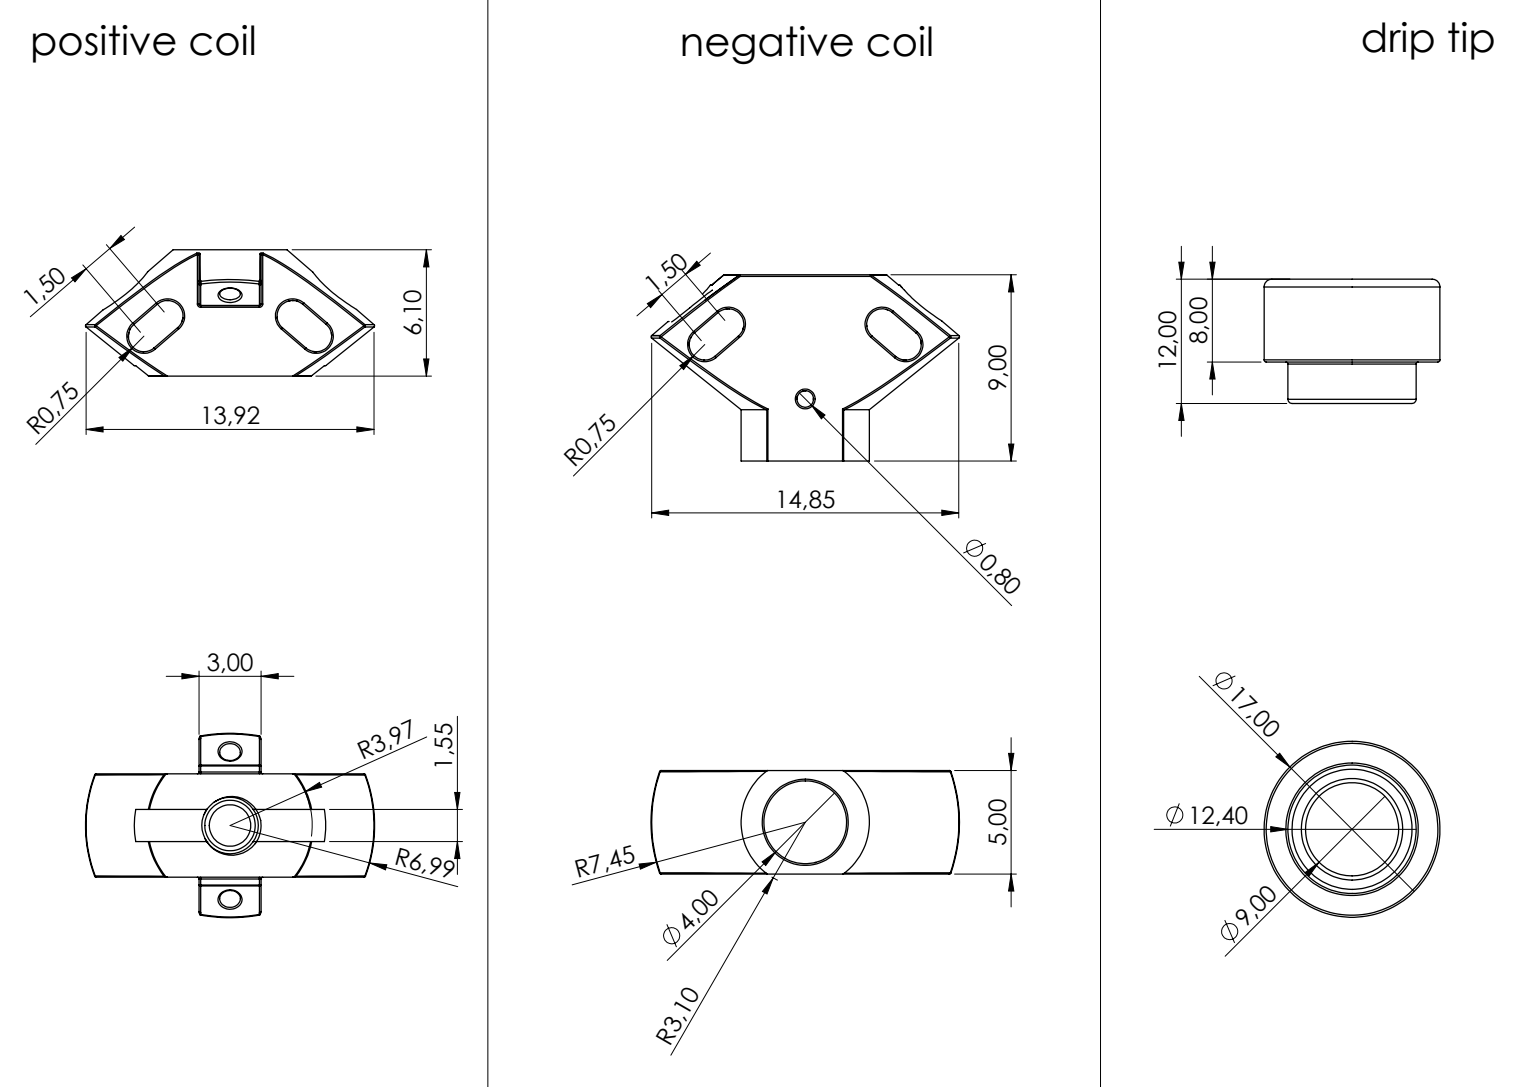
ISO-10303-21;
HEADER;
FILE_DESCRIPTION (('STEP AP214'),
    '1' );
FILE_NAME ('positive coil.step',
    '2026-10-05T20:10:51',
    ( '' ),
    ( '' ),
    'SwSTEP 2.0',
    'SolidWorks 2020',
    '' );
FILE_SCHEMA (( 'AUTOMOTIVE_DESIGN' ));
ENDSEC;

DATA;
#3=ORIENTED_EDGE ( 'NONE', *, *, #96141, .T. ) ;
#13=CARTESIAN_POINT ( 'NONE',  ( -4.869349725602420520, 8.832658446511480577, 1.040834085586084257E-14 ) ) ;
#16=CARTESIAN_POINT ( 'NONE',  ( 5.233084105194869551, 6.167981546557892436, -1.082531754730548412 ) ) ;
#20=CARTESIAN_POINT ( 'NONE',  ( -4.460796234096120472, 5.163016013655583158, 1.199719254218462483 ) ) ;
#28=CARTESIAN_POINT ( 'NONE',  ( -8.474009703741204547, 9.845098394908269768, -1.199719254218446718 ) ) ;
#29=CARTESIAN_POINT ( 'NONE',  ( 5.666418135507635512, 8.698239360479199433, 1.199719254218462483 ) ) ;
#31=CARTESIAN_POINT ( 'NONE',  ( -9.158696461231359720, 10.64389961198009615, 1.199719254218462483 ) ) ;
#33=CARTESIAN_POINT ( 'NONE',  ( 5.118366684358879759, 5.930181538962194132, 1.199719254218462483 ) ) ;
#36=CARTESIAN_POINT ( 'NONE',  ( 0.6823417656249882723, -0.5947916663252492686, 1.181850606188755259 ) ) ;
#39=CARTESIAN_POINT ( 'NONE',  ( 6.954969614130424027, 11.05795561655343384, 1.040834085586084257E-14 ) ) ;
#45=CARTESIAN_POINT ( 'NONE',  ( 10.37162432432990755, 11.20257592124748136, -0.7216878364870257245 ) ) ;
#49=( BOUNDED_SURFACE ( )  B_SPLINE_SURFACE ( 3, 2, ( 
 ( #54801, #106802, #172831 ),
 ( #26553, #190122, #173916 ),
 ( #25490, #91596, #38551 ),
 ( #157648, #9245, #191177 ),
 ( #108952, #72088, #42845 ),
 ( #4939, #71015, #22263 ) ),
 .UNSPECIFIED., .F., .F., .T. ) 
 B_SPLINE_SURFACE_WITH_KNOTS ( ( 4, 2, 4 ),
 ( 3, 3 ),
 ( 0.0001465838689801548850, 0.0002810652682710442613, 0.0004155466675619336647 ),
 ( 0.000000000000000000, 1.000000000000000000 ),
 .UNSPECIFIED. ) 
 GEOMETRIC_REPRESENTATION_ITEM ( )  RATIONAL_B_SPLINE_SURFACE ( (
 ( 1.000000000000000000, 0.8789000212895399233, 1.000000000000000000),
 ( 1.000000000000000000, 0.9073166784884888481, 1.000000000000000000),
 ( 1.000000000000000000, 0.9160359019619195298, 1.000000000000000000),
 ( 1.000000000000000000, 0.8858134948703222378, 1.000000000000000000),
 ( 1.000000000000000000, 0.8506312074210943264, 1.000000000000000000),
 ( 1.000000000000000000, 0.8104931255412257673, 1.000000000000000000) ) ) 
 REPRESENTATION_ITEM ( '' )  SURFACE ( )  );
#64=CARTESIAN_POINT ( 'NONE',  ( 1.499999999999989120, 0.05625000068281565957, 0.000000000000000000 ) ) ;
#71=CARTESIAN_POINT ( 'NONE',  ( 8.540746701604824409, 12.05162268759261224, -1.199719254218446718 ) ) ;
#75=CARTESIAN_POINT ( 'NONE',  ( 4.253507506385319381, 5.985511395581417204, 1.599625672291267398 ) ) ;
#76=CARTESIAN_POINT ( 'NONE',  ( -6.887178846062123938, 8.097758744236356776, -1.082531754730544860 ) ) ;
#77=CARTESIAN_POINT ( 'NONE',  ( -5.762141863986474100, 6.090740110424618159, 0.6348889758391648153 ) ) ;
#80=CARTESIAN_POINT ( 'NONE',  ( -8.830438121202295321, 9.196599317691152464, -0.7998128361456291469 ) ) ;
#81=CARTESIAN_POINT ( 'NONE',  ( -4.460269348771590536, 5.266364330730674226, 1.082531754730558626 ) ) ;
#84=CARTESIAN_POINT ( 'NONE',  ( -0.7500000000000006661, -0.6104166659838470288, -1.299038105676652011 ) ) ;
#91=CARTESIAN_POINT ( 'NONE',  ( -3.592547517496929466, 7.135129837147637488, -0.7216878364870257245 ) ) ;
#94=CARTESIAN_POINT ( 'NONE',  ( 4.014365637759117256, 7.575528411784208771, 0.2883143100938356240 ) ) ;
#99=CARTESIAN_POINT ( 'NONE',  ( -8.859363311525973117, 12.42334206583395328, -1.199719254218446718 ) ) ;
#100=CARTESIAN_POINT ( 'NONE',  ( 8.308449207076147758, 8.587612251210650527, -0.7998128361456281477 ) ) ;
#104=CARTESIAN_POINT ( 'NONE',  ( -0.7500000000000215383, 5.191666666666685082, 1.299038105676671107 ) ) ;
#109=CARTESIAN_POINT ( 'NONE',  ( -8.565000355531095622, 11.01558638625153286, -1.599625672291263179 ) ) ;
#112=ORIENTED_EDGE ( 'NONE', *, *, #89227, .T. ) ;
#114=CARTESIAN_POINT ( 'NONE',  ( 5.843727902690005749, 6.776436293681846301, -1.199719254218445830 ) ) ;
#132=CARTESIAN_POINT ( 'NONE',  ( 6.286176778230493589, 10.48562334124426698, 0.7998128361456462443 ) ) ;
#134=CARTESIAN_POINT ( 'NONE',  ( -5.434120640978981065, 5.234228924097238611, -0.7998128361456221525 ) ) ;
#136=AXIS2_PLACEMENT_3D ( 'NONE', #150027, #130648, #82874 ) ;
#142=CARTESIAN_POINT ( 'NONE',  ( -1.500000000000015099, -0.5479166659838513587, 0.8660254037844403729 ) ) ;
#146=CARTESIAN_POINT ( 'NONE',  ( 4.403700966340357681, 4.032072637018845107, -0.7998128361456211532 ) ) ;
#148=CARTESIAN_POINT ( 'NONE',  ( -3.216308754939891212, 4.775446185561722956, -1.599625672291262513 ) ) ;
#154=CARTESIAN_POINT ( 'NONE',  ( 5.178851490740207453, 5.144340948726102702, 0.7216878364870317197 ) ) ;
#157=CARTESIAN_POINT ( 'NONE',  ( -1.364683531250010295, 5.301041667008085767, -0.7879004041258300672 ) ) ;
#159=CARTESIAN_POINT ( 'NONE',  ( 4.541618270453549044, 5.361271406026338227, -1.082531754730548412 ) ) ;
#167=CARTESIAN_POINT ( 'NONE',  ( -6.137267537028628261, 5.996416355291856348, 0.05987573180751305790 ) ) ;
#170=CARTESIAN_POINT ( 'NONE',  ( 0.6823417656249899377, 5.738541667008087543, -1.181850606188754593 ) ) ;
#177=CARTESIAN_POINT ( 'NONE',  ( 1.499999999999990896, 4.275000000000021672, 1.214306433183764966E-14 ) ) ;
#185=CARTESIAN_POINT ( 'NONE',  ( -1.201851678989727383E-14, 5.009375000341421469, -1.575800808251660134 ) ) ;
#187=CARTESIAN_POINT ( 'NONE',  ( 4.964256800898067645, 8.943383367689749619, 0.7998128361456462443 ) ) ;
#188=CARTESIAN_POINT ( 'NONE',  ( -8.154339323615371171, 11.60081407993821045, 1.199719254218453823 ) ) ;
#194=CARTESIAN_POINT ( 'NONE',  ( -1.402160292154681736E-14, -1.115624999658584082, 1.575800808251672791 ) ) ;
#198=CARTESIAN_POINT ( 'NONE',  ( 3.823036128929238942, 7.404033217152015567, 1.040834085586084257E-14 ) ) ;
#201=CARTESIAN_POINT ( 'NONE',  ( 7.443063144222396232, 11.62739806832741785, 1.040834085586084257E-14 ) ) ;
#206=CARTESIAN_POINT ( 'NONE',  ( -1.500000000000011324, 3.702083334016152971, 0.8660254037844403729 ) ) ;
#208=CARTESIAN_POINT ( 'NONE',  ( -3.554208825076827782, 7.298327395898266623, 0.7998128361456341429 ) ) ;
#209=CARTESIAN_POINT ( 'NONE',  ( 5.300874872818843286, 5.286701561151180506, 0.7216878364870317197 ) ) ;
#217=CARTESIAN_POINT ( 'NONE',  ( 3.011882680530176604, 6.665613560593854459, 0.7998128361456341429 ) ) ;
#221=CARTESIAN_POINT ( 'NONE',  ( 2.706824224222692088, 6.309712028235118453, 0.7998128361456362523 ) ) ;
#232=CARTESIAN_POINT ( 'NONE',  ( 2.279325334093329936, 5.605928279738464859, -0.5932882675315593879 ) ) ;
#233=CARTESIAN_POINT ( 'NONE',  ( 4.809732914444119878, 6.735689552132856583, -1.248430568442916888 ) ) ;
#236=CARTESIAN_POINT ( 'NONE',  ( 9.673906298550626559, 11.24497775551929557, 1.199719254218452047 ) ) ;
#243=CARTESIAN_POINT ( 'NONE',  ( 5.775410249741494972, 8.721433810464993996, -1.082531754730537088 ) ) ;
#244=CARTESIAN_POINT ( 'NONE',  ( -10.49364770729726359, 11.34493653470939023, 0.7216878364870438212 ) ) ;
#250=CARTESIAN_POINT ( 'NONE',  ( -4.009460741339347045, 5.700790169694431420, -1.599625672291256295 ) ) ;
#254=ORIENTED_EDGE ( 'NONE', *, *, #20526, .T. ) ;
#261=ADVANCED_FACE ( 'NONE', ( #76746 ), #62774, .T. ) ;
#263=CARTESIAN_POINT ( 'NONE',  ( 6.114015800945279189, 6.016301931502064271, 0.06476946160361742033 ) ) ;
#270=CARTESIAN_POINT ( 'NONE',  ( -7.537970219518066450, 11.73812298950569044, -0.7216878364870267237 ) ) ;
#274=CARTESIAN_POINT ( 'NONE',  ( 6.805303039055573322, 10.02693841461847057, 1.199719254218460707 ) ) ;
#275=CARTESIAN_POINT ( 'NONE',  ( -4.680589345215810049, 6.483773540883647435, -1.599625672291256517 ) ) ;
#277=CARTESIAN_POINT ( 'NONE',  ( 4.054051625686104998, 4.688480637177271149, -1.199719254218446718 ) ) ;
#279=CARTESIAN_POINT ( 'NONE',  ( -5.063080299699540987, 7.994345218703034384, 1.199719254218464037 ) ) ;
#280=CARTESIAN_POINT ( 'NONE',  ( 4.196412238629597447, 4.854568018944682706, -1.199719254218452047 ) ) ;
#282=CARTESIAN_POINT ( 'NONE',  ( -6.227272627378437342, 6.159572908229946187, -0.7998128361456291469 ) ) ;
#284=ADVANCED_FACE ( 'NONE', ( #194766 ), #46403, .F. ) ;
#286=CARTESIAN_POINT ( 'NONE',  ( 8.809047120577066181, 11.30030761213851953, 1.599625672291281386 ) ) ;
#287=CARTESIAN_POINT ( 'NONE',  ( 0.5718752940412629160, 6.816535892783741168, 3.722047857044940233 ) ) ;
#289=CARTESIAN_POINT ( 'NONE',  ( 4.000033042702237474, 7.827758669039140749, -0.08873751906842038129 ) ) ;
#290=CARTESIAN_POINT ( 'NONE',  ( 6.344852701515477200, 6.504675694630598137, -0.7216878364870257245 ) ) ;
#295=CARTESIAN_POINT ( 'NONE',  ( 1.123270288254022198, 3.158552654332631882, -0.7749999999939810591 ) ) ;
#297=CARTESIAN_POINT ( 'NONE',  ( 7.036318535368067728, 10.19249347702934294, -1.082531754730537976 ) ) ;
#300=CARTESIAN_POINT ( 'NONE',  ( -8.597841969360544567, 13.18256606422934674, 0.7998128361456341429 ) ) ;
#301=CARTESIAN_POINT ( 'NONE',  ( -8.389798128758148010, 8.682519326506312751, 0.7998128361456462443 ) ) ;
#306=DIRECTION ( 'NONE',  ( -5.578564026256490882E-16, -1.000000000000000000, -9.066213480720158442E-32 ) ) ;
#309=CARTESIAN_POINT ( 'NONE',  ( 4.227444969362701421, 3.826440640544909400, 1.214306433183764966E-14 ) ) ;
#314=CARTESIAN_POINT ( 'NONE',  ( 5.034155109375821446, 4.767602470560229122, -0.7998128361456221525 ) ) ;
#318=CARTESIAN_POINT ( 'NONE',  ( -0.7500000000000215383, 3.722916667349487785, 1.299038105676671107 ) ) ;
#324=CARTESIAN_POINT ( 'NONE',  ( -1.500000000000013101, 1.670833333333355153, 0.8660254037844403729 ) ) ;
#325=CARTESIAN_POINT ( 'NONE',  ( 7.149227073107712549, 7.235186428247455837, -0.7998128361456281477 ) ) ;
#326=CARTESIAN_POINT ( 'NONE',  ( 3.348500752450929596, 6.850408611260650815, 0.7216878364870317197 ) ) ;
#329=CARTESIAN_POINT ( 'NONE',  ( 8.758204044748010730, 9.320252261735261001, 0.7216878364870438212 ) ) ;
#333=CARTESIAN_POINT ( 'NONE',  ( -4.548924232584923288, 5.265832011892554121, -1.199719254218446718 ) ) ;
#334=CARTESIAN_POINT ( 'NONE',  ( 1.499999999999990896, 5.306250000682820378, 1.214306433183764966E-14 ) ) ;
#335=CARTESIAN_POINT ( 'NONE',  ( 1.364683531249986537, -0.8447916663252468261, -0.7879004041258309554 ) ) ;
#339=CARTESIAN_POINT ( 'NONE',  ( 3.497113557321089861, 6.167384019261527683, -1.199719254218446718 ) ) ;
#341=CARTESIAN_POINT ( 'NONE',  ( -1.402160292154681736E-14, -1.178124999658576311, 1.575800808251672791 ) ) ;
#349=CARTESIAN_POINT ( 'NONE',  ( -7.039708073993679704, 9.236078724457858158, 1.599625672291283607 ) ) ;
#350=CARTESIAN_POINT ( 'NONE',  ( 5.681030059326015014, 6.586622143090519188, -1.199719254218445830 ) ) ;
#353=CARTESIAN_POINT ( 'NONE',  ( -1.364683531250000748, -0.4906249996585801409, 0.000000000000000000 ) ) ;
#360=CARTESIAN_POINT ( 'NONE',  ( -5.585069213825653023, 8.603332285183535433, -1.199719254218440723 ) ) ;
#364=CARTESIAN_POINT ( 'NONE',  ( 9.378489572351044856, 11.96465713920816043, -1.599625672291262513 ) ) ;
#366=CARTESIAN_POINT ( 'NONE',  ( 9.413438726589914651, 9.876766690643398405, 0.000000000000000000 ) ) ;
#368=CARTESIAN_POINT ( 'NONE',  ( -3.765413976293358278, 5.416068943807445635, 1.599625672291267398 ) ) ;
#369=CARTESIAN_POINT ( 'NONE',  ( -8.532158741701643123, 8.848606708273724308, 0.7998128361456462443 ) ) ;
#372=CARTESIAN_POINT ( 'NONE',  ( -4.265659997730736563, 7.487761795085347671, 1.069252549957976361 ) ) ;
#373=CARTESIAN_POINT ( 'NONE',  ( -1.364683531250014514, 0.4885416670080875434, -0.7879004041258289570 ) ) ;
#377=CARTESIAN_POINT ( 'NONE',  ( 9.083599731475992201, 9.699880562917908122, 0.7216878364870438212 ) ) ;
#380=CARTESIAN_POINT ( 'NONE',  ( 5.005985031943777308, 6.863401842066294556, -1.599625672291256295 ) ) ;
#399=CARTESIAN_POINT ( 'NONE',  ( 9.480175724453529185, 12.08329098332774265, 1.599625672291279388 ) ) ;
#400=CARTESIAN_POINT ( 'NONE',  ( -3.511198596259299087, 6.271927390929313617, -7.499999999999997335 ) ) ;
#403=CARTESIAN_POINT ( 'NONE',  ( -3.899941742225307539, 7.701682465904834629, 0.7998128361456341429 ) ) ;
#409=CARTESIAN_POINT ( 'NONE',  ( -1.500000000000013101, 3.660416667349488673, -0.8660254037844313801 ) ) ;
#410=CARTESIAN_POINT ( 'NONE',  ( 9.413438726589914651, 9.876766690643398405, 0.000000000000000000 ) ) ;
#415=CARTESIAN_POINT ( 'NONE',  ( -9.287498920561160887, 10.79416914786490089, -1.199719254218441611 ) ) ;
#417=CARTESIAN_POINT ( 'NONE',  ( -0.6823417656250003738, 2.467708333674753618, -1.181850606188749264 ) ) ;
#419=CARTESIAN_POINT ( 'NONE',  ( -5.738979324000901272, 5.917037536912919116, 2.440165351842437769 ) ) ;
#423=CARTESIAN_POINT ( 'NONE',  ( -4.464712657601869417, 4.103252943490596216, 0.7998128361456341429 ) ) ;
#428=CARTESIAN_POINT ( 'NONE',  ( 0.6823417656249882723, 1.238541667008083547, -1.181850606188749264 ) ) ;
#429=AXIS2_PLACEMENT_3D ( 'NONE', #143118, #44524, #58621 ) ;
#434=CARTESIAN_POINT ( 'NONE',  ( -1.364683531250014514, 1.488541667008084435, -0.7879004041258289570 ) ) ;
#437=CARTESIAN_POINT ( 'NONE',  ( -5.575427483717760424, 7.527751369135936343, 1.599625672291269396 ) ) ;
#438=CARTESIAN_POINT ( 'NONE',  ( 7.450369105909416589, 8.650851030771185890, -1.199719254218441611 ) ) ;
#439=CARTESIAN_POINT ( 'NONE',  ( -0.9999999999999988898, 5.868705557303652398, -4.125226524755048807 ) ) ;
#441=CARTESIAN_POINT ( 'NONE',  ( 0.7499999999999902300, 3.733333333333352488, 1.299038105676669330 ) ) ;
#442=EDGE_CURVE ( 'NONE', #108282, #170224, #25846, .T. ) ;
#443=CARTESIAN_POINT ( 'NONE',  ( -1.364683531250012516, 2.301041667008087988, -0.7879004041258289570 ) ) ;
#446=CARTESIAN_POINT ( 'NONE',  ( -3.795919822146315514, 7.372397525905186377, -0.7216878364870545903 ) ) ;
#447=CARTESIAN_POINT ( 'NONE',  ( -3.931501358282937009, 7.530575984731317618, 0.7216878364870317197 ) ) ;
#450=CARTESIAN_POINT ( 'NONE',  ( 5.422898255786183341, 7.349800603215774331, -1.443375672974051449 ) ) ;
#453=CARTESIAN_POINT ( 'NONE',  ( -8.045874094706015001, 11.47427131287732927, -1.199719254218446718 ) ) ;
#454=CARTESIAN_POINT ( 'NONE',  ( -9.110716038703348119, 12.61262389758715408, 1.082531754730560403 ) ) ;
#456=CARTESIAN_POINT ( 'NONE',  ( -0.6823417656249969321, 5.217708333674756283, -1.181850606188749264 ) ) ;
#461=CARTESIAN_POINT ( 'NONE',  ( -5.856759170979136897, 9.776710099543576504, 0.000000000000000000 ) ) ;
#463=CARTESIAN_POINT ( 'NONE',  ( 1.364683531249986537, -0.2822916663252520997, -0.7879004041258309554 ) ) ;
#466=CARTESIAN_POINT ( 'NONE',  ( 6.480434237652115570, 10.50433101066207442, 0.7216878364870438212 ) ) ;
#472=CARTESIAN_POINT ( 'NONE',  ( -4.238987453163843178, 3.980249526191325771, 0.4947463914901452098 ) ) ;
#476=AXIS2_PLACEMENT_3D ( 'NONE', #130364, #209367, #32780 ) ;
#483=CARTESIAN_POINT ( 'NONE',  ( 7.474622759835693131, 7.614814729430110951, -0.7998128361456281477 ) ) ;
#484=CARTESIAN_POINT ( 'NONE',  ( -5.579343907223557331, 6.467988298970945849, 1.199719254218450271 ) ) ;
#488=CARTESIAN_POINT ( 'NONE',  ( 6.005898860729467437, 7.069598761348265370, -1.082531754730543083 ) ) ;
#489=CARTESIAN_POINT ( 'NONE',  ( -1.402160292154681736E-14, 0.7593750003414168059, -1.575800808251659024 ) ) ;
#490=CARTESIAN_POINT ( 'NONE',  ( 4.365362273920252889, 4.195270195769483124, 0.7216878364870317197 ) ) ;
#491=CARTESIAN_POINT ( 'NONE',  ( -8.890396042259075315, 11.39521468743417998, -1.599625672291263179 ) ) ;
#507=CARTESIAN_POINT ( 'NONE',  ( 6.877010230629674759, 9.046264573866535486, 1.599625672291281386 ) ) ;
#508=CARTESIAN_POINT ( 'NONE',  ( 6.174848896020108668, 9.291408581077091000, 1.199719254218460707 ) ) ;
#517=CARTESIAN_POINT ( 'NONE',  ( 8.886479618753304166, 12.45497775759917758, -1.199719254218446718 ) ) ;
#519=CARTESIAN_POINT ( 'NONE',  ( -6.087774667736030487, 7.061157519568837415, 1.199719254218450271 ) ) ;
#520=CARTESIAN_POINT ( 'NONE',  ( 1.123270288254022198, 2.908552654332631437, -0.7749999999939810591 ) ) ;
#524=CARTESIAN_POINT ( 'NONE',  ( -1.499999999999997780, 4.681250000682819490, 1.214306433183764966E-14 ) ) ;
#530=CARTESIAN_POINT ( 'NONE',  ( -8.948018195339354719, 12.42280974699582607, 1.082531754730560403 ) ) ;
#533=CARTESIAN_POINT ( 'NONE',  ( 5.666418135507635512, 8.698239360479199433, 1.199719254218462483 ) ) ;
#534=CARTESIAN_POINT ( 'NONE',  ( 1.364683531249990311, 5.363541667008086655, 0.7879004041258499402 ) ) ;
#538=ADVANCED_FACE ( 'NONE', ( #17059 ), #84921, .T. ) ;
#540=CARTESIAN_POINT ( 'NONE',  ( 3.334942598837264960, 6.834590765378040444, 1.214306433183764966E-14 ) ) ;
#541=CARTESIAN_POINT ( 'NONE',  ( -6.693975156845199059, 8.832723654451292816, 1.599625672291283607 ) ) ;
#546=CARTESIAN_POINT ( 'NONE',  ( -7.802881099864745984, 9.062115023719057305, -1.199719254218446718 ) ) ;
#547=CARTESIAN_POINT ( 'NONE',  ( -4.111146893441842920, 5.819424013814012753, 1.599625672291267398 ) ) ;
#555=CARTESIAN_POINT ( 'NONE',  ( 6.959412922516382771, 7.013736585890911535, 0.7998128361456341429 ) ) ;
#568=CARTESIAN_POINT ( 'NONE',  ( -1.364683531250000748, 0.3218750003414205807, 0.000000000000000000 ) ) ;
#569=CARTESIAN_POINT ( 'NONE',  ( 2.496672843210871129, 6.064535417054653266, -0.7998128361456291469 ) ) ;
#570=CARTESIAN_POINT ( 'NONE',  ( 5.681030059326015014, 6.586622143090519188, -1.199719254218445830 ) ) ;
#573=CARTESIAN_POINT ( 'NONE',  ( -7.754900677336769022, 9.110100880723427608, 1.082531754730558626 ) ) ;
#576=CARTESIAN_POINT ( 'NONE',  ( 6.656690234629796699, 6.868486149930637552, 1.040834085586084257E-14 ) ) ;
#577=CARTESIAN_POINT ( 'NONE',  ( -7.659993601596720936, 8.999375959026737704, -1.082531754730543083 ) ) ;
#579=ORIENTED_EDGE ( 'NONE', *, *, #182370, .T. ) ;
#581=CARTESIAN_POINT ( 'NONE',  ( 5.587931867126699537, 9.671004278289832001, -0.7998128361456291469 ) ) ;
#586=CARTESIAN_POINT ( 'NONE',  ( -0.6823417656249969321, 3.217708333674754062, -1.181850606188749264 ) ) ;
#591=CARTESIAN_POINT ( 'NONE',  ( 7.202405917357655341, 9.425892875049191488, 1.599625672291281386 ) ) ;
#595=CARTESIAN_POINT ( 'NONE',  ( -8.015895134177625891, 10.37496362800581018, 1.599625672291295375 ) ) ;
#601=CARTESIAN_POINT ( 'NONE',  ( 9.589694723567584234, 10.08239868711733855, -0.7998128361456281477 ) ) ;
#604=CARTESIAN_POINT ( 'NONE',  ( -8.690940161559884913, 10.09818392903003748, 1.199719254218462483 ) ) ;
#607=CARTESIAN_POINT ( 'NONE',  ( 4.459584003380381745, 7.054591843250856975, -1.127873490090089748 ) ) ;
#608=CARTESIAN_POINT ( 'NONE',  ( -4.288456660624211381, 3.897620947016656956, 1.214306433183764966E-14 ) ) ;
#613=CARTESIAN_POINT ( 'NONE',  ( 5.289652487626049115, 9.323011668872403845, 0.7998128361456462443 ) ) ;
#615=CARTESIAN_POINT ( 'NONE',  ( 4.852928918687680948, 7.749168607522574526, 1.199719254218462483 ) ) ;
#616=CARTESIAN_POINT ( 'NONE',  ( -4.047760499819613500, 7.578451897646762525, -0.3740945913360635977 ) ) ;
#617=CARTESIAN_POINT ( 'NONE',  ( 5.508690485854129903, 5.321227076451600091, 1.040834085586084257E-14 ) ) ;
#619=CARTESIAN_POINT ( 'NONE',  ( -7.754900677336769022, 9.110100880723427608, 1.082531754730558626 ) ) ;
#628=CARTESIAN_POINT ( 'NONE',  ( -4.379705010876359772, 7.173806194452361673, -1.050513582990858064 ) ) ;
#630=ADVANCED_FACE ( 'NONE', ( #146201 ), #63852, .T. ) ;
#632=DIRECTION ( 'NONE',  ( 1.207943261119674327E-30, 2.168404344971008079E-15, 1.000000000000000000 ) ) ;
#633=CARTESIAN_POINT ( 'NONE',  ( 5.355107487717867265, 5.349972945200037522, 1.040834085586084257E-14 ) ) ;
#643=CARTESIAN_POINT ( 'NONE',  ( -8.134528978075012517, 12.43410820782212767, 1.040834085586084257E-14 ) ) ;
#650=CARTESIAN_POINT ( 'NONE',  ( -8.148087131688679818, 12.44992605370473804, -0.7216878364870267237 ) ) ;
#657=CARTESIAN_POINT ( 'NONE',  ( -0.7500000000000215383, 2.722916667349486897, 1.299038105676671107 ) ) ;
#659=CARTESIAN_POINT ( 'NONE',  ( -5.850506979496850057, 6.784345216623154151, -1.199719254218446718 ) ) ;
#663=CARTESIAN_POINT ( 'NONE',  ( -9.508345801885592863, 9.987491611821676329, 0.7998128361456462443 ) ) ;
#667=CARTESIAN_POINT ( 'NONE',  ( 6.311484202361478779, 7.322151976631905868, -1.199719254218446718 ) ) ;
#674=CARTESIAN_POINT ( 'NONE',  ( 7.584896871841365851, 10.93646455286856956, -1.199719254218446718 ) ) ;
#680=CARTESIAN_POINT ( 'NONE',  ( -6.317736394288148816, 8.393778431468064127, 1.443375672974078761 ) ) ;
#683=CARTESIAN_POINT ( 'NONE',  ( 1.284279953904121641, 3.077889714876734573, -0.7749999999999892530 ) ) ;
#686=CARTESIAN_POINT ( 'NONE',  ( -1.364683531250010295, 5.488541667008087543, -0.7879004041258300672 ) ) ;
#690=CARTESIAN_POINT ( 'NONE',  ( -3.511198595814942980, 5.119484333249288532, 1.443375672974064550 ) ) ;
#692=EDGE_CURVE ( 'NONE', #173454, #209728, #53694, .T. ) ;
#693=CARTESIAN_POINT ( 'NONE',  ( 9.694243528971124846, 11.26870452434320491, 1.199719254218450271 ) ) ;
#695=CARTESIAN_POINT ( 'NONE',  ( -9.398826802771548472, 11.98838390803207865, -1.599625672291263179 ) ) ;
#698=CARTESIAN_POINT ( 'NONE',  ( 0.6823417656249882723, 1.676041667008083769, -1.181850606188749264 ) ) ;
#701=CARTESIAN_POINT ( 'NONE',  ( 4.172158584703322681, 5.890604320285754980, -1.599625672291256295 ) ) ;
#706=FACE_OUTER_BOUND ( 'NONE', #213489, .T. ) ;
#707=DIRECTION ( 'NONE',  ( 0.6507913734559627184, 0.7592566023653016805, 0.000000000000000000 ) ) ;
#708=CARTESIAN_POINT ( 'NONE',  ( 9.856414487010592751, 10.60149777770828194, 0.7216878364870438212 ) ) ;
#709=CARTESIAN_POINT ( 'NONE',  ( -1.201851678989727383E-14, 3.993750000682817713, 1.732050807568877637 ) ) ;
#710=CARTESIAN_POINT ( 'NONE',  ( -7.619319141200077361, 9.912291636198670375, 1.443375672974090751 ) ) ;
#712=CARTESIAN_POINT ( 'NONE',  ( 0.4301767877893971637, 8.007958762483859516, 1.954153227243374813 ) ) ;
#714=CARTESIAN_POINT ( 'NONE',  ( -8.670602931139386627, 10.07445716020612103, 1.199719254218462483 ) ) ;
#715=CARTESIAN_POINT ( 'NONE',  ( -3.592547517496929466, 7.135129837147637488, -0.7216878364870257245 ) ) ;
#716=CARTESIAN_POINT ( 'NONE',  ( -0.6823417656250212460, 3.363541667008085323, 1.181850606188767472 ) ) ;
#732=CARTESIAN_POINT ( 'NONE',  ( -1.436838838544753694, 7.449283400311743186, 4.203727439823589762 ) ) ;
#735=CARTESIAN_POINT ( 'NONE',  ( 0.6823417656249899377, 3.988541667008085767, -1.181850606188754593 ) ) ;
#742=CARTESIAN_POINT ( 'NONE',  ( 10.08456733046637765, 10.65975006183261087, 0.000000000000000000 ) ) ;
#745=CARTESIAN_POINT ( 'NONE',  ( -1.201851678989727383E-14, 2.321875000341416584, 1.575800808251672791 ) ) ;
#747=CARTESIAN_POINT ( 'NONE',  ( -7.592202833972775622, 8.920286730132099606, 1.082531754730558626 ) ) ;
#755=CARTESIAN_POINT ( 'NONE',  ( 5.054492339796319733, 4.791329239384148231, -0.7998128361456211532 ) ) ;
#759=CARTESIAN_POINT ( 'NONE',  ( 10.38962578677386084, 11.01565159419135043, 0.000000000000000000 ) ) ;
#763=ORIENTED_EDGE ( 'NONE', *, *, #8087, .T. ) ;
#765=CARTESIAN_POINT ( 'NONE',  ( -8.123306592882240551, 12.62894145833798376, 0.000000000000000000 ) ) ;
#767=CARTESIAN_POINT ( 'NONE',  ( 5.784525094524856748, 9.900363043587685041, 1.040834085586084257E-14 ) ) ;
#769=CARTESIAN_POINT ( 'NONE',  ( 5.327991180046175224, 5.318337252916401248, -0.7216878364870207285 ) ) ;
#778=CARTESIAN_POINT ( 'NONE',  ( -5.409340102172518705, 9.254721185935849803, 0.000000000000000000 ) ) ;
#779=CARTESIAN_POINT ( 'NONE',  ( 4.310602774141044868, 7.116454772218158809, -1.199719254218452047 ) ) ;
#782=CARTESIAN_POINT ( 'NONE',  ( -7.537443334193545397, 10.88110209227943770, -1.199719254218446718 ) ) ;
#787=CARTESIAN_POINT ( 'NONE',  ( -4.620631424159025613, 4.285158171140619032, -0.7998128361456221525 ) ) ;
#791=CARTESIAN_POINT ( 'NONE',  ( 8.235688245297327015, 11.69572115523387268, -1.199719254218446718 ) ) ;
#792=DIRECTION ( 'NONE',  ( -0.5265943820737358783, 0.4485553919928856326, 0.7221470882600643515 ) ) ;
#798=CARTESIAN_POINT ( 'NONE',  ( 3.145128448690309053, 4.692402494937224056, -1.443375672974057666 ) ) ;
#801=CARTESIAN_POINT ( 'NONE',  ( -2.740719608256871442, 6.349256642941639051, 0.7998128361456341429 ) ) ;
#802=CYLINDRICAL_SURFACE ( 'NONE', #123024, 1.250000000000000000 ) ;
#804=CARTESIAN_POINT ( 'NONE',  ( -9.332089804907933939, 9.781859615347734405, 1.040834085586084257E-14 ) ) ;
#808=CARTESIAN_POINT ( 'NONE',  ( 7.131225611108085616, 10.30321839872603462, 1.082531754730558626 ) ) ;
#809=CARTESIAN_POINT ( 'NONE',  ( -1.001543065824772872E-14, 5.634375000341417028, 1.575800808251672791 ) ) ;
#812=CARTESIAN_POINT ( 'NONE',  ( 4.518945272056516416, 4.166524327021037699, 0.7998128361456341429 ) ) ;
#813=CARTESIAN_POINT ( 'NONE',  ( 5.928835565505618632, 6.052265235248638575, -0.5446974197955555264 ) ) ;
#815=CARTESIAN_POINT ( 'NONE',  ( -5.377780486114890124, 9.425827667109372143, 0.000000000000000000 ) ) ;
#818=CARTESIAN_POINT ( 'NONE',  ( 1.123270288250311610, 3.110197346350006331, 0.7749999999993734123 ) ) ;
#827=CARTESIAN_POINT ( 'NONE',  ( -1.364683531250012516, 3.592708333674750509, 0.7879004041258379498 ) ) ;
#828=CARTESIAN_POINT ( 'NONE',  ( 8.971744963941056028, 11.49012176272984931, 1.599625672291281386 ) ) ;
#830=CARTESIAN_POINT ( 'NONE',  ( -5.938108093105513241, 6.030140318152288792, 0.7216878364870317197 ) ) ;
#832=CYLINDRICAL_SURFACE ( 'NONE', #156750, 1.250000000000000000 ) ;
#835=CARTESIAN_POINT ( 'NONE',  ( -4.080641047588907888, 6.744203074620265248, -1.082531754730548412 ) ) ;
#844=CARTESIAN_POINT ( 'NONE',  ( 2.849184837166184536, 6.475799410002530898, 0.7998128361456362523 ) ) ;
#854=CARTESIAN_POINT ( 'NONE',  ( 3.832150974156964818, 7.622593236491780999, 1.040834085586084257E-14 ) ) ;
#859=CARTESIAN_POINT ( 'NONE',  ( -6.144869935491728441, 8.192100896205577243, -1.599625672291263179 ) ) ;
#863=CARTESIAN_POINT ( 'NONE',  ( 7.637320603199683866, 7.804628880021436288, -0.7998128361456281477 ) ) ;
#866=CARTESIAN_POINT ( 'NONE',  ( -4.791917227426195858, 7.677988301050826969, -1.199719254218452047 ) ) ;
#867=CARTESIAN_POINT ( 'NONE',  ( 5.463572716182819811, 8.357623354646536384, 1.082531754730558626 ) ) ;
#868=CARTESIAN_POINT ( 'NONE',  ( -1.402160292154681736E-14, 1.837500000000019895, -1.732050807568863648 ) ) ;
#870=CARTESIAN_POINT ( 'NONE',  ( -2.761056838677368397, 6.372983411765559048, 0.7998128361456341429 ) ) ;
#873=CARTESIAN_POINT ( 'NONE',  ( -6.261168011412601153, 6.199117522936475666, 1.040834085586084257E-14 ) ) ;
#876=CARTESIAN_POINT ( 'NONE',  ( 1.364683531249988535, 3.905208333674751842, -0.7879004041258239610 ) ) ;
#878=CARTESIAN_POINT ( 'NONE',  ( -5.260200412422208593, 7.159986452624450770, -1.443375672974053447 ) ) ;
#884=CARTESIAN_POINT ( 'NONE',  ( 5.005985031943777308, 6.863401842066294556, -1.599625672291256295 ) ) ;
#887=CARTESIAN_POINT ( 'NONE',  ( 1.364683531249988535, 2.176041667008087543, 0.7879004041258500513 ) ) ;
#889=CARTESIAN_POINT ( 'NONE',  ( 2.737856954955798727, 5.281584649835344258, 1.199719254218452047 ) ) ;
#891=CARTESIAN_POINT ( 'NONE',  ( -1.402160292154681736E-14, 0.5093750003414236893, -1.575800808251659024 ) ) ;
#894=CARTESIAN_POINT ( 'NONE',  ( -4.081167932913447594, 4.720116328942494555, -1.199719254218452047 ) ) ;
#895=CARTESIAN_POINT ( 'NONE',  ( -6.439759776366783761, 8.536139043893143707, 1.443375672974078761 ) ) ;
#898=CARTESIAN_POINT ( 'NONE',  ( -1.364683531250012516, 3.530208333674758059, 0.7879004041258379498 ) ) ;
#906=CARTESIAN_POINT ( 'NONE',  ( -6.141480396866151992, 9.148515648777049591, 1.082531754730548412 ) ) ;
#909=CARTESIAN_POINT ( 'NONE',  ( 4.758470758277942636, 5.183766117661583017, 0.9120521451414279612 ) ) ;
#912=CARTESIAN_POINT ( 'NONE',  ( -1.499999999999997780, 5.150000000000022560, 1.214306433183764966E-14 ) ) ;
#914=CARTESIAN_POINT ( 'NONE',  ( -6.765155463094763455, 8.915767345075790828, 1.443375672974078761 ) ) ;
#927=CARTESIAN_POINT ( 'NONE',  ( -5.961834861707238531, 7.978559976790334574, -1.599625672291263179 ) ) ;
#929=CARTESIAN_POINT ( 'NONE',  ( -0.7500000000000006661, -0.8916666666666448471, -1.299038105676652011 ) ) ;
#930=CARTESIAN_POINT ( 'NONE',  ( 9.571693261567954636, 12.19006144329456731, 1.443375672974076540 ) ) ;
#932=EDGE_CURVE ( 'NONE', #104450, #135613, #77272, .T. ) ;
#935=CARTESIAN_POINT ( 'NONE',  ( 4.008406971134620633, 7.828225232965717595, 0.7998128361456321445 ) ) ;
#943=CARTESIAN_POINT ( 'NONE',  ( -3.633221978782299910, 5.261844946711204507, -1.443375672974053447 ) ) ;
#946=CARTESIAN_POINT ( 'NONE',  ( -0.02418498125556165293, 7.070485378046342362, 4.060647170728404198 ) ) ;
#947=CARTESIAN_POINT ( 'NONE',  ( 3.159844690031233583, 6.439914444440794306, -0.7080165339683067716 ) ) ;
#950=CARTESIAN_POINT ( 'NONE',  ( 1.364683531249988535, 2.113541667008087099, 0.7879004041258500513 ) ) ;
#951=CARTESIAN_POINT ( 'NONE',  ( 9.151390499099949949, 12.66007743471656788, -1.082531754730543971 ) ) ;
#952=CARTESIAN_POINT ( 'NONE',  ( -7.283754839039664475, 9.520799950344851936, -1.599625672291263179 ) ) ;
#956=CARTESIAN_POINT ( 'NONE',  ( 7.494959990256193194, 7.638541498254023843, -0.7998128361456281477 ) ) ;
#957=CARTESIAN_POINT ( 'NONE',  ( -7.874588291438845644, 8.081441182967111558, -0.7998128361456291469 ) ) ;
#960=CARTESIAN_POINT ( 'NONE',  ( -1.402160292154681736E-14, -0.5062499993171791779, 1.732050807568877637 ) ) ;
#963=CARTESIAN_POINT ( 'NONE',  ( 8.920901888111997025, 10.47043562662792304, 1.082531754730549967 ) ) ;
#966=CARTESIAN_POINT ( 'NONE',  ( -1.364683531250012516, 1.342708333674755616, 0.7879004041258379498 ) ) ;
#968=CARTESIAN_POINT ( 'NONE',  ( 3.404766800216717737, 6.348112014766642552, 1.069586989871921467 ) ) ;
#969=CARTESIAN_POINT ( 'NONE',  ( 5.897433631820129918, 8.863794422890064695, -1.082531754730537976 ) ) ;
#972=CARTESIAN_POINT ( 'NONE',  ( -3.280709984826970516, 6.771319382366015383, 0.7216878364870317197 ) ) ;
#974=CARTESIAN_POINT ( 'NONE',  ( -1.364683531250010295, 5.238541667008086655, -0.7879004041258300672 ) ) ;
#985=CARTESIAN_POINT ( 'NONE',  ( 7.416473721875251890, 8.611306416064660851, 1.199719254218462483 ) ) ;
#989=CARTESIAN_POINT ( 'NONE',  ( 4.304877467538922531, 4.981110786005563007, 1.199719254218464037 ) ) ;
#995=ORIENTED_EDGE ( 'NONE', *, *, #65741, .T. ) ;
#996=CARTESIAN_POINT ( 'NONE',  ( 4.528060117284222308, 8.226561203566173930, 0.7216878364870438212 ) ) ;
#997=CARTESIAN_POINT ( 'NONE',  ( -1.402160292154681736E-14, 0.7593750003414168059, -1.575800808251659024 ) ) ;
#999=CARTESIAN_POINT ( 'NONE',  ( 9.459838494033030898, 12.05956421450382088, 1.599625672291281386 ) ) ;
#1000=DIRECTION ( 'NONE',  ( 1.207943261119674327E-30, 2.168404344971008079E-15, 1.000000000000000000 ) ) ;
#1002=DIRECTION ( 'NONE',  ( 0.000000000000000000, 0.7999999999999973799, -0.6000000000000034195 ) ) ;
#1004=CARTESIAN_POINT ( 'NONE',  ( -0.7500000000000006661, -0.1416666666666441254, -1.299038105676652011 ) ) ;
#1005=CARTESIAN_POINT ( 'NONE',  ( 8.111855979677986994, 8.358253485912799263, 1.040834085586084257E-14 ) ) ;
#1006=CARTESIAN_POINT ( 'NONE',  ( -8.636707547105197946, 10.03491254549959777, -1.199719254218446718 ) ) ;
#1009=CARTESIAN_POINT ( 'NONE',  ( -1.201851678989727383E-14, 1.321875000341419248, 1.575800808251672791 ) ) ;
#1010=CARTESIAN_POINT ( 'NONE',  ( -0.7500000000000215383, 2.191666666666689078, 1.299038105676671107 ) ) ;
#1012=CARTESIAN_POINT ( 'NONE',  ( 5.007038802148489509, 4.735966778795008381, 0.7998128361456341429 ) ) ;
#1020=CARTESIAN_POINT ( 'NONE',  ( 0.7499999999999867883, -0.9020833326505162120, -1.299038105676652011 ) ) ;
#1021=CARTESIAN_POINT ( 'NONE',  ( -6.482770005628665011, 10.71498210654212002, 0.7998128361456481317 ) ) ;
#1022=CARTESIAN_POINT ( 'NONE',  ( -5.599154252763867134, 5.634694171087028636, 0.000000000000000000 ) ) ;
#1029=ORIENTED_EDGE ( 'NONE', *, *, #159807, .F. ) ;
#1030=CARTESIAN_POINT ( 'NONE',  ( 6.425674737872927089, 9.584038729905381970, -1.199719254218440723 ) ) ;
#1032=DIRECTION ( 'NONE',  ( -5.176899690512889973E-31, 0.6299249119529756191, -0.7766560405359864694 ) ) ;
#1035=CARTESIAN_POINT ( 'NONE',  ( 5.300874872818821082, 9.128178418356554857, 0.7216878364870438212 ) ) ;
#1040=CARTESIAN_POINT ( 'NONE',  ( -5.859094939400033120, 9.987361195942037639, -0.7998128361456231517 ) ) ;
#1041=CARTESIAN_POINT ( 'NONE',  ( 4.813308228051395687, 5.574280006603454574, 1.199719254218462483 ) ) ;
#1047=CARTESIAN_POINT ( 'NONE',  ( 8.839552966430002101, 11.33589776563360019, -1.443375672974052559 ) ) ;
#1048=ORIENTED_EDGE ( 'NONE', *, *, #68958, .F. ) ;
#1056=( BOUNDED_CURVE ( )  B_SPLINE_CURVE ( 2, ( #102050, #170239, #187553, #185416, #85797, #37034, #69520 ),
 .UNSPECIFIED., .F., .T. ) 
 B_SPLINE_CURVE_WITH_KNOTS ( ( 3, 2, 2, 3 ),
 ( 0.000000000000000000, 0.005952380952380876590, 0.01190476190476175318, 0.01785714285714263064 ),
 .UNSPECIFIED. ) 
 CURVE ( )  GEOMETRIC_REPRESENTATION_ITEM ( )  RATIONAL_B_SPLINE_CURVE ( ( 1.000000000000000000, 0.8660254037844387076, 1.000000000000000000, 0.8660254037844387076, 1.000000000000000000, 0.8660254037844438146, 0.9999999999999948930 ) ) 
 REPRESENTATION_ITEM ( '' )  );
#1057=CARTESIAN_POINT ( 'NONE',  ( -4.039966587192274083, 5.736380323189513852, 1.443375672974064550 ) ) ;
#1058=CARTESIAN_POINT ( 'NONE',  ( 9.273413882067330860, 9.921330405274451536, -0.7216878364870257245 ) ) ;
#1061=CARTESIAN_POINT ( 'NONE',  ( -5.311043488251275591, 7.219303374425030562, -1.599625672291256295 ) ) ;
#1067=CARTESIAN_POINT ( 'NONE',  ( -5.181187258716735577, 9.196468901811520880, 0.7998128361456481317 ) ) ;
#1068=CARTESIAN_POINT ( 'NONE',  ( -1.284279953904132077, 2.878360285806111474, -0.7749999999999935829 ) ) ;
#1070=CARTESIAN_POINT ( 'NONE',  ( 5.447384925931444855, 6.422658924545643799, -1.238017914293283228 ) ) ;
#1082=CARTESIAN_POINT ( 'NONE',  ( -5.473741331615264549, 7.409117525016355010, -1.599625672291256295 ) ) ;
#1085=CARTESIAN_POINT ( 'NONE',  ( 4.365362273920244007, 6.116008624372160973, 1.443375672974062551 ) ) ;
#1088=CARTESIAN_POINT ( 'NONE',  ( -3.563261906135796409, 6.332667919118538435, 2.500000000000011102 ) ) ;
#1091=CARTESIAN_POINT ( 'NONE',  ( -3.598799709423620374, 6.286017863381107240, 1.199719254218464037 ) ) ;
#1101=CARTESIAN_POINT ( 'NONE',  ( -8.688077508258798431, 9.030511935923748013, -0.7998128361456291469 ) ) ;
#1102=CARTESIAN_POINT ( 'NONE',  ( 5.124091990960999432, 8.065525525174782828, -1.199719254218452047 ) ) ;
#1105=CARTESIAN_POINT ( 'NONE',  ( -7.472515219426274946, 11.86968485597268064, 0.000000000000000000 ) ) ;
#1106=CARTESIAN_POINT ( 'NONE',  ( 4.310602774141044868, 7.116454772218158809, -1.199719254218452047 ) ) ;
#1109=CARTESIAN_POINT ( 'NONE',  ( -1.402160292154681736E-14, 0.5093750003414236893, -1.575800808251659024 ) ) ;
#1110=VERTEX_POINT ( 'NONE', #18511 ) ;
#1112=CARTESIAN_POINT ( 'NONE',  ( 8.771762198361678031, 9.336070107617867819, 1.040834085586084257E-14 ) ) ;
#1131=CARTESIAN_POINT ( 'NONE',  ( -3.297657676621885692, 4.870353260857385180, 1.599625672291267398 ) ) ;
#1138=CARTESIAN_POINT ( 'NONE',  ( -1.402160292154681736E-14, -0.2562499993171780122, 1.732050807568877637 ) ) ;
#1143=CARTESIAN_POINT ( 'NONE',  ( -1.500000000000001110, 5.379166666666693075, -0.8660254037844372643 ) ) ;
#1144=CARTESIAN_POINT ( 'NONE',  ( -1.270904146967337889, 3.209693569853256268, 0.7750000000000083489 ) ) ;
#1146=CARTESIAN_POINT ( 'NONE',  ( 8.269583629331492602, 11.73526576994040482, 1.199719254218450271 ) ) ;
#1150=CARTESIAN_POINT ( 'NONE',  ( 3.662674053986138656, 7.424870162959149589, 0.7998128361456321445 ) ) ;
#1151=CARTESIAN_POINT ( 'NONE',  ( -5.558479791922849245, 9.428717490644563881, 0.7216878364870458196 ) ) ;
#1152=CARTESIAN_POINT ( 'NONE',  ( -5.907986510169434879, 6.002582827494773454, 0.1128355114666315662 ) ) ;
#1153=CARTESIAN_POINT ( 'NONE',  ( 10.56588178375152864, 11.22128359066528169, -0.7998128361456281477 ) ) ;
#1154=CIRCLE ( 'NONE', #42813, 0.07999999999999994615 ) ;
#1156=CARTESIAN_POINT ( 'NONE',  ( -6.995117189646935962, 10.24838825697502109, 1.199719254218453823 ) ) ;
#1157=CARTESIAN_POINT ( 'NONE',  ( -3.090895833791289071, 6.549869539491048442, 1.040834085586084257E-14 ) ) ;
#1160=CARTESIAN_POINT ( 'NONE',  ( 1.499999999999987121, 0.03541666734948738238, 0.8660254037844524744 ) ) ;
#1167=CARTESIAN_POINT ( 'NONE',  ( -4.568734577680887199, 6.353276312092901890, -1.443375672974051449 ) ) ;
#1170=CARTESIAN_POINT ( 'NONE',  ( 4.010558181858147719, 7.580895019428740333, -0.2605091080661054437 ) ) ;
#1176=CARTESIAN_POINT ( 'NONE',  ( -4.243338890952904841, 5.973648010910253880, -1.443375672974051449 ) ) ;
#1177=CARTESIAN_POINT ( 'NONE',  ( 8.127223016387999266, 11.56917838817298616, 1.199719254218460707 ) ) ;
#1183=EDGE_LOOP ( 'NONE', ( #24674, #45547, #19701, #34320, #64094 ) ) ;
#1185=CARTESIAN_POINT ( 'NONE',  ( -2.252626078164912560, 5.779814191167667481, 0.7998128361456341429 ) ) ;
#1186=CARTESIAN_POINT ( 'NONE',  ( -7.458957065812611198, 11.85386701009007204, 0.7998128361456481317 ) ) ;
#1190=CARTESIAN_POINT ( 'NONE',  ( 5.626797444871351139, 6.523350759560078593, 1.199719254218462483 ) ) ;
#1195=CARTESIAN_POINT ( 'NONE',  ( -1.284279953904156280, 2.921639714193936754, 0.7750000000000117906 ) ) ;
#1198=DIRECTION ( 'NONE',  ( 0.000000000000000000, 8.546850786086437571E-32, 1.000000000000000000 ) ) ;
#1199=VERTEX_POINT ( 'NONE', #148536 ) ;
#1207=CARTESIAN_POINT ( 'NONE',  ( 8.633844893804129228, 8.967240552393299424, -0.7998128361456211532 ) ) ;
#1209=CARTESIAN_POINT ( 'NONE',  ( -3.438964519360665051, 7.163875705896082913, -0.7998128361456281477 ) ) ;
#1215=CARTESIAN_POINT ( 'NONE',  ( -1.402160292154681736E-14, -1.256249999317182953, 1.732050807568877637 ) ) ;
#1219=CARTESIAN_POINT ( 'NONE',  ( 4.856179778084614540, 5.010200168423447842, 0.6077543439236311462 ) ) ;
#1220=CARTESIAN_POINT ( 'NONE',  ( 4.976006071415387311, 5.764094157194782575, 1.199719254218462483 ) ) ;
#1222=CARTESIAN_POINT ( 'NONE',  ( -4.810445574750349174, 4.506608013497163334, 0.7998128361456341429 ) ) ;
#1228=CARTESIAN_POINT ( 'NONE',  ( 4.365362273920230685, 8.036747052974847705, 0.7216878364870298324 ) ) ;
#1231=CARTESIAN_POINT ( 'NONE',  ( 7.659993601596707613, 9.959745173328078849, -1.443375672974058777 ) ) ;
#1232=CARTESIAN_POINT ( 'NONE',  ( 0.6823417656249917140, 4.405208333674755394, 1.181850606188765695 ) ) ;
#1234=CARTESIAN_POINT ( 'NONE',  ( 3.131570294632282092, 5.636953862837537521, -1.082531754730543971 ) ) ;
#1242=CARTESIAN_POINT ( 'NONE',  ( -6.137326611691442224, 5.996379759157309586, -0.05818935505210766357 ) ) ;
#1244=CARTESIAN_POINT ( 'NONE',  ( -1.364683531250010295, 5.342708333674750953, 0.7879004041258379498 ) ) ;
#1252=CARTESIAN_POINT ( 'NONE',  ( -0.7500000000000249800, -1.058333333333314030, 1.299038105676659116 ) ) ;
#1261=CARTESIAN_POINT ( 'NONE',  ( 1.364683531249990311, 4.446875000341417028, 1.214306433183764966E-14 ) ) ;
#1263=CARTESIAN_POINT ( 'NONE',  ( 6.100279051144945619, 9.204410428722734849, -1.199719254218440723 ) ) ;
#1264=CARTESIAN_POINT ( 'NONE',  ( -7.991641480251377772, 11.41099992934688956, 1.199719254218453823 ) ) ;
#1272=CARTESIAN_POINT ( 'NONE',  ( -1.500000000000011324, 4.420833333333352044, 0.8660254037844403729 ) ) ;
#1278=CARTESIAN_POINT ( 'NONE',  ( 8.514157279702022407, 10.95626946445095307, -1.443375672974063439 ) ) ;
#1283=CARTESIAN_POINT ( 'NONE',  ( 1.499999999999987121, 3.327083334016150751, -0.8660254037844262731 ) ) ;
#1285=CARTESIAN_POINT ( 'NONE',  ( -5.576481253922474401, 5.400316305864651056, -0.7998128361456221525 ) ) ;
#1286=CARTESIAN_POINT ( 'NONE',  ( 4.378920427089557421, 5.171457255435017331, -1.082531754730548412 ) ) ;
#1287=CARTESIAN_POINT ( 'NONE',  ( -1.420000000000001039, 6.280000000000042881, -2.899999999999995470 ) ) ;
#1294=CARTESIAN_POINT ( 'NONE',  ( 4.172158584703322681, 5.890604320285754980, -1.599625672291256295 ) ) ;
#1297=CARTESIAN_POINT ( 'NONE',  ( 4.924636110261782385, 6.768494766770632332, 1.599625672291267398 ) ) ;
#1309=CARTESIAN_POINT ( 'NONE',  ( 5.762717851902044330, 6.056246448182416309, -0.5943541797442238872 ) ) ;
#1311=CARTESIAN_POINT ( 'NONE',  ( 9.999301985278609806, 11.62460605670194447, 1.199719254218452047 ) ) ;
#1317=CARTESIAN_POINT ( 'NONE',  ( -1.364683531250014514, -1.219791666325248602, 0.7879004041258379498 ) ) ;
#1319=CARTESIAN_POINT ( 'NONE',  ( 6.399085315970131305, 8.488685506763726352, -1.443375672974057666 ) ) ;
#1320=CARTESIAN_POINT ( 'NONE',  ( -9.653042183249970876, 11.32459930428888306, -1.082531754730539753 ) ) ;
#1326=CARTESIAN_POINT ( 'NONE',  ( -4.939248034080176097, 4.656877549381960080, 1.214306433183764966E-14 ) ) ;
#1338=CARTESIAN_POINT ( 'NONE',  ( 6.115167699822185554, 6.015585554489271125, 0.01814796302670486361 ) ) ;
#1339=CARTESIAN_POINT ( 'NONE',  ( -4.281104764355953662, 5.612007818275039917, -1.265243560071245055 ) ) ;
#1345=CARTESIAN_POINT ( 'NONE',  ( -8.839552966430012759, 10.37552855133225904, -1.082531754730543971 ) ) ;
#1349=CARTESIAN_POINT ( 'NONE',  ( 8.111855979677986994, 8.358253485912799263, 1.040834085586084257E-14 ) ) ;
#1350=CARTESIAN_POINT ( 'NONE',  ( -3.922452899745962451, 7.727945483012266692, -0.5281491603440056082 ) ) ;
#1352=CARTESIAN_POINT ( 'NONE',  ( 4.813308228051395687, 5.574280006603454574, 1.199719254218462483 ) ) ;
#1354=CARTESIAN_POINT ( 'NONE',  ( -4.629219384062206011, 7.488174150459498968, -1.199719254218452047 ) ) ;
#1356=CARTESIAN_POINT ( 'NONE',  ( -6.742482464697739708, 6.760651051769146491, 0.7998128361456341429 ) ) ;
#1359=CARTESIAN_POINT ( 'NONE',  ( 10.06423010004587759, 10.63602329300870153, 0.000000000000000000 ) ) ;
#1360=CARTESIAN_POINT ( 'NONE',  ( 0.4934552264687537271, 6.857579847919138771, 3.660192259447391461 ) ) ;
#1363=CARTESIAN_POINT ( 'NONE',  ( 4.033840454514115770, 7.781623563118116316, -0.4120627063678127255 ) ) ;
#1364=CARTESIAN_POINT ( 'NONE',  ( 6.182154858151487353, 6.314861544039274577, -0.7216878364870257245 ) ) ;
#1366=CARTESIAN_POINT ( 'NONE',  ( -2.081668171172168513E-14, 6.487495393664096888, 3.100011470320013451 ) ) ;
#1368=CARTESIAN_POINT ( 'NONE',  ( -1.198337723683057465, 3.300000000000024691, 0.6661986840810731891 ) ) ;
#1369=CARTESIAN_POINT ( 'NONE',  ( 1.123270288250309834, 3.221052654332833054, -0.7749999999993620881 ) ) ;
#1372=CARTESIAN_POINT ( 'NONE',  ( 8.893785580440313865, 9.478430720042945623, 1.040834085586084257E-14 ) ) ;
#1377=CARTESIAN_POINT ( 'NONE',  ( -7.527801604085656351, 9.805521176231838609, 1.599625672291295375 ) ) ;
#1386=CARTESIAN_POINT ( 'NONE',  ( 9.541187415715040032, 12.15447128979948310, -1.599625672291262513 ) ) ;
#1389=CARTESIAN_POINT ( 'NONE',  ( 5.522248639467795428, 5.337044922334209573, -0.7998128361456231517 ) ) ;
#1392=CARTESIAN_POINT ( 'NONE',  ( 1.499999999999989120, 4.535416667349484676, 0.8660254037844524744 ) ) ;
#1398=CARTESIAN_POINT ( 'NONE',  ( 0.7499999999999902300, 1.983333333333357817, 1.299038105676669330 ) ) ;
#1399=CARTESIAN_POINT ( 'NONE',  ( 5.612185521052973414, 8.634967976948757951, -1.199719254218440723 ) ) ;
#1400=CARTESIAN_POINT ( 'NONE',  ( 4.406036734316882253, 6.163462161501577441, -1.443375672974051449 ) ) ;
#1404=CARTESIAN_POINT ( 'NONE',  ( 8.771762198361678031, 9.336070107617867819, 1.040834085586084257E-14 ) ) ;
#1411=CARTESIAN_POINT ( 'NONE',  ( -5.752737250900127997, 5.605948302338584099, 0.000000000000000000 ) ) ;
#1412=CARTESIAN_POINT ( 'NONE',  ( 1.499999999999989120, 4.285416667349482900, 0.8660254037844524744 ) ) ;
#1413=CARTESIAN_POINT ( 'NONE',  ( -0.6823417656250246877, -0.1989583329919109023, 1.181850606188755259 ) ) ;
#1417=CARTESIAN_POINT ( 'NONE',  ( 5.020596955762157698, 4.751784624677624080, 1.040834085586084257E-14 ) ) ;
#1419=CARTESIAN_POINT ( 'NONE',  ( -1.001543065824772872E-14, 4.884375000341420581, 1.575800808251672791 ) ) ;
#1424=CARTESIAN_POINT ( 'NONE',  ( -3.755245360860945958, 7.324943987738942397, -0.7216878364870454865 ) ) ;
#1426=CARTESIAN_POINT ( 'NONE',  ( -7.714753101375940503, 8.959299025482085455, 1.199719254218462483 ) ) ;
#1427=CARTESIAN_POINT ( 'NONE',  ( 6.114890974963323345, 7.092793211334054604, 1.199719254218462483 ) ) ;
#1430=CARTESIAN_POINT ( 'NONE',  ( -0.6823417656250003738, -0.5322916663252491576, -1.181850606188749264 ) ) ;
#1436=CARTESIAN_POINT ( 'NONE',  ( -5.181187258716735577, 9.196468901811520880, 0.7998128361456481317 ) ) ;
#1441=CARTESIAN_POINT ( 'NONE',  ( 10.22692794340986921, 10.82583744360002243, 0.000000000000000000 ) ) ;
#1443=CARTESIAN_POINT ( 'NONE',  ( -2.981903720001798597, 5.566305875722335372, -1.199719254218446718 ) ) ;
#1444=CARTESIAN_POINT ( 'NONE',  ( -7.670162217029145246, 9.971608557999250166, 1.599625672291295375 ) ) ;
#1447=CARTESIAN_POINT ( 'NONE',  ( -5.011569529345123897, 6.785514760743092566, 1.449221747052743092 ) ) ;
#1452=CARTESIAN_POINT ( 'NONE',  ( 8.622622508611357262, 9.162073802909148412, -0.7216878364870197293 ) ) ;
#1455=CARTESIAN_POINT ( 'NONE',  ( 3.832150974156964818, 7.622593236491780999, 1.040834085586084257E-14 ) ) ;
#1474=ORIENTED_EDGE ( 'NONE', *, *, #92359, .T. ) ;
#1476=CARTESIAN_POINT ( 'NONE',  ( -3.411848212133334446, 7.132240014130862171, 0.7998128361456341429 ) ) ;
#1477=CARTESIAN_POINT ( 'NONE',  ( -7.133561379084627063, 11.47423870890741782, 0.7998128361456481317 ) ) ;
#1478=FACE_OUTER_BOUND ( 'NONE', #174070, .T. ) ;
#1483=CARTESIAN_POINT ( 'NONE',  ( -1.500000000000013101, 2.410416667349482456, -0.8660254037844313801 ) ) ;
#1484=CARTESIAN_POINT ( 'NONE',  ( 10.71502147350184231, 11.39527989537399755, 0.000000000000000000 ) ) ;
#1488=CARTESIAN_POINT ( 'NONE',  ( -9.179033691651859783, 10.66762638080401260, 1.199719254218462483 ) ) ;
#1489=CARTESIAN_POINT ( 'NONE',  ( 1.438880590755393429, 3.300000000000025135, 0.4368907704009279414 ) ) ;
#1490=CARTESIAN_POINT ( 'NONE',  ( -0.6823417656250212460, 2.551041667008084435, 1.181850606188767472 ) ) ;
#1492=FACE_OUTER_BOUND ( 'NONE', #13832, .T. ) ;
#1497=CARTESIAN_POINT ( 'NONE',  ( -10.49364770729726359, 11.34493653470939023, 0.7216878364870438212 ) ) ;
#1501=CARTESIAN_POINT ( 'NONE',  ( -1.201851678989727383E-14, 2.134375000341423689, 1.575800808251672791 ) ) ;
#1506=CARTESIAN_POINT ( 'NONE',  ( -0.6823417656250212460, 1.301041667008083547, 1.181850606188755259 ) ) ;
#1508=CARTESIAN_POINT ( 'NONE',  ( -5.819474248763749635, 7.812472595022922128, -1.599625672291256295 ) ) ;
#1509=CARTESIAN_POINT ( 'NONE',  ( 8.076906825439115423, 10.44614393447756129, -1.599625672291262513 ) ) ;
#1510=CARTESIAN_POINT ( 'NONE',  ( 5.217190183160311356, 4.981143389975473568, -0.7998128361456211532 ) ) ;
#1511=EDGE_CURVE ( 'NONE', #26662, #152681, #56567, .T. ) ;
#1512=CIRCLE ( 'NONE', #164066, 0.7499999999999997780 ) ;
#1514=CARTESIAN_POINT ( 'NONE',  ( -0.7499999999999972244, 3.858333333333359594, -1.299038105676652011 ) ) ;
#1516=CARTESIAN_POINT ( 'NONE',  ( -1.201851678989727383E-14, 3.009375000341419248, -1.575800808251660134 ) ) ;
#1523=CARTESIAN_POINT ( 'NONE',  ( 5.178851490740193242, 8.025448591630130579, 1.082531754730558626 ) ) ;
#1526=CARTESIAN_POINT ( 'NONE',  ( -9.352427035328430449, 9.805586384171650849, 1.040834085586084257E-14 ) ) ;
#1527=CARTESIAN_POINT ( 'NONE',  ( -9.978437869977950569, 11.70422760547153906, -1.082531754730539753 ) ) ;
#1529=CARTESIAN_POINT ( 'NONE',  ( 1.364683531249990311, 4.384375000341417028, 1.214306433183764966E-14 ) ) ;
#1533=DIRECTION ( 'NONE',  ( 1.000000000000000000, -5.578564026256504688E-16, -1.232595164407830946E-31 ) ) ;
#1534=CARTESIAN_POINT ( 'NONE',  ( -7.673551755210395342, 8.054824590608001600, 1.040834085586084257E-14 ) ) ;
#1536=CARTESIAN_POINT ( 'NONE',  ( 1.499999999999990896, 5.025000000000022560, 1.214306433183764966E-14 ) ) ;
#1539=CARTESIAN_POINT ( 'NONE',  ( 7.565086526745395723, 10.80938946696957004, -1.082531754730543083 ) ) ;
#1545=CARTESIAN_POINT ( 'NONE',  ( 3.511198595814932766, 5.119484333249288532, 1.443375672974066548 ) ) ;
#1548=CARTESIAN_POINT ( 'NONE',  ( 8.690413276235306128, 13.08263988900915109, -0.7216878364870267237 ) ) ;
#1555=CARTESIAN_POINT ( 'NONE',  ( 7.287671262545424966, 8.461036880179857889, -1.199719254218451159 ) ) ;
#1557=CARTESIAN_POINT ( 'NONE',  ( -4.880045225915050189, 7.780804299287790826, 1.199719254218464037 ) ) ;
#1561=CARTESIAN_POINT ( 'NONE',  ( 5.951666246274803562, 7.006327377817825663, 1.082531754730558626 ) ) ;
#1562=CARTESIAN_POINT ( 'NONE',  ( -1.201851678989727383E-14, 0.8843750003414173610, 1.575800808251672791 ) ) ;
#1563=CARTESIAN_POINT ( 'NONE',  ( -3.164938793786285842, 5.779846795137578930, -1.199719254218452935 ) ) ;
#1579=CARTESIAN_POINT ( 'NONE',  ( 7.633404179693907388, 8.864391950186421454, -1.199719254218441611 ) ) ;
#1580=CARTESIAN_POINT ( 'NONE',  ( 5.445571254183207088, 9.504916896522420444, -0.7998128361456281477 ) ) ;
#1586=CARTESIAN_POINT ( 'NONE',  ( 1.492681600543877440, 8.694743381153815065, 2.590460435319994481 ) ) ;
#1591=CARTESIAN_POINT ( 'NONE',  ( -4.791917227426195858, 7.677988301050826969, -1.199719254218452047 ) ) ;
#1593=CARTESIAN_POINT ( 'NONE',  ( -4.009460741339347045, 5.700790169694431420, -1.599625672291256295 ) ) ;
#1598=CARTESIAN_POINT ( 'NONE',  ( -1.001543065824772872E-14, 4.743750000682821266, 1.732050807568877637 ) ) ;
#1599=EDGE_CURVE ( 'NONE', #159704, #117563, #86721, .T. ) ;
#1602=AXIS2_PLACEMENT_3D ( 'NONE', #73848, #139942, #205969 ) ;
#1604=CARTESIAN_POINT ( 'NONE',  ( -8.351459436338023679, 12.68719374246231624, -0.7216878364870267237 ) ) ;
#1607=AXIS2_PLACEMENT_3D ( 'NONE', #102862, #87673, #121322 ) ;
#1608=CARTESIAN_POINT ( 'NONE',  ( 6.796715079152391148, 6.823922435299587974, 0.7998128361456341429 ) ) ;
#1609=CARTESIAN_POINT ( 'NONE',  ( 1.364683531249990311, 4.634375000341417916, 1.214306433183764966E-14 ) ) ;
#1615=CARTESIAN_POINT ( 'NONE',  ( 3.999292125906894313, 7.609665213625947722, 0.7216878364870317197 ) ) ;
#1616=CARTESIAN_POINT ( 'NONE',  ( -6.021792782764022078, 10.17717534653336209, -0.7998128361456291469 ) ) ;
#1617=ORIENTED_EDGE ( 'NONE', *, *, #48198, .T. ) ;
#1618=ORIENTED_EDGE ( 'NONE', *, *, #202081, .T. ) ;
#1622=CARTESIAN_POINT ( 'NONE',  ( -8.694856585065634746, 9.038420858865048757, 0.7998128361456462443 ) ) ;
#1623=CARTESIAN_POINT ( 'NONE',  ( -5.250031796989778066, 7.148123067953287446, 1.599625672291267398 ) ) ;
#1630=CARTESIAN_POINT ( 'NONE',  ( 6.693975156845185737, 8.832723654451292816, 1.599625672291281386 ) ) ;
#1637=PLANE ( 'NONE',  #210177 ) ;
#1642=VERTEX_POINT ( 'NONE', #153866 ) ;
#1644=CARTESIAN_POINT ( 'NONE',  ( -1.001543065824772872E-14, 5.712500000000021672, 1.732050807568877637 ) ) ;
#1645=CARTESIAN_POINT ( 'NONE',  ( 3.521367211247359741, 5.131347717920458962, -1.599625672291262513 ) ) ;
#1646=CARTESIAN_POINT ( 'NONE',  ( 4.981731378017507872, 7.899438143407371271, -1.199719254218452047 ) ) ;
#1648=CARTESIAN_POINT ( 'NONE',  ( -7.456621297836087514, 9.722477485607340597, 1.443375672974090751 ) ) ;
#1649=CARTESIAN_POINT ( 'NONE',  ( -2.493766133720152212, 8.265889183060426859, -2.456386456769293236 ) ) ;
#1650=CARTESIAN_POINT ( 'NONE',  ( 6.317736394288140822, 7.433409217166723870, 1.082531754730558626 ) ) ;
#1651=CARTESIAN_POINT ( 'NONE',  ( -8.365017589507372620, 9.821903944922480534, 1.082531754730558626 ) ) ;
#1656=CARTESIAN_POINT ( 'NONE',  ( 6.642605195691581699, 9.837124264027149678, 1.199719254218462483 ) ) ;
#1661=CARTESIAN_POINT ( 'NONE',  ( -2.305169766234572926, 5.485456815665096464, -0.7666753726264395885 ) ) ;
#1662=CARTESIAN_POINT ( 'NONE',  ( -1.201851678989727383E-14, 3.446875000341421469, -1.575800808251660134 ) ) ;
#1669=CARTESIAN_POINT ( 'NONE',  ( 8.392660782059197189, 9.750191319612612872, 1.199719254218462483 ) ) ;
#1673=CARTESIAN_POINT ( 'NONE',  ( -9.040589502214116280, 9.441775928871617651, 0.7998128361456462443 ) ) ;
#1677=CARTESIAN_POINT ( 'NONE',  ( 1.499999999999990896, 4.306250000682819490, 1.214306433183764966E-14 ) ) ;
#1679=CARTESIAN_POINT ( 'NONE',  ( 9.728138913005292210, 11.30824913904973705, -1.199719254218440723 ) ) ;
#1682=CARTESIAN_POINT ( 'NONE',  ( -6.692921386640485082, 10.96015871772258521, -0.7998128361456291469 ) ) ;
#1688=CARTESIAN_POINT ( 'NONE',  ( 5.859090863903361424, 5.997168572722006097, -0.3086645125121977862 ) ) ;
#1689=CARTESIAN_POINT ( 'NONE',  ( -3.898132859128961236, 4.506575409527250997, -1.199719254218452047 ) ) ;
#1694=CARTESIAN_POINT ( 'NONE',  ( 7.637320603199683866, 7.804628880021436288, -0.7998128361456281477 ) ) ;
#1696=CARTESIAN_POINT ( 'NONE',  ( 7.623762449586013901, 7.788811034138823253, 1.040834085586084257E-14 ) ) ;
#1697=CARTESIAN_POINT ( 'NONE',  ( -4.209440762792112878, 7.367024337791516331, -0.8326445619948764643 ) ) ;
#1698=CARTESIAN_POINT ( 'NONE',  ( 3.662674053986138656, 7.424870162959149589, 0.7998128361456321445 ) ) ;
#1700=CARTESIAN_POINT ( 'NONE',  ( -8.026063749610061748, 9.426457798375635022, -1.082531754730543971 ) ) ;
#1707=CARTESIAN_POINT ( 'NONE',  ( -4.018125071768071876, 7.621166010707856486, 0.1319346992594405132 ) ) ;
#1711=CARTESIAN_POINT ( 'NONE',  ( 5.178851490740193242, 8.025448591630130579, 1.082531754730558626 ) ) ;
#1715=CARTESIAN_POINT ( 'NONE',  ( -9.775065565328603157, 11.46695991671396087, -1.082531754730537976 ) ) ;
#1720=CARTESIAN_POINT ( 'NONE',  ( -9.124274191872636663, 11.66807252865000244, -1.443375672974058777 ) ) ;
#1722=ORIENTED_EDGE ( 'NONE', *, *, #196542, .T. ) ;
#1727=CARTESIAN_POINT ( 'NONE',  ( -10.26315909542058336, 11.07603315418659840, -0.7216878364870267237 ) ) ;
#1732=EDGE_LOOP ( 'NONE', ( #72750, #180023, #184227, #175031, #33412, #31755 ) ) ;
#1734=CARTESIAN_POINT ( 'NONE',  ( -0.7500000000000215383, 3.222916667349487341, 1.299038105676671107 ) ) ;
#1736=CARTESIAN_POINT ( 'NONE',  ( -5.042743069279040036, 7.970618449879118828, 1.199719254218464037 ) ) ;
#1739=CARTESIAN_POINT ( 'NONE',  ( -8.402302512167102222, 10.82577223566020841, -1.599625672291263179 ) ) ;
#1740=CARTESIAN_POINT ( 'NONE',  ( 7.084367489069545069E-14, 8.210952333604106812, 2.038660652713624177 ) ) ;
#1744=CARTESIAN_POINT ( 'NONE',  ( 5.438792177376376991, 9.497007973581119700, 1.040834085586084257E-14 ) ) ;
#1749=CARTESIAN_POINT ( 'NONE',  ( 7.750457368506414646, 12.19395069656619945, 0.7998128361456462443 ) ) ;
#1756=CARTESIAN_POINT ( 'NONE',  ( -6.724481002698120768, 9.828683022247721723, -1.082531754730538864 ) ) ;
#1759=CARTESIAN_POINT ( 'NONE',  ( -1.201851678989727383E-14, 5.009375000341421469, -1.575800808251660134 ) ) ;
#1767=CARTESIAN_POINT ( 'NONE',  ( -2.765500147063310266, 6.170241238308400433, 1.040834085586084257E-14 ) ) ;
#1770=CARTESIAN_POINT ( 'NONE',  ( 8.374132434735052755, 12.92157160716627295, -0.7998128361456352531 ) ) ;
#1772=CARTESIAN_POINT ( 'NONE',  ( -1.127943160727153060, 2.800000000000024691, -0.7749999999999935829 ) ) ;
#1776=CARTESIAN_POINT ( 'NONE',  ( 1.364683531249988535, 2.113541667008087099, 0.7879004041258500513 ) ) ;
#1778=CARTESIAN_POINT ( 'NONE',  ( 5.508690485854129903, 5.321227076451600091, 1.040834085586084257E-14 ) ) ;
#1786=DIRECTION ( 'NONE',  ( -5.578564026256490882E-16, -1.000000000000000000, -9.066213480720158442E-32 ) ) ;
#1787=CARTESIAN_POINT ( 'NONE',  ( -5.897433632264490910, 9.824163637709826702, 0.000000000000000000 ) ) ;
#1789=CARTESIAN_POINT ( 'NONE',  ( -0.004619473214107579565, 7.151453204069600389, 1.999995854215794511 ) ) ;
#1792=CARTESIAN_POINT ( 'NONE',  ( -8.320953590485107298, 10.73086516036454618, 1.599625672291269396 ) ) ;
#1793=CARTESIAN_POINT ( 'NONE',  ( -3.565431210269599749, 7.103494145382415859, 0.7216878364870317197 ) ) ;
#1794=CARTESIAN_POINT ( 'NONE',  ( 0.6823417656249899377, 2.655208333674753618, 1.181850606188767472 ) ) ;
#1812=CARTESIAN_POINT ( 'NONE',  ( 0.6823417656249917140, 4.655208333674755394, 1.181850606188765695 ) ) ;
#1820=CARTESIAN_POINT ( 'NONE',  ( 9.260382613333817403, 10.76253345609967660, -1.199719254218446718 ) ) ;
#1823=CARTESIAN_POINT ( 'NONE',  ( 0.6823417656249899377, 2.092708333674753174, 1.181850606188767472 ) ) ;
#1826=CARTESIAN_POINT ( 'NONE',  ( -8.541273586929371220, 9.067166727613487964, 0.7216878364870438212 ) ) ;
#1834=CARTESIAN_POINT ( 'NONE',  ( 5.138703914779377158, 5.953908307786102583, 1.199719254218462483 ) ) ;
#1839=CARTESIAN_POINT ( 'NONE',  ( -0.7500000000000006661, 2.858333333333358706, -1.299038105676652011 ) ) ;
#1843=ORIENTED_EDGE ( 'NONE', *, *, #58178, .F. ) ;
#1845=CARTESIAN_POINT ( 'NONE',  ( -3.490334480514268645, 6.159475096320226939, -1.199719254218452935 ) ) ;
#1846=CARTESIAN_POINT ( 'NONE',  ( 8.132193210098487057, 8.381980254736715708, 1.040834085586084257E-14 ) ) ;
#1848=CARTESIAN_POINT ( 'NONE',  ( 5.151735183068521629, 5.112705256442466428, 1.040834085586084257E-14 ) ) ;
#1857=CARTESIAN_POINT ( 'NONE',  ( -6.209271165378811297, 10.18797409300986878, 0.7216878364870458196 ) ) ;
#1858=CARTESIAN_POINT ( 'NONE',  ( 4.635998460869027227, 7.496083073400806818, -1.199719254218452047 ) ) ;
#1861=CARTESIAN_POINT ( 'NONE',  ( -6.984421689334302741, 11.30024240419870374, 0.000000000000000000 ) ) ;
#1865=CARTESIAN_POINT ( 'NONE',  ( -2.937312835655025101, 6.578615408239493867, 1.040834085586084257E-14 ) ) ;
#1868=CARTESIAN_POINT ( 'NONE',  ( 8.829384350997564468, 11.32403438096243775, 1.599625672291281386 ) ) ;
#1869=CARTESIAN_POINT ( 'NONE',  ( 3.246287715468270108, 5.874753870433235825, 1.199719254218450271 ) ) ;
#1878=CARTESIAN_POINT ( 'NONE',  ( -5.766295404513795297, 5.621766148221195358, 0.7998128361456341429 ) ) ;
#1879=CARTESIAN_POINT ( 'NONE',  ( -1.364683531249997417, 5.759375000341418804, 1.214306433183764966E-14 ) ) ;
#1881=CARTESIAN_POINT ( 'NONE',  ( -8.402302512167102222, 10.82577223566020841, -1.599625672291263179 ) ) ;
#1886=CARTESIAN_POINT ( 'NONE',  ( 8.432808358020029260, 8.940623960552603222, 0.7216878364870438212 ) ) ;
#1889=CARTESIAN_POINT ( 'NONE',  ( 3.499976210622149253, 7.235056012367825140, 0.7998128361456321445 ) ) ;
#1890=CARTESIAN_POINT ( 'NONE',  ( 5.969672231941198781, 6.017005441543672895, -0.3686804784870336693 ) ) ;
#1891=CARTESIAN_POINT ( 'NONE',  ( 5.691725559638619814, 5.534767995866836543, 1.040834085586084257E-14 ) ) ;
#1893=CARTESIAN_POINT ( 'NONE',  ( -5.540478329478883524, 9.615641817700700145, 0.000000000000000000 ) ) ;
#1901=EDGE_CURVE ( 'NONE', #91287, #146442, #53074, .T. ) ;
#1904=CARTESIAN_POINT ( 'NONE',  ( -1.402160292154681736E-14, 2.009375000341422801, -1.575800808251660134 ) ) ;
#1905=CARTESIAN_POINT ( 'NONE',  ( 7.879259827836241570, 12.34422023245099176, 1.040834085586084257E-14 ) ) ;
#1907=CARTESIAN_POINT ( 'NONE',  ( -5.436456409399874623, 5.444880020495701523, 0.000000000000000000 ) ) ;
#1909=CARTESIAN_POINT ( 'NONE',  ( 4.202664430556261266, 4.005456045178151570, 0.7216878364870317197 ) ) ;
#1910=CARTESIAN_POINT ( 'NONE',  ( -5.463572716182839351, 7.397254140345190798, 1.443375672974064550 ) ) ;
#1918=CARTESIAN_POINT ( 'NONE',  ( 5.671388329218120639, 5.511041227042920099, 1.040834085586084257E-14 ) ) ;
#1922=EDGE_CURVE ( 'NONE', #174777, #97759, #198409, .T. ) ;
#1929=CARTESIAN_POINT ( 'NONE',  ( 3.683011284406639607, 7.448596931783069586, 0.7998128361456321445 ) ) ;
#1932=( BOUNDED_CURVE ( )  B_SPLINE_CURVE ( 2, ( #75134, #139079, #40511, #104435, #26365, #138007, #141242 ),
 .UNSPECIFIED., .F., .T. ) 
 B_SPLINE_CURVE_WITH_KNOTS ( ( 3, 2, 2, 3 ),
 ( 0.1874999999999999722, 0.1916666666666665964, 0.1958333333333332205, 0.1999999999999998446 ),
 .UNSPECIFIED. ) 
 CURVE ( )  GEOMETRIC_REPRESENTATION_ITEM ( )  RATIONAL_B_SPLINE_CURVE ( ( 1.000000000000000888, 0.8660254037844378194, 1.000000000000000000, 0.8660254037844387076, 1.000000000000000000, 0.8660254037844440367, 0.9999999999999946709 ) ) 
 REPRESENTATION_ITEM ( '' )  );
#1933=CARTESIAN_POINT ( 'NONE',  ( -5.494078562035765501, 7.432844293840273231, -1.599625672291256295 ) ) ;
#1937=CARTESIAN_POINT ( 'NONE',  ( 6.908042961362778733, 8.018137195466769285, 1.199719254218462483 ) ) ;
#1940=CARTESIAN_POINT ( 'NONE',  ( -5.925076824372040640, 6.871343368977510302, 1.199719254218450271 ) ) ;
#1941=CARTESIAN_POINT ( 'NONE',  ( -1.201851678989727383E-14, 2.837500000000024780, -1.732050807568863648 ) ) ;
#1942=CARTESIAN_POINT ( 'NONE',  ( -3.276266675996675204, 6.974061555304760240, -0.7998128361456281477 ) ) ;
#1945=CARTESIAN_POINT ( 'NONE',  ( -4.574986769607567894, 7.424902766929059261, 1.199719254218464037 ) ) ;
#1947=CARTESIAN_POINT ( 'NONE',  ( -1.364683531250012516, 2.780208333674754506, 0.7879004041258379498 ) ) ;
#1950=CARTESIAN_POINT ( 'NONE',  ( -6.236387472606166327, 6.378132927569716060, -0.7216878364870278340 ) ) ;
#1956=CARTESIAN_POINT ( 'NONE',  ( 3.818592820543298405, 7.606775390609172405, -0.7998128361456221525 ) ) ;
#1958=CARTESIAN_POINT ( 'NONE',  ( 0.6823417656249899377, 2.655208333674753618, 1.181850606188767472 ) ) ;
#1961=CARTESIAN_POINT ( 'NONE',  ( 0.6823417656249864960, -1.011458332991911568, -1.181850606188749264 ) ) ;
#1964=CARTESIAN_POINT ( 'NONE',  ( -4.406563619641430840, 5.099744630125142564, -1.199719254218446718 ) ) ;
#1965=CARTESIAN_POINT ( 'NONE',  ( -7.551528372687420720, 8.872833191965849409, 1.082531754730558626 ) ) ;
#1967=CARTESIAN_POINT ( 'NONE',  ( -1.364683531250012516, 2.488541667008088876, -0.7879004041258289570 ) ) ;
#1975=CARTESIAN_POINT ( 'NONE',  ( -7.009202228140751778, 9.200488570962775725, -1.443375672974058777 ) ) ;
#1981=CARTESIAN_POINT ( 'NONE',  ( -5.192409643909507544, 9.001635651295671892, 0.7216878364870458196 ) ) ;
#1994=CARTESIAN_POINT ( 'NONE',  ( -5.904739593951539689, 6.847616600153594746, 1.199719254218450271 ) ) ;
#1996=CARTESIAN_POINT ( 'NONE',  ( -1.500000000000001332, -0.5999999999999755529, 0.000000000000000000 ) ) ;
#1997=CARTESIAN_POINT ( 'NONE',  ( 2.523789150438203510, 6.096171108819874007, 0.7998128361456462443 ) ) ;
#2001=CARTESIAN_POINT ( 'NONE',  ( 6.765682348419287173, 7.852049813699357728, 1.199719254218462483 ) ) ;
#2007=CARTESIAN_POINT ( 'NONE',  ( -3.443407828190963915, 6.961133532957338943, 0.7216878364870317197 ) ) ;
#2014=CARTESIAN_POINT ( 'NONE',  ( 0.6823417656249899377, 2.592708333674753618, 1.181850606188767472 ) ) ;
#2015=CARTESIAN_POINT ( 'NONE',  ( 9.368320956918608999, 11.95279375453699622, 1.443375672974076540 ) ) ;
#2016=CARTESIAN_POINT ( 'NONE',  ( -7.015454420067433361, 10.27211502579893754, 1.199719254218453823 ) ) ;
#2019=CARTESIAN_POINT ( 'NONE',  ( 7.308008492965924141, 8.484763649003774333, -1.199719254218451159 ) ) ;
#2020=CARTESIAN_POINT ( 'NONE',  ( -5.703176172842872482, 9.805455968292021041, 0.000000000000000000 ) ) ;
#2021=CARTESIAN_POINT ( 'NONE',  ( -1.445184293213162663, 8.696352241143832984, 2.614796098495217436 ) ) ;
#2023=CARTESIAN_POINT ( 'NONE',  ( 0.7499999999999885647, -1.235416665983847473, 1.299038105676657340 ) ) ;
#2025=CARTESIAN_POINT ( 'NONE',  ( 6.792271770766432404, 10.86814146596211472, 1.040834085586084257E-14 ) ) ;
#2028=CARTESIAN_POINT ( 'NONE',  ( 1.364683531249986537, 0.4260416670080872659, 0.7879004041258500513 ) ) ;
#2031=CARTESIAN_POINT ( 'NONE',  ( 7.741342523278707866, 8.133913820021057006, 0.7216878364870458196 ) ) ;
#2033=CARTESIAN_POINT ( 'NONE',  ( -5.924549939491850381, 6.014322472269677533, 0.000000000000000000 ) ) ;
#2035=CARTESIAN_POINT ( 'NONE',  ( -0.6823417656250212460, 3.301041667008085323, 1.181850606188767472 ) ) ;
#2039=CARTESIAN_POINT ( 'NONE',  ( -4.985647801523292344, 6.839675073242382553, -1.599625672291256295 ) ) ;
#2040=CARTESIAN_POINT ( 'NONE',  ( -4.662544117754887196, 7.086110115384146368, -1.393066284953614620 ) ) ;
#2046=CARTESIAN_POINT ( 'NONE',  ( 6.174848896020108668, 9.291408581077091000, 1.199719254218460707 ) ) ;
#2050=CARTESIAN_POINT ( 'NONE',  ( -0.7500000000000006661, 2.858333333333358706, -1.299038105676652011 ) ) ;
#2056=CARTESIAN_POINT ( 'NONE',  ( 6.209271165378815738, 7.306866450105836464, -1.082531754730543083 ) ) ;
#2057=CARTESIAN_POINT ( 'NONE',  ( -1.402160292154681736E-14, 0.5093750003414236893, -1.575800808251659024 ) ) ;
#2061=CARTESIAN_POINT ( 'NONE',  ( 9.378489572351044856, 11.96465713920816043, -1.599625672291262513 ) ) ;
#2062=CARTESIAN_POINT ( 'NONE',  ( -1.201851678989727383E-14, 2.821875000341418360, 1.575800808251672791 ) ) ;
#2068=CARTESIAN_POINT ( 'NONE',  ( -1.500000000000013101, 0.1708333333333560411, 0.8660254037844403729 ) ) ;
#2069=CARTESIAN_POINT ( 'NONE',  ( 5.750629710490689384, 9.860818428881154674, -0.7998128361456291469 ) ) ;
#2070=CARTESIAN_POINT ( 'NONE',  ( -7.991641480251377772, 11.41099992934688956, 1.199719254218453823 ) ) ;
#2072=CARTESIAN_POINT ( 'NONE',  ( 1.364683531249986537, 0.6135416670080880985, 0.7879004041258500513 ) ) ;
#2073=CARTESIAN_POINT ( 'NONE',  ( -1.500000000000011324, 2.920833333333352932, 0.8660254037844403729 ) ) ;
#2075=CARTESIAN_POINT ( 'NONE',  ( 3.928111819657337911, 5.605883094398769195, 1.599625672291267398 ) ) ;
#2082=CARTESIAN_POINT ( 'NONE',  ( -1.402160292154681736E-14, -0.1312499993171854229, -1.732050807568870754 ) ) ;
#2083=CARTESIAN_POINT ( 'NONE',  ( -8.342344591110322227, 8.627156865917170236, -0.7998128361456291469 ) ) ;
#2084=CARTESIAN_POINT ( 'NONE',  ( -4.772106882330241717, 5.630174786549132726, -1.082531754730544860 ) ) ;
#2086=CARTESIAN_POINT ( 'NONE',  ( 6.938893903907228378E-15, 10.64264068711930733, 1.214306433183764966E-14 ) ) ;
#2091=VERTEX_POINT ( 'NONE', #146970 ) ;
#2092=EDGE_CURVE ( 'NONE', #108467, #7144, #178391, .T. ) ;
#2093=CARTESIAN_POINT ( 'NONE',  ( 6.938021921891177612, 9.117444880338284818, -1.599625672291262513 ) ) ;
#2097=CARTESIAN_POINT ( 'NONE',  ( 5.599154252319471503, 9.476171027773981237, -0.7216878364870267237 ) ) ;
#2102=CARTESIAN_POINT ( 'NONE',  ( -8.345207244411405156, 9.694828859023472134, 1.199719254218462483 ) ) ;
#2103=CARTESIAN_POINT ( 'NONE',  ( 5.678167406024951624, 5.518950149984223508, 0.7998128361456341429 ) ) ;
#2107=CARTESIAN_POINT ( 'NONE',  ( 3.995705304526904200, 7.602062626508213405, -0.07732544726959944548 ) ) ;
#2108=CARTESIAN_POINT ( 'NONE',  ( 8.107412671292022921, 12.40247251657532956, 0.7216878364870438212 ) ) ;
#2115=CARTESIAN_POINT ( 'NONE',  ( -5.287316719649550301, 5.270883715786984780, 0.7216878364870317197 ) ) ;
#2116=CARTESIAN_POINT ( 'NONE',  ( 9.408995418203971894, 11.03987807840189816, 1.082531754730549967 ) ) ;
#2119=CARTESIAN_POINT ( 'NONE',  ( -6.566226467720086113, 6.555019055295208119, 1.040834085586084257E-14 ) ) ;
#2125=CARTESIAN_POINT ( 'NONE',  ( -7.832860060393135093, 10.16142270859057462, 1.599625672291295375 ) ) ;
#2128=EDGE_CURVE ( 'NONE', #10132, #104455, #80771, .T. ) ;
#2130=ORIENTED_EDGE ( 'NONE', *, *, #75894, .F. ) ;
#2140=CARTESIAN_POINT ( 'NONE',  ( -4.530395885260773525, 8.437212299446219532, 0.7998128361456481317 ) ) ;
#2143=CARTESIAN_POINT ( 'NONE',  ( 3.863710590214593399, 7.451486755318259547, 1.040834085586084257E-14 ) ) ;
#2149=CARTESIAN_POINT ( 'NONE',  ( -4.517891501851816649, 6.293959390292322986, -1.599625672291256295 ) ) ;
#2152=CARTESIAN_POINT ( 'NONE',  ( 3.946537740505243974, 2.817530495244580102, -0.7749999999999935829 ) ) ;
#2155=CARTESIAN_POINT ( 'NONE',  ( -10.15235809853472126, 10.73883929124566983, -0.7998128361456291469 ) ) ;
#2156=CARTESIAN_POINT ( 'NONE',  ( 7.461064606222022277, 7.598996883547496139, 1.040834085586084257E-14 ) ) ;
#2159=CARTESIAN_POINT ( 'NONE',  ( -7.797910906154257304, 12.24931315715533486, 0.000000000000000000 ) ) ;
#2160=CARTESIAN_POINT ( 'NONE',  ( 5.443762371086860341, 6.309809840144842141, 1.199719254218462483 ) ) ;
#2162=CARTESIAN_POINT ( 'NONE',  ( -1.364683531250000748, -0.1781249996585798634, 0.000000000000000000 ) ) ;
#2164=EDGE_LOOP ( 'NONE', ( #182900, #30650 ) ) ;
#2166=CARTESIAN_POINT ( 'NONE',  ( 7.402388683381404988, 10.61957531637824204, -1.082531754730537976 ) ) ;
#2176=CARTESIAN_POINT ( 'NONE',  ( -0.03975248801529755738, 6.418311689316416491, -3.191082252424501498 ) ) ;
#2195=CARTESIAN_POINT ( 'NONE',  ( -0.7500000000000006661, -0.3604166659838467512, -1.299038105676652011 ) ) ;
#2200=CARTESIAN_POINT ( 'NONE',  ( 1.230761180058546289, 3.021116465842660581, -0.7749999999999874767 ) ) ;
#2201=CARTESIAN_POINT ( 'NONE',  ( 4.175548122884573665, 3.973820352894515295, 1.214306433183764966E-14 ) ) ;
#2203=CARTESIAN_POINT ( 'NONE',  ( 9.240045382913317340, 10.73880668727576015, -1.199719254218446718 ) ) ;
#2204=CARTESIAN_POINT ( 'NONE',  ( 3.469446951953614189E-15, 5.227586206896610577, 1.214306433183764966E-14 ) ) ;
#2208=CARTESIAN_POINT ( 'NONE',  ( 3.472859903394816872, 7.203420320602605287, -0.7998128361456291469 ) ) ;
#2209=CARTESIAN_POINT ( 'NONE',  ( -7.266807147244793263, 8.540658428949452485, 1.082531754730549967 ) ) ;
#2210=CARTESIAN_POINT ( 'NONE',  ( -5.912397865540070185, 5.999963284693008880, 0.01096864257240509621 ) ) ;
#2214=CARTESIAN_POINT ( 'NONE',  ( -6.496328159242330536, 10.73079995242472862, 0.000000000000000000 ) ) ;
#2215=CARTESIAN_POINT ( 'NONE',  ( -4.650083499362882122, 6.448183387388563226, 1.443375672974064550 ) ) ;
#2219=CARTESIAN_POINT ( 'NONE',  ( 1.499999999999987121, 0.07708333401615156955, -0.8660254037844323793 ) ) ;
#2226=CARTESIAN_POINT ( 'NONE',  ( -5.233084104750526322, 5.207612331738130429, 0.000000000000000000 ) ) ;
#2229=CARTESIAN_POINT ( 'NONE',  ( 3.995022045461748217, 7.603044914155053569, 0.06581304817247432548 ) ) ;
#2234=CARTESIAN_POINT ( 'NONE',  ( -4.582292731294565158, 4.448355729372827305, 1.214306433183764966E-14 ) ) ;
#2235=CARTESIAN_POINT ( 'NONE',  ( 9.284636267260101050, 9.726497154758602548, -0.7998128361456281477 ) ) ;
#2244=CARTESIAN_POINT ( 'NONE',  ( -3.952365473583647315, 4.569846793057691592, 1.199719254218462483 ) ) ;
#2246=CARTESIAN_POINT ( 'NONE',  ( -8.727698198895085469, 11.20540053684285553, -1.599625672291263179 ) ) ;
#2251=CARTESIAN_POINT ( 'NONE',  ( 5.705283713252285338, 5.550585841749444249, -0.7998128361456211532 ) ) ;
#2267=CARTESIAN_POINT ( 'NONE',  ( 8.959240580532112475, 9.346868853575953651, -0.7998128361456221525 ) ) ;
#2269=CARTESIAN_POINT ( 'NONE',  ( -3.601662362724658895, 7.353689856487406473, -0.7998128361456281477 ) ) ;
#2275=CARTESIAN_POINT ( 'NONE',  ( -0.7500000000000006661, -1.110416665983847473, -1.299038105676652011 ) ) ;
#2279=CARTESIAN_POINT ( 'NONE',  ( 5.040934186182656873, 4.775511393501539636, 1.040834085586084257E-14 ) ) ;
#2281=CARTESIAN_POINT ( 'NONE',  ( -5.610376637956639101, 5.439860920571172542, 0.000000000000000000 ) ) ;
#2287=CARTESIAN_POINT ( 'NONE',  ( 6.832946231607457399, 7.074118146404578589, -0.7216878364870257245 ) ) ;
#2289=VERTEX_POINT ( 'NONE', #198859 ) ;
#2290=CARTESIAN_POINT ( 'NONE',  ( 8.446366511189332016, 9.916811020218137429, -1.082531754730543083 ) ) ;
#2291=CARTESIAN_POINT ( 'NONE',  ( -1.001543065824772872E-14, 5.134375000341421469, 1.575800808251672791 ) ) ;
#2293=CARTESIAN_POINT ( 'NONE',  ( 3.321384445223597659, 6.818772919495430074, -0.7216878364870267237 ) ) ;
#2297=CARTESIAN_POINT ( 'NONE',  ( 5.358717427693826529, 6.320109463822404905, -1.084804798701855422 ) ) ;
#2301=CARTESIAN_POINT ( 'NONE',  ( -5.796211742468360129, 6.069872997065163922, -0.5622600474686073602 ) ) ;
#2305=CARTESIAN_POINT ( 'NONE',  ( -1.364683531250010295, 5.092708333674757171, 0.7879004041258379498 ) ) ;
#2321=CARTESIAN_POINT ( 'NONE',  ( -0.6823417656249969321, 5.280208333674756283, -1.181850606188749264 ) ) ;
#2323=CARTESIAN_POINT ( 'NONE',  ( 5.438792177376376991, 9.497007973581119700, 1.040834085586084257E-14 ) ) ;
#2325=CARTESIAN_POINT ( 'NONE',  ( -7.669108446824431269, 12.09904362127053545, -0.7998128361456291469 ) ) ;
#2326=CARTESIAN_POINT ( 'NONE',  ( 1.931788062848141441E-13, 7.054063922337705073, -3.955400951015614730 ) ) ;
#2328=DIRECTION ( 'NONE',  ( 0.7071067811865489050, -0.7071067811865462405, -6.410781031902101009E-32 ) ) ;
#2331=CARTESIAN_POINT ( 'NONE',  ( 1.499999999999990896, 4.775000000000022560, 1.214306433183764966E-14 ) ) ;
#2335=DIRECTION ( 'NONE',  ( 1.000000000000000000, 0.000000000000000000, 0.000000000000000000 ) ) ;
#2338=CARTESIAN_POINT ( 'NONE',  ( 8.351459436338029008, 10.76645531385962862, -1.443375672974063439 ) ) ;
#2344=CARTESIAN_POINT ( 'NONE',  ( -0.7500000000000006661, 2.889583334016148974, -1.299038105676652011 ) ) ;
#2346=CARTESIAN_POINT ( 'NONE',  ( -5.199715606040888005, 6.025088614257851027, -1.199719254218446718 ) ) ;
#2347=CARTESIAN_POINT ( 'NONE',  ( 2.670593071767634719, 6.059516317130127838, -0.7216878364870267237 ) ) ;
#2348=CARTESIAN_POINT ( 'NONE',  ( -8.771762197917311710, 13.17754696430482042, 0.7216878364870317197 ) ) ;
#2355=CARTESIAN_POINT ( 'NONE',  ( 2.998324526916512411, 6.649795714711241423, 0.000000000000000000 ) ) ;
#2356=CARTESIAN_POINT ( 'NONE',  ( -1.203941962966158297, 2.947768152887754400, -0.7749999999999944711 ) ) ;
#2358=( BOUNDED_CURVE ( )  B_SPLINE_CURVE ( 2, ( #63130, #78303, #129294, #209348, #192038, #177957, #128227 ),
 .UNSPECIFIED., .F., .T. ) 
 B_SPLINE_CURVE_WITH_KNOTS ( ( 3, 2, 2, 3 ),
 ( 0.1607142857142856152, 0.1666666666666666297, 0.1726190476190476719, 0.1785714285714287142 ),
 .UNSPECIFIED. ) 
 CURVE ( )  GEOMETRIC_REPRESENTATION_ITEM ( )  RATIONAL_B_SPLINE_CURVE ( ( 1.000000000000002442, 0.8660254037844361541, 1.000000000000000000, 0.8660254037844387076, 1.000000000000000000, 0.8660254037844355990, 1.000000000000003109 ) ) 
 REPRESENTATION_ITEM ( '' )  );
#2359=LINE ( 'NONE', #202702, #32917 ) ;
#2360=CARTESIAN_POINT ( 'NONE',  ( 3.194917754314666514, 6.879154480009089134, 0.7998128361456321445 ) ) ;
#2371=CARTESIAN_POINT ( 'NONE',  ( 5.000138648025401977, 6.582195279309941860, -1.237349059142704988 ) ) ;
#2372=AXIS2_PLACEMENT_3D ( 'NONE', #8636, #206834, #154907 ) ;
#2374=CARTESIAN_POINT ( 'NONE',  ( 8.218213668177886788, 12.73966637951625813, 0.7998128361456462443 ) ) ;
#2380=CARTESIAN_POINT ( 'NONE',  ( 6.832946231607457399, 7.074118146404578589, -0.7216878364870257245 ) ) ;
#2381=B_SPLINE_CURVE_WITH_KNOTS ( 'NONE', 3,
 ( #62739, #78993, #77931, #47596, #28118, #113710, #147221 ),
 .UNSPECIFIED., .F., .F.,
 ( 4, 3, 4 ),
 ( 0.000000000000000000, 6.254153400238295828E-05, 0.0001620526076657094038 ),
 .UNSPECIFIED. ) ;
#2382=CARTESIAN_POINT ( 'NONE',  ( -2.279742385392243165, 5.811449882932888222, -0.7998128361456281477 ) ) ;
#2387=CARTESIAN_POINT ( 'NONE',  ( -5.739179097286464248, 5.590130456455974617, -0.7998128361456221525 ) ) ;
#2397=CARTESIAN_POINT ( 'NONE',  ( 8.934986926605834157, 10.38290515491702770, -1.199719254218446718 ) ) ;
#2398=CARTESIAN_POINT ( 'NONE',  ( 6.101957686160805139, 6.023808750328159434, -0.2146407016825630509 ) ) ;
#2400=CARTESIAN_POINT ( 'NONE',  ( 4.578903193113299963, 6.365139696764064325, 1.599625672291267398 ) ) ;
#2406=CARTESIAN_POINT ( 'NONE',  ( -7.998947442382709383, 12.27592974951444660, 0.7216878364870478180 ) ) ;
#2412=CARTESIAN_POINT ( 'NONE',  ( 7.775764792637399836, 9.030479331953833011, -1.199719254218441611 ) ) ;
#2414=CARTESIAN_POINT ( 'NONE',  ( -3.411848212133334446, 7.132240014130863059, 0.7998128361456341429 ) ) ;
#2415=CARTESIAN_POINT ( 'NONE',  ( 2.679707916995359263, 6.278076336469897711, -0.7998128361456291469 ) ) ;
#2417=CARTESIAN_POINT ( 'NONE',  ( -6.250472511100020334, 7.250971670160158311, 1.199719254218450271 ) ) ;
#2418=CARTESIAN_POINT ( 'NONE',  ( 4.304877467538922531, 4.981110786005563007, 1.199719254218464037 ) ) ;
#2421=CARTESIAN_POINT ( 'NONE',  ( 7.242026607993941489, 11.60078147596829901, 0.7998128361456462443 ) ) ;
#2425=CARTESIAN_POINT ( 'NONE',  ( 4.104435073692848768, 7.689436668370499106, -0.6928796192886893524 ) ) ;
#2426=CARTESIAN_POINT ( 'NONE',  ( 6.832946231607457399, 7.074118146404578589, -0.7216878364870257245 ) ) ;
#2428=DIRECTION ( 'NONE',  ( 0.7797859179643625849, -0.6260462619842693810, -1.666848690107906998E-15 ) ) ;
#2435=CARTESIAN_POINT ( 'NONE',  ( 7.659993601596707613, 9.959745173328078849, -1.443375672974058777 ) ) ;
#2439=CARTESIAN_POINT ( 'NONE',  ( -7.153898609505128015, 11.49796547773133604, 0.7998128361456481317 ) ) ;
#2448=CARTESIAN_POINT ( 'NONE',  ( 9.622536337397022521, 12.24937836509514710, 1.599625672291281386 ) ) ;
#2451=CARTESIAN_POINT ( 'NONE',  ( 4.364835388595708743, 7.179726155748598515, 1.199719254218462483 ) ) ;
#2454=CARTESIAN_POINT ( 'NONE',  ( -1.201851678989727383E-14, 3.868750000682817713, -1.732050807568863648 ) ) ;
#2460=CARTESIAN_POINT ( 'NONE',  ( -0.7500000000000006661, 1.108333333333356929, -1.299038105676652011 ) ) ;
#2461=CARTESIAN_POINT ( 'NONE',  ( 5.262536180398716290, 9.291375977107183104, -0.7998128361456291469 ) ) ;
#2462=CARTESIAN_POINT ( 'NONE',  ( 4.433153041544209749, 7.155467067568137551, -1.082531754730548412 ) ) ;
#2466=CARTESIAN_POINT ( 'NONE',  ( 7.782016984564049444, 11.06247500109133064, 1.082531754730557072 ) ) ;
#2473=CARTESIAN_POINT ( 'NONE',  ( -5.928993247877788697, 5.811580298812519807, 0.7998128361456341429 ) ) ;
#2474=CARTESIAN_POINT ( 'NONE',  ( -1.500000000000011324, 3.702083334016152971, 0.8660254037844403729 ) ) ;
#2475=CARTESIAN_POINT ( 'NONE',  ( -0.6823417656250003738, -0.2822916663252489355, -1.181850606188749264 ) ) ;
#2482=CARTESIAN_POINT ( 'NONE',  ( 1.364683531249988535, 4.176041667008081326, 0.7879004041258500513 ) ) ;
#2485=CARTESIAN_POINT ( 'NONE',  ( -4.586165880992525423, 5.350526861157986147, -7.499999999999997335 ) ) ;
#2488=CARTESIAN_POINT ( 'NONE',  ( 5.605114358992040913, 6.317488171369740613, -1.123711807521186490 ) ) ;
#2490=CARTESIAN_POINT ( 'NONE',  ( -8.688077508258798431, 9.030511935923748013, -0.7998128361456291469 ) ) ;
#2491=CARTESIAN_POINT ( 'NONE',  ( 5.982172092127724383, 8.002286745614243912, -1.599625672291262513 ) ) ;
#2494=CARTESIAN_POINT ( 'NONE',  ( 1.364683531249986981, -1.115624999658580752, 0.000000000000000000 ) ) ;
#2496=ORIENTED_EDGE ( 'NONE', *, *, #183589, .T. ) ;
#2500=EDGE_CURVE ( 'NONE', #54417, #1642, #189065, .T. ) ;
#2502=CARTESIAN_POINT ( 'NONE',  ( -6.175902666224832416, 7.163973517805802160, -1.199719254218446718 ) ) ;
#2507=CARTESIAN_POINT ( 'NONE',  ( 8.041957671200231417, 12.53403438304231976, 1.040834085586084257E-14 ) ) ;
#2510=CARTESIAN_POINT ( 'NONE',  ( -2.428882075142555497, 5.985446187641602300, 1.040834085586084257E-14 ) ) ;
#2511=CARTESIAN_POINT ( 'NONE',  ( -8.290974629956718189, 9.631557475493025322, -1.199719254218446718 ) ) ;
#2513=CARTESIAN_POINT ( 'NONE',  ( -4.201283080389795366, 7.561618497949153195, 0.9685097419542560981 ) ) ;
#2514=CARTESIAN_POINT ( 'NONE',  ( -0.6823417656250246877, -0.4489583329919111243, 1.181850606188755259 ) ) ;
#2518=CARTESIAN_POINT ( 'NONE',  ( 9.097157885089661278, 9.715698408800516717, 1.040834085586084257E-14 ) ) ;
#2521=CARTESIAN_POINT ( 'NONE',  ( 4.656335691289526402, 7.519809842224722374, -1.199719254218452047 ) ) ;
#2538=CARTESIAN_POINT ( 'NONE',  ( 4.229780737783593203, 4.037091736943370535, -0.7216878364870188411 ) ) ;
#2542=CARTESIAN_POINT ( 'NONE',  ( -5.274285450916075035, 6.112086766612214284, 1.199719254218450271 ) ) ;
#2543=CARTESIAN_POINT ( 'NONE',  ( -9.006694118179950692, 9.402231314165087284, 1.040834085586084257E-14 ) ) ;
#2548=CARTESIAN_POINT ( 'NONE',  ( -0.7500000000000215383, 1.472916667349486008, 1.299038105676659116 ) ) ;
#2549=CARTESIAN_POINT ( 'NONE',  ( 9.565441069641300587, 11.11843498845840905, -1.199719254218440723 ) ) ;
#2554=CARTESIAN_POINT ( 'NONE',  ( -9.504429378379839477, 11.04725468198666150, 1.199719254218462483 ) ) ;
#2555=CARTESIAN_POINT ( 'NONE',  ( 1.499999999999990896, 5.025000000000022560, 1.214306433183764966E-14 ) ) ;
#2556=CARTESIAN_POINT ( 'NONE',  ( -1.364683531250012516, 2.030208333674750953, 0.7879004041258379498 ) ) ;
#2558=CARTESIAN_POINT ( 'NONE',  ( -5.690973801483992567, 5.856266416790857576, 2.499999999999998668 ) ) ;
#2566=CARTESIAN_POINT ( 'NONE',  ( -3.277320446201389181, 4.846626492033466072, 1.599625672291267398 ) ) ;
#2570=CARTESIAN_POINT ( 'NONE',  ( 1.364683531249988757, 0.6968750003414209138, 0.000000000000000000 ) ) ;
#2577=CARTESIAN_POINT ( 'NONE',  ( 1.364683531249988757, 1.634375000341421691, 0.000000000000000000 ) ) ;
#2579=CARTESIAN_POINT ( 'NONE',  ( -6.575868197828002693, 7.630599971342813426, 1.199719254218450271 ) ) ;
#2580=CARTESIAN_POINT ( 'NONE',  ( 7.079328764629950754, 11.41096732537697633, 0.7998128361456462443 ) ) ;
#2581=CARTESIAN_POINT ( 'NONE',  ( -1.284279953904156280, 2.921639714193936754, 0.7750000000000117906 ) ) ;
#2582=CARTESIAN_POINT ( 'NONE',  ( 4.819033534653518025, 7.709623992816043270, -1.199719254218452047 ) ) ;
#2584=CARTESIAN_POINT ( 'NONE',  ( -0.7500000000000215383, 3.191666666666689967, 1.299038105676671107 ) ) ;
#2586=CARTESIAN_POINT ( 'NONE',  ( -1.364683531250012516, 0.8427083336747532849, 0.7879004041258379498 ) ) ;
#2589=CARTESIAN_POINT ( 'NONE',  ( -3.782361668532609134, 7.356579680022602652, 1.040834085586084257E-14 ) ) ;
#2594=CARTESIAN_POINT ( 'NONE',  ( 5.748293942514166588, 7.729428904398431222, -1.443375672974057666 ) ) ;
#2597=CARTESIAN_POINT ( 'NONE',  ( -8.748035429315585532, 11.22912730566677553, -1.599625672291263179 ) ) ;
#2598=CARTESIAN_POINT ( 'NONE',  ( -2.916975605234527702, 6.554888639415577423, 1.040834085586084257E-14 ) ) ;
#2604=CARTESIAN_POINT ( 'NONE',  ( -6.019457014343129408, 9.966524250134902729, 0.000000000000000000 ) ) ;
#2606=CARTESIAN_POINT ( 'NONE',  ( 0.7499999999999920064, 4.983333333333353821, 1.299038105676669330 ) ) ;
#2609=CARTESIAN_POINT ( 'NONE',  ( 8.934460041725669655, 9.525884258209195821, 1.040834085586084257E-14 ) ) ;
#2614=CARTESIAN_POINT ( 'NONE',  ( -4.217958839219735800, 3.978389137448586244, 0.5316758947214468289 ) ) ;
#2622=CARTESIAN_POINT ( 'NONE',  ( 6.612626235163189925, 8.737816579155630592, -1.599625672291262513 ) ) ;
#2623=CARTESIAN_POINT ( 'NONE',  ( -6.417086777969760902, 6.381022750586497594, 0.7998128361456341429 ) ) ;
#2625=FACE_OUTER_BOUND ( 'NONE', #17021, .T. ) ;
#2627=CARTESIAN_POINT ( 'NONE',  ( 0.6823417656249882723, -0.3447916663252489911, 1.181850606188755259 ) ) ;
#2628=CARTESIAN_POINT ( 'NONE',  ( 2.846849069189655967, 5.304779099821139710, -1.082531754730543083 ) ) ;
#2629=CARTESIAN_POINT ( 'NONE',  ( -2.676845263694313637, 5.210404343363602919, -1.199719254218446718 ) ) ;
#2642=ORIENTED_EDGE ( 'NONE', *, *, #49219, .T. ) ;
#2645=DIRECTION ( 'NONE',  ( -5.578564026256490882E-16, -1.000000000000000000, -9.066213480720158442E-32 ) ) ;
#2646=CARTESIAN_POINT ( 'NONE',  ( 5.282873410819217241, 9.315102745931094219, -0.7998128361456281477 ) ) ;
#2652=CARTESIAN_POINT ( 'NONE',  ( 1.536019160937515116, 8.701056780447510519, 2.509677374737102618 ) ) ;
#2655=DIRECTION ( 'NONE',  ( -7.387867266669436732E-31, -1.000000000000000000, 8.546850786086437571E-32 ) ) ;
#2658=CARTESIAN_POINT ( 'NONE',  ( -4.577849422908604637, 8.492574760035358494, -0.7998128361456281477 ) ) ;
#2659=VECTOR ( 'NONE', #54397, 1000.000000000000000 ) ;
#2661=CARTESIAN_POINT ( 'NONE',  ( -4.253507506385335368, 5.985511395581417204, 1.599625672291267398 ) ) ;
#2671=CARTESIAN_POINT ( 'NONE',  ( -9.002250809794000830, 11.52571191622492464, -1.443375672974059665 ) ) ;
#2675=CARTESIAN_POINT ( 'NONE',  ( 7.447506452608354088, 7.583179037664891098, 0.7998128361456341429 ) ) ;
#2676=CARTESIAN_POINT ( 'NONE',  ( 1.364683531249988535, 4.905208333674756283, -0.7879004041258300672 ) ) ;
#2683=CARTESIAN_POINT ( 'NONE',  ( 5.083944415000174466, 7.914723669933440675, -1.082531754730549078 ) ) ;
#2684=CARTESIAN_POINT ( 'NONE',  ( -6.989391883044787868, 8.113044270762433285, -1.199719254218446718 ) ) ;
#2687=CARTESIAN_POINT ( 'NONE',  ( -7.965578943228732278, 9.251929174310385307, -1.199719254218446718 ) ) ;
#2688=CARTESIAN_POINT ( 'NONE',  ( -3.927058049452637700, 7.733318157670055371, -0.7998128361456281477 ) ) ;
#2696=CARTESIAN_POINT ( 'NONE',  ( 5.940443861082012944, 10.08226827123770697, 0.7998128361456462443 ) ) ;
#2703=CARTESIAN_POINT ( 'NONE',  ( -1.500000000000051514, 3.920833333333356485, 0.8660254037844170583 ) ) ;
#2709=CARTESIAN_POINT ( 'NONE',  ( -1.500000000000011324, 5.629166666666693963, -0.8660254037844313801 ) ) ;
#2710=CARTESIAN_POINT ( 'NONE',  ( 2.361091307074211887, 5.906356958228550447, 0.7998128361456462443 ) ) ;
#2711=CARTESIAN_POINT ( 'NONE',  ( 6.654354466208897811, 6.657835053532175529, 0.7998128361456341429 ) ) ;
#2714=CARTESIAN_POINT ( 'NONE',  ( -6.710922849084449915, 10.77323439066645783, 0.000000000000000000 ) ) ;
#2716=CARTESIAN_POINT ( 'NONE',  ( 5.748293942514166588, 7.729428904398431222, -1.443375672974057666 ) ) ;
#2717=CARTESIAN_POINT ( 'NONE',  ( -9.300530188850304469, 9.952966096521256745, 1.040834085586084257E-14 ) ) ;
#2718=EDGE_CURVE ( 'NONE', #5398, #119510, #136351, .T. ) ;
#2721=CARTESIAN_POINT ( 'NONE',  ( 7.564559641420864899, 10.91273778404466199, -1.199719254218446718 ) ) ;
#2726=CARTESIAN_POINT ( 'NONE',  ( -1.201851678989727383E-14, 4.071875000341425022, 1.575800808251672791 ) ) ;
#2730=B_SPLINE_CURVE_WITH_KNOTS ( 'NONE', 3,
 ( #213653, #83672, #34915, #98882, #85818, #65279, #135648, #200607, #84749, #49067 ),
 .UNSPECIFIED., .F., .F.,
 ( 4, 3, 3, 4 ),
 ( 0.000000000000000000, 4.502046072368915222E-05, 9.004093402560281781E-05, 0.0001800865003231029719 ),
 .UNSPECIFIED. ) ;
#2733=CARTESIAN_POINT ( 'NONE',  ( 8.772289083241844310, 10.19309100432570148, -1.199719254218446718 ) ) ;
#2737=CARTESIAN_POINT ( 'NONE',  ( -8.503988664269602538, 10.94440607977979063, 1.599625672291269396 ) ) ;
#2743=CARTESIAN_POINT ( 'NONE',  ( 9.999301985278609806, 11.62460605670194447, 1.199719254218452047 ) ) ;
#2746=CARTESIAN_POINT ( 'NONE',  ( -7.828943636887387925, 11.22118577875556156, 1.199719254218453823 ) ) ;
#2751=CARTESIAN_POINT ( 'NONE',  ( 5.449628763635895545, 6.258197423388296876, 1.014392677442396806 ) ) ;
#2754=CARTESIAN_POINT ( 'NONE',  ( -4.451154503988200339, 4.087435097607984957, 1.214306433183764966E-14 ) ) ;
#2758=CARTESIAN_POINT ( 'NONE',  ( 7.287671262545424966, 8.461036880179857889, -1.199719254218451159 ) ) ;
#2760=CARTESIAN_POINT ( 'NONE',  ( 7.135668919494039031, 7.219368582364847242, 1.040834085586084257E-14 ) ) ;
#2761=CARTESIAN_POINT ( 'NONE',  ( 4.904298879841284098, 6.744767997946721216, 1.599625672291267398 ) ) ;
#2763=CARTESIAN_POINT ( 'NONE',  ( -7.375272376154081932, 10.58793962461302485, -1.082531754730543971 ) ) ;
#2770=CARTESIAN_POINT ( 'NONE',  ( -4.328009424535094851, 7.229878788426305825, -0.9977569098220413490 ) ) ;
#2771=CARTESIAN_POINT ( 'NONE',  ( -1.364683531250000748, -1.178124999658580752, 0.000000000000000000 ) ) ;
#2774=AXIS2_PLACEMENT_3D ( 'NONE', #61267, #40770, #7156 ) ;
#2775=CARTESIAN_POINT ( 'NONE',  ( 4.636525346193557162, 7.392734756325715750, -1.082531754730549078 ) ) ;
#2784=CARTESIAN_POINT ( 'NONE',  ( -9.666600336419303829, 11.34041714965307968, 1.082531754730558626 ) ) ;
#2792=CARTESIAN_POINT ( 'NONE',  ( -9.788623718942277563, 10.52240854829523187, 1.040834085586084257E-14 ) ) ;
#2799=CARTESIAN_POINT ( 'NONE',  ( -1.201851678989727383E-14, 3.368750000682815049, -1.732050807568863648 ) ) ;
#2801=CARTESIAN_POINT ( 'NONE',  ( -4.706651882238427120, 8.642844295920152575, 1.040834085586084257E-14 ) ) ;
#2804=CARTESIAN_POINT ( 'NONE',  ( -8.320953590485107298, 10.73086516036454618, 1.599625672291269396 ) ) ;
#2808=CARTESIAN_POINT ( 'NONE',  ( 5.937581207780954884, 9.014596278131406848, -1.199719254218440723 ) ) ;
#2812=CARTESIAN_POINT ( 'NONE',  ( 9.585778300061798873, 11.14216175728232550, -1.199719254218440723 ) ) ;
#2815=ADVANCED_FACE ( 'NONE', ( #11520 ), #165360, .T. ) ;
#2819=CARTESIAN_POINT ( 'NONE',  ( -7.537970219518083326, 9.817384560903001045, -1.443375672974059665 ) ) ;
#2822=CARTESIAN_POINT ( 'NONE',  ( -0.6823417656249969321, 5.530208333674756283, -1.181850606188749264 ) ) ;
#2831=CARTESIAN_POINT ( 'NONE',  ( -3.429849674132948500, 5.024577257953626308, -1.443375672974051449 ) ) ;
#2833=CARTESIAN_POINT ( 'NONE',  ( 10.18233705906309972, 11.83814697611718714, 1.199719254218450271 ) ) ;
#2835=CARTESIAN_POINT ( 'NONE',  ( -9.829825065107822724, 11.42688298316931572, 1.199719254218462483 ) ) ;
#2839=CARTESIAN_POINT ( 'NONE',  ( 0.6823417656249882723, 2.426041667008084435, -1.181850606188749264 ) ) ;
#2840=FACE_OUTER_BOUND ( 'NONE', #99831, .T. ) ;
#2841=CARTESIAN_POINT ( 'NONE',  ( 4.955668840994886359, 5.740367388370866131, 1.199719254218462483 ) ) ;
#2850=CARTESIAN_POINT ( 'NONE',  ( -6.805829924380121909, 8.963220883242035697, 1.443375672974078761 ) ) ;
#2855=CARTESIAN_POINT ( 'NONE',  ( -7.700141177557535244, 11.07091624287075859, -1.199719254218446718 ) ) ;
#2856=CARTESIAN_POINT ( 'NONE',  ( -3.863710589770277259, 6.491117540498504646, 1.082531754730560403 ) ) ;
#2857=CARTESIAN_POINT ( 'NONE',  ( 0.6823417656249882723, 1.988541667008083991, -1.181850606188749264 ) ) ;
#2877=CARTESIAN_POINT ( 'NONE',  ( 1.364683531249988535, 3.176041667008084435, 0.7879004041258500513 ) ) ;
#2881=DIRECTION ( 'NONE',  ( 0.7592566023653005702, -0.6507913734559639396, 0.000000000000000000 ) ) ;
#2884=CARTESIAN_POINT ( 'NONE',  ( 9.154780037725547714, 11.70366268214508487, 1.599625672291279388 ) ) ;
#2887=CARTESIAN_POINT ( 'NONE',  ( 1.364683531249988535, 2.363541667008088432, 0.7879004041258500513 ) ) ;
#2895=VERTEX_POINT ( 'NONE', #94937 ) ;
#2897=CARTESIAN_POINT ( 'NONE',  ( 3.330499290451326200, 7.037332938835193730, -0.7998128361456291469 ) ) ;
#2901=CARTESIAN_POINT ( 'NONE',  ( 8.530051201292206287, 13.10347683481629488, 0.000000000000000000 ) ) ;
#2909=CARTESIAN_POINT ( 'NONE',  ( -2.788173145904702555, 6.404619103530779789, -0.7998128361456281477 ) ) ;
#2910=CARTESIAN_POINT ( 'NONE',  ( 8.609591239877852686, 10.00327685373437347, -1.199719254218445830 ) ) ;
#2913=CARTESIAN_POINT ( 'NONE',  ( 4.433153041544209749, 7.155467067568137551, -1.082531754730548412 ) ) ;
#2923=CARTESIAN_POINT ( 'NONE',  ( -5.897433632264490910, 9.824163637709826702, 0.000000000000000000 ) ) ;
#2925=CARTESIAN_POINT ( 'NONE',  ( 3.811813743736467419, 7.598866467667865443, 1.040834085586084257E-14 ) ) ;
#2929=CARTESIAN_POINT ( 'NONE',  ( -8.971744963941075568, 11.49012176272984931, 1.599625672291269396 ) ) ;
#2934=CARTESIAN_POINT ( 'NONE',  ( -4.471491734408701291, 4.111161866431900513, 1.214306433183764966E-14 ) ) ;
#2936=CARTESIAN_POINT ( 'NONE',  ( 9.911173986789782120, 11.52179005846497972, -1.199719254218440723 ) ) ;
#2937=CARTESIAN_POINT ( 'NONE',  ( 2.544126380858701797, 6.119897877643793116, 0.7998128361456462443 ) ) ;
#2939=ORIENTED_EDGE ( 'NONE', *, *, #137004, .T. ) ;
#2943=CARTESIAN_POINT ( 'NONE',  ( 3.633221978782282147, 5.261844946711204507, -1.443375672974057666 ) ) ;
#2946=CARTESIAN_POINT ( 'NONE',  ( -4.069418662396130593, 7.899405539437467816, -0.7998128361456281477 ) ) ;
#2949=CARTESIAN_POINT ( 'NONE',  ( -10.30827686509187835, 10.92074451889568643, 1.040834085586084257E-14 ) ) ;
#2955=CARTESIAN_POINT ( 'NONE',  ( 7.443063144222396232, 11.62739806832741785, 1.040834085586084257E-14 ) ) ;
#2956=CARTESIAN_POINT ( 'NONE',  ( -0.6823417656249969321, 5.280208333674756283, -1.181850606188749264 ) ) ;
#2958=CARTESIAN_POINT ( 'NONE',  ( 5.196852952739813070, 4.957416621151553571, -0.7998128361456221525 ) ) ;
#2960=CARTESIAN_POINT ( 'NONE',  ( 5.854423403002611437, 5.724582146458163656, 1.040834085586084257E-14 ) ) ;
#2962=CARTESIAN_POINT ( 'NONE',  ( -5.876569516519495551, 8.943415971659659292, 1.199719254218452047 ) ) ;
#2974=CARTESIAN_POINT ( 'NONE',  ( -1.364683531250012516, 2.801041667008090652, -0.7879004041258289570 ) ) ;
#2976=CARTESIAN_POINT ( 'NONE',  ( 8.218213668177886788, 12.73966637951625813, 0.7998128361456462443 ) ) ;
#2978=CARTESIAN_POINT ( 'NONE',  ( -4.094199201646926412, 7.720390135322642067, 0.7216878364870317197 ) ) ;
#2980=CARTESIAN_POINT ( 'NONE',  ( -4.243338890952892406, 7.894386439512932618, -0.7216878364870257245 ) ) ;
#2985=EDGE_LOOP ( 'NONE', ( #132684, #96087, #82644, #101049 ) ) ;
#2987=CARTESIAN_POINT ( 'NONE',  ( 5.332434488876471868, 5.115595079977664383, 0.7998128361456341429 ) ) ;
#2996=CARTESIAN_POINT ( 'NONE',  ( 6.602984505055297326, 7.662235663108029726, 1.199719254218462483 ) ) ;
#3000=CARTESIAN_POINT ( 'NONE',  ( -6.413170354464012846, 7.440785820751486312, 1.199719254218450271 ) ) ;
#3004=CARTESIAN_POINT ( 'NONE',  ( 7.019370843573166319, 9.212351955633947043, 1.599625672291281386 ) ) ;
#3006=CARTESIAN_POINT ( 'NONE',  ( -5.331380718671772101, 7.243030143248949670, -1.599625672291256295 ) ) ;
#3007=CARTESIAN_POINT ( 'NONE',  ( 6.927853306458752414, 7.184843067064434763, 0.7216878364870317197 ) ) ;
#3008=CARTESIAN_POINT ( 'NONE',  ( 4.945911955618520928, 6.845357471522081738, 1.424928946000488583 ) ) ;
#3009=CARTESIAN_POINT ( 'NONE',  ( -2.788173145904702555, 6.404619103530779789, -0.7998128361456281477 ) ) ;
#3012=CARTESIAN_POINT ( 'NONE',  ( -4.412288926243578935, 7.235088616337731260, 1.199719254218464037 ) ) ;
#3017=CARTESIAN_POINT ( 'NONE',  ( 1.364683531249986537, 1.905208333674750287, -0.7879004041258239610 ) ) ;
#3019=CARTESIAN_POINT ( 'NONE',  ( -4.256897045010916258, 7.910204285913967404, 0.7216878364870317197 ) ) ;
#3022=ORIENTED_EDGE ( 'NONE', *, *, #119577, .T. ) ;
#3025=CARTESIAN_POINT ( 'NONE',  ( 4.482942347612929979, 8.381849838857084123, 1.040834085586084257E-14 ) ) ;
#3028=CARTESIAN_POINT ( 'NONE',  ( -0.6823417656250003738, 2.530208333674753618, -1.181850606188749264 ) ) ;
#3031=CARTESIAN_POINT ( 'NONE',  ( -1.364683531250000748, -0.9281249996585805295, 0.000000000000000000 ) ) ;
#3035=CARTESIAN_POINT ( 'NONE',  ( -4.295235737431041478, 3.905529869957963029, -0.7998128361456221525 ) ) ;
#3036=CARTESIAN_POINT ( 'NONE',  ( -7.171900071504745178, 9.390302721554109056, -1.443375672974058777 ) ) ;
#3038=CARTESIAN_POINT ( 'NONE',  ( 1.364683531249988535, 3.405208333674749621, -0.7879004041258239610 ) ) ;
#3045=CARTESIAN_POINT ( 'NONE',  ( -8.148087131688699358, 8.608449196499371681, -0.7216878364870267237 ) ) ;
#3050=CARTESIAN_POINT ( 'NONE',  ( -6.846504384776758378, 9.010674420371453053, -1.443375672974058777 ) ) ;
#3062=CARTESIAN_POINT ( 'NONE',  ( -5.259673527097670664, 8.223703984000886535, -1.199719254218446718 ) ) ;
#3064=CARTESIAN_POINT ( 'NONE',  ( -1.500000000000015099, 0.1291666666666918539, -0.8660254037844383745 ) ) ;
#3065=CARTESIAN_POINT ( 'NONE',  ( 4.142179624174931796, 4.791296635414242111, 1.199719254218464037 ) ) ;
#3069=CARTESIAN_POINT ( 'NONE',  ( 6.063521013809720195, 8.097193820909906137, 1.599625672291281386 ) ) ;
#3074=CARTESIAN_POINT ( 'NONE',  ( -4.446711195602252253, 6.210915699667823198, -1.443375672974053447 ) ) ;
#3079=CARTESIAN_POINT ( 'NONE',  ( -0.5167901049056953244, 6.690130572215640115, 3.553507429615057056 ) ) ;
#3080=CARTESIAN_POINT ( 'NONE',  ( 3.194898696050481934, 6.432863918183953089, -0.8190951789856844023 ) ) ;
#3083=CARTESIAN_POINT ( 'NONE',  ( -1.364683531250012516, 2.488541667008088876, -0.7879004041258289570 ) ) ;
#3085=CARTESIAN_POINT ( 'NONE',  ( -8.202846631467911820, 9.528741477256060577, 1.199719254218462483 ) ) ;
#3087=CARTESIAN_POINT ( 'NONE',  ( 6.500244582748090139, 9.671036882259738121, 1.199719254218460707 ) ) ;
#3088=CARTESIAN_POINT ( 'NONE',  ( -7.389357414647957256, 8.579670724299436557, 1.199719254218450271 ) ) ;
#3091=CARTESIAN_POINT ( 'NONE',  ( -1.364683531250010295, 5.738541667008088432, -0.7879004041258300672 ) ) ;
#3094=CARTESIAN_POINT ( 'NONE',  ( 7.782016984564054773, 10.10210578678999482, 1.443375672974076540 ) ) ;
#3097=CARTESIAN_POINT ( 'NONE',  ( -0.6823417656250212460, 0.8635416670080899859, 1.181850606188755259 ) ) ;
#3099=CARTESIAN_POINT ( 'NONE',  ( 6.412643469139427843, 10.42524178073059993, -0.7216878364870267237 ) ) ;
#3102=CARTESIAN_POINT ( 'NONE',  ( -5.910991785878183080, 5.998504626387068051, -0.7216878364870278340 ) ) ;
#3104=CARTESIAN_POINT ( 'NONE',  ( -1.364683531250012516, 3.988541667008088876, -0.7879004041258300672 ) ) ;
#3108=CARTESIAN_POINT ( 'NONE',  ( -5.371001409308059138, 9.417918744168066070, -0.7998128361456231517 ) ) ;
#3109=CARTESIAN_POINT ( 'NONE',  ( -0.6823417656249969321, 5.780208333674756283, -1.181850606188749264 ) ) ;
#3117=CARTESIAN_POINT ( 'NONE',  ( 6.259060471003163428, 10.45398764947904624, -0.7998128361456291469 ) ) ;
#3120=CARTESIAN_POINT ( 'NONE',  ( -1.500000000000013101, 3.129166666666689967, -0.8660254037844313801 ) ) ;
#3126=VERTEX_POINT ( 'NONE', #76233 ) ;
#3127=CARTESIAN_POINT ( 'NONE',  ( 5.016153647376196290, 8.796003655340152605, 0.7216878364870438212 ) ) ;
#3128=CARTESIAN_POINT ( 'NONE',  ( -1.402160292154681736E-14, -0.3656249996585805295, 1.575800808251672791 ) ) ;
#3130=CARTESIAN_POINT ( 'NONE',  ( 3.837121167867449945, 4.435395103055503441, 1.199719254218464037 ) ) ;
#3136=CARTESIAN_POINT ( 'NONE',  ( 1.499999999999987121, 0.7541666666666868579, 0.8660254037844524744 ) ) ;
#3137=CARTESIAN_POINT ( 'NONE',  ( 6.076025397218672630, 10.24044673006381245, -0.7998128361456291469 ) ) ;
#3138=CARTESIAN_POINT ( 'NONE',  ( -9.124801077197171040, 10.60435499727357289, -1.199719254218441611 ) ) ;
#3141=CARTESIAN_POINT ( 'NONE',  ( 0.6823417656249899377, 1.342708333674752508, 1.181850606188755259 ) ) ;
#3143=CARTESIAN_POINT ( 'NONE',  ( -0.7500000000000215383, 1.691666666666688634, 1.299038105676659116 ) ) ;
#3145=CARTESIAN_POINT ( 'NONE',  ( 5.009901455449552010, 5.803638771901306725, -1.199719254218452047 ) ) ;
#3151=CARTESIAN_POINT ( 'NONE',  ( 0.7499999999999885647, -0.9854166659838472508, 1.299038105676657340 ) ) ;
#3152=CARTESIAN_POINT ( 'NONE',  ( -8.532158741701643123, 8.848606708273724308, 0.7998128361456462443 ) ) ;
#3153=CARTESIAN_POINT ( 'NONE',  ( -5.965224400332865606, 7.022145224218852455, 1.082531754730549967 ) ) ;
#3161=CARTESIAN_POINT ( 'NONE',  ( 6.414979237560321401, 10.63589287712906462, 1.040834085586084257E-14 ) ) ;
#3165=CARTESIAN_POINT ( 'NONE',  ( 7.429504990164394584, 7.770103364721017591, 1.040834085586084257E-14 ) ) ;
#3169=CARTESIAN_POINT ( 'NONE',  ( -7.157815033010924921, 10.43820240756634199, 1.199719254218453823 ) ) ;
#3170=CARTESIAN_POINT ( 'NONE',  ( 5.738125327081736060, 7.717565519727259904, 1.599625672291267398 ) ) ;
#3173=CARTESIAN_POINT ( 'NONE',  ( 4.088303131848604721, 7.475188365022519932, -0.6044521916458069910 ) ) ;
#3174=CARTESIAN_POINT ( 'NONE',  ( 2.333974999846879061, 5.874721266463329705, -0.7998128361456291469 ) ) ;
#3182=CARTESIAN_POINT ( 'NONE',  ( -4.446711195602252253, 6.210915699667823198, -1.443375672974053447 ) ) ;
#3183=CARTESIAN_POINT ( 'NONE',  ( 8.812436659202669276, 10.34389285956704363, -1.082531754730543083 ) ) ;
#3186=CARTESIAN_POINT ( 'NONE',  ( -5.687809136132860210, 6.594531066031826150, -1.199719254218446718 ) ) ;
#3192=CARTESIAN_POINT ( 'NONE',  ( -6.170932472514347289, 10.35117165124207972, 0.000000000000000000 ) ) ;
#3196=( BOUNDED_CURVE ( )  B_SPLINE_CURVE ( 2, ( #79841, #46301, #211960, #66750, #180542, #83028, #683 ),
 .UNSPECIFIED., .F., .T. ) 
 B_SPLINE_CURVE_WITH_KNOTS ( ( 3, 2, 2, 3 ),
 ( 0.3602265381971914149, 0.3630952380952380820, 0.3690476190476190688, 0.3719163189456657359 ),
 .UNSPECIFIED. ) 
 CURVE ( )  GEOMETRIC_REPRESENTATION_ITEM ( )  RATIONAL_B_SPLINE_CURVE ( ( 0.9331000818465633451, 0.9354320710352566071, 1.000000000000000000, 0.8660254037844387076, 1.000000000000000000, 0.9354320710352564960, 0.9331000818465632340 ) ) 
 REPRESENTATION_ITEM ( '' )  );
#3199=ORIENTED_EDGE ( 'NONE', *, *, #79298, .T. ) ;
#3209=CARTESIAN_POINT ( 'NONE',  ( -7.705111371268023923, 7.883718109434487253, 1.040834085586084257E-14 ) ) ;
#3213=CARTESIAN_POINT ( 'NONE',  ( 5.178851490740207453, 5.144340948726102702, 0.7216878364870317197 ) ) ;
#3219=CARTESIAN_POINT ( 'NONE',  ( -5.610376637956639101, 5.439860920571172542, 0.000000000000000000 ) ) ;
#3223=CARTESIAN_POINT ( 'NONE',  ( 8.543609354905870035, 13.11929468069890525, 0.7998128361456462443 ) ) ;
#3228=CARTESIAN_POINT ( 'NONE',  ( -7.669108446824431269, 12.09904362127053545, -0.7998128361456291469 ) ) ;
#3229=CARTESIAN_POINT ( 'NONE',  ( 5.750629710490689384, 9.860818428881154674, -0.7998128361456291469 ) ) ;
#3234=CARTESIAN_POINT ( 'NONE',  ( -9.215791728987058562, 11.77484298861683598, -1.599625672291263179 ) ) ;
#3237=CARTESIAN_POINT ( 'NONE',  ( 1.364683531249986537, -0.3239583329919163424, 0.7879004041258500513 ) ) ;
#3239=ORIENTED_EDGE ( 'NONE', *, *, #70073, .T. ) ;
#3241=CARTESIAN_POINT ( 'NONE',  ( 7.429504990608736037, 11.61158022244479682, -0.7216878364870267237 ) ) ;
#3247=CARTESIAN_POINT ( 'NONE',  ( -0.3380113051594444973, 6.991913160484415357, -3.863100633853273624 ) ) ;
#3267=CARTESIAN_POINT ( 'NONE',  ( -1.500000000000001332, -0.5687499993171779566, 0.000000000000000000 ) ) ;
#3271=CARTESIAN_POINT ( 'NONE',  ( 9.836604141914616406, 11.43479190611061647, 1.199719254218452047 ) ) ;
#3276=CARTESIAN_POINT ( 'NONE',  ( 9.836604141914616406, 11.43479190611061647, 1.199719254218452047 ) ) ;
#3281=CARTESIAN_POINT ( 'NONE',  ( 5.118366684358879759, 5.930181538962194132, 1.199719254218462483 ) ) ;
#3282=CARTESIAN_POINT ( 'NONE',  ( -1.364683531249997417, 2.821875000341422801, 1.214306433183764966E-14 ) ) ;
#3284=CARTESIAN_POINT ( 'NONE',  ( -5.877243123607416742, 6.020912620514094371, 0.3151507616369741416 ) ) ;
#3285=CARTESIAN_POINT ( 'NONE',  ( 8.353795204314554468, 12.89784483834236184, -0.7998128361456352531 ) ) ;
#3287=CARTESIAN_POINT ( 'NONE',  ( -8.453672473320708036, 9.821371626084353323, -1.199719254218446718 ) ) ;
#3288=CARTESIAN_POINT ( 'NONE',  ( -3.429849674132936066, 6.945315686556313040, -0.7216878364870257245 ) ) ;
#3291=CARTESIAN_POINT ( 'NONE',  ( -6.728924311084075960, 6.744833205886536120, 1.040834085586084257E-14 ) ) ;
#3293=CARTESIAN_POINT ( 'NONE',  ( -1.402160292154681736E-14, 0.6187500006828180465, -1.732050807568863648 ) ) ;
#3300=CARTESIAN_POINT ( 'NONE',  ( -5.572037945092175981, 5.603058478803387032, 0.7216878364870317197 ) ) ;
#3302=CARTESIAN_POINT ( 'NONE',  ( 4.034853869772982549, 7.546986718285443985, 0.4065704115671017749 ) ) ;
#3306=CARTESIAN_POINT ( 'NONE',  ( -5.070386261386537363, 5.017798181146802428, 1.214306433183764966E-14 ) ) ;
#3307=CARTESIAN_POINT ( 'NONE',  ( 8.235688245297327015, 11.69572115523387268, -1.199719254218446718 ) ) ;
#3317=CARTESIAN_POINT ( 'NONE',  ( -8.286004436246233951, 12.81875560892930466, 1.040834085586084257E-14 ) ) ;
#3322=CARTESIAN_POINT ( 'NONE',  ( 6.505214776458575265, 6.483838748823460563, 1.040834085586084257E-14 ) ) ;
#3325=ORIENTED_EDGE ( 'NONE', *, *, #12700, .F. ) ;
#3326=ORIENTED_EDGE ( 'NONE', *, *, #166535, .F. ) ;
#3328=CARTESIAN_POINT ( 'NONE',  ( 4.729096653068339151, 4.411700938201493116, -0.7998128361456211532 ) ) ;
#3330=VERTEX_POINT ( 'NONE', #125077 ) ;
#3334=CARTESIAN_POINT ( 'NONE',  ( -2.064209525776537379, 8.524375063532971808, 2.459883114193454734 ) ) ;
#3339=CARTESIAN_POINT ( 'NONE',  ( 6.923409998072794558, 11.22906209772695618, 1.040834085586084257E-14 ) ) ;
#3342=CARTESIAN_POINT ( 'NONE',  ( -5.436983294280064882, 6.301900917203534291, 1.199719254218450271 ) ) ;
#3348=CARTESIAN_POINT ( 'NONE',  ( -1.500000000000015099, -0.8395833326505166561, -0.8660254037844383745 ) ) ;
#3351=ORIENTED_EDGE ( 'NONE', *, *, #39947, .F. ) ;
#3352=CARTESIAN_POINT ( 'NONE',  ( -3.946537740505278613, 2.817530495244580102, 0.7750000000000135669 ) ) ;
#3353=CARTESIAN_POINT ( 'NONE',  ( 3.517450787741589036, 6.191110788085444128, -1.199719254218446718 ) ) ;
#3354=CARTESIAN_POINT ( 'NONE',  ( -5.284980951228653190, 5.060232619388524533, 0.000000000000000000 ) ) ;
#3359=ADVANCED_FACE ( 'NONE', ( #193180 ), #42332, .T. ) ;
#3361=CARTESIAN_POINT ( 'NONE',  ( 4.663641653420880218, 8.384739662392275861, -0.7216878364870207285 ) ) ;
#3364=CARTESIAN_POINT ( 'NONE',  ( 7.036318535368067728, 10.19249347702934294, -1.082531754730537976 ) ) ;
#3365=CARTESIAN_POINT ( 'NONE',  ( 1.364683531249990311, 4.946875000341417916, 1.214306433183764966E-14 ) ) ;
#3367=CARTESIAN_POINT ( 'NONE',  ( 5.138177029454847222, 6.057256624861201644, 1.082531754730560403 ) ) ;
#3372=CARTESIAN_POINT ( 'NONE',  ( 5.299301323368958094, 6.361497809228795930, -1.122821758042211959 ) ) ;
#3375=CARTESIAN_POINT ( 'NONE',  ( -4.797329538616279976, 6.965272035667838146, 1.434408638962878957 ) ) ;
#3378=CARTESIAN_POINT ( 'NONE',  ( 1.364683531249988535, 5.467708333674750953, -0.7879004041258300672 ) ) ;
#3382=CARTESIAN_POINT ( 'NONE',  ( -10.01677656239806247, 10.58066083241955901, 0.7998128361456462443 ) ) ;
#3392=CARTESIAN_POINT ( 'NONE',  ( 4.690757960648234359, 4.574898496952131133, 0.7216878364870317197 ) ) ;
#3394=CARTESIAN_POINT ( 'NONE',  ( 0.6823417656249899377, 4.988541667008086655, -1.181850606188754593 ) ) ;
#3396=CARTESIAN_POINT ( 'NONE',  ( 6.479907352327590964, 9.647310113435821677, 1.199719254218462483 ) ) ;
#3397=CARTESIAN_POINT ( 'NONE',  ( -10.31505594189871111, 10.92865344183699428, -0.7998128361456291469 ) ) ;
#3398=CYLINDRICAL_SURFACE ( 'NONE', #154398, 1.500000000000000222 ) ;
#3401=ORIENTED_EDGE ( 'NONE', *, *, #139587, .T. ) ;
#3403=CARTESIAN_POINT ( 'NONE',  ( 1.499999999999990896, 5.025000000000022560, 1.214306433183764966E-14 ) ) ;
#3404=CARTESIAN_POINT ( 'NONE',  ( 5.684946482831785275, 5.526859072925533134, -0.7998128361456231517 ) ) ;
#3407=EDGE_CURVE ( 'NONE', #7144, #39666, #210193, .T. ) ;
#3412=CARTESIAN_POINT ( 'NONE',  ( 7.293923454472077239, 10.49303254931736262, 1.082531754730558626 ) ) ;
#3417=CARTESIAN_POINT ( 'NONE',  ( 1.499999999999989120, 3.035416667349485564, 0.8660254037844524744 ) ) ;
#3419=CARTESIAN_POINT ( 'NONE',  ( -4.554649539187067830, 7.401175998105142817, 1.199719254218464037 ) ) ;
#3420=CARTESIAN_POINT ( 'NONE',  ( 4.541618270453549044, 5.361271406026338227, -1.082531754730548412 ) ) ;
#3421=DIRECTION ( 'NONE',  ( 0.8079921913844798631, -2.168404344971001295E-14, -0.5891931929865669160 ) ) ;
#3429=CARTESIAN_POINT ( 'NONE',  ( 5.933664784275179294, 10.07435934829639912, -0.7998128361456291469 ) ) ;
#3430=CARTESIAN_POINT ( 'NONE',  ( 4.578903193113299963, 6.365139696764064325, 1.599625672291267398 ) ) ;
#3431=CARTESIAN_POINT ( 'NONE',  ( -3.094265954482842140, 2.800000000000024691, -2.490342512183689294 ) ) ;
#3434=CARTESIAN_POINT ( 'NONE',  ( 4.517891501851804215, 6.293959390292322986, -1.599625672291255185 ) ) ;
#3436=ORIENTED_EDGE ( 'NONE', *, *, #120152, .T. ) ;
#3444=DIRECTION ( 'NONE',  ( -1.000000000000000000, 4.984021416236792516E-16, 0.000000000000000000 ) ) ;
#3445=CARTESIAN_POINT ( 'NONE',  ( 5.808322585208748556, 6.028124808163927817, -0.4837759047566763670 ) ) ;
#3447=CARTESIAN_POINT ( 'NONE',  ( 10.37606763316019531, 10.99983374830873650, 0.7998128361456462443 ) ) ;
#3453=CARTESIAN_POINT ( 'NONE',  ( 5.490689023854504747, 9.349628261231513804, 1.040834085586084257E-14 ) ) ;
#3454=CARTESIAN_POINT ( 'NONE',  ( -2.819205876637805641, 5.376491725131008259, -1.199719254218446718 ) ) ;
#3459=CARTESIAN_POINT ( 'NONE',  ( -4.822949958159302497, 6.649860922651058992, -1.599625672291256295 ) ) ;
#3465=B_SPLINE_CURVE_WITH_KNOTS ( 'NONE', 3,
 ( #152853, #149657, #133439, #18570, #199446, #35891, #54290, #84648, #20692, #202640, #150737, #134505, #101968, #4430, #2297, #68374, #151797, #3372 ),
 .UNSPECIFIED., .F., .F.,
 ( 4, 2, 2, 2, 2, 2, 2, 2, 4 ),
 ( 0.7195170131146431114, 0.7275020556221073464, 0.7354870981295715815, 0.7434721406370357055, 0.7514571831444999406, 0.7594422256519641756, 0.7674272681594282997, 0.7754123106668925347, 0.7833973531743566587 ),
 .UNSPECIFIED. ) ;
#3470=CARTESIAN_POINT ( 'NONE',  ( 8.748035429315576650, 11.22912730566677553, -1.599625672291255185 ) ) ;
#3471=CARTESIAN_POINT ( 'NONE',  ( 5.971451247601332391, 6.106144735068791185, -0.6754856502540294017 ) ) ;
#3478=CARTESIAN_POINT ( 'NONE',  ( -8.026063749610043985, 12.30756544127966912, -0.7216878364870267237 ) ) ;
#3480=CARTESIAN_POINT ( 'NONE',  ( 3.511198596259284876, 6.271927390929313617, -1.052294140492317842 ) ) ;
#3482=CARTESIAN_POINT ( 'NONE',  ( 8.599949509769960088, 8.927695937686774386, 1.040834085586084257E-14 ) ) ;
#3486=CARTESIAN_POINT ( 'NONE',  ( -6.911959384868566758, 6.958374125301778790, 1.040834085586084257E-14 ) ) ;
#3490=CARTESIAN_POINT ( 'NONE',  ( 8.218213668177886788, 12.73966637951625813, 0.7998128361456462443 ) ) ;
#3494=CARTESIAN_POINT ( 'NONE',  ( 4.021084497595363239, 7.798870403269500429, 0.3307836955792880507 ) ) ;
#3496=CARTESIAN_POINT ( 'NONE',  ( 5.666945020832177882, 6.674152614801420746, 1.082531754730558626 ) ) ;
#3504=CARTESIAN_POINT ( 'NONE',  ( 9.070041577417981671, 9.684062716516882219, -0.7216878364870197293 ) ) ;
#3507=CARTESIAN_POINT ( 'NONE',  ( -9.013473194986783454, 9.410140237106395134, -0.7998128361456291469 ) ) ;
#3509=CARTESIAN_POINT ( 'NONE',  ( 1.419999999999989049, 6.280000000000042881, -2.873333333333328632 ) ) ;
#3516=CARTESIAN_POINT ( 'NONE',  ( 4.241003122976366058, 3.842258486427521103, -0.7998128361456211532 ) ) ;
#3519=CARTESIAN_POINT ( 'NONE',  ( 4.955668840994886359, 5.740367388370866131, 1.199719254218462483 ) ) ;
#3522=CARTESIAN_POINT ( 'NONE',  ( 1.499999999999989120, 4.285416667349482900, 0.8660254037844524744 ) ) ;
#3528=CARTESIAN_POINT ( 'NONE',  ( 0.7499999999999885647, 1.816666666666688634, -1.299038105676652899 ) ) ;
#3529=CARTESIAN_POINT ( 'NONE',  ( 6.531277313481192337, 8.642909503859968368, 1.599625672291281386 ) ) ;
#3530=CARTESIAN_POINT ( 'NONE',  ( 4.867013957181530515, 5.740899707208986236, -1.082531754730548412 ) ) ;
#3536=CARTESIAN_POINT ( 'NONE',  ( 8.270110514656026979, 10.67154823856396817, 1.443375672974076540 ) ) ;
#3544=CARTESIAN_POINT ( 'NONE',  ( -4.218558352146454915, 8.073401844146177453, 1.040834085586084257E-14 ) ) ;
#3546=CARTESIAN_POINT ( 'NONE',  ( 1.499999999999987121, 3.577083334016152527, -0.8660254037844262731 ) ) ;
#3547=CARTESIAN_POINT ( 'NONE',  ( 0.6823417656249899377, 5.738541667008087543, -1.181850606188754593 ) ) ;
#3552=CARTESIAN_POINT ( 'NONE',  ( 1.364683531249990311, 3.946875000341417028, 1.214306433183764966E-14 ) ) ;
#3555=DIRECTION ( 'NONE',  ( -5.578564026256490882E-16, -1.000000000000000000, -9.066213480720158442E-32 ) ) ;
#3559=CARTESIAN_POINT ( 'NONE',  ( -9.027031348600448979, 9.425958082989001952, 1.040834085586084257E-14 ) ) ;
#3560=CARTESIAN_POINT ( 'NONE',  ( 5.632522751473472589, 8.658694745772667289, -1.199719254218440723 ) ) ;
#3562=CARTESIAN_POINT ( 'NONE',  ( -1.602468905319636405E-14, -1.053124999658583638, -1.575800808251665908 ) ) ;
#3567=CARTESIAN_POINT ( 'NONE',  ( -4.720210035852093533, 8.658662141802762946, -0.7998128361456281477 ) ) ;
#3570=CARTESIAN_POINT ( 'NONE',  ( 10.24048609702354717, 10.84165528948263457, -0.7998128361456281477 ) ) ;
#3573=CARTESIAN_POINT ( 'NONE',  ( 7.567422294721922960, 11.98040977715095323, 0.7998128361456462443 ) ) ;
#3575=CARTESIAN_POINT ( 'NONE',  ( -3.928111819657352566, 5.605883094398769195, 1.599625672291267398 ) ) ;
#3576=CARTESIAN_POINT ( 'NONE',  ( -6.184490626128011925, 10.36698949712469364, -0.7998128361456291469 ) ) ;
#3579=CARTESIAN_POINT ( 'NONE',  ( -4.031038109533945146, 7.773819255970239261, -0.5157005294549130703 ) ) ;
#3584=CARTESIAN_POINT ( 'NONE',  ( 8.446366511633696561, 8.956441806435218922, 1.040834085586084257E-14 ) ) ;
#3600=ORIENTED_EDGE ( 'NONE', *, *, #25641, .F. ) ;
#3613=CARTESIAN_POINT ( 'NONE',  ( -0.7500000000000006661, 2.139583334016155636, -1.299038105676652011 ) ) ;
#3614=CARTESIAN_POINT ( 'NONE',  ( 8.204655514564224816, 12.72384853363364066, 1.040834085586084257E-14 ) ) ;
#3618=CARTESIAN_POINT ( 'NONE',  ( -8.306341666666730461, 12.84248237775322643, 1.040834085586084257E-14 ) ) ;
#3620=CARTESIAN_POINT ( 'NONE',  ( 1.364683531249986537, 1.655208333674748955, -0.7879004041258239610 ) ) ;
#3627=CARTESIAN_POINT ( 'NONE',  ( -9.490344339885973923, 12.09515436799890331, -1.443375672974059665 ) ) ;
#3632=CARTESIAN_POINT ( 'NONE',  ( 1.364683531249986537, 0.4677083336747514530, -0.7879004041258309554 ) ) ;
#3637=CARTESIAN_POINT ( 'NONE',  ( -1.201851678989727383E-14, 1.071875000341418138, 1.575800808251672791 ) ) ;
#3639=CARTESIAN_POINT ( 'NONE',  ( -6.093499974338126179, 9.196501505781426999, -1.199719254218440723 ) ) ;
#3640=CARTESIAN_POINT ( 'NONE',  ( 6.726816770674637347, 10.99970333242910669, -0.7998128361456291469 ) ) ;
#3641=CARTESIAN_POINT ( 'NONE',  ( 5.366329872910639232, 5.155139694684188534, 1.040834085586084257E-14 ) ) ;
#3642=CARTESIAN_POINT ( 'NONE',  ( 6.003563092752934871, 5.898578451166879510, 0.7998128361456341429 ) ) ;
#3644=CARTESIAN_POINT ( 'NONE',  ( 0.7499999999999920064, 4.233333333333352932, 1.299038105676669330 ) ) ;
#3646=CARTESIAN_POINT ( 'NONE',  ( 0.6823417656249882723, 1.988541667008083991, -1.181850606188749264 ) ) ;
#3649=EDGE_CURVE ( 'NONE', #171443, #25476, #165651, .T. ) ;
#3653=CARTESIAN_POINT ( 'NONE',  ( 6.507550544879468823, 6.694489845221929691, -0.7216878364870257245 ) ) ;
#3656=CARTESIAN_POINT ( 'NONE',  ( -7.316596452869116973, 11.68777962832266049, 0.7998128361456481317 ) ) ;
#3657=CARTESIAN_POINT ( 'NONE',  ( -5.603597561149804562, 5.431951997629870910, 0.7998128361456341429 ) ) ;
#3662=CARTESIAN_POINT ( 'NONE',  ( -7.578644679914719795, 9.864838098032418401, 1.443375672974090751 ) ) ;
#3664=CARTESIAN_POINT ( 'NONE',  ( 1.499999999999990896, 5.275000000000022560, 1.214306433183764966E-14 ) ) ;
#3667=CARTESIAN_POINT ( 'NONE',  ( 9.110716038703335684, 9.731516254683127087, -0.7216878364870197293 ) ) ;
#3682=CARTESIAN_POINT ( 'NONE',  ( 8.148087131688683371, 10.52918762510205042, -1.443375672974063439 ) ) ;
#3683=CARTESIAN_POINT ( 'NONE',  ( 7.949158136313996259, 8.168439335321471262, 1.040834085586084257E-14 ) ) ;
#3684=CARTESIAN_POINT ( 'NONE',  ( -4.205000198532790279, 8.057583998263570635, 0.7998128361456341429 ) ) ;
#3687=CARTESIAN_POINT ( 'NONE',  ( 5.572037945092146671, 8.484166121707415797, -1.082531754730543971 ) ) ;
#3688=CARTESIAN_POINT ( 'NONE',  ( 1.364683531249986537, -0.5322916663252452718, -0.7879004041258309554 ) ) ;
#3689=CARTESIAN_POINT ( 'NONE',  ( 2.901081683644319842, 5.368050483351580304, 1.082531754730548412 ) ) ;
#3691=CARTESIAN_POINT ( 'NONE',  ( -10.63367255181986160, 11.30037282007833532, 1.040834085586084257E-14 ) ) ;
#3706=CARTESIAN_POINT ( 'NONE',  ( 8.145751363712157911, 8.397798100619326078, -0.7998128361456281477 ) ) ;
#3709=ORIENTED_EDGE ( 'NONE', *, *, #84508, .T. ) ;
#3718=CARTESIAN_POINT ( 'NONE',  ( -5.331380718671772101, 7.243030143248949670, -1.599625672291256295 ) ) ;
#3719=CIRCLE ( 'NONE', #173397, 1.500000000000000222 ) ;
#3721=CARTESIAN_POINT ( 'NONE',  ( -4.334856428067329404, 6.080418470877079429, -1.599625672291256295 ) ) ;
#3731=CARTESIAN_POINT ( 'NONE',  ( -3.090368948911150770, 5.692848642783215674, 1.199719254218462483 ) ) ;
#3734=CARTESIAN_POINT ( 'NONE',  ( 5.937581207780954884, 9.014596278131406848, -1.199719254218440723 ) ) ;
#3735=CARTESIAN_POINT ( 'NONE',  ( 0.6823417656249899377, 4.926041667008086655, -1.181850606188754593 ) ) ;
#3741=CARTESIAN_POINT ( 'NONE',  ( 4.812781342726850653, 8.558735966582574406, 0.7216878364870438212 ) ) ;
#3742=CARTESIAN_POINT ( 'NONE',  ( -5.696397096036042385, 9.797547045350714967, -0.7998128361456231517 ) ) ;
#3745=CARTESIAN_POINT ( 'NONE',  ( -8.681298431451969222, 9.022603012982438386, 1.040834085586084257E-14 ) ) ;
#3746=CARTESIAN_POINT ( 'NONE',  ( -4.900382456335551140, 7.804531068111707270, 1.199719254218464037 ) ) ;
#3748=B_SPLINE_CURVE_WITH_KNOTS ( 'NONE', 3,
 ( #3480, #53326, #137797, #55461 ),
 .UNSPECIFIED., .F., .F.,
 ( 4, 4 ),
 ( 0.000000000000000000, 0.0007855215049759376551 ),
 .UNSPECIFIED. ) ;
#3754=CARTESIAN_POINT ( 'NONE',  ( 8.260995669428309540, 8.532249790621511565, 0.7998128361456481317 ) ) ;
#3767=CARTESIAN_POINT ( 'NONE',  ( -1.500000000000011324, 5.420833333333356485, 0.8660254037844403729 ) ) ;
#3768=CARTESIAN_POINT ( 'NONE',  ( 4.681643115420508039, 4.356338477612361260, 0.7998128361456341429 ) ) ;
#3769=CARTESIAN_POINT ( 'NONE',  ( 4.482942347612929979, 8.381849838857084123, 1.040834085586084257E-14 ) ) ;
#3772=CARTESIAN_POINT ( 'NONE',  ( -7.782016984564068096, 10.10210578678999482, 1.443375672974090751 ) ) ;
#3773=CARTESIAN_POINT ( 'NONE',  ( 5.666945020832170776, 7.634521829102760115, 1.443375672974062551 ) ) ;
#3775=CARTESIAN_POINT ( 'NONE',  ( -8.148087131688692253, 9.568818410800712826, -1.082531754730543083 ) ) ;
#3779=CARTESIAN_POINT ( 'NONE',  ( 6.753933077901968396, 11.03133902419432566, 0.7998128361456462443 ) ) ;
#3784=CARTESIAN_POINT ( 'NONE',  ( 1.364683531249988535, 2.863541667008082658, 0.7879004041258500513 ) ) ;
#3790=CARTESIAN_POINT ( 'NONE',  ( 8.880754312151170282, 10.31963377138658089, 1.199719254218453823 ) ) ;
#3795=CARTESIAN_POINT ( 'NONE',  ( -7.991641480251377772, 11.41099992934688956, 1.199719254218453823 ) ) ;
#3799=CARTESIAN_POINT ( 'NONE',  ( 1.500000000000001332, 4.285416667349482900, 0.8660254037844450359 ) ) ;
#3801=CARTESIAN_POINT ( 'NONE',  ( 8.516493047678546091, 13.08765898893368629, -0.7998128361456352531 ) ) ;
#3804=CARTESIAN_POINT ( 'NONE',  ( -10.17947440576205054, 10.77047498301088346, 0.7998128361456462443 ) ) ;
#3810=CARTESIAN_POINT ( 'NONE',  ( 5.740253418993177981, 6.070215967746060315, 0.6401420356763661834 ) ) ;
#3812=CARTESIAN_POINT ( 'NONE',  ( -10.48008955368359629, 11.32911868882677986, 1.040834085586084257E-14 ) ) ;
#3817=CARTESIAN_POINT ( 'NONE',  ( 6.642605195691581699, 9.837124264027149678, 1.199719254218462483 ) ) ;
#3819=CARTESIAN_POINT ( 'NONE',  ( 5.425234023762710578, 9.481190127698507553, -0.7998128361456291469 ) ) ;
#3820=CARTESIAN_POINT ( 'NONE',  ( 5.847644326195776010, 5.716673223516856694, -0.7998128361456281477 ) ) ;
#3822=CARTESIAN_POINT ( 'NONE',  ( -8.514157279702033065, 9.995900250149611921, -1.082531754730543971 ) ) ;
#3830=CARTESIAN_POINT ( 'NONE',  ( -4.397708481796120950, 7.154691356138512148, -1.067048916732843411 ) ) ;
#3833=CARTESIAN_POINT ( 'NONE',  ( 5.585596099150174965, 7.539614753807099667, -1.443375672974057666 ) ) ;
#3835=AXIS2_PLACEMENT_3D ( 'NONE', #173719, #205098, #39419 ) ;
#3851=CARTESIAN_POINT ( 'NONE',  ( -8.473482818416657736, 12.82955435488738516, -0.7216878364870267237 ) ) ;
#3856=CARTESIAN_POINT ( 'NONE',  ( 6.825640269476072497, 10.05066518344239412, 1.199719254218460707 ) ) ;
#3860=CARTESIAN_POINT ( 'NONE',  ( -0.7500000000000006661, 2.139583334016155636, -1.299038105676652011 ) ) ;
#3862=CARTESIAN_POINT ( 'NONE',  ( -4.855791571988752331, 8.816840600628864877, 0.7998128361456481317 ) ) ;
#3865=CARTESIAN_POINT ( 'NONE',  ( -9.155833807930273238, 9.576227618873799585, -0.7998128361456291469 ) ) ;
#3866=CARTESIAN_POINT ( 'NONE',  ( -3.307826292054345974, 6.802955074131202373, -0.7216878364870574769 ) ) ;
#3869=CARTESIAN_POINT ( 'NONE',  ( 5.289652487626049115, 9.323011668872403845, 0.7998128361456462443 ) ) ;
#3871=CARTESIAN_POINT ( 'NONE',  ( -5.391338639728555648, 9.441645512991978961, -0.7998128361456231517 ) ) ;
#3873=CARTESIAN_POINT ( 'NONE',  ( 9.531545685607134999, 11.07889037375188401, 1.199719254218450271 ) ) ;
#3874=CARTESIAN_POINT ( 'NONE',  ( 0.6823417656249899377, 5.676041667008087543, -1.181850606188754593 ) ) ;
#3875=CARTESIAN_POINT ( 'NONE',  ( -5.914749137557818059, 6.074338953224275528, -0.6118981238392419142 ) ) ;
#3883=CARTESIAN_POINT ( 'NONE',  ( -6.995644074971465010, 10.14503993989993091, 1.082531754730549967 ) ) ;
#3886=CARTESIAN_POINT ( 'NONE',  ( 1.364683531249990311, 4.676041667008083103, 0.7879004041258500513 ) ) ;
#3891=CARTESIAN_POINT ( 'NONE',  ( -1.001543065824772872E-14, 5.321875000341422357, 1.575800808251672791 ) ) ;
#3893=CARTESIAN_POINT ( 'NONE',  ( -4.297571505407598025, 5.076550180139354218, 1.082531754730558626 ) ) ;
#3895=CARTESIAN_POINT ( 'NONE',  ( 8.224992744984721327, 12.74757530245756243, 1.040834085586084257E-14 ) ) ;
#3896=CARTESIAN_POINT ( 'NONE',  ( -0.6823417656249969321, 5.780208333674756283, -1.181850606188749264 ) ) ;
#3897=CARTESIAN_POINT ( 'NONE',  ( -8.469039510030723861, 13.03229652834454733, 1.040834085586084257E-14 ) ) ;
#3899=CARTESIAN_POINT ( 'NONE',  ( 1.220000000000002194, 5.900000000000022560, 1.214306433183764966E-14 ) ) ;
#3901=ADVANCED_FACE ( 'NONE', ( #93117 ), #122745, .T. ) ;
#3902=CARTESIAN_POINT ( 'NONE',  ( -0.6823417656250212460, 2.051041667008083991, 1.181850606188767472 ) ) ;
#3903=CARTESIAN_POINT ( 'NONE',  ( -4.460269349215930212, 4.305995116947750390, 1.214306433183764966E-14 ) ) ;
#3904=CARTESIAN_POINT ( 'NONE',  ( 5.671388329218120639, 5.511041227042920099, 1.040834085586084257E-14 ) ) ;
#3909=CARTESIAN_POINT ( 'NONE',  ( -3.001048869802147134, 2.786623193720125791, -2.499999999999995115 ) ) ;
#3910=DIRECTION ( 'NONE',  ( 0.000000000000000000, -0.7999999999999973799, -0.6000000000000034195 ) ) ;
#3911=CARTESIAN_POINT ( 'NONE',  ( 9.693716643646590470, 12.33242205571964512, 1.443375672974076540 ) ) ;
#3913=CARTESIAN_POINT ( 'NONE',  ( -7.361714222540411967, 11.53249099303175385, 0.000000000000000000 ) ) ;
#3919=CARTESIAN_POINT ( 'NONE',  ( -9.494787648271923786, 9.971673765939062406, 1.040834085586084257E-14 ) ) ;
#3920=CARTESIAN_POINT ( 'NONE',  ( -5.897433631820158340, 5.982686779986042147, 0.7216878364870317197 ) ) ;
#3921=CARTESIAN_POINT ( 'NONE',  ( -1.364683531250000748, 2.321875000341422357, 1.214306433183764966E-14 ) ) ;
#3922=CARTESIAN_POINT ( 'NONE',  ( -1.001543065824772872E-14, 4.462500000000024336, 1.732050807568877637 ) ) ;
#3935=ORIENTED_EDGE ( 'NONE', *, *, #52342, .F. ) ;
#3939=CARTESIAN_POINT ( 'NONE',  ( 2.034713692888018954, 8.461455076002922127, -2.499999999999988898 ) ) ;
#3944=B_SPLINE_CURVE_WITH_KNOTS ( 'NONE', 3,
 ( #102434, #103511, #37433, #116615, #169570, #166371, #21151, #197796, #87257, #35291 ),
 .UNSPECIFIED., .F., .F.,
 ( 4, 3, 3, 4 ),
 ( 0.000000000000000000, 6.251636445012719089E-05, 0.0001877505388839963824, 0.0003462489540127104736 ),
 .UNSPECIFIED. ) ;
#3945=CARTESIAN_POINT ( 'NONE',  ( 0.6823417656249882723, 2.488541667008084435, -1.181850606188749264 ) ) ;
#3949=DIRECTION ( 'NONE',  ( 0.6507913734559640506, -0.7592566023653004592, 0.000000000000000000 ) ) ;
#3952=CARTESIAN_POINT ( 'NONE',  ( 8.585337585951586803, 11.03931315507545108, -1.599625672291255185 ) ) ;
#3955=CARTESIAN_POINT ( 'NONE',  ( -1.402160292154681736E-14, 1.446875000341420137, -1.575800808251659024 ) ) ;
#3957=ORIENTED_EDGE ( 'NONE', *, *, #138240, .F. ) ;
#3965=CARTESIAN_POINT ( 'NONE',  ( 6.342516933094585418, 6.294024598232139667, 1.040834085586084257E-14 ) ) ;
#3970=CARTESIAN_POINT ( 'NONE',  ( 4.017950238124170959, 5.837568840759415068, 1.364652132238639348 ) ) ;
#3975=VERTEX_POINT ( 'NONE', #81812 ) ;
#3977=CARTESIAN_POINT ( 'NONE',  ( -4.457933580795036654, 4.095344020549286590, -0.7998128361456221525 ) ) ;
#3978=CARTESIAN_POINT ( 'NONE',  ( 6.923409998072794558, 11.22906209772695618, 1.040834085586084257E-14 ) ) ;
#3981=CARTESIAN_POINT ( 'NONE',  ( 5.517805330637495231, 6.500156309574290248, -1.082531754730543083 ) ) ;
#3991=CARTESIAN_POINT ( 'NONE',  ( -8.541273586929371220, 9.067166727613487964, 0.7216878364870438212 ) ) ;
#3993=CARTESIAN_POINT ( 'NONE',  ( 6.311484202361478779, 7.322151976631905868, -1.199719254218446718 ) ) ;
#3996=CARTESIAN_POINT ( 'NONE',  ( -8.622095623286845978, 12.14652976288826913, 1.199719254218462483 ) ) ;
#4001=CARTESIAN_POINT ( 'NONE',  ( -4.810445574750349174, 4.506608013497163334, 0.7998128361456341429 ) ) ;
#4003=CARTESIAN_POINT ( 'NONE',  ( 10.23370702021670020, 10.83374636654133383, 0.7998128361456462443 ) ) ;
#4004=CARTESIAN_POINT ( 'NONE',  ( 3.167801447087334576, 6.847518788243868393, -0.7998128361456291469 ) ) ;
#4006=ORIENTED_EDGE ( 'NONE', *, *, #98111, .F. ) ;
#4010=CARTESIAN_POINT ( 'NONE',  ( 3.877268743828270470, 5.546566172598190292, 1.443375672974062551 ) ) ;
#4013=CARTESIAN_POINT ( 'NONE',  ( -5.752737250900127997, 5.605948302338584099, 0.000000000000000000 ) ) ;
#4016=CARTESIAN_POINT ( 'NONE',  ( -8.299562589859897699, 12.83457345481192036, -0.7998128361456281477 ) ) ;
#4021=CARTESIAN_POINT ( 'NONE',  ( 7.280365300858406385, 11.43758391773608984, 1.040834085586084257E-14 ) ) ;
#4022=CARTESIAN_POINT ( 'NONE',  ( -1.364683531250010740, 5.342708333674750953, 0.7879004041258379498 ) ) ;
#4024=CARTESIAN_POINT ( 'NONE',  ( 3.822509244049070887, 6.547012320444182798, -1.199719254218452047 ) ) ;
#4033=CARTESIAN_POINT ( 'NONE',  ( 3.998552357014331982, 7.829812261164016185, 1.248643980066187585E-14 ) ) ;
#4038=CARTESIAN_POINT ( 'NONE',  ( -1.364683531250012516, 2.842708333674754506, 0.7879004041258379498 ) ) ;
#4040=CARTESIAN_POINT ( 'NONE',  ( 8.594979316059474073, 12.11489407112305372, 1.199719254218450271 ) ) ;
#4043=CARTESIAN_POINT ( 'NONE',  ( -5.016153647376219382, 6.875265226737464985, 1.443375672974064550 ) ) ;
#4045=CARTESIAN_POINT ( 'NONE',  ( -5.056828107772860292, 6.922718763866881453, -1.443375672974051449 ) ) ;
#4050=CARTESIAN_POINT ( 'NONE',  ( 5.443762371086860341, 6.309809840144842141, 1.199719254218462483 ) ) ;
#4060=CARTESIAN_POINT ( 'NONE',  ( 4.984594031318565932, 8.967110136513669616, 0.7998128361456462443 ) ) ;
#4066=CARTESIAN_POINT ( 'NONE',  ( -4.388035272317281077, 8.271124917678806199, 0.7998128361456481317 ) ) ;
#4070=CARTESIAN_POINT ( 'NONE',  ( 6.317209508963599340, 9.457495962844502557, 1.199719254218462483 ) ) ;
#4073=CARTESIAN_POINT ( 'NONE',  ( -5.605406444246153974, 8.627059054007450101, -1.199719254218440723 ) ) ;
#4074=CARTESIAN_POINT ( 'NONE',  ( 6.493992390821439642, 7.639041213122241381, -1.082531754730543971 ) ) ;
#4075=CARTESIAN_POINT ( 'NONE',  ( 4.666586266758273815, 7.089143983547513628, 1.366926838653566012 ) ) ;
#4076=CARTESIAN_POINT ( 'NONE',  ( -3.249150368769345043, 6.942425863539538611, 0.7998128361456341429 ) ) ;
#4079=CARTESIAN_POINT ( 'NONE',  ( -4.089755892816631544, 7.923132308261379819, -0.7998128361456281477 ) ) ;
#4082=CARTESIAN_POINT ( 'NONE',  ( 1.364683531249988757, 2.134375000341422357, 1.214306433183764966E-14 ) ) ;
#4084=CARTESIAN_POINT ( 'NONE',  ( -4.772106882330227506, 7.550913215151819458, -1.082531754730549967 ) ) ;
#4091=CARTESIAN_POINT ( 'NONE',  ( 7.156006149914539982, 7.243095351188763686, 1.040834085586084257E-14 ) ) ;
#4094=CARTESIAN_POINT ( 'NONE',  ( -0.6823417656249969321, 3.280208333674754062, -1.181850606188749264 ) ) ;
#4101=CARTESIAN_POINT ( 'NONE',  ( -4.783329267523015460, 4.474972321731942593, -0.7998128361456221525 ) ) ;
#4102=VECTOR ( 'NONE', #211672, 1000.000000000000000 ) ;
#4103=CARTESIAN_POINT ( 'NONE',  ( -8.310784975052689205, 8.798263347090697906, -0.7216878364870267237 ) ) ;
#4105=CARTESIAN_POINT ( 'NONE',  ( -1.364683531250012516, 2.988541667008091096, -0.7879004041258289570 ) ) ;
#4112=CARTESIAN_POINT ( 'NONE',  ( -5.843201017365469596, 9.760892253660966134, 0.7216878364870458196 ) ) ;
#4114=CARTESIAN_POINT ( 'NONE',  ( -1.201851678989727383E-14, 2.993750000682821266, 1.732050807568877637 ) ) ;
#4116=CARTESIAN_POINT ( 'NONE',  ( -7.497295758232736418, 7.849192594134070333, -0.7216878364870267237 ) ) ;
#4122=CARTESIAN_POINT ( 'NONE',  ( -1.500000000000011324, 5.410416667349489117, -0.8660254037844313801 ) ) ;
#4130=CARTESIAN_POINT ( 'NONE',  ( -6.552668314106420588, 6.539201209412602189, -0.7998128361456291469 ) ) ;
#4133=CARTESIAN_POINT ( 'NONE',  ( 3.714044015139744914, 6.420469553383295391, 1.199719254218462483 ) ) ;
#4138=CARTESIAN_POINT ( 'NONE',  ( 6.993308306550549247, 7.053281200597435685, 1.040834085586084257E-14 ) ) ;
#4142=CARTESIAN_POINT ( 'NONE',  ( -4.555176424511596878, 7.297827681030051750, 1.082531754730560403 ) ) ;
#4148=ORIENTED_EDGE ( 'NONE', *, *, #189189, .F. ) ;
#4151=CARTESIAN_POINT ( 'NONE',  ( 1.364683531249988535, 1.363541667008083769, 0.7879004041258500513 ) ) ;
#4153=CARTESIAN_POINT ( 'NONE',  ( -6.353967546298838087, 10.56471257065732416, 0.000000000000000000 ) ) ;
#4155=CARTESIAN_POINT ( 'NONE',  ( 7.253775878511261155, 8.421492265473332850, 1.199719254218462483 ) ) ;
#4157=CARTESIAN_POINT ( 'NONE',  ( -6.353967546298838087, 10.56471257065732416, 0.000000000000000000 ) ) ;
#4160=CARTESIAN_POINT ( 'NONE',  ( -1.402160292154681736E-14, -0.8812499993171809543, -1.732050807568870754 ) ) ;
#4162=CARTESIAN_POINT ( 'NONE',  ( 7.443063144222396232, 11.62739806832741785, 1.040834085586084257E-14 ) ) ;
#4165=CARTESIAN_POINT ( 'NONE',  ( -0.6823417656250003738, -0.9697916663252494907, -1.181850606188749264 ) ) ;
#4167=CARTESIAN_POINT ( 'NONE',  ( 7.253248993186720561, 10.44557901115111065, 1.082531754730558626 ) ) ;
#4170=CARTESIAN_POINT ( 'NONE',  ( -5.639828713604883248, 6.642516923036197340, 1.082531754730548412 ) ) ;
#4173=CARTESIAN_POINT ( 'NONE',  ( -0.6823417656250212460, 3.051041667008084879, 1.181850606188767472 ) ) ;
#4177=CARTESIAN_POINT ( 'NONE',  ( -5.194745412330402878, 9.212286747694129474, 0.000000000000000000 ) ) ;
#4184=CARTESIAN_POINT ( 'NONE',  ( 7.584896871841365851, 10.93646455286856956, -1.199719254218446718 ) ) ;
#4188=CARTESIAN_POINT ( 'NONE',  ( -1.500000000000013101, 1.920833333333356263, 0.8660254037844403729 ) ) ;
#4194=CARTESIAN_POINT ( 'NONE',  ( 5.287316719649520991, 8.151991358691011769, -1.082531754730549078 ) ) ;
#4195=CARTESIAN_POINT ( 'NONE',  ( 1.364683531249984538, -1.032291666325247714, -0.7879004041258309554 ) ) ;
#4197=CARTESIAN_POINT ( 'NONE',  ( 3.891353782322113375, 4.498666486585943147, -1.199719254218446718 ) ) ;
#4204=CARTESIAN_POINT ( 'NONE',  ( -0.7500000000000006661, 1.108333333333356929, -1.299038105676652011 ) ) ;
#4205=CARTESIAN_POINT ( 'NONE',  ( 7.401861798056875053, 10.72292363345333399, -1.199719254218441611 ) ) ;
#4206=CARTESIAN_POINT ( 'NONE',  ( -7.804689982961090955, 12.25722208009664094, 0.7998128361456481317 ) ) ;
#4208=CARTESIAN_POINT ( 'NONE',  ( -0.6823417656250003738, -0.5322916663252491576, -1.181850606188749264 ) ) ;
#4209=CARTESIAN_POINT ( 'NONE',  ( -1.500000000000013101, 1.379166666666689745, -0.8660254037844313801 ) ) ;
#4211=CARTESIAN_POINT ( 'NONE',  ( 5.443762371086860341, 6.309809840144842141, 1.199719254218462483 ) ) ;
#4218=CARTESIAN_POINT ( 'NONE',  ( -1.364683531250010295, 5.530208333674751842, 0.7879004041258379498 ) ) ;
#4220=CARTESIAN_POINT ( 'NONE',  ( -8.843996274815957293, 9.212417163573759282, 1.040834085586084257E-14 ) ) ;
#4221=CARTESIAN_POINT ( 'NONE',  ( -5.016153647376219382, 6.875265226737464985, 1.443375672974064550 ) ) ;
#4225=CARTESIAN_POINT ( 'NONE',  ( 4.040754838981084340, 7.538853419981225379, -0.4347147375480670539 ) ) ;
#4228=CARTESIAN_POINT ( 'NONE',  ( 6.740374924288304648, 11.01552117831172062, 1.040834085586084257E-14 ) ) ;
#4229=CARTESIAN_POINT ( 'NONE',  ( -4.456559383047711265, 7.083366476587958260, -1.119882773345021842 ) ) ;
#4230=VECTOR ( 'NONE', #185116, 1000.000000000000114 ) ;
#4231=CARTESIAN_POINT ( 'NONE',  ( 6.795661308947685164, 8.951357498570873261, -1.599625672291262513 ) ) ;
#4232=CARTESIAN_POINT ( 'NONE',  ( 6.602457619730760285, 8.725953194484466380, 1.443375672974076540 ) ) ;
#4236=CARTESIAN_POINT ( 'NONE',  ( -9.020252271793614440, 9.418049160047695878, 0.7998128361456462443 ) ) ;
#4237=CARTESIAN_POINT ( 'NONE',  ( 5.518332215962025167, 6.396807992499198292, -1.199719254218445830 ) ) ;
#4239=CARTESIAN_POINT ( 'NONE',  ( 4.065672160753666553, 7.505179260319745360, -0.5311146244057519672 ) ) ;
#4240=CARTESIAN_POINT ( 'NONE',  ( 10.56143847536557878, 11.42402576412244386, 0.000000000000000000 ) ) ;
#4245=VECTOR ( 'NONE', #197041, 1000.000000000000227 ) ;
#4249=CARTESIAN_POINT ( 'NONE',  ( -3.578989364327652467, 6.158942777482099729, 1.082531754730560403 ) ) ;
#4250=CARTESIAN_POINT ( 'NONE',  ( 9.951321562750607086, 11.67259191370631477, -1.082531754730537088 ) ) ;
#4253=CARTESIAN_POINT ( 'NONE',  ( -6.718228810771495141, 7.796687353110217877, 1.199719254218450271 ) ) ;
#4256=CARTESIAN_POINT ( 'NONE',  ( 5.427887300360813683, 4.356806483369909166, 2.440341253675380351 ) ) ;
#4258=CARTESIAN_POINT ( 'NONE',  ( -7.507464373665155399, 9.781794407407920389, 1.599625672291295375 ) ) ;
#4261=CARTESIAN_POINT ( 'NONE',  ( 7.084367489069545069E-14, 8.210952333604106812, 2.038660652713624177 ) ) ;
#4272=CARTESIAN_POINT ( 'NONE',  ( -5.994676475536691029, 10.14553965476814845, 0.7998128361456481317 ) ) ;
#4275=CARTESIAN_POINT ( 'NONE',  ( 5.992340707560163793, 6.093411701682730275, 0.7216878364870317197 ) ) ;
#4277=CIRCLE ( 'NONE', #159863, 0.8299999999999999600 ) ;
#4280=CARTESIAN_POINT ( 'NONE',  ( -3.588104209110990706, 7.337872010604796991, 1.040834085586084257E-14 ) ) ;
#4281=( BOUNDED_SURFACE ( )  B_SPLINE_SURFACE ( 1, 2, ( 
 ( #60722, #125819, #11968, #92201, #191780, #158251, #174510, #8773, #194993, #46627, #45566, #13027, #144166, #43436, #208033, #74856, #109560, #9839, #193920, #140958, #160365, #126885, #175564, #75915, #206969, #94324, #192843, #27155, #210158, #93259, #159293, #10892, #76967, #58599, #112750, #178762, #111683, #79104, #61799, #127968, #124754, #143094, #209087, #145222, #44502, #177690, #29301, #110619, #190714, #176619, #95395, #161447, #129016, #181921, #213352, #214388, #200296, #96461, #197117, #63923, #162511, #84434, #50874, #33551, #116996, #14082, #180869, #182996, #48755, #179819, #64974, #148387, #32490, #51949, #30375, #196073, #98564, #67087, #97517, #147324, #150523, #118071, #80172, #146278, #164625, #66017, #212290, #130078, #2084, #31438, #132166, #47705, #113820, #34613, #149440, #163573, #133221, #15156, #82294, #68157, #81242, #199227, #18356, #49805, #131128, #115931, #114868, #16210, #198172, #99624, #165690, #134291, #17279, #83355, #1022, #100683, #166761, #172096, #121287, #171015, #56205, #120213, #203488, #35676, #19421, #151586, #138534, #86571, #36740, #135343, #187263, #153712, #204557, #188325, #89799, #104974, #37820, #57274, #152634, #102826, #20485, #4221, #154779, #201357, #72432, #39966, #185114, #70290, #168881, #186187, #54077, #52998, #38889, #22612, #103898, #101754, #69224, #88720, #136406, #202422, #184058, #139614, #205636, #169945, #23689, #122369, #21531, #106073, #87641, #155844, #6363, #167821, #85499, #5281, #71358, #137474, #3153, #55141, #7430, #73511, #119134, #58336, #9577, #60457, #126614, #42109, #95120, #26887, #123436, #191513, #207769, #124492, #190451, #160098, #24754, #45295, #78829, #108222, #90856, #177419, #175301, #74590, #189398, #142820, #77775, #144950, #12755, #174247, #161169, #127693, #210956, #44232, #140693, #76703, #25819, #91929, #41040, #110353, #107149, #157989, #143895, #75654, #176356, #141761, #193653, #94057, #173174, #109291, #11701, #27964, #59396, #61527, #125552, #156920, #43178, #92990, #159035, #10628, #8509, #206709, #208827, #192577, #209889, #111415, #29037, #84169, #99367, #100419, #182727, #113549, #166490, #163300, #165419, #97246, #34346, #194719, #63661, #149170, #18081, #179552, #13824, #146007, #31173, #132956, #164362, #114611, #130858, #46358, #150258, #14881, #80975, #147065, #112478, #213086, #79898, #17015, #178487, #131900, #98299, #64716, #212017, #30097, #214124, #32227, #196854, #197907, #129815, #48493, #195797, #47434, #62583, #128745, #96187, #83091, #198959, #49536, #747, #162238, #180602, #15947, #116727, #82030, #115662, #181656, #148124, #65753, #33282, #66813, #50602, #57812, #156394, #187802, #188875, #174795, #67885, #171557, #35411, #134030, #58884, #25306, #7980, #91408, #200037, #155318, #157468, #23153, #154257, #39430, #122917, #6902, #26371, #1826, #170489, #72979, #41591, #71903, #121831, #125039, #92483, #51689, #117811, #139082, #40515, #183801, #101489, #190995, #5830, #106618, #22073, #88185, #9063, #123975, #138012, #107703, #204027, #56752, #42661, #55675, #173729, #207256, #24223, #105523, #90325, #89268, #205109, #172647, #74069, #140162, #108770, #206185, #189942, #75138, #141247, #210454, #146569, #95682, #145518, #30668, #94611, #177981, #10120, #208315, #126101, #113043, #61018, #11182, #109838, #161736, #128251, #179049, #162801, #64226, #79401, #12252, #31733, #127176, #77261, #45859, #62092, #78329, #142304, #114116, #193145, #129318, #175853, #46925, #14378, #159584, #44795, #143375, #160654, #28521, #27442, #13327, #211517, #144451, #76195, #43724, #63153, #110900, #209374, #158523, #180109, #59945, #176906, #212587, #96751, #194214, #80470, #111980, #130368, #195294, #192061, #93540, #29596, #196358, #47999, #65259, #116227, #17569, #199529, #184352, #32786, #198462, #34897, #100970, #16507, #69523, #1320, #97806, #165983, #182218, #98862, #164914, #134588, #213633, #19721, #53300, #82589, #131406, #151880, #149743, #49047, #163869, #117295, #52236, #119432, #201650, #148676, #135630, #102054, #185419, #18651, #115167, #51172, #244, #66316, #15445, #84730, #81534, #132460 ),
 ( #50106, #33841, #67381, #99922, #147615, #197406, #83653, #181162, #133522, #183292, #167059, #150819, #200588, #2382, #3454, #68460, #118363, #35974, #168120, #85800, #157216, #169179, #38122, #123732, #8813, #87935, #202723, #120513, #154008, #107454, #6662, #71655, #20772, #207006, #5575, #58637, #137769, #74890, #170242, #124790, #73817, #140998, #37037, #203787, #103121, #55433, #139911, #121585, #86867, #152933, #104195, #189694, #4510, #187557, #54376, #186491, #39185, #173481, #138836, #89021, #105273, #70582, #136698, #171310, #7732, #21827, #205942, #41346, #22904, #155073, #72739, #204852, #56507, #122668, #188630, #23984, #40261, #106373, #172396, #90087, #156150, #57574, #25058, #91160, #146310, #109595, #30414, #145260, #192881, #79143, #60763, #96498, #161486, #174548, #212324, #27190, #143130, #94360, #158285, #209126, #110654, #78078, #62890, #125856, #77004, #128002, #193956, #175601, #162548, #160402, #190750, #44538, #126924, #191813, #43477, #13064, #92235, #112787, #63963, #93296, #9875, #14118, #28268, #142053, #42414, #210199, #211266, #108519, #80210, #159332, #26123, #195032, #75951, #111720, #208068, #144203, #10928, #176655, #59693, #177728, #12004, #61835, #129058, #45603, #29340, #95433, #46666, #178798, #3186, #115970, #100719, #50910, #114907, #68194, #180905, #113860, #197153, #48790, #85530, #1061, #131162, #130118, #179855, #198207, #196108, #184092, #35711, #31478, #97553, #165728, #181958, #118107, #67126, #117038, #2119, #66056, #149478, #47744, #163611, #15192, #84467, #32528, #98603, #81283, #133259, #99659, #150559, #134326, #101788, #183033, #49842, #147359, #164664, #16246, #82332, #148424, #66031, #213386, #132200, #65010, #18390, #33587, #199266, #17316, #83394, #34649, #166796, #200332, #51982, #167857, #19454, #151620, #37853, #136439, #20520, #69257, #173207, #24787, #23721, #205668, #56240, #106105, #90890, #103932, #4253, #123469, #38921, #122399, #188357, #169976, #135374, #54109, #72467, #105005, #39997, #6394, #21564, #171044, #156949, #201392, #87670, #102859, #53030, #189432, #89828, #138567, #155876, #119163, #5310, #7465, #153742, #70322, #71391, #187295, #137503, #185149, #36773, #86603, #203520, #172127, #202455, #186222, #41074, #168915, #152669, #120244, #55174, #22643, #121319, #88751, #107181, #154808, #204588, #73544, #139647, #57306, #127728, #42141, #111449, #178521, #60488, #62616, #59428, #45330, #210989, #27996, #30131, #126646, #128778, #125586, #177454, #194755, #94093, #96220, #160132, #9609, #8541, #206740, #76735, #74623, #46392, #112509, #58371, #124525, #44264, #192611, #140727, #11731, #209923, #95151, #159067, #77807, #190482, #108256, #174277, #29068, #191546, #75686, #25852, #143928, #110386, #161203, #12789, #91962, #61562, #142853, #158021, #43211, #141796, #109327, #175335, #26917, #207800, #93026, #10663, #78863, #208857, #193686, #176391, #144984, #97282, #63694, #99400, #131934, #130894, #83127, #163337, #196888, #14916, #113584, #162271, #51724, #117846, #116766, #84206, #149207, #198994, #183838, #48526, #81010, #1861, #197944, #782, #66849, #114646, #13858, #147098, #165453, #49572, #132993, #17048, #180639, #115697, #35447, #79935, #32264, #195831, #146040, #67922, #182764, #50640, #34381, #212054, #98331, #100454, #164397, #213122, #15980, #65784, #82065, #129848, #47469, #179586, #148157, #166527, #64752, #214158, #134066, #31208, #181689, #33319, #18118, #150294, #200075, #201134, #7206, #102603, #203271, #52772, #135118, #188104, #6135, #118909, #204327, #155621, #152417, #138312, #89572, #121068, #57054, #187036, #168657, #101527, #85273, #169725, #189182, #73279, #139383, #151360, #2929, #137251, #153488, #205416, #38668, #88495, #39734, #37594, #104747, #167596, #69001, #184892, #55985, #3996, #20262, #36516, #170795, #71133, #122137, #105839, #123218, #22386, #21314, #19195, #70065, #86346, #136178, #202196, #53852, #119985, #185962, #103677, #171866, #87421, #154556, #54917, #5058, #72204, #23460, #10419, #109072, #25604, #208611, #124277, #91716, #190235, #140476, #40819, #193452, #45096, #27751, #77563 ) ),
 .UNSPECIFIED., .F., .F., .T. ) 
 B_SPLINE_SURFACE_WITH_KNOTS ( ( 2, 2 ),
 ( 3, 2, 2, 2, 2, 2, 2, 2, 2, 2, 2, 2, 2, 2, 2, 2, 2, 2, 2, 2, 2, 2, 2, 2, 2, 2, 2, 2, 2, 2, 2, 2, 2, 2, 2, 2, 2, 2, 2, 2, 2, 2, 2, 2, 2, 2, 2, 2, 2, 2, 2, 2, 2, 2, 2, 2, 2, 2, 2, 2, 2, 2, 2, 2, 2, 2, 2, 2, 2, 2, 2, 2, 2, 2, 2, 2, 2, 2, 2, 2, 2, 2, 2, 2, 2, 2, 2, 2, 2, 2, 2, 2, 2, 2, 2, 2, 2, 2, 2, 2, 2, 2, 2, 2, 2, 2, 2, 2, 2, 2, 2, 2, 2, 2, 2, 2, 2, 2, 2, 2, 2, 2, 2, 2, 2, 2, 2, 2, 2, 2, 2, 2, 2, 2, 2, 2, 2, 2, 2, 2, 2, 2, 2, 2, 2, 2, 2, 2, 2, 2, 2, 2, 2, 2, 2, 2, 2, 2, 2, 2, 2, 2, 2, 2, 2, 2, 2, 2, 2, 2, 2, 2, 2, 2, 2, 2, 2, 2, 2, 2, 2, 2, 2, 2, 2, 2, 2, 2, 2, 2, 2, 2, 2, 2, 2, 2, 2, 2, 2, 2, 2, 2, 2, 2, 2, 2, 2, 2, 2, 2, 2, 2, 2, 2, 2, 2, 2, 2, 2, 2, 2, 2, 2, 2, 2, 2, 2, 2, 2, 2, 2, 2, 2, 2, 2, 2, 2, 2, 2, 2, 3 ),
 ( 0.000000000000000000, 1.000000000000000000 ),
 ( 0.000000000000000000, 0.004166666666666666609, 0.008333333333333333218, 0.01250000000000000069, 0.01666666666666666644, 0.02083333333333333218, 0.02500000000000000139, 0.02916666666666666713, 0.03333333333333333287, 0.03749999999999999861, 0.04166666666666666435, 0.04583333333333333010, 0.05000000000000000278, 0.05416666666666666852, 0.05833333333333333426, 0.06250000000000000000, 0.06666666666666666574, 0.07083333333333333148, 0.07499999999999999722, 0.07916666666666666297, 0.08333333333333332871, 0.08749999999999999445, 0.09166666666666666019, 0.09583333333333333981, 0.1000000000000000056, 0.1041666666666666713, 0.1083333333333333370, 0.1125000000000000028, 0.1166666666666666685, 0.1208333333333333343, 0.1250000000000000000, 0.1291666666666666796, 0.1333333333333333315, 0.1375000000000000111, 0.1416666666666666630, 0.1458333333333333426, 0.1499999999999999944, 0.1541666666666666741, 0.1583333333333333259, 0.1625000000000000056, 0.1666666666666666574, 0.1708333333333333370, 0.1749999999999999889, 0.1791666666666666685, 0.1833333333333333204, 0.1875000000000000000, 0.1916666666666666796, 0.1958333333333333315, 0.2000000000000000111, 0.2041666666666666630, 0.2083333333333333426, 0.2124999999999999944, 0.2166666666666666741, 0.2208333333333333259, 0.2250000000000000056, 0.2291666666666666574, 0.2333333333333333370, 0.2374999999999999889, 0.2416666666666666685, 0.2458333333333333204, 0.2500000000000000000, 0.2541666666666666519, 0.2583333333333333592, 0.2625000000000000111, 0.2666666666666666630, 0.2708333333333333148, 0.2750000000000000222, 0.2791666666666666741, 0.2833333333333333259, 0.2874999999999999778, 0.2916666666666666852, 0.2958333333333333370, 0.2999999999999999889, 0.3041666666666666408, 0.3083333333333333481, 0.3125000000000000000, 0.3166666666666666519, 0.3208333333333333592, 0.3250000000000000111, 0.3291666666666666630, 0.3333333333333333148, 0.3375000000000000222, 0.3416666666666666741, 0.3458333333333333259, 0.3499999999999999778, 0.3541666666666666852, 0.3583333333333333370, 0.3624999999999999889, 0.3666666666666666408, 0.3708333333333333481, 0.3750000000000000000, 0.3791666666666666519, 0.3833333333333333592, 0.3875000000000000111, 0.3916666666666666630, 0.3958333333333333148, 0.4000000000000000222, 0.4041666666666666741, 0.4083333333333333259, 0.4124999999999999778, 0.4166666666666666852, 0.4208333333333333370, 0.4249999999999999889, 0.4291666666666666408, 0.4333333333333333481, 0.4375000000000000000, 0.4416666666666666519, 0.4458333333333333592, 0.4500000000000000111, 0.4541666666666666630, 0.4583333333333333148, 0.4625000000000000222, 0.4666666666666666741, 0.4708333333333333259, 0.4749999999999999778, 0.4791666666666666852, 0.4833333333333333370, 0.4874999999999999889, 0.4916666666666666408, 0.4958333333333333481, 0.5000000000000000000, 0.5041666666666666519, 0.5083333333333333037, 0.5124999999999999556, 0.5166666666666667185, 0.5208333333333333703, 0.5250000000000000222, 0.5291666666666666741, 0.5333333333333333259, 0.5374999999999999778, 0.5416666666666666297, 0.5458333333333332815, 0.5500000000000000444, 0.5541666666666666963, 0.5583333333333333481, 0.5625000000000000000, 0.5666666666666666519, 0.5708333333333333037, 0.5749999999999999556, 0.5791666666666667185, 0.5833333333333333703, 0.5875000000000000222, 0.5916666666666666741, 0.5958333333333333259, 0.5999999999999999778, 0.6041666666666666297, 0.6083333333333332815, 0.6125000000000000444, 0.6166666666666666963, 0.6208333333333333481, 0.6250000000000000000, 0.6291666666666666519, 0.6333333333333333037, 0.6374999999999999556, 0.6416666666666667185, 0.6458333333333333703, 0.6500000000000000222, 0.6541666666666666741, 0.6583333333333333259, 0.6624999999999999778, 0.6666666666666666297, 0.6708333333333332815, 0.6750000000000000444, 0.6791666666666666963, 0.6833333333333333481, 0.6875000000000000000, 0.6916666666666666519, 0.6958333333333333037, 0.6999999999999999556, 0.7041666666666667185, 0.7083333333333333703, 0.7125000000000000222, 0.7166666666666666741, 0.7208333333333333259, 0.7249999999999999778, 0.7291666666666666297, 0.7333333333333332815, 0.7375000000000000444, 0.7416666666666666963, 0.7458333333333333481, 0.7500000000000000000, 0.7541666666666666519, 0.7583333333333333037, 0.7624999999999999556, 0.7666666666666667185, 0.7708333333333333703, 0.7750000000000000222, 0.7791666666666666741, 0.7833333333333333259, 0.7874999999999999778, 0.7916666666666666297, 0.7958333333333332815, 0.8000000000000000444, 0.8041666666666666963, 0.8083333333333333481, 0.8125000000000000000, 0.8166666666666666519, 0.8208333333333333037, 0.8249999999999999556, 0.8291666666666667185, 0.8333333333333333703, 0.8375000000000000222, 0.8416666666666666741, 0.8458333333333333259, 0.8499999999999999778, 0.8541666666666666297, 0.8583333333333332815, 0.8625000000000000444, 0.8666666666666666963, 0.8708333333333333481, 0.8750000000000000000, 0.8791666666666666519, 0.8833333333333333037, 0.8874999999999999556, 0.8916666666666667185, 0.8958333333333333703, 0.9000000000000000222, 0.9041666666666666741, 0.9083333333333333259, 0.9124999999999999778, 0.9166666666666666297, 0.9208333333333332815, 0.9250000000000000444, 0.9291666666666666963, 0.9333333333333333481, 0.9375000000000000000, 0.9416666666666666519, 0.9458333333333333037, 0.9499999999999999556, 0.9541666666666667185, 0.9583333333333333703, 0.9625000000000000222, 0.9666666666666666741, 0.9708333333333333259, 0.9749999999999999778, 0.9791666666666666297, 0.9833333333333332815, 0.9875000000000000444, 0.9916666666666666963, 0.9958333333333333481, 1.000000000000000000 ),
 .UNSPECIFIED. ) 
 GEOMETRIC_REPRESENTATION_ITEM ( )  RATIONAL_B_SPLINE_SURFACE ( (
 ( 1.000000000000000000, 0.8660254037844387076, 1.000000000000000000, 0.8660254037844387076, 1.000000000000000000, 0.8660254037844387076, 1.000000000000000000, 0.8660254037844387076, 1.000000000000000000, 0.8660254037844387076, 1.000000000000000000, 0.8660254037844387076, 1.000000000000000000, 0.8660254037844387076, 1.000000000000000000, 0.8660254037844387076, 1.000000000000000000, 0.8660254037844387076, 1.000000000000000000, 0.8660254037844387076, 1.000000000000000000, 0.8660254037844387076, 1.000000000000000000, 0.8660254037844387076, 1.000000000000000000, 0.8660254037844387076, 1.000000000000000000, 0.8660254037844387076, 1.000000000000000000, 0.8660254037844387076, 1.000000000000000000, 0.8660254037844387076, 1.000000000000000000, 0.8660254037844387076, 1.000000000000000000, 0.8660254037844387076, 1.000000000000000000, 0.8660254037844387076, 1.000000000000000000, 0.8660254037844387076, 1.000000000000000000, 0.8660254037844387076, 1.000000000000000000, 0.8660254037844387076, 1.000000000000000000, 0.8660254037844387076, 1.000000000000000000, 0.8660254037844387076, 1.000000000000000000, 0.8660254037844387076, 1.000000000000000000, 0.8660254037844387076, 1.000000000000000000, 0.8660254037844387076, 1.000000000000000000, 0.8660254037844387076, 1.000000000000000000, 0.8660254037844387076, 1.000000000000000000, 0.8660254037844387076, 1.000000000000000000, 0.8660254037844387076, 1.000000000000000000, 0.8660254037844387076, 1.000000000000000000, 0.8660254037844387076, 1.000000000000000000, 0.8660254037844387076, 1.000000000000000000, 0.8660254037844387076, 1.000000000000000000, 0.8660254037844387076, 1.000000000000000000, 0.8660254037844387076, 1.000000000000000000, 0.8660254037844387076, 1.000000000000000000, 0.8660254037844387076, 1.000000000000000000, 0.8660254037844387076, 1.000000000000000000, 0.8660254037844387076, 1.000000000000000000, 0.8660254037844387076, 1.000000000000000000, 0.8660254037844387076, 1.000000000000000000, 0.8660254037844387076, 1.000000000000000000, 0.8660254037844387076, 1.000000000000000000, 0.8660254037844387076, 1.000000000000000000, 0.8660254037844387076, 1.000000000000000000, 0.8660254037844387076, 1.000000000000000000, 0.8660254037844387076, 1.000000000000000000, 0.8660254037844387076, 1.000000000000000000, 0.8660254037844387076, 1.000000000000000000, 0.8660254037844387076, 1.000000000000000000, 0.8660254037844387076, 1.000000000000000000, 0.8660254037844387076, 1.000000000000000000, 0.8660254037844387076, 1.000000000000000000, 0.8660254037844387076, 1.000000000000000000, 0.8660254037844387076, 1.000000000000000000, 0.8660254037844387076, 1.000000000000000000, 0.8660254037844387076, 1.000000000000000000, 0.8660254037844387076, 1.000000000000000000, 0.8660254037844387076, 1.000000000000000000, 0.8660254037844387076, 1.000000000000000000, 0.8660254037844387076, 1.000000000000000000, 0.8660254037844387076, 1.000000000000000000, 0.8660254037844387076, 1.000000000000000000, 0.8660254037844387076, 1.000000000000000000, 0.8660254037844387076, 1.000000000000000000, 0.8660254037844387076, 1.000000000000000000, 0.8660254037844387076, 1.000000000000000000, 0.8660254037844387076, 1.000000000000000000, 0.8660254037844387076, 1.000000000000000000, 0.8660254037844387076, 1.000000000000000000, 0.8660254037844387076, 1.000000000000000000, 0.8660254037844387076, 1.000000000000000000, 0.8660254037844387076, 1.000000000000000000, 0.8660254037844387076, 1.000000000000000000, 0.8660254037844387076, 1.000000000000000000, 0.8660254037844387076, 1.000000000000000000, 0.8660254037844387076, 1.000000000000000000, 0.8660254037844387076, 1.000000000000000000, 0.8660254037844387076, 1.000000000000000000, 0.8660254037844387076, 1.000000000000000000, 0.8660254037844387076, 1.000000000000000000, 0.8660254037844387076, 1.000000000000000000, 0.8660254037844387076, 1.000000000000000000, 0.8660254037844387076, 1.000000000000000000, 0.8660254037844387076, 1.000000000000000000, 0.8660254037844387076, 1.000000000000000000, 0.8660254037844387076, 1.000000000000000000, 0.8660254037844387076, 1.000000000000000000, 0.8660254037844387076, 1.000000000000000000, 0.8660254037844387076, 1.000000000000000000, 0.8660254037844387076, 1.000000000000000000, 0.8660254037844387076, 1.000000000000000000, 0.8660254037844387076, 1.000000000000000000, 0.8660254037844387076, 1.000000000000000000, 0.8660254037844387076, 1.000000000000000000, 0.8660254037844387076, 1.000000000000000000, 0.8660254037844387076, 1.000000000000000000, 0.8660254037844387076, 1.000000000000000000, 0.8660254037844387076, 1.000000000000000000, 0.8660254037844387076, 1.000000000000000000, 0.8660254037844387076, 1.000000000000000000, 0.8660254037844387076, 1.000000000000000000, 0.8660254037844387076, 1.000000000000000000, 0.8660254037844387076, 1.000000000000000000, 0.8660254037844387076, 1.000000000000000000, 0.8660254037844387076, 1.000000000000000000, 0.8660254037844387076, 1.000000000000000000, 0.8660254037844387076, 1.000000000000000000, 0.8660254037844387076, 1.000000000000000000, 0.8660254037844387076, 1.000000000000000000, 0.8660254037844387076, 1.000000000000000000, 0.8660254037844387076, 1.000000000000000000, 0.8660254037844387076, 1.000000000000000000, 0.8660254037844387076, 1.000000000000000000, 0.8660254037844387076, 1.000000000000000000, 0.8660254037844387076, 1.000000000000000000, 0.8660254037844387076, 1.000000000000000000, 0.8660254037844387076, 1.000000000000000000, 0.8660254037844387076, 1.000000000000000000, 0.8660254037844387076, 1.000000000000000000, 0.8660254037844387076, 1.000000000000000000, 0.8660254037844387076, 1.000000000000000000, 0.8660254037844387076, 1.000000000000000000, 0.8660254037844387076, 1.000000000000000000, 0.8660254037844387076, 1.000000000000000000, 0.8660254037844387076, 1.000000000000000000, 0.8660254037844387076, 1.000000000000000000, 0.8660254037844387076, 1.000000000000000000, 0.8660254037844387076, 1.000000000000000000, 0.8660254037844387076, 1.000000000000000000, 0.8660254037844387076, 1.000000000000000000, 0.8660254037844387076, 1.000000000000000000, 0.8660254037844387076, 1.000000000000000000, 0.8660254037844387076, 1.000000000000000000, 0.8660254037844387076, 1.000000000000000000, 0.8660254037844387076, 1.000000000000000000, 0.8660254037844387076, 1.000000000000000000, 0.8660254037844387076, 1.000000000000000000, 0.8660254037844387076, 1.000000000000000000, 0.8660254037844387076, 1.000000000000000000, 0.8660254037844387076, 1.000000000000000000, 0.8660254037844387076, 1.000000000000000000, 0.8660254037844387076, 1.000000000000000000, 0.8660254037844387076, 1.000000000000000000, 0.8660254037844387076, 1.000000000000000000, 0.8660254037844387076, 1.000000000000000000, 0.8660254037844387076, 1.000000000000000000, 0.8660254037844387076, 1.000000000000000000, 0.8660254037844387076, 1.000000000000000000, 0.8660254037844387076, 1.000000000000000000, 0.8660254037844387076, 1.000000000000000000, 0.8660254037844387076, 1.000000000000000000, 0.8660254037844387076, 1.000000000000000000, 0.8660254037844387076, 1.000000000000000000, 0.8660254037844387076, 1.000000000000000000, 0.8660254037844387076, 1.000000000000000000, 0.8660254037844387076, 1.000000000000000000, 0.8660254037844387076, 1.000000000000000000, 0.8660254037844387076, 1.000000000000000000, 0.8660254037844387076, 1.000000000000000000, 0.8660254037844387076, 1.000000000000000000, 0.8660254037844387076, 1.000000000000000000, 0.8660254037844387076, 1.000000000000000000, 0.8660254037844387076, 1.000000000000000000, 0.8660254037844387076, 1.000000000000000000, 0.8660254037844387076, 1.000000000000000000, 0.8660254037844387076, 1.000000000000000000, 0.8660254037844387076, 1.000000000000000000, 0.8660254037844387076, 1.000000000000000000, 0.8660254037844387076, 1.000000000000000000, 0.8660254037844387076, 1.000000000000000000, 0.8660254037844387076, 1.000000000000000000, 0.8660254037844387076, 1.000000000000000000, 0.8660254037844387076, 1.000000000000000000, 0.8660254037844387076, 1.000000000000000000, 0.8660254037844387076, 1.000000000000000000, 0.8660254037844387076, 1.000000000000000000, 0.8660254037844387076, 1.000000000000000000, 0.8660254037844387076, 1.000000000000000000, 0.8660254037844387076, 1.000000000000000000, 0.8660254037844387076, 1.000000000000000000, 0.8660254037844387076, 1.000000000000000000, 0.8660254037844387076, 1.000000000000000000, 0.8660254037844387076, 1.000000000000000000, 0.8660254037844387076, 1.000000000000000000, 0.8660254037844387076, 1.000000000000000000, 0.8660254037844387076, 1.000000000000000000, 0.8660254037844387076, 1.000000000000000000, 0.8660254037844387076, 1.000000000000000000, 0.8660254037844387076, 1.000000000000000000, 0.8660254037844387076, 1.000000000000000000, 0.8660254037844387076, 1.000000000000000000, 0.8660254037844387076, 1.000000000000000000, 0.8660254037844387076, 1.000000000000000000, 0.8660254037844387076, 1.000000000000000000, 0.8660254037844387076, 1.000000000000000000, 0.8660254037844387076, 1.000000000000000000, 0.8660254037844387076, 1.000000000000000000, 0.8660254037844387076, 1.000000000000000000, 0.8660254037844387076, 1.000000000000000000, 0.8660254037844387076, 1.000000000000000000, 0.8660254037844387076, 1.000000000000000000, 0.8660254037844387076, 1.000000000000000000, 0.8660254037844387076, 1.000000000000000000, 0.8660254037844387076, 1.000000000000000000, 0.8660254037844387076, 1.000000000000000000, 0.8660254037844387076, 1.000000000000000000, 0.8660254037844387076, 1.000000000000000000, 0.8660254037844387076, 1.000000000000000000, 0.8660254037844387076, 1.000000000000000000, 0.8660254037844387076, 1.000000000000000000, 0.8660254037844387076, 1.000000000000000000, 0.8660254037844387076, 1.000000000000000000, 0.8660254037844387076, 1.000000000000000000, 0.8660254037844387076, 1.000000000000000000, 0.8660254037844387076, 1.000000000000000000, 0.8660254037844387076, 1.000000000000000000, 0.8660254037844387076, 1.000000000000000000, 0.8660254037844387076, 1.000000000000000000, 0.8660254037844387076, 1.000000000000000000, 0.8660254037844387076, 1.000000000000000000, 0.8660254037844387076, 1.000000000000000000, 0.8660254037844387076, 1.000000000000000000, 0.8660254037844387076, 1.000000000000000000, 0.8660254037844387076, 1.000000000000000000, 0.8660254037844387076, 1.000000000000000000, 0.8660254037844387076, 1.000000000000000000, 0.8660254037844387076, 1.000000000000000000, 0.8660254037844387076, 1.000000000000000000, 0.8660254037844387076, 1.000000000000000000, 0.8660254037844387076, 1.000000000000000000, 0.8660254037844387076, 1.000000000000000000, 0.8660254037844387076, 1.000000000000000000, 0.8660254037844387076, 1.000000000000000000, 0.8660254037844387076, 1.000000000000000000, 0.8660254037844387076, 1.000000000000000000, 0.8660254037844387076, 1.000000000000000000, 0.8660254037844387076, 1.000000000000000000),
 ( 1.000000000000000000, 0.8660254037844387076, 1.000000000000000000, 0.8660254037844387076, 1.000000000000000000, 0.8660254037844387076, 1.000000000000000000, 0.8660254037844387076, 1.000000000000000000, 0.8660254037844387076, 1.000000000000000000, 0.8660254037844387076, 1.000000000000000000, 0.8660254037844387076, 1.000000000000000000, 0.8660254037844387076, 1.000000000000000000, 0.8660254037844387076, 1.000000000000000000, 0.8660254037844387076, 1.000000000000000000, 0.8660254037844387076, 1.000000000000000000, 0.8660254037844387076, 1.000000000000000000, 0.8660254037844387076, 1.000000000000000000, 0.8660254037844387076, 1.000000000000000000, 0.8660254037844387076, 1.000000000000000000, 0.8660254037844387076, 1.000000000000000000, 0.8660254037844387076, 1.000000000000000000, 0.8660254037844387076, 1.000000000000000000, 0.8660254037844387076, 1.000000000000000000, 0.8660254037844387076, 1.000000000000000000, 0.8660254037844387076, 1.000000000000000000, 0.8660254037844387076, 1.000000000000000000, 0.8660254037844387076, 1.000000000000000000, 0.8660254037844387076, 1.000000000000000000, 0.8660254037844387076, 1.000000000000000000, 0.8660254037844387076, 1.000000000000000000, 0.8660254037844387076, 1.000000000000000000, 0.8660254037844387076, 1.000000000000000000, 0.8660254037844387076, 1.000000000000000000, 0.8660254037844387076, 1.000000000000000000, 0.8660254037844387076, 1.000000000000000000, 0.8660254037844387076, 1.000000000000000000, 0.8660254037844387076, 1.000000000000000000, 0.8660254037844387076, 1.000000000000000000, 0.8660254037844387076, 1.000000000000000000, 0.8660254037844387076, 1.000000000000000000, 0.8660254037844387076, 1.000000000000000000, 0.8660254037844387076, 1.000000000000000000, 0.8660254037844387076, 1.000000000000000000, 0.8660254037844387076, 1.000000000000000000, 0.8660254037844387076, 1.000000000000000000, 0.8660254037844387076, 1.000000000000000000, 0.8660254037844387076, 1.000000000000000000, 0.8660254037844387076, 1.000000000000000000, 0.8660254037844387076, 1.000000000000000000, 0.8660254037844387076, 1.000000000000000000, 0.8660254037844387076, 1.000000000000000000, 0.8660254037844387076, 1.000000000000000000, 0.8660254037844387076, 1.000000000000000000, 0.8660254037844387076, 1.000000000000000000, 0.8660254037844387076, 1.000000000000000000, 0.8660254037844387076, 1.000000000000000000, 0.8660254037844387076, 1.000000000000000000, 0.8660254037844387076, 1.000000000000000000, 0.8660254037844387076, 1.000000000000000000, 0.8660254037844387076, 1.000000000000000000, 0.8660254037844387076, 1.000000000000000000, 0.8660254037844387076, 1.000000000000000000, 0.8660254037844387076, 1.000000000000000000, 0.8660254037844387076, 1.000000000000000000, 0.8660254037844387076, 1.000000000000000000, 0.8660254037844387076, 1.000000000000000000, 0.8660254037844387076, 1.000000000000000000, 0.8660254037844387076, 1.000000000000000000, 0.8660254037844387076, 1.000000000000000000, 0.8660254037844387076, 1.000000000000000000, 0.8660254037844387076, 1.000000000000000000, 0.8660254037844387076, 1.000000000000000000, 0.8660254037844387076, 1.000000000000000000, 0.8660254037844387076, 1.000000000000000000, 0.8660254037844387076, 1.000000000000000000, 0.8660254037844387076, 1.000000000000000000, 0.8660254037844387076, 1.000000000000000000, 0.8660254037844387076, 1.000000000000000000, 0.8660254037844387076, 1.000000000000000000, 0.8660254037844387076, 1.000000000000000000, 0.8660254037844387076, 1.000000000000000000, 0.8660254037844387076, 1.000000000000000000, 0.8660254037844387076, 1.000000000000000000, 0.8660254037844387076, 1.000000000000000000, 0.8660254037844387076, 1.000000000000000000, 0.8660254037844387076, 1.000000000000000000, 0.8660254037844387076, 1.000000000000000000, 0.8660254037844387076, 1.000000000000000000, 0.8660254037844387076, 1.000000000000000000, 0.8660254037844387076, 1.000000000000000000, 0.8660254037844387076, 1.000000000000000000, 0.8660254037844387076, 1.000000000000000000, 0.8660254037844387076, 1.000000000000000000, 0.8660254037844387076, 1.000000000000000000, 0.8660254037844387076, 1.000000000000000000, 0.8660254037844387076, 1.000000000000000000, 0.8660254037844387076, 1.000000000000000000, 0.8660254037844387076, 1.000000000000000000, 0.8660254037844387076, 1.000000000000000000, 0.8660254037844387076, 1.000000000000000000, 0.8660254037844387076, 1.000000000000000000, 0.8660254037844387076, 1.000000000000000000, 0.8660254037844387076, 1.000000000000000000, 0.8660254037844387076, 1.000000000000000000, 0.8660254037844387076, 1.000000000000000000, 0.8660254037844387076, 1.000000000000000000, 0.8660254037844387076, 1.000000000000000000, 0.8660254037844387076, 1.000000000000000000, 0.8660254037844387076, 1.000000000000000000, 0.8660254037844387076, 1.000000000000000000, 0.8660254037844387076, 1.000000000000000000, 0.8660254037844387076, 1.000000000000000000, 0.8660254037844387076, 1.000000000000000000, 0.8660254037844387076, 1.000000000000000000, 0.8660254037844387076, 1.000000000000000000, 0.8660254037844387076, 1.000000000000000000, 0.8660254037844387076, 1.000000000000000000, 0.8660254037844387076, 1.000000000000000000, 0.8660254037844387076, 1.000000000000000000, 0.8660254037844387076, 1.000000000000000000, 0.8660254037844387076, 1.000000000000000000, 0.8660254037844387076, 1.000000000000000000, 0.8660254037844387076, 1.000000000000000000, 0.8660254037844387076, 1.000000000000000000, 0.8660254037844387076, 1.000000000000000000, 0.8660254037844387076, 1.000000000000000000, 0.8660254037844387076, 1.000000000000000000, 0.8660254037844387076, 1.000000000000000000, 0.8660254037844387076, 1.000000000000000000, 0.8660254037844387076, 1.000000000000000000, 0.8660254037844387076, 1.000000000000000000, 0.8660254037844387076, 1.000000000000000000, 0.8660254037844387076, 1.000000000000000000, 0.8660254037844387076, 1.000000000000000000, 0.8660254037844387076, 1.000000000000000000, 0.8660254037844387076, 1.000000000000000000, 0.8660254037844387076, 1.000000000000000000, 0.8660254037844387076, 1.000000000000000000, 0.8660254037844387076, 1.000000000000000000, 0.8660254037844387076, 1.000000000000000000, 0.8660254037844387076, 1.000000000000000000, 0.8660254037844387076, 1.000000000000000000, 0.8660254037844387076, 1.000000000000000000, 0.8660254037844387076, 1.000000000000000000, 0.8660254037844387076, 1.000000000000000000, 0.8660254037844387076, 1.000000000000000000, 0.8660254037844387076, 1.000000000000000000, 0.8660254037844387076, 1.000000000000000000, 0.8660254037844387076, 1.000000000000000000, 0.8660254037844387076, 1.000000000000000000, 0.8660254037844387076, 1.000000000000000000, 0.8660254037844387076, 1.000000000000000000, 0.8660254037844387076, 1.000000000000000000, 0.8660254037844387076, 1.000000000000000000, 0.8660254037844387076, 1.000000000000000000, 0.8660254037844387076, 1.000000000000000000, 0.8660254037844387076, 1.000000000000000000, 0.8660254037844387076, 1.000000000000000000, 0.8660254037844387076, 1.000000000000000000, 0.8660254037844387076, 1.000000000000000000, 0.8660254037844387076, 1.000000000000000000, 0.8660254037844387076, 1.000000000000000000, 0.8660254037844387076, 1.000000000000000000, 0.8660254037844387076, 1.000000000000000000, 0.8660254037844387076, 1.000000000000000000, 0.8660254037844387076, 1.000000000000000000, 0.8660254037844387076, 1.000000000000000000, 0.8660254037844387076, 1.000000000000000000, 0.8660254037844387076, 1.000000000000000000, 0.8660254037844387076, 1.000000000000000000, 0.8660254037844387076, 1.000000000000000000, 0.8660254037844387076, 1.000000000000000000, 0.8660254037844387076, 1.000000000000000000, 0.8660254037844387076, 1.000000000000000000, 0.8660254037844387076, 1.000000000000000000, 0.8660254037844387076, 1.000000000000000000, 0.8660254037844387076, 1.000000000000000000, 0.8660254037844387076, 1.000000000000000000, 0.8660254037844387076, 1.000000000000000000, 0.8660254037844387076, 1.000000000000000000, 0.8660254037844387076, 1.000000000000000000, 0.8660254037844387076, 1.000000000000000000, 0.8660254037844387076, 1.000000000000000000, 0.8660254037844387076, 1.000000000000000000, 0.8660254037844387076, 1.000000000000000000, 0.8660254037844387076, 1.000000000000000000, 0.8660254037844387076, 1.000000000000000000, 0.8660254037844387076, 1.000000000000000000, 0.8660254037844387076, 1.000000000000000000, 0.8660254037844387076, 1.000000000000000000, 0.8660254037844387076, 1.000000000000000000, 0.8660254037844387076, 1.000000000000000000, 0.8660254037844387076, 1.000000000000000000, 0.8660254037844387076, 1.000000000000000000, 0.8660254037844387076, 1.000000000000000000, 0.8660254037844387076, 1.000000000000000000, 0.8660254037844387076, 1.000000000000000000, 0.8660254037844387076, 1.000000000000000000, 0.8660254037844387076, 1.000000000000000000, 0.8660254037844387076, 1.000000000000000000, 0.8660254037844387076, 1.000000000000000000, 0.8660254037844387076, 1.000000000000000000, 0.8660254037844387076, 1.000000000000000000, 0.8660254037844387076, 1.000000000000000000, 0.8660254037844387076, 1.000000000000000000, 0.8660254037844387076, 1.000000000000000000, 0.8660254037844387076, 1.000000000000000000, 0.8660254037844387076, 1.000000000000000000, 0.8660254037844387076, 1.000000000000000000, 0.8660254037844387076, 1.000000000000000000, 0.8660254037844387076, 1.000000000000000000, 0.8660254037844387076, 1.000000000000000000, 0.8660254037844387076, 1.000000000000000000, 0.8660254037844387076, 1.000000000000000000, 0.8660254037844387076, 1.000000000000000000, 0.8660254037844387076, 1.000000000000000000, 0.8660254037844387076, 1.000000000000000000, 0.8660254037844387076, 1.000000000000000000, 0.8660254037844387076, 1.000000000000000000, 0.8660254037844387076, 1.000000000000000000, 0.8660254037844387076, 1.000000000000000000, 0.8660254037844387076, 1.000000000000000000, 0.8660254037844387076, 1.000000000000000000, 0.8660254037844387076, 1.000000000000000000, 0.8660254037844387076, 1.000000000000000000, 0.8660254037844387076, 1.000000000000000000, 0.8660254037844387076, 1.000000000000000000, 0.8660254037844387076, 1.000000000000000000, 0.8660254037844387076, 1.000000000000000000, 0.8660254037844387076, 1.000000000000000000, 0.8660254037844387076, 1.000000000000000000, 0.8660254037844387076, 1.000000000000000000, 0.8660254037844387076, 1.000000000000000000, 0.8660254037844387076, 1.000000000000000000, 0.8660254037844387076, 1.000000000000000000, 0.8660254037844387076, 1.000000000000000000, 0.8660254037844387076, 1.000000000000000000, 0.8660254037844387076, 1.000000000000000000, 0.8660254037844387076, 1.000000000000000000, 0.8660254037844387076, 1.000000000000000000, 0.8660254037844387076, 1.000000000000000000, 0.8660254037844387076, 1.000000000000000000, 0.8660254037844387076, 1.000000000000000000, 0.8660254037844387076, 1.000000000000000000) ) ) 
 REPRESENTATION_ITEM ( '' )  SURFACE ( )  );
#4289=CARTESIAN_POINT ( 'NONE',  ( -7.492852449846775897, 11.89341162479659531, 0.000000000000000000 ) ) ;
#4290=CARTESIAN_POINT ( 'NONE',  ( 7.637320603199683866, 7.804628880021436288, -0.7998128361456281477 ) ) ;
#4294=CARTESIAN_POINT ( 'NONE',  ( -10.64723070543352712, 11.31619066596094392, 0.7998128361456462443 ) ) ;
#4297=CARTESIAN_POINT ( 'NONE',  ( 1.364683531249986537, -0.5322916663252452718, -0.7879004041258309554 ) ) ;
#4301=CARTESIAN_POINT ( 'NONE',  ( 9.083599731475988648, 10.66024977721925104, 1.082531754730549967 ) ) ;
#4307=CARTESIAN_POINT ( 'NONE',  ( -0.5161058020549844638, 6.726351010739881175, -3.601801347653132090 ) ) ;
#4315=VERTEX_POINT ( 'NONE', #187828 ) ;
#4328=CARTESIAN_POINT ( 'NONE',  ( 0.7499999999999885647, -0.7354166659838470288, 1.299038105676657340 ) ) ;
#4332=CARTESIAN_POINT ( 'NONE',  ( 8.028399517586572998, 12.51821653715971472, -0.7998128361456352531 ) ) ;
#4334=CARTESIAN_POINT ( 'NONE',  ( 4.175484721775176489, 3.976419294354625933, -0.06592222766770190756 ) ) ;
#4337=CARTESIAN_POINT ( 'NONE',  ( 3.728655938958122196, 4.308852335994623139, -1.199719254218446718 ) ) ;
#4338=EDGE_CURVE ( 'NONE', #17872, #210292, #167413, .T. ) ;
#4343=CARTESIAN_POINT ( 'NONE',  ( 4.150767584078112193, 7.994312614733129152, 0.7998128361456321445 ) ) ;
#4344=CARTESIAN_POINT ( 'NONE',  ( 0.6823417656249899377, 3.238541667008085323, -1.181850606188754593 ) ) ;
#4345=CARTESIAN_POINT ( 'NONE',  ( -5.899175937014327076, 6.007822909898694164, -0.1935691424272238670 ) ) ;
#4348=CARTESIAN_POINT ( 'NONE',  ( -6.509886312855995172, 10.74661779830734254, -0.7998128361456291469 ) ) ;
#4349=CARTESIAN_POINT ( 'NONE',  ( -4.568734577680887199, 6.353276312092901890, -1.443375672974051449 ) ) ;
#4352=CARTESIAN_POINT ( 'NONE',  ( -4.882907879216086933, 8.848476292394087395, -0.7998128361456281477 ) ) ;
#4354=CARTESIAN_POINT ( 'NONE',  ( 0.7499999999999885647, 0.3479166673494848983, -1.299038105676652899 ) ) ;
#4362=CARTESIAN_POINT ( 'NONE',  ( -3.538314903042294457, 6.111489239315849531, 1.082531754730560403 ) ) ;
#4366=CARTESIAN_POINT ( 'NONE',  ( -3.917943204224921150, 5.594019709727598766, -1.443375672974051449 ) ) ;
#4368=CARTESIAN_POINT ( 'NONE',  ( 7.262363838414439776, 11.62450824479221900, 0.7998128361456462443 ) ) ;
#4382=CARTESIAN_POINT ( 'NONE',  ( 5.681030059326015014, 6.586622143090519188, -1.199719254218445830 ) ) ;
#4388=CARTESIAN_POINT ( 'NONE',  ( 2.679707916995359263, 6.278076336469897711, -0.7998128361456291469 ) ) ;
#4398=CARTESIAN_POINT ( 'NONE',  ( 8.392660782059197189, 9.750191319612612872, 1.199719254218462483 ) ) ;
#4400=CARTESIAN_POINT ( 'NONE',  ( -5.922214171070950606, 5.803671375871217286, -0.7998128361456291469 ) ) ;
#4401=CARTESIAN_POINT ( 'NONE',  ( -4.911285141672522059, 4.693790260148114513, 0.3511878651327460243 ) ) ;
#4402=CARTESIAN_POINT ( 'NONE',  ( 1.166320357434693644, 2.840374313856441013, 0.7750000000000117906 ) ) ;
#4407=CARTESIAN_POINT ( 'NONE',  ( -1.001543065824772872E-14, 5.571875000341416140, 1.575800808251672791 ) ) ;
#4409=ORIENTED_EDGE ( 'NONE', *, *, #182370, .F. ) ;
#4411=CARTESIAN_POINT ( 'NONE',  ( 4.487912541323413329, 5.194651705420806564, 1.199719254218462483 ) ) ;
#4412=CARTESIAN_POINT ( 'NONE',  ( -4.303823697334223652, 7.108545849276850959, -1.199719254218452047 ) ) ;
#4418=CARTESIAN_POINT ( 'NONE',  ( 6.507550544879468823, 6.694489845221929691, -0.7216878364870257245 ) ) ;
#4422=CARTESIAN_POINT ( 'NONE',  ( 8.893785580440313865, 9.478430720042945623, 1.040834085586084257E-14 ) ) ;
#4423=CARTESIAN_POINT ( 'NONE',  ( -1.364683531250012516, 3.801041667008087099, -0.7879004041258300672 ) ) ;
#4425=CARTESIAN_POINT ( 'NONE',  ( 5.490689023410166847, 5.508151403507724808, -0.7216878364870207285 ) ) ;
#4430=CARTESIAN_POINT ( 'NONE',  ( 5.374112064994988280, 6.309506852805883526, -1.073983825876674514 ) ) ;
#4433=CARTESIAN_POINT ( 'NONE',  ( -4.670247306389155639, 7.079074041166477649, 1.395957953274113983 ) ) ;
#4439=CARTESIAN_POINT ( 'NONE',  ( -9.667127221743832877, 11.23706883257798772, 1.199719254218462483 ) ) ;
#4449=CARTESIAN_POINT ( 'NONE',  ( 3.606105671554957759, 4.269840040644637291, -1.082531754730543083 ) ) ;
#4450=CARTESIAN_POINT ( 'NONE',  ( -1.201851678989727383E-14, 3.259375000341420581, -1.575800808251660134 ) ) ;
#4452=CARTESIAN_POINT ( 'NONE',  ( 7.287671262545424966, 8.461036880179857889, -1.199719254218451159 ) ) ;
#4453=CARTESIAN_POINT ( 'NONE',  ( -10.17947440576205054, 10.77047498301088346, 0.7998128361456462443 ) ) ;
#4459=CARTESIAN_POINT ( 'NONE',  ( 1.499999999999987121, 4.795833333333353821, -0.8660254037844323793 ) ) ;
#4460=CARTESIAN_POINT ( 'NONE',  ( 4.822949958159288286, 6.649860922651058992, -1.599625672291256295 ) ) ;
#4465=CARTESIAN_POINT ( 'NONE',  ( 8.107412671292031803, 11.44210330227398487, 1.082531754730557072 ) ) ;
#4471=CARTESIAN_POINT ( 'NONE',  ( -0.7500000000000215383, 3.972916667349481123, 1.299038105676671107 ) ) ;
#4473=CARTESIAN_POINT ( 'NONE',  ( -3.906720819032141190, 7.709591388846142479, -0.7998128361456281477 ) ) ;
#4474=CARTESIAN_POINT ( 'NONE',  ( 2.860407222358956503, 6.280966159486672140, 0.7216878364870338292 ) ) ;
#4483=CARTESIAN_POINT ( 'NONE',  ( 8.606728586576791074, 8.935604860628076906, 0.7998128361456462443 ) ) ;
#4484=CARTESIAN_POINT ( 'NONE',  ( 3.499976210622149253, 7.235056012367825140, 0.7998128361456321445 ) ) ;
#4485=CARTESIAN_POINT ( 'NONE',  ( -1.420000000000077423, 7.240846818246208905, 4.154462424328226433 ) ) ;
#4488=CARTESIAN_POINT ( 'NONE',  ( 5.529027716274630855, 5.344953845275508542, 1.040834085586084257E-14 ) ) ;
#4495=ORIENTED_EDGE ( 'NONE', *, *, #87710, .F. ) ;
#4496=CARTESIAN_POINT ( 'NONE',  ( 9.134442807305049428, 11.67993591332117376, 1.599625672291281386 ) ) ;
#4501=CARTESIAN_POINT ( 'NONE',  ( 5.096651299933133039, 6.508523278119453082, -1.213691435513279293 ) ) ;
#4507=CARTESIAN_POINT ( 'NONE',  ( -0.7500000000000215383, 3.191666666666689967, 1.299038105676671107 ) ) ;
#4509=CARTESIAN_POINT ( 'NONE',  ( 7.307481608085759639, 7.627742752295940676, 1.040834085586084257E-14 ) ) ;
#4510=CARTESIAN_POINT ( 'NONE',  ( -4.386226389220933441, 5.076017861301227008, -1.199719254218446718 ) ) ;
#4516=CARTESIAN_POINT ( 'NONE',  ( -5.416646063859567484, 6.278174148379618735, 1.199719254218450271 ) ) ;
#4522=ORIENTED_EDGE ( 'NONE', *, *, #24691, .F. ) ;
#4527=CARTESIAN_POINT ( 'NONE',  ( 8.235688245297327015, 11.69572115523387268, -1.199719254218446718 ) ) ;
#4528=CARTESIAN_POINT ( 'NONE',  ( 6.006184860439112150, 6.084034629330242971, -0.5924424362405518174 ) ) ;
#4530=AXIS2_PLACEMENT_3D ( 'NONE', #162845, #130413, #147660 ) ;
#4535=CARTESIAN_POINT ( 'NONE',  ( -9.869972641068651242, 11.57768483841065787, 1.082531754730558626 ) ) ;
#4539=CARTESIAN_POINT ( 'NONE',  ( 8.749089199520284410, 9.101692242395490240, 0.7998128361456481317 ) ) ;
#4543=CARTESIAN_POINT ( 'NONE',  ( 4.864678189204997949, 4.569879397027603929, 0.7998128361456341429 ) ) ;
#4545=CARTESIAN_POINT ( 'NONE',  ( -6.925517538482230506, 6.974191971184389160, 0.7998128361456341429 ) ) ;
#4546=CARTESIAN_POINT ( 'NONE',  ( 3.499976210622149253, 7.235056012367825140, 0.7998128361456321445 ) ) ;
#4551=CARTESIAN_POINT ( 'NONE',  ( 8.191097360950562845, 12.70803068775103739, -0.7998128361456352531 ) ) ;
#4555=CARTESIAN_POINT ( 'NONE',  ( 4.414360472080629094, 7.100309700288360837, -1.094782333960819809 ) ) ;
#4557=CARTESIAN_POINT ( 'NONE',  ( 6.046573322014824114, 7.117052299514516456, -1.082531754730543083 ) ) ;
#4564=CARTESIAN_POINT ( 'NONE',  ( 8.934460041281305109, 10.48625347199211966, -1.082531754730543083 ) ) ;
#4567=ORIENTED_EDGE ( 'NONE', *, *, #168015, .F. ) ;
#4570=CARTESIAN_POINT ( 'NONE',  ( -8.864333505236459132, 9.236143932397675727, 1.040834085586084257E-14 ) ) ;
#4578=AXIS2_PLACEMENT_3D ( 'NONE', #160731, #176983, #30744 ) ;
#4579=CARTESIAN_POINT ( 'NONE',  ( 10.55232363013785246, 11.20546574478267132, 0.000000000000000000 ) ) ;
#4583=CARTESIAN_POINT ( 'NONE',  ( 4.684505768721569652, 5.424010470718658716, -1.199719254218452047 ) ) ;
#4586=CARTESIAN_POINT ( 'NONE',  ( 1.499999999999989120, 2.285416667349482012, 0.8660254037844524744 ) ) ;
#4590=VERTEX_POINT ( 'NONE', #141275 ) ;
#4592=CARTESIAN_POINT ( 'NONE',  ( 1.499999999999987121, 1.795833333333355819, -0.8660254037844253849 ) ) ;
#4593=CARTESIAN_POINT ( 'NONE',  ( 8.776205506747620788, 9.133327934160710981, -0.7998128361456221525 ) ) ;
#4594=CARTESIAN_POINT ( 'NONE',  ( 4.270455198180219902, 6.965652916976816655, -1.082531754730548412 ) ) ;
#4598=CARTESIAN_POINT ( 'NONE',  ( 7.754900677336718395, 11.99120852362745460, -0.7216878364870267237 ) ) ;
#4603=CARTESIAN_POINT ( 'NONE',  ( -5.739179097286464248, 5.590130456455974617, -0.7998128361456221525 ) ) ;
#4604=CARTESIAN_POINT ( 'NONE',  ( -1.201851678989727383E-14, 3.368750000682815049, -1.732050807568863648 ) ) ;
#4606=CARTESIAN_POINT ( 'NONE',  ( 0.6823417656249899377, 4.988541667008086655, -1.181850606188754593 ) ) ;
#4611=CARTESIAN_POINT ( 'NONE',  ( -1.364683531250012516, 3.551041667008086211, -0.7879004041258300672 ) ) ;
#4614=EDGE_CURVE ( 'NONE', #59123, #6715, #158549, .T. ) ;
#4620=CARTESIAN_POINT ( 'NONE',  ( -7.181014916732457287, 11.52960116949655678, -0.7998128361456291469 ) ) ;
#4621=CARTESIAN_POINT ( 'NONE',  ( 7.156006149914539982, 7.243095351188763686, 1.040834085586084257E-14 ) ) ;
#4629=CARTESIAN_POINT ( 'NONE',  ( -5.696397096036042385, 9.797547045350714967, -0.7998128361456231517 ) ) ;
#4632=CARTESIAN_POINT ( 'NONE',  ( 10.22692794340986921, 10.82583744360002243, 0.000000000000000000 ) ) ;
#4634=CARTESIAN_POINT ( 'NONE',  ( 10.06423010004587759, 10.63602329300870153, 0.000000000000000000 ) ) ;
#4638=CARTESIAN_POINT ( 'NONE',  ( -3.730464822054482710, 7.503959392372201442, 1.040834085586084257E-14 ) ) ;
#4640=CARTESIAN_POINT ( 'NONE',  ( -6.984421689334302741, 11.30024240419870374, 0.000000000000000000 ) ) ;
#4644=CARTESIAN_POINT ( 'NONE',  ( -4.021356766390437265, 7.786759281977493785, -0.4705729632344165525 ) ) ;
#4651=CARTESIAN_POINT ( 'NONE',  ( 6.491656622844908853, 6.468020902940851968, 0.7998128361456341429 ) ) ;
#4664=ORIENTED_EDGE ( 'NONE', *, *, #12460, .T. ) ;
#4673=CARTESIAN_POINT ( 'NONE',  ( -9.508345801885592863, 9.987491611821676329, 0.7998128361456462443 ) ) ;
#4674=DIRECTION ( 'NONE',  ( -0.01538971728768980148, -0.9998815712882226370, 0.000000000000000000 ) ) ;
#4678=CARTESIAN_POINT ( 'NONE',  ( -1.500000000000013101, 1.702083334016151417, 0.8660254037844403729 ) ) ;
#4679=CARTESIAN_POINT ( 'NONE',  ( 10.56588178375152864, 11.22128359066528169, -0.7998128361456281477 ) ) ;
#4683=CARTESIAN_POINT ( 'NONE',  ( -9.561524646135538319, 12.17819805862340310, -1.599625672291263179 ) ) ;
#4685=CARTESIAN_POINT ( 'NONE',  ( -1.364683531250000748, 1.509375000341421691, 0.000000000000000000 ) ) ;
#4689=CARTESIAN_POINT ( 'NONE',  ( -4.277761160311629673, 4.949475094240346706, 1.199719254218462483 ) ) ;
#4691=CYLINDRICAL_SURFACE ( 'NONE', #142641, 0.07999999999999998779 ) ;
#4694=CARTESIAN_POINT ( 'NONE',  ( -0.6823417656250246877, 0.6135416670080897639, 1.181850606188755259 ) ) ;
#4699=CARTESIAN_POINT ( 'NONE',  ( 0.6823417656249882723, -0.07395833299191079124, -1.181850606188749264 ) ) ;
#4701=CIRCLE ( 'NONE', #32417, 0.08000000000000016820 ) ;
#4703=CARTESIAN_POINT ( 'NONE',  ( -7.250913225210214641, 7.353820272367037170, 0.7998128361456341429 ) ) ;
#4704=CARTESIAN_POINT ( 'NONE',  ( 7.076466111328892694, 10.34329533227067799, -1.199719254218441611 ) ) ;
#4706=CARTESIAN_POINT ( 'NONE',  ( 4.981731378017507872, 7.899438143407371271, -1.199719254218452047 ) ) ;
#4708=CARTESIAN_POINT ( 'NONE',  ( -1.201851678989727383E-14, 3.337500000000019007, -1.732050807568863648 ) ) ;
#4711=CARTESIAN_POINT ( 'NONE',  ( 1.364683531249986537, 1.176041667008082658, 0.7879004041258500513 ) ) ;
#4717=CARTESIAN_POINT ( 'NONE',  ( 6.155038550924150087, 7.243595066575396757, 1.082531754730558626 ) ) ;
#4720=CARTESIAN_POINT ( 'NONE',  ( -9.203287345578106127, 9.631590079462940324, 0.7998128361456462443 ) ) ;
#4721=CARTESIAN_POINT ( 'NONE',  ( -3.928111819657352566, 5.605883094398769195, 1.599625672291267398 ) ) ;
#4725=CARTESIAN_POINT ( 'NONE',  ( 6.938893903907228378E-15, 10.64264068711930733, 1.214306433183764966E-14 ) ) ;
#4726=CARTESIAN_POINT ( 'NONE',  ( -7.171900071504729191, 11.31104115015678779, -0.7216878364870267237 ) ) ;
#4728=CARTESIAN_POINT ( 'NONE',  ( -1.201851678989727383E-14, 4.837500000000018119, -1.732050807568863648 ) ) ;
#4732=CARTESIAN_POINT ( 'NONE',  ( 9.734391104931955141, 10.45913716528321125, 0.7216878364870438212 ) ) ;
#4738=CARTESIAN_POINT ( 'NONE',  ( -1.408440994509095656, 7.230285460703086642, -4.273713947604043994 ) ) ;
#4743=DIRECTION ( 'NONE',  ( -7.387867266669436732E-31, 1.000000000000000000, 8.546850786086424434E-32 ) ) ;
#4744=CARTESIAN_POINT ( 'NONE',  ( 6.588899466117086767, 10.63087377720454363, 1.040834085586084257E-14 ) ) ;
#4746=CARTESIAN_POINT ( 'NONE',  ( 7.124973419181436007, 8.271222729588529887, -1.199719254218446718 ) ) ;
#4747=CARTESIAN_POINT ( 'NONE',  ( -4.283486466913726254, 7.084819080452935403, -1.199719254218452047 ) ) ;
#4752=CARTESIAN_POINT ( 'NONE',  ( 4.202664430556257713, 4.965825259479493603, 1.082531754730560403 ) ) ;
#4754=CARTESIAN_POINT ( 'NONE',  ( -2.611917148927046295, 6.198987107056845858, 1.040834085586084257E-14 ) ) ;
#4768=CARTESIAN_POINT ( 'NONE',  ( 8.229962938695207342, 9.560377169021284871, 1.199719254218462483 ) ) ;
#4772=EDGE_CURVE ( 'NONE', #10129, #60515, #159749, .T. ) ;
#4780=CARTESIAN_POINT ( 'NONE',  ( -4.062639585589296942, 7.891496616496157301, 0.7998128361456341429 ) ) ;
#4782=CARTESIAN_POINT ( 'NONE',  ( -5.427341564172148303, 5.226320001155936090, 0.000000000000000000 ) ) ;
#4786=CARTESIAN_POINT ( 'NONE',  ( -4.865483722010302436, 4.987817560565853903, 0.6172052690934929364 ) ) ;
#4791=CARTESIAN_POINT ( 'NONE',  ( -4.600294193738529103, 4.261431402316699035, -0.7998128361456221525 ) ) ;
#4794=CARTESIAN_POINT ( 'NONE',  ( 7.070740804726770357, 8.207951346058097286, 1.199719254218462483 ) ) ;
#4795=CARTESIAN_POINT ( 'NONE',  ( -1.001543065824772872E-14, 4.321875000341417916, 1.575800808251672791 ) ) ;
#4801=CARTESIAN_POINT ( 'NONE',  ( 6.304178240230120522, 6.457222156464352381, -0.7216878364870257245 ) ) ;
#4803=CARTESIAN_POINT ( 'NONE',  ( -6.995117189646935962, 10.24838825697502109, 1.199719254218453823 ) ) ;
#4806=CARTESIAN_POINT ( 'NONE',  ( -5.994676475536691029, 10.14553965476814845, 0.7998128361456481317 ) ) ;
#4807=CARTESIAN_POINT ( 'NONE',  ( -4.466521540698216164, 7.298359999868178960, -1.199719254218452047 ) ) ;
#4815=CARTESIAN_POINT ( 'NONE',  ( 7.263417608619159083, 9.497073181520933716, -1.599625672291262513 ) ) ;
#4831=CARTESIAN_POINT ( 'NONE',  ( -1.402160292154681736E-14, -0.9906249996585834161, -1.575800808251665908 ) ) ;
#4832=CARTESIAN_POINT ( 'NONE',  ( 3.714044015139744914, 6.420469553383295391, 1.199719254218462483 ) ) ;
#4833=CARTESIAN_POINT ( 'NONE',  ( 5.575427483717746213, 7.527751369135936343, 1.599625672291267398 ) ) ;
#4835=CARTESIAN_POINT ( 'NONE',  ( -7.348156068926747331, 11.51667314714914347, 0.7216878364870458196 ) ) ;
#4837=CARTESIAN_POINT ( 'NONE',  ( 4.853455804012203778, 8.606189504748821051, 0.7216878364870438212 ) ) ;
#4838=CARTESIAN_POINT ( 'NONE',  ( -8.310784975052682100, 10.71900177569337487, -1.443375672974058777 ) ) ;
#4842=CARTESIAN_POINT ( 'NONE',  ( 8.586391356156291010, 8.911878091804165791, 0.7998128361456481317 ) ) ;
#4849=CARTESIAN_POINT ( 'NONE',  ( 1.364683531249988757, 2.134375000341422357, 1.214306433183764966E-14 ) ) ;
#4855=EDGE_CURVE ( 'NONE', #38245, #21699, #58544, .T. ) ;
#4856=CARTESIAN_POINT ( 'NONE',  ( 7.248805684800777804, 11.60869039890961218, 1.040834085586084257E-14 ) ) ;
#4859=CARTESIAN_POINT ( 'NONE',  ( -8.045874094706015001, 11.47427131287732927, -1.199719254218446718 ) ) ;
#4863=CARTESIAN_POINT ( 'NONE',  ( 5.299301323368958094, 6.361497809228795930, -1.122821758042211959 ) ) ;
#4865=CARTESIAN_POINT ( 'NONE',  ( 9.541187415715040032, 12.15447128979948310, -1.599625672291262513 ) ) ;
#4869=CARTESIAN_POINT ( 'NONE',  ( -8.992082194361570302, 11.51384853155376220, 1.599625672291269396 ) ) ;
#4871=CARTESIAN_POINT ( 'NONE',  ( -4.911894908834722351, 4.738238661368090909, 0.4458799699701230246 ) ) ;
#4874=CARTESIAN_POINT ( 'NONE',  ( 5.490683550995299811, 6.230756917952954055, 0.9772120879164881702 ) ) ;
#4876=CARTESIAN_POINT ( 'NONE',  ( -2.930533758848195447, 6.570706485298192234, -0.7998128361456281477 ) ) ;
#4880=CARTESIAN_POINT ( 'NONE',  ( 6.775324078527185989, 8.927630729746953264, -1.599625672291262513 ) ) ;
#4882=CARTESIAN_POINT ( 'NONE',  ( 6.474182045725470402, 7.511966127223233869, -1.199719254218446718 ) ) ;
#4884=CARTESIAN_POINT ( 'NONE',  ( 3.486418057008484617, 7.219238166485217434, 1.040834085586084257E-14 ) ) ;
#4886=CARTESIAN_POINT ( 'NONE',  ( -8.351459436338041442, 9.806086099558291025, -1.082531754730543971 ) ) ;
#4894=CARTESIAN_POINT ( 'NONE',  ( -5.603170282960403092, 6.190551086330195574, -0.8764620106105174280 ) ) ;
#4897=CARTESIAN_POINT ( 'NONE',  ( 4.039966587192250103, 7.657118751792200584, 0.7216878364870298324 ) ) ;
#4918=CARTESIAN_POINT ( 'NONE',  ( 6.286176778230493589, 10.48562334124426698, 0.7998128361456462443 ) ) ;
#4920=ORIENTED_EDGE ( 'NONE', *, *, #33691, .F. ) ;
#4922=CARTESIAN_POINT ( 'NONE',  ( -0.7500000000000215383, 1.722916667349486008, 1.299038105676659116 ) ) ;
#4923=PLANE ( 'NONE',  #80079 ) ;
#4924=CARTESIAN_POINT ( 'NONE',  ( -4.720210035852093533, 8.658662141802762946, -0.7998128361456281477 ) ) ;
#4928=CARTESIAN_POINT ( 'NONE',  ( -7.974166903131914452, 12.45494515362926435, -0.7998128361456281477 ) ) ;
#4929=CARTESIAN_POINT ( 'NONE',  ( -1.500000000000079936, 7.240846818246208905, 4.154462424328226433 ) ) ;
#4932=CARTESIAN_POINT ( 'NONE',  ( 5.913327553854682783, 10.05063257947248800, -0.7998128361456291469 ) ) ;
#4934=CARTESIAN_POINT ( 'NONE',  ( -7.226659571283968297, 8.389856573708110332, 1.199719254218450271 ) ) ;
#4936=CARTESIAN_POINT ( 'NONE',  ( 7.747594715205354809, 11.12627870345989756, -1.199719254218446718 ) ) ;
#4939=CARTESIAN_POINT ( 'NONE',  ( -1.499999999998184563, 8.627523663849279600, 2.580000000000257643 ) ) ;
#4943=CARTESIAN_POINT ( 'NONE',  ( -6.887178846062116833, 9.058127958537705027, -1.443375672974059665 ) ) ;
#4946=CARTESIAN_POINT ( 'NONE',  ( 0.6823417656249917140, 4.405208333674755394, 1.181850606188765695 ) ) ;
#4955=CARTESIAN_POINT ( 'NONE',  ( -3.077337680177623103, 6.534051693608437184, 0.7216878364870317197 ) ) ;
#4957=CARTESIAN_POINT ( 'NONE',  ( 2.833290915131624566, 6.249330467721451399, -0.7216878364870267237 ) ) ;
#4958=CARTESIAN_POINT ( 'NONE',  ( 0.6823417656249917140, 5.655208333674749177, 1.181850606188765695 ) ) ;
#4959=CARTESIAN_POINT ( 'NONE',  ( 8.283668668269706714, 8.766627655843896250, 1.040834085586084257E-14 ) ) ;
#4963=CARTESIAN_POINT ( 'NONE',  ( 1.364683531249986537, 0.6135416670080880985, 0.7879004041258500513 ) ) ;
#4964=CARTESIAN_POINT ( 'NONE',  ( -4.311129659465605002, 4.131998812239033647, 0.7216878364870317197 ) ) ;
#4965=CARTESIAN_POINT ( 'NONE',  ( 4.822949958159288286, 6.649860922651058992, -1.599625672291256295 ) ) ;
#4971=CARTESIAN_POINT ( 'NONE',  ( 3.307826292054301121, 4.882216645528547616, -1.443375672974057666 ) ) ;
#4974=CARTESIAN_POINT ( 'NONE',  ( -7.537970219518066450, 11.73812298950569044, -0.7216878364870267237 ) ) ;
#4979=CARTESIAN_POINT ( 'NONE',  ( -7.971304249830880373, 11.38727316052296601, 1.199719254218453823 ) ) ;
#4981=CARTESIAN_POINT ( 'NONE',  ( -4.568734577680875653, 8.274014740695587733, -0.7216878364870257245 ) ) ;
#4982=CARTESIAN_POINT ( 'NONE',  ( -0.6823417656250212460, 1.613541667008083769, 1.181850606188755259 ) ) ;
#5000=ORIENTED_EDGE ( 'NONE', *, *, #203502, .F. ) ;
#5002=EDGE_CURVE ( 'NONE', #213175, #71915, #22342, .T. ) ;
#5009=AXIS2_PLACEMENT_3D ( 'NONE', #84193, #213107, #67910 ) ;
#5010=CARTESIAN_POINT ( 'NONE',  ( 0.6823417656249882723, 2.988541667008084879, -1.181850606188754593 ) ) ;
#5012=B_SPLINE_CURVE_WITH_KNOTS ( 'NONE', 3,
 ( #205696, #87693, #55201, #187322, #71419 ),
 .UNSPECIFIED., .F., .F.,
 ( 4, 1, 4 ),
 ( 0.003096135707997031087, 0.003151720136792417887, 0.003207304565587804253 ),
 .UNSPECIFIED. ) ;
#5021=CARTESIAN_POINT ( 'NONE',  ( -1.201851678989727383E-14, 1.071875000341418138, 1.575800808251672791 ) ) ;
#5023=EDGE_LOOP ( 'NONE', ( #156828, #125984, #201892, #90334 ) ) ;
#5029=ORIENTED_EDGE ( 'NONE', *, *, #163609, .T. ) ;
#5031=CARTESIAN_POINT ( 'NONE',  ( 3.994848817520957773, 7.812407387083109001, 1.040834085586084257E-14 ) ) ;
#5041=CARTESIAN_POINT ( 'NONE',  ( -3.623053363349869382, 5.249981562040033189, 1.599625672291267398 ) ) ;
#5042=CARTESIAN_POINT ( 'NONE',  ( 7.639129486296027061, 10.99973593639901814, 1.199719254218460707 ) ) ;
#5054=CARTESIAN_POINT ( 'NONE',  ( -6.399085315970132193, 10.40942393536641397, -0.7216878364870278340 ) ) ;
#5058=CARTESIAN_POINT ( 'NONE',  ( -9.459838494033043332, 12.05956421450382088, 1.599625672291281386 ) ) ;
#5063=CARTESIAN_POINT ( 'NONE',  ( -4.135400547368138113, 4.783387712472935149, 1.199719254218462483 ) ) ;
#5065=CARTESIAN_POINT ( 'NONE',  ( 8.550388431712704573, 13.12720360364021133, 0.000000000000000000 ) ) ;
#5067=CARTESIAN_POINT ( 'NONE',  ( 5.203632029546647608, 4.965325544092860532, 1.040834085586084257E-14 ) ) ;
#5073=CARTESIAN_POINT ( 'NONE',  ( 4.528060117284244512, 4.385084346360807572, 0.7216878364870317197 ) ) ;
#5075=CARTESIAN_POINT ( 'NONE',  ( -3.581325132304157943, 7.329963087663487364, -0.7998128361456281477 ) ) ;
#5078=CARTESIAN_POINT ( 'NONE',  ( -8.622095623286845978, 12.14652976288826913, 1.199719254218462483 ) ) ;
#5084=CARTESIAN_POINT ( 'NONE',  ( 9.246297574839983824, 9.889694713509232571, 0.7216878364870438212 ) ) ;
#5085=CARTESIAN_POINT ( 'NONE',  ( -1.364683531249997417, 3.571875000341423245, 1.214306433183764966E-14 ) ) ;
#5087=CARTESIAN_POINT ( 'NONE',  ( 5.820528018968444961, 5.685037531751635953, 0.7998128361456341429 ) ) ;
#5096=DIRECTION ( 'NONE',  ( 1.000000000000000000, 0.000000000000000000, 0.000000000000000000 ) ) ;
#5100=CARTESIAN_POINT ( 'NONE',  ( -1.402160292154681736E-14, 2.259375000341416140, -1.575800808251660134 ) ) ;
#5102=CARTESIAN_POINT ( 'NONE',  ( 2.205172540517054802, 5.724451730578533848, 1.040834085586084257E-14 ) ) ;
#5104=CARTESIAN_POINT ( 'NONE',  ( -4.934804725694231564, 5.819988937140460727, -1.082531754730544860 ) ) ;
#5105=DIRECTION ( 'NONE',  ( 0.7592566023653005702, 0.6507913734559639396, 0.000000000000000000 ) ) ;
#5107=CARTESIAN_POINT ( 'NONE',  ( -4.067082893975237035, 7.688754443039000464, 1.040834085586084257E-14 ) ) ;
#5111=CARTESIAN_POINT ( 'NONE',  ( 4.137209430464448445, 7.978494768850520558, 1.040834085586084257E-14 ) ) ;
#5123=CARTESIAN_POINT ( 'NONE',  ( 5.494078562035752178, 7.432844293840273231, -1.599625672291262513 ) ) ;
#5126=CARTESIAN_POINT ( 'NONE',  ( -2.117044542028253318, 5.621635732341564662, -0.7998128361456281477 ) ) ;
#5128=CARTESIAN_POINT ( 'NONE',  ( -5.117312914154178216, 8.057616602233474978, -1.199719254218452047 ) ) ;
#5132=CARTESIAN_POINT ( 'NONE',  ( 5.777746017718023097, 9.892454120646377191, 0.7998128361456462443 ) ) ;
#5134=CARTESIAN_POINT ( 'NONE',  ( -7.335124800193271177, 8.516399340768996851, -1.199719254218452935 ) ) ;
#5135=CARTESIAN_POINT ( 'NONE',  ( 6.765155463094759014, 7.955398130774449683, 1.082531754730558626 ) ) ;
#5136=CARTESIAN_POINT ( 'NONE',  ( 4.765179230921094522, 7.000095391635957398, 1.399907146243694722 ) ) ;
#5137=CARTESIAN_POINT ( 'NONE',  ( -4.249591082879585535, 7.045274465746411252, 1.199719254218464037 ) ) ;
#5140=CARTESIAN_POINT ( 'NONE',  ( -6.226218857173722476, 8.287007971501239467, 1.599625672291283607 ) ) ;
#5144=CARTESIAN_POINT ( 'NONE',  ( 1.364683531249988535, 1.613541667008084879, 0.7879004041258500513 ) ) ;
#5146=CARTESIAN_POINT ( 'NONE',  ( -4.555176424511596878, 7.297827681030051750, 1.082531754730560403 ) ) ;
#5152=CARTESIAN_POINT ( 'NONE',  ( 6.830610463186557624, 6.863467050006115677, 1.040834085586084257E-14 ) ) ;
#5155=CARTESIAN_POINT ( 'NONE',  ( -5.911504460181634002, 6.000493611234613667, 0.05175081109743372154 ) ) ;
#5156=CARTESIAN_POINT ( 'NONE',  ( 1.364683531249988535, 1.926041667008086211, 0.7879004041258500513 ) ) ;
#5158=DIRECTION ( 'NONE',  ( -5.578564026256490882E-16, -1.000000000000000000, -9.066213480720158442E-32 ) ) ;
#5159=CARTESIAN_POINT ( 'NONE',  ( -0.4963857527936129665, 7.354535952643655783, 1.939768365030048125 ) ) ;
#5164=CARTESIAN_POINT ( 'NONE',  ( -5.610376637956639101, 5.439860920571172542, 0.000000000000000000 ) ) ;
#5166=CARTESIAN_POINT ( 'NONE',  ( -7.985389288324710400, 8.418635045908049008, -0.7216878364870267237 ) ) ;
#5175=CARTESIAN_POINT ( 'NONE',  ( -7.171900071504729191, 11.31104115015678779, -0.7216878364870267237 ) ) ;
#5179=CARTESIAN_POINT ( 'NONE',  ( -6.277061933002790362, 8.346324893301817482, 1.443375672974078761 ) ) ;
#5182=ORIENTED_EDGE ( 'NONE', *, *, #52572, .T. ) ;
#5185=CARTESIAN_POINT ( 'NONE',  ( -0.7500000000000215383, 5.222916667349482012, 1.299038105676671107 ) ) ;
#5193=CARTESIAN_POINT ( 'NONE',  ( -4.394814349124112951, 8.279033840620114049, -0.7998128361456281477 ) ) ;
#5196=CARTESIAN_POINT ( 'NONE',  ( 4.708759422647839976, 4.387974169377582001, -0.7998128361456211532 ) ) ;
#5200=CARTESIAN_POINT ( 'NONE',  ( 5.849453209292126310, 8.911780279894442103, 1.199719254218462483 ) ) ;
#5206=CARTESIAN_POINT ( 'NONE',  ( -3.958617665510266725, 7.562211676496538360, -0.7216878364870267237 ) ) ;
#5213=CARTESIAN_POINT ( 'NONE',  ( -1.364683531250014514, 0.7385416670080887647, -0.7879004041258289570 ) ) ;
#5214=CARTESIAN_POINT ( 'NONE',  ( 2.280903940472752467, 5.594607745005274246, -0.6109567437776646237 ) ) ;
#5215=CARTESIAN_POINT ( 'NONE',  ( -7.330154606482786050, 11.70359747420527619, 0.000000000000000000 ) ) ;
#5217=CARTESIAN_POINT ( 'NONE',  ( 7.202405917357655341, 9.425892875049191488, 1.599625672291281386 ) ) ;
#5219=CARTESIAN_POINT ( 'NONE',  ( -8.552495972122143186, 8.872333477097637200, 0.7998128361456462443 ) ) ;
#5222=CARTESIAN_POINT ( 'NONE',  ( -1.364683531249997417, 4.509375000341424133, 1.214306433183764966E-14 ) ) ;
#5225=CARTESIAN_POINT ( 'NONE',  ( 9.083599731475988648, 10.66024977721925104, 1.082531754730549967 ) ) ;
#5228=CARTESIAN_POINT ( 'NONE',  ( -1.402160292154681736E-14, -0.6156249996585817508, 1.575800808251672791 ) ) ;
#5230=CARTESIAN_POINT ( 'NONE',  ( 8.744645890689993095, 9.304434415334227992, -0.7216878364870197293 ) ) ;
#5233=CARTESIAN_POINT ( 'NONE',  ( -4.880572111239580124, 7.677455982212699759, 1.082531754730560403 ) ) ;
#5235=CARTESIAN_POINT ( 'NONE',  ( -1.364683531250012516, 2.988541667008091096, -0.7879004041258289570 ) ) ;
#5239=CARTESIAN_POINT ( 'NONE',  ( -6.742482464697739708, 6.760651051769146491, 0.7998128361456341429 ) ) ;
#5247=CARTESIAN_POINT ( 'NONE',  ( 6.774270308322468459, 11.05506579301824743, 0.7998128361456462443 ) ) ;
#5253=EDGE_LOOP ( 'NONE', ( #32865, #102273, #31606, #108392, #176513 ) ) ;
#5254=CARTESIAN_POINT ( 'NONE',  ( 6.317736394288135493, 8.393778431468064127, 1.443375672974076540 ) ) ;
#5263=CARTESIAN_POINT ( 'NONE',  ( 1.499999999999989120, 0.5250000000000185629, 0.000000000000000000 ) ) ;
#5264=CARTESIAN_POINT ( 'NONE',  ( 7.588813295347141441, 9.876701482703580837, -1.599625672291262513 ) ) ;
#5265=CARTESIAN_POINT ( 'NONE',  ( -9.450196763925152510, 10.98398329845622001, -1.199719254218441611 ) ) ;
#5267=CARTESIAN_POINT ( 'NONE',  ( -1.364683531250000748, -0.7406249996585803075, 0.000000000000000000 ) ) ;
#5268=CARTESIAN_POINT ( 'NONE',  ( -1.500000000000001332, 1.400000000000019229, 0.000000000000000000 ) ) ;
#5270=CARTESIAN_POINT ( 'NONE',  ( 4.904298879841284098, 6.744767997946721216, 1.599625672291267398 ) ) ;
#5278=CARTESIAN_POINT ( 'NONE',  ( -1.201851678989727383E-14, 5.196875000341422357, -1.575800808251660134 ) ) ;
#5280=CARTESIAN_POINT ( 'NONE',  ( -7.914208982075130905, 10.25632978388623684, -1.599625672291263179 ) ) ;
#5281=CARTESIAN_POINT ( 'NONE',  ( -6.399085315970155285, 6.567947078161039620, -0.7216878364870278340 ) ) ;
#5288=CARTESIAN_POINT ( 'NONE',  ( 8.450809820019639318, 8.753699632978056755, -0.7998128361456291469 ) ) ;
#5292=CARTESIAN_POINT ( 'NONE',  ( 7.917598520256366790, 8.339545816494993602, 1.040834085586084257E-14 ) ) ;
#5295=CARTESIAN_POINT ( 'NONE',  ( -6.984421689334302741, 11.30024240419870374, 0.000000000000000000 ) ) ;
#5296=CARTESIAN_POINT ( 'NONE',  ( 6.681470773436232413, 6.689470745297396270, -0.7998128361456281477 ) ) ;
#5299=CARTESIAN_POINT ( 'NONE',  ( 2.737856954955798727, 5.281584649835344258, 1.199719254218452047 ) ) ;
#5305=CARTESIAN_POINT ( 'NONE',  ( -4.609409038966234995, 7.361099064560491456, -1.082531754730549967 ) ) ;
#5307=CARTESIAN_POINT ( 'NONE',  ( 9.490344339885973923, 12.09515436799890331, -1.443375672974057666 ) ) ;
#5310=CARTESIAN_POINT ( 'NONE',  ( -7.043624497499477499, 8.176315654292865887, 1.199719254218450271 ) ) ;
#5315=CARTESIAN_POINT ( 'NONE',  ( -6.496328159242330536, 10.73079995242472862, 0.000000000000000000 ) ) ;
#5320=ORIENTED_EDGE ( 'NONE', *, *, #70130, .T. ) ;
#5331=CARTESIAN_POINT ( 'NONE',  ( -7.881367368245678406, 8.089350105908421185, 0.7998128361456602331 ) ) ;
#5334=CARTESIAN_POINT ( 'NONE',  ( 5.748293942514166588, 7.729428904398431222, -1.443375672974057666 ) ) ;
#5335=ORIENTED_EDGE ( 'NONE', *, *, #197116, .T. ) ;
#5339=CARTESIAN_POINT ( 'NONE',  ( -4.843287188579803448, 6.673587691474970107, -1.599625672291256295 ) ) ;
#5342=CARTESIAN_POINT ( 'NONE',  ( -6.126860945727902852, 6.002842251083519542, -0.2255282439200041456 ) ) ;
#5344=CARTESIAN_POINT ( 'NONE',  ( -6.287230548435221777, 8.358188277972981695, -1.599625672291263179 ) ) ;
#5345=CARTESIAN_POINT ( 'NONE',  ( -5.913158477246164502, 5.999510931274985026, -0.08576477159101922321 ) ) ;
#5350=CARTESIAN_POINT ( 'NONE',  ( -9.667127221743832877, 11.23706883257798772, 1.199719254218462483 ) ) ;
#5351=CARTESIAN_POINT ( 'NONE',  ( 5.926885707468349196, 10.06645042535509660, 1.040834085586084257E-14 ) ) ;
#5354=CARTESIAN_POINT ( 'NONE',  ( -9.646789991323334590, 11.21334206375407305, 1.199719254218462483 ) ) ;
#5362=CARTESIAN_POINT ( 'NONE',  ( 8.242994207428692377, 12.56065097540143327, -0.7216878364870328300 ) ) ;
#5369=ORIENTED_EDGE ( 'NONE', *, *, #11637, .F. ) ;
#5386=CARTESIAN_POINT ( 'NONE',  ( -3.704402285031864306, 5.344888637335695414, -1.599625672291256295 ) ) ;
#5393=CARTESIAN_POINT ( 'NONE',  ( 0.7499999999999867883, -0.6520833326505159899, -1.299038105676652899 ) ) ;
#5398=VERTEX_POINT ( 'NONE', #94559 ) ;
#5399=CARTESIAN_POINT ( 'NONE',  ( 1.483013432599449732, 7.294277089886982424, -4.259227663826814059 ) ) ;
#5401=CARTESIAN_POINT ( 'NONE',  ( -3.633221978782290140, 6.222214161012547429, -1.082531754730549967 ) ) ;
#5402=CARTESIAN_POINT ( 'NONE',  ( 3.785751206713845018, 5.439795712631356750, 1.599625672291267398 ) ) ;
#5403=LINE ( 'NONE', #55263, #76976 ) ;
#5404=DIRECTION ( 'NONE',  ( 1.000000000000000000, 0.000000000000000000, 0.000000000000000000 ) ) ;
#5407=CARTESIAN_POINT ( 'NONE',  ( 4.798696304233017074, 7.685897223992134819, -1.199719254218452047 ) ) ;
#5408=CARTESIAN_POINT ( 'NONE',  ( -1.364683531250012516, 2.801041667008090652, -0.7879004041258289570 ) ) ;
#5409=CARTESIAN_POINT ( 'NONE',  ( -4.361599125657974696, 7.193191237876310318, 1.033186747995703758 ) ) ;
#5410=CARTESIAN_POINT ( 'NONE',  ( 4.371348721082305211, 3.994328350884451151, -0.09103173162486978554 ) ) ;
#5412=CARTESIAN_POINT ( 'NONE',  ( -8.616370316684697883, 10.01118577667568132, -1.199719254218446718 ) ) ;
#5414=CARTESIAN_POINT ( 'NONE',  ( -3.267151830768946663, 6.755501535964989479, -0.7216878364870257245 ) ) ;
#5417=CARTESIAN_POINT ( 'NONE',  ( -6.175902666224832416, 7.163973517805802160, -1.199719254218446718 ) ) ;
#5419=CARTESIAN_POINT ( 'NONE',  ( -0.6823417656249969321, 5.467708333674756283, -1.181850606188749264 ) ) ;
#5427=CARTESIAN_POINT ( 'NONE',  ( -5.870317324592821073, 6.911420302522161663, -1.082531754730543083 ) ) ;
#5431=CARTESIAN_POINT ( 'NONE',  ( -4.907688418022547516, 4.827984030555475314, 1.214306433183764966E-14 ) ) ;
#5433=CARTESIAN_POINT ( 'NONE',  ( 9.745613490124728884, 10.26430391476735338, 0.7998128361456462443 ) ) ;
#5443=CARTESIAN_POINT ( 'NONE',  ( -2.819205876637805641, 5.376491725131008259, -1.199719254218446718 ) ) ;
#5444=CARTESIAN_POINT ( 'NONE',  ( -10.13202086811422475, 10.71511252242175161, -0.7998128361456291469 ) ) ;
#5449=CARTESIAN_POINT ( 'NONE',  ( 6.226218857173709154, 8.287007971501239467, 1.599625672291281386 ) ) ;
#5453=DIRECTION ( 'NONE',  ( -1.000000000000000000, 5.782411586589355667E-16, 0.000000000000000000 ) ) ;
#5454=CARTESIAN_POINT ( 'NONE',  ( 2.706824224222692088, 6.309712028235118453, 0.7998128361456362523 ) ) ;
#5464=CARTESIAN_POINT ( 'NONE',  ( 7.747594715205354809, 11.12627870345989756, -1.199719254218446718 ) ) ;
#5465=CARTESIAN_POINT ( 'NONE',  ( -5.870844209917351009, 6.808071985447069707, -1.199719254218446718 ) ) ;
#5472=AXIS2_PLACEMENT_3D ( 'NONE', #139402, #59195, #174049 ) ;
#5473=CARTESIAN_POINT ( 'NONE',  ( -1.364683531249997417, 4.509375000341424133, 1.214306433183764966E-14 ) ) ;
#5478=CARTESIAN_POINT ( 'NONE',  ( 3.167801447087334576, 6.847518788243868393, -0.7998128361456291469 ) ) ;
#5479=CARTESIAN_POINT ( 'NONE',  ( -5.447678794592645701, 5.250046769979851646, 0.000000000000000000 ) ) ;
#5485=CARTESIAN_POINT ( 'NONE',  ( 6.805829924380118356, 7.042482454639357847, 0.7216878364870317197 ) ) ;
#5487=CARTESIAN_POINT ( 'NONE',  ( 7.253248993186724114, 9.485209796849769504, 1.443375672974076540 ) ) ;
#5488=CARTESIAN_POINT ( 'NONE',  ( -0.6823417656249969321, 4.030208333674754506, -1.181850606188749264 ) ) ;
#5490=CARTESIAN_POINT ( 'NONE',  ( 4.406036734316882253, 6.163462161501577441, -1.443375672974051449 ) ) ;
#5494=CARTESIAN_POINT ( 'NONE',  ( 4.161361007603033180, 7.399433999391101580, -0.7812420967184935394 ) ) ;
#5497=CARTESIAN_POINT ( 'NONE',  ( -4.201283080389795366, 7.561618497949153195, 0.9685097419542560981 ) ) ;
#5502=VECTOR ( 'NONE', #213164, 1000.000000000000000 ) ;
#5504=CARTESIAN_POINT ( 'NONE',  ( -9.022061154889962964, 12.61315621642528129, -1.199719254218446718 ) ) ;
#5513=CARTESIAN_POINT ( 'NONE',  ( 4.365362273920252889, 4.195270195769483124, 0.7216878364870317197 ) ) ;
#5514=EDGE_CURVE ( 'NONE', #6079, #59123, #30565, .T. ) ;
#5515=CARTESIAN_POINT ( 'NONE',  ( -1.364683531250012516, 3.092708333674755838, 0.7879004041258379498 ) ) ;
#5517=CARTESIAN_POINT ( 'NONE',  ( 7.450369105909416589, 8.650851030771185890, -1.199719254218441611 ) ) ;
#5523=CARTESIAN_POINT ( 'NONE',  ( 1.499999999999989120, 5.004166666666691299, 0.8660254037844524744 ) ) ;
#5524=CARTESIAN_POINT ( 'NONE',  ( 4.741601036477289810, 6.554953847355395880, 1.599625672291267398 ) ) ;
#5527=CARTESIAN_POINT ( 'NONE',  ( 0.6823417656249899377, 2.905208333674754062, 1.181850606188765695 ) ) ;
#5528=CARTESIAN_POINT ( 'NONE',  ( 1.364683531249988535, 3.655208333674750509, -0.7879004041258239610 ) ) ;
#5531=CARTESIAN_POINT ( 'NONE',  ( 10.39874063200158893, 11.23421161353111586, 0.000000000000000000 ) ) ;
#5536=CARTESIAN_POINT ( 'NONE',  ( -1.201851678989727383E-14, 2.243750000682818158, 1.732050807568877637 ) ) ;
#5538=CARTESIAN_POINT ( 'NONE',  ( -5.530836599371015794, 8.540060901653093950, 1.199719254218452047 ) ) ;
#5539=CARTESIAN_POINT ( 'NONE',  ( 5.463572716182834910, 5.476515711742504067, 0.7216878364870317197 ) ) ;
#5547=CARTESIAN_POINT ( 'NONE',  ( 7.039708073993665494, 9.236078724457858158, 1.599625672291281386 ) ) ;
#5548=CARTESIAN_POINT ( 'NONE',  ( 4.147904930777053245, 6.926640621626830807, -1.199719254218452047 ) ) ;
#5549=DIRECTION ( 'NONE',  ( 1.000000000000000000, 0.000000000000000000, 0.000000000000000000 ) ) ;
#5552=CARTESIAN_POINT ( 'NONE',  ( 4.599240423533799138, 6.388866465587984322, 1.599625672291267398 ) ) ;
#5554=VERTEX_POINT ( 'NONE', #31681 ) ;
#5560=CARTESIAN_POINT ( 'NONE',  ( 10.22692794340986921, 10.82583744360002243, 0.000000000000000000 ) ) ;
#5566=CARTESIAN_POINT ( 'NONE',  ( 5.421662447778366811, 6.277071961296246450, 1.037714289653376198 ) ) ;
#5572=CARTESIAN_POINT ( 'NONE',  ( 1.084637062511528693, 3.242628807292008197, 1.105835307554807301 ) ) ;
#5574=CARTESIAN_POINT ( 'NONE',  ( 7.632877294813741109, 8.007371053478589573, 1.040834085586084257E-14 ) ) ;
#5575=CARTESIAN_POINT ( 'NONE',  ( -3.090368948911150770, 5.692848642783215674, 1.199719254218462483 ) ) ;
#5580=CARTESIAN_POINT ( 'NONE',  ( -4.229253852459088137, 7.021547696922494808, 1.199719254218464037 ) ) ;
#5588=CARTESIAN_POINT ( 'NONE',  ( -1.201851678989727383E-14, 3.243750000682814161, 1.732050807568877637 ) ) ;
#5593=CARTESIAN_POINT ( 'NONE',  ( 9.073431116043567002, 11.60875560684942265, -1.599625672291262513 ) ) ;
#5600=CARTESIAN_POINT ( 'NONE',  ( -9.815740026613960723, 11.51441345488021106, -1.082531754730539753 ) ) ;
#5604=CARTESIAN_POINT ( 'NONE',  ( 8.320953590485093088, 10.73086516036454618, 1.599625672291281386 ) ) ;
#5608=CARTESIAN_POINT ( 'NONE',  ( -6.847031270101295419, 7.946956888995021728, -1.199719254218446718 ) ) ;
#5609=CARTESIAN_POINT ( 'NONE',  ( 3.714044015139744914, 6.420469553383295391, 1.199719254218462483 ) ) ;
#5611=AXIS2_PLACEMENT_3D ( 'NONE', #38582, #22291, #88404 ) ;
#5614=CARTESIAN_POINT ( 'NONE',  ( 10.40318394038753702, 11.03146944007395724, -0.7998128361456281477 ) ) ;
#5615=FACE_OUTER_BOUND ( 'NONE', #172724, .T. ) ;
#5616=ORIENTED_EDGE ( 'NONE', *, *, #174895, .T. ) ;
#5619=CARTESIAN_POINT ( 'NONE',  ( 1.364683531249986537, 2.717708333674754062, -0.7879004041258239610 ) ) ;
#5622=CARTESIAN_POINT ( 'NONE',  ( 7.158341918335438869, 7.453746447587225710, -0.7216878364870257245 ) ) ;
#5629=CARTESIAN_POINT ( 'NONE',  ( 8.744645890689993095, 9.304434415334227992, -0.7216878364870197293 ) ) ;
#5630=ORIENTED_EDGE ( 'NONE', *, *, #14825, .T. ) ;
#5633=CARTESIAN_POINT ( 'NONE',  ( -9.352427035328430449, 9.805586384171650849, 1.040834085586084257E-14 ) ) ;
#5639=ADVANCED_FACE ( 'NONE', ( #29543 ), #18874, .T. ) ;
#5643=CARTESIAN_POINT ( 'NONE',  ( 4.379447312414087357, 5.068108938359919158, -1.199719254218452047 ) ) ;
#5647=CARTESIAN_POINT ( 'NONE',  ( 4.497554271431305040, 6.270232621468402989, -1.599625672291256295 ) ) ;
#5650=AXIS2_PLACEMENT_3D ( 'NONE', #135606, #134562, #118340 ) ;
#5651=CARTESIAN_POINT ( 'NONE',  ( -1.499999999999997780, 3.431250000682818602, 1.214306433183764966E-14 ) ) ;
#5657=CARTESIAN_POINT ( 'NONE',  ( -1.500000000000001332, -0.09999999999997510880, 0.000000000000000000 ) ) ;
#5658=CARTESIAN_POINT ( 'NONE',  ( 6.642605195691581699, 9.837124264027149678, 1.199719254218462483 ) ) ;
#5659=CARTESIAN_POINT ( 'NONE',  ( 6.168596704093459060, 7.259412911939593371, -1.082531754730543083 ) ) ;
#5662=VECTOR ( 'NONE', #18240, 1000.000000000000000 ) ;
#5664=CARTESIAN_POINT ( 'NONE',  ( 10.07334494527360569, 10.85458331234846696, 0.000000000000000000 ) ) ;
#5669=CARTESIAN_POINT ( 'NONE',  ( -5.915435094264120508, 5.795762452929912101, 0.000000000000000000 ) ) ;
#5671=CARTESIAN_POINT ( 'NONE',  ( 1.499999999999987121, 2.327083334016154303, -0.8660254037844262731 ) ) ;
#5672=CARTESIAN_POINT ( 'NONE',  ( 1.364683531249986537, -1.136458332991912235, 0.7879004041258500513 ) ) ;
#5677=CARTESIAN_POINT ( 'NONE',  ( 0.6823417656249917140, 4.155208333674755394, 1.181850606188765695 ) ) ;
#5687=CARTESIAN_POINT ( 'NONE',  ( -7.018317073368468328, 11.33978701890523233, -0.7998128361456291469 ) ) ;
#5688=CARTESIAN_POINT ( 'NONE',  ( 5.307127064745490230, 8.279066444590018392, -1.199719254218452935 ) ) ;
#5697=CARTESIAN_POINT ( 'NONE',  ( -8.030507057996002729, 8.263346410617135263, 1.040834085586084257E-14 ) ) ;
#5702=CARTESIAN_POINT ( 'NONE',  ( 7.716561984472250835, 12.15440608185967086, 1.040834085586084257E-14 ) ) ;
#5705=CARTESIAN_POINT ( 'NONE',  ( -4.765854690403601879, 5.518917546014321829, 1.199719254218462483 ) ) ;
#5706=CARTESIAN_POINT ( 'NONE',  ( -8.350932551013499960, 11.83017284523606172, -1.199719254218446718 ) ) ;
#5709=CARTESIAN_POINT ( 'NONE',  ( -4.002915605954192380, 7.811702849818844108, -0.3674259761444337302 ) ) ;
#5716=CARTESIAN_POINT ( 'NONE',  ( 6.993308306550549247, 7.053281200597435685, 1.040834085586084257E-14 ) ) ;
#5719=CARTESIAN_POINT ( 'NONE',  ( 5.905025204062885003, 4.805319369733568102, 2.500000000000011102 ) ) ;
#5736=ORIENTED_EDGE ( 'NONE', *, *, #67524, .T. ) ;
#5738=( BOUNDED_SURFACE ( )  B_SPLINE_SURFACE ( 1, 2, ( 
 ( #81026, #99416, #83145, #798, #64770, #15996, #197961, #133011, #49590, #165470, #130912, #116782, #101542, #182779, #17066, #34397, #18132, #134080, #200088, #117860, #183852, #35464, #39750, #85288, #208365, #126149, #201149, #154573, #151374, #153503, #204342, #6149, #92533, #38683, #175902, #5073, #71148, #169739, #26421, #2943, #137265, #21328, #86360, #168672, #174844, #192112, #37609, #202212, #203285, #105855, #158573, #185976, #59996, #87435, #20276, #188119, #69015, #4010, #10172, #53866, #54932, #142355, #76246, #43776, #72219, #109889, #135132, #138326, #119999, #56000, #121084, #52787, #118926, #184906, #88511, #36530, #152431, #122151, #102617, #187051, #104762, #170811, #22402, #70080, #136194, #103690, #61067, #147663, #46972, #209422, #144498, #143426, #110949, #146613, #211564, #63198, #195340, #113088, #127226, #159637, #162848, #179094, #112026, #77313, #196404, #161783, #30716, #93593, #45908, #212631, #15492, #114162, #145565, #12297, #14426, #78377, #176956, #193195, #178028, #27493, #44843, #28572, #31781, #94660, #131452, #130417, #81580, #210505, #29646, #95731, #129362, #64272, #96799, #160703, #11234, #62140, #128300, #194262, #13374, #79448, #80516, #48049, #180155, #97853, #163916, #115214, #213680, #65303, #197453, #49094, #199575, #136742, #181204, #149790, #3496, #70631, #51219, #1364, #66361, #54419, #202769, #148720, #103165, #183340, #119478, #67426, #32832, #98909, #134631, #290, #169226, #168166, #167108, #133569, #20818, #86914, #164961, #118412, #68503, #16553, #132507, #152982, #4557, #50150, #85846, #82636, #198506, #116274, #185466, #182263, #150864, #184397, #36017, #33888, #117343, #34945, #102096, #101017, #18695, #99966, #19764, #166031, #151923, #84777, #52283, #2426, #200635, #69566, #17616, #37086, #135676, #201701, #53344, #83702, #21874, #122715, #156198, #170286, #92284, #157263, #104240, #74933, #186538, #87981, #38167, #71703, #40311, #141043, #190796, #5622, #139960, #124829, #42456, #137815, #188677, #121633, #154055, #203834, #55480, #106418, #187602, #171358, #39229, #90131, #108564, #205983, #174592, #75996, #73865, #158329, #25100, #138883, #58682, #204901, #26166, #173527, #9922, #57619, #105321, #7774, #123776, #56555, #189736, #6706, #22952, #89066, #172441, #41388, #155124, #142101, #24028, #8854, #72783, #120560, #208114, #207050, #107499, #91202, #210243, #78120, #95481, #96543, #13114, #60809, #191860, #159377, #125902, #93341, #160445, #44584, #12052, #176697, #175647, #126970, #61879, #147405, #110697, #109644, #28310, #195079, #14164, #59743, #179901, #97598, #27233, #129105, #43521, #128044, #178846, #46717, #64012, #79192, #10976, #193999, #45648, #144250, #212371, #77049, #111765, #177772, #192928, #143179, #146358, #163657, #29387, #94406, #161529, #80259, #130160, #145307, #31524, #211312, #209171, #162590, #62937, #112830, #196152, #30457, #47792, #113906, #15239, #81326, #134377, #119216, #65054, #200381, #33634, #118155, #1112, #131210, #185199, #180951, #2166, #213431, #39, #52029, #167906, #67173, #18441, #149526, #117083, #36824, #32574, #184139, #98650, #102905, #84518, #164707, #116017, #114951, #82380, #35763, #183082, #34694, #166845, #150606, #16295, #197198, #101838, #68243, #83446, #48837, #19504, #133308, #85580, #148471, #17362, #151670, #201440, #3241, #100763, #198253, #69307, #49893, #66103, #132245, #199313, #182003, #99707, #165779, #135419, #50959, #168964, #53081, #20568, #86651, #4301, #54159, #70372, #103983, #72522, #173260, #8592, #37907, #172183, #157006, #74674, #170026, #154862, #153793, #136487, #120298, #202509, #6444, #186271, #203574, #21612, #122452, #140777, #23773, #206792, #108309, #106157, #190538, #57357, #171099, #90940, #22690, #58424, #205722, #124577, #89878, #137556, #40048, #155930, #88803, #7515, #38975, #87720, #5362, #138618, #73597, #71444, #42194, #204641, #41127, #55225, #152719, #107239, #174329, #121371, #187346, #56292, #25905, #105061, #188411, #189484, #139699, #123520, #24841, #191599, #179643, #195887, #59481, #13910, #94147, #30186, #192664, #92015, #9661, #45387 ),
 ( #175386, #211043, #158073, #125638, #113638, #96276, #75737, #61616, #29121, #161257, #26972, #110440, #44318, #12844, #176442, #11787, #43261, #95208, #47525, #78918, #77861, #177509, #143984, #209975, #127786, #142911, #162326, #60545, #126703, #145040, #141850, #207855, #160186, #193741, #109379, #79992, #62669, #111503, #28054, #146096, #212107, #93077, #128828, #194810, #159119, #10720, #63744, #129903, #76789, #46446, #208911, #112567, #178578, #183892, #118965, #844, #182823, #100512, #180693, #49628, #198002, #166587, #131993, #165512, #196943, #34439, #201189, #18176, #17104, #116821, #83182, #149265, #66909, #82120, #101581, #214215, #65844, #84263, #31263, #147152, #33374, #133049, #81066, #2987, #67977, #14969, #200129, #97337, #213177, #163395, #48583, #199051, #51782, #167649, #130953, #50697, #35504, #19250, #114699, #99455, #32318, #64806, #98386, #164450, #150348, #16037, #148213, #115753, #1918, #85330, #134120, #151413, #52828, #117899, #69054, #135174, #181744, #123273, #203322, #106979, #23518, #173004, #56040, #169779, #72259, #204384, #54973, #122196, #71188, #20317, #4050, #170849, #138367, #36570, #40874, #187089, #73334, #87476, #184943, #139437, #189235, #21368, #86403, #121125, #140528, #102656, #153542, #7258, #74428, #38723, #5111, #70120, #58170, #206540, #152470, #24585, #104804, #90692, #137305, #168713, #136231, #188158, #202254, #53905, #120040, #186014, #156754, #37650, #154611, #39791, #105898, #103728, #22439, #88550, #6190, #8343, #171922, #89624, #155676, #205472, #57104, #28873, #193503, #128594, #77613, #211865, #192416, #44071, #208664, #62431, #124328, #110190, #60295, #125383, #207606, #210806, #162081, #76543, #26727, #176200, #144799, #78673, #10469, #29945, #126453, #59225, #12601, #190288, #43014, #194560, #92829, #27801, #178336, #46205, #13670, #45144, #96030, #41945, #111256, #158873, #94958, #93899, #108058, #79742, #91765, #127531, #174083, #191349, #177259, #112321, #159938, #143736, #11543, #209730, #145859, #157821, #161006, #9417, #25655, #61373, #75488, #142654, #141599, #109127, #175141, #33127, #99207, #16849, #82932, #97093, #195642, #198795, #149005, #147960, #113390, #17910, #197747, #581, #129658, #81876, #182556, #51514, #150085, #181499, #48340, #50444, #114451, #146912, #163146, #213973, #63504, #14730, #80822, #67713, #212930, #167394, #166321, #117639, #32067, #65593, #131742, #165256, #100252, #66647, #64566, #47278, #130709, #179399, #196700, #164203, #180450, #98156, #34180, #31019, #15790, #85066, #1656, #151152, #132792, #116563, #83996, #133864, #49385, #115504, #183631, #199871, #35238, #101313, #18985, #172737, #154342, #137032, #88277, #203059, #120852, #38456, #53635, #73068, #185748, #37381, #204114, #90419, #118699, #4842, #104533, #52568, #188964, #39519, #200920, #171648, #68793, #184685, #134913, #168451, #54702, #23245, #139167, #102384, #22162, #6988, #205198, #20050, #70921, #3779, #36305, #86138, #152209, #186826, #69853, #119768, #135963, #170579, #56839, #5920, #123012, #24313, #71992, #40606, #121924, #21099, #155405, #87202, #106711, #55766, #2721, #138104, #201979, #187891, #105619, #153267, #89357, #103456, #169518, #190032, #142397, #43818, #8077, #12340, #158617, #44887, #58974, #156488, #110993, #160745, #141340, #57903, #174886, #112069, #74165, #125129, #193240, #45949, #26466, #191087, #41685, #29688, #178070, #124067, #78420, #10214, #94704, #42756, #140258, #206280, #109933, #107796, #144542, #143469, #208405, #108860, #210549, #62185, #173821, #93633, #175942, #25399, #91499, #128342, #194308, #157560, #76288, #60039, #92575, #9153, #75230, #126192, #192155, #207354, #27538, #28614, #159675, #11277, #77356, #209466, #176998, #61109, #127269, #4332, #180201, #179137, #201471, #186303, #14470, #102938, #212672, #97899, #152750, #119247, #136520, #19537, #70401, #161828, #85614, #130458, #3271, #163958, #13415, #202538, #63241, #98953, #95771, #96840, #151702, #53114, #15536, #115256, #31823, #213723, #54187, #129403, #69338, #195383, #120327, #181249, #47015, #64313, #211605, #30760, #135449, #65346, #131493 ) ),
 .UNSPECIFIED., .F., .F., .T. ) 
 B_SPLINE_SURFACE_WITH_KNOTS ( ( 2, 2 ),
 ( 3, 2, 2, 2, 2, 2, 2, 2, 2, 2, 2, 2, 2, 2, 2, 2, 2, 2, 2, 2, 2, 2, 2, 2, 2, 2, 2, 2, 2, 2, 2, 2, 2, 2, 2, 2, 2, 2, 2, 2, 2, 2, 2, 2, 2, 2, 2, 2, 2, 2, 2, 2, 2, 2, 2, 2, 2, 2, 2, 2, 2, 2, 2, 2, 2, 2, 2, 2, 2, 2, 2, 2, 2, 2, 2, 2, 2, 2, 2, 2, 2, 2, 2, 2, 2, 2, 2, 2, 2, 2, 2, 2, 2, 2, 2, 2, 2, 2, 2, 2, 2, 2, 2, 2, 2, 2, 2, 2, 2, 2, 2, 2, 2, 2, 2, 2, 2, 2, 2, 2, 2, 2, 2, 2, 2, 2, 2, 2, 2, 2, 2, 2, 2, 2, 2, 2, 2, 2, 2, 2, 2, 2, 2, 2, 2, 2, 2, 2, 2, 2, 2, 2, 2, 2, 2, 2, 2, 2, 2, 2, 2, 2, 2, 2, 2, 2, 2, 2, 2, 2, 2, 2, 2, 2, 2, 2, 2, 2, 2, 2, 2, 2, 2, 2, 2, 2, 2, 2, 2, 2, 2, 2, 2, 2, 2, 2, 2, 2, 2, 2, 2, 2, 2, 2, 2, 2, 2, 2, 2, 2, 2, 2, 2, 2, 2, 2, 2, 2, 2, 2, 2, 2, 2, 2, 2, 2, 2, 2, 2, 2, 2, 2, 2, 2, 2, 2, 2, 2, 2, 2, 3 ),
 ( 0.000000000000000000, 1.000000000000000000 ),
 ( 0.000000000000000000, 0.004166666666666666609, 0.008333333333333333218, 0.01250000000000000069, 0.01666666666666666644, 0.02083333333333333218, 0.02500000000000000139, 0.02916666666666666713, 0.03333333333333333287, 0.03749999999999999861, 0.04166666666666666435, 0.04583333333333333010, 0.05000000000000000278, 0.05416666666666666852, 0.05833333333333333426, 0.06250000000000000000, 0.06666666666666666574, 0.07083333333333333148, 0.07499999999999999722, 0.07916666666666666297, 0.08333333333333332871, 0.08749999999999999445, 0.09166666666666666019, 0.09583333333333333981, 0.1000000000000000056, 0.1041666666666666713, 0.1083333333333333370, 0.1125000000000000028, 0.1166666666666666685, 0.1208333333333333343, 0.1250000000000000000, 0.1291666666666666796, 0.1333333333333333315, 0.1375000000000000111, 0.1416666666666666630, 0.1458333333333333426, 0.1499999999999999944, 0.1541666666666666741, 0.1583333333333333259, 0.1625000000000000056, 0.1666666666666666574, 0.1708333333333333370, 0.1749999999999999889, 0.1791666666666666685, 0.1833333333333333204, 0.1875000000000000000, 0.1916666666666666796, 0.1958333333333333315, 0.2000000000000000111, 0.2041666666666666630, 0.2083333333333333426, 0.2124999999999999944, 0.2166666666666666741, 0.2208333333333333259, 0.2250000000000000056, 0.2291666666666666574, 0.2333333333333333370, 0.2374999999999999889, 0.2416666666666666685, 0.2458333333333333204, 0.2500000000000000000, 0.2541666666666666519, 0.2583333333333333592, 0.2625000000000000111, 0.2666666666666666630, 0.2708333333333333148, 0.2750000000000000222, 0.2791666666666666741, 0.2833333333333333259, 0.2874999999999999778, 0.2916666666666666852, 0.2958333333333333370, 0.2999999999999999889, 0.3041666666666666408, 0.3083333333333333481, 0.3125000000000000000, 0.3166666666666666519, 0.3208333333333333592, 0.3250000000000000111, 0.3291666666666666630, 0.3333333333333333148, 0.3375000000000000222, 0.3416666666666666741, 0.3458333333333333259, 0.3499999999999999778, 0.3541666666666666852, 0.3583333333333333370, 0.3624999999999999889, 0.3666666666666666408, 0.3708333333333333481, 0.3750000000000000000, 0.3791666666666666519, 0.3833333333333333592, 0.3875000000000000111, 0.3916666666666666630, 0.3958333333333333148, 0.4000000000000000222, 0.4041666666666666741, 0.4083333333333333259, 0.4124999999999999778, 0.4166666666666666852, 0.4208333333333333370, 0.4249999999999999889, 0.4291666666666666408, 0.4333333333333333481, 0.4375000000000000000, 0.4416666666666666519, 0.4458333333333333592, 0.4500000000000000111, 0.4541666666666666630, 0.4583333333333333148, 0.4625000000000000222, 0.4666666666666666741, 0.4708333333333333259, 0.4749999999999999778, 0.4791666666666666852, 0.4833333333333333370, 0.4874999999999999889, 0.4916666666666666408, 0.4958333333333333481, 0.5000000000000000000, 0.5041666666666666519, 0.5083333333333333037, 0.5124999999999999556, 0.5166666666666667185, 0.5208333333333333703, 0.5250000000000000222, 0.5291666666666666741, 0.5333333333333333259, 0.5374999999999999778, 0.5416666666666666297, 0.5458333333333332815, 0.5500000000000000444, 0.5541666666666666963, 0.5583333333333333481, 0.5625000000000000000, 0.5666666666666666519, 0.5708333333333333037, 0.5749999999999999556, 0.5791666666666667185, 0.5833333333333333703, 0.5875000000000000222, 0.5916666666666666741, 0.5958333333333333259, 0.5999999999999999778, 0.6041666666666666297, 0.6083333333333332815, 0.6125000000000000444, 0.6166666666666666963, 0.6208333333333333481, 0.6250000000000000000, 0.6291666666666666519, 0.6333333333333333037, 0.6374999999999999556, 0.6416666666666667185, 0.6458333333333333703, 0.6500000000000000222, 0.6541666666666666741, 0.6583333333333333259, 0.6624999999999999778, 0.6666666666666666297, 0.6708333333333332815, 0.6750000000000000444, 0.6791666666666666963, 0.6833333333333333481, 0.6875000000000000000, 0.6916666666666666519, 0.6958333333333333037, 0.6999999999999999556, 0.7041666666666667185, 0.7083333333333333703, 0.7125000000000000222, 0.7166666666666666741, 0.7208333333333333259, 0.7249999999999999778, 0.7291666666666666297, 0.7333333333333332815, 0.7375000000000000444, 0.7416666666666666963, 0.7458333333333333481, 0.7500000000000000000, 0.7541666666666666519, 0.7583333333333333037, 0.7624999999999999556, 0.7666666666666667185, 0.7708333333333333703, 0.7750000000000000222, 0.7791666666666666741, 0.7833333333333333259, 0.7874999999999999778, 0.7916666666666666297, 0.7958333333333332815, 0.8000000000000000444, 0.8041666666666666963, 0.8083333333333333481, 0.8125000000000000000, 0.8166666666666666519, 0.8208333333333333037, 0.8249999999999999556, 0.8291666666666667185, 0.8333333333333333703, 0.8375000000000000222, 0.8416666666666666741, 0.8458333333333333259, 0.8499999999999999778, 0.8541666666666666297, 0.8583333333333332815, 0.8625000000000000444, 0.8666666666666666963, 0.8708333333333333481, 0.8750000000000000000, 0.8791666666666666519, 0.8833333333333333037, 0.8874999999999999556, 0.8916666666666667185, 0.8958333333333333703, 0.9000000000000000222, 0.9041666666666666741, 0.9083333333333333259, 0.9124999999999999778, 0.9166666666666666297, 0.9208333333333332815, 0.9250000000000000444, 0.9291666666666666963, 0.9333333333333333481, 0.9375000000000000000, 0.9416666666666666519, 0.9458333333333333037, 0.9499999999999999556, 0.9541666666666667185, 0.9583333333333333703, 0.9625000000000000222, 0.9666666666666666741, 0.9708333333333333259, 0.9749999999999999778, 0.9791666666666666297, 0.9833333333333332815, 0.9875000000000000444, 0.9916666666666666963, 0.9958333333333333481, 1.000000000000000000 ),
 .UNSPECIFIED. ) 
 GEOMETRIC_REPRESENTATION_ITEM ( )  RATIONAL_B_SPLINE_SURFACE ( (
 ( 1.000000000000000000, 0.8660254037844387076, 1.000000000000000000, 0.8660254037844387076, 1.000000000000000000, 0.8660254037844387076, 1.000000000000000000, 0.8660254037844387076, 1.000000000000000000, 0.8660254037844387076, 1.000000000000000000, 0.8660254037844387076, 1.000000000000000000, 0.8660254037844387076, 1.000000000000000000, 0.8660254037844387076, 1.000000000000000000, 0.8660254037844387076, 1.000000000000000000, 0.8660254037844387076, 1.000000000000000000, 0.8660254037844387076, 1.000000000000000000, 0.8660254037844387076, 1.000000000000000000, 0.8660254037844387076, 1.000000000000000000, 0.8660254037844387076, 1.000000000000000000, 0.8660254037844387076, 1.000000000000000000, 0.8660254037844387076, 1.000000000000000000, 0.8660254037844387076, 1.000000000000000000, 0.8660254037844387076, 1.000000000000000000, 0.8660254037844387076, 1.000000000000000000, 0.8660254037844387076, 1.000000000000000000, 0.8660254037844387076, 1.000000000000000000, 0.8660254037844387076, 1.000000000000000000, 0.8660254037844387076, 1.000000000000000000, 0.8660254037844387076, 1.000000000000000000, 0.8660254037844387076, 1.000000000000000000, 0.8660254037844387076, 1.000000000000000000, 0.8660254037844387076, 1.000000000000000000, 0.8660254037844387076, 1.000000000000000000, 0.8660254037844387076, 1.000000000000000000, 0.8660254037844387076, 1.000000000000000000, 0.8660254037844387076, 1.000000000000000000, 0.8660254037844387076, 1.000000000000000000, 0.8660254037844387076, 1.000000000000000000, 0.8660254037844387076, 1.000000000000000000, 0.8660254037844387076, 1.000000000000000000, 0.8660254037844387076, 1.000000000000000000, 0.8660254037844387076, 1.000000000000000000, 0.8660254037844387076, 1.000000000000000000, 0.8660254037844387076, 1.000000000000000000, 0.8660254037844387076, 1.000000000000000000, 0.8660254037844387076, 1.000000000000000000, 0.8660254037844387076, 1.000000000000000000, 0.8660254037844387076, 1.000000000000000000, 0.8660254037844387076, 1.000000000000000000, 0.8660254037844387076, 1.000000000000000000, 0.8660254037844387076, 1.000000000000000000, 0.8660254037844387076, 1.000000000000000000, 0.8660254037844387076, 1.000000000000000000, 0.8660254037844387076, 1.000000000000000000, 0.8660254037844387076, 1.000000000000000000, 0.8660254037844387076, 1.000000000000000000, 0.8660254037844387076, 1.000000000000000000, 0.8660254037844387076, 1.000000000000000000, 0.8660254037844387076, 1.000000000000000000, 0.8660254037844387076, 1.000000000000000000, 0.8660254037844387076, 1.000000000000000000, 0.8660254037844387076, 1.000000000000000000, 0.8660254037844387076, 1.000000000000000000, 0.8660254037844387076, 1.000000000000000000, 0.8660254037844387076, 1.000000000000000000, 0.8660254037844387076, 1.000000000000000000, 0.8660254037844387076, 1.000000000000000000, 0.8660254037844387076, 1.000000000000000000, 0.8660254037844387076, 1.000000000000000000, 0.8660254037844387076, 1.000000000000000000, 0.8660254037844387076, 1.000000000000000000, 0.8660254037844387076, 1.000000000000000000, 0.8660254037844387076, 1.000000000000000000, 0.8660254037844387076, 1.000000000000000000, 0.8660254037844387076, 1.000000000000000000, 0.8660254037844387076, 1.000000000000000000, 0.8660254037844387076, 1.000000000000000000, 0.8660254037844387076, 1.000000000000000000, 0.8660254037844387076, 1.000000000000000000, 0.8660254037844387076, 1.000000000000000000, 0.8660254037844387076, 1.000000000000000000, 0.8660254037844387076, 1.000000000000000000, 0.8660254037844387076, 1.000000000000000000, 0.8660254037844387076, 1.000000000000000000, 0.8660254037844387076, 1.000000000000000000, 0.8660254037844387076, 1.000000000000000000, 0.8660254037844387076, 1.000000000000000000, 0.8660254037844387076, 1.000000000000000000, 0.8660254037844387076, 1.000000000000000000, 0.8660254037844387076, 1.000000000000000000, 0.8660254037844387076, 1.000000000000000000, 0.8660254037844387076, 1.000000000000000000, 0.8660254037844387076, 1.000000000000000000, 0.8660254037844387076, 1.000000000000000000, 0.8660254037844387076, 1.000000000000000000, 0.8660254037844387076, 1.000000000000000000, 0.8660254037844387076, 1.000000000000000000, 0.8660254037844387076, 1.000000000000000000, 0.8660254037844387076, 1.000000000000000000, 0.8660254037844387076, 1.000000000000000000, 0.8660254037844387076, 1.000000000000000000, 0.8660254037844387076, 1.000000000000000000, 0.8660254037844387076, 1.000000000000000000, 0.8660254037844387076, 1.000000000000000000, 0.8660254037844387076, 1.000000000000000000, 0.8660254037844387076, 1.000000000000000000, 0.8660254037844387076, 1.000000000000000000, 0.8660254037844387076, 1.000000000000000000, 0.8660254037844387076, 1.000000000000000000, 0.8660254037844387076, 1.000000000000000000, 0.8660254037844387076, 1.000000000000000000, 0.8660254037844387076, 1.000000000000000000, 0.8660254037844387076, 1.000000000000000000, 0.8660254037844387076, 1.000000000000000000, 0.8660254037844387076, 1.000000000000000000, 0.8660254037844387076, 1.000000000000000000, 0.8660254037844387076, 1.000000000000000000, 0.8660254037844387076, 1.000000000000000000, 0.8660254037844387076, 1.000000000000000000, 0.8660254037844387076, 1.000000000000000000, 0.8660254037844387076, 1.000000000000000000, 0.8660254037844387076, 1.000000000000000000, 0.8660254037844387076, 1.000000000000000000, 0.8660254037844387076, 1.000000000000000000, 0.8660254037844387076, 1.000000000000000000, 0.8660254037844387076, 1.000000000000000000, 0.8660254037844387076, 1.000000000000000000, 0.8660254037844387076, 1.000000000000000000, 0.8660254037844387076, 1.000000000000000000, 0.8660254037844387076, 1.000000000000000000, 0.8660254037844387076, 1.000000000000000000, 0.8660254037844387076, 1.000000000000000000, 0.8660254037844387076, 1.000000000000000000, 0.8660254037844387076, 1.000000000000000000, 0.8660254037844387076, 1.000000000000000000, 0.8660254037844387076, 1.000000000000000000, 0.8660254037844387076, 1.000000000000000000, 0.8660254037844387076, 1.000000000000000000, 0.8660254037844387076, 1.000000000000000000, 0.8660254037844387076, 1.000000000000000000, 0.8660254037844387076, 1.000000000000000000, 0.8660254037844387076, 1.000000000000000000, 0.8660254037844387076, 1.000000000000000000, 0.8660254037844387076, 1.000000000000000000, 0.8660254037844387076, 1.000000000000000000, 0.8660254037844387076, 1.000000000000000000, 0.8660254037844387076, 1.000000000000000000, 0.8660254037844387076, 1.000000000000000000, 0.8660254037844387076, 1.000000000000000000, 0.8660254037844387076, 1.000000000000000000, 0.8660254037844387076, 1.000000000000000000, 0.8660254037844387076, 1.000000000000000000, 0.8660254037844387076, 1.000000000000000000, 0.8660254037844387076, 1.000000000000000000, 0.8660254037844387076, 1.000000000000000000, 0.8660254037844387076, 1.000000000000000000, 0.8660254037844387076, 1.000000000000000000, 0.8660254037844387076, 1.000000000000000000, 0.8660254037844387076, 1.000000000000000000, 0.8660254037844387076, 1.000000000000000000, 0.8660254037844387076, 1.000000000000000000, 0.8660254037844387076, 1.000000000000000000, 0.8660254037844387076, 1.000000000000000000, 0.8660254037844387076, 1.000000000000000000, 0.8660254037844387076, 1.000000000000000000, 0.8660254037844387076, 1.000000000000000000, 0.8660254037844387076, 1.000000000000000000, 0.8660254037844387076, 1.000000000000000000, 0.8660254037844387076, 1.000000000000000000, 0.8660254037844387076, 1.000000000000000000, 0.8660254037844387076, 1.000000000000000000, 0.8660254037844387076, 1.000000000000000000, 0.8660254037844387076, 1.000000000000000000, 0.8660254037844387076, 1.000000000000000000, 0.8660254037844387076, 1.000000000000000000, 0.8660254037844387076, 1.000000000000000000, 0.8660254037844387076, 1.000000000000000000, 0.8660254037844387076, 1.000000000000000000, 0.8660254037844387076, 1.000000000000000000, 0.8660254037844387076, 1.000000000000000000, 0.8660254037844387076, 1.000000000000000000, 0.8660254037844387076, 1.000000000000000000, 0.8660254037844387076, 1.000000000000000000, 0.8660254037844387076, 1.000000000000000000, 0.8660254037844387076, 1.000000000000000000, 0.8660254037844387076, 1.000000000000000000, 0.8660254037844387076, 1.000000000000000000, 0.8660254037844387076, 1.000000000000000000, 0.8660254037844387076, 1.000000000000000000, 0.8660254037844387076, 1.000000000000000000, 0.8660254037844387076, 1.000000000000000000, 0.8660254037844387076, 1.000000000000000000, 0.8660254037844387076, 1.000000000000000000, 0.8660254037844387076, 1.000000000000000000, 0.8660254037844387076, 1.000000000000000000, 0.8660254037844387076, 1.000000000000000000, 0.8660254037844387076, 1.000000000000000000, 0.8660254037844387076, 1.000000000000000000, 0.8660254037844387076, 1.000000000000000000, 0.8660254037844387076, 1.000000000000000000, 0.8660254037844387076, 1.000000000000000000, 0.8660254037844387076, 1.000000000000000000, 0.8660254037844387076, 1.000000000000000000, 0.8660254037844387076, 1.000000000000000000, 0.8660254037844387076, 1.000000000000000000, 0.8660254037844387076, 1.000000000000000000, 0.8660254037844387076, 1.000000000000000000, 0.8660254037844387076, 1.000000000000000000, 0.8660254037844387076, 1.000000000000000000, 0.8660254037844387076, 1.000000000000000000, 0.8660254037844387076, 1.000000000000000000, 0.8660254037844387076, 1.000000000000000000, 0.8660254037844387076, 1.000000000000000000, 0.8660254037844387076, 1.000000000000000000, 0.8660254037844387076, 1.000000000000000000, 0.8660254037844387076, 1.000000000000000000, 0.8660254037844387076, 1.000000000000000000, 0.8660254037844387076, 1.000000000000000000, 0.8660254037844387076, 1.000000000000000000, 0.8660254037844387076, 1.000000000000000000, 0.8660254037844387076, 1.000000000000000000, 0.8660254037844387076, 1.000000000000000000, 0.8660254037844387076, 1.000000000000000000, 0.8660254037844387076, 1.000000000000000000, 0.8660254037844387076, 1.000000000000000000, 0.8660254037844387076, 1.000000000000000000, 0.8660254037844387076, 1.000000000000000000, 0.8660254037844387076, 1.000000000000000000, 0.8660254037844387076, 1.000000000000000000, 0.8660254037844387076, 1.000000000000000000, 0.8660254037844387076, 1.000000000000000000, 0.8660254037844387076, 1.000000000000000000, 0.8660254037844387076, 1.000000000000000000, 0.8660254037844387076, 1.000000000000000000, 0.8660254037844387076, 1.000000000000000000, 0.8660254037844387076, 1.000000000000000000, 0.8660254037844387076, 1.000000000000000000, 0.8660254037844387076, 1.000000000000000000, 0.8660254037844387076, 1.000000000000000000, 0.8660254037844387076, 1.000000000000000000, 0.8660254037844387076, 1.000000000000000000, 0.8660254037844387076, 1.000000000000000000, 0.8660254037844387076, 1.000000000000000000, 0.8660254037844387076, 1.000000000000000000, 0.8660254037844387076, 1.000000000000000000),
 ( 1.000000000000000000, 0.8660254037844387076, 1.000000000000000000, 0.8660254037844387076, 1.000000000000000000, 0.8660254037844387076, 1.000000000000000000, 0.8660254037844387076, 1.000000000000000000, 0.8660254037844387076, 1.000000000000000000, 0.8660254037844387076, 1.000000000000000000, 0.8660254037844387076, 1.000000000000000000, 0.8660254037844387076, 1.000000000000000000, 0.8660254037844387076, 1.000000000000000000, 0.8660254037844387076, 1.000000000000000000, 0.8660254037844387076, 1.000000000000000000, 0.8660254037844387076, 1.000000000000000000, 0.8660254037844387076, 1.000000000000000000, 0.8660254037844387076, 1.000000000000000000, 0.8660254037844387076, 1.000000000000000000, 0.8660254037844387076, 1.000000000000000000, 0.8660254037844387076, 1.000000000000000000, 0.8660254037844387076, 1.000000000000000000, 0.8660254037844387076, 1.000000000000000000, 0.8660254037844387076, 1.000000000000000000, 0.8660254037844387076, 1.000000000000000000, 0.8660254037844387076, 1.000000000000000000, 0.8660254037844387076, 1.000000000000000000, 0.8660254037844387076, 1.000000000000000000, 0.8660254037844387076, 1.000000000000000000, 0.8660254037844387076, 1.000000000000000000, 0.8660254037844387076, 1.000000000000000000, 0.8660254037844387076, 1.000000000000000000, 0.8660254037844387076, 1.000000000000000000, 0.8660254037844387076, 1.000000000000000000, 0.8660254037844387076, 1.000000000000000000, 0.8660254037844387076, 1.000000000000000000, 0.8660254037844387076, 1.000000000000000000, 0.8660254037844387076, 1.000000000000000000, 0.8660254037844387076, 1.000000000000000000, 0.8660254037844387076, 1.000000000000000000, 0.8660254037844387076, 1.000000000000000000, 0.8660254037844387076, 1.000000000000000000, 0.8660254037844387076, 1.000000000000000000, 0.8660254037844387076, 1.000000000000000000, 0.8660254037844387076, 1.000000000000000000, 0.8660254037844387076, 1.000000000000000000, 0.8660254037844387076, 1.000000000000000000, 0.8660254037844387076, 1.000000000000000000, 0.8660254037844387076, 1.000000000000000000, 0.8660254037844387076, 1.000000000000000000, 0.8660254037844387076, 1.000000000000000000, 0.8660254037844387076, 1.000000000000000000, 0.8660254037844387076, 1.000000000000000000, 0.8660254037844387076, 1.000000000000000000, 0.8660254037844387076, 1.000000000000000000, 0.8660254037844387076, 1.000000000000000000, 0.8660254037844387076, 1.000000000000000000, 0.8660254037844387076, 1.000000000000000000, 0.8660254037844387076, 1.000000000000000000, 0.8660254037844387076, 1.000000000000000000, 0.8660254037844387076, 1.000000000000000000, 0.8660254037844387076, 1.000000000000000000, 0.8660254037844387076, 1.000000000000000000, 0.8660254037844387076, 1.000000000000000000, 0.8660254037844387076, 1.000000000000000000, 0.8660254037844387076, 1.000000000000000000, 0.8660254037844387076, 1.000000000000000000, 0.8660254037844387076, 1.000000000000000000, 0.8660254037844387076, 1.000000000000000000, 0.8660254037844387076, 1.000000000000000000, 0.8660254037844387076, 1.000000000000000000, 0.8660254037844387076, 1.000000000000000000, 0.8660254037844387076, 1.000000000000000000, 0.8660254037844387076, 1.000000000000000000, 0.8660254037844387076, 1.000000000000000000, 0.8660254037844387076, 1.000000000000000000, 0.8660254037844387076, 1.000000000000000000, 0.8660254037844387076, 1.000000000000000000, 0.8660254037844387076, 1.000000000000000000, 0.8660254037844387076, 1.000000000000000000, 0.8660254037844387076, 1.000000000000000000, 0.8660254037844387076, 1.000000000000000000, 0.8660254037844387076, 1.000000000000000000, 0.8660254037844387076, 1.000000000000000000, 0.8660254037844387076, 1.000000000000000000, 0.8660254037844387076, 1.000000000000000000, 0.8660254037844387076, 1.000000000000000000, 0.8660254037844387076, 1.000000000000000000, 0.8660254037844387076, 1.000000000000000000, 0.8660254037844387076, 1.000000000000000000, 0.8660254037844387076, 1.000000000000000000, 0.8660254037844387076, 1.000000000000000000, 0.8660254037844387076, 1.000000000000000000, 0.8660254037844387076, 1.000000000000000000, 0.8660254037844387076, 1.000000000000000000, 0.8660254037844387076, 1.000000000000000000, 0.8660254037844387076, 1.000000000000000000, 0.8660254037844387076, 1.000000000000000000, 0.8660254037844387076, 1.000000000000000000, 0.8660254037844387076, 1.000000000000000000, 0.8660254037844387076, 1.000000000000000000, 0.8660254037844387076, 1.000000000000000000, 0.8660254037844387076, 1.000000000000000000, 0.8660254037844387076, 1.000000000000000000, 0.8660254037844387076, 1.000000000000000000, 0.8660254037844387076, 1.000000000000000000, 0.8660254037844387076, 1.000000000000000000, 0.8660254037844387076, 1.000000000000000000, 0.8660254037844387076, 1.000000000000000000, 0.8660254037844387076, 1.000000000000000000, 0.8660254037844387076, 1.000000000000000000, 0.8660254037844387076, 1.000000000000000000, 0.8660254037844387076, 1.000000000000000000, 0.8660254037844387076, 1.000000000000000000, 0.8660254037844387076, 1.000000000000000000, 0.8660254037844387076, 1.000000000000000000, 0.8660254037844387076, 1.000000000000000000, 0.8660254037844387076, 1.000000000000000000, 0.8660254037844387076, 1.000000000000000000, 0.8660254037844387076, 1.000000000000000000, 0.8660254037844387076, 1.000000000000000000, 0.8660254037844387076, 1.000000000000000000, 0.8660254037844387076, 1.000000000000000000, 0.8660254037844387076, 1.000000000000000000, 0.8660254037844387076, 1.000000000000000000, 0.8660254037844387076, 1.000000000000000000, 0.8660254037844387076, 1.000000000000000000, 0.8660254037844387076, 1.000000000000000000, 0.8660254037844387076, 1.000000000000000000, 0.8660254037844387076, 1.000000000000000000, 0.8660254037844387076, 1.000000000000000000, 0.8660254037844387076, 1.000000000000000000, 0.8660254037844387076, 1.000000000000000000, 0.8660254037844387076, 1.000000000000000000, 0.8660254037844387076, 1.000000000000000000, 0.8660254037844387076, 1.000000000000000000, 0.8660254037844387076, 1.000000000000000000, 0.8660254037844387076, 1.000000000000000000, 0.8660254037844387076, 1.000000000000000000, 0.8660254037844387076, 1.000000000000000000, 0.8660254037844387076, 1.000000000000000000, 0.8660254037844387076, 1.000000000000000000, 0.8660254037844387076, 1.000000000000000000, 0.8660254037844387076, 1.000000000000000000, 0.8660254037844387076, 1.000000000000000000, 0.8660254037844387076, 1.000000000000000000, 0.8660254037844387076, 1.000000000000000000, 0.8660254037844387076, 1.000000000000000000, 0.8660254037844387076, 1.000000000000000000, 0.8660254037844387076, 1.000000000000000000, 0.8660254037844387076, 1.000000000000000000, 0.8660254037844387076, 1.000000000000000000, 0.8660254037844387076, 1.000000000000000000, 0.8660254037844387076, 1.000000000000000000, 0.8660254037844387076, 1.000000000000000000, 0.8660254037844387076, 1.000000000000000000, 0.8660254037844387076, 1.000000000000000000, 0.8660254037844387076, 1.000000000000000000, 0.8660254037844387076, 1.000000000000000000, 0.8660254037844387076, 1.000000000000000000, 0.8660254037844387076, 1.000000000000000000, 0.8660254037844387076, 1.000000000000000000, 0.8660254037844387076, 1.000000000000000000, 0.8660254037844387076, 1.000000000000000000, 0.8660254037844387076, 1.000000000000000000, 0.8660254037844387076, 1.000000000000000000, 0.8660254037844387076, 1.000000000000000000, 0.8660254037844387076, 1.000000000000000000, 0.8660254037844387076, 1.000000000000000000, 0.8660254037844387076, 1.000000000000000000, 0.8660254037844387076, 1.000000000000000000, 0.8660254037844387076, 1.000000000000000000, 0.8660254037844387076, 1.000000000000000000, 0.8660254037844387076, 1.000000000000000000, 0.8660254037844387076, 1.000000000000000000, 0.8660254037844387076, 1.000000000000000000, 0.8660254037844387076, 1.000000000000000000, 0.8660254037844387076, 1.000000000000000000, 0.8660254037844387076, 1.000000000000000000, 0.8660254037844387076, 1.000000000000000000, 0.8660254037844387076, 1.000000000000000000, 0.8660254037844387076, 1.000000000000000000, 0.8660254037844387076, 1.000000000000000000, 0.8660254037844387076, 1.000000000000000000, 0.8660254037844387076, 1.000000000000000000, 0.8660254037844387076, 1.000000000000000000, 0.8660254037844387076, 1.000000000000000000, 0.8660254037844387076, 1.000000000000000000, 0.8660254037844387076, 1.000000000000000000, 0.8660254037844387076, 1.000000000000000000, 0.8660254037844387076, 1.000000000000000000, 0.8660254037844387076, 1.000000000000000000, 0.8660254037844387076, 1.000000000000000000, 0.8660254037844387076, 1.000000000000000000, 0.8660254037844387076, 1.000000000000000000, 0.8660254037844387076, 1.000000000000000000, 0.8660254037844387076, 1.000000000000000000, 0.8660254037844387076, 1.000000000000000000, 0.8660254037844387076, 1.000000000000000000, 0.8660254037844387076, 1.000000000000000000, 0.8660254037844387076, 1.000000000000000000, 0.8660254037844387076, 1.000000000000000000, 0.8660254037844387076, 1.000000000000000000, 0.8660254037844387076, 1.000000000000000000, 0.8660254037844387076, 1.000000000000000000, 0.8660254037844387076, 1.000000000000000000, 0.8660254037844387076, 1.000000000000000000, 0.8660254037844387076, 1.000000000000000000, 0.8660254037844387076, 1.000000000000000000, 0.8660254037844387076, 1.000000000000000000, 0.8660254037844387076, 1.000000000000000000, 0.8660254037844387076, 1.000000000000000000, 0.8660254037844387076, 1.000000000000000000, 0.8660254037844387076, 1.000000000000000000, 0.8660254037844387076, 1.000000000000000000, 0.8660254037844387076, 1.000000000000000000, 0.8660254037844387076, 1.000000000000000000, 0.8660254037844387076, 1.000000000000000000, 0.8660254037844387076, 1.000000000000000000, 0.8660254037844387076, 1.000000000000000000, 0.8660254037844387076, 1.000000000000000000, 0.8660254037844387076, 1.000000000000000000, 0.8660254037844387076, 1.000000000000000000, 0.8660254037844387076, 1.000000000000000000, 0.8660254037844387076, 1.000000000000000000, 0.8660254037844387076, 1.000000000000000000, 0.8660254037844387076, 1.000000000000000000, 0.8660254037844387076, 1.000000000000000000, 0.8660254037844387076, 1.000000000000000000, 0.8660254037844387076, 1.000000000000000000, 0.8660254037844387076, 1.000000000000000000, 0.8660254037844387076, 1.000000000000000000, 0.8660254037844387076, 1.000000000000000000, 0.8660254037844387076, 1.000000000000000000, 0.8660254037844387076, 1.000000000000000000, 0.8660254037844387076, 1.000000000000000000, 0.8660254037844387076, 1.000000000000000000, 0.8660254037844387076, 1.000000000000000000, 0.8660254037844387076, 1.000000000000000000, 0.8660254037844387076, 1.000000000000000000, 0.8660254037844387076, 1.000000000000000000, 0.8660254037844387076, 1.000000000000000000, 0.8660254037844387076, 1.000000000000000000, 0.8660254037844387076, 1.000000000000000000) ) ) 
 REPRESENTATION_ITEM ( '' )  SURFACE ( )  );
#5739=CARTESIAN_POINT ( 'NONE',  ( -8.299562589859897699, 12.83457345481192036, -0.7998128361456281477 ) ) ;
#5745=CARTESIAN_POINT ( 'NONE',  ( 1.499999999999987121, 1.535416667349486453, 0.8660254037844524744 ) ) ;
#5746=CARTESIAN_POINT ( 'NONE',  ( 9.836604141914616406, 11.43479190611061647, 1.199719254218452047 ) ) ;
#5750=CYLINDRICAL_SURFACE ( 'NONE', #104934, 0.08000000000000020983 ) ;
#5752=CARTESIAN_POINT ( 'NONE',  ( 1.364683531249988757, 0.3843750003414206362, 0.000000000000000000 ) ) ;
#5758=CARTESIAN_POINT ( 'NONE',  ( -3.741160322367112379, 6.452105245148518797, 1.199719254218464037 ) ) ;
#5760=CARTESIAN_POINT ( 'NONE',  ( 1.579999999999985860, -1.099999999999982991, -2.579999999999990301 ) ) ;
#5763=CARTESIAN_POINT ( 'NONE',  ( -0.6823417656250003738, -0.2197916663252488800, -1.181850606188749264 ) ) ;
#5769=CARTESIAN_POINT ( 'NONE',  ( 0.6823417656249882723, 0.9260416670080831025, -1.181850606188749264 ) ) ;
#5770=AXIS2_PLACEMENT_3D ( 'NONE', #198618, #116383, #196517 ) ;
#5772=CARTESIAN_POINT ( 'NONE',  ( -7.063961727919978451, 8.200042423116789436, 1.199719254218450271 ) ) ;
#5773=CARTESIAN_POINT ( 'NONE',  ( 7.130698725783555680, 10.40656671580112658, 1.199719254218460707 ) ) ;
#5774=CARTESIAN_POINT ( 'NONE',  ( 4.436542580169809291, 6.199052314996659874, 1.599625672291267175 ) ) ;
#5778=CARTESIAN_POINT ( 'NONE',  ( -0.6823417656250212460, 1.613541667008083769, 1.181850606188755259 ) ) ;
#5785=CARTESIAN_POINT ( 'NONE',  ( 7.022760382198770301, 8.255937203062467589, -1.082531754730543083 ) ) ;
#5788=CARTESIAN_POINT ( 'NONE',  ( -6.744291347794091784, 9.955758108146730123, -1.199719254218440723 ) ) ;
#5789=CARTESIAN_POINT ( 'NONE',  ( -4.711622075948912247, 5.455646162483875017, -1.199719254218446718 ) ) ;
#5790=CARTESIAN_POINT ( 'NONE',  ( -4.199533704925234368, 7.510932310329544670, -0.9222493318717175370 ) ) ;
#5794=CARTESIAN_POINT ( 'NONE',  ( 5.382223794500827552, 7.302347065049529462, -1.443375672974051449 ) ) ;
#5795=CARTESIAN_POINT ( 'NONE',  ( -7.904040366642703930, 10.24446639921506552, 1.443375672974090751 ) ) ;
#5797=CARTESIAN_POINT ( 'NONE',  ( -1.201851678989727383E-14, 5.087500000000019007, -1.732050807568863648 ) ) ;
#5801=CARTESIAN_POINT ( 'NONE',  ( 9.897088948295946764, 10.64895131587453569, 0.7216878364870438212 ) ) ;
#5807=AXIS2_PLACEMENT_3D ( 'NONE', #106904, #86320, #6112 ) ;
#5813=ADVANCED_FACE ( 'NONE', ( #155960 ), #129697, .T. ) ;
#5818=CARTESIAN_POINT ( 'NONE',  ( 8.554831740098663317, 9.082984572977682802, 0.7216878364870458196 ) ) ;
#5819=CARTESIAN_POINT ( 'NONE',  ( 6.252281394196331554, 10.44607872653774372, 1.040834085586084257E-14 ) ) ;
#5820=CARTESIAN_POINT ( 'NONE',  ( -5.961834861707238531, 7.978559976790334574, -1.599625672291263179 ) ) ;
#5825=EDGE_CURVE ( 'NONE', #57442, #6079, #12173, .T. ) ;
#5827=CARTESIAN_POINT ( 'NONE',  ( 4.148431816101584957, 6.823292304551739740, -1.082531754730548412 ) ) ;
#5829=CARTESIAN_POINT ( 'NONE',  ( -3.785751206713858785, 5.439795712631356750, 1.599625672291267398 ) ) ;
#5830=CARTESIAN_POINT ( 'NONE',  ( -7.321039761699444703, 10.52466824108257804, 1.082531754730549967 ) ) ;
#5833=EDGE_CURVE ( 'NONE', #17518, #146015, #43134, .T. ) ;
#5848=CARTESIAN_POINT ( 'NONE',  ( 6.435316467980822353, 10.65961964595298817, 1.040834085586084257E-14 ) ) ;
#5858=CARTESIAN_POINT ( 'NONE',  ( -6.898401231254901234, 6.942556279419168419, -0.7998128361456291469 ) ) ;
#5860=CARTESIAN_POINT ( 'NONE',  ( -2.605138072120212200, 6.191078184115536232, -0.7998128361456281477 ) ) ;
#5864=CARTESIAN_POINT ( 'NONE',  ( -4.812789021178021542, 5.101776157678782120, 0.9029685044427698815 ) ) ;
#5869=CARTESIAN_POINT ( 'NONE',  ( -3.066115294984855133, 6.728884944124295053, 0.7998128361456341429 ) ) ;
#5872=CARTESIAN_POINT ( 'NONE',  ( 8.450809820019639318, 8.753699632978056755, -0.7998128361456291469 ) ) ;
#5873=CARTESIAN_POINT ( 'NONE',  ( -1.364683531250010740, 4.030208333674752730, 0.7879004041258379498 ) ) ;
#5879=CARTESIAN_POINT ( 'NONE',  ( 6.277061933002788585, 6.425586464699131639, 0.7216878364870317197 ) ) ;
#5880=CARTESIAN_POINT ( 'NONE',  ( -6.886651960737580680, 10.12184548991413457, -1.199719254218440723 ) ) ;
#5883=CARTESIAN_POINT ( 'NONE',  ( -6.997979842947967377, 11.31606025008131233, -0.7998128361456291469 ) ) ;
#5885=CARTESIAN_POINT ( 'NONE',  ( -4.412288926243578935, 7.235088616337731260, 1.199719254218464037 ) ) ;
#5893=CARTESIAN_POINT ( 'NONE',  ( 6.317209508963599340, 9.457495962844502557, 1.199719254218462483 ) ) ;
#5903=CARTESIAN_POINT ( 'NONE',  ( -0.2871295479482242619, 7.105992221059546310, -1.980474574527449239 ) ) ;
#5906=ORIENTED_EDGE ( 'NONE', *, *, #198196, .F. ) ;
#5908=CARTESIAN_POINT ( 'NONE',  ( -0.6823417656250246877, -1.136458332991911790, 1.181850606188755259 ) ) ;
#5909=CARTESIAN_POINT ( 'NONE',  ( 6.159481859310094620, 6.080483678816896109, 1.040834085586084257E-14 ) ) ;
#5910=CARTESIAN_POINT ( 'NONE',  ( 6.277588818327314080, 7.282607361925381717, 1.199719254218462483 ) ) ;
#5912=CARTESIAN_POINT ( 'NONE',  ( -8.866669273657352690, 9.446795028796142191, 0.7216878364870438212 ) ) ;
#5914=CARTESIAN_POINT ( 'NONE',  ( 6.968527767744104651, 8.192665819532020777, 1.082531754730558626 ) ) ;
#5915=CARTESIAN_POINT ( 'NONE',  ( -7.659993601596710278, 10.92011438762942355, -1.082531754730543083 ) ) ;
#5918=ORIENTED_EDGE ( 'NONE', *, *, #36887, .T. ) ;
#5920=CARTESIAN_POINT ( 'NONE',  ( 6.889514614038635187, 11.18951748302043114, -0.7998128361456291469 ) ) ;
#5926=CARTESIAN_POINT ( 'NONE',  ( -1.364683531250000748, 2.009375000341421913, 1.214306433183764966E-14 ) ) ;
#5932=CARTESIAN_POINT ( 'NONE',  ( 9.094822116668764167, 9.505047312402055582, 0.7998128361456462443 ) ) ;
#5936=CARTESIAN_POINT ( 'NONE',  ( -10.34217224912604571, 10.96028913360221502, 0.7998128361456462443 ) ) ;
#5942=CARTESIAN_POINT ( 'NONE',  ( 9.028840231696797503, 12.62106513936658203, -1.199719254218446718 ) ) ;
#5946=CARTESIAN_POINT ( 'NONE',  ( -9.854078719034067291, 10.39084668182823634, 0.7998128361456462443 ) ) ;
#5951=CARTESIAN_POINT ( 'NONE',  ( 5.378845419373885051, 6.306261619127770501, 1.070519943709395960 ) ) ;
#5953=CARTESIAN_POINT ( 'NONE',  ( -3.066115294984855133, 6.728884944124295053, 0.7998128361456341429 ) ) ;
#5957=CARTESIAN_POINT ( 'NONE',  ( 7.610204295972345712, 7.772993188256215547, 0.7998128361456341429 ) ) ;
#5959=CARTESIAN_POINT ( 'NONE',  ( 5.587931867126699537, 9.671004278289832001, -0.7998128361456291469 ) ) ;
#5962=AXIS2_PLACEMENT_3D ( 'NONE', #45770, #62003, #127084 ) ;
#5963=CARTESIAN_POINT ( 'NONE',  ( -7.809133291791416909, 11.09411069285655493, 1.082531754730549967 ) ) ;
#5971=CARTESIAN_POINT ( 'NONE',  ( -5.796211742468360129, 6.069872997065163922, -0.5622600474686073602 ) ) ;
#5973=CARTESIAN_POINT ( 'NONE',  ( 4.934804725694211136, 6.780358151441803649, -1.443375672974051449 ) ) ;
#5977=ADVANCED_FACE ( 'NONE', ( #194125 ), #211187, .F. ) ;
#5986=ORIENTED_EDGE ( 'NONE', *, *, #186211, .T. ) ;
#5996=CARTESIAN_POINT ( 'NONE',  ( 6.760712154708803823, 11.03924794713562818, 1.040834085586084257E-14 ) ) ;
#6000=CARTESIAN_POINT ( 'NONE',  ( -0.7500000000000006661, 1.139583334016154526, -1.299038105676652011 ) ) ;
#6001=FACE_OUTER_BOUND ( 'NONE', #149072, .T. ) ;
#6002=CARTESIAN_POINT ( 'NONE',  ( -5.194745412330402878, 9.212286747694129474, 0.000000000000000000 ) ) ;
#6006=CARTESIAN_POINT ( 'NONE',  ( -9.917953063596627317, 11.52969898140628047, -1.199719254218441611 ) ) ;
#6007=CARTESIAN_POINT ( 'NONE',  ( -1.490514837427357131, 7.209629588552680879, 4.246172784736861772 ) ) ;
#6010=CARTESIAN_POINT ( 'NONE',  ( 0.7499999999999920064, 5.514583334016151639, 1.299038105676669330 ) ) ;
#6011=CARTESIAN_POINT ( 'NONE',  ( 7.019370843573166319, 9.212351955633947043, 1.599625672291281386 ) ) ;
#6015=CARTESIAN_POINT ( 'NONE',  ( -5.540478329478883524, 9.615641817700700145, 0.000000000000000000 ) ) ;
#6017=CARTESIAN_POINT ( 'NONE',  ( 5.111635199556411102, 6.706590097621358382, -1.441599559997795321 ) ) ;
#6018=CARTESIAN_POINT ( 'NONE',  ( -5.070386261386537363, 5.017798181146802428, 1.214306433183764966E-14 ) ) ;
#6023=CARTESIAN_POINT ( 'NONE',  ( -7.131225611108100715, 9.342849184424693476, 1.443375672974078761 ) ) ;
#6028=CARTESIAN_POINT ( 'NONE',  ( 1.364683531249988535, 3.967708333674751842, -0.7879004041258239610 ) ) ;
#6034=CARTESIAN_POINT ( 'NONE',  ( -0.6823417656250212460, 4.551041667008086655, 1.181850606188767472 ) ) ;
#6037=CARTESIAN_POINT ( 'NONE',  ( 4.338245966248566177, 4.163634503485842409, 1.214306433183764966E-14 ) ) ;
#6038=CARTESIAN_POINT ( 'NONE',  ( -1.201851678989727383E-14, 5.509375000341415252, -1.575800808251660134 ) ) ;
#6044=CARTESIAN_POINT ( 'NONE',  ( -1.364683531250014514, 1.238541667008091096, -0.7879004041258289570 ) ) ;
#6045=CARTESIAN_POINT ( 'NONE',  ( -2.494337075234348777, 5.853884321174607663, -0.7216878364870267237 ) ) ;
#6046=CARTESIAN_POINT ( 'NONE',  ( 5.820528018968444961, 5.685037531751635953, 0.7998128361456341429 ) ) ;
#6050=FACE_OUTER_BOUND ( 'NONE', #40063, .T. ) ;
#6053=CARTESIAN_POINT ( 'NONE',  ( 5.029711800989886683, 4.970344644017389513, 1.040834085586084257E-14 ) ) ;
#6056=CARTESIAN_POINT ( 'NONE',  ( -9.002250809794013264, 9.604973487622245898, -0.7216878364870267237 ) ) ;
#6061=CARTESIAN_POINT ( 'NONE',  ( -8.459397779922852578, 11.95671561229694824, 1.199719254218453823 ) ) ;
#6063=CARTESIAN_POINT ( 'NONE',  ( -6.710922848640111127, 6.931757532942661726, 0.7216878364870317197 ) ) ;
#6065=CARTESIAN_POINT ( 'NONE',  ( 1.364683531249986537, 2.717708333674754062, -0.7879004041258239610 ) ) ;
#6079=VERTEX_POINT ( 'NONE', #186414 ) ;
#6083=CARTESIAN_POINT ( 'NONE',  ( -3.789667630219657912, 4.380032642466370696, 1.199719254218462483 ) ) ;
#6087=CARTESIAN_POINT ( 'NONE',  ( -1.201851678989727383E-14, 2.634375000341417916, 1.575800808251672791 ) ) ;
#6098=CARTESIAN_POINT ( 'NONE',  ( 1.364683531249986537, 0.6552083336747522857, -0.7879004041258239610 ) ) ;
#6107=CARTESIAN_POINT ( 'NONE',  ( 5.867981556616276073, 5.740399992340775803, -0.7998128361456281477 ) ) ;
#6110=ORIENTED_EDGE ( 'NONE', *, *, #176940, .T. ) ;
#6112=DIRECTION ( 'NONE',  ( 0.1674078377056216482, 0.000000000000000000, 0.9858877298530133171 ) ) ;
#6114=CARTESIAN_POINT ( 'NONE',  ( 8.606728586576791074, 8.935604860628076906, 0.7998128361456462443 ) ) ;
#6119=CARTESIAN_POINT ( 'NONE',  ( 7.476431642932036326, 10.80992178580769014, 1.199719254218460707 ) ) ;
#6125=ORIENTED_EDGE ( 'NONE', *, *, #20625, .T. ) ;
#6127=CYLINDRICAL_SURFACE ( 'NONE', #144539, 1.500000000000000222 ) ;
#6131=CARTESIAN_POINT ( 'NONE',  ( -8.188761592974058701, 8.655902734665618325, -0.7216878364870278340 ) ) ;
#6135=CARTESIAN_POINT ( 'NONE',  ( -8.727698198895085469, 11.20540053684285553, -1.599625672291263179 ) ) ;
#6139=CARTESIAN_POINT ( 'NONE',  ( -3.276266675996675204, 6.974061555304760240, -0.7998128361456281477 ) ) ;
#6141=CARTESIAN_POINT ( 'NONE',  ( 8.452618703115982512, 11.94880668935564216, 1.199719254218450271 ) ) ;
#6143=CARTESIAN_POINT ( 'NONE',  ( 5.840865249388943248, 5.708764300575555062, 0.7998128361456341429 ) ) ;
#6149=CARTESIAN_POINT ( 'NONE',  ( 2.575685996916329046, 5.948791396470269888, 0.7216878364870438212 ) ) ;
#6151=CARTESIAN_POINT ( 'NONE',  ( -5.901876940650454095, 5.779944607047298177, -0.7998128361456291469 ) ) ;
#6154=B_SPLINE_CURVE_WITH_KNOTS ( 'NONE', 3,
 ( #90588, #58065, #41844, #107956, #208558, #175039, #76445, #91666, #9314, #75390 ),
 .UNSPECIFIED., .F., .F.,
 ( 4, 3, 3, 4 ),
 ( 0.000000000000000000, 4.502046072369012122E-05, 9.004093402560476938E-05, 0.0001800865003230942441 ),
 .UNSPECIFIED. ) ;
#6155=CARTESIAN_POINT ( 'NONE',  ( -9.809487834687324437, 11.40315621434539395, 1.199719254218462483 ) ) ;
#6161=CARTESIAN_POINT ( 'NONE',  ( 9.422553571817644524, 10.09532670998316384, 0.000000000000000000 ) ) ;
#6162=CARTESIAN_POINT ( 'NONE',  ( -1.364683531250012516, 3.551041667008085323, -0.7879004041258300672 ) ) ;
#6164=CARTESIAN_POINT ( 'NONE',  ( 3.147464216666835402, 6.823792019419957278, -0.7998128361456291469 ) ) ;
#6168=( BOUNDED_CURVE ( )  B_SPLINE_CURVE ( 2, ( #149856, #1424, #202829, #120623, #183402, #82696, #35006 ),
 .UNSPECIFIED., .F., .T. ) 
 B_SPLINE_CURVE_WITH_KNOTS ( ( 3, 2, 2, 3 ),
 ( 0.2250000000000001998, 0.2291666666666668517, 0.2333333333333335313, 0.2375000000000001832 ),
 .UNSPECIFIED. ) 
 CURVE ( )  GEOMETRIC_REPRESENTATION_ITEM ( )  RATIONAL_B_SPLINE_CURVE ( ( 0.9999999999999937828, 0.8660254037844449249, 1.000000000000000000, 0.8660254037844387076, 1.000000000000000000, 0.8660254037844324904, 1.000000000000006217 ) ) 
 REPRESENTATION_ITEM ( '' )  );
#6180=CARTESIAN_POINT ( 'NONE',  ( -1.201851678989727383E-14, 2.134375000341423689, 1.575800808251672791 ) ) ;
#6182=CARTESIAN_POINT ( 'NONE',  ( 3.460355519985863548, 5.060167411448709629, 1.599625672291267398 ) ) ;
#6184=CARTESIAN_POINT ( 'NONE',  ( -6.236387472606166327, 6.378132927569716060, -0.7216878364870278340 ) ) ;
#6185=CARTESIAN_POINT ( 'NONE',  ( 3.551873057100287223, 5.166937871415542283, 1.443375672974062551 ) ) ;
#6186=CARTESIAN_POINT ( 'NONE',  ( -6.548225005276122168, 6.741943382351338165, 0.7216878364870317197 ) ) ;
#6187=DIRECTION ( 'NONE',  ( 5.578564026256490882E-16, 1.000000000000000000, 9.066213480720158442E-32 ) ) ;
#6190=CARTESIAN_POINT ( 'NONE',  ( 4.462605117192430804, 8.358123070033169455, 1.040834085586084257E-14 ) ) ;
#6200=CARTESIAN_POINT ( 'NONE',  ( 6.440286661691305703, 7.472421512516709718, 1.199719254218462483 ) ) ;
#6201=SURFACE_SIDE_STYLE ('',( #206551 ) ) ;
#6205=CARTESIAN_POINT ( 'NONE',  ( -5.554036483092550824, 9.631459663583308739, -0.7998128361456231517 ) ) ;
#6209=CARTESIAN_POINT ( 'NONE',  ( 6.968000882419564945, 10.21675256520979858, 1.199719254218460707 ) ) ;
#6211=CARTESIAN_POINT ( 'NONE',  ( -5.228640796364566690, 9.251831362400652736, -0.7998128361456231517 ) ) ;
#6212=CARTESIAN_POINT ( 'NONE',  ( 6.765155463094751909, 8.915767345075790828, 1.443375672974076540 ) ) ;
#6213=CARTESIAN_POINT ( 'NONE',  ( 4.247106804623488330, 7.517614509530361033, 0.9983198370346995087 ) ) ;
#6215=CARTESIAN_POINT ( 'NONE',  ( -4.086893239515592136, 6.855460315155083251, 1.199719254218464037 ) ) ;
#6219=CARTESIAN_POINT ( 'NONE',  ( -6.413170354464012846, 7.440785820751486312, 1.199719254218450271 ) ) ;
#6222=CARTESIAN_POINT ( 'NONE',  ( 1.364683531249986537, 1.405208333674755838, -0.7879004041258239610 ) ) ;
#6224=CARTESIAN_POINT ( 'NONE',  ( -5.694061328059534688, 8.626526735169329996, 1.082531754730548412 ) ) ;
#6230=CARTESIAN_POINT ( 'NONE',  ( 7.006866460164219212, 7.069099046480051385, -0.7998128361456281477 ) ) ;
#6232=FACE_OUTER_BOUND ( 'NONE', #129039, .T. ) ;
#6233=CARTESIAN_POINT ( 'NONE',  ( -1.402160292154681736E-14, 1.009375000341417916, -1.575800808251659024 ) ) ;
#6237=CARTESIAN_POINT ( 'NONE',  ( 4.067082894419602468, 3.847277586352047862, -0.7216878364870188411 ) ) ;
#6240=EDGE_CURVE ( 'NONE', #180436, #147186, #129871, .T. ) ;
#6241=CARTESIAN_POINT ( 'NONE',  ( -3.262708522383007903, 6.958243709422141876, 1.040834085586084257E-14 ) ) ;
#6242=CARTESIAN_POINT ( 'NONE',  ( -7.687109908824056426, 8.070642436490613747, 0.7216878364870438212 ) ) ;
#6252=CARTESIAN_POINT ( 'NONE',  ( -8.148087131688692253, 10.52918762510205042, -1.443375672974058777 ) ) ;
#6254=CARTESIAN_POINT ( 'NONE',  ( -7.334597915313094241, 9.580116872663850813, 1.040834085586084257E-14 ) ) ;
#6256=CARTESIAN_POINT ( 'NONE',  ( -8.636180661780672452, 9.177891648273343250, -0.7216878364870267237 ) ) ;
#6262=CARTESIAN_POINT ( 'NONE',  ( -0.7499999999999972244, 5.389583334016151639, -1.299038105676652899 ) ) ;
#6270=CARTESIAN_POINT ( 'NONE',  ( -7.393273838153706201, 7.519907654134449615, 0.7998128361456341429 ) ) ;
#6273=CARTESIAN_POINT ( 'NONE',  ( 3.659811400685081040, 6.357198169852855685, -1.199719254218446718 ) ) ;
#6277=CARTESIAN_POINT ( 'NONE',  ( 6.440286661691305703, 7.472421512516709718, 1.199719254218462483 ) ) ;
#6282=CARTESIAN_POINT ( 'NONE',  ( -3.619663825168619731, 7.166765529431275539, 1.040834085586084257E-14 ) ) ;
#6289=LINE ( 'NONE', #205566, #12324 ) ;
#6292=CARTESIAN_POINT ( 'NONE',  ( -0.6823417656250212460, 1.051041667008083325, 1.181850606188755259 ) ) ;
#6294=CARTESIAN_POINT ( 'NONE',  ( -9.203287345578106127, 9.631590079462940324, 0.7998128361456462443 ) ) ;
#6296=CARTESIAN_POINT ( 'NONE',  ( 8.633844893804129228, 8.967240552393299424, -0.7998128361456211532 ) ) ;
#6298=CARTESIAN_POINT ( 'NONE',  ( -7.316596452869116973, 11.68777962832266049, 0.7998128361456481317 ) ) ;
#6301=B_SPLINE_CURVE_WITH_KNOTS ( 'NONE', 3,
 ( #149473, #168910, #166791, #150553, #202449, #74359, #67121, #54104, #50905, #35706, #84462, #172938, #186217, #140462, #115963, #100714, #99654, #165723, #133254, #117033, #183028, #34644, #18385, #68188, #200326, #101783, #167850, #138143 ),
 .UNSPECIFIED., .F., .F.,
 ( 4, 3, 3, 3, 3, 3, 3, 3, 3, 4 ),
 ( 0.000000000000000000, 1.600956980237147682E-05, 1.644526376030698057E-05, 3.791386034648869355E-05, 4.420234518516011314E-05, 5.951836916331200894E-05, 6.580566471116502784E-05, 8.237066101204505307E-05, 0.0001137110868648263224, 0.0001607716038169918046 ),
 .UNSPECIFIED. ) ;
#6302=CARTESIAN_POINT ( 'NONE',  ( -0.6823417656249969321, 5.217708333674756283, -1.181850606188749264 ) ) ;
#6304=CARTESIAN_POINT ( 'NONE',  ( 9.408995418203971894, 11.03987807840189816, 1.082531754730549967 ) ) ;
#6308=CARTESIAN_POINT ( 'NONE',  ( -1.499999999999997780, 5.900000000000023448, 1.214306433183764966E-14 ) ) ;
#6310=CARTESIAN_POINT ( 'NONE',  ( -2.081668171172168513E-14, 2.800000000000024691, 2.500000000000011102 ) ) ;
#6311=CARTESIAN_POINT ( 'NONE',  ( 6.249945625775433555, 10.23542763013927726, -0.7216878364870267237 ) ) ;
#6314=CARTESIAN_POINT ( 'NONE',  ( -4.921246572080546500, 8.685278734161874681, 1.214306433183764966E-14 ) ) ;
#6316=CARTESIAN_POINT ( 'NONE',  ( 1.364683531249990311, 2.884375000341422801, 1.214306433183764966E-14 ) ) ;
#6320=CARTESIAN_POINT ( 'NONE',  ( -7.217017841176048165, 7.314275657660511243, 1.040834085586084257E-14 ) ) ;
#6327=CARTESIAN_POINT ( 'NONE',  ( 7.690499447449630210, 9.995335326823163058, 1.599625672291281386 ) ) ;
#6330=CARTESIAN_POINT ( 'NONE',  ( -0.7500000000000006661, 1.358333333333357151, -1.299038105676652011 ) ) ;
#6332=VECTOR ( 'NONE', #120431, 1000.000000000000000 ) ;
#6337=CARTESIAN_POINT ( 'NONE',  ( 6.805829924380118356, 7.042482454639357847, 0.7216878364870317197 ) ) ;
#6338=CARTESIAN_POINT ( 'NONE',  ( -1.364683531250000748, -1.178124999658580752, 0.000000000000000000 ) ) ;
#6340=CARTESIAN_POINT ( 'NONE',  ( 3.029357257649615054, 5.621668336311468117, -1.199719254218446718 ) ) ;
#6345=CARTESIAN_POINT ( 'NONE',  ( 6.428537391173986038, 10.65171072301167854, 0.7998128361456462443 ) ) ;
#6346=CARTESIAN_POINT ( 'NONE',  ( -8.829384350997580455, 11.32403438096243775, 1.599625672291269396 ) ) ;
#6348=EDGE_CURVE ( 'NONE', #47677, #152385, #64088, .T. ) ;
#6349=CARTESIAN_POINT ( 'NONE',  ( -1.402160292154681736E-14, 0.07187500034142156602, 1.575800808251672791 ) ) ;
#6350=CARTESIAN_POINT ( 'NONE',  ( 0.7499999999999885647, 0.9833333333333569293, 1.299038105676657340 ) ) ;
#6352=CARTESIAN_POINT ( 'NONE',  ( 4.985647801523278133, 6.839675073242382553, -1.599625672291256295 ) ) ;
#6357=( BOUNDED_SURFACE ( )  B_SPLINE_SURFACE ( 1, 2, ( 
 ( #155486, #185829, #87284, #186904, #171728, #54784, #37460, #140335, #122004, #71000, #137113, #205278, #106787, #56917, #172815, #203142, #206354, #38536, #24387, #57981, #124144, #63317, #107871, #76362, #144612, #211681, #126272, #142469, #207424, #195460, #129478, #9230, #173897, #60113, #145683, #11349, #75302, #59043, #108937, #25473, #160823, #141417, #43892, #91580, #78495, #111067, #157632, #174958, #125201, #191164, #26540, #92648, #178147, #44959, #177073, #61183, #158690, #42831, #10288, #208477, #192229, #77430, #110006, #79564, #176019, #193313, #27611, #12415, #161902, #93711, #143547, #29761, #159752, #209541, #94775, #127343, #28689, #210627, #62253, #128414, #194381, #46024, #112144, #95846, #13489, #132615, #48164, #212751, #181323, #67543, #117461, #146733, #66475, #51335, #183454, #1476, #34005, #165081, #148830, #35059, #49212, #197568, #80641, #50269, #114276, #101130, #180273, #167218, #18805, #31897, #16672, #198622, #133685, #84890, #150977, #65418, #2542, #100079, #68617, #149909, #116387, #96914, #97974, #131567, #182375, #147779, #162965, #134742, #115332, #196521, #164033, #403, #199690, #32951, #99025, #14544, #47089, #15608, #113207, #64385, #82757, #179212, #30837, #81696, #83816, #130530, #166141, #213795, #17728, #76895, #93189, #105168, #200749, #156032, #27081, #107342, #171206, #88914, #204748, #52398, #42300, #22800, #139805, #118525, #174437, #206896, #159221, #56399, #39082, #10821, #122560, #188522, #59587, #187454, #40153, #154968, #6553, #72631, #141949, #138730, #173364, #106266, #172288, #207961, #23876, #24946, #140884, #58527, #157111, #89982, #7622, #73708, #205833, #57466, #91050, #123625, #175494, #189589, #74784, #41235, #108414, #43364, #8700, #124682, #125744, #190640, #26013, #92124, #158176, #9769, #75842, #191705, #109486, #146202, #11895, #144091, #64910, #180799, #14012, #210087, #94253, #62778, #163499, #213284, #28157, #162436, #147252, #131059, #97443, #130009, #46556, #30299, #197047, #145148, #79032, #176547, #212217, #61726, #48684, #127894, #114800, #32424, #193845, #112676, #80098, #15082, #98491, #164555, #161372, #16140, #196000, #143019, #31367, #63853, #192769, #45495, #12954, #47634, #29231, #44428, #209014, #211154, #77969, #111611, #96384, #81173, #128941, #194918, #110545, #60650, #177622, #126813, #160292, #178686, #95323, #113745, #179749, #119065, #186121, #100614, #50801, #181847, #169876, #37755, #198105, #82225, #34544, #120143, #200230, #49734, #33484, #83285, #148316, #135276, #115862, #18281, #214315, #52931, #85432, #103828, #149370, #132095, #65947, #952, #67018, #152566, #99556, #133154, #165621, #36671, #136335, #151517, #4153, #166690, #199156, #17209, #185047, #116929, #182928, #201290, #84364, #150455, #2016, #68085, #134220, #51880, #118003, #183992, #35606, #101683, #167752, #19352, #3085, #168815, #70224, #69156, #102760, #20419, #202355, #86501, #54005, #91871, #154713, #141704, #89732, #155780, #7365, #106009, #174187, #21466, #73442, #172031, #22547, #139546, #9520, #170947, #187195, #74530, #205572, #57210, #71290, #122302, #207715, #23623, #104907, #124432, #109234, #6294, #25758, #123370, #90793, #38823, #189337, #40976, #88653, #107087, #173109, #72368, #43119, #153645, #24689, #156857, #138469, #157927, #5215, #75592, #140630, #8442, #137402, #206643, #58276, #190390, #42048, #108159, #59338, #125492, #203420, #191454, #87575, #55076, #204491, #121225, #56141, #188259, #39900, #142763, #47381, #196800, #61470, #45242, #147011, #209833, #95063, #10574, #129760, #161112, #46307, #26830, #193600, #79847, #163249, #113494, #78776, #160041, #162185, #213035, #128694, #12698, #11645, #211966, #145956, #144897, #77716, #63605, #143838, #110294, #127635, #13771, #210905, #62532, #76648, #111359, #80922, #177364, #44174, #195744, #48442, #94002, #179500, #194662, #30043, #192520, #112423, #178437, #176302, #96132, #31122, #28978, #175244, #92933, #97196, #14831, #126560, #64664, #158977, #130810, #208768, #60396, #27905, #116669, #133971, #50547, #18022, #167498, #35351, #19096, #98248, #20159, #199979, #81977, #16955 ),
 ( #34289, #51626, #180550, #132897, #85175, #102496, #201033, #84108, #99312, #101427, #86246, #67824, #166431, #165362, #151259, #2831, #150197, #83036, #68900, #149111, #49485, #690, #135019, #168560, #117751, #36418, #66756, #33229, #164304, #52676, #136075, #202091, #118807, #198901, #182667, #100361, #1767, #15893, #115606, #183741, #114557, #184792, #32171, #152316, #3893, #69965, #148065, #214071, #65697, #131844, #197854, #181601, #53749, #71033, #137146, #37495, #119882, #87316, #153383, #4955, #21212, #185860, #103571, #169629, #50689, #149258, #131986, #164442, #30177, #112558, #214207, #147144, #64799, #211036, #47518, #66902, #31256, #96267, #49621, #34432, #79985, #165504, #48576, #16029, #178571, #213170, #130943, #162319, #114692, #180685, #212100, #182815, #78909, #163388, #32311, #13904, #17097, #145033, #835, #65837, #82113, #62662, #14961, #98378, #97330, #196936, #197994, #148206, #115746, #128821, #133042, #181735, #194803, #63737, #33367, #83175, #81059, #99448, #46439, #199042, #161250, #113629, #116814, #12837, #195880, #146088, #129895, #179636, #20311, #186009, #166580, #118960, #5107, #88545, #187085, #4045, #85324, #87471, #72255, #53899, #152465, #151407, #137301, #71183, #70114, #2980, #203318, #69049, #35497, #135169, #54968, #154607, #103723, #22435, #52823, #19244, #84256, #121121, #122190, #188155, #153537, #201184, #184938, #36565, #102651, #1910, #101575, #168707, #100505, #86397, #18168, #120035, #136226, #202248, #38718, #6186, #150341, #37644, #169773, #138362, #67969, #104799, #170845, #21363, #204380, #56036, #134112, #200121, #51775, #117893, #183885, #167643, #205467, #44067, #25650, #27797, #189231, #208660, #190284, #91761, #89619, #159934, #40870, #142650, #155672, #58166, #209725, #39787, #8338, #76539, #143732, #124324, #74423, #139432, #127527, #61369, #7254, #105893, #206536, #77607, #157815, #73330, #57100, #106975, #171918, #92824, #123267, #41941, #23514, #10465, #43009, #173000, #24581, #90688, #156749, #140523, #108054, #110185, #174079, #9413, #75484, #141595, #207602, #192412, #59221, #125379, #191344, #109122, #175136, #26723, #158869, #60290, #126449, #176196, #93895, #11538, #165252, #46200, #64561, #211861, #32062, #33123, #112317, #163142, #49381, #162077, #13666, #180446, #80817, #212926, #82928, #181494, #164198, #196696, #62425, #194556, #115499, #16845, #130705, #178332, #144795, #113386, #213969, #99202, #78669, #48336, #197743, #149000, #147956, #98150, #97089, #146907, #577, #195638, #129653, #12596, #114446, #29940, #66643, #96026, #193498, #45140, #79738, #14725, #15786, #65589, #111252, #177255, #63499, #28869, #81871, #94954, #131737, #161002, #210802, #145854, #47272, #128590, #179395, #31015, #120849, #134909, #67709, #35234, #20047, #100248, #104530, #199867, #3775, #151148, #185744, #186822, #51510, #102379, #203054, #101309, #167390, #119765, #86134, #152206, #22157, #38450, #103453, #135960, #1651, #133858, #54698, #170576, #69850, #117635, #83992, #52564, #153263, #88272, #17906, #201975, #137028, #154339, #87199, #37378, #36302, #53632, #5915, #200916, #68790, #166316, #169513, #183626, #132787, #18980, #198790, #50439, #85063, #168448, #21095, #4838, #116559, #182552, #2717, #34176, #70917, #150080, #118695, #184680, #121919, #205194, #90415, #9150, #172734, #187887, #60035, #74160, #6985, #188961, #173818, #26462, #8074, #124064, #39515, #192151, #73065, #174882, #105614, #156485, #27535, #71989, #40602, #108856, #175939, #140254, #106708, #171644, #159672, #93630, #23241, #138100, #24310, #109928, #190029, #89353, #155402, #139164, #204111, #125126, #56835, #206277, #55763, #42752, #75226, #123007, #57899, #41682, #107792, #25396, #91495, #142393, #157555, #141337, #207351, #58971, #191084, #10211, #92571, #158614, #76285, #208402, #126188, #43815, #28611, #94701, #61106, #194304, #195379, #179132, #63238, #210546, #48088, #196443, #129400, #62181, #114200, #128339, #160741, #45946, #180198, #65343, #14465, #147701, #178066, #144537, #209462, #31819, #32872, #98949, #64309, #112066, #29684, #95768, #161823, #127265, #12336 ) ),
 .UNSPECIFIED., .F., .F., .T. ) 
 B_SPLINE_SURFACE_WITH_KNOTS ( ( 2, 2 ),
 ( 3, 2, 2, 2, 2, 2, 2, 2, 2, 2, 2, 2, 2, 2, 2, 2, 2, 2, 2, 2, 2, 2, 2, 2, 2, 2, 2, 2, 2, 2, 2, 2, 2, 2, 2, 2, 2, 2, 2, 2, 2, 2, 2, 2, 2, 2, 2, 2, 2, 2, 2, 2, 2, 2, 2, 2, 2, 2, 2, 2, 2, 2, 2, 2, 2, 2, 2, 2, 2, 2, 2, 2, 2, 2, 2, 2, 2, 2, 2, 2, 2, 2, 2, 2, 2, 2, 2, 2, 2, 2, 2, 2, 2, 2, 2, 2, 2, 2, 2, 2, 2, 2, 2, 2, 2, 2, 2, 2, 2, 2, 2, 2, 2, 2, 2, 2, 2, 2, 2, 2, 2, 2, 2, 2, 2, 2, 2, 2, 2, 2, 2, 2, 2, 2, 2, 2, 2, 2, 2, 2, 2, 2, 2, 2, 2, 2, 2, 2, 2, 2, 2, 2, 2, 2, 2, 2, 2, 2, 2, 2, 2, 2, 2, 2, 2, 2, 2, 2, 2, 2, 2, 2, 2, 2, 2, 2, 2, 2, 2, 2, 2, 2, 2, 2, 2, 2, 2, 2, 2, 2, 2, 2, 2, 2, 2, 2, 2, 2, 2, 2, 2, 2, 2, 2, 2, 2, 2, 2, 2, 2, 2, 2, 2, 2, 2, 2, 2, 2, 2, 2, 2, 2, 2, 2, 2, 2, 2, 2, 2, 2, 2, 2, 2, 2, 2, 2, 2, 2, 2, 2, 3 ),
 ( 0.000000000000000000, 1.000000000000000000 ),
 ( 0.000000000000000000, 0.004166666666666666609, 0.008333333333333333218, 0.01250000000000000069, 0.01666666666666666644, 0.02083333333333333218, 0.02500000000000000139, 0.02916666666666666713, 0.03333333333333333287, 0.03749999999999999861, 0.04166666666666666435, 0.04583333333333333010, 0.05000000000000000278, 0.05416666666666666852, 0.05833333333333333426, 0.06250000000000000000, 0.06666666666666666574, 0.07083333333333333148, 0.07499999999999999722, 0.07916666666666666297, 0.08333333333333332871, 0.08749999999999999445, 0.09166666666666666019, 0.09583333333333333981, 0.1000000000000000056, 0.1041666666666666713, 0.1083333333333333370, 0.1125000000000000028, 0.1166666666666666685, 0.1208333333333333343, 0.1250000000000000000, 0.1291666666666666796, 0.1333333333333333315, 0.1375000000000000111, 0.1416666666666666630, 0.1458333333333333426, 0.1499999999999999944, 0.1541666666666666741, 0.1583333333333333259, 0.1625000000000000056, 0.1666666666666666574, 0.1708333333333333370, 0.1749999999999999889, 0.1791666666666666685, 0.1833333333333333204, 0.1875000000000000000, 0.1916666666666666796, 0.1958333333333333315, 0.2000000000000000111, 0.2041666666666666630, 0.2083333333333333426, 0.2124999999999999944, 0.2166666666666666741, 0.2208333333333333259, 0.2250000000000000056, 0.2291666666666666574, 0.2333333333333333370, 0.2374999999999999889, 0.2416666666666666685, 0.2458333333333333204, 0.2500000000000000000, 0.2541666666666666519, 0.2583333333333333592, 0.2625000000000000111, 0.2666666666666666630, 0.2708333333333333148, 0.2750000000000000222, 0.2791666666666666741, 0.2833333333333333259, 0.2874999999999999778, 0.2916666666666666852, 0.2958333333333333370, 0.2999999999999999889, 0.3041666666666666408, 0.3083333333333333481, 0.3125000000000000000, 0.3166666666666666519, 0.3208333333333333592, 0.3250000000000000111, 0.3291666666666666630, 0.3333333333333333148, 0.3375000000000000222, 0.3416666666666666741, 0.3458333333333333259, 0.3499999999999999778, 0.3541666666666666852, 0.3583333333333333370, 0.3624999999999999889, 0.3666666666666666408, 0.3708333333333333481, 0.3750000000000000000, 0.3791666666666666519, 0.3833333333333333592, 0.3875000000000000111, 0.3916666666666666630, 0.3958333333333333148, 0.4000000000000000222, 0.4041666666666666741, 0.4083333333333333259, 0.4124999999999999778, 0.4166666666666666852, 0.4208333333333333370, 0.4249999999999999889, 0.4291666666666666408, 0.4333333333333333481, 0.4375000000000000000, 0.4416666666666666519, 0.4458333333333333592, 0.4500000000000000111, 0.4541666666666666630, 0.4583333333333333148, 0.4625000000000000222, 0.4666666666666666741, 0.4708333333333333259, 0.4749999999999999778, 0.4791666666666666852, 0.4833333333333333370, 0.4874999999999999889, 0.4916666666666666408, 0.4958333333333333481, 0.5000000000000000000, 0.5041666666666666519, 0.5083333333333333037, 0.5124999999999999556, 0.5166666666666667185, 0.5208333333333333703, 0.5250000000000000222, 0.5291666666666666741, 0.5333333333333333259, 0.5374999999999999778, 0.5416666666666666297, 0.5458333333333332815, 0.5500000000000000444, 0.5541666666666666963, 0.5583333333333333481, 0.5625000000000000000, 0.5666666666666666519, 0.5708333333333333037, 0.5749999999999999556, 0.5791666666666667185, 0.5833333333333333703, 0.5875000000000000222, 0.5916666666666666741, 0.5958333333333333259, 0.5999999999999999778, 0.6041666666666666297, 0.6083333333333332815, 0.6125000000000000444, 0.6166666666666666963, 0.6208333333333333481, 0.6250000000000000000, 0.6291666666666666519, 0.6333333333333333037, 0.6374999999999999556, 0.6416666666666667185, 0.6458333333333333703, 0.6500000000000000222, 0.6541666666666666741, 0.6583333333333333259, 0.6624999999999999778, 0.6666666666666666297, 0.6708333333333332815, 0.6750000000000000444, 0.6791666666666666963, 0.6833333333333333481, 0.6875000000000000000, 0.6916666666666666519, 0.6958333333333333037, 0.6999999999999999556, 0.7041666666666667185, 0.7083333333333333703, 0.7125000000000000222, 0.7166666666666666741, 0.7208333333333333259, 0.7249999999999999778, 0.7291666666666666297, 0.7333333333333332815, 0.7375000000000000444, 0.7416666666666666963, 0.7458333333333333481, 0.7500000000000000000, 0.7541666666666666519, 0.7583333333333333037, 0.7624999999999999556, 0.7666666666666667185, 0.7708333333333333703, 0.7750000000000000222, 0.7791666666666666741, 0.7833333333333333259, 0.7874999999999999778, 0.7916666666666666297, 0.7958333333333332815, 0.8000000000000000444, 0.8041666666666666963, 0.8083333333333333481, 0.8125000000000000000, 0.8166666666666666519, 0.8208333333333333037, 0.8249999999999999556, 0.8291666666666667185, 0.8333333333333333703, 0.8375000000000000222, 0.8416666666666666741, 0.8458333333333333259, 0.8499999999999999778, 0.8541666666666666297, 0.8583333333333332815, 0.8625000000000000444, 0.8666666666666666963, 0.8708333333333333481, 0.8750000000000000000, 0.8791666666666666519, 0.8833333333333333037, 0.8874999999999999556, 0.8916666666666667185, 0.8958333333333333703, 0.9000000000000000222, 0.9041666666666666741, 0.9083333333333333259, 0.9124999999999999778, 0.9166666666666666297, 0.9208333333333332815, 0.9250000000000000444, 0.9291666666666666963, 0.9333333333333333481, 0.9375000000000000000, 0.9416666666666666519, 0.9458333333333333037, 0.9499999999999999556, 0.9541666666666667185, 0.9583333333333333703, 0.9625000000000000222, 0.9666666666666666741, 0.9708333333333333259, 0.9749999999999999778, 0.9791666666666666297, 0.9833333333333332815, 0.9875000000000000444, 0.9916666666666666963, 0.9958333333333333481, 1.000000000000000000 ),
 .UNSPECIFIED. ) 
 GEOMETRIC_REPRESENTATION_ITEM ( )  RATIONAL_B_SPLINE_SURFACE ( (
 ( 1.000000000000000000, 0.8660254037844387076, 1.000000000000000000, 0.8660254037844387076, 1.000000000000000000, 0.8660254037844387076, 1.000000000000000000, 0.8660254037844387076, 1.000000000000000000, 0.8660254037844387076, 1.000000000000000000, 0.8660254037844387076, 1.000000000000000000, 0.8660254037844387076, 1.000000000000000000, 0.8660254037844387076, 1.000000000000000000, 0.8660254037844387076, 1.000000000000000000, 0.8660254037844387076, 1.000000000000000000, 0.8660254037844387076, 1.000000000000000000, 0.8660254037844387076, 1.000000000000000000, 0.8660254037844387076, 1.000000000000000000, 0.8660254037844387076, 1.000000000000000000, 0.8660254037844387076, 1.000000000000000000, 0.8660254037844387076, 1.000000000000000000, 0.8660254037844387076, 1.000000000000000000, 0.8660254037844387076, 1.000000000000000000, 0.8660254037844387076, 1.000000000000000000, 0.8660254037844387076, 1.000000000000000000, 0.8660254037844387076, 1.000000000000000000, 0.8660254037844387076, 1.000000000000000000, 0.8660254037844387076, 1.000000000000000000, 0.8660254037844387076, 1.000000000000000000, 0.8660254037844387076, 1.000000000000000000, 0.8660254037844387076, 1.000000000000000000, 0.8660254037844387076, 1.000000000000000000, 0.8660254037844387076, 1.000000000000000000, 0.8660254037844387076, 1.000000000000000000, 0.8660254037844387076, 1.000000000000000000, 0.8660254037844387076, 1.000000000000000000, 0.8660254037844387076, 1.000000000000000000, 0.8660254037844387076, 1.000000000000000000, 0.8660254037844387076, 1.000000000000000000, 0.8660254037844387076, 1.000000000000000000, 0.8660254037844387076, 1.000000000000000000, 0.8660254037844387076, 1.000000000000000000, 0.8660254037844387076, 1.000000000000000000, 0.8660254037844387076, 1.000000000000000000, 0.8660254037844387076, 1.000000000000000000, 0.8660254037844387076, 1.000000000000000000, 0.8660254037844387076, 1.000000000000000000, 0.8660254037844387076, 1.000000000000000000, 0.8660254037844387076, 1.000000000000000000, 0.8660254037844387076, 1.000000000000000000, 0.8660254037844387076, 1.000000000000000000, 0.8660254037844387076, 1.000000000000000000, 0.8660254037844387076, 1.000000000000000000, 0.8660254037844387076, 1.000000000000000000, 0.8660254037844387076, 1.000000000000000000, 0.8660254037844387076, 1.000000000000000000, 0.8660254037844387076, 1.000000000000000000, 0.8660254037844387076, 1.000000000000000000, 0.8660254037844387076, 1.000000000000000000, 0.8660254037844387076, 1.000000000000000000, 0.8660254037844387076, 1.000000000000000000, 0.8660254037844387076, 1.000000000000000000, 0.8660254037844387076, 1.000000000000000000, 0.8660254037844387076, 1.000000000000000000, 0.8660254037844387076, 1.000000000000000000, 0.8660254037844387076, 1.000000000000000000, 0.8660254037844387076, 1.000000000000000000, 0.8660254037844387076, 1.000000000000000000, 0.8660254037844387076, 1.000000000000000000, 0.8660254037844387076, 1.000000000000000000, 0.8660254037844387076, 1.000000000000000000, 0.8660254037844387076, 1.000000000000000000, 0.8660254037844387076, 1.000000000000000000, 0.8660254037844387076, 1.000000000000000000, 0.8660254037844387076, 1.000000000000000000, 0.8660254037844387076, 1.000000000000000000, 0.8660254037844387076, 1.000000000000000000, 0.8660254037844387076, 1.000000000000000000, 0.8660254037844387076, 1.000000000000000000, 0.8660254037844387076, 1.000000000000000000, 0.8660254037844387076, 1.000000000000000000, 0.8660254037844387076, 1.000000000000000000, 0.8660254037844387076, 1.000000000000000000, 0.8660254037844387076, 1.000000000000000000, 0.8660254037844387076, 1.000000000000000000, 0.8660254037844387076, 1.000000000000000000, 0.8660254037844387076, 1.000000000000000000, 0.8660254037844387076, 1.000000000000000000, 0.8660254037844387076, 1.000000000000000000, 0.8660254037844387076, 1.000000000000000000, 0.8660254037844387076, 1.000000000000000000, 0.8660254037844387076, 1.000000000000000000, 0.8660254037844387076, 1.000000000000000000, 0.8660254037844387076, 1.000000000000000000, 0.8660254037844387076, 1.000000000000000000, 0.8660254037844387076, 1.000000000000000000, 0.8660254037844387076, 1.000000000000000000, 0.8660254037844387076, 1.000000000000000000, 0.8660254037844387076, 1.000000000000000000, 0.8660254037844387076, 1.000000000000000000, 0.8660254037844387076, 1.000000000000000000, 0.8660254037844387076, 1.000000000000000000, 0.8660254037844387076, 1.000000000000000000, 0.8660254037844387076, 1.000000000000000000, 0.8660254037844387076, 1.000000000000000000, 0.8660254037844387076, 1.000000000000000000, 0.8660254037844387076, 1.000000000000000000, 0.8660254037844387076, 1.000000000000000000, 0.8660254037844387076, 1.000000000000000000, 0.8660254037844387076, 1.000000000000000000, 0.8660254037844387076, 1.000000000000000000, 0.8660254037844387076, 1.000000000000000000, 0.8660254037844387076, 1.000000000000000000, 0.8660254037844387076, 1.000000000000000000, 0.8660254037844387076, 1.000000000000000000, 0.8660254037844387076, 1.000000000000000000, 0.8660254037844387076, 1.000000000000000000, 0.8660254037844387076, 1.000000000000000000, 0.8660254037844387076, 1.000000000000000000, 0.8660254037844387076, 1.000000000000000000, 0.8660254037844387076, 1.000000000000000000, 0.8660254037844387076, 1.000000000000000000, 0.8660254037844387076, 1.000000000000000000, 0.8660254037844387076, 1.000000000000000000, 0.8660254037844387076, 1.000000000000000000, 0.8660254037844387076, 1.000000000000000000, 0.8660254037844387076, 1.000000000000000000, 0.8660254037844387076, 1.000000000000000000, 0.8660254037844387076, 1.000000000000000000, 0.8660254037844387076, 1.000000000000000000, 0.8660254037844387076, 1.000000000000000000, 0.8660254037844387076, 1.000000000000000000, 0.8660254037844387076, 1.000000000000000000, 0.8660254037844387076, 1.000000000000000000, 0.8660254037844387076, 1.000000000000000000, 0.8660254037844387076, 1.000000000000000000, 0.8660254037844387076, 1.000000000000000000, 0.8660254037844387076, 1.000000000000000000, 0.8660254037844387076, 1.000000000000000000, 0.8660254037844387076, 1.000000000000000000, 0.8660254037844387076, 1.000000000000000000, 0.8660254037844387076, 1.000000000000000000, 0.8660254037844387076, 1.000000000000000000, 0.8660254037844387076, 1.000000000000000000, 0.8660254037844387076, 1.000000000000000000, 0.8660254037844387076, 1.000000000000000000, 0.8660254037844387076, 1.000000000000000000, 0.8660254037844387076, 1.000000000000000000, 0.8660254037844387076, 1.000000000000000000, 0.8660254037844387076, 1.000000000000000000, 0.8660254037844387076, 1.000000000000000000, 0.8660254037844387076, 1.000000000000000000, 0.8660254037844387076, 1.000000000000000000, 0.8660254037844387076, 1.000000000000000000, 0.8660254037844387076, 1.000000000000000000, 0.8660254037844387076, 1.000000000000000000, 0.8660254037844387076, 1.000000000000000000, 0.8660254037844387076, 1.000000000000000000, 0.8660254037844387076, 1.000000000000000000, 0.8660254037844387076, 1.000000000000000000, 0.8660254037844387076, 1.000000000000000000, 0.8660254037844387076, 1.000000000000000000, 0.8660254037844387076, 1.000000000000000000, 0.8660254037844387076, 1.000000000000000000, 0.8660254037844387076, 1.000000000000000000, 0.8660254037844387076, 1.000000000000000000, 0.8660254037844387076, 1.000000000000000000, 0.8660254037844387076, 1.000000000000000000, 0.8660254037844387076, 1.000000000000000000, 0.8660254037844387076, 1.000000000000000000, 0.8660254037844387076, 1.000000000000000000, 0.8660254037844387076, 1.000000000000000000, 0.8660254037844387076, 1.000000000000000000, 0.8660254037844387076, 1.000000000000000000, 0.8660254037844387076, 1.000000000000000000, 0.8660254037844387076, 1.000000000000000000, 0.8660254037844387076, 1.000000000000000000, 0.8660254037844387076, 1.000000000000000000, 0.8660254037844387076, 1.000000000000000000, 0.8660254037844387076, 1.000000000000000000, 0.8660254037844387076, 1.000000000000000000, 0.8660254037844387076, 1.000000000000000000, 0.8660254037844387076, 1.000000000000000000, 0.8660254037844387076, 1.000000000000000000, 0.8660254037844387076, 1.000000000000000000, 0.8660254037844387076, 1.000000000000000000, 0.8660254037844387076, 1.000000000000000000, 0.8660254037844387076, 1.000000000000000000, 0.8660254037844387076, 1.000000000000000000, 0.8660254037844387076, 1.000000000000000000, 0.8660254037844387076, 1.000000000000000000, 0.8660254037844387076, 1.000000000000000000, 0.8660254037844387076, 1.000000000000000000, 0.8660254037844387076, 1.000000000000000000, 0.8660254037844387076, 1.000000000000000000, 0.8660254037844387076, 1.000000000000000000, 0.8660254037844387076, 1.000000000000000000, 0.8660254037844387076, 1.000000000000000000, 0.8660254037844387076, 1.000000000000000000, 0.8660254037844387076, 1.000000000000000000, 0.8660254037844387076, 1.000000000000000000, 0.8660254037844387076, 1.000000000000000000, 0.8660254037844387076, 1.000000000000000000, 0.8660254037844387076, 1.000000000000000000, 0.8660254037844387076, 1.000000000000000000, 0.8660254037844387076, 1.000000000000000000, 0.8660254037844387076, 1.000000000000000000, 0.8660254037844387076, 1.000000000000000000, 0.8660254037844387076, 1.000000000000000000, 0.8660254037844387076, 1.000000000000000000, 0.8660254037844387076, 1.000000000000000000, 0.8660254037844387076, 1.000000000000000000, 0.8660254037844387076, 1.000000000000000000, 0.8660254037844387076, 1.000000000000000000, 0.8660254037844387076, 1.000000000000000000, 0.8660254037844387076, 1.000000000000000000, 0.8660254037844387076, 1.000000000000000000, 0.8660254037844387076, 1.000000000000000000, 0.8660254037844387076, 1.000000000000000000, 0.8660254037844387076, 1.000000000000000000, 0.8660254037844387076, 1.000000000000000000, 0.8660254037844387076, 1.000000000000000000, 0.8660254037844387076, 1.000000000000000000, 0.8660254037844387076, 1.000000000000000000, 0.8660254037844387076, 1.000000000000000000, 0.8660254037844387076, 1.000000000000000000, 0.8660254037844387076, 1.000000000000000000, 0.8660254037844387076, 1.000000000000000000, 0.8660254037844387076, 1.000000000000000000, 0.8660254037844387076, 1.000000000000000000, 0.8660254037844387076, 1.000000000000000000, 0.8660254037844387076, 1.000000000000000000, 0.8660254037844387076, 1.000000000000000000, 0.8660254037844387076, 1.000000000000000000, 0.8660254037844387076, 1.000000000000000000, 0.8660254037844387076, 1.000000000000000000, 0.8660254037844387076, 1.000000000000000000, 0.8660254037844387076, 1.000000000000000000, 0.8660254037844387076, 1.000000000000000000, 0.8660254037844387076, 1.000000000000000000, 0.8660254037844387076, 1.000000000000000000, 0.8660254037844387076, 1.000000000000000000, 0.8660254037844387076, 1.000000000000000000, 0.8660254037844387076, 1.000000000000000000, 0.8660254037844387076, 1.000000000000000000),
 ( 1.000000000000000000, 0.8660254037844387076, 1.000000000000000000, 0.8660254037844387076, 1.000000000000000000, 0.8660254037844387076, 1.000000000000000000, 0.8660254037844387076, 1.000000000000000000, 0.8660254037844387076, 1.000000000000000000, 0.8660254037844387076, 1.000000000000000000, 0.8660254037844387076, 1.000000000000000000, 0.8660254037844387076, 1.000000000000000000, 0.8660254037844387076, 1.000000000000000000, 0.8660254037844387076, 1.000000000000000000, 0.8660254037844387076, 1.000000000000000000, 0.8660254037844387076, 1.000000000000000000, 0.8660254037844387076, 1.000000000000000000, 0.8660254037844387076, 1.000000000000000000, 0.8660254037844387076, 1.000000000000000000, 0.8660254037844387076, 1.000000000000000000, 0.8660254037844387076, 1.000000000000000000, 0.8660254037844387076, 1.000000000000000000, 0.8660254037844387076, 1.000000000000000000, 0.8660254037844387076, 1.000000000000000000, 0.8660254037844387076, 1.000000000000000000, 0.8660254037844387076, 1.000000000000000000, 0.8660254037844387076, 1.000000000000000000, 0.8660254037844387076, 1.000000000000000000, 0.8660254037844387076, 1.000000000000000000, 0.8660254037844387076, 1.000000000000000000, 0.8660254037844387076, 1.000000000000000000, 0.8660254037844387076, 1.000000000000000000, 0.8660254037844387076, 1.000000000000000000, 0.8660254037844387076, 1.000000000000000000, 0.8660254037844387076, 1.000000000000000000, 0.8660254037844387076, 1.000000000000000000, 0.8660254037844387076, 1.000000000000000000, 0.8660254037844387076, 1.000000000000000000, 0.8660254037844387076, 1.000000000000000000, 0.8660254037844387076, 1.000000000000000000, 0.8660254037844387076, 1.000000000000000000, 0.8660254037844387076, 1.000000000000000000, 0.8660254037844387076, 1.000000000000000000, 0.8660254037844387076, 1.000000000000000000, 0.8660254037844387076, 1.000000000000000000, 0.8660254037844387076, 1.000000000000000000, 0.8660254037844387076, 1.000000000000000000, 0.8660254037844387076, 1.000000000000000000, 0.8660254037844387076, 1.000000000000000000, 0.8660254037844387076, 1.000000000000000000, 0.8660254037844387076, 1.000000000000000000, 0.8660254037844387076, 1.000000000000000000, 0.8660254037844387076, 1.000000000000000000, 0.8660254037844387076, 1.000000000000000000, 0.8660254037844387076, 1.000000000000000000, 0.8660254037844387076, 1.000000000000000000, 0.8660254037844387076, 1.000000000000000000, 0.8660254037844387076, 1.000000000000000000, 0.8660254037844387076, 1.000000000000000000, 0.8660254037844387076, 1.000000000000000000, 0.8660254037844387076, 1.000000000000000000, 0.8660254037844387076, 1.000000000000000000, 0.8660254037844387076, 1.000000000000000000, 0.8660254037844387076, 1.000000000000000000, 0.8660254037844387076, 1.000000000000000000, 0.8660254037844387076, 1.000000000000000000, 0.8660254037844387076, 1.000000000000000000, 0.8660254037844387076, 1.000000000000000000, 0.8660254037844387076, 1.000000000000000000, 0.8660254037844387076, 1.000000000000000000, 0.8660254037844387076, 1.000000000000000000, 0.8660254037844387076, 1.000000000000000000, 0.8660254037844387076, 1.000000000000000000, 0.8660254037844387076, 1.000000000000000000, 0.8660254037844387076, 1.000000000000000000, 0.8660254037844387076, 1.000000000000000000, 0.8660254037844387076, 1.000000000000000000, 0.8660254037844387076, 1.000000000000000000, 0.8660254037844387076, 1.000000000000000000, 0.8660254037844387076, 1.000000000000000000, 0.8660254037844387076, 1.000000000000000000, 0.8660254037844387076, 1.000000000000000000, 0.8660254037844387076, 1.000000000000000000, 0.8660254037844387076, 1.000000000000000000, 0.8660254037844387076, 1.000000000000000000, 0.8660254037844387076, 1.000000000000000000, 0.8660254037844387076, 1.000000000000000000, 0.8660254037844387076, 1.000000000000000000, 0.8660254037844387076, 1.000000000000000000, 0.8660254037844387076, 1.000000000000000000, 0.8660254037844387076, 1.000000000000000000, 0.8660254037844387076, 1.000000000000000000, 0.8660254037844387076, 1.000000000000000000, 0.8660254037844387076, 1.000000000000000000, 0.8660254037844387076, 1.000000000000000000, 0.8660254037844387076, 1.000000000000000000, 0.8660254037844387076, 1.000000000000000000, 0.8660254037844387076, 1.000000000000000000, 0.8660254037844387076, 1.000000000000000000, 0.8660254037844387076, 1.000000000000000000, 0.8660254037844387076, 1.000000000000000000, 0.8660254037844387076, 1.000000000000000000, 0.8660254037844387076, 1.000000000000000000, 0.8660254037844387076, 1.000000000000000000, 0.8660254037844387076, 1.000000000000000000, 0.8660254037844387076, 1.000000000000000000, 0.8660254037844387076, 1.000000000000000000, 0.8660254037844387076, 1.000000000000000000, 0.8660254037844387076, 1.000000000000000000, 0.8660254037844387076, 1.000000000000000000, 0.8660254037844387076, 1.000000000000000000, 0.8660254037844387076, 1.000000000000000000, 0.8660254037844387076, 1.000000000000000000, 0.8660254037844387076, 1.000000000000000000, 0.8660254037844387076, 1.000000000000000000, 0.8660254037844387076, 1.000000000000000000, 0.8660254037844387076, 1.000000000000000000, 0.8660254037844387076, 1.000000000000000000, 0.8660254037844387076, 1.000000000000000000, 0.8660254037844387076, 1.000000000000000000, 0.8660254037844387076, 1.000000000000000000, 0.8660254037844387076, 1.000000000000000000, 0.8660254037844387076, 1.000000000000000000, 0.8660254037844387076, 1.000000000000000000, 0.8660254037844387076, 1.000000000000000000, 0.8660254037844387076, 1.000000000000000000, 0.8660254037844387076, 1.000000000000000000, 0.8660254037844387076, 1.000000000000000000, 0.8660254037844387076, 1.000000000000000000, 0.8660254037844387076, 1.000000000000000000, 0.8660254037844387076, 1.000000000000000000, 0.8660254037844387076, 1.000000000000000000, 0.8660254037844387076, 1.000000000000000000, 0.8660254037844387076, 1.000000000000000000, 0.8660254037844387076, 1.000000000000000000, 0.8660254037844387076, 1.000000000000000000, 0.8660254037844387076, 1.000000000000000000, 0.8660254037844387076, 1.000000000000000000, 0.8660254037844387076, 1.000000000000000000, 0.8660254037844387076, 1.000000000000000000, 0.8660254037844387076, 1.000000000000000000, 0.8660254037844387076, 1.000000000000000000, 0.8660254037844387076, 1.000000000000000000, 0.8660254037844387076, 1.000000000000000000, 0.8660254037844387076, 1.000000000000000000, 0.8660254037844387076, 1.000000000000000000, 0.8660254037844387076, 1.000000000000000000, 0.8660254037844387076, 1.000000000000000000, 0.8660254037844387076, 1.000000000000000000, 0.8660254037844387076, 1.000000000000000000, 0.8660254037844387076, 1.000000000000000000, 0.8660254037844387076, 1.000000000000000000, 0.8660254037844387076, 1.000000000000000000, 0.8660254037844387076, 1.000000000000000000, 0.8660254037844387076, 1.000000000000000000, 0.8660254037844387076, 1.000000000000000000, 0.8660254037844387076, 1.000000000000000000, 0.8660254037844387076, 1.000000000000000000, 0.8660254037844387076, 1.000000000000000000, 0.8660254037844387076, 1.000000000000000000, 0.8660254037844387076, 1.000000000000000000, 0.8660254037844387076, 1.000000000000000000, 0.8660254037844387076, 1.000000000000000000, 0.8660254037844387076, 1.000000000000000000, 0.8660254037844387076, 1.000000000000000000, 0.8660254037844387076, 1.000000000000000000, 0.8660254037844387076, 1.000000000000000000, 0.8660254037844387076, 1.000000000000000000, 0.8660254037844387076, 1.000000000000000000, 0.8660254037844387076, 1.000000000000000000, 0.8660254037844387076, 1.000000000000000000, 0.8660254037844387076, 1.000000000000000000, 0.8660254037844387076, 1.000000000000000000, 0.8660254037844387076, 1.000000000000000000, 0.8660254037844387076, 1.000000000000000000, 0.8660254037844387076, 1.000000000000000000, 0.8660254037844387076, 1.000000000000000000, 0.8660254037844387076, 1.000000000000000000, 0.8660254037844387076, 1.000000000000000000, 0.8660254037844387076, 1.000000000000000000, 0.8660254037844387076, 1.000000000000000000, 0.8660254037844387076, 1.000000000000000000, 0.8660254037844387076, 1.000000000000000000, 0.8660254037844387076, 1.000000000000000000, 0.8660254037844387076, 1.000000000000000000, 0.8660254037844387076, 1.000000000000000000, 0.8660254037844387076, 1.000000000000000000, 0.8660254037844387076, 1.000000000000000000, 0.8660254037844387076, 1.000000000000000000, 0.8660254037844387076, 1.000000000000000000, 0.8660254037844387076, 1.000000000000000000, 0.8660254037844387076, 1.000000000000000000, 0.8660254037844387076, 1.000000000000000000, 0.8660254037844387076, 1.000000000000000000, 0.8660254037844387076, 1.000000000000000000, 0.8660254037844387076, 1.000000000000000000, 0.8660254037844387076, 1.000000000000000000, 0.8660254037844387076, 1.000000000000000000, 0.8660254037844387076, 1.000000000000000000, 0.8660254037844387076, 1.000000000000000000, 0.8660254037844387076, 1.000000000000000000, 0.8660254037844387076, 1.000000000000000000, 0.8660254037844387076, 1.000000000000000000, 0.8660254037844387076, 1.000000000000000000, 0.8660254037844387076, 1.000000000000000000, 0.8660254037844387076, 1.000000000000000000, 0.8660254037844387076, 1.000000000000000000, 0.8660254037844387076, 1.000000000000000000, 0.8660254037844387076, 1.000000000000000000, 0.8660254037844387076, 1.000000000000000000, 0.8660254037844387076, 1.000000000000000000, 0.8660254037844387076, 1.000000000000000000, 0.8660254037844387076, 1.000000000000000000, 0.8660254037844387076, 1.000000000000000000, 0.8660254037844387076, 1.000000000000000000, 0.8660254037844387076, 1.000000000000000000, 0.8660254037844387076, 1.000000000000000000, 0.8660254037844387076, 1.000000000000000000, 0.8660254037844387076, 1.000000000000000000, 0.8660254037844387076, 1.000000000000000000, 0.8660254037844387076, 1.000000000000000000, 0.8660254037844387076, 1.000000000000000000, 0.8660254037844387076, 1.000000000000000000, 0.8660254037844387076, 1.000000000000000000, 0.8660254037844387076, 1.000000000000000000, 0.8660254037844387076, 1.000000000000000000, 0.8660254037844387076, 1.000000000000000000, 0.8660254037844387076, 1.000000000000000000, 0.8660254037844387076, 1.000000000000000000, 0.8660254037844387076, 1.000000000000000000, 0.8660254037844387076, 1.000000000000000000, 0.8660254037844387076, 1.000000000000000000, 0.8660254037844387076, 1.000000000000000000, 0.8660254037844387076, 1.000000000000000000, 0.8660254037844387076, 1.000000000000000000, 0.8660254037844387076, 1.000000000000000000, 0.8660254037844387076, 1.000000000000000000, 0.8660254037844387076, 1.000000000000000000, 0.8660254037844387076, 1.000000000000000000, 0.8660254037844387076, 1.000000000000000000, 0.8660254037844387076, 1.000000000000000000, 0.8660254037844387076, 1.000000000000000000, 0.8660254037844387076, 1.000000000000000000, 0.8660254037844387076, 1.000000000000000000) ) ) 
 REPRESENTATION_ITEM ( '' )  SURFACE ( )  );
#6360=CARTESIAN_POINT ( 'NONE',  ( -1.364683531250010295, 5.030208333674757171, 0.7879004041258379498 ) ) ;
#6362=CARTESIAN_POINT ( 'NONE',  ( -8.507905087775398556, 9.884643009614800135, 1.199719254218462483 ) ) ;
#6363=CARTESIAN_POINT ( 'NONE',  ( -4.934804725694220906, 7.740727365743146571, -1.082531754730549967 ) ) ;
#6371=VERTEX_POINT ( 'NONE', #122593 ) ;
#6372=CARTESIAN_POINT ( 'NONE',  ( 6.968000882419564945, 10.21675256520979858, 1.199719254218460707 ) ) ;
#6374=EDGE_CURVE ( 'NONE', #25036, #199311, #105200, .T. ) ;
#6376=CARTESIAN_POINT ( 'NONE',  ( 7.578644679914713578, 8.904468883731073703, 1.082531754730558626 ) ) ;
#6379=CARTESIAN_POINT ( 'NONE',  ( -7.507464373665155399, 9.781794407407920389, 1.599625672291295375 ) ) ;
#6380=CARTESIAN_POINT ( 'NONE',  ( 3.994848817520957773, 7.812407387083109001, 1.040834085586084257E-14 ) ) ;
#6384=CARTESIAN_POINT ( 'NONE',  ( 3.871016551901614200, 4.474939717762034697, -1.199719254218446718 ) ) ;
#6387=CARTESIAN_POINT ( 'NONE',  ( -4.036335974549790429, 7.671137949187412985, -0.4422704879359267149 ) ) ;
#6390=CARTESIAN_POINT ( 'NONE',  ( -4.609409038966245653, 6.400729850259146758, -1.443375672974053447 ) ) ;
#6391=CARTESIAN_POINT ( 'NONE',  ( 9.327646496521982300, 11.90534021740758064, -1.443375672974057666 ) ) ;
#6394=CARTESIAN_POINT ( 'NONE',  ( -7.393273838153706201, 7.519907654134449615, 0.7998128361456341429 ) ) ;
#6399=CARTESIAN_POINT ( 'NONE',  ( -7.309817376062285099, 11.67987070538135264, 0.000000000000000000 ) ) ;
#6401=DIRECTION ( 'NONE',  ( -0.6507913734559640506, -0.7592566023653004592, 0.000000000000000000 ) ) ;
#6404=CARTESIAN_POINT ( 'NONE',  ( 4.904298879841284098, 6.744767997946721216, 1.599625672291267398 ) ) ;
#6416=CARTESIAN_POINT ( 'NONE',  ( -6.531277313481209212, 8.642909503859968368, 1.599625672291283607 ) ) ;
#6419=CARTESIAN_POINT ( 'NONE',  ( 4.690757960648213931, 8.416375354157496602, 0.7216878364870438212 ) ) ;
#6424=CARTESIAN_POINT ( 'NONE',  ( -4.141125853970233806, 6.918731698685530063, -1.199719254218452047 ) ) ;
#6428=CARTESIAN_POINT ( 'NONE',  ( -6.663996196316808174, 7.733415969579778171, -1.199719254218446718 ) ) ;
#6434=CARTESIAN_POINT ( 'NONE',  ( -7.828943636887387925, 11.22118577875556156, 1.199719254218453823 ) ) ;
#6435=CARTESIAN_POINT ( 'NONE',  ( 7.124973419181436007, 8.271222729588529887, -1.199719254218446718 ) ) ;
#6437=CARTESIAN_POINT ( 'NONE',  ( -3.850152436600983386, 4.554561266531622188, 1.082531754730560403 ) ) ;
#6438=CARTESIAN_POINT ( 'NONE',  ( -8.784793466650835825, 12.33634391347959713, 1.199719254218462483 ) ) ;
#6440=CARTESIAN_POINT ( 'NONE',  ( -1.402160292154681736E-14, -0.9906249996585834161, -1.575800808251665908 ) ) ;
#6444=CARTESIAN_POINT ( 'NONE',  ( 8.839552966430002101, 11.33589776563360019, -1.443375672974052559 ) ) ;
#6451=EDGE_CURVE ( 'NONE', #135502, #92250, #102553, .T. ) ;
#6465=CARTESIAN_POINT ( 'NONE',  ( -3.623053363349869382, 5.249981562040033189, 1.599625672291267398 ) ) ;
#6469=CARTESIAN_POINT ( 'NONE',  ( -3.972702704004144714, 4.593573561881607148, 1.199719254218462483 ) ) ;
#6473=CARTESIAN_POINT ( 'NONE',  ( 1.499999999999987121, -0.7145833326505161009, 0.8660254037844524744 ) ) ;
#6476=CARTESIAN_POINT ( 'NONE',  ( -2.819732761962335577, 5.273143408055916304, -1.082531754730543971 ) ) ;
#6478=CARTESIAN_POINT ( 'NONE',  ( 2.833104737058811384, 6.457039293210589115, -0.1487728517625390434 ) ) ;
#6479=ORIENTED_EDGE ( 'NONE', *, *, #122849, .F. ) ;
#6482=CARTESIAN_POINT ( 'NONE',  ( 4.552840656090682891, 4.206068941727564514, 1.214306433183764966E-14 ) ) ;
#6483=CARTESIAN_POINT ( 'NONE',  ( -3.416291520519271874, 6.929497840673697340, 1.040834085586084257E-14 ) ) ;
#6487=CARTESIAN_POINT ( 'NONE',  ( 10.34450801710256584, 11.17094022948226240, 0.7216878364870438212 ) ) ;
#6490=CARTESIAN_POINT ( 'NONE',  ( -1.201851678989727383E-14, 3.259375000341420581, -1.575800808251660134 ) ) ;
#6493=CARTESIAN_POINT ( 'NONE',  ( -8.483651433849100698, 10.92067931095586886, 1.599625672291269396 ) ) ;
#6494=CARTESIAN_POINT ( 'NONE',  ( -4.406036734316898240, 6.163462161501577441, -1.443375672974051449 ) ) ;
#6496=CARTESIAN_POINT ( 'NONE',  ( -6.013204822860843457, 6.974159367214481264, -1.199719254218446718 ) ) ;
#6498=CARTESIAN_POINT ( 'NONE',  ( -1.364683531250010295, 5.238541667008086655, -0.7879004041258300672 ) ) ;
#6506=CARTESIAN_POINT ( 'NONE',  ( -5.002595493318215070, 7.819816594637776674, 1.082531754730560403 ) ) ;
#6511=CARTESIAN_POINT ( 'NONE',  ( -3.728129053633589152, 7.293308295973741195, 0.7216878364870317197 ) ) ;
#6513=CARTESIAN_POINT ( 'NONE',  ( 10.07100917685271035, 10.64393221595000938, 0.7998128361456462443 ) ) ;
#6518=ORIENTED_EDGE ( 'NONE', *, *, #122619, .T. ) ;
#6522=CARTESIAN_POINT ( 'NONE',  ( -4.386226389220933441, 5.076017861301227008, -1.199719254218446718 ) ) ;
#6523=CARTESIAN_POINT ( 'NONE',  ( -8.947491310014823895, 12.52615806407091803, 1.199719254218462483 ) ) ;
#6528=CARTESIAN_POINT ( 'NONE',  ( 5.198661835836162481, 8.152523677529138979, 1.199719254218462483 ) ) ;
#6533=CARTESIAN_POINT ( 'NONE',  ( 4.241003122976366058, 3.842258486427521103, -0.7998128361456211532 ) ) ;
#6544=CARTESIAN_POINT ( 'NONE',  ( 7.422199028477372451, 10.74665040227725044, -1.199719254218441611 ) ) ;
#6545=CARTESIAN_POINT ( 'NONE',  ( -4.303823697334223652, 7.108545849276850959, -1.199719254218452047 ) ) ;
#6547=CARTESIAN_POINT ( 'NONE',  ( 0.7499999999999902300, 4.097916667349481123, -1.299038105676658228 ) ) ;
#6551=CARTESIAN_POINT ( 'NONE',  ( 1.364683531249990311, 4.634375000341417916, 1.214306433183764966E-14 ) ) ;
#6553=CARTESIAN_POINT ( 'NONE',  ( -6.087774667736030487, 7.061157519568837415, 1.199719254218450271 ) ) ;
#6556=CARTESIAN_POINT ( 'NONE',  ( 4.924636110261782385, 6.768494766770632332, 1.599625672291267398 ) ) ;
#6557=CARTESIAN_POINT ( 'NONE',  ( -3.601662362724658895, 7.353689856487406473, -0.7998128361456281477 ) ) ;
#6563=CARTESIAN_POINT ( 'NONE',  ( 7.646435448427411963, 8.023188899361205273, -0.7216878364870257245 ) ) ;
#6566=CARTESIAN_POINT ( 'NONE',  ( 6.263503779389103521, 10.25124547602188763, 1.040834085586084257E-14 ) ) ;
#6567=CARTESIAN_POINT ( 'NONE',  ( 1.364683531249988535, 2.967708333674755394, -0.7879004041258239610 ) ) ;
#6569=CARTESIAN_POINT ( 'NONE',  ( 4.650083499362864359, 7.408552601689905259, 1.082531754730558626 ) ) ;
#6577=CARTESIAN_POINT ( 'NONE',  ( -4.265659997730736563, 7.487761795085347671, 1.069252549957976361 ) ) ;
#6580=AXIS2_PLACEMENT_3D ( 'NONE', #81953, #126534, #44147 ) ;
#6584=CARTESIAN_POINT ( 'NONE',  ( -9.450196763925152510, 10.98398329845622001, -1.199719254218441611 ) ) ;
#6589=CARTESIAN_POINT ( 'NONE',  ( -2.676845263694313637, 5.210404343363602919, -1.199719254218446718 ) ) ;
#6594=CARTESIAN_POINT ( 'NONE',  ( 3.389175213736292047, 5.937492935125556315, 1.082531754730558626 ) ) ;
#6595=CARTESIAN_POINT ( 'NONE',  ( -1.364683531250012516, 3.801041667008087099, -0.7879004041258300672 ) ) ;
#6597=CARTESIAN_POINT ( 'NONE',  ( 8.437251666405968464, 8.737881787095446384, 1.040834085586084257E-14 ) ) ;
#6605=CARTESIAN_POINT ( 'NONE',  ( 1.499999999999987121, 3.295833333333354709, -0.8660254037844262731 ) ) ;
#6606=CARTESIAN_POINT ( 'NONE',  ( 4.039439701867726384, 6.800097854565950506, 1.199719254218462483 ) ) ;
#6609=CARTESIAN_POINT ( 'NONE',  ( -0.9486429539237359876, 2.855410930033766004, 1.028101543438980858 ) ) ;
#6611=CARTESIAN_POINT ( 'NONE',  ( -0.6823417656250212460, 4.301041667008085767, 1.181850606188767472 ) ) ;
#6613=CARTESIAN_POINT ( 'NONE',  ( 8.080296364064698977, 12.37083682481011060, -0.7216878364870328300 ) ) ;
#6618=CARTESIAN_POINT ( 'NONE',  ( 0.7499999999999902300, 2.264583334016148530, 1.299038105676669330 ) ) ;
#6620=CARTESIAN_POINT ( 'NONE',  ( -5.636439174979254396, 7.598931675607687453, -1.599625672291256295 ) ) ;
#6622=CARTESIAN_POINT ( 'NONE',  ( 5.626270559546826533, 5.666329862333828515, 0.7216878364870317197 ) ) ;
#6629=EDGE_LOOP ( 'NONE', ( #142802, #100215, #187967, #175350, #153356, #26686 ) ) ;
#6631=CARTESIAN_POINT ( 'NONE',  ( 7.904567251967224095, 9.180748867838630645, 1.199719254218462483 ) ) ;
#6632=CARTESIAN_POINT ( 'NONE',  ( 3.988069740714122791, 7.804498464141805592, 0.7998128361456321445 ) ) ;
#6633=DIRECTION ( 'NONE',  ( -0.000000000000000000, -8.546850786086437571E-32, -1.000000000000000000 ) ) ;
#6636=CARTESIAN_POINT ( 'NONE',  ( 4.482942347612929979, 8.381849838857084123, 1.040834085586084257E-14 ) ) ;
#6638=EDGE_LOOP ( 'NONE', ( #124575, #65665, #31410, #32397, #104320, #120467, #203236, #199464, #168970 ) ) ;
#6644=CARTESIAN_POINT ( 'NONE',  ( 9.541187415715040032, 12.15447128979948310, -1.599625672291262513 ) ) ;
#6650=CARTESIAN_POINT ( 'NONE',  ( 5.197613018050254219, 6.434050360596694773, 1.175743713691650871 ) ) ;
#6661=CARTESIAN_POINT ( 'NONE',  ( 7.049876689426101350, 9.247942109129029475, -1.443375672974057666 ) ) ;
#6662=CARTESIAN_POINT ( 'NONE',  ( -4.613852347352193739, 4.277249248199312071, 1.214306433183764966E-14 ) ) ;
#6666=CARTESIAN_POINT ( 'NONE',  ( -6.078132937628113908, 5.985576603521232109, 1.040834085586084257E-14 ) ) ;
#6674=CARTESIAN_POINT ( 'NONE',  ( -1.123270288250342919, 3.096052654332833054, 0.7749999999993751887 ) ) ;
#6679=CARTESIAN_POINT ( 'NONE',  ( 8.992082194361556091, 11.51384853155376220, 1.599625672291279388 ) ) ;
#6682=VERTEX_POINT ( 'NONE', #90015 ) ;
#6688=CARTESIAN_POINT ( 'NONE',  ( -10.49364770729726359, 11.34493653470939023, 0.7216878364870438212 ) ) ;
#6693=CARTESIAN_POINT ( 'NONE',  ( 7.727257484784855635, 11.10255193463598111, -1.199719254218446718 ) ) ;
#6697=CARTESIAN_POINT ( 'NONE',  ( -6.388916700537716764, 8.476822122092563916, 1.599625672291283607 ) ) ;
#6698=CARTESIAN_POINT ( 'NONE',  ( 3.472859903394816872, 7.203420320602605287, -0.7998128361456291469 ) ) ;
#6704=CARTESIAN_POINT ( 'NONE',  ( -1.364683531250012516, 2.301041667008087988, -0.7879004041258289570 ) ) ;
#6706=CARTESIAN_POINT ( 'NONE',  ( 7.619319141200072920, 7.991553207595983643, 0.7216878364870317197 ) ) ;
#6713=VERTEX_POINT ( 'NONE', #10856 ) ;
#6714=CARTESIAN_POINT ( 'NONE',  ( 9.558135107509954764, 10.25350516829085379, -0.7216878364870257245 ) ) ;
#6715=VERTEX_POINT ( 'NONE', #191743 ) ;
#6718=CARTESIAN_POINT ( 'NONE',  ( -8.130085669689073313, 12.63685038127928806, 0.7998128361456481317 ) ) ;
#6726=CARTESIAN_POINT ( 'NONE',  ( 4.325214697959421706, 5.004837554829479451, 1.199719254218462483 ) ) ;
#6732=CARTESIAN_POINT ( 'NONE',  ( 4.798696304233017074, 7.685897223992134819, -1.199719254218452047 ) ) ;
#6735=CARTESIAN_POINT ( 'NONE',  ( 0.7499999999999902300, 2.764583334016148974, 1.299038105676669330 ) ) ;
#6741=CARTESIAN_POINT ( 'NONE',  ( 1.499999999999987566, 0.02500000000001806333, 0.000000000000000000 ) ) ;
#6742=CARTESIAN_POINT ( 'NONE',  ( 7.182068686937156166, 9.402166106225269715, 1.599625672291281386 ) ) ;
#6743=CARTESIAN_POINT ( 'NONE',  ( 1.364683531249986537, -0.09479166632524321789, -0.7879004041258309554 ) ) ;
#6746=EDGE_CURVE ( 'NONE', #154836, #212421, #35941, .T. ) ;
#6747=CARTESIAN_POINT ( 'NONE',  ( 9.598809568795314107, 10.30095870645710754, -0.7216878364870257245 ) ) ;
#6753=CARTESIAN_POINT ( 'NONE',  ( -5.259673527097670664, 8.223703984000886535, -1.199719254218446718 ) ) ;
#6754=( BOUNDED_SURFACE ( )  B_SPLINE_SURFACE ( 3, 2, ( 
 ( #121485, #174439, #123627 ),
 ( #71557, #189591, #42302 ),
 ( #108417, #41237, #122562 ),
 ( #43366, #24950, #107344 ) ),
 .UNSPECIFIED., .F., .F., .T. ) 
 B_SPLINE_SURFACE_WITH_KNOTS ( ( 4, 4 ),
 ( 3, 3 ),
 ( 5.985662991026288423E-05, 0.0001887152224066689804 ),
 ( 0.000000000000000000, 1.000000000000000000 ),
 .UNSPECIFIED. ) 
 GEOMETRIC_REPRESENTATION_ITEM ( )  RATIONAL_B_SPLINE_SURFACE ( (
 ( 1.000000000000000000, 0.8739472344185998942, 1.000000000000000000),
 ( 1.000000000000000000, 0.8497613059193734886, 1.000000000000000000),
 ( 1.000000000000000000, 0.8164163343283138419, 1.000000000000000000),
 ( 1.000000000000000000, 0.7779734834199523164, 1.000000000000000000) ) ) 
 REPRESENTATION_ITEM ( '' )  SURFACE ( )  );
#6755=CARTESIAN_POINT ( 'NONE',  ( -0.7500000000000006661, 2.389583334016155636, -1.299038105676652011 ) ) ;
#6756=CARTESIAN_POINT ( 'NONE',  ( -1.364683531250010295, 4.842708333674756283, 0.7879004041258379498 ) ) ;
#6761=CARTESIAN_POINT ( 'NONE',  ( 1.364683531249988535, 3.717708333674750953, -0.7879004041258239610 ) ) ;
#6768=CARTESIAN_POINT ( 'NONE',  ( -8.259941899223614215, 10.65968485389279508, -1.599625672291263179 ) ) ;
#6769=CARTESIAN_POINT ( 'NONE',  ( 5.309989718046547402, 9.346738437696316737, 0.7998128361456462443 ) ) ;
#6772=ORIENTED_EDGE ( 'NONE', *, *, #124997, .T. ) ;
#6776=CARTESIAN_POINT ( 'NONE',  ( -6.775324078527193983, 8.927630729746953264, -1.599625672291263179 ) ) ;
#6781=CARTESIAN_POINT ( 'NONE',  ( 3.999819011231439347, 4.625209253646830554, 1.199719254218464037 ) ) ;
#6784=CARTESIAN_POINT ( 'NONE',  ( -3.581325132304157943, 7.329963087663487364, -0.7998128361456281477 ) ) ;
#6785=CARTESIAN_POINT ( 'NONE',  ( -7.971304249830880373, 11.38727316052296601, 1.199719254218453823 ) ) ;
#6788=CARTESIAN_POINT ( 'NONE',  ( -4.351531800032816477, 7.393666969396889499, -1.175081553336376317 ) ) ;
#6795=CARTESIAN_POINT ( 'NONE',  ( 4.469384193999260901, 8.366031992974468423, -0.7998128361456231517 ) ) ;
#6796=VECTOR ( 'NONE', #78584, 1000.000000000000000 ) ;
#6814=CARTESIAN_POINT ( 'NONE',  ( 3.633221978782282147, 5.261844946711204507, -1.443375672974057666 ) ) ;
#6818=CARTESIAN_POINT ( 'NONE',  ( -9.104463846776669200, 10.58062822844965645, -1.199719254218441611 ) ) ;
#6824=CARTESIAN_POINT ( 'NONE',  ( 1.499999999999989120, 1.785416667349487563, 0.8660254037844524744 ) ) ;
#6826=DIRECTION ( 'NONE',  ( 0.000000000000000000, 8.546850786086437571E-32, 1.000000000000000000 ) ) ;
#6829=CARTESIAN_POINT ( 'NONE',  ( -8.292783513053063160, 12.82666453187061073, 0.7998128361456481317 ) ) ;
#6831=CARTESIAN_POINT ( 'NONE',  ( -1.402160292154681736E-14, 0.9468750003414176941, -1.575800808251659024 ) ) ;
#6832=CARTESIAN_POINT ( 'NONE',  ( -1.001543065824772872E-14, 5.462500000000020783, 1.732050807568877637 ) ) ;
#6838=CARTESIAN_POINT ( 'NONE',  ( -3.958090780185743451, 6.705190779270287393, -1.199719254218452047 ) ) ;
#6843=CARTESIAN_POINT ( 'NONE',  ( 1.364683531249986537, -0.03229166632525094088, -0.7879004041258309554 ) ) ;
#6848=CARTESIAN_POINT ( 'NONE',  ( 1.364683531249986537, 0.1552083336747499542, -0.7879004041258309554 ) ) ;
#6850=CARTESIAN_POINT ( 'NONE',  ( -7.823218330285243383, 9.085841792542966644, -1.199719254218446718 ) ) ;
#6851=CARTESIAN_POINT ( 'NONE',  ( 9.565441069641300587, 11.11843498845840905, -1.199719254218440723 ) ) ;
#6855=CARTESIAN_POINT ( 'NONE',  ( 1.364683531249988757, 1.696875000341414808, 0.000000000000000000 ) ) ;
#6863=CARTESIAN_POINT ( 'NONE',  ( 7.321039761699430493, 7.643560598178549270, -0.7216878364870257245 ) ) ;
#6866=CARTESIAN_POINT ( 'NONE',  ( -3.578462479003122976, 6.262291094557191684, 1.199719254218464037 ) ) ;
#6867=CARTESIAN_POINT ( 'NONE',  ( -4.213005119291713285, 7.494488749433884323, -0.9457084323257232139 ) ) ;
#6868=CARTESIAN_POINT ( 'NONE',  ( -1.201851678989727383E-14, 5.618750000682818602, -1.732050807568863648 ) ) ;
#6871=ADVANCED_FACE ( 'NONE', ( #110582 ), #56223, .T. ) ;
#6872=CARTESIAN_POINT ( 'NONE',  ( 6.616015773344440021, 6.821032611764393572, 1.040834085586084257E-14 ) ) ;
#6873=CARTESIAN_POINT ( 'NONE',  ( -7.158341917891067219, 11.29522330427417565, 0.000000000000000000 ) ) ;
#6875=CARTESIAN_POINT ( 'NONE',  ( -1.499999999999997780, 3.900000000000021672, 1.214306433183764966E-14 ) ) ;
#6879=CARTESIAN_POINT ( 'NONE',  ( 7.917598520700710019, 12.18102267421877727, -0.7216878364870328300 ) ) ;
#6891=CARTESIAN_POINT ( 'NONE',  ( 6.927853306458731986, 11.02631992426980112, 0.7216878364870438212 ) ) ;
#6893=CARTESIAN_POINT ( 'NONE',  ( 8.158255747121103241, 10.54105100977322174, 1.599625672291281386 ) ) ;
#6894=CARTESIAN_POINT ( 'NONE',  ( -5.555090253297260361, 7.504024600312024340, 1.599625672291269396 ) ) ;
#6900=CARTESIAN_POINT ( 'NONE',  ( 4.365362273920244007, 6.116008624372160973, 1.443375672974062551 ) ) ;
#6901=VERTEX_POINT ( 'NONE', #90103 ) ;
#6902=CARTESIAN_POINT ( 'NONE',  ( -8.514157279702036618, 9.035531035848267223, -0.7216878364870278340 ) ) ;
#6929=CARTESIAN_POINT ( 'NONE',  ( -5.982172092127739482, 8.002286745614243912, -1.599625672291263179 ) ) ;
#6934=CARTESIAN_POINT ( 'NONE',  ( -4.786163832636268545, 5.147994549525747310, 0.9918565312223650565 ) ) ;
#6940=CARTESIAN_POINT ( 'NONE',  ( -5.115504031057831469, 4.862509545855891346, 0.7998128361456341429 ) ) ;
#6943=CARTESIAN_POINT ( 'NONE',  ( 7.263417608619159083, 9.497073181520933716, -1.599625672291262513 ) ) ;
#6946=CARTESIAN_POINT ( 'NONE',  ( 6.055847235078346991, 6.052673195394750572, 0.4411178842869938888 ) ) ;
#6951=CARTESIAN_POINT ( 'NONE',  ( 5.965224399888476192, 6.061776009399090448, 1.040834085586084257E-14 ) ) ;
#6952=CARTESIAN_POINT ( 'NONE',  ( -7.857113714319432063, 9.125386407249497012, 1.199719254218462483 ) ) ;
#6955=CARTESIAN_POINT ( 'NONE',  ( -9.006694118179950692, 9.402231314165087284, 1.040834085586084257E-14 ) ) ;
#6956=CARTESIAN_POINT ( 'NONE',  ( -6.911959384868566758, 6.958374125301778790, 1.040834085586084257E-14 ) ) ;
#6960=CARTESIAN_POINT ( 'NONE',  ( 1.499999999999995115, 3.327083334016150307, -0.8660254037844217212 ) ) ;
#6963=CARTESIAN_POINT ( 'NONE',  ( 8.751951852821344247, 10.16936423550178503, -1.199719254218446718 ) ) ;
#6964=CARTESIAN_POINT ( 'NONE',  ( -2.163990585822766377, 5.468480083527750502, -0.4581612399152222848 ) ) ;
#6970=DIRECTION ( 'NONE',  ( 0.7592566023652994600, 0.6507913734559651608, 0.000000000000000000 ) ) ;
#6973=CARTESIAN_POINT ( 'NONE',  ( -0.3461162505576212411, 7.159215625956849571, -1.970439023737479811 ) ) ;
#6976=VERTEX_POINT ( 'NONE', #122685 ) ;
#6977=CARTESIAN_POINT ( 'NONE',  ( 0.7499999999999920064, 4.483333333333352932, 1.299038105676669330 ) ) ;
#6978=CARTESIAN_POINT ( 'NONE',  ( 5.066996723205273057, 6.934582148538044777, 1.599625672291267398 ) ) ;
#6979=CARTESIAN_POINT ( 'NONE',  ( 6.765682348419287173, 7.852049813699357728, 1.199719254218462483 ) ) ;
#6981=CARTESIAN_POINT ( 'NONE',  ( -9.192064960385334160, 9.826423329978791088, 0.7216878364870438212 ) ) ;
#6984=CARTESIAN_POINT ( 'NONE',  ( 6.399085315970131305, 8.488685506763726352, -1.443375672974057666 ) ) ;
#6985=CARTESIAN_POINT ( 'NONE',  ( -9.015808962963337336, 10.58116054728778366, 1.082531754730558626 ) ) ;
#6988=CARTESIAN_POINT ( 'NONE',  ( 7.751511138711133064, 10.06651563329490529, -1.599625672291262513 ) ) ;
#6994=CARTESIAN_POINT ( 'NONE',  ( 1.364683531249986537, 1.905208333674750287, -0.7879004041258239610 ) ) ;
#7001=CARTESIAN_POINT ( 'NONE',  ( 8.992082194361556091, 11.51384853155376220, 1.599625672291279388 ) ) ;
#7005=CARTESIAN_POINT ( 'NONE',  ( -8.859363311525973117, 12.42334206583395328, -1.199719254218446718 ) ) ;
#7013=CARTESIAN_POINT ( 'NONE',  ( 4.403700966340357681, 4.032072637018845107, -0.7998128361456211532 ) ) ;
#7016=CARTESIAN_POINT ( 'NONE',  ( -9.179033691651859783, 10.66762638080401260, 1.199719254218462483 ) ) ;
#7019=CARTESIAN_POINT ( 'NONE',  ( 7.235247531187115833, 11.59287255302699648, -0.7998128361456291469 ) ) ;
#7021=CARTESIAN_POINT ( 'NONE',  ( 4.574835874639041400, 6.943354005153362429, 1.191215277921169324 ) ) ;
#7022=CARTESIAN_POINT ( 'NONE',  ( 1.123270288250309834, 3.221052654332833054, -0.7749999999993620881 ) ) ;
#7023=CARTESIAN_POINT ( 'NONE',  ( -5.427341564172148303, 5.226320001155936090, 0.000000000000000000 ) ) ;
#7027=CARTESIAN_POINT ( 'NONE',  ( 8.101160479365381306, 9.410107633136481908, -1.199719254218446718 ) ) ;
#7029=CARTESIAN_POINT ( 'NONE',  ( 7.613066949273408213, 8.840665181362512115, -1.199719254218441611 ) ) ;
#7031=CARTESIAN_POINT ( 'NONE',  ( -8.297226821883391779, 11.66355314463053006, 1.082531754730549967 ) ) ;
#7039=CARTESIAN_POINT ( 'NONE',  ( -4.595871994550918771, 6.958256438637705266, -1.193191807407071536 ) ) ;
#7040=EDGE_CURVE ( 'NONE', #45871, #120076, #40428, .T. ) ;
#7042=CARTESIAN_POINT ( 'NONE',  ( 6.561783159334121152, 8.678499657355050800, -1.443375672974057666 ) ) ;
#7044=CARTESIAN_POINT ( 'NONE',  ( 9.908311333488716954, 10.45411806535867782, 0.7998128361456462443 ) ) ;
#7064=CARTESIAN_POINT ( 'NONE',  ( 6.584456157731144899, 10.83361595066169514, -0.7998128361456291469 ) ) ;
#7066=VERTEX_POINT ( 'NONE', #97574 ) ;
#7068=CARTESIAN_POINT ( 'NONE',  ( 0.7499999999999885647, 1.597916667349486008, -1.299038105676652899 ) ) ;
#7070=CARTESIAN_POINT ( 'NONE',  ( -5.343885102080728977, 9.386283052402845328, 0.7998128361456481317 ) ) ;
#7072=ORIENTED_EDGE ( 'NONE', *, *, #63358, .T. ) ;
#7073=CARTESIAN_POINT ( 'NONE',  ( -10.64723070543352712, 11.31619066596094392, 0.7998128361456462443 ) ) ;
#7074=CARTESIAN_POINT ( 'NONE',  ( -1.420000000000079865, 7.176846818246208848, 4.202462424328226476 ) ) ;
#7078=CARTESIAN_POINT ( 'NONE',  ( 8.423693512792301163, 8.722063941212843119, 0.7998128361456481317 ) ) ;
#7082=CARTESIAN_POINT ( 'NONE',  ( -8.199983978166823562, 8.461069484149769337, -0.7998128361456291469 ) ) ;
#7084=CARTESIAN_POINT ( 'NONE',  ( -0.6823417656250212460, 4.051041667008085767, 1.181850606188767472 ) ) ;
#7090=CARTESIAN_POINT ( 'NONE',  ( -7.022760382198764084, 11.13704484596649635, 0.7216878364870458196 ) ) ;
#7094=CARTESIAN_POINT ( 'NONE',  ( -0.6823417656249969321, 4.780208333674755394, -1.181850606188749264 ) ) ;
#7095=AXIS2_PLACEMENT_3D ( 'NONE', #116290, #164979, #97873 ) ;
#7101=CARTESIAN_POINT ( 'NONE',  ( 0.6823417656249899377, 4.676041667008086655, -1.181850606188754593 ) ) ;
#7102=CARTESIAN_POINT ( 'NONE',  ( -5.274285450916075035, 6.112086766612214284, 1.199719254218450271 ) ) ;
#7103=CARTESIAN_POINT ( 'NONE',  ( 6.474182045725470402, 7.511966127223233869, -1.199719254218446718 ) ) ;
#7106=CARTESIAN_POINT ( 'NONE',  ( 4.378920427089557421, 5.171457255435017331, -1.082531754730548412 ) ) ;
#7107=CARTESIAN_POINT ( 'NONE',  ( -1.364683531250010295, 5.592708333674750953, 0.7879004041258379498 ) ) ;
#7111=DIRECTION ( 'NONE',  ( 5.578564026256490882E-16, 1.000000000000000000, 9.066213480720158442E-32 ) ) ;
#7113=CARTESIAN_POINT ( 'NONE',  ( -0.6823417656250212460, 1.301041667008083547, 1.181850606188755259 ) ) ;
#7114=CARTESIAN_POINT ( 'NONE',  ( -3.307826292054316664, 4.882216645528547616, -1.443375672974059665 ) ) ;
#7115=CARTESIAN_POINT ( 'NONE',  ( 5.148345644887269756, 7.029489223833707001, -1.599625672291256295 ) ) ;
#7116=EDGE_LOOP ( 'NONE', ( #145175, #143722, #160934, #141114, #2642, #68990 ) ) ;
#7121=CARTESIAN_POINT ( 'NONE',  ( 4.867013957625893283, 4.780530493426062399, 1.040834085586084257E-14 ) ) ;
#7124=CARTESIAN_POINT ( 'NONE',  ( -7.944714827928056167, 10.29191993738131927, 1.443375672974090751 ) ) ;
#7129=CARTESIAN_POINT ( 'NONE',  ( -10.08065090696061716, 11.71951313199760136, -1.199719254218441611 ) ) ;
#7131=CARTESIAN_POINT ( 'NONE',  ( -4.731432421044865499, 8.463828891286912182, -0.7216878364870257245 ) ) ;
#7133=CARTESIAN_POINT ( 'NONE',  ( 1.364683531249988757, 0.9468750003414211358, 0.000000000000000000 ) ) ;
#7134=CARTESIAN_POINT ( 'NONE',  ( -1.420000000000001039, 6.120000000000041851, -2.579999999999995630 ) ) ;
#7142=CARTESIAN_POINT ( 'NONE',  ( 10.40996301719436090, 11.03937836301526687, 0.000000000000000000 ) ) ;
#7144=VERTEX_POINT ( 'NONE', #78096 ) ;
#7156=DIRECTION ( 'NONE',  ( -1.000000000000000000, 6.505213034913026604E-16, 0.000000000000000000 ) ) ;
#7158=CARTESIAN_POINT ( 'NONE',  ( 1.364683531249986537, 2.717708333674754062, -0.7879004041258239610 ) ) ;
#7160=ORIENTED_EDGE ( 'NONE', *, *, #59177, .F. ) ;
#7169=CARTESIAN_POINT ( 'NONE',  ( -1.364683531250012516, 0.7802083336747528408, 0.7879004041258379498 ) ) ;
#7174=ORIENTED_EDGE ( 'NONE', *, *, #42629, .F. ) ;
#7178=CARTESIAN_POINT ( 'NONE',  ( 4.843287188579786573, 6.673587691474970107, -1.599625672291256295 ) ) ;
#7186=CARTESIAN_POINT ( 'NONE',  ( 7.633404179693907388, 8.864391950186421454, -1.199719254218441611 ) ) ;
#7187=CARTESIAN_POINT ( 'NONE',  ( 4.080641032480825103, 5.783833874167997102, -1.249999999999999334 ) ) ;
#7189=CARTESIAN_POINT ( 'NONE',  ( 7.086107841436786181, 11.41887624831828418, 1.040834085586084257E-14 ) ) ;
#7191=CARTESIAN_POINT ( 'NONE',  ( 1.522480120926855029, 8.691153603980712461, -2.524399069149761310 ) ) ;
#7197=ADVANCED_FACE ( 'NONE', ( #129079 ), #61913, .T. ) ;
#7201=CARTESIAN_POINT ( 'NONE',  ( -7.321039761699444703, 10.52466824108257804, 1.082531754730549967 ) ) ;
#7206=CARTESIAN_POINT ( 'NONE',  ( -8.646349277213090545, 11.11049346154719508, 1.599625672291269396 ) ) ;
#7208=CARTESIAN_POINT ( 'NONE',  ( -4.180211397942203533, 3.976498670287245130, -0.5934635338003064753 ) ) ;
#7212=CARTESIAN_POINT ( 'NONE',  ( 8.563946585326370098, 13.14302144952281814, 0.7998128361456462443 ) ) ;
#7214=CARTESIAN_POINT ( 'NONE',  ( 3.734381245560244089, 6.444196322207211836, 1.199719254218462483 ) ) ;
#7221=CARTESIAN_POINT ( 'NONE',  ( -6.878064000834399394, 6.918829510595249310, -0.7998128361456291469 ) ) ;
#7223=CARTESIAN_POINT ( 'NONE',  ( -8.890396042259075315, 11.39521468743417998, -1.599625672291263179 ) ) ;
#7229=CARTESIAN_POINT ( 'NONE',  ( 9.436111725431318931, 10.11114455586577776, -0.7216878364870257245 ) ) ;
#7230=CARTESIAN_POINT ( 'NONE',  ( -1.201851678989727383E-14, 4.134375000341417028, 1.575800808251672791 ) ) ;
#7232=VECTOR ( 'NONE', #21262, 1000.000000000000114 ) ;
#7233=CARTESIAN_POINT ( 'NONE',  ( 6.498435699651741615, 6.475929825882159818, -0.7998128361456281477 ) ) ;
#7234=CARTESIAN_POINT ( 'NONE',  ( 5.477130869796502211, 5.492333557625114437, 1.040834085586084257E-14 ) ) ;
#7247=CARTESIAN_POINT ( 'NONE',  ( -0.6823417656250212460, 1.863541667008083991, 1.181850606188755259 ) ) ;
#7249=CARTESIAN_POINT ( 'NONE',  ( 3.999819011231439347, 4.625209253646830554, 1.199719254218464037 ) ) ;
#7252=CARTESIAN_POINT ( 'NONE',  ( -6.290620087060847965, 7.401773525401500464, 1.082531754730549967 ) ) ;
#7253=CARTESIAN_POINT ( 'NONE',  ( 5.029711800989886683, 4.970344644017389513, 1.040834085586084257E-14 ) ) ;
#7254=CARTESIAN_POINT ( 'NONE',  ( -5.205967797523171292, 9.017453497178271604, 0.000000000000000000 ) ) ;
#7258=CARTESIAN_POINT ( 'NONE',  ( 5.148345644887269756, 7.029489223833707001, -1.599625672291256295 ) ) ;
#7264=CARTESIAN_POINT ( 'NONE',  ( -1.364683531249997417, 5.759375000341418804, 1.214306433183764966E-14 ) ) ;
#7269=CARTESIAN_POINT ( 'NONE',  ( 6.169123589417988995, 7.156064594864501416, -1.199719254218445830 ) ) ;
#7270=FILL_AREA_STYLE_COLOUR ( '', #179735 ) ;
#7272=CARTESIAN_POINT ( 'NONE',  ( -7.549192604710863286, 7.701812881784464437, -0.7998128361456291469 ) ) ;
#7276=CARTESIAN_POINT ( 'NONE',  ( 8.125414133291656071, 8.374071331795406081, -0.7998128361456291469 ) ) ;
#7279=CARTESIAN_POINT ( 'NONE',  ( -6.256197817702116026, 9.386315656372753224, -1.199719254218440723 ) ) ;
#7280=CARTESIAN_POINT ( 'NONE',  ( 5.287316719205157334, 9.112360572473935605, 1.040834085586084257E-14 ) ) ;
#7281=CARTESIAN_POINT ( 'NONE',  ( 4.279786810092509164, 7.480689796721937235, 1.046525044888670486 ) ) ;
#7282=CARTESIAN_POINT ( 'NONE',  ( -6.098470168048611306, 6.009303372345148553, 1.040834085586084257E-14 ) ) ;
#7285=CARTESIAN_POINT ( 'NONE',  ( -5.656776405399756236, 7.622658444431597680, -1.599625672291256295 ) ) ;
#7291=CARTESIAN_POINT ( 'NONE',  ( 0.6823417656249882723, 1.926041667008083991, -1.181850606188749264 ) ) ;
#7293=CARTESIAN_POINT ( 'NONE',  ( -5.666945020832185875, 7.634521829102760115, 1.443375672974064550 ) ) ;
#7298=CARTESIAN_POINT ( 'NONE',  ( 6.657217119509961201, 7.725507046638470321, -1.199719254218446718 ) ) ;
#7301=VECTOR ( 'NONE', #176467, 1000.000000000000000 ) ;
#7302=CARTESIAN_POINT ( 'NONE',  ( -5.833005281931015418, 6.047509994665502653, 0.4702358434125544773 ) ) ;
#7303=CARTESIAN_POINT ( 'NONE',  ( 1.364683531249986537, 1.467708333674748289, -0.7879004041258239610 ) ) ;
#7306=CARTESIAN_POINT ( 'NONE',  ( 3.958617665510264949, 5.641473247893851628, -1.443375672974051449 ) ) ;
#7309=CARTESIAN_POINT ( 'NONE',  ( -3.588104209110990706, 7.337872010604796991, 1.040834085586084257E-14 ) ) ;
#7311=CARTESIAN_POINT ( 'NONE',  ( -8.500599125644013654, 9.019713189447241319, 0.7216878364870438212 ) ) ;
#7320=CARTESIAN_POINT ( 'NONE',  ( -6.954969613686107444, 10.09758640173367894, 1.082531754730549967 ) ) ;
#7323=CARTESIAN_POINT ( 'NONE',  ( -1.084637062511556005, 2.963621193390831632, 1.105835307554803082 ) ) ;
#7326=CARTESIAN_POINT ( 'NONE',  ( -7.985389288324703294, 9.379004260209384825, -1.082531754730543083 ) ) ;
#7332=CARTESIAN_POINT ( 'NONE',  ( 1.499999999999991118, 5.535416667349481123, 0.8660254037844524744 ) ) ;
#7334=CARTESIAN_POINT ( 'NONE',  ( -0.7499999999999972244, 5.139583334016151639, -1.299038105676652899 ) ) ;
#7340=CARTESIAN_POINT ( 'NONE',  ( -7.691553217654356622, 7.867900263551875994, -0.7998128361456291469 ) ) ;
#7343=CARTESIAN_POINT ( 'NONE',  ( 3.497113557321089861, 6.167384019261527683, -1.199719254218446718 ) ) ;
#7347=CARTESIAN_POINT ( 'NONE',  ( 7.820355676984174664, 8.018169799436671852, -0.7998128361456281477 ) ) ;
#7352=CARTESIAN_POINT ( 'NONE',  ( -5.802526556968872207, 6.832331073627524454, 1.082531754730548412 ) ) ;
#7363=CARTESIAN_POINT ( 'NONE',  ( -1.364683531250012516, 0.5302083336747518416, 0.7879004041258379498 ) ) ;
#7365=CARTESIAN_POINT ( 'NONE',  ( -7.340850106795412167, 10.65174332698158643, 1.199719254218453823 ) ) ;
#7367=CARTESIAN_POINT ( 'NONE',  ( 6.936968151686458306, 11.24487994360957188, 0.7998128361456462443 ) ) ;
#7369=CARTESIAN_POINT ( 'NONE',  ( -7.004758919754800139, 11.32396917302262018, 0.000000000000000000 ) ) ;
#7372=CARTESIAN_POINT ( 'NONE',  ( -1.364683531250010295, 5.280208333674758059, 0.7879004041258379498 ) ) ;
#7374=CARTESIAN_POINT ( 'NONE',  ( 7.782016984564043227, 12.02284421539267356, 0.7216878364870438212 ) ) ;
#7377=CARTESIAN_POINT ( 'NONE',  ( -1.201851678989727383E-14, 5.837500000000023448, -1.732050807568863648 ) ) ;
#7380=CARTESIAN_POINT ( 'NONE',  ( 7.958272981097359811, 9.347368568444167636, -1.082531754730537976 ) ) ;
#7383=CARTESIAN_POINT ( 'NONE',  ( -4.419594888374909658, 8.100018436505289188, 0.7216878364870458196 ) ) ;
#7385=CARTESIAN_POINT ( 'NONE',  ( 0.6823417656249899377, 1.842708333674752952, 1.181850606188755259 ) ) ;
#7389=CARTESIAN_POINT ( 'NONE',  ( -6.205881626753225966, 8.263281202677319470, 1.599625672291283607 ) ) ;
#7390=CARTESIAN_POINT ( 'NONE',  ( 0.6823417656249917140, 4.905208333674755394, 1.181850606188765695 ) ) ;
#7396=CARTESIAN_POINT ( 'NONE',  ( 8.945682426918439845, 9.331051007693339727, 1.040834085586084257E-14 ) ) ;
#7399=CARTESIAN_POINT ( 'NONE',  ( 1.499999999999987121, 1.254166666666689300, 0.8660254037844524744 ) ) ;
#7402=CARTESIAN_POINT ( 'NONE',  ( 1.284279953904121641, 3.284610286488902187, 0.7750000000000135669 ) ) ;
#7405=CARTESIAN_POINT ( 'NONE',  ( 7.293923454472080792, 9.532663335016016148, 1.443375672974076540 ) ) ;
#7406=AXIS2_PLACEMENT_3D ( 'NONE', #155832, #139600, #188311 ) ;
#7413=CARTESIAN_POINT ( 'NONE',  ( 8.749089199520284410, 9.101692242395490240, 0.7998128361456481317 ) ) ;
#7414=CARTESIAN_POINT ( 'NONE',  ( -10.65400978224035811, 11.32409958890225710, 1.040834085586084257E-14 ) ) ;
#7416=DIRECTION ( 'NONE',  ( -0.6507913734559640506, -0.7592566023653004592, 0.000000000000000000 ) ) ;
#7417=CARTESIAN_POINT ( 'NONE',  ( -1.364683531250014514, 0.2802083336747505649, 0.7879004041258379498 ) ) ;
#7418=CARTESIAN_POINT ( 'NONE',  ( -1.500000000000013101, 1.170833333333352710, 0.8660254037844403729 ) ) ;
#7420=CARTESIAN_POINT ( 'NONE',  ( 4.150767584078112193, 7.994312614733129152, 0.7998128361456321445 ) ) ;
#7423=CARTESIAN_POINT ( 'NONE',  ( 3.563261906135759993, 6.332667919118538435, -2.500000000000000444 ) ) ;
#7427=CARTESIAN_POINT ( 'NONE',  ( -1.364683531250012516, 4.488541667008090208, -0.7879004041258300672 ) ) ;
#7429=CARTESIAN_POINT ( 'NONE',  ( -8.402302512167102222, 10.82577223566020841, -1.599625672291263179 ) ) ;
#7430=CARTESIAN_POINT ( 'NONE',  ( -5.043269954603569083, 7.867270132804026872, 1.082531754730560403 ) ) ;
#7439=CARTESIAN_POINT ( 'NONE',  ( 8.098297826064319693, 8.342435640030188893, 0.7998128361456481317 ) ) ;
#7440=CARTESIAN_POINT ( 'NONE',  ( -3.917943204224951348, 7.514758138330256187, -0.7216878364870535911 ) ) ;
#7443=CARTESIAN_POINT ( 'NONE',  ( 6.602457619730756733, 9.686322408785807525, 1.082531754730558626 ) ) ;
#7447=CARTESIAN_POINT ( 'NONE',  ( -9.671043645249580933, 10.17730576241299900, 0.7998128361456462443 ) ) ;
#7449=CARTESIAN_POINT ( 'NONE',  ( 6.667912619822566000, 6.673652899414787676, 1.040834085586084257E-14 ) ) ;
#7452=CARTESIAN_POINT ( 'NONE',  ( 2.521453382017309952, 5.885520012421409319, 0.000000000000000000 ) ) ;
#7454=CARTESIAN_POINT ( 'NONE',  ( 2.672928840188529609, 6.270167413528593414, 0.000000000000000000 ) ) ;
#7461=CARTESIAN_POINT ( 'NONE',  ( -5.748293942514186128, 6.769059690097084747, -1.082531754730544860 ) ) ;
#7462=CARTESIAN_POINT ( 'NONE',  ( 2.347533153460546806, 5.890539112345938300, 0.000000000000000000 ) ) ;
#7465=CARTESIAN_POINT ( 'NONE',  ( -6.531277313481209212, 8.642909503859968368, 1.599625672291283607 ) ) ;
#7470=CARTESIAN_POINT ( 'NONE',  ( -8.158255747121117452, 10.54105100977322174, 1.599625672291295375 ) ) ;
#7472=FACE_OUTER_BOUND ( 'NONE', #34916, .T. ) ;
#7474=CARTESIAN_POINT ( 'NONE',  ( 5.606460214450851964, 6.499623990736163037, 1.199719254218462483 ) ) ;
#7475=CARTESIAN_POINT ( 'NONE',  ( -3.733524485140106819, 7.410126666105433024, -2.499999999999995559 ) ) ;
#7485=CARTESIAN_POINT ( 'NONE',  ( -5.910464900553636269, 8.982960586366182554, -1.199719254218440723 ) ) ;
#7488=CARTESIAN_POINT ( 'NONE',  ( 4.528060117284222308, 8.226561203566173930, 0.7216878364870438212 ) ) ;
#7492=CARTESIAN_POINT ( 'NONE',  ( -5.925076824372040640, 6.871343368977510302, 1.199719254218450271 ) ) ;
#7496=CARTESIAN_POINT ( 'NONE',  ( -6.501298352952815662, 7.543601818988450169, -1.199719254218446718 ) ) ;
#7501=DIRECTION ( 'NONE',  ( -5.578564026256490882E-16, -1.000000000000000000, -9.066213480720158442E-32 ) ) ;
#7502=CARTESIAN_POINT ( 'NONE',  ( -10.64045162862669081, 11.30828174301964140, -0.7998128361456221525 ) ) ;
#7503=CARTESIAN_POINT ( 'NONE',  ( 7.344766530301147789, 9.591980256816594164, 1.599625672291281386 ) ) ;
#7508=CARTESIAN_POINT ( 'NONE',  ( -5.590823505525904125, 6.198478227408987351, -0.8910005059661347815 ) ) ;
#7511=CARTESIAN_POINT ( 'NONE',  ( -1.364683531250000748, -1.178124999658580752, 0.000000000000000000 ) ) ;
#7515=CARTESIAN_POINT ( 'NONE',  ( 9.625925876022625616, 11.29296361252366765, -1.082531754730537088 ) ) ;
#7521=CARTESIAN_POINT ( 'NONE',  ( -5.618132639473230050, 6.180982067432974070, -0.8581683403942765853 ) ) ;
#7535=CARTESIAN_POINT ( 'NONE',  ( -3.541704441667874903, 5.155074486744371853, -1.599625672291256295 ) ) ;
#7538=CARTESIAN_POINT ( 'NONE',  ( -2.272963308585411735, 5.803540959991587478, 0.7998128361456341429 ) ) ;
#7543=CARTESIAN_POINT ( 'NONE',  ( -1.402160292154681736E-14, -0.5062499993171791779, 1.732050807568877637 ) ) ;
#7546=CARTESIAN_POINT ( 'NONE',  ( -2.168941388506379742, 5.474256019991960542, -0.7216878364870267237 ) ) ;
#7549=ORIENTED_EDGE ( 'NONE', *, *, #36887, .F. ) ;
#7552=CARTESIAN_POINT ( 'NONE',  ( 2.866659414285625651, 5.431854185720147221, -1.199719254218446718 ) ) ;
#7555=CARTESIAN_POINT ( 'NONE',  ( 9.693716643646595799, 11.37205284141829686, 1.082531754730548412 ) ) ;
#7558=CARTESIAN_POINT ( 'NONE',  ( -1.201851678989727383E-14, 3.134375000341420137, 1.575800808251672791 ) ) ;
#7561=CARTESIAN_POINT ( 'NONE',  ( -7.995557903757128493, 10.35123685918189729, 1.599625672291295375 ) ) ;
#7562=CARTESIAN_POINT ( 'NONE',  ( -6.534666851662457532, 6.726125536468730459, 1.040834085586084257E-14 ) ) ;
#7564=CARTESIAN_POINT ( 'NONE',  ( -5.045605722580076780, 9.038290442985410067, -0.7998128361456231517 ) ) ;
#7566=CARTESIAN_POINT ( 'NONE',  ( -1.364683531249997417, 5.759375000341418804, 1.214306433183764966E-14 ) ) ;
#7575=CARTESIAN_POINT ( 'NONE',  ( -5.382223794500845315, 6.341977850748185652, -1.082531754730543971 ) ) ;
#7580=CARTESIAN_POINT ( 'NONE',  ( -3.429849674132936066, 6.945315686556313040, -0.7216878364870257245 ) ) ;
#7582=CARTESIAN_POINT ( 'NONE',  ( 10.24726517383036928, 10.84956421242393887, 0.000000000000000000 ) ) ;
#7591=CARTESIAN_POINT ( 'NONE',  ( -4.762992037102518950, 4.451245552908022596, -0.7998128361456221525 ) ) ;
#7592=DIRECTION ( 'NONE',  ( -5.578564026256483980E-16, -1.000000000000000000, 2.168404344971008079E-15 ) ) ;
#7597=CARTESIAN_POINT ( 'NONE',  ( 8.188761592974039161, 10.57664116326830595, -1.443375672974063439 ) ) ;
#7598=CARTESIAN_POINT ( 'NONE',  ( 5.819474248763732760, 7.812472595022922128, -1.599625672291262513 ) ) ;
#7603=CARTESIAN_POINT ( 'NONE',  ( 4.566398809704347528, 4.221886787610169556, -0.7998128361456211532 ) ) ;
#7606=ORIENTED_EDGE ( 'NONE', *, *, #7783, .F. ) ;
#7615=CARTESIAN_POINT ( 'NONE',  ( -4.726989112658928072, 8.666571064744069020, 1.040834085586084257E-14 ) ) ;
#7620=CARTESIAN_POINT ( 'NONE',  ( 1.364683531249990311, 4.884375000341417916, 1.214306433183764966E-14 ) ) ;
#7622=CARTESIAN_POINT ( 'NONE',  ( -5.225778143063529946, 8.184159369294361497, 1.199719254218452047 ) ) ;
#7625=CARTESIAN_POINT ( 'NONE',  ( 5.005985031943777308, 6.863401842066294556, -1.599625672291256295 ) ) ;
#7626=CARTESIAN_POINT ( 'NONE',  ( -6.247609857798938293, 6.183299677053865295, -0.7998128361456291469 ) ) ;
#7632=CARTESIAN_POINT ( 'NONE',  ( 7.456621297836082185, 7.801739057004660971, 0.7216878364870317197 ) ) ;
#7634=( BOUNDED_CURVE ( )  B_SPLINE_CURVE ( 3, ( #196803, #35354, #132900, #198905 ),
 .UNSPECIFIED., .F., .T. ) 
 B_SPLINE_CURVE_WITH_KNOTS ( ( 4, 4 ),
 ( 4.082329036743152173, 4.712388980384690562 ),
 .UNSPECIFIED. ) 
 CURVE ( )  GEOMETRIC_REPRESENTATION_ITEM ( )  RATIONAL_B_SPLINE_CURVE ( ( 1.000000000000000000, 0.9671913951488351202, 0.9671913951488351202, 1.000000000000000000 ) ) 
 REPRESENTATION_ITEM ( '' )  );
#7635=CARTESIAN_POINT ( 'NONE',  ( 6.439759776366765998, 9.496508258194486629, 1.082531754730558626 ) ) ;
#7636=CARTESIAN_POINT ( 'NONE',  ( 1.364683531249988535, 3.676041667008087099, 0.7879004041258500513 ) ) ;
#7638=CARTESIAN_POINT ( 'NONE',  ( 5.965224399888476192, 6.061776009399090448, 1.040834085586084257E-14 ) ) ;
#7648=CARTESIAN_POINT ( 'NONE',  ( -4.902910567894817717, 6.875085367926331514, 1.448488056007392721 ) ) ;
#7656=CARTESIAN_POINT ( 'NONE',  ( -10.47775378526269918, 11.11846759242831872, -0.7998128361456221525 ) ) ;
#7658=CARTESIAN_POINT ( 'NONE',  ( 2.737856954955798727, 5.281584649835344258, 1.199719254218452047 ) ) ;
#7666=CARTESIAN_POINT ( 'NONE',  ( 2.711267533052988732, 6.106969855296372707, -0.7216878364870267237 ) ) ;
#7667=CARTESIAN_POINT ( 'NONE',  ( 1.364683531249988535, 3.926041667008087543, 0.7879004041258500513 ) ) ;
#7669=CARTESIAN_POINT ( 'NONE',  ( 7.130698725783555680, 10.40656671580112658, 1.199719254218460707 ) ) ;
#7670=CARTESIAN_POINT ( 'NONE',  ( -9.317477881089553549, 11.89347683273641820, 1.599625672291281386 ) ) ;
#7672=CARTESIAN_POINT ( 'NONE',  ( -3.228813138348844536, 6.918699094715619502, 0.7998128361456341429 ) ) ;
#7677=CARTESIAN_POINT ( 'NONE',  ( -1.201851678989727383E-14, 3.462500000000019895, 1.732050807568877637 ) ) ;
#7678=CARTESIAN_POINT ( 'NONE',  ( 6.322179702674084467, 6.270297829408224111, 1.040834085586084257E-14 ) ) ;
#7681=CARTESIAN_POINT ( 'NONE',  ( 1.499999999999990896, 8.627523663848672086, 2.580000000000004068 ) ) ;
#7682=CARTESIAN_POINT ( 'NONE',  ( 0.6823417656249899377, 4.426041667008086655, -1.181850606188754593 ) ) ;
#7684=CARTESIAN_POINT ( 'NONE',  ( 8.256552361042350796, 12.57646882128404187, 1.040834085586084257E-14 ) ) ;
#7690=CARTESIAN_POINT ( 'NONE',  ( -1.500000000000013101, 1.452083334016150085, 0.8660254037844403729 ) ) ;
#7692=CARTESIAN_POINT ( 'NONE',  ( -6.891622154448065807, 6.934647356477856128, 1.040834085586084257E-14 ) ) ;
#7701=CARTESIAN_POINT ( 'NONE',  ( 7.955937213120826357, 8.176348258262782664, 0.7998128361456481317 ) ) ;
#7702=CARTESIAN_POINT ( 'NONE',  ( 5.657830175604453338, 5.495223381160312393, 0.7998128361456341429 ) ) ;
#7707=CARTESIAN_POINT ( 'NONE',  ( 4.819033534653518025, 7.709623992816043270, -1.199719254218452047 ) ) ;
#7709=ORIENTED_EDGE ( 'NONE', *, *, #85341, .T. ) ;
#7714=CARTESIAN_POINT ( 'NONE',  ( 10.16199982864259788, 11.81442020729326536, 1.199719254218452047 ) ) ;
#7719=CARTESIAN_POINT ( 'NONE',  ( 4.911299649074239326, 6.652374229206746037, 1.248453844233877286 ) ) ;
#7731=CARTESIAN_POINT ( 'NONE',  ( 6.155038550924139429, 9.164333495178082600, 1.082531754730558626 ) ) ;
#7732=CARTESIAN_POINT ( 'NONE',  ( -4.548924232584923288, 5.265832011892554121, -1.199719254218446718 ) ) ;
#7735=CARTESIAN_POINT ( 'NONE',  ( -6.067437437315529536, 7.037430750744921859, 1.199719254218450271 ) ) ;
#7748=DIRECTION ( 'NONE',  ( 5.578564026256490882E-16, 1.000000000000000000, 2.168404344971008079E-15 ) ) ;
#7749=CARTESIAN_POINT ( 'NONE',  ( 9.236128959407556849, 11.79856975744075598, -1.599625672291262513 ) ) ;
#7752=CARTESIAN_POINT ( 'NONE',  ( 3.145128448690309053, 4.692402494937224056, -1.443375672974057666 ) ) ;
#7757=CARTESIAN_POINT ( 'NONE',  ( -9.002250809794000830, 11.52571191622492464, -1.443375672974059665 ) ) ;
#7760=CARTESIAN_POINT ( 'NONE',  ( 7.401861798056875053, 10.72292363345333399, -1.199719254218441611 ) ) ;
#7764=CARTESIAN_POINT ( 'NONE',  ( -5.768104287610143821, 8.816873204598778102, -1.199719254218440723 ) ) ;
#7765=CARTESIAN_POINT ( 'NONE',  ( 5.183294799126148433, 4.941598775268944976, 1.040834085586084257E-14 ) ) ;
#7767=CARTESIAN_POINT ( 'NONE',  ( 10.71502147350184231, 11.39527989537399755, 0.000000000000000000 ) ) ;
#7768=CARTESIAN_POINT ( 'NONE',  ( -3.687454593236990430, 4.364747115940301292, 1.082531754730560403 ) ) ;
#7771=CARTESIAN_POINT ( 'NONE',  ( -0.6823417656250003738, 3.030208333674754062, -1.181850606188749264 ) ) ;
#7774=CARTESIAN_POINT ( 'NONE',  ( 5.666945020832160118, 9.555260257705446847, 0.7216878364870438212 ) ) ;
#7782=CARTESIAN_POINT ( 'NONE',  ( 10.19536832735223975, 10.99694392477354477, 0.000000000000000000 ) ) ;
#7783=EDGE_CURVE ( 'NONE', #179842, #192556, #181951, .T. ) ;
#7788=CARTESIAN_POINT ( 'NONE',  ( -9.504429378379839477, 11.04725468198666150, 1.199719254218462483 ) ) ;
#7789=CARTESIAN_POINT ( 'NONE',  ( 3.511198596259284876, 6.271927390929313617, -1.052294140492317842 ) ) ;
#7797=CARTESIAN_POINT ( 'NONE',  ( 5.366329872910639232, 5.155139694684188534, 1.040834085586084257E-14 ) ) ;
#7804=CARTESIAN_POINT ( 'NONE',  ( 4.852928918687680948, 7.749168607522574526, 1.199719254218462483 ) ) ;
#7807=CARTESIAN_POINT ( 'NONE',  ( 1.499999999999989120, 3.056250000682818158, 1.214306433183764966E-14 ) ) ;
#7813=CARTESIAN_POINT ( 'NONE',  ( 0.7499999999999885647, 1.066666666666687968, -1.299038105676652899 ) ) ;
#7814=CARTESIAN_POINT ( 'NONE',  ( 8.586391356156291010, 8.911878091804165791, 0.7998128361456481317 ) ) ;
#7815=CARTESIAN_POINT ( 'NONE',  ( -1.364683531250000748, -0.2406249996585799189, 0.000000000000000000 ) ) ;
#7818=CARTESIAN_POINT ( 'NONE',  ( 9.585251415181632595, 10.28514086057449184, 0.000000000000000000 ) ) ;
#7824=CARTESIAN_POINT ( 'NONE',  ( -5.205440912643032547, 8.160432600470439723, 1.199719254218452047 ) ) ;
#7825=CARTESIAN_POINT ( 'NONE',  ( -1.500000000000011324, 3.202083334016150307, 0.8660254037844403729 ) ) ;
#7826=CARTESIAN_POINT ( 'NONE',  ( -0.6823417656250246877, -1.198958332991911790, 1.181850606188755259 ) ) ;
#7830=EDGE_CURVE ( 'NONE', #166540, #80549, #114491, .T. ) ;
#7843=CARTESIAN_POINT ( 'NONE',  ( -9.352427035328430449, 9.805586384171650849, 1.040834085586084257E-14 ) ) ;
#7844=CARTESIAN_POINT ( 'NONE',  ( 5.296431564432884542, 9.330920591813708143, 1.040834085586084257E-14 ) ) ;
#7852=CARTESIAN_POINT ( 'NONE',  ( -7.694415870955439551, 8.935572256658169010, 1.199719254218462483 ) ) ;
#7858=CARTESIAN_POINT ( 'NONE',  ( 10.53876547652418338, 11.18964789890005918, 0.7998128361456462443 ) ) ;
#7861=CARTESIAN_POINT ( 'NONE',  ( -4.391951695823077984, 7.211361847513815704, 1.199719254218464037 ) ) ;
#7862=CARTESIAN_POINT ( 'NONE',  ( -7.645908563102897126, 11.00764485934031889, 1.199719254218453823 ) ) ;
#7865=CARTESIAN_POINT ( 'NONE',  ( -4.212224785787594961, 7.548845203666256332, -0.9872405639642158892 ) ) ;
#7872=CARTESIAN_POINT ( 'NONE',  ( 4.821896187954575197, 8.777295985922343391, 0.7998128361456462443 ) ) ;
#7874=CARTESIAN_POINT ( 'NONE',  ( 3.642672431166742886, 3.097590952613315185, 2.447572309175040761 ) ) ;
#7889=CARTESIAN_POINT ( 'NONE',  ( 6.471393748265519719, 5.229711127717882491, -2.419999999999995932 ) ) ;
#7891=CARTESIAN_POINT ( 'NONE',  ( 2.399429999938675007, 5.743159399996332404, 0.000000000000000000 ) ) ;
#7895=CARTESIAN_POINT ( 'NONE',  ( -9.643927338022246332, 10.14567007064778004, -0.7998128361456291469 ) ) ;
#7900=CARTESIAN_POINT ( 'NONE',  ( -1.402160292154681736E-14, 0.3687500006828169363, -1.732050807568870754 ) ) ;
#7905=CARTESIAN_POINT ( 'NONE',  ( -8.482597663644387609, 13.04811437422715414, -0.7998128361456281477 ) ) ;
#7907=CARTESIAN_POINT ( 'NONE',  ( 1.364683531249986537, 0.3635416670080869328, 0.7879004041258500513 ) ) ;
#7908=CARTESIAN_POINT ( 'NONE',  ( -2.482948226198870678, 5.072301959192136778, -2.419999999999995044 ) ) ;
#7916=CARTESIAN_POINT ( 'NONE',  ( -4.009460741339347045, 5.700790169694431420, -1.599625672291256295 ) ) ;
#7918=CARTESIAN_POINT ( 'NONE',  ( 1.499999999989245048, 7.854386371692742230, -3.680172642288968010 ) ) ;
#7920=CARTESIAN_POINT ( 'NONE',  ( -0.7500000000000249800, -0.3083333333333132531, 1.299038105676659116 ) ) ;
#7922=CARTESIAN_POINT ( 'NONE',  ( -1.364683531250014514, -0.6989583329919100141, -0.7879004041258359514 ) ) ;
#7927=CARTESIAN_POINT ( 'NONE',  ( -1.402160292154681736E-14, 0.4468750003414233563, -1.575800808251665908 ) ) ;
#7929=CARTESIAN_POINT ( 'NONE',  ( -8.040148788103921973, 9.338927326664741457, 1.199719254218462483 ) ) ;
#7930=CARTESIAN_POINT ( 'NONE',  ( 7.892817981449907982, 12.36003807833360391, 0.7998128361456462443 ) ) ;
#7931=CARTESIAN_POINT ( 'NONE',  ( 4.976006071415387311, 5.764094157194782575, 1.199719254218462483 ) ) ;
#7934=CARTESIAN_POINT ( 'NONE',  ( 0.6823417656249864960, -0.5114583329919111243, -1.181850606188749264 ) ) ;
#7942=CARTESIAN_POINT ( 'NONE',  ( 6.263503779833467178, 9.290876262238963790, -1.082531754730537088 ) ) ;
#7945=CARTESIAN_POINT ( 'NONE',  ( -5.148345644887285744, 7.029489223833707001, -1.599625672291256295 ) ) ;
#7946=CARTESIAN_POINT ( 'NONE',  ( -4.251504296082277534, 7.448701262369814557, -1.004931253576486272 ) ) ;
#7949=FACE_OUTER_BOUND ( 'NONE', #105805, .T. ) ;
#7950=CARTESIAN_POINT ( 'NONE',  ( -7.307481607641392429, 11.46921960898288972, 0.7216878364870458196 ) ) ;
#7952=CARTESIAN_POINT ( 'NONE',  ( -1.001543065824772872E-14, 4.212500000000023448, 1.732050807568877637 ) ) ;
#7956=CARTESIAN_POINT ( 'NONE',  ( 7.443063144222396232, 11.62739806832741785, 1.040834085586084257E-14 ) ) ;
#7967=CARTESIAN_POINT ( 'NONE',  ( -2.398572866711294438, 5.287202466803544887, -0.8077998227820496480 ) ) ;
#7970=CARTESIAN_POINT ( 'NONE',  ( 8.419250203962011625, 8.924806114151579095, -0.7216878364870267237 ) ) ;
#7971=CARTESIAN_POINT ( 'NONE',  ( 8.535021395002688749, 9.916278701380017324, 1.199719254218462483 ) ) ;
#7975=CARTESIAN_POINT ( 'NONE',  ( 4.690757960648231695, 5.535267711253469614, 1.082531754730560403 ) ) ;
#7978=CARTESIAN_POINT ( 'NONE',  ( 4.528060117284240071, 5.345453560662148718, 1.082531754730560403 ) ) ;
#7980=CARTESIAN_POINT ( 'NONE',  ( -7.917598520700757980, 9.299915031314755609, 1.082531754730558626 ) ) ;
#8000=EDGE_LOOP ( 'NONE', ( #169777, #110513, #206840, #203741 ) ) ;
#8005=DIRECTION ( 'NONE',  ( -4.336808689941987759E-15, -0.6000000000000035305, -0.7999999999999976019 ) ) ;
#8007=CARTESIAN_POINT ( 'NONE',  ( -0.07432994781761058378, 7.051017997671326754, -3.950880802765572408 ) ) ;
#8009=CARTESIAN_POINT ( 'NONE',  ( -5.930802130974132780, 9.006687355190106103, -1.199719254218440723 ) ) ;
#8012=CARTESIAN_POINT ( 'NONE',  ( 6.498435699651741615, 6.475929825882159818, -0.7998128361456281477 ) ) ;
#8021=CARTESIAN_POINT ( 'NONE',  ( -2.916975605234527702, 6.554888639415577423, 1.040834085586084257E-14 ) ) ;
#8025=CARTESIAN_POINT ( 'NONE',  ( 7.935599982700328958, 8.152621489438862667, 0.7998128361456481317 ) ) ;
#8026=CARTESIAN_POINT ( 'NONE',  ( 1.364683531249990311, 3.384375000341416140, 1.214306433183764966E-14 ) ) ;
#8028=CARTESIAN_POINT ( 'NONE',  ( 5.430717995911492402, 6.471920874811950775, 1.294091166901890633 ) ) ;
#8034=CARTESIAN_POINT ( 'NONE',  ( 6.439759776366775768, 7.575769829591800786, 1.082531754730558626 ) ) ;
#8035=CARTESIAN_POINT ( 'NONE',  ( -6.821723845970312894, 11.11042825360738284, 0.000000000000000000 ) ) ;
#8039=CARTESIAN_POINT ( 'NONE',  ( -8.345207244411405156, 9.694828859023472134, 1.199719254218462483 ) ) ;
#8041=CARTESIAN_POINT ( 'NONE',  ( -5.551173829791513192, 8.563787670477010394, 1.199719254218452047 ) ) ;
#8048=B_SPLINE_CURVE_WITH_KNOTS ( 'NONE', 3,
 ( #16100, #150411, #909, #66978 ),
 .UNSPECIFIED., .F., .F.,
 ( 4, 4 ),
 ( 0.000000000000000000, 0.0003450753579246922977 ),
 .UNSPECIFIED. ) ;
#8049=CARTESIAN_POINT ( 'NONE',  ( 7.456094412511537151, 10.78619501698377370, 1.199719254218460707 ) ) ;
#8067=CARTESIAN_POINT ( 'NONE',  ( 1.499999999999987121, 4.545833333333352932, -0.8660254037844323793 ) ) ;
#8068=CARTESIAN_POINT ( 'NONE',  ( 5.332434488876471868, 5.115595079977664383, 0.7998128361456341429 ) ) ;
#8069=CARTESIAN_POINT ( 'NONE',  ( 6.982612806237943559, 8.105135347821125436, -1.199719254218446718 ) ) ;
#8071=CARTESIAN_POINT ( 'NONE',  ( -7.863365906246061243, 10.19701286208565705, -1.443375672974059665 ) ) ;
#8073=CARTESIAN_POINT ( 'NONE',  ( 5.327991180490514012, 9.159814110640187579, 1.040834085586084257E-14 ) ) ;
#8074=CARTESIAN_POINT ( 'NONE',  ( -7.646435447983039424, 11.86466575604815787, 0.000000000000000000 ) ) ;
#8077=CARTESIAN_POINT ( 'NONE',  ( 7.727257484784855635, 11.10255193463598111, -1.199719254218446718 ) ) ;
#8082=CARTESIAN_POINT ( 'NONE',  ( -2.314109536355652530, 5.457892750589173225, -0.8025987720412944837 ) ) ;
#8083=CARTESIAN_POINT ( 'NONE',  ( 1.364683531249988535, 2.363541667008088432, 0.7879004041258500513 ) ) ;
#8087=EDGE_CURVE ( 'NONE', #191425, #2091, #133614, .T. ) ;
#8089=CARTESIAN_POINT ( 'NONE',  ( -0.6823417656250003738, -0.7822916663252423852, -1.181850606188749264 ) ) ;
#8091=CARTESIAN_POINT ( 'NONE',  ( 8.940712233207955606, 12.51824914112961729, 1.199719254218450271 ) ) ;
#8094=CARTESIAN_POINT ( 'NONE',  ( -10.49131193887636826, 11.13428543831092909, 1.040834085586084257E-14 ) ) ;
#8100=CARTESIAN_POINT ( 'NONE',  ( 3.571683402196252910, 6.254382171615883834, 1.199719254218462483 ) ) ;
#8104=CARTESIAN_POINT ( 'NONE',  ( -8.154339323615371171, 11.60081407993821045, 1.199719254218453823 ) ) ;
#8106=EDGE_CURVE ( 'NONE', #179696, #186824, #27111, .T. ) ;
#8108=CARTESIAN_POINT ( 'NONE',  ( 8.127223016387999266, 11.56917838817298616, 1.199719254218460707 ) ) ;
#8110=CARTESIAN_POINT ( 'NONE',  ( 4.768780016659259324, 6.770301073365750710, 1.244442160714388068 ) ) ;
#8112=CARTESIAN_POINT ( 'NONE',  ( -4.939248034080176097, 4.656877549381960080, 1.214306433183764966E-14 ) ) ;
#8116=CARTESIAN_POINT ( 'NONE',  ( 8.749089199520284410, 9.101692242395490240, 0.7998128361456481317 ) ) ;
#8118=CARTESIAN_POINT ( 'NONE',  ( 8.125414133291656071, 8.374071331795406081, -0.7998128361456291469 ) ) ;
#8121=CARTESIAN_POINT ( 'NONE',  ( -8.351459436338030784, 11.72682452816096976, -1.082531754730543971 ) ) ;
#8129=CARTESIAN_POINT ( 'NONE',  ( -4.639453055371920875, 6.917948375795638150, -1.210149155198399828 ) ) ;
#8130=CARTESIAN_POINT ( 'NONE',  ( -0.6823417656250212460, 1.301041667008083547, 1.181850606188755259 ) ) ;
#8132=CARTESIAN_POINT ( 'NONE',  ( 5.002595493762530765, 8.780185809457538681, 1.040834085586084257E-14 ) ) ;
#8142=CIRCLE ( 'NONE', #91200, 6.959052028703005099 ) ;
#8152=CARTESIAN_POINT ( 'NONE',  ( -4.559605246071192219, 3.300000000000025135, -0.7749999999999935829 ) ) ;
#8154=CARTESIAN_POINT ( 'NONE',  ( 9.935427640716063991, 10.48575375712389679, -0.7998128361456281477 ) ) ;
#8156=ORIENTED_EDGE ( 'NONE', *, *, #203953, .T. ) ;
#8159=CARTESIAN_POINT ( 'NONE',  ( -7.206322340863467346, 8.366129804884193888, 1.199719254218450271 ) ) ;
#8162=CARTESIAN_POINT ( 'NONE',  ( -7.811469059767924605, 12.26513100303794168, -0.7998128361456281477 ) ) ;
#8163=CARTESIAN_POINT ( 'NONE',  ( -1.468321960012643590, 7.242494692102438236, 4.289992922803264719 ) ) ;
#8167=CARTESIAN_POINT ( 'NONE',  ( 6.265839547809997079, 10.46189657242035587, 0.7998128361456462443 ) ) ;
#8170=CARTESIAN_POINT ( 'NONE',  ( -6.714312387265696458, 8.856450423275211037, 1.599625672291283607 ) ) ;
#8172=CARTESIAN_POINT ( 'NONE',  ( -1.364683531250010295, 5.030208333674757171, 0.7879004041258379498 ) ) ;
#8175=CARTESIAN_POINT ( 'NONE',  ( 2.889785579457926801, 6.440540434672812786, -0.3822207396134719715 ) ) ;
#8178=CARTESIAN_POINT ( 'NONE',  ( -8.866669273657352690, 9.446795028796142191, 0.7216878364870438212 ) ) ;
#8182=CARTESIAN_POINT ( 'NONE',  ( -1.364683531249997417, 4.071875000341417028, 1.214306433183764966E-14 ) ) ;
#8188=CARTESIAN_POINT ( 'NONE',  ( 1.364683531249988535, 4.113541667008088432, 0.7879004041258500513 ) ) ;
#8189=CARTESIAN_POINT ( 'NONE',  ( -3.249150368769345043, 6.942425863539538611, 0.7998128361456341429 ) ) ;
#8190=CARTESIAN_POINT ( 'NONE',  ( 7.298366762858032430, 7.409182732956175244, 1.040834085586084257E-14 ) ) ;
#8193=CARTESIAN_POINT ( 'NONE',  ( 3.836594282542914236, 5.499112634431936542, 1.443375672974062551 ) ) ;
#8194=CARTESIAN_POINT ( 'NONE',  ( 1.364683531249988535, 3.926041667008087543, 0.7879004041258500513 ) ) ;
#8198=CARTESIAN_POINT ( 'NONE',  ( -1.364683531250014514, 0.2385416670080863499, -0.7879004041258359514 ) ) ;
#8199=CARTESIAN_POINT ( 'NONE',  ( -5.585596099150199834, 5.618876325204420930, -0.7216878364870207285 ) ) ;
#8200=CARTESIAN_POINT ( 'NONE',  ( 4.313465427442102929, 8.184126765324453601, 0.7998128361456462443 ) ) ;
#8203=CARTESIAN_POINT ( 'NONE',  ( 2.273349394227877074, 5.683342515206170731, 0.4597581080974435519 ) ) ;
#8204=CARTESIAN_POINT ( 'NONE',  ( 3.714570900464274850, 6.317121236308204324, 1.082531754730558626 ) ) ;
#8207=CARTESIAN_POINT ( 'NONE',  ( -7.185458225562757484, 11.32685899655781903, 0.7216878364870458196 ) ) ;
#8212=CARTESIAN_POINT ( 'NONE',  ( -8.272446282632566650, 12.80293776304669962, 0.7998128361456481317 ) ) ;
#8213=CARTESIAN_POINT ( 'NONE',  ( -4.839897649954225223, 7.630002444046455778, 1.082531754730560403 ) ) ;
#8215=CARTESIAN_POINT ( 'NONE',  ( -1.201851678989727383E-14, 1.384375000341419693, 1.575800808251672791 ) ) ;
#8225=CARTESIAN_POINT ( 'NONE',  ( 9.642873567817520808, 12.27310513391906532, 1.599625672291279388 ) ) ;
#8229=CARTESIAN_POINT ( 'NONE',  ( 8.934460041281305109, 10.48625347199211966, -1.082531754730543083 ) ) ;
#8236=EDGE_CURVE ( 'NONE', #60515, #145094, #31973, .T. ) ;
#8239=CARTESIAN_POINT ( 'NONE',  ( -2.656508033273816238, 5.186677574539687363, -1.199719254218446718 ) ) ;
#8240=DIRECTION ( 'NONE',  ( 0.000000000000000000, 8.546850786086437571E-32, 1.000000000000000000 ) ) ;
#8242=CARTESIAN_POINT ( 'NONE',  ( -1.364683531250000748, 1.321875000341421469, 0.000000000000000000 ) ) ;
#8251=CARTESIAN_POINT ( 'NONE',  ( -0.6823417656250003738, 1.717708333674752730, -1.181850606188749264 ) ) ;
#8261=CARTESIAN_POINT ( 'NONE',  ( 4.330940004561544043, 7.140181541042074365, -1.199719254218452047 ) ) ;
#8267=CARTESIAN_POINT ( 'NONE',  ( 4.650083499807235121, 5.295740330745369207, 1.082471891955963716 ) ) ;
#8269=CARTESIAN_POINT ( 'NONE',  ( 8.457588896826466751, 8.761608555919362828, 1.040834085586084257E-14 ) ) ;
#8272=CARTESIAN_POINT ( 'NONE',  ( 7.425061681778431399, 11.81432239538354345, 0.7998128361456462443 ) ) ;
#8274=CARTESIAN_POINT ( 'NONE',  ( 1.530444406200885954, 8.694995975526813581, -2.517029436271772003 ) ) ;
#8277=ORIENTED_EDGE ( 'NONE', *, *, #163792, .T. ) ;
#8284=CARTESIAN_POINT ( 'NONE',  ( -7.537970219518075332, 10.77775377520434574, -1.082531754730543971 ) ) ;
#8296=CARTESIAN_POINT ( 'NONE',  ( 2.670593071767634719, 6.059516317130127838, -0.7216878364870267237 ) ) ;
#8298=CARTESIAN_POINT ( 'NONE',  ( 5.138703914779377158, 5.953908307786102583, 1.199719254218462483 ) ) ;
#8306=CARTESIAN_POINT ( 'NONE',  ( -5.850506979496850057, 6.784345216623154151, -1.199719254218446718 ) ) ;
#8308=CARTESIAN_POINT ( 'NONE',  ( -4.135400547368138113, 4.783387712472935149, 1.199719254218462483 ) ) ;
#8314=CARTESIAN_POINT ( 'NONE',  ( 9.571693261567965294, 10.26932301469188857, 0.7216878364870438212 ) ) ;
#8316=CARTESIAN_POINT ( 'NONE',  ( -1.364683531250012516, 4.051041667008088432, -0.7879004041258300672 ) ) ;
#8318=CARTESIAN_POINT ( 'NONE',  ( 4.852928918687680948, 7.749168607522574526, 1.199719254218462483 ) ) ;
#8332=CARTESIAN_POINT ( 'NONE',  ( 1.364683531249988535, 1.426041667008083991, 0.7879004041258500513 ) ) ;
#8334=CARTESIAN_POINT ( 'NONE',  ( 3.785751206713845018, 5.439795712631356750, 1.599625672291267398 ) ) ;
#8336=CARTESIAN_POINT ( 'NONE',  ( -4.419594888374909658, 8.100018436505289188, 0.7216878364870458196 ) ) ;
#8337=CARTESIAN_POINT ( 'NONE',  ( 2.548569689688999329, 5.917155704705049146, -0.7216878364870267237 ) ) ;
#8338=CARTESIAN_POINT ( 'NONE',  ( -6.521108698048783126, 7.670676904887464786, -1.082531754730543083 ) ) ;
#8343=CARTESIAN_POINT ( 'NONE',  ( 4.476163270806094552, 8.373940915915776273, 0.7998128361456462443 ) ) ;
#8348=FACE_OUTER_BOUND ( 'NONE', #113636, .T. ) ;
#8352=CARTESIAN_POINT ( 'NONE',  ( 6.500244582748090139, 9.671036882259738121, 1.199719254218460707 ) ) ;
#8355=CARTESIAN_POINT ( 'NONE',  ( -5.703176172842872482, 9.805455968292021041, 0.000000000000000000 ) ) ;
#8359=CARTESIAN_POINT ( 'NONE',  ( 9.101601193475611140, 9.512956235343358102, -0.7998128361456221525 ) ) ;
#8362=CARTESIAN_POINT ( 'NONE',  ( -5.551173829791513192, 8.563787670477010394, 1.199719254218452047 ) ) ;
#8364=CARTESIAN_POINT ( 'NONE',  ( 7.090551149822728938, 10.25576486055978442, 1.082531754730558626 ) ) ;
#8365=CARTESIAN_POINT ( 'NONE',  ( 4.051511279158463985, 7.758049153162790645, -0.5006740859710266944 ) ) ;
#8366=CARTESIAN_POINT ( 'NONE',  ( -4.761938266897808525, 6.578680616179308771, 1.599625672291267398 ) ) ;
#8372=CARTESIAN_POINT ( 'NONE',  ( 8.757677159423465696, 12.30470822171437284, 1.199719254218450271 ) ) ;
#8373=FACE_OUTER_BOUND ( 'NONE', #100184, .T. ) ;
#8374=CARTESIAN_POINT ( 'NONE',  ( 1.364683531249986537, 0.3635416670080869328, 0.7879004041258500513 ) ) ;
#8376=CARTESIAN_POINT ( 'NONE',  ( -4.772106882330223954, 8.511282429453158827, -0.7216878364870267237 ) ) ;
#8383=CARTESIAN_POINT ( 'NONE',  ( -5.911556925646939575, 6.000462466000660022, -0.05029327469607651480 ) ) ;
#8384=CARTESIAN_POINT ( 'NONE',  ( -0.6823417656250212460, 0.8635416670080899859, 1.181850606188755259 ) ) ;
#8387=CARTESIAN_POINT ( 'NONE',  ( 2.223174002961016082, 5.537527403522402025, -0.7216878364870267237 ) ) ;
#8390=CARTESIAN_POINT ( 'NONE',  ( -5.434120640978981065, 5.234228924097238611, -0.7998128361456221525 ) ) ;
#8392=CARTESIAN_POINT ( 'NONE',  ( -8.798878505144665851, 9.367705798864669475, -0.7216878364870267237 ) ) ;
#8399=CARTESIAN_POINT ( 'NONE',  ( -6.832946231163084860, 10.91559500309152675, 0.000000000000000000 ) ) ;
#8404=CARTESIAN_POINT ( 'NONE',  ( -8.310784975052685652, 9.758632561392040827, -1.082531754730543083 ) ) ;
#8410=CARTESIAN_POINT ( 'NONE',  ( 1.499999999999989120, 5.327083334016152527, -0.8660254037844323793 ) ) ;
#8412=CARTESIAN_POINT ( 'NONE',  ( 1.499999999999964695, 5.077083334016150751, -0.8660254037844461461 ) ) ;
#8418=CARTESIAN_POINT ( 'NONE',  ( -5.845536785786364931, 9.971543350059432598, 0.000000000000000000 ) ) ;
#8421=CARTESIAN_POINT ( 'NONE',  ( 4.364835388595708743, 7.179726155748598515, 1.199719254218462483 ) ) ;
#8425=CARTESIAN_POINT ( 'NONE',  ( 7.121056995675668411, 9.330985799753529264, -1.599625672291262513 ) ) ;
#8430=CARTESIAN_POINT ( 'NONE',  ( -4.270455198624581783, 7.926022131796578662, 1.040834085586084257E-14 ) ) ;
#8440=CARTESIAN_POINT ( 'NONE',  ( -1.364683531250012516, 1.280208333674755172, 0.7879004041258379498 ) ) ;
#8442=CARTESIAN_POINT ( 'NONE',  ( -8.422639742587602285, 10.84949900448412841, -1.599625672291263179 ) ) ;
#8445=CARTESIAN_POINT ( 'NONE',  ( 8.959240580532112475, 9.346868853575953651, -0.7998128361456221525 ) ) ;
#8447=CARTESIAN_POINT ( 'NONE',  ( -9.352427035328430449, 9.805586384171650849, 1.040834085586084257E-14 ) ) ;
#8450=CARTESIAN_POINT ( 'NONE',  ( 1.364683531249990311, 5.113541667008084879, 0.7879004041258500513 ) ) ;
#8451=CARTESIAN_POINT ( 'NONE',  ( 8.242994207428692377, 12.56065097540143327, -0.7216878364870328300 ) ) ;
#8454=CARTESIAN_POINT ( 'NONE',  ( 0.6823417656249864960, -0.5114583329919111243, -1.181850606188749264 ) ) ;
#8457=CARTESIAN_POINT ( 'NONE',  ( 9.042925270190638187, 9.652427024751663254, 0.7216878364870458196 ) ) ;
#8461=CARTESIAN_POINT ( 'NONE',  ( -5.260200412422200600, 8.120355666925794580, -1.082531754730544860 ) ) ;
#8463=CARTESIAN_POINT ( 'NONE',  ( 1.364683531249986537, 1.655208333674748955, -0.7879004041258239610 ) ) ;
#8465=FACE_OUTER_BOUND ( 'NONE', #74080, .T. ) ;
#8467=CARTESIAN_POINT ( 'NONE',  ( -8.179646747746328828, 8.437342715325849341, -0.7998128361456291469 ) ) ;
#8468=CARTESIAN_POINT ( 'NONE',  ( -1.201851678989727383E-14, 5.009375000341421469, -1.575800808251660134 ) ) ;
#8473=CARTESIAN_POINT ( 'NONE',  ( 7.099665995050449041, 11.43469409420089455, 0.7998128361456462443 ) ) ;
#8477=CARTESIAN_POINT ( 'NONE',  ( -1.500000000000013101, 1.170833333333352710, 0.8660254037844403729 ) ) ;
#8480=CARTESIAN_POINT ( 'NONE',  ( -0.4241069589250067162, 7.990617654048622676, -1.998204128839461191 ) ) ;
#8483=CARTESIAN_POINT ( 'NONE',  ( 7.348156068926750883, 8.635565504245116486, -1.082531754730537976 ) ) ;
#8485=CARTESIAN_POINT ( 'NONE',  ( 10.07100917685271035, 10.64393221595000938, 0.7998128361456462443 ) ) ;
#8493=CARTESIAN_POINT ( 'NONE',  ( 8.646349277213076334, 11.11049346154719508, 1.599625672291281386 ) ) ;
#8494=CARTESIAN_POINT ( 'NONE',  ( -9.992522908471816123, 11.61669713376064372, 1.199719254218462483 ) ) ;
#8497=CARTESIAN_POINT ( 'NONE',  ( -1.402160292154681736E-14, 0.5718750003414239114, 1.575800808251672791 ) ) ;
#8498=CARTESIAN_POINT ( 'NONE',  ( -1.402160292154681736E-14, 0.4625000000000214495, 1.732050807568877637 ) ) ;
#8507=CARTESIAN_POINT ( 'NONE',  ( -1.201851678989727383E-14, 4.696875000341419693, -1.575800808251660134 ) ) ;
#8509=CARTESIAN_POINT ( 'NONE',  ( -5.856759171423528088, 8.816340885760650892, 1.082531754730548412 ) ) ;
#8518=CARTESIAN_POINT ( 'NONE',  ( 9.237182729612253951, 9.671134694169463586, 0.7998128361456462443 ) ) ;
#8519=CARTESIAN_POINT ( 'NONE',  ( -6.080807945883922372, 5.988697446486341391, 0.1578021610283755760 ) ) ;
#8524=CARTESIAN_POINT ( 'NONE',  ( -7.133561379084627063, 11.47423870890741782, 0.7998128361456481317 ) ) ;
#8525=CARTESIAN_POINT ( 'NONE',  ( 5.147291874682557555, 9.156924287104992288, 0.7998128361456462443 ) ) ;
#8526=CARTESIAN_POINT ( 'NONE',  ( 0.007473969438204840048, 8.279395425053873936, 1.999986034896453324 ) ) ;
#8527=CARTESIAN_POINT ( 'NONE',  ( 3.511198595814932766, 5.119484333249288532, 1.443375672974066548 ) ) ;
#8530=CARTESIAN_POINT ( 'NONE',  ( 3.985207087413062066, 6.736826471035503694, -1.199719254218452047 ) ) ;
#8536=CARTESIAN_POINT ( 'NONE',  ( -4.880572111239580124, 7.677455982212699759, 1.082531754730560403 ) ) ;
#8537=CARTESIAN_POINT ( 'NONE',  ( 10.38518247838791986, 11.21839376764850726, 0.7216878364870438212 ) ) ;
#8541=CARTESIAN_POINT ( 'NONE',  ( -7.694415870955439551, 8.935572256658169010, 1.199719254218462483 ) ) ;
#8546=CARTESIAN_POINT ( 'NONE',  ( -6.984421689334302741, 11.30024240419870374, 0.000000000000000000 ) ) ;
#8547=ADVANCED_FACE ( 'NONE', ( #163769 ), #81440, .F. ) ;
#8552=CARTESIAN_POINT ( 'NONE',  ( 4.741601036477289810, 6.554953847355395880, 1.599625672291267398 ) ) ;
#8563=CARTESIAN_POINT ( 'NONE',  ( -6.008234629150358330, 10.16135750065076060, 0.000000000000000000 ) ) ;
#8566=CARTESIAN_POINT ( 'NONE',  ( 6.317736394288140822, 7.433409217166723870, 1.082531754730558626 ) ) ;
#8568=CARTESIAN_POINT ( 'NONE',  ( -1.436717746206722213, 7.422220963915807879, 4.237135035833794916 ) ) ;
#8569=DIRECTION ( 'NONE',  ( 1.000000000000000000, 0.000000000000000000, 0.000000000000000000 ) ) ;
#8570=CARTESIAN_POINT ( 'NONE',  ( 5.352771719296971042, 5.139321848801576387, 0.7998128361456341429 ) ) ;
#8572=CARTESIAN_POINT ( 'NONE',  ( -6.247609857798938293, 6.183299677053865295, -0.7998128361456291469 ) ) ;
#8581=CARTESIAN_POINT ( 'NONE',  ( -9.642873567817536795, 12.27310513391906532, 1.599625672291281386 ) ) ;
#8582=CARTESIAN_POINT ( 'NONE',  ( 7.564559641420864899, 10.91273778404466199, -1.199719254218446718 ) ) ;
#8584=CARTESIAN_POINT ( 'NONE',  ( -2.168941388506379742, 5.474256019991960542, -0.7216878364870267237 ) ) ;
#8586=CARTESIAN_POINT ( 'NONE',  ( -4.822091459260241741, 6.758233420496813082, -1.248138317850192580 ) ) ;
#8588=CARTESIAN_POINT ( 'NONE',  ( 2.280903940472752467, 5.594607745005274246, -0.6109567437776646237 ) ) ;
#8592=CARTESIAN_POINT ( 'NONE',  ( 8.215877900201359552, 11.56864606933486606, -1.082531754730543083 ) ) ;
#8611=CARTESIAN_POINT ( 'NONE',  ( -2.923754682041362241, 6.562797562356882608, 0.7998128361456341429 ) ) ;
#8613=CARTESIAN_POINT ( 'NONE',  ( -1.500000000000011324, 3.670833333333356485, 0.8660254037844403729 ) ) ;
#8615=CARTESIAN_POINT ( 'NONE',  ( -3.460355519985875983, 5.060167411448709629, 1.599625672291267398 ) ) ;
#8619=CARTESIAN_POINT ( 'NONE',  ( 0.6823417656249917140, 5.092708333674749177, 1.181850606188765695 ) ) ;
#8622=AXIS2_PLACEMENT_3D ( 'NONE', #210944, #14869, #130846 ) ;
#8623=CARTESIAN_POINT ( 'NONE',  ( -2.304522924643024773, 5.632434478818063361, 0.7216878364870317197 ) ) ;
#8629=CARTESIAN_POINT ( 'NONE',  ( 2.218730694130720771, 5.740269576461138890, 0.7998128361456462443 ) ) ;
#8633=CARTESIAN_POINT ( 'NONE',  ( 9.205623113554612047, 12.72334881824701469, 1.082531754730546636 ) ) ;
#8635=CARTESIAN_POINT ( 'NONE',  ( -1.364683531250014514, 1.801041667008085767, -0.7879004041258289570 ) ) ;
#8636=CARTESIAN_POINT ( 'NONE',  ( 1.419999999999990603, 6.280000000000042881, 2.873333333333337070 ) ) ;
#8637=EDGE_CURVE ( 'NONE', #190586, #5554, #143562, .T. ) ;
#8639=CARTESIAN_POINT ( 'NONE',  ( -8.402302512167102222, 10.82577223566020841, -1.599625672291263179 ) ) ;
#8640=CARTESIAN_POINT ( 'NONE',  ( -5.463572716182839351, 7.397254140345190798, 1.443375672974064550 ) ) ;
#8645=CARTESIAN_POINT ( 'NONE',  ( -1.402160292154681736E-14, -1.006249999317181620, 1.732050807568877637 ) ) ;
#8653=CARTESIAN_POINT ( 'NONE',  ( -4.514501963226242864, 7.250374142863800664, 1.082531754730560403 ) ) ;
#8655=CARTESIAN_POINT ( 'NONE',  ( -0.4644214298786696893, 7.369507887681775671, -4.459343850242297513 ) ) ;
#8659=CARTESIAN_POINT ( 'NONE',  ( -3.917943204224914933, 6.554388924028945240, -1.082531754730548412 ) ) ;
#8661=CARTESIAN_POINT ( 'NONE',  ( 8.940712233207955606, 12.51824914112961729, 1.199719254218450271 ) ) ;
#8669=CARTESIAN_POINT ( 'NONE',  ( -3.255929445576174697, 6.950334786480840243, -0.7998128361456281477 ) ) ;
#8670=CARTESIAN_POINT ( 'NONE',  ( -6.114675100508033978, 6.010327456751344499, 0.3238074992715953559 ) ) ;
#8675=CARTESIAN_POINT ( 'NONE',  ( 7.592202833972727660, 11.80139437303613015, -0.7216878364870267237 ) ) ;
#8676=CARTESIAN_POINT ( 'NONE',  ( 5.133733721068893807, 9.141106441222381918, 1.040834085586084257E-14 ) ) ;
#8681=CARTESIAN_POINT ( 'NONE',  ( 5.190073875932979419, 4.949507698210251938, 0.7998128361456341429 ) ) ;
#8690=CARTESIAN_POINT ( 'NONE',  ( 8.127223016387999266, 11.56917838817298616, 1.199719254218460707 ) ) ;
#8691=CARTESIAN_POINT ( 'NONE',  ( -6.413170354464012846, 7.440785820751486312, 1.199719254218450271 ) ) ;
#8692=ADVANCED_FACE ( 'NONE', ( #31634 ), #41057, .T. ) ;
#8695=DIRECTION ( 'NONE',  ( 0.000000000000000000, 8.546850786086437571E-32, 1.000000000000000000 ) ) ;
#8698=CARTESIAN_POINT ( 'NONE',  ( 1.364683531249990311, 4.384375000341417028, 1.214306433183764966E-14 ) ) ;
#8699=CARTESIAN_POINT ( 'NONE',  ( 8.717529583462646059, 11.19353715217169309, 1.443375672974076540 ) ) ;
#8700=CARTESIAN_POINT ( 'NONE',  ( -5.388475986427523345, 8.373973519885682393, 1.199719254218452047 ) ) ;
#8703=CARTESIAN_POINT ( 'NONE',  ( 3.994848817520957773, 7.812407387083109001, 1.040834085586084257E-14 ) ) ;
#8704=CARTESIAN_POINT ( 'NONE',  ( -5.762378981008047241, 6.681529218386182301, 1.199719254218450271 ) ) ;
#8710=CARTESIAN_POINT ( 'NONE',  ( 6.155038550924144758, 8.203964280876741455, 1.443375672974076540 ) ) ;
#8712=CARTESIAN_POINT ( 'NONE',  ( 6.927853306458743532, 9.105581495667113501, 1.443375672974076540 ) ) ;
#8713=CARTESIAN_POINT ( 'NONE',  ( 0.6823417656249899377, 3.988541667008085767, -1.181850606188754593 ) ) ;
#8715=CARTESIAN_POINT ( 'NONE',  ( 4.460269348771534581, 8.147471973634706544, -0.7216878364870207285 ) ) ;
#8718=CARTESIAN_POINT ( 'NONE',  ( -4.148431816101615155, 3.942184661647709198, 0.7216878364870317197 ) ) ;
#8721=AXIS2_PLACEMENT_3D ( 'NONE', #55363, #53229, #151811 ) ;
#8728=CARTESIAN_POINT ( 'NONE',  ( -4.212224785787594961, 7.548845203666256332, -0.9872405639642158892 ) ) ;
#8736=CARTESIAN_POINT ( 'NONE',  ( 5.464099601507359516, 6.333536608968757697, 1.199719254218462483 ) ) ;
#8738=CARTESIAN_POINT ( 'NONE',  ( -3.050221372950322252, 5.542046787541873520, 1.082531754730560403 ) ) ;
#8747=CARTESIAN_POINT ( 'NONE',  ( 3.714570900464269076, 7.277490450609545469, 0.7216878364870298324 ) ) ;
#8748=CARTESIAN_POINT ( 'NONE',  ( 1.364683531249988535, 2.926041667008082658, 0.7879004041258500513 ) ) ;
#8750=CARTESIAN_POINT ( 'NONE',  ( 7.832860060393120882, 10.16142270859057462, 1.599625672291281386 ) ) ;
#8751=CARTESIAN_POINT ( 'NONE',  ( -10.15522075183580419, 11.80651128435196462, 1.199719254218462483 ) ) ;
#8758=CARTESIAN_POINT ( 'NONE',  ( 1.499999999999989120, 2.775000000000020339, 1.214306433183764966E-14 ) ) ;
#8759=CARTESIAN_POINT ( 'NONE',  ( 5.099838337034727331, 9.101561826515851550, -0.7998128361456281477 ) ) ;
#8763=CARTESIAN_POINT ( 'NONE',  ( 1.364683531249988535, 3.405208333674749621, -0.7879004041258239610 ) ) ;
#8766=CARTESIAN_POINT ( 'NONE',  ( 7.944714827928033962, 12.21265836598400689, 0.7216878364870438212 ) ) ;
#8770=CARTESIAN_POINT ( 'NONE',  ( 1.499999999999987121, 1.827083334016151861, -0.8660254037844253849 ) ) ;
#8772=CARTESIAN_POINT ( 'NONE',  ( -6.742482464697739708, 6.760651051769146491, 0.7998128361456341429 ) ) ;
#8773=CARTESIAN_POINT ( 'NONE',  ( -4.148431816101615155, 3.942184661647709198, 0.7216878364870317197 ) ) ;
#8781=CARTESIAN_POINT ( 'NONE',  ( 6.484877546038077867, 6.460111979999551224, 1.040834085586084257E-14 ) ) ;
#8782=DIRECTION ( 'NONE',  ( 4.462851221005182648E-16, 0.7999999999999986011, 0.6000000000000019762 ) ) ;
#8786=CARTESIAN_POINT ( 'NONE',  ( 6.681470773436232413, 6.689470745297396270, -0.7998128361456281477 ) ) ;
#8793=CARTESIAN_POINT ( 'NONE',  ( 4.227444969362701421, 3.826440640544909400, 1.214306433183764966E-14 ) ) ;
#8798=CARTESIAN_POINT ( 'NONE',  ( 5.702249273124194495, 6.094009171513759426, 0.7094654760324905496 ) ) ;
#8804=FACE_OUTER_BOUND ( 'NONE', #114369, .T. ) ;
#8808=CARTESIAN_POINT ( 'NONE',  ( -1.519470924986878968, 8.761764328395900137, -2.483655442635856136 ) ) ;
#8810=CARTESIAN_POINT ( 'NONE',  ( 5.992340707560141588, 9.934888558888093968, 0.7216878364870438212 ) ) ;
#8813=CARTESIAN_POINT ( 'NONE',  ( -2.428882075142555497, 5.985446187641602300, 1.040834085586084257E-14 ) ) ;
#8818=CARTESIAN_POINT ( 'NONE',  ( -5.368138756007025947, 8.350246751061767725, 1.199719254218452047 ) ) ;
#8837=CARTESIAN_POINT ( 'NONE',  ( -2.819205876637805641, 5.376491725131008259, -1.199719254218446718 ) ) ;
#8840=CARTESIAN_POINT ( 'NONE',  ( 9.023114925094663619, 10.48572115315399245, 1.199719254218453823 ) ) ;
#8844=CARTESIAN_POINT ( 'NONE',  ( -7.202405917357668663, 9.425892875049191488, 1.599625672291295375 ) ) ;
#8845=CARTESIAN_POINT ( 'NONE',  ( 5.169736645512481132, 4.925780929386339935, 0.7998128361456341429 ) ) ;
#8847=CARTESIAN_POINT ( 'NONE',  ( 3.323720213644492993, 7.029424015893889433, 1.040834085586084257E-14 ) ) ;
#8848=CARTESIAN_POINT ( 'NONE',  ( -2.304522924643024773, 5.632434478818063361, 0.7216878364870317197 ) ) ;
#8851=CARTESIAN_POINT ( 'NONE',  ( -0.6823417656250003738, 2.280208333674753174, -1.181850606188749264 ) ) ;
#8852=VERTEX_POINT ( 'NONE', #183553 ) ;
#8854=CARTESIAN_POINT ( 'NONE',  ( 5.829642864196151741, 9.745074408296771296, 0.7216878364870438212 ) ) ;
#8861=ORIENTED_EDGE ( 'NONE', *, *, #44771, .T. ) ;
#8862=CARTESIAN_POINT ( 'NONE',  ( 7.727784369665023689, 11.95957283134381477, 1.040834085586084257E-14 ) ) ;
#8867=CARTESIAN_POINT ( 'NONE',  ( -7.883176251342026042, 11.28445716228600126, -1.199719254218446718 ) ) ;
#8884=CARTESIAN_POINT ( 'NONE',  ( -0.7500000000000006661, 3.139583334016149418, -1.299038105676652011 ) ) ;
#8888=EDGE_LOOP ( 'NONE', ( #204730, #101929, #36498, #178099 ) ) ;
#8890=CARTESIAN_POINT ( 'NONE',  ( 0.7499999999999885647, 0.7333333333333567072, 1.299038105676657340 ) ) ;
#8891=CARTESIAN_POINT ( 'NONE',  ( 8.749089199520284410, 9.101692242395490240, 0.7998128361456481317 ) ) ;
#8892=CARTESIAN_POINT ( 'NONE',  ( 0.6823417656249864960, -0.5739583329919112353, -1.181850606188749264 ) ) ;
#8895=CARTESIAN_POINT ( 'NONE',  ( 9.734391104931951588, 11.41950637958454706, 1.082531754730548412 ) ) ;
#8896=CARTESIAN_POINT ( 'NONE',  ( -6.155038550924159857, 8.203964280876741455, 1.443375672974078761 ) ) ;
#8901=CARTESIAN_POINT ( 'NONE',  ( -5.392392409933270514, 7.314210449720692786, 1.599625672291269396 ) ) ;
#8904=CARTESIAN_POINT ( 'NONE',  ( -0.7500000000000006661, 3.139583334016149418, -1.299038105676652011 ) ) ;
#8905=CARTESIAN_POINT ( 'NONE',  ( 1.364683531249988535, 3.967708333674751842, -0.7879004041258239610 ) ) ;
#8913=LINE ( 'NONE', #74994, #118908 ) ;
#8918=CARTESIAN_POINT ( 'NONE',  ( -9.826962411806732689, 10.35921099006301382, -0.7998128361456291469 ) ) ;
#8920=CARTESIAN_POINT ( 'NONE',  ( 7.806797523370503811, 8.002351953554066810, 1.040834085586084257E-14 ) ) ;
#8921=CARTESIAN_POINT ( 'NONE',  ( 1.419999999999999485, 7.140846818246212813, 4.154462424328221104 ) ) ;
#8927=CARTESIAN_POINT ( 'NONE',  ( -8.616370316684697883, 10.01118577667568132, -1.199719254218446718 ) ) ;
#8930=ADVANCED_FACE ( 'NONE', ( #200843 ), #104458, .F. ) ;
#8933=CARTESIAN_POINT ( 'NONE',  ( 2.205172540517054802, 5.724451730578533848, 1.040834085586084257E-14 ) ) ;
#8936=ORIENTED_EDGE ( 'NONE', *, *, #6348, .T. ) ;
#8937=CARTESIAN_POINT ( 'NONE',  ( -5.440899717785814715, 5.242137847038546461, 0.7998128361456341429 ) ) ;
#8938=CARTESIAN_POINT ( 'NONE',  ( -8.188234707649510113, 11.64035869464474082, -1.199719254218446718 ) ) ;
#8948=CARTESIAN_POINT ( 'NONE',  ( 5.147291874682557555, 9.156924287104992288, 0.7998128361456462443 ) ) ;
#8949=EDGE_CURVE ( 'NONE', #43706, #168291, #35160, .T. ) ;
#8972=CARTESIAN_POINT ( 'NONE',  ( 4.690757960648234359, 4.574898496952131133, 0.7216878364870317197 ) ) ;
#8976=CARTESIAN_POINT ( 'NONE',  ( -9.982881178363895103, 10.54111621771303753, 1.040834085586084257E-14 ) ) ;
#8979=CARTESIAN_POINT ( 'NONE',  ( 9.368847842243145152, 10.88907622316056312, 1.199719254218453823 ) ) ;
#8983=CARTESIAN_POINT ( 'NONE',  ( 5.096922329222960180, 6.645262723539179461, 1.370935683266294003 ) ) ;
#8987=CARTESIAN_POINT ( 'NONE',  ( 4.363950690066983107, 4.004001632660354915, -0.1812806842866887536 ) ) ;
#8988=CARTESIAN_POINT ( 'NONE',  ( -1.364683531250014514, 0.2802083336747505649, 0.7879004041258379498 ) ) ;
#8994=CARTESIAN_POINT ( 'NONE',  ( -5.278201874421821316, 5.052323696447222900, 0.7998128361456341429 ) ) ;
#8997=CARTESIAN_POINT ( 'NONE',  ( -1.402160292154681736E-14, 0.2125000000000202283, 1.732050807568877637 ) ) ;
#8999=CARTESIAN_POINT ( 'NONE',  ( 0.7499999999999920064, 5.733333333333353821, 1.299038105676669330 ) ) ;
#9004=CARTESIAN_POINT ( 'NONE',  ( 1.364683531249986537, 0.6135416670080880985, 0.7879004041258500513 ) ) ;
#9006=CARTESIAN_POINT ( 'NONE',  ( -7.335124800193271177, 8.516399340768996851, -1.199719254218452935 ) ) ;
#9007=CARTESIAN_POINT ( 'NONE',  ( 7.404724451357931336, 11.79059562655963056, 0.7998128361456462443 ) ) ;
#9012=CARTESIAN_POINT ( 'NONE',  ( 1.364683531249986537, -0.5739583329919174526, 0.7879004041258500513 ) ) ;
#9023=CARTESIAN_POINT ( 'NONE',  ( 7.646435448427411963, 8.023188899361205273, -0.7216878364870257245 ) ) ;
#9026=CARTESIAN_POINT ( 'NONE',  ( -5.362413449404877852, 6.214902764849178141, -1.199719254218446718 ) ) ;
#9031=CARTESIAN_POINT ( 'NONE',  ( -2.103486388414573138, 5.605817886458954291, 1.040834085586084257E-14 ) ) ;
#9032=CARTESIAN_POINT ( 'NONE',  ( 4.473827502385202770, 8.163289819517311585, 1.040834085586084257E-14 ) ) ;
#9033=CARTESIAN_POINT ( 'NONE',  ( -7.497295758232712437, 11.69066945133944380, -0.7216878364870267237 ) ) ;
#9035=CARTESIAN_POINT ( 'NONE',  ( 0.7499999999999902300, 3.816666666666690411, -1.299038105676658228 ) ) ;
#9039=CARTESIAN_POINT ( 'NONE',  ( 9.259855728453651125, 9.905512559391842942, 1.040834085586084257E-14 ) ) ;
#9053=CARTESIAN_POINT ( 'NONE',  ( 7.849807752188022292, 11.14156422998596696, -1.082531754730543083 ) ) ;
#9056=CARTESIAN_POINT ( 'NONE',  ( 8.697719238366680372, 10.10609285197134533, 1.199719254218462483 ) ) ;
#9060=CARTESIAN_POINT ( 'NONE',  ( 4.609409038966229666, 6.400729850259146758, -1.443375672974051449 ) ) ;
#9061=ORIENTED_EDGE ( 'NONE', *, *, #16612, .F. ) ;
#9063=CARTESIAN_POINT ( 'NONE',  ( -7.375272376154081932, 10.58793962461302485, -1.082531754730543971 ) ) ;
#9067=CARTESIAN_POINT ( 'NONE',  ( -3.521367211247373508, 5.131347717920458962, -1.599625672291256295 ) ) ;
#9091=CARTESIAN_POINT ( 'NONE',  ( -7.549192604710863286, 7.701812881784464437, -0.7998128361456291469 ) ) ;
#9092=CIRCLE ( 'NONE', #5650, 0.1599999999999999756 ) ;
#9094=CARTESIAN_POINT ( 'NONE',  ( 1.257518954444996062, 2.841479010054028365, -0.7749999999999926947 ) ) ;
#9096=CARTESIAN_POINT ( 'NONE',  ( 5.799137018343234473, 7.788745826199009237, -1.599625672291262513 ) ) ;
#9104=CARTESIAN_POINT ( 'NONE',  ( -5.590039407536138150, 5.416134151747256986, 0.000000000000000000 ) ) ;
#9107=CARTESIAN_POINT ( 'NONE',  ( 6.938021921891177612, 9.117444880338284818, -1.599625672291262513 ) ) ;
#9108=CARTESIAN_POINT ( 'NONE',  ( 6.520158902582592120, 5.290451655907108197, -2.438235897557449849 ) ) ;
#9110=CARTESIAN_POINT ( 'NONE',  ( 5.577782935947014131, 6.368007920784547693, 1.193350709755973682 ) ) ;
#9117=CARTESIAN_POINT ( 'NONE',  ( 5.734735788456138295, 8.673980272298743799, -1.082531754730537976 ) ) ;
#9118=CARTESIAN_POINT ( 'NONE',  ( -7.212047647465563038, 10.50147379109678880, -1.199719254218446718 ) ) ;
#9121=CARTESIAN_POINT ( 'NONE',  ( -7.320512876374914768, 10.62801655815766999, 1.199719254218453823 ) ) ;
#9122=CARTESIAN_POINT ( 'NONE',  ( -6.358937740009323214, 7.377514437221045718, -1.199719254218446718 ) ) ;
#9130=CARTESIAN_POINT ( 'NONE',  ( 7.995557903757111617, 10.35123685918189729, 1.599625672291281386 ) ) ;
#9145=CARTESIAN_POINT ( 'NONE',  ( -1.499999999999997780, 4.400000000000021672, 1.214306433183764966E-14 ) ) ;
#9146=CARTESIAN_POINT ( 'NONE',  ( 5.996784015946103885, 5.890669528225568996, 1.040834085586084257E-14 ) ) ;
#9147=CARTESIAN_POINT ( 'NONE',  ( 5.296431564432884542, 9.330920591813708143, 1.040834085586084257E-14 ) ) ;
#9149=CARTESIAN_POINT ( 'NONE',  ( 6.073689629242148058, 8.109057205581079231, -1.443375672974057666 ) ) ;
#9150=CARTESIAN_POINT ( 'NONE',  ( -8.473482818416670170, 10.90881592628469932, -1.443375672974058777 ) ) ;
#9153=CARTESIAN_POINT ( 'NONE',  ( 8.890396042259068210, 11.39521468743417998, -1.599625672291257406 ) ) ;
#9158=CARTESIAN_POINT ( 'NONE',  ( -1.201851678989727383E-14, 0.8218750003414171390, 1.575800808251672791 ) ) ;
#9163=CARTESIAN_POINT ( 'NONE',  ( -0.6823417656250246877, -0.6989583329919113464, 1.181850606188755259 ) ) ;
#9165=CARTESIAN_POINT ( 'NONE',  ( 10.55910270694468345, 11.21337466772398095, 0.7998128361456462443 ) ) ;
#9169=CARTESIAN_POINT ( 'NONE',  ( -8.371269781434001800, 11.85389961405997816, -1.199719254218446718 ) ) ;
#9175=CARTESIAN_POINT ( 'NONE',  ( 4.891794496432329886, 4.601515088792824670, -0.7998128361456211532 ) ) ;
#9179=AXIS2_PLACEMENT_3D ( 'NONE', #210281, #64048, #29426 ) ;
#9180=B_SPLINE_CURVE_WITH_KNOTS ( 'NONE', 3,
 ( #116797, #165484, #67950, #813, #1890, #66881, #86378, #133025, #33348, #17081 ),
 .UNSPECIFIED., .F., .F.,
 ( 4, 2, 2, 2, 4 ),
 ( 0.000000000000000000, 0.0005402298572614764672, 0.001080459714522952934, 0.001620689571784429510, 0.002160919429045905869 ),
 .UNSPECIFIED. ) ;
#9181=CARTESIAN_POINT ( 'NONE',  ( -4.134873662043608178, 4.886736029548026217, 1.082531754730558626 ) ) ;
#9184=CARTESIAN_POINT ( 'NONE',  ( 9.935427640716063991, 10.48575375712389679, -0.7998128361456281477 ) ) ;
#9186=CARTESIAN_POINT ( 'NONE',  ( 4.285325189395043033, 7.238007417033815116, 0.9681492361576886641 ) ) ;
#9188=CARTESIAN_POINT ( 'NONE',  ( -5.413783410558481002, 5.210502155273325720, -0.7998128361456221525 ) ) ;
#9192=CARTESIAN_POINT ( 'NONE',  ( 6.428537391173986038, 10.65171072301167854, 0.7998128361456462443 ) ) ;
#9194=CARTESIAN_POINT ( 'NONE',  ( 7.775764792637399836, 9.030479331953833011, -1.199719254218441611 ) ) ;
#9197=CARTESIAN_POINT ( 'NONE',  ( -8.188761592974040937, 11.53701037756964887, -1.082531754730543971 ) ) ;
#9199=FACE_OUTER_BOUND ( 'NONE', #151864, .T. ) ;
#9204=CARTESIAN_POINT ( 'NONE',  ( -5.077710034904439951, 6.555083676148210081, -1.223860624452234980 ) ) ;
#9205=CARTESIAN_POINT ( 'NONE',  ( -1.402160292154681736E-14, 1.446875000341420137, -1.575800808251659024 ) ) ;
#9207=CARTESIAN_POINT ( 'NONE',  ( 6.100805936469477331, 9.101062111647635788, -1.082531754730537088 ) ) ;
#9221=CARTESIAN_POINT ( 'NONE',  ( -10.15469386651127515, 11.90985960142705657, 1.082531754730558626 ) ) ;
#9226=CARTESIAN_POINT ( 'NONE',  ( 8.772289083241844310, 10.19309100432570148, -1.199719254218446718 ) ) ;
#9228=ORIENTED_EDGE ( 'NONE', *, *, #160649, .T. ) ;
#9230=CARTESIAN_POINT ( 'NONE',  ( -4.647747731386360215, 4.316793862905830892, 0.7998128361456341429 ) ) ;
#9231=CARTESIAN_POINT ( 'NONE',  ( -5.845536785786364931, 9.971543350059432598, 0.000000000000000000 ) ) ;
#9234=CARTESIAN_POINT ( 'NONE',  ( -9.001723924469462901, 12.58942944760136484, -1.199719254218446718 ) ) ;
#9237=CARTESIAN_POINT ( 'NONE',  ( -0.7500000000000215383, 4.222916667349481123, 1.299038105676671107 ) ) ;
#9238=CARTESIAN_POINT ( 'NONE',  ( 8.101160479365381306, 9.410107633136481908, -1.199719254218446718 ) ) ;
#9241=CARTESIAN_POINT ( 'NONE',  ( -7.690499447449645309, 9.995335326823163058, 1.599625672291295375 ) ) ;
#9243=CARTESIAN_POINT ( 'NONE',  ( -0.6823417656249969321, 4.467708333674755394, -1.181850606188749264 ) ) ;
#9245=CARTESIAN_POINT ( 'NONE',  ( -1.495221130952461897, 8.717880658893493617, 2.557745341056316679 ) ) ;
#9250=CARTESIAN_POINT ( 'NONE',  ( -7.049876689426097798, 11.16868053773170821, -0.7216878364870267237 ) ) ;
#9254=CARTESIAN_POINT ( 'NONE',  ( -1.364683531250012516, 2.842708333674754506, 0.7879004041258379498 ) ) ;
#9261=CARTESIAN_POINT ( 'NONE',  ( 1.364683531249990311, 4.384375000341417028, 1.214306433183764966E-14 ) ) ;
#9262=CARTESIAN_POINT ( 'NONE',  ( -4.355193658487827690, 6.104145239700998538, -1.599625672291256295 ) ) ;
#9263=CARTESIAN_POINT ( 'NONE',  ( 6.799577732453452761, 7.891594428405881878, -1.199719254218446718 ) ) ;
#9266=CARTESIAN_POINT ( 'NONE',  ( -0.6823417656250212460, 4.363541667008085767, 1.181850606188767472 ) ) ;
#9271=CARTESIAN_POINT ( 'NONE',  ( -1.402160292154681736E-14, -0.4281249996585808071, 1.575800808251672791 ) ) ;
#9273=CARTESIAN_POINT ( 'NONE',  ( -4.067082894419624672, 6.728385229256075739, 1.082531754730560403 ) ) ;
#9274=CARTESIAN_POINT ( 'NONE',  ( 3.825371897350130723, 7.614684313550482031, 0.7998128361456321445 ) ) ;
#9279=CARTESIAN_POINT ( 'NONE',  ( 3.470524135418292300, 5.072030796119872953, -1.443375672974057666 ) ) ;
#9282=CARTESIAN_POINT ( 'NONE',  ( -8.337901282724359930, 12.67137589657970409, 1.040834085586084257E-14 ) ) ;
#9287=CARTESIAN_POINT ( 'NONE',  ( -10.63367255181986160, 11.30037282007833532, 1.040834085586084257E-14 ) ) ;
#9288=CARTESIAN_POINT ( 'NONE',  ( -6.087247782411500552, 7.164505836643929371, 1.082531754730549967 ) ) ;
#9290=CARTESIAN_POINT ( 'NONE',  ( 1.364683531249988535, 1.426041667008083991, 0.7879004041258500513 ) ) ;
#9300=ORIENTED_EDGE ( 'NONE', *, *, #159807, .T. ) ;
#9302=CARTESIAN_POINT ( 'NONE',  ( 7.551528372687370094, 11.75394083486988528, -0.7216878364870267237 ) ) ;
#9306=ORIENTED_EDGE ( 'NONE', *, *, #154040, .F. ) ;
#9310=CARTESIAN_POINT ( 'NONE',  ( 2.869522067586683711, 6.499526178826442013, 0.7998128361456362523 ) ) ;
#9312=CARTESIAN_POINT ( 'NONE',  ( -2.578021764892882040, 6.159442492350315490, 0.7998128361456341429 ) ) ;
#9314=CARTESIAN_POINT ( 'NONE',  ( 1.150196859685076012, 3.185958678954800227, 0.7750000000000135669 ) ) ;
#9316=CARTESIAN_POINT ( 'NONE',  ( -1.364683531250012516, 1.092708333674754506, 0.7879004041258379498 ) ) ;
#9326=( BOUNDED_CURVE ( )  B_SPLINE_CURVE ( 2, ( #61882, #147407, #146360, #179903, #211315, #78123, #80261 ),
 .UNSPECIFIED., .F., .T. ) 
 B_SPLINE_CURVE_WITH_KNOTS ( ( 3, 2, 2, 3 ),
 ( 0.2125000000000000222, 0.2166666666666667573, 0.2208333333333334647, 0.2250000000000001998 ),
 .UNSPECIFIED. ) 
 CURVE ( )  GEOMETRIC_REPRESENTATION_ITEM ( )  RATIONAL_B_SPLINE_CURVE ( ( 0.9999999999999991118, 0.8660254037844395958, 1.000000000000000000, 0.8660254037844387076, 1.000000000000000000, 0.8660254037844324904, 1.000000000000006217 ) ) 
 REPRESENTATION_ITEM ( '' )  );
#9337=CARTESIAN_POINT ( 'NONE',  ( 6.993308306550549247, 7.053281200597435685, 1.040834085586084257E-14 ) ) ;
#9340=ORIENTED_EDGE ( 'NONE', *, *, #45325, .T. ) ;
#9344=CARTESIAN_POINT ( 'NONE',  ( 8.118635056484817980, 8.366162408854107113, 0.7998128361456481317 ) ) ;
#9348=CARTESIAN_POINT ( 'NONE',  ( 8.992082194361556091, 11.51384853155376220, 1.599625672291279388 ) ) ;
#9359=CARTESIAN_POINT ( 'NONE',  ( -7.348156068926747331, 11.51667314714914347, 0.7216878364870458196 ) ) ;
#9372=CARTESIAN_POINT ( 'NONE',  ( 2.521453382017309952, 5.885520012421409319, 0.000000000000000000 ) ) ;
#9380=CARTESIAN_POINT ( 'NONE',  ( -4.855791571988752331, 8.816840600628864877, 0.7998128361456481317 ) ) ;
#9382=CARTESIAN_POINT ( 'NONE',  ( -3.327636637150278798, 5.969660945728899826, -1.199719254218452935 ) ) ;
#9389=CARTESIAN_POINT ( 'NONE',  ( 1.364683531249990311, 3.696875000341416584, 1.214306433183764966E-14 ) ) ;
#9391=CARTESIAN_POINT ( 'NONE',  ( 6.159481859310094620, 6.080483678816896109, 1.040834085586084257E-14 ) ) ;
#9406=CARTESIAN_POINT ( 'NONE',  ( 1.364683531249986537, 0.7177083336747527298, -0.7879004041258239610 ) ) ;
#9408=CARTESIAN_POINT ( 'NONE',  ( 4.192495815123822744, 5.914331089109666983, -1.599625672291255185 ) ) ;
#9409=CIRCLE ( 'NONE', #158169, 0.07999999999999993228 ) ;
#9411=CARTESIAN_POINT ( 'NONE',  ( -5.260200412422200600, 8.120355666925794580, -1.082531754730544860 ) ) ;
#9412=CARTESIAN_POINT ( 'NONE',  ( 4.717874267875568961, 4.606534188717351874, -0.7216878364870188411 ) ) ;
#9413=CARTESIAN_POINT ( 'NONE',  ( -5.517805330637490790, 9.381263952478319013, 0.7216878364870458196 ) ) ;
#9415=ORIENTED_EDGE ( 'NONE', *, *, #36946, .F. ) ;
#9417=CARTESIAN_POINT ( 'NONE',  ( 6.368579470117202490, 8.453095353268645695, 1.599625672291281386 ) ) ;
#9427=CARTESIAN_POINT ( 'NONE',  ( 5.147291874682557555, 9.156924287104992288, 0.7998128361456462443 ) ) ;
#9430=CARTESIAN_POINT ( 'NONE',  ( -5.364222332501225488, 9.410009821226765325, 0.7998128361456481317 ) ) ;
#9434=CARTESIAN_POINT ( 'NONE',  ( 8.320953590485093088, 10.73086516036454618, 1.599625672291281386 ) ) ;
#9436=CARTESIAN_POINT ( 'NONE',  ( -7.365103760721662951, 9.615707025640515937, 1.599625672291295375 ) ) ;
#9437=CYLINDRICAL_SURFACE ( 'NONE', #140955, 1.500000000000000222 ) ;
#9438=CARTESIAN_POINT ( 'NONE',  ( 8.066738210006686671, 9.473911335505048825, 1.082531754730558626 ) ) ;
#9439=CARTESIAN_POINT ( 'NONE',  ( 4.000033042702237474, 7.827758669039140749, -0.08873751906842038129 ) ) ;
#9440=CARTESIAN_POINT ( 'NONE',  ( -4.843287188579803448, 6.673587691474970107, -1.599625672291256295 ) ) ;
#9444=CARTESIAN_POINT ( 'NONE',  ( 4.123651276850781144, 7.962676922967908411, -0.7998128361456221525 ) ) ;
#9446=CARTESIAN_POINT ( 'NONE',  ( 8.540746701604824409, 12.05162268759261224, -1.199719254218446718 ) ) ;
#9447=CARTESIAN_POINT ( 'NONE',  ( -5.028543871580710700, 6.592580098690584478, 1.235119876028653918 ) ) ;
#9448=CARTESIAN_POINT ( 'NONE',  ( -3.913718639709061087, 2.801499522163740430, -0.7749999999999944711 ) ) ;
#9449=CARTESIAN_POINT ( 'NONE',  ( 1.364683531249986537, 0.4052083336747511200, -0.7879004041258309554 ) ) ;
#9451=CARTESIAN_POINT ( 'NONE',  ( -6.588899466561478846, 6.789396920517583922, 0.7216878364870317197 ) ) ;
#9458=CARTESIAN_POINT ( 'NONE',  ( -5.532833371615617502, 6.236068886146576951, 0.9535701153140889730 ) ) ;
#9459=CARTESIAN_POINT ( 'NONE',  ( 1.364683531249986537, 1.176041667008082658, 0.7879004041258500513 ) ) ;
#9462=CARTESIAN_POINT ( 'NONE',  ( 2.711267533052988732, 6.106969855296372707, -0.7216878364870267237 ) ) ;
#9467=CARTESIAN_POINT ( 'NONE',  ( -9.151390499099978371, 9.778969791812544443, 0.7216878364870438212 ) ) ;
#9474=CARTESIAN_POINT ( 'NONE',  ( -8.812436658758329600, 9.383523644747281622, 1.040834085586084257E-14 ) ) ;
#9475=CARTESIAN_POINT ( 'NONE',  ( -1.150222622689996532, 3.108395032273046255, 0.7749999999993751887 ) ) ;
#9478=DIRECTION ( 'NONE',  ( 1.000000000000000000, 0.000000000000000000, 0.000000000000000000 ) ) ;
#9480=VERTEX_POINT ( 'NONE', #213114 ) ;
#9481=CARTESIAN_POINT ( 'NONE',  ( -7.985389288324710400, 8.418635045908049008, -0.7216878364870267237 ) ) ;
#9486=CARTESIAN_POINT ( 'NONE',  ( 1.499999999999990896, 4.806250000682819490, 1.214306433183764966E-14 ) ) ;
#9495=CARTESIAN_POINT ( 'NONE',  ( -6.938021921891187382, 9.117444880338284818, -1.599625672291263179 ) ) ;
#9499=CARTESIAN_POINT ( 'NONE',  ( 4.473300617505036492, 7.306268922809479704, -1.199719254218452047 ) ) ;
#9504=CARTESIAN_POINT ( 'NONE',  ( 8.308449207076147758, 8.587612251210650527, -0.7998128361456281477 ) ) ;
#9511=CARTESIAN_POINT ( 'NONE',  ( -6.588899466561478846, 6.789396920517583922, 0.7216878364870317197 ) ) ;
#9520=CARTESIAN_POINT ( 'NONE',  ( -9.027031348600448979, 9.425958082989001952, 1.040834085586084257E-14 ) ) ;
#9522=CARTESIAN_POINT ( 'NONE',  ( 8.932124273304774320, 9.315233161810734686, 0.7998128361456462443 ) ) ;
#9523=CARTESIAN_POINT ( 'NONE',  ( -1.402160292154681736E-14, -0.2874999999999741096, 1.732050807568877637 ) ) ;
#9524=CARTESIAN_POINT ( 'NONE',  ( -6.991200766141138168, 11.30815132714001159, 0.7998128361456481317 ) ) ;
#9527=CARTESIAN_POINT ( 'NONE',  ( 1.364683531249988535, 4.363541667008090208, 0.7879004041258500513 ) ) ;
#9528=CARTESIAN_POINT ( 'NONE',  ( 8.866669273657322492, 12.32790267170016207, -1.082531754730543083 ) ) ;
#9531=CARTESIAN_POINT ( 'NONE',  ( -1.500000000000011324, 5.629166666666693963, -0.8660254037844313801 ) ) ;
#9533=CARTESIAN_POINT ( 'NONE',  ( 8.229436053370669413, 10.62409470039771442, 1.443375672974076540 ) ) ;
#9536=CARTESIAN_POINT ( 'NONE',  ( -6.317736394288148816, 8.393778431468064127, 1.443375672974078761 ) ) ;
#9538=CARTESIAN_POINT ( 'NONE',  ( 1.364683531249988535, 1.363541667008083769, 0.7879004041258500513 ) ) ;
#9540=FACE_OUTER_BOUND ( 'NONE', #165967, .T. ) ;
#9543=CARTESIAN_POINT ( 'NONE',  ( -5.669280788808708671, 9.765911353585494226, 0.7998128361456481317 ) ) ;
#9544=CARTESIAN_POINT ( 'NONE',  ( 1.364683531249990311, 5.196875000341417916, 1.214306433183764966E-14 ) ) ;
#9550=CARTESIAN_POINT ( 'NONE',  ( 8.235688245297327015, 11.69572115523387268, -1.199719254218446718 ) ) ;
#9553=CARTESIAN_POINT ( 'NONE',  ( 0.7499999999999902300, 1.733333333333357595, 1.299038105676657340 ) ) ;
#9556=CARTESIAN_POINT ( 'NONE',  ( -0.3124725659140401568, 7.215207000027771045, -2.082817582596259154 ) ) ;
#9558=CARTESIAN_POINT ( 'NONE',  ( 5.992340707560141588, 9.934888558888093968, 0.7216878364870438212 ) ) ;
#9565=CARTESIAN_POINT ( 'NONE',  ( 7.404724451357931336, 11.79059562655963056, 0.7998128361456462443 ) ) ;
#9566=CARTESIAN_POINT ( 'NONE',  ( -10.47775378526269918, 11.11846759242831872, -0.7998128361456221525 ) ) ;
#9569=CARTESIAN_POINT ( 'NONE',  ( 0.6823417656249882723, -1.157291666325249713, 1.181850606188755259 ) ) ;
#9575=CARTESIAN_POINT ( 'NONE',  ( -0.6823417656250212460, 4.051041667008085767, 1.181850606188767472 ) ) ;
#9577=CARTESIAN_POINT ( 'NONE',  ( -5.097502569058210753, 7.930541516334467467, -1.082531754730549967 ) ) ;
#9587=CARTESIAN_POINT ( 'NONE',  ( 7.727257484784855635, 11.10255193463598111, -1.199719254218446718 ) ) ;
#9588=CARTESIAN_POINT ( 'NONE',  ( 6.471393748265519719, 5.229711127717882491, -2.499999999999995115 ) ) ;
#9589=CARTESIAN_POINT ( 'NONE',  ( 5.299301323368958094, 6.361497809228795930, -1.122821758042211959 ) ) ;
#9593=CARTESIAN_POINT ( 'NONE',  ( -8.158255747121117452, 10.54105100977322174, 1.599625672291295375 ) ) ;
#9594=CARTESIAN_POINT ( 'NONE',  ( 7.156006149914539982, 7.243095351188763686, 1.040834085586084257E-14 ) ) ;
#9597=CARTESIAN_POINT ( 'NONE',  ( 3.714044015139744914, 6.420469553383295391, 1.199719254218462483 ) ) ;
#9601=CARTESIAN_POINT ( 'NONE',  ( -4.143499164831425219, 7.564990639293021957, -0.8130116771524699137 ) ) ;
#9605=CARTESIAN_POINT ( 'NONE',  ( -5.151735183512911043, 6.073074471262228435, 1.082531754730548412 ) ) ;
#9606=CARTESIAN_POINT ( 'NONE',  ( 4.521807925357579805, 5.234196320127330715, -1.199719254218452047 ) ) ;
#9609=CARTESIAN_POINT ( 'NONE',  ( -8.206763054973658100, 8.468978407091068306, 0.7998128361456602331 ) ) ;
#9614=CARTESIAN_POINT ( 'NONE',  ( -7.808606406466886973, 11.19745900993164511, 1.199719254218453823 ) ) ;
#9617=CARTESIAN_POINT ( 'NONE',  ( 8.229962938695207342, 9.560377169021284871, 1.199719254218462483 ) ) ;
#9618=CARTESIAN_POINT ( 'NONE',  ( 5.769158057814842699, 6.689438141327490150, 1.199719254218462483 ) ) ;
#9629=CARTESIAN_POINT ( 'NONE',  ( -8.681298431451969222, 9.022603012982438386, 1.040834085586084257E-14 ) ) ;
#9632=CARTESIAN_POINT ( 'NONE',  ( 5.450014563013511726, 8.341805509282339770, -1.082531754730543083 ) ) ;
#9634=CARTESIAN_POINT ( 'NONE',  ( -1.440240048133426987, 7.355731858844955617, 4.317885097512588644 ) ) ;
#9637=CARTESIAN_POINT ( 'NONE',  ( -5.168682875307782254, 7.053215992657626110, -1.599625672291256295 ) ) ;
#9647=CARTESIAN_POINT ( 'NONE',  ( -8.455481356417053007, 13.01647868246193518, 0.7998128361456341429 ) ) ;
#9648=CARTESIAN_POINT ( 'NONE',  ( 7.130698725783555680, 10.40656671580112658, 1.199719254218460707 ) ) ;
#9650=CARTESIAN_POINT ( 'NONE',  ( -4.311129659465605002, 4.131998812239033647, 0.7216878364870317197 ) ) ;
#9652=CARTESIAN_POINT ( 'NONE',  ( -5.312752313518235958, 6.384578190230367767, -1.125208257168613502 ) ) ;
#9661=CARTESIAN_POINT ( 'NONE',  ( 10.54788032175191326, 11.40820791823982994, 0.7216878364870317197 ) ) ;
#9680=CARTESIAN_POINT ( 'NONE',  ( -3.653032323878261600, 6.349289246911547835, -1.199719254218452047 ) ) ;
#9681=CARTESIAN_POINT ( 'NONE',  ( 4.812781342726855982, 7.598366752281232372, 1.082531754730558626 ) ) ;
#9682=CARTESIAN_POINT ( 'NONE',  ( -1.201851678989727383E-14, 4.087500000000022560, -1.732050807568863648 ) ) ;
#9684=CARTESIAN_POINT ( 'NONE',  ( -2.625475302540713152, 6.214804952939456228, -0.7998128361456281477 ) ) ;
#9689=CARTESIAN_POINT ( 'NONE',  ( 1.364683531249988535, 5.155208333674749177, -0.7879004041258300672 ) ) ;
#9692=CARTESIAN_POINT ( 'NONE',  ( -3.470524135418306511, 5.072030796119872953, -1.443375672974053447 ) ) ;
#9697=CARTESIAN_POINT ( 'NONE',  ( 5.678167406024951624, 5.518950149984223508, 0.7998128361456341429 ) ) ;
#9699=CYLINDRICAL_SURFACE ( 'NONE', #69895, 0.08000000000000041800 ) ;
#9701=CARTESIAN_POINT ( 'NONE',  ( 10.37162432432990755, 11.20257592124748136, -0.7216878364870257245 ) ) ;
#9704=CARTESIAN_POINT ( 'NONE',  ( -1.364683531250000748, 1.071875000341421247, 0.000000000000000000 ) ) ;
#9708=CARTESIAN_POINT ( 'NONE',  ( -8.296699936558862731, 11.76690146170562201, 1.199719254218453823 ) ) ;
#9709=CARTESIAN_POINT ( 'NONE',  ( -4.378920427089552092, 8.052564898339037214, 0.7216878364870317197 ) ) ;
#9713=CARTESIAN_POINT ( 'NONE',  ( -1.402160292154681736E-14, -0.8812499993171809543, -1.732050807568870754 ) ) ;
#9721=CARTESIAN_POINT ( 'NONE',  ( -5.870317324592829067, 5.951051088220814300, -0.7216878364870197293 ) ) ;
#9726=CARTESIAN_POINT ( 'NONE',  ( -3.890826896997578999, 7.483122446565064756, 0.7216878364870317197 ) ) ;
#9728=CARTESIAN_POINT ( 'NONE',  ( 9.480175724453529185, 12.08329098332774265, 1.599625672291279388 ) ) ;
#9737=CARTESIAN_POINT ( 'NONE',  ( -4.925689880466507908, 4.641059703499347044, -0.7998128361456221525 ) ) ;
#9738=CARTESIAN_POINT ( 'NONE',  ( -6.025283891683315574, 6.066383424671776936, 0.6274445299816646671 ) ) ;
#9744=CARTESIAN_POINT ( 'NONE',  ( 7.782016984564043227, 12.02284421539267356, 0.7216878364870438212 ) ) ;
#9745=CARTESIAN_POINT ( 'NONE',  ( 5.795220594837462436, 8.848508896363995291, -1.199719254218440723 ) ) ;
#9749=CARTESIAN_POINT ( 'NONE',  ( 4.192495815123822744, 5.914331089109666983, -1.599625672291255185 ) ) ;
#9750=CARTESIAN_POINT ( 'NONE',  ( -0.3138284133838390444, 8.211984188054007205, -1.978018658440992006 ) ) ;
#9751=ORIENTED_EDGE ( 'NONE', *, *, #107896, .F. ) ;
#9760=CARTESIAN_POINT ( 'NONE',  ( -6.847031270101295419, 7.946956888995021728, -1.199719254218446718 ) ) ;
#9766=CARTESIAN_POINT ( 'NONE',  ( 1.364683531249988535, 4.905208333674756283, -0.7879004041258300672 ) ) ;
#9767=CARTESIAN_POINT ( 'NONE',  ( 9.205623113554628034, 9.842241175342985926, 0.7216878364870458196 ) ) ;
#9769=CARTESIAN_POINT ( 'NONE',  ( -7.061099074618889304, 7.132370430010492868, -0.7998128361456291469 ) ) ;
#9772=CARTESIAN_POINT ( 'NONE',  ( 4.171104814498611368, 8.018039383557042044, 0.7998128361456321445 ) ) ;
#9773=CARTESIAN_POINT ( 'NONE',  ( -4.737684612971557740, 7.614716917520386374, 1.199719254218464037 ) ) ;
#9780=CARTESIAN_POINT ( 'NONE',  ( 5.002595493762530765, 8.780185809457538681, 1.040834085586084257E-14 ) ) ;
#9782=CARTESIAN_POINT ( 'NONE',  ( 0.6823417656249882723, 1.488541667008083547, -1.181850606188749264 ) ) ;
#9784=CARTESIAN_POINT ( 'NONE',  ( 5.409340101728155936, 8.294351971116089572, -1.082531754730543971 ) ) ;
#9786=CARTESIAN_POINT ( 'NONE',  ( -2.331639231870358930, 5.664070170583284103, -0.7216878364870267237 ) ) ;
#9792=CARTESIAN_POINT ( 'NONE',  ( -3.975603406396657213, 7.849426279905078019, -0.02588959144292704573 ) ) ;
#9799=CARTESIAN_POINT ( 'NONE',  ( 6.817052309572890323, 6.847649204123507083, 0.7998128361456341429 ) ) ;
#9810=CARTESIAN_POINT ( 'NONE',  ( 4.853455804012228647, 4.764712647543454693, 0.7216878364870317197 ) ) ;
#9811=CARTESIAN_POINT ( 'NONE',  ( -1.364683531250012516, 2.551041667008089320, -0.7879004041258289570 ) ) ;
#9813=CARTESIAN_POINT ( 'NONE',  ( 8.101160479365381306, 9.410107633136481908, -1.199719254218446718 ) ) ;
#9814=CARTESIAN_POINT ( 'NONE',  ( -10.65400978224035811, 11.32409958890225710, 1.040834085586084257E-14 ) ) ;
#9816=CARTESIAN_POINT ( 'NONE',  ( 3.008927249609713250, 6.454239524612553680, -0.03298405530798137475 ) ) ;
#9821=CARTESIAN_POINT ( 'NONE',  ( -1.499999999999997780, 3.150000000000020783, 1.214306433183764966E-14 ) ) ;
#9822=CARTESIAN_POINT ( 'NONE',  ( 6.986529229743720926, 7.045372277656132276, -0.7998128361456281477 ) ) ;
#9823=CARTESIAN_POINT ( 'NONE',  ( -7.874588291438845644, 8.081441182967111558, -0.7998128361456291469 ) ) ;
#9827=CARTESIAN_POINT ( 'NONE',  ( 0.6823417656249882723, 2.426041667008084435, -1.181850606188749264 ) ) ;
#9829=CARTESIAN_POINT ( 'NONE',  ( 3.195971524519376494, 4.751719416737803847, -1.599625672291262513 ) ) ;
#9834=CARTESIAN_POINT ( 'NONE',  ( -3.294268138440636928, 6.787137228248626641, 1.040834085586084257E-14 ) ) ;
#9835=CARTESIAN_POINT ( 'NONE',  ( 1.499999999999989120, 2.056250000682817269, 1.214306433183764966E-14 ) ) ;
#9838=CARTESIAN_POINT ( 'NONE',  ( -6.501298352952815662, 7.543601818988450169, -1.199719254218446718 ) ) ;
#9839=CARTESIAN_POINT ( 'NONE',  ( -4.284013352238274841, 4.100363120473813794, -0.7216878364870207285 ) ) ;
#9848=CARTESIAN_POINT ( 'NONE',  ( 6.311484202361478779, 7.322151976631905868, -1.199719254218446718 ) ) ;
#9852=CARTESIAN_POINT ( 'NONE',  ( 5.789495288235341874, 6.713164910151406595, 1.199719254218462483 ) ) ;
#9857=CARTESIAN_POINT ( 'NONE',  ( 4.729096653068339151, 4.411700938201493116, -0.7998128361456211532 ) ) ;
#9861=CARTESIAN_POINT ( 'NONE',  ( 5.726377019126981160, 6.078880280049443918, 0.6665230057388837892 ) ) ;
#9862=CIRCLE ( 'NONE', #82522, 1.250000000000000222 ) ;
#9872=CARTESIAN_POINT ( 'NONE',  ( -4.140316941461365197, 3.976524957527992843, 0.4412079600669023272 ) ) ;
#9873=CARTESIAN_POINT ( 'NONE',  ( 7.293923454472080792, 9.532663335016016148, 1.443375672974076540 ) ) ;
#9875=CARTESIAN_POINT ( 'NONE',  ( -3.730464822054482710, 7.503959392372201442, 1.040834085586084257E-14 ) ) ;
#9876=CARTESIAN_POINT ( 'NONE',  ( -0.4786071537202271076, 6.664221364234077960, 3.365248248540958276 ) ) ;
#9878=CARTESIAN_POINT ( 'NONE',  ( 8.281332899848809603, 8.555976559445431562, 0.7998128361456481317 ) ) ;
#9880=CARTESIAN_POINT ( 'NONE',  ( -5.473741331615264549, 7.409117525016355010, -1.599625672291256295 ) ) ;
#9881=EDGE_CURVE ( 'NONE', #124240, #145532, #176599, .T. ) ;
#9893=CARTESIAN_POINT ( 'NONE',  ( 9.480175724453529185, 12.08329098332774265, 1.599625672291279388 ) ) ;
#9894=CARTESIAN_POINT ( 'NONE',  ( -3.958090780185743451, 6.705190779270287393, -1.199719254218452047 ) ) ;
#9897=CARTESIAN_POINT ( 'NONE',  ( 3.063779527008304360, 6.518233848244248563, 0.7216878364870317197 ) ) ;
#9900=DIRECTION ( 'NONE',  ( -4.462851221005182648E-16, -0.7999999999999986011, 0.6000000000000019762 ) ) ;
#9903=CARTESIAN_POINT ( 'NONE',  ( -2.927671105547157371, 5.503034492191895666, 1.199719254218462483 ) ) ;
#9906=CARTESIAN_POINT ( 'NONE',  ( 7.456094412511537151, 10.78619501698377370, 1.199719254218460707 ) ) ;
#9911=CARTESIAN_POINT ( 'NONE',  ( -8.376239975144482486, 8.666701480623698828, 1.040834085586084257E-14 ) ) ;
#9912=CARTESIAN_POINT ( 'NONE',  ( 5.847644326195776010, 5.716673223516856694, -0.7998128361456281477 ) ) ;
#9915=( BOUNDED_SURFACE ( )  B_SPLINE_SURFACE ( 1, 2, ( 
 ( #122541, #6533, #136575, #154949, #20650, #72612, #138711, #56378, #185290, #35848, #156016, #36913, #135505, #188502, #202596, #151757, #106244, #203663, #105148, #170114, #137644, #169053, #172270, #23856, #89964, #7603, #186361, #54248, #52115, #55314, #118242, #184225, #19598, #167993, #101927, #86740, #70459, #3328, #201528, #171188, #152809, #4388, #120386, #5454, #37996, #104068, #21701, #87813, #153885, #121463, #187433, #22777, #39062, #27062, #75823, #10805, #177602, #110529, #76879, #109467, #24927, #159204, #144074, #210069, #43347, #74763, #61709, #175474, #95304, #91031, #108394, #8681, #205813, #143000, #123605, #9749, #57445, #25994, #208998, #92103, #140865, #191687, #206878, #125726, #124665, #127877, #190622, #157092, #58510, #193827, #189570, #42281, #60634, #59566, #28141, #192752, #174418, #41215, #158157, #141932, #126797, #45476, #207945, #93167, #44409, #161353, #176529, #94236, #160274, #11877, #77953, #111592, #29214, #173346, #12935, #139786, #107322, #211138, #30281, #212199, #147239, #164538, #15062, #16124, #62760, #163480, #145131, #179734, #98473, #31352, #13998, #131041, #146184, #64894, #63836, #83267, #129994, #96368, #195983, #935, #128920, #47615, #82207, #213267, #181831, #132080, #113729, #194901, #97427, #80083, #214298, #67002, #81154, #197030, #48667, #100599, #114784, #180782, #162421, #32407, #148301, #65931, #198089, #112660, #149355, #99539, #49716, #46539, #115845, #33464, #165603, #17192, #133139, #199138, #50783, #116911, #182911, #34527, #166675, #79015, #178669, #121209, #52915, #38806, #187178, #170930, #85416, #68066, #188241, #151499, #101668, #22527, #168798, #117986, #88636, #21452, #137389, #202337, #169863, #135262, #104888, #154694, #6277, #72349, #4138, #86486, #138451, #87560, #204472, #56125, #51864, #200212, #122283, #3069, #102743, #134202, #105992, #203405, #150438, #18265, #183978, #37738, #84349, #35589, #167737, #39881, #2001, #153628, #20405, #55058, #19337, #120130, #152551, #103814, #69139, #201275, #5200, #53989, #119048, #71275, #185032, #36658, #136319, #70206, #186106, #207698, #127619, #57192, #140615, #40957, #23604, #77699, #205553, #139527, #11625, #156838, #42031, #73426, #45227, #142745, #89713, #172012, #123352, #191436, #155763, #7347, #189319, #209817, #107065, #26813, #108143, #208753, #143820, #59319, #174169, #43103, #61452, #60379, #109217, #141685, #173090, #175228, #176285, #27887, #75576, #24671, #93984, #125476, #193583, #90777, #206627, #8425, #74511, #92915, #58257, #25741, #124413, #190371, #158961, #91852, #157909, #9504, #10556, #76630, #126542, #160026, #192504, #44155, #110276, #33212, #28959, #13756, #114539, #31106, #214054, #164288, #96113, #95044, #79830, #112407, #32155, #99296, #113477, #63587, #145940, #132883, #47363, #179484, #128679, #194648, #46290, #64650, #195727, #144883, #115589, #131829, #178418, #161094, #62514, #30028, #97179, #196785, #163233, #49470, #15876, #81961, #14815, #180533, #165343, #197838, #80906, #65682, #211952, #181583, #16938, #83019, #162169, #12683, #66740, #129744, #146997, #149092, #213014, #210889, #674, #98233, #148046, #130790, #48426, #198885, #111342, #177347, #78759, #137125, #36401, #118789, #4936, #119863, #203154, #41505, #54798, #102479, #184775, #71012, #185841, #120947, #173650, #84094, #18004, #107619, #35332, #135003, #166409, #141167, #21193, #182651, #50531, #150181, #69946, #116654, #100345, #67806, #91327, #34273, #37473, #201014, #87296, #25224, #152300, #52661, #136058, #157387, #153365, #202071, #20142, #1749, #53731, #189862, #8979, #168545, #199962, #75053, #86229, #133955, #51610, #19079, #117734, #183723, #103551, #101411, #3873, #167484, #151243, #169611, #2812, #85160, #68884, #59866, #193055, #191978, #211436, #43645, #10042, #126018, #129235, #124955, #109759, #210370, #127092, #95604, #45777, #175768, #190917, #27361, #208234, #128166, #195207, #209288, #159501, #93462, #14290, #143297, #60935, #76116, #142221, #11099, #160567, #77175, #26288, #63067, #13247, #44709, #42581, #158441, #110816, #176821, #78247, #28436, #145436, #111894, #177898 ),
 ( #62010, #30584, #46844, #112958, #94529, #12175, #29511, #108685, #144370, #194127, #161652, #58800, #79320, #80385, #178969, #96666, #162718, #207176, #174714, #92402, #81454, #82503, #64141, #181078, #83571, #212500, #134502, #213552, #1234, #149653, #132373, #148590, #164833, #184262, #130285, #116140, #97724, #68370, #31647, #196273, #114032, #99835, #100888, #98778, #65175, #47920, #117210, #67296, #35888, #200506, #150733, #163782, #165901, #199442, #180026, #182129, #48964, #133435, #15361, #115082, #198375, #52149, #159, #118277, #147531, #131330, #18566, #183207, #33758, #101964, #34813, #17485, #197324, #84642, #16423, #168030, #32696, #2293, #19634, #146481, #66226, #50016, #51085, #166975, #203700, #169089, #138745, #5490, #135542, #56415, #204763, #36954, #201567, #152850, #171221, #188538, #173380, #4425, #89998, #106282, #87849, #137679, #202636, #70495, #71571, #55346, #3367, #54286, #41250, #73723, #103034, #53213, #22816, #172303, #121498, #139819, #122576, #153920, #104104, #69436, #186397, #151793, #88929, #38034, #154984, #20688, #40168, #86779, #23892, #85705, #170154, #156049, #7638, #205849, #187470, #120423, #136611, #21740, #57482, #185331, #6569, #119344, #123641, #39100, #72649, #189604, #105185, #107358, #43379, #62795, #157126, #209031, #190655, #161390, #124697, #91066, #206912, #192786, #193862, #191723, #158193, #8715, #210103, #94269, #128957, #12973, #29248, #42316, #44444, #77986, #74800, #60666, #141964, #160309, #140901, #207976, #10836, #145165, #27097, #211170, #174452, #26028, #111627, #61743, #126829, #79049, #127910, #110562, #92138, #177640, #109500, #194936, #108432, #95340, #46573, #112692, #9784, #58542, #144109, #45511, #143036, #75856, #24964, #159235, #59603, #125761, #175507, #93204, #76910, #176564, #28173, #11913, #51894, #97459, #182943, #199171, #180813, #16155, #81189, #163514, #164570, #82240, #96402, #147267, #134236, #166706, #130025, #80114, #49751, #50817, #98508, #18297, #969, #32440, #197063, #162452, #64926, #30317, #115878, #131075, #33499, #196016, #67034, #113763, #133171, #178703, #48701, #116943, #149386, #34559, #148331, #213299, #179767, #31383, #100629, #63870, #114815, #14028, #15101, #132112, #84383, #150470, #214331, #2031, #65963, #198120, #146219, #181863, #99572, #165636, #47652, #17224, #83301, #68100, #200244, #212237, #122318, #138484, #52944, #35620, #69170, #36687, #186135, #203437, #54021, #56155, #22563, #170963, #202372, #187210, #39915, #204506, #120160, #6311, #152581, #188275, #72385, #106024, #185062, #167769, #73460, #102773, #201304, #172046, #37770, #3099, #23639, #121240, #88669, #87590, #55091, #20433, #89747, #155796, #7380, #139561, #103844, #169892, #205588, #38839, #118017, #184006, #151531, #85446, #101699, #168829, #21481, #19366, #135290, #154728, #119082, #86516, #4167, #137418, #70237, #136352, #153662, #5230, #71305, #104922, #141718, #27921, #177378, #158992, #207727, #142777, #95078, #94016, #208783, #26843, #156871, #76663, #61485, #127650, #175258, #206657, #193614, #92947, #12714, #8457, #25773, #140644, #123385, #60413, #40990, #59350, #189350, #157941, #126574, #9533, #58290, #109250, #124446, #43136, #42061, #45255, #108175, #74545, #190405, #111374, #107101, #174201, #192534, #191469, #160055, #110308, #91886, #173124, #75607, #125506, #44188, #28992, #10588, #176316, #11659, #78788, #77732, #24705, #57225, #90807, #143854, #144911, #209846, #161127, #34304, #62544, #65712, #80934, #181615, #116685, #98261, #147024, #81991, #100378, #33244, #148079, #180563, #96147, #15908, #708, #66772, #114571, #145968, #132913, #32185, #166449, #162198, #179515, #79859, #128707, #214084, #194676, #213048, #46320, #97210, #131860, #163262, #211980, #48458, #63619, #196815, #195756, #198918, #47394, #13785, #129774, #50564, #112436, #113507, #197867, #130823, #99326, #49499, #31135, #178449, #14844, #64676, #115619, #182684, #164318, #165377, #16970, #18040, #83051, #149126, #84127, #210918, #30057, #103588, #20176, #183759, #154476, #170710, #85192, #67842, #101443, #68917, #3911, #21230, #86263, #88408 ) ),
 .UNSPECIFIED., .F., .F., .T. ) 
 B_SPLINE_SURFACE_WITH_KNOTS ( ( 2, 2 ),
 ( 3, 2, 2, 2, 2, 2, 2, 2, 2, 2, 2, 2, 2, 2, 2, 2, 2, 2, 2, 2, 2, 2, 2, 2, 2, 2, 2, 2, 2, 2, 2, 2, 2, 2, 2, 2, 2, 2, 2, 2, 2, 2, 2, 2, 2, 2, 2, 2, 2, 2, 2, 2, 2, 2, 2, 2, 2, 2, 2, 2, 2, 2, 2, 2, 2, 2, 2, 2, 2, 2, 2, 2, 2, 2, 2, 2, 2, 2, 2, 2, 2, 2, 2, 2, 2, 2, 2, 2, 2, 2, 2, 2, 2, 2, 2, 2, 2, 2, 2, 2, 2, 2, 2, 2, 2, 2, 2, 2, 2, 2, 2, 2, 2, 2, 2, 2, 2, 2, 2, 2, 2, 2, 2, 2, 2, 2, 2, 2, 2, 2, 2, 2, 2, 2, 2, 2, 2, 2, 2, 2, 2, 2, 2, 2, 2, 2, 2, 2, 2, 2, 2, 2, 2, 2, 2, 2, 2, 2, 2, 2, 2, 2, 2, 2, 2, 2, 2, 2, 2, 2, 2, 2, 2, 2, 2, 2, 2, 2, 2, 2, 2, 2, 2, 2, 2, 2, 2, 2, 2, 2, 2, 2, 2, 2, 2, 2, 2, 2, 2, 2, 2, 2, 2, 2, 2, 2, 2, 2, 2, 2, 2, 2, 2, 2, 2, 2, 2, 2, 2, 2, 2, 2, 2, 2, 2, 2, 2, 2, 2, 2, 2, 2, 2, 2, 2, 2, 2, 2, 2, 2, 3 ),
 ( 0.000000000000000000, 1.000000000000000000 ),
 ( 0.000000000000000000, 0.004166666666666666609, 0.008333333333333333218, 0.01250000000000000069, 0.01666666666666666644, 0.02083333333333333218, 0.02500000000000000139, 0.02916666666666666713, 0.03333333333333333287, 0.03749999999999999861, 0.04166666666666666435, 0.04583333333333333010, 0.05000000000000000278, 0.05416666666666666852, 0.05833333333333333426, 0.06250000000000000000, 0.06666666666666666574, 0.07083333333333333148, 0.07499999999999999722, 0.07916666666666666297, 0.08333333333333332871, 0.08749999999999999445, 0.09166666666666666019, 0.09583333333333333981, 0.1000000000000000056, 0.1041666666666666713, 0.1083333333333333370, 0.1125000000000000028, 0.1166666666666666685, 0.1208333333333333343, 0.1250000000000000000, 0.1291666666666666796, 0.1333333333333333315, 0.1375000000000000111, 0.1416666666666666630, 0.1458333333333333426, 0.1499999999999999944, 0.1541666666666666741, 0.1583333333333333259, 0.1625000000000000056, 0.1666666666666666574, 0.1708333333333333370, 0.1749999999999999889, 0.1791666666666666685, 0.1833333333333333204, 0.1875000000000000000, 0.1916666666666666796, 0.1958333333333333315, 0.2000000000000000111, 0.2041666666666666630, 0.2083333333333333426, 0.2124999999999999944, 0.2166666666666666741, 0.2208333333333333259, 0.2250000000000000056, 0.2291666666666666574, 0.2333333333333333370, 0.2374999999999999889, 0.2416666666666666685, 0.2458333333333333204, 0.2500000000000000000, 0.2541666666666666519, 0.2583333333333333592, 0.2625000000000000111, 0.2666666666666666630, 0.2708333333333333148, 0.2750000000000000222, 0.2791666666666666741, 0.2833333333333333259, 0.2874999999999999778, 0.2916666666666666852, 0.2958333333333333370, 0.2999999999999999889, 0.3041666666666666408, 0.3083333333333333481, 0.3125000000000000000, 0.3166666666666666519, 0.3208333333333333592, 0.3250000000000000111, 0.3291666666666666630, 0.3333333333333333148, 0.3375000000000000222, 0.3416666666666666741, 0.3458333333333333259, 0.3499999999999999778, 0.3541666666666666852, 0.3583333333333333370, 0.3624999999999999889, 0.3666666666666666408, 0.3708333333333333481, 0.3750000000000000000, 0.3791666666666666519, 0.3833333333333333592, 0.3875000000000000111, 0.3916666666666666630, 0.3958333333333333148, 0.4000000000000000222, 0.4041666666666666741, 0.4083333333333333259, 0.4124999999999999778, 0.4166666666666666852, 0.4208333333333333370, 0.4249999999999999889, 0.4291666666666666408, 0.4333333333333333481, 0.4375000000000000000, 0.4416666666666666519, 0.4458333333333333592, 0.4500000000000000111, 0.4541666666666666630, 0.4583333333333333148, 0.4625000000000000222, 0.4666666666666666741, 0.4708333333333333259, 0.4749999999999999778, 0.4791666666666666852, 0.4833333333333333370, 0.4874999999999999889, 0.4916666666666666408, 0.4958333333333333481, 0.5000000000000000000, 0.5041666666666666519, 0.5083333333333333037, 0.5124999999999999556, 0.5166666666666667185, 0.5208333333333333703, 0.5250000000000000222, 0.5291666666666666741, 0.5333333333333333259, 0.5374999999999999778, 0.5416666666666666297, 0.5458333333333332815, 0.5500000000000000444, 0.5541666666666666963, 0.5583333333333333481, 0.5625000000000000000, 0.5666666666666666519, 0.5708333333333333037, 0.5749999999999999556, 0.5791666666666667185, 0.5833333333333333703, 0.5875000000000000222, 0.5916666666666666741, 0.5958333333333333259, 0.5999999999999999778, 0.6041666666666666297, 0.6083333333333332815, 0.6125000000000000444, 0.6166666666666666963, 0.6208333333333333481, 0.6250000000000000000, 0.6291666666666666519, 0.6333333333333333037, 0.6374999999999999556, 0.6416666666666667185, 0.6458333333333333703, 0.6500000000000000222, 0.6541666666666666741, 0.6583333333333333259, 0.6624999999999999778, 0.6666666666666666297, 0.6708333333333332815, 0.6750000000000000444, 0.6791666666666666963, 0.6833333333333333481, 0.6875000000000000000, 0.6916666666666666519, 0.6958333333333333037, 0.6999999999999999556, 0.7041666666666667185, 0.7083333333333333703, 0.7125000000000000222, 0.7166666666666666741, 0.7208333333333333259, 0.7249999999999999778, 0.7291666666666666297, 0.7333333333333332815, 0.7375000000000000444, 0.7416666666666666963, 0.7458333333333333481, 0.7500000000000000000, 0.7541666666666666519, 0.7583333333333333037, 0.7624999999999999556, 0.7666666666666667185, 0.7708333333333333703, 0.7750000000000000222, 0.7791666666666666741, 0.7833333333333333259, 0.7874999999999999778, 0.7916666666666666297, 0.7958333333333332815, 0.8000000000000000444, 0.8041666666666666963, 0.8083333333333333481, 0.8125000000000000000, 0.8166666666666666519, 0.8208333333333333037, 0.8249999999999999556, 0.8291666666666667185, 0.8333333333333333703, 0.8375000000000000222, 0.8416666666666666741, 0.8458333333333333259, 0.8499999999999999778, 0.8541666666666666297, 0.8583333333333332815, 0.8625000000000000444, 0.8666666666666666963, 0.8708333333333333481, 0.8750000000000000000, 0.8791666666666666519, 0.8833333333333333037, 0.8874999999999999556, 0.8916666666666667185, 0.8958333333333333703, 0.9000000000000000222, 0.9041666666666666741, 0.9083333333333333259, 0.9124999999999999778, 0.9166666666666666297, 0.9208333333333332815, 0.9250000000000000444, 0.9291666666666666963, 0.9333333333333333481, 0.9375000000000000000, 0.9416666666666666519, 0.9458333333333333037, 0.9499999999999999556, 0.9541666666666667185, 0.9583333333333333703, 0.9625000000000000222, 0.9666666666666666741, 0.9708333333333333259, 0.9749999999999999778, 0.9791666666666666297, 0.9833333333333332815, 0.9875000000000000444, 0.9916666666666666963, 0.9958333333333333481, 1.000000000000000000 ),
 .UNSPECIFIED. ) 
 GEOMETRIC_REPRESENTATION_ITEM ( )  RATIONAL_B_SPLINE_SURFACE ( (
 ( 1.000000000000000000, 0.8660254037844387076, 1.000000000000000000, 0.8660254037844387076, 1.000000000000000000, 0.8660254037844387076, 1.000000000000000000, 0.8660254037844387076, 1.000000000000000000, 0.8660254037844387076, 1.000000000000000000, 0.8660254037844387076, 1.000000000000000000, 0.8660254037844387076, 1.000000000000000000, 0.8660254037844387076, 1.000000000000000000, 0.8660254037844387076, 1.000000000000000000, 0.8660254037844387076, 1.000000000000000000, 0.8660254037844387076, 1.000000000000000000, 0.8660254037844387076, 1.000000000000000000, 0.8660254037844387076, 1.000000000000000000, 0.8660254037844387076, 1.000000000000000000, 0.8660254037844387076, 1.000000000000000000, 0.8660254037844387076, 1.000000000000000000, 0.8660254037844387076, 1.000000000000000000, 0.8660254037844387076, 1.000000000000000000, 0.8660254037844387076, 1.000000000000000000, 0.8660254037844387076, 1.000000000000000000, 0.8660254037844387076, 1.000000000000000000, 0.8660254037844387076, 1.000000000000000000, 0.8660254037844387076, 1.000000000000000000, 0.8660254037844387076, 1.000000000000000000, 0.8660254037844387076, 1.000000000000000000, 0.8660254037844387076, 1.000000000000000000, 0.8660254037844387076, 1.000000000000000000, 0.8660254037844387076, 1.000000000000000000, 0.8660254037844387076, 1.000000000000000000, 0.8660254037844387076, 1.000000000000000000, 0.8660254037844387076, 1.000000000000000000, 0.8660254037844387076, 1.000000000000000000, 0.8660254037844387076, 1.000000000000000000, 0.8660254037844387076, 1.000000000000000000, 0.8660254037844387076, 1.000000000000000000, 0.8660254037844387076, 1.000000000000000000, 0.8660254037844387076, 1.000000000000000000, 0.8660254037844387076, 1.000000000000000000, 0.8660254037844387076, 1.000000000000000000, 0.8660254037844387076, 1.000000000000000000, 0.8660254037844387076, 1.000000000000000000, 0.8660254037844387076, 1.000000000000000000, 0.8660254037844387076, 1.000000000000000000, 0.8660254037844387076, 1.000000000000000000, 0.8660254037844387076, 1.000000000000000000, 0.8660254037844387076, 1.000000000000000000, 0.8660254037844387076, 1.000000000000000000, 0.8660254037844387076, 1.000000000000000000, 0.8660254037844387076, 1.000000000000000000, 0.8660254037844387076, 1.000000000000000000, 0.8660254037844387076, 1.000000000000000000, 0.8660254037844387076, 1.000000000000000000, 0.8660254037844387076, 1.000000000000000000, 0.8660254037844387076, 1.000000000000000000, 0.8660254037844387076, 1.000000000000000000, 0.8660254037844387076, 1.000000000000000000, 0.8660254037844387076, 1.000000000000000000, 0.8660254037844387076, 1.000000000000000000, 0.8660254037844387076, 1.000000000000000000, 0.8660254037844387076, 1.000000000000000000, 0.8660254037844387076, 1.000000000000000000, 0.8660254037844387076, 1.000000000000000000, 0.8660254037844387076, 1.000000000000000000, 0.8660254037844387076, 1.000000000000000000, 0.8660254037844387076, 1.000000000000000000, 0.8660254037844387076, 1.000000000000000000, 0.8660254037844387076, 1.000000000000000000, 0.8660254037844387076, 1.000000000000000000, 0.8660254037844387076, 1.000000000000000000, 0.8660254037844387076, 1.000000000000000000, 0.8660254037844387076, 1.000000000000000000, 0.8660254037844387076, 1.000000000000000000, 0.8660254037844387076, 1.000000000000000000, 0.8660254037844387076, 1.000000000000000000, 0.8660254037844387076, 1.000000000000000000, 0.8660254037844387076, 1.000000000000000000, 0.8660254037844387076, 1.000000000000000000, 0.8660254037844387076, 1.000000000000000000, 0.8660254037844387076, 1.000000000000000000, 0.8660254037844387076, 1.000000000000000000, 0.8660254037844387076, 1.000000000000000000, 0.8660254037844387076, 1.000000000000000000, 0.8660254037844387076, 1.000000000000000000, 0.8660254037844387076, 1.000000000000000000, 0.8660254037844387076, 1.000000000000000000, 0.8660254037844387076, 1.000000000000000000, 0.8660254037844387076, 1.000000000000000000, 0.8660254037844387076, 1.000000000000000000, 0.8660254037844387076, 1.000000000000000000, 0.8660254037844387076, 1.000000000000000000, 0.8660254037844387076, 1.000000000000000000, 0.8660254037844387076, 1.000000000000000000, 0.8660254037844387076, 1.000000000000000000, 0.8660254037844387076, 1.000000000000000000, 0.8660254037844387076, 1.000000000000000000, 0.8660254037844387076, 1.000000000000000000, 0.8660254037844387076, 1.000000000000000000, 0.8660254037844387076, 1.000000000000000000, 0.8660254037844387076, 1.000000000000000000, 0.8660254037844387076, 1.000000000000000000, 0.8660254037844387076, 1.000000000000000000, 0.8660254037844387076, 1.000000000000000000, 0.8660254037844387076, 1.000000000000000000, 0.8660254037844387076, 1.000000000000000000, 0.8660254037844387076, 1.000000000000000000, 0.8660254037844387076, 1.000000000000000000, 0.8660254037844387076, 1.000000000000000000, 0.8660254037844387076, 1.000000000000000000, 0.8660254037844387076, 1.000000000000000000, 0.8660254037844387076, 1.000000000000000000, 0.8660254037844387076, 1.000000000000000000, 0.8660254037844387076, 1.000000000000000000, 0.8660254037844387076, 1.000000000000000000, 0.8660254037844387076, 1.000000000000000000, 0.8660254037844387076, 1.000000000000000000, 0.8660254037844387076, 1.000000000000000000, 0.8660254037844387076, 1.000000000000000000, 0.8660254037844387076, 1.000000000000000000, 0.8660254037844387076, 1.000000000000000000, 0.8660254037844387076, 1.000000000000000000, 0.8660254037844387076, 1.000000000000000000, 0.8660254037844387076, 1.000000000000000000, 0.8660254037844387076, 1.000000000000000000, 0.8660254037844387076, 1.000000000000000000, 0.8660254037844387076, 1.000000000000000000, 0.8660254037844387076, 1.000000000000000000, 0.8660254037844387076, 1.000000000000000000, 0.8660254037844387076, 1.000000000000000000, 0.8660254037844387076, 1.000000000000000000, 0.8660254037844387076, 1.000000000000000000, 0.8660254037844387076, 1.000000000000000000, 0.8660254037844387076, 1.000000000000000000, 0.8660254037844387076, 1.000000000000000000, 0.8660254037844387076, 1.000000000000000000, 0.8660254037844387076, 1.000000000000000000, 0.8660254037844387076, 1.000000000000000000, 0.8660254037844387076, 1.000000000000000000, 0.8660254037844387076, 1.000000000000000000, 0.8660254037844387076, 1.000000000000000000, 0.8660254037844387076, 1.000000000000000000, 0.8660254037844387076, 1.000000000000000000, 0.8660254037844387076, 1.000000000000000000, 0.8660254037844387076, 1.000000000000000000, 0.8660254037844387076, 1.000000000000000000, 0.8660254037844387076, 1.000000000000000000, 0.8660254037844387076, 1.000000000000000000, 0.8660254037844387076, 1.000000000000000000, 0.8660254037844387076, 1.000000000000000000, 0.8660254037844387076, 1.000000000000000000, 0.8660254037844387076, 1.000000000000000000, 0.8660254037844387076, 1.000000000000000000, 0.8660254037844387076, 1.000000000000000000, 0.8660254037844387076, 1.000000000000000000, 0.8660254037844387076, 1.000000000000000000, 0.8660254037844387076, 1.000000000000000000, 0.8660254037844387076, 1.000000000000000000, 0.8660254037844387076, 1.000000000000000000, 0.8660254037844387076, 1.000000000000000000, 0.8660254037844387076, 1.000000000000000000, 0.8660254037844387076, 1.000000000000000000, 0.8660254037844387076, 1.000000000000000000, 0.8660254037844387076, 1.000000000000000000, 0.8660254037844387076, 1.000000000000000000, 0.8660254037844387076, 1.000000000000000000, 0.8660254037844387076, 1.000000000000000000, 0.8660254037844387076, 1.000000000000000000, 0.8660254037844387076, 1.000000000000000000, 0.8660254037844387076, 1.000000000000000000, 0.8660254037844387076, 1.000000000000000000, 0.8660254037844387076, 1.000000000000000000, 0.8660254037844387076, 1.000000000000000000, 0.8660254037844387076, 1.000000000000000000, 0.8660254037844387076, 1.000000000000000000, 0.8660254037844387076, 1.000000000000000000, 0.8660254037844387076, 1.000000000000000000, 0.8660254037844387076, 1.000000000000000000, 0.8660254037844387076, 1.000000000000000000, 0.8660254037844387076, 1.000000000000000000, 0.8660254037844387076, 1.000000000000000000, 0.8660254037844387076, 1.000000000000000000, 0.8660254037844387076, 1.000000000000000000, 0.8660254037844387076, 1.000000000000000000, 0.8660254037844387076, 1.000000000000000000, 0.8660254037844387076, 1.000000000000000000, 0.8660254037844387076, 1.000000000000000000, 0.8660254037844387076, 1.000000000000000000, 0.8660254037844387076, 1.000000000000000000, 0.8660254037844387076, 1.000000000000000000, 0.8660254037844387076, 1.000000000000000000, 0.8660254037844387076, 1.000000000000000000, 0.8660254037844387076, 1.000000000000000000, 0.8660254037844387076, 1.000000000000000000, 0.8660254037844387076, 1.000000000000000000, 0.8660254037844387076, 1.000000000000000000, 0.8660254037844387076, 1.000000000000000000, 0.8660254037844387076, 1.000000000000000000, 0.8660254037844387076, 1.000000000000000000, 0.8660254037844387076, 1.000000000000000000, 0.8660254037844387076, 1.000000000000000000, 0.8660254037844387076, 1.000000000000000000, 0.8660254037844387076, 1.000000000000000000, 0.8660254037844387076, 1.000000000000000000, 0.8660254037844387076, 1.000000000000000000, 0.8660254037844387076, 1.000000000000000000, 0.8660254037844387076, 1.000000000000000000, 0.8660254037844387076, 1.000000000000000000, 0.8660254037844387076, 1.000000000000000000, 0.8660254037844387076, 1.000000000000000000, 0.8660254037844387076, 1.000000000000000000, 0.8660254037844387076, 1.000000000000000000, 0.8660254037844387076, 1.000000000000000000, 0.8660254037844387076, 1.000000000000000000, 0.8660254037844387076, 1.000000000000000000, 0.8660254037844387076, 1.000000000000000000, 0.8660254037844387076, 1.000000000000000000, 0.8660254037844387076, 1.000000000000000000, 0.8660254037844387076, 1.000000000000000000, 0.8660254037844387076, 1.000000000000000000, 0.8660254037844387076, 1.000000000000000000, 0.8660254037844387076, 1.000000000000000000, 0.8660254037844387076, 1.000000000000000000, 0.8660254037844387076, 1.000000000000000000, 0.8660254037844387076, 1.000000000000000000, 0.8660254037844387076, 1.000000000000000000, 0.8660254037844387076, 1.000000000000000000, 0.8660254037844387076, 1.000000000000000000, 0.8660254037844387076, 1.000000000000000000, 0.8660254037844387076, 1.000000000000000000, 0.8660254037844387076, 1.000000000000000000, 0.8660254037844387076, 1.000000000000000000, 0.8660254037844387076, 1.000000000000000000, 0.8660254037844387076, 1.000000000000000000, 0.8660254037844387076, 1.000000000000000000, 0.8660254037844387076, 1.000000000000000000, 0.8660254037844387076, 1.000000000000000000, 0.8660254037844387076, 1.000000000000000000, 0.8660254037844387076, 1.000000000000000000, 0.8660254037844387076, 1.000000000000000000, 0.8660254037844387076, 1.000000000000000000, 0.8660254037844387076, 1.000000000000000000),
 ( 1.000000000000000000, 0.8660254037844387076, 1.000000000000000000, 0.8660254037844387076, 1.000000000000000000, 0.8660254037844387076, 1.000000000000000000, 0.8660254037844387076, 1.000000000000000000, 0.8660254037844387076, 1.000000000000000000, 0.8660254037844387076, 1.000000000000000000, 0.8660254037844387076, 1.000000000000000000, 0.8660254037844387076, 1.000000000000000000, 0.8660254037844387076, 1.000000000000000000, 0.8660254037844387076, 1.000000000000000000, 0.8660254037844387076, 1.000000000000000000, 0.8660254037844387076, 1.000000000000000000, 0.8660254037844387076, 1.000000000000000000, 0.8660254037844387076, 1.000000000000000000, 0.8660254037844387076, 1.000000000000000000, 0.8660254037844387076, 1.000000000000000000, 0.8660254037844387076, 1.000000000000000000, 0.8660254037844387076, 1.000000000000000000, 0.8660254037844387076, 1.000000000000000000, 0.8660254037844387076, 1.000000000000000000, 0.8660254037844387076, 1.000000000000000000, 0.8660254037844387076, 1.000000000000000000, 0.8660254037844387076, 1.000000000000000000, 0.8660254037844387076, 1.000000000000000000, 0.8660254037844387076, 1.000000000000000000, 0.8660254037844387076, 1.000000000000000000, 0.8660254037844387076, 1.000000000000000000, 0.8660254037844387076, 1.000000000000000000, 0.8660254037844387076, 1.000000000000000000, 0.8660254037844387076, 1.000000000000000000, 0.8660254037844387076, 1.000000000000000000, 0.8660254037844387076, 1.000000000000000000, 0.8660254037844387076, 1.000000000000000000, 0.8660254037844387076, 1.000000000000000000, 0.8660254037844387076, 1.000000000000000000, 0.8660254037844387076, 1.000000000000000000, 0.8660254037844387076, 1.000000000000000000, 0.8660254037844387076, 1.000000000000000000, 0.8660254037844387076, 1.000000000000000000, 0.8660254037844387076, 1.000000000000000000, 0.8660254037844387076, 1.000000000000000000, 0.8660254037844387076, 1.000000000000000000, 0.8660254037844387076, 1.000000000000000000, 0.8660254037844387076, 1.000000000000000000, 0.8660254037844387076, 1.000000000000000000, 0.8660254037844387076, 1.000000000000000000, 0.8660254037844387076, 1.000000000000000000, 0.8660254037844387076, 1.000000000000000000, 0.8660254037844387076, 1.000000000000000000, 0.8660254037844387076, 1.000000000000000000, 0.8660254037844387076, 1.000000000000000000, 0.8660254037844387076, 1.000000000000000000, 0.8660254037844387076, 1.000000000000000000, 0.8660254037844387076, 1.000000000000000000, 0.8660254037844387076, 1.000000000000000000, 0.8660254037844387076, 1.000000000000000000, 0.8660254037844387076, 1.000000000000000000, 0.8660254037844387076, 1.000000000000000000, 0.8660254037844387076, 1.000000000000000000, 0.8660254037844387076, 1.000000000000000000, 0.8660254037844387076, 1.000000000000000000, 0.8660254037844387076, 1.000000000000000000, 0.8660254037844387076, 1.000000000000000000, 0.8660254037844387076, 1.000000000000000000, 0.8660254037844387076, 1.000000000000000000, 0.8660254037844387076, 1.000000000000000000, 0.8660254037844387076, 1.000000000000000000, 0.8660254037844387076, 1.000000000000000000, 0.8660254037844387076, 1.000000000000000000, 0.8660254037844387076, 1.000000000000000000, 0.8660254037844387076, 1.000000000000000000, 0.8660254037844387076, 1.000000000000000000, 0.8660254037844387076, 1.000000000000000000, 0.8660254037844387076, 1.000000000000000000, 0.8660254037844387076, 1.000000000000000000, 0.8660254037844387076, 1.000000000000000000, 0.8660254037844387076, 1.000000000000000000, 0.8660254037844387076, 1.000000000000000000, 0.8660254037844387076, 1.000000000000000000, 0.8660254037844387076, 1.000000000000000000, 0.8660254037844387076, 1.000000000000000000, 0.8660254037844387076, 1.000000000000000000, 0.8660254037844387076, 1.000000000000000000, 0.8660254037844387076, 1.000000000000000000, 0.8660254037844387076, 1.000000000000000000, 0.8660254037844387076, 1.000000000000000000, 0.8660254037844387076, 1.000000000000000000, 0.8660254037844387076, 1.000000000000000000, 0.8660254037844387076, 1.000000000000000000, 0.8660254037844387076, 1.000000000000000000, 0.8660254037844387076, 1.000000000000000000, 0.8660254037844387076, 1.000000000000000000, 0.8660254037844387076, 1.000000000000000000, 0.8660254037844387076, 1.000000000000000000, 0.8660254037844387076, 1.000000000000000000, 0.8660254037844387076, 1.000000000000000000, 0.8660254037844387076, 1.000000000000000000, 0.8660254037844387076, 1.000000000000000000, 0.8660254037844387076, 1.000000000000000000, 0.8660254037844387076, 1.000000000000000000, 0.8660254037844387076, 1.000000000000000000, 0.8660254037844387076, 1.000000000000000000, 0.8660254037844387076, 1.000000000000000000, 0.8660254037844387076, 1.000000000000000000, 0.8660254037844387076, 1.000000000000000000, 0.8660254037844387076, 1.000000000000000000, 0.8660254037844387076, 1.000000000000000000, 0.8660254037844387076, 1.000000000000000000, 0.8660254037844387076, 1.000000000000000000, 0.8660254037844387076, 1.000000000000000000, 0.8660254037844387076, 1.000000000000000000, 0.8660254037844387076, 1.000000000000000000, 0.8660254037844387076, 1.000000000000000000, 0.8660254037844387076, 1.000000000000000000, 0.8660254037844387076, 1.000000000000000000, 0.8660254037844387076, 1.000000000000000000, 0.8660254037844387076, 1.000000000000000000, 0.8660254037844387076, 1.000000000000000000, 0.8660254037844387076, 1.000000000000000000, 0.8660254037844387076, 1.000000000000000000, 0.8660254037844387076, 1.000000000000000000, 0.8660254037844387076, 1.000000000000000000, 0.8660254037844387076, 1.000000000000000000, 0.8660254037844387076, 1.000000000000000000, 0.8660254037844387076, 1.000000000000000000, 0.8660254037844387076, 1.000000000000000000, 0.8660254037844387076, 1.000000000000000000, 0.8660254037844387076, 1.000000000000000000, 0.8660254037844387076, 1.000000000000000000, 0.8660254037844387076, 1.000000000000000000, 0.8660254037844387076, 1.000000000000000000, 0.8660254037844387076, 1.000000000000000000, 0.8660254037844387076, 1.000000000000000000, 0.8660254037844387076, 1.000000000000000000, 0.8660254037844387076, 1.000000000000000000, 0.8660254037844387076, 1.000000000000000000, 0.8660254037844387076, 1.000000000000000000, 0.8660254037844387076, 1.000000000000000000, 0.8660254037844387076, 1.000000000000000000, 0.8660254037844387076, 1.000000000000000000, 0.8660254037844387076, 1.000000000000000000, 0.8660254037844387076, 1.000000000000000000, 0.8660254037844387076, 1.000000000000000000, 0.8660254037844387076, 1.000000000000000000, 0.8660254037844387076, 1.000000000000000000, 0.8660254037844387076, 1.000000000000000000, 0.8660254037844387076, 1.000000000000000000, 0.8660254037844387076, 1.000000000000000000, 0.8660254037844387076, 1.000000000000000000, 0.8660254037844387076, 1.000000000000000000, 0.8660254037844387076, 1.000000000000000000, 0.8660254037844387076, 1.000000000000000000, 0.8660254037844387076, 1.000000000000000000, 0.8660254037844387076, 1.000000000000000000, 0.8660254037844387076, 1.000000000000000000, 0.8660254037844387076, 1.000000000000000000, 0.8660254037844387076, 1.000000000000000000, 0.8660254037844387076, 1.000000000000000000, 0.8660254037844387076, 1.000000000000000000, 0.8660254037844387076, 1.000000000000000000, 0.8660254037844387076, 1.000000000000000000, 0.8660254037844387076, 1.000000000000000000, 0.8660254037844387076, 1.000000000000000000, 0.8660254037844387076, 1.000000000000000000, 0.8660254037844387076, 1.000000000000000000, 0.8660254037844387076, 1.000000000000000000, 0.8660254037844387076, 1.000000000000000000, 0.8660254037844387076, 1.000000000000000000, 0.8660254037844387076, 1.000000000000000000, 0.8660254037844387076, 1.000000000000000000, 0.8660254037844387076, 1.000000000000000000, 0.8660254037844387076, 1.000000000000000000, 0.8660254037844387076, 1.000000000000000000, 0.8660254037844387076, 1.000000000000000000, 0.8660254037844387076, 1.000000000000000000, 0.8660254037844387076, 1.000000000000000000, 0.8660254037844387076, 1.000000000000000000, 0.8660254037844387076, 1.000000000000000000, 0.8660254037844387076, 1.000000000000000000, 0.8660254037844387076, 1.000000000000000000, 0.8660254037844387076, 1.000000000000000000, 0.8660254037844387076, 1.000000000000000000, 0.8660254037844387076, 1.000000000000000000, 0.8660254037844387076, 1.000000000000000000, 0.8660254037844387076, 1.000000000000000000, 0.8660254037844387076, 1.000000000000000000, 0.8660254037844387076, 1.000000000000000000, 0.8660254037844387076, 1.000000000000000000, 0.8660254037844387076, 1.000000000000000000, 0.8660254037844387076, 1.000000000000000000, 0.8660254037844387076, 1.000000000000000000, 0.8660254037844387076, 1.000000000000000000, 0.8660254037844387076, 1.000000000000000000, 0.8660254037844387076, 1.000000000000000000, 0.8660254037844387076, 1.000000000000000000, 0.8660254037844387076, 1.000000000000000000, 0.8660254037844387076, 1.000000000000000000, 0.8660254037844387076, 1.000000000000000000, 0.8660254037844387076, 1.000000000000000000, 0.8660254037844387076, 1.000000000000000000, 0.8660254037844387076, 1.000000000000000000, 0.8660254037844387076, 1.000000000000000000, 0.8660254037844387076, 1.000000000000000000, 0.8660254037844387076, 1.000000000000000000, 0.8660254037844387076, 1.000000000000000000, 0.8660254037844387076, 1.000000000000000000, 0.8660254037844387076, 1.000000000000000000, 0.8660254037844387076, 1.000000000000000000, 0.8660254037844387076, 1.000000000000000000, 0.8660254037844387076, 1.000000000000000000, 0.8660254037844387076, 1.000000000000000000, 0.8660254037844387076, 1.000000000000000000, 0.8660254037844387076, 1.000000000000000000, 0.8660254037844387076, 1.000000000000000000, 0.8660254037844387076, 1.000000000000000000, 0.8660254037844387076, 1.000000000000000000, 0.8660254037844387076, 1.000000000000000000, 0.8660254037844387076, 1.000000000000000000, 0.8660254037844387076, 1.000000000000000000, 0.8660254037844387076, 1.000000000000000000, 0.8660254037844387076, 1.000000000000000000, 0.8660254037844387076, 1.000000000000000000, 0.8660254037844387076, 1.000000000000000000, 0.8660254037844387076, 1.000000000000000000, 0.8660254037844387076, 1.000000000000000000, 0.8660254037844387076, 1.000000000000000000, 0.8660254037844387076, 1.000000000000000000, 0.8660254037844387076, 1.000000000000000000, 0.8660254037844387076, 1.000000000000000000, 0.8660254037844387076, 1.000000000000000000, 0.8660254037844387076, 1.000000000000000000, 0.8660254037844387076, 1.000000000000000000, 0.8660254037844387076, 1.000000000000000000, 0.8660254037844387076, 1.000000000000000000, 0.8660254037844387076, 1.000000000000000000, 0.8660254037844387076, 1.000000000000000000, 0.8660254037844387076, 1.000000000000000000, 0.8660254037844387076, 1.000000000000000000, 0.8660254037844387076, 1.000000000000000000, 0.8660254037844387076, 1.000000000000000000) ) ) 
 REPRESENTATION_ITEM ( '' )  SURFACE ( )  );
#9919=CARTESIAN_POINT ( 'NONE',  ( -0.6823417656250003738, 2.030208333674753174, -1.181850606188749264 ) ) ;
#9922=CARTESIAN_POINT ( 'NONE',  ( 6.100805936469477331, 9.101062111647635788, -1.082531754730537088 ) ) ;
#9930=CARTESIAN_POINT ( 'NONE',  ( 9.869972640624258275, 10.61731562359089587, 0.000000000000000000 ) ) ;
#9935=CARTESIAN_POINT ( 'NONE',  ( -7.818248136574758256, 12.27303992597924420, 0.000000000000000000 ) ) ;
#9951=CARTESIAN_POINT ( 'NONE',  ( -1.402160292154681736E-14, 0.8687500006828192678, -1.732050807568863648 ) ) ;
#9956=CARTESIAN_POINT ( 'NONE',  ( -1.402160292154681736E-14, 0.08750000000001964540, -1.732050807568870754 ) ) ;
#9957=CARTESIAN_POINT ( 'NONE',  ( 9.074484886248265880, 9.481320543578137361, 0.7998128361456462443 ) ) ;
#9958=ADVANCED_FACE ( 'NONE', ( #60171 ), #27673, .T. ) ;
#9959=CARTESIAN_POINT ( 'NONE',  ( 0.6823417656249882723, -0.9072916663252494907, 1.181850606188755259 ) ) ;
#9962=CARTESIAN_POINT ( 'NONE',  ( 2.683624340501134853, 5.218313266304903664, -1.199719254218446718 ) ) ;
#9963=CARTESIAN_POINT ( 'NONE',  ( -5.748293942514180799, 7.729428904398431222, -1.443375672974052559 ) ) ;
#9968=CARTESIAN_POINT ( 'NONE',  ( -6.718228810771495141, 7.796687353110217877, 1.199719254218450271 ) ) ;
#9970=CARTESIAN_POINT ( 'NONE',  ( -1.500000000000013101, 2.702083334016155636, 0.8660254037844403729 ) ) ;
#9983=CARTESIAN_POINT ( 'NONE',  ( -9.450196763925152510, 10.98398329845622001, -1.199719254218441611 ) ) ;
#9984=CARTESIAN_POINT ( 'NONE',  ( 5.933664784275179294, 10.07435934829639912, -0.7998128361456291469 ) ) ;
#9992=CARTESIAN_POINT ( 'NONE',  ( -8.182509401047415309, 9.505014708432145909, 1.199719254218462483 ) ) ;
#9998=CARTESIAN_POINT ( 'NONE',  ( 2.679707916995359263, 6.278076336469897711, -0.7998128361456291469 ) ) ;
#10002=( BOUNDED_CURVE ( )  B_SPLINE_CURVE ( 2, ( #183760, #167517, #32186, #709, #65713, #15909, #67843 ),
 .UNSPECIFIED., .F., .T. ) 
 B_SPLINE_CURVE_WITH_KNOTS ( ( 3, 2, 2, 3 ),
 ( 0.2321428571428570953, 0.2380952380952381098, 0.2440476190476191798, 0.2500000000000002220 ),
 .UNSPECIFIED. ) 
 CURVE ( )  GEOMETRIC_REPRESENTATION_ITEM ( )  RATIONAL_B_SPLINE_CURVE ( ( 1.000000000000001332, 0.8660254037844374864, 1.000000000000000000, 0.8660254037844387076, 1.000000000000000000, 0.8660254037844337116, 1.000000000000005107 ) ) 
 REPRESENTATION_ITEM ( '' )  );
#10003=CARTESIAN_POINT ( 'NONE',  ( -7.808606406466886973, 11.19745900993164511, 1.199719254218453823 ) ) ;
#10006=CARTESIAN_POINT ( 'NONE',  ( -5.768665591941109838, 6.232869020846472097, -1.039980349891131972 ) ) ;
#10013=CARTESIAN_POINT ( 'NONE',  ( 7.481401836642521452, 7.622723652371411696, 1.040834085586084257E-14 ) ) ;
#10015=CIRCLE ( 'NONE', #162180, 0.07999999999999990452 ) ;
#10032=CARTESIAN_POINT ( 'NONE',  ( -1.580000000000001625, -1.099999999999976108, -2.499999999999989342 ) ) ;
#10034=CARTESIAN_POINT ( 'NONE',  ( 3.050221373394638835, 6.502416002361635528, 0.000000000000000000 ) ) ;
#10039=CARTESIAN_POINT ( 'NONE',  ( -8.646349277213090545, 11.11049346154719508, 1.599625672291269396 ) ) ;
#10042=CARTESIAN_POINT ( 'NONE',  ( 9.694243528971124846, 11.26870452434320491, 1.199719254218450271 ) ) ;
#10045=DIRECTION ( 'NONE',  ( 0.1431542804991169926, 0.000000000000000000, 0.9897003849523248187 ) ) ;
#10051=CARTESIAN_POINT ( 'NONE',  ( -0.6823417656250246877, 0.05104166700808931978, 1.181850606188755259 ) ) ;
#10055=CARTESIAN_POINT ( 'NONE',  ( -4.497554271431319250, 6.270232621468402989, -1.599625672291256295 ) ) ;
#10059=CARTESIAN_POINT ( 'NONE',  ( -0.7500000000000006661, 0.3583333333333563187, -1.299038105676652011 ) ) ;
#10061=CARTESIAN_POINT ( 'NONE',  ( -1.364683531250014514, -0.9489583329919112353, -0.7879004041258359514 ) ) ;
#10066=CARTESIAN_POINT ( 'NONE',  ( -1.364683531250014514, -0.9697916663252473812, 0.7879004041258379498 ) ) ;
#10068=CARTESIAN_POINT ( 'NONE',  ( -6.042130013184518589, 10.20090211535728031, -0.7998128361456291469 ) ) ;
#10069=CARTESIAN_POINT ( 'NONE',  ( 7.214910300766615769, 11.56914578420308715, -0.7998128361456291469 ) ) ;
#10073=VERTEX_POINT ( 'NONE', #160883 ) ;
#10075=CARTESIAN_POINT ( 'NONE',  ( -1.364683531250014514, 0.3010416670080866552, -0.7879004041258359514 ) ) ;
#10084=CARTESIAN_POINT ( 'NONE',  ( 5.775410249741494972, 8.721433810464993996, -1.082531754730537088 ) ) ;
#10087=CARTESIAN_POINT ( 'NONE',  ( -6.403528624356093601, 6.365204904703887223, 1.040834085586084257E-14 ) ) ;
#10089=CARTESIAN_POINT ( 'NONE',  ( 0.7499999999999920064, 5.514583334016151639, 1.299038105676669330 ) ) ;
#10091=CARTESIAN_POINT ( 'NONE',  ( -4.437596350374534815, 4.071617251725375475, -0.7998128361456221525 ) ) ;
#10092=CARTESIAN_POINT ( 'NONE',  ( 6.114364089638795186, 7.196141528409145671, 1.082531754730558626 ) ) ;
#10093=CARTESIAN_POINT ( 'NONE',  ( -8.419250203962027612, 11.80591375705560608, 1.082531754730549967 ) ) ;
#10098=CARTESIAN_POINT ( 'NONE',  ( 4.369805582306193870, 3.992528022312320957, 1.214306433183764966E-14 ) ) ;
#10103=CIRCLE ( 'NONE', #17033, 4.624999999999993783 ) ;
#10114=CARTESIAN_POINT ( 'NONE',  ( 7.670162217029129259, 9.971608557999250166, 1.599625672291281386 ) ) ;
#10116=CARTESIAN_POINT ( 'NONE',  ( -4.038971567461725698, 3.986455684509185193, -0.5169845646830102392 ) ) ;
#10118=CARTESIAN_POINT ( 'NONE',  ( 5.043269954603547767, 4.986162489899998995, -0.7216878364870197293 ) ) ;
#10120=CARTESIAN_POINT ( 'NONE',  ( -8.731087737520713432, 10.24898578427137963, 1.082531754730558626 ) ) ;
#10129=VERTEX_POINT ( 'NONE', #40745 ) ;
#10132=VERTEX_POINT ( 'NONE', #150779 ) ;
#10134=ORIENTED_EDGE ( 'NONE', *, *, #77070, .F. ) ;
#10148=CARTESIAN_POINT ( 'NONE',  ( -6.684333426737305572, 7.757142738403693727, -1.199719254218446718 ) ) ;
#10153=CARTESIAN_POINT ( 'NONE',  ( 6.471319392424407901, 6.444294134116939077, 0.7998128361456341429 ) ) ;
#10159=CARTESIAN_POINT ( 'NONE',  ( -3.411848212133334446, 7.132240014130862171, 0.7998128361456341429 ) ) ;
#10163=ADVANCED_FACE ( 'NONE', ( #183253 ), #132422, .F. ) ;
#10165=CARTESIAN_POINT ( 'NONE',  ( -5.928993247877788697, 5.811580298812519807, 0.7998128361456341429 ) ) ;
#10168=CARTESIAN_POINT ( 'NONE',  ( 8.925345196497941558, 9.307324238869423283, 1.040834085586084257E-14 ) ) ;
#10169=CARTESIAN_POINT ( 'NONE',  ( -0.6823417656250212460, 3.301041667008085323, 1.181850606188767472 ) ) ;
#10171=CARTESIAN_POINT ( 'NONE',  ( 5.529887635128906354, 6.401445659467410287, 1.229860404580757072 ) ) ;
#10172=CARTESIAN_POINT ( 'NONE',  ( 4.365362273920250225, 5.155639410070820716, 1.082531754730560403 ) ) ;
#10178=CARTESIAN_POINT ( 'NONE',  ( 5.463572716182812705, 9.317992568947877530, 0.7216878364870438212 ) ) ;
#10179=CARTESIAN_POINT ( 'NONE',  ( -8.134002093194872884, 11.57708731111429401, 1.199719254218453823 ) ) ;
#10183=CARTESIAN_POINT ( 'NONE',  ( -8.830438121202295321, 9.196599317691152464, -0.7998128361456291469 ) ) ;
#10184=CARTESIAN_POINT ( 'NONE',  ( -5.819474248763749635, 7.812472595022922128, -1.599625672291256295 ) ) ;
#10191=CARTESIAN_POINT ( 'NONE',  ( 7.507464373665139412, 9.781794407407920389, 1.599625672291281386 ) ) ;
#10199=CARTESIAN_POINT ( 'NONE',  ( -1.499999999999997780, 5.181250000682820378, 1.214306433183764966E-14 ) ) ;
#10203=EDGE_LOOP ( 'NONE', ( #213866, #160272, #58142, #76607 ) ) ;
#10204=CARTESIAN_POINT ( 'NONE',  ( 0.7499999999999920064, 4.733333333333352932, 1.299038105676669330 ) ) ;
#10205=CARTESIAN_POINT ( 'NONE',  ( 3.988069740714122791, 7.804498464141805592, 0.7998128361456321445 ) ) ;
#10206=CARTESIAN_POINT ( 'NONE',  ( 5.635385404774530649, 9.726366738878972740, 0.7998128361456462443 ) ) ;
#10210=CARTESIAN_POINT ( 'NONE',  ( 6.805829924380108586, 8.963220883242035697, 1.443375672974076540 ) ) ;
#10211=CARTESIAN_POINT ( 'NONE',  ( -9.205623113554631587, 11.76297960394566466, 1.443375672974076540 ) ) ;
#10214=CARTESIAN_POINT ( 'NONE',  ( 8.565000355531088516, 11.01558638625153286, -1.599625672291257406 ) ) ;
#10217=CARTESIAN_POINT ( 'NONE',  ( -2.442440228756222353, 6.001264033524212671, -0.7998128361456281477 ) ) ;
#10220=CARTESIAN_POINT ( 'NONE',  ( -1.364683531250014514, 0.4885416670080875434, -0.7879004041258289570 ) ) ;
#10225=CARTESIAN_POINT ( 'NONE',  ( 0.6823417656249882723, -0.07395833299191079124, -1.181850606188749264 ) ) ;
#10228=CARTESIAN_POINT ( 'NONE',  ( 8.075853055234393452, 12.57357899774884658, 0.7998128361456462443 ) ) ;
#10231=CARTESIAN_POINT ( 'NONE',  ( -9.667127221743832877, 11.23706883257798772, 1.199719254218462483 ) ) ;
#10236=CARTESIAN_POINT ( 'NONE',  ( 4.111146893441827821, 5.819424013814004759, 1.599625672291267398 ) ) ;
#10243=CARTESIAN_POINT ( 'NONE',  ( 9.433775957010412938, 9.900493459467314850, 0.000000000000000000 ) ) ;
#10246=CARTESIAN_POINT ( 'NONE',  ( -4.717347382551060342, 7.590990148696470818, 1.199719254218464037 ) ) ;
#10250=CARTESIAN_POINT ( 'NONE',  ( 6.968000882419564945, 10.21675256520979858, 1.199719254218460707 ) ) ;
#10252=CARTESIAN_POINT ( 'NONE',  ( 6.089583550832340819, 10.25626457594641749, 1.040834085586084257E-14 ) ) ;
#10257=CARTESIAN_POINT ( 'NONE',  ( -9.002250809793991948, 12.48608113052627289, -1.082531754730543971 ) ) ;
#10263=CARTESIAN_POINT ( 'NONE',  ( -6.123425537405413621, 6.005001634332811200, 0.2246051741978810634 ) ) ;
#10264=CARTESIAN_POINT ( 'NONE',  ( -0.6823417656250003738, 1.217708333674752286, -1.181850606188749264 ) ) ;
#10266=CARTESIAN_POINT ( 'NONE',  ( 5.829642864196157070, 8.784705193995428374, 1.082531754730558626 ) ) ;
#10284=CARTESIAN_POINT ( 'NONE',  ( 9.433775957010412938, 9.900493459467314850, 0.000000000000000000 ) ) ;
#10288=CARTESIAN_POINT ( 'NONE',  ( -3.436101866059630527, 6.096203712789787232, 1.199719254218462483 ) ) ;
#10289=CARTESIAN_POINT ( 'NONE',  ( -6.124532705071231931, 8.168374127381657246, -1.599625672291263179 ) ) ;
#10294=CARTESIAN_POINT ( 'NONE',  ( -0.7500000000000215383, 4.722916667349482012, 1.299038105676671107 ) ) ;
#10295=CARTESIAN_POINT ( 'NONE',  ( 8.938903350111612411, 9.323142084752035430, -0.7998128361456221525 ) ) ;
#10299=CARTESIAN_POINT ( 'NONE',  ( -6.679363233026820446, 10.94434087183997129, 0.000000000000000000 ) ) ;
#10301=CARTESIAN_POINT ( 'NONE',  ( 0.6823417656249899377, 5.176041667008086655, -1.181850606188754593 ) ) ;
#10306=CARTESIAN_POINT ( 'NONE',  ( -7.700668062882072284, 10.00719871149432549, -1.443375672974059665 ) ) ;
#10310=CARTESIAN_POINT ( 'NONE',  ( 0.6823417656249882723, 2.738541667008084879, -1.181850606188749264 ) ) ;
#10318=CARTESIAN_POINT ( 'NONE',  ( 1.364683531249990311, 3.884375000341417028, 1.214306433183764966E-14 ) ) ;
#10319=CARTESIAN_POINT ( 'NONE',  ( -4.111146893441842920, 5.819424013814012753, 1.599625672291267398 ) ) ;
#10320=CARTESIAN_POINT ( 'NONE',  ( 7.311924916471702396, 7.425000578838787391, -0.7998128361456281477 ) ) ;
#10323=CARTESIAN_POINT ( 'NONE',  ( -1.201851678989727383E-14, 3.884375000341423689, 1.575800808251672791 ) ) ;
#10326=CARTESIAN_POINT ( 'NONE',  ( -1.402160292154681736E-14, -0.05312499965857903073, -1.575800808251665908 ) ) ;
#10327=CARTESIAN_POINT ( 'NONE',  ( -4.229780737783618072, 6.918199379847403740, 1.082531754730560403 ) ) ;
#10330=CARTESIAN_POINT ( 'NONE',  ( 4.717874267875568961, 4.606534188717351874, -0.7216878364870188411 ) ) ;
#10333=CARTESIAN_POINT ( 'NONE',  ( -9.544576954340667996, 11.19805653722800365, 1.082531754730558626 ) ) ;
#10337=CARTESIAN_POINT ( 'NONE',  ( -10.32183501870554387, 10.93656236477829502, 0.7998128361456462443 ) ) ;
#10338=CARTESIAN_POINT ( 'NONE',  ( -5.219525951136837705, 9.033271343060892633, -0.7216878364870207285 ) ) ;
#10340=CARTESIAN_POINT ( 'NONE',  ( 0.6823417656249882723, 1.238541667008083547, -1.181850606188749264 ) ) ;
#10347=CARTESIAN_POINT ( 'NONE',  ( -1.402160292154681736E-14, -0.7406249996585823059, -1.575800808251665908 ) ) ;
#10350=ADVANCED_FACE ( 'NONE', ( #105229 ), #71614, .T. ) ;
#10351=CARTESIAN_POINT ( 'NONE',  ( 2.372313692266983853, 5.711523707712699682, 0.7216878364870438212 ) ) ;
#10356=CARTESIAN_POINT ( 'NONE',  ( 8.473482818416664841, 10.90881592628469932, -1.443375672974063439 ) ) ;
#10366=CARTESIAN_POINT ( 'NONE',  ( -3.684065054611367351, 5.321161868511784299, -1.599625672291256295 ) ) ;
#10368=FACE_OUTER_BOUND ( 'NONE', #10203, .T. ) ;
#10369=CARTESIAN_POINT ( 'NONE',  ( 1.364683531249988535, 1.676041667008085101, 0.7879004041258500513 ) ) ;
#10377=CARTESIAN_POINT ( 'NONE',  ( -1.499999999999997780, 5.650000000000023448, 1.214306433183764966E-14 ) ) ;
#10390=CARTESIAN_POINT ( 'NONE',  ( 5.819474248763732760, 7.812472595022922128, -1.599625672291262513 ) ) ;
#10393=ORIENTED_EDGE ( 'NONE', *, *, #121074, .F. ) ;
#10398=CARTESIAN_POINT ( 'NONE',  ( 7.072549687823125097, 11.40305840243567381, -0.7998128361456291469 ) ) ;
#10401=CARTESIAN_POINT ( 'NONE',  ( 9.935427640716063991, 10.48575375712389679, -0.7998128361456281477 ) ) ;
#10403=CARTESIAN_POINT ( 'NONE',  ( -3.045082456892887812, 6.452177443058107364, 0.6540759397886571902 ) ) ;
#10406=ORIENTED_EDGE ( 'NONE', *, *, #104659, .T. ) ;
#10407=LINE ( 'NONE', #28811, #27850 ) ;
#10410=CARTESIAN_POINT ( 'NONE',  ( -0.5511734105799743766, 7.507429961897361892, 1.922562588595814415 ) ) ;
#10414=CARTESIAN_POINT ( 'NONE',  ( -7.212574532790087645, 11.35849468832304154, -0.7216878364870267237 ) ) ;
#10419=CARTESIAN_POINT ( 'NONE',  ( -8.448702279610222021, 13.00856975952063088, 1.040834085586084257E-14 ) ) ;
#10420=CARTESIAN_POINT ( 'NONE',  ( 5.497994985541524215, 6.373081223675282736, -1.199719254218445830 ) ) ;
#10426=CARTESIAN_POINT ( 'NONE',  ( 2.358755538653318773, 5.695705861830088423, 1.040834085586084257E-14 ) ) ;
#10435=CARTESIAN_POINT ( 'NONE',  ( -6.715366157470410435, 6.729015360003925750, -0.7998128361456291469 ) ) ;
#10437=CARTESIAN_POINT ( 'NONE',  ( -4.243865776277440993, 4.909930479533815451, -1.199719254218446718 ) ) ;
#10442=CARTESIAN_POINT ( 'NONE',  ( 1.419999999999990603, 6.280000000000042881, 2.500000000000000444 ) ) ;
#10445=CARTESIAN_POINT ( 'NONE',  ( 6.010342169559767633, 5.906487374108181143, -0.7998128361456281477 ) ) ;
#10447=CARTESIAN_POINT ( 'NONE',  ( 1.567286081490169902, 8.684911043814580012, 2.501016734198271418 ) ) ;
#10459=CARTESIAN_POINT ( 'NONE',  ( -1.201851678989727383E-14, 1.884375000341422135, 1.575800808251672791 ) ) ;
#10461=CARTESIAN_POINT ( 'NONE',  ( 3.083589872104280705, 5.684939719841914929, 1.199719254218450271 ) ) ;
#10463=CARTESIAN_POINT ( 'NONE',  ( -7.049876689426121779, 7.327203680526343632, -0.7216878364870278340 ) ) ;
#10464=CARTESIAN_POINT ( 'NONE',  ( 4.121315508874254796, 5.831287398485176077, -1.443375672974051449 ) ) ;
#10465=CARTESIAN_POINT ( 'NONE',  ( -5.382223794500827552, 9.223085493652217082, -0.7216878364870207285 ) ) ;
#10469=CARTESIAN_POINT ( 'NONE',  ( 6.419949431270806528, 7.448694743692793274, 1.199719254218462483 ) ) ;
#10474=CARTESIAN_POINT ( 'NONE',  ( 1.364683531249990311, 5.134375000341417916, 1.214306433183764966E-14 ) ) ;
#10479=CARTESIAN_POINT ( 'NONE',  ( 6.283314124929436417, 9.417951348137970413, -1.199719254218440723 ) ) ;
#10480=SHAPE_REPRESENTATION_RELATIONSHIP ( 'NONE' , 'NONE' ,  #113740, #127801 ) ;
#10482=CARTESIAN_POINT ( 'NONE',  ( -7.386494761346872551, 7.511998731193139989, -0.7998128361456291469 ) ) ;
#10488=CARTESIAN_POINT ( 'NONE',  ( 7.391166297744269365, 11.77477778067701664, 1.040834085586084257E-14 ) ) ;
#10491=CARTESIAN_POINT ( 'NONE',  ( -8.552495972122143186, 8.872333477097637200, 0.7998128361456462443 ) ) ;
#10493=CARTESIAN_POINT ( 'NONE',  ( 7.253248993186724114, 9.485209796849769504, 1.443375672974076540 ) ) ;
#10494=CARTESIAN_POINT ( 'NONE',  ( 4.166517013042797757, 7.612504677086913141, -0.8493068020909979587 ) ) ;
#10495=CARTESIAN_POINT ( 'NONE',  ( -8.514157279702020631, 11.91663867875229776, -1.082531754730543971 ) ) ;
#10500=CARTESIAN_POINT ( 'NONE',  ( 3.811813743736467419, 7.598866467667865443, 1.040834085586084257E-14 ) ) ;
#10502=CARTESIAN_POINT ( 'NONE',  ( 8.378048858240820351, 11.86180853700128601, -1.199719254218446718 ) ) ;
#10503=CARTESIAN_POINT ( 'NONE',  ( -5.724176140219916498, 6.114206214821067853, 0.7043541215260868960 ) ) ;
#10505=CARTESIAN_POINT ( 'NONE',  ( 1.364683531249988757, 0.6343750003414208027, 0.000000000000000000 ) ) ;
#10507=CARTESIAN_POINT ( 'NONE',  ( -7.076992996653451939, 7.358839372291564374, 0.7216878364870317197 ) ) ;
#10513=CARTESIAN_POINT ( 'NONE',  ( -4.409122955247444686, 7.142713865425108111, 1.076920909521961622 ) ) ;
#10514=CARTESIAN_POINT ( 'NONE',  ( 1.364683531249988757, -0.5531249996585801965, 0.000000000000000000 ) ) ;
#10517=CARTESIAN_POINT ( 'NONE',  ( 3.145128448690309053, 4.692402494937224056, -1.443375672974057666 ) ) ;
#10522=CARTESIAN_POINT ( 'NONE',  ( -7.497295758232720431, 10.73030023703809555, -1.082531754730543083 ) ) ;
#10528=CARTESIAN_POINT ( 'NONE',  ( -8.961576348508641487, 11.47825837805867799, -1.443375672974058777 ) ) ;
#10529=ADVANCED_FACE ( 'NONE', ( #92194 ), #212283, .F. ) ;
#10535=CARTESIAN_POINT ( 'NONE',  ( -7.009202228140739344, 11.12122699956546334, -0.7216878364870267237 ) ) ;
#10539=CARTESIAN_POINT ( 'NONE',  ( 1.364683531249990311, 5.676041667008088432, 0.7879004041258500513 ) ) ;
#10540=CARTESIAN_POINT ( 'NONE',  ( -0.7500000000000215383, 3.972916667349481123, 1.299038105676671107 ) ) ;
#10541=CARTESIAN_POINT ( 'NONE',  ( 5.889294496748854968, 6.159041356224602026, -0.8323295365256941913 ) ) ;
#10547=CARTESIAN_POINT ( 'NONE',  ( -5.533699252672048985, 9.607732894759390518, -0.7998128361456231517 ) ) ;
#10548=CARTESIAN_POINT ( 'NONE',  ( -3.009396220815599321, 6.452359640394901952, 0.6004564335717228474 ) ) ;
#10551=CARTESIAN_POINT ( 'NONE',  ( 5.229694566569264680, 7.124396299129368337, 1.599625672291267398 ) ) ;
#10556=CARTESIAN_POINT ( 'NONE',  ( 7.796102023057898123, 9.054206100777749455, -1.199719254218441611 ) ) ;
#10563=CARTESIAN_POINT ( 'NONE',  ( -5.260200412422200600, 8.120355666925794580, -1.082531754730544860 ) ) ;
#10574=CARTESIAN_POINT ( 'NONE',  ( -9.826962411806732689, 10.35921099006301382, -0.7998128361456291469 ) ) ;
#10576=CARTESIAN_POINT ( 'NONE',  ( 9.257519960032755790, 9.694861462993381807, 0.7998128361456462443 ) ) ;
#10577=CARTESIAN_POINT ( 'NONE',  ( -0.7500000000000215383, 0.1916666666666871910, 1.299038105676659116 ) ) ;
#10578=CARTESIAN_POINT ( 'NONE',  ( -9.176171038350775078, 9.599954387697719582, -0.7998128361456291469 ) ) ;
#10581=CARTESIAN_POINT ( 'NONE',  ( -0.6823417656249969321, 3.217708333674754062, -1.181850606188749264 ) ) ;
#10582=CARTESIAN_POINT ( 'NONE',  ( 2.900554798319789906, 5.471398800426671372, 1.199719254218452047 ) ) ;
#10585=CARTESIAN_POINT ( 'NONE',  ( -1.001543065824772872E-14, 5.462500000000020783, 1.732050807568877637 ) ) ;
#10588=CARTESIAN_POINT ( 'NONE',  ( 8.066738210006674237, 11.39464976410773467, 1.082531754730558626 ) ) ;
#10590=CARTESIAN_POINT ( 'NONE',  ( -7.212574532790102744, 8.477387045419011002, -1.082531754730550855 ) ) ;
#10592=CARTESIAN_POINT ( 'NONE',  ( -1.364683531250012516, 2.488541667008088876, -0.7879004041258289570 ) ) ;
#10596=CARTESIAN_POINT ( 'NONE',  ( -8.342344591110322227, 8.627156865917170236, -0.7998128361456291469 ) ) ;
#10597=CARTESIAN_POINT ( 'NONE',  ( -1.364683531249997417, 5.321875000341417916, 1.214306433183764966E-14 ) ) ;
#10601=( BOUNDED_SURFACE ( )  B_SPLINE_SURFACE ( 1, 2, ( 
 ( #75386, #139333, #8239, #24473, #125285, #60191, #126351, #73226, #6083, #122087, #138263, #74322, #56997, #191245, #140419, #109018, #206437, #104693, #106872, #172899, #175037, #55932, #90587, #154505, #192311, #124227, #190186, #41842, #207508, #107954, #170744, #157715, #173981, #25553, #42909, #9312, #141500, #26623, #158771, #10366, #22329, #72154, #188049, #39680, #105789, #171815, #78573, #15691, #45040, #159833, #47175, #176097, #93794, #195538, #212829, #12501, #196597, #31974, #110085, #129553, #30918, #98053, #11433, #178229, #127424, #77509, #14625, #96994, #144693, #43970, #27697, #211762, #143629, #130609, #80720, #48240, #210706, #128493, #114353, #163046, #209624, #81777, #164107, #62334, #147859, #213875, #193396, #146811, #161981, #180349, #61265, #194461, #111153, #113288, #112222, #13572, #63400, #28771, #177153, #94853, #160904, #29844, #65497, #46104, #179295, #95926, #131645, #79645, #145761, #64467, #67618, #84968, #53536, #19953, #52473, #101211, #70822, #99106, #199770, #82835, #118599, #165157, #4747, #50344, #184587, #116465, #103359, #36205, #167297, #100157, #16750, #117536, #66551, #148910, #168358, #102281, #83894, #197647, #115410, #151060, #484, #69761, #86037, #135867, #166220, #133762, #201886, #152113, #132693, #169422, #37286, #149984, #185655, #21005, #198700, #3684, #18883, #119668, #33028, #17810, #182457, #134817, #51415, #2623, #68694, #34085, #1557, #183531, #35137, #200822, #87102, #153172, #49294, #181403, #29318, #136938, #155311, #6894, #72972, #24215, #210176, #176636, #209102, #40508, #13044, #38354, #139077, #172639, #205101, #90317, #110634, #56742, #10908, #39422, #202965, #105516, #122910, #159311, #120753, #193937, #188868, #45584, #187794, #28248, #94341, #61816, #106612, #5820, #76984, #143110, #111701, #60740, #138003, #186731, #71895, #104432, #88177, #95413, #204020, #126902, #44518, #171550, #170480, #78060, #160383, #22065, #55668, #11983, #23145, #177708, #54605, #89261, #192860, #144185, #127984, #161464, #154248, #121824, #214404, #183013, #63942, #164644, #113840, #212307, #14100, #197133, #99639, #97534, #162527, #163591, #147340, #50891, #16227, #80190, #62869, #146295, #195012, #30392, #34630, #130097, #82310, #198188, #179836, #112768, #17296, #181938, #46645, #196091, #49823, #47723, #117014, #145239, #31457, #64989, #81261, #213368, #165707, #1040, #79123, #66034, #100700, #15174, #148405, #131144, #48771, #114886, #180885, #83373, #178780, #132182, #96480, #166777, #32507, #115948, #98582, #199244, #33568, #149457, #67103, #133239, #211244, #129036, #51965, #203504, #71374, #119149, #18373, #150538, #186203, #134306, #104989, #55156, #171030, #201374, #102842, #22626, #137489, #118088, #204573, #72450, #185131, #6379, #138550, #101769, #121303, #136422, #88736, #68176, #53015, #184074, #169959, #86586, #202438, #37838, #3169, #200314, #69240, #35693, #152652, #154792, #167837, #87657, #84450, #122385, #2102, #36757, #168898, #20501, #120230, #56222, #187277, #153726, #54093, #106090, #19435, #4236, #103914, #70306, #21546, #38905, #5295, #188342, #135357, #85515, #39981, #151601, #207784, #155860, #11716, #9593, #77790, #8524, #208842, #126629, #94073, #160114, #73527, #26902, #172112, #61542, #23705, #190466, #42125, #108238, #59411, #27980, #60472, #93006, #75669, #45312, #139629, #174262, #125568, #25834, #191529, #142836, #91943, #43193, #74605, #89815, #140709, #158005, #109306, #7447, #143911, #141777, #209904, #206724, #192593, #44247, #127708, #175316, #41056, #159051, #10643, #193669, #76719, #173190, #205652, #107165, #57289, #123452, #189414, #24770, #110368, #176374, #58351, #90873, #156935, #124507, #12771, #112492, #82047, #79915, #83110, #177435, #162252, #97262, #113565, #179568, #131915, #33299, #111430, #32243, #765, #96203, #196870, #146023, #30113, #46373, #14898, #197924, #210971, #98314, #78845, #132975, #178503, #164378, #13839, #17032, #15963, #80992, #212034, #144965, #31189, #194735, #62599, #148140, #214142, #63676, #29052, #95135, #64733, #128761, #49552, #65768, #115678, #129830, #195813, #181672, #99384 ),
 ( #165436, #47450, #163316, #198977, #161185, #149190, #147080, #213102, #130877, #48508, #66832, #114628, #180618, #68981, #53835, #118889, #71117, #3977, #85252, #36500, #185943, #102578, #86326, #151340, #152398, #20241, #202178, #19177, #52754, #70045, #54898, #184874, #35431, #5041, #67904, #100439, #136160, #116748, #34365, #168639, #119966, #101508, #37576, #21297, #182747, #103656, #169707, #153468, #167578, #2909, #137233, #87402, #134049, #203255, #50622, #51708, #200058, #166510, #18100, #84188, #150275, #135100, #1845, #201114, #117829, #183820, #92677, #157664, #76393, #10319, #11383, #143579, #106820, #142502, #141451, #110038, #73174, #58011, #123122, #174988, #91614, #207457, #42861, #8189, #139282, #74274, #56950, #9262, #159782, #205312, #158722, #23358, #127374, #89468, #41793, #107906, #173933, #125236, #93743, #60144, #208510, #59076, #111099, #189081, #25505, #191195, #75333, #108969, #126302, #26573, #192261, #140367, #155521, #206385, #43923, #176050, #7102, #77461, #27643, #209572, #124176, #61217, #193346, #44990, #40714, #172849, #24420, #90533, #156597, #190139, #178180, #160856, #46055, #78526, #128446, #66507, #113241, #130562, #147812, #30869, #48195, #79597, #177105, #145716, #96947, #212782, #12448, #16704, #14578, #82790, #13525, #213831, #131599, #99057, #195490, #112175, #47125, #162997, #148863, #114307, #29795, #144643, #95879, #210659, #194412, #132648, #161934, #180305, #81730, #211714, #62286, #115366, #65449, #63351, #129509, #197601, #179245, #437, #28721, #80674, #146764, #64418, #196552, #49244, #165112, #94807, #98008, #198652, #31927, #164063, #15642, #181355, #32981, #50301, #136891, #1508, #37243, #83850, #137959, #183484, #103314, #35093, #22023, #169376, #19910, #18837, #149940, #36162, #199724, #67574, #87058, #20960, #2579, #116419, #34039, #69718, #17762, #202918, #153130, #54562, #84922, #200780, #120708, #4703, #185612, #102241, #70777, #186683, #104388, #88132, #51370, #38311, #85995, #170435, #166173, #151010, #133719, #53490, #184542, #152069, #135821, #101164, #117493, #167251, #68649, #168313, #154203, #134772, #5772, #182410, #71851, #100112, #52432, #118558, #3639, #201846, #203979, #119627, #124983, #173678, #143323, #171508, #57764, #91354, #157415, #93488, #42607, #206134, #9006, #142247, #75081, #190943, #140107, #108715, #58829, #158468, #123925, #25253, #174742, #55626, #141194, #90275, #27388, #56700, #23101, #26316, #187750, #105475, #207205, #10068, #24172, #208260, #43670, #121783, #92428, #76144, #175796, #156344, #189893, #159527, #59893, #122867, #126043, #39379, #6850, #155269, #192005, #109788, #41535, #11126, #188828, #77204, #89217, #72928, #139034, #205058, #107646, #40463, #106566, #172594, #7929, #74017, #95633, #213582, #112988, #80415, #14323, #211462, #96702, #180055, #128196, #63097, #82534, #60963, #97755, #16453, #210399, #31677, #64171, #147560, #131357, #115112, #163813, #48994, #32726, #197352, #178998, #146513, #161682, #212531, #12202, #209316, #129266, #79350, #62043, #65205, #194157, #46874, #45805, #15390, #127120, #130314, #81483, #181110, #29541, #30613, #195237, #98807, #164860, #193088, #111926, #110844, #78272, #28464, #162750, #177927, #44738, #196302, #176850, #47948, #94557, #114063, #160597, #144398, #13276, #145467, #198406, #186427, #118305, #150762, #68400, #36982, #99866, #38066, #1264, #151824, #53243, #183237, #182157, #86809, #103065, #50050, #149683, #119373, #117237, #120452, #188, #199470, #134528, #2325, #200534, #169121, #70523, #148620, #69466, #104135, #133467, #19663, #34841, #67323, #83601, #52180, #20716, #33787, #135571, #116171, #170181, #51112, #201595, #100916, #54314, #185360, #184292, #167004, #165929, #35917, #17514, #18595, #152875, #4453, #84674, #66256, #132404, #101993, #168061, #136640, #202664, #21769, #85739, #3397, #174484, #140932, #157160, #7670, #206946, #74833, #75890, #208011, #171250, #58576, #205880, #26061, #137707, #122605, #187499, #24996, #156084, #57514, #107393, #72679, #203728, #138775, #121530, #73756, #9814, #55375, #8751, #87877, #191755, #153950, #106311 ) ),
 .UNSPECIFIED., .F., .F., .F. ) 
 B_SPLINE_SURFACE_WITH_KNOTS ( ( 2, 2 ),
 ( 3, 2, 2, 2, 2, 2, 2, 2, 2, 2, 2, 2, 2, 2, 2, 2, 2, 2, 2, 2, 2, 2, 2, 2, 2, 2, 2, 2, 2, 2, 2, 2, 2, 2, 2, 2, 2, 2, 2, 2, 2, 2, 2, 2, 2, 2, 2, 2, 2, 2, 2, 2, 2, 2, 2, 2, 2, 2, 2, 2, 2, 2, 2, 2, 2, 2, 2, 2, 2, 2, 2, 2, 2, 2, 2, 2, 2, 2, 2, 2, 2, 2, 2, 2, 2, 2, 2, 2, 2, 2, 2, 2, 2, 2, 2, 2, 2, 2, 2, 2, 2, 2, 2, 2, 2, 2, 2, 2, 2, 2, 2, 2, 2, 2, 2, 2, 2, 2, 2, 2, 2, 2, 2, 2, 2, 2, 2, 2, 2, 2, 2, 2, 2, 2, 2, 2, 2, 2, 2, 2, 2, 2, 2, 2, 2, 2, 2, 2, 2, 2, 2, 2, 2, 2, 2, 2, 2, 2, 2, 2, 2, 2, 2, 2, 2, 2, 2, 2, 2, 2, 2, 2, 2, 2, 2, 2, 2, 2, 2, 2, 2, 2, 2, 2, 2, 2, 2, 2, 2, 2, 2, 2, 2, 2, 2, 2, 2, 2, 2, 2, 2, 2, 2, 2, 2, 2, 2, 2, 2, 2, 2, 2, 2, 2, 2, 2, 2, 2, 2, 2, 2, 2, 2, 2, 2, 2, 2, 2, 2, 2, 2, 2, 2, 2, 2, 2, 2, 2, 2, 2, 3 ),
 ( 0.000000000000000000, 1.000000000000000000 ),
 ( 0.000000000000000000, 0.004166666666666666609, 0.008333333333333333218, 0.01250000000000000069, 0.01666666666666666644, 0.02083333333333333218, 0.02500000000000000139, 0.02916666666666666713, 0.03333333333333333287, 0.03749999999999999861, 0.04166666666666666435, 0.04583333333333333010, 0.05000000000000000278, 0.05416666666666666852, 0.05833333333333333426, 0.06250000000000000000, 0.06666666666666666574, 0.07083333333333333148, 0.07499999999999999722, 0.07916666666666666297, 0.08333333333333332871, 0.08749999999999999445, 0.09166666666666666019, 0.09583333333333333981, 0.1000000000000000056, 0.1041666666666666713, 0.1083333333333333370, 0.1125000000000000028, 0.1166666666666666685, 0.1208333333333333343, 0.1250000000000000000, 0.1291666666666666796, 0.1333333333333333315, 0.1375000000000000111, 0.1416666666666666630, 0.1458333333333333426, 0.1499999999999999944, 0.1541666666666666741, 0.1583333333333333259, 0.1625000000000000056, 0.1666666666666666574, 0.1708333333333333370, 0.1749999999999999889, 0.1791666666666666685, 0.1833333333333333204, 0.1875000000000000000, 0.1916666666666666796, 0.1958333333333333315, 0.2000000000000000111, 0.2041666666666666630, 0.2083333333333333426, 0.2124999999999999944, 0.2166666666666666741, 0.2208333333333333259, 0.2250000000000000056, 0.2291666666666666574, 0.2333333333333333370, 0.2374999999999999889, 0.2416666666666666685, 0.2458333333333333204, 0.2500000000000000000, 0.2541666666666666519, 0.2583333333333333592, 0.2625000000000000111, 0.2666666666666666630, 0.2708333333333333148, 0.2750000000000000222, 0.2791666666666666741, 0.2833333333333333259, 0.2874999999999999778, 0.2916666666666666852, 0.2958333333333333370, 0.2999999999999999889, 0.3041666666666666408, 0.3083333333333333481, 0.3125000000000000000, 0.3166666666666666519, 0.3208333333333333592, 0.3250000000000000111, 0.3291666666666666630, 0.3333333333333333148, 0.3375000000000000222, 0.3416666666666666741, 0.3458333333333333259, 0.3499999999999999778, 0.3541666666666666852, 0.3583333333333333370, 0.3624999999999999889, 0.3666666666666666408, 0.3708333333333333481, 0.3750000000000000000, 0.3791666666666666519, 0.3833333333333333592, 0.3875000000000000111, 0.3916666666666666630, 0.3958333333333333148, 0.4000000000000000222, 0.4041666666666666741, 0.4083333333333333259, 0.4124999999999999778, 0.4166666666666666852, 0.4208333333333333370, 0.4249999999999999889, 0.4291666666666666408, 0.4333333333333333481, 0.4375000000000000000, 0.4416666666666666519, 0.4458333333333333592, 0.4500000000000000111, 0.4541666666666666630, 0.4583333333333333148, 0.4625000000000000222, 0.4666666666666666741, 0.4708333333333333259, 0.4749999999999999778, 0.4791666666666666852, 0.4833333333333333370, 0.4874999999999999889, 0.4916666666666666408, 0.4958333333333333481, 0.5000000000000000000, 0.5041666666666666519, 0.5083333333333333037, 0.5124999999999999556, 0.5166666666666667185, 0.5208333333333333703, 0.5250000000000000222, 0.5291666666666666741, 0.5333333333333333259, 0.5374999999999999778, 0.5416666666666666297, 0.5458333333333332815, 0.5500000000000000444, 0.5541666666666666963, 0.5583333333333333481, 0.5625000000000000000, 0.5666666666666666519, 0.5708333333333333037, 0.5749999999999999556, 0.5791666666666667185, 0.5833333333333333703, 0.5875000000000000222, 0.5916666666666666741, 0.5958333333333333259, 0.5999999999999999778, 0.6041666666666666297, 0.6083333333333332815, 0.6125000000000000444, 0.6166666666666666963, 0.6208333333333333481, 0.6250000000000000000, 0.6291666666666666519, 0.6333333333333333037, 0.6374999999999999556, 0.6416666666666667185, 0.6458333333333333703, 0.6500000000000000222, 0.6541666666666666741, 0.6583333333333333259, 0.6624999999999999778, 0.6666666666666666297, 0.6708333333333332815, 0.6750000000000000444, 0.6791666666666666963, 0.6833333333333333481, 0.6875000000000000000, 0.6916666666666666519, 0.6958333333333333037, 0.6999999999999999556, 0.7041666666666667185, 0.7083333333333333703, 0.7125000000000000222, 0.7166666666666666741, 0.7208333333333333259, 0.7249999999999999778, 0.7291666666666666297, 0.7333333333333332815, 0.7375000000000000444, 0.7416666666666666963, 0.7458333333333333481, 0.7500000000000000000, 0.7541666666666666519, 0.7583333333333333037, 0.7624999999999999556, 0.7666666666666667185, 0.7708333333333333703, 0.7750000000000000222, 0.7791666666666666741, 0.7833333333333333259, 0.7874999999999999778, 0.7916666666666666297, 0.7958333333333332815, 0.8000000000000000444, 0.8041666666666666963, 0.8083333333333333481, 0.8125000000000000000, 0.8166666666666666519, 0.8208333333333333037, 0.8249999999999999556, 0.8291666666666667185, 0.8333333333333333703, 0.8375000000000000222, 0.8416666666666666741, 0.8458333333333333259, 0.8499999999999999778, 0.8541666666666666297, 0.8583333333333332815, 0.8625000000000000444, 0.8666666666666666963, 0.8708333333333333481, 0.8750000000000000000, 0.8791666666666666519, 0.8833333333333333037, 0.8874999999999999556, 0.8916666666666667185, 0.8958333333333333703, 0.9000000000000000222, 0.9041666666666666741, 0.9083333333333333259, 0.9124999999999999778, 0.9166666666666666297, 0.9208333333333332815, 0.9250000000000000444, 0.9291666666666666963, 0.9333333333333333481, 0.9375000000000000000, 0.9416666666666666519, 0.9458333333333333037, 0.9499999999999999556, 0.9541666666666667185, 0.9583333333333333703, 0.9625000000000000222, 0.9666666666666666741, 0.9708333333333333259, 0.9749999999999999778, 0.9791666666666666297, 0.9833333333333332815, 0.9875000000000000444, 0.9916666666666666963, 0.9958333333333333481, 1.000000000000000000 ),
 .UNSPECIFIED. ) 
 GEOMETRIC_REPRESENTATION_ITEM ( )  RATIONAL_B_SPLINE_SURFACE ( (
 ( 1.000000000000000000, 0.8660254037844387076, 1.000000000000000000, 0.8660254037844387076, 1.000000000000000000, 0.8660254037844387076, 1.000000000000000000, 0.8660254037844387076, 1.000000000000000000, 0.8660254037844387076, 1.000000000000000000, 0.8660254037844387076, 1.000000000000000000, 0.8660254037844387076, 1.000000000000000000, 0.8660254037844387076, 1.000000000000000000, 0.8660254037844387076, 1.000000000000000000, 0.8660254037844387076, 1.000000000000000000, 0.8660254037844387076, 1.000000000000000000, 0.8660254037844387076, 1.000000000000000000, 0.8660254037844387076, 1.000000000000000000, 0.8660254037844387076, 1.000000000000000000, 0.8660254037844387076, 1.000000000000000000, 0.8660254037844387076, 1.000000000000000000, 0.8660254037844387076, 1.000000000000000000, 0.8660254037844387076, 1.000000000000000000, 0.8660254037844387076, 1.000000000000000000, 0.8660254037844387076, 1.000000000000000000, 0.8660254037844387076, 1.000000000000000000, 0.8660254037844387076, 1.000000000000000000, 0.8660254037844387076, 1.000000000000000000, 0.8660254037844387076, 1.000000000000000000, 0.8660254037844387076, 1.000000000000000000, 0.8660254037844387076, 1.000000000000000000, 0.8660254037844387076, 1.000000000000000000, 0.8660254037844387076, 1.000000000000000000, 0.8660254037844387076, 1.000000000000000000, 0.8660254037844387076, 1.000000000000000000, 0.8660254037844387076, 1.000000000000000000, 0.8660254037844387076, 1.000000000000000000, 0.8660254037844387076, 1.000000000000000000, 0.8660254037844387076, 1.000000000000000000, 0.8660254037844387076, 1.000000000000000000, 0.8660254037844387076, 1.000000000000000000, 0.8660254037844387076, 1.000000000000000000, 0.8660254037844387076, 1.000000000000000000, 0.8660254037844387076, 1.000000000000000000, 0.8660254037844387076, 1.000000000000000000, 0.8660254037844387076, 1.000000000000000000, 0.8660254037844387076, 1.000000000000000000, 0.8660254037844387076, 1.000000000000000000, 0.8660254037844387076, 1.000000000000000000, 0.8660254037844387076, 1.000000000000000000, 0.8660254037844387076, 1.000000000000000000, 0.8660254037844387076, 1.000000000000000000, 0.8660254037844387076, 1.000000000000000000, 0.8660254037844387076, 1.000000000000000000, 0.8660254037844387076, 1.000000000000000000, 0.8660254037844387076, 1.000000000000000000, 0.8660254037844387076, 1.000000000000000000, 0.8660254037844387076, 1.000000000000000000, 0.8660254037844387076, 1.000000000000000000, 0.8660254037844387076, 1.000000000000000000, 0.8660254037844387076, 1.000000000000000000, 0.8660254037844387076, 1.000000000000000000, 0.8660254037844387076, 1.000000000000000000, 0.8660254037844387076, 1.000000000000000000, 0.8660254037844387076, 1.000000000000000000, 0.8660254037844387076, 1.000000000000000000, 0.8660254037844387076, 1.000000000000000000, 0.8660254037844387076, 1.000000000000000000, 0.8660254037844387076, 1.000000000000000000, 0.8660254037844387076, 1.000000000000000000, 0.8660254037844387076, 1.000000000000000000, 0.8660254037844387076, 1.000000000000000000, 0.8660254037844387076, 1.000000000000000000, 0.8660254037844387076, 1.000000000000000000, 0.8660254037844387076, 1.000000000000000000, 0.8660254037844387076, 1.000000000000000000, 0.8660254037844387076, 1.000000000000000000, 0.8660254037844387076, 1.000000000000000000, 0.8660254037844387076, 1.000000000000000000, 0.8660254037844387076, 1.000000000000000000, 0.8660254037844387076, 1.000000000000000000, 0.8660254037844387076, 1.000000000000000000, 0.8660254037844387076, 1.000000000000000000, 0.8660254037844387076, 1.000000000000000000, 0.8660254037844387076, 1.000000000000000000, 0.8660254037844387076, 1.000000000000000000, 0.8660254037844387076, 1.000000000000000000, 0.8660254037844387076, 1.000000000000000000, 0.8660254037844387076, 1.000000000000000000, 0.8660254037844387076, 1.000000000000000000, 0.8660254037844387076, 1.000000000000000000, 0.8660254037844387076, 1.000000000000000000, 0.8660254037844387076, 1.000000000000000000, 0.8660254037844387076, 1.000000000000000000, 0.8660254037844387076, 1.000000000000000000, 0.8660254037844387076, 1.000000000000000000, 0.8660254037844387076, 1.000000000000000000, 0.8660254037844387076, 1.000000000000000000, 0.8660254037844387076, 1.000000000000000000, 0.8660254037844387076, 1.000000000000000000, 0.8660254037844387076, 1.000000000000000000, 0.8660254037844387076, 1.000000000000000000, 0.8660254037844387076, 1.000000000000000000, 0.8660254037844387076, 1.000000000000000000, 0.8660254037844387076, 1.000000000000000000, 0.8660254037844387076, 1.000000000000000000, 0.8660254037844387076, 1.000000000000000000, 0.8660254037844387076, 1.000000000000000000, 0.8660254037844387076, 1.000000000000000000, 0.8660254037844387076, 1.000000000000000000, 0.8660254037844387076, 1.000000000000000000, 0.8660254037844387076, 1.000000000000000000, 0.8660254037844387076, 1.000000000000000000, 0.8660254037844387076, 1.000000000000000000, 0.8660254037844387076, 1.000000000000000000, 0.8660254037844387076, 1.000000000000000000, 0.8660254037844387076, 1.000000000000000000, 0.8660254037844387076, 1.000000000000000000, 0.8660254037844387076, 1.000000000000000000, 0.8660254037844387076, 1.000000000000000000, 0.8660254037844387076, 1.000000000000000000, 0.8660254037844387076, 1.000000000000000000, 0.8660254037844387076, 1.000000000000000000, 0.8660254037844387076, 1.000000000000000000, 0.8660254037844387076, 1.000000000000000000, 0.8660254037844387076, 1.000000000000000000, 0.8660254037844387076, 1.000000000000000000, 0.8660254037844387076, 1.000000000000000000, 0.8660254037844387076, 1.000000000000000000, 0.8660254037844387076, 1.000000000000000000, 0.8660254037844387076, 1.000000000000000000, 0.8660254037844387076, 1.000000000000000000, 0.8660254037844387076, 1.000000000000000000, 0.8660254037844387076, 1.000000000000000000, 0.8660254037844387076, 1.000000000000000000, 0.8660254037844387076, 1.000000000000000000, 0.8660254037844387076, 1.000000000000000000, 0.8660254037844387076, 1.000000000000000000, 0.8660254037844387076, 1.000000000000000000, 0.8660254037844387076, 1.000000000000000000, 0.8660254037844387076, 1.000000000000000000, 0.8660254037844387076, 1.000000000000000000, 0.8660254037844387076, 1.000000000000000000, 0.8660254037844387076, 1.000000000000000000, 0.8660254037844387076, 1.000000000000000000, 0.8660254037844387076, 1.000000000000000000, 0.8660254037844387076, 1.000000000000000000, 0.8660254037844387076, 1.000000000000000000, 0.8660254037844387076, 1.000000000000000000, 0.8660254037844387076, 1.000000000000000000, 0.8660254037844387076, 1.000000000000000000, 0.8660254037844387076, 1.000000000000000000, 0.8660254037844387076, 1.000000000000000000, 0.8660254037844387076, 1.000000000000000000, 0.8660254037844387076, 1.000000000000000000, 0.8660254037844387076, 1.000000000000000000, 0.8660254037844387076, 1.000000000000000000, 0.8660254037844387076, 1.000000000000000000, 0.8660254037844387076, 1.000000000000000000, 0.8660254037844387076, 1.000000000000000000, 0.8660254037844387076, 1.000000000000000000, 0.8660254037844387076, 1.000000000000000000, 0.8660254037844387076, 1.000000000000000000, 0.8660254037844387076, 1.000000000000000000, 0.8660254037844387076, 1.000000000000000000, 0.8660254037844387076, 1.000000000000000000, 0.8660254037844387076, 1.000000000000000000, 0.8660254037844387076, 1.000000000000000000, 0.8660254037844387076, 1.000000000000000000, 0.8660254037844387076, 1.000000000000000000, 0.8660254037844387076, 1.000000000000000000, 0.8660254037844387076, 1.000000000000000000, 0.8660254037844387076, 1.000000000000000000, 0.8660254037844387076, 1.000000000000000000, 0.8660254037844387076, 1.000000000000000000, 0.8660254037844387076, 1.000000000000000000, 0.8660254037844387076, 1.000000000000000000, 0.8660254037844387076, 1.000000000000000000, 0.8660254037844387076, 1.000000000000000000, 0.8660254037844387076, 1.000000000000000000, 0.8660254037844387076, 1.000000000000000000, 0.8660254037844387076, 1.000000000000000000, 0.8660254037844387076, 1.000000000000000000, 0.8660254037844387076, 1.000000000000000000, 0.8660254037844387076, 1.000000000000000000, 0.8660254037844387076, 1.000000000000000000, 0.8660254037844387076, 1.000000000000000000, 0.8660254037844387076, 1.000000000000000000, 0.8660254037844387076, 1.000000000000000000, 0.8660254037844387076, 1.000000000000000000, 0.8660254037844387076, 1.000000000000000000, 0.8660254037844387076, 1.000000000000000000, 0.8660254037844387076, 1.000000000000000000, 0.8660254037844387076, 1.000000000000000000, 0.8660254037844387076, 1.000000000000000000, 0.8660254037844387076, 1.000000000000000000, 0.8660254037844387076, 1.000000000000000000, 0.8660254037844387076, 1.000000000000000000, 0.8660254037844387076, 1.000000000000000000, 0.8660254037844387076, 1.000000000000000000, 0.8660254037844387076, 1.000000000000000000, 0.8660254037844387076, 1.000000000000000000, 0.8660254037844387076, 1.000000000000000000, 0.8660254037844387076, 1.000000000000000000, 0.8660254037844387076, 1.000000000000000000, 0.8660254037844387076, 1.000000000000000000, 0.8660254037844387076, 1.000000000000000000, 0.8660254037844387076, 1.000000000000000000, 0.8660254037844387076, 1.000000000000000000, 0.8660254037844387076, 1.000000000000000000, 0.8660254037844387076, 1.000000000000000000, 0.8660254037844387076, 1.000000000000000000, 0.8660254037844387076, 1.000000000000000000, 0.8660254037844387076, 1.000000000000000000, 0.8660254037844387076, 1.000000000000000000, 0.8660254037844387076, 1.000000000000000000, 0.8660254037844387076, 1.000000000000000000, 0.8660254037844387076, 1.000000000000000000, 0.8660254037844387076, 1.000000000000000000, 0.8660254037844387076, 1.000000000000000000, 0.8660254037844387076, 1.000000000000000000, 0.8660254037844387076, 1.000000000000000000, 0.8660254037844387076, 1.000000000000000000, 0.8660254037844387076, 1.000000000000000000, 0.8660254037844387076, 1.000000000000000000, 0.8660254037844387076, 1.000000000000000000, 0.8660254037844387076, 1.000000000000000000, 0.8660254037844387076, 1.000000000000000000, 0.8660254037844387076, 1.000000000000000000, 0.8660254037844387076, 1.000000000000000000, 0.8660254037844387076, 1.000000000000000000, 0.8660254037844387076, 1.000000000000000000, 0.8660254037844387076, 1.000000000000000000, 0.8660254037844387076, 1.000000000000000000, 0.8660254037844387076, 1.000000000000000000, 0.8660254037844387076, 1.000000000000000000, 0.8660254037844387076, 1.000000000000000000, 0.8660254037844387076, 1.000000000000000000, 0.8660254037844387076, 1.000000000000000000, 0.8660254037844387076, 1.000000000000000000, 0.8660254037844387076, 1.000000000000000000, 0.8660254037844387076, 1.000000000000000000, 0.8660254037844387076, 1.000000000000000000, 0.8660254037844387076, 1.000000000000000000, 0.8660254037844387076, 1.000000000000000000),
 ( 1.000000000000000000, 0.8660254037844387076, 1.000000000000000000, 0.8660254037844387076, 1.000000000000000000, 0.8660254037844387076, 1.000000000000000000, 0.8660254037844387076, 1.000000000000000000, 0.8660254037844387076, 1.000000000000000000, 0.8660254037844387076, 1.000000000000000000, 0.8660254037844387076, 1.000000000000000000, 0.8660254037844387076, 1.000000000000000000, 0.8660254037844387076, 1.000000000000000000, 0.8660254037844387076, 1.000000000000000000, 0.8660254037844387076, 1.000000000000000000, 0.8660254037844387076, 1.000000000000000000, 0.8660254037844387076, 1.000000000000000000, 0.8660254037844387076, 1.000000000000000000, 0.8660254037844387076, 1.000000000000000000, 0.8660254037844387076, 1.000000000000000000, 0.8660254037844387076, 1.000000000000000000, 0.8660254037844387076, 1.000000000000000000, 0.8660254037844387076, 1.000000000000000000, 0.8660254037844387076, 1.000000000000000000, 0.8660254037844387076, 1.000000000000000000, 0.8660254037844387076, 1.000000000000000000, 0.8660254037844387076, 1.000000000000000000, 0.8660254037844387076, 1.000000000000000000, 0.8660254037844387076, 1.000000000000000000, 0.8660254037844387076, 1.000000000000000000, 0.8660254037844387076, 1.000000000000000000, 0.8660254037844387076, 1.000000000000000000, 0.8660254037844387076, 1.000000000000000000, 0.8660254037844387076, 1.000000000000000000, 0.8660254037844387076, 1.000000000000000000, 0.8660254037844387076, 1.000000000000000000, 0.8660254037844387076, 1.000000000000000000, 0.8660254037844387076, 1.000000000000000000, 0.8660254037844387076, 1.000000000000000000, 0.8660254037844387076, 1.000000000000000000, 0.8660254037844387076, 1.000000000000000000, 0.8660254037844387076, 1.000000000000000000, 0.8660254037844387076, 1.000000000000000000, 0.8660254037844387076, 1.000000000000000000, 0.8660254037844387076, 1.000000000000000000, 0.8660254037844387076, 1.000000000000000000, 0.8660254037844387076, 1.000000000000000000, 0.8660254037844387076, 1.000000000000000000, 0.8660254037844387076, 1.000000000000000000, 0.8660254037844387076, 1.000000000000000000, 0.8660254037844387076, 1.000000000000000000, 0.8660254037844387076, 1.000000000000000000, 0.8660254037844387076, 1.000000000000000000, 0.8660254037844387076, 1.000000000000000000, 0.8660254037844387076, 1.000000000000000000, 0.8660254037844387076, 1.000000000000000000, 0.8660254037844387076, 1.000000000000000000, 0.8660254037844387076, 1.000000000000000000, 0.8660254037844387076, 1.000000000000000000, 0.8660254037844387076, 1.000000000000000000, 0.8660254037844387076, 1.000000000000000000, 0.8660254037844387076, 1.000000000000000000, 0.8660254037844387076, 1.000000000000000000, 0.8660254037844387076, 1.000000000000000000, 0.8660254037844387076, 1.000000000000000000, 0.8660254037844387076, 1.000000000000000000, 0.8660254037844387076, 1.000000000000000000, 0.8660254037844387076, 1.000000000000000000, 0.8660254037844387076, 1.000000000000000000, 0.8660254037844387076, 1.000000000000000000, 0.8660254037844387076, 1.000000000000000000, 0.8660254037844387076, 1.000000000000000000, 0.8660254037844387076, 1.000000000000000000, 0.8660254037844387076, 1.000000000000000000, 0.8660254037844387076, 1.000000000000000000, 0.8660254037844387076, 1.000000000000000000, 0.8660254037844387076, 1.000000000000000000, 0.8660254037844387076, 1.000000000000000000, 0.8660254037844387076, 1.000000000000000000, 0.8660254037844387076, 1.000000000000000000, 0.8660254037844387076, 1.000000000000000000, 0.8660254037844387076, 1.000000000000000000, 0.8660254037844387076, 1.000000000000000000, 0.8660254037844387076, 1.000000000000000000, 0.8660254037844387076, 1.000000000000000000, 0.8660254037844387076, 1.000000000000000000, 0.8660254037844387076, 1.000000000000000000, 0.8660254037844387076, 1.000000000000000000, 0.8660254037844387076, 1.000000000000000000, 0.8660254037844387076, 1.000000000000000000, 0.8660254037844387076, 1.000000000000000000, 0.8660254037844387076, 1.000000000000000000, 0.8660254037844387076, 1.000000000000000000, 0.8660254037844387076, 1.000000000000000000, 0.8660254037844387076, 1.000000000000000000, 0.8660254037844387076, 1.000000000000000000, 0.8660254037844387076, 1.000000000000000000, 0.8660254037844387076, 1.000000000000000000, 0.8660254037844387076, 1.000000000000000000, 0.8660254037844387076, 1.000000000000000000, 0.8660254037844387076, 1.000000000000000000, 0.8660254037844387076, 1.000000000000000000, 0.8660254037844387076, 1.000000000000000000, 0.8660254037844387076, 1.000000000000000000, 0.8660254037844387076, 1.000000000000000000, 0.8660254037844387076, 1.000000000000000000, 0.8660254037844387076, 1.000000000000000000, 0.8660254037844387076, 1.000000000000000000, 0.8660254037844387076, 1.000000000000000000, 0.8660254037844387076, 1.000000000000000000, 0.8660254037844387076, 1.000000000000000000, 0.8660254037844387076, 1.000000000000000000, 0.8660254037844387076, 1.000000000000000000, 0.8660254037844387076, 1.000000000000000000, 0.8660254037844387076, 1.000000000000000000, 0.8660254037844387076, 1.000000000000000000, 0.8660254037844387076, 1.000000000000000000, 0.8660254037844387076, 1.000000000000000000, 0.8660254037844387076, 1.000000000000000000, 0.8660254037844387076, 1.000000000000000000, 0.8660254037844387076, 1.000000000000000000, 0.8660254037844387076, 1.000000000000000000, 0.8660254037844387076, 1.000000000000000000, 0.8660254037844387076, 1.000000000000000000, 0.8660254037844387076, 1.000000000000000000, 0.8660254037844387076, 1.000000000000000000, 0.8660254037844387076, 1.000000000000000000, 0.8660254037844387076, 1.000000000000000000, 0.8660254037844387076, 1.000000000000000000, 0.8660254037844387076, 1.000000000000000000, 0.8660254037844387076, 1.000000000000000000, 0.8660254037844387076, 1.000000000000000000, 0.8660254037844387076, 1.000000000000000000, 0.8660254037844387076, 1.000000000000000000, 0.8660254037844387076, 1.000000000000000000, 0.8660254037844387076, 1.000000000000000000, 0.8660254037844387076, 1.000000000000000000, 0.8660254037844387076, 1.000000000000000000, 0.8660254037844387076, 1.000000000000000000, 0.8660254037844387076, 1.000000000000000000, 0.8660254037844387076, 1.000000000000000000, 0.8660254037844387076, 1.000000000000000000, 0.8660254037844387076, 1.000000000000000000, 0.8660254037844387076, 1.000000000000000000, 0.8660254037844387076, 1.000000000000000000, 0.8660254037844387076, 1.000000000000000000, 0.8660254037844387076, 1.000000000000000000, 0.8660254037844387076, 1.000000000000000000, 0.8660254037844387076, 1.000000000000000000, 0.8660254037844387076, 1.000000000000000000, 0.8660254037844387076, 1.000000000000000000, 0.8660254037844387076, 1.000000000000000000, 0.8660254037844387076, 1.000000000000000000, 0.8660254037844387076, 1.000000000000000000, 0.8660254037844387076, 1.000000000000000000, 0.8660254037844387076, 1.000000000000000000, 0.8660254037844387076, 1.000000000000000000, 0.8660254037844387076, 1.000000000000000000, 0.8660254037844387076, 1.000000000000000000, 0.8660254037844387076, 1.000000000000000000, 0.8660254037844387076, 1.000000000000000000, 0.8660254037844387076, 1.000000000000000000, 0.8660254037844387076, 1.000000000000000000, 0.8660254037844387076, 1.000000000000000000, 0.8660254037844387076, 1.000000000000000000, 0.8660254037844387076, 1.000000000000000000, 0.8660254037844387076, 1.000000000000000000, 0.8660254037844387076, 1.000000000000000000, 0.8660254037844387076, 1.000000000000000000, 0.8660254037844387076, 1.000000000000000000, 0.8660254037844387076, 1.000000000000000000, 0.8660254037844387076, 1.000000000000000000, 0.8660254037844387076, 1.000000000000000000, 0.8660254037844387076, 1.000000000000000000, 0.8660254037844387076, 1.000000000000000000, 0.8660254037844387076, 1.000000000000000000, 0.8660254037844387076, 1.000000000000000000, 0.8660254037844387076, 1.000000000000000000, 0.8660254037844387076, 1.000000000000000000, 0.8660254037844387076, 1.000000000000000000, 0.8660254037844387076, 1.000000000000000000, 0.8660254037844387076, 1.000000000000000000, 0.8660254037844387076, 1.000000000000000000, 0.8660254037844387076, 1.000000000000000000, 0.8660254037844387076, 1.000000000000000000, 0.8660254037844387076, 1.000000000000000000, 0.8660254037844387076, 1.000000000000000000, 0.8660254037844387076, 1.000000000000000000, 0.8660254037844387076, 1.000000000000000000, 0.8660254037844387076, 1.000000000000000000, 0.8660254037844387076, 1.000000000000000000, 0.8660254037844387076, 1.000000000000000000, 0.8660254037844387076, 1.000000000000000000, 0.8660254037844387076, 1.000000000000000000, 0.8660254037844387076, 1.000000000000000000, 0.8660254037844387076, 1.000000000000000000, 0.8660254037844387076, 1.000000000000000000, 0.8660254037844387076, 1.000000000000000000, 0.8660254037844387076, 1.000000000000000000, 0.8660254037844387076, 1.000000000000000000, 0.8660254037844387076, 1.000000000000000000, 0.8660254037844387076, 1.000000000000000000, 0.8660254037844387076, 1.000000000000000000, 0.8660254037844387076, 1.000000000000000000, 0.8660254037844387076, 1.000000000000000000, 0.8660254037844387076, 1.000000000000000000, 0.8660254037844387076, 1.000000000000000000, 0.8660254037844387076, 1.000000000000000000, 0.8660254037844387076, 1.000000000000000000, 0.8660254037844387076, 1.000000000000000000, 0.8660254037844387076, 1.000000000000000000, 0.8660254037844387076, 1.000000000000000000, 0.8660254037844387076, 1.000000000000000000, 0.8660254037844387076, 1.000000000000000000, 0.8660254037844387076, 1.000000000000000000, 0.8660254037844387076, 1.000000000000000000, 0.8660254037844387076, 1.000000000000000000, 0.8660254037844387076, 1.000000000000000000, 0.8660254037844387076, 1.000000000000000000, 0.8660254037844387076, 1.000000000000000000, 0.8660254037844387076, 1.000000000000000000, 0.8660254037844387076, 1.000000000000000000, 0.8660254037844387076, 1.000000000000000000, 0.8660254037844387076, 1.000000000000000000, 0.8660254037844387076, 1.000000000000000000, 0.8660254037844387076, 1.000000000000000000, 0.8660254037844387076, 1.000000000000000000, 0.8660254037844387076, 1.000000000000000000, 0.8660254037844387076, 1.000000000000000000, 0.8660254037844387076, 1.000000000000000000, 0.8660254037844387076, 1.000000000000000000, 0.8660254037844387076, 1.000000000000000000, 0.8660254037844387076, 1.000000000000000000, 0.8660254037844387076, 1.000000000000000000, 0.8660254037844387076, 1.000000000000000000, 0.8660254037844387076, 1.000000000000000000, 0.8660254037844387076, 1.000000000000000000, 0.8660254037844387076, 1.000000000000000000, 0.8660254037844387076, 1.000000000000000000, 0.8660254037844387076, 1.000000000000000000, 0.8660254037844387076, 1.000000000000000000, 0.8660254037844387076, 1.000000000000000000, 0.8660254037844387076, 1.000000000000000000, 0.8660254037844387076, 1.000000000000000000) ) ) 
 REPRESENTATION_ITEM ( '' )  SURFACE ( )  );
#10603=CARTESIAN_POINT ( 'NONE',  ( 7.560643217915098191, 11.97250085420964716, -0.7998128361456291469 ) ) ;
#10606=CARTESIAN_POINT ( 'NONE',  ( 1.499999999999989120, 1.025000000000019007, 0.000000000000000000 ) ) ;
#10611=CARTESIAN_POINT ( 'NONE',  ( 8.062294901620731480, 12.55776115186623620, 1.040834085586084257E-14 ) ) ;
#10617=CARTESIAN_POINT ( 'NONE',  ( -5.070386261386537363, 5.017798181146802428, 1.214306433183764966E-14 ) ) ;
#10620=CARTESIAN_POINT ( 'NONE',  ( 0.6823417656249864960, -1.073958332991911568, -1.181850606188749264 ) ) ;
#10626=CARTESIAN_POINT ( 'NONE',  ( 1.364683531249988535, 4.363541667008090208, 0.7879004041258500513 ) ) ;
#10628=CARTESIAN_POINT ( 'NONE',  ( -6.317736394288148816, 8.393778431468064127, 1.443375672974078761 ) ) ;
#10637=CARTESIAN_POINT ( 'NONE',  ( 7.914208982075123799, 10.25632978388623684, -1.599625672291262513 ) ) ;
#10638=CARTESIAN_POINT ( 'NONE',  ( 6.520158902582594784, 5.290451655907107309, -2.438235897557449405 ) ) ;
#10643=CARTESIAN_POINT ( 'NONE',  ( -9.820183334999905256, 10.35130206712171130, 1.040834085586084257E-14 ) ) ;
#10644=( BOUNDED_SURFACE ( )  B_SPLINE_SURFACE ( 3, 1, ( 
 ( #149942, #116421 ),
 ( #439, #65451 ),
 ( #66508, #100114 ),
 ( #148865, #49245 ),
 ( #132649, #50303 ),
 ( #81732, #198654 ),
 ( #85997, #147814 ) ),
 .UNSPECIFIED., .T., .F., .T. ) 
 B_SPLINE_SURFACE_WITH_KNOTS ( ( 4, 3, 4 ),
 ( 2, 2 ),
 ( 0.000000000000000000, 0.5000000000000000000, 1.000000000000000000 ),
 ( 0.000000000000000000, 1.000000000000000000 ),
 .UNSPECIFIED. ) 
 GEOMETRIC_REPRESENTATION_ITEM ( )  RATIONAL_B_SPLINE_SURFACE ( (
 ( 1.000000000000000000, 1.000000000000000000),
 ( 0.3333333333333333703, 0.3333333333333333703),
 ( 0.3333333333333333703, 0.3333333333333333703),
 ( 1.000000000000000000, 1.000000000000000000),
 ( 0.3333333333333333703, 0.3333333333333333703),
 ( 0.3333333333333333703, 0.3333333333333333703),
 ( 1.000000000000000000, 1.000000000000000000) ) ) 
 REPRESENTATION_ITEM ( '' )  SURFACE ( )  );
#10645=CARTESIAN_POINT ( 'NONE',  ( 5.686755365928134687, 8.721966129303114101, 1.199719254218462483 ) ) ;
#10647=CARTESIAN_POINT ( 'NONE',  ( 3.755245360860917536, 5.404205559136275205, -1.443375672974051449 ) ) ;
#10649=CARTESIAN_POINT ( 'NONE',  ( 3.822509244049070887, 6.547012320444182798, -1.199719254218452047 ) ) ;
#10652=EDGE_CURVE ( 'NONE', #108753, #32719, #85310, .T. ) ;
#10659=CARTESIAN_POINT ( 'NONE',  ( -4.921246572080546500, 8.685278734161874681, 1.214306433183764966E-14 ) ) ;
#10660=CARTESIAN_POINT ( 'NONE',  ( 3.928111819657337911, 5.605883094398769195, 1.599625672291267398 ) ) ;
#10663=CARTESIAN_POINT ( 'NONE',  ( -7.157815033010924921, 10.43820240756634199, 1.199719254218453823 ) ) ;
#10668=CARTESIAN_POINT ( 'NONE',  ( -8.507905087775398556, 9.884643009614800135, 1.199719254218462483 ) ) ;
#10672=CARTESIAN_POINT ( 'NONE',  ( 6.123478934866503742, 10.29580919065294431, 0.7998128361456462443 ) ) ;
#10674=CARTESIAN_POINT ( 'NONE',  ( 4.985647801523278133, 6.839675073242382553, -1.599625672291256295 ) ) ;
#10686=CARTESIAN_POINT ( 'NONE',  ( -7.640183256500752584, 8.872300873127729304, -1.199719254218446718 ) ) ;
#10690=CARTESIAN_POINT ( 'NONE',  ( 6.534666852106798096, 7.686494751288491578, -1.082531754730543083 ) ) ;
#10695=CARTESIAN_POINT ( 'NONE',  ( -6.762819695118240659, 6.784377820593065600, 0.7998128361456341429 ) ) ;
#10707=LINE ( 'NONE', #189472, #61281 ) ;
#10709=CARTESIAN_POINT ( 'NONE',  ( 6.913768267964901071, 10.15348118167935709, -1.199719254218441611 ) ) ;
#10713=CARTESIAN_POINT ( 'NONE',  ( -4.869203491162207520, 6.719169366249152731, -1.250126817991310757 ) ) ;
#10720=CARTESIAN_POINT ( 'NONE',  ( 3.765413976293345844, 5.416068943807445635, 1.599625672291267398 ) ) ;
#10726=CARTESIAN_POINT ( 'NONE',  ( -5.697837992078444991, 6.130623284354489222, -0.7472135431472062272 ) ) ;
#10739=CARTESIAN_POINT ( 'NONE',  ( -3.411848212133334446, 7.132240014130862171, 0.7998128361456341429 ) ) ;
#10740=CARTESIAN_POINT ( 'NONE',  ( 4.487385655998873624, 7.218738451098584363, 1.082531754730558626 ) ) ;
#10741=CARTESIAN_POINT ( 'NONE',  ( -1.500000000000013101, 3.379166666666691299, -0.8660254037844313801 ) ) ;
#10743=CARTESIAN_POINT ( 'NONE',  ( -3.653032323878261600, 6.349289246911547835, -1.199719254218452047 ) ) ;
#10744=DIRECTION ( 'NONE',  ( 0.7592566023653005702, 0.6507913734559639396, 0.000000000000000000 ) ) ;
#10747=CARTESIAN_POINT ( 'NONE',  ( -1.364683531250010295, 4.780208333674755394, 0.7879004041258379498 ) ) ;
#10750=CARTESIAN_POINT ( 'NONE',  ( -3.145128448690317935, 5.652771709238564313, -1.082531754730549967 ) ) ;
#10753=CARTESIAN_POINT ( 'NONE',  ( 1.499999999999821032, 7.388542872122531691, -4.154462424328212222 ) ) ;
#10754=CARTESIAN_POINT ( 'NONE',  ( 4.436542580169809291, 6.199052314996659874, 1.599625672291267398 ) ) ;
#10759=CARTESIAN_POINT ( 'NONE',  ( -1.364683531250012516, 1.592708333674756727, 0.7879004041258379498 ) ) ;
#10762=CARTESIAN_POINT ( 'NONE',  ( -8.286004436246233951, 12.81875560892930466, 1.040834085586084257E-14 ) ) ;
#10763=CARTESIAN_POINT ( 'NONE',  ( -5.707619481228822345, 7.681975366232176583, -1.443375672974051449 ) ) ;
#10767=CARTESIAN_POINT ( 'NONE',  ( 0.6823417656249917140, 4.342708333674755394, 1.181850606188765695 ) ) ;
#10776=CARTESIAN_POINT ( 'NONE',  ( -5.165293336682207581, 8.009630745229104676, 1.082531754730548412 ) ) ;
#10780=CARTESIAN_POINT ( 'NONE',  ( -6.060131475184148186, 6.172500930577367484, 0.7216878364870317197 ) ) ;
#10783=CARTESIAN_POINT ( 'NONE',  ( 8.992082194361556091, 11.51384853155376220, 1.599625672291279388 ) ) ;
#10788=FACE_OUTER_BOUND ( 'NONE', #93961, .T. ) ;
#10793=CARTESIAN_POINT ( 'NONE',  ( -3.418627288940168096, 7.140148937072163804, -0.7998128361456281477 ) ) ;
#10796=CARTESIAN_POINT ( 'NONE',  ( 1.499999999999985123, 0.2958333333333566517, -0.8660254037844323793 ) ) ;
#10797=ORIENTED_EDGE ( 'NONE', *, *, #174895, .F. ) ;
#10799=CARTESIAN_POINT ( 'NONE',  ( 9.408995418203971894, 11.03987807840189816, 1.082531754730549967 ) ) ;
#10800=CARTESIAN_POINT ( 'NONE',  ( 7.741869408603235136, 8.990934717247309749, 1.199719254218462483 ) ) ;
#10803=VERTEX_POINT ( 'NONE', #7423 ) ;
#10805=CARTESIAN_POINT ( 'NONE',  ( 2.869522067586683711, 6.499526178826442013, 0.7998128361456362523 ) ) ;
#10813=CARTESIAN_POINT ( 'NONE',  ( -6.144869935491728441, 8.192100896205577243, -1.599625672291263179 ) ) ;
#10819=CARTESIAN_POINT ( 'NONE',  ( -1.201851678989727383E-14, 2.946875000341419248, -1.575800808251660134 ) ) ;
#10820=CARTESIAN_POINT ( 'NONE',  ( 9.056483423804305488, 9.668244870634271848, 1.040834085586084257E-14 ) ) ;
#10821=CARTESIAN_POINT ( 'NONE',  ( -4.415151579544611238, 8.302760609444034046, -0.7998128361456281477 ) ) ;
#10824=CARTESIAN_POINT ( 'NONE',  ( 4.761938266897790761, 6.578680616179308771, 1.599625672291267398 ) ) ;
#10825=CARTESIAN_POINT ( 'NONE',  ( -6.437424008390261854, 6.404749519410410485, 0.7998128361456341429 ) ) ;
#10831=CARTESIAN_POINT ( 'NONE',  ( 5.666945020832167224, 8.594891043404107478, 1.082531754730558626 ) ) ;
#10834=CARTESIAN_POINT ( 'NONE',  ( 1.364683531249986537, 1.717708333674749399, -0.7879004041258239610 ) ) ;
#10836=CARTESIAN_POINT ( 'NONE',  ( 5.138177029454836564, 7.977995053463880382, 1.082531754730558626 ) ) ;
#10838=CARTESIAN_POINT ( 'NONE',  ( -2.494337075234348777, 5.853884321174607663, -0.7216878364870267237 ) ) ;
#10845=CARTESIAN_POINT ( 'NONE',  ( -3.992976280936286759, 7.825322551632388546, 0.2949607357299148802 ) ) ;
#10851=CIRCLE ( 'NONE', #104268, 0.08000000000000020983 ) ;
#10853=CARTESIAN_POINT ( 'NONE',  ( 5.524057522564145728, 8.532151978711786100, 1.199719254218462483 ) ) ;
#10856=CARTESIAN_POINT ( 'NONE',  ( -3.337985173046072340, 6.383183490859034137, 0.8077998227833966816 ) ) ;
#10864=CARTESIAN_POINT ( 'NONE',  ( 4.202664430556254160, 5.926194473780837413, 1.443375672974062551 ) ) ;
#10865=CARTESIAN_POINT ( 'NONE',  ( 1.364683531249988757, 2.196875000341415252, 1.214306433183764966E-14 ) ) ;
#10867=CARTESIAN_POINT ( 'NONE',  ( 7.076466111328892694, 10.34329533227067799, -1.199719254218441611 ) ) ;
#10869=CARTESIAN_POINT ( 'NONE',  ( 0.6823417656249899377, 3.176041667008085323, -1.181850606188754593 ) ) ;
#10870=CARTESIAN_POINT ( 'NONE',  ( -3.879604511804807032, 7.677955697080921738, 0.7998128361456341429 ) ) ;
#10874=CARTESIAN_POINT ( 'NONE',  ( -0.7499999999999972244, 3.358333333333359150, -1.299038105676652011 ) ) ;
#10875=CARTESIAN_POINT ( 'NONE',  ( 4.638861114170084399, 8.563755066507100722, 0.7998128361456462443 ) ) ;
#10876=CARTESIAN_POINT ( 'NONE',  ( -7.202405917357668663, 9.425892875049191488, 1.599625672291295375 ) ) ;
#10879=CARTESIAN_POINT ( 'NONE',  ( -3.084802633888621859, 6.542760806271256335, 0.3243353321068309092 ) ) ;
#10880=CARTESIAN_POINT ( 'NONE',  ( -1.201851678989727383E-14, 3.071875000341420137, 1.575800808251672791 ) ) ;
#10882=CARTESIAN_POINT ( 'NONE',  ( 10.05978679165993483, 11.79913468076720306, 1.082531754730548412 ) ) ;
#10888=CARTESIAN_POINT ( 'NONE',  ( -0.7500000000000215383, 0.4729166673494850093, 1.299038105676659116 ) ) ;
#10891=CARTESIAN_POINT ( 'NONE',  ( -7.393273838153706201, 7.519907654134449615, 0.7998128361456341429 ) ) ;
#10892=CARTESIAN_POINT ( 'NONE',  ( -4.473827502829599290, 4.321812962830357208, 0.7216878364870317197 ) ) ;
#10900=CARTESIAN_POINT ( 'NONE',  ( 6.661133543015731462, 6.665743976473484267, -0.7998128361456281477 ) ) ;
#10903=CARTESIAN_POINT ( 'NONE',  ( 6.342516933094585418, 6.294024598232139667, 1.040834085586084257E-14 ) ) ;
#10908=CARTESIAN_POINT ( 'NONE',  ( -4.706651882238427120, 8.642844295920152575, 1.040834085586084257E-14 ) ) ;
#10910=CARTESIAN_POINT ( 'NONE',  ( 4.891794496432329886, 4.601515088792824670, -0.7998128361456211532 ) ) ;
#10914=CARTESIAN_POINT ( 'NONE',  ( -4.650083499807243115, 5.295740330745369207, -1.052294140492322283 ) ) ;
#10915=CARTESIAN_POINT ( 'NONE',  ( 4.632932323280743780, 6.889805956345480986, 1.213532624337316124 ) ) ;
#10925=CARTESIAN_POINT ( 'NONE',  ( -4.559605246071217088, 3.300000000000025135, 0.7750000000000135669 ) ) ;
#10926=CARTESIAN_POINT ( 'NONE',  ( 9.083599731475992201, 9.699880562917908122, 0.7216878364870438212 ) ) ;
#10928=CARTESIAN_POINT ( 'NONE',  ( -5.525111292768871252, 6.404716915440499037, -1.199719254218446718 ) ) ;
#10929=DIRECTION ( 'NONE',  ( 1.000000000000000000, 0.000000000000000000, 0.000000000000000000 ) ) ;
#10931=CARTESIAN_POINT ( 'NONE',  ( 8.959240580532112475, 9.346868853575953651, -0.7998128361456221525 ) ) ;
#10933=CARTESIAN_POINT ( 'NONE',  ( -5.205440912643032547, 8.160432600470439723, 1.199719254218452047 ) ) ;
#10946=DIRECTION ( 'NONE',  ( 0.000000000000000000, -2.168404344971008079E-15, 1.000000000000000000 ) ) ;
#10947=CARTESIAN_POINT ( 'NONE',  ( 8.238550898598388628, 12.76339314834017102, 0.7998128361456462443 ) ) ;
#10948=CARTESIAN_POINT ( 'NONE',  ( -4.120788623549732854, 6.895004929861607401, -1.199719254218452047 ) ) ;
#10951=CARTESIAN_POINT ( 'NONE',  ( 4.690757960648234359, 4.574898496952131133, 0.7216878364870317197 ) ) ;
#10956=CARTESIAN_POINT ( 'NONE',  ( 4.867013957181530515, 5.740899707208986236, -1.082531754730548412 ) ) ;
#10957=CARTESIAN_POINT ( 'NONE',  ( -3.602716132929368875, 5.226254793216122074, 1.599625672291267398 ) ) ;
#10960=CARTESIAN_POINT ( 'NONE',  ( 7.730120138085914583, 12.17022392774227768, 0.7998128361456462443 ) ) ;
#10964=VECTOR ( 'NONE', #31462, 1000.000000000000000 ) ;
#10966=CARTESIAN_POINT ( 'NONE',  ( -7.497822643557261024, 8.706213491360317747, -1.199719254218446718 ) ) ;
#10967=CARTESIAN_POINT ( 'NONE',  ( 5.823390672269506574, 6.752709524857930745, -1.199719254218446718 ) ) ;
#10969=CARTESIAN_POINT ( 'NONE',  ( 4.955668840994886359, 5.740367388370866131, 1.199719254218462483 ) ) ;
#10973=CARTESIAN_POINT ( 'NONE',  ( 1.364683531249986537, 1.217708333674754950, -0.7879004041258239610 ) ) ;
#10976=CARTESIAN_POINT ( 'NONE',  ( 8.283668668269706714, 8.766627655843892697, 1.040834085586084257E-14 ) ) ;
#10983=CARTESIAN_POINT ( 'NONE',  ( 8.392133896734652154, 12.73464727959172293, 0.7216878364870438212 ) ) ;
#10989=CARTESIAN_POINT ( 'NONE',  ( -8.962103233833181193, 10.41454084668224489, -1.199719254218446718 ) ) ;
#11007=CARTESIAN_POINT ( 'NONE',  ( 0.7499999999999902300, 1.264583334016147642, 1.299038105676657340 ) ) ;
#11013=AXIS2_PLACEMENT_3D ( 'NONE', #208059, #142044, #22898 ) ;
#11014=CARTESIAN_POINT ( 'NONE',  ( -0.7500000000000006661, -0.6416666666666446250, -1.299038105676652011 ) ) ;
#11015=CARTESIAN_POINT ( 'NONE',  ( 8.320953590485093088, 10.73086516036454618, 1.599625672291281386 ) ) ;
#11016=CARTESIAN_POINT ( 'NONE',  ( -1.402160292154681736E-14, -0.4281249996585808071, 1.575800808251672791 ) ) ;
#11019=CARTESIAN_POINT ( 'NONE',  ( 4.695201269034174452, 4.372156323494968966, 1.214306433183764966E-14 ) ) ;
#11020=CARTESIAN_POINT ( 'NONE',  ( -5.585596099150182958, 8.499983968108443477, -1.082531754730544860 ) ) ;
#11024=CARTESIAN_POINT ( 'NONE',  ( -7.718669524881690336, 7.899535955317097624, 0.7998128361456462443 ) ) ;
#11025=EDGE_LOOP ( 'NONE', ( #127296, #55478, #5029, #135031, #55241 ) ) ;
#11026=CARTESIAN_POINT ( 'NONE',  ( -1.500000000000013101, 1.452083334016150085, 0.8660254037844403729 ) ) ;
#11038=CARTESIAN_POINT ( 'NONE',  ( -2.931280137532493946, 6.571577260429871892, 0.3558765841190729140 ) ) ;
#11039=CARTESIAN_POINT ( 'NONE',  ( -9.365985188942097750, 9.821404230054264772, 0.7998128361456462443 ) ) ;
#11040=CARTESIAN_POINT ( 'NONE',  ( 7.467843683028853263, 7.606905806488803101, 0.7998128361456341429 ) ) ;
#11044=ORIENTED_EDGE ( 'NONE', *, *, #114672, .F. ) ;
#11048=CARTESIAN_POINT ( 'NONE',  ( -9.155833807930273238, 9.576227618873799585, -0.7998128361456291469 ) ) ;
#11055=CARTESIAN_POINT ( 'NONE',  ( 4.701980345841006326, 4.380065246436280368, 0.7998128361456341429 ) ) ;
#11060=CARTESIAN_POINT ( 'NONE',  ( -5.687809136132860210, 6.594531066031826150, -1.199719254218446718 ) ) ;
#11061=CARTESIAN_POINT ( 'NONE',  ( -10.62011439820619429, 11.28455497419572318, -0.7998128361456221525 ) ) ;
#11064=CARTESIAN_POINT ( 'NONE',  ( -5.789674969154799733, 6.218922551941099108, -1.014761583188450000 ) ) ;
#11072=CARTESIAN_POINT ( 'NONE',  ( 7.253775878511261155, 8.421492265473332850, 1.199719254218462483 ) ) ;
#11075=DIRECTION ( 'NONE',  ( 1.000000000000000000, 0.000000000000000000, 0.000000000000000000 ) ) ;
#11077=VECTOR ( 'NONE', #8695, 1000.000000000000000 ) ;
#11082=CARTESIAN_POINT ( 'NONE',  ( -1.201851678989727383E-14, 1.743750000682815493, 1.732050807568877637 ) ) ;
#11093=CARTESIAN_POINT ( 'NONE',  ( 3.877268743828276243, 4.586196958296845594, 1.082531754730560403 ) ) ;
#11096=ORIENTED_EDGE ( 'NONE', *, *, #111969, .T. ) ;
#11097=CARTESIAN_POINT ( 'NONE',  ( -9.972185678051314284, 11.59297036493672017, 1.199719254218462483 ) ) ;
#11099=CARTESIAN_POINT ( 'NONE',  ( 9.480175724453529185, 12.08329098332774265, 1.599625672291279388 ) ) ;
#11109=CARTESIAN_POINT ( 'NONE',  ( -1.364683531250014514, -1.219791666325248602, 0.7879004041258379498 ) ) ;
#11114=CARTESIAN_POINT ( 'NONE',  ( -5.915435094264120508, 5.795762452929912101, 0.000000000000000000 ) ) ;
#11117=CARTESIAN_POINT ( 'NONE',  ( 0.7499999999999885647, -0.5166666666666444030, 1.299038105676657340 ) ) ;
#11119=CARTESIAN_POINT ( 'NONE',  ( -1.402160292154681736E-14, -0.4906249996585810846, -1.575800808251665908 ) ) ;
#11124=CARTESIAN_POINT ( 'NONE',  ( -0.6823417656250246877, -0.4489583329919111243, 1.181850606188755259 ) ) ;
#11126=CARTESIAN_POINT ( 'NONE',  ( -7.365103760721662951, 9.615707025640515937, 1.599625672291295375 ) ) ;
#11128=CARTESIAN_POINT ( 'NONE',  ( 9.915090410295563927, 10.46202698829998567, -0.7998128361456281477 ) ) ;
#11132=ORIENTED_EDGE ( 'NONE', *, *, #47186, .F. ) ;
#11134=CARTESIAN_POINT ( 'NONE',  ( 1.364683531249986537, -0.2822916663252520997, -0.7879004041258309554 ) ) ;
#11141=CARTESIAN_POINT ( 'NONE',  ( 6.805829924380105034, 9.923590097543378619, 1.082531754730558626 ) ) ;
#11144=CARTESIAN_POINT ( 'NONE',  ( -4.069418662396130593, 7.899405539437467816, -0.7998128361456281477 ) ) ;
#11146=CARTESIAN_POINT ( 'NONE',  ( -0.7500000000000215383, 4.472916667349482012, 1.299038105676671107 ) ) ;
#11149=CARTESIAN_POINT ( 'NONE',  ( 6.358410854684775515, 8.441231968597481483, -1.443375672974058777 ) ) ;
#11150=CARTESIAN_POINT ( 'NONE',  ( -7.971831134711019118, 12.24429405723079967, 0.000000000000000000 ) ) ;
#11156=CARTESIAN_POINT ( 'NONE',  ( 4.383363735919856730, 4.008345868194933104, -0.7998128361456211532 ) ) ;
#11161=CIRCLE ( 'NONE', #159920, 3.971937515251341644 ) ;
#11172=EDGE_CURVE ( 'NONE', #205805, #2289, #107528, .T. ) ;
#11174=CARTESIAN_POINT ( 'NONE',  ( 7.426115451983150706, 9.686887332112256388, -1.599625672291262513 ) ) ;
#11180=CARTESIAN_POINT ( 'NONE',  ( 6.493992391265805075, 6.678671999339316656, 1.040834085586084257E-14 ) ) ;
#11182=CARTESIAN_POINT ( 'NONE',  ( -7.375272376154077492, 11.54830883891436422, -0.7216878364870267237 ) ) ;
#11203=CARTESIAN_POINT ( 'NONE',  ( 4.499531974119707733, 7.248992493261455117, -1.273121237324711386 ) ) ;
#11212=CARTESIAN_POINT ( 'NONE',  ( -8.853111120043687166, 9.430977182913531820, 1.040834085586084257E-14 ) ) ;
#11216=CARTESIAN_POINT ( 'NONE',  ( 6.634017235788401301, 6.634108284708264414, 0.7998128361456341429 ) ) ;
#11218=CARTESIAN_POINT ( 'NONE',  ( 2.218730694130720771, 5.740269576461138890, 0.7998128361456462443 ) ) ;
#11220=CARTESIAN_POINT ( 'NONE',  ( -3.249150368769345043, 6.942425863539538611, 0.7998128361456341429 ) ) ;
#11225=CARTESIAN_POINT ( 'NONE',  ( -5.037017762676898158, 5.835274463666530131, -1.199719254218446718 ) ) ;
#11229=CARTESIAN_POINT ( 'NONE',  ( 8.749089199520284410, 9.101692242395490240, 0.7998128361456481317 ) ) ;
#11230=CARTESIAN_POINT ( 'NONE',  ( 0.02270195696656561457, 6.343288419976386372, 3.091051226635131322 ) ) ;
#11233=CARTESIAN_POINT ( 'NONE',  ( 4.556571072163061231, 7.192851904033680910, 1.311937382574361877 ) ) ;
#11234=CARTESIAN_POINT ( 'NONE',  ( 5.395781948558860286, 6.357795697149212444, -1.082531754730542195 ) ) ;
#11242=CARTESIAN_POINT ( 'NONE',  ( 7.429504990164394584, 7.770103364721017591, 1.040834085586084257E-14 ) ) ;
#11243=CARTESIAN_POINT ( 'NONE',  ( -7.995557903757128493, 10.35123685918189729, 1.599625672291295375 ) ) ;
#11246=CARTESIAN_POINT ( 'NONE',  ( -10.30827686509187835, 10.92074451889568643, 1.040834085586084257E-14 ) ) ;
#11247=CARTESIAN_POINT ( 'NONE',  ( -6.684333426737305572, 7.757142738403693727, -1.199719254218446718 ) ) ;
#11255=CARTESIAN_POINT ( 'NONE',  ( 7.130698725783555680, 10.40656671580112658, 1.199719254218460707 ) ) ;
#11258=( BOUNDED_CURVE ( )  B_SPLINE_CURVE ( 2, ( #117538, #83897, #184589, #186733, #101214, #103361, #38356 ),
 .UNSPECIFIED., .F., .T. ) 
 B_SPLINE_CURVE_WITH_KNOTS ( ( 3, 2, 2, 3 ),
 ( 0.1071428571428572341, 0.1130952380952381098, 0.1190476190476189855, 0.1249999999999998612 ),
 .UNSPECIFIED. ) 
 CURVE ( )  GEOMETRIC_REPRESENTATION_ITEM ( )  RATIONAL_B_SPLINE_CURVE ( ( 0.9999999999999977796, 0.8660254037844409281, 1.000000000000000000, 0.8660254037844387076, 1.000000000000000000, 0.8660254037844418162, 0.9999999999999968914 ) ) 
 REPRESENTATION_ITEM ( '' )  );
#11263=CARTESIAN_POINT ( 'NONE',  ( -1.500000000000011324, 5.452083334016153415, 0.8660254037844403729 ) ) ;
#11269=CARTESIAN_POINT ( 'NONE',  ( -1.500000000000011324, 2.920833333333352932, 0.8660254037844403729 ) ) ;
#11270=CARTESIAN_POINT ( 'NONE',  ( 5.931855901178834323, 6.879252291918818152, 1.199719254218462483 ) ) ;
#11273=CARTESIAN_POINT ( 'NONE',  ( 7.619319141200063150, 9.912291636198670375, 1.443375672974076540 ) ) ;
#11277=CARTESIAN_POINT ( 'NONE',  ( 10.05067194643221207, 10.62020544712608938, 0.7998128361456462443 ) ) ;
#11280=DIRECTION ( 'NONE',  ( 0.000000000000000000, 8.546850786086437571E-32, 1.000000000000000000 ) ) ;
#11282=CARTESIAN_POINT ( 'NONE',  ( -0.6823417656250212460, 1.301041667008083547, 1.181850606188755259 ) ) ;
#11287=CARTESIAN_POINT ( 'NONE',  ( 1.364683531249986537, -0.6364583329919177856, 0.7879004041258500513 ) ) ;
#11289=CARTESIAN_POINT ( 'NONE',  ( 9.423080456697809026, 10.95234760669099749, -1.199719254218446718 ) ) ;
#11292=CARTESIAN_POINT ( 'NONE',  ( -2.941756144040970522, 5.415504020480993219, -1.082531754730543083 ) ) ;
#11295=CARTESIAN_POINT ( 'NONE',  ( -6.911959384868566758, 6.958374125301778790, 1.040834085586084257E-14 ) ) ;
#11298=CARTESIAN_POINT ( 'NONE',  ( 4.355193658487811703, 6.104145239700998538, -1.599625672291255185 ) ) ;
#11305=CARTESIAN_POINT ( 'NONE',  ( 9.759171643738394408, 10.28012176064996197, 0.000000000000000000 ) ) ;
#11308=CARTESIAN_POINT ( 'NONE',  ( -4.283486466913726254, 7.084819080452935403, -1.199719254218452047 ) ) ;
#11312=CARTESIAN_POINT ( 'NONE',  ( 9.887974103068218668, 10.43039129653476493, 0.7998128361456462443 ) ) ;
#11314=CARTESIAN_POINT ( 'NONE',  ( 6.968000882419564945, 10.21675256520979858, 1.199719254218460707 ) ) ;
#11315=CARTESIAN_POINT ( 'NONE',  ( 4.879410147971470657, 4.944948943068641967, -0.7687999843507594688 ) ) ;
#11317=CARTESIAN_POINT ( 'NONE',  ( -4.288456660624211381, 3.897620947016656956, 1.214306433183764966E-14 ) ) ;
#11325=CARTESIAN_POINT ( 'NONE',  ( -6.131443063645894753, 6.000026256920684808, -0.1528826387674747100 ) ) ;
#11326=CARTESIAN_POINT ( 'NONE',  ( -1.364683531250014514, 1.738541667008085545, -0.7879004041258289570 ) ) ;
#11329=CARTESIAN_POINT ( 'NONE',  ( 6.832946231607457399, 7.074118146404578589, -0.7216878364870257245 ) ) ;
#11345=CARTESIAN_POINT ( 'NONE',  ( 9.610031953988080744, 10.10612545594124967, -0.7998128361456281477 ) ) ;
#11347=VERTEX_POINT ( 'NONE', #171008 ) ;
#11349=CARTESIAN_POINT ( 'NONE',  ( -2.598358995313378550, 6.183169261174235487, 0.7998128361456341429 ) ) ;
#11350=CARTESIAN_POINT ( 'NONE',  ( -6.509886312855995172, 10.74661779830734254, -0.7998128361456291469 ) ) ;
#11355=CARTESIAN_POINT ( 'NONE',  ( -1.500000000000011324, 4.702083334016148974, 0.8660254037844403729 ) ) ;
#11356=CARTESIAN_POINT ( 'NONE',  ( 7.239163954692881653, 10.53310948286200599, -1.199719254218441611 ) ) ;
#11358=ORIENTED_EDGE ( 'NONE', *, *, #33313, .T. ) ;
#11361=CARTESIAN_POINT ( 'NONE',  ( -6.340409392685171674, 10.54889472477470846, 0.7998128361456481317 ) ) ;
#11363=CARTESIAN_POINT ( 'NONE',  ( -1.364683531250010295, 4.030208333674751842, 0.7879004041258379498 ) ) ;
#11368=CARTESIAN_POINT ( 'NONE',  ( -8.188761592974040937, 11.53701037756964887, -1.082531754730543971 ) ) ;
#11372=CARTESIAN_POINT ( 'NONE',  ( -1.364683531250012516, 2.592708333674753174, 0.7879004041258379498 ) ) ;
#11380=CARTESIAN_POINT ( 'NONE',  ( -0.6823417656250212460, 3.051041667008084879, 1.181850606188767472 ) ) ;
#11383=CARTESIAN_POINT ( 'NONE',  ( -3.598799709423620374, 6.286017863381107240, 1.199719254218464037 ) ) ;
#11384=CARTESIAN_POINT ( 'NONE',  ( 6.449928391799196525, 8.548002428564306143, -1.599625672291262513 ) ) ;
#11387=CARTESIAN_POINT ( 'NONE',  ( -0.6823417656250212460, 3.613541667008085767, 1.181850606188767472 ) ) ;
#11390=CARTESIAN_POINT ( 'NONE',  ( -0.6823417656250246877, 0.05104166700808931978, 1.181850606188755259 ) ) ;
#11391=CARTESIAN_POINT ( 'NONE',  ( -5.273758566035884776, 5.255065869904374409, 0.000000000000000000 ) ) ;
#11395=CARTESIAN_POINT ( 'NONE',  ( 5.694061328059515148, 5.745419092265303007, -0.7216878364870207285 ) ) ;
#11398=CARTESIAN_POINT ( 'NONE',  ( -6.690058733339450114, 9.892486724616283311, 1.199719254218452047 ) ) ;
#11399=CARTESIAN_POINT ( 'NONE',  ( -8.026063749610047537, 11.34719622697832264, -1.082531754730543971 ) ) ;
#11405=B_SPLINE_CURVE_WITH_KNOTS ( 'NONE', 3,
 ( #7967, #139073, #56739, #123964 ),
 .UNSPECIFIED., .F., .F.,
 ( 4, 4 ),
 ( 0.002059939351769829192, 0.002341702326271049867 ),
 .UNSPECIFIED. ) ;
#11406=CARTESIAN_POINT ( 'NONE',  ( -9.001723924469462901, 12.58942944760136484, -1.199719254218446718 ) ) ;
#11407=CARTESIAN_POINT ( 'NONE',  ( -7.063434842595444962, 8.303390740191881392, 1.082531754730549967 ) ) ;
#11409=CARTESIAN_POINT ( 'NONE',  ( 1.364683531249986537, 0.9260416670080896528, 0.7879004041258500513 ) ) ;
#11423=CARTESIAN_POINT ( 'NONE',  ( 8.880227426826646564, 9.462612874160329923, 0.7216878364870458196 ) ) ;
#11431=CARTESIAN_POINT ( 'NONE',  ( 4.310602774141044868, 7.116454772218158809, -1.199719254218452047 ) ) ;
#11433=CARTESIAN_POINT ( 'NONE',  ( -3.469997250093771246, 6.135748327496311383, -1.199719254218452935 ) ) ;
#11436=CARTESIAN_POINT ( 'NONE',  ( 1.403499169903295263, 7.376709478543810761, -4.304123474983216902 ) ) ;
#11437=CARTESIAN_POINT ( 'NONE',  ( 1.364683531249986537, 1.217708333674754950, -0.7879004041258239610 ) ) ;
#11439=CARTESIAN_POINT ( 'NONE',  ( -8.239604668803112375, 10.63595808506888396, -1.599625672291263179 ) ) ;
#11443=EDGE_CURVE ( 'NONE', #166897, #157452, #130929, .T. ) ;
#11457=CARTESIAN_POINT ( 'NONE',  ( 2.276512373593124305, 5.629777788065645439, 0.5132344841170741745 ) ) ;
#11460=CARTESIAN_POINT ( 'NONE',  ( 5.120175567455225618, 9.125288595339771547, -0.7998128361456281477 ) ) ;
#11467=CARTESIAN_POINT ( 'NONE',  ( 9.094822116668764167, 9.505047312402055582, 0.7998128361456462443 ) ) ;
#11472=CARTESIAN_POINT ( 'NONE',  ( 7.886038904643079661, 12.35212915539230139, -0.7998128361456352531 ) ) ;
#11478=CARTESIAN_POINT ( 'NONE',  ( 9.480175724453529185, 12.08329098332774265, 1.599625672291279388 ) ) ;
#11480=CARTESIAN_POINT ( 'NONE',  ( -0.4491468415841158301, 7.944909564338812125, 1.993991491228178869 ) ) ;
#11485=CARTESIAN_POINT ( 'NONE',  ( -9.666600336863641729, 10.38004793587015584, 1.040834085586084257E-14 ) ) ;
#11491=CARTESIAN_POINT ( 'NONE',  ( 3.960953433486789521, 7.772862772376584850, -0.7998128361456221525 ) ) ;
#11497=EDGE_CURVE ( 'NONE', #109299, #83910, #150502, .T. ) ;
#11499=CARTESIAN_POINT ( 'NONE',  ( 5.002595493318194642, 4.938708951733754127, -0.7216878364870197293 ) ) ;
#11507=CARTESIAN_POINT ( 'NONE',  ( -4.205000198532790279, 8.057583998263570635, 0.7998128361456341429 ) ) ;
#11509=CARTESIAN_POINT ( 'NONE',  ( -3.948449050077848632, 5.629609863222681199, 1.599625672291267398 ) ) ;
#11514=CARTESIAN_POINT ( 'NONE',  ( 2.359223927328457648E-13, 7.078193277237625480, 2.121339347286388843 ) ) ;
#11517=AXIS2_PLACEMENT_3D ( 'NONE', #25231, #45785, #141173 ) ;
#11518=CARTESIAN_POINT ( 'NONE',  ( 6.322179702674084467, 6.270297829408224111, 1.040834085586084257E-14 ) ) ;
#11520=FACE_OUTER_BOUND ( 'NONE', #148034, .T. ) ;
#11531=CARTESIAN_POINT ( 'NONE',  ( 1.364683531249986537, 1.967708333674750731, -0.7879004041258239610 ) ) ;
#11532=CARTESIAN_POINT ( 'NONE',  ( 3.871016551901614200, 4.474939717762034697, -1.199719254218446718 ) ) ;
#11533=CARTESIAN_POINT ( 'NONE',  ( 5.203632029546647608, 4.965325544092860532, 1.040834085586084257E-14 ) ) ;
#11535=CARTESIAN_POINT ( 'NONE',  ( -6.561783159334137139, 8.678499657355050800, -1.443375672974059665 ) ) ;
#11536=CARTESIAN_POINT ( 'NONE',  ( 4.039966587192257208, 6.696749537490852333, 1.082531754730558626 ) ) ;
#11538=CARTESIAN_POINT ( 'NONE',  ( -6.683806541412768532, 8.820860269780128604, -1.443375672974058777 ) ) ;
#11543=CARTESIAN_POINT ( 'NONE',  ( 5.774883364416965037, 8.824782127540085952, -1.199719254218440723 ) ) ;
#11545=CARTESIAN_POINT ( 'NONE',  ( 6.471393748265540147, 5.229711127717882491, 2.420000000000010587 ) ) ;
#11548=CARTESIAN_POINT ( 'NONE',  ( 0.6823417656249917140, 4.842708333674755394, 1.181850606188765695 ) ) ;
#11552=CARTESIAN_POINT ( 'NONE',  ( 7.983053520348166288, 8.207983950027992748, -0.7998128361456281477 ) ) ;
#11556=CARTESIAN_POINT ( 'NONE',  ( -8.525379664894808585, 8.840697785332414682, -0.7998128361456291469 ) ) ;
#11561=CARTESIAN_POINT ( 'NONE',  ( 8.483651433849084711, 10.92067931095586886, 1.599625672291281386 ) ) ;
#11564=CARTESIAN_POINT ( 'NONE',  ( -6.177711549321182716, 10.35908057418338402, 0.7998128361456481317 ) ) ;
#11565=DIRECTION ( 'NONE',  ( 1.000000000000000000, 0.000000000000000000, 0.000000000000000000 ) ) ;
#11566=CARTESIAN_POINT ( 'NONE',  ( 8.568389893712330618, 9.098802418860289620, 1.040834085586084257E-14 ) ) ;
#11567=CARTESIAN_POINT ( 'NONE',  ( 4.250508905105749413, 7.277302409985156650, -0.9232175757047023090 ) ) ;
#11568=CARTESIAN_POINT ( 'NONE',  ( -8.758204044748012507, 11.24099069033793974, 1.443375672974064550 ) ) ;
#11573=CARTESIAN_POINT ( 'NONE',  ( 4.473300617505036492, 7.306268922809479704, -1.199719254218452047 ) ) ;
#11575=CARTESIAN_POINT ( 'NONE',  ( 8.594979316059474073, 12.11489407112305372, 1.199719254218450271 ) ) ;
#11576=CARTESIAN_POINT ( 'NONE',  ( -5.638288519115033814, 6.168138913823901781, 0.8326226707794943671 ) ) ;
#11577=CARTESIAN_POINT ( 'NONE',  ( -1.364683531250014514, 0.2385416670080863499, -0.7879004041258359514 ) ) ;
#11579=CARTESIAN_POINT ( 'NONE',  ( -6.670248388243482651, 9.765411638717282017, 1.082531754730548412 ) ) ;
#11584=CARTESIAN_POINT ( 'NONE',  ( -4.653572958549120564, 6.905085616583060748, 1.214936962016188726 ) ) ;
#11585=CARTESIAN_POINT ( 'NONE',  ( -1.364683531250014514, -0.1572916663252435232, 0.7879004041258379498 ) ) ;
#11588=CARTESIAN_POINT ( 'NONE',  ( 2.684151225825664788, 5.114964949229812596, -1.082531754730543083 ) ) ;
#11592=CARTESIAN_POINT ( 'NONE',  ( -8.527715432871366019, 10.01171809551380143, 1.082531754730558626 ) ) ;
#11597=CARTESIAN_POINT ( 'NONE',  ( -9.178506806327330736, 10.77097469787910455, 1.082531754730558626 ) ) ;
#11603=ORIENTED_EDGE ( 'NONE', *, *, #137720, .T. ) ;
#11604=CARTESIAN_POINT ( 'NONE',  ( -8.148087131688683371, 11.48955683940339867, -1.082531754730543083 ) ) ;
#11608=CARTESIAN_POINT ( 'NONE',  ( 1.364683531249988535, 5.717708333674752730, -0.7879004041258300672 ) ) ;
#11609=CARTESIAN_POINT ( 'NONE',  ( -0.7499999999999972244, 3.639583334016149863, -1.299038105676652011 ) ) ;
#11610=CARTESIAN_POINT ( 'NONE',  ( 5.997902985473373860, 6.089292839903872157, -0.6134941253506603909 ) ) ;
#11616=CARTESIAN_POINT ( 'NONE',  ( -7.507464373665155399, 9.781794407407920389, 1.599625672291295375 ) ) ;
#11619=CARTESIAN_POINT ( 'NONE',  ( 3.798255590122797898, 7.583048621785260401, -0.7998128361456221525 ) ) ;
#11625=CARTESIAN_POINT ( 'NONE',  ( 7.145310649601935182, 8.294949498412453437, -1.199719254218446718 ) ) ;
#11626=CARTESIAN_POINT ( 'NONE',  ( -4.911920813620073822, 4.715216669348689216, 0.3991582675463816177 ) ) ;
#11634=CARTESIAN_POINT ( 'NONE',  ( -6.290620087060847965, 7.401773525401500464, 1.082531754730549967 ) ) ;
#11637=EDGE_CURVE ( 'NONE', #69998, #31219, #69047, .T. ) ;
#11638=CARTESIAN_POINT ( 'NONE',  ( -4.498292041426138255, 5.425847295072050436, 1.271850428444160963 ) ) ;
#11645=CARTESIAN_POINT ( 'NONE',  ( -9.504429378379839477, 11.04725468198666150, 1.199719254218462483 ) ) ;
#11647=CARTESIAN_POINT ( 'NONE',  ( 9.271078113646423091, 9.710679308875986848, 1.040834085586084257E-14 ) ) ;
#11648=CARTESIAN_POINT ( 'NONE',  ( 0.7499999999999867883, -0.4333333333333133641, -1.299038105676652899 ) ) ;
#11649=CARTESIAN_POINT ( 'NONE',  ( -7.343712760096452463, 11.71941532008788833, -0.7998128361456291469 ) ) ;
#11652=CARTESIAN_POINT ( 'NONE',  ( -1.364683531250012516, 3.280208333674756727, 0.7879004041258379498 ) ) ;
#11653=CARTESIAN_POINT ( 'NONE',  ( 4.304877467538922531, 4.981110786005563007, 1.199719254218464037 ) ) ;
#11656=CARTESIAN_POINT ( 'NONE',  ( 0.7499999999999920064, 5.233333333333353821, 1.299038105676669330 ) ) ;
#11659=CARTESIAN_POINT ( 'NONE',  ( 9.042925270190632858, 10.61279623905300085, 1.082531754730549967 ) ) ;
#11662=CARTESIAN_POINT ( 'NONE',  ( -5.409340102172518705, 9.254721185935849803, 0.000000000000000000 ) ) ;
#11663=CARTESIAN_POINT ( 'NONE',  ( -0.6823417656250003738, 1.967708333674753174, -1.181850606188749264 ) ) ;
#11667=CARTESIAN_POINT ( 'NONE',  ( -6.989391883044787868, 8.113044270762433285, -1.199719254218446718 ) ) ;
#11668=CARTESIAN_POINT ( 'NONE',  ( -1.201851678989727383E-14, 4.134375000341417028, 1.575800808251672791 ) ) ;
#11673=CARTESIAN_POINT ( 'NONE',  ( 8.880754312151170282, 10.31963377138658089, 1.199719254218453823 ) ) ;
#11676=CARTESIAN_POINT ( 'NONE',  ( 1.499999999999985123, 0.5458333333333577064, -0.8660254037844253849 ) ) ;
#11680=ORIENTED_EDGE ( 'NONE', *, *, #196609, .F. ) ;
#11681=CARTESIAN_POINT ( 'NONE',  ( 9.911173986789782120, 11.52179005846497972, -1.199719254218440723 ) ) ;
#11684=AXIS2_PLACEMENT_3D ( 'NONE', #22954, #191862, #43523 ) ;
#11686=CARTESIAN_POINT ( 'NONE',  ( 7.727257484784855635, 11.10255193463598111, -1.199719254218446718 ) ) ;
#11687=CARTESIAN_POINT ( 'NONE',  ( -1.538487831126141625, 8.695753106490483830, 2.511613306591230721 ) ) ;
#11691=CARTESIAN_POINT ( 'NONE',  ( -1.001543065824772872E-14, 5.384375000341415252, 1.575800808251672791 ) ) ;
#11696=CARTESIAN_POINT ( 'NONE',  ( 8.503988664269582998, 10.94440607977979063, 1.599625672291281386 ) ) ;
#11699=CARTESIAN_POINT ( 'NONE',  ( -1.364683531250012516, 3.530208333674758059, 0.7879004041258379498 ) ) ;
#11701=CARTESIAN_POINT ( 'NONE',  ( -5.246642258808529746, 9.064907035344523578, 0.000000000000000000 ) ) ;
#11707=CARTESIAN_POINT ( 'NONE',  ( 3.460355519985863548, 5.060167411448709629, 1.599625672291267398 ) ) ;
#11710=CARTESIAN_POINT ( 'NONE',  ( 9.185812768458653466, 10.67553530374532045, 1.199719254218453823 ) ) ;
#11711=CARTESIAN_POINT ( 'NONE',  ( 6.511106444361000278, 5.279176164185798825, -2.499999999999995559 ) ) ;
#11716=CARTESIAN_POINT ( 'NONE',  ( -8.670602931139386627, 10.07445716020612103, 1.199719254218462483 ) ) ;
#11717=CARTESIAN_POINT ( 'NONE',  ( 6.657217119509961201, 7.725507046638470321, -1.199719254218446718 ) ) ;
#11720=CARTESIAN_POINT ( 'NONE',  ( 3.659811400685081040, 6.357198169852855685, -1.199719254218446718 ) ) ;
#11727=CARTESIAN_POINT ( 'NONE',  ( -5.083944415444539899, 8.875092884753202682, 0.000000000000000000 ) ) ;
#11728=CARTESIAN_POINT ( 'NONE',  ( 2.822068529938852155, 6.444163718237301275, -0.7998128361456291469 ) ) ;
#11731=CARTESIAN_POINT ( 'NONE',  ( -8.369460898337653276, 8.658792557682392754, 0.7998128361456462443 ) ) ;
#11738=CARTESIAN_POINT ( 'NONE',  ( -9.809487834687324437, 11.40315621434539395, 1.199719254218462483 ) ) ;
#11742=CARTESIAN_POINT ( 'NONE',  ( 8.959240580532112475, 9.346868853575953651, -0.7998128361456221525 ) ) ;
#11745=VERTEX_POINT ( 'NONE', #158635 ) ;
#11755=CARTESIAN_POINT ( 'NONE',  ( -8.843996274815957293, 9.212417163573759282, 1.040834085586084257E-14 ) ) ;
#11759=CARTESIAN_POINT ( 'NONE',  ( 5.938108093105483931, 8.911247961056314892, -1.082531754730537088 ) ) ;
#11761=CARTESIAN_POINT ( 'NONE',  ( -1.451998047846444262, 7.315968950355187239, 4.301760722574934803 ) ) ;
#11764=CARTESIAN_POINT ( 'NONE',  ( -5.656776405399756236, 7.622658444431597680, -1.599625672291256295 ) ) ;
#11774=CARTESIAN_POINT ( 'NONE',  ( 0.7499999999999902300, 5.566666666666685082, -1.299038105676658228 ) ) ;
#11775=CARTESIAN_POINT ( 'NONE',  ( 9.101601193475611140, 9.512956235343358102, -0.7998128361456221525 ) ) ;
#11777=CARTESIAN_POINT ( 'NONE',  ( -4.284013352238262407, 6.021101549076499637, -1.443375672974053447 ) ) ;
#11780=CARTESIAN_POINT ( 'NONE',  ( -5.157125652413038885, 6.495829312680758250, -1.199528311315662510 ) ) ;
#11787=CARTESIAN_POINT ( 'NONE',  ( 3.358669367883368118, 4.941533567329135401, -1.599625672291262513 ) ) ;
#11794=CARTESIAN_POINT ( 'NONE',  ( 5.054492339796319733, 4.791329239384148231, -0.7998128361456211532 ) ) ;
#11799=CARTESIAN_POINT ( 'NONE',  ( -1.364683531250012516, 3.551041667008086211, -0.7879004041258300672 ) ) ;
#11804=CARTESIAN_POINT ( 'NONE',  ( 4.449046963578762615, 8.342305224150557308, -0.7998128361456231517 ) ) ;
#11808=CARTESIAN_POINT ( 'NONE',  ( -5.111587607552082524, 5.922272616020886282, 1.199719254218450271 ) ) ;
#11809=CARTESIAN_POINT ( 'NONE',  ( 6.114364089638798738, 6.235772314107808079, 0.7216878364870317197 ) ) ;
#11810=CARTESIAN_POINT ( 'NONE',  ( 0.7499999999999902300, 4.066666666666690411, -1.299038105676658228 ) ) ;
#11812=CARTESIAN_POINT ( 'NONE',  ( -3.815730167242251003, 6.539103397502874948, -1.199719254218452047 ) ) ;
#11813=CARTESIAN_POINT ( 'NONE',  ( -0.007473969438131279966, 8.279395425053861501, -1.999986034896452436 ) ) ;
#11815=CARTESIAN_POINT ( 'NONE',  ( -1.201851678989727383E-14, 4.946875000341420581, -1.575800808251660134 ) ) ;
#11818=CARTESIAN_POINT ( 'NONE',  ( -2.982430605326321427, 6.423326772948587227, -0.7216878364870267237 ) ) ;
#11822=CARTESIAN_POINT ( 'NONE',  ( 5.203632029546647608, 4.965325544092860532, 1.040834085586084257E-14 ) ) ;
#11825=CARTESIAN_POINT ( 'NONE',  ( 4.911089278408375947, 4.764320510802636299, 0.1685941148131786249 ) ) ;
#11827=CARTESIAN_POINT ( 'NONE',  ( -1.201851678989727383E-14, 1.884375000341422135, 1.575800808251672791 ) ) ;
#11831=CARTESIAN_POINT ( 'NONE',  ( -8.136864746495904299, 12.64475930422059768, -0.7998128361456281477 ) ) ;
#11832=CARTESIAN_POINT ( 'NONE',  ( -4.053524740361572398, 7.672936597156388316, 0.7216878364870317197 ) ) ;
#11835=VERTEX_POINT ( 'NONE', #209484 ) ;
#11836=CARTESIAN_POINT ( 'NONE',  ( 0.6823417656249917140, 3.842708333674754506, 1.181850606188765695 ) ) ;
#11839=AXIS2_PLACEMENT_3D ( 'NONE', #150815, #54373, #120511 ) ;
#11845=CARTESIAN_POINT ( 'NONE',  ( -6.710922848640111127, 6.931757532942661726, 0.7216878364870317197 ) ) ;
#11847=CARTESIAN_POINT ( 'NONE',  ( -2.193105066167322370, 5.702484939155337607, -2.500000000000000444 ) ) ;
#11851=CARTESIAN_POINT ( 'NONE',  ( -6.222829318548141586, 6.362315081168691044, 0.7216878364870317197 ) ) ;
#11855=PLANE ( 'NONE',  #28189 ) ;
#11865=CARTESIAN_POINT ( 'NONE',  ( -5.148345644887285744, 7.029489223833707001, -1.599625672291256295 ) ) ;
#11866=CARTESIAN_POINT ( 'NONE',  ( -5.958368452836739770, 6.108636665014236300, 0.7718718275001738016 ) ) ;
#11868=CARTESIAN_POINT ( 'NONE',  ( 1.499999999999987121, 0.7958333333333510451, -0.8660254037844253849 ) ) ;
#11870=CARTESIAN_POINT ( 'NONE',  ( 9.761507412159302177, 10.49077285704843199, -0.7216878364870257245 ) ) ;
#11871=CARTESIAN_POINT ( 'NONE',  ( 5.960781091502512119, 10.10599504006161986, 0.7998128361456462443 ) ) ;
#11876=FACE_OUTER_BOUND ( 'NONE', #59289, .T. ) ;
#11877=CARTESIAN_POINT ( 'NONE',  ( 5.705283713252285338, 5.550585841749444249, -0.7998128361456211532 ) ) ;
#11878=CARTESIAN_POINT ( 'NONE',  ( -0.5528008270655216938, 7.812676398891195362, -1.922238454054859824 ) ) ;
#11885=CARTESIAN_POINT ( 'NONE',  ( -4.889686956022917919, 8.856385215335397021, 1.214306433183764966E-14 ) ) ;
#11893=CARTESIAN_POINT ( 'NONE',  ( 1.364683531249988535, 3.863541667008087543, 0.7879004041258500513 ) ) ;
#11894=CARTESIAN_POINT ( 'NONE',  ( 8.934460041281305109, 10.48625347199211966, -1.082531754730543083 ) ) ;
#11895=CARTESIAN_POINT ( 'NONE',  ( -5.551173829791513192, 8.563787670477010394, 1.199719254218452047 ) ) ;
#11898=CARTESIAN_POINT ( 'NONE',  ( 6.307567778855705853, 8.381915046796901692, -1.599625672291262513 ) ) ;
#11899=CARTESIAN_POINT ( 'NONE',  ( -4.466521540698216164, 7.298359999868178960, -1.199719254218452047 ) ) ;
#11903=CARTESIAN_POINT ( 'NONE',  ( 1.499999999999987121, 0.2854166673494805684, 0.8660254037844524744 ) ) ;
#11907=CARTESIAN_POINT ( 'NONE',  ( 7.375272376154084597, 9.627570410311676596, -1.443375672974057666 ) ) ;
#11911=CARTESIAN_POINT ( 'NONE',  ( 1.364683531249988535, 2.426041667008088432, 0.7879004041258500513 ) ) ;
#11913=CARTESIAN_POINT ( 'NONE',  ( 5.138177029454829459, 8.938364267765221527, 0.7216878364870438212 ) ) ;
#11916=CARTESIAN_POINT ( 'NONE',  ( -2.982430605326328532, 5.462957558647244305, -1.082531754730543971 ) ) ;
#11918=CARTESIAN_POINT ( 'NONE',  ( -1.364683531250010295, 5.530208333674751842, 0.7879004041258379498 ) ) ;
#11923=VERTEX_POINT ( 'NONE', #126211 ) ;
#11924=CARTESIAN_POINT ( 'NONE',  ( -4.338732707277040745, 7.407397761066524922, -1.160996969951762159 ) ) ;
#11930=( BOUNDED_CURVE ( )  B_SPLINE_CURVE ( 2, ( #138777, #188571, #106313, #55377, #172336, #185362, #136642, #23925, #202666, #20718, #54316, #121532, #21770, #39131, #90030, #7672, #139852, #205882, #105214, #173417, #24998, #120454, #87879, #186429, #69468, #53245, #137709, #104137, #170183, #36984, #135573, #71600, #152877, #155015, #171252, #57516, #22847, #123674, #189636, #41287, #107395, #201597, #11947, #209063, #46607, #124733, #194970, #58578, #190692, #59637, #61779, #143069, #96437, #210136, #125795, #94303, #176598, #76944, #108466, #191757, #159270, #174486, #127946, #10870, #126864, #30352, #13006 ),
 .UNSPECIFIED., .F., .T. ) 
 B_SPLINE_CURVE_WITH_KNOTS ( ( 3, 2, 2, 2, 2, 2, 2, 2, 2, 2, 2, 2, 2, 2, 2, 2, 2, 2, 2, 2, 2, 2, 2, 2, 2, 2, 2, 2, 2, 2, 2, 2, 2, 3 ),
 ( 0.1422369605164285622, 0.1458333333333333426, 0.1499999999999999944, 0.1541666666666666741, 0.1583333333333333259, 0.1625000000000000056, 0.1666666666666666574, 0.1708333333333333370, 0.1749999999999999889, 0.1791666666666666685, 0.1833333333333333204, 0.1875000000000000000, 0.1916666666666666796, 0.1958333333333333315, 0.2000000000000000111, 0.2041666666666666630, 0.2083333333333333426, 0.2124999999999999944, 0.2166666666666666741, 0.2208333333333333259, 0.2250000000000000056, 0.2291666666666666574, 0.2333333333333333370, 0.2374999999999999889, 0.2416666666666666685, 0.2458333333333333204, 0.2500000000000000000, 0.2541666666666666519, 0.2583333333333333592, 0.2625000000000000111, 0.2666666666666666630, 0.2708333333333333148, 0.2750000000000000222, 0.2785089426034975113 ),
 .UNSPECIFIED. ) 
 CURVE ( )  GEOMETRIC_REPRESENTATION_ITEM ( )  RATIONAL_B_SPLINE_CURVE ( ( 0.9683452906431839757, 0.8843625769634950728, 1.000000000000000000, 0.8660254037844387076, 1.000000000000000000, 0.8660254037844387076, 1.000000000000000000, 0.8660254037844387076, 1.000000000000000000, 0.8660254037844387076, 1.000000000000000000, 0.8660254037844387076, 1.000000000000000000, 0.8660254037844387076, 1.000000000000000000, 0.8660254037844387076, 1.000000000000000000, 0.8660254037844387076, 1.000000000000000000, 0.8660254037844387076, 1.000000000000000000, 0.8660254037844387076, 1.000000000000000000, 0.8660254037844387076, 1.000000000000000000, 0.8660254037844387076, 1.000000000000000000, 0.8660254037844387076, 1.000000000000000000, 0.8660254037844387076, 1.000000000000000000, 0.8660254037844387076, 1.000000000000000000, 0.8660254037844387076, 1.000000000000000000, 0.8660254037844387076, 1.000000000000000000, 0.8660254037844387076, 1.000000000000000000, 0.8660254037844387076, 1.000000000000000000, 0.8660254037844387076, 1.000000000000000000, 0.8660254037844387076, 1.000000000000000000, 0.8660254037844387076, 1.000000000000000000, 0.8660254037844387076, 1.000000000000000000, 0.8660254037844387076, 1.000000000000000000, 0.8660254037844387076, 1.000000000000000000, 0.8660254037844387076, 1.000000000000000000, 0.8660254037844387076, 1.000000000000000000, 0.8660254037844387076, 1.000000000000000000, 0.8660254037844387076, 1.000000000000000000, 0.8660254037844387076, 1.000000000000000000, 0.8660254037844387076, 1.000000000000000000, 0.8871737995726820536, 0.9643799166510427234 ) ) 
 REPRESENTATION_ITEM ( '' )  );
#11940=ORIENTED_EDGE ( 'NONE', *, *, #26674, .T. ) ;
#11942=CARTESIAN_POINT ( 'NONE',  ( 5.192409644353875642, 5.160158794608717514, 1.040834085586084257E-14 ) ) ;
#11943=CARTESIAN_POINT ( 'NONE',  ( -1.402160292154681736E-14, 1.759375000341421469, -1.575800808251659024 ) ) ;
#11944=CARTESIAN_POINT ( 'NONE',  ( 8.158255747121103241, 10.54105100977322174, 1.599625672291281386 ) ) ;
#11946=CARTESIAN_POINT ( 'NONE',  ( 1.499999999999990896, 3.806250000682819046, 1.214306433183764966E-14 ) ) ;
#11947=CARTESIAN_POINT ( 'NONE',  ( -4.120788623549732854, 6.895004929861607401, -1.199719254218452047 ) ) ;
#11950=CARTESIAN_POINT ( 'NONE',  ( 1.499999999999989120, 2.025000000000019895, 1.214306433183764966E-14 ) ) ;
#11951=CARTESIAN_POINT ( 'NONE',  ( 6.419949431270806528, 7.448694743692793274, 1.199719254218462483 ) ) ;
#11952=CARTESIAN_POINT ( 'NONE',  ( -7.660520486921249983, 8.896027641951645748, -1.199719254218446718 ) ) ;
#11956=CARTESIAN_POINT ( 'NONE',  ( 0.6823417656249899377, 2.342708333674753618, 1.181850606188767472 ) ) ;
#11959=CARTESIAN_POINT ( 'NONE',  ( 4.369805582306193870, 3.992528022312320957, 1.214306433183764966E-14 ) ) ;
#11965=CARTESIAN_POINT ( 'NONE',  ( -0.7500000000000006661, 0.3895833340161539149, -1.299038105676652011 ) ) ;
#11967=CARTESIAN_POINT ( 'NONE',  ( -7.230575994789712801, 7.330093503543126054, 0.7998128361456341429 ) ) ;
#11968=CARTESIAN_POINT ( 'NONE',  ( -2.657034918598345730, 5.083329257464595408, -1.082531754730543971 ) ) ;
#11976=CARTESIAN_POINT ( 'NONE',  ( 4.638861114170084399, 8.563755066507100722, 0.7998128361456462443 ) ) ;
#11980=CARTESIAN_POINT ( 'NONE',  ( 6.602984505055297326, 7.662235663108029726, 1.199719254218462483 ) ) ;
#11981=DIRECTION ( 'NONE',  ( 1.207943261119674327E-30, 2.168404344971008079E-15, 1.000000000000000000 ) ) ;
#11983=CARTESIAN_POINT ( 'NONE',  ( -5.181187258716735577, 9.196468901811520880, 0.7998128361456481317 ) ) ;
#11985=CARTESIAN_POINT ( 'NONE',  ( 4.542145155778077203, 5.257923088951247159, -1.199719254218452047 ) ) ;
#11991=CARTESIAN_POINT ( 'NONE',  ( 4.139348914150634329, 7.410017372392475821, 0.7316189255667099323 ) ) ;
#11997=CARTESIAN_POINT ( 'NONE',  ( -3.931501358282930791, 7.530575984731325612, 0.7216878364870262796 ) ) ;
#11999=CARTESIAN_POINT ( 'NONE',  ( 1.419999999999990603, 8.627523663848661428, -2.579999999999989413 ) ) ;
#12002=CARTESIAN_POINT ( 'NONE',  ( 6.792271770766432404, 10.86814146596211472, 1.040834085586084257E-14 ) ) ;
#12004=CARTESIAN_POINT ( 'NONE',  ( -5.579343907223557331, 6.467988298970945849, 1.199719254218450271 ) ) ;
#12008=CARTESIAN_POINT ( 'NONE',  ( 7.283754839039659146, 9.520799950344851936, -1.599625672291262513 ) ) ;
#12010=CARTESIAN_POINT ( 'NONE',  ( -6.417086777969760902, 6.381022750586497594, 0.7998128361456341429 ) ) ;
#12026=CARTESIAN_POINT ( 'NONE',  ( -4.985647801523292344, 6.839675073242382553, -1.599625672291256295 ) ) ;
#12029=CARTESIAN_POINT ( 'NONE',  ( 5.016153647376217606, 4.954526798134778254, 0.7216878364870317197 ) ) ;
#12032=CARTESIAN_POINT ( 'NONE',  ( -4.457933580795036654, 4.095344020549286590, -0.7998128361456221525 ) ) ;
#12033=CARTESIAN_POINT ( 'NONE',  ( -5.088387723830502196, 4.830873854090670605, -0.7998128361456221525 ) ) ;
#12036=( GEOMETRIC_REPRESENTATION_CONTEXT ( 3 ) GLOBAL_UNCERTAINTY_ASSIGNED_CONTEXT ( ( #66933 ) ) GLOBAL_UNIT_ASSIGNED_CONTEXT ( ( #170220, #120491, #168099 ) ) REPRESENTATION_CONTEXT ( 'NONE', 'WORKASPACE' ) );
#12037=CARTESIAN_POINT ( 'NONE',  ( 7.703003830858588863, 12.13858823597705872, -0.7998128361456291469 ) ) ;
#12040=CARTESIAN_POINT ( 'NONE',  ( -5.865874016206865882, 9.995270118883347266, 0.000000000000000000 ) ) ;
#12041=CARTESIAN_POINT ( 'NONE',  ( 6.498435699651741615, 6.475929825882159818, -0.7998128361456281477 ) ) ;
#12047=CARTESIAN_POINT ( 'NONE',  ( -1.402160292154681736E-14, 1.509375000341420359, -1.575800808251659024 ) ) ;
#12049=ORIENTED_EDGE ( 'NONE', *, *, #172459, .F. ) ;
#12052=CARTESIAN_POINT ( 'NONE',  ( 7.510853912290742507, 8.825379654836435606, -1.082531754730537976 ) ) ;
#12060=AXIS2_PLACEMENT_3D ( 'NONE', #146329, #96517, #65028 ) ;
#12061=CARTESIAN_POINT ( 'NONE',  ( 8.554831740098642001, 12.92446143018304916, 0.7216878364870438212 ) ) ;
#12068=CARTESIAN_POINT ( 'NONE',  ( -10.50487009249003378, 11.15010328419353947, 0.7998128361456462443 ) ) ;
#12069=CARTESIAN_POINT ( 'NONE',  ( 3.284841267552055299, 6.405332120898776793, -0.9495590844852130896 ) ) ;
#12077=CARTESIAN_POINT ( 'NONE',  ( 1.284279953904121641, 3.300000000000018030, -0.7749999999999892530 ) ) ;
#12084=CARTESIAN_POINT ( 'NONE',  ( -1.500000000000013101, 1.952083334016152527, 0.8660254037844403729 ) ) ;
#12090=CARTESIAN_POINT ( 'NONE',  ( 1.499999999999987566, -0.4749999999999823808, 0.000000000000000000 ) ) ;
#12091=CARTESIAN_POINT ( 'NONE',  ( 9.250740883225924804, 9.686952540052077509, 1.040834085586084257E-14 ) ) ;
#12095=CARTESIAN_POINT ( 'NONE',  ( 2.496672843210871129, 6.064535417054653266, -0.7998128361456291469 ) ) ;
#12096=CARTESIAN_POINT ( 'NONE',  ( -6.073689629242160493, 8.109057205581079231, -1.443375672974059665 ) ) ;
#12100=CARTESIAN_POINT ( 'NONE',  ( -6.612626235163205024, 8.737816579155630592, -1.599625672291263179 ) ) ;
#12101=VERTEX_POINT ( 'NONE', #105638 ) ;
#12102=CARTESIAN_POINT ( 'NONE',  ( -1.500000000000013101, 1.702083334016151417, 0.8660254037844403729 ) ) ;
#12114=CARTESIAN_POINT ( 'NONE',  ( -2.440104460335327463, 5.790612937125752424, 1.040834085586084257E-14 ) ) ;
#12115=CARTESIAN_POINT ( 'NONE',  ( 6.286176778230493589, 10.48562334124426698, 0.7998128361456462443 ) ) ;
#12119=ORIENTED_EDGE ( 'NONE', *, *, #82075, .T. ) ;
#12123=CARTESIAN_POINT ( 'NONE',  ( -6.496328159242330536, 10.73079995242472862, 0.000000000000000000 ) ) ;
#12130=CARTESIAN_POINT ( 'NONE',  ( 3.357615597678655917, 7.068968630600412695, 0.7998128361456321445 ) ) ;
#12135=CARTESIAN_POINT ( 'NONE',  ( -9.378489572351046633, 11.96465713920816043, -1.599625672291263179 ) ) ;
#12138=CARTESIAN_POINT ( 'NONE',  ( -4.764280463835226520, 6.994423760310605864, -1.426210198329436851 ) ) ;
#12147=CARTESIAN_POINT ( 'NONE',  ( 5.957918438201454059, 9.038323046955323292, -1.199719254218440723 ) ) ;
#12149=VERTEX_POINT ( 'NONE', #205215 ) ;
#12158=CARTESIAN_POINT ( 'NONE',  ( -1.500000000000013101, 0.2020833340161521663, 0.8660254037844403729 ) ) ;
#12161=CARTESIAN_POINT ( 'NONE',  ( -4.115954692286631023, 7.559005856764831499, 0.7081028429081294151 ) ) ;
#12170=CARTESIAN_POINT ( 'NONE',  ( 5.016153647376205171, 6.875265226737464985, 1.443375672974062551 ) ) ;
#12172=VERTEX_POINT ( 'NONE', #175960 ) ;
#12173=LINE ( 'NONE', #128164, #133224 ) ;
#12175=CARTESIAN_POINT ( 'NONE',  ( 2.345197385039651472, 5.679888015947478941, -0.7216878364870267237 ) ) ;
#12184=CARTESIAN_POINT ( 'NONE',  ( 1.364683531249986537, -0.5947916663252456049, -0.7879004041258309554 ) ) ;
#12189=CARTESIAN_POINT ( 'NONE',  ( -5.148345644887285744, 7.029489223833707001, -1.599625672291256295 ) ) ;
#12192=CARTESIAN_POINT ( 'NONE',  ( 1.499999999999987566, 0.02500000000001806333, 0.000000000000000000 ) ) ;
#12194=CARTESIAN_POINT ( 'NONE',  ( -1.500000000000011324, 5.670833333333358262, 0.8660254037844403729 ) ) ;
#12200=CARTESIAN_POINT ( 'NONE',  ( 1.364683531249986537, -0.8447916663252468261, -0.7879004041258309554 ) ) ;
#12202=CARTESIAN_POINT ( 'NONE',  ( -7.395082721250053837, 10.71501471051202614, -1.199719254218446718 ) ) ;
#12208=CARTESIAN_POINT ( 'NONE',  ( 1.364683531249986537, 0.2177083336747502595, -0.7879004041258309554 ) ) ;
#12212=CARTESIAN_POINT ( 'NONE',  ( -4.907894938888499148, 6.474487383728022571, 2.499999999999999112 ) ) ;
#12215=CARTESIAN_POINT ( 'NONE',  ( 7.293923454472080792, 9.532663335016016148, 1.443375672974076540 ) ) ;
#12219=CARTESIAN_POINT ( 'NONE',  ( -0.7500000000000215383, 4.222916667349481123, 1.299038105676671107 ) ) ;
#12221=CARTESIAN_POINT ( 'NONE',  ( -3.079673448598517549, 6.744702790006905424, 1.040834085586084257E-14 ) ) ;
#12222=CARTESIAN_POINT ( 'NONE',  ( 7.104109303436412226, 7.390475063538369582, 1.040834085586084257E-14 ) ) ;
#12223=CARTESIAN_POINT ( 'NONE',  ( -7.958272981097355370, 12.22847621134819285, 0.7216878364870458196 ) ) ;
#12229=CARTESIAN_POINT ( 'NONE',  ( 9.897088948295943212, 11.60932053017587506, 1.082531754730548412 ) ) ;
#12231=CARTESIAN_POINT ( 'NONE',  ( 2.378026000468616452, 5.267601517901375097, 0.8449283794987967333 ) ) ;
#12242=ORIENTED_EDGE ( 'NONE', *, *, #7783, .T. ) ;
#12244=CARTESIAN_POINT ( 'NONE',  ( 7.889955328148847258, 11.29236608522730911, -1.199719254218446718 ) ) ;
#12249=CARTESIAN_POINT ( 'NONE',  ( -1.402160292154681736E-14, -0.1781249996585796136, 1.575800808251672791 ) ) ;
#12250=CARTESIAN_POINT ( 'NONE',  ( 4.636525346193557162, 7.392734756325715750, -1.082531754730549078 ) ) ;
#12251=ORIENTED_EDGE ( 'NONE', *, *, #442, .T. ) ;
#12252=CARTESIAN_POINT ( 'NONE',  ( -8.432808358020034589, 10.86136238915529084, 1.443375672974064550 ) ) ;
#12264=VERTEX_POINT ( 'NONE', #173837 ) ;
#12271=CARTESIAN_POINT ( 'NONE',  ( 4.675513026854819287, 7.080785086760167601, -1.371149936167876282 ) ) ;
#12278=CARTESIAN_POINT ( 'NONE',  ( -7.619319141200077361, 9.912291636198670375, 1.443375672974090751 ) ) ;
#12280=DIRECTION ( 'NONE',  ( -0.8002608041566210417, 0.5996521035822340862, 0.000000000000000000 ) ) ;
#12282=CARTESIAN_POINT ( 'NONE',  ( 7.284808609244363353, 7.393364887073558656, 0.7998128361456341429 ) ) ;
#12284=CARTESIAN_POINT ( 'NONE',  ( -5.447678794592645701, 5.250046769979851646, 0.000000000000000000 ) ) ;
#12285=CARTESIAN_POINT ( 'NONE',  ( -5.000000000000000888, 0.2350621082554960051, -0.7749999999999935829 ) ) ;
#12288=CARTESIAN_POINT ( 'NONE',  ( -5.752737250900127997, 5.605948302338584099, 0.000000000000000000 ) ) ;
#12292=CARTESIAN_POINT ( 'NONE',  ( 4.059776932288224671, 6.823824623389866950, 1.199719254218462483 ) ) ;
#12293=CARTESIAN_POINT ( 'NONE',  ( 9.088043039861931405, 9.497138389460751284, 1.040834085586084257E-14 ) ) ;
#12294=CARTESIAN_POINT ( 'NONE',  ( 4.650083499807233345, 5.295740330745369207, -7.499999999999997335 ) ) ;
#12296=CARTESIAN_POINT ( 'NONE',  ( 5.132834705836428313, 6.694876404991986441, 1.408819685294822932 ) ) ;
#12297=CARTESIAN_POINT ( 'NONE',  ( 3.687454593236936251, 7.245854758844324728, -0.7216878364870267237 ) ) ;
#12304=CARTESIAN_POINT ( 'NONE',  ( 7.104109303436412226, 7.390475063538369582, 1.040834085586084257E-14 ) ) ;
#12305=CARTESIAN_POINT ( 'NONE',  ( -8.296699936558862731, 11.76690146170562201, 1.199719254218453823 ) ) ;
#12308=CARTESIAN_POINT ( 'NONE',  ( -9.429859533504656000, 10.96025652963230534, -1.199719254218441611 ) ) ;
#12309=CARTESIAN_POINT ( 'NONE',  ( -6.042130013184518589, 10.20090211535728031, -0.7998128361456291469 ) ) ;
#12314=CARTESIAN_POINT ( 'NONE',  ( 1.566565198595117892, 8.754658464387805594, -2.463935442259830744 ) ) ;
#12317=CARTESIAN_POINT ( 'NONE',  ( 9.185812768458653466, 10.67553530374532045, 1.199719254218453823 ) ) ;
#12321=CARTESIAN_POINT ( 'NONE',  ( 3.171717870593107058, 5.787755718078879674, -1.199719254218446718 ) ) ;
#12324=VECTOR ( 'NONE', #175241, 1000.000000000000000 ) ;
#12325=CARTESIAN_POINT ( 'NONE',  ( 1.499999999999990896, 5.306250000682820378, 1.214306433183764966E-14 ) ) ;
#12331=CARTESIAN_POINT ( 'NONE',  ( -1.500000000000011324, 3.420833333333355597, 0.8660254037844403729 ) ) ;
#12332=CARTESIAN_POINT ( 'NONE',  ( 6.972971076130050072, 7.029554431773520129, 1.040834085586084257E-14 ) ) ;
#12335=CARTESIAN_POINT ( 'NONE',  ( 7.619319141200070256, 8.951922421897323900, 1.082531754730558626 ) ) ;
#12336=CARTESIAN_POINT ( 'NONE',  ( -8.785320351530977234, 13.19336481018743079, 1.040834085586084257E-14 ) ) ;
#12340=CARTESIAN_POINT ( 'NONE',  ( 7.214910300766615769, 11.56914578420308715, -0.7998128361456291469 ) ) ;
#12343=CARTESIAN_POINT ( 'NONE',  ( -3.307299406729781399, 5.945934176904983381, -1.199719254218452935 ) ) ;
#12344=CARTESIAN_POINT ( 'NONE',  ( -0.7499999999999972244, 4.889583334016150751, -1.299038105676652899 ) ) ;
#12345=CARTESIAN_POINT ( 'NONE',  ( -1.402160292154681736E-14, 0.6968750003414164729, -1.575800808251659024 ) ) ;
#12350=CARTESIAN_POINT ( 'NONE',  ( -1.364683531250014514, -0.2614583329919080157, -0.7879004041258359514 ) ) ;
#12356=CARTESIAN_POINT ( 'NONE',  ( -3.375617059678305054, 5.921675088724528635, 1.082531754730560403 ) ) ;
#12360=CARTESIAN_POINT ( 'NONE',  ( -7.549192604710863286, 7.701812881784464437, -0.7998128361456291469 ) ) ;
#12363=CARTESIAN_POINT ( 'NONE',  ( 5.515469562660962666, 5.329135999392899947, 0.7998128361456341429 ) ) ;
#12370=CARTESIAN_POINT ( 'NONE',  ( 10.07387183015377197, 11.71160420905630062, -1.199719254218440723 ) ) ;
#12373=CARTESIAN_POINT ( 'NONE',  ( -5.555090253297260361, 7.504024600312024340, 1.599625672291269396 ) ) ;
#12377=CARTESIAN_POINT ( 'NONE',  ( 9.399880572976245574, 9.860948844760784482, 0.7998128361456462443 ) ) ;
#12379=CARTESIAN_POINT ( 'NONE',  ( 7.751511138711133064, 10.06651563329490529, -1.599625672291262513 ) ) ;
#12382=CARTESIAN_POINT ( 'NONE',  ( -3.789667630219657912, 4.380032642466370696, 1.199719254218462483 ) ) ;
#12385=CARTESIAN_POINT ( 'NONE',  ( -6.531277313481209212, 8.642909503859968368, 1.599625672291283607 ) ) ;
#12389=CARTESIAN_POINT ( 'NONE',  ( -6.024621019446552594, 6.066914679173425640, 0.6088392743194663836 ) ) ;
#12390=CARTESIAN_POINT ( 'NONE',  ( 1.364683531249986537, -0.1364583329919154264, 0.7879004041258500513 ) ) ;
#12393=CARTESIAN_POINT ( 'NONE',  ( 7.131225611108096274, 8.382479970123348778, 1.082531754730558626 ) ) ;
#12411=CARTESIAN_POINT ( 'NONE',  ( 7.248805684800777804, 11.60869039890961218, 1.040834085586084257E-14 ) ) ;
#12415=CARTESIAN_POINT ( 'NONE',  ( -5.135841261478327979, 4.886236314679810455, 0.7998128361456341429 ) ) ;
#12416=CARTESIAN_POINT ( 'NONE',  ( -8.830438121202295321, 9.196599317691152464, -0.7998128361456291469 ) ) ;
#12418=ORIENTED_EDGE ( 'NONE', *, *, #20075, .F. ) ;
#12421=CARTESIAN_POINT ( 'NONE',  ( -1.001543065824772872E-14, 4.243750000682819490, 1.732050807568877637 ) ) ;
#12422=CARTESIAN_POINT ( 'NONE',  ( 9.101601193475611140, 9.512956235343358102, -0.7998128361456221525 ) ) ;
#12425=CARTESIAN_POINT ( 'NONE',  ( -8.715193815486133033, 9.062147627688959872, 0.7998128361456462443 ) ) ;
#12427=CARTESIAN_POINT ( 'NONE',  ( -1.201851678989727383E-14, 3.696875000341422801, -1.575800808251660134 ) ) ;
#12433=CARTESIAN_POINT ( 'NONE',  ( -9.815740026613967828, 10.55404424057886636, -0.7216878364870267237 ) ) ;
#12438=CARTESIAN_POINT ( 'NONE',  ( -1.402160292154681736E-14, 2.259375000341416140, -1.575800808251660134 ) ) ;
#12445=CARTESIAN_POINT ( 'NONE',  ( -1.201851678989727383E-14, 2.696875000341417916, -1.575800808251660134 ) ) ;
#12448=CARTESIAN_POINT ( 'NONE',  ( -4.629219384062206011, 7.488174150459498968, -1.199719254218452047 ) ) ;
#12449=CARTESIAN_POINT ( 'NONE',  ( 7.613066949273408213, 8.840665181362512115, -1.199719254218441611 ) ) ;
#12451=( BOUNDED_CURVE ( )  B_SPLINE_CURVE ( 2, ( #177571, #78985, #154125, #123848, #23024 ),
 .UNSPECIFIED., .F., .T. ) 
 B_SPLINE_CURVE_WITH_KNOTS ( ( 3, 2, 3 ),
 ( 0.01092446968156909545, 0.01250000000000000069, 0.01386088777671199215 ),
 .UNSPECIFIED. ) 
 CURVE ( )  GEOMETRIC_REPRESENTATION_ITEM ( )  RATIONAL_B_SPLINE_CURVE ( ( 0.9369925407309220855, 0.9493405508230827738, 1.000000000000000000, 0.9562421463088763840, 0.9410680661649857282 ) ) 
 REPRESENTATION_ITEM ( '' )  );
#12454=ADVANCED_FACE ( 'NONE', ( #206049 ), #109701, .T. ) ;
#12455=CARTESIAN_POINT ( 'NONE',  ( 0.6823417656249917140, 4.405208333674755394, 1.181850606188765695 ) ) ;
#12458=CARTESIAN_POINT ( 'NONE',  ( 1.364683531249988757, 0.1343750003414204142, 0.000000000000000000 ) ) ;
#12459=CARTESIAN_POINT ( 'NONE',  ( -4.934804725694236893, 4.859619722839116918, -0.7216878364870207285 ) ) ;
#12460=EDGE_CURVE ( 'NONE', #141559, #71915, #153009, .T. ) ;
#12463=CARTESIAN_POINT ( 'NONE',  ( 5.368665641331531013, 5.365790791082654998, -0.7216878364870207285 ) ) ;
#12466=CARTESIAN_POINT ( 'NONE',  ( -8.311311860377216476, 9.655284244316948872, -1.199719254218446718 ) ) ;
#12467=CARTESIAN_POINT ( 'NONE',  ( -9.083599731475995753, 11.62061899152058686, 1.443375672974064550 ) ) ;
#12469=CARTESIAN_POINT ( 'NONE',  ( 1.364683531249990311, 5.613541667008087543, 0.7879004041258500513 ) ) ;
#12475=CARTESIAN_POINT ( 'NONE',  ( -6.195713011320790109, 9.211787032307496403, -1.082531754730537976 ) ) ;
#12477=CARTESIAN_POINT ( 'NONE',  ( -1.364683531250000748, -0.9281249996585805295, 0.000000000000000000 ) ) ;
#12490=CARTESIAN_POINT ( 'NONE',  ( 1.499999999999987121, -0.2458333333333099502, 0.8660254037844524744 ) ) ;
#12491=CARTESIAN_POINT ( 'NONE',  ( 7.578644679914702031, 10.82520731233375955, 1.082531754730558626 ) ) ;
#12495=VERTEX_POINT ( 'NONE', #106481 ) ;
#12499=CARTESIAN_POINT ( 'NONE',  ( 5.636439174979242850, 7.598931675607687453, -1.599625672291262513 ) ) ;
#12501=CARTESIAN_POINT ( 'NONE',  ( -4.952806187693842510, 4.672695395264567786, 0.7998128361456341429 ) ) ;
#12503=CARTESIAN_POINT ( 'NONE',  ( 1.499999999999981126, 3.504166666666683749, 0.8660254037844571373 ) ) ;
#12504=CARTESIAN_POINT ( 'NONE',  ( 5.020596955762157698, 4.751784624677624080, 1.040834085586084257E-14 ) ) ;
#12505=CARTESIAN_POINT ( 'NONE',  ( -1.364683531250000748, 2.071875000341422357, 1.214306433183764966E-14 ) ) ;
#12507=CARTESIAN_POINT ( 'NONE',  ( -9.671043645249580933, 10.17730576241299900, 0.7998128361456462443 ) ) ;
#12513=LINE ( 'NONE', #129565, #6796 ) ;
#12521=ORIENTED_EDGE ( 'NONE', *, *, #31725, .F. ) ;
#12525=CARTESIAN_POINT ( 'NONE',  ( 5.147291874682557555, 9.156924287104992288, 0.7998128361456462443 ) ) ;
#12534=( BOUNDED_SURFACE ( )  B_SPLINE_SURFACE ( 3, 2, ( 
 ( #121731, #72874, #172539 ),
 ( #5719, #71796, #138980 ),
 ( #124930, #205003, #56649 ),
 ( #122811, #156290, #188770 ),
 ( #24124, #90226, #7874 ),
 ( #73962, #140056, #123870 ) ),
 .UNSPECIFIED., .F., .F., .T. ) 
 B_SPLINE_SURFACE_WITH_KNOTS ( ( 4, 2, 4 ),
 ( 3, 3 ),
 ( 0.000000000000000000, 0.002122857551078452965, 0.004245715102156905930 ),
 ( 0.000000000000000000, 1.000000000000000000 ),
 .UNSPECIFIED. ) 
 GEOMETRIC_REPRESENTATION_ITEM ( )  RATIONAL_B_SPLINE_SURFACE ( (
 ( 1.000000000000000000, 0.7806433624857582743, 1.000000000000000000),
 ( 1.000000000000000000, 0.7860453980259710649, 1.000000000000000000),
 ( 1.000000000000000000, 0.7924770197564218188, 1.000000000000000000),
 ( 1.000000000000000000, 0.8094762427233131996, 1.000000000000000000),
 ( 1.000000000000000000, 0.8200718518785218292, 1.000000000000000000),
 ( 1.000000000000000000, 0.8343063410434344851, 1.000000000000000000) ) ) 
 REPRESENTATION_ITEM ( '' )  SURFACE ( )  );
#12535=CARTESIAN_POINT ( 'NONE',  ( 7.913155211870404493, 12.38376484715752213, 0.7998128361456462443 ) ) ;
#12544=CARTESIAN_POINT ( 'NONE',  ( -9.842856333841300653, 10.58567993234409421, 0.7216878364870438212 ) ) ;
#12549=CARTESIAN_POINT ( 'NONE',  ( 4.473300617505036492, 7.306268922809479704, -1.199719254218452047 ) ) ;
#12556=CARTESIAN_POINT ( 'NONE',  ( 3.185802909086937973, 6.660594460669327255, 0.7216878364870317197 ) ) ;
#12564=CARTESIAN_POINT ( 'NONE',  ( -5.682838942422375084, 9.781729199468104596, 0.000000000000000000 ) ) ;
#12565=DIRECTION ( 'NONE',  ( 1.224646799147360603E-16, 1.000000000000000000, -8.546850786086437571E-32 ) ) ;
#12567=CARTESIAN_POINT ( 'NONE',  ( -4.308793891044708779, 3.921347715840572956, 1.214306433183764966E-14 ) ) ;
#12575=CARTESIAN_POINT ( 'NONE',  ( 6.531277313481192337, 8.642909503859968368, 1.599625672291281386 ) ) ;
#12583=CARTESIAN_POINT ( 'NONE',  ( -1.123270288254055060, 3.033552654332631437, 0.7749999999939940487 ) ) ;
#12588=CARTESIAN_POINT ( 'NONE',  ( 1.364683531249986537, -0.3239583329919163424, 0.7879004041258500513 ) ) ;
#12590=CARTESIAN_POINT ( 'NONE',  ( 3.867100128395839942, 5.534702787927018974, -1.599625672291255185 ) ) ;
#12592=CARTESIAN_POINT ( 'NONE',  ( -6.019457014787517046, 9.006155036351978893, 1.082531754730548412 ) ) ;
#12595=CARTESIAN_POINT ( 'NONE',  ( 5.680503174445848735, 5.729601246382692636, 1.040834085586084257E-14 ) ) ;
#12596=CARTESIAN_POINT ( 'NONE',  ( -8.175203438916030407, 8.640084888264587093, 0.7216878364870578100 ) ) ;
#12601=CARTESIAN_POINT ( 'NONE',  ( 6.474182045725470402, 7.511966127223233869, -1.199719254218446718 ) ) ;
#12606=CARTESIAN_POINT ( 'NONE',  ( -1.364683531249997417, 4.759375000341424133, 1.214306433183764966E-14 ) ) ;
#12610=CARTESIAN_POINT ( 'NONE',  ( 6.388916700537700777, 8.476822122092563916, 1.599625672291281386 ) ) ;
#12614=CARTESIAN_POINT ( 'NONE',  ( -7.985916173649233230, 9.275655943134292869, -1.199719254218446718 ) ) ;
#12619=CARTESIAN_POINT ( 'NONE',  ( 8.426556166093362776, 9.789735934319136135, -1.199719254218446718 ) ) ;
#12622=CARTESIAN_POINT ( 'NONE',  ( -6.581593504430098385, 9.765943957555402122, -1.199719254218440723 ) ) ;
#12624=CARTESIAN_POINT ( 'NONE',  ( 3.404766800216717737, 6.348112014766642552, 1.069586989871921467 ) ) ;
#12625=CARTESIAN_POINT ( 'NONE',  ( 8.392133896734671694, 8.893170422386358354, 0.7216878364870458196 ) ) ;
#12626=CARTESIAN_POINT ( 'NONE',  ( 4.005937425286727027, 7.819599604358462130, 0.1919598339409686050 ) ) ;
#12627=CARTESIAN_POINT ( 'NONE',  ( -9.978437869977959451, 10.74385839117019614, -0.7216878364870267237 ) ) ;
#12630=CARTESIAN_POINT ( 'NONE',  ( 3.250441568315368457, 6.417235977211314335, -0.9123035412251535581 ) ) ;
#12632=CARTESIAN_POINT ( 'NONE',  ( 5.666418135507635512, 8.698239360479199433, 1.199719254218462483 ) ) ;
#12634=CARTESIAN_POINT ( 'NONE',  ( 5.286789834324991055, 8.255339675766103724, -1.199719254218452935 ) ) ;
#12635=CARTESIAN_POINT ( 'NONE',  ( -5.155981903556834389, 6.496760599866445496, 1.199444197134313272 ) ) ;
#12636=CARTESIAN_POINT ( 'NONE',  ( 4.630273154266905777, 5.360739087188218122, 1.199719254218464037 ) ) ;
#12639=CARTESIAN_POINT ( 'NONE',  ( -6.561783159334137139, 8.678499657355050800, -1.443375672974059665 ) ) ;
#12645=CARTESIAN_POINT ( 'NONE',  ( -4.609732581575539889, 6.945374051331699938, 1.198810113796699328 ) ) ;
#12646=CARTESIAN_POINT ( 'NONE',  ( 0.6823417656249882723, -0.2614583329919109578, -1.181850606188749264 ) ) ;
#12649=CARTESIAN_POINT ( 'NONE',  ( 3.863710590214593399, 7.451486755318259547, 1.040834085586084257E-14 ) ) ;
#12653=CARTESIAN_POINT ( 'NONE',  ( -7.971831134711019118, 12.24429405723079967, 0.000000000000000000 ) ) ;
#12657=CARTESIAN_POINT ( 'NONE',  ( -8.636180661780660017, 11.09863007687603087, -1.443375672974058777 ) ) ;
#12664=CARTESIAN_POINT ( 'NONE',  ( -7.605760987142072160, 10.85684300409898384, 1.082531754730549967 ) ) ;
#12668=CARTESIAN_POINT ( 'NONE',  ( -1.500000000000013101, 3.660416667349488673, -0.8660254037844313801 ) ) ;
#12669=CARTESIAN_POINT ( 'NONE',  ( 5.018332763094478288, 6.785885375482345161, -1.424093192218821136 ) ) ;
#12672=ORIENTED_EDGE ( 'NONE', *, *, #61478, .T. ) ;
#12674=CARTESIAN_POINT ( 'NONE',  ( -8.019811557683421910, 9.315200557840817908, 1.199719254218462483 ) ) ;
#12678=CARTESIAN_POINT ( 'NONE',  ( 3.499976210622149253, 7.235056012367825140, 0.7998128361456321445 ) ) ;
#12683=CARTESIAN_POINT ( 'NONE',  ( 8.015895134177609904, 10.37496362800581018, 1.599625672291281386 ) ) ;
#12690=CARTESIAN_POINT ( 'NONE',  ( -5.409340102172518705, 9.254721185935849803, 0.000000000000000000 ) ) ;
#12693=CARTESIAN_POINT ( 'NONE',  ( -5.908535366263003574, 4.807949608181244727, -2.499999999999995115 ) ) ;
#12698=CARTESIAN_POINT ( 'NONE',  ( -10.01677656239806247, 10.58066083241955901, 0.7998128361456462443 ) ) ;
#12700=EDGE_CURVE ( 'NONE', #95577, #60775, #94466, .T. ) ;
#12701=CARTESIAN_POINT ( 'NONE',  ( 9.420217803396747414, 9.884675613584706255, 0.7998128361456462443 ) ) ;
#12702=CARTESIAN_POINT ( 'NONE',  ( 0.7499999999999867883, -0.9333333333333138082, -1.299038105676652011 ) ) ;
#12703=CARTESIAN_POINT ( 'NONE',  ( -9.341731535015849630, 10.85744053139533349, 1.199719254218462483 ) ) ;
#12706=CARTESIAN_POINT ( 'NONE',  ( -0.6823417656250212460, 3.801041667008085767, 1.181850606188767472 ) ) ;
#12708=CARTESIAN_POINT ( 'NONE',  ( 2.659370686574860976, 6.254349567645977714, -0.7998128361456291469 ) ) ;
#12712=DIRECTION ( 'NONE',  ( -0.7592566023653016805, -0.6507913734559627184, 0.000000000000000000 ) ) ;
#12714=CARTESIAN_POINT ( 'NONE',  ( 8.554831740098659765, 10.04335378727902395, 1.082531754730558626 ) ) ;
#12717=CARTESIAN_POINT ( 'NONE',  ( -7.375272376154101472, 7.706831981708990753, -0.7216878364870278340 ) ) ;
#12719=CARTESIAN_POINT ( 'NONE',  ( -1.364683531250000748, 1.009375000341421247, 0.000000000000000000 ) ) ;
#12723=CARTESIAN_POINT ( 'NONE',  ( -7.694415870955439551, 8.935572256658169010, 1.199719254218462483 ) ) ;
#12724=CARTESIAN_POINT ( 'NONE',  ( -4.758548728272219641, 4.653987725846768342, 0.7216878364870317197 ) ) ;
#12725=CARTESIAN_POINT ( 'NONE',  ( -1.364683531250012516, 3.051041667008083547, -0.7879004041258289570 ) ) ;
#12730=CARTESIAN_POINT ( 'NONE',  ( 8.585337585951586803, 11.03931315507545108, -1.599625672291255185 ) ) ;
#12736=CARTESIAN_POINT ( 'NONE',  ( 9.748476143425788720, 11.33197590787365172, -1.199719254218440723 ) ) ;
#12741=CARTESIAN_POINT ( 'NONE',  ( 9.752392566931574081, 10.27221283770866300, -0.7998128361456281477 ) ) ;
#12742=CARTESIAN_POINT ( 'NONE',  ( -1.573645197550657349, 8.680485584337372273, 2.500000000000011102 ) ) ;
#12746=CARTESIAN_POINT ( 'NONE',  ( -1.364683531250012516, 5.051041667008085767, -0.7879004041258300672 ) ) ;
#12750=CARTESIAN_POINT ( 'NONE',  ( 7.086107841436786181, 11.41887624831828418, 1.040834085586084257E-14 ) ) ;
#12753=CARTESIAN_POINT ( 'NONE',  ( 0.6823417656249917140, 3.592708333674754506, 1.181850606188765695 ) ) ;
#12755=CARTESIAN_POINT ( 'NONE',  ( -5.422898255786193111, 8.310169817517122581, -1.082531754730544860 ) ) ;
#12757=CARTESIAN_POINT ( 'NONE',  ( 1.474199074347493310, 7.377996015708387034, 4.279257749350846574 ) ) ;
#12761=CARTESIAN_POINT ( 'NONE',  ( 2.517010073631369860, 6.088262185878572375, -0.7998128361456281477 ) ) ;
#12764=CARTESIAN_POINT ( 'NONE',  ( 7.553864141108259211, 11.96459193126834464, 1.040834085586084257E-14 ) ) ;
#12765=CARTESIAN_POINT ( 'NONE',  ( 4.957044826796043857, 6.512741263610869247, -2.500000000000437428 ) ) ;
#12771=CARTESIAN_POINT ( 'NONE',  ( -8.459397779922852578, 11.95671561229694824, 1.199719254218453823 ) ) ;
#12772=CARTESIAN_POINT ( 'NONE',  ( 5.900823170445728572, 7.907379670318584353, 1.599625672291267398 ) ) ;
#12774=CARTESIAN_POINT ( 'NONE',  ( 4.650083499362880346, 4.527444958785877382, 0.7216878364870317197 ) ) ;
#12776=CARTESIAN_POINT ( 'NONE',  ( 5.847644326195776010, 5.716673223516856694, -0.7998128361456281477 ) ) ;
#12785=CARTESIAN_POINT ( 'NONE',  ( -7.049876689426121779, 7.327203680526343632, -0.7216878364870278340 ) ) ;
#12786=CARTESIAN_POINT ( 'NONE',  ( 3.497113557321089861, 6.167384019261527683, -1.199719254218446718 ) ) ;
#12789=CARTESIAN_POINT ( 'NONE',  ( -6.995117189646935962, 10.24838825697502109, 1.199719254218453823 ) ) ;
#12795=CARTESIAN_POINT ( 'NONE',  ( -9.622536337397040285, 12.24937836509514710, 1.599625672291281386 ) ) ;
#12796=CARTESIAN_POINT ( 'NONE',  ( 1.150222622689965446, 3.097854968409793130, 0.7749999999993734123 ) ) ;
#12799=CARTESIAN_POINT ( 'NONE',  ( 6.936968151686458306, 11.24487994360957188, 0.7998128361456462443 ) ) ;
#12800=CARTESIAN_POINT ( 'NONE',  ( 4.774442650306744085, 8.721933525333202653, -0.7998128361456281477 ) ) ;
#12812=CARTESIAN_POINT ( 'NONE',  ( -6.835281999583978418, 11.12624609948998966, -0.7998128361456291469 ) ) ;
#12816=CARTESIAN_POINT ( 'NONE',  ( 7.321039761699430493, 7.643560598178549270, -0.7216878364870257245 ) ) ;
#12818=DIRECTION ( 'NONE',  ( 0.000000000000000000, 8.546850786086437571E-32, 1.000000000000000000 ) ) ;
#12820=CARTESIAN_POINT ( 'NONE',  ( -6.600121851754250812, 6.594563670001734046, 0.7998128361456341429 ) ) ;
#12824=DIRECTION ( 'NONE',  ( 0.6507913734559627184, -0.7592566023653016805, 0.000000000000000000 ) ) ;
#12830=CARTESIAN_POINT ( 'NONE',  ( 0.6823417656249917140, 4.155208333674755394, 1.181850606188765695 ) ) ;
#12831=CARTESIAN_POINT ( 'NONE',  ( 3.998264212729667033, 7.812795105822084807, 0.04491226807220529554 ) ) ;
#12832=CARTESIAN_POINT ( 'NONE',  ( 6.726816770674637347, 10.99970333242910669, -0.7998128361456291469 ) ) ;
#12834=CARTESIAN_POINT ( 'NONE',  ( -3.145128448690317935, 5.652771709238564313, -1.082531754730549967 ) ) ;
#12837=CARTESIAN_POINT ( 'NONE',  ( -4.894130264408866893, 6.732904613275549899, -1.443375672974051449 ) ) ;
#12844=CARTESIAN_POINT ( 'NONE',  ( 4.383363735919856730, 4.008345868194933104, -0.7998128361456211532 ) ) ;
#12851=CARTESIAN_POINT ( 'NONE',  ( 3.246287715468270108, 5.874753870433235825, 1.199719254218450271 ) ) ;
#12856=CARTESIAN_POINT ( 'NONE',  ( -0.6823417656249969321, 4.530208333674755394, -1.181850606188749264 ) ) ;
#12862=CARTESIAN_POINT ( 'NONE',  ( 6.661133543015731462, 6.665743976473484267, -0.7998128361456281477 ) ) ;
#12866=CARTESIAN_POINT ( 'NONE',  ( -4.894657149733403045, 5.669187081899118574, -1.199719254218446718 ) ) ;
#12867=CARTESIAN_POINT ( 'NONE',  ( 5.138177029454836564, 7.977995053463880382, 1.082531754730558626 ) ) ;
#12868=CARTESIAN_POINT ( 'NONE',  ( -1.499999999999997780, 4.150000000000021672, 1.214306433183764966E-14 ) ) ;
#12870=CARTESIAN_POINT ( 'NONE',  ( -5.610376637956639101, 5.439860920571172542, 0.000000000000000000 ) ) ;
#12873=CARTESIAN_POINT ( 'NONE',  ( 0.6823417656249917140, 4.842708333674755394, 1.181850606188765695 ) ) ;
#12876=CARTESIAN_POINT ( 'NONE',  ( -3.741687207691642314, 6.348756928073427730, 1.082531754730560403 ) ) ;
#12879=ORIENTED_EDGE ( 'NONE', *, *, #207859, .T. ) ;
#12881=DIRECTION ( 'NONE',  ( 0.7797859179643623628, 0.6260462619842697141, 0.000000000000000000 ) ) ;
#12882=CARTESIAN_POINT ( 'NONE',  ( 5.691725559638619814, 5.534767995866836543, 1.040834085586084257E-14 ) ) ;
#12885=CARTESIAN_POINT ( 'NONE',  ( -1.364683531250012516, 3.592708333674750509, 0.7879004041258379498 ) ) ;
#12889=CARTESIAN_POINT ( 'NONE',  ( 0.6823417656249882723, 1.238541667008083547, -1.181850606188749264 ) ) ;
#12891=CARTESIAN_POINT ( 'NONE',  ( -8.947491310014823895, 12.52615806407091803, 1.199719254218462483 ) ) ;
#12892=CARTESIAN_POINT ( 'NONE',  ( -7.185458225118419584, 7.485382138834033583, 1.040834085586084257E-14 ) ) ;
#12896=CARTESIAN_POINT ( 'NONE',  ( 1.364683531249990311, 4.134375000341417028, 1.214306433183764966E-14 ) ) ;
#12904=CARTESIAN_POINT ( 'NONE',  ( -7.348156068482412095, 7.675196289425353591, 1.040834085586084257E-14 ) ) ;
#12911=CARTESIAN_POINT ( 'NONE',  ( -6.209271164934474285, 6.346497235286081562, 1.040834085586084257E-14 ) ) ;
#12922=CARTESIAN_POINT ( 'NONE',  ( 4.132297641190314508, 7.622816840561035256, -0.7610026044957002300 ) ) ;
#12924=CARTESIAN_POINT ( 'NONE',  ( -6.091691091241777656, 6.001394449403842479, 0.7998128361456341429 ) ) ;
#12926=CARTESIAN_POINT ( 'NONE',  ( 0.7499999999999885647, 1.066666666666687968, -1.299038105676652899 ) ) ;
#12928=CARTESIAN_POINT ( 'NONE',  ( 8.703971430293332645, 12.13808852110884118, -1.082531754730543083 ) ) ;
#12929=CARTESIAN_POINT ( 'NONE',  ( 7.145310649601935182, 8.294949498412453437, -1.199719254218446718 ) ) ;
#12934=DIRECTION ( 'NONE',  ( -0.9755242178752412396, 0.1319352118352180581, 0.1759136157802891343 ) ) ;
#12935=CARTESIAN_POINT ( 'NONE',  ( 3.669453130792974971, 7.432779085900453886, 1.040834085586084257E-14 ) ) ;
#12937=CARTESIAN_POINT ( 'NONE',  ( -0.2914054381963274709, 8.170846587879108114, -1.980990740193308675 ) ) ;
#12938=EDGE_LOOP ( 'NONE', ( #193587, #178495, #123906, #201563, #24468, #210579 ) ) ;
#12944=CARTESIAN_POINT ( 'NONE',  ( -4.039966587192274083, 5.736380323189513852, 1.443375672974064550 ) ) ;
#12946=AXIS2_PLACEMENT_3D ( 'NONE', #173418, #193900, #126865 ) ;
#12949=CARTESIAN_POINT ( 'NONE',  ( 5.335766472694944973, 4.384919054141800387, -2.499999999999995115 ) ) ;
#12952=CARTESIAN_POINT ( 'NONE',  ( -1.201851678989727383E-14, 3.071875000341420137, 1.575800808251672791 ) ) ;
#12953=CARTESIAN_POINT ( 'NONE',  ( 7.876924059415351564, 12.13356913605253240, -0.7216878364870267237 ) ) ;
#12954=CARTESIAN_POINT ( 'NONE',  ( -7.172426956829277778, 8.326585190177668849, -1.199719254218452935 ) ) ;
#12958=CARTESIAN_POINT ( 'NONE',  ( 5.900823170445728572, 7.907379670318584353, 1.599625672291267398 ) ) ;
#12959=CARTESIAN_POINT ( 'NONE',  ( -5.065942953000576843, 9.062017211809330064, -0.7998128361456231517 ) ) ;
#12964=CARTESIAN_POINT ( 'NONE',  ( 0.7499999999999885647, 0.3479166673494848983, -1.299038105676652899 ) ) ;
#12968=CARTESIAN_POINT ( 'NONE',  ( 7.971831135155394321, 8.402817200543854170, -0.7216878364870267237 ) ) ;
#12971=CARTESIAN_POINT ( 'NONE',  ( 1.364683531249986537, 2.467708333674753174, -0.7879004041258239610 ) ) ;
#12973=CARTESIAN_POINT ( 'NONE',  ( 5.463572716182824252, 7.397254140345190798, 1.443375672974062551 ) ) ;
#12976=CARTESIAN_POINT ( 'NONE',  ( -4.609409038966253647, 4.479991421656468908, -0.7216878364870207285 ) ) ;
#12984=CARTESIAN_POINT ( 'NONE',  ( -4.031038109533945146, 7.773819255970239261, -0.5157005294549130703 ) ) ;
#12990=CARTESIAN_POINT ( 'NONE',  ( 5.133733721068893807, 9.141106441222381918, 1.040834085586084257E-14 ) ) ;
#12993=CARTESIAN_POINT ( 'NONE',  ( 2.361091307074211887, 5.906356958228550447, 0.7998128361456462443 ) ) ;
#13001=CARTESIAN_POINT ( 'NONE',  ( 3.212919216758630014, 6.692230152952963529, 0.000000000000000000 ) ) ;
#13002=CARTESIAN_POINT ( 'NONE',  ( 1.364683531249986537, 1.967708333674750731, -0.7879004041258239610 ) ) ;
#13003=CARTESIAN_POINT ( 'NONE',  ( 9.023114925094663619, 10.48572115315399245, 1.199719254218453823 ) ) ;
#13005=CARTESIAN_POINT ( 'NONE',  ( 0.9486429539266817423, 3.167910930033676298, -1.028101543437250465 ) ) ;
#13006=CARTESIAN_POINT ( 'NONE',  ( -4.303094902415906198, 7.389312076987425648, -1.073240500945132236 ) ) ;
#13009=CARTESIAN_POINT ( 'NONE',  ( -0.7500000000000215383, 1.941666666666688634, 1.299038105676659116 ) ) ;
#13010=CARTESIAN_POINT ( 'NONE',  ( 6.498435699651741615, 6.475929825882159818, -0.7998128361456281477 ) ) ;
#13011=CARTESIAN_POINT ( 'NONE',  ( -6.551614543901706611, 8.666636272683888365, 1.599625672291283607 ) ) ;
#13015=CARTESIAN_POINT ( 'NONE',  ( -0.6823417656249969321, 3.217708333674754062, -1.181850606188749264 ) ) ;
#13016=CARTESIAN_POINT ( 'NONE',  ( -1.500000000000013101, 3.879166666666685970, -0.8660254037844313801 ) ) ;
#13018=CARTESIAN_POINT ( 'NONE',  ( 3.816783937446950770, 4.411668334231586996, 1.199719254218464037 ) ) ;
#13024=CARTESIAN_POINT ( 'NONE',  ( -1.500000000000013101, 0.2020833340161521663, 0.8660254037844403729 ) ) ;
#13026=CARTESIAN_POINT ( 'NONE',  ( -6.775324078527193983, 8.927630729746953264, -1.599625672291263179 ) ) ;
#13027=CARTESIAN_POINT ( 'NONE',  ( -2.304522924643024773, 5.632434478818063361, 0.7216878364870317197 ) ) ;
#13035=CARTESIAN_POINT ( 'NONE',  ( 4.625302960556422427, 8.547937220624488575, 1.040834085586084257E-14 ) ) ;
#13038=CARTESIAN_POINT ( 'NONE',  ( 6.993308306550549247, 7.053281200597435685, 1.040834085586084257E-14 ) ) ;
#13044=CARTESIAN_POINT ( 'NONE',  ( -6.175902666224832416, 7.163973517805802160, -1.199719254218446718 ) ) ;
#13046=CARTESIAN_POINT ( 'NONE',  ( 3.517450787741589036, 6.191110788085444128, -1.199719254218446718 ) ) ;
#13050=CARTESIAN_POINT ( 'NONE',  ( -4.711399975388157024, 5.243183351676022674, -1.000706908094962433 ) ) ;
#13052=CARTESIAN_POINT ( 'NONE',  ( 4.847318722290685500, 6.704483692258053296, 1.249926399124022147 ) ) ;
#13061=CARTESIAN_POINT ( 'NONE',  ( -4.117449517434937256, 3.977532912766735151, 0.4210360159884243281 ) ) ;
#13062=CARTESIAN_POINT ( 'NONE',  ( 8.432808358020025707, 9.900993174853955026, 1.082531754730558626 ) ) ;
#13064=CARTESIAN_POINT ( 'NONE',  ( -5.766295404513795297, 5.621766148221195358, 0.7998128361456341429 ) ) ;
#13069=CARTESIAN_POINT ( 'NONE',  ( -6.398558430645608475, 9.552403038140164782, -1.199719254218440723 ) ) ;
#13084=CARTESIAN_POINT ( 'NONE',  ( 4.065119107856408398, 3.982580166312400749, -0.7566012008942292200 ) ) ;
#13085=CARTESIAN_POINT ( 'NONE',  ( -3.554208825076827782, 7.298327395898266623, 0.7998128361456341429 ) ) ;
#13088=B_SPLINE_CURVE_WITH_KNOTS ( 'NONE', 3,
 ( #43907, #194396, #79581, #82776 ),
 .UNSPECIFIED., .F., .F.,
 ( 4, 4 ),
 ( 2.669248499352272927E-16, 7.241384396125430216E-05 ),
 .UNSPECIFIED. ) ;
#13089=CARTESIAN_POINT ( 'NONE',  ( 2.901081683644312736, 6.328419697652925002, 0.7216878364870338292 ) ) ;
#13093=CARTESIAN_POINT ( 'NONE',  ( -3.002240950422295995, 5.590032644546251817, -1.199719254218452935 ) ) ;
#13094=CARTESIAN_POINT ( 'NONE',  ( -3.578462479003122976, 6.262291094557191684, 1.199719254218464037 ) ) ;
#13098=CARTESIAN_POINT ( 'NONE',  ( 8.971744963941056028, 11.49012176272984931, 1.599625672291281386 ) ) ;
#13103=CARTESIAN_POINT ( 'NONE',  ( -8.864333505236459132, 9.236143932397675727, 1.040834085586084257E-14 ) ) ;
#13104=CARTESIAN_POINT ( 'NONE',  ( 5.555090253297246150, 7.504024600312024340, 1.599625672291267398 ) ) ;
#13108=CARTESIAN_POINT ( 'NONE',  ( 4.684505768721569652, 5.424010470718658716, -1.199719254218452047 ) ) ;
#13110=CARTESIAN_POINT ( 'NONE',  ( -4.624999999999992895, 3.300000000000025135, 1.214306433183764966E-14 ) ) ;
#13111=CARTESIAN_POINT ( 'NONE',  ( 1.364683531249988757, 1.196875000341421469, 0.000000000000000000 ) ) ;
#13112=ORIENTED_EDGE ( 'NONE', *, *, #188476, .F. ) ;
#13114=CARTESIAN_POINT ( 'NONE',  ( 5.978782553946477840, 9.919070713005490703, 1.040834085586084257E-14 ) ) ;
#13121=CARTESIAN_POINT ( 'NONE',  ( 4.690757960648224589, 6.495636925554817864, 1.443375672974062551 ) ) ;
#13128=CARTESIAN_POINT ( 'NONE',  ( -3.325722479477156934, 7.699077257575940081, 2.499999999999999112 ) ) ;
#13130=CARTESIAN_POINT ( 'NONE',  ( -8.292783513053063160, 12.82666453187061073, 0.7998128361456481317 ) ) ;
#13138=AXIS2_PLACEMENT_3D ( 'NONE', #37985, #7592, #185280 ) ;
#13147=CARTESIAN_POINT ( 'NONE',  ( -1.500000000000013101, 2.160416667349489561, -0.8660254037844313801 ) ) ;
#13153=CARTESIAN_POINT ( 'NONE',  ( -1.500000000000015099, -0.6208333333333116988, -0.8660254037844383745 ) ) ;
#13154=CARTESIAN_POINT ( 'NONE',  ( 7.214910300766615769, 11.56914578420308715, -0.7998128361456291469 ) ) ;
#13155=CARTESIAN_POINT ( 'NONE',  ( 0.6823417656249882723, -1.157291666325249713, 1.181850606188755259 ) ) ;
#13159=CARTESIAN_POINT ( 'NONE',  ( 2.900554798319789906, 5.471398800426671372, 1.199719254218452047 ) ) ;
#13160=CARTESIAN_POINT ( 'NONE',  ( -7.239690840017442675, 7.548653522882887934, 0.7216878364870317197 ) ) ;
#13164=CARTESIAN_POINT ( 'NONE',  ( -5.669280788808708671, 9.765911353585494226, 0.7998128361456481317 ) ) ;
#13167=CARTESIAN_POINT ( 'NONE',  ( -1.402160292154681736E-14, 1.618750000682814827, -1.732050807568863648 ) ) ;
#13175=CARTESIAN_POINT ( 'NONE',  ( -2.779058300676980675, 5.225689869889666106, -1.082531754730543083 ) ) ;
#13179=CARTESIAN_POINT ( 'NONE',  ( 4.618273733618881494, 6.903169301580018846, 1.208453198238930382 ) ) ;
#13184=CARTESIAN_POINT ( 'NONE',  ( -9.480175724453545172, 12.08329098332774265, 1.599625672291281386 ) ) ;
#13185=CARTESIAN_POINT ( 'NONE',  ( 7.690499447449630210, 9.995335326823163058, 1.599625672291281386 ) ) ;
#13193=CARTESIAN_POINT ( 'NONE',  ( -6.835281999583978418, 11.12624609948998966, -0.7998128361456291469 ) ) ;
#13199=CARTESIAN_POINT ( 'NONE',  ( 4.599240423533799138, 6.388866465587984322, 1.599625672291267398 ) ) ;
#13205=CARTESIAN_POINT ( 'NONE',  ( -9.001723924469462901, 12.58942944760136484, -1.199719254218446718 ) ) ;
#13209=CARTESIAN_POINT ( 'NONE',  ( -5.969600656924041182, 6.101865228085409321, -0.7346798775042752139 ) ) ;
#13218=CARTESIAN_POINT ( 'NONE',  ( 6.632963465583686435, 8.761543347979550589, -1.599625672291262513 ) ) ;
#13228=CARTESIAN_POINT ( 'NONE',  ( 0.7499999999999885647, 0.01458333401615358182, 1.299038105676657340 ) ) ;
#13233=CARTESIAN_POINT ( 'NONE',  ( 7.334597915313080918, 9.580116872663850813, 1.040834085586084257E-14 ) ) ;
#13235=CARTESIAN_POINT ( 'NONE',  ( -3.623053363349869382, 5.249981562040033189, 1.599625672291267398 ) ) ;
#13240=FACE_OUTER_BOUND ( 'NONE', #186738, .T. ) ;
#13242=CARTESIAN_POINT ( 'NONE',  ( 5.368665641331531013, 5.365790791082654998, -0.7216878364870207285 ) ) ;
#13245=CARTESIAN_POINT ( 'NONE',  ( 1.364683531249988535, 5.717708333674752730, -0.7879004041258300672 ) ) ;
#13247=CARTESIAN_POINT ( 'NONE',  ( 10.07387183015377197, 11.71160420905630062, -1.199719254218440723 ) ) ;
#13257=CARTESIAN_POINT ( 'NONE',  ( -1.402160292154681736E-14, -0.5531249996585814177, -1.575800808251665908 ) ) ;
#13261=CARTESIAN_POINT ( 'NONE',  ( -6.579784621333750749, 6.570836901177822931, 0.7998128361456341429 ) ) ;
#13265=CARTESIAN_POINT ( 'NONE',  ( 0.7499999999999920064, 5.233333333333353821, 1.299038105676669330 ) ) ;
#13273=CARTESIAN_POINT ( 'NONE',  ( -1.402160292154681736E-14, -0.5531249996585814177, -1.575800808251665908 ) ) ;
#13275=CARTESIAN_POINT ( 'NONE',  ( 6.986529229743720926, 7.045372277656132276, -0.7998128361456281477 ) ) ;
#13276=CARTESIAN_POINT ( 'NONE',  ( -7.330154606482786050, 11.70359747420527619, 0.000000000000000000 ) ) ;
#13279=ADVANCED_FACE ( 'NONE', ( #131843 ), #136074, .T. ) ;
#13280=CARTESIAN_POINT ( 'NONE',  ( -1.420000000000021911, 6.280000000000042881, 2.873333333333347728 ) ) ;
#13284=CARTESIAN_POINT ( 'NONE',  ( 1.364683531249986537, -1.073958332991911790, 0.7879004041258500513 ) ) ;
#13291=CARTESIAN_POINT ( 'NONE',  ( 7.375272376154084597, 9.627570410311676596, -1.443375672974057666 ) ) ;
#13295=CARTESIAN_POINT ( 'NONE',  ( -1.500000000000011324, 4.702083334016148974, 0.8660254037844403729 ) ) ;
#13297=CARTESIAN_POINT ( 'NONE',  ( -3.684065054611367351, 5.321161868511784299, -1.599625672291256295 ) ) ;
#13298=CARTESIAN_POINT ( 'NONE',  ( 6.493992390821439642, 7.639041213122241381, -1.082531754730543971 ) ) ;
#13299=CARTESIAN_POINT ( 'NONE',  ( -9.951321562306267410, 10.71222269888655987, 1.040834085586084257E-14 ) ) ;
#13305=CARTESIAN_POINT ( 'NONE',  ( 9.571693261567961741, 11.22969222899322617, 1.082531754730548412 ) ) ;
#13307=CARTESIAN_POINT ( 'NONE',  ( 4.650610384687404952, 5.384465856012134566, 1.199719254218462483 ) ) ;
#13317=CARTESIAN_POINT ( 'NONE',  ( -1.201851678989727383E-14, 3.259375000341420581, -1.575800808251660134 ) ) ;
#13319=ORIENTED_EDGE ( 'NONE', *, *, #200558, .T. ) ;
#13321=CARTESIAN_POINT ( 'NONE',  ( 8.646349277213076334, 11.11049346154719508, 1.599625672291281386 ) ) ;
#13324=CARTESIAN_POINT ( 'NONE',  ( -0.6823417656250003738, 0.4677083336747517306, -1.181850606188749264 ) ) ;
#13325=CARTESIAN_POINT ( 'NONE',  ( 4.338245966692901412, 8.005111361209628740, -0.7216878364870197293 ) ) ;
#13327=CARTESIAN_POINT ( 'NONE',  ( -9.653042183249972652, 10.36423008998754192, -0.7216878364870267237 ) ) ;
#13332=CARTESIAN_POINT ( 'NONE',  ( -5.101945877444165944, 4.846691699973280976, 0.000000000000000000 ) ) ;
#13334=( BOUNDED_SURFACE ( )  B_SPLINE_SURFACE ( 3, 2, ( 
 ( #16974, #1789, #47401 ),
 ( #113513, #34307, #129781 ),
 ( #114576, #63627, #15914 ),
 ( #64682, #150217, #130828 ),
 ( #81997, #79865, #132917 ),
 ( #182689, #33248, #131865 ),
 ( #196820, #148084, #48462 ),
 ( #145974, #214089, #198922 ),
 ( #195762, #194684, #100382 ),
 ( #49504, #112442, #147031 ),
 ( #96153, #712, #128713 ),
 ( #166454, #163267, #180568 ),
 ( #83055, #32190, #65717 ),
 ( #213053, #99332, #116690 ) ),
 .UNSPECIFIED., .F., .F., .T. ) 
 B_SPLINE_SURFACE_WITH_KNOTS ( ( 4, 2, 2, 2, 2, 2, 4 ),
 ( 3, 3 ),
 ( 0.000000000000000000, 0.0002390010041311323369, 0.0004780020082622646739, 0.0009560040165245293478, 0.001195005020655661712, 0.001434006024786793967, 0.001912008033049058696 ),
 ( 0.000000000000000000, 1.000000000000000000 ),
 .UNSPECIFIED. ) 
 GEOMETRIC_REPRESENTATION_ITEM ( )  RATIONAL_B_SPLINE_SURFACE ( (
 ( 1.000000000000000000, 0.4915962107220576138, 1.000000000000000000),
 ( 1.000000000000000000, 0.4903111309377842786, 1.000000000000000000),
 ( 1.000000000000000000, 0.5057854813392340665, 1.000000000000000000),
 ( 1.000000000000000000, 0.5532305778937406382, 1.000000000000000000),
 ( 1.000000000000000000, 0.5846576190772416748, 1.000000000000000000),
 ( 1.000000000000000000, 0.6796638612371262989, 1.000000000000000000),
 ( 1.000000000000000000, 0.7435379557940102746, 1.000000000000000000),
 ( 1.000000000000000000, 0.8106661767825046327, 1.000000000000000000),
 ( 1.000000000000000000, 0.8285023559304793839, 1.000000000000000000),
 ( 1.000000000000000000, 0.8541358093762889681, 1.000000000000000000),
 ( 1.000000000000000000, 0.8615977546921151919, 1.000000000000000000),
 ( 1.000000000000000000, 0.8740883989870674720, 1.000000000000000000),
 ( 1.000000000000000000, 0.8700938199806586004, 1.000000000000000000),
 ( 1.000000000000000000, 0.8708456909032173954, 1.000000000000000000) ) ) 
 REPRESENTATION_ITEM ( '' )  SURFACE ( )  );
#13346=CARTESIAN_POINT ( 'NONE',  ( 4.800107077129743161, 6.969409711611327829, -1.408023891483715317 ) ) ;
#13351=CARTESIAN_POINT ( 'NONE',  ( -4.495875322732098667, 7.242909153342021789, -1.312876762094741245 ) ) ;
#13354=CARTESIAN_POINT ( 'NONE',  ( -7.375272376154081932, 10.58793962461302485, -1.082531754730543971 ) ) ;
#13359=CARTESIAN_POINT ( 'NONE',  ( 6.856673000209174695, 9.022537805042615489, 1.599625672291281386 ) ) ;
#13363=CARTESIAN_POINT ( 'NONE',  ( -4.141125853970233806, 6.918731698685530063, -1.199719254218452047 ) ) ;
#13367=CARTESIAN_POINT ( 'NONE',  ( -4.283486466913726254, 7.084819080452935403, -1.199719254218452047 ) ) ;
#13370=CARTESIAN_POINT ( 'NONE',  ( 7.588813295347141441, 9.876701482703580837, -1.599625672291262513 ) ) ;
#13373=CARTESIAN_POINT ( 'NONE',  ( 4.401803827585060169, 7.348580664174646060, 1.190671039528957253 ) ) ;
#13374=CARTESIAN_POINT ( 'NONE',  ( 4.026408433578586354, 7.641300905909586660, 1.040834085586084257E-14 ) ) ;
#13381=CARTESIAN_POINT ( 'NONE',  ( 6.385527161912102123, 9.433236874664039817, -1.082531754730537976 ) ) ;
#13384=CARTESIAN_POINT ( 'NONE',  ( -9.053093885623068715, 11.58502883802551153, -1.599625672291263179 ) ) ;
#13385=CARTESIAN_POINT ( 'NONE',  ( -7.874588291438845644, 8.081441182967111558, -0.7998128361456291469 ) ) ;
#13392=CARTESIAN_POINT ( 'NONE',  ( 7.703003830858588863, 12.13858823597705872, -0.7998128361456291469 ) ) ;
#13393=TOROIDAL_SURFACE ( 'NONE', #155201, 0.8300000000000010703, 0.08000000000000000167 ) ;
#13397=CARTESIAN_POINT ( 'NONE',  ( 3.440018289565364817, 5.036440642624797626, 1.599625672291267398 ) ) ;
#13400=CARTESIAN_POINT ( 'NONE',  ( -1.201851678989727383E-14, 5.118750000682815937, -1.732050807568863648 ) ) ;
#13406=CARTESIAN_POINT ( 'NONE',  ( -1.500000000000013101, 2.420833333333359150, 0.8660254037844403729 ) ) ;
#13407=CARTESIAN_POINT ( 'NONE',  ( 4.476163270806094552, 8.373940915915776273, 0.7998128361456462443 ) ) ;
#13410=CARTESIAN_POINT ( 'NONE',  ( 7.456621297836072415, 9.722477485607340597, 1.443375672974076540 ) ) ;
#13411=CIRCLE ( 'NONE', #82676, 0.07999999999999971023 ) ;
#13415=CARTESIAN_POINT ( 'NONE',  ( 10.38962578677386084, 11.01565159419135043, 0.000000000000000000 ) ) ;
#13417=CARTESIAN_POINT ( 'NONE',  ( 1.499999999999964695, 5.295833333333357373, -0.8660254037844461461 ) ) ;
#13418=CARTESIAN_POINT ( 'NONE',  ( -3.765413976293358278, 5.416068943807445635, 1.599625672291267398 ) ) ;
#13419=CARTESIAN_POINT ( 'NONE',  ( -1.500000000000011324, 5.410416667349489117, -0.8660254037844313801 ) ) ;
#13420=CARTESIAN_POINT ( 'NONE',  ( 1.364683531249986537, 0.3635416670080869328, 0.7879004041258500513 ) ) ;
#13424=CARTESIAN_POINT ( 'NONE',  ( 5.007038802148489509, 4.735966778795008381, 0.7998128361456341429 ) ) ;
#13426=CARTESIAN_POINT ( 'NONE',  ( -0.6823417656250212460, 5.613541667008087543, 1.181850606188767472 ) ) ;
#13428=CARTESIAN_POINT ( 'NONE',  ( 5.055452015064900273, 6.750733944905253914, 1.449865234212225351 ) ) ;
#13435=CARTESIAN_POINT ( 'NONE',  ( -8.064402442030170093, 8.302891025323665630, 0.7998128361456602331 ) ) ;
#13438=CARTESIAN_POINT ( 'NONE',  ( 4.157546660884947620, 8.002221537674429896, 1.040834085586084257E-14 ) ) ;
#13441=B_SPLINE_CURVE_WITH_KNOTS ( 'NONE', 3,
 ( #76491, #176151, #111205, #106927 ),
 .UNSPECIFIED., .F., .F.,
 ( 4, 4 ),
 ( 0.001235641190896625326, 0.001582017824277171924 ),
 .UNSPECIFIED. ) ;
#13443=ORIENTED_EDGE ( 'NONE', *, *, #49082, .F. ) ;
#13445=CARTESIAN_POINT ( 'NONE',  ( 9.531545685607134999, 11.07889037375188401, 1.199719254218450271 ) ) ;
#13449=CARTESIAN_POINT ( 'NONE',  ( -5.928993247877788697, 5.811580298812519807, 0.7998128361456341429 ) ) ;
#13453=CARTESIAN_POINT ( 'NONE',  ( 9.901532256681887745, 10.44620914241737530, 0.000000000000000000 ) ) ;
#13455=CARTESIAN_POINT ( 'NONE',  ( 8.483651433849084711, 10.92067931095586886, 1.599625672291281386 ) ) ;
#13456=CARTESIAN_POINT ( 'NONE',  ( 4.081882008079450230, 3.980588341361369853, -0.7346435760097062007 ) ) ;
#13458=CARTESIAN_POINT ( 'NONE',  ( -9.490344339885977476, 11.13478515369756217, -1.082531754730539753 ) ) ;
#13459=CARTESIAN_POINT ( 'NONE',  ( -6.449928391799210736, 8.548002428564306143, -1.599625672291263179 ) ) ;
#13463=CARTESIAN_POINT ( 'NONE',  ( -6.127725819454865608, 6.002332559294505820, -0.1884722350499398735 ) ) ;
#13464=CARTESIAN_POINT ( 'NONE',  ( -1.364683531250012516, 0.5302083336747518416, 0.7879004041258379498 ) ) ;
#13467=CARTESIAN_POINT ( 'NONE',  ( 7.212574532790092974, 9.437756259720353924, -1.443375672974057666 ) ) ;
#13485=CARTESIAN_POINT ( 'NONE',  ( 9.585778300061798873, 11.14216175728232550, -1.199719254218440723 ) ) ;
#13489=CARTESIAN_POINT ( 'NONE',  ( -3.262708522383007903, 6.958243709422141876, 1.040834085586084257E-14 ) ) ;
#13490=CARTESIAN_POINT ( 'NONE',  ( -8.044065211609668253, 8.279164256499745633, 0.7998128361456602331 ) ) ;
#13497=CARTESIAN_POINT ( 'NONE',  ( -0.7500000000000215383, 3.722916667349487785, 1.299038105676671107 ) ) ;
#13498=CARTESIAN_POINT ( 'NONE',  ( 7.404724451357931336, 11.79059562655963056, 0.7998128361456462443 ) ) ;
#13503=CARTESIAN_POINT ( 'NONE',  ( -7.340850106795412167, 10.65174332698158643, 1.199719254218453823 ) ) ;
#13505=CARTESIAN_POINT ( 'NONE',  ( 1.364683531249990311, 3.134375000341423245, 1.214306433183764966E-14 ) ) ;
#13511=CARTESIAN_POINT ( 'NONE',  ( -7.687109909268394325, 11.91211929421440097, 0.000000000000000000 ) ) ;
#13515=CARTESIAN_POINT ( 'NONE',  ( -1.201851678989727383E-14, 1.634375000341421025, 1.575800808251672791 ) ) ;
#13522=CARTESIAN_POINT ( 'NONE',  ( -1.201851678989727383E-14, 3.571875000341422357, 1.575800808251672791 ) ) ;
#13525=CARTESIAN_POINT ( 'NONE',  ( -6.261168011412601153, 6.199117522936475666, 1.040834085586084257E-14 ) ) ;
#13526=CARTESIAN_POINT ( 'NONE',  ( 7.935599982700328958, 8.152621489438862667, 0.7998128361456481317 ) ) ;
#13531=CARTESIAN_POINT ( 'NONE',  ( 0.6823417656249899377, 2.655208333674753618, 1.181850606188767472 ) ) ;
#13534=CARTESIAN_POINT ( 'NONE',  ( -0.6823417656250246877, -0.9489583329919115684, 1.181850606188755259 ) ) ;
#13535=CARTESIAN_POINT ( 'NONE',  ( -4.433153041988574294, 8.115836282387899558, 1.040834085586084257E-14 ) ) ;
#13538=CARTESIAN_POINT ( 'NONE',  ( 5.531363484695522637, 5.555604941673978558, -0.7216878364870207285 ) ) ;
#13541=CARTESIAN_POINT ( 'NONE',  ( -6.530223543276495235, 10.77034456713125188, -0.7998128361456291469 ) ) ;
#13542=CARTESIAN_POINT ( 'NONE',  ( -8.622622508611375025, 12.04318144581317895, 1.082531754730560403 ) ) ;
#13547=CARTESIAN_POINT ( 'NONE',  ( -5.368665640887164692, 9.207267647769599606, 0.000000000000000000 ) ) ;
#13549=CARTESIAN_POINT ( 'NONE',  ( -1.402160292154681736E-14, -0.7406249996585823059, -1.575800808251665908 ) ) ;
#13552=CARTESIAN_POINT ( 'NONE',  ( 8.134528978519385944, 8.592631351135175066, -0.7216878364870267237 ) ) ;
#13563=CARTESIAN_POINT ( 'NONE',  ( 10.18181017373857600, 10.98112607889092907, 0.7216878364870438212 ) ) ;
#13567=ORIENTED_EDGE ( 'NONE', *, *, #109130, .T. ) ;
#13571=CARTESIAN_POINT ( 'NONE',  ( 4.611744806942754238, 8.532119374741881757, -0.7998128361456231517 ) ) ;
#13572=CARTESIAN_POINT ( 'NONE',  ( -3.391510981712833939, 7.108513245306943062, 0.7998128361456341429 ) ) ;
#13576=CARTESIAN_POINT ( 'NONE',  ( 5.870317324592803310, 7.871789516823500144, -1.443375672974057666 ) ) ;
#13577=CARTESIAN_POINT ( 'NONE',  ( -0.6823417656250246877, 0.6135416670080897639, 1.181850606188755259 ) ) ;
#13579=CARTESIAN_POINT ( 'NONE',  ( -10.13202086811422475, 10.71511252242175161, -0.7998128361456291469 ) ) ;
#13596=CARTESIAN_POINT ( 'NONE',  ( 4.957477724091233995, 8.935474444748447098, -0.7998128361456281477 ) ) ;
#13599=VERTEX_POINT ( 'NONE', #72105 ) ;
#13605=CARTESIAN_POINT ( 'NONE',  ( 10.55910270694468345, 11.21337466772398095, 0.7998128361456462443 ) ) ;
#13607=CARTESIAN_POINT ( 'NONE',  ( -3.789667630219657912, 4.380032642466370696, 1.199719254218462483 ) ) ;
#13613=CARTESIAN_POINT ( 'NONE',  ( -0.1598595594940371567, 7.033953395470809333, 1.994736385849470883 ) ) ;
#13619=CARTESIAN_POINT ( 'NONE',  ( -9.056483424248693126, 10.62861408545402675, 1.082531754730558626 ) ) ;
#13623=CARTESIAN_POINT ( 'NONE',  ( 4.449046963578762615, 8.342305224150557308, -0.7998128361456231517 ) ) ;
#13629=CARTESIAN_POINT ( 'NONE',  ( 4.975479186090852046, 6.827811688571220117, 1.443375672974062551 ) ) ;
#13637=CARTESIAN_POINT ( 'NONE',  ( -5.520141099058386125, 9.591915048876776595, 0.000000000000000000 ) ) ;
#13638=CARTESIAN_POINT ( 'NONE',  ( -3.262708522383007903, 6.958243709422141876, 1.040834085586084257E-14 ) ) ;
#13639=LINE ( 'NONE', #130678, #154252 ) ;
#13646=CARTESIAN_POINT ( 'NONE',  ( 6.419949431270806528, 7.448694743692793274, 1.199719254218462483 ) ) ;
#13648=CARTESIAN_POINT ( 'NONE',  ( 1.530509776559449753, 8.694755902745800569, 2.517145264428167106 ) ) ;
#13660=CARTESIAN_POINT ( 'NONE',  ( 0.6823417656249882723, -0.2614583329919109578, -1.181850606188749264 ) ) ;
#13662=CARTESIAN_POINT ( 'NONE',  ( 5.867981556616276073, 5.740399992340775803, -0.7998128361456281477 ) ) ;
#13664=CARTESIAN_POINT ( 'NONE',  ( -5.734735788900501952, 9.634349487118505806, 0.000000000000000000 ) ) ;
#13665=CARTESIAN_POINT ( 'NONE',  ( 5.504247177468186258, 6.484338464210099851, 1.082531754730558626 ) ) ;
#13666=CARTESIAN_POINT ( 'NONE',  ( -6.358410854684783509, 9.401601182898824405, -1.082531754730537976 ) ) ;
#13670=CARTESIAN_POINT ( 'NONE',  ( 6.582647274634798151, 7.638508894284114170, 1.199719254218462483 ) ) ;
#13677=CARTESIAN_POINT ( 'NONE',  ( 1.364683531249988535, 4.363541667008090208, 0.7879004041258500513 ) ) ;
#13681=CARTESIAN_POINT ( 'NONE',  ( 7.609150525767641504, 9.900428251527500834, -1.599625672291262513 ) ) ;
#13685=CARTESIAN_POINT ( 'NONE',  ( -8.148614017013223076, 9.465470093725620870, -1.199719254218446718 ) ) ;
#13690=CARTESIAN_POINT ( 'NONE',  ( 7.703003830858588863, 12.13858823597705872, -0.7998128361456291469 ) ) ;
#13693=CARTESIAN_POINT ( 'NONE',  ( -7.121056995675673740, 9.330985799753529264, -1.599625672291263179 ) ) ;
#13694=CARTESIAN_POINT ( 'NONE',  ( 0.4082588578520087719, 6.973322098160817717, 3.931096130881035489 ) ) ;
#13696=CARTESIAN_POINT ( 'NONE',  ( 5.611280047485872835, 6.151892252731265387, -0.8436193503846599606 ) ) ;
#13697=CARTESIAN_POINT ( 'NONE',  ( -8.337901282724359930, 12.67137589657970409, 1.040834085586084257E-14 ) ) ;
#13699=CARTESIAN_POINT ( 'NONE',  ( 3.284841267552055299, 6.405332120898776793, -0.9495590844852130896 ) ) ;
#13702=CARTESIAN_POINT ( 'NONE',  ( 6.311484202361478779, 7.322151976631905868, -1.199719254218446718 ) ) ;
#13704=CARTESIAN_POINT ( 'NONE',  ( 6.311484202361478779, 7.322151976631905868, -1.199719254218446718 ) ) ;
#13705=CARTESIAN_POINT ( 'NONE',  ( -4.305726085941478765, 7.254707473775878768, 0.9719050602644065950 ) ) ;
#13706=CARTESIAN_POINT ( 'NONE',  ( 4.359110081993588182, 5.044382169536003602, -1.199719254218452047 ) ) ;
#13708=CARTESIAN_POINT ( 'NONE',  ( -6.968527767744110868, 9.153035033833367251, 1.443375672974078761 ) ) ;
#13713=CARTESIAN_POINT ( 'NONE',  ( -4.235850332497944848, 7.335353122692886529, 0.8760575672057471230 ) ) ;
#13714=CARTESIAN_POINT ( 'NONE',  ( -1.364683531250012516, 0.5927083336747520637, 0.7879004041258379498 ) ) ;
#13717=CARTESIAN_POINT ( 'NONE',  ( 3.212919216758630014, 6.692230152952963529, 0.000000000000000000 ) ) ;
#13722=CARTESIAN_POINT ( 'NONE',  ( -9.788623718942277563, 10.52240854829523187, 1.040834085586084257E-14 ) ) ;
#13728=CARTESIAN_POINT ( 'NONE',  ( -9.625925875578284163, 10.33259439770390564, 1.040834085586084257E-14 ) ) ;
#13735=CARTESIAN_POINT ( 'NONE',  ( -7.307481607641392429, 11.46921960898288972, 0.7216878364870458196 ) ) ;
#13740=CARTESIAN_POINT ( 'NONE',  ( 0.7499999999999902300, 4.347916667349481123, -1.299038105676658228 ) ) ;
#13741=CARTESIAN_POINT ( 'NONE',  ( 5.389300372041062381, 6.501875383066589187, -1.316743393031569509 ) ) ;
#13744=VERTEX_POINT ( 'NONE', #123124 ) ;
#13746=CARTESIAN_POINT ( 'NONE',  ( -8.453672473320708036, 9.821371626084353323, -1.199719254218446718 ) ) ;
#13748=DIRECTION ( 'NONE',  ( -5.578564026256490882E-16, -1.000000000000000000, -9.066213480720158442E-32 ) ) ;
#13751=CARTESIAN_POINT ( 'NONE',  ( 4.313465427442102929, 8.184126765324453601, 0.7998128361456462443 ) ) ;
#13756=CARTESIAN_POINT ( 'NONE',  ( 8.444030743212801227, 8.745790710036752458, 0.7998128361456462443 ) ) ;
#13761=CARTESIAN_POINT ( 'NONE',  ( -6.616015773788831211, 7.781401826584148473, 1.082531754730549967 ) ) ;
#13768=CARTESIAN_POINT ( 'NONE',  ( 3.551873057100290776, 7.087676300018209474, 0.7216878364870409346 ) ) ;
#13771=CARTESIAN_POINT ( 'NONE',  ( -10.15235809853472126, 10.73883929124566983, -0.7998128361456291469 ) ) ;
#13773=B_SPLINE_CURVE_WITH_KNOTS ( 'NONE', 3,
 ( #52355, #101086, #54487, #18762, #17687, #103239 ),
 .UNSPECIFIED., .F., .F.,
 ( 4, 2, 4 ),
 ( 0.000000000000000000, 0.0004994260320849895846, 0.0009988520641699791692 ),
 .UNSPECIFIED. ) ;
#13774=CARTESIAN_POINT ( 'NONE',  ( 9.121938423896107651, 9.536683004167278099, -0.7998128361456221525 ) ) ;
#13775=CARTESIAN_POINT ( 'NONE',  ( -0.7500000000000006661, -0.1416666666666441254, -1.299038105676652011 ) ) ;
#13776=CARTESIAN_POINT ( 'NONE',  ( -9.515124878692420296, 9.995400534762978850, 1.040834085586084257E-14 ) ) ;
#13777=LINE ( 'NONE', #171770, #34015 ) ;
#13779=CARTESIAN_POINT ( 'NONE',  ( 0.6823417656249917140, 4.092708333674755394, 1.181850606188765695 ) ) ;
#13780=CARTESIAN_POINT ( 'NONE',  ( 4.518945272056516416, 4.166524327021037699, 0.7998128361456341429 ) ) ;
#13782=DIRECTION ( 'NONE',  ( -5.578564026256490882E-16, -1.000000000000000000, -9.066213480720158442E-32 ) ) ;
#13785=CARTESIAN_POINT ( 'NONE',  ( 10.19536832735223975, 10.99694392477354477, 0.000000000000000000 ) ) ;
#13788=CARTESIAN_POINT ( 'NONE',  ( -7.212574532790110737, 7.517017831117667193, -0.7216878364870278340 ) ) ;
#13789=CARTESIAN_POINT ( 'NONE',  ( 0.6823417656249882723, 0.9260416670080831025, -1.181850606188749264 ) ) ;
#13793=CARTESIAN_POINT ( 'NONE',  ( -8.843996274815957293, 9.212417163573759282, 1.040834085586084257E-14 ) ) ;
#13794=CARTESIAN_POINT ( 'NONE',  ( -3.429849674132942727, 5.984946472254969230, -1.082531754730549078 ) ) ;
#13795=CARTESIAN_POINT ( 'NONE',  ( -0.6823417656249969321, 4.030208333674754506, -1.181850606188749264 ) ) ;
#13802=CARTESIAN_POINT ( 'NONE',  ( 9.935427640716063991, 10.48575375712389679, -0.7998128361456281477 ) ) ;
#13805=EDGE_CURVE ( 'NONE', #54853, #69998, #61985, .T. ) ;
#13816=CARTESIAN_POINT ( 'NONE',  ( 0.6823417656249917140, 3.905208333674754950, 1.181850606188765695 ) ) ;
#13819=CARTESIAN_POINT ( 'NONE',  ( 1.123270288250309834, 2.971052654332832610, -0.7749999999993620881 ) ) ;
#13820=CARTESIAN_POINT ( 'NONE',  ( 9.447334110624092673, 9.916311305349925220, -0.7998128361456281477 ) ) ;
#13822=CARTESIAN_POINT ( 'NONE',  ( 1.364683531249988535, 3.655208333674750509, -0.7879004041258239610 ) ) ;
#13824=CARTESIAN_POINT ( 'NONE',  ( -7.104109303880803417, 8.350844278358124484, 1.082531754730549967 ) ) ;
#13826=CARTESIAN_POINT ( 'NONE',  ( 1.485618637124549890, 7.335443175656853221, 4.255655007286210711 ) ) ;
#13830=CARTESIAN_POINT ( 'NONE',  ( 2.191614386903386613, 5.708633884695917260, -0.7998128361456281477 ) ) ;
#13832=EDGE_LOOP ( 'NONE', ( #176733, #106427, #67677, #90976, #85784, #12418 ) ) ;
#13833=CARTESIAN_POINT ( 'NONE',  ( 10.37606763316019531, 10.99983374830873650, 0.7998128361456462443 ) ) ;
#13839=CARTESIAN_POINT ( 'NONE',  ( -8.839026081105473054, 12.39961529701003684, -1.199719254218446718 ) ) ;
#13840=CARTESIAN_POINT ( 'NONE',  ( 7.308008492965924141, 8.484763649003774333, -1.199719254218451159 ) ) ;
#13842=CARTESIAN_POINT ( 'NONE',  ( 4.826339496340538382, 4.733076955259818419, 1.040834085586084257E-14 ) ) ;
#13846=ORIENTED_EDGE ( 'NONE', *, *, #144073, .F. ) ;
#13854=CARTESIAN_POINT ( 'NONE',  ( -6.575341312947811545, 6.773579074634973551, 1.040834085586084257E-14 ) ) ;
#13855=CARTESIAN_POINT ( 'NONE',  ( 4.467575310902914154, 5.170924936596891008, 1.199719254218464037 ) ) ;
#13858=CARTESIAN_POINT ( 'NONE',  ( -9.155833807930273238, 9.576227618873799585, -0.7998128361456291469 ) ) ;
#13862=CARTESIAN_POINT ( 'NONE',  ( -9.134442807305063639, 11.67993591332117376, 1.599625672291281386 ) ) ;
#13867=CARTESIAN_POINT ( 'NONE',  ( 8.121497709785879593, 9.433834401960398353, -1.199719254218445830 ) ) ;
#13868=CARTESIAN_POINT ( 'NONE',  ( 6.094553744542824170, 7.069066442510145265, 1.199719254218462483 ) ) ;
#13879=CARTESIAN_POINT ( 'NONE',  ( -6.984421689334302741, 11.30024240419870374, 0.000000000000000000 ) ) ;
#13883=CARTESIAN_POINT ( 'NONE',  ( 5.666945020832160118, 9.555260257705446847, 0.7216878364870438212 ) ) ;
#13885=CARTESIAN_POINT ( 'NONE',  ( 4.695201269034174452, 4.372156323494968966, 1.214306433183764966E-14 ) ) ;
#13888=CARTESIAN_POINT ( 'NONE',  ( -6.911959384868566758, 6.958374125301778790, 1.040834085586084257E-14 ) ) ;
#13897=CARTESIAN_POINT ( 'NONE',  ( -1.001543065824772872E-14, 4.384375000341417916, 1.575800808251672791 ) ) ;
#13898=CARTESIAN_POINT ( 'NONE',  ( 5.738979324004444216, 5.917037536917005625, 2.440165351819284290 ) ) ;
#13899=CARTESIAN_POINT ( 'NONE',  ( 8.809047120577066181, 11.30030761213851953, 1.599625672291281386 ) ) ;
#13902=CARTESIAN_POINT ( 'NONE',  ( -4.609409038966253647, 4.479991421656468908, -0.7216878364870207285 ) ) ;
#13903=CARTESIAN_POINT ( 'NONE',  ( -6.385527162356468445, 10.39360608948380538, 1.040834085586084257E-14 ) ) ;
#13904=CARTESIAN_POINT ( 'NONE',  ( -3.565431210269599749, 7.103494145382415859, 0.7216878364870317197 ) ) ;
#13910=CARTESIAN_POINT ( 'NONE',  ( 8.581948047770334043, 12.95609712246668899, 0.000000000000000000 ) ) ;
#13919=CARTESIAN_POINT ( 'NONE',  ( 4.680589345215795838, 6.483773540883647435, -1.599625672291256295 ) ) ;
#13923=CARTESIAN_POINT ( 'NONE',  ( 0.6823417656249899377, 3.738541667008085767, -1.181850606188754593 ) ) ;
#13928=CARTESIAN_POINT ( 'NONE',  ( 5.148345644887269756, 7.029489223833707001, -1.599625672291256295 ) ) ;
#13931=CARTESIAN_POINT ( 'NONE',  ( -5.434120640978981065, 5.234228924097238611, -0.7998128361456221525 ) ) ;
#13932=CARTESIAN_POINT ( 'NONE',  ( -1.201851678989727383E-14, 1.962500000000020783, 1.732050807568877637 ) ) ;
#13934=CARTESIAN_POINT ( 'NONE',  ( -4.599240423533815125, 6.388866465587984322, 1.599625672291267398 ) ) ;
#13935=CARTESIAN_POINT ( 'NONE',  ( 0.2718889520039936558, 8.158259021453691417, -2.022062967018519064 ) ) ;
#13937=CARTESIAN_POINT ( 'NONE',  ( 0.6823417656249899377, 2.842708333674753618, 1.181850606188765695 ) ) ;
#13940=CARTESIAN_POINT ( 'NONE',  ( -4.365362273920257330, 6.116008624372160973, 1.443375672974064550 ) ) ;
#13946=CARTESIAN_POINT ( 'NONE',  ( 5.054492339796319733, 4.791329239384148231, -0.7998128361456211532 ) ) ;
#13949=CARTESIAN_POINT ( 'NONE',  ( 0.5451294565930948632, 6.857673063737054875, -3.776897418316011557 ) ) ;
#13950=CARTESIAN_POINT ( 'NONE',  ( -1.364683531250012516, 4.301041667008089320, -0.7879004041258300672 ) ) ;
#13952=CARTESIAN_POINT ( 'NONE',  ( 5.205967797967502975, 5.175976640491358083, -0.7216878364870503715 ) ) ;
#13954=CARTESIAN_POINT ( 'NONE',  ( -1.364683531250000748, 0.5718750003414208027, 0.000000000000000000 ) ) ;
#13956=CARTESIAN_POINT ( 'NONE',  ( -10.63367255181986160, 11.30037282007833532, 1.040834085586084257E-14 ) ) ;
#13957=CARTESIAN_POINT ( 'NONE',  ( -4.894130264408858899, 8.653643041878236630, -0.7216878364870207285 ) ) ;
#13961=CARTESIAN_POINT ( 'NONE',  ( -1.001543065824772872E-14, 4.321875000341417916, 1.575800808251672791 ) ) ;
#13969=CARTESIAN_POINT ( 'NONE',  ( -5.368665640887164692, 9.207267647769599606, 0.000000000000000000 ) ) ;
#13974=CARTESIAN_POINT ( 'NONE',  ( -6.697364695026446491, 6.915939687060050467, 1.040834085586084257E-14 ) ) ;
#13980=EDGE_CURVE ( 'NONE', #73877, #17090, #13411, .T. ) ;
#13984=CARTESIAN_POINT ( 'NONE',  ( 1.458514304043815102, 8.731595392684152301, -2.560210433951503273 ) ) ;
#13988=CARTESIAN_POINT ( 'NONE',  ( -4.205000198532790279, 8.057583998263570635, 0.7998128361456341429 ) ) ;
#13991=CARTESIAN_POINT ( 'NONE',  ( -1.500000000000001332, 0.4000000000000253353, 0.000000000000000000 ) ) ;
#13993=CARTESIAN_POINT ( 'NONE',  ( 4.369805582306193870, 3.992528022312320957, 1.214306433183764966E-14 ) ) ;
#13994=CARTESIAN_POINT ( 'NONE',  ( 8.118635056484817980, 8.366162408854107113, 0.7998128361456481317 ) ) ;
#13997=CARTESIAN_POINT ( 'NONE',  ( -2.428612866367529932E-14, 2.800000000000024691, 0.7750000000000117906 ) ) ;
#13998=CARTESIAN_POINT ( 'NONE',  ( 5.464099601507359516, 6.333536608968757697, 1.199719254218462483 ) ) ;
#13999=CARTESIAN_POINT ( 'NONE',  ( -0.4680205011783908353, 8.035366863023629236, -1.945178226287664902 ) ) ;
#14004=CARTESIAN_POINT ( 'NONE',  ( -4.121315508874269007, 5.831287398485176077, -1.443375672974053447 ) ) ;
#14006=CARTESIAN_POINT ( 'NONE',  ( 3.642672431166743330, 3.097590952613315185, -2.447572309175019889 ) ) ;
#14010=CARTESIAN_POINT ( 'NONE',  ( 1.364683531249988535, 3.155208333674756283, -0.7879004041258239610 ) ) ;
#14012=CARTESIAN_POINT ( 'NONE',  ( -5.605406444246153974, 8.627059054007450101, -1.199719254218440723 ) ) ;
#14015=CARTESIAN_POINT ( 'NONE',  ( 6.169123589417988995, 7.156064594864501416, -1.199719254218445830 ) ) ;
#14016=CARTESIAN_POINT ( 'NONE',  ( -6.039267359883488950, 9.133230122250985517, 1.199719254218452047 ) ) ;
#14019=CARTESIAN_POINT ( 'NONE',  ( 1.499999999999989120, -0.1937499993171845625, 0.000000000000000000 ) ) ;
#14023=CARTESIAN_POINT ( 'NONE',  ( 7.293923454472080792, 9.532663335016016148, 1.443375672974076540 ) ) ;
#14026=CARTESIAN_POINT ( 'NONE',  ( 1.364683531249988535, 1.676041667008085101, 0.7879004041258500513 ) ) ;
#14028=CARTESIAN_POINT ( 'NONE',  ( 5.761852095683461350, 9.665985178365305686, -0.7216878364870267237 ) ) ;
#14031=CARTESIAN_POINT ( 'NONE',  ( -3.850152436600983386, 4.554561266531622188, 1.082531754730560403 ) ) ;
#14033=CARTESIAN_POINT ( 'NONE',  ( -0.6823417656249969321, 4.217708333674755394, -1.181850606188749264 ) ) ;
#14038=CARTESIAN_POINT ( 'NONE',  ( -4.613696345000219523, 7.131516869168907924, -1.371494837298018243 ) ) ;
#14044=CARTESIAN_POINT ( 'NONE',  ( 5.296431564432884542, 9.330920591813708143, 1.040834085586084257E-14 ) ) ;
#14047=CARTESIAN_POINT ( 'NONE',  ( 3.171717870593107058, 5.787755718078879674, -1.199719254218446718 ) ) ;
#14053=VERTEX_POINT ( 'NONE', #98010 ) ;
#14055=CARTESIAN_POINT ( 'NONE',  ( 3.850152436600926542, 7.435668909435648288, -0.7216878364870197293 ) ) ;
#14056=TOROIDAL_SURFACE ( 'NONE', #114504, 0.8299999999999998490, 0.08000000000000000167 ) ;
#14057=CARTESIAN_POINT ( 'NONE',  ( -0.6823417656250003738, 1.530208333674752730, -1.181850606188749264 ) ) ;
#14058=CARTESIAN_POINT ( 'NONE',  ( 9.576136569953906275, 10.06658084123472641, 0.000000000000000000 ) ) ;
#14061=CARTESIAN_POINT ( 'NONE',  ( -0.6823417656249969321, 3.217708333674754062, -1.181850606188749264 ) ) ;
#14065=CARTESIAN_POINT ( 'NONE',  ( -0.7500000000000215383, 2.441666666666689078, 1.299038105676671107 ) ) ;
#14066=CARTESIAN_POINT ( 'NONE',  ( 6.449928391799196525, 8.548002428564306143, -1.599625672291262513 ) ) ;
#14067=CARTESIAN_POINT ( 'NONE',  ( -8.040148788103921973, 9.338927326664741457, 1.199719254218462483 ) ) ;
#14070=CARTESIAN_POINT ( 'NONE',  ( 1.364683531249986537, 2.655208333674754062, -0.7879004041258239610 ) ) ;
#14071=CARTESIAN_POINT ( 'NONE',  ( -1.402160292154681736E-14, 2.587500000000023892, -1.732050807568863648 ) ) ;
#14073=CARTESIAN_POINT ( 'NONE',  ( 3.765413976293345844, 5.416068943807445635, 1.599625672291267398 ) ) ;
#14078=FACE_OUTER_BOUND ( 'NONE', #25305, .T. ) ;
#14079=CARTESIAN_POINT ( 'NONE',  ( 0.7499999999999902300, 1.264583334016147642, 1.299038105676657340 ) ) ;
#14081=CARTESIAN_POINT ( 'NONE',  ( -5.856232286098998152, 8.919689202835742847, 1.199719254218452047 ) ) ;
#14082=CARTESIAN_POINT ( 'NONE',  ( -4.934804725694236893, 4.859619722839116918, -0.7216878364870207285 ) ) ;
#14088=VERTEX_POINT ( 'NONE', #134774 ) ;
#14089=CARTESIAN_POINT ( 'NONE',  ( 5.113396490648394632, 9.117379672398465473, 1.040834085586084257E-14 ) ) ;
#14091=EDGE_CURVE ( 'NONE', #80549, #69931, #47329, .T. ) ;
#14094=CARTESIAN_POINT ( 'NONE',  ( 7.142447996300871793, 7.227277505306155092, 0.7998128361456341429 ) ) ;
#14095=CARTESIAN_POINT ( 'NONE',  ( 8.500599125643985232, 11.90082083235127008, -1.082531754730543083 ) ) ;
#14100=CARTESIAN_POINT ( 'NONE',  ( -6.989391883044787868, 8.113044270762433285, -1.199719254218446718 ) ) ;
#14101=CARTESIAN_POINT ( 'NONE',  ( 4.701980345841006326, 4.380065246436280368, 0.7998128361456341429 ) ) ;
#14107=CARTESIAN_POINT ( 'NONE',  ( 4.863282293121215183, 6.691362709583676072, 1.250037515303052738 ) ) ;
#14108=CARTESIAN_POINT ( 'NONE',  ( 10.08690309888728187, 10.87040115823107911, -0.7216878364870257245 ) ) ;
#14113=CARTESIAN_POINT ( 'NONE',  ( 5.048048446811987944, 4.783811364235761587, -0.4196793407983526181 ) ) ;
#14115=CARTESIAN_POINT ( 'NONE',  ( -3.714570900464290393, 5.356752022006865843, 1.443375672974064550 ) ) ;
#14116=CARTESIAN_POINT ( 'NONE',  ( 7.104109303880752790, 11.23195192126214970, -0.7216878364870267237 ) ) ;
#14118=CARTESIAN_POINT ( 'NONE',  ( -3.744022975668147790, 7.519777238254810925, -0.7998128361456281477 ) ) ;
#14124=CARTESIAN_POINT ( 'NONE',  ( -7.881367368245678406, 8.089350105908421185, 0.7998128361456602331 ) ) ;
#14139=CARTESIAN_POINT ( 'NONE',  ( 1.485661138090796918, 7.335467742080692410, -4.255596723435695949 ) ) ;
#14140=CARTESIAN_POINT ( 'NONE',  ( -6.555530967407501741, 7.606873202518897870, 1.199719254218450271 ) ) ;
#14143=CARTESIAN_POINT ( 'NONE',  ( 4.555176424511575561, 4.416720038126027426, -0.7216878364870188411 ) ) ;
#14144=ORIENTED_EDGE ( 'NONE', *, *, #16612, .T. ) ;
#14146=DIRECTION ( 'NONE',  ( -0.6507913734559640506, -0.7592566023653004592, 0.000000000000000000 ) ) ;
#14148=ADVANCED_FACE ( 'NONE', ( #165114 ), #10644, .T. ) ;
#14152=CARTESIAN_POINT ( 'NONE',  ( 7.879259827836241570, 12.34422023245099176, 1.040834085586084257E-14 ) ) ;
#14155=CARTESIAN_POINT ( 'NONE',  ( -7.015454420067433361, 10.27211502579893754, 1.199719254218453823 ) ) ;
#14156=CARTESIAN_POINT ( 'NONE',  ( 4.462605117192430804, 8.358123070033169455, 1.040834085586084257E-14 ) ) ;
#14159=CARTESIAN_POINT ( 'NONE',  ( 3.662674053986138656, 7.424870162959149589, 0.7998128361456321445 ) ) ;
#14161=CARTESIAN_POINT ( 'NONE',  ( 0.6823417656249899377, 1.655208333674752730, 1.181850606188755259 ) ) ;
#14164=CARTESIAN_POINT ( 'NONE',  ( 8.120970824905713314, 8.576813505252564696, 1.040834085586084257E-14 ) ) ;
#14168=EDGE_CURVE ( 'NONE', #23324, #85368, #93570, .T. ) ;
#14172=CARTESIAN_POINT ( 'NONE',  ( 10.68346185744421462, 11.56638637654751989, 0.000000000000000000 ) ) ;
#14179=CARTESIAN_POINT ( 'NONE',  ( -2.060660350337629509, 8.500464906089689521, 2.499999999999999556 ) ) ;
#14195=CARTESIAN_POINT ( 'NONE',  ( -1.500000000000015099, 0.9104166673494835660, -0.8660254037844313801 ) ) ;
#14201=CARTESIAN_POINT ( 'NONE',  ( 1.499999999999987121, -0.9958333333333134751, 0.8660254037844524744 ) ) ;
#14202=CARTESIAN_POINT ( 'NONE',  ( 7.079328764629950754, 11.41096732537697633, 0.7998128361456462443 ) ) ;
#14206=CARTESIAN_POINT ( 'NONE',  ( 2.347533153460546806, 5.890539112345938300, 0.000000000000000000 ) ) ;
#14207=CARTESIAN_POINT ( 'NONE',  ( -6.073689629242151611, 10.02979563418376685, -0.7216878364870278340 ) ) ;
#14211=CARTESIAN_POINT ( 'NONE',  ( -5.194745412330402878, 9.212286747694129474, 0.000000000000000000 ) ) ;
#14214=CARTESIAN_POINT ( 'NONE',  ( -1.499999999999997780, 1.681250000682817047, 0.000000000000000000 ) ) ;
#14221=CARTESIAN_POINT ( 'NONE',  ( -9.642873567817536795, 12.27310513391906532, 1.599625672291281386 ) ) ;
#14223=CARTESIAN_POINT ( 'NONE',  ( 4.244147651705390878, 7.284590634535035747, 0.9143829328417275581 ) ) ;
#14228=CARTESIAN_POINT ( 'NONE',  ( -8.292783513053063160, 12.82666453187061073, 0.7998128361456481317 ) ) ;
#14229=CARTESIAN_POINT ( 'NONE',  ( 6.923409998072794558, 11.22906209772695618, 1.040834085586084257E-14 ) ) ;
#14233=DIRECTION ( 'NONE',  ( 1.000000000000000000, -4.985516615831701596E-16, 0.000000000000000000 ) ) ;
#14238=CARTESIAN_POINT ( 'NONE',  ( -8.483651433849100698, 10.92067931095586886, 1.599625672291269396 ) ) ;
#14244=CARTESIAN_POINT ( 'NONE',  ( 4.436542580169809291, 6.199052314996659874, 1.599625672291267398 ) ) ;
#14266=CARTESIAN_POINT ( 'NONE',  ( -5.623934791570306402, 5.455678766453782913, 0.7998128361456341429 ) ) ;
#14273=CARTESIAN_POINT ( 'NONE',  ( -0.7500000000000249800, -0.2770833326505156569, 1.299038105676659116 ) ) ;
#14277=CARTESIAN_POINT ( 'NONE',  ( 2.367870383881045981, 5.914265881169853856, 0.000000000000000000 ) ) ;
#14279=CARTESIAN_POINT ( 'NONE',  ( -2.300079615812729905, 5.835176651756807331, -0.7998128361456281477 ) ) ;
#14285=CARTESIAN_POINT ( 'NONE',  ( 3.714570900464274850, 6.317121236308204324, 1.082531754730558626 ) ) ;
#14288=CARTESIAN_POINT ( 'NONE',  ( 0.6823417656249899377, 5.488541667008087543, -1.181850606188754593 ) ) ;
#14290=CARTESIAN_POINT ( 'NONE',  ( 8.886479618753304166, 12.45497775759917758, -1.199719254218446718 ) ) ;
#14298=CARTESIAN_POINT ( 'NONE',  ( -5.679923764332232672, 6.292470487948599533, 1.134535232271353999 ) ) ;
#14302=CARTESIAN_POINT ( 'NONE',  ( 1.364683531249986537, -0.8864583329919110133, 0.7879004041258500513 ) ) ;
#14306=CARTESIAN_POINT ( 'NONE',  ( -6.403528624356093601, 6.365204904703887223, 1.040834085586084257E-14 ) ) ;
#14310=CARTESIAN_POINT ( 'NONE',  ( 1.499999999999990896, 4.775000000000022560, 1.214306433183764966E-14 ) ) ;
#14316=EDGE_LOOP ( 'NONE', ( #108492, #41932, #194808, #161749 ) ) ;
#14319=CARTESIAN_POINT ( 'NONE',  ( 1.364683531249986981, -1.115624999658580752, 0.000000000000000000 ) ) ;
#14321=CARTESIAN_POINT ( 'NONE',  ( 5.829115978871627135, 8.888053511070525659, 1.199719254218462483 ) ) ;
#14323=CARTESIAN_POINT ( 'NONE',  ( -7.069687034522070590, 10.33538640932937724, -1.199719254218440723 ) ) ;
#14324=CARTESIAN_POINT ( 'NONE',  ( 10.21336978979620191, 10.81001959771741205, 0.7998128361456462443 ) ) ;
#14327=CARTESIAN_POINT ( 'NONE',  ( 0.9999999999999833467, 8.600000000000013856, 0.4000000000000014655 ) ) ;
#14332=CARTESIAN_POINT ( 'NONE',  ( -0.7499999999999972244, 5.358333333333353821, -1.299038105676652011 ) ) ;
#14338=ORIENTED_EDGE ( 'NONE', *, *, #36355, .F. ) ;
#14341=CARTESIAN_POINT ( 'NONE',  ( 6.616015773788773480, 10.66250946948817813, -0.7216878364870267237 ) ) ;
#14346=CARTESIAN_POINT ( 'NONE',  ( 1.499999999999990896, 5.056250000682820378, 1.214306433183764966E-14 ) ) ;
#14348=CARTESIAN_POINT ( 'NONE',  ( -4.603156847039612920, 5.329103395422994716, 1.199719254218462483 ) ) ;
#14349=CARTESIAN_POINT ( 'NONE',  ( 5.300874872818828187, 8.167809204055208383, 1.082531754730558626 ) ) ;
#14350=CARTESIAN_POINT ( 'NONE',  ( -7.795575137733361970, 12.03866206075687018, 0.7216878364870458196 ) ) ;
#14356=CARTESIAN_POINT ( 'NONE',  ( 10.39874063200158893, 11.23421161353111586, 0.000000000000000000 ) ) ;
#14357=AXIS2_PLACEMENT_3D ( 'NONE', #75561, #209803, #77685 ) ;
#14362=ORIENTED_EDGE ( 'NONE', *, *, #14825, .F. ) ;
#14372=CARTESIAN_POINT ( 'NONE',  ( 9.725276259704228821, 10.24057714594344048, 0.7998128361456462443 ) ) ;
#14374=CARTESIAN_POINT ( 'NONE',  ( -1.364683531249997417, 5.821875000341418804, 1.214306433183764966E-14 ) ) ;
#14376=CARTESIAN_POINT ( 'NONE',  ( 0.6823417656249882723, -0.6572916663252492686, 1.181850606188755259 ) ) ;
#14377=CARTESIAN_POINT ( 'NONE',  ( 5.422898255786183341, 7.349800603215774331, -1.443375672974051449 ) ) ;
#14378=CARTESIAN_POINT ( 'NONE',  ( -8.134528978519403708, 11.47373899403920205, 1.082531754730549967 ) ) ;
#14383=CARTESIAN_POINT ( 'NONE',  ( -4.790108344329849110, 4.482881244673243337, 0.7998128361456341429 ) ) ;
#14398=CARTESIAN_POINT ( 'NONE',  ( 4.983022828693913553, 6.814620138096638691, -1.425645453754071257 ) ) ;
#14401=CARTESIAN_POINT ( 'NONE',  ( 5.671388329218120639, 5.511041227042920099, 1.040834085586084257E-14 ) ) ;
#14404=( BOUNDED_SURFACE ( )  B_SPLINE_SURFACE ( 3, 1, ( 
 ( #189815, #93415 ),
 ( #41465, #209242 ),
 ( #158396, #60886 ),
 ( #125974, #54755 ),
 ( #76072, #44658 ),
 ( #27311, #110773 ),
 ( #142171, #59821 ) ),
 .UNSPECIFIED., .T., .F., .T. ) 
 B_SPLINE_SURFACE_WITH_KNOTS ( ( 4, 3, 4 ),
 ( 2, 2 ),
 ( 0.000000000000000000, 0.5000000000000000000, 1.000000000000000000 ),
 ( 0.000000000000000000, 1.000000000000000000 ),
 .UNSPECIFIED. ) 
 GEOMETRIC_REPRESENTATION_ITEM ( )  RATIONAL_B_SPLINE_SURFACE ( (
 ( 1.000000000000000000, 1.000000000000000000),
 ( 0.3333333333333333703, 0.3333333333333333703),
 ( 0.3333333333333333703, 0.3333333333333333703),
 ( 1.000000000000000000, 1.000000000000000000),
 ( 0.3333333333333333703, 0.3333333333333333703),
 ( 0.3333333333333333703, 0.3333333333333333703),
 ( 1.000000000000000000, 1.000000000000000000) ) ) 
 REPRESENTATION_ITEM ( '' )  SURFACE ( )  );
#14407=CARTESIAN_POINT ( 'NONE',  ( -7.537970219518083326, 9.817384560903001045, -1.443375672974059665 ) ) ;
#14412=CARTESIAN_POINT ( 'NONE',  ( 6.799577732453452761, 7.891594428405881878, -1.199719254218446718 ) ) ;
#14414=CARTESIAN_POINT ( 'NONE',  ( -5.759516327706960759, 5.613857225279885732, -0.7998128361456221525 ) ) ;
#14416=CARTESIAN_POINT ( 'NONE',  ( -6.410307701162927252, 6.373113827645189744, -0.7998128361456291469 ) ) ;
#14419=CARTESIAN_POINT ( 'NONE',  ( -6.389970470742427189, 6.349387058821269747, -0.7998128361456291469 ) ) ;
#14422=CARTESIAN_POINT ( 'NONE',  ( 7.239163954692881653, 10.53310948286200599, -1.199719254218441611 ) ) ;
#14423=CARTESIAN_POINT ( 'NONE',  ( -0.7500000000000215383, 3.472916667349487785, 1.299038105676671107 ) ) ;
#14425=CARTESIAN_POINT ( 'NONE',  ( 4.954777096267108050, 6.838018505022927407, 1.425084580847448379 ) ) ;
#14426=CARTESIAN_POINT ( 'NONE',  ( 3.701012746850603996, 7.261672604726938651, 1.040834085586084257E-14 ) ) ;
#14434=CARTESIAN_POINT ( 'NONE',  ( 6.114364089638775646, 10.07724917131317355, 0.7216878364870438212 ) ) ;
#14437=CARTESIAN_POINT ( 'NONE',  ( -9.267161690140662600, 10.77044237904097734, -1.199719254218441611 ) ) ;
#14438=CARTESIAN_POINT ( 'NONE',  ( -7.739006755302186846, 7.923262724141010516, 0.7998128361456462443 ) ) ;
#14444=CARTESIAN_POINT ( 'NONE',  ( 1.579999999999990523, 8.674529973577531194, -2.499999999999989342 ) ) ;
#14447=CARTESIAN_POINT ( 'NONE',  ( 9.077347539549325717, 10.54899253668443393, -1.199719254218446718 ) ) ;
#14451=CARTESIAN_POINT ( 'NONE',  ( 4.521807925357579805, 5.234196320127330715, -1.199719254218452047 ) ) ;
#14454=CARTESIAN_POINT ( 'NONE',  ( -1.500000000000011324, 4.910416667349486453, -0.8660254037844313801 ) ) ;
#14460=CARTESIAN_POINT ( 'NONE',  ( -1.500000000000013101, 3.629166666666692187, -0.8660254037844313801 ) ) ;
#14461=CARTESIAN_POINT ( 'NONE',  ( 6.148786358997489820, 7.132337826040578754, -1.199719254218446718 ) ) ;
#14463=CARTESIAN_POINT ( 'NONE',  ( -0.7499999999999972244, 4.858333333333353821, -1.299038105676652011 ) ) ;
#14464=CARTESIAN_POINT ( 'NONE',  ( 6.968527767744093993, 10.11340424813470662, 1.082531754730558626 ) ) ;
#14465=CARTESIAN_POINT ( 'NONE',  ( -9.070041577417988776, 12.56517035942090388, 1.082531754730558626 ) ) ;
#14470=CARTESIAN_POINT ( 'NONE',  ( 9.673906298550626559, 11.24497775551929557, 1.199719254218452047 ) ) ;
#14473=CARTESIAN_POINT ( 'NONE',  ( -3.795392936821753604, 6.515376628678959392, -1.199719254218452047 ) ) ;
#14474=CARTESIAN_POINT ( 'NONE',  ( -1.001543065824772872E-14, 5.243750000682815937, 1.732050807568877637 ) ) ;
#14475=CARTESIAN_POINT ( 'NONE',  ( -1.364683531250000748, -0.2406249996585799189, 0.000000000000000000 ) ) ;
#14479=CARTESIAN_POINT ( 'NONE',  ( 3.659811400685081040, 6.357198169852855685, -1.199719254218446718 ) ) ;
#14481=CARTESIAN_POINT ( 'NONE',  ( 0.6823417656249899377, 5.238541667008086655, -1.181850606188754593 ) ) ;
#14490=CARTESIAN_POINT ( 'NONE',  ( -7.202405917357668663, 9.425892875049191488, 1.599625672291295375 ) ) ;
#14493=CARTESIAN_POINT ( 'NONE',  ( 5.005985031943777308, 6.863401842066294556, -1.599625672291256295 ) ) ;
#14499=CARTESIAN_POINT ( 'NONE',  ( 8.778014389843965759, 12.32843499053828928, 1.199719254218450271 ) ) ;
#14502=CARTESIAN_POINT ( 'NONE',  ( -4.904298879841297421, 6.744767997946721216, 1.599625672291267398 ) ) ;
#14507=CARTESIAN_POINT ( 'NONE',  ( 9.752392566931574081, 10.27221283770866300, -0.7998128361456281477 ) ) ;
#14509=CARTESIAN_POINT ( 'NONE',  ( 7.052212457402625922, 11.37933163361175382, -0.7998128361456291469 ) ) ;
#14512=CARTESIAN_POINT ( 'NONE',  ( -8.948018195339354719, 12.42280974699582607, 1.082531754730560403 ) ) ;
#14513=CARTESIAN_POINT ( 'NONE',  ( -6.398558430645608475, 9.552403038140164782, -1.199719254218440723 ) ) ;
#14517=CARTESIAN_POINT ( 'NONE',  ( -5.364460139690476304, 6.514416944181776081, 1.355983593732257741 ) ) ;
#14518=CARTESIAN_POINT ( 'NONE',  ( -0.6823417656250003738, 0.4677083336747517306, -1.181850606188749264 ) ) ;
#14522=CARTESIAN_POINT ( 'NONE',  ( 6.751597309925441159, 9.860318714012938912, -1.082531754730537088 ) ) ;
#14540=CARTESIAN_POINT ( 'NONE',  ( 9.561524646135536543, 12.17819805862340310, -1.599625672291262513 ) ) ;
#14544=CARTESIAN_POINT ( 'NONE',  ( -5.005985031943793295, 6.863401842066301661, -1.599625672291256295 ) ) ;
#14545=CARTESIAN_POINT ( 'NONE',  ( -6.157374318900681764, 10.33535380535947290, 0.7998128361456481317 ) ) ;
#14549=B_SPLINE_CURVE_WITH_KNOTS ( 'NONE', 3,
 ( #147638, #45883, #95706, #65282, #112004, #82613, #13351, #63176, #129341, #195319, #46950, #213656 ),
 .UNSPECIFIED., .F., .F.,
 ( 4, 2, 2, 2, 2, 4 ),
 ( 0.0001305756608390105640, 0.1066250804225375576, 0.2131195851842360989, 0.2663668375650854458, 0.3196140899459348206, 0.4261085947076337366 ),
 .UNSPECIFIED. ) ;
#14552=CARTESIAN_POINT ( 'NONE',  ( 1.499999999999989120, 3.285416667349486897, 0.8660254037844524744 ) ) ;
#14553=CARTESIAN_POINT ( 'NONE',  ( 8.320953590485093088, 10.73086516036454618, 1.599625672291281386 ) ) ;
#14555=CARTESIAN_POINT ( 'NONE',  ( -7.831806290188425557, 12.28885777186185990, -0.7998128361456281477 ) ) ;
#14557=CARTESIAN_POINT ( 'NONE',  ( 0.6823417656249917140, 3.842708333674754506, 1.181850606188765695 ) ) ;
#14564=CARTESIAN_POINT ( 'NONE',  ( -10.16825202056928390, 10.96530823352674133, 0.7216878364870438212 ) ) ;
#14568=CARTESIAN_POINT ( 'NONE',  ( 0.6823417656249882723, 0.9885416670080832136, -1.181850606188749264 ) ) ;
#14576=CARTESIAN_POINT ( 'NONE',  ( -1.364683531249997417, 3.259375000341423245, 1.214306433183764966E-14 ) ) ;
#14578=CARTESIAN_POINT ( 'NONE',  ( -5.708146366553361162, 6.618257834855742594, -1.199719254218446718 ) ) ;
#14581=CARTESIAN_POINT ( 'NONE',  ( 0.6823417656249899377, 2.905208333674754062, 1.181850606188765695 ) ) ;
#14585=DIRECTION ( 'NONE',  ( -0.6507913734559642727, -0.7592566023653003482, -2.775557561562895049E-17 ) ) ;
#14586=CARTESIAN_POINT ( 'NONE',  ( -4.717874267875590277, 7.487641831621378863, 1.082531754730560403 ) ) ;
#14587=EDGE_CURVE ( 'NONE', #57016, #37648, #11930, .T. ) ;
#14590=CARTESIAN_POINT ( 'NONE',  ( 5.233084105194869551, 6.167981546557892436, -1.082531754730548412 ) ) ;
#14594=CARTESIAN_POINT ( 'NONE',  ( -6.353967546298838087, 10.56471257065732416, 0.000000000000000000 ) ) ;
#14595=CARTESIAN_POINT ( 'NONE',  ( -4.302014814237876017, 3.913438792899272212, 0.7998128361456341429 ) ) ;
#14596=CARTESIAN_POINT ( 'NONE',  ( 0.6823417656249899377, 5.426041667008087543, -1.181850606188754593 ) ) ;
#14601=CARTESIAN_POINT ( 'NONE',  ( -7.036318535368094373, 7.311385834125318617, 0.7216878364870317197 ) ) ;
#14603=CARTESIAN_POINT ( 'NONE',  ( 1.364683531249984538, -1.032291666325247714, -0.7879004041258309554 ) ) ;
#14607=CARTESIAN_POINT ( 'NONE',  ( 6.141480397310468575, 10.10888486359680982, 1.040834085586084257E-14 ) ) ;
#14617=CARTESIAN_POINT ( 'NONE',  ( 8.825994812371966702, 12.28044913353391898, -1.082531754730543083 ) ) ;
#14621=ORIENTED_EDGE ( 'NONE', *, *, #185057, .F. ) ;
#14624=CARTESIAN_POINT ( 'NONE',  ( 6.043183783389218355, 8.073467052085995022, 1.599625672291267398 ) ) ;
#14625=CARTESIAN_POINT ( 'NONE',  ( -5.101945877444165944, 4.846691699973280976, 0.000000000000000000 ) ) ;
#14629=CARTESIAN_POINT ( 'NONE',  ( 1.484505139761094883, 7.334797934598051405, 4.257182005875050024 ) ) ;
#14630=CARTESIAN_POINT ( 'NONE',  ( 4.460269348771534581, 8.147471973634706544, -0.7216878364870207285 ) ) ;
#14631=CARTESIAN_POINT ( 'NONE',  ( -0.6823417656250003738, 0.5302083336747518416, -1.181850606188749264 ) ) ;
#14632=LINE ( 'NONE', #62339, #18849 ) ;
#14633=CARTESIAN_POINT ( 'NONE',  ( -9.053093885623068715, 11.58502883802551153, -1.599625672291263179 ) ) ;
#14653=CARTESIAN_POINT ( 'NONE',  ( 7.644099680006512187, 7.812537802962739697, 1.040834085586084257E-14 ) ) ;
#14660=CARTESIAN_POINT ( 'NONE',  ( 9.121938423896107651, 9.536683004167278099, -0.7998128361456221525 ) ) ;
#14664=CARTESIAN_POINT ( 'NONE',  ( 8.224992744984721327, 12.74757530245756243, 1.040834085586084257E-14 ) ) ;
#14666=CARTESIAN_POINT ( 'NONE',  ( -2.266184231778562541, 5.795632037050281404, 1.040834085586084257E-14 ) ) ;
#14670=CARTESIAN_POINT ( 'NONE',  ( -0.4829820140311024135, 7.516281308464804134, 1.942130999994731377 ) ) ;
#14675=CARTESIAN_POINT ( 'NONE',  ( -8.514157279702020631, 11.91663867875229776, -1.082531754730543971 ) ) ;
#14679=CARTESIAN_POINT ( 'NONE',  ( 5.986088515633498197, 6.942523675449257858, -1.199719254218446718 ) ) ;
#14686=CARTESIAN_POINT ( 'NONE',  ( 4.270455198180219902, 6.965652916976816655, -1.082531754730548412 ) ) ;
#14690=ORIENTED_EDGE ( 'NONE', *, *, #149161, .F. ) ;
#14694=CARTESIAN_POINT ( 'NONE',  ( -5.696397096036042385, 9.797547045350714967, -0.7998128361456231517 ) ) ;
#14695=CARTESIAN_POINT ( 'NONE',  ( -4.731959306369413198, 5.479372931307791461, -1.199719254218446718 ) ) ;
#14705=CARTESIAN_POINT ( 'NONE',  ( 6.474182045725470402, 7.511966127223233869, -1.199719254218446718 ) ) ;
#14719=CARTESIAN_POINT ( 'NONE',  ( 0.6823417656249882723, -0.09479166632524876901, 1.181850606188755259 ) ) ;
#14721=CARTESIAN_POINT ( 'NONE',  ( 4.168242161197552420, 6.950367390450747251, -1.199719254218452047 ) ) ;
#14723=CARTESIAN_POINT ( 'NONE',  ( -6.724481002698130538, 7.907944593645035880, -1.082531754730544860 ) ) ;
#14724=CARTESIAN_POINT ( 'NONE',  ( 4.189106276942576201, 7.831115056500907556, 1.040834085586084257E-14 ) ) ;
#14725=CARTESIAN_POINT ( 'NONE',  ( -7.334597914868735025, 9.580116872145431728, -1.443375672974058777 ) ) ;
#14730=CARTESIAN_POINT ( 'NONE',  ( 5.777746017718023097, 9.892454120646377191, 0.7998128361456462443 ) ) ;
#14734=B_SPLINE_CURVE_WITH_KNOTS ( 'NONE', 3,
 ( #17284, #70295, #67092, #4225, #164631, #54082, #150528, #165695, #53003, #16215 ),
 .UNSPECIFIED., .F., .F.,
 ( 4, 2, 2, 2, 4 ),
 ( 0.03215845547981503738, 0.04524000524079174745, 0.05832155500176845753, 0.08448465452372194706, 0.1368108535676289816 ),
 .UNSPECIFIED. ) ;
#14735=CARTESIAN_POINT ( 'NONE',  ( -5.097502569058221411, 6.009803087731781623, -1.082531754730544860 ) ) ;
#14736=CARTESIAN_POINT ( 'NONE',  ( 1.364683531249992088, 5.634375000341417916, 1.214306433183764966E-14 ) ) ;
#14740=CARTESIAN_POINT ( 'NONE',  ( 8.281332899848809603, 8.555976559445431562, 0.7998128361456481317 ) ) ;
#14744=CARTESIAN_POINT ( 'NONE',  ( -7.446452682403657874, 9.710614100936176385, -1.599625672291263179 ) ) ;
#14750=CARTESIAN_POINT ( 'NONE',  ( 8.106885785967500979, 11.54545161934907682, 1.199719254218460707 ) ) ;
#14751=CYLINDRICAL_SURFACE ( 'NONE', #162988, 0.07999999999999998779 ) ;
#14753=CARTESIAN_POINT ( 'NONE',  ( -7.340850106795412167, 10.65174332698158643, 1.199719254218453823 ) ) ;
#14757=CARTESIAN_POINT ( 'NONE',  ( 5.815065281910236195, 6.023992952839542170, -0.4647386070683479642 ) ) ;
#14758=CARTESIAN_POINT ( 'NONE',  ( -10.30383355670593737, 11.12348669235284504, -0.7216878364870267237 ) ) ;
#14763=CARTESIAN_POINT ( 'NONE',  ( 6.257251587906815793, 7.258880593101466161, 1.199719254218462483 ) ) ;
#14765=CARTESIAN_POINT ( 'NONE',  ( 5.066996723205273057, 6.934582148538044777, 1.599625672291267398 ) ) ;
#14766=CARTESIAN_POINT ( 'NONE',  ( -4.014213326890253342, 7.626914324717730231, 0.01912188359321290165 ) ) ;
#14767=CARTESIAN_POINT ( 'NONE',  ( 3.602716132929354664, 5.226254793216122074, 1.599625672291267398 ) ) ;
#14769=CARTESIAN_POINT ( 'NONE',  ( -7.049876689426113785, 8.287572894827684777, -1.082531754730544860 ) ) ;
#14774=CARTESIAN_POINT ( 'NONE',  ( -4.159863475130535448, 7.428450666093093346, 0.7365534166655554049 ) ) ;
#14775=CARTESIAN_POINT ( 'NONE',  ( 0.6823417656249882723, -0.09479166632524876901, 1.181850606188755259 ) ) ;
#14778=CARTESIAN_POINT ( 'NONE',  ( 4.284013352238246419, 6.021101549076499637, -1.443375672974051449 ) ) ;
#14779=CARTESIAN_POINT ( 'NONE',  ( 1.499999999999987121, 3.577083334016152971, -0.8660254037844263841 ) ) ;
#14782=CARTESIAN_POINT ( 'NONE',  ( -8.310784975052669665, 12.63974020429606249, -0.7216878364870267237 ) ) ;
#14784=AXIS2_PLACEMENT_3D ( 'NONE', #48429, #132885, #183726 ) ;
#14788=CARTESIAN_POINT ( 'NONE',  ( -8.880227426826648340, 11.38335130276301754, 1.443375672974064550 ) ) ;
#14794=ORIENTED_EDGE ( 'NONE', *, *, #95866, .F. ) ;
#14795=CARTESIAN_POINT ( 'NONE',  ( -6.982085920913410071, 11.08959130780024260, 0.7216878364870458196 ) ) ;
#14800=CARTESIAN_POINT ( 'NONE',  ( -0.6823417656249969321, 4.780208333674755394, -1.181850606188749264 ) ) ;
#14801=CARTESIAN_POINT ( 'NONE',  ( -1.499999999999997780, 2.681250000682818158, 1.214306433183764966E-14 ) ) ;
#14806=CARTESIAN_POINT ( 'NONE',  ( -6.157374318900681764, 10.33535380535947290, 0.7998128361456481317 ) ) ;
#14809=CARTESIAN_POINT ( 'NONE',  ( 4.611744806942754238, 8.532119374741881757, -0.7998128361456231517 ) ) ;
#14815=CARTESIAN_POINT ( 'NONE',  ( 8.392660782059197189, 9.750191319612612872, 1.199719254218462483 ) ) ;
#14818=CYLINDRICAL_SURFACE ( 'NONE', #208509, 0.08000000000000020983 ) ;
#14821=CARTESIAN_POINT ( 'NONE',  ( -7.388830529767770550, 7.722649827591604677, 1.040834085586084257E-14 ) ) ;
#14824=CARTESIAN_POINT ( 'NONE',  ( -1.364683531250010295, 5.551041667008087543, -0.7879004041258300672 ) ) ;
#14825=EDGE_CURVE ( 'NONE', #58688, #185939, #54952, .T. ) ;
#14831=CARTESIAN_POINT ( 'NONE',  ( -10.47775378526269918, 11.11846759242831872, -0.7998128361456221525 ) ) ;
#14833=CARTESIAN_POINT ( 'NONE',  ( 7.574201371528760163, 11.98831870009225931, 1.040834085586084257E-14 ) ) ;
#14835=CARTESIAN_POINT ( 'NONE',  ( -9.826962411806732689, 10.35921099006301382, -0.7998128361456291469 ) ) ;
#14838=CARTESIAN_POINT ( 'NONE',  ( -1.364683531249997417, 3.759375000341423689, 1.214306433183764966E-14 ) ) ;
#14839=CARTESIAN_POINT ( 'NONE',  ( 9.029367117021314115, 12.51771682229149008, -1.082531754730543083 ) ) ;
#14844=CARTESIAN_POINT ( 'NONE',  ( 10.34450801710256584, 11.17094022948226240, 0.7216878364870438212 ) ) ;
#14846=CARTESIAN_POINT ( 'NONE',  ( -7.429504990608782222, 8.730472579540773381, 1.082531754730549967 ) ) ;
#14847=CARTESIAN_POINT ( 'NONE',  ( -1.402160292154681736E-14, 0.6968750003414164729, -1.575800808251659024 ) ) ;
#14851=CARTESIAN_POINT ( 'NONE',  ( -7.751511138711140170, 10.06651563329490529, -1.599625672291263179 ) ) ;
#14852=CARTESIAN_POINT ( 'NONE',  ( -4.921246571636213929, 4.843801876438091902, 0.7216878364870317197 ) ) ;
#14853=CARTESIAN_POINT ( 'NONE',  ( 1.364683531249990311, 3.446875000341416584, 1.214306433183764966E-14 ) ) ;
#14862=ORIENTED_EDGE ( 'NONE', *, *, #48534, .F. ) ;
#14869=DIRECTION ( 'NONE',  ( -1.735552045436534953E-14, 0.6004703560067730095, 0.7996470168499969500 ) ) ;
#14871=CARTESIAN_POINT ( 'NONE',  ( -1.001543065824772872E-14, 4.384375000341417916, 1.575800808251672791 ) ) ;
#14876=CARTESIAN_POINT ( 'NONE',  ( 8.555358625423188812, 9.940005470203933768, 1.199719254218462483 ) ) ;
#14879=CARTESIAN_POINT ( 'NONE',  ( 1.364683531249988535, 3.113541667008083991, 0.7879004041258500513 ) ) ;
#14881=CARTESIAN_POINT ( 'NONE',  ( -7.700668062882084719, 8.086460282891644979, -0.7216878364870278340 ) ) ;
#14887=CARTESIAN_POINT ( 'NONE',  ( 3.785751206713845018, 5.439795712631356750, 1.599625672291267398 ) ) ;
#14889=ORIENTED_EDGE ( 'NONE', *, *, #91598, .T. ) ;
#14890=CARTESIAN_POINT ( 'NONE',  ( 8.727698198895078363, 11.20540053684285553, -1.599625672291257406 ) ) ;
#14898=CARTESIAN_POINT ( 'NONE',  ( -10.30827686509187835, 10.92074451889568643, 1.040834085586084257E-14 ) ) ;
#14899=CARTESIAN_POINT ( 'NONE',  ( 6.608709811657416999, 9.797579649320619311, -1.199719254218440723 ) ) ;
#14901=CARTESIAN_POINT ( 'NONE',  ( 5.355107487273504496, 6.310342158982962246, -1.082531754730543083 ) ) ;
#14912=CARTESIAN_POINT ( 'NONE',  ( -5.694061328059534688, 8.626526735169329996, 1.082531754730548412 ) ) ;
#14913=CARTESIAN_POINT ( 'NONE',  ( 3.337278367258157630, 7.045241861776501580, 0.7998128361456341429 ) ) ;
#14916=CARTESIAN_POINT ( 'NONE',  ( -6.821723845970312894, 11.11042825360738284, 0.000000000000000000 ) ) ;
#14918=DIRECTION ( 'NONE',  ( -5.578564026256490882E-16, -1.000000000000000000, -9.066213480720158442E-32 ) ) ;
#14921=CARTESIAN_POINT ( 'NONE',  ( -9.996439331977562404, 10.55693406359564790, 0.7998128361456462443 ) ) ;
#14922=DIRECTION ( 'NONE',  ( -0.7592566023652994600, 0.6507913734559651608, 0.000000000000000000 ) ) ;
#14923=CARTESIAN_POINT ( 'NONE',  ( 5.531363484695498656, 5.555604941674001651, -0.7216878364870402685 ) ) ;
#14924=CARTESIAN_POINT ( 'NONE',  ( 9.772729797352075920, 10.29593960653257234, -0.7998128361456281477 ) ) ;
#14925=DIRECTION ( 'NONE',  ( 0.7592566023653005702, -0.6507913734559639396, 0.000000000000000000 ) ) ;
#14931=DIRECTION ( 'NONE',  ( 6.314299915563594049E-62, 8.546850786086437571E-32, 1.000000000000000000 ) ) ;
#14936=CARTESIAN_POINT ( 'NONE',  ( -9.481229494658258261, 9.955855920056455588, -0.7998128361456291469 ) ) ;
#14941=CARTESIAN_POINT ( 'NONE',  ( 7.782016984564065432, 8.181367358187307204, 0.7216878364870458196 ) ) ;
#14943=CARTESIAN_POINT ( 'NONE',  ( 2.171277156482887882, 5.684907115872006145, -0.7998128361456291469 ) ) ;
#14944=CARTESIAN_POINT ( 'NONE',  ( -5.599154252763867134, 5.634694171087028636, 0.000000000000000000 ) ) ;
#14946=CARTESIAN_POINT ( 'NONE',  ( -6.196239896645333367, 7.187700286629718605, -1.199719254218446718 ) ) ;
#14955=CARTESIAN_POINT ( 'NONE',  ( -1.364683531249997417, 3.571875000341423245, 1.214306433183764966E-14 ) ) ;
#14957=CARTESIAN_POINT ( 'NONE',  ( 7.567422294721922960, 11.98040977715095323, 0.7998128361456462443 ) ) ;
#14959=CARTESIAN_POINT ( 'NONE',  ( -5.111060722671894929, 5.065251719313053513, 0.000000000000000000 ) ) ;
#14960=DIRECTION ( 'NONE',  ( 0.6507913734559640506, -0.7592566023653004592, 0.000000000000000000 ) ) ;
#14961=CARTESIAN_POINT ( 'NONE',  ( -5.558479791478509568, 5.587240632920778438, 0.000000000000000000 ) ) ;
#14962=( BOUNDED_CURVE ( )  B_SPLINE_CURVE ( 2, ( #137176, #72136, #55909, #3922, #203200, #86274, #74301 ),
 .UNSPECIFIED., .F., .T. ) 
 B_SPLINE_CURVE_WITH_KNOTS ( ( 3, 2, 2, 3 ),
 ( 0.1964285714285713413, 0.2023809523809523836, 0.2083333333333334536, 0.2142857142857144681 ),
 .UNSPECIFIED. ) 
 CURVE ( )  GEOMETRIC_REPRESENTATION_ITEM ( )  RATIONAL_B_SPLINE_CURVE ( ( 1.000000000000001776, 0.8660254037844368202, 1.000000000000000000, 0.8660254037844387076, 1.000000000000000000, 0.8660254037844343777, 1.000000000000004441 ) ) 
 REPRESENTATION_ITEM ( '' )  );
#14969=CARTESIAN_POINT ( 'NONE',  ( 5.359550796103802028, 5.147230771742885125, -0.7998128361456231517 ) ) ;
#14974=B_SPLINE_CURVE_WITH_KNOTS ( 'NONE', 3,
 ( #194320, #161840, #15547, #13428, #181262, #146671, #49153, #113144, #79504, #115270, #211618, #179150, #30774, #64328 ),
 .UNSPECIFIED., .F., .F.,
 ( 4, 2, 2, 2, 2, 2, 4 ),
 ( 0.5002398796579472506, 0.5986944666282260075, 0.6971490535985047643, 0.7956036405687834101, 0.8202172873113531271, 0.8448309340539227330, 0.8940582275390620559 ),
 .UNSPECIFIED. ) ;
#14978=CARTESIAN_POINT ( 'NONE',  ( 3.981290663907289140, 7.796589541200495965, -0.7998128361456221525 ) ) ;
#14983=CARTESIAN_POINT ( 'NONE',  ( 1.364683531249990311, 3.696875000341416584, 1.214306433183764966E-14 ) ) ;
#14989=CARTESIAN_POINT ( 'NONE',  ( 6.287230548435207567, 8.358188277972981695, -1.599625672291262513 ) ) ;
#14991=CARTESIAN_POINT ( 'NONE',  ( -6.358937740009323214, 7.377514437221045718, -1.199719254218446718 ) ) ;
#14993=CARTESIAN_POINT ( 'NONE',  ( -0.7500000000000006661, 1.858333333333357595, -1.299038105676652011 ) ) ;
#14996=CARTESIAN_POINT ( 'NONE',  ( -4.436542580169821726, 6.199052314996659874, 1.599625672291267398 ) ) ;
#15001=CARTESIAN_POINT ( 'NONE',  ( -1.364683531250012516, 2.738541667008090208, -0.7879004041258289570 ) ) ;
#15003=CARTESIAN_POINT ( 'NONE',  ( -3.118012141462980669, 6.581505231774690046, 0.7216878364870317197 ) ) ;
#15010=CARTESIAN_POINT ( 'NONE',  ( 6.328958779480917229, 6.278206752349526631, 0.7998128361456341429 ) ) ;
#15015=CARTESIAN_POINT ( 'NONE',  ( -0.6823417656250212460, 4.363541667008085767, 1.181850606188767472 ) ) ;
#15019=CARTESIAN_POINT ( 'NONE',  ( -0.6823417656250246877, -0.3864583329919110688, 1.181850606188755259 ) ) ;
#15022=CARTESIAN_POINT ( 'NONE',  ( -9.484092147959342967, 11.02352791316275216, 1.199719254218462483 ) ) ;
#15023=CARTESIAN_POINT ( 'NONE',  ( -5.870317324592811303, 8.832158731124840401, -1.082531754730537976 ) ) ;
#15027=CARTESIAN_POINT ( 'NONE',  ( -0.6823417656249969321, 4.967708333674755394, -1.181850606188749264 ) ) ;
#15035=CARTESIAN_POINT ( 'NONE',  ( -5.870317324592812191, 7.871789516823500144, -1.443375672974051449 ) ) ;
#15041=CARTESIAN_POINT ( 'NONE',  ( -5.300874872818844175, 7.207439989753867238, 1.443375672974064550 ) ) ;
#15044=CARTESIAN_POINT ( 'NONE',  ( -2.130563195606704152, 5.637407494849765222, -0.3975762604357975238 ) ) ;
#15045=CARTESIAN_POINT ( 'NONE',  ( -1.420000000000077423, 7.388542872122504157, 4.154462424328221104 ) ) ;
#15052=CARTESIAN_POINT ( 'NONE',  ( 4.057778671964185513, 7.726788352570485685, -0.5270377139656738930 ) ) ;
#15054=CARTESIAN_POINT ( 'NONE',  ( 0.5086597423466597823, 6.727065972568171404, -3.461085622288095021 ) ) ;
#15055=CARTESIAN_POINT ( 'NONE',  ( -5.766295404513795297, 5.621766148221195358, 0.7998128361456341429 ) ) ;
#15057=CARTESIAN_POINT ( 'NONE',  ( -0.7500000000000006661, -0.3916666666666443475, -1.299038105676652011 ) ) ;
#15058=CARTESIAN_POINT ( 'NONE',  ( 9.734391104931951588, 11.41950637958454706, 1.082531754730548412 ) ) ;
#15059=CARTESIAN_POINT ( 'NONE',  ( 7.630541526392844887, 7.796719957080126662, 0.7998128361456341429 ) ) ;
#15062=CARTESIAN_POINT ( 'NONE',  ( 5.355634372598031767, 6.206993841907870291, -1.199719254218445830 ) ) ;
#15070=CARTESIAN_POINT ( 'NONE',  ( -3.958617665510283601, 4.681104033592509595, -1.082531754730549967 ) ) ;
#15074=CARTESIAN_POINT ( 'NONE',  ( 3.642287698956710340, 3.120124397464730581, -2.499999999999995115 ) ) ;
#15075=VECTOR ( 'NONE', #63072, 1000.000000000000227 ) ;
#15076=CARTESIAN_POINT ( 'NONE',  ( -0.3986307598441150568, 6.926362299646860343, 3.868483066195463227 ) ) ;
#15080=CARTESIAN_POINT ( 'NONE',  ( 1.364683531249990311, 3.884375000341417028, 1.214306433183764966E-14 ) ) ;
#15081=CARTESIAN_POINT ( 'NONE',  ( 9.531018800282598846, 12.14260790512831889, 1.443375672974076540 ) ) ;
#15082=CARTESIAN_POINT ( 'NONE',  ( -7.549192604710863286, 7.701812881784464437, -0.7998128361456291469 ) ) ;
#15086=CARTESIAN_POINT ( 'NONE',  ( 6.063521013809720195, 8.097193820909906137, 1.599625672291281386 ) ) ;
#15087=CARTESIAN_POINT ( 'NONE',  ( -5.364222332501225488, 9.410009821226765325, 0.7998128361456481317 ) ) ;
#15088=CARTESIAN_POINT ( 'NONE',  ( -1.445103857048130047, 8.688264192037886247, 2.625611233228264840 ) ) ;
#15090=CARTESIAN_POINT ( 'NONE',  ( -1.500000000000001332, -0.06874999931718445145, 0.000000000000000000 ) ) ;
#15094=CARTESIAN_POINT ( 'NONE',  ( 6.629573927402440781, 10.67832731537079383, 1.040834085586084257E-14 ) ) ;
#15098=CARTESIAN_POINT ( 'NONE',  ( 1.364683531249986537, 1.217708333674754950, -0.7879004041258239610 ) ) ;
#15101=CARTESIAN_POINT ( 'NONE',  ( 5.775410249297131315, 9.681803024247919609, 1.040834085586084257E-14 ) ) ;
#15104=CARTESIAN_POINT ( 'NONE',  ( -4.961921032921567054, 4.891255414604337659, 0.7216878364870317197 ) ) ;
#15106=CARTESIAN_POINT ( 'NONE',  ( 1.364683531249988535, 4.405208333674754506, -0.7879004041258300672 ) ) ;
#15110=CARTESIAN_POINT ( 'NONE',  ( -5.657660137730037953, 6.307591819868396676, -1.155748867827746995 ) ) ;
#15116=CARTESIAN_POINT ( 'NONE',  ( 7.156006149914539982, 7.243095351188763686, 1.040834085586084257E-14 ) ) ;
#15119=CARTESIAN_POINT ( 'NONE',  ( 4.684505768721569652, 5.424010470718658716, -1.199719254218452047 ) ) ;
#15120=EDGE_CURVE ( 'NONE', #23582, #57442, #17256, .T. ) ;
#15128=CARTESIAN_POINT ( 'NONE',  ( 4.365362273920238678, 7.076377838673507448, 1.082531754730558626 ) ) ;
#15129=CARTESIAN_POINT ( 'NONE',  ( 1.364683531249988757, 0.6968750003414209138, 0.000000000000000000 ) ) ;
#15135=CARTESIAN_POINT ( 'NONE',  ( 1.499999999999987121, 1.295833333333353377, -0.8660254037844253849 ) ) ;
#15136=CARTESIAN_POINT ( 'NONE',  ( 5.289652487626049115, 9.323011668872403845, 0.7998128361456462443 ) ) ;
#15137=CARTESIAN_POINT ( 'NONE',  ( -8.311311860377216476, 9.655284244316948872, -1.199719254218446718 ) ) ;
#15140=EDGE_CURVE ( 'NONE', #62825, #21505, #10015, .T. ) ;
#15141=B_SPLINE_CURVE_WITH_KNOTS ( 'NONE', 3,
 ( #55799, #155437, #104566, #204144, #173851, #108894, #191119, #124100, #43850, #93666, #26497, #172770 ),
 .UNSPECIFIED., .F., .F.,
 ( 4, 2, 2, 2, 2, 4 ),
 ( 2.082684362675771891E-18, 0.0006884729345724524986, 0.001376945869144903046, 0.002065418803717353376, 0.002409655271003578649, 0.002753891738289803923 ),
 .UNSPECIFIED. ) ;
#15143=CARTESIAN_POINT ( 'NONE',  ( 1.364683531249988757, 1.134375000341421247, 0.000000000000000000 ) ) ;
#15145=CARTESIAN_POINT ( 'NONE',  ( -1.500000000000013101, 3.129166666666689967, -0.8660254037844313801 ) ) ;
#15147=CARTESIAN_POINT ( 'NONE',  ( 4.955668840994886359, 5.740367388370866131, 1.199719254218462483 ) ) ;
#15154=CARTESIAN_POINT ( 'NONE',  ( 0.7499999999999885647, -0.4854166659838468623, 1.299038105676657340 ) ) ;
#15155=CARTESIAN_POINT ( 'NONE',  ( -7.477485413136760073, 8.682486722536401302, -1.199719254218446718 ) ) ;
#15156=CARTESIAN_POINT ( 'NONE',  ( -3.470524135418294520, 6.992769224722559684, -0.7216878364870267237 ) ) ;
#15163=CARTESIAN_POINT ( 'NONE',  ( 6.908042961362778733, 8.018137195466769285, 1.199719254218462483 ) ) ;
#15167=CARTESIAN_POINT ( 'NONE',  ( 7.806797523370503811, 8.002351953554066810, 1.040834085586084257E-14 ) ) ;
#15168=CARTESIAN_POINT ( 'NONE',  ( 7.415946836550703303, 11.59576237604377091, 0.7216878364870438212 ) ) ;
#15174=CARTESIAN_POINT ( 'NONE',  ( -8.016948904382338981, 8.247528564734524892, -0.7998128361456291469 ) ) ;
#15175=CARTESIAN_POINT ( 'NONE',  ( 5.138703914779377158, 5.953908307786102583, 1.199719254218462483 ) ) ;
#15179=CARTESIAN_POINT ( 'NONE',  ( 4.895304229855391043, 6.665267352516039523, 1.249363049274658799 ) ) ;
#15180=CARTESIAN_POINT ( 'NONE',  ( 9.897088948295946764, 10.64895131587453569, 0.7216878364870438212 ) ) ;
#15185=CARTESIAN_POINT ( 'NONE',  ( 4.879410147971469769, 4.944948943068641967, -0.7687999843507594688 ) ) ;
#15188=CARTESIAN_POINT ( 'NONE',  ( -2.480778921620681921, 5.838066475291996404, 1.040834085586084257E-14 ) ) ;
#15189=CARTESIAN_POINT ( 'NONE',  ( 8.270110514656026979, 10.67154823856396817, 1.443375672974076540 ) ) ;
#15192=CARTESIAN_POINT ( 'NONE',  ( -4.530395885260773525, 8.437212299446219532, 0.7998128361456481317 ) ) ;
#15198=CARTESIAN_POINT ( 'NONE',  ( -5.357443255694392725, 9.402100898285455699, 0.000000000000000000 ) ) ;
#15212=FACE_OUTER_BOUND ( 'NONE', #194035, .T. ) ;
#15214=CARTESIAN_POINT ( 'NONE',  ( -6.124532705071231931, 8.168374127381657246, -1.599625672291263179 ) ) ;
#15218=CARTESIAN_POINT ( 'NONE',  ( 5.205967797967541166, 5.175976640491323444, -0.7216878364870197293 ) ) ;
#15222=CARTESIAN_POINT ( 'NONE',  ( -2.839543107058306592, 5.400218493954923815, -1.199719254218446718 ) ) ;
#15225=CARTESIAN_POINT ( 'NONE',  ( 8.041957671200231417, 12.53403438304231976, 1.040834085586084257E-14 ) ) ;
#15228=CARTESIAN_POINT ( 'NONE',  ( -9.040589502214116280, 9.441775928871617651, 0.7998128361456462443 ) ) ;
#15229=CARTESIAN_POINT ( 'NONE',  ( 4.937140493670735708, 8.911747675924535983, -0.7998128361456281477 ) ) ;
#15233=CARTESIAN_POINT ( 'NONE',  ( 4.578903193113299963, 6.365139696764064325, 1.599625672291267175 ) ) ;
#15236=CARTESIAN_POINT ( 'NONE',  ( 0.6823417656249882723, 1.238541667008083547, -1.181850606188749264 ) ) ;
#15239=CARTESIAN_POINT ( 'NONE',  ( 7.239690840017413365, 10.42976116578691403, -1.082531754730537976 ) ) ;
#15246=CARTESIAN_POINT ( 'NONE',  ( 8.717529583462633624, 13.11427558077437894, 0.7216878364870438212 ) ) ;
#15247=EDGE_CURVE ( 'NONE', #28244, #23747, #137843, .T. ) ;
#15249=CARTESIAN_POINT ( 'NONE',  ( 4.800089777832203808, 5.120415418395356077, -0.7784788408505428636 ) ) ;
#15267=CARTESIAN_POINT ( 'NONE',  ( -0.7500000000000006661, 0.1395833340161536928, -1.299038105676652011 ) ) ;
#15273=CARTESIAN_POINT ( 'NONE',  ( -1.402160292154681736E-14, -0.4124999999999747202, -1.732050807568870754 ) ) ;
#15274=CARTESIAN_POINT ( 'NONE',  ( 9.890836756369282057, 11.49806328964105617, -1.199719254218440723 ) ) ;
#15279=CARTESIAN_POINT ( 'NONE',  ( 4.039439701867726384, 6.800097854565950506, 1.199719254218462483 ) ) ;
#15280=CARTESIAN_POINT ( 'NONE',  ( -5.721177635286839092, 9.618531641235897212, 0.7216878364870458196 ) ) ;
#15281=EDGE_CURVE ( 'NONE', #14053, #135613, #88336, .T. ) ;
#15285=CARTESIAN_POINT ( 'NONE',  ( -6.287230548435221777, 8.358188277972981695, -1.599625672291263179 ) ) ;
#15289=CARTESIAN_POINT ( 'NONE',  ( -1.500000000000015099, 0.6604166673494823447, -0.8660254037844313801 ) ) ;
#15296=CARTESIAN_POINT ( 'NONE',  ( -3.592547517496941900, 5.214391408544949869, -1.443375672974051449 ) ) ;
#15302=CARTESIAN_POINT ( 'NONE',  ( -2.941756144040970522, 5.415504020480993219, -1.082531754730543083 ) ) ;
#15303=CARTESIAN_POINT ( 'NONE',  ( 6.272618624616828953, 10.46980549536166016, 1.040834085586084257E-14 ) ) ;
#15308=ORIENTED_EDGE ( 'NONE', *, *, #52716, .T. ) ;
#15311=CARTESIAN_POINT ( 'NONE',  ( -7.700141177557535244, 11.07091624287075859, -1.199719254218446718 ) ) ;
#15317=CARTESIAN_POINT ( 'NONE',  ( 4.273844736805816780, 6.009238164405336313, 1.599625672291267398 ) ) ;
#15321=CARTESIAN_POINT ( 'NONE',  ( -9.459838494033043332, 12.05956421450382088, 1.599625672291281386 ) ) ;
#15325=VERTEX_POINT ( 'NONE', #148364 ) ;
#15334=CARTESIAN_POINT ( 'NONE',  ( 6.934105498385400246, 10.17720795050327354, -1.199719254218441611 ) ) ;
#15336=CARTESIAN_POINT ( 'NONE',  ( -4.111146893441842920, 5.819424013814012753, 1.599625672291267398 ) ) ;
#15343=CARTESIAN_POINT ( 'NONE',  ( -1.402160292154681736E-14, -0.3812499993171785673, -1.732050807568870754 ) ) ;
#15347=CARTESIAN_POINT ( 'NONE',  ( 3.297657676621871925, 4.870353260857385180, 1.599625672291267398 ) ) ;
#15349=CARTESIAN_POINT ( 'NONE',  ( -3.110706179331648169, 5.716575411607132118, 1.199719254218462483 ) ) ;
#15356=CARTESIAN_POINT ( 'NONE',  ( 4.690757960648224589, 6.495636925554817864, 1.443375672974062551 ) ) ;
#15359=CARTESIAN_POINT ( 'NONE',  ( -0.6823417656249969321, 5.780208333674756283, -1.181850606188749264 ) ) ;
#15361=CARTESIAN_POINT ( 'NONE',  ( 4.487385655998885170, 5.298000022495898520, 1.082531754730560403 ) ) ;
#15369=CARTESIAN_POINT ( 'NONE',  ( -5.656850995454980158, 6.308143005704411443, 1.156498089891801140 ) ) ;
#15371=CARTESIAN_POINT ( 'NONE',  ( 0.6823417656249882723, -1.157291666325249713, 1.181850606188755259 ) ) ;
#15378=CARTESIAN_POINT ( 'NONE',  ( 1.499999999999987121, 4.295833333333352044, -0.8660254037844323793 ) ) ;
#15386=CARTESIAN_POINT ( 'NONE',  ( -1.364683531250012516, 4.051041667008088432, -0.7879004041258300672 ) ) ;
#15388=CARTESIAN_POINT ( 'NONE',  ( 4.950698647284403009, 8.927565521807144577, 1.040834085586084257E-14 ) ) ;
#15390=CARTESIAN_POINT ( 'NONE',  ( -6.991200766141138168, 11.30815132714001159, 0.7998128361456481317 ) ) ;
#15392=CARTESIAN_POINT ( 'NONE',  ( 10.40318394038753702, 11.03146944007395724, -0.7998128361456281477 ) ) ;
#15398=CARTESIAN_POINT ( 'NONE',  ( -1.499999999999997780, 5.650000000000023448, 1.214306433183764966E-14 ) ) ;
#15403=CARTESIAN_POINT ( 'NONE',  ( 4.161361007603033180, 7.399433999391101580, -0.7812420967184935394 ) ) ;
#15406=CARTESIAN_POINT ( 'NONE',  ( 8.161645285746708112, 9.584636257201740506, -1.082531754730543083 ) ) ;
#15411=CARTESIAN_POINT ( 'NONE',  ( -1.500000000000011324, 5.202083334016151639, 0.8660254037844403729 ) ) ;
#15413=CARTESIAN_POINT ( 'NONE',  ( -4.765854690403601879, 5.518917546014321829, 1.199719254218462483 ) ) ;
#15414=CARTESIAN_POINT ( 'NONE',  ( 6.277061933002777927, 8.346324893301817482, 1.443375672974076540 ) ) ;
#15415=CARTESIAN_POINT ( 'NONE',  ( -9.693716643646601128, 12.33242205571964512, 1.443375672974076540 ) ) ;
#15422=CARTESIAN_POINT ( 'NONE',  ( 4.334856428067313416, 6.080418470877079429, -1.599625672291256295 ) ) ;
#15424=CARTESIAN_POINT ( 'NONE',  ( 2.693266070609028784, 6.293894182352508970, 0.000000000000000000 ) ) ;
#15436=CARTESIAN_POINT ( 'NONE',  ( 2.275802642753376404, 5.638713387891790774, -0.5397176953658294751 ) ) ;
#15439=CARTESIAN_POINT ( 'NONE',  ( 7.879259827836241570, 12.34422023245099176, 1.040834085586084257E-14 ) ) ;
#15443=CARTESIAN_POINT ( 'NONE',  ( 0.6823417656249864960, -0.5739583329919112353, -1.181850606188749264 ) ) ;
#15444=CARTESIAN_POINT ( 'NONE',  ( 4.473827502829567315, 7.202920605734387749, -1.082531754730548412 ) ) ;
#15445=CARTESIAN_POINT ( 'NONE',  ( -9.571693261567968847, 12.19006144329456731, 1.443375672974076540 ) ) ;
#15451=CARTESIAN_POINT ( 'NONE',  ( -2.903417451620861289, 6.539070793532962611, 0.7998128361456341429 ) ) ;
#15465=CARTESIAN_POINT ( 'NONE',  ( 5.722549628727856330, 6.269105753387675506, -1.057781258018471782 ) ) ;
#15469=CARTESIAN_POINT ( 'NONE',  ( 5.522248639467795428, 5.337044922334209573, -0.7998128361456231517 ) ) ;
#15474=CARTESIAN_POINT ( 'NONE',  ( -7.212574532790092974, 10.39812547402169862, -1.082531754730543971 ) ) ;
#15478=CARTESIAN_POINT ( 'NONE',  ( 7.287671262545424966, 8.461036880179857889, -1.199719254218451159 ) ) ;
#15479=CYLINDRICAL_SURFACE ( 'NONE', #152461, 0.08000000000000041800 ) ;
#15481=CARTESIAN_POINT ( 'NONE',  ( -4.574986769607567894, 7.424902766929059261, 1.199719254218464037 ) ) ;
#15482=CARTESIAN_POINT ( 'NONE',  ( 3.440018289565364817, 5.036440642624797626, 1.599625672291267398 ) ) ;
#15485=CARTESIAN_POINT ( 'NONE',  ( -6.566226467720086113, 6.555019055295208119, 1.040834085586084257E-14 ) ) ;
#15488=CARTESIAN_POINT ( 'NONE',  ( 8.540746701604824409, 12.05162268759261224, -1.199719254218446718 ) ) ;
#15491=CARTESIAN_POINT ( 'NONE',  ( 4.170588824514860349, 7.607689953969209995, 0.8569815457360376865 ) ) ;
#15492=CARTESIAN_POINT ( 'NONE',  ( 5.070386261830877928, 5.978167395966564435, -1.082531754730548412 ) ) ;
#15496=CARTESIAN_POINT ( 'NONE',  ( 3.946537740505224878, 2.817530495244566335, 0.7750000000000135669 ) ) ;
#15499=CARTESIAN_POINT ( 'NONE',  ( 7.904040366642695048, 9.284097184913720824, 1.082531754730558626 ) ) ;
#15502=CARTESIAN_POINT ( 'NONE',  ( -9.917953063596627317, 11.52969898140628047, -1.199719254218441611 ) ) ;
#15503=CARTESIAN_POINT ( 'NONE',  ( -7.172426956829277778, 8.326585190177668849, -1.199719254218452935 ) ) ;
#15509=CARTESIAN_POINT ( 'NONE',  ( 2.189521126745244128, 5.706191747844753692, 0.2764223219648713759 ) ) ;
#15513=CARTESIAN_POINT ( 'NONE',  ( 8.914649696185335870, 10.35917838609310593, -1.199719254218446718 ) ) ;
#15517=CARTESIAN_POINT ( 'NONE',  ( 4.857899112398166075, 4.561970474086296079, 1.040834085586084257E-14 ) ) ;
#15520=CARTESIAN_POINT ( 'NONE',  ( -1.201851678989727383E-14, 3.993750000682817713, 1.732050807568877637 ) ) ;
#15526=CARTESIAN_POINT ( 'NONE',  ( 1.499999999999989120, 3.025000000000020783, 1.214306433183764966E-14 ) ) ;
#15527=CARTESIAN_POINT ( 'NONE',  ( 5.124091990960999432, 8.065525525174782828, -1.199719254218452047 ) ) ;
#15531=CARTESIAN_POINT ( 'NONE',  ( 6.643132081016111634, 9.733775946952057723, 1.082531754730558626 ) ) ;
#15536=CARTESIAN_POINT ( 'NONE',  ( 8.920375002787457319, 12.49452237230570084, 1.199719254218450271 ) ) ;
#15538=CARTESIAN_POINT ( 'NONE',  ( -4.603156847039612920, 5.329103395422994716, 1.199719254218462483 ) ) ;
#15539=CARTESIAN_POINT ( 'NONE',  ( 1.364683531249986537, -0.09479166632524321789, -0.7879004041258309554 ) ) ;
#15543=CARTESIAN_POINT ( 'NONE',  ( 4.681643115420508039, 4.356338477612361260, 0.7998128361456341429 ) ) ;
#15545=CARTESIAN_POINT ( 'NONE',  ( -0.6823417656249969321, 4.780208333674755394, -1.181850606188749264 ) ) ;
#15547=CARTESIAN_POINT ( 'NONE',  ( 5.499899648425819798, 6.417811729657633357, 1.282877755774240791 ) ) ;
#15552=CARTESIAN_POINT ( 'NONE',  ( -7.121056995675673740, 9.330985799753529264, -1.599625672291263179 ) ) ;
#15554=CARTESIAN_POINT ( 'NONE',  ( 4.924636110261782385, 6.768494766770632332, 1.599625672291267398 ) ) ;
#15557=CARTESIAN_POINT ( 'NONE',  ( 1.364683531249986537, 0.1135416670080857532, 0.7879004041258500513 ) ) ;
#15561=CARTESIAN_POINT ( 'NONE',  ( 8.536830278099042602, 13.11138575775759563, -0.7998128361456352531 ) ) ;
#15564=CARTESIAN_POINT ( 'NONE',  ( -5.910464900553636269, 8.982960586366182554, -1.199719254218440723 ) ) ;
#15568=CARTESIAN_POINT ( 'NONE',  ( 8.483651433849084711, 10.92067931095586886, 1.599625672291281386 ) ) ;
#15570=CARTESIAN_POINT ( 'NONE',  ( 8.402302512167096893, 10.82577223566020841, -1.599625672291268286 ) ) ;
#15572=CARTESIAN_POINT ( 'NONE',  ( -2.930533758848195447, 6.570706485298192234, -0.7998128361456281477 ) ) ;
#15573=CARTESIAN_POINT ( 'NONE',  ( -6.693975156845199059, 8.832723654451292816, 1.599625672291283607 ) ) ;
#15577=CARTESIAN_POINT ( 'NONE',  ( -4.081306271799089558, 7.708262650413779227, 0.6970576149333465032 ) ) ;
#15578=CARTESIAN_POINT ( 'NONE',  ( 0.6823417656249882723, 0.09270833367475139752, 1.181850606188755259 ) ) ;
#15582=CARTESIAN_POINT ( 'NONE',  ( 6.643132081016117851, 8.773406732650713025, 1.443375672974076540 ) ) ;
#15585=CARTESIAN_POINT ( 'NONE',  ( 3.845709127770629010, 7.638411082374393146, 0.7998128361456321445 ) ) ;
#15604=CARTESIAN_POINT ( 'NONE',  ( 8.238550898598388628, 12.76339314834017102, 0.7998128361456462443 ) ) ;
#15608=CARTESIAN_POINT ( 'NONE',  ( -6.084912014434944894, 5.993485526462540847, -0.7998128361456291469 ) ) ;
#15609=CARTESIAN_POINT ( 'NONE',  ( -8.193204901359996128, 8.453160561208463264, 1.040834085586084257E-14 ) ) ;
#15611=ORIENTED_EDGE ( 'NONE', *, *, #136238, .T. ) ;
#15615=CARTESIAN_POINT ( 'NONE',  ( -1.201851678989727383E-14, 2.868750000682821266, -1.732050807568863648 ) ) ;
#15616=CARTESIAN_POINT ( 'NONE',  ( 8.727698198895078363, 11.20540053684285553, -1.599625672291257406 ) ) ;
#15620=CARTESIAN_POINT ( 'NONE',  ( -7.330154606482786050, 11.70359747420527619, 0.000000000000000000 ) ) ;
#15622=CARTESIAN_POINT ( 'NONE',  ( -1.201851678989727383E-14, 3.196875000341420137, -1.575800808251660134 ) ) ;
#15628=CARTESIAN_POINT ( 'NONE',  ( -5.558479791478509568, 5.587240632920778438, 0.000000000000000000 ) ) ;
#15631=CARTESIAN_POINT ( 'NONE',  ( -8.622622508611375025, 12.04318144581317895, 1.082531754730560403 ) ) ;
#15635=CARTESIAN_POINT ( 'NONE',  ( -1.364683531250012516, 1.842708333674749843, 0.7879004041258379498 ) ) ;
#15640=CARTESIAN_POINT ( 'NONE',  ( 0.6823417656249899377, 2.592708333674753618, 1.181850606188767472 ) ) ;
#15642=CARTESIAN_POINT ( 'NONE',  ( -5.225778143063529946, 8.184159369294361497, 1.199719254218452047 ) ) ;
#15643=CARTESIAN_POINT ( 'NONE',  ( 7.396136491454752715, 8.587579647240744407, 1.199719254218462483 ) ) ;
#15644=CARTESIAN_POINT ( 'NONE',  ( -1.244150428499027239, 2.902476754118171520, 0.7750000000000117906 ) ) ;
#15646=CARTESIAN_POINT ( 'NONE',  ( 1.499999999999989120, 4.504166666666688634, 0.8660254037844524744 ) ) ;
#15647=CARTESIAN_POINT ( 'NONE',  ( -1.201851678989727383E-14, 3.134375000341420137, 1.575800808251672791 ) ) ;
#15652=CARTESIAN_POINT ( 'NONE',  ( -5.043269954603569083, 7.867270132804026872, 1.082531754730560403 ) ) ;
#15656=CARTESIAN_POINT ( 'NONE',  ( 3.524756749872944628, 7.056040608253000279, -0.7216878364870267237 ) ) ;
#15659=CARTESIAN_POINT ( 'NONE',  ( -7.934546212495630968, 10.28005655271014795, -1.599625672291263179 ) ) ;
#15660=CARTESIAN_POINT ( 'NONE',  ( -8.487040972474682476, 12.84537220128841817, 0.7216878364870338292 ) ) ;
#15662=CARTESIAN_POINT ( 'NONE',  ( -1.364683531249997417, 5.259375000341425022, 1.214306433183764966E-14 ) ) ;
#15667=CARTESIAN_POINT ( 'NONE',  ( -8.161645285302366659, 8.624267042381978499, 1.040834085586084257E-14 ) ) ;
#15669=CARTESIAN_POINT ( 'NONE',  ( 0.6823417656249864960, -0.7614583329919113464, -1.181850606188749264 ) ) ;
#15672=CARTESIAN_POINT ( 'NONE',  ( 8.622622508611357262, 9.162073802909148412, -0.7216878364870197293 ) ) ;
#15682=CARTESIAN_POINT ( 'NONE',  ( 8.175203438916005538, 11.52119253116861586, -1.082531754730543083 ) ) ;
#15690=CARTESIAN_POINT ( 'NONE',  ( 6.661133543015731462, 6.665743976473484267, -0.7998128361456281477 ) ) ;
#15691=CARTESIAN_POINT ( 'NONE',  ( -2.740719608256871442, 6.349256642941639051, 0.7998128361456341429 ) ) ;
#15693=CARTESIAN_POINT ( 'NONE',  ( -1.499999999999997780, 3.400000000000021227, 1.214306433183764966E-14 ) ) ;
#15695=CIRCLE ( 'NONE', #136790, 0.7499999999999997780 ) ;
#15696=CARTESIAN_POINT ( 'NONE',  ( 4.812781342726850653, 8.558735966582574406, 0.7216878364870438212 ) ) ;
#15697=CARTESIAN_POINT ( 'NONE',  ( -0.6823417656250212460, 0.8635416670080899859, 1.181850606188755259 ) ) ;
#15699=CARTESIAN_POINT ( 'NONE',  ( -9.917953063596627317, 11.52969898140628047, -1.199719254218441611 ) ) ;
#15713=DIRECTION ( 'NONE',  ( 1.000000000000000000, -7.387867266669436732E-31, 0.000000000000000000 ) ) ;
#15717=CARTESIAN_POINT ( 'NONE',  ( 7.091078035147269532, 8.231678114882006625, 1.199719254218462483 ) ) ;
#15718=CARTESIAN_POINT ( 'NONE',  ( 5.608269097547198712, 9.694731047113750222, -0.7998128361456281477 ) ) ;
#15729=CARTESIAN_POINT ( 'NONE',  ( -2.927671105547157371, 5.503034492191895666, 1.199719254218462483 ) ) ;
#15740=CARTESIAN_POINT ( 'NONE',  ( -9.544576954340667996, 11.19805653722800365, 1.082531754730558626 ) ) ;
#15743=CARTESIAN_POINT ( 'NONE',  ( 6.972971076130050072, 7.029554431773520129, 1.040834085586084257E-14 ) ) ;
#15750=CARTESIAN_POINT ( 'NONE',  ( 3.484082288587588838, 7.008587070086755411, -0.7216878364870267237 ) ) ;
#15757=CARTESIAN_POINT ( 'NONE',  ( -6.826694039680798021, 7.923230120171105284, -1.199719254218446718 ) ) ;
#15758=CARTESIAN_POINT ( 'NONE',  ( -3.411848212133334446, 7.132240014130862171, 0.7998128361456341429 ) ) ;
#15767=CARTESIAN_POINT ( 'NONE',  ( 5.829115978871627135, 8.888053511070525659, 1.199719254218462483 ) ) ;
#15778=CARTESIAN_POINT ( 'NONE',  ( -1.402160292154681736E-14, 0.2593750003414224681, -1.575800808251665908 ) ) ;
#15779=CARTESIAN_POINT ( 'NONE',  ( 4.005544317833563461, 6.760553239859419250, -1.199719254218452047 ) ) ;
#15782=CARTESIAN_POINT ( 'NONE',  ( -6.643132081016132062, 8.773406732650713025, 1.443375672974078761 ) ) ;
#15784=CARTESIAN_POINT ( 'NONE',  ( 4.473827502829567315, 7.202920605734387749, -1.082531754730548412 ) ) ;
#15785=B_SPLINE_CURVE_WITH_KNOTS ( 'NONE', 3,
 ( #148899, #51405, #19942, #18872, #472, #16737, #200813, #84956, #199761, #2614 ),
 .UNSPECIFIED., .F., .F.,
 ( 4, 3, 3, 4 ),
 ( 1.661478437462647650E-14, 3.125169445508157778E-05, 5.676984422619956599E-05, 8.229491417181853481E-05 ),
 .UNSPECIFIED. ) ;
#15786=CARTESIAN_POINT ( 'NONE',  ( -7.822691444960713447, 9.189190109618056823, -1.082531754730543083 ) ) ;
#15790=CARTESIAN_POINT ( 'NONE',  ( 6.089583550832340819, 10.25626457594641749, 1.040834085586084257E-14 ) ) ;
#15795=CARTESIAN_POINT ( 'NONE',  ( -0.6823417656250212460, 3.551041667008085323, 1.181850606188767472 ) ) ;
#15799=CARTESIAN_POINT ( 'NONE',  ( 8.620286740190458374, 8.951422706510690830, 1.040834085586084257E-14 ) ) ;
#15803=CARTESIAN_POINT ( 'NONE',  ( -6.530223543276495235, 10.77034456713125188, -0.7998128361456291469 ) ) ;
#15809=CARTESIAN_POINT ( 'NONE',  ( 9.185812768458653466, 10.67553530374532045, 1.199719254218453823 ) ) ;
#15812=CARTESIAN_POINT ( 'NONE',  ( -8.341290820905609138, 10.75459192918846618, 1.599625672291269396 ) ) ;
#15815=CARTESIAN_POINT ( 'NONE',  ( 5.373129273518238769, 6.310201232541126970, -1.074510414011679016 ) ) ;
#15816=CARTESIAN_POINT ( 'NONE',  ( -4.060830702492950195, 4.696389560118578999, -1.199719254218452047 ) ) ;
#15821=CARTESIAN_POINT ( 'NONE',  ( 5.612185521052973414, 8.634967976948757951, -1.199719254218440723 ) ) ;
#15823=CARTESIAN_POINT ( 'NONE',  ( 4.150767584078112193, 7.994312614733129152, 0.7998128361456321445 ) ) ;
#15824=CARTESIAN_POINT ( 'NONE',  ( -4.037324417950741484, 7.593329901778307800, 0.3124507474575183297 ) ) ;
#15825=CARTESIAN_POINT ( 'NONE',  ( 2.672928840188529609, 6.270167413528593414, 0.000000000000000000 ) ) ;
#15827=CARTESIAN_POINT ( 'NONE',  ( -6.344852701515500293, 9.385783337534627790, 1.082531754730548412 ) ) ;
#15833=CARTESIAN_POINT ( 'NONE',  ( -4.145235801320589886, 7.447099624555288067, -0.7035710955675591460 ) ) ;
#15834=CARTESIAN_POINT ( 'NONE',  ( -1.402160292154681736E-14, -0.9906249996585834161, -1.575800808251665908 ) ) ;
#15837=CARTESIAN_POINT ( 'NONE',  ( 3.701012746850603996, 7.261672604726938651, 1.040834085586084257E-14 ) ) ;
#15842=CARTESIAN_POINT ( 'NONE',  ( -8.554831740098665094, 11.00372300158037042, 1.443375672974064550 ) ) ;
#15848=CARTESIAN_POINT ( 'NONE',  ( -9.232739420781982176, 12.75498451001223010, 1.082531754730558626 ) ) ;
#15856=CARTESIAN_POINT ( 'NONE',  ( -8.880227426826648340, 11.38335130276301754, 1.443375672974064550 ) ) ;
#15861=( BOUNDED_CURVE ( )  B_SPLINE_CURVE ( 2, ( #42415, #161487, #126925 ),
 .UNSPECIFIED., .F., .T. ) 
 B_SPLINE_CURVE_WITH_KNOTS ( ( 3, 3 ),
 ( 0.1249999999999998751, 0.1276624645066395392 ),
 .UNSPECIFIED. ) 
 CURVE ( )  GEOMETRIC_REPRESENTATION_ITEM ( )  RATIONAL_B_SPLINE_CURVE ( ( 1.000000000000003997, 0.9143913742683281720, 0.9381891137235824907 ) ) 
 REPRESENTATION_ITEM ( '' )  );
#15863=CARTESIAN_POINT ( 'NONE',  ( 1.499999999999989120, 2.535416667349483344, 0.8660254037844524744 ) ) ;
#15867=CARTESIAN_POINT ( 'NONE',  ( -8.681298431451969222, 9.022603012982438386, 1.040834085586084257E-14 ) ) ;
#15871=CARTESIAN_POINT ( 'NONE',  ( 7.122110765880372618, 7.203550736482235095, 0.7998128361456341429 ) ) ;
#15873=CARTESIAN_POINT ( 'NONE',  ( 1.499999999999987566, 6.120000000000041851, -2.499999999999995115 ) ) ;
#15876=CARTESIAN_POINT ( 'NONE',  ( 7.313733799568044702, 10.62010763521636214, 1.199719254218460707 ) ) ;
#15880=CIRCLE ( 'NONE', #136973, 0.7500000000000011102 ) ;
#15883=CARTESIAN_POINT ( 'NONE',  ( -5.558479791922849245, 9.428717490644563881, 0.7216878364870458196 ) ) ;
#15886=CARTESIAN_POINT ( 'NONE',  ( -1.364683531250010295, 5.301041667008085767, -0.7879004041258300672 ) ) ;
#15889=FACE_OUTER_BOUND ( 'NONE', #110188, .T. ) ;
#15893=CARTESIAN_POINT ( 'NONE',  ( -2.779058300676974014, 6.186059084191009916, -0.7216878364870257245 ) ) ;
#15895=CARTESIAN_POINT ( 'NONE',  ( 9.748476143425788720, 11.33197590787365172, -1.199719254218440723 ) ) ;
#15897=CARTESIAN_POINT ( 'NONE',  ( -9.236128959407555072, 11.79856975744075598, -1.599625672291263179 ) ) ;
#15901=CARTESIAN_POINT ( 'NONE',  ( 1.364683531249988757, 2.134375000341422357, 1.214306433183764966E-14 ) ) ;
#15903=CARTESIAN_POINT ( 'NONE',  ( 3.472859903394816872, 7.203420320602605287, -0.7998128361456291469 ) ) ;
#15908=CARTESIAN_POINT ( 'NONE',  ( 9.368320956918614328, 10.99242454023565507, 1.082531754730549967 ) ) ;
#15909=CARTESIAN_POINT ( 'NONE',  ( -1.500000000000043299, 3.952083334016152971, 0.8660254037844216102 ) ) ;
#15910=CARTESIAN_POINT ( 'NONE',  ( -5.910991785878158211, 9.839981483592442402, -0.7216878364870278340 ) ) ;
#15912=CARTESIAN_POINT ( 'NONE',  ( -1.364683531250014514, 0.2802083336747505649, 0.7879004041258379498 ) ) ;
#15914=CARTESIAN_POINT ( 'NONE',  ( 0.1471985351164479261, 7.029189141431359644, 1.995741298138908659 ) ) ;
#15916=CARTESIAN_POINT ( 'NONE',  ( -7.537443334193545397, 10.88110209227943770, -1.199719254218446718 ) ) ;
#15917=CARTESIAN_POINT ( 'NONE',  ( -3.755245360860939297, 4.443836344834937613, -1.082531754730548412 ) ) ;
#15918=CARTESIAN_POINT ( 'NONE',  ( -1.364683531249997417, 4.071875000341417028, 1.214306433183764966E-14 ) ) ;
#15931=EDGE_CURVE ( 'NONE', #108458, #76077, #15785, .T. ) ;
#15935=CARTESIAN_POINT ( 'NONE',  ( -1.566570994388993832, 8.685985410138266971, 2.500753655585676416 ) ) ;
#15936=CARTESIAN_POINT ( 'NONE',  ( 1.364683531249988535, 4.217708333674752730, -0.7879004041258239610 ) ) ;
#15941=CARTESIAN_POINT ( 'NONE',  ( 7.736899214892750010, 12.17813285068358020, 1.040834085586084257E-14 ) ) ;
#15944=CARTESIAN_POINT ( 'NONE',  ( -0.6823417656250003738, 2.467708333674753618, -1.181850606188749264 ) ) ;
#15947=CARTESIAN_POINT ( 'NONE',  ( -6.209271165378811297, 10.18797409300986878, 0.7216878364870458196 ) ) ;
#15953=CARTESIAN_POINT ( 'NONE',  ( 3.897079088924235712, 6.634010472798538949, 1.199719254218462483 ) ) ;
#15956=CARTESIAN_POINT ( 'NONE',  ( 10.55232363013785246, 11.20546574478267132, 0.000000000000000000 ) ) ;
#15963=CARTESIAN_POINT ( 'NONE',  ( -9.917953063596627317, 11.52969898140628047, -1.199719254218441611 ) ) ;
#15964=CARTESIAN_POINT ( 'NONE',  ( 8.294891053462476904, 8.571794405328034827, 1.040834085586084257E-14 ) ) ;
#15966=CARTESIAN_POINT ( 'NONE',  ( 5.300874872818840622, 6.247070775452521652, 1.082531754730560403 ) ) ;
#15974=LINE ( 'NONE', #47463, #199100 ) ;
#15975=CARTESIAN_POINT ( 'NONE',  ( -6.344852701515500293, 9.385783337534627790, 1.082531754730548412 ) ) ;
#15977=CARTESIAN_POINT ( 'NONE',  ( 3.472859903394816872, 7.203420320602605287, -0.7998128361456291469 ) ) ;
#15980=CARTESIAN_POINT ( 'NONE',  ( -8.402302512167102222, 10.82577223566020841, -1.599625672291263179 ) ) ;
#15985=CARTESIAN_POINT ( 'NONE',  ( -7.784352752540590004, 12.23349531127272094, 0.7998128361456481317 ) ) ;
#15989=CARTESIAN_POINT ( 'NONE',  ( 9.610031953988080744, 10.10612545594124967, -0.7998128361456281477 ) ) ;
#15990=CARTESIAN_POINT ( 'NONE',  ( -3.325722479476970861, 7.699077257576049327, -2.499999999999995115 ) ) ;
#15996=CARTESIAN_POINT ( 'NONE',  ( 2.223174002961016082, 5.537527403522402025, -0.7216878364870267237 ) ) ;
#15999=CARTESIAN_POINT ( 'NONE',  ( -4.129789846611330972, 3.920435697242382833, -0.2706067644339962830 ) ) ;
#16001=CARTESIAN_POINT ( 'NONE',  ( -9.643927338022246332, 10.14567007064778004, -0.7998128361456291469 ) ) ;
#16005=CARTESIAN_POINT ( 'NONE',  ( 6.588899466561449536, 9.670504563421618016, -1.082531754730537088 ) ) ;
#16007=CARTESIAN_POINT ( 'NONE',  ( 4.857899112398166075, 4.561970474086296079, 1.040834085586084257E-14 ) ) ;
#16009=CARTESIAN_POINT ( 'NONE',  ( 5.192936529234042808, 6.017179691316550283, -1.199719254218452047 ) ) ;
#16011=CARTESIAN_POINT ( 'NONE',  ( -6.364663046611467756, 9.512858423433634414, 1.199719254218452047 ) ) ;
#16014=AXIS2_PLACEMENT_3D ( 'NONE', #40234, #6633, #5549 ) ;
#16021=CARTESIAN_POINT ( 'NONE',  ( -1.364683531249997417, 4.321875000341417028, 1.214306433183764966E-14 ) ) ;
#16022=CARTESIAN_POINT ( 'NONE',  ( -4.312804375668592982, 3.926026614568435935, 0.2365836213946782007 ) ) ;
#16023=CARTESIAN_POINT ( 'NONE',  ( 8.860417081730671995, 10.29590700256267155, 1.199719254218453823 ) ) ;
#16027=CARTESIAN_POINT ( 'NONE',  ( -2.806174608348664723, 6.217694776474651519, 1.040834085586084257E-14 ) ) ;
#16029=CARTESIAN_POINT ( 'NONE',  ( -3.402733366905605905, 6.913679994791092298, 0.7216878364870317197 ) ) ;
#16033=ORIENTED_EDGE ( 'NONE', *, *, #99218, .T. ) ;
#16037=CARTESIAN_POINT ( 'NONE',  ( 4.578903193113299963, 6.365139696764064325, 1.599625672291267398 ) ) ;
#16046=CARTESIAN_POINT ( 'NONE',  ( 5.515469562660962666, 5.329135999392899947, 0.7998128361456341429 ) ) ;
#16050=CARTESIAN_POINT ( 'NONE',  ( -1.364683531250010295, 3.842708333674751398, 0.7879004041258379498 ) ) ;
#16055=CARTESIAN_POINT ( 'NONE',  ( 5.276094334012385367, 9.307193822989793475, 1.040834085586084257E-14 ) ) ;
#16057=CARTESIAN_POINT ( 'NONE',  ( -5.762378981008047241, 6.681529218386182301, 1.199719254218450271 ) ) ;
#16058=CARTESIAN_POINT ( 'NONE',  ( 6.792271770322100721, 7.026664608238323950, -0.7216878364870257245 ) ) ;
#16059=CARTESIAN_POINT ( 'NONE',  ( 1.499999999999989120, 2.775000000000020339, 1.214306433183764966E-14 ) ) ;
#16062=CARTESIAN_POINT ( 'NONE',  ( -4.415151579544611238, 8.302760609444034046, -0.7998128361456281477 ) ) ;
#16065=CARTESIAN_POINT ( 'NONE',  ( 1.364683531249988535, 3.363541667008084879, 0.7879004041258500513 ) ) ;
#16067=CARTESIAN_POINT ( 'NONE',  ( -3.714570900464290393, 5.356752022006865843, 1.443375672974064550 ) ) ;
#16070=ORIENTED_EDGE ( 'NONE', *, *, #32218, .T. ) ;
#16072=CARTESIAN_POINT ( 'NONE',  ( -1.451998047843676476, 7.315968950353781253, 4.301760722578348073 ) ) ;
#16073=CARTESIAN_POINT ( 'NONE',  ( 3.845709127770629010, 7.638411082374393146, 0.7998128361456321445 ) ) ;
#16074=CARTESIAN_POINT ( 'NONE',  ( 0.7499999999999885647, 3.066666666666689522, -1.299038105676658228 ) ) ;
#16077=CARTESIAN_POINT ( 'NONE',  ( -1.364683531250010295, 3.842708333674751398, 0.7879004041258379498 ) ) ;
#16079=CARTESIAN_POINT ( 'NONE',  ( 3.195971524519376494, 4.751719416737803847, -1.599625672291262513 ) ) ;
#16081=CARTESIAN_POINT ( 'NONE',  ( -1.364683531250012516, 0.5927083336747520637, 0.7879004041258379498 ) ) ;
#16084=CARTESIAN_POINT ( 'NONE',  ( -2.937312835655025101, 6.578615408239493867, 1.040834085586084257E-14 ) ) ;
#16085=CARTESIAN_POINT ( 'NONE',  ( -5.816084710138169633, 8.768887347594400694, 1.082531754730548412 ) ) ;
#16088=EDGE_LOOP ( 'NONE', ( #104066, #153254, #75735 ) ) ;
#16089=CARTESIAN_POINT ( 'NONE',  ( -1.364683531250012516, 3.238541667008084879, -0.7879004041258289570 ) ) ;
#16097=CARTESIAN_POINT ( 'NONE',  ( -6.927853306458756855, 9.105581495667113501, 1.443375672974078761 ) ) ;
#16100=CARTESIAN_POINT ( 'NONE',  ( 4.650083499807235121, 5.295740330745369207, 1.082471891955963716 ) ) ;
#16104=CARTESIAN_POINT ( 'NONE',  ( -6.033015167956805591, 8.061603667414825480, -1.443375672974058777 ) ) ;
#16111=CONICAL_SURFACE ( 'NONE', #68053, 4.000000000000000000, 0.8960553845713404852 ) ;
#16112=DIRECTION ( 'NONE',  ( 0.000000000000000000, 8.546850786086437571E-32, 1.000000000000000000 ) ) ;
#16113=EDGE_LOOP ( 'NONE', ( #16490, #12251, #70332, #82896 ) ) ;
#16117=CARTESIAN_POINT ( 'NONE',  ( -5.915435094264120508, 5.795762452929912101, 0.000000000000000000 ) ) ;
#16119=CARTESIAN_POINT ( 'NONE',  ( 0.7499999999999885647, -0.7666666666666446250, 1.299038105676657340 ) ) ;
#16120=CARTESIAN_POINT ( 'NONE',  ( 2.171277156482887882, 5.684907115872006145, -0.7998128361456291469 ) ) ;
#16121=CARTESIAN_POINT ( 'NONE',  ( 8.444030743212801227, 8.745790710036752458, 0.7998128361456462443 ) ) ;
#16123=CARTESIAN_POINT ( 'NONE',  ( 4.111308439460083619, 3.971718457827854376, 0.3900462783498518937 ) ) ;
#16124=CARTESIAN_POINT ( 'NONE',  ( 4.843287188579786573, 6.673587691474970107, -1.599625672291256295 ) ) ;
#16130=CARTESIAN_POINT ( 'NONE',  ( -4.460269349215930212, 4.305995116947750390, 1.214306433183764966E-14 ) ) ;
#16132=AXIS2_PLACEMENT_3D ( 'NONE', #53453, #200745, #84886 ) ;
#16138=CARTESIAN_POINT ( 'NONE',  ( 1.364683531249988757, 2.384375000341422357, 1.214306433183764966E-14 ) ) ;
#16139=CARTESIAN_POINT ( 'NONE',  ( 9.612367721964607981, 12.23751498042398289, -1.443375672974058777 ) ) ;
#16140=CARTESIAN_POINT ( 'NONE',  ( -6.551614543901706611, 8.666636272683888365, 1.599625672291283607 ) ) ;
#16143=CARTESIAN_POINT ( 'NONE',  ( 7.305145839664861640, 7.417091655897478653, 0.7998128361456341429 ) ) ;
#16144=CARTESIAN_POINT ( 'NONE',  ( -6.911959384868566758, 6.958374125301778790, 1.040834085586084257E-14 ) ) ;
#16147=CARTESIAN_POINT ( 'NONE',  ( -0.7500000000000249800, -1.027083332650516212, 1.299038105676659116 ) ) ;
#16150=CARTESIAN_POINT ( 'NONE',  ( 7.456621297836072415, 9.722477485607340597, 1.443375672974076540 ) ) ;
#16153=CARTESIAN_POINT ( 'NONE',  ( -1.402160292154681736E-14, 0.7593750003414168059, -1.575800808251659024 ) ) ;
#16155=CARTESIAN_POINT ( 'NONE',  ( 7.117667457050084856, 7.406292909420979953, -0.7216878364870257245 ) ) ;
#16158=CARTESIAN_POINT ( 'NONE',  ( -4.934804725694231564, 5.819988937140460727, -1.082531754730544860 ) ) ;
#16161=CARTESIAN_POINT ( 'NONE',  ( 1.364683531249990311, 4.863541667008084879, 0.7879004041258500513 ) ) ;
#16165=CARTESIAN_POINT ( 'NONE',  ( -5.688173390364544169, 6.286868445634342883, -1.126660468825124273 ) ) ;
#16172=CARTESIAN_POINT ( 'NONE',  ( 8.308449207076147758, 8.587612251210650527, -0.7998128361456281477 ) ) ;
#16175=CARTESIAN_POINT ( 'NONE',  ( 4.172158584703322681, 5.890604320285754980, -1.599625672291256295 ) ) ;
#16182=CARTESIAN_POINT ( 'NONE',  ( 6.019457014787495730, 6.125047393447951016, -0.7216878364870257245 ) ) ;
#16184=CARTESIAN_POINT ( 'NONE',  ( -1.364683531250014514, 0.3427083336747508424, 0.7879004041258379498 ) ) ;
#16186=CARTESIAN_POINT ( 'NONE',  ( 10.05353459973327368, 11.68787744023238417, -1.199719254218440723 ) ) ;
#16192=CARTESIAN_POINT ( 'NONE',  ( -1.402160292154681736E-14, 1.837500000000019895, -1.732050807568863648 ) ) ;
#16193=CARTESIAN_POINT ( 'NONE',  ( 6.962275575817444384, 8.081408578997208991, -1.199719254218446718 ) ) ;
#16194=CARTESIAN_POINT ( 'NONE',  ( -7.527801604085656351, 9.805521176231838609, 1.599625672291295375 ) ) ;
#16198=CARTESIAN_POINT ( 'NONE',  ( 1.364683531249988535, 1.363541667008083769, 0.7879004041258500513 ) ) ;
#16199=CARTESIAN_POINT ( 'NONE',  ( -1.500000000000013101, 2.379166666666686414, -0.8660254037844313801 ) ) ;
#16201=CARTESIAN_POINT ( 'NONE',  ( 3.659811400685081040, 6.357198169852855685, -1.199719254218446718 ) ) ;
#16204=CARTESIAN_POINT ( 'NONE',  ( -1.001543065824772872E-14, 4.493750000682820378, 1.732050807568877637 ) ) ;
#16208=CARTESIAN_POINT ( 'NONE',  ( -1.402160292154681736E-14, -0.006249999317184824418, 1.732050807568877637 ) ) ;
#16209=CARTESIAN_POINT ( 'NONE',  ( -6.509886312855995172, 10.74661779830734254, -0.7998128361456291469 ) ) ;
#16210=CARTESIAN_POINT ( 'NONE',  ( -3.606105671554953318, 7.150947683548662503, 0.7216878364870317197 ) ) ;
#16215=CARTESIAN_POINT ( 'NONE',  ( 4.008199524592567897, 7.584238231759597326, 0.2402771892247856922 ) ) ;
#16218=CARTESIAN_POINT ( 'NONE',  ( 5.750629710490689384, 9.860818428881154674, -0.7998128361456291469 ) ) ;
#16222=CARTESIAN_POINT ( 'NONE',  ( 7.253775878511261155, 8.421492265473332850, 1.199719254218462483 ) ) ;
#16223=CARTESIAN_POINT ( 'NONE',  ( 8.798878505144646311, 11.28844422746735532, -1.443375672974052559 ) ) ;
#16227=CARTESIAN_POINT ( 'NONE',  ( -5.520141099058386125, 9.591915048876776595, 0.000000000000000000 ) ) ;
#16228=CARTESIAN_POINT ( 'NONE',  ( 3.330499290451326200, 7.037332938835193730, -0.7998128361456291469 ) ) ;
#16233=LINE ( 'NONE', #148410, #62770 ) ;
#16235=CARTESIAN_POINT ( 'NONE',  ( 8.242994207428692377, 12.56065097540143327, -0.7216878364870328300 ) ) ;
#16242=CARTESIAN_POINT ( 'NONE',  ( -3.280709984826970516, 6.771319382366015383, 0.7216878364870317197 ) ) ;
#16243=CARTESIAN_POINT ( 'NONE',  ( 9.259855728453651125, 9.905512559391842942, 1.040834085586084257E-14 ) ) ;
#16246=CARTESIAN_POINT ( 'NONE',  ( -4.720210035852093533, 8.658662141802762946, -0.7998128361456281477 ) ) ;
#16253=CARTESIAN_POINT ( 'NONE',  ( -7.542413527904030524, 7.693903958843159252, 1.040834085586084257E-14 ) ) ;
#16259=ORIENTED_EDGE ( 'NONE', *, *, #137350, .F. ) ;
#16268=CARTESIAN_POINT ( 'NONE',  ( -6.403528624356093601, 6.365204904703887223, 1.040834085586084257E-14 ) ) ;
#16271=CARTESIAN_POINT ( 'NONE',  ( 5.192409644353875642, 5.160158794608717514, 1.040834085586084257E-14 ) ) ;
#16275=( BOUNDED_CURVE ( )  B_SPLINE_CURVE ( 2, ( #155853, #7440, #153721, #4229, #203497 ),
 .UNSPECIFIED., .F., .T. ) 
 B_SPLINE_CURVE_WITH_KNOTS ( ( 3, 2, 3 ),
 ( 0.2500000000000002776, 0.2541666666666667074, 0.2546568312040279891 ),
 .UNSPECIFIED. ) 
 CURVE ( )  GEOMETRIC_REPRESENTATION_ITEM ( )  RATIONAL_B_SPLINE_CURVE ( ( 0.9999999999999911182, 0.8660254037844475894, 1.000000000000000000, 0.9842392969666786673, 0.9721867560345496262 ) ) 
 REPRESENTATION_ITEM ( '' )  );
#16277=CARTESIAN_POINT ( 'NONE',  ( -3.948449050077848632, 5.629609863222681199, 1.599625672291267398 ) ) ;
#16283=CARTESIAN_POINT ( 'NONE',  ( -6.516665389662827934, 10.75452672124865217, 0.000000000000000000 ) ) ;
#16284=CARTESIAN_POINT ( 'NONE',  ( 5.276094334012385367, 9.307193822989793475, 1.040834085586084257E-14 ) ) ;
#16287=CARTESIAN_POINT ( 'NONE',  ( -7.645908563102897126, 11.00764485934031889, 1.199719254218453823 ) ) ;
#16289=CARTESIAN_POINT ( 'NONE',  ( 3.649115900372475796, 7.409052317076538330, 1.040834085586084257E-14 ) ) ;
#16292=CARTESIAN_POINT ( 'NONE',  ( 1.364683531249986537, -0.5739583329919174526, 0.7879004041258500513 ) ) ;
#16295=CARTESIAN_POINT ( 'NONE',  ( 7.727784370109387346, 10.99920361756089093, -1.082531754730543083 ) ) ;
#16304=CARTESIAN_POINT ( 'NONE',  ( -6.007394966791244961, 6.077829431809393945, -0.6506939885215150543 ) ) ;
#16315=CARTESIAN_POINT ( 'NONE',  ( -2.123823618835070537, 5.629544655282869847, 1.040834085586084257E-14 ) ) ;
#16324=CARTESIAN_POINT ( 'NONE',  ( 1.499999999999987121, 0.5770833340161539704, -0.8660254037844253849 ) ) ;
#16331=CARTESIAN_POINT ( 'NONE',  ( 8.204655514564224816, 12.72384853363364066, 1.040834085586084257E-14 ) ) ;
#16332=EDGE_CURVE ( 'NONE', #110797, #23962, #158502, .T. ) ;
#16333=CARTESIAN_POINT ( 'NONE',  ( -0.7500000000000215383, 5.222916667349482012, 1.299038105676671107 ) ) ;
#16338=CARTESIAN_POINT ( 'NONE',  ( 4.416205349749311004, 6.175325546172740765, 1.599625672291267398 ) ) ;
#16339=CARTESIAN_POINT ( 'NONE',  ( -7.131225611108100715, 9.342849184424693476, 1.443375672974078761 ) ) ;
#16340=CARTESIAN_POINT ( 'NONE',  ( -5.890076507333620981, 6.013243542187837853, -0.2543948676220365024 ) ) ;
#16343=CARTESIAN_POINT ( 'NONE',  ( -8.681298431451969222, 9.022603012982438386, 1.040834085586084257E-14 ) ) ;
#16344=CARTESIAN_POINT ( 'NONE',  ( -4.907688418022547516, 4.827984030555475314, 1.214306433183764966E-14 ) ) ;
#16347=CARTESIAN_POINT ( 'NONE',  ( 1.499999999999989120, 0.05625000068281565957, 0.000000000000000000 ) ) ;
#16356=CARTESIAN_POINT ( 'NONE',  ( -3.348500752450953577, 4.929670182657964084, 1.443375672974062551 ) ) ;
#16364=CARTESIAN_POINT ( 'NONE',  ( -10.34217224912604571, 10.96028913360221502, 0.7998128361456462443 ) ) ;
#16365=CARTESIAN_POINT ( 'NONE',  ( 8.067265095331215718, 9.370563018429956870, 1.199719254218462483 ) ) ;
#16375=CARTESIAN_POINT ( 'NONE',  ( -9.104463846776669200, 10.58062822844965645, -1.199719254218441611 ) ) ;
#16380=CARTESIAN_POINT ( 'NONE',  ( 4.320244504248938355, 8.192035688265757898, 1.040834085586084257E-14 ) ) ;
#16383=ORIENTED_EDGE ( 'NONE', *, *, #115804, .T. ) ;
#16398=CARTESIAN_POINT ( 'NONE',  ( 7.416473721875251890, 8.611306416064660851, 1.199719254218462483 ) ) ;
#16400=CARTESIAN_POINT ( 'NONE',  ( -4.273844736805832767, 6.009238164405336313, 1.599625672291267398 ) ) ;
#16406=CARTESIAN_POINT ( 'NONE',  ( 0.7499999999999885647, -1.235416665983847473, 1.299038105676657340 ) ) ;
#16409=CARTESIAN_POINT ( 'NONE',  ( -1.558944071570950163, 8.694263516232775046, -2.499999999999761080 ) ) ;
#16410=CARTESIAN_POINT ( 'NONE',  ( 2.517010073631369860, 6.088262185878572375, -0.7998128361456281477 ) ) ;
#16412=CARTESIAN_POINT ( 'NONE',  ( -4.973143418114339021, 4.696422164088486895, 0.7998128361456341429 ) ) ;
#16418=CARTESIAN_POINT ( 'NONE',  ( 5.694061328059515148, 5.745419092265303007, -0.7216878364870207285 ) ) ;
#16421=CARTESIAN_POINT ( 'NONE',  ( -1.364683531250010295, 5.342708333674750953, 0.7879004041258379498 ) ) ;
#16423=CARTESIAN_POINT ( 'NONE',  ( 4.704316113817540668, 5.551085556617666228, -1.082531754730548412 ) ) ;
#16433=CARTESIAN_POINT ( 'NONE',  ( -6.121777486219434294, 6.006025806897081765, -0.2357381234046468377 ) ) ;
#16435=CARTESIAN_POINT ( 'NONE',  ( 0.6823417656249899377, 5.238541667008086655, -1.181850606188754593 ) ) ;
#16442=CARTESIAN_POINT ( 'NONE',  ( 0.7499999999999920064, 4.733333333333352932, 1.299038105676669330 ) ) ;
#16449=CARTESIAN_POINT ( 'NONE',  ( -1.201851678989727383E-14, 4.759375000341419693, -1.575800808251660134 ) ) ;
#16452=CARTESIAN_POINT ( 'NONE',  ( 5.799137018343234473, 7.788745826199009237, -1.599625672291262513 ) ) ;
#16453=CARTESIAN_POINT ( 'NONE',  ( -6.665805079413154921, 10.92852302595736447, 0.7998128361456481317 ) ) ;
#16460=CARTESIAN_POINT ( 'NONE',  ( 1.499999999999989120, 5.254166666666684193, 0.8660254037844524744 ) ) ;
#16468=CARTESIAN_POINT ( 'NONE',  ( 7.456621297836061757, 11.64321591421002644, 0.7216878364870438212 ) ) ;
#16473=CARTESIAN_POINT ( 'NONE',  ( -1.499999999999997780, 3.181250000682818602, 1.214306433183764966E-14 ) ) ;
#16475=CARTESIAN_POINT ( 'NONE',  ( -4.613852347352193739, 4.277249248199312071, 1.214306433183764966E-14 ) ) ;
#16476=CARTESIAN_POINT ( 'NONE',  ( 3.023105065722948126, 6.470780310077995701, 0.7216878364870338292 ) ) ;
#16484=CARTESIAN_POINT ( 'NONE',  ( 2.835626683552519012, 6.459981564119914310, 0.000000000000000000 ) ) ;
#16485=CARTESIAN_POINT ( 'NONE',  ( -1.230761180058552950, 2.935133534840178804, -0.7749999999999988010 ) ) ;
#16487=CARTESIAN_POINT ( 'NONE',  ( 2.679707916995359263, 6.278076336469897711, -0.7998128361456291469 ) ) ;
#16490=ORIENTED_EDGE ( 'NONE', *, *, #103236, .F. ) ;
#16498=CARTESIAN_POINT ( 'NONE',  ( 5.237746300327911442, 6.405127287353401755, -1.156737470277836355 ) ) ;
#16502=CARTESIAN_POINT ( 'NONE',  ( 9.134442807305049428, 11.67993591332117376, 1.599625672291281386 ) ) ;
#16505=CARTESIAN_POINT ( 'NONE',  ( -1.364683531250000748, 0.2593750003414205252, 0.000000000000000000 ) ) ;
#16506=CARTESIAN_POINT ( 'NONE',  ( 5.327991180490514012, 9.159814110640187579, 1.040834085586084257E-14 ) ) ;
#16507=CARTESIAN_POINT ( 'NONE',  ( -8.676855123066012254, 12.10645282934361866, -1.082531754730543971 ) ) ;
#16513=CARTESIAN_POINT ( 'NONE',  ( -3.144601563365788444, 5.756120026313656268, -1.199719254218452935 ) ) ;
#16525=CARTESIAN_POINT ( 'NONE',  ( 6.001708393183096568, 6.086876045059843143, 0.6039332608892417076 ) ) ;
#16529=CARTESIAN_POINT ( 'NONE',  ( 5.332434488876471868, 5.115595079977664383, 0.7998128361456341429 ) ) ;
#16531=DIRECTION ( 'NONE',  ( -5.578564026256490882E-16, -1.000000000000000000, -9.066213480720158442E-32 ) ) ;
#16534=CARTESIAN_POINT ( 'NONE',  ( -7.212574532790087645, 11.35849468832304154, -0.7216878364870267237 ) ) ;
#16538=CARTESIAN_POINT ( 'NONE',  ( 5.262536180398716290, 9.291375977107183104, -0.7998128361456291469 ) ) ;
#16539=CARTESIAN_POINT ( 'NONE',  ( -5.220052836461385404, 6.048815383081766583, -1.199719254218446718 ) ) ;
#16543=CARTESIAN_POINT ( 'NONE',  ( -4.238895582566952314, 8.097128612970093897, 1.040834085586084257E-14 ) ) ;
#16544=CARTESIAN_POINT ( 'NONE',  ( 3.009020027229115879, 5.597941567487558778, -1.199719254218446718 ) ) ;
#16546=CARTESIAN_POINT ( 'NONE',  ( -5.042743069279040036, 7.970618449879118828, 1.199719254218464037 ) ) ;
#16549=CARTESIAN_POINT ( 'NONE',  ( 8.483651433849084711, 10.92067931095586886, 1.599625672291281386 ) ) ;
#16552=CARTESIAN_POINT ( 'NONE',  ( 4.193481561896174270, 7.343914482741291216, -0.8359065270147625348 ) ) ;
#16553=CARTESIAN_POINT ( 'NONE',  ( 6.480434237652135998, 6.662854153456708950, 0.7216878364870317197 ) ) ;
#16555=LINE ( 'NONE', #161785, #177448 ) ;
#16558=CARTESIAN_POINT ( 'NONE',  ( 6.938893903907228378E-15, 10.64264068711930733, 1.214306433183764966E-14 ) ) ;
#16561=CARTESIAN_POINT ( 'NONE',  ( 8.093854517234030155, 8.545177812968924869, -0.7216878364870267237 ) ) ;
#16566=CARTESIAN_POINT ( 'NONE',  ( -6.177711549321182716, 10.35908057418338402, 0.7998128361456481317 ) ) ;
#16570=CARTESIAN_POINT ( 'NONE',  ( 4.074186250656476993, 7.493853916489129574, -0.5595503573846259959 ) ) ;
#16574=CARTESIAN_POINT ( 'NONE',  ( 9.673906298550626559, 11.24497775551929557, 1.199719254218452047 ) ) ;
#16578=CARTESIAN_POINT ( 'NONE',  ( 4.467575310902914154, 5.170924936596891008, 1.199719254218464037 ) ) ;
#16582=CARTESIAN_POINT ( 'NONE',  ( 1.499999999999990896, 4.306250000682819490, 1.214306433183764966E-14 ) ) ;
#16588=CARTESIAN_POINT ( 'NONE',  ( 1.499999999999987121, 1.545833333333354487, -0.8660254037844253849 ) ) ;
#16589=CARTESIAN_POINT ( 'NONE',  ( 6.205881626753210867, 8.263281202677319470, 1.599625672291281386 ) ) ;
#16590=CARTESIAN_POINT ( 'NONE',  ( 5.002595493318194642, 4.938708951733754127, -0.7216878364870197293 ) ) ;
#16593=CARTESIAN_POINT ( 'NONE',  ( 8.948018195339340508, 9.541702104091804415, -0.7216878364870197293 ) ) ;
#16600=CARTESIAN_POINT ( 'NONE',  ( -4.416205349749324327, 6.175325546172740765, 1.599625672291267398 ) ) ;
#16601=CARTESIAN_POINT ( 'NONE',  ( -1.500000000000011324, 5.202083334016151639, 0.8660254037844403729 ) ) ;
#16603=CARTESIAN_POINT ( 'NONE',  ( -0.6823417656250003738, -0.03229166632524871350, -1.181850606188749264 ) ) ;
#16607=CARTESIAN_POINT ( 'NONE',  ( 4.359110081993588182, 5.044382169536003602, -1.199719254218452047 ) ) ;
#16609=CARTESIAN_POINT ( 'NONE',  ( -1.364683531250000748, -1.240624999658580752, 0.000000000000000000 ) ) ;
#16612=EDGE_CURVE ( 'NONE', #6901, #173454, #104421, .T. ) ;
#16613=CARTESIAN_POINT ( 'NONE',  ( 10.73535870392234237, 11.41900666419791399, 0.000000000000000000 ) ) ;
#16617=CARTESIAN_POINT ( 'NONE',  ( -6.201965203247477909, 9.323044272842313518, 1.199719254218452047 ) ) ;
#16619=CARTESIAN_POINT ( 'NONE',  ( 4.680589345215795838, 6.483773540883647435, -1.599625672291256295 ) ) ;
#16622=CARTESIAN_POINT ( 'NONE',  ( 1.364683531249986537, -0.5947916663252456049, -0.7879004041258309554 ) ) ;
#16626=CARTESIAN_POINT ( 'NONE',  ( 8.910733272679570049, 11.41894145625809820, -1.599625672291255185 ) ) ;
#16629=CARTESIAN_POINT ( 'NONE',  ( -5.961834861707238531, 7.978559976790334574, -1.599625672291263179 ) ) ;
#16633=CARTESIAN_POINT ( 'NONE',  ( 9.541187415715040032, 12.15447128979948310, -1.599625672291262513 ) ) ;
#16635=CARTESIAN_POINT ( 'NONE',  ( 8.925345196497941558, 9.307324238869423283, 1.040834085586084257E-14 ) ) ;
#16637=AXIS2_PLACEMENT_3D ( 'NONE', #21550, #87660, #55160 ) ;
#16638=CARTESIAN_POINT ( 'NONE',  ( -4.451154503988200339, 4.087435097607984957, 1.214306433183764966E-14 ) ) ;
#16639=CARTESIAN_POINT ( 'NONE',  ( -8.016948904382338981, 8.247528564734524892, -0.7998128361456291469 ) ) ;
#16642=CARTESIAN_POINT ( 'NONE',  ( -4.565105001785453531, 7.177652750280781646, 1.346018956990787885 ) ) ;
#16643=CARTESIAN_POINT ( 'NONE',  ( -0.6823417656250003738, 0.9677083336747521747, -1.181850606188749264 ) ) ;
#16647=CARTESIAN_POINT ( 'NONE',  ( 5.816084710582486217, 9.729256562414162701, 1.040834085586084257E-14 ) ) ;
#16650=CARTESIAN_POINT ( 'NONE',  ( 5.843727902690005749, 6.776436293681846301, -1.199719254218445830 ) ) ;
#16669=CARTESIAN_POINT ( 'NONE',  ( 10.73535870392234237, 11.41900666419791399, 0.000000000000000000 ) ) ;
#16672=CARTESIAN_POINT ( 'NONE',  ( -4.141125853970233806, 6.918731698685530063, -1.199719254218452047 ) ) ;
#16673=CARTESIAN_POINT ( 'NONE',  ( -7.320512876374914768, 10.62801655815766999, 1.199719254218453823 ) ) ;
#16679=CARTESIAN_POINT ( 'NONE',  ( 0.7499999999999902300, 3.597916667349487785, -1.299038105676658228 ) ) ;
#16680=CARTESIAN_POINT ( 'NONE',  ( 9.077347539549325717, 10.54899253668443393, -1.199719254218446718 ) ) ;
#16684=CARTESIAN_POINT ( 'NONE',  ( -9.016335848287868160, 10.47781223021269170, 1.199719254218462483 ) ) ;
#16686=CARTESIAN_POINT ( 'NONE',  ( -1.364683531250012516, 2.738541667008090208, -0.7879004041258289570 ) ) ;
#16688=DIRECTION ( 'NONE',  ( 1.000000000000000000, 0.000000000000000000, 0.000000000000000000 ) ) ;
#16692=CARTESIAN_POINT ( 'NONE',  ( -3.735435015764967837, 4.316761258935923884, -1.199719254218452047 ) ) ;
#16697=CARTESIAN_POINT ( 'NONE',  ( 1.364683531249986537, 1.217708333674754950, -0.7879004041258239610 ) ) ;
#16702=CARTESIAN_POINT ( 'NONE',  ( -1.402160292154681736E-14, 1.696875000341421469, -1.575800808251659024 ) ) ;
#16704=CARTESIAN_POINT ( 'NONE',  ( -5.168682875307782254, 7.053215992657626110, -1.599625672291256295 ) ) ;
#16705=CARTESIAN_POINT ( 'NONE',  ( 7.800018446563675489, 7.994443030612759848, -0.7998128361456281477 ) ) ;
#16706=CARTESIAN_POINT ( 'NONE',  ( -1.257539916218630927, 2.908837156058346807, 0.7750000000000117906 ) ) ;
#16708=CARTESIAN_POINT ( 'NONE',  ( 1.499999999999987121, 4.795833333333353821, -0.8660254037844323793 ) ) ;
#16709=CARTESIAN_POINT ( 'NONE',  ( 1.364683531249988535, 2.426041667008088432, 0.7879004041258500513 ) ) ;
#16713=CARTESIAN_POINT ( 'NONE',  ( -5.910991785878175975, 6.958873840688411860, -1.082531754730544860 ) ) ;
#16716=CARTESIAN_POINT ( 'NONE',  ( 4.799223189557548785, 7.582548906917042864, -1.082531754730549078 ) ) ;
#16719=CARTESIAN_POINT ( 'NONE',  ( -9.016335848287868160, 10.47781223021269170, 1.199719254218462483 ) ) ;
#16720=CARTESIAN_POINT ( 'NONE',  ( -10.03267048443264109, 11.76749898900197877, 1.082531754730558626 ) ) ;
#16721=CARTESIAN_POINT ( 'NONE',  ( 1.579999999999989413, 6.280000000000042881, -2.579999999999995630 ) ) ;
#16722=CARTESIAN_POINT ( 'NONE',  ( -1.364683531250010295, 5.488541667008087543, -0.7879004041258300672 ) ) ;
#16727=CARTESIAN_POINT ( 'NONE',  ( -6.168596704093453731, 10.14052055484361325, 0.7216878364870458196 ) ) ;
#16729=CARTESIAN_POINT ( 'NONE',  ( -1.402160292154681736E-14, -0.1156249996585793222, 1.575800808251672791 ) ) ;
#16732=CARTESIAN_POINT ( 'NONE',  ( 7.456621297836067086, 10.68284669990868174, 1.082531754730558626 ) ) ;
#16734=CARTESIAN_POINT ( 'NONE',  ( -3.402733366905634327, 6.913679994791067429, 0.7216878364870540352 ) ) ;
#16737=CARTESIAN_POINT ( 'NONE',  ( -4.234859498635395347, 3.979834430640218468, 0.5021729129214658194 ) ) ;
#16741=CARTESIAN_POINT ( 'NONE',  ( 8.039621902779343188, 12.32338328664385507, -0.7216878364870328300 ) ) ;
#16749=CARTESIAN_POINT ( 'NONE',  ( 7.447506452608354088, 7.583179037664891098, 0.7998128361456341429 ) ) ;
#16750=CARTESIAN_POINT ( 'NONE',  ( -4.391951695823077984, 7.211361847513815704, 1.199719254218464037 ) ) ;
#16755=CARTESIAN_POINT ( 'NONE',  ( 6.466876083594112146, 6.647036307055676829, -0.7216878364870257245 ) ) ;
#16756=CARTESIAN_POINT ( 'NONE',  ( -1.402160292154681736E-14, 0.2593750003414224681, -1.575800808251665908 ) ) ;
#16757=CARTESIAN_POINT ( 'NONE',  ( 4.216222584169931231, 4.021273891060765493, 1.214306433183764966E-14 ) ) ;
#16758=CARTESIAN_POINT ( 'NONE',  ( -7.797910906154257304, 12.24931315715533486, 0.000000000000000000 ) ) ;
#16775=CARTESIAN_POINT ( 'NONE',  ( 8.118635056484817980, 8.366162408854107113, 0.7998128361456481317 ) ) ;
#16776=CARTESIAN_POINT ( 'NONE',  ( 6.795661308947685164, 8.951357498570873261, -1.599625672291262513 ) ) ;
#16779=VERTEX_POINT ( 'NONE', #94588 ) ;
#16787=CARTESIAN_POINT ( 'NONE',  ( -3.899941742225307539, 7.701682465904834629, 0.7998128361456341429 ) ) ;
#16797=CARTESIAN_POINT ( 'NONE',  ( -10.03267048443264109, 11.76749898900197877, 1.082531754730558626 ) ) ;
#16800=CARTESIAN_POINT ( 'NONE',  ( 7.122110765880372618, 7.203550736482235095, 0.7998128361456341429 ) ) ;
#16806=CARTESIAN_POINT ( 'NONE',  ( 3.673896439178918172, 6.269667698141953238, 1.082531754730558626 ) ) ;
#16808=CARTESIAN_POINT ( 'NONE',  ( -6.531277313481209212, 8.642909503859968368, 1.599625672291283607 ) ) ;
#16814=CARTESIAN_POINT ( 'NONE',  ( -5.194745412330402878, 9.212286747694129474, 0.000000000000000000 ) ) ;
#16815=CARTESIAN_POINT ( 'NONE',  ( -4.680589345215810049, 6.483773540883647435, -1.599625672291256295 ) ) ;
#16822=VECTOR ( 'NONE', #209264, 1000.000000000000114 ) ;
#16823=CARTESIAN_POINT ( 'NONE',  ( 6.311484202361478779, 7.322151976631905868, -1.199719254218446718 ) ) ;
#16838=CARTESIAN_POINT ( 'NONE',  ( -1.364683531250014514, 0.05104166700808546175, -0.7879004041258359514 ) ) ;
#16839=CARTESIAN_POINT ( 'NONE',  ( 3.765413976293345844, 5.416068943807445635, 1.599625672291267398 ) ) ;
#16840=CARTESIAN_POINT ( 'NONE',  ( 3.493197133815315603, 7.227147089426516402, -0.7998128361456291469 ) ) ;
#16842=CARTESIAN_POINT ( 'NONE',  ( -8.541273586929371220, 9.067166727613487964, 0.7216878364870438212 ) ) ;
#16844=CARTESIAN_POINT ( 'NONE',  ( 4.690757960648213931, 8.416375354157496602, 0.7216878364870438212 ) ) ;
#16845=CARTESIAN_POINT ( 'NONE',  ( -6.033015167956794933, 9.982342096017511324, -0.7216878364870267237 ) ) ;
#16849=CARTESIAN_POINT ( 'NONE',  ( 5.452350330990040739, 9.512825819463730070, 0.7998128361456462443 ) ) ;
#16856=CARTESIAN_POINT ( 'NONE',  ( -1.364683531249997417, 3.259375000341423245, 1.214306433183764966E-14 ) ) ;
#16862=CARTESIAN_POINT ( 'NONE',  ( 7.771848369131631351, 10.09024240211882351, -1.599625672291262513 ) ) ;
#16866=CARTESIAN_POINT ( 'NONE',  ( -9.124801077197171040, 10.60435499727357289, -1.199719254218441611 ) ) ;
#16871=CARTESIAN_POINT ( 'NONE',  ( 9.297140650669039275, 11.86975006391249643, 1.599625672291281386 ) ) ;
#16874=CARTESIAN_POINT ( 'NONE',  ( -7.557780564614042795, 10.90482886110335414, -1.199719254218446718 ) ) ;
#16877=CARTESIAN_POINT ( 'NONE',  ( 4.825424889954152086, 6.722588627200480893, -1.249340337910074705 ) ) ;
#16878=CARTESIAN_POINT ( 'NONE',  ( -3.358669367883384105, 4.941533567329135401, -1.599625672291262513 ) ) ;
#16881=CARTESIAN_POINT ( 'NONE',  ( -1.500000000000079270, 7.360305807095733677, 4.205660139708331080 ) ) ;
#16883=CARTESIAN_POINT ( 'NONE',  ( 5.099838337034727331, 9.101561826515851550, -0.7998128361456281477 ) ) ;
#16885=CARTESIAN_POINT ( 'NONE',  ( 4.313465427442102929, 8.184126765324453601, 0.7998128361456462443 ) ) ;
#16886=CARTESIAN_POINT ( 'NONE',  ( -4.055583655087145800, 7.567422049930973671, -0.4132208808486706464 ) ) ;
#16887=CARTESIAN_POINT ( 'NONE',  ( 4.334856428067313416, 6.080418470877079429, -1.599625672291256295 ) ) ;
#16889=CARTESIAN_POINT ( 'NONE',  ( -7.022760382198764084, 11.13704484596649635, 0.7216878364870458196 ) ) ;
#16896=CARTESIAN_POINT ( 'NONE',  ( -4.295541959788370612, 7.266047401097770475, -0.9601269197386901322 ) ) ;
#16897=CARTESIAN_POINT ( 'NONE',  ( 0.6823417656249882723, -0.8447916663252494907, 1.181850606188755259 ) ) ;
#16900=CARTESIAN_POINT ( 'NONE',  ( 4.853455804012222430, 5.725081861844796727, 1.082531754730560403 ) ) ;
#16904=CARTESIAN_POINT ( 'NONE',  ( -8.961576348508641487, 11.47825837805867799, -1.443375672974058777 ) ) ;
#16909=DIRECTION ( 'NONE',  ( 1.000000000000000000, 0.000000000000000000, 0.000000000000000000 ) ) ;
#16911=CARTESIAN_POINT ( 'NONE',  ( -10.10046125205659173, 10.88621900359527572, -0.7216878364870267237 ) ) ;
#16917=CARTESIAN_POINT ( 'NONE',  ( -7.809133291347029271, 12.05447990663947877, 0.000000000000000000 ) ) ;
#16921=VERTEX_POINT ( 'NONE', #161716 ) ;
#16923=CARTESIAN_POINT ( 'NONE',  ( -1.201851678989727383E-14, 2.493750000682819046, 1.732050807568877637 ) ) ;
#16925=CARTESIAN_POINT ( 'NONE',  ( -5.205440912643032547, 8.160432600470439723, 1.199719254218452047 ) ) ;
#16929=CARTESIAN_POINT ( 'NONE',  ( -7.537443334193545397, 10.88110209227943770, -1.199719254218446718 ) ) ;
#16932=CARTESIAN_POINT ( 'NONE',  ( 5.717788096661236885, 7.693838750903348789, 1.599625672291267398 ) ) ;
#16938=CARTESIAN_POINT ( 'NONE',  ( 6.923409998072794558, 11.22906209772695618, 1.040834085586084257E-14 ) ) ;
#16941=CARTESIAN_POINT ( 'NONE',  ( -4.821467422361007671, 5.083637263933393768, -0.9394917190213262215 ) ) ;
#16945=CARTESIAN_POINT ( 'NONE',  ( -7.714226216495749355, 8.102278128774251797, 1.040834085586084257E-14 ) ) ;
#16948=CARTESIAN_POINT ( 'NONE',  ( 1.364683531249988535, 5.467708333674750953, -0.7879004041258300672 ) ) ;
#16955=CARTESIAN_POINT ( 'NONE',  ( -8.631737353394710155, 13.22211067893587533, 1.040834085586084257E-14 ) ) ;
#16957=CARTESIAN_POINT ( 'NONE',  ( 8.561083932025322696, 12.07534945641652158, -1.199719254218446718 ) ) ;
#16962=CARTESIAN_POINT ( 'NONE',  ( -0.6823417656250212460, 2.301041667008084435, 1.181850606188767472 ) ) ;
#16963=CARTESIAN_POINT ( 'NONE',  ( 4.521807925357579805, 5.234196320127330715, -1.199719254218452047 ) ) ;
#16970=CARTESIAN_POINT ( 'NONE',  ( 8.527715432871318058, 12.89282573841782664, -0.7216878364870338292 ) ) ;
#16972=CARTESIAN_POINT ( 'NONE',  ( -8.365017589951714072, 8.861534731139549592, 1.040834085586084257E-14 ) ) ;
#16974=CARTESIAN_POINT ( 'NONE',  ( -0.006158830626143650504, 7.078243236992579845, 2.121324627965421872 ) ) ;
#16976=CARTESIAN_POINT ( 'NONE',  ( -6.659026002606323047, 10.92061410301605662, 0.000000000000000000 ) ) ;
#16977=CARTESIAN_POINT ( 'NONE',  ( -4.243338890952901288, 6.934017225211593249, -1.082531754730548412 ) ) ;
#16978=CARTESIAN_POINT ( 'NONE',  ( 1.364683531249988535, 3.676041667008087099, 0.7879004041258500513 ) ) ;
#16981=EDGE_CURVE ( 'NONE', #80197, #96352, #199150, .T. ) ;
#16991=ORIENTED_EDGE ( 'NONE', *, *, #170571, .T. ) ;
#16995=EDGE_CURVE ( 'NONE', #54853, #25107, #50771, .T. ) ;
#17003=CARTESIAN_POINT ( 'NONE',  ( -1.364683531250012516, 4.051041667008088432, -0.7879004041258300672 ) ) ;
#17010=CARTESIAN_POINT ( 'NONE',  ( 8.666686507633574621, 11.13422023037111330, 1.599625672291281386 ) ) ;
#17011=CARTESIAN_POINT ( 'NONE',  ( -5.436456409399874623, 5.444880020495701523, 0.000000000000000000 ) ) ;
#17013=CARTESIAN_POINT ( 'NONE',  ( 1.364683531249986537, 1.905208333674750287, -0.7879004041258239610 ) ) ;
#17015=CARTESIAN_POINT ( 'NONE',  ( -5.883875478650828050, 9.808345791827219884, 0.7216878364870458196 ) ) ;
#17021=EDGE_LOOP ( 'NONE', ( #64383, #144286, #151370 ) ) ;
#17023=CARTESIAN_POINT ( 'NONE',  ( 4.192495815123822744, 5.914331089109666983, -1.599625672291255185 ) ) ;
#17025=CARTESIAN_POINT ( 'NONE',  ( 9.728138913005292210, 11.30824913904973705, -1.199719254218440723 ) ) ;
#17026=CARTESIAN_POINT ( 'NONE',  ( -1.201851678989727383E-14, 2.837500000000024336, -1.732050807568863648 ) ) ;
#17032=CARTESIAN_POINT ( 'NONE',  ( -9.378489572351046633, 11.96465713920816043, -1.599625672291263179 ) ) ;
#17033=AXIS2_PLACEMENT_3D ( 'NONE', #135425, #185207, #52036 ) ;
#17034=CARTESIAN_POINT ( 'NONE',  ( 7.741869408603235136, 8.990934717247309749, 1.199719254218462483 ) ) ;
#17036=CARTESIAN_POINT ( 'NONE',  ( 4.568734577680873876, 6.353276312092901890, -1.443375672974051449 ) ) ;
#17044=CARTESIAN_POINT ( 'NONE',  ( -7.212574532790102744, 8.477387045419011002, -1.082531754730550855 ) ) ;
#17045=CARTESIAN_POINT ( 'NONE',  ( 3.323720213644492993, 7.029424015893889433, 1.040834085586084257E-14 ) ) ;
#17048=CARTESIAN_POINT ( 'NONE',  ( -7.645908563102897126, 11.00764485934031889, 1.199719254218453823 ) ) ;
#17053=CARTESIAN_POINT ( 'NONE',  ( -4.647747731386360215, 4.316793862905830892, 0.7998128361456341429 ) ) ;
#17055=FACE_OUTER_BOUND ( 'NONE', #20642, .T. ) ;
#17057=CARTESIAN_POINT ( 'NONE',  ( 9.745613490124728884, 10.26430391476735338, 0.7998128361456462443 ) ) ;
#17059=FACE_OUTER_BOUND ( 'NONE', #62667, .T. ) ;
#17062=ORIENTED_EDGE ( 'NONE', *, *, #43825, .F. ) ;
#17066=CARTESIAN_POINT ( 'NONE',  ( 3.768803514918948938, 4.459654191235965293, -1.082531754730543083 ) ) ;
#17069=CARTESIAN_POINT ( 'NONE',  ( -4.765854690403601879, 5.518917546014321829, 1.199719254218462483 ) ) ;
#17072=CARTESIAN_POINT ( 'NONE',  ( -8.134002093194872884, 11.57708731111429401, 1.199719254218453823 ) ) ;
#17076=CARTESIAN_POINT ( 'NONE',  ( 7.076992996653421741, 10.23994701519558781, -1.082531754730537976 ) ) ;
#17077=CARTESIAN_POINT ( 'NONE',  ( 1.364683531249990311, 5.426041667008087543, 0.7879004041258499402 ) ) ;
#17080=CARTESIAN_POINT ( 'NONE',  ( 2.361091307074211887, 5.906356958228550447, 0.7998128361456462443 ) ) ;
#17081=CARTESIAN_POINT ( 'NONE',  ( 5.756345505848640798, 6.148709499980903992, 0.8262799378709930753 ) ) ;
#17083=CARTESIAN_POINT ( 'NONE',  ( -6.093499974338126179, 9.196501505781426999, -1.199719254218440723 ) ) ;
#17090=VERTEX_POINT ( 'NONE', #80449 ) ;
#17092=CARTESIAN_POINT ( 'NONE',  ( 1.364683531249988535, 4.176041667008081326, 0.7879004041258500513 ) ) ;
#17093=CARTESIAN_POINT ( 'NONE',  ( 7.892817981449907982, 12.36003807833360391, 0.7998128361456462443 ) ) ;
#17095=CARTESIAN_POINT ( 'NONE',  ( -4.989037340148921196, 5.883260320670900434, 1.082531754730560403 ) ) ;
#17097=CARTESIAN_POINT ( 'NONE',  ( -3.578989363883261277, 7.119311991265024453, 1.040834085586084257E-14 ) ) ;
#17104=CARTESIAN_POINT ( 'NONE',  ( 3.551346171775753735, 6.230655402791975384, 1.199719254218462483 ) ) ;
#17114=CARTESIAN_POINT ( 'NONE',  ( 5.789495288235341874, 6.713164910151406595, 1.199719254218462483 ) ) ;
#17119=CARTESIAN_POINT ( 'NONE',  ( -4.415151579544611238, 8.302760609444034046, -0.7998128361456281477 ) ) ;
#17124=CARTESIAN_POINT ( 'NONE',  ( 5.829115978871627135, 8.888053511070525659, 1.199719254218462483 ) ) ;
#17125=EDGE_CURVE ( 'NONE', #108467, #143793, #102559, .T. ) ;
#17128=CARTESIAN_POINT ( 'NONE',  ( -4.388035272317281077, 8.271124917678806199, 0.7998128361456481317 ) ) ;
#17129=CARTESIAN_POINT ( 'NONE',  ( -0.7500000000000006661, 1.608333333333357373, -1.299038105676652011 ) ) ;
#17130=CARTESIAN_POINT ( 'NONE',  ( -5.284980951228653190, 5.060232619388524533, 0.000000000000000000 ) ) ;
#17133=CARTESIAN_POINT ( 'NONE',  ( -5.949330478298285207, 5.835307067636438028, 0.7998128361456341429 ) ) ;
#17136=CARTESIAN_POINT ( 'NONE',  ( 0.6823417656249917140, 3.592708333674754506, 1.181850606188765695 ) ) ;
#17138=CARTESIAN_POINT ( 'NONE',  ( -4.853455804012230423, 6.685451076146141425, 1.443375672974064550 ) ) ;
#17144=CARTESIAN_POINT ( 'NONE',  ( 4.143988507271280319, 7.986403691791820414, -0.7998128361456221525 ) ) ;
#17147=CARTESIAN_POINT ( 'NONE',  ( -1.201851678989727383E-14, 2.634375000341417916, 1.575800808251672791 ) ) ;
#17149=CARTESIAN_POINT ( 'NONE',  ( 2.333974999846879061, 5.874721266463329705, -0.7998128361456291469 ) ) ;
#17151=CARTESIAN_POINT ( 'NONE',  ( -1.364683531250014514, -0.6572916663252459379, 0.7879004041258379498 ) ) ;
#17152=DIRECTION ( 'NONE',  ( 0.000000000000000000, 0.000000000000000000, 1.000000000000000000 ) ) ;
#17155=CARTESIAN_POINT ( 'NONE',  ( -2.839543107058306592, 5.400218493954923815, -1.199719254218446718 ) ) ;
#17157=CARTESIAN_POINT ( 'NONE',  ( -7.524412065460066579, 7.880828285899290186, 0.7216878364870317197 ) ) ;
#17161=CARTESIAN_POINT ( 'NONE',  ( -0.6823417656250212460, 3.301041667008085323, 1.181850606188767472 ) ) ;
#17169=CARTESIAN_POINT ( 'NONE',  ( -6.466876083594135238, 9.528143949959703818, 1.082531754730548412 ) ) ;
#17175=CARTESIAN_POINT ( 'NONE',  ( -6.005898860729463884, 9.950706404252290582, 0.7216878364870458196 ) ) ;
#17186=CARTESIAN_POINT ( 'NONE',  ( -5.368138756007025947, 8.350246751061767725, 1.199719254218452047 ) ) ;
#17188=CARTESIAN_POINT ( 'NONE',  ( -1.402160292154681736E-14, -0.6624999999999758860, -1.732050807568870754 ) ) ;
#17189=CARTESIAN_POINT ( 'NONE',  ( 10.56143847536557878, 11.42402576412244386, 0.000000000000000000 ) ) ;
#17192=CARTESIAN_POINT ( 'NONE',  ( 5.494078562035752178, 7.432844293840273231, -1.599625672291262513 ) ) ;
#17199=CARTESIAN_POINT ( 'NONE',  ( -2.494337075234348777, 5.853884321174607663, -0.7216878364870267237 ) ) ;
#17207=CARTESIAN_POINT ( 'NONE',  ( -1.364683531250012516, 2.238541667008087988, -0.7879004041258289570 ) ) ;
#17208=CARTESIAN_POINT ( 'NONE',  ( 9.747949258101261449, 11.43532422494874368, -1.082531754730537088 ) ) ;
#17209=CARTESIAN_POINT ( 'NONE',  ( -7.446452682403657874, 9.710614100936176385, -1.599625672291263179 ) ) ;
#17212=CARTESIAN_POINT ( 'NONE',  ( 6.877010230629674759, 9.046264573866535486, 1.599625672291281386 ) ) ;
#17213=CARTESIAN_POINT ( 'NONE',  ( -5.377780486114890124, 9.425827667109372143, 0.000000000000000000 ) ) ;
#17216=CARTESIAN_POINT ( 'NONE',  ( -0.7500000000000006661, -0.6104166659838470288, -1.299038105676652011 ) ) ;
#17219=CARTESIAN_POINT ( 'NONE',  ( 7.266807147244743526, 11.42176607185347414, -0.7216878364870267237 ) ) ;
#17222=CARTESIAN_POINT ( 'NONE',  ( -1.201851678989727383E-14, 0.8843750003414173610, 1.575800808251672791 ) ) ;
#17224=CARTESIAN_POINT ( 'NONE',  ( 5.951666246274784910, 9.887435020721849099, 0.7216878364870438212 ) ) ;
#17228=CARTESIAN_POINT ( 'NONE',  ( -4.121315508874262790, 6.791656612786516334, -1.082531754730549967 ) ) ;
#17230=CARTESIAN_POINT ( 'NONE',  ( -1.001543065824772872E-14, 4.321875000341417916, 1.575800808251672791 ) ) ;
#17234=CARTESIAN_POINT ( 'NONE',  ( -5.856132087369688044, 6.175168335346238990, -0.9273813317931516309 ) ) ;
#17241=CARTESIAN_POINT ( 'NONE',  ( 6.109920781252839994, 10.27999134477033216, 1.040834085586084257E-14 ) ) ;
#17244=CARTESIAN_POINT ( 'NONE',  ( 4.857899112398166075, 4.561970474086296079, 1.040834085586084257E-14 ) ) ;
#17249=VERTEX_POINT ( 'NONE', #212567 ) ;
#17250=CARTESIAN_POINT ( 'NONE',  ( 6.182154858151487353, 6.314861544039274577, -0.7216878364870257245 ) ) ;
#17252=CARTESIAN_POINT ( 'NONE',  ( 1.364683531249986537, 1.217708333674754950, -0.7879004041258239610 ) ) ;
#17255=CARTESIAN_POINT ( 'NONE',  ( 8.367353357928214663, 12.91366268422496688, 1.040834085586084257E-14 ) ) ;
#17256=LINE ( 'NONE', #164601, #107026 ) ;
#17260=CARTESIAN_POINT ( 'NONE',  ( -0.7500000000000006661, 0.1083333333333560966, -1.299038105676652011 ) ) ;
#17261=CARTESIAN_POINT ( 'NONE',  ( 7.786460292950004636, 7.978625184730144149, 1.040834085586084257E-14 ) ) ;
#17262=CARTESIAN_POINT ( 'NONE',  ( -8.148614017013223076, 9.465470093725620870, -1.199719254218446718 ) ) ;
#17266=CARTESIAN_POINT ( 'NONE',  ( -1.402160292154681736E-14, 1.196875000341419026, -1.575800808251659024 ) ) ;
#17267=CARTESIAN_POINT ( 'NONE',  ( -1.201851678989727383E-14, 2.462500000000023004, 1.732050807568877637 ) ) ;
#17269=CARTESIAN_POINT ( 'NONE',  ( 4.009460741339333723, 5.700790169694431420, -1.599625672291256295 ) ) ;
#17277=CARTESIAN_POINT ( 'NONE',  ( -1.500000000000001332, -0.06874999931718445145, 0.000000000000000000 ) ) ;
#17278=CARTESIAN_POINT ( 'NONE',  ( -6.886651960737580680, 10.12184548991413457, -1.199719254218440723 ) ) ;
#17279=CARTESIAN_POINT ( 'NONE',  ( -5.097502569058221411, 6.009803087731781623, -1.082531754730544860 ) ) ;
#17284=CARTESIAN_POINT ( 'NONE',  ( 4.074186250656476993, 7.493853916489129574, -0.5595503573846259959 ) ) ;
#17287=CARTESIAN_POINT ( 'NONE',  ( 5.601490020740366838, 9.686822124172440596, 1.040834085586084257E-14 ) ) ;
#17289=PLANE ( 'NONE',  #106917 ) ;
#17291=CARTESIAN_POINT ( 'NONE',  ( 7.416473721875251890, 8.611306416064660851, 1.199719254218462483 ) ) ;
#17292=CARTESIAN_POINT ( 'NONE',  ( 7.443063143778065438, 7.785921210603627962, -0.7216878364870257245 ) ) ;
#17296=CARTESIAN_POINT ( 'NONE',  ( -5.682838942422375084, 9.781729199468104596, 0.000000000000000000 ) ) ;
#17297=CARTESIAN_POINT ( 'NONE',  ( 4.005544317833563461, 6.760553239859419250, -1.199719254218452047 ) ) ;
#17302=CARTESIAN_POINT ( 'NONE',  ( 4.008122245411202655, 7.584344604122328803, -0.2404964666735086298 ) ) ;
#17303=CARTESIAN_POINT ( 'NONE',  ( 8.920901888111989919, 11.43080484092926241, 1.443375672974076540 ) ) ;
#17304=VERTEX_POINT ( 'NONE', #186466 ) ;
#17312=CARTESIAN_POINT ( 'NONE',  ( -3.877268743828284681, 5.546566172598190292, 1.443375672974064550 ) ) ;
#17313=CARTESIAN_POINT ( 'NONE',  ( 9.408995418203975447, 10.07950886410055524, 0.7216878364870438212 ) ) ;
#17316=CARTESIAN_POINT ( 'NONE',  ( -4.855791571988752331, 8.816840600628864877, 0.7998128361456481317 ) ) ;
#17321=CARTESIAN_POINT ( 'NONE',  ( -7.206322340863467346, 8.366129804884193888, 1.199719254218450271 ) ) ;
#17336=CARTESIAN_POINT ( 'NONE',  ( -5.422371370461663176, 8.413518134592214537, -1.199719254218446718 ) ) ;
#17339=CARTESIAN_POINT ( 'NONE',  ( 3.701012746850603996, 7.261672604726938651, 1.040834085586084257E-14 ) ) ;
#17342=CARTESIAN_POINT ( 'NONE',  ( 3.022498986271238586, 2.800000000000017586, -2.499999999999995115 ) ) ;
#17344=CARTESIAN_POINT ( 'NONE',  ( -4.731959306369413198, 5.479372931307791461, -1.199719254218446718 ) ) ;
#17351=CARTESIAN_POINT ( 'NONE',  ( -7.853197290813634268, 10.18514947741448573, 1.599625672291295375 ) ) ;
#17352=CARTESIAN_POINT ( 'NONE',  ( 5.289652487626049115, 9.323011668872403845, 0.7998128361456462443 ) ) ;
#17355=CARTESIAN_POINT ( 'NONE',  ( -8.320953590485107298, 10.73086516036454618, 1.599625672291269396 ) ) ;
#17356=CARTESIAN_POINT ( 'NONE',  ( 4.364835388595708743, 7.179726155748598515, 1.199719254218462483 ) ) ;
#17358=CARTESIAN_POINT ( 'NONE',  ( 2.064209525776505849, 8.524375063532966479, -2.459883114193431197 ) ) ;
#17359=CARTESIAN_POINT ( 'NONE',  ( -1.402160292154681736E-14, 0.2593750003414224681, -1.575800808251665908 ) ) ;
#17362=CARTESIAN_POINT ( 'NONE',  ( 8.812436659202669276, 10.34389285956704363, -1.082531754730543083 ) ) ;
#17378=EDGE_CURVE ( 'NONE', #82863, #33705, #209850, .T. ) ;
#17389=CARTESIAN_POINT ( 'NONE',  ( -1.402160292154681736E-14, 0.6187500006828180465, -1.732050807568863648 ) ) ;
#17395=CARTESIAN_POINT ( 'NONE',  ( 8.378048858240820351, 11.86180853700128601, -1.199719254218446718 ) ) ;
#17400=CARTESIAN_POINT ( 'NONE',  ( 4.660252114795294887, 6.460046772059735432, -1.599625672291256295 ) ) ;
#17401=CARTESIAN_POINT ( 'NONE',  ( -8.202319746587722449, 8.671720580548228696, 1.040834085586084257E-14 ) ) ;
#17402=CARTESIAN_POINT ( 'NONE',  ( -5.908080316777766683, 6.002527095666024159, -0.1116623552285273685 ) ) ;
#17403=CARTESIAN_POINT ( 'NONE',  ( 10.16199982864259788, 11.81442020729326536, 1.199719254218452047 ) ) ;
#17405=CARTESIAN_POINT ( 'NONE',  ( -7.802881099864745984, 9.062115023719057305, -1.199719254218446718 ) ) ;
#17407=CARTESIAN_POINT ( 'NONE',  ( -3.999292125906916073, 5.688926785023260102, 1.443375672974064550 ) ) ;
#17410=CARTESIAN_POINT ( 'NONE',  ( -1.402160292154681736E-14, 0.2437500006828163535, 1.732050807568877637 ) ) ;
#17417=CARTESIAN_POINT ( 'NONE',  ( -3.917943204224914933, 6.554388924028945240, -1.082531754730548412 ) ) ;
#17421=CARTESIAN_POINT ( 'NONE',  ( 4.038955833855768063, 7.541343398062151593, 0.4257906834902285276 ) ) ;
#17426=CARTESIAN_POINT ( 'NONE',  ( -4.744990574658554117, 4.638169879964154418, 1.214306433183764966E-14 ) ) ;
#17427=CARTESIAN_POINT ( 'NONE',  ( 7.584896871841365851, 10.93646455286856956, -1.199719254218446718 ) ) ;
#17436=CARTESIAN_POINT ( 'NONE',  ( -7.808606406466886973, 11.19745900993164511, 1.199719254218453823 ) ) ;
#17441=CARTESIAN_POINT ( 'NONE',  ( 6.017121246366603060, 5.914396297049491658, 1.040834085586084257E-14 ) ) ;
#17442=AXIS2_PLACEMENT_3D ( 'NONE', #29341, #96499, #10929 ) ;
#17446=ORIENTED_EDGE ( 'NONE', *, *, #140681, .F. ) ;
#17447=CARTESIAN_POINT ( 'NONE',  ( 2.892933200463445154, 6.441114558253461908, 0.3893011784570130640 ) ) ;
#17450=CARTESIAN_POINT ( 'NONE',  ( 1.499999999999990896, 5.275000000000022560, 1.214306433183764966E-14 ) ) ;
#17459=CARTESIAN_POINT ( 'NONE',  ( 8.067265095331215718, 9.370563018429956870, 1.199719254218462483 ) ) ;
#17461=CARTESIAN_POINT ( 'NONE',  ( -3.411848212133334446, 7.132240014130862171, 0.7998128361456341429 ) ) ;
#17462=EDGE_LOOP ( 'NONE', ( #99648, #51992, #11358, #213136 ) ) ;
#17468=CARTESIAN_POINT ( 'NONE',  ( 1.499999999999987566, -0.6937499993171849511, 0.000000000000000000 ) ) ;
#17471=CARTESIAN_POINT ( 'NONE',  ( -5.586852281741751192, 6.234037913494448802, 1.005928974618113481 ) ) ;
#17472=CARTESIAN_POINT ( 'NONE',  ( 3.344057444064992168, 7.053150784717805877, 1.040834085586084257E-14 ) ) ;
#17474=CARTESIAN_POINT ( 'NONE',  ( -4.029797971759847997, 5.724516938518342535, -1.599625672291256295 ) ) ;
#17480=CARTESIAN_POINT ( 'NONE',  ( 6.155038550924150087, 7.243595066575396757, 1.082531754730558626 ) ) ;
#17483=CARTESIAN_POINT ( 'NONE',  ( -1.364683531250012516, 4.551041667008082214, -0.7879004041258300672 ) ) ;
#17485=CARTESIAN_POINT ( 'NONE',  ( 5.138177029454852551, 5.096887410559856946, 0.7216878364870317197 ) ) ;
#17493=CARTESIAN_POINT ( 'NONE',  ( -5.747036748294815922, 6.247280920146251582, 1.064921034751656226 ) ) ;
#17496=CARTESIAN_POINT ( 'NONE',  ( -1.364683531249997417, 5.071875000341417916, 1.214306433183764966E-14 ) ) ;
#17511=CARTESIAN_POINT ( 'NONE',  ( 1.364683531249990311, 4.926041667008083991, 0.7879004041258500513 ) ) ;
#17513=CARTESIAN_POINT ( 'NONE',  ( 4.937140493670735708, 8.911747675924535983, -0.7998128361456281477 ) ) ;
#17514=CARTESIAN_POINT ( 'NONE',  ( -9.612894607289142357, 11.17379744904754801, -1.199719254218441611 ) ) ;
#17518=VERTEX_POINT ( 'NONE', #171291 ) ;
#17520=CARTESIAN_POINT ( 'NONE',  ( -1.364683531250000748, -0.9281249996585805295, 0.000000000000000000 ) ) ;
#17527=CARTESIAN_POINT ( 'NONE',  ( 8.920901888111997025, 10.47043562662792304, 1.082531754730549967 ) ) ;
#17531=CARTESIAN_POINT ( 'NONE',  ( 0.7499999999999902300, 3.514583334016149863, 1.299038105676669330 ) ) ;
#17533=CARTESIAN_POINT ( 'NONE',  ( -4.741601036477307574, 6.554953847355395880, 1.599625672291267398 ) ) ;
#17534=CARTESIAN_POINT ( 'NONE',  ( 3.158686601859607368, 6.628958768904106513, -0.7216878364870267237 ) ) ;
#17542=CARTESIAN_POINT ( 'NONE',  ( 5.196852952739813070, 4.957416621151553571, -0.7998128361456221525 ) ) ;
#17546=CARTESIAN_POINT ( 'NONE',  ( -1.123270288250339366, 3.283552654332833054, 0.7749999999993804067 ) ) ;
#17547=CARTESIAN_POINT ( 'NONE',  ( 3.669453130792974971, 7.432779085900453886, 1.040834085586084257E-14 ) ) ;
#17557=FACE_OUTER_BOUND ( 'NONE', #140145, .T. ) ;
#17558=B_SPLINE_CURVE_WITH_KNOTS ( 'NONE', 3,
 ( #11514, #94932, #128566, #61344, #212905 ),
 .UNSPECIFIED., .F., .F.,
 ( 4, 1, 4 ),
 ( 0.000000000000000000, 3.079525422856393096E-06, 6.159050845712786192E-06 ),
 .UNSPECIFIED. ) ;
#17559=CARTESIAN_POINT ( 'NONE',  ( 5.298667053604809496, 6.361919491657284986, -1.123377533431538566 ) ) ;
#17561=CARTESIAN_POINT ( 'NONE',  ( 8.594979316059474073, 12.11489407112305372, 1.199719254218450271 ) ) ;
#17568=CARTESIAN_POINT ( 'NONE',  ( 5.829642864196157070, 8.784705193995428374, 1.082531754730558626 ) ) ;
#17569=CARTESIAN_POINT ( 'NONE',  ( -10.00555417720528872, 10.77549408293541866, 0.7216878364870438212 ) ) ;
#17575=CARTESIAN_POINT ( 'NONE',  ( -3.602716132929368875, 5.226254793216122074, 1.599625672291267398 ) ) ;
#17577=CARTESIAN_POINT ( 'NONE',  ( -4.183485216215332869, 3.563207579971354289, 2.499999999999998668 ) ) ;
#17587=CARTESIAN_POINT ( 'NONE',  ( 5.756168354352870331, 6.246635012430203027, 1.018728318139457523 ) ) ;
#17591=CARTESIAN_POINT ( 'NONE',  ( 3.310162060030825248, 7.013606170011280838, -0.7998128361456291469 ) ) ;
#17596=CARTESIAN_POINT ( 'NONE',  ( -8.026063749610047537, 11.34719622697832264, -1.082531754730543971 ) ) ;
#17601=CARTESIAN_POINT ( 'NONE',  ( 8.437251666405968464, 8.737881787095446384, 1.040834085586084257E-14 ) ) ;
#17602=CARTESIAN_POINT ( 'NONE',  ( -4.436542580169821726, 6.199052314996659874, 1.599625672291267175 ) ) ;
#17604=CARTESIAN_POINT ( 'NONE',  ( 4.355193658487811703, 6.104145239700998538, -1.599625672291255185 ) ) ;
#17606=CARTESIAN_POINT ( 'NONE',  ( -6.423865854776591000, 6.388931673527803667, 1.040834085586084257E-14 ) ) ;
#17608=CARTESIAN_POINT ( 'NONE',  ( -4.042302355168801320, 7.867769847672247074, 0.7998128361456341429 ) ) ;
#17611=CARTESIAN_POINT ( 'NONE',  ( 8.052653171512838881, 11.48218023581863001, -1.199719254218446718 ) ) ;
#17615=CARTESIAN_POINT ( 'NONE',  ( 4.513260471453858003, 7.001907027245110271, -1.160773635454902530 ) ) ;
#17616=CARTESIAN_POINT ( 'NONE',  ( 5.450014563013511726, 8.341805509282339770, -1.082531754730543083 ) ) ;
#17620=DIRECTION ( 'NONE',  ( 1.000000000000000000, 0.000000000000000000, 0.000000000000000000 ) ) ;
#17621=CARTESIAN_POINT ( 'NONE',  ( -1.387358672536802340, 7.315968950354509559, 4.254625267136455058 ) ) ;
#17624=CARTESIAN_POINT ( 'NONE',  ( 6.100805936025112786, 10.06143132543056673, 1.040834085586084257E-14 ) ) ;
#17628=CARTESIAN_POINT ( 'NONE',  ( -8.311311860377216476, 9.655284244316948872, -1.199719254218446718 ) ) ;
#17632=CARTESIAN_POINT ( 'NONE',  ( 4.008199524592567897, 7.584238231759597326, 0.2402771892247856922 ) ) ;
#17637=CARTESIAN_POINT ( 'NONE',  ( 3.029357257649615054, 5.621668336311468117, -1.199719254218446718 ) ) ;
#17640=CARTESIAN_POINT ( 'NONE',  ( -6.775324078527193983, 8.927630729746953264, -1.599625672291263179 ) ) ;
#17642=CARTESIAN_POINT ( 'NONE',  ( 5.332434488876471868, 5.115595079977664383, 0.7998128361456341429 ) ) ;
#17646=CARTESIAN_POINT ( 'NONE',  ( 1.499999999999989120, 4.785416667349486453, 0.8660254037844524744 ) ) ;
#17653=CARTESIAN_POINT ( 'NONE',  ( -1.500000000000013101, 2.170833333333357373, 0.8660254037844403729 ) ) ;
#17654=CARTESIAN_POINT ( 'NONE',  ( 6.856673000209174695, 9.022537805042615489, 1.599625672291281386 ) ) ;
#17655=CARTESIAN_POINT ( 'NONE',  ( 3.484082288587588838, 7.008587070086755411, -0.7216878364870267237 ) ) ;
#17659=CARTESIAN_POINT ( 'NONE',  ( 7.429504990608736037, 11.61158022244479682, -0.7216878364870267237 ) ) ;
#17664=CARTESIAN_POINT ( 'NONE',  ( -5.742041750587549842, 6.657802449562273850, 1.199719254218450271 ) ) ;
#17665=CARTESIAN_POINT ( 'NONE',  ( 0.7499999999999902300, 4.597916667349482012, -1.299038105676658228 ) ) ;
#17666=CARTESIAN_POINT ( 'NONE',  ( -1.364683531250014514, 0.03020833367475737191, 0.7879004041258379498 ) ) ;
#17670=CARTESIAN_POINT ( 'NONE',  ( 5.009901455449552010, 5.803638771901306725, -1.199719254218452047 ) ) ;
#17672=CARTESIAN_POINT ( 'NONE',  ( 1.364683531249990311, 5.676041667008088432, 0.7879004041258500513 ) ) ;
#17679=CARTESIAN_POINT ( 'NONE',  ( -6.364663046611467756, 9.512858423433634414, 1.199719254218452047 ) ) ;
#17680=CARTESIAN_POINT ( 'NONE',  ( 3.655894977179307226, 7.416961240017848844, -0.7998128361456291469 ) ) ;
#17683=CARTESIAN_POINT ( 'NONE',  ( 0.6823417656249882723, -0.4072916663252490466, 1.181850606188755259 ) ) ;
#17685=ORIENTED_EDGE ( 'NONE', *, *, #82075, .F. ) ;
#17687=CARTESIAN_POINT ( 'NONE',  ( 2.272459710430874580, 5.681424495331688362, -0.3682267578792697282 ) ) ;
#17689=CARTESIAN_POINT ( 'NONE',  ( -6.663996196316808174, 7.733415969579778171, -1.199719254218446718 ) ) ;
#17692=CARTESIAN_POINT ( 'NONE',  ( 10.05353459973327368, 11.68787744023238417, -1.199719254218440723 ) ) ;
#17694=CARTESIAN_POINT ( 'NONE',  ( 9.053093885623066939, 11.58502883802551153, -1.599625672291262513 ) ) ;
#17696=CARTESIAN_POINT ( 'NONE',  ( -2.266184231778562541, 5.795632037050281404, 1.040834085586084257E-14 ) ) ;
#17697=CARTESIAN_POINT ( 'NONE',  ( -7.212047647465563038, 10.50147379109678880, -1.199719254218446718 ) ) ;
#17700=CARTESIAN_POINT ( 'NONE',  ( -4.670247306389155639, 7.079074041166477649, 1.395957953274113983 ) ) ;
#17701=CARTESIAN_POINT ( 'NONE',  ( -1.402160292154681736E-14, -0.9281249996585830830, 1.575800808251672791 ) ) ;
#17705=CARTESIAN_POINT ( 'NONE',  ( 8.026063749610047537, 10.38682701267698150, -1.443375672974057666 ) ) ;
#17709=CARTESIAN_POINT ( 'NONE',  ( 0.003079562121058774214, 7.078201604703558303, -2.121336893758704711 ) ) ;
#17711=VECTOR ( 'NONE', #30583, 1000.000000000000000 ) ;
#17724=CARTESIAN_POINT ( 'NONE',  ( 10.08456733046637765, 10.65975006183261087, 0.000000000000000000 ) ) ;
#17728=CARTESIAN_POINT ( 'NONE',  ( -5.708146366553361162, 6.618257834855742594, -1.199719254218446718 ) ) ;
#17733=CARTESIAN_POINT ( 'NONE',  ( -0.7499999999999972244, 3.639583334016149863, -1.299038105676652011 ) ) ;
#17734=CARTESIAN_POINT ( 'NONE',  ( 8.530051201292206287, 13.10347683481629488, 0.000000000000000000 ) ) ;
#17739=CARTESIAN_POINT ( 'NONE',  ( -7.167456763118792651, 11.51378332361394818, 0.000000000000000000 ) ) ;
#17741=CARTESIAN_POINT ( 'NONE',  ( 1.364683531249986537, 2.405208333674752286, -0.7879004041258239610 ) ) ;
#17744=VERTEX_POINT ( 'NONE', #137748 ) ;
#17748=CARTESIAN_POINT ( 'NONE',  ( -2.656508033273816238, 5.186677574539687363, -1.199719254218446718 ) ) ;
#17753=CARTESIAN_POINT ( 'NONE',  ( -1.201851678989727383E-14, 0.8843750003414173610, 1.575800808251672791 ) ) ;
#17760=CARTESIAN_POINT ( 'NONE',  ( 1.364683531249986537, 1.905208333674750287, -0.7879004041258239610 ) ) ;
#17762=CARTESIAN_POINT ( 'NONE',  ( -5.052384799386910430, 9.046199365926717917, 1.214306433183764966E-14 ) ) ;
#17763=CARTESIAN_POINT ( 'NONE',  ( 9.088043039861931405, 9.497138389460751284, 1.040834085586084257E-14 ) ) ;
#17764=CARTESIAN_POINT ( 'NONE',  ( 5.203632029546647608, 4.965325544092860532, 1.040834085586084257E-14 ) ) ;
#17766=CARTESIAN_POINT ( 'NONE',  ( -1.201851678989727383E-14, 3.587500000000020339, -1.732050807568863648 ) ) ;
#17768=CARTESIAN_POINT ( 'NONE',  ( -1.364683531250000748, 2.321875000341422357, 1.214306433183764966E-14 ) ) ;
#17775=CARTESIAN_POINT ( 'NONE',  ( 4.528060117284222308, 8.226561203566173930, 0.7216878364870438212 ) ) ;
#17778=CARTESIAN_POINT ( 'NONE',  ( -7.181014916732457287, 11.52960116949655678, -0.7998128361456291469 ) ) ;
#17779=CARTESIAN_POINT ( 'NONE',  ( -2.252626078164912560, 5.779814191167667481, 0.7998128361456341429 ) ) ;
#17781=CARTESIAN_POINT ( 'NONE',  ( -1.364683531250010295, 3.780208333674750953, 0.7879004041258379498 ) ) ;
#17786=CARTESIAN_POINT ( 'NONE',  ( -8.310784975052689205, 8.798263347090697906, -0.7216878364870267237 ) ) ;
#17788=CARTESIAN_POINT ( 'NONE',  ( -0.7500000000000215383, 5.691666666666685082, 1.299038105676671107 ) ) ;
#17791=CARTESIAN_POINT ( 'NONE',  ( 8.026063749610047537, 10.38682701267698150, -1.443375672974057666 ) ) ;
#17798=B_SPLINE_CURVE_WITH_KNOTS ( 'NONE', 3,
 ( #202185, #87413, #102590, #20252 ),
 .UNSPECIFIED., .F., .F.,
 ( 4, 4 ),
 ( 8.516827915682558025E-05, 0.0002597075693988114926 ),
 .UNSPECIFIED. ) ;
#17801=CIRCLE ( 'NONE', #104275, 6.961139734775127152 ) ;
#17802=CARTESIAN_POINT ( 'NONE',  ( 8.392133896734652154, 12.73464727959172293, 0.7216878364870438212 ) ) ;
#17809=CARTESIAN_POINT ( 'NONE',  ( 6.775324078527185989, 8.927630729746953264, -1.599625672291262513 ) ) ;
#17810=CARTESIAN_POINT ( 'NONE',  ( -5.311043488251275591, 7.219303374425030562, -1.599625672291256295 ) ) ;
#17812=DIRECTION ( 'NONE',  ( 0.6507913734559640506, -0.7592566023653004592, 0.000000000000000000 ) ) ;
#17813=CARTESIAN_POINT ( 'NONE',  ( 5.246642258364164313, 8.104537820524768676, -1.082531754730549078 ) ) ;
#17814=EDGE_CURVE ( 'NONE', #67975, #189420, #118890, .T. ) ;
#17816=CARTESIAN_POINT ( 'NONE',  ( 1.364683531249986537, 0.6760416670080884316, 0.7879004041258500513 ) ) ;
#17817=CARTESIAN_POINT ( 'NONE',  ( 3.307826292054301121, 4.882216645528547616, -1.443375672974057666 ) ) ;
#17818=CARTESIAN_POINT ( 'NONE',  ( -8.136864746495904299, 12.64475930422059768, -0.7998128361456281477 ) ) ;
#17827=ORIENTED_EDGE ( 'NONE', *, *, #2718, .F. ) ;
#17835=CARTESIAN_POINT ( 'NONE',  ( 5.621827251160867789, 9.710548892996357040, 1.040834085586084257E-14 ) ) ;
#17836=CARTESIAN_POINT ( 'NONE',  ( 7.644099680006512187, 7.812537802962739697, 1.040834085586084257E-14 ) ) ;
#17847=CARTESIAN_POINT ( 'NONE',  ( -5.762378981008047241, 6.681529218386182301, 1.199719254218450271 ) ) ;
#17849=CARTESIAN_POINT ( 'NONE',  ( -2.578021764892882040, 6.159442492350315490, 0.7998128361456341429 ) ) ;
#17860=CARTESIAN_POINT ( 'NONE',  ( -9.490344339885973923, 12.09515436799890331, -1.443375672974059665 ) ) ;
#17863=CARTESIAN_POINT ( 'NONE',  ( 5.449487677688982679, 8.445153826357429949, -1.199719254218446718 ) ) ;
#17864=CARTESIAN_POINT ( 'NONE',  ( -1.364683531249997417, 5.009375000341425022, 1.214306433183764966E-14 ) ) ;
#17870=CARTESIAN_POINT ( 'NONE',  ( 3.972175818679561043, 7.578029521860726092, -0.7216878364870197293 ) ) ;
#17871=CARTESIAN_POINT ( 'NONE',  ( -5.994676475536691029, 10.14553965476814845, 0.7998128361456481317 ) ) ;
#17872=VERTEX_POINT ( 'NONE', #167721 ) ;
#17873=ORIENTED_EDGE ( 'NONE', *, *, #6374, .F. ) ;
#17876=CARTESIAN_POINT ( 'NONE',  ( -6.509886312855995172, 10.74661779830734254, -0.7998128361456291469 ) ) ;
#17878=CARTESIAN_POINT ( 'NONE',  ( -5.117312914154178216, 8.057616602233474978, -1.199719254218452047 ) ) ;
#17885=CARTESIAN_POINT ( 'NONE',  ( 6.089583550832340819, 10.25626457594641749, 1.040834085586084257E-14 ) ) ;
#17898=CARTESIAN_POINT ( 'NONE',  ( 0.7499999999999902300, 5.566666666666685082, -1.299038105676658228 ) ) ;
#17899=CARTESIAN_POINT ( 'NONE',  ( 3.225950485047770933, 5.851027101609320269, 1.199719254218450271 ) ) ;
#17900=CARTESIAN_POINT ( 'NONE',  ( 5.192936529234042808, 6.017179691316550283, -1.199719254218452047 ) ) ;
#17903=CARTESIAN_POINT ( 'NONE',  ( -8.378575743565381373, 8.877352577022161739, 0.7216878364870438212 ) ) ;
#17905=CARTESIAN_POINT ( 'NONE',  ( 5.666945020832177882, 6.674152614801420746, 1.082531754730558626 ) ) ;
#17906=CARTESIAN_POINT ( 'NONE',  ( -8.975134502122321223, 9.573337795338607847, 1.040834085586084257E-14 ) ) ;
#17910=CARTESIAN_POINT ( 'NONE',  ( 6.612626235163189925, 8.737816579155630592, -1.599625672291262513 ) ) ;
#17915=CARTESIAN_POINT ( 'NONE',  ( -1.364683531249997417, 3.759375000341423689, 1.214306433183764966E-14 ) ) ;
#17922=CARTESIAN_POINT ( 'NONE',  ( 7.313733799568044702, 10.62010763521636214, 1.199719254218460707 ) ) ;
#17926=CARTESIAN_POINT ( 'NONE',  ( -8.178592977541617515, 10.56477777859713463, 1.599625672291295375 ) ) ;
#17931=CARTESIAN_POINT ( 'NONE',  ( 10.06423010004587759, 10.63602329300870153, 0.000000000000000000 ) ) ;
#17934=CARTESIAN_POINT ( 'NONE',  ( -9.501566725078754772, 9.979582688880366703, -0.7998128361456291469 ) ) ;
#17939=CARTESIAN_POINT ( 'NONE',  ( 5.786614514570532997, 6.041473168147688533, -0.5398422057949890940 ) ) ;
#17940=CARTESIAN_POINT ( 'NONE',  ( -2.103486388414573138, 5.605817886458954291, 1.040834085586084257E-14 ) ) ;
#17945=CARTESIAN_POINT ( 'NONE',  ( 7.070740804726770357, 8.207951346058097286, 1.199719254218462483 ) ) ;
#17947=CARTESIAN_POINT ( 'NONE',  ( 6.043183783389218355, 8.073467052085995022, 1.599625672291267398 ) ) ;
#17948=CARTESIAN_POINT ( 'NONE',  ( -4.167783244592077274, 7.418453011031667543, -0.7534271236282058526 ) ) ;
#17949=CARTESIAN_POINT ( 'NONE',  ( 3.147464216666835402, 6.823792019419957278, -0.7998128361456291469 ) ) ;
#17951=CARTESIAN_POINT ( 'NONE',  ( -8.514157279702036618, 9.035531035848267223, -0.7216878364870278340 ) ) ;
#17952=AXIS2_PLACEMENT_3D ( 'NONE', #170064, #50998, #153834 ) ;
#17960=CARTESIAN_POINT ( 'NONE',  ( -4.072711641797504001, 7.543564457389225986, 0.4874124537386469447 ) ) ;
#17961=CARTESIAN_POINT ( 'NONE',  ( 0.6823417656249864960, -1.011458332991911568, -1.181850606188749264 ) ) ;
#17964=CARTESIAN_POINT ( 'NONE',  ( 5.843201017809841247, 5.919415396974013532, 1.040834085586084257E-14 ) ) ;
#17974=CARTESIAN_POINT ( 'NONE',  ( -9.531018800282611281, 12.14260790512831889, 1.443375672974076540 ) ) ;
#17981=CARTESIAN_POINT ( 'NONE',  ( -9.449669878600623463, 11.08733161553131197, -1.082531754730537976 ) ) ;
#17988=CARTESIAN_POINT ( 'NONE',  ( 1.499999999999987121, 3.327083334016150751, -0.8660254037844262731 ) ) ;
#17990=CARTESIAN_POINT ( 'NONE',  ( -5.799137018343247796, 7.788745826199009237, -1.599625672291256295 ) ) ;
#17992=ORIENTED_EDGE ( 'NONE', *, *, #38172, .F. ) ;
#17994=CARTESIAN_POINT ( 'NONE',  ( -7.648771216403934758, 12.07531685244661723, -0.7998128361456291469 ) ) ;
#17998=CARTESIAN_POINT ( 'NONE',  ( 6.471319392424407901, 6.444294134116939077, 0.7998128361456341429 ) ) ;
#18004=CARTESIAN_POINT ( 'NONE',  ( 7.910292558569346433, 11.31609285405122556, -1.199719254218446718 ) ) ;
#18006=CARTESIAN_POINT ( 'NONE',  ( 3.673896439623290266, 4.156855427197417185, 1.000000000000011324 ) ) ;
#18011=CARTESIAN_POINT ( 'NONE',  ( -7.456621297836087514, 9.722477485607340597, 1.443375672974090751 ) ) ;
#18014=CARTESIAN_POINT ( 'NONE',  ( -0.6823417656250212460, 5.113541667008086655, 1.181850606188767472 ) ) ;
#18022=CARTESIAN_POINT ( 'NONE',  ( -10.10098813738111545, 11.74323990082152491, -1.199719254218441611 ) ) ;
#18024=CARTESIAN_POINT ( 'NONE',  ( 10.26082332744404368, 10.86538205830655279, -0.7998128361456281477 ) ) ;
#18026=CARTESIAN_POINT ( 'NONE',  ( -8.455481356417053007, 13.01647868246193518, 0.7998128361456341429 ) ) ;
#18030=CARTESIAN_POINT ( 'NONE',  ( -1.364683531250014514, 1.988541667008086655, -0.7879004041258289570 ) ) ;
#18032=CARTESIAN_POINT ( 'NONE',  ( 3.337278367258157630, 7.045241861776501580, 0.7998128361456341429 ) ) ;
#18039=CARTESIAN_POINT ( 'NONE',  ( 2.901081683644319842, 5.368050483351580304, 1.082531754730548412 ) ) ;
#18040=CARTESIAN_POINT ( 'NONE',  ( 8.541273586484978253, 12.90864358430044589, 0.000000000000000000 ) ) ;
#18042=CARTESIAN_POINT ( 'NONE',  ( -7.131225611108100715, 9.342849184424693476, 1.443375672974078761 ) ) ;
#18044=FACE_OUTER_BOUND ( 'NONE', #77963, .T. ) ;
#18047=CARTESIAN_POINT ( 'NONE',  ( -8.833300774503376473, 10.26427131079744193, 1.199719254218462483 ) ) ;
#18048=CARTESIAN_POINT ( 'NONE',  ( -5.273758565591545988, 6.215435083687305351, 1.082531754730546636 ) ) ;
#18049=CARTESIAN_POINT ( 'NONE',  ( 0.6823417656249882723, 2.238541667008084435, -1.181850606188749264 ) ) ;
#18054=ADVANCED_FACE ( 'NONE', ( #162152 ), #60635, .F. ) ;
#18060=EDGE_LOOP ( 'NONE', ( #148558, #78337, #41757, #56181 ) ) ;
#18068=EDGE_CURVE ( 'NONE', #85365, #116525, #109609, .T. ) ;
#18069=CARTESIAN_POINT ( 'NONE',  ( -0.6823417656249969321, 4.780208333674755394, -1.181850606188749264 ) ) ;
#18073=ADVANCED_FACE ( 'NONE', ( #146392 ), #16111, .T. ) ;
#18077=CARTESIAN_POINT ( 'NONE',  ( 9.043452155515161905, 10.50944792197790889, 1.199719254218453823 ) ) ;
#18079=CARTESIAN_POINT ( 'NONE',  ( -1.364683531249997417, 2.509375000341422357, 1.214306433183764966E-14 ) ) ;
#18081=CARTESIAN_POINT ( 'NONE',  ( -7.551528373131759508, 7.912463978182924684, 1.040834085586084257E-14 ) ) ;
#18089=CARTESIAN_POINT ( 'NONE',  ( 3.357615597678655917, 7.068968630600412695, 0.7998128361456321445 ) ) ;
#18093=CARTESIAN_POINT ( 'NONE',  ( 8.809047120577066181, 11.30030761213851953, 1.599625672291281386 ) ) ;
#18100=CARTESIAN_POINT ( 'NONE',  ( -3.436101866059630527, 6.096203712789787232, 1.199719254218462483 ) ) ;
#18102=CARTESIAN_POINT ( 'NONE',  ( 8.444030743212801227, 8.745790710036752458, 0.7998128361456462443 ) ) ;
#18105=CARTESIAN_POINT ( 'NONE',  ( 3.782361668088245921, 6.396210465202840645, -1.082531754730548412 ) ) ;
#18114=CARTESIAN_POINT ( 'NONE',  ( -7.537970219518089543, 8.857015346601659900, -1.082531754730543971 ) ) ;
#18115=CARTESIAN_POINT ( 'NONE',  ( 5.671388329218120639, 5.511041227042920099, 1.040834085586084257E-14 ) ) ;
#18118=CARTESIAN_POINT ( 'NONE',  ( -9.643927338022246332, 10.14567007064778004, -0.7998128361456291469 ) ) ;
#18123=CARTESIAN_POINT ( 'NONE',  ( -4.460796234096120472, 5.163016013655583158, 1.199719254218462483 ) ) ;
#18125=CARTESIAN_POINT ( 'NONE',  ( 8.289920859751990889, 11.75899253876431416, 1.199719254218450271 ) ) ;
#18126=CARTESIAN_POINT ( 'NONE',  ( 3.032219910950674890, 6.689340329417765574, 0.7998128361456321445 ) ) ;
#18132=CARTESIAN_POINT ( 'NONE',  ( 2.846849069189655967, 5.304779099821139710, -1.082531754730543083 ) ) ;
#18135=CARTESIAN_POINT ( 'NONE',  ( -4.120788623549732854, 6.895004929861607401, -1.199719254218452047 ) ) ;
#18138=CARTESIAN_POINT ( 'NONE',  ( -7.160677686311960777, 11.50587440067263678, -0.7998128361456291469 ) ) ;
#18144=CARTESIAN_POINT ( 'NONE',  ( 6.914295153289432783, 10.05013286460426691, -1.082531754730537976 ) ) ;
#18148=CARTESIAN_POINT ( 'NONE',  ( 3.358669367883368118, 4.941533567329135401, -1.599625672291262513 ) ) ;
#18150=CARTESIAN_POINT ( 'NONE',  ( 3.655894977179307226, 7.416961240017848844, -0.7998128361456291469 ) ) ;
#18152=CARTESIAN_POINT ( 'NONE',  ( -7.711890448074853133, 7.891627032375787998, -0.7998128361456291469 ) ) ;
#18162=CARTESIAN_POINT ( 'NONE',  ( -1.364683531250012516, 2.092708333674750953, 0.7879004041258379498 ) ) ;
#18163=CARTESIAN_POINT ( 'NONE',  ( 9.399880572976245574, 9.860948844760784482, 0.7998128361456462443 ) ) ;
#18165=CARTESIAN_POINT ( 'NONE',  ( -3.456965981804629884, 6.976951378839947537, 1.040834085586084257E-14 ) ) ;
#18166=DIRECTION ( 'NONE',  ( 0.6507913734559640506, -0.7592566023653004592, 0.000000000000000000 ) ) ;
#18168=CARTESIAN_POINT ( 'NONE',  ( -5.056828107772852299, 7.883087978168217269, -1.082531754730548412 ) ) ;
#18176=CARTESIAN_POINT ( 'NONE',  ( 3.011882680530176604, 6.665613560593854459, 0.7998128361456341429 ) ) ;
#18186=CARTESIAN_POINT ( 'NONE',  ( 3.493197133815315603, 7.227147089426516402, -0.7998128361456291469 ) ) ;
#18191=CARTESIAN_POINT ( 'NONE',  ( -6.749261541504576911, 6.768559974710451677, 1.040834085586084257E-14 ) ) ;
#18195=CARTESIAN_POINT ( 'NONE',  ( 4.950698647284403009, 8.927565521807144577, 1.040834085586084257E-14 ) ) ;
#18198=CARTESIAN_POINT ( 'NONE',  ( -5.738125327081750271, 7.717565519727259904, 1.599625672291269396 ) ) ;
#18199=CARTESIAN_POINT ( 'NONE',  ( 1.499999999999989120, 1.525000000000019451, 0.000000000000000000 ) ) ;
#18202=CARTESIAN_POINT ( 'NONE',  ( -4.243865776277440993, 4.909930479533815451, -1.199719254218446718 ) ) ;
#18205=CARTESIAN_POINT ( 'NONE',  ( -5.494078562035765501, 7.432844293840273231, -1.599625672291256295 ) ) ;
#18207=( BOUNDED_SURFACE ( )  B_SPLINE_SURFACE ( 3, 2, ( 
 ( #210225, #48819, #195059 ),
 ( #145290, #161512, #78104 ),
 ( #113889, #192909, #213415 ),
 ( #144231, #44565, #131194 ) ),
 .UNSPECIFIED., .F., .F., .F. ) 
 B_SPLINE_SURFACE_WITH_KNOTS ( ( 4, 4 ),
 ( 3, 3 ),
 ( 3.059570999471135089, 3.223614307708988491 ),
 ( 0.000000000000000000, 1.000000000000000000 ),
 .UNSPECIFIED. ) 
 GEOMETRIC_REPRESENTATION_ITEM ( )  RATIONAL_B_SPLINE_SURFACE ( (
 ( 1.000000000000000000, 0.6179932349766422695, 1.000000000000000000),
 ( 1.000000000000000000, 0.6282795510881240553, 1.000000000000000000),
 ( 1.000000000000000000, 0.6282795510880839762, 1.000000000000000000),
 ( 1.000000000000000000, 0.6179932349765423494, 1.000000000000000000) ) ) 
 REPRESENTATION_ITEM ( '' )  SURFACE ( )  );
#18208=CARTESIAN_POINT ( 'NONE',  ( 1.364683531249988535, 3.113541667008083991, 0.7879004041258500513 ) ) ;
#18210=CARTESIAN_POINT ( 'NONE',  ( -4.392478581147607031, 7.108013530438723748, 1.082531754730560403 ) ) ;
#18216=CARTESIAN_POINT ( 'NONE',  ( 6.518772930072240790, 6.499656594706071822, -0.7998128361456281477 ) ) ;
#18218=CARTESIAN_POINT ( 'NONE',  ( -0.6823417656250212460, 2.363541667008084435, 1.181850606188767472 ) ) ;
#18220=CARTESIAN_POINT ( 'NONE',  ( 4.356247428692526569, 3.976710176429713250, 0.7998128361456341429 ) ) ;
#18227=CARTESIAN_POINT ( 'NONE',  ( -3.541704441667874903, 5.155074486744371853, -1.599625672291256295 ) ) ;
#18228=CARTESIAN_POINT ( 'NONE',  ( -7.009202228140751778, 9.200488570962775725, -1.443375672974058777 ) ) ;
#18230=CARTESIAN_POINT ( 'NONE',  ( -0.6823417656250003738, 2.717708333674753618, -1.181850606188749264 ) ) ;
#18238=CARTESIAN_POINT ( 'NONE',  ( -7.334597914868741242, 8.619747657844088806, -1.082531754730543083 ) ) ;
#18240=DIRECTION ( 'NONE',  ( 7.387867266669436732E-31, -1.000000000000000000, -8.546850786086424434E-32 ) ) ;
#18244=CARTESIAN_POINT ( 'NONE',  ( -5.856759170979136897, 9.776710099543576504, 0.000000000000000000 ) ) ;
#18250=CARTESIAN_POINT ( 'NONE',  ( 1.579999999999989413, 6.280000000000042881, -2.499999999999995115 ) ) ;
#18253=CARTESIAN_POINT ( 'NONE',  ( 1.452308200714679032, 8.721976639181708180, -2.576600914284014276 ) ) ;
#18258=CARTESIAN_POINT ( 'NONE',  ( -6.043183783389232566, 8.073467052085995022, 1.599625672291269396 ) ) ;
#18260=CARTESIAN_POINT ( 'NONE',  ( -1.402160292154681736E-14, -1.037499999999977662, 1.732050807568877637 ) ) ;
#18261=CARTESIAN_POINT ( 'NONE',  ( 2.737856954955798727, 5.281584649835344258, 1.199719254218452047 ) ) ;
#18265=CARTESIAN_POINT ( 'NONE',  ( 6.144869935491714230, 8.192100896205568361, -1.599625672291262513 ) ) ;
#18273=CARTESIAN_POINT ( 'NONE',  ( -5.097502569058221411, 6.009803087731781623, -1.082531754730544860 ) ) ;
#18276=CARTESIAN_POINT ( 'NONE',  ( 0.1100172516835694753, 7.047065462479300990, 3.945011421254984718 ) ) ;
#18279=CARTESIAN_POINT ( 'NONE',  ( 1.364683531249986537, 1.905208333674750287, -0.7879004041258239610 ) ) ;
#18280=CARTESIAN_POINT ( 'NONE',  ( 10.20892648096591770, 11.01276177065614981, -0.7216878364870257245 ) ) ;
#18281=CARTESIAN_POINT ( 'NONE',  ( -8.227100285394159940, 8.492705175914988303, 0.7998128361456602331 ) ) ;
#18284=CARTESIAN_POINT ( 'NONE',  ( 6.174848896020108668, 9.291408581077091000, 1.199719254218460707 ) ) ;
#18285=CARTESIAN_POINT ( 'NONE',  ( -7.877450944739929461, 9.149113176073413456, 1.199719254218462483 ) ) ;
#18286=CARTESIAN_POINT ( 'NONE',  ( -1.448804818547335449, 8.711467014680348342, 2.592604518246293122 ) ) ;
#18288=CARTESIAN_POINT ( 'NONE',  ( -0.7500000000000006661, -1.110416665983847473, -1.299038105676652011 ) ) ;
#18290=CARTESIAN_POINT ( 'NONE',  ( 7.700668062882064291, 10.00719871149432549, -1.443375672974057666 ) ) ;
#18294=CARTESIAN_POINT ( 'NONE',  ( 0.6823417656249882723, 0.7385416670080829915, -1.181850606188749264 ) ) ;
#18297=CARTESIAN_POINT ( 'NONE',  ( 6.358410854684775515, 8.441231968597481483, -1.443375672974058777 ) ) ;
#18300=CARTESIAN_POINT ( 'NONE',  ( -5.273758566035884776, 5.255065869904374409, 0.000000000000000000 ) ) ;
#18302=CARTESIAN_POINT ( 'NONE',  ( -1.201851678989727383E-14, 3.821875000341423689, 1.575800808251672791 ) ) ;
#18304=LINE ( 'NONE', #179773, #32426 ) ;
#18306=CARTESIAN_POINT ( 'NONE',  ( -5.752737250900127997, 5.605948302338584099, 0.000000000000000000 ) ) ;
#18307=CARTESIAN_POINT ( 'NONE',  ( -6.007394967034264788, 6.077829431587280062, -0.6506939886842719734 ) ) ;
#18312=EDGE_CURVE ( 'NONE', #46131, #158010, #140792, .T. ) ;
#18316=CARTESIAN_POINT ( 'NONE',  ( 7.633404179693907388, 8.864391950186421454, -1.199719254218441611 ) ) ;
#18320=CARTESIAN_POINT ( 'NONE',  ( -1.402160292154681736E-14, 2.087500000000021227, -1.732050807568863648 ) ) ;
#18326=CARTESIAN_POINT ( 'NONE',  ( 6.480434237652124452, 8.583592582059388576, 1.443375672974076540 ) ) ;
#18327=CARTESIAN_POINT ( 'NONE',  ( 0.6823417656249899377, 0.9052083336747520637, 1.181850606188755259 ) ) ;
#18329=CARTESIAN_POINT ( 'NONE',  ( 10.56588178375152864, 11.22128359066528169, -0.7998128361456281477 ) ) ;
#18330=CARTESIAN_POINT ( 'NONE',  ( 0.6823417656249899377, 2.842708333674753618, 1.181850606188765695 ) ) ;
#18337=CARTESIAN_POINT ( 'NONE',  ( 1.499999999999985123, 0.5458333333333577064, -0.8660254037844253849 ) ) ;
#18338=CARTESIAN_POINT ( 'NONE',  ( 6.100279051144945619, 9.204410428722734849, -1.199719254218440723 ) ) ;
#18339=CARTESIAN_POINT ( 'NONE',  ( -6.367525699912501835, 10.58053041653993098, -0.7998128361456291469 ) ) ;
#18342=CARTESIAN_POINT ( 'NONE',  ( 0.6823417656249882723, 0.6760416670080898749, -1.181850606188749264 ) ) ;
#18343=CARTESIAN_POINT ( 'NONE',  ( -1.500000000000013101, 2.629166666666687746, -0.8660254037844313801 ) ) ;
#18345=CARTESIAN_POINT ( 'NONE',  ( 3.337278367258157630, 7.045241861776501580, 0.7998128361456341429 ) ) ;
#18349=CARTESIAN_POINT ( 'NONE',  ( -1.499999999999997780, 4.431250000682819490, 1.214306433183764966E-14 ) ) ;
#18354=CARTESIAN_POINT ( 'NONE',  ( -1.402160292154681736E-14, -1.256249999317182953, 1.732050807568877637 ) ) ;
#18355=CARTESIAN_POINT ( 'NONE',  ( -6.561256274009600986, 9.742217188731485678, -1.199719254218440723 ) ) ;
#18356=CARTESIAN_POINT ( 'NONE',  ( -5.436456409399874623, 5.444880020495701523, 0.000000000000000000 ) ) ;
#18364=CARTESIAN_POINT ( 'NONE',  ( 7.935599982700328958, 8.152621489438862667, 0.7998128361456481317 ) ) ;
#18369=CARTESIAN_POINT ( 'NONE',  ( 6.548225005276093746, 9.623051025255367819, -1.082531754730537976 ) ) ;
#18370=FACE_OUTER_BOUND ( 'NONE', #201264, .T. ) ;
#18373=CARTESIAN_POINT ( 'NONE',  ( -8.355902744723985975, 8.642974711799791265, 1.040834085586084257E-14 ) ) ;
#18374=CARTESIAN_POINT ( 'NONE',  ( 5.366329872910639232, 5.155139694684188534, 1.040834085586084257E-14 ) ) ;
#18378=CARTESIAN_POINT ( 'NONE',  ( 9.571693261567961741, 11.22969222899322617, 1.082531754730548412 ) ) ;
#18385=CARTESIAN_POINT ( 'NONE',  ( -1.510809298642995957, 8.679800937805021377, -2.538927604451439723 ) ) ;
#18386=CARTESIAN_POINT ( 'NONE',  ( -4.365362273920257330, 6.116008624372160973, 1.443375672974064550 ) ) ;
#18387=CARTESIAN_POINT ( 'NONE',  ( 8.270110514656021650, 11.63191745286530576, 1.082531754730557072 ) ) ;
#18390=CARTESIAN_POINT ( 'NONE',  ( -6.392833124043511894, 7.417059051927569868, 1.199719254218450271 ) ) ;
#18396=CARTESIAN_POINT ( 'NONE',  ( -6.021792782764022078, 10.17717534653336209, -0.7998128361456291469 ) ) ;
#18401=VERTEX_POINT ( 'NONE', #166883 ) ;
#18410=DIRECTION ( 'NONE',  ( 1.000000000000000000, 0.000000000000000000, 0.000000000000000000 ) ) ;
#18412=CARTESIAN_POINT ( 'NONE',  ( -5.018489415352746619, 9.006654751220198207, 0.7998128361456481317 ) ) ;
#18416=CARTESIAN_POINT ( 'NONE',  ( 4.012850279964918165, 7.625483060026979842, -0.7216878364870197293 ) ) ;
#18421=CARTESIAN_POINT ( 'NONE',  ( -3.867100128395853709, 5.534702787927018974, -1.599625672291256295 ) ) ;
#18430=CARTESIAN_POINT ( 'NONE',  ( -8.585337585951595685, 11.03931315507545108, -1.599625672291263179 ) ) ;
#18431=CARTESIAN_POINT ( 'NONE',  ( 5.829115978871627135, 8.888053511070525659, 1.199719254218462483 ) ) ;
#18434=CARTESIAN_POINT ( 'NONE',  ( -8.109748439268576803, 12.61312361245537517, 0.7998128361456481317 ) ) ;
#18438=CARTESIAN_POINT ( 'NONE',  ( -0.6823417656250003738, 0.2802083336747515641, -1.181850606188749264 ) ) ;
#18441=CARTESIAN_POINT ( 'NONE',  ( 8.432808358020025707, 9.900993174853955026, 1.082531754730558626 ) ) ;
#18466=CARTESIAN_POINT ( 'NONE',  ( 0.7499999999999885647, 0.5979166673494851203, -1.299038105676652899 ) ) ;
#18471=CARTESIAN_POINT ( 'NONE',  ( 1.284279953904119864, 3.046639714193936754, -0.7749999999999910294 ) ) ;
#18472=CARTESIAN_POINT ( 'NONE',  ( -1.203907071533418582, 3.243479746939698316, 0.7750000000000100142 ) ) ;
#18474=CARTESIAN_POINT ( 'NONE',  ( 10.22692794340986921, 10.82583744360002243, 0.000000000000000000 ) ) ;
#18475=CARTESIAN_POINT ( 'NONE',  ( 1.500000000000018430, 5.285416667349480235, 0.8660254037844364872 ) ) ;
#18479=CARTESIAN_POINT ( 'NONE',  ( 5.281064527722868718, 6.119995689553514140, 1.199719254218462483 ) ) ;
#18480=CARTESIAN_POINT ( 'NONE',  ( -7.402388683381436074, 7.738467673474211495, 0.7216878364870317197 ) ) ;
#18481=CARTESIAN_POINT ( 'NONE',  ( -5.826669560333386677, 6.051347404617407832, -0.4878656478981869826 ) ) ;
#18486=CARTESIAN_POINT ( 'NONE',  ( -6.723954117373590833, 9.932031339322813679, -1.199719254218440723 ) ) ;
#18487=CARTESIAN_POINT ( 'NONE',  ( -5.233084104750526322, 5.207612331738130429, 0.000000000000000000 ) ) ;
#18490=CARTESIAN_POINT ( 'NONE',  ( -1.500000000000013101, 0.4520833340161533598, 0.8660254037844403729 ) ) ;
#18498=CARTESIAN_POINT ( 'NONE',  ( -5.056828107772866510, 5.962349549565537643, -1.082531754730543971 ) ) ;
#18501=CARTESIAN_POINT ( 'NONE',  ( 4.018854549923576158, 7.569224129587659888, 0.3183394790292719545 ) ) ;
#18507=CARTESIAN_POINT ( 'NONE',  ( -3.253593677155282471, 6.739683690082376444, 1.040834085586084257E-14 ) ) ;
#18508=CARTESIAN_POINT ( 'NONE',  ( 8.910733272679570049, 11.41894145625809820, -1.599625672291255185 ) ) ;
#18511=CARTESIAN_POINT ( 'NONE',  ( -0.1021852871783679312, 7.053056311350174745, -4.037408415133499240 ) ) ;
#18518=CARTESIAN_POINT ( 'NONE',  ( -8.971744963941075568, 11.49012176272984931, 1.599625672291269396 ) ) ;
#18523=CARTESIAN_POINT ( 'NONE',  ( 5.301401758143367893, 6.143722458377430584, 1.199719254218462483 ) ) ;
#18526=VERTEX_POINT ( 'NONE', #152754 ) ;
#18539=CARTESIAN_POINT ( 'NONE',  ( 7.609150525767641504, 9.900428251527500834, -1.599625672291262513 ) ) ;
#18541=CARTESIAN_POINT ( 'NONE',  ( -4.086893239515592136, 6.855460315155083251, 1.199719254218464037 ) ) ;
#18547=CARTESIAN_POINT ( 'NONE',  ( -1.402160292154681736E-14, -0.7562499993171803991, 1.732050807568877637 ) ) ;
#18551=CARTESIAN_POINT ( 'NONE',  ( 5.366329872910639232, 5.155139694684188534, 1.040834085586084257E-14 ) ) ;
#18553=CARTESIAN_POINT ( 'NONE',  ( -5.122283107864663343, 4.870418468797203637, 0.000000000000000000 ) ) ;
#18559=CARTESIAN_POINT ( 'NONE',  ( 5.666945020832170776, 7.634521829102760115, 1.443375672974062551 ) ) ;
#18560=EDGE_CURVE ( 'NONE', #18526, #210539, #142283, .T. ) ;
#18563=CARTESIAN_POINT ( 'NONE',  ( 8.256552360598020002, 8.734991963560254646, -0.7216878364870267237 ) ) ;
#18564=CARTESIAN_POINT ( 'NONE',  ( 0.6823417656249917140, 4.155208333674755394, 1.181850606188765695 ) ) ;
#18566=CARTESIAN_POINT ( 'NONE',  ( 3.172244755473273781, 6.644776614786712443, 0.000000000000000000 ) ) ;
#18570=CARTESIAN_POINT ( 'NONE',  ( 5.583956936972517937, 6.169539715420659931, -0.8775874851904285068 ) ) ;
#18573=CARTESIAN_POINT ( 'NONE',  ( -5.998154408198820953, 6.083692137903044639, 0.6724663025347333845 ) ) ;
#18576=CARTESIAN_POINT ( 'NONE',  ( 0.6823417656249899377, 4.738541667008086655, -1.181850606188754593 ) ) ;
#18589=ORIENTED_EDGE ( 'NONE', *, *, #125125, .F. ) ;
#18592=CARTESIAN_POINT ( 'NONE',  ( -1.364683531250010295, 4.342708333674753618, 0.7879004041258379498 ) ) ;
#18594=CARTESIAN_POINT ( 'NONE',  ( 7.949158136313996259, 8.168439335321471262, 1.040834085586084257E-14 ) ) ;
#18595=CARTESIAN_POINT ( 'NONE',  ( -10.15235809853472126, 10.73883929124566983, -0.7998128361456291469 ) ) ;
#18596=CARTESIAN_POINT ( 'NONE',  ( 1.445377862185226014, 8.715816065047345518, 2.588769565374623660 ) ) ;
#18602=CARTESIAN_POINT ( 'NONE',  ( -1.201851678989727383E-14, 3.837500000000021227, -1.732050807568863648 ) ) ;
#18606=CYLINDRICAL_SURFACE ( 'NONE', #160072, 1.500000000000000222 ) ;
#18609=CARTESIAN_POINT ( 'NONE',  ( 9.246297574839983824, 9.889694713509232571, 0.7216878364870438212 ) ) ;
#18614=CARTESIAN_POINT ( 'NONE',  ( -1.500000000000011324, 3.202083334016150307, 0.8660254037844403729 ) ) ;
#18616=CARTESIAN_POINT ( 'NONE',  ( -5.752737250900127997, 5.605948302338584099, 0.000000000000000000 ) ) ;
#18618=CARTESIAN_POINT ( 'NONE',  ( 4.975479186090860928, 4.907073259968533385, 0.7216878364870317197 ) ) ;
#18626=CARTESIAN_POINT ( 'NONE',  ( 3.388648328411762556, 6.040841252200647382, 1.199719254218462483 ) ) ;
#18630=CARTESIAN_POINT ( 'NONE',  ( 6.017121246366603060, 5.914396297049491658, 1.040834085586084257E-14 ) ) ;
#18632=CARTESIAN_POINT ( 'NONE',  ( 7.334597915313080918, 9.580116872663850813, 1.040834085586084257E-14 ) ) ;
#18641=CARTESIAN_POINT ( 'NONE',  ( 4.731797659388218946, 6.802130194288283249, -1.238660871931380303 ) ) ;
#18643=CARTESIAN_POINT ( 'NONE',  ( 8.204655514564224816, 12.72384853363364066, 1.040834085586084257E-14 ) ) ;
#18648=ADVANCED_FACE ( 'NONE', ( #190306 ), #9437, .F. ) ;
#18649=CARTESIAN_POINT ( 'NONE',  ( 4.839897650398541806, 8.590371658866210680, 1.040834085586084257E-14 ) ) ;
#18651=CARTESIAN_POINT ( 'NONE',  ( -9.978437869977950569, 11.70422760547153906, -1.082531754730539753 ) ) ;
#18656=CARTESIAN_POINT ( 'NONE',  ( -5.915435094264120508, 5.795762452929912101, 0.000000000000000000 ) ) ;
#18667=CARTESIAN_POINT ( 'NONE',  ( 8.289920859751990889, 11.75899253876431416, 1.199719254218450271 ) ) ;
#18668=CARTESIAN_POINT ( 'NONE',  ( 6.025359521845701671, 6.071890788804434891, 0.5399204162177869692 ) ) ;
#18673=CARTESIAN_POINT ( 'NONE',  ( 3.499976210622149253, 7.235056012367825140, 0.7998128361456321445 ) ) ;
#18678=CARTESIAN_POINT ( 'NONE',  ( -7.361714222540411967, 11.53249099303175385, 0.000000000000000000 ) ) ;
#18682=CARTESIAN_POINT ( 'NONE',  ( 5.940443861082012944, 10.08226827123770697, 0.7998128361456462443 ) ) ;
#18685=CARTESIAN_POINT ( 'NONE',  ( -5.708146366553361162, 6.618257834855742594, -1.199719254218446718 ) ) ;
#18686=CARTESIAN_POINT ( 'NONE',  ( 2.347533153460546806, 5.890539112345938300, 0.000000000000000000 ) ) ;
#18690=CARTESIAN_POINT ( 'NONE',  ( 7.391166297744269365, 11.77477778067701664, 1.040834085586084257E-14 ) ) ;
#18694=CARTESIAN_POINT ( 'NONE',  ( 4.007117460063951420, 7.817974094756804604, -0.2064290434495383852 ) ) ;
#18695=CARTESIAN_POINT ( 'NONE',  ( 4.839897650398541806, 8.590371658866210680, 1.040834085586084257E-14 ) ) ;
#18697=CARTESIAN_POINT ( 'NONE',  ( 0.4267829560204765005, 6.608306969908364081, 3.280653110164307495 ) ) ;
#18700=ORIENTED_EDGE ( 'NONE', *, *, #181594, .F. ) ;
#18701=CARTESIAN_POINT ( 'NONE',  ( 7.524412065460039933, 10.76193592880331984, -1.082531754730537976 ) ) ;
#18705=CARTESIAN_POINT ( 'NONE',  ( -7.720478407978036195, 11.09464301169468037, -1.199719254218446718 ) ) ;
#18713=CARTESIAN_POINT ( 'NONE',  ( 2.703961570921634028, 5.242040035128820108, -1.199719254218446718 ) ) ;
#18717=CARTESIAN_POINT ( 'NONE',  ( 4.822949958159288286, 6.649860922651058992, -1.599625672291256295 ) ) ;
#18720=CARTESIAN_POINT ( 'NONE',  ( -0.7499999999999972244, 3.889583334016149863, -1.299038105676652011 ) ) ;
#18726=CARTESIAN_POINT ( 'NONE',  ( -1.500000000000013101, 1.920833333333356263, 0.8660254037844403729 ) ) ;
#18727=CARTESIAN_POINT ( 'NONE',  ( 6.636879889089462026, 7.701780277814560982, -1.199719254218446718 ) ) ;
#18728=CARTESIAN_POINT ( 'NONE',  ( 5.816084710138150093, 5.887779704690372817, -0.7216878364870257245 ) ) ;
#18733=CARTESIAN_POINT ( 'NONE',  ( 8.595506201384008449, 11.05117653974661529, 1.443375672974076540 ) ) ;
#18739=CARTESIAN_POINT ( 'NONE',  ( -4.066556009095094737, 6.831733546331167695, 1.199719254218464037 ) ) ;
#18740=CARTESIAN_POINT ( 'NONE',  ( -1.500000000000013101, 3.910416667349482012, -0.8660254037844313801 ) ) ;
#18741=CARTESIAN_POINT ( 'NONE',  ( -1.364683531250000748, -0.4906249996585801409, 0.000000000000000000 ) ) ;
#18745=CARTESIAN_POINT ( 'NONE',  ( 10.50720586046655391, 11.36075438007358507, 0.7216878364870438212 ) ) ;
#18747=CARTESIAN_POINT ( 'NONE',  ( 0.6823417656249917140, 3.655208333674754506, 1.181850606188765695 ) ) ;
#18750=CARTESIAN_POINT ( 'NONE',  ( 1.499999999999990896, 5.056250000682820378, 1.214306433183764966E-14 ) ) ;
#18755=CARTESIAN_POINT ( 'NONE',  ( -7.527801604085656351, 9.805521176231838609, 1.599625672291295375 ) ) ;
#18756=CARTESIAN_POINT ( 'NONE',  ( 5.819474248763732760, 7.812472595022922128, -1.599625672291262513 ) ) ;
#18758=CARTESIAN_POINT ( 'NONE',  ( 0.6823417656249882723, -0.6572916663252492686, 1.181850606188755259 ) ) ;
#18762=CARTESIAN_POINT ( 'NONE',  ( 2.273078772964581606, 5.704048046545305617, -0.2041365465368546461 ) ) ;
#18765=CARTESIAN_POINT ( 'NONE',  ( -5.368138756007025947, 8.350246751061767725, 1.199719254218452047 ) ) ;
#18770=CARTESIAN_POINT ( 'NONE',  ( 10.07778825365955733, 10.65184113889131012, -0.7998128361456281477 ) ) ;
#18772=CARTESIAN_POINT ( 'NONE',  ( -4.440459003675619520, 5.139289244831666714, 1.199719254218462483 ) ) ;
#18773=CARTESIAN_POINT ( 'NONE',  ( -6.672584156219988571, 10.93643194889866521, -0.7998128361456291469 ) ) ;
#18775=CARTESIAN_POINT ( 'NONE',  ( -4.645415345243833372, 7.101964347008438594, 1.385782282575825919 ) ) ;
#18776=CARTESIAN_POINT ( 'NONE',  ( -1.402160292154681736E-14, -0.3031249996585801965, -1.575800808251665908 ) ) ;
#18780=CARTESIAN_POINT ( 'NONE',  ( 8.948018195339340508, 9.541702104091804415, -0.7216878364870197293 ) ) ;
#18783=CARTESIAN_POINT ( 'NONE',  ( 4.306686350635271054, 8.176217842383143974, -0.7998128361456221525 ) ) ;
#18789=CIRCLE ( 'NONE', #139908, 6.959052028703005099 ) ;
#18802=CARTESIAN_POINT ( 'NONE',  ( 4.202664430556261266, 4.005456045178151570, 0.7216878364870317197 ) ) ;
#18805=CARTESIAN_POINT ( 'NONE',  ( -3.588104209110990706, 7.337872010604796991, 1.040834085586084257E-14 ) ) ;
#18810=CARTESIAN_POINT ( 'NONE',  ( -0.7499999999999972244, 3.389583334016149863, -1.299038105676652011 ) ) ;
#18811=CARTESIAN_POINT ( 'NONE',  ( 8.971744963941056028, 11.49012176272984931, 1.599625672291281386 ) ) ;
#18815=CARTESIAN_POINT ( 'NONE',  ( -10.00321840878439339, 10.56484298653695397, 1.040834085586084257E-14 ) ) ;
#18817=CARTESIAN_POINT ( 'NONE',  ( -1.402160292154681736E-14, 2.446875000341416584, -1.575800808251660134 ) ) ;
#18819=( BOUNDED_CURVE ( )  B_SPLINE_CURVE ( 2, ( #24188, #205075, #23117, #71867, #168333, #69736, #170455 ),
 .UNSPECIFIED., .F., .T. ) 
 B_SPLINE_CURVE_WITH_KNOTS ( ( 3, 2, 2, 3 ),
 ( 0.3784226669537131271, 0.3809523809523809312, 0.3869047619047619180, 0.3894344759034296666 ),
 .UNSPECIFIED. ) 
 CURVE ( )  GEOMETRIC_REPRESENTATION_ITEM ( )  RATIONAL_B_SPLINE_CURVE ( ( 0.9345202395942608931, 0.9430618748659213013, 1.000000000000000000, 0.8660254037844387076, 1.000000000000000000, 0.9430618748659225226, 0.9345202395942613371 ) ) 
 REPRESENTATION_ITEM ( '' )  );
#18821=ORIENTED_EDGE ( 'NONE', *, *, #137465, .T. ) ;
#18826=CARTESIAN_POINT ( 'NONE',  ( -2.117044542028253318, 5.621635732341564662, -0.7998128361456281477 ) ) ;
#18830=CARTESIAN_POINT ( 'NONE',  ( 1.364683531249986537, 0.1760416670080860446, 0.7879004041258500513 ) ) ;
#18835=CARTESIAN_POINT ( 'NONE',  ( -1.364683531250012516, 1.780208333674757615, 0.7879004041258379498 ) ) ;
#18837=CARTESIAN_POINT ( 'NONE',  ( -4.903245109636583443, 8.872203061218007392, -0.7998128361456281477 ) ) ;
#18838=CARTESIAN_POINT ( 'NONE',  ( 6.903072767652295383, 11.20533532890304684, 1.040834085586084257E-14 ) ) ;
#18840=CARTESIAN_POINT ( 'NONE',  ( 5.843727902690005749, 6.776436293681846301, -1.199719254218445830 ) ) ;
#18843=CARTESIAN_POINT ( 'NONE',  ( 1.499999999999989120, 3.254166666666690855, 0.8660254037844524744 ) ) ;
#18845=CARTESIAN_POINT ( 'NONE',  ( 1.364683531249988757, 1.946875000341415030, 0.000000000000000000 ) ) ;
#18848=DIRECTION ( 'NONE',  ( -5.578564026256490882E-16, -1.000000000000000000, -9.066213480720158442E-32 ) ) ;
#18849=VECTOR ( 'NONE', #45045, 1000.000000000000000 ) ;
#18852=CARTESIAN_POINT ( 'NONE',  ( 4.853455804012203778, 8.606189504748821051, 0.7216878364870438212 ) ) ;
#18855=CARTESIAN_POINT ( 'NONE',  ( -6.991200766141138168, 11.30815132714001159, 0.7998128361456481317 ) ) ;
#18856=CARTESIAN_POINT ( 'NONE',  ( -4.060830702492950195, 4.696389560118578999, -1.199719254218452047 ) ) ;
#18862=CARTESIAN_POINT ( 'NONE',  ( -7.998947441938374148, 8.434452891790657603, 1.040834085586084257E-14 ) ) ;
#18864=CARTESIAN_POINT ( 'NONE',  ( 0.7499999999999920064, 4.733333333333352932, 1.299038105676669330 ) ) ;
#18867=CARTESIAN_POINT ( 'NONE',  ( 7.117667457494414762, 11.24776976714476184, 1.040834085586084257E-14 ) ) ;
#18872=CARTESIAN_POINT ( 'NONE',  ( -4.243057018770354460, 3.980691995439412878, 0.4872899543362524954 ) ) ;
#18873=CARTESIAN_POINT ( 'NONE',  ( 4.514501963226220660, 4.369266499959774563, -0.7216878364870197293 ) ) ;
#18874=( BOUNDED_SURFACE ( )  B_SPLINE_SURFACE ( 3, 1, ( 
 ( #27392, #112989 ),
 ( #93492, #179001 ),
 ( #30616, #96705 ),
 ( #128200, #159532 ),
 ( #95635, #79353 ),
 ( #162754, #14327 ),
 ( #145471, #211466 ) ),
 .UNSPECIFIED., .T., .F., .T. ) 
 B_SPLINE_SURFACE_WITH_KNOTS ( ( 4, 3, 4 ),
 ( 2, 2 ),
 ( 0.000000000000000000, 0.5000000000000000000, 1.000000000000000000 ),
 ( 0.000000000000000000, 1.000000000000000000 ),
 .UNSPECIFIED. ) 
 GEOMETRIC_REPRESENTATION_ITEM ( )  RATIONAL_B_SPLINE_SURFACE ( (
 ( 1.000000000000000000, 1.000000000000000000),
 ( 0.3333333333333333703, 0.3333333333333333703),
 ( 0.3333333333333333703, 0.3333333333333333703),
 ( 1.000000000000000000, 1.000000000000000000),
 ( 0.3333333333333333703, 0.3333333333333333703),
 ( 0.3333333333333333703, 0.3333333333333333703),
 ( 1.000000000000000000, 1.000000000000000000) ) ) 
 REPRESENTATION_ITEM ( '' )  SURFACE ( )  );
#18882=CARTESIAN_POINT ( 'NONE',  ( 6.089583550832340819, 10.25626457594641749, 1.040834085586084257E-14 ) ) ;
#18883=CARTESIAN_POINT ( 'NONE',  ( -4.218558352146454915, 8.073401844146177453, 1.040834085586084257E-14 ) ) ;
#18888=CARTESIAN_POINT ( 'NONE',  ( 6.439759776366775768, 7.575769829591800786, 1.082531754730558626 ) ) ;
#18889=CARTESIAN_POINT ( 'NONE',  ( -1.402160292154681736E-14, -0.9906249996585834161, -1.575800808251665908 ) ) ;
#18890=CARTESIAN_POINT ( 'NONE',  ( 2.738383840280328663, 5.178236332760252303, 1.082531754730548412 ) ) ;
#18891=CARTESIAN_POINT ( 'NONE',  ( -9.622536337397040285, 12.24937836509514710, 1.599625672291281386 ) ) ;
#18907=CARTESIAN_POINT ( 'NONE',  ( 7.793239369756836510, 7.986534107671458216, 0.7998128361456341429 ) ) ;
#18917=CARTESIAN_POINT ( 'NONE',  ( -0.5341596719058562259, 6.871489935936940796, 3.795319914582534704 ) ) ;
#18919=CARTESIAN_POINT ( 'NONE',  ( -5.382750679825375251, 6.238629533673094585, -1.199719254218446718 ) ) ;
#18921=CARTESIAN_POINT ( 'NONE',  ( -5.278201874421821316, 5.052323696447222900, 0.7998128361456341429 ) ) ;
#18931=CARTESIAN_POINT ( 'NONE',  ( -8.514157279702017078, 12.87700789305364069, -0.7216878364870267237 ) ) ;
#18935=CARTESIAN_POINT ( 'NONE',  ( 6.419949431270806528, 7.448694743692793274, 1.199719254218462483 ) ) ;
#18936=CARTESIAN_POINT ( 'NONE',  ( 1.364683531249990311, 4.134375000341417028, 1.214306433183764966E-14 ) ) ;
#18941=B_SPLINE_CURVE_WITH_KNOTS ( 'NONE', 1,
 ( #202880, #21987 ),
 .UNSPECIFIED., .F., .F.,
 ( 2, 2 ),
 ( 0.000000000000000000, 0.9297416518164913768 ),
 .UNSPECIFIED. ) ;
#18943=CARTESIAN_POINT ( 'NONE',  ( 4.161989969270883272, 7.799479364217271282, 0.7216878364870317197 ) ) ;
#18944=CARTESIAN_POINT ( 'NONE',  ( -6.775324078527193983, 8.927630729746953264, -1.599625672291263179 ) ) ;
#18947=VECTOR ( 'NONE', #81634, 1000.000000000000000 ) ;
#18949=CARTESIAN_POINT ( 'NONE',  ( -6.832419346282942563, 10.05857410638369487, 1.199719254218453823 ) ) ;
#18950=CARTESIAN_POINT ( 'NONE',  ( -6.437424008390261854, 6.404749519410410485, 0.7998128361456341429 ) ) ;
#18957=CARTESIAN_POINT ( 'NONE',  ( 7.019370843573166319, 9.212351955633947043, 1.599625672291281386 ) ) ;
#18965=CARTESIAN_POINT ( 'NONE',  ( 0.7499999999999902300, 3.983333333333352488, 1.299038105676669330 ) ) ;
#18972=CARTESIAN_POINT ( 'NONE',  ( -1.001543065824772872E-14, 5.212500000000019895, 1.732050807568877637 ) ) ;
#18973=CARTESIAN_POINT ( 'NONE',  ( 4.844340958784499662, 4.546152628203684820, 0.7998128361456341429 ) ) ;
#18974=CARTESIAN_POINT ( 'NONE',  ( 5.198661835836162481, 8.152523677529138979, 1.199719254218462483 ) ) ;
#18976=CARTESIAN_POINT ( 'NONE',  ( -7.619319141200077361, 9.912291636198670375, 1.443375672974090751 ) ) ;
#18979=CARTESIAN_POINT ( 'NONE',  ( 6.507550544879468823, 6.694489845221929691, -0.7216878364870257245 ) ) ;
#18980=CARTESIAN_POINT ( 'NONE',  ( -8.229436053370685400, 10.62409470039771442, 1.443375672974090751 ) ) ;
#18982=AXIS2_PLACEMENT_3D ( 'NONE', #16721, #148882, #151030 ) ;
#18983=ORIENTED_EDGE ( 'NONE', *, *, #122619, .F. ) ;
#18985=CARTESIAN_POINT ( 'NONE',  ( 6.805303039055573322, 10.02693841461847057, 1.199719254218460707 ) ) ;
#18990=CARTESIAN_POINT ( 'NONE',  ( -1.364683531250010295, 4.030208333674751842, 0.7879004041258379498 ) ) ;
#18998=CARTESIAN_POINT ( 'NONE',  ( 8.259941899223605333, 10.65968485389279508, -1.599625672291268286 ) ) ;
#19001=CARTESIAN_POINT ( 'NONE',  ( -7.343712760096452463, 11.71941532008788833, -0.7998128361456291469 ) ) ;
#19007=CARTESIAN_POINT ( 'NONE',  ( 10.05353459973327368, 11.68787744023238417, -1.199719254218440723 ) ) ;
#19010=CARTESIAN_POINT ( 'NONE',  ( -7.181014916732457287, 11.52960116949655678, -0.7998128361456291469 ) ) ;
#19016=CARTESIAN_POINT ( 'NONE',  ( 5.892130686423356245, 5.977214202646935703, -0.03562020706840245132 ) ) ;
#19017=CARTESIAN_POINT ( 'NONE',  ( -4.790108344329849110, 4.482881244673243337, 0.7998128361456341429 ) ) ;
#19021=CARTESIAN_POINT ( 'NONE',  ( 5.587931867126699537, 9.671004278289832001, -0.7998128361456291469 ) ) ;
#19023=CARTESIAN_POINT ( 'NONE',  ( 5.452350330990040739, 9.512825819463730070, 0.7998128361456462443 ) ) ;
#19024=CARTESIAN_POINT ( 'NONE',  ( 4.310602774141044868, 7.116454772218158809, -1.199719254218452047 ) ) ;
#19026=CARTESIAN_POINT ( 'NONE',  ( -7.321039761699444703, 10.52466824108257804, 1.082531754730549967 ) ) ;
#19033=CARTESIAN_POINT ( 'NONE',  ( -4.053570677780473197, 7.570253647979210854, -0.4034679714342986889 ) ) ;
#19034=EDGE_CURVE ( 'NONE', #59141, #16779, #45477, .T. ) ;
#19035=CARTESIAN_POINT ( 'NONE',  ( -1.364683531250014514, -0.9489583329919112353, -0.7879004041258359514 ) ) ;
#19039=CARTESIAN_POINT ( 'NONE',  ( 6.670248388243460447, 6.884303995813253252, -0.7216878364870257245 ) ) ;
#19049=CARTESIAN_POINT ( 'NONE',  ( -8.771762197917311710, 13.17754696430482042, 0.7216878364870317197 ) ) ;
#19052=EDGE_CURVE ( 'NONE', #210292, #17872, #80252, .T. ) ;
#19058=CARTESIAN_POINT ( 'NONE',  ( -9.124274191872636663, 11.66807252865000244, -1.443375672974058777 ) ) ;
#19063=ORIENTED_EDGE ( 'NONE', *, *, #192235, .F. ) ;
#19065=CARTESIAN_POINT ( 'NONE',  ( -1.500000000000011324, 3.202083334016150307, 0.8660254037844403729 ) ) ;
#19067=CARTESIAN_POINT ( 'NONE',  ( -5.392392409933270514, 7.314210449720692786, 1.599625672291269396 ) ) ;
#19070=CARTESIAN_POINT ( 'NONE',  ( -8.483651433849100698, 10.92067931095586886, 1.599625672291269396 ) ) ;
#19075=CARTESIAN_POINT ( 'NONE',  ( 7.935599982700328958, 8.152621489438862667, 0.7998128361456481317 ) ) ;
#19079=CARTESIAN_POINT ( 'NONE',  ( 7.886038904643079661, 12.35212915539230139, -0.7998128361456352531 ) ) ;
#19086=CARTESIAN_POINT ( 'NONE',  ( -6.887178846062109727, 10.01849717283904262, -1.082531754730537976 ) ) ;
#19089=CARTESIAN_POINT ( 'NONE',  ( 1.364683531249990311, 5.176041667008085767, 0.7879004041258500513 ) ) ;
#19093=CARTESIAN_POINT ( 'NONE',  ( -1.001543065824772872E-14, 5.571875000341416140, 1.575800808251672791 ) ) ;
#19096=CARTESIAN_POINT ( 'NONE',  ( -10.66756793585402363, 11.33991743478486391, 0.7998128361456462443 ) ) ;
#19099=CARTESIAN_POINT ( 'NONE',  ( 8.563946585326370098, 13.14302144952281814, 0.7998128361456462443 ) ) ;
#19100=CARTESIAN_POINT ( 'NONE',  ( 1.403499169903295263, 7.376709478543810761, -4.304123474983216902 ) ) ;
#19101=CARTESIAN_POINT ( 'NONE',  ( -9.480175724453545172, 12.08329098332774265, 1.599625672291281386 ) ) ;
#19105=CARTESIAN_POINT ( 'NONE',  ( -1.364683531250000748, 1.759375000341421913, 0.000000000000000000 ) ) ;
#19106=CARTESIAN_POINT ( 'NONE',  ( -2.304522924643024773, 5.632434478818063361, 0.7216878364870317197 ) ) ;
#19107=CARTESIAN_POINT ( 'NONE',  ( 4.009460741339333723, 5.700790169694431420, -1.599625672291256295 ) ) ;
#19114=CARTESIAN_POINT ( 'NONE',  ( -2.282425430171015623, 5.569261388197155327, -0.5172846513131660329 ) ) ;
#19115=CARTESIAN_POINT ( 'NONE',  ( -6.832946231607472498, 9.955225789308602913, 1.082531754730549967 ) ) ;
#19117=CARTESIAN_POINT ( 'NONE',  ( 4.151089631643987587, 2.978105173886053336, 0.7750000000000117906 ) ) ;
#19120=CARTESIAN_POINT ( 'NONE',  ( -9.345647958521597687, 9.797677461230342999, 0.7998128361456462443 ) ) ;
#19122=CARTESIAN_POINT ( 'NONE',  ( -4.894130264408866893, 6.732904613275549899, -1.443375672974051449 ) ) ;
#19123=CARTESIAN_POINT ( 'NONE',  ( -1.364683531250014514, 2.051041667008086655, -0.7879004041258289570 ) ) ;
#19145=CARTESIAN_POINT ( 'NONE',  ( 0.6823417656249899377, 3.488541667008085323, -1.181850606188754593 ) ) ;
#19154=CARTESIAN_POINT ( 'NONE',  ( 8.062294901620731480, 12.55776115186623620, 1.040834085586084257E-14 ) ) ;
#19157=CARTESIAN_POINT ( 'NONE',  ( 0.6823417656249899377, 2.592708333674753618, 1.181850606188767472 ) ) ;
#19167=CARTESIAN_POINT ( 'NONE',  ( 5.691725559638619814, 5.534767995866836543, 1.040834085586084257E-14 ) ) ;
#19177=CARTESIAN_POINT ( 'NONE',  ( -3.541704441667874903, 5.155074486744371853, -1.599625672291256295 ) ) ;
#19178=CARTESIAN_POINT ( 'NONE',  ( 7.259501185113382604, 10.55683625168592243, -1.199719254218441611 ) ) ;
#19181=CARTESIAN_POINT ( 'NONE',  ( 5.463572716182829581, 6.436884926043849653, 1.082531754730560403 ) ) ;
#19187=ADVANCED_FACE ( 'NONE', ( #146937 ), #182583, .F. ) ;
#19190=CARTESIAN_POINT ( 'NONE',  ( -7.876924059859742755, 8.292092279365579799, 1.040834085586084257E-14 ) ) ;
#19192=CARTESIAN_POINT ( 'NONE',  ( 4.364835388595708743, 7.179726155748598515, 1.199719254218462483 ) ) ;
#19195=CARTESIAN_POINT ( 'NONE',  ( -9.809487834687324437, 11.40315621434539395, 1.199719254218462483 ) ) ;
#19200=CARTESIAN_POINT ( 'NONE',  ( -4.322352044658376968, 3.937165561723182883, 0.7998128361456341429 ) ) ;
#19202=CARTESIAN_POINT ( 'NONE',  ( 10.26082332744404368, 10.86538205830655279, -0.7998128361456281477 ) ) ;
#19203=CARTESIAN_POINT ( 'NONE',  ( 5.054492339796319733, 4.791329239384148231, -0.7998128361456211532 ) ) ;
#19212=CARTESIAN_POINT ( 'NONE',  ( -5.427341564172148303, 5.226320001155936090, 0.000000000000000000 ) ) ;
#19215=CARTESIAN_POINT ( 'NONE',  ( -8.350932551013499960, 11.83017284523606172, -1.199719254218446718 ) ) ;
#19221=CARTESIAN_POINT ( 'NONE',  ( 8.270110514656037637, 8.750809809961280550, 0.7216878364870458196 ) ) ;
#19222=CARTESIAN_POINT ( 'NONE',  ( -1.364683531249997417, 5.821875000341418804, 1.214306433183764966E-14 ) ) ;
#19224=CARTESIAN_POINT ( 'NONE',  ( 3.551346171775753735, 6.230655402791975384, 1.199719254218462483 ) ) ;
#19226=CARTESIAN_POINT ( 'NONE',  ( 4.680589345215795838, 6.483773540883647435, -1.599625672291256295 ) ) ;
#19228=CARTESIAN_POINT ( 'NONE',  ( -7.497822643557261024, 8.706213491360317747, -1.199719254218446718 ) ) ;
#19230=CARTESIAN_POINT ( 'NONE',  ( -1.426546532658534927, 7.396047039057213723, 4.272878514717270093 ) ) ;
#19236=EDGE_CURVE ( 'NONE', #214357, #6682, #162749, .T. ) ;
#19239=CARTESIAN_POINT ( 'NONE',  ( -0.6823417656250212460, 2.613541667008084879, 1.181850606188767472 ) ) ;
#19240=CARTESIAN_POINT ( 'NONE',  ( 9.378489572351044856, 11.96465713920816043, -1.599625672291262513 ) ) ;
#19242=CARTESIAN_POINT ( 'NONE',  ( -5.612712406377534435, 5.650512016969639895, 0.7216878364870317197 ) ) ;
#19244=CARTESIAN_POINT ( 'NONE',  ( -4.378920427089552092, 8.052564898339037214, 0.7216878364870317197 ) ) ;
#19250=CARTESIAN_POINT ( 'NONE',  ( 5.522248639467795428, 5.337044922334209573, -0.7998128361456231517 ) ) ;
#19260=CARTESIAN_POINT ( 'NONE',  ( 5.307127064745490230, 8.279066444590018392, -1.199719254218452935 ) ) ;
#19264=CARTESIAN_POINT ( 'NONE',  ( -6.033542053281340856, 6.997886136038390603, -1.199719254218446718 ) ) ;
#19268=CARTESIAN_POINT ( 'NONE',  ( 7.076466111328892694, 10.34329533227067799, -1.199719254218441611 ) ) ;
#19271=CARTESIAN_POINT ( 'NONE',  ( -4.225337428953291230, 8.081310767087481750, 0.7998128361456341429 ) ) ;
#19272=CARTESIAN_POINT ( 'NONE',  ( 6.114364089638782751, 9.116879957011832403, 1.082531754730558626 ) ) ;
#19273=CARTESIAN_POINT ( 'NONE',  ( 5.061713581663421557, 6.751138122384800155, 1.419579013000639378 ) ) ;
#19274=CARTESIAN_POINT ( 'NONE',  ( -5.298539104842322267, 5.076050465271134016, 0.7998128361456341429 ) ) ;
#19277=CARTESIAN_POINT ( 'NONE',  ( -5.545448523189368650, 6.428443684264421698, -1.199719254218446718 ) ) ;
#19280=CARTESIAN_POINT ( 'NONE',  ( 1.364683531249988535, 2.113541667008087099, 0.7879004041258500513 ) ) ;
#19283=CARTESIAN_POINT ( 'NONE',  ( -5.585596099150199834, 5.618876325204420930, -0.7216878364870207285 ) ) ;
#19289=CARTESIAN_POINT ( 'NONE',  ( 6.179819089730593795, 6.104210447640811665, 1.040834085586084257E-14 ) ) ;
#19292=CARTESIAN_POINT ( 'NONE',  ( -1.201851678989727383E-14, 3.384375000341421469, 1.575800808251672791 ) ) ;
#19298=CARTESIAN_POINT ( 'NONE',  ( -2.611917148927046295, 6.198987107056845858, 1.040834085586084257E-14 ) ) ;
#19299=AXIS2_PLACEMENT_3D ( 'NONE', #141920, #189557, #140853 ) ;
#19300=CARTESIAN_POINT ( 'NONE',  ( -6.521108698048772467, 9.591415333490143524, -1.082531754730537976 ) ) ;
#19303=CARTESIAN_POINT ( 'NONE',  ( 1.364683531249988535, 3.113541667008083991, 0.7879004041258500513 ) ) ;
#19311=CARTESIAN_POINT ( 'NONE',  ( -7.253248993186740989, 9.485209796849769504, 1.443375672974090751 ) ) ;
#19318=CARTESIAN_POINT ( 'NONE',  ( -5.870317324592811303, 8.832158731124840401, -1.082531754730537976 ) ) ;
#19327=VERTEX_POINT ( 'NONE', #4871 ) ;
#19330=CARTESIAN_POINT ( 'NONE',  ( -5.799137018343247796, 7.788745826199009237, -1.599625672291256295 ) ) ;
#19333=CARTESIAN_POINT ( 'NONE',  ( 5.034155109375821446, 4.767602470560229122, -0.7998128361456221525 ) ) ;
#19337=CARTESIAN_POINT ( 'NONE',  ( 6.819914962873951936, 7.915321197229798322, -1.199719254218446718 ) ) ;
#19342=CARTESIAN_POINT ( 'NONE',  ( -4.989037340148921196, 5.883260320670900434, 1.082531754730560403 ) ) ;
#19346=CARTESIAN_POINT ( 'NONE',  ( -0.4925365349140243265, 6.683082350101194002, 3.393863156617258792 ) ) ;
#19350=CARTESIAN_POINT ( 'NONE',  ( -1.364683531250014514, 1.488541667008084435, -0.7879004041258289570 ) ) ;
#19352=CARTESIAN_POINT ( 'NONE',  ( -8.715193815486133033, 9.062147627688959872, 0.7998128361456462443 ) ) ;
#19354=CARTESIAN_POINT ( 'NONE',  ( 7.969495366734495434, 8.192166104145387706, 1.040834085586084257E-14 ) ) ;
#19355=CARTESIAN_POINT ( 'NONE',  ( -7.714753101375940503, 8.959299025482085455, 1.199719254218462483 ) ) ;
#19358=CARTESIAN_POINT ( 'NONE',  ( -1.500000000000015099, -0.3395833326505143801, -0.8660254037844383745 ) ) ;
#19360=CARTESIAN_POINT ( 'NONE',  ( 8.026063749610047537, 10.38682701267698150, -1.443375672974057666 ) ) ;
#19363=CARTESIAN_POINT ( 'NONE',  ( 1.364683531249988757, 0.4468750003414206917, 0.000000000000000000 ) ) ;
#19366=CARTESIAN_POINT ( 'NONE',  ( 7.659993601596707613, 9.959745173328078849, -1.443375672974058777 ) ) ;
#19369=CARTESIAN_POINT ( 'NONE',  ( -4.609409038966245653, 6.400729850259146758, -1.443375672974053447 ) ) ;
#19371=CARTESIAN_POINT ( 'NONE',  ( 0.6823417656249899377, 3.092708333674754062, 1.181850606188765695 ) ) ;
#19375=CARTESIAN_POINT ( 'NONE',  ( -5.343885102080728977, 9.386283052402845328, 0.7998128361456481317 ) ) ;
#19376=CARTESIAN_POINT ( 'NONE',  ( -0.6823417656250212460, 5.613541667008087543, 1.181850606188767472 ) ) ;
#19383=CARTESIAN_POINT ( 'NONE',  ( 7.793239369756836510, 7.986534107671458216, 0.7998128361456341429 ) ) ;
#19386=CARTESIAN_POINT ( 'NONE',  ( -1.499999999999997780, 2.150000000000019895, 1.214306433183764966E-14 ) ) ;
#19392=CARTESIAN_POINT ( 'NONE',  ( 5.829642864196157070, 8.784705193995428374, 1.082531754730558626 ) ) ;
#19393=CARTESIAN_POINT ( 'NONE',  ( 0.6823417656249882723, 0.2385416670080825474, -1.181850606188749264 ) ) ;
#19394=VECTOR ( 'NONE', #184475, 1000.000000000000000 ) ;
#19396=CARTESIAN_POINT ( 'NONE',  ( 2.218730694130720771, 5.740269576461138890, 0.7998128361456462443 ) ) ;
#19404=CARTESIAN_POINT ( 'NONE',  ( -1.402160292154681736E-14, 0.2125000000000202283, 1.732050807568877637 ) ) ;
#19405=CARTESIAN_POINT ( 'NONE',  ( 8.925345196497941558, 9.307324238869423283, 1.040834085586084257E-14 ) ) ;
#19406=CARTESIAN_POINT ( 'NONE',  ( -9.854078719034067291, 10.39084668182823634, 0.7998128361456462443 ) ) ;
#19408=CARTESIAN_POINT ( 'NONE',  ( 1.364683531249988757, 1.884375000341421913, 0.000000000000000000 ) ) ;
#19409=ORIENTED_EDGE ( 'NONE', *, *, #153621, .T. ) ;
#19410=CARTESIAN_POINT ( 'NONE',  ( -0.7500000000000006661, 1.608333333333357373, -1.299038105676652011 ) ) ;
#19412=CARTESIAN_POINT ( 'NONE',  ( 3.714044015139744914, 6.420469553383295391, 1.199719254218462483 ) ) ;
#19419=CARTESIAN_POINT ( 'NONE',  ( 0.7499999999999885647, 0.01458333401615358182, 1.299038105676657340 ) ) ;
#19420=CARTESIAN_POINT ( 'NONE',  ( -7.670162217029145246, 9.971608557999250166, 1.599625672291295375 ) ) ;
#19421=CARTESIAN_POINT ( 'NONE',  ( -5.260200412422213923, 6.199617238323108737, -1.082531754730544860 ) ) ;
#19428=CARTESIAN_POINT ( 'NONE',  ( 7.884230021546724920, 9.157022099014721306, 1.199719254218462483 ) ) ;
#19431=CARTESIAN_POINT ( 'NONE',  ( 5.287316719205157334, 9.112360572473935605, 1.040834085586084257E-14 ) ) ;
#19435=CARTESIAN_POINT ( 'NONE',  ( -9.006694118179950692, 9.402231314165087284, 1.040834085586084257E-14 ) ) ;
#19436=CARTESIAN_POINT ( 'NONE',  ( 3.493197133815315603, 7.227147089426516402, -0.7998128361456291469 ) ) ;
#19439=CARTESIAN_POINT ( 'NONE',  ( 4.003835517601626925, 7.590433450137844318, -0.2001945245787856709 ) ) ;
#19440=CARTESIAN_POINT ( 'NONE',  ( 2.849184837166184536, 6.475799410002530898, 0.7998128361456362523 ) ) ;
#19441=ORIENTED_EDGE ( 'NONE', *, *, #159575, .T. ) ;
#19450=CARTESIAN_POINT ( 'NONE',  ( -5.260200412422220140, 5.239248024021764039, -0.7216878364870207285 ) ) ;
#19451=CARTESIAN_POINT ( 'NONE',  ( 8.053180056837369705, 11.37883191874353805, -1.082531754730543083 ) ) ;
#19454=CARTESIAN_POINT ( 'NONE',  ( -7.054319997812058318, 7.124461507069184130, 1.040834085586084257E-14 ) ) ;
#19455=CARTESIAN_POINT ( 'NONE',  ( 0.000000000000000000, 2.880000000000021210, 1.214306433183764966E-14 ) ) ;
#19459=CARTESIAN_POINT ( 'NONE',  ( 4.322341018716207017, 3.567520274870273678, 2.444429072473035536 ) ) ;
#19461=CARTESIAN_POINT ( 'NONE',  ( -7.374745490829552885, 10.69128794168811680, -1.199719254218446718 ) ) ;
#19464=CARTESIAN_POINT ( 'NONE',  ( 5.493163732433528068, 6.391633739925519642, -1.208849031437130961 ) ) ;
#19475=CARTESIAN_POINT ( 'NONE',  ( -6.856673000209188906, 9.022537805042615489, 1.599625672291283607 ) ) ;
#19479=CARTESIAN_POINT ( 'NONE',  ( 4.446711195602238931, 6.210915699667823198, -1.443375672974051449 ) ) ;
#19484=CARTESIAN_POINT ( 'NONE',  ( -4.111146893441842920, 5.819424013814012753, 1.599625672291267398 ) ) ;
#19493=CARTESIAN_POINT ( 'NONE',  ( -10.16591625214838679, 10.75465713712827487, 1.040834085586084257E-14 ) ) ;
#19494=CARTESIAN_POINT ( 'NONE',  ( 5.286789834324991055, 8.255339675766103724, -1.199719254218452935 ) ) ;
#19497=CARTESIAN_POINT ( 'NONE',  ( -8.448702279610222021, 13.00856975952063088, 1.040834085586084257E-14 ) ) ;
#19500=CARTESIAN_POINT ( 'NONE',  ( 0.6823417656249882723, 0.4052083336747516751, 1.181850606188755259 ) ) ;
#19504=CARTESIAN_POINT ( 'NONE',  ( 8.758204044748005401, 10.28062147603659504, 1.082531754730549967 ) ) ;
#19510=EDGE_CURVE ( 'NONE', #137701, #137589, #67164, .T. ) ;
#19512=CARTESIAN_POINT ( 'NONE',  ( -0.08896015503664653212, 7.049507384514471120, -3.948637857580538313 ) ) ;
#19519=VERTEX_POINT ( 'NONE', #120880 ) ;
#19533=CARTESIAN_POINT ( 'NONE',  ( 1.499999999999987121, -0.4645833326505149907, 0.8660254037844524744 ) ) ;
#19537=CARTESIAN_POINT ( 'NONE',  ( 8.191097360950562845, 12.70803068775103739, -0.7998128361456352531 ) ) ;
#19542=CARTESIAN_POINT ( 'NONE',  ( 10.07778825365955733, 10.65184113889131012, -0.7998128361456281477 ) ) ;
#19547=CARTESIAN_POINT ( 'NONE',  ( 2.849184837166184536, 6.475799410002530898, 0.7998128361456362523 ) ) ;
#19548=CARTESIAN_POINT ( 'NONE',  ( -1.201851678989727383E-14, 2.134375000341423689, 1.575800808251672791 ) ) ;
#19549=CARTESIAN_POINT ( 'NONE',  ( -5.881612045648562770, 6.018300081020916181, 0.2952277700727298781 ) ) ;
#19553=CARTESIAN_POINT ( 'NONE',  ( -6.821723845970312894, 11.11042825360738284, 0.000000000000000000 ) ) ;
#19554=CARTESIAN_POINT ( 'NONE',  ( -3.755245360860925086, 6.364574773437617239, -1.082531754730548412 ) ) ;
#19559=CARTESIAN_POINT ( 'NONE',  ( -1.500000000000015099, -0.5895833326505155458, -0.8660254037844383745 ) ) ;
#19568=CARTESIAN_POINT ( 'NONE',  ( -4.731432421044883263, 5.582721248382882528, -1.082531754730543971 ) ) ;
#19571=CARTESIAN_POINT ( 'NONE',  ( 4.012968703617612931, 7.577496623363801476, 0.2782505873175616373 ) ) ;
#19576=CARTESIAN_POINT ( 'NONE',  ( -4.460269348771590536, 5.266364330730674226, 1.082531754730558626 ) ) ;
#19577=CARTESIAN_POINT ( 'NONE',  ( 8.341290820905593151, 10.75459192918846618, 1.599625672291281386 ) ) ;
#19586=CARTESIAN_POINT ( 'NONE',  ( -4.060830702492950195, 4.696389560118578999, -1.199719254218452047 ) ) ;
#19587=CARTESIAN_POINT ( 'NONE',  ( -8.611400122974211868, 13.19838391011195888, 1.040834085586084257E-14 ) ) ;
#19592=CARTESIAN_POINT ( 'NONE',  ( 5.331380718671758778, 7.243030143248949670, -1.599625672291256295 ) ) ;
#19598=CARTESIAN_POINT ( 'NONE',  ( 3.083589872104280705, 5.684939719841914929, 1.199719254218450271 ) ) ;
#19609=CARTESIAN_POINT ( 'NONE',  ( 9.271078113646423091, 9.710679308875986848, 1.040834085586084257E-14 ) ) ;
#19611=CARTESIAN_POINT ( 'NONE',  ( -4.466521540698216164, 7.298359999868178960, -1.199719254218452047 ) ) ;
#19616=CARTESIAN_POINT ( 'NONE',  ( 1.364683531249990311, 5.363541667008086655, 0.7879004041258500513 ) ) ;
#19620=CARTESIAN_POINT ( 'NONE',  ( 4.878236342818665250, 4.585697242910212523, 1.040834085586084257E-14 ) ) ;
#19621=CARTESIAN_POINT ( 'NONE',  ( -5.786632634934295361, 5.645492917045106473, 0.7998128361456341429 ) ) ;
#19628=CARTESIAN_POINT ( 'NONE',  ( 5.585596099150174965, 7.539614753807099667, -1.443375672974057666 ) ) ;
#19631=CARTESIAN_POINT ( 'NONE',  ( 8.120970824461352322, 9.537182719035495637, -1.082531754730543083 ) ) ;
#19632=CARTESIAN_POINT ( 'NONE',  ( -0.6823417656250212460, 4.113541667008085767, 1.181850606188767472 ) ) ;
#19634=CARTESIAN_POINT ( 'NONE',  ( 3.334942598837264960, 6.834590765378040444, 1.214306433183764966E-14 ) ) ;
#19636=CARTESIAN_POINT ( 'NONE',  ( -5.599154252763867134, 5.634694171087028636, 0.000000000000000000 ) ) ;
#19642=CARTESIAN_POINT ( 'NONE',  ( -4.338283617754775889, 7.407916770541659091, 1.160293660280581785 ) ) ;
#19644=CARTESIAN_POINT ( 'NONE',  ( -1.364683531250010295, 4.842708333674756283, 0.7879004041258379498 ) ) ;
#19647=EDGE_CURVE ( 'NONE', #143793, #163734, #175460, .T. ) ;
#19649=CARTESIAN_POINT ( 'NONE',  ( -8.371269781434001800, 11.85389961405997816, -1.199719254218446718 ) ) ;
#19659=CARTESIAN_POINT ( 'NONE',  ( 4.541618270897912701, 4.400902192243413502, 1.214306433183764966E-14 ) ) ;
#19660=CARTESIAN_POINT ( 'NONE',  ( -1.364683531250010295, 4.842708333674756283, 0.7879004041258379498 ) ) ;
#19662=CARTESIAN_POINT ( 'NONE',  ( 5.615048174354031474, 9.702639970055050966, 0.7998128361456462443 ) ) ;
#19663=CARTESIAN_POINT ( 'NONE',  ( -8.829384350997580455, 11.32403438096243775, 1.599625672291269396 ) ) ;
#19669=CARTESIAN_POINT ( 'NONE',  ( 1.499999999999987121, 4.545833333333352932, -0.8660254037844323793 ) ) ;
#19670=CARTESIAN_POINT ( 'NONE',  ( 5.769158057814842699, 6.689438141327490150, 1.199719254218462483 ) ) ;
#19673=CARTESIAN_POINT ( 'NONE',  ( -0.7499999999999972244, 5.858333333333353821, -1.299038105676652011 ) ) ;
#19675=CARTESIAN_POINT ( 'NONE',  ( 7.280365300858406385, 11.43758391773608984, 1.040834085586084257E-14 ) ) ;
#19680=( BOUNDED_CURVE ( )  B_SPLINE_CURVE ( 2, ( #121893, #139139, #55738, #171621, #56809, #6960, #169489 ),
 .UNSPECIFIED., .F., .T. ) 
 B_SPLINE_CURVE_WITH_KNOTS ( ( 3, 2, 2, 3 ),
 ( 0.3214285714285716744, 0.3273809523809525501, 0.3333333333333334259, 0.3392857142857143571 ),
 .UNSPECIFIED. ) 
 CURVE ( )  GEOMETRIC_REPRESENTATION_ITEM ( )  RATIONAL_B_SPLINE_CURVE ( ( 0.9999999999999950040, 0.8660254037844437036, 1.000000000000000000, 0.8660254037844387076, 1.000000000000000000, 0.8660254037844374864, 1.000000000000001332 ) ) 
 REPRESENTATION_ITEM ( '' )  );
#19681=CARTESIAN_POINT ( 'NONE',  ( -0.7499999999999972244, 3.389583334016149863, -1.299038105676652011 ) ) ;
#19684=CARTESIAN_POINT ( 'NONE',  ( -5.525111292768871252, 6.404716915440499037, -1.199719254218446718 ) ) ;
#19685=CARTESIAN_POINT ( 'NONE',  ( 3.836594282542914236, 5.499112634431936542, 1.443375672974062551 ) ) ;
#19686=CARTESIAN_POINT ( 'NONE',  ( -10.29027540264791440, 11.10766884595181203, 0.7216878364870438212 ) ) ;
#19694=CARTESIAN_POINT ( 'NONE',  ( 7.121056995675668411, 9.330985799753529264, -1.599625672291262513 ) ) ;
#19695=CARTESIAN_POINT ( 'NONE',  ( 4.359110081993588182, 5.044382169536003602, -1.199719254218452047 ) ) ;
#19696=DIRECTION ( 'NONE',  ( 0.000000000000000000, 0.7999999999999973799, -0.6000000000000034195 ) ) ;
#19699=CARTESIAN_POINT ( 'NONE',  ( 4.976006071415387311, 5.764094157194782575, 1.199719254218462483 ) ) ;
#19701=ORIENTED_EDGE ( 'NONE', *, *, #126447, .F. ) ;
#19711=CARTESIAN_POINT ( 'NONE',  ( 5.191320393234815533, 6.438618948542633724, -1.178512179637403623 ) ) ;
#19714=EDGE_CURVE ( 'NONE', #164705, #138703, #64510, .T. ) ;
#19720=CARTESIAN_POINT ( 'NONE',  ( 4.853455804012203778, 8.606189504748821051, 0.7216878364870438212 ) ) ;
#19721=CARTESIAN_POINT ( 'NONE',  ( -8.337901282724359930, 12.67137589657970409, 1.040834085586084257E-14 ) ) ;
#19726=CARTESIAN_POINT ( 'NONE',  ( -3.391510981712833939, 7.108513245306943062, 0.7998128361456341429 ) ) ;
#19729=CARTESIAN_POINT ( 'NONE',  ( -5.335766472694970730, 4.384919054141817263, 2.499999999999998668 ) ) ;
#19737=CARTESIAN_POINT ( 'NONE',  ( 9.759171643738394408, 10.28012176064996197, 0.000000000000000000 ) ) ;
#19738=CARTESIAN_POINT ( 'NONE',  ( 5.922464229660435286, 6.137557782886555735, -0.7752440879994120237 ) ) ;
#19739=FACE_OUTER_BOUND ( 'NONE', #21516, .T. ) ;
#19744=CARTESIAN_POINT ( 'NONE',  ( -7.199016379176422120, 11.34267684244042584, 0.000000000000000000 ) ) ;
#19749=CARTESIAN_POINT ( 'NONE',  ( 8.046927864910717432, 9.346836249606042202, 1.199719254218462483 ) ) ;
#19752=CARTESIAN_POINT ( 'NONE',  ( 3.408985558832261731, 6.064568021024562938, 1.199719254218462483 ) ) ;
#19754=CARTESIAN_POINT ( 'NONE',  ( -5.876569516519495551, 8.943415971659659292, 1.199719254218452047 ) ) ;
#19755=CARTESIAN_POINT ( 'NONE',  ( 3.358669367883368118, 4.941533567329135401, -1.599625672291262513 ) ) ;
#19758=CARTESIAN_POINT ( 'NONE',  ( 8.971744963941056028, 11.49012176272984931, 1.599625672291281386 ) ) ;
#19759=CARTESIAN_POINT ( 'NONE',  ( 0.7499999999999885647, 3.566666666666690411, -1.299038105676658228 ) ) ;
#19762=CARTESIAN_POINT ( 'NONE',  ( 4.085089063302896228, 7.714230733137671159, -0.6301764584765887633 ) ) ;
#19764=CARTESIAN_POINT ( 'NONE',  ( 5.341549334104184865, 8.215262742221458581, 1.082531754730558626 ) ) ;
#19768=VECTOR ( 'NONE', #210248, 1000.000000000000000 ) ;
#19772=CARTESIAN_POINT ( 'NONE',  ( 9.056483423804305488, 9.668244870634271848, 1.040834085586084257E-14 ) ) ;
#19776=CARTESIAN_POINT ( 'NONE',  ( -7.018317073368468328, 11.33978701890523233, -0.7998128361456291469 ) ) ;
#19782=CARTESIAN_POINT ( 'NONE',  ( -1.420000000000001039, 7.176846818246207960, -4.202462424328208712 ) ) ;
#19785=CARTESIAN_POINT ( 'NONE',  ( 8.757677159423465696, 12.30470822171437284, 1.199719254218450271 ) ) ;
#19789=CARTESIAN_POINT ( 'NONE',  ( 5.281064527722868718, 6.119995689553514140, 1.199719254218462483 ) ) ;
#19792=CARTESIAN_POINT ( 'NONE',  ( -1.201851678989727383E-14, 4.618750000682821266, -1.732050807568863648 ) ) ;
#19798=CARTESIAN_POINT ( 'NONE',  ( -0.7500000000000006661, 2.108333333333357817, -1.299038105676652011 ) ) ;
#19799=CARTESIAN_POINT ( 'NONE',  ( 5.587931867126699537, 9.671004278289832001, -0.7998128361456291469 ) ) ;
#19800=CARTESIAN_POINT ( 'NONE',  ( 5.490689023410166847, 5.508151403507724808, -0.7216878364870207285 ) ) ;
#19804=CARTESIAN_POINT ( 'NONE',  ( 8.432808358020016826, 10.86136238915529084, 1.443375672974076540 ) ) ;
#19810=CARTESIAN_POINT ( 'NONE',  ( -6.227272627378437342, 6.159572908229946187, -0.7998128361456291469 ) ) ;
#19811=CARTESIAN_POINT ( 'NONE',  ( 0.7499999999999902300, 3.847916667349481123, -1.299038105676658228 ) ) ;
#19812=CARTESIAN_POINT ( 'NONE',  ( -1.364683531250000748, -0.9906249996585805295, 0.000000000000000000 ) ) ;
#19816=CARTESIAN_POINT ( 'NONE',  ( 8.541273586484978253, 12.90864358430044589, 0.000000000000000000 ) ) ;
#19819=CARTESIAN_POINT ( 'NONE',  ( 1.364683531249988535, 3.467708333674749621, -0.7879004041258239610 ) ) ;
#19826=CARTESIAN_POINT ( 'NONE',  ( -8.877891658850122880, 9.251961778280284321, 0.7998128361456462443 ) ) ;
#19827=CARTESIAN_POINT ( 'NONE',  ( 6.830610463186557624, 6.863467050006115677, 1.040834085586084257E-14 ) ) ;
#19830=CARTESIAN_POINT ( 'NONE',  ( -1.402160292154681736E-14, -0.8031249996585825279, -1.575800808251665908 ) ) ;
#19836=CARTESIAN_POINT ( 'NONE',  ( -5.422371370461663176, 8.413518134592214537, -1.199719254218446718 ) ) ;
#19839=CARTESIAN_POINT ( 'NONE',  ( 9.297140650669039275, 11.86975006391249643, 1.599625672291281386 ) ) ;
#19841=CARTESIAN_POINT ( 'NONE',  ( 9.887974103068218668, 10.43039129653476493, 0.7998128361456462443 ) ) ;
#19844=CARTESIAN_POINT ( 'NONE',  ( -3.253066792275140173, 5.882662793374543675, 1.199719254218462483 ) ) ;
#19845=CARTESIAN_POINT ( 'NONE',  ( -8.507905087775398556, 9.884643009614800135, 1.199719254218462483 ) ) ;
#19848=CARTESIAN_POINT ( 'NONE',  ( -4.103288207896339301, 7.680416417065718093, 0.7589585138018557497 ) ) ;
#19849=CARTESIAN_POINT ( 'NONE',  ( -1.364683531250014514, -1.011458332991911568, -0.7879004041258359514 ) ) ;
#19853=CARTESIAN_POINT ( 'NONE',  ( 7.131225611108085616, 10.30321839872603462, 1.082531754730558626 ) ) ;
#19856=CARTESIAN_POINT ( 'NONE',  ( 4.794779880727245036, 8.745660294157122649, -0.7998128361456281477 ) ) ;
#19879=CARTESIAN_POINT ( 'NONE',  ( -8.320953590485107298, 10.73086516036454618, 1.599625672291269396 ) ) ;
#19884=CARTESIAN_POINT ( 'NONE',  ( 1.499999999999987121, 1.827083334016151861, -0.8660254037844253849 ) ) ;
#19885=CARTESIAN_POINT ( 'NONE',  ( 9.915090410295563927, 10.46202698829998567, -0.7998128361456281477 ) ) ;
#19890=LINE ( 'NONE', #201825, #193665 ) ;
#19891=CARTESIAN_POINT ( 'NONE',  ( -1.402160292154681736E-14, 1.696875000341421469, -1.575800808251659024 ) ) ;
#19893=ORIENTED_EDGE ( 'NONE', *, *, #141538, .F. ) ;
#19897=CARTESIAN_POINT ( 'NONE',  ( -3.090368948911150770, 5.692848642783215674, 1.199719254218462483 ) ) ;
#19899=CARTESIAN_POINT ( 'NONE',  ( 1.500000000000001110, 7.438721522839136568, -4.195160983902596286 ) ) ;
#19902=CARTESIAN_POINT ( 'NONE',  ( -0.6823417656250246877, -0.1364583329919108468, 1.181850606188755259 ) ) ;
#19908=CARTESIAN_POINT ( 'NONE',  ( -1.364683531250012516, 1.530208333674756505, 0.7879004041258379498 ) ) ;
#19910=CARTESIAN_POINT ( 'NONE',  ( -4.889686956022917919, 8.856385215335397021, 1.214306433183764966E-14 ) ) ;
#19911=CARTESIAN_POINT ( 'NONE',  ( 7.670162217029129259, 9.971608557999250166, 1.599625672291281386 ) ) ;
#19912=CARTESIAN_POINT ( 'NONE',  ( -1.203941962966186052, 2.883481847795091202, 0.7750000000000083489 ) ) ;
#19913=CARTESIAN_POINT ( 'NONE',  ( 4.157546660884947620, 8.002221537674429896, 1.040834085586084257E-14 ) ) ;
#19915=CARTESIAN_POINT ( 'NONE',  ( -1.001543065824772872E-14, 4.212500000000023448, 1.732050807568877637 ) ) ;
#19917=CARTESIAN_POINT ( 'NONE',  ( -1.364683531250014514, 1.551041667008084435, -0.7879004041258289570 ) ) ;
#19923=CARTESIAN_POINT ( 'NONE',  ( 4.202664430556241726, 7.846932902383524144, 0.7216878364870298324 ) ) ;
#19926=CARTESIAN_POINT ( 'NONE',  ( -8.341290820905609138, 10.75459192918846618, 1.599625672291269396 ) ) ;
#19927=CARTESIAN_POINT ( 'NONE',  ( -2.903417451620861289, 6.539070793532962611, 0.7998128361456341429 ) ) ;
#19930=FACE_OUTER_BOUND ( 'NONE', #64730, .T. ) ;
#19931=B_SPLINE_CURVE_WITH_KNOTS ( 'NONE', 3,
 ( #1366, #86916, #182265, #18697, #200637, #134633, #84779, #37088, #152984, #199577 ),
 .UNSPECIFIED., .F., .F.,
 ( 4, 2, 2, 2, 4 ),
 ( 0.000000000000000000, 0.0003729762227911204739, 0.0007459524455822409477, 0.001118928668373361367, 0.001491904891164481895 ),
 .UNSPECIFIED. ) ;
#19932=CARTESIAN_POINT ( 'NONE',  ( -7.497295758232731089, 8.809561808435409702, -1.082531754730543083 ) ) ;
#19934=CARTESIAN_POINT ( 'NONE',  ( -0.7499999999999972244, 4.858333333333353821, -1.299038105676652011 ) ) ;
#19937=CARTESIAN_POINT ( 'NONE',  ( 9.097157885089661278, 9.715698408800516717, 1.040834085586084257E-14 ) ) ;
#19942=CARTESIAN_POINT ( 'NONE',  ( -4.248040861160308879, 3.981233870717535872, 0.4781583390340860551 ) ) ;
#19951=CARTESIAN_POINT ( 'NONE',  ( 9.070041577417981671, 9.684062716516882219, -0.7216878364870197293 ) ) ;
#19952=CARTESIAN_POINT ( 'NONE',  ( 7.800018446563675489, 7.994443030612759848, -0.7998128361456281477 ) ) ;
#19953=CARTESIAN_POINT ( 'NONE',  ( -5.739179097286464248, 5.590130456455974617, -0.7998128361456221525 ) ) ;
#19955=DIRECTION ( 'NONE',  ( 0.7592566023653005702, 0.6507913734559639396, 0.000000000000000000 ) ) ;
#19957=CARTESIAN_POINT ( 'NONE',  ( -1.364683531250014514, -0.6572916663252459379, 0.7879004041258379498 ) ) ;
#19958=CARTESIAN_POINT ( 'NONE',  ( 2.684151225825664788, 5.114964949229812596, -1.082531754730543083 ) ) ;
#19961=CARTESIAN_POINT ( 'NONE',  ( -4.457933580795036654, 4.095344020549286590, -0.7998128361456221525 ) ) ;
#19967=ADVANCED_FACE ( 'NONE', ( #123507 ), #92000, .F. ) ;
#19977=CARTESIAN_POINT ( 'NONE',  ( 5.957918438201454059, 9.038323046955323292, -1.199719254218440723 ) ) ;
#19989=CARTESIAN_POINT ( 'NONE',  ( -4.737684612971557740, 7.614716917520386374, 1.199719254218464037 ) ) ;
#19992=CARTESIAN_POINT ( 'NONE',  ( -3.255929445576174697, 6.950334786480840243, -0.7998128361456281477 ) ) ;
#20001=CARTESIAN_POINT ( 'NONE',  ( -4.437596350374534815, 4.071617251725375475, -0.7998128361456221525 ) ) ;
#20005=CARTESIAN_POINT ( 'NONE',  ( 4.625302960556422427, 8.547937220624488575, 1.040834085586084257E-14 ) ) ;
#20006=CARTESIAN_POINT ( 'NONE',  ( 1.364683531249990311, 5.113541667008084879, 0.7879004041258499402 ) ) ;
#20012=CARTESIAN_POINT ( 'NONE',  ( 5.707619481228810798, 7.681975366232176583, -1.443375672974057666 ) ) ;
#20013=CARTESIAN_POINT ( 'NONE',  ( -6.368579470117215813, 8.453095353268645695, 1.599625672291283607 ) ) ;
#20016=CARTESIAN_POINT ( 'NONE',  ( -8.182509401047415309, 9.505014708432145909, 1.199719254218462483 ) ) ;
#20017=CARTESIAN_POINT ( 'NONE',  ( -6.410307701162927252, 6.373113827645189744, -0.7998128361456291469 ) ) ;
#20024=CARTESIAN_POINT ( 'NONE',  ( 6.076025397218672630, 10.24044673006381245, -0.7998128361456291469 ) ) ;
#20040=CARTESIAN_POINT ( 'NONE',  ( -0.6823417656250246877, -0.8864583329919115684, 1.181850606188755259 ) ) ;
#20041=CARTESIAN_POINT ( 'NONE',  ( 2.686486993802192913, 6.285985259411197568, 0.7998128361456362523 ) ) ;
#20042=CARTESIAN_POINT ( 'NONE',  ( 4.957477724091233995, 8.935474444748447098, -0.7998128361456281477 ) ) ;
#20044=CARTESIAN_POINT ( 'NONE',  ( -8.703971430293361067, 9.256980878204810637, 0.7216878364870438212 ) ) ;
#20046=CARTESIAN_POINT ( 'NONE',  ( 6.480434237652135998, 6.662854153456708950, 0.7216878364870317197 ) ) ;
#20047=CARTESIAN_POINT ( 'NONE',  ( -6.670248387799091461, 10.72578085250020585, 0.000000000000000000 ) ) ;
#20050=CARTESIAN_POINT ( 'NONE',  ( 6.726816770674637347, 10.99970333242910669, -0.7998128361456291469 ) ) ;
#20055=CARTESIAN_POINT ( 'NONE',  ( -1.402160292154681736E-14, 1.946875000341422579, -1.575800808251660134 ) ) ;
#20060=CARTESIAN_POINT ( 'NONE',  ( 8.446893396513862839, 9.813462703143045474, -1.199719254218445830 ) ) ;
#20064=CARTESIAN_POINT ( 'NONE',  ( -8.528242318195895066, 9.908369778438709474, 1.199719254218462483 ) ) ;
#20068=CARTESIAN_POINT ( 'NONE',  ( -1.001543065824772872E-14, 4.243750000682819490, 1.732050807568877637 ) ) ;
#20070=CARTESIAN_POINT ( 'NONE',  ( 2.544126380858701797, 6.119897877643793116, 0.7998128361456462443 ) ) ;
#20073=CARTESIAN_POINT ( 'NONE',  ( -8.208571938070008400, 11.66408546346865016, -1.199719254218446718 ) ) ;
#20075=EDGE_CURVE ( 'NONE', #204725, #33202, #10707, .T. ) ;
#20079=CARTESIAN_POINT ( 'NONE',  ( 5.841717777309253457, 6.007722996832359996, 0.3783690319567531435 ) ) ;
#20081=AXIS2_PLACEMENT_3D ( 'NONE', #49852, #150567, #181967 ) ;
#20082=CARTESIAN_POINT ( 'NONE',  ( -3.307299406729781399, 5.945934176904983381, -1.199719254218452935 ) ) ;
#20086=CARTESIAN_POINT ( 'NONE',  ( 8.288111976655649471, 8.563885482386732306, -0.7998128361456291469 ) ) ;
#20088=CARTESIAN_POINT ( 'NONE',  ( 6.449928391799196525, 8.548002428564306143, -1.599625672291262513 ) ) ;
#20090=CARTESIAN_POINT ( 'NONE',  ( 5.522248639467795428, 5.337044922334209573, -0.7998128361456231517 ) ) ;
#20092=CARTESIAN_POINT ( 'NONE',  ( -8.690413276679693766, 9.241163032322203819, 1.040834085586084257E-14 ) ) ;
#20099=CARTESIAN_POINT ( 'NONE',  ( -4.362038794589177648, 7.192753374110822051, -1.033456106840037192 ) ) ;
#20103=CARTESIAN_POINT ( 'NONE',  ( 4.338245966692901412, 8.005111361209628740, -0.7216878364870197293 ) ) ;
#20107=CARTESIAN_POINT ( 'NONE',  ( -9.531018800282611281, 12.14260790512831889, 1.443375672974076540 ) ) ;
#20113=CARTESIAN_POINT ( 'NONE',  ( -8.297226821439000588, 12.62392235841345389, 1.040834085586084257E-14 ) ) ;
#20121=CARTESIAN_POINT ( 'NONE',  ( -8.310784975052669665, 12.63974020429606249, -0.7216878364870267237 ) ) ;
#20125=CARTESIAN_POINT ( 'NONE',  ( 6.909851844459134362, 11.21324425184434936, -0.7998128361456291469 ) ) ;
#20129=CARTESIAN_POINT ( 'NONE',  ( 0.7499999999999885647, 1.097916667349485564, -1.299038105676652899 ) ) ;
#20131=CARTESIAN_POINT ( 'NONE',  ( -4.381256195510448315, 8.263215994737505454, 1.040834085586084257E-14 ) ) ;
#20134=CARTESIAN_POINT ( 'NONE',  ( -7.458957065812611198, 11.85386701009007204, 0.7998128361456481317 ) ) ;
#20135=CARTESIAN_POINT ( 'NONE',  ( -5.260200412422217475, 5.239248024021766703, -0.7216878364870237261 ) ) ;
#20138=CARTESIAN_POINT ( 'NONE',  ( 5.425234023762710578, 9.481190127698507553, -0.7998128361456291469 ) ) ;
#20140=CARTESIAN_POINT ( 'NONE',  ( -5.377780486114890124, 9.425827667109372143, 0.000000000000000000 ) ) ;
#20142=CARTESIAN_POINT ( 'NONE',  ( 7.736899214892750010, 12.17813285068358020, 1.040834085586084257E-14 ) ) ;
#20150=CARTESIAN_POINT ( 'NONE',  ( -6.670248388243482651, 9.765411638717282017, 1.082531754730548412 ) ) ;
#20153=CARTESIAN_POINT ( 'NONE',  ( -0.6823417656249969321, 4.280208333674755394, -1.181850606188749264 ) ) ;
#20157=CARTESIAN_POINT ( 'NONE',  ( -0.6823417656249969321, 5.217708333674756283, -1.181850606188749264 ) ) ;
#20159=CARTESIAN_POINT ( 'NONE',  ( -9.642873567817536795, 12.27310513391906532, 1.599625672291281386 ) ) ;
#20161=CARTESIAN_POINT ( 'NONE',  ( 4.189106276498237413, 3.989638198777126110, -0.7216878364870188411 ) ) ;
#20162=CARTESIAN_POINT ( 'NONE',  ( -0.6823417656250212460, 4.863541667008086655, 1.181850606188767472 ) ) ;
#20165=DIRECTION ( 'NONE',  ( 0.7592566023653016805, -0.6507913734559627184, 0.000000000000000000 ) ) ;
#20167=CARTESIAN_POINT ( 'NONE',  ( -1.364683531250014514, 1.488541667008084435, -0.7879004041258289570 ) ) ;
#20168=CARTESIAN_POINT ( 'NONE',  ( -4.121315508874276112, 4.870918184183829602, -1.082531754730549967 ) ) ;
#20169=CARTESIAN_POINT ( 'NONE',  ( 5.657830175604453338, 5.495223381160312393, 0.7998128361456341429 ) ) ;
#20172=DIRECTION ( 'NONE',  ( 5.176899690512889973E-31, -0.6000000000000035305, 0.7999999999999974909 ) ) ;
#20174=CARTESIAN_POINT ( 'NONE',  ( -3.600749563572677836, 3.160087278256992427, -2.499999999999995115 ) ) ;
#20175=CARTESIAN_POINT ( 'NONE',  ( 4.229780737783593203, 4.037091736943370535, -0.7216878364870188411 ) ) ;
#20176=CARTESIAN_POINT ( 'NONE',  ( 10.53432216769390095, 11.39239007183880581, -0.7216878364870257245 ) ) ;
#20178=CARTESIAN_POINT ( 'NONE',  ( -8.568389894156720032, 10.05917163368005163, 1.082531754730558626 ) ) ;
#20180=CARTESIAN_POINT ( 'NONE',  ( 4.559605246071184226, 3.300000000000025135, 0.7750000000000135669 ) ) ;
#20183=CARTESIAN_POINT ( 'NONE',  ( -9.481229494658258261, 9.955855920056455588, -0.7998128361456291469 ) ) ;
#20184=CARTESIAN_POINT ( 'NONE',  ( -3.402733366905605905, 6.913679994791092298, 0.7216878364870317197 ) ) ;
#20185=CARTESIAN_POINT ( 'NONE',  ( -1.201851678989727383E-14, 1.884375000341422135, 1.575800808251672791 ) ) ;
#20194=ORIENTED_EDGE ( 'NONE', *, *, #121776, .F. ) ;
#20204=CARTESIAN_POINT ( 'NONE',  ( -7.334597915313094241, 9.580116872663850813, 1.040834085586084257E-14 ) ) ;
#20209=CARTESIAN_POINT ( 'NONE',  ( -0.6823417656250212460, 3.363541667008085323, 1.181850606188767472 ) ) ;
#20216=CARTESIAN_POINT ( 'NONE',  ( 9.745613490124728884, 10.26430391476735338, 0.7998128361456462443 ) ) ;
#20219=CARTESIAN_POINT ( 'NONE',  ( 0.6823417656249882723, 0.9260416670080831025, -1.181850606188749264 ) ) ;
#20230=CARTESIAN_POINT ( 'NONE',  ( 3.867100128395839942, 5.534702787927018974, -1.599625672291255185 ) ) ;
#20234=CARTESIAN_POINT ( 'NONE',  ( 10.71502147350184231, 11.39527989537399755, 0.000000000000000000 ) ) ;
#20241=CARTESIAN_POINT ( 'NONE',  ( -2.462777459176719308, 6.024990802348131780, -0.7998128361456281477 ) ) ;
#20242=CARTESIAN_POINT ( 'NONE',  ( 7.853197290813620945, 10.18514947741448573, 1.599625672291281386 ) ) ;
#20245=CARTESIAN_POINT ( 'NONE',  ( 5.978782553502139940, 6.077593855281705260, -0.7216878364870257245 ) ) ;
#20250=ORIENTED_EDGE ( 'NONE', *, *, #29169, .T. ) ;
#20252=CARTESIAN_POINT ( 'NONE',  ( 1.499999999999821032, 7.388542872122531691, -4.154462424328212222 ) ) ;
#20255=FACE_OUTER_BOUND ( 'NONE', #177544, .T. ) ;
#20256=CARTESIAN_POINT ( 'NONE',  ( -7.890482213473404727, 8.307910125248191946, 0.7216878364870578100 ) ) ;
#20258=CARTESIAN_POINT ( 'NONE',  ( 6.322179702674084467, 6.270297829408224111, 1.040834085586084257E-14 ) ) ;
#20262=CARTESIAN_POINT ( 'NONE',  ( -8.109748439268576803, 12.61312361245537517, 0.7998128361456481317 ) ) ;
#20267=CARTESIAN_POINT ( 'NONE',  ( -2.435661151949389147, 5.993355110582911038, 0.7998128361456341429 ) ) ;
#20269=CARTESIAN_POINT ( 'NONE',  ( 9.423080456697809026, 10.95234760669099749, -1.199719254218446718 ) ) ;
#20270=CARTESIAN_POINT ( 'NONE',  ( 3.541704441667858472, 5.155074486744371853, -1.599625672291262513 ) ) ;
#20276=CARTESIAN_POINT ( 'NONE',  ( 2.887523530030648988, 6.312601851770308414, 0.000000000000000000 ) ) ;
#20279=CARTESIAN_POINT ( 'NONE',  ( -4.741601036477307574, 6.554953847355395880, 1.599625672291267398 ) ) ;
#20282=CARTESIAN_POINT ( 'NONE',  ( -9.110189153378817295, 12.71597221466224603, 1.199719254218462483 ) ) ;
#20288=CARTESIAN_POINT ( 'NONE',  ( 7.293923454472077239, 10.49303254931736262, 1.082531754730558626 ) ) ;
#20291=CARTESIAN_POINT ( 'NONE',  ( 3.798255590122797898, 7.583048621785260401, -0.7998128361456221525 ) ) ;
#20305=CARTESIAN_POINT ( 'NONE',  ( -1.201851678989727383E-14, 2.634375000341417916, 1.575800808251672791 ) ) ;
#20307=CARTESIAN_POINT ( 'NONE',  ( 10.40318394038753702, 11.03146944007395724, -0.7998128361456281477 ) ) ;
#20309=CARTESIAN_POINT ( 'NONE',  ( -5.097502569058215194, 6.970172302033127210, -1.443375672974053447 ) ) ;
#20311=CARTESIAN_POINT ( 'NONE',  ( -5.436456408955534947, 6.405249234278626247, 1.082531754730546636 ) ) ;
#20317=CARTESIAN_POINT ( 'NONE',  ( 4.904298879841284098, 6.744767997946721216, 1.599625672291267398 ) ) ;
#20327=CARTESIAN_POINT ( 'NONE',  ( 6.681470773436232413, 6.689470745297396270, -0.7998128361456281477 ) ) ;
#20331=CARTESIAN_POINT ( 'NONE',  ( -6.063521013809733518, 8.097193820909906137, 1.599625672291283607 ) ) ;
#20335=CARTESIAN_POINT ( 'NONE',  ( 8.098297826064319693, 8.342435640030188893, 0.7998128361456481317 ) ) ;
#20337=CARTESIAN_POINT ( 'NONE',  ( -6.632963465583701534, 8.761543347979550589, -1.599625672291263179 ) ) ;
#20340=CARTESIAN_POINT ( 'NONE',  ( 6.602457619730767391, 7.765583980183128787, 1.082531754730558626 ) ) ;
#20341=CARTESIAN_POINT ( 'NONE',  ( 4.388746605030885206, 7.362284722717403085, 1.177686187499202619 ) ) ;
#20342=CARTESIAN_POINT ( 'NONE',  ( -4.647747731386360215, 4.316793862905830892, 0.7998128361456341429 ) ) ;
#20345=CARTESIAN_POINT ( 'NONE',  ( -4.564291269294938225, 8.476756914152748124, 1.040834085586084257E-14 ) ) ;
#20349=CARTESIAN_POINT ( 'NONE',  ( 0.6823417656249899377, 2.592708333674753618, 1.181850606188767472 ) ) ;
#20351=CARTESIAN_POINT ( 'NONE',  ( -5.924549939491850381, 6.014322472269677533, 0.000000000000000000 ) ) ;
#20356=CARTESIAN_POINT ( 'NONE',  ( 4.559605246071182449, 3.300000000000025135, -0.7749999999999944711 ) ) ;
#20357=CARTESIAN_POINT ( 'NONE',  ( 6.817052309572890323, 6.847649204123507083, 0.7998128361456341429 ) ) ;
#20361=CARTESIAN_POINT ( 'NONE',  ( 0.6823417656249882723, 2.238541667008084435, -1.181850606188749264 ) ) ;
#20368=CARTESIAN_POINT ( 'NONE',  ( -4.029797971759847997, 5.724516938518342535, -1.599625672291256295 ) ) ;
#20369=CARTESIAN_POINT ( 'NONE',  ( -6.683806541412762314, 9.781229484081471526, -1.082531754730537976 ) ) ;
#20371=CARTESIAN_POINT ( 'NONE',  ( -0.6823417656249969321, 3.217708333674754062, -1.181850606188749264 ) ) ;
#20378=CARTESIAN_POINT ( 'NONE',  ( -7.673551755210395342, 8.054824590608001600, 1.040834085586084257E-14 ) ) ;
#20383=CARTESIAN_POINT ( 'NONE',  ( -6.900736999231456004, 8.113576589600553390, 1.082531754730549967 ) ) ;
#20393=ORIENTED_EDGE ( 'NONE', *, *, #50263, .F. ) ;
#20397=CARTESIAN_POINT ( 'NONE',  ( -5.042743069279040036, 7.970618449879118828, 1.199719254218464037 ) ) ;
#20400=TOROIDAL_SURFACE ( 'NONE', #148296, 0.8299999999999998490, 0.08000000000000000167 ) ;
#20401=CARTESIAN_POINT ( 'NONE',  ( 4.844340958784499662, 4.546152628203684820, 0.7998128361456341429 ) ) ;
#20403=CARTESIAN_POINT ( 'NONE',  ( -1.483456582845284810, 7.293967155395466584, -4.258619948150268009 ) ) ;
#20405=CARTESIAN_POINT ( 'NONE',  ( 7.318703993278529829, 7.432909501780090800, 1.040834085586084257E-14 ) ) ;
#20409=CARTESIAN_POINT ( 'NONE',  ( -5.422898255786209099, 5.429062174613087599, -0.7216878364870207285 ) ) ;
#20414=CARTESIAN_POINT ( 'NONE',  ( 3.100381309523608131, 6.448533663283696704, -0.4548243241709319928 ) ) ;
#20417=CARTESIAN_POINT ( 'NONE',  ( -0.6823417656250212460, 2.051041667008083991, 1.181850606188767472 ) ) ;
#20419=CARTESIAN_POINT ( 'NONE',  ( -6.692921386640485082, 10.96015871772258521, -0.7998128361456291469 ) ) ;
#20421=CARTESIAN_POINT ( 'NONE',  ( 6.608709811657416999, 9.797579649320619311, -1.199719254218440723 ) ) ;
#20423=CARTESIAN_POINT ( 'NONE',  ( -8.040148788103921973, 9.338927326664741457, 1.199719254218462483 ) ) ;
#20426=CARTESIAN_POINT ( 'NONE',  ( 1.499999999999987566, -1.193749999317185395, 0.000000000000000000 ) ) ;
#20428=CARTESIAN_POINT ( 'NONE',  ( 9.097157885089661278, 9.715698408800516717, 1.040834085586084257E-14 ) ) ;
#20430=CARTESIAN_POINT ( 'NONE',  ( 0.6823417656249882723, -0.8447916663252494907, 1.181850606188755259 ) ) ;
#20433=CARTESIAN_POINT ( 'NONE',  ( 8.392133896734671694, 8.893170422386358354, 0.7216878364870458196 ) ) ;
#20436=CARTESIAN_POINT ( 'NONE',  ( -5.910991785878175975, 6.958873840688411860, -1.082531754730544860 ) ) ;
#20438=CARTESIAN_POINT ( 'NONE',  ( -0.6823417656250212460, 3.551041667008085323, 1.181850606188767472 ) ) ;
#20443=CARTESIAN_POINT ( 'NONE',  ( -4.543954038874438162, 8.453030145328826350, 1.040834085586084257E-14 ) ) ;
#20444=FACE_OUTER_BOUND ( 'NONE', #41048, .T. ) ;
#20450=CARTESIAN_POINT ( 'NONE',  ( 8.284195553149872993, 9.623648552551724578, -1.199719254218445830 ) ) ;
#20453=CARTESIAN_POINT ( 'NONE',  ( 0.7499999999999885647, 3.066666666666689522, -1.299038105676658228 ) ) ;
#20455=EDGE_CURVE ( 'NONE', #78710, #163734, #138660, .T. ) ;
#20457=CARTESIAN_POINT ( 'NONE',  ( 1.499999999999961586, 5.327083334016154303, -0.8660254037844482555 ) ) ;
#20460=CARTESIAN_POINT ( 'NONE',  ( 5.504247177468175600, 8.405076892812779477, 1.082531754730558626 ) ) ;
#20461=CARTESIAN_POINT ( 'NONE',  ( 0.6823417656249882723, -1.094791666325249713, 1.181850606188755259 ) ) ;
#20463=CARTESIAN_POINT ( 'NONE',  ( 10.53876547652418338, 11.18964789890005918, 0.7998128361456462443 ) ) ;
#20467=CARTESIAN_POINT ( 'NONE',  ( -0.7500000000000215383, 0.4416666666666874130, 1.299038105676659116 ) ) ;
#20468=CARTESIAN_POINT ( 'NONE',  ( 7.832860060393120882, 10.16142270859057462, 1.599625672291281386 ) ) ;
#20469=CARTESIAN_POINT ( 'NONE',  ( -8.154339323615371171, 11.60081407993821045, 1.199719254218453823 ) ) ;
#20471=CARTESIAN_POINT ( 'NONE',  ( -0.6823417656250246877, -0.1989583329919109023, 1.181850606188755259 ) ) ;
#20472=CARTESIAN_POINT ( 'NONE',  ( 1.499999999999985123, 0.5458333333333577064, -0.8660254037844253849 ) ) ;
#20475=CARTESIAN_POINT ( 'NONE',  ( 6.634017235788401301, 6.634108284708264414, 0.7998128361456341429 ) ) ;
#20482=CARTESIAN_POINT ( 'NONE',  ( 0.6823417656249917140, 5.342708333674749177, 1.181850606188765695 ) ) ;
#20484=CARTESIAN_POINT ( 'NONE',  ( -7.263417608619167076, 9.497073181520933716, -1.599625672291263179 ) ) ;
#20485=CARTESIAN_POINT ( 'NONE',  ( -5.477130870240893401, 6.452702772444876445, 1.082531754730548412 ) ) ;
#20493=CARTESIAN_POINT ( 'NONE',  ( 8.263858322729371153, 9.599921783727809910, -1.199719254218446718 ) ) ;
#20494=CARTESIAN_POINT ( 'NONE',  ( -3.470524135418306066, 6.992769224722549914, -0.7216878364870351614 ) ) ;
#20497=CARTESIAN_POINT ( 'NONE',  ( 6.385527161912102123, 9.433236874664039817, -1.082531754730537976 ) ) ;
#20501=CARTESIAN_POINT ( 'NONE',  ( -6.808165692356648258, 11.09461040772476714, 0.7998128361456481317 ) ) ;
#20502=CARTESIAN_POINT ( 'NONE',  ( 5.464099601507359516, 6.333536608968757697, 1.199719254218462483 ) ) ;
#20505=CARTESIAN_POINT ( 'NONE',  ( 4.010558181858147719, 7.580895019428740333, -0.2605091080661054437 ) ) ;
#20506=CARTESIAN_POINT ( 'NONE',  ( 3.009020027229115879, 5.597941567487558778, -1.199719254218446718 ) ) ;
#20507=VERTEX_POINT ( 'NONE', #59517 ) ;
#20514=CARTESIAN_POINT ( 'NONE',  ( -4.121315508874269007, 5.831287398485176077, -1.443375672974053447 ) ) ;
#20515=CARTESIAN_POINT ( 'NONE',  ( 9.734391104931951588, 11.41950637958454706, 1.082531754730548412 ) ) ;
#20520=CARTESIAN_POINT ( 'NONE',  ( -5.530836599371015794, 8.540060901653093950, 1.199719254218452047 ) ) ;
#20525=CARTESIAN_POINT ( 'NONE',  ( -6.184490626128011925, 10.36698949712469364, -0.7998128361456291469 ) ) ;
#20526=EDGE_CURVE ( 'NONE', #56362, #6371, #108347, .T. ) ;
#20540=CARTESIAN_POINT ( 'NONE',  ( -6.449928391799210736, 8.548002428564306143, -1.599625672291263179 ) ) ;
#20543=CARTESIAN_POINT ( 'NONE',  ( 5.829642864196168617, 6.863966765392747860, 1.082531754730558626 ) ) ;
#20548=CARTESIAN_POINT ( 'NONE',  ( -3.924195396151603177, 6.665646164563756138, 1.199719254218464037 ) ) ;
#20556=CARTESIAN_POINT ( 'NONE',  ( -9.528683032306089373, 10.01121838064558744, 0.7998128361456462443 ) ) ;
#20557=CARTESIAN_POINT ( 'NONE',  ( 7.721532178182734185, 8.967207948423393304, 1.199719254218462483 ) ) ;
#20561=CARTESIAN_POINT ( 'NONE',  ( -10.63367255181986160, 11.30037282007833532, 1.040834085586084257E-14 ) ) ;
#20564=CARTESIAN_POINT ( 'NONE',  ( -1.402160292154681736E-14, -0.2406249996585799189, -1.575800808251665908 ) ) ;
#20568=CARTESIAN_POINT ( 'NONE',  ( 8.107412671292031803, 11.44210330227398487, 1.082531754730557072 ) ) ;
#20593=CARTESIAN_POINT ( 'NONE',  ( -1.001543065824772872E-14, 5.321875000341422357, 1.575800808251672791 ) ) ;
#20597=DIRECTION ( 'NONE',  ( 0.000000000000000000, 8.546850786086437571E-32, 1.000000000000000000 ) ) ;
#20598=ORIENTED_EDGE ( 'NONE', *, *, #27948, .T. ) ;
#20601=CARTESIAN_POINT ( 'NONE',  ( 9.083072846151447166, 12.68433652289702884, 1.199719254218450271 ) ) ;
#20606=CARTESIAN_POINT ( 'NONE',  ( 5.606460214450851964, 6.499623990736163037, 1.199719254218462483 ) ) ;
#20607=CARTESIAN_POINT ( 'NONE',  ( 1.364683531249988535, 2.676041667008082214, 0.7879004041258500513 ) ) ;
#20608=CARTESIAN_POINT ( 'NONE',  ( 10.53876547652418338, 11.18964789890005918, 0.7998128361456462443 ) ) ;
#20610=CARTESIAN_POINT ( 'NONE',  ( -9.006694118179950692, 9.402231314165087284, 1.040834085586084257E-14 ) ) ;
#20611=CARTESIAN_POINT ( 'NONE',  ( -3.592547517496929466, 7.135129837147637488, -0.7216878364870257245 ) ) ;
#20614=CARTESIAN_POINT ( 'NONE',  ( -7.230575994789712801, 7.330093503543126054, 0.7998128361456341429 ) ) ;
#20616=CARTESIAN_POINT ( 'NONE',  ( 0.7499999999999885647, -0.4854166659838468623, 1.299038105676657340 ) ) ;
#20623=CARTESIAN_POINT ( 'NONE',  ( -3.836594282542926226, 5.499112634431936542, 1.443375672974064550 ) ) ;
#20625=EDGE_CURVE ( 'NONE', #119323, #138593, #180742, .T. ) ;
#20628=CARTESIAN_POINT ( 'NONE',  ( -5.246642258364192735, 5.223430177620739023, 0.7216878364870317197 ) ) ;
#20630=CARTESIAN_POINT ( 'NONE',  ( 8.748035429315576650, 11.22912730566677553, -1.599625672291255185 ) ) ;
#20639=CARTESIAN_POINT ( 'NONE',  ( -9.215791728987058562, 11.77484298861683598, -1.599625672291263179 ) ) ;
#20642=EDGE_LOOP ( 'NONE', ( #93306, #213462, #168074, #204382 ) ) ;
#20644=CARTESIAN_POINT ( 'NONE',  ( 4.873266149108180123, 7.772895376346490970, 1.199719254218462483 ) ) ;
#20650=CARTESIAN_POINT ( 'NONE',  ( 2.703961570921634028, 5.242040035128820108, -1.199719254218446718 ) ) ;
#20652=ORIENTED_EDGE ( 'NONE', *, *, #148219, .T. ) ;
#20660=CARTESIAN_POINT ( 'NONE',  ( 6.774270308322468459, 11.05506579301824743, 0.7998128361456462443 ) ) ;
#20662=CARTESIAN_POINT ( 'NONE',  ( -6.410307701162927252, 6.373113827645189744, -0.7998128361456291469 ) ) ;
#20663=AXIS2_PLACEMENT_3D ( 'NONE', #117657, #67729, #133880 ) ;
#20666=CARTESIAN_POINT ( 'NONE',  ( -5.558479791478509568, 5.587240632920778438, 0.000000000000000000 ) ) ;
#20670=CARTESIAN_POINT ( 'NONE',  ( 1.499999999999985123, -0.6729166659838520248, -0.8660254037844323793 ) ) ;
#20675=CARTESIAN_POINT ( 'NONE',  ( 2.869522067586683711, 6.499526178826442013, 0.7998128361456362523 ) ) ;
#20676=CARTESIAN_POINT ( 'NONE',  ( -3.764360206088648297, 7.543504007078730922, -0.7998128361456281477 ) ) ;
#20682=CARTESIAN_POINT ( 'NONE',  ( 4.338245966692901412, 8.005111361209628740, -0.7216878364870197293 ) ) ;
#20685=CARTESIAN_POINT ( 'NONE',  ( 6.900736999231407154, 10.99468423250458038, -0.7216878364870267237 ) ) ;
#20686=CARTESIAN_POINT ( 'NONE',  ( 1.364683531249990311, 3.696875000341416584, 1.214306433183764966E-14 ) ) ;
#20688=CARTESIAN_POINT ( 'NONE',  ( 3.972175818679561043, 7.578029521860726092, -0.7216878364870197293 ) ) ;
#20692=CARTESIAN_POINT ( 'NONE',  ( 5.491164291198047387, 6.230432265623782939, -0.9768187426044780963 ) ) ;
#20695=CARTESIAN_POINT ( 'NONE',  ( -4.232483270035822365, 7.525443216328503659, 1.020073867034466675 ) ) ;
#20701=CARTESIAN_POINT ( 'NONE',  ( -9.989660255170729641, 10.54902514065433827, -0.7998128361456291469 ) ) ;
#20706=DIRECTION ( 'NONE',  ( -0.4243160830846597342, 0.9055141421511274658, 0.000000000000000000 ) ) ;
#20711=CARTESIAN_POINT ( 'NONE',  ( 3.551873057100287223, 5.166937871415542283, 1.443375672974062551 ) ) ;
#20713=CARTESIAN_POINT ( 'NONE',  ( -1.201851678989727383E-14, 2.759375000341417916, -1.575800808251660134 ) ) ;
#20715=CARTESIAN_POINT ( 'NONE',  ( 5.601490020740366838, 9.686822124172440596, 1.040834085586084257E-14 ) ) ;
#20716=CARTESIAN_POINT ( 'NONE',  ( -8.371269781434001800, 11.85389961405997816, -1.199719254218446718 ) ) ;
#20718=CARTESIAN_POINT ( 'NONE',  ( -5.251085567194492043, 5.020688004682003047, -0.7998128361456221525 ) ) ;
#20719=VERTEX_POINT ( 'NONE', #22730 ) ;
#20721=CARTESIAN_POINT ( 'NONE',  ( -0.7499999999999972244, 5.108333333333353821, -1.299038105676652011 ) ) ;
#20722=CARTESIAN_POINT ( 'NONE',  ( 4.497554271431305040, 6.270232621468402989, -1.599625672291256295 ) ) ;
#20728=CARTESIAN_POINT ( 'NONE',  ( 9.422553571817644524, 10.09532670998316384, 0.000000000000000000 ) ) ;
#20733=CARTESIAN_POINT ( 'NONE',  ( 0.7499999999999902300, 3.847916667349481123, -1.299038105676658228 ) ) ;
#20735=CARTESIAN_POINT ( 'NONE',  ( -4.578903193113314174, 6.365139696764064325, 1.599625672291267398 ) ) ;
#20736=CARTESIAN_POINT ( 'NONE',  ( 2.833290915131624566, 6.249330467721451399, -0.7216878364870267237 ) ) ;
#20745=CARTESIAN_POINT ( 'NONE',  ( 6.988338112840064120, 10.24047933403371502, 1.199719254218460707 ) ) ;
#20746=CARTESIAN_POINT ( 'NONE',  ( 4.527533231959700366, 7.369540306339926516, 1.199719254218462483 ) ) ;
#20750=CARTESIAN_POINT ( 'NONE',  ( 3.493197133815315603, 7.227147089426516402, -0.7998128361456291469 ) ) ;
#20759=CARTESIAN_POINT ( 'NONE',  ( 9.728138913005292210, 11.30824913904973705, -1.199719254218440723 ) ) ;
#20764=CARTESIAN_POINT ( 'NONE',  ( 5.794097129154974546, 6.036864960932135205, -0.5213279746436976225 ) ) ;
#20768=CARTESIAN_POINT ( 'NONE',  ( -5.775410249741537605, 5.840326167560951909, 0.7216878364870206175 ) ) ;
#20770=CARTESIAN_POINT ( 'NONE',  ( 5.992340707560147806, 8.974519344586754599, 1.082531754730558626 ) ) ;
#20771=EDGE_CURVE ( 'NONE', #106155, #173996, #152598, .T. ) ;
#20772=CARTESIAN_POINT ( 'NONE',  ( -4.115063316947640715, 4.759660943649018705, 1.199719254218462483 ) ) ;
#20777=CARTESIAN_POINT ( 'NONE',  ( -3.716906668440817185, 7.488141546489591072, 0.7998128361456341429 ) ) ;
#20780=CARTESIAN_POINT ( 'NONE',  ( -4.222669843016490177, 3.519858668466411267, 2.499999999999998668 ) ) ;
#20790=CARTESIAN_POINT ( 'NONE',  ( 7.750457368506414646, 12.19395069656619945, 0.7998128361456462443 ) ) ;
#20791=CARTESIAN_POINT ( 'NONE',  ( 5.809489818682099127, 6.211223759639540987, 0.9523037572534819306 ) ) ;
#20798=CARTESIAN_POINT ( 'NONE',  ( -9.327646496521992958, 9.984601788804893019, -0.7216878364870267237 ) ) ;
#20802=CARTESIAN_POINT ( 'NONE',  ( 7.507464373665139412, 9.781794407407920389, 1.599625672291281386 ) ) ;
#20805=CARTESIAN_POINT ( 'NONE',  ( 3.517450787741589036, 6.191110788085444128, -1.199719254218446718 ) ) ;
#20807=CARTESIAN_POINT ( 'NONE',  ( -7.386494761346872551, 7.511998731193139989, -0.7998128361456291469 ) ) ;
#20808=CARTESIAN_POINT ( 'NONE',  ( 3.310162060030825248, 7.013606170011280838, -0.7998128361456291469 ) ) ;
#20812=CARTESIAN_POINT ( 'NONE',  ( 10.53876547652418338, 11.18964789890005918, 0.7998128361456462443 ) ) ;
#20816=CARTESIAN_POINT ( 'NONE',  ( 4.166517013042797757, 7.612504677086913141, -0.8493068020909979587 ) ) ;
#20818=CARTESIAN_POINT ( 'NONE',  ( 4.514501963670558560, 8.210743357683563559, 1.040834085586084257E-14 ) ) ;
#20824=CARTESIAN_POINT ( 'NONE',  ( 8.148087131688683371, 10.52918762510205042, -1.443375672974063439 ) ) ;
#20828=CARTESIAN_POINT ( 'NONE',  ( -8.853638004923878313, 10.28799807962136548, 1.199719254218462483 ) ) ;
#20837=CARTESIAN_POINT ( 'NONE',  ( 2.354312230267378236, 5.898448035287240820, -0.7998128361456281477 ) ) ;
#20841=CARTESIAN_POINT ( 'NONE',  ( 4.473300617505036492, 7.306268922809479704, -1.199719254218452047 ) ) ;
#20844=CARTESIAN_POINT ( 'NONE',  ( -0.7499999999999972244, 3.389583334016149863, -1.299038105676652011 ) ) ;
#20850=CARTESIAN_POINT ( 'NONE',  ( -1.500000000000013101, 1.379166666666689745, -0.8660254037844313801 ) ) ;
#20851=CARTESIAN_POINT ( 'NONE',  ( 7.786460292950004636, 7.978625184730144149, 1.040834085586084257E-14 ) ) ;
#20852=CARTESIAN_POINT ( 'NONE',  ( 5.463572716182834910, 5.476515711742504067, 0.7216878364870317197 ) ) ;
#20856=CARTESIAN_POINT ( 'NONE',  ( 7.293923454472069245, 11.45340176361870199, 0.7216878364870438212 ) ) ;
#20862=CARTESIAN_POINT ( 'NONE',  ( -3.879604511804807032, 7.677955697080923514, 0.7998128361456341429 ) ) ;
#20863=CARTESIAN_POINT ( 'NONE',  ( -0.7500000000000215383, 3.472916667349487785, 1.299038105676671107 ) ) ;
#20864=CARTESIAN_POINT ( 'NONE',  ( -1.364683531249997417, 5.821875000341418804, 1.214306433183764966E-14 ) ) ;
#20869=CARTESIAN_POINT ( 'NONE',  ( -0.6823417656250212460, 3.363541667008085323, 1.181850606188767472 ) ) ;
#20876=CARTESIAN_POINT ( 'NONE',  ( -7.153898609505128015, 11.49796547773133604, 0.7998128361456481317 ) ) ;
#20877=CARTESIAN_POINT ( 'NONE',  ( 6.331821432781979730, 7.345878745455822312, -1.199719254218445830 ) ) ;
#20879=CARTESIAN_POINT ( 'NONE',  ( -0.6823417656250246877, -0.9489583329919115684, 1.181850606188755259 ) ) ;
#20886=CARTESIAN_POINT ( 'NONE',  ( -7.369020184227459858, 8.555943955475521889, 1.199719254218450271 ) ) ;
#20889=ADVANCED_FACE ( 'NONE', ( #194853 ), #171337, .T. ) ;
#20890=CARTESIAN_POINT ( 'NONE',  ( 8.530051201292206287, 13.10347683481629488, 0.000000000000000000 ) ) ;
#20892=CARTESIAN_POINT ( 'NONE',  ( 8.378048858240820351, 11.86180853700128601, -1.199719254218446718 ) ) ;
#20894=CARTESIAN_POINT ( 'NONE',  ( -4.172158584703340445, 5.890604320285754980, -1.599625672291256295 ) ) ;
#20895=CARTESIAN_POINT ( 'NONE',  ( -7.483210719738908168, 10.81783070874899799, 1.199719254218453823 ) ) ;
#20898=CARTESIAN_POINT ( 'NONE',  ( -4.244195945626527688, 7.512047922924973697, -1.038054094898384294 ) ) ;
#20899=CARTESIAN_POINT ( 'NONE',  ( -1.402160292154681736E-14, -0.6781249996585819728, 1.575800808251672791 ) ) ;
#20903=CARTESIAN_POINT ( 'NONE',  ( 8.161645285746708112, 9.584636257201740506, -1.082531754730543083 ) ) ;
#20906=CARTESIAN_POINT ( 'NONE',  ( 4.632082037363250748, 8.555846143565791095, -0.7998128361456231517 ) ) ;
#20930=CARTESIAN_POINT ( 'NONE',  ( -9.332089804907933939, 9.781859615347734405, 1.040834085586084257E-14 ) ) ;
#20935=CARTESIAN_POINT ( 'NONE',  ( -1.201851678989727383E-14, 1.743750000682815493, 1.732050807568877637 ) ) ;
#20936=CARTESIAN_POINT ( 'NONE',  ( 7.892817981449907982, 12.36003807833360391, 0.7998128361456462443 ) ) ;
#20941=CARTESIAN_POINT ( 'NONE',  ( -9.398826802771548472, 11.98838390803207865, -1.599625672291263179 ) ) ;
#20943=CARTESIAN_POINT ( 'NONE',  ( -1.364683531250000748, 1.759375000341421913, 0.000000000000000000 ) ) ;
#20945=ORIENTED_EDGE ( 'NONE', *, *, #85279, .T. ) ;
#20948=CARTESIAN_POINT ( 'NONE',  ( -9.978437869977950569, 11.70422760547153906, -1.082531754730539753 ) ) ;
#20953=CARTESIAN_POINT ( 'NONE',  ( -1.364683531250000748, -0.1781249996585798634, 0.000000000000000000 ) ) ;
#20958=CARTESIAN_POINT ( 'NONE',  ( -0.6823417656250003738, 1.217708333674752286, -1.181850606188749264 ) ) ;
#20960=CARTESIAN_POINT ( 'NONE',  ( -7.088215381846223906, 7.164006121775713609, 0.7998128361456341429 ) ) ;
#20961=CARTESIAN_POINT ( 'NONE',  ( 6.414979237560321401, 10.63589287712906462, 1.040834085586084257E-14 ) ) ;
#20962=CARTESIAN_POINT ( 'NONE',  ( 4.843287188579786573, 6.673587691474970107, -1.599625672291256517 ) ) ;
#20964=CARTESIAN_POINT ( 'NONE',  ( 6.179819089730593795, 6.104210447640811665, 1.040834085586084257E-14 ) ) ;
#20966=CARTESIAN_POINT ( 'NONE',  ( -1.201851678989727383E-14, 4.087500000000022560, -1.732050807568863648 ) ) ;
#20968=CARTESIAN_POINT ( 'NONE',  ( 0.6823417656249899377, 1.655208333674752730, 1.181850606188755259 ) ) ;
#20975=CARTESIAN_POINT ( 'NONE',  ( 4.677199807034550183, 8.400557508274889784, 1.040834085586084257E-14 ) ) ;
#20978=CARTESIAN_POINT ( 'NONE',  ( -7.503547950159405566, 10.84155747757291266, 1.199719254218453823 ) ) ;
#20979=CARTESIAN_POINT ( 'NONE',  ( -4.578903193113314174, 6.365139696764064325, 1.599625672291267398 ) ) ;
#20982=CARTESIAN_POINT ( 'NONE',  ( -1.126385703232235747, 3.299232110657536410, -0.7749999999999935829 ) ) ;
#20984=CARTESIAN_POINT ( 'NONE',  ( -8.066738210006693777, 10.43428054980638997, 1.443375672974090751 ) ) ;
#20986=CARTESIAN_POINT ( 'NONE',  ( -1.001543065824772872E-14, 4.712500000000017231, 1.732050807568877637 ) ) ;
#20990=CARTESIAN_POINT ( 'NONE',  ( 7.768458830950378591, 12.00702636951006497, 1.040834085586084257E-14 ) ) ;
#20991=CARTESIAN_POINT ( 'NONE',  ( -6.120066830577914452, 5.977401641919705355, -0.003186534051367873044 ) ) ;
#20992=AXIS2_PLACEMENT_3D ( 'NONE', #108520, #208069, #209127 ) ;
#21003=CARTESIAN_POINT ( 'NONE',  ( 8.229436053370669413, 10.62409470039771442, 1.443375672974076540 ) ) ;
#21004=CARTESIAN_POINT ( 'NONE',  ( 7.786460292950004636, 7.978625184730144149, 1.040834085586084257E-14 ) ) ;
#21005=CARTESIAN_POINT ( 'NONE',  ( -5.229694566569281555, 7.124396299129368337, 1.599625672291267398 ) ) ;
#21008=CARTESIAN_POINT ( 'NONE',  ( -1.402160292154681736E-14, -0.6156249996585817508, 1.575800808251672791 ) ) ;
#21009=CARTESIAN_POINT ( 'NONE',  ( 2.575685996916329046, 5.948791396470269888, 0.7216878364870438212 ) ) ;
#21011=CARTESIAN_POINT ( 'NONE',  ( -2.435661151949389147, 5.993355110582911038, 0.7998128361456341429 ) ) ;
#21029=CARTESIAN_POINT ( 'NONE',  ( 8.015895134177609904, 10.37496362800581018, 1.599625672291281386 ) ) ;
#21041=CARTESIAN_POINT ( 'NONE',  ( -5.656776405399756236, 7.622658444431597680, -1.599625672291256295 ) ) ;
#21044=CARTESIAN_POINT ( 'NONE',  ( -4.548924232584923288, 5.265832011892554121, -1.199719254218446718 ) ) ;
#21049=DIRECTION ( 'NONE',  ( 0.000000000000000000, 1.000000000000000000, 0.000000000000000000 ) ) ;
#21053=CARTESIAN_POINT ( 'NONE',  ( -4.925689880466507908, 4.641059703499347044, -0.7998128361456221525 ) ) ;
#21056=CARTESIAN_POINT ( 'NONE',  ( 7.775764792637399836, 9.030479331953833011, -1.199719254218441611 ) ) ;
#21057=CARTESIAN_POINT ( 'NONE',  ( -1.364683531250010740, 4.780208333674755394, 0.7879004041258379498 ) ) ;
#21063=CARTESIAN_POINT ( 'NONE',  ( 5.843201017365476702, 6.879784610756938257, -1.082531754730543083 ) ) ;
#21064=CARTESIAN_POINT ( 'NONE',  ( -6.344325816190970357, 9.489131654609717970, 1.199719254218452047 ) ) ;
#21067=CARTESIAN_POINT ( 'NONE',  ( -6.669721502918952716, 9.868759955792373972, 1.199719254218452047 ) ) ;
#21068=CARTESIAN_POINT ( 'NONE',  ( -6.247609857798938293, 6.183299677053865295, -0.7998128361456291469 ) ) ;
#21074=CARTESIAN_POINT ( 'NONE',  ( 7.949158136313996259, 8.168439335321471262, 1.040834085586084257E-14 ) ) ;
#21088=CARTESIAN_POINT ( 'NONE',  ( -1.364683531250014514, -1.157291666325248158, 0.7879004041258379498 ) ) ;
#21089=CARTESIAN_POINT ( 'NONE',  ( 3.497113557321089861, 6.167384019261527683, -1.199719254218446718 ) ) ;
#21090=CARTESIAN_POINT ( 'NONE',  ( 5.738125327081736060, 7.717565519727259904, 1.599625672291267398 ) ) ;
#21092=CARTESIAN_POINT ( 'NONE',  ( -8.405692050792730186, 9.869357483088723626, 1.082531754730558626 ) ) ;
#21094=CARTESIAN_POINT ( 'NONE',  ( 6.832946231607457399, 7.074118146404578589, -0.7216878364870257245 ) ) ;
#21095=CARTESIAN_POINT ( 'NONE',  ( -7.822691444960700125, 11.10992853822074444, -1.082531754730543083 ) ) ;
#21099=CARTESIAN_POINT ( 'NONE',  ( 9.074484886248265880, 9.481320543578137361, 0.7998128361456462443 ) ) ;
#21104=CARTESIAN_POINT ( 'NONE',  ( -1.402160292154681736E-14, 2.196875000341423689, -1.575800808251660134 ) ) ;
#21110=CARTESIAN_POINT ( 'NONE',  ( 8.178592977541601527, 10.56477777859713463, 1.599625672291281386 ) ) ;
#21113=CARTESIAN_POINT ( 'NONE',  ( -6.991200766141138168, 11.30815132714001159, 0.7998128361456481317 ) ) ;
#21117=CARTESIAN_POINT ( 'NONE',  ( -0.4634916963857253491, 7.369626292149035862, -4.459501722865316431 ) ) ;
#21119=CARTESIAN_POINT ( 'NONE',  ( 9.459838494033030898, 12.05956421450382088, 1.599625672291281386 ) ) ;
#21123=CARTESIAN_POINT ( 'NONE',  ( -10.00321840878439339, 10.56484298653695397, 1.040834085586084257E-14 ) ) ;
#21130=CARTESIAN_POINT ( 'NONE',  ( 5.849792259110643933, 6.002811869646802911, -0.3480847251615213356 ) ) ;
#21131=CARTESIAN_POINT ( 'NONE',  ( 1.244150428498992600, 3.277476754118171964, -0.7749999999999874767 ) ) ;
#21132=CARTESIAN_POINT ( 'NONE',  ( -3.567766978690493307, 7.314145241780881435, 1.040834085586084257E-14 ) ) ;
#21137=CARTESIAN_POINT ( 'NONE',  ( 5.777746017718023097, 9.892454120646377191, 0.7998128361456462443 ) ) ;
#21139=CARTESIAN_POINT ( 'NONE',  ( 6.612626235163189925, 8.737816579155630592, -1.599625672291262513 ) ) ;
#21140=CARTESIAN_POINT ( 'NONE',  ( 5.684946482831785275, 5.526859072925533134, -0.7998128361456231517 ) ) ;
#21142=CARTESIAN_POINT ( 'NONE',  ( -7.700668062882072284, 10.00719871149432549, -1.443375672974059665 ) ) ;
#21149=CARTESIAN_POINT ( 'NONE',  ( -5.251027302601237956, 6.428042375187708934, -1.158707231040608576 ) ) ;
#21151=CARTESIAN_POINT ( 'NONE',  ( 4.015246738442954211, 7.790260991562450776, 0.2862651747304548744 ) ) ;
#21152=CARTESIAN_POINT ( 'NONE',  ( 6.005898861173831094, 6.109229547565340646, 1.040834085586084257E-14 ) ) ;
#21158=CARTESIAN_POINT ( 'NONE',  ( -10.26315909542058336, 11.07603315418659840, -0.7216878364870267237 ) ) ;
#21165=ORIENTED_EDGE ( 'NONE', *, *, #202366, .T. ) ;
#21176=CARTESIAN_POINT ( 'NONE',  ( 8.959240580532112475, 9.346868853575953651, -0.7998128361456221525 ) ) ;
#21178=ORIENTED_EDGE ( 'NONE', *, *, #206094, .T. ) ;
#21180=CARTESIAN_POINT ( 'NONE',  ( -1.500000000000013101, 1.910416667349488451, -0.8660254037844313801 ) ) ;
#21182=CARTESIAN_POINT ( 'NONE',  ( -4.530395885260773525, 8.437212299446219532, 0.7998128361456481317 ) ) ;
#21186=CARTESIAN_POINT ( 'NONE',  ( -10.15913717534155047, 10.74674821418697057, 0.7998128361456462443 ) ) ;
#21189=CARTESIAN_POINT ( 'NONE',  ( 6.287230548435207567, 8.358188277972981695, -1.599625672291262513 ) ) ;
#21191=CARTESIAN_POINT ( 'NONE',  ( -7.888146445052511169, 8.097259028849730811, 1.040834085586084257E-14 ) ) ;
#21193=CARTESIAN_POINT ( 'NONE',  ( 9.043452155515161905, 10.50944792197790889, 1.199719254218453823 ) ) ;
#21194=CARTESIAN_POINT ( 'NONE',  ( -1.364683531250010295, 5.530208333674751842, 0.7879004041258379498 ) ) ;
#21196=CARTESIAN_POINT ( 'NONE',  ( -4.816538118508267630, 5.092449105792602460, -0.9495590845017554127 ) ) ;
#21201=CARTESIAN_POINT ( 'NONE',  ( -8.080296364064746939, 9.489729181906076505, 1.082531754730558626 ) ) ;
#21204=CARTESIAN_POINT ( 'NONE',  ( 1.364683531249988535, 4.217708333674752730, -0.7879004041258239610 ) ) ;
#21212=CARTESIAN_POINT ( 'NONE',  ( -3.090895833791289071, 6.549869539491048442, 1.040834085586084257E-14 ) ) ;
#21214=CARTESIAN_POINT ( 'NONE',  ( 3.429849674132933846, 5.024577257953626308, -1.443375672974058777 ) ) ;
#21215=CARTESIAN_POINT ( 'NONE',  ( -1.364683531250012516, 5.051041667008085767, -0.7879004041258300672 ) ) ;
#21216=CARTESIAN_POINT ( 'NONE',  ( -8.967828540435322182, 12.54988483289483980, 1.199719254218462483 ) ) ;
#21220=CARTESIAN_POINT ( 'NONE',  ( -1.201851678989727383E-14, 1.071875000341418138, 1.575800808251672791 ) ) ;
#21221=CARTESIAN_POINT ( 'NONE',  ( -4.785665035943912571, 4.685623418130398399, 1.214306433183764966E-14 ) ) ;
#21222=CARTESIAN_POINT ( 'NONE',  ( 5.847644326195776010, 5.716673223516856694, -0.7998128361456281477 ) ) ;
#21225=CARTESIAN_POINT ( 'NONE',  ( 4.772106882330221289, 6.590544000850480089, -1.443375672974051449 ) ) ;
#21229=CARTESIAN_POINT ( 'NONE',  ( 3.226477370372305753, 4.787309570232886280, 1.443375672974062551 ) ) ;
#21230=CARTESIAN_POINT ( 'NONE',  ( 10.18181017373857067, 11.94149529319227909, 1.082531754730548412 ) ) ;
#21232=CARTESIAN_POINT ( 'NONE',  ( -9.015808963407680565, 9.620791333504852716, 1.040834085586084257E-14 ) ) ;
#21237=CARTESIAN_POINT ( 'NONE',  ( -9.833741488613570780, 10.36711991300432345, 0.7998128361456462443 ) ) ;
#21238=CARTESIAN_POINT ( 'NONE',  ( -5.056828107772866510, 5.962349549565537643, -1.082531754730543971 ) ) ;
#21239=CARTESIAN_POINT ( 'NONE',  ( 0.6823417656249899377, 1.655208333674752730, 1.181850606188755259 ) ) ;
#21245=CARTESIAN_POINT ( 'NONE',  ( 9.911173986789782120, 11.52179005846497972, -1.199719254218440723 ) ) ;
#21247=ORIENTED_EDGE ( 'NONE', *, *, #191462, .F. ) ;
#21260=CARTESIAN_POINT ( 'NONE',  ( 2.535011536075336913, 5.133042487381361596, -2.419999999999995044 ) ) ;
#21262=DIRECTION ( 'NONE',  ( -0.7592566023653004592, -0.6507913734559639396, -0.000000000000000000 ) ) ;
#21263=CARTESIAN_POINT ( 'NONE',  ( -1.364683531249997417, 3.071875000341423245, 1.214306433183764966E-14 ) ) ;
#21265=ADVANCED_FACE ( 'NONE', ( #6232 ), #72939, .T. ) ;
#21272=CARTESIAN_POINT ( 'NONE',  ( 0.000000000000000000, 2.800000000000024691, -0.7749999999999935829 ) ) ;
#21274=CARTESIAN_POINT ( 'NONE',  ( -1.364683531250000748, 1.259375000341421469, 0.000000000000000000 ) ) ;
#21283=ORIENTED_EDGE ( 'NONE', *, *, #113401, .T. ) ;
#21285=CARTESIAN_POINT ( 'NONE',  ( 4.547870462380197765, 7.393267075163835855, 1.199719254218462483 ) ) ;
#21293=CARTESIAN_POINT ( 'NONE',  ( 6.662942426112080874, 9.860851032851066122, 1.199719254218460707 ) ) ;
#21295=ORIENTED_EDGE ( 'NONE', *, *, #201653, .T. ) ;
#21297=CARTESIAN_POINT ( 'NONE',  ( -4.810445574750349174, 4.506608013497163334, 0.7998128361456341429 ) ) ;
#21298=CARTESIAN_POINT ( 'NONE',  ( 7.609150525767641504, 9.900428251527500834, -1.599625672291262513 ) ) ;
#21310=CARTESIAN_POINT ( 'NONE',  ( -7.700668062882072284, 10.00719871149432549, -1.443375672974059665 ) ) ;
#21314=CARTESIAN_POINT ( 'NONE',  ( -10.32183501870554387, 10.93656236477829502, 0.7998128361456462443 ) ) ;
#21319=CARTESIAN_POINT ( 'NONE',  ( -3.110706179331648169, 5.716575411607132118, 1.199719254218462483 ) ) ;
#21321=CARTESIAN_POINT ( 'NONE',  ( 7.886038904643079661, 12.35212915539230139, -0.7998128361456352531 ) ) ;
#21322=CARTESIAN_POINT ( 'NONE',  ( 5.040934186182656873, 4.775511393501539636, 1.040834085586084257E-14 ) ) ;
#21328=CARTESIAN_POINT ( 'NONE',  ( 2.711267533052988732, 6.106969855296372707, -0.7216878364870267237 ) ) ;
#21331=CARTESIAN_POINT ( 'NONE',  ( -4.578903193113314174, 6.365139696764064325, 1.599625672291267398 ) ) ;
#21334=CARTESIAN_POINT ( 'NONE',  ( -9.053093885623068715, 11.58502883802551153, -1.599625672291263179 ) ) ;
#21339=CARTESIAN_POINT ( 'NONE',  ( 6.954969614130424027, 11.05795561655343384, 1.040834085586084257E-14 ) ) ;
#21340=CARTESIAN_POINT ( 'NONE',  ( -0.6823417656250212460, 3.613541667008085767, 1.181850606188767472 ) ) ;
#21342=CARTESIAN_POINT ( 'NONE',  ( 5.183294799126148433, 4.941598775268944976, 1.040834085586084257E-14 ) ) ;
#21348=CARTESIAN_POINT ( 'NONE',  ( 1.123270288250311610, 3.172697346350006331, 0.7749999999993734123 ) ) ;
#21352=CARTESIAN_POINT ( 'NONE',  ( 4.161989969715272686, 4.726297878971393196, 2.420000000000010587 ) ) ;
#21355=ORIENTED_EDGE ( 'NONE', *, *, #65262, .F. ) ;
#21357=CARTESIAN_POINT ( 'NONE',  ( -1.364683531250012516, 3.092708333674755838, 0.7879004041258379498 ) ) ;
#21359=CARTESIAN_POINT ( 'NONE',  ( 8.516493047678546091, 13.08765898893368629, -0.7998128361456352531 ) ) ;
#21361=CARTESIAN_POINT ( 'NONE',  ( -5.599154252763867134, 5.634694171087028636, 0.000000000000000000 ) ) ;
#21363=CARTESIAN_POINT ( 'NONE',  ( -5.707619481228822345, 7.681975366232176583, -1.443375672974051449 ) ) ;
#21368=CARTESIAN_POINT ( 'NONE',  ( 5.066996723205273057, 6.934582148538044777, 1.599625672291267398 ) ) ;
#21374=DIRECTION ( 'NONE',  ( 1.000000000000000000, -5.578564026256504688E-16, 0.000000000000000000 ) ) ;
#21378=CARTESIAN_POINT ( 'NONE',  ( 4.333802657862601215, 8.207853534148366492, 0.7998128361456462443 ) ) ;
#21383=CARTESIAN_POINT ( 'NONE',  ( -7.223796917982883592, 7.322184580601816428, -0.7998128361456291469 ) ) ;
#21387=CARTESIAN_POINT ( 'NONE',  ( 7.613066949273408213, 8.840665181362512115, -1.199719254218441611 ) ) ;
#21390=CARTESIAN_POINT ( 'NONE',  ( -6.551614543901706611, 8.666636272683888365, 1.599625672291283607 ) ) ;
#21391=CARTESIAN_POINT ( 'NONE',  ( 5.612712405933139692, 9.491988873656591608, 1.040834085586084257E-14 ) ) ;
#21392=CARTESIAN_POINT ( 'NONE',  ( 4.798800619506367049, 6.970516071510092893, 1.407892184351482889 ) ) ;
#21393=CARTESIAN_POINT ( 'NONE',  ( -3.164938793786285842, 5.779846795137578930, -1.199719254218452935 ) ) ;
#21396=CARTESIAN_POINT ( 'NONE',  ( -5.738125327081750271, 7.717565519727259904, 1.599625672291269396 ) ) ;
#21400=CARTESIAN_POINT ( 'NONE',  ( -1.364683531250012516, 1.780208333674757615, 0.7879004041258379498 ) ) ;
#21402=CARTESIAN_POINT ( 'NONE',  ( -5.761852096127856981, 5.824508321678349532, 0.000000000000000000 ) ) ;
#21408=CARTESIAN_POINT ( 'NONE',  ( 4.808338034340912337, 8.761478140039733020, 1.040834085586084257E-14 ) ) ;
#21410=CARTESIAN_POINT ( 'NONE',  ( -5.912397865540070185, 5.999963284693008880, 0.01096864257240509621 ) ) ;
#21411=CARTESIAN_POINT ( 'NONE',  ( 1.364683531249990311, 3.196875000341416140, 1.214306433183764966E-14 ) ) ;
#21414=CARTESIAN_POINT ( 'NONE',  ( 1.364683531249986537, -0.8239583329919186738, 0.7879004041258500513 ) ) ;
#21418=CARTESIAN_POINT ( 'NONE',  ( -4.731959306369413198, 5.479372931307791461, -1.199719254218446718 ) ) ;
#21419=CARTESIAN_POINT ( 'NONE',  ( -6.033015167956794933, 9.982342096017511324, -0.7216878364870267237 ) ) ;
#21427=CARTESIAN_POINT ( 'NONE',  ( -8.324343128666356506, 8.814081192973304724, 1.040834085586084257E-14 ) ) ;
#21431=CARTESIAN_POINT ( 'NONE',  ( -7.822691444960716112, 8.228820895316715678, -0.7216878364870267237 ) ) ;
#21445=CARTESIAN_POINT ( 'NONE',  ( -4.367698041896780126, 8.247398148854895084, 0.7998128361456481317 ) ) ;
#21446=CARTESIAN_POINT ( 'NONE',  ( 3.023105066167310895, 5.702484939155337607, -2.419999999999995044 ) ) ;
#21447=CARTESIAN_POINT ( 'NONE',  ( 4.009460741339333723, 5.700790169694431420, -1.599625672291256295 ) ) ;
#21448=CIRCLE ( 'NONE', #142580, 0.07999999999999991840 ) ;
#21452=CARTESIAN_POINT ( 'NONE',  ( 5.819474248763732760, 7.812472595022922128, -1.599625672291262513 ) ) ;
#21457=CARTESIAN_POINT ( 'NONE',  ( -3.945059511896602089, 7.546393830613923548, 1.040834085586084257E-14 ) ) ;
#21460=CARTESIAN_POINT ( 'NONE',  ( -4.278334434596112068, 3.985349064379731576, -0.2033706498285611231 ) ) ;
#21464=CARTESIAN_POINT ( 'NONE',  ( -1.201851678989727383E-14, 1.071875000341418138, 1.575800808251672791 ) ) ;
#21465=CARTESIAN_POINT ( 'NONE',  ( -6.471393748265538370, 5.229711127717889596, -2.419999999999995044 ) ) ;
#21466=CARTESIAN_POINT ( 'NONE',  ( -6.855619230004478482, 11.14997286831390788, -0.7998128361456291469 ) ) ;
#21468=CARTESIAN_POINT ( 'NONE',  ( 6.096362627639171805, 10.26417349888772179, -0.7998128361456291469 ) ) ;
#21470=CARTESIAN_POINT ( 'NONE',  ( -8.227100285394159940, 8.492705175914988303, 0.7998128361456602331 ) ) ;
#21473=CARTESIAN_POINT ( 'NONE',  ( -1.201851678989727383E-14, 4.946875000341420581, -1.575800808251660134 ) ) ;
#21475=CARTESIAN_POINT ( 'NONE',  ( 6.954969614130424027, 11.05795561655343384, 1.040834085586084257E-14 ) ) ;
#21478=CARTESIAN_POINT ( 'NONE',  ( 0.6823417656249882723, -0.09479166632524876901, 1.181850606188755259 ) ) ;
#21481=CARTESIAN_POINT ( 'NONE',  ( 8.120970824461352322, 9.537182719035495637, -1.082531754730543083 ) ) ;
#21483=CARTESIAN_POINT ( 'NONE',  ( 6.520158902582616101, 5.290451655907108197, 2.438235897557466281 ) ) ;
#21484=CARTESIAN_POINT ( 'NONE',  ( -5.178851490740209229, 7.065079377328788546, 1.443375672974064550 ) ) ;
#21486=CARTESIAN_POINT ( 'NONE',  ( -1.364683531250012516, 3.238541667008084879, -0.7879004041258289570 ) ) ;
#21490=CARTESIAN_POINT ( 'NONE',  ( -4.530395885260773525, 8.437212299446219532, 0.7998128361456481317 ) ) ;
#21491=CARTESIAN_POINT ( 'NONE',  ( -1.201851678989727383E-14, 5.759375000341417028, -1.575800808251660801 ) ) ;
#21499=CARTESIAN_POINT ( 'NONE',  ( 7.934546212495622086, 10.28005655271014795, -1.599625672291262513 ) ) ;
#21505=VERTEX_POINT ( 'NONE', #97687 ) ;
#21506=CARTESIAN_POINT ( 'NONE',  ( 6.697364695470787943, 7.876308901879812474, -1.082531754730543083 ) ) ;
#21511=CARTESIAN_POINT ( 'NONE',  ( 1.499999999999987121, 0.7958333333333510451, -0.8660254037844253849 ) ) ;
#21512=CARTESIAN_POINT ( 'NONE',  ( 6.913768267964901071, 10.15348118167935709, -1.199719254218441611 ) ) ;
#21513=CARTESIAN_POINT ( 'NONE',  ( -8.045874094706015001, 11.47427131287732927, -1.199719254218446718 ) ) ;
#21515=CARTESIAN_POINT ( 'NONE',  ( -1.402160292154681736E-14, -0.6781249996585819728, 1.575800808251672791 ) ) ;
#21516=EDGE_LOOP ( 'NONE', ( #109719, #67136, #1048, #182706 ) ) ;
#21517=CARTESIAN_POINT ( 'NONE',  ( -0.7500000000000215383, 0.9416666666666878571, 1.299038105676659116 ) ) ;
#21519=CARTESIAN_POINT ( 'NONE',  ( 3.811813743736467419, 7.598866467667865443, 1.040834085586084257E-14 ) ) ;
#21527=CARTESIAN_POINT ( 'NONE',  ( -1.201851678989727383E-14, 5.696875000341416140, -1.575800808251660134 ) ) ;
#21530=CARTESIAN_POINT ( 'NONE',  ( -8.320953590485107298, 10.73086516036454618, 1.599625672291269396 ) ) ;
#21531=CARTESIAN_POINT ( 'NONE',  ( -4.880572111239580124, 7.677455982212699759, 1.082531754730560403 ) ) ;
#21540=CARTESIAN_POINT ( 'NONE',  ( 6.588372581236919601, 9.773852880496709972, -1.199719254218440723 ) ) ;
#21543=CARTESIAN_POINT ( 'NONE',  ( 7.904040366642699489, 8.323727970612377902, 0.7216878364870458196 ) ) ;
#21546=CARTESIAN_POINT ( 'NONE',  ( -7.483210719738908168, 10.81783070874899799, 1.199719254218453823 ) ) ;
#21547=CARTESIAN_POINT ( 'NONE',  ( 5.035963992472171746, 7.962709526937818083, 1.199719254218462483 ) ) ;
#21548=PLANE ( 'NONE',  #204533 ) ;
#21549=CARTESIAN_POINT ( 'NONE',  ( 4.351804119862229037, 4.179452349368450115, -0.7216878364870188411 ) ) ;
#21550=CARTESIAN_POINT ( 'NONE',  ( -1.420000000000056550, 7.388542872122504157, -4.154462424328204229 ) ) ;
#21551=CARTESIAN_POINT ( 'NONE',  ( 4.220665892555866883, 3.818531717603609987, -0.7998128361456211532 ) ) ;
#21552=VERTEX_POINT ( 'NONE', #32659 ) ;
#21559=EDGE_CURVE ( 'NONE', #189420, #63704, #191329, .T. ) ;
#21560=CARTESIAN_POINT ( 'NONE',  ( -4.107757355260591936, 7.736207981205250661, 1.040834085586084257E-14 ) ) ;
#21561=CARTESIAN_POINT ( 'NONE',  ( 9.029367117021314115, 12.51771682229149008, -1.082531754730543083 ) ) ;
#21564=CARTESIAN_POINT ( 'NONE',  ( -6.880926654135487652, 7.986501503701545879, 1.199719254218450271 ) ) ;
#21568=CARTESIAN_POINT ( 'NONE',  ( -7.857113714319432063, 9.125386407249497012, 1.199719254218462483 ) ) ;
#21583=CARTESIAN_POINT ( 'NONE',  ( -5.696397096036042385, 9.797547045350714967, -0.7998128361456231517 ) ) ;
#21586=CARTESIAN_POINT ( 'NONE',  ( 6.670248388243460447, 6.884303995813253252, -0.7216878364870257245 ) ) ;
#21592=CARTESIAN_POINT ( 'NONE',  ( -5.005985031943793295, 6.863401842066301661, -1.599625672291256295 ) ) ;
#21596=CARTESIAN_POINT ( 'NONE',  ( -6.392833124043511894, 7.417059051927569868, 1.199719254218450271 ) ) ;
#21597=CARTESIAN_POINT ( 'NONE',  ( 1.084637062511527361, 3.307371192708035590, -1.105835307554789759 ) ) ;
#21602=CARTESIAN_POINT ( 'NONE',  ( -9.124801077197171040, 10.60435499727357289, -1.199719254218441611 ) ) ;
#21603=CARTESIAN_POINT ( 'NONE',  ( 5.764187864104357573, 9.876636274763768597, 1.040834085586084257E-14 ) ) ;
#21606=CARTESIAN_POINT ( 'NONE',  ( -9.378489572351046633, 11.96465713920816043, -1.599625672291263179 ) ) ;
#21610=VERTEX_POINT ( 'NONE', #17450 ) ;
#21612=CARTESIAN_POINT ( 'NONE',  ( 7.931156674314368438, 12.19684052010138586, 1.040834085586084257E-14 ) ) ;
#21620=CARTESIAN_POINT ( 'NONE',  ( -0.5448033855394223135, 6.555371112116565868, -3.373828149488691253 ) ) ;
#21631=CARTESIAN_POINT ( 'NONE',  ( -4.731959306369413198, 5.479372931307791461, -1.199719254218446718 ) ) ;
#21639=CARTESIAN_POINT ( 'NONE',  ( 1.499999999999987121, -0.9645833326505173222, 0.8660254037844524744 ) ) ;
#21643=CARTESIAN_POINT ( 'NONE',  ( 2.838652716839808576, 6.463511936288419690, 0.1785095769484796591 ) ) ;
#21645=CARTESIAN_POINT ( 'NONE',  ( 1.499999999999819256, 7.176846818246210624, -4.202462424328214041 ) ) ;
#21648=CARTESIAN_POINT ( 'NONE',  ( -3.131570295076647525, 6.597323077657299528, 1.040834085586084257E-14 ) ) ;
#21649=CARTESIAN_POINT ( 'NONE',  ( 4.566398809704347528, 4.221886787610169556, -0.7998128361456211532 ) ) ;
#21654=CARTESIAN_POINT ( 'NONE',  ( 5.983225862332436584, 5.874851682342960402, 0.7998128361456341429 ) ) ;
#21655=CARTESIAN_POINT ( 'NONE',  ( -0.6823417656250003738, 2.280208333674753174, -1.181850606188749264 ) ) ;
#21656=ADVANCED_FACE ( 'NONE', ( #65140 ), #13393, .T. ) ;
#21657=CARTESIAN_POINT ( 'NONE',  ( -4.409122955247444686, 7.142713865425108111, 1.076920909521961622 ) ) ;
#21658=CARTESIAN_POINT ( 'NONE',  ( 9.459838494033030898, 12.05956421450382088, 1.599625672291281386 ) ) ;
#21660=CARTESIAN_POINT ( 'NONE',  ( -8.941766003412679353, 10.39081407785832845, -1.199719254218446718 ) ) ;
#21661=CARTESIAN_POINT ( 'NONE',  ( -5.734735788456164940, 5.792872629394710593, 0.7216878364870317197 ) ) ;
#21664=CARTESIAN_POINT ( 'NONE',  ( -6.566226467720086113, 6.555019055295208119, 1.040834085586084257E-14 ) ) ;
#21666=CARTESIAN_POINT ( 'NONE',  ( 1.499999999999985123, -0.9229166659838452524, -0.8660254037844323793 ) ) ;
#21674=CARTESIAN_POINT ( 'NONE',  ( -4.378920427089552092, 8.052564898339037214, 0.7216878364870317197 ) ) ;
#21675=DIRECTION ( 'NONE',  ( -0.6507913734559640506, -0.7592566023653004592, 0.000000000000000000 ) ) ;
#21676=FACE_OUTER_BOUND ( 'NONE', #108148, .T. ) ;
#21678=CARTESIAN_POINT ( 'NONE',  ( -3.755245360860925086, 6.364574773437617239, -1.082531754730548412 ) ) ;
#21680=CARTESIAN_POINT ( 'NONE',  ( 9.420217803396747414, 9.884675613584706255, 0.7998128361456462443 ) ) ;
#21686=ORIENTED_EDGE ( 'NONE', *, *, #186211, .F. ) ;
#21690=CARTESIAN_POINT ( 'NONE',  ( -9.646789991323334590, 11.21334206375407305, 1.199719254218462483 ) ) ;
#21696=CARTESIAN_POINT ( 'NONE',  ( 6.063521013809720195, 8.097193820909906137, 1.599625672291281386 ) ) ;
#21699=VERTEX_POINT ( 'NONE', #48926 ) ;
#21700=CYLINDRICAL_SURFACE ( 'NONE', #190671, 0.08000000000000041800 ) ;
#21701=CARTESIAN_POINT ( 'NONE',  ( 4.325214697959421706, 5.004837554829479451, 1.199719254218462483 ) ) ;
#21712=CARTESIAN_POINT ( 'NONE',  ( 9.284636267260101050, 9.726497154758602548, -0.7998128361456281477 ) ) ;
#21714=CARTESIAN_POINT ( 'NONE',  ( -4.062639585589296942, 7.891496616496157301, 0.7998128361456341429 ) ) ;
#21721=CARTESIAN_POINT ( 'NONE',  ( 1.364683531249990311, 5.134375000341417916, 1.214306433183764966E-14 ) ) ;
#21726=DIRECTION ( 'NONE',  ( 0.7592566023653004592, 0.6507913734559639396, 0.000000000000000000 ) ) ;
#21727=CARTESIAN_POINT ( 'NONE',  ( 4.813308228051395687, 5.574280006603454574, 1.199719254218462483 ) ) ;
#21728=CARTESIAN_POINT ( 'NONE',  ( -3.249150368769345043, 6.942425863539538611, 0.7998128361456341429 ) ) ;
#21729=CARTESIAN_POINT ( 'NONE',  ( 3.019342412789784547, 6.452475500722323787, 0.1501914610189964416 ) ) ;
#21735=CARTESIAN_POINT ( 'NONE',  ( 5.260200412422194383, 7.159986452624450770, -1.443375672974051449 ) ) ;
#21737=CARTESIAN_POINT ( 'NONE',  ( 6.426201622753093368, 10.44105962661321563, 1.040834085586084257E-14 ) ) ;
#21738=CARTESIAN_POINT ( 'NONE',  ( 0.6823417656249899377, 3.488541667008085323, -1.181850606188754593 ) ) ;
#21740=CARTESIAN_POINT ( 'NONE',  ( 4.134873662043553111, 7.767843672452050541, -0.7216878364870197293 ) ) ;
#21742=CARTESIAN_POINT ( 'NONE',  ( -0.02984615528259876305, 7.053682067332115224, -3.954834431657083371 ) ) ;
#21749=CARTESIAN_POINT ( 'NONE',  ( -5.328671718129330159, 6.540706332611327944, 1.372188321006672540 ) ) ;
#21755=CARTESIAN_POINT ( 'NONE',  ( -8.992082194361570302, 11.51384853155376220, 1.599625672291269396 ) ) ;
#21760=FACE_OUTER_BOUND ( 'NONE', #172155, .T. ) ;
#21763=EDGE_LOOP ( 'NONE', ( #111698, #171731, #28810, #155056, #176706 ) ) ;
#21765=CARTESIAN_POINT ( 'NONE',  ( 2.548569689688999329, 5.917155704705049146, -0.7216878364870267237 ) ) ;
#21766=CARTESIAN_POINT ( 'NONE',  ( 0.6823417656249899377, 3.488541667008085323, -1.181850606188754593 ) ) ;
#21768=CARTESIAN_POINT ( 'NONE',  ( 7.613066949273408213, 8.840665181362512115, -1.199719254218441611 ) ) ;
#21769=CARTESIAN_POINT ( 'NONE',  ( -9.236128959407555072, 11.79856975744075598, -1.599625672291263179 ) ) ;
#21770=CARTESIAN_POINT ( 'NONE',  ( -4.765854690403601879, 5.518917546014321829, 1.199719254218462483 ) ) ;
#21771=LINE ( 'NONE', #55378, #206684 ) ;
#21774=CARTESIAN_POINT ( 'NONE',  ( -0.7500000000000215383, 4.191666666666690411, 1.299038105676671107 ) ) ;
#21775=CARTESIAN_POINT ( 'NONE',  ( 5.983225862332436584, 5.874851682342960402, 0.7998128361456341429 ) ) ;
#21778=DIRECTION ( 'NONE',  ( 1.000000000000000000, 0.000000000000000000, 0.000000000000000000 ) ) ;
#21779=CARTESIAN_POINT ( 'NONE',  ( 1.364683531249988535, 3.363541667008084879, 0.7879004041258500513 ) ) ;
#21782=CARTESIAN_POINT ( 'NONE',  ( 7.931156674314368438, 12.19684052010138586, 1.040834085586084257E-14 ) ) ;
#21787=CARTESIAN_POINT ( 'NONE',  ( 1.499999999999987121, 1.535416667349486453, 0.8660254037844524744 ) ) ;
#21789=CARTESIAN_POINT ( 'NONE',  ( -6.043183783389232566, 8.073467052085995022, 1.599625672291269396 ) ) ;
#21790=CARTESIAN_POINT ( 'NONE',  ( 5.653386866774156694, 5.697965554099049257, -0.7216878364870207285 ) ) ;
#21800=CARTESIAN_POINT ( 'NONE',  ( 7.470706336329915764, 8.674577799595093452, -1.199719254218441611 ) ) ;
#21801=CARTESIAN_POINT ( 'NONE',  ( 5.834086172582112262, 5.700855377634248100, 1.040834085586084257E-14 ) ) ;
#21805=CARTESIAN_POINT ( 'NONE',  ( 5.352771719296971042, 5.139321848801576387, 0.7998128361456341429 ) ) ;
#21813=CARTESIAN_POINT ( 'NONE',  ( 8.757677159423465696, 12.30470822171437284, 1.199719254218450271 ) ) ;
#21818=CARTESIAN_POINT ( 'NONE',  ( 5.782412516234797017, 6.044064802175099338, 0.5499171889626064402 ) ) ;
#21824=CARTESIAN_POINT ( 'NONE',  ( -5.896220218617790110, 6.102442225045867197, -0.7164689422466080648 ) ) ;
#21825=CARTESIAN_POINT ( 'NONE',  ( 6.290620087060792009, 10.28288116830553101, -0.7216878364870267237 ) ) ;
#21827=CARTESIAN_POINT ( 'NONE',  ( -5.088387723830502196, 4.830873854090670605, -0.7998128361456221525 ) ) ;
#21832=CARTESIAN_POINT ( 'NONE',  ( -6.064574784014443942, 5.969758757638621738, -0.7998128361456291469 ) ) ;
#21834=CARTESIAN_POINT ( 'NONE',  ( -3.600749563572741785, 3.160087278256925813, 2.499999999999998668 ) ) ;
#21839=CARTESIAN_POINT ( 'NONE',  ( -3.941149012854040290, 4.002721280689181427, -0.7037892630772435432 ) ) ;
#21844=CARTESIAN_POINT ( 'NONE',  ( 7.899597058256738968, 12.36794700127490820, 1.040834085586084257E-14 ) ) ;
#21848=AXIS2_PLACEMENT_3D ( 'NONE', #51394, #202940, #88153 ) ;
#21853=CARTESIAN_POINT ( 'NONE',  ( -10.14113571334194930, 10.93367254176152059, -0.7216878364870267237 ) ) ;
#21857=CARTESIAN_POINT ( 'NONE',  ( 7.914208982075123799, 10.25632978388623684, -1.599625672291262513 ) ) ;
#21861=CARTESIAN_POINT ( 'NONE',  ( -7.576308911938196999, 7.733448573549685179, 0.7998128361456462443 ) ) ;
#21862=CARTESIAN_POINT ( 'NONE',  ( 2.998324526916512411, 6.649795714711241423, 0.000000000000000000 ) ) ;
#21868=CARTESIAN_POINT ( 'NONE',  ( 8.543609354905870035, 13.11929468069890525, 0.7998128361456462443 ) ) ;
#21869=CARTESIAN_POINT ( 'NONE',  ( -4.297571505851936813, 4.116180966356429494, 1.214306433183764966E-14 ) ) ;
#21872=CARTESIAN_POINT ( 'NONE',  ( -0.6823417656250212460, 2.363541667008084435, 1.181850606188767472 ) ) ;
#21874=CARTESIAN_POINT ( 'NONE',  ( 6.480434237652132445, 7.623223367758051872, 1.082531754730558626 ) ) ;
#21882=CARTESIAN_POINT ( 'NONE',  ( 8.731087737076324018, 9.288616569451617622, 1.040834085586084257E-14 ) ) ;
#21886=CARTESIAN_POINT ( 'NONE',  ( -6.842061076390810292, 11.13415502243129218, 0.000000000000000000 ) ) ;
#21895=CARTESIAN_POINT ( 'NONE',  ( 10.16199982864259788, 11.81442020729326536, 1.199719254218452047 ) ) ;
#21899=CARTESIAN_POINT ( 'NONE',  ( 3.161022370280501814, 6.839609865302569425, 0.000000000000000000 ) ) ;
#21902=CARTESIAN_POINT ( 'NONE',  ( -1.201851678989727383E-14, 2.993750000682821266, 1.732050807568877637 ) ) ;
#21908=CARTESIAN_POINT ( 'NONE',  ( -1.402160292154681736E-14, -0.03749999999998095135, 1.732050807568877637 ) ) ;
#21909=CARTESIAN_POINT ( 'NONE',  ( 8.450809820019639318, 8.753699632978056755, -0.7998128361456291469 ) ) ;
#21910=CARTESIAN_POINT ( 'NONE',  ( 6.616015773344440021, 6.821032611764393572, 1.040834085586084257E-14 ) ) ;
#21914=CARTESIAN_POINT ( 'NONE',  ( 10.41229878561526512, 11.25002945941372623, -0.7216878364870257245 ) ) ;
#21919=CARTESIAN_POINT ( 'NONE',  ( -5.416646063859567484, 6.278174148379618735, 1.199719254218450271 ) ) ;
#21921=CARTESIAN_POINT ( 'NONE',  ( -1.500000000000013101, 4.160416667349482900, -0.8660254037844313801 ) ) ;
#21922=CARTESIAN_POINT ( 'NONE',  ( 1.364683531249984538, -1.094791666325247936, -0.7879004041258309554 ) ) ;
#21927=CARTESIAN_POINT ( 'NONE',  ( -1.364683531250012516, 4.301041667008089320, -0.7879004041258300672 ) ) ;
#21930=EDGE_CURVE ( 'NONE', #196589, #192824, #157450, .T. ) ;
#21931=FACE_OUTER_BOUND ( 'NONE', #84845, .T. ) ;
#21936=CARTESIAN_POINT ( 'NONE',  ( -7.853197290813634268, 10.18514947741448573, 1.599625672291295375 ) ) ;
#21937=CARTESIAN_POINT ( 'NONE',  ( 5.795220594837462436, 8.848508896363995291, -1.199719254218440723 ) ) ;
#21945=CARTESIAN_POINT ( 'NONE',  ( -7.705111371268023923, 7.883718109434487253, 1.040834085586084257E-14 ) ) ;
#21950=CARTESIAN_POINT ( 'NONE',  ( 7.553864141108259211, 11.96459193126834464, 1.040834085586084257E-14 ) ) ;
#21952=ORIENTED_EDGE ( 'NONE', *, *, #101780, .F. ) ;
#21954=CARTESIAN_POINT ( 'NONE',  ( -5.576481253922474401, 5.400316305864651056, -0.7998128361456221525 ) ) ;
#21956=CARTESIAN_POINT ( 'NONE',  ( -8.239604668803112375, 10.63595808506888396, -1.599625672291263179 ) ) ;
#21960=CARTESIAN_POINT ( 'NONE',  ( -4.061770719603903679, 7.733366158448967909, -0.6361108440643822304 ) ) ;
#21961=CARTESIAN_POINT ( 'NONE',  ( -0.6823417656250246877, -0.6989583329919113464, 1.181850606188755259 ) ) ;
#21967=CARTESIAN_POINT ( 'NONE',  ( 5.144429221381498607, 8.089252293998699272, -1.199719254218452047 ) ) ;
#21984=DIRECTION ( 'NONE',  ( 0.3502638921866464417, -1.953969548649013438E-16, 0.9366510587354618389 ) ) ;
#21987=CARTESIAN_POINT ( 'NONE',  ( 4.161361007603033180, 7.399433999391101580, -0.7812420967184935394 ) ) ;
#21988=ORIENTED_EDGE ( 'NONE', *, *, #119470, .F. ) ;
#21990=CARTESIAN_POINT ( 'NONE',  ( -8.286004436246233951, 12.81875560892930466, 1.040834085586084257E-14 ) ) ;
#21996=CARTESIAN_POINT ( 'NONE',  ( -1.500000000000001332, 1.181250000682816603, 0.000000000000000000 ) ) ;
#21997=CARTESIAN_POINT ( 'NONE',  ( 8.432281472695482449, 11.92507992053172572, 1.199719254218450271 ) ) ;
#22003=CARTESIAN_POINT ( 'NONE',  ( -1.201851678989727383E-14, 2.321875000341416584, 1.575800808251672791 ) ) ;
#22005=ORIENTED_EDGE ( 'NONE', *, *, #207859, .F. ) ;
#22010=CARTESIAN_POINT ( 'NONE',  ( -4.066556009095094737, 6.831733546331167695, 1.199719254218464037 ) ) ;
#22015=CARTESIAN_POINT ( 'NONE',  ( -1.364683531250014514, 0.8010416670080889867, -0.7879004041258289570 ) ) ;
#22020=CARTESIAN_POINT ( 'NONE',  ( -1.364683531250012516, 0.7802083336747528408, 0.7879004041258379498 ) ) ;
#22023=CARTESIAN_POINT ( 'NONE',  ( -5.388475986427523345, 8.373973519885682393, 1.199719254218452047 ) ) ;
#22024=CARTESIAN_POINT ( 'NONE',  ( 7.426115451983150706, 9.686887332112256388, -1.599625672291262513 ) ) ;
#22025=CARTESIAN_POINT ( 'NONE',  ( 4.222474775652216294, 7.013638773981186958, 1.199719254218462483 ) ) ;
#22026=CARTESIAN_POINT ( 'NONE',  ( -1.001543065824772872E-14, 4.462500000000024336, 1.732050807568877637 ) ) ;
#22029=CARTESIAN_POINT ( 'NONE',  ( 0.6823417656249882723, 1.238541667008083547, -1.181850606188749264 ) ) ;
#22035=CARTESIAN_POINT ( 'NONE',  ( 7.795575138177731844, 8.197185204069915798, 1.040834085586084257E-14 ) ) ;
#22038=CARTESIAN_POINT ( 'NONE',  ( -6.042130013184518589, 10.20090211535728031, -0.7998128361456291469 ) ) ;
#22039=CARTESIAN_POINT ( 'NONE',  ( -3.415764635639130020, 6.072476943965863683, 1.199719254218462483 ) ) ;
#22044=CARTESIAN_POINT ( 'NONE',  ( -8.975134502122321223, 9.573337795338607847, 1.040834085586084257E-14 ) ) ;
#22046=CARTESIAN_POINT ( 'NONE',  ( -1.001543065824772872E-14, 5.212500000000019895, 1.732050807568877637 ) ) ;
#22050=CARTESIAN_POINT ( 'NONE',  ( 9.761507412159302177, 10.49077285704843199, -0.7216878364870257245 ) ) ;
#22057=CARTESIAN_POINT ( 'NONE',  ( -1.483013432599996628, 7.294277089886567644, -4.259227663825902788 ) ) ;
#22063=CARTESIAN_POINT ( 'NONE',  ( 8.880227426826646564, 9.462612874160329923, 0.7216878364870458196 ) ) ;
#22064=CARTESIAN_POINT ( 'NONE',  ( 7.263417608619159083, 9.497073181520933716, -1.599625672291262513 ) ) ;
#22065=CARTESIAN_POINT ( 'NONE',  ( -6.205881626753225966, 8.263281202677319470, 1.599625672291283607 ) ) ;
#22068=LINE ( 'NONE', #23148, #97424 ) ;
#22069=CARTESIAN_POINT ( 'NONE',  ( 0.6823417656249882723, -1.094791666325249713, 1.181850606188755259 ) ) ;
#22070=CARTESIAN_POINT ( 'NONE',  ( 3.375617060122621194, 6.882044303544283537, 1.040834085586084257E-14 ) ) ;
#22072=CARTESIAN_POINT ( 'NONE',  ( -4.647747731386360215, 4.316793862905830892, 0.7998128361456341429 ) ) ;
#22073=CARTESIAN_POINT ( 'NONE',  ( -6.873620692448438874, 10.96304854125777695, 0.000000000000000000 ) ) ;
#22088=CARTESIAN_POINT ( 'NONE',  ( 6.760712154708803823, 11.03924794713562818, 1.040834085586084257E-14 ) ) ;
#22100=CARTESIAN_POINT ( 'NONE',  ( -6.307567778855718288, 8.381915046796901692, -1.599625672291263179 ) ) ;
#22102=CARTESIAN_POINT ( 'NONE',  ( -4.277761160311629673, 4.949475094240346706, 1.199719254218462483 ) ) ;
#22114=CARTESIAN_POINT ( 'NONE',  ( -2.767835915484202047, 6.380892334706859792, -0.7998128361456281477 ) ) ;
#22117=CARTESIAN_POINT ( 'NONE',  ( 5.601490020740366838, 9.686822124172440596, 1.040834085586084257E-14 ) ) ;
#22118=CARTESIAN_POINT ( 'NONE',  ( -1.201851678989727383E-14, 4.071875000341425022, 1.575800808251672791 ) ) ;
#22124=CARTESIAN_POINT ( 'NONE',  ( 4.134873662043553111, 7.767843672452050541, -0.7216878364870197293 ) ) ;
#22125=CARTESIAN_POINT ( 'NONE',  ( -6.832419346282942563, 10.05857410638369487, 1.199719254218453823 ) ) ;
#22128=CARTESIAN_POINT ( 'NONE',  ( -8.044065211609668253, 8.279164256499745633, 0.7998128361456602331 ) ) ;
#22129=CARTESIAN_POINT ( 'NONE',  ( -5.494078562035765501, 7.432844293840273231, -1.599625672291256295 ) ) ;
#22136=CARTESIAN_POINT ( 'NONE',  ( 7.935599982700328958, 8.152621489438862667, 0.7998128361456481317 ) ) ;
#22137=CARTESIAN_POINT ( 'NONE',  ( -2.398572866711294438, 5.287202466803545775, -0.8077998227820496480 ) ) ;
#22150=CARTESIAN_POINT ( 'NONE',  ( 1.364683531249986537, -0.8239583329919186738, 0.7879004041258500513 ) ) ;
#22151=CARTESIAN_POINT ( 'NONE',  ( 6.145923705696426431, 6.064665832934283962, 0.7998128361456341429 ) ) ;
#22152=CARTESIAN_POINT ( 'NONE',  ( 4.645640190976921602, 8.571663989448405019, 1.040834085586084257E-14 ) ) ;
#22154=CARTESIAN_POINT ( 'NONE',  ( -9.164948653158003111, 9.794787638213568570, -0.7216878364870267237 ) ) ;
#22156=CARTESIAN_POINT ( 'NONE',  ( 7.144783764721768904, 7.437928601704619780, 1.040834085586084257E-14 ) ) ;
#22157=CARTESIAN_POINT ( 'NONE',  ( -8.310784975052685652, 9.758632561392040827, -1.082531754730543083 ) ) ;
#22162=CARTESIAN_POINT ( 'NONE',  ( 8.263858322729371153, 9.599921783727809910, -1.199719254218446718 ) ) ;
#22169=CARTESIAN_POINT ( 'NONE',  ( -0.6823417656250003738, 2.967708333674754062, -1.181850606188749264 ) ) ;
#22176=CARTESIAN_POINT ( 'NONE',  ( 7.411503528164766763, 11.79850454950093841, 1.040834085586084257E-14 ) ) ;
#22180=CARTESIAN_POINT ( 'NONE',  ( -8.696665468161981494, 12.23352791524263239, -1.199719254218446718 ) ) ;
#22185=( BOUNDED_CURVE ( )  B_SPLINE_CURVE ( 2, ( #78018, #210135, #14061, #113793, #10869, #13005, #63900 ),
 .UNSPECIFIED., .F., .T. ) 
 B_SPLINE_CURVE_WITH_KNOTS ( ( 3, 2, 2, 3 ),
 ( 0.3605655240965703334, 0.3630952380952380820, 0.3690476190476190688, 0.3715773330463134627 ),
 .UNSPECIFIED. ) 
 CURVE ( )  GEOMETRIC_REPRESENTATION_ITEM ( )  RATIONAL_B_SPLINE_CURVE ( ( 0.9345202395942613371, 0.9430618748659225226, 1.000000000000000000, 0.8660254037844387076, 1.000000000000000000, 0.9430618748653227801, 0.9345202395940813700 ) ) 
 REPRESENTATION_ITEM ( '' )  );
#22187=CARTESIAN_POINT ( 'NONE',  ( 9.083072846151447166, 12.68433652289702884, 1.199719254218450271 ) ) ;
#22191=CARTESIAN_POINT ( 'NONE',  ( -9.775592450653132204, 11.36361159963886891, -1.199719254218441611 ) ) ;
#22197=CARTESIAN_POINT ( 'NONE',  ( 5.886971415934090679, 5.980320297827544707, -0.1280069804882408846 ) ) ;
#22198=CARTESIAN_POINT ( 'NONE',  ( 1.284279953904119864, 3.296639714193937198, -0.7749999999999910294 ) ) ;
#22199=CARTESIAN_POINT ( 'NONE',  ( -5.101945877444165944, 4.846691699973280976, 0.000000000000000000 ) ) ;
#22203=CARTESIAN_POINT ( 'NONE',  ( 7.623762449586013901, 7.788811034138823253, 1.040834085586084257E-14 ) ) ;
#22205=CARTESIAN_POINT ( 'NONE',  ( 5.615048174354031474, 9.702639970055050966, 0.7998128361456462443 ) ) ;
#22208=CARTESIAN_POINT ( 'NONE',  ( -8.595506201384022660, 11.05117653974661529, 1.443375672974064550 ) ) ;
#22216=CARTESIAN_POINT ( 'NONE',  ( -5.013591113304329383, 6.604120902668014992, -1.237928687022475494 ) ) ;
#22218=CARTESIAN_POINT ( 'NONE',  ( 4.799223189557548785, 7.582548906917042864, -1.082531754730549078 ) ) ;
#22241=LINE ( 'NONE', #189041, #28887 ) ;
#22243=CARTESIAN_POINT ( 'NONE',  ( 7.796102023057898123, 9.054206100777749455, -1.199719254218441611 ) ) ;
#22247=CARTESIAN_POINT ( 'NONE',  ( -1.500000000000013101, 1.452083334016150085, 0.8660254037844403729 ) ) ;
#22249=CARTESIAN_POINT ( 'NONE',  ( -6.612626235163205024, 8.737816579155630592, -1.599625672291263179 ) ) ;
#22252=CARTESIAN_POINT ( 'NONE',  ( -8.272446282632566650, 12.80293776304669962, 0.7998128361456481317 ) ) ;
#22256=CARTESIAN_POINT ( 'NONE',  ( 1.499999999999989120, 5.577083334016153415, -0.8660254037844323793 ) ) ;
#22257=CARTESIAN_POINT ( 'NONE',  ( 6.317209508963599340, 9.457495962844502557, 1.199719254218462483 ) ) ;
#22260=CARTESIAN_POINT ( 'NONE',  ( -7.711890448074853133, 7.891627032375787998, -0.7998128361456291469 ) ) ;
#22262=CARTESIAN_POINT ( 'NONE',  ( 6.015607636943825831, 6.078019264660407650, -0.5714835875584244329 ) ) ;
#22263=CARTESIAN_POINT ( 'NONE',  ( -1.445103857046265317, 8.688264192038502642, 2.625611233228785313 ) ) ;
#22267=CARTESIAN_POINT ( 'NONE',  ( -6.724481002698115439, 10.78905223654906109, -0.7216878364870267237 ) ) ;
#22271=CARTESIAN_POINT ( 'NONE',  ( 0.6823417656249899377, 3.988541667008085767, -1.181850606188754593 ) ) ;
#22277=CARTESIAN_POINT ( 'NONE',  ( -0.6823417656250212460, 4.051041667008085767, 1.181850606188767472 ) ) ;
#22280=CARTESIAN_POINT ( 'NONE',  ( 2.521453382017309952, 5.885520012421409319, 0.000000000000000000 ) ) ;
#22286=CARTESIAN_POINT ( 'NONE',  ( -1.364683531250000748, 0.7593750003414210248, 0.000000000000000000 ) ) ;
#22287=CARTESIAN_POINT ( 'NONE',  ( -2.480778921620681921, 5.838066475291996404, 1.040834085586084257E-14 ) ) ;
#22288=CARTESIAN_POINT ( 'NONE',  ( 6.173040012923759257, 6.096301524699504704, -0.7998128361456281477 ) ) ;
#22291=DIRECTION ( 'NONE',  ( 0.5038915848679205167, -0.5182601445718857391, 0.6910135260959974213 ) ) ;
#22294=CARTESIAN_POINT ( 'NONE',  ( 3.714570900464285064, 4.396382807705524698, 1.082531754730560403 ) ) ;
#22297=CARTESIAN_POINT ( 'NONE',  ( -7.537970219518075332, 10.77775377520434574, -1.082531754730543971 ) ) ;
#22304=CARTESIAN_POINT ( 'NONE',  ( -9.996439331977562404, 10.55693406359564790, 0.7998128361456462443 ) ) ;
#22305=CARTESIAN_POINT ( 'NONE',  ( -5.165293336682207581, 8.009630745229104676, 1.082531754730548412 ) ) ;
#22307=CARTESIAN_POINT ( 'NONE',  ( 0.6823417656249882723, 1.488541667008083547, -1.181850606188749264 ) ) ;
#22314=CARTESIAN_POINT ( 'NONE',  ( 9.480175724453529185, 12.08329098332774265, 1.599625672291279388 ) ) ;
#22329=CARTESIAN_POINT ( 'NONE',  ( -4.223528545856940042, 4.886203710709899006, -1.199719254218446718 ) ) ;
#22331=CARTESIAN_POINT ( 'NONE',  ( -3.931431380944478082, 2.807600633707135529, 0.7750000000000135669 ) ) ;
#22333=CARTESIAN_POINT ( 'NONE',  ( -1.201851678989727383E-14, 2.759375000341417916, -1.575800808251660134 ) ) ;
#22342=B_SPLINE_CURVE_WITH_KNOTS ( 'NONE', 3,
 ( #145167, #146221, #30319, #164573, #194938, #47654 ),
 .UNSPECIFIED., .F., .F.,
 ( 4, 2, 4 ),
 ( 7.273049277091636640E-18, 9.878339706010669664E-05, 0.0001975667941202061020 ),
 .UNSPECIFIED. ) ;
#22344=CARTESIAN_POINT ( 'NONE',  ( -0.6823417656250212460, 1.801041667008083991, 1.181850606188755259 ) ) ;
#22351=ORIENTED_EDGE ( 'NONE', *, *, #175516, .F. ) ;
#22356=CARTESIAN_POINT ( 'NONE',  ( 5.681030059326015014, 6.586622143090519188, -1.199719254218445830 ) ) ;
#22359=ORIENTED_EDGE ( 'NONE', *, *, #121776, .T. ) ;
#22363=CARTESIAN_POINT ( 'NONE',  ( 6.435316467980822353, 10.65961964595298817, 1.040834085586084257E-14 ) ) ;
#22366=CARTESIAN_POINT ( 'NONE',  ( 7.248805684800777804, 11.60869039890961218, 1.040834085586084257E-14 ) ) ;
#22373=ORIENTED_EDGE ( 'NONE', *, *, #119838, .T. ) ;
#22381=CARTESIAN_POINT ( 'NONE',  ( -6.860062538834774237, 10.94723069537516302, 0.7216878364870458196 ) ) ;
#22386=CARTESIAN_POINT ( 'NONE',  ( -10.30827686509187835, 10.92074451889568643, 1.040834085586084257E-14 ) ) ;
#22390=CARTESIAN_POINT ( 'NONE',  ( -3.978428010606240850, 6.728917548094202949, -1.199719254218452047 ) ) ;
#22393=CARTESIAN_POINT ( 'NONE',  ( 3.267151830768944443, 4.834763107362302748, -1.443375672974058777 ) ) ;
#22394=ADVANCED_FACE ( 'NONE', ( #194639 ), #162160, .F. ) ;
#22396=CARTESIAN_POINT ( 'NONE',  ( 4.487912541323413329, 5.194651705420806564, 1.199719254218462483 ) ) ;
#22402=CARTESIAN_POINT ( 'NONE',  ( 4.690757960648231695, 5.535267711253469614, 1.082531754730560403 ) ) ;
#22404=CARTESIAN_POINT ( 'NONE',  ( -3.795392936821753604, 6.515376628678959392, -1.199719254218452047 ) ) ;
#22407=CARTESIAN_POINT ( 'NONE',  ( -8.947491310014823895, 12.52615806407091803, 1.199719254218462483 ) ) ;
#22413=CARTESIAN_POINT ( 'NONE',  ( 7.456621297836061757, 11.64321591421002644, 0.7216878364870438212 ) ) ;
#22414=CARTESIAN_POINT ( 'NONE',  ( -1.201851678989727383E-14, 3.759375000341423245, -1.575800808251660134 ) ) ;
#22416=CARTESIAN_POINT ( 'NONE',  ( 4.147904930777053245, 6.926640621626830807, -1.199719254218452047 ) ) ;
#22424=DIRECTION ( 'NONE',  ( -0.6507913734559642727, -0.7592566023653003482, -2.775557561562895049E-17 ) ) ;
#22429=CARTESIAN_POINT ( 'NONE',  ( 1.364683531249988535, 2.176041667008087543, 0.7879004041258500513 ) ) ;
#22431=CARTESIAN_POINT ( 'NONE',  ( 10.05353459973327368, 11.68787744023238417, -1.199719254218440723 ) ) ;
#22433=CARTESIAN_POINT ( 'NONE',  ( -5.260200412422208593, 7.159986452624450770, -1.443375672974053447 ) ) ;
#22434=CARTESIAN_POINT ( 'NONE',  ( 4.216222584169931231, 4.021273891060765493, 1.214306433183764966E-14 ) ) ;
#22435=CARTESIAN_POINT ( 'NONE',  ( -5.300874872818844175, 7.207439989753867238, 1.443375672974064550 ) ) ;
#22439=CARTESIAN_POINT ( 'NONE',  ( 4.961394147597008697, 7.875711374583454827, -1.199719254218452047 ) ) ;
#22441=CARTESIAN_POINT ( 'NONE',  ( -2.965583170617148046, 6.450339737514259930, -0.2656679274986517014 ) ) ;
#22449=EDGE_CURVE ( 'NONE', #86628, #54687, #193576, .T. ) ;
#22450=CARTESIAN_POINT ( 'NONE',  ( 5.900823170445728572, 7.907379670318584353, 1.599625672291267398 ) ) ;
#22453=CARTESIAN_POINT ( 'NONE',  ( -2.279742385392243165, 5.811449882932888222, -0.7998128361456281477 ) ) ;
#22455=CARTESIAN_POINT ( 'NONE',  ( -6.039267359883488950, 9.133230122250985517, 1.199719254218452047 ) ) ;
#22459=CARTESIAN_POINT ( 'NONE',  ( 6.414979237560321401, 10.63589287712906462, 1.040834085586084257E-14 ) ) ;
#22462=CARTESIAN_POINT ( 'NONE',  ( -5.982172092127739482, 8.002286745614243912, -1.599625672291263179 ) ) ;
#22463=CARTESIAN_POINT ( 'NONE',  ( 6.195713011320782115, 8.251417818006149929, -1.443375672974057666 ) ) ;
#22464=CARTESIAN_POINT ( 'NONE',  ( 5.379472278790374595, 6.509029678566758292, 1.321781506194243727 ) ) ;
#22465=CARTESIAN_POINT ( 'NONE',  ( -4.791917227426195858, 7.677988301050826969, -1.199719254218452047 ) ) ;
#22469=CARTESIAN_POINT ( 'NONE',  ( -6.738566041191992539, 7.820414121934134322, 1.199719254218450271 ) ) ;
#22472=CARTESIAN_POINT ( 'NONE',  ( -1.364683531250014514, 1.488541667008084435, -0.7879004041258289570 ) ) ;
#22474=CARTESIAN_POINT ( 'NONE',  ( -6.155038550924159857, 8.203964280876741455, 1.443375672974078761 ) ) ;
#22478=ORIENTED_EDGE ( 'NONE', *, *, #46917, .T. ) ;
#22480=CARTESIAN_POINT ( 'NONE',  ( 6.494519276145969577, 7.535692896047149425, -1.199719254218446718 ) ) ;
#22482=CARTESIAN_POINT ( 'NONE',  ( -5.912409256564314930, 5.999956524776160371, -0.009440138123966573813 ) ) ;
#22483=CARTESIAN_POINT ( 'NONE',  ( -1.364683531250000748, 1.071875000341421247, 0.000000000000000000 ) ) ;
#22486=CARTESIAN_POINT ( 'NONE',  ( -0.08635228504281292072, 7.011029804986348424, 1.999717945518313611 ) ) ;
#22489=CARTESIAN_POINT ( 'NONE',  ( -5.135841261478327979, 4.886236314679810455, 0.7998128361456341429 ) ) ;
#22490=CARTESIAN_POINT ( 'NONE',  ( -6.168596704093453731, 10.14052055484361325, 0.7216878364870458196 ) ) ;
#22499=CARTESIAN_POINT ( 'NONE',  ( -7.117667457050096402, 10.28740055232499984, 1.082531754730549967 ) ) ;
#22500=EDGE_CURVE ( 'NONE', #11347, #121606, #103548, .T. ) ;
#22506=CARTESIAN_POINT ( 'NONE',  ( -6.629573926958124197, 9.717958100551031819, 1.082531754730548412 ) ) ;
#22512=FACE_OUTER_BOUND ( 'NONE', #134740, .T. ) ;
#22516=VERTEX_POINT ( 'NONE', #79820 ) ;
#22520=CARTESIAN_POINT ( 'NONE',  ( -5.994676475536691029, 10.14553965476814845, 0.7998128361456481317 ) ) ;
#22523=CARTESIAN_POINT ( 'NONE',  ( 3.337278367258157630, 7.045241861776501580, 0.7998128361456341429 ) ) ;
#22527=CARTESIAN_POINT ( 'NONE',  ( 6.817052309572890323, 6.847649204123507083, 0.7998128361456341429 ) ) ;
#22533=CARTESIAN_POINT ( 'NONE',  ( -5.938108093105513241, 6.030140318152288792, 0.7216878364870317197 ) ) ;
#22545=CARTESIAN_POINT ( 'NONE',  ( -0.6823417656250246877, 0.5510416670080897639, 1.181850606188755259 ) ) ;
#22546=DIRECTION ( 'NONE',  ( -1.000000000000000000, 7.109522442527899011E-16, 0.000000000000000000 ) ) ;
#22547=CARTESIAN_POINT ( 'NONE',  ( -8.474009703741204547, 9.845098394908269768, -1.199719254218446718 ) ) ;
#22549=CARTESIAN_POINT ( 'NONE',  ( 6.747154001095143627, 11.02343010125301959, -0.7998128361456291469 ) ) ;
#22551=CARTESIAN_POINT ( 'NONE',  ( -6.877010230629689858, 9.046264573866535486, 1.599625672291283607 ) ) ;
#22554=CARTESIAN_POINT ( 'NONE',  ( 0.6823417656249899377, 5.176041667008086655, -1.181850606188754593 ) ) ;
#22555=AXIS2_PLACEMENT_3D ( 'NONE', #16558, #149795, #183345 ) ;
#22557=CARTESIAN_POINT ( 'NONE',  ( 9.734391104931951588, 11.41950637958454706, 1.082531754730548412 ) ) ;
#22560=CARTESIAN_POINT ( 'NONE',  ( 1.364683531249988757, -0.8031249996585804185, 0.000000000000000000 ) ) ;
#22563=CARTESIAN_POINT ( 'NONE',  ( 7.578644679914713578, 8.904468883731073703, 1.082531754730558626 ) ) ;
#22566=CARTESIAN_POINT ( 'NONE',  ( -6.290620087060847965, 7.401773525401500464, 1.082531754730549967 ) ) ;
#22568=CARTESIAN_POINT ( 'NONE',  ( -1.364683531250012516, 2.738541667008090208, -0.7879004041258289570 ) ) ;
#22572=CARTESIAN_POINT ( 'NONE',  ( -5.018489415352746619, 9.006654751220198207, 0.7998128361456481317 ) ) ;
#22578=CARTESIAN_POINT ( 'NONE',  ( 9.284636267260101050, 9.726497154758602548, -0.7998128361456281477 ) ) ;
#22581=CARTESIAN_POINT ( 'NONE',  ( -0.7500000000000215383, 2.441666666666689078, 1.299038105676671107 ) ) ;
#22584=CARTESIAN_POINT ( 'NONE',  ( -0.7499999999999972244, 5.389583334016151639, -1.299038105676652899 ) ) ;
#22587=CARTESIAN_POINT ( 'NONE',  ( 5.938108093105483931, 8.911247961056314892, -1.082531754730537088 ) ) ;
#22588=CARTESIAN_POINT ( 'NONE',  ( -1.364683531250014514, -0.4072916663252447167, 0.7879004041258379498 ) ) ;
#22590=CARTESIAN_POINT ( 'NONE',  ( 3.460355519985863548, 5.060167411448709629, 1.599625672291267398 ) ) ;
#22596=CARTESIAN_POINT ( 'NONE',  ( -1.500000000000001332, -0.5999999999999755529, 0.000000000000000000 ) ) ;
#22597=CARTESIAN_POINT ( 'NONE',  ( 7.344766530301147789, 9.591980256816594164, 1.599625672291281386 ) ) ;
#22598=CARTESIAN_POINT ( 'NONE',  ( -10.15235809853472126, 10.73883929124566983, -0.7998128361456291469 ) ) ;
#22600=CARTESIAN_POINT ( 'NONE',  ( 1.364683531249988757, 0.3843750003414206362, 0.000000000000000000 ) ) ;
#22601=CARTESIAN_POINT ( 'NONE',  ( 1.499999999999987121, 0.7541666666666868579, 0.8660254037844524744 ) ) ;
#22603=CARTESIAN_POINT ( 'NONE',  ( 6.335737856287750880, 6.286115675290828264, -0.7998128361456281477 ) ) ;
#22609=CARTESIAN_POINT ( 'NONE',  ( -1.364683531250010295, 5.280208333674758059, 0.7879004041258379498 ) ) ;
#22611=CARTESIAN_POINT ( 'NONE',  ( -7.320512876374914768, 10.62801655815766999, 1.199719254218453823 ) ) ;
#22612=CARTESIAN_POINT ( 'NONE',  ( -5.178851490740209229, 7.065079377328788546, 1.443375672974064550 ) ) ;
#22620=CARTESIAN_POINT ( 'NONE',  ( 8.288111976655649471, 8.563885482386732306, -0.7998128361456291469 ) ) ;
#22624=( BOUNDED_SURFACE ( )  B_SPLINE_SURFACE ( 3, 2, ( 
 ( #113739, #35600, #18276 ),
 ( #946, #69149, #97438 ),
 ( #67011, #133147, #199149 ),
 ( #50794, #15076, #31362 ),
 ( #84358, #182922, #34537 ),
 ( #101676, #3079, #47629 ),
 ( #167746, #100608, #19346 ),
 ( #81166, #131054, #170939 ),
 ( #73436, #135268, #156851 ),
 ( #139539, #86495, #203415 ) ),
 .UNSPECIFIED., .F., .F., .F. ) 
 B_SPLINE_SURFACE_WITH_KNOTS ( ( 4, 2, 2, 2, 4 ),
 ( 3, 3 ),
 ( 0.001823043507466968506, 0.002278804384346605483, 0.002734565261226242026, 0.003190326138105878569, 0.003646087014985515545 ),
 ( 0.000000000000000000, 1.000000000000000000 ),
 .UNSPECIFIED. ) 
 GEOMETRIC_REPRESENTATION_ITEM ( )  RATIONAL_B_SPLINE_SURFACE ( (
 ( 1.000000000000000000, 0.8267197332287864464, 1.000000000000000000),
 ( 1.000000000000000000, 0.8323584916099276976, 1.000000000000000000),
 ( 1.000000000000000000, 0.8280586474256576013, 1.000000000000000000),
 ( 1.000000000000000000, 0.7975649039268305485, 1.000000000000000000),
 ( 1.000000000000000000, 0.7708027761888249785, 1.000000000000000000),
 ( 1.000000000000000000, 0.7027005163579342906, 1.000000000000000000),
 ( 1.000000000000000000, 0.6615630608851112981, 1.000000000000000000),
 ( 1.000000000000000000, 0.5955151780456100497, 1.000000000000000000),
 ( 1.000000000000000000, 0.5705924789361177529, 1.000000000000000000),
 ( 1.000000000000000000, 0.5626093260850774103, 1.000000000000000000) ) ) 
 REPRESENTATION_ITEM ( '' )  SURFACE ( )  );
#22626=CARTESIAN_POINT ( 'NONE',  ( -7.426115451983156923, 9.686887332112256388, -1.599625672291263179 ) ) ;
#22627=CARTESIAN_POINT ( 'NONE',  ( 4.710568305744190276, 7.583081225755162968, 1.199719254218462483 ) ) ;
#22629=DIRECTION ( 'NONE',  ( 0.6507913734559651608, 0.7592566023652994600, 1.725633230170963543E-31 ) ) ;
#22630=CARTESIAN_POINT ( 'NONE',  ( 4.708759422647839976, 4.387974169377582001, -0.7998128361456211532 ) ) ;
#22631=ORIENTED_EDGE ( 'NONE', *, *, #65958, .F. ) ;
#22638=CARTESIAN_POINT ( 'NONE',  ( -5.775410249741523394, 5.840326167560965231, 0.7216878364870317197 ) ) ;
#22640=CARTESIAN_POINT ( 'NONE',  ( 2.184835310096557404, 5.700724961754617404, 1.040834085586084257E-14 ) ) ;
#22643=CARTESIAN_POINT ( 'NONE',  ( -6.775324078527193983, 8.927630729746953264, -1.599625672291263179 ) ) ;
#22647=CARTESIAN_POINT ( 'NONE',  ( -6.669721502918952716, 9.868759955792373972, 1.199719254218452047 ) ) ;
#22651=CARTESIAN_POINT ( 'NONE',  ( 5.148345644887269756, 7.029489223833707001, -1.599625672291256295 ) ) ;
#22652=ORIENTED_EDGE ( 'NONE', *, *, #5514, .F. ) ;
#22663=CARTESIAN_POINT ( 'NONE',  ( -6.989391883044787868, 8.113044270762433285, -1.199719254218446718 ) ) ;
#22666=CARTESIAN_POINT ( 'NONE',  ( 5.260200412422194383, 7.159986452624450770, -1.443375672974051449 ) ) ;
#22670=CARTESIAN_POINT ( 'NONE',  ( -3.737243898861318137, 7.511868315313511069, 0.7998128361456341429 ) ) ;
#22674=CARTESIAN_POINT ( 'NONE',  ( -5.530836599371015794, 8.540060901653093950, 1.199719254218452047 ) ) ;
#22680=CARTESIAN_POINT ( 'NONE',  ( -8.829384350997580455, 11.32403438096243775, 1.599625672291269396 ) ) ;
#22681=CARTESIAN_POINT ( 'NONE',  ( 7.775764792637399836, 9.030479331953833011, -1.199719254218441611 ) ) ;
#22683=CARTESIAN_POINT ( 'NONE',  ( -2.480778921620681921, 5.838066475291996404, 1.040834085586084257E-14 ) ) ;
#22684=CARTESIAN_POINT ( 'NONE',  ( -7.784352752540590004, 12.23349531127272094, 0.7998128361456481317 ) ) ;
#22688=ORIENTED_EDGE ( 'NONE', *, *, #20771, .F. ) ;
#22690=CARTESIAN_POINT ( 'NONE',  ( 8.080296364064698977, 12.37083682481011060, -0.7216878364870328300 ) ) ;
#22694=DIRECTION ( 'NONE',  ( 0.000000000000000000, 8.546850786086437571E-32, 1.000000000000000000 ) ) ;
#22697=AXIS2_PLACEMENT_3D ( 'NONE', #27581, #93679, #159721 ) ;
#22711=B_SPLINE_CURVE_WITH_KNOTS ( 'NONE', 3,
 ( #166807, #1070, #183042, #202464, #19464, #35721, #200340, #115979, #201401, #169984 ),
 .UNSPECIFIED., .F., .F.,
 ( 4, 3, 3, 4 ),
 ( 2.763748478102358283E-14, 6.251571079173980452E-05, 0.0001250313277099753971, 0.0002424569244162144992 ),
 .UNSPECIFIED. ) ;
#22713=CARTESIAN_POINT ( 'NONE',  ( -4.081167932913447594, 4.720116328942494555, -1.199719254218452047 ) ) ;
#22716=CARTESIAN_POINT ( 'NONE',  ( -4.457933580795036654, 4.095344020549286590, -0.7998128361456221525 ) ) ;
#22720=CARTESIAN_POINT ( 'NONE',  ( -1.402160292154681736E-14, -0.8812499993171809543, -1.732050807568870754 ) ) ;
#22725=ORIENTED_EDGE ( 'NONE', *, *, #117255, .T. ) ;
#22728=CARTESIAN_POINT ( 'NONE',  ( 4.390142812726693045, 4.016254791136236513, 1.214306433183764966E-14 ) ) ;
#22730=CARTESIAN_POINT ( 'NONE',  ( 1.284279953904119864, 3.046639714193936754, -0.7749999999999910294 ) ) ;
#22732=CARTESIAN_POINT ( 'NONE',  ( 5.473741331615251227, 7.409117525016355010, -1.599625672291262513 ) ) ;
#22733=CARTESIAN_POINT ( 'NONE',  ( -1.364683531250012516, 3.051041667008083547, -0.7879004041258289570 ) ) ;
#22736=CARTESIAN_POINT ( 'NONE',  ( -7.323375529675950624, 11.69568855126397011, -0.7998128361456291469 ) ) ;
#22737=CARTESIAN_POINT ( 'NONE',  ( -3.904385050611244079, 7.498940292447679568, 1.040834085586084257E-14 ) ) ;
#22739=CARTESIAN_POINT ( 'NONE',  ( -5.422371370461663176, 8.413518134592214537, -1.199719254218446718 ) ) ;
#22741=CARTESIAN_POINT ( 'NONE',  ( -1.364683531249997417, 5.259375000341425022, 1.214306433183764966E-14 ) ) ;
#22749=CARTESIAN_POINT ( 'NONE',  ( -4.351804119862249465, 7.060559992272473551, 1.082531754730560403 ) ) ;
#22754=CARTESIAN_POINT ( 'NONE',  ( -3.741687207247254676, 7.309126141856352454, 1.040834085586084257E-14 ) ) ;
#22757=CARTESIAN_POINT ( 'NONE',  ( 3.673896439623286714, 4.156855427197417185, -2.419999999999995044 ) ) ;
#22763=ORIENTED_EDGE ( 'NONE', *, *, #178800, .F. ) ;
#22766=EDGE_CURVE ( 'NONE', #121840, #148633, #160275, .T. ) ;
#22767=CARTESIAN_POINT ( 'NONE',  ( 1.931788062848141441E-13, 7.054063922337705073, -3.955400951015614730 ) ) ;
#22768=CARTESIAN_POINT ( 'NONE',  ( -4.711622075948912247, 5.455646162483875017, -1.199719254218446718 ) ) ;
#22769=CARTESIAN_POINT ( 'NONE',  ( -9.809487834687324437, 11.40315621434539395, 1.199719254218462483 ) ) ;
#22773=CARTESIAN_POINT ( 'NONE',  ( 5.144429221381498607, 8.089252293998699272, -1.199719254218452047 ) ) ;
#22777=CARTESIAN_POINT ( 'NONE',  ( 3.867100128395839942, 5.534702787927018974, -1.599625672291255185 ) ) ;
#22780=ORIENTED_EDGE ( 'NONE', *, *, #34390, .F. ) ;
#22788=CARTESIAN_POINT ( 'NONE',  ( 8.284195553149872993, 9.623648552551724578, -1.199719254218445830 ) ) ;
#22789=CARTESIAN_POINT ( 'NONE',  ( -5.786632634934295361, 5.645492917045106473, 0.7998128361456341429 ) ) ;
#22792=CARTESIAN_POINT ( 'NONE',  ( 1.499999999999990896, 4.056250000682819490, 1.214306433183764966E-14 ) ) ;
#22797=CARTESIAN_POINT ( 'NONE',  ( -1.201851678989727383E-14, 4.946875000341420581, -1.575800808251660134 ) ) ;
#22800=CARTESIAN_POINT ( 'NONE',  ( -6.410307701162927252, 6.373113827645189744, -0.7998128361456291469 ) ) ;
#22803=CARTESIAN_POINT ( 'NONE',  ( 4.222474775652216294, 7.013638773981186958, 1.199719254218462483 ) ) ;
#22804=CARTESIAN_POINT ( 'NONE',  ( -3.978428010606240850, 6.728917548094202949, -1.199719254218452047 ) ) ;
#22810=CARTESIAN_POINT ( 'NONE',  ( 7.632877294813741109, 8.007371053478589573, 1.040834085586084257E-14 ) ) ;
#22812=( BOUNDED_CURVE ( )  B_SPLINE_CURVE ( 2, ( #83134, #144991, #114652, #82071, #214165, #162277, #46398 ),
 .UNSPECIFIED., .F., .T. ) 
 B_SPLINE_CURVE_WITH_KNOTS ( ( 3, 2, 2, 3 ),
 ( 0.3784226669537131271, 0.3809523809523809312, 0.3869047619047619180, 0.3894344759034563674 ),
 .UNSPECIFIED. ) 
 CURVE ( )  GEOMETRIC_REPRESENTATION_ITEM ( )  RATIONAL_B_SPLINE_CURVE ( ( 0.9345202395942608931, 0.9430618748659213013, 1.000000000000000000, 0.8660254037844387076, 1.000000000000000000, 0.9430618748653214478, 0.9345202395940808149 ) ) 
 REPRESENTATION_ITEM ( '' )  );
#22813=CARTESIAN_POINT ( 'NONE',  ( 5.761852095683461350, 9.665985178365305686, -0.7216878364870267237 ) ) ;
#22814=CARTESIAN_POINT ( 'NONE',  ( 1.364683531249990311, 3.946875000341417028, 1.214306433183764966E-14 ) ) ;
#22816=CARTESIAN_POINT ( 'NONE',  ( 4.270455198180219902, 6.965652916976816655, -1.082531754730548412 ) ) ;
#22824=CARTESIAN_POINT ( 'NONE',  ( -5.364460139690476304, 6.514416944181776081, 1.355983593732257741 ) ) ;
#22831=CARTESIAN_POINT ( 'NONE',  ( -7.818248136574758256, 12.27303992597924420, 0.000000000000000000 ) ) ;
#22836=CARTESIAN_POINT ( 'NONE',  ( -3.216308754939891212, 4.775446185561722956, -1.599625672291262513 ) ) ;
#22841=CARTESIAN_POINT ( 'NONE',  ( 4.704316114261903436, 4.590716342834741504, 1.214306433183764966E-14 ) ) ;
#22842=CARTESIAN_POINT ( 'NONE',  ( -0.6823417656249969321, 3.530208333674754506, -1.181850606188749264 ) ) ;
#22844=CARTESIAN_POINT ( 'NONE',  ( 5.764187864104357573, 9.876636274763768597, 1.040834085586084257E-14 ) ) ;
#22845=LINE ( 'NONE', #204794, #191991 ) ;
#22847=CARTESIAN_POINT ( 'NONE',  ( -5.091250377131585125, 5.898545847196970726, 1.199719254218450271 ) ) ;
#22850=ORIENTED_EDGE ( 'NONE', *, *, #66705, .F. ) ;
#22852=CARTESIAN_POINT ( 'NONE',  ( 0.7499999999999902300, 5.066666666666684193, -1.299038105676658228 ) ) ;
#22853=CARTESIAN_POINT ( 'NONE',  ( 5.671388329218120639, 5.511041227042920099, 1.040834085586084257E-14 ) ) ;
#22856=CARTESIAN_POINT ( 'NONE',  ( 1.364683531249990311, 4.134375000341417028, 1.214306433183764966E-14 ) ) ;
#22860=CARTESIAN_POINT ( 'NONE',  ( 8.920901888111989919, 11.43080484092926241, 1.443375672974076540 ) ) ;
#22865=CARTESIAN_POINT ( 'NONE',  ( -0.7500000000000215383, 1.472916667349486008, 1.299038105676659116 ) ) ;
#22867=CARTESIAN_POINT ( 'NONE',  ( -4.530395885260773525, 8.437212299446219532, 0.7998128361456481317 ) ) ;
#22868=CARTESIAN_POINT ( 'NONE',  ( 4.161989969270892153, 6.839110149915929249, 1.082531754730558626 ) ) ;
#22876=CARTESIAN_POINT ( 'NONE',  ( 6.421758314367153275, 10.64380180007036891, -0.7998128361456291469 ) ) ;
#22877=CARTESIAN_POINT ( 'NONE',  ( 5.820528018968444961, 5.685037531751635953, 0.7998128361456341429 ) ) ;
#22878=DIRECTION ( 'NONE',  ( 5.176899690512889097E-31, -0.6000000000000018652, 0.7999999999999984901 ) ) ;
#22881=CARTESIAN_POINT ( 'NONE',  ( 5.361359679200154105, 8.342337828120466980, 1.199719254218462483 ) ) ;
#22888=CARTESIAN_POINT ( 'NONE',  ( 10.53876547652418338, 11.18964789890005918, 0.7998128361456462443 ) ) ;
#22893=CARTESIAN_POINT ( 'NONE',  ( 5.543269800280802073, 6.196057874731542015, 0.9238780061134096444 ) ) ;
#22894=EDGE_CURVE ( 'NONE', #178259, #184579, #127154, .T. ) ;
#22898=DIRECTION ( 'NONE',  ( 0.9366510587354612838, 0.000000000000000000, -0.3502638921866474409 ) ) ;
#22903=CARTESIAN_POINT ( 'NONE',  ( 6.561783159334121152, 8.678499657355050800, -1.443375672974057666 ) ) ;
#22904=CARTESIAN_POINT ( 'NONE',  ( -4.603156847039612920, 5.329103395422994716, 1.199719254218462483 ) ) ;
#22910=CARTESIAN_POINT ( 'NONE',  ( -3.906720819032141190, 7.709591388846142479, -0.7998128361456281477 ) ) ;
#22923=CARTESIAN_POINT ( 'NONE',  ( 7.235247531187115833, 11.59287255302699648, -0.7998128361456291469 ) ) ;
#22925=CARTESIAN_POINT ( 'NONE',  ( 2.684151225825664788, 5.114964949229812596, -1.082531754730543083 ) ) ;
#22931=CARTESIAN_POINT ( 'NONE',  ( -9.408995418203979000, 12.00024729270324286, 1.443375672974076540 ) ) ;
#22935=CARTESIAN_POINT ( 'NONE',  ( 6.903072767652295383, 11.20533532890304684, 1.040834085586084257E-14 ) ) ;
#22940=CARTESIAN_POINT ( 'NONE',  ( -4.889686956022917919, 8.856385215335397021, 1.214306433183764966E-14 ) ) ;
#22941=CARTESIAN_POINT ( 'NONE',  ( 5.007038802148489509, 4.735966778795008381, 0.7998128361456341429 ) ) ;
#22945=CARTESIAN_POINT ( 'NONE',  ( 9.541187415715040032, 12.15447128979948310, -1.599625672291262513 ) ) ;
#22950=CARTESIAN_POINT ( 'NONE',  ( 0.6823417656249882723, 2.988541667008084879, -1.181850606188754593 ) ) ;
#22952=CARTESIAN_POINT ( 'NONE',  ( 7.632877294813741109, 8.007371053478589573, 1.040834085586084257E-14 ) ) ;
#22954=CARTESIAN_POINT ( 'NONE',  ( 3.621833129746810265, 4.096114899008192367, -2.419999999999995044 ) ) ;
#22960=CARTESIAN_POINT ( 'NONE',  ( 7.741342523278686549, 11.97539067722642869, 0.7216878364870438212 ) ) ;
#22961=ORIENTED_EDGE ( 'NONE', *, *, #202925, .T. ) ;
#22964=CARTESIAN_POINT ( 'NONE',  ( -7.669108446824431269, 12.09904362127053545, -0.7998128361456291469 ) ) ;
#22972=CARTESIAN_POINT ( 'NONE',  ( 3.005103603723342953, 6.657704637652544832, -0.7998128361456291469 ) ) ;
#22978=CARTESIAN_POINT ( 'NONE',  ( 5.717788096661236885, 7.693838750903348789, 1.599625672291267398 ) ) ;
#22981=CARTESIAN_POINT ( 'NONE',  ( 0.7499999999999885647, 3.097916667349487341, -1.299038105676658228 ) ) ;
#22985=ORIENTED_EDGE ( 'NONE', *, *, #51647, .T. ) ;
#22987=CARTESIAN_POINT ( 'NONE',  ( -0.7500000000000006661, 0.6083333333333564852, -1.299038105676652011 ) ) ;
#22988=CARTESIAN_POINT ( 'NONE',  ( 6.751070424600909448, 9.963667031088037973, -1.199719254218441611 ) ) ;
#22989=CARTESIAN_POINT ( 'NONE',  ( 1.364683531249986537, -0.3447916663252443836, -0.7879004041258309554 ) ) ;
#22993=CARTESIAN_POINT ( 'NONE',  ( 8.378575743565351175, 11.75846021992619406, -1.082531754730543083 ) ) ;
#22998=CARTESIAN_POINT ( 'NONE',  ( -7.054319997812058318, 7.124461507069184130, 1.040834085586084257E-14 ) ) ;
#22999=CARTESIAN_POINT ( 'NONE',  ( 0.7499999999999902300, 2.514583334016148974, 1.299038105676669330 ) ) ;
#23000=CARTESIAN_POINT ( 'NONE',  ( 0.6823417656249917140, 5.655208333674749177, 1.181850606188765695 ) ) ;
#23005=CARTESIAN_POINT ( 'NONE',  ( -0.6823417656249969321, 3.780208333674754506, -1.181850606188749264 ) ) ;
#23014=CARTESIAN_POINT ( 'NONE',  ( -3.129460678718345878, 6.444905630999884671, -0.7687999843507524744 ) ) ;
#23015=CARTESIAN_POINT ( 'NONE',  ( -6.503107236049161521, 10.73870887536603291, 0.7998128361456481317 ) ) ;
#23016=CARTESIAN_POINT ( 'NONE',  ( 6.662942426112080874, 9.860851032851066122, 1.199719254218460707 ) ) ;
#23024=CARTESIAN_POINT ( 'NONE',  ( 2.273349394227877074, 5.683342515206170731, 0.4597581080974435519 ) ) ;
#23026=CARTESIAN_POINT ( 'NONE',  ( -5.845536785786364931, 9.971543350059432598, 0.000000000000000000 ) ) ;
#23031=CARTESIAN_POINT ( 'NONE',  ( 10.55232363013785246, 11.20546574478267132, 0.000000000000000000 ) ) ;
#23034=CARTESIAN_POINT ( 'NONE',  ( -3.632695093457760649, 6.325562478087638496, -1.199719254218452047 ) ) ;
#23035=CARTESIAN_POINT ( 'NONE',  ( -8.158255747121117452, 10.54105100977322174, 1.599625672291295375 ) ) ;
#23038=CARTESIAN_POINT ( 'NONE',  ( -3.976739547089790161, 7.847837856468413698, 0.08243740857501527519 ) ) ;
#23045=CARTESIAN_POINT ( 'NONE',  ( 6.602984505055297326, 7.662235663108029726, 1.199719254218462483 ) ) ;
#23060=ADVANCED_FACE ( 'NONE', ( #104618 ), #125884, .T. ) ;
#23065=CARTESIAN_POINT ( 'NONE',  ( 3.877268743828270470, 5.546566172598190292, 1.443375672974062551 ) ) ;
#23069=CARTESIAN_POINT ( 'NONE',  ( -8.971744963941075568, 11.49012176272984931, 1.599625672291269396 ) ) ;
#23075=CARTESIAN_POINT ( 'NONE',  ( -1.402160292154681736E-14, 1.368750000682821710, -1.732050807568863648 ) ) ;
#23080=CARTESIAN_POINT ( 'NONE',  ( -10.34217224912604571, 10.96028913360221502, 0.7998128361456462443 ) ) ;
#23081=CARTESIAN_POINT ( 'NONE',  ( -3.701970883082869701, 7.364863713882350282, -2.499999999999995559 ) ) ;
#23082=CARTESIAN_POINT ( 'NONE',  ( -1.402160292154681736E-14, 1.196875000341419026, -1.575800808251659024 ) ) ;
#23088=CARTESIAN_POINT ( 'NONE',  ( -3.093231602212184850, 6.760520635889515795, -0.7998128361456281477 ) ) ;
#23090=CARTESIAN_POINT ( 'NONE',  ( 4.132297641190314508, 7.622816840561035256, -0.7610026044957002300 ) ) ;
#23093=CARTESIAN_POINT ( 'NONE',  ( 1.364683531249988757, 0.4468750003414206917, 0.000000000000000000 ) ) ;
#23099=CARTESIAN_POINT ( 'NONE',  ( -1.364683531250000748, 0.5093750003414208027, 0.000000000000000000 ) ) ;
#23101=CARTESIAN_POINT ( 'NONE',  ( -7.552055258011950656, 8.769484874890757453, 1.199719254218462483 ) ) ;
#23102=CARTESIAN_POINT ( 'NONE',  ( 10.07778825365955733, 10.65184113889131012, -0.7998128361456281477 ) ) ;
#23103=CARTESIAN_POINT ( 'NONE',  ( 3.845709127770629010, 7.638411082374393146, 0.7998128361456321445 ) ) ;
#23107=CARTESIAN_POINT ( 'NONE',  ( 1.364683531249988535, 1.426041667008083991, 0.7879004041258500513 ) ) ;
#23113=CARTESIAN_POINT ( 'NONE',  ( 5.666945020832167224, 8.594891043404107478, 1.082531754730558626 ) ) ;
#23116=CARTESIAN_POINT ( 'NONE',  ( -3.903858165731105778, 6.641919395739846799, 1.199719254218464037 ) ) ;
#23117=CARTESIAN_POINT ( 'NONE',  ( 0.6823417656249899377, 3.155208333674754062, 1.181850606188765695 ) ) ;
#23121=CARTESIAN_POINT ( 'NONE',  ( 6.141480396866128899, 6.267408005873028820, -0.7216878364870257245 ) ) ;
#23122=CARTESIAN_POINT ( 'NONE',  ( -7.443063143778079649, 10.66702885350765584, 1.082531754730549967 ) ) ;
#23124=CARTESIAN_POINT ( 'NONE',  ( 0.7499999999999902300, 4.316666666666691299, -1.299038105676658228 ) ) ;
#23128=CARTESIAN_POINT ( 'NONE',  ( 8.595506201384008449, 11.05117653974661529, 1.443375672974076540 ) ) ;
#23142=CARTESIAN_POINT ( 'NONE',  ( 7.199016378732056687, 10.38230762762066384, -1.082531754730537976 ) ) ;
#23144=CARTESIAN_POINT ( 'NONE',  ( 7.401861798056875053, 10.72292363345333399, -1.199719254218441611 ) ) ;
#23145=CARTESIAN_POINT ( 'NONE',  ( -5.194745412330402878, 9.212286747694129474, 0.000000000000000000 ) ) ;
#23148=CARTESIAN_POINT ( 'NONE',  ( -1.580000000000022276, 8.758163473637745611, 2.500000000000011102 ) ) ;
#23149=CARTESIAN_POINT ( 'NONE',  ( 6.954969613686092345, 7.216478758829655504, -0.7216878364870257245 ) ) ;
#23151=CARTESIAN_POINT ( 'NONE',  ( 3.212919216758630014, 6.692230152952963529, 0.000000000000000000 ) ) ;
#23153=CARTESIAN_POINT ( 'NONE',  ( -6.561783159334121152, 10.59923808595773664, -0.7216878364870278340 ) ) ;
#23170=CARTESIAN_POINT ( 'NONE',  ( 8.294891053462476904, 8.571794405328034827, 1.040834085586084257E-14 ) ) ;
#23180=CARTESIAN_POINT ( 'NONE',  ( -6.925517538482230506, 6.974191971184389160, 0.7998128361456341429 ) ) ;
#23182=CARTESIAN_POINT ( 'NONE',  ( -5.766295404513795297, 5.621766148221195358, 0.7998128361456341429 ) ) ;
#23191=CARTESIAN_POINT ( 'NONE',  ( -3.684065054611367351, 5.321161868511784299, -1.599625672291256295 ) ) ;
#23195=CARTESIAN_POINT ( 'NONE',  ( 7.613066949273408213, 8.840665181362512115, -1.199719254218441611 ) ) ;
#23196=CARTESIAN_POINT ( 'NONE',  ( -1.364683531250012516, 3.530208333674758059, 0.7879004041258379498 ) ) ;
#23199=CARTESIAN_POINT ( 'NONE',  ( 6.114332400817464652, 6.016105027659348181, -0.05221600309115309591 ) ) ;
#23205=CARTESIAN_POINT ( 'NONE',  ( 5.626270559546821204, 6.626699076635176766, 1.082531754730560403 ) ) ;
#23206=CARTESIAN_POINT ( 'NONE',  ( -7.320512876374914768, 10.62801655815766999, 1.199719254218453823 ) ) ;
#23210=CARTESIAN_POINT ( 'NONE',  ( -7.751511138711140170, 10.06651563329490529, -1.599625672291263179 ) ) ;
#23211=CARTESIAN_POINT ( 'NONE',  ( -7.009729113465285266, 8.136771039586342624, -1.199719254218446718 ) ) ;
#23215=CARTESIAN_POINT ( 'NONE',  ( 4.901740149399201663, 4.849955969763177777, 0.6350953998956505586 ) ) ;
#23218=CARTESIAN_POINT ( 'NONE',  ( 8.372323551638698902, 9.726464550788689323, 1.199719254218462483 ) ) ;
#23233=ORIENTED_EDGE ( 'NONE', *, *, #77263, .F. ) ;
#23235=CARTESIAN_POINT ( 'NONE',  ( -0.7499999999999972244, 4.358333333333352932, -1.299038105676652011 ) ) ;
#23236=CARTESIAN_POINT ( 'NONE',  ( 5.522248639467795428, 5.337044922334209573, -0.7998128361456231517 ) ) ;
#23237=CARTESIAN_POINT ( 'NONE',  ( 6.063521013809720195, 8.097193820909906137, 1.599625672291281386 ) ) ;
#23239=CARTESIAN_POINT ( 'NONE',  ( -7.199016379176422120, 11.34267684244042584, 0.000000000000000000 ) ) ;
#23240=CARTESIAN_POINT ( 'NONE',  ( 6.887178846062110615, 9.058127958537705027, -1.443375672974057666 ) ) ;
#23241=CARTESIAN_POINT ( 'NONE',  ( -9.788623718942277563, 10.52240854829523187, 1.040834085586084257E-14 ) ) ;
#23245=CARTESIAN_POINT ( 'NONE',  ( 8.749089199520284410, 9.101692242395490240, 0.7998128361456481317 ) ) ;
#23250=CARTESIAN_POINT ( 'NONE',  ( -0.6823417656250003738, 1.967708333674753174, -1.181850606188749264 ) ) ;
#23256=CARTESIAN_POINT ( 'NONE',  ( 7.639129486296027061, 10.99973593639901814, 1.199719254218460707 ) ) ;
#23260=CARTESIAN_POINT ( 'NONE',  ( -8.306341666666730461, 12.84248237775322643, 1.040834085586084257E-14 ) ) ;
#23266=CARTESIAN_POINT ( 'NONE',  ( 3.891353782322113375, 4.498666486585943147, -1.199719254218446718 ) ) ;
#23270=CARTESIAN_POINT ( 'NONE',  ( -7.804689982961090955, 12.25722208009664094, 0.7998128361456481317 ) ) ;
#23274=CARTESIAN_POINT ( 'NONE',  ( 7.584896871841365851, 10.93646455286856956, -1.199719254218446718 ) ) ;
#23276=CARTESIAN_POINT ( 'NONE',  ( 5.681948419994366617, 6.106813310819505070, 0.7427411415691799190 ) ) ;
#23278=CARTESIAN_POINT ( 'NONE',  ( -4.253507506385335368, 5.985511395581417204, 1.599625672291267398 ) ) ;
#23282=CARTESIAN_POINT ( 'NONE',  ( 9.237182729612253951, 9.671134694169463586, 0.7998128361456462443 ) ) ;
#23284=CARTESIAN_POINT ( 'NONE',  ( 6.588372581236919601, 9.773852880496709972, -1.199719254218440723 ) ) ;
#23288=CARTESIAN_POINT ( 'NONE',  ( -9.680158490477310806, 10.39586578175276266, 0.7216878364870438212 ) ) ;
#23297=CARTESIAN_POINT ( 'NONE',  ( -5.219871119622601086, 6.450327202623305389, -1.173442693870077935 ) ) ;
#23299=CARTESIAN_POINT ( 'NONE',  ( 6.236387472606139681, 8.298871356172400127, -1.443375672974057666 ) ) ;
#23301=VECTOR ( 'NONE', #2328, 1000.000000000000000 ) ;
#23304=DIRECTION ( 'NONE',  ( 0.000000000000000000, 8.546850786086437571E-32, 1.000000000000000000 ) ) ;
#23318=CARTESIAN_POINT ( 'NONE',  ( -9.612367721964606204, 12.23751498042398289, -1.443375672974058777 ) ) ;
#23320=DIRECTION ( 'NONE',  ( 0.9829311923673916818, -0.1839735607939843032, 0.000000000000000000 ) ) ;
#23322=CARTESIAN_POINT ( 'NONE',  ( 9.108380270282433244, 9.520865158284665952, 1.040834085586084257E-14 ) ) ;
#23324=VERTEX_POINT ( 'NONE', #141169 ) ;
#23326=CARTESIAN_POINT ( 'NONE',  ( 1.499999999999987121, 1.827083334016151861, -0.8660254037844253849 ) ) ;
#23327=CARTESIAN_POINT ( 'NONE',  ( -7.366157530926372488, 7.488271962369228874, -0.7998128361456291469 ) ) ;
#23330=CARTESIAN_POINT ( 'NONE',  ( -8.296699936558862731, 11.76690146170562201, 1.199719254218453823 ) ) ;
#23333=CARTESIAN_POINT ( 'NONE',  ( -1.201851678989727383E-14, 5.368750000682816825, -1.732050807568863648 ) ) ;
#23334=CARTESIAN_POINT ( 'NONE',  ( 5.829115978871627135, 8.888053511070525659, 1.199719254218462483 ) ) ;
#23337=CARTESIAN_POINT ( 'NONE',  ( -7.660520486921249983, 8.896027641951645748, -1.199719254218446718 ) ) ;
#23339=CARTESIAN_POINT ( 'NONE',  ( 0.6823417656249917140, 5.092708333674749177, 1.181850606188765695 ) ) ;
#23345=CARTESIAN_POINT ( 'NONE',  ( -8.839552966430023417, 9.415159337030921449, -0.7216878364870267237 ) ) ;
#23350=CARTESIAN_POINT ( 'NONE',  ( 0.6823417656249899377, 4.488541667008086655, -1.181850606188754593 ) ) ;
#23357=CARTESIAN_POINT ( 'NONE',  ( -1.001543065824772872E-14, 4.821875000341419693, 1.575800808251672791 ) ) ;
#23358=CARTESIAN_POINT ( 'NONE',  ( -5.461236948206312114, 5.265864615862458464, 0.7998128361456341429 ) ) ;
#23359=CARTESIAN_POINT ( 'NONE',  ( 5.615048174354031474, 9.702639970055050966, 0.7998128361456462443 ) ) ;
#23362=CARTESIAN_POINT ( 'NONE',  ( 4.826339496340538382, 4.733076955259818419, 1.040834085586084257E-14 ) ) ;
#23363=CARTESIAN_POINT ( 'NONE',  ( 0.6823417656249917140, 5.155208333674749177, 1.181850606188765695 ) ) ;
#23369=CARTESIAN_POINT ( 'NONE',  ( -0.6823417656250246877, 0.5510416670080897639, 1.181850606188755259 ) ) ;
#23370=CARTESIAN_POINT ( 'NONE',  ( -4.121315508874280553, 3.910548969882488901, -0.7216878364870207285 ) ) ;
#23371=CARTESIAN_POINT ( 'NONE',  ( 4.310602774141044868, 7.116454772218158809, -1.199719254218452047 ) ) ;
#23377=CARTESIAN_POINT ( 'NONE',  ( 4.880572111239557920, 4.796348339308675435, -0.7216878364870197293 ) ) ;
#23380=CARTESIAN_POINT ( 'NONE',  ( -8.839552966430023417, 9.415159337030921449, -0.7216878364870267237 ) ) ;
#23384=CARTESIAN_POINT ( 'NONE',  ( -8.947491310014823895, 12.52615806407091803, 1.199719254218462483 ) ) ;
#23385=CARTESIAN_POINT ( 'NONE',  ( -5.599154252319524794, 6.595063384869953360, 1.082531754730546636 ) ) ;
#23387=CARTESIAN_POINT ( 'NONE',  ( 0.6823417656249882723, 0.1552083336747514530, 1.181850606188755259 ) ) ;
#23388=B_SPLINE_CURVE_WITH_KNOTS ( 'NONE', 3,
 ( #193811, #128905, #177584, #207927, #161336, #194886, #93150, #140849, #159187, #141915, #76863, #126779, #142982, #13984, #18253, #164526, #50772, #64882, #98462 ),
 .UNSPECIFIED., .F., .F.,
 ( 4, 3, 3, 3, 3, 3, 4 ),
 ( 0.000000000000000000, 4.552787399504174405E-05, 9.164501444053742372E-05, 0.0001336247809766562765, 0.0001748474261958513174, 0.0002334031072667115464, 0.0002737127687883765038 ),
 .UNSPECIFIED. ) ;
#23404=CARTESIAN_POINT ( 'NONE',  ( 3.294945724223596883, 7.655198976062512983, -2.499999999999994671 ) ) ;
#23411=CARTESIAN_POINT ( 'NONE',  ( -1.364683531250012516, 3.551041667008086211, -0.7879004041258300672 ) ) ;
#23421=CARTESIAN_POINT ( 'NONE',  ( 1.364683531249988757, 1.134375000341421247, 0.000000000000000000 ) ) ;
#23431=CARTESIAN_POINT ( 'NONE',  ( 4.819033534653518025, 7.709623992816043270, -1.199719254218452047 ) ) ;
#23439=CARTESIAN_POINT ( 'NONE',  ( 8.145751363712157911, 8.397798100619326078, -0.7998128361456281477 ) ) ;
#23444=CARTESIAN_POINT ( 'NONE',  ( 6.909851844459134362, 11.21324425184434936, -0.7998128361456291469 ) ) ;
#23446=CARTESIAN_POINT ( 'NONE',  ( -3.040408649313822931, 6.452285303259204241, 0.6472276285178559796 ) ) ;
#23455=CARTESIAN_POINT ( 'NONE',  ( -8.405692050792730186, 9.869357483088723626, 1.082531754730558626 ) ) ;
#23460=CARTESIAN_POINT ( 'NONE',  ( -8.435144125996554720, 12.99275191363802229, 0.7998128361456341429 ) ) ;
#23467=CARTESIAN_POINT ( 'NONE',  ( -5.108724954250998707, 4.854600622914589714, -0.7998128361456221525 ) ) ;
#23470=CARTESIAN_POINT ( 'NONE',  ( 9.935427640716063991, 10.48575375712389679, -0.7998128361456281477 ) ) ;
#23472=CARTESIAN_POINT ( 'NONE',  ( 3.344057444064992168, 7.053150784717805877, 1.040834085586084257E-14 ) ) ;
#23474=( BOUNDED_CURVE ( )  B_SPLINE_CURVE ( 2, ( #156716, #91732, #26692 ),
 .UNSPECIFIED., .F., .T. ) 
 B_SPLINE_CURVE_WITH_KNOTS ( ( 3, 3 ),
 ( 0.2750000000000000777, 0.2780234451730101974 ),
 .UNSPECIFIED. ) 
 CURVE ( )  GEOMETRIC_REPRESENTATION_ITEM ( )  RATIONAL_B_SPLINE_CURVE ( ( 0.9999999999999982236, 0.9027844369038582339, 0.9466533178002750626 ) ) 
 REPRESENTATION_ITEM ( '' )  );
#23480=CARTESIAN_POINT ( 'NONE',  ( -6.728924311084075960, 6.744833205886536120, 1.040834085586084257E-14 ) ) ;
#23483=CARTESIAN_POINT ( 'NONE',  ( -8.462260433223891098, 13.02438760540324481, -0.7998128361456281477 ) ) ;
#23484=CYLINDRICAL_SURFACE ( 'NONE', #5472, 0.07999999999999998779 ) ;
#23489=CARTESIAN_POINT ( 'NONE',  ( 8.812436659202669276, 10.34389285956704363, -1.082531754730543083 ) ) ;
#23491=CARTESIAN_POINT ( 'NONE',  ( -1.364683531249997417, 4.571875000341417028, 1.214306433183764966E-14 ) ) ;
#23493=CARTESIAN_POINT ( 'NONE',  ( 3.472859903394816872, 7.203420320602605287, -0.7998128361456291469 ) ) ;
#23494=CARTESIAN_POINT ( 'NONE',  ( 6.959052028703007764, 5.167241622962437830, 1.214306433183764966E-14 ) ) ;
#23508=CARTESIAN_POINT ( 'NONE',  ( -1.364683531250012516, 0.8427083336747532849, 0.7879004041258379498 ) ) ;
#23510=CARTESIAN_POINT ( 'NONE',  ( 2.920892028740289081, 5.495125569250587816, 1.199719254218452047 ) ) ;
#23512=CARTESIAN_POINT ( 'NONE',  ( -6.588899466561478846, 6.789396920517583922, 0.7216878364870317197 ) ) ;
#23513=CARTESIAN_POINT ( 'NONE',  ( 3.714570900464278846, 5.356752022006865843, 1.443375672974062551 ) ) ;
#23514=CARTESIAN_POINT ( 'NONE',  ( -5.368665640887164692, 9.207267647769599606, 0.000000000000000000 ) ) ;
#23518=CARTESIAN_POINT ( 'NONE',  ( 5.834086172582112262, 5.700855377634248100, 1.040834085586084257E-14 ) ) ;
#23527=CARTESIAN_POINT ( 'NONE',  ( 5.952193131599331721, 6.902979060742733708, 1.199719254218462483 ) ) ;
#23529=CARTESIAN_POINT ( 'NONE',  ( -7.562750758324527922, 7.717630727667075696, 1.040834085586084257E-14 ) ) ;
#23533=CARTESIAN_POINT ( 'NONE',  ( 6.856673000209174695, 9.022537805042615489, 1.599625672291281386 ) ) ;
#23535=CARTESIAN_POINT ( 'NONE',  ( -6.201965203247477909, 9.323044272842313518, 1.199719254218452047 ) ) ;
#23536=CARTESIAN_POINT ( 'NONE',  ( 6.602457619730760285, 8.725953194484466380, 1.443375672974076540 ) ) ;
#23537=CARTESIAN_POINT ( 'NONE',  ( 5.430717995911492402, 6.471920874811950775, 1.294091166901890633 ) ) ;
#23538=CARTESIAN_POINT ( 'NONE',  ( -5.949330478298285207, 5.835307067636438028, 0.7998128361456341429 ) ) ;
#23541=CARTESIAN_POINT ( 'NONE',  ( -6.144869935491728441, 8.192100896205577243, -1.599625672291263179 ) ) ;
#23546=CARTESIAN_POINT ( 'NONE',  ( -1.201851678989727383E-14, 2.321875000341416584, 1.575800808251672791 ) ) ;
#23549=CARTESIAN_POINT ( 'NONE',  ( -6.399085315970151733, 7.528316292462387871, -1.082531754730544860 ) ) ;
#23556=CARTESIAN_POINT ( 'NONE',  ( 6.993308306550549247, 7.053281200597435685, 1.040834085586084257E-14 ) ) ;
#23558=CARTESIAN_POINT ( 'NONE',  ( -5.894595317363360287, 6.010551413984606128, 0.2245382864616944640 ) ) ;
#23559=CARTESIAN_POINT ( 'NONE',  ( 1.364683531249988757, 1.946875000341415030, 0.000000000000000000 ) ) ;
#23562=CARTESIAN_POINT ( 'NONE',  ( 4.704316114261903436, 4.590716342834741504, 1.214306433183764966E-14 ) ) ;
#23565=CARTESIAN_POINT ( 'NONE',  ( -5.623934791570306402, 5.455678766453782913, 0.7998128361456341429 ) ) ;
#23567=CARTESIAN_POINT ( 'NONE',  ( -8.812436658758329600, 9.383523644747281622, 1.040834085586084257E-14 ) ) ;
#23577=CARTESIAN_POINT ( 'NONE',  ( -7.171900071504738072, 10.35067193585544665, -1.082531754730543083 ) ) ;
#23582=VERTEX_POINT ( 'NONE', #87029 ) ;
#23583=CARTESIAN_POINT ( 'NONE',  ( -7.415946836550729948, 9.675023947441092176, 1.443375672974090751 ) ) ;
#23590=CARTESIAN_POINT ( 'NONE',  ( 4.612443543746578278, 7.139628114692022187, -1.342220757880496995 ) ) ;
#23593=ORIENTED_EDGE ( 'NONE', *, *, #66049, .F. ) ;
#23596=CARTESIAN_POINT ( 'NONE',  ( -7.043624497499477499, 8.176315654292865887, 1.199719254218450271 ) ) ;
#23599=CARTESIAN_POINT ( 'NONE',  ( 4.681643115420508039, 4.356338477612361260, 0.7998128361456341429 ) ) ;
#23604=CARTESIAN_POINT ( 'NONE',  ( 7.091078035147269532, 8.231678114882006625, 1.199719254218462483 ) ) ;
#23609=CARTESIAN_POINT ( 'NONE',  ( -6.236387472606158333, 7.338502141871059870, -1.082531754730544860 ) ) ;
#23621=CARTESIAN_POINT ( 'NONE',  ( -1.364683531250014514, 0.9885416670080898749, -0.7879004041258289570 ) ) ;
#23623=CARTESIAN_POINT ( 'NONE',  ( -8.097244055859620815, 10.46987070330147063, -1.599625672291263179 ) ) ;
#23626=CARTESIAN_POINT ( 'NONE',  ( 8.308449207076147758, 8.587612251210650527, -0.7998128361456281477 ) ) ;
#23628=CARTESIAN_POINT ( 'NONE',  ( -8.528242318195895066, 9.908369778438709474, 1.199719254218462483 ) ) ;
#23631=CARTESIAN_POINT ( 'NONE',  ( -1.364683531250010295, 4.280208333674753618, 0.7879004041258379498 ) ) ;
#23633=CARTESIAN_POINT ( 'NONE',  ( 7.931156674314368438, 12.19684052010138586, 1.040834085586084257E-14 ) ) ;
#23636=CARTESIAN_POINT ( 'NONE',  ( 1.364683531249986537, -0.07395833299191513499, 0.7879004041258500513 ) ) ;
#23638=DIRECTION ( 'NONE',  ( 1.000000000000000000, -6.165071176878339540E-16, 0.000000000000000000 ) ) ;
#23639=CARTESIAN_POINT ( 'NONE',  ( 6.426201622753093368, 10.44105962661321563, 1.040834085586084257E-14 ) ) ;
#23642=CARTESIAN_POINT ( 'NONE',  ( -4.094199201646926412, 7.720390135322642067, 0.7216878364870317197 ) ) ;
#23644=CARTESIAN_POINT ( 'NONE',  ( -1.364683531250012516, 1.530208333674756505, 0.7879004041258379498 ) ) ;
#23648=CARTESIAN_POINT ( 'NONE',  ( -4.882907879216086933, 8.848476292394087395, -0.7998128361456281477 ) ) ;
#23650=AXIS2_PLACEMENT_3D ( 'NONE', #81982, #31127, #64669 ) ;
#23655=CARTESIAN_POINT ( 'NONE',  ( 8.959240580532112475, 9.346868853575953651, -0.7998128361456221525 ) ) ;
#23658=CARTESIAN_POINT ( 'NONE',  ( -1.500000000000015099, 0.8791666666666874130, -0.8660254037844313801 ) ) ;
#23662=CARTESIAN_POINT ( 'NONE',  ( -1.499999999999997780, 5.431250000682820378, 1.214306433183764966E-14 ) ) ;
#23664=ORIENTED_EDGE ( 'NONE', *, *, #81050, .T. ) ;
#23665=CARTESIAN_POINT ( 'NONE',  ( 6.968527767744104651, 8.192665819532020777, 1.082531754730558626 ) ) ;
#23667=ORIENTED_EDGE ( 'NONE', *, *, #11443, .F. ) ;
#23672=CARTESIAN_POINT ( 'NONE',  ( 6.252281394196331554, 10.44607872653774372, 1.040834085586084257E-14 ) ) ;
#23673=CARTESIAN_POINT ( 'NONE',  ( -7.343712760096452463, 11.71941532008788833, -0.7998128361456291469 ) ) ;
#23676=CARTESIAN_POINT ( 'NONE',  ( 1.364683531249986537, -0.5947916663252456049, -0.7879004041258309554 ) ) ;
#23677=CARTESIAN_POINT ( 'NONE',  ( -1.201851678989727383E-14, 0.7125000000000225597, 1.732050807568877637 ) ) ;
#23679=CARTESIAN_POINT ( 'NONE',  ( 3.974511587100456822, 7.788680618259193444, 1.040834085586084257E-14 ) ) ;
#23686=CARTESIAN_POINT ( 'NONE',  ( 1.364683531249990311, 4.884375000341417916, 1.214306433183764966E-14 ) ) ;
#23688=CARTESIAN_POINT ( 'NONE',  ( -7.832860060393135093, 10.16142270859057462, 1.599625672291295375 ) ) ;
#23689=CARTESIAN_POINT ( 'NONE',  ( -5.802526556968872207, 6.832331073627524454, 1.082531754730548412 ) ) ;
#23698=CARTESIAN_POINT ( 'NONE',  ( 8.274553823041976841, 8.548067636504127265, 1.040834085586084257E-14 ) ) ;
#23700=CARTESIAN_POINT ( 'NONE',  ( 2.889785579457927245, 6.440540434672811898, -0.3822207396134719715 ) ) ;
#23702=CARTESIAN_POINT ( 'NONE',  ( 6.873620692004076105, 10.00267932643801672, -1.082531754730537976 ) ) ;
#23705=CARTESIAN_POINT ( 'NONE',  ( -8.833300774503376473, 10.26427131079744193, 1.199719254218462483 ) ) ;
#23707=CARTESIAN_POINT ( 'NONE',  ( 6.505214776458575265, 6.483838748823460563, 1.040834085586084257E-14 ) ) ;
#23709=CARTESIAN_POINT ( 'NONE',  ( 2.507895228403643539, 5.869702166538802501, -0.7216878364870267237 ) ) ;
#23711=CARTESIAN_POINT ( 'NONE',  ( 3.171717870593107058, 5.787755718078879674, -1.199719254218446718 ) ) ;
#23714=CARTESIAN_POINT ( 'NONE',  ( -3.131570295076647525, 6.597323077657299528, 1.040834085586084257E-14 ) ) ;
#23717=CARTESIAN_POINT ( 'NONE',  ( -4.392478581147607031, 7.108013530438723748, 1.082531754730560403 ) ) ;
#23718=CARTESIAN_POINT ( 'NONE',  ( 3.708318708537623021, 4.285125567170706695, -1.199719254218446718 ) ) ;
#23721=CARTESIAN_POINT ( 'NONE',  ( -5.585069213825653023, 8.603332285183535433, -1.199719254218440723 ) ) ;
#23727=CARTESIAN_POINT ( 'NONE',  ( -7.296259222448620463, 11.66405285949874759, 0.7998128361456481317 ) ) ;
#23732=CARTESIAN_POINT ( 'NONE',  ( 4.123651276850781144, 7.962676922967908411, -0.7998128361456221525 ) ) ;
#23743=CARTESIAN_POINT ( 'NONE',  ( -5.181187258716735577, 9.196468901811520880, 0.7998128361456481317 ) ) ;
#23746=CARTESIAN_POINT ( 'NONE',  ( 6.493992391265805075, 6.678671999339316656, 1.040834085586084257E-14 ) ) ;
#23747=VERTEX_POINT ( 'NONE', #209290 ) ;
#23752=CARTESIAN_POINT ( 'NONE',  ( -5.250031796989778066, 7.148123067953287446, 1.599625672291267398 ) ) ;
#23755=CARTESIAN_POINT ( 'NONE',  ( 3.895595285070167169, 2.800000000000017586, -0.7749999999999935829 ) ) ;
#23756=CARTESIAN_POINT ( 'NONE',  ( -7.366157530926372488, 7.488271962369228874, -0.7998128361456291469 ) ) ;
#23762=FACE_OUTER_BOUND ( 'NONE', #36121, .T. ) ;
#23763=CARTESIAN_POINT ( 'NONE',  ( 7.019370843573166319, 9.212351955633947043, 1.599625672291281386 ) ) ;
#23773=CARTESIAN_POINT ( 'NONE',  ( 8.920901888111989919, 11.43080484092926241, 1.443375672974076540 ) ) ;
#23779=CARTESIAN_POINT ( 'NONE',  ( -3.240269673027908137, 6.421702286726624465, 0.6780825091596647258 ) ) ;
#23792=CARTESIAN_POINT ( 'NONE',  ( -3.948449050077848632, 5.629609863222681199, 1.599625672291267398 ) ) ;
#23796=CARTESIAN_POINT ( 'NONE',  ( -2.785310492603665367, 5.336947110424484109, 1.199719254218462483 ) ) ;
#23800=CARTESIAN_POINT ( 'NONE',  ( -1.500000000000001332, -1.318749999317178734, 0.000000000000000000 ) ) ;
#23803=CARTESIAN_POINT ( 'NONE',  ( -3.633221978782304351, 4.301475732409860697, -1.082531754730549967 ) ) ;
#23808=CARTESIAN_POINT ( 'NONE',  ( 2.530568227245037605, 6.104080031761181857, 0.000000000000000000 ) ) ;
#23813=CARTESIAN_POINT ( 'NONE',  ( 1.419999999999989049, 6.280000000000042881, -2.579999999999995630 ) ) ;
#23815=CARTESIAN_POINT ( 'NONE',  ( -0.6823417656250003738, 2.530208333674753618, -1.181850606188749264 ) ) ;
#23816=PLANE ( 'NONE',  #95825 ) ;
#23818=CARTESIAN_POINT ( 'NONE',  ( -9.267161690140662600, 10.77044237904097734, -1.199719254218441611 ) ) ;
#23819=CARTESIAN_POINT ( 'NONE',  ( -5.897433631820158340, 5.982686779986042147, 0.7216878364870317197 ) ) ;
#23821=CARTESIAN_POINT ( 'NONE',  ( -5.530836599371015794, 8.540060901653093950, 1.199719254218452047 ) ) ;
#23823=CARTESIAN_POINT ( 'NONE',  ( -1.500000000000001332, -1.068749999317178290, 0.000000000000000000 ) ) ;
#23831=CARTESIAN_POINT ( 'NONE',  ( -4.080641047588902559, 7.704572288921609058, -0.7216878364870257245 ) ) ;
#23835=CARTESIAN_POINT ( 'NONE',  ( -4.026408433134269771, 6.680931691089825541, 1.082531754730560403 ) ) ;
#23837=CARTESIAN_POINT ( 'NONE',  ( 8.401248741962376698, 12.95320729893149370, 0.7998128361456462443 ) ) ;
#23846=CARTESIAN_POINT ( 'NONE',  ( -4.009460741339347045, 5.700790169694431420, -1.599625672291256295 ) ) ;
#23847=CARTESIAN_POINT ( 'NONE',  ( -8.299562589859897699, 12.83457345481192036, -0.7998128361456281477 ) ) ;
#23852=CARTESIAN_POINT ( 'NONE',  ( 6.667912619822566000, 6.673652899414787676, 1.040834085586084257E-14 ) ) ;
#23856=CARTESIAN_POINT ( 'NONE',  ( 4.539282502477016479, 4.190251095844947926, 0.7998128361456341429 ) ) ;
#23867=CARTESIAN_POINT ( 'NONE',  ( 7.397945374551106568, 11.78268670361832093, -0.7998128361456291469 ) ) ;
#23868=CARTESIAN_POINT ( 'NONE',  ( -5.494078562035765501, 7.432844293840273231, -1.599625672291256295 ) ) ;
#23874=CARTESIAN_POINT ( 'NONE',  ( 1.364683531249990311, 5.113541667008084879, 0.7879004041258500513 ) ) ;
#23876=CARTESIAN_POINT ( 'NONE',  ( -6.196239896645333367, 7.187700286629718605, -1.199719254218446718 ) ) ;
#23879=CARTESIAN_POINT ( 'NONE',  ( 4.599240423533799138, 6.388866465587984322, 1.599625672291267398 ) ) ;
#23880=CARTESIAN_POINT ( 'NONE',  ( -5.412729640353771465, 7.337937218544611895, 1.599625672291269396 ) ) ;
#23886=CARTESIAN_POINT ( 'NONE',  ( 6.155038550924139429, 9.164333495178082600, 1.082531754730558626 ) ) ;
#23889=CARTESIAN_POINT ( 'NONE',  ( 7.605760987142057061, 7.975735361194951523, -0.7216878364870267237 ) ) ;
#23890=CARTESIAN_POINT ( 'NONE',  ( -0.6823417656250212460, 3.113541667008084879, 1.181850606188767472 ) ) ;
#23892=CARTESIAN_POINT ( 'NONE',  ( 4.487385655998873624, 7.218738451098584363, 1.082531754730558626 ) ) ;
#23900=CARTESIAN_POINT ( 'NONE',  ( -5.391143034427437364, 6.494952464278877180, 1.342996321926675396 ) ) ;
#23906=( BOUNDED_SURFACE ( )  B_SPLINE_SURFACE ( 1, 2, ( 
 ( #47775, #193982, #110680, #129087, #31508, #45630, #128028, #94387, #80242, #46698, #97583, #81312, #197182, #212354, #15222, #114935, #111747, #12032, #177753, #95463, #147388, #178829, #112815, #211294, #60792, #32555, #13093, #179884, #79173, #65037, #180933, #62919, #30441, #96526, #162574, #146340, #63994, #130146, #196136, #98631, #143159, #176680, #164691, #77030, #126951, #103961, #186249, #37884, #149507, #70351, #185180, #18421, #119194, #100745, #136468, #201421, #20, #16277, #67153, #183062, #134356, #198236, #34675, #150586, #118135, #102887, #165759, #117064, #167884, #19484, #1091, #202487, #200361, #82361, #84496, #166827, #17344, #83426, #53059, #132227, #152699, #148451, #133289, #49873, #54139, #68225, #181986, #66084, #35741, #36804, #115998, #120275, #199295, #33618, #20548, #99688, #151649, #50940, #184121, #2149, #52009, #101816, #3219, #85560, #69286, #168946, #135398, #86632, #4280, #206768, #6424, #141829, #158051, #42172, #38954, #107215, #191576, #72498, #153771, #22670, #88782, #139677, #204620, #5339, #125617, #138597, #43239, #56272, #207831, #154839, #170004, #58402, #59459, #75715, #122430, #21592, #188387, #124557, #40024, #87696, #71422, #171074, #156983, #190515, #137533, #106136, #105036, #9637, #205700, #8572, #74652, #172159, #203549, #23752, #173237, #57335, #140757, #24817, #89856, #123499, #55204, #121349, #155907, #187325, #7492, #73576, #108288, #90919, #174307, #189463, #41106, #25882, #91992, #44296, #77838, #12820, #111479, #130926, #109356, #60520, #177486, #146071, #176421, #11764, #14946, #196919, #175367, #10695, #29100, #145017, #76766, #208889, #81043, #110418, #211022, #126681, #142888, #195863, #13888, #192643, #212084, #64784, #161233, #163371, #160164, #63722, #97312, #128805, #26949, #194787, #28028, #93057, #159095, #95184, #94126, #147128, #213154, #143960, #209955, #62646, #78894, #61592, #127763, #193719, #45362, #96250, #79967, #46423, #112540, #178552, #129880, #30162, #162303, #47504, #113613, #179618, #31238, #167627, #2962, #150326, #815, #118944, #33351, #131965, #115730, #99433, #181721, #180670, #165486, #82096, #117878, #32296, #1893, #182797, #17083, #65818, #98362, #18152, #116799, #83160, #67952, #197977, #149240, #49606, #148189, #48558, #201166, #52806, #35483, #85306, #114677, #66883, #164427, #133027, #16011, #199026, #214191, #50673, #34416, #100488, #19228, #166563, #135150, #84239, #134097, #200105, #183868, #51756, #101560, #151392, #69033, #193361, #111116, #78541, #98024, #129524, #79611, #95896, #11398, #197615, #210673, #212796, #45006, #130578, #31940, #28736, #62301, #94821, #29811, #112190, #177119, #179262, #14594, #161949, #93756, #127388, #30884, #128460, #144658, #115380, #49259, #27661, #160872, #81746, #196568, #13541, #48210, #178194, #147828, #64434, #77476, #159795, #194428, #46069, #145730, #209587, #211730, #63368, #195504, #114322, #12466, #47140, #96963, #163011, #113257, #213847, #80690, #143595, #146781, #180320, #164079, #15659, #65465, #61233, #131616, #136908, #34054, #148880, #20978, #18855, #132664, #181374, #200797, #135838, #202935, #70795, #166189, #4720, #185627, #153145, #102257, #198669, #134790, #17778, #100127, #54578, #168331, #99075, #1526, #201863, #67590, #19926, #83866, #3656, #149957, #32998, #169393, #53509, #50316, #118574, #165128, #133735, #16719, #199742, #51388, #151028, #117509, #82804, #453, #183502, #66521, #37260, #116434, #86012, #182427, #52448, #35110, #101181, #167270, #152086, #84939, #2597, #119644, #68666, #69734, #184560, #103330, #36181, #87075, #202651, #22831, #169104, #19649, #104120, #6584, #20701, #119358, #3382, #55361, #21755, #72663, #56432, #172319, #187485, #120438, #139837, #86794, #185346, #103051, #152861, #4439, #35903, #70509, #69451, #154999, #101978, #121513, #87863, #136624, #201581, #168047, #203713, #153935, #54300, #39115, #53227, #186412, #36968, #135557, #52164, #156069, #7656, #138761, #188554, #105198, #88945, #73740, #38049, #170167, #106298, #5504, #171235, #204778, #71584, #118291, #137693, #122591, #40185, #23909, #90013, #184277 ),
 ( #85722, #151809, #112445, #210927, #15917, #205865, #157145, #62553, #31144, #58562, #111384, #114580, #82000, #57499, #107377, #128716, #30067, #173400, #91085, #180571, #206933, #96157, #8738, #24982, #80942, #113516, #74819, #97218, #164327, #46330, #124716, #45264, #29001, #177387, #189621, #161136, #140919, #163270, #41269, #63630, #162208, #95088, #190675, #12724, #145977, #178458, #78797, #129784, #144920, #194688, #13794, #79868, #123658, #98269, #211989, #14852, #130831, #195765, #147034, #47404, #179524, #213056, #48465, #64686, #196823, #32193, #116693, #214092, #132920, #151285, #183767, #201059, #85201, #182692, #117776, #103596, #65720, #100386, #181622, #131868, #202117, #168584, #2856, #20184, #197876, #84135, #86271, #166457, #83058, #34310, #51653, #150223, #169653, #148087, #99335, #1793, #184817, #715, #50571, #53777, #21238, #49507, #115627, #67850, #35377, #33251, #165384, #119910, #149134, #101452, #16977, #66780, #152342, #52700, #198925, #36447, #18048, #200004, #185886, #133998, #102522, #136101, #167524, #19122, #68925, #135046, #118831, #3920, #69989, #37520, #141473, #207480, #137174, #203198, #123150, #139309, #75361, #24449, #74298, #173957, #23385, #58037, #204255, #54845, #205338, #41819, #55906, #154484, #38594, #90562, #56976, #107932, #91638, #59100, #8213, #155551, #175010, #122063, #72133, #156623, #189107, #140394, #206413, #188027, #40740, #42884, #153411, #39657, #120995, #4981, #125260, #25530, #124201, #157690, #71058, #89497, #9288, #105765, #22305, #171790, #106846, #7131, #108993, #87344, #104671, #73203, #190165, #6063, #172877, #191220, #186962, #170719, #88417, #138241, #62309, #208531, #126324, #146789, #27669, #128468, #192283, #60167, #113266, #145738, #43943, #129532, #196576, #78550, #80698, #77484, #63376, #14601, #46077, #48218, #112197, #93764, #26597, #10338, #94828, #114331, #212805, #64442, #76412, #142522, #194436, #144667, #130586, #178203, #13547, #179270, #177127, #211738, #143603, #110059, #210680, #195513, #209596, #159803, #176071, #29820, #95904, #47149, #30894, #92698, #161957, #160880, #158744, #61240, #11407, #127397, #193369, #45014, #111124, #28744, #12475, #96971, #79619, #163019, #1534, #148888, #115388, #81754, #117515, #149965, #461, #101188, #181382, #66530, #33005, #131624, #180326, #69739, #135844, #134796, #102262, #167277, #2604, #201867, #132672, #99084, #19932, #67596, #18862, #84946, #198678, #31948, #165136, #16727, #50323, #82811, #164086, #116441, #197623, #68673, #15667, #35117, #133742, #182435, #34062, #147836, #183508, #199750, #100133, #151035, #166195, #17786, #83873, #49267, #98032, #53515, #213853, #200802, #168337, #52453, #118578, #65474, #51395, #184566, #86018, #36186, #152091, #3662, #88155, #185633, #104410, #122890, #155290, #172617, #56722, #154223, #89239, #75107, #37266, #71872, #153151, #103336, #173702, #140132, #188849, #206158, #169398, #55648, #57786, #137982, #54585, #5795, #23122, #121804, #141218, #119649, #70801, #187771, #156366, #186705, #22044, #25277, #207228, #20984, #87081, #39403, #6873, #4726, #136914, #91379, #120732, #72951, #202941, #38333, #123946, #24193, #170459, #7950, #203999, #171529, #157439, #105497, #74042, #107673, #139053, #205080, #40485, #106589, #90296, #189915, #41560, #9033, #113012, #179021, #108740, #174767, #94579, #110871, #46897, #210423, #45827, #145491, #209341, #29564, #175821, #26342, #109812, #42631, #126071, #192032, #28488, #93512, #92455, #14350, #27414, #80440, #159553, #96723, #43695, #146539, #162772, #63123, #30639, #194182, #10093, #12223, #11150, #77227, #58852, #111948, #190965, #143346, #13299, #60989, #177950, #127142, #129287, #95656, #125008, #44763, #161707, #79372, #193114, #211486, #176876, #158494, #160622, #78296, #144421, #62065, #76167, #142272, #128220, #208283, #195263, #59914, #131379, #19686, #34863, #35938, #118329, #49016, #102018, #98833, #100937, #32751, #184314, #130338, #213602, #84698, #168086, #115135, #163836, #81505, #181130, #68424, #99889, #50075, #66281, #196327, #85764, #164883, #183259, #15415, #167024, #2348, #65228 ) ),
 .UNSPECIFIED., .F., .F., .F. ) 
 B_SPLINE_SURFACE_WITH_KNOTS ( ( 2, 2 ),
 ( 3, 2, 2, 2, 2, 2, 2, 2, 2, 2, 2, 2, 2, 2, 2, 2, 2, 2, 2, 2, 2, 2, 2, 2, 2, 2, 2, 2, 2, 2, 2, 2, 2, 2, 2, 2, 2, 2, 2, 2, 2, 2, 2, 2, 2, 2, 2, 2, 2, 2, 2, 2, 2, 2, 2, 2, 2, 2, 2, 2, 2, 2, 2, 2, 2, 2, 2, 2, 2, 2, 2, 2, 2, 2, 2, 2, 2, 2, 2, 2, 2, 2, 2, 2, 2, 2, 2, 2, 2, 2, 2, 2, 2, 2, 2, 2, 2, 2, 2, 2, 2, 2, 2, 2, 2, 2, 2, 2, 2, 2, 2, 2, 2, 2, 2, 2, 2, 2, 2, 2, 2, 2, 2, 2, 2, 2, 2, 2, 2, 2, 2, 2, 2, 2, 2, 2, 2, 2, 2, 2, 2, 2, 2, 2, 2, 2, 2, 2, 2, 2, 2, 2, 2, 2, 2, 2, 2, 2, 2, 2, 2, 2, 2, 2, 2, 2, 2, 2, 2, 2, 2, 2, 2, 2, 2, 2, 2, 2, 2, 2, 2, 2, 2, 2, 2, 2, 2, 2, 2, 2, 2, 2, 2, 2, 2, 2, 2, 2, 2, 2, 2, 2, 2, 2, 2, 2, 2, 2, 2, 2, 2, 2, 2, 2, 2, 2, 2, 2, 2, 2, 2, 2, 2, 2, 2, 2, 2, 2, 2, 2, 2, 2, 2, 2, 2, 2, 2, 2, 2, 2, 3 ),
 ( 0.000000000000000000, 1.000000000000000000 ),
 ( 0.000000000000000000, 0.004166666666666666609, 0.008333333333333333218, 0.01250000000000000069, 0.01666666666666666644, 0.02083333333333333218, 0.02500000000000000139, 0.02916666666666666713, 0.03333333333333333287, 0.03749999999999999861, 0.04166666666666666435, 0.04583333333333333010, 0.05000000000000000278, 0.05416666666666666852, 0.05833333333333333426, 0.06250000000000000000, 0.06666666666666666574, 0.07083333333333333148, 0.07499999999999999722, 0.07916666666666666297, 0.08333333333333332871, 0.08749999999999999445, 0.09166666666666666019, 0.09583333333333333981, 0.1000000000000000056, 0.1041666666666666713, 0.1083333333333333370, 0.1125000000000000028, 0.1166666666666666685, 0.1208333333333333343, 0.1250000000000000000, 0.1291666666666666796, 0.1333333333333333315, 0.1375000000000000111, 0.1416666666666666630, 0.1458333333333333426, 0.1499999999999999944, 0.1541666666666666741, 0.1583333333333333259, 0.1625000000000000056, 0.1666666666666666574, 0.1708333333333333370, 0.1749999999999999889, 0.1791666666666666685, 0.1833333333333333204, 0.1875000000000000000, 0.1916666666666666796, 0.1958333333333333315, 0.2000000000000000111, 0.2041666666666666630, 0.2083333333333333426, 0.2124999999999999944, 0.2166666666666666741, 0.2208333333333333259, 0.2250000000000000056, 0.2291666666666666574, 0.2333333333333333370, 0.2374999999999999889, 0.2416666666666666685, 0.2458333333333333204, 0.2500000000000000000, 0.2541666666666666519, 0.2583333333333333592, 0.2625000000000000111, 0.2666666666666666630, 0.2708333333333333148, 0.2750000000000000222, 0.2791666666666666741, 0.2833333333333333259, 0.2874999999999999778, 0.2916666666666666852, 0.2958333333333333370, 0.2999999999999999889, 0.3041666666666666408, 0.3083333333333333481, 0.3125000000000000000, 0.3166666666666666519, 0.3208333333333333592, 0.3250000000000000111, 0.3291666666666666630, 0.3333333333333333148, 0.3375000000000000222, 0.3416666666666666741, 0.3458333333333333259, 0.3499999999999999778, 0.3541666666666666852, 0.3583333333333333370, 0.3624999999999999889, 0.3666666666666666408, 0.3708333333333333481, 0.3750000000000000000, 0.3791666666666666519, 0.3833333333333333592, 0.3875000000000000111, 0.3916666666666666630, 0.3958333333333333148, 0.4000000000000000222, 0.4041666666666666741, 0.4083333333333333259, 0.4124999999999999778, 0.4166666666666666852, 0.4208333333333333370, 0.4249999999999999889, 0.4291666666666666408, 0.4333333333333333481, 0.4375000000000000000, 0.4416666666666666519, 0.4458333333333333592, 0.4500000000000000111, 0.4541666666666666630, 0.4583333333333333148, 0.4625000000000000222, 0.4666666666666666741, 0.4708333333333333259, 0.4749999999999999778, 0.4791666666666666852, 0.4833333333333333370, 0.4874999999999999889, 0.4916666666666666408, 0.4958333333333333481, 0.5000000000000000000, 0.5041666666666666519, 0.5083333333333333037, 0.5124999999999999556, 0.5166666666666667185, 0.5208333333333333703, 0.5250000000000000222, 0.5291666666666666741, 0.5333333333333333259, 0.5374999999999999778, 0.5416666666666666297, 0.5458333333333332815, 0.5500000000000000444, 0.5541666666666666963, 0.5583333333333333481, 0.5625000000000000000, 0.5666666666666666519, 0.5708333333333333037, 0.5749999999999999556, 0.5791666666666667185, 0.5833333333333333703, 0.5875000000000000222, 0.5916666666666666741, 0.5958333333333333259, 0.5999999999999999778, 0.6041666666666666297, 0.6083333333333332815, 0.6125000000000000444, 0.6166666666666666963, 0.6208333333333333481, 0.6250000000000000000, 0.6291666666666666519, 0.6333333333333333037, 0.6374999999999999556, 0.6416666666666667185, 0.6458333333333333703, 0.6500000000000000222, 0.6541666666666666741, 0.6583333333333333259, 0.6624999999999999778, 0.6666666666666666297, 0.6708333333333332815, 0.6750000000000000444, 0.6791666666666666963, 0.6833333333333333481, 0.6875000000000000000, 0.6916666666666666519, 0.6958333333333333037, 0.6999999999999999556, 0.7041666666666667185, 0.7083333333333333703, 0.7125000000000000222, 0.7166666666666666741, 0.7208333333333333259, 0.7249999999999999778, 0.7291666666666666297, 0.7333333333333332815, 0.7375000000000000444, 0.7416666666666666963, 0.7458333333333333481, 0.7500000000000000000, 0.7541666666666666519, 0.7583333333333333037, 0.7624999999999999556, 0.7666666666666667185, 0.7708333333333333703, 0.7750000000000000222, 0.7791666666666666741, 0.7833333333333333259, 0.7874999999999999778, 0.7916666666666666297, 0.7958333333333332815, 0.8000000000000000444, 0.8041666666666666963, 0.8083333333333333481, 0.8125000000000000000, 0.8166666666666666519, 0.8208333333333333037, 0.8249999999999999556, 0.8291666666666667185, 0.8333333333333333703, 0.8375000000000000222, 0.8416666666666666741, 0.8458333333333333259, 0.8499999999999999778, 0.8541666666666666297, 0.8583333333333332815, 0.8625000000000000444, 0.8666666666666666963, 0.8708333333333333481, 0.8750000000000000000, 0.8791666666666666519, 0.8833333333333333037, 0.8874999999999999556, 0.8916666666666667185, 0.8958333333333333703, 0.9000000000000000222, 0.9041666666666666741, 0.9083333333333333259, 0.9124999999999999778, 0.9166666666666666297, 0.9208333333333332815, 0.9250000000000000444, 0.9291666666666666963, 0.9333333333333333481, 0.9375000000000000000, 0.9416666666666666519, 0.9458333333333333037, 0.9499999999999999556, 0.9541666666666667185, 0.9583333333333333703, 0.9625000000000000222, 0.9666666666666666741, 0.9708333333333333259, 0.9749999999999999778, 0.9791666666666666297, 0.9833333333333332815, 0.9875000000000000444, 0.9916666666666666963, 0.9958333333333333481, 1.000000000000000000 ),
 .UNSPECIFIED. ) 
 GEOMETRIC_REPRESENTATION_ITEM ( )  RATIONAL_B_SPLINE_SURFACE ( (
 ( 1.000000000000000000, 0.8660254037844387076, 1.000000000000000000, 0.8660254037844387076, 1.000000000000000000, 0.8660254037844387076, 1.000000000000000000, 0.8660254037844387076, 1.000000000000000000, 0.8660254037844387076, 1.000000000000000000, 0.8660254037844387076, 1.000000000000000000, 0.8660254037844387076, 1.000000000000000000, 0.8660254037844387076, 1.000000000000000000, 0.8660254037844387076, 1.000000000000000000, 0.8660254037844387076, 1.000000000000000000, 0.8660254037844387076, 1.000000000000000000, 0.8660254037844387076, 1.000000000000000000, 0.8660254037844387076, 1.000000000000000000, 0.8660254037844387076, 1.000000000000000000, 0.8660254037844387076, 1.000000000000000000, 0.8660254037844387076, 1.000000000000000000, 0.8660254037844387076, 1.000000000000000000, 0.8660254037844387076, 1.000000000000000000, 0.8660254037844387076, 1.000000000000000000, 0.8660254037844387076, 1.000000000000000000, 0.8660254037844387076, 1.000000000000000000, 0.8660254037844387076, 1.000000000000000000, 0.8660254037844387076, 1.000000000000000000, 0.8660254037844387076, 1.000000000000000000, 0.8660254037844387076, 1.000000000000000000, 0.8660254037844387076, 1.000000000000000000, 0.8660254037844387076, 1.000000000000000000, 0.8660254037844387076, 1.000000000000000000, 0.8660254037844387076, 1.000000000000000000, 0.8660254037844387076, 1.000000000000000000, 0.8660254037844387076, 1.000000000000000000, 0.8660254037844387076, 1.000000000000000000, 0.8660254037844387076, 1.000000000000000000, 0.8660254037844387076, 1.000000000000000000, 0.8660254037844387076, 1.000000000000000000, 0.8660254037844387076, 1.000000000000000000, 0.8660254037844387076, 1.000000000000000000, 0.8660254037844387076, 1.000000000000000000, 0.8660254037844387076, 1.000000000000000000, 0.8660254037844387076, 1.000000000000000000, 0.8660254037844387076, 1.000000000000000000, 0.8660254037844387076, 1.000000000000000000, 0.8660254037844387076, 1.000000000000000000, 0.8660254037844387076, 1.000000000000000000, 0.8660254037844387076, 1.000000000000000000, 0.8660254037844387076, 1.000000000000000000, 0.8660254037844387076, 1.000000000000000000, 0.8660254037844387076, 1.000000000000000000, 0.8660254037844387076, 1.000000000000000000, 0.8660254037844387076, 1.000000000000000000, 0.8660254037844387076, 1.000000000000000000, 0.8660254037844387076, 1.000000000000000000, 0.8660254037844387076, 1.000000000000000000, 0.8660254037844387076, 1.000000000000000000, 0.8660254037844387076, 1.000000000000000000, 0.8660254037844387076, 1.000000000000000000, 0.8660254037844387076, 1.000000000000000000, 0.8660254037844387076, 1.000000000000000000, 0.8660254037844387076, 1.000000000000000000, 0.8660254037844387076, 1.000000000000000000, 0.8660254037844387076, 1.000000000000000000, 0.8660254037844387076, 1.000000000000000000, 0.8660254037844387076, 1.000000000000000000, 0.8660254037844387076, 1.000000000000000000, 0.8660254037844387076, 1.000000000000000000, 0.8660254037844387076, 1.000000000000000000, 0.8660254037844387076, 1.000000000000000000, 0.8660254037844387076, 1.000000000000000000, 0.8660254037844387076, 1.000000000000000000, 0.8660254037844387076, 1.000000000000000000, 0.8660254037844387076, 1.000000000000000000, 0.8660254037844387076, 1.000000000000000000, 0.8660254037844387076, 1.000000000000000000, 0.8660254037844387076, 1.000000000000000000, 0.8660254037844387076, 1.000000000000000000, 0.8660254037844387076, 1.000000000000000000, 0.8660254037844387076, 1.000000000000000000, 0.8660254037844387076, 1.000000000000000000, 0.8660254037844387076, 1.000000000000000000, 0.8660254037844387076, 1.000000000000000000, 0.8660254037844387076, 1.000000000000000000, 0.8660254037844387076, 1.000000000000000000, 0.8660254037844387076, 1.000000000000000000, 0.8660254037844387076, 1.000000000000000000, 0.8660254037844387076, 1.000000000000000000, 0.8660254037844387076, 1.000000000000000000, 0.8660254037844387076, 1.000000000000000000, 0.8660254037844387076, 1.000000000000000000, 0.8660254037844387076, 1.000000000000000000, 0.8660254037844387076, 1.000000000000000000, 0.8660254037844387076, 1.000000000000000000, 0.8660254037844387076, 1.000000000000000000, 0.8660254037844387076, 1.000000000000000000, 0.8660254037844387076, 1.000000000000000000, 0.8660254037844387076, 1.000000000000000000, 0.8660254037844387076, 1.000000000000000000, 0.8660254037844387076, 1.000000000000000000, 0.8660254037844387076, 1.000000000000000000, 0.8660254037844387076, 1.000000000000000000, 0.8660254037844387076, 1.000000000000000000, 0.8660254037844387076, 1.000000000000000000, 0.8660254037844387076, 1.000000000000000000, 0.8660254037844387076, 1.000000000000000000, 0.8660254037844387076, 1.000000000000000000, 0.8660254037844387076, 1.000000000000000000, 0.8660254037844387076, 1.000000000000000000, 0.8660254037844387076, 1.000000000000000000, 0.8660254037844387076, 1.000000000000000000, 0.8660254037844387076, 1.000000000000000000, 0.8660254037844387076, 1.000000000000000000, 0.8660254037844387076, 1.000000000000000000, 0.8660254037844387076, 1.000000000000000000, 0.8660254037844387076, 1.000000000000000000, 0.8660254037844387076, 1.000000000000000000, 0.8660254037844387076, 1.000000000000000000, 0.8660254037844387076, 1.000000000000000000, 0.8660254037844387076, 1.000000000000000000, 0.8660254037844387076, 1.000000000000000000, 0.8660254037844387076, 1.000000000000000000, 0.8660254037844387076, 1.000000000000000000, 0.8660254037844387076, 1.000000000000000000, 0.8660254037844387076, 1.000000000000000000, 0.8660254037844387076, 1.000000000000000000, 0.8660254037844387076, 1.000000000000000000, 0.8660254037844387076, 1.000000000000000000, 0.8660254037844387076, 1.000000000000000000, 0.8660254037844387076, 1.000000000000000000, 0.8660254037844387076, 1.000000000000000000, 0.8660254037844387076, 1.000000000000000000, 0.8660254037844387076, 1.000000000000000000, 0.8660254037844387076, 1.000000000000000000, 0.8660254037844387076, 1.000000000000000000, 0.8660254037844387076, 1.000000000000000000, 0.8660254037844387076, 1.000000000000000000, 0.8660254037844387076, 1.000000000000000000, 0.8660254037844387076, 1.000000000000000000, 0.8660254037844387076, 1.000000000000000000, 0.8660254037844387076, 1.000000000000000000, 0.8660254037844387076, 1.000000000000000000, 0.8660254037844387076, 1.000000000000000000, 0.8660254037844387076, 1.000000000000000000, 0.8660254037844387076, 1.000000000000000000, 0.8660254037844387076, 1.000000000000000000, 0.8660254037844387076, 1.000000000000000000, 0.8660254037844387076, 1.000000000000000000, 0.8660254037844387076, 1.000000000000000000, 0.8660254037844387076, 1.000000000000000000, 0.8660254037844387076, 1.000000000000000000, 0.8660254037844387076, 1.000000000000000000, 0.8660254037844387076, 1.000000000000000000, 0.8660254037844387076, 1.000000000000000000, 0.8660254037844387076, 1.000000000000000000, 0.8660254037844387076, 1.000000000000000000, 0.8660254037844387076, 1.000000000000000000, 0.8660254037844387076, 1.000000000000000000, 0.8660254037844387076, 1.000000000000000000, 0.8660254037844387076, 1.000000000000000000, 0.8660254037844387076, 1.000000000000000000, 0.8660254037844387076, 1.000000000000000000, 0.8660254037844387076, 1.000000000000000000, 0.8660254037844387076, 1.000000000000000000, 0.8660254037844387076, 1.000000000000000000, 0.8660254037844387076, 1.000000000000000000, 0.8660254037844387076, 1.000000000000000000, 0.8660254037844387076, 1.000000000000000000, 0.8660254037844387076, 1.000000000000000000, 0.8660254037844387076, 1.000000000000000000, 0.8660254037844387076, 1.000000000000000000, 0.8660254037844387076, 1.000000000000000000, 0.8660254037844387076, 1.000000000000000000, 0.8660254037844387076, 1.000000000000000000, 0.8660254037844387076, 1.000000000000000000, 0.8660254037844387076, 1.000000000000000000, 0.8660254037844387076, 1.000000000000000000, 0.8660254037844387076, 1.000000000000000000, 0.8660254037844387076, 1.000000000000000000, 0.8660254037844387076, 1.000000000000000000, 0.8660254037844387076, 1.000000000000000000, 0.8660254037844387076, 1.000000000000000000, 0.8660254037844387076, 1.000000000000000000, 0.8660254037844387076, 1.000000000000000000, 0.8660254037844387076, 1.000000000000000000, 0.8660254037844387076, 1.000000000000000000, 0.8660254037844387076, 1.000000000000000000, 0.8660254037844387076, 1.000000000000000000, 0.8660254037844387076, 1.000000000000000000, 0.8660254037844387076, 1.000000000000000000, 0.8660254037844387076, 1.000000000000000000, 0.8660254037844387076, 1.000000000000000000, 0.8660254037844387076, 1.000000000000000000, 0.8660254037844387076, 1.000000000000000000, 0.8660254037844387076, 1.000000000000000000, 0.8660254037844387076, 1.000000000000000000, 0.8660254037844387076, 1.000000000000000000, 0.8660254037844387076, 1.000000000000000000, 0.8660254037844387076, 1.000000000000000000, 0.8660254037844387076, 1.000000000000000000, 0.8660254037844387076, 1.000000000000000000, 0.8660254037844387076, 1.000000000000000000, 0.8660254037844387076, 1.000000000000000000, 0.8660254037844387076, 1.000000000000000000, 0.8660254037844387076, 1.000000000000000000, 0.8660254037844387076, 1.000000000000000000, 0.8660254037844387076, 1.000000000000000000, 0.8660254037844387076, 1.000000000000000000, 0.8660254037844387076, 1.000000000000000000, 0.8660254037844387076, 1.000000000000000000, 0.8660254037844387076, 1.000000000000000000, 0.8660254037844387076, 1.000000000000000000, 0.8660254037844387076, 1.000000000000000000, 0.8660254037844387076, 1.000000000000000000, 0.8660254037844387076, 1.000000000000000000, 0.8660254037844387076, 1.000000000000000000, 0.8660254037844387076, 1.000000000000000000, 0.8660254037844387076, 1.000000000000000000, 0.8660254037844387076, 1.000000000000000000, 0.8660254037844387076, 1.000000000000000000, 0.8660254037844387076, 1.000000000000000000, 0.8660254037844387076, 1.000000000000000000, 0.8660254037844387076, 1.000000000000000000, 0.8660254037844387076, 1.000000000000000000, 0.8660254037844387076, 1.000000000000000000, 0.8660254037844387076, 1.000000000000000000, 0.8660254037844387076, 1.000000000000000000, 0.8660254037844387076, 1.000000000000000000, 0.8660254037844387076, 1.000000000000000000, 0.8660254037844387076, 1.000000000000000000, 0.8660254037844387076, 1.000000000000000000, 0.8660254037844387076, 1.000000000000000000, 0.8660254037844387076, 1.000000000000000000, 0.8660254037844387076, 1.000000000000000000, 0.8660254037844387076, 1.000000000000000000, 0.8660254037844387076, 1.000000000000000000, 0.8660254037844387076, 1.000000000000000000, 0.8660254037844387076, 1.000000000000000000, 0.8660254037844387076, 1.000000000000000000, 0.8660254037844387076, 1.000000000000000000, 0.8660254037844387076, 1.000000000000000000, 0.8660254037844387076, 1.000000000000000000, 0.8660254037844387076, 1.000000000000000000),
 ( 1.000000000000000000, 0.8660254037844387076, 1.000000000000000000, 0.8660254037844387076, 1.000000000000000000, 0.8660254037844387076, 1.000000000000000000, 0.8660254037844387076, 1.000000000000000000, 0.8660254037844387076, 1.000000000000000000, 0.8660254037844387076, 1.000000000000000000, 0.8660254037844387076, 1.000000000000000000, 0.8660254037844387076, 1.000000000000000000, 0.8660254037844387076, 1.000000000000000000, 0.8660254037844387076, 1.000000000000000000, 0.8660254037844387076, 1.000000000000000000, 0.8660254037844387076, 1.000000000000000000, 0.8660254037844387076, 1.000000000000000000, 0.8660254037844387076, 1.000000000000000000, 0.8660254037844387076, 1.000000000000000000, 0.8660254037844387076, 1.000000000000000000, 0.8660254037844387076, 1.000000000000000000, 0.8660254037844387076, 1.000000000000000000, 0.8660254037844387076, 1.000000000000000000, 0.8660254037844387076, 1.000000000000000000, 0.8660254037844387076, 1.000000000000000000, 0.8660254037844387076, 1.000000000000000000, 0.8660254037844387076, 1.000000000000000000, 0.8660254037844387076, 1.000000000000000000, 0.8660254037844387076, 1.000000000000000000, 0.8660254037844387076, 1.000000000000000000, 0.8660254037844387076, 1.000000000000000000, 0.8660254037844387076, 1.000000000000000000, 0.8660254037844387076, 1.000000000000000000, 0.8660254037844387076, 1.000000000000000000, 0.8660254037844387076, 1.000000000000000000, 0.8660254037844387076, 1.000000000000000000, 0.8660254037844387076, 1.000000000000000000, 0.8660254037844387076, 1.000000000000000000, 0.8660254037844387076, 1.000000000000000000, 0.8660254037844387076, 1.000000000000000000, 0.8660254037844387076, 1.000000000000000000, 0.8660254037844387076, 1.000000000000000000, 0.8660254037844387076, 1.000000000000000000, 0.8660254037844387076, 1.000000000000000000, 0.8660254037844387076, 1.000000000000000000, 0.8660254037844387076, 1.000000000000000000, 0.8660254037844387076, 1.000000000000000000, 0.8660254037844387076, 1.000000000000000000, 0.8660254037844387076, 1.000000000000000000, 0.8660254037844387076, 1.000000000000000000, 0.8660254037844387076, 1.000000000000000000, 0.8660254037844387076, 1.000000000000000000, 0.8660254037844387076, 1.000000000000000000, 0.8660254037844387076, 1.000000000000000000, 0.8660254037844387076, 1.000000000000000000, 0.8660254037844387076, 1.000000000000000000, 0.8660254037844387076, 1.000000000000000000, 0.8660254037844387076, 1.000000000000000000, 0.8660254037844387076, 1.000000000000000000, 0.8660254037844387076, 1.000000000000000000, 0.8660254037844387076, 1.000000000000000000, 0.8660254037844387076, 1.000000000000000000, 0.8660254037844387076, 1.000000000000000000, 0.8660254037844387076, 1.000000000000000000, 0.8660254037844387076, 1.000000000000000000, 0.8660254037844387076, 1.000000000000000000, 0.8660254037844387076, 1.000000000000000000, 0.8660254037844387076, 1.000000000000000000, 0.8660254037844387076, 1.000000000000000000, 0.8660254037844387076, 1.000000000000000000, 0.8660254037844387076, 1.000000000000000000, 0.8660254037844387076, 1.000000000000000000, 0.8660254037844387076, 1.000000000000000000, 0.8660254037844387076, 1.000000000000000000, 0.8660254037844387076, 1.000000000000000000, 0.8660254037844387076, 1.000000000000000000, 0.8660254037844387076, 1.000000000000000000, 0.8660254037844387076, 1.000000000000000000, 0.8660254037844387076, 1.000000000000000000, 0.8660254037844387076, 1.000000000000000000, 0.8660254037844387076, 1.000000000000000000, 0.8660254037844387076, 1.000000000000000000, 0.8660254037844387076, 1.000000000000000000, 0.8660254037844387076, 1.000000000000000000, 0.8660254037844387076, 1.000000000000000000, 0.8660254037844387076, 1.000000000000000000, 0.8660254037844387076, 1.000000000000000000, 0.8660254037844387076, 1.000000000000000000, 0.8660254037844387076, 1.000000000000000000, 0.8660254037844387076, 1.000000000000000000, 0.8660254037844387076, 1.000000000000000000, 0.8660254037844387076, 1.000000000000000000, 0.8660254037844387076, 1.000000000000000000, 0.8660254037844387076, 1.000000000000000000, 0.8660254037844387076, 1.000000000000000000, 0.8660254037844387076, 1.000000000000000000, 0.8660254037844387076, 1.000000000000000000, 0.8660254037844387076, 1.000000000000000000, 0.8660254037844387076, 1.000000000000000000, 0.8660254037844387076, 1.000000000000000000, 0.8660254037844387076, 1.000000000000000000, 0.8660254037844387076, 1.000000000000000000, 0.8660254037844387076, 1.000000000000000000, 0.8660254037844387076, 1.000000000000000000, 0.8660254037844387076, 1.000000000000000000, 0.8660254037844387076, 1.000000000000000000, 0.8660254037844387076, 1.000000000000000000, 0.8660254037844387076, 1.000000000000000000, 0.8660254037844387076, 1.000000000000000000, 0.8660254037844387076, 1.000000000000000000, 0.8660254037844387076, 1.000000000000000000, 0.8660254037844387076, 1.000000000000000000, 0.8660254037844387076, 1.000000000000000000, 0.8660254037844387076, 1.000000000000000000, 0.8660254037844387076, 1.000000000000000000, 0.8660254037844387076, 1.000000000000000000, 0.8660254037844387076, 1.000000000000000000, 0.8660254037844387076, 1.000000000000000000, 0.8660254037844387076, 1.000000000000000000, 0.8660254037844387076, 1.000000000000000000, 0.8660254037844387076, 1.000000000000000000, 0.8660254037844387076, 1.000000000000000000, 0.8660254037844387076, 1.000000000000000000, 0.8660254037844387076, 1.000000000000000000, 0.8660254037844387076, 1.000000000000000000, 0.8660254037844387076, 1.000000000000000000, 0.8660254037844387076, 1.000000000000000000, 0.8660254037844387076, 1.000000000000000000, 0.8660254037844387076, 1.000000000000000000, 0.8660254037844387076, 1.000000000000000000, 0.8660254037844387076, 1.000000000000000000, 0.8660254037844387076, 1.000000000000000000, 0.8660254037844387076, 1.000000000000000000, 0.8660254037844387076, 1.000000000000000000, 0.8660254037844387076, 1.000000000000000000, 0.8660254037844387076, 1.000000000000000000, 0.8660254037844387076, 1.000000000000000000, 0.8660254037844387076, 1.000000000000000000, 0.8660254037844387076, 1.000000000000000000, 0.8660254037844387076, 1.000000000000000000, 0.8660254037844387076, 1.000000000000000000, 0.8660254037844387076, 1.000000000000000000, 0.8660254037844387076, 1.000000000000000000, 0.8660254037844387076, 1.000000000000000000, 0.8660254037844387076, 1.000000000000000000, 0.8660254037844387076, 1.000000000000000000, 0.8660254037844387076, 1.000000000000000000, 0.8660254037844387076, 1.000000000000000000, 0.8660254037844387076, 1.000000000000000000, 0.8660254037844387076, 1.000000000000000000, 0.8660254037844387076, 1.000000000000000000, 0.8660254037844387076, 1.000000000000000000, 0.8660254037844387076, 1.000000000000000000, 0.8660254037844387076, 1.000000000000000000, 0.8660254037844387076, 1.000000000000000000, 0.8660254037844387076, 1.000000000000000000, 0.8660254037844387076, 1.000000000000000000, 0.8660254037844387076, 1.000000000000000000, 0.8660254037844387076, 1.000000000000000000, 0.8660254037844387076, 1.000000000000000000, 0.8660254037844387076, 1.000000000000000000, 0.8660254037844387076, 1.000000000000000000, 0.8660254037844387076, 1.000000000000000000, 0.8660254037844387076, 1.000000000000000000, 0.8660254037844387076, 1.000000000000000000, 0.8660254037844387076, 1.000000000000000000, 0.8660254037844387076, 1.000000000000000000, 0.8660254037844387076, 1.000000000000000000, 0.8660254037844387076, 1.000000000000000000, 0.8660254037844387076, 1.000000000000000000, 0.8660254037844387076, 1.000000000000000000, 0.8660254037844387076, 1.000000000000000000, 0.8660254037844387076, 1.000000000000000000, 0.8660254037844387076, 1.000000000000000000, 0.8660254037844387076, 1.000000000000000000, 0.8660254037844387076, 1.000000000000000000, 0.8660254037844387076, 1.000000000000000000, 0.8660254037844387076, 1.000000000000000000, 0.8660254037844387076, 1.000000000000000000, 0.8660254037844387076, 1.000000000000000000, 0.8660254037844387076, 1.000000000000000000, 0.8660254037844387076, 1.000000000000000000, 0.8660254037844387076, 1.000000000000000000, 0.8660254037844387076, 1.000000000000000000, 0.8660254037844387076, 1.000000000000000000, 0.8660254037844387076, 1.000000000000000000, 0.8660254037844387076, 1.000000000000000000, 0.8660254037844387076, 1.000000000000000000, 0.8660254037844387076, 1.000000000000000000, 0.8660254037844387076, 1.000000000000000000, 0.8660254037844387076, 1.000000000000000000, 0.8660254037844387076, 1.000000000000000000, 0.8660254037844387076, 1.000000000000000000, 0.8660254037844387076, 1.000000000000000000, 0.8660254037844387076, 1.000000000000000000, 0.8660254037844387076, 1.000000000000000000, 0.8660254037844387076, 1.000000000000000000, 0.8660254037844387076, 1.000000000000000000, 0.8660254037844387076, 1.000000000000000000, 0.8660254037844387076, 1.000000000000000000, 0.8660254037844387076, 1.000000000000000000, 0.8660254037844387076, 1.000000000000000000, 0.8660254037844387076, 1.000000000000000000, 0.8660254037844387076, 1.000000000000000000, 0.8660254037844387076, 1.000000000000000000, 0.8660254037844387076, 1.000000000000000000, 0.8660254037844387076, 1.000000000000000000, 0.8660254037844387076, 1.000000000000000000, 0.8660254037844387076, 1.000000000000000000, 0.8660254037844387076, 1.000000000000000000, 0.8660254037844387076, 1.000000000000000000, 0.8660254037844387076, 1.000000000000000000, 0.8660254037844387076, 1.000000000000000000, 0.8660254037844387076, 1.000000000000000000, 0.8660254037844387076, 1.000000000000000000, 0.8660254037844387076, 1.000000000000000000, 0.8660254037844387076, 1.000000000000000000, 0.8660254037844387076, 1.000000000000000000, 0.8660254037844387076, 1.000000000000000000, 0.8660254037844387076, 1.000000000000000000, 0.8660254037844387076, 1.000000000000000000, 0.8660254037844387076, 1.000000000000000000, 0.8660254037844387076, 1.000000000000000000, 0.8660254037844387076, 1.000000000000000000, 0.8660254037844387076, 1.000000000000000000, 0.8660254037844387076, 1.000000000000000000, 0.8660254037844387076, 1.000000000000000000, 0.8660254037844387076, 1.000000000000000000, 0.8660254037844387076, 1.000000000000000000, 0.8660254037844387076, 1.000000000000000000, 0.8660254037844387076, 1.000000000000000000, 0.8660254037844387076, 1.000000000000000000, 0.8660254037844387076, 1.000000000000000000, 0.8660254037844387076, 1.000000000000000000, 0.8660254037844387076, 1.000000000000000000, 0.8660254037844387076, 1.000000000000000000, 0.8660254037844387076, 1.000000000000000000, 0.8660254037844387076, 1.000000000000000000, 0.8660254037844387076, 1.000000000000000000, 0.8660254037844387076, 1.000000000000000000, 0.8660254037844387076, 1.000000000000000000, 0.8660254037844387076, 1.000000000000000000, 0.8660254037844387076, 1.000000000000000000, 0.8660254037844387076, 1.000000000000000000) ) ) 
 REPRESENTATION_ITEM ( '' )  SURFACE ( )  );
#23909=CARTESIAN_POINT ( 'NONE',  ( -9.130526383799315582, 12.73969898348616070, 1.199719254218462483 ) ) ;
#23918=CARTESIAN_POINT ( 'NONE',  ( 3.307826292054301121, 4.882216645528547616, -1.443375672974057666 ) ) ;
#23919=CARTESIAN_POINT ( 'NONE',  ( -1.201851678989727383E-14, 3.134375000341420137, 1.575800808251672791 ) ) ;
#23921=CARTESIAN_POINT ( 'NONE',  ( 6.238723240582662477, 10.43026088065513513, -0.7998128361456291469 ) ) ;
#23925=CARTESIAN_POINT ( 'NONE',  ( -4.172158584703340445, 5.890604320285754980, -1.599625672291256517 ) ) ;
#23929=CARTESIAN_POINT ( 'NONE',  ( -1.201851678989727383E-14, 3.087500000000026112, -1.732050807568863648 ) ) ;
#23930=CARTESIAN_POINT ( 'NONE',  ( 4.286349120214771879, 8.152491073559232859, -0.7998128361456221525 ) ) ;
#23933=CARTESIAN_POINT ( 'NONE',  ( -1.499999999999997780, 5.900000000000023448, 1.214306433183764966E-14 ) ) ;
#23935=CARTESIAN_POINT ( 'NONE',  ( 1.364683531249988535, 4.113541667008088432, 0.7879004041258500513 ) ) ;
#23937=CARTESIAN_POINT ( 'NONE',  ( 10.05978679165993839, 10.83876546646586014, 0.7216878364870438212 ) ) ;
#23942=CARTESIAN_POINT ( 'NONE',  ( 1.499999999999989120, 2.556250000682817713, 1.214306433183764966E-14 ) ) ;
#23944=CARTESIAN_POINT ( 'NONE',  ( -6.338600509588822263, 7.353787668397130162, -1.199719254218446718 ) ) ;
#23945=CARTESIAN_POINT ( 'NONE',  ( 4.324687812634882000, 7.028924300507257250, 1.082531754730558626 ) ) ;
#23946=DIRECTION ( 'NONE',  ( -1.000000000000000000, 8.673617379884035472E-16, 0.000000000000000000 ) ) ;
#23955=CARTESIAN_POINT ( 'NONE',  ( 7.202405917357655341, 9.425892875049191488, 1.599625672291281386 ) ) ;
#23956=CARTESIAN_POINT ( 'NONE',  ( 5.118366684358879759, 5.930181538962194132, 1.199719254218462483 ) ) ;
#23960=CARTESIAN_POINT ( 'NONE',  ( 4.547870462380197765, 7.393267075163835855, 1.199719254218462483 ) ) ;
#23962=VERTEX_POINT ( 'NONE', #81711 ) ;
#23967=CARTESIAN_POINT ( 'NONE',  ( 10.40318394038753702, 11.03146944007395724, -0.7998128361456281477 ) ) ;
#23972=CARTESIAN_POINT ( 'NONE',  ( 5.007133299032078710, 6.576657384445655730, 1.236533897214306066 ) ) ;
#23983=CARTESIAN_POINT ( 'NONE',  ( 6.480434237652121787, 9.543961796360731498, 1.082531754730558626 ) ) ;
#23984=CARTESIAN_POINT ( 'NONE',  ( -4.172158584703340445, 5.890604320285754980, -1.599625672291256295 ) ) ;
#23988=CARTESIAN_POINT ( 'NONE',  ( -5.880485940025243607, 7.883652901494672349, 1.599625672291269396 ) ) ;
#23994=ORIENTED_EDGE ( 'NONE', *, *, #126096, .T. ) ;
#23999=CARTESIAN_POINT ( 'NONE',  ( 1.579999999999991189, 8.674529973577531194, 2.420000000000000373 ) ) ;
#24005=ORIENTED_EDGE ( 'NONE', *, *, #143969, .F. ) ;
#24007=CARTESIAN_POINT ( 'NONE',  ( 4.214603523450839440, 3.811458953647739900, -0.4421859227901690503 ) ) ;
#24010=CARTESIAN_POINT ( 'NONE',  ( -2.764973262183167968, 5.313220341600567664, 1.199719254218462483 ) ) ;
#24014=CARTESIAN_POINT ( 'NONE',  ( 7.052212457402625922, 11.37933163361175382, -0.7998128361456291469 ) ) ;
#24016=CARTESIAN_POINT ( 'NONE',  ( -0.5569645644277303465, 2.800000000000026468, 1.258719724711860666 ) ) ;
#24018=CARTESIAN_POINT ( 'NONE',  ( -6.521635583373313061, 7.567328587812373719, -1.199719254218446718 ) ) ;
#24019=CARTESIAN_POINT ( 'NONE',  ( 3.388648328411762556, 6.040841252200647382, 1.199719254218462483 ) ) ;
#24023=CARTESIAN_POINT ( 'NONE',  ( 8.757677159423465696, 12.30470822171437284, 1.199719254218450271 ) ) ;
#24026=CARTESIAN_POINT ( 'NONE',  ( -1.364683531249997417, 3.321875000341423245, 1.214306433183764966E-14 ) ) ;
#24028=CARTESIAN_POINT ( 'NONE',  ( 5.816084710582486217, 9.729256562414162701, 1.040834085586084257E-14 ) ) ;
#24036=CARTESIAN_POINT ( 'NONE',  ( 8.500599125643985232, 11.90082083235127008, -1.082531754730543083 ) ) ;
#24037=VERTEX_POINT ( 'NONE', #2555 ) ;
#24041=CARTESIAN_POINT ( 'NONE',  ( -10.16591625214838679, 10.75465713712827487, 1.040834085586084257E-14 ) ) ;
#24046=B_SPLINE_CURVE_WITH_KNOTS ( 'NONE', 3,
 ( #156683, #141534, #208595, #190220, #91700, #41879, #105825, #74358, #60227, #7191, #58102, #209661, #39718, #8274, #76476, #143668, #124261, #140461, #139369, #127464, #61302, #207542, #157752, #24514, #142587 ),
 .UNSPECIFIED., .F., .F.,
 ( 4, 3, 3, 3, 3, 3, 3, 3, 4 ),
 ( 0.000000000000000000, 2.847723191052623255E-05, 6.630505566358953792E-05, 8.958118362427201905E-05, 9.621695898307930904E-05, 0.0001106671188294701110, 0.0001194291616091197475, 0.0001339184197518206642, 0.0001602236158699481391 ),
 .UNSPECIFIED. ) ;
#24050=CARTESIAN_POINT ( 'NONE',  ( 3.194917754314666514, 6.879154480009089134, 0.7998128361456321445 ) ) ;
#24058=CARTESIAN_POINT ( 'NONE',  ( 5.473741331615251227, 7.409117525016355010, -1.599625672291262513 ) ) ;
#24061=CARTESIAN_POINT ( 'NONE',  ( -1.499999999999997780, 2.431250000682817713, 1.214306433183764966E-14 ) ) ;
#24067=CARTESIAN_POINT ( 'NONE',  ( -1.201851678989727383E-14, 0.7125000000000225597, 1.732050807568877637 ) ) ;
#24068=CARTESIAN_POINT ( 'NONE',  ( 8.046927864910717432, 9.346836249606042202, 1.199719254218462483 ) ) ;
#24069=CARTESIAN_POINT ( 'NONE',  ( 1.364683531249986537, 0.1552083336747499542, -0.7879004041258309554 ) ) ;
#24072=CARTESIAN_POINT ( 'NONE',  ( 9.463228032658635769, 11.10314946193233965, -1.082531754730543083 ) ) ;
#24078=CARTESIAN_POINT ( 'NONE',  ( -6.742482464697739708, 6.760651051769146491, 0.7998128361456341429 ) ) ;
#24079=CARTESIAN_POINT ( 'NONE',  ( 1.499999999999987121, 3.077083334016149863, -0.8660254037844262731 ) ) ;
#24080=CARTESIAN_POINT ( 'NONE',  ( -1.364683531250010295, 5.592708333674750953, 0.7879004041258379498 ) ) ;
#24093=CARTESIAN_POINT ( 'NONE',  ( -8.317037166979361018, 11.79062823052953668, 1.199719254218453823 ) ) ;
#24094=( BOUNDED_CURVE ( )  B_SPLINE_CURVE ( 2, ( #158557, #44828, #211550, #142340, #59980, #210488, #28555, #78361, #125075, #62125, #195327, #128285, #112012, #79434, #191031, #179081, #101004, #198493, #166017, #114148, #148706, #84763, #98894, #32820, #130402, #99952, #97838, #167093, #163903, #17602, #180140, #2414, #117327, #131437, #83687, #213666, #68491, #116260, #64258, #65290, #212618, #82622, #50137, #162835, #182249, #51205, #164947, #275, #16539, #14414, #197440, #183325, #196391, #115200, #52268, #96784, #49081, #133553, #200621, #181193, #66348, #81563, #149775, #134619, #33874, #132491, #147647, #199561, #67412, #1350, #34931 ),
 .UNSPECIFIED., .F., .T. ) 
 B_SPLINE_CURVE_WITH_KNOTS ( ( 3, 2, 2, 2, 2, 2, 2, 2, 2, 2, 2, 2, 2, 2, 2, 2, 2, 2, 2, 2, 2, 2, 2, 2, 2, 2, 2, 2, 2, 2, 2, 2, 2, 2, 2, 3 ),
 ( 0.1345121972684862333, 0.1375000000000000111, 0.1416666666666666630, 0.1458333333333333426, 0.1499999999999999944, 0.1541666666666666741, 0.1583333333333333259, 0.1625000000000000056, 0.1666666666666666574, 0.1708333333333333370, 0.1749999999999999889, 0.1791666666666666685, 0.1833333333333333204, 0.1875000000000000000, 0.1916666666666666796, 0.1958333333333333315, 0.2000000000000000111, 0.2041666666666666630, 0.2083333333333333426, 0.2124999999999999944, 0.2166666666666666741, 0.2208333333333333259, 0.2250000000000000056, 0.2291666666666666574, 0.2333333333333333370, 0.2374999999999999889, 0.2416666666666666685, 0.2458333333333333204, 0.2500000000000000000, 0.2541666666666666519, 0.2583333333333333592, 0.2625000000000000111, 0.2666666666666666630, 0.2708333333333333148, 0.2750000000000000222, 0.2778825950481893514 ),
 .UNSPECIFIED. ) 
 CURVE ( )  GEOMETRIC_REPRESENTATION_ITEM ( )  RATIONAL_B_SPLINE_CURVE ( ( 0.9456386119408557445, 0.9039304805136860743, 1.000000000000000000, 0.8660254037844387076, 1.000000000000000000, 0.8660254037844387076, 1.000000000000000000, 0.8660254037844387076, 1.000000000000000000, 0.8660254037844387076, 1.000000000000000000, 0.8660254037844387076, 1.000000000000000000, 0.8660254037844387076, 1.000000000000000000, 0.8660254037844387076, 1.000000000000000000, 0.8660254037844387076, 1.000000000000000000, 0.8660254037844387076, 1.000000000000000000, 0.8660254037844387076, 1.000000000000000000, 0.8660254037844387076, 1.000000000000000000, 0.8660254037844387076, 1.000000000000000000, 0.8660254037844387076, 1.000000000000000000, 0.8660254037844387076, 1.000000000000000000, 0.8660254037844387076, 1.000000000000000000, 0.8660254037844387076, 1.000000000000000000, 0.8660254037844387076, 1.000000000000000000, 0.8660254037844387076, 1.000000000000000000, 0.8660254037844387076, 1.000000000000000000, 0.8660254037844387076, 1.000000000000000000, 0.8660254037844387076, 1.000000000000000000, 0.8660254037844387076, 1.000000000000000000, 0.8660254037844387076, 1.000000000000000000, 0.8660254037844387076, 1.000000000000000000, 0.8660254037844387076, 1.000000000000000000, 0.8660254037844387076, 1.000000000000000000, 0.8660254037844387076, 1.000000000000000000, 0.8660254037844387076, 1.000000000000000000, 0.8660254037844387076, 1.000000000000000000, 0.8660254037844387076, 1.000000000000000000, 0.8660254037844387076, 1.000000000000000000, 0.8660254037844387076, 1.000000000000000000, 0.8660254037844387076, 1.000000000000000000, 0.9073133181678055825, 0.9428721579752517012 ) ) 
 REPRESENTATION_ITEM ( '' )  );
#24095=CARTESIAN_POINT ( 'NONE',  ( 6.388916700537700777, 8.476822122092563916, 1.599625672291281386 ) ) ;
#24102=CARTESIAN_POINT ( 'NONE',  ( -6.531277313481209212, 8.642909503859968368, 1.599625672291283607 ) ) ;
#24107=CARTESIAN_POINT ( 'NONE',  ( 4.241003122976366058, 3.842258486427521103, -0.7998128361456211532 ) ) ;
#24108=CYLINDRICAL_SURFACE ( 'NONE', #112877, 2.000000000000000000 ) ;
#24110=CARTESIAN_POINT ( 'NONE',  ( -4.578903193113314174, 6.365139696764064325, 1.599625672291267398 ) ) ;
#24111=CARTESIAN_POINT ( 'NONE',  ( -8.809047120577080392, 11.30030761213851953, 1.599625672291269396 ) ) ;
#24114=CARTESIAN_POINT ( 'NONE',  ( -4.119491766144414591, 7.660190618428146081, -0.8001636830725885607 ) ) ;
#24124=CARTESIAN_POINT ( 'NONE',  ( 3.600749563572445133, 3.160087278257350807, 2.499999999999998668 ) ) ;
#24139=CARTESIAN_POINT ( 'NONE',  ( 2.887523530030648988, 6.312601851770308414, 0.000000000000000000 ) ) ;
#24143=CARTESIAN_POINT ( 'NONE',  ( -8.565000355531095622, 11.01558638625153286, -1.599625672291263179 ) ) ;
#24147=CARTESIAN_POINT ( 'NONE',  ( -1.402160292154681736E-14, 2.368750000682818602, -1.732050807568863648 ) ) ;
#24149=CARTESIAN_POINT ( 'NONE',  ( -1.420000000000021911, 6.120000000000041851, 2.500000000000011102 ) ) ;
#24152=CARTESIAN_POINT ( 'NONE',  ( -10.50487009249003378, 11.15010328419353947, 0.7998128361456462443 ) ) ;
#24154=CARTESIAN_POINT ( 'NONE',  ( -1.364683531250014514, 0.4885416670080875434, -0.7879004041258289570 ) ) ;
#24160=CARTESIAN_POINT ( 'NONE',  ( -5.101945877444165944, 4.846691699973280976, 0.000000000000000000 ) ) ;
#24162=CARTESIAN_POINT ( 'NONE',  ( 1.499999999999990896, 8.627523663848663205, -2.579999999999991189 ) ) ;
#24165=CARTESIAN_POINT ( 'NONE',  ( 0.6823417656249882723, -1.094791666325249713, 1.181850606188755259 ) ) ;
#24170=CARTESIAN_POINT ( 'NONE',  ( 0.6823417656249882723, -0.1572916663252488245, 1.181850606188755259 ) ) ;
#24172=CARTESIAN_POINT ( 'NONE',  ( -6.581593504430098385, 9.765943957555402122, -1.199719254218440723 ) ) ;
#24173=CARTESIAN_POINT ( 'NONE',  ( 9.562578416340237197, 10.05076299535211781, 0.7998128361456462443 ) ) ;
#24174=CARTESIAN_POINT ( 'NONE',  ( 5.691725559638619814, 5.534767995866836543, 1.040834085586084257E-14 ) ) ;
#24178=CARTESIAN_POINT ( 'NONE',  ( -0.6823417656250003738, -0.2197916663252488800, -1.181850606188749264 ) ) ;
#24184=CARTESIAN_POINT ( 'NONE',  ( 6.480434237652124452, 8.583592582059388576, 1.443375672974076540 ) ) ;
#24187=CARTESIAN_POINT ( 'NONE',  ( -4.985647801523292344, 6.839675073242382553, -1.599625672291256295 ) ) ;
#24188=CARTESIAN_POINT ( 'NONE',  ( 1.123270288250311610, 3.172697346350006331, 0.7749999999993734123 ) ) ;
#24189=CARTESIAN_POINT ( 'NONE',  ( -1.500000000000011324, 5.452083334016153415, 0.8660254037844403729 ) ) ;
#24192=CARTESIAN_POINT ( 'NONE',  ( 6.439759776366780208, 6.615400615290456088, 0.7216878364870317197 ) ) ;
#24193=CARTESIAN_POINT ( 'NONE',  ( -8.229436053370685400, 10.62409470039771442, 1.443375672974090751 ) ) ;
#24195=CARTESIAN_POINT ( 'NONE',  ( -1.499999999999997780, 4.400000000000021672, 1.214306433183764966E-14 ) ) ;
#24199=CARTESIAN_POINT ( 'NONE',  ( 9.585251415181632595, 10.28514086057449184, 0.000000000000000000 ) ) ;
#24212=CARTESIAN_POINT ( 'NONE',  ( 7.904040366642689719, 10.24446639921506552, 1.443375672974076540 ) ) ;
#24214=CARTESIAN_POINT ( 'NONE',  ( 8.776205506747620788, 9.133327934160710981, -0.7998128361456221525 ) ) ;
#24215=CARTESIAN_POINT ( 'NONE',  ( -4.530395885260773525, 8.437212299446219532, 0.7998128361456481317 ) ) ;
#24219=CARTESIAN_POINT ( 'NONE',  ( 9.103410076571945453, 12.70806329172093818, 1.199719254218450271 ) ) ;
#24221=CARTESIAN_POINT ( 'NONE',  ( 3.985733972737593778, 6.633478153960411738, -1.082531754730548412 ) ) ;
#24223=CARTESIAN_POINT ( 'NONE',  ( -7.036318535812428721, 11.15286269184909784, 0.000000000000000000 ) ) ;
#24241=EDGE_CURVE ( 'NONE', #52497, #71497, #180577, .T. ) ;
#24247=CARTESIAN_POINT ( 'NONE',  ( 1.284279953904125193, 3.003360285806104368, 0.7750000000000065725 ) ) ;
#24251=CARTESIAN_POINT ( 'NONE',  ( -6.388916700537716764, 8.476822122092563916, 1.599625672291283607 ) ) ;
#24254=CARTESIAN_POINT ( 'NONE',  ( 5.931855901178834323, 6.879252291918818152, 1.199719254218462483 ) ) ;
#24264=CARTESIAN_POINT ( 'NONE',  ( -2.591579918506545344, 6.175260338232929413, 1.040834085586084257E-14 ) ) ;
#24267=CARTESIAN_POINT ( 'NONE',  ( 8.423693512792301163, 8.722063941212843119, 0.7998128361456481317 ) ) ;
#24268=CARTESIAN_POINT ( 'NONE',  ( 0.6823417656249899377, 3.426041667008085323, -1.181850606188754593 ) ) ;
#24270=CARTESIAN_POINT ( 'NONE',  ( 5.545980446453017798, 6.390169355917580951, 1.218016560845627483 ) ) ;
#24275=CARTESIAN_POINT ( 'NONE',  ( 6.114364089638782751, 9.116879957011832403, 1.082531754730558626 ) ) ;
#24276=CARTESIAN_POINT ( 'NONE',  ( -6.723954117373590833, 9.932031339322813679, -1.199719254218440723 ) ) ;
#24279=CARTESIAN_POINT ( 'NONE',  ( -8.507905087775398556, 9.884643009614800135, 1.199719254218462483 ) ) ;
#24280=CARTESIAN_POINT ( 'NONE',  ( -6.144869935491728441, 8.192100896205577243, -1.599625672291263179 ) ) ;
#24287=CARTESIAN_POINT ( 'NONE',  ( 7.914208982075123799, 10.25632978388623684, -1.599625672291262513 ) ) ;
#24303=CARTESIAN_POINT ( 'NONE',  ( -1.201851678989727383E-14, 3.962500000000022116, 1.732050807568877637 ) ) ;
#24304=CARTESIAN_POINT ( 'NONE',  ( 5.847644326195776010, 5.716673223516856694, -0.7998128361456281477 ) ) ;
#24305=CARTESIAN_POINT ( 'NONE',  ( 6.012151052656117933, 9.101594430485762999, 1.199719254218460707 ) ) ;
#24307=CARTESIAN_POINT ( 'NONE',  ( -7.524412065904404479, 11.72230514362308185, 0.000000000000000000 ) ) ;
#24309=CARTESIAN_POINT ( 'NONE',  ( 5.802526556968819804, 9.713438716531550554, -0.7216878364870267237 ) ) ;
#24310=CARTESIAN_POINT ( 'NONE',  ( -9.341204649691320583, 10.96078884847042545, 1.082531754730558626 ) ) ;
#24313=CARTESIAN_POINT ( 'NONE',  ( 6.916630921265960019, 11.22115317478565188, 0.7998128361456462443 ) ) ;
#24319=CARTESIAN_POINT ( 'NONE',  ( 1.364683531249990311, 2.634375000341422801, 1.214306433183764966E-14 ) ) ;
#24325=CARTESIAN_POINT ( 'NONE',  ( 10.23370702021670020, 10.83374636654133383, 0.7998128361456462443 ) ) ;
#24329=CARTESIAN_POINT ( 'NONE',  ( -9.154780037725563702, 11.70366268214508487, 1.599625672291281386 ) ) ;
#24335=CARTESIAN_POINT ( 'NONE',  ( 4.192495815123822744, 5.914331089109666983, -1.599625672291255185 ) ) ;
#24338=CARTESIAN_POINT ( 'NONE',  ( -7.994504133552415404, 12.47867192245318435, -0.7998128361456281477 ) ) ;
#24341=CARTESIAN_POINT ( 'NONE',  ( 8.609591239877852686, 10.00327685373437347, -1.199719254218445830 ) ) ;
#24343=CARTESIAN_POINT ( 'NONE',  ( 4.839368334287259543, 6.711050605271530856, 1.249743143419468350 ) ) ;
#24345=CARTESIAN_POINT ( 'NONE',  ( -4.440459003675619520, 5.139289244831666714, 1.199719254218462483 ) ) ;
#24349=CARTESIAN_POINT ( 'NONE',  ( 7.076466111328892694, 10.34329533227067799, -1.199719254218441611 ) ) ;
#24351=CARTESIAN_POINT ( 'NONE',  ( 7.507464373665139412, 9.781794407407920389, 1.599625672291281386 ) ) ;
#24354=CARTESIAN_POINT ( 'NONE',  ( -7.863365906246048809, 12.11775129068834289, -0.7216878364870267237 ) ) ;
#24361=CARTESIAN_POINT ( 'NONE',  ( -5.061731940678604325, 6.567192784585701659, -1.227863150880079246 ) ) ;
#24362=CARTESIAN_POINT ( 'NONE',  ( -1.201851678989727383E-14, 2.071875000341422801, 1.575800808251672791 ) ) ;
#24364=CARTESIAN_POINT ( 'NONE',  ( 5.992340707560147806, 8.974519344586754599, 1.082531754730558626 ) ) ;
#24379=CARTESIAN_POINT ( 'NONE',  ( 3.511198596259283544, 6.271927390929313617, -7.499999999999997335 ) ) ;
#24383=CARTESIAN_POINT ( 'NONE',  ( 8.666686507633574621, 11.13422023037111330, 1.599625672291281386 ) ) ;
#24385=ORIENTED_EDGE ( 'NONE', *, *, #96265, .F. ) ;
#24387=CARTESIAN_POINT ( 'NONE',  ( -4.471491734408701291, 4.111161866431900513, 1.214306433183764966E-14 ) ) ;
#24388=CARTESIAN_POINT ( 'NONE',  ( -6.205881626753225966, 8.263281202677319470, 1.599625672291283607 ) ) ;
#24391=CARTESIAN_POINT ( 'NONE',  ( -7.947050595904583403, 12.42330946186405249, 0.7998128361456481317 ) ) ;
#24395=FACE_OUTER_BOUND ( 'NONE', #27943, .T. ) ;
#24396=CARTESIAN_POINT ( 'NONE',  ( 8.586391356156291010, 8.911878091804165791, 0.7998128361456481317 ) ) ;
#24399=CARTESIAN_POINT ( 'NONE',  ( -6.690058733339450114, 9.892486724616283311, 1.199719254218452047 ) ) ;
#24401=CARTESIAN_POINT ( 'NONE',  ( -0.6823417656250212460, 5.301041667008086655, 1.181850606188767472 ) ) ;
#24407=CARTESIAN_POINT ( 'NONE',  ( -8.676855123066030018, 9.225345186439589895, -0.7216878364870267237 ) ) ;
#24412=CARTESIAN_POINT ( 'NONE',  ( -1.201851678989727383E-14, 4.509375000341417916, -1.575800808251660134 ) ) ;
#24419=CARTESIAN_POINT ( 'NONE',  ( 0.6823417656249917140, 4.842708333674755394, 1.181850606188765695 ) ) ;
#24420=CARTESIAN_POINT ( 'NONE',  ( -5.935772324684618795, 5.819489221753827657, 0.000000000000000000 ) ) ;
#24421=CARTESIAN_POINT ( 'NONE',  ( 7.623762449586013901, 7.788811034138823253, 1.040834085586084257E-14 ) ) ;
#24425=CARTESIAN_POINT ( 'NONE',  ( 4.487385655998885170, 5.298000022495898520, 1.082531754730560403 ) ) ;
#24426=CARTESIAN_POINT ( 'NONE',  ( -1.364683531250010295, 5.092708333674757171, 0.7879004041258379498 ) ) ;
#24432=CARTESIAN_POINT ( 'NONE',  ( 1.364683531249988757, 1.134375000341421247, 0.000000000000000000 ) ) ;
#24433=CARTESIAN_POINT ( 'NONE',  ( -3.470524135418294520, 6.992769224722559684, -0.7216878364870267237 ) ) ;
#24435=CARTESIAN_POINT ( 'NONE',  ( 4.299907273828439180, 8.168308919441841454, 1.040834085586084257E-14 ) ) ;
#24439=CARTESIAN_POINT ( 'NONE',  ( 4.853455804012228647, 4.764712647543454693, 0.7216878364870317197 ) ) ;
#24442=CARTESIAN_POINT ( 'NONE',  ( -8.026063749610056419, 10.38682701267698150, -1.443375672974059665 ) ) ;
#24447=B_SPLINE_CURVE_WITH_KNOTS ( 'NONE', 3,
 ( #24792, #12796, #143935, #205674, #26923, #142861, #126653, #90895, #107188, #209930 ),
 .UNSPECIFIED., .F., .F.,
 ( 4, 3, 3, 4 ),
 ( 0.000000000000000000, 8.893179197954895123E-05, 0.0001334007970840213895, 0.0001778705873658962123 ),
 .UNSPECIFIED. ) ;
#24448=CARTESIAN_POINT ( 'NONE',  ( -9.755255220232635693, 11.33988483081495957, -1.199719254218441611 ) ) ;
#24449=CARTESIAN_POINT ( 'NONE',  ( -6.033015167956818026, 6.140865238812146742, -0.7216878364870267237 ) ) ;
#24451=CARTESIAN_POINT ( 'NONE',  ( -0.6823417656250003738, 1.030208333674752286, -1.181850606188749264 ) ) ;
#24463=CARTESIAN_POINT ( 'NONE',  ( 7.415946836550703303, 11.59576237604377091, 0.7216878364870438212 ) ) ;
#24468=ORIENTED_EDGE ( 'NONE', *, *, #113441, .T. ) ;
#24473=CARTESIAN_POINT ( 'NONE',  ( -3.195971524519394702, 4.751719416737803847, -1.599625672291262513 ) ) ;
#24476=CARTESIAN_POINT ( 'NONE',  ( -1.364683531250014514, 2.051041667008086655, -0.7879004041258289570 ) ) ;
#24487=CARTESIAN_POINT ( 'NONE',  ( 0.6823417656249899377, 1.592708333674752730, 1.181850606188755259 ) ) ;
#24499=CARTESIAN_POINT ( 'NONE',  ( 4.306686350635271054, 8.176217842383143974, -0.7998128361456221525 ) ) ;
#24501=EDGE_CURVE ( 'NONE', #209728, #173454, #200462, .T. ) ;
#24508=CARTESIAN_POINT ( 'NONE',  ( 8.444030743212801227, 8.745790710036752458, 0.7998128361456462443 ) ) ;
#24512=CARTESIAN_POINT ( 'NONE',  ( 7.587759525142423911, 12.00413654597487501, 0.7998128361456462443 ) ) ;
#24514=CARTESIAN_POINT ( 'NONE',  ( 1.573645197550626484, 8.680485584337372273, -2.499999999999989342 ) ) ;
#24517=VERTEX_POINT ( 'NONE', #102224 ) ;
#24525=CARTESIAN_POINT ( 'NONE',  ( -7.036318535812428721, 11.15286269184909784, 0.000000000000000000 ) ) ;
#24533=CARTESIAN_POINT ( 'NONE',  ( -4.185765024244170185, 3.976674809167545011, -0.5846519713818258968 ) ) ;
#24537=CARTESIAN_POINT ( 'NONE',  ( 3.917943204224906939, 5.594019709727598766, -1.443375672974051449 ) ) ;
#24539=CARTESIAN_POINT ( 'NONE',  ( 4.436542580169809291, 6.199052314996659874, 1.599625672291267398 ) ) ;
#24546=CARTESIAN_POINT ( 'NONE',  ( -6.403528624356093601, 6.365204904703887223, 1.040834085586084257E-14 ) ) ;
#24548=CARTESIAN_POINT ( 'NONE',  ( -3.755772246185468788, 4.340488027759846545, -1.199719254218452047 ) ) ;
#24554=CARTESIAN_POINT ( 'NONE',  ( 9.585251415181632595, 10.28514086057449184, 0.000000000000000000 ) ) ;
#24555=ORIENTED_EDGE ( 'NONE', *, *, #41976, .F. ) ;
#24556=CARTESIAN_POINT ( 'NONE',  ( -1.364683531249997417, 4.821875000341417916, 1.214306433183764966E-14 ) ) ;
#24559=CARTESIAN_POINT ( 'NONE',  ( 5.717788096661236885, 7.693838750903348789, 1.599625672291267398 ) ) ;
#24574=CARTESIAN_POINT ( 'NONE',  ( -0.6823417656250003738, 0.7802083336747520637, -1.181850606188749264 ) ) ;
#24576=CARTESIAN_POINT ( 'NONE',  ( 2.530568227245037605, 6.104080031761181857, 0.000000000000000000 ) ) ;
#24578=CARTESIAN_POINT ( 'NONE',  ( -4.595850885352567694, 8.305650432979225783, 1.040834085586084257E-14 ) ) ;
#24579=EDGE_CURVE ( 'NONE', #154420, #6976, #19890, .T. ) ;
#24580=CARTESIAN_POINT ( 'NONE',  ( 4.202664430556257713, 4.965825259479493603, 1.082531754730560403 ) ) ;
#24581=CARTESIAN_POINT ( 'NONE',  ( -6.846504384776765484, 8.050305206070113684, -1.082531754730543083 ) ) ;
#24585=CARTESIAN_POINT ( 'NONE',  ( 6.308621549060418054, 6.254479983525607523, 0.7998128361456341429 ) ) ;
#24595=CARTESIAN_POINT ( 'NONE',  ( 6.226218857173709154, 8.287007971501239467, 1.599625672291281386 ) ) ;
#24598=CARTESIAN_POINT ( 'NONE',  ( -7.009729113465285266, 8.136771039586342624, -1.199719254218446718 ) ) ;
#24602=CARTESIAN_POINT ( 'NONE',  ( 9.088043039861931405, 9.497138389460751284, 1.040834085586084257E-14 ) ) ;
#24604=CARTESIAN_POINT ( 'NONE',  ( -7.549192604710863286, 7.701812881784464437, -0.7998128361456291469 ) ) ;
#24606=CARTESIAN_POINT ( 'NONE',  ( 6.087247782411444597, 10.04561347954795281, -0.7216878364870267237 ) ) ;
#24607=CARTESIAN_POINT ( 'NONE',  ( 4.009205846845453003, 7.815100513429686480, -0.2297154615349787654 ) ) ;
#24608=CARTESIAN_POINT ( 'NONE',  ( -5.087333953625788219, 6.958308917361963886, 1.599625672291267398 ) ) ;
#24615=CARTESIAN_POINT ( 'NONE',  ( 8.191097360950562845, 12.70803068775103739, -0.7998128361456352531 ) ) ;
#24616=CARTESIAN_POINT ( 'NONE',  ( 4.227444969362701421, 3.826440640544909400, 1.214306433183764966E-14 ) ) ;
#24617=CARTESIAN_POINT ( 'NONE',  ( 0.6823417656249899377, 0.5927083336747518416, 1.181850606188755259 ) ) ;
#24619=CARTESIAN_POINT ( 'NONE',  ( -5.504247177468192476, 7.444707678511436555, 1.443375672974064550 ) ) ;
#24626=CARTESIAN_POINT ( 'NONE',  ( -5.693503466768185639, 6.133329901302775333, 0.7540896269448340572 ) ) ;
#24627=CARTESIAN_POINT ( 'NONE',  ( -1.201851678989727383E-14, 1.134375000341418582, 1.575800808251672791 ) ) ;
#24630=CARTESIAN_POINT ( 'NONE',  ( 4.202664430556261266, 4.005456045178151570, 0.7216878364870317197 ) ) ;
#24633=CARTESIAN_POINT ( 'NONE',  ( -3.737243898861318137, 7.511868315313511069, 0.7998128361456341429 ) ) ;
#24635=CARTESIAN_POINT ( 'NONE',  ( -6.846504384776750385, 10.93141284897413890, -0.7216878364870267237 ) ) ;
#24642=CARTESIAN_POINT ( 'NONE',  ( -7.985389288324697965, 10.33937347451072775, -1.443375672974058777 ) ) ;
#24646=EDGE_CURVE ( 'NONE', #77611, #155158, #170223, .T. ) ;
#24649=CARTESIAN_POINT ( 'NONE',  ( -6.819388077549415783, 10.89977715720891815, 0.7216878364870458196 ) ) ;
#24655=CARTESIAN_POINT ( 'NONE',  ( -1.499999999999997780, 5.181250000682820378, 1.214306433183764966E-14 ) ) ;
#24663=CARTESIAN_POINT ( 'NONE',  ( -6.775324078527193983, 8.927630729746953264, -1.599625672291263179 ) ) ;
#24666=CARTESIAN_POINT ( 'NONE',  ( 4.822949958159288286, 6.649860922651058992, -1.599625672291256295 ) ) ;
#24671=CARTESIAN_POINT ( 'NONE',  ( 7.039708073993665494, 9.236078724457858158, 1.599625672291281386 ) ) ;
#24674=ORIENTED_EDGE ( 'NONE', *, *, #41280, .F. ) ;
#24677=CARTESIAN_POINT ( 'NONE',  ( -6.575341312947811545, 6.773579074634973551, 1.040834085586084257E-14 ) ) ;
#24680=CARTESIAN_POINT ( 'NONE',  ( 0.006768871532346317291, 8.210909518262139883, 2.038649385027042626 ) ) ;
#24687=CARTESIAN_POINT ( 'NONE',  ( -1.364683531250012516, 0.7802083336747528408, 0.7879004041258379498 ) ) ;
#24689=CARTESIAN_POINT ( 'NONE',  ( -8.853638004923878313, 10.28799807962136548, 1.199719254218462483 ) ) ;
#24691=EDGE_CURVE ( 'NONE', #179842, #145502, #201276, .T. ) ;
#24692=CARTESIAN_POINT ( 'NONE',  ( 7.796102023057898123, 9.054206100777749455, -1.199719254218441611 ) ) ;
#24694=CARTESIAN_POINT ( 'NONE',  ( -7.720478407978036195, 11.09464301169468037, -1.199719254218446718 ) ) ;
#24697=CARTESIAN_POINT ( 'NONE',  ( 1.364683531249988535, 5.405208333674750953, -0.7879004041258300672 ) ) ;
#24699=CARTESIAN_POINT ( 'NONE',  ( 7.605760987586388744, 11.81721221891873697, 1.040834085586084257E-14 ) ) ;
#24702=CARTESIAN_POINT ( 'NONE',  ( -1.364683531250014514, -0.1989583329919157317, -0.7879004041258359514 ) ) ;
#24705=CARTESIAN_POINT ( 'NONE',  ( 9.558135107509954764, 10.25350516829085379, -0.7216878364870257245 ) ) ;
#24708=CARTESIAN_POINT ( 'NONE',  ( -6.426201623197489887, 6.599582769926260362, 0.7216878364870317197 ) ) ;
#24710=CARTESIAN_POINT ( 'NONE',  ( -1.364683531250012516, 2.530208333674753174, 0.7879004041258379498 ) ) ;
#24714=CARTESIAN_POINT ( 'NONE',  ( -6.693975156845199059, 8.832723654451292816, 1.599625672291283607 ) ) ;
#24715=CARTESIAN_POINT ( 'NONE',  ( -0.6823417656250212460, 4.613541667008086655, 1.181850606188767472 ) ) ;
#24721=CARTESIAN_POINT ( 'NONE',  ( 7.771848369131631351, 10.09024240211882351, -1.599625672291262513 ) ) ;
#24724=CARTESIAN_POINT ( 'NONE',  ( 0.7499999999999902300, 1.233333333333357151, 1.299038105676657340 ) ) ;
#24729=VERTEX_POINT ( 'NONE', #105454 ) ;
#24730=CARTESIAN_POINT ( 'NONE',  ( 6.263503779833467178, 9.290876262238963790, -1.082531754730537088 ) ) ;
#24732=CARTESIAN_POINT ( 'NONE',  ( 8.886479618753304166, 12.45497775759917758, -1.199719254218446718 ) ) ;
#24734=CARTESIAN_POINT ( 'NONE',  ( 4.162516854595432747, 4.815023404238158555, 1.199719254218464037 ) ) ;
#24735=ORIENTED_EDGE ( 'NONE', *, *, #211914, .F. ) ;
#24740=CARTESIAN_POINT ( 'NONE',  ( 7.703003830858588863, 12.13858823597705872, -0.7998128361456291469 ) ) ;
#24741=CARTESIAN_POINT ( 'NONE',  ( -1.510814038188236452, 8.678413394653590629, 2.539834060596353638 ) ) ;
#24744=CARTESIAN_POINT ( 'NONE',  ( -1.364683531250014514, -0.2614583329919080157, -0.7879004041258359514 ) ) ;
#24745=CARTESIAN_POINT ( 'NONE',  ( 1.499999999999987121, 0.5041666666666856367, 0.8660254037844524744 ) ) ;
#24752=CARTESIAN_POINT ( 'NONE',  ( -1.364683531250010295, 4.780208333674755394, 0.7879004041258379498 ) ) ;
#24754=CARTESIAN_POINT ( 'NONE',  ( -5.260200412422200600, 8.120355666925794580, -1.082531754730544860 ) ) ;
#24762=ORIENTED_EDGE ( 'NONE', *, *, #162536, .T. ) ;
#24763=CARTESIAN_POINT ( 'NONE',  ( 8.535021395002688749, 9.916278701380017324, 1.199719254218462483 ) ) ;
#24767=CARTESIAN_POINT ( 'NONE',  ( 6.412643469139427843, 10.42524178073059993, -0.7216878364870267237 ) ) ;
#24770=CARTESIAN_POINT ( 'NONE',  ( -8.890396042259075315, 11.39521468743417998, -1.599625672291263179 ) ) ;
#24771=CARTESIAN_POINT ( 'NONE',  ( 5.133733721068893807, 9.141106441222381918, 1.040834085586084257E-14 ) ) ;
#24774=CARTESIAN_POINT ( 'NONE',  ( 3.348500752450942031, 4.929670182657964084, 1.443375672974066548 ) ) ;
#24776=CARTESIAN_POINT ( 'NONE',  ( 4.955668840994886359, 5.740367388370866131, 1.199719254218462483 ) ) ;
#24783=CARTESIAN_POINT ( 'NONE',  ( -3.795919822146277767, 7.372397525905215687, -0.7216878364870267237 ) ) ;
#24784=CARTESIAN_POINT ( 'NONE',  ( 3.277320446201373638, 4.846626492033466072, 1.599625672291267398 ) ) ;
#24787=CARTESIAN_POINT ( 'NONE',  ( -5.045605722580076780, 9.038290442985410067, -0.7998128361456231517 ) ) ;
#24791=CARTESIAN_POINT ( 'NONE',  ( -9.806625181386236179, 10.33548422123910449, -0.7998128361456291469 ) ) ;
#24792=CARTESIAN_POINT ( 'NONE',  ( 1.123270288250311610, 3.110197346350006331, 0.7749999999993734123 ) ) ;
#24796=CARTESIAN_POINT ( 'NONE',  ( 4.150767584078112193, 7.994312614733129152, 0.7998128361456321445 ) ) ;
#24808=CARTESIAN_POINT ( 'NONE',  ( -6.170932472514347289, 10.35117165124207972, 0.000000000000000000 ) ) ;
#24811=CARTESIAN_POINT ( 'NONE',  ( 5.422898255786183341, 7.349800603215774331, -1.443375672974051449 ) ) ;
#24812=ORIENTED_EDGE ( 'NONE', *, *, #117742, .F. ) ;
#24814=CARTESIAN_POINT ( 'NONE',  ( -1.474248253921377483, 7.378028154548616158, 4.279201940598175824 ) ) ;
#24817=CARTESIAN_POINT ( 'NONE',  ( -4.252453736180621391, 8.112946458852704268, -0.7998128361456281477 ) ) ;
#24827=DIRECTION ( 'NONE',  ( 6.314299915563594049E-62, 8.546850786086437571E-32, 1.000000000000000000 ) ) ;
#24828=CARTESIAN_POINT ( 'NONE',  ( -8.859363311525973117, 12.42334206583395328, -1.199719254218446718 ) ) ;
#24829=CARTESIAN_POINT ( 'NONE',  ( 6.642605195691581699, 9.837124264027149678, 1.199719254218462483 ) ) ;
#24833=CARTESIAN_POINT ( 'NONE',  ( -1.500000000000022204, 10.00000000000000178, 4.154462424328226433 ) ) ;
#24834=CARTESIAN_POINT ( 'NONE',  ( -4.362038794589177648, 7.192753374110822051, -1.033456106840037192 ) ) ;
#24837=CARTESIAN_POINT ( 'NONE',  ( 0.6823417656249864960, -0.7614583329919113464, -1.181850606188749264 ) ) ;
#24841=CARTESIAN_POINT ( 'NONE',  ( 10.41229878561526512, 11.25002945941372623, -0.7216878364870257245 ) ) ;
#24847=CARTESIAN_POINT ( 'NONE',  ( -5.689683820183289775, 6.135727912364857595, -0.7597814889456652176 ) ) ;
#24858=CARTESIAN_POINT ( 'NONE',  ( -2.839543107058306592, 5.400218493954923815, -1.199719254218446718 ) ) ;
#24859=CARTESIAN_POINT ( 'NONE',  ( 0.7499999999999885647, 3.066666666666689522, -1.299038105676658228 ) ) ;
#24862=CARTESIAN_POINT ( 'NONE',  ( -3.327636637150278798, 5.969660945728899826, -1.199719254218452935 ) ) ;
#24866=CARTESIAN_POINT ( 'NONE',  ( -1.500000000000001332, -1.068749999317178290, 0.000000000000000000 ) ) ;
#24869=CARTESIAN_POINT ( 'NONE',  ( -4.121315508874280553, 3.910548969882488901, -0.7216878364870207285 ) ) ;
#24874=CARTESIAN_POINT ( 'NONE',  ( 2.354312230267378236, 5.898448035287240820, -0.7998128361456281477 ) ) ;
#24877=CARTESIAN_POINT ( 'NONE',  ( -1.499999999999993339, 10.64264068711930733, 1.232676135170975238E-14 ) ) ;
#24878=CARTESIAN_POINT ( 'NONE',  ( 10.07334494482924292, 11.81495252613139257, -1.082531754730537088 ) ) ;
#24880=CARTESIAN_POINT ( 'NONE',  ( 1.364683531249986537, 0.6760416670080884316, 0.7879004041258500513 ) ) ;
#24883=CARTESIAN_POINT ( 'NONE',  ( -6.984421689334302741, 11.30024240419870374, 0.000000000000000000 ) ) ;
#24884=CARTESIAN_POINT ( 'NONE',  ( -5.707619481228832115, 6.721606151930833661, -1.082531754730543971 ) ) ;
#24886=CARTESIAN_POINT ( 'NONE',  ( -7.217017841176048165, 7.314275657660511243, 1.040834085586084257E-14 ) ) ;
#24888=CARTESIAN_POINT ( 'NONE',  ( 1.364683531249988535, 5.155208333674749177, -0.7879004041258300672 ) ) ;
#24896=CARTESIAN_POINT ( 'NONE',  ( -5.544921637864833386, 7.492161215640853023, -1.443375672974051449 ) ) ;
#24898=EDGE_CURVE ( 'NONE', #210539, #197889, #154889, .T. ) ;
#24900=DIRECTION ( 'NONE',  ( 0.000000000000000000, 0.000000000000000000, -1.000000000000000000 ) ) ;
#24902=CARTESIAN_POINT ( 'NONE',  ( -3.904385050611244079, 7.498940292447679568, 1.040834085586084257E-14 ) ) ;
#24904=CARTESIAN_POINT ( 'NONE',  ( 8.211434591371064684, 12.73175745657494851, -0.7998128361456352531 ) ) ;
#24915=CARTESIAN_POINT ( 'NONE',  ( -3.253066792275140173, 5.882662793374543675, 1.199719254218462483 ) ) ;
#24916=CARTESIAN_POINT ( 'NONE',  ( -4.285806009943333272, 7.464806705703632694, 1.099619435331932404 ) ) ;
#24920=CARTESIAN_POINT ( 'NONE',  ( 7.605760987586388744, 11.81721221891873697, 1.040834085586084257E-14 ) ) ;
#24921=CARTESIAN_POINT ( 'NONE',  ( 6.144869935491714230, 8.192100896205568361, -1.599625672291262513 ) ) ;
#24927=CARTESIAN_POINT ( 'NONE',  ( 5.040934186182656873, 4.775511393501539636, 1.040834085586084257E-14 ) ) ;
#24938=CARTESIAN_POINT ( 'NONE',  ( -7.386494761346872551, 7.511998731193139989, -0.7998128361456291469 ) ) ;
#24944=CARTESIAN_POINT ( 'NONE',  ( -0.6823417656250212460, 4.051041667008085767, 1.181850606188767472 ) ) ;
#24945=CARTESIAN_POINT ( 'NONE',  ( 9.259855728009286580, 10.86588177317476855, -1.082531754730543083 ) ) ;
#24946=CARTESIAN_POINT ( 'NONE',  ( -6.735703387890906946, 6.752742128827836865, -0.7998128361456291469 ) ) ;
#24948=B_SPLINE_CURVE_WITH_KNOTS ( 'NONE', 3,
 ( #181619, #66776, #80939, #165381, #178455, #50568, #46326, #30064 ),
 .UNSPECIFIED., .F., .F.,
 ( 4, 2, 2, 4 ),
 ( 0.000000000000000000, 0.0006693095108161682119, 0.001003964266224251396, 0.001338619021632334689 ),
 .UNSPECIFIED. ) ;
#24950=CARTESIAN_POINT ( 'NONE',  ( -1.500000000000057288, 7.438721522839117029, -4.195160983902607832 ) ) ;
#24951=CARTESIAN_POINT ( 'NONE',  ( 5.867981556616276073, 5.740399992340775803, -0.7998128361456281477 ) ) ;
#24952=CARTESIAN_POINT ( 'NONE',  ( -4.791917227426195858, 7.677988301050826969, -1.199719254218452047 ) ) ;
#24957=EDGE_CURVE ( 'NONE', #205506, #104139, #169891, .T. ) ;
#24959=CARTESIAN_POINT ( 'NONE',  ( 5.666945020832160118, 9.555260257705446847, 0.7216878364870438212 ) ) ;
#24961=CARTESIAN_POINT ( 'NONE',  ( 7.768458830506048685, 8.165549511786275971, -0.7216878364870267237 ) ) ;
#24962=CARTESIAN_POINT ( 'NONE',  ( 1.364683531249988535, 3.467708333674749621, -0.7879004041258239610 ) ) ;
#24964=CARTESIAN_POINT ( 'NONE',  ( 6.439759776366775768, 7.575769829591800786, 1.082531754730558626 ) ) ;
#24966=CARTESIAN_POINT ( 'NONE',  ( -4.121315508874280553, 3.910548969882488901, -0.7216878364870207285 ) ) ;
#24968=CARTESIAN_POINT ( 'NONE',  ( 0.6823417656249899377, 5.426041667008087543, -1.181850606188754593 ) ) ;
#24973=CARTESIAN_POINT ( 'NONE',  ( -4.002466101043451019, 7.812316210466456745, 0.3644823170804913914 ) ) ;
#24974=DIRECTION ( 'NONE',  ( 0.000000000000000000, 8.546850786086437571E-32, 1.000000000000000000 ) ) ;
#24980=CARTESIAN_POINT ( 'NONE',  ( 4.547870462380197765, 7.393267075163835855, 1.199719254218462483 ) ) ;
#24982=CARTESIAN_POINT ( 'NONE',  ( -2.589244150085650009, 5.964609241834465614, 0.7216878364870317197 ) ) ;
#24987=CARTESIAN_POINT ( 'NONE',  ( -4.620631424159025613, 4.285158171140619032, -0.7998128361456221525 ) ) ;
#24992=CARTESIAN_POINT ( 'NONE',  ( 5.666945020832181434, 5.713783400500082266, 0.7216878364870317197 ) ) ;
#24993=CARTESIAN_POINT ( 'NONE',  ( -1.364683531250012516, 3.551041667008086211, -0.7879004041258300672 ) ) ;
#24995=CARTESIAN_POINT ( 'NONE',  ( 6.564118927310645724, 10.80988918183778225, -0.7998128361456291469 ) ) ;
#24996=CARTESIAN_POINT ( 'NONE',  ( -9.480175724453545172, 12.08329098332774265, 1.599625672291281386 ) ) ;
#24997=CARTESIAN_POINT ( 'NONE',  ( 1.519470924986870308, 8.761764328395914347, 2.483655442635868571 ) ) ;
#24998=CARTESIAN_POINT ( 'NONE',  ( -4.874319919312905647, 5.645460313075203018, -1.199719254218446718 ) ) ;
#25003=CARTESIAN_POINT ( 'NONE',  ( -1.499999999999997780, 2.900000000000020783, 1.214306433183764966E-14 ) ) ;
#25004=CARTESIAN_POINT ( 'NONE',  ( 7.149227073107712549, 7.235186428247455837, -0.7998128361456281477 ) ) ;
#25008=CARTESIAN_POINT ( 'NONE',  ( 1.364683531249990311, 3.634375000341416584, 1.214306433183764966E-14 ) ) ;
#25010=CARTESIAN_POINT ( 'NONE',  ( 9.734391104931951588, 11.41950637958454706, 1.082531754730548412 ) ) ;
#25015=CARTESIAN_POINT ( 'NONE',  ( -0.7500000000000006661, 2.389583334016155636, -1.299038105676652011 ) ) ;
#25017=CARTESIAN_POINT ( 'NONE',  ( -5.096975683733680818, 8.033889833409558534, -1.199719254218452047 ) ) ;
#25027=CARTESIAN_POINT ( 'NONE',  ( 7.135668919494039031, 7.219368582364847242, 1.040834085586084257E-14 ) ) ;
#25032=CARTESIAN_POINT ( 'NONE',  ( 6.179819089730593795, 6.104210447640811665, 1.040834085586084257E-14 ) ) ;
#25036=VERTEX_POINT ( 'NONE', #184005 ) ;
#25039=CARTESIAN_POINT ( 'NONE',  ( 8.703444544968814256, 12.24143683818393313, -1.199719254218446718 ) ) ;
#25044=CARTESIAN_POINT ( 'NONE',  ( 5.744750223003346257, 6.067414509003485001, 0.6312745094601609486 ) ) ;
#25054=CARTESIAN_POINT ( 'NONE',  ( -1.445377862185231344, 8.715816065047343741, -2.588769565374613002 ) ) ;
#25056=CARTESIAN_POINT ( 'NONE',  ( 7.131225611108088280, 9.342849184424693476, 1.443375672974076540 ) ) ;
#25058=CARTESIAN_POINT ( 'NONE',  ( -3.741160322367112379, 6.452105245148518797, 1.199719254218464037 ) ) ;
#25062=CARTESIAN_POINT ( 'NONE',  ( -7.054319997812058318, 7.124461507069184130, 1.040834085586084257E-14 ) ) ;
#25066=ORIENTED_EDGE ( 'NONE', *, *, #77767, .T. ) ;
#25074=CARTESIAN_POINT ( 'NONE',  ( 10.58621901417202515, 11.24501035948919991, -0.7998128361456281477 ) ) ;
#25080=CARTESIAN_POINT ( 'NONE',  ( -3.277320446201389181, 4.846626492033466072, 1.599625672291267398 ) ) ;
#25084=CARTESIAN_POINT ( 'NONE',  ( 8.914649696185335870, 10.35917838609310593, -1.199719254218446718 ) ) ;
#25085=CIRCLE ( 'NONE', #114987, 1.500000000000000222 ) ;
#25090=CARTESIAN_POINT ( 'NONE',  ( -6.581593504430098385, 9.765943957555402122, -1.199719254218440723 ) ) ;
#25091=CARTESIAN_POINT ( 'NONE',  ( 4.172158584703322681, 5.890604320285754980, -1.599625672291256295 ) ) ;
#25093=( BOUNDED_CURVE ( )  B_SPLINE_CURVE ( 2, ( #97409, #15044, #94213 ),
 .UNSPECIFIED., .F., .T. ) 
 B_SPLINE_CURVE_WITH_KNOTS ( ( 3, 3 ),
 ( 0.000000000000000000, 0.002220828379238357509 ),
 .UNSPECIFIED. ) 
 CURVE ( )  GEOMETRIC_REPRESENTATION_ITEM ( )  RATIONAL_B_SPLINE_CURVE ( ( 1.000000000000000000, 0.9285916995105956140, 0.9333044775364149892 ) ) 
 REPRESENTATION_ITEM ( '' )  );
#25094=CARTESIAN_POINT ( 'NONE',  ( 3.147464216666835402, 6.823792019419957278, -0.7998128361456291469 ) ) ;
#25095=CARTESIAN_POINT ( 'NONE',  ( -3.226477370372317743, 4.787309570232886280, 1.443375672974064550 ) ) ;
#25098=CARTESIAN_POINT ( 'NONE',  ( 1.364683531249988757, 2.446875000341415696, 1.214306433183764966E-14 ) ) ;
#25100=CARTESIAN_POINT ( 'NONE',  ( 6.968527767744104651, 8.192665819532020777, 1.082531754730558626 ) ) ;
#25107=VERTEX_POINT ( 'NONE', #51893 ) ;
#25108=CARTESIAN_POINT ( 'NONE',  ( 8.961576348508637935, 11.47825837805867799, -1.443375672974052559 ) ) ;
#25114=CARTESIAN_POINT ( 'NONE',  ( -7.980945979938748103, 12.46285407657057220, 0.000000000000000000 ) ) ;
#25129=CARTESIAN_POINT ( 'NONE',  ( 6.810273232766058449, 6.839740281182199233, 1.040834085586084257E-14 ) ) ;
#25132=CARTESIAN_POINT ( 'NONE',  ( 1.499999999999989120, 2.806250000682818158, 1.214306433183764966E-14 ) ) ;
#25138=CARTESIAN_POINT ( 'NONE',  ( 1.499999999999987121, 0.7541666666666868579, 0.8660254037844524744 ) ) ;
#25139=CARTESIAN_POINT ( 'NONE',  ( 7.884230021546724920, 9.157022099014721306, 1.199719254218462483 ) ) ;
#25140=CARTESIAN_POINT ( 'NONE',  ( -1.364683531250014514, 0.03020833367475737191, 0.7879004041258379498 ) ) ;
#25143=CARTESIAN_POINT ( 'NONE',  ( 8.703971430293332645, 12.13808852110884118, -1.082531754730543083 ) ) ;
#25144=CARTESIAN_POINT ( 'NONE',  ( -5.205967797967562483, 8.057084283395347768, 1.082531754730548412 ) ) ;
#25150=CARTESIAN_POINT ( 'NONE',  ( -5.045605722580076780, 9.038290442985410067, -0.7998128361456231517 ) ) ;
#25151=VERTEX_POINT ( 'NONE', #168828 ) ;
#25152=CARTESIAN_POINT ( 'NONE',  ( -1.500000000000013101, 2.660416667349483788, -0.8660254037844313801 ) ) ;
#25153=CARTESIAN_POINT ( 'NONE',  ( -0.6823417656250212460, 4.113541667008085767, 1.181850606188767472 ) ) ;
#25169=CARTESIAN_POINT ( 'NONE',  ( -7.804689982961090955, 12.25722208009664094, 0.7998128361456481317 ) ) ;
#25170=CARTESIAN_POINT ( 'NONE',  ( 7.481401836642521452, 7.622723652371411696, 1.040834085586084257E-14 ) ) ;
#25178=CARTESIAN_POINT ( 'NONE',  ( -7.528855374290365887, 7.678086112960552434, -0.7998128361456291469 ) ) ;
#25184=CARTESIAN_POINT ( 'NONE',  ( 10.05353459973327368, 11.68787744023238417, -1.199719254218440723 ) ) ;
#25185=CARTESIAN_POINT ( 'NONE',  ( -3.906720819032141190, 7.709591388846142479, -0.7998128361456281477 ) ) ;
#25187=CARTESIAN_POINT ( 'NONE',  ( -8.646349277213090545, 11.11049346154719508, 1.599625672291269396 ) ) ;
#25214=DIRECTION ( 'NONE',  ( 0.9366510587354612838, 0.000000000000000000, -0.3502638921866474409 ) ) ;
#25216=CARTESIAN_POINT ( 'NONE',  ( 2.385871846325007706, 5.727341554113725586, -0.7216878364870267237 ) ) ;
#25221=CARTESIAN_POINT ( 'NONE',  ( -9.267161690140662600, 10.77044237904097734, -1.199719254218441611 ) ) ;
#25222=CARTESIAN_POINT ( 'NONE',  ( -1.500000000000043299, 4.170833333333358262, 0.8660254037844216102 ) ) ;
#25224=CARTESIAN_POINT ( 'NONE',  ( 9.745613490124728884, 10.26430391476735338, 0.7998128361456462443 ) ) ;
#25227=ADVANCED_FACE ( 'NONE', ( #141717 ), #204006, .T. ) ;
#25231=CARTESIAN_POINT ( 'NONE',  ( 6.938893903907228378E-15, 10.64264068711930733, 1.214306433183764966E-14 ) ) ;
#25233=CARTESIAN_POINT ( 'NONE',  ( -0.6823417656250003738, 0.9677083336747521747, -1.181850606188749264 ) ) ;
#25241=CARTESIAN_POINT ( 'NONE',  ( -5.264643720808155791, 5.036505850564608089, 0.000000000000000000 ) ) ;
#25244=CARTESIAN_POINT ( 'NONE',  ( -1.500000000000001332, -0.09999999999997510880, 0.000000000000000000 ) ) ;
#25246=CARTESIAN_POINT ( 'NONE',  ( -1.201851678989727383E-14, 5.837500000000023448, -1.732050807568863648 ) ) ;
#25251=CARTESIAN_POINT ( 'NONE',  ( -1.364683531250014514, 0.4885416670080875434, -0.7879004041258289570 ) ) ;
#25253=CARTESIAN_POINT ( 'NONE',  ( -5.879432169820529630, 10.01108796476595764, -0.7998128361456221525 ) ) ;
#25254=CARTESIAN_POINT ( 'NONE',  ( 7.703003830858588863, 12.13858823597705872, -0.7998128361456291469 ) ) ;
#25260=CARTESIAN_POINT ( 'NONE',  ( -1.402160292154681736E-14, -0.1156249996585793222, 1.575800808251672791 ) ) ;
#25268=CARTESIAN_POINT ( 'NONE',  ( 5.314433026876846711, 9.143996264757578984, -0.7216878364870267237 ) ) ;
#25271=CARTESIAN_POINT ( 'NONE',  ( -4.232116505760120440, 8.089219690028791376, -0.7998128361456281477 ) ) ;
#25276=CARTESIAN_POINT ( 'NONE',  ( 5.680503174001485078, 6.689970460165617361, -1.082531754730543083 ) ) ;
#25277=CARTESIAN_POINT ( 'NONE',  ( -8.988692655735990300, 9.589155641221221771, 0.7216878364870438212 ) ) ;
#25279=CARTESIAN_POINT ( 'NONE',  ( 1.499999999999990896, 3.775000000000021227, 1.214306433183764966E-14 ) ) ;
#25284=CARTESIAN_POINT ( 'NONE',  ( 9.571693261567965294, 10.26932301469188857, 0.7216878364870438212 ) ) ;
#25295=CARTESIAN_POINT ( 'NONE',  ( -1.364683531249997417, 5.790625000341422357, 1.214306433183764966E-14 ) ) ;
#25297=CARTESIAN_POINT ( 'NONE',  ( 9.259855728009286580, 10.86588177317476855, -1.082531754730543083 ) ) ;
#25299=CARTESIAN_POINT ( 'NONE',  ( 8.589254009457354400, 9.979550084910457031, -1.199719254218446718 ) ) ;
#25302=CARTESIAN_POINT ( 'NONE',  ( -4.133872419145380839, 3.976560215030992662, -0.5735765104555013982 ) ) ;
#25303=DIRECTION ( 'NONE',  ( 0.6507913734559652719, 0.7592566023652995710, 1.725633230170963762E-31 ) ) ;
#25304=CARTESIAN_POINT ( 'NONE',  ( 5.016153647376212277, 5.914896012436124728, 1.082531754730558626 ) ) ;
#25305=EDGE_LOOP ( 'NONE', ( #169051, #142565, #213254 ) ) ;
#25306=CARTESIAN_POINT ( 'NONE',  ( -8.378575743565381373, 8.877352577022161739, 0.7216878364870438212 ) ) ;
#25310=CARTESIAN_POINT ( 'NONE',  ( -2.927671105547157371, 5.503034492191895666, 1.199719254218462483 ) ) ;
#25312=VECTOR ( 'NONE', #25466, 1000.000000000000000 ) ;
#25335=CARTESIAN_POINT ( 'NONE',  ( -6.470265622219711688, 8.571729197388226140, -1.599625672291263179 ) ) ;
#25337=CARTESIAN_POINT ( 'NONE',  ( 1.270904146967301473, 2.834693569853255823, -0.7749999999999910294 ) ) ;
#25339=CARTESIAN_POINT ( 'NONE',  ( 6.796715079152391148, 6.823922435299587974, 0.7998128361456341429 ) ) ;
#25340=DIRECTION ( 'NONE',  ( -5.578564026256490882E-16, -1.000000000000000000, -9.066213480720158442E-32 ) ) ;
#25348=CARTESIAN_POINT ( 'NONE',  ( -5.264643720808155791, 5.036505850564608089, 0.000000000000000000 ) ) ;
#25351=CARTESIAN_POINT ( 'NONE',  ( 5.777746017718023097, 9.892454120646377191, 0.7998128361456462443 ) ) ;
#25352=CARTESIAN_POINT ( 'NONE',  ( -1.364683531249997417, 3.759375000341423689, 1.214306433183764966E-14 ) ) ;
#25354=CARTESIAN_POINT ( 'NONE',  ( 5.379472278790374595, 6.509029678566758292, 1.321781506194243727 ) ) ;
#25356=CARTESIAN_POINT ( 'NONE',  ( 1.387358672534390935, 7.315968950353690659, -4.254625267138188782 ) ) ;
#25360=CARTESIAN_POINT ( 'NONE',  ( 5.138177029454829459, 8.938364267765221527, 0.7216878364870438212 ) ) ;
#25361=CARTESIAN_POINT ( 'NONE',  ( -6.333630315878337136, 10.54098580183340772, 0.000000000000000000 ) ) ;
#25365=CARTESIAN_POINT ( 'NONE',  ( -6.835281999583978418, 11.12624609948998966, -0.7998128361456291469 ) ) ;
#25366=CARTESIAN_POINT ( 'NONE',  ( -5.713871673155502151, 8.753601821068331290, 1.199719254218452047 ) ) ;
#25373=CARTESIAN_POINT ( 'NONE',  ( 7.781490099239519509, 11.16582331816642260, 1.199719254218460707 ) ) ;
#25389=CARTESIAN_POINT ( 'NONE',  ( 1.499999999999990896, 4.275000000000021672, 1.214306433183764966E-14 ) ) ;
#25390=CARTESIAN_POINT ( 'NONE',  ( 5.443762371086860341, 6.309809840144842141, 1.199719254218462483 ) ) ;
#25391=CARTESIAN_POINT ( 'NONE',  ( 7.657657833620182153, 7.828355648845348291, -0.7998128361456281477 ) ) ;
#25393=CARTESIAN_POINT ( 'NONE',  ( -8.514157279702033065, 9.995900250149611921, -1.082531754730543971 ) ) ;
#25395=CARTESIAN_POINT ( 'NONE',  ( 7.321039761699430493, 7.643560598178549270, -0.7216878364870257245 ) ) ;
#25396=CARTESIAN_POINT ( 'NONE',  ( -8.148087131688679818, 12.44992605370473804, -0.7216878364870267237 ) ) ;
#25399=CARTESIAN_POINT ( 'NONE',  ( 7.730120138085914583, 12.17022392774227768, 0.7998128361456462443 ) ) ;
#25402=CARTESIAN_POINT ( 'NONE',  ( 1.364683531249988757, 1.134375000341421247, 0.000000000000000000 ) ) ;
#25407=CARTESIAN_POINT ( 'NONE',  ( 0.6823417656249864960, -1.073958332991911568, -1.181850606188749264 ) ) ;
#25409=CARTESIAN_POINT ( 'NONE',  ( 8.778014389843965759, 12.32843499053828928, 1.199719254218450271 ) ) ;
#25412=CARTESIAN_POINT ( 'NONE',  ( -10.65400978224035811, 11.32409958890225710, 1.040834085586084257E-14 ) ) ;
#25418=CARTESIAN_POINT ( 'NONE',  ( 5.030238685870051185, 5.827365540725222282, -1.199719254218452047 ) ) ;
#25421=CARTESIAN_POINT ( 'NONE',  ( -9.561524646135538319, 12.17819805862340310, -1.599625672291263179 ) ) ;
#25424=CARTESIAN_POINT ( 'NONE',  ( 8.097244055859613709, 10.46987070330147063, -1.599625672291262513 ) ) ;
#25426=CARTESIAN_POINT ( 'NONE',  ( 4.847318722290685500, 6.704483692258053296, 1.249926399124022147 ) ) ;
#25428=CARTESIAN_POINT ( 'NONE',  ( -3.554208825076827782, 7.298327395898266623, 0.7998128361456341429 ) ) ;
#25432=CARTESIAN_POINT ( 'NONE',  ( 6.903072767652295383, 11.20533532890304684, 1.040834085586084257E-14 ) ) ;
#25434=CARTESIAN_POINT ( 'NONE',  ( 7.935599982700328958, 8.152621489438862667, 0.7998128361456481317 ) ) ;
#25437=CARTESIAN_POINT ( 'NONE',  ( -9.327646496521989405, 10.94497100310623594, -1.082531754730539753 ) ) ;
#25439=DIRECTION ( 'NONE',  ( 1.000000000000000000, 0.000000000000000000, 0.000000000000000000 ) ) ;
#25444=CARTESIAN_POINT ( 'NONE',  ( -5.526577223899823643, 6.240148858909590146, -0.9599604131041916677 ) ) ;
#25445=CARTESIAN_POINT ( 'NONE',  ( -0.6823417656250003738, 1.717708333674752730, -1.181850606188749264 ) ) ;
#25447=CARTESIAN_POINT ( 'NONE',  ( 7.022760382198770301, 8.255937203062467589, -1.082531754730543083 ) ) ;
#25454=CIRCLE ( 'NONE', #73857, 0.08000000000000020983 ) ;
#25466=DIRECTION ( 'NONE',  ( 0.6507913734559640506, -0.7592566023653004592, 0.000000000000000000 ) ) ;
#25468=CARTESIAN_POINT ( 'NONE',  ( 8.178592977541601527, 10.56477777859713463, 1.599625672291281386 ) ) ;
#25473=CARTESIAN_POINT ( 'NONE',  ( -3.704402285031864306, 5.344888637335695414, -1.599625672291256295 ) ) ;
#25474=CARTESIAN_POINT ( 'NONE',  ( -5.585069213825653023, 8.603332285183535433, -1.199719254218440723 ) ) ;
#25476=VERTEX_POINT ( 'NONE', #114570 ) ;
#25477=CARTESIAN_POINT ( 'NONE',  ( -9.622536337397040285, 12.24937836509514710, 1.599625672291281386 ) ) ;
#25482=CARTESIAN_POINT ( 'NONE',  ( -1.500000000000013101, 4.160416667349482900, -0.8660254037844313801 ) ) ;
#25483=CARTESIAN_POINT ( 'NONE',  ( 6.968000882419564945, 10.21675256520979858, 1.199719254218460707 ) ) ;
#25486=CARTESIAN_POINT ( 'NONE',  ( -8.525379664894808585, 8.840697785332414682, -0.7998128361456291469 ) ) ;
#25488=CARTESIAN_POINT ( 'NONE',  ( -1.364683531249997417, 4.509375000341424133, 1.214306433183764966E-14 ) ) ;
#25490=CARTESIAN_POINT ( 'NONE',  ( -1.536181705502190908, 8.701161256998856786, 2.509509933406568472 ) ) ;
#25494=CARTESIAN_POINT ( 'NONE',  ( -8.270110514656041190, 10.67154823856396817, 1.443375672974090751 ) ) ;
#25498=CARTESIAN_POINT ( 'NONE',  ( 1.364683531249988535, 3.176041667008084435, 0.7879004041258500513 ) ) ;
#25504=CARTESIAN_POINT ( 'NONE',  ( -1.201851678989727383E-14, 4.696875000341419693, -1.575800808251660134 ) ) ;
#25505=CARTESIAN_POINT ( 'NONE',  ( -5.111587607552082524, 5.922272616020886282, 1.199719254218450271 ) ) ;
#25506=CARTESIAN_POINT ( 'NONE',  ( 6.124532705071213279, 8.168374127381657246, -1.599625672291262513 ) ) ;
#25510=CARTESIAN_POINT ( 'NONE',  ( -1.201851678989727383E-14, 4.509375000341417916, -1.575800808251660134 ) ) ;
#25511=CARTESIAN_POINT ( 'NONE',  ( -1.284279953904132077, 3.159610286488902187, -0.7749999999999935829 ) ) ;
#25515=CARTESIAN_POINT ( 'NONE',  ( 1.364683531249986537, 0.1552083336747499542, -0.7879004041258309554 ) ) ;
#25516=CARTESIAN_POINT ( 'NONE',  ( -4.365362273920257330, 6.116008624372160973, 1.443375672974064550 ) ) ;
#25517=CARTESIAN_POINT ( 'NONE',  ( 5.996784015946103885, 5.890669528225568996, 1.040834085586084257E-14 ) ) ;
#25521=CARTESIAN_POINT ( 'NONE',  ( 5.178851490740207453, 5.144340948726102702, 0.7216878364870317197 ) ) ;
#25524=CARTESIAN_POINT ( 'NONE',  ( -9.666600336863641729, 10.38004793587015584, 1.040834085586084257E-14 ) ) ;
#25529=CARTESIAN_POINT ( 'NONE',  ( -8.448702279610222021, 13.00856975952063088, 1.040834085586084257E-14 ) ) ;
#25530=CARTESIAN_POINT ( 'NONE',  ( -5.544921637864833386, 7.492161215640853023, -1.443375672974051449 ) ) ;
#25532=CARTESIAN_POINT ( 'NONE',  ( -0.6823417656250003738, 0.5302083336747518416, -1.181850606188749264 ) ) ;
#25544=CARTESIAN_POINT ( 'NONE',  ( 8.446366511189332016, 9.916811020218137429, -1.082531754730543083 ) ) ;
#25551=CARTESIAN_POINT ( 'NONE',  ( 3.192055101013606233, 5.811482486902795230, -1.199719254218446718 ) ) ;
#25553=CARTESIAN_POINT ( 'NONE',  ( -3.602716132929368875, 5.226254793216122074, 1.599625672291267398 ) ) ;
#25557=CARTESIAN_POINT ( 'NONE',  ( -1.364683531250012516, 2.092708333674750953, 0.7879004041258379498 ) ) ;
#25576=CARTESIAN_POINT ( 'NONE',  ( 4.171104814498611368, 8.018039383557042044, 0.7998128361456321445 ) ) ;
#25583=CARTESIAN_POINT ( 'NONE',  ( 6.584456157731144899, 10.83361595066169514, -0.7998128361456291469 ) ) ;
#25586=CARTESIAN_POINT ( 'NONE',  ( 7.411503528164766763, 11.79850454950093841, 1.040834085586084257E-14 ) ) ;
#25588=CARTESIAN_POINT ( 'NONE',  ( -3.049795748596713985, 6.452024942755530290, 0.6608969203207606391 ) ) ;
#25593=EDGE_CURVE ( 'NONE', #44776, #189774, #207435, .T. ) ;
#25598=CARTESIAN_POINT ( 'NONE',  ( -8.188761592974046266, 10.57664116326830595, -1.443375672974059665 ) ) ;
#25604=CARTESIAN_POINT ( 'NONE',  ( -9.001723924469462901, 12.58942944760136484, -1.199719254218446718 ) ) ;
#25611=CARTESIAN_POINT ( 'NONE',  ( 2.345197385039651472, 5.679888015947478941, -0.7216878364870267237 ) ) ;
#25619=CARTESIAN_POINT ( 'NONE',  ( -5.880485940025243607, 7.883652901494672349, 1.599625672291269396 ) ) ;
#25621=CARTESIAN_POINT ( 'NONE',  ( -2.774614992291035698, 6.388801257648172971, 1.040834085586084257E-14 ) ) ;
#25628=CARTESIAN_POINT ( 'NONE',  ( 0.6823417656249899377, 3.738541667008085767, -1.181850606188754593 ) ) ;
#25630=CARTESIAN_POINT ( 'NONE',  ( 4.137209430464448445, 7.978494768850520558, 1.040834085586084257E-14 ) ) ;
#25632=CARTESIAN_POINT ( 'NONE',  ( 1.501328131443582459, 8.653248444470666101, 2.562127481693529774 ) ) ;
#25641=EDGE_CURVE ( 'NONE', #16921, #112218, #141773, .T. ) ;
#25644=CARTESIAN_POINT ( 'NONE',  ( -1.402160292154681736E-14, 0.7593750003414168059, -1.575800808251659024 ) ) ;
#25646=CARTESIAN_POINT ( 'NONE',  ( 5.217190183160311356, 4.981143389975473568, -0.7998128361456211532 ) ) ;
#25648=CARTESIAN_POINT ( 'NONE',  ( -6.914295153289458540, 7.169025221700239925, 0.7216878364870317197 ) ) ;
#25649=CARTESIAN_POINT ( 'NONE',  ( 3.877268743828270470, 5.546566172598190292, 1.443375672974062551 ) ) ;
#25650=CARTESIAN_POINT ( 'NONE',  ( -5.382223794500835545, 8.262716279350872384, -1.082531754730543971 ) ) ;
#25655=CARTESIAN_POINT ( 'NONE',  ( 6.908042961362778733, 8.018137195466769285, 1.199719254218462483 ) ) ;
#25665=CARTESIAN_POINT ( 'NONE',  ( 6.470265622219697477, 8.571729197388226140, -1.599625672291262513 ) ) ;
#25666=FILL_AREA_STYLE ('',( #7270 ) ) ;
#25669=CARTESIAN_POINT ( 'NONE',  ( -6.958359152311683893, 9.141171649162195934, -1.599625672291263179 ) ) ;
#25673=CARTESIAN_POINT ( 'NONE',  ( 9.264299036839600987, 9.702770385934682551, -0.7998128361456281477 ) ) ;
#25676=CARTESIAN_POINT ( 'NONE',  ( -8.037286134802835491, 8.271255333558444889, -0.7998128361456291469 ) ) ;
#25678=CARTESIAN_POINT ( 'NONE',  ( 8.242994206984347372, 8.719174117677642499, 1.040834085586084257E-14 ) ) ;
#25679=CARTESIAN_POINT ( 'NONE',  ( 3.999262108721039155, 7.828827674157968985, 0.07552679838754294828 ) ) ;
#25680=CARTESIAN_POINT ( 'NONE',  ( -4.599240423533815125, 6.388866465587984322, 1.599625672291267398 ) ) ;
#25687=CARTESIAN_POINT ( 'NONE',  ( 7.716561984472250835, 12.15440608185967086, 1.040834085586084257E-14 ) ) ;
#25688=CARTESIAN_POINT ( 'NONE',  ( -5.076477019373391464, 6.555905325687263030, 1.224675693024103174 ) ) ;
#25690=CARTESIAN_POINT ( 'NONE',  ( 1.364683531249986537, 1.113541667008082658, 0.7879004041258500513 ) ) ;
#25692=CARTESIAN_POINT ( 'NONE',  ( -6.724481002698138532, 6.947575379343695623, -0.7216878364870278340 ) ) ;
#25699=CARTESIAN_POINT ( 'NONE',  ( -5.906331710381417466, 6.003565991635761989, -0.1321356564752910190 ) ) ;
#25700=CARTESIAN_POINT ( 'NONE',  ( 0.6823417656249899377, 1.405208333674752508, 1.181850606188755259 ) ) ;
#25703=CARTESIAN_POINT ( 'NONE',  ( 4.039966587192267866, 4.776011108888172707, 1.082531754730560403 ) ) ;
#25708=CARTESIAN_POINT ( 'NONE',  ( -7.659993601596710278, 10.92011438762942355, -1.082531754730543083 ) ) ;
#25715=CARTESIAN_POINT ( 'NONE',  ( -6.656690234185426824, 10.70996300661758660, 0.7216878364870458196 ) ) ;
#25718=CARTESIAN_POINT ( 'NONE',  ( 6.938893903907228378E-15, 10.64264068711930733, 1.214306433183764966E-14 ) ) ;
#25721=CARTESIAN_POINT ( 'NONE',  ( -6.521108698048772467, 9.591415333490143524, -1.082531754730537976 ) ) ;
#25726=CARTESIAN_POINT ( 'NONE',  ( -1.499999999999997780, 3.681250000682819046, 1.214306433183764966E-14 ) ) ;
#25733=CARTESIAN_POINT ( 'NONE',  ( -7.379715684540041565, 7.504089808251839244, 1.040834085586084257E-14 ) ) ;
#25735=CARTESIAN_POINT ( 'NONE',  ( -1.499999999999993339, 10.64264068711930733, 1.232676135170975238E-14 ) ) ;
#25738=CARTESIAN_POINT ( 'NONE',  ( 3.811813743736467419, 7.598866467667865443, 1.040834085586084257E-14 ) ) ;
#25741=CARTESIAN_POINT ( 'NONE',  ( 6.123478934866503742, 10.29580919065294431, 0.7998128361456462443 ) ) ;
#25748=CARTESIAN_POINT ( 'NONE',  ( -4.744990575102892905, 8.479646737687938085, 0.7216878364870458196 ) ) ;
#25751=CARTESIAN_POINT ( 'NONE',  ( -4.543684818008837389, 5.386939200858302357, 1.243851604716961212 ) ) ;
#25753=ADVANCED_FACE ( 'NONE', ( #83050 ), #115618, .T. ) ;
#25758=CARTESIAN_POINT ( 'NONE',  ( -8.690940161559884913, 10.09818392903003748, 1.199719254218462483 ) ) ;
#25761=CARTESIAN_POINT ( 'NONE',  ( 6.923409998072794558, 11.22906209772695618, 1.040834085586084257E-14 ) ) ;
#25762=CARTESIAN_POINT ( 'NONE',  ( -1.500000000000015099, 0.1291666666666918539, -0.8660254037844383745 ) ) ;
#25763=CARTESIAN_POINT ( 'NONE',  ( -6.828502922777144768, 11.11833717654868892, 0.7998128361456481317 ) ) ;
#25766=CARTESIAN_POINT ( 'NONE',  ( -1.201851678989727383E-14, 4.196875000341417028, -1.575800808251660134 ) ) ;
#25768=CARTESIAN_POINT ( 'NONE',  ( 10.05978679165993839, 10.83876546646586014, 0.7216878364870438212 ) ) ;
#25771=CARTESIAN_POINT ( 'NONE',  ( -1.500000000000011324, 5.670833333333358262, 0.8660254037844403729 ) ) ;
#25773=CARTESIAN_POINT ( 'NONE',  ( 9.056483423804305488, 9.668244870634271848, 1.040834085586084257E-14 ) ) ;
#25777=CARTESIAN_POINT ( 'NONE',  ( -7.076992996653451939, 7.358839372291564374, 0.7216878364870317197 ) ) ;
#25779=CARTESIAN_POINT ( 'NONE',  ( -1.364683531250000748, 1.759375000341421913, 0.000000000000000000 ) ) ;
#25783=CARTESIAN_POINT ( 'NONE',  ( -7.542413527904030524, 7.693903958843159252, 1.040834085586084257E-14 ) ) ;
#25785=CARTESIAN_POINT ( 'NONE',  ( 1.364683531249990311, 4.946875000341417916, 1.214306433183764966E-14 ) ) ;
#25791=CARTESIAN_POINT ( 'NONE',  ( 8.829384350997564468, 11.32403438096243775, 1.599625672291281386 ) ) ;
#25795=CARTESIAN_POINT ( 'NONE',  ( -0.7500000000000215383, 1.191666666666688190, 1.299038105676659116 ) ) ;
#25800=CARTESIAN_POINT ( 'NONE',  ( 6.100805936469477331, 9.101062111647635788, -1.082531754730537088 ) ) ;
#25807=CARTESIAN_POINT ( 'NONE',  ( 9.101601193475611140, 9.512956235343358102, -0.7998128361456221525 ) ) ;
#25808=CARTESIAN_POINT ( 'NONE',  ( -10.49131193887636826, 11.13428543831092909, 1.040834085586084257E-14 ) ) ;
#25810=CARTESIAN_POINT ( 'NONE',  ( 0.6823417656249917140, 5.655208333674749177, 1.181850606188765695 ) ) ;
#25817=CARTESIAN_POINT ( 'NONE',  ( 1.364683531249990311, 4.134375000341417028, 1.214306433183764966E-14 ) ) ;
#25819=CARTESIAN_POINT ( 'NONE',  ( -5.531363484695544841, 8.436712584578003771, 1.082531754730548412 ) ) ;
#25828=CARTESIAN_POINT ( 'NONE',  ( 7.456094412511537151, 10.78619501698377370, 1.199719254218460707 ) ) ;
#25834=CARTESIAN_POINT ( 'NONE',  ( -8.483651433849100698, 10.92067931095586886, 1.599625672291269396 ) ) ;
#25836=CARTESIAN_POINT ( 'NONE',  ( 6.331821432781979730, 7.345878745455822312, -1.199719254218445830 ) ) ;
#25838=B_SPLINE_CURVE_WITH_KNOTS ( 'NONE', 3,
 ( #116827, #182829, #168720, #114705, #34444, #100519, #115759, #131999, #135180, #86409 ),
 .UNSPECIFIED., .F., .F.,
 ( 4, 3, 3, 4 ),
 ( 0.000000000000000000, 4.502046072368877275E-05, 9.004093402560205887E-05, 0.0001800865003231008306 ),
 .UNSPECIFIED. ) ;
#25841=CARTESIAN_POINT ( 'NONE',  ( 4.497554271431305040, 6.270232621468402989, -1.599625672291256295 ) ) ;
#25845=CARTESIAN_POINT ( 'NONE',  ( -4.199533704925234368, 7.510932310329544670, -0.9222493318717175370 ) ) ;
#25846=CIRCLE ( 'NONE', #146962, 0.07999999999999994615 ) ;
#25848=CARTESIAN_POINT ( 'NONE',  ( -5.599154252763867134, 5.634694171087028636, 0.000000000000000000 ) ) ;
#25849=CARTESIAN_POINT ( 'NONE',  ( 3.171717870593107058, 5.787755718078879674, -1.199719254218446718 ) ) ;
#25852=CARTESIAN_POINT ( 'NONE',  ( -8.518600588087975822, 8.832788862391110385, 1.040834085586084257E-14 ) ) ;
#25857=CARTESIAN_POINT ( 'NONE',  ( -6.970863535720637216, 11.28442455831609337, 0.7998128361456481317 ) ) ;
#25861=CARTESIAN_POINT ( 'NONE',  ( 7.365103760721646076, 9.615707025640515937, 1.599625672291281386 ) ) ;
#25862=CARTESIAN_POINT ( 'NONE',  ( 3.960953433486789521, 7.772862772376584850, -0.7998128361456221525 ) ) ;
#25865=ORIENTED_EDGE ( 'NONE', *, *, #200558, .F. ) ;
#25872=PLANE ( 'NONE',  #212739 ) ;
#25873=CARTESIAN_POINT ( 'NONE',  ( -8.369460898337653276, 8.658792557682392754, 0.7998128361456462443 ) ) ;
#25877=CARTESIAN_POINT ( 'NONE',  ( 7.022760382198770301, 8.255937203062467589, -1.082531754730543083 ) ) ;
#25882=CARTESIAN_POINT ( 'NONE',  ( -5.494078562035765501, 7.432844293840273231, -1.599625672291256295 ) ) ;
#25891=CARTESIAN_POINT ( 'NONE',  ( -8.469039510030723861, 13.03229652834454733, 1.040834085586084257E-14 ) ) ;
#25892=CARTESIAN_POINT ( 'NONE',  ( 7.618792255875527886, 10.97600916757510170, 1.199719254218460707 ) ) ;
#25894=CARTESIAN_POINT ( 'NONE',  ( -3.633221978782304351, 4.301475732409860697, -1.082531754730549967 ) ) ;
#25897=CARTESIAN_POINT ( 'NONE',  ( -4.553630449417391368, 6.998240405024593436, -1.173447104293420473 ) ) ;
#25900=CARTESIAN_POINT ( 'NONE',  ( 1.364683531249986537, -1.073958332991911790, 0.7879004041258500513 ) ) ;
#25905=CARTESIAN_POINT ( 'NONE',  ( 8.432808358020004391, 12.78210081775797669, 0.7216878364870438212 ) ) ;
#25911=CARTESIAN_POINT ( 'NONE',  ( -4.161989969715295778, 4.726297878971393196, 2.420000000000010587 ) ) ;
#25926=CARTESIAN_POINT ( 'NONE',  ( -4.783329267523015460, 4.474972321731942593, -0.7998128361456221525 ) ) ;
#25928=CARTESIAN_POINT ( 'NONE',  ( 4.134873662043553111, 7.767843672452050541, -0.7216878364870197293 ) ) ;
#25929=CARTESIAN_POINT ( 'NONE',  ( -1.201851678989727383E-14, 3.462500000000019895, 1.732050807568877637 ) ) ;
#25931=CARTESIAN_POINT ( 'NONE',  ( -4.634189577772691138, 4.300976017023221409, 1.214306433183764966E-14 ) ) ;
#25935=CARTESIAN_POINT ( 'NONE',  ( 1.364683531249990311, 4.863541667008084879, 0.7879004041258500513 ) ) ;
#25939=CARTESIAN_POINT ( 'NONE',  ( -2.467220768007014176, 5.822248629409386922, 0.7216878364870317197 ) ) ;
#25944=CARTESIAN_POINT ( 'NONE',  ( 5.542585869888291938, 5.360771691158120689, -0.7998128361456211532 ) ) ;
#25948=CARTESIAN_POINT ( 'NONE',  ( 9.042925270190622200, 12.53353466765568669, 1.082531754730546636 ) ) ;
#25950=CARTESIAN_POINT ( 'NONE',  ( 1.364683531249988535, 1.426041667008083991, 0.7879004041258500513 ) ) ;
#25953=CARTESIAN_POINT ( 'NONE',  ( -9.155833807930273238, 9.576227618873799585, -0.7998128361456291469 ) ) ;
#25954=CARTESIAN_POINT ( 'NONE',  ( -4.568734577680880093, 7.313645526394248364, -1.082531754730548412 ) ) ;
#25959=CARTESIAN_POINT ( 'NONE',  ( 0.6823417656249899377, 5.676041667008087543, -1.181850606188754593 ) ) ;
#25967=CARTESIAN_POINT ( 'NONE',  ( -3.917943204224913156, 7.514758138330285497, -0.7216878364870257245 ) ) ;
#25972=CARTESIAN_POINT ( 'NONE',  ( -4.894130264408866893, 6.732904613275549899, -1.443375672974051449 ) ) ;
#25974=CARTESIAN_POINT ( 'NONE',  ( 9.317477881089539338, 11.89347683273640932, 1.599625672291279388 ) ) ;
#25983=CARTESIAN_POINT ( 'NONE',  ( -2.754277761870538299, 6.365074488824250309, 1.040834085586084257E-14 ) ) ;
#25984=CARTESIAN_POINT ( 'NONE',  ( -5.163658976018723479, 6.664880576339902163, 1.429021111749773532 ) ) ;
#25989=CARTESIAN_POINT ( 'NONE',  ( 9.300530189294644146, 10.91333531134101165, -1.082531754730543083 ) ) ;
#25990=CARTESIAN_POINT ( 'NONE',  ( 7.318703993278529829, 7.432909501780090800, 1.040834085586084257E-14 ) ) ;
#25994=CARTESIAN_POINT ( 'NONE',  ( 3.167801447087334576, 6.847518788243868393, -0.7998128361456291469 ) ) ;
#25995=CARTESIAN_POINT ( 'NONE',  ( -0.4210486379899329723, 7.995128625469242856, -1.998698746375223045 ) ) ;
#26003=CARTESIAN_POINT ( 'NONE',  ( -7.061099074618889304, 7.132370430010492868, -0.7998128361456291469 ) ) ;
#26011=CARTESIAN_POINT ( 'NONE',  ( -1.201851678989727383E-14, 4.696875000341419693, -1.575800808251660134 ) ) ;
#26012=CARTESIAN_POINT ( 'NONE',  ( 7.253248993186713456, 11.40594822545244824, 0.7216878364870438212 ) ) ;
#26013=CARTESIAN_POINT ( 'NONE',  ( -5.442708600882160574, 8.437244903416123876, -1.199719254218446718 ) ) ;
#26016=CARTESIAN_POINT ( 'NONE',  ( 4.680589345215795838, 6.483773540883647435, -1.599625672291256295 ) ) ;
#26017=CARTESIAN_POINT ( 'NONE',  ( -4.564291269294938225, 8.476756914152748124, 1.040834085586084257E-14 ) ) ;
#26023=CARTESIAN_POINT ( 'NONE',  ( 5.653386867218496370, 9.539442411822841805, 1.040834085586084257E-14 ) ) ;
#26025=CARTESIAN_POINT ( 'NONE',  ( 8.080296363620359301, 8.529359967086321603, 1.040834085586084257E-14 ) ) ;
#26026=CARTESIAN_POINT ( 'NONE',  ( -1.364683531250014514, 1.551041667008084435, -0.7879004041258289570 ) ) ;
#26028=CARTESIAN_POINT ( 'NONE',  ( 6.629573926958101993, 6.836850457647000390, -0.7216878364870257245 ) ) ;
#26032=CARTESIAN_POINT ( 'NONE',  ( -1.364683531250010295, 5.488541667008087543, -0.7879004041258300672 ) ) ;
#26037=CARTESIAN_POINT ( 'NONE',  ( -4.021356766390437265, 7.786759281977493785, -0.4705729632344165525 ) ) ;
#26044=CARTESIAN_POINT ( 'NONE',  ( 4.333802657862601215, 8.207853534148366492, 0.7998128361456462443 ) ) ;
#26050=EDGE_CURVE ( 'NONE', #108697, #163734, #79575, .T. ) ;
#26056=CARTESIAN_POINT ( 'NONE',  ( 5.043269954603547767, 4.986162489899998995, -0.7216878364870197293 ) ) ;
#26057=CARTESIAN_POINT ( 'NONE',  ( 0.6823417656249882723, 2.488541667008084435, -1.181850606188749264 ) ) ;
#26059=CARTESIAN_POINT ( 'NONE',  ( 8.599949509769960088, 8.927695937686774386, 1.040834085586084257E-14 ) ) ;
#26060=ADVANCED_FACE ( 'NONE', ( #84126 ), #119901, .F. ) ;
#26061=CARTESIAN_POINT ( 'NONE',  ( -10.47775378526269918, 11.11846759242831872, -0.7998128361456221525 ) ) ;
#26068=CARTESIAN_POINT ( 'NONE',  ( -1.500000000000011324, 2.920833333333352932, 0.8660254037844403729 ) ) ;
#26069=CARTESIAN_POINT ( 'NONE',  ( 6.823831386379729302, 6.855558127064808716, -0.7998128361456281477 ) ) ;
#26070=CARTESIAN_POINT ( 'NONE',  ( -6.795661308947694934, 8.951357498570873261, -1.599625672291263179 ) ) ;
#26074=CARTESIAN_POINT ( 'NONE',  ( -1.364683531250012516, 3.238541667008084879, -0.7879004041258289570 ) ) ;
#26077=CARTESIAN_POINT ( 'NONE',  ( 10.38518247838791986, 11.21839376764850726, 0.7216878364870438212 ) ) ;
#26081=CARTESIAN_POINT ( 'NONE',  ( -4.663641653420935285, 5.503632019488245319, 1.082531754730560403 ) ) ;
#26082=CARTESIAN_POINT ( 'NONE',  ( -0.7500000000000006661, 1.639583334016154970, -1.299038105676652011 ) ) ;
#26085=CARTESIAN_POINT ( 'NONE',  ( -5.961834861707238531, 7.978559976790334574, -1.599625672291263179 ) ) ;
#26094=CARTESIAN_POINT ( 'NONE',  ( 4.313465427442102929, 8.184126765324453601, 0.7998128361456462443 ) ) ;
#26098=CARTESIAN_POINT ( 'NONE',  ( 6.830610463186557624, 6.863467050006115677, 1.040834085586084257E-14 ) ) ;
#26105=CARTESIAN_POINT ( 'NONE',  ( 2.367870383881045981, 5.914265881169853856, 0.000000000000000000 ) ) ;
#26110=CARTESIAN_POINT ( 'NONE',  ( 5.449628763635895545, 6.258197423388296876, 1.014392677442396806 ) ) ;
#26116=AXIS2_PLACEMENT_3D ( 'NONE', #48784, #98595, #150551 ) ;
#26121=CARTESIAN_POINT ( 'NONE',  ( 6.643132081016111634, 9.733775946952057723, 1.082531754730558626 ) ) ;
#26123=CARTESIAN_POINT ( 'NONE',  ( -4.391951695823077984, 7.211361847513815704, 1.199719254218464037 ) ) ;
#26125=AXIS2_PLACEMENT_3D ( 'NONE', #32040, #36276, #182524 ) ;
#26128=CARTESIAN_POINT ( 'NONE',  ( -6.555530967407501741, 7.606873202518897870, 1.199719254218450271 ) ) ;
#26131=ADVANCED_FACE ( 'NONE', ( #117767 ), #183758, .F. ) ;
#26143=CARTESIAN_POINT ( 'NONE',  ( 4.041704886938696006, 3.985977791876626597, -0.7864694415971177355 ) ) ;
#26146=CARTESIAN_POINT ( 'NONE',  ( 3.389175213736292047, 5.937492935125556315, 1.082531754730558626 ) ) ;
#26152=CARTESIAN_POINT ( 'NONE',  ( -3.090368948911150770, 5.692848642783215674, 1.199719254218462483 ) ) ;
#26155=CARTESIAN_POINT ( 'NONE',  ( 8.697719238366680372, 10.10609285197134533, 1.199719254218462483 ) ) ;
#26159=CARTESIAN_POINT ( 'NONE',  ( -8.525379664894808585, 8.840697785332414682, -0.7998128361456291469 ) ) ;
#26160=CARTESIAN_POINT ( 'NONE',  ( 4.690231075323689325, 7.559354456931247412, 1.199719254218462483 ) ) ;
#26162=CARTESIAN_POINT ( 'NONE',  ( 5.332434488876471868, 5.115595079977664383, 0.7998128361456341429 ) ) ;
#26164=CARTESIAN_POINT ( 'NONE',  ( -0.6823417656250212460, 2.113541667008083991, 1.181850606188767472 ) ) ;
#26166=CARTESIAN_POINT ( 'NONE',  ( 7.022760382198770301, 8.255937203062467589, -1.082531754730543083 ) ) ;
#26171=ADVANCED_FACE ( 'NONE', ( #168574 ), #113223, .T. ) ;
#26172=B_SPLINE_CURVE_WITH_KNOTS ( 'NONE', 3,
 ( #49136, #44884, #211601, #47011, #110990, #30757, #96836, #176994, #162885, #80556, #146655, #212668, #130455, #69610 ),
 .UNSPECIFIED., .F., .F.,
 ( 4, 2, 2, 2, 2, 2, 4 ),
 ( 0.001720018798322700722, 0.002147110083253294267, 0.002360655725718589087, 0.002574201368183881306, 0.003001292653114468779, 0.003214838295579761432, 0.003428383938045054084 ),
 .UNSPECIFIED. ) ;
#26176=CARTESIAN_POINT ( 'NONE',  ( 9.205623113554615600, 11.76297960394566466, 1.443375672974076540 ) ) ;
#26182=CARTESIAN_POINT ( 'NONE',  ( -10.00321840878439339, 10.56484298653695397, 1.040834085586084257E-14 ) ) ;
#26199=CARTESIAN_POINT ( 'NONE',  ( -1.499999999999997780, 1.681250000682817047, 0.000000000000000000 ) ) ;
#26203=ORIENTED_EDGE ( 'NONE', *, *, #24579, .T. ) ;
#26205=CARTESIAN_POINT ( 'NONE',  ( -1.402160292154681736E-14, 0.2125000000000202283, 1.732050807568877637 ) ) ;
#26206=CARTESIAN_POINT ( 'NONE',  ( 7.263417608619159083, 9.497073181520933716, -1.599625672291262513 ) ) ;
#26207=CARTESIAN_POINT ( 'NONE',  ( 1.364683531249988757, -0.6156249996585803075, 0.000000000000000000 ) ) ;
#26210=CARTESIAN_POINT ( 'NONE',  ( 8.866669273657322492, 12.32790267170016207, -1.082531754730543083 ) ) ;
#26211=CARTESIAN_POINT ( 'NONE',  ( -5.422898255786193111, 8.310169817517122581, -1.082531754730544860 ) ) ;
#26214=VECTOR ( 'NONE', #13782, 1000.000000000000000 ) ;
#26216=CARTESIAN_POINT ( 'NONE',  ( -5.042743069279040036, 7.970618449879118828, 1.199719254218464037 ) ) ;
#26219=CARTESIAN_POINT ( 'NONE',  ( -1.201851678989727383E-14, 1.993750000682816381, 1.732050807568877637 ) ) ;
#26231=CARTESIAN_POINT ( 'NONE',  ( -9.287498920561160887, 10.79416914786490089, -1.199719254218441611 ) ) ;
#26232=CARTESIAN_POINT ( 'NONE',  ( 5.947222937888848371, 10.09017719417900416, 1.040834085586084257E-14 ) ) ;
#26239=CARTESIAN_POINT ( 'NONE',  ( -8.670602931139386627, 10.07445716020612103, 1.199719254218462483 ) ) ;
#26244=CARTESIAN_POINT ( 'NONE',  ( 8.530051201292206287, 13.10347683481629488, 0.000000000000000000 ) ) ;
#26248=CARTESIAN_POINT ( 'NONE',  ( -7.147119532698295252, 11.49005655479003174, 0.000000000000000000 ) ) ;
#26252=CARTESIAN_POINT ( 'NONE',  ( -5.703190497605960196, 6.276721696052339539, -1.111643793752248754 ) ) ;
#26256=B_SPLINE_CURVE_WITH_KNOTS ( 'NONE', 3,
 ( #175143, #60297, #22441, #98158, #61375, #97095 ),
 .UNSPECIFIED., .F., .F.,
 ( 4, 2, 4 ),
 ( 0.000000000000000000, 0.0006533415270788660040, 0.001306683054157732008 ),
 .UNSPECIFIED. ) ;
#26260=CARTESIAN_POINT ( 'NONE',  ( 7.145310649601935182, 8.294949498412453437, -1.199719254218446718 ) ) ;
#26281=CARTESIAN_POINT ( 'NONE',  ( 4.528060117284244512, 4.385084346360807572, 0.7216878364870317197 ) ) ;
#26286=CARTESIAN_POINT ( 'NONE',  ( -8.459397779922852578, 11.95671561229694824, 1.199719254218453823 ) ) ;
#26288=CARTESIAN_POINT ( 'NONE',  ( 10.57266086055835075, 11.22919251360659310, 0.000000000000000000 ) ) ;
#26291=CARTESIAN_POINT ( 'NONE',  ( 4.892426280589802445, 6.808304349406905764, 1.389186069060392104 ) ) ;
#26296=CARTESIAN_POINT ( 'NONE',  ( -0.6823417656250003738, 1.217708333674752286, -1.181850606188749264 ) ) ;
#26298=EDGE_LOOP ( 'NONE', ( #159425, #60743 ) ) ;
#26302=CARTESIAN_POINT ( 'NONE',  ( -3.228813138348844536, 6.918699094715619502, 0.7998128361456341429 ) ) ;
#26303=CARTESIAN_POINT ( 'NONE',  ( 3.609978820808554811, 4.211641957610042120, 2.420000000000023022 ) ) ;
#26305=CARTESIAN_POINT ( 'NONE',  ( -0.7500000000000249800, -0.05833333333331303105, 1.299038105676659116 ) ) ;
#26307=CARTESIAN_POINT ( 'NONE',  ( -1.364683531250000748, -0.9281249996585805295, 0.000000000000000000 ) ) ;
#26313=CARTESIAN_POINT ( 'NONE',  ( 0.6823417656249882723, -0.3239583329919110133, -1.181850606188749264 ) ) ;
#26316=CARTESIAN_POINT ( 'NONE',  ( -7.039708073993679704, 9.236078724457858158, 1.599625672291283607 ) ) ;
#26317=CARTESIAN_POINT ( 'NONE',  ( 9.725276259704228821, 10.24057714594344048, 0.7998128361456462443 ) ) ;
#26322=CARTESIAN_POINT ( 'NONE',  ( -0.6823417656250003738, 0.5302083336747518416, -1.181850606188749264 ) ) ;
#26328=PRODUCT ( 'positive coil', 'positive coil', '', ( #166342 ) ) ;
#26332=CARTESIAN_POINT ( 'NONE',  ( 6.399085315970131305, 8.488685506763726352, -1.443375672974057666 ) ) ;
#26335=CARTESIAN_POINT ( 'NONE',  ( -5.850506979496850057, 6.784345216623154151, -1.199719254218446718 ) ) ;
#26341=CARTESIAN_POINT ( 'NONE',  ( 4.622967192135525316, 8.337286124226029216, -0.7216878364870207285 ) ) ;
#26342=CARTESIAN_POINT ( 'NONE',  ( -8.636180661780660017, 11.09863007687603087, -1.443375672974058777 ) ) ;
#26347=CARTESIAN_POINT ( 'NONE',  ( 4.207107738942202246, 3.802713871720993399, 1.214306433183764966E-14 ) ) ;
#26352=ORIENTED_EDGE ( 'NONE', *, *, #129464, .F. ) ;
#26359=CARTESIAN_POINT ( 'NONE',  ( 8.961576348508637935, 11.47825837805867799, -1.443375672974052559 ) ) ;
#26362=CARTESIAN_POINT ( 'NONE',  ( 8.925345196497941558, 9.307324238869423283, 1.040834085586084257E-14 ) ) ;
#26365=CARTESIAN_POINT ( 'NONE',  ( -4.026408433134269771, 6.680931691089825541, 1.082531754730560403 ) ) ;
#26367=AXIS2_PLACEMENT_3D ( 'NONE', #37386, #151156, #154347 ) ;
#26368=DIRECTION ( 'NONE',  ( -1.000000000000000000, 7.109522442527899011E-16, 0.000000000000000000 ) ) ;
#26369=CARTESIAN_POINT ( 'NONE',  ( 5.666945020832181434, 5.713783400500082266, 0.7216878364870317197 ) ) ;
#26371=CARTESIAN_POINT ( 'NONE',  ( -8.527715433315703919, 9.051348881730875817, 1.040834085586084257E-14 ) ) ;
#26375=CARTESIAN_POINT ( 'NONE',  ( -2.764973262183167968, 5.313220341600567664, 1.199719254218462483 ) ) ;
#26381=ORIENTED_EDGE ( 'NONE', *, *, #24691, .T. ) ;
#26397=CARTESIAN_POINT ( 'NONE',  ( 0.1639926229446086736, 8.277376109547596172, 1.999401122995874358 ) ) ;
#26401=CARTESIAN_POINT ( 'NONE',  ( -5.819474248763749635, 7.812472595022922128, -1.599625672291256295 ) ) ;
#26405=CARTESIAN_POINT ( 'NONE',  ( 4.449046963578762615, 8.342305224150557308, -0.7998128361456231517 ) ) ;
#26408=AXIS2_PLACEMENT_3D ( 'NONE', #72582, #21675, #155988 ) ;
#26409=CARTESIAN_POINT ( 'NONE',  ( 3.728655938958122196, 4.308852335994623139, -1.199719254218446718 ) ) ;
#26414=CARTESIAN_POINT ( 'NONE',  ( -4.416205349749324327, 6.175325546172740765, 1.599625672291267398 ) ) ;
#26417=CARTESIAN_POINT ( 'NONE',  ( 7.751511138711133064, 10.06651563329490529, -1.599625672291262513 ) ) ;
#26418=CARTESIAN_POINT ( 'NONE',  ( -1.201851678989727383E-14, 3.321875000341421025, 1.575800808251672791 ) ) ;
#26420=CARTESIAN_POINT ( 'NONE',  ( 5.966167892564917530, 6.109520806784549229, 0.6870465322655286977 ) ) ;
#26421=CARTESIAN_POINT ( 'NONE',  ( 4.094199201646931741, 4.839282492418613302, -1.082531754730543083 ) ) ;
#26429=CARTESIAN_POINT ( 'NONE',  ( 6.765155463094759014, 7.955398130774449683, 1.082531754730558626 ) ) ;
#26430=CARTESIAN_POINT ( 'NONE',  ( -8.646349277213090545, 11.11049346154719508, 1.599625672291269396 ) ) ;
#26433=CARTESIAN_POINT ( 'NONE',  ( -8.025536864285518490, 11.45054454405341282, -1.199719254218446718 ) ) ;
#26434=CARTESIAN_POINT ( 'NONE',  ( -5.228640796364566690, 9.251831362400652736, -0.7998128361456231517 ) ) ;
#26442=CARTESIAN_POINT ( 'NONE',  ( 8.076906825439115423, 10.44614393447756129, -1.599625672291262513 ) ) ;
#26448=CARTESIAN_POINT ( 'NONE',  ( 2.198393463710220264, 5.716542807637226886, 0.7998128361456462443 ) ) ;
#26456=CARTESIAN_POINT ( 'NONE',  ( 1.499999999999989120, 4.754166666666689522, 0.8660254037844524744 ) ) ;
#26457=CARTESIAN_POINT ( 'NONE',  ( 3.662674053986138656, 7.424870162959149589, 0.7998128361456321445 ) ) ;
#26458=CARTESIAN_POINT ( 'NONE',  ( 7.156006149914539982, 7.243095351188763686, 1.040834085586084257E-14 ) ) ;
#26461=CARTESIAN_POINT ( 'NONE',  ( 7.470179451449751262, 7.817556902887268677, 1.040834085586084257E-14 ) ) ;
#26462=CARTESIAN_POINT ( 'NONE',  ( -7.632877294369372123, 11.84884791016554573, 0.7216878364870458196 ) ) ;
#26466=CARTESIAN_POINT ( 'NONE',  ( 7.944187942603509356, 11.35563746875774882, 1.199719254218460707 ) ) ;
#26470=DIRECTION ( 'NONE',  ( 0.000000000000000000, 8.546850786086437571E-32, 1.000000000000000000 ) ) ;
#26471=CARTESIAN_POINT ( 'NONE',  ( -0.6823417656250003738, 0.7177083336747519526, -1.181850606188749264 ) ) ;
#26476=CARTESIAN_POINT ( 'NONE',  ( 0.6823417656249882723, -0.3239583329919110133, -1.181850606188749264 ) ) ;
#26478=CARTESIAN_POINT ( 'NONE',  ( 9.103410076571945453, 12.70806329172093818, 1.199719254218450271 ) ) ;
#26482=CARTESIAN_POINT ( 'NONE',  ( -9.561524646135538319, 12.17819805862340310, -1.599625672291263179 ) ) ;
#26487=CARTESIAN_POINT ( 'NONE',  ( 5.203632029546647608, 4.965325544092860532, 1.040834085586084257E-14 ) ) ;
#26495=CARTESIAN_POINT ( 'NONE',  ( 8.718056468787178659, 10.12981962079525289, 1.199719254218462483 ) ) ;
#26497=CARTESIAN_POINT ( 'NONE',  ( 1.145612256460542211, 2.800000000000024247, -0.9666182179050045731 ) ) ;
#26498=CARTESIAN_POINT ( 'NONE',  ( -4.822949958159302497, 6.649860922651058992, -1.599625672291256295 ) ) ;
#26502=CARTESIAN_POINT ( 'NONE',  ( 9.101601193475611140, 9.512956235343358102, -0.7998128361456221525 ) ) ;
#26504=CARTESIAN_POINT ( 'NONE',  ( 6.428537391173986038, 10.65171072301167854, 0.7998128361456462443 ) ) ;
#26507=CARTESIAN_POINT ( 'NONE',  ( -9.056483424248693126, 10.62861408545402675, 1.082531754730558626 ) ) ;
#26513=ADVANCED_FACE ( 'NONE', ( #100685 ), #182998, .T. ) ;
#26515=CARTESIAN_POINT ( 'NONE',  ( -6.118227108790639690, 6.008232112836603633, 0.2598000991895776934 ) ) ;
#26516=CARTESIAN_POINT ( 'NONE',  ( 1.364683531249988757, 1.384375000341421469, 0.000000000000000000 ) ) ;
#26518=CARTESIAN_POINT ( 'NONE',  ( 6.643132081016124069, 7.813037518349371879, 1.082531754730558626 ) ) ;
#26536=CARTESIAN_POINT ( 'NONE',  ( 7.072549687823125097, 11.40305840243567381, -0.7998128361456291469 ) ) ;
#26538=ORIENTED_EDGE ( 'NONE', *, *, #175957, .T. ) ;
#26540=CARTESIAN_POINT ( 'NONE',  ( -3.327636637150278798, 5.969660945728899826, -1.199719254218452935 ) ) ;
#26541=CARTESIAN_POINT ( 'NONE',  ( -5.693534442735004752, 8.729875052244421951, 1.199719254218452047 ) ) ;
#26546=CARTESIAN_POINT ( 'NONE',  ( -1.499999999999997780, 3.931250000682819046, 1.214306433183764966E-14 ) ) ;
#26547=CARTESIAN_POINT ( 'NONE',  ( 8.911787042884274257, 9.291506392986812912, 0.7998128361456462443 ) ) ;
#26550=CARTESIAN_POINT ( 'NONE',  ( -6.852756576703439961, 10.08230087520760954, 1.199719254218453823 ) ) ;
#26552=CARTESIAN_POINT ( 'NONE',  ( -1.201851678989727383E-14, 4.696875000341419693, -1.575800808251660134 ) ) ;
#26553=CARTESIAN_POINT ( 'NONE',  ( -1.558973042057849590, 8.694236233169934991, 2.500000000000010658 ) ) ;
#26554=CARTESIAN_POINT ( 'NONE',  ( 2.861609313207599925, 6.434901926071078471, -0.3141389326147243088 ) ) ;
#26558=CARTESIAN_POINT ( 'NONE',  ( -9.354762803749327560, 10.01623748057011376, 0.7216878364870438212 ) ) ;
#26562=CARTESIAN_POINT ( 'NONE',  ( 1.364683531249988535, 3.467708333674749621, -0.7879004041258239610 ) ) ;
#26571=CARTESIAN_POINT ( 'NONE',  ( 1.364683531249990311, 4.884375000341417916, 1.214306433183764966E-14 ) ) ;
#26573=CARTESIAN_POINT ( 'NONE',  ( -3.601662362724658895, 7.353689856487406473, -0.7998128361456281477 ) ) ;
#26574=CARTESIAN_POINT ( 'NONE',  ( 6.986529229743720926, 7.045372277656132276, -0.7998128361456281477 ) ) ;
#26578=CARTESIAN_POINT ( 'NONE',  ( -1.364683531249997417, 4.071875000341417028, 1.214306433183764966E-14 ) ) ;
#26582=CARTESIAN_POINT ( 'NONE',  ( -1.402160292154681736E-14, -0.1781249996585796136, 1.575800808251672791 ) ) ;
#26584=CARTESIAN_POINT ( 'NONE',  ( -2.982430605326321427, 6.423326772948587227, -0.7216878364870267237 ) ) ;
#26588=CARTESIAN_POINT ( 'NONE',  ( 3.226477370372302644, 5.747678784534228313, 1.082531754730546636 ) ) ;
#26591=CARTESIAN_POINT ( 'NONE',  ( -9.815740026613967828, 10.55404424057886636, -0.7216878364870267237 ) ) ;
#26597=CARTESIAN_POINT ( 'NONE',  ( -5.205967797523171292, 9.017453497178271604, 0.000000000000000000 ) ) ;
#26599=CARTESIAN_POINT ( 'NONE',  ( -1.364683531250012516, 1.342708333674755616, 0.7879004041258379498 ) ) ;
#26605=CARTESIAN_POINT ( 'NONE',  ( -0.6823417656250003738, 0.03020833367475134201, -1.181850606188749264 ) ) ;
#26609=CARTESIAN_POINT ( 'NONE',  ( 3.728129053633592704, 4.412200653069714207, -1.082531754730543083 ) ) ;
#26613=CARTESIAN_POINT ( 'NONE',  ( 1.499999999999985123, -0.9541666666666493990, -0.8660254037844323793 ) ) ;
#26614=CARTESIAN_POINT ( 'NONE',  ( 9.219181267168295335, 9.858059021225592744, 1.040834085586084257E-14 ) ) ;
#26623=CARTESIAN_POINT ( 'NONE',  ( -2.605138072120212200, 6.191078184115536232, -0.7998128361456281477 ) ) ;
#26626=CARTESIAN_POINT ( 'NONE',  ( -3.895595285070201808, 2.800000000000024691, 0.7750000000000135669 ) ) ;
#26627=CARTESIAN_POINT ( 'NONE',  ( 1.364683531249988535, 1.926041667008086211, 0.7879004041258500513 ) ) ;
#26641=CARTESIAN_POINT ( 'NONE',  ( -0.5451172737955251035, 6.555825640206980331, -3.374434186942578684 ) ) ;
#26648=CARTESIAN_POINT ( 'NONE',  ( 6.063521013809720195, 8.097193820909906137, 1.599625672291281386 ) ) ;
#26653=CARTESIAN_POINT ( 'NONE',  ( 3.009610312849396951, 6.452363523749469643, -0.06592220986071165023 ) ) ;
#26657=CARTESIAN_POINT ( 'NONE',  ( 7.574201371528760163, 11.98831870009225931, 1.040834085586084257E-14 ) ) ;
#26662=VERTEX_POINT ( 'NONE', #34615 ) ;
#26663=CARTESIAN_POINT ( 'NONE',  ( 10.55910270694468345, 11.21337466772398095, 0.7998128361456462443 ) ) ;
#26665=LINE ( 'NONE', #90629, #134168 ) ;
#26669=CARTESIAN_POINT ( 'NONE',  ( -9.192064960385334160, 9.826423329978791088, 0.7216878364870438212 ) ) ;
#26674=EDGE_CURVE ( 'NONE', #45840, #15325, #53000, .T. ) ;
#26677=CARTESIAN_POINT ( 'NONE',  ( 3.798255590122797898, 7.583048621785260401, -0.7998128361456221525 ) ) ;
#26683=CARTESIAN_POINT ( 'NONE',  ( 4.487385655998888723, 4.337630808194552934, 0.7216878364870317197 ) ) ;
#26686=ORIENTED_EDGE ( 'NONE', *, *, #212483, .F. ) ;
#26691=CARTESIAN_POINT ( 'NONE',  ( -5.259673527097670664, 8.223703984000886535, -1.199719254218446718 ) ) ;
#26692=CARTESIAN_POINT ( 'NONE',  ( -4.229020061460118107, 7.343517960532632394, -0.8650006913940473385 ) ) ;
#26693=CARTESIAN_POINT ( 'NONE',  ( -4.810445574750349174, 4.506608013497163334, 0.7998128361456341429 ) ) ;
#26699=CARTESIAN_POINT ( 'NONE',  ( 1.084637062511532246, 2.992628807292006865, 1.105835307554805524 ) ) ;
#26700=CARTESIAN_POINT ( 'NONE',  ( -1.364683531250012516, 3.342708333674756727, 0.7879004041258379498 ) ) ;
#26702=CARTESIAN_POINT ( 'NONE',  ( 5.473741331615251227, 7.409117525016355010, -1.599625672291262513 ) ) ;
#26704=CARTESIAN_POINT ( 'NONE',  ( 1.534404370307017595, 8.695807324171010322, 2.514078760162040904 ) ) ;
#26716=CARTESIAN_POINT ( 'NONE',  ( 0.6823417656249899377, 1.655208333674752730, 1.181850606188755259 ) ) ;
#26718=CARTESIAN_POINT ( 'NONE',  ( 4.650610384687404952, 5.384465856012134566, 1.199719254218462483 ) ) ;
#26719=AXIS2_PLACEMENT_3D ( 'NONE', #191667, #174400, #96351 ) ;
#26721=CARTESIAN_POINT ( 'NONE',  ( -5.802526556968872207, 6.832331073627524454, 1.082531754730548412 ) ) ;
#26722=CARTESIAN_POINT ( 'NONE',  ( 3.172244755917638770, 5.684407401003788607, -1.082531754730543083 ) ) ;
#26723=CARTESIAN_POINT ( 'NONE',  ( -6.602457619730773608, 8.725953194484466380, 1.443375672974078761 ) ) ;
#26724=ADVANCED_FACE ( 'NONE', ( #70292 ), #202424, .F. ) ;
#26727=CARTESIAN_POINT ( 'NONE',  ( 4.788000803920411386, 8.737751371215816576, 1.040834085586084257E-14 ) ) ;
#26732=CARTESIAN_POINT ( 'NONE',  ( 1.364683531249988535, 5.655208333674751842, -0.7879004041258300672 ) ) ;
#26737=CARTESIAN_POINT ( 'NONE',  ( 7.467843683028853263, 7.606905806488803101, 0.7998128361456341429 ) ) ;
#26739=CARTESIAN_POINT ( 'NONE',  ( -6.527360889975461156, 9.702672574024962415, 1.199719254218452047 ) ) ;
#26744=CARTESIAN_POINT ( 'NONE',  ( 8.697719238366680372, 10.10609285197134533, 1.199719254218462483 ) ) ;
#26748=CARTESIAN_POINT ( 'NONE',  ( -8.538937818508475885, 8.856515631215026829, 1.040834085586084257E-14 ) ) ;
#26750=CARTESIAN_POINT ( 'NONE',  ( 6.927853306458743532, 9.105581495667113501, 1.443375672974076540 ) ) ;
#26751=CARTESIAN_POINT ( 'NONE',  ( 4.078932850288060408, 7.722175824222965446, -0.6089670364913578604 ) ) ;
#26752=CARTESIAN_POINT ( 'NONE',  ( -3.438964519360665051, 7.163875705896082913, -0.7998128361456281477 ) ) ;
#26756=CARTESIAN_POINT ( 'NONE',  ( 6.484877546038077867, 6.460111979999551224, 1.040834085586084257E-14 ) ) ;
#26758=CARTESIAN_POINT ( 'NONE',  ( 8.890396042259068210, 11.39521468743417998, -1.599625672291257406 ) ) ;
#26759=CARTESIAN_POINT ( 'NONE',  ( -4.774234299259712877, 6.798759937490593153, 1.242976086189879759 ) ) ;
#26761=CARTESIAN_POINT ( 'NONE',  ( 1.364683531249988757, 0.3843750003414206362, 0.000000000000000000 ) ) ;
#26763=CARTESIAN_POINT ( 'NONE',  ( -5.097502569058207200, 8.890910730635814829, -0.7216878364870207285 ) ) ;
#26770=CARTESIAN_POINT ( 'NONE',  ( -5.028543871580710700, 6.592580098690584478, 1.235119876028653918 ) ) ;
#26771=CARTESIAN_POINT ( 'NONE',  ( -1.402160292154681736E-14, 0.6343750003414162508, 1.575800808251672791 ) ) ;
#26773=CARTESIAN_POINT ( 'NONE',  ( 3.334942599281629949, 5.874221551595115720, -1.082531754730543083 ) ) ;
#26777=CARTESIAN_POINT ( 'NONE',  ( -8.487040972030346353, 9.003895343564625620, 1.040834085586084257E-14 ) ) ;
#26782=CARTESIAN_POINT ( 'NONE',  ( -8.554831740098665094, 11.00372300158037042, 1.443375672974064550 ) ) ;
#26783=CARTESIAN_POINT ( 'NONE',  ( -1.217358635584816495, 3.139784080462332927, 0.7750000000000083489 ) ) ;
#26784=EDGE_LOOP ( 'NONE', ( #63024, #33922, #49454, #195898 ) ) ;
#26788=VERTEX_POINT ( 'NONE', #68160 ) ;
#26789=CARTESIAN_POINT ( 'NONE',  ( -8.324343128666356506, 8.814081192973304724, 1.040834085586084257E-14 ) ) ;
#26793=CARTESIAN_POINT ( 'NONE',  ( -1.364683531249997417, 5.571875000341417916, 1.214306433183764966E-14 ) ) ;
#26794=CARTESIAN_POINT ( 'NONE',  ( -1.201851678989727383E-14, 4.118750000682818602, -1.732050807568863648 ) ) ;
#26795=CARTESIAN_POINT ( 'NONE',  ( 4.408913874118179699, 7.341020650511065782, -1.198271334459002802 ) ) ;
#26804=CARTESIAN_POINT ( 'NONE',  ( -5.506582945444718824, 9.576097202994168001, 0.7998128361456481317 ) ) ;
#26808=CARTESIAN_POINT ( 'NONE',  ( 5.497994985541524215, 6.373081223675282736, -1.199719254218445830 ) ) ;
#26813=CARTESIAN_POINT ( 'NONE',  ( 5.770966940911189447, 9.884545197705074671, -0.7998128361456291469 ) ) ;
#26819=CARTESIAN_POINT ( 'NONE',  ( -5.205967797967562483, 8.057084283395347768, 1.082531754730548412 ) ) ;
#26826=DIRECTION ( 'NONE',  ( 1.000000000000000000, 0.000000000000000000, 0.000000000000000000 ) ) ;
#26830=CARTESIAN_POINT ( 'NONE',  ( -8.829384350997580455, 11.32403438096243775, 1.599625672291269396 ) ) ;
#26832=CARTESIAN_POINT ( 'NONE',  ( 6.272618624616828953, 10.46980549536166016, 1.040834085586084257E-14 ) ) ;
#26833=CARTESIAN_POINT ( 'NONE',  ( 0.7499999999999885647, -0.5166666666666444030, 1.299038105676657340 ) ) ;
#26834=CARTESIAN_POINT ( 'NONE',  ( -7.557780564614042795, 10.90482886110335414, -1.199719254218446718 ) ) ;
#26837=CARTESIAN_POINT ( 'NONE',  ( 0.6823417656249917140, 3.842708333674754506, 1.181850606188765695 ) ) ;
#26838=CARTESIAN_POINT ( 'NONE',  ( 4.356247428692526569, 3.976710176429713250, 0.7998128361456341429 ) ) ;
#26841=CARTESIAN_POINT ( 'NONE',  ( -1.001543065824772872E-14, 5.212500000000019895, 1.732050807568877637 ) ) ;
#26843=CARTESIAN_POINT ( 'NONE',  ( 8.907343734053986495, 9.494248565925552441, -0.7216878364870197293 ) ) ;
#26846=CARTESIAN_POINT ( 'NONE',  ( -5.748293942514169252, 9.650167333001109071, -0.7216878364870207285 ) ) ;
#26848=CARTESIAN_POINT ( 'NONE',  ( 0.6823417656249882723, 2.676041667008084879, -1.181850606188749264 ) ) ;
#26850=CYLINDRICAL_SURFACE ( 'NONE', #195076, 0.7499999999999997780 ) ;
#26852=CARTESIAN_POINT ( 'NONE',  ( -6.449928391799210736, 8.548002428564306143, -1.599625672291263179 ) ) ;
#26853=CARTESIAN_POINT ( 'NONE',  ( -0.6823417656250212460, 5.363541667008087543, 1.181850606188767472 ) ) ;
#26859=CARTESIAN_POINT ( 'NONE',  ( 9.097684769969825780, 10.57271930550834860, -1.199719254218446718 ) ) ;
#26862=CARTESIAN_POINT ( 'NONE',  ( 1.499999999999987121, 1.295833333333353377, -0.8660254037844253849 ) ) ;
#26866=ORIENTED_EDGE ( 'NONE', *, *, #124486, .T. ) ;
#26867=CARTESIAN_POINT ( 'NONE',  ( 6.588899466561449536, 9.670504563421618016, -1.082531754730537088 ) ) ;
#26868=AXIS2_PLACEMENT_3D ( 'NONE', #115909, #165667, #194971 ) ;
#26869=CARTESIAN_POINT ( 'NONE',  ( 9.073431116043567002, 11.60875560684942265, -1.599625672291262513 ) ) ;
#26874=CARTESIAN_POINT ( 'NONE',  ( 7.944187942603509356, 11.35563746875774882, 1.199719254218460707 ) ) ;
#26875=CARTESIAN_POINT ( 'NONE',  ( -5.056828107772880720, 5.001980335264189392, -0.7216878364870142892 ) ) ;
#26877=EDGE_CURVE ( 'NONE', #182051, #73782, #170053, .T. ) ;
#26879=CARTESIAN_POINT ( 'NONE',  ( -1.201851678989727383E-14, 5.509375000341415252, -1.575800808251660134 ) ) ;
#26885=CARTESIAN_POINT ( 'NONE',  ( -1.364683531249997417, 4.009375000341424133, 1.214306433183764966E-14 ) ) ;
#26887=CARTESIAN_POINT ( 'NONE',  ( -6.588899466561478846, 6.789396920517583922, 0.7216878364870317197 ) ) ;
#26893=CARTESIAN_POINT ( 'NONE',  ( 3.891353782322113375, 4.498666486585943147, -1.199719254218446718 ) ) ;
#26896=CARTESIAN_POINT ( 'NONE',  ( 8.925345196497941558, 9.307324238869423283, 1.040834085586084257E-14 ) ) ;
#26902=CARTESIAN_POINT ( 'NONE',  ( -9.318531651294266638, 9.766041769465124034, -0.7998128361456291469 ) ) ;
#26903=CARTESIAN_POINT ( 'NONE',  ( 4.808338034340912337, 8.761478140039733020, 1.040834085586084257E-14 ) ) ;
#26905=CARTESIAN_POINT ( 'NONE',  ( 4.677199806590210507, 4.559080650551097236, -0.7216878364870197293 ) ) ;
#26906=CARTESIAN_POINT ( 'NONE',  ( 4.090809663021327758, 5.795697244990093644, 1.599625672291267398 ) ) ;
#26913=CARTESIAN_POINT ( 'NONE',  ( -5.748293942514180799, 7.729428904398431222, -1.443375672974052559 ) ) ;
#26914=CARTESIAN_POINT ( 'NONE',  ( 3.009020027229115879, 5.597941567487558778, -1.199719254218446718 ) ) ;
#26917=CARTESIAN_POINT ( 'NONE',  ( -8.694856585065634746, 9.038420858865048757, 0.7998128361456462443 ) ) ;
#26920=CARTESIAN_POINT ( 'NONE',  ( -1.123270288250318494, 3.235197346350006331, -0.7749999999993560929 ) ) ;
#26922=CARTESIAN_POINT ( 'NONE',  ( -8.995998617867369873, 10.45408546138876993, 1.199719254218462483 ) ) ;
#26923=CARTESIAN_POINT ( 'NONE',  ( 1.217358635584785631, 3.066465920220505570, 0.7750000000000065725 ) ) ;
#26926=CARTESIAN_POINT ( 'NONE',  ( 8.294891053462476904, 8.571794405328034827, 1.040834085586084257E-14 ) ) ;
#26927=CARTESIAN_POINT ( 'NONE',  ( 6.010342169559767633, 5.906487374108181143, -0.7998128361456281477 ) ) ;
#26939=CARTESIAN_POINT ( 'NONE',  ( -6.832419346282942563, 10.05857410638369487, 1.199719254218453823 ) ) ;
#26944=CARTESIAN_POINT ( 'NONE',  ( 5.666945020832167224, 8.594891043404107478, 1.082531754730558626 ) ) ;
#26946=CARTESIAN_POINT ( 'NONE',  ( -4.080641048033267992, 5.783833860837341412, 1.214306433183764966E-14 ) ) ;
#26949=CARTESIAN_POINT ( 'NONE',  ( -6.521635583373313061, 7.567328587812373719, -1.199719254218446718 ) ) ;
#26958=CARTESIAN_POINT ( 'NONE',  ( 8.372323551638698902, 9.726464550788689323, 1.199719254218462483 ) ) ;
#26962=CARTESIAN_POINT ( 'NONE',  ( -5.125485847170801357, 6.519186964134095597, -1.210412105186658094 ) ) ;
#26972=CARTESIAN_POINT ( 'NONE',  ( 3.816783937446950770, 4.411668334231586996, 1.199719254218464037 ) ) ;
#26978=CARTESIAN_POINT ( 'NONE',  ( -5.651877628014641886, 6.159505484824964405, -0.8148192377588457935 ) ) ;
#26989=CARTESIAN_POINT ( 'NONE',  ( -6.084912014434944894, 5.993485526462540847, -0.7998128361456291469 ) ) ;
#26990=CARTESIAN_POINT ( 'NONE',  ( 5.951666246274807115, 6.045958163516475636, 0.7216878364870317197 ) ) ;
#26991=CARTESIAN_POINT ( 'NONE',  ( 1.499999999999990896, 3.775000000000021227, 1.214306433183764966E-14 ) ) ;
#26994=CYLINDRICAL_SURFACE ( 'NONE', #201710, 1.250000000000000000 ) ;
#26998=CARTESIAN_POINT ( 'NONE',  ( -0.6823417656249969321, 4.717708333674755394, -1.181850606188749264 ) ) ;
#27001=CARTESIAN_POINT ( 'NONE',  ( -4.121315508874276112, 4.870918184183829602, -1.082531754730549967 ) ) ;
#27006=CARTESIAN_POINT ( 'NONE',  ( 2.842405760359353106, 6.467890487061221272, -0.7998128361456291469 ) ) ;
#27007=CARTESIAN_POINT ( 'NONE',  ( -1.284279953904135407, 3.128360285806111474, -0.7749999999999892530 ) ) ;
#27008=DIRECTION ( 'NONE',  ( -0.6507913734559658270, 0.7592566023652989049, 0.000000000000000000 ) ) ;
#27013=CARTESIAN_POINT ( 'NONE',  ( 0.6823417656249882723, 1.738541667008083991, -1.181850606188749264 ) ) ;
#27016=CARTESIAN_POINT ( 'NONE',  ( -10.13202086811422475, 10.71511252242175161, -0.7998128361456291469 ) ) ;
#27017=CARTESIAN_POINT ( 'NONE',  ( -5.165293336682207581, 8.009630745229104676, 1.082531754730548412 ) ) ;
#27021=CARTESIAN_POINT ( 'NONE',  ( -1.364683531249997417, 4.759375000341424133, 1.214306433183764966E-14 ) ) ;
#27029=CARTESIAN_POINT ( 'NONE',  ( -5.056828107772848746, 8.843457192469559303, -0.7216878364870207285 ) ) ;
#27034=CARTESIAN_POINT ( 'NONE',  ( -5.707619481228832115, 6.721606151930833661, -1.082531754730543971 ) ) ;
#27036=CARTESIAN_POINT ( 'NONE',  ( 10.01963921569910632, 11.64833282552586091, 1.199719254218450271 ) ) ;
#27044=CARTESIAN_POINT ( 'NONE',  ( 4.108043207509617822, 7.655708725298683071, -0.6976724544028364283 ) ) ;
#27047=CARTESIAN_POINT ( 'NONE',  ( -4.277761160311629673, 4.949475094240346706, 1.199719254218462483 ) ) ;
#27050=CARTESIAN_POINT ( 'NONE',  ( 1.499999999999989120, 0.5250000000000185629, 0.000000000000000000 ) ) ;
#27054=CARTESIAN_POINT ( 'NONE',  ( 9.422553571817644524, 10.09532670998316384, 0.000000000000000000 ) ) ;
#27055=CARTESIAN_POINT ( 'NONE',  ( 6.096362627639171805, 10.26417349888772179, -0.7998128361456291469 ) ) ;
#27060=( BOUNDED_CURVE ( )  B_SPLINE_CURVE ( 2, ( #154230, #206965, #26081, #118585, #92196, #158245, #9834 ),
 .UNSPECIFIED., .F., .T. ) 
 B_SPLINE_CURVE_WITH_KNOTS ( ( 3, 2, 2, 3 ),
 ( 0.1625000000000003941, 0.1666666666666670182, 0.1708333333333336701, 0.1750000000000002942 ),
 .UNSPECIFIED. ) 
 CURVE ( )  GEOMETRIC_REPRESENTATION_ITEM ( )  RATIONAL_B_SPLINE_CURVE ( ( 0.9999999999999874545, 0.8660254037844512531, 1.000000000000000000, 0.8660254037844387076, 1.000000000000000000, 0.8660254037844289376, 1.000000000000009770 ) ) 
 REPRESENTATION_ITEM ( '' )  );
#27062=CARTESIAN_POINT ( 'NONE',  ( 2.842405760359353106, 6.467890487061221272, -0.7998128361456291469 ) ) ;
#27063=CARTESIAN_POINT ( 'NONE',  ( -0.06360284778254256255, 7.077111424250725591, -2.121658048144599018 ) ) ;
#27072=CARTESIAN_POINT ( 'NONE',  ( -6.388916700537716764, 8.476822122092563916, 1.599625672291283607 ) ) ;
#27079=CARTESIAN_POINT ( 'NONE',  ( -1.364683531250012516, 3.280208333674756727, 0.7879004041258379498 ) ) ;
#27080=CARTESIAN_POINT ( 'NONE',  ( 7.904040366642678173, 12.16520482781775137, 0.7216878364870438212 ) ) ;
#27081=CARTESIAN_POINT ( 'NONE',  ( -4.737684612971557740, 7.614716917520386374, 1.199719254218464037 ) ) ;
#27084=CARTESIAN_POINT ( 'NONE',  ( 4.333802657862601215, 8.207853534148366492, 0.7998128361456462443 ) ) ;
#27085=CARTESIAN_POINT ( 'NONE',  ( -5.168682875307782254, 7.053215992657626110, -1.599625672291256295 ) ) ;
#27092=CARTESIAN_POINT ( 'NONE',  ( 5.639828713604826405, 9.523624565940227882, -0.7216878364870267237 ) ) ;
#27095=CARTESIAN_POINT ( 'NONE',  ( -1.364683531250012516, 2.592708333674753174, 0.7879004041258379498 ) ) ;
#27097=CARTESIAN_POINT ( 'NONE',  ( 6.114364089638795186, 7.196141528409145671, 1.082531754730558626 ) ) ;
#27099=CARTESIAN_POINT ( 'NONE',  ( -4.500943810056945438, 5.313817868896925312, 1.082531754730560403 ) ) ;
#27101=CARTESIAN_POINT ( 'NONE',  ( 1.364683531249990311, 5.363541667008086655, 0.7879004041258500513 ) ) ;
#27106=CARTESIAN_POINT ( 'NONE',  ( -4.144866890078757748, 7.628995377423835045, -0.8586628004631415845 ) ) ;
#27111=( BOUNDED_CURVE ( )  B_SPLINE_CURVE ( 2, ( #41203, #204716, #87800, #203650, #107310, #56365, #173334 ),
 .UNSPECIFIED., .F., .T. ) 
 B_SPLINE_CURVE_WITH_KNOTS ( ( 3, 2, 2, 3 ),
 ( 0.1500000000000002165, 0.1541666666666668961, 0.1583333333333335480, 0.1625000000000002276 ),
 .UNSPECIFIED. ) 
 CURVE ( )  GEOMETRIC_REPRESENTATION_ITEM ( )  RATIONAL_B_SPLINE_CURVE ( ( 0.9999999999999928946, 0.8660254037844458130, 1.000000000000000000, 0.8660254037844387076, 1.000000000000000000, 0.8660254037844316022, 1.000000000000007105 ) ) 
 REPRESENTATION_ITEM ( '' )  );
#27114=CARTESIAN_POINT ( 'NONE',  ( 5.469824908109481854, 8.468880595181346393, -1.199719254218446718 ) ) ;
#27117=CARTESIAN_POINT ( 'NONE',  ( 4.220665892555866883, 3.818531717603609987, -0.7998128361456211532 ) ) ;
#27125=CARTESIAN_POINT ( 'NONE',  ( 5.178851490740207453, 5.144340948726102702, 0.7216878364870317197 ) ) ;
#27126=CARTESIAN_POINT ( 'NONE',  ( -1.364683531250012516, 2.342708333674752286, 0.7879004041258379498 ) ) ;
#27128=CARTESIAN_POINT ( 'NONE',  ( 8.938903350111612411, 9.323142084752035430, -0.7998128361456221525 ) ) ;
#27135=CARTESIAN_POINT ( 'NONE',  ( 0.7499999999999885647, 2.566666666666689522, -1.299038105676658228 ) ) ;
#27136=CARTESIAN_POINT ( 'NONE',  ( 6.124532705071213279, 8.168374127381657246, -1.599625672291262513 ) ) ;
#27137=CARTESIAN_POINT ( 'NONE',  ( -6.527360889975461156, 9.702672574024962415, 1.199719254218452047 ) ) ;
#27142=CARTESIAN_POINT ( 'NONE',  ( 1.364683531249990311, 3.134375000341423245, 1.214306433183764966E-14 ) ) ;
#27145=CARTESIAN_POINT ( 'NONE',  ( 2.737856954955798727, 5.281584649835344258, 1.199719254218452047 ) ) ;
#27151=CARTESIAN_POINT ( 'NONE',  ( 1.499999999999987121, 0.7854166673494828999, 0.8660254037844524744 ) ) ;
#27154=CARTESIAN_POINT ( 'NONE',  ( -7.043624497499477499, 8.176315654292865887, 1.199719254218450271 ) ) ;
#27155=CARTESIAN_POINT ( 'NONE',  ( -3.470524135418306511, 5.072030796119872953, -1.443375672974053447 ) ) ;
#27161=VERTEX_POINT ( 'NONE', #60459 ) ;
#27163=CARTESIAN_POINT ( 'NONE',  ( 6.308621549060418054, 6.254479983525607523, 0.7998128361456341429 ) ) ;
#27167=CARTESIAN_POINT ( 'NONE',  ( 4.008406971134620633, 7.828225232965717595, 0.7998128361456321445 ) ) ;
#27171=CARTESIAN_POINT ( 'NONE',  ( 2.544126380858701797, 6.119897877643793116, 0.7998128361456462443 ) ) ;
#27172=ORIENTED_EDGE ( 'NONE', *, *, #692, .F. ) ;
#27177=CARTESIAN_POINT ( 'NONE',  ( 4.006694938150886287, 7.586369203660299654, 0.2279062292016853508 ) ) ;
#27187=CARTESIAN_POINT ( 'NONE',  ( -3.226477370372317743, 4.787309570232886280, 1.443375672974064550 ) ) ;
#27188=CARTESIAN_POINT ( 'NONE',  ( 8.595506201384013778, 10.09080732544527592, 1.082531754730558626 ) ) ;
#27190=CARTESIAN_POINT ( 'NONE',  ( -3.391510981712833939, 7.108513245306943062, 0.7998128361456341429 ) ) ;
#27191=CYLINDRICAL_SURFACE ( 'NONE', #17442, 1.500000000000000222 ) ;
#27193=CARTESIAN_POINT ( 'NONE',  ( 8.945682426918439845, 9.331051007693339727, 1.040834085586084257E-14 ) ) ;
#27195=CARTESIAN_POINT ( 'NONE',  ( -4.934277840369690971, 7.844075682818238526, -1.199719254218452047 ) ) ;
#27209=CARTESIAN_POINT ( 'NONE',  ( -4.069418662396130593, 7.899405539437467816, -0.7998128361456281477 ) ) ;
#27212=CARTESIAN_POINT ( 'NONE',  ( 4.378920427533921078, 4.211088041652093494, 1.214306433183764966E-14 ) ) ;
#27216=DIRECTION ( 'NONE',  ( -5.176899690512889973E-31, 0.6299249119529756191, 0.7766560405359864694 ) ) ;
#27217=CARTESIAN_POINT ( 'NONE',  ( -3.765413976293358278, 5.416068943807445635, 1.599625672291267398 ) ) ;
#27220=CARTESIAN_POINT ( 'NONE',  ( 9.887974103068218668, 10.43039129653476493, 0.7998128361456462443 ) ) ;
#27223=CIRCLE ( 'NONE', #58311, 0.1599999999999999756 ) ;
#27225=CARTESIAN_POINT ( 'NONE',  ( -7.725448601688521322, 7.907444878258402809, 1.040834085586084257E-14 ) ) ;
#27226=CARTESIAN_POINT ( 'NONE',  ( 4.286349120214771879, 8.152491073559232859, -0.7998128361456221525 ) ) ;
#27228=CARTESIAN_POINT ( 'NONE',  ( 4.253507506385319381, 5.985511395581417204, 1.599625672291267175 ) ) ;
#27230=CARTESIAN_POINT ( 'NONE',  ( 0.6823417656249882723, 0.9885416670080832136, -1.181850606188749264 ) ) ;
#27233=CARTESIAN_POINT ( 'NONE',  ( 6.751597309925441159, 9.860318714012938912, -1.082531754730537088 ) ) ;
#27236=B_SPLINE_CURVE_WITH_KNOTS ( 'NONE', 3,
 ( #54114, #71395, #4256, #19459, #200335, #203523 ),
 .UNSPECIFIED., .F., .F.,
 ( 4, 2, 4 ),
 ( 0.000000000000000000, 0.002037565947615824213, 0.004075131895231648427 ),
 .UNSPECIFIED. ) ;
#27241=CARTESIAN_POINT ( 'NONE',  ( 8.825994812371966702, 12.28044913353391898, -1.082531754730543083 ) ) ;
#27247=CARTESIAN_POINT ( 'NONE',  ( -10.17947440576205054, 10.77047498301088346, 0.7998128361456462443 ) ) ;
#27264=CARTESIAN_POINT ( 'NONE',  ( -1.500000000000013101, 1.452083334016150085, 0.8660254037844403729 ) ) ;
#27268=ORIENTED_EDGE ( 'NONE', *, *, #47118, .T. ) ;
#27271=CARTESIAN_POINT ( 'NONE',  ( 7.889955328148847258, 11.29236608522730911, -1.199719254218446718 ) ) ;
#27272=CARTESIAN_POINT ( 'NONE',  ( -1.364683531250000748, -0.9906249996585805295, 0.000000000000000000 ) ) ;
#27275=CARTESIAN_POINT ( 'NONE',  ( 10.05978679165993483, 11.79913468076720306, 1.082531754730548412 ) ) ;
#27276=CARTESIAN_POINT ( 'NONE',  ( -5.246642258808529746, 9.064907035344523578, 0.000000000000000000 ) ) ;
#27278=CARTESIAN_POINT ( 'NONE',  ( 1.220000000000003526, 6.400000000000022560, 1.229247124133362667E-14 ) ) ;
#27282=CARTESIAN_POINT ( 'NONE',  ( -6.566226467720086113, 6.555019055295208119, 1.040834085586084257E-14 ) ) ;
#27284=CARTESIAN_POINT ( 'NONE',  ( -1.499999999999997780, 2.681250000682818158, 1.214306433183764966E-14 ) ) ;
#27297=CARTESIAN_POINT ( 'NONE',  ( -7.479294296233107708, 11.87759377891399204, 0.7998128361456481317 ) ) ;
#27298=CARTESIAN_POINT ( 'NONE',  ( 7.644099680006512187, 7.812537802962739697, 1.040834085586084257E-14 ) ) ;
#27299=CARTESIAN_POINT ( 'NONE',  ( -6.471393748265538370, 5.229711127717889596, -2.499999999999995115 ) ) ;
#27301=B_SPLINE_CURVE_WITH_KNOTS ( 'NONE', 3,
 ( #65400, #85945, #17709, #82739, #167198 ),
 .UNSPECIFIED., .F., .F.,
 ( 4, 1, 4 ),
 ( 7.342161860471412858E-17, 3.079525422763246153E-06, 6.159050845453070644E-06 ),
 .UNSPECIFIED. ) ;
#27307=CARTESIAN_POINT ( 'NONE',  ( -8.505042434474312074, 8.816971016508505343, -0.7998128361456291469 ) ) ;
#27311=CARTESIAN_POINT ( 'NONE',  ( -1.000000000000017097, 5.868705557303652398, 4.125226524755080781 ) ) ;
#27314=CARTESIAN_POINT ( 'NONE',  ( 8.367353357928214663, 12.91366268422496688, 1.040834085586084257E-14 ) ) ;
#27320=CARTESIAN_POINT ( 'NONE',  ( -4.055860508782465068, 7.883587693554856557, 1.040834085586084257E-14 ) ) ;
#27321=CARTESIAN_POINT ( 'NONE',  ( -10.14557902172788495, 10.73093036830436553, 1.040834085586084257E-14 ) ) ;
#27324=CARTESIAN_POINT ( 'NONE',  ( -5.775737613422593952, 6.228167737865282660, -1.031624843267029190 ) ) ;
#27332=CARTESIAN_POINT ( 'NONE',  ( 7.494959990256193194, 7.638541498254023843, -0.7998128361456281477 ) ) ;
#27341=CARTESIAN_POINT ( 'NONE',  ( 1.499999999999989120, 1.806250000682817269, 0.000000000000000000 ) ) ;
#27352=ADVANCED_FACE ( 'NONE', ( #95122 ), #214299, .T. ) ;
#27353=DIRECTION ( 'NONE',  ( 0.000000000000000000, 0.000000000000000000, -1.000000000000000000 ) ) ;
#27355=CARTESIAN_POINT ( 'NONE',  ( 4.039966587192259873, 5.736380323189513852, 1.443375672974062551 ) ) ;
#27359=CARTESIAN_POINT ( 'NONE',  ( 0.6823417656249917140, 5.655208333674749177, 1.181850606188765695 ) ) ;
#27361=CARTESIAN_POINT ( 'NONE',  ( 9.317477881089539338, 11.89347683273640932, 1.599625672291279388 ) ) ;
#27365=CARTESIAN_POINT ( 'NONE',  ( -3.094265954482870118, 2.800000000000024691, 2.490342512183699508 ) ) ;
#27371=CARTESIAN_POINT ( 'NONE',  ( -1.364683531250000748, 0.5093750003414208027, 0.000000000000000000 ) ) ;
#27376=CARTESIAN_POINT ( 'NONE',  ( -4.608882153641705059, 7.464447381635583412, -1.199719254218452047 ) ) ;
#27378=CARTESIAN_POINT ( 'NONE',  ( 0.7499999999999885647, -0.2666666666666442365, 1.299038105676657340 ) ) ;
#27380=CARTESIAN_POINT ( 'NONE',  ( -0.7500000000000215383, 5.691666666666685082, 1.299038105676671107 ) ) ;
#27386=CARTESIAN_POINT ( 'NONE',  ( 0.6823417656249899377, 5.488541667008087543, -1.181850606188754593 ) ) ;
#27388=CARTESIAN_POINT ( 'NONE',  ( -8.050844288416501016, 8.287073179441051707, 1.040834085586084257E-14 ) ) ;
#27390=CARTESIAN_POINT ( 'NONE',  ( 8.646349277213076334, 11.11049346154719508, 1.599625672291281386 ) ) ;
#27392=CARTESIAN_POINT ( 'NONE',  ( 0.000000000000000000, 5.868705557303649734, -4.125226524755057689 ) ) ;
#27396=CARTESIAN_POINT ( 'NONE',  ( 0.6823417656249882723, 0.1552083336747514530, 1.181850606188755259 ) ) ;
#27402=EDGE_CURVE ( 'NONE', #159043, #103805, #203550, .T. ) ;
#27405=CARTESIAN_POINT ( 'NONE',  ( 7.456621297836078632, 8.762108271306003004, 1.082531754730558626 ) ) ;
#27408=CARTESIAN_POINT ( 'NONE',  ( -3.906720819032141190, 7.709591388846142479, -0.7998128361456281477 ) ) ;
#27410=CARTESIAN_POINT ( 'NONE',  ( -1.499999999999997780, 4.931250000682820378, 1.214306433183764966E-14 ) ) ;
#27413=CARTESIAN_POINT ( 'NONE',  ( 5.138177029454829459, 8.938364267765221527, 0.7216878364870438212 ) ) ;
#27414=CARTESIAN_POINT ( 'NONE',  ( -7.809133291347029271, 12.05447990663947877, 0.000000000000000000 ) ) ;
#27419=CARTESIAN_POINT ( 'NONE',  ( 2.184835310096557404, 5.700724961754617404, 1.040834085586084257E-14 ) ) ;
#27420=CARTESIAN_POINT ( 'NONE',  ( -1.499999999999997780, 3.931250000682819046, 1.214306433183764966E-14 ) ) ;
#27422=DIRECTION ( 'NONE',  ( 0.9366510587354612838, 2.168404344971001926E-14, 0.3502638921866474409 ) ) ;
#27435=CARTESIAN_POINT ( 'NONE',  ( 7.995557903757111617, 10.35123685918189729, 1.599625672291281386 ) ) ;
#27437=CARTESIAN_POINT ( 'NONE',  ( 4.202664430556254160, 5.926194473780837413, 1.443375672974062551 ) ) ;
#27440=CARTESIAN_POINT ( 'NONE',  ( 4.514501963670558560, 8.210743357683563559, 1.040834085586084257E-14 ) ) ;
#27442=CARTESIAN_POINT ( 'NONE',  ( -9.164948653157999559, 10.75515685251491504, -1.082531754730539753 ) ) ;
#27446=CARTESIAN_POINT ( 'NONE',  ( -4.060830702492950195, 4.696389560118578999, -1.199719254218452047 ) ) ;
#27451=ORIENTED_EDGE ( 'NONE', *, *, #180525, .T. ) ;
#27468=CARTESIAN_POINT ( 'NONE',  ( 0.007473969438204840048, 8.279395425053873936, 1.999986034896453324 ) ) ;
#27471=CARTESIAN_POINT ( 'NONE',  ( -6.548225005720456515, 10.58342024007512983, 0.000000000000000000 ) ) ;
#27476=CARTESIAN_POINT ( 'NONE',  ( 5.636439174979242850, 7.598931675607687453, -1.599625672291262513 ) ) ;
#27477=FACE_OUTER_BOUND ( 'NONE', #63136, .T. ) ;
#27479=CARTESIAN_POINT ( 'NONE',  ( 3.297657676621871925, 4.870353260857385180, 1.599625672291267398 ) ) ;
#27481=CARTESIAN_POINT ( 'NONE',  ( -4.894657149733403045, 5.669187081899118574, -1.199719254218446718 ) ) ;
#27486=CARTESIAN_POINT ( 'NONE',  ( -3.879604511804807032, 7.677955697080923514, 0.7998128361456341429 ) ) ;
#27489=CARTESIAN_POINT ( 'NONE',  ( 8.101160479365381306, 9.410107633136481908, -1.199719254218446718 ) ) ;
#27490=CARTESIAN_POINT ( 'NONE',  ( -1.201851678989727383E-14, 3.821875000341422801, 1.575800808251672791 ) ) ;
#27492=CARTESIAN_POINT ( 'NONE',  ( 5.327099315257549428, 6.547468694062620997, 1.346473575380419563 ) ) ;
#27493=CARTESIAN_POINT ( 'NONE',  ( 5.666945020832181434, 5.713783400500082266, 0.7216878364870317197 ) ) ;
#27500=CARTESIAN_POINT ( 'NONE',  ( 7.117667457050084856, 7.406292909420979953, -0.7216878364870257245 ) ) ;
#27501=CARTESIAN_POINT ( 'NONE',  ( -8.727698198895085469, 11.20540053684285553, -1.599625672291263179 ) ) ;
#27504=CARTESIAN_POINT ( 'NONE',  ( -8.239604668803112375, 10.63595808506888396, -1.599625672291263179 ) ) ;
#27505=CARTESIAN_POINT ( 'NONE',  ( -5.364222332501225488, 9.410009821226765325, 0.7998128361456481317 ) ) ;
#27513=CARTESIAN_POINT ( 'NONE',  ( 7.228468454380276853, 11.58496363008569574, 1.040834085586084257E-14 ) ) ;
#27518=DIRECTION ( 'NONE',  ( -0.7592566023652971285, -0.6507913734559680474, 0.000000000000000000 ) ) ;
#27521=CARTESIAN_POINT ( 'NONE',  ( -1.001543065824772872E-14, 5.243750000682815937, 1.732050807568877637 ) ) ;
#27525=VERTEX_POINT ( 'NONE', #141516 ) ;
#27526=CARTESIAN_POINT ( 'NONE',  ( -1.001543065824772872E-14, 4.212500000000023448, 1.732050807568877637 ) ) ;
#27527=CARTESIAN_POINT ( 'NONE',  ( 4.801558957534076022, 8.753569217098425170, 0.7998128361456462443 ) ) ;
#27528=B_SPLINE_CURVE_WITH_KNOTS ( 'NONE', 3,
 ( #79666, #211784, #160928, #28792, #63422, #131665, #78595, #197668, #11457, #178252 ),
 .UNSPECIFIED., .F., .F.,
 ( 4, 3, 3, 4 ),
 ( 1.626303258728287225E-19, 4.381009615557519019E-05, 0.0001116909227615702350, 0.0001805408983559123135 ),
 .UNSPECIFIED. ) ;
#27529=EDGE_CURVE ( 'NONE', #1110, #188860, #115784, .T. ) ;
#27533=CARTESIAN_POINT ( 'NONE',  ( 8.120970824905713314, 8.576813505252564696, 1.040834085586084257E-14 ) ) ;
#27534=ADVANCED_FACE ( 'NONE', ( #92741 ), #57018, .T. ) ;
#27535=CARTESIAN_POINT ( 'NONE',  ( -9.178506806327330736, 10.77097469787910455, 1.082531754730558626 ) ) ;
#27538=CARTESIAN_POINT ( 'NONE',  ( 8.432281472695482449, 11.92507992053172572, 1.199719254218450271 ) ) ;
#27541=CARTESIAN_POINT ( 'NONE',  ( -3.602716132929368875, 5.226254793216122074, 1.599625672291267398 ) ) ;
#27543=CARTESIAN_POINT ( 'NONE',  ( -1.201851678989727383E-14, 1.571875000341420581, 1.575800808251672791 ) ) ;
#27548=CARTESIAN_POINT ( 'NONE',  ( 1.364683531249986537, -0.3864583329919166199, 0.7879004041258500513 ) ) ;
#27550=CARTESIAN_POINT ( 'NONE',  ( 9.368847842243145152, 10.88907622316056312, 1.199719254218453823 ) ) ;
#27554=CARTESIAN_POINT ( 'NONE',  ( -3.809477975315625375, 4.507107728365378208, 1.082531754730558626 ) ) ;
#27557=CARTESIAN_POINT ( 'NONE',  ( -4.889686956022917919, 8.856385215335397021, 1.214306433183764966E-14 ) ) ;
#27560=CARTESIAN_POINT ( 'NONE',  ( 3.167801447087334576, 6.847518788243868393, -0.7998128361456291469 ) ) ;
#27566=CARTESIAN_POINT ( 'NONE',  ( 9.260382613333817403, 10.76253345609967660, -1.199719254218446718 ) ) ;
#27569=CARTESIAN_POINT ( 'NONE',  ( -4.741601036477307574, 6.554953847355395880, 1.599625672291267398 ) ) ;
#27573=CARTESIAN_POINT ( 'NONE',  ( 6.414979237560321401, 10.63589287712906462, 1.040834085586084257E-14 ) ) ;
#27575=CARTESIAN_POINT ( 'NONE',  ( 8.101160479365381306, 9.410107633136481908, -1.199719254218446718 ) ) ;
#27578=CARTESIAN_POINT ( 'NONE',  ( -4.274898507010545856, 3.881803101134051470, -0.7998128361456221525 ) ) ;
#27581=CARTESIAN_POINT ( 'NONE',  ( -3.023105066167326882, 5.702484939155337607, -7.499999999999997335 ) ) ;
#27586=CARTESIAN_POINT ( 'NONE',  ( -5.789194372615304118, 6.219231786955013774, 1.015549131865096211 ) ) ;
#27587=CARTESIAN_POINT ( 'NONE',  ( -1.364683531250014514, 1.238541667008091096, -0.7879004041258289570 ) ) ;
#27590=CARTESIAN_POINT ( 'NONE',  ( 5.775410249741494972, 8.721433810464993996, -1.082531754730537088 ) ) ;
#27607=CARTESIAN_POINT ( 'NONE',  ( 8.503988664269582998, 10.94440607977979063, 1.599625672291281386 ) ) ;
#27611=CARTESIAN_POINT ( 'NONE',  ( -5.122283107864663343, 4.870418468797203637, 0.000000000000000000 ) ) ;
#27612=CARTESIAN_POINT ( 'NONE',  ( -8.182509401047415309, 9.505014708432145909, 1.199719254218462483 ) ) ;
#27614=ORIENTED_EDGE ( 'NONE', *, *, #40619, .F. ) ;
#27617=CARTESIAN_POINT ( 'NONE',  ( -1.201851678989727383E-14, 4.368750000682820378, -1.732050807568863648 ) ) ;
#27618=CARTESIAN_POINT ( 'NONE',  ( 6.414979237560321401, 10.63589287712906462, 1.040834085586084257E-14 ) ) ;
#27622=CARTESIAN_POINT ( 'NONE',  ( -7.069687034522070590, 10.33538640932937724, -1.199719254218440723 ) ) ;
#27624=CARTESIAN_POINT ( 'NONE',  ( 1.364683531249990311, 4.134375000341417028, 1.214306433183764966E-14 ) ) ;
#27629=CARTESIAN_POINT ( 'NONE',  ( -9.490344339885981029, 10.17441593939621924, -0.7216878364870267237 ) ) ;
#27633=CARTESIAN_POINT ( 'NONE',  ( -1.364683531250012516, 2.301041667008087988, -0.7879004041258289570 ) ) ;
#27641=CARTESIAN_POINT ( 'NONE',  ( 0.6823417656249899377, 2.342708333674753618, 1.181850606188767472 ) ) ;
#27643=CARTESIAN_POINT ( 'NONE',  ( -4.249591082879585535, 7.045274465746411252, 1.199719254218464037 ) ) ;
#27644=CARTESIAN_POINT ( 'NONE',  ( 6.100279051144945619, 9.204410428722734849, -1.199719254218440723 ) ) ;
#27648=CARTESIAN_POINT ( 'NONE',  ( 1.364683531249990311, 3.696875000341416584, 1.214306433183764966E-14 ) ) ;
#27653=CARTESIAN_POINT ( 'NONE',  ( 1.364683531249986981, -1.115624999658580752, 0.000000000000000000 ) ) ;
#27654=CARTESIAN_POINT ( 'NONE',  ( -4.446711195602252253, 6.210915699667823198, -1.443375672974053447 ) ) ;
#27658=CARTESIAN_POINT ( 'NONE',  ( 4.378920427533921078, 4.211088041652093494, 1.214306433183764966E-14 ) ) ;
#27661=CARTESIAN_POINT ( 'NONE',  ( -7.527801604085656351, 9.805521176231838609, 1.599625672291295375 ) ) ;
#27662=CARTESIAN_POINT ( 'NONE',  ( -10.30383355670593737, 11.12348669235284504, -0.7216878364870267237 ) ) ;
#27668=CARTESIAN_POINT ( 'NONE',  ( -9.809487834687324437, 11.40315621434539395, 1.199719254218462483 ) ) ;
#27669=CARTESIAN_POINT ( 'NONE',  ( -6.860062538390436337, 7.105753837651378468, 1.040834085586084257E-14 ) ) ;
#27671=CARTESIAN_POINT ( 'NONE',  ( -1.402160292154681736E-14, 0.7593750003414168059, -1.575800808251659024 ) ) ;
#27673=PLANE ( 'NONE',  #176250 ) ;
#27677=CARTESIAN_POINT ( 'NONE',  ( -0.6823417656250003738, -0.9697916663252494907, -1.181850606188749264 ) ) ;
#27684=CARTESIAN_POINT ( 'NONE',  ( -0.7500000000000249800, -0.5583333333333134751, 1.299038105676659116 ) ) ;
#27685=CARTESIAN_POINT ( 'NONE',  ( 7.361714222096048310, 10.57212177821199184, -1.082531754730537976 ) ) ;
#27689=ORIENTED_EDGE ( 'NONE', *, *, #82128, .F. ) ;
#27692=AXIS2_PLACEMENT_3D ( 'NONE', #12285, #62128, #142345 ) ;
#27694=CARTESIAN_POINT ( 'NONE',  ( 5.015626762051672571, 7.938982758113895422, 1.199719254218462483 ) ) ;
#27697=CARTESIAN_POINT ( 'NONE',  ( -3.578462479003122976, 6.262291094557191684, 1.199719254218464037 ) ) ;
#27701=CARTESIAN_POINT ( 'NONE',  ( 1.364683531249988535, 1.426041667008083991, 0.7879004041258500513 ) ) ;
#27703=CARTESIAN_POINT ( 'NONE',  ( -7.486073373039941359, 11.88550270185529278, -0.7998128361456291469 ) ) ;
#27719=CARTESIAN_POINT ( 'NONE',  ( -4.299226640135908717, 7.262029271172127487, -0.9639859114825770625 ) ) ;
#27722=CARTESIAN_POINT ( 'NONE',  ( 6.819914962873951936, 7.915321197229798322, -1.199719254218446718 ) ) ;
#27729=CARTESIAN_POINT ( 'NONE',  ( 7.313733799568044702, 10.62010763521636214, 1.199719254218460707 ) ) ;
#27730=CARTESIAN_POINT ( 'NONE',  ( -5.886439722289627419, 6.118937485343679761, -0.7679415244158314113 ) ) ;
#27732=( BOUNDED_SURFACE ( )  B_SPLINE_SURFACE ( 1, 2, ( 
 ( #156997, #8584, #206781, #59471, #25894, #125630, #43250, #58414, #126694, #175377, #142901, #92004, #188401, #124568, #190528, #108299, #44308, #158064, #88795, #9650, #6437, #109369, #93067, #204633, #22683, #154853, #72513, #56284, #40038, #106149, #172173, #131983, #161248, #94138, #177500, #29113, #48573, #197991, #12834, #130941, #111493, #13902, #179632, #97329, #95196, #110430, #147142, #148204, #16027, #78908, #214204, #211034, #180683, #79983, #145030, #96264, #62660, #196934, #82111, #128818, #61606, #193732, #194801, #32309, #212098, #162316, #178568, #160177, #31254, #65835, #46437, #195878, #112555, #146086, #176434, #30175, #163385, #164439, #14959, #81057, #47516, #213168, #63735, #28045, #129893, #113628, #77850, #11777, #143973, #209966, #127776, #64797, #45377, #114691, #98376, #152463, #18165, #166578, #184937, #69046, #5104, #100503, #1907, #167640, #17095, #67967, #183883, #151405, #136224, #199039, #150339, #201182, #52820, #182813, #21361, #19242, #102649, #118958, #36561, #168705, #50687, #86394, #165502, #186007, #71180, #103720, #83174, #202245, #117891, #116812, #200119, #70111, #134110, #34429, #84253, #85322, #51772, #137299, #49619, #830, #35495, #4043, #101573, #2978, #169771, #115744, #135166, #20309, #53896, #120032, #149257, #66900, #87468, #37642, #153535, #133040, #181733, #33365, #99447, #22433, #39785, #6184, #138360, #106973, #26721, #188153, #191340, #8336, #158867, #74421, #204378, #203316, #187083, #57098, #76537, #43006, #109119, #38716, #41939, #105890, #24578, #171916, #56034, #73328, #54966, #190281, #174076, #23512, #170843, #40868, #157812, #89617, #122187, #154605, #9411, #108051, #175133, #155668, #206534, #172997, #7252, #139430, #205465, #123264, #189229, #90685, #156746, #104796, #140520, #72252, #88543, #25648, #207599, #58164, #124322, #91759, #75482, #141593, #59219, #125377, #92822, #10463, #121118, #209721, #93893, #142648, #161000, #179392, #159932, #94952, #29938, #28865, #14723, #178330, #31012, #80814, #126446, #112315, #129651, #111250, #208657, #127525, #193496, #210800, #45138, #61367, #177253, #96022, #98146, #60287, #12592, #176194, #192409, #164195, #44065, #11535, #62423, #97087, #78666, #144793, #48332, #15782, #162074, #128588, #13664, #194554, #110183, #27795, #114442, #143728, #79736, #77605, #46197, #146905, #145852, #211859, #63496, #195636, #47269, #113384, #180443, #163140, #130702, #212924, #64558, #196693, #32059, #81867, #65586, #150076, #169510, #135957, #201972, #131733, #134907, #198787, #117632, #66639, #148997, #166313, #147953, #68787, #52561, #50436, #49378, #133854, #36299, #116555, #573, #33120, #102375, #200913, #53630, #132784, #85060, #51507, #182549, #34173, #100245, #17903, #83988, #1648, #67706, #197739, #199864, #99198, #115496, #118693, #86131, #183623, #35231, #16842, #181491, #18976, #101306, #167386, #2714, #82924, #151146, #184677, #165249, #213966, #168445, #20044, #152204, #3772, #69846, #119762, #185741, #37375, #103450, #8071, #153260, #89351, #40599, #5912, #21092, #88269, #154337, #39513, #71986, #138095, #204108, #155399, #25393, #87196, #121916, #120845, #137025, #107789, #54694, #206273, #23239, #55760, #105611, #140251, #187885, #22154, #171642, #6981, #73062, #170573, #188959, #4835, #139161, #203052, #205191, #56832, #124061, #70915, #123003, #173814, #106705, #172729, #74157, #57897, #24307, #186819, #41678, #38447, #104527, #90412, #156482, #190026, #91492, #79769, #47304, #110216, #127558, #93923, #60318, #96055, #128620, #193527, #145883, #159963, #45169, #11568, #176223, #158899, #177286, #195669, #27825, #111281, #46232, #28901, #31045, #194586, #113418, #97121, #142679, #112349, #211892, #94986, #10495, #143760, #209755, #12627, #61396, #77638, #161032, #178362, #114479, #76568, #78698, #192441, #208690, #212955, #126477, #163173, #144825, #210832, #62457, #179425, #29969, #162108, #13697, #63531, #129685, #180477, #44096, #14758, #80849, #146940, #64594, #130733, #196726, #32094, #48366, #100283, #199900, #166349, #65620, #197773, #3812, #99235, #51546, #49410, #131769, #184713, #181526 ),
 ( #17940, #185780, #152240, #69884, #147989, #151182, #608, #133893, #82959, #165284, #182587, #164228, #85097, #68823, #118728, #16878, #1689, #167425, #2754, #149032, #119801, #134945, #135996, #202010, #66675, #53669, #198827, #35267, #15816, #117670, #200951, #132823, #36337, #98180, #50472, #115531, #33154, #116593, #168483, #183663, #150116, #84026, #81901, #19017, #213999, #34210, #101344, #67743, #52600, #102415, #20082, #86170, #91534, #90455, #8112, #188998, #24345, #171681, #103490, #170612, #55800, #4876, #75259, #125161, #207384, #59005, #22199, #157593, #206313, #39552, #140294, #5953, #154376, #172771, #56871, #37414, #88312, #204145, #155438, #70955, #121955, #23278, #139200, #124102, #186859, #138136, #40641, #106744, #72024, #9188, #7023, #156521, #74200, #57937, #190065, #38489, #41717, #153300, #173852, #169551, #104567, #137065, #141373, #89390, #187921, #73099, #107827, #25428, #21132, #87236, #205230, #203090, #54735, #120885, #105653, #123047, #144571, #27569, #43851, #162922, #112102, #108895, #11308, #26498, #79525, #178105, #158648, #13449, #93667, #14502, #179169, #63274, #60070, #128372, #212706, #159709, #174918, #109965, #175976, #129436, #64347, #77386, #80594, #94734, #29721, #194339, #95803, #45981, #126226, #145643, #92605, #113165, #146690, #143502, #10246, #30793, #177030, #209499, #28647, #161859, #211638, #195419, #47049, #111025, #191120, #96872, #42786, #76322, #142427, #210585, #61139, #127301, #208436, #192187, #193272, #44917, #160780, #12373, #78453, #62215, #167176, #181279, #102170, #118485, #2502, #213754, #67501, #151995, #32905, #114234, #197526, #49170, #68574, #3567, #98983, #150939, #131523, #33963, #199646, #117418, #115288, #130493, #18765, #168237, #36086, #165036, #19836, #16629, #133647, #196480, #149868, #183415, #82713, #134701, #85922, #148790, #81651, #65377, #360, #200706, #17689, #182335, #198578, #180232, #51293, #48122, #66432, #1436, #132575, #166103, #31855, #50225, #35018, #184469, #101089, #84849, #52357, #97931, #116344, #163989, #100040, #83775, #15564, #147738, #157339, #25178, #91280, #202841, #123850, #24102, #71774, #172517, #38238, #186612, #204979, #89141, #69641, #120634, #21945, #187673, #37164, #88055, #203909, #171436, #156270, #4629, #170360, #6776, #72851, #54490, #41463, #104311, #20886, #153053, #154127, #140033, #23026, #121711, #137890, #53413, #138958, #107572, #5697, #155195, #55556, #105398, #189813, #39303, #56624, #173606, #122789, #40387, #188748, #106491, #90206, #135749, #7852, #73939, #103242, #201773, #119550, #185536, #169302, #206058, #86983, #57693, #70701, #136814, #191929, #125972, #144322, #28384, #178919, #59818, #175715, #127042, #190869, #27307, #143249, #110769, #95552, #158394, #109711, #160519, #12123, #142169, #195160, #193002, #61957, #78195, #210320, #128115, #9992, #45726, #124906, #145387, #30534, #76069, #42533, #63012, #209239, #93412, #60883, #194073, #111845, #177850, #29462, #44655, #46795, #13193, #112908, #161604, #174665, #176769, #43593, #208185, #96614, #79270, #141117, #159450, #58754, #211386, #129182, #108637, #8927, #11048, #75008, #207128, #26239, #92356, #77127, #94479, #213505, #146433, #15311, #81400, #100839, #184215, #65126, #183162, #163730, #66176, #17436, #149601, #147483, #35838, #199390, #200456, #68322, #131284, #52102, #48911, #99785, #14238, #182076, #1186, #197271, #34766, #49967, #109, #16375, #212447, #83520, #118231, #115031, #33708, #181030, #198327, #134453, #32647, #67250, #2246, #133385, #51036, #165851, #117159, #82454, #80332, #98724, #164783, #130233, #162668, #64091, #196226, #47868, #148543, #113979, #166924, #132321, #18518, #116086, #84596, #150684, #179976, #31597, #97673, #54237, #5444, #69386, #120375, #21690, #203653, #188492, #36902, #202585, #39053, #105138, #20639, #73676, #71523, #154939, #171178, #22769, #88885, #102984, #138700, #3317, #23847, #57433, #169042, #135494, #156005, #87802, #186350, #153875, #72600, #6523, #204718, #122531, #137634, #139775, #106234, #205802, #56368, #53165, #55303, #152798, #86728, #123594, #40124, #19587 ) ),
 .UNSPECIFIED., .F., .F., .T. ) 
 B_SPLINE_SURFACE_WITH_KNOTS ( ( 2, 2 ),
 ( 3, 2, 2, 2, 2, 2, 2, 2, 2, 2, 2, 2, 2, 2, 2, 2, 2, 2, 2, 2, 2, 2, 2, 2, 2, 2, 2, 2, 2, 2, 2, 2, 2, 2, 2, 2, 2, 2, 2, 2, 2, 2, 2, 2, 2, 2, 2, 2, 2, 2, 2, 2, 2, 2, 2, 2, 2, 2, 2, 2, 2, 2, 2, 2, 2, 2, 2, 2, 2, 2, 2, 2, 2, 2, 2, 2, 2, 2, 2, 2, 2, 2, 2, 2, 2, 2, 2, 2, 2, 2, 2, 2, 2, 2, 2, 2, 2, 2, 2, 2, 2, 2, 2, 2, 2, 2, 2, 2, 2, 2, 2, 2, 2, 2, 2, 2, 2, 2, 2, 2, 2, 2, 2, 2, 2, 2, 2, 2, 2, 2, 2, 2, 2, 2, 2, 2, 2, 2, 2, 2, 2, 2, 2, 2, 2, 2, 2, 2, 2, 2, 2, 2, 2, 2, 2, 2, 2, 2, 2, 2, 2, 2, 2, 2, 2, 2, 2, 2, 2, 2, 2, 2, 2, 2, 2, 2, 2, 2, 2, 2, 2, 2, 2, 2, 2, 2, 2, 2, 2, 2, 2, 2, 2, 2, 2, 2, 2, 2, 2, 2, 2, 2, 2, 2, 2, 2, 2, 2, 2, 2, 2, 2, 2, 2, 2, 2, 2, 2, 2, 2, 2, 2, 2, 2, 2, 2, 2, 2, 2, 2, 2, 2, 2, 2, 2, 2, 2, 2, 2, 2, 3 ),
 ( 0.000000000000000000, 1.000000000000000000 ),
 ( 0.000000000000000000, 0.004166666666666666609, 0.008333333333333333218, 0.01250000000000000069, 0.01666666666666666644, 0.02083333333333333218, 0.02500000000000000139, 0.02916666666666666713, 0.03333333333333333287, 0.03749999999999999861, 0.04166666666666666435, 0.04583333333333333010, 0.05000000000000000278, 0.05416666666666666852, 0.05833333333333333426, 0.06250000000000000000, 0.06666666666666666574, 0.07083333333333333148, 0.07499999999999999722, 0.07916666666666666297, 0.08333333333333332871, 0.08749999999999999445, 0.09166666666666666019, 0.09583333333333333981, 0.1000000000000000056, 0.1041666666666666713, 0.1083333333333333370, 0.1125000000000000028, 0.1166666666666666685, 0.1208333333333333343, 0.1250000000000000000, 0.1291666666666666796, 0.1333333333333333315, 0.1375000000000000111, 0.1416666666666666630, 0.1458333333333333426, 0.1499999999999999944, 0.1541666666666666741, 0.1583333333333333259, 0.1625000000000000056, 0.1666666666666666574, 0.1708333333333333370, 0.1749999999999999889, 0.1791666666666666685, 0.1833333333333333204, 0.1875000000000000000, 0.1916666666666666796, 0.1958333333333333315, 0.2000000000000000111, 0.2041666666666666630, 0.2083333333333333426, 0.2124999999999999944, 0.2166666666666666741, 0.2208333333333333259, 0.2250000000000000056, 0.2291666666666666574, 0.2333333333333333370, 0.2374999999999999889, 0.2416666666666666685, 0.2458333333333333204, 0.2500000000000000000, 0.2541666666666666519, 0.2583333333333333592, 0.2625000000000000111, 0.2666666666666666630, 0.2708333333333333148, 0.2750000000000000222, 0.2791666666666666741, 0.2833333333333333259, 0.2874999999999999778, 0.2916666666666666852, 0.2958333333333333370, 0.2999999999999999889, 0.3041666666666666408, 0.3083333333333333481, 0.3125000000000000000, 0.3166666666666666519, 0.3208333333333333592, 0.3250000000000000111, 0.3291666666666666630, 0.3333333333333333148, 0.3375000000000000222, 0.3416666666666666741, 0.3458333333333333259, 0.3499999999999999778, 0.3541666666666666852, 0.3583333333333333370, 0.3624999999999999889, 0.3666666666666666408, 0.3708333333333333481, 0.3750000000000000000, 0.3791666666666666519, 0.3833333333333333592, 0.3875000000000000111, 0.3916666666666666630, 0.3958333333333333148, 0.4000000000000000222, 0.4041666666666666741, 0.4083333333333333259, 0.4124999999999999778, 0.4166666666666666852, 0.4208333333333333370, 0.4249999999999999889, 0.4291666666666666408, 0.4333333333333333481, 0.4375000000000000000, 0.4416666666666666519, 0.4458333333333333592, 0.4500000000000000111, 0.4541666666666666630, 0.4583333333333333148, 0.4625000000000000222, 0.4666666666666666741, 0.4708333333333333259, 0.4749999999999999778, 0.4791666666666666852, 0.4833333333333333370, 0.4874999999999999889, 0.4916666666666666408, 0.4958333333333333481, 0.5000000000000000000, 0.5041666666666666519, 0.5083333333333333037, 0.5124999999999999556, 0.5166666666666667185, 0.5208333333333333703, 0.5250000000000000222, 0.5291666666666666741, 0.5333333333333333259, 0.5374999999999999778, 0.5416666666666666297, 0.5458333333333332815, 0.5500000000000000444, 0.5541666666666666963, 0.5583333333333333481, 0.5625000000000000000, 0.5666666666666666519, 0.5708333333333333037, 0.5749999999999999556, 0.5791666666666667185, 0.5833333333333333703, 0.5875000000000000222, 0.5916666666666666741, 0.5958333333333333259, 0.5999999999999999778, 0.6041666666666666297, 0.6083333333333332815, 0.6125000000000000444, 0.6166666666666666963, 0.6208333333333333481, 0.6250000000000000000, 0.6291666666666666519, 0.6333333333333333037, 0.6374999999999999556, 0.6416666666666667185, 0.6458333333333333703, 0.6500000000000000222, 0.6541666666666666741, 0.6583333333333333259, 0.6624999999999999778, 0.6666666666666666297, 0.6708333333333332815, 0.6750000000000000444, 0.6791666666666666963, 0.6833333333333333481, 0.6875000000000000000, 0.6916666666666666519, 0.6958333333333333037, 0.6999999999999999556, 0.7041666666666667185, 0.7083333333333333703, 0.7125000000000000222, 0.7166666666666666741, 0.7208333333333333259, 0.7249999999999999778, 0.7291666666666666297, 0.7333333333333332815, 0.7375000000000000444, 0.7416666666666666963, 0.7458333333333333481, 0.7500000000000000000, 0.7541666666666666519, 0.7583333333333333037, 0.7624999999999999556, 0.7666666666666667185, 0.7708333333333333703, 0.7750000000000000222, 0.7791666666666666741, 0.7833333333333333259, 0.7874999999999999778, 0.7916666666666666297, 0.7958333333333332815, 0.8000000000000000444, 0.8041666666666666963, 0.8083333333333333481, 0.8125000000000000000, 0.8166666666666666519, 0.8208333333333333037, 0.8249999999999999556, 0.8291666666666667185, 0.8333333333333333703, 0.8375000000000000222, 0.8416666666666666741, 0.8458333333333333259, 0.8499999999999999778, 0.8541666666666666297, 0.8583333333333332815, 0.8625000000000000444, 0.8666666666666666963, 0.8708333333333333481, 0.8750000000000000000, 0.8791666666666666519, 0.8833333333333333037, 0.8874999999999999556, 0.8916666666666667185, 0.8958333333333333703, 0.9000000000000000222, 0.9041666666666666741, 0.9083333333333333259, 0.9124999999999999778, 0.9166666666666666297, 0.9208333333333332815, 0.9250000000000000444, 0.9291666666666666963, 0.9333333333333333481, 0.9375000000000000000, 0.9416666666666666519, 0.9458333333333333037, 0.9499999999999999556, 0.9541666666666667185, 0.9583333333333333703, 0.9625000000000000222, 0.9666666666666666741, 0.9708333333333333259, 0.9749999999999999778, 0.9791666666666666297, 0.9833333333333332815, 0.9875000000000000444, 0.9916666666666666963, 0.9958333333333333481, 1.000000000000000000 ),
 .UNSPECIFIED. ) 
 GEOMETRIC_REPRESENTATION_ITEM ( )  RATIONAL_B_SPLINE_SURFACE ( (
 ( 1.000000000000000000, 0.8660254037844387076, 1.000000000000000000, 0.8660254037844387076, 1.000000000000000000, 0.8660254037844387076, 1.000000000000000000, 0.8660254037844387076, 1.000000000000000000, 0.8660254037844387076, 1.000000000000000000, 0.8660254037844387076, 1.000000000000000000, 0.8660254037844387076, 1.000000000000000000, 0.8660254037844387076, 1.000000000000000000, 0.8660254037844387076, 1.000000000000000000, 0.8660254037844387076, 1.000000000000000000, 0.8660254037844387076, 1.000000000000000000, 0.8660254037844387076, 1.000000000000000000, 0.8660254037844387076, 1.000000000000000000, 0.8660254037844387076, 1.000000000000000000, 0.8660254037844387076, 1.000000000000000000, 0.8660254037844387076, 1.000000000000000000, 0.8660254037844387076, 1.000000000000000000, 0.8660254037844387076, 1.000000000000000000, 0.8660254037844387076, 1.000000000000000000, 0.8660254037844387076, 1.000000000000000000, 0.8660254037844387076, 1.000000000000000000, 0.8660254037844387076, 1.000000000000000000, 0.8660254037844387076, 1.000000000000000000, 0.8660254037844387076, 1.000000000000000000, 0.8660254037844387076, 1.000000000000000000, 0.8660254037844387076, 1.000000000000000000, 0.8660254037844387076, 1.000000000000000000, 0.8660254037844387076, 1.000000000000000000, 0.8660254037844387076, 1.000000000000000000, 0.8660254037844387076, 1.000000000000000000, 0.8660254037844387076, 1.000000000000000000, 0.8660254037844387076, 1.000000000000000000, 0.8660254037844387076, 1.000000000000000000, 0.8660254037844387076, 1.000000000000000000, 0.8660254037844387076, 1.000000000000000000, 0.8660254037844387076, 1.000000000000000000, 0.8660254037844387076, 1.000000000000000000, 0.8660254037844387076, 1.000000000000000000, 0.8660254037844387076, 1.000000000000000000, 0.8660254037844387076, 1.000000000000000000, 0.8660254037844387076, 1.000000000000000000, 0.8660254037844387076, 1.000000000000000000, 0.8660254037844387076, 1.000000000000000000, 0.8660254037844387076, 1.000000000000000000, 0.8660254037844387076, 1.000000000000000000, 0.8660254037844387076, 1.000000000000000000, 0.8660254037844387076, 1.000000000000000000, 0.8660254037844387076, 1.000000000000000000, 0.8660254037844387076, 1.000000000000000000, 0.8660254037844387076, 1.000000000000000000, 0.8660254037844387076, 1.000000000000000000, 0.8660254037844387076, 1.000000000000000000, 0.8660254037844387076, 1.000000000000000000, 0.8660254037844387076, 1.000000000000000000, 0.8660254037844387076, 1.000000000000000000, 0.8660254037844387076, 1.000000000000000000, 0.8660254037844387076, 1.000000000000000000, 0.8660254037844387076, 1.000000000000000000, 0.8660254037844387076, 1.000000000000000000, 0.8660254037844387076, 1.000000000000000000, 0.8660254037844387076, 1.000000000000000000, 0.8660254037844387076, 1.000000000000000000, 0.8660254037844387076, 1.000000000000000000, 0.8660254037844387076, 1.000000000000000000, 0.8660254037844387076, 1.000000000000000000, 0.8660254037844387076, 1.000000000000000000, 0.8660254037844387076, 1.000000000000000000, 0.8660254037844387076, 1.000000000000000000, 0.8660254037844387076, 1.000000000000000000, 0.8660254037844387076, 1.000000000000000000, 0.8660254037844387076, 1.000000000000000000, 0.8660254037844387076, 1.000000000000000000, 0.8660254037844387076, 1.000000000000000000, 0.8660254037844387076, 1.000000000000000000, 0.8660254037844387076, 1.000000000000000000, 0.8660254037844387076, 1.000000000000000000, 0.8660254037844387076, 1.000000000000000000, 0.8660254037844387076, 1.000000000000000000, 0.8660254037844387076, 1.000000000000000000, 0.8660254037844387076, 1.000000000000000000, 0.8660254037844387076, 1.000000000000000000, 0.8660254037844387076, 1.000000000000000000, 0.8660254037844387076, 1.000000000000000000, 0.8660254037844387076, 1.000000000000000000, 0.8660254037844387076, 1.000000000000000000, 0.8660254037844387076, 1.000000000000000000, 0.8660254037844387076, 1.000000000000000000, 0.8660254037844387076, 1.000000000000000000, 0.8660254037844387076, 1.000000000000000000, 0.8660254037844387076, 1.000000000000000000, 0.8660254037844387076, 1.000000000000000000, 0.8660254037844387076, 1.000000000000000000, 0.8660254037844387076, 1.000000000000000000, 0.8660254037844387076, 1.000000000000000000, 0.8660254037844387076, 1.000000000000000000, 0.8660254037844387076, 1.000000000000000000, 0.8660254037844387076, 1.000000000000000000, 0.8660254037844387076, 1.000000000000000000, 0.8660254037844387076, 1.000000000000000000, 0.8660254037844387076, 1.000000000000000000, 0.8660254037844387076, 1.000000000000000000, 0.8660254037844387076, 1.000000000000000000, 0.8660254037844387076, 1.000000000000000000, 0.8660254037844387076, 1.000000000000000000, 0.8660254037844387076, 1.000000000000000000, 0.8660254037844387076, 1.000000000000000000, 0.8660254037844387076, 1.000000000000000000, 0.8660254037844387076, 1.000000000000000000, 0.8660254037844387076, 1.000000000000000000, 0.8660254037844387076, 1.000000000000000000, 0.8660254037844387076, 1.000000000000000000, 0.8660254037844387076, 1.000000000000000000, 0.8660254037844387076, 1.000000000000000000, 0.8660254037844387076, 1.000000000000000000, 0.8660254037844387076, 1.000000000000000000, 0.8660254037844387076, 1.000000000000000000, 0.8660254037844387076, 1.000000000000000000, 0.8660254037844387076, 1.000000000000000000, 0.8660254037844387076, 1.000000000000000000, 0.8660254037844387076, 1.000000000000000000, 0.8660254037844387076, 1.000000000000000000, 0.8660254037844387076, 1.000000000000000000, 0.8660254037844387076, 1.000000000000000000, 0.8660254037844387076, 1.000000000000000000, 0.8660254037844387076, 1.000000000000000000, 0.8660254037844387076, 1.000000000000000000, 0.8660254037844387076, 1.000000000000000000, 0.8660254037844387076, 1.000000000000000000, 0.8660254037844387076, 1.000000000000000000, 0.8660254037844387076, 1.000000000000000000, 0.8660254037844387076, 1.000000000000000000, 0.8660254037844387076, 1.000000000000000000, 0.8660254037844387076, 1.000000000000000000, 0.8660254037844387076, 1.000000000000000000, 0.8660254037844387076, 1.000000000000000000, 0.8660254037844387076, 1.000000000000000000, 0.8660254037844387076, 1.000000000000000000, 0.8660254037844387076, 1.000000000000000000, 0.8660254037844387076, 1.000000000000000000, 0.8660254037844387076, 1.000000000000000000, 0.8660254037844387076, 1.000000000000000000, 0.8660254037844387076, 1.000000000000000000, 0.8660254037844387076, 1.000000000000000000, 0.8660254037844387076, 1.000000000000000000, 0.8660254037844387076, 1.000000000000000000, 0.8660254037844387076, 1.000000000000000000, 0.8660254037844387076, 1.000000000000000000, 0.8660254037844387076, 1.000000000000000000, 0.8660254037844387076, 1.000000000000000000, 0.8660254037844387076, 1.000000000000000000, 0.8660254037844387076, 1.000000000000000000, 0.8660254037844387076, 1.000000000000000000, 0.8660254037844387076, 1.000000000000000000, 0.8660254037844387076, 1.000000000000000000, 0.8660254037844387076, 1.000000000000000000, 0.8660254037844387076, 1.000000000000000000, 0.8660254037844387076, 1.000000000000000000, 0.8660254037844387076, 1.000000000000000000, 0.8660254037844387076, 1.000000000000000000, 0.8660254037844387076, 1.000000000000000000, 0.8660254037844387076, 1.000000000000000000, 0.8660254037844387076, 1.000000000000000000, 0.8660254037844387076, 1.000000000000000000, 0.8660254037844387076, 1.000000000000000000, 0.8660254037844387076, 1.000000000000000000, 0.8660254037844387076, 1.000000000000000000, 0.8660254037844387076, 1.000000000000000000, 0.8660254037844387076, 1.000000000000000000, 0.8660254037844387076, 1.000000000000000000, 0.8660254037844387076, 1.000000000000000000, 0.8660254037844387076, 1.000000000000000000, 0.8660254037844387076, 1.000000000000000000, 0.8660254037844387076, 1.000000000000000000, 0.8660254037844387076, 1.000000000000000000, 0.8660254037844387076, 1.000000000000000000, 0.8660254037844387076, 1.000000000000000000, 0.8660254037844387076, 1.000000000000000000, 0.8660254037844387076, 1.000000000000000000, 0.8660254037844387076, 1.000000000000000000, 0.8660254037844387076, 1.000000000000000000, 0.8660254037844387076, 1.000000000000000000, 0.8660254037844387076, 1.000000000000000000, 0.8660254037844387076, 1.000000000000000000, 0.8660254037844387076, 1.000000000000000000, 0.8660254037844387076, 1.000000000000000000, 0.8660254037844387076, 1.000000000000000000, 0.8660254037844387076, 1.000000000000000000, 0.8660254037844387076, 1.000000000000000000, 0.8660254037844387076, 1.000000000000000000, 0.8660254037844387076, 1.000000000000000000, 0.8660254037844387076, 1.000000000000000000, 0.8660254037844387076, 1.000000000000000000, 0.8660254037844387076, 1.000000000000000000, 0.8660254037844387076, 1.000000000000000000, 0.8660254037844387076, 1.000000000000000000, 0.8660254037844387076, 1.000000000000000000, 0.8660254037844387076, 1.000000000000000000, 0.8660254037844387076, 1.000000000000000000, 0.8660254037844387076, 1.000000000000000000, 0.8660254037844387076, 1.000000000000000000, 0.8660254037844387076, 1.000000000000000000, 0.8660254037844387076, 1.000000000000000000, 0.8660254037844387076, 1.000000000000000000, 0.8660254037844387076, 1.000000000000000000, 0.8660254037844387076, 1.000000000000000000, 0.8660254037844387076, 1.000000000000000000, 0.8660254037844387076, 1.000000000000000000, 0.8660254037844387076, 1.000000000000000000, 0.8660254037844387076, 1.000000000000000000, 0.8660254037844387076, 1.000000000000000000, 0.8660254037844387076, 1.000000000000000000, 0.8660254037844387076, 1.000000000000000000, 0.8660254037844387076, 1.000000000000000000, 0.8660254037844387076, 1.000000000000000000, 0.8660254037844387076, 1.000000000000000000, 0.8660254037844387076, 1.000000000000000000, 0.8660254037844387076, 1.000000000000000000, 0.8660254037844387076, 1.000000000000000000, 0.8660254037844387076, 1.000000000000000000, 0.8660254037844387076, 1.000000000000000000, 0.8660254037844387076, 1.000000000000000000, 0.8660254037844387076, 1.000000000000000000, 0.8660254037844387076, 1.000000000000000000, 0.8660254037844387076, 1.000000000000000000, 0.8660254037844387076, 1.000000000000000000, 0.8660254037844387076, 1.000000000000000000, 0.8660254037844387076, 1.000000000000000000, 0.8660254037844387076, 1.000000000000000000, 0.8660254037844387076, 1.000000000000000000, 0.8660254037844387076, 1.000000000000000000, 0.8660254037844387076, 1.000000000000000000, 0.8660254037844387076, 1.000000000000000000, 0.8660254037844387076, 1.000000000000000000, 0.8660254037844387076, 1.000000000000000000, 0.8660254037844387076, 1.000000000000000000, 0.8660254037844387076, 1.000000000000000000, 0.8660254037844387076, 1.000000000000000000, 0.8660254037844387076, 1.000000000000000000, 0.8660254037844387076, 1.000000000000000000, 0.8660254037844387076, 1.000000000000000000),
 ( 1.000000000000000000, 0.8660254037844387076, 1.000000000000000000, 0.8660254037844387076, 1.000000000000000000, 0.8660254037844387076, 1.000000000000000000, 0.8660254037844387076, 1.000000000000000000, 0.8660254037844387076, 1.000000000000000000, 0.8660254037844387076, 1.000000000000000000, 0.8660254037844387076, 1.000000000000000000, 0.8660254037844387076, 1.000000000000000000, 0.8660254037844387076, 1.000000000000000000, 0.8660254037844387076, 1.000000000000000000, 0.8660254037844387076, 1.000000000000000000, 0.8660254037844387076, 1.000000000000000000, 0.8660254037844387076, 1.000000000000000000, 0.8660254037844387076, 1.000000000000000000, 0.8660254037844387076, 1.000000000000000000, 0.8660254037844387076, 1.000000000000000000, 0.8660254037844387076, 1.000000000000000000, 0.8660254037844387076, 1.000000000000000000, 0.8660254037844387076, 1.000000000000000000, 0.8660254037844387076, 1.000000000000000000, 0.8660254037844387076, 1.000000000000000000, 0.8660254037844387076, 1.000000000000000000, 0.8660254037844387076, 1.000000000000000000, 0.8660254037844387076, 1.000000000000000000, 0.8660254037844387076, 1.000000000000000000, 0.8660254037844387076, 1.000000000000000000, 0.8660254037844387076, 1.000000000000000000, 0.8660254037844387076, 1.000000000000000000, 0.8660254037844387076, 1.000000000000000000, 0.8660254037844387076, 1.000000000000000000, 0.8660254037844387076, 1.000000000000000000, 0.8660254037844387076, 1.000000000000000000, 0.8660254037844387076, 1.000000000000000000, 0.8660254037844387076, 1.000000000000000000, 0.8660254037844387076, 1.000000000000000000, 0.8660254037844387076, 1.000000000000000000, 0.8660254037844387076, 1.000000000000000000, 0.8660254037844387076, 1.000000000000000000, 0.8660254037844387076, 1.000000000000000000, 0.8660254037844387076, 1.000000000000000000, 0.8660254037844387076, 1.000000000000000000, 0.8660254037844387076, 1.000000000000000000, 0.8660254037844387076, 1.000000000000000000, 0.8660254037844387076, 1.000000000000000000, 0.8660254037844387076, 1.000000000000000000, 0.8660254037844387076, 1.000000000000000000, 0.8660254037844387076, 1.000000000000000000, 0.8660254037844387076, 1.000000000000000000, 0.8660254037844387076, 1.000000000000000000, 0.8660254037844387076, 1.000000000000000000, 0.8660254037844387076, 1.000000000000000000, 0.8660254037844387076, 1.000000000000000000, 0.8660254037844387076, 1.000000000000000000, 0.8660254037844387076, 1.000000000000000000, 0.8660254037844387076, 1.000000000000000000, 0.8660254037844387076, 1.000000000000000000, 0.8660254037844387076, 1.000000000000000000, 0.8660254037844387076, 1.000000000000000000, 0.8660254037844387076, 1.000000000000000000, 0.8660254037844387076, 1.000000000000000000, 0.8660254037844387076, 1.000000000000000000, 0.8660254037844387076, 1.000000000000000000, 0.8660254037844387076, 1.000000000000000000, 0.8660254037844387076, 1.000000000000000000, 0.8660254037844387076, 1.000000000000000000, 0.8660254037844387076, 1.000000000000000000, 0.8660254037844387076, 1.000000000000000000, 0.8660254037844387076, 1.000000000000000000, 0.8660254037844387076, 1.000000000000000000, 0.8660254037844387076, 1.000000000000000000, 0.8660254037844387076, 1.000000000000000000, 0.8660254037844387076, 1.000000000000000000, 0.8660254037844387076, 1.000000000000000000, 0.8660254037844387076, 1.000000000000000000, 0.8660254037844387076, 1.000000000000000000, 0.8660254037844387076, 1.000000000000000000, 0.8660254037844387076, 1.000000000000000000, 0.8660254037844387076, 1.000000000000000000, 0.8660254037844387076, 1.000000000000000000, 0.8660254037844387076, 1.000000000000000000, 0.8660254037844387076, 1.000000000000000000, 0.8660254037844387076, 1.000000000000000000, 0.8660254037844387076, 1.000000000000000000, 0.8660254037844387076, 1.000000000000000000, 0.8660254037844387076, 1.000000000000000000, 0.8660254037844387076, 1.000000000000000000, 0.8660254037844387076, 1.000000000000000000, 0.8660254037844387076, 1.000000000000000000, 0.8660254037844387076, 1.000000000000000000, 0.8660254037844387076, 1.000000000000000000, 0.8660254037844387076, 1.000000000000000000, 0.8660254037844387076, 1.000000000000000000, 0.8660254037844387076, 1.000000000000000000, 0.8660254037844387076, 1.000000000000000000, 0.8660254037844387076, 1.000000000000000000, 0.8660254037844387076, 1.000000000000000000, 0.8660254037844387076, 1.000000000000000000, 0.8660254037844387076, 1.000000000000000000, 0.8660254037844387076, 1.000000000000000000, 0.8660254037844387076, 1.000000000000000000, 0.8660254037844387076, 1.000000000000000000, 0.8660254037844387076, 1.000000000000000000, 0.8660254037844387076, 1.000000000000000000, 0.8660254037844387076, 1.000000000000000000, 0.8660254037844387076, 1.000000000000000000, 0.8660254037844387076, 1.000000000000000000, 0.8660254037844387076, 1.000000000000000000, 0.8660254037844387076, 1.000000000000000000, 0.8660254037844387076, 1.000000000000000000, 0.8660254037844387076, 1.000000000000000000, 0.8660254037844387076, 1.000000000000000000, 0.8660254037844387076, 1.000000000000000000, 0.8660254037844387076, 1.000000000000000000, 0.8660254037844387076, 1.000000000000000000, 0.8660254037844387076, 1.000000000000000000, 0.8660254037844387076, 1.000000000000000000, 0.8660254037844387076, 1.000000000000000000, 0.8660254037844387076, 1.000000000000000000, 0.8660254037844387076, 1.000000000000000000, 0.8660254037844387076, 1.000000000000000000, 0.8660254037844387076, 1.000000000000000000, 0.8660254037844387076, 1.000000000000000000, 0.8660254037844387076, 1.000000000000000000, 0.8660254037844387076, 1.000000000000000000, 0.8660254037844387076, 1.000000000000000000, 0.8660254037844387076, 1.000000000000000000, 0.8660254037844387076, 1.000000000000000000, 0.8660254037844387076, 1.000000000000000000, 0.8660254037844387076, 1.000000000000000000, 0.8660254037844387076, 1.000000000000000000, 0.8660254037844387076, 1.000000000000000000, 0.8660254037844387076, 1.000000000000000000, 0.8660254037844387076, 1.000000000000000000, 0.8660254037844387076, 1.000000000000000000, 0.8660254037844387076, 1.000000000000000000, 0.8660254037844387076, 1.000000000000000000, 0.8660254037844387076, 1.000000000000000000, 0.8660254037844387076, 1.000000000000000000, 0.8660254037844387076, 1.000000000000000000, 0.8660254037844387076, 1.000000000000000000, 0.8660254037844387076, 1.000000000000000000, 0.8660254037844387076, 1.000000000000000000, 0.8660254037844387076, 1.000000000000000000, 0.8660254037844387076, 1.000000000000000000, 0.8660254037844387076, 1.000000000000000000, 0.8660254037844387076, 1.000000000000000000, 0.8660254037844387076, 1.000000000000000000, 0.8660254037844387076, 1.000000000000000000, 0.8660254037844387076, 1.000000000000000000, 0.8660254037844387076, 1.000000000000000000, 0.8660254037844387076, 1.000000000000000000, 0.8660254037844387076, 1.000000000000000000, 0.8660254037844387076, 1.000000000000000000, 0.8660254037844387076, 1.000000000000000000, 0.8660254037844387076, 1.000000000000000000, 0.8660254037844387076, 1.000000000000000000, 0.8660254037844387076, 1.000000000000000000, 0.8660254037844387076, 1.000000000000000000, 0.8660254037844387076, 1.000000000000000000, 0.8660254037844387076, 1.000000000000000000, 0.8660254037844387076, 1.000000000000000000, 0.8660254037844387076, 1.000000000000000000, 0.8660254037844387076, 1.000000000000000000, 0.8660254037844387076, 1.000000000000000000, 0.8660254037844387076, 1.000000000000000000, 0.8660254037844387076, 1.000000000000000000, 0.8660254037844387076, 1.000000000000000000, 0.8660254037844387076, 1.000000000000000000, 0.8660254037844387076, 1.000000000000000000, 0.8660254037844387076, 1.000000000000000000, 0.8660254037844387076, 1.000000000000000000, 0.8660254037844387076, 1.000000000000000000, 0.8660254037844387076, 1.000000000000000000, 0.8660254037844387076, 1.000000000000000000, 0.8660254037844387076, 1.000000000000000000, 0.8660254037844387076, 1.000000000000000000, 0.8660254037844387076, 1.000000000000000000, 0.8660254037844387076, 1.000000000000000000, 0.8660254037844387076, 1.000000000000000000, 0.8660254037844387076, 1.000000000000000000, 0.8660254037844387076, 1.000000000000000000, 0.8660254037844387076, 1.000000000000000000, 0.8660254037844387076, 1.000000000000000000, 0.8660254037844387076, 1.000000000000000000, 0.8660254037844387076, 1.000000000000000000, 0.8660254037844387076, 1.000000000000000000, 0.8660254037844387076, 1.000000000000000000, 0.8660254037844387076, 1.000000000000000000, 0.8660254037844387076, 1.000000000000000000, 0.8660254037844387076, 1.000000000000000000, 0.8660254037844387076, 1.000000000000000000, 0.8660254037844387076, 1.000000000000000000, 0.8660254037844387076, 1.000000000000000000, 0.8660254037844387076, 1.000000000000000000, 0.8660254037844387076, 1.000000000000000000, 0.8660254037844387076, 1.000000000000000000, 0.8660254037844387076, 1.000000000000000000, 0.8660254037844387076, 1.000000000000000000, 0.8660254037844387076, 1.000000000000000000, 0.8660254037844387076, 1.000000000000000000, 0.8660254037844387076, 1.000000000000000000, 0.8660254037844387076, 1.000000000000000000, 0.8660254037844387076, 1.000000000000000000, 0.8660254037844387076, 1.000000000000000000, 0.8660254037844387076, 1.000000000000000000, 0.8660254037844387076, 1.000000000000000000, 0.8660254037844387076, 1.000000000000000000, 0.8660254037844387076, 1.000000000000000000, 0.8660254037844387076, 1.000000000000000000, 0.8660254037844387076, 1.000000000000000000, 0.8660254037844387076, 1.000000000000000000, 0.8660254037844387076, 1.000000000000000000, 0.8660254037844387076, 1.000000000000000000, 0.8660254037844387076, 1.000000000000000000, 0.8660254037844387076, 1.000000000000000000, 0.8660254037844387076, 1.000000000000000000, 0.8660254037844387076, 1.000000000000000000, 0.8660254037844387076, 1.000000000000000000, 0.8660254037844387076, 1.000000000000000000, 0.8660254037844387076, 1.000000000000000000, 0.8660254037844387076, 1.000000000000000000, 0.8660254037844387076, 1.000000000000000000, 0.8660254037844387076, 1.000000000000000000, 0.8660254037844387076, 1.000000000000000000, 0.8660254037844387076, 1.000000000000000000, 0.8660254037844387076, 1.000000000000000000, 0.8660254037844387076, 1.000000000000000000, 0.8660254037844387076, 1.000000000000000000, 0.8660254037844387076, 1.000000000000000000, 0.8660254037844387076, 1.000000000000000000, 0.8660254037844387076, 1.000000000000000000, 0.8660254037844387076, 1.000000000000000000, 0.8660254037844387076, 1.000000000000000000, 0.8660254037844387076, 1.000000000000000000, 0.8660254037844387076, 1.000000000000000000, 0.8660254037844387076, 1.000000000000000000, 0.8660254037844387076, 1.000000000000000000, 0.8660254037844387076, 1.000000000000000000, 0.8660254037844387076, 1.000000000000000000, 0.8660254037844387076, 1.000000000000000000) ) ) 
 REPRESENTATION_ITEM ( '' )  SURFACE ( )  );
#27733=CARTESIAN_POINT ( 'NONE',  ( 7.910292558569346433, 11.31609285405122556, -1.199719254218446718 ) ) ;
#27735=CARTESIAN_POINT ( 'NONE',  ( -3.026510298046701575, 6.452477208712732448, 0.6266050759124314196 ) ) ;
#27739=CARTESIAN_POINT ( 'NONE',  ( 10.01963921569910632, 11.64833282552586091, 1.199719254218450271 ) ) ;
#27740=DIRECTION ( 'NONE',  ( -1.000000000000000000, 5.578564026256504688E-16, 0.000000000000000000 ) ) ;
#27746=CARTESIAN_POINT ( 'NONE',  ( -7.646435448427427062, 10.90429654226522693, 1.082531754730549967 ) ) ;
#27751=CARTESIAN_POINT ( 'NONE',  ( -8.597841969360544567, 13.18256606422934674, 0.7998128361456341429 ) ) ;
#27752=CARTESIAN_POINT ( 'NONE',  ( 6.647575389402066826, 6.649926130590872120, 1.040834085586084257E-14 ) ) ;
#27758=CARTESIAN_POINT ( 'NONE',  ( 4.514501963226220660, 4.369266499959774563, -0.7216878364870197293 ) ) ;
#27766=CARTESIAN_POINT ( 'NONE',  ( -6.742482464697739708, 6.760651051769146491, 0.7998128361456341429 ) ) ;
#27768=CARTESIAN_POINT ( 'NONE',  ( -4.973143418114339021, 4.696422164088486895, 0.7998128361456341429 ) ) ;
#27773=DIRECTION ( 'NONE',  ( 0.000000000000000000, 8.546850786086437571E-32, 1.000000000000000000 ) ) ;
#27776=CARTESIAN_POINT ( 'NONE',  ( 6.661133543015731462, 6.665743976473484267, -0.7998128361456281477 ) ) ;
#27778=CARTESIAN_POINT ( 'NONE',  ( 1.571977147778452544, 8.681624870483057421, 2.500282472944442613 ) ) ;
#27790=CARTESIAN_POINT ( 'NONE',  ( 0.6823417656249882723, 0.9885416670080832136, -1.181850606188749264 ) ) ;
#27792=CARTESIAN_POINT ( 'NONE',  ( 3.005103603723342953, 6.657704637652544832, -0.7998128361456291469 ) ) ;
#27795=CARTESIAN_POINT ( 'NONE',  ( -6.724481002698126098, 8.868313807946373473, -1.443375672974059665 ) ) ;
#27796=CARTESIAN_POINT ( 'NONE',  ( 3.470524135418292300, 5.072030796119872953, -1.443375672974057666 ) ) ;
#27797=CARTESIAN_POINT ( 'NONE',  ( -5.870317324592812191, 7.871789516823500144, -1.443375672974051449 ) ) ;
#27799=ORIENTED_EDGE ( 'NONE', *, *, #159108, .F. ) ;
#27801=CARTESIAN_POINT ( 'NONE',  ( 4.964256800898067645, 8.943383367689749619, 0.7998128361456462443 ) ) ;
#27806=CARTESIAN_POINT ( 'NONE',  ( 1.364683531249990311, 4.634375000341417916, 1.214306433183764966E-14 ) ) ;
#27810=CARTESIAN_POINT ( 'NONE',  ( 6.446011968293428041, 9.607765498729298415, -1.199719254218440723 ) ) ;
#27814=CARTESIAN_POINT ( 'NONE',  ( -6.204827856548512877, 10.39071626594860476, -0.7998128361456291469 ) ) ;
#27819=CARTESIAN_POINT ( 'NONE',  ( 7.832860060393120882, 10.16142270859057462, 1.599625672291281386 ) ) ;
#27821=CARTESIAN_POINT ( 'NONE',  ( -6.530223543276495235, 10.77034456713125188, -0.7998128361456291469 ) ) ;
#27822=DIRECTION ( 'NONE',  ( -5.578564026256490882E-16, -1.000000000000000000, -9.066213480720158442E-32 ) ) ;
#27823=CARTESIAN_POINT ( 'NONE',  ( 6.426201622753093368, 10.44105962661321563, 1.040834085586084257E-14 ) ) ;
#27824=CARTESIAN_POINT ( 'NONE',  ( 4.184706906298553797, 7.590773377710720915, -0.8858016571234141878 ) ) ;
#27825=CARTESIAN_POINT ( 'NONE',  ( -8.351459436338030784, 11.72682452816096976, -1.082531754730543971 ) ) ;
#27831=CARTESIAN_POINT ( 'NONE',  ( 6.173040012923759257, 6.096301524699504704, -0.7998128361456281477 ) ) ;
#27833=CARTESIAN_POINT ( 'NONE',  ( 8.106885785967500979, 11.54545161934907682, 1.199719254218460707 ) ) ;
#27834=CARTESIAN_POINT ( 'NONE',  ( -5.443780329924999606, 6.294985656096041993, 1.034245658874383578 ) ) ;
#27835=CARTESIAN_POINT ( 'NONE',  ( 4.356247428692526569, 3.976710176429713250, 0.7998128361456341429 ) ) ;
#27836=CARTESIAN_POINT ( 'NONE',  ( -0.6823417656250246877, 0.3010416670080895418, 1.181850606188755259 ) ) ;
#27838=CARTESIAN_POINT ( 'NONE',  ( -5.572037945536512105, 9.444535336527177805, 0.000000000000000000 ) ) ;
#27839=ORIENTED_EDGE ( 'NONE', *, *, #61445, .T. ) ;
#27844=CARTESIAN_POINT ( 'NONE',  ( -4.638859928512265363, 6.918491158249495676, 1.209939204767721987 ) ) ;
#27845=CARTESIAN_POINT ( 'NONE',  ( -0.6823417656250246877, 0.6135416670080897639, 1.181850606188755259 ) ) ;
#27848=CARTESIAN_POINT ( 'NONE',  ( 2.901081683644312736, 6.328419697652925002, 0.7216878364870338292 ) ) ;
#27850=VECTOR ( 'NONE', #128531, 1000.000000000000114 ) ;
#27853=CARTESIAN_POINT ( 'NONE',  ( -7.578644679914719795, 9.864838098032418401, 1.443375672974090751 ) ) ;
#27858=CARTESIAN_POINT ( 'NONE',  ( -7.985389288324692636, 11.29974268881207067, -1.082531754730543083 ) ) ;
#27862=CARTESIAN_POINT ( 'NONE',  ( 8.283668668269706714, 8.766627655843896250, 1.040834085586084257E-14 ) ) ;
#27865=CARTESIAN_POINT ( 'NONE',  ( -8.148087131688692253, 10.52918762510205042, -1.443375672974058777 ) ) ;
#27870=CARTESIAN_POINT ( 'NONE',  ( -1.364683531250010295, 4.842708333674756283, 0.7879004041258379498 ) ) ;
#27871=CARTESIAN_POINT ( 'NONE',  ( -1.201851678989727383E-14, 3.743750000682817269, 1.732050807568877637 ) ) ;
#27872=CARTESIAN_POINT ( 'NONE',  ( 5.302928268938337020, 6.565392180301311775, -1.356678214699511775 ) ) ;
#27876=ORIENTED_EDGE ( 'NONE', *, *, #97341, .T. ) ;
#27878=CARTESIAN_POINT ( 'NONE',  ( -8.843996274815957293, 9.212417163573759282, 1.040834085586084257E-14 ) ) ;
#27879=DIRECTION ( 'NONE',  ( 0.000000000000000000, 8.546850786086437571E-32, 1.000000000000000000 ) ) ;
#27882=CARTESIAN_POINT ( 'NONE',  ( 5.847644326195776010, 5.716673223516856694, -0.7998128361456281477 ) ) ;
#27884=CARTESIAN_POINT ( 'NONE',  ( 3.673896439623286714, 4.156855427197417185, -0.9999999999999940048 ) ) ;
#27887=CARTESIAN_POINT ( 'NONE',  ( 5.960781091502512119, 10.10599504006161986, 0.7998128361456462443 ) ) ;
#27896=CARTESIAN_POINT ( 'NONE',  ( -5.910991785878170646, 7.919243054989755670, -1.443375672974059665 ) ) ;
#27899=LINE ( 'NONE', #127629, #57661 ) ;
#27902=CYLINDRICAL_SURFACE ( 'NONE', #116300, 1.250000000000000000 ) ;
#27905=CARTESIAN_POINT ( 'NONE',  ( -8.469039510030723861, 13.03229652834454733, 1.040834085586084257E-14 ) ) ;
#27907=CARTESIAN_POINT ( 'NONE',  ( 9.908311333488716954, 10.45411806535867782, 0.7998128361456462443 ) ) ;
#27908=CARTESIAN_POINT ( 'NONE',  ( 1.499999999999989120, 0.2750000000000182854, 0.000000000000000000 ) ) ;
#27909=CARTESIAN_POINT ( 'NONE',  ( -9.528683032306089373, 10.01121838064558744, 0.7998128361456462443 ) ) ;
#27913=CARTESIAN_POINT ( 'NONE',  ( 1.364683531249988535, 4.113541667008088432, 0.7879004041258500513 ) ) ;
#27914=CARTESIAN_POINT ( 'NONE',  ( 4.220665892555866883, 3.818531717603609987, -0.7998128361456211532 ) ) ;
#27917=CARTESIAN_POINT ( 'NONE',  ( -1.500000000000011324, 4.879166666666690411, -0.8660254037844313801 ) ) ;
#27921=CARTESIAN_POINT ( 'NONE',  ( 6.900736999231407154, 10.99468423250458038, -0.7216878364870267237 ) ) ;
#27924=CARTESIAN_POINT ( 'NONE',  ( -6.155038550924159857, 8.203964280876741455, 1.443375672974078761 ) ) ;
#27926=CARTESIAN_POINT ( 'NONE',  ( -0.6823417656250003738, 2.217708333674753174, -1.181850606188749264 ) ) ;
#27930=CARTESIAN_POINT ( 'NONE',  ( -7.854251061018346469, 8.057714414143200443, -0.7998128361456291469 ) ) ;
#27932=CARTESIAN_POINT ( 'NONE',  ( 1.364683531249990311, 4.196875000341417028, 1.214306433183764966E-14 ) ) ;
#27937=CARTESIAN_POINT ( 'NONE',  ( 8.934986926605834157, 10.38290515491702770, -1.199719254218446718 ) ) ;
#27940=CARTESIAN_POINT ( 'NONE',  ( 1.499999999999987121, 0.7541666666666868579, 0.8660254037844524744 ) ) ;
#27943=EDGE_LOOP ( 'NONE', ( #92721, #122147, #75961, #69505 ) ) ;
#27944=CARTESIAN_POINT ( 'NONE',  ( 9.935427640716063991, 10.48575375712389679, -0.7998128361456281477 ) ) ;
#27948=EDGE_CURVE ( 'NONE', #169987, #179933, #149191, .T. ) ;
#27951=CARTESIAN_POINT ( 'NONE',  ( 7.065770611016287006, 11.39514947949436774, 1.040834085586084257E-14 ) ) ;
#27952=CARTESIAN_POINT ( 'NONE',  ( -9.829825065107822724, 11.42688298316931572, 1.199719254218462483 ) ) ;
#27955=CARTESIAN_POINT ( 'NONE',  ( -1.364683531249997417, 5.821875000341418804, 1.214306433183764966E-14 ) ) ;
#27959=CARTESIAN_POINT ( 'NONE',  ( 7.964525173024008531, 11.37936423758166526, 1.199719254218460707 ) ) ;
#27962=CARTESIAN_POINT ( 'NONE',  ( 1.364683531249988535, 3.613541667008086211, 0.7879004041258500513 ) ) ;
#27964=CARTESIAN_POINT ( 'NONE',  ( -5.260200412422196159, 9.080724881227137502, -0.7216878364870207285 ) ) ;
#27973=CARTESIAN_POINT ( 'NONE',  ( 7.564559641420864899, 10.91273778404466199, -1.199719254218446718 ) ) ;
#27974=CARTESIAN_POINT ( 'NONE',  ( 4.856179778084614540, 5.010200168423447842, 0.6077543439236311462 ) ) ;
#27976=VECTOR ( 'NONE', #131648, 1000.000000000000000 ) ;
#27980=CARTESIAN_POINT ( 'NONE',  ( -7.323375529675950624, 11.69568855126397011, -0.7998128361456291469 ) ) ;
#27981=CARTESIAN_POINT ( 'NONE',  ( 7.494959990256193194, 7.638541498254023843, -0.7998128361456281477 ) ) ;
#27984=CARTESIAN_POINT ( 'NONE',  ( 4.467575310902914154, 5.170924936596891008, 1.199719254218464037 ) ) ;
#27986=AXIS2_PLACEMENT_3D ( 'NONE', #167124, #306, #69583 ) ;
#27992=CARTESIAN_POINT ( 'NONE',  ( -5.260200412422200600, 8.120355666925794580, -1.082531754730544860 ) ) ;
#27993=CARTESIAN_POINT ( 'NONE',  ( 4.684505768721569652, 5.424010470718658716, -1.199719254218452047 ) ) ;
#27996=CARTESIAN_POINT ( 'NONE',  ( -7.019370843573183194, 9.212351955633947043, 1.599625672291283607 ) ) ;
#28002=CARTESIAN_POINT ( 'NONE',  ( -8.670602931139386627, 10.07445716020612103, 1.199719254218462483 ) ) ;
#28006=CARTESIAN_POINT ( 'NONE',  ( 7.796102023057898123, 9.054206100777749455, -1.199719254218441611 ) ) ;
#28007=CARTESIAN_POINT ( 'NONE',  ( -6.471393748263779777, 5.229711127719298247, -2.499999999999995115 ) ) ;
#28018=CARTESIAN_POINT ( 'NONE',  ( -7.049349804101573191, 10.31165964050546258, -1.199719254218440723 ) ) ;
#28023=CARTESIAN_POINT ( 'NONE',  ( 5.165293337126522388, 8.969999960048859577, 1.040834085586084257E-14 ) ) ;
#28025=CARTESIAN_POINT ( 'NONE',  ( -1.436838838544810093, 7.449283400311735193, 4.203727439823581769 ) ) ;
#28028=CARTESIAN_POINT ( 'NONE',  ( -7.074657228232555717, 7.148188275893099686, 1.040834085586084257E-14 ) ) ;
#28031=CARTESIAN_POINT ( 'NONE',  ( -1.499999999999998002, 8.226407212580417294, -3.114167208185186553 ) ) ;
#28042=CARTESIAN_POINT ( 'NONE',  ( 8.938903350111612411, 9.323142084752035430, -0.7998128361456221525 ) ) ;
#28045=CARTESIAN_POINT ( 'NONE',  ( -3.280709984826970516, 6.771319382366015383, 0.7216878364870317197 ) ) ;
#28046=LINE ( 'NONE', #24833, #28564 ) ;
#28047=CARTESIAN_POINT ( 'NONE',  ( -5.029675114306419559, 6.591709307070120261, -1.234896939913838754 ) ) ;
#28054=CARTESIAN_POINT ( 'NONE',  ( 4.196412238629597447, 4.854568018944682706, -1.199719254218452047 ) ) ;
#28061=CARTESIAN_POINT ( 'NONE',  ( 5.203632029546647608, 4.965325544092860532, 1.040834085586084257E-14 ) ) ;
#28072=CARTESIAN_POINT ( 'NONE',  ( -3.438964519360665051, 7.163875705896082913, -0.7998128361456281477 ) ) ;
#28074=CARTESIAN_POINT ( 'NONE',  ( 6.466876083594112146, 6.647036307055676829, -0.7216878364870257245 ) ) ;
#28075=CARTESIAN_POINT ( 'NONE',  ( -1.499999999999997780, 3.150000000000020783, 1.214306433183764966E-14 ) ) ;
#28077=CARTESIAN_POINT ( 'NONE',  ( -3.249150368769345043, 6.942425863539538611, 0.7998128361456341429 ) ) ;
#28079=CARTESIAN_POINT ( 'NONE',  ( 1.364683531249990311, 4.613541667008083103, 0.7879004041258500513 ) ) ;
#28082=CARTESIAN_POINT ( 'NONE',  ( -4.012850279964973232, 4.744375417122949301, 1.082531754730560403 ) ) ;
#28087=CARTESIAN_POINT ( 'NONE',  ( 5.529027716274630855, 5.344953845275508542, 1.040834085586084257E-14 ) ) ;
#28090=CARTESIAN_POINT ( 'NONE',  ( 0.2198916526692429596, 6.505559487570201860, -3.126830488621899384 ) ) ;
#28093=CARTESIAN_POINT ( 'NONE',  ( -1.364683531250000748, 1.571875000341421691, 0.000000000000000000 ) ) ;
#28096=CARTESIAN_POINT ( 'NONE',  ( -8.784793466650835825, 12.33634391347959713, 1.199719254218462483 ) ) ;
#28098=CARTESIAN_POINT ( 'NONE',  ( -6.249945625775490399, 7.354319987235250267, 1.082531754730549967 ) ) ;
#28102=CARTESIAN_POINT ( 'NONE',  ( 1.364683531249988535, 3.863541667008087543, 0.7879004041258500513 ) ) ;
#28110=CARTESIAN_POINT ( 'NONE',  ( -5.870317324592811303, 8.832158731124840401, -1.082531754730537976 ) ) ;
#28116=CARTESIAN_POINT ( 'NONE',  ( -4.378920427089552092, 8.052564898339037214, 0.7216878364870317197 ) ) ;
#28118=CARTESIAN_POINT ( 'NONE',  ( -4.707509334217570007, 5.241700920597089031, 1.110557563554106952 ) ) ;
#28129=CARTESIAN_POINT ( 'NONE',  ( -5.752737250900127997, 5.605948302338584099, 0.000000000000000000 ) ) ;
#28130=CARTESIAN_POINT ( 'NONE',  ( -5.792162442946777290, 6.216820166843662676, 1.023959129923063260 ) ) ;
#28132=CARTESIAN_POINT ( 'NONE',  ( -1.500000000000015099, 0.6291666666666863028, -0.8660254037844313801 ) ) ;
#28134=CARTESIAN_POINT ( 'NONE',  ( 7.768458830950378591, 12.00702636951006497, 1.040834085586084257E-14 ) ) ;
#28135=CARTESIAN_POINT ( 'NONE',  ( 6.123478934866503742, 10.29580919065294431, 0.7998128361456462443 ) ) ;
#28141=CARTESIAN_POINT ( 'NONE',  ( 4.976006071415387311, 5.764094157194782575, 1.199719254218462483 ) ) ;
#28142=CARTESIAN_POINT ( 'NONE',  ( -0.4909524369919514020, 7.516007857510251355, -2.014442075801170073 ) ) ;
#28149=CARTESIAN_POINT ( 'NONE',  ( -5.201524489137236529, 9.220195670635433771, 0.7998128361456481317 ) ) ;
#28155=CARTESIAN_POINT ( 'NONE',  ( -0.6823417656249969321, 3.967708333674754950, -1.181850606188749264 ) ) ;
#28156=CARTESIAN_POINT ( 'NONE',  ( 8.148087131688683371, 10.52918762510205042, -1.443375672974063439 ) ) ;
#28157=CARTESIAN_POINT ( 'NONE',  ( -6.738566041191992539, 7.820414121934134322, 1.199719254218450271 ) ) ;
#28160=CARTESIAN_POINT ( 'NONE',  ( 7.318703993278529829, 7.432909501780090800, 1.040834085586084257E-14 ) ) ;
#28161=CARTESIAN_POINT ( 'NONE',  ( -4.089755892816631544, 7.923132308261379819, -0.7998128361456281477 ) ) ;
#28165=CARTESIAN_POINT ( 'NONE',  ( -1.500000000000015099, -0.08958333265051321437, -0.8660254037844383745 ) ) ;
#28168=CARTESIAN_POINT ( 'NONE',  ( 7.348156068926750883, 8.635565504245116486, -1.082531754730537976 ) ) ;
#28171=CARTESIAN_POINT ( 'NONE',  ( -1.364683531250012516, 2.342708333674752286, 0.7879004041258379498 ) ) ;
#28173=CARTESIAN_POINT ( 'NONE',  ( 5.124618875841165710, 8.922546421882614709, 1.040834085586084257E-14 ) ) ;
#28175=CARTESIAN_POINT ( 'NONE',  ( -3.633221978782299910, 5.261844946711204507, -1.443375672974053447 ) ) ;
#28178=CARTESIAN_POINT ( 'NONE',  ( 1.364683531249988535, 5.655208333674751842, -0.7879004041258300672 ) ) ;
#28184=CARTESIAN_POINT ( 'NONE',  ( -3.976739547089790161, 7.847837856468413698, 0.08243740857501527519 ) ) ;
#28189=AXIS2_PLACEMENT_3D ( 'NONE', #125705, #210049, #175453 ) ;
#28192=CARTESIAN_POINT ( 'NONE',  ( 4.984594031318565932, 8.967110136513669616, 0.7998128361456462443 ) ) ;
#28204=CARTESIAN_POINT ( 'NONE',  ( 4.609409038966229666, 6.400729850259146758, -1.443375672974051449 ) ) ;
#28205=CARTESIAN_POINT ( 'NONE',  ( -1.364683531250012516, 2.592708333674753174, 0.7879004041258379498 ) ) ;
#28206=CARTESIAN_POINT ( 'NONE',  ( 7.884230021546724920, 9.157022099014721306, 1.199719254218462483 ) ) ;
#28210=FACE_OUTER_BOUND ( 'NONE', #8888, .T. ) ;
#28211=EDGE_CURVE ( 'NONE', #38245, #152353, #33045, .T. ) ;
#28214=CARTESIAN_POINT ( 'NONE',  ( -1.500000000000013101, 3.629166666666692187, -0.8660254037844313801 ) ) ;
#28215=CARTESIAN_POINT ( 'NONE',  ( 5.880485940025228508, 7.883652901494672349, 1.599625672291267398 ) ) ;
#28216=CARTESIAN_POINT ( 'NONE',  ( -6.714312387265696458, 8.856450423275211037, 1.599625672291283607 ) ) ;
#28220=CARTESIAN_POINT ( 'NONE',  ( -1.201851678989727383E-14, 3.196875000341420137, -1.575800808251660134 ) ) ;
#28222=CARTESIAN_POINT ( 'NONE',  ( 4.033714395265605823, 4.664753868353354704, -1.199719254218446718 ) ) ;
#28228=CARTESIAN_POINT ( 'NONE',  ( 1.499999999999989120, 0.5562500006828161592, 0.000000000000000000 ) ) ;
#28230=CARTESIAN_POINT ( 'NONE',  ( -5.506582945444718824, 9.576097202994168001, 0.7998128361456481317 ) ) ;
#28239=CARTESIAN_POINT ( 'NONE',  ( 5.229694566569264680, 7.124396299129368337, 1.599625672291267398 ) ) ;
#28243=CARTESIAN_POINT ( 'NONE',  ( 7.657657833620182153, 7.828355648845348291, -0.7998128361456281477 ) ) ;
#28244=VERTEX_POINT ( 'NONE', #184605 ) ;
#28248=CARTESIAN_POINT ( 'NONE',  ( -4.855791571988752331, 8.816840600628864877, 0.7998128361456481317 ) ) ;
#28249=EDGE_LOOP ( 'NONE', ( #44108, #63980, #98141, #104247, #95306, #50558 ) ) ;
#28250=CARTESIAN_POINT ( 'NONE',  ( 3.837121167867449945, 4.435395103055503441, 1.199719254218464037 ) ) ;
#28256=CARTESIAN_POINT ( 'NONE',  ( 4.002655450416458649, 7.592114961386800864, 0.1875155472659401079 ) ) ;
#28265=CARTESIAN_POINT ( 'NONE',  ( -4.297571505851936813, 4.116180966356429494, 1.214306433183764966E-14 ) ) ;
#28266=CARTESIAN_POINT ( 'NONE',  ( 8.270110514656034084, 9.711179024262627024, 1.082531754730558626 ) ) ;
#28268=CARTESIAN_POINT ( 'NONE',  ( -4.283486466913726254, 7.084819080452935403, -1.199719254218452047 ) ) ;
#28271=CARTESIAN_POINT ( 'NONE',  ( 6.611572464958476836, 10.86525164242692298, 0.7998128361456462443 ) ) ;
#28273=CARTESIAN_POINT ( 'NONE',  ( -5.799137018343247796, 7.788745826199009237, -1.599625672291256295 ) ) ;
#28284=CARTESIAN_POINT ( 'NONE',  ( 10.72180055030867329, 11.40318881831530540, 0.7998128361456341429 ) ) ;
#28285=CARTESIAN_POINT ( 'NONE',  ( -5.590039407536138150, 5.416134151747256986, 0.000000000000000000 ) ) ;
#28288=CARTESIAN_POINT ( 'NONE',  ( 3.633221978782282147, 5.261844946711204507, -1.443375672974057666 ) ) ;
#28293=CARTESIAN_POINT ( 'NONE',  ( -4.009460741339347045, 5.700790169694431420, -1.599625672291256295 ) ) ;
#28296=CARTESIAN_POINT ( 'NONE',  ( 10.06423010004587759, 10.63602329300870153, 0.000000000000000000 ) ) ;
#28300=CARTESIAN_POINT ( 'NONE',  ( -8.362681821530818738, 8.650883634741092010, -0.7998128361456291469 ) ) ;
#28301=CARTESIAN_POINT ( 'NONE',  ( 6.335737856287750880, 6.286115675290828264, -0.7998128361456281477 ) ) ;
#28304=CARTESIAN_POINT ( 'NONE',  ( 5.345992642490140057, 5.131412925860272090, 1.040834085586084257E-14 ) ) ;
#28307=CARTESIAN_POINT ( 'NONE',  ( -1.364683531250000748, 0.8218750003414210248, 0.000000000000000000 ) ) ;
#28308=ORIENTED_EDGE ( 'NONE', *, *, #22894, .F. ) ;
#28310=CARTESIAN_POINT ( 'NONE',  ( 7.619319141200070256, 8.951922421897323900, 1.082531754730558626 ) ) ;
#28311=ORIENTED_EDGE ( 'NONE', *, *, #51004, .T. ) ;
#28317=CARTESIAN_POINT ( 'NONE',  ( 10.34450801710256584, 11.17094022948226240, 0.7216878364870438212 ) ) ;
#28325=CARTESIAN_POINT ( 'NONE',  ( -10.15522075183580419, 11.80651128435196462, 1.199719254218462483 ) ) ;
#28334=CARTESIAN_POINT ( 'NONE',  ( -1.123270288249905713, 3.300000000000025135, 0.7750000000000119016 ) ) ;
#28343=CARTESIAN_POINT ( 'NONE',  ( 0.7499999999999885647, 1.597916667349486008, -1.299038105676652899 ) ) ;
#28348=CARTESIAN_POINT ( 'NONE',  ( -1.402160292154681736E-14, -0.6624999999999758860, -1.732050807568870754 ) ) ;
#28349=CARTESIAN_POINT ( 'NONE',  ( 7.242026607993941489, 11.60078147596829901, 0.7998128361456462443 ) ) ;
#28354=CARTESIAN_POINT ( 'NONE',  ( 3.358669367883368118, 4.941533567329135401, -1.599625672291262513 ) ) ;
#28355=CARTESIAN_POINT ( 'NONE',  ( -5.585596099150191840, 7.539614753807099667, -1.443375672974052559 ) ) ;
#28359=CARTESIAN_POINT ( 'NONE',  ( -7.555971681517696936, 7.709721804725773175, 0.7998128361456462443 ) ) ;
#28361=CARTESIAN_POINT ( 'NONE',  ( 1.499999999999989120, 1.785416667349487563, 0.8660254037844524744 ) ) ;
#28376=CARTESIAN_POINT ( 'NONE',  ( -8.666686507633592385, 11.13422023037111330, 1.599625672291269396 ) ) ;
#28377=CARTESIAN_POINT ( 'NONE',  ( 8.444030743212801227, 8.745790710036752458, 0.7998128361456462443 ) ) ;
#28384=CARTESIAN_POINT ( 'NONE',  ( -6.320072162264675164, 10.52516795595079557, 0.7998128361456481317 ) ) ;
#28392=CARTESIAN_POINT ( 'NONE',  ( 3.330499290451326200, 7.037332938835193730, -0.7998128361456291469 ) ) ;
#28396=ORIENTED_EDGE ( 'NONE', *, *, #95435, .T. ) ;
#28397=CARTESIAN_POINT ( 'NONE',  ( -10.30827686509187835, 10.92074451889568643, 1.040834085586084257E-14 ) ) ;
#28400=CARTESIAN_POINT ( 'NONE',  ( -5.194998520284300980, 6.641152480062820551, -1.419077516013200313 ) ) ;
#28401=ORIENTED_EDGE ( 'NONE', *, *, #99577, .F. ) ;
#28409=CARTESIAN_POINT ( 'NONE',  ( 6.174848896020108668, 9.291408581077091000, 1.199719254218460707 ) ) ;
#28419=CARTESIAN_POINT ( 'NONE',  ( 1.499999999999987121, 0.8270833340161471980, -0.8660254037844253849 ) ) ;
#28431=CARTESIAN_POINT ( 'NONE',  ( 3.362058906508953449, 6.866226457661676719, -0.7216878364870267237 ) ) ;
#28436=CARTESIAN_POINT ( 'NONE',  ( 9.642873567817520808, 12.27310513391906532, 1.599625672291279388 ) ) ;
#28446=CARTESIAN_POINT ( 'NONE',  ( 1.364683531249986981, -1.115624999658580752, 0.000000000000000000 ) ) ;
#28451=CARTESIAN_POINT ( 'NONE',  ( -4.394814349124112951, 8.279033840620114049, -0.7998128361456281477 ) ) ;
#28453=CARTESIAN_POINT ( 'NONE',  ( -1.402160292154681736E-14, -0.6624999999999758860, -1.732050807568870754 ) ) ;
#28455=CARTESIAN_POINT ( 'NONE',  ( -1.201851678989727383E-14, 5.337500000000020783, -1.732050807568863648 ) ) ;
#28461=CARTESIAN_POINT ( 'NONE',  ( -1.001543065824772872E-14, 5.384375000341415252, 1.575800808251672791 ) ) ;
#28464=CARTESIAN_POINT ( 'NONE',  ( -7.181014916732457287, 11.52960116949655678, -0.7998128361456291469 ) ) ;
#28471=CARTESIAN_POINT ( 'NONE',  ( -1.402160292154681736E-14, 0.1343750003414218575, 1.575800808251672791 ) ) ;
#28479=CARTESIAN_POINT ( 'NONE',  ( 8.283668668269706714, 8.766627655843892697, 1.040834085586084257E-14 ) ) ;
#28482=CARTESIAN_POINT ( 'NONE',  ( -5.687809136132860210, 6.594531066031826150, -1.199719254218446718 ) ) ;
#28484=CARTESIAN_POINT ( 'NONE',  ( 1.499999999999989120, 5.035416667349487341, 0.8660254037844524744 ) ) ;
#28486=CARTESIAN_POINT ( 'NONE',  ( -4.009460741339347045, 5.700790169694431420, -1.599625672291256295 ) ) ;
#28487=CARTESIAN_POINT ( 'NONE',  ( 5.788968402910802169, 8.737251655829183505, 1.082531754730558626 ) ) ;
#28488=CARTESIAN_POINT ( 'NONE',  ( -9.178506806327330736, 10.77097469787910455, 1.082531754730558626 ) ) ;
#28494=CARTESIAN_POINT ( 'NONE',  ( 2.900554798319789906, 5.471398800426671372, 1.199719254218452047 ) ) ;
#28498=TOROIDAL_SURFACE ( 'NONE', #166873, 0.8299999999999998490, 0.08000000000000000167 ) ;
#28509=EDGE_LOOP ( 'NONE', ( #176987, #95263, #69460, #132137 ) ) ;
#28512=CARTESIAN_POINT ( 'NONE',  ( 9.752392566931574081, 10.27221283770866300, -0.7998128361456281477 ) ) ;
#28514=CARTESIAN_POINT ( 'NONE',  ( -1.500000000000021760, 7.809254910133661909, 3.635752117228817859 ) ) ;
#28517=CARTESIAN_POINT ( 'NONE',  ( -1.364683531250000748, -0.4906249996585801409, 0.000000000000000000 ) ) ;
#28518=CARTESIAN_POINT ( 'NONE',  ( 5.395781948558860286, 6.357795697149212444, -1.082531754730542195 ) ) ;
#28521=CARTESIAN_POINT ( 'NONE',  ( -8.676855123066019360, 11.14608361504227574, -1.443375672974059665 ) ) ;
#28541=CARTESIAN_POINT ( 'NONE',  ( 5.337709665475443011, 6.539638787446115487, -1.341754179669167213 ) ) ;
#28550=CARTESIAN_POINT ( 'NONE',  ( -8.378575743565381373, 8.877352577022161739, 0.7216878364870438212 ) ) ;
#28554=CARTESIAN_POINT ( 'NONE',  ( 6.745345117998789775, 7.828323044875442172, 1.199719254218462483 ) ) ;
#28555=CARTESIAN_POINT ( 'NONE',  ( -3.598799709423620374, 6.286017863381107240, 1.199719254218464037 ) ) ;
#28558=CARTESIAN_POINT ( 'NONE',  ( -5.057354993097396445, 5.859001232490445688, -1.199719254218446718 ) ) ;
#28563=CARTESIAN_POINT ( 'NONE',  ( -5.440899717785814715, 5.242137847038546461, 0.7998128361456341429 ) ) ;
#28564=VECTOR ( 'NONE', #190529, 1000.000000000000000 ) ;
#28567=CARTESIAN_POINT ( 'NONE',  ( 4.517891501851804215, 6.293959390292322986, -1.599625672291255185 ) ) ;
#28568=CARTESIAN_POINT ( 'NONE',  ( 7.401861798056875053, 10.72292363345333399, -1.199719254218441611 ) ) ;
#28571=CARTESIAN_POINT ( 'NONE',  ( 4.081185262901700028, 7.719248740676039056, 0.6171906885068592086 ) ) ;
#28572=CARTESIAN_POINT ( 'NONE',  ( 5.694061328059515148, 5.745419092265303007, -0.7216878364870207285 ) ) ;
#28579=CARTESIAN_POINT ( 'NONE',  ( 6.602457619730767391, 7.765583980183128787, 1.082531754730558626 ) ) ;
#28581=CARTESIAN_POINT ( 'NONE',  ( -9.345647958521597687, 9.797677461230342999, 0.7998128361456462443 ) ) ;
#28584=CARTESIAN_POINT ( 'NONE',  ( -9.321394304595349567, 10.83371376257142416, 1.199719254218462483 ) ) ;
#28585=CARTESIAN_POINT ( 'NONE',  ( -7.823218330285243383, 9.085841792542966644, -1.199719254218446718 ) ) ;
#28594=CARTESIAN_POINT ( 'NONE',  ( 9.240045382913317340, 10.73880668727576015, -1.199719254218446718 ) ) ;
#28598=CARTESIAN_POINT ( 'NONE',  ( 2.900554798319789906, 5.471398800426671372, 1.199719254218452047 ) ) ;
#28601=CARTESIAN_POINT ( 'NONE',  ( 1.499999999999990896, 5.556250000682820378, 1.214306433183764966E-14 ) ) ;
#28607=CARTESIAN_POINT ( 'NONE',  ( 1.499999999999987121, 2.545833333333351156, -0.8660254037844262731 ) ) ;
#28608=CARTESIAN_POINT ( 'NONE',  ( 5.229694566569264680, 7.124396299129368337, 1.599625672291267398 ) ) ;
#28610=CARTESIAN_POINT ( 'NONE',  ( 7.131225611108085616, 10.30321839872603462, 1.082531754730558626 ) ) ;
#28611=CARTESIAN_POINT ( 'NONE',  ( -9.775065565328603157, 11.46695991671396087, -1.082531754730537976 ) ) ;
#28614=CARTESIAN_POINT ( 'NONE',  ( 8.971744963941056028, 11.49012176272984931, 1.599625672291281386 ) ) ;
#28617=CARTESIAN_POINT ( 'NONE',  ( -4.440459003675619520, 5.139289244831666714, 1.199719254218462483 ) ) ;
#28618=CARTESIAN_POINT ( 'NONE',  ( 0.7499999999999902300, 5.097916667349482012, -1.299038105676658228 ) ) ;
#28619=EDGE_CURVE ( 'NONE', #180436, #179865, #149607, .T. ) ;
#28620=CARTESIAN_POINT ( 'NONE',  ( 1.364683531249986537, 1.655208333674748955, -0.7879004041258239610 ) ) ;
#28625=CARTESIAN_POINT ( 'NONE',  ( -0.6823417656250003738, -1.032291666325242607, -1.181850606188749264 ) ) ;
#28628=CARTESIAN_POINT ( 'NONE',  ( 9.073431116043567002, 11.60875560684942265, -1.599625672291262513 ) ) ;
#28632=CARTESIAN_POINT ( 'NONE',  ( -4.297571505407598025, 5.076550180139354218, 1.082531754730558626 ) ) ;
#28635=CARTESIAN_POINT ( 'NONE',  ( -5.388475986427523345, 8.373973519885682393, 1.199719254218452047 ) ) ;
#28638=CARTESIAN_POINT ( 'NONE',  ( 4.379447312414087357, 5.068108938359919158, -1.199719254218452047 ) ) ;
#28642=ORIENTED_EDGE ( 'NONE', *, *, #100675, .F. ) ;
#28644=CARTESIAN_POINT ( 'NONE',  ( 9.480175724453529185, 12.08329098332774265, 1.599625672291279388 ) ) ;
#28647=CARTESIAN_POINT ( 'NONE',  ( -4.771579997005698459, 7.654261532226910525, -1.199719254218452047 ) ) ;
#28651=CARTESIAN_POINT ( 'NONE',  ( 7.892817981449907982, 12.36003807833360391, 0.7998128361456462443 ) ) ;
#28653=CARTESIAN_POINT ( 'NONE',  ( 7.391166297744269365, 11.77477778067701664, 1.040834085586084257E-14 ) ) ;
#28654=CARTESIAN_POINT ( 'NONE',  ( 4.888763274855682184, 4.911624973226616397, -0.7238686217227735531 ) ) ;
#28657=CARTESIAN_POINT ( 'NONE',  ( -2.117044542028253318, 5.621635732341564662, -0.7998128361456281477 ) ) ;
#28660=CARTESIAN_POINT ( 'NONE',  ( -7.694415870955439551, 8.935572256658169010, 1.199719254218462483 ) ) ;
#28663=AXIS2_PLACEMENT_3D ( 'NONE', #103076, #201605, #185370 ) ;
#28665=CARTESIAN_POINT ( 'NONE',  ( -6.126391799051042142, 6.003160260013642890, 0.2011063304240209848 ) ) ;
#28666=CARTESIAN_POINT ( 'NONE',  ( 0.6823417656249882723, 1.426041667008083547, -1.181850606188749264 ) ) ;
#28669=CARTESIAN_POINT ( 'NONE',  ( 6.968527767744093993, 10.11340424813470662, 1.082531754730558626 ) ) ;
#28685=CARTESIAN_POINT ( 'NONE',  ( 7.411503528164766763, 11.79850454950093841, 1.040834085586084257E-14 ) ) ;
#28689=CARTESIAN_POINT ( 'NONE',  ( -4.731959306369413198, 5.479372931307791461, -1.199719254218446718 ) ) ;
#28690=CARTESIAN_POINT ( 'NONE',  ( -8.355902744723985975, 8.642974711799791265, 1.040834085586084257E-14 ) ) ;
#28695=CARTESIAN_POINT ( 'NONE',  ( 0.7499999999999920064, 4.764583334016150751, 1.299038105676669330 ) ) ;
#28696=CARTESIAN_POINT ( 'NONE',  ( 8.697719238366680372, 10.10609285197134533, 1.199719254218462483 ) ) ;
#28700=CARTESIAN_POINT ( 'NONE',  ( -8.701635661872465732, 9.046329781806354831, 1.040834085586084257E-14 ) ) ;
#28702=CARTESIAN_POINT ( 'NONE',  ( -0.6823417656250212460, 3.801041667008085767, 1.181850606188767472 ) ) ;
#28705=CARTESIAN_POINT ( 'NONE',  ( -3.741687207247254676, 7.309126141856352454, 1.040834085586084257E-14 ) ) ;
#28707=CARTESIAN_POINT ( 'NONE',  ( -7.998947442382709383, 12.27592974951444660, 0.7216878364870478180 ) ) ;
#28711=CARTESIAN_POINT ( 'NONE',  ( -1.201851678989727383E-14, 3.384375000341421469, 1.575800808251672791 ) ) ;
#28718=CARTESIAN_POINT ( 'NONE',  ( -1.201851678989727383E-14, 3.446875000341421469, -1.575800808251660134 ) ) ;
#28721=CARTESIAN_POINT ( 'NONE',  ( -5.063080299699540987, 7.994345218703034384, 1.199719254218464037 ) ) ;
#28722=CARTESIAN_POINT ( 'NONE',  ( 6.425674737872927089, 9.584038729905381970, -1.199719254218440723 ) ) ;
#28725=CARTESIAN_POINT ( 'NONE',  ( -1.364683531249997417, 3.821875000341416584, 1.214306433183764966E-14 ) ) ;
#28728=CARTESIAN_POINT ( 'NONE',  ( 1.364683531249986537, -0.3447916663252443836, -0.7879004041258309554 ) ) ;
#28729=CARTESIAN_POINT ( 'NONE',  ( -4.772106882330241717, 5.630174786549132726, -1.082531754730544860 ) ) ;
#28733=CARTESIAN_POINT ( 'NONE',  ( 4.446711195602238931, 6.210915699667823198, -1.443375672974051449 ) ) ;
#28736=CARTESIAN_POINT ( 'NONE',  ( -8.362681821530818738, 8.650883634741092010, -0.7998128361456291469 ) ) ;
#28737=CARTESIAN_POINT ( 'NONE',  ( -9.680158490477310806, 10.39586578175276266, 0.7216878364870438212 ) ) ;
#28739=CARTESIAN_POINT ( 'NONE',  ( -0.7500000000000215383, 4.941666666666684193, 1.299038105676671107 ) ) ;
#28744=CARTESIAN_POINT ( 'NONE',  ( -5.707619481228814351, 9.602713794834864203, -0.7216878364870207285 ) ) ;
#28746=CARTESIAN_POINT ( 'NONE',  ( 1.364683531249986537, -0.5739583329919174526, 0.7879004041258500513 ) ) ;
#28759=CARTESIAN_POINT ( 'NONE',  ( -1.402160292154681736E-14, -0.5374999999999753308, 1.732050807568877637 ) ) ;
#28760=CARTESIAN_POINT ( 'NONE',  ( 7.090551149822722721, 11.21613407486112379, 0.7216878364870438212 ) ) ;
#28770=CARTESIAN_POINT ( 'NONE',  ( 6.823831386379729302, 6.855558127064808716, -0.7998128361456281477 ) ) ;
#28771=CARTESIAN_POINT ( 'NONE',  ( -3.418627288940168096, 7.140148937072163804, -0.7998128361456281477 ) ) ;
#28775=CARTESIAN_POINT ( 'NONE',  ( -1.201851678989727383E-14, 1.634375000341421025, 1.575800808251672791 ) ) ;
#28777=CARTESIAN_POINT ( 'NONE',  ( -9.104463846776669200, 10.58062822844965645, -1.199719254218441611 ) ) ;
#28785=B_SPLINE_CURVE_WITH_KNOTS ( 'NONE', 3,
 ( #56690, #57753, #140096, #136880, #123913, #120698, #40452, #54551, #206123, #152059 ),
 .UNSPECIFIED., .F., .F.,
 ( 4, 2, 2, 2, 4 ),
 ( 0.000000000000000000, 0.0003777850654088144890, 0.0007555701308176289779, 0.001133355196226443467, 0.001511140261635257956 ),
 .UNSPECIFIED. ) ;
#28792=CARTESIAN_POINT ( 'NONE',  ( 2.288037425052380058, 5.553570322680376314, 0.4296897185159433974 ) ) ;
#28795=CARTESIAN_POINT ( 'NONE',  ( 6.388916700537700777, 8.476822122092563916, 1.599625672291281386 ) ) ;
#28801=CARTESIAN_POINT ( 'NONE',  ( 8.769426429940780920, 9.125419011219408461, 0.7998128361456462443 ) ) ;
#28804=CARTESIAN_POINT ( 'NONE',  ( 9.260382613333817403, 10.76253345609967660, -1.199719254218446718 ) ) ;
#28810=ORIENTED_EDGE ( 'NONE', *, *, #120432, .F. ) ;
#28811=CARTESIAN_POINT ( 'NONE',  ( -1.499999999999997780, 6.344000000000043826, -2.958666666666662337 ) ) ;
#28813=CARTESIAN_POINT ( 'NONE',  ( -0.004619473214107579565, 7.151453204069600389, 1.999995854215794511 ) ) ;
#28818=CARTESIAN_POINT ( 'NONE',  ( -9.829298180227631576, 10.56986208646148384, 1.040834085586084257E-14 ) ) ;
#28823=CARTESIAN_POINT ( 'NONE',  ( 4.798696304233017074, 7.685897223992134819, -1.199719254218452047 ) ) ;
#28828=CARTESIAN_POINT ( 'NONE',  ( 4.053524740361575063, 4.791828954252362216, -1.082531754730543083 ) ) ;
#28832=ORIENTED_EDGE ( 'NONE', *, *, #186592, .T. ) ;
#28837=CARTESIAN_POINT ( 'NONE',  ( -6.205881626753225966, 8.263281202677319470, 1.599625672291283607 ) ) ;
#28839=CARTESIAN_POINT ( 'NONE',  ( -2.300079615812729905, 5.835176651756807331, -0.7998128361456281477 ) ) ;
#28844=CARTESIAN_POINT ( 'NONE',  ( 0.006800380015298257419, 7.009756401597622144, -1.999988438674496383 ) ) ;
#28847=CARTESIAN_POINT ( 'NONE',  ( 6.449928391799196525, 8.548002428564306143, -1.599625672291262513 ) ) ;
#28859=ORIENTED_EDGE ( 'NONE', *, *, #99914, .T. ) ;
#28861=CARTESIAN_POINT ( 'NONE',  ( 0.6823417656249882723, -0.01145833299191073573, -1.181850606188749264 ) ) ;
#28863=CARTESIAN_POINT ( 'NONE',  ( 2.842405760359353106, 6.467890487061221272, -0.7998128361456291469 ) ) ;
#28865=CARTESIAN_POINT ( 'NONE',  ( -6.236387472606153892, 8.298871356172400127, -1.443375672974059665 ) ) ;
#28866=CARTESIAN_POINT ( 'NONE',  ( 5.517805331081858888, 5.539787095791365523, 1.040834085586084257E-14 ) ) ;
#28869=CARTESIAN_POINT ( 'NONE',  ( -7.415946836550729948, 9.675023947441092176, 1.443375672974090751 ) ) ;
#28873=CARTESIAN_POINT ( 'NONE',  ( 6.661133543015731462, 6.665743976473484267, -0.7998128361456281477 ) ) ;
#28880=CARTESIAN_POINT ( 'NONE',  ( -1.364683531250010295, 5.238541667008086655, -0.7879004041258300672 ) ) ;
#28885=CARTESIAN_POINT ( 'NONE',  ( 5.472687561410540802, 9.536552588287639409, 0.7998128361456462443 ) ) ;
#28887=VECTOR ( 'NONE', #23320, 999.9999999999998863 ) ;
#28889=CARTESIAN_POINT ( 'NONE',  ( -6.852756576703439961, 10.08230087520760954, 1.199719254218453823 ) ) ;
#28894=CARTESIAN_POINT ( 'NONE',  ( 7.130698725783555680, 10.40656671580112658, 1.199719254218460707 ) ) ;
#28897=CARTESIAN_POINT ( 'NONE',  ( -8.202846631467911820, 9.528741477256060577, 1.199719254218462483 ) ) ;
#28899=CARTESIAN_POINT ( 'NONE',  ( 8.066738210006692000, 8.513542121203711233, 0.7216878364870458196 ) ) ;
#28900=CARTESIAN_POINT ( 'NONE',  ( 4.046752668985390322, 7.764364035880440440, -0.4786816536347000550 ) ) ;
#28901=CARTESIAN_POINT ( 'NONE',  ( -9.815740026613967828, 10.55404424057886636, -0.7216878364870267237 ) ) ;
#28906=CARTESIAN_POINT ( 'NONE',  ( 5.286789834324991055, 8.255339675766103724, -1.199719254218452935 ) ) ;
#28908=CARTESIAN_POINT ( 'NONE',  ( 8.218213668177886788, 12.73966637951625813, 0.7998128361456462443 ) ) ;
#28909=CARTESIAN_POINT ( 'NONE',  ( -4.525130642185515306, 7.025754810433701536, 1.158151338111103046 ) ) ;
#28910=CARTESIAN_POINT ( 'NONE',  ( 3.551346171775753735, 6.230655402791975384, 1.199719254218462483 ) ) ;
#28912=CARTESIAN_POINT ( 'NONE',  ( -6.317736394288148816, 8.393778431468064127, 1.443375672974078761 ) ) ;
#28918=CARTESIAN_POINT ( 'NONE',  ( -4.322081814030608982, 7.236479734952984799, 0.9908985150933833363 ) ) ;
#28919=CARTESIAN_POINT ( 'NONE',  ( 0.6823417656249882723, 0.7385416670080829915, -1.181850606188749264 ) ) ;
#28922=CARTESIAN_POINT ( 'NONE',  ( 3.714570900464269076, 7.277490450609545469, 0.7216878364870298324 ) ) ;
#28926=CARTESIAN_POINT ( 'NONE',  ( -8.148087131688679818, 12.44992605370473804, -0.7216878364870267237 ) ) ;
#28932=CARTESIAN_POINT ( 'NONE',  ( -9.286972035236635392, 9.937148250638648150, -0.7216878364870267237 ) ) ;
#28939=CARTESIAN_POINT ( 'NONE',  ( -8.798878505144658746, 10.32807501316600884, -1.082531754730543083 ) ) ;
#28943=CARTESIAN_POINT ( 'NONE',  ( -1.364683531249997417, 5.821875000341418804, 1.214306433183764966E-14 ) ) ;
#28944=CARTESIAN_POINT ( 'NONE',  ( 0.7499999999999902300, 3.764583334016149863, 1.299038105676669330 ) ) ;
#28945=CARTESIAN_POINT ( 'NONE',  ( 4.912861335034773624, 6.872882102868723919, -1.423633489635463878 ) ) ;
#28950=CARTESIAN_POINT ( 'NONE',  ( -8.179646747746328828, 8.437342715325849341, -0.7998128361456291469 ) ) ;
#28951=CARTESIAN_POINT ( 'NONE',  ( -1.499999999999997780, 6.280000000000042881, -2.499999999999995115 ) ) ;
#28954=CARTESIAN_POINT ( 'NONE',  ( 4.660252114795294887, 6.460046772059735432, -1.599625672291256295 ) ) ;
#28959=CARTESIAN_POINT ( 'NONE',  ( 7.904567251967224095, 9.180748867838630645, 1.199719254218462483 ) ) ;
#28960=CARTESIAN_POINT ( 'NONE',  ( 1.499999999999990896, 3.556250000682818602, 1.214306433183764966E-14 ) ) ;
#28968=CARTESIAN_POINT ( 'NONE',  ( -7.076992996653451939, 7.358839372291564374, 0.7216878364870317197 ) ) ;
#28974=DIRECTION ( 'NONE',  ( 0.7592566023653005702, 0.6507913734559639396, 0.000000000000000000 ) ) ;
#28978=CARTESIAN_POINT ( 'NONE',  ( -8.319899820280397762, 12.85830022363583147, -0.7998128361456281477 ) ) ;
#28980=CARTESIAN_POINT ( 'NONE',  ( 8.666686507633574621, 11.13422023037111330, 1.599625672291281386 ) ) ;
#28981=CARTESIAN_POINT ( 'NONE',  ( -1.402160292154681736E-14, -0.03749999999998095135, 1.732050807568877637 ) ) ;
#28982=CARTESIAN_POINT ( 'NONE',  ( -7.669108446824431269, 12.09904362127053545, -0.7998128361456291469 ) ) ;
#28985=CARTESIAN_POINT ( 'NONE',  ( -1.364683531250010295, 3.780208333674750953, 0.7879004041258379498 ) ) ;
#28986=CARTESIAN_POINT ( 'NONE',  ( 10.38518247838791986, 11.21839376764850726, 0.7216878364870438212 ) ) ;
#28989=CARTESIAN_POINT ( 'NONE',  ( 1.499999999999987121, 4.545833333333352932, -0.8660254037844323793 ) ) ;
#28992=CARTESIAN_POINT ( 'NONE',  ( 7.578644679914694926, 11.78557652663510424, 0.7216878364870438212 ) ) ;
#28995=CARTESIAN_POINT ( 'NONE',  ( -6.887178846062128379, 7.137389529935019183, -0.7216878364870278340 ) ) ;
#28996=CARTESIAN_POINT ( 'NONE',  ( 1.364683531249986537, 0.6552083336747522857, -0.7879004041258239610 ) ) ;
#29000=CARTESIAN_POINT ( 'NONE',  ( -6.561256274009600986, 9.742217188731485678, -1.199719254218440723 ) ) ;
#29001=CARTESIAN_POINT ( 'NONE',  ( -4.134873662043608178, 4.886736029548026217, 1.082531754730558626 ) ) ;
#29002=CARTESIAN_POINT ( 'NONE',  ( 0.6823417656249899377, 4.738541667008086655, -1.181850606188754593 ) ) ;
#29008=CARTESIAN_POINT ( 'NONE',  ( 9.531545685607134999, 11.07889037375188401, 1.199719254218450271 ) ) ;
#29012=CARTESIAN_POINT ( 'NONE',  ( -0.07118442604936793539, 7.078193277237627257, -2.121339347286375965 ) ) ;
#29016=CARTESIAN_POINT ( 'NONE',  ( 8.374132434735052755, 12.92157160716627295, -0.7998128361456352531 ) ) ;
#29022=CARTESIAN_POINT ( 'NONE',  ( 7.567422294721922960, 11.98040977715095323, 0.7998128361456462443 ) ) ;
#29023=CARTESIAN_POINT ( 'NONE',  ( -1.541006503187426269, 8.695732182938039401, 2.510084419394989386 ) ) ;
#29025=CONICAL_SURFACE ( 'NONE', #184688, 1.219999999999999751, 0.7853981633974463916 ) ;
#29027=CARTESIAN_POINT ( 'NONE',  ( -1.602468905319636405E-14, -1.053124999658583638, -1.575800808251665908 ) ) ;
#29030=ADVANCED_FACE ( 'NONE', ( #180907 ), #47746, .F. ) ;
#29032=CARTESIAN_POINT ( 'NONE',  ( 7.853197290813620945, 10.18514947741448573, 1.599625672291281386 ) ) ;
#29035=CARTESIAN_POINT ( 'NONE',  ( -0.6823417656250212460, 3.301041667008085323, 1.181850606188767472 ) ) ;
#29037=CARTESIAN_POINT ( 'NONE',  ( -6.887178846062123938, 8.097758744236356776, -1.082531754730544860 ) ) ;
#29046=CARTESIAN_POINT ( 'NONE',  ( 9.074484886248265880, 9.481320543578137361, 0.7998128361456462443 ) ) ;
#29047=CARTESIAN_POINT ( 'NONE',  ( 5.738979324002048799, 5.917037536914529383, -2.440165351833862850 ) ) ;
#29052=CARTESIAN_POINT ( 'NONE',  ( -9.001723924469462901, 12.58942944760136484, -1.199719254218446718 ) ) ;
#29053=CARTESIAN_POINT ( 'NONE',  ( 7.006866460164219212, 7.069099046480051385, -0.7998128361456281477 ) ) ;
#29056=CARTESIAN_POINT ( 'NONE',  ( 4.253507506385319381, 5.985511395581417204, 1.599625672291267398 ) ) ;
#29063=VECTOR ( 'NONE', #81964, 1000.000000000000000 ) ;
#29064=CARTESIAN_POINT ( 'NONE',  ( -6.236387472606153892, 8.298871356172400127, -1.443375672974059665 ) ) ;
#29065=CARTESIAN_POINT ( 'NONE',  ( 3.388648328411762556, 6.040841252200647382, 1.199719254218462483 ) ) ;
#29068=CARTESIAN_POINT ( 'NONE',  ( -7.426115451983156923, 9.686887332112256388, -1.599625672291263179 ) ) ;
#29074=CARTESIAN_POINT ( 'NONE',  ( -7.974166903131914452, 12.45494515362926435, -0.7998128361456281477 ) ) ;
#29078=CARTESIAN_POINT ( 'NONE',  ( 6.448874621594486989, 10.67543749183559143, 0.7998128361456462443 ) ) ;
#29080=CARTESIAN_POINT ( 'NONE',  ( 6.311484202361478779, 7.322151976631905868, -1.199719254218446718 ) ) ;
#29083=ORIENTED_EDGE ( 'NONE', *, *, #76301, .T. ) ;
#29090=CARTESIAN_POINT ( 'NONE',  ( -4.138764970217294170, 3.930906674782672194, 0.2071306710573931620 ) ) ;
#29092=CARTESIAN_POINT ( 'NONE',  ( -8.667740277838301921, 9.006785167099828016, -0.7998128361456291469 ) ) ;
#29096=CARTESIAN_POINT ( 'NONE',  ( 7.619319141200072920, 7.991553207595983643, 0.7216878364870317197 ) ) ;
#29098=CARTESIAN_POINT ( 'NONE',  ( -5.612712406377478480, 5.650512016969688744, 0.7216878364870735751 ) ) ;
#29100=CARTESIAN_POINT ( 'NONE',  ( -6.250472511100020334, 7.250971670160158311, 1.199719254218450271 ) ) ;
#29104=CARTESIAN_POINT ( 'NONE',  ( -1.484505139761352455, 7.334797934598009661, -4.257182005874962094 ) ) ;
#29110=CARTESIAN_POINT ( 'NONE',  ( 3.999470987966422086, 7.812499711282003823, 0.08775337862014347123 ) ) ;
#29111=CARTESIAN_POINT ( 'NONE',  ( 8.589254009457354400, 9.979550084910457031, -1.199719254218446718 ) ) ;
#29113=CARTESIAN_POINT ( 'NONE',  ( -2.629918611371007575, 6.012062780000711371, 0.7216878364870317197 ) ) ;
#29115=CARTESIAN_POINT ( 'NONE',  ( -5.486276195386677657, 6.266678140956847720, -0.9979454321464575894 ) ) ;
#29121=CARTESIAN_POINT ( 'NONE',  ( 2.737856954955798727, 5.281584649835344258, 1.199719254218452047 ) ) ;
#29128=CARTESIAN_POINT ( 'NONE',  ( 4.162516854595432747, 4.815023404238158555, 1.199719254218464037 ) ) ;
#29132=CARTESIAN_POINT ( 'NONE',  ( -1.364683531250012516, 3.342708333674756727, 0.7879004041258379498 ) ) ;
#29137=CARTESIAN_POINT ( 'NONE',  ( 5.636439174979242850, 7.598931675607687453, -1.599625672291262513 ) ) ;
#29142=CARTESIAN_POINT ( 'NONE',  ( -4.843287188579803448, 6.673587691474970107, -1.599625672291256295 ) ) ;
#29143=CARTESIAN_POINT ( 'NONE',  ( 5.463572716182824252, 7.397254140345190798, 1.443375672974062551 ) ) ;
#29144=CARTESIAN_POINT ( 'NONE',  ( -1.499999999999997780, 3.900000000000021672, 1.214306433183764966E-14 ) ) ;
#29146=CARTESIAN_POINT ( 'NONE',  ( -3.978428010606240850, 6.728917548094202949, -1.199719254218452047 ) ) ;
#29147=CARTESIAN_POINT ( 'NONE',  ( -0.006768871532362320982, 8.210909518262125673, -2.038649385027043071 ) ) ;
#29149=CARTESIAN_POINT ( 'NONE',  ( -1.201851678989727383E-14, 3.946875000341423689, -1.575800808251660134 ) ) ;
#29152=CARTESIAN_POINT ( 'NONE',  ( -3.958617665510279160, 5.641473247893851628, -1.443375672974053447 ) ) ;
#29157=CARTESIAN_POINT ( 'NONE',  ( 3.517450787741589036, 6.191110788085444128, -1.199719254218446718 ) ) ;
#29159=CARTESIAN_POINT ( 'NONE',  ( 0.5972946108512422470, 6.677937114322130441, -3.537249485762780310 ) ) ;
#29160=CARTESIAN_POINT ( 'NONE',  ( 1.364683531249990311, 4.696875000341417916, 1.214306433183764966E-14 ) ) ;
#29162=CARTESIAN_POINT ( 'NONE',  ( 3.823036129373602154, 6.443664003369091731, -1.082531754730548412 ) ) ;
#29164=CARTESIAN_POINT ( 'NONE',  ( -1.402160292154681736E-14, 1.259375000341419248, -1.575800808251659024 ) ) ;
#29168=CARTESIAN_POINT ( 'NONE',  ( -9.972185678051314284, 11.59297036493672017, 1.199719254218462483 ) ) ;
#29169=EDGE_CURVE ( 'NONE', #71915, #192824, #118494, .T. ) ;
#29170=CARTESIAN_POINT ( 'NONE',  ( -7.510853911846401942, 7.865010440016681592, 1.040834085586084257E-14 ) ) ;
#29174=CARTESIAN_POINT ( 'NONE',  ( 1.364683531249990311, 4.863541667008084879, 0.7879004041258500513 ) ) ;
#29183=CARTESIAN_POINT ( 'NONE',  ( -5.043269954159181445, 8.827639346586952485, 1.214306433183764966E-14 ) ) ;
#29189=CARTESIAN_POINT ( 'NONE',  ( -5.544921637864833386, 7.492161215640853023, -1.443375672974051449 ) ) ;
#29193=( BOUNDED_CURVE ( )  B_SPLINE_CURVE ( 2, ( #114272, #162961, #80637, #146729, #130526 ),
 .UNSPECIFIED., .F., .T. ) 
 B_SPLINE_CURVE_WITH_KNOTS ( ( 3, 2, 3 ),
 ( 0.1113702160535958580, 0.1125000000000000028, 0.1138193015819521647 ),
 .UNSPECIFIED. ) 
 CURVE ( )  GEOMETRIC_REPRESENTATION_ITEM ( )  RATIONAL_B_SPLINE_CURVE ( ( 0.9470460506485154362, 0.9636730364727235099, 1.000000000000000000, 0.9575793047851379747, 0.9420221409164253323 ) ) 
 REPRESENTATION_ITEM ( '' )  );
#29199=ORIENTED_EDGE ( 'NONE', *, *, #81687, .F. ) ;
#29202=CARTESIAN_POINT ( 'NONE',  ( 0.2498445108307164875, 7.025621425018297117, -3.913348414359987704 ) ) ;
#29203=CARTESIAN_POINT ( 'NONE',  ( -3.730464822054482710, 7.503959392372201442, 1.040834085586084257E-14 ) ) ;
#29206=CARTESIAN_POINT ( 'NONE',  ( 0.7499999999999885647, 1.316666666666688190, -1.299038105676652899 ) ) ;
#29208=CARTESIAN_POINT ( 'NONE',  ( 8.595506201384004896, 12.01154575404795466, 1.082531754730546636 ) ) ;
#29209=CARTESIAN_POINT ( 'NONE',  ( 5.933664784275179294, 10.07435934829639912, -0.7998128361456291469 ) ) ;
#29212=EDGE_LOOP ( 'NONE', ( #53456, #56487, #144213, #37866 ) ) ;
#29213=CARTESIAN_POINT ( 'NONE',  ( -0.1263102688159843667, 6.427441598446242743, 3.069922131261606513 ) ) ;
#29214=CARTESIAN_POINT ( 'NONE',  ( 4.168242161197552420, 6.950367390450747251, -1.199719254218452047 ) ) ;
#29215=CARTESIAN_POINT ( 'NONE',  ( -0.2638905955354677868, 7.233311467405415307, -1.984662505942582422 ) ) ;
#29222=CARTESIAN_POINT ( 'NONE',  ( -5.063080299699540987, 7.994345218703034384, 1.199719254218464037 ) ) ;
#29225=CARTESIAN_POINT ( 'NONE',  ( 5.946383829937739840, 4.757679660029577207, -2.499999999999690470 ) ) ;
#29229=CARTESIAN_POINT ( 'NONE',  ( 1.364683531249990311, 2.884375000341422801, 1.214306433183764966E-14 ) ) ;
#29230=CARTESIAN_POINT ( 'NONE',  ( 7.402388682937041331, 11.57994453016116587, 1.040834085586084257E-14 ) ) ;
#29231=CARTESIAN_POINT ( 'NONE',  ( -7.725448601688521322, 7.907444878258402809, 1.040834085586084257E-14 ) ) ;
#29234=CARTESIAN_POINT ( 'NONE',  ( 7.006866460164219212, 7.069099046480051385, -0.7998128361456281477 ) ) ;
#29235=CARTESIAN_POINT ( 'NONE',  ( -5.819474248763749635, 7.812472595022922128, -1.599625672291256295 ) ) ;
#29239=CARTESIAN_POINT ( 'NONE',  ( 1.499999999999987121, 0.7854166673494828999, 0.8660254037844524744 ) ) ;
#29243=CARTESIAN_POINT ( 'NONE',  ( 7.619319141200070256, 8.951922421897323900, 1.082531754730558626 ) ) ;
#29246=CARTESIAN_POINT ( 'NONE',  ( 1.364683531249988535, 1.926041667008086211, 0.7879004041258500513 ) ) ;
#29248=CARTESIAN_POINT ( 'NONE',  ( 5.951666246274803562, 7.006327377817825663, 1.082531754730558626 ) ) ;
#29250=CARTESIAN_POINT ( 'NONE',  ( -4.460269349215930212, 4.305995116947750390, 1.214306433183764966E-14 ) ) ;
#29258=CARTESIAN_POINT ( 'NONE',  ( -3.976064435573588796, 7.848781721302746206, 0.05846302465613295585 ) ) ;
#29264=CARTESIAN_POINT ( 'NONE',  ( 5.849453209292126310, 8.911780279894442103, 1.199719254218462483 ) ) ;
#29267=CARTESIAN_POINT ( 'NONE',  ( 4.090809663021327758, 5.795697244990093644, 1.599625672291267398 ) ) ;
#29275=CARTESIAN_POINT ( 'NONE',  ( 4.202664430556247055, 6.886563688082179446, 1.082531754730558626 ) ) ;
#29277=CARTESIAN_POINT ( 'NONE',  ( 1.364683531249986537, 2.217708333674751398, -0.7879004041258239610 ) ) ;
#29278=CARTESIAN_POINT ( 'NONE',  ( 7.377608144130607393, 11.75895993479440982, -0.7998128361456291469 ) ) ;
#29279=CARTESIAN_POINT ( 'NONE',  ( -1.420000000000001039, 6.200000000000045475, -2.873333333333329520 ) ) ;
#29283=CARTESIAN_POINT ( 'NONE',  ( -0.7500000000000215383, 1.691666666666688634, 1.299038105676659116 ) ) ;
#29284=CARTESIAN_POINT ( 'NONE',  ( 5.931855901178834323, 6.879252291918818152, 1.199719254218462483 ) ) ;
#29285=CARTESIAN_POINT ( 'NONE',  ( -5.865874016206865882, 9.995270118883347266, 0.000000000000000000 ) ) ;
#29288=CARTESIAN_POINT ( 'NONE',  ( 5.477130869796502211, 5.492333557625114437, 1.040834085586084257E-14 ) ) ;
#29289=CARTESIAN_POINT ( 'NONE',  ( 1.364683531249986537, 2.155208333674751398, -0.7879004041258239610 ) ) ;
#29291=CARTESIAN_POINT ( 'NONE',  ( 0.7499999999999885647, 3.316666666666689967, -1.299038105676658228 ) ) ;
#29293=CARTESIAN_POINT ( 'NONE',  ( 3.063252641683779753, 5.661212951017999373, 1.199719254218450271 ) ) ;
#29298=CARTESIAN_POINT ( 'NONE',  ( -1.500000000000013101, 0.4520833340161533598, 0.8660254037844403729 ) ) ;
#29300=CARTESIAN_POINT ( 'NONE',  ( -6.235860587281615075, 9.362588887548838557, -1.199719254218440723 ) ) ;
#29301=CARTESIAN_POINT ( 'NONE',  ( -3.253593677599670109, 5.779314476299451719, 1.082531754730560403 ) ) ;
#29307=ORIENTED_EDGE ( 'NONE', *, *, #183234, .F. ) ;
#29309=CARTESIAN_POINT ( 'NONE',  ( 6.043183783389218355, 8.073467052085995022, 1.599625672291267398 ) ) ;
#29313=CARTESIAN_POINT ( 'NONE',  ( 5.309989718046547402, 9.346738437696316737, 0.7998128361456462443 ) ) ;
#29318=CARTESIAN_POINT ( 'NONE',  ( -6.566226467720086113, 6.555019055295208119, 1.040834085586084257E-14 ) ) ;
#29320=CARTESIAN_POINT ( 'NONE',  ( 2.706824224222692088, 6.309712028235118453, 0.7998128361456362523 ) ) ;
#29326=CARTESIAN_POINT ( 'NONE',  ( 4.196871964084724738, 7.339766560697110975, 0.8424661700066529146 ) ) ;
#29333=LINE ( 'NONE', #78071, #133470 ) ;
#29336=CARTESIAN_POINT ( 'NONE',  ( -4.105300466841341311, 3.978332001433686926, 0.4115170502265364516 ) ) ;
#29338=CARTESIAN_POINT ( 'NONE',  ( 6.629573927402440781, 10.67832731537079383, 1.040834085586084257E-14 ) ) ;
#29340=CARTESIAN_POINT ( 'NONE',  ( -4.055860508782465068, 7.883587693554856557, 1.040834085586084257E-14 ) ) ;
#29341=CARTESIAN_POINT ( 'NONE',  ( 6.938893903907228378E-15, 10.64264068711930733, 1.214306433183764966E-14 ) ) ;
#29345=CARTESIAN_POINT ( 'NONE',  ( -5.194745412330402878, 9.212286747694129474, 0.000000000000000000 ) ) ;
#29361=CARTESIAN_POINT ( 'NONE',  ( -6.227272627378437342, 6.159572908229946187, -0.7998128361456291469 ) ) ;
#29364=CARTESIAN_POINT ( 'NONE',  ( 2.711267533052988732, 6.106969855296372707, -0.7216878364870267237 ) ) ;
#29368=FACE_OUTER_BOUND ( 'NONE', #145751, .T. ) ;
#29369=CARTESIAN_POINT ( 'NONE',  ( -4.762992037102518950, 4.451245552908022596, -0.7998128361456221525 ) ) ;
#29373=CARTESIAN_POINT ( 'NONE',  ( 9.728138913005292210, 11.30824913904973705, -1.199719254218440723 ) ) ;
#29376=CARTESIAN_POINT ( 'NONE',  ( -7.823218330285243383, 9.085841792542966644, -1.199719254218446718 ) ) ;
#29377=CARTESIAN_POINT ( 'NONE',  ( 4.449046963578762615, 8.342305224150557308, -0.7998128361456231517 ) ) ;
#29380=CARTESIAN_POINT ( 'NONE',  ( 4.053524740805938720, 3.831459740469437936, 1.214306433183764966E-14 ) ) ;
#29384=CARTESIAN_POINT ( 'NONE',  ( 1.364683531249986537, 0.7177083336747527298, -0.7879004041258239610 ) ) ;
#29387=CARTESIAN_POINT ( 'NONE',  ( 8.446366511633696561, 8.956441806435218922, 1.040834085586084257E-14 ) ) ;
#29388=ORIENTED_EDGE ( 'NONE', *, *, #103873, .F. ) ;
#29396=CARTESIAN_POINT ( 'NONE',  ( 3.701012746850603996, 7.261672604726938651, 1.040834085586084257E-14 ) ) ;
#29402=LINE ( 'NONE', #81340, #191209 ) ;
#29405=CARTESIAN_POINT ( 'NONE',  ( 1.284279953904126748, 10.64264068711930733, 0.7750000000000013545 ) ) ;
#29420=CARTESIAN_POINT ( 'NONE',  ( -0.7500000000000215383, 1.722916667349486008, 1.299038105676659116 ) ) ;
#29426=DIRECTION ( 'NONE',  ( 0.000000000000000000, 0.000000000000000000, 1.000000000000000000 ) ) ;
#29427=CARTESIAN_POINT ( 'NONE',  ( 8.751951852821344247, 10.16936423550178503, -1.199719254218446718 ) ) ;
#29431=CARTESIAN_POINT ( 'NONE',  ( 3.277320446201373638, 4.846626492033466072, 1.599625672291267398 ) ) ;
#29432=CARTESIAN_POINT ( 'NONE',  ( -5.694061328059534688, 8.626526735169329996, 1.082531754730548412 ) ) ;
#29436=CARTESIAN_POINT ( 'NONE',  ( -5.533699252672048985, 9.607732894759390518, -0.7998128361456231517 ) ) ;
#29440=CARTESIAN_POINT ( 'NONE',  ( 1.499999999999989120, 1.806250000682817269, 0.000000000000000000 ) ) ;
#29447=CARTESIAN_POINT ( 'NONE',  ( -10.49131193887636826, 11.13428543831092909, 1.040834085586084257E-14 ) ) ;
#29449=CARTESIAN_POINT ( 'NONE',  ( 4.525353972290461435, 6.990290696447242880, 1.167197606177571734 ) ) ;
#29454=CARTESIAN_POINT ( 'NONE',  ( -10.49131193887636826, 11.13428543831092909, 1.040834085586084257E-14 ) ) ;
#29455=CARTESIAN_POINT ( 'NONE',  ( 8.633844893804129228, 8.967240552393299424, -0.7998128361456211532 ) ) ;
#29462=CARTESIAN_POINT ( 'NONE',  ( -7.320512876374914768, 10.62801655815766999, 1.199719254218453823 ) ) ;
#29467=CARTESIAN_POINT ( 'NONE',  ( 5.678167406024951624, 5.518950149984223508, 0.7998128361456341429 ) ) ;
#29473=CARTESIAN_POINT ( 'NONE',  ( -9.592557376868645846, 11.15007068022363157, -1.199719254218441611 ) ) ;
#29476=CARTESIAN_POINT ( 'NONE',  ( -5.904496024515287544, 6.143719773163115683, -0.8530293227379917020 ) ) ;
#29493=CARTESIAN_POINT ( 'NONE',  ( -1.402160292154681736E-14, 0.1187500006828157706, -1.732050807568870754 ) ) ;
#29499=CARTESIAN_POINT ( 'NONE',  ( -4.308793891044708779, 3.921347715840572956, 1.214306433183764966E-14 ) ) ;
#29506=CARTESIAN_POINT ( 'NONE',  ( 5.504247177468186258, 6.484338464210099851, 1.082531754730558626 ) ) ;
#29508=ORIENTED_EDGE ( 'NONE', *, *, #53132, .T. ) ;
#29509=DIRECTION ( 'NONE',  ( -1.000000000000000000, 5.578564026256504688E-16, 1.479114197289397135E-31 ) ) ;
#29511=CARTESIAN_POINT ( 'NONE',  ( 2.358755538653318773, 5.695705861830088423, 1.040834085586084257E-14 ) ) ;
#29520=CARTESIAN_POINT ( 'NONE',  ( -0.6823417656250246877, -0.4489583329919111243, 1.181850606188755259 ) ) ;
#29525=CARTESIAN_POINT ( 'NONE',  ( -3.744022975668147790, 7.519777238254810925, -0.7998128361456281477 ) ) ;
#29526=LINE ( 'NONE', #26303, #177245 ) ;
#29528=CARTESIAN_POINT ( 'NONE',  ( -1.402160292154681736E-14, -0.2874999999999741096, 1.732050807568877637 ) ) ;
#29530=CARTESIAN_POINT ( 'NONE',  ( -1.500000000000011324, 4.879166666666690411, -0.8660254037844313801 ) ) ;
#29538=CARTESIAN_POINT ( 'NONE',  ( -1.201851678989727383E-14, 5.759375000341417028, -1.575800808251660801 ) ) ;
#29540=CARTESIAN_POINT ( 'NONE',  ( 6.311484202361478779, 7.322151976631905868, -1.199719254218446718 ) ) ;
#29541=CARTESIAN_POINT ( 'NONE',  ( -8.636707547105197946, 10.03491254549959777, -1.199719254218446718 ) ) ;
#29543=FACE_OUTER_BOUND ( 'NONE', #79119, .T. ) ;
#29547=CARTESIAN_POINT ( 'NONE',  ( -1.364683531250014514, -0.6572916663252459379, 0.7879004041258379498 ) ) ;
#29552=ORIENTED_EDGE ( 'NONE', *, *, #69670, .F. ) ;
#29556=CARTESIAN_POINT ( 'NONE',  ( 7.958272981541723468, 8.386999354661243800, 1.040834085586084257E-14 ) ) ;
#29560=CARTESIAN_POINT ( 'NONE',  ( 1.499999999999989120, 4.285416667349482900, 0.8660254037844524744 ) ) ;
#29562=CARTESIAN_POINT ( 'NONE',  ( -3.415764635639130020, 6.072476943965863683, 1.199719254218462483 ) ) ;
#29563=CARTESIAN_POINT ( 'NONE',  ( 6.060131475184119765, 9.053608573481392696, -1.082531754730537976 ) ) ;
#29564=CARTESIAN_POINT ( 'NONE',  ( -7.659993601596706725, 11.88048360193076647, -0.7216878364870267237 ) ) ;
#29570=CARTESIAN_POINT ( 'NONE',  ( 4.532503425670185493, 4.182342172903648070, 1.214306433183764966E-14 ) ) ;
#29572=CARTESIAN_POINT ( 'NONE',  ( 3.018661757337009810, 6.673522483535157868, 0.000000000000000000 ) ) ;
#29579=DIRECTION ( 'NONE',  ( -0.6507913734559640506, -0.7592566023653004592, 0.000000000000000000 ) ) ;
#29583=CARTESIAN_POINT ( 'NONE',  ( -0.9486429539237212216, 3.288339070649073381, -1.028101543438966425 ) ) ;
#29587=CARTESIAN_POINT ( 'NONE',  ( 9.915090410295563927, 10.46202698829998567, -0.7998128361456281477 ) ) ;
#29593=CARTESIAN_POINT ( 'NONE',  ( 1.364683531249986537, -0.3864583329919166199, 0.7879004041258500513 ) ) ;
#29594=CARTESIAN_POINT ( 'NONE',  ( 4.799223189557548785, 7.582548906917042864, -1.082531754730549078 ) ) ;
#29596=CARTESIAN_POINT ( 'NONE',  ( -8.514157279702020631, 11.91663867875229776, -1.082531754730543971 ) ) ;
#29601=CARTESIAN_POINT ( 'NONE',  ( -4.437596350374534815, 4.071617251725375475, -0.7998128361456221525 ) ) ;
#29606=ORIENTED_EDGE ( 'NONE', *, *, #146212, .T. ) ;
#29615=CARTESIAN_POINT ( 'NONE',  ( 5.285422529909848066, 6.578444217690160301, -1.363614577128515082 ) ) ;
#29616=DIRECTION ( 'NONE',  ( -5.578564026256490882E-16, -1.000000000000000000, -9.066213480720158442E-32 ) ) ;
#29625=CARTESIAN_POINT ( 'NONE',  ( -7.917598520700757980, 9.299915031314755609, 1.082531754730558626 ) ) ;
#29629=CARTESIAN_POINT ( 'NONE',  ( 6.908042961362778733, 8.018137195466769285, 1.199719254218462483 ) ) ;
#29632=CARTESIAN_POINT ( 'NONE',  ( -4.599240423533815125, 6.388866465587984322, 1.599625672291267398 ) ) ;
#29635=AXIS2_PLACEMENT_3D ( 'NONE', #106432, #135689, #169241 ) ;
#29637=CARTESIAN_POINT ( 'NONE',  ( -3.405069135326500351, 7.124331091189553433, 1.040834085586084257E-14 ) ) ;
#29640=CARTESIAN_POINT ( 'NONE',  ( 4.273844736805816780, 6.009238164405336313, 1.599625672291267398 ) ) ;
#29642=CARTESIAN_POINT ( 'NONE',  ( 9.250740883225924804, 9.686952540052077509, 1.040834085586084257E-14 ) ) ;
#29645=CARTESIAN_POINT ( 'NONE',  ( 4.093767505759832837, 7.703081727663242617, 0.6588811006658854552 ) ) ;
#29646=CARTESIAN_POINT ( 'NONE',  ( 4.365362273920238678, 7.076377838673507448, 1.082531754730558626 ) ) ;
#29653=CARTESIAN_POINT ( 'NONE',  ( 7.578644679914706472, 9.864838098032418401, 1.443375672974076540 ) ) ;
#29656=CARTESIAN_POINT ( 'NONE',  ( -9.996439331977562404, 10.55693406359564790, 0.7998128361456462443 ) ) ;
#29657=CARTESIAN_POINT ( 'NONE',  ( -6.958359152311683893, 9.141171649162195934, -1.599625672291263179 ) ) ;
#29663=FACE_OUTER_BOUND ( 'NONE', #170730, .T. ) ;
#29666=CARTESIAN_POINT ( 'NONE',  ( 7.716561984472250835, 12.15440608185967086, 1.040834085586084257E-14 ) ) ;
#29670=CARTESIAN_POINT ( 'NONE',  ( 2.361091307074211887, 5.906356958228550447, 0.7998128361456462443 ) ) ;
#29673=CARTESIAN_POINT ( 'NONE',  ( -0.7500000000000215383, 5.222916667349482012, 1.299038105676671107 ) ) ;
#29679=CARTESIAN_POINT ( 'NONE',  ( 0.7499999999999902300, 2.483333333333351156, 1.299038105676669330 ) ) ;
#29680=CARTESIAN_POINT ( 'NONE',  ( 5.636439174979242850, 7.598931675607687453, -1.599625672291262513 ) ) ;
#29683=CARTESIAN_POINT ( 'NONE',  ( 7.212574532790092974, 9.437756259720353924, -1.443375672974057666 ) ) ;
#29684=CARTESIAN_POINT ( 'NONE',  ( -10.15469386651127515, 11.90985960142705657, 1.082531754730558626 ) ) ;
#29688=CARTESIAN_POINT ( 'NONE',  ( 9.562578416340237197, 10.05076299535211781, 0.7998128361456462443 ) ) ;
#29691=CARTESIAN_POINT ( 'NONE',  ( -4.762992037102518950, 4.451245552908022596, -0.7998128361456221525 ) ) ;
#29692=B_SPLINE_CURVE_WITH_KNOTS ( 'NONE', 3,
 ( #164537, #49715, #131040, #65930, #132079, #16123, #133137, #148300 ),
 .UNSPECIFIED., .F., .F.,
 ( 4, 2, 2, 4 ),
 ( 2.179219396325681589E-18, 0.0002925934901276173745, 0.0005851869802552325806, 0.001170373960510463426 ),
 .UNSPECIFIED. ) ;
#29693=CARTESIAN_POINT ( 'NONE',  ( 1.499999999999989120, 5.077083334016151639, -0.8660254037844323793 ) ) ;
#29694=CARTESIAN_POINT ( 'NONE',  ( 0.6823417656249899377, 1.092708333674752286, 1.181850606188755259 ) ) ;
#29699=CARTESIAN_POINT ( 'NONE',  ( -1.364683531250010295, 5.801041667008088432, -0.7879004041258300672 ) ) ;
#29709=CARTESIAN_POINT ( 'NONE',  ( -6.714312387265696458, 8.856450423275211037, 1.599625672291283607 ) ) ;
#29712=CARTESIAN_POINT ( 'NONE',  ( 5.355634372598031767, 6.206993841907870291, -1.199719254218445830 ) ) ;
#29716=ORIENTED_EDGE ( 'NONE', *, *, #87363, .F. ) ;
#29721=CARTESIAN_POINT ( 'NONE',  ( -4.055860508782465068, 7.883587693554856557, 1.040834085586084257E-14 ) ) ;
#29725=CARTESIAN_POINT ( 'NONE',  ( 8.890396042259068210, 11.39521468743417998, -1.599625672291257406 ) ) ;
#29727=CARTESIAN_POINT ( 'NONE',  ( 7.404724451357931336, 11.79059562655963056, 0.7998128361456462443 ) ) ;
#29730=CARTESIAN_POINT ( 'NONE',  ( -9.815740026613960723, 11.51441345488021106, -1.082531754730539753 ) ) ;
#29731=CARTESIAN_POINT ( 'NONE',  ( -5.669280788808708671, 9.765911353585494226, 0.7998128361456481317 ) ) ;
#29735=CARTESIAN_POINT ( 'NONE',  ( -6.131331467106510225, 6.000095466447766590, 0.1540833971661673130 ) ) ;
#29736=CARTESIAN_POINT ( 'NONE',  ( -1.364683531250012516, 0.7802083336747528408, 0.7879004041258379498 ) ) ;
#29739=CARTESIAN_POINT ( 'NONE',  ( 6.480434237652121787, 9.543961796360731498, 1.082531754730558626 ) ) ;
#29757=CARTESIAN_POINT ( 'NONE',  ( 10.07100917685271035, 10.64393221595000938, 0.7998128361456462443 ) ) ;
#29759=ORIENTED_EDGE ( 'NONE', *, *, #51124, .T. ) ;
#29761=CARTESIAN_POINT ( 'NONE',  ( -3.086452525405351643, 6.752611712948207057, 0.7998128361456341429 ) ) ;
#29762=CARTESIAN_POINT ( 'NONE',  ( -7.426115451983156923, 9.686887332112256388, -1.599625672291263179 ) ) ;
#29768=CARTESIAN_POINT ( 'NONE',  ( 1.499999999999989120, 4.577083334016148974, -0.8660254037844323793 ) ) ;
#29769=CARTESIAN_POINT ( 'NONE',  ( 9.426996880203592610, 9.892584536526015881, -0.7998128361456281477 ) ) ;
#29773=CARTESIAN_POINT ( 'NONE',  ( -7.557780564614042795, 10.90482886110335414, -1.199719254218446718 ) ) ;
#29775=CARTESIAN_POINT ( 'NONE',  ( -1.364683531249997417, 3.259375000341423245, 1.214306433183764966E-14 ) ) ;
#29778=CARTESIAN_POINT ( 'NONE',  ( -4.650083499362883011, 6.448183387388563226, 1.443375672974064550 ) ) ;
#29780=CARTESIAN_POINT ( 'NONE',  ( -9.056483424248693126, 10.62861408545402675, 1.082531754730558626 ) ) ;
#29785=CARTESIAN_POINT ( 'NONE',  ( 1.364683531249988535, 2.926041667008082658, 0.7879004041258500513 ) ) ;
#29792=CARTESIAN_POINT ( 'NONE',  ( -1.364683531250012516, 2.530208333674753174, 0.7879004041258379498 ) ) ;
#29795=CARTESIAN_POINT ( 'NONE',  ( -5.870844209917351009, 6.808071985447069707, -1.199719254218446718 ) ) ;
#29796=CARTESIAN_POINT ( 'NONE',  ( 7.100719765255169236, 9.307259030929609267, -1.599625672291262513 ) ) ;
#29799=CARTESIAN_POINT ( 'NONE',  ( 1.364683531249990311, 3.196875000341416140, 1.214306433183764966E-14 ) ) ;
#29802=CARTESIAN_POINT ( 'NONE',  ( 0.6823417656249864960, -0.8239583329919114574, -1.181850606188749264 ) ) ;
#29803=CARTESIAN_POINT ( 'NONE',  ( -4.419594888374909658, 8.100018436505289188, 0.7216878364870458196 ) ) ;
#29804=EDGE_CURVE ( 'NONE', #140464, #188755, #170307, .T. ) ;
#29807=CARTESIAN_POINT ( 'NONE',  ( 4.473827502829567315, 7.202920605734387749, -1.082531754730548412 ) ) ;
#29811=CARTESIAN_POINT ( 'NONE',  ( -7.877450944739929461, 9.149113176073413456, 1.199719254218462483 ) ) ;
#29812=CARTESIAN_POINT ( 'NONE',  ( -10.16825202056928390, 10.96530823352674133, 0.7216878364870438212 ) ) ;
#29815=CARTESIAN_POINT ( 'NONE',  ( -0.6823417656250212460, 5.051041667008086655, 1.181850606188767472 ) ) ;
#29820=CARTESIAN_POINT ( 'NONE',  ( -5.517805330637490790, 9.381263952478319013, 0.7216878364870458196 ) ) ;
#29822=CARTESIAN_POINT ( 'NONE',  ( -0.6823417656250246877, -0.3864583329919110688, 1.181850606188755259 ) ) ;
#29835=CARTESIAN_POINT ( 'NONE',  ( 9.883530794237934458, 10.63313346947350269, -0.7216878364870257245 ) ) ;
#29843=CARTESIAN_POINT ( 'NONE',  ( 6.796715079152391148, 6.823922435299587974, 0.7998128361456341429 ) ) ;
#29844=CARTESIAN_POINT ( 'NONE',  ( -5.576481253922474401, 5.400316305864651056, -0.7998128361456221525 ) ) ;
#29849=CARTESIAN_POINT ( 'NONE',  ( 1.364683531249986537, 0.9260416670080896528, 0.7879004041258500513 ) ) ;
#29850=CARTESIAN_POINT ( 'NONE',  ( 6.004977026901663351, 6.084690627017792508, 0.6157370554833795362 ) ) ;
#29851=CARTESIAN_POINT ( 'NONE',  ( -10.08065090696061716, 11.71951313199760136, -1.199719254218441611 ) ) ;
#29869=CARTESIAN_POINT ( 'NONE',  ( 5.469824908109481854, 8.468880595181346393, -1.199719254218446718 ) ) ;
#29875=CARTESIAN_POINT ( 'NONE',  ( 8.015895134177609904, 10.37496362800581018, 1.599625672291281386 ) ) ;
#29876=CARTESIAN_POINT ( 'NONE',  ( -3.094265954482870118, 2.800000000000024691, 2.490342512183699508 ) ) ;
#29878=CARTESIAN_POINT ( 'NONE',  ( 9.480175724453529185, 12.08329098332774265, 1.599625672291279388 ) ) ;
#29880=CARTESIAN_POINT ( 'NONE',  ( -2.103486388414573138, 5.605817886458954291, 1.040834085586084257E-14 ) ) ;
#29884=CARTESIAN_POINT ( 'NONE',  ( 3.987613135628201633, 7.732542241470636846, 0.05202909940443302406 ) ) ;
#29885=CARTESIAN_POINT ( 'NONE',  ( -0.4229270055063389377, 8.019365653748030454, 1.955756443285257218 ) ) ;
#29890=CARTESIAN_POINT ( 'NONE',  ( -7.510853912290736289, 11.70648729774046792, 0.7216878364870458196 ) ) ;
#29894=CARTESIAN_POINT ( 'NONE',  ( 4.476163270806094552, 8.373940915915776273, 0.7998128361456462443 ) ) ;
#29901=CARTESIAN_POINT ( 'NONE',  ( 4.487385655998873624, 7.218738451098584363, 1.082531754730558626 ) ) ;
#29909=CARTESIAN_POINT ( 'NONE',  ( -5.530836599371015794, 8.540060901653093950, 1.199719254218452047 ) ) ;
#29912=CARTESIAN_POINT ( 'NONE',  ( -5.461236948206312114, 5.265864615862458464, 0.7998128361456341429 ) ) ;
#29920=CARTESIAN_POINT ( 'NONE',  ( 6.287230548435207567, 8.358188277972981695, -1.599625672291262513 ) ) ;
#29934=CARTESIAN_POINT ( 'NONE',  ( 1.364683531249986537, 0.4677083336747514530, -0.7879004041258309554 ) ) ;
#29936=CARTESIAN_POINT ( 'NONE',  ( 5.854423403002611437, 5.724582146458163656, 1.040834085586084257E-14 ) ) ;
#29938=CARTESIAN_POINT ( 'NONE',  ( -5.748293942514172805, 8.689798118699771479, -1.082531754730538864 ) ) ;
#29939=CARTESIAN_POINT ( 'NONE',  ( 5.856759171423504107, 5.935233242856626568, -0.7216878364870257245 ) ) ;
#29940=CARTESIAN_POINT ( 'NONE',  ( -7.253248993186740989, 9.485209796849769504, 1.443375672974090751 ) ) ;
#29945=CARTESIAN_POINT ( 'NONE',  ( 6.959412922516382771, 7.013736585890911535, 0.7998128361456341429 ) ) ;
#29950=CARTESIAN_POINT ( 'NONE',  ( -0.6823417656250212460, 4.551041667008086655, 1.181850606188767472 ) ) ;
#29954=CARTESIAN_POINT ( 'NONE',  ( 8.229962938695207342, 9.560377169021284871, 1.199719254218462483 ) ) ;
#29957=CARTESIAN_POINT ( 'NONE',  ( -7.690499447449645309, 9.995335326823163058, 1.599625672291295375 ) ) ;
#29962=CARTESIAN_POINT ( 'NONE',  ( 9.915090410295563927, 10.46202698829998567, -0.7998128361456281477 ) ) ;
#29964=CARTESIAN_POINT ( 'NONE',  ( -6.503107236049161521, 10.73870887536603291, 0.7998128361456481317 ) ) ;
#29968=CARTESIAN_POINT ( 'NONE',  ( 5.458613854904844409, 6.252117202148153474, -1.007154897844428687 ) ) ;
#29969=CARTESIAN_POINT ( 'NONE',  ( -8.785320351975364872, 12.23299559640450518, 1.082531754730560403 ) ) ;
#29974=CARTESIAN_POINT ( 'NONE',  ( 5.438792177376376991, 9.497007973581119700, 1.040834085586084257E-14 ) ) ;
#29976=CARTESIAN_POINT ( 'NONE',  ( 4.788000803920411386, 8.737751371215816576, 1.040834085586084257E-14 ) ) ;
#29977=CARTESIAN_POINT ( 'NONE',  ( -4.295139169456660078, 7.266651303919805294, 0.9588947021764819834 ) ) ;
#29978=CARTESIAN_POINT ( 'NONE',  ( 3.011882680530176604, 6.665613560593854459, 0.7998128361456341429 ) ) ;
#29981=CARTESIAN_POINT ( 'NONE',  ( -7.375272376154096143, 8.667201196010339004, -1.082531754730544860 ) ) ;
#29986=CARTESIAN_POINT ( 'NONE',  ( -4.338815981289680934, 7.218015932674029855, 1.009429000442535918 ) ) ;
#29987=CARTESIAN_POINT ( 'NONE',  ( 0.6823417656249899377, 0.6552083336747518416, 1.181850606188755259 ) ) ;
#29990=CARTESIAN_POINT ( 'NONE',  ( 4.202664430556254160, 5.926194473780837413, 1.443375672974062551 ) ) ;
#29993=ADVANCED_FACE ( 'NONE', ( #179588 ), #46394, .F. ) ;
#29995=CARTESIAN_POINT ( 'NONE',  ( -7.632877294369372123, 11.84884791016554573, 0.7216878364870458196 ) ) ;
#30001=CARTESIAN_POINT ( 'NONE',  ( -8.093854517234044366, 11.42628545587295186, 1.082531754730549967 ) ) ;
#30009=CARTESIAN_POINT ( 'NONE',  ( -9.124274191872640216, 10.70770331434866485, -1.082531754730537976 ) ) ;
#30014=CARTESIAN_POINT ( 'NONE',  ( -0.7500000000000215383, 4.472916667349482012, 1.299038105676671107 ) ) ;
#30015=CARTESIAN_POINT ( 'NONE',  ( 5.841900715481964212, 6.189949835993628469, -0.9061318016433889122 ) ) ;
#30019=CARTESIAN_POINT ( 'NONE',  ( -8.355902744723985975, 8.642974711799791265, 1.040834085586084257E-14 ) ) ;
#30022=CARTESIAN_POINT ( 'NONE',  ( 4.625302960556422427, 8.547937220624488575, 1.040834085586084257E-14 ) ) ;
#30028=CARTESIAN_POINT ( 'NONE',  ( 7.771848369131631351, 10.09024240211882351, -1.599625672291262513 ) ) ;
#30034=CARTESIAN_POINT ( 'NONE',  ( -5.246642258808529746, 9.064907035344523578, 0.000000000000000000 ) ) ;
#30037=CARTESIAN_POINT ( 'NONE',  ( -3.619250341048971809, 3.172667246362773863, -2.499999999999999556 ) ) ;
#30040=CARTESIAN_POINT ( 'NONE',  ( 3.538314903486612817, 7.071858454135611538, 1.040834085586084257E-14 ) ) ;
#30043=CARTESIAN_POINT ( 'NONE',  ( -10.32861409551237486, 10.94447128771960287, 1.040834085586084257E-14 ) ) ;
#30045=CARTESIAN_POINT ( 'NONE',  ( 9.759171643738394408, 10.28012176064996197, 0.000000000000000000 ) ) ;
#30046=CARTESIAN_POINT ( 'NONE',  ( -1.500000000000001332, -0.5999999999999755529, 0.000000000000000000 ) ) ;
#30047=CARTESIAN_POINT ( 'NONE',  ( -8.829384350997580455, 11.32403438096243775, 1.599625672291269396 ) ) ;
#30050=CARTESIAN_POINT ( 'NONE',  ( -0.6823417656250003738, 2.967708333674754062, -1.181850606188749264 ) ) ;
#30051=CARTESIAN_POINT ( 'NONE',  ( 8.595506201383999567, 12.97191496834930113, 0.7216878364870438212 ) ) ;
#30057=CARTESIAN_POINT ( 'NONE',  ( 10.50720586046655391, 11.36075438007358507, 0.7216878364870438212 ) ) ;
#30060=CARTESIAN_POINT ( 'NONE',  ( -5.531363484695544841, 8.436712584578003771, 1.082531754730548412 ) ) ;
#30062=CARTESIAN_POINT ( 'NONE',  ( 1.364683531249986537, 1.113541667008082658, 0.7879004041258500513 ) ) ;
#30064=CARTESIAN_POINT ( 'NONE',  ( -3.511198596259319960, 6.271927390929313617, 1.082471891955974153 ) ) ;
#30066=CARTESIAN_POINT ( 'NONE',  ( -6.821723845970312894, 11.11042825360738284, 0.000000000000000000 ) ) ;
#30067=CARTESIAN_POINT ( 'NONE',  ( -3.917943204224928699, 4.633650495426258509, -1.082531754730548412 ) ) ;
#30068=CARTESIAN_POINT ( 'NONE',  ( 0.6823417656249899377, 3.988541667008085767, -1.181850606188754593 ) ) ;
#30074=CARTESIAN_POINT ( 'NONE',  ( 7.574201371528760163, 11.98831870009225931, 1.040834085586084257E-14 ) ) ;
#30078=CARTESIAN_POINT ( 'NONE',  ( -0.1400748609342543360, 7.098713645440452247, -2.115199198882514953 ) ) ;
#30088=CARTESIAN_POINT ( 'NONE',  ( -1.402160292154681736E-14, -0.9281249996585830830, 1.575800808251672791 ) ) ;
#30090=EDGE_CURVE ( 'NONE', #135613, #80197, #150485, .T. ) ;
#30092=CARTESIAN_POINT ( 'NONE',  ( -4.037141169473096980, 7.765219724388391143, 0.5542112752373774542 ) ) ;
#30093=CARTESIAN_POINT ( 'NONE',  ( 8.097244055859613709, 10.46987070330147063, -1.599625672291262513 ) ) ;
#30095=CARTESIAN_POINT ( 'NONE',  ( -1.364683531250012516, 3.238541667008084879, -0.7879004041258289570 ) ) ;
#30097=CARTESIAN_POINT ( 'NONE',  ( -7.863365906246074566, 8.276274433482971205, -0.7216878364870278340 ) ) ;
#30103=CARTESIAN_POINT ( 'NONE',  ( 4.241003122976366058, 3.842258486427521103, -0.7998128361456211532 ) ) ;
#30106=CARTESIAN_POINT ( 'NONE',  ( 9.215791728987056786, 11.77484298861683598, -1.599625672291262513 ) ) ;
#30113=CARTESIAN_POINT ( 'NONE',  ( -9.755255220232635693, 11.33988483081495957, -1.199719254218441611 ) ) ;
#30114=CARTESIAN_POINT ( 'NONE',  ( 7.969495366734495434, 8.192166104145387706, 1.040834085586084257E-14 ) ) ;
#30116=CARTESIAN_POINT ( 'NONE',  ( 4.812781342726870193, 4.717259109377208048, 0.7216878364870317197 ) ) ;
#30127=CARTESIAN_POINT ( 'NONE',  ( -5.965224400332865606, 7.022145224218852455, 1.082531754730549967 ) ) ;
#30128=CARTESIAN_POINT ( 'NONE',  ( 4.334856428067313416, 6.080418470877079429, -1.599625672291256295 ) ) ;
#30131=CARTESIAN_POINT ( 'NONE',  ( -6.507023659554960204, 9.678945805201045971, 1.199719254218452047 ) ) ;
#30137=CARTESIAN_POINT ( 'NONE',  ( -9.429859533504656000, 10.96025652963230534, -1.199719254218441611 ) ) ;
#30141=CARTESIAN_POINT ( 'NONE',  ( 6.771407655021410399, 9.987393799911945536, -1.199719254218441611 ) ) ;
#30153=CARTESIAN_POINT ( 'NONE',  ( -8.646349277213090545, 11.11049346154719508, 1.599625672291269396 ) ) ;
#30157=CARTESIAN_POINT ( 'NONE',  ( 5.829642864196157070, 8.784705193995428374, 1.082531754730558626 ) ) ;
#30159=CARTESIAN_POINT ( 'NONE',  ( 4.142179624174931796, 4.791296635414242111, 1.199719254218464037 ) ) ;
#30160=LINE ( 'NONE', #78892, #130930 ) ;
#30162=CARTESIAN_POINT ( 'NONE',  ( -6.307567778855718288, 8.381915046796901692, -1.599625672291263179 ) ) ;
#30171=CARTESIAN_POINT ( 'NONE',  ( 0.6823417656249899377, 4.238541667008085767, -1.181850606188754593 ) ) ;
#30173=CARTESIAN_POINT ( 'NONE',  ( 7.228468454380276853, 11.58496363008569574, 1.040834085586084257E-14 ) ) ;
#30175=CARTESIAN_POINT ( 'NONE',  ( -4.121315508874269007, 5.831287398485176077, -1.443375672974053447 ) ) ;
#30177=CARTESIAN_POINT ( 'NONE',  ( -4.622967192135580383, 5.456178481322002227, 1.082531754730558626 ) ) ;
#30182=VERTEX_POINT ( 'NONE', #51726 ) ;
#30186=CARTESIAN_POINT ( 'NONE',  ( 9.083599731475976213, 12.58098820582193689, 1.082531754730546636 ) ) ;
#30194=CARTESIAN_POINT ( 'NONE',  ( 3.408985558832261731, 6.064568021024562938, 1.199719254218462483 ) ) ;
#30199=CARTESIAN_POINT ( 'NONE',  ( -1.364683531249997417, 3.821875000341416584, 1.214306433183764966E-14 ) ) ;
#30206=CARTESIAN_POINT ( 'NONE',  ( 5.286789834324991055, 8.255339675766103724, -1.199719254218452935 ) ) ;
#30209=CARTESIAN_POINT ( 'NONE',  ( -4.412288926243578935, 7.235088616337731260, 1.199719254218464037 ) ) ;
#30211=CARTESIAN_POINT ( 'NONE',  ( -1.499999999999997780, 2.400000000000020339, 1.214306433183764966E-14 ) ) ;
#30214=CARTESIAN_POINT ( 'NONE',  ( -5.298539104842322267, 5.076050465271134016, 0.7998128361456341429 ) ) ;
#30218=CARTESIAN_POINT ( 'NONE',  ( 0.6823417656249899377, 5.176041667008086655, -1.181850606188754593 ) ) ;
#30221=CARTESIAN_POINT ( 'NONE',  ( -2.819732761962332024, 6.233512622357263666, -0.7216878364870267237 ) ) ;
#30224=ORIENTED_EDGE ( 'NONE', *, *, #204793, .F. ) ;
#30227=CARTESIAN_POINT ( 'NONE',  ( 3.344057444064992168, 7.053150784717805877, 1.040834085586084257E-14 ) ) ;
#30229=CARTESIAN_POINT ( 'NONE',  ( 0.4131705840078804814, 6.915508634455322046, -3.854011512607138812 ) ) ;
#30230=CARTESIAN_POINT ( 'NONE',  ( -1.364683531250010295, 4.592708333674755394, 0.7879004041258379498 ) ) ;
#30235=CARTESIAN_POINT ( 'NONE',  ( -1.364683531250000748, 0.07187500034142035865, 0.000000000000000000 ) ) ;
#30239=CARTESIAN_POINT ( 'NONE',  ( -10.32183501870554387, 10.93656236477829502, 0.7998128361456462443 ) ) ;
#30240=CARTESIAN_POINT ( 'NONE',  ( -5.544921637864824504, 8.452530429942200385, -1.082531754730543971 ) ) ;
#30244=CARTESIAN_POINT ( 'NONE',  ( 0.6823417656249917140, 4.092708333674755394, 1.181850606188765695 ) ) ;
#30252=CARTESIAN_POINT ( 'NONE',  ( -5.205967797523171292, 9.017453497178271604, 0.000000000000000000 ) ) ;
#30257=CARTESIAN_POINT ( 'NONE',  ( -6.358410854684796831, 6.520493539994793863, -0.7216878364870267237 ) ) ;
#30270=CARTESIAN_POINT ( 'NONE',  ( -4.660252114795309097, 6.460046772059735432, -1.599625672291256295 ) ) ;
#30274=CARTESIAN_POINT ( 'NONE',  ( 0.7499999999999867883, 0.3166666666666873020, -1.299038105676652899 ) ) ;
#30276=CARTESIAN_POINT ( 'NONE',  ( 2.683624340501134853, 5.218313266304903664, -1.199719254218446718 ) ) ;
#30277=CARTESIAN_POINT ( 'NONE',  ( 7.470706336329915764, 8.674577799595093452, -1.199719254218441611 ) ) ;
#30280=SPHERICAL_SURFACE ( 'NONE', #176783, 0.08000000000000000167 ) ;
#30281=CARTESIAN_POINT ( 'NONE',  ( 5.301401758143367893, 6.143722458377430584, 1.199719254218462483 ) ) ;
#30283=( BOUNDED_CURVE ( )  B_SPLINE_CURVE ( 2, ( #63454, #62381, #33083, #179350, #97047, #131695, #115462, #98107, #144749, #128545, #165211, #212886, #82885, #64517, #130662, #48292, #148962, #114404, #164159, #534, #66601, #193454, #154298, #132747, #83947, #200877, #169472, #168409, #150038, #166272, #135916, #20006, #134870, #86090, #52522, #100206, #17864, #38408, #133812, #152166, #3735, #2676, #118654, #85021, #184640, #103411, #201934, #21057, #153225, #36258, #186782, #136988, #183582, #53591, #1609, #69810, #35189, #199826, #104490, #119725, #50397, #182507, #185704, #102337, #37338, #87154, #51467, #68748, #198750, #4795, #70874, #101265, #67668, #203015, #167349, #54657, #120805, #117591, #18936, #170533, #151110, #22118, #88230, #5873, #116517, #34137, #93590, #108817, #109886, #192109, #122962, #175899, #172690, #27490, #73025, #158570, #25352, #41637, #39472, #56793, #139123, #107751, #40559, #207305, #205150, #106665, #188921, #23196, #71946, #90373, #174841, #89312, #24268, #156442, #8026, #74116, #59993, #26418, #10169, #55721, #173777 ),
 .UNSPECIFIED., .F., .T. ) 
 B_SPLINE_CURVE_WITH_KNOTS ( ( 3, 2, 2, 2, 2, 2, 2, 2, 2, 2, 2, 2, 2, 2, 2, 2, 2, 2, 2, 2, 2, 2, 2, 2, 2, 2, 2, 2, 2, 2, 2, 2, 2, 2, 2, 2, 2, 2, 2, 2, 2, 2, 2, 2, 2, 2, 2, 2, 2, 2, 2, 2, 2, 2, 2, 2, 2, 2, 2, 2, 3 ),
 ( 0.000000000000000000, 0.005952380952380951183, 0.01190476190476190237, 0.01785714285714285615, 0.02380952380952380473, 0.02976190476190476025, 0.03571428571428571230, 0.04166666666666666435, 0.04761904761904760947, 0.05357142857142856845, 0.05952380952380952051, 0.06547619047619047949, 0.07142857142857142461, 0.07738095238095238360, 0.08333333333333332871, 0.08928571428571428770, 0.09523809523809521893, 0.1011904761904762057, 0.1071428571428571369, 0.1130952380952380959, 0.1190476190476190410, 0.1250000000000000000, 0.1309523809523809590, 0.1369047619047619180, 0.1428571428571428492, 0.1488095238095238082, 0.1547619047619047672, 0.1607142857142857262, 0.1666666666666666574, 0.1726190476190476164, 0.1785714285714285754, 0.1845238095238095621, 0.1904761904761904379, 0.1964285714285714246, 0.2023809523809524114, 0.2083333333333333426, 0.2142857142857142738, 0.2202380952380952328, 0.2261904761904761918, 0.2321428571428571508, 0.2380952380952380820, 0.2440476190476190133, 0.2500000000000000000, 0.2559523809523809312, 0.2619047619047619180, 0.2678571428571428492, 0.2738095238095238360, 0.2797619047619047672, 0.2857142857142856984, 0.2916666666666666852, 0.2976190476190476164, 0.3035714285714285476, 0.3095238095238095344, 0.3154761904761904656, 0.3214285714285714524, 0.3273809523809523836, 0.3333333333333333148, 0.3392857142857143016, 0.3452380952380952328, 0.3511904761904761640, 0.3537201901891439126 ),
 .UNSPECIFIED. ) 
 CURVE ( )  GEOMETRIC_REPRESENTATION_ITEM ( )  RATIONAL_B_SPLINE_CURVE ( ( 1.000000000000000000, 0.8660254037844387076, 1.000000000000000000, 0.8660254037844387076, 1.000000000000000000, 0.8660254037844387076, 1.000000000000000000, 0.8660254037844387076, 1.000000000000000000, 0.8660254037844387076, 1.000000000000000000, 0.8660254037844387076, 1.000000000000000000, 0.8660254037844387076, 1.000000000000000000, 0.8660254037844387076, 1.000000000000000000, 0.8660254037844387076, 1.000000000000000000, 0.8660254037844387076, 1.000000000000000000, 0.8660254037844387076, 1.000000000000000000, 0.8660254037844387076, 1.000000000000000000, 0.8660254037844387076, 1.000000000000000000, 0.8660254037844387076, 1.000000000000000000, 0.8660254037844387076, 1.000000000000000000, 0.8660254037844387076, 1.000000000000000000, 0.8660254037844387076, 1.000000000000000000, 0.8660254037844387076, 1.000000000000000000, 0.8660254037844387076, 1.000000000000000000, 0.8660254037844387076, 1.000000000000000000, 0.8660254037844387076, 1.000000000000000000, 0.8660254037844387076, 1.000000000000000000, 0.8660254037844387076, 1.000000000000000000, 0.8660254037844387076, 1.000000000000000000, 0.8660254037844387076, 1.000000000000000000, 0.8660254037844387076, 1.000000000000000000, 0.8660254037844387076, 1.000000000000000000, 0.8660254037844387076, 1.000000000000000000, 0.8660254037844387076, 1.000000000000000000, 0.8660254037844387076, 1.000000000000000000, 0.8660254037844387076, 1.000000000000000000, 0.8660254037844387076, 1.000000000000000000, 0.8660254037844387076, 1.000000000000000000, 0.8660254037844387076, 1.000000000000000000, 0.8660254037844387076, 1.000000000000000000, 0.8660254037844387076, 1.000000000000000000, 0.8660254037844387076, 1.000000000000000000, 0.8660254037844387076, 1.000000000000000000, 0.8660254037844387076, 1.000000000000000000, 0.8660254037844387076, 1.000000000000000000, 0.8660254037844387076, 1.000000000000000000, 0.8660254037844387076, 1.000000000000000000, 0.8660254037844387076, 1.000000000000000000, 0.8660254037844387076, 1.000000000000000000, 0.8660254037844387076, 1.000000000000000000, 0.8660254037844387076, 1.000000000000000000, 0.8660254037844387076, 1.000000000000000000, 0.8660254037844387076, 1.000000000000000000, 0.8660254037844387076, 1.000000000000000000, 0.8660254037844387076, 1.000000000000000000, 0.8660254037844387076, 1.000000000000000000, 0.8660254037844387076, 1.000000000000000000, 0.8660254037844387076, 1.000000000000000000, 0.8660254037844387076, 1.000000000000000000, 0.8660254037844387076, 1.000000000000000000, 0.8660254037844387076, 1.000000000000000000, 0.8660254037844387076, 1.000000000000000000, 0.8660254037844387076, 1.000000000000000000, 0.8660254037844387076, 1.000000000000000000, 0.9430618748659230777, 0.9345202395942615592 ) ) 
 REPRESENTATION_ITEM ( '' )  );
#30284=CARTESIAN_POINT ( 'NONE',  ( -0.5029403714634873568, 7.727853499550840333, -1.993913793680506696 ) ) ;
#30285=ORIENTED_EDGE ( 'NONE', *, *, #63218, .F. ) ;
#30290=CARTESIAN_POINT ( 'NONE',  ( -2.467220768007014176, 5.822248629409386922, 0.7216878364870317197 ) ) ;
#30297=CARTESIAN_POINT ( 'NONE',  ( -0.6823417656249969321, 3.467708333674754506, -1.181850606188749264 ) ) ;
#30298=CARTESIAN_POINT ( 'NONE',  ( 10.03267048398825168, 10.80712977418221676, 0.000000000000000000 ) ) ;
#30299=CARTESIAN_POINT ( 'NONE',  ( -6.307567778855718288, 8.381915046796901692, -1.599625672291263179 ) ) ;
#30302=CARTESIAN_POINT ( 'NONE',  ( 6.331821432781979730, 7.345878745455822312, -1.199719254218445830 ) ) ;
#30303=CARTESIAN_POINT ( 'NONE',  ( -7.063961727919978451, 8.200042423116789436, 1.199719254218450271 ) ) ;
#30308=CARTESIAN_POINT ( 'NONE',  ( 0.7499999999999867883, -0.1520833326505155458, -1.299038105676652899 ) ) ;
#30311=CARTESIAN_POINT ( 'NONE',  ( 8.595506201384020883, 9.130438111143927671, 0.7216878364870438212 ) ) ;
#30315=CARTESIAN_POINT ( 'NONE',  ( -1.402160292154681736E-14, 1.759375000341421469, -1.575800808251659024 ) ) ;
#30317=CARTESIAN_POINT ( 'NONE',  ( 6.439759776366769550, 8.536139043893143707, 1.443375672974076540 ) ) ;
#30319=CARTESIAN_POINT ( 'NONE',  ( -3.256827568602408185, 6.415910372102921144, -0.7556650801423603347 ) ) ;
#30320=CARTESIAN_POINT ( 'NONE',  ( -4.622967192579922724, 4.495809267539077503, 1.214306433183764966E-14 ) ) ;
#30322=CARTESIAN_POINT ( 'NONE',  ( -1.364683531250012516, 4.238541667008090208, -0.7879004041258300672 ) ) ;
#30329=CARTESIAN_POINT ( 'NONE',  ( -5.409091473909686698, 6.481950958801420803, -1.333638828535830045 ) ) ;
#30335=CARTESIAN_POINT ( 'NONE',  ( 5.282873410819217241, 9.315102745931094219, -0.7998128361456281477 ) ) ;
#30338=CARTESIAN_POINT ( 'NONE',  ( 3.011882680530176604, 6.665613560593854459, 0.7998128361456341429 ) ) ;
#30347=CARTESIAN_POINT ( 'NONE',  ( 5.856759171423504107, 5.935233242856626568, -0.7216878364870257245 ) ) ;
#30348=CARTESIAN_POINT ( 'NONE',  ( 0.6823417656249899377, 2.405208333674753618, 1.181850606188767472 ) ) ;
#30349=CARTESIAN_POINT ( 'NONE',  ( 9.562578416340237197, 10.05076299535211781, 0.7998128361456462443 ) ) ;
#30352=CARTESIAN_POINT ( 'NONE',  ( -3.904308432943693230, 7.706776938409620747, -0.6575030929269864988 ) ) ;
#30355=CARTESIAN_POINT ( 'NONE',  ( 1.499999999999987121, 2.045833333333356929, -0.8660254037844262731 ) ) ;
#30356=CARTESIAN_POINT ( 'NONE',  ( 5.764187864104357573, 9.876636274763768597, 1.040834085586084257E-14 ) ) ;
#30357=CARTESIAN_POINT ( 'NONE',  ( -9.027031348600448979, 9.425958082989001952, 1.040834085586084257E-14 ) ) ;
#30361=EDGE_CURVE ( 'NONE', #11347, #185972, #49413, .T. ) ;
#30362=CARTESIAN_POINT ( 'NONE',  ( 0.6823417656249899377, 2.842708333674753618, 1.181850606188765695 ) ) ;
#30363=CARTESIAN_POINT ( 'NONE',  ( -1.500000000000013101, 4.129166666666687746, -0.8660254037844313801 ) ) ;
#30365=CARTESIAN_POINT ( 'NONE',  ( 2.686486993802192913, 6.285985259411197568, 0.7998128361456362523 ) ) ;
#30371=CARTESIAN_POINT ( 'NONE',  ( -0.7500000000000006661, 1.139583334016154526, -1.299038105676652011 ) ) ;
#30373=CARTESIAN_POINT ( 'NONE',  ( -6.856673000209188906, 9.022537805042615489, 1.599625672291283607 ) ) ;
#30375=CARTESIAN_POINT ( 'NONE',  ( -3.633221978782290140, 6.222214161012547429, -1.082531754730549967 ) ) ;
#30382=CARTESIAN_POINT ( 'NONE',  ( 7.311924916471702396, 7.425000578838787391, -0.7998128361456281477 ) ) ;
#30386=CARTESIAN_POINT ( 'NONE',  ( 6.012151052656117933, 9.101594430485762999, 1.199719254218460707 ) ) ;
#30387=CARTESIAN_POINT ( 'NONE',  ( 8.934460041281305109, 10.48625347199211966, -1.082531754730543083 ) ) ;
#30392=CARTESIAN_POINT ( 'NONE',  ( -7.691553217654356622, 7.867900263551875994, -0.7998128361456291469 ) ) ;
#30395=CARTESIAN_POINT ( 'NONE',  ( 4.552840656090682891, 4.206068941727564514, 1.214306433183764966E-14 ) ) ;
#30401=CARTESIAN_POINT ( 'NONE',  ( 4.307253300151457687, 7.213791655154011551, 0.9935852123437900474 ) ) ;
#30411=CARTESIAN_POINT ( 'NONE',  ( -2.657034918598345730, 5.083329257464595408, -1.082531754730543971 ) ) ;
#30412=CARTESIAN_POINT ( 'NONE',  ( 6.466876084038451822, 10.48851316477946582, 1.040834085586084257E-14 ) ) ;
#30414=CARTESIAN_POINT ( 'NONE',  ( -3.795392936821753604, 6.515376628678959392, -1.199719254218452047 ) ) ;
#30418=CARTESIAN_POINT ( 'NONE',  ( -6.880926654135487652, 7.986501503701545879, 1.199719254218450271 ) ) ;
#30423=ORIENTED_EDGE ( 'NONE', *, *, #140820, .T. ) ;
#30433=CARTESIAN_POINT ( 'NONE',  ( -4.232116505760120440, 8.089219690028791376, -0.7998128361456281477 ) ) ;
#30436=CARTESIAN_POINT ( 'NONE',  ( 3.009546912553647147, 5.494593250412460606, -1.082531754730543083 ) ) ;
#30441=CARTESIAN_POINT ( 'NONE',  ( -4.135400547368138113, 4.783387712472935149, 1.199719254218462483 ) ) ;
#30445=CARTESIAN_POINT ( 'NONE',  ( 8.218213668177886788, 12.73966637951625813, 0.7998128361456462443 ) ) ;
#30449=CARTESIAN_POINT ( 'NONE',  ( -7.503547950159405566, 10.84155747757291266, 1.199719254218453823 ) ) ;
#30450=CARTESIAN_POINT ( 'NONE',  ( 4.299907273828439180, 8.168308919441841454, 1.040834085586084257E-14 ) ) ;
#30454=CARTESIAN_POINT ( 'NONE',  ( -1.364683531250012516, 1.592708333674756727, 0.7879004041258379498 ) ) ;
#30457=CARTESIAN_POINT ( 'NONE',  ( 8.622622508611357262, 9.162073802909148412, -0.7216878364870197293 ) ) ;
#30473=CARTESIAN_POINT ( 'NONE',  ( -8.306341666666730461, 12.84248237775322643, 1.040834085586084257E-14 ) ) ;
#30481=CARTESIAN_POINT ( 'NONE',  ( 5.120175567455225618, 9.125288595339771547, -0.7998128361456281477 ) ) ;
#30488=CARTESIAN_POINT ( 'NONE',  ( 1.499999999999989120, 2.056250000682817269, 1.214306433183764966E-14 ) ) ;
#30492=VERTEX_POINT ( 'NONE', #175090 ) ;
#30494=CARTESIAN_POINT ( 'NONE',  ( -1.500000000000001332, -0.3499999999999753308, 0.000000000000000000 ) ) ;
#30495=CARTESIAN_POINT ( 'NONE',  ( 7.995557903757111617, 10.35123685918189729, 1.599625672291281386 ) ) ;
#30502=CARTESIAN_POINT ( 'NONE',  ( 3.171717870593107058, 5.787755718078879674, -1.199719254218446718 ) ) ;
#30503=CARTESIAN_POINT ( 'NONE',  ( -5.734735788900501952, 9.634349487118505806, 0.000000000000000000 ) ) ;
#30507=CARTESIAN_POINT ( 'NONE',  ( -5.859094939400033120, 9.987361195942037639, -0.7998128361456231517 ) ) ;
#30510=CARTESIAN_POINT ( 'NONE',  ( -0.7500000000000006661, 1.139583334016154526, -1.299038105676652011 ) ) ;
#30517=CARTESIAN_POINT ( 'NONE',  ( -3.755245360860939297, 4.443836344834937613, -1.082531754730548412 ) ) ;
#30519=CARTESIAN_POINT ( 'NONE',  ( 4.307253300151457687, 7.213791655154011551, 0.9935852123437900474 ) ) ;
#30522=EDGE_CURVE ( 'NONE', #61877, #96829, #123009, .T. ) ;
#30525=CARTESIAN_POINT ( 'NONE',  ( -8.306341666666730461, 12.84248237775322643, 1.040834085586084257E-14 ) ) ;
#30526=CARTESIAN_POINT ( 'NONE',  ( 7.422199028477372451, 10.74665040227725044, -1.199719254218441611 ) ) ;
#30527=DIRECTION ( 'NONE',  ( 5.578564026256490882E-16, 1.000000000000000000, 9.066213480720158442E-32 ) ) ;
#30534=CARTESIAN_POINT ( 'NONE',  ( -6.659026002606323047, 10.92061410301605662, 0.000000000000000000 ) ) ;
#30540=CARTESIAN_POINT ( 'NONE',  ( 4.704842999142070603, 5.447737239542574272, -1.199719254218452047 ) ) ;
#30544=EDGE_LOOP ( 'NONE', ( #42490, #193144, #178946, #88016 ) ) ;
#30545=CARTESIAN_POINT ( 'NONE',  ( -4.069418662396130593, 7.899405539437467816, -0.7998128361456281477 ) ) ;
#30546=CARTESIAN_POINT ( 'NONE',  ( -8.109748439268576803, 12.61312361245537517, 0.7998128361456481317 ) ) ;
#30557=CARTESIAN_POINT ( 'NONE',  ( 6.825640269476072497, 10.05066518344239412, 1.199719254218460707 ) ) ;
#30559=CARTESIAN_POINT ( 'NONE',  ( -3.653032323878261600, 6.349289246911547835, -1.199719254218452047 ) ) ;
#30562=CARTESIAN_POINT ( 'NONE',  ( 5.630352418794719149, 6.139657267270441920, -0.8181431533968346326 ) ) ;
#30565=CIRCLE ( 'NONE', #85893, 0.08000000000000020983 ) ;
#30567=CARTESIAN_POINT ( 'NONE',  ( 0.7499999999999885647, -0.2354166659838466402, 1.299038105676657340 ) ) ;
#30573=CARTESIAN_POINT ( 'NONE',  ( -2.137381772448751605, 5.645362501165475777, -0.7998128361456281477 ) ) ;
#30579=CARTESIAN_POINT ( 'NONE',  ( 5.341549334104200852, 5.334155099317434257, 0.7216878364870317197 ) ) ;
#30582=CARTESIAN_POINT ( 'NONE',  ( -1.364683531250010295, 5.592708333674750953, 0.7879004041258379498 ) ) ;
#30583=DIRECTION ( 'NONE',  ( 5.578564026256490882E-16, 1.000000000000000000, 9.066213480720158442E-32 ) ) ;
#30584=CARTESIAN_POINT ( 'NONE',  ( 4.189106276498237413, 3.989638198777126110, -0.7216878364870188411 ) ) ;
#30594=CARTESIAN_POINT ( 'NONE',  ( -1.364683531250014514, -0.5114583329919092369, -0.7879004041258359514 ) ) ;
#30598=CARTESIAN_POINT ( 'NONE',  ( -3.879604511804807032, 7.677955697080923514, 0.7998128361456341429 ) ) ;
#30602=CARTESIAN_POINT ( 'NONE',  ( -1.500000000000011324, 4.629166666666689522, -0.8660254037844313801 ) ) ;
#30610=CARTESIAN_POINT ( 'NONE',  ( 1.364683531249984538, -1.094791666325247936, -0.7879004041258309554 ) ) ;
#30612=CARTESIAN_POINT ( 'NONE',  ( 6.908042961362778733, 8.018137195466769285, 1.199719254218462483 ) ) ;
#30613=CARTESIAN_POINT ( 'NONE',  ( -9.176171038350775078, 9.599954387697719582, -0.7998128361456291469 ) ) ;
#30616=CARTESIAN_POINT ( 'NONE',  ( -0.9999999999999988898, 6.468705557303653819, -4.925226524755048629 ) ) ;
#30620=CARTESIAN_POINT ( 'NONE',  ( -0.7500000000000215383, 5.441666666666685082, 1.299038105676671107 ) ) ;
#30624=CARTESIAN_POINT ( 'NONE',  ( 4.465192238825641979, 7.096428296808035441, -1.166435484173217629 ) ) ;
#30626=EDGE_LOOP ( 'NONE', ( #180949, #134007, #137222, #70638 ) ) ;
#30627=ORIENTED_EDGE ( 'NONE', *, *, #27402, .T. ) ;
#30629=CARTESIAN_POINT ( 'NONE',  ( 6.480434237652115570, 10.50433101066207442, 0.7216878364870438212 ) ) ;
#30634=CARTESIAN_POINT ( 'NONE',  ( 0.7499999999999902300, 5.347916667349482012, -1.299038105676658228 ) ) ;
#30636=CARTESIAN_POINT ( 'NONE',  ( -3.090368948911150770, 5.692848642783215674, 1.199719254218462483 ) ) ;
#30638=CARTESIAN_POINT ( 'NONE',  ( 5.246642258364164313, 8.104537820524768676, -1.082531754730549078 ) ) ;
#30639=CARTESIAN_POINT ( 'NONE',  ( -9.341204649691320583, 10.96078884847042545, 1.082531754730558626 ) ) ;
#30645=CARTESIAN_POINT ( 'NONE',  ( 3.358669367883368118, 4.941533567329135401, -1.599625672291262513 ) ) ;
#30650=ORIENTED_EDGE ( 'NONE', *, *, #70571, .T. ) ;
#30661=CARTESIAN_POINT ( 'NONE',  ( 8.751951852821344247, 10.16936423550178503, -1.199719254218446718 ) ) ;
#30666=CARTESIAN_POINT ( 'NONE',  ( 1.364683531249986537, 0.1552083336747499542, -0.7879004041258309554 ) ) ;
#30667=CARTESIAN_POINT ( 'NONE',  ( 4.772106882330221289, 6.590544000850479200, -1.443375672974051449 ) ) ;
#30668=CARTESIAN_POINT ( 'NONE',  ( -9.164948653158003111, 9.794787638213568570, -0.7216878364870267237 ) ) ;
#30673=CARTESIAN_POINT ( 'NONE',  ( -4.277761160311629673, 4.949475094240346706, 1.199719254218462483 ) ) ;
#30681=ORIENTED_EDGE ( 'NONE', *, *, #7830, .F. ) ;
#30688=B_SPLINE_CURVE_WITH_KNOTS ( 'NONE', 3,
 ( #91695, #107986, #123201, #27730 ),
 .UNSPECIFIED., .F., .F.,
 ( 4, 4 ),
 ( 0.0009695358052320346897, 0.001130783094531867799 ),
 .UNSPECIFIED. ) ;
#30689=CARTESIAN_POINT ( 'NONE',  ( 5.178766244632133642, 6.659365504414815895, -1.397763381526682336 ) ) ;
#30692=CARTESIAN_POINT ( 'NONE',  ( 5.657830175604453338, 5.495223381160312393, 0.7998128361456341429 ) ) ;
#30697=CARTESIAN_POINT ( 'NONE',  ( -8.690413276679693766, 9.241163032322203819, 1.040834085586084257E-14 ) ) ;
#30702=CARTESIAN_POINT ( 'NONE',  ( 5.612185521052973414, 8.634967976948757951, -1.199719254218440723 ) ) ;
#30703=CARTESIAN_POINT ( 'NONE',  ( 3.023105066167310895, 5.702484939155337607, -2.419999999999995044 ) ) ;
#30705=CARTESIAN_POINT ( 'NONE',  ( -6.600121851754250812, 6.594563670001734046, 0.7998128361456341429 ) ) ;
#30708=CARTESIAN_POINT ( 'NONE',  ( -5.742041750587549842, 6.657802449562273850, 1.199719254218450271 ) ) ;
#30712=CARTESIAN_POINT ( 'NONE',  ( 6.401421083946654100, 10.62007503124645957, -0.7998128361456291469 ) ) ;
#30715=CARTESIAN_POINT ( 'NONE',  ( 5.061713581663421557, 6.751138122384800155, 1.419579013000639378 ) ) ;
#30716=CARTESIAN_POINT ( 'NONE',  ( 5.016153647376212277, 5.914896012436124728, 1.082531754730558626 ) ) ;
#30724=CARTESIAN_POINT ( 'NONE',  ( 7.415946836550722843, 8.714654733139752807, 1.082531754730558626 ) ) ;
#30727=CARTESIAN_POINT ( 'NONE',  ( -8.296699936558862731, 11.76690146170562201, 1.199719254218453823 ) ) ;
#30728=CARTESIAN_POINT ( 'NONE',  ( -8.050844288416501016, 8.287073179441051707, 1.040834085586084257E-14 ) ) ;
#30736=CARTESIAN_POINT ( 'NONE',  ( 8.646349277213076334, 11.11049346154719508, 1.599625672291281386 ) ) ;
#30741=CARTESIAN_POINT ( 'NONE',  ( 4.871457266011829823, 4.577788319968905562, -0.7998128361456221525 ) ) ;
#30744=DIRECTION ( 'NONE',  ( 1.000000000000000000, 0.000000000000000000, 0.000000000000000000 ) ) ;
#30750=CARTESIAN_POINT ( 'NONE',  ( -0.7500000000000215383, 2.941666666666689522, 1.299038105676671107 ) ) ;
#30751=CARTESIAN_POINT ( 'NONE',  ( 4.123651276850781144, 7.962676922967908411, -0.7998128361456221525 ) ) ;
#30755=CARTESIAN_POINT ( 'NONE',  ( 6.805829924380097040, 10.88395931184472154, 0.7216878364870438212 ) ) ;
#30757=CARTESIAN_POINT ( 'NONE',  ( 0.4967775439448678942, 7.792564024146675372, 1.990974371293808165 ) ) ;
#30760=CARTESIAN_POINT ( 'NONE',  ( 9.622536337397022521, 12.24937836509514710, 1.599625672291281386 ) ) ;
#30763=CARTESIAN_POINT ( 'NONE',  ( -3.255929445576174697, 6.950334786480840243, -0.7998128361456281477 ) ) ;
#30764=CARTESIAN_POINT ( 'NONE',  ( -1.201851678989727383E-14, 5.118750000682815937, -1.732050807568863648 ) ) ;
#30765=CARTESIAN_POINT ( 'NONE',  ( -1.364683531250014514, -0.5114583329919092369, -0.7879004041258359514 ) ) ;
#30769=CARTESIAN_POINT ( 'NONE',  ( 2.835626683552519012, 6.459981564119914310, 0.000000000000000000 ) ) ;
#30770=B_SPLINE_CURVE_WITH_KNOTS ( 'NONE', 3,
 ( #100742, #81310, #150583, #179881, #66081, #198233, #147386, #49869 ),
 .UNSPECIFIED., .F., .F.,
 ( 4, 2, 2, 4 ),
 ( 0.000000000000000000, 0.002997375907120273901, 0.004496063860680410418, 0.005994751814240547802 ),
 .UNSPECIFIED. ) ;
#30772=CARTESIAN_POINT ( 'NONE',  ( 1.364683531249990311, 5.196875000341417916, 1.214306433183764966E-14 ) ) ;
#30774=CARTESIAN_POINT ( 'NONE',  ( 3.998552503512865730, 7.829812139846150210, 0.1485553033222472286 ) ) ;
#30781=CARTESIAN_POINT ( 'NONE',  ( -6.527360889975461156, 9.702672574024962415, 1.199719254218452047 ) ) ;
#30784=CARTESIAN_POINT ( 'NONE',  ( 3.981290663907289140, 7.796589541200495965, -0.7998128361456221525 ) ) ;
#30790=CARTESIAN_POINT ( 'NONE',  ( 10.01963921569910632, 11.64833282552586091, 1.199719254218450271 ) ) ;
#30793=CARTESIAN_POINT ( 'NONE',  ( -4.205000198532790279, 8.057583998263570635, 0.7998128361456341429 ) ) ;
#30797=CARTESIAN_POINT ( 'NONE',  ( 7.781490099239519509, 11.16582331816642260, 1.199719254218460707 ) ) ;
#30799=CARTESIAN_POINT ( 'NONE',  ( 7.214910300766615769, 11.56914578420308715, -0.7998128361456291469 ) ) ;
#30802=CARTESIAN_POINT ( 'NONE',  ( -9.707274797704657843, 11.38787068781932987, 1.082531754730558626 ) ) ;
#30803=CARTESIAN_POINT ( 'NONE',  ( -6.775324078527193983, 8.927630729746953264, -1.599625672291263179 ) ) ;
#30807=CARTESIAN_POINT ( 'NONE',  ( -5.867374215541069304, 6.167859493020809047, 0.9100554989533160555 ) ) ;
#30808=CARTESIAN_POINT ( 'NONE',  ( 1.364683531249986537, 0.4052083336747511200, -0.7879004041258309554 ) ) ;
#30813=CARTESIAN_POINT ( 'NONE',  ( 7.131225611108088280, 9.342849184424693476, 1.443375672974076540 ) ) ;
#30816=CARTESIAN_POINT ( 'NONE',  ( 6.030679399980265920, 5.930214142932100252, -0.7998128361456281477 ) ) ;
#30821=EDGE_CURVE ( 'NONE', #201912, #84679, #205772, .T. ) ;
#30833=CARTESIAN_POINT ( 'NONE',  ( 8.062294901620731480, 12.55776115186623620, 1.040834085586084257E-14 ) ) ;
#30837=CARTESIAN_POINT ( 'NONE',  ( -4.574986769607567894, 7.424902766929059261, 1.199719254218464037 ) ) ;
#30838=CARTESIAN_POINT ( 'NONE',  ( -6.669721502918952716, 9.868759955792373972, 1.199719254218452047 ) ) ;
#30844=CARTESIAN_POINT ( 'NONE',  ( 0.7499999999999885647, 3.347916667349487341, -1.299038105676658228 ) ) ;
#30845=CARTESIAN_POINT ( 'NONE',  ( 7.618792255875527886, 10.97600916757510170, 1.199719254218460707 ) ) ;
#30848=CARTESIAN_POINT ( 'NONE',  ( -7.492852449846775897, 11.89341162479659531, 0.000000000000000000 ) ) ;
#30850=CARTESIAN_POINT ( 'NONE',  ( -1.364683531249997417, 3.009375000341422801, 1.214306433183764966E-14 ) ) ;
#30856=CARTESIAN_POINT ( 'NONE',  ( -9.829298180227631576, 10.56986208646148384, 1.040834085586084257E-14 ) ) ;
#30860=CARTESIAN_POINT ( 'NONE',  ( -0.6823417656250212460, 1.113541667008083325, 1.181850606188755259 ) ) ;
#30867=CARTESIAN_POINT ( 'NONE',  ( -0.6823417656250212460, 3.551041667008085323, 1.181850606188767472 ) ) ;
#30869=CARTESIAN_POINT ( 'NONE',  ( -6.112028321662274166, 6.025121218227761588, 0.7998128361456341429 ) ) ;
#30870=CARTESIAN_POINT ( 'NONE',  ( 6.479907352327590964, 9.647310113435821677, 1.199719254218462483 ) ) ;
#30873=CARTESIAN_POINT ( 'NONE',  ( 1.364683531249988535, 2.967708333674755394, -0.7879004041258239610 ) ) ;
#30877=CARTESIAN_POINT ( 'NONE',  ( 1.364683531249988757, -0.3656249996585800299, 0.000000000000000000 ) ) ;
#30878=CARTESIAN_POINT ( 'NONE',  ( -4.121315508874255684, 7.752025827087861920, -0.7216878364870267237 ) ) ;
#30881=CARTESIAN_POINT ( 'NONE',  ( 4.609409038966229666, 6.400729850259146758, -1.443375672974051449 ) ) ;
#30884=CARTESIAN_POINT ( 'NONE',  ( -7.985916173649233230, 9.275655943134292869, -1.199719254218446718 ) ) ;
#30886=CARTESIAN_POINT ( 'NONE',  ( -2.578021764892882040, 6.159442492350315490, 0.7998128361456341429 ) ) ;
#30888=CARTESIAN_POINT ( 'NONE',  ( 1.364683531249990311, 5.363541667008086655, 0.7879004041258500513 ) ) ;
#30894=CARTESIAN_POINT ( 'NONE',  ( -6.033015167956800262, 9.021972881716168402, -1.082531754730537976 ) ) ;
#30896=CARTESIAN_POINT ( 'NONE',  ( 1.364683531249988757, -0.5531249996585801965, 0.000000000000000000 ) ) ;
#30899=CARTESIAN_POINT ( 'NONE',  ( 7.022760382198770301, 8.255937203062467589, -1.082531754730543083 ) ) ;
#30904=( BOUNDED_SURFACE ( )  B_SPLINE_SURFACE ( 1, 2, ( 
 ( #137579, #207879, #205745, #125659, #204665, #190560, #203597, #124600, #71466, #188436, #23796, #7538, #191621, #90963, #43283, #174352, #107260, #22716, #171122, #109404, #6469, #8615, #58446, #40070, #187369, #92039, #108332, #75761, #55249, #139722, #25931, #56314, #72545, #88830, #57377, #155953, #73622, #9684, #153818, #74697, #123541, #121396, #106181, #138643, #172206, #89901, #189505, #38999, #41151, #173280, #24862, #140801, #206812, #141870, #208934, #146120, #192688, #96299, #160211, #210001, #45411, #77888, #176464, #126727, #63769, #212133, #193765, #147177, #145068, #213203, #144009, #129928, #76814, #195916, #10743, #61643, #177534, #161284, #64832, #30214, #130978, #113664, #46470, #28077, #44342, #196969, #11812, #162354, #47553, #127811, #110464, #31287, #179668, #14996, #142933, #78943, #97363, #111528, #29146, #94171, #211071, #95235, #12870, #163421, #48606, #13934, #62694, #180721, #128855, #194836, #112593, #178605, #80017, #60568, #81089, #114724, #93100, #159141, #132019, #136261, #148238, #85359, #198029, #35533, #99482, #149292, #199078, #17133, #115781, #65870, #3012, #151441, #133080, #32345, #164475, #200155, #19277, #69082, #53934, #66938, #181770, #86431, #1945, #135202, #49658, #4079, #152496, #50724, #34469, #201219, #873, #52860, #116849, #68007, #202281, #98411, #33403, #183921, #100540, #150375, #51809, #83209, #82146, #182850, #165540, #166615, #168742, #214240, #101609, #16062, #120070, #18205, #84289, #167676, #134147, #117927, #118993, #184972, #36597, #102684, #20345, #70150, #188185, #7285, #122225, #139468, #159696, #39820, #153571, #21396, #60058, #126213, #105928, #73362, #169807, #103758, #208424, #175962, #11295, #210569, #6219, #121153, #28635, #155704, #27557, #71216, #160765, #94722, #72288, #171952, #93653, #154638, #77374, #138396, #192175, #144559, #37681, #137333, #43836, #23541, #89650, #109952, #170877, #87507, #22469, #5140, #143489, #111013, #203349, #209486, #186046, #78439, #55002, #204414, #61127, #187118, #38750, #104832, #127287, #193258, #88580, #62203, #56068, #44905, #177018, #12360, #81639, #98971, #196467, #95790, #178091, #213741, #65364, #48109, #163977, #112090, #182324, #180220, #33953, #179157, #165023, #29709, #16617, #45969, #96860, #212693, #114221, #100028, #131511, #166091, #148779, #147724, #211626, #79511, #17679, #195406, #197514, #32893, #162908, #161847, #66422, #82698, #50215, #13435, #31842, #349, #30781, #47036, #145629, #97918, #130476, #15552, #132565, #83765, #49158, #115274, #1426, #14490, #113151, #80580, #146678, #64335, #63261, #181267, #129423, #198566, #116334, #149858, #128359, #194327, #120625, #167168, #54479, #55546, #118475, #52347, #171427, #70692, #68565, #136805, #67489, #18755, #84839, #23015, #202831, #134692, #186601, #133635, #150929, #2490, #71764, #170351, #137880, #200696, #36078, #184460, #69631, #151985, #102161, #38228, #168229, #104302, #185526, #19826, #199637, #21936, #39293, #155186, #89132, #51283, #85911, #135740, #169291, #88046, #3559, #201762, #117408, #183404, #154117, #35008, #53403, #5687, #203900, #121700, #187664, #105388, #101079, #119541, #86975, #37151, #103231, #20876, #153045, #4620, #124898, #6768, #75000, #91270, #7843, #11039, #140024, #58745, #206050, #90198, #60875, #159441, #73931, #191920, #41454, #190861, #141109, #175707, #176760, #110761, #57685, #27297, #42524, #107562, #108629, #123841, #93404, #174656, #77118, #143241, #72844, #28376, #209230, #127034, #172509, #207120, #56616, #44647, #26231, #8918, #92348, #208176, #189803, #173597, #24093, #25169, #204970, #157327, #158387, #142160, #9983, #76061, #59809, #125964, #94470, #43585, #138949, #109702, #122780, #192993, #188740, #40379, #106482, #156262, #46785, #82442, #61948, #78188, #164774, #33698, #144314, #210312, #213495, #147474, #148532, #211377, #145379, #16364, #113970, #64080, #160511, #14228, #30525, #161595, #99, #79262, #212438, #63003, #29454, #66165, #98715, #13184, #131273, #195151, #130223, #80323, #115021, #116076, #49957, #129174, #181018, #196217, #112899, #47858, #178910, #32638, #179967 ),
 ( #197261, #132310, #128107, #146424, #198317, #96605, #162657, #111837, #31589, #97664, #163722, #182066, #12114, #81390, #15302, #194065, #65117, #48901, #45718, #177840, #95544, #83509, #52091, #51026, #35827, #134442, #199379, #203639, #101905, #120363, #2234, #54225, #166913, #68311, #118218, #84586, #183151, #133374, #70436, #152786, #200445, #99775, #17426, #53153, #86717, #136552, #121440, #184204, #34754, #153862, #69376, #4366, #117147, #71510, #5431, #167970, #19576, #202573, #85649, #186338, #151736, #135484, #55290, #165840, #100828, #36891, #3306, #201506, #119282, #150673, #149592, #185268, #18507, #102973, #21678, #1176, #169031, #67240, #187409, #20628, #37973, #104046, #170092, #87788, #137622, #7580, #8659, #208975, #105125, #138688, #190600, #107300, #157070, #58487, #23835, #88872, #89942, #72587, #173324, #175450, #154926, #108371, #39040, #142974, #171165, #57420, #174394, #6511, #22754, #204705, #124643, #42258, #56355, #126770, #122518, #41193, #74738, #189545, #206855, #9726, #24902, #188481, #40111, #25972, #92078, #91008, #140843, #106222, #93142, #158135, #159179, #155993, #75801, #172248, #141909, #73665, #139764, #123582, #207921, #10780, #59541, #76855, #125702, #191661, #205790, #43325, #60611, #109443, #27034, #97406, #12911, #11851, #131020, #15041, #114765, #28116, #178646, #147219, #95279, #45452, #144049, #30257, #194878, #46514, #213244, #98454, #113708, #112637, #65913, #161327, #111568, #29189, #78991, #145107, #176504, #211113, #210045, #128897, #62737, #77929, #82188, #96343, #64874, #162398, #197012, #177576, #13974, #80061, #146162, #61684, #127853, #163461, #31329, #212177, #192728, #110504, #63812, #179712, #81133, #214280, #129972, #193803, #32389, #195959, #48648, #47593, #164519, #16104, #180762, #148281, #44382, #94210, #160250, #199118, #134182, #1981, #149334, #119028, #83249, #185010, #35567, #84328, #198070, #36637, #103794, #5179, #87539, #153608, #50761, #200191, #19318, #102721, #116891, #51844, #132060, #49698, #20383, #115826, #133119, #168778, #201254, #70185, #53969, #37716, #86467, #4116, #151480, #182890, #117963, #152531, #136297, #85394, #101648, #181813, #183957, #68045, #34507, #202319, #100580, #167715, #166653, #914, #186085, #120106, #18244, #169844, #150414, #3050, #69119, #21431, #33445, #99522, #135240, #165581, #52894, #17175, #66981, #56105, #25721, #107041, #75553, #9481, #71254, #92894, #91830, #141664, #22506, #139506, #121187, #109195, #40936, #73403, #205533, #58235, #122262, #188220, #88616, #39860, #55038, #138433, #204451, #206606, #155741, #140595, #74489, #105969, #26789, #171991, #175207, #23583, #158939, #108121, #137368, #191415, #89690, #203385, #7326, #207675, #187156, #38785, #59294, #104866, #170911, #154671, #124392, #190350, #125453, #57170, #123332, #6256, #42012, #72327, #174148, #189296, #173068, #24649, #43082, #157889, #90756, #156817, #8404, #194625, #45207, #62494, #209796, #179461, #46268, #14795, #163213, #10535, #32135, #31085, #80886, #176264, #78738, #60358, #48408, #112385, #12664, #144862, #211932, #61431, #127598, #27865, #193564, #208731, #77678, #143799, #145920, #95023, #79808, #13735, #111321, #180515, #177325, #114520, #28939, #98216, #47342, #76608, #130770, #161073, #142722, #210869, #146976, #126521, #192482, #212993, #44134, #110255, #93962, #63566, #129723, #64631, #128659, #178397, #160003, #195707, #11604, #113456, #30009, #96093, #162148, #196765, #97158, #168523, #165323, #132860, #16917, #166390, #34250, #181564, #151223, #115568, #2792, #67784, #116633, #15856, #68863, #136036, #37451, #119842, #185820, #82997, #17981, #51587, #134982, #149073, #84070, #164267, #81942, #52638, #148026, #650, #200992, #19058, #102457, #86207, #69924, #118766, #36379, #183702, #66716, #150159, #184751, #20121, #117711, #133934, #214036, #1727, #100323, #198864, #152278, #50511, #199939, #182628, #33192, #3851, #202049, #35310, #53709, #101387, #167462, #85136, #65661, #131809, #197818, #49449, #99275, #189038, #40676, #23318, #139237, #87274, #157624, #155477, #9221, #154413, #140327, #153342, #74234 ) ),
 .UNSPECIFIED., .F., .F., .T. ) 
 B_SPLINE_SURFACE_WITH_KNOTS ( ( 2, 2 ),
 ( 3, 2, 2, 2, 2, 2, 2, 2, 2, 2, 2, 2, 2, 2, 2, 2, 2, 2, 2, 2, 2, 2, 2, 2, 2, 2, 2, 2, 2, 2, 2, 2, 2, 2, 2, 2, 2, 2, 2, 2, 2, 2, 2, 2, 2, 2, 2, 2, 2, 2, 2, 2, 2, 2, 2, 2, 2, 2, 2, 2, 2, 2, 2, 2, 2, 2, 2, 2, 2, 2, 2, 2, 2, 2, 2, 2, 2, 2, 2, 2, 2, 2, 2, 2, 2, 2, 2, 2, 2, 2, 2, 2, 2, 2, 2, 2, 2, 2, 2, 2, 2, 2, 2, 2, 2, 2, 2, 2, 2, 2, 2, 2, 2, 2, 2, 2, 2, 2, 2, 2, 2, 2, 2, 2, 2, 2, 2, 2, 2, 2, 2, 2, 2, 2, 2, 2, 2, 2, 2, 2, 2, 2, 2, 2, 2, 2, 2, 2, 2, 2, 2, 2, 2, 2, 2, 2, 2, 2, 2, 2, 2, 2, 2, 2, 2, 2, 2, 2, 2, 2, 2, 2, 2, 2, 2, 2, 2, 2, 2, 2, 2, 2, 2, 2, 2, 2, 2, 2, 2, 2, 2, 2, 2, 2, 2, 2, 2, 2, 2, 2, 2, 2, 2, 2, 2, 2, 2, 2, 2, 2, 2, 2, 2, 2, 2, 2, 2, 2, 2, 2, 2, 2, 2, 2, 2, 2, 2, 2, 2, 2, 2, 2, 2, 2, 2, 2, 2, 2, 2, 2, 3 ),
 ( 0.000000000000000000, 1.000000000000000000 ),
 ( 0.000000000000000000, 0.004166666666666666609, 0.008333333333333333218, 0.01250000000000000069, 0.01666666666666666644, 0.02083333333333333218, 0.02500000000000000139, 0.02916666666666666713, 0.03333333333333333287, 0.03749999999999999861, 0.04166666666666666435, 0.04583333333333333010, 0.05000000000000000278, 0.05416666666666666852, 0.05833333333333333426, 0.06250000000000000000, 0.06666666666666666574, 0.07083333333333333148, 0.07499999999999999722, 0.07916666666666666297, 0.08333333333333332871, 0.08749999999999999445, 0.09166666666666666019, 0.09583333333333333981, 0.1000000000000000056, 0.1041666666666666713, 0.1083333333333333370, 0.1125000000000000028, 0.1166666666666666685, 0.1208333333333333343, 0.1250000000000000000, 0.1291666666666666796, 0.1333333333333333315, 0.1375000000000000111, 0.1416666666666666630, 0.1458333333333333426, 0.1499999999999999944, 0.1541666666666666741, 0.1583333333333333259, 0.1625000000000000056, 0.1666666666666666574, 0.1708333333333333370, 0.1749999999999999889, 0.1791666666666666685, 0.1833333333333333204, 0.1875000000000000000, 0.1916666666666666796, 0.1958333333333333315, 0.2000000000000000111, 0.2041666666666666630, 0.2083333333333333426, 0.2124999999999999944, 0.2166666666666666741, 0.2208333333333333259, 0.2250000000000000056, 0.2291666666666666574, 0.2333333333333333370, 0.2374999999999999889, 0.2416666666666666685, 0.2458333333333333204, 0.2500000000000000000, 0.2541666666666666519, 0.2583333333333333592, 0.2625000000000000111, 0.2666666666666666630, 0.2708333333333333148, 0.2750000000000000222, 0.2791666666666666741, 0.2833333333333333259, 0.2874999999999999778, 0.2916666666666666852, 0.2958333333333333370, 0.2999999999999999889, 0.3041666666666666408, 0.3083333333333333481, 0.3125000000000000000, 0.3166666666666666519, 0.3208333333333333592, 0.3250000000000000111, 0.3291666666666666630, 0.3333333333333333148, 0.3375000000000000222, 0.3416666666666666741, 0.3458333333333333259, 0.3499999999999999778, 0.3541666666666666852, 0.3583333333333333370, 0.3624999999999999889, 0.3666666666666666408, 0.3708333333333333481, 0.3750000000000000000, 0.3791666666666666519, 0.3833333333333333592, 0.3875000000000000111, 0.3916666666666666630, 0.3958333333333333148, 0.4000000000000000222, 0.4041666666666666741, 0.4083333333333333259, 0.4124999999999999778, 0.4166666666666666852, 0.4208333333333333370, 0.4249999999999999889, 0.4291666666666666408, 0.4333333333333333481, 0.4375000000000000000, 0.4416666666666666519, 0.4458333333333333592, 0.4500000000000000111, 0.4541666666666666630, 0.4583333333333333148, 0.4625000000000000222, 0.4666666666666666741, 0.4708333333333333259, 0.4749999999999999778, 0.4791666666666666852, 0.4833333333333333370, 0.4874999999999999889, 0.4916666666666666408, 0.4958333333333333481, 0.5000000000000000000, 0.5041666666666666519, 0.5083333333333333037, 0.5124999999999999556, 0.5166666666666667185, 0.5208333333333333703, 0.5250000000000000222, 0.5291666666666666741, 0.5333333333333333259, 0.5374999999999999778, 0.5416666666666666297, 0.5458333333333332815, 0.5500000000000000444, 0.5541666666666666963, 0.5583333333333333481, 0.5625000000000000000, 0.5666666666666666519, 0.5708333333333333037, 0.5749999999999999556, 0.5791666666666667185, 0.5833333333333333703, 0.5875000000000000222, 0.5916666666666666741, 0.5958333333333333259, 0.5999999999999999778, 0.6041666666666666297, 0.6083333333333332815, 0.6125000000000000444, 0.6166666666666666963, 0.6208333333333333481, 0.6250000000000000000, 0.6291666666666666519, 0.6333333333333333037, 0.6374999999999999556, 0.6416666666666667185, 0.6458333333333333703, 0.6500000000000000222, 0.6541666666666666741, 0.6583333333333333259, 0.6624999999999999778, 0.6666666666666666297, 0.6708333333333332815, 0.6750000000000000444, 0.6791666666666666963, 0.6833333333333333481, 0.6875000000000000000, 0.6916666666666666519, 0.6958333333333333037, 0.6999999999999999556, 0.7041666666666667185, 0.7083333333333333703, 0.7125000000000000222, 0.7166666666666666741, 0.7208333333333333259, 0.7249999999999999778, 0.7291666666666666297, 0.7333333333333332815, 0.7375000000000000444, 0.7416666666666666963, 0.7458333333333333481, 0.7500000000000000000, 0.7541666666666666519, 0.7583333333333333037, 0.7624999999999999556, 0.7666666666666667185, 0.7708333333333333703, 0.7750000000000000222, 0.7791666666666666741, 0.7833333333333333259, 0.7874999999999999778, 0.7916666666666666297, 0.7958333333333332815, 0.8000000000000000444, 0.8041666666666666963, 0.8083333333333333481, 0.8125000000000000000, 0.8166666666666666519, 0.8208333333333333037, 0.8249999999999999556, 0.8291666666666667185, 0.8333333333333333703, 0.8375000000000000222, 0.8416666666666666741, 0.8458333333333333259, 0.8499999999999999778, 0.8541666666666666297, 0.8583333333333332815, 0.8625000000000000444, 0.8666666666666666963, 0.8708333333333333481, 0.8750000000000000000, 0.8791666666666666519, 0.8833333333333333037, 0.8874999999999999556, 0.8916666666666667185, 0.8958333333333333703, 0.9000000000000000222, 0.9041666666666666741, 0.9083333333333333259, 0.9124999999999999778, 0.9166666666666666297, 0.9208333333333332815, 0.9250000000000000444, 0.9291666666666666963, 0.9333333333333333481, 0.9375000000000000000, 0.9416666666666666519, 0.9458333333333333037, 0.9499999999999999556, 0.9541666666666667185, 0.9583333333333333703, 0.9625000000000000222, 0.9666666666666666741, 0.9708333333333333259, 0.9749999999999999778, 0.9791666666666666297, 0.9833333333333332815, 0.9875000000000000444, 0.9916666666666666963, 0.9958333333333333481, 1.000000000000000000 ),
 .UNSPECIFIED. ) 
 GEOMETRIC_REPRESENTATION_ITEM ( )  RATIONAL_B_SPLINE_SURFACE ( (
 ( 1.000000000000000000, 0.8660254037844387076, 1.000000000000000000, 0.8660254037844387076, 1.000000000000000000, 0.8660254037844387076, 1.000000000000000000, 0.8660254037844387076, 1.000000000000000000, 0.8660254037844387076, 1.000000000000000000, 0.8660254037844387076, 1.000000000000000000, 0.8660254037844387076, 1.000000000000000000, 0.8660254037844387076, 1.000000000000000000, 0.8660254037844387076, 1.000000000000000000, 0.8660254037844387076, 1.000000000000000000, 0.8660254037844387076, 1.000000000000000000, 0.8660254037844387076, 1.000000000000000000, 0.8660254037844387076, 1.000000000000000000, 0.8660254037844387076, 1.000000000000000000, 0.8660254037844387076, 1.000000000000000000, 0.8660254037844387076, 1.000000000000000000, 0.8660254037844387076, 1.000000000000000000, 0.8660254037844387076, 1.000000000000000000, 0.8660254037844387076, 1.000000000000000000, 0.8660254037844387076, 1.000000000000000000, 0.8660254037844387076, 1.000000000000000000, 0.8660254037844387076, 1.000000000000000000, 0.8660254037844387076, 1.000000000000000000, 0.8660254037844387076, 1.000000000000000000, 0.8660254037844387076, 1.000000000000000000, 0.8660254037844387076, 1.000000000000000000, 0.8660254037844387076, 1.000000000000000000, 0.8660254037844387076, 1.000000000000000000, 0.8660254037844387076, 1.000000000000000000, 0.8660254037844387076, 1.000000000000000000, 0.8660254037844387076, 1.000000000000000000, 0.8660254037844387076, 1.000000000000000000, 0.8660254037844387076, 1.000000000000000000, 0.8660254037844387076, 1.000000000000000000, 0.8660254037844387076, 1.000000000000000000, 0.8660254037844387076, 1.000000000000000000, 0.8660254037844387076, 1.000000000000000000, 0.8660254037844387076, 1.000000000000000000, 0.8660254037844387076, 1.000000000000000000, 0.8660254037844387076, 1.000000000000000000, 0.8660254037844387076, 1.000000000000000000, 0.8660254037844387076, 1.000000000000000000, 0.8660254037844387076, 1.000000000000000000, 0.8660254037844387076, 1.000000000000000000, 0.8660254037844387076, 1.000000000000000000, 0.8660254037844387076, 1.000000000000000000, 0.8660254037844387076, 1.000000000000000000, 0.8660254037844387076, 1.000000000000000000, 0.8660254037844387076, 1.000000000000000000, 0.8660254037844387076, 1.000000000000000000, 0.8660254037844387076, 1.000000000000000000, 0.8660254037844387076, 1.000000000000000000, 0.8660254037844387076, 1.000000000000000000, 0.8660254037844387076, 1.000000000000000000, 0.8660254037844387076, 1.000000000000000000, 0.8660254037844387076, 1.000000000000000000, 0.8660254037844387076, 1.000000000000000000, 0.8660254037844387076, 1.000000000000000000, 0.8660254037844387076, 1.000000000000000000, 0.8660254037844387076, 1.000000000000000000, 0.8660254037844387076, 1.000000000000000000, 0.8660254037844387076, 1.000000000000000000, 0.8660254037844387076, 1.000000000000000000, 0.8660254037844387076, 1.000000000000000000, 0.8660254037844387076, 1.000000000000000000, 0.8660254037844387076, 1.000000000000000000, 0.8660254037844387076, 1.000000000000000000, 0.8660254037844387076, 1.000000000000000000, 0.8660254037844387076, 1.000000000000000000, 0.8660254037844387076, 1.000000000000000000, 0.8660254037844387076, 1.000000000000000000, 0.8660254037844387076, 1.000000000000000000, 0.8660254037844387076, 1.000000000000000000, 0.8660254037844387076, 1.000000000000000000, 0.8660254037844387076, 1.000000000000000000, 0.8660254037844387076, 1.000000000000000000, 0.8660254037844387076, 1.000000000000000000, 0.8660254037844387076, 1.000000000000000000, 0.8660254037844387076, 1.000000000000000000, 0.8660254037844387076, 1.000000000000000000, 0.8660254037844387076, 1.000000000000000000, 0.8660254037844387076, 1.000000000000000000, 0.8660254037844387076, 1.000000000000000000, 0.8660254037844387076, 1.000000000000000000, 0.8660254037844387076, 1.000000000000000000, 0.8660254037844387076, 1.000000000000000000, 0.8660254037844387076, 1.000000000000000000, 0.8660254037844387076, 1.000000000000000000, 0.8660254037844387076, 1.000000000000000000, 0.8660254037844387076, 1.000000000000000000, 0.8660254037844387076, 1.000000000000000000, 0.8660254037844387076, 1.000000000000000000, 0.8660254037844387076, 1.000000000000000000, 0.8660254037844387076, 1.000000000000000000, 0.8660254037844387076, 1.000000000000000000, 0.8660254037844387076, 1.000000000000000000, 0.8660254037844387076, 1.000000000000000000, 0.8660254037844387076, 1.000000000000000000, 0.8660254037844387076, 1.000000000000000000, 0.8660254037844387076, 1.000000000000000000, 0.8660254037844387076, 1.000000000000000000, 0.8660254037844387076, 1.000000000000000000, 0.8660254037844387076, 1.000000000000000000, 0.8660254037844387076, 1.000000000000000000, 0.8660254037844387076, 1.000000000000000000, 0.8660254037844387076, 1.000000000000000000, 0.8660254037844387076, 1.000000000000000000, 0.8660254037844387076, 1.000000000000000000, 0.8660254037844387076, 1.000000000000000000, 0.8660254037844387076, 1.000000000000000000, 0.8660254037844387076, 1.000000000000000000, 0.8660254037844387076, 1.000000000000000000, 0.8660254037844387076, 1.000000000000000000, 0.8660254037844387076, 1.000000000000000000, 0.8660254037844387076, 1.000000000000000000, 0.8660254037844387076, 1.000000000000000000, 0.8660254037844387076, 1.000000000000000000, 0.8660254037844387076, 1.000000000000000000, 0.8660254037844387076, 1.000000000000000000, 0.8660254037844387076, 1.000000000000000000, 0.8660254037844387076, 1.000000000000000000, 0.8660254037844387076, 1.000000000000000000, 0.8660254037844387076, 1.000000000000000000, 0.8660254037844387076, 1.000000000000000000, 0.8660254037844387076, 1.000000000000000000, 0.8660254037844387076, 1.000000000000000000, 0.8660254037844387076, 1.000000000000000000, 0.8660254037844387076, 1.000000000000000000, 0.8660254037844387076, 1.000000000000000000, 0.8660254037844387076, 1.000000000000000000, 0.8660254037844387076, 1.000000000000000000, 0.8660254037844387076, 1.000000000000000000, 0.8660254037844387076, 1.000000000000000000, 0.8660254037844387076, 1.000000000000000000, 0.8660254037844387076, 1.000000000000000000, 0.8660254037844387076, 1.000000000000000000, 0.8660254037844387076, 1.000000000000000000, 0.8660254037844387076, 1.000000000000000000, 0.8660254037844387076, 1.000000000000000000, 0.8660254037844387076, 1.000000000000000000, 0.8660254037844387076, 1.000000000000000000, 0.8660254037844387076, 1.000000000000000000, 0.8660254037844387076, 1.000000000000000000, 0.8660254037844387076, 1.000000000000000000, 0.8660254037844387076, 1.000000000000000000, 0.8660254037844387076, 1.000000000000000000, 0.8660254037844387076, 1.000000000000000000, 0.8660254037844387076, 1.000000000000000000, 0.8660254037844387076, 1.000000000000000000, 0.8660254037844387076, 1.000000000000000000, 0.8660254037844387076, 1.000000000000000000, 0.8660254037844387076, 1.000000000000000000, 0.8660254037844387076, 1.000000000000000000, 0.8660254037844387076, 1.000000000000000000, 0.8660254037844387076, 1.000000000000000000, 0.8660254037844387076, 1.000000000000000000, 0.8660254037844387076, 1.000000000000000000, 0.8660254037844387076, 1.000000000000000000, 0.8660254037844387076, 1.000000000000000000, 0.8660254037844387076, 1.000000000000000000, 0.8660254037844387076, 1.000000000000000000, 0.8660254037844387076, 1.000000000000000000, 0.8660254037844387076, 1.000000000000000000, 0.8660254037844387076, 1.000000000000000000, 0.8660254037844387076, 1.000000000000000000, 0.8660254037844387076, 1.000000000000000000, 0.8660254037844387076, 1.000000000000000000, 0.8660254037844387076, 1.000000000000000000, 0.8660254037844387076, 1.000000000000000000, 0.8660254037844387076, 1.000000000000000000, 0.8660254037844387076, 1.000000000000000000, 0.8660254037844387076, 1.000000000000000000, 0.8660254037844387076, 1.000000000000000000, 0.8660254037844387076, 1.000000000000000000, 0.8660254037844387076, 1.000000000000000000, 0.8660254037844387076, 1.000000000000000000, 0.8660254037844387076, 1.000000000000000000, 0.8660254037844387076, 1.000000000000000000, 0.8660254037844387076, 1.000000000000000000, 0.8660254037844387076, 1.000000000000000000, 0.8660254037844387076, 1.000000000000000000, 0.8660254037844387076, 1.000000000000000000, 0.8660254037844387076, 1.000000000000000000, 0.8660254037844387076, 1.000000000000000000, 0.8660254037844387076, 1.000000000000000000, 0.8660254037844387076, 1.000000000000000000, 0.8660254037844387076, 1.000000000000000000, 0.8660254037844387076, 1.000000000000000000, 0.8660254037844387076, 1.000000000000000000, 0.8660254037844387076, 1.000000000000000000, 0.8660254037844387076, 1.000000000000000000, 0.8660254037844387076, 1.000000000000000000, 0.8660254037844387076, 1.000000000000000000, 0.8660254037844387076, 1.000000000000000000, 0.8660254037844387076, 1.000000000000000000, 0.8660254037844387076, 1.000000000000000000, 0.8660254037844387076, 1.000000000000000000, 0.8660254037844387076, 1.000000000000000000, 0.8660254037844387076, 1.000000000000000000, 0.8660254037844387076, 1.000000000000000000, 0.8660254037844387076, 1.000000000000000000, 0.8660254037844387076, 1.000000000000000000, 0.8660254037844387076, 1.000000000000000000, 0.8660254037844387076, 1.000000000000000000, 0.8660254037844387076, 1.000000000000000000, 0.8660254037844387076, 1.000000000000000000, 0.8660254037844387076, 1.000000000000000000, 0.8660254037844387076, 1.000000000000000000, 0.8660254037844387076, 1.000000000000000000, 0.8660254037844387076, 1.000000000000000000, 0.8660254037844387076, 1.000000000000000000, 0.8660254037844387076, 1.000000000000000000, 0.8660254037844387076, 1.000000000000000000, 0.8660254037844387076, 1.000000000000000000, 0.8660254037844387076, 1.000000000000000000, 0.8660254037844387076, 1.000000000000000000, 0.8660254037844387076, 1.000000000000000000, 0.8660254037844387076, 1.000000000000000000, 0.8660254037844387076, 1.000000000000000000, 0.8660254037844387076, 1.000000000000000000, 0.8660254037844387076, 1.000000000000000000, 0.8660254037844387076, 1.000000000000000000, 0.8660254037844387076, 1.000000000000000000, 0.8660254037844387076, 1.000000000000000000, 0.8660254037844387076, 1.000000000000000000, 0.8660254037844387076, 1.000000000000000000, 0.8660254037844387076, 1.000000000000000000, 0.8660254037844387076, 1.000000000000000000, 0.8660254037844387076, 1.000000000000000000, 0.8660254037844387076, 1.000000000000000000, 0.8660254037844387076, 1.000000000000000000, 0.8660254037844387076, 1.000000000000000000, 0.8660254037844387076, 1.000000000000000000, 0.8660254037844387076, 1.000000000000000000, 0.8660254037844387076, 1.000000000000000000, 0.8660254037844387076, 1.000000000000000000, 0.8660254037844387076, 1.000000000000000000, 0.8660254037844387076, 1.000000000000000000, 0.8660254037844387076, 1.000000000000000000, 0.8660254037844387076, 1.000000000000000000),
 ( 1.000000000000000000, 0.8660254037844387076, 1.000000000000000000, 0.8660254037844387076, 1.000000000000000000, 0.8660254037844387076, 1.000000000000000000, 0.8660254037844387076, 1.000000000000000000, 0.8660254037844387076, 1.000000000000000000, 0.8660254037844387076, 1.000000000000000000, 0.8660254037844387076, 1.000000000000000000, 0.8660254037844387076, 1.000000000000000000, 0.8660254037844387076, 1.000000000000000000, 0.8660254037844387076, 1.000000000000000000, 0.8660254037844387076, 1.000000000000000000, 0.8660254037844387076, 1.000000000000000000, 0.8660254037844387076, 1.000000000000000000, 0.8660254037844387076, 1.000000000000000000, 0.8660254037844387076, 1.000000000000000000, 0.8660254037844387076, 1.000000000000000000, 0.8660254037844387076, 1.000000000000000000, 0.8660254037844387076, 1.000000000000000000, 0.8660254037844387076, 1.000000000000000000, 0.8660254037844387076, 1.000000000000000000, 0.8660254037844387076, 1.000000000000000000, 0.8660254037844387076, 1.000000000000000000, 0.8660254037844387076, 1.000000000000000000, 0.8660254037844387076, 1.000000000000000000, 0.8660254037844387076, 1.000000000000000000, 0.8660254037844387076, 1.000000000000000000, 0.8660254037844387076, 1.000000000000000000, 0.8660254037844387076, 1.000000000000000000, 0.8660254037844387076, 1.000000000000000000, 0.8660254037844387076, 1.000000000000000000, 0.8660254037844387076, 1.000000000000000000, 0.8660254037844387076, 1.000000000000000000, 0.8660254037844387076, 1.000000000000000000, 0.8660254037844387076, 1.000000000000000000, 0.8660254037844387076, 1.000000000000000000, 0.8660254037844387076, 1.000000000000000000, 0.8660254037844387076, 1.000000000000000000, 0.8660254037844387076, 1.000000000000000000, 0.8660254037844387076, 1.000000000000000000, 0.8660254037844387076, 1.000000000000000000, 0.8660254037844387076, 1.000000000000000000, 0.8660254037844387076, 1.000000000000000000, 0.8660254037844387076, 1.000000000000000000, 0.8660254037844387076, 1.000000000000000000, 0.8660254037844387076, 1.000000000000000000, 0.8660254037844387076, 1.000000000000000000, 0.8660254037844387076, 1.000000000000000000, 0.8660254037844387076, 1.000000000000000000, 0.8660254037844387076, 1.000000000000000000, 0.8660254037844387076, 1.000000000000000000, 0.8660254037844387076, 1.000000000000000000, 0.8660254037844387076, 1.000000000000000000, 0.8660254037844387076, 1.000000000000000000, 0.8660254037844387076, 1.000000000000000000, 0.8660254037844387076, 1.000000000000000000, 0.8660254037844387076, 1.000000000000000000, 0.8660254037844387076, 1.000000000000000000, 0.8660254037844387076, 1.000000000000000000, 0.8660254037844387076, 1.000000000000000000, 0.8660254037844387076, 1.000000000000000000, 0.8660254037844387076, 1.000000000000000000, 0.8660254037844387076, 1.000000000000000000, 0.8660254037844387076, 1.000000000000000000, 0.8660254037844387076, 1.000000000000000000, 0.8660254037844387076, 1.000000000000000000, 0.8660254037844387076, 1.000000000000000000, 0.8660254037844387076, 1.000000000000000000, 0.8660254037844387076, 1.000000000000000000, 0.8660254037844387076, 1.000000000000000000, 0.8660254037844387076, 1.000000000000000000, 0.8660254037844387076, 1.000000000000000000, 0.8660254037844387076, 1.000000000000000000, 0.8660254037844387076, 1.000000000000000000, 0.8660254037844387076, 1.000000000000000000, 0.8660254037844387076, 1.000000000000000000, 0.8660254037844387076, 1.000000000000000000, 0.8660254037844387076, 1.000000000000000000, 0.8660254037844387076, 1.000000000000000000, 0.8660254037844387076, 1.000000000000000000, 0.8660254037844387076, 1.000000000000000000, 0.8660254037844387076, 1.000000000000000000, 0.8660254037844387076, 1.000000000000000000, 0.8660254037844387076, 1.000000000000000000, 0.8660254037844387076, 1.000000000000000000, 0.8660254037844387076, 1.000000000000000000, 0.8660254037844387076, 1.000000000000000000, 0.8660254037844387076, 1.000000000000000000, 0.8660254037844387076, 1.000000000000000000, 0.8660254037844387076, 1.000000000000000000, 0.8660254037844387076, 1.000000000000000000, 0.8660254037844387076, 1.000000000000000000, 0.8660254037844387076, 1.000000000000000000, 0.8660254037844387076, 1.000000000000000000, 0.8660254037844387076, 1.000000000000000000, 0.8660254037844387076, 1.000000000000000000, 0.8660254037844387076, 1.000000000000000000, 0.8660254037844387076, 1.000000000000000000, 0.8660254037844387076, 1.000000000000000000, 0.8660254037844387076, 1.000000000000000000, 0.8660254037844387076, 1.000000000000000000, 0.8660254037844387076, 1.000000000000000000, 0.8660254037844387076, 1.000000000000000000, 0.8660254037844387076, 1.000000000000000000, 0.8660254037844387076, 1.000000000000000000, 0.8660254037844387076, 1.000000000000000000, 0.8660254037844387076, 1.000000000000000000, 0.8660254037844387076, 1.000000000000000000, 0.8660254037844387076, 1.000000000000000000, 0.8660254037844387076, 1.000000000000000000, 0.8660254037844387076, 1.000000000000000000, 0.8660254037844387076, 1.000000000000000000, 0.8660254037844387076, 1.000000000000000000, 0.8660254037844387076, 1.000000000000000000, 0.8660254037844387076, 1.000000000000000000, 0.8660254037844387076, 1.000000000000000000, 0.8660254037844387076, 1.000000000000000000, 0.8660254037844387076, 1.000000000000000000, 0.8660254037844387076, 1.000000000000000000, 0.8660254037844387076, 1.000000000000000000, 0.8660254037844387076, 1.000000000000000000, 0.8660254037844387076, 1.000000000000000000, 0.8660254037844387076, 1.000000000000000000, 0.8660254037844387076, 1.000000000000000000, 0.8660254037844387076, 1.000000000000000000, 0.8660254037844387076, 1.000000000000000000, 0.8660254037844387076, 1.000000000000000000, 0.8660254037844387076, 1.000000000000000000, 0.8660254037844387076, 1.000000000000000000, 0.8660254037844387076, 1.000000000000000000, 0.8660254037844387076, 1.000000000000000000, 0.8660254037844387076, 1.000000000000000000, 0.8660254037844387076, 1.000000000000000000, 0.8660254037844387076, 1.000000000000000000, 0.8660254037844387076, 1.000000000000000000, 0.8660254037844387076, 1.000000000000000000, 0.8660254037844387076, 1.000000000000000000, 0.8660254037844387076, 1.000000000000000000, 0.8660254037844387076, 1.000000000000000000, 0.8660254037844387076, 1.000000000000000000, 0.8660254037844387076, 1.000000000000000000, 0.8660254037844387076, 1.000000000000000000, 0.8660254037844387076, 1.000000000000000000, 0.8660254037844387076, 1.000000000000000000, 0.8660254037844387076, 1.000000000000000000, 0.8660254037844387076, 1.000000000000000000, 0.8660254037844387076, 1.000000000000000000, 0.8660254037844387076, 1.000000000000000000, 0.8660254037844387076, 1.000000000000000000, 0.8660254037844387076, 1.000000000000000000, 0.8660254037844387076, 1.000000000000000000, 0.8660254037844387076, 1.000000000000000000, 0.8660254037844387076, 1.000000000000000000, 0.8660254037844387076, 1.000000000000000000, 0.8660254037844387076, 1.000000000000000000, 0.8660254037844387076, 1.000000000000000000, 0.8660254037844387076, 1.000000000000000000, 0.8660254037844387076, 1.000000000000000000, 0.8660254037844387076, 1.000000000000000000, 0.8660254037844387076, 1.000000000000000000, 0.8660254037844387076, 1.000000000000000000, 0.8660254037844387076, 1.000000000000000000, 0.8660254037844387076, 1.000000000000000000, 0.8660254037844387076, 1.000000000000000000, 0.8660254037844387076, 1.000000000000000000, 0.8660254037844387076, 1.000000000000000000, 0.8660254037844387076, 1.000000000000000000, 0.8660254037844387076, 1.000000000000000000, 0.8660254037844387076, 1.000000000000000000, 0.8660254037844387076, 1.000000000000000000, 0.8660254037844387076, 1.000000000000000000, 0.8660254037844387076, 1.000000000000000000, 0.8660254037844387076, 1.000000000000000000, 0.8660254037844387076, 1.000000000000000000, 0.8660254037844387076, 1.000000000000000000, 0.8660254037844387076, 1.000000000000000000, 0.8660254037844387076, 1.000000000000000000, 0.8660254037844387076, 1.000000000000000000, 0.8660254037844387076, 1.000000000000000000, 0.8660254037844387076, 1.000000000000000000, 0.8660254037844387076, 1.000000000000000000, 0.8660254037844387076, 1.000000000000000000, 0.8660254037844387076, 1.000000000000000000, 0.8660254037844387076, 1.000000000000000000, 0.8660254037844387076, 1.000000000000000000, 0.8660254037844387076, 1.000000000000000000, 0.8660254037844387076, 1.000000000000000000, 0.8660254037844387076, 1.000000000000000000, 0.8660254037844387076, 1.000000000000000000, 0.8660254037844387076, 1.000000000000000000, 0.8660254037844387076, 1.000000000000000000, 0.8660254037844387076, 1.000000000000000000, 0.8660254037844387076, 1.000000000000000000, 0.8660254037844387076, 1.000000000000000000, 0.8660254037844387076, 1.000000000000000000, 0.8660254037844387076, 1.000000000000000000, 0.8660254037844387076, 1.000000000000000000, 0.8660254037844387076, 1.000000000000000000, 0.8660254037844387076, 1.000000000000000000, 0.8660254037844387076, 1.000000000000000000, 0.8660254037844387076, 1.000000000000000000, 0.8660254037844387076, 1.000000000000000000, 0.8660254037844387076, 1.000000000000000000, 0.8660254037844387076, 1.000000000000000000, 0.8660254037844387076, 1.000000000000000000, 0.8660254037844387076, 1.000000000000000000, 0.8660254037844387076, 1.000000000000000000, 0.8660254037844387076, 1.000000000000000000, 0.8660254037844387076, 1.000000000000000000, 0.8660254037844387076, 1.000000000000000000, 0.8660254037844387076, 1.000000000000000000, 0.8660254037844387076, 1.000000000000000000, 0.8660254037844387076, 1.000000000000000000, 0.8660254037844387076, 1.000000000000000000, 0.8660254037844387076, 1.000000000000000000, 0.8660254037844387076, 1.000000000000000000, 0.8660254037844387076, 1.000000000000000000, 0.8660254037844387076, 1.000000000000000000, 0.8660254037844387076, 1.000000000000000000, 0.8660254037844387076, 1.000000000000000000, 0.8660254037844387076, 1.000000000000000000, 0.8660254037844387076, 1.000000000000000000, 0.8660254037844387076, 1.000000000000000000, 0.8660254037844387076, 1.000000000000000000, 0.8660254037844387076, 1.000000000000000000, 0.8660254037844387076, 1.000000000000000000, 0.8660254037844387076, 1.000000000000000000, 0.8660254037844387076, 1.000000000000000000, 0.8660254037844387076, 1.000000000000000000, 0.8660254037844387076, 1.000000000000000000, 0.8660254037844387076, 1.000000000000000000, 0.8660254037844387076, 1.000000000000000000, 0.8660254037844387076, 1.000000000000000000, 0.8660254037844387076, 1.000000000000000000, 0.8660254037844387076, 1.000000000000000000, 0.8660254037844387076, 1.000000000000000000, 0.8660254037844387076, 1.000000000000000000, 0.8660254037844387076, 1.000000000000000000, 0.8660254037844387076, 1.000000000000000000, 0.8660254037844387076, 1.000000000000000000, 0.8660254037844387076, 1.000000000000000000) ) ) 
 REPRESENTATION_ITEM ( '' )  SURFACE ( )  );
#30910=EDGE_LOOP ( 'NONE', ( #50609, #100398, #203760, #160946, #3436, #102690 ) ) ;
#30917=CARTESIAN_POINT ( 'NONE',  ( 5.099838337034727331, 9.101561826515851550, -0.7998128361456281477 ) ) ;
#30918=CARTESIAN_POINT ( 'NONE',  ( -2.916975605234527702, 6.554888639415577423, 1.040834085586084257E-14 ) ) ;
#30922=CARTESIAN_POINT ( 'NONE',  ( 4.758548728272192108, 7.535095368750792666, -1.082531754730549078 ) ) ;
#30923=CARTESIAN_POINT ( 'NONE',  ( 1.364683531249986537, -0.07395833299191513499, 0.7879004041258500513 ) ) ;
#30925=CARTESIAN_POINT ( 'NONE',  ( -7.974166903131914452, 12.45494515362926435, -0.7998128361456281477 ) ) ;
#30939=CARTESIAN_POINT ( 'NONE',  ( -4.229020061460118107, 7.343517960532633282, -0.8650006913940473385 ) ) ;
#30943=CARTESIAN_POINT ( 'NONE',  ( 7.481401836642521452, 7.622723652371411696, 1.040834085586084257E-14 ) ) ;
#30950=CARTESIAN_POINT ( 'NONE',  ( 8.959240580532112475, 9.346868853575953651, -0.7998128361456221525 ) ) ;
#30954=CARTESIAN_POINT ( 'NONE',  ( 10.42352117080803708, 11.05519620889787724, -0.7998128361456281477 ) ) ;
#30956=CARTESIAN_POINT ( 'NONE',  ( 1.499999999999987121, 3.795833333333357373, -0.8660254037844263841 ) ) ;
#30962=CARTESIAN_POINT ( 'NONE',  ( -0.4996389044604229723, 7.815212647110488575, 1.937417588921823919 ) ) ;
#30967=CARTESIAN_POINT ( 'NONE',  ( -10.33094986393327197, 11.15512238411806578, 0.7216878364870438212 ) ) ;
#30971=CARTESIAN_POINT ( 'NONE',  ( 6.335737856287750880, 6.286115675290828264, -0.7998128361456281477 ) ) ;
#30977=CARTESIAN_POINT ( 'NONE',  ( 5.490689023410166847, 5.508151403507724808, -0.7216878364870207285 ) ) ;
#30985=CARTESIAN_POINT ( 'NONE',  ( -6.612626235163205024, 8.737816579155630592, -1.599625672291263179 ) ) ;
#30986=CARTESIAN_POINT ( 'NONE',  ( -5.382750679825375251, 6.238629533673094585, -1.199719254218446718 ) ) ;
#30991=CARTESIAN_POINT ( 'NONE',  ( 0.5512317429218656084, 7.510131493957763915, -1.922545642343834738 ) ) ;
#30995=CARTESIAN_POINT ( 'NONE',  ( 6.368579470117202490, 8.453095353268645695, 1.599625672291281386 ) ) ;
#31008=CARTESIAN_POINT ( 'NONE',  ( -0.6823417656250246877, 0.3635416670080895973, 1.181850606188755259 ) ) ;
#31010=CARTESIAN_POINT ( 'NONE',  ( 3.330499290451326200, 7.037332938835193730, -0.7998128361456291469 ) ) ;
#31012=CARTESIAN_POINT ( 'NONE',  ( -7.226132686403777150, 7.532835677000276675, 1.040834085586084257E-14 ) ) ;
#31014=CARTESIAN_POINT ( 'NONE',  ( 3.362058906508953449, 6.866226457661676719, -0.7216878364870267237 ) ) ;
#31015=CARTESIAN_POINT ( 'NONE',  ( -8.500599125644013654, 9.019713189447241319, 0.7216878364870438212 ) ) ;
#31017=EDGE_LOOP ( 'NONE', ( #116832, #45027, #165860, #134297, #63937 ) ) ;
#31019=CARTESIAN_POINT ( 'NONE',  ( 6.076025397218672630, 10.24044673006381245, -0.7998128361456291469 ) ) ;
#31024=CARTESIAN_POINT ( 'NONE',  ( 1.364683531249990311, 5.613541667008087543, 0.7879004041258500513 ) ) ;
#31029=CARTESIAN_POINT ( 'NONE',  ( 7.958799866421889746, 9.244020251369077457, -1.199719254218441611 ) ) ;
#31033=CARTESIAN_POINT ( 'NONE',  ( -6.906989191158078079, 10.14557225873805812, -1.199719254218440723 ) ) ;
#31039=CARTESIAN_POINT ( 'NONE',  ( 8.565000355531088516, 11.01558638625153286, -1.599625672291257406 ) ) ;
#31041=CARTESIAN_POINT ( 'NONE',  ( -9.016335848287868160, 10.47781223021269170, 1.199719254218462483 ) ) ;
#31044=CARTESIAN_POINT ( 'NONE',  ( 5.808322585208748556, 6.028124808163927817, -0.4837759047566763670 ) ) ;
#31045=CARTESIAN_POINT ( 'NONE',  ( -9.829298180227631576, 10.56986208646148384, 1.040834085586084257E-14 ) ) ;
#31050=CARTESIAN_POINT ( 'NONE',  ( 5.961834861707224320, 7.978559976790334574, -1.599625672291262513 ) ) ;
#31052=CARTESIAN_POINT ( 'NONE',  ( 5.392392409933256303, 7.314210449720692786, 1.599625672291267398 ) ) ;
#31053=CARTESIAN_POINT ( 'NONE',  ( -4.073306942994160629, 7.542743630792291043, -0.4897309385070089394 ) ) ;
#31054=CARTESIAN_POINT ( 'NONE',  ( 2.659370686574860976, 6.254349567645977714, -0.7998128361456291469 ) ) ;
#31056=CARTESIAN_POINT ( 'NONE',  ( -7.429504990608782222, 8.730472579540773381, 1.082531754730549967 ) ) ;
#31061=CARTESIAN_POINT ( 'NONE',  ( -5.076477019373391464, 6.555905325687263030, 1.224675693024103174 ) ) ;
#31063=CARTESIAN_POINT ( 'NONE',  ( -1.364683531250000748, -0.1781249996585798634, 0.000000000000000000 ) ) ;
#31066=CARTESIAN_POINT ( 'NONE',  ( 4.202664430556247055, 6.886563688082179446, 1.082531754730558626 ) ) ;
#31070=CARTESIAN_POINT ( 'NONE',  ( -9.015808962963337336, 10.58116054728778366, 1.082531754730558626 ) ) ;
#31077=CARTESIAN_POINT ( 'NONE',  ( -9.802181872555943087, 10.53822639417784046, 0.7216878364870438212 ) ) ;
#31078=DIRECTION ( 'NONE',  ( -0.9055141421511233579, 0.4243160830846685050, -2.454401000341485681E-15 ) ) ;
#31079=ORIENTED_EDGE ( 'NONE', *, *, #198311, .T. ) ;
#31081=EDGE_CURVE ( 'NONE', #136958, #93339, #30283, .T. ) ;
#31085=CARTESIAN_POINT ( 'NONE',  ( -7.985389288324697965, 10.33937347451072775, -1.443375672974058777 ) ) ;
#31090=CARTESIAN_POINT ( 'NONE',  ( -1.364683531250010295, 5.342708333674750953, 0.7879004041258379498 ) ) ;
#31091=CARTESIAN_POINT ( 'NONE',  ( -1.500000000000013101, 2.702083334016155636, 0.8660254037844403729 ) ) ;
#31092=CARTESIAN_POINT ( 'NONE',  ( 5.354985324346148268, 6.526937442883553153, -1.333766491515418817 ) ) ;
#31097=CARTESIAN_POINT ( 'NONE',  ( -6.886651960737580680, 10.12184548991413457, -1.199719254218440723 ) ) ;
#31100=CARTESIAN_POINT ( 'NONE',  ( 6.484877546038077867, 6.460111979999551224, 1.040834085586084257E-14 ) ) ;
#31101=ORIENTED_EDGE ( 'NONE', *, *, #101284, .T. ) ;
#31106=CARTESIAN_POINT ( 'NONE',  ( 8.471147050440139381, 8.777426401801974976, -0.7998128361456281477 ) ) ;
#31112=CARTESIAN_POINT ( 'NONE',  ( -5.992340707560165569, 8.014150130285418783, 1.443375672974064550 ) ) ;
#31115=CARTESIAN_POINT ( 'NONE',  ( -1.364683531249997417, 5.321875000341417916, 1.214306433183764966E-14 ) ) ;
#31116=CIRCLE ( 'NONE', #152157, 0.08000000000000020983 ) ;
#31119=CARTESIAN_POINT ( 'NONE',  ( -5.426287360647527258, 6.306760859481674864, -1.047964138152550406 ) ) ;
#31122=CARTESIAN_POINT ( 'NONE',  ( -8.306341666666730461, 12.84248237775322643, 1.040834085586084257E-14 ) ) ;
#31124=CARTESIAN_POINT ( 'NONE',  ( 7.639129486296027061, 10.99973593639901814, 1.199719254218460707 ) ) ;
#31126=CARTESIAN_POINT ( 'NONE',  ( -8.479735010343349089, 11.98044238112085758, 1.199719254218453823 ) ) ;
#31127=DIRECTION ( 'NONE',  ( -0.7592566023653005702, 0.6507913734559640506, 0.000000000000000000 ) ) ;
#31129=CARTESIAN_POINT ( 'NONE',  ( 1.364683531249990311, 4.134375000341417028, 1.214306433183764966E-14 ) ) ;
#31130=CARTESIAN_POINT ( 'NONE',  ( 4.695201269034174452, 4.372156323494968966, 1.214306433183764966E-14 ) ) ;
#31135=CARTESIAN_POINT ( 'NONE',  ( 9.368320956918608999, 11.95279375453699622, 1.443375672974076540 ) ) ;
#31137=CARTESIAN_POINT ( 'NONE',  ( -6.222829318992474157, 10.20379193889247382, 0.000000000000000000 ) ) ;
#31138=CARTESIAN_POINT ( 'NONE',  ( -1.364683531250012516, 1.030208333674754062, 0.7879004041258379498 ) ) ;
#31142=CARTESIAN_POINT ( 'NONE',  ( -8.857554428429624593, 9.228235009456373206, 0.7998128361456462443 ) ) ;
#31144=CARTESIAN_POINT ( 'NONE',  ( -3.809477975315625375, 4.507107728365378208, 1.082531754730558626 ) ) ;
#31145=CARTESIAN_POINT ( 'NONE',  ( 0.6823417656249899377, 3.155208333674754062, 1.181850606188765695 ) ) ;
#31163=CARTESIAN_POINT ( 'NONE',  ( -1.364683531250012516, 4.551041667008082214, -0.7879004041258300672 ) ) ;
#31168=CARTESIAN_POINT ( 'NONE',  ( 7.934546212495622086, 10.28005655271014795, -1.599625672291262513 ) ) ;
#31171=CARTESIAN_POINT ( 'NONE',  ( 1.364683531249986537, 2.655208333674754062, -0.7879004041258239610 ) ) ;
#31173=CARTESIAN_POINT ( 'NONE',  ( -6.182154858151506893, 9.195969186943299789, 1.082531754730548412 ) ) ;
#31175=CARTESIAN_POINT ( 'NONE',  ( 1.436838838544552299, 7.449283400311791148, 4.203727439823582657 ) ) ;
#31179=CARTESIAN_POINT ( 'NONE',  ( 2.530568227245037605, 6.104080031761181857, 0.000000000000000000 ) ) ;
#31182=CARTESIAN_POINT ( 'NONE',  ( 9.378489572351044856, 11.96465713920816043, -1.599625672291262513 ) ) ;
#31183=CARTESIAN_POINT ( 'NONE',  ( -1.499999999999993339, 10.64264068711930733, 1.232676135170975238E-14 ) ) ;
#31189=CARTESIAN_POINT ( 'NONE',  ( -9.972185678051314284, 11.59297036493672017, 1.199719254218462483 ) ) ;
#31190=CARTESIAN_POINT ( 'NONE',  ( 7.955937213120826357, 8.176348258262782664, 0.7998128361456481317 ) ) ;
#31204=CARTESIAN_POINT ( 'NONE',  ( -6.887178846062128379, 7.137389529935019183, -0.7216878364870278340 ) ) ;
#31205=CARTESIAN_POINT ( 'NONE',  ( 6.173040012923759257, 6.096301524699504704, -0.7998128361456281477 ) ) ;
#31208=CARTESIAN_POINT ( 'NONE',  ( -8.025536864285518490, 11.45054454405341282, -1.199719254218446718 ) ) ;
#31212=CARTESIAN_POINT ( 'NONE',  ( -1.499999999999993339, 10.64264068711930733, 1.232676135170975238E-14 ) ) ;
#31213=CARTESIAN_POINT ( 'NONE',  ( -10.47097470845587175, 11.11055866948701443, 1.040834085586084257E-14 ) ) ;
#31215=CARTESIAN_POINT ( 'NONE',  ( -4.303094902415906198, 7.389312076987425648, -1.073240500945132236 ) ) ;
#31216=CARTESIAN_POINT ( 'NONE',  ( 8.178592977541601527, 10.56477777859713463, 1.599625672291281386 ) ) ;
#31219=VERTEX_POINT ( 'NONE', #9108 ) ;
#31228=CARTESIAN_POINT ( 'NONE',  ( -9.158696461231359720, 10.64389961198009615, 1.199719254218462483 ) ) ;
#31232=CARTESIAN_POINT ( 'NONE',  ( 6.805829924380105034, 9.923590097543378619, 1.082531754730558626 ) ) ;
#31235=CARTESIAN_POINT ( 'NONE',  ( 3.979481780810941949, 4.601482484822914998, 1.199719254218464037 ) ) ;
#31238=CARTESIAN_POINT ( 'NONE',  ( -6.901263884555985051, 8.010228272525461435, 1.199719254218450271 ) ) ;
#31249=CARTESIAN_POINT ( 'NONE',  ( -0.6823417656249969321, 3.780208333674754506, -1.181850606188749264 ) ) ;
#31251=CARTESIAN_POINT ( 'NONE',  ( 8.320953590485093088, 10.73086516036454618, 1.599625672291281386 ) ) ;
#31254=CARTESIAN_POINT ( 'NONE',  ( -4.500943810056945438, 5.313817868896925312, 1.082531754730560403 ) ) ;
#31256=CARTESIAN_POINT ( 'NONE',  ( -4.731432421044883263, 5.582721248382882528, -1.082531754730543971 ) ) ;
#31263=CARTESIAN_POINT ( 'NONE',  ( 3.161022370280501814, 6.839609865302569425, 0.000000000000000000 ) ) ;
#31271=EDGE_CURVE ( 'NONE', #43706, #30492, #74559, .T. ) ;
#31272=CARTESIAN_POINT ( 'NONE',  ( 4.171104814498611368, 8.018039383557042044, 0.7998128361456321445 ) ) ;
#31276=CARTESIAN_POINT ( 'NONE',  ( 0.6823417656249899377, 4.238541667008085767, -1.181850606188754593 ) ) ;
#31281=CARTESIAN_POINT ( 'NONE',  ( 6.986529229743720926, 7.045372277656132276, -0.7998128361456281477 ) ) ;
#31283=CARTESIAN_POINT ( 'NONE',  ( -4.355193658487827690, 6.104145239700998538, -1.599625672291256295 ) ) ;
#31284=CARTESIAN_POINT ( 'NONE',  ( 0.7499999999999902300, 1.983333333333357817, 1.299038105676669330 ) ) ;
#31287=CARTESIAN_POINT ( 'NONE',  ( -5.461236948206312114, 5.265864615862458464, 0.7998128361456341429 ) ) ;
#31291=CARTESIAN_POINT ( 'NONE',  ( 1.364683531249988535, 2.613541667008089764, 0.7879004041258500513 ) ) ;
#31293=CARTESIAN_POINT ( 'NONE',  ( -4.948362879307902418, 4.875437568721725512, 1.214306433183764966E-14 ) ) ;
#31299=CARTESIAN_POINT ( 'NONE',  ( 6.342516933094585418, 6.294024598232139667, 1.040834085586084257E-14 ) ) ;
#31303=CARTESIAN_POINT ( 'NONE',  ( -0.6823417656249969321, 4.530208333674755394, -1.181850606188749264 ) ) ;
#31306=CARTESIAN_POINT ( 'NONE',  ( -1.402160292154681736E-14, 0.3843750003414230232, 1.575800808251672791 ) ) ;
#31308=CARTESIAN_POINT ( 'NONE',  ( -9.001723924469462901, 12.58942944760136484, -1.199719254218446718 ) ) ;
#31309=CARTESIAN_POINT ( 'NONE',  ( -5.368665640887164692, 9.207267647769599606, 0.000000000000000000 ) ) ;
#31311=CARTESIAN_POINT ( 'NONE',  ( -1.403499169902660437, 7.376709478543006071, -4.304123474984413278 ) ) ;
#31313=CARTESIAN_POINT ( 'NONE',  ( -1.364683531249997417, 4.009375000341424133, 1.214306433183764966E-14 ) ) ;
#31323=CARTESIAN_POINT ( 'NONE',  ( -5.327991180046197428, 8.199444895820425572, 1.082531754730548412 ) ) ;
#31325=EDGE_CURVE ( 'NONE', #24517, #153088, #195337, .T. ) ;
#31329=CARTESIAN_POINT ( 'NONE',  ( -4.880572110795192486, 8.637825195995631589, 1.214306433183764966E-14 ) ) ;
#31343=CARTESIAN_POINT ( 'NONE',  ( 0.08888683327021307257, 6.492044364012829583, -3.106763327641859362 ) ) ;
#31344=CARTESIAN_POINT ( 'NONE',  ( -3.893162665418476109, 7.693773542963529444, 1.040834085586084257E-14 ) ) ;
#31347=CARTESIAN_POINT ( 'NONE',  ( -1.402160292154681736E-14, 1.337500000000025446, -1.732050807568863648 ) ) ;
#31348=CARTESIAN_POINT ( 'NONE',  ( 9.246297574839974942, 11.81043314211192019, 1.443375672974076540 ) ) ;
#31349=CARTESIAN_POINT ( 'NONE',  ( 6.877010230629674759, 9.046264573866535486, 1.599625672291281386 ) ) ;
#31352=CARTESIAN_POINT ( 'NONE',  ( 4.924636110261782385, 6.768494766770632332, 1.599625672291267398 ) ) ;
#31358=CARTESIAN_POINT ( 'NONE',  ( -2.955314298098991266, 6.391691081183366485, 0.7216878364870317197 ) ) ;
#31361=CARTESIAN_POINT ( 'NONE',  ( 4.222669843016465308, 3.519858668466394835, -2.499999999999995115 ) ) ;
#31362=CARTESIAN_POINT ( 'NONE',  ( -0.3833105440376022299, 6.967102400362891856, 3.825703835310487300 ) ) ;
#31365=CARTESIAN_POINT ( 'NONE',  ( -1.201851678989727383E-14, 2.696875000341417916, -1.575800808251660134 ) ) ;
#31366=CARTESIAN_POINT ( 'NONE',  ( 10.04622863760192963, 10.82294762006482713, -0.7216878364870257245 ) ) ;
#31367=CARTESIAN_POINT ( 'NONE',  ( -5.540478329478883524, 9.615641817700700145, 0.000000000000000000 ) ) ;
#31370=CARTESIAN_POINT ( 'NONE',  ( 5.819474248763732760, 7.812472595022922128, -1.599625672291262513 ) ) ;
#31371=CARTESIAN_POINT ( 'NONE',  ( -7.223796917982883592, 7.322184580601816428, -0.7998128361456291469 ) ) ;
#31375=CARTESIAN_POINT ( 'NONE',  ( 1.499999999999987121, 0.5354166673494816786, 0.8660254037844524744 ) ) ;
#31378=CARTESIAN_POINT ( 'NONE',  ( 8.459924665247367415, 8.972259652317825740, -0.7216878364870267237 ) ) ;
#31381=CARTESIAN_POINT ( 'NONE',  ( 0.6823417656249882723, 0.2385416670080825474, -1.181850606188749264 ) ) ;
#31383=CARTESIAN_POINT ( 'NONE',  ( 7.605760987142057061, 7.975735361194951523, -0.7216878364870267237 ) ) ;
#31386=CARTESIAN_POINT ( 'NONE',  ( -4.785665035943912571, 4.685623418130398399, 1.214306433183764966E-14 ) ) ;
#31388=CARTESIAN_POINT ( 'NONE',  ( 0.6823417656249899377, 4.426041667008086655, -1.181850606188754593 ) ) ;
#31392=CARTESIAN_POINT ( 'NONE',  ( -5.338497050760650176, 6.533440992188984886, -1.368045069562271010 ) ) ;
#31400=B_SPLINE_CURVE_WITH_KNOTS ( 'NONE', 3,
 ( #76121, #205032, #40440, #174718, #43648, #8983, #26291, #58805, #89193, #190921, #41510, #59869 ),
 .UNSPECIFIED., .F., .F.,
 ( 4, 2, 2, 2, 2, 4 ),
 ( 0.002160919429045905869, 0.002539139494017131175, 0.002917359558988356916, 0.003673799688930807529, 0.004430239818873258142, 0.005186679948815707888 ),
 .UNSPECIFIED. ) ;
#31401=CARTESIAN_POINT ( 'NONE',  ( 7.657657833620182153, 7.828355648845348291, -0.7998128361456281477 ) ) ;
#31404=CARTESIAN_POINT ( 'NONE',  ( 5.034155109375821446, 4.767602470560229122, -0.7998128361456221525 ) ) ;
#31410=ORIENTED_EDGE ( 'NONE', *, *, #43730, .F. ) ;
#31412=CARTESIAN_POINT ( 'NONE',  ( 4.663641653420880218, 8.384739662392275861, -0.7216878364870207285 ) ) ;
#31413=CARTESIAN_POINT ( 'NONE',  ( 1.364683531249986537, 0.4677083336747514530, -0.7879004041258309554 ) ) ;
#31419=CARTESIAN_POINT ( 'NONE',  ( -1.499999999999997780, 1.650000000000019451, 0.000000000000000000 ) ) ;
#31420=CARTESIAN_POINT ( 'NONE',  ( 5.937581207780954884, 9.014596278131406848, -1.199719254218440723 ) ) ;
#31421=CARTESIAN_POINT ( 'NONE',  ( -7.690499447449645309, 9.995335326823163058, 1.599625672291295375 ) ) ;
#31425=CARTESIAN_POINT ( 'NONE',  ( -0.6823417656250003738, 1.217708333674752286, -1.181850606188749264 ) ) ;
#31427=CARTESIAN_POINT ( 'NONE',  ( -1.402160292154681736E-14, 2.337500000000022560, -1.732050807568863648 ) ) ;
#31429=CARTESIAN_POINT ( 'NONE',  ( 4.359110081993588182, 5.044382169536003602, -1.199719254218452047 ) ) ;
#31436=CARTESIAN_POINT ( 'NONE',  ( -1.402160292154681736E-14, 1.118750000682820378, -1.732050807568863648 ) ) ;
#31437=CARTESIAN_POINT ( 'NONE',  ( -6.398558430645608475, 9.552403038140164782, -1.199719254218440723 ) ) ;
#31438=CARTESIAN_POINT ( 'NONE',  ( -5.260200412422220140, 5.239248024021764039, -0.7216878364870207285 ) ) ;
#31444=ORIENTED_EDGE ( 'NONE', *, *, #186498, .T. ) ;
#31445=CARTESIAN_POINT ( 'NONE',  ( 5.099838337034727331, 9.101561826515851550, -0.7998128361456281477 ) ) ;
#31450=CARTESIAN_POINT ( 'NONE',  ( 6.714312387265682247, 8.856450423275211037, 1.599625672291281386 ) ) ;
#31451=CARTESIAN_POINT ( 'NONE',  ( 7.714226216051361718, 11.94375498546120795, -0.7216878364870267237 ) ) ;
#31457=CARTESIAN_POINT ( 'NONE',  ( -7.369020184227459858, 8.555943955475521889, 1.199719254218450271 ) ) ;
#31458=CARTESIAN_POINT ( 'NONE',  ( 3.832150974156964818, 7.622593236491780999, 1.040834085586084257E-14 ) ) ;
#31462=DIRECTION ( 'NONE',  ( 1.207943261119674327E-30, 2.168404344971008079E-15, -1.000000000000000000 ) ) ;
#31463=CARTESIAN_POINT ( 'NONE',  ( 4.067670533747345551, 7.502496534258641603, 0.5382987142239087364 ) ) ;
#31464=CARTESIAN_POINT ( 'NONE',  ( 7.944714827928033962, 12.21265836598400689, 0.7216878364870438212 ) ) ;
#31465=EDGE_LOOP ( 'NONE', ( #155483, #128240, #20598, #120185 ) ) ;
#31474=CARTESIAN_POINT ( 'NONE',  ( -2.494337075234348777, 5.853884321174607663, -0.7216878364870267237 ) ) ;
#31475=CARTESIAN_POINT ( 'NONE',  ( 8.649738815838679429, 10.15407870897571563, -1.082531754730543083 ) ) ;
#31478=CARTESIAN_POINT ( 'NONE',  ( -4.367698041896780126, 8.247398148854895084, 0.7998128361456481317 ) ) ;
#31479=CARTESIAN_POINT ( 'NONE',  ( -5.083944415000194894, 5.033616027029421680, 0.7216878364870371598 ) ) ;
#31484=CARTESIAN_POINT ( 'NONE',  ( -5.693534442735004752, 8.729875052244421951, 1.199719254218452047 ) ) ;
#31491=( BOUNDED_CURVE ( )  B_SPLINE_CURVE ( 2, ( #81099, #113674, #213213, #64842, #114733, #32356, #77898 ),
 .UNSPECIFIED., .F., .T. ) 
 B_SPLINE_CURVE_WITH_KNOTS ( ( 3, 2, 2, 3 ),
 ( 0.1874999999999999722, 0.1916666666666666796, 0.1958333333333333870, 0.2000000000000000944 ),
 .UNSPECIFIED. ) 
 CURVE ( )  GEOMETRIC_REPRESENTATION_ITEM ( )  RATIONAL_B_SPLINE_CURVE ( ( 1.000000000000000888, 0.8660254037844378194, 1.000000000000000000, 0.8660254037844387076, 1.000000000000000000, 0.8660254037844360431, 1.000000000000002665 ) ) 
 REPRESENTATION_ITEM ( '' )  );
#31492=ORIENTED_EDGE ( 'NONE', *, *, #166617, .F. ) ;
#31501=CARTESIAN_POINT ( 'NONE',  ( -6.043183783389232566, 8.073467052085995022, 1.599625672291269396 ) ) ;
#31504=CARTESIAN_POINT ( 'NONE',  ( 3.985733972737593778, 6.633478153960411738, -1.082531754730548412 ) ) ;
#31506=( BOUNDED_CURVE ( )  B_SPLINE_CURVE ( 2, ( #120740, #100140, #202949, #54593, #186714, #16734, #82820 ),
 .UNSPECIFIED., .F., .T. ) 
 B_SPLINE_CURVE_WITH_KNOTS ( ( 3, 2, 2, 3 ),
 ( 0.1625000000000001443, 0.1666666666666666852, 0.1708333333333332260, 0.1749999999999997669 ),
 .UNSPECIFIED. ) 
 CURVE ( )  GEOMETRIC_REPRESENTATION_ITEM ( )  RATIONAL_B_SPLINE_CURVE ( ( 0.9999999999999955591, 0.8660254037844431485, 1.000000000000000000, 0.8660254037844387076, 1.000000000000000000, 0.8660254037844458130, 0.9999999999999928946 ) ) 
 REPRESENTATION_ITEM ( '' )  );
#31508=CARTESIAN_POINT ( 'NONE',  ( -3.755772246185468788, 4.340488027759846545, -1.199719254218452047 ) ) ;
#31510=CARTESIAN_POINT ( 'NONE',  ( 3.673896439623286714, 4.156855427197417185, -7.499999999999997335 ) ) ;
#31511=CARTESIAN_POINT ( 'NONE',  ( 8.757677159423465696, 12.30470822171437284, 1.199719254218450271 ) ) ;
#31514=CARTESIAN_POINT ( 'NONE',  ( -9.352427035328430449, 9.805586384171650849, 1.040834085586084257E-14 ) ) ;
#31515=CARTESIAN_POINT ( 'NONE',  ( 5.799137018343234473, 7.788745826199009237, -1.599625672291262513 ) ) ;
#31517=AXIS2_PLACEMENT_3D ( 'NONE', #132563, #102159, #168227 ) ;
#31518=CARTESIAN_POINT ( 'NONE',  ( 3.499976210622149253, 7.235056012367826028, 0.7998128361456321445 ) ) ;
#31521=CARTESIAN_POINT ( 'NONE',  ( 1.364683531249988535, 1.926041667008086211, 0.7879004041258500513 ) ) ;
#31524=CARTESIAN_POINT ( 'NONE',  ( 6.629573927402440781, 10.67832731537079383, 1.040834085586084257E-14 ) ) ;
#31531=CARTESIAN_POINT ( 'NONE',  ( 8.880227426826630577, 12.34372051706435869, 1.082531754730546636 ) ) ;
#31539=CARTESIAN_POINT ( 'NONE',  ( -9.775592450653132204, 11.36361159963886891, -1.199719254218441611 ) ) ;
#31546=CARTESIAN_POINT ( 'NONE',  ( -4.510196435976065565, 7.040407170307378060, -1.149263043085164915 ) ) ;
#31553=CARTESIAN_POINT ( 'NONE',  ( -0.7500000000000215383, 0.7229166673494852313, 1.299038105676659116 ) ) ;
#31560=CARTESIAN_POINT ( 'NONE',  ( 7.914208982075123799, 10.25632978388623684, -1.599625672291262513 ) ) ;
#31562=CARTESIAN_POINT ( 'NONE',  ( 1.364683531249984538, -1.094791666325247936, -0.7879004041258309554 ) ) ;
#31565=CARTESIAN_POINT ( 'NONE',  ( 9.083599731475976213, 12.58098820582193689, 1.082531754730546636 ) ) ;
#31566=CARTESIAN_POINT ( 'NONE',  ( -6.073689629242158716, 9.069426419882418600, -1.082531754730538864 ) ) ;
#31570=CARTESIAN_POINT ( 'NONE',  ( -5.747767057189642870, 8.793146435774861658, -1.199719254218440723 ) ) ;
#31573=CARTESIAN_POINT ( 'NONE',  ( -0.7500000000000006661, 0.8895833340161543035, -1.299038105676652011 ) ) ;
#31581=CARTESIAN_POINT ( 'NONE',  ( -4.419594887930571758, 4.258541578781506409, 1.214306433183764966E-14 ) ) ;
#31584=EDGE_CURVE ( 'NONE', #138847, #162407, #139411, .T. ) ;
#31585=CARTESIAN_POINT ( 'NONE',  ( 4.159596813995052322, 7.384974941181836172, -0.7733407813514819873 ) ) ;
#31589=CARTESIAN_POINT ( 'NONE',  ( -3.809477975315625375, 4.507107728365378208, 1.082531754730558626 ) ) ;
#31590=CARTESIAN_POINT ( 'NONE',  ( 8.294891053462476904, 8.571794405328034827, 1.040834085586084257E-14 ) ) ;
#31597=CARTESIAN_POINT ( 'NONE',  ( -8.513630394377489807, 12.01998699582738972, -1.199719254218446718 ) ) ;
#31602=CARTESIAN_POINT ( 'NONE',  ( 2.869522067586683711, 6.499526178826442013, 0.7998128361456362523 ) ) ;
#31606=ORIENTED_EDGE ( 'NONE', *, *, #51124, .F. ) ;
#31608=CARTESIAN_POINT ( 'NONE',  ( -10.45741655484220267, 11.09474082360439873, -0.7998128361456221525 ) ) ;
#31622=CARTESIAN_POINT ( 'NONE',  ( 6.662942426112080874, 9.860851032851066122, 1.199719254218460707 ) ) ;
#31624=CARTESIAN_POINT ( 'NONE',  ( -4.959585264500673496, 4.680604318205876524, 1.214306433183764966E-14 ) ) ;
#31626=CARTESIAN_POINT ( 'NONE',  ( 5.516820392445955790, 6.318161192665863624, -1.127043001766608432 ) ) ;
#31630=CARTESIAN_POINT ( 'NONE',  ( 0.7499999999999885647, 0.7645833340161543035, 1.299038105676657340 ) ) ;
#31633=CARTESIAN_POINT ( 'NONE',  ( -1.458525620005792334, 8.740196138359387135, -2.548959422809881747 ) ) ;
#31634=FACE_OUTER_BOUND ( 'NONE', #172255, .T. ) ;
#31636=CARTESIAN_POINT ( 'NONE',  ( -3.297657676621885692, 4.870353260857385180, 1.599625672291267398 ) ) ;
#31642=CARTESIAN_POINT ( 'NONE',  ( 5.517805331081858888, 5.539787095791365523, 1.040834085586084257E-14 ) ) ;
#31645=CARTESIAN_POINT ( 'NONE',  ( 1.364683531249992088, 5.446875000341417916, 1.214306433183764966E-14 ) ) ;
#31647=CARTESIAN_POINT ( 'NONE',  ( 4.216222583725566686, 4.981643104843690217, -1.082531754730548412 ) ) ;
#31651=ADVANCED_FACE ( 'NONE', ( #210502 ), #141026, .T. ) ;
#31656=CARTESIAN_POINT ( 'NONE',  ( -6.082092046053040768, 6.030765914320626919, 0.4329532585971782033 ) ) ;
#31658=CARTESIAN_POINT ( 'NONE',  ( 1.364683531249984538, -1.094791666325247936, -0.7879004041258309554 ) ) ;
#31666=CARTESIAN_POINT ( 'NONE',  ( -0.7500000000000215383, 5.191666666666685082, 1.299038105676671107 ) ) ;
#31674=CARTESIAN_POINT ( 'NONE',  ( -1.364683531249997417, 4.821875000341417916, 1.214306433183764966E-14 ) ) ;
#31676=CARTESIAN_POINT ( 'NONE',  ( 5.774883364416965037, 8.824782127540085952, -1.199719254218440723 ) ) ;
#31677=CARTESIAN_POINT ( 'NONE',  ( -6.692921386640485082, 10.96015871772258521, -0.7998128361456291469 ) ) ;
#31678=DIRECTION ( 'NONE',  ( -0.8079921913640178976, 0.000000000000000000, -0.5891931930146276919 ) ) ;
#31681=CARTESIAN_POINT ( 'NONE',  ( 5.151735183068521629, 5.112705256442466428, 1.040834085586084257E-14 ) ) ;
#31683=ORIENTED_EDGE ( 'NONE', *, *, #203502, .T. ) ;
#31685=CARTESIAN_POINT ( 'NONE',  ( -1.364683531250014514, -1.157291666325248158, 0.7879004041258379498 ) ) ;
#31689=DIRECTION ( 'NONE',  ( -5.578564026256490882E-16, -1.000000000000000000, -9.066213480720158442E-32 ) ) ;
#31693=CARTESIAN_POINT ( 'NONE',  ( 6.480434237652121787, 9.543961796360731498, 1.082531754730558626 ) ) ;
#31697=CARTESIAN_POINT ( 'NONE',  ( -1.500000000000011324, 4.452083334016148086, 0.8660254037844403729 ) ) ;
#31699=CARTESIAN_POINT ( 'NONE',  ( -2.754277761870538299, 6.365074488824250309, 1.040834085586084257E-14 ) ) ;
#31700=CARTESIAN_POINT ( 'NONE',  ( 5.111060722227499298, 8.906728576000002562, -0.7216878364870267237 ) ) ;
#31707=CARTESIAN_POINT ( 'NONE',  ( 0.000000000000000000, -1.099999999999982991, -2.499999999999995115 ) ) ;
#31708=CARTESIAN_POINT ( 'NONE',  ( 2.523789150438203510, 6.096171108819874007, 0.7998128361456462443 ) ) ;
#31716=ORIENTED_EDGE ( 'NONE', *, *, #121204, .T. ) ;
#31721=CARTESIAN_POINT ( 'NONE',  ( 2.280077068888842540, 5.600296667721481825, -0.6021448391562183033 ) ) ;
#31725=EDGE_CURVE ( 'NONE', #102537, #168291, #185226, .T. ) ;
#31727=CARTESIAN_POINT ( 'NONE',  ( 9.887974103068218668, 10.43039129653476493, 0.7998128361456462443 ) ) ;
#31731=CARTESIAN_POINT ( 'NONE',  ( -1.364683531250014514, 0.03020833367475737191, 0.7879004041258379498 ) ) ;
#31732=CARTESIAN_POINT ( 'NONE',  ( 5.829642864196171281, 5.903597551091405826, 0.7216878364870317197 ) ) ;
#31733=CARTESIAN_POINT ( 'NONE',  ( -7.971831135155409420, 11.28392484344787405, 1.082531754730549967 ) ) ;
#31738=CARTESIAN_POINT ( 'NONE',  ( -3.093231602212184850, 6.760520635889515795, -0.7998128361456281477 ) ) ;
#31746=ORIENTED_EDGE ( 'NONE', *, *, #196609, .T. ) ;
#31753=CARTESIAN_POINT ( 'NONE',  ( 4.860569815253008130, 6.917139861862701800, -1.418536646215622365 ) ) ;
#31755=ORIENTED_EDGE ( 'NONE', *, *, #52269, .T. ) ;
#31757=CARTESIAN_POINT ( 'NONE',  ( 3.714044015139744914, 6.420469553383295391, 1.199719254218462483 ) ) ;
#31762=CARTESIAN_POINT ( 'NONE',  ( -9.029367117021344313, 9.636609179387466639, 0.7216878364870438212 ) ) ;
#31767=CARTESIAN_POINT ( 'NONE',  ( 6.775324078527185989, 8.927630729746953264, -1.599625672291262513 ) ) ;
#31768=FACE_OUTER_BOUND ( 'NONE', #56104, .T. ) ;
#31770=CARTESIAN_POINT ( 'NONE',  ( -3.899941742225307539, 7.701682465904834629, 0.7998128361456341429 ) ) ;
#31771=CARTESIAN_POINT ( 'NONE',  ( 3.521367211247359741, 5.131347717920458962, -1.599625672291262513 ) ) ;
#31774=CARTESIAN_POINT ( 'NONE',  ( -6.254388934605767503, 6.191208599995166040, 0.7998128361456341429 ) ) ;
#31777=CARTESIAN_POINT ( 'NONE',  ( 9.402743226277308963, 10.92862083786708816, -1.199719254218446718 ) ) ;
#31778=CARTESIAN_POINT ( 'NONE',  ( -1.499999999999997780, 3.431250000682818602, 1.214306433183764966E-14 ) ) ;
#31780=CARTESIAN_POINT ( 'NONE',  ( 4.291011075107065587, 7.468133931351726318, 1.062205608224401576 ) ) ;
#31781=CARTESIAN_POINT ( 'NONE',  ( 5.233084105194869551, 6.167981546557892436, -1.082531754730548412 ) ) ;
#31788=CARTESIAN_POINT ( 'NONE',  ( 6.765155463094746580, 9.876136559377135526, 1.082531754730558626 ) ) ;
#31792=CARTESIAN_POINT ( 'NONE',  ( -8.286004436246233951, 12.81875560892930466, 1.040834085586084257E-14 ) ) ;
#31793=CARTESIAN_POINT ( 'NONE',  ( -8.376239975144482486, 8.666701480623698828, 1.040834085586084257E-14 ) ) ;
#31798=CARTESIAN_POINT ( 'NONE',  ( 2.184835310096557404, 5.700724961754617404, 1.040834085586084257E-14 ) ) ;
#31801=CARTESIAN_POINT ( 'NONE',  ( 7.553864141108259211, 11.96459193126834464, 1.040834085586084257E-14 ) ) ;
#31805=CARTESIAN_POINT ( 'NONE',  ( 5.169736645512481132, 4.925780929386339935, 0.7998128361456341429 ) ) ;
#31808=CARTESIAN_POINT ( 'NONE',  ( -0.7499999999999972244, 3.639583334016149863, -1.299038105676652011 ) ) ;
#31814=CARTESIAN_POINT ( 'NONE',  ( 1.499999999999989120, 3.275000000000020783, 1.214306433183764966E-14 ) ) ;
#31815=CARTESIAN_POINT ( 'NONE',  ( 5.555090253297246150, 7.504024600312024340, 1.599625672291267398 ) ) ;
#31818=CARTESIAN_POINT ( 'NONE',  ( 6.968527767744098433, 9.153035033833367251, 1.443375672974076540 ) ) ;
#31819=CARTESIAN_POINT ( 'NONE',  ( -9.612367721964606204, 12.23751498042398289, -1.443375672974058777 ) ) ;
#31823=CARTESIAN_POINT ( 'NONE',  ( 9.999301985278609806, 11.62460605670194447, 1.199719254218452047 ) ) ;
#31825=CARTESIAN_POINT ( 'NONE',  ( -2.591579918506545344, 6.175260338232929413, 1.040834085586084257E-14 ) ) ;
#31826=CARTESIAN_POINT ( 'NONE',  ( -1.500000000000011324, 5.660416667349481123, -0.8660254037844313801 ) ) ;
#31827=CARTESIAN_POINT ( 'NONE',  ( 1.364683531249988757, -0.8656249996585805295, 0.000000000000000000 ) ) ;
#31831=CARTESIAN_POINT ( 'NONE',  ( 4.334856428067313416, 6.080418470877079429, -1.599625672291256295 ) ) ;
#31834=CARTESIAN_POINT ( 'NONE',  ( -1.364683531250010295, 5.301041667008085767, -0.7879004041258300672 ) ) ;
#31842=CARTESIAN_POINT ( 'NONE',  ( -7.552055258011950656, 8.769484874890757453, 1.199719254218462483 ) ) ;
#31844=CARTESIAN_POINT ( 'NONE',  ( 4.710568305744190276, 7.583081225755162968, 1.199719254218462483 ) ) ;
#31847=CARTESIAN_POINT ( 'NONE',  ( -1.402160292154681736E-14, 0.9468750003414176941, -1.575800808251659024 ) ) ;
#31852=CARTESIAN_POINT ( 'NONE',  ( 9.561524646135536543, 12.17819805862340310, -1.599625672291262513 ) ) ;
#31855=CARTESIAN_POINT ( 'NONE',  ( -5.747767057189642870, 8.793146435774861658, -1.199719254218440723 ) ) ;
#31860=CARTESIAN_POINT ( 'NONE',  ( 8.106885785967500979, 11.54545161934907682, 1.199719254218460707 ) ) ;
#31862=CARTESIAN_POINT ( 'NONE',  ( 7.781490099239519509, 11.16582331816642260, 1.199719254218460707 ) ) ;
#31863=CARTESIAN_POINT ( 'NONE',  ( 1.387358672531572079, 7.315968950354051259, 4.254625267138675504 ) ) ;
#31864=CARTESIAN_POINT ( 'NONE',  ( -8.337901282724359930, 12.67137589657970409, 1.040834085586084257E-14 ) ) ;
#31865=CARTESIAN_POINT ( 'NONE',  ( -6.008234629150358330, 10.16135750065076060, 0.000000000000000000 ) ) ;
#31868=CARTESIAN_POINT ( 'NONE',  ( -4.300870446666812619, 7.448604017583265957, 1.116033750828262949 ) ) ;
#31869=CARTESIAN_POINT ( 'NONE',  ( -1.364683531250014514, 0.9885416670080898749, -0.7879004041258289570 ) ) ;
#31873=CARTESIAN_POINT ( 'NONE',  ( 6.290620087060792009, 10.28288116830553101, -0.7216878364870267237 ) ) ;
#31876=CARTESIAN_POINT ( 'NONE',  ( 4.493637847925535667, 7.329995691633395261, -1.199719254218452047 ) ) ;
#31889=CARTESIAN_POINT ( 'NONE',  ( -4.080641047588907888, 6.744203074620265248, -1.082531754730548412 ) ) ;
#31897=CARTESIAN_POINT ( 'NONE',  ( -3.601662362724658895, 7.353689856487406473, -0.7998128361456281477 ) ) ;
#31898=CARTESIAN_POINT ( 'NONE',  ( -6.496328159242330536, 10.73079995242472862, 0.000000000000000000 ) ) ;
#31904=CARTESIAN_POINT ( 'NONE',  ( 1.499999999999987121, 2.827083334016148530, -0.8660254037844262731 ) ) ;
#31905=CARTESIAN_POINT ( 'NONE',  ( 9.074484886248265880, 9.481320543578137361, 0.7998128361456462443 ) ) ;
#31909=CARTESIAN_POINT ( 'NONE',  ( -8.422639742587602285, 10.84949900448412841, -1.599625672291263179 ) ) ;
#31911=CARTESIAN_POINT ( 'NONE',  ( -1.364683531250012516, 3.280208333674756727, 0.7879004041258379498 ) ) ;
#31913=CARTESIAN_POINT ( 'NONE',  ( -6.511106444361044687, 5.279176164185805042, 2.499999999999998668 ) ) ;
#31916=CARTESIAN_POINT ( 'NONE',  ( -9.517460647113315630, 10.20605163116143821, 0.7216878364870438212 ) ) ;
#31920=CARTESIAN_POINT ( 'NONE',  ( -0.6823417656250003738, 2.030208333674753174, -1.181850606188749264 ) ) ;
#31925=CARTESIAN_POINT ( 'NONE',  ( 1.364683531249990311, 3.134375000341423245, 1.214306433183764966E-14 ) ) ;
#31927=CARTESIAN_POINT ( 'NONE',  ( -6.250472511100020334, 7.250971670160158311, 1.199719254218450271 ) ) ;
#31928=CARTESIAN_POINT ( 'NONE',  ( 5.777746017718023097, 9.892454120646377191, 0.7998128361456462443 ) ) ;
#31930=CARTESIAN_POINT ( 'NONE',  ( -1.201851678989727383E-14, 2.634375000341417916, 1.575800808251672791 ) ) ;
#31934=CARTESIAN_POINT ( 'NONE',  ( -5.260200412422208593, 7.159986452624450770, -1.443375672974053447 ) ) ;
#31937=CARTESIAN_POINT ( 'NONE',  ( 3.877268743828266029, 6.506935386899531437, 1.082531754730558626 ) ) ;
#31940=CARTESIAN_POINT ( 'NONE',  ( -7.823218330285243383, 9.085841792542966644, -1.199719254218446718 ) ) ;
#31941=CARTESIAN_POINT ( 'NONE',  ( -2.117044542028253318, 5.621635732341564662, -0.7998128361456281477 ) ) ;
#31943=CARTESIAN_POINT ( 'NONE',  ( -0.6823417656249969321, 5.717708333674756283, -1.181850606188749264 ) ) ;
#31948=CARTESIAN_POINT ( 'NONE',  ( -7.090551149822745813, 9.295395646258437949, 1.443375672974078761 ) ) ;
#31950=CARTESIAN_POINT ( 'NONE',  ( -1.364683531250014514, -0.1989583329919157317, -0.7879004041258359514 ) ) ;
#31954=CARTESIAN_POINT ( 'NONE',  ( 7.727784370109387346, 10.99920361756089093, -1.082531754730543083 ) ) ;
#31963=CARTESIAN_POINT ( 'NONE',  ( 9.856414487010592751, 10.60149777770828194, 0.7216878364870438212 ) ) ;
#31970=EDGE_CURVE ( 'NONE', #40394, #99491, #208638, .T. ) ;
#31971=CARTESIAN_POINT ( 'NONE',  ( 6.647575389402066826, 6.649926130590872120, 1.040834085586084257E-14 ) ) ;
#31973=B_SPLINE_CURVE_WITH_KNOTS ( 'NONE', 3,
 ( #22767, #128909, #29202, #194890, #95292, #15054, #61696, #94224, #80071, #31343 ),
 .UNSPECIFIED., .F., .F.,
 ( 4, 2, 2, 2, 4 ),
 ( 0.001600703253539966127, 0.001978746783904330314, 0.002356790314268694501, 0.002734833844633058689, 0.003112877374997422876 ),
 .UNSPECIFIED. ) ;
#31974=CARTESIAN_POINT ( 'NONE',  ( -3.928111819657352566, 5.605883094398769195, 1.599625672291267398 ) ) ;
#31979=CARTESIAN_POINT ( 'NONE',  ( 5.409340101728155936, 8.294351971116089572, -1.082531754730543971 ) ) ;
#31980=CARTESIAN_POINT ( 'NONE',  ( 1.364683531249986537, 0.9677083336747538400, -0.7879004041258239610 ) ) ;
#31982=CARTESIAN_POINT ( 'NONE',  ( -8.513630394377489807, 12.01998699582738972, -1.199719254218446718 ) ) ;
#31993=CARTESIAN_POINT ( 'NONE',  ( -4.251935539942575559, 7.316435789055923955, -0.9001278212061183392 ) ) ;
#31997=CARTESIAN_POINT ( 'NONE',  ( 7.470706336329915764, 8.674577799595093452, -1.199719254218441611 ) ) ;
#31998=CARTESIAN_POINT ( 'NONE',  ( 6.120616281565444794, 9.228137197546649517, -1.199719254218440723 ) ) ;
#32001=ORIENTED_EDGE ( 'NONE', *, *, #209714, .T. ) ;
#32007=CARTESIAN_POINT ( 'NONE',  ( 8.238550898598388628, 12.76339314834017102, 0.7998128361456462443 ) ) ;
#32012=LINE ( 'NONE', #66591, #96992 ) ;
#32013=CARTESIAN_POINT ( 'NONE',  ( 0.000000000000000000, 2.800000000000024691, 1.214306433183764966E-14 ) ) ;
#32014=CARTESIAN_POINT ( 'NONE',  ( -0.2935777296395137848, 7.111227605955122044, 1.979479841891082170 ) ) ;
#32018=CARTESIAN_POINT ( 'NONE',  ( -8.188761592974033832, 12.49737959187099179, -0.7216878364870267237 ) ) ;
#32021=CARTESIAN_POINT ( 'NONE',  ( 5.799137018343234473, 7.788745826199009237, -1.599625672291262513 ) ) ;
#32027=CARTESIAN_POINT ( 'NONE',  ( 5.029711800545521250, 5.930713857800314237, -1.082531754730549078 ) ) ;
#32034=CARTESIAN_POINT ( 'NONE',  ( -7.043624497499477499, 8.176315654292865887, 1.199719254218450271 ) ) ;
#32035=CARTESIAN_POINT ( 'NONE',  ( -3.276266675996675204, 6.974061555304760240, -0.7998128361456281477 ) ) ;
#32040=CARTESIAN_POINT ( 'NONE',  ( 0.000000000000000000, 2.880000000000021210, 1.214306433183764966E-14 ) ) ;
#32044=CARTESIAN_POINT ( 'NONE',  ( 5.774883364416965037, 8.824782127540085952, -1.199719254218440723 ) ) ;
#32049=CARTESIAN_POINT ( 'NONE',  ( 1.217323170181688008, 3.111755683774203085, -0.7749999999999910294 ) ) ;
#32055=CARTESIAN_POINT ( 'NONE',  ( -1.364683531250014514, 0.3427083336747508424, 0.7879004041258379498 ) ) ;
#32056=CARTESIAN_POINT ( 'NONE',  ( 2.171277156482887882, 5.684907115872006145, -0.7998128361456291469 ) ) ;
#32057=CARTESIAN_POINT ( 'NONE',  ( 5.355634372598031767, 6.206993841907870291, -1.199719254218445830 ) ) ;
#32059=CARTESIAN_POINT ( 'NONE',  ( -6.507550544879489252, 9.575597488125954015, 1.082531754730548412 ) ) ;
#32060=CARTESIAN_POINT ( 'NONE',  ( -5.796211742350026341, 6.069872996917573538, -0.5622600474562855499 ) ) ;
#32061=CARTESIAN_POINT ( 'NONE',  ( 5.016153647376212277, 5.914896012436124728, 1.082531754730558626 ) ) ;
#32062=CARTESIAN_POINT ( 'NONE',  ( -7.226132685959434809, 8.493204890783200511, 1.082531754730549967 ) ) ;
#32067=CARTESIAN_POINT ( 'NONE',  ( 7.450369105909416589, 8.650851030771185890, -1.199719254218441611 ) ) ;
#32070=ADVANCED_FACE ( 'NONE', ( #5615 ), #117619, .T. ) ;
#32073=CARTESIAN_POINT ( 'NONE',  ( -1.201851678989727383E-14, 3.696875000341422801, -1.575800808251660134 ) ) ;
#32077=CARTESIAN_POINT ( 'NONE',  ( 8.782984583554449998, 9.141236857102018831, 1.040834085586084257E-14 ) ) ;
#32080=CARTESIAN_POINT ( 'NONE',  ( -8.227100285394159940, 8.492705175914988303, 0.7998128361456602331 ) ) ;
#32086=CARTESIAN_POINT ( 'NONE',  ( 8.269583629331492602, 11.73526576994040482, 1.199719254218450271 ) ) ;
#32087=CARTESIAN_POINT ( 'NONE',  ( 4.122904863638303219, 7.664607755345567597, -0.7618067034359333745 ) ) ;
#32089=CARTESIAN_POINT ( 'NONE',  ( -6.679363233026820446, 10.94434087183997129, 0.000000000000000000 ) ) ;
#32093=CARTESIAN_POINT ( 'NONE',  ( 5.387724311900628393, 6.300193624175450147, -1.063853923354351361 ) ) ;
#32094=CARTESIAN_POINT ( 'NONE',  ( -8.487040972474682476, 12.84537220128841817, 0.7216878364870338292 ) ) ;
#32100=CARTESIAN_POINT ( 'NONE',  ( 6.908042961362778733, 8.018137195466769285, 1.199719254218462483 ) ) ;
#32102=CARTESIAN_POINT ( 'NONE',  ( 4.462605117192430804, 8.358123070033169455, 1.040834085586084257E-14 ) ) ;
#32103=CARTESIAN_POINT ( 'NONE',  ( -4.338815981289680934, 7.218015932674029855, 1.009429000442535918 ) ) ;
#32104=CARTESIAN_POINT ( 'NONE',  ( 4.033714395265605823, 4.664753868353354704, -1.199719254218446718 ) ) ;
#32106=CARTESIAN_POINT ( 'NONE',  ( -7.537970219518089543, 8.857015346601659900, -1.082531754730543971 ) ) ;
#32112=CARTESIAN_POINT ( 'NONE',  ( -4.014146127519945928, 7.627013291057631150, 0.008764090477326666462 ) ) ;
#32113=CARTESIAN_POINT ( 'NONE',  ( 1.364683531249986537, -0.8239583329919186738, 0.7879004041258500513 ) ) ;
#32116=CARTESIAN_POINT ( 'NONE',  ( 3.551873057100283226, 6.127307085716883428, 1.082531754730558626 ) ) ;
#32121=CARTESIAN_POINT ( 'NONE',  ( -9.449669878600623463, 11.08733161553131197, -1.082531754730537976 ) ) ;
#32128=CARTESIAN_POINT ( 'NONE',  ( -8.148087131688679818, 12.44992605370473804, -0.7216878364870267237 ) ) ;
#32135=CARTESIAN_POINT ( 'NONE',  ( -7.497295758232720431, 10.73030023703809555, -1.082531754730543083 ) ) ;
#32141=CARTESIAN_POINT ( 'NONE',  ( -0.7500000000000006661, 2.639583334016156080, -1.299038105676652011 ) ) ;
#32145=CARTESIAN_POINT ( 'NONE',  ( -7.640183256500752584, 8.872300873127729304, -1.199719254218446718 ) ) ;
#32149=CARTESIAN_POINT ( 'NONE',  ( 4.964256800898067645, 8.943383367689749619, 0.7998128361456462443 ) ) ;
#32152=CARTESIAN_POINT ( 'NONE',  ( -4.293142477272898994, 3.903087733106795021, 0.2764223219648706542 ) ) ;
#32155=CARTESIAN_POINT ( 'NONE',  ( 6.988338112840064120, 10.24047933403371502, 1.199719254218460707 ) ) ;
#32159=CARTESIAN_POINT ( 'NONE',  ( -2.200615117903204077, 5.615171720908647579, 1.040834085586084257E-14 ) ) ;
#32162=CARTESIAN_POINT ( 'NONE',  ( -7.049876689426113785, 8.287572894827684777, -1.082531754730544860 ) ) ;
#32165=CARTESIAN_POINT ( 'NONE',  ( 0.6823417656249899377, 4.988541667008086655, -1.181850606188754593 ) ) ;
#32168=CARTESIAN_POINT ( 'NONE',  ( -1.387358672527355008, 7.251968950354660493, 4.302625267139497112 ) ) ;
#32171=CARTESIAN_POINT ( 'NONE',  ( -4.744990574658554117, 4.638169879964154418, 1.214306433183764966E-14 ) ) ;
#32173=CARTESIAN_POINT ( 'NONE',  ( 8.829384350997564468, 11.32403438096243775, 1.599625672291281386 ) ) ;
#32175=CARTESIAN_POINT ( 'NONE',  ( -8.157201976916404362, 12.66848607304450702, -0.7998128361456281477 ) ) ;
#32178=CARTESIAN_POINT ( 'NONE',  ( -1.201851678989727383E-14, 2.071875000341422801, 1.575800808251672791 ) ) ;
#32179=CARTESIAN_POINT ( 'NONE',  ( 4.630273154266905777, 5.360739087188218122, 1.199719254218464037 ) ) ;
#32183=CARTESIAN_POINT ( 'NONE',  ( -6.509799877575631832, 5.178456542363093718, -2.499999999999995115 ) ) ;
#32185=CARTESIAN_POINT ( 'NONE',  ( 8.500599125643985232, 11.90082083235127008, -1.082531754730543083 ) ) ;
#32186=CARTESIAN_POINT ( 'NONE',  ( 0.7499999999999920064, 4.014583334016149863, 1.299038105676669330 ) ) ;
#32187=CARTESIAN_POINT ( 'NONE',  ( -7.863365906246068349, 9.236643647784308797, -1.082531754730543971 ) ) ;
#32188=CARTESIAN_POINT ( 'NONE',  ( 1.364683531249988757, 0.8843750003414210248, 0.000000000000000000 ) ) ;
#32190=CARTESIAN_POINT ( 'NONE',  ( 0.1495493664682667478, 8.232402834745700559, 1.999498275786589119 ) ) ;
#32192=CARTESIAN_POINT ( 'NONE',  ( -7.995557903757128493, 10.35123685918189729, 1.599625672291295375 ) ) ;
#32193=CARTESIAN_POINT ( 'NONE',  ( -5.056828107772872727, 5.001980335264194721, -0.7216878364870197293 ) ) ;
#32194=CARTESIAN_POINT ( 'NONE',  ( -1.364683531250010295, 3.842708333674751398, 0.7879004041258379498 ) ) ;
#32206=VERTEX_POINT ( 'NONE', #34061 ) ;
#32216=CARTESIAN_POINT ( 'NONE',  ( 1.364683531249990311, 4.196875000341417028, 1.214306433183764966E-14 ) ) ;
#32218=EDGE_CURVE ( 'NONE', #162762, #201902, #71870, .T. ) ;
#32222=CARTESIAN_POINT ( 'NONE',  ( 8.392660782059197189, 9.750191319612612872, 1.199719254218462483 ) ) ;
#32225=CARTESIAN_POINT ( 'NONE',  ( -1.364683531250000748, 2.259375000341422357, 1.214306433183764966E-14 ) ) ;
#32227=CARTESIAN_POINT ( 'NONE',  ( -7.890482213473404727, 8.307910125248191946, 0.7216878364870578100 ) ) ;
#32233=CARTESIAN_POINT ( 'NONE',  ( 3.167801447087334576, 6.847518788243868393, -0.7998128361456291469 ) ) ;
#32236=CARTESIAN_POINT ( 'NONE',  ( 10.24048609702354717, 10.84165528948263457, -0.7998128361456281477 ) ) ;
#32243=CARTESIAN_POINT ( 'NONE',  ( -8.109748439268576803, 12.61312361245537517, 0.7998128361456481317 ) ) ;
#32244=CARTESIAN_POINT ( 'NONE',  ( 7.579171565239241737, 8.801120566655981747, 1.199719254218462483 ) ) ;
#32246=CARTESIAN_POINT ( 'NONE',  ( 3.836594282542909795, 6.459481848733281240, 1.082531754730558626 ) ) ;
#32259=CARTESIAN_POINT ( 'NONE',  ( -6.480434237652138663, 8.583592582059388576, 1.443375672974078761 ) ) ;
#32260=CARTESIAN_POINT ( 'NONE',  ( 4.985647801523278133, 6.839675073242382553, -1.599625672291256295 ) ) ;
#32264=CARTESIAN_POINT ( 'NONE',  ( -8.239604668803112375, 10.63595808506888396, -1.599625672291263179 ) ) ;
#32269=CARTESIAN_POINT ( 'NONE',  ( -9.969323024750229578, 10.52529837183042716, -0.7998128361456291469 ) ) ;
#32273=CARTESIAN_POINT ( 'NONE',  ( 7.910292558569346433, 11.31609285405122556, -1.199719254218446718 ) ) ;
#32286=CARTESIAN_POINT ( 'NONE',  ( -8.995998617867369873, 10.45408546138876993, 1.199719254218462483 ) ) ;
#32290=CARTESIAN_POINT ( 'NONE',  ( 7.375272376154084597, 9.627570410311676596, -1.443375672974057666 ) ) ;
#32292=CARTESIAN_POINT ( 'NONE',  ( 2.737856954955798727, 5.281584649835344258, 1.199719254218452047 ) ) ;
#32294=CARTESIAN_POINT ( 'NONE',  ( 3.520313441042647540, 7.258782781191745137, 0.7998128361456321445 ) ) ;
#32296=CARTESIAN_POINT ( 'NONE',  ( -5.526920175865215334, 9.599823971818089774, 0.7998128361456481317 ) ) ;
#32299=LINE ( 'NONE', #164429, #169323 ) ;
#32305=CARTESIAN_POINT ( 'NONE',  ( 1.364683531249988535, 3.467708333674749621, -0.7879004041258239610 ) ) ;
#32306=CARTESIAN_POINT ( 'NONE',  ( -4.308793891044708779, 3.921347715840572956, 1.214306433183764966E-14 ) ) ;
#32307=CARTESIAN_POINT ( 'NONE',  ( 7.944187942603509356, 11.35563746875774882, 1.199719254218460707 ) ) ;
#32309=CARTESIAN_POINT ( 'NONE',  ( -3.958617665510279160, 5.641473247893851628, -1.443375672974053447 ) ) ;
#32311=CARTESIAN_POINT ( 'NONE',  ( -4.026408433134269771, 6.680931691089825541, 1.082531754730560403 ) ) ;
#32318=CARTESIAN_POINT ( 'NONE',  ( 3.985207087413062066, 6.736826471035503694, -1.199719254218452047 ) ) ;
#32326=CARTESIAN_POINT ( 'NONE',  ( 4.599240423533799138, 6.388866465587984322, 1.599625672291267398 ) ) ;
#32331=CARTESIAN_POINT ( 'NONE',  ( -1.364683531250012516, 4.551041667008082214, -0.7879004041258300672 ) ) ;
#32336=CARTESIAN_POINT ( 'NONE',  ( 7.124973419181436007, 8.271222729588529887, -1.199719254218446718 ) ) ;
#32338=CARTESIAN_POINT ( 'NONE',  ( -6.250472511100020334, 7.250971670160158311, 1.199719254218450271 ) ) ;
#32339=EDGE_CURVE ( 'NONE', #52497, #33202, #212030, .T. ) ;
#32341=CARTESIAN_POINT ( 'NONE',  ( 4.812781342726850653, 8.558735966582574406, 0.7216878364870438212 ) ) ;
#32342=CARTESIAN_POINT ( 'NONE',  ( -1.500000000000013101, 2.129166666666693519, -0.8660254037844313801 ) ) ;
#32345=CARTESIAN_POINT ( 'NONE',  ( -3.927058049452637700, 7.733318157670055371, -0.7998128361456281477 ) ) ;
#32346=CARTESIAN_POINT ( 'NONE',  ( 0.4996389044603895546, 7.815212647110186595, -1.937417588921664047 ) ) ;
#32349=CARTESIAN_POINT ( 'NONE',  ( -0.6823417656250212460, 3.801041667008085767, 1.181850606188767472 ) ) ;
#32351=CARTESIAN_POINT ( 'NONE',  ( -5.111060722671894929, 5.065251719313053513, 0.000000000000000000 ) ) ;
#32356=CARTESIAN_POINT ( 'NONE',  ( -3.443407828190952813, 6.961133532957347825, 0.7216878364870233931 ) ) ;
#32358=CARTESIAN_POINT ( 'NONE',  ( 5.626797444871351139, 6.523350759560078593, 1.199719254218462483 ) ) ;
#32362=CARTESIAN_POINT ( 'NONE',  ( -1.201851678989727383E-14, 4.134375000341417028, 1.575800808251672791 ) ) ;
#32364=CARTESIAN_POINT ( 'NONE',  ( 4.532503425670185493, 4.182342172903648070, 1.214306433183764966E-14 ) ) ;
#32366=CARTESIAN_POINT ( 'NONE',  ( 0.6823417656249864960, -0.5114583329919111243, -1.181850606188749264 ) ) ;
#32369=CARTESIAN_POINT ( 'NONE',  ( -2.950870989268691957, 6.594433254122103349, -0.7998128361456281477 ) ) ;
#32371=CARTESIAN_POINT ( 'NONE',  ( -5.219525951136837705, 9.033271343060892633, -0.7216878364870207285 ) ) ;
#32375=CARTESIAN_POINT ( 'NONE',  ( -1.201851678989727383E-14, 2.571875000341417472, 1.575800808251672791 ) ) ;
#32383=CARTESIAN_POINT ( 'NONE',  ( -7.998947441938374148, 8.434452891790657603, 1.040834085586084257E-14 ) ) ;
#32389=CARTESIAN_POINT ( 'NONE',  ( -5.490689023410187275, 8.389259046411751797, 1.082531754730548412 ) ) ;
#32397=ORIENTED_EDGE ( 'NONE', *, *, #124309, .T. ) ;
#32400=CARTESIAN_POINT ( 'NONE',  ( -5.687809136132860210, 6.594531066031826150, -1.199719254218446718 ) ) ;
#32402=CARTESIAN_POINT ( 'NONE',  ( 1.499999999999985123, -0.7041666666666481778, -0.8660254037844323793 ) ) ;
#32403=CARTESIAN_POINT ( 'NONE',  ( 10.54788032175191326, 11.40820791823982994, 0.7216878364870317197 ) ) ;
#32404=CARTESIAN_POINT ( 'NONE',  ( 7.958799866421889746, 9.244020251369077457, -1.199719254218441611 ) ) ;
#32407=CARTESIAN_POINT ( 'NONE',  ( 5.331380718671758778, 7.243030143248949670, -1.599625672291256295 ) ) ;
#32413=CARTESIAN_POINT ( 'NONE',  ( -3.551873057100300990, 5.166937871415542283, 1.443375672974064550 ) ) ;
#32415=ADVANCED_FACE ( 'NONE', ( #19930 ), #83872, .F. ) ;
#32417=AXIS2_PLACEMENT_3D ( 'NONE', #92406, #158445, #10045 ) ;
#32422=CARTESIAN_POINT ( 'NONE',  ( 1.364683531249988757, 2.134375000341422357, 1.214306433183764966E-14 ) ) ;
#32424=CARTESIAN_POINT ( 'NONE',  ( -5.391338639728555648, 9.441645512991978961, -0.7998128361456231517 ) ) ;
#32426=VECTOR ( 'NONE', #114822, 1000.000000000000000 ) ;
#32428=CARTESIAN_POINT ( 'NONE',  ( 6.226218857173709154, 8.287007971501239467, 1.599625672291281386 ) ) ;
#32429=CARTESIAN_POINT ( 'NONE',  ( -6.388916700537716764, 8.476822122092563916, 1.599625672291283607 ) ) ;
#32432=CARTESIAN_POINT ( 'NONE',  ( -1.500000000000013101, 0.9520833340161557468, 0.8660254037844403729 ) ) ;
#32435=CARTESIAN_POINT ( 'NONE',  ( 7.456621297836078632, 8.762108271306003004, 1.082531754730558626 ) ) ;
#32438=CARTESIAN_POINT ( 'NONE',  ( -1.402160292154681736E-14, 0.2593750003414224681, -1.575800808251665908 ) ) ;
#32440=CARTESIAN_POINT ( 'NONE',  ( 5.436456408955479880, 9.286356877182658565, -0.7216878364870267237 ) ) ;
#32443=CARTESIAN_POINT ( 'NONE',  ( -5.477130870240893401, 6.452702772444876445, 1.082531754730548412 ) ) ;
#32445=CARTESIAN_POINT ( 'NONE',  ( 0.6823417656249899377, 4.926041667008086655, -1.181850606188754593 ) ) ;
#32455=CARTESIAN_POINT ( 'NONE',  ( 6.120616281565444794, 9.228137197546649517, -1.199719254218440723 ) ) ;
#32458=CARTESIAN_POINT ( 'NONE',  ( 4.871457266011829823, 4.577788319968905562, -0.7998128361456221525 ) ) ;
#32465=CARTESIAN_POINT ( 'NONE',  ( 5.843201017809841247, 5.919415396974013532, 1.040834085586084257E-14 ) ) ;
#32466=CARTESIAN_POINT ( 'NONE',  ( -1.364683531250012516, 1.092708333674754506, 0.7879004041258379498 ) ) ;
#32471=CARTESIAN_POINT ( 'NONE',  ( -1.201851678989727383E-14, 1.712500000000019229, 1.732050807568877637 ) ) ;
#32472=CARTESIAN_POINT ( 'NONE',  ( 7.474622759835693131, 7.614814729430110951, -0.7998128361456281477 ) ) ;
#32473=CARTESIAN_POINT ( 'NONE',  ( -8.365544474831901667, 9.718555627847388578, 1.199719254218462483 ) ) ;
#32477=CARTESIAN_POINT ( 'NONE',  ( -1.201851678989727383E-14, 1.571875000341420581, 1.575800808251672791 ) ) ;
#32478=CARTESIAN_POINT ( 'NONE',  ( -1.500000000000013101, 1.879166666666692187, -0.8660254037844313801 ) ) ;
#32481=CARTESIAN_POINT ( 'NONE',  ( 4.253507506385319381, 5.985511395581417204, 1.599625672291267398 ) ) ;
#32488=CARTESIAN_POINT ( 'NONE',  ( -0.7500000000000006661, -0.1104166659838465292, -1.299038105676652011 ) ) ;
#32489=CARTESIAN_POINT ( 'NONE',  ( -8.345207244411405156, 9.694828859023472134, 1.199719254218462483 ) ) ;
#32490=CARTESIAN_POINT ( 'NONE',  ( -3.131570295076647525, 6.597323077657299528, 1.040834085586084257E-14 ) ) ;
#32498=CARTESIAN_POINT ( 'NONE',  ( 7.233438648090761980, 8.397765496649418182, 1.199719254218462483 ) ) ;
#32501=CARTESIAN_POINT ( 'NONE',  ( -1.436838838544753694, 7.449283400311743186, 4.203727439823589762 ) ) ;
#32502=CARTESIAN_POINT ( 'NONE',  ( 5.849453209292126310, 8.911780279894442103, 1.199719254218462483 ) ) ;
#32503=CARTESIAN_POINT ( 'NONE',  ( 10.04622863760192963, 10.82294762006482713, -0.7216878364870257245 ) ) ;
#32507=CARTESIAN_POINT ( 'NONE',  ( -7.640183256500752584, 8.872300873127729304, -1.199719254218446718 ) ) ;
#32508=CARTESIAN_POINT ( 'NONE',  ( 4.222474775652216294, 7.013638773981186958, 1.199719254218462483 ) ) ;
#32514=CARTESIAN_POINT ( 'NONE',  ( 7.782016984564043227, 12.02284421539267356, 0.7216878364870438212 ) ) ;
#32523=CARTESIAN_POINT ( 'NONE',  ( -4.663641653420935285, 5.503632019488245319, 1.082531754730560403 ) ) ;
#32524=CARTESIAN_POINT ( 'NONE',  ( 7.605760987586388744, 11.81721221891873697, 1.040834085586084257E-14 ) ) ;
#32528=CARTESIAN_POINT ( 'NONE',  ( -4.557512192488103686, 8.468847991211438497, -0.7998128361456281477 ) ) ;
#32534=CARTESIAN_POINT ( 'NONE',  ( -5.669280788808708671, 9.765911353585494226, 0.7998128361456481317 ) ) ;
#32538=ORIENTED_EDGE ( 'NONE', *, *, #101958, .T. ) ;
#32547=CARTESIAN_POINT ( 'NONE',  ( -5.555090253297260361, 7.504024600312024340, 1.599625672291269396 ) ) ;
#32550=CARTESIAN_POINT ( 'NONE',  ( 4.907688418466886304, 5.788353245375237321, -1.082531754730548412 ) ) ;
#32555=CARTESIAN_POINT ( 'NONE',  ( -2.462777459176719308, 6.024990802348131780, -0.7998128361456281477 ) ) ;
#32561=CARTESIAN_POINT ( 'NONE',  ( -7.178152263431422320, 10.46192917639026554, 1.199719254218453823 ) ) ;
#32562=CARTESIAN_POINT ( 'NONE',  ( 6.124532705071213279, 8.168374127381657246, -1.599625672291262513 ) ) ;
#32566=CARTESIAN_POINT ( 'NONE',  ( -8.670602931139386627, 10.07445716020612103, 1.199719254218462483 ) ) ;
#32570=CARTESIAN_POINT ( 'NONE',  ( 1.364683531249988757, 0.1968750003414204697, 0.000000000000000000 ) ) ;
#32574=CARTESIAN_POINT ( 'NONE',  ( 8.487040972474689582, 9.964264558384387627, -1.082531754730543083 ) ) ;
#32602=CARTESIAN_POINT ( 'NONE',  ( -1.402160292154681736E-14, 0.3687500006828169363, -1.732050807568870754 ) ) ;
#32609=CARTESIAN_POINT ( 'NONE',  ( 8.971744963941056028, 11.49012176272984931, 1.599625672291281386 ) ) ;
#32612=CARTESIAN_POINT ( 'NONE',  ( 5.009901455449552010, 5.803638771901306725, -1.199719254218452047 ) ) ;
#32613=CARTESIAN_POINT ( 'NONE',  ( -6.561783159334130922, 9.638868871656395498, -1.082531754730538864 ) ) ;
#32617=CARTESIAN_POINT ( 'NONE',  ( -6.235860587281615075, 9.362588887548838557, -1.199719254218440723 ) ) ;
#32618=CARTESIAN_POINT ( 'NONE',  ( -4.270455198180246548, 4.084545274072787890, 0.7216878364870317197 ) ) ;
#32622=CARTESIAN_POINT ( 'NONE',  ( -1.500000000000015099, 1.160416667349484898, -0.8660254037844313801 ) ) ;
#32629=CARTESIAN_POINT ( 'NONE',  ( -2.765500147063310266, 6.170241238308400433, 1.040834085586084257E-14 ) ) ;
#32630=AXIS2_PLACEMENT_3D ( 'NONE', #91669, #76448, #142555 ) ;
#32634=CARTESIAN_POINT ( 'NONE',  ( 4.073938026035560434, 7.494178044256873505, -0.5588469191320240004 ) ) ;
#32638=CARTESIAN_POINT ( 'NONE',  ( -8.618179199781044630, 13.20629283305325963, 0.7998128361456341429 ) ) ;
#32639=CARTESIAN_POINT ( 'NONE',  ( 6.598014311344812199, 10.84943379654430906, 1.040834085586084257E-14 ) ) ;
#32647=CARTESIAN_POINT ( 'NONE',  ( -7.648771216403934758, 12.07531685244661723, -0.7998128361456291469 ) ) ;
#32652=CARTESIAN_POINT ( 'NONE',  ( 5.515469562660962666, 5.329135999392899947, 0.7998128361456341429 ) ) ;
#32659=CARTESIAN_POINT ( 'NONE',  ( 1.499999999999990896, 8.627523663848661428, -2.579999999999989413 ) ) ;
#32660=ORIENTED_EDGE ( 'NONE', *, *, #6374, .T. ) ;
#32668=CARTESIAN_POINT ( 'NONE',  ( 6.109920781252839994, 10.27999134477033216, 1.040834085586084257E-14 ) ) ;
#32671=CARTESIAN_POINT ( 'NONE',  ( -4.460796234096120472, 5.163016013655583158, 1.199719254218462483 ) ) ;
#32679=CARTESIAN_POINT ( 'NONE',  ( -1.201851678989727383E-14, 0.7437500006828187127, 1.732050807568877637 ) ) ;
#32682=CARTESIAN_POINT ( 'NONE',  ( -1.566597853259662276, 8.754643479813401186, -2.463935000415734322 ) ) ;
#32683=CARTESIAN_POINT ( 'NONE',  ( 3.460355519985863548, 5.060167411448709629, 1.599625672291267398 ) ) ;
#32685=CARTESIAN_POINT ( 'NONE',  ( -4.959585264500673496, 4.680604318205876524, 1.214306433183764966E-14 ) ) ;
#32691=CARTESIAN_POINT ( 'NONE',  ( 5.843201017809841247, 5.919415396974013532, 1.040834085586084257E-14 ) ) ;
#32694=CARTESIAN_POINT ( 'NONE',  ( -0.6823417656249969321, 4.280208333674755394, -1.181850606188749264 ) ) ;
#32696=CARTESIAN_POINT ( 'NONE',  ( 3.782361668088245921, 6.396210465202840645, -1.082531754730548412 ) ) ;
#32704=CARTESIAN_POINT ( 'NONE',  ( -5.988731108142371085, 6.089685199429741402, 0.6933981374793452002 ) ) ;
#32707=CARTESIAN_POINT ( 'NONE',  ( 0.6823417656249917140, 5.155208333674749177, 1.181850606188765695 ) ) ;
#32714=CARTESIAN_POINT ( 'NONE',  ( -1.001543065824772872E-14, 4.712500000000017231, 1.732050807568877637 ) ) ;
#32719=VERTEX_POINT ( 'NONE', #171527 ) ;
#32721=CARTESIAN_POINT ( 'NONE',  ( 1.499999999999990896, 4.275000000000021672, 1.214306433183764966E-14 ) ) ;
#32722=CARTESIAN_POINT ( 'NONE',  ( -1.364683531250012516, 5.051041667008085767, -0.7879004041258300672 ) ) ;
#32724=CARTESIAN_POINT ( 'NONE',  ( 5.636439174979242850, 7.598931675607687453, -1.599625672291262513 ) ) ;
#32726=CARTESIAN_POINT ( 'NONE',  ( -8.365544474831901667, 9.718555627847388578, 1.199719254218462483 ) ) ;
#32728=CARTESIAN_POINT ( 'NONE',  ( 8.594979316059474073, 12.11489407112305372, 1.199719254218450271 ) ) ;
#32734=CARTESIAN_POINT ( 'NONE',  ( 1.364683531249986537, -0.8239583329919186738, 0.7879004041258500513 ) ) ;
#32738=CARTESIAN_POINT ( 'NONE',  ( 5.097642140193346272, 6.530873256209153155, -1.245904388912087324 ) ) ;
#32739=VERTEX_POINT ( 'NONE', #187769 ) ;
#32742=CARTESIAN_POINT ( 'NONE',  ( 8.948018195339340508, 9.541702104091804415, -0.7216878364870197293 ) ) ;
#32747=CARTESIAN_POINT ( 'NONE',  ( -1.201851678989727383E-14, 3.868750000682817713, -1.732050807568863648 ) ) ;
#32749=CARTESIAN_POINT ( 'NONE',  ( -4.334856428067329404, 6.080418470877079429, -1.599625672291256295 ) ) ;
#32750=CARTESIAN_POINT ( 'NONE',  ( 2.995988758495615745, 6.439144618312774959, -0.7216878364870267237 ) ) ;
#32751=CARTESIAN_POINT ( 'NONE',  ( -9.449669878600616357, 12.04770082983265844, -1.443375672974058777 ) ) ;
#32758=CARTESIAN_POINT ( 'NONE',  ( 3.765413976293345844, 5.416068943807445635, 1.599625672291267398 ) ) ;
#32761=ADVANCED_FACE ( 'NONE', ( #7949 ), #161870, .T. ) ;
#32763=CARTESIAN_POINT ( 'NONE',  ( 4.542145155778077203, 5.257923088951247159, -1.199719254218452047 ) ) ;
#32778=CARTESIAN_POINT ( 'NONE',  ( 10.05067194643221207, 10.62020544712608938, 0.7998128361456462443 ) ) ;
#32780=DIRECTION ( 'NONE',  ( -1.000000000000000000, 5.578564026256490882E-16, 2.058387550816952846E-48 ) ) ;
#32783=CARTESIAN_POINT ( 'NONE',  ( 0.6823417656249882723, -0.4072916663252490466, 1.181850606188755259 ) ) ;
#32784=CARTESIAN_POINT ( 'NONE',  ( 5.165293337126522388, 8.969999960048859577, 1.040834085586084257E-14 ) ) ;
#32786=CARTESIAN_POINT ( 'NONE',  ( -8.622622508611375025, 12.04318144581317895, 1.082531754730560403 ) ) ;
#32793=CARTESIAN_POINT ( 'NONE',  ( -5.413783410558481002, 5.210502155273325720, -0.7998128361456221525 ) ) ;
#32806=CARTESIAN_POINT ( 'NONE',  ( 4.757767692435503015, 7.006667324785019524, -1.397933448811568224 ) ) ;
#32809=CARTESIAN_POINT ( 'NONE',  ( 4.147904930777053245, 6.926640621626830807, -1.199719254218452047 ) ) ;
#32814=CARTESIAN_POINT ( 'NONE',  ( -7.700668062882065179, 10.96756792579566664, -1.082531754730543971 ) ) ;
#32819=CARTESIAN_POINT ( 'NONE',  ( 6.938021921891177612, 9.117444880338284818, -1.599625672291262513 ) ) ;
#32820=CARTESIAN_POINT ( 'NONE',  ( -4.355193658487826802, 6.104145239700998538, -1.599625672291256517 ) ) ;
#32822=CARTESIAN_POINT ( 'NONE',  ( -5.575427483717760424, 7.527751369135936343, 1.599625672291269396 ) ) ;
#32823=CARTESIAN_POINT ( 'NONE',  ( 4.220665892555866883, 3.818531717603609987, -0.7998128361456211532 ) ) ;
#32825=CARTESIAN_POINT ( 'NONE',  ( -4.706651882238427120, 8.642844295920152575, 1.040834085586084257E-14 ) ) ;
#32828=CARTESIAN_POINT ( 'NONE',  ( 7.944187942603509356, 11.35563746875774882, 1.199719254218460707 ) ) ;
#32831=CARTESIAN_POINT ( 'NONE',  ( 4.137223920935246824, 7.648466568186386816, 0.7801199165378830402 ) ) ;
#32832=CARTESIAN_POINT ( 'NONE',  ( 5.829642864196168617, 6.863966765392747860, 1.082531754730558626 ) ) ;
#32834=CARTESIAN_POINT ( 'NONE',  ( 5.639828713160493834, 5.682147708216442439, 1.040834085586084257E-14 ) ) ;
#32840=CARTESIAN_POINT ( 'NONE',  ( 6.873620692004076105, 10.00267932643801672, -1.082531754730537976 ) ) ;
#32843=CARTESIAN_POINT ( 'NONE',  ( -8.435144125996554720, 12.99275191363802229, 0.7998128361456341429 ) ) ;
#32844=CARTESIAN_POINT ( 'NONE',  ( -5.879432169820529630, 10.01108796476595764, -0.7998128361456221525 ) ) ;
#32846=ADVANCED_FACE ( 'NONE', ( #154182 ), #5750, .T. ) ;
#32851=CARTESIAN_POINT ( 'NONE',  ( 8.283668668269706714, 8.766627655843896250, 1.040834085586084257E-14 ) ) ;
#32854=CARTESIAN_POINT ( 'NONE',  ( 8.860417081730671995, 10.29590700256267155, 1.199719254218453823 ) ) ;
#32858=CARTESIAN_POINT ( 'NONE',  ( 4.532503425670185493, 4.182342172903648070, 1.214306433183764966E-14 ) ) ;
#32861=CARTESIAN_POINT ( 'NONE',  ( 0.7499999999999920064, 4.264583334016150751, 1.299038105676669330 ) ) ;
#32865=ORIENTED_EDGE ( 'NONE', *, *, #27529, .F. ) ;
#32867=CARTESIAN_POINT ( 'NONE',  ( -0.7500000000000215383, 3.691666666666690411, 1.299038105676671107 ) ) ;
#32868=CARTESIAN_POINT ( 'NONE',  ( 5.991813822235618758, 9.077867661661846554, 1.199719254218462483 ) ) ;
#32871=CARTESIAN_POINT ( 'NONE',  ( 7.605760987586388744, 11.81721221891873697, 1.040834085586084257E-14 ) ) ;
#32872=CARTESIAN_POINT ( 'NONE',  ( -10.10046125205658463, 11.84658821789661509, -1.082531754730537976 ) ) ;
#32873=CIRCLE ( 'NONE', #181598, 0.07999999999999994615 ) ;
#32878=CARTESIAN_POINT ( 'NONE',  ( -4.386226389220933441, 5.076017861301227008, -1.199719254218446718 ) ) ;
#32880=CARTESIAN_POINT ( 'NONE',  ( 1.364683531249986537, 0.1135416670080857532, 0.7879004041258500513 ) ) ;
#32884=CARTESIAN_POINT ( 'NONE',  ( 5.495132332240461714, 5.305409230568988832, 0.7998128361456341429 ) ) ;
#32886=CARTESIAN_POINT ( 'NONE',  ( 1.364683531249986537, -1.136458332991912235, 0.7879004041258500513 ) ) ;
#32893=CARTESIAN_POINT ( 'NONE',  ( -5.879432169820529630, 10.01108796476595764, -0.7998128361456221525 ) ) ;
#32895=CARTESIAN_POINT ( 'NONE',  ( 4.168242161197552420, 6.950367390450747251, -1.199719254218452047 ) ) ;
#32898=CARTESIAN_POINT ( 'NONE',  ( -0.6823417656250246877, -0.4489583329919111243, 1.181850606188755259 ) ) ;
#32902=CARTESIAN_POINT ( 'NONE',  ( 9.103410076571945453, 12.70806329172093818, 1.199719254218450271 ) ) ;
#32905=CARTESIAN_POINT ( 'NONE',  ( -6.230135280679522936, 7.227244901336242755, 1.199719254218450271 ) ) ;
#32910=CARTESIAN_POINT ( 'NONE',  ( 8.646349277213076334, 11.11049346154719508, 1.599625672291281386 ) ) ;
#32912=CARTESIAN_POINT ( 'NONE',  ( 8.076906825439115423, 10.44614393447756129, -1.599625672291262513 ) ) ;
#32914=CARTESIAN_POINT ( 'NONE',  ( -2.754277761870538299, 6.365074488824250309, 1.040834085586084257E-14 ) ) ;
#32915=CARTESIAN_POINT ( 'NONE',  ( -7.718669524881690336, 7.899535955317097624, 0.7998128361456462443 ) ) ;
#32917=VECTOR ( 'NONE', #165961, 1000.000000000000000 ) ;
#32919=CARTESIAN_POINT ( 'NONE',  ( -4.612682051294048513, 7.132468998681293471, 1.371008595254997964 ) ) ;
#32920=CARTESIAN_POINT ( 'NONE',  ( 1.364683531249988757, 0.6343750003414208027, 0.000000000000000000 ) ) ;
#32924=CARTESIAN_POINT ( 'NONE',  ( 5.992340707560141588, 9.934888558888093968, 0.7216878364870438212 ) ) ;
#32927=ADVANCED_FACE ( 'NONE', ( #191985 ), #41513, .F. ) ;
#32947=CARTESIAN_POINT ( 'NONE',  ( 10.07387183015377197, 11.71160420905630062, -1.199719254218440723 ) ) ;
#32951=CARTESIAN_POINT ( 'NONE',  ( -3.927058049452637700, 7.733318157670055371, -0.7998128361456281477 ) ) ;
#32952=CARTESIAN_POINT ( 'NONE',  ( -8.995998617867369873, 10.45408546138876993, 1.199719254218462483 ) ) ;
#32958=CARTESIAN_POINT ( 'NONE',  ( 1.499999999999987121, 2.577083334016147198, -0.8660254037844262731 ) ) ;
#32959=CARTESIAN_POINT ( 'NONE',  ( 7.377608144130607393, 11.75895993479440982, -0.7998128361456291469 ) ) ;
#32962=CARTESIAN_POINT ( 'NONE',  ( -9.691380875670077444, 10.20103253123691189, 0.7998128361456462443 ) ) ;
#32964=CARTESIAN_POINT ( 'NONE',  ( -1.364683531249997417, 3.759375000341423689, 1.214306433183764966E-14 ) ) ;
#32970=CARTESIAN_POINT ( 'NONE',  ( -7.700668062882059850, 11.92793714009701311, -0.7216878364870267237 ) ) ;
#32974=CARTESIAN_POINT ( 'NONE',  ( -1.364683531250014514, 2.051041667008086655, -0.7879004041258289570 ) ) ;
#32979=CARTESIAN_POINT ( 'NONE',  ( -1.364683531250000748, 1.759375000341421913, 0.000000000000000000 ) ) ;
#32981=CARTESIAN_POINT ( 'NONE',  ( -4.726989112658928072, 8.666571064744069020, 1.040834085586084257E-14 ) ) ;
#32982=CARTESIAN_POINT ( 'NONE',  ( 7.558834334818744338, 8.777393797832065303, 1.199719254218462483 ) ) ;
#32983=CARTESIAN_POINT ( 'NONE',  ( -1.230761180058581372, 2.896116465842660137, 0.7750000000000117906 ) ) ;
#32985=CARTESIAN_POINT ( 'NONE',  ( 0.7499999999999902300, 5.566666666666685082, -1.299038105676658228 ) ) ;
#32986=CARTESIAN_POINT ( 'NONE',  ( 1.364683531249986537, 2.717708333674754062, -0.7879004041258239610 ) ) ;
#32990=CARTESIAN_POINT ( 'NONE',  ( -5.748293942514186128, 6.769059690097084747, -1.082531754730544860 ) ) ;
#32995=CARTESIAN_POINT ( 'NONE',  ( 5.843201017809841247, 5.919415396974013532, 1.040834085586084257E-14 ) ) ;
#32998=CARTESIAN_POINT ( 'NONE',  ( -7.343712760096452463, 11.71941532008788833, -0.7998128361456291469 ) ) ;
#32999=CARTESIAN_POINT ( 'NONE',  ( -4.277761160311629673, 4.949475094240346706, 1.199719254218462483 ) ) ;
#33001=CARTESIAN_POINT ( 'NONE',  ( 1.364683531249988535, 5.655208333674751842, -0.7879004041258300672 ) ) ;
#33005=CARTESIAN_POINT ( 'NONE',  ( -7.334597914868741242, 8.619747657844088806, -1.082531754730543083 ) ) ;
#33007=CARTESIAN_POINT ( 'NONE',  ( -0.6823417656250003738, -0.2197916663252488800, -1.181850606188749264 ) ) ;
#33010=CARTESIAN_POINT ( 'NONE',  ( 6.792271770766432404, 10.86814146596211472, 1.040834085586084257E-14 ) ) ;
#33016=CARTESIAN_POINT ( 'NONE',  ( 2.507895228403643539, 5.869702166538802501, -0.7216878364870267237 ) ) ;
#33020=CARTESIAN_POINT ( 'NONE',  ( 8.337901282279995385, 11.71100668175994386, -1.082531754730543083 ) ) ;
#33027=CARTESIAN_POINT ( 'NONE',  ( 6.124532705071213279, 8.168374127381657246, -1.599625672291262513 ) ) ;
#33028=CARTESIAN_POINT ( 'NONE',  ( -4.771579997005698459, 7.654261532226910525, -1.199719254218452047 ) ) ;
#33032=CARTESIAN_POINT ( 'NONE',  ( 4.487385655998867406, 8.179107665399927285, 0.7216878364870438212 ) ) ;
#33033=CARTESIAN_POINT ( 'NONE',  ( -1.364683531250014514, 0.8010416670080889867, -0.7879004041258289570 ) ) ;
#33035=CARTESIAN_POINT ( 'NONE',  ( -7.784352752540590004, 12.23349531127272094, 0.7998128361456481317 ) ) ;
#33045=LINE ( 'NONE', #83911, #187624 ) ;
#33054=CARTESIAN_POINT ( 'NONE',  ( 5.960781091502512119, 10.10599504006161986, 0.7998128361456462443 ) ) ;
#33055=CARTESIAN_POINT ( 'NONE',  ( 5.472687561410540802, 9.536552588287639409, 0.7998128361456462443 ) ) ;
#33066=CARTESIAN_POINT ( 'NONE',  ( -4.225337428953291230, 8.081310767087481750, 0.7998128361456341429 ) ) ;
#33067=CARTESIAN_POINT ( 'NONE',  ( -4.274898507010545856, 3.881803101134051470, -0.7998128361456221525 ) ) ;
#33072=CARTESIAN_POINT ( 'NONE',  ( 1.483013432599452175, 7.294277089886983312, 4.259227663826820276 ) ) ;
#33079=CARTESIAN_POINT ( 'NONE',  ( -8.026063749610043985, 12.30756544127966912, -0.7216878364870267237 ) ) ;
#33082=CARTESIAN_POINT ( 'NONE',  ( 5.612185521052973414, 8.634967976948757951, -1.199719254218440723 ) ) ;
#33083=CARTESIAN_POINT ( 'NONE',  ( -0.6823417656249969321, 5.717708333674756283, -1.181850606188749264 ) ) ;
#33089=CARTESIAN_POINT ( 'NONE',  ( 4.704316113817540668, 5.551085556617666228, -1.082531754730548412 ) ) ;
#33090=CARTESIAN_POINT ( 'NONE',  ( -5.747767057189642870, 8.793146435774861658, -1.199719254218440723 ) ) ;
#33095=CARTESIAN_POINT ( 'NONE',  ( -7.555971681517696936, 7.709721804725773175, 0.7998128361456462443 ) ) ;
#33096=CARTESIAN_POINT ( 'NONE',  ( -3.598799709423620374, 6.286017863381107240, 1.199719254218464037 ) ) ;
#33101=CARTESIAN_POINT ( 'NONE',  ( -8.283668668269720925, 8.766627655843896250, 1.056142170575426150E-14 ) ) ;
#33104=CARTESIAN_POINT ( 'NONE',  ( 5.449487677688982679, 8.445153826357429949, -1.199719254218446718 ) ) ;
#33116=CARTESIAN_POINT ( 'NONE',  ( -0.6823417656250246877, -0.3864583329919110688, 1.181850606188755259 ) ) ;
#33117=CARTESIAN_POINT ( 'NONE',  ( 3.928111819657337911, 5.605883094398769195, 1.599625672291267398 ) ) ;
#33118=CARTESIAN_POINT ( 'NONE',  ( 6.030679399980265920, 5.930214142932100252, -0.7998128361456281477 ) ) ;
#33120=CARTESIAN_POINT ( 'NONE',  ( -7.293923454472094114, 9.532663335016016148, 1.443375672974090751 ) ) ;
#33122=CARTESIAN_POINT ( 'NONE',  ( 5.504247177468179153, 7.444707678511436555, 1.443375672974062551 ) ) ;
#33123=CARTESIAN_POINT ( 'NONE',  ( -6.765155463094763455, 8.915767345075790828, 1.443375672974078761 ) ) ;
#33127=CARTESIAN_POINT ( 'NONE',  ( 5.425234023762710578, 9.481190127698507553, -0.7998128361456291469 ) ) ;
#33132=CARTESIAN_POINT ( 'NONE',  ( -1.201851678989727383E-14, 3.321875000341421025, 1.575800808251672791 ) ) ;
#33137=CARTESIAN_POINT ( 'NONE',  ( 7.904567251967224095, 9.180748867838630645, 1.199719254218462483 ) ) ;
#33141=CARTESIAN_POINT ( 'NONE',  ( -9.826962411806732689, 10.35921099006301382, -0.7998128361456291469 ) ) ;
#33147=CARTESIAN_POINT ( 'NONE',  ( 8.703444544968814256, 12.24143683818393313, -1.199719254218446718 ) ) ;
#33148=CARTESIAN_POINT ( 'NONE',  ( 1.499999999999821032, 7.240846818246208905, -4.154462424328212222 ) ) ;
#33150=CARTESIAN_POINT ( 'NONE',  ( -9.203287345578106127, 9.631590079462940324, 0.7998128361456462443 ) ) ;
#33153=CARTESIAN_POINT ( 'NONE',  ( 5.678179657697552507, 6.109196432984326464, -0.7486794562398890740 ) ) ;
#33154=CARTESIAN_POINT ( 'NONE',  ( -2.591579918506545344, 6.175260338232929413, 1.040834085586084257E-14 ) ) ;
#33159=CARTESIAN_POINT ( 'NONE',  ( 6.810273232766058449, 6.839740281182199233, 1.040834085586084257E-14 ) ) ;
#33161=CARTESIAN_POINT ( 'NONE',  ( 5.880485940025228508, 7.883652901494672349, 1.599625672291267398 ) ) ;
#33162=CARTESIAN_POINT ( 'NONE',  ( -4.015022313999534909, 7.625723350685065682, -0.07359193599470841007 ) ) ;
#33163=CARTESIAN_POINT ( 'NONE',  ( 3.171717870593107058, 5.787755718078879674, -1.199719254218446718 ) ) ;
#33165=CARTESIAN_POINT ( 'NONE',  ( -6.873620692448438874, 10.96304854125777695, 0.000000000000000000 ) ) ;
#33172=CARTESIAN_POINT ( 'NONE',  ( -4.068573627943592008, 7.549288226164498461, -0.4708643921484123585 ) ) ;
#33173=CARTESIAN_POINT ( 'NONE',  ( -1.364683531250014514, -0.6989583329919100141, -0.7879004041258359514 ) ) ;
#33176=CARTESIAN_POINT ( 'NONE',  ( 5.666945020832181434, 5.713783400500082266, 0.7216878364870317197 ) ) ;
#33181=CARTESIAN_POINT ( 'NONE',  ( -7.985389288324685531, 12.26011190311341537, -0.7216878364870267237 ) ) ;
#33186=CARTESIAN_POINT ( 'NONE',  ( -8.609064354553318310, 12.98773281371349775, 0.7216878364870317197 ) ) ;
#33192=CARTESIAN_POINT ( 'NONE',  ( -8.459924664802993988, 12.81373650900478189, 1.040834085586084257E-14 ) ) ;
#33199=CARTESIAN_POINT ( 'NONE',  ( 1.499999999999989120, 2.785416667349484676, 0.8660254037844524744 ) ) ;
#33200=CARTESIAN_POINT ( 'NONE',  ( 5.029711800989886683, 4.970344644017389513, 1.040834085586084257E-14 ) ) ;
#33202=VERTEX_POINT ( 'NONE', #135551 ) ;
#33204=CARTESIAN_POINT ( 'NONE',  ( -7.133561379084627063, 11.47423870890741782, 0.7998128361456481317 ) ) ;
#33205=CARTESIAN_POINT ( 'NONE',  ( -4.772106882330241717, 5.630174786549132726, -1.082531754730544860 ) ) ;
#33207=CARTESIAN_POINT ( 'NONE',  ( 4.299907273828439180, 8.168308919441841454, 1.040834085586084257E-14 ) ) ;
#33212=CARTESIAN_POINT ( 'NONE',  ( 7.365103760721646076, 9.615707025640515937, 1.599625672291281386 ) ) ;
#33213=CARTESIAN_POINT ( 'NONE',  ( -3.023105066167323329, 5.702484939155337607, -2.500000000000000444 ) ) ;
#33215=FACE_OUTER_BOUND ( 'NONE', #120667, .T. ) ;
#33219=CARTESIAN_POINT ( 'NONE',  ( -7.212574532790102744, 8.477387045419011002, -1.082531754730550855 ) ) ;
#33222=CARTESIAN_POINT ( 'NONE',  ( 1.364683531249988535, 5.717708333674752730, -0.7879004041258300672 ) ) ;
#33225=CARTESIAN_POINT ( 'NONE',  ( -1.364683531249997417, 5.509375000341417916, 1.214306433183764966E-14 ) ) ;
#33229=CARTESIAN_POINT ( 'NONE',  ( -3.592547517496941900, 5.214391408544949869, -1.443375672974051449 ) ) ;
#33231=CARTESIAN_POINT ( 'NONE',  ( 9.561524646135536543, 12.17819805862340310, -1.599625672291262513 ) ) ;
#33236=CARTESIAN_POINT ( 'NONE',  ( -1.364683531250014514, 1.738541667008085545, -0.7879004041258289570 ) ) ;
#33237=VECTOR ( 'NONE', #56520, 1000.000000000000000 ) ;
#33238=CARTESIAN_POINT ( 'NONE',  ( 5.009901455449552010, 5.803638771901306725, -1.199719254218452047 ) ) ;
#33242=CARTESIAN_POINT ( 'NONE',  ( -6.518203450479830963, 5.167241622962447600, -2.437504649502885812 ) ) ;
#33243=DIRECTION ( 'NONE',  ( 0.6507913734559627184, -0.7592566023653016805, 0.000000000000000000 ) ) ;
#33244=CARTESIAN_POINT ( 'NONE',  ( 7.890482213029013536, 12.14938698193514277, 1.040834085586084257E-14 ) ) ;
#33246=CARTESIAN_POINT ( 'NONE',  ( -8.514157279702036618, 9.035531035848267223, -0.7216878364870278340 ) ) ;
#33248=CARTESIAN_POINT ( 'NONE',  ( 0.4020909550005648536, 7.366597533580820034, 1.962779437971595931 ) ) ;
#33250=CARTESIAN_POINT ( 'NONE',  ( -8.667740277838301921, 9.006785167099828016, -0.7998128361456291469 ) ) ;
#33251=CARTESIAN_POINT ( 'NONE',  ( -4.650083499362882122, 6.448183387388563226, 1.443375672974064550 ) ) ;
#33252=CARTESIAN_POINT ( 'NONE',  ( -1.364683531249997417, 2.821875000341422801, 1.214306433183764966E-14 ) ) ;
#33271=CARTESIAN_POINT ( 'NONE',  ( 1.364683531249990311, 4.696875000341417916, 1.214306433183764966E-14 ) ) ;
#33275=CARTESIAN_POINT ( 'NONE',  ( -6.518203450479830963, 5.167241622962448488, -2.437504649502885368 ) ) ;
#33278=CARTESIAN_POINT ( 'NONE',  ( 9.073431116043567002, 11.60875560684942265, -1.599625672291262513 ) ) ;
#33280=CARTESIAN_POINT ( 'NONE',  ( -1.364683531250012516, 2.030208333674750953, 0.7879004041258379498 ) ) ;
#33282=CARTESIAN_POINT ( 'NONE',  ( -8.202319746587722449, 8.671720580548228696, 1.040834085586084257E-14 ) ) ;
#33289=CARTESIAN_POINT ( 'NONE',  ( 3.354752944377597856, 6.001296637494123232, -1.199719254218446718 ) ) ;
#33292=CARTESIAN_POINT ( 'NONE',  ( 8.594979316059474073, 12.11489407112305372, 1.199719254218450271 ) ) ;
#33293=CARTESIAN_POINT ( 'NONE',  ( -1.284279953904132077, 2.878360285806111474, -0.7749999999999936939 ) ) ;
#33299=CARTESIAN_POINT ( 'NONE',  ( -9.134442807305063639, 11.67993591332117376, 1.599625672291281386 ) ) ;
#33300=CARTESIAN_POINT ( 'NONE',  ( 7.806797523370503811, 8.002351953554066810, 1.040834085586084257E-14 ) ) ;
#33302=CARTESIAN_POINT ( 'NONE',  ( 3.985733972293228344, 7.593847367743336463, 1.040834085586084257E-14 ) ) ;
#33313=EDGE_CURVE ( 'NONE', #171893, #109221, #72658, .T. ) ;
#33314=CARTESIAN_POINT ( 'NONE',  ( -5.572037945536512105, 9.444535336527177805, 0.000000000000000000 ) ) ;
#33315=AXIS2_PLACEMENT_3D ( 'NONE', #194564, #178340, #96034 ) ;
#33316=CARTESIAN_POINT ( 'NONE',  ( 4.741601036477289810, 6.554953847355395880, 1.599625672291267398 ) ) ;
#33319=CARTESIAN_POINT ( 'NONE',  ( -9.104463846776669200, 10.58062822844965645, -1.199719254218441611 ) ) ;
#33324=CARTESIAN_POINT ( 'NONE',  ( -10.48453286206953727, 11.12637651536962125, 0.7998128361456462443 ) ) ;
#33327=CARTESIAN_POINT ( 'NONE',  ( 8.585337585951586803, 11.03931315507545108, -1.599625672291255185 ) ) ;
#33328=CARTESIAN_POINT ( 'NONE',  ( 4.390142812726693045, 4.016254791136236513, 1.214306433183764966E-14 ) ) ;
#33330=ORIENTED_EDGE ( 'NONE', *, *, #199925, .F. ) ;
#33334=DIRECTION ( 'NONE',  ( -0.6507913734559642727, 0.7592566023653003482, 2.775557561562893816E-17 ) ) ;
#33337=CARTESIAN_POINT ( 'NONE',  ( -3.469997250093771246, 6.135748327496311383, -1.199719254218452935 ) ) ;
#33340=CARTESIAN_POINT ( 'NONE',  ( -8.727698198895085469, 11.20540053684285553, -1.599625672291263179 ) ) ;
#33344=CARTESIAN_POINT ( 'NONE',  ( 5.992340707560141588, 9.934888558888093968, 0.7216878364870438212 ) ) ;
#33345=CARTESIAN_POINT ( 'NONE',  ( -0.6823417656250212460, 5.113541667008086655, 1.181850606188767472 ) ) ;
#33347=CARTESIAN_POINT ( 'NONE',  ( 3.195971524519376494, 4.751719416737803847, -1.599625672291262513 ) ) ;
#33348=CARTESIAN_POINT ( 'NONE',  ( 5.843238758086321205, 6.086642049024201917, 0.6823498365625046969 ) ) ;
#33349=CARTESIAN_POINT ( 'NONE',  ( 4.976006071415387311, 5.764094157194782575, 1.199719254218462483 ) ) ;
#33351=CARTESIAN_POINT ( 'NONE',  ( -5.930802130974132780, 9.006687355190106103, -1.199719254218440723 ) ) ;
#33355=CIRCLE ( 'NONE', #16014, 0.7500000000000011102 ) ;
#33361=CARTESIAN_POINT ( 'NONE',  ( 0.6823417656249899377, 4.488541667008086655, -1.181850606188754593 ) ) ;
#33362=CARTESIAN_POINT ( 'NONE',  ( 7.703003830858588863, 12.13858823597705872, -0.7998128361456291469 ) ) ;
#33365=CARTESIAN_POINT ( 'NONE',  ( -4.284013352238250860, 7.941839977679187257, -0.7216878364870267237 ) ) ;
#33367=CARTESIAN_POINT ( 'NONE',  ( -5.721177634842498527, 5.777054783512106440, 0.000000000000000000 ) ) ;
#33374=CARTESIAN_POINT ( 'NONE',  ( 3.714044015139744914, 6.420469553383295391, 1.199719254218462483 ) ) ;
#33384=CARTESIAN_POINT ( 'NONE',  ( 6.003563092752934871, 5.898578451166879510, 0.7998128361456341429 ) ) ;
#33385=VERTEX_POINT ( 'NONE', #186406 ) ;
#33390=CARTESIAN_POINT ( 'NONE',  ( -1.364683531250010295, 4.592708333674755394, 0.7879004041258379498 ) ) ;
#33395=CARTESIAN_POINT ( 'NONE',  ( 7.233438648090761980, 8.397765496649418182, 1.199719254218462483 ) ) ;
#33397=CARTESIAN_POINT ( 'NONE',  ( -4.713430959045263435, 8.650753218861462202, 0.7998128361456481317 ) ) ;
#33398=CARTESIAN_POINT ( 'NONE',  ( 4.975479186090839612, 8.748550117173898855, 0.7216878364870438212 ) ) ;
#33399=CARTESIAN_POINT ( 'NONE',  ( 1.499999999999987121, 1.754166666666691521, 0.8660254037844524744 ) ) ;
#33400=CARTESIAN_POINT ( 'NONE',  ( -4.796887421136680985, 4.490790167614548523, 1.214306433183764966E-14 ) ) ;
#33403=CARTESIAN_POINT ( 'NONE',  ( -4.238895582566952314, 8.097128612970093897, 1.040834085586084257E-14 ) ) ;
#33407=CARTESIAN_POINT ( 'NONE',  ( -1.364683531250012516, 3.280208333674756727, 0.7879004041258379498 ) ) ;
#33409=CARTESIAN_POINT ( 'NONE',  ( -2.968872451712654126, 6.407508927065978632, 1.040834085586084257E-14 ) ) ;
#33412=ORIENTED_EDGE ( 'NONE', *, *, #101217, .T. ) ;
#33415=CARTESIAN_POINT ( 'NONE',  ( 4.843287188579786573, 6.673587691474970107, -1.599625672291256295 ) ) ;
#33417=UNCERTAINTY_MEASURE_WITH_UNIT (LENGTH_MEASURE( 1.000000000000000082E-05 ), #37663, 'distance_accuracy_value', 'NONE');
#33419=CARTESIAN_POINT ( 'NONE',  ( -0.6823417656250212460, 2.863541667008084879, 1.181850606188767472 ) ) ;
#33421=CARTESIAN_POINT ( 'NONE',  ( 2.184835310096557404, 5.700724961754617404, 1.040834085586084257E-14 ) ) ;
#33423=CARTESIAN_POINT ( 'NONE',  ( -1.402160292154681736E-14, -0.6156249996585817508, 1.575800808251672791 ) ) ;
#33424=DIRECTION ( 'NONE',  ( -1.000000000000000000, 5.578564026256504688E-16, -1.232595164407830946E-31 ) ) ;
#33427=CARTESIAN_POINT ( 'NONE',  ( -2.300079615812729905, 5.835176651756807331, -0.7998128361456281477 ) ) ;
#33428=CARTESIAN_POINT ( 'NONE',  ( -7.497295758232736418, 7.849192594134070333, -0.7216878364870267237 ) ) ;
#33432=CARTESIAN_POINT ( 'NONE',  ( 1.364683531249988535, 3.613541667008086211, 0.7879004041258500513 ) ) ;
#33440=CARTESIAN_POINT ( 'NONE',  ( -7.171900071504748730, 8.429933507252760805, -1.082531754730549078 ) ) ;
#33442=LINE ( 'NONE', #195955, #5662 ) ;
#33445=CARTESIAN_POINT ( 'NONE',  ( -7.836249598574384301, 8.244638741199329601, 1.040834085586084257E-14 ) ) ;
#33458=CARTESIAN_POINT ( 'NONE',  ( -4.530395885260773525, 8.437212299446219532, 0.7998128361456481317 ) ) ;
#33460=CARTESIAN_POINT ( 'NONE',  ( -1.402160292154681736E-14, -0.9124999999999769962, -1.732050807568870754 ) ) ;
#33461=CARTESIAN_POINT ( 'NONE',  ( 2.361091307074211887, 5.906356958228550447, 0.7998128361456462443 ) ) ;
#33464=CARTESIAN_POINT ( 'NONE',  ( 6.518772930072240790, 6.499656594706071822, -0.7998128361456281477 ) ) ;
#33472=CARTESIAN_POINT ( 'NONE',  ( -4.311129659465605002, 4.131998812239033647, 0.7216878364870317197 ) ) ;
#33481=CARTESIAN_POINT ( 'NONE',  ( 1.364683531249990311, 2.634375000341422801, 1.214306433183764966E-14 ) ) ;
#33482=CARTESIAN_POINT ( 'NONE',  ( 9.205623113554615600, 11.76297960394566466, 1.443375672974076540 ) ) ;
#33484=CARTESIAN_POINT ( 'NONE',  ( -6.581593504430098385, 9.765943957555402122, -1.199719254218440723 ) ) ;
#33487=CARTESIAN_POINT ( 'NONE',  ( 7.470706336329915764, 8.674577799595093452, -1.199719254218441611 ) ) ;
#33488=CARTESIAN_POINT ( 'NONE',  ( -7.088215381846223906, 7.164006121775713609, 0.7998128361456341429 ) ) ;
#33489=CARTESIAN_POINT ( 'NONE',  ( -1.452308200714708342, 8.721976639181708180, 2.576600914284036037 ) ) ;
#33491=CARTESIAN_POINT ( 'NONE',  ( -0.6823417656249969321, 5.717708333674756283, -1.181850606188749264 ) ) ;
#33494=CARTESIAN_POINT ( 'NONE',  ( 6.805829924380097040, 10.88395931184472154, 0.7216878364870438212 ) ) ;
#33497=CARTESIAN_POINT ( 'NONE',  ( 1.364683531249988757, 0.9468750003414211358, 0.000000000000000000 ) ) ;
#33499=CARTESIAN_POINT ( 'NONE',  ( 7.429504990164394584, 7.770103364721017591, 1.040834085586084257E-14 ) ) ;
#33503=CARTESIAN_POINT ( 'NONE',  ( -3.456965981804629884, 6.976951378839947537, 1.040834085586084257E-14 ) ) ;
#33505=CARTESIAN_POINT ( 'NONE',  ( -1.364683531250010295, 4.530208333674754506, 0.7879004041258379498 ) ) ;
#33509=CARTESIAN_POINT ( 'NONE',  ( -5.594971466091354095, 6.350553869658721595, -1.210626573312810761 ) ) ;
#33516=CARTESIAN_POINT ( 'NONE',  ( 6.662942426112080874, 9.860851032851066122, 1.199719254218460707 ) ) ;
#33519=CARTESIAN_POINT ( 'NONE',  ( 4.546061579283848353, 4.198160018786257552, -0.7998128361456211532 ) ) ;
#33525=CARTESIAN_POINT ( 'NONE',  ( 5.341549334104188418, 7.254893527920112994, 1.443375672974062551 ) ) ;
#33526=AXIS2_PLACEMENT_3D ( 'NONE', #63822, #16112, #117973 ) ;
#33527=CARTESIAN_POINT ( 'NONE',  ( -1.364683531250000748, 0.3218750003414205807, 0.000000000000000000 ) ) ;
#33533=CARTESIAN_POINT ( 'NONE',  ( 1.499999999999985123, 0.2958333333333566517, -0.8660254037844323793 ) ) ;
#33534=CARTESIAN_POINT ( 'NONE',  ( 7.311924916471702396, 7.425000578838787391, -0.7998128361456281477 ) ) ;
#33535=CARTESIAN_POINT ( 'NONE',  ( -6.828502922777144768, 11.11833717654868892, 0.7998128361456481317 ) ) ;
#33539=CARTESIAN_POINT ( 'NONE',  ( -1.364683531250000748, 1.009375000341421247, 0.000000000000000000 ) ) ;
#33540=CARTESIAN_POINT ( 'NONE',  ( -1.201851678989727383E-14, 2.962500000000025224, 1.732050807568877637 ) ) ;
#33542=CARTESIAN_POINT ( 'NONE',  ( 5.118366684358879759, 5.930181538962194132, 1.199719254218462483 ) ) ;
#33549=CARTESIAN_POINT ( 'NONE',  ( 0.7499999999999867883, -1.152083332650516434, -1.299038105676652011 ) ) ;
#33550=CARTESIAN_POINT ( 'NONE',  ( -8.019811557683421910, 9.315200557840817908, 1.199719254218462483 ) ) ;
#33551=CARTESIAN_POINT ( 'NONE',  ( -3.958617665510279160, 5.641473247893851628, -1.443375672974053447 ) ) ;
#33560=CARTESIAN_POINT ( 'NONE',  ( 5.829115978871627135, 8.888053511070525659, 1.199719254218462483 ) ) ;
#33564=CARTESIAN_POINT ( 'NONE',  ( 5.924549939047454750, 9.855799328956630134, -0.7216878364870267237 ) ) ;
#33568=CARTESIAN_POINT ( 'NONE',  ( -7.694415870955439551, 8.935572256658169010, 1.199719254218462483 ) ) ;
#33569=CARTESIAN_POINT ( 'NONE',  ( 3.842846474469570062, 6.570739089268092137, -1.199719254218452047 ) ) ;
#33575=CARTESIAN_POINT ( 'NONE',  ( 9.083599731475983319, 11.62061899152058686, 1.443375672974076540 ) ) ;
#33582=CARTESIAN_POINT ( 'NONE',  ( -3.470524135418300737, 6.032400010421219427, -1.082531754730549967 ) ) ;
#33583=CARTESIAN_POINT ( 'NONE',  ( 8.432808358020015049, 11.82173160345663376, 1.082531754730546636 ) ) ;
#33585=B_SPLINE_CURVE_WITH_KNOTS ( 'NONE', 3,
 ( #97028, #116500, #51449, #118636, #200856, #81811, #134850, #101247 ),
 .UNSPECIFIED., .F., .F.,
 ( 4, 2, 2, 4 ),
 ( 1.951563910473858677E-18, 0.0002925934901276177539, 0.0005851869802552335563, 0.001170373960510464294 ),
 .UNSPECIFIED. ) ;
#33587=CARTESIAN_POINT ( 'NONE',  ( -5.880485940025243607, 7.883652901494672349, 1.599625672291269396 ) ) ;
#33593=CARTESIAN_POINT ( 'NONE',  ( -6.989391883044787868, 8.113044270762433285, -1.199719254218446718 ) ) ;
#33599=CYLINDRICAL_SURFACE ( 'NONE', #37536, 0.08000000000000020983 ) ;
#33610=CARTESIAN_POINT ( 'NONE',  ( -6.392833124043511894, 7.417059051927569868, 1.199719254218450271 ) ) ;
#33613=CARTESIAN_POINT ( 'NONE',  ( 5.016153647376212277, 5.914896012436124728, 1.082531754730558626 ) ) ;
#33618=CARTESIAN_POINT ( 'NONE',  ( -4.436542580169821726, 6.199052314996659874, 1.599625672291267398 ) ) ;
#33622=CARTESIAN_POINT ( 'NONE',  ( 9.622536337397022521, 12.24937836509514710, 1.599625672291281386 ) ) ;
#33625=CARTESIAN_POINT ( 'NONE',  ( -8.799405390469187793, 10.22472669609091689, -1.199719254218446718 ) ) ;
#33626=CARTESIAN_POINT ( 'NONE',  ( 5.449487677688982679, 8.445153826357429949, -1.199719254218446718 ) ) ;
#33628=CARTESIAN_POINT ( 'NONE',  ( -6.984421689334302741, 11.30024240419870374, 0.000000000000000000 ) ) ;
#33631=CARTESIAN_POINT ( 'NONE',  ( 1.364683531249986537, -0.03229166632525094088, -0.7879004041258309554 ) ) ;
#33634=CARTESIAN_POINT ( 'NONE',  ( 8.270110514656034084, 9.711179024262627024, 1.082531754730558626 ) ) ;
#33639=CARTESIAN_POINT ( 'NONE',  ( -5.593146208820614973, 6.196971745715879720, -0.8885217884838312319 ) ) ;
#33658=AXIS2_PLACEMENT_3D ( 'NONE', #7889, #21984, #25214 ) ;
#33659=CARTESIAN_POINT ( 'NONE',  ( -1.500000000000015099, 0.1604166673494879791, -0.8660254037844383745 ) ) ;
#33666=CARTESIAN_POINT ( 'NONE',  ( 7.567422294721922960, 11.98040977715095323, 0.7998128361456462443 ) ) ;
#33672=CARTESIAN_POINT ( 'NONE',  ( 5.172599298813543633, 5.993452922492633839, -1.199719254218452047 ) ) ;
#33673=CARTESIAN_POINT ( 'NONE',  ( -5.585596099150174965, 9.460353182409786399, -0.7216878364870207285 ) ) ;
#33675=CARTESIAN_POINT ( 'NONE',  ( -5.892944143475336460, 6.011535633345318708, 0.2346759862181871381 ) ) ;
#33678=CARTESIAN_POINT ( 'NONE',  ( -8.019811557683421910, 9.315200557840817908, 1.199719254218462483 ) ) ;
#33679=CARTESIAN_POINT ( 'NONE',  ( -4.758548728272219641, 4.653987725846768342, 0.7216878364870317197 ) ) ;
#33682=CARTESIAN_POINT ( 'NONE',  ( -0.7500000000000006661, 0.1395833340161536928, -1.299038105676652011 ) ) ;
#33690=CARTESIAN_POINT ( 'NONE',  ( -5.558479791478509568, 5.587240632920778438, 0.000000000000000000 ) ) ;
#33691=EDGE_CURVE ( 'NONE', #179865, #133314, #105193, .T. ) ;
#33698=CARTESIAN_POINT ( 'NONE',  ( -8.130085669689073313, 12.63685038127928806, 0.7998128361456481317 ) ) ;
#33699=CARTESIAN_POINT ( 'NONE',  ( 9.271078113646423091, 9.710679308875986848, 1.040834085586084257E-14 ) ) ;
#33705=VERTEX_POINT ( 'NONE', #204772 ) ;
#33707=CARTESIAN_POINT ( 'NONE',  ( -1.608462485350629301, 8.735270501766756013, 2.463594439587650342 ) ) ;
#33708=CARTESIAN_POINT ( 'NONE',  ( -8.646349277213090545, 11.11049346154719508, 1.599625672291269396 ) ) ;
#33713=CARTESIAN_POINT ( 'NONE',  ( 3.994848817520957773, 7.812407387083109001, 1.040834085586084257E-14 ) ) ;
#33718=CARTESIAN_POINT ( 'NONE',  ( -3.619250341049077946, 3.172667246362661064, 2.500000000000011102 ) ) ;
#33731=CARTESIAN_POINT ( 'NONE',  ( 7.527801604085637699, 9.805521176231838609, 1.599625672291281386 ) ) ;
#33733=CARTESIAN_POINT ( 'NONE',  ( -4.436542580169821726, 6.199052314996659874, 1.599625672291267398 ) ) ;
#33738=CARTESIAN_POINT ( 'NONE',  ( -1.500000000000015099, -0.5895833326505155458, -0.8660254037844383745 ) ) ;
#33743=CARTESIAN_POINT ( 'NONE',  ( 5.352771719296971042, 5.139321848801576387, 0.7998128361456341429 ) ) ;
#33745=CARTESIAN_POINT ( 'NONE',  ( -2.950870989268691957, 6.594433254122103349, -0.7998128361456281477 ) ) ;
#33752=CARTESIAN_POINT ( 'NONE',  ( 6.005898861173831094, 6.109229547565340646, 1.040834085586084257E-14 ) ) ;
#33755=CARTESIAN_POINT ( 'NONE',  ( 7.076992996209058973, 11.20031622897851165, 1.040834085586084257E-14 ) ) ;
#33756=CARTESIAN_POINT ( 'NONE',  ( -0.6823417656249969321, 4.780208333674755394, -1.181850606188749264 ) ) ;
#33758=CARTESIAN_POINT ( 'NONE',  ( 3.673896439178918172, 6.269667698141953238, 1.082531754730558626 ) ) ;
#33766=CARTESIAN_POINT ( 'NONE',  ( -5.641245921709659328, 6.318796091258308323, 1.170641968482153850 ) ) ;
#33769=CARTESIAN_POINT ( 'NONE',  ( -0.6823417656250212460, 5.113541667008086655, 1.181850606188767472 ) ) ;
#33784=CARTESIAN_POINT ( 'NONE',  ( -1.201851678989727383E-14, 4.259375000341417028, -1.575800808251660134 ) ) ;
#33786=CARTESIAN_POINT ( 'NONE',  ( 7.311924916471702396, 7.425000578838787391, -0.7998128361456281477 ) ) ;
#33787=CARTESIAN_POINT ( 'NONE',  ( -8.910733272679575379, 11.41894145625809820, -1.599625672291263179 ) ) ;
#33794=CARTESIAN_POINT ( 'NONE',  ( 1.499999999999989120, 5.795833333333350268, -0.8660254037844323793 ) ) ;
#33799=ORIENTED_EDGE ( 'NONE', *, *, #442, .F. ) ;
#33801=CARTESIAN_POINT ( 'NONE',  ( 7.944714827928039291, 11.25228915168265864, 1.082531754730557072 ) ) ;
#33804=CARTESIAN_POINT ( 'NONE',  ( 7.334597915313080918, 9.580116872663850813, 1.040834085586084257E-14 ) ) ;
#33806=CARTESIAN_POINT ( 'NONE',  ( -1.201851678989727383E-14, 3.743750000682817269, 1.732050807568877637 ) ) ;
#33808=CARTESIAN_POINT ( 'NONE',  ( -4.822949958159302497, 6.649860922651058992, -1.599625672291256295 ) ) ;
#33809=CARTESIAN_POINT ( 'NONE',  ( 3.999292125906905859, 5.688926785023260102, 1.443375672974062551 ) ) ;
#33818=CARTESIAN_POINT ( 'NONE',  ( 2.849184837166184536, 6.475799410002530898, 0.7998128361456362523 ) ) ;
#33825=DIRECTION ( 'NONE',  ( -0.6507913734559640506, -0.7592566023653004592, 0.000000000000000000 ) ) ;
#33833=CARTESIAN_POINT ( 'NONE',  ( 5.206864636422387171, 6.427350532134703087, -1.171562478298654231 ) ) ;
#33836=CARTESIAN_POINT ( 'NONE',  ( 10.70146331988817323, 11.37946204949139251, 0.7998128361456341429 ) ) ;
#33839=CARTESIAN_POINT ( 'NONE',  ( -1.364683531250014514, -1.011458332991911568, -0.7879004041258359514 ) ) ;
#33840=CARTESIAN_POINT ( 'NONE',  ( 6.155038550924150087, 7.243595066575396757, 1.082531754730558626 ) ) ;
#33841=CARTESIAN_POINT ( 'NONE',  ( -2.117044542028253318, 5.621635732341564662, -0.7998128361456281477 ) ) ;
#33847=CARTESIAN_POINT ( 'NONE',  ( -3.228813138348844536, 6.918699094715619502, 0.7998128361456341429 ) ) ;
#33859=CARTESIAN_POINT ( 'NONE',  ( 5.904500254309781759, 6.149185751451256898, 0.8064407133735688182 ) ) ;
#33860=CARTESIAN_POINT ( 'NONE',  ( -1.420000000000001039, 6.200000000000045475, -2.899999999999995470 ) ) ;
#33864=CARTESIAN_POINT ( 'NONE',  ( 3.822509244049070887, 6.547012320444182798, -1.199719254218452047 ) ) ;
#33869=CARTESIAN_POINT ( 'NONE',  ( -9.164948653157999559, 10.75515685251491504, -1.082531754730539753 ) ) ;
#33873=CARTESIAN_POINT ( 'NONE',  ( 8.423693512792301163, 8.722063941212843119, 0.7998128361456481317 ) ) ;
#33874=CARTESIAN_POINT ( 'NONE',  ( -5.436983294280064882, 6.301900917203534291, 1.199719254218450271 ) ) ;
#33877=CARTESIAN_POINT ( 'NONE',  ( -4.225337428953291230, 8.081310767087481750, 0.7998128361456341429 ) ) ;
#33881=CARTESIAN_POINT ( 'NONE',  ( -4.717347382551060342, 7.590990148696470818, 1.199719254218464037 ) ) ;
#33884=CARTESIAN_POINT ( 'NONE',  ( 7.865701674222579598, 12.32840238656838139, -0.7998128361456352531 ) ) ;
#33885=CARTESIAN_POINT ( 'NONE',  ( 0.5337978311145309407, 6.541559214916611076, 3.355412286555431667 ) ) ;
#33887=CARTESIAN_POINT ( 'NONE',  ( 3.999262108721039155, 7.828827674157968985, 0.07552679838754294828 ) ) ;
#33888=CARTESIAN_POINT ( 'NONE',  ( 6.670248388243460447, 6.884303995813253252, -0.7216878364870257245 ) ) ;
#33892=DIRECTION ( 'NONE',  ( -0.000000000000000000, -8.546850786086437571E-32, -1.000000000000000000 ) ) ;
#33896=CARTESIAN_POINT ( 'NONE',  ( 7.009202228140744673, 9.200488570962775725, -1.443375672974058777 ) ) ;
#33899=CARTESIAN_POINT ( 'NONE',  ( 5.974412749747233242, 4.760129193867229880, -2.438793960827100094 ) ) ;
#33900=CARTESIAN_POINT ( 'NONE',  ( -9.027031348600448979, 9.425958082989001952, 1.040834085586084257E-14 ) ) ;
#33909=CARTESIAN_POINT ( 'NONE',  ( 2.367870383881045981, 5.914265881169853856, 0.000000000000000000 ) ) ;
#33914=CARTESIAN_POINT ( 'NONE',  ( 5.508690485854129903, 5.321227076451600091, 1.040834085586084257E-14 ) ) ;
#33918=CARTESIAN_POINT ( 'NONE',  ( 1.499999999999987121, 4.077083334016147198, -0.8660254037844323793 ) ) ;
#33922=ORIENTED_EDGE ( 'NONE', *, *, #125247, .T. ) ;
#33924=B_SPLINE_CURVE_WITH_KNOTS ( 'NONE', 3,
 ( #108060, #174085, #141601, #109129 ),
 .UNSPECIFIED., .F., .F.,
 ( 4, 4 ),
 ( 0.001582017824277145253, 0.002341702326271046831 ),
 .UNSPECIFIED. ) ;
#33925=CARTESIAN_POINT ( 'NONE',  ( 1.499999999999989120, 2.025000000000019895, 1.214306433183764966E-14 ) ) ;
#33926=CARTESIAN_POINT ( 'NONE',  ( 6.317209508963599340, 9.457495962844502557, 1.199719254218462483 ) ) ;
#33927=CARTESIAN_POINT ( 'NONE',  ( 3.646780131951580461, 7.198401220678078971, -0.7216878364870267237 ) ) ;
#33930=CARTESIAN_POINT ( 'NONE',  ( 8.785320351975350661, 9.351887953500479966, -0.7216878364870197293 ) ) ;
#33937=CARTESIAN_POINT ( 'NONE',  ( -4.985647801523292344, 6.839675073242382553, -1.599625672291256295 ) ) ;
#33938=CARTESIAN_POINT ( 'NONE',  ( 1.499999999999987121, 3.327083334016150751, -0.8660254037844262731 ) ) ;
#33939=CARTESIAN_POINT ( 'NONE',  ( -1.364683531250014514, -0.4697916663252449943, 0.7879004041258379498 ) ) ;
#33943=CARTESIAN_POINT ( 'NONE',  ( 3.714044015139744914, 6.420469553383295391, 1.199719254218462483 ) ) ;
#33945=CARTESIAN_POINT ( 'NONE',  ( 0.6823417656249899377, 5.738541667008087543, -1.181850606188754593 ) ) ;
#33949=CARTESIAN_POINT ( 'NONE',  ( 3.469446951953614189E-15, 6.400000000000023448, 1.214306433183764966E-14 ) ) ;
#33953=CARTESIAN_POINT ( 'NONE',  ( -7.725448601688521322, 7.907444878258402809, 1.040834085586084257E-14 ) ) ;
#33954=CARTESIAN_POINT ( 'NONE',  ( 4.819033534653518025, 7.709623992816043270, -1.199719254218452047 ) ) ;
#33957=CARTESIAN_POINT ( 'NONE',  ( 1.364683531249988757, -0.3656249996585800299, 0.000000000000000000 ) ) ;
#33963=CARTESIAN_POINT ( 'NONE',  ( -6.878064000834399394, 6.918829510595249310, -0.7998128361456291469 ) ) ;
#33966=CARTESIAN_POINT ( 'NONE',  ( 9.890836756369282057, 11.49806328964105617, -1.199719254218440723 ) ) ;
#33968=CARTESIAN_POINT ( 'NONE',  ( 9.077347539549325717, 10.54899253668443393, -1.199719254218446718 ) ) ;
#33972=CARTESIAN_POINT ( 'NONE',  ( -3.090368948911150770, 5.692848642783215674, 1.199719254218462483 ) ) ;
#33973=CARTESIAN_POINT ( 'NONE',  ( -6.320072162264675164, 10.52516795595079557, 0.7998128361456481317 ) ) ;
#33976=CARTESIAN_POINT ( 'NONE',  ( -4.144643181316929770, 7.629267798522465505, 0.8581763667485035052 ) ) ;
#33977=CARTESIAN_POINT ( 'NONE',  ( -0.6823417656250212460, 1.051041667008083325, 1.181850606188755259 ) ) ;
#33981=CARTESIAN_POINT ( 'NONE',  ( 8.487040972474689582, 9.964264558384387627, -1.082531754730543083 ) ) ;
#33983=CARTESIAN_POINT ( 'NONE',  ( 5.168682875307768931, 7.053215992657626110, -1.599625672291256295 ) ) ;
#34001=CARTESIAN_POINT ( 'NONE',  ( 10.09812548408005384, 10.67556790771522124, -0.7998128361456281477 ) ) ;
#34005=CARTESIAN_POINT ( 'NONE',  ( -3.425406365747000859, 7.148057860013469877, 1.040834085586084257E-14 ) ) ;
#34006=CARTESIAN_POINT ( 'NONE',  ( -9.169391961543940539, 9.592045464756413509, 1.040834085586084257E-14 ) ) ;
#34011=CARTESIAN_POINT ( 'NONE',  ( 1.499999999999989120, 2.785416667349484676, 0.8660254037844524744 ) ) ;
#34012=CARTESIAN_POINT ( 'NONE',  ( 8.866142388332804103, 12.43125098877526113, -1.199719254218446718 ) ) ;
#34015=VECTOR ( 'NONE', #7111, 1000.000000000000000 ) ;
#34017=CARTESIAN_POINT ( 'NONE',  ( -7.479294296233107708, 11.87759377891399204, 0.7998128361456481317 ) ) ;
#34019=CARTESIAN_POINT ( 'NONE',  ( 0.6823417656249882723, 1.926041667008083991, -1.181850606188749264 ) ) ;
#34027=CARTESIAN_POINT ( 'NONE',  ( -10.46653140006992899, 11.31330084294416771, -0.7216878364870267237 ) ) ;
#34030=CIRCLE ( 'NONE', #124121, 0.7500000000000011102 ) ;
#34032=CARTESIAN_POINT ( 'NONE',  ( 1.364683531249986537, 1.717708333674749399, -0.7879004041258239610 ) ) ;
#34037=CARTESIAN_POINT ( 'NONE',  ( 0.6823417656249899377, 1.592708333674752730, 1.181850606188755259 ) ) ;
#34039=CARTESIAN_POINT ( 'NONE',  ( -5.551173829791513192, 8.563787670477010394, 1.199719254218452047 ) ) ;
#34040=CARTESIAN_POINT ( 'NONE',  ( 8.925345196497941558, 9.307324238869423283, 1.040834085586084257E-14 ) ) ;
#34041=CARTESIAN_POINT ( 'NONE',  ( 4.111146893441827821, 5.819424013814004759, 1.599625672291267175 ) ) ;
#34043=CARTESIAN_POINT ( 'NONE',  ( -1.499999999999997780, 4.400000000000021672, 1.214306433183764966E-14 ) ) ;
#34045=CARTESIAN_POINT ( 'NONE',  ( 0.6823417656249899377, 3.238541667008085323, -1.181850606188754593 ) ) ;
#34051=CARTESIAN_POINT ( 'NONE',  ( 6.656690234629796699, 6.868486149930637552, 1.040834085586084257E-14 ) ) ;
#34054=CARTESIAN_POINT ( 'NONE',  ( -8.528242318195895066, 9.908369778438709474, 1.199719254218462483 ) ) ;
#34055=CARTESIAN_POINT ( 'NONE',  ( -10.48008955368359629, 11.32911868882677986, 1.040834085586084257E-14 ) ) ;
#34057=CARTESIAN_POINT ( 'NONE',  ( 0.6823417656249917140, 4.842708333674755394, 1.181850606188765695 ) ) ;
#34061=CARTESIAN_POINT ( 'NONE',  ( 1.387358672525639269, 7.251968950354889643, 4.302625267139791987 ) ) ;
#34062=CARTESIAN_POINT ( 'NONE',  ( -6.792271770322117597, 9.907772251142352715, 1.082531754730549967 ) ) ;
#34064=CARTESIAN_POINT ( 'NONE',  ( -1.201851678989727383E-14, 5.837500000000023448, -1.732050807568863648 ) ) ;
#34067=CARTESIAN_POINT ( 'NONE',  ( 8.432808358020029260, 8.940623960552603222, 0.7216878364870438212 ) ) ;
#34077=CARTESIAN_POINT ( 'NONE',  ( 9.042925270190632858, 10.61279623905300085, 1.082531754730549967 ) ) ;
#34084=CARTESIAN_POINT ( 'NONE',  ( 7.935599982700328958, 8.152621489438862667, 0.7998128361456481317 ) ) ;
#34085=CARTESIAN_POINT ( 'NONE',  ( -5.392392409933270514, 7.314210449720692786, 1.599625672291269396 ) ) ;
#34090=CARTESIAN_POINT ( 'NONE',  ( 6.114364089638798738, 6.235772314107808079, 0.7216878364870317197 ) ) ;
#34091=CARTESIAN_POINT ( 'NONE',  ( -1.364683531250014514, 0.05104166700808546175, -0.7879004041258359514 ) ) ;
#34092=CARTESIAN_POINT ( 'NONE',  ( 3.470524135418292300, 5.072030796119872953, -1.443375672974057666 ) ) ;
#34093=CARTESIAN_POINT ( 'NONE',  ( -9.646789991323334590, 11.21334206375407305, 1.199719254218462483 ) ) ;
#34108=CARTESIAN_POINT ( 'NONE',  ( 5.947222937888848371, 10.09017719417900416, 1.040834085586084257E-14 ) ) ;
#34109=CARTESIAN_POINT ( 'NONE',  ( 5.296431564432884542, 9.330920591813708143, 1.040834085586084257E-14 ) ) ;
#34119=CARTESIAN_POINT ( 'NONE',  ( 10.07387183015377197, 11.71160420905630062, -1.199719254218440723 ) ) ;
#34121=CARTESIAN_POINT ( 'NONE',  ( -4.303823697334223652, 7.108545849276850959, -1.199719254218452047 ) ) ;
#34122=CARTESIAN_POINT ( 'NONE',  ( -2.930533758848195447, 6.570706485298192234, -0.7998128361456281477 ) ) ;
#34128=CARTESIAN_POINT ( 'NONE',  ( 1.451998047839293315, 7.315968950356647404, 4.301760722583980900 ) ) ;
#34133=CARTESIAN_POINT ( 'NONE',  ( -4.288456660624211381, 3.897620947016656956, 1.214306433183764966E-14 ) ) ;
#34136=CARTESIAN_POINT ( 'NONE',  ( 6.986529229743720926, 7.045372277656132276, -0.7998128361456281477 ) ) ;
#34137=CARTESIAN_POINT ( 'NONE',  ( -1.364683531250012516, 3.988541667008088432, -0.7879004041258300672 ) ) ;
#34143=CARTESIAN_POINT ( 'NONE',  ( 3.836594282542902246, 7.419851063034623273, 0.7216878364870317197 ) ) ;
#34144=CARTESIAN_POINT ( 'NONE',  ( -5.682838942422375084, 9.781729199468104596, 0.000000000000000000 ) ) ;
#34146=VERTEX_POINT ( 'NONE', #205859 ) ;
#34149=CARTESIAN_POINT ( 'NONE',  ( -7.507464373665155399, 9.781794407407920389, 1.599625672291295375 ) ) ;
#34150=CARTESIAN_POINT ( 'NONE',  ( -5.274285450916075035, 6.112086766612214284, 1.199719254218450271 ) ) ;
#34151=FACE_OUTER_BOUND ( 'NONE', #195204, .T. ) ;
#34158=CARTESIAN_POINT ( 'NONE',  ( 8.111855979677986994, 8.358253485912799263, 1.040834085586084257E-14 ) ) ;
#34164=CARTESIAN_POINT ( 'NONE',  ( -1.217323170181719538, 2.986755683774202197, 0.7750000000000152323 ) ) ;
#34169=CARTESIAN_POINT ( 'NONE',  ( -1.500000000000011324, 5.379166666666692187, -0.8660254037844313801 ) ) ;
#34170=CARTESIAN_POINT ( 'NONE',  ( 3.063252641683779753, 5.661212951017999373, 1.199719254218450271 ) ) ;
#34171=CARTESIAN_POINT ( 'NONE',  ( 4.157546660884947620, 8.002221537674429896, 1.040834085586084257E-14 ) ) ;
#34173=CARTESIAN_POINT ( 'NONE',  ( -8.351459436338048548, 8.845716885256940998, -0.7216878364870278340 ) ) ;
#34174=CARTESIAN_POINT ( 'NONE',  ( -5.914749137557818059, 6.074338953224275528, -0.6118981238392419142 ) ) ;
#34175=CARTESIAN_POINT ( 'NONE',  ( 5.287316719649520991, 8.151991358691011769, -1.082531754730549078 ) ) ;
#34176=CARTESIAN_POINT ( 'NONE',  ( -9.314088342463968218, 9.968783942403868892, 0.7216878364870438212 ) ) ;
#34180=CARTESIAN_POINT ( 'NONE',  ( 6.588372581236919601, 9.773852880496709972, -1.199719254218440723 ) ) ;
#34183=CARTESIAN_POINT ( 'NONE',  ( -2.301756715112211360, 5.497064121812672788, -0.7511966642406193717 ) ) ;
#34184=CARTESIAN_POINT ( 'NONE',  ( 1.364683531249988535, 3.155208333674756283, -0.7879004041258239610 ) ) ;
#34190=ADVANCED_FACE ( 'NONE', ( #206924 ), #61754, .T. ) ;
#34191=CARTESIAN_POINT ( 'NONE',  ( 6.760712154708803823, 11.03924794713562818, 1.040834085586084257E-14 ) ) ;
#34194=CARTESIAN_POINT ( 'NONE',  ( -8.636707547105197946, 10.03491254549959777, -1.199719254218446718 ) ) ;
#34200=CARTESIAN_POINT ( 'NONE',  ( 10.07778825365955733, 10.65184113889131012, -0.7998128361456281477 ) ) ;
#34201=CARTESIAN_POINT ( 'NONE',  ( -1.580000000000001625, -1.099999999999982991, -2.579999999999989413 ) ) ;
#34203=CARTESIAN_POINT ( 'NONE',  ( -9.040589502214116280, 9.441775928871617651, 0.7998128361456462443 ) ) ;
#34209=CARTESIAN_POINT ( 'NONE',  ( 4.739561450132447007, 6.795411536013346243, -1.240012687728889951 ) ) ;
#34210=CARTESIAN_POINT ( 'NONE',  ( -3.765413976293358278, 5.416068943807445635, 1.599625672291267398 ) ) ;
#34215=CARTESIAN_POINT ( 'NONE',  ( 6.938021921891177612, 9.117444880338284818, -1.599625672291262513 ) ) ;
#34217=CARTESIAN_POINT ( 'NONE',  ( 4.299907273828439180, 8.168308919441841454, 1.040834085586084257E-14 ) ) ;
#34218=CARTESIAN_POINT ( 'NONE',  ( -4.124570878694319376, 7.473888947179561981, -0.6522657496016289747 ) ) ;
#34219=CARTESIAN_POINT ( 'NONE',  ( 5.657830175604453338, 5.495223381160312393, 0.7998128361456341429 ) ) ;
#34221=CARTESIAN_POINT ( 'NONE',  ( -6.832946231607472498, 9.955225789308602913, 1.082531754730549967 ) ) ;
#34229=CARTESIAN_POINT ( 'NONE',  ( -4.236586233130071655, 7.334480220043515075, -0.8772045297030308664 ) ) ;
#34230=CARTESIAN_POINT ( 'NONE',  ( -1.402160292154681736E-14, -1.115624999658584082, 1.575800808251672791 ) ) ;
#34232=CARTESIAN_POINT ( 'NONE',  ( -1.419999999999997708, 6.280000000000035776, -3.469446951953614189E-15 ) ) ;
#34233=CARTESIAN_POINT ( 'NONE',  ( 6.019457014787495730, 6.125047393447951016, -0.7216878364870257245 ) ) ;
#34237=CARTESIAN_POINT ( 'NONE',  ( -10.58855478214856660, 11.45566145536924552, -0.7216878364870217277 ) ) ;
#34244=CARTESIAN_POINT ( 'NONE',  ( -10.12757755928392456, 10.91785469536048758, 0.7216878364870438212 ) ) ;
#34246=EDGE_CURVE ( 'NONE', #202349, #152273, #34030, .T. ) ;
#34250=CARTESIAN_POINT ( 'NONE',  ( -8.310784975052671442, 11.67937098999472667, -1.082531754730543083 ) ) ;
#34256=ORIENTED_EDGE ( 'NONE', *, *, #20771, .T. ) ;
#34258=CARTESIAN_POINT ( 'NONE',  ( 1.499999999999989120, 2.285416667349482012, 0.8660254037844524744 ) ) ;
#34260=CARTESIAN_POINT ( 'NONE',  ( -6.043183783389232566, 8.073467052085995022, 1.599625672291269396 ) ) ;
#34263=CARTESIAN_POINT ( 'NONE',  ( -9.671043645249580933, 10.17730576241299900, 0.7998128361456462443 ) ) ;
#34265=CARTESIAN_POINT ( 'NONE',  ( -1.499999999999990896, 4.410416667349482900, -0.8660254037844429265 ) ) ;
#34266=CARTESIAN_POINT ( 'NONE',  ( 5.666418135507635512, 8.698239360479199433, 1.199719254218462483 ) ) ;
#34273=CARTESIAN_POINT ( 'NONE',  ( 7.587759525142423911, 12.00413654597487501, 0.7998128361456462443 ) ) ;
#34278=CARTESIAN_POINT ( 'NONE',  ( -5.897433632264490910, 9.824163637709826702, 0.000000000000000000 ) ) ;
#34281=CARTESIAN_POINT ( 'NONE',  ( -1.001543065824772872E-14, 5.134375000341421469, 1.575800808251672791 ) ) ;
#34285=CARTESIAN_POINT ( 'NONE',  ( 0.6823417656249917140, 5.092708333674749177, 1.181850606188765695 ) ) ;
#34289=CARTESIAN_POINT ( 'NONE',  ( -2.277406616971334508, 5.600798786534425311, 1.040834085586084257E-14 ) ) ;
#34291=CARTESIAN_POINT ( 'NONE',  ( 9.911173986789782120, 11.52179005846497972, -1.199719254218440723 ) ) ;
#34293=DIRECTION ( 'NONE',  ( -1.000000000000000000, 5.459311322609750190E-16, -1.776356839400250465E-15 ) ) ;
#34296=CARTESIAN_POINT ( 'NONE',  ( -1.364683531250012516, 2.280208333674751842, 0.7879004041258379498 ) ) ;
#34298=CARTESIAN_POINT ( 'NONE',  ( 5.007038802148489509, 4.735966778795008381, 0.7998128361456341429 ) ) ;
#34304=CARTESIAN_POINT ( 'NONE',  ( 8.229436053370667636, 11.58446391469906267, 1.082531754730558626 ) ) ;
#34305=CARTESIAN_POINT ( 'NONE',  ( -7.266807147244793263, 8.540658428949452485, 1.082531754730549967 ) ) ;
#34307=CARTESIAN_POINT ( 'NONE',  ( 0.04711431077958990604, 7.150937050890798119, 2.000088718513667541 ) ) ;
#34309=CARTESIAN_POINT ( 'NONE',  ( -7.965578943228732278, 9.251929174310385307, -1.199719254218446718 ) ) ;
#34310=CARTESIAN_POINT ( 'NONE',  ( -5.382223794500852421, 5.381608636446842731, -0.7216878364870197293 ) ) ;
#34311=CARTESIAN_POINT ( 'NONE',  ( -1.201851678989727383E-14, 3.134375000341420137, 1.575800808251672791 ) ) ;
#34317=ADVANCED_FACE ( 'NONE', ( #706 ), #102363, .T. ) ;
#34320=ORIENTED_EDGE ( 'NONE', *, *, #49219, .F. ) ;
#34333=CARTESIAN_POINT ( 'NONE',  ( -1.364683531249997417, 3.821875000341416584, 1.214306433183764966E-14 ) ) ;
#34341=CARTESIAN_POINT ( 'NONE',  ( 8.238550898598388628, 12.76339314834017102, 0.7998128361456462443 ) ) ;
#34344=CARTESIAN_POINT ( 'NONE',  ( -0.6823417656250003738, 2.717708333674753618, -1.181850606188749264 ) ) ;
#34346=CARTESIAN_POINT ( 'NONE',  ( -6.073689629242158716, 9.069426419882418600, -1.082531754730538864 ) ) ;
#34354=CARTESIAN_POINT ( 'NONE',  ( 3.018661757337009810, 6.673522483535157868, 0.000000000000000000 ) ) ;
#34358=CARTESIAN_POINT ( 'NONE',  ( 9.752392566931574081, 10.27221283770866300, -0.7998128361456281477 ) ) ;
#34365=CARTESIAN_POINT ( 'NONE',  ( -3.164938793786285842, 5.779846795137578930, -1.199719254218452935 ) ) ;
#34366=CARTESIAN_POINT ( 'NONE',  ( 6.096362627639171805, 10.26417349888772179, -0.7998128361456291469 ) ) ;
#34368=CARTESIAN_POINT ( 'NONE',  ( 5.490689023410166847, 5.508151403507724808, -0.7216878364870207285 ) ) ;
#34372=EDGE_LOOP ( 'NONE', ( #209373, #178150, #31079 ) ) ;
#34377=CARTESIAN_POINT ( 'NONE',  ( -6.046573322014817897, 9.998159942418544333, 0.7216878364870458196 ) ) ;
#34378=CARTESIAN_POINT ( 'NONE',  ( 3.499976210622149253, 7.235056012367825140, 0.7998128361456321445 ) ) ;
#34381=CARTESIAN_POINT ( 'NONE',  ( -8.320953590485107298, 10.73086516036454618, 1.599625672291269396 ) ) ;
#34386=CARTESIAN_POINT ( 'NONE',  ( -4.959585264500673496, 4.680604318205876524, 1.214306433183764966E-14 ) ) ;
#34389=CARTESIAN_POINT ( 'NONE',  ( 9.121938423896107651, 9.536683004167278099, -0.7998128361456221525 ) ) ;
#34390=EDGE_CURVE ( 'NONE', #11745, #81936, #27223, .T. ) ;
#34391=CARTESIAN_POINT ( 'NONE',  ( 2.381428537494710618, 5.930083727052461562, 0.7998128361456462443 ) ) ;
#34397=CARTESIAN_POINT ( 'NONE',  ( 3.307826292054301121, 4.882216645528547616, -1.443375672974057666 ) ) ;
#34400=CARTESIAN_POINT ( 'NONE',  ( -5.579343907223557331, 6.467988298970945849, 1.199719254218450271 ) ) ;
#34403=CARTESIAN_POINT ( 'NONE',  ( -6.970863535720637216, 11.28442455831609337, 0.7998128361456481317 ) ) ;
#34408=CARTESIAN_POINT ( 'NONE',  ( 7.510853912290742507, 8.825379654836435606, -1.082531754730537976 ) ) ;
#34409=CARTESIAN_POINT ( 'NONE',  ( -1.201851678989727383E-14, 5.009375000341421469, -1.575800808251660134 ) ) ;
#34412=CARTESIAN_POINT ( 'NONE',  ( 4.383363735919856730, 4.008345868194933104, -0.7998128361456211532 ) ) ;
#34414=CARTESIAN_POINT ( 'NONE',  ( 3.506755287428983792, 7.242964935309132990, 1.040834085586084257E-14 ) ) ;
#34416=CARTESIAN_POINT ( 'NONE',  ( -6.418895661066105873, 9.576129806964074120, -1.199719254218440723 ) ) ;
#34424=ORIENTED_EDGE ( 'NONE', *, *, #59430, .F. ) ;
#34426=CARTESIAN_POINT ( 'NONE',  ( -1.364683531249997417, 3.321875000341423245, 1.214306433183764966E-14 ) ) ;
#34427=CARTESIAN_POINT ( 'NONE',  ( 9.589694723567584234, 10.08239868711733855, -0.7998128361456281477 ) ) ;
#34429=CARTESIAN_POINT ( 'NONE',  ( -3.958617665510266725, 7.562211676496538360, -0.7216878364870267237 ) ) ;
#34431=FACE_OUTER_BOUND ( 'NONE', #41439, .T. ) ;
#34432=CARTESIAN_POINT ( 'NONE',  ( -5.246642258364192735, 5.223430177620739023, 0.7216878364870317197 ) ) ;
#34439=CARTESIAN_POINT ( 'NONE',  ( 2.984766373302843778, 6.633977868828633717, -0.7998128361456291469 ) ) ;
#34444=CARTESIAN_POINT ( 'NONE',  ( 1.230728480726492879, 2.976239941806479550, 0.7750000000000100142 ) ) ;
#34448=EDGE_CURVE ( 'NONE', #48080, #83910, #107231, .T. ) ;
#34449=CARTESIAN_POINT ( 'NONE',  ( 4.059776932288224671, 6.823824623389866950, 1.199719254218462483 ) ) ;
#34455=CARTESIAN_POINT ( 'NONE',  ( -6.521635583373313061, 7.567328587812373719, -1.199719254218446718 ) ) ;
#34460=CARTESIAN_POINT ( 'NONE',  ( 6.419949431270806528, 7.448694743692793274, 1.199719254218462483 ) ) ;
#34463=CARTESIAN_POINT ( 'NONE',  ( -4.574986769607567894, 7.424902766929059261, 1.199719254218464037 ) ) ;
#34465=CARTESIAN_POINT ( 'NONE',  ( -1.499999999999997780, 1.650000000000019451, 0.000000000000000000 ) ) ;
#34466=CARTESIAN_POINT ( 'NONE',  ( -3.110706179331648169, 5.716575411607132118, 1.199719254218462483 ) ) ;
#34469=CARTESIAN_POINT ( 'NONE',  ( -5.708146366553361162, 6.618257834855742594, -1.199719254218446718 ) ) ;
#34471=CARTESIAN_POINT ( 'NONE',  ( 1.364683531249988535, 2.863541667008082658, 0.7879004041258500513 ) ) ;
#34473=CARTESIAN_POINT ( 'NONE',  ( -5.314433026876900001, 6.262888621853549331, 1.082531754730548412 ) ) ;
#34476=EDGE_LOOP ( 'NONE', ( #163636, #29606, #89777, #64062 ) ) ;
#34479=CARTESIAN_POINT ( 'NONE',  ( 3.994848817520957773, 7.812407387083109001, 1.040834085586084257E-14 ) ) ;
#34481=CARTESIAN_POINT ( 'NONE',  ( 0.6823417656249899377, 2.155208333674753174, 1.181850606188767472 ) ) ;
#34483=CARTESIAN_POINT ( 'NONE',  ( 4.142179624174931796, 4.791296635414242111, 1.199719254218464037 ) ) ;
#34485=CARTESIAN_POINT ( 'NONE',  ( 0.6823417656249882723, 0.4885416670080827695, -1.181850606188749264 ) ) ;
#34488=CARTESIAN_POINT ( 'NONE',  ( -2.774614992291035698, 6.388801257648172971, 1.040834085586084257E-14 ) ) ;
#34489=CARTESIAN_POINT ( 'NONE',  ( -5.843201017365469596, 9.760892253660966134, 0.7216878364870458196 ) ) ;
#34492=CARTESIAN_POINT ( 'NONE',  ( 0.6823417656249899377, 2.592708333674753618, 1.181850606188767472 ) ) ;
#34500=CARTESIAN_POINT ( 'NONE',  ( -7.009202228140755331, 8.240119356661432803, -1.082531754730543083 ) ) ;
#34507=CARTESIAN_POINT ( 'NONE',  ( -7.171900071504748730, 8.429933507252760805, -1.082531754730549078 ) ) ;
#34520=CARTESIAN_POINT ( 'NONE',  ( -4.882907879216086933, 8.848476292394087395, -0.7998128361456281477 ) ) ;
#34522=CARTESIAN_POINT ( 'NONE',  ( 0.7499999999999867883, -0.6833333333333135862, -1.299038105676652899 ) ) ;
#34523=CARTESIAN_POINT ( 'NONE',  ( 4.546061579283848353, 4.198160018786257552, -0.7998128361456211532 ) ) ;
#34527=CARTESIAN_POINT ( 'NONE',  ( 5.575427483717746213, 7.527751369135936343, 1.599625672291267398 ) ) ;
#34534=CARTESIAN_POINT ( 'NONE',  ( -4.948362879307902418, 4.875437568721725512, 1.214306433183764966E-14 ) ) ;
#34537=CARTESIAN_POINT ( 'NONE',  ( -0.4612990374432109908, 6.901512110099052855, 3.726810127985829446 ) ) ;
#34538=CARTESIAN_POINT ( 'NONE',  ( 3.176271558300056697, 6.436868453234527720, -0.7638679071477995075 ) ) ;
#34542=CARTESIAN_POINT ( 'NONE',  ( -1.364683531249997417, 2.509375000341422357, 1.214306433183764966E-14 ) ) ;
#34543=CARTESIAN_POINT ( 'NONE',  ( 9.042925270190625753, 11.57316545335434199, 1.443375672974076540 ) ) ;
#34544=CARTESIAN_POINT ( 'NONE',  ( -6.527360889975461156, 9.702672574024962415, 1.199719254218452047 ) ) ;
#34547=CARTESIAN_POINT ( 'NONE',  ( 5.472687561410540802, 9.536552588287639409, 0.7998128361456462443 ) ) ;
#34548=CARTESIAN_POINT ( 'NONE',  ( -6.744291347794091784, 9.955758108146730123, -1.199719254218440723 ) ) ;
#34551=CARTESIAN_POINT ( 'NONE',  ( 0.7499999999999867883, -0.9020833326505162120, -1.299038105676652011 ) ) ;
#34553=CARTESIAN_POINT ( 'NONE',  ( 7.280365300858406385, 11.43758391773608984, 1.040834085586084257E-14 ) ) ;
#34556=CARTESIAN_POINT ( 'NONE',  ( 0.6823417656249882723, 1.238541667008083547, -1.181850606188749264 ) ) ;
#34559=CARTESIAN_POINT ( 'NONE',  ( 6.602457619730760285, 8.725953194484466380, 1.443375672974076540 ) ) ;
#34562=CARTESIAN_POINT ( 'NONE',  ( -3.958617665510266725, 7.562211676496538360, -0.7216878364870267237 ) ) ;
#34564=CARTESIAN_POINT ( 'NONE',  ( -1.201851678989727383E-14, 4.696875000341419693, -1.575800808251660134 ) ) ;
#34568=CARTESIAN_POINT ( 'NONE',  ( -5.766295404513795297, 5.621766148221195358, 0.7998128361456341429 ) ) ;
#34575=CARTESIAN_POINT ( 'NONE',  ( 5.608269097547198712, 9.694731047113750222, -0.7998128361456281477 ) ) ;
#34579=CARTESIAN_POINT ( 'NONE',  ( 0.7499999999999902300, 2.983333333333351600, 1.299038105676669330 ) ) ;
#34584=ORIENTED_EDGE ( 'NONE', *, *, #184415, .F. ) ;
#34585=CARTESIAN_POINT ( 'NONE',  ( 5.992340707560160240, 7.053780915984068756, 1.082531754730558626 ) ) ;
#34586=CARTESIAN_POINT ( 'NONE',  ( 1.364683531249988757, 1.196875000341421469, 0.000000000000000000 ) ) ;
#34589=CARTESIAN_POINT ( 'NONE',  ( 10.55232363013785246, 11.20546574478267132, 0.000000000000000000 ) ) ;
#34591=VERTEX_POINT ( 'NONE', #8203 ) ;
#34594=( BOUNDED_CURVE ( )  B_SPLINE_CURVE ( 2, ( #113648, #198012, #98396, #82130, #61626 ),
 .UNSPECIFIED., .F., .T. ) 
 B_SPLINE_CURVE_WITH_KNOTS ( ( 3, 2, 3 ),
 ( 0.1116300932268876750, 0.1125000000000000028, 0.1135379806157290616 ),
 .UNSPECIFIED. ) 
 CURVE ( )  GEOMETRIC_REPRESENTATION_ITEM ( )  RATIONAL_B_SPLINE_CURVE ( ( 0.9557375992087471239, 0.9720291019185025583, 1.000000000000000000, 0.9666248718707487475, 0.9498782570434030070 ) ) 
 REPRESENTATION_ITEM ( '' )  );
#34597=CARTESIAN_POINT ( 'NONE',  ( 1.499999999999987121, 1.045833333333352266, -0.8660254037844253849 ) ) ;
#34598=CARTESIAN_POINT ( 'NONE',  ( 6.262976894508937242, 9.394224579314053969, -1.199719254218440723 ) ) ;
#34599=CARTESIAN_POINT ( 'NONE',  ( -8.538937818508475885, 8.856515631215026829, 1.040834085586084257E-14 ) ) ;
#34601=CARTESIAN_POINT ( 'NONE',  ( -1.364683531250014514, 0.7385416670080887647, -0.7879004041258289570 ) ) ;
#34602=CARTESIAN_POINT ( 'NONE',  ( -1.500000000000013101, 2.129166666666693519, -0.8660254037844313801 ) ) ;
#34604=CARTESIAN_POINT ( 'NONE',  ( 3.161022370280501814, 6.839609865302569425, 0.000000000000000000 ) ) ;
#34611=CARTESIAN_POINT ( 'NONE',  ( 1.499999999999987566, -1.193749999317185395, 0.000000000000000000 ) ) ;
#34612=CARTESIAN_POINT ( 'NONE',  ( -8.206763054973658100, 8.468978407091068306, 0.7998128361456602331 ) ) ;
#34613=CARTESIAN_POINT ( 'NONE',  ( -4.365362273920257330, 6.116008624372160973, 1.443375672974064550 ) ) ;
#34615=CARTESIAN_POINT ( 'NONE',  ( -1.123270288250342919, 3.096052654332833054, 0.7749999999993751887 ) ) ;
#34622=CARTESIAN_POINT ( 'NONE',  ( 7.637320603199683866, 7.804628880021436288, -0.7998128361456281477 ) ) ;
#34623=FACE_OUTER_BOUND ( 'NONE', #87542, .T. ) ;
#34626=CARTESIAN_POINT ( 'NONE',  ( 7.280365300414074703, 7.596107060012304402, -0.7216878364870257245 ) ) ;
#34630=CARTESIAN_POINT ( 'NONE',  ( -7.705111371268023923, 7.883718109434487253, 1.040834085586084257E-14 ) ) ;
#34631=CARTESIAN_POINT ( 'NONE',  ( 3.167801447087334576, 6.847518788243868393, -0.7998128361456291469 ) ) ;
#34635=CARTESIAN_POINT ( 'NONE',  ( 4.025675347721991315, 7.559696154190033823, -0.3592088497781486534 ) ) ;
#34636=CARTESIAN_POINT ( 'NONE',  ( 8.093854517678360949, 12.38665467069271386, 1.040834085586084257E-14 ) ) ;
#34644=CARTESIAN_POINT ( 'NONE',  ( -1.515977770626737664, 8.685538819012460721, -2.532029653471351338 ) ) ;
#34645=CARTESIAN_POINT ( 'NONE',  ( -4.785665035943912571, 4.685623418130398399, 1.214306433183764966E-14 ) ) ;
#34646=CARTESIAN_POINT ( 'NONE',  ( 9.585251415181632595, 10.28514086057449184, 0.000000000000000000 ) ) ;
#34649=CARTESIAN_POINT ( 'NONE',  ( -4.882907879216086933, 8.848476292394087395, -0.7998128361456281477 ) ) ;
#34655=CARTESIAN_POINT ( 'NONE',  ( -6.659026002606323047, 10.92061410301605662, 0.000000000000000000 ) ) ;
#34658=CARTESIAN_POINT ( 'NONE',  ( -0.2656570211550942084, 7.171539594011602681, 2.094714161149640042 ) ) ;
#34668=CARTESIAN_POINT ( 'NONE',  ( -4.394814349124112951, 8.279033840620114049, -0.7998128361456281477 ) ) ;
#34671=CARTESIAN_POINT ( 'NONE',  ( 4.934804725694211136, 6.780358151441803649, -1.443375672974051449 ) ) ;
#34675=CARTESIAN_POINT ( 'NONE',  ( -3.490334480514268645, 6.159475096320226939, -1.199719254218452935 ) ) ;
#34683=CARTESIAN_POINT ( 'NONE',  ( -9.027031348600448979, 9.425958082989001952, 1.040834085586084257E-14 ) ) ;
#34684=CARTESIAN_POINT ( 'NONE',  ( 6.449928391799196525, 8.548002428564306143, -1.599625672291262513 ) ) ;
#34687=CARTESIAN_POINT ( 'NONE',  ( -8.459397779922852578, 11.95671561229694824, 1.199719254218453823 ) ) ;
#34691=CARTESIAN_POINT ( 'NONE',  ( -1.402160292154681736E-14, 0.009375000341421267647, -1.575800808251665908 ) ) ;
#34694=CARTESIAN_POINT ( 'NONE',  ( 9.110716038703335684, 9.731516254683127087, -0.7216878364870197293 ) ) ;
#34713=CARTESIAN_POINT ( 'NONE',  ( -2.300079615812729905, 5.835176651756807331, -0.7998128361456281477 ) ) ;
#34719=CARTESIAN_POINT ( 'NONE',  ( 1.499999999999989120, 0.8062500006828163812, 0.000000000000000000 ) ) ;
#34726=CARTESIAN_POINT ( 'NONE',  ( 9.673906298550626559, 11.24497775551929557, 1.199719254218452047 ) ) ;
#34731=CARTESIAN_POINT ( 'NONE',  ( 3.310162060030825248, 7.013606170011280838, -0.7998128361456291469 ) ) ;
#34732=CARTESIAN_POINT ( 'NONE',  ( -7.551528373131759508, 7.912463978182924684, 1.040834085586084257E-14 ) ) ;
#34734=CARTESIAN_POINT ( 'NONE',  ( 4.363950690066983107, 4.004001632660354915, -0.1812806842866887536 ) ) ;
#34736=CARTESIAN_POINT ( 'NONE',  ( -7.212047647465563038, 10.50147379109678880, -1.199719254218446718 ) ) ;
#34737=CARTESIAN_POINT ( 'NONE',  ( -3.511198595814942980, 5.119484333249288532, 1.443375672974064550 ) ) ;
#34740=CARTESIAN_POINT ( 'NONE',  ( 0.7499999999999885647, 0.5145833340161540814, 1.299038105676657340 ) ) ;
#34747=CARTESIAN_POINT ( 'NONE',  ( -3.741687207247254676, 7.309126141856352454, 1.040834085586084257E-14 ) ) ;
#34754=CARTESIAN_POINT ( 'NONE',  ( -2.928197990427299668, 6.360055388899728435, 1.040834085586084257E-14 ) ) ;
#34755=CARTESIAN_POINT ( 'NONE',  ( 7.964525173024008531, 11.37936423758166526, 1.199719254218460707 ) ) ;
#34766=CARTESIAN_POINT ( 'NONE',  ( -7.486073373039941359, 11.88550270185529278, -0.7998128361456291469 ) ) ;
#34769=ORIENTED_EDGE ( 'NONE', *, *, #165987, .F. ) ;
#34771=CARTESIAN_POINT ( 'NONE',  ( 4.330940004561544043, 7.140181541042074365, -1.199719254218452047 ) ) ;
#34779=ORIENTED_EDGE ( 'NONE', *, *, #87971, .F. ) ;
#34787=CARTESIAN_POINT ( 'NONE',  ( 7.446452682403650769, 9.710614100936176385, -1.599625672291262513 ) ) ;
#34789=CARTESIAN_POINT ( 'NONE',  ( -4.623494077460110319, 5.352830164246910272, 1.199719254218462483 ) ) ;
#34796=CARTESIAN_POINT ( 'NONE',  ( -0.6823417656249969321, 5.467708333674756283, -1.181850606188749264 ) ) ;
#34799=CARTESIAN_POINT ( 'NONE',  ( 4.517891501851804215, 6.293959390292322986, -1.599625672291255185 ) ) ;
#34801=CARTESIAN_POINT ( 'NONE',  ( -3.113568832632681360, 6.784247404713427798, -0.7998128361456281477 ) ) ;
#34807=CARTESIAN_POINT ( 'NONE',  ( 4.677199807034550183, 8.400557508274889784, 1.040834085586084257E-14 ) ) ;
#34809=ORIENTED_EDGE ( 'NONE', *, *, #75894, .T. ) ;
#34810=CARTESIAN_POINT ( 'NONE',  ( 7.199016378732056687, 10.38230762762066384, -1.082531754730537976 ) ) ;
#34811=CARTESIAN_POINT ( 'NONE',  ( 1.364683531249988535, 4.217708333674752730, -0.7879004041258239610 ) ) ;
#34813=CARTESIAN_POINT ( 'NONE',  ( 4.650083499362875017, 5.487814173087225633, 1.082531754730560403 ) ) ;
#34819=CARTESIAN_POINT ( 'NONE',  ( -6.138273485042783584, 5.995793210058552702, 0.01269068828805425264 ) ) ;
#34822=CARTESIAN_POINT ( 'NONE',  ( -1.364683531249997417, 4.821875000341417916, 1.214306433183764966E-14 ) ) ;
#34838=CARTESIAN_POINT ( 'NONE',  ( 1.364683531249990311, 5.196875000341417916, 1.214306433183764966E-14 ) ) ;
#34840=CARTESIAN_POINT ( 'NONE',  ( 7.623762449586013901, 7.788811034138823253, 1.040834085586084257E-14 ) ) ;
#34841=CARTESIAN_POINT ( 'NONE',  ( -8.317037166979361018, 11.79062823052953668, 1.199719254218453823 ) ) ;
#34847=CARTESIAN_POINT ( 'NONE',  ( 0.7499999999999902300, 4.816666666666684193, -1.299038105676658228 ) ) ;
#34853=CARTESIAN_POINT ( 'NONE',  ( 9.110716038703335684, 9.731516254683127087, -0.7216878364870197293 ) ) ;
#34859=CARTESIAN_POINT ( 'NONE',  ( -1.201851678989727383E-14, 2.993750000682821266, 1.732050807568877637 ) ) ;
#34861=CARTESIAN_POINT ( 'NONE',  ( -5.928993247877788697, 5.811580298812519807, 0.7998128361456341429 ) ) ;
#34862=CARTESIAN_POINT ( 'NONE',  ( 4.406036734316882253, 6.163462161501577441, -1.443375672974051449 ) ) ;
#34863=CARTESIAN_POINT ( 'NONE',  ( -9.829298179783291900, 11.53023130024440768, 1.082531754730558626 ) ) ;
#34870=CARTESIAN_POINT ( 'NONE',  ( 5.345992642490140057, 5.131412925860272090, 1.040834085586084257E-14 ) ) ;
#34874=CARTESIAN_POINT ( 'NONE',  ( 5.515469562660962666, 5.329135999392899947, 0.7998128361456341429 ) ) ;
#34876=ORIENTED_EDGE ( 'NONE', *, *, #68027, .T. ) ;
#34886=CARTESIAN_POINT ( 'NONE',  ( 4.968100067739229075, 6.607231601306259527, -1.242533411653036879 ) ) ;
#34890=CARTESIAN_POINT ( 'NONE',  ( 9.028840231696797503, 12.62106513936658203, -1.199719254218446718 ) ) ;
#34895=CARTESIAN_POINT ( 'NONE',  ( 0.6823417656249864960, -1.073958332991911568, -1.181850606188749264 ) ) ;
#34896=CARTESIAN_POINT ( 'NONE',  ( 5.910991785878156435, 7.919243054989755670, -1.443375672974057666 ) ) ;
#34897=CARTESIAN_POINT ( 'NONE',  ( -8.175203439360366531, 12.48156174598837787, 1.040834085586084257E-14 ) ) ;
#34903=CARTESIAN_POINT ( 'NONE',  ( -5.576481253922474401, 5.400316305864651056, -0.7998128361456221525 ) ) ;
#34905=CARTESIAN_POINT ( 'NONE',  ( -3.001048869802169783, 2.786623193720129343, 2.499999999999998668 ) ) ;
#34913=CARTESIAN_POINT ( 'NONE',  ( 9.596473800374404561, 10.09030761005864285, 0.000000000000000000 ) ) ;
#34914=CARTESIAN_POINT ( 'NONE',  ( 6.095406204355903412, 6.027892130464396203, -0.2603320317973931153 ) ) ;
#34915=CARTESIAN_POINT ( 'NONE',  ( -1.257518954445011827, 3.114770990628817682, -0.7749999999999918066 ) ) ;
#34916=EDGE_LOOP ( 'NONE', ( #190349, #208983 ) ) ;
#34924=CARTESIAN_POINT ( 'NONE',  ( -9.327646496521989405, 10.94497100310623594, -1.082531754730539753 ) ) ;
#34928=CARTESIAN_POINT ( 'NONE',  ( 6.103141704446003679, 10.27208242182903142, 0.7998128361456462443 ) ) ;
#34931=CARTESIAN_POINT ( 'NONE',  ( -4.199533704925234368, 7.510932310329544670, -0.9222493318717175370 ) ) ;
#34932=AXIS2_PLACEMENT_3D ( 'NONE', #149730, #132453, #116218 ) ;
#34933=CARTESIAN_POINT ( 'NONE',  ( 4.704842999142070603, 5.447737239542574272, -1.199719254218452047 ) ) ;
#34935=CARTESIAN_POINT ( 'NONE',  ( -6.749261541504576911, 6.768559974710451677, 1.040834085586084257E-14 ) ) ;
#34936=CARTESIAN_POINT ( 'NONE',  ( 3.708318708537623021, 4.285125567170706695, -1.199719254218446718 ) ) ;
#34939=CARTESIAN_POINT ( 'NONE',  ( 9.901532256681887745, 10.44620914241737530, 0.000000000000000000 ) ) ;
#34944=CARTESIAN_POINT ( 'NONE',  ( 4.026147685736890303, 7.792003671190927960, 0.3652107146706294882 ) ) ;
#34945=CARTESIAN_POINT ( 'NONE',  ( 5.748293942514166588, 7.729428904398431222, -1.443375672974057666 ) ) ;
#34948=CARTESIAN_POINT ( 'NONE',  ( -1.352264364406415176, 3.300000000000026024, -0.2254051929223724882 ) ) ;
#34952=CARTESIAN_POINT ( 'NONE',  ( 7.741342523278692767, 11.01502146292508044, 1.082531754730558626 ) ) ;
#34955=CARTESIAN_POINT ( 'NONE',  ( -10.13488352141530768, 11.78278451552804817, 1.199719254218462483 ) ) ;
#34956=CARTESIAN_POINT ( 'NONE',  ( -6.828502922777144768, 11.11833717654868892, 0.7998128361456481317 ) ) ;
#34966=CARTESIAN_POINT ( 'NONE',  ( 2.866659414285625651, 5.431854185720147221, -1.199719254218446718 ) ) ;
#34970=CARTESIAN_POINT ( 'NONE',  ( 5.834086172582112262, 5.700855377634248100, 1.040834085586084257E-14 ) ) ;
#34974=CARTESIAN_POINT ( 'NONE',  ( -1.500000000000013101, 4.160416667349482900, -0.8660254037844313801 ) ) ;
#34981=CARTESIAN_POINT ( 'NONE',  ( 1.499999999999989120, 1.275000000000019229, 0.000000000000000000 ) ) ;
#34982=CARTESIAN_POINT ( 'NONE',  ( 5.452350330990040739, 9.512825819463730070, 0.7998128361456462443 ) ) ;
#34983=CARTESIAN_POINT ( 'NONE',  ( 3.158686601859607368, 6.628958768904106513, -0.7216878364870267237 ) ) ;
#34987=CARTESIAN_POINT ( 'NONE',  ( 7.592202833972727660, 11.80139437303613015, -0.7216878364870267237 ) ) ;
#34993=CARTESIAN_POINT ( 'NONE',  ( -4.741601036477307574, 6.554953847355395880, 1.599625672291267398 ) ) ;
#34994=CARTESIAN_POINT ( 'NONE',  ( 1.499999999999990896, 3.806250000682819046, 1.214306433183764966E-14 ) ) ;
#34995=CARTESIAN_POINT ( 'NONE',  ( -1.364683531250000748, -0.7406249996585803075, 0.000000000000000000 ) ) ;
#34999=CARTESIAN_POINT ( 'NONE',  ( 4.009460741339333723, 5.700790169694431420, -1.599625672291256295 ) ) ;
#35001=CARTESIAN_POINT ( 'NONE',  ( 1.364683531249988535, 3.676041667008087099, 0.7879004041258500513 ) ) ;
#35006=CARTESIAN_POINT ( 'NONE',  ( -5.721177634842498527, 5.777054783512106440, 0.000000000000000000 ) ) ;
#35008=CARTESIAN_POINT ( 'NONE',  ( -6.991200766141138168, 11.30815132714001159, 0.7998128361456481317 ) ) ;
#35009=CARTESIAN_POINT ( 'NONE',  ( 5.198661835836162481, 8.152523677529138979, 1.199719254218462483 ) ) ;
#35011=CARTESIAN_POINT ( 'NONE',  ( -1.364683531250014514, -0.9697916663252473812, 0.7879004041258379498 ) ) ;
#35018=CARTESIAN_POINT ( 'NONE',  ( -6.826694039680798021, 7.923230120171105284, -1.199719254218446718 ) ) ;
#35023=CARTESIAN_POINT ( 'NONE',  ( 8.565000355531088516, 11.01558638625153286, -1.599625672291257406 ) ) ;
#35025=CARTESIAN_POINT ( 'NONE',  ( -4.925689880466507908, 4.641059703499347044, -0.7998128361456221525 ) ) ;
#35026=CARTESIAN_POINT ( 'NONE',  ( -6.832419346282942563, 10.05857410638369487, 1.199719254218453823 ) ) ;
#35028=CARTESIAN_POINT ( 'NONE',  ( -5.229776604766065873, 6.614552831964506829, 1.409540066939333425 ) ) ;
#35029=CARTESIAN_POINT ( 'NONE',  ( 0.6823417656249882723, -0.3239583329919110133, -1.181850606188749264 ) ) ;
#35033=CARTESIAN_POINT ( 'NONE',  ( 7.863365906246055914, 10.19701286208565705, -1.443375672974057666 ) ) ;
#35036=CARTESIAN_POINT ( 'NONE',  ( 5.464099601507359516, 6.333536608968757697, 1.199719254218462483 ) ) ;
#35055=CARTESIAN_POINT ( 'NONE',  ( 3.606105671554957759, 4.269840040644637291, -1.082531754730543083 ) ) ;
#35059=CARTESIAN_POINT ( 'NONE',  ( -4.517891501851816649, 6.293959390292322986, -1.599625672291256295 ) ) ;
#35060=CARTESIAN_POINT ( 'NONE',  ( -6.835281999583978418, 11.12624609948998966, -0.7998128361456291469 ) ) ;
#35065=CARTESIAN_POINT ( 'NONE',  ( 0.7499999999999885647, 3.097916667349487341, -1.299038105676658228 ) ) ;
#35066=CARTESIAN_POINT ( 'NONE',  ( 8.378048858240820351, 11.86180853700128601, -1.199719254218446718 ) ) ;
#35071=CARTESIAN_POINT ( 'NONE',  ( -8.371269781434001800, 11.85389961405997816, -1.199719254218446718 ) ) ;
#35073=CARTESIAN_POINT ( 'NONE',  ( -1.364683531250012516, 2.530208333674753174, 0.7879004041258379498 ) ) ;
#35080=CARTESIAN_POINT ( 'NONE',  ( -3.195971524519394702, 4.751719416737803847, -1.599625672291262513 ) ) ;
#35084=CARTESIAN_POINT ( 'NONE',  ( 1.364683531249986537, 1.467708333674748289, -0.7879004041258239610 ) ) ;
#35085=AXIS2_PLACEMENT_3D ( 'NONE', #112466, #86034, #193643 ) ;
#35091=CARTESIAN_POINT ( 'NONE',  ( 0.6823417656249899377, 2.092708333674753174, 1.181850606188767472 ) ) ;
#35093=CARTESIAN_POINT ( 'NONE',  ( -5.900823170445743671, 7.907379670318584353, 1.599625672291269396 ) ) ;
#35094=CARTESIAN_POINT ( 'NONE',  ( 8.776205506747620788, 9.133327934160710981, -0.7998128361456221525 ) ) ;
#35096=CARTESIAN_POINT ( 'NONE',  ( 5.412729640353754590, 7.337937218544611895, 1.599625672291267398 ) ) ;
#35098=CARTESIAN_POINT ( 'NONE',  ( -0.7499999999999972244, 3.358333333333359150, -1.299038105676652011 ) ) ;
#35100=CARTESIAN_POINT ( 'NONE',  ( -0.6823417656250212460, 1.863541667008083991, 1.181850606188755259 ) ) ;
#35103=CARTESIAN_POINT ( 'NONE',  ( -1.015412733742047324, 2.800000000000017586, 0.9313266920541376503 ) ) ;
#35107=CARTESIAN_POINT ( 'NONE',  ( 5.666945020832170776, 7.634521829102760115, 1.443375672974062551 ) ) ;
#35110=CARTESIAN_POINT ( 'NONE',  ( -8.154339323615371171, 11.60081407993821045, 1.199719254218453823 ) ) ;
#35111=CARTESIAN_POINT ( 'NONE',  ( -9.490344339885973923, 12.09515436799890331, -1.443375672974059665 ) ) ;
#35117=CARTESIAN_POINT ( 'NONE',  ( -8.175203438916030407, 8.640084888264587093, 0.7216878364870578100 ) ) ;
#35119=CARTESIAN_POINT ( 'NONE',  ( -0.7499999999999972244, 5.858333333333353821, -1.299038105676652011 ) ) ;
#35122=CARTESIAN_POINT ( 'NONE',  ( 7.104109303880752790, 11.23195192126214970, -0.7216878364870267237 ) ) ;
#35124=CARTESIAN_POINT ( 'NONE',  ( -4.218512253981381299, 3.978430757497701364, -0.5307291018261834914 ) ) ;
#35136=CARTESIAN_POINT ( 'NONE',  ( 6.588372581236919601, 9.773852880496709972, -1.199719254218440723 ) ) ;
#35137=CARTESIAN_POINT ( 'NONE',  ( -4.381256195510448315, 8.263215994737505454, 1.040834085586084257E-14 ) ) ;
#35139=CARTESIAN_POINT ( 'NONE',  ( -1.420000000000021911, 6.280000000000042881, 2.580000000000011173 ) ) ;
#35141=CARTESIAN_POINT ( 'NONE',  ( 6.941411460072420603, 7.200660912947041581, 1.040834085586084257E-14 ) ) ;
#35142=CARTESIAN_POINT ( 'NONE',  ( -0.6823417656250246877, -0.3864583329919110688, 1.181850606188755259 ) ) ;
#35143=CARTESIAN_POINT ( 'NONE',  ( 3.714570900464285064, 4.396382807705524698, 1.082531754730560403 ) ) ;
#35144=CARTESIAN_POINT ( 'NONE',  ( -8.611400122974211868, 13.19838391011195888, 1.040834085586084257E-14 ) ) ;
#35157=ORIENTED_EDGE ( 'NONE', *, *, #154124, .F. ) ;
#35160=LINE ( 'NONE', #39444, #186151 ) ;
#35161=CARTESIAN_POINT ( 'NONE',  ( 6.795661308947685164, 8.951357498570873261, -1.599625672291262513 ) ) ;
#35162=CARTESIAN_POINT ( 'NONE',  ( 6.958359152311676787, 9.141171649162195934, -1.599625672291262513 ) ) ;
#35171=CARTESIAN_POINT ( 'NONE',  ( -0.4421172008954280530, 6.952755576498319989, 3.903674101997708146 ) ) ;
#35173=CARTESIAN_POINT ( 'NONE',  ( -5.575427483717760424, 7.527751369135936343, 1.599625672291269396 ) ) ;
#35175=CARTESIAN_POINT ( 'NONE',  ( -3.632695093457760649, 6.325562478087638496, -1.199719254218452047 ) ) ;
#35180=CARTESIAN_POINT ( 'NONE',  ( 1.387358672530662584, 7.251968950356647348, 4.302625267142138554 ) ) ;
#35183=PRODUCT_DEFINITION_CONTEXT ( 'detailed design', #51947, 'design' ) ;
#35185=CARTESIAN_POINT ( 'NONE',  ( -2.764973262183167968, 5.313220341600567664, 1.199719254218462483 ) ) ;
#35188=CARTESIAN_POINT ( 'NONE',  ( 7.149227073107712549, 7.235186428247455837, -0.7998128361456281477 ) ) ;
#35189=CARTESIAN_POINT ( 'NONE',  ( 0.6823417656249917140, 4.592708333674755394, 1.181850606188765695 ) ) ;
#35197=CARTESIAN_POINT ( 'NONE',  ( 4.622967192135525316, 8.337286124226029216, -0.7216878364870207285 ) ) ;
#35198=CARTESIAN_POINT ( 'NONE',  ( -6.008234629150358330, 10.16135750065076060, 0.000000000000000000 ) ) ;
#35199=ORIENTED_EDGE ( 'NONE', *, *, #137619, .F. ) ;
#35202=CARTESIAN_POINT ( 'NONE',  ( -7.182068686937172153, 9.402166106225269715, 1.599625672291283607 ) ) ;
#35203=CARTESIAN_POINT ( 'NONE',  ( -5.738125327081750271, 7.717565519727259904, 1.599625672291269396 ) ) ;
#35212=CARTESIAN_POINT ( 'NONE',  ( 6.262976894508937242, 9.394224579314053969, -1.199719254218440723 ) ) ;
#35226=CARTESIAN_POINT ( 'NONE',  ( -1.364683531250000748, -1.178124999658580752, 0.000000000000000000 ) ) ;
#35227=CARTESIAN_POINT ( 'NONE',  ( 3.388648328411762556, 6.040841252200647382, 1.199719254218462483 ) ) ;
#35228=CARTESIAN_POINT ( 'NONE',  ( 5.331380718671758778, 7.243030143248949670, -1.599625672291256295 ) ) ;
#35231=CARTESIAN_POINT ( 'NONE',  ( -8.527715433315703919, 9.051348881730875817, 1.040834085586084257E-14 ) ) ;
#35233=CARTESIAN_POINT ( 'NONE',  ( 4.528060117284222308, 8.226561203566173930, 0.7216878364870438212 ) ) ;
#35234=CARTESIAN_POINT ( 'NONE',  ( -6.656690234185426824, 10.70996300661758660, 0.7216878364870458196 ) ) ;
#35238=CARTESIAN_POINT ( 'NONE',  ( 6.252281394196331554, 10.44607872653774372, 1.040834085586084257E-14 ) ) ;
#35243=CARTESIAN_POINT ( 'NONE',  ( -0.6823417656250212460, 3.051041667008084879, 1.181850606188767472 ) ) ;
#35249=CARTESIAN_POINT ( 'NONE',  ( 8.503988664269582998, 10.94440607977979063, 1.599625672291281386 ) ) ;
#35252=CARTESIAN_POINT ( 'NONE',  ( -8.962103233833181193, 10.41454084668224489, -1.199719254218446718 ) ) ;
#35258=CARTESIAN_POINT ( 'NONE',  ( 8.543609354905870035, 13.11929468069890525, 0.7998128361456462443 ) ) ;
#35261=CARTESIAN_POINT ( 'NONE',  ( -7.004758919754800139, 11.32396917302262018, 0.000000000000000000 ) ) ;
#35266=CARTESIAN_POINT ( 'NONE',  ( 5.790052644182137165, 6.039355072771209088, 0.5314338945540015846 ) ) ;
#35267=CARTESIAN_POINT ( 'NONE',  ( -3.521367211247373508, 5.131347717920458962, -1.599625672291256295 ) ) ;
#35272=CARTESIAN_POINT ( 'NONE',  ( 5.452350330990040739, 9.512825819463730070, 0.7998128361456462443 ) ) ;
#35274=CARTESIAN_POINT ( 'NONE',  ( 6.775324078527185989, 8.927630729746953264, -1.599625672291262513 ) ) ;
#35275=CARTESIAN_POINT ( 'NONE',  ( -4.339127873110165901, 7.217636166161084610, -1.009937615098016606 ) ) ;
#35277=CARTESIAN_POINT ( 'NONE',  ( 5.497994985541524215, 6.373081223675282736, -1.199719254218445830 ) ) ;
#35279=CARTESIAN_POINT ( 'NONE',  ( -6.399085315970132193, 10.40942393536641397, -0.7216878364870278340 ) ) ;
#35288=CARTESIAN_POINT ( 'NONE',  ( -4.054949276293840832, 7.568305524423037056, 0.4105793130844727079 ) ) ;
#35289=CARTESIAN_POINT ( 'NONE',  ( 4.232984923718338344, 7.533997312158466464, -0.9744250676351111640 ) ) ;
#35291=CARTESIAN_POINT ( 'NONE',  ( 4.001749955438753226, 7.811071542261023737, 0.1299566359906061952 ) ) ;
#35292=CARTESIAN_POINT ( 'NONE',  ( 5.260200412422194383, 7.159986452624450770, -1.443375672974051449 ) ) ;
#35296=CARTESIAN_POINT ( 'NONE',  ( -10.61567108937589765, 11.48729714713446803, 0.7216878364870438212 ) ) ;
#35302=CARTESIAN_POINT ( 'NONE',  ( -8.622622508166983835, 13.00355065959610279, 1.040834085586084257E-14 ) ) ;
#35310=CARTESIAN_POINT ( 'NONE',  ( -9.449669878600616357, 12.04770082983265844, -1.443375672974058777 ) ) ;
#35317=CARTESIAN_POINT ( 'NONE',  ( 1.499999999999989120, 3.535416667349488229, 0.8660254037844524744 ) ) ;
#35318=CARTESIAN_POINT ( 'NONE',  ( -6.175902666224832416, 7.163973517805802160, -1.199719254218446718 ) ) ;
#35322=CARTESIAN_POINT ( 'NONE',  ( -8.507905087775398556, 9.884643009614800135, 1.199719254218462483 ) ) ;
#35326=CARTESIAN_POINT ( 'NONE',  ( 7.450369105909416589, 8.650851030771185890, -1.199719254218441611 ) ) ;
#35332=CARTESIAN_POINT ( 'NONE',  ( 7.411503528164766763, 11.79850454950093841, 1.040834085586084257E-14 ) ) ;
#35338=CARTESIAN_POINT ( 'NONE',  ( -8.053180056837398126, 8.497724275839514618, 0.7216878364870578100 ) ) ;
#35342=CARTESIAN_POINT ( 'NONE',  ( -0.6823417656249969321, 5.780208333674756283, -1.181850606188749264 ) ) ;
#35347=CARTESIAN_POINT ( 'NONE',  ( -0.6823417656250212460, 5.551041667008087543, 1.181850606188767472 ) ) ;
#35351=CARTESIAN_POINT ( 'NONE',  ( -10.65400978224035811, 11.32409958890225710, 1.040834085586084257E-14 ) ) ;
#35353=CARTESIAN_POINT ( 'NONE',  ( 8.536830278099042602, 13.11138575775759563, -0.7998128361456352531 ) ) ;
#35354=CARTESIAN_POINT ( 'NONE',  ( 1.483456582845025240, 7.293967155395495006, 4.258619948150350609 ) ) ;
#35355=CARTESIAN_POINT ( 'NONE',  ( -10.65400978224035811, 11.32409958890225710, 1.040834085586084257E-14 ) ) ;
#35357=DIRECTION ( 'NONE',  ( 0.6507913734559627184, 0.7592566023653016805, 0.000000000000000000 ) ) ;
#35359=CARTESIAN_POINT ( 'NONE',  ( -0.6823417656250212460, 1.801041667008083991, 1.181850606188755259 ) ) ;
#35360=CARTESIAN_POINT ( 'NONE',  ( -2.765500147507697459, 5.209872024525476597, 1.082531754730560403 ) ) ;
#35361=CARTESIAN_POINT ( 'NONE',  ( 3.334415713957098681, 5.977569868670206787, -1.199719254218446718 ) ) ;
#35370=CARTESIAN_POINT ( 'NONE',  ( -7.714226216495749355, 8.102278128774251797, 1.040834085586084257E-14 ) ) ;
#35376=CARTESIAN_POINT ( 'NONE',  ( -7.645908563102897126, 11.00764485934031889, 1.199719254218453823 ) ) ;
#35377=CARTESIAN_POINT ( 'NONE',  ( -5.111060722227552588, 6.025620933095978238, 1.082531754730546636 ) ) ;
#35378=CARTESIAN_POINT ( 'NONE',  ( 1.364683531249990311, 2.696875000341415696, 1.214306433183764966E-14 ) ) ;
#35396=CARTESIAN_POINT ( 'NONE',  ( -3.621833129746846680, 4.096114899008192367, 2.500000000000011102 ) ) ;
#35397=CARTESIAN_POINT ( 'NONE',  ( -1.364683531249997417, 4.071875000341417028, 1.214306433183764966E-14 ) ) ;
#35401=CARTESIAN_POINT ( 'NONE',  ( -4.322341018716196359, 3.567520274870279007, -2.444429072473030651 ) ) ;
#35405=CARTESIAN_POINT ( 'NONE',  ( 9.759171643738394408, 10.28012176064996197, 0.000000000000000000 ) ) ;
#35408=CARTESIAN_POINT ( 'NONE',  ( -1.201851678989727383E-14, 1.821875000341421691, 1.575800808251672791 ) ) ;
#35411=CARTESIAN_POINT ( 'NONE',  ( -7.863365906246068349, 9.236643647784308797, -1.082531754730543971 ) ) ;
#35417=EDGE_LOOP ( 'NONE', ( #16033, #128581, #169667 ) ) ;
#35419=CARTESIAN_POINT ( 'NONE',  ( 4.379447312414087357, 5.068108938359919158, -1.199719254218452047 ) ) ;
#35431=CARTESIAN_POINT ( 'NONE',  ( -4.135400547368138113, 4.783387712472935149, 1.199719254218462483 ) ) ;
#35435=CARTESIAN_POINT ( 'NONE',  ( 4.487385655998873624, 7.218738451098584363, 1.082531754730558626 ) ) ;
#35442=CARTESIAN_POINT ( 'NONE',  ( -7.537970219518091319, 7.896646132300314314, -0.7216878364870278340 ) ) ;
#35444=CARTESIAN_POINT ( 'NONE',  ( 5.495132332240461714, 5.305409230568988832, 0.7998128361456341429 ) ) ;
#35447=CARTESIAN_POINT ( 'NONE',  ( -7.160677686311960777, 11.50587440067263678, -0.7998128361456291469 ) ) ;
#35449=CARTESIAN_POINT ( 'NONE',  ( 2.295757763869426871, 5.519548059767960702, 0.4031905389056070765 ) ) ;
#35453=CARTESIAN_POINT ( 'NONE',  ( -2.286521462199063492, 5.819358805874190743, 1.040834085586084257E-14 ) ) ;
#35456=CARTESIAN_POINT ( 'NONE',  ( 7.397945374551106568, 11.78268670361832093, -0.7998128361456291469 ) ) ;
#35458=CARTESIAN_POINT ( 'NONE',  ( 2.530568227245037605, 6.104080031761181857, 0.000000000000000000 ) ) ;
#35464=CARTESIAN_POINT ( 'NONE',  ( 3.389175213736297820, 4.977123720824209840, 1.443375672974062551 ) ) ;
#35467=CARTESIAN_POINT ( 'NONE',  ( -3.879604511804807032, 7.677955697080923514, 0.7998128361456341429 ) ) ;
#35470=CARTESIAN_POINT ( 'NONE',  ( -8.971744963941075568, 11.49012176272984931, 1.599625672291269396 ) ) ;
#35475=CARTESIAN_POINT ( 'NONE',  ( 7.131225611108088280, 9.342849184424693476, 1.443375672974076540 ) ) ;
#35478=AXIS2_PLACEMENT_3D ( 'NONE', #97284, #14918, #147100 ) ;
#35479=CARTESIAN_POINT ( 'NONE',  ( 3.161022370280501814, 6.839609865302569425, 0.000000000000000000 ) ) ;
#35481=CARTESIAN_POINT ( 'NONE',  ( 5.030238685870051185, 5.827365540725222282, -1.199719254218452047 ) ) ;
#35483=CARTESIAN_POINT ( 'NONE',  ( -7.335124800193271177, 8.516399340768996851, -1.199719254218452935 ) ) ;
#35492=CARTESIAN_POINT ( 'NONE',  ( -1.201851678989727383E-14, 2.884375000341418804, 1.575800808251672791 ) ) ;
#35493=CARTESIAN_POINT ( 'NONE',  ( 8.380911511541880188, 12.92948053010758258, 0.7998128361456462443 ) ) ;
#35495=CARTESIAN_POINT ( 'NONE',  ( -5.477130870240893401, 6.452702772444876445, 1.082531754730548412 ) ) ;
#35496=CARTESIAN_POINT ( 'NONE',  ( 3.389175213736297820, 4.977123720824209840, 1.443375672974062551 ) ) ;
#35497=CARTESIAN_POINT ( 'NONE',  ( -5.707619481228832115, 6.721606151930833661, -1.082531754730543971 ) ) ;
#35504=CARTESIAN_POINT ( 'NONE',  ( 5.508690485854129903, 5.321227076451600091, 1.040834085586084257E-14 ) ) ;
#35513=CARTESIAN_POINT ( 'NONE',  ( 5.524057522564145728, 8.532151978711786100, 1.199719254218462483 ) ) ;
#35518=CARTESIAN_POINT ( 'NONE',  ( -6.925517538482230506, 6.974191971184389160, 0.7998128361456341429 ) ) ;
#35522=CARTESIAN_POINT ( 'NONE',  ( 7.447506452608354088, 7.583179037664891098, 0.7998128361456341429 ) ) ;
#35524=ADVANCED_FACE ( 'NONE', ( #195003 ), #212299, .F. ) ;
#35526=CARTESIAN_POINT ( 'NONE',  ( -4.401593425930945713, 8.286942763561420122, 1.040834085586084257E-14 ) ) ;
#35527=CARTESIAN_POINT ( 'NONE',  ( 6.033015167956792268, 8.061603667414825480, -1.443375672974057666 ) ) ;
#35528=CARTESIAN_POINT ( 'NONE',  ( 4.469394083494863779, 7.278994484577430590, 1.251062204184281379 ) ) ;
#35530=CARTESIAN_POINT ( 'NONE',  ( -4.946027110887008860, 4.664786472323266153, -0.7998128361456221525 ) ) ;
#35533=CARTESIAN_POINT ( 'NONE',  ( -4.843287188579803448, 6.673587691474970107, -1.599625672291256295 ) ) ;
#35536=CARTESIAN_POINT ( 'NONE',  ( 1.364683531249986537, 2.155208333674751398, -0.7879004041258239610 ) ) ;
#35538=CARTESIAN_POINT ( 'NONE',  ( -4.880572111239580124, 7.677455982212699759, 1.082531754730560403 ) ) ;
#35544=CARTESIAN_POINT ( 'NONE',  ( 4.469384193999260901, 8.366031992974468423, -0.7998128361456231517 ) ) ;
#35546=CARTESIAN_POINT ( 'NONE',  ( -1.201851678989727383E-14, 3.134375000341420137, 1.575800808251672791 ) ) ;
#35549=CARTESIAN_POINT ( 'NONE',  ( 1.364683531249986981, -1.053124999658580752, 0.000000000000000000 ) ) ;
#35552=CARTESIAN_POINT ( 'NONE',  ( -4.620631424159025613, 4.285158171140619032, -0.7998128361456221525 ) ) ;
#35553=CARTESIAN_POINT ( 'NONE',  ( -7.388830529323428209, 8.683019041374528513, 1.082531754730549967 ) ) ;
#35555=CARTESIAN_POINT ( 'NONE',  ( 1.364683531249990311, 3.134375000341423245, 1.214306433183764966E-14 ) ) ;
#35562=CARTESIAN_POINT ( 'NONE',  ( -7.659993601596720936, 8.999375959026737704, -1.082531754730543083 ) ) ;
#35567=CARTESIAN_POINT ( 'NONE',  ( -6.683806541412776525, 7.860491055478785682, -1.082531754730543083 ) ) ;
#35578=ORIENTED_EDGE ( 'NONE', *, *, #31325, .F. ) ;
#35582=CARTESIAN_POINT ( 'NONE',  ( -5.045605722580076780, 9.038290442985410067, -0.7998128361456231517 ) ) ;
#35584=CARTESIAN_POINT ( 'NONE',  ( -1.500000000000001332, -1.099999999999976108, 0.000000000000000000 ) ) ;
#35585=CARTESIAN_POINT ( 'NONE',  ( 5.196852952739813070, 4.957416621151553571, -0.7998128361456221525 ) ) ;
#35589=CARTESIAN_POINT ( 'NONE',  ( 5.147291874682557555, 9.156924287104992288, 0.7998128361456462443 ) ) ;
#35595=CARTESIAN_POINT ( 'NONE',  ( -3.795919822146277767, 7.372397525905215687, -0.7216878364870267237 ) ) ;
#35600=CARTESIAN_POINT ( 'NONE',  ( 0.1144128442461203460, 7.018241394329717942, 3.990988525772905859 ) ) ;
#35601=CARTESIAN_POINT ( 'NONE',  ( 3.132295304332796348, 6.444579696763526933, -0.6078999513244928155 ) ) ;
#35604=CARTESIAN_POINT ( 'NONE',  ( 1.364683531249988535, 1.863541667008086211, 0.7879004041258500513 ) ) ;
#35606=CARTESIAN_POINT ( 'NONE',  ( -8.148614017013223076, 9.465470093725620870, -1.199719254218446718 ) ) ;
#35608=CARTESIAN_POINT ( 'NONE',  ( 5.784525094524856748, 9.900363043587685041, 1.040834085586084257E-14 ) ) ;
#35609=CARTESIAN_POINT ( 'NONE',  ( -8.064402442030170093, 8.302891025323665630, 0.7998128361456602331 ) ) ;
#35612=CARTESIAN_POINT ( 'NONE',  ( 0.6823417656249899377, 5.676041667008087543, -1.181850606188754593 ) ) ;
#35614=CARTESIAN_POINT ( 'NONE',  ( 8.785320351975350661, 9.351887953500479966, -0.7216878364870197293 ) ) ;
#35618=CARTESIAN_POINT ( 'NONE',  ( -1.364683531250014514, 0.3010416670080866552, -0.7879004041258359514 ) ) ;
#35620=CARTESIAN_POINT ( 'NONE',  ( 7.009202228140744673, 9.200488570962775725, -1.443375672974058777 ) ) ;
#35623=CARTESIAN_POINT ( 'NONE',  ( -5.450014563013544588, 5.460697866378308341, 0.7216878364870317197 ) ) ;
#35625=CARTESIAN_POINT ( 'NONE',  ( -1.364683531249997417, 3.009375000341422801, 1.214306433183764966E-14 ) ) ;
#35629=CARTESIAN_POINT ( 'NONE',  ( -5.693534442735004752, 8.729875052244421951, 1.199719254218452047 ) ) ;
#35637=CARTESIAN_POINT ( 'NONE',  ( 6.272618624616828953, 10.46980549536166016, 1.040834085586084257E-14 ) ) ;
#35641=CARTESIAN_POINT ( 'NONE',  ( 1.499999999999989120, 2.504166666666687302, 0.8660254037844524744 ) ) ;
#35647=CARTESIAN_POINT ( 'NONE',  ( 6.073689629242148058, 8.109057205581079231, -1.443375672974057666 ) ) ;
#35648=CARTESIAN_POINT ( 'NONE',  ( -0.6823417656250003738, 0.7802083336747520637, -1.181850606188749264 ) ) ;
#35657=CARTESIAN_POINT ( 'NONE',  ( -1.500000000000013101, 0.6708333333333583726, 0.8660254037844403729 ) ) ;
#35658=CARTESIAN_POINT ( 'NONE',  ( 7.751511138711133064, 10.06651563329490529, -1.599625672291262513 ) ) ;
#35659=CARTESIAN_POINT ( 'NONE',  ( -8.479735010343349089, 11.98044238112085758, 1.199719254218453823 ) ) ;
#35661=CARTESIAN_POINT ( 'NONE',  ( -1.201851678989727383E-14, 0.8218750003414171390, 1.575800808251672791 ) ) ;
#35663=CARTESIAN_POINT ( 'NONE',  ( -1.500000000000013101, 2.420833333333359150, 0.8660254037844403729 ) ) ;
#35665=CARTESIAN_POINT ( 'NONE',  ( 4.039439701867726384, 6.800097854565950506, 1.199719254218462483 ) ) ;
#35674=CARTESIAN_POINT ( 'NONE',  ( 1.499999999999987566, -0.6937499993171849511, 0.000000000000000000 ) ) ;
#35675=CARTESIAN_POINT ( 'NONE',  ( -8.182509401047415309, 9.505014708432145909, 1.199719254218462483 ) ) ;
#35676=CARTESIAN_POINT ( 'NONE',  ( -4.772106882330234612, 6.590544000850479200, -1.443375672974053447 ) ) ;
#35684=CARTESIAN_POINT ( 'NONE',  ( 7.558834334818744338, 8.777393797832065303, 1.199719254218462483 ) ) ;
#35685=CIRCLE ( 'NONE', #184419, 0.07999999999999998779 ) ;
#35689=CARTESIAN_POINT ( 'NONE',  ( 7.307481607641395094, 8.588111966078864512, -1.082531754730537976 ) ) ;
#35690=DIRECTION ( 'NONE',  ( -5.578564026256490882E-16, -1.000000000000000000, -9.066213480720158442E-32 ) ) ;
#35693=CARTESIAN_POINT ( 'NONE',  ( -6.672584156219988571, 10.93643194889866521, -0.7998128361456291469 ) ) ;
#35694=CARTESIAN_POINT ( 'NONE',  ( 4.059776932288224671, 6.823824623389866950, 1.199719254218462483 ) ) ;
#35699=CARTESIAN_POINT ( 'NONE',  ( 10.23604278863759909, 11.04439746293979496, 0.000000000000000000 ) ) ;
#35705=CARTESIAN_POINT ( 'NONE',  ( 2.274369412726469530, 5.658954245771043112, 0.5045856980266817393 ) ) ;
#35706=CARTESIAN_POINT ( 'NONE',  ( -1.548913609767783806, 8.694120146927671655, -2.506286796689249030 ) ) ;
#35707=CARTESIAN_POINT ( 'NONE',  ( -3.443407828190963915, 6.961133532957338943, 0.7216878364870317197 ) ) ;
#35708=CARTESIAN_POINT ( 'NONE',  ( 8.080296364064698977, 12.37083682481011060, -0.7216878364870328300 ) ) ;
#35711=CARTESIAN_POINT ( 'NONE',  ( -4.880045225915050189, 7.780804299287790826, 1.199719254218464037 ) ) ;
#35718=CARTESIAN_POINT ( 'NONE',  ( -8.681298431451969222, 9.022603012982438386, 1.040834085586084257E-14 ) ) ;
#35721=CARTESIAN_POINT ( 'NONE',  ( 5.508226607891452353, 6.381517327172165466, -1.198580242432255583 ) ) ;
#35733=CARTESIAN_POINT ( 'NONE',  ( -4.880045225915050189, 7.780804299287790826, 1.199719254218464037 ) ) ;
#35736=CARTESIAN_POINT ( 'NONE',  ( 4.853455804012216213, 6.685451076146141425, 1.443375672974062551 ) ) ;
#35741=CARTESIAN_POINT ( 'NONE',  ( -4.894657149733403045, 5.669187081899118574, -1.199719254218446718 ) ) ;
#35751=CARTESIAN_POINT ( 'NONE',  ( -8.748035429315585532, 11.22912730566677553, -1.599625672291263179 ) ) ;
#35752=CARTESIAN_POINT ( 'NONE',  ( 4.611744806942754238, 8.532119374741881757, -0.7998128361456231517 ) ) ;
#35755=CARTESIAN_POINT ( 'NONE',  ( -8.435144125996554720, 12.99275191363802229, 0.7998128361456341429 ) ) ;
#35759=CARTESIAN_POINT ( 'NONE',  ( 1.364683531249988757, -0.3031249996585799744, 0.000000000000000000 ) ) ;
#35763=CARTESIAN_POINT ( 'NONE',  ( 9.083599731475992201, 9.699880562917908122, 0.7216878364870438212 ) ) ;
#35771=CARTESIAN_POINT ( 'NONE',  ( -0.4536928783070027782, 6.573802805905836877, -3.398403741207694395 ) ) ;
#35789=CARTESIAN_POINT ( 'NONE',  ( -1.402160292154681736E-14, 0.1187500006828157706, -1.732050807568870754 ) ) ;
#35795=CARTESIAN_POINT ( 'NONE',  ( -1.244123718695710368, 3.223244533904601195, 0.7750000000000100142 ) ) ;
#35797=CARTESIAN_POINT ( 'NONE',  ( 8.041957671200231417, 12.53403438304231976, 1.040834085586084257E-14 ) ) ;
#35802=CARTESIAN_POINT ( 'NONE',  ( 3.011882680530176604, 6.665613560593854459, 0.7998128361456341429 ) ) ;
#35803=CARTESIAN_POINT ( 'NONE',  ( -1.201851678989727383E-14, 2.384375000341416584, 1.575800808251672791 ) ) ;
#35808=CARTESIAN_POINT ( 'NONE',  ( -7.832860060393135093, 10.16142270859057462, 1.599625672291295375 ) ) ;
#35809=CARTESIAN_POINT ( 'NONE',  ( -5.070386261386537363, 5.017798181146802428, 1.214306433183764966E-14 ) ) ;
#35812=ORIENTED_EDGE ( 'NONE', *, *, #50840, .F. ) ;
#35813=CARTESIAN_POINT ( 'NONE',  ( -0.7500000000000249800, -0.5270833326505158789, 1.299038105676659116 ) ) ;
#35821=CARTESIAN_POINT ( 'NONE',  ( -3.267151830768946663, 6.755501535964989479, -0.7216878364870257245 ) ) ;
#35823=CARTESIAN_POINT ( 'NONE',  ( 4.128490713069958851, 7.423566268403333446, -0.7082486411538677640 ) ) ;
#35827=CARTESIAN_POINT ( 'NONE',  ( -2.602802303699316866, 5.980427087717073320, 1.040834085586084257E-14 ) ) ;
#35828=CARTESIAN_POINT ( 'NONE',  ( 7.099665995050449041, 11.43469409420089455, 0.7998128361456462443 ) ) ;
#35835=ORIENTED_EDGE ( 'NONE', *, *, #109210, .F. ) ;
#35837=CARTESIAN_POINT ( 'NONE',  ( -3.440018289565379028, 5.036440642624797626, 1.599625672291267398 ) ) ;
#35838=CARTESIAN_POINT ( 'NONE',  ( -7.323375529675950624, 11.69568855126397011, -0.7998128361456291469 ) ) ;
#35842=CARTESIAN_POINT ( 'NONE',  ( 6.193377243344257543, 6.120028293523423812, -0.7998128361456281477 ) ) ;
#35845=EDGE_LOOP ( 'NONE', ( #51045, #178776, #21247, #35835 ) ) ;
#35847=CARTESIAN_POINT ( 'NONE',  ( -6.471393748265563239, 5.229711127717889596, 2.499999999999998668 ) ) ;
#35848=CARTESIAN_POINT ( 'NONE',  ( 3.297657676621871925, 4.870353260857385180, 1.599625672291267398 ) ) ;
#35859=CARTESIAN_POINT ( 'NONE',  ( 8.718056468787178659, 10.12981962079525289, 1.199719254218462483 ) ) ;
#35861=CARTESIAN_POINT ( 'NONE',  ( -3.764360206088648297, 7.543504007078730922, -0.7998128361456281477 ) ) ;
#35862=ORIENTED_EDGE ( 'NONE', *, *, #16332, .T. ) ;
#35871=CARTESIAN_POINT ( 'NONE',  ( 1.364683531249988535, 5.405208333674750953, -0.7879004041258300672 ) ) ;
#35874=CARTESIAN_POINT ( 'NONE',  ( -5.272649268605510642, 6.486664981949695985, 1.286175789206098319 ) ) ;
#35875=CARTESIAN_POINT ( 'NONE',  ( 3.520313441042647540, 7.258782781191745137, 0.7998128361456321445 ) ) ;
#35876=CARTESIAN_POINT ( 'NONE',  ( -4.141125853970233806, 6.918731698685530063, -1.199719254218452047 ) ) ;
#35882=CARTESIAN_POINT ( 'NONE',  ( 4.189106276942576201, 7.831115056500907556, 1.040834085586084257E-14 ) ) ;
#35885=CARTESIAN_POINT ( 'NONE',  ( 7.334597914868727919, 9.580116872145431728, -1.443375672974058777 ) ) ;
#35886=CARTESIAN_POINT ( 'NONE',  ( -1.364683531250010295, 4.092708333674751842, 0.7879004041258379498 ) ) ;
#35888=CARTESIAN_POINT ( 'NONE',  ( 4.826339496340538382, 4.733076955259818419, 1.040834085586084257E-14 ) ) ;
#35891=CARTESIAN_POINT ( 'NONE',  ( 5.545987530334119953, 6.194280231554463612, -0.9208864965579254269 ) ) ;
#35894=CARTESIAN_POINT ( 'NONE',  ( -4.695247098932518348, 7.056227087241170537, 1.405392365797274445 ) ) ;
#35897=CARTESIAN_POINT ( 'NONE',  ( 1.364683531249988535, 4.967708333674756283, -0.7879004041258300672 ) ) ;
#35903=CARTESIAN_POINT ( 'NONE',  ( -9.154780037725563702, 11.70366268214508487, 1.599625672291281386 ) ) ;
#35913=CARTESIAN_POINT ( 'NONE',  ( 3.389175213736297820, 4.977123720824209840, 1.443375672974062551 ) ) ;
#35914=CARTESIAN_POINT ( 'NONE',  ( 1.364683531249988535, 4.426041667008082214, 0.7879004041258500513 ) ) ;
#35916=CARTESIAN_POINT ( 'NONE',  ( 6.642605195691581699, 9.837124264027149678, 1.199719254218462483 ) ) ;
#35917=CARTESIAN_POINT ( 'NONE',  ( -9.073431116043565225, 11.60875560684942265, -1.599625672291263179 ) ) ;
#35923=CARTESIAN_POINT ( 'NONE',  ( 0.7499999999999920064, 4.233333333333352932, 1.299038105676669330 ) ) ;
#35927=CARTESIAN_POINT ( 'NONE',  ( 1.441115678601017747, 8.287243072884294293, 3.161846531485674738 ) ) ;
#35929=CARTESIAN_POINT ( 'NONE',  ( 8.920901888112002354, 9.510066412326583674, 0.7216878364870438212 ) ) ;
#35934=CARTESIAN_POINT ( 'NONE',  ( 0.7499999999999885647, 3.097916667349487341, -1.299038105676658228 ) ) ;
#35936=CARTESIAN_POINT ( 'NONE',  ( -3.893162665418476109, 7.693773542963529444, 1.040834085586084257E-14 ) ) ;
#35937=CARTESIAN_POINT ( 'NONE',  ( 2.697709378994964879, 6.091152008895348580, 0.7216878364870338292 ) ) ;
#35938=CARTESIAN_POINT ( 'NONE',  ( -9.368320956918621434, 11.95279375453699622, 1.443375672974076540 ) ) ;
#35941=CIRCLE ( 'NONE', #42934, 6.959052028703005099 ) ;
#35947=CARTESIAN_POINT ( 'NONE',  ( 7.969495366734495434, 8.192166104145387706, 1.040834085586084257E-14 ) ) ;
#35948=CARTESIAN_POINT ( 'NONE',  ( 2.984766373302843778, 6.633977868828633717, -0.7998128361456291469 ) ) ;
#35952=CARTESIAN_POINT ( 'NONE',  ( 4.059776932288224671, 6.823824623389866950, 1.199719254218462483 ) ) ;
#35954=ORIENTED_EDGE ( 'NONE', *, *, #41280, .T. ) ;
#35965=CARTESIAN_POINT ( 'NONE',  ( 5.737025562671778545, 6.072208551910874164, -0.6475843906825241580 ) ) ;
#35967=CARTESIAN_POINT ( 'NONE',  ( 8.543609354905870035, 13.11929468069890525, 0.7998128361456462443 ) ) ;
#35971=CARTESIAN_POINT ( 'NONE',  ( 1.284279953904121641, 3.253360285806104812, 0.7750000000000135669 ) ) ;
#35973=CARTESIAN_POINT ( 'NONE',  ( 6.073689629242148058, 8.109057205581079231, -1.443375672974057666 ) ) ;
#35974=CARTESIAN_POINT ( 'NONE',  ( -4.437596350374534815, 4.071617251725375475, -0.7998128361456221525 ) ) ;
#35979=CARTESIAN_POINT ( 'NONE',  ( -4.218558352146454915, 8.073401844146177453, 1.040834085586084257E-14 ) ) ;
#35989=ADVANCED_FACE ( 'NONE', ( #167831 ), #17289, .F. ) ;
#35990=CARTESIAN_POINT ( 'NONE',  ( 7.801827329660018684, 11.18955008699033726, 1.199719254218460707 ) ) ;
#35991=CARTESIAN_POINT ( 'NONE',  ( 6.080382892099663650, 6.037283676876850969, 0.3399492115118609714 ) ) ;
#35993=DIRECTION ( 'NONE',  ( 0.000000000000000000, 8.546850786086437571E-32, 1.000000000000000000 ) ) ;
#35996=CARTESIAN_POINT ( 'NONE',  ( -9.842856333841300653, 10.58567993234409421, 0.7216878364870438212 ) ) ;
#36000=CARTESIAN_POINT ( 'NONE',  ( 7.263417608619159083, 9.497073181520933716, -1.599625672291262513 ) ) ;
#36003=CARTESIAN_POINT ( 'NONE',  ( 4.216749469050096621, 4.878294787768598262, -1.199719254218452047 ) ) ;
#36005=CARTESIAN_POINT ( 'NONE',  ( -5.052384799386910430, 9.046199365926717917, 1.214306433183764966E-14 ) ) ;
#36006=CARTESIAN_POINT ( 'NONE',  ( 2.496672843210871129, 6.064535417054653266, -0.7998128361456291469 ) ) ;
#36011=CARTESIAN_POINT ( 'NONE',  ( 8.041957671200231417, 12.53403438304231976, 1.040834085586084257E-14 ) ) ;
#36012=CARTESIAN_POINT ( 'NONE',  ( 1.499999999999989120, 3.525000000000021227, 1.214306433183764966E-14 ) ) ;
#36015=CARTESIAN_POINT ( 'NONE',  ( 4.016789712308713511, 7.804715019974644008, -0.2988979438510626085 ) ) ;
#36017=CARTESIAN_POINT ( 'NONE',  ( 6.656690234629796699, 6.868486149930637552, 1.040834085586084257E-14 ) ) ;
#36025=CARTESIAN_POINT ( 'NONE',  ( 8.392133896734662812, 10.81390885098904420, 1.443375672974076540 ) ) ;
#36028=CARTESIAN_POINT ( 'NONE',  ( -6.503107236049161521, 10.73870887536603291, 0.7998128361456481317 ) ) ;
#36037=CARTESIAN_POINT ( 'NONE',  ( 8.516493047678546091, 13.08765898893368629, -0.7998128361456352531 ) ) ;
#36041=CARTESIAN_POINT ( 'NONE',  ( 5.996784015946103885, 5.890669528225568996, 1.040834085586084257E-14 ) ) ;
#36044=CARTESIAN_POINT ( 'NONE',  ( 1.499999999999989120, 4.327083334016148086, -0.8660254037844323793 ) ) ;
#36050=CARTESIAN_POINT ( 'NONE',  ( -1.500000000000013101, 1.879166666666692187, -0.8660254037844313801 ) ) ;
#36051=CARTESIAN_POINT ( 'NONE',  ( 7.311924916471702396, 7.425000578838787391, -0.7998128361456281477 ) ) ;
#36052=CARTESIAN_POINT ( 'NONE',  ( 3.172244755473273781, 6.644776614786712443, 0.000000000000000000 ) ) ;
#36056=CARTESIAN_POINT ( 'NONE',  ( 7.619319141200057821, 10.87266085050000974, 1.082531754730557072 ) ) ;
#36063=CARTESIAN_POINT ( 'NONE',  ( -6.254388934605767503, 6.191208599995166040, 0.7998128361456341429 ) ) ;
#36064=CARTESIAN_POINT ( 'NONE',  ( 1.499999999999990896, 4.056250000682819490, 1.214306433183764966E-14 ) ) ;
#36065=CARTESIAN_POINT ( 'NONE',  ( 0.6823417656249917140, 5.155208333674749177, 1.181850606188765695 ) ) ;
#36069=CARTESIAN_POINT ( 'NONE',  ( 9.124274191872634887, 11.66807252865000244, -1.443375672974058777 ) ) ;
#36071=CARTESIAN_POINT ( 'NONE',  ( -1.364683531250010295, 4.342708333674753618, 0.7879004041258379498 ) ) ;
#36078=CARTESIAN_POINT ( 'NONE',  ( -7.178152263431422320, 10.46192917639026554, 1.199719254218453823 ) ) ;
#36079=CARTESIAN_POINT ( 'NONE',  ( 7.142447996300871793, 7.227277505306155092, 0.7998128361456341429 ) ) ;
#36081=CARTESIAN_POINT ( 'NONE',  ( 1.364683531249988757, -0.1156249996585798079, 0.000000000000000000 ) ) ;
#36086=CARTESIAN_POINT ( 'NONE',  ( -4.869349725602420520, 8.832658446511480577, 1.040834085586084257E-14 ) ) ;
#36089=CARTESIAN_POINT ( 'NONE',  ( 9.083072846151447166, 12.68433652289702884, 1.199719254218450271 ) ) ;
#36091=CARTESIAN_POINT ( 'NONE',  ( 9.378489572351044856, 11.96465713920816043, -1.599625672291262513 ) ) ;
#36093=EDGE_LOOP ( 'NONE', ( #167937, #17062, #7606 ) ) ;
#36094=CARTESIAN_POINT ( 'NONE',  ( -3.440018289565379028, 5.036440642624797626, 1.599625672291267398 ) ) ;
#36095=CARTESIAN_POINT ( 'NONE',  ( -6.333630315878337136, 10.54098580183340772, 0.000000000000000000 ) ) ;
#36097=CARTESIAN_POINT ( 'NONE',  ( -4.061425534073997312, 7.733864674645915649, 0.6335290845049870168 ) ) ;
#36098=CARTESIAN_POINT ( 'NONE',  ( -1.364683531250000748, -1.240624999658580752, 0.000000000000000000 ) ) ;
#36102=CARTESIAN_POINT ( 'NONE',  ( 7.782016984564049444, 11.06247500109133064, 1.082531754730557072 ) ) ;
#36105=CARTESIAN_POINT ( 'NONE',  ( 7.156006149914539982, 7.243095351188763686, 1.040834085586084257E-14 ) ) ;
#36121=EDGE_LOOP ( 'NONE', ( #144154, #198195, #38278, #71698 ) ) ;
#36129=CARTESIAN_POINT ( 'NONE',  ( -7.914208982075130905, 10.25632978388623684, -1.599625672291263179 ) ) ;
#36131=CYLINDRICAL_SURFACE ( 'NONE', #75128, 1.250000000000000000 ) ;
#36135=CARTESIAN_POINT ( 'NONE',  ( -1.201851678989727383E-14, 1.243750000682821044, 1.732050807568877637 ) ) ;
#36136=CARTESIAN_POINT ( 'NONE',  ( 8.218213668177886788, 12.73966637951625813, 0.7998128361456462443 ) ) ;
#36140=CARTESIAN_POINT ( 'NONE',  ( -8.618179199781044630, 13.20629283305325963, 0.7998128361456341429 ) ) ;
#36141=DIRECTION ( 'NONE',  ( -1.000000000000000000, 7.109522442527899011E-16, 0.000000000000000000 ) ) ;
#36142=CARTESIAN_POINT ( 'NONE',  ( -1.364683531250000748, 2.009375000341421913, 1.214306433183764966E-14 ) ) ;
#36150=CARTESIAN_POINT ( 'NONE',  ( -4.600294193738529103, 4.261431402316699035, -0.7998128361456221525 ) ) ;
#36155=CARTESIAN_POINT ( 'NONE',  ( 1.364683531249986537, 0.7177083336747527298, -0.7879004041258239610 ) ) ;
#36160=CARTESIAN_POINT ( 'NONE',  ( -0.6823417656250003738, 1.967708333674753174, -1.181850606188749264 ) ) ;
#36162=CARTESIAN_POINT ( 'NONE',  ( -5.982172092127739482, 8.002286745614243912, -1.599625672291263179 ) ) ;
#36163=CARTESIAN_POINT ( 'NONE',  ( 6.968000882419564945, 10.21675256520979858, 1.199719254218460707 ) ) ;
#36164=CARTESIAN_POINT ( 'NONE',  ( 4.273844736805817668, 6.009238164405336313, 1.599625672291267175 ) ) ;
#36165=CARTESIAN_POINT ( 'NONE',  ( 5.789495288235341874, 6.713164910151406595, 1.199719254218462483 ) ) ;
#36168=CARTESIAN_POINT ( 'NONE',  ( -0.7500000000000215383, 3.941666666666690411, 1.299038105676671107 ) ) ;
#36171=CARTESIAN_POINT ( 'NONE',  ( 0.6823417656249882723, 0.7385416670080829915, -1.181850606188749264 ) ) ;
#36174=CARTESIAN_POINT ( 'NONE',  ( -1.123270288249902160, 2.800000000000024691, 0.7750000000000117906 ) ) ;
#36178=CARTESIAN_POINT ( 'NONE',  ( 5.666945020832177882, 6.674152614801420746, 1.082531754730558626 ) ) ;
#36181=CARTESIAN_POINT ( 'NONE',  ( -8.829384350997580455, 11.32403438096243775, 1.599625672291269396 ) ) ;
#36182=CARTESIAN_POINT ( 'NONE',  ( -5.037017762676898158, 5.835274463666530131, -1.199719254218446718 ) ) ;
#36186=CARTESIAN_POINT ( 'NONE',  ( -8.500599125644013654, 9.019713189447241319, 0.7216878364870438212 ) ) ;
#36188=CARTESIAN_POINT ( 'NONE',  ( 1.499999999999989120, 5.295833333333356485, -0.8660254037844323793 ) ) ;
#36191=CARTESIAN_POINT ( 'NONE',  ( 8.948018195339340508, 9.541702104091804415, -0.7216878364870197293 ) ) ;
#36199=CARTESIAN_POINT ( 'NONE',  ( 10.50720586046655391, 11.36075438007358507, 0.7216878364870438212 ) ) ;
#36204=CARTESIAN_POINT ( 'NONE',  ( 5.615048174354031474, 9.702639970055050966, 0.7998128361456462443 ) ) ;
#36205=CARTESIAN_POINT ( 'NONE',  ( -5.928993247877788697, 5.811580298812519807, 0.7998128361456341429 ) ) ;
#36209=CARTESIAN_POINT ( 'NONE',  ( 5.124618875841165710, 8.922546421882614709, 1.040834085586084257E-14 ) ) ;
#36210=CARTESIAN_POINT ( 'NONE',  ( -1.402160292154681736E-14, -0.8656249996585829720, 1.575800808251672791 ) ) ;
#36211=CARTESIAN_POINT ( 'NONE',  ( 3.633221978782282147, 5.261844946711204507, -1.443375672974057666 ) ) ;
#36213=CARTESIAN_POINT ( 'NONE',  ( -4.471491734408701291, 4.111161866431900513, 1.214306433183764966E-14 ) ) ;
#36228=CARTESIAN_POINT ( 'NONE',  ( 7.467843683028853263, 7.606905806488803101, 0.7998128361456341429 ) ) ;
#36241=CARTESIAN_POINT ( 'NONE',  ( -5.949330478298285207, 5.835307067636438028, 0.7998128361456341429 ) ) ;
#36243=CARTESIAN_POINT ( 'NONE',  ( -3.602716132929368875, 5.226254793216122074, 1.599625672291267398 ) ) ;
#36253=CARTESIAN_POINT ( 'NONE',  ( -2.428882075142555497, 5.985446187641602300, 1.040834085586084257E-14 ) ) ;
#36257=CARTESIAN_POINT ( 'NONE',  ( 5.276094334012385367, 9.307193822989793475, 1.040834085586084257E-14 ) ) ;
#36258=CARTESIAN_POINT ( 'NONE',  ( -1.364683531250012516, 4.738541667008091984, -0.7879004041258300672 ) ) ;
#36260=B_SPLINE_CURVE_WITH_KNOTS ( 'NONE', 3,
 ( #25845, #9601, #188349, #6387, #39988, #156943, #190475, #106098, #172120, #63434 ),
 .UNSPECIFIED., .F., .F.,
 ( 4, 2, 2, 2, 4 ),
 ( 0.000000000000000000, 0.0003993275742951113514, 0.0007986551485902227028, 0.001197982722885334054, 0.001597310297180445406 ),
 .UNSPECIFIED. ) ;
#36264=EDGE_CURVE ( 'NONE', #11923, #121448, #160579, .T. ) ;
#36266=CARTESIAN_POINT ( 'NONE',  ( 4.148431815657221300, 7.783661518334664464, 1.040834085586084257E-14 ) ) ;
#36267=CARTESIAN_POINT ( 'NONE',  ( -7.881367368245678406, 8.089350105908421185, 0.7998128361456602331 ) ) ;
#36269=AXIS2_PLACEMENT_3D ( 'NONE', #2485, #208170, #191914 ) ;
#36271=CARTESIAN_POINT ( 'NONE',  ( -8.667740277838301921, 9.006785167099828016, -0.7998128361456291469 ) ) ;
#36272=CARTESIAN_POINT ( 'NONE',  ( -5.436983294280064882, 6.301900917203534291, 1.199719254218450271 ) ) ;
#36276=DIRECTION ( 'NONE',  ( 5.578564026256490882E-16, 1.000000000000000000, 9.066213480720158442E-32 ) ) ;
#36279=CARTESIAN_POINT ( 'NONE',  ( 6.154511665599609493, 9.267681812253174556, 1.199719254218462483 ) ) ;
#36289=VECTOR ( 'NONE', #203220, 1000.000000000000114 ) ;
#36295=CARTESIAN_POINT ( 'NONE',  ( 1.364683531249986981, -1.053124999658580752, 0.000000000000000000 ) ) ;
#36296=CARTESIAN_POINT ( 'NONE',  ( 4.708759422647839976, 4.387974169377582001, -0.7998128361456211532 ) ) ;
#36297=CARTESIAN_POINT ( 'NONE',  ( 6.518772930072240790, 6.499656594706071822, -0.7998128361456281477 ) ) ;
#36299=CARTESIAN_POINT ( 'NONE',  ( -8.202319746587722449, 8.671720580548228696, 1.040834085586084257E-14 ) ) ;
#36301=CARTESIAN_POINT ( 'NONE',  ( 4.365362273920230685, 8.036747052974847705, 0.7216878364870298324 ) ) ;
#36302=CARTESIAN_POINT ( 'NONE',  ( -7.158341917891067219, 11.29522330427417565, 0.000000000000000000 ) ) ;
#36305=CARTESIAN_POINT ( 'NONE',  ( 7.293396569147545527, 10.59638086639245280, 1.199719254218460707 ) ) ;
#36310=CARTESIAN_POINT ( 'NONE',  ( -0.6823417656250212460, 4.301041667008085767, 1.181850606188767472 ) ) ;
#36317=CARTESIAN_POINT ( 'NONE',  ( 7.560643217915098191, 11.97250085420964716, -0.7998128361456291469 ) ) ;
#36320=CARTESIAN_POINT ( 'NONE',  ( -8.585337585951595685, 11.03931315507545108, -1.599625672291263179 ) ) ;
#36326=CARTESIAN_POINT ( 'NONE',  ( 4.566398809704347528, 4.221886787610169556, -0.7998128361456211532 ) ) ;
#36329=CARTESIAN_POINT ( 'NONE',  ( -8.371269781434001800, 11.85389961405997816, -1.199719254218446718 ) ) ;
#36335=CARTESIAN_POINT ( 'NONE',  ( 5.757945239960298167, 6.059206896687658883, 0.6045188873357760784 ) ) ;
#36337=CARTESIAN_POINT ( 'NONE',  ( -4.115063316947640715, 4.759660943649018705, 1.199719254218462483 ) ) ;
#36341=CARTESIAN_POINT ( 'NONE',  ( 8.274553823041976841, 8.548067636504127265, 1.040834085586084257E-14 ) ) ;
#36343=CARTESIAN_POINT ( 'NONE',  ( 5.262536180398716290, 9.291375977107183104, -0.7998128361456291469 ) ) ;
#36344=CARTESIAN_POINT ( 'NONE',  ( 3.337278367258157630, 7.045241861776501580, 0.7998128361456341429 ) ) ;
#36346=CARTESIAN_POINT ( 'NONE',  ( -7.483737605063437215, 10.71448239167390604, 1.082531754730549967 ) ) ;
#36353=B_SPLINE_CURVE_WITH_KNOTS ( 'NONE', 3,
 ( #198629, #102220, #185587, #149917 ),
 .UNSPECIFIED., .F., .F.,
 ( 4, 4 ),
 ( 4.091847515137629478E-16, 0.0006466603606995657751 ),
 .UNSPECIFIED. ) ;
#36354=CARTESIAN_POINT ( 'NONE',  ( -4.192242263785030509, 7.388029550104924681, -0.8017062249071702507 ) ) ;
#36355=EDGE_CURVE ( 'NONE', #112883, #70347, #58099, .T. ) ;
#36358=CARTESIAN_POINT ( 'NONE',  ( 4.514501963670558560, 8.210743357683563559, 1.040834085586084257E-14 ) ) ;
#36360=CARTESIAN_POINT ( 'NONE',  ( 7.723341061279088038, 12.16231500480096983, -0.7998128361456291469 ) ) ;
#36370=CARTESIAN_POINT ( 'NONE',  ( -8.581948047326017459, 11.99572790764693409, 1.082531754730558626 ) ) ;
#36379=CARTESIAN_POINT ( 'NONE',  ( -9.666600336419303829, 11.34041714965307968, 1.082531754730558626 ) ) ;
#36383=CARTESIAN_POINT ( 'NONE',  ( 7.690499447449630210, 9.995335326823163058, 1.599625672291281386 ) ) ;
#36387=CARTESIAN_POINT ( 'NONE',  ( 1.499999999999989120, 1.306250000682816825, 0.000000000000000000 ) ) ;
#36389=CARTESIAN_POINT ( 'NONE',  ( -6.905180308061733996, 6.950465202360470052, 0.7998128361456341429 ) ) ;
#36392=CARTESIAN_POINT ( 'NONE',  ( -9.006694118179950692, 9.402231314165087284, 1.040834085586084257E-14 ) ) ;
#36397=CARTESIAN_POINT ( 'NONE',  ( 7.786460292950004636, 7.978625184730144149, 1.040834085586084257E-14 ) ) ;
#36401=CARTESIAN_POINT ( 'NONE',  ( 8.772289083241844310, 10.19309100432570148, -1.199719254218446718 ) ) ;
#36404=CARTESIAN_POINT ( 'NONE',  ( -4.830635273601783020, 5.066023441139620331, -0.9190199222270474255 ) ) ;
#36408=CARTESIAN_POINT ( 'NONE',  ( -6.046573322014817897, 9.998159942418544333, 0.7216878364870458196 ) ) ;
#36411=CARTESIAN_POINT ( 'NONE',  ( -1.201851678989727383E-14, 4.134375000341417028, 1.575800808251672791 ) ) ;
#36415=CARTESIAN_POINT ( 'NONE',  ( 0.6823417656249917140, 5.342708333674749177, 1.181850606188765695 ) ) ;
#36418=CARTESIAN_POINT ( 'NONE',  ( -2.616360457312984167, 5.996244933599686355, -0.7216878364870257245 ) ) ;
#36421=ADVANCED_FACE ( 'NONE', ( #133530 ), #132772, .T. ) ;
#36422=CARTESIAN_POINT ( 'NONE',  ( 10.24726517383036928, 10.84956421242393887, 0.000000000000000000 ) ) ;
#36423=CARTESIAN_POINT ( 'NONE',  ( -1.001543065824772872E-14, 4.884375000341420581, 1.575800808251672791 ) ) ;
#36428=CARTESIAN_POINT ( 'NONE',  ( 0.6823417656249882723, 1.926041667008083991, -1.181850606188749264 ) ) ;
#36429=CARTESIAN_POINT ( 'NONE',  ( -3.226477370372317743, 4.787309570232886280, 1.443375672974064550 ) ) ;
#36431=CARTESIAN_POINT ( 'NONE',  ( 3.499976210622149253, 7.235056012367825140, 0.7998128361456321445 ) ) ;
#36436=DIRECTION ( 'NONE',  ( 0.000000000000000000, 8.546850786086437571E-32, 1.000000000000000000 ) ) ;
#36437=CARTESIAN_POINT ( 'NONE',  ( 4.202664430556261266, 4.005456045178151570, 0.7216878364870317197 ) ) ;
#36440=CARTESIAN_POINT ( 'NONE',  ( -7.863365906246061243, 10.19701286208565705, -1.443375672974059665 ) ) ;
#36446=CARTESIAN_POINT ( 'NONE',  ( -8.727698198895085469, 11.20540053684285553, -1.599625672291263179 ) ) ;
#36447=CARTESIAN_POINT ( 'NONE',  ( -5.734735788456164940, 5.792872629394710593, 0.7216878364870317197 ) ) ;
#36448=CARTESIAN_POINT ( 'NONE',  ( 1.364683531249988535, 2.176041667008087543, 0.7879004041258500513 ) ) ;
#36462=ORIENTED_EDGE ( 'NONE', *, *, #175516, .T. ) ;
#36464=CARTESIAN_POINT ( 'NONE',  ( 1.483456582844651095, 7.293967155396083868, -4.258619948151496359 ) ) ;
#36470=CARTESIAN_POINT ( 'NONE',  ( 0.6823417656249899377, 2.655208333674753618, 1.181850606188767472 ) ) ;
#36478=CARTESIAN_POINT ( 'NONE',  ( 9.317477881089539338, 11.89347683273640932, 1.599625672291279388 ) ) ;
#36481=CARTESIAN_POINT ( 'NONE',  ( 1.364683531249988535, 1.613541667008084879, 0.7879004041258500513 ) ) ;
#36488=ORIENTED_EDGE ( 'NONE', *, *, #159575, .F. ) ;
#36490=CARTESIAN_POINT ( 'NONE',  ( 3.680148631105580215, 6.380924938676771241, -1.199719254218446718 ) ) ;
#36494=CARTESIAN_POINT ( 'NONE',  ( 10.16199982864259788, 11.81442020729326536, 1.199719254218452047 ) ) ;
#36498=ORIENTED_EDGE ( 'NONE', *, *, #85279, .F. ) ;
#36500=CARTESIAN_POINT ( 'NONE',  ( -4.485049888022365927, 4.126979712314507331, 0.7998128361456341429 ) ) ;
#36501=CARTESIAN_POINT ( 'NONE',  ( 6.774270308322468459, 11.05506579301824743, 0.7998128361456462443 ) ) ;
#36504=CARTESIAN_POINT ( 'NONE',  ( 4.243338890952890630, 5.973648010910253880, -1.443375672974051449 ) ) ;
#36510=CYLINDRICAL_SURFACE ( 'NONE', #46543, 1.250000000000000000 ) ;
#36511=CARTESIAN_POINT ( 'NONE',  ( -7.551528373131759508, 7.912463978182924684, 1.040834085586084257E-14 ) ) ;
#36513=CARTESIAN_POINT ( 'NONE',  ( 6.308621549060418054, 6.254479983525607523, 0.7998128361456341429 ) ) ;
#36516=CARTESIAN_POINT ( 'NONE',  ( -8.123306592882240551, 12.62894145833798376, 0.000000000000000000 ) ) ;
#36521=CARTESIAN_POINT ( 'NONE',  ( -3.623053363349869382, 5.249981562040033189, 1.599625672291267398 ) ) ;
#36523=CARTESIAN_POINT ( 'NONE',  ( 7.913155211870404493, 12.38376484715752213, 0.7998128361456462443 ) ) ;
#36524=CARTESIAN_POINT ( 'NONE',  ( 4.729096653068339151, 4.411700938201493116, -0.7998128361456211532 ) ) ;
#36530=CARTESIAN_POINT ( 'NONE',  ( 4.121315508874254796, 5.831287398485176077, -1.443375672974051449 ) ) ;
#36533=CARTESIAN_POINT ( 'NONE',  ( -5.739179097286464248, 5.590130456455974617, -0.7998128361456221525 ) ) ;
#36536=CARTESIAN_POINT ( 'NONE',  ( -9.622536337397040285, 12.24937836509514710, 1.599625672291281386 ) ) ;
#36541=CARTESIAN_POINT ( 'NONE',  ( 7.266807147244743526, 11.42176607185347414, -0.7216878364870267237 ) ) ;
#36542=CARTESIAN_POINT ( 'NONE',  ( -1.364683531250010740, 5.551041667008087543, -0.7879004041258300672 ) ) ;
#36544=CARTESIAN_POINT ( 'NONE',  ( 4.741601036477289810, 6.554953847355395880, 1.599625672291267398 ) ) ;
#36557=CARTESIAN_POINT ( 'NONE',  ( 1.364683531249986537, 2.467708333674753174, -0.7879004041258239610 ) ) ;
#36559=CARTESIAN_POINT ( 'NONE',  ( 9.083072846151447166, 12.68433652289702884, 1.199719254218450271 ) ) ;
#36561=CARTESIAN_POINT ( 'NONE',  ( -4.229780737783618072, 6.918199379847403740, 1.082531754730560403 ) ) ;
#36565=CARTESIAN_POINT ( 'NONE',  ( -6.385527161912131433, 6.552129231760014605, 0.7216878364870317197 ) ) ;
#36568=ORIENTED_EDGE ( 'NONE', *, *, #60217, .F. ) ;
#36570=CARTESIAN_POINT ( 'NONE',  ( 6.010342169559767633, 5.906487374108181143, -0.7998128361456281477 ) ) ;
#36580=CARTESIAN_POINT ( 'NONE',  ( 5.656776405399742025, 7.622658444431597680, -1.599625672291262513 ) ) ;
#36582=CARTESIAN_POINT ( 'NONE',  ( -2.103486388414573138, 5.605817886458954291, 1.040834085586084257E-14 ) ) ;
#36584=CARTESIAN_POINT ( 'NONE',  ( -7.074657228232555717, 7.148188275893099686, 1.040834085586084257E-14 ) ) ;
#36588=CARTESIAN_POINT ( 'NONE',  ( 7.935599982700328958, 8.152621489438862667, 0.7998128361456481317 ) ) ;
#36591=CARTESIAN_POINT ( 'NONE',  ( -5.819474248763749635, 7.812472595022922128, -1.599625672291256295 ) ) ;
#36592=CARTESIAN_POINT ( 'NONE',  ( 6.954969613686092345, 7.216478758829655504, -0.7216878364870257245 ) ) ;
#36593=CARTESIAN_POINT ( 'NONE',  ( 4.170588824514860349, 7.607689953969209995, 0.8569815457360376865 ) ) ;
#36594=CARTESIAN_POINT ( 'NONE',  ( -4.111146893441842920, 5.819424013814012753, 1.599625672291267398 ) ) ;
#36597=CARTESIAN_POINT ( 'NONE',  ( -5.063080299699540987, 7.994345218703034384, 1.199719254218464037 ) ) ;
#36600=CARTESIAN_POINT ( 'NONE',  ( -1.364683531249997417, 2.509375000341422357, 1.214306433183764966E-14 ) ) ;
#36603=CARTESIAN_POINT ( 'NONE',  ( -4.433153041988574294, 8.115836282387899558, 1.040834085586084257E-14 ) ) ;
#36610=CARTESIAN_POINT ( 'NONE',  ( 5.147291874682557555, 9.156924287104992288, 0.7998128361456462443 ) ) ;
#36613=CARTESIAN_POINT ( 'NONE',  ( -0.6823417656250003738, 2.280208333674753174, -1.181850606188749264 ) ) ;
#36616=CARTESIAN_POINT ( 'NONE',  ( 1.364683531249984538, -1.032291666325247714, -0.7879004041258309554 ) ) ;
#36617=CARTESIAN_POINT ( 'NONE',  ( 5.843201017809841247, 5.919415396974013532, 1.040834085586084257E-14 ) ) ;
#36619=CARTESIAN_POINT ( 'NONE',  ( -4.298098390732130625, 4.973201863064262263, 1.199719254218462483 ) ) ;
#36621=CARTESIAN_POINT ( 'NONE',  ( -7.714226216051410567, 9.062647342557177410, 1.082531754730558626 ) ) ;
#36624=CARTESIAN_POINT ( 'NONE',  ( -0.6823417656249969321, 3.467708333674754506, -1.181850606188749264 ) ) ;
#36631=CARTESIAN_POINT ( 'NONE',  ( -6.792271770322117597, 9.907772251142352715, 1.082531754730549967 ) ) ;
#36635=EDGE_CURVE ( 'NONE', #65489, #108697, #146700, .T. ) ;
#36637=CARTESIAN_POINT ( 'NONE',  ( -7.199016378732087773, 7.501199984716642177, 0.7216878364870317197 ) ) ;
#36650=CARTESIAN_POINT ( 'NONE',  ( -6.718228810771495141, 7.796687353110217877, 1.199719254218450271 ) ) ;
#36652=CARTESIAN_POINT ( 'NONE',  ( -1.500000000000013101, -0.07916666666664513852, 0.8660254037844403729 ) ) ;
#36653=CARTESIAN_POINT ( 'NONE',  ( 2.984766373302843778, 6.633977868828633717, -0.7998128361456291469 ) ) ;
#36655=ADVANCED_FACE ( 'NONE', ( #42421 ), #125864, .F. ) ;
#36658=CARTESIAN_POINT ( 'NONE',  ( 7.494959990256193194, 7.638541498254023843, -0.7998128361456281477 ) ) ;
#36662=CARTESIAN_POINT ( 'NONE',  ( -5.016153647376219382, 6.875265226737464985, 1.443375672974064550 ) ) ;
#36669=CARTESIAN_POINT ( 'NONE',  ( 0.6823417656249882723, 1.426041667008083547, -1.181850606188749264 ) ) ;
#36671=CARTESIAN_POINT ( 'NONE',  ( -7.365103760721662951, 9.615707025640515937, 1.599625672291295375 ) ) ;
#36674=CARTESIAN_POINT ( 'NONE',  ( 8.145751363712157911, 8.397798100619326078, -0.7998128361456281477 ) ) ;
#36676=CARTESIAN_POINT ( 'NONE',  ( -7.446452682403657874, 9.710614100936176385, -1.599625672291263179 ) ) ;
#36679=CARTESIAN_POINT ( 'NONE',  ( -0.6823417656250212460, 5.551041667008087543, 1.181850606188767472 ) ) ;
#36682=CARTESIAN_POINT ( 'NONE',  ( 7.565086526745395723, 10.80938946696957004, -1.082531754730543083 ) ) ;
#36684=CARTESIAN_POINT ( 'NONE',  ( -1.364683531250014514, -0.6989583329919100141, -0.7879004041258359514 ) ) ;
#36687=CARTESIAN_POINT ( 'NONE',  ( 6.087247782411444597, 10.04561347954795281, -0.7216878364870267237 ) ) ;
#36690=CARTESIAN_POINT ( 'NONE',  ( -3.619663825168619731, 7.166765529431275539, 1.040834085586084257E-14 ) ) ;
#36693=CARTESIAN_POINT ( 'NONE',  ( -1.364683531249997417, 3.759375000341423689, 1.214306433183764966E-14 ) ) ;
#36697=CARTESIAN_POINT ( 'NONE',  ( -5.799137018343247796, 7.788745826199009237, -1.599625672291256295 ) ) ;
#36698=DIRECTION ( 'NONE',  ( -0.3502638921866460531, 1.953969548649011466E-16, -0.9366510587354619499 ) ) ;
#36704=CARTESIAN_POINT ( 'NONE',  ( 7.820355676984174664, 8.018169799436671852, -0.7998128361456281477 ) ) ;
#36707=CARTESIAN_POINT ( 'NONE',  ( 1.499999999999989120, 3.004166666666689522, 0.8660254037844524744 ) ) ;
#36713=CARTESIAN_POINT ( 'NONE',  ( 5.829642864196162400, 7.824335979694092558, 1.443375672974062551 ) ) ;
#36714=CARTESIAN_POINT ( 'NONE',  ( 1.364683531249986537, -0.2822916663252520997, -0.7879004041258309554 ) ) ;
#36715=CIRCLE ( 'NONE', #5611, 0.08000000000000004330 ) ;
#36717=CARTESIAN_POINT ( 'NONE',  ( 8.530051201292206287, 13.10347683481629488, 0.000000000000000000 ) ) ;
#36722=CARTESIAN_POINT ( 'NONE',  ( -1.402160292154681736E-14, 1.087500000000024336, -1.732050807568863648 ) ) ;
#36723=CARTESIAN_POINT ( 'NONE',  ( 7.076466111328892694, 10.34329533227067799, -1.199719254218441611 ) ) ;
#36724=CARTESIAN_POINT ( 'NONE',  ( -8.341290820905609138, 10.75459192918846618, 1.599625672291269396 ) ) ;
#36726=CARTESIAN_POINT ( 'NONE',  ( 1.364683531249986537, 0.1135416670080857532, 0.7879004041258500513 ) ) ;
#36727=CARTESIAN_POINT ( 'NONE',  ( 0.7499999999999885647, 0.5666666666666875241, -1.299038105676652899 ) ) ;
#36729=CARTESIAN_POINT ( 'NONE',  ( 5.522248639467795428, 5.337044922334209573, -0.7998128361456231517 ) ) ;
#36737=CARTESIAN_POINT ( 'NONE',  ( -1.500000000000015099, -0.3395833326505143801, -0.8660254037844383745 ) ) ;
#36739=CARTESIAN_POINT ( 'NONE',  ( -7.751511138711140170, 10.06651563329490529, -1.599625672291263179 ) ) ;
#36740=CARTESIAN_POINT ( 'NONE',  ( -5.314433026876900001, 6.262888621853549331, 1.082531754730548412 ) ) ;
#36742=DIRECTION ( 'NONE',  ( 7.387867266669436732E-31, -1.000000000000000000, -8.546850786086424434E-32 ) ) ;
#36748=CARTESIAN_POINT ( 'NONE',  ( 7.670162217029129259, 9.971608557999250166, 1.599625672291281386 ) ) ;
#36752=CARTESIAN_POINT ( 'NONE',  ( 6.656690234185433042, 7.828855363713562276, -1.082531754730543971 ) ) ;
#36757=CARTESIAN_POINT ( 'NONE',  ( -7.832860060393135093, 10.16142270859057462, 1.599625672291295375 ) ) ;
#36758=CARTESIAN_POINT ( 'NONE',  ( 4.493637847925535667, 7.329995691633395261, -1.199719254218452047 ) ) ;
#36760=CARTESIAN_POINT ( 'NONE',  ( 4.050410598061423784, 7.525715715152009544, -0.4746587800704554772 ) ) ;
#36761=CARTESIAN_POINT ( 'NONE',  ( 3.440018289565364817, 5.036440642624797626, 1.599625672291267398 ) ) ;
#36769=CARTESIAN_POINT ( 'NONE',  ( -3.606105671554953318, 7.150947683548662503, 0.7216878364870317197 ) ) ;
#36770=CARTESIAN_POINT ( 'NONE',  ( 9.137832345930652522, 10.72352116074969075, -1.082531754730543083 ) ) ;
#36773=CARTESIAN_POINT ( 'NONE',  ( -7.152089726408780379, 8.302858421353754181, -1.199719254218446718 ) ) ;
#36776=AXIS2_PLACEMENT_3D ( 'NONE', #123488, #204609, #141818 ) ;
#36779=CARTESIAN_POINT ( 'NONE',  ( -8.179646747746328828, 8.437342715325849341, -0.7998128361456291469 ) ) ;
#36795=CARTESIAN_POINT ( 'NONE',  ( -5.845536785786364931, 9.971543350059432598, 0.000000000000000000 ) ) ;
#36798=CARTESIAN_POINT ( 'NONE',  ( 6.019457014787495730, 6.125047393447951016, -0.7216878364870257245 ) ) ;
#36801=CARTESIAN_POINT ( 'NONE',  ( -3.122962944146551845, 6.587281168238894757, 0.4581612399161954507 ) ) ;
#36804=CARTESIAN_POINT ( 'NONE',  ( -5.434120640978981065, 5.234228924097238611, -0.7998128361456221525 ) ) ;
#36812=CARTESIAN_POINT ( 'NONE',  ( -9.016335848287868160, 10.47781223021269170, 1.199719254218462483 ) ) ;
#36813=CARTESIAN_POINT ( 'NONE',  ( 7.396136491454752715, 8.587579647240744407, 1.199719254218462483 ) ) ;
#36817=CARTESIAN_POINT ( 'NONE',  ( -10.47097470845587175, 11.11055866948701443, 1.040834085586084257E-14 ) ) ;
#36820=CARTESIAN_POINT ( 'NONE',  ( -0.6823417656250003738, 0.03020833367475134201, -1.181850606188749264 ) ) ;
#36824=CARTESIAN_POINT ( 'NONE',  ( 8.948018195339340508, 9.541702104091804415, -0.7216878364870197293 ) ) ;
#36835=DIRECTION ( 'NONE',  ( 0.6507913734559640506, -0.7592566023653004592, 0.000000000000000000 ) ) ;
#36838=ORIENTED_EDGE ( 'NONE', *, *, #144102, .F. ) ;
#36843=CARTESIAN_POINT ( 'NONE',  ( -3.216308754939891212, 4.775446185561722956, -1.599625672291262513 ) ) ;
#36850=CARTESIAN_POINT ( 'NONE',  ( 1.499999999999987566, -0.6937499993171849511, 0.000000000000000000 ) ) ;
#36854=FACE_OUTER_BOUND ( 'NONE', #144248, .T. ) ;
#36857=CARTESIAN_POINT ( 'NONE',  ( -1.257518954445032477, 3.216479010054028809, 0.7750000000000100142 ) ) ;
#36859=CARTESIAN_POINT ( 'NONE',  ( 4.864678189204997949, 4.569879397027603929, 0.7998128361456341429 ) ) ;
#36864=CARTESIAN_POINT ( 'NONE',  ( 4.313465427442102929, 8.184126765324453601, 0.7998128361456462443 ) ) ;
#36865=CARTESIAN_POINT ( 'NONE',  ( -0.6823417656250003738, 2.780208333674753618, -1.181850606188749264 ) ) ;
#36866=CARTESIAN_POINT ( 'NONE',  ( -5.901845825571131243, 6.006233656505717278, 0.1738135011533047114 ) ) ;
#36870=CARTESIAN_POINT ( 'NONE',  ( -8.532158741701643123, 8.848606708273724308, 0.7998128361456462443 ) ) ;
#36871=CARTESIAN_POINT ( 'NONE',  ( -5.246642258364192735, 5.223430177620739023, 0.7216878364870317197 ) ) ;
#36875=CARTESIAN_POINT ( 'NONE',  ( -6.043183783389232566, 8.073467052085995022, 1.599625672291269396 ) ) ;
#36877=CARTESIAN_POINT ( 'NONE',  ( 0.7499999999999867883, -0.1520833326505155458, -1.299038105676652899 ) ) ;
#36884=CARTESIAN_POINT ( 'NONE',  ( -2.941756144040963417, 6.375873234782333476, -0.7216878364870257245 ) ) ;
#36887=EDGE_CURVE ( 'NONE', #168810, #69998, #78087, .T. ) ;
#36891=CARTESIAN_POINT ( 'NONE',  ( -5.056828107772872727, 5.001980335264194721, -0.7216878364870197293 ) ) ;
#36893=CARTESIAN_POINT ( 'NONE',  ( 9.423080456697809026, 10.95234760669099749, -1.199719254218446718 ) ) ;
#36901=CARTESIAN_POINT ( 'NONE',  ( -3.358669367883384105, 4.941533567329135401, -1.599625672291262513 ) ) ;
#36902=CARTESIAN_POINT ( 'NONE',  ( -8.109748439268576803, 12.61312361245537517, 0.7998128361456481317 ) ) ;
#36907=CARTESIAN_POINT ( 'NONE',  ( 4.656335691289526402, 7.519809842224722374, -1.199719254218452047 ) ) ;
#36913=CARTESIAN_POINT ( 'NONE',  ( 4.376584659113025744, 4.000436945253625254, 0.7998128361456341429 ) ) ;
#36924=CARTESIAN_POINT ( 'NONE',  ( 8.229962938695207342, 9.560377169021284871, 1.199719254218462483 ) ) ;
#36926=CARTESIAN_POINT ( 'NONE',  ( -4.924636110261798372, 6.768494766770632332, 1.599625672291267398 ) ) ;
#36933=CARTESIAN_POINT ( 'NONE',  ( -1.602468905319636405E-14, -1.131249999317182064, -1.732050807568870754 ) ) ;
#36938=CARTESIAN_POINT ( 'NONE',  ( 1.262825079187945398, 3.294887467576579798, 0.7750000000000100142 ) ) ;
#36939=CARTESIAN_POINT ( 'NONE',  ( 2.679707916995359263, 6.278076336469897711, -0.7998128361456291469 ) ) ;
#36940=CARTESIAN_POINT ( 'NONE',  ( -5.111587607552082524, 5.922272616020886282, 1.199719254218450271 ) ) ;
#36946=EDGE_CURVE ( 'NONE', #116745, #121840, #87170, .T. ) ;
#36948=CARTESIAN_POINT ( 'NONE',  ( 5.883875478650832491, 6.927238148923188454, -1.082531754730543083 ) ) ;
#36951=CARTESIAN_POINT ( 'NONE',  ( 8.419250203962011625, 8.924806114151579095, -0.7216878364870267237 ) ) ;
#36952=CARTESIAN_POINT ( 'NONE',  ( -1.001543065824772872E-14, 4.884375000341420581, 1.575800808251672791 ) ) ;
#36954=CARTESIAN_POINT ( 'NONE',  ( 3.511198595814921219, 7.040222761851976152, 0.7216878364870317197 ) ) ;
#36958=EDGE_CURVE ( 'NONE', #211239, #85368, #22711, .T. ) ;
#36961=CARTESIAN_POINT ( 'NONE',  ( 1.499999999999990896, 5.775000000000023448, 1.040834085586084257E-14 ) ) ;
#36962=CARTESIAN_POINT ( 'NONE',  ( -4.867404985860277478, 6.905081695904778272, 1.445136279841979121 ) ) ;
#36964=CARTESIAN_POINT ( 'NONE',  ( 1.364683531249990311, 5.676041667008088432, 0.7879004041258500513 ) ) ;
#36968=CARTESIAN_POINT ( 'NONE',  ( -8.319899820280397762, 12.85830022363583147, -0.7998128361456281477 ) ) ;
#36978=CARTESIAN_POINT ( 'NONE',  ( 2.562127843302666186, 5.932973550587659517, 0.000000000000000000 ) ) ;
#36979=CARTESIAN_POINT ( 'NONE',  ( 0.6823417656249899377, 2.905208333674754062, 1.181850606188765695 ) ) ;
#36981=CARTESIAN_POINT ( 'NONE',  ( 7.019370843573166319, 9.212351955633947043, 1.599625672291281386 ) ) ;
#36982=CARTESIAN_POINT ( 'NONE',  ( -9.528683032306089373, 10.01121838064558744, 0.7998128361456462443 ) ) ;
#36983=DIRECTION ( 'NONE',  ( 1.000000000000000000, 0.000000000000000000, 0.000000000000000000 ) ) ;
#36984=CARTESIAN_POINT ( 'NONE',  ( -3.418627288940168096, 7.140148937072163804, -0.7998128361456282587 ) ) ;
#36989=CARTESIAN_POINT ( 'NONE',  ( -1.500000000000011324, 4.170833333333359150, 0.8660254037844403729 ) ) ;
#36990=CARTESIAN_POINT ( 'NONE',  ( 4.147904930777053245, 6.926640621626830807, -1.199719254218452047 ) ) ;
#36994=CARTESIAN_POINT ( 'NONE',  ( 8.053180056837369705, 11.37883191874353805, -1.082531754730543083 ) ) ;
#36999=CARTESIAN_POINT ( 'NONE',  ( -0.7500000000000006661, 3.139583334016149418, -1.299038105676652011 ) ) ;
#37002=CARTESIAN_POINT ( 'NONE',  ( -5.091250377131585125, 5.898545847196970726, 1.199719254218450271 ) ) ;
#37003=CARTESIAN_POINT ( 'NONE',  ( 3.619663824724254741, 6.206396314611513532, -1.082531754730543971 ) ) ;
#37011=CARTESIAN_POINT ( 'NONE',  ( 7.096803341749390981, 10.36702210109460154, -1.199719254218441611 ) ) ;
#37012=CARTESIAN_POINT ( 'NONE',  ( 3.798255590122797898, 7.583048621785260401, -0.7998128361456221525 ) ) ;
#37013=CARTESIAN_POINT ( 'NONE',  ( -1.150222622689967888, 2.972854968409793575, -0.7749999999993613109 ) ) ;
#37015=DIRECTION ( 'NONE',  ( -5.578564026256490882E-16, -1.000000000000000000, -9.066213480720158442E-32 ) ) ;
#37017=ORIENTED_EDGE ( 'NONE', *, *, #56788, .T. ) ;
#37022=CARTESIAN_POINT ( 'NONE',  ( 9.887974103068218668, 10.43039129653476493, 0.7998128361456462443 ) ) ;
#37023=DIRECTION ( 'NONE',  ( -7.387867266669436732E-31, 1.000000000000000000, -8.546850786086437571E-32 ) ) ;
#37027=CARTESIAN_POINT ( 'NONE',  ( 5.770924896911269641, 6.051163903260999177, -0.5763553215429690901 ) ) ;
#37033=CIRCLE ( 'NONE', #175432, 0.08000000000000020983 ) ;
#37034=CARTESIAN_POINT ( 'NONE',  ( 1.499999999999956257, 5.577083334016155192, -0.8660254037844512531 ) ) ;
#37036=CARTESIAN_POINT ( 'NONE',  ( 6.982085921357777281, 7.248114451113292667, 1.040834085586084257E-14 ) ) ;
#37037=CARTESIAN_POINT ( 'NONE',  ( -4.776550190716183586, 4.467063398790632966, 1.214306433183764966E-14 ) ) ;
#37043=CARTESIAN_POINT ( 'NONE',  ( -5.752737250900127997, 5.605948302338584099, 0.000000000000000000 ) ) ;
#37056=CARTESIAN_POINT ( 'NONE',  ( 7.964525173024008531, 11.37936423758166526, 1.199719254218460707 ) ) ;
#37057=CARTESIAN_POINT ( 'NONE',  ( 5.951559787436734084, 6.118878616701469042, 0.7174803059855124898 ) ) ;
#37064=CARTESIAN_POINT ( 'NONE',  ( -8.676855123066019360, 11.14608361504227574, -1.443375672974059665 ) ) ;
#37069=CARTESIAN_POINT ( 'NONE',  ( 7.130698725783555680, 10.40656671580112658, 1.199719254218460707 ) ) ;
#37073=EDGE_CURVE ( 'NONE', #69090, #92214, #40847, .T. ) ;
#37074=CARTESIAN_POINT ( 'NONE',  ( 4.542145155778077203, 5.257923088951247159, -1.199719254218452047 ) ) ;
#37076=CARTESIAN_POINT ( 'NONE',  ( -7.237355071596549116, 7.338002426484427687, 1.040834085586084257E-14 ) ) ;
#37077=CARTESIAN_POINT ( 'NONE',  ( 5.684946482831785275, 5.526859072925533134, -0.7998128361456231517 ) ) ;
#37080=CARTESIAN_POINT ( 'NONE',  ( 10.55232363013785246, 11.20546574478267132, 0.000000000000000000 ) ) ;
#37084=CARTESIAN_POINT ( 'NONE',  ( 4.024405658984873568, 7.794362949307388710, 0.3537781459504486525 ) ) ;
#37086=CARTESIAN_POINT ( 'NONE',  ( 4.989037340148863464, 8.764367963574922982, -0.7216878364870257245 ) ) ;
#37088=CARTESIAN_POINT ( 'NONE',  ( 0.3384194684227018746, 6.989896059384769877, 3.860023792759414096 ) ) ;
#37095=CARTESIAN_POINT ( 'NONE',  ( 8.392133896734668141, 9.853539636687704828, 1.082531754730558626 ) ) ;
#37100=CARTESIAN_POINT ( 'NONE',  ( -9.365985188942097750, 9.821404230054264772, 0.7998128361456462443 ) ) ;
#37110=CARTESIAN_POINT ( 'NONE',  ( 2.381428537494710618, 5.930083727052461562, 0.7998128361456462443 ) ) ;
#37114=CARTESIAN_POINT ( 'NONE',  ( 5.497994985541524215, 6.373081223675282736, -1.199719254218445830 ) ) ;
#37117=CARTESIAN_POINT ( 'NONE',  ( 1.499999999999990896, 3.306250000682818602, 1.214306433183764966E-14 ) ) ;
#37123=CARTESIAN_POINT ( 'NONE',  ( 1.499999999999989120, 2.275000000000019895, 1.214306433183764966E-14 ) ) ;
#37124=CARTESIAN_POINT ( 'NONE',  ( 6.962275575817444384, 8.081408578997208991, -1.199719254218446718 ) ) ;
#37125=CARTESIAN_POINT ( 'NONE',  ( 4.650083499362867911, 6.448183387388563226, 1.443375672974062551 ) ) ;
#37129=CARTESIAN_POINT ( 'NONE',  ( 7.117667457494414762, 11.24776976714476184, 1.040834085586084257E-14 ) ) ;
#37134=CARTESIAN_POINT ( 'NONE',  ( -5.850506979496850057, 6.784345216623154151, -1.199719254218446718 ) ) ;
#37136=CARTESIAN_POINT ( 'NONE',  ( 1.499999999999990896, 4.556250000682819490, 1.214306433183764966E-14 ) ) ;
#37137=CARTESIAN_POINT ( 'NONE',  ( -1.364683531250012516, 5.051041667008085767, -0.7879004041258300672 ) ) ;
#37142=CARTESIAN_POINT ( 'NONE',  ( -1.364683531249997417, 3.571875000341423245, 1.214306433183764966E-14 ) ) ;
#37145=CARTESIAN_POINT ( 'NONE',  ( 1.419999999999989049, 6.120000000000041851, -2.579999999999995630 ) ) ;
#37151=CARTESIAN_POINT ( 'NONE',  ( -8.178592977541617515, 10.56477777859713463, 1.599625672291295375 ) ) ;
#37153=CARTESIAN_POINT ( 'NONE',  ( 5.686755365928134687, 8.721966129303114101, 1.199719254218462483 ) ) ;
#37157=CARTESIAN_POINT ( 'NONE',  ( 1.364683531249988757, -0.6156249996585803075, 0.000000000000000000 ) ) ;
#37164=CARTESIAN_POINT ( 'NONE',  ( -7.206322340863467346, 8.366129804884193888, 1.199719254218450271 ) ) ;
#37167=CARTESIAN_POINT ( 'NONE',  ( 9.728138913005292210, 11.30824913904973705, -1.199719254218440723 ) ) ;
#37169=CARTESIAN_POINT ( 'NONE',  ( 9.215791728987056786, 11.77484298861683598, -1.599625672291262513 ) ) ;
#37170=( BOUNDED_SURFACE ( )  B_SPLINE_SURFACE ( 3, 1, ( 
 ( #91947, #137492 ),
 ( #173193, #41061 ),
 ( #202441, #120233 ),
 ( #58356, #190469 ),
 ( #172116, #171033 ),
 ( #140713, #107168 ),
 ( #38909, #203508 ) ),
 .UNSPECIFIED., .T., .F., .F. ) 
 B_SPLINE_SURFACE_WITH_KNOTS ( ( 4, 3, 4 ),
 ( 2, 2 ),
 ( 0.000000000000000000, 0.5000000000000000000, 1.000000000000000000 ),
 ( 0.000000000000000000, 1.000000000000000000 ),
 .UNSPECIFIED. ) 
 GEOMETRIC_REPRESENTATION_ITEM ( )  RATIONAL_B_SPLINE_SURFACE ( (
 ( 1.000000000000000000, 1.000000000000000000),
 ( 0.3333333333333333703, 0.3333333333333333703),
 ( 0.3333333333333333703, 0.3333333333333333703),
 ( 1.000000000000000000, 1.000000000000000000),
 ( 0.3333333333333333703, 0.3333333333333333703),
 ( 0.3333333333333333703, 0.3333333333333333703),
 ( 1.000000000000000000, 1.000000000000000000) ) ) 
 REPRESENTATION_ITEM ( '' )  SURFACE ( )  );
#37174=CARTESIAN_POINT ( 'NONE',  ( -4.090809663021341969, 5.795697244990093644, 1.599625672291267398 ) ) ;
#37175=CARTESIAN_POINT ( 'NONE',  ( -7.507464373665155399, 9.781794407407920389, 1.599625672291295375 ) ) ;
#37178=CARTESIAN_POINT ( 'NONE',  ( -4.277728075731661583, 7.474117497184462167, -1.086723757153153835 ) ) ;
#37179=CARTESIAN_POINT ( 'NONE',  ( -1.364683531250014514, -1.219791666325248602, 0.7879004041258379498 ) ) ;
#37183=CARTESIAN_POINT ( 'NONE',  ( 8.649738815838679429, 10.15407870897571563, -1.082531754730543083 ) ) ;
#37209=CARTESIAN_POINT ( 'NONE',  ( -9.494787648271923786, 9.971673765939062406, 1.040834085586084257E-14 ) ) ;
#37215=CARTESIAN_POINT ( 'NONE',  ( -1.500000000000013101, 2.202083334016153859, 0.8660254037844403729 ) ) ;
#37216=CARTESIAN_POINT ( 'NONE',  ( 9.378489572351044856, 11.96465713920816043, -1.599625672291262513 ) ) ;
#37220=CARTESIAN_POINT ( 'NONE',  ( -9.154780037725563702, 11.70366268214508487, 1.599625672291281386 ) ) ;
#37222=CARTESIAN_POINT ( 'NONE',  ( 0.6823417656249882723, 2.426041667008084435, -1.181850606188749264 ) ) ;
#37224=ORIENTED_EDGE ( 'NONE', *, *, #52716, .F. ) ;
#37230=CARTESIAN_POINT ( 'NONE',  ( -4.223528545856940042, 4.886203710709899006, -1.199719254218446718 ) ) ;
#37235=CARTESIAN_POINT ( 'NONE',  ( -1.364683531250000748, -0.4281249996585800854, 0.000000000000000000 ) ) ;
#37241=CARTESIAN_POINT ( 'NONE',  ( 0.6823417656249882723, 1.426041667008083547, -1.181850606188749264 ) ) ;
#37243=CARTESIAN_POINT ( 'NONE',  ( -6.358937740009323214, 7.377514437221045718, -1.199719254218446718 ) ) ;
#37244=CARTESIAN_POINT ( 'NONE',  ( 8.423693512792301163, 8.722063941212843119, 0.7998128361456481317 ) ) ;
#37245=CARTESIAN_POINT ( 'NONE',  ( 5.355634372598031767, 6.206993841907870291, -1.199719254218445830 ) ) ;
#37247=CARTESIAN_POINT ( 'NONE',  ( 5.005985031943777308, 6.863401842066294556, -1.599625672291256295 ) ) ;
#37249=CARTESIAN_POINT ( 'NONE',  ( 1.499999999999987121, 3.545833333333356041, -0.8660254037844262731 ) ) ;
#37251=CARTESIAN_POINT ( 'NONE',  ( 1.364683531249986537, 1.217708333674754950, -0.7879004041258239610 ) ) ;
#37257=CARTESIAN_POINT ( 'NONE',  ( 6.493992391265805075, 6.678671999339316656, 1.040834085586084257E-14 ) ) ;
#37260=CARTESIAN_POINT ( 'NONE',  ( -9.664264568442742842, 10.16939683947169115, -0.7998128361456291469 ) ) ;
#37261=CARTESIAN_POINT ( 'NONE',  ( -3.567766978690493307, 7.314145241780881435, 1.040834085586084257E-14 ) ) ;
#37266=CARTESIAN_POINT ( 'NONE',  ( -8.202319746143382773, 9.632089794331152532, 1.082531754730558626 ) ) ;
#37268=CARTESIAN_POINT ( 'NONE',  ( -1.500000000000011324, 4.670833333333353821, 0.8660254037844403729 ) ) ;
#37271=CARTESIAN_POINT ( 'NONE',  ( 7.605760987586388744, 11.81721221891873697, 1.040834085586084257E-14 ) ) ;
#37279=CARTESIAN_POINT ( 'NONE',  ( 8.541273586484978253, 12.90864358430044589, 0.000000000000000000 ) ) ;
#37284=CARTESIAN_POINT ( 'NONE',  ( 6.602457619730749627, 10.64669162308715222, 0.7216878364870438212 ) ) ;
#37285=CARTESIAN_POINT ( 'NONE',  ( 5.587931867126699537, 9.671004278289832001, -0.7998128361456291469 ) ) ;
#37286=CARTESIAN_POINT ( 'NONE',  ( -6.240830780992103755, 6.175390754112560110, 1.040834085586084257E-14 ) ) ;
#37291=CARTESIAN_POINT ( 'NONE',  ( 2.887523530030648988, 6.312601851770308414, 0.000000000000000000 ) ) ;
#37293=CARTESIAN_POINT ( 'NONE',  ( -3.623053363349869382, 5.249981562040033189, 1.599625672291267398 ) ) ;
#37308=CARTESIAN_POINT ( 'NONE',  ( 6.774270308322468459, 11.05506579301824743, 0.7998128361456462443 ) ) ;
#37313=CARTESIAN_POINT ( 'NONE',  ( 1.495402192688908727, 8.717956978849549898, 2.557532308801792720 ) ) ;
#37319=CARTESIAN_POINT ( 'NONE',  ( -3.913499895838973508, 7.717500311787445000, 1.040834085586084257E-14 ) ) ;
#37320=CIRCLE ( 'NONE', #182655, 0.07999999999999994615 ) ;
#37322=CARTESIAN_POINT ( 'NONE',  ( -4.874319919312905647, 5.645460313075203018, -1.199719254218446718 ) ) ;
#37324=CARTESIAN_POINT ( 'NONE',  ( 6.938893903907228378E-15, 10.64264068711930733, 1.214306433183764966E-14 ) ) ;
#37332=CARTESIAN_POINT ( 'NONE',  ( -3.469997250093771246, 6.135748327496311383, -1.199719254218452935 ) ) ;
#37337=CARTESIAN_POINT ( 'NONE',  ( 8.260995669428309540, 8.532249790621511565, 0.7998128361456481317 ) ) ;
#37338=CARTESIAN_POINT ( 'NONE',  ( 0.6823417656249899377, 4.426041667008086655, -1.181850606188754593 ) ) ;
#37344=CARTESIAN_POINT ( 'NONE',  ( 6.792271770322100721, 7.026664608238323950, -0.7216878364870257245 ) ) ;
#37345=CARTESIAN_POINT ( 'NONE',  ( -5.371001409308059138, 9.417918744168066070, -0.7998128361456231517 ) ) ;
#37348=CARTESIAN_POINT ( 'NONE',  ( -6.723954117373590833, 9.932031339322813679, -1.199719254218440723 ) ) ;
#37349=CARTESIAN_POINT ( 'NONE',  ( -4.577849422908604637, 8.492574760035358494, -0.7998128361456281477 ) ) ;
#37350=CYLINDRICAL_SURFACE ( 'NONE', #67917, 0.7500000000000011102 ) ;
#37353=CARTESIAN_POINT ( 'NONE',  ( 1.499999999999822586, 7.388542872122531691, 4.154462424328221104 ) ) ;
#37356=CARTESIAN_POINT ( 'NONE',  ( 6.913768267964901071, 10.15348118167935709, -1.199719254218441611 ) ) ;
#37370=CARTESIAN_POINT ( 'NONE',  ( 1.499999999999990896, 5.275000000000022560, 1.214306433183764966E-14 ) ) ;
#37371=CARTESIAN_POINT ( 'NONE',  ( 4.172158584703322681, 5.890604320285754980, -1.599625672291256295 ) ) ;
#37372=CARTESIAN_POINT ( 'NONE',  ( 5.952193131599331721, 6.902979060742733708, 1.199719254218462483 ) ) ;
#37373=VECTOR ( 'NONE', #35690, 1000.000000000000000 ) ;
#37375=CARTESIAN_POINT ( 'NONE',  ( -6.887178846062105286, 10.97886638714038554, -0.7216878364870267237 ) ) ;
#37377=CARTESIAN_POINT ( 'NONE',  ( 6.643132081016125845, 6.852668304048034287, 0.7216878364870317197 ) ) ;
#37378=CARTESIAN_POINT ( 'NONE',  ( -7.144783764277399030, 11.27940545839156528, 0.7216878364870458196 ) ) ;
#37381=CARTESIAN_POINT ( 'NONE',  ( 6.428537391173986038, 10.65171072301167854, 0.7998128361456462443 ) ) ;
#37386=CARTESIAN_POINT ( 'NONE',  ( 4.161989969715248705, 4.726297878971393196, -2.500000000000000444 ) ) ;
#37387=CARTESIAN_POINT ( 'NONE',  ( -1.364683531250012516, 2.488541667008088876, -0.7879004041258289570 ) ) ;
#37393=CARTESIAN_POINT ( 'NONE',  ( 7.235247531187115833, 11.59287255302699648, -0.7998128361456291469 ) ) ;
#37396=CARTESIAN_POINT ( 'NONE',  ( -9.664264568442742842, 10.16939683947169115, -0.7998128361456291469 ) ) ;
#37401=( BOUNDED_CURVE ( )  B_SPLINE_CURVE ( 2, ( #24616, #41977, #56073 ),
 .UNSPECIFIED., .F., .T. ) 
 B_SPLINE_CURVE_WITH_KNOTS ( ( 3, 3 ),
 ( 0.000000000000000000, 0.002220828379238361412 ),
 .UNSPECIFIED. ) 
 CURVE ( )  GEOMETRIC_REPRESENTATION_ITEM ( )  RATIONAL_B_SPLINE_CURVE ( ( 1.000000000000000000, 0.9285916995105953919, 0.9333044775364149892 ) ) 
 REPRESENTATION_ITEM ( '' )  );
#37403=CARTESIAN_POINT ( 'NONE',  ( 8.866142388332804103, 12.43125098877526113, -1.199719254218446718 ) ) ;
#37407=CARTESIAN_POINT ( 'NONE',  ( -8.859363311525973117, 12.42334206583395328, -1.199719254218446718 ) ) ;
#37412=CARTESIAN_POINT ( 'NONE',  ( 5.639205186016292615, 6.133955845365204773, 0.8069632701028349731 ) ) ;
#37414=CARTESIAN_POINT ( 'NONE',  ( -4.172158584703340445, 5.890604320285754980, -1.599625672291256295 ) ) ;
#37418=CARTESIAN_POINT ( 'NONE',  ( 6.262976894508937242, 9.394224579314053969, -1.199719254218440723 ) ) ;
#37420=CARTESIAN_POINT ( 'NONE',  ( 5.612185521052973414, 8.634967976948757951, -1.199719254218440723 ) ) ;
#37421=CARTESIAN_POINT ( 'NONE',  ( 3.811813743736467419, 7.598866467667865443, 1.040834085586084257E-14 ) ) ;
#37423=CARTESIAN_POINT ( 'NONE',  ( -7.537970219518083326, 9.817384560903001045, -1.443375672974059665 ) ) ;
#37431=CARTESIAN_POINT ( 'NONE',  ( -5.704936041347759001, 6.126156357109620032, -0.7369488182252960096 ) ) ;
#37433=CARTESIAN_POINT ( 'NONE',  ( 4.036703073083682369, 7.757870032734638599, 0.4269520307091502209 ) ) ;
#37435=CARTESIAN_POINT ( 'NONE',  ( 5.341549334104188418, 7.254893527920112994, 1.443375672974062551 ) ) ;
#37451=CARTESIAN_POINT ( 'NONE',  ( -7.971831134711019118, 12.24429405723079967, 0.000000000000000000 ) ) ;
#37455=CARTESIAN_POINT ( 'NONE',  ( 9.094822116668764167, 9.505047312402055582, 0.7998128361456462443 ) ) ;
#37459=CARTESIAN_POINT ( 'NONE',  ( -1.500000000000013101, 2.160416667349489561, -0.8660254037844313801 ) ) ;
#37460=CARTESIAN_POINT ( 'NONE',  ( -4.308793891044708779, 3.921347715840572956, 1.214306433183764966E-14 ) ) ;
#37461=CARTESIAN_POINT ( 'NONE',  ( -6.013204822860843457, 6.974159367214481264, -1.199719254218446718 ) ) ;
#37464=CARTESIAN_POINT ( 'NONE',  ( -9.169391961543940539, 9.592045464756413509, 1.040834085586084257E-14 ) ) ;
#37467=EDGE_CURVE ( 'NONE', #180436, #115335, #190491, .T. ) ;
#37469=CARTESIAN_POINT ( 'NONE',  ( 7.949158136313996259, 8.168439335321471262, 1.040834085586084257E-14 ) ) ;
#37471=CARTESIAN_POINT ( 'NONE',  ( -6.039267359883488950, 9.133230122250985517, 1.199719254218452047 ) ) ;
#37473=CARTESIAN_POINT ( 'NONE',  ( 8.127223016387999266, 11.56917838817298616, 1.199719254218460707 ) ) ;
#37474=CARTESIAN_POINT ( 'NONE',  ( -1.364683531250010295, 5.488541667008087543, -0.7879004041258300672 ) ) ;
#37476=CARTESIAN_POINT ( 'NONE',  ( -4.837049282416619356, 5.053169767094015441, -0.9039271902641244916 ) ) ;
#37481=CARTESIAN_POINT ( 'NONE',  ( -8.541273586929371220, 9.067166727613487964, 0.7216878364870438212 ) ) ;
#37484=CARTESIAN_POINT ( 'NONE',  ( -0.6823417656250212460, 4.613541667008086655, 1.181850606188767472 ) ) ;
#37490=CARTESIAN_POINT ( 'NONE',  ( -1.001543065824772872E-14, 5.071875000341421469, 1.575800808251672791 ) ) ;
#37495=CARTESIAN_POINT ( 'NONE',  ( -4.921246571636213929, 4.843801876438091902, 0.7216878364870317197 ) ) ;
#37497=CARTESIAN_POINT ( 'NONE',  ( 3.890826896997583884, 4.602014803661035103, -1.082531754730543083 ) ) ;
#37498=CARTESIAN_POINT ( 'NONE',  ( -1.364683531249997417, 5.071875000341417916, 1.214306433183764966E-14 ) ) ;
#37503=CARTESIAN_POINT ( 'NONE',  ( 0.6823417656249882723, 1.176041667008083325, -1.181850606188749264 ) ) ;
#37504=CARTESIAN_POINT ( 'NONE',  ( -2.819732761962332024, 6.233512622357263666, -0.7216878364870267237 ) ) ;
#37505=CARTESIAN_POINT ( 'NONE',  ( 4.449046963578762615, 8.342305224150557308, -0.7998128361456231517 ) ) ;
#37508=CARTESIAN_POINT ( 'NONE',  ( 4.311129659465574804, 7.013106455143060636, -1.082531754730548412 ) ) ;
#37514=CARTESIAN_POINT ( 'NONE',  ( -7.971831135155409420, 11.28392484344787405, 1.082531754730549967 ) ) ;
#37519=CARTESIAN_POINT ( 'NONE',  ( -9.104463846776669200, 10.58062822844965645, -1.199719254218441611 ) ) ;
#37520=CARTESIAN_POINT ( 'NONE',  ( -4.975479186090865369, 6.827811688571220117, 1.443375672974064550 ) ) ;
#37521=CARTESIAN_POINT ( 'NONE',  ( -0.6823417656250003738, 1.780208333674752952, -1.181850606188749264 ) ) ;
#37536=AXIS2_PLACEMENT_3D ( 'NONE', #148434, #66067, #166809 ) ;
#37544=CARTESIAN_POINT ( 'NONE',  ( -1.201851678989727383E-14, 3.259375000341420581, -1.575800808251660134 ) ) ;
#37551=CARTESIAN_POINT ( 'NONE',  ( 10.23370702021670020, 10.83374636654133383, 0.7998128361456462443 ) ) ;
#37554=CARTESIAN_POINT ( 'NONE',  ( -1.364683531250014514, 1.488541667008084435, -0.7879004041258289570 ) ) ;
#37560=ORIENTED_EDGE ( 'NONE', *, *, #113892, .T. ) ;
#37565=CARTESIAN_POINT ( 'NONE',  ( 5.494078562035752178, 7.432844293840273231, -1.599625672291262513 ) ) ;
#37568=ORIENTED_EDGE ( 'NONE', *, *, #8637, .T. ) ;
#37572=CARTESIAN_POINT ( 'NONE',  ( 6.272618624616828953, 10.46980549536166016, 1.040834085586084257E-14 ) ) ;
#37576=CARTESIAN_POINT ( 'NONE',  ( -4.796887421136680985, 4.490790167614548523, 1.214306433183764966E-14 ) ) ;
#37577=CARTESIAN_POINT ( 'NONE',  ( 8.945682426918439845, 9.331051007693339727, 1.040834085586084257E-14 ) ) ;
#37582=ORIENTED_EDGE ( 'NONE', *, *, #38322, .F. ) ;
#37590=CARTESIAN_POINT ( 'NONE',  ( -6.887178846062105286, 10.97886638714038554, -0.7216878364870267237 ) ) ;
#37594=CARTESIAN_POINT ( 'NONE',  ( -9.592557376868645846, 11.15007068022363157, -1.199719254218441611 ) ) ;
#37599=CARTESIAN_POINT ( 'NONE',  ( -2.611917148927046295, 6.198987107056845858, 1.040834085586084257E-14 ) ) ;
#37602=CARTESIAN_POINT ( 'NONE',  ( 10.18233705906309972, 11.83814697611718714, 1.199719254218450271 ) ) ;
#37603=CARTESIAN_POINT ( 'NONE',  ( 3.354752944377597856, 6.001296637494123232, -1.199719254218446718 ) ) ;
#37609=CARTESIAN_POINT ( 'NONE',  ( 4.202664430556257713, 4.965825259479493603, 1.082531754730560403 ) ) ;
#37612=CARTESIAN_POINT ( 'NONE',  ( -4.066556009095094737, 6.831733546331167695, 1.199719254218464037 ) ) ;
#37615=CARTESIAN_POINT ( 'NONE',  ( -10.13202086811422475, 10.71511252242175161, -0.7998128361456291469 ) ) ;
#37620=CARTESIAN_POINT ( 'NONE',  ( 8.649738815838679429, 10.15407870897571563, -1.082531754730543083 ) ) ;
#37621=CARTESIAN_POINT ( 'NONE',  ( 1.364683531249992088, 5.446875000341417916, 1.214306433183764966E-14 ) ) ;
#37623=CARTESIAN_POINT ( 'NONE',  ( 4.310602774141044868, 7.116454772218158809, -1.199719254218452047 ) ) ;
#37638=CARTESIAN_POINT ( 'NONE',  ( -0.6823417656250003738, 2.280208333674753174, -1.181850606188749264 ) ) ;
#37640=CARTESIAN_POINT ( 'NONE',  ( 2.866659414285625651, 5.431854185720147221, -1.199719254218446718 ) ) ;
#37642=CARTESIAN_POINT ( 'NONE',  ( -5.178851490740209229, 7.065079377328788546, 1.443375672974064550 ) ) ;
#37644=CARTESIAN_POINT ( 'NONE',  ( -5.626270559546828309, 7.587068290936515247, 1.443375672974064550 ) ) ;
#37648=VERTEX_POINT ( 'NONE', #31215 ) ;
#37650=CARTESIAN_POINT ( 'NONE',  ( 6.471319392424407901, 6.444294134116939077, 0.7998128361456341429 ) ) ;
#37662=CARTESIAN_POINT ( 'NONE',  ( 5.738125327081736060, 7.717565519727259904, 1.599625672291267398 ) ) ;
#37663=( LENGTH_UNIT ( ) NAMED_UNIT ( * ) SI_UNIT ( .MILLI., .METRE. ) );
#37665=CARTESIAN_POINT ( 'NONE',  ( -3.952365473583647315, 4.569846793057691592, 1.199719254218462483 ) ) ;
#37667=CARTESIAN_POINT ( 'NONE',  ( -5.412729640353771465, 7.337937218544611895, 1.599625672291269396 ) ) ;
#37671=CARTESIAN_POINT ( 'NONE',  ( 7.182068686937156166, 9.402166106225269715, 1.599625672291281386 ) ) ;
#37674=CARTESIAN_POINT ( 'NONE',  ( -7.237355071596549116, 7.338002426484427687, 1.040834085586084257E-14 ) ) ;
#37675=CARTESIAN_POINT ( 'NONE',  ( 5.300874872818821082, 9.128178418356554857, 0.7216878364870438212 ) ) ;
#37676=CARTESIAN_POINT ( 'NONE',  ( 4.867170269011318773, 6.911508770089412224, 1.419371323323643130 ) ) ;
#37677=CARTESIAN_POINT ( 'NONE',  ( -4.406563619641430840, 5.099744630125142564, -1.199719254218446718 ) ) ;
#37681=CARTESIAN_POINT ( 'NONE',  ( -5.052384799386910430, 9.046199365926717917, 1.214306433183764966E-14 ) ) ;
#37684=CARTESIAN_POINT ( 'NONE',  ( -1.364683531250012516, 2.488541667008088876, -0.7879004041258289570 ) ) ;
#37686=CARTESIAN_POINT ( 'NONE',  ( -4.270455198624581783, 7.926022131796578662, 1.040834085586084257E-14 ) ) ;
#37693=CARTESIAN_POINT ( 'NONE',  ( 6.114890974963323345, 7.092793211334054604, 1.199719254218462483 ) ) ;
#37697=CARTESIAN_POINT ( 'NONE',  ( 1.364683531249988757, 2.446875000341415696, 1.214306433183764966E-14 ) ) ;
#37704=CARTESIAN_POINT ( 'NONE',  ( -5.596818484342970912, 5.424043074688562172, -0.7998128361456221525 ) ) ;
#37705=CARTESIAN_POINT ( 'NONE',  ( -6.019457014343129408, 9.966524250134902729, 0.000000000000000000 ) ) ;
#37713=CARTESIAN_POINT ( 'NONE',  ( -6.819388077549415783, 10.89977715720891815, 0.7216878364870458196 ) ) ;
#37716=CARTESIAN_POINT ( 'NONE',  ( -6.521108698048779573, 8.631046119188804155, -1.443375672974058777 ) ) ;
#37729=CARTESIAN_POINT ( 'NONE',  ( -4.855791571988752331, 8.816840600628864877, 0.7998128361456481317 ) ) ;
#37734=CARTESIAN_POINT ( 'NONE',  ( 4.172158584703322681, 5.890604320285754980, -1.599625672291256295 ) ) ;
#37738=CARTESIAN_POINT ( 'NONE',  ( 5.120175567455225618, 9.125288595339771547, -0.7998128361456281477 ) ) ;
#37744=CARTESIAN_POINT ( 'NONE',  ( -5.273758566035884776, 5.255065869904374409, 0.000000000000000000 ) ) ;
#37752=CARTESIAN_POINT ( 'NONE',  ( -1.364683531250000748, 1.009375000341421247, 0.000000000000000000 ) ) ;
#37754=B_SPLINE_CURVE_WITH_KNOTS ( 'NONE', 3,
 ( #70798, #136911, #74037, #139049 ),
 .UNSPECIFIED., .F., .F.,
 ( 4, 4 ),
 ( 0.000000000000000000, 0.002003498272494338549 ),
 .UNSPECIFIED. ) ;
#37755=CARTESIAN_POINT ( 'NONE',  ( -8.064402442030170093, 8.302891025323665630, 0.7998128361456602331 ) ) ;
#37757=CARTESIAN_POINT ( 'NONE',  ( 6.446011968293428041, 9.607765498729298415, -1.199719254218440723 ) ) ;
#37759=CARTESIAN_POINT ( 'NONE',  ( -6.256197817702116026, 9.386315656372753224, -1.199719254218440723 ) ) ;
#37762=CARTESIAN_POINT ( 'NONE',  ( 0.6823417656249899377, 4.676041667008086655, -1.181850606188754593 ) ) ;
#37765=CARTESIAN_POINT ( 'NONE',  ( 7.944714827928039291, 11.25228915168265864, 1.082531754730557072 ) ) ;
#37768=CARTESIAN_POINT ( 'NONE',  ( -1.402160292154681736E-14, -0.4906249996585810846, -1.575800808251665908 ) ) ;
#37770=CARTESIAN_POINT ( 'NONE',  ( 6.873620692004076105, 10.00267932643801672, -1.082531754730537976 ) ) ;
#37773=CARTESIAN_POINT ( 'NONE',  ( -6.412643469583822586, 6.583764924043652655, 1.040834085586084257E-14 ) ) ;
#37775=CARTESIAN_POINT ( 'NONE',  ( -1.364683531249997417, 4.009375000341424133, 1.214306433183764966E-14 ) ) ;
#37779=CARTESIAN_POINT ( 'NONE',  ( -5.880485940025243607, 7.883652901494672349, 1.599625672291269396 ) ) ;
#37780=CARTESIAN_POINT ( 'NONE',  ( -1.364683531250010295, 5.551041667008087543, -0.7879004041258300672 ) ) ;
#37787=CARTESIAN_POINT ( 'NONE',  ( 6.611572464958476836, 10.86525164242692298, 0.7998128361456462443 ) ) ;
#37790=CARTESIAN_POINT ( 'NONE',  ( 1.499999999999989120, 2.525000000000020339, 1.214306433183764966E-14 ) ) ;
#37793=FACE_OUTER_BOUND ( 'NONE', #66991, .T. ) ;
#37796=CARTESIAN_POINT ( 'NONE',  ( 4.989037340148863464, 8.764367963574922982, -0.7216878364870257245 ) ) ;
#37797=CARTESIAN_POINT ( 'NONE',  ( 1.364683531249986537, -0.8239583329919186738, 0.7879004041258500513 ) ) ;
#37804=CARTESIAN_POINT ( 'NONE',  ( 0.7499999999999885647, 0.8166666666666877461, -1.299038105676652899 ) ) ;
#37805=CARTESIAN_POINT ( 'NONE',  ( 8.288111976655649471, 8.563885482386732306, -0.7998128361456291469 ) ) ;
#37806=CARTESIAN_POINT ( 'NONE',  ( -10.00321840878439339, 10.56484298653695397, 1.040834085586084257E-14 ) ) ;
#37808=CARTESIAN_POINT ( 'NONE',  ( 0.6823417656249864960, -0.5739583329919112353, -1.181850606188749264 ) ) ;
#37809=CARTESIAN_POINT ( 'NONE',  ( 1.499999999999989120, 1.775000000000019673, 0.000000000000000000 ) ) ;
#37811=CARTESIAN_POINT ( 'NONE',  ( 6.322179702674084467, 6.270297829408224111, 1.040834085586084257E-14 ) ) ;
#37817=CARTESIAN_POINT ( 'NONE',  ( -1.364683531249997417, 5.759375000341418804, 1.214306433183764966E-14 ) ) ;
#37819=CARTESIAN_POINT ( 'NONE',  ( -8.076906825439122528, 10.44614393447756129, -1.599625672291263179 ) ) ;
#37820=CARTESIAN_POINT ( 'NONE',  ( -5.422898255786203769, 6.389431388914436738, -1.082531754730544860 ) ) ;
#37828=CARTESIAN_POINT ( 'NONE',  ( 6.238723240582662477, 10.43026088065513513, -0.7998128361456291469 ) ) ;
#37833=CARTESIAN_POINT ( 'NONE',  ( 5.770966940911189447, 9.884545197705074671, -0.7998128361456291469 ) ) ;
#37834=CARTESIAN_POINT ( 'NONE',  ( 6.277061933002774374, 9.306694107603160404, 1.082531754730558626 ) ) ;
#37836=( BOUNDED_SURFACE ( )  B_SPLINE_SURFACE ( 1, 2, ( 
 ( #89235, #75103, #172613, #6868, #190961, #122886, #42626, #188845, #10089, #76163, #40481, #24189, #90292, #57782, #123943, #60984, #30634, #209336, #96719, #161702, #210419, #109808, #162768, #15411, #131374, #213598, #65224, #176872, #45823, #145487, #14346, #28484, #111944, #43691, #175817, #146535, #27410, #44759, #80436, #113007, #196323, #180074, #163832, #212554, #81501, #127138, #93508, #13295, #64193, #47967, #211482, #79368, #159549, #177946, #128216, #110867, #193110, #130334, #11146, #31697, #94575, #97772, #114083, #160618, #147579, #78290, #95652, #29560, #77223, #143342, #12219, #144417, #62061, #63118, #194178, #129283, #195258, #46893, #179017, #201612, #135591, #197370, #4471, #151840, #53261, #148640, #51134, #32747, #20733, #167020, #199488, #117256, #184310, #33806, #99885, #206, #165947, #181126, #50071, #116192, #66276, #183255, #198425, #182177, #17531, #152892, #83620, #86828, #149702, #70542, #19681, #49012, #103082, #1283, #115131, #67341, #98829, #164878, #169138, #18614, #16473, #200551, #36999, #82553, #35934, #132424, #102013, #3417, #84694, #34859, #133486, #100933, #85760, #150781, #2344, #68420, #134547, #52198, #118324, #168082, #69483, #119392, #185380, #139869, #190710, #186447, #189653, #71616, #41304, #91117, #23942, #188588, #204813, #120474, #57534, #153969, #205900, #87896, #25015, #140954, #137729, #105231, #203749, #138793, #6618, #5536, #123691, #55393, #107412, #40220, #88978, #202686, #173436, #108482, #9835, #92197, #158246, #121548, #56464, #90046, #157176, #187519, #122626, #136661, #54335, #8770, #38083, #39150, #74853, #206966, #58595, #124750, #42371, #174506, #26082, #171272, #104155, #106330, #170203, #21787, #156105, #172352, #22865, #7690, #72698, #155033, #73773, #112747, #191776, #212286, #159289, #130076, #14079, #143090, #46624, #110616, #127965, #210154, #30371, #31436, #179817, #60719, #96458, #45563, #176616, #193917, #126882, #162508, #111680, #80169, #146275, #75911, #97514, #63920, #196071, #27151, #144162, #125814, #113817, #177687, #78038, #61796, #62851, #192840, #44499, #93255, #28228, #59657, #209082, #94321, #10888, #29298, #76963, #160362, #11965, #163571, #95392, #142014, #43432, #129013, #161443, #194990, #47703, #13024, #79101, #145219, #109556, #211225, #178759, #208029, #175560, #118069, #19419, #16208, #198170, #82291, #17277, #99622, #32488, #2082, #180867, #68155, #133219, #181917, #81240, #134289, #201354, #102823, #185111, #36737, #148384, #83353, #116994, #200294, #214385, #149438, #15154, #147322, #184055, #213349, #66015, #51946, #84432, #167819, #151584, #135340, #35674, #52995, #98562, #64972, #199225, #101752, #85497, #182994, #50872, #131125, #1020, #165688, #132164, #164623, #3151, #197114, #69221, #49803, #119131, #48753, #115929, #114866, #33549, #67085, #34611, #100680, #166758, #18354, #150521, #189395, #138531 ),
 ( #37817, #120209, #58334, #21527, #172094, #73508, #203485, #202419, #107147, #205633, #90854, #4218, #154776, #123433, #71355, #87638, #186184, #57271, #136403, #70287, #20482, #74588, #89796, #22609, #42107, #137471, #153709, #5278, #55138, #121283, #152631, #187259, #103894, #122366, #140691, #6360, #168878, #41037, #124490, #169942, #190449, #38886, #23686, #139611, #104971, #54074, #173173, #24752, #156918, #171012, #72429, #8507, #88717, #204554, #56203, #206707, #188322, #39962, #86569, #106070, #155842, #7427, #195794, #76701, #175299, #159033, #142818, #10626, #91927, #60455, #59394, #61525, #79896, #94055, #108220, #128743, #63659, #157987, #25817, #208825, #62581, #174245, #9575, #126612, #26885, #125550, #75652, #46356, #192575, #141759, #176354, #95118, #144948, #129813, #44230, #43176, #162236, #77773, #161167, #207767, #146005, #13822, #110351, #27962, #12753, #160096, #78827, #11699, #143893, #191511, #109289, #92988, #45293, #209887, #127691, #193651, #111413, #177417, #29035, #210954, #194717, #30095, #112476, #178485, #96185, #212015, #47432, #14879, #85230, #198957, #116725, #80972, #132954, #50600, #97244, #135079, #163298, #49534, #83089, #147063, #213083, #167556, #48491, #64714, #130857, #182725, #34344, #181654, #149168, #31171, #101486, #99365, #19157, #98297, #84167, #196853, #18079, #179550, #15944, #131897, #115660, #151319, #100417, #2887, #67881, #745, #114609, #180600, #32225, #150255, #164360, #183798, #82028, #68959, #200034, #148121, #1823, #214122, #165417, #33280, #134027, #113547, #65751, #197905, #51686, #17013, #66811, #166488, #117808, #35408, #22344, #205376, #139346, #201092, #8251, #155584, #57013, #152376, #54878, #36481, #24487, #170756, #203234, #121032, #188063, #37554, #103634, #3955, #169686, #184853, #53814, #119943, #70022, #186999, #202154, #185919, #21274, #156659, #87380, #90599, #153448, #77258, #23421, #52733, #106887, #5021, #118867, #71095, #102556, #168617, #172913, #88457, #20219, #204289, #40781, #86306, #39692, #136138, #105803, #7169, #154517, #38630, #104707, #137212, #122099, #6098, #55946, #72167, #89532, #123183, #138275, #171827, #73239, #189143, #13324, #160651, #130366, #94608, #196356, #46923, #95679, #209371, #47997, #115165, #16505, #98860, #164912, #62089, #145515, #30666, #114114, #128247, #211514, #143372, #61015, #31731, #127173, #144448, #180107, #212585, #81532, #65257, #49045, #97804, #181159, #12249, #193142, #113041, #163865, #147613, #96749, #179047, #44791, #63151, #79398, #29593, #32783, #110897, #176903, #162799, #28517, #146566, #197404, #78326, #15443, #210451, #213631, #131404, #14376, #195291, #129315, #194211, #64224, #45856, #111977, #177978, #161733, #80466, #83651, #51170, #149740, #84728, #167057, #99920, #69521, #33839, #135628, #200586, #34895, #148674, #201648, #54374, #170240, #38120, #104192, #1317, #150816 ) ),
 .UNSPECIFIED., .F., .F., .T. ) 
 B_SPLINE_SURFACE_WITH_KNOTS ( ( 2, 2 ),
 ( 3, 2, 2, 2, 2, 2, 2, 2, 2, 2, 2, 2, 2, 2, 2, 2, 2, 2, 2, 2, 2, 2, 2, 2, 2, 2, 2, 2, 2, 2, 2, 2, 2, 2, 2, 2, 2, 2, 2, 2, 2, 2, 2, 2, 2, 2, 2, 2, 2, 2, 2, 2, 2, 2, 2, 2, 2, 2, 2, 2, 2, 2, 2, 2, 2, 2, 2, 2, 2, 2, 2, 2, 2, 2, 2, 2, 2, 2, 2, 2, 2, 2, 2, 2, 2, 2, 2, 2, 2, 2, 2, 2, 2, 2, 2, 2, 2, 2, 2, 2, 2, 2, 2, 2, 2, 2, 2, 2, 2, 2, 2, 2, 2, 2, 2, 2, 2, 2, 2, 2, 2, 2, 2, 2, 2, 2, 2, 2, 2, 2, 2, 2, 2, 2, 2, 2, 2, 2, 2, 2, 2, 2, 2, 2, 2, 2, 2, 2, 2, 2, 2, 2, 2, 2, 2, 2, 2, 2, 2, 2, 2, 2, 2, 2, 2, 2, 2, 2, 3 ),
 ( 0.000000000000000000, 1.000000000000000000 ),
 ( 0.000000000000000000, 0.005952380952380952051, 0.01190476190476190410, 0.01785714285714285615, 0.02380952380952380820, 0.02976190476190476025, 0.03571428571428571230, 0.04166666666666666435, 0.04761904761904761640, 0.05357142857142856845, 0.05952380952380952051, 0.06547619047619047949, 0.07142857142857142461, 0.07738095238095238360, 0.08333333333333332871, 0.08928571428571428770, 0.09523809523809523281, 0.1011904761904761918, 0.1071428571428571369, 0.1130952380952380959, 0.1190476190476190410, 0.1250000000000000000, 0.1309523809523809590, 0.1369047619047619180, 0.1428571428571428492, 0.1488095238095238082, 0.1547619047619047672, 0.1607142857142857262, 0.1666666666666666574, 0.1726190476190476164, 0.1785714285714285754, 0.1845238095238095344, 0.1904761904761904656, 0.1964285714285714246, 0.2023809523809523836, 0.2083333333333333426, 0.2142857142857142738, 0.2202380952380952328, 0.2261904761904761918, 0.2321428571428571508, 0.2380952380952380820, 0.2440476190476190410, 0.2500000000000000000, 0.2559523809523809312, 0.2619047619047619180, 0.2678571428571428492, 0.2738095238095238360, 0.2797619047619047672, 0.2857142857142856984, 0.2916666666666666852, 0.2976190476190476164, 0.3035714285714285476, 0.3095238095238095344, 0.3154761904761904656, 0.3214285714285714524, 0.3273809523809523836, 0.3333333333333333148, 0.3392857142857143016, 0.3452380952380952328, 0.3511904761904761640, 0.3571428571428571508, 0.3630952380952380820, 0.3690476190476190688, 0.3750000000000000000, 0.3809523809523809312, 0.3869047619047619180, 0.3928571428571428492, 0.3988095238095238360, 0.4047619047619047672, 0.4107142857142856984, 0.4166666666666666852, 0.4226190476190476164, 0.4285714285714285476, 0.4345238095238095344, 0.4404761904761904656, 0.4464285714285714524, 0.4523809523809523836, 0.4583333333333333148, 0.4642857142857143016, 0.4702380952380952328, 0.4761904761904761640, 0.4821428571428571508, 0.4880952380952380820, 0.4940476190476190688, 0.5000000000000000000, 0.5059523809523809312, 0.5119047619047618625, 0.5178571428571429047, 0.5238095238095238360, 0.5297619047619047672, 0.5357142857142856984, 0.5416666666666666297, 0.5476190476190476719, 0.5535714285714286031, 0.5595238095238095344, 0.5654761904761904656, 0.5714285714285713969, 0.5773809523809523281, 0.5833333333333333703, 0.5892857142857143016, 0.5952380952380952328, 0.6011904761904761640, 0.6071428571428570953, 0.6130952380952381375, 0.6190476190476190688, 0.6250000000000000000, 0.6309523809523809312, 0.6369047619047618625, 0.6428571428571429047, 0.6488095238095238360, 0.6547619047619047672, 0.6607142857142856984, 0.6666666666666666297, 0.6726190476190476719, 0.6785714285714286031, 0.6845238095238095344, 0.6904761904761904656, 0.6964285714285713969, 0.7023809523809523281, 0.7083333333333333703, 0.7142857142857143016, 0.7202380952380952328, 0.7261904761904761640, 0.7321428571428570953, 0.7380952380952381375, 0.7440476190476190688, 0.7500000000000000000, 0.7559523809523809312, 0.7619047619047618625, 0.7678571428571429047, 0.7738095238095238360, 0.7797619047619047672, 0.7857142857142856984, 0.7916666666666666297, 0.7976190476190476719, 0.8035714285714286031, 0.8095238095238095344, 0.8154761904761904656, 0.8214285714285713969, 0.8273809523809523281, 0.8333333333333333703, 0.8392857142857143016, 0.8452380952380952328, 0.8511904761904761640, 0.8571428571428570953, 0.8630952380952381375, 0.8690476190476190688, 0.8750000000000000000, 0.8809523809523809312, 0.8869047619047618625, 0.8928571428571429047, 0.8988095238095238360, 0.9047619047619047672, 0.9107142857142856984, 0.9166666666666666297, 0.9226190476190476719, 0.9285714285714286031, 0.9345238095238095344, 0.9404761904761904656, 0.9464285714285713969, 0.9523809523809523281, 0.9583333333333333703, 0.9642857142857143016, 0.9702380952380952328, 0.9761904761904761640, 0.9821428571428570953, 0.9880952380952381375, 0.9940476190476190688, 1.000000000000000000 ),
 .UNSPECIFIED. ) 
 GEOMETRIC_REPRESENTATION_ITEM ( )  RATIONAL_B_SPLINE_SURFACE ( (
 ( 1.000000000000000000, 0.8660254037844387076, 1.000000000000000000, 0.8660254037844387076, 1.000000000000000000, 0.8660254037844387076, 1.000000000000000000, 0.8660254037844387076, 1.000000000000000000, 0.8660254037844387076, 1.000000000000000000, 0.8660254037844387076, 1.000000000000000000, 0.8660254037844387076, 1.000000000000000000, 0.8660254037844387076, 1.000000000000000000, 0.8660254037844387076, 1.000000000000000000, 0.8660254037844387076, 1.000000000000000000, 0.8660254037844387076, 1.000000000000000000, 0.8660254037844387076, 1.000000000000000000, 0.8660254037844387076, 1.000000000000000000, 0.8660254037844387076, 1.000000000000000000, 0.8660254037844387076, 1.000000000000000000, 0.8660254037844387076, 1.000000000000000000, 0.8660254037844387076, 1.000000000000000000, 0.8660254037844387076, 1.000000000000000000, 0.8660254037844387076, 1.000000000000000000, 0.8660254037844387076, 1.000000000000000000, 0.8660254037844387076, 1.000000000000000000, 0.8660254037844387076, 1.000000000000000000, 0.8660254037844387076, 1.000000000000000000, 0.8660254037844387076, 1.000000000000000000, 0.8660254037844387076, 1.000000000000000000, 0.8660254037844387076, 1.000000000000000000, 0.8660254037844387076, 1.000000000000000000, 0.8660254037844387076, 1.000000000000000000, 0.8660254037844387076, 1.000000000000000000, 0.8660254037844387076, 1.000000000000000000, 0.8660254037844387076, 1.000000000000000000, 0.8660254037844387076, 1.000000000000000000, 0.8660254037844387076, 1.000000000000000000, 0.8660254037844387076, 1.000000000000000000, 0.8660254037844387076, 1.000000000000000000, 0.8660254037844387076, 1.000000000000000000, 0.8660254037844387076, 1.000000000000000000, 0.8660254037844387076, 1.000000000000000000, 0.8660254037844387076, 1.000000000000000000, 0.8660254037844387076, 1.000000000000000000, 0.8660254037844387076, 1.000000000000000000, 0.8660254037844387076, 1.000000000000000000, 0.8660254037844387076, 1.000000000000000000, 0.8660254037844387076, 1.000000000000000000, 0.8660254037844387076, 1.000000000000000000, 0.8660254037844387076, 1.000000000000000000, 0.8660254037844387076, 1.000000000000000000, 0.8660254037844387076, 1.000000000000000000, 0.8660254037844387076, 1.000000000000000000, 0.8660254037844387076, 1.000000000000000000, 0.8660254037844387076, 1.000000000000000000, 0.8660254037844387076, 1.000000000000000000, 0.8660254037844387076, 1.000000000000000000, 0.8660254037844387076, 1.000000000000000000, 0.8660254037844387076, 1.000000000000000000, 0.8660254037844387076, 1.000000000000000000, 0.8660254037844387076, 1.000000000000000000, 0.8660254037844387076, 1.000000000000000000, 0.8660254037844387076, 1.000000000000000000, 0.8660254037844387076, 1.000000000000000000, 0.8660254037844387076, 1.000000000000000000, 0.8660254037844387076, 1.000000000000000000, 0.8660254037844387076, 1.000000000000000000, 0.8660254037844387076, 1.000000000000000000, 0.8660254037844387076, 1.000000000000000000, 0.8660254037844387076, 1.000000000000000000, 0.8660254037844387076, 1.000000000000000000, 0.8660254037844387076, 1.000000000000000000, 0.8660254037844387076, 1.000000000000000000, 0.8660254037844387076, 1.000000000000000000, 0.8660254037844387076, 1.000000000000000000, 0.8660254037844387076, 1.000000000000000000, 0.8660254037844387076, 1.000000000000000000, 0.8660254037844387076, 1.000000000000000000, 0.8660254037844387076, 1.000000000000000000, 0.8660254037844387076, 1.000000000000000000, 0.8660254037844387076, 1.000000000000000000, 0.8660254037844387076, 1.000000000000000000, 0.8660254037844387076, 1.000000000000000000, 0.8660254037844387076, 1.000000000000000000, 0.8660254037844387076, 1.000000000000000000, 0.8660254037844387076, 1.000000000000000000, 0.8660254037844387076, 1.000000000000000000, 0.8660254037844387076, 1.000000000000000000, 0.8660254037844387076, 1.000000000000000000, 0.8660254037844387076, 1.000000000000000000, 0.8660254037844387076, 1.000000000000000000, 0.8660254037844387076, 1.000000000000000000, 0.8660254037844387076, 1.000000000000000000, 0.8660254037844387076, 1.000000000000000000, 0.8660254037844387076, 1.000000000000000000, 0.8660254037844387076, 1.000000000000000000, 0.8660254037844387076, 1.000000000000000000, 0.8660254037844387076, 1.000000000000000000, 0.8660254037844387076, 1.000000000000000000, 0.8660254037844387076, 1.000000000000000000, 0.8660254037844387076, 1.000000000000000000, 0.8660254037844387076, 1.000000000000000000, 0.8660254037844387076, 1.000000000000000000, 0.8660254037844387076, 1.000000000000000000, 0.8660254037844387076, 1.000000000000000000, 0.8660254037844387076, 1.000000000000000000, 0.8660254037844387076, 1.000000000000000000, 0.8660254037844387076, 1.000000000000000000, 0.8660254037844387076, 1.000000000000000000, 0.8660254037844387076, 1.000000000000000000, 0.8660254037844387076, 1.000000000000000000, 0.8660254037844387076, 1.000000000000000000, 0.8660254037844387076, 1.000000000000000000, 0.8660254037844387076, 1.000000000000000000, 0.8660254037844387076, 1.000000000000000000, 0.8660254037844387076, 1.000000000000000000, 0.8660254037844387076, 1.000000000000000000, 0.8660254037844387076, 1.000000000000000000, 0.8660254037844387076, 1.000000000000000000, 0.8660254037844387076, 1.000000000000000000, 0.8660254037844387076, 1.000000000000000000, 0.8660254037844387076, 1.000000000000000000, 0.8660254037844387076, 1.000000000000000000, 0.8660254037844387076, 1.000000000000000000, 0.8660254037844387076, 1.000000000000000000, 0.8660254037844387076, 1.000000000000000000, 0.8660254037844387076, 1.000000000000000000, 0.8660254037844387076, 1.000000000000000000, 0.8660254037844387076, 1.000000000000000000, 0.8660254037844387076, 1.000000000000000000, 0.8660254037844387076, 1.000000000000000000, 0.8660254037844387076, 1.000000000000000000, 0.8660254037844387076, 1.000000000000000000, 0.8660254037844387076, 1.000000000000000000, 0.8660254037844387076, 1.000000000000000000, 0.8660254037844387076, 1.000000000000000000, 0.8660254037844387076, 1.000000000000000000, 0.8660254037844387076, 1.000000000000000000, 0.8660254037844387076, 1.000000000000000000, 0.8660254037844387076, 1.000000000000000000, 0.8660254037844387076, 1.000000000000000000, 0.8660254037844387076, 1.000000000000000000, 0.8660254037844387076, 1.000000000000000000, 0.8660254037844387076, 1.000000000000000000, 0.8660254037844387076, 1.000000000000000000, 0.8660254037844387076, 1.000000000000000000, 0.8660254037844387076, 1.000000000000000000, 0.8660254037844387076, 1.000000000000000000, 0.8660254037844387076, 1.000000000000000000, 0.8660254037844387076, 1.000000000000000000, 0.8660254037844387076, 1.000000000000000000, 0.8660254037844387076, 1.000000000000000000, 0.8660254037844387076, 1.000000000000000000, 0.8660254037844387076, 1.000000000000000000, 0.8660254037844387076, 1.000000000000000000, 0.8660254037844387076, 1.000000000000000000, 0.8660254037844387076, 1.000000000000000000, 0.8660254037844387076, 1.000000000000000000, 0.8660254037844387076, 1.000000000000000000, 0.8660254037844387076, 1.000000000000000000, 0.8660254037844387076, 1.000000000000000000, 0.8660254037844387076, 1.000000000000000000, 0.8660254037844387076, 1.000000000000000000, 0.8660254037844387076, 1.000000000000000000, 0.8660254037844387076, 1.000000000000000000, 0.8660254037844387076, 1.000000000000000000, 0.8660254037844387076, 1.000000000000000000, 0.8660254037844387076, 1.000000000000000000, 0.8660254037844387076, 1.000000000000000000, 0.8660254037844387076, 1.000000000000000000, 0.8660254037844387076, 1.000000000000000000, 0.8660254037844387076, 1.000000000000000000),
 ( 1.000000000000000000, 0.8660254037844387076, 1.000000000000000000, 0.8660254037844387076, 1.000000000000000000, 0.8660254037844387076, 1.000000000000000000, 0.8660254037844387076, 1.000000000000000000, 0.8660254037844387076, 1.000000000000000000, 0.8660254037844387076, 1.000000000000000000, 0.8660254037844387076, 1.000000000000000000, 0.8660254037844387076, 1.000000000000000000, 0.8660254037844387076, 1.000000000000000000, 0.8660254037844387076, 1.000000000000000000, 0.8660254037844387076, 1.000000000000000000, 0.8660254037844387076, 1.000000000000000000, 0.8660254037844387076, 1.000000000000000000, 0.8660254037844387076, 1.000000000000000000, 0.8660254037844387076, 1.000000000000000000, 0.8660254037844387076, 1.000000000000000000, 0.8660254037844387076, 1.000000000000000000, 0.8660254037844387076, 1.000000000000000000, 0.8660254037844387076, 1.000000000000000000, 0.8660254037844387076, 1.000000000000000000, 0.8660254037844387076, 1.000000000000000000, 0.8660254037844387076, 1.000000000000000000, 0.8660254037844387076, 1.000000000000000000, 0.8660254037844387076, 1.000000000000000000, 0.8660254037844387076, 1.000000000000000000, 0.8660254037844387076, 1.000000000000000000, 0.8660254037844387076, 1.000000000000000000, 0.8660254037844387076, 1.000000000000000000, 0.8660254037844387076, 1.000000000000000000, 0.8660254037844387076, 1.000000000000000000, 0.8660254037844387076, 1.000000000000000000, 0.8660254037844387076, 1.000000000000000000, 0.8660254037844387076, 1.000000000000000000, 0.8660254037844387076, 1.000000000000000000, 0.8660254037844387076, 1.000000000000000000, 0.8660254037844387076, 1.000000000000000000, 0.8660254037844387076, 1.000000000000000000, 0.8660254037844387076, 1.000000000000000000, 0.8660254037844387076, 1.000000000000000000, 0.8660254037844387076, 1.000000000000000000, 0.8660254037844387076, 1.000000000000000000, 0.8660254037844387076, 1.000000000000000000, 0.8660254037844387076, 1.000000000000000000, 0.8660254037844387076, 1.000000000000000000, 0.8660254037844387076, 1.000000000000000000, 0.8660254037844387076, 1.000000000000000000, 0.8660254037844387076, 1.000000000000000000, 0.8660254037844387076, 1.000000000000000000, 0.8660254037844387076, 1.000000000000000000, 0.8660254037844387076, 1.000000000000000000, 0.8660254037844387076, 1.000000000000000000, 0.8660254037844387076, 1.000000000000000000, 0.8660254037844387076, 1.000000000000000000, 0.8660254037844387076, 1.000000000000000000, 0.8660254037844387076, 1.000000000000000000, 0.8660254037844387076, 1.000000000000000000, 0.8660254037844387076, 1.000000000000000000, 0.8660254037844387076, 1.000000000000000000, 0.8660254037844387076, 1.000000000000000000, 0.8660254037844387076, 1.000000000000000000, 0.8660254037844387076, 1.000000000000000000, 0.8660254037844387076, 1.000000000000000000, 0.8660254037844387076, 1.000000000000000000, 0.8660254037844387076, 1.000000000000000000, 0.8660254037844387076, 1.000000000000000000, 0.8660254037844387076, 1.000000000000000000, 0.8660254037844387076, 1.000000000000000000, 0.8660254037844387076, 1.000000000000000000, 0.8660254037844387076, 1.000000000000000000, 0.8660254037844387076, 1.000000000000000000, 0.8660254037844387076, 1.000000000000000000, 0.8660254037844387076, 1.000000000000000000, 0.8660254037844387076, 1.000000000000000000, 0.8660254037844387076, 1.000000000000000000, 0.8660254037844387076, 1.000000000000000000, 0.8660254037844387076, 1.000000000000000000, 0.8660254037844387076, 1.000000000000000000, 0.8660254037844387076, 1.000000000000000000, 0.8660254037844387076, 1.000000000000000000, 0.8660254037844387076, 1.000000000000000000, 0.8660254037844387076, 1.000000000000000000, 0.8660254037844387076, 1.000000000000000000, 0.8660254037844387076, 1.000000000000000000, 0.8660254037844387076, 1.000000000000000000, 0.8660254037844387076, 1.000000000000000000, 0.8660254037844387076, 1.000000000000000000, 0.8660254037844387076, 1.000000000000000000, 0.8660254037844387076, 1.000000000000000000, 0.8660254037844387076, 1.000000000000000000, 0.8660254037844387076, 1.000000000000000000, 0.8660254037844387076, 1.000000000000000000, 0.8660254037844387076, 1.000000000000000000, 0.8660254037844387076, 1.000000000000000000, 0.8660254037844387076, 1.000000000000000000, 0.8660254037844387076, 1.000000000000000000, 0.8660254037844387076, 1.000000000000000000, 0.8660254037844387076, 1.000000000000000000, 0.8660254037844387076, 1.000000000000000000, 0.8660254037844387076, 1.000000000000000000, 0.8660254037844387076, 1.000000000000000000, 0.8660254037844387076, 1.000000000000000000, 0.8660254037844387076, 1.000000000000000000, 0.8660254037844387076, 1.000000000000000000, 0.8660254037844387076, 1.000000000000000000, 0.8660254037844387076, 1.000000000000000000, 0.8660254037844387076, 1.000000000000000000, 0.8660254037844387076, 1.000000000000000000, 0.8660254037844387076, 1.000000000000000000, 0.8660254037844387076, 1.000000000000000000, 0.8660254037844387076, 1.000000000000000000, 0.8660254037844387076, 1.000000000000000000, 0.8660254037844387076, 1.000000000000000000, 0.8660254037844387076, 1.000000000000000000, 0.8660254037844387076, 1.000000000000000000, 0.8660254037844387076, 1.000000000000000000, 0.8660254037844387076, 1.000000000000000000, 0.8660254037844387076, 1.000000000000000000, 0.8660254037844387076, 1.000000000000000000, 0.8660254037844387076, 1.000000000000000000, 0.8660254037844387076, 1.000000000000000000, 0.8660254037844387076, 1.000000000000000000, 0.8660254037844387076, 1.000000000000000000, 0.8660254037844387076, 1.000000000000000000, 0.8660254037844387076, 1.000000000000000000, 0.8660254037844387076, 1.000000000000000000, 0.8660254037844387076, 1.000000000000000000, 0.8660254037844387076, 1.000000000000000000, 0.8660254037844387076, 1.000000000000000000, 0.8660254037844387076, 1.000000000000000000, 0.8660254037844387076, 1.000000000000000000, 0.8660254037844387076, 1.000000000000000000, 0.8660254037844387076, 1.000000000000000000, 0.8660254037844387076, 1.000000000000000000, 0.8660254037844387076, 1.000000000000000000, 0.8660254037844387076, 1.000000000000000000, 0.8660254037844387076, 1.000000000000000000, 0.8660254037844387076, 1.000000000000000000, 0.8660254037844387076, 1.000000000000000000, 0.8660254037844387076, 1.000000000000000000, 0.8660254037844387076, 1.000000000000000000, 0.8660254037844387076, 1.000000000000000000, 0.8660254037844387076, 1.000000000000000000, 0.8660254037844387076, 1.000000000000000000, 0.8660254037844387076, 1.000000000000000000, 0.8660254037844387076, 1.000000000000000000, 0.8660254037844387076, 1.000000000000000000, 0.8660254037844387076, 1.000000000000000000, 0.8660254037844387076, 1.000000000000000000, 0.8660254037844387076, 1.000000000000000000, 0.8660254037844387076, 1.000000000000000000, 0.8660254037844387076, 1.000000000000000000, 0.8660254037844387076, 1.000000000000000000, 0.8660254037844387076, 1.000000000000000000, 0.8660254037844387076, 1.000000000000000000, 0.8660254037844387076, 1.000000000000000000, 0.8660254037844387076, 1.000000000000000000, 0.8660254037844387076, 1.000000000000000000, 0.8660254037844387076, 1.000000000000000000, 0.8660254037844387076, 1.000000000000000000, 0.8660254037844387076, 1.000000000000000000, 0.8660254037844387076, 1.000000000000000000, 0.8660254037844387076, 1.000000000000000000, 0.8660254037844387076, 1.000000000000000000, 0.8660254037844387076, 1.000000000000000000, 0.8660254037844387076, 1.000000000000000000, 0.8660254037844387076, 1.000000000000000000, 0.8660254037844387076, 1.000000000000000000, 0.8660254037844387076, 1.000000000000000000) ) ) 
 REPRESENTATION_ITEM ( '' )  SURFACE ( )  );
#37838=CARTESIAN_POINT ( 'NONE',  ( -7.670162217029145246, 9.971608557999250166, 1.599625672291295375 ) ) ;
#37839=CARTESIAN_POINT ( 'NONE',  ( 4.482942347612929979, 8.381849838857084123, 1.040834085586084257E-14 ) ) ;
#37841=DIRECTION ( 'NONE',  ( -0.7592566023652994600, 0.6507913734559651608, 0.000000000000000000 ) ) ;
#37842=CARTESIAN_POINT ( 'NONE',  ( 2.683624340501134853, 5.218313266304903664, -1.199719254218446718 ) ) ;
#37847=CARTESIAN_POINT ( 'NONE',  ( -1.284279953904125193, 10.64264068711930733, 0.7750000000000117906 ) ) ;
#37849=CARTESIAN_POINT ( 'NONE',  ( -3.931501358282937009, 7.530575984731317618, 0.7216878364870317197 ) ) ;
#37850=CARTESIAN_POINT ( 'NONE',  ( 8.595506201383999567, 12.97191496834930113, 0.7216878364870438212 ) ) ;
#37853=CARTESIAN_POINT ( 'NONE',  ( -6.555530967407501741, 7.606873202518897870, 1.199719254218450271 ) ) ;
#37857=CARTESIAN_POINT ( 'NONE',  ( 3.913718639709028668, 2.801499522163732880, 0.7750000000000135669 ) ) ;
#37859=CARTESIAN_POINT ( 'NONE',  ( -7.670162217029145246, 9.971608557999250166, 1.599625672291295375 ) ) ;
#37864=ORIENTED_EDGE ( 'NONE', *, *, #11497, .F. ) ;
#37866=ORIENTED_EDGE ( 'NONE', *, *, #109624, .F. ) ;
#37877=CARTESIAN_POINT ( 'NONE',  ( -7.206322340863467346, 8.366129804884193888, 1.199719254218450271 ) ) ;
#37880=CARTESIAN_POINT ( 'NONE',  ( 5.666945020832170776, 7.634521829102760115, 1.443375672974062551 ) ) ;
#37884=CARTESIAN_POINT ( 'NONE',  ( -2.761056838677368397, 6.372983411765559048, 0.7998128361456341429 ) ) ;
#37888=CARTESIAN_POINT ( 'NONE',  ( -4.869349725602420520, 8.832658446511480577, 1.040834085586084257E-14 ) ) ;
#37894=CARTESIAN_POINT ( 'NONE',  ( -7.883176251342026042, 11.28445716228600126, -1.199719254218446718 ) ) ;
#37895=CARTESIAN_POINT ( 'NONE',  ( 6.317209508963599340, 9.457495962844502557, 1.199719254218462483 ) ) ;
#37899=CARTESIAN_POINT ( 'NONE',  ( -10.15913717534155047, 10.74674821418697057, 0.7998128361456462443 ) ) ;
#37902=CARTESIAN_POINT ( 'NONE',  ( 1.364683531249986537, -0.7822916663252464931, -0.7879004041258309554 ) ) ;
#37907=CARTESIAN_POINT ( 'NONE',  ( 7.754900677336718395, 11.99120852362745460, -0.7216878364870267237 ) ) ;
#37913=CARTESIAN_POINT ( 'NONE',  ( -5.473998445134435009, 6.274837103192765220, -1.008633756803478443 ) ) ;
#37916=CARTESIAN_POINT ( 'NONE',  ( -0.5637493975453833350, 6.831070374499072173, -3.741427165998697291 ) ) ;
#37928=CARTESIAN_POINT ( 'NONE',  ( -3.867100128395853709, 5.534702787927018974, -1.599625672291256295 ) ) ;
#37935=CARTESIAN_POINT ( 'NONE',  ( 0.7499999999999867883, -1.152083332650516434, -1.299038105676652011 ) ) ;
#37944=CARTESIAN_POINT ( 'NONE',  ( 3.192055101013606233, 5.811482486902795230, -1.199719254218446718 ) ) ;
#37949=CARTESIAN_POINT ( 'NONE',  ( 5.148345644887269756, 7.029489223833707001, -1.599625672291256295 ) ) ;
#37950=CARTESIAN_POINT ( 'NONE',  ( -0.6823417656250212460, 2.363541667008084435, 1.181850606188767472 ) ) ;
#37951=CARTESIAN_POINT ( 'NONE',  ( -4.964471428385745178, 6.642511170548884181, 1.245120630419704888 ) ) ;
#37954=CARTESIAN_POINT ( 'NONE',  ( -8.369460898337653276, 8.658792557682392754, 0.7998128361456462443 ) ) ;
#37955=CARTESIAN_POINT ( 'NONE',  ( -5.707619481228834779, 5.761236937629489852, -0.7216878364870197293 ) ) ;
#37958=CARTESIAN_POINT ( 'NONE',  ( -6.905180308061733996, 6.950465202360470052, 0.7998128361456341429 ) ) ;
#37960=CARTESIAN_POINT ( 'NONE',  ( 1.499999999999987566, -0.9437499993171851731, 0.000000000000000000 ) ) ;
#37968=CARTESIAN_POINT ( 'NONE',  ( -4.026408433134269771, 6.680931691089825541, 1.082531754730560403 ) ) ;
#37969=FACE_OUTER_BOUND ( 'NONE', #60819, .T. ) ;
#37973=CARTESIAN_POINT ( 'NONE',  ( -4.785665035499573783, 5.645992631913323123, 1.082531754730558626 ) ) ;
#37975=CARTESIAN_POINT ( 'NONE',  ( 9.206149998879153529, 10.69926207256923689, 1.199719254218453823 ) ) ;
#37984=CARTESIAN_POINT ( 'NONE',  ( -2.279742385392243165, 5.811449882932888222, -0.7998128361456281477 ) ) ;
#37985=CARTESIAN_POINT ( 'NONE',  ( 8.499999999999980460, 6.200000000000038369, 2.900000000000013678 ) ) ;
#37990=CARTESIAN_POINT ( 'NONE',  ( 5.494078562035752178, 7.432844293840273231, -1.599625672291262513 ) ) ;
#37996=CARTESIAN_POINT ( 'NONE',  ( 3.246287715468270108, 5.874753870433235825, 1.199719254218450271 ) ) ;
#37998=ORIENTED_EDGE ( 'NONE', *, *, #70571, .F. ) ;
#38006=CARTESIAN_POINT ( 'NONE',  ( 7.476431642932036326, 10.80992178580769014, 1.199719254218460707 ) ) ;
#38008=CARTESIAN_POINT ( 'NONE',  ( -4.574986769607567894, 7.424902766929059261, 1.199719254218464037 ) ) ;
#38015=CARTESIAN_POINT ( 'NONE',  ( -0.7500000000000249800, -1.027083332650516212, 1.299038105676659116 ) ) ;
#38019=B_SPLINE_CURVE_WITH_KNOTS ( 'NONE', 3,
 ( #72736, #25054, #108516, #8808, #74886, #122664 ),
 .UNSPECIFIED., .F., .F.,
 ( 4, 2, 4 ),
 ( 0.000000000000000000, 0.0001363166885564070553, 0.0002726333771128141106 ),
 .UNSPECIFIED. ) ;
#38021=CARTESIAN_POINT ( 'NONE',  ( 3.194917754314666514, 6.879154480009089134, 0.7998128361456321445 ) ) ;
#38022=CARTESIAN_POINT ( 'NONE',  ( -5.773074481320628948, 5.629675071162500544, 0.000000000000000000 ) ) ;
#38028=CARTESIAN_POINT ( 'NONE',  ( 6.046573322014824114, 7.117052299514516456, -1.082531754730543083 ) ) ;
#38031=CARTESIAN_POINT ( 'NONE',  ( 7.524412065460039933, 10.76193592880331984, -1.082531754730537976 ) ) ;
#38032=CARTESIAN_POINT ( 'NONE',  ( -1.201851678989727383E-14, 4.009375000341416140, -1.575800808251660134 ) ) ;
#38033=CARTESIAN_POINT ( 'NONE',  ( 1.419999999999990603, 6.120000000000041851, 2.500000000000000444 ) ) ;
#38034=CARTESIAN_POINT ( 'NONE',  ( 4.894130264408854458, 6.732904613275549899, -1.443375672974051449 ) ) ;
#38042=CARTESIAN_POINT ( 'NONE',  ( -5.120997767102647202, 6.698429628811411796, 1.435921996857256300 ) ) ;
#38043=ADVANCED_FACE ( 'NONE', ( #189476 ), #27732, .T. ) ;
#38049=CARTESIAN_POINT ( 'NONE',  ( -8.455481356417053007, 13.01647868246193518, 0.7998128361456341429 ) ) ;
#38060=CARTESIAN_POINT ( 'NONE',  ( 4.202664430556261266, 4.005456045178151570, 0.7216878364870317197 ) ) ;
#38062=CARTESIAN_POINT ( 'NONE',  ( 0.6823417656249899377, 3.155208333674754062, 1.181850606188765695 ) ) ;
#38064=CARTESIAN_POINT ( 'NONE',  ( 7.396136491454752715, 8.587579647240744407, 1.199719254218462483 ) ) ;
#38066=CARTESIAN_POINT ( 'NONE',  ( -8.503988664269602538, 10.94440607977979063, 1.599625672291269396 ) ) ;
#38071=CARTESIAN_POINT ( 'NONE',  ( -0.7500000000000215383, 3.941666666666690411, 1.299038105676671107 ) ) ;
#38072=CARTESIAN_POINT ( 'NONE',  ( 5.229694566569264680, 7.124396299129368337, 1.599625672291267398 ) ) ;
#38075=CARTESIAN_POINT ( 'NONE',  ( 1.364683531249990311, 3.384375000341416140, 1.214306433183764966E-14 ) ) ;
#38078=CARTESIAN_POINT ( 'NONE',  ( 9.747949258545622442, 10.47495501116581984, 0.000000000000000000 ) ) ;
#38083=CARTESIAN_POINT ( 'NONE',  ( 1.499999999999989120, 1.806250000682817269, 0.000000000000000000 ) ) ;
#38085=CARTESIAN_POINT ( 'NONE',  ( -6.227272627378437342, 6.159572908229946187, -0.7998128361456291469 ) ) ;
#38087=CARTESIAN_POINT ( 'NONE',  ( 3.823036128929238942, 7.404033217152015567, 1.040834085586084257E-14 ) ) ;
#38096=CARTESIAN_POINT ( 'NONE',  ( 6.283314124929436417, 9.417951348137970413, -1.199719254218440723 ) ) ;
#38097=CARTESIAN_POINT ( 'NONE',  ( 5.522248639467795428, 5.337044922334209573, -0.7998128361456231517 ) ) ;
#38100=CARTESIAN_POINT ( 'NONE',  ( 1.123270288250308280, 2.922697346350005887, 0.7749999999993786304 ) ) ;
#38101=CARTESIAN_POINT ( 'NONE',  ( 4.761938266897790761, 6.578680616179308771, 1.599625672291267398 ) ) ;
#38107=ORIENTED_EDGE ( 'NONE', *, *, #146747, .T. ) ;
#38108=CARTESIAN_POINT ( 'NONE',  ( 9.565441069641300587, 11.11843498845840905, -1.199719254218440723 ) ) ;
#38113=CARTESIAN_POINT ( 'NONE',  ( 5.890517129559706078, 5.978185313570312687, -0.07684424279984919393 ) ) ;
#38117=DIRECTION ( 'NONE',  ( 5.578564026256490882E-16, 1.000000000000000000, 9.066213480720158442E-32 ) ) ;
#38118=CARTESIAN_POINT ( 'NONE',  ( -4.392478581147607031, 7.108013530438723748, 1.082531754730560403 ) ) ;
#38120=CARTESIAN_POINT ( 'NONE',  ( -1.402160292154681736E-14, -1.178124999658576311, 1.575800808251672791 ) ) ;
#38121=CARTESIAN_POINT ( 'NONE',  ( 7.619319141200072920, 7.991553207595983643, 0.7216878364870317197 ) ) ;
#38122=CARTESIAN_POINT ( 'NONE',  ( -2.927671105547157371, 5.503034492191895666, 1.199719254218462483 ) ) ;
#38127=CARTESIAN_POINT ( 'NONE',  ( -5.525111292768871252, 6.404716915440499037, -1.199719254218446718 ) ) ;
#38129=ADVANCED_FACE ( 'NONE', ( #121452 ), #167982, .T. ) ;
#38134=EDGE_LOOP ( 'NONE', ( #213338, #5000 ) ) ;
#38135=CARTESIAN_POINT ( 'NONE',  ( 1.084637062511528693, 3.273878807974804683, 1.105835307554807301 ) ) ;
#38140=CARTESIAN_POINT ( 'NONE',  ( 8.585337585951586803, 11.03931315507545108, -1.599625672291255185 ) ) ;
#38144=LINE ( 'NONE', #87957, #2659 ) ;
#38149=CARTESIAN_POINT ( 'NONE',  ( -10.00555417720528872, 10.77549408293541866, 0.7216878364870438212 ) ) ;
#38153=CARTESIAN_POINT ( 'NONE',  ( 6.753933077901968396, 11.03133902419432566, 0.7998128361456462443 ) ) ;
#38155=CARTESIAN_POINT ( 'NONE',  ( -0.02374884625625755044, 2.800000000000025135, 1.413344025506580337 ) ) ;
#38157=CARTESIAN_POINT ( 'NONE',  ( -6.901263884555985051, 8.010228272525461435, 1.199719254218450271 ) ) ;
#38158=CARTESIAN_POINT ( 'NONE',  ( 3.551346171775753735, 6.230655402791975384, 1.199719254218462483 ) ) ;
#38161=CARTESIAN_POINT ( 'NONE',  ( 10.21336978979620191, 10.81001959771741205, 0.7998128361456462443 ) ) ;
#38162=CARTESIAN_POINT ( 'NONE',  ( 0.3697396242580934245, 6.943430631093202798, 3.891240841457444866 ) ) ;
#38165=CARTESIAN_POINT ( 'NONE',  ( 4.499659979152191625, 7.015106111828595559, -1.153029749421132566 ) ) ;
#38167=CARTESIAN_POINT ( 'NONE',  ( 5.666945020832167224, 8.594891043404107478, 1.082531754730558626 ) ) ;
#38172=EDGE_CURVE ( 'NONE', #83910, #154420, #58803, .T. ) ;
#38175=ORIENTED_EDGE ( 'NONE', *, *, #178570, .F. ) ;
#38176=CARTESIAN_POINT ( 'NONE',  ( 7.415946836550712185, 10.63539316174243865, 1.082531754730558626 ) ) ;
#38180=CARTESIAN_POINT ( 'NONE',  ( -8.552495972122143186, 8.872333477097637200, 0.7998128361456462443 ) ) ;
#38181=CYLINDRICAL_SURFACE ( 'NONE', #29635, 0.7499999999999997780 ) ;
#38189=CARTESIAN_POINT ( 'NONE',  ( 2.758194185376297902, 5.305311418659259814, 1.199719254218452047 ) ) ;
#38193=CARTESIAN_POINT ( 'NONE',  ( 5.359550796103802028, 5.147230771742885125, -0.7998128361456231517 ) ) ;
#38196=CARTESIAN_POINT ( 'NONE',  ( -1.499999999999997780, 2.181250000682817713, 1.214306433183764966E-14 ) ) ;
#38202=CARTESIAN_POINT ( 'NONE',  ( 0.7499999999999902300, 1.733333333333357595, 1.299038105676657340 ) ) ;
#38203=CARTESIAN_POINT ( 'NONE',  ( 8.288111976655649471, 8.563885482386732306, -0.7998128361456291469 ) ) ;
#38204=CARTESIAN_POINT ( 'NONE',  ( 4.650083499362875017, 5.487814173087225633, 1.082531754730560403 ) ) ;
#38209=CARTESIAN_POINT ( 'NONE',  ( 8.242994207428692377, 12.56065097540143327, -0.7216878364870328300 ) ) ;
#38214=CARTESIAN_POINT ( 'NONE',  ( -3.906720819032141190, 7.709591388846142479, -0.7998128361456281477 ) ) ;
#38215=CARTESIAN_POINT ( 'NONE',  ( -1.201851678989727383E-14, 3.743750000682817269, 1.732050807568877637 ) ) ;
#38216=CARTESIAN_POINT ( 'NONE',  ( -0.6823417656250212460, 5.613541667008087543, 1.181850606188767472 ) ) ;
#38221=CARTESIAN_POINT ( 'NONE',  ( 0.6823417656249899377, 4.488541667008086655, -1.181850606188754593 ) ) ;
#38228=CARTESIAN_POINT ( 'NONE',  ( -7.771848369131641121, 10.09024240211882351, -1.599625672291263179 ) ) ;
#38229=CARTESIAN_POINT ( 'NONE',  ( 6.819914962873951936, 7.915321197229798322, -1.199719254218446718 ) ) ;
#38238=CARTESIAN_POINT ( 'NONE',  ( -5.520141099058386125, 9.591915048876776595, 0.000000000000000000 ) ) ;
#38243=CARTESIAN_POINT ( 'NONE',  ( 10.05067194643221207, 10.62020544712608938, 0.7998128361456462443 ) ) ;
#38245=VERTEX_POINT ( 'NONE', #69425 ) ;
#38246=CARTESIAN_POINT ( 'NONE',  ( -3.418627288940168096, 7.140148937072163804, -0.7998128361456281477 ) ) ;
#38247=CARTESIAN_POINT ( 'NONE',  ( -8.505042434474312074, 8.816971016508505343, -0.7998128361456291469 ) ) ;
#38251=CARTESIAN_POINT ( 'NONE',  ( -4.371234765837696656, 7.372762773471292164, -1.195546268109607846 ) ) ;
#38252=CARTESIAN_POINT ( 'NONE',  ( 1.364683531249988757, -0.6156249996585803075, 0.000000000000000000 ) ) ;
#38258=CARTESIAN_POINT ( 'NONE',  ( 5.952193131599331721, 6.902979060742733708, 1.199719254218462483 ) ) ;
#38278=ORIENTED_EDGE ( 'NONE', *, *, #113945, .F. ) ;
#38280=CARTESIAN_POINT ( 'NONE',  ( -7.635213062790267458, 12.05949900656400686, 0.000000000000000000 ) ) ;
#38285=CARTESIAN_POINT ( 'NONE',  ( -0.7500000000000215383, 1.222916667349485564, 1.299038105676659116 ) ) ;
#38286=CARTESIAN_POINT ( 'NONE',  ( 10.05353459973327368, 11.68787744023238417, -1.199719254218440723 ) ) ;
#38292=CARTESIAN_POINT ( 'NONE',  ( 1.364683531249988757, 1.384375000341421469, 0.000000000000000000 ) ) ;
#38298=CARTESIAN_POINT ( 'NONE',  ( -2.754277761870538299, 6.365074488824250309, 1.040834085586084257E-14 ) ) ;
#38303=CARTESIAN_POINT ( 'NONE',  ( 1.364683531249988757, -0.05312499965857975237, 0.000000000000000000 ) ) ;
#38309=CARTESIAN_POINT ( 'NONE',  ( -1.402160292154681736E-14, 0.5718750003414239114, 1.575800808251672791 ) ) ;
#38311=CARTESIAN_POINT ( 'NONE',  ( -6.307567778855718288, 8.381915046796901692, -1.599625672291263179 ) ) ;
#38312=CARTESIAN_POINT ( 'NONE',  ( 7.456094412511537151, 10.78619501698377370, 1.199719254218460707 ) ) ;
#38313=CARTESIAN_POINT ( 'NONE',  ( 4.168242161197552420, 6.950367390450747251, -1.199719254218452047 ) ) ;
#38315=CARTESIAN_POINT ( 'NONE',  ( 6.030679399980265920, 5.930214142932100252, -0.7998128361456281477 ) ) ;
#38316=CARTESIAN_POINT ( 'NONE',  ( 1.499999999999989120, 4.004166666666685970, 0.8660254037844524744 ) ) ;
#38318=CARTESIAN_POINT ( 'NONE',  ( -1.402160292154681736E-14, 1.009375000341417916, -1.575800808251659024 ) ) ;
#38322=EDGE_CURVE ( 'NONE', #70347, #185939, #159703, .T. ) ;
#38325=CARTESIAN_POINT ( 'NONE',  ( 6.805829924380108586, 8.963220883242035697, 1.443375672974076540 ) ) ;
#38328=CARTESIAN_POINT ( 'NONE',  ( -7.389357414647957256, 8.579670724299436557, 1.199719254218450271 ) ) ;
#38329=CARTESIAN_POINT ( 'NONE',  ( -5.251085567194491155, 5.020688004682002159, -0.7998128361456221525 ) ) ;
#38333=CARTESIAN_POINT ( 'NONE',  ( -9.151390499099978371, 9.778969791812544443, 0.7216878364870438212 ) ) ;
#38335=CARTESIAN_POINT ( 'NONE',  ( -0.7499999999999972244, 5.358333333333353821, -1.299038105676652011 ) ) ;
#38340=CARTESIAN_POINT ( 'NONE',  ( 9.910647101909615841, 10.66476916175714607, 0.000000000000000000 ) ) ;
#38348=CARTESIAN_POINT ( 'NONE',  ( 9.693716643646590470, 12.33242205571964512, 1.443375672974076540 ) ) ;
#38352=CARTESIAN_POINT ( 'NONE',  ( 9.205623113554628034, 9.842241175342985926, 0.7216878364870458196 ) ) ;
#38353=CARTESIAN_POINT ( 'NONE',  ( 8.288111976655649471, 8.563885482386732306, -0.7998128361456291469 ) ) ;
#38354=CARTESIAN_POINT ( 'NONE',  ( -6.715366157470410435, 6.729015360003925750, -0.7998128361456291469 ) ) ;
#38356=CARTESIAN_POINT ( 'NONE',  ( 1.499999999999990896, 5.025000000000022560, 1.214306433183765124E-14 ) ) ;
#38358=CARTESIAN_POINT ( 'NONE',  ( 1.364683531249988757, -0.5531249996585801965, 0.000000000000000000 ) ) ;
#38359=CARTESIAN_POINT ( 'NONE',  ( 2.250290310188348464, 5.569163095287620990, 0.7216878364870438212 ) ) ;
#38361=CARTESIAN_POINT ( 'NONE',  ( -2.625475302540713152, 6.214804952939456228, -0.7998128361456281477 ) ) ;
#38378=CARTESIAN_POINT ( 'NONE',  ( 7.958799866421889746, 9.244020251369077457, -1.199719254218441611 ) ) ;
#38383=CARTESIAN_POINT ( 'NONE',  ( -1.284279953904152949, 2.952889714876734573, 0.7750000000000152323 ) ) ;
#38390=CARTESIAN_POINT ( 'NONE',  ( -4.889686956022917919, 8.856385215335397021, 1.214306433183764966E-14 ) ) ;
#38393=CARTESIAN_POINT ( 'NONE',  ( -3.903858165731105778, 6.641919395739846799, 1.199719254218464037 ) ) ;
#38404=CARTESIAN_POINT ( 'NONE',  ( -2.754277761870538299, 6.365074488824250309, 1.040834085586084257E-14 ) ) ;
#38407=CARTESIAN_POINT ( 'NONE',  ( 6.238723240582662477, 10.43026088065513513, -0.7998128361456291469 ) ) ;
#38408=CARTESIAN_POINT ( 'NONE',  ( -1.364683531250012516, 4.988541667008084879, -0.7879004041258300672 ) ) ;
#38415=CARTESIAN_POINT ( 'NONE',  ( 6.331294547457450683, 7.449227062530913379, -1.082531754730543083 ) ) ;
#38416=CARTESIAN_POINT ( 'NONE',  ( -8.993135964566285168, 9.386413468282476913, -0.7998128361456291469 ) ) ;
#38418=( BOUNDED_CURVE ( )  B_SPLINE_CURVE ( 2, ( #190798, #39231, #71704, #187604, #172443, #142103, #123778 ),
 .UNSPECIFIED., .F., .T. ) 
 B_SPLINE_CURVE_WITH_KNOTS ( ( 3, 2, 2, 3 ),
 ( 0.1428571428571429880, 0.1488095238095238637, 0.1547619047619047394, 0.1607142857142856152 ),
 .UNSPECIFIED. ) 
 CURVE ( )  GEOMETRIC_REPRESENTATION_ITEM ( )  RATIONAL_B_SPLINE_CURVE ( ( 0.9999999999999968914, 0.8660254037844418162, 1.000000000000000000, 0.8660254037844387076, 1.000000000000000000, 0.8660254037844412611, 0.9999999999999974465 ) ) 
 REPRESENTATION_ITEM ( '' )  );
#38420=CARTESIAN_POINT ( 'NONE',  ( -6.507023659554960204, 9.678945805201045971, 1.199719254218452047 ) ) ;
#38421=CARTESIAN_POINT ( 'NONE',  ( -4.737684612971557740, 7.614716917520386374, 1.199719254218464037 ) ) ;
#38426=CARTESIAN_POINT ( 'NONE',  ( -2.334365499475838046, 5.399177108899520405, -0.7827922733892430651 ) ) ;
#38429=CARTESIAN_POINT ( 'NONE',  ( 7.344766530301147789, 9.591980256816594164, 1.599625672291281386 ) ) ;
#38432=( BOUNDED_CURVE ( )  B_SPLINE_CURVE ( 2, ( #59468, #155918, #160174, #125627, #11774, #74661, #208899 ),
 .UNSPECIFIED., .F., .T. ) 
 B_SPLINE_CURVE_WITH_KNOTS ( ( 3, 2, 2, 3 ),
 ( 0.03571428571428574700, 0.04166666666666662272, 0.04761904761904750538, 0.05357142857142838110 ),
 .UNSPECIFIED. ) 
 CURVE ( )  GEOMETRIC_REPRESENTATION_ITEM ( )  RATIONAL_B_SPLINE_CURVE ( ( 0.9999999999999992228, 0.8660254037844394848, 1.000000000000000000, 0.8660254037844387076, 1.000000000000000000, 0.8660254037844429265, 0.9999999999999957812 ) ) 
 REPRESENTATION_ITEM ( '' )  );
#38443=CARTESIAN_POINT ( 'NONE',  ( 0.7499999999999920064, 5.733333333333353821, 1.299038105676669330 ) ) ;
#38444=CARTESIAN_POINT ( 'NONE',  ( 4.364835388595708743, 7.179726155748598515, 1.199719254218462483 ) ) ;
#38445=CARTESIAN_POINT ( 'NONE',  ( 6.979750152936881058, 7.037463354714830643, 0.7998128361456341429 ) ) ;
#38447=CARTESIAN_POINT ( 'NONE',  ( -8.514157279702027736, 10.95626946445095307, -1.443375672974059665 ) ) ;
#38448=LINE ( 'NONE', #88270, #156679 ) ;
#38449=CARTESIAN_POINT ( 'NONE',  ( 5.639828713604826405, 9.523624565940227882, -0.7216878364870267237 ) ) ;
#38450=CARTESIAN_POINT ( 'NONE',  ( -8.798878505144665851, 9.367705798864669475, -0.7216878364870267237 ) ) ;
#38451=CIRCLE ( 'NONE', #180396, 0.07999999999999998779 ) ;
#38456=CARTESIAN_POINT ( 'NONE',  ( 7.426115451983150706, 9.686887332112256388, -1.599625672291262513 ) ) ;
#38462=CARTESIAN_POINT ( 'NONE',  ( -1.364683531250012516, 2.280208333674751842, 0.7879004041258379498 ) ) ;
#38469=CARTESIAN_POINT ( 'NONE',  ( 8.127223016387999266, 11.56917838817298616, 1.199719254218460707 ) ) ;
#38473=CARTESIAN_POINT ( 'NONE',  ( -7.831806290188425557, 12.28885777186185990, -0.7998128361456281477 ) ) ;
#38479=CARTESIAN_POINT ( 'NONE',  ( 3.192055101013606233, 5.811482486902795230, -1.199719254218446718 ) ) ;
#38483=CARTESIAN_POINT ( 'NONE',  ( -9.398826802771548472, 11.98838390803207865, -1.599625672291263179 ) ) ;
#38488=CARTESIAN_POINT ( 'NONE',  ( 5.890592889100787488, 5.978139607520936316, 0.07745371066007235294 ) ) ;
#38489=CARTESIAN_POINT ( 'NONE',  ( -3.391510981712833939, 7.108513245306943062, 0.7998128361456341429 ) ) ;
#38493=CARTESIAN_POINT ( 'NONE',  ( 7.721532178182734185, 8.967207948423393304, 1.199719254218462483 ) ) ;
#38495=CARTESIAN_POINT ( 'NONE',  ( 6.908042961362778733, 8.018137195466769285, 1.199719254218462483 ) ) ;
#38496=CARTESIAN_POINT ( 'NONE',  ( 3.472859903394816872, 7.203420320602605287, -0.7998128361456291469 ) ) ;
#38498=CARTESIAN_POINT ( 'NONE',  ( -8.188761592974046266, 10.57664116326830595, -1.443375672974059665 ) ) ;
#38507=CARTESIAN_POINT ( 'NONE',  ( -4.684235067853224521, 6.877467941869524815, -1.224209591347114046 ) ) ;
#38509=CARTESIAN_POINT ( 'NONE',  ( 6.155038550924150087, 7.243595066575396757, 1.082531754730558626 ) ) ;
#38531=CARTESIAN_POINT ( 'NONE',  ( 7.771848369131631351, 10.09024240211882351, -1.599625672291262513 ) ) ;
#38535=CARTESIAN_POINT ( 'NONE',  ( -1.500000000000013101, 1.410416667349486008, -0.8660254037844313801 ) ) ;
#38536=CARTESIAN_POINT ( 'NONE',  ( -4.457933580795036654, 4.095344020549286590, -0.7998128361456221525 ) ) ;
#38537=CARTESIAN_POINT ( 'NONE',  ( -6.555530967407501741, 7.606873202518897870, 1.199719254218450271 ) ) ;
#38539=ORIENTED_EDGE ( 'NONE', *, *, #185325, .T. ) ;
#38540=CARTESIAN_POINT ( 'NONE',  ( -10.29471871147821282, 10.90492667301307605, -0.7998128361456291469 ) ) ;
#38544=CARTESIAN_POINT ( 'NONE',  ( -1.499999999999997780, 5.681250000682820378, 1.214306433183764966E-14 ) ) ;
#38545=CARTESIAN_POINT ( 'NONE',  ( 7.396136491454752715, 8.587579647240744407, 1.199719254218462483 ) ) ;
#38547=CARTESIAN_POINT ( 'NONE',  ( -7.576308911938196999, 7.733448573549685179, 0.7998128361456462443 ) ) ;
#38549=CARTESIAN_POINT ( 'NONE',  ( 0.6823417656249899377, 5.426041667008087543, -1.181850606188754593 ) ) ;
#38550=CARTESIAN_POINT ( 'NONE',  ( 1.284279953904121641, 3.253360285806104812, 0.7750000000000135669 ) ) ;
#38551=CARTESIAN_POINT ( 'NONE',  ( -1.519536625744598579, 8.761901799250109590, 2.483436355453746192 ) ) ;
#38557=CARTESIAN_POINT ( 'NONE',  ( -7.592202833972775622, 8.920286730132099606, 1.082531754730558626 ) ) ;
#38561=CARTESIAN_POINT ( 'NONE',  ( -1.201851678989727383E-14, 4.759375000341419693, -1.575800808251660134 ) ) ;
#38568=CARTESIAN_POINT ( 'NONE',  ( 1.364683531249990311, 4.634375000341417916, 1.214306433183764966E-14 ) ) ;
#38572=CARTESIAN_POINT ( 'NONE',  ( 2.860407222358963608, 5.320596945185329218, 1.082531754730548412 ) ) ;
#38573=CARTESIAN_POINT ( 'NONE',  ( 0.6823417656249917140, 5.405208333674749177, 1.181850606188765695 ) ) ;
#38578=CARTESIAN_POINT ( 'NONE',  ( 1.364683531249988757, 0.8843750003414210248, 0.000000000000000000 ) ) ;
#38579=CARTESIAN_POINT ( 'NONE',  ( -2.657034918598338180, 6.043698471765932112, -0.7216878364870267237 ) ) ;
#38580=CARTESIAN_POINT ( 'NONE',  ( 5.769158057814842699, 6.689438141327490150, 1.199719254218462483 ) ) ;
#38582=CARTESIAN_POINT ( 'NONE',  ( 1.387358672533454351, 7.315968950353815892, -4.254625267138348654 ) ) ;
#38585=CARTESIAN_POINT ( 'NONE',  ( 4.053524740805938720, 3.831459740469437936, 1.214306433183764966E-14 ) ) ;
#38588=CARTESIAN_POINT ( 'NONE',  ( -7.782016984564068096, 10.10210578678999482, 1.443375672974090751 ) ) ;
#38593=CARTESIAN_POINT ( 'NONE',  ( -9.969323024750229578, 10.52529837183042716, -0.7998128361456291469 ) ) ;
#38594=CARTESIAN_POINT ( 'NONE',  ( -5.707619481228832115, 6.721606151930833661, -1.082531754730543971 ) ) ;
#38595=CARTESIAN_POINT ( 'NONE',  ( -1.364683531250012516, 1.842708333674749843, 0.7879004041258379498 ) ) ;
#38616=CARTESIAN_POINT ( 'NONE',  ( -1.445103857048130047, 8.688264192037886247, 2.625611233228264840 ) ) ;
#38618=CARTESIAN_POINT ( 'NONE',  ( -1.499999999999997780, 4.650000000000022560, 1.214306433183764966E-14 ) ) ;
#38619=CARTESIAN_POINT ( 'NONE',  ( -1.364683531249997417, 3.571875000341423245, 1.214306433183764966E-14 ) ) ;
#38630=CARTESIAN_POINT ( 'NONE',  ( -1.364683531250014514, 0.7385416670080887647, -0.7879004041258289570 ) ) ;
#38638=ORIENTED_EDGE ( 'NONE', *, *, #206116, .F. ) ;
#38640=CARTESIAN_POINT ( 'NONE',  ( 4.493637847925535667, 7.329995691633395261, -1.199719254218452047 ) ) ;
#38648=CARTESIAN_POINT ( 'NONE',  ( 6.109920781252839994, 10.27999134477033216, 1.040834085586084257E-14 ) ) ;
#38651=CARTESIAN_POINT ( 'NONE',  ( 7.747594715205354809, 11.12627870345989756, -1.199719254218446718 ) ) ;
#38664=CARTESIAN_POINT ( 'NONE',  ( -6.995644074971465010, 10.14503993989993091, 1.082531754730549967 ) ) ;
#38668=CARTESIAN_POINT ( 'NONE',  ( -7.974166903131914452, 12.45494515362926435, -0.7998128361456281477 ) ) ;
#38673=CARTESIAN_POINT ( 'NONE',  ( -3.113568832632681360, 6.784247404713427798, -0.7998128361456281477 ) ) ;
#38675=CARTESIAN_POINT ( 'NONE',  ( 10.73535870392234237, 11.41900666419791399, 0.000000000000000000 ) ) ;
#38677=CARTESIAN_POINT ( 'NONE',  ( 2.354312230267378236, 5.898448035287240820, -0.7998128361456281477 ) ) ;
#38683=CARTESIAN_POINT ( 'NONE',  ( 3.551873057100287223, 5.166937871415542283, 1.443375672974062551 ) ) ;
#38685=CARTESIAN_POINT ( 'NONE',  ( -4.391951695823077984, 7.211361847513815704, 1.199719254218464037 ) ) ;
#38686=DIRECTION ( 'NONE',  ( 0.7592566023653005702, -0.6507913734559639396, 0.000000000000000000 ) ) ;
#38688=CARTESIAN_POINT ( 'NONE',  ( -8.784793466650835825, 12.33634391347959713, 1.199719254218462483 ) ) ;
#38695=CARTESIAN_POINT ( 'NONE',  ( 8.595506201384020883, 9.130438111143927671, 0.7216878364870438212 ) ) ;
#38696=CARTESIAN_POINT ( 'NONE',  ( 1.364683531249988535, 4.467708333674754506, -0.7879004041258300672 ) ) ;
#38698=CARTESIAN_POINT ( 'NONE',  ( 5.281064527722868718, 6.119995689553514140, 1.199719254218462483 ) ) ;
#38712=CARTESIAN_POINT ( 'NONE',  ( 0.6823417656249882723, 2.988541667008084879, -1.181850606188754593 ) ) ;
#38714=CARTESIAN_POINT ( 'NONE',  ( 2.758194185376297902, 5.305311418659259814, 1.199719254218452047 ) ) ;
#38716=CARTESIAN_POINT ( 'NONE',  ( -5.504247177468192476, 7.444707678511436555, 1.443375672974064550 ) ) ;
#38717=CARTESIAN_POINT ( 'NONE',  ( 3.606105671554957759, 4.269840040644637291, -1.082531754730543083 ) ) ;
#38718=CARTESIAN_POINT ( 'NONE',  ( -6.534666851662457532, 6.726125536468730459, 1.040834085586084257E-14 ) ) ;
#38723=CARTESIAN_POINT ( 'NONE',  ( 4.123651276850781144, 7.962676922967908411, -0.7998128361456221525 ) ) ;
#38729=CYLINDRICAL_SURFACE ( 'NONE', #123781, 0.08000000000000020983 ) ;
#38733=CARTESIAN_POINT ( 'NONE',  ( 6.817052309572890323, 6.847649204123507083, 0.7998128361456341429 ) ) ;
#38735=CARTESIAN_POINT ( 'NONE',  ( -3.735435015764967837, 4.316761258935923884, -1.199719254218452047 ) ) ;
#38737=CARTESIAN_POINT ( 'NONE',  ( -5.388475986427523345, 8.373973519885682393, 1.199719254218452047 ) ) ;
#38741=CARTESIAN_POINT ( 'NONE',  ( 7.287671262545424966, 8.461036880179857889, -1.199719254218451159 ) ) ;
#38743=CARTESIAN_POINT ( 'NONE',  ( -7.250913225210214641, 7.353820272367037170, 0.7998128361456341429 ) ) ;
#38745=CARTESIAN_POINT ( 'NONE',  ( 6.114364089638786304, 8.156510742710487705, 1.443375672974076540 ) ) ;
#38746=CARTESIAN_POINT ( 'NONE',  ( 4.602920755658417740, 7.148668813305413039, 1.337190490212318839 ) ) ;
#38747=CARTESIAN_POINT ( 'NONE',  ( -4.737684612971557740, 7.614716917520386374, 1.199719254218464037 ) ) ;
#38750=CARTESIAN_POINT ( 'NONE',  ( -6.901263884555985051, 8.010228272525461435, 1.199719254218450271 ) ) ;
#38754=CARTESIAN_POINT ( 'NONE',  ( 0.6823417656249882723, 1.676041667008083769, -1.181850606188749264 ) ) ;
#38756=CARTESIAN_POINT ( 'NONE',  ( -5.083944415444539899, 8.875092884753202682, 0.000000000000000000 ) ) ;
#38761=CARTESIAN_POINT ( 'NONE',  ( 6.331821432781979730, 7.345878745455822312, -1.199719254218445830 ) ) ;
#38763=CARTESIAN_POINT ( 'NONE',  ( -5.890076507333620981, 6.013243542187837853, -0.2543948676220365024 ) ) ;
#38764=CARTESIAN_POINT ( 'NONE',  ( 1.364683531249986537, 0.9677083336747538400, -0.7879004041258239610 ) ) ;
#38767=CARTESIAN_POINT ( 'NONE',  ( -1.402160292154681736E-14, -0.7406249996585823059, -1.575800808251665908 ) ) ;
#38770=CARTESIAN_POINT ( 'NONE',  ( -5.057354993097396445, 5.859001232490445688, -1.199719254218446718 ) ) ;
#38772=CARTESIAN_POINT ( 'NONE',  ( -7.659993601596726265, 8.039006744725394782, -0.7216878364870267237 ) ) ;
#38780=CARTESIAN_POINT ( 'NONE',  ( -7.659993601596713830, 9.959745173328078849, -1.443375672974058777 ) ) ;
#38785=CARTESIAN_POINT ( 'NONE',  ( -8.500599125644013654, 9.019713189447241319, 0.7216878364870438212 ) ) ;
#38791=CARTESIAN_POINT ( 'NONE',  ( 0.7499999999999920064, 5.514583334016151639, 1.299038105676669330 ) ) ;
#38792=CARTESIAN_POINT ( 'NONE',  ( 4.298292216229534723, 7.460037067547172107, -1.072071942351945584 ) ) ;
#38793=FACE_OUTER_BOUND ( 'NONE', #43723, .T. ) ;
#38796=ORIENTED_EDGE ( 'NONE', *, *, #43620, .T. ) ;
#38799=CARTESIAN_POINT ( 'NONE',  ( -6.287230548435221777, 8.358188277972981695, -1.599625672291263179 ) ) ;
#38801=CARTESIAN_POINT ( 'NONE',  ( 3.310162060030825248, 7.013606170011280838, -0.7998128361456291469 ) ) ;
#38804=CARTESIAN_POINT ( 'NONE',  ( 4.882711408206717785, 4.933808380148556161, 0.6288647573781755984 ) ) ;
#38806=CARTESIAN_POINT ( 'NONE',  ( 5.656776405399742025, 7.622658444431597680, -1.599625672291262513 ) ) ;
#38809=CARTESIAN_POINT ( 'NONE',  ( -5.599154252763867134, 5.634694171087028636, 0.000000000000000000 ) ) ;
#38815=CARTESIAN_POINT ( 'NONE',  ( -4.218512253981381299, 3.978430757497701364, -0.5307291018261834914 ) ) ;
#38821=CARTESIAN_POINT ( 'NONE',  ( -0.6823417656250003738, 0.7177083336747519526, -1.181850606188749264 ) ) ;
#38823=CARTESIAN_POINT ( 'NONE',  ( -7.153898609505128015, 11.49796547773133604, 0.7998128361456481317 ) ) ;
#38825=CARTESIAN_POINT ( 'NONE',  ( 7.934546212495622086, 10.28005655271014795, -1.599625672291262513 ) ) ;
#38827=CARTESIAN_POINT ( 'NONE',  ( -6.906989191158078079, 10.14557225873805812, -1.199719254218440723 ) ) ;
#38830=CARTESIAN_POINT ( 'NONE',  ( -1.364683531249997417, 4.759375000341424133, 1.214306433183764966E-14 ) ) ;
#38831=EDGE_CURVE ( 'NONE', #62825, #17090, #135887, .T. ) ;
#38833=CARTESIAN_POINT ( 'NONE',  ( 8.703971430293332645, 12.13808852110884118, -1.082531754730543083 ) ) ;
#38836=CARTESIAN_POINT ( 'NONE',  ( 1.364683531249986537, -0.2822916663252520997, -0.7879004041258309554 ) ) ;
#38839=CARTESIAN_POINT ( 'NONE',  ( 6.602457619730749627, 10.64669162308715222, 0.7216878364870438212 ) ) ;
#38842=CARTESIAN_POINT ( 'NONE',  ( -5.829642864196175722, 7.824335979694092558, 1.443375672974064550 ) ) ;
#38844=CARTESIAN_POINT ( 'NONE',  ( -1.364683531250012516, 2.780208333674754506, 0.7879004041258379498 ) ) ;
#38848=CARTESIAN_POINT ( 'NONE',  ( -6.555530967407501741, 7.606873202518897870, 1.199719254218450271 ) ) ;
#38855=CARTESIAN_POINT ( 'NONE',  ( 6.923409998072794558, 11.22906209772695618, 1.040834085586084257E-14 ) ) ;
#38858=CARTESIAN_POINT ( 'NONE',  ( -1.201851678989727383E-14, 2.712500000000023892, 1.732050807568877637 ) ) ;
#38865=CARTESIAN_POINT ( 'NONE',  ( 5.178851490740187913, 8.985817805931475277, 0.7216878364870438212 ) ) ;
#38866=CARTESIAN_POINT ( 'NONE',  ( 0.6823417656249864960, -0.7614583329919113464, -1.181850606188749264 ) ) ;
#38872=CARTESIAN_POINT ( 'NONE',  ( -0.7500000000000249800, -0.8083333333333136972, 1.299038105676659116 ) ) ;
#38873=CARTESIAN_POINT ( 'NONE',  ( 7.775764792637399836, 9.030479331953833011, -1.199719254218441611 ) ) ;
#38874=CARTESIAN_POINT ( 'NONE',  ( -9.515124878692420296, 9.995400534762978850, 1.040834085586084257E-14 ) ) ;
#38877=CARTESIAN_POINT ( 'NONE',  ( -1.364683531250014514, 0.03020833367475737191, 0.7879004041258379498 ) ) ;
#38878=CARTESIAN_POINT ( 'NONE',  ( -1.500000000000013101, 1.629166666666691077, -0.8660254037844313801 ) ) ;
#38880=CARTESIAN_POINT ( 'NONE',  ( 5.497994985541524215, 6.373081223675282736, -1.199719254218445830 ) ) ;
#38886=CARTESIAN_POINT ( 'NONE',  ( 1.364683531249988535, 4.905208333674756283, -0.7879004041258300672 ) ) ;
#38888=CARTESIAN_POINT ( 'NONE',  ( -8.670602931139386627, 10.07445716020612103, 1.199719254218462483 ) ) ;
#38889=CARTESIAN_POINT ( 'NONE',  ( -5.639828713604883248, 6.642516923036197340, 1.082531754730548412 ) ) ;
#38897=CARTESIAN_POINT ( 'NONE',  ( 7.293396569147545527, 10.59638086639245280, 1.199719254218460707 ) ) ;
#38902=CARTESIAN_POINT ( 'NONE',  ( 7.632877294369377452, 8.967740267261513409, -1.082531754730537976 ) ) ;
#38905=CARTESIAN_POINT ( 'NONE',  ( -6.970863535720637216, 11.28442455831609337, 0.7998128361456481317 ) ) ;
#38906=CARTESIAN_POINT ( 'NONE',  ( 5.952193131599331721, 6.902979060742733708, 1.199719254218462483 ) ) ;
#38909=CARTESIAN_POINT ( 'NONE',  ( -2.081668171172168513E-14, 5.868705557303649734, 4.125226524755077229 ) ) ;
#38910=CARTESIAN_POINT ( 'NONE',  ( 2.510230996824538430, 6.080353262937265413, 0.000000000000000000 ) ) ;
#38916=CARTESIAN_POINT ( 'NONE',  ( 2.273753298029672187, 5.671309185932734032, 0.4822658753677200871 ) ) ;
#38917=CARTESIAN_POINT ( 'NONE',  ( -4.284013352238255301, 6.981470763377843447, -1.082531754730549967 ) ) ;
#38918=CARTESIAN_POINT ( 'NONE',  ( 2.737856954955798727, 5.281584649835344258, 1.199719254218452047 ) ) ;
#38921=CARTESIAN_POINT ( 'NONE',  ( -5.693534442735004752, 8.729875052244421951, 1.199719254218452047 ) ) ;
#38926=CARTESIAN_POINT ( 'NONE',  ( -7.426115451983156923, 9.686887332112256388, -1.599625672291263179 ) ) ;
#38931=CARTESIAN_POINT ( 'NONE',  ( 5.996784015946103885, 5.890669528225568996, 1.040834085586084257E-14 ) ) ;
#38944=CARTESIAN_POINT ( 'NONE',  ( -8.044065211609668253, 8.279164256499745633, 0.7998128361456602331 ) ) ;
#38948=CARTESIAN_POINT ( 'NONE',  ( 5.016153647376201619, 7.835634441038803466, 1.082531754730558626 ) ) ;
#38954=CARTESIAN_POINT ( 'NONE',  ( -5.773074481320628948, 5.629675071162500544, 0.000000000000000000 ) ) ;
#38958=CARTESIAN_POINT ( 'NONE',  ( -7.230575994789712801, 7.330093503543126054, 0.7998128361456341429 ) ) ;
#38964=CARTESIAN_POINT ( 'NONE',  ( -9.664264568442742842, 10.16939683947169115, -0.7998128361456291469 ) ) ;
#38965=CARTESIAN_POINT ( 'NONE',  ( 7.949158136313996259, 8.168439335321471262, 1.040834085586084257E-14 ) ) ;
#38968=CARTESIAN_POINT ( 'NONE',  ( -10.62011439820619429, 11.28455497419572318, -0.7998128361456221525 ) ) ;
#38971=CARTESIAN_POINT ( 'NONE',  ( -1.364683531250014514, -1.157291666325248158, 0.7879004041258379498 ) ) ;
#38973=EDGE_LOOP ( 'NONE', ( #133862, #116237 ) ) ;
#38975=CARTESIAN_POINT ( 'NONE',  ( 9.164948653157988900, 11.71552606681625619, -1.443375672974057666 ) ) ;
#38984=CARTESIAN_POINT ( 'NONE',  ( -0.2214363961139278192, 7.035828811087419865, -3.928328033908623507 ) ) ;
#38996=CARTESIAN_POINT ( 'NONE',  ( -4.471491734408701291, 4.111161866431900513, 1.214306433183764966E-14 ) ) ;
#38999=CARTESIAN_POINT ( 'NONE',  ( -2.761056838677368397, 6.372983411765559048, 0.7998128361456341429 ) ) ;
#39004=CARTESIAN_POINT ( 'NONE',  ( -0.6823417656250212460, 5.551041667008087543, 1.181850606188767472 ) ) ;
#39012=CARTESIAN_POINT ( 'NONE',  ( 9.541187415715040032, 12.15447128979948310, -1.599625672291262513 ) ) ;
#39013=DIRECTION ( 'NONE',  ( -0.7592566023652994600, -0.6507913734559651608, -0.000000000000000000 ) ) ;
#39017=CARTESIAN_POINT ( 'NONE',  ( 5.986088515633498197, 6.942523675449257858, -1.199719254218446718 ) ) ;
#39018=CARTESIAN_POINT ( 'NONE',  ( -0.6823417656250212460, 2.613541667008084879, 1.181850606188767472 ) ) ;
#39022=CARTESIAN_POINT ( 'NONE',  ( -7.537443334193545397, 10.88110209227943770, -1.199719254218446718 ) ) ;
#39023=CARTESIAN_POINT ( 'NONE',  ( -5.219525951136856357, 6.152163700156858539, -1.082531754730543971 ) ) ;
#39025=CARTESIAN_POINT ( 'NONE',  ( -6.715366157470410435, 6.729015360003925750, -0.7998128361456291469 ) ) ;
#39027=CARTESIAN_POINT ( 'NONE',  ( -1.500000000000015099, -1.047916665983845919, 0.8660254037844403729 ) ) ;
#39035=CARTESIAN_POINT ( 'NONE',  ( -6.371969008298464132, 6.536311385877402458, 1.040834085586084257E-14 ) ) ;
#39040=CARTESIAN_POINT ( 'NONE',  ( -5.558479791478509568, 5.587240632920778438, 0.000000000000000000 ) ) ;
#39042=CARTESIAN_POINT ( 'NONE',  ( 9.561524646135536543, 12.17819805862340310, -1.599625672291262513 ) ) ;
#39044=DIRECTION ( 'NONE',  ( -5.578564026256490882E-16, -1.000000000000000000, -9.066213480720158442E-32 ) ) ;
#39053=CARTESIAN_POINT ( 'NONE',  ( -8.136864746495904299, 12.64475930422059768, -0.7998128361456281477 ) ) ;
#39057=CARTESIAN_POINT ( 'NONE',  ( 6.440286661691305703, 7.472421512516709718, 1.199719254218462483 ) ) ;
#39061=SPHERICAL_SURFACE ( 'NONE', #83374, 0.08000000000000000167 ) ;
#39062=CARTESIAN_POINT ( 'NONE',  ( 3.354752944377597856, 6.001296637494123232, -1.199719254218446718 ) ) ;
#39073=CARTESIAN_POINT ( 'NONE',  ( 6.584456157731144899, 10.83361595066169514, -0.7998128361456291469 ) ) ;
#39074=CARTESIAN_POINT ( 'NONE',  ( -6.261168011412601153, 6.199117522936475666, 1.040834085586084257E-14 ) ) ;
#39076=CARTESIAN_POINT ( 'NONE',  ( -1.499999999999984901, 4.160416667349482900, -0.8660254037844477004 ) ) ;
#39080=CARTESIAN_POINT ( 'NONE',  ( -1.201851678989727383E-14, 4.446875000341417916, -1.575800808251660134 ) ) ;
#39082=CARTESIAN_POINT ( 'NONE',  ( -4.401593425930945713, 8.286942763561420122, 1.040834085586084257E-14 ) ) ;
#39086=CARTESIAN_POINT ( 'NONE',  ( 4.306686350635271054, 8.176217842383143974, -0.7998128361456221525 ) ) ;
#39087=CARTESIAN_POINT ( 'NONE',  ( -4.599240423533815125, 6.388866465587984322, 1.599625672291267398 ) ) ;
#39094=CARTESIAN_POINT ( 'NONE',  ( 4.989037340148863464, 8.764367963574922982, -0.7216878364870257245 ) ) ;
#39097=CARTESIAN_POINT ( 'NONE',  ( 5.938108092661121162, 9.871617174839238729, 1.040834085586084257E-14 ) ) ;
#39098=CARTESIAN_POINT ( 'NONE',  ( -1.364683531250012516, 3.342708333674756727, 0.7879004041258379498 ) ) ;
#39100=CARTESIAN_POINT ( 'NONE',  ( 6.114364089638798738, 6.235772314107808079, 0.7216878364870317197 ) ) ;
#39108=CARTESIAN_POINT ( 'NONE',  ( -4.243318646243602998, 7.513047557524930475, 1.036732258902311354 ) ) ;
#39115=CARTESIAN_POINT ( 'NONE',  ( -8.805130697071332335, 12.36007068230351358, 1.199719254218462483 ) ) ;
#39120=CARTESIAN_POINT ( 'NONE',  ( -2.123823618835070537, 5.629544655282869847, 1.040834085586084257E-14 ) ) ;
#39125=CARTESIAN_POINT ( 'NONE',  ( 3.226477370372302644, 5.747678784534228313, 1.082531754730546636 ) ) ;
#39126=CARTESIAN_POINT ( 'NONE',  ( -0.6823417656249969321, 3.780208333674754506, -1.181850606188749264 ) ) ;
#39128=CARTESIAN_POINT ( 'NONE',  ( 7.721532178182734185, 8.967207948423393304, 1.199719254218462483 ) ) ;
#39130=CARTESIAN_POINT ( 'NONE',  ( 1.566537053174811955, 8.754671357082440153, 2.463935854687016480 ) ) ;
#39131=CARTESIAN_POINT ( 'NONE',  ( -4.253507506385334480, 5.985511395581417204, 1.599625672291267175 ) ) ;
#39132=CARTESIAN_POINT ( 'NONE',  ( 1.000000000000003553, 6.120000000000020535, 1.214306433183764966E-14 ) ) ;
#39135=CARTESIAN_POINT ( 'NONE',  ( -1.201851678989727383E-14, 4.587500000000025224, -1.732050807568863648 ) ) ;
#39136=CARTESIAN_POINT ( 'NONE',  ( 4.904298879841284098, 6.744767997946721216, 1.599625672291267398 ) ) ;
#39141=CARTESIAN_POINT ( 'NONE',  ( -1.001543065824772872E-14, 4.571875000341418804, 1.575800808251672791 ) ) ;
#39145=CARTESIAN_POINT ( 'NONE',  ( 9.300530189294644146, 10.91333531134101165, -1.082531754730543083 ) ) ;
#39150=CARTESIAN_POINT ( 'NONE',  ( 1.499999999999989120, 1.785416667349487563, 0.8660254037844524744 ) ) ;
#39152=CARTESIAN_POINT ( 'NONE',  ( -7.054319997812058318, 7.124461507069184130, 1.040834085586084257E-14 ) ) ;
#39153=CARTESIAN_POINT ( 'NONE',  ( 4.975479186090857375, 5.867442474269873642, 1.082531754730560403 ) ) ;
#39161=CARTESIAN_POINT ( 'NONE',  ( 8.444030743212801227, 8.745790710036752458, 0.7998128361456462443 ) ) ;
#39162=CARTESIAN_POINT ( 'NONE',  ( 4.202137545231717120, 6.989912005157271402, 1.199719254218462483 ) ) ;
#39165=CARTESIAN_POINT ( 'NONE',  ( 6.166260936116925606, 6.088392601758203071, 0.7998128361456341429 ) ) ;
#39171=ORIENTED_EDGE ( 'NONE', *, *, #100675, .T. ) ;
#39172=CARTESIAN_POINT ( 'NONE',  ( 10.07778825365955733, 10.65184113889131012, -0.7998128361456281477 ) ) ;
#39177=CARTESIAN_POINT ( 'NONE',  ( 5.228900738148710481, 6.411469580122314049, 1.161126877744517838 ) ) ;
#39183=CARTESIAN_POINT ( 'NONE',  ( -1.284279953904152949, 3.171639714193937198, 0.7750000000000152323 ) ) ;
#39184=CARTESIAN_POINT ( 'NONE',  ( 5.653386867218496370, 9.539442411822841805, 1.040834085586084257E-14 ) ) ;
#39185=CARTESIAN_POINT ( 'NONE',  ( -4.440459003675619520, 5.139289244831666714, 1.199719254218462483 ) ) ;
#39189=CARTESIAN_POINT ( 'NONE',  ( -6.240830780992103755, 6.175390754112560110, 1.040834085586084257E-14 ) ) ;
#39200=CARTESIAN_POINT ( 'NONE',  ( 10.07100917685271035, 10.64393221595000938, 0.7998128361456462443 ) ) ;
#39203=ORIENTED_EDGE ( 'NONE', *, *, #190382, .F. ) ;
#39208=CARTESIAN_POINT ( 'NONE',  ( 3.484082288587600384, 7.008587070086744752, -0.7216878364870351614 ) ) ;
#39209=CARTESIAN_POINT ( 'NONE',  ( -8.175203439360366531, 12.48156174598837787, 1.040834085586084257E-14 ) ) ;
#39213=CARTESIAN_POINT ( 'NONE',  ( 9.250740883225924804, 9.686952540052077509, 1.040834085586084257E-14 ) ) ;
#39215=CARTESIAN_POINT ( 'NONE',  ( -0.6385288935052398918, 2.800000000000018474, 1.214618717626907207 ) ) ;
#39217=CARTESIAN_POINT ( 'NONE',  ( -7.088215381846223906, 7.164006121775713609, 0.7998128361456341429 ) ) ;
#39218=CARTESIAN_POINT ( 'NONE',  ( 4.416205349749311004, 6.175325546172740765, 1.599625672291267398 ) ) ;
#39223=CARTESIAN_POINT ( 'NONE',  ( 8.367353357928214663, 12.91366268422496688, 1.040834085586084257E-14 ) ) ;
#39227=CARTESIAN_POINT ( 'NONE',  ( -0.6823417656250003738, 2.530208333674753618, -1.181850606188749264 ) ) ;
#39229=CARTESIAN_POINT ( 'NONE',  ( 6.860062538834778678, 8.066123052471139587, -1.082531754730543083 ) ) ;
#39231=CARTESIAN_POINT ( 'NONE',  ( -1.499999999999990896, 4.660416667349485564, -0.8660254037844429265 ) ) ;
#39237=CARTESIAN_POINT ( 'NONE',  ( 8.229436053370669413, 10.62409470039771442, 1.443375672974076540 ) ) ;
#39242=CARTESIAN_POINT ( 'NONE',  ( -8.910733272679575379, 11.41894145625809820, -1.599625672291263179 ) ) ;
#39251=CARTESIAN_POINT ( 'NONE',  ( 3.018661757337009810, 6.673522483535157868, 0.000000000000000000 ) ) ;
#39256=CARTESIAN_POINT ( 'NONE',  ( 5.311043488251262268, 7.219303374425030562, -1.599625672291256295 ) ) ;
#39259=CARTESIAN_POINT ( 'NONE',  ( -0.7500000000000006661, 2.639583334016156080, -1.299038105676652011 ) ) ;
#39265=CARTESIAN_POINT ( 'NONE',  ( -0.7500000000000215383, 0.9416666666666878571, 1.299038105676659116 ) ) ;
#39266=CARTESIAN_POINT ( 'NONE',  ( 8.260995669428309540, 8.532249790621511565, 0.7998128361456481317 ) ) ;
#39267=CARTESIAN_POINT ( 'NONE',  ( -1.364683531250014514, -0.4697916663252449943, 0.7879004041258379498 ) ) ;
#39271=CARTESIAN_POINT ( 'NONE',  ( 9.734391104931955141, 10.45913716528321125, 0.7216878364870438212 ) ) ;
#39276=CARTESIAN_POINT ( 'NONE',  ( -5.473741331615264549, 7.409117525016355010, -1.599625672291256295 ) ) ;
#39277=CARTESIAN_POINT ( 'NONE',  ( 1.499999999999989120, 2.535416667349483344, 0.8660254037844524744 ) ) ;
#39278=CARTESIAN_POINT ( 'NONE',  ( -0.6823417656249969321, 5.530208333674756283, -1.181850606188749264 ) ) ;
#39283=CARTESIAN_POINT ( 'NONE',  ( -0.6823417656250212460, 4.613541667008086655, 1.181850606188767472 ) ) ;
#39284=B_SPLINE_CURVE_WITH_KNOTS ( 'NONE', 3,
 ( #130056, #178737, #196050, #96436, #145200, #209062, #60699, #47682, #176597, #211206 ),
 .UNSPECIFIED., .F., .F.,
 ( 4, 2, 2, 2, 4 ),
 ( 0.0001025101613542923196, 0.0005630481886794980444, 0.001023586216004703647, 0.001484124243329909250, 0.001944662270655115070 ),
 .UNSPECIFIED. ) ;
#39293=CARTESIAN_POINT ( 'NONE',  ( -7.340850106795412167, 10.65174332698158643, 1.199719254218453823 ) ) ;
#39295=CARTESIAN_POINT ( 'NONE',  ( 5.147291874682557555, 9.156924287104992288, 0.7998128361456462443 ) ) ;
#39303=CARTESIAN_POINT ( 'NONE',  ( -5.994676475536691029, 10.14553965476814845, 0.7998128361456481317 ) ) ;
#39308=CARTESIAN_POINT ( 'NONE',  ( 3.379006598303866848, 4.965260336153046516, -1.599625672291262513 ) ) ;
#39311=CARTESIAN_POINT ( 'NONE',  ( -5.199715606040888005, 6.025088614257851027, -1.199719254218446718 ) ) ;
#39313=CARTESIAN_POINT ( 'NONE',  ( -7.648771216403934758, 12.07531685244661723, -0.7998128361456291469 ) ) ;
#39316=CARTESIAN_POINT ( 'NONE',  ( -4.127707017443506210, 7.650024674618332021, -0.8198546088712642677 ) ) ;
#39323=CARTESIAN_POINT ( 'NONE',  ( 4.984594031318565932, 8.967110136513669616, 0.7998128361456462443 ) ) ;
#39352=CARTESIAN_POINT ( 'NONE',  ( 0.7499999999999885647, 2.347916667349486453, -1.299038105676652899 ) ) ;
#39354=CARTESIAN_POINT ( 'NONE',  ( -3.189213936345698830, 2.817530495244580102, 2.450448857954578230 ) ) ;
#39357=CARTESIAN_POINT ( 'NONE',  ( -9.022061154889962964, 12.61315621642528129, -1.199719254218446718 ) ) ;
#39358=CARTESIAN_POINT ( 'NONE',  ( -3.294945724223601768, 7.655198976062505878, -2.499999999999995115 ) ) ;
#39359=CARTESIAN_POINT ( 'NONE',  ( 0.6823417656249899377, 1.342708333674752508, 1.181850606188755259 ) ) ;
#39366=CARTESIAN_POINT ( 'NONE',  ( -4.090809663021341969, 5.795697244990093644, 1.599625672291267398 ) ) ;
#39371=CARTESIAN_POINT ( 'NONE',  ( 0.6823417656249882723, 0.7385416670080829915, -1.181850606188749264 ) ) ;
#39376=CARTESIAN_POINT ( 'NONE',  ( -1.402160292154681736E-14, 0.6968750003414164729, -1.575800808251659024 ) ) ;
#39379=CARTESIAN_POINT ( 'NONE',  ( -7.283754839039664475, 9.520799950344851936, -1.599625672291263179 ) ) ;
#39380=CARTESIAN_POINT ( 'NONE',  ( 9.511208455186636712, 11.05516360492796935, 1.199719254218453823 ) ) ;
#39384=CARTESIAN_POINT ( 'NONE',  ( -1.201851678989727383E-14, 0.8843750003414173610, 1.575800808251672791 ) ) ;
#39392=CARTESIAN_POINT ( 'NONE',  ( 6.805829924380114804, 8.002851668940699881, 1.082531754730558626 ) ) ;
#39395=CARTESIAN_POINT ( 'NONE',  ( -7.335124800193271177, 8.516399340768996851, -1.199719254218452935 ) ) ;
#39396=CARTESIAN_POINT ( 'NONE',  ( -4.090809663021341969, 5.795697244990093644, 1.599625672291267398 ) ) ;
#39398=FACE_OUTER_BOUND ( 'NONE', #83528, .T. ) ;
#39401=CARTESIAN_POINT ( 'NONE',  ( -2.428882075142555497, 5.985446187641602300, 1.040834085586084257E-14 ) ) ;
#39402=CARTESIAN_POINT ( 'NONE',  ( 6.277061933002788585, 6.425586464699131639, 0.7216878364870317197 ) ) ;
#39403=CARTESIAN_POINT ( 'NONE',  ( -7.144783764277399030, 11.27940545839156528, 0.7216878364870458196 ) ) ;
#39405=CARTESIAN_POINT ( 'NONE',  ( -1.201851678989727383E-14, 4.337500000000023448, -1.732050807568863648 ) ) ;
#39409=CARTESIAN_POINT ( 'NONE',  ( 8.053180056837369705, 11.37883191874353805, -1.082531754730543083 ) ) ;
#39419=DIRECTION ( 'NONE',  ( 0.6507913734559627184, -0.7592566023653016805, 0.000000000000000000 ) ) ;
#39420=CARTESIAN_POINT ( 'NONE',  ( 8.893785580440313865, 9.478430720042945623, 1.040834085586084257E-14 ) ) ;
#39421=CARTESIAN_POINT ( 'NONE',  ( 8.263858322729371153, 9.599921783727809910, -1.199719254218446718 ) ) ;
#39422=CARTESIAN_POINT ( 'NONE',  ( -4.720210035852093533, 8.658662141802762946, -0.7998128361456281477 ) ) ;
#39424=CARTESIAN_POINT ( 'NONE',  ( -3.673896439623302257, 4.156855427197417185, -0.9999999999999991118 ) ) ;
#39426=CARTESIAN_POINT ( 'NONE',  ( 6.033015167956792268, 8.061603667414825480, -1.443375672974057666 ) ) ;
#39427=CARTESIAN_POINT ( 'NONE',  ( 1.364683531249986537, -0.5739583329919174526, 0.7879004041258500513 ) ) ;
#39428=CARTESIAN_POINT ( 'NONE',  ( 3.050221373394638835, 6.502416002361635528, 0.000000000000000000 ) ) ;
#39430=CARTESIAN_POINT ( 'NONE',  ( -7.537970219518083326, 9.817384560903001045, -1.443375672974059665 ) ) ;
#39444=CARTESIAN_POINT ( 'NONE',  ( 1.500000000000007105, 10.64264068711930733, 1.214306433183764966E-14 ) ) ;
#39445=CARTESIAN_POINT ( 'NONE',  ( 7.609150525767641504, 9.900428251527500834, -1.599625672291262513 ) ) ;
#39456=CARTESIAN_POINT ( 'NONE',  ( -6.226218857173722476, 8.287007971501239467, 1.599625672291283607 ) ) ;
#39459=CARTESIAN_POINT ( 'NONE',  ( -4.608882153641705059, 7.464447381635583412, -1.199719254218452047 ) ) ;
#39468=CARTESIAN_POINT ( 'NONE',  ( -5.088387723830502196, 4.830873854090670605, -0.7998128361456221525 ) ) ;
#39471=CARTESIAN_POINT ( 'NONE',  ( 7.019370843573166319, 9.212351955633947043, 1.599625672291281386 ) ) ;
#39472=CARTESIAN_POINT ( 'NONE',  ( -0.6823417656249969321, 3.717708333674754506, -1.181850606188749264 ) ) ;
#39474=CARTESIAN_POINT ( 'NONE',  ( 5.756168354352870331, 6.246635012430203027, 1.018728318139457523 ) ) ;
#39479=CARTESIAN_POINT ( 'NONE',  ( 5.951666246274803562, 7.006327377817825663, 1.082531754730558626 ) ) ;
#39480=CARTESIAN_POINT ( 'NONE',  ( -7.182068686937172153, 9.402166106225269715, 1.599625672291283607 ) ) ;
#39484=CARTESIAN_POINT ( 'NONE',  ( -8.565000355531095622, 11.01558638625153286, -1.599625672291263179 ) ) ;
#39485=CARTESIAN_POINT ( 'NONE',  ( -6.250472511100020334, 7.250971670160158311, 1.199719254218450271 ) ) ;
#39489=CARTESIAN_POINT ( 'NONE',  ( 4.903883154387664867, 4.836367890058183683, 0.6143738762558150768 ) ) ;
#39493=CARTESIAN_POINT ( 'NONE',  ( 7.242026607993941489, 11.60078147596829901, 0.7998128361456462443 ) ) ;
#39508=CARTESIAN_POINT ( 'NONE',  ( -1.500000000000011324, 4.629166666666689522, -0.8660254037844313801 ) ) ;
#39509=CARTESIAN_POINT ( 'NONE',  ( 4.334856428067313416, 6.080418470877079429, -1.599625672291256295 ) ) ;
#39510=CARTESIAN_POINT ( 'NONE',  ( 6.681470773436232413, 6.689470745297396270, -0.7998128361456281477 ) ) ;
#39513=CARTESIAN_POINT ( 'NONE',  ( -7.022760382198764084, 11.13704484596649635, 0.7216878364870458196 ) ) ;
#39514=CARTESIAN_POINT ( 'NONE',  ( 5.178851490740187913, 8.985817805931475277, 0.7216878364870438212 ) ) ;
#39515=CARTESIAN_POINT ( 'NONE',  ( -8.148087131688683371, 11.48955683940339867, -1.082531754730543083 ) ) ;
#39519=CARTESIAN_POINT ( 'NONE',  ( 7.588813295347141441, 9.876701482703580837, -1.599625672291262513 ) ) ;
#39526=CARTESIAN_POINT ( 'NONE',  ( 1.364683531249986537, 2.655208333674754062, -0.7879004041258239610 ) ) ;
#39532=CARTESIAN_POINT ( 'NONE',  ( 8.609591239877852686, 10.00327685373437347, -1.199719254218445830 ) ) ;
#39535=CARTESIAN_POINT ( 'NONE',  ( -10.16591625214838679, 10.75465713712827487, 1.040834085586084257E-14 ) ) ;
#39541=CARTESIAN_POINT ( 'NONE',  ( 10.70146331988817323, 11.37946204949139251, 0.7998128361456341429 ) ) ;
#39545=CARTESIAN_POINT ( 'NONE',  ( -10.16591625214838679, 10.75465713712827487, 1.040834085586084257E-14 ) ) ;
#39547=CARTESIAN_POINT ( 'NONE',  ( 4.816116650875026828, 5.094466954826537552, -0.7651464576672448725 ) ) ;
#39548=CARTESIAN_POINT ( 'NONE',  ( 9.206149998879153529, 10.69926207256923689, 1.199719254218453823 ) ) ;
#39550=CARTESIAN_POINT ( 'NONE',  ( 5.869075745953527878, 5.991122463535357490, 0.2593076673842714119 ) ) ;
#39551=CARTESIAN_POINT ( 'NONE',  ( 1.203941962966152968, 3.258481847795084541, -0.7749999999999840350 ) ) ;
#39552=CARTESIAN_POINT ( 'NONE',  ( -4.090809663021341969, 5.795697244990093644, 1.599625672291267398 ) ) ;
#39556=CARTESIAN_POINT ( 'NONE',  ( 6.740374924288304648, 11.01552117831172062, 1.040834085586084257E-14 ) ) ;
#39558=CARTESIAN_POINT ( 'NONE',  ( 6.205881626753210867, 8.263281202677319470, 1.599625672291281386 ) ) ;
#39561=CARTESIAN_POINT ( 'NONE',  ( -8.514157279702027736, 10.95626946445095307, -1.443375672974059665 ) ) ;
#39569=CARTESIAN_POINT ( 'NONE',  ( -5.552734181323573992, 6.223089306236814444, -0.9332588772281782408 ) ) ;
#39571=CARTESIAN_POINT ( 'NONE',  ( 6.480434237652124452, 8.583592582059388576, 1.443375672974076540 ) ) ;
#39591=ADVANCED_FACE ( 'NONE', ( #196805 ), #115611, .T. ) ;
#39593=CARTESIAN_POINT ( 'NONE',  ( 6.988338112840064120, 10.24047933403371502, 1.199719254218460707 ) ) ;
#39597=CARTESIAN_POINT ( 'NONE',  ( 0.7499999999999902300, 1.014583334016154526, 1.299038105676657340 ) ) ;
#39598=CARTESIAN_POINT ( 'NONE',  ( -5.357443255694392725, 9.402100898285455699, 0.000000000000000000 ) ) ;
#39600=ORIENTED_EDGE ( 'NONE', *, *, #157816, .T. ) ;
#39601=CARTESIAN_POINT ( 'NONE',  ( -10.13488352141530768, 11.78278451552804817, 1.199719254218462483 ) ) ;
#39605=CARTESIAN_POINT ( 'NONE',  ( 8.111855979677986994, 8.358253485912799263, 1.040834085586084257E-14 ) ) ;
#39609=CARTESIAN_POINT ( 'NONE',  ( -7.039708073993679704, 9.236078724457858158, 1.599625672291283607 ) ) ;
#39611=CARTESIAN_POINT ( 'NONE',  ( 1.364683531249988535, 4.405208333674754506, -0.7879004041258300672 ) ) ;
#39616=CARTESIAN_POINT ( 'NONE',  ( -7.036318535812428721, 11.15286269184909784, 0.000000000000000000 ) ) ;
#39620=CARTESIAN_POINT ( 'NONE',  ( -1.364683531249997417, 4.821875000341417916, 1.214306433183764966E-14 ) ) ;
#39626=CARTESIAN_POINT ( 'NONE',  ( 1.364683531249988535, 3.655208333674750509, -0.7879004041258239610 ) ) ;
#39630=CARTESIAN_POINT ( 'NONE',  ( 3.755245360860917536, 5.404205559136275205, -1.443375672974051449 ) ) ;
#39631=CARTESIAN_POINT ( 'NONE',  ( 1.364683531249988535, 5.217708333674750065, -0.7879004041258300672 ) ) ;
#39638=CARTESIAN_POINT ( 'NONE',  ( -1.364683531250012516, 1.030208333674754062, 0.7879004041258379498 ) ) ;
#39639=CARTESIAN_POINT ( 'NONE',  ( -3.416291520963659512, 5.969128626890772615, 1.082531754730560403 ) ) ;
#39640=CARTESIAN_POINT ( 'NONE',  ( 4.202137545231717120, 6.989912005157271402, 1.199719254218462483 ) ) ;
#39643=CARTESIAN_POINT ( 'NONE',  ( -1.500000000000001332, -1.099999999999982991, 0.000000000000000000 ) ) ;
#39646=CARTESIAN_POINT ( 'NONE',  ( 5.043269954603547767, 4.986162489899998995, -0.7216878364870197293 ) ) ;
#39649=CARTESIAN_POINT ( 'NONE',  ( -7.199016379176422120, 11.34267684244042584, 0.000000000000000000 ) ) ;
#39655=CARTESIAN_POINT ( 'NONE',  ( -8.350932551013499960, 11.83017284523606172, -1.199719254218446718 ) ) ;
#39657=CARTESIAN_POINT ( 'NONE',  ( -4.541618270453545492, 8.242379048930368768, 0.7216878364870458196 ) ) ;
#39659=CARTESIAN_POINT ( 'NONE',  ( 1.364683531249986537, 0.2177083336747502595, -0.7879004041258309554 ) ) ;
#39666=VERTEX_POINT ( 'NONE', #48448 ) ;
#39674=ORIENTED_EDGE ( 'NONE', *, *, #34390, .T. ) ;
#39680=CARTESIAN_POINT ( 'NONE',  ( -4.790108344329849110, 4.482881244673243337, 0.7998128361456341429 ) ) ;
#39683=CARTESIAN_POINT ( 'NONE',  ( -1.364683531249997417, 3.321875000341423245, 1.214306433183764966E-14 ) ) ;
#39692=CARTESIAN_POINT ( 'NONE',  ( 0.6823417656249899377, 0.8427083336747520637, 1.181850606188755259 ) ) ;
#39703=CARTESIAN_POINT ( 'NONE',  ( 5.250031796989762967, 7.148123067953287446, 1.599625672291267398 ) ) ;
#39711=CARTESIAN_POINT ( 'NONE',  ( 7.579171565239241737, 8.801120566655981747, 1.199719254218462483 ) ) ;
#39715=CARTESIAN_POINT ( 'NONE',  ( 7.771848369131631351, 10.09024240211882351, -1.599625672291262513 ) ) ;
#39718=CARTESIAN_POINT ( 'NONE',  ( 1.527007413433539407, 8.693555224946434734, -2.520068491016797196 ) ) ;
#39729=CARTESIAN_POINT ( 'NONE',  ( -8.839552966430023417, 9.415159337030921449, -0.7216878364870267237 ) ) ;
#39734=CARTESIAN_POINT ( 'NONE',  ( -9.053093885623068715, 11.58502883802551153, -1.599625672291263179 ) ) ;
#39739=CARTESIAN_POINT ( 'NONE',  ( -4.843287188579803448, 6.673587691474970107, -1.599625672291256295 ) ) ;
#39742=CARTESIAN_POINT ( 'NONE',  ( 8.886479618753304166, 12.45497775759917758, -1.199719254218446718 ) ) ;
#39744=CARTESIAN_POINT ( 'NONE',  ( 4.924636110261782385, 6.768494766770632332, 1.599625672291267398 ) ) ;
#39750=CARTESIAN_POINT ( 'NONE',  ( 3.877268743828276243, 4.586196958296845594, 1.082531754730560403 ) ) ;
#39752=CARTESIAN_POINT ( 'NONE',  ( -4.232116505760120440, 8.089219690028791376, -0.7998128361456281477 ) ) ;
#39755=CARTESIAN_POINT ( 'NONE',  ( -8.839026081105473054, 12.39961529701003684, -1.199719254218446718 ) ) ;
#39761=CARTESIAN_POINT ( 'NONE',  ( 6.941411460516762943, 11.04213777067082702, -0.7216878364870267237 ) ) ;
#39762=ORIENTED_EDGE ( 'NONE', *, *, #116366, .T. ) ;
#39763=CARTESIAN_POINT ( 'NONE',  ( -0.6823417656249969321, 4.780208333674755394, -1.181850606188749264 ) ) ;
#39765=CARTESIAN_POINT ( 'NONE',  ( 3.876741858503734761, 6.610283703974623393, 1.199719254218462483 ) ) ;
#39780=CARTESIAN_POINT ( 'NONE',  ( -1.364683531250014514, 1.051041667008090208, -0.7879004041258289570 ) ) ;
#39782=CARTESIAN_POINT ( 'NONE',  ( 2.703961570921634028, 5.242040035128820108, -1.199719254218446718 ) ) ;
#39785=CARTESIAN_POINT ( 'NONE',  ( -5.748293942514186128, 6.769059690097084747, -1.082531754730544860 ) ) ;
#39786=CARTESIAN_POINT ( 'NONE',  ( 3.199361063144961825, 6.676412307070352270, -0.7216878364870267237 ) ) ;
#39787=CARTESIAN_POINT ( 'NONE',  ( -6.033015167956805591, 8.061603667414825480, -1.443375672974058777 ) ) ;
#39791=CARTESIAN_POINT ( 'NONE',  ( 6.498435699651741615, 6.475929825882159818, -0.7998128361456281477 ) ) ;
#39801=CARTESIAN_POINT ( 'NONE',  ( 6.667912619822566000, 6.673652899414787676, 1.040834085586084257E-14 ) ) ;
#39805=CARTESIAN_POINT ( 'NONE',  ( 4.028709946750490545, 3.988235255965033588, -0.8025987720412866011 ) ) ;
#39807=CARTESIAN_POINT ( 'NONE',  ( -6.201965203247477909, 9.323044272842313518, 1.199719254218452047 ) ) ;
#39811=CARTESIAN_POINT ( 'NONE',  ( 7.263417608619159083, 9.497073181520933716, -1.599625672291262513 ) ) ;
#39814=CARTESIAN_POINT ( 'NONE',  ( -7.226659571283968297, 8.389856573708110332, 1.199719254218450271 ) ) ;
#39815=CARTESIAN_POINT ( 'NONE',  ( 7.754900676892376055, 8.149731665903665601, 1.040834085586084257E-14 ) ) ;
#39816=CARTESIAN_POINT ( 'NONE',  ( 4.350666953118342839, 7.402852620340107492, 1.136566098749042242 ) ) ;
#39817=CARTESIAN_POINT ( 'NONE',  ( -3.737243898861318137, 7.511868315313511069, 0.7998128361456341429 ) ) ;
#39820=CARTESIAN_POINT ( 'NONE',  ( -6.762819695118240659, 6.784377820593065600, 0.7998128361456341429 ) ) ;
#39825=CARTESIAN_POINT ( 'NONE',  ( -1.364683531250012516, 2.030208333674750953, 0.7879004041258379498 ) ) ;
#39827=CARTESIAN_POINT ( 'NONE',  ( -5.748293942514172805, 8.689798118699771479, -1.082531754730538864 ) ) ;
#39833=CARTESIAN_POINT ( 'NONE',  ( 5.198661835836162481, 8.152523677529138979, 1.199719254218462483 ) ) ;
#39836=CARTESIAN_POINT ( 'NONE',  ( -5.881612045648562770, 6.018300081020916181, 0.2952277700727298781 ) ) ;
#39837=CARTESIAN_POINT ( 'NONE',  ( 0.6823417656249882723, 1.238541667008083547, -1.181850606188749264 ) ) ;
#39844=CARTESIAN_POINT ( 'NONE',  ( -3.601662362724658895, 7.353689856487406473, -0.7998128361456281477 ) ) ;
#39846=CARTESIAN_POINT ( 'NONE',  ( -8.392133896734675247, 10.81390885098904420, 1.443375672974064550 ) ) ;
#39855=CARTESIAN_POINT ( 'NONE',  ( -7.876924059415400414, 9.252461493148505411, 1.082531754730558626 ) ) ;
#39857=CARTESIAN_POINT ( 'NONE',  ( 1.284279953904121641, 3.034610286488902187, 0.7750000000000117906 ) ) ;
#39860=CARTESIAN_POINT ( 'NONE',  ( -7.253248993186740989, 9.485209796849769504, 1.443375672974090751 ) ) ;
#39866=CARTESIAN_POINT ( 'NONE',  ( 1.499999999999989120, 5.077083334016151639, -0.8660254037844323793 ) ) ;
#39867=CARTESIAN_POINT ( 'NONE',  ( 4.521492410791133842, 7.227233577430748568, -1.288726771885986055 ) ) ;
#39874=CARTESIAN_POINT ( 'NONE',  ( -6.368579470117215813, 8.453095353268645695, 1.599625672291283607 ) ) ;
#39877=CARTESIAN_POINT ( 'NONE',  ( 5.522248639467795428, 5.337044922334209573, -0.7998128361456231517 ) ) ;
#39881=CARTESIAN_POINT ( 'NONE',  ( 6.226218857173709154, 8.287007971501239467, 1.599625672291281386 ) ) ;
#39887=CARTESIAN_POINT ( 'NONE',  ( -5.748293942514180799, 7.729428904398431222, -1.443375672974052559 ) ) ;
#39894=CARTESIAN_POINT ( 'NONE',  ( 4.022871489700263758, 7.776595455899835585, -0.3464378842543735515 ) ) ;
#39896=VECTOR ( 'NONE', #82026, 1000.000000000000000 ) ;
#39898=CARTESIAN_POINT ( 'NONE',  ( 0.6823417656249882723, 0.3427083336747516196, 1.181850606188755259 ) ) ;
#39900=CARTESIAN_POINT ( 'NONE',  ( -9.179033691651859783, 10.66762638080401260, 1.199719254218462483 ) ) ;
#39902=CARTESIAN_POINT ( 'NONE',  ( 6.598014311344812199, 10.84943379654430906, 1.040834085586084257E-14 ) ) ;
#39904=CARTESIAN_POINT ( 'NONE',  ( -7.690499447449645309, 9.995335326823163058, 1.599625672291295375 ) ) ;
#39907=CARTESIAN_POINT ( 'NONE',  ( -1.201851678989727383E-14, 4.696875000341419693, -1.575800808251660134 ) ) ;
#39910=CARTESIAN_POINT ( 'NONE',  ( 9.137832345930652522, 10.72352116074969075, -1.082531754730543083 ) ) ;
#39913=CARTESIAN_POINT ( 'NONE',  ( -1.402160292154681736E-14, -0.8656249996585829720, 1.575800808251672791 ) ) ;
#39915=CARTESIAN_POINT ( 'NONE',  ( 7.632877294369377452, 8.967740267261513409, -1.082531754730537976 ) ) ;
#39917=CARTESIAN_POINT ( 'NONE',  ( 1.419999999999990603, 6.200000000000045475, 2.873333333333337070 ) ) ;
#39918=CARTESIAN_POINT ( 'NONE',  ( -6.087247782855839340, 6.204136622861004646, 0.000000000000000000 ) ) ;
#39921=CARTESIAN_POINT ( 'NONE',  ( -0.6823417656250003738, 2.717708333674753618, -1.181850606188749264 ) ) ;
#39925=CARTESIAN_POINT ( 'NONE',  ( -6.043183783389232566, 8.073467052085995022, 1.599625672291269396 ) ) ;
#39931=CARTESIAN_POINT ( 'NONE',  ( 8.772289083241844310, 10.19309100432570148, -1.199719254218446718 ) ) ;
#39934=CARTESIAN_POINT ( 'NONE',  ( -1.500000000000013101, 0.9208333333333594828, 0.8660254037844403729 ) ) ;
#39940=CARTESIAN_POINT ( 'NONE',  ( 7.307481608085759639, 7.627742752295940676, 1.040834085586084257E-14 ) ) ;
#39942=CARTESIAN_POINT ( 'NONE',  ( 2.866659414285625651, 5.431854185720147221, -1.199719254218446718 ) ) ;
#39947=EDGE_CURVE ( 'NONE', #159976, #205805, #13777, .T. ) ;
#39949=CARTESIAN_POINT ( 'NONE',  ( 0.006158830626129541130, 7.078243236992583398, -2.121324627965408993 ) ) ;
#39950=CARTESIAN_POINT ( 'NONE',  ( 8.762647353133951711, 9.117510088278095282, 1.040834085586084257E-14 ) ) ;
#39951=CARTESIAN_POINT ( 'NONE',  ( -8.422639742587602285, 10.84949900448412841, -1.599625672291263179 ) ) ;
#39953=CYLINDRICAL_SURFACE ( 'NONE', #94039, 1.250000000000000000 ) ;
#39954=CARTESIAN_POINT ( 'NONE',  ( 1.364683531249986537, 0.1552083336747499542, -0.7879004041258309554 ) ) ;
#39955=CARTESIAN_POINT ( 'NONE',  ( -1.402160292154681736E-14, 1.837500000000019895, -1.732050807568863648 ) ) ;
#39957=CARTESIAN_POINT ( 'NONE',  ( 5.660692828905515839, 6.562895374266609849, -1.199719254218445830 ) ) ;
#39962=CARTESIAN_POINT ( 'NONE',  ( -1.001543065824772872E-14, 4.571875000341418804, 1.575800808251672791 ) ) ;
#39964=CARTESIAN_POINT ( 'NONE',  ( -7.296259222448620463, 11.66405285949874759, 0.7998128361456481317 ) ) ;
#39966=CARTESIAN_POINT ( 'NONE',  ( -4.121315508874255684, 7.752025827087861920, -0.7216878364870267237 ) ) ;
#39975=CARTESIAN_POINT ( 'NONE',  ( 8.125414133291656071, 8.374071331795406081, -0.7998128361456291469 ) ) ;
#39978=CARTESIAN_POINT ( 'NONE',  ( 6.263503779389103521, 10.25124547602188763, 1.040834085586084257E-14 ) ) ;
#39981=CARTESIAN_POINT ( 'NONE',  ( -8.616370316684697883, 10.01118577667568132, -1.199719254218446718 ) ) ;
#39982=CARTESIAN_POINT ( 'NONE',  ( 6.006425746053997372, 6.966250444273174303, -1.199719254218445830 ) ) ;
#39985=CARTESIAN_POINT ( 'NONE',  ( 3.846762897975340767, 5.510976019103107859, -1.599625672291256295 ) ) ;
#39988=CARTESIAN_POINT ( 'NONE',  ( -4.016479854857874621, 7.690552166905142428, -0.3130353517275369368 ) ) ;
#39992=CARTESIAN_POINT ( 'NONE',  ( -4.555176424511596878, 7.297827681030051750, 1.082531754730560403 ) ) ;
#39994=CARTESIAN_POINT ( 'NONE',  ( 2.846322183865124700, 5.408127416896231665, -1.199719254218446718 ) ) ;
#39997=CARTESIAN_POINT ( 'NONE',  ( -7.379715684540041565, 7.504089808251839244, 1.040834085586084257E-14 ) ) ;
#39998=CARTESIAN_POINT ( 'NONE',  ( -3.083288183660637838, 6.450096981798545848, -0.7078863735355921394 ) ) ;
#40002=CARTESIAN_POINT ( 'NONE',  ( -9.006694118179950692, 9.402231314165087284, 1.040834085586084257E-14 ) ) ;
#40006=CARTESIAN_POINT ( 'NONE',  ( 3.649115900372475796, 7.409052317076538330, 1.040834085586084257E-14 ) ) ;
#40007=CARTESIAN_POINT ( 'NONE',  ( -4.957044826794452241, 6.512741263612475962, -2.499999999999995115 ) ) ;
#40016=CARTESIAN_POINT ( 'NONE',  ( -1.123270288250342919, 2.846052654332832610, 0.7749999999993751887 ) ) ;
#40017=CARTESIAN_POINT ( 'NONE',  ( -7.555971681517696936, 7.709721804725773175, 0.7998128361456462443 ) ) ;
#40020=CARTESIAN_POINT ( 'NONE',  ( 6.046573322014824114, 7.117052299514516456, -1.082531754730543083 ) ) ;
#40024=CARTESIAN_POINT ( 'NONE',  ( -6.098470168048611306, 6.009303372345148553, 1.040834085586084257E-14 ) ) ;
#40028=CARTESIAN_POINT ( 'NONE',  ( -7.067878151425722955, 7.140279352951794500, 0.7998128361456341429 ) ) ;
#40029=CARTESIAN_POINT ( 'NONE',  ( -5.868066076333878556, 6.026401760103492045, 0.3561039394813777514 ) ) ;
#40034=CARTESIAN_POINT ( 'NONE',  ( -7.818248136574758256, 12.27303992597924420, 0.000000000000000000 ) ) ;
#40035=CARTESIAN_POINT ( 'NONE',  ( 6.238723240582662477, 10.43026088065513513, -0.7998128361456291469 ) ) ;
#40038=CARTESIAN_POINT ( 'NONE',  ( -3.958617665510283601, 4.681104033592509595, -1.082531754730549967 ) ) ;
#40048=CARTESIAN_POINT ( 'NONE',  ( 10.05978679165993839, 10.83876546646586014, 0.7216878364870438212 ) ) ;
#40053=EDGE_LOOP ( 'NONE', ( #153906, #187955, #200470 ) ) ;
#40054=CARTESIAN_POINT ( 'NONE',  ( 1.387358672525637715, 7.251968950354889643, -4.302625267139783993 ) ) ;
#40063=EDGE_LOOP ( 'NONE', ( #145473, #127716, #81646, #187436, #138281 ) ) ;
#40068=CARTESIAN_POINT ( 'NONE',  ( -3.273404022695637572, 5.906389562198459231, 1.199719254218462483 ) ) ;
#40070=CARTESIAN_POINT ( 'NONE',  ( -2.435661151949389147, 5.993355110582911038, 0.7998128361456341429 ) ) ;
#40074=CARTESIAN_POINT ( 'NONE',  ( -1.364683531249997417, 5.509375000341417916, 1.214306433183764966E-14 ) ) ;
#40082=CARTESIAN_POINT ( 'NONE',  ( 10.70146331988817323, 11.37946204949139251, 0.7998128361456341429 ) ) ;
#40086=CARTESIAN_POINT ( 'NONE',  ( 9.368320956918608999, 11.95279375453699622, 1.443375672974076540 ) ) ;
#40088=CARTESIAN_POINT ( 'NONE',  ( 0.6823417656249882723, 1.988541667008083991, -1.181850606188749264 ) ) ;
#40089=CARTESIAN_POINT ( 'NONE',  ( 1.499999999999989120, 3.754166666666685082, 0.8660254037844522523 ) ) ;
#40091=CARTESIAN_POINT ( 'NONE',  ( -8.646349277213090545, 11.11049346154719508, 1.599625672291269396 ) ) ;
#40092=CARTESIAN_POINT ( 'NONE',  ( -4.351804119862249465, 7.060559992272473551, 1.082531754730560403 ) ) ;
#40094=CARTESIAN_POINT ( 'NONE',  ( -4.530395885260773525, 8.437212299446219532, 0.7998128361456481317 ) ) ;
#40096=CARTESIAN_POINT ( 'NONE',  ( -1.364683531249997417, 5.509375000341417916, 1.214306433183764966E-14 ) ) ;
#40105=CARTESIAN_POINT ( 'NONE',  ( -5.924549939047510705, 6.974691686052601369, 1.082531754730549967 ) ) ;
#40107=CYLINDRICAL_SURFACE ( 'NONE', #26408, 1.250000000000000000 ) ;
#40111=CARTESIAN_POINT ( 'NONE',  ( -4.406036734316890247, 7.123831375802920363, -1.082531754730548412 ) ) ;
#40113=CARTESIAN_POINT ( 'NONE',  ( 9.103410076571945453, 12.70806329172093818, 1.199719254218450271 ) ) ;
#40123=CARTESIAN_POINT ( 'NONE',  ( -2.916975605234527702, 6.554888639415577423, 1.040834085586084257E-14 ) ) ;
#40124=CARTESIAN_POINT ( 'NONE',  ( -8.597841969360544567, 13.18256606422934674, 0.7998128361456341429 ) ) ;
#40129=CARTESIAN_POINT ( 'NONE',  ( 4.469384193999260901, 8.366031992974468423, -0.7998128361456231517 ) ) ;
#40133=DIRECTION ( 'NONE',  ( 1.000000000000000000, 0.000000000000000000, 0.000000000000000000 ) ) ;
#40143=CARTESIAN_POINT ( 'NONE',  ( 8.259941899223605333, 10.65968485389279508, -1.599625672291268286 ) ) ;
#40144=CARTESIAN_POINT ( 'NONE',  ( -5.168682875307782254, 7.053215992657626110, -1.599625672291256295 ) ) ;
#40147=CARTESIAN_POINT ( 'NONE',  ( -3.673896439623305810, 4.156855427197417185, -7.499999999999991118 ) ) ;
#40151=CARTESIAN_POINT ( 'NONE',  ( 0.6823417656249917140, 5.092708333674749177, 1.181850606188765695 ) ) ;
#40153=CARTESIAN_POINT ( 'NONE',  ( -6.586563698140583512, 6.578745824119123675, 1.040834085586084257E-14 ) ) ;
#40155=FACE_OUTER_BOUND ( 'NONE', #16113, .T. ) ;
#40156=CARTESIAN_POINT ( 'NONE',  ( 5.138703914779377158, 5.953908307786102583, 1.199719254218462483 ) ) ;
#40157=CARTESIAN_POINT ( 'NONE',  ( -6.274726165026268454, 6.214935368819085149, 0.7998128361456341429 ) ) ;
#40163=CARTESIAN_POINT ( 'NONE',  ( 5.816084710582486217, 9.729256562414162701, 1.040834085586084257E-14 ) ) ;
#40165=CARTESIAN_POINT ( 'NONE',  ( 5.951666246274784910, 9.887435020721849099, 0.7216878364870438212 ) ) ;
#40166=CARTESIAN_POINT ( 'NONE',  ( 1.364683531249988535, 3.426041667008085323, 0.7879004041258500513 ) ) ;
#40168=CARTESIAN_POINT ( 'NONE',  ( 3.985733972293228344, 7.593847367743336463, 1.040834085586084257E-14 ) ) ;
#40172=EDGE_CURVE ( 'NONE', #38245, #10803, #155098, .T. ) ;
#40177=CARTESIAN_POINT ( 'NONE',  ( -4.061425534073997312, 7.733864674645915649, 0.6335290845049870168 ) ) ;
#40185=CARTESIAN_POINT ( 'NONE',  ( -9.642873567817536795, 12.27310513391906532, 1.599625672291281386 ) ) ;
#40187=CARTESIAN_POINT ( 'NONE',  ( 2.198393463710220264, 5.716542807637226886, 0.7998128361456462443 ) ) ;
#40195=CARTESIAN_POINT ( 'NONE',  ( 2.412988153552339643, 5.758977245878946327, 0.7216878364870438212 ) ) ;
#40197=CARTESIAN_POINT ( 'NONE',  ( 0.6823417656249917140, 3.905208333674754950, 1.181850606188765695 ) ) ;
#40199=CARTESIAN_POINT ( 'NONE',  ( 6.916630921265960019, 11.22115317478565188, 0.7998128361456462443 ) ) ;
#40204=DIRECTION ( 'NONE',  ( 1.000000000000000000, -5.578564026256504688E-16, 0.000000000000000000 ) ) ;
#40207=CARTESIAN_POINT ( 'NONE',  ( -1.500000000000011324, 3.670833333333356485, 0.8660254037844403729 ) ) ;
#40208=CARTESIAN_POINT ( 'NONE',  ( 5.311043488251262268, 7.219303374425030562, -1.599625672291256295 ) ) ;
#40212=CARTESIAN_POINT ( 'NONE',  ( -0.6823417656250212460, 3.801041667008085767, 1.181850606188767472 ) ) ;
#40215=CARTESIAN_POINT ( 'NONE',  ( 8.093854517678360949, 12.38665467069271386, 1.040834085586084257E-14 ) ) ;
#40220=CARTESIAN_POINT ( 'NONE',  ( -1.500000000000013101, 2.160416667349489561, -0.8660254037844313801 ) ) ;
#40222=CARTESIAN_POINT ( 'NONE',  ( -4.205000198532790279, 8.057583998263570635, 0.7998128361456341429 ) ) ;
#40223=CARTESIAN_POINT ( 'NONE',  ( 3.673896439178911066, 7.230036912443299713, 0.7216878364870317197 ) ) ;
#40224=CARTESIAN_POINT ( 'NONE',  ( -4.912887863224139728, 4.752532773970169266, -0.2786491325915474437 ) ) ;
#40232=CARTESIAN_POINT ( 'NONE',  ( 6.109920781252839994, 10.27999134477033216, 1.040834085586084257E-14 ) ) ;
#40233=CARTESIAN_POINT ( 'NONE',  ( 4.150767584078112193, 7.994312614733129152, 0.7998128361456321445 ) ) ;
#40234=CARTESIAN_POINT ( 'NONE',  ( -3.023105066167323329, 5.702484939155337607, -2.420000000000000373 ) ) ;
#40237=CARTESIAN_POINT ( 'NONE',  ( 4.306686350635271054, 8.176217842383143974, -0.7998128361456221525 ) ) ;
#40244=CARTESIAN_POINT ( 'NONE',  ( 8.218213668177886788, 12.73966637951625813, 0.7998128361456462443 ) ) ;
#40249=CARTESIAN_POINT ( 'NONE',  ( 5.856753424380153561, 5.998585917076054486, 0.3190708477142957245 ) ) ;
#40254=LINE ( 'NONE', #139903, #166572 ) ;
#40260=CARTESIAN_POINT ( 'NONE',  ( 7.022760382198770301, 8.255937203062467589, -1.082531754730543083 ) ) ;
#40261=CARTESIAN_POINT ( 'NONE',  ( -4.711622075948912247, 5.455646162483875017, -1.199719254218446718 ) ) ;
#40265=CARTESIAN_POINT ( 'NONE',  ( -5.032047568966410367, 9.022472597102808578, 1.214306433183764966E-14 ) ) ;
#40273=VERTEX_POINT ( 'NONE', #3899 ) ;
#40274=CARTESIAN_POINT ( 'NONE',  ( 1.499999999999822586, 7.240846818246208905, 4.154462424328221104 ) ) ;
#40287=CARTESIAN_POINT ( 'NONE',  ( -8.663296969452339624, 13.05100419776235299, 1.040834085586084257E-14 ) ) ;
#40291=CARTESIAN_POINT ( 'NONE',  ( 9.077347539549325717, 10.54899253668443393, -1.199719254218446718 ) ) ;
#40296=CARTESIAN_POINT ( 'NONE',  ( -4.726989112658928072, 8.666571064744069020, 1.040834085586084257E-14 ) ) ;
#40297=CARTESIAN_POINT ( 'NONE',  ( 5.671388329218120639, 5.511041227042920099, 1.040834085586084257E-14 ) ) ;
#40305=CARTESIAN_POINT ( 'NONE',  ( -4.148431816101615155, 3.942184661647709198, 0.7216878364870317197 ) ) ;
#40308=CARTESIAN_POINT ( 'NONE',  ( -1.402160292154681736E-14, 2.509375000341417028, -1.575800808251660134 ) ) ;
#40309=ORIENTED_EDGE ( 'NONE', *, *, #184415, .T. ) ;
#40311=CARTESIAN_POINT ( 'NONE',  ( 6.643132081016124069, 7.813037518349371879, 1.082531754730558626 ) ) ;
#40320=CARTESIAN_POINT ( 'NONE',  ( 7.890482213029013536, 12.14938698193514277, 1.040834085586084257E-14 ) ) ;
#40326=CARTESIAN_POINT ( 'NONE',  ( -8.422639742587602285, 10.84949900448412841, -1.599625672291263179 ) ) ;
#40334=CARTESIAN_POINT ( 'NONE',  ( 3.680148631105580215, 6.380924938676771241, -1.199719254218446718 ) ) ;
#40341=CARTESIAN_POINT ( 'NONE',  ( 6.145923705696426431, 6.064665832934283962, 0.7998128361456341429 ) ) ;
#40344=CARTESIAN_POINT ( 'NONE',  ( -0.7500000000000215383, 2.472916667349486897, 1.299038105676671107 ) ) ;
#40350=CARTESIAN_POINT ( 'NONE',  ( 1.499999999999987566, -0.2249999999999821587, 0.000000000000000000 ) ) ;
#40351=CARTESIAN_POINT ( 'NONE',  ( 6.414979237560321401, 10.63589287712906462, 1.040834085586084257E-14 ) ) ;
#40353=CARTESIAN_POINT ( 'NONE',  ( -1.364683531250014514, -0.5114583329919092369, -0.7879004041258359514 ) ) ;
#40357=CARTESIAN_POINT ( 'NONE',  ( 7.782016984564043227, 12.02284421539267356, 0.7216878364870438212 ) ) ;
#40362=CARTESIAN_POINT ( 'NONE',  ( -5.032047568966410367, 9.022472597102808578, 1.214306433183764966E-14 ) ) ;
#40363=CARTESIAN_POINT ( 'NONE',  ( -1.499999999999997780, 2.181250000682817713, 1.214306433183764966E-14 ) ) ;
#40365=CARTESIAN_POINT ( 'NONE',  ( -1.364683531250010295, 5.551041667008087543, -0.7879004041258300672 ) ) ;
#40379=CARTESIAN_POINT ( 'NONE',  ( -9.073431116043565225, 11.60875560684942265, -1.599625672291263179 ) ) ;
#40380=CARTESIAN_POINT ( 'NONE',  ( 5.459129407796876166, 9.520734742405036144, 1.040834085586084257E-14 ) ) ;
#40387=CARTESIAN_POINT ( 'NONE',  ( -7.100719765255177229, 9.307259030929609267, -1.599625672291263179 ) ) ;
#40392=CARTESIAN_POINT ( 'NONE',  ( 8.543609354905870035, 13.11929468069890525, 0.7998128361456462443 ) ) ;
#40394=VERTEX_POINT ( 'NONE', #111917 ) ;
#40396=CARTESIAN_POINT ( 'NONE',  ( -3.716906668440817185, 7.488141546489591072, 0.7998128361456341429 ) ) ;
#40397=( BOUNDED_CURVE ( )  B_SPLINE_CURVE ( 2, ( #2589, #446, #180313, #163004, #182419, #117503, #118568 ),
 .UNSPECIFIED., .F., .T. ) 
 B_SPLINE_CURVE_WITH_KNOTS ( ( 3, 2, 2, 3 ),
 ( 0.2500000000000002776, 0.2541666666666668184, 0.2583333333333333592, 0.2624999999999999001 ),
 .UNSPECIFIED. ) 
 CURVE ( )  GEOMETRIC_REPRESENTATION_ITEM ( )  RATIONAL_B_SPLINE_CURVE ( ( 0.9999999999999911182, 0.8660254037844475894, 1.000000000000000000, 0.8660254037844387076, 1.000000000000000000, 0.8660254037844422603, 0.9999999999999964473 ) ) 
 REPRESENTATION_ITEM ( '' )  );
#40398=CARTESIAN_POINT ( 'NONE',  ( -9.321394304595349567, 10.83371376257142416, 1.199719254218462483 ) ) ;
#40401=CARTESIAN_POINT ( 'NONE',  ( -4.418902842294746947, 7.322973332268160718, -1.241058569461401362 ) ) ;
#40408=CARTESIAN_POINT ( 'NONE',  ( 5.361359679200154105, 8.342337828120466980, 1.199719254218462483 ) ) ;
#40426=CARTESIAN_POINT ( 'NONE',  ( 3.063779527008304360, 6.518233848244248563, 0.7216878364870317197 ) ) ;
#40428=B_SPLINE_CURVE_WITH_KNOTS ( 'NONE', 3,
 ( #141016, #58655, #26143, #92256, #158302, #147381, #13084, #210217, #81304, #63986 ),
 .UNSPECIFIED., .F., .F.,
 ( 4, 3, 3, 4 ),
 ( 1.060539725738902859E-15, 3.125190826550851492E-05, 5.893811830794473683E-05, 8.663425284181113851E-05 ),
 .UNSPECIFIED. ) ;
#40431=CARTESIAN_POINT ( 'NONE',  ( -9.134442807305063639, 11.67993591332117376, 1.599625672291281386 ) ) ;
#40435=AXIS2_PLACEMENT_3D ( 'NONE', #177959, #208291, #79381 ) ;
#40438=CARTESIAN_POINT ( 'NONE',  ( 1.499999999999987121, 2.327083334016154303, -0.8660254037844262731 ) ) ;
#40440=CARTESIAN_POINT ( 'NONE',  ( 5.622977593387656015, 6.244972703327866803, 1.018919728668438385 ) ) ;
#40443=CARTESIAN_POINT ( 'NONE',  ( -10.66756793585402363, 11.33991743478486391, 0.7998128361456462443 ) ) ;
#40445=CARTESIAN_POINT ( 'NONE',  ( -0.6823417656250212460, 1.051041667008083325, 1.181850606188755259 ) ) ;
#40450=CARTESIAN_POINT ( 'NONE',  ( -5.088387723830502196, 4.830873854090670605, -0.7998128361456221525 ) ) ;
#40452=CARTESIAN_POINT ( 'NONE',  ( -0.4734754237523640663, 6.885074608495208359, -3.701908037242890526 ) ) ;
#40455=CARTESIAN_POINT ( 'NONE',  ( -1.364683531250012516, 0.5927083336747520637, 0.7879004041258379498 ) ) ;
#40460=CARTESIAN_POINT ( 'NONE',  ( 1.364683531249988757, 0.1343750003414204142, 0.000000000000000000 ) ) ;
#40463=CARTESIAN_POINT ( 'NONE',  ( -8.525379664894808585, 8.840697785332414682, -0.7998128361456291469 ) ) ;
#40464=CARTESIAN_POINT ( 'NONE',  ( 8.727698198895078363, 11.20540053684285553, -1.599625672291257406 ) ) ;
#40465=CARTESIAN_POINT ( 'NONE',  ( 5.030238685870051185, 5.827365540725222282, -1.199719254218452047 ) ) ;
#40469=CARTESIAN_POINT ( 'NONE',  ( -1.402160292154681736E-14, -0.3656249996585805295, 1.575800808251672791 ) ) ;
#40476=CARTESIAN_POINT ( 'NONE',  ( 5.653386867218496370, 9.539442411822841805, 1.040834085586084257E-14 ) ) ;
#40479=CARTESIAN_POINT ( 'NONE',  ( -3.228813138348844536, 6.918699094715619502, 0.7998128361456341429 ) ) ;
#40481=CARTESIAN_POINT ( 'NONE',  ( -0.7500000000000215383, 5.472916667349482900, 1.299038105676671107 ) ) ;
#40484=CARTESIAN_POINT ( 'NONE',  ( 4.460269348771534581, 8.147471973634706544, -0.7216878364870207285 ) ) ;
#40485=CARTESIAN_POINT ( 'NONE',  ( -8.853111119599343937, 10.39134639669645566, 1.082531754730558626 ) ) ;
#40487=CARTESIAN_POINT ( 'NONE',  ( 1.499999999999990896, 4.525000000000021672, 1.214306433183764966E-14 ) ) ;
#40491=CARTESIAN_POINT ( 'NONE',  ( 8.270110514656026979, 10.67154823856396817, 1.443375672974076540 ) ) ;
#40505=CARTESIAN_POINT ( 'NONE',  ( 6.914295152845067349, 11.01050207838719075, 1.040834085586084257E-14 ) ) ;
#40507=CARTESIAN_POINT ( 'NONE',  ( 6.916630921265960019, 11.22115317478565188, 0.7998128361456462443 ) ) ;
#40508=CARTESIAN_POINT ( 'NONE',  ( -5.636439174979254396, 7.598931675607687453, -1.599625672291256295 ) ) ;
#40511=CARTESIAN_POINT ( 'NONE',  ( -4.948362878863562742, 5.835806782504650236, 1.082531754730558626 ) ) ;
#40512=FACE_OUTER_BOUND ( 'NONE', #154942, .T. ) ;
#40513=CARTESIAN_POINT ( 'NONE',  ( 4.582292731738905722, 5.408724944192588424, -1.082531754730548412 ) ) ;
#40515=CARTESIAN_POINT ( 'NONE',  ( -8.690413276679693766, 9.241163032322203819, 1.040834085586084257E-14 ) ) ;
#40539=CARTESIAN_POINT ( 'NONE',  ( 0.3190191529055473874, 8.208688096292709346, 1.977123213039587268 ) ) ;
#40543=CARTESIAN_POINT ( 'NONE',  ( -5.768104287610143821, 8.816873204598778102, -1.199719254218440723 ) ) ;
#40546=CARTESIAN_POINT ( 'NONE',  ( 5.503720292143644777, 8.508425209887878538, 1.199719254218462483 ) ) ;
#40549=CARTESIAN_POINT ( 'NONE',  ( -4.874313559192080092, 4.961021341527962036, 0.5169845646830675268 ) ) ;
#40555=CARTESIAN_POINT ( 'NONE',  ( -4.440459003675619520, 5.139289244831666714, 1.199719254218462483 ) ) ;
#40558=CARTESIAN_POINT ( 'NONE',  ( 5.926885707468349196, 10.06645042535509660, 1.040834085586084257E-14 ) ) ;
#40559=CARTESIAN_POINT ( 'NONE',  ( 1.364683531249990311, 3.634375000341416584, 1.214306433183764966E-14 ) ) ;
#40561=CARTESIAN_POINT ( 'NONE',  ( 6.108345433475511399, 6.019830046288782377, 0.1574382575924727079 ) ) ;
#40566=CARTESIAN_POINT ( 'NONE',  ( 5.450014562569148957, 9.302174723065263606, 1.040834085586084257E-14 ) ) ;
#40568=CARTESIAN_POINT ( 'NONE',  ( -6.808165692356648258, 11.09461040772476714, 0.7998128361456481317 ) ) ;
#40572=CARTESIAN_POINT ( 'NONE',  ( -8.941766003412679353, 10.39081407785832845, -1.199719254218446718 ) ) ;
#40573=CARTESIAN_POINT ( 'NONE',  ( -5.388475986427523345, 8.373973519885682393, 1.199719254218452047 ) ) ;
#40580=CARTESIAN_POINT ( 'NONE',  ( 6.564118927310645724, 10.80988918183778225, -0.7998128361456291469 ) ) ;
#40591=CARTESIAN_POINT ( 'NONE',  ( -0.5654481856765094516, 7.808910395760659817, -1.918425245283294611 ) ) ;
#40595=CARTESIAN_POINT ( 'NONE',  ( 0.7499999999999902300, 4.066666666666690411, -1.299038105676658228 ) ) ;
#40596=CARTESIAN_POINT ( 'NONE',  ( 5.684946482831785275, 5.526859072925533134, -0.7998128361456231517 ) ) ;
#40597=CARTESIAN_POINT ( 'NONE',  ( 7.481401836642521452, 7.622723652371411696, 1.040834085586084257E-14 ) ) ;
#40599=CARTESIAN_POINT ( 'NONE',  ( -8.853111120043687166, 9.430977182913531820, 1.040834085586084257E-14 ) ) ;
#40601=CARTESIAN_POINT ( 'NONE',  ( 5.829642864196157070, 8.784705193995428374, 1.082531754730558626 ) ) ;
#40602=CARTESIAN_POINT ( 'NONE',  ( -8.256552360598034213, 11.61609960646427986, 1.082531754730549967 ) ) ;
#40606=CARTESIAN_POINT ( 'NONE',  ( 7.995557903757111617, 10.35123685918189729, 1.599625672291281386 ) ) ;
#40613=CARTESIAN_POINT ( 'NONE',  ( -0.6823417656250003738, 2.717708333674753618, -1.181850606188749264 ) ) ;
#40619=EDGE_CURVE ( 'NONE', #145502, #56116, #155246, .T. ) ;
#40620=CARTESIAN_POINT ( 'NONE',  ( 9.585778300061798873, 11.14216175728232550, -1.199719254218440723 ) ) ;
#40624=CARTESIAN_POINT ( 'NONE',  ( -8.479735010343349089, 11.98044238112085758, 1.199719254218453823 ) ) ;
#40630=CARTESIAN_POINT ( 'NONE',  ( 4.542145155778077203, 5.257923088951247159, -1.199719254218452047 ) ) ;
#40633=CARTESIAN_POINT ( 'NONE',  ( -7.980945979938748103, 12.46285407657057220, 0.000000000000000000 ) ) ;
#40637=CARTESIAN_POINT ( 'NONE',  ( 8.880754312151170282, 10.31963377138658089, 1.199719254218453823 ) ) ;
#40639=CARTESIAN_POINT ( 'NONE',  ( 4.707534831891463156, 6.823246043637223757, 1.233988984638714426 ) ) ;
#40641=CARTESIAN_POINT ( 'NONE',  ( -3.795392936821753604, 6.515376628678959392, -1.199719254218452047 ) ) ;
#40645=CARTESIAN_POINT ( 'NONE',  ( 8.697719238366680372, 10.10609285197134533, 1.199719254218462483 ) ) ;
#40647=CARTESIAN_POINT ( 'NONE',  ( 8.613507663383630941, 8.943513783569379427, -0.7998128361456221525 ) ) ;
#40650=AXIS2_PLACEMENT_3D ( 'NONE', #174703, #76106, #142210 ) ;
#40651=CARTESIAN_POINT ( 'NONE',  ( -7.700668062882065179, 10.96756792579566664, -1.082531754730543971 ) ) ;
#40659=CARTESIAN_POINT ( 'NONE',  ( -4.916882227542496153, 6.680427897100001289, -1.249109758411016236 ) ) ;
#40660=CARTESIAN_POINT ( 'NONE',  ( 1.364683531249986537, 1.405208333674755838, -0.7879004041258239610 ) ) ;
#40662=CARTESIAN_POINT ( 'NONE',  ( 6.371969008742804697, 7.496680600697164465, -1.082531754730543083 ) ) ;
#40676=CARTESIAN_POINT ( 'NONE',  ( -9.124274191872631334, 12.62844174295135069, -1.082531754730543083 ) ) ;
#40680=CARTESIAN_POINT ( 'NONE',  ( 9.257519960032755790, 9.694861462993381807, 0.7998128361456462443 ) ) ;
#40682=EDGE_LOOP ( 'NONE', ( #94591, #94491, #190620, #23593 ) ) ;
#40685=CARTESIAN_POINT ( 'NONE',  ( -5.747767057189642870, 8.793146435774861658, -1.199719254218440723 ) ) ;
#40688=CARTESIAN_POINT ( 'NONE',  ( -9.541187415715041809, 12.15447128979948310, -1.599625672291263179 ) ) ;
#40692=CARTESIAN_POINT ( 'NONE',  ( -1.500000000000011324, 5.202083334016151639, 0.8660254037844403729 ) ) ;
#40693=CARTESIAN_POINT ( 'NONE',  ( 7.076466111328892694, 10.34329533227067799, -1.199719254218441611 ) ) ;
#40696=CARTESIAN_POINT ( 'NONE',  ( -8.227100285394159940, 8.492705175914988303, 0.7998128361456602331 ) ) ;
#40698=CARTESIAN_POINT ( 'NONE',  ( 0.6823417656249917140, 4.842708333674755394, 1.181850606188765695 ) ) ;
#40703=CARTESIAN_POINT ( 'NONE',  ( -7.321039761699444703, 10.52466824108257804, 1.082531754730549967 ) ) ;
#40707=CARTESIAN_POINT ( 'NONE',  ( 1.364683531249988535, 3.926041667008087543, 0.7879004041258500513 ) ) ;
#40713=CARTESIAN_POINT ( 'NONE',  ( -1.364683531250010295, 4.780208333674755394, 0.7879004041258379498 ) ) ;
#40714=CARTESIAN_POINT ( 'NONE',  ( -5.382750679825375251, 6.238629533673094585, -1.199719254218446718 ) ) ;
#40715=CARTESIAN_POINT ( 'NONE',  ( 5.438792177376376991, 9.497007973581119700, 1.040834085586084257E-14 ) ) ;
#40718=CARTESIAN_POINT ( 'NONE',  ( 2.995988758495615745, 6.439144618312774959, -0.7216878364870267237 ) ) ;
#40719=CARTESIAN_POINT ( 'NONE',  ( 1.364683531249990311, 4.946875000341417916, 1.214306433183764966E-14 ) ) ;
#40725=CARTESIAN_POINT ( 'NONE',  ( -0.6823417656250246877, 0.3010416670080895418, 1.181850606188755259 ) ) ;
#40726=CARTESIAN_POINT ( 'NONE',  ( -5.124618876285560454, 5.081069565195661220, 0.7216878364870317197 ) ) ;
#40727=CARTESIAN_POINT ( 'NONE',  ( 4.364835388595708743, 7.179726155748598515, 1.199719254218462483 ) ) ;
#40731=CARTESIAN_POINT ( 'NONE',  ( 3.877268743828270470, 5.546566172598190292, 1.443375672974062551 ) ) ;
#40734=CARTESIAN_POINT ( 'NONE',  ( -7.646435448427427062, 10.90429654226522693, 1.082531754730549967 ) ) ;
#40736=CARTESIAN_POINT ( 'NONE',  ( -1.001543065824772872E-14, 4.962500000000019007, 1.732050807568877637 ) ) ;
#40739=CARTESIAN_POINT ( 'NONE',  ( -9.297140650669053485, 11.86975006391249643, 1.599625672291281386 ) ) ;
#40740=CARTESIAN_POINT ( 'NONE',  ( -5.924549939047510705, 6.974691686052601369, 1.082531754730549967 ) ) ;
#40742=CARTESIAN_POINT ( 'NONE',  ( 1.364683531249986537, 1.176041667008082658, 0.7879004041258500513 ) ) ;
#40745=CARTESIAN_POINT ( 'NONE',  ( -0.08896015503664694846, 7.049507384514476449, -3.948637857580539201 ) ) ;
#40751=CARTESIAN_POINT ( 'NONE',  ( 8.886479618753304166, 12.45497775759917758, -1.199719254218446718 ) ) ;
#40753=VECTOR ( 'NONE', #16531, 1000.000000000000000 ) ;
#40755=CARTESIAN_POINT ( 'NONE',  ( 8.310784975052673218, 10.71900177569337487, -1.443375672974063439 ) ) ;
#40770=DIRECTION ( 'NONE',  ( 5.578564026256490882E-16, 1.000000000000000000, 9.066213480720158442E-32 ) ) ;
#40772=CARTESIAN_POINT ( 'NONE',  ( -0.6823417656250212460, 2.363541667008084435, 1.181850606188767472 ) ) ;
#40781=CARTESIAN_POINT ( 'NONE',  ( 1.364683531249988757, 0.8843750003414210248, 0.000000000000000000 ) ) ;
#40788=VERTEX_POINT ( 'NONE', #67313 ) ;
#40792=CARTESIAN_POINT ( 'NONE',  ( 3.683011284406639607, 7.448596931783069586, 0.7998128361456321445 ) ) ;
#40800=CARTESIAN_POINT ( 'NONE',  ( 6.123478934866503742, 10.29580919065294431, 0.7998128361456462443 ) ) ;
#40803=CARTESIAN_POINT ( 'NONE',  ( 7.736899214892750010, 12.17813285068358020, 1.040834085586084257E-14 ) ) ;
#40805=DIRECTION ( 'NONE',  ( 0.01240427322301438165, -0.9999230640433337536, 0.000000000000000000 ) ) ;
#40808=ORIENTED_EDGE ( 'NONE', *, *, #6746, .F. ) ;
#40814=CARTESIAN_POINT ( 'NONE',  ( -8.676855123066030018, 9.225345186439589895, -0.7216878364870267237 ) ) ;
#40819=CARTESIAN_POINT ( 'NONE',  ( -10.13488352141530768, 11.78278451552804817, 1.199719254218462483 ) ) ;
#40821=CARTESIAN_POINT ( 'NONE',  ( -4.191371940688026321, 3.976852638198642875, -0.5757558571073126963 ) ) ;
#40825=CARTESIAN_POINT ( 'NONE',  ( 8.062294901620731480, 12.55776115186623620, 1.040834085586084257E-14 ) ) ;
#40828=CARTESIAN_POINT ( 'NONE',  ( 5.854423403002611437, 5.724582146458163656, 1.040834085586084257E-14 ) ) ;
#40835=CARTESIAN_POINT ( 'NONE',  ( -6.552668314106420588, 6.539201209412602189, -0.7998128361456291469 ) ) ;
#40837=CARTESIAN_POINT ( 'NONE',  ( -4.634189577772691138, 4.300976017023221409, 1.214306433183764966E-14 ) ) ;
#40843=CARTESIAN_POINT ( 'NONE',  ( 8.487040972474689582, 9.964264558384387627, -1.082531754730543083 ) ) ;
#40845=CARTESIAN_POINT ( 'NONE',  ( -0.6823417656250212460, 4.113541667008085767, 1.181850606188767472 ) ) ;
#40847=CIRCLE ( 'NONE', #20081, 1.500000000000000222 ) ;
#40848=CARTESIAN_POINT ( 'NONE',  ( 5.931855901178834323, 6.879252291918818152, 1.199719254218462483 ) ) ;
#40864=CARTESIAN_POINT ( 'NONE',  ( 0.6823417656249899377, 1.155208333674752286, 1.181850606188755259 ) ) ;
#40866=CARTESIAN_POINT ( 'NONE',  ( 3.734381245560244089, 6.444196322207211836, 1.199719254218462483 ) ) ;
#40868=CARTESIAN_POINT ( 'NONE',  ( -5.666945020832185875, 7.634521829102760115, 1.443375672974064550 ) ) ;
#40869=CARTESIAN_POINT ( 'NONE',  ( 4.853455804012228647, 4.764712647543454693, 0.7216878364870317197 ) ) ;
#40870=CARTESIAN_POINT ( 'NONE',  ( -5.490689023410187275, 8.389259046411751797, 1.082531754730548412 ) ) ;
#40872=ORIENTED_EDGE ( 'NONE', *, *, #164153, .T. ) ;
#40874=CARTESIAN_POINT ( 'NONE',  ( 5.497994985541524215, 6.373081223675282736, -1.199719254218445830 ) ) ;
#40885=CARTESIAN_POINT ( 'NONE',  ( 7.332262146892202459, 7.448727347662698506, -0.7998128361456281477 ) ) ;
#40887=CARTESIAN_POINT ( 'NONE',  ( -7.739006755302186846, 7.923262724141010516, 0.7998128361456462443 ) ) ;
#40892=CARTESIAN_POINT ( 'NONE',  ( 5.913327553854682783, 10.05063257947248800, -0.7998128361456291469 ) ) ;
#40894=CARTESIAN_POINT ( 'NONE',  ( -5.065942953000576843, 9.062017211809330064, -0.7998128361456231517 ) ) ;
#40895=CARTESIAN_POINT ( 'NONE',  ( 6.765155463094746580, 9.876136559377135526, 1.082531754730558626 ) ) ;
#40896=CARTESIAN_POINT ( 'NONE',  ( 4.104435073692848768, 7.689436668370499106, -0.6928796192886893524 ) ) ;
#40897=CARTESIAN_POINT ( 'NONE',  ( -5.762378981008047241, 6.681529218386182301, 1.199719254218450271 ) ) ;
#40903=CARTESIAN_POINT ( 'NONE',  ( 9.378489572351044856, 11.96465713920816043, -1.599625672291262513 ) ) ;
#40905=CARTESIAN_POINT ( 'NONE',  ( -1.364683531250014514, 0.2802083336747505649, 0.7879004041258379498 ) ) ;
#40907=CARTESIAN_POINT ( 'NONE',  ( -7.239690840017442675, 7.548653522882887934, 0.7216878364870317197 ) ) ;
#40913=CARTESIAN_POINT ( 'NONE',  ( -5.889415777131212337, 6.013640170854067435, 0.2549476635474844932 ) ) ;
#40914=CARTESIAN_POINT ( 'NONE',  ( -1.402160292154681736E-14, 1.509375000341420359, -1.575800808251659024 ) ) ;
#40917=CARTESIAN_POINT ( 'NONE',  ( 3.063779527008311021, 5.557864633942907417, 1.082531754730546636 ) ) ;
#40920=CARTESIAN_POINT ( 'NONE',  ( -4.761938266897808525, 6.578680616179308771, 1.599625672291267398 ) ) ;
#40923=CARTESIAN_POINT ( 'NONE',  ( -7.741342523278709642, 10.05465224862374285, 1.443375672974090751 ) ) ;
#40932=CARTESIAN_POINT ( 'NONE',  ( -8.148087131688692253, 9.568818410800712826, -1.082531754730543083 ) ) ;
#40936=CARTESIAN_POINT ( 'NONE',  ( -6.683806541412762314, 9.781229484081471526, -1.082531754730537976 ) ) ;
#40942=CARTESIAN_POINT ( 'NONE',  ( -1.001543065824772872E-14, 4.993750000682814161, 1.732050807568877637 ) ) ;
#40943=CARTESIAN_POINT ( 'NONE',  ( 4.800107077129743161, 6.969409711611327829, -1.408023891483715317 ) ) ;
#40944=CARTESIAN_POINT ( 'NONE',  ( -3.563261906135796409, 6.332667919118538435, 2.420000000000010587 ) ) ;
#40950=CARTESIAN_POINT ( 'NONE',  ( -7.881367368245678406, 8.089350105908421185, 0.7998128361456602331 ) ) ;
#40953=CARTESIAN_POINT ( 'NONE',  ( 5.657830175604453338, 5.495223381160312393, 0.7998128361456341429 ) ) ;
#40957=CARTESIAN_POINT ( 'NONE',  ( 6.551614543901692400, 8.666636272683888365, 1.599625672291281386 ) ) ;
#40965=CARTESIAN_POINT ( 'NONE',  ( -4.446711195602239819, 8.131654128270509929, -0.7216878364870267237 ) ) ;
#40974=CARTESIAN_POINT ( 'NONE',  ( 0.6823417656249899377, 0.8427083336747520637, 1.181850606188755259 ) ) ;
#40976=CARTESIAN_POINT ( 'NONE',  ( -7.181014916732457287, 11.52960116949655678, -0.7998128361456291469 ) ) ;
#40978=CARTESIAN_POINT ( 'NONE',  ( 8.294891053462476904, 8.571794405328034827, 1.040834085586084257E-14 ) ) ;
#40980=CARTESIAN_POINT ( 'NONE',  ( -7.153898609505128015, 11.49796547773133604, 0.7998128361456481317 ) ) ;
#40983=CARTESIAN_POINT ( 'NONE',  ( 1.364683531249988535, 5.155208333674749177, -0.7879004041258300672 ) ) ;
#40984=CARTESIAN_POINT ( 'NONE',  ( 9.924205255523292024, 10.68058700763975466, -0.7216878364870257245 ) ) ;
#40987=CARTESIAN_POINT ( 'NONE',  ( -0.6823417656250246877, -0.6364583329919113464, 1.181850606188755259 ) ) ;
#40990=CARTESIAN_POINT ( 'NONE',  ( 7.687109908824030668, 10.95175007939464606, -1.082531754730543083 ) ) ;
#40992=CARTESIAN_POINT ( 'NONE',  ( 4.951116456854005143, 6.538279688806404089, 2.442614223628301495 ) ) ;
#40993=CARTESIAN_POINT ( 'NONE',  ( -6.073689629242165822, 7.148687991279732756, -1.082531754730544860 ) ) ;
#40995=CARTESIAN_POINT ( 'NONE',  ( 1.364683531249988757, 2.384375000341422357, 1.214306433183764966E-14 ) ) ;
#40999=CARTESIAN_POINT ( 'NONE',  ( -7.705111371268023923, 7.883718109434487253, 1.040834085586084257E-14 ) ) ;
#41000=CARTESIAN_POINT ( 'NONE',  ( 1.364683531249988535, 4.717708333674756283, -0.7879004041258300672 ) ) ;
#41007=CARTESIAN_POINT ( 'NONE',  ( 7.086107841436786181, 11.41887624831828418, 1.040834085586084257E-14 ) ) ;
#41010=CARTESIAN_POINT ( 'NONE',  ( -1.402160292154681736E-14, 1.087500000000024336, -1.732050807568863648 ) ) ;
#41014=CARTESIAN_POINT ( 'NONE',  ( 0.7499999999999902300, 5.347916667349482012, -1.299038105676658228 ) ) ;
#41016=ORIENTED_EDGE ( 'NONE', *, *, #73284, .T. ) ;
#41017=CARTESIAN_POINT ( 'NONE',  ( 7.782016984564065432, 8.181367358187307204, 0.7216878364870458196 ) ) ;
#41019=CARTESIAN_POINT ( 'NONE',  ( 9.561524646135536543, 12.17819805862340310, -1.599625672291262513 ) ) ;
#41021=CARTESIAN_POINT ( 'NONE',  ( 2.544126380858701797, 6.119897877643793116, 0.7998128361456462443 ) ) ;
#41026=CARTESIAN_POINT ( 'NONE',  ( 8.727698198895078363, 11.20540053684285553, -1.599625672291257406 ) ) ;
#41029=CARTESIAN_POINT ( 'NONE',  ( -1.364683531250014514, 0.4885416670080875434, -0.7879004041258289570 ) ) ;
#41030=CARTESIAN_POINT ( 'NONE',  ( 1.499999999999989120, 1.025000000000019007, 0.000000000000000000 ) ) ;
#41037=CARTESIAN_POINT ( 'NONE',  ( -1.364683531250012516, 4.988541667008084879, -0.7879004041258300672 ) ) ;
#41039=CARTESIAN_POINT ( 'NONE',  ( -9.155833807930273238, 9.576227618873799585, -0.7998128361456291469 ) ) ;
#41040=CARTESIAN_POINT ( 'NONE',  ( -5.083944415444539899, 8.875092884753202682, 0.000000000000000000 ) ) ;
#41048=EDGE_LOOP ( 'NONE', ( #21686, #169818, #71922, #166517 ) ) ;
#41049=CARTESIAN_POINT ( 'NONE',  ( 8.106885785967500979, 11.54545161934907682, 1.199719254218460707 ) ) ;
#41053=CARTESIAN_POINT ( 'NONE',  ( 6.087247782411444597, 10.04561347954795281, -0.7216878364870267237 ) ) ;
#41056=CARTESIAN_POINT ( 'NONE',  ( -9.267161690140662600, 10.77044237904097734, -1.199719254218441611 ) ) ;
#41057=( BOUNDED_SURFACE ( )  B_SPLINE_SURFACE ( 1, 2, ( 
 ( #210357, #79306, #177884, #97711, #128152, #195194, #132360, #160554, #148577, #15347, #198362, #61996, #48951, #146, #115069, #181065, #194112, #45762, #14277, #111880, #114017, #32683, #130271, #129220, #164819, #50002, #161638, #196260, #98763, #16410, #145422, #82490, #211423, #46831, #116126, #112944, #80372, #146467, #212486, #64128, #180013, #36939, #119330, #51070, #120409, #183193, #134488, #185317, #19620, #203688, #153908, #85692, #86765, #103021, #169076, #20675, #71558, #100874, #4411, #70482, #2279, #151780, #166961, #136598, #3353, #200491, #69423, #202622, #152836, #54272, #186384, #168017, #137666, #55334, #135529, #201553, #121486, #5478, #53199, #38021, #104092, #170141, #21727, #33743, #18551, #87837, #99821, #68355, #165887, #84628, #17472, #83556, #52136, #149638, #1220, #67282, #133421, #199427, #117195, #34799, #150719, #118264, #184248, #35875, #101950, #23879, #40156, #207964, #41238, #125747, #107345, #26016, #143022, #173367, #60653, #42303, #22803, #10824, #209017, #56402, #206899, #24951, #156036, #190643, #91053, #76898, #88917, #159223, #154971, #6556, #89985, #92127, #157114, #187458, #174440, #7625, #58530, #140887, #8703, #72636, #73710, #123628, #158179, #139808, #124685, #93192, #74787, #108418, #138733, #172291, #188525, #9772, #109489, #75845, #122563, #105172, #106269, #205836, #141952, #204751, #57469, #39086, #171209, #27084, #59590, #189592, #191709, #43367, #175496, #179753, #97446, #214318, #44431, #62781, #176550, #80101, #113749, #162439, #161375, #197050, #82228, #192772, #14015, #213287, #196003, #126816, #64913, #61729, #193848, #164558, #111614, #148319, #177626, #79036, #30302, #31370, #130012, #212221, #144095, #131062, #127897, #12958, #63856, #112679, #145151, #29234, #147255, #45498, #163502, #128944, #48688, #211157, #95326, #15086, #194922, #178689, #47637, #110548, #77972, #46559, #81176, #96388, #146205, #114803, #180802, #32428, #98494, #16143, #28160, #94256, #160295, #11898, #210090, #70226, #116932, #136337, #133158, #149373, #99559, #182931, #83288, #956, #183994, #103830, #50804, #135278, #120146, #34547, #84370, #67022, #65950, #49738, #134222, #199159, #100618, #115865, #87577, #150458, #166693, #85434, #18284, #54007, #4155, #200232, #198108, #51882, #2019, #68088, #186123, #118005, #35608, #168817, #101686, #17212, #202357, #167755, #19354, #181850, #33487, #151519, #37757, #169878, #132099, #52933, #3087, #69158, #201292, #119068, #165624, #36674, #185049, #102762, #20421, #21468, #86503, #152568, #153648, #5217, #123372, #104909, #40978, #23626, #24692, #189339, #187197, #138471, #26832, #74532, #90795, #55078, #156859, #191457, #188262, #42050, #91873, #203423, #107089, #71292, #72371, #124434, #57212, #43122, #206645, #204493, #109236, #6296, #173111, #174189, #157929, #73444, #39902, #175246, #121227, #106011, #125494, #75594, #137404, #58278, #172033, #89734, #154715, #22549, #170950, #190392, #56143, #155783, #88655, #9522, #140632, #8445, #92935, #38825, #108162, #122304, #25761, #7367, #141706, #207717, #139548, #205575, #59340, #13774, #178439, #208770, #96135, #130812, #127637, #195746, #31124, #142765, #128696, #10576, #11647, #63607, #210907, #196802, #145958, #77719, #48445, #160043, #62534, #113496, #97198, #12701, #193602, #114559, #111361, #143841, #179503, #209835, #47383, #95066, #163251, #177366, #94004, #211968, #161114, #194664, #162187, #158979, #110296, #78778, #14833, #144899, #61472, #28980, #46309, #112425, #30045, #79849, #129763, #147014, #45244, #80924, #213037, #64666, #180552, #32173, #76650, #27907, #192522, #60400, #176304, #126562, #44176, #136077, #83038, #167501, #152318, #149113, #116671, #99314, #98250, #81979, #166433, #165364, #16957, #148067, #119885, #182669, #115608, #117753, #693, #86248, #36422, #18024, #15895, #84111, #66758, #181603, #3895, #132899, #100363, #201035, #198904, #49487, #102498, #50549, #34291, #214073, #150199, #1770, #69967, #67826, #133973, #118809, #199981, #135021, #51628, #184794, #183743, #33231, #151261, #35353, #101429, #19099, #164307, #85177, #2833, #52678, #68902 ),
 ( #168562, #20161, #131847, #202094, #53752, #185862, #65699, #197856, #38572, #73180, #74278, #104647, #6037, #120969, #37497, #21214, #55882, #170693, #22280, #87318, #41797, #138217, #203175, #155526, #186939, #140372, #90537, #122040, #153385, #188004, #88392, #54820, #206389, #154459, #204230, #106824, #72108, #137148, #156602, #39630, #105739, #4957, #71036, #171766, #58016, #8193, #103573, #56954, #23362, #89472, #7106, #139286, #205316, #40718, #123126, #189085, #172854, #124180, #24425, #190143, #169631, #16590, #134666, #116309, #52319, #34983, #36052, #200669, #198542, #149830, #38204, #85884, #102132, #66396, #168201, #202807, #199612, #53379, #103204, #326, #118448, #82672, #83738, #135712, #68538, #54456, #3530, #1400, #120599, #17655, #184435, #185500, #169266, #51255, #182299, #20852, #151960, #19800, #104278, #148756, #69605, #33927, #201738, #101054, #119514, #37125, #50188, #67461, #132544, #86950, #153019, #100001, #4594, #186576, #117380, #70668, #136778, #166068, #133607, #183377, #167143, #18728, #84812, #150901, #2462, #92036, #145065, #174349, #10740, #127808, #45408, #26990, #59499, #211068, #125656, #158093, #193762, #25928, #209998, #109401, #111524, #191618, #108329, #11809, #175407, #76810, #110461, #170322, #121674, #93097, #61640, #159138, #9681, #43280, #208930, #60565, #142930, #126724, #192685, #161280, #44339, #75758, #77884, #177530, #141867, #29143, #176461, #42212, #203874, #28074, #190557, #94167, #160208, #62691, #144006, #95232, #12867, #128850, #194833, #46467, #21910, #154091, #5659, #71739, #137853, #55518, #200150, #32341, #195912, #49653, #98407, #68002, #112590, #16058, #162351, #65864, #181765, #47549, #178602, #33398, #867, #80013, #118988, #3007, #204409, #36592, #4074, #35527, #101603, #86426, #171947, #122219, #51804, #38745, #20340, #136256, #201214, #69077, #151436, #22463, #184966, #155698, #7280, #37675, #153566, #135197, #5135, #102679, #168737, #72283, #120064, #56062, #186040, #104826, #73357, #103752, #139461, #121148, #167671, #89645, #117922, #52854, #71211, #169802, #152491, #54996, #21391, #183916, #19272, #23536, #85354, #70144, #202276, #170872, #87501, #53927, #88575, #137327, #203344, #187112, #154632, #6212, #138391, #188180, #39815, #105922, #158897, #111279, #191371, #175163, #173025, #190307, #206564, #26750, #127556, #60316, #140551, #123292, #124350, #74447, #208687, #24606, #91786, #177284, #57126, #45167, #126475, #28899, #78696, #192439, #94984, #44094, #176221, #205492, #189256, #141620, #40895, #10493, #110214, #92851, #25678, #61394, #161030, #107000, #76566, #77636, #27823, #90715, #143758, #58191, #41965, #12625, #108077, #156777, #174106, #157842, #109150, #93921, #159961, #142677, #8364, #209753, #9438, #75508, #11566, #43038, #207629, #59247, #193525, #125405, #142541, #126340, #76433, #177143, #206427, #110075, #176087, #107944, #125274, #58051, #27685, #191236, #91652, #42899, #93784, #208547, #159820, #11423, #59117, #172888, #25544, #111143, #205353, #193385, #192300, #28760, #12491, #43959, #45029, #77499, #143618, #139322, #56987, #75375, #189120, #92715, #209612, #175027, #173970, #61255, #94844, #123160, #26614, #127413, #160895, #40755, #106861, #74312, #124216, #24463, #190178, #90576, #41833, #157705, #109008, #156636, #8229, #10356, #140409, #9302, #141489, #207495, #158761, #64457, #34077, #198692, #130601, #131637, #81769, #213867, #15682, #116456, #145754, #49284, #115403, #47167, #196590, #211754, #181396, #114345, #96986, #180342, #33020, #147849, #99097, #165150, #212821, #182449, #100146, #31963, #98046, #29835, #164099, #129546, #63392, #16741, #65490, #82826, #197640, #148902, #78564, #132685, #144684, #50336, #128484, #210695, #62324, #161973, #46095, #112211, #113281, #178220, #95919, #13563, #79635, #195528, #179287, #163037, #14617, #136929, #152105, #17802, #54599, #68688, #103349, #185648, #86031, #117528, #184580, #168352, #120747, #134810, #37279, #204014, #69754, #201879, #183522, #36199, #84960, #53528, #154239, #153165, #151049, #1548, #102274, #101203, #186721, #38348, #135858, #104425, #119662 ) ),
 .UNSPECIFIED., .F., .F., .T. ) 
 B_SPLINE_SURFACE_WITH_KNOTS ( ( 2, 2 ),
 ( 3, 2, 2, 2, 2, 2, 2, 2, 2, 2, 2, 2, 2, 2, 2, 2, 2, 2, 2, 2, 2, 2, 2, 2, 2, 2, 2, 2, 2, 2, 2, 2, 2, 2, 2, 2, 2, 2, 2, 2, 2, 2, 2, 2, 2, 2, 2, 2, 2, 2, 2, 2, 2, 2, 2, 2, 2, 2, 2, 2, 2, 2, 2, 2, 2, 2, 2, 2, 2, 2, 2, 2, 2, 2, 2, 2, 2, 2, 2, 2, 2, 2, 2, 2, 2, 2, 2, 2, 2, 2, 2, 2, 2, 2, 2, 2, 2, 2, 2, 2, 2, 2, 2, 2, 2, 2, 2, 2, 2, 2, 2, 2, 2, 2, 2, 2, 2, 2, 2, 2, 2, 2, 2, 2, 2, 2, 2, 2, 2, 2, 2, 2, 2, 2, 2, 2, 2, 2, 2, 2, 2, 2, 2, 2, 2, 2, 2, 2, 2, 2, 2, 2, 2, 2, 2, 2, 2, 2, 2, 2, 2, 2, 2, 2, 2, 2, 2, 2, 2, 2, 2, 2, 2, 2, 2, 2, 2, 2, 2, 2, 2, 2, 2, 2, 2, 2, 2, 2, 2, 2, 2, 2, 2, 2, 2, 2, 2, 2, 2, 2, 2, 2, 2, 2, 2, 2, 2, 2, 2, 2, 2, 2, 2, 2, 2, 2, 2, 2, 2, 2, 2, 2, 2, 2, 2, 2, 2, 2, 2, 2, 2, 2, 2, 2, 2, 2, 2, 2, 2, 2, 3 ),
 ( 0.000000000000000000, 1.000000000000000000 ),
 ( 0.000000000000000000, 0.004166666666666666609, 0.008333333333333333218, 0.01250000000000000069, 0.01666666666666666644, 0.02083333333333333218, 0.02500000000000000139, 0.02916666666666666713, 0.03333333333333333287, 0.03749999999999999861, 0.04166666666666666435, 0.04583333333333333010, 0.05000000000000000278, 0.05416666666666666852, 0.05833333333333333426, 0.06250000000000000000, 0.06666666666666666574, 0.07083333333333333148, 0.07499999999999999722, 0.07916666666666666297, 0.08333333333333332871, 0.08749999999999999445, 0.09166666666666666019, 0.09583333333333333981, 0.1000000000000000056, 0.1041666666666666713, 0.1083333333333333370, 0.1125000000000000028, 0.1166666666666666685, 0.1208333333333333343, 0.1250000000000000000, 0.1291666666666666796, 0.1333333333333333315, 0.1375000000000000111, 0.1416666666666666630, 0.1458333333333333426, 0.1499999999999999944, 0.1541666666666666741, 0.1583333333333333259, 0.1625000000000000056, 0.1666666666666666574, 0.1708333333333333370, 0.1749999999999999889, 0.1791666666666666685, 0.1833333333333333204, 0.1875000000000000000, 0.1916666666666666796, 0.1958333333333333315, 0.2000000000000000111, 0.2041666666666666630, 0.2083333333333333426, 0.2124999999999999944, 0.2166666666666666741, 0.2208333333333333259, 0.2250000000000000056, 0.2291666666666666574, 0.2333333333333333370, 0.2374999999999999889, 0.2416666666666666685, 0.2458333333333333204, 0.2500000000000000000, 0.2541666666666666519, 0.2583333333333333592, 0.2625000000000000111, 0.2666666666666666630, 0.2708333333333333148, 0.2750000000000000222, 0.2791666666666666741, 0.2833333333333333259, 0.2874999999999999778, 0.2916666666666666852, 0.2958333333333333370, 0.2999999999999999889, 0.3041666666666666408, 0.3083333333333333481, 0.3125000000000000000, 0.3166666666666666519, 0.3208333333333333592, 0.3250000000000000111, 0.3291666666666666630, 0.3333333333333333148, 0.3375000000000000222, 0.3416666666666666741, 0.3458333333333333259, 0.3499999999999999778, 0.3541666666666666852, 0.3583333333333333370, 0.3624999999999999889, 0.3666666666666666408, 0.3708333333333333481, 0.3750000000000000000, 0.3791666666666666519, 0.3833333333333333592, 0.3875000000000000111, 0.3916666666666666630, 0.3958333333333333148, 0.4000000000000000222, 0.4041666666666666741, 0.4083333333333333259, 0.4124999999999999778, 0.4166666666666666852, 0.4208333333333333370, 0.4249999999999999889, 0.4291666666666666408, 0.4333333333333333481, 0.4375000000000000000, 0.4416666666666666519, 0.4458333333333333592, 0.4500000000000000111, 0.4541666666666666630, 0.4583333333333333148, 0.4625000000000000222, 0.4666666666666666741, 0.4708333333333333259, 0.4749999999999999778, 0.4791666666666666852, 0.4833333333333333370, 0.4874999999999999889, 0.4916666666666666408, 0.4958333333333333481, 0.5000000000000000000, 0.5041666666666666519, 0.5083333333333333037, 0.5124999999999999556, 0.5166666666666667185, 0.5208333333333333703, 0.5250000000000000222, 0.5291666666666666741, 0.5333333333333333259, 0.5374999999999999778, 0.5416666666666666297, 0.5458333333333332815, 0.5500000000000000444, 0.5541666666666666963, 0.5583333333333333481, 0.5625000000000000000, 0.5666666666666666519, 0.5708333333333333037, 0.5749999999999999556, 0.5791666666666667185, 0.5833333333333333703, 0.5875000000000000222, 0.5916666666666666741, 0.5958333333333333259, 0.5999999999999999778, 0.6041666666666666297, 0.6083333333333332815, 0.6125000000000000444, 0.6166666666666666963, 0.6208333333333333481, 0.6250000000000000000, 0.6291666666666666519, 0.6333333333333333037, 0.6374999999999999556, 0.6416666666666667185, 0.6458333333333333703, 0.6500000000000000222, 0.6541666666666666741, 0.6583333333333333259, 0.6624999999999999778, 0.6666666666666666297, 0.6708333333333332815, 0.6750000000000000444, 0.6791666666666666963, 0.6833333333333333481, 0.6875000000000000000, 0.6916666666666666519, 0.6958333333333333037, 0.6999999999999999556, 0.7041666666666667185, 0.7083333333333333703, 0.7125000000000000222, 0.7166666666666666741, 0.7208333333333333259, 0.7249999999999999778, 0.7291666666666666297, 0.7333333333333332815, 0.7375000000000000444, 0.7416666666666666963, 0.7458333333333333481, 0.7500000000000000000, 0.7541666666666666519, 0.7583333333333333037, 0.7624999999999999556, 0.7666666666666667185, 0.7708333333333333703, 0.7750000000000000222, 0.7791666666666666741, 0.7833333333333333259, 0.7874999999999999778, 0.7916666666666666297, 0.7958333333333332815, 0.8000000000000000444, 0.8041666666666666963, 0.8083333333333333481, 0.8125000000000000000, 0.8166666666666666519, 0.8208333333333333037, 0.8249999999999999556, 0.8291666666666667185, 0.8333333333333333703, 0.8375000000000000222, 0.8416666666666666741, 0.8458333333333333259, 0.8499999999999999778, 0.8541666666666666297, 0.8583333333333332815, 0.8625000000000000444, 0.8666666666666666963, 0.8708333333333333481, 0.8750000000000000000, 0.8791666666666666519, 0.8833333333333333037, 0.8874999999999999556, 0.8916666666666667185, 0.8958333333333333703, 0.9000000000000000222, 0.9041666666666666741, 0.9083333333333333259, 0.9124999999999999778, 0.9166666666666666297, 0.9208333333333332815, 0.9250000000000000444, 0.9291666666666666963, 0.9333333333333333481, 0.9375000000000000000, 0.9416666666666666519, 0.9458333333333333037, 0.9499999999999999556, 0.9541666666666667185, 0.9583333333333333703, 0.9625000000000000222, 0.9666666666666666741, 0.9708333333333333259, 0.9749999999999999778, 0.9791666666666666297, 0.9833333333333332815, 0.9875000000000000444, 0.9916666666666666963, 0.9958333333333333481, 1.000000000000000000 ),
 .UNSPECIFIED. ) 
 GEOMETRIC_REPRESENTATION_ITEM ( )  RATIONAL_B_SPLINE_SURFACE ( (
 ( 1.000000000000000000, 0.8660254037844387076, 1.000000000000000000, 0.8660254037844387076, 1.000000000000000000, 0.8660254037844387076, 1.000000000000000000, 0.8660254037844387076, 1.000000000000000000, 0.8660254037844387076, 1.000000000000000000, 0.8660254037844387076, 1.000000000000000000, 0.8660254037844387076, 1.000000000000000000, 0.8660254037844387076, 1.000000000000000000, 0.8660254037844387076, 1.000000000000000000, 0.8660254037844387076, 1.000000000000000000, 0.8660254037844387076, 1.000000000000000000, 0.8660254037844387076, 1.000000000000000000, 0.8660254037844387076, 1.000000000000000000, 0.8660254037844387076, 1.000000000000000000, 0.8660254037844387076, 1.000000000000000000, 0.8660254037844387076, 1.000000000000000000, 0.8660254037844387076, 1.000000000000000000, 0.8660254037844387076, 1.000000000000000000, 0.8660254037844387076, 1.000000000000000000, 0.8660254037844387076, 1.000000000000000000, 0.8660254037844387076, 1.000000000000000000, 0.8660254037844387076, 1.000000000000000000, 0.8660254037844387076, 1.000000000000000000, 0.8660254037844387076, 1.000000000000000000, 0.8660254037844387076, 1.000000000000000000, 0.8660254037844387076, 1.000000000000000000, 0.8660254037844387076, 1.000000000000000000, 0.8660254037844387076, 1.000000000000000000, 0.8660254037844387076, 1.000000000000000000, 0.8660254037844387076, 1.000000000000000000, 0.8660254037844387076, 1.000000000000000000, 0.8660254037844387076, 1.000000000000000000, 0.8660254037844387076, 1.000000000000000000, 0.8660254037844387076, 1.000000000000000000, 0.8660254037844387076, 1.000000000000000000, 0.8660254037844387076, 1.000000000000000000, 0.8660254037844387076, 1.000000000000000000, 0.8660254037844387076, 1.000000000000000000, 0.8660254037844387076, 1.000000000000000000, 0.8660254037844387076, 1.000000000000000000, 0.8660254037844387076, 1.000000000000000000, 0.8660254037844387076, 1.000000000000000000, 0.8660254037844387076, 1.000000000000000000, 0.8660254037844387076, 1.000000000000000000, 0.8660254037844387076, 1.000000000000000000, 0.8660254037844387076, 1.000000000000000000, 0.8660254037844387076, 1.000000000000000000, 0.8660254037844387076, 1.000000000000000000, 0.8660254037844387076, 1.000000000000000000, 0.8660254037844387076, 1.000000000000000000, 0.8660254037844387076, 1.000000000000000000, 0.8660254037844387076, 1.000000000000000000, 0.8660254037844387076, 1.000000000000000000, 0.8660254037844387076, 1.000000000000000000, 0.8660254037844387076, 1.000000000000000000, 0.8660254037844387076, 1.000000000000000000, 0.8660254037844387076, 1.000000000000000000, 0.8660254037844387076, 1.000000000000000000, 0.8660254037844387076, 1.000000000000000000, 0.8660254037844387076, 1.000000000000000000, 0.8660254037844387076, 1.000000000000000000, 0.8660254037844387076, 1.000000000000000000, 0.8660254037844387076, 1.000000000000000000, 0.8660254037844387076, 1.000000000000000000, 0.8660254037844387076, 1.000000000000000000, 0.8660254037844387076, 1.000000000000000000, 0.8660254037844387076, 1.000000000000000000, 0.8660254037844387076, 1.000000000000000000, 0.8660254037844387076, 1.000000000000000000, 0.8660254037844387076, 1.000000000000000000, 0.8660254037844387076, 1.000000000000000000, 0.8660254037844387076, 1.000000000000000000, 0.8660254037844387076, 1.000000000000000000, 0.8660254037844387076, 1.000000000000000000, 0.8660254037844387076, 1.000000000000000000, 0.8660254037844387076, 1.000000000000000000, 0.8660254037844387076, 1.000000000000000000, 0.8660254037844387076, 1.000000000000000000, 0.8660254037844387076, 1.000000000000000000, 0.8660254037844387076, 1.000000000000000000, 0.8660254037844387076, 1.000000000000000000, 0.8660254037844387076, 1.000000000000000000, 0.8660254037844387076, 1.000000000000000000, 0.8660254037844387076, 1.000000000000000000, 0.8660254037844387076, 1.000000000000000000, 0.8660254037844387076, 1.000000000000000000, 0.8660254037844387076, 1.000000000000000000, 0.8660254037844387076, 1.000000000000000000, 0.8660254037844387076, 1.000000000000000000, 0.8660254037844387076, 1.000000000000000000, 0.8660254037844387076, 1.000000000000000000, 0.8660254037844387076, 1.000000000000000000, 0.8660254037844387076, 1.000000000000000000, 0.8660254037844387076, 1.000000000000000000, 0.8660254037844387076, 1.000000000000000000, 0.8660254037844387076, 1.000000000000000000, 0.8660254037844387076, 1.000000000000000000, 0.8660254037844387076, 1.000000000000000000, 0.8660254037844387076, 1.000000000000000000, 0.8660254037844387076, 1.000000000000000000, 0.8660254037844387076, 1.000000000000000000, 0.8660254037844387076, 1.000000000000000000, 0.8660254037844387076, 1.000000000000000000, 0.8660254037844387076, 1.000000000000000000, 0.8660254037844387076, 1.000000000000000000, 0.8660254037844387076, 1.000000000000000000, 0.8660254037844387076, 1.000000000000000000, 0.8660254037844387076, 1.000000000000000000, 0.8660254037844387076, 1.000000000000000000, 0.8660254037844387076, 1.000000000000000000, 0.8660254037844387076, 1.000000000000000000, 0.8660254037844387076, 1.000000000000000000, 0.8660254037844387076, 1.000000000000000000, 0.8660254037844387076, 1.000000000000000000, 0.8660254037844387076, 1.000000000000000000, 0.8660254037844387076, 1.000000000000000000, 0.8660254037844387076, 1.000000000000000000, 0.8660254037844387076, 1.000000000000000000, 0.8660254037844387076, 1.000000000000000000, 0.8660254037844387076, 1.000000000000000000, 0.8660254037844387076, 1.000000000000000000, 0.8660254037844387076, 1.000000000000000000, 0.8660254037844387076, 1.000000000000000000, 0.8660254037844387076, 1.000000000000000000, 0.8660254037844387076, 1.000000000000000000, 0.8660254037844387076, 1.000000000000000000, 0.8660254037844387076, 1.000000000000000000, 0.8660254037844387076, 1.000000000000000000, 0.8660254037844387076, 1.000000000000000000, 0.8660254037844387076, 1.000000000000000000, 0.8660254037844387076, 1.000000000000000000, 0.8660254037844387076, 1.000000000000000000, 0.8660254037844387076, 1.000000000000000000, 0.8660254037844387076, 1.000000000000000000, 0.8660254037844387076, 1.000000000000000000, 0.8660254037844387076, 1.000000000000000000, 0.8660254037844387076, 1.000000000000000000, 0.8660254037844387076, 1.000000000000000000, 0.8660254037844387076, 1.000000000000000000, 0.8660254037844387076, 1.000000000000000000, 0.8660254037844387076, 1.000000000000000000, 0.8660254037844387076, 1.000000000000000000, 0.8660254037844387076, 1.000000000000000000, 0.8660254037844387076, 1.000000000000000000, 0.8660254037844387076, 1.000000000000000000, 0.8660254037844387076, 1.000000000000000000, 0.8660254037844387076, 1.000000000000000000, 0.8660254037844387076, 1.000000000000000000, 0.8660254037844387076, 1.000000000000000000, 0.8660254037844387076, 1.000000000000000000, 0.8660254037844387076, 1.000000000000000000, 0.8660254037844387076, 1.000000000000000000, 0.8660254037844387076, 1.000000000000000000, 0.8660254037844387076, 1.000000000000000000, 0.8660254037844387076, 1.000000000000000000, 0.8660254037844387076, 1.000000000000000000, 0.8660254037844387076, 1.000000000000000000, 0.8660254037844387076, 1.000000000000000000, 0.8660254037844387076, 1.000000000000000000, 0.8660254037844387076, 1.000000000000000000, 0.8660254037844387076, 1.000000000000000000, 0.8660254037844387076, 1.000000000000000000, 0.8660254037844387076, 1.000000000000000000, 0.8660254037844387076, 1.000000000000000000, 0.8660254037844387076, 1.000000000000000000, 0.8660254037844387076, 1.000000000000000000, 0.8660254037844387076, 1.000000000000000000, 0.8660254037844387076, 1.000000000000000000, 0.8660254037844387076, 1.000000000000000000, 0.8660254037844387076, 1.000000000000000000, 0.8660254037844387076, 1.000000000000000000, 0.8660254037844387076, 1.000000000000000000, 0.8660254037844387076, 1.000000000000000000, 0.8660254037844387076, 1.000000000000000000, 0.8660254037844387076, 1.000000000000000000, 0.8660254037844387076, 1.000000000000000000, 0.8660254037844387076, 1.000000000000000000, 0.8660254037844387076, 1.000000000000000000, 0.8660254037844387076, 1.000000000000000000, 0.8660254037844387076, 1.000000000000000000, 0.8660254037844387076, 1.000000000000000000, 0.8660254037844387076, 1.000000000000000000, 0.8660254037844387076, 1.000000000000000000, 0.8660254037844387076, 1.000000000000000000, 0.8660254037844387076, 1.000000000000000000, 0.8660254037844387076, 1.000000000000000000, 0.8660254037844387076, 1.000000000000000000, 0.8660254037844387076, 1.000000000000000000, 0.8660254037844387076, 1.000000000000000000, 0.8660254037844387076, 1.000000000000000000, 0.8660254037844387076, 1.000000000000000000, 0.8660254037844387076, 1.000000000000000000, 0.8660254037844387076, 1.000000000000000000, 0.8660254037844387076, 1.000000000000000000, 0.8660254037844387076, 1.000000000000000000, 0.8660254037844387076, 1.000000000000000000, 0.8660254037844387076, 1.000000000000000000, 0.8660254037844387076, 1.000000000000000000, 0.8660254037844387076, 1.000000000000000000, 0.8660254037844387076, 1.000000000000000000, 0.8660254037844387076, 1.000000000000000000, 0.8660254037844387076, 1.000000000000000000, 0.8660254037844387076, 1.000000000000000000, 0.8660254037844387076, 1.000000000000000000, 0.8660254037844387076, 1.000000000000000000, 0.8660254037844387076, 1.000000000000000000, 0.8660254037844387076, 1.000000000000000000, 0.8660254037844387076, 1.000000000000000000, 0.8660254037844387076, 1.000000000000000000, 0.8660254037844387076, 1.000000000000000000, 0.8660254037844387076, 1.000000000000000000, 0.8660254037844387076, 1.000000000000000000, 0.8660254037844387076, 1.000000000000000000, 0.8660254037844387076, 1.000000000000000000, 0.8660254037844387076, 1.000000000000000000, 0.8660254037844387076, 1.000000000000000000, 0.8660254037844387076, 1.000000000000000000, 0.8660254037844387076, 1.000000000000000000, 0.8660254037844387076, 1.000000000000000000, 0.8660254037844387076, 1.000000000000000000, 0.8660254037844387076, 1.000000000000000000, 0.8660254037844387076, 1.000000000000000000, 0.8660254037844387076, 1.000000000000000000, 0.8660254037844387076, 1.000000000000000000, 0.8660254037844387076, 1.000000000000000000, 0.8660254037844387076, 1.000000000000000000, 0.8660254037844387076, 1.000000000000000000, 0.8660254037844387076, 1.000000000000000000, 0.8660254037844387076, 1.000000000000000000, 0.8660254037844387076, 1.000000000000000000, 0.8660254037844387076, 1.000000000000000000, 0.8660254037844387076, 1.000000000000000000, 0.8660254037844387076, 1.000000000000000000, 0.8660254037844387076, 1.000000000000000000, 0.8660254037844387076, 1.000000000000000000, 0.8660254037844387076, 1.000000000000000000, 0.8660254037844387076, 1.000000000000000000, 0.8660254037844387076, 1.000000000000000000, 0.8660254037844387076, 1.000000000000000000, 0.8660254037844387076, 1.000000000000000000),
 ( 1.000000000000000000, 0.8660254037844387076, 1.000000000000000000, 0.8660254037844387076, 1.000000000000000000, 0.8660254037844387076, 1.000000000000000000, 0.8660254037844387076, 1.000000000000000000, 0.8660254037844387076, 1.000000000000000000, 0.8660254037844387076, 1.000000000000000000, 0.8660254037844387076, 1.000000000000000000, 0.8660254037844387076, 1.000000000000000000, 0.8660254037844387076, 1.000000000000000000, 0.8660254037844387076, 1.000000000000000000, 0.8660254037844387076, 1.000000000000000000, 0.8660254037844387076, 1.000000000000000000, 0.8660254037844387076, 1.000000000000000000, 0.8660254037844387076, 1.000000000000000000, 0.8660254037844387076, 1.000000000000000000, 0.8660254037844387076, 1.000000000000000000, 0.8660254037844387076, 1.000000000000000000, 0.8660254037844387076, 1.000000000000000000, 0.8660254037844387076, 1.000000000000000000, 0.8660254037844387076, 1.000000000000000000, 0.8660254037844387076, 1.000000000000000000, 0.8660254037844387076, 1.000000000000000000, 0.8660254037844387076, 1.000000000000000000, 0.8660254037844387076, 1.000000000000000000, 0.8660254037844387076, 1.000000000000000000, 0.8660254037844387076, 1.000000000000000000, 0.8660254037844387076, 1.000000000000000000, 0.8660254037844387076, 1.000000000000000000, 0.8660254037844387076, 1.000000000000000000, 0.8660254037844387076, 1.000000000000000000, 0.8660254037844387076, 1.000000000000000000, 0.8660254037844387076, 1.000000000000000000, 0.8660254037844387076, 1.000000000000000000, 0.8660254037844387076, 1.000000000000000000, 0.8660254037844387076, 1.000000000000000000, 0.8660254037844387076, 1.000000000000000000, 0.8660254037844387076, 1.000000000000000000, 0.8660254037844387076, 1.000000000000000000, 0.8660254037844387076, 1.000000000000000000, 0.8660254037844387076, 1.000000000000000000, 0.8660254037844387076, 1.000000000000000000, 0.8660254037844387076, 1.000000000000000000, 0.8660254037844387076, 1.000000000000000000, 0.8660254037844387076, 1.000000000000000000, 0.8660254037844387076, 1.000000000000000000, 0.8660254037844387076, 1.000000000000000000, 0.8660254037844387076, 1.000000000000000000, 0.8660254037844387076, 1.000000000000000000, 0.8660254037844387076, 1.000000000000000000, 0.8660254037844387076, 1.000000000000000000, 0.8660254037844387076, 1.000000000000000000, 0.8660254037844387076, 1.000000000000000000, 0.8660254037844387076, 1.000000000000000000, 0.8660254037844387076, 1.000000000000000000, 0.8660254037844387076, 1.000000000000000000, 0.8660254037844387076, 1.000000000000000000, 0.8660254037844387076, 1.000000000000000000, 0.8660254037844387076, 1.000000000000000000, 0.8660254037844387076, 1.000000000000000000, 0.8660254037844387076, 1.000000000000000000, 0.8660254037844387076, 1.000000000000000000, 0.8660254037844387076, 1.000000000000000000, 0.8660254037844387076, 1.000000000000000000, 0.8660254037844387076, 1.000000000000000000, 0.8660254037844387076, 1.000000000000000000, 0.8660254037844387076, 1.000000000000000000, 0.8660254037844387076, 1.000000000000000000, 0.8660254037844387076, 1.000000000000000000, 0.8660254037844387076, 1.000000000000000000, 0.8660254037844387076, 1.000000000000000000, 0.8660254037844387076, 1.000000000000000000, 0.8660254037844387076, 1.000000000000000000, 0.8660254037844387076, 1.000000000000000000, 0.8660254037844387076, 1.000000000000000000, 0.8660254037844387076, 1.000000000000000000, 0.8660254037844387076, 1.000000000000000000, 0.8660254037844387076, 1.000000000000000000, 0.8660254037844387076, 1.000000000000000000, 0.8660254037844387076, 1.000000000000000000, 0.8660254037844387076, 1.000000000000000000, 0.8660254037844387076, 1.000000000000000000, 0.8660254037844387076, 1.000000000000000000, 0.8660254037844387076, 1.000000000000000000, 0.8660254037844387076, 1.000000000000000000, 0.8660254037844387076, 1.000000000000000000, 0.8660254037844387076, 1.000000000000000000, 0.8660254037844387076, 1.000000000000000000, 0.8660254037844387076, 1.000000000000000000, 0.8660254037844387076, 1.000000000000000000, 0.8660254037844387076, 1.000000000000000000, 0.8660254037844387076, 1.000000000000000000, 0.8660254037844387076, 1.000000000000000000, 0.8660254037844387076, 1.000000000000000000, 0.8660254037844387076, 1.000000000000000000, 0.8660254037844387076, 1.000000000000000000, 0.8660254037844387076, 1.000000000000000000, 0.8660254037844387076, 1.000000000000000000, 0.8660254037844387076, 1.000000000000000000, 0.8660254037844387076, 1.000000000000000000, 0.8660254037844387076, 1.000000000000000000, 0.8660254037844387076, 1.000000000000000000, 0.8660254037844387076, 1.000000000000000000, 0.8660254037844387076, 1.000000000000000000, 0.8660254037844387076, 1.000000000000000000, 0.8660254037844387076, 1.000000000000000000, 0.8660254037844387076, 1.000000000000000000, 0.8660254037844387076, 1.000000000000000000, 0.8660254037844387076, 1.000000000000000000, 0.8660254037844387076, 1.000000000000000000, 0.8660254037844387076, 1.000000000000000000, 0.8660254037844387076, 1.000000000000000000, 0.8660254037844387076, 1.000000000000000000, 0.8660254037844387076, 1.000000000000000000, 0.8660254037844387076, 1.000000000000000000, 0.8660254037844387076, 1.000000000000000000, 0.8660254037844387076, 1.000000000000000000, 0.8660254037844387076, 1.000000000000000000, 0.8660254037844387076, 1.000000000000000000, 0.8660254037844387076, 1.000000000000000000, 0.8660254037844387076, 1.000000000000000000, 0.8660254037844387076, 1.000000000000000000, 0.8660254037844387076, 1.000000000000000000, 0.8660254037844387076, 1.000000000000000000, 0.8660254037844387076, 1.000000000000000000, 0.8660254037844387076, 1.000000000000000000, 0.8660254037844387076, 1.000000000000000000, 0.8660254037844387076, 1.000000000000000000, 0.8660254037844387076, 1.000000000000000000, 0.8660254037844387076, 1.000000000000000000, 0.8660254037844387076, 1.000000000000000000, 0.8660254037844387076, 1.000000000000000000, 0.8660254037844387076, 1.000000000000000000, 0.8660254037844387076, 1.000000000000000000, 0.8660254037844387076, 1.000000000000000000, 0.8660254037844387076, 1.000000000000000000, 0.8660254037844387076, 1.000000000000000000, 0.8660254037844387076, 1.000000000000000000, 0.8660254037844387076, 1.000000000000000000, 0.8660254037844387076, 1.000000000000000000, 0.8660254037844387076, 1.000000000000000000, 0.8660254037844387076, 1.000000000000000000, 0.8660254037844387076, 1.000000000000000000, 0.8660254037844387076, 1.000000000000000000, 0.8660254037844387076, 1.000000000000000000, 0.8660254037844387076, 1.000000000000000000, 0.8660254037844387076, 1.000000000000000000, 0.8660254037844387076, 1.000000000000000000, 0.8660254037844387076, 1.000000000000000000, 0.8660254037844387076, 1.000000000000000000, 0.8660254037844387076, 1.000000000000000000, 0.8660254037844387076, 1.000000000000000000, 0.8660254037844387076, 1.000000000000000000, 0.8660254037844387076, 1.000000000000000000, 0.8660254037844387076, 1.000000000000000000, 0.8660254037844387076, 1.000000000000000000, 0.8660254037844387076, 1.000000000000000000, 0.8660254037844387076, 1.000000000000000000, 0.8660254037844387076, 1.000000000000000000, 0.8660254037844387076, 1.000000000000000000, 0.8660254037844387076, 1.000000000000000000, 0.8660254037844387076, 1.000000000000000000, 0.8660254037844387076, 1.000000000000000000, 0.8660254037844387076, 1.000000000000000000, 0.8660254037844387076, 1.000000000000000000, 0.8660254037844387076, 1.000000000000000000, 0.8660254037844387076, 1.000000000000000000, 0.8660254037844387076, 1.000000000000000000, 0.8660254037844387076, 1.000000000000000000, 0.8660254037844387076, 1.000000000000000000, 0.8660254037844387076, 1.000000000000000000, 0.8660254037844387076, 1.000000000000000000, 0.8660254037844387076, 1.000000000000000000, 0.8660254037844387076, 1.000000000000000000, 0.8660254037844387076, 1.000000000000000000, 0.8660254037844387076, 1.000000000000000000, 0.8660254037844387076, 1.000000000000000000, 0.8660254037844387076, 1.000000000000000000, 0.8660254037844387076, 1.000000000000000000, 0.8660254037844387076, 1.000000000000000000, 0.8660254037844387076, 1.000000000000000000, 0.8660254037844387076, 1.000000000000000000, 0.8660254037844387076, 1.000000000000000000, 0.8660254037844387076, 1.000000000000000000, 0.8660254037844387076, 1.000000000000000000, 0.8660254037844387076, 1.000000000000000000, 0.8660254037844387076, 1.000000000000000000, 0.8660254037844387076, 1.000000000000000000, 0.8660254037844387076, 1.000000000000000000, 0.8660254037844387076, 1.000000000000000000, 0.8660254037844387076, 1.000000000000000000, 0.8660254037844387076, 1.000000000000000000, 0.8660254037844387076, 1.000000000000000000, 0.8660254037844387076, 1.000000000000000000, 0.8660254037844387076, 1.000000000000000000, 0.8660254037844387076, 1.000000000000000000, 0.8660254037844387076, 1.000000000000000000, 0.8660254037844387076, 1.000000000000000000, 0.8660254037844387076, 1.000000000000000000, 0.8660254037844387076, 1.000000000000000000, 0.8660254037844387076, 1.000000000000000000, 0.8660254037844387076, 1.000000000000000000, 0.8660254037844387076, 1.000000000000000000, 0.8660254037844387076, 1.000000000000000000, 0.8660254037844387076, 1.000000000000000000, 0.8660254037844387076, 1.000000000000000000, 0.8660254037844387076, 1.000000000000000000, 0.8660254037844387076, 1.000000000000000000, 0.8660254037844387076, 1.000000000000000000, 0.8660254037844387076, 1.000000000000000000, 0.8660254037844387076, 1.000000000000000000, 0.8660254037844387076, 1.000000000000000000, 0.8660254037844387076, 1.000000000000000000, 0.8660254037844387076, 1.000000000000000000, 0.8660254037844387076, 1.000000000000000000, 0.8660254037844387076, 1.000000000000000000, 0.8660254037844387076, 1.000000000000000000, 0.8660254037844387076, 1.000000000000000000, 0.8660254037844387076, 1.000000000000000000, 0.8660254037844387076, 1.000000000000000000, 0.8660254037844387076, 1.000000000000000000, 0.8660254037844387076, 1.000000000000000000, 0.8660254037844387076, 1.000000000000000000, 0.8660254037844387076, 1.000000000000000000, 0.8660254037844387076, 1.000000000000000000, 0.8660254037844387076, 1.000000000000000000, 0.8660254037844387076, 1.000000000000000000, 0.8660254037844387076, 1.000000000000000000, 0.8660254037844387076, 1.000000000000000000, 0.8660254037844387076, 1.000000000000000000, 0.8660254037844387076, 1.000000000000000000, 0.8660254037844387076, 1.000000000000000000, 0.8660254037844387076, 1.000000000000000000, 0.8660254037844387076, 1.000000000000000000, 0.8660254037844387076, 1.000000000000000000, 0.8660254037844387076, 1.000000000000000000, 0.8660254037844387076, 1.000000000000000000, 0.8660254037844387076, 1.000000000000000000, 0.8660254037844387076, 1.000000000000000000, 0.8660254037844387076, 1.000000000000000000, 0.8660254037844387076, 1.000000000000000000) ) ) 
 REPRESENTATION_ITEM ( '' )  SURFACE ( )  );
#41059=CARTESIAN_POINT ( 'NONE',  ( 4.981731378017507872, 7.899438143407371271, -1.199719254218452047 ) ) ;
#41061=CARTESIAN_POINT ( 'NONE',  ( 0.9999999999999833467, 8.600000000000013856, -0.3999999999999832023 ) ) ;
#41062=CARTESIAN_POINT ( 'NONE',  ( 10.54788032175191326, 11.40820791823982994, 0.7216878364870317197 ) ) ;
#41068=AXIS2_PLACEMENT_3D ( 'NONE', #202249, #6187, #167644 ) ;
#41070=CARTESIAN_POINT ( 'NONE',  ( -5.314433026876900001, 6.262888621853549331, 1.082531754730548412 ) ) ;
#41071=CARTESIAN_POINT ( 'NONE',  ( 4.546061579283848353, 4.198160018786257552, -0.7998128361456211532 ) ) ;
#41074=CARTESIAN_POINT ( 'NONE',  ( -6.181627972826976958, 9.299317504018391745, 1.199719254218452047 ) ) ;
#41079=CARTESIAN_POINT ( 'NONE',  ( -7.486073373039941359, 11.88550270185529278, -0.7998128361456291469 ) ) ;
#41084=ADVANCED_FACE ( 'NONE', ( #21760 ), #108145, .T. ) ;
#41085=CARTESIAN_POINT ( 'NONE',  ( 5.986088515633498197, 6.942523675449257858, -1.199719254218446718 ) ) ;
#41095=CARTESIAN_POINT ( 'NONE',  ( -6.398558430645608475, 9.552403038140164782, -1.199719254218440723 ) ) ;
#41099=CARTESIAN_POINT ( 'NONE',  ( 6.507550544879468823, 6.694489845221929691, -0.7216878364870257245 ) ) ;
#41102=DIRECTION ( 'NONE',  ( 0.7592566023652993490, 0.6507913734559652719, -8.881784197001246407E-16 ) ) ;
#41104=CARTESIAN_POINT ( 'NONE',  ( 4.273844736805816780, 6.009238164405336313, 1.599625672291267398 ) ) ;
#41106=CARTESIAN_POINT ( 'NONE',  ( -4.954615070790188369, 7.867802451642154082, -1.199719254218452047 ) ) ;
#41109=CARTESIAN_POINT ( 'NONE',  ( -1.499999999999997780, 5.431250000682820378, 1.214306433183764966E-14 ) ) ;
#41115=CARTESIAN_POINT ( 'NONE',  ( 6.511106444361020706, 5.279176164185798825, 2.500000000000011546 ) ) ;
#41116=CARTESIAN_POINT ( 'NONE',  ( 6.588372581236919601, 9.773852880496709972, -1.199719254218440723 ) ) ;
#41120=CARTESIAN_POINT ( 'NONE',  ( -5.343048727742272241, 6.363526295613923800, -1.106837213068444292 ) ) ;
#41127=CARTESIAN_POINT ( 'NONE',  ( 10.22248463502393001, 11.02857961705718282, 0.7216878364870438212 ) ) ;
#41133=DIRECTION ( 'NONE',  ( 1.000000000000000000, 0.000000000000000000, 0.000000000000000000 ) ) ;
#41148=CARTESIAN_POINT ( 'NONE',  ( -3.113568832632681360, 6.784247404713427798, -0.7998128361456281477 ) ) ;
#41151=CARTESIAN_POINT ( 'NONE',  ( -2.774614992291035698, 6.388801257648172971, 1.040834085586084257E-14 ) ) ;
#41155=CARTESIAN_POINT ( 'NONE',  ( 1.499999999999985123, -0.9229166659838452524, -0.8660254037844323793 ) ) ;
#41158=CARTESIAN_POINT ( 'NONE',  ( -2.155383234892699562, 5.458438174109348395, 1.040834085586084257E-14 ) ) ;
#41163=CARTESIAN_POINT ( 'NONE',  ( 8.543609354905870035, 13.11929468069890525, 0.7998128361456462443 ) ) ;
#41170=CARTESIAN_POINT ( 'NONE',  ( 1.364683531249988757, 0.6968750003414209138, 0.000000000000000000 ) ) ;
#41174=CARTESIAN_POINT ( 'NONE',  ( -6.997979842947967377, 11.31606025008131233, -0.7998128361456291469 ) ) ;
#41176=CARTESIAN_POINT ( 'NONE',  ( -6.371969008298464132, 6.536311385877402458, 1.040834085586084257E-14 ) ) ;
#41178=CARTESIAN_POINT ( 'NONE',  ( -5.585069213825653023, 8.603332285183535433, -1.199719254218440723 ) ) ;
#41180=CARTESIAN_POINT ( 'NONE',  ( 1.364683531249988535, 5.405208333674750953, -0.7879004041258300672 ) ) ;
#41188=CARTESIAN_POINT ( 'NONE',  ( -5.599154252319524794, 6.595063384869953360, 1.082531754730546636 ) ) ;
#41193=CARTESIAN_POINT ( 'NONE',  ( -5.734735788456164940, 5.792872629394710593, 0.7216878364870317197 ) ) ;
#41195=CARTESIAN_POINT ( 'NONE',  ( 10.39640486358069360, 11.02356051713265650, 0.7998128361456462443 ) ) ;
#41203=CARTESIAN_POINT ( 'NONE',  ( 5.029711800989886683, 4.970344644017389513, 1.040834085586084257E-14 ) ) ;
#41204=CARTESIAN_POINT ( 'NONE',  ( -3.093231602212184850, 6.760520635889515795, -0.7998128361456281477 ) ) ;
#41209=CARTESIAN_POINT ( 'NONE',  ( 8.934460041725669655, 9.525884258209195821, 1.040834085586084257E-14 ) ) ;
#41210=CARTESIAN_POINT ( 'NONE',  ( 7.169564303528210836, 7.258913197071374945, -0.7998128361456281477 ) ) ;
#41215=CARTESIAN_POINT ( 'NONE',  ( 5.542585869888291938, 5.360771691158120689, -0.7998128361456211532 ) ) ;
#41227=CARTESIAN_POINT ( 'NONE',  ( 9.260382613333817403, 10.76253345609967660, -1.199719254218446718 ) ) ;
#41228=CARTESIAN_POINT ( 'NONE',  ( -7.237355071596549116, 7.338002426484427687, 1.040834085586084257E-14 ) ) ;
#41231=ORIENTED_EDGE ( 'NONE', *, *, #183348, .F. ) ;
#41233=CARTESIAN_POINT ( 'NONE',  ( 1.364683531249988535, 4.113541667008088432, 0.7879004041258500513 ) ) ;
#41235=CARTESIAN_POINT ( 'NONE',  ( -6.925517538482230506, 6.974191971184389160, 0.7998128361456341429 ) ) ;
#41237=CARTESIAN_POINT ( 'NONE',  ( -1.492392680118208803, 7.408236896935049387, -4.235501437639352496 ) ) ;
#41238=CARTESIAN_POINT ( 'NONE',  ( 5.691725559638619814, 5.534767995866836543, 1.040834085586084257E-14 ) ) ;
#41239=CARTESIAN_POINT ( 'NONE',  ( -6.735703387890906946, 6.752742128827836865, -0.7998128361456291469 ) ) ;
#41245=CARTESIAN_POINT ( 'NONE',  ( 6.805829924380114804, 8.002851668940699881, 1.082531754730558626 ) ) ;
#41247=CARTESIAN_POINT ( 'NONE',  ( 6.602457619730760285, 8.725953194484466380, 1.443375672974076540 ) ) ;
#41248=CARTESIAN_POINT ( 'NONE',  ( -1.364683531250012516, 2.801041667008090652, -0.7879004041258289570 ) ) ;
#41250=CARTESIAN_POINT ( 'NONE',  ( 5.639828713160493834, 5.682147708216442439, 1.040834085586084257E-14 ) ) ;
#41259=CARTESIAN_POINT ( 'NONE',  ( -4.461457896923207933, 7.279594253155052819, -1.276495073192641883 ) ) ;
#41269=CARTESIAN_POINT ( 'NONE',  ( -3.267151830768952880, 5.795132321663641228, -1.082531754730549078 ) ) ;
#41274=CARTESIAN_POINT ( 'NONE',  ( -2.435661151949389147, 5.993355110582911038, 0.7998128361456341429 ) ) ;
#41279=CARTESIAN_POINT ( 'NONE',  ( 4.121315508874254796, 5.831287398485176077, -1.443375672974051449 ) ) ;
#41280=EDGE_CURVE ( 'NONE', #205506, #154674, #48064, .T. ) ;
#41281=CARTESIAN_POINT ( 'NONE',  ( 1.364683531249990311, 3.946875000341417028, 1.214306433183764966E-14 ) ) ;
#41283=CARTESIAN_POINT ( 'NONE',  ( 6.252281394196331554, 10.44607872653774372, 1.040834085586084257E-14 ) ) ;
#41287=CARTESIAN_POINT ( 'NONE',  ( -3.554208825076827782, 7.298327395898266623, 0.7998128361456341429 ) ) ;
#41291=CARTESIAN_POINT ( 'NONE',  ( 0.7499999999999902300, 2.983333333333351600, 1.299038105676669330 ) ) ;
#41292=CARTESIAN_POINT ( 'NONE',  ( 5.657830175604453338, 5.495223381160312393, 0.7998128361456341429 ) ) ;
#41296=CARTESIAN_POINT ( 'NONE',  ( -1.364683531249997417, 4.009375000341424133, 1.214306433183764966E-14 ) ) ;
#41299=CARTESIAN_POINT ( 'NONE',  ( 9.246297574839980271, 10.85006392781057905, 1.082531754730549967 ) ) ;
#41304=CARTESIAN_POINT ( 'NONE',  ( 0.7499999999999885647, 2.597916667349486897, -1.299038105676658228 ) ) ;
#41306=CARTESIAN_POINT ( 'NONE',  ( -4.394814349124112951, 8.279033840620114049, -0.7998128361456281477 ) ) ;
#41316=CARTESIAN_POINT ( 'NONE',  ( 3.662674053986138656, 7.424870162959149589, 0.7998128361456321445 ) ) ;
#41318=CARTESIAN_POINT ( 'NONE',  ( 4.496500501226593727, 8.397667684739696270, 0.7998128361456462443 ) ) ;
#41320=ORIENTED_EDGE ( 'NONE', *, *, #164628, .T. ) ;
#41324=ORIENTED_EDGE ( 'NONE', *, *, #166876, .T. ) ;
#41325=CARTESIAN_POINT ( 'NONE',  ( 8.378048858240820351, 11.86180853700128601, -1.199719254218446718 ) ) ;
#41331=CARTESIAN_POINT ( 'NONE',  ( 5.838973523318124137, 6.009393772954500612, 0.3882124113597507087 ) ) ;
#41343=CARTESIAN_POINT ( 'NONE',  ( 7.646435448427411963, 8.023188899361205273, -0.7216878364870257245 ) ) ;
#41346=CARTESIAN_POINT ( 'NONE',  ( -5.115504031057831469, 4.862509545855891346, 0.7998128361456341429 ) ) ;
#41350=CARTESIAN_POINT ( 'NONE',  ( -4.381256195510448315, 8.263215994737505454, 1.040834085586084257E-14 ) ) ;
#41363=CARTESIAN_POINT ( 'NONE',  ( 10.73535870392234237, 11.41900666419791399, 0.000000000000000000 ) ) ;
#41372=CARTESIAN_POINT ( 'NONE',  ( -4.288456660624211381, 3.897620947016656956, 1.214306433183764966E-14 ) ) ;
#41376=CARTESIAN_POINT ( 'NONE',  ( 7.228468454380276853, 11.58496363008569574, 1.040834085586084257E-14 ) ) ;
#41380=CARTESIAN_POINT ( 'NONE',  ( -6.714312387265696458, 8.856450423275211037, 1.599625672291283607 ) ) ;
#41381=CARTESIAN_POINT ( 'NONE',  ( 3.147464216666835402, 6.823792019419957278, -0.7998128361456291469 ) ) ;
#41383=CARTESIAN_POINT ( 'NONE',  ( 8.353795204314554468, 12.89784483834236184, -0.7998128361456352531 ) ) ;
#41386=CARTESIAN_POINT ( 'NONE',  ( 1.364683531249988535, 3.176041667008084435, 0.7879004041258500513 ) ) ;
#41388=CARTESIAN_POINT ( 'NONE',  ( 6.724481002698112775, 8.868313807946373473, -1.443375672974057666 ) ) ;
#41396=CARTESIAN_POINT ( 'NONE',  ( 9.707274797260268429, 10.42750147299956964, 0.000000000000000000 ) ) ;
#41401=CARTESIAN_POINT ( 'NONE',  ( -9.989660255170729641, 10.54902514065433827, -0.7998128361456291469 ) ) ;
#41418=CARTESIAN_POINT ( 'NONE',  ( 6.148786358997489820, 7.132337826040578754, -1.199719254218446718 ) ) ;
#41421=CARTESIAN_POINT ( 'NONE',  ( -1.500000000000013101, 2.660416667349483788, -0.8660254037844313801 ) ) ;
#41427=CARTESIAN_POINT ( 'NONE',  ( -1.500000000000001332, 0.9000000000000187850, 0.000000000000000000 ) ) ;
#41428=CARTESIAN_POINT ( 'NONE',  ( 6.564118927310645724, 10.80988918183778225, -0.7998128361456291469 ) ) ;
#41429=CARTESIAN_POINT ( 'NONE',  ( 1.364683531249986537, -0.6364583329919177856, 0.7879004041258500513 ) ) ;
#41432=CARTESIAN_POINT ( 'NONE',  ( 10.08690309888728187, 10.87040115823107911, -0.7216878364870257245 ) ) ;
#41437=CARTESIAN_POINT ( 'NONE',  ( -6.392833124043511894, 7.417059051927569868, 1.199719254218450271 ) ) ;
#41439=EDGE_LOOP ( 'NONE', ( #141924, #102034 ) ) ;
#41440=CARTESIAN_POINT ( 'NONE',  ( 0.7499999999999885647, 2.597916667349486897, -1.299038105676658228 ) ) ;
#41441=CARTESIAN_POINT ( 'NONE',  ( -1.364683531249997417, 4.571875000341417028, 1.214306433183764966E-14 ) ) ;
#41450=ORIENTED_EDGE ( 'NONE', *, *, #101458, .T. ) ;
#41452=CARTESIAN_POINT ( 'NONE',  ( -7.815970093360414158E-14, 8.210952333604092601, -2.038660652713623733 ) ) ;
#41453=CARTESIAN_POINT ( 'NONE',  ( -2.944427096284358836, 6.586915378973714930, -0.4196793407983508972 ) ) ;
#41454=CARTESIAN_POINT ( 'NONE',  ( -8.962103233833181193, 10.41454084668224489, -1.199719254218446718 ) ) ;
#41455=CARTESIAN_POINT ( 'NONE',  ( 7.039708073993665494, 9.236078724457858158, 1.599625672291281386 ) ) ;
#41463=CARTESIAN_POINT ( 'NONE',  ( -7.867809214632013770, 8.073532260025807261, 1.040834085586084257E-14 ) ) ;
#41465=CARTESIAN_POINT ( 'NONE',  ( 0.9999999999999833467, 5.868705557303652398, 4.125226524755083446 ) ) ;
#41468=CARTESIAN_POINT ( 'NONE',  ( 4.403700966340357681, 4.032072637018845107, -0.7998128361456211532 ) ) ;
#41471=CARTESIAN_POINT ( 'NONE',  ( -3.255929445576174697, 6.950334786480840243, -0.7998128361456281477 ) ) ;
#41472=CARTESIAN_POINT ( 'NONE',  ( -8.670602931139386627, 10.07445716020612103, 1.199719254218462483 ) ) ;
#41475=CARTESIAN_POINT ( 'NONE',  ( -4.009952404978103679, 7.802135278885950598, 0.4104602055842437314 ) ) ;
#41482=CARTESIAN_POINT ( 'NONE',  ( 7.806797523370503811, 8.002351953554066810, 1.040834085586084257E-14 ) ) ;
#41499=CARTESIAN_POINT ( 'NONE',  ( 2.738383840280320669, 6.138605547061593448, 0.7216878364870338292 ) ) ;
#41503=CARTESIAN_POINT ( 'NONE',  ( -9.646789991323334590, 11.21334206375407305, 1.199719254218462483 ) ) ;
#41505=CARTESIAN_POINT ( 'NONE',  ( 7.262363838414439776, 11.62450824479221900, 0.7998128361456462443 ) ) ;
#41510=CARTESIAN_POINT ( 'NONE',  ( 4.037628742901151924, 7.560846779974220055, 0.4916741515407979102 ) ) ;
#41513=CYLINDRICAL_SURFACE ( 'NONE', #11517, 1.500000000000000222 ) ;
#41515=CARTESIAN_POINT ( 'NONE',  ( -1.364683531250012516, 1.280208333674755172, 0.7879004041258379498 ) ) ;
#41519=STYLED_ITEM ( 'NONE', ( #204397 ), #127801 ) ;
#41522=CARTESIAN_POINT ( 'NONE',  ( -3.066115294984855133, 6.728884944124295053, 0.7998128361456341429 ) ) ;
#41523=FACE_OUTER_BOUND ( 'NONE', #74723, .T. ) ;
#41525=CARTESIAN_POINT ( 'NONE',  ( -1.500000000000015099, -0.1208333333333093396, -0.8660254037844383745 ) ) ;
#41527=CARTESIAN_POINT ( 'NONE',  ( -1.499999999999997780, 5.900000000000023448, 1.214306433183764966E-14 ) ) ;
#41533=CARTESIAN_POINT ( 'NONE',  ( 1.364683531249986537, 0.4052083336747511200, -0.7879004041258309554 ) ) ;
#41535=CARTESIAN_POINT ( 'NONE',  ( -7.877450944739929461, 9.149113176073413456, 1.199719254218462483 ) ) ;
#41536=CARTESIAN_POINT ( 'NONE',  ( 7.889955328148847258, 11.29236608522730911, -1.199719254218446718 ) ) ;
#41537=CARTESIAN_POINT ( 'NONE',  ( 3.832150974156964818, 7.622593236491780999, 1.040834085586084257E-14 ) ) ;
#41541=CARTESIAN_POINT ( 'NONE',  ( 0.6823417656249882723, -0.2614583329919109578, -1.181850606188749264 ) ) ;
#41547=B_SPLINE_CURVE_WITH_KNOTS ( 'NONE', 3,
 ( #66334, #1339, #81552, #132480 ),
 .UNSPECIFIED., .F., .F.,
 ( 4, 4 ),
 ( 0.000000000000000000, 0.0007854274309115643520 ),
 .UNSPECIFIED. ) ;
#41551=CARTESIAN_POINT ( 'NONE',  ( 5.992340707560147806, 8.974519344586754599, 1.082531754730558626 ) ) ;
#41554=CARTESIAN_POINT ( 'NONE',  ( -5.901876940650454095, 5.779944607047298177, -0.7998128361456291469 ) ) ;
#41559=CARTESIAN_POINT ( 'NONE',  ( 4.487385655998867406, 8.179107665399927285, 0.7216878364870438212 ) ) ;
#41560=CARTESIAN_POINT ( 'NONE',  ( -7.483737604619046913, 11.67485160545682987, 0.000000000000000000 ) ) ;
#41562=CARTESIAN_POINT ( 'NONE',  ( -1.201851678989727383E-14, 3.837500000000021227, -1.732050807568863648 ) ) ;
#41566=CARTESIAN_POINT ( 'NONE',  ( 8.920901888111997025, 10.47043562662792304, 1.082531754730549967 ) ) ;
#41574=EDGE_CURVE ( 'NONE', #21699, #9480, #154400, .T. ) ;
#41579=CARTESIAN_POINT ( 'NONE',  ( 9.042925270190638187, 9.652427024751663254, 0.7216878364870458196 ) ) ;
#41581=CARTESIAN_POINT ( 'NONE',  ( 7.884230021546724920, 9.157022099014721306, 1.199719254218462483 ) ) ;
#41583=CARTESIAN_POINT ( 'NONE',  ( 3.212919216758630014, 6.692230152952963529, 0.000000000000000000 ) ) ;
#41586=CARTESIAN_POINT ( 'NONE',  ( 8.536830278099042602, 13.11138575775759563, -0.7998128361456352531 ) ) ;
#41588=DIRECTION ( 'NONE',  ( -0.7592566023652993490, 0.6507913734559652719, 0.000000000000000000 ) ) ;
#41589=CARTESIAN_POINT ( 'NONE',  ( 3.524756749872944628, 7.056040608253000279, -0.7216878364870267237 ) ) ;
#41590=ORIENTED_EDGE ( 'NONE', *, *, #107353, .T. ) ;
#41591=CARTESIAN_POINT ( 'NONE',  ( -7.158341918335454857, 10.33485409049125003, 1.082531754730549967 ) ) ;
#41596=CARTESIAN_POINT ( 'NONE',  ( -2.117044542028253318, 5.621635732341564662, -0.7998128361456281477 ) ) ;
#41619=CARTESIAN_POINT ( 'NONE',  ( -7.413611068574208041, 7.543634422958360730, 0.7998128361456341429 ) ) ;
#41623=CARTESIAN_POINT ( 'NONE',  ( 5.124091990960999432, 8.065525525174782828, -1.199719254218452047 ) ) ;
#41633=CARTESIAN_POINT ( 'NONE',  ( -3.242371291962510504, 6.934516940598226320, 1.040834085586084257E-14 ) ) ;
#41636=CARTESIAN_POINT ( 'NONE',  ( 7.233438648090761980, 8.397765496649418182, 1.199719254218462483 ) ) ;
#41637=CARTESIAN_POINT ( 'NONE',  ( -1.364683531250012516, 3.738541667008087099, -0.7879004041258300672 ) ) ;
#41639=CARTESIAN_POINT ( 'NONE',  ( 6.001708393183096568, 6.086876045059843143, 0.6039332608892417076 ) ) ;
#41645=CARTESIAN_POINT ( 'NONE',  ( 5.463572716182819811, 8.357623354646536384, 1.082531754730558626 ) ) ;
#41646=CARTESIAN_POINT ( 'NONE',  ( -7.802881099864745984, 9.062115023719057305, -1.199719254218446718 ) ) ;
#41649=CARTESIAN_POINT ( 'NONE',  ( -8.843996274815957293, 9.212417163573759282, 1.040834085586084257E-14 ) ) ;
#41650=CARTESIAN_POINT ( 'NONE',  ( -5.900823170445743671, 7.907379670318584353, 1.599625672291269396 ) ) ;
#41655=EDGE_CURVE ( 'NONE', #103805, #91287, #27301, .T. ) ;
#41658=CARTESIAN_POINT ( 'NONE',  ( 8.239604668803105270, 10.63595808506888396, -1.599625672291268286 ) ) ;
#41674=CARTESIAN_POINT ( 'NONE',  ( 0.7499999999999920064, 4.983333333333353821, 1.299038105676669330 ) ) ;
#41675=CARTESIAN_POINT ( 'NONE',  ( 5.834086172582112262, 5.700855377634248100, 1.040834085586084257E-14 ) ) ;
#41676=CARTESIAN_POINT ( 'NONE',  ( 7.494959990256193194, 7.638541498254023843, -0.7998128361456281477 ) ) ;
#41678=CARTESIAN_POINT ( 'NONE',  ( -8.026063749610047537, 11.34719622697832264, -1.082531754730543971 ) ) ;
#41679=CARTESIAN_POINT ( 'NONE',  ( 4.379563740902463920, 4.008367186281499350, -0.1129952432600847406 ) ) ;
#41680=CARTESIAN_POINT ( 'NONE',  ( 5.653386867218496370, 9.539442411822841805, 1.040834085586084257E-14 ) ) ;
#41682=CARTESIAN_POINT ( 'NONE',  ( -8.120970824461345217, 12.41829036193951730, 0.7216878364870458196 ) ) ;
#41685=CARTESIAN_POINT ( 'NONE',  ( 9.023114925094663619, 10.48572115315399245, 1.199719254218453823 ) ) ;
#41689=CARTESIAN_POINT ( 'NONE',  ( -1.402160292154681736E-14, 1.696875000341421469, -1.575800808251659024 ) ) ;
#41694=CARTESIAN_POINT ( 'NONE',  ( -0.6823417656250246877, 0.05104166700808931978, 1.181850606188755259 ) ) ;
#41696=CARTESIAN_POINT ( 'NONE',  ( 9.935427640716063991, 10.48575375712389679, -0.7998128361456281477 ) ) ;
#41700=CARTESIAN_POINT ( 'NONE',  ( -9.398826802771548472, 11.98838390803207865, -1.599625672291263179 ) ) ;
#41706=CARTESIAN_POINT ( 'NONE',  ( 3.330499290451326200, 7.037332938835193730, -0.7998128361456291469 ) ) ;
#41709=B_SPLINE_CURVE_WITH_KNOTS ( 'NONE', 3,
 ( #143632, #128496, #14629, #164110 ),
 .UNSPECIFIED., .F., .F.,
 ( 4, 4 ),
 ( 1.569810930355607827E-17, 0.0001726908832627367966 ),
 .UNSPECIFIED. ) ;
#41710=CARTESIAN_POINT ( 'NONE',  ( -2.887523529586332405, 5.352232636950553513, 1.082531754730560403 ) ) ;
#41713=CARTESIAN_POINT ( 'NONE',  ( 7.411503528164766763, 11.79850454950093841, 1.040834085586084257E-14 ) ) ;
#41715=CARTESIAN_POINT ( 'NONE',  ( 5.007133299032078710, 6.576657384445655730, 1.236533897214306066 ) ) ;
#41717=CARTESIAN_POINT ( 'NONE',  ( -3.405069135326500351, 7.124331091189553433, 1.040834085586084257E-14 ) ) ;
#41721=CARTESIAN_POINT ( 'NONE',  ( 7.239163954692881653, 10.53310948286200599, -1.199719254218441611 ) ) ;
#41723=CARTESIAN_POINT ( 'NONE',  ( 6.265839547809997079, 10.46189657242035587, 0.7998128361456462443 ) ) ;
#41726=CARTESIAN_POINT ( 'NONE',  ( -8.026063749610047537, 11.34719622697832264, -1.082531754730543971 ) ) ;
#41733=CARTESIAN_POINT ( 'NONE',  ( -5.584559075236136039, 6.202510182859402477, -0.8982034194818852013 ) ) ;
#41734=CARTESIAN_POINT ( 'NONE',  ( -1.364683531250012516, 1.280208333674755172, 0.7879004041258379498 ) ) ;
#41736=CARTESIAN_POINT ( 'NONE',  ( 5.341549334104176872, 9.175631956522799726, 0.7216878364870438212 ) ) ;
#41744=DIRECTION ( 'NONE',  ( 1.000000000000000000, 0.000000000000000000, 0.000000000000000000 ) ) ;
#41755=CARTESIAN_POINT ( 'NONE',  ( 7.899597058256738968, 12.36794700127490820, 1.040834085586084257E-14 ) ) ;
#41757=ORIENTED_EDGE ( 'NONE', *, *, #170416, .T. ) ;
#41760=CARTESIAN_POINT ( 'NONE',  ( -7.854251061018346469, 8.057714414143200443, -0.7998128361456291469 ) ) ;
#41762=ORIENTED_EDGE ( 'NONE', *, *, #25593, .F. ) ;
#41763=CARTESIAN_POINT ( 'NONE',  ( -8.459397779922852578, 11.95671561229694824, 1.199719254218453823 ) ) ;
#41767=CARTESIAN_POINT ( 'NONE',  ( -1.500000000000011324, 4.660416667349484676, -0.8660254037844313801 ) ) ;
#41768=CARTESIAN_POINT ( 'NONE',  ( 7.100719765255169236, 9.307259030929609267, -1.599625672291262513 ) ) ;
#41772=CARTESIAN_POINT ( 'NONE',  ( -7.985916173649233230, 9.275655943134292869, -1.199719254218446718 ) ) ;
#41774=CARTESIAN_POINT ( 'NONE',  ( -1.001543065824772872E-14, 4.571875000341418804, 1.575800808251672791 ) ) ;
#41777=CARTESIAN_POINT ( 'NONE',  ( 2.854315967138055132, 6.433244981884085334, -0.2941531795266367211 ) ) ;
#41780=CARTESIAN_POINT ( 'NONE',  ( -7.537970219518075332, 10.77775377520434574, -1.082531754730543971 ) ) ;
#41785=CARTESIAN_POINT ( 'NONE',  ( 0.6823417656249899377, 2.905208333674754062, 1.181850606188765695 ) ) ;
#41792=CARTESIAN_POINT ( 'NONE',  ( 0.6823417656249899377, 3.926041667008085767, -1.181850606188754593 ) ) ;
#41793=CARTESIAN_POINT ( 'NONE',  ( -3.924195396151603177, 6.665646164563756138, 1.199719254218464037 ) ) ;
#41794=CARTESIAN_POINT ( 'NONE',  ( 7.447506452608354088, 7.583179037664891098, 0.7998128361456341429 ) ) ;
#41797=CARTESIAN_POINT ( 'NONE',  ( 3.023105065722954787, 5.510411095776657220, 1.082531754730546636 ) ) ;
#41798=CARTESIAN_POINT ( 'NONE',  ( 0.6823417656249899377, 3.488541667008085323, -1.181850606188754593 ) ) ;
#41799=DIRECTION ( 'NONE',  ( 1.000000000000000000, -3.135042426464105837E-15, 0.000000000000000000 ) ) ;
#41803=CARTESIAN_POINT ( 'NONE',  ( -0.6823417656250003738, 0.9677083336747521747, -1.181850606188749264 ) ) ;
#41804=CARTESIAN_POINT ( 'NONE',  ( -4.934804725694231564, 5.819988937140460727, -1.082531754730544860 ) ) ;
#41805=CARTESIAN_POINT ( 'NONE',  ( 6.145923705696426431, 6.064665832934283962, 0.7998128361456341429 ) ) ;
#41810=CARTESIAN_POINT ( 'NONE',  ( 4.365362273920250225, 5.155639410070820716, 1.082531754730560403 ) ) ;
#41813=CARTESIAN_POINT ( 'NONE',  ( -10.00555417720528872, 10.77549408293541866, 0.7216878364870438212 ) ) ;
#41818=CARTESIAN_POINT ( 'NONE',  ( -10.15913717534155047, 10.74674821418697057, 0.7998128361456462443 ) ) ;
#41819=CARTESIAN_POINT ( 'NONE',  ( -4.243338890952892406, 7.894386439512932618, -0.7216878364870257245 ) ) ;
#41821=CARTESIAN_POINT ( 'NONE',  ( -1.402160292154681736E-14, 0.6343750003414162508, 1.575800808251672791 ) ) ;
#41833=CARTESIAN_POINT ( 'NONE',  ( 8.880227426826641235, 10.42298208846167284, 1.082531754730549967 ) ) ;
#41842=CARTESIAN_POINT ( 'NONE',  ( -3.521367211247373508, 5.131347717920458962, -1.599625672291256295 ) ) ;
#41844=CARTESIAN_POINT ( 'NONE',  ( 1.257518954444997838, 3.239770990628810576, 0.7750000000000152323 ) ) ;
#41847=CARTESIAN_POINT ( 'NONE',  ( 0.6823417656249899377, 1.155208333674752286, 1.181850606188755259 ) ) ;
#41863=ORIENTED_EDGE ( 'NONE', *, *, #189117, .F. ) ;
#41867=CARTESIAN_POINT ( 'NONE',  ( 5.168682875307768931, 7.053215992657626110, -1.599625672291256295 ) ) ;
#41874=CARTESIAN_POINT ( 'NONE',  ( 8.067265095331215718, 9.370563018429956870, 1.199719254218462483 ) ) ;
#41877=CARTESIAN_POINT ( 'NONE',  ( 8.127223016387999266, 11.56917838817298616, 1.199719254218460707 ) ) ;
#41879=CARTESIAN_POINT ( 'NONE',  ( 1.506030227042737701, 8.670273769332156988, -2.548074190919165094 ) ) ;
#41883=ORIENTED_EDGE ( 'NONE', *, *, #19647, .T. ) ;
#41889=CARTESIAN_POINT ( 'NONE',  ( -8.378575743565381373, 8.877352577022161739, 0.7216878364870438212 ) ) ;
#41901=CARTESIAN_POINT ( 'NONE',  ( 4.677199806590210507, 4.559080650551097236, -0.7216878364870197293 ) ) ;
#41909=CARTESIAN_POINT ( 'NONE',  ( -6.230135280679522936, 7.227244901336242755, 1.199719254218450271 ) ) ;
#41911=CARTESIAN_POINT ( 'NONE',  ( -3.785751206713858785, 5.439795712631356750, 1.599625672291267398 ) ) ;
#41912=FACE_OUTER_BOUND ( 'NONE', #166768, .T. ) ;
#41917=CARTESIAN_POINT ( 'NONE',  ( 8.107412671292031803, 11.44210330227398487, 1.082531754730557072 ) ) ;
#41919=CARTESIAN_POINT ( 'NONE',  ( -1.364683531249997417, 3.821875000341416584, 1.214306433183764966E-14 ) ) ;
#41922=CARTESIAN_POINT ( 'NONE',  ( 4.449046963578762615, 8.342305224150557308, -0.7998128361456231517 ) ) ;
#41932=ORIENTED_EDGE ( 'NONE', *, *, #53132, .F. ) ;
#41934=CARTESIAN_POINT ( 'NONE',  ( -1.364683531250012516, 1.092708333674754506, 0.7879004041258379498 ) ) ;
#41936=CARTESIAN_POINT ( 'NONE',  ( 4.487912541323413329, 5.194651705420806564, 1.199719254218462483 ) ) ;
#41939=CARTESIAN_POINT ( 'NONE',  ( -5.043269954603569083, 7.867270132804026872, 1.082531754730560403 ) ) ;
#41940=CARTESIAN_POINT ( 'NONE',  ( 4.528060117284244512, 4.385084346360807572, 0.7216878364870317197 ) ) ;
#41941=CARTESIAN_POINT ( 'NONE',  ( -5.355107487273497391, 9.191449801886996340, 0.7216878364870458196 ) ) ;
#41945=CARTESIAN_POINT ( 'NONE',  ( 7.149227073107712549, 7.235186428247455837, -0.7998128361456281477 ) ) ;
#41950=CARTESIAN_POINT ( 'NONE',  ( -1.201851678989727383E-14, 5.696875000341416140, -1.575800808251660134 ) ) ;
#41954=CARTESIAN_POINT ( 'NONE',  ( 7.820355676984174664, 8.018169799436671852, -0.7998128361456281477 ) ) ;
#41956=CARTESIAN_POINT ( 'NONE',  ( -5.865874016206865882, 9.995270118883347266, 0.000000000000000000 ) ) ;
#41960=CARTESIAN_POINT ( 'NONE',  ( 8.589254009457354400, 9.979550084910457031, -1.199719254218446718 ) ) ;
#41963=CARTESIAN_POINT ( 'NONE',  ( -5.540478329478883524, 9.615641817700700145, 0.000000000000000000 ) ) ;
#41965=CARTESIAN_POINT ( 'NONE',  ( 7.904040366642695048, 9.284097184913720824, 1.082531754730558626 ) ) ;
#41966=CARTESIAN_POINT ( 'NONE',  ( 4.420695050690802930, 7.093836324768183488, -1.099706215833176515 ) ) ;
#41967=CARTESIAN_POINT ( 'NONE',  ( -4.680589345215810049, 6.483773540883647435, -1.599625672291256295 ) ) ;
#41974=CARTESIAN_POINT ( 'NONE',  ( 8.971744963941056028, 11.49012176272984931, 1.599625672291281386 ) ) ;
#41975=CARTESIAN_POINT ( 'NONE',  ( -5.471750928372196121, 6.276313537582185909, 1.010767274114855008 ) ) ;
#41976=EDGE_CURVE ( 'NONE', #133576, #140589, #34594, .T. ) ;
#41977=CARTESIAN_POINT ( 'NONE',  ( 4.234184546134326155, 3.834303480111807882, -0.3975762604357939156 ) ) ;
#41978=CARTESIAN_POINT ( 'NONE',  ( -1.402160292154681736E-14, 0.6968750003414164729, -1.575800808251659024 ) ) ;
#41980=CARTESIAN_POINT ( 'NONE',  ( -5.097502569058210753, 7.930541516334467467, -1.082531754730549967 ) ) ;
#41989=CARTESIAN_POINT ( 'NONE',  ( -5.590496338642190643, 6.198678163000841401, 0.8915474099989786350 ) ) ;
#41990=CARTESIAN_POINT ( 'NONE',  ( 0.6823417656249899377, 1.155208333674752286, 1.181850606188755259 ) ) ;
#41994=CARTESIAN_POINT ( 'NONE',  ( 3.877268743828276243, 4.586196958296845594, 1.082531754730560403 ) ) ;
#41999=CARTESIAN_POINT ( 'NONE',  ( -7.171900071504729191, 11.31104115015678779, -0.7216878364870267237 ) ) ;
#42006=CARTESIAN_POINT ( 'NONE',  ( -6.358410854684777291, 10.36197039720016022, -0.7216878364870267237 ) ) ;
#42012=CARTESIAN_POINT ( 'NONE',  ( -8.649738815394339753, 9.193709494155953621, 1.040834085586084257E-14 ) ) ;
#42017=CARTESIAN_POINT ( 'NONE',  ( 1.499999999999990896, 4.306250000682819490, 1.214306433183764966E-14 ) ) ;
#42018=CARTESIAN_POINT ( 'NONE',  ( 4.477916600690244664, 7.270601638097409669, -1.256879854437189969 ) ) ;
#42022=ORIENTED_EDGE ( 'NONE', *, *, #24501, .T. ) ;
#42025=CARTESIAN_POINT ( 'NONE',  ( -6.826694039680798021, 7.923230120171105284, -1.199719254218446718 ) ) ;
#42027=CARTESIAN_POINT ( 'NONE',  ( 4.985647801523278133, 6.839675073242382553, -1.599625672291256295 ) ) ;
#42031=CARTESIAN_POINT ( 'NONE',  ( 6.120616281565444794, 9.228137197546649517, -1.199719254218440723 ) ) ;
#42032=CARTESIAN_POINT ( 'NONE',  ( -4.911999630574282349, 4.728820931584174048, 0.4272946817465201885 ) ) ;
#42039=CARTESIAN_POINT ( 'NONE',  ( -6.399085315970155285, 6.567947078161039620, -0.7216878364870278340 ) ) ;
#42048=CARTESIAN_POINT ( 'NONE',  ( -9.016335848287868160, 10.47781223021269170, 1.199719254218462483 ) ) ;
#42050=CARTESIAN_POINT ( 'NONE',  ( 8.471147050440139381, 8.777426401801974976, -0.7998128361456281477 ) ) ;
#42051=CARTESIAN_POINT ( 'NONE',  ( 1.499999999999987566, -0.2249999999999821587, 0.000000000000000000 ) ) ;
#42052=CARTESIAN_POINT ( 'NONE',  ( -9.040589502214116280, 9.441775928871617651, 0.7998128361456462443 ) ) ;
#42054=CARTESIAN_POINT ( 'NONE',  ( -1.364683531249997417, 4.259375000341424133, 1.214306433183764966E-14 ) ) ;
#42055=CARTESIAN_POINT ( 'NONE',  ( 9.585251415181632595, 10.28514086057449184, 0.000000000000000000 ) ) ;
#42059=CARTESIAN_POINT ( 'NONE',  ( 0.7499999999999902300, 5.316666666666685082, -1.299038105676658228 ) ) ;
#42061=CARTESIAN_POINT ( 'NONE',  ( 8.771762197917315262, 10.29643932140079166, -1.082531754730543083 ) ) ;
#42064=CARTESIAN_POINT ( 'NONE',  ( -6.575341312947811545, 6.773579074634973551, 1.040834085586084257E-14 ) ) ;
#42066=CARTESIAN_POINT ( 'NONE',  ( 1.364683531249988535, 2.113541667008087099, 0.7879004041258500513 ) ) ;
#42070=CARTESIAN_POINT ( 'NONE',  ( -6.398558430645608475, 9.552403038140164782, -1.199719254218440723 ) ) ;
#42072=CARTESIAN_POINT ( 'NONE',  ( -1.364683531250012516, 4.801041667008083991, -0.7879004041258300672 ) ) ;
#42081=CARTESIAN_POINT ( 'NONE',  ( -1.201851678989727383E-14, 1.462500000000018119, 1.732050807568877637 ) ) ;
#42084=CARTESIAN_POINT ( 'NONE',  ( -0.4396008313320713401, 7.377972292137100929, -2.042906170116811637 ) ) ;
#42086=CARTESIAN_POINT ( 'NONE',  ( 5.653386867218496370, 9.539442411822841805, 1.040834085586084257E-14 ) ) ;
#42088=CARTESIAN_POINT ( 'NONE',  ( 9.423080456697809026, 10.95234760669099749, -1.199719254218446718 ) ) ;
#42095=CARTESIAN_POINT ( 'NONE',  ( 7.553864141108259211, 11.96459193126834464, 1.040834085586084257E-14 ) ) ;
#42096=CARTESIAN_POINT ( 'NONE',  ( -8.805130697071332335, 12.36007068230351358, 1.199719254218462483 ) ) ;
#42098=CARTESIAN_POINT ( 'NONE',  ( -4.911316915444452036, 4.694531097513658935, -0.3529309010900701926 ) ) ;
#42100=CARTESIAN_POINT ( 'NONE',  ( -0.6823417656250246877, -1.198958332991911790, 1.181850606188755259 ) ) ;
#42105=CARTESIAN_POINT ( 'NONE',  ( 4.074186250656476993, 7.493853916489129574, -0.5595503573846259959 ) ) ;
#42107=CARTESIAN_POINT ( 'NONE',  ( -1.364683531249997417, 5.259375000341425022, 1.214306433183764966E-14 ) ) ;
#42109=CARTESIAN_POINT ( 'NONE',  ( -6.561783159334145132, 6.757761228752363181, -0.7216878364870278340 ) ) ;
#42119=CARTESIAN_POINT ( 'NONE',  ( 7.052212457402625922, 11.37933163361175382, -0.7998128361456291469 ) ) ;
#42121=CARTESIAN_POINT ( 'NONE',  ( 5.816084710138182068, 5.887779704690343507, -0.7216878364870008555 ) ) ;
#42125=CARTESIAN_POINT ( 'NONE',  ( -7.808606406466886973, 11.19745900993164511, 1.199719254218453823 ) ) ;
#42126=CARTESIAN_POINT ( 'NONE',  ( 5.524057522564145728, 8.532151978711786100, 1.199719254218462483 ) ) ;
#42129=CARTESIAN_POINT ( 'NONE',  ( 4.175548122884573665, 3.973820352894515295, 1.214306433183764966E-14 ) ) ;
#42131=CARTESIAN_POINT ( 'NONE',  ( 3.876741858503734761, 6.610283703974623393, 1.199719254218462483 ) ) ;
#42132=ORIENTED_EDGE ( 'NONE', *, *, #177985, .T. ) ;
#42137=CARTESIAN_POINT ( 'NONE',  ( -6.399085315970155285, 6.567947078161039620, -0.7216878364870278340 ) ) ;
#42138=CARTESIAN_POINT ( 'NONE',  ( 8.270110514656016321, 12.59228666716665401, 0.7216878364870438212 ) ) ;
#42141=CARTESIAN_POINT ( 'NONE',  ( -5.859094939400033120, 9.987361195942037639, -0.7998128361456231517 ) ) ;
#42146=CARTESIAN_POINT ( 'NONE',  ( -8.025536864285518490, 11.45054454405341282, -1.199719254218446718 ) ) ;
#42150=CARTESIAN_POINT ( 'NONE',  ( 7.527801604085637699, 9.805521176231838609, 1.599625672291281386 ) ) ;
#42151=CARTESIAN_POINT ( 'NONE',  ( 4.822949958159288286, 6.649860922651058992, -1.599625672291256295 ) ) ;
#42163=CARTESIAN_POINT ( 'NONE',  ( -6.995117189646935962, 10.24838825697502109, 1.199719254218453823 ) ) ;
#42166=CARTESIAN_POINT ( 'NONE',  ( 6.263503779833467178, 9.290876262238963790, -1.082531754730537088 ) ) ;
#42168=CARTESIAN_POINT ( 'NONE',  ( -1.500000000000077494, 7.388542872122511262, 4.154462424328213110 ) ) ;
#42170=CARTESIAN_POINT ( 'NONE',  ( 5.379888026524302980, 5.170957540566797128, -0.7998128361456211532 ) ) ;
#42172=CARTESIAN_POINT ( 'NONE',  ( -5.759516327706961647, 5.613857225279885732, -0.7998128361456221525 ) ) ;
#42174=DIRECTION ( 'NONE',  ( -0.9782075119097244364, 0.1245777785627091433, -0.1661037047502772757 ) ) ;
#42182=CARTESIAN_POINT ( 'NONE',  ( 8.751951852821344247, 10.16936423550178503, -1.199719254218446718 ) ) ;
#42187=CARTESIAN_POINT ( 'NONE',  ( -4.684235067853224521, 6.877467941869524815, -1.224209591347114046 ) ) ;
#42194=CARTESIAN_POINT ( 'NONE',  ( 9.246297574839974942, 11.81043314211192019, 1.443375672974076540 ) ) ;
#42211=CARTESIAN_POINT ( 'NONE',  ( -2.611917148927046295, 6.198987107056845858, 1.040834085586084257E-14 ) ) ;
#42212=CARTESIAN_POINT ( 'NONE',  ( 6.439759776366780208, 6.615400615290456088, 0.7216878364870317197 ) ) ;
#42213=CARTESIAN_POINT ( 'NONE',  ( -1.500000000000013101, 3.879166666666685970, -0.8660254037844313801 ) ) ;
#42220=CARTESIAN_POINT ( 'NONE',  ( -0.6823417656250212460, 4.051041667008085767, 1.181850606188767472 ) ) ;
#42223=CARTESIAN_POINT ( 'NONE',  ( -3.389175213736311587, 4.977123720824209840, 1.443375672974064550 ) ) ;
#42228=CARTESIAN_POINT ( 'NONE',  ( 5.040934186182656873, 4.775511393501539636, 1.040834085586084257E-14 ) ) ;
#42232=CARTESIAN_POINT ( 'NONE',  ( 9.286972035236624734, 11.85788667924133399, -1.443375672974058777 ) ) ;
#42235=CARTESIAN_POINT ( 'NONE',  ( -0.6823417656250003738, 1.780208333674752952, -1.181850606188749264 ) ) ;
#42236=CARTESIAN_POINT ( 'NONE',  ( -1.499999999999997780, 3.650000000000021227, 1.214306433183764966E-14 ) ) ;
#42239=CARTESIAN_POINT ( 'NONE',  ( -8.025536864285518490, 11.45054454405341282, -1.199719254218446718 ) ) ;
#42240=CARTESIAN_POINT ( 'NONE',  ( -4.568734577680875653, 8.274014740695587733, -0.7216878364870257245 ) ) ;
#42244=CARTESIAN_POINT ( 'NONE',  ( 0.6823417656249899377, 5.176041667008086655, -1.181850606188754593 ) ) ;
#42252=CARTESIAN_POINT ( 'NONE',  ( -4.568734577680880093, 7.313645526394248364, -1.082531754730548412 ) ) ;
#42255=ADVANCED_FACE ( 'NONE', ( #107596 ), #12534, .T. ) ;
#42258=CARTESIAN_POINT ( 'NONE',  ( -4.731432421044877934, 6.543090462684225450, -1.443375672974051449 ) ) ;
#42260=CARTESIAN_POINT ( 'NONE',  ( 9.642873567817520808, 12.27310513391906532, 1.599625672291279388 ) ) ;
#42269=CARTESIAN_POINT ( 'NONE',  ( -4.416205349749324327, 6.175325546172740765, 1.599625672291267398 ) ) ;
#42274=CARTESIAN_POINT ( 'NONE',  ( 10.05978679165993839, 10.83876546646586014, 0.7216878364870438212 ) ) ;
#42275=CARTESIAN_POINT ( 'NONE',  ( 4.496500501226593727, 8.397667684739696270, 0.7998128361456462443 ) ) ;
#42278=VERTEX_POINT ( 'NONE', #173627 ) ;
#42281=CARTESIAN_POINT ( 'NONE',  ( 3.357615597678655917, 7.068968630600412695, 0.7998128361456321445 ) ) ;
#42283=CARTESIAN_POINT ( 'NONE',  ( 1.419999999999989049, 6.200000000000045475, -2.873333333333328632 ) ) ;
#42292=CARTESIAN_POINT ( 'NONE',  ( -4.876128802409253282, 8.840567369452784874, 0.7998128361456481317 ) ) ;
#42294=ORIENTED_EDGE ( 'NONE', *, *, #126911, .F. ) ;
#42298=CARTESIAN_POINT ( 'NONE',  ( 1.364683531249990311, 4.613541667008083103, 0.7879004041258500513 ) ) ;
#42299=CARTESIAN_POINT ( 'NONE',  ( 8.961576348508637935, 11.47825837805867799, -1.443375672974052559 ) ) ;
#42300=CARTESIAN_POINT ( 'NONE',  ( -5.870844209917351009, 6.808071985447069707, -1.199719254218446718 ) ) ;
#42302=CARTESIAN_POINT ( 'NONE',  ( -1.426714497269032655, 7.396188545894244015, -4.272650097712488382 ) ) ;
#42303=CARTESIAN_POINT ( 'NONE',  ( 3.683011284406639607, 7.448596931783069586, 0.7998128361456321445 ) ) ;
#42304=CARTESIAN_POINT ( 'NONE',  ( -4.238895582566952314, 8.097128612970093897, 1.040834085586084257E-14 ) ) ;
#42310=CARTESIAN_POINT ( 'NONE',  ( 6.561783159334121152, 8.678499657355050800, -1.443375672974057666 ) ) ;
#42311=EDGE_CURVE ( 'NONE', #195242, #136958, #190892, .T. ) ;
#42313=CARTESIAN_POINT ( 'NONE',  ( 6.548225005276093746, 9.623051025255367819, -1.082531754730537976 ) ) ;
#42314=CARTESIAN_POINT ( 'NONE',  ( 1.364683531249990311, 3.196875000341416140, 1.214306433183764966E-14 ) ) ;
#42316=CARTESIAN_POINT ( 'NONE',  ( 6.439759776366780208, 6.615400615290456088, 0.7216878364870317197 ) ) ;
#42321=CARTESIAN_POINT ( 'NONE',  ( -0.6823417656250212460, 5.551041667008087543, 1.181850606188767472 ) ) ;
#42323=DIRECTION ( 'NONE',  ( -0.7592566023653004592, -0.6507913734559639396, -0.000000000000000000 ) ) ;
#42325=CARTESIAN_POINT ( 'NONE',  ( -4.022959435666734862, 7.784601250164370434, 0.4788606935734913694 ) ) ;
#42328=AXIS2_PLACEMENT_3D ( 'NONE', #2086, #167823, #54079 ) ;
#42330=CARTESIAN_POINT ( 'NONE',  ( 1.499999999999821032, 7.388542872122531691, -4.154462424328212222 ) ) ;
#42332=( BOUNDED_SURFACE ( )  B_SPLINE_SURFACE ( 1, 2, ( 
 ( #108807, #174830, #26409, #59982, #208351, #126135, #192097, #11218, #175888, #27479, #93579, #143412, #139113, #106654, #209406, #61053, #127212, #172681, #81564, #182251, #79435, #98895, #148707, #113077, #196392, #129349, #277, #48035, #96786, #114149, #66349, #147650, #132493, #78363, #210490, #128286, #194248, #201686, #36003, #117329, #119464, #2415, #84765, #86902, #67413, #53331, #107213, #4543, #124555, #101005, #73574, #102084, #69553, #169214, #166018, #183327, #19752, #205698, #85833, #167094, #184384, #185452, #37074, #168153, #20805, #151911, #156981, #200622, #150851, #139675, #173235, #52271, #90917, #118398, #34933, #199563, #152969, #57333, #123497, #189461, #206766, #41104, #1352, #8570, #74650, #42170, #58400, #17604, #149776, #190513, #83688, #133554, #51207, #183866, #33349, #130924, #182795, #180668, #35481, #51754, #99431, #179616, #34414, #32294, #196917, #101558, #164425, #100486, #1891, #98360, #16009, #19226, #166561, #18150, #97310, #81041, #84237, #85304, #151390, #47502, #2960, #135148, #113611, #147126, #114256, #196500, #1455, #15585, #65398, #180252, #35036, #166123, #50245, #30816, #96895, #380, #31876, #66454, #181300, #116365, #198598, #212728, #81672, #52377, #100059, #182355, #80619, #33983, #2521, #131544, #67520, #117438, #147758, #83795, #197546, #99003, #162944, #165058, #16650, #133665, #199666, #18783, #68594, #200726, #82735, #140052, #38258, #4651, #156288, #136834, #169322, #205001, #103261, #6795, #120652, #56645, #202860, #53433, #203927, #185557, #172537, #122809, #104332, #102190, #21967, #20906, #119570, #90224, #87002, #186631, #72872, #153074, #135770, #188768, #70721, #54508, #168257, #19856, #88075, #7872, #40408, #184488, #171456, #154149, #5716, #71793, #55575, #69662, #155214, #121729, #187694, #39323, #106510, #105418, #23045, #57711, #36105, #89161, #138978, #73960, #206077, #85943, #93434, #8948, #42555, #145409, #44680, #60907, #173625, #110792, #95575, #92376, #160541, #61982, #107593, #159474, #141140, #190889, #189833, #191948, #10013, #27332, #176794, #128136, #12147, #78220, #194100, #79291, #43614, #76089, #161625, #142191, #108658, #111867, #26260, #13218, #109732, #123868, #208206, #58773, #28409, #175739, #11072, #94503, #41482, #207150, #124928, #99808, #131304, #64114, #81423, #98748, #164805, #65148, #16398, #197295, #51058, #97696, #130256, #116109, #67270, #114003, #133408, #196247, #146455, #96636, #179998, #80356, #212470, #181052, #100862, #47891, #112930, #49990, #32668, #150705, #31622, #63039, #46816, #48936, #199413, #117182, #178943, #183183, #147504, #213525, #82476, #132, #30557, #163754, #84616, #132345, #66200, #162690, #198350, #34787, #15334, #165873, #149625, #115055, #182100, #33731, #17459, #129206, #83544, #1207, #166947, #18539, #195183, #39073, #105159, #171198, #172280, #70469, #36924, #188513, #169063, #201538, #22788, #69409, #88906, #152822, #154958, #20660, #151769, #55323, #4398, #54259, #153895, #2267, #168003, #136586, #6544, #202606, #3339, #86752, #38006, #104078, #120396, #170127, #186371, #204739, #103007, #135516, #121474, #72622, #53186, #138721, #119314, #85681, #35859, #185301, #19609, #21712, #87823, #40143, #5464, #52125, #203674, #71544, #89974, #137654, #68343, #200479, #187445, #56388, #122552, #118254, #106256, #23867, #134477, #184235, #101938, #210078, #127885, #141941, #73698, #59577, #108403, #173356, #193836, #92112, #191695, #44418, #8690, #107332, #205824, #109475, #175483, #123616, #41227, #93178, #204962, #36360, #197799, #151205, #105675, #171702, #203113, #7044, #107847, #27944, #42088, #157967, #156897, #61509, #192558, #76687, #144935, #57251, #175282, #8485, #92972, #59378, #159017, #26869, #207751, #140670, #10611, #108202, #125534, #44214, #173150, #60437, #209869, #110335, #12736, #43161, #123411, #176338, #107127, #95101, #78811, #206685, #94040, #191493, #109274, #160079, #11681, #161149, #24732, #29016, #90834, #77755, #143877, #127674, #193634, #189376, #45276, #111397, #177401, #41019, #211253, #41586, #141243, #129044, #24219, #91405, #207252, #58879, #172115 ),
 ( #42129, #136425, #124510, #205655, #108241, #186206, #57291, #103918, #123455, #24774, #104992, #154796, #206727, #21549, #71378, #55159, #72453, #23709, #7452, #189417, #156938, #8527, #74608, #140712, #58355, #96206, #159053, #76723, #47453, #126632, #97265, #192596, #176377, #127712, #194739, #12774, #78848, #26905, #162256, #10647, #110372, #46376, #209908, #141779, #129833, #61545, #112495, #30116, #13842, #79918, #113568, #94078, #146028, #63679, #160117, #193672, #77794, #207787, #45315, #111435, #177438, #59415, #125571, #191532, #43196, #109309, #175319, #93010, #84191, #64737, #198980, #101511, #1848, #118894, #149194, #36504, #18105, #213105, #201118, #184879, #32246, #182750, #83113, #131919, #166513, #769, #52760, #130880, #135104, #196874, #48511, #214145, #67907, #66835, #163320, #150278, #65771, #34368, #116751, #17036, #114631, #197929, #99387, #134053, #49555, #100442, #68986, #132978, #50625, #180623, #148143, #164382, #200061, #85256, #51713, #98317, #80995, #82050, #15966, #117832, #115681, #181675, #14901, #147083, #2913, #183823, #33302, #165439, #35435, #167582, #19181, #151344, #168643, #20245, #3981, #102583, #86331, #152402, #145765, #113292, #179301, #81781, #147864, #34090, #182461, #165160, #95930, #100161, #30922, #163051, #133766, #80724, #51420, #146815, #48244, #213880, #82838, #99110, #181406, #96998, #166225, #14630, #196603, #33032, #65501, #117541, #1561, #131649, #148913, #16755, #488, #66556, #199774, #212834, #132698, #198704, #64471, #197652, #130612, #50349, #49299, #114358, #115414, #116469, #17813, #83899, #149989, #15696, #98057, #67622, #183535, #180353, #47179, #161986, #164111, #13576, #31979, #79649, #211766, #63404, #129557, #195543, #18888, #69764, #35141, #23149, #101216, #39426, #3687, #119673, #36209, #52476, #102288, #167301, #168361, #53540, #186735, #120226, #36752, #135353, #203500, #115944, #19431, #1035, #151597, #134302, #201370, #85511, #83367, #34626, #137486, #185127, #53010, #165703, #119145, #87655, #84446, #152647, #202434, #99635, #3165, #17292, #183009, #181933, #118083, #2097, #69236, #102838, #54088, #4232, #70302, #136418, #71370, #184070, #150534, #153723, #68171, #100695, #186199, #166773, #37834, #51961, #103911, #200310, #50887, #168894, #35689, #167832, #20497, #33564, #67099, #101765, #169956, #86582, #117010, #21543, #5292, #149453, #133235, #199240, #18369, #41053, #72446, #88733, #7443, #189411, #6376, #107162, #154789, #138547, #38902, #56219, #171027, #122382, #39978, #173187, #188339, #187274, #73524, #106086, #90870, #172109, #55153, #104986, #23702, #24767, #121300, #155857, #89812, #139626, #205649, #57286, #123449, #7970, #172637, #154245, #152110, #88173, #4744, #37284, #74060, #136935, #171546, #5818, #189934, #140152, #71893, #72970, #23142, #155309, #89259, #123966, #87100, #56740, #122908, #202963, #138001, #153169, #188866, #55666, #186728, #121822, #40505, #6891, #106609, #24212, #187791, #22063, #39420, #105514, #104430, #185653, #139075, #70820, #54603, #90315, #135863, #156386, #206176, #41579, #107694, #19951, #86035, #3682, #69759, #53534, #119666, #103357, #169419, #21003, #120751, #38352, #170477, #214400, #75129, #148401, #9053, #141238, #76186, #15168, #96474, #49819, #163586, #142294, #47717, #130090, #30387, #58872, #208305, #112762, #81256, #59935, #196085, #82306, #162522, #146290, #207246, #158514, #174785, #212302, #98577, #31451, #108760, #91399, #126090, #42650, #179831, #125029, #192051, #66029, #25297, #16223, #97529, #132178, #157459, #147335, #198184, #213364, #64985, #43715, #178775, #164639, #190986, #26359, #14095, #80185, #63935, #113833, #131141, #197129, #114882, #48767, #180882, #32503, #190576, #36069, #168217, #141886, #88846, #59518, #154903, #56333, #7555, #90983, #107277, #189521, #118465, #42232, #102151, #204682, #172223, #200686, #72563, #40086, #157045, #6487, #57393, #9701, #89917, #73642, #68556, #138661, #19816, #139740, #25948, #173296, #122492, #18745, #188454, #184451, #24878, #134683, #106197, #75779, #167158, #158111, #8633, #207895, #191636, #74714, #125676 ) ),
 .UNSPECIFIED., .F., .F., .T. ) 
 B_SPLINE_SURFACE_WITH_KNOTS ( ( 2, 2 ),
 ( 3, 2, 2, 2, 2, 2, 2, 2, 2, 2, 2, 2, 2, 2, 2, 2, 2, 2, 2, 2, 2, 2, 2, 2, 2, 2, 2, 2, 2, 2, 2, 2, 2, 2, 2, 2, 2, 2, 2, 2, 2, 2, 2, 2, 2, 2, 2, 2, 2, 2, 2, 2, 2, 2, 2, 2, 2, 2, 2, 2, 2, 2, 2, 2, 2, 2, 2, 2, 2, 2, 2, 2, 2, 2, 2, 2, 2, 2, 2, 2, 2, 2, 2, 2, 2, 2, 2, 2, 2, 2, 2, 2, 2, 2, 2, 2, 2, 2, 2, 2, 2, 2, 2, 2, 2, 2, 2, 2, 2, 2, 2, 2, 2, 2, 2, 2, 2, 2, 2, 2, 2, 2, 2, 2, 2, 2, 2, 2, 2, 2, 2, 2, 2, 2, 2, 2, 2, 2, 2, 2, 2, 2, 2, 2, 2, 2, 2, 2, 2, 2, 2, 2, 2, 2, 2, 2, 2, 2, 2, 2, 2, 2, 2, 2, 2, 2, 2, 2, 2, 2, 2, 2, 2, 2, 2, 2, 2, 2, 2, 2, 2, 2, 2, 2, 2, 2, 2, 2, 2, 2, 2, 2, 2, 2, 2, 2, 2, 2, 2, 2, 2, 2, 2, 2, 2, 2, 2, 2, 2, 2, 2, 2, 2, 2, 2, 2, 2, 2, 2, 2, 2, 2, 2, 2, 2, 2, 2, 2, 2, 2, 2, 2, 2, 2, 2, 2, 2, 2, 2, 2, 3 ),
 ( 0.000000000000000000, 1.000000000000000000 ),
 ( 0.000000000000000000, 0.004166666666666666609, 0.008333333333333333218, 0.01250000000000000069, 0.01666666666666666644, 0.02083333333333333218, 0.02500000000000000139, 0.02916666666666666713, 0.03333333333333333287, 0.03749999999999999861, 0.04166666666666666435, 0.04583333333333333010, 0.05000000000000000278, 0.05416666666666666852, 0.05833333333333333426, 0.06250000000000000000, 0.06666666666666666574, 0.07083333333333333148, 0.07499999999999999722, 0.07916666666666666297, 0.08333333333333332871, 0.08749999999999999445, 0.09166666666666666019, 0.09583333333333333981, 0.1000000000000000056, 0.1041666666666666713, 0.1083333333333333370, 0.1125000000000000028, 0.1166666666666666685, 0.1208333333333333343, 0.1250000000000000000, 0.1291666666666666796, 0.1333333333333333315, 0.1375000000000000111, 0.1416666666666666630, 0.1458333333333333426, 0.1499999999999999944, 0.1541666666666666741, 0.1583333333333333259, 0.1625000000000000056, 0.1666666666666666574, 0.1708333333333333370, 0.1749999999999999889, 0.1791666666666666685, 0.1833333333333333204, 0.1875000000000000000, 0.1916666666666666796, 0.1958333333333333315, 0.2000000000000000111, 0.2041666666666666630, 0.2083333333333333426, 0.2124999999999999944, 0.2166666666666666741, 0.2208333333333333259, 0.2250000000000000056, 0.2291666666666666574, 0.2333333333333333370, 0.2374999999999999889, 0.2416666666666666685, 0.2458333333333333204, 0.2500000000000000000, 0.2541666666666666519, 0.2583333333333333592, 0.2625000000000000111, 0.2666666666666666630, 0.2708333333333333148, 0.2750000000000000222, 0.2791666666666666741, 0.2833333333333333259, 0.2874999999999999778, 0.2916666666666666852, 0.2958333333333333370, 0.2999999999999999889, 0.3041666666666666408, 0.3083333333333333481, 0.3125000000000000000, 0.3166666666666666519, 0.3208333333333333592, 0.3250000000000000111, 0.3291666666666666630, 0.3333333333333333148, 0.3375000000000000222, 0.3416666666666666741, 0.3458333333333333259, 0.3499999999999999778, 0.3541666666666666852, 0.3583333333333333370, 0.3624999999999999889, 0.3666666666666666408, 0.3708333333333333481, 0.3750000000000000000, 0.3791666666666666519, 0.3833333333333333592, 0.3875000000000000111, 0.3916666666666666630, 0.3958333333333333148, 0.4000000000000000222, 0.4041666666666666741, 0.4083333333333333259, 0.4124999999999999778, 0.4166666666666666852, 0.4208333333333333370, 0.4249999999999999889, 0.4291666666666666408, 0.4333333333333333481, 0.4375000000000000000, 0.4416666666666666519, 0.4458333333333333592, 0.4500000000000000111, 0.4541666666666666630, 0.4583333333333333148, 0.4625000000000000222, 0.4666666666666666741, 0.4708333333333333259, 0.4749999999999999778, 0.4791666666666666852, 0.4833333333333333370, 0.4874999999999999889, 0.4916666666666666408, 0.4958333333333333481, 0.5000000000000000000, 0.5041666666666666519, 0.5083333333333333037, 0.5124999999999999556, 0.5166666666666667185, 0.5208333333333333703, 0.5250000000000000222, 0.5291666666666666741, 0.5333333333333333259, 0.5374999999999999778, 0.5416666666666666297, 0.5458333333333332815, 0.5500000000000000444, 0.5541666666666666963, 0.5583333333333333481, 0.5625000000000000000, 0.5666666666666666519, 0.5708333333333333037, 0.5749999999999999556, 0.5791666666666667185, 0.5833333333333333703, 0.5875000000000000222, 0.5916666666666666741, 0.5958333333333333259, 0.5999999999999999778, 0.6041666666666666297, 0.6083333333333332815, 0.6125000000000000444, 0.6166666666666666963, 0.6208333333333333481, 0.6250000000000000000, 0.6291666666666666519, 0.6333333333333333037, 0.6374999999999999556, 0.6416666666666667185, 0.6458333333333333703, 0.6500000000000000222, 0.6541666666666666741, 0.6583333333333333259, 0.6624999999999999778, 0.6666666666666666297, 0.6708333333333332815, 0.6750000000000000444, 0.6791666666666666963, 0.6833333333333333481, 0.6875000000000000000, 0.6916666666666666519, 0.6958333333333333037, 0.6999999999999999556, 0.7041666666666667185, 0.7083333333333333703, 0.7125000000000000222, 0.7166666666666666741, 0.7208333333333333259, 0.7249999999999999778, 0.7291666666666666297, 0.7333333333333332815, 0.7375000000000000444, 0.7416666666666666963, 0.7458333333333333481, 0.7500000000000000000, 0.7541666666666666519, 0.7583333333333333037, 0.7624999999999999556, 0.7666666666666667185, 0.7708333333333333703, 0.7750000000000000222, 0.7791666666666666741, 0.7833333333333333259, 0.7874999999999999778, 0.7916666666666666297, 0.7958333333333332815, 0.8000000000000000444, 0.8041666666666666963, 0.8083333333333333481, 0.8125000000000000000, 0.8166666666666666519, 0.8208333333333333037, 0.8249999999999999556, 0.8291666666666667185, 0.8333333333333333703, 0.8375000000000000222, 0.8416666666666666741, 0.8458333333333333259, 0.8499999999999999778, 0.8541666666666666297, 0.8583333333333332815, 0.8625000000000000444, 0.8666666666666666963, 0.8708333333333333481, 0.8750000000000000000, 0.8791666666666666519, 0.8833333333333333037, 0.8874999999999999556, 0.8916666666666667185, 0.8958333333333333703, 0.9000000000000000222, 0.9041666666666666741, 0.9083333333333333259, 0.9124999999999999778, 0.9166666666666666297, 0.9208333333333332815, 0.9250000000000000444, 0.9291666666666666963, 0.9333333333333333481, 0.9375000000000000000, 0.9416666666666666519, 0.9458333333333333037, 0.9499999999999999556, 0.9541666666666667185, 0.9583333333333333703, 0.9625000000000000222, 0.9666666666666666741, 0.9708333333333333259, 0.9749999999999999778, 0.9791666666666666297, 0.9833333333333332815, 0.9875000000000000444, 0.9916666666666666963, 0.9958333333333333481, 1.000000000000000000 ),
 .UNSPECIFIED. ) 
 GEOMETRIC_REPRESENTATION_ITEM ( )  RATIONAL_B_SPLINE_SURFACE ( (
 ( 1.000000000000000000, 0.8660254037844387076, 1.000000000000000000, 0.8660254037844387076, 1.000000000000000000, 0.8660254037844387076, 1.000000000000000000, 0.8660254037844387076, 1.000000000000000000, 0.8660254037844387076, 1.000000000000000000, 0.8660254037844387076, 1.000000000000000000, 0.8660254037844387076, 1.000000000000000000, 0.8660254037844387076, 1.000000000000000000, 0.8660254037844387076, 1.000000000000000000, 0.8660254037844387076, 1.000000000000000000, 0.8660254037844387076, 1.000000000000000000, 0.8660254037844387076, 1.000000000000000000, 0.8660254037844387076, 1.000000000000000000, 0.8660254037844387076, 1.000000000000000000, 0.8660254037844387076, 1.000000000000000000, 0.8660254037844387076, 1.000000000000000000, 0.8660254037844387076, 1.000000000000000000, 0.8660254037844387076, 1.000000000000000000, 0.8660254037844387076, 1.000000000000000000, 0.8660254037844387076, 1.000000000000000000, 0.8660254037844387076, 1.000000000000000000, 0.8660254037844387076, 1.000000000000000000, 0.8660254037844387076, 1.000000000000000000, 0.8660254037844387076, 1.000000000000000000, 0.8660254037844387076, 1.000000000000000000, 0.8660254037844387076, 1.000000000000000000, 0.8660254037844387076, 1.000000000000000000, 0.8660254037844387076, 1.000000000000000000, 0.8660254037844387076, 1.000000000000000000, 0.8660254037844387076, 1.000000000000000000, 0.8660254037844387076, 1.000000000000000000, 0.8660254037844387076, 1.000000000000000000, 0.8660254037844387076, 1.000000000000000000, 0.8660254037844387076, 1.000000000000000000, 0.8660254037844387076, 1.000000000000000000, 0.8660254037844387076, 1.000000000000000000, 0.8660254037844387076, 1.000000000000000000, 0.8660254037844387076, 1.000000000000000000, 0.8660254037844387076, 1.000000000000000000, 0.8660254037844387076, 1.000000000000000000, 0.8660254037844387076, 1.000000000000000000, 0.8660254037844387076, 1.000000000000000000, 0.8660254037844387076, 1.000000000000000000, 0.8660254037844387076, 1.000000000000000000, 0.8660254037844387076, 1.000000000000000000, 0.8660254037844387076, 1.000000000000000000, 0.8660254037844387076, 1.000000000000000000, 0.8660254037844387076, 1.000000000000000000, 0.8660254037844387076, 1.000000000000000000, 0.8660254037844387076, 1.000000000000000000, 0.8660254037844387076, 1.000000000000000000, 0.8660254037844387076, 1.000000000000000000, 0.8660254037844387076, 1.000000000000000000, 0.8660254037844387076, 1.000000000000000000, 0.8660254037844387076, 1.000000000000000000, 0.8660254037844387076, 1.000000000000000000, 0.8660254037844387076, 1.000000000000000000, 0.8660254037844387076, 1.000000000000000000, 0.8660254037844387076, 1.000000000000000000, 0.8660254037844387076, 1.000000000000000000, 0.8660254037844387076, 1.000000000000000000, 0.8660254037844387076, 1.000000000000000000, 0.8660254037844387076, 1.000000000000000000, 0.8660254037844387076, 1.000000000000000000, 0.8660254037844387076, 1.000000000000000000, 0.8660254037844387076, 1.000000000000000000, 0.8660254037844387076, 1.000000000000000000, 0.8660254037844387076, 1.000000000000000000, 0.8660254037844387076, 1.000000000000000000, 0.8660254037844387076, 1.000000000000000000, 0.8660254037844387076, 1.000000000000000000, 0.8660254037844387076, 1.000000000000000000, 0.8660254037844387076, 1.000000000000000000, 0.8660254037844387076, 1.000000000000000000, 0.8660254037844387076, 1.000000000000000000, 0.8660254037844387076, 1.000000000000000000, 0.8660254037844387076, 1.000000000000000000, 0.8660254037844387076, 1.000000000000000000, 0.8660254037844387076, 1.000000000000000000, 0.8660254037844387076, 1.000000000000000000, 0.8660254037844387076, 1.000000000000000000, 0.8660254037844387076, 1.000000000000000000, 0.8660254037844387076, 1.000000000000000000, 0.8660254037844387076, 1.000000000000000000, 0.8660254037844387076, 1.000000000000000000, 0.8660254037844387076, 1.000000000000000000, 0.8660254037844387076, 1.000000000000000000, 0.8660254037844387076, 1.000000000000000000, 0.8660254037844387076, 1.000000000000000000, 0.8660254037844387076, 1.000000000000000000, 0.8660254037844387076, 1.000000000000000000, 0.8660254037844387076, 1.000000000000000000, 0.8660254037844387076, 1.000000000000000000, 0.8660254037844387076, 1.000000000000000000, 0.8660254037844387076, 1.000000000000000000, 0.8660254037844387076, 1.000000000000000000, 0.8660254037844387076, 1.000000000000000000, 0.8660254037844387076, 1.000000000000000000, 0.8660254037844387076, 1.000000000000000000, 0.8660254037844387076, 1.000000000000000000, 0.8660254037844387076, 1.000000000000000000, 0.8660254037844387076, 1.000000000000000000, 0.8660254037844387076, 1.000000000000000000, 0.8660254037844387076, 1.000000000000000000, 0.8660254037844387076, 1.000000000000000000, 0.8660254037844387076, 1.000000000000000000, 0.8660254037844387076, 1.000000000000000000, 0.8660254037844387076, 1.000000000000000000, 0.8660254037844387076, 1.000000000000000000, 0.8660254037844387076, 1.000000000000000000, 0.8660254037844387076, 1.000000000000000000, 0.8660254037844387076, 1.000000000000000000, 0.8660254037844387076, 1.000000000000000000, 0.8660254037844387076, 1.000000000000000000, 0.8660254037844387076, 1.000000000000000000, 0.8660254037844387076, 1.000000000000000000, 0.8660254037844387076, 1.000000000000000000, 0.8660254037844387076, 1.000000000000000000, 0.8660254037844387076, 1.000000000000000000, 0.8660254037844387076, 1.000000000000000000, 0.8660254037844387076, 1.000000000000000000, 0.8660254037844387076, 1.000000000000000000, 0.8660254037844387076, 1.000000000000000000, 0.8660254037844387076, 1.000000000000000000, 0.8660254037844387076, 1.000000000000000000, 0.8660254037844387076, 1.000000000000000000, 0.8660254037844387076, 1.000000000000000000, 0.8660254037844387076, 1.000000000000000000, 0.8660254037844387076, 1.000000000000000000, 0.8660254037844387076, 1.000000000000000000, 0.8660254037844387076, 1.000000000000000000, 0.8660254037844387076, 1.000000000000000000, 0.8660254037844387076, 1.000000000000000000, 0.8660254037844387076, 1.000000000000000000, 0.8660254037844387076, 1.000000000000000000, 0.8660254037844387076, 1.000000000000000000, 0.8660254037844387076, 1.000000000000000000, 0.8660254037844387076, 1.000000000000000000, 0.8660254037844387076, 1.000000000000000000, 0.8660254037844387076, 1.000000000000000000, 0.8660254037844387076, 1.000000000000000000, 0.8660254037844387076, 1.000000000000000000, 0.8660254037844387076, 1.000000000000000000, 0.8660254037844387076, 1.000000000000000000, 0.8660254037844387076, 1.000000000000000000, 0.8660254037844387076, 1.000000000000000000, 0.8660254037844387076, 1.000000000000000000, 0.8660254037844387076, 1.000000000000000000, 0.8660254037844387076, 1.000000000000000000, 0.8660254037844387076, 1.000000000000000000, 0.8660254037844387076, 1.000000000000000000, 0.8660254037844387076, 1.000000000000000000, 0.8660254037844387076, 1.000000000000000000, 0.8660254037844387076, 1.000000000000000000, 0.8660254037844387076, 1.000000000000000000, 0.8660254037844387076, 1.000000000000000000, 0.8660254037844387076, 1.000000000000000000, 0.8660254037844387076, 1.000000000000000000, 0.8660254037844387076, 1.000000000000000000, 0.8660254037844387076, 1.000000000000000000, 0.8660254037844387076, 1.000000000000000000, 0.8660254037844387076, 1.000000000000000000, 0.8660254037844387076, 1.000000000000000000, 0.8660254037844387076, 1.000000000000000000, 0.8660254037844387076, 1.000000000000000000, 0.8660254037844387076, 1.000000000000000000, 0.8660254037844387076, 1.000000000000000000, 0.8660254037844387076, 1.000000000000000000, 0.8660254037844387076, 1.000000000000000000, 0.8660254037844387076, 1.000000000000000000, 0.8660254037844387076, 1.000000000000000000, 0.8660254037844387076, 1.000000000000000000, 0.8660254037844387076, 1.000000000000000000, 0.8660254037844387076, 1.000000000000000000, 0.8660254037844387076, 1.000000000000000000, 0.8660254037844387076, 1.000000000000000000, 0.8660254037844387076, 1.000000000000000000, 0.8660254037844387076, 1.000000000000000000, 0.8660254037844387076, 1.000000000000000000, 0.8660254037844387076, 1.000000000000000000, 0.8660254037844387076, 1.000000000000000000, 0.8660254037844387076, 1.000000000000000000, 0.8660254037844387076, 1.000000000000000000, 0.8660254037844387076, 1.000000000000000000, 0.8660254037844387076, 1.000000000000000000, 0.8660254037844387076, 1.000000000000000000, 0.8660254037844387076, 1.000000000000000000, 0.8660254037844387076, 1.000000000000000000, 0.8660254037844387076, 1.000000000000000000, 0.8660254037844387076, 1.000000000000000000, 0.8660254037844387076, 1.000000000000000000, 0.8660254037844387076, 1.000000000000000000, 0.8660254037844387076, 1.000000000000000000, 0.8660254037844387076, 1.000000000000000000, 0.8660254037844387076, 1.000000000000000000, 0.8660254037844387076, 1.000000000000000000, 0.8660254037844387076, 1.000000000000000000, 0.8660254037844387076, 1.000000000000000000, 0.8660254037844387076, 1.000000000000000000, 0.8660254037844387076, 1.000000000000000000, 0.8660254037844387076, 1.000000000000000000, 0.8660254037844387076, 1.000000000000000000, 0.8660254037844387076, 1.000000000000000000, 0.8660254037844387076, 1.000000000000000000, 0.8660254037844387076, 1.000000000000000000, 0.8660254037844387076, 1.000000000000000000, 0.8660254037844387076, 1.000000000000000000, 0.8660254037844387076, 1.000000000000000000, 0.8660254037844387076, 1.000000000000000000, 0.8660254037844387076, 1.000000000000000000, 0.8660254037844387076, 1.000000000000000000, 0.8660254037844387076, 1.000000000000000000, 0.8660254037844387076, 1.000000000000000000, 0.8660254037844387076, 1.000000000000000000, 0.8660254037844387076, 1.000000000000000000, 0.8660254037844387076, 1.000000000000000000, 0.8660254037844387076, 1.000000000000000000, 0.8660254037844387076, 1.000000000000000000, 0.8660254037844387076, 1.000000000000000000, 0.8660254037844387076, 1.000000000000000000, 0.8660254037844387076, 1.000000000000000000, 0.8660254037844387076, 1.000000000000000000, 0.8660254037844387076, 1.000000000000000000, 0.8660254037844387076, 1.000000000000000000, 0.8660254037844387076, 1.000000000000000000, 0.8660254037844387076, 1.000000000000000000, 0.8660254037844387076, 1.000000000000000000, 0.8660254037844387076, 1.000000000000000000, 0.8660254037844387076, 1.000000000000000000, 0.8660254037844387076, 1.000000000000000000, 0.8660254037844387076, 1.000000000000000000, 0.8660254037844387076, 1.000000000000000000, 0.8660254037844387076, 1.000000000000000000, 0.8660254037844387076, 1.000000000000000000, 0.8660254037844387076, 1.000000000000000000, 0.8660254037844387076, 1.000000000000000000, 0.8660254037844387076, 1.000000000000000000, 0.8660254037844387076, 1.000000000000000000, 0.8660254037844387076, 1.000000000000000000, 0.8660254037844387076, 1.000000000000000000),
 ( 1.000000000000000000, 0.8660254037844387076, 1.000000000000000000, 0.8660254037844387076, 1.000000000000000000, 0.8660254037844387076, 1.000000000000000000, 0.8660254037844387076, 1.000000000000000000, 0.8660254037844387076, 1.000000000000000000, 0.8660254037844387076, 1.000000000000000000, 0.8660254037844387076, 1.000000000000000000, 0.8660254037844387076, 1.000000000000000000, 0.8660254037844387076, 1.000000000000000000, 0.8660254037844387076, 1.000000000000000000, 0.8660254037844387076, 1.000000000000000000, 0.8660254037844387076, 1.000000000000000000, 0.8660254037844387076, 1.000000000000000000, 0.8660254037844387076, 1.000000000000000000, 0.8660254037844387076, 1.000000000000000000, 0.8660254037844387076, 1.000000000000000000, 0.8660254037844387076, 1.000000000000000000, 0.8660254037844387076, 1.000000000000000000, 0.8660254037844387076, 1.000000000000000000, 0.8660254037844387076, 1.000000000000000000, 0.8660254037844387076, 1.000000000000000000, 0.8660254037844387076, 1.000000000000000000, 0.8660254037844387076, 1.000000000000000000, 0.8660254037844387076, 1.000000000000000000, 0.8660254037844387076, 1.000000000000000000, 0.8660254037844387076, 1.000000000000000000, 0.8660254037844387076, 1.000000000000000000, 0.8660254037844387076, 1.000000000000000000, 0.8660254037844387076, 1.000000000000000000, 0.8660254037844387076, 1.000000000000000000, 0.8660254037844387076, 1.000000000000000000, 0.8660254037844387076, 1.000000000000000000, 0.8660254037844387076, 1.000000000000000000, 0.8660254037844387076, 1.000000000000000000, 0.8660254037844387076, 1.000000000000000000, 0.8660254037844387076, 1.000000000000000000, 0.8660254037844387076, 1.000000000000000000, 0.8660254037844387076, 1.000000000000000000, 0.8660254037844387076, 1.000000000000000000, 0.8660254037844387076, 1.000000000000000000, 0.8660254037844387076, 1.000000000000000000, 0.8660254037844387076, 1.000000000000000000, 0.8660254037844387076, 1.000000000000000000, 0.8660254037844387076, 1.000000000000000000, 0.8660254037844387076, 1.000000000000000000, 0.8660254037844387076, 1.000000000000000000, 0.8660254037844387076, 1.000000000000000000, 0.8660254037844387076, 1.000000000000000000, 0.8660254037844387076, 1.000000000000000000, 0.8660254037844387076, 1.000000000000000000, 0.8660254037844387076, 1.000000000000000000, 0.8660254037844387076, 1.000000000000000000, 0.8660254037844387076, 1.000000000000000000, 0.8660254037844387076, 1.000000000000000000, 0.8660254037844387076, 1.000000000000000000, 0.8660254037844387076, 1.000000000000000000, 0.8660254037844387076, 1.000000000000000000, 0.8660254037844387076, 1.000000000000000000, 0.8660254037844387076, 1.000000000000000000, 0.8660254037844387076, 1.000000000000000000, 0.8660254037844387076, 1.000000000000000000, 0.8660254037844387076, 1.000000000000000000, 0.8660254037844387076, 1.000000000000000000, 0.8660254037844387076, 1.000000000000000000, 0.8660254037844387076, 1.000000000000000000, 0.8660254037844387076, 1.000000000000000000, 0.8660254037844387076, 1.000000000000000000, 0.8660254037844387076, 1.000000000000000000, 0.8660254037844387076, 1.000000000000000000, 0.8660254037844387076, 1.000000000000000000, 0.8660254037844387076, 1.000000000000000000, 0.8660254037844387076, 1.000000000000000000, 0.8660254037844387076, 1.000000000000000000, 0.8660254037844387076, 1.000000000000000000, 0.8660254037844387076, 1.000000000000000000, 0.8660254037844387076, 1.000000000000000000, 0.8660254037844387076, 1.000000000000000000, 0.8660254037844387076, 1.000000000000000000, 0.8660254037844387076, 1.000000000000000000, 0.8660254037844387076, 1.000000000000000000, 0.8660254037844387076, 1.000000000000000000, 0.8660254037844387076, 1.000000000000000000, 0.8660254037844387076, 1.000000000000000000, 0.8660254037844387076, 1.000000000000000000, 0.8660254037844387076, 1.000000000000000000, 0.8660254037844387076, 1.000000000000000000, 0.8660254037844387076, 1.000000000000000000, 0.8660254037844387076, 1.000000000000000000, 0.8660254037844387076, 1.000000000000000000, 0.8660254037844387076, 1.000000000000000000, 0.8660254037844387076, 1.000000000000000000, 0.8660254037844387076, 1.000000000000000000, 0.8660254037844387076, 1.000000000000000000, 0.8660254037844387076, 1.000000000000000000, 0.8660254037844387076, 1.000000000000000000, 0.8660254037844387076, 1.000000000000000000, 0.8660254037844387076, 1.000000000000000000, 0.8660254037844387076, 1.000000000000000000, 0.8660254037844387076, 1.000000000000000000, 0.8660254037844387076, 1.000000000000000000, 0.8660254037844387076, 1.000000000000000000, 0.8660254037844387076, 1.000000000000000000, 0.8660254037844387076, 1.000000000000000000, 0.8660254037844387076, 1.000000000000000000, 0.8660254037844387076, 1.000000000000000000, 0.8660254037844387076, 1.000000000000000000, 0.8660254037844387076, 1.000000000000000000, 0.8660254037844387076, 1.000000000000000000, 0.8660254037844387076, 1.000000000000000000, 0.8660254037844387076, 1.000000000000000000, 0.8660254037844387076, 1.000000000000000000, 0.8660254037844387076, 1.000000000000000000, 0.8660254037844387076, 1.000000000000000000, 0.8660254037844387076, 1.000000000000000000, 0.8660254037844387076, 1.000000000000000000, 0.8660254037844387076, 1.000000000000000000, 0.8660254037844387076, 1.000000000000000000, 0.8660254037844387076, 1.000000000000000000, 0.8660254037844387076, 1.000000000000000000, 0.8660254037844387076, 1.000000000000000000, 0.8660254037844387076, 1.000000000000000000, 0.8660254037844387076, 1.000000000000000000, 0.8660254037844387076, 1.000000000000000000, 0.8660254037844387076, 1.000000000000000000, 0.8660254037844387076, 1.000000000000000000, 0.8660254037844387076, 1.000000000000000000, 0.8660254037844387076, 1.000000000000000000, 0.8660254037844387076, 1.000000000000000000, 0.8660254037844387076, 1.000000000000000000, 0.8660254037844387076, 1.000000000000000000, 0.8660254037844387076, 1.000000000000000000, 0.8660254037844387076, 1.000000000000000000, 0.8660254037844387076, 1.000000000000000000, 0.8660254037844387076, 1.000000000000000000, 0.8660254037844387076, 1.000000000000000000, 0.8660254037844387076, 1.000000000000000000, 0.8660254037844387076, 1.000000000000000000, 0.8660254037844387076, 1.000000000000000000, 0.8660254037844387076, 1.000000000000000000, 0.8660254037844387076, 1.000000000000000000, 0.8660254037844387076, 1.000000000000000000, 0.8660254037844387076, 1.000000000000000000, 0.8660254037844387076, 1.000000000000000000, 0.8660254037844387076, 1.000000000000000000, 0.8660254037844387076, 1.000000000000000000, 0.8660254037844387076, 1.000000000000000000, 0.8660254037844387076, 1.000000000000000000, 0.8660254037844387076, 1.000000000000000000, 0.8660254037844387076, 1.000000000000000000, 0.8660254037844387076, 1.000000000000000000, 0.8660254037844387076, 1.000000000000000000, 0.8660254037844387076, 1.000000000000000000, 0.8660254037844387076, 1.000000000000000000, 0.8660254037844387076, 1.000000000000000000, 0.8660254037844387076, 1.000000000000000000, 0.8660254037844387076, 1.000000000000000000, 0.8660254037844387076, 1.000000000000000000, 0.8660254037844387076, 1.000000000000000000, 0.8660254037844387076, 1.000000000000000000, 0.8660254037844387076, 1.000000000000000000, 0.8660254037844387076, 1.000000000000000000, 0.8660254037844387076, 1.000000000000000000, 0.8660254037844387076, 1.000000000000000000, 0.8660254037844387076, 1.000000000000000000, 0.8660254037844387076, 1.000000000000000000, 0.8660254037844387076, 1.000000000000000000, 0.8660254037844387076, 1.000000000000000000, 0.8660254037844387076, 1.000000000000000000, 0.8660254037844387076, 1.000000000000000000, 0.8660254037844387076, 1.000000000000000000, 0.8660254037844387076, 1.000000000000000000, 0.8660254037844387076, 1.000000000000000000, 0.8660254037844387076, 1.000000000000000000, 0.8660254037844387076, 1.000000000000000000, 0.8660254037844387076, 1.000000000000000000, 0.8660254037844387076, 1.000000000000000000, 0.8660254037844387076, 1.000000000000000000, 0.8660254037844387076, 1.000000000000000000, 0.8660254037844387076, 1.000000000000000000, 0.8660254037844387076, 1.000000000000000000, 0.8660254037844387076, 1.000000000000000000, 0.8660254037844387076, 1.000000000000000000, 0.8660254037844387076, 1.000000000000000000, 0.8660254037844387076, 1.000000000000000000, 0.8660254037844387076, 1.000000000000000000, 0.8660254037844387076, 1.000000000000000000, 0.8660254037844387076, 1.000000000000000000, 0.8660254037844387076, 1.000000000000000000, 0.8660254037844387076, 1.000000000000000000, 0.8660254037844387076, 1.000000000000000000, 0.8660254037844387076, 1.000000000000000000, 0.8660254037844387076, 1.000000000000000000, 0.8660254037844387076, 1.000000000000000000, 0.8660254037844387076, 1.000000000000000000, 0.8660254037844387076, 1.000000000000000000, 0.8660254037844387076, 1.000000000000000000, 0.8660254037844387076, 1.000000000000000000, 0.8660254037844387076, 1.000000000000000000, 0.8660254037844387076, 1.000000000000000000, 0.8660254037844387076, 1.000000000000000000, 0.8660254037844387076, 1.000000000000000000, 0.8660254037844387076, 1.000000000000000000, 0.8660254037844387076, 1.000000000000000000, 0.8660254037844387076, 1.000000000000000000, 0.8660254037844387076, 1.000000000000000000, 0.8660254037844387076, 1.000000000000000000, 0.8660254037844387076, 1.000000000000000000, 0.8660254037844387076, 1.000000000000000000, 0.8660254037844387076, 1.000000000000000000, 0.8660254037844387076, 1.000000000000000000, 0.8660254037844387076, 1.000000000000000000, 0.8660254037844387076, 1.000000000000000000, 0.8660254037844387076, 1.000000000000000000, 0.8660254037844387076, 1.000000000000000000, 0.8660254037844387076, 1.000000000000000000, 0.8660254037844387076, 1.000000000000000000, 0.8660254037844387076, 1.000000000000000000, 0.8660254037844387076, 1.000000000000000000, 0.8660254037844387076, 1.000000000000000000, 0.8660254037844387076, 1.000000000000000000, 0.8660254037844387076, 1.000000000000000000, 0.8660254037844387076, 1.000000000000000000, 0.8660254037844387076, 1.000000000000000000, 0.8660254037844387076, 1.000000000000000000, 0.8660254037844387076, 1.000000000000000000, 0.8660254037844387076, 1.000000000000000000, 0.8660254037844387076, 1.000000000000000000, 0.8660254037844387076, 1.000000000000000000, 0.8660254037844387076, 1.000000000000000000, 0.8660254037844387076, 1.000000000000000000, 0.8660254037844387076, 1.000000000000000000, 0.8660254037844387076, 1.000000000000000000, 0.8660254037844387076, 1.000000000000000000, 0.8660254037844387076, 1.000000000000000000, 0.8660254037844387076, 1.000000000000000000, 0.8660254037844387076, 1.000000000000000000, 0.8660254037844387076, 1.000000000000000000, 0.8660254037844387076, 1.000000000000000000, 0.8660254037844387076, 1.000000000000000000, 0.8660254037844387076, 1.000000000000000000) ) ) 
 REPRESENTATION_ITEM ( '' )  SURFACE ( )  );
#42334=CARTESIAN_POINT ( 'NONE',  ( 4.482942347612929979, 8.381849838857084123, 1.040834085586084257E-14 ) ) ;
#42345=CARTESIAN_POINT ( 'NONE',  ( 5.029711800989886683, 4.970344644017389513, 1.040834085586084257E-14 ) ) ;
#42346=CARTESIAN_POINT ( 'NONE',  ( 0.6823417656249899377, 2.155208333674753174, 1.181850606188767472 ) ) ;
#42348=CARTESIAN_POINT ( 'NONE',  ( 8.762647353133951711, 9.117510088278095282, 1.040834085586084257E-14 ) ) ;
#42352=CIRCLE ( 'NONE', #177152, 0.08000000000000041800 ) ;
#42357=CARTESIAN_POINT ( 'NONE',  ( 0.7499999999999885647, 2.816666666666689522, -1.299038105676658228 ) ) ;
#42358=CARTESIAN_POINT ( 'NONE',  ( 6.647575389402066826, 6.649926130590872120, 1.040834085586084257E-14 ) ) ;
#42361=CARTESIAN_POINT ( 'NONE',  ( 1.499999999999990896, 5.775000000000023448, 1.040834085586084414E-14 ) ) ;
#42363=CARTESIAN_POINT ( 'NONE',  ( 1.364683531249988757, 2.384375000341422357, 1.214306433183764966E-14 ) ) ;
#42365=CARTESIAN_POINT ( 'NONE',  ( 9.924205255523292024, 10.68058700763975466, -0.7216878364870257245 ) ) ;
#42371=CARTESIAN_POINT ( 'NONE',  ( -1.499999999999997780, 1.681250000682817047, 0.000000000000000000 ) ) ;
#42374=CARTESIAN_POINT ( 'NONE',  ( -4.855791571988752331, 8.816840600628864877, 0.7998128361456481317 ) ) ;
#42375=EDGE_CURVE ( 'NONE', #177940, #105963, #113885, .T. ) ;
#42384=CARTESIAN_POINT ( 'NONE',  ( 5.341022448779654930, 8.318611059296550536, 1.199719254218462483 ) ) ;
#42385=CONICAL_SURFACE ( 'NONE', #211793, 7.034482758620711706, 0.8621700546672336207 ) ;
#42389=CARTESIAN_POINT ( 'NONE',  ( 4.645640190976921602, 8.571663989448405019, 1.040834085586084257E-14 ) ) ;
#42394=CARTESIAN_POINT ( 'NONE',  ( 4.715538499454675403, 4.395883092318884522, 1.214306433183764966E-14 ) ) ;
#42399=CARTESIAN_POINT ( 'NONE',  ( 5.891550962509589873, 5.977563058329811163, 0.05700887847147687038 ) ) ;
#42412=CARTESIAN_POINT ( 'NONE',  ( 5.666945020832160118, 9.555260257705446847, 0.7216878364870438212 ) ) ;
#42414=CARTESIAN_POINT ( 'NONE',  ( -5.362413449404877852, 6.214902764849178141, -1.199719254218446718 ) ) ;
#42415=CARTESIAN_POINT ( 'NONE',  ( 4.989037339704528229, 4.922891105851139315, 1.040834085586084257E-14 ) ) ;
#42418=CARTESIAN_POINT ( 'NONE',  ( -4.882907879216086933, 8.848476292394087395, -0.7998128361456281477 ) ) ;
#42421=FACE_OUTER_BOUND ( 'NONE', #82580, .T. ) ;
#42431=CARTESIAN_POINT ( 'NONE',  ( 8.387690588348714726, 12.93738945304888333, 1.040834085586084257E-14 ) ) ;
#42439=CARTESIAN_POINT ( 'NONE',  ( -10.33094986393327197, 11.15512238411806578, 0.7216878364870438212 ) ) ;
#42443=CARTESIAN_POINT ( 'NONE',  ( 7.567422294721922960, 11.98040977715095323, 0.7998128361456462443 ) ) ;
#42444=AXIS2_PLACEMENT_3D ( 'NONE', #120941, #103545, #169606 ) ;
#42448=CARTESIAN_POINT ( 'NONE',  ( -5.689618019229208734, 9.789638122409414223, 0.7998128361456481317 ) ) ;
#42449=CARTESIAN_POINT ( 'NONE',  ( 4.961394147597008697, 7.875711374583454827, -1.199719254218452047 ) ) ;
#42451=CARTESIAN_POINT ( 'NONE',  ( 3.686212053427321056, 6.121915856213854923, 1.284222742053100941 ) ) ;
#42452=CARTESIAN_POINT ( 'NONE',  ( -3.795919822146293754, 4.491289883001181593, -1.082531754730549967 ) ) ;
#42454=CARTESIAN_POINT ( 'NONE',  ( 1.364683531249988757, 2.196875000341415252, 1.214306433183764966E-14 ) ) ;
#42456=CARTESIAN_POINT ( 'NONE',  ( 5.775410249741494972, 8.721433810464993996, -1.082531754730537088 ) ) ;
#42463=CARTESIAN_POINT ( 'NONE',  ( 8.202319746143333035, 12.51319743723517952, -0.7216878364870328300 ) ) ;
#42468=CARTESIAN_POINT ( 'NONE',  ( -9.691380875670077444, 10.20103253123691189, 0.7998128361456462443 ) ) ;
#42486=CARTESIAN_POINT ( 'NONE',  ( -1.402160292154681736E-14, 1.868750000682816381, -1.732050807568863648 ) ) ;
#42490=ORIENTED_EDGE ( 'NONE', *, *, #192621, .T. ) ;
#42492=CARTESIAN_POINT ( 'NONE',  ( 0.7499999999999885647, 0.8166666666666877461, -1.299038105676652899 ) ) ;
#42493=CARTESIAN_POINT ( 'NONE',  ( 7.396136491454752715, 8.587579647240744407, 1.199719254218462483 ) ) ;
#42495=CARTESIAN_POINT ( 'NONE',  ( -1.402160292154681736E-14, 0.1968750003414221628, -1.575800808251665908 ) ) ;
#42499=CARTESIAN_POINT ( 'NONE',  ( 9.625925876022625616, 11.29296361252366765, -1.082531754730537088 ) ) ;
#42500=CARTESIAN_POINT ( 'NONE',  ( -7.076992996653451939, 7.358839372291564374, 0.7216878364870317197 ) ) ;
#42506=CARTESIAN_POINT ( 'NONE',  ( -5.636439174979254396, 7.598931675607687453, -1.599625672291256295 ) ) ;
#42508=CARTESIAN_POINT ( 'NONE',  ( 1.499999999999989120, 2.035416667349480679, 0.8660254037844524744 ) ) ;
#42509=CARTESIAN_POINT ( 'NONE',  ( -1.201851678989727383E-14, 4.759375000341419693, -1.575800808251660134 ) ) ;
#42524=CARTESIAN_POINT ( 'NONE',  ( -7.492852449846775897, 11.89341162479659531, 0.000000000000000000 ) ) ;
#42525=CARTESIAN_POINT ( 'NONE',  ( 8.145751363712157911, 8.397798100619326078, -0.7998128361456281477 ) ) ;
#42530=B_SPLINE_CURVE_WITH_KNOTS ( 'NONE', 3,
 ( #184341, #15436, #100958, #198451, #165972, #114106, #148666, #232, #31721, #50097 ),
 .UNSPECIFIED., .F., .F.,
 ( 4, 3, 3, 4 ),
 ( 1.084202172485514786E-19, 3.125153504173336036E-05, 6.280295210142521956E-05, 9.436679189892625938E-05 ),
 .UNSPECIFIED. ) ;
#42533=CARTESIAN_POINT ( 'NONE',  ( -7.212047647465563038, 10.50147379109678880, -1.199719254218446718 ) ) ;
#42537=ORIENTED_EDGE ( 'NONE', *, *, #155510, .T. ) ;
#42540=CARTESIAN_POINT ( 'NONE',  ( 4.054051625686104998, 4.688480637177271149, -1.199719254218446718 ) ) ;
#42542=ORIENTED_EDGE ( 'NONE', *, *, #54037, .F. ) ;
#42544=CARTESIAN_POINT ( 'NONE',  ( -9.508345801885592863, 9.987491611821676329, 0.7998128361456462443 ) ) ;
#42547=CARTESIAN_POINT ( 'NONE',  ( -5.285102783734889620, 6.572932445422958736, -1.390504041276509062 ) ) ;
#42555=CARTESIAN_POINT ( 'NONE',  ( 5.686755365928134687, 8.721966129303114101, 1.199719254218462483 ) ) ;
#42574=CARTESIAN_POINT ( 'NONE',  ( 4.880572111239557920, 4.796348339308675435, -0.7216878364870197293 ) ) ;
#42579=CARTESIAN_POINT ( 'NONE',  ( -10.32183501870554387, 10.93656236477829502, 0.7998128361456462443 ) ) ;
#42581=CARTESIAN_POINT ( 'NONE',  ( 9.049177462117294013, 12.64479190819049670, -1.199719254218446718 ) ) ;
#42590=CARTESIAN_POINT ( 'NONE',  ( -1.402160292154681736E-14, 0.1968750003414221628, -1.575800808251665908 ) ) ;
#42596=CARTESIAN_POINT ( 'NONE',  ( -4.603156847039612920, 5.329103395422994716, 1.199719254218462483 ) ) ;
#42598=CARTESIAN_POINT ( 'NONE',  ( 0.7499999999999867883, -0.1833333333333131421, -1.299038105676652899 ) ) ;
#42600=CARTESIAN_POINT ( 'NONE',  ( 1.499999999999989120, 5.504166666666685970, 0.8660254037844524744 ) ) ;
#42605=CARTESIAN_POINT ( 'NONE',  ( -0.6823417656250246877, -0.1989583329919109023, 1.181850606188755259 ) ) ;
#42607=CARTESIAN_POINT ( 'NONE',  ( -6.256197817702116026, 9.386315656372753224, -1.199719254218440723 ) ) ;
#42608=CARTESIAN_POINT ( 'NONE',  ( 7.540305987494599016, 11.94877408538573427, -0.7998128361456291469 ) ) ;
#42613=CARTESIAN_POINT ( 'NONE',  ( 1.364683531249988757, 0.6968750003414209138, 0.000000000000000000 ) ) ;
#42621=CARTESIAN_POINT ( 'NONE',  ( 6.155038550924144758, 8.203964280876741455, 1.443375672974076540 ) ) ;
#42624=CARTESIAN_POINT ( 'NONE',  ( -4.218558352146454915, 8.073401844146177453, 1.040834085586084257E-14 ) ) ;
#42626=CARTESIAN_POINT ( 'NONE',  ( 1.499999999999990896, 5.556250000682820378, 1.214306433183764966E-14 ) ) ;
#42629=EDGE_CURVE ( 'NONE', #50158, #211239, #202984, .T. ) ;
#42630=CARTESIAN_POINT ( 'NONE',  ( 6.005898860729467437, 7.069598761348265370, -1.082531754730543083 ) ) ;
#42631=CARTESIAN_POINT ( 'NONE',  ( -9.612367721964622191, 10.31677655182129527, -0.7216878364870267237 ) ) ;
#42633=CARTESIAN_POINT ( 'NONE',  ( -1.500000000000011324, 4.170833333333359150, 0.8660254037844403729 ) ) ;
#42638=CARTESIAN_POINT ( 'NONE',  ( 9.625925876022625616, 11.29296361252366765, -1.082531754730537088 ) ) ;
#42641=DIRECTION ( 'NONE',  ( 0.7071067811865465735, 0.7071067811865483499, 8.659560562354921765E-17 ) ) ;
#42645=CARTESIAN_POINT ( 'NONE',  ( -4.355418974009601207, 3.138960640472630459, -0.7749999999999935829 ) ) ;
#42649=ORIENTED_EDGE ( 'NONE', *, *, #180280, .T. ) ;
#42650=CARTESIAN_POINT ( 'NONE',  ( 8.717529583462646059, 11.19353715217169309, 1.443375672974076540 ) ) ;
#42652=CARTESIAN_POINT ( 'NONE',  ( 8.762647353133951711, 9.117510088278095282, 1.040834085586084257E-14 ) ) ;
#42657=ADVANCED_FACE ( 'NONE', ( #47897 ), #20400, .T. ) ;
#42659=CARTESIAN_POINT ( 'NONE',  ( 4.853455804012228647, 4.764712647543454693, 0.7216878364870317197 ) ) ;
#42661=CARTESIAN_POINT ( 'NONE',  ( -8.405692050792730186, 9.869357483088723626, 1.082531754730558626 ) ) ;
#42665=CARTESIAN_POINT ( 'NONE',  ( -2.103486388414573138, 5.605817886458954291, 1.040834085586084257E-14 ) ) ;
#42674=VERTEX_POINT ( 'NONE', #175743 ) ;
#42676=B_SPLINE_CURVE_WITH_KNOTS ( 'NONE', 3,
 ( #169828, #84307, #150392, #87524, #51825, #134163, #56087, #104848, #5159, #170894, #200172, #137351, #22486, #203368 ),
 .UNSPECIFIED., .F., .F.,
 ( 4, 2, 2, 2, 2, 2, 4 ),
 ( 0.001872291076883575130, 0.002107054070182344009, 0.002341817063481112671, 0.002811343050078650863, 0.003280869036676186019, 0.003515632029974954248, 0.003750395023273722043 ),
 .UNSPECIFIED. ) ;
#42684=VECTOR ( 'NONE', #202834, 1000.000000000000114 ) ;
#42688=CARTESIAN_POINT ( 'NONE',  ( 0.3461162505575273163, 7.159215625956777629, 1.970439023737499351 ) ) ;
#42693=CARTESIAN_POINT ( 'NONE',  ( -7.576308911938196999, 7.733448573549685179, 0.7998128361456462443 ) ) ;
#42695=DIRECTION ( 'NONE',  ( -0.5996521035822321988, -0.8002608041566222630, 0.000000000000000000 ) ) ;
#42697=CARTESIAN_POINT ( 'NONE',  ( 6.419949431270806528, 7.448694743692793274, 1.199719254218462483 ) ) ;
#42705=CARTESIAN_POINT ( 'NONE',  ( -3.730464822054482710, 7.503959392372201442, 1.040834085586084257E-14 ) ) ;
#42708=CARTESIAN_POINT ( 'NONE',  ( 6.591235234537977661, 10.84152487360300299, 0.7998128361456462443 ) ) ;
#42711=CARTESIAN_POINT ( 'NONE',  ( 6.103366240126457676, 6.022929404904433071, 0.2034074856576886248 ) ) ;
#42717=CARTESIAN_POINT ( 'NONE',  ( 5.897433631820129918, 8.863794422890064695, -1.082531754730537976 ) ) ;
#42718=CARTESIAN_POINT ( 'NONE',  ( -8.694856585065634746, 9.038420858865048757, 0.7998128361456462443 ) ) ;
#42721=CARTESIAN_POINT ( 'NONE',  ( -7.374745490829552885, 10.69128794168811680, -1.199719254218446718 ) ) ;
#42722=CARTESIAN_POINT ( 'NONE',  ( -7.237355071596549116, 7.338002426484427687, 1.040834085586084257E-14 ) ) ;
#42729=CARTESIAN_POINT ( 'NONE',  ( 8.697719238366680372, 10.10609285197134533, 1.199719254218462483 ) ) ;
#42734=AXIS2_PLACEMENT_3D ( 'NONE', #80554, #64307, #146652 ) ;
#42736=CARTESIAN_POINT ( 'NONE',  ( 2.184835310096557404, 5.700724961754617404, 1.040834085586084257E-14 ) ) ;
#42745=CARTESIAN_POINT ( 'NONE',  ( -1.001543065824772872E-14, 4.462500000000024336, 1.732050807568877637 ) ) ;
#42746=CARTESIAN_POINT ( 'NONE',  ( 3.635557746758808495, 7.393234471193928847, -0.7998128361456291469 ) ) ;
#42747=CARTESIAN_POINT ( 'NONE',  ( 6.120616281565444794, 9.228137197546649517, -1.199719254218440723 ) ) ;
#42751=CARTESIAN_POINT ( 'NONE',  ( 6.643132081016124069, 7.813037518349371879, 1.082531754730558626 ) ) ;
#42752=CARTESIAN_POINT ( 'NONE',  ( -9.964879715919934711, 10.72804054476916313, 0.7216878364870438212 ) ) ;
#42756=CARTESIAN_POINT ( 'NONE',  ( 7.540305987494599016, 11.94877408538573427, -0.7998128361456291469 ) ) ;
#42761=CARTESIAN_POINT ( 'NONE',  ( 1.364683531249986537, 1.405208333674755838, -0.7879004041258239610 ) ) ;
#42766=CARTESIAN_POINT ( 'NONE',  ( -1.364683531250000748, -0.7406249996585803075, 0.000000000000000000 ) ) ;
#42768=CARTESIAN_POINT ( 'NONE',  ( 9.236128959407556849, 11.79856975744075598, -1.599625672291262513 ) ) ;
#42772=CARTESIAN_POINT ( 'NONE',  ( -10.17947440576205054, 10.77047498301088346, 0.7998128361456462443 ) ) ;
#42778=CARTESIAN_POINT ( 'NONE',  ( 3.520313441042647540, 7.258782781191745137, 0.7998128361456321445 ) ) ;
#42783=CARTESIAN_POINT ( 'NONE',  ( 7.248805684800777804, 11.60869039890961218, 1.040834085586084257E-14 ) ) ;
#42786=CARTESIAN_POINT ( 'NONE',  ( -4.880045225915050189, 7.780804299287790826, 1.199719254218464037 ) ) ;
#42790=CARTESIAN_POINT ( 'NONE',  ( 6.401421083946654100, 10.62007503124645957, -0.7998128361456291469 ) ) ;
#42792=CARTESIAN_POINT ( 'NONE',  ( 7.396136491454752715, 8.587579647240744407, 1.199719254218462483 ) ) ;
#42795=CARTESIAN_POINT ( 'NONE',  ( -9.327646496521992958, 9.984601788804893019, -0.7216878364870267237 ) ) ;
#42803=CARTESIAN_POINT ( 'NONE',  ( -5.355516094498059765, 6.520963868127283014, 1.360184235745926618 ) ) ;
#42804=CARTESIAN_POINT ( 'NONE',  ( -0.6823417656250003738, 2.217708333674753174, -1.181850606188749264 ) ) ;
#42807=CARTESIAN_POINT ( 'NONE',  ( 5.151735183512854199, 8.954182114166247430, -0.7216878364870257245 ) ) ;
#42813=AXIS2_PLACEMENT_3D ( 'NONE', #131454, #2428, #103167 ) ;
#42815=EDGE_CURVE ( 'NONE', #185401, #195170, #163761, .T. ) ;
#42823=CARTESIAN_POINT ( 'NONE',  ( 4.704316113817540668, 5.551085556617666228, -1.082531754730548412 ) ) ;
#42827=CARTESIAN_POINT ( 'NONE',  ( 7.560643217915098191, 11.97250085420964716, -0.7998128361456291469 ) ) ;
#42829=EDGE_LOOP ( 'NONE', ( #178922, #66633, #198179 ) ) ;
#42831=CARTESIAN_POINT ( 'NONE',  ( -3.948449050077848632, 5.629609863222681199, 1.599625672291267398 ) ) ;
#42832=CARTESIAN_POINT ( 'NONE',  ( -7.369020184227459858, 8.555943955475521889, 1.199719254218450271 ) ) ;
#42837=CARTESIAN_POINT ( 'NONE',  ( -1.201851678989727383E-14, 3.993750000682817713, 1.732050807568877637 ) ) ;
#42838=CARTESIAN_POINT ( 'NONE',  ( 6.753933077901968396, 11.03133902419432566, 0.7998128361456462443 ) ) ;
#42841=CARTESIAN_POINT ( 'NONE',  ( -7.446452682403657874, 9.710614100936176385, -1.599625672291263179 ) ) ;
#42843=CARTESIAN_POINT ( 'NONE',  ( -1.201851678989727383E-14, 5.196875000341422357, -1.575800808251660134 ) ) ;
#42845=CARTESIAN_POINT ( 'NONE',  ( -1.445368642221011024, 8.714907460504111469, 2.589984629573252928 ) ) ;
#42849=CARTESIAN_POINT ( 'NONE',  ( -9.341204650135658483, 10.00041963468749984, 1.040834085586084257E-14 ) ) ;
#42853=CARTESIAN_POINT ( 'NONE',  ( -1.364683531250012516, 2.551041667008089320, -0.7879004041258289570 ) ) ;
#42860=CARTESIAN_POINT ( 'NONE',  ( -0.6823417656249969321, 3.967708333674754950, -1.181850606188749264 ) ) ;
#42861=CARTESIAN_POINT ( 'NONE',  ( -3.761497552787613330, 6.475832013972435242, 1.199719254218464037 ) ) ;
#42862=CARTESIAN_POINT ( 'NONE',  ( 5.276094334012385367, 9.307193822989793475, 1.040834085586084257E-14 ) ) ;
#42866=CARTESIAN_POINT ( 'NONE',  ( -1.001543065824772872E-14, 4.384375000341417916, 1.575800808251672791 ) ) ;
#42870=CARTESIAN_POINT ( 'NONE',  ( 1.364683531249988757, -0.1156249996585798079, 0.000000000000000000 ) ) ;
#42871=CARTESIAN_POINT ( 'NONE',  ( -3.470524135418300737, 6.032400010421219427, -1.082531754730549967 ) ) ;
#42875=CARTESIAN_POINT ( 'NONE',  ( 2.575685996916329046, 5.948791396470269888, 0.7216878364870438212 ) ) ;
#42878=CARTESIAN_POINT ( 'NONE',  ( -9.653042183249970876, 11.32459930428888306, -1.082531754730539753 ) ) ;
#42882=CARTESIAN_POINT ( 'NONE',  ( -9.110189153378817295, 12.71597221466224603, 1.199719254218462483 ) ) ;
#42884=CARTESIAN_POINT ( 'NONE',  ( -5.463572716182839351, 7.397254140345190798, 1.443375672974064550 ) ) ;
#42886=CARTESIAN_POINT ( 'NONE',  ( 1.364683531249986537, 1.217708333674754950, -0.7879004041258239610 ) ) ;
#42892=CARTESIAN_POINT ( 'NONE',  ( 1.364683531249988757, -0.3031249996585799744, 0.000000000000000000 ) ) ;
#42897=ORIENTED_EDGE ( 'NONE', *, *, #161474, .T. ) ;
#42899=CARTESIAN_POINT ( 'NONE',  ( 6.927853306458731986, 11.02631992426980112, 0.7216878364870438212 ) ) ;
#42909=CARTESIAN_POINT ( 'NONE',  ( -3.090368948911150770, 5.692848642783215674, 1.199719254218462483 ) ) ;
#42913=CARTESIAN_POINT ( 'NONE',  ( 0.6823417656249882723, 1.738541667008083991, -1.181850606188749264 ) ) ;
#42932=CARTESIAN_POINT ( 'NONE',  ( 4.496500501226593727, 8.397667684739696270, 0.7998128361456462443 ) ) ;
#42934=AXIS2_PLACEMENT_3D ( 'NONE', #158213, #140921, #43398 ) ;
#42940=CARTESIAN_POINT ( 'NONE',  ( 8.097244055859613709, 10.46987070330147063, -1.599625672291262513 ) ) ;
#42944=CARTESIAN_POINT ( 'NONE',  ( 8.062294901620731480, 12.55776115186623620, 1.040834085586084257E-14 ) ) ;
#42946=CARTESIAN_POINT ( 'NONE',  ( -3.020739592526671125, 6.452503409769998477, 0.6179323767311885041 ) ) ;
#42958=CARTESIAN_POINT ( 'NONE',  ( -8.893785580884703279, 10.43879993486270585, 1.082531754730558626 ) ) ;
#42966=CARTESIAN_POINT ( 'NONE',  ( -5.132810702184136709, 6.527128546466574477, -1.246928735940135313 ) ) ;
#42971=CARTESIAN_POINT ( 'NONE',  ( 4.324687812634892659, 5.108185871904570519, 1.082531754730560403 ) ) ;
#42979=CARTESIAN_POINT ( 'NONE',  ( -6.240830780992103755, 6.175390754112560110, 1.040834085586084257E-14 ) ) ;
#42981=CARTESIAN_POINT ( 'NONE',  ( -2.676845263694313637, 5.210404343363602919, -1.199719254218446718 ) ) ;
#42987=CARTESIAN_POINT ( 'NONE',  ( -1.201851678989727383E-14, 3.634375000341422357, 1.575800808251672791 ) ) ;
#42989=CARTESIAN_POINT ( 'NONE',  ( 5.823390672269506574, 6.752709524857930745, -1.199719254218446718 ) ) ;
#42990=CARTESIAN_POINT ( 'NONE',  ( 1.504932104232256984, 8.664796307965634270, 2.552344783041808451 ) ) ;
#43002=CARTESIAN_POINT ( 'NONE',  ( 1.364683531249988535, 1.926041667008086211, 0.7879004041258500513 ) ) ;
#43004=CARTESIAN_POINT ( 'NONE',  ( 2.693266070609028784, 6.293894182352508970, 0.000000000000000000 ) ) ;
#43006=CARTESIAN_POINT ( 'NONE',  ( -6.426201623197489887, 6.599582769926260362, 0.7216878364870317197 ) ) ;
#43008=CARTESIAN_POINT ( 'NONE',  ( 4.419594888374914099, 5.218910793601261311, -1.082531754730548412 ) ) ;
#43009=CARTESIAN_POINT ( 'NONE',  ( -5.870317324592811303, 8.832158731124840401, -1.082531754730537976 ) ) ;
#43014=CARTESIAN_POINT ( 'NONE',  ( 5.449487677688982679, 8.445153826357429949, -1.199719254218446718 ) ) ;
#43019=CARTESIAN_POINT ( 'NONE',  ( -0.6823417656249969321, 4.967708333674755394, -1.181850606188749264 ) ) ;
#43024=CARTESIAN_POINT ( 'NONE',  ( 7.793239369756836510, 7.986534107671458216, 0.7998128361456341429 ) ) ;
#43025=( NAMED_UNIT ( * ) PLANE_ANGLE_UNIT ( ) SI_UNIT ( $, .RADIAN. ) );
#43028=CARTESIAN_POINT ( 'NONE',  ( -7.172426956829277778, 8.326585190177668849, -1.199719254218452935 ) ) ;
#43033=CARTESIAN_POINT ( 'NONE',  ( 7.401861798056875053, 10.72292363345333399, -1.199719254218441611 ) ) ;
#43036=CARTESIAN_POINT ( 'NONE',  ( -7.202405917357668663, 9.425892875049191488, 1.599625672291295375 ) ) ;
#43038=CARTESIAN_POINT ( 'NONE',  ( 8.581948047326003248, 9.114620264742901767, -0.7216878364870197293 ) ) ;
#43039=CARTESIAN_POINT ( 'NONE',  ( 4.064005108223194718, 7.741596126659699983, 0.5534810405699239766 ) ) ;
#43040=CARTESIAN_POINT ( 'NONE',  ( -4.466521540698216164, 7.298359999868178960, -1.199719254218452047 ) ) ;
#43044=CARTESIAN_POINT ( 'NONE',  ( 4.527533231959700366, 7.369540306339926516, 1.199719254218462483 ) ) ;
#43046=CARTESIAN_POINT ( 'NONE',  ( 9.725276259704228821, 10.24057714594344048, 0.7998128361456462443 ) ) ;
#43047=CARTESIAN_POINT ( 'NONE',  ( -5.626640144655740805, 6.175545741207232098, 0.8476793345565808435 ) ) ;
#43049=CARTESIAN_POINT ( 'NONE',  ( -0.6823417656250003738, 1.217708333674752286, -1.181850606188749264 ) ) ;
#43051=CARTESIAN_POINT ( 'NONE',  ( -6.453317930424837812, 7.591587675992828466, 1.082531754730549967 ) ) ;
#43057=CARTESIAN_POINT ( 'NONE',  ( -5.899211624428097878, 6.007801130575932014, 0.1941222073163356709 ) ) ;
#43058=CARTESIAN_POINT ( 'NONE',  ( -1.364683531250000748, 1.821875000341421913, 0.000000000000000000 ) ) ;
#43061=CARTESIAN_POINT ( 'NONE',  ( 3.795919822146273326, 5.451659097302528068, -1.443375672974051449 ) ) ;
#43066=CARTESIAN_POINT ( 'NONE',  ( -8.636180661780672452, 9.177891648273343250, -0.7216878364870267237 ) ) ;
#43069=EDGE_CURVE ( 'NONE', #176773, #166897, #123353, .T. ) ;
#43074=CARTESIAN_POINT ( 'NONE',  ( -7.307481607641392429, 11.46921960898288972, 0.7216878364870458196 ) ) ;
#43081=ORIENTED_EDGE ( 'NONE', *, *, #48451, .F. ) ;
#43082=CARTESIAN_POINT ( 'NONE',  ( -6.832946231163084860, 10.91559500309152675, 0.000000000000000000 ) ) ;
#43087=CARTESIAN_POINT ( 'NONE',  ( -1.001543065824772872E-14, 4.743750000682822154, 1.732050807568877637 ) ) ;
#43094=CARTESIAN_POINT ( 'NONE',  ( -6.507023659554960204, 9.678945805201045971, 1.199719254218452047 ) ) ;
#43098=CARTESIAN_POINT ( 'NONE',  ( 6.145923705696426431, 6.064665832934283962, 0.7998128361456341429 ) ) ;
#43103=CARTESIAN_POINT ( 'NONE',  ( 7.955937213120826357, 8.176348258262782664, 0.7998128361456481317 ) ) ;
#43110=CARTESIAN_POINT ( 'NONE',  ( -4.582292731738899505, 8.289832587096611860, 0.7216878364870458196 ) ) ;
#43113=CARTESIAN_POINT ( 'NONE',  ( 3.375617060122621194, 6.882044303544283537, 1.040834085586084257E-14 ) ) ;
#43119=CARTESIAN_POINT ( 'NONE',  ( -9.352427035328430449, 9.805586384171650849, 1.040834085586084257E-14 ) ) ;
#43122=CARTESIAN_POINT ( 'NONE',  ( 7.527801604085637699, 9.805521176231838609, 1.599625672291281386 ) ) ;
#43123=CARTESIAN_POINT ( 'NONE',  ( 0.7499999999999867883, -0.1833333333333131421, -1.299038105676652899 ) ) ;
#43124=CARTESIAN_POINT ( 'NONE',  ( -8.636707547105197946, 10.03491254549959777, -1.199719254218446718 ) ) ;
#43127=CARTESIAN_POINT ( 'NONE',  ( 0.6823417656249917140, 3.342708333674754506, 1.181850606188765695 ) ) ;
#43128=CARTESIAN_POINT ( 'NONE',  ( 10.22248463502393001, 11.02857961705718282, 0.7216878364870438212 ) ) ;
#43131=CARTESIAN_POINT ( 'NONE',  ( 1.499999999999991118, 5.754166666666685970, 0.8660254037844524744 ) ) ;
#43134=B_SPLINE_CURVE_WITH_KNOTS ( 'NONE', 3,
 ( #109756, #176819, #46842, #62008 ),
 .UNSPECIFIED., .F., .F.,
 ( 4, 4 ),
 ( 0.0006335992342242843800, 0.001020988003094342074 ),
 .UNSPECIFIED. ) ;
#43136=CARTESIAN_POINT ( 'NONE',  ( 9.232739420781973294, 9.873876867108206667, -0.7216878364870257245 ) ) ;
#43140=CARTESIAN_POINT ( 'NONE',  ( -5.422898255786186006, 9.270539031818461950, -0.7216878364870207285 ) ) ;
#43142=CARTESIAN_POINT ( 'NONE',  ( -1.364683531250014514, 1.988541667008086655, -0.7879004041258289570 ) ) ;
#43146=CARTESIAN_POINT ( 'NONE',  ( -5.506582945444718824, 9.576097202994168001, 0.7998128361456481317 ) ) ;
#43147=CARTESIAN_POINT ( 'NONE',  ( -1.364683531250010295, 4.342708333674753618, 0.7879004041258379498 ) ) ;
#43152=CARTESIAN_POINT ( 'NONE',  ( 8.127223016387999266, 11.56917838817298616, 1.199719254218460707 ) ) ;
#43156=CARTESIAN_POINT ( 'NONE',  ( -0.7500000000000006661, 1.608333333333357373, -1.299038105676652011 ) ) ;
#43159=ORIENTED_EDGE ( 'NONE', *, *, #192264, .F. ) ;
#43160=CARTESIAN_POINT ( 'NONE',  ( 7.944714827928056167, 8.371181508778631652, 0.7216878364870458196 ) ) ;
#43161=CARTESIAN_POINT ( 'NONE',  ( 9.236128959407556849, 11.79856975744075598, -1.599625672291262513 ) ) ;
#43166=CARTESIAN_POINT ( 'NONE',  ( 8.589254009457354400, 9.979550084910457031, -1.199719254218446718 ) ) ;
#43167=CARTESIAN_POINT ( 'NONE',  ( -10.34217224912604571, 10.96028913360221502, 0.7998128361456462443 ) ) ;
#43170=CARTESIAN_POINT ( 'NONE',  ( -1.364683531250010295, 5.342708333674750953, 0.7879004041258379498 ) ) ;
#43176=CARTESIAN_POINT ( 'NONE',  ( -1.364683531250010295, 3.780208333674750953, 0.7879004041258379498 ) ) ;
#43178=CARTESIAN_POINT ( 'NONE',  ( -7.226132686403777150, 7.532835677000276675, 1.040834085586084257E-14 ) ) ;
#43187=CARTESIAN_POINT ( 'NONE',  ( 9.413438726589914651, 9.876766690643398405, 0.000000000000000000 ) ) ;
#43193=CARTESIAN_POINT ( 'NONE',  ( -7.486073373039941359, 11.88550270185529278, -0.7998128361456291469 ) ) ;
#43194=CARTESIAN_POINT ( 'NONE',  ( 5.819474248763732760, 7.812472595022922128, -1.599625672291262513 ) ) ;
#43196=CARTESIAN_POINT ( 'NONE',  ( 3.619663824724254741, 6.206396314611513532, -1.082531754730543971 ) ) ;
#43198=CARTESIAN_POINT ( 'NONE',  ( 4.172158584703322681, 5.890604320285754980, -1.599625672291256295 ) ) ;
#43207=CARTESIAN_POINT ( 'NONE',  ( -6.751597309925468693, 6.979211071108916364, 0.7216878364870317197 ) ) ;
#43208=CARTESIAN_POINT ( 'NONE',  ( 4.681643115420508039, 4.356338477612361260, 0.7998128361456341429 ) ) ;
#43211=CARTESIAN_POINT ( 'NONE',  ( -7.588813295347149435, 9.876701482703580837, -1.599625672291263179 ) ) ;
#43215=CARTESIAN_POINT ( 'NONE',  ( -7.645908563102897126, 11.00764485934031889, 1.199719254218453823 ) ) ;
#43219=CARTESIAN_POINT ( 'NONE',  ( 6.934105498385400246, 10.17720795050327354, -1.199719254218441611 ) ) ;
#43220=CARTESIAN_POINT ( 'NONE',  ( 6.322179702674084467, 6.270297829408224111, 1.040834085586084257E-14 ) ) ;
#43232=CARTESIAN_POINT ( 'NONE',  ( -6.157374318900681764, 10.33535380535947290, 0.7998128361456481317 ) ) ;
#43235=CARTESIAN_POINT ( 'NONE',  ( 5.327991180490514012, 9.159814110640187579, 1.040834085586084257E-14 ) ) ;
#43239=CARTESIAN_POINT ( 'NONE',  ( -5.935772324684618795, 5.819489221753827657, 0.000000000000000000 ) ) ;
#43247=CARTESIAN_POINT ( 'NONE',  ( -10.34217224912604571, 10.96028913360221502, 0.7998128361456462443 ) ) ;
#43248=CARTESIAN_POINT ( 'NONE',  ( 7.293396569147545527, 10.59638086639245280, 1.199719254218460707 ) ) ;
#43250=CARTESIAN_POINT ( 'NONE',  ( -4.134873662487946966, 3.926366815765101936, 1.214306433183764966E-14 ) ) ;
#43251=VECTOR ( 'NONE', #129882, 1000.000000000000000 ) ;
#43253=CARTESIAN_POINT ( 'NONE',  ( -4.639453055371920875, 6.917948375795638150, -1.210149155198399828 ) ) ;
#43261=CARTESIAN_POINT ( 'NONE',  ( 2.846322183865124700, 5.408127416896231665, -1.199719254218446718 ) ) ;
#43265=FACE_OUTER_BOUND ( 'NONE', #66542, .T. ) ;
#43279=CARTESIAN_POINT ( 'NONE',  ( -4.680589345215810049, 6.483773540883647435, -1.599625672291256295 ) ) ;
#43280=CARTESIAN_POINT ( 'NONE',  ( 5.300874872818830852, 7.207439989753867238, 1.443375672974062551 ) ) ;
#43281=CARTESIAN_POINT ( 'NONE',  ( 1.499999999999989120, 3.754166666666685082, 0.8660254037844524744 ) ) ;
#43283=CARTESIAN_POINT ( 'NONE',  ( -2.839543107058306592, 5.400218493954923815, -1.199719254218446718 ) ) ;
#43285=EDGE_CURVE ( 'NONE', #19327, #140589, #89084, .T. ) ;
#43288=CARTESIAN_POINT ( 'NONE',  ( 0.6823417656249899377, 4.426041667008086655, -1.181850606188754593 ) ) ;
#43292=CARTESIAN_POINT ( 'NONE',  ( -2.643476764984671767, 6.027880625883323518, 1.040834085586084257E-14 ) ) ;
#43296=CARTESIAN_POINT ( 'NONE',  ( 3.680148631105580215, 6.380924938676771241, -1.199719254218446718 ) ) ;
#43299=CARTESIAN_POINT ( 'NONE',  ( 3.931431380944446108, 2.807600633707128424, -0.7749999999999935829 ) ) ;
#43302=CARTESIAN_POINT ( 'NONE',  ( 1.364683531249988757, 0.9468750003414211358, 0.000000000000000000 ) ) ;
#43305=CARTESIAN_POINT ( 'NONE',  ( -10.64723070543352712, 11.31619066596094392, 0.7998128361456462443 ) ) ;
#43306=CARTESIAN_POINT ( 'NONE',  ( -6.521108698048791119, 6.710307690586118312, -0.7216878364870267237 ) ) ;
#43311=CARTESIAN_POINT ( 'NONE',  ( -0.6823417656249969321, 4.467708333674755394, -1.181850606188749264 ) ) ;
#43320=CARTESIAN_POINT ( 'NONE',  ( -4.839897649954225223, 7.630002444046455778, 1.082531754730560403 ) ) ;
#43325=CARTESIAN_POINT ( 'NONE',  ( -4.243338890952892406, 7.894386439512932618, -0.7216878364870257245 ) ) ;
#43327=CARTESIAN_POINT ( 'NONE',  ( 9.531545685607134999, 11.07889037375188401, 1.199719254218450271 ) ) ;
#43336=CARTESIAN_POINT ( 'NONE',  ( -3.795392936821753604, 6.515376628678959392, -1.199719254218452047 ) ) ;
#43339=CARTESIAN_POINT ( 'NONE',  ( 0.7499999999999902300, 1.233333333333357151, 1.299038105676657340 ) ) ;
#43341=CARTESIAN_POINT ( 'NONE',  ( 8.351459436338029008, 10.76645531385962862, -1.443375672974063439 ) ) ;
#43342=CARTESIAN_POINT ( 'NONE',  ( 5.282873410819217241, 9.315102745931094219, -0.7998128361456281477 ) ) ;
#43347=CARTESIAN_POINT ( 'NONE',  ( 3.517450787741589036, 6.191110788085444128, -1.199719254218446718 ) ) ;
#43348=CARTESIAN_POINT ( 'NONE',  ( -0.4301767877894160375, 8.007958762483717408, -1.954153227243214719 ) ) ;
#43355=CARTESIAN_POINT ( 'NONE',  ( -6.901263884555985051, 8.010228272525461435, 1.199719254218450271 ) ) ;
#43362=CARTESIAN_POINT ( 'NONE',  ( -0.6823417656249969321, 4.717708333674755394, -1.181850606188749264 ) ) ;
#43363=CARTESIAN_POINT ( 'NONE',  ( 8.337901282279995385, 11.71100668175994386, -1.082531754730543083 ) ) ;
#43364=CARTESIAN_POINT ( 'NONE',  ( -5.900823170445743671, 7.907379670318584353, 1.599625672291269396 ) ) ;
#43366=CARTESIAN_POINT ( 'NONE',  ( -1.500000000000056621, 7.388542872122511262, -4.154462424328199788 ) ) ;
#43367=CARTESIAN_POINT ( 'NONE',  ( 6.491656622844908853, 6.468020902940851968, 0.7998128361456341429 ) ) ;
#43368=CARTESIAN_POINT ( 'NONE',  ( -6.586563698140583512, 6.578745824119123675, 1.040834085586084257E-14 ) ) ;
#43374=CARTESIAN_POINT ( 'NONE',  ( 5.178851490740187913, 8.985817805931475277, 0.7216878364870438212 ) ) ;
#43377=CARTESIAN_POINT ( 'NONE',  ( -1.201851678989727383E-14, 1.384375000341419693, 1.575800808251672791 ) ) ;
#43379=CARTESIAN_POINT ( 'NONE',  ( 4.758548728272192108, 7.535095368750792666, -1.082531754730549078 ) ) ;
#43381=CARTESIAN_POINT ( 'NONE',  ( -4.121315508874276112, 4.870918184183829602, -1.082531754730549967 ) ) ;
#43388=CARTESIAN_POINT ( 'NONE',  ( -4.233332884224245696, 7.524468121203685023, -1.021403520103405294 ) ) ;
#43395=CARTESIAN_POINT ( 'NONE',  ( 7.332262146892202459, 7.448727347662698506, -0.7998128361456281477 ) ) ;
#43398=DIRECTION ( 'NONE',  ( 1.000000000000000000, -4.985516615831701596E-16, 0.000000000000000000 ) ) ;
#43404=ORIENTED_EDGE ( 'NONE', *, *, #80530, .T. ) ;
#43406=CARTESIAN_POINT ( 'NONE',  ( 4.907688418466886304, 5.788353245375237321, -1.082531754730548412 ) ) ;
#43407=CARTESIAN_POINT ( 'NONE',  ( -1.201851678989727383E-14, 2.634375000341417916, 1.575800808251672791 ) ) ;
#43409=CARTESIAN_POINT ( 'NONE',  ( 6.428537391173986038, 10.65171072301167854, 0.7998128361456462443 ) ) ;
#43418=CARTESIAN_POINT ( 'NONE',  ( 0.7499999999999902300, 3.816666666666690411, -1.299038105676658228 ) ) ;
#43419=CARTESIAN_POINT ( 'NONE',  ( 6.043183783389218355, 8.073467052085995022, 1.599625672291267398 ) ) ;
#43420=CARTESIAN_POINT ( 'NONE',  ( -7.121056995675673740, 9.330985799753529264, -1.599625672291263179 ) ) ;
#43423=CARTESIAN_POINT ( 'NONE',  ( -1.201851678989727383E-14, 5.837500000000023448, -1.732050807568863648 ) ) ;
#43424=CARTESIAN_POINT ( 'NONE',  ( -1.364683531250012516, 3.030208333674755394, 0.7879004041258379498 ) ) ;
#43426=CARTESIAN_POINT ( 'NONE',  ( 3.277320446201373638, 4.846626492033466072, 1.599625672291267398 ) ) ;
#43432=CARTESIAN_POINT ( 'NONE',  ( 1.499999999999989120, 0.3062500006828158816, 0.000000000000000000 ) ) ;
#43435=CARTESIAN_POINT ( 'NONE',  ( -4.934277840369690971, 7.844075682818238526, -1.199719254218452047 ) ) ;
#43436=CARTESIAN_POINT ( 'NONE',  ( -2.331639231870358930, 5.664070170583284103, -0.7216878364870267237 ) ) ;
#43444=CARTESIAN_POINT ( 'NONE',  ( 6.498435699651741615, 6.475929825882159818, -0.7998128361456281477 ) ) ;
#43449=CARTESIAN_POINT ( 'NONE',  ( 5.035963992472171746, 7.962709526937818083, 1.199719254218462483 ) ) ;
#43456=CARTESIAN_POINT ( 'NONE',  ( 3.728655938958122196, 4.308852335994623139, -1.199719254218446718 ) ) ;
#43462=CARTESIAN_POINT ( 'NONE',  ( 5.244386534325491844, 6.400378350754194479, 1.153371672928265479 ) ) ;
#43474=CARTESIAN_POINT ( 'NONE',  ( -5.905617501100172362, 6.087552950387692619, -0.6644227375040656636 ) ) ;
#43475=CARTESIAN_POINT ( 'NONE',  ( 7.266807147244743526, 11.42176607185347414, -0.7216878364870267237 ) ) ;
#43477=CARTESIAN_POINT ( 'NONE',  ( -5.752737250900127997, 5.605948302338584099, 0.000000000000000000 ) ) ;
#43481=CARTESIAN_POINT ( 'NONE',  ( 8.932124273304774320, 9.315233161810734686, 0.7998128361456462443 ) ) ;
#43483=CARTESIAN_POINT ( 'NONE',  ( -4.693093728624763372, 8.627026450037540428, 0.7998128361456481317 ) ) ;
#43486=DIRECTION ( 'NONE',  ( 1.000000000000000000, 0.000000000000000000, 0.000000000000000000 ) ) ;
#43496=CARTESIAN_POINT ( 'NONE',  ( 9.642873567817520808, 12.27310513391906532, 1.599625672291279388 ) ) ;
#43497=CARTESIAN_POINT ( 'NONE',  ( -5.579343907223557331, 6.467988298970945849, 1.199719254218450271 ) ) ;
#43500=CARTESIAN_POINT ( 'NONE',  ( 2.412988153552339643, 5.758977245878946327, 0.7216878364870438212 ) ) ;
#43505=CARTESIAN_POINT ( 'NONE',  ( -4.603156847039612920, 5.329103395422994716, 1.199719254218462483 ) ) ;
#43508=CARTESIAN_POINT ( 'NONE',  ( 7.781490099239519509, 11.16582331816642260, 1.199719254218460707 ) ) ;
#43512=CARTESIAN_POINT ( 'NONE',  ( -6.201965203247477909, 9.323044272842313518, 1.199719254218452047 ) ) ;
#43513=CARTESIAN_POINT ( 'NONE',  ( 5.148345644887269756, 7.029489223833707001, -1.599625672291256295 ) ) ;
#43518=CARTESIAN_POINT ( 'NONE',  ( 0.6823417656249899377, 1.905208333674752952, 1.181850606188755259 ) ) ;
#43521=CARTESIAN_POINT ( 'NONE',  ( 6.304178240674458422, 10.29869901418813782, 1.040834085586084257E-14 ) ) ;
#43523=DIRECTION ( 'NONE',  ( 0.6507913734559596097, 0.7592566023653043450, 0.000000000000000000 ) ) ;
#43527=VERTEX_POINT ( 'NONE', #48427 ) ;
#43528=CARTESIAN_POINT ( 'NONE',  ( 9.747949258101261449, 11.43532422494874368, -1.082531754730537088 ) ) ;
#43534=CARTESIAN_POINT ( 'NONE',  ( -8.479735010343349089, 11.98044238112085758, 1.199719254218453823 ) ) ;
#43544=CARTESIAN_POINT ( 'NONE',  ( -1.123270288250339588, 3.283552654332833054, 0.7749999999993804067 ) ) ;
#43552=CARTESIAN_POINT ( 'NONE',  ( -1.402160292154681736E-14, 2.118750000682816825, -1.732050807568863648 ) ) ;
#43556=ORIENTED_EDGE ( 'NONE', *, *, #213928, .T. ) ;
#43558=CARTESIAN_POINT ( 'NONE',  ( -0.7500000000000006661, -0.8916666666666448471, -1.299038105676652011 ) ) ;
#43559=CARTESIAN_POINT ( 'NONE',  ( 8.052653171512838881, 11.48218023581863001, -1.199719254218446718 ) ) ;
#43560=CARTESIAN_POINT ( 'NONE',  ( -1.364683531250000748, -0.7406249996585803075, 0.000000000000000000 ) ) ;
#43563=CARTESIAN_POINT ( 'NONE',  ( 8.595506201383999567, 12.97191496834930113, 0.7216878364870438212 ) ) ;
#43564=CARTESIAN_POINT ( 'NONE',  ( -6.453317930424837812, 7.591587675992828466, 1.082531754730549967 ) ) ;
#43569=CARTESIAN_POINT ( 'NONE',  ( -6.905180308061733996, 6.950465202360470052, 0.7998128361456341429 ) ) ;
#43570=AXIS2_PLACEMENT_3D ( 'NONE', #135747, #83773, #166100 ) ;
#43571=CARTESIAN_POINT ( 'NONE',  ( 1.499999999999989120, 3.056250000682818158, 1.214306433183764966E-14 ) ) ;
#43579=ORIENTED_EDGE ( 'NONE', *, *, #54015, .T. ) ;
#43585=CARTESIAN_POINT ( 'NONE',  ( -8.992082194361570302, 11.51384853155376220, 1.599625672291269396 ) ) ;
#43586=CARTESIAN_POINT ( 'NONE',  ( 7.657657833620182153, 7.828355648845348291, -0.7998128361456281477 ) ) ;
#43593=CARTESIAN_POINT ( 'NONE',  ( -9.006694118179950692, 9.402231314165087284, 1.040834085586084257E-14 ) ) ;
#43598=CARTESIAN_POINT ( 'NONE',  ( 2.530568227245037605, 6.104080031761181857, 0.000000000000000000 ) ) ;
#43602=CARTESIAN_POINT ( 'NONE',  ( -9.158696461231359720, 10.64389961198009615, 1.199719254218462483 ) ) ;
#43604=VECTOR ( 'NONE', #62529, 1000.000000000000000 ) ;
#43606=CARTESIAN_POINT ( 'NONE',  ( -5.391520587109122076, 6.494678753518896563, -1.342800935913717852 ) ) ;
#43614=CARTESIAN_POINT ( 'NONE',  ( 6.012151052656117933, 9.101594430485762999, 1.199719254218460707 ) ) ;
#43620=EDGE_CURVE ( 'NONE', #147186, #119686, #96675, .T. ) ;
#43624=CARTESIAN_POINT ( 'NONE',  ( 1.499999999999989120, 1.785416667349487563, 0.8660254037844524744 ) ) ;
#43635=CARTESIAN_POINT ( 'NONE',  ( -1.420000000000021911, 6.120000000000041851, 2.580000000000011173 ) ) ;
#43637=CARTESIAN_POINT ( 'NONE',  ( 2.873965376416980355, 6.296784005887697155, -0.7216878364870267237 ) ) ;
#43645=CARTESIAN_POINT ( 'NONE',  ( 9.154780037725547714, 11.70366268214508487, 1.599625672291279388 ) ) ;
#43648=CARTESIAN_POINT ( 'NONE',  ( 5.375201043168952530, 6.430740811364754173, 1.235622880962461201 ) ) ;
#43653=CARTESIAN_POINT ( 'NONE',  ( 0.6823417656249882723, 0.1760416670080894308, -1.181850606188749264 ) ) ;
#43658=CARTESIAN_POINT ( 'NONE',  ( -3.906720819032141190, 7.709591388846142479, -0.7998128361456281477 ) ) ;
#43661=CARTESIAN_POINT ( 'NONE',  ( -1.500000000000015099, -0.6208333333333116988, -0.8660254037844383745 ) ) ;
#43663=CARTESIAN_POINT ( 'NONE',  ( -0.6823417656250246877, -0.6364583329919113464, 1.181850606188755259 ) ) ;
#43668=CARTESIAN_POINT ( 'NONE',  ( -1.402160292154681736E-14, -0.6781249996585819728, 1.575800808251672791 ) ) ;
#43670=CARTESIAN_POINT ( 'NONE',  ( -7.660520486921249983, 8.896027641951645748, -1.199719254218446718 ) ) ;
#43672=CARTESIAN_POINT ( 'NONE',  ( 8.565000355531088516, 11.01558638625153286, -1.599625672291257406 ) ) ;
#43678=CARTESIAN_POINT ( 'NONE',  ( -1.364683531250014514, -0.1989583329919157317, -0.7879004041258359514 ) ) ;
#43685=CARTESIAN_POINT ( 'NONE',  ( 6.127922243696800386, 10.09306701771420656, -0.7216878364870267237 ) ) ;
#43689=CARTESIAN_POINT ( 'NONE',  ( -4.283486466913726254, 7.084819080452935403, -1.199719254218452047 ) ) ;
#43691=CARTESIAN_POINT ( 'NONE',  ( -1.001543065824772872E-14, 4.993750000682814161, 1.732050807568877637 ) ) ;
#43694=CARTESIAN_POINT ( 'NONE',  ( 4.433153041544209749, 7.155467067568137551, -1.082531754730548412 ) ) ;
#43695=CARTESIAN_POINT ( 'NONE',  ( -9.286972035236630063, 10.89751746493999107, -1.082531754730537976 ) ) ;
#43700=CARTESIAN_POINT ( 'NONE',  ( 10.24960094225127172, 11.06021530882240356, -0.7216878364870257245 ) ) ;
#43706=VERTEX_POINT ( 'NONE', #28960 ) ;
#43715=CARTESIAN_POINT ( 'NONE',  ( 9.856414487010592751, 10.60149777770828194, 0.7216878364870438212 ) ) ;
#43718=CARTESIAN_POINT ( 'NONE',  ( 6.889514614038635187, 11.18951748302043114, -0.7998128361456291469 ) ) ;
#43722=CARTESIAN_POINT ( 'NONE',  ( 4.663641653420880218, 8.384739662392275861, -0.7216878364870207285 ) ) ;
#43723=EDGE_LOOP ( 'NONE', ( #214133, #57195, #6772 ) ) ;
#43724=CARTESIAN_POINT ( 'NONE',  ( -8.758204044748012507, 11.24099069033793974, 1.443375672974064550 ) ) ;
#43728=CARTESIAN_POINT ( 'NONE',  ( -2.266184231778562541, 5.795632037050281404, 1.040834085586084257E-14 ) ) ;
#43730=EDGE_CURVE ( 'NONE', #40788, #168810, #60670, .T. ) ;
#43755=CARTESIAN_POINT ( 'NONE',  ( -8.527715433315703919, 9.051348881730875817, 1.040834085586084257E-14 ) ) ;
#43760=CARTESIAN_POINT ( 'NONE',  ( 4.801558957534076022, 8.753569217098425170, 0.7998128361456462443 ) ) ;
#43765=CARTESIAN_POINT ( 'NONE',  ( -3.815730167242251003, 6.539103397502874948, -1.199719254218452047 ) ) ;
#43769=CARTESIAN_POINT ( 'NONE',  ( -5.739179097286464248, 5.590130456455974617, -0.7998128361456221525 ) ) ;
#43772=CARTESIAN_POINT ( 'NONE',  ( 7.670162217029129259, 9.971608557999250166, 1.599625672291281386 ) ) ;
#43775=CARTESIAN_POINT ( 'NONE',  ( 5.624517712206933417, 6.335738387217328516, 1.153896037602806013 ) ) ;
#43776=CARTESIAN_POINT ( 'NONE',  ( 3.958617665510264949, 5.641473247893851628, -1.443375672974051449 ) ) ;
#43784=CARTESIAN_POINT ( 'NONE',  ( 6.358410854684775515, 8.441231968597481483, -1.443375672974058777 ) ) ;
#43785=CARTESIAN_POINT ( 'NONE',  ( -8.188234707649510113, 11.64035869464474082, -1.199719254218446718 ) ) ;
#43789=CARTESIAN_POINT ( 'NONE',  ( -7.808606406466886973, 11.19745900993164511, 1.199719254218453823 ) ) ;
#43790=CARTESIAN_POINT ( 'NONE',  ( -6.470265622219711688, 8.571729197388226140, -1.599625672291263179 ) ) ;
#43797=CARTESIAN_POINT ( 'NONE',  ( 6.414979237560321401, 10.63589287712906462, 1.040834085586084257E-14 ) ) ;
#43804=FACE_OUTER_BOUND ( 'NONE', #152053, .T. ) ;
#43809=CARTESIAN_POINT ( 'NONE',  ( 0.7499999999999902300, 4.816666666666684193, -1.299038105676658228 ) ) ;
#43810=CARTESIAN_POINT ( 'NONE',  ( 4.299907273828439180, 8.168308919441841454, 1.040834085586084257E-14 ) ) ;
#43811=CARTESIAN_POINT ( 'NONE',  ( 6.470265622219697477, 8.571729197388226140, -1.599625672291262513 ) ) ;
#43813=CARTESIAN_POINT ( 'NONE',  ( 4.363950690066983107, 4.004001632660354915, -0.1812806842866887536 ) ) ;
#43814=CARTESIAN_POINT ( 'NONE',  ( 7.293923454472080792, 9.532663335016016148, 1.443375672974076540 ) ) ;
#43815=CARTESIAN_POINT ( 'NONE',  ( -9.286972035236626510, 11.85788667924133399, -1.443375672974058777 ) ) ;
#43818=CARTESIAN_POINT ( 'NONE',  ( 8.239604668803105270, 10.63595808506888396, -1.599625672291268286 ) ) ;
#43820=CARTESIAN_POINT ( 'NONE',  ( -4.600294193738529103, 4.261431402316699035, -0.7998128361456221525 ) ) ;
#43821=CARTESIAN_POINT ( 'NONE',  ( -1.364683531250012516, 1.530208333674756505, 0.7879004041258379498 ) ) ;
#43825=EDGE_CURVE ( 'NONE', #192556, #13744, #200356, .T. ) ;
#43827=CARTESIAN_POINT ( 'NONE',  ( -1.402160292154681736E-14, -0.4281249996585808071, 1.575800808251672791 ) ) ;
#43829=CARTESIAN_POINT ( 'NONE',  ( 9.561524646135536543, 12.17819805862340310, -1.599625672291262513 ) ) ;
#43833=CARTESIAN_POINT ( 'NONE',  ( -3.267151830768959098, 4.834763107362302748, -1.443375672974058777 ) ) ;
#43836=CARTESIAN_POINT ( 'NONE',  ( -5.605406444246153974, 8.627059054007450101, -1.199719254218440723 ) ) ;
#43839=CARTESIAN_POINT ( 'NONE',  ( 4.650610384687404952, 5.384465856012134566, 1.199719254218462483 ) ) ;
#43845=ADVANCED_FACE ( 'NONE', ( #67807 ), #167531, .F. ) ;
#43848=CARTESIAN_POINT ( 'NONE',  ( 9.596473800374404561, 10.09030761005864285, 0.000000000000000000 ) ) ;
#43850=CARTESIAN_POINT ( 'NONE',  ( 0.8858701160440104472, 2.800000000000024247, -1.189311836856266735 ) ) ;
#43851=CARTESIAN_POINT ( 'NONE',  ( -4.229253852459088137, 7.021547696922494808, 1.199719254218464037 ) ) ;
#43855=CARTESIAN_POINT ( 'NONE',  ( 7.065770611016287006, 11.39514947949436774, 1.040834085586084257E-14 ) ) ;
#43857=CARTESIAN_POINT ( 'NONE',  ( 8.586391356156291010, 8.911878091804165791, 0.7998128361456481317 ) ) ;
#43860=CARTESIAN_POINT ( 'NONE',  ( -3.195971524519394702, 4.751719416737803847, -1.599625672291262513 ) ) ;
#43866=CARTESIAN_POINT ( 'NONE',  ( -5.937252720508472414, 6.122620518184580973, 0.7955437839095025332 ) ) ;
#43867=CARTESIAN_POINT ( 'NONE',  ( -1.364683531250012516, 2.030208333674750953, 0.7879004041258379498 ) ) ;
#43870=CARTESIAN_POINT ( 'NONE',  ( 4.826339496784873617, 8.574553812983598533, -0.7216878364870257245 ) ) ;
#43884=CARTESIAN_POINT ( 'NONE',  ( 5.151735183068521629, 5.112705256442466428, 1.040834085586084257E-14 ) ) ;
#43888=CARTESIAN_POINT ( 'NONE',  ( 9.420217803396747414, 9.884675613584706255, 0.7998128361456462443 ) ) ;
#43892=CARTESIAN_POINT ( 'NONE',  ( -4.796887421136680985, 4.490790167614548523, 1.214306433183764966E-14 ) ) ;
#43893=CARTESIAN_POINT ( 'NONE',  ( -6.398558430645608475, 9.552403038140164782, -1.199719254218440723 ) ) ;
#43898=CARTESIAN_POINT ( 'NONE',  ( 0.7499999999999902300, 4.097916667349481123, -1.299038105676658228 ) ) ;
#43899=CARTESIAN_POINT ( 'NONE',  ( 8.749089199520284410, 9.101692242395490240, 0.7998128361456481317 ) ) ;
#43902=CARTESIAN_POINT ( 'NONE',  ( -6.530223543276495235, 10.77034456713125188, -0.7998128361456291469 ) ) ;
#43904=CARTESIAN_POINT ( 'NONE',  ( 1.364683531249988535, 4.155208333674753618, -0.7879004041258239610 ) ) ;
#43907=CARTESIAN_POINT ( 'NONE',  ( -3.094265954482842140, 2.800000000000024691, -2.490342512183689294 ) ) ;
#43909=CARTESIAN_POINT ( 'NONE',  ( -8.026063749610047537, 11.34719622697832264, -1.082531754730543971 ) ) ;
#43913=CARTESIAN_POINT ( 'NONE',  ( 1.364683531249986537, 2.467708333674753174, -0.7879004041258239610 ) ) ;
#43921=CARTESIAN_POINT ( 'NONE',  ( 1.364683531249990311, 3.384375000341416140, 1.214306433183764966E-14 ) ) ;
#43923=CARTESIAN_POINT ( 'NONE',  ( -5.773074481320628948, 5.629675071162500544, 0.000000000000000000 ) ) ;
#43924=CARTESIAN_POINT ( 'NONE',  ( 5.449487677688982679, 8.445153826357429949, -1.199719254218446718 ) ) ;
#43927=CARTESIAN_POINT ( 'NONE',  ( 1.364683531249990311, 4.696875000341417916, 1.214306433183764966E-14 ) ) ;
#43930=CARTESIAN_POINT ( 'NONE',  ( -1.602468905319636405E-14, -1.053124999658583638, -1.575800808251665908 ) ) ;
#43931=CARTESIAN_POINT ( 'NONE',  ( -4.446711195602255806, 5.250546485366484717, -1.082531754730544860 ) ) ;
#43934=CARTESIAN_POINT ( 'NONE',  ( 3.497640442645619796, 6.064035702186436616, -1.082531754730543083 ) ) ;
#43937=CARTESIAN_POINT ( 'NONE',  ( -9.327646496521984076, 11.90534021740758064, -1.443375672974059665 ) ) ;
#43942=CARTESIAN_POINT ( 'NONE',  ( -8.123306592882240551, 12.62894145833798376, 0.000000000000000000 ) ) ;
#43943=CARTESIAN_POINT ( 'NONE',  ( -5.043269954159181445, 8.827639346586952485, 1.214306433183764966E-14 ) ) ;
#43945=CARTESIAN_POINT ( 'NONE',  ( -1.364683531250014514, 0.3010416670080866552, -0.7879004041258359514 ) ) ;
#43951=CARTESIAN_POINT ( 'NONE',  ( -1.402160292154681736E-14, -0.8656249996585829720, 1.575800808251672791 ) ) ;
#43958=CARTESIAN_POINT ( 'NONE',  ( -1.402160292154681736E-14, -0.4124999999999747202, -1.732050807568870754 ) ) ;
#43959=CARTESIAN_POINT ( 'NONE',  ( 8.066738210006679566, 10.43428054980638997, 1.443375672974076540 ) ) ;
#43968=CARTESIAN_POINT ( 'NONE',  ( 5.281064527722868718, 6.119995689553514140, 1.199719254218462483 ) ) ;
#43970=CARTESIAN_POINT ( 'NONE',  ( -4.090809663021341969, 5.795697244990093644, 1.599625672291267398 ) ) ;
#43973=CARTESIAN_POINT ( 'NONE',  ( -1.402160292154681736E-14, 1.759375000341421469, -1.575800808251659024 ) ) ;
#43983=EDGE_LOOP ( 'NONE', ( #61017, #13443, #126013, #22351 ) ) ;
#43993=CARTESIAN_POINT ( 'NONE',  ( 5.198661835836162481, 8.152523677529138979, 1.199719254218462483 ) ) ;
#44002=CARTESIAN_POINT ( 'NONE',  ( 9.423080456697809026, 10.95234760669099749, -1.199719254218446718 ) ) ;
#44010=CARTESIAN_POINT ( 'NONE',  ( -0.1341411654175228285, 8.212692222353540572, 2.039118504324687553 ) ) ;
#44014=CARTESIAN_POINT ( 'NONE',  ( -7.863365906246048809, 12.11775129068834289, -0.7216878364870267237 ) ) ;
#44021=CARTESIAN_POINT ( 'NONE',  ( 5.015626762051672571, 7.938982758113895422, 1.199719254218462483 ) ) ;
#44022=CARTESIAN_POINT ( 'NONE',  ( -4.218512253981381299, 3.978430757497701364, -0.5307291018261834914 ) ) ;
#44027=CARTESIAN_POINT ( 'NONE',  ( 4.378920427089557421, 5.171457255435017331, -1.082531754730548412 ) ) ;
#44035=CARTESIAN_POINT ( 'NONE',  ( -5.368138756007025947, 8.350246751061767725, 1.199719254218452047 ) ) ;
#44037=CARTESIAN_POINT ( 'NONE',  ( -4.946027110887008860, 4.664786472323266153, -0.7998128361456221525 ) ) ;
#44042=CARTESIAN_POINT ( 'NONE',  ( 0.5160254906862444813, 7.984099418343982180, -1.935262202534223208 ) ) ;
#44046=CARTESIAN_POINT ( 'NONE',  ( 5.660692828905515839, 6.562895374266609849, -1.199719254218445830 ) ) ;
#44048=CARTESIAN_POINT ( 'NONE',  ( 1.515977770626730781, 8.685538819012467826, 2.532029653471363773 ) ) ;
#44053=TOROIDAL_SURFACE ( 'NONE', #40650, 0.8300000000000010703, 0.08000000000000000167 ) ;
#44060=CARTESIAN_POINT ( 'NONE',  ( -0.6823417656250003738, 1.030208333674752286, -1.181850606188749264 ) ) ;
#44062=CARTESIAN_POINT ( 'NONE',  ( 4.379447312414087357, 5.068108938359919158, -1.199719254218452047 ) ) ;
#44065=CARTESIAN_POINT ( 'NONE',  ( -6.073689629242158716, 9.069426419882418600, -1.082531754730538864 ) ) ;
#44066=CARTESIAN_POINT ( 'NONE',  ( 3.212919216758630014, 6.692230152952963529, 0.000000000000000000 ) ) ;
#44067=CARTESIAN_POINT ( 'NONE',  ( -4.894130264408858899, 8.653643041878236630, -0.7216878364870207285 ) ) ;
#44071=CARTESIAN_POINT ( 'NONE',  ( 4.638861114170084399, 8.563755066507100722, 0.7998128361456462443 ) ) ;
#44076=CARTESIAN_POINT ( 'NONE',  ( -1.364683531250010295, 4.530208333674754506, 0.7879004041258379498 ) ) ;
#44081=CARTESIAN_POINT ( 'NONE',  ( 6.337546739384100292, 9.481222731668410120, 1.199719254218460707 ) ) ;
#44083=CARTESIAN_POINT ( 'NONE',  ( -6.191269702934848240, 10.37489842006599616, 0.000000000000000000 ) ) ;
#44088=CARTESIAN_POINT ( 'NONE',  ( 9.237182729612253951, 9.671134694169463586, 0.7998128361456462443 ) ) ;
#44091=CARTESIAN_POINT ( 'NONE',  ( -6.906989191158078079, 10.14557225873805812, -1.199719254218440723 ) ) ;
#44094=CARTESIAN_POINT ( 'NONE',  ( 7.171900071504736296, 9.390302721554109056, -1.443375672974058777 ) ) ;
#44095=CARTESIAN_POINT ( 'NONE',  ( 4.067188154045468629, 7.737431308562400467, -0.5659913801023385149 ) ) ;
#44096=CARTESIAN_POINT ( 'NONE',  ( -9.815740026613960723, 11.51441345488021106, -1.082531754730539753 ) ) ;
#44101=CARTESIAN_POINT ( 'NONE',  ( 5.497994985541524215, 6.373081223675282736, -1.199719254218445830 ) ) ;
#44103=CARTESIAN_POINT ( 'NONE',  ( 8.432281472695482449, 11.92507992053172572, 1.199719254218450271 ) ) ;
#44104=CARTESIAN_POINT ( 'NONE',  ( -5.672026259827416261, 6.146810915570031675, 0.7861540255039052294 ) ) ;
#44105=CARTESIAN_POINT ( 'NONE',  ( -0.6823417656250003738, 0.7177083336747519526, -1.181850606188749264 ) ) ;
#44107=CARTESIAN_POINT ( 'NONE',  ( -6.182154858151506893, 9.195969186943299789, 1.082531754730548412 ) ) ;
#44108=ORIENTED_EDGE ( 'NONE', *, *, #98529, .F. ) ;
#44113=CARTESIAN_POINT ( 'NONE',  ( -4.274576072154308903, 7.290118009659216192, 0.9321895248279310486 ) ) ;
#44114=CARTESIAN_POINT ( 'NONE',  ( 0.6823417656249882723, 0.1552083336747514530, 1.181850606188755259 ) ) ;
#44117=CARTESIAN_POINT ( 'NONE',  ( 3.226477370372302644, 5.747678784534228313, 1.082531754730546636 ) ) ;
#44121=CARTESIAN_POINT ( 'NONE',  ( -8.365017589507372620, 9.821903944922480534, 1.082531754730558626 ) ) ;
#44128=CARTESIAN_POINT ( 'NONE',  ( -9.951321562306267410, 10.71222269888655987, 1.040834085586084257E-14 ) ) ;
#44134=CARTESIAN_POINT ( 'NONE',  ( -8.961576348508652146, 10.51788916375733685, -1.082531754730543083 ) ) ;
#44138=CARTESIAN_POINT ( 'NONE',  ( 1.364683531249988535, 5.467708333674750953, -0.7879004041258300672 ) ) ;
#44139=CARTESIAN_POINT ( 'NONE',  ( 0.7499999999999902300, 4.847916667349482012, -1.299038105676658228 ) ) ;
#44140=CARTESIAN_POINT ( 'NONE',  ( 5.125043568333415678, 6.701081866602433657, -1.409791652392645700 ) ) ;
#44144=ORIENTED_EDGE ( 'NONE', *, *, #30090, .T. ) ;
#44146=CARTESIAN_POINT ( 'NONE',  ( -8.182509401047415309, 9.505014708432145909, 1.199719254218462483 ) ) ;
#44147=DIRECTION ( 'NONE',  ( 1.000000000000000000, 0.000000000000000000, 0.000000000000000000 ) ) ;
#44150=CARTESIAN_POINT ( 'NONE',  ( 5.834086172582112262, 5.700855377634248100, 1.040834085586084257E-14 ) ) ;
#44155=CARTESIAN_POINT ( 'NONE',  ( 6.286176778230493589, 10.48562334124426698, 0.7998128361456462443 ) ) ;
#44163=CARTESIAN_POINT ( 'NONE',  ( -5.422898255786193111, 8.310169817517122581, -1.082531754730544860 ) ) ;
#44167=EDGE_CURVE ( 'NONE', #166401, #73904, #42676, .T. ) ;
#44174=CARTESIAN_POINT ( 'NONE',  ( -8.143643823302737061, 12.65266822716189843, 0.000000000000000000 ) ) ;
#44176=CARTESIAN_POINT ( 'NONE',  ( 8.398386088661320414, 11.88553530582519357, -1.199719254218446718 ) ) ;
#44177=CARTESIAN_POINT ( 'NONE',  ( -1.500000000000001332, -0.8499999999999757749, 0.000000000000000000 ) ) ;
#44178=CARTESIAN_POINT ( 'NONE',  ( -7.771848369131641121, 10.09024240211882351, -1.599625672291263179 ) ) ;
#44181=CARTESIAN_POINT ( 'NONE',  ( -1.364683531250012516, 3.530208333674758059, 0.7879004041258379498 ) ) ;
#44182=CARTESIAN_POINT ( 'NONE',  ( 3.063252641683779753, 5.661212951017999373, 1.199719254218450271 ) ) ;
#44185=CARTESIAN_POINT ( 'NONE',  ( -1.001543065824772872E-14, 4.962500000000019007, 1.732050807568877637 ) ) ;
#44188=CARTESIAN_POINT ( 'NONE',  ( 7.565086526301031178, 11.76975868075249387, 1.040834085586084257E-14 ) ) ;
#44191=CARTESIAN_POINT ( 'NONE',  ( -6.914295153289458540, 7.169025221700239925, 0.7216878364870317197 ) ) ;
#44193=CARTESIAN_POINT ( 'NONE',  ( 0.6823417656249899377, 2.092708333674753174, 1.181850606188767472 ) ) ;
#44195=CARTESIAN_POINT ( 'NONE',  ( 4.161989969715261140, 4.726297878971393196, -7.499999999999991118 ) ) ;
#44197=CARTESIAN_POINT ( 'NONE',  ( -7.314787569772770226, 8.492672571945082183, -1.199719254218452935 ) ) ;
#44198=CARTESIAN_POINT ( 'NONE',  ( -0.6823417656250212460, 4.863541667008086655, 1.181850606188767472 ) ) ;
#44205=CARTESIAN_POINT ( 'NONE',  ( 8.398386088661320414, 11.88553530582519357, -1.199719254218446718 ) ) ;
#44208=CARTESIAN_POINT ( 'NONE',  ( -1.500000000000013101, 1.670833333333355153, 0.8660254037844403729 ) ) ;
#44213=ADVANCED_FACE ( 'NONE', ( #88597 ), #73261, .T. ) ;
#44214=CARTESIAN_POINT ( 'NONE',  ( 9.154780037725547714, 11.70366268214508487, 1.599625672291279388 ) ) ;
#44219=CARTESIAN_POINT ( 'NONE',  ( -1.522480120926886116, 8.691153603980712461, 2.524399069149781294 ) ) ;
#44221=CARTESIAN_POINT ( 'NONE',  ( -4.910230551782461816, 4.674830742458788713, -0.3039354299698590056 ) ) ;
#44222=CARTESIAN_POINT ( 'NONE',  ( -0.6823417656250246877, -0.9489583329919115684, 1.181850606188755259 ) ) ;
#44226=CARTESIAN_POINT ( 'NONE',  ( -4.013798184412302739, 7.796799554311066416, 0.4460873486146191835 ) ) ;
#44227=CARTESIAN_POINT ( 'NONE',  ( 8.782984583554449998, 9.141236857102018831, 1.040834085586084257E-14 ) ) ;
#44230=CARTESIAN_POINT ( 'NONE',  ( -0.6823417656250212460, 3.801041667008085767, 1.181850606188767472 ) ) ;
#44232=CARTESIAN_POINT ( 'NONE',  ( -6.914295153289458540, 7.169025221700239925, 0.7216878364870317197 ) ) ;
#44238=CARTESIAN_POINT ( 'NONE',  ( 4.376584659113025744, 4.000436945253625254, 0.7998128361456341429 ) ) ;
#44241=CARTESIAN_POINT ( 'NONE',  ( 8.697719238366680372, 10.10609285197134533, 1.199719254218462483 ) ) ;
#44247=CARTESIAN_POINT ( 'NONE',  ( -7.648771216403934758, 12.07531685244661723, -0.7998128361456291469 ) ) ;
#44248=CARTESIAN_POINT ( 'NONE',  ( 6.307567778855705853, 8.381915046796901692, -1.599625672291262513 ) ) ;
#44252=CARTESIAN_POINT ( 'NONE',  ( 5.172599298813543633, 5.993452922492633839, -1.199719254218452047 ) ) ;
#44253=ORIENTED_EDGE ( 'NONE', *, *, #45961, .F. ) ;
#44259=CARTESIAN_POINT ( 'NONE',  ( -6.426201623197489887, 6.599582769926260362, 0.7216878364870317197 ) ) ;
#44260=CARTESIAN_POINT ( 'NONE',  ( 3.334415713957098681, 5.977569868670206787, -1.199719254218446718 ) ) ;
#44264=CARTESIAN_POINT ( 'NONE',  ( -7.802881099864745984, 9.062115023719057305, -1.199719254218446718 ) ) ;
#44267=B_SPLINE_CURVE_WITH_KNOTS ( 'NONE', 3,
 ( #167486, #49472, #165345, #202074, #37476, #66742, #36404, #131831, #16941, #21196 ),
 .UNSPECIFIED., .F., .F.,
 ( 4, 3, 3, 4 ),
 ( 7.376790794998995890E-17, 3.125231531348378344E-05, 6.250486059666306160E-05, 0.0001052831138300465999 ),
 .UNSPECIFIED. ) ;
#44271=CARTESIAN_POINT ( 'NONE',  ( -9.318531651294266638, 9.766041769465124034, -0.7998128361456291469 ) ) ;
#44275=CARTESIAN_POINT ( 'NONE',  ( 7.771848369131631351, 10.09024240211882351, -1.599625672291262513 ) ) ;
#44276=CARTESIAN_POINT ( 'NONE',  ( 5.717788096661236885, 7.693838750903348789, 1.599625672291267398 ) ) ;
#44287=CARTESIAN_POINT ( 'NONE',  ( -8.518600588087975822, 8.832788862391110385, 1.040834085586084257E-14 ) ) ;
#44291=CARTESIAN_POINT ( 'NONE',  ( 4.989037340148863464, 8.764367963574922982, -0.7216878364870257245 ) ) ;
#44294=CARTESIAN_POINT ( 'NONE',  ( 1.000000000000003553, 6.400000000000022560, 1.214306433183764966E-14 ) ) ;
#44296=CARTESIAN_POINT ( 'NONE',  ( -6.573005544526917099, 6.562927978236513304, -0.7998128361456291469 ) ) ;
#44306=CARTESIAN_POINT ( 'NONE',  ( 7.588813295347141441, 9.876701482703580837, -1.599625672291262513 ) ) ;
#44308=CARTESIAN_POINT ( 'NONE',  ( -3.795919822146293754, 4.491289883001181593, -1.082531754730549967 ) ) ;
#44310=CARTESIAN_POINT ( 'NONE',  ( -5.251027302601237956, 6.428042375187708934, -1.158707231040608576 ) ) ;
#44318=CARTESIAN_POINT ( 'NONE',  ( 4.369805582306193870, 3.992528022312320957, 1.214306433183764966E-14 ) ) ;
#44325=CARTESIAN_POINT ( 'NONE',  ( 3.167801447087334576, 6.847518788243868393, -0.7998128361456291469 ) ) ;
#44337=CARTESIAN_POINT ( 'NONE',  ( -6.112028321662274166, 6.025121218227761588, 0.7998128361456341429 ) ) ;
#44339=CARTESIAN_POINT ( 'NONE',  ( 4.921246571636183731, 7.724909519342112674, -1.082531754730549078 ) ) ;
#44340=CARTESIAN_POINT ( 'NONE',  ( -1.201851678989727383E-14, 3.712500000000020339, 1.732050807568877637 ) ) ;
#44342=CARTESIAN_POINT ( 'NONE',  ( -3.262708522383007903, 6.958243709422141876, 1.040834085586084257E-14 ) ) ;
#44343=CARTESIAN_POINT ( 'NONE',  ( -1.420000000000056550, 7.240846818246208905, -4.154462424328208670 ) ) ;
#44346=CARTESIAN_POINT ( 'NONE',  ( -0.6823417656249969321, 4.467708333674755394, -1.181850606188749264 ) ) ;
#44349=CARTESIAN_POINT ( 'NONE',  ( -4.148431816101615155, 3.942184661647709198, 0.7216878364870317197 ) ) ;
#44354=CARTESIAN_POINT ( 'NONE',  ( 3.032219910950674890, 6.689340329417765574, 0.7998128361456321445 ) ) ;
#44361=CARTESIAN_POINT ( 'NONE',  ( -1.402160292154681736E-14, 0.7593750003414168059, -1.575800808251659024 ) ) ;
#44364=CARTESIAN_POINT ( 'NONE',  ( -9.982881178363895103, 10.54111621771303753, 1.040834085586084257E-14 ) ) ;
#44365=CARTESIAN_POINT ( 'NONE',  ( -4.080641047588902559, 7.704572288921609058, -0.7216878364870257245 ) ) ;
#44369=CARTESIAN_POINT ( 'NONE',  ( -0.6823417656249969321, 4.717708333674755394, -1.181850606188749264 ) ) ;
#44377=CARTESIAN_POINT ( 'NONE',  ( -6.534666851662457532, 6.726125536468730459, 1.040834085586084257E-14 ) ) ;
#44382=CARTESIAN_POINT ( 'NONE',  ( -7.022760381754429737, 7.295567988242705582, 1.040834085586084257E-14 ) ) ;
#44386=( BOUNDED_CURVE ( )  B_SPLINE_CURVE ( 2, ( #128057, #45663, #113919, #110710, #147419, #94419, #160458 ),
 .UNSPECIFIED., .F., .F. ) 
 B_SPLINE_CURVE_WITH_KNOTS ( ( 3, 2, 2, 3 ),
 ( 0.1999999999999999556, 0.2041666666666666630, 0.2083333333333333981, 0.2125000000000001055 ),
 .UNSPECIFIED. ) 
 CURVE ( )  GEOMETRIC_REPRESENTATION_ITEM ( )  RATIONAL_B_SPLINE_CURVE ( ( 1.000000000000001776, 0.8660254037844369313, 1.000000000000000000, 0.8660254037844387076, 1.000000000000000000, 0.8660254037844351549, 1.000000000000003553 ) ) 
 REPRESENTATION_ITEM ( '' )  );
#44390=CARTESIAN_POINT ( 'NONE',  ( 5.341549334104194635, 6.294524313618772737, 1.082531754730558626 ) ) ;
#44396=CARTESIAN_POINT ( 'NONE',  ( -3.079673448598517549, 6.744702790006905424, 1.040834085586084257E-14 ) ) ;
#44399=CARTESIAN_POINT ( 'NONE',  ( 0.7499999999999885647, 0.8166666666666877461, -1.299038105676652899 ) ) ;
#44400=EDGE_LOOP ( 'NONE', ( #102833, #3199, #16383, #206716 ) ) ;
#44403=CARTESIAN_POINT ( 'NONE',  ( 8.242994207428692377, 12.56065097540143327, -0.7216878364870328300 ) ) ;
#44404=CARTESIAN_POINT ( 'NONE',  ( 7.969495366734495434, 8.192166104145387706, 1.040834085586084257E-14 ) ) ;
#44409=CARTESIAN_POINT ( 'NONE',  ( 4.059776932288224671, 6.823824623389866950, 1.199719254218462483 ) ) ;
#44411=CARTESIAN_POINT ( 'NONE',  ( -0.5473748313345772054, 7.493086169160624976, -1.923660786605011497 ) ) ;
#44418=CARTESIAN_POINT ( 'NONE',  ( 7.587759525142423911, 12.00413654597487501, 0.7998128361456462443 ) ) ;
#44420=CARTESIAN_POINT ( 'NONE',  ( -4.740547266272593596, 8.682388910626682943, -0.7998128361456281477 ) ) ;
#44426=CARTESIAN_POINT ( 'NONE',  ( 1.364683531249988535, 3.405208333674749621, -0.7879004041258239610 ) ) ;
#44427=CARTESIAN_POINT ( 'NONE',  ( 7.849807752188022292, 11.14156422998596696, -1.082531754730543083 ) ) ;
#44428=CARTESIAN_POINT ( 'NONE',  ( -7.739006755302186846, 7.923262724141010516, 0.7998128361456462443 ) ) ;
#44431=CARTESIAN_POINT ( 'NONE',  ( 4.981731378017507872, 7.899438143407371271, -1.199719254218452047 ) ) ;
#44432=CARTESIAN_POINT ( 'NONE',  ( -6.112028321662274166, 6.025121218227761588, 0.7998128361456341429 ) ) ;
#44436=CARTESIAN_POINT ( 'NONE',  ( 1.499999999999987121, 1.035416667349484232, 0.8660254037844524744 ) ) ;
#44439=CARTESIAN_POINT ( 'NONE',  ( 7.998947442382716488, 9.394822106610419610, -1.082531754730543083 ) ) ;
#44442=CARTESIAN_POINT ( 'NONE',  ( -1.402160292154681736E-14, 2.259375000341416140, -1.575800808251660134 ) ) ;
#44444=CARTESIAN_POINT ( 'NONE',  ( 6.453317929980448397, 6.631218461173066459, 1.040834085586084257E-14 ) ) ;
#44447=CARTESIAN_POINT ( 'NONE',  ( -2.982430605326321427, 6.423326772948587227, -0.7216878364870267237 ) ) ;
#44455=CARTESIAN_POINT ( 'NONE',  ( -4.038103646828244742, 7.764432012698684105, 0.5462726908427618655 ) ) ;
#44463=CARTESIAN_POINT ( 'NONE',  ( 6.388916700537700777, 8.476822122092563916, 1.599625672291281386 ) ) ;
#44466=CARTESIAN_POINT ( 'NONE',  ( 2.846322183865124700, 5.408127416896231665, -1.199719254218446718 ) ) ;
#44474=CARTESIAN_POINT ( 'NONE',  ( 5.016153647376212277, 5.914896012436124728, 1.082531754730558626 ) ) ;
#44475=CARTESIAN_POINT ( 'NONE',  ( -1.364683531250012516, 2.301041667008087988, -0.7879004041258289570 ) ) ;
#44476=CARTESIAN_POINT ( 'NONE',  ( 7.588813295347141441, 9.876701482703580837, -1.599625672291262513 ) ) ;
#44484=CARTESIAN_POINT ( 'NONE',  ( 0.7499999999999902300, 3.483333333333352044, 1.299038105676669330 ) ) ;
#44485=CARTESIAN_POINT ( 'NONE',  ( 5.799137018343234473, 7.788745826199009237, -1.599625672291262513 ) ) ;
#44486=CARTESIAN_POINT ( 'NONE',  ( -6.852756576703439961, 10.08230087520760954, 1.199719254218453823 ) ) ;
#44490=CARTESIAN_POINT ( 'NONE',  ( -1.364683531249997417, 3.009375000341422801, 1.214306433183764966E-14 ) ) ;
#44493=CARTESIAN_POINT ( 'NONE',  ( 3.440018289565364817, 5.036440642624797626, 1.599625672291267398 ) ) ;
#44499=CARTESIAN_POINT ( 'NONE',  ( 0.7499999999999885647, 0.5979166673494851203, -1.299038105676652899 ) ) ;
#44501=CARTESIAN_POINT ( 'NONE',  ( -5.181187258716735577, 9.196468901811520880, 0.7998128361456481317 ) ) ;
#44502=CARTESIAN_POINT ( 'NONE',  ( -4.175548123328963079, 4.934189567714277302, 1.082531754730560403 ) ) ;
#44510=CARTESIAN_POINT ( 'NONE',  ( 6.322179702674084467, 6.270297829408224111, 1.040834085586084257E-14 ) ) ;
#44511=CARTESIAN_POINT ( 'NONE',  ( -1.420000000000001039, 6.280000000000042881, -2.873333333333329520 ) ) ;
#44514=CARTESIAN_POINT ( 'NONE',  ( 4.984594031318565932, 8.967110136513669616, 0.7998128361456462443 ) ) ;
#44518=CARTESIAN_POINT ( 'NONE',  ( -6.663996196316808174, 7.733415969579778171, -1.199719254218446718 ) ) ;
#44519=CARTESIAN_POINT ( 'NONE',  ( 3.704402285031850539, 5.344888637335695414, -1.599625672291262513 ) ) ;
#44524=DIRECTION ( 'NONE',  ( 0.6507913734559640506, -0.7592566023653004592, 0.000000000000000000 ) ) ;
#44525=CARTESIAN_POINT ( 'NONE',  ( 4.574835874639041400, 6.943354005153362429, 1.191215277921169324 ) ) ;
#44533=CARTESIAN_POINT ( 'NONE',  ( -2.467220768007014176, 5.822248629409386922, 0.7216878364870317197 ) ) ;
#44534=CARTESIAN_POINT ( 'NONE',  ( 7.619319141200063150, 9.912291636198670375, 1.443375672974076540 ) ) ;
#44538=CARTESIAN_POINT ( 'NONE',  ( -4.660252114795309097, 6.460046772059735432, -1.599625672291256295 ) ) ;
#44539=CARTESIAN_POINT ( 'NONE',  ( -0.3384797366876900471, 6.551676121695759747, 3.195407356336833260 ) ) ;
#44541=CARTESIAN_POINT ( 'NONE',  ( 8.769426429940780920, 9.125419011219408461, 0.7998128361456462443 ) ) ;
#44543=CARTESIAN_POINT ( 'NONE',  ( -5.636439174979254396, 7.598931675607687453, -1.599625672291256295 ) ) ;
#44556=CARTESIAN_POINT ( 'NONE',  ( 10.24726517383036928, 10.84956421242393887, 0.000000000000000000 ) ) ;
#44557=CARTESIAN_POINT ( 'NONE',  ( -4.229253852459088137, 7.021547696922494808, 1.199719254218464037 ) ) ;
#44560=CARTESIAN_POINT ( 'NONE',  ( 3.958617665510264949, 5.641473247893851628, -1.443375672974051449 ) ) ;
#44565=CARTESIAN_POINT ( 'NONE',  ( -1.408489644590935175, 7.311701683603598845, 4.382268911471428829 ) ) ;
#44566=CARTESIAN_POINT ( 'NONE',  ( -2.754277761870538299, 6.365074488824250309, 1.040834085586084257E-14 ) ) ;
#44570=CARTESIAN_POINT ( 'NONE',  ( 9.999301985278609806, 11.62460605670194447, 1.199719254218452047 ) ) ;
#44575=CARTESIAN_POINT ( 'NONE',  ( -7.874588291438845644, 8.081441182967111558, -0.7998128361456291469 ) ) ;
#44576=CARTESIAN_POINT ( 'NONE',  ( 4.822949958159288286, 6.649860922651058992, -1.599625672291256295 ) ) ;
#44578=CARTESIAN_POINT ( 'NONE',  ( 5.196852952739812181, 4.957416621151552683, -0.7998128361456221525 ) ) ;
#44581=CARTESIAN_POINT ( 'NONE',  ( -1.364683531250012516, 0.8427083336747532849, 0.7879004041258379498 ) ) ;
#44584=CARTESIAN_POINT ( 'NONE',  ( 7.971831135155394321, 8.402817200543854170, -0.7216878364870267237 ) ) ;
#44590=ORIENTED_EDGE ( 'NONE', *, *, #7040, .T. ) ;
#44591=CARTESIAN_POINT ( 'NONE',  ( 9.422553571373278203, 11.05569592376608945, -1.082531754730543083 ) ) ;
#44597=CARTESIAN_POINT ( 'NONE',  ( -9.480175724453545172, 12.08329098332774265, 1.599625672291281386 ) ) ;
#44606=DIRECTION ( 'NONE',  ( 1.224646799147360603E-16, 1.000000000000000000, -8.546850786086437571E-32 ) ) ;
#44614=CARTESIAN_POINT ( 'NONE',  ( -1.500000000000013101, 1.660416667349487119, -0.8660254037844313801 ) ) ;
#44620=CARTESIAN_POINT ( 'NONE',  ( -0.7500000000000249800, -0.5583333333333134751, 1.299038105676659116 ) ) ;
#44621=CARTESIAN_POINT ( 'NONE',  ( 8.372323551638698902, 9.726464550788689323, 1.199719254218462483 ) ) ;
#44622=CARTESIAN_POINT ( 'NONE',  ( -1.364683531250014514, -1.219791666325248602, 0.7879004041258379498 ) ) ;
#44625=CARTESIAN_POINT ( 'NONE',  ( 2.184835310096557404, 5.700724961754617404, 1.040834085586084257E-14 ) ) ;
#44626=CARTESIAN_POINT ( 'NONE',  ( -5.368665641331555882, 8.246898433986675769, 1.082531754730548412 ) ) ;
#44631=CARTESIAN_POINT ( 'NONE',  ( -7.019370843573183194, 9.212351955633947043, 1.599625672291283607 ) ) ;
#44633=VERTEX_POINT ( 'NONE', #100892 ) ;
#44634=CARTESIAN_POINT ( 'NONE',  ( -0.7500000000000215383, 1.472916667349486008, 1.299038105676659116 ) ) ;
#44647=CARTESIAN_POINT ( 'NONE',  ( -8.748035429315585532, 11.22912730566677553, -1.599625672291263179 ) ) ;
#44648=CARTESIAN_POINT ( 'NONE',  ( 5.282873410819217241, 9.315102745931094219, -0.7998128361456281477 ) ) ;
#44655=CARTESIAN_POINT ( 'NONE',  ( -6.808165692356648258, 11.09461040772476714, 0.7998128361456481317 ) ) ;
#44658=CARTESIAN_POINT ( 'NONE',  ( -1.000000000000017097, 9.200000000000018829, 0.4000000000000144551 ) ) ;
#44662=CARTESIAN_POINT ( 'NONE',  ( 3.734381245560244089, 6.444196322207211836, 1.199719254218462483 ) ) ;
#44668=CARTESIAN_POINT ( 'NONE',  ( -9.972185678051314284, 11.59297036493672017, 1.199719254218462483 ) ) ;
#44671=CARTESIAN_POINT ( 'NONE',  ( -5.067137445304809695, 6.740953878067043270, -1.444057985504534125 ) ) ;
#44680=CARTESIAN_POINT ( 'NONE',  ( 6.765682348419287173, 7.852049813699357728, 1.199719254218462483 ) ) ;
#44683=AXIS2_PLACEMENT_3D ( 'NONE', #53748, #150196, #119881 ) ;
#44686=DIRECTION ( 'NONE',  ( -5.578564026256490882E-16, -1.000000000000000000, -9.066213480720158442E-32 ) ) ;
#44691=CARTESIAN_POINT ( 'NONE',  ( -0.7500000000000006661, 0.8895833340161543035, -1.299038105676652011 ) ) ;
#44694=CARTESIAN_POINT ( 'NONE',  ( -1.506334365903787775, 8.679455619938881483, -2.541882285198141300 ) ) ;
#44703=CARTESIAN_POINT ( 'NONE',  ( 3.212919216758630014, 6.692230152952963529, 0.000000000000000000 ) ) ;
#44707=CARTESIAN_POINT ( 'NONE',  ( -8.947491310014823895, 12.52615806407091803, 1.199719254218462483 ) ) ;
#44709=CARTESIAN_POINT ( 'NONE',  ( 9.561524646135536543, 12.17819805862340310, -1.599625672291262513 ) ) ;
#44718=CARTESIAN_POINT ( 'NONE',  ( 1.364683531249986537, -0.09479166632524321789, -0.7879004041258309554 ) ) ;
#44723=CARTESIAN_POINT ( 'NONE',  ( -5.066996723205291708, 6.934582148538044777, 1.599625672291267398 ) ) ;
#44726=AXIS2_PLACEMENT_3D ( 'NONE', #173488, #77012, #43486 ) ;
#44727=CARTESIAN_POINT ( 'NONE',  ( 0.7499999999999885647, 0.2333333333333562076, 1.299038105676657340 ) ) ;
#44729=CARTESIAN_POINT ( 'NONE',  ( 1.364683531249986537, -0.5739583329919174526, 0.7879004041258500513 ) ) ;
#44735=CIRCLE ( 'NONE', #176141, 1.000000000000000000 ) ;
#44736=CARTESIAN_POINT ( 'NONE',  ( 0.6823417656249917140, 5.405208333674749177, 1.181850606188765695 ) ) ;
#44738=CARTESIAN_POINT ( 'NONE',  ( -8.799405390469187793, 10.22472669609091689, -1.199719254218446718 ) ) ;
#44743=EDGE_LOOP ( 'NONE', ( #174783, #12672, #21165, #182775, #136680 ) ) ;
#44745=CARTESIAN_POINT ( 'NONE',  ( -0.6823417656250246877, 0.3635416670080895973, 1.181850606188755259 ) ) ;
#44754=CARTESIAN_POINT ( 'NONE',  ( 7.049876689426101350, 9.247942109129029475, -1.443375672974057666 ) ) ;
#44757=CARTESIAN_POINT ( 'NONE',  ( -4.608882153641705059, 7.464447381635583412, -1.199719254218452047 ) ) ;
#44759=CARTESIAN_POINT ( 'NONE',  ( -1.500000000000011324, 4.910416667349486453, -0.8660254037844313801 ) ) ;
#44761=CARTESIAN_POINT ( 'NONE',  ( -4.939248034080176097, 4.656877549381960080, 1.214306433183764966E-14 ) ) ;
#44762=CARTESIAN_POINT ( 'NONE',  ( 6.941411460072420603, 7.200660912947041581, 1.040834085586084257E-14 ) ) ;
#44763=CARTESIAN_POINT ( 'NONE',  ( -8.148087131688679818, 12.44992605370473804, -0.7216878364870267237 ) ) ;
#44769=CARTESIAN_POINT ( 'NONE',  ( 2.198393463710220264, 5.716542807637226886, 0.7998128361456462443 ) ) ;
#44771=EDGE_CURVE ( 'NONE', #50158, #121448, #3465, .T. ) ;
#44775=CARTESIAN_POINT ( 'NONE',  ( -1.500000000000055511, 7.240846818246208905, -4.154462424328210446 ) ) ;
#44776=VERTEX_POINT ( 'NONE', #200509 ) ;
#44786=CARTESIAN_POINT ( 'NONE',  ( 7.727257484784855635, 11.10255193463598111, -1.199719254218446718 ) ) ;
#44788=CARTESIAN_POINT ( 'NONE',  ( -1.500000000000021982, 7.388542872122518368, 4.154462424328226433 ) ) ;
#44791=CARTESIAN_POINT ( 'NONE',  ( 0.6823417656249882723, -0.3239583329919110133, -1.181850606188749264 ) ) ;
#44792=CARTESIAN_POINT ( 'NONE',  ( 4.853455804012212660, 7.645820290447483458, 1.082531754730558626 ) ) ;
#44795=CARTESIAN_POINT ( 'NONE',  ( -7.687109909268394325, 11.91211929421440097, 0.000000000000000000 ) ) ;
#44807=ORIENTED_EDGE ( 'NONE', *, *, #208519, .T. ) ;
#44815=CARTESIAN_POINT ( 'NONE',  ( 4.492266506575326446, 7.256230230409263626, -1.267781117195718288 ) ) ;
#44820=( BOUNDED_SURFACE ( )  B_SPLINE_SURFACE ( 3, 2, ( 
 ( #98483, #113738, #148310 ),
 ( #177614, #29225, #164548 ),
 ( #95317, #212209, #12949 ),
 ( #179743, #31361, #163492 ),
 ( #14006, #15074, #79027 ),
 ( #145143, #211149, #81165 ) ),
 .UNSPECIFIED., .F., .F., .T. ) 
 B_SPLINE_SURFACE_WITH_KNOTS ( ( 4, 2, 4 ),
 ( 3, 3 ),
 ( 0.000000000000000000, 0.002122857551078453833, 0.004245715102156907665 ),
 ( 0.000000000000000000, 1.000000000000000000 ),
 .UNSPECIFIED. ) 
 GEOMETRIC_REPRESENTATION_ITEM ( )  RATIONAL_B_SPLINE_SURFACE ( (
 ( 1.000000000000000000, 0.7806433624857551656, 1.000000000000000000),
 ( 1.000000000000000000, 0.7860453980259762830, 1.000000000000000000),
 ( 1.000000000000000000, 0.7924770197564222629, 1.000000000000000000),
 ( 1.000000000000000000, 0.8094762427233136437, 1.000000000000000000),
 ( 1.000000000000000000, 0.8200718518785207189, 1.000000000000000000),
 ( 1.000000000000000000, 0.8343063410434355953, 1.000000000000000000) ) ) 
 REPRESENTATION_ITEM ( '' )  SURFACE ( )  );
#44823=CARTESIAN_POINT ( 'NONE',  ( -7.375272376154093479, 9.627570410311676596, -1.443375672974059665 ) ) ;
#44827=CARTESIAN_POINT ( 'NONE',  ( 5.438792177376376991, 9.497007973581119700, 1.040834085586084257E-14 ) ) ;
#44828=CARTESIAN_POINT ( 'NONE',  ( -5.112968612895188336, 4.859551557999480131, -0.5494739808295947547 ) ) ;
#44831=CARTESIAN_POINT ( 'NONE',  ( -3.438964519360665051, 7.163875705896082913, -0.7998128361456281477 ) ) ;
#44835=CARTESIAN_POINT ( 'NONE',  ( -4.446184310277715213, 7.274633231044262516, -1.199719254218452047 ) ) ;
#44838=CARTESIAN_POINT ( 'NONE',  ( 5.030238685870051185, 5.827365540725222282, -1.199719254218452047 ) ) ;
#44839=CARTESIAN_POINT ( 'NONE',  ( 7.564559641420864899, 10.91273778404466199, -1.199719254218446718 ) ) ;
#44840=CARTESIAN_POINT ( 'NONE',  ( 0.4405300623744661803, 6.460114622649768990, 3.246819496866228505 ) ) ;
#44842=CARTESIAN_POINT ( 'NONE',  ( 4.121712324234096059, 7.667736414601909800, 0.7403736254629582625 ) ) ;
#44843=CARTESIAN_POINT ( 'NONE',  ( 5.680503174445848735, 5.729601246382692636, 1.040834085586084257E-14 ) ) ;
#44845=CARTESIAN_POINT ( 'NONE',  ( 4.161989969270892153, 6.839110149915929249, 1.082531754730558626 ) ) ;
#44850=CARTESIAN_POINT ( 'NONE',  ( 5.788968402910795064, 9.697620870130524651, 0.7216878364870438212 ) ) ;
#44851=CARTESIAN_POINT ( 'NONE',  ( -7.808606406466886973, 11.19745900993164511, 1.199719254218453823 ) ) ;
#44854=CARTESIAN_POINT ( 'NONE',  ( -8.188234707649510113, 11.64035869464474082, -1.199719254218446718 ) ) ;
#44856=CARTESIAN_POINT ( 'NONE',  ( -4.889686956022917919, 8.856385215335397021, 1.214306433183764966E-14 ) ) ;
#44864=CARTESIAN_POINT ( 'NONE',  ( 7.730120138085914583, 12.17022392774227768, 0.7998128361456462443 ) ) ;
#44868=CARTESIAN_POINT ( 'NONE',  ( 5.183294799126148433, 4.941598775268944976, 1.040834085586084257E-14 ) ) ;
#44872=CARTESIAN_POINT ( 'NONE',  ( 1.499999999999989120, 5.577083334016153415, -0.8660254037844323793 ) ) ;
#44878=CARTESIAN_POINT ( 'NONE',  ( -0.7500000000000006661, 2.608333333333358262, -1.299038105676652011 ) ) ;
#44879=CARTESIAN_POINT ( 'NONE',  ( 5.880485940025228508, 7.883652901494672349, 1.599625672291267398 ) ) ;
#44883=CARTESIAN_POINT ( 'NONE',  ( 6.914295153289432783, 10.05013286460426691, -1.082531754730537976 ) ) ;
#44884=CARTESIAN_POINT ( 'NONE',  ( 0.1467296397388196671, 8.209138825498294878, 2.038183423090501378 ) ) ;
#44887=CARTESIAN_POINT ( 'NONE',  ( 7.242026607993941489, 11.60078147596829901, 0.7998128361456462443 ) ) ;
#44890=CARTESIAN_POINT ( 'NONE',  ( -3.684065054611367351, 5.321161868511784299, -1.599625672291256295 ) ) ;
#44892=CARTESIAN_POINT ( 'NONE',  ( -0.6823417656250003738, 0.4677083336747517306, -1.181850606188749264 ) ) ;
#44897=CARTESIAN_POINT ( 'NONE',  ( -1.364683531250000748, -0.2406249996585799189, 0.000000000000000000 ) ) ;
#44899=CARTESIAN_POINT ( 'NONE',  ( 7.736899214892750010, 12.17813285068358020, 1.040834085586084257E-14 ) ) ;
#44902=CARTESIAN_POINT ( 'NONE',  ( -4.243338890952911058, 5.013278796608906518, -1.082531754730543971 ) ) ;
#44905=CARTESIAN_POINT ( 'NONE',  ( -6.470265622219711688, 8.571729197388226140, -1.599625672291263179 ) ) ;
#44908=CARTESIAN_POINT ( 'NONE',  ( 3.018661757337009810, 6.673522483535157868, 0.000000000000000000 ) ) ;
#44914=CARTESIAN_POINT ( 'NONE',  ( 8.048736748007069508, 12.54194330598362406, -0.7998128361456352531 ) ) ;
#44917=CARTESIAN_POINT ( 'NONE',  ( -6.579784621333750749, 6.570836901177822931, 0.7998128361456341429 ) ) ;
#44921=CARTESIAN_POINT ( 'NONE',  ( 9.576136569953906275, 10.06658084123472641, 0.000000000000000000 ) ) ;
#44923=CARTESIAN_POINT ( 'NONE',  ( 9.426996880203592610, 9.892584536526015881, -0.7998128361456281477 ) ) ;
#44926=CARTESIAN_POINT ( 'NONE',  ( -9.110716038703348119, 12.61262389758715408, 1.082531754730560403 ) ) ;
#44929=CARTESIAN_POINT ( 'NONE',  ( -7.555971681517696936, 7.709721804725773175, 0.7998128361456462443 ) ) ;
#44933=CARTESIAN_POINT ( 'NONE',  ( -6.138286310890375574, 5.995785266799176227, -0.01092221066891288506 ) ) ;
#44934=CARTESIAN_POINT ( 'NONE',  ( 1.364683531249988757, 1.634375000341421691, 0.000000000000000000 ) ) ;
#44937=CARTESIAN_POINT ( 'NONE',  ( 7.782016984564060103, 9.141736572488651902, 1.082531754730558626 ) ) ;
#44955=CARTESIAN_POINT ( 'NONE',  ( 7.099665995050449041, 11.43469409420089455, 0.7998128361456462443 ) ) ;
#44957=VERTEX_POINT ( 'NONE', #5494 ) ;
#44959=CARTESIAN_POINT ( 'NONE',  ( -4.946027110887008860, 4.664786472323266153, -0.7998128361456221525 ) ) ;
#44960=CARTESIAN_POINT ( 'NONE',  ( -6.021792782764022078, 10.17717534653336209, -0.7998128361456291469 ) ) ;
#44965=CARTESIAN_POINT ( 'NONE',  ( -1.499999999999997780, 4.181250000682819490, 1.214306433183764966E-14 ) ) ;
#44966=CARTESIAN_POINT ( 'NONE',  ( 7.884230021546724920, 9.157022099014721306, 1.199719254218462483 ) ) ;
#44970=VECTOR ( 'NONE', #69169, 1000.000000000000000 ) ;
#44971=CARTESIAN_POINT ( 'NONE',  ( -7.395082721250053837, 10.71501471051202614, -1.199719254218446718 ) ) ;
#44973=CARTESIAN_POINT ( 'NONE',  ( 0.6823417656249899377, 2.842708333674753618, 1.181850606188765695 ) ) ;
#44977=CARTESIAN_POINT ( 'NONE',  ( -9.083599731475995753, 11.62061899152058686, 1.443375672974064550 ) ) ;
#44981=CARTESIAN_POINT ( 'NONE',  ( 0.6823417656249899377, 2.655208333674753618, 1.181850606188767472 ) ) ;
#44988=CARTESIAN_POINT ( 'NONE',  ( -0.6823417656250212460, 2.301041667008084435, 1.181850606188767472 ) ) ;
#44990=CARTESIAN_POINT ( 'NONE',  ( -4.843287188579803448, 6.673587691474970107, -1.599625672291256295 ) ) ;
#44991=CARTESIAN_POINT ( 'NONE',  ( 5.764187864104357573, 9.876636274763768597, 1.040834085586084257E-14 ) ) ;
#44994=CARTESIAN_POINT ( 'NONE',  ( 1.364683531249988535, 4.467708333674754506, -0.7879004041258300672 ) ) ;
#44997=CARTESIAN_POINT ( 'NONE',  ( -1.364683531250014514, 0.03020833367475737191, 0.7879004041258379498 ) ) ;
#44998=CARTESIAN_POINT ( 'NONE',  ( -3.606105671554953318, 7.150947683548662503, 0.7216878364870317197 ) ) ;
#45002=CARTESIAN_POINT ( 'NONE',  ( 4.636525346193557162, 7.392734756325715750, -1.082531754730549078 ) ) ;
#45006=CARTESIAN_POINT ( 'NONE',  ( -6.744291347794091784, 9.955758108146730123, -1.199719254218440723 ) ) ;
#45007=CARTESIAN_POINT ( 'NONE',  ( -8.595506201384022660, 11.05117653974661529, 1.443375672974064550 ) ) ;
#45013=CARTESIAN_POINT ( 'NONE',  ( -8.462260433223891098, 13.02438760540324481, -0.7998128361456281477 ) ) ;
#45014=CARTESIAN_POINT ( 'NONE',  ( -5.680503174001480637, 9.571078103069643461, 0.7216878364870458196 ) ) ;
#45016=CARTESIAN_POINT ( 'NONE',  ( 1.364683531249986537, -0.7822916663252464931, -0.7879004041258309554 ) ) ;
#45027=ORIENTED_EDGE ( 'NONE', *, *, #204793, .T. ) ;
#45029=CARTESIAN_POINT ( 'NONE',  ( 8.554831740098659765, 10.04335378727902395, 1.082531754730558626 ) ) ;
#45035=ORIENTED_EDGE ( 'NONE', *, *, #149161, .T. ) ;
#45038=CARTESIAN_POINT ( 'NONE',  ( 6.962275575817444384, 8.081408578997208991, -1.199719254218446718 ) ) ;
#45040=CARTESIAN_POINT ( 'NONE',  ( -2.754277761870538299, 6.365074488824250309, 1.040834085586084257E-14 ) ) ;
#45044=CARTESIAN_POINT ( 'NONE',  ( -0.6823417656250003738, 2.030208333674753174, -1.181850606188749264 ) ) ;
#45045=DIRECTION ( 'NONE',  ( 0.6507913734559640506, -0.7592566023653004592, 0.000000000000000000 ) ) ;
#45046=CARTESIAN_POINT ( 'NONE',  ( -6.984421689334302741, 11.30024240419870374, 0.000000000000000000 ) ) ;
#45066=CARTESIAN_POINT ( 'NONE',  ( 6.144869935491714230, 8.192100896205568361, -1.599625672291262513 ) ) ;
#45073=CARTESIAN_POINT ( 'NONE',  ( 8.229962938695207342, 9.560377169021284871, 1.199719254218462483 ) ) ;
#45077=CARTESIAN_POINT ( 'NONE',  ( 8.048736748007069508, 12.54194330598362406, -0.7998128361456352531 ) ) ;
#45079=CARTESIAN_POINT ( 'NONE',  ( -2.819205876637805641, 5.376491725131008259, -1.199719254218446718 ) ) ;
#45083=CARTESIAN_POINT ( 'NONE',  ( 8.550388431712704573, 13.12720360364021133, 0.000000000000000000 ) ) ;
#45084=CARTESIAN_POINT ( 'NONE',  ( 4.059580577656426215, 7.665954309842628156, -0.5688408669104396687 ) ) ;
#45085=CARTESIAN_POINT ( 'NONE',  ( -0.2184521437216538908, 7.205153265248401162, 1.990034439536109145 ) ) ;
#45091=CARTESIAN_POINT ( 'NONE',  ( -8.351459436338030784, 11.72682452816096976, -1.082531754730543971 ) ) ;
#45096=CARTESIAN_POINT ( 'NONE',  ( -9.110189153378817295, 12.71597221466224603, 1.199719254218462483 ) ) ;
#45097=CARTESIAN_POINT ( 'NONE',  ( 5.823390672269506574, 6.752709524857930745, -1.199719254218446718 ) ) ;
#45103=CARTESIAN_POINT ( 'NONE',  ( 2.535011535630975477, 5.901337858304024131, 0.7216878364870438212 ) ) ;
#45111=CARTESIAN_POINT ( 'NONE',  ( -5.357443255694392725, 9.402100898285455699, 0.000000000000000000 ) ) ;
#45113=CARTESIAN_POINT ( 'NONE',  ( -3.490334480514268645, 6.159475096320226939, -1.199719254218452935 ) ) ;
#45118=CARTESIAN_POINT ( 'NONE',  ( -1.284279953904156280, 2.921639714193936754, 0.7750000000000117906 ) ) ;
#45121=CARTESIAN_POINT ( 'NONE',  ( 4.625302960556422427, 8.547937220624488575, 1.040834085586084257E-14 ) ) ;
#45123=DIRECTION ( 'NONE',  ( 0.000000000000000000, 8.546850786086437571E-32, 1.000000000000000000 ) ) ;
#45132=ORIENTED_EDGE ( 'NONE', *, *, #208519, .F. ) ;
#45134=CARTESIAN_POINT ( 'NONE',  ( -1.402160292154681736E-14, 0.009375000341421267647, -1.575800808251665908 ) ) ;
#45136=CARTESIAN_POINT ( 'NONE',  ( 4.729096653068339151, 4.411700938201493116, -0.7998128361456211532 ) ) ;
#45138=CARTESIAN_POINT ( 'NONE',  ( -6.887178846062123938, 8.097758744236356776, -1.082531754730544860 ) ) ;
#45139=CARTESIAN_POINT ( 'NONE',  ( 4.039966587192250103, 7.657118751792200584, 0.7216878364870298324 ) ) ;
#45140=CARTESIAN_POINT ( 'NONE',  ( -6.358410854684777291, 10.36197039720016022, -0.7216878364870267237 ) ) ;
#45144=CARTESIAN_POINT ( 'NONE',  ( 7.122110765880372618, 7.203550736482235095, 0.7998128361456341429 ) ) ;
#45149=CARTESIAN_POINT ( 'NONE',  ( -1.001543065824772872E-14, 4.571875000341418804, 1.575800808251672791 ) ) ;
#45153=CARTESIAN_POINT ( 'NONE',  ( 7.416473721875251890, 8.611306416064660851, 1.199719254218462483 ) ) ;
#45156=CARTESIAN_POINT ( 'NONE',  ( -6.177711549321182716, 10.35908057418338402, 0.7998128361456481317 ) ) ;
#45161=CARTESIAN_POINT ( 'NONE',  ( 7.293396569147545527, 10.59638086639245280, 1.199719254218460707 ) ) ;
#45164=CARTESIAN_POINT ( 'NONE',  ( -8.362681821530818738, 8.650883634741092010, -0.7998128361456291469 ) ) ;
#45167=CARTESIAN_POINT ( 'NONE',  ( 7.090551149822735155, 9.295395646258437949, 1.443375672974076540 ) ) ;
#45168=CARTESIAN_POINT ( 'NONE',  ( 4.061730550730160871, 7.744580798899280971, -0.5443347154160914636 ) ) ;
#45169=CARTESIAN_POINT ( 'NONE',  ( -9.219181267612684749, 10.81842823604534765, 1.082531754730558626 ) ) ;
#45174=CARTESIAN_POINT ( 'NONE',  ( 6.962275575817444384, 8.081408578997208991, -1.199719254218446718 ) ) ;
#45176=CARTESIAN_POINT ( 'NONE',  ( 10.24048609702354717, 10.84165528948263457, -0.7998128361456281477 ) ) ;
#45177=CARTESIAN_POINT ( 'NONE',  ( -4.698067037153471404, 6.865000302791745668, 1.228424997642649563 ) ) ;
#45178=CARTESIAN_POINT ( 'NONE',  ( 4.681643115420508039, 4.356338477612361260, 0.7998128361456341429 ) ) ;
#45180=CARTESIAN_POINT ( 'NONE',  ( -6.643132081016132062, 8.773406732650713025, 1.443375672974078761 ) ) ;
#45186=CARTESIAN_POINT ( 'NONE',  ( -4.820845164874406841, 6.759277571458118139, 1.248045366310134741 ) ) ;
#45187=CARTESIAN_POINT ( 'NONE',  ( 1.364683531249988757, -0.05312499965857975237, 0.000000000000000000 ) ) ;
#45190=CARTESIAN_POINT ( 'NONE',  ( 4.880572111239557920, 4.796348339308675435, -0.7216878364870197293 ) ) ;
#45192=ADVANCED_FACE ( 'NONE', ( #2840 ), #130296, .T. ) ;
#45195=CARTESIAN_POINT ( 'NONE',  ( -7.795575137733361970, 12.03866206075687018, 0.7216878364870458196 ) ) ;
#45201=CARTESIAN_POINT ( 'NONE',  ( -9.964879715919934711, 10.72804054476916313, 0.7216878364870438212 ) ) ;
#45207=CARTESIAN_POINT ( 'NONE',  ( -8.812436658758329600, 9.383523644747281622, 1.040834085586084257E-14 ) ) ;
#45211=CARTESIAN_POINT ( 'NONE',  ( 1.364683531249992088, 5.696875000341418804, 1.214306433183764966E-14 ) ) ;
#45212=CARTESIAN_POINT ( 'NONE',  ( -1.500000000000013101, 4.160416667349482900, -0.8660254037844313801 ) ) ;
#45213=CARTESIAN_POINT ( 'NONE',  ( 5.250185332887272516, 6.604911474350376288, -1.376424501724478944 ) ) ;
#45218=CARTESIAN_POINT ( 'NONE',  ( -6.184490626128011925, 10.36698949712469364, -0.7998128361456291469 ) ) ;
#45221=DIRECTION ( 'NONE',  ( 1.000000000000000000, 0.000000000000000000, 0.000000000000000000 ) ) ;
#45222=CARTESIAN_POINT ( 'NONE',  ( 3.472859903394816872, 7.203420320602605287, -0.7998128361456291469 ) ) ;
#45227=CARTESIAN_POINT ( 'NONE',  ( 5.621827251160867789, 9.710548892996357040, 1.040834085586084257E-14 ) ) ;
#45234=CARTESIAN_POINT ( 'NONE',  ( -5.734735788900501952, 9.634349487118505806, 0.000000000000000000 ) ) ;
#45239=CARTESIAN_POINT ( 'NONE',  ( -5.889704870869313602, 5.973669892210054400, 0.3102931194572235429 ) ) ;
#45242=CARTESIAN_POINT ( 'NONE',  ( -7.669108446824431269, 12.09904362127053545, -0.7998128361456291469 ) ) ;
#45244=CARTESIAN_POINT ( 'NONE',  ( 8.235688245297327015, 11.69572115523387268, -1.199719254218446718 ) ) ;
#45245=CARTESIAN_POINT ( 'NONE',  ( -1.500000000000015099, -0.8291666666666407393, 0.8660254037844403729 ) ) ;
#45246=CARTESIAN_POINT ( 'NONE',  ( -9.677822722056413696, 10.18521468535430685, 1.040834085586084257E-14 ) ) ;
#45249=CARTESIAN_POINT ( 'NONE',  ( 0.6823417656249899377, 3.926041667008085767, -1.181850606188754593 ) ) ;
#45250=CARTESIAN_POINT ( 'NONE',  ( 8.568389894156670294, 12.94027927658408217, -0.7216878364870257245 ) ) ;
#45253=CARTESIAN_POINT ( 'NONE',  ( 1.499999999999989120, 5.795833333333350268, -0.8660254037844323793 ) ) ;
#45255=CARTESIAN_POINT ( 'NONE',  ( 8.310784975052673218, 10.71900177569337487, -1.443375672974063439 ) ) ;
#45258=CARTESIAN_POINT ( 'NONE',  ( -7.388830529767770550, 7.722649827591604677, 1.040834085586084257E-14 ) ) ;
#45259=CARTESIAN_POINT ( 'NONE',  ( 0.6823417656249882723, 2.426041667008084435, -1.181850606188749264 ) ) ;
#45263=CARTESIAN_POINT ( 'NONE',  ( -7.640183256500752584, 8.872300873127729304, -1.199719254218446718 ) ) ;
#45264=CARTESIAN_POINT ( 'NONE',  ( -4.595850884908229794, 4.464173575255435011, 0.7216878364870317197 ) ) ;
#45265=CARTESIAN_POINT ( 'NONE',  ( 0.6823417656249917140, 4.655208333674755394, 1.181850606188765695 ) ) ;
#45270=CARTESIAN_POINT ( 'NONE',  ( 9.908311333488716954, 10.45411806535867782, 0.7998128361456462443 ) ) ;
#45276=CARTESIAN_POINT ( 'NONE',  ( 10.57266086055835075, 11.22919251360659310, 0.000000000000000000 ) ) ;
#45281=CARTESIAN_POINT ( 'NONE',  ( 8.052653171512838881, 11.48218023581863001, -1.199719254218446718 ) ) ;
#45282=CARTESIAN_POINT ( 'NONE',  ( -1.525408907393426716, 8.692885148323941991, 2.521481920632497431 ) ) ;
#45286=CARTESIAN_POINT ( 'NONE',  ( 1.364683531249992088, 5.446875000341417916, 1.214306433183764966E-14 ) ) ;
#45290=CARTESIAN_POINT ( 'NONE',  ( 8.796542737168120851, 9.157054702984622097, -0.7998128361456211532 ) ) ;
#45291=CARTESIAN_POINT ( 'NONE',  ( 4.161361007603033180, 7.399433999391101580, -0.7812420967184935394 ) ) ;
#45293=CARTESIAN_POINT ( 'NONE',  ( 0.6823417656249899377, 3.426041667008085323, -1.181850606188754593 ) ) ;
#45295=CARTESIAN_POINT ( 'NONE',  ( -5.748293942514180799, 7.729428904398431222, -1.443375672974052559 ) ) ;
#45302=CARTESIAN_POINT ( 'NONE',  ( 2.758194185376297902, 5.305311418659259814, 1.199719254218452047 ) ) ;
#45305=CARTESIAN_POINT ( 'NONE',  ( 8.914649696185335870, 10.35917838609310593, -1.199719254218446718 ) ) ;
#45312=CARTESIAN_POINT ( 'NONE',  ( -9.481229494658258261, 9.955855920056455588, -0.7998128361456291469 ) ) ;
#45313=CARTESIAN_POINT ( 'NONE',  ( 7.630541526392844887, 7.796719957080126662, 0.7998128361456341429 ) ) ;
#45315=CARTESIAN_POINT ( 'NONE',  ( 4.487385655998885170, 5.298000022495898520, 1.082531754730560403 ) ) ;
#45317=CARTESIAN_POINT ( 'NONE',  ( 3.472859903394816872, 7.203420320602605287, -0.7998128361456291469 ) ) ;
#45325=EDGE_CURVE ( 'NONE', #17304, #154836, #143198, .T. ) ;
#45326=CARTESIAN_POINT ( 'NONE',  ( -7.076992996653451939, 7.358839372291564374, 0.7216878364870317197 ) ) ;
#45327=CARTESIAN_POINT ( 'NONE',  ( 3.846762897975340767, 5.510976019103107859, -1.599625672291256295 ) ) ;
#45330=CARTESIAN_POINT ( 'NONE',  ( -8.044065211609668253, 8.279164256499745633, 0.7998128361456602331 ) ) ;
#45336=CARTESIAN_POINT ( 'NONE',  ( -10.15913717534155047, 10.74674821418697057, 0.7998128361456462443 ) ) ;
#45340=CARTESIAN_POINT ( 'NONE',  ( 6.286176778230493589, 10.48562334124426698, 0.7998128361456462443 ) ) ;
#45341=CARTESIAN_POINT ( 'NONE',  ( 4.611744806942754238, 8.532119374741881757, -0.7998128361456231517 ) ) ;
#45342=CARTESIAN_POINT ( 'NONE',  ( -2.060660350336243063, 8.500464906087067618, -2.499999999999995559 ) ) ;
#45353=CARTESIAN_POINT ( 'NONE',  ( -7.426115451983156923, 9.686887332112256388, -1.599625672291263179 ) ) ;
#45357=CARTESIAN_POINT ( 'NONE',  ( 6.073689629242148058, 8.109057205581079231, -1.443375672974057666 ) ) ;
#45362=CARTESIAN_POINT ( 'NONE',  ( -6.738566041191992539, 7.820414121934134322, 1.199719254218450271 ) ) ;
#45374=CARTESIAN_POINT ( 'NONE',  ( 2.456316247939566821, 8.205176026796580757, 2.499999999999998668 ) ) ;
#45375=CARTESIAN_POINT ( 'NONE',  ( 7.426115451983150706, 9.686887332112256388, -1.599625672291262513 ) ) ;
#45377=CARTESIAN_POINT ( 'NONE',  ( -4.826339496784927796, 5.693446170079573321, 1.082531754730560403 ) ) ;
#45379=CARTESIAN_POINT ( 'NONE',  ( -4.957065645985164970, 6.648394846229956023, -1.245809975726259067 ) ) ;
#45380=( BOUNDED_CURVE ( )  B_SPLINE_CURVE ( 2, ( #100799, #18475, #147442, #68280, #16333, #82415, #148504 ),
 .UNSPECIFIED., .F., .T. ) 
 B_SPLINE_CURVE_WITH_KNOTS ( ( 3, 2, 2, 3 ),
 ( 0.05357142857142838110, 0.05952380952380941642, 0.06547619047619046562, 0.07142857142857149400 ),
 .UNSPECIFIED. ) 
 CURVE ( )  GEOMETRIC_REPRESENTATION_ITEM ( )  RATIONAL_B_SPLINE_CURVE ( ( 1.000000000000004219, 0.8660254037844345998, 1.000000000000000000, 0.8660254037844387076, 1.000000000000000000, 0.8660254037844371533, 1.000000000000001554 ) ) 
 REPRESENTATION_ITEM ( '' )  );
#45387=CARTESIAN_POINT ( 'NONE',  ( 10.56143847536557878, 11.42402576412244386, 0.000000000000000000 ) ) ;
#45393=CARTESIAN_POINT ( 'NONE',  ( 2.517010073631369860, 6.088262185878572375, -0.7998128361456281477 ) ) ;
#45397=CARTESIAN_POINT ( 'NONE',  ( 0.6823417656249899377, 3.488541667008085323, -1.181850606188754593 ) ) ;
#45398=( BOUNDED_SURFACE ( )  B_SPLINE_SURFACE ( 1, 2, ( 
 ( #189606, #73725, #75858, #139822, #107362, #24966, #157129, #8718, #74802, #140903, #206915, #58545, #92142, #9786, #61745, #177642, #125763, #196019, #112695, #176566, #14031, #191725, #96405, #63873, #160312, #10838, #11916, #210105, #113766, #79051, #29250, #110564, #144111, #59607, #161392, #130028, #97461, #95342, #193865, #28175, #43381, #12976, #30320, #109502, #143038, #178705, #179769, #80117, #162455, #175509, #127912, #47655, #209033, #77989, #31386, #141967, #62798, #163517, #212240, #45514, #146222, #44447, #145168, #211173, #128960, #194939, #46576, #15104, #27099, #207979, #93207, #111629, #94271, #60668, #159237, #76912, #126832, #192789, #164574, #198124, #48704, #99575, #67038, #972, #135292, #119085, #69173, #50821, #166710, #181867, #18300, #98512, #81193, #149390, #165640, #82244, #33503, #201307, #148335, #132114, #16158, #84386, #185065, #35623, #51897, #115882, #133175, #199175, #36690, #214335, #17228, #19369, #197066, #65965, #114818, #116947, #49755, #101701, #182946, #85449, #167771, #213303, #118020, #102776, #147270, #52947, #180816, #150473, #83303, #68103, #168832, #151534, #184009, #34562, #64928, #134239, #100633, #3102, #2033, #131078, #32443, #200246, #138487, #23642, #123388, #104925, #204509, #155799, #56158, #188278, #39918, #54024, #4170, #21484, #156874, #86519, #140647, #120162, #122321, #169895, #170966, #203440, #74548, #73463, #107104, #106027, #5233, #7383, #124449, #89750, #87593, #139564, #20436, #186138, #37773, #24708, #103847, #70240, #206660, #153665, #205591, #136355, #57228, #189353, #40993, #58293, #42064, #173127, #71308, #152584, #137421, #121243, #90810, #172049, #8461, #190408, #108178, #202375, #55094, #187213, #22566, #38842, #88671, #154731, #6314, #72388, #208786, #59353, #177381, #28995, #192537, #44191, #110311, #61488, #30060, #210921, #95082, #77736, #47397, #75610, #176319, #209849, #174204, #25777, #161130, #27924, #94019, #111377, #109253, #91889, #160058, #127653, #157944, #13788, #144914, #60417, #46323, #9536, #128710, #96150, #11662, #43140, #143857, #193617, #145971, #12717, #45258, #142780, #78791, #141721, #62547, #162201, #129778, #194680, #112439, #126577, #207730, #178452, #79862, #125509, #175261, #211983, #63623, #195759, #191472, #26846, #92950, #158996, #10590, #76666, #35370, #113510, #34305, #2850, #183761, #115621, #1787, #15910, #198920, #132915, #182686, #116687, #66774, #84129, #14846, #50566, #166451, #83053, #81993, #114573, #148081, #213050, #201052, #68919, #196817, #147027, #150215, #18042, #214086, #179519, #31137, #100380, #51646, #167518, #48459, #180565, #65714, #197869, #199997, #67844, #19115, #97212, #135039, #131862, #101445, #85194, #32187, #133990, #16972, #117770, #163264, #49501, #151278, #80936, #64678, #130825, #98263, #164321, #181617, #33246, #99328, #165379, #149129, #710, #120989, #122057, #170712, #140387, #168577, #54838, #88410, #52694, #118825, #55900, #186956, #38588, #204248, #202111, #184811, #104665, #154478, #36440, #106840, #23380, #87336, #139303, #102515, #7124, #189101, #71052, #136095, #137168, #22297, #24442, #188021, #6056, #21232, #72127, #20178, #138234, #40734, #8207, #39649, #105758, #153403, #86265, #171784, #155545, #152336, #53771, #89490, #90554, #205332, #73197, #3913, #56970, #172871, #119904, #203192, #156617, #69983, #123143, #74292, #185878, #37514, #103590, #169647, #4974, #11399, #61234, #209588, #159796, #177120, #107926, #143596, #45007, #176065, #108986, #207475, #175005, #91632, #79612, #95897, #75354, #25524, #28737, #111117, #92692, #206406, #124195, #77477, #144659, #46070, #141467, #59094, #26591, #76407, #78542, #94822, #112191, #190158, #161950, #158738, #194429, #178196, #125254, #160873, #110052, #210674, #41813, #10333, #12467, #13542, #127389, #62302, #193362, #191215, #173950, #42878, #128461, #142516, #29812, #208525, #60161, #157684, #58031, #9282, #126316, #192276, #43937, #93757, #27662, #182428, #47141, #131617, #67591, #212797, #15660, #133736, #145731, #66522, #35111, #1527, #147829, #34055, #48211, #16720, #165129, #454, #148881, #99076 ),
 ( #198670, #31941, #211731, #63369, #82805, #83867, #199743, #14595, #80691, #114323, #81747, #17779, #50317, #51389, #129525, #101182, #98025, #117510, #183503, #146782, #116435, #49260, #149958, #195505, #180321, #100128, #167271, #132665, #18856, #166190, #130579, #113258, #196569, #179263, #64435, #30886, #164080, #213848, #96964, #163012, #65466, #197616, #115381, #181375, #32999, #155285, #121798, #154217, #202936, #172611, #200798, #87076, #120727, #84940, #151029, #88150, #153146, #4721, #22039, #19927, #2598, #70796, #186700, #68667, #139048, #55642, #119645, #171523, #134791, #39396, #6866, #103331, #168332, #169394, #136909, #56716, #5789, #38329, #53510, #54579, #52449, #104405, #72945, #40479, #170454, #71866, #185628, #118575, #137975, #187766, #184561, #86013, #105491, #122885, #23116, #89233, #152087, #205074, #188843, #106583, #36182, #102258, #203994, #3657, #69735, #20979, #135839, #201864, #37261, #110864, #143340, #190959, #93506, #157433, #142266, #76161, #59909, #126063, #208277, #109806, #74035, #192026, #43689, #92449, #9026, #41554, #75101, #206153, #94573, #176870, #189909, #57780, #175815, #27408, #141211, #24187, #156360, #159547, #209334, #193108, #107667, #173695, #207222, #125002, #77221, #11144, #44757, #7945, #28482, #58846, #127136, #90291, #91373, #60982, #140126, #123941, #42624, #25271, #108734, #174762, #26335, #158488, #10087, #202557, #53135, #54209, #89926, #86702, #123567, #170077, #71496, #102957, #6496, #72571, #21664, #87770, #153846, #105108, #73650, #40094, #138671, #121423, #90991, #119266, #5417, #39025, #3291, #69359, #204691, #137607, #203623, #154912, #152771, #135467, #55274, #171148, #201489, #57402, #188463, #37958, #155977, #185251, #172233, #139749, #187393, #4352, #22739, #88857, #189530, #56341, #122502, #186323, #106207, #36875, #23821, #205774, #173307, #7564, #41178, #104031, #169016, #107285, #24886, #20614, #70420, #120347, #136538, #101272, #168416, #53598, #33090, #183590, #82893, #83955, #116523, #201943, #200884, #20013, #51474, #132753, #134877, #37345, #151117, #148968, #2684, #147919, #99164, #165217, #152173, #16808, #197707, #119733, #181460, #118664, #131702, #68755, #52530, #86099, #185711, #169480, #184647, #541, #213935, #66607, #34144, #3742, #117598, #18944, #167357, #85029, #65556, #36267, #102345, #150045, #21064, #49349, #69817, #115468, #135924, #182514, #50405, #198756, #166282, #133820, #67676, #103419, #100214, #17871, #35198, #1616, #199833, #172698, #104497, #87161, #155367, #171613, #88238, #39480, #207316, #154308, #138064, #170540, #24276, #125095, #41646, #57867, #121884, #139131, #6952, #191053, #22125, #187854, #25361, #203022, #5880, #120812, #205159, #71954, #107760, #122970, #91461, #173786, #4803, #124030, #108826, #153232, #58938, #54664, #90382, #204077, #74126, #42718, #157523, #189996, #188930, #174851, #140221, #73033, #9118, #89320, #75193, #141305, #105579, #56801, #156451, #70883, #23206, #40568, #8035, #106675, #206241, #136995, #186789, #38416, #55729, #60004, #78386, #11243, #198246, #62149, #33628, #116009, #158580, #66095, #50952, #92540, #149519, #208372, #32566, #93601, #16287, #133300, #49885, #132238, #128308, #67166, #82373, #160711, #165772, #28581, #181996, #17355, #44851, #144506, #98642, #99701, #110957, #210513, #164700, #194270, #45916, #112035, #126157, #159646, #83437, #178037, #1105, #199306, #192120, #148463, #175910, #176964, #209430, #117076, #31, #26430, #10179, #77321, #76254, #142363, #43785, #27501, #109898, #143434, #61075, #127234, #193204, #94669, #12305, #22684, #2159, #153785, #166838, #103976, #186264, #203567, #154854, #204634, #87713, #68236, #34687, #134370, #69299, #187339, #86644, #54152, #202501, #120290, #100756, #37899, #5354, #185192, #56285, #18434, #71436, #84510, #137548, #3234, #85572, #150597, #201433, #168957, #102898, #88796, #6438, #171090, #152711, #170018, #135411, #21606, #200374, #183075, #36817, #53073, #184132, #119207, #72515, #35755, #19497, #52022, #55219, #138611, #121364, #38968, #20561, #4294, #70365, #118147, #101830, #105054, #167898 ) ),
 .UNSPECIFIED., .F., .F., .F. ) 
 B_SPLINE_SURFACE_WITH_KNOTS ( ( 2, 2 ),
 ( 3, 2, 2, 2, 2, 2, 2, 2, 2, 2, 2, 2, 2, 2, 2, 2, 2, 2, 2, 2, 2, 2, 2, 2, 2, 2, 2, 2, 2, 2, 2, 2, 2, 2, 2, 2, 2, 2, 2, 2, 2, 2, 2, 2, 2, 2, 2, 2, 2, 2, 2, 2, 2, 2, 2, 2, 2, 2, 2, 2, 2, 2, 2, 2, 2, 2, 2, 2, 2, 2, 2, 2, 2, 2, 2, 2, 2, 2, 2, 2, 2, 2, 2, 2, 2, 2, 2, 2, 2, 2, 2, 2, 2, 2, 2, 2, 2, 2, 2, 2, 2, 2, 2, 2, 2, 2, 2, 2, 2, 2, 2, 2, 2, 2, 2, 2, 2, 2, 2, 2, 2, 2, 2, 2, 2, 2, 2, 2, 2, 2, 2, 2, 2, 2, 2, 2, 2, 2, 2, 2, 2, 2, 2, 2, 2, 2, 2, 2, 2, 2, 2, 2, 2, 2, 2, 2, 2, 2, 2, 2, 2, 2, 2, 2, 2, 2, 2, 2, 2, 2, 2, 2, 2, 2, 2, 2, 2, 2, 2, 2, 2, 2, 2, 2, 2, 2, 2, 2, 2, 2, 2, 2, 2, 2, 2, 2, 2, 2, 2, 2, 2, 2, 2, 2, 2, 2, 2, 2, 2, 2, 2, 2, 2, 2, 2, 2, 2, 2, 2, 2, 2, 2, 2, 2, 2, 2, 2, 2, 2, 2, 2, 2, 2, 2, 2, 2, 2, 2, 2, 2, 3 ),
 ( 0.000000000000000000, 1.000000000000000000 ),
 ( 0.000000000000000000, 0.004166666666666666609, 0.008333333333333333218, 0.01250000000000000069, 0.01666666666666666644, 0.02083333333333333218, 0.02500000000000000139, 0.02916666666666666713, 0.03333333333333333287, 0.03749999999999999861, 0.04166666666666666435, 0.04583333333333333010, 0.05000000000000000278, 0.05416666666666666852, 0.05833333333333333426, 0.06250000000000000000, 0.06666666666666666574, 0.07083333333333333148, 0.07499999999999999722, 0.07916666666666666297, 0.08333333333333332871, 0.08749999999999999445, 0.09166666666666666019, 0.09583333333333333981, 0.1000000000000000056, 0.1041666666666666713, 0.1083333333333333370, 0.1125000000000000028, 0.1166666666666666685, 0.1208333333333333343, 0.1250000000000000000, 0.1291666666666666796, 0.1333333333333333315, 0.1375000000000000111, 0.1416666666666666630, 0.1458333333333333426, 0.1499999999999999944, 0.1541666666666666741, 0.1583333333333333259, 0.1625000000000000056, 0.1666666666666666574, 0.1708333333333333370, 0.1749999999999999889, 0.1791666666666666685, 0.1833333333333333204, 0.1875000000000000000, 0.1916666666666666796, 0.1958333333333333315, 0.2000000000000000111, 0.2041666666666666630, 0.2083333333333333426, 0.2124999999999999944, 0.2166666666666666741, 0.2208333333333333259, 0.2250000000000000056, 0.2291666666666666574, 0.2333333333333333370, 0.2374999999999999889, 0.2416666666666666685, 0.2458333333333333204, 0.2500000000000000000, 0.2541666666666666519, 0.2583333333333333592, 0.2625000000000000111, 0.2666666666666666630, 0.2708333333333333148, 0.2750000000000000222, 0.2791666666666666741, 0.2833333333333333259, 0.2874999999999999778, 0.2916666666666666852, 0.2958333333333333370, 0.2999999999999999889, 0.3041666666666666408, 0.3083333333333333481, 0.3125000000000000000, 0.3166666666666666519, 0.3208333333333333592, 0.3250000000000000111, 0.3291666666666666630, 0.3333333333333333148, 0.3375000000000000222, 0.3416666666666666741, 0.3458333333333333259, 0.3499999999999999778, 0.3541666666666666852, 0.3583333333333333370, 0.3624999999999999889, 0.3666666666666666408, 0.3708333333333333481, 0.3750000000000000000, 0.3791666666666666519, 0.3833333333333333592, 0.3875000000000000111, 0.3916666666666666630, 0.3958333333333333148, 0.4000000000000000222, 0.4041666666666666741, 0.4083333333333333259, 0.4124999999999999778, 0.4166666666666666852, 0.4208333333333333370, 0.4249999999999999889, 0.4291666666666666408, 0.4333333333333333481, 0.4375000000000000000, 0.4416666666666666519, 0.4458333333333333592, 0.4500000000000000111, 0.4541666666666666630, 0.4583333333333333148, 0.4625000000000000222, 0.4666666666666666741, 0.4708333333333333259, 0.4749999999999999778, 0.4791666666666666852, 0.4833333333333333370, 0.4874999999999999889, 0.4916666666666666408, 0.4958333333333333481, 0.5000000000000000000, 0.5041666666666666519, 0.5083333333333333037, 0.5124999999999999556, 0.5166666666666667185, 0.5208333333333333703, 0.5250000000000000222, 0.5291666666666666741, 0.5333333333333333259, 0.5374999999999999778, 0.5416666666666666297, 0.5458333333333332815, 0.5500000000000000444, 0.5541666666666666963, 0.5583333333333333481, 0.5625000000000000000, 0.5666666666666666519, 0.5708333333333333037, 0.5749999999999999556, 0.5791666666666667185, 0.5833333333333333703, 0.5875000000000000222, 0.5916666666666666741, 0.5958333333333333259, 0.5999999999999999778, 0.6041666666666666297, 0.6083333333333332815, 0.6125000000000000444, 0.6166666666666666963, 0.6208333333333333481, 0.6250000000000000000, 0.6291666666666666519, 0.6333333333333333037, 0.6374999999999999556, 0.6416666666666667185, 0.6458333333333333703, 0.6500000000000000222, 0.6541666666666666741, 0.6583333333333333259, 0.6624999999999999778, 0.6666666666666666297, 0.6708333333333332815, 0.6750000000000000444, 0.6791666666666666963, 0.6833333333333333481, 0.6875000000000000000, 0.6916666666666666519, 0.6958333333333333037, 0.6999999999999999556, 0.7041666666666667185, 0.7083333333333333703, 0.7125000000000000222, 0.7166666666666666741, 0.7208333333333333259, 0.7249999999999999778, 0.7291666666666666297, 0.7333333333333332815, 0.7375000000000000444, 0.7416666666666666963, 0.7458333333333333481, 0.7500000000000000000, 0.7541666666666666519, 0.7583333333333333037, 0.7624999999999999556, 0.7666666666666667185, 0.7708333333333333703, 0.7750000000000000222, 0.7791666666666666741, 0.7833333333333333259, 0.7874999999999999778, 0.7916666666666666297, 0.7958333333333332815, 0.8000000000000000444, 0.8041666666666666963, 0.8083333333333333481, 0.8125000000000000000, 0.8166666666666666519, 0.8208333333333333037, 0.8249999999999999556, 0.8291666666666667185, 0.8333333333333333703, 0.8375000000000000222, 0.8416666666666666741, 0.8458333333333333259, 0.8499999999999999778, 0.8541666666666666297, 0.8583333333333332815, 0.8625000000000000444, 0.8666666666666666963, 0.8708333333333333481, 0.8750000000000000000, 0.8791666666666666519, 0.8833333333333333037, 0.8874999999999999556, 0.8916666666666667185, 0.8958333333333333703, 0.9000000000000000222, 0.9041666666666666741, 0.9083333333333333259, 0.9124999999999999778, 0.9166666666666666297, 0.9208333333333332815, 0.9250000000000000444, 0.9291666666666666963, 0.9333333333333333481, 0.9375000000000000000, 0.9416666666666666519, 0.9458333333333333037, 0.9499999999999999556, 0.9541666666666667185, 0.9583333333333333703, 0.9625000000000000222, 0.9666666666666666741, 0.9708333333333333259, 0.9749999999999999778, 0.9791666666666666297, 0.9833333333333332815, 0.9875000000000000444, 0.9916666666666666963, 0.9958333333333333481, 1.000000000000000000 ),
 .UNSPECIFIED. ) 
 GEOMETRIC_REPRESENTATION_ITEM ( )  RATIONAL_B_SPLINE_SURFACE ( (
 ( 1.000000000000000000, 0.8660254037844387076, 1.000000000000000000, 0.8660254037844387076, 1.000000000000000000, 0.8660254037844387076, 1.000000000000000000, 0.8660254037844387076, 1.000000000000000000, 0.8660254037844387076, 1.000000000000000000, 0.8660254037844387076, 1.000000000000000000, 0.8660254037844387076, 1.000000000000000000, 0.8660254037844387076, 1.000000000000000000, 0.8660254037844387076, 1.000000000000000000, 0.8660254037844387076, 1.000000000000000000, 0.8660254037844387076, 1.000000000000000000, 0.8660254037844387076, 1.000000000000000000, 0.8660254037844387076, 1.000000000000000000, 0.8660254037844387076, 1.000000000000000000, 0.8660254037844387076, 1.000000000000000000, 0.8660254037844387076, 1.000000000000000000, 0.8660254037844387076, 1.000000000000000000, 0.8660254037844387076, 1.000000000000000000, 0.8660254037844387076, 1.000000000000000000, 0.8660254037844387076, 1.000000000000000000, 0.8660254037844387076, 1.000000000000000000, 0.8660254037844387076, 1.000000000000000000, 0.8660254037844387076, 1.000000000000000000, 0.8660254037844387076, 1.000000000000000000, 0.8660254037844387076, 1.000000000000000000, 0.8660254037844387076, 1.000000000000000000, 0.8660254037844387076, 1.000000000000000000, 0.8660254037844387076, 1.000000000000000000, 0.8660254037844387076, 1.000000000000000000, 0.8660254037844387076, 1.000000000000000000, 0.8660254037844387076, 1.000000000000000000, 0.8660254037844387076, 1.000000000000000000, 0.8660254037844387076, 1.000000000000000000, 0.8660254037844387076, 1.000000000000000000, 0.8660254037844387076, 1.000000000000000000, 0.8660254037844387076, 1.000000000000000000, 0.8660254037844387076, 1.000000000000000000, 0.8660254037844387076, 1.000000000000000000, 0.8660254037844387076, 1.000000000000000000, 0.8660254037844387076, 1.000000000000000000, 0.8660254037844387076, 1.000000000000000000, 0.8660254037844387076, 1.000000000000000000, 0.8660254037844387076, 1.000000000000000000, 0.8660254037844387076, 1.000000000000000000, 0.8660254037844387076, 1.000000000000000000, 0.8660254037844387076, 1.000000000000000000, 0.8660254037844387076, 1.000000000000000000, 0.8660254037844387076, 1.000000000000000000, 0.8660254037844387076, 1.000000000000000000, 0.8660254037844387076, 1.000000000000000000, 0.8660254037844387076, 1.000000000000000000, 0.8660254037844387076, 1.000000000000000000, 0.8660254037844387076, 1.000000000000000000, 0.8660254037844387076, 1.000000000000000000, 0.8660254037844387076, 1.000000000000000000, 0.8660254037844387076, 1.000000000000000000, 0.8660254037844387076, 1.000000000000000000, 0.8660254037844387076, 1.000000000000000000, 0.8660254037844387076, 1.000000000000000000, 0.8660254037844387076, 1.000000000000000000, 0.8660254037844387076, 1.000000000000000000, 0.8660254037844387076, 1.000000000000000000, 0.8660254037844387076, 1.000000000000000000, 0.8660254037844387076, 1.000000000000000000, 0.8660254037844387076, 1.000000000000000000, 0.8660254037844387076, 1.000000000000000000, 0.8660254037844387076, 1.000000000000000000, 0.8660254037844387076, 1.000000000000000000, 0.8660254037844387076, 1.000000000000000000, 0.8660254037844387076, 1.000000000000000000, 0.8660254037844387076, 1.000000000000000000, 0.8660254037844387076, 1.000000000000000000, 0.8660254037844387076, 1.000000000000000000, 0.8660254037844387076, 1.000000000000000000, 0.8660254037844387076, 1.000000000000000000, 0.8660254037844387076, 1.000000000000000000, 0.8660254037844387076, 1.000000000000000000, 0.8660254037844387076, 1.000000000000000000, 0.8660254037844387076, 1.000000000000000000, 0.8660254037844387076, 1.000000000000000000, 0.8660254037844387076, 1.000000000000000000, 0.8660254037844387076, 1.000000000000000000, 0.8660254037844387076, 1.000000000000000000, 0.8660254037844387076, 1.000000000000000000, 0.8660254037844387076, 1.000000000000000000, 0.8660254037844387076, 1.000000000000000000, 0.8660254037844387076, 1.000000000000000000, 0.8660254037844387076, 1.000000000000000000, 0.8660254037844387076, 1.000000000000000000, 0.8660254037844387076, 1.000000000000000000, 0.8660254037844387076, 1.000000000000000000, 0.8660254037844387076, 1.000000000000000000, 0.8660254037844387076, 1.000000000000000000, 0.8660254037844387076, 1.000000000000000000, 0.8660254037844387076, 1.000000000000000000, 0.8660254037844387076, 1.000000000000000000, 0.8660254037844387076, 1.000000000000000000, 0.8660254037844387076, 1.000000000000000000, 0.8660254037844387076, 1.000000000000000000, 0.8660254037844387076, 1.000000000000000000, 0.8660254037844387076, 1.000000000000000000, 0.8660254037844387076, 1.000000000000000000, 0.8660254037844387076, 1.000000000000000000, 0.8660254037844387076, 1.000000000000000000, 0.8660254037844387076, 1.000000000000000000, 0.8660254037844387076, 1.000000000000000000, 0.8660254037844387076, 1.000000000000000000, 0.8660254037844387076, 1.000000000000000000, 0.8660254037844387076, 1.000000000000000000, 0.8660254037844387076, 1.000000000000000000, 0.8660254037844387076, 1.000000000000000000, 0.8660254037844387076, 1.000000000000000000, 0.8660254037844387076, 1.000000000000000000, 0.8660254037844387076, 1.000000000000000000, 0.8660254037844387076, 1.000000000000000000, 0.8660254037844387076, 1.000000000000000000, 0.8660254037844387076, 1.000000000000000000, 0.8660254037844387076, 1.000000000000000000, 0.8660254037844387076, 1.000000000000000000, 0.8660254037844387076, 1.000000000000000000, 0.8660254037844387076, 1.000000000000000000, 0.8660254037844387076, 1.000000000000000000, 0.8660254037844387076, 1.000000000000000000, 0.8660254037844387076, 1.000000000000000000, 0.8660254037844387076, 1.000000000000000000, 0.8660254037844387076, 1.000000000000000000, 0.8660254037844387076, 1.000000000000000000, 0.8660254037844387076, 1.000000000000000000, 0.8660254037844387076, 1.000000000000000000, 0.8660254037844387076, 1.000000000000000000, 0.8660254037844387076, 1.000000000000000000, 0.8660254037844387076, 1.000000000000000000, 0.8660254037844387076, 1.000000000000000000, 0.8660254037844387076, 1.000000000000000000, 0.8660254037844387076, 1.000000000000000000, 0.8660254037844387076, 1.000000000000000000, 0.8660254037844387076, 1.000000000000000000, 0.8660254037844387076, 1.000000000000000000, 0.8660254037844387076, 1.000000000000000000, 0.8660254037844387076, 1.000000000000000000, 0.8660254037844387076, 1.000000000000000000, 0.8660254037844387076, 1.000000000000000000, 0.8660254037844387076, 1.000000000000000000, 0.8660254037844387076, 1.000000000000000000, 0.8660254037844387076, 1.000000000000000000, 0.8660254037844387076, 1.000000000000000000, 0.8660254037844387076, 1.000000000000000000, 0.8660254037844387076, 1.000000000000000000, 0.8660254037844387076, 1.000000000000000000, 0.8660254037844387076, 1.000000000000000000, 0.8660254037844387076, 1.000000000000000000, 0.8660254037844387076, 1.000000000000000000, 0.8660254037844387076, 1.000000000000000000, 0.8660254037844387076, 1.000000000000000000, 0.8660254037844387076, 1.000000000000000000, 0.8660254037844387076, 1.000000000000000000, 0.8660254037844387076, 1.000000000000000000, 0.8660254037844387076, 1.000000000000000000, 0.8660254037844387076, 1.000000000000000000, 0.8660254037844387076, 1.000000000000000000, 0.8660254037844387076, 1.000000000000000000, 0.8660254037844387076, 1.000000000000000000, 0.8660254037844387076, 1.000000000000000000, 0.8660254037844387076, 1.000000000000000000, 0.8660254037844387076, 1.000000000000000000, 0.8660254037844387076, 1.000000000000000000, 0.8660254037844387076, 1.000000000000000000, 0.8660254037844387076, 1.000000000000000000, 0.8660254037844387076, 1.000000000000000000, 0.8660254037844387076, 1.000000000000000000, 0.8660254037844387076, 1.000000000000000000, 0.8660254037844387076, 1.000000000000000000, 0.8660254037844387076, 1.000000000000000000, 0.8660254037844387076, 1.000000000000000000, 0.8660254037844387076, 1.000000000000000000, 0.8660254037844387076, 1.000000000000000000, 0.8660254037844387076, 1.000000000000000000, 0.8660254037844387076, 1.000000000000000000, 0.8660254037844387076, 1.000000000000000000, 0.8660254037844387076, 1.000000000000000000, 0.8660254037844387076, 1.000000000000000000, 0.8660254037844387076, 1.000000000000000000, 0.8660254037844387076, 1.000000000000000000, 0.8660254037844387076, 1.000000000000000000, 0.8660254037844387076, 1.000000000000000000, 0.8660254037844387076, 1.000000000000000000, 0.8660254037844387076, 1.000000000000000000, 0.8660254037844387076, 1.000000000000000000, 0.8660254037844387076, 1.000000000000000000, 0.8660254037844387076, 1.000000000000000000, 0.8660254037844387076, 1.000000000000000000, 0.8660254037844387076, 1.000000000000000000, 0.8660254037844387076, 1.000000000000000000, 0.8660254037844387076, 1.000000000000000000, 0.8660254037844387076, 1.000000000000000000, 0.8660254037844387076, 1.000000000000000000, 0.8660254037844387076, 1.000000000000000000, 0.8660254037844387076, 1.000000000000000000, 0.8660254037844387076, 1.000000000000000000, 0.8660254037844387076, 1.000000000000000000, 0.8660254037844387076, 1.000000000000000000, 0.8660254037844387076, 1.000000000000000000, 0.8660254037844387076, 1.000000000000000000, 0.8660254037844387076, 1.000000000000000000, 0.8660254037844387076, 1.000000000000000000, 0.8660254037844387076, 1.000000000000000000, 0.8660254037844387076, 1.000000000000000000, 0.8660254037844387076, 1.000000000000000000, 0.8660254037844387076, 1.000000000000000000, 0.8660254037844387076, 1.000000000000000000, 0.8660254037844387076, 1.000000000000000000, 0.8660254037844387076, 1.000000000000000000, 0.8660254037844387076, 1.000000000000000000, 0.8660254037844387076, 1.000000000000000000, 0.8660254037844387076, 1.000000000000000000, 0.8660254037844387076, 1.000000000000000000, 0.8660254037844387076, 1.000000000000000000, 0.8660254037844387076, 1.000000000000000000, 0.8660254037844387076, 1.000000000000000000, 0.8660254037844387076, 1.000000000000000000, 0.8660254037844387076, 1.000000000000000000, 0.8660254037844387076, 1.000000000000000000, 0.8660254037844387076, 1.000000000000000000, 0.8660254037844387076, 1.000000000000000000, 0.8660254037844387076, 1.000000000000000000, 0.8660254037844387076, 1.000000000000000000, 0.8660254037844387076, 1.000000000000000000, 0.8660254037844387076, 1.000000000000000000, 0.8660254037844387076, 1.000000000000000000, 0.8660254037844387076, 1.000000000000000000, 0.8660254037844387076, 1.000000000000000000, 0.8660254037844387076, 1.000000000000000000, 0.8660254037844387076, 1.000000000000000000, 0.8660254037844387076, 1.000000000000000000, 0.8660254037844387076, 1.000000000000000000, 0.8660254037844387076, 1.000000000000000000, 0.8660254037844387076, 1.000000000000000000, 0.8660254037844387076, 1.000000000000000000, 0.8660254037844387076, 1.000000000000000000, 0.8660254037844387076, 1.000000000000000000),
 ( 1.000000000000000000, 0.8660254037844387076, 1.000000000000000000, 0.8660254037844387076, 1.000000000000000000, 0.8660254037844387076, 1.000000000000000000, 0.8660254037844387076, 1.000000000000000000, 0.8660254037844387076, 1.000000000000000000, 0.8660254037844387076, 1.000000000000000000, 0.8660254037844387076, 1.000000000000000000, 0.8660254037844387076, 1.000000000000000000, 0.8660254037844387076, 1.000000000000000000, 0.8660254037844387076, 1.000000000000000000, 0.8660254037844387076, 1.000000000000000000, 0.8660254037844387076, 1.000000000000000000, 0.8660254037844387076, 1.000000000000000000, 0.8660254037844387076, 1.000000000000000000, 0.8660254037844387076, 1.000000000000000000, 0.8660254037844387076, 1.000000000000000000, 0.8660254037844387076, 1.000000000000000000, 0.8660254037844387076, 1.000000000000000000, 0.8660254037844387076, 1.000000000000000000, 0.8660254037844387076, 1.000000000000000000, 0.8660254037844387076, 1.000000000000000000, 0.8660254037844387076, 1.000000000000000000, 0.8660254037844387076, 1.000000000000000000, 0.8660254037844387076, 1.000000000000000000, 0.8660254037844387076, 1.000000000000000000, 0.8660254037844387076, 1.000000000000000000, 0.8660254037844387076, 1.000000000000000000, 0.8660254037844387076, 1.000000000000000000, 0.8660254037844387076, 1.000000000000000000, 0.8660254037844387076, 1.000000000000000000, 0.8660254037844387076, 1.000000000000000000, 0.8660254037844387076, 1.000000000000000000, 0.8660254037844387076, 1.000000000000000000, 0.8660254037844387076, 1.000000000000000000, 0.8660254037844387076, 1.000000000000000000, 0.8660254037844387076, 1.000000000000000000, 0.8660254037844387076, 1.000000000000000000, 0.8660254037844387076, 1.000000000000000000, 0.8660254037844387076, 1.000000000000000000, 0.8660254037844387076, 1.000000000000000000, 0.8660254037844387076, 1.000000000000000000, 0.8660254037844387076, 1.000000000000000000, 0.8660254037844387076, 1.000000000000000000, 0.8660254037844387076, 1.000000000000000000, 0.8660254037844387076, 1.000000000000000000, 0.8660254037844387076, 1.000000000000000000, 0.8660254037844387076, 1.000000000000000000, 0.8660254037844387076, 1.000000000000000000, 0.8660254037844387076, 1.000000000000000000, 0.8660254037844387076, 1.000000000000000000, 0.8660254037844387076, 1.000000000000000000, 0.8660254037844387076, 1.000000000000000000, 0.8660254037844387076, 1.000000000000000000, 0.8660254037844387076, 1.000000000000000000, 0.8660254037844387076, 1.000000000000000000, 0.8660254037844387076, 1.000000000000000000, 0.8660254037844387076, 1.000000000000000000, 0.8660254037844387076, 1.000000000000000000, 0.8660254037844387076, 1.000000000000000000, 0.8660254037844387076, 1.000000000000000000, 0.8660254037844387076, 1.000000000000000000, 0.8660254037844387076, 1.000000000000000000, 0.8660254037844387076, 1.000000000000000000, 0.8660254037844387076, 1.000000000000000000, 0.8660254037844387076, 1.000000000000000000, 0.8660254037844387076, 1.000000000000000000, 0.8660254037844387076, 1.000000000000000000, 0.8660254037844387076, 1.000000000000000000, 0.8660254037844387076, 1.000000000000000000, 0.8660254037844387076, 1.000000000000000000, 0.8660254037844387076, 1.000000000000000000, 0.8660254037844387076, 1.000000000000000000, 0.8660254037844387076, 1.000000000000000000, 0.8660254037844387076, 1.000000000000000000, 0.8660254037844387076, 1.000000000000000000, 0.8660254037844387076, 1.000000000000000000, 0.8660254037844387076, 1.000000000000000000, 0.8660254037844387076, 1.000000000000000000, 0.8660254037844387076, 1.000000000000000000, 0.8660254037844387076, 1.000000000000000000, 0.8660254037844387076, 1.000000000000000000, 0.8660254037844387076, 1.000000000000000000, 0.8660254037844387076, 1.000000000000000000, 0.8660254037844387076, 1.000000000000000000, 0.8660254037844387076, 1.000000000000000000, 0.8660254037844387076, 1.000000000000000000, 0.8660254037844387076, 1.000000000000000000, 0.8660254037844387076, 1.000000000000000000, 0.8660254037844387076, 1.000000000000000000, 0.8660254037844387076, 1.000000000000000000, 0.8660254037844387076, 1.000000000000000000, 0.8660254037844387076, 1.000000000000000000, 0.8660254037844387076, 1.000000000000000000, 0.8660254037844387076, 1.000000000000000000, 0.8660254037844387076, 1.000000000000000000, 0.8660254037844387076, 1.000000000000000000, 0.8660254037844387076, 1.000000000000000000, 0.8660254037844387076, 1.000000000000000000, 0.8660254037844387076, 1.000000000000000000, 0.8660254037844387076, 1.000000000000000000, 0.8660254037844387076, 1.000000000000000000, 0.8660254037844387076, 1.000000000000000000, 0.8660254037844387076, 1.000000000000000000, 0.8660254037844387076, 1.000000000000000000, 0.8660254037844387076, 1.000000000000000000, 0.8660254037844387076, 1.000000000000000000, 0.8660254037844387076, 1.000000000000000000, 0.8660254037844387076, 1.000000000000000000, 0.8660254037844387076, 1.000000000000000000, 0.8660254037844387076, 1.000000000000000000, 0.8660254037844387076, 1.000000000000000000, 0.8660254037844387076, 1.000000000000000000, 0.8660254037844387076, 1.000000000000000000, 0.8660254037844387076, 1.000000000000000000, 0.8660254037844387076, 1.000000000000000000, 0.8660254037844387076, 1.000000000000000000, 0.8660254037844387076, 1.000000000000000000, 0.8660254037844387076, 1.000000000000000000, 0.8660254037844387076, 1.000000000000000000, 0.8660254037844387076, 1.000000000000000000, 0.8660254037844387076, 1.000000000000000000, 0.8660254037844387076, 1.000000000000000000, 0.8660254037844387076, 1.000000000000000000, 0.8660254037844387076, 1.000000000000000000, 0.8660254037844387076, 1.000000000000000000, 0.8660254037844387076, 1.000000000000000000, 0.8660254037844387076, 1.000000000000000000, 0.8660254037844387076, 1.000000000000000000, 0.8660254037844387076, 1.000000000000000000, 0.8660254037844387076, 1.000000000000000000, 0.8660254037844387076, 1.000000000000000000, 0.8660254037844387076, 1.000000000000000000, 0.8660254037844387076, 1.000000000000000000, 0.8660254037844387076, 1.000000000000000000, 0.8660254037844387076, 1.000000000000000000, 0.8660254037844387076, 1.000000000000000000, 0.8660254037844387076, 1.000000000000000000, 0.8660254037844387076, 1.000000000000000000, 0.8660254037844387076, 1.000000000000000000, 0.8660254037844387076, 1.000000000000000000, 0.8660254037844387076, 1.000000000000000000, 0.8660254037844387076, 1.000000000000000000, 0.8660254037844387076, 1.000000000000000000, 0.8660254037844387076, 1.000000000000000000, 0.8660254037844387076, 1.000000000000000000, 0.8660254037844387076, 1.000000000000000000, 0.8660254037844387076, 1.000000000000000000, 0.8660254037844387076, 1.000000000000000000, 0.8660254037844387076, 1.000000000000000000, 0.8660254037844387076, 1.000000000000000000, 0.8660254037844387076, 1.000000000000000000, 0.8660254037844387076, 1.000000000000000000, 0.8660254037844387076, 1.000000000000000000, 0.8660254037844387076, 1.000000000000000000, 0.8660254037844387076, 1.000000000000000000, 0.8660254037844387076, 1.000000000000000000, 0.8660254037844387076, 1.000000000000000000, 0.8660254037844387076, 1.000000000000000000, 0.8660254037844387076, 1.000000000000000000, 0.8660254037844387076, 1.000000000000000000, 0.8660254037844387076, 1.000000000000000000, 0.8660254037844387076, 1.000000000000000000, 0.8660254037844387076, 1.000000000000000000, 0.8660254037844387076, 1.000000000000000000, 0.8660254037844387076, 1.000000000000000000, 0.8660254037844387076, 1.000000000000000000, 0.8660254037844387076, 1.000000000000000000, 0.8660254037844387076, 1.000000000000000000, 0.8660254037844387076, 1.000000000000000000, 0.8660254037844387076, 1.000000000000000000, 0.8660254037844387076, 1.000000000000000000, 0.8660254037844387076, 1.000000000000000000, 0.8660254037844387076, 1.000000000000000000, 0.8660254037844387076, 1.000000000000000000, 0.8660254037844387076, 1.000000000000000000, 0.8660254037844387076, 1.000000000000000000, 0.8660254037844387076, 1.000000000000000000, 0.8660254037844387076, 1.000000000000000000, 0.8660254037844387076, 1.000000000000000000, 0.8660254037844387076, 1.000000000000000000, 0.8660254037844387076, 1.000000000000000000, 0.8660254037844387076, 1.000000000000000000, 0.8660254037844387076, 1.000000000000000000, 0.8660254037844387076, 1.000000000000000000, 0.8660254037844387076, 1.000000000000000000, 0.8660254037844387076, 1.000000000000000000, 0.8660254037844387076, 1.000000000000000000, 0.8660254037844387076, 1.000000000000000000, 0.8660254037844387076, 1.000000000000000000, 0.8660254037844387076, 1.000000000000000000, 0.8660254037844387076, 1.000000000000000000, 0.8660254037844387076, 1.000000000000000000, 0.8660254037844387076, 1.000000000000000000, 0.8660254037844387076, 1.000000000000000000, 0.8660254037844387076, 1.000000000000000000, 0.8660254037844387076, 1.000000000000000000, 0.8660254037844387076, 1.000000000000000000, 0.8660254037844387076, 1.000000000000000000, 0.8660254037844387076, 1.000000000000000000, 0.8660254037844387076, 1.000000000000000000, 0.8660254037844387076, 1.000000000000000000, 0.8660254037844387076, 1.000000000000000000, 0.8660254037844387076, 1.000000000000000000, 0.8660254037844387076, 1.000000000000000000, 0.8660254037844387076, 1.000000000000000000, 0.8660254037844387076, 1.000000000000000000, 0.8660254037844387076, 1.000000000000000000, 0.8660254037844387076, 1.000000000000000000, 0.8660254037844387076, 1.000000000000000000, 0.8660254037844387076, 1.000000000000000000, 0.8660254037844387076, 1.000000000000000000, 0.8660254037844387076, 1.000000000000000000, 0.8660254037844387076, 1.000000000000000000, 0.8660254037844387076, 1.000000000000000000, 0.8660254037844387076, 1.000000000000000000, 0.8660254037844387076, 1.000000000000000000, 0.8660254037844387076, 1.000000000000000000, 0.8660254037844387076, 1.000000000000000000, 0.8660254037844387076, 1.000000000000000000, 0.8660254037844387076, 1.000000000000000000, 0.8660254037844387076, 1.000000000000000000, 0.8660254037844387076, 1.000000000000000000, 0.8660254037844387076, 1.000000000000000000, 0.8660254037844387076, 1.000000000000000000, 0.8660254037844387076, 1.000000000000000000, 0.8660254037844387076, 1.000000000000000000, 0.8660254037844387076, 1.000000000000000000, 0.8660254037844387076, 1.000000000000000000, 0.8660254037844387076, 1.000000000000000000, 0.8660254037844387076, 1.000000000000000000, 0.8660254037844387076, 1.000000000000000000, 0.8660254037844387076, 1.000000000000000000, 0.8660254037844387076, 1.000000000000000000, 0.8660254037844387076, 1.000000000000000000, 0.8660254037844387076, 1.000000000000000000, 0.8660254037844387076, 1.000000000000000000, 0.8660254037844387076, 1.000000000000000000, 0.8660254037844387076, 1.000000000000000000, 0.8660254037844387076, 1.000000000000000000, 0.8660254037844387076, 1.000000000000000000) ) ) 
 REPRESENTATION_ITEM ( '' )  SURFACE ( )  );
#45403=CARTESIAN_POINT ( 'NONE',  ( 5.015626762051672571, 7.938982758113895422, 1.199719254218462483 ) ) ;
#45407=CARTESIAN_POINT ( 'NONE',  ( -3.601662362724658895, 7.353689856487406473, -0.7998128361456281477 ) ) ;
#45408=CARTESIAN_POINT ( 'NONE',  ( 5.463572716182829581, 6.436884926043849653, 1.082531754730560403 ) ) ;
#45409=CARTESIAN_POINT ( 'NONE',  ( 1.499999999999989120, 3.004166666666689522, 0.8660254037844524744 ) ) ;
#45411=CARTESIAN_POINT ( 'NONE',  ( -2.937312835655025101, 6.578615408239493867, 1.040834085586084257E-14 ) ) ;
#45412=CARTESIAN_POINT ( 'NONE',  ( 0.006800380015300722461, 7.009756401597622144, -1.999988438675401881 ) ) ;
#45413=( BOUNDED_CURVE ( )  B_SPLINE_CURVE ( 2, ( #30040, #13768, #96126, #127632, #160038, #61466, #128690 ),
 .UNSPECIFIED., .F., .T. ) 
 B_SPLINE_CURVE_WITH_KNOTS ( ( 3, 2, 2, 3 ),
 ( 0.2125000000000001055, 0.2166666666666668128, 0.2208333333333334925, 0.2250000000000001998 ),
 .UNSPECIFIED. ) 
 CURVE ( )  GEOMETRIC_REPRESENTATION_ITEM ( )  RATIONAL_B_SPLINE_CURVE ( ( 0.9999999999999964473, 0.8660254037844422603, 1.000000000000000000, 0.8660254037844387076, 1.000000000000000000, 0.8660254037844324904, 1.000000000000006217 ) ) 
 REPRESENTATION_ITEM ( '' )  );
#45415=CARTESIAN_POINT ( 'NONE',  ( 0.6823417656249917140, 4.342708333674755394, 1.181850606188765695 ) ) ;
#45418=CARTESIAN_POINT ( 'NONE',  ( -4.284013352238265959, 5.060732334775157604, -1.082531754730544860 ) ) ;
#45423=CARTESIAN_POINT ( 'NONE',  ( 5.515469562660962666, 5.329135999392899947, 0.7998128361456341429 ) ) ;
#45430=CARTESIAN_POINT ( 'NONE',  ( -1.364683531250014514, 1.051041667008090208, -0.7879004041258289570 ) ) ;
#45433=CARTESIAN_POINT ( 'NONE',  ( -9.215791728987058562, 11.77484298861683598, -1.599625672291263179 ) ) ;
#45435=CARTESIAN_POINT ( 'NONE',  ( -6.222829318548141586, 6.362315081168691044, 0.7216878364870317197 ) ) ;
#45439=CARTESIAN_POINT ( 'NONE',  ( 1.364683531249990311, 4.634375000341417916, 1.214306433183764966E-14 ) ) ;
#45447=CARTESIAN_POINT ( 'NONE',  ( -6.738039155867462604, 7.923762439009225389, 1.082531754730549967 ) ) ;
#45452=CARTESIAN_POINT ( 'NONE',  ( -5.382223794500843539, 7.302347065049529462, -1.443375672974051449 ) ) ;
#45464=CARTESIAN_POINT ( 'NONE',  ( -5.066996723205291708, 6.934582148538044777, 1.599625672291267398 ) ) ;
#45467=CARTESIAN_POINT ( 'NONE',  ( -1.500000000000013101, 1.420833333333354043, 0.8660254037844403729 ) ) ;
#45469=CARTESIAN_POINT ( 'NONE',  ( 9.924205255523292024, 10.68058700763975466, -0.7216878364870257245 ) ) ;
#45470=CARTESIAN_POINT ( 'NONE',  ( 6.551614543901692400, 8.666636272683888365, 1.599625672291281386 ) ) ;
#45476=CARTESIAN_POINT ( 'NONE',  ( 3.493197133815315603, 7.227147089426516402, -0.7998128361456291469 ) ) ;
#45477=( BOUNDED_CURVE ( )  B_SPLINE_CURVE ( 2, ( #21648, #153831, #5401, #58190, #80846, #181523, #145880 ),
 .UNSPECIFIED., .F., .T. ) 
 B_SPLINE_CURVE_WITH_KNOTS ( ( 3, 2, 2, 3 ),
 ( 0.1500000000000002165, 0.1541666666666669516, 0.1583333333333336590, 0.1625000000000003941 ),
 .UNSPECIFIED. ) 
 CURVE ( )  GEOMETRIC_REPRESENTATION_ITEM ( )  RATIONAL_B_SPLINE_CURVE ( ( 0.9999999999999928946, 0.8660254037844458130, 1.000000000000000000, 0.8660254037844387076, 1.000000000000000000, 0.8660254037844261621, 1.000000000000012434 ) ) 
 REPRESENTATION_ITEM ( '' )  );
#45478=CARTESIAN_POINT ( 'NONE',  ( -0.006768871532359400575, 8.210909518262125673, -2.038649385027044403 ) ) ;
#45486=CARTESIAN_POINT ( 'NONE',  ( -5.280010757518168063, 8.247430752824802980, -1.199719254218446718 ) ) ;
#45488=ORIENTED_EDGE ( 'NONE', *, *, #30522, .F. ) ;
#45492=CARTESIAN_POINT ( 'NONE',  ( -1.364683531250012516, 3.030208333674755394, 0.7879004041258379498 ) ) ;
#45493=CARTESIAN_POINT ( 'NONE',  ( 8.609064354553323639, 10.10662517080946543, -1.082531754730543083 ) ) ;
#45495=CARTESIAN_POINT ( 'NONE',  ( -6.632963465583701534, 8.761543347979550589, -1.599625672291263179 ) ) ;
#45498=CARTESIAN_POINT ( 'NONE',  ( 5.982172092127724383, 8.002286745614243912, -1.599625672291262513 ) ) ;
#45499=CARTESIAN_POINT ( 'NONE',  ( -7.061099074618889304, 7.132370430010492868, -0.7998128361456291469 ) ) ;
#45503=CARTESIAN_POINT ( 'NONE',  ( -1.201851678989727383E-14, 0.9937500006828198229, 1.732050807568877637 ) ) ;
#45506=CARTESIAN_POINT ( 'NONE',  ( 8.107412671292042461, 9.521364873671299023, 1.082531754730558626 ) ) ;
#45509=CARTESIAN_POINT ( 'NONE',  ( -0.6823417656250003738, 2.030208333674753174, -1.181850606188749264 ) ) ;
#45511=CARTESIAN_POINT ( 'NONE',  ( 4.975479186090839612, 8.748550117173898855, 0.7216878364870438212 ) ) ;
#45514=CARTESIAN_POINT ( 'NONE',  ( -2.955314298098991266, 6.391691081183366485, 0.7216878364870317197 ) ) ;
#45519=CARTESIAN_POINT ( 'NONE',  ( -1.499999999999993339, 10.64264068711930733, 1.232676135170975238E-14 ) ) ;
#45522=CARTESIAN_POINT ( 'NONE',  ( -3.975508435578610555, 7.849559089036333148, -0.01386331990411299175 ) ) ;
#45527=AXIS2_PLACEMENT_3D ( 'NONE', #15045, #115831, #81138 ) ;
#45529=CARTESIAN_POINT ( 'NONE',  ( 6.657217119509961201, 7.725507046638470321, -1.199719254218446718 ) ) ;
#45533=CARTESIAN_POINT ( 'NONE',  ( 4.681643115420508039, 4.356338477612361260, 0.7998128361456341429 ) ) ;
#45541=CARTESIAN_POINT ( 'NONE',  ( 3.362058906508953449, 6.866226457661676719, -0.7216878364870267237 ) ) ;
#45542=CARTESIAN_POINT ( 'NONE',  ( 0.6823417656249882723, 1.738541667008083991, -1.181850606188749264 ) ) ;
#45543=CARTESIAN_POINT ( 'NONE',  ( 8.914649696185335870, 10.35917838609310593, -1.199719254218446718 ) ) ;
#45547=ORIENTED_EDGE ( 'NONE', *, *, #70130, .F. ) ;
#45550=CARTESIAN_POINT ( 'NONE',  ( -1.201851678989727383E-14, 2.462500000000023004, 1.732050807568877637 ) ) ;
#45551=CARTESIAN_POINT ( 'NONE',  ( 4.476163270806094552, 8.373940915915776273, 0.7998128361456462443 ) ) ;
#45552=CARTESIAN_POINT ( 'NONE',  ( -5.540478329478883524, 9.615641817700700145, 0.000000000000000000 ) ) ;
#45556=CARTESIAN_POINT ( 'NONE',  ( -1.364683531250012516, 2.280208333674751842, 0.7879004041258379498 ) ) ;
#45559=CARTESIAN_POINT ( 'NONE',  ( 2.198393463710220264, 5.716542807637226886, 0.7998128361456462443 ) ) ;
#45563=CARTESIAN_POINT ( 'NONE',  ( 1.499999999999987121, 1.035416667349484232, 0.8660254037844524744 ) ) ;
#45565=CARTESIAN_POINT ( 'NONE',  ( -7.206322340863467346, 8.366129804884193888, 1.199719254218450271 ) ) ;
#45566=CARTESIAN_POINT ( 'NONE',  ( -2.765500147507697459, 5.209872024525476597, 1.082531754730560403 ) ) ;
#45575=CARTESIAN_POINT ( 'NONE',  ( 6.474182045725470402, 7.511966127223233869, -1.199719254218446718 ) ) ;
#45579=CARTESIAN_POINT ( 'NONE',  ( 5.133733721068893807, 9.141106441222381918, 1.040834085586084257E-14 ) ) ;
#45584=CARTESIAN_POINT ( 'NONE',  ( -5.880485940025243607, 7.883652901494672349, 1.599625672291269396 ) ) ;
#45586=CARTESIAN_POINT ( 'NONE',  ( 4.054051625686104998, 4.688480637177271149, -1.199719254218446718 ) ) ;
#45591=CARTESIAN_POINT ( 'NONE',  ( 4.352817808933668431, 7.164511876539561896, 1.041257065902738477 ) ) ;
#45600=CARTESIAN_POINT ( 'NONE',  ( -4.284013352238274841, 4.100363120473813794, -0.7216878364870207285 ) ) ;
#45601=CARTESIAN_POINT ( 'NONE',  ( 6.941411460516762943, 11.04213777067082702, -0.7216878364870267237 ) ) ;
#45603=CARTESIAN_POINT ( 'NONE',  ( -4.042302355168801320, 7.867769847672247074, 0.7998128361456341429 ) ) ;
#45608=CARTESIAN_POINT ( 'NONE',  ( -8.016948904382338981, 8.247528564734524892, -0.7998128361456291469 ) ) ;
#45622=CARTESIAN_POINT ( 'NONE',  ( 1.403499169901393673, 7.376709478541975784, -4.304123474986169207 ) ) ;
#45623=CARTESIAN_POINT ( 'NONE',  ( -5.687809136132860210, 6.594531066031826150, -1.199719254218446718 ) ) ;
#45626=CARTESIAN_POINT ( 'NONE',  ( 4.365362273920252889, 4.195270195769483124, 0.7216878364870317197 ) ) ;
#45630=CARTESIAN_POINT ( 'NONE',  ( -4.295235737431041478, 3.905529869957963029, -0.7998128361456221525 ) ) ;
#45631=CARTESIAN_POINT ( 'NONE',  ( -4.790108344329849110, 4.482881244673243337, 0.7998128361456341429 ) ) ;
#45634=CARTESIAN_POINT ( 'NONE',  ( 9.134442807305049428, 11.67993591332117376, 1.599625672291281386 ) ) ;
#45638=CARTESIAN_POINT ( 'NONE',  ( -7.365103760721662951, 9.615707025640515937, 1.599625672291295375 ) ) ;
#45639=CARTESIAN_POINT ( 'NONE',  ( 5.986088515633498197, 6.942523675449257858, -1.199719254218446718 ) ) ;
#45642=CARTESIAN_POINT ( 'NONE',  ( 4.630273154266905777, 5.360739087188218122, 1.199719254218464037 ) ) ;
#45644=DIRECTION ( 'NONE',  ( 0.000000000000000000, 1.000000000000000000, -8.546850786086437571E-32 ) ) ;
#45645=CARTESIAN_POINT ( 'NONE',  ( -1.364683531250000748, 1.821875000341421913, 0.000000000000000000 ) ) ;
#45648=CARTESIAN_POINT ( 'NONE',  ( 7.836249599018724865, 9.205007956019091608, -1.082531754730537976 ) ) ;
#45656=CARTESIAN_POINT ( 'NONE',  ( 8.690413276235306128, 13.08263988900915109, -0.7216878364870267237 ) ) ;
#45663=CARTESIAN_POINT ( 'NONE',  ( 5.368665641331539007, 5.365790791082648781, -0.7216878364870152884 ) ) ;
#45665=CARTESIAN_POINT ( 'NONE',  ( -10.34217224912604571, 10.96028913360221502, 0.7998128361456462443 ) ) ;
#45682=CARTESIAN_POINT ( 'NONE',  ( -1.500000000000013101, 1.410416667349486008, -0.8660254037844313801 ) ) ;
#45688=AXIS2_PLACEMENT_3D ( 'NONE', #172420, #27216, #155103 ) ;
#45690=CARTESIAN_POINT ( 'NONE',  ( 7.456094412511537151, 10.78619501698377370, 1.199719254218460707 ) ) ;
#45695=CARTESIAN_POINT ( 'NONE',  ( 2.333974999846879061, 5.874721266463329705, -0.7998128361456291469 ) ) ;
#45696=CARTESIAN_POINT ( 'NONE',  ( -6.399085315970151733, 7.528316292462387871, -1.082531754730544860 ) ) ;
#45700=CARTESIAN_POINT ( 'NONE',  ( -5.343885102080728977, 9.386283052402845328, 0.7998128361456481317 ) ) ;
#45702=CARTESIAN_POINT ( 'NONE',  ( 0.7499999999999885647, 1.847916667349486231, -1.299038105676652899 ) ) ;
#45709=CARTESIAN_POINT ( 'NONE',  ( -4.297571505407598025, 5.076550180139354218, 1.082531754730558626 ) ) ;
#45710=ADVANCED_FACE ( 'NONE', ( #142400 ), #113573, .T. ) ;
#45713=CARTESIAN_POINT ( 'NONE',  ( 4.124567353486244592, 7.428622122647839277, 0.6979301818166357974 ) ) ;
#45718=CARTESIAN_POINT ( 'NONE',  ( -4.419594887930571758, 4.258541578781506409, 1.214306433183764966E-14 ) ) ;
#45719=CARTESIAN_POINT ( 'NONE',  ( 6.584456157731144899, 10.83361595066169514, -0.7998128361456291469 ) ) ;
#45726=CARTESIAN_POINT ( 'NONE',  ( -7.670162217029145246, 9.971608557999250166, 1.599625672291295375 ) ) ;
#45733=CARTESIAN_POINT ( 'NONE',  ( 5.138703914779377158, 5.953908307786102583, 1.199719254218462483 ) ) ;
#45737=CARTESIAN_POINT ( 'NONE',  ( -8.839026081105473054, 12.39961529701003684, -1.199719254218446718 ) ) ;
#45740=CARTESIAN_POINT ( 'NONE',  ( -5.856132087369688044, 6.175168335346238990, -0.9273813317931516309 ) ) ;
#45750=ORIENTED_EDGE ( 'NONE', *, *, #188907, .F. ) ;
#45757=CARTESIAN_POINT ( 'NONE',  ( -0.7500000000000249800, 0.2229166673494847872, 1.299038105676659116 ) ) ;
#45762=CARTESIAN_POINT ( 'NONE',  ( 2.354312230267378236, 5.898448035287240820, -0.7998128361456281477 ) ) ;
#45764=CARTESIAN_POINT ( 'NONE',  ( -9.459838494033043332, 12.05956421450382088, 1.599625672291281386 ) ) ;
#45770=CARTESIAN_POINT ( 'NONE',  ( -1.387358672534699799, 7.315968950353656020, 4.254625267138158584 ) ) ;
#45772=CARTESIAN_POINT ( 'NONE',  ( 5.070386261830877928, 5.978167395966564435, -1.082531754730548412 ) ) ;
#45774=EDGE_LOOP ( 'NONE', ( #183929, #146447, #139733, #150545 ) ) ;
#45775=CARTESIAN_POINT ( 'NONE',  ( -8.462260433223891098, 13.02438760540324481, -0.7998128361456281477 ) ) ;
#45777=CARTESIAN_POINT ( 'NONE',  ( 8.224992744984721327, 12.74757530245756243, 1.040834085586084257E-14 ) ) ;
#45785=DIRECTION ( 'NONE',  ( -5.578564026256490882E-16, -1.000000000000000000, -9.066213480720158442E-32 ) ) ;
#45787=CARTESIAN_POINT ( 'NONE',  ( -1.402160292154681736E-14, -0.3031249996585801965, -1.575800808251665908 ) ) ;
#45791=CARTESIAN_POINT ( 'NONE',  ( -6.566226467720086113, 6.555019055295208119, 1.040834085586084257E-14 ) ) ;
#45793=CARTESIAN_POINT ( 'NONE',  ( -0.7500000000000249800, -0.8083333333333136972, 1.299038105676659116 ) ) ;
#45795=CARTESIAN_POINT ( 'NONE',  ( -0.7500000000000215383, 4.191666666666690411, 1.299038105676671107 ) ) ;
#45802=CARTESIAN_POINT ( 'NONE',  ( -1.364683531249997417, 5.821875000341418804, 1.214306433183764966E-14 ) ) ;
#45804=CARTESIAN_POINT ( 'NONE',  ( 5.717788096661236885, 7.693838750903348789, 1.599625672291267398 ) ) ;
#45805=CARTESIAN_POINT ( 'NONE',  ( -7.503547950159405566, 10.84155747757291266, 1.199719254218453823 ) ) ;
#45806=CARTESIAN_POINT ( 'NONE',  ( 10.22692794340986921, 10.82583744360002243, 0.000000000000000000 ) ) ;
#45812=CARTESIAN_POINT ( 'NONE',  ( 0.6823417656249864960, -1.011458332991911568, -1.181850606188749264 ) ) ;
#45819=CARTESIAN_POINT ( 'NONE',  ( 5.978782553946477840, 9.919070713005490703, 1.040834085586084257E-14 ) ) ;
#45823=CARTESIAN_POINT ( 'NONE',  ( 0.7499999999999902300, 5.097916667349482012, -1.299038105676658228 ) ) ;
#45825=CARTESIAN_POINT ( 'NONE',  ( -4.790108344329849110, 4.482881244673243337, 0.7998128361456341429 ) ) ;
#45826=CARTESIAN_POINT ( 'NONE',  ( 7.429504990164394584, 7.770103364721017591, 1.040834085586084257E-14 ) ) ;
#45827=CARTESIAN_POINT ( 'NONE',  ( -8.093854517234044366, 11.42628545587295186, 1.082531754730549967 ) ) ;
#45833=CARTESIAN_POINT ( 'NONE',  ( 4.518945272056516416, 4.166524327021037699, 0.7998128361456341429 ) ) ;
#45835=CARTESIAN_POINT ( 'NONE',  ( 3.948449050077836642, 5.629609863222681199, 1.599625672291267398 ) ) ;
#45840=VERTEX_POINT ( 'NONE', #153555 ) ;
#45844=CARTESIAN_POINT ( 'NONE',  ( -4.909967638851771454, 4.671257834700952571, -0.2941531795261614346 ) ) ;
#45849=ORIENTED_EDGE ( 'NONE', *, *, #177010, .F. ) ;
#45851=CARTESIAN_POINT ( 'NONE',  ( 7.716561984472250835, 12.15440608185967086, 1.040834085586084257E-14 ) ) ;
#45856=CARTESIAN_POINT ( 'NONE',  ( -1.364683531250014514, -0.7614583329919104582, -0.7879004041258359514 ) ) ;
#45857=CARTESIAN_POINT ( 'NONE',  ( 6.155038550924155416, 6.283225852274053835, 0.7216878364870317197 ) ) ;
#45859=CARTESIAN_POINT ( 'NONE',  ( -7.537970219518066450, 11.73812298950569044, -0.7216878364870267237 ) ) ;
#45869=ORIENTED_EDGE ( 'NONE', *, *, #126844, .T. ) ;
#45871=VERTEX_POINT ( 'NONE', #39805 ) ;
#45878=CARTESIAN_POINT ( 'NONE',  ( 4.536316240020330071, 7.212700717958764329, -1.298556639521078582 ) ) ;
#45883=CARTESIAN_POINT ( 'NONE',  ( -5.884810976140032679, 6.155599488313971079, -0.9398637431582609336 ) ) ;
#45886=CARTESIAN_POINT ( 'NONE',  ( -6.860062538834774237, 10.94723069537516302, 0.7216878364870458196 ) ) ;
#45890=CARTESIAN_POINT ( 'NONE',  ( 7.474622759835693131, 7.614814729430110951, -0.7998128361456281477 ) ) ;
#45891=DIRECTION ( 'NONE',  ( 0.6507913734559640506, -0.7592566023653004592, 0.000000000000000000 ) ) ;
#45893=CARTESIAN_POINT ( 'NONE',  ( -5.786632634934295361, 5.645492917045106473, 0.7998128361456341429 ) ) ;
#45896=ADVANCED_FACE ( 'NONE', ( #122209 ), #188388, .T. ) ;
#45899=CARTESIAN_POINT ( 'NONE',  ( -5.579343907223557331, 6.467988298970945849, 1.199719254218450271 ) ) ;
#45903=CARTESIAN_POINT ( 'NONE',  ( 5.515469562660962666, 5.329135999392899947, 0.7998128361456341429 ) ) ;
#45904=CARTESIAN_POINT ( 'NONE',  ( 7.618792255875527886, 10.97600916757510170, 1.199719254218460707 ) ) ;
#45907=CARTESIAN_POINT ( 'NONE',  ( 4.919437264989244163, 6.867374270256937585, 1.424029350978267550 ) ) ;
#45908=CARTESIAN_POINT ( 'NONE',  ( 5.517805331081858888, 5.539787095791365523, 1.040834085586084257E-14 ) ) ;
#45910=DIRECTION ( 'NONE',  ( 3.347138415753903010E-16, 0.6000000000000018652, -0.7999999999999984901 ) ) ;
#45915=CARTESIAN_POINT ( 'NONE',  ( 6.575341312503417690, 10.61505593132193326, -0.7216878364870267237 ) ) ;
#45916=CARTESIAN_POINT ( 'NONE',  ( -9.494787648271923786, 9.971673765939062406, 1.040834085586084257E-14 ) ) ;
#45919=CARTESIAN_POINT ( 'NONE',  ( -7.648771216403934758, 12.07531685244661723, -0.7998128361456291469 ) ) ;
#45920=CARTESIAN_POINT ( 'NONE',  ( -7.389357414647957256, 8.579670724299436557, 1.199719254218450271 ) ) ;
#45928=CARTESIAN_POINT ( 'NONE',  ( 8.052653171512838881, 11.48218023581863001, -1.199719254218446718 ) ) ;
#45929=CARTESIAN_POINT ( 'NONE',  ( 0.7499999999999902300, 4.066666666666690411, -1.299038105676658228 ) ) ;
#45933=CARTESIAN_POINT ( 'NONE',  ( 3.979481780810941949, 4.601482484822914998, 1.199719254218464037 ) ) ;
#45936=CARTESIAN_POINT ( 'NONE',  ( 0.7499999999999920064, 5.514583334016151639, 1.299038105676669330 ) ) ;
#45942=CARTESIAN_POINT ( 'NONE',  ( -1.402160292154681736E-14, 2.587500000000023892, -1.732050807568863648 ) ) ;
#45943=CARTESIAN_POINT ( 'NONE',  ( 6.796715079152391148, 6.823922435299587974, 0.7998128361456341429 ) ) ;
#45945=CARTESIAN_POINT ( 'NONE',  ( 6.155038550924133212, 10.12470270947942730, 0.7216878364870438212 ) ) ;
#45946=CARTESIAN_POINT ( 'NONE',  ( -10.45297324601190425, 11.29748299654313470, 0.7216878364870438212 ) ) ;
#45949=CARTESIAN_POINT ( 'NONE',  ( 7.404724451357931336, 11.79059562655963056, 0.7998128361456462443 ) ) ;
#45951=CARTESIAN_POINT ( 'NONE',  ( 3.566600549852601887, 6.224440002135039229, 1.211718802956414764 ) ) ;
#45952=CARTESIAN_POINT ( 'NONE',  ( -4.090809663021341969, 5.795697244990093644, 1.599625672291267398 ) ) ;
#45953=CARTESIAN_POINT ( 'NONE',  ( 1.499999999999991118, 5.285416667349480235, 0.8660254037844524744 ) ) ;
#45954=CARTESIAN_POINT ( 'NONE',  ( 1.364683531249988757, 1.384375000341421469, 0.000000000000000000 ) ) ;
#45959=CARTESIAN_POINT ( 'NONE',  ( 0.6823417656249882723, -0.9072916663252494907, 1.181850606188755259 ) ) ;
#45961=EDGE_CURVE ( 'NONE', #150994, #55454, #149816, .T. ) ;
#45962=CARTESIAN_POINT ( 'NONE',  ( 9.642873567817520808, 12.27310513391906532, 1.599625672291279388 ) ) ;
#45969=CARTESIAN_POINT ( 'NONE',  ( -5.689618019229208734, 9.789638122409414223, 0.7998128361456481317 ) ) ;
#45972=CARTESIAN_POINT ( 'NONE',  ( 4.385172619016207918, 7.203452924572514959, 1.199719254218462483 ) ) ;
#45981=CARTESIAN_POINT ( 'NONE',  ( -5.148345644887285744, 7.029489223833707001, -1.599625672291256295 ) ) ;
#45985=CARTESIAN_POINT ( 'NONE',  ( 7.228468454380276853, 11.58496363008569574, 1.040834085586084257E-14 ) ) ;
#45987=CARTESIAN_POINT ( 'NONE',  ( 8.751951852821344247, 10.16936423550178503, -1.199719254218446718 ) ) ;
#45988=EDGE_CURVE ( 'NONE', #73877, #21505, #153508, .T. ) ;
#45991=CARTESIAN_POINT ( 'NONE',  ( -10.14113571334194930, 10.93367254176152059, -0.7216878364870267237 ) ) ;
#45993=CARTESIAN_POINT ( 'NONE',  ( -8.030507057996002729, 8.263346410617135263, 1.040834085586084257E-14 ) ) ;
#45998=CARTESIAN_POINT ( 'NONE',  ( -6.136354103119505687, 5.996982182489118962, -0.08184359936842452998 ) ) ;
#45999=CARTESIAN_POINT ( 'NONE',  ( -1.364683531250014514, -0.2197916663252438285, 0.7879004041258379498 ) ) ;
#46002=CARTESIAN_POINT ( 'NONE',  ( 5.829642864196151741, 9.745074408296771296, 0.7216878364870438212 ) ) ;
#46010=ADVANCED_FACE ( 'NONE', ( #147053 ), #145995, .F. ) ;
#46015=CARTESIAN_POINT ( 'NONE',  ( 5.165293336682155179, 5.128523102325101668, -0.7216878364870420448 ) ) ;
#46020=CARTESIAN_POINT ( 'NONE',  ( 10.57266086055835075, 11.22919251360659310, 0.000000000000000000 ) ) ;
#46024=CARTESIAN_POINT ( 'NONE',  ( -4.273844736805832767, 6.009238164405336313, 1.599625672291267398 ) ) ;
#46025=CARTESIAN_POINT ( 'NONE',  ( -8.857554428429624593, 9.228235009456373206, 0.7998128361456462443 ) ) ;
#46027=ORIENTED_EDGE ( 'NONE', *, *, #138422, .F. ) ;
#46030=CARTESIAN_POINT ( 'NONE',  ( 0.7499999999999902300, 3.764583334016149863, 1.299038105676669330 ) ) ;
#46031=CARTESIAN_POINT ( 'NONE',  ( 8.402302512167096893, 10.82577223566020841, -1.599625672291268286 ) ) ;
#46034=CARTESIAN_POINT ( 'NONE',  ( -7.004758919754800139, 11.32396917302262018, 0.000000000000000000 ) ) ;
#46036=CARTESIAN_POINT ( 'NONE',  ( -1.364683531250012516, 3.238541667008084879, -0.7879004041258289570 ) ) ;
#46041=CARTESIAN_POINT ( 'NONE',  ( -8.920901888112002354, 11.43080484092926241, 1.443375672974064550 ) ) ;
#46045=CARTESIAN_POINT ( 'NONE',  ( -1.364683531249997417, 3.071875000341423245, 1.214306433183764966E-14 ) ) ;
#46052=CARTESIAN_POINT ( 'NONE',  ( 1.364683531249988535, 3.155208333674756283, -0.7879004041258239610 ) ) ;
#46055=CARTESIAN_POINT ( 'NONE',  ( -3.913499895838973508, 7.717500311787445000, 1.040834085586084257E-14 ) ) ;
#46058=CARTESIAN_POINT ( 'NONE',  ( -1.201851678989727383E-14, 3.634375000341422357, 1.575800808251672791 ) ) ;
#46061=CARTESIAN_POINT ( 'NONE',  ( -1.402160292154681736E-14, -0.3031249996585801965, -1.575800808251665908 ) ) ;
#46062=CARTESIAN_POINT ( 'NONE',  ( -4.446711195602245148, 7.171284913969171448, -1.082531754730549967 ) ) ;
#46066=CARTESIAN_POINT ( 'NONE',  ( 3.362058906508953449, 6.866226457661676719, -0.7216878364870267237 ) ) ;
#46069=CARTESIAN_POINT ( 'NONE',  ( -7.690499447449645309, 9.995335326823163058, 1.599625672291295375 ) ) ;
#46070=CARTESIAN_POINT ( 'NONE',  ( -8.351459436338030784, 11.72682452816096976, -1.082531754730543971 ) ) ;
#46072=CARTESIAN_POINT ( 'NONE',  ( 0.6823417656249917140, 4.592708333674755394, 1.181850606188765695 ) ) ;
#46075=CARTESIAN_POINT ( 'NONE',  ( 1.499999999999990896, 6.344000000000043826, 2.958666666666670331 ) ) ;
#46077=CARTESIAN_POINT ( 'NONE',  ( -6.575341312503472757, 7.733948288417905381, 1.082531754730549967 ) ) ;
#46079=CARTESIAN_POINT ( 'NONE',  ( -0.6823417656250003738, 0.03020833367475134201, -1.181850606188749264 ) ) ;
#46087=( BOUNDED_CURVE ( )  B_SPLINE_CURVE ( 2, ( #23933, #168073, #19673, #43423, #126873, #60709, #42361 ),
 .UNSPECIFIED., .F., .T. ) 
 B_SPLINE_CURVE_WITH_KNOTS ( ( 3, 2, 2, 3 ),
 ( 0.000000000000000000, 0.005952380952380876590, 0.01190476190476175318, 0.01785714285714263064 ),
 .UNSPECIFIED. ) 
 CURVE ( )  GEOMETRIC_REPRESENTATION_ITEM ( )  RATIONAL_B_SPLINE_CURVE ( ( 1.000000000000000000, 0.8660254037844387076, 1.000000000000000000, 0.8660254037844387076, 1.000000000000000000, 0.8660254037844438146, 0.9999999999999948930 ) ) 
 REPRESENTATION_ITEM ( '' )  );
#46090=CARTESIAN_POINT ( 'NONE',  ( 2.358755538653318773, 5.695705861830088423, 1.040834085586084257E-14 ) ) ;
#46094=CARTESIAN_POINT ( 'NONE',  ( -1.500000000000015099, -1.079166666666641961, 0.8660254037844403729 ) ) ;
#46095=CARTESIAN_POINT ( 'NONE',  ( 8.215877899756996783, 12.52901528311778989, 1.040834085586084257E-14 ) ) ;
#46103=CARTESIAN_POINT ( 'NONE',  ( 7.135668919494039031, 7.219368582364847242, 1.040834085586084257E-14 ) ) ;
#46104=CARTESIAN_POINT ( 'NONE',  ( -5.603597561149804562, 5.431951997629870910, 0.7998128361456341429 ) ) ;
#46108=CARTESIAN_POINT ( 'NONE',  ( -1.364683531250014514, 0.5510416670080878765, -0.7879004041258289570 ) ) ;
#46109=CARTESIAN_POINT ( 'NONE',  ( 6.115103934187892776, 6.015625209457229339, 1.345820777640227805E-10 ) ) ;
#46110=CARTESIAN_POINT ( 'NONE',  ( -8.272446282632566650, 12.80293776304669962, 0.7998128361456481317 ) ) ;
#46116=CARTESIAN_POINT ( 'NONE',  ( 1.499999999999990896, 5.775000000000023448, 1.040834085586084257E-14 ) ) ;
#46128=CARTESIAN_POINT ( 'NONE',  ( 6.494519276145969577, 7.535692896047149425, -1.199719254218446718 ) ) ;
#46131=VERTEX_POINT ( 'NONE', #112464 ) ;
#46135=CARTESIAN_POINT ( 'NONE',  ( 6.598014311344812199, 10.84943379654430906, 1.040834085586084257E-14 ) ) ;
#46136=CARTESIAN_POINT ( 'NONE',  ( 1.499999999999991118, 8.673756432004008587, 2.614717076620604264 ) ) ;
#46139=CARTESIAN_POINT ( 'NONE',  ( 9.049177462117294013, 12.64479190819049670, -1.199719254218446718 ) ) ;
#46154=CARTESIAN_POINT ( 'NONE',  ( -7.375272376154077492, 11.54830883891436422, -0.7216878364870267237 ) ) ;
#46158=CARTESIAN_POINT ( 'NONE',  ( 5.931855901178834323, 6.879252291918818152, 1.199719254218462483 ) ) ;
#46164=CARTESIAN_POINT ( 'NONE',  ( 4.839897649954202130, 4.748894801142428790, -0.7216878364870197293 ) ) ;
#46172=CARTESIAN_POINT ( 'NONE',  ( -5.747767057189642870, 8.793146435774861658, -1.199719254218440723 ) ) ;
#46173=CARTESIAN_POINT ( 'NONE',  ( -3.438964519360665051, 7.163875705896082913, -0.7998128361456281477 ) ) ;
#46174=DIRECTION ( 'NONE',  ( 5.578564026256490882E-16, 1.000000000000000000, 9.066213480720158442E-32 ) ) ;
#46181=CARTESIAN_POINT ( 'NONE',  ( 5.438792177376376991, 9.497007973581119700, 1.040834085586084257E-14 ) ) ;
#46189=CARTESIAN_POINT ( 'NONE',  ( 1.284279953904121641, 3.077889714876734573, -0.7749999999999892530 ) ) ;
#46193=CARTESIAN_POINT ( 'NONE',  ( 1.364683531249988757, 0.4468750003414206917, 0.000000000000000000 ) ) ;
#46195=CARTESIAN_POINT ( 'NONE',  ( 4.599240423533799138, 6.388866465587984322, 1.599625672291267398 ) ) ;
#46197=CARTESIAN_POINT ( 'NONE',  ( -7.266807147244793263, 8.540658428949452485, 1.082531754730549967 ) ) ;
#46198=CARTESIAN_POINT ( 'NONE',  ( 4.690757960648224589, 6.495636925554817864, 1.443375672974062551 ) ) ;
#46200=CARTESIAN_POINT ( 'NONE',  ( -7.659993601596726265, 8.039006744725394782, -0.7216878364870267237 ) ) ;
#46205=CARTESIAN_POINT ( 'NONE',  ( 6.043183783389218355, 8.073467052085995022, 1.599625672291267398 ) ) ;
#46211=CARTESIAN_POINT ( 'NONE',  ( -1.364683531249997417, 5.509375000341417916, 1.214306433183764966E-14 ) ) ;
#46216=CARTESIAN_POINT ( 'NONE',  ( 7.096803341749390981, 10.36702210109460154, -1.199719254218441611 ) ) ;
#46220=CARTESIAN_POINT ( 'NONE',  ( -8.715193815486133033, 9.062147627688959872, 0.7998128361456462443 ) ) ;
#46225=CARTESIAN_POINT ( 'NONE',  ( 6.903072767652295383, 11.20533532890304684, 1.040834085586084257E-14 ) ) ;
#46226=CARTESIAN_POINT ( 'NONE',  ( -3.197497122698730099, 6.431928158754200986, 0.6077543439236172684 ) ) ;
#46228=CARTESIAN_POINT ( 'NONE',  ( -6.191269702934848240, 10.37489842006599616, 0.000000000000000000 ) ) ;
#46229=CARTESIAN_POINT ( 'NONE',  ( 3.022498986271238586, 2.800000000000017586, -2.499999999999995115 ) ) ;
#46231=CARTESIAN_POINT ( 'NONE',  ( 5.283544098290614777, 6.372568566219670494, -1.132182188465682859 ) ) ;
#46232=CARTESIAN_POINT ( 'NONE',  ( -9.327646496521989405, 10.94497100310623594, -1.082531754730539753 ) ) ;
#46236=CARTESIAN_POINT ( 'NONE',  ( 7.284808609244363353, 7.393364887073558656, 0.7998128361456341429 ) ) ;
#46238=CARTESIAN_POINT ( 'NONE',  ( 4.476163270806094552, 8.373940915915776273, 0.7998128361456462443 ) ) ;
#46239=CARTESIAN_POINT ( 'NONE',  ( -4.016817522127867690, 7.623078265842172740, -0.1143880650965305862 ) ) ;
#46240=CARTESIAN_POINT ( 'NONE',  ( 4.172158584703322681, 5.890604320285754980, -1.599625672291256295 ) ) ;
#46242=CARTESIAN_POINT ( 'NONE',  ( -5.409340102172518705, 9.254721185935849803, 0.000000000000000000 ) ) ;
#46247=CARTESIAN_POINT ( 'NONE',  ( -5.195561487237588594, 6.467898337602993486, 1.183867312878450484 ) ) ;
#46248=CARTESIAN_POINT ( 'NONE',  ( -0.6823417656250003738, 0.5302083336747518416, -1.181850606188749264 ) ) ;
#46251=CARTESIAN_POINT ( 'NONE',  ( 5.504247177468190699, 5.523969249908757817, 0.7216878364870317197 ) ) ;
#46255=CARTESIAN_POINT ( 'NONE',  ( -7.931156673870055407, 11.23647130528163096, 1.082531754730549967 ) ) ;
#46260=CARTESIAN_POINT ( 'NONE',  ( -7.483737604619046913, 11.67485160545682987, 0.000000000000000000 ) ) ;
#46261=CARTESIAN_POINT ( 'NONE',  ( 0.000000000000000000, 2.800000000000024691, 1.214306433183764966E-14 ) ) ;
#46262=ADVANCED_FACE ( 'NONE', ( #190188, #126353 ), #110089, .F. ) ;
#46268=CARTESIAN_POINT ( 'NONE',  ( -7.443063143778079649, 10.66702885350765584, 1.082531754730549967 ) ) ;
#46273=CARTESIAN_POINT ( 'NONE',  ( -1.364683531250010295, 5.301041667008085767, -0.7879004041258300672 ) ) ;
#46274=CARTESIAN_POINT ( 'NONE',  ( -1.499999999999997780, 3.931250000682819046, 1.214306433183764966E-14 ) ) ;
#46275=CARTESIAN_POINT ( 'NONE',  ( 5.803731464950218744, 6.215061796778338810, -0.9591748237987550718 ) ) ;
#46278=ORIENTED_EDGE ( 'NONE', *, *, #119577, .F. ) ;
#46281=CARTESIAN_POINT ( 'NONE',  ( -6.821723845970312894, 11.11042825360738284, 0.000000000000000000 ) ) ;
#46282=DIRECTION ( 'NONE',  ( 1.000000000000000000, 0.000000000000000000, 0.000000000000000000 ) ) ;
#46285=CARTESIAN_POINT ( 'NONE',  ( 6.810273232766058449, 6.839740281182199233, 1.040834085586084257E-14 ) ) ;
#46290=CARTESIAN_POINT ( 'NONE',  ( 6.598014311344812199, 10.84943379654430906, 1.040834085586084257E-14 ) ) ;
#46291=DIRECTION ( 'NONE',  ( 0.000000000000000000, 8.546850786086437571E-32, 1.000000000000000000 ) ) ;
#46298=CARTESIAN_POINT ( 'NONE',  ( -5.097502569058207200, 8.890910730635814829, -0.7216878364870207285 ) ) ;
#46301=CARTESIAN_POINT ( 'NONE',  ( -1.084637062511545347, 3.148878807974804239, -1.105835307554788649 ) ) ;
#46304=ADVANCED_FACE ( 'NONE', ( #10368 ), #123963, .F. ) ;
#46307=CARTESIAN_POINT ( 'NONE',  ( -9.341731535015849630, 10.85744053139533349, 1.199719254218462483 ) ) ;
#46309=CARTESIAN_POINT ( 'NONE',  ( 9.206149998879153529, 10.69926207256923689, 1.199719254218453823 ) ) ;
#46310=CARTESIAN_POINT ( 'NONE',  ( 0.7499999999999885647, -1.016666666666644847, 1.299038105676657340 ) ) ;
#46311=CARTESIAN_POINT ( 'NONE',  ( -7.655550293210764856, 12.08322577538792331, 0.000000000000000000 ) ) ;
#46314=CARTESIAN_POINT ( 'NONE',  ( 1.364683531249988535, 3.113541667008083991, 0.7879004041258500513 ) ) ;
#46315=CARTESIAN_POINT ( 'NONE',  ( 3.358669367883368118, 4.941533567329135401, -1.599625672291262513 ) ) ;
#46320=CARTESIAN_POINT ( 'NONE',  ( 10.04622863760192963, 10.82294762006482713, -0.7216878364870257245 ) ) ;
#46323=CARTESIAN_POINT ( 'NONE',  ( -6.778713617152821058, 7.971215977175476475, 1.082531754730549967 ) ) ;
#46324=CARTESIAN_POINT ( 'NONE',  ( 0.6823417656249899377, 0.5927083336747518416, 1.181850606188755259 ) ) ;
#46326=CARTESIAN_POINT ( 'NONE',  ( -3.578934198120170329, 6.213868303620019518, 1.151059397407709239 ) ) ;
#46328=CARTESIAN_POINT ( 'NONE',  ( -6.645467848992654858, 10.90479625713344625, 0.7998128361456481317 ) ) ;
#46330=CARTESIAN_POINT ( 'NONE',  ( -4.568734577680899633, 4.432537883490215158, -0.7216878364870207285 ) ) ;
#46331=CARTESIAN_POINT ( 'NONE',  ( 0.6823417656249917140, 3.655208333674754506, 1.181850606188765695 ) ) ;
#46337=CARTESIAN_POINT ( 'NONE',  ( 8.615316546479974136, 12.13862083994696839, 1.199719254218450271 ) ) ;
#46342=EDGE_LOOP ( 'NONE', ( #161148, #91583, #213793, #91136 ) ) ;
#46350=CARTESIAN_POINT ( 'NONE',  ( 1.364683531249986537, -1.136458332991912235, 0.7879004041258500513 ) ) ;
#46354=CARTESIAN_POINT ( 'NONE',  ( 6.747154001095143627, 11.02343010125301959, -0.7998128361456291469 ) ) ;
#46356=CARTESIAN_POINT ( 'NONE',  ( -1.201851678989727383E-14, 3.946875000341423689, -1.575800808251660134 ) ) ;
#46358=CARTESIAN_POINT ( 'NONE',  ( -6.724481002698126098, 8.868313807946373473, -1.443375672974059665 ) ) ;
#46364=CARTESIAN_POINT ( 'NONE',  ( 4.729096653068339151, 4.411700938201493116, -0.7998128361456211532 ) ) ;
#46366=ORIENTED_EDGE ( 'NONE', *, *, #158371, .F. ) ;
#46367=CARTESIAN_POINT ( 'NONE',  ( 10.05067194643221207, 10.62020544712608938, 0.7998128361456462443 ) ) ;
#46368=CARTESIAN_POINT ( 'NONE',  ( 4.786522169170392971, 5.141580351323886688, 0.8077998227834035649 ) ) ;
#46373=CARTESIAN_POINT ( 'NONE',  ( -10.29471871147821282, 10.90492667301307605, -0.7998128361456291469 ) ) ;
#46374=CARTESIAN_POINT ( 'NONE',  ( 6.120616281565444794, 9.228137197546649517, -1.199719254218440723 ) ) ;
#46376=CARTESIAN_POINT ( 'NONE',  ( 2.833290915131624566, 6.249330467721451399, -0.7216878364870267237 ) ) ;
#46380=EDGE_CURVE ( 'NONE', #21699, #12264, #141235, .T. ) ;
#46385=CARTESIAN_POINT ( 'NONE',  ( -1.438721403204643368, 7.870009100113813716, -3.684356824106938877 ) ) ;
#46388=CARTESIAN_POINT ( 'NONE',  ( -6.778713617152821058, 7.971215977175476475, 1.082531754730549967 ) ) ;
#46389=CARTESIAN_POINT ( 'NONE',  ( 3.174580523894166006, 6.855427711185178019, 0.7998128361456341429 ) ) ;
#46392=CARTESIAN_POINT ( 'NONE',  ( -6.170932472514347289, 10.35117165124207972, 0.000000000000000000 ) ) ;
#46394=CYLINDRICAL_SURFACE ( 'NONE', #35478, 1.500000000000000222 ) ;
#46397=CARTESIAN_POINT ( 'NONE',  ( -9.833741488613570780, 10.36711991300432345, 0.7998128361456462443 ) ) ;
#46398=CARTESIAN_POINT ( 'NONE',  ( -1.123270288254055060, 3.033552654332631437, 0.7749999999939939377 ) ) ;
#46401=CARTESIAN_POINT ( 'NONE',  ( 8.606728586576791074, 8.935604860628076906, 0.7998128361456462443 ) ) ;
#46403=CYLINDRICAL_SURFACE ( 'NONE', #119321, 1.250000000000000000 ) ;
#46414=CARTESIAN_POINT ( 'NONE',  ( -8.941766003412679353, 10.39081407785832845, -1.199719254218446718 ) ) ;
#46418=CARTESIAN_POINT ( 'NONE',  ( 5.612712406377503349, 8.531619659873665995, -1.082531754730543083 ) ) ;
#46420=CARTESIAN_POINT ( 'NONE',  ( 3.521367211247359741, 5.131347717920458962, -1.599625672291262513 ) ) ;
#46423=CARTESIAN_POINT ( 'NONE',  ( -5.201524489137236529, 9.220195670635433771, 0.7998128361456481317 ) ) ;
#46433=CARTESIAN_POINT ( 'NONE',  ( -0.6823417656250212460, 4.613541667008086655, 1.181850606188767472 ) ) ;
#46434=CARTESIAN_POINT ( 'NONE',  ( 4.007721930888963335, 7.796164093330856026, -0.2192809687468954827 ) ) ;
#46435=CARTESIAN_POINT ( 'NONE',  ( 8.076906825439115423, 10.44614393447756129, -1.599625672291262513 ) ) ;
#46437=CARTESIAN_POINT ( 'NONE',  ( -3.578989364327652467, 6.158942777482099729, 1.082531754730560403 ) ) ;
#46439=CARTESIAN_POINT ( 'NONE',  ( -4.351804119862249465, 7.060559992272473551, 1.082531754730560403 ) ) ;
#46444=ORIENTED_EDGE ( 'NONE', *, *, #47557, .T. ) ;
#46446=CARTESIAN_POINT ( 'NONE',  ( 4.871457266011829823, 4.577788319968905562, -0.7998128361456221525 ) ) ;
#46453=CARTESIAN_POINT ( 'NONE',  ( 4.701980345841006326, 4.380065246436280368, 0.7998128361456341429 ) ) ;
#46457=CARTESIAN_POINT ( 'NONE',  ( -1.364683531249997417, 4.071875000341417028, 1.214306433183764966E-14 ) ) ;
#46462=CARTESIAN_POINT ( 'NONE',  ( 4.611744806942754238, 8.532119374741881757, -0.7998128361456231517 ) ) ;
#46466=CARTESIAN_POINT ( 'NONE',  ( -3.815730167242251003, 6.539103397502874948, -1.199719254218452047 ) ) ;
#46467=CARTESIAN_POINT ( 'NONE',  ( 6.602457619730771832, 6.805214765881779648, 0.7216878364870317197 ) ) ;
#46468=CARTESIAN_POINT ( 'NONE',  ( -1.500000000000013101, 2.879166666666688634, -0.8660254037844313801 ) ) ;
#46470=CARTESIAN_POINT ( 'NONE',  ( -3.761497552787613330, 6.475832013972435242, 1.199719254218464037 ) ) ;
#46471=CARTESIAN_POINT ( 'NONE',  ( 0.4942839625836501494, 7.528790859548413650, -2.012357903315102448 ) ) ;
#46473=CARTESIAN_POINT ( 'NONE',  ( 1.364683531249990311, 5.134375000341417916, 1.214306433183764966E-14 ) ) ;
#46476=CARTESIAN_POINT ( 'NONE',  ( -4.609409038966248318, 5.440360635957812718, -1.082531754730544860 ) ) ;
#46481=DIRECTION ( 'NONE',  ( -0.6260462619842731558, 0.7797859179643593652, 0.000000000000000000 ) ) ;
#46482=CARTESIAN_POINT ( 'NONE',  ( 4.542145155778077203, 5.257923088951247159, -1.199719254218452047 ) ) ;
#46483=CARTESIAN_POINT ( 'NONE',  ( -1.201851678989727383E-14, 3.087500000000026112, -1.732050807568863648 ) ) ;
#46485=CARTESIAN_POINT ( 'NONE',  ( -0.1021852871783673899, 7.053056311350172969, -4.037408415133502793 ) ) ;
#46486=CARTESIAN_POINT ( 'NONE',  ( -1.364683531250012516, 4.051041667008088432, -0.7879004041258300672 ) ) ;
#46490=CARTESIAN_POINT ( 'NONE',  ( 1.364683531249988757, 0.4468750003414206917, 0.000000000000000000 ) ) ;
#46493=CARTESIAN_POINT ( 'NONE',  ( -10.30827686509187835, 10.92074451889568643, 1.040834085586084257E-14 ) ) ;
#46494=CARTESIAN_POINT ( 'NONE',  ( -7.171900071504754060, 7.469564292951421436, -0.7216878364870267237 ) ) ;
#46497=ORIENTED_EDGE ( 'NONE', *, *, #47186, .T. ) ;
#46498=CARTESIAN_POINT ( 'NONE',  ( -1.364683531250012516, 4.988541667008084879, -0.7879004041258300672 ) ) ;
#46508=CARTESIAN_POINT ( 'NONE',  ( -6.873620692004104527, 7.121571683533994168, 0.7216878364870317197 ) ) ;
#46514=CARTESIAN_POINT ( 'NONE',  ( -6.385527161912131433, 6.552129231760014605, 0.7216878364870317197 ) ) ;
#46527=EDGE_CURVE ( 'NONE', #55695, #166004, #6154, .T. ) ;
#46529=CARTESIAN_POINT ( 'NONE',  ( -5.901876940650454095, 5.779944607047298177, -0.7998128361456291469 ) ) ;
#46532=CARTESIAN_POINT ( 'NONE',  ( -1.402160292154681736E-14, 0.3375000000000208389, -1.732050807568870754 ) ) ;
#46534=CARTESIAN_POINT ( 'NONE',  ( 7.944714827928039291, 11.25228915168265864, 1.082531754730557072 ) ) ;
#46535=CARTESIAN_POINT ( 'NONE',  ( 6.283314124929436417, 9.417951348137970413, -1.199719254218440723 ) ) ;
#46539=CARTESIAN_POINT ( 'NONE',  ( 6.491656622844908853, 6.468020902940851968, 0.7998128361456341429 ) ) ;
#46543=AXIS2_PLACEMENT_3D ( 'NONE', #102595, #168651, #86339 ) ;
#46547=CARTESIAN_POINT ( 'NONE',  ( -3.877268743828284681, 5.546566172598190292, 1.443375672974064550 ) ) ;
#46554=CARTESIAN_POINT ( 'NONE',  ( 0.6823417656249899377, 2.842708333674753618, 1.181850606188765695 ) ) ;
#46555=CARTESIAN_POINT ( 'NONE',  ( 7.727784369665023689, 11.95957283134381477, 1.040834085586084257E-14 ) ) ;
#46556=CARTESIAN_POINT ( 'NONE',  ( -5.768104287610143821, 8.816873204598778102, -1.199719254218440723 ) ) ;
#46559=CARTESIAN_POINT ( 'NONE',  ( 6.144869935491714230, 8.192100896205568361, -1.599625672291262513 ) ) ;
#46560=CARTESIAN_POINT ( 'NONE',  ( -6.307567778855718288, 8.381915046796901692, -1.599625672291263179 ) ) ;
#46564=CARTESIAN_POINT ( 'NONE',  ( 1.499999999999989120, 0.5562500006828161592, 0.000000000000000000 ) ) ;
#46568=CARTESIAN_POINT ( 'NONE',  ( 6.887178846062110615, 9.058127958537705027, -1.443375672974057666 ) ) ;
#46571=CARTESIAN_POINT ( 'NONE',  ( -0.6823417656250003738, 2.530208333674753618, -1.181850606188749264 ) ) ;
#46573=CARTESIAN_POINT ( 'NONE',  ( 6.331294547457450683, 7.449227062530913379, -1.082531754730543083 ) ) ;
#46576=CARTESIAN_POINT ( 'NONE',  ( -4.948362879307902418, 4.875437568721725512, 1.214306433183764966E-14 ) ) ;
#46578=CARTESIAN_POINT ( 'NONE',  ( -0.6823417656249969321, 4.467708333674755394, -1.181850606188749264 ) ) ;
#46583=ORIENTED_EDGE ( 'NONE', *, *, #97341, .F. ) ;
#46584=CARTESIAN_POINT ( 'NONE',  ( -4.764280463835226520, 6.994423760310605864, -1.426210198329436851 ) ) ;
#46590=CARTESIAN_POINT ( 'NONE',  ( 7.644099680006512187, 7.812537802962739697, 1.040834085586084257E-14 ) ) ;
#46593=CARTESIAN_POINT ( 'NONE',  ( 4.695201269034174452, 4.372156323494968966, 1.214306433183764966E-14 ) ) ;
#46600=ORIENTED_EDGE ( 'NONE', *, *, #128539, .T. ) ;
#46602=CARTESIAN_POINT ( 'NONE',  ( 6.168596704537822717, 6.299043698156668647, 1.040834085586084257E-14 ) ) ;
#46603=CARTESIAN_POINT ( 'NONE',  ( -0.6823417656250212460, 1.613541667008083769, 1.181850606188755259 ) ) ;
#46604=CARTESIAN_POINT ( 'NONE',  ( 7.404724451357931336, 11.79059562655963056, 0.7998128361456462443 ) ) ;
#46607=CARTESIAN_POINT ( 'NONE',  ( -5.199715606040888005, 6.025088614257851027, -1.199719254218446718 ) ) ;
#46610=CARTESIAN_POINT ( 'NONE',  ( 0.7499999999999902300, 2.233333333333351156, 1.299038105676669330 ) ) ;
#46611=CARTESIAN_POINT ( 'NONE',  ( 6.693975156845185737, 8.832723654451292816, 1.599625672291281386 ) ) ;
#46612=CARTESIAN_POINT ( 'NONE',  ( -8.850775351622791831, 9.220326086515070685, -0.7998128361456291469 ) ) ;
#46616=CARTESIAN_POINT ( 'NONE',  ( -0.6823417656250212460, 2.551041667008084435, 1.181850606188767472 ) ) ;
#46617=ORIENTED_EDGE ( 'NONE', *, *, #140381, .F. ) ;
#46618=CARTESIAN_POINT ( 'NONE',  ( -0.7499999999999972244, 3.608333333333359150, -1.299038105676652011 ) ) ;
#46620=CARTESIAN_POINT ( 'NONE',  ( 2.184835310096557404, 5.700724961754617404, 1.040834085586084257E-14 ) ) ;
#46624=CARTESIAN_POINT ( 'NONE',  ( -0.7500000000000215383, 1.222916667349485564, 1.299038105676659116 ) ) ;
#46626=CARTESIAN_POINT ( 'NONE',  ( -7.369020184227459858, 8.555943955475521889, 1.199719254218450271 ) ) ;
#46627=CARTESIAN_POINT ( 'NONE',  ( -3.226477370372317743, 4.787309570232886280, 1.443375672974064550 ) ) ;
#46633=EDGE_LOOP ( 'NONE', ( #20250, #159314, #154609, #4664 ) ) ;
#46635=CARTESIAN_POINT ( 'NONE',  ( 4.449046963578762615, 8.342305224150557308, -0.7998128361456231517 ) ) ;
#46639=CARTESIAN_POINT ( 'NONE',  ( 6.470265622219697477, 8.571729197388226140, -1.599625672291262513 ) ) ;
#46645=CARTESIAN_POINT ( 'NONE',  ( -6.235860587281615075, 9.362588887548838557, -1.199719254218440723 ) ) ;
#46647=CARTESIAN_POINT ( 'NONE',  ( 3.999819011231439347, 4.625209253646830554, 1.199719254218464037 ) ) ;
#46653=CARTESIAN_POINT ( 'NONE',  ( 4.722716239034094876, 6.809985054512954328, 1.237095216770202954 ) ) ;
#46663=CARTESIAN_POINT ( 'NONE',  ( -2.643476764984671767, 6.027880625883323518, 1.040834085586084257E-14 ) ) ;
#46664=CARTESIAN_POINT ( 'NONE',  ( 8.026063749610047537, 10.38682701267698150, -1.443375672974057666 ) ) ;
#46666=CARTESIAN_POINT ( 'NONE',  ( -4.608882153641705059, 7.464447381635583412, -1.199719254218452047 ) ) ;
#46671=CARTESIAN_POINT ( 'NONE',  ( -6.507023659554960204, 9.678945805201045971, 1.199719254218452047 ) ) ;
#46687=B_SPLINE_CURVE_WITH_KNOTS ( 'NONE', 3,
 ( #66759, #179504, #150200, #19100 ),
 .UNSPECIFIED., .F., .F.,
 ( 4, 4 ),
 ( 2.884874348012686430E-17, 0.0001292189244443286045 ),
 .UNSPECIFIED. ) ;
#46688=CARTESIAN_POINT ( 'NONE',  ( -1.436838838544729491, 7.449283400311743186, -4.203727439823575551 ) ) ;
#46690=CARTESIAN_POINT ( 'NONE',  ( -5.229694566569281555, 7.124396299129368337, 1.599625672291267398 ) ) ;
#46693=CARTESIAN_POINT ( 'NONE',  ( 4.528060117284240071, 5.345453560662148718, 1.082531754730560403 ) ) ;
#46695=CARTESIAN_POINT ( 'NONE',  ( -1.420000000000001039, 6.280000000000042881, -2.579999999999995630 ) ) ;
#46696=( BOUNDED_CURVE ( )  B_SPLINE_CURVE ( 1, ( #38100, #151858 ),
 .UNSPECIFIED., .F., .T. ) 
 B_SPLINE_CURVE_WITH_KNOTS ( ( 2, 2 ),
 ( 0.000000000000000000, 6.249999999999788711E-05 ),
 .UNSPECIFIED. ) 
 CURVE ( )  GEOMETRIC_REPRESENTATION_ITEM ( )  RATIONAL_B_SPLINE_CURVE ( ( 0.9345202395942817652, 0.9345202395942817652 ) ) 
 REPRESENTATION_ITEM ( '' )  );
#46698=CARTESIAN_POINT ( 'NONE',  ( -3.297657676621885692, 4.870353260857385180, 1.599625672291267398 ) ) ;
#46702=CARTESIAN_POINT ( 'NONE',  ( 9.348510611822643313, 10.86534945433664134, 1.199719254218453823 ) ) ;
#46706=CARTESIAN_POINT ( 'NONE',  ( -7.004758919754800139, 11.32396917302262018, 0.000000000000000000 ) ) ;
#46707=CARTESIAN_POINT ( 'NONE',  ( 4.635998460869027227, 7.496083073400806818, -1.199719254218452047 ) ) ;
#46710=CARTESIAN_POINT ( 'NONE',  ( 3.337278367258157630, 7.045241861776501580, 0.7998128361456341429 ) ) ;
#46714=CARTESIAN_POINT ( 'NONE',  ( 1.364683531249988757, 1.696875000341414808, 0.000000000000000000 ) ) ;
#46717=CARTESIAN_POINT ( 'NONE',  ( 7.293923454472080792, 9.532663335016016148, 1.443375672974076540 ) ) ;
#46734=CARTESIAN_POINT ( 'NONE',  ( -10.65400978224035811, 11.32409958890225710, 1.040834085586084257E-14 ) ) ;
#46749=CARTESIAN_POINT ( 'NONE',  ( 1.499999999999987121, 1.535416667349486453, 0.8660254037844524744 ) ) ;
#46754=EDGE_LOOP ( 'NONE', ( #29759, #71144, #123331, #151956, #84549, #145919 ) ) ;
#46756=CARTESIAN_POINT ( 'NONE',  ( -1.500000000000001332, -0.8499999999999757749, 0.000000000000000000 ) ) ;
#46757=CARTESIAN_POINT ( 'NONE',  ( 8.076906825439115423, 10.44614393447756129, -1.599625672291262513 ) ) ;
#46762=CARTESIAN_POINT ( 'NONE',  ( 4.196412238629597447, 4.854568018944682706, -1.199719254218452047 ) ) ;
#46763=CARTESIAN_POINT ( 'NONE',  ( -5.897433632264490910, 9.824163637709826702, 0.000000000000000000 ) ) ;
#46767=CARTESIAN_POINT ( 'NONE',  ( -5.520141099058386125, 9.591915048876776595, 0.000000000000000000 ) ) ;
#46769=ORIENTED_EDGE ( 'NONE', *, *, #43069, .T. ) ;
#46770=CARTESIAN_POINT ( 'NONE',  ( -0.7500000000000215383, 0.7229166673494852313, 1.299038105676659116 ) ) ;
#46777=CARTESIAN_POINT ( 'NONE',  ( -10.15522075183580419, 11.80651128435196462, 1.199719254218462483 ) ) ;
#46780=CARTESIAN_POINT ( 'NONE',  ( 4.895304229855391043, 6.665267352516039523, 1.249363049274658799 ) ) ;
#46785=CARTESIAN_POINT ( 'NONE',  ( -10.16591625214838679, 10.75465713712827487, 1.040834085586084257E-14 ) ) ;
#46786=CARTESIAN_POINT ( 'NONE',  ( 8.796542737168120851, 9.157054702984622097, -0.7998128361456211532 ) ) ;
#46795=CARTESIAN_POINT ( 'NONE',  ( -6.821723845970312894, 11.11042825360738284, 0.000000000000000000 ) ) ;
#46801=CARTESIAN_POINT ( 'NONE',  ( 4.487912541323413329, 5.194651705420806564, 1.199719254218462483 ) ) ;
#46805=CARTESIAN_POINT ( 'NONE',  ( -8.597841969360544567, 13.18256606422934674, 0.7998128361456341429 ) ) ;
#46808=CARTESIAN_POINT ( 'NONE',  ( -5.085529380082158823, 6.726364094520411285, -1.441608068093344741 ) ) ;
#46816=CARTESIAN_POINT ( 'NONE',  ( 7.741869408603235136, 8.990934717247309749, 1.199719254218462483 ) ) ;
#46818=CARTESIAN_POINT ( 'NONE',  ( -3.574546055497324737, 7.322054164722185732, 0.7998128361456341429 ) ) ;
#46827=CARTESIAN_POINT ( 'NONE',  ( 1.499999999999987121, 0.3270833340161527492, -0.8660254037844323793 ) ) ;
#46831=CARTESIAN_POINT ( 'NONE',  ( 3.623053363349855172, 5.249981562040033189, 1.599625672291267398 ) ) ;
#46833=CARTESIAN_POINT ( 'NONE',  ( -2.435661151949389147, 5.993355110582911038, 0.7998128361456341429 ) ) ;
#46839=CARTESIAN_POINT ( 'NONE',  ( 5.355107487717867265, 5.349972945200037522, 1.040834085586084257E-14 ) ) ;
#46841=ORIENTED_EDGE ( 'NONE', *, *, #165880, .T. ) ;
#46842=CARTESIAN_POINT ( 'NONE',  ( -4.900701038327225589, 4.857544330914580044, 0.2781515650015027319 ) ) ;
#46844=CARTESIAN_POINT ( 'NONE',  ( 3.728129053633592704, 4.412200653069714207, -1.082531754730543083 ) ) ;
#46846=CARTESIAN_POINT ( 'NONE',  ( 2.857890832048201712, 6.434070695103256021, -0.3041713968356236086 ) ) ;
#46854=CARTESIAN_POINT ( 'NONE',  ( -0.6823417656250003738, -1.032291666325242607, -1.181850606188749264 ) ) ;
#46859=CARTESIAN_POINT ( 'NONE',  ( -3.730464822054482710, 7.503959392372201442, 1.040834085586084257E-14 ) ) ;
#46863=CARTESIAN_POINT ( 'NONE',  ( -1.500000000000011324, 4.670833333333353821, 0.8660254037844403729 ) ) ;
#46870=CARTESIAN_POINT ( 'NONE',  ( 0.7499999999999902300, 4.316666666666691299, -1.299038105676658228 ) ) ;
#46871=CARTESIAN_POINT ( 'NONE',  ( -1.602468905319636405E-14, -1.053124999658583638, -1.575800808251665908 ) ) ;
#46873=CARTESIAN_POINT ( 'NONE',  ( 5.289652487626049115, 9.323011668872403845, 0.7998128361456462443 ) ) ;
#46874=CARTESIAN_POINT ( 'NONE',  ( -8.015895134177625891, 10.37496362800581018, 1.599625672291295375 ) ) ;
#46881=CARTESIAN_POINT ( 'NONE',  ( -0.6823417656250003738, -0.9697916663252494907, -1.181850606188749264 ) ) ;
#46889=CARTESIAN_POINT ( 'NONE',  ( 7.537970219518073556, 9.817384560903001045, -1.443375672974057666 ) ) ;
#46893=CARTESIAN_POINT ( 'NONE',  ( 1.499999999999987121, 4.077083334016147198, -0.8660254037844323793 ) ) ;
#46895=CARTESIAN_POINT ( 'NONE',  ( -3.765413976293358278, 5.416068943807445635, 1.599625672291267398 ) ) ;
#46896=CARTESIAN_POINT ( 'NONE',  ( 5.599154252319471503, 9.476171027773981237, -0.7216878364870267237 ) ) ;
#46897=CARTESIAN_POINT ( 'NONE',  ( -9.015808962963337336, 10.58116054728778366, 1.082531754730558626 ) ) ;
#46900=B_SPLINE_CURVE_WITH_KNOTS ( 'NONE', 3,
 ( #27974, #126624, #109301, #46368 ),
 .UNSPECIFIED., .F., .F.,
 ( 4, 4 ),
 ( 0.001812203442042620034, 0.002059939351771558277 ),
 .UNSPECIFIED. ) ;
#46904=CARTESIAN_POINT ( 'NONE',  ( 8.595506201383999567, 12.97191496834930113, 0.7216878364870438212 ) ) ;
#46914=CARTESIAN_POINT ( 'NONE',  ( 1.123270288250309612, 3.221052654332833054, -0.7749999999993620881 ) ) ;
#46917=EDGE_CURVE ( 'NONE', #168291, #160543, #129033, .T. ) ;
#46919=CARTESIAN_POINT ( 'NONE',  ( 7.944187942603509356, 11.35563746875774882, 1.199719254218460707 ) ) ;
#46923=CARTESIAN_POINT ( 'NONE',  ( 1.364683531249986537, 0.3635416670080869328, 0.7879004041258500513 ) ) ;
#46924=CARTESIAN_POINT ( 'NONE',  ( 6.331294547901813452, 6.488857848747989543, 1.040834085586084257E-14 ) ) ;
#46925=CARTESIAN_POINT ( 'NONE',  ( -8.595506201384022660, 11.05117653974661529, 1.443375672974064550 ) ) ;
#46930=CARTESIAN_POINT ( 'NONE',  ( -3.578462479003122976, 6.262291094557191684, 1.199719254218464037 ) ) ;
#46936=ORIENTED_EDGE ( 'NONE', *, *, #165880, .F. ) ;
#46938=ORIENTED_EDGE ( 'NONE', *, *, #207112, .F. ) ;
#46945=CARTESIAN_POINT ( 'NONE',  ( 4.930363510330384003, 6.858250545851714008, -1.424563464522425882 ) ) ;
#46948=CARTESIAN_POINT ( 'NONE',  ( 1.608462485350599769, 8.735270501766756013, 2.463594439587641904 ) ) ;
#46950=CARTESIAN_POINT ( 'NONE',  ( -3.975509539288551775, 7.849563252032789151, -0.3275587863690732071 ) ) ;
#46953=CARTESIAN_POINT ( 'NONE',  ( -6.832946231607472498, 9.955225789308602913, 1.082531754730549967 ) ) ;
#46957=CARTESIAN_POINT ( 'NONE',  ( 6.368579470117202490, 8.453095353268645695, 1.599625672291281386 ) ) ;
#46959=DIRECTION ( 'NONE',  ( 0.7592566023653005702, 0.6507913734559639396, 0.000000000000000000 ) ) ;
#46961=CARTESIAN_POINT ( 'NONE',  ( -4.412288926243578935, 7.235088616337731260, 1.199719254218464037 ) ) ;
#46963=CIRCLE ( 'NONE', #195691, 0.07999999999999983513 ) ;
#46964=CARTESIAN_POINT ( 'NONE',  ( -4.218558352146454915, 8.073401844146177453, 1.040834085586084257E-14 ) ) ;
#46968=CARTESIAN_POINT ( 'NONE',  ( 8.158255747121103241, 10.54105100977322174, 1.599625672291281386 ) ) ;
#46971=CARTESIAN_POINT ( 'NONE',  ( 4.044190953901719787, 7.767772900817621284, 0.4663397696828552874 ) ) ;
#46972=CARTESIAN_POINT ( 'NONE',  ( 3.823036129373602154, 6.443664003369091731, -1.082531754730548412 ) ) ;
#46980=CARTESIAN_POINT ( 'NONE',  ( 7.253248993186731219, 8.524840582548424806, 1.082531754730558626 ) ) ;
#46983=CARTESIAN_POINT ( 'NONE',  ( -8.136864746495904299, 12.64475930422059768, -0.7998128361456281477 ) ) ;
#46984=CARTESIAN_POINT ( 'NONE',  ( -6.015013705957189316, 10.16926642359206134, 0.7998128361456481317 ) ) ;
#46992=CARTESIAN_POINT ( 'NONE',  ( 8.402302512167096893, 10.82577223566020841, -1.599625672291268286 ) ) ;
#46996=CARTESIAN_POINT ( 'NONE',  ( 4.546061579283848353, 4.198160018786257552, -0.7998128361456211532 ) ) ;
#47000=CARTESIAN_POINT ( 'NONE',  ( -1.001543065824772872E-14, 5.493750000682816825, 1.732050807568877637 ) ) ;
#47006=CARTESIAN_POINT ( 'NONE',  ( 1.499999999999989120, 3.004166666666689522, 0.8660254037844524744 ) ) ;
#47007=CARTESIAN_POINT ( 'NONE',  ( 4.150767584078112193, 7.994312614733129152, 0.7998128361456321445 ) ) ;
#47010=CARTESIAN_POINT ( 'NONE',  ( 8.161645285746708112, 9.584636257201740506, -1.082531754730543083 ) ) ;
#47011=CARTESIAN_POINT ( 'NONE',  ( 0.4241069589249533700, 7.990617654048686624, 1.998204128839474958 ) ) ;
#47015=CARTESIAN_POINT ( 'NONE',  ( 8.530051201292206287, 13.10347683481629488, 0.000000000000000000 ) ) ;
#47018=CARTESIAN_POINT ( 'NONE',  ( -4.776550190716183586, 4.467063398790632966, 1.214306433183764966E-14 ) ) ;
#47019=CARTESIAN_POINT ( 'NONE',  ( -1.001543065824772872E-14, 5.493750000682816825, 1.732050807568877637 ) ) ;
#47020=CARTESIAN_POINT ( 'NONE',  ( 0.6823417656249899377, 1.592708333674752730, 1.181850606188755259 ) ) ;
#47024=CARTESIAN_POINT ( 'NONE',  ( 4.695201269034174452, 4.372156323494968966, 1.214306433183764966E-14 ) ) ;
#47026=CARTESIAN_POINT ( 'NONE',  ( -0.6823417656249969321, 5.530208333674756283, -1.181850606188749264 ) ) ;
#47036=CARTESIAN_POINT ( 'NONE',  ( -6.015013705957189316, 10.16926642359206134, 0.7998128361456481317 ) ) ;
#47039=CARTESIAN_POINT ( 'NONE',  ( 5.840865249388943248, 5.708764300575555062, 0.7998128361456341429 ) ) ;
#47046=CARTESIAN_POINT ( 'NONE',  ( 8.992082194361556091, 11.51384853155376220, 1.599625672291279388 ) ) ;
#47049=CARTESIAN_POINT ( 'NONE',  ( -6.403528624356093601, 6.365204904703887223, 1.040834085586084257E-14 ) ) ;
#47053=CARTESIAN_POINT ( 'NONE',  ( 8.052653171512838881, 11.48218023581863001, -1.199719254218446718 ) ) ;
#47055=CARTESIAN_POINT ( 'NONE',  ( 7.239163954692881653, 10.53310948286200599, -1.199719254218441611 ) ) ;
#47058=CARTESIAN_POINT ( 'NONE',  ( -8.622622508611375025, 12.04318144581317895, 1.082531754730560403 ) ) ;
#47059=CARTESIAN_POINT ( 'NONE',  ( -5.357443255694392725, 9.402100898285455699, 0.000000000000000000 ) ) ;
#47063=CARTESIAN_POINT ( 'NONE',  ( -5.511734814698080243, 6.408623376260899285, 1.272316098655206229 ) ) ;
#47064=CARTESIAN_POINT ( 'NONE',  ( -0.6823417656250246877, 0.5510416670080897639, 1.181850606188755259 ) ) ;
#47068=CARTESIAN_POINT ( 'NONE',  ( 7.293923454472087897, 8.572294120714675003, 1.082531754730558626 ) ) ;
#47081=CARTESIAN_POINT ( 'NONE',  ( 3.321384445223568793, 6.818772919495456719, -0.7216878364870045193 ) ) ;
#47085=CARTESIAN_POINT ( 'NONE',  ( 8.452618703115982512, 11.94880668935564216, 1.199719254218450271 ) ) ;
#47089=CARTESIAN_POINT ( 'NONE',  ( -5.545448523189368650, 6.428443684264421698, -1.199719254218446718 ) ) ;
#47090=CARTESIAN_POINT ( 'NONE',  ( -7.100719765255177229, 9.307259030929609267, -1.599625672291263179 ) ) ;
#47098=CARTESIAN_POINT ( 'NONE',  ( 0.7499999999999902300, 2.764583334016148974, 1.299038105676669330 ) ) ;
#47099=CARTESIAN_POINT ( 'NONE',  ( 7.564559641420864899, 10.91273778404466199, -1.199719254218446718 ) ) ;
#47103=CARTESIAN_POINT ( 'NONE',  ( -7.343712760096452463, 11.71941532008788833, -0.7998128361456291469 ) ) ;
#47105=CARTESIAN_POINT ( 'NONE',  ( -0.6823417656250212460, 3.551041667008085323, 1.181850606188767472 ) ) ;
#47110=CARTESIAN_POINT ( 'NONE',  ( -9.842856333841300653, 10.58567993234409421, 0.7216878364870438212 ) ) ;
#47114=CARTESIAN_POINT ( 'NONE',  ( 1.364683531249988757, 1.946875000341415030, 0.000000000000000000 ) ) ;
#47118=EDGE_CURVE ( 'NONE', #164652, #3975, #69602, .T. ) ;
#47122=CARTESIAN_POINT ( 'NONE',  ( -0.6823417656250003738, 2.467708333674753618, -1.181850606188749264 ) ) ;
#47125=CARTESIAN_POINT ( 'NONE',  ( -4.238895582566952314, 8.097128612970093897, 1.040834085586084257E-14 ) ) ;
#47126=CARTESIAN_POINT ( 'NONE',  ( 6.751070424600909448, 9.963667031088037973, -1.199719254218441611 ) ) ;
#47130=CARTESIAN_POINT ( 'NONE',  ( -0.6823417656250212460, 2.363541667008084435, 1.181850606188767472 ) ) ;
#47133=CARTESIAN_POINT ( 'NONE',  ( -0.6823417656250003738, -0.5322916663252491576, -1.181850606188749264 ) ) ;
#47134=CARTESIAN_POINT ( 'NONE',  ( -4.934804725694224459, 6.780358151441803649, -1.443375672974053447 ) ) ;
#47137=CARTESIAN_POINT ( 'NONE',  ( 4.853455804012216213, 6.685451076146141425, 1.443375672974062551 ) ) ;
#47140=CARTESIAN_POINT ( 'NONE',  ( -8.850775351622791831, 9.220326086515070685, -0.7998128361456291469 ) ) ;
#47141=CARTESIAN_POINT ( 'NONE',  ( -10.33094986393327197, 11.15512238411806578, 0.7216878364870438212 ) ) ;
#47144=CARTESIAN_POINT ( 'NONE',  ( -1.364683531250012516, 4.988541667008084879, -0.7879004041258300672 ) ) ;
#47149=CARTESIAN_POINT ( 'NONE',  ( -5.544921637864820951, 9.412899644243539754, -0.7216878364870207285 ) ) ;
#47151=CARTESIAN_POINT ( 'NONE',  ( -1.364683531250000748, -0.6781249996585803075, 0.000000000000000000 ) ) ;
#47155=CARTESIAN_POINT ( 'NONE',  ( 7.049876689426101350, 9.247942109129029475, -1.443375672974057666 ) ) ;
#47167=CARTESIAN_POINT ( 'NONE',  ( 8.717529583462646059, 11.19353715217169309, 1.443375672974076540 ) ) ;
#47174=CARTESIAN_POINT ( 'NONE',  ( 4.625302960556422427, 8.547937220624488575, 1.040834085586084257E-14 ) ) ;
#47175=CARTESIAN_POINT ( 'NONE',  ( -3.307299406729781399, 5.945934176904983381, -1.199719254218452935 ) ) ;
#47179=CARTESIAN_POINT ( 'NONE',  ( 6.778713616708431644, 7.010846762355714468, 1.040834085586084257E-14 ) ) ;
#47180=CARTESIAN_POINT ( 'NONE',  ( -1.402160292154681736E-14, -0.1156249996585793222, 1.575800808251672791 ) ) ;
#47182=CARTESIAN_POINT ( 'NONE',  ( -9.429859533504656000, 10.96025652963230534, -1.199719254218441611 ) ) ;
#47186=EDGE_CURVE ( 'NONE', #86388, #24037, #11258, .T. ) ;
#47201=CARTESIAN_POINT ( 'NONE',  ( 6.844168616800228477, 6.879284895888727824, -0.7998128361456281477 ) ) ;
#47207=CARTESIAN_POINT ( 'NONE',  ( 7.259501185113382604, 10.55683625168592243, -1.199719254218441611 ) ) ;
#47212=CARTESIAN_POINT ( 'NONE',  ( 8.374132434735052755, 12.92157160716627295, -0.7998128361456352531 ) ) ;
#47217=CARTESIAN_POINT ( 'NONE',  ( -0.2791710057858245442, 8.178600120975007215, 1.982899171336969912 ) ) ;
#47222=CARTESIAN_POINT ( 'NONE',  ( -8.568389894156720032, 10.05917163368005163, 1.082531754730558626 ) ) ;
#47226=CARTESIAN_POINT ( 'NONE',  ( 4.123651276850781144, 7.962676922967908411, -0.7998128361456221525 ) ) ;
#47228=ADVANCED_FACE ( 'NONE', ( #2625 ), #104434, .F. ) ;
#47235=CARTESIAN_POINT ( 'NONE',  ( 4.406036734316882253, 6.163462161501577441, -1.443375672974051449 ) ) ;
#47243=CARTESIAN_POINT ( 'NONE',  ( -6.989391883044787868, 8.113044270762433285, -1.199719254218446718 ) ) ;
#47245=CARTESIAN_POINT ( 'NONE',  ( -3.764360206088648297, 7.543504007078730922, -0.7998128361456281477 ) ) ;
#47254=CARTESIAN_POINT ( 'NONE',  ( 5.425234023762710578, 9.481190127698507553, -0.7998128361456291469 ) ) ;
#47266=CARTESIAN_POINT ( 'NONE',  ( 0.6823417656249882723, 0.4052083336747516751, 1.181850606188755259 ) ) ;
#47267=CARTESIAN_POINT ( 'NONE',  ( 4.493637847925535667, 7.329995691633395261, -1.199719254218452047 ) ) ;
#47269=CARTESIAN_POINT ( 'NONE',  ( -6.399085315970137522, 9.449054721065074602, -1.082531754730538864 ) ) ;
#47270=CIRCLE ( 'NONE', #74925, 0.07999999999999994615 ) ;
#47271=CARTESIAN_POINT ( 'NONE',  ( 4.528060117284232966, 6.305822774963486310, 1.443375672974062551 ) ) ;
#47272=CARTESIAN_POINT ( 'NONE',  ( -7.985389288324703294, 9.379004260209384825, -1.082531754730543083 ) ) ;
#47278=CARTESIAN_POINT ( 'NONE',  ( 7.019370843573166319, 9.212351955633947043, 1.599625672291281386 ) ) ;
#47284=CARTESIAN_POINT ( 'NONE',  ( -0.6823417656250212460, 5.301041667008086655, 1.181850606188767472 ) ) ;
#47288=CARTESIAN_POINT ( 'NONE',  ( 8.606728586576791074, 8.935604860628076906, 0.7998128361456462443 ) ) ;
#47291=CARTESIAN_POINT ( 'NONE',  ( -7.609150525767646833, 9.900428251527500834, -1.599625672291263179 ) ) ;
#47296=CARTESIAN_POINT ( 'NONE',  ( 9.562578416340237197, 10.05076299535211781, 0.7998128361456462443 ) ) ;
#47299=CARTESIAN_POINT ( 'NONE',  ( -8.259941899223614215, 10.65968485389279508, -1.599625672291263179 ) ) ;
#47303=CARTESIAN_POINT ( 'NONE',  ( 5.770924896911269641, 6.051163903260999177, -0.5763553215429690901 ) ) ;
#47304=CARTESIAN_POINT ( 'NONE',  ( -8.134528978519403708, 11.47373899403920205, 1.082531754730549967 ) ) ;
#47309=CARTESIAN_POINT ( 'NONE',  ( 4.611744806942754238, 8.532119374741881757, -0.7998128361456231517 ) ) ;
#47311=CARTESIAN_POINT ( 'NONE',  ( 6.094553744542824170, 7.069066442510145265, 1.199719254218462483 ) ) ;
#47312=CARTESIAN_POINT ( 'NONE',  ( -4.118090981180881016, 7.482401814132296103, -0.6348448669579254133 ) ) ;
#47313=CARTESIAN_POINT ( 'NONE',  ( 3.928111819657337911, 5.605883094398769195, 1.599625672291267398 ) ) ;
#47316=CARTESIAN_POINT ( 'NONE',  ( -6.019457014787517046, 9.006155036351978893, 1.082531754730548412 ) ) ;
#47321=CARTESIAN_POINT ( 'NONE',  ( -4.774234299259712877, 6.798759937490593153, 1.242976086189879759 ) ) ;
#47322=CARTESIAN_POINT ( 'NONE',  ( -0.6823417656250246877, 0.1135416670080893753, 1.181850606188755259 ) ) ;
#47324=CARTESIAN_POINT ( 'NONE',  ( 4.528060117284232966, 6.305822774963486310, 1.443375672974062551 ) ) ;
#47328=CARTESIAN_POINT ( 'NONE',  ( -8.961576348508652146, 10.51788916375733685, -1.082531754730543083 ) ) ;
#47329=B_SPLINE_CURVE_WITH_KNOTS ( 'NONE', 3,
 ( #82791, #99059, #133721, #19912, #151012, #32983, #15644, #16706, #181357, #2581 ),
 .UNSPECIFIED., .F., .F.,
 ( 4, 3, 3, 4 ),
 ( 0.000000000000000000, 8.893179197954989991E-05, 0.0001334007970840231242, 0.0001778705873658994649 ),
 .UNSPECIFIED. ) ;
#47334=CARTESIAN_POINT ( 'NONE',  ( -9.286972035236630063, 10.89751746493999107, -1.082531754730537976 ) ) ;
#47335=CARTESIAN_POINT ( 'NONE',  ( 1.579999999999989413, 8.674529973577531194, -2.419999999999988827 ) ) ;
#47341=ORIENTED_EDGE ( 'NONE', *, *, #98243, .F. ) ;
#47342=CARTESIAN_POINT ( 'NONE',  ( -9.300530188850304469, 9.952966096521256745, 1.040834085586084257E-14 ) ) ;
#47346=CARTESIAN_POINT ( 'NONE',  ( -1.001543065824772872E-14, 4.884375000341420581, 1.575800808251672791 ) ) ;
#47347=CARTESIAN_POINT ( 'NONE',  ( 1.499999999999989120, 3.035416667349485564, 0.8660254037844524744 ) ) ;
#47348=CARTESIAN_POINT ( 'NONE',  ( 5.563869425686542414, 6.377698570463163463, -1.204193420357344557 ) ) ;
#47349=FACE_OUTER_BOUND ( 'NONE', #133779, .T. ) ;
#47353=CARTESIAN_POINT ( 'NONE',  ( -7.802881099864745984, 9.062115023719057305, -1.199719254218446718 ) ) ;
#47357=CARTESIAN_POINT ( 'NONE',  ( 5.555090253297246150, 7.504024600312024340, 1.599625672291267398 ) ) ;
#47363=CARTESIAN_POINT ( 'NONE',  ( 8.121497709785879593, 9.433834401960398353, -1.199719254218445830 ) ) ;
#47367=LINE ( 'NONE', #32159, #129512 ) ;
#47370=CARTESIAN_POINT ( 'NONE',  ( -7.239690840017442675, 7.548653522882887934, 0.7216878364870317197 ) ) ;
#47374=CARTESIAN_POINT ( 'NONE',  ( -1.364683531249997417, 5.571875000341417916, 1.214306433183764966E-14 ) ) ;
#47381=CARTESIAN_POINT ( 'NONE',  ( -8.154339323615371171, 11.60081407993821045, 1.199719254218453823 ) ) ;
#47383=CARTESIAN_POINT ( 'NONE',  ( 7.411503528164766763, 11.79850454950093841, 1.040834085586084257E-14 ) ) ;
#47385=CARTESIAN_POINT ( 'NONE',  ( -9.667127221743832877, 11.23706883257798772, 1.199719254218462483 ) ) ;
#47388=CARTESIAN_POINT ( 'NONE',  ( -1.364683531249997417, 3.009375000341422801, 1.214306433183764966E-14 ) ) ;
#47389=CARTESIAN_POINT ( 'NONE',  ( 2.523789150438203510, 6.096171108819874007, 0.7998128361456462443 ) ) ;
#47394=CARTESIAN_POINT ( 'NONE',  ( 10.18181017373857600, 10.98112607889092907, 0.7216878364870438212 ) ) ;
#47397=CARTESIAN_POINT ( 'NONE',  ( -5.585596099150182958, 8.499983968108443477, -1.082531754730544860 ) ) ;
#47398=AXIS2_PLACEMENT_3D ( 'NONE', #116048, #169001, #182036 ) ;
#47399=CARTESIAN_POINT ( 'NONE',  ( -1.364683531250012516, 0.5302083336747518416, 0.7879004041258379498 ) ) ;
#47401=CARTESIAN_POINT ( 'NONE',  ( -0.006800380015323652903, 7.009756401597622144, 1.999988438675414759 ) ) ;
#47403=CARTESIAN_POINT ( 'NONE',  ( -8.019811557683421910, 9.315200557840817908, 1.199719254218462483 ) ) ;
#47404=CARTESIAN_POINT ( 'NONE',  ( -3.077337680177623103, 6.534051693608437184, 0.7216878364870317197 ) ) ;
#47405=CARTESIAN_POINT ( 'NONE',  ( 1.364683531249988535, 2.926041667008082658, 0.7879004041258500513 ) ) ;
#47410=CARTESIAN_POINT ( 'NONE',  ( 7.750457368506414646, 12.19395069656619945, 0.7998128361456462443 ) ) ;
#47423=CARTESIAN_POINT ( 'NONE',  ( 1.364683531249990311, 3.696875000341416584, 1.214306433183764966E-14 ) ) ;
#47429=CARTESIAN_POINT ( 'NONE',  ( 7.476431642932036326, 10.80992178580769014, 1.199719254218460707 ) ) ;
#47432=CARTESIAN_POINT ( 'NONE',  ( 1.364683531249990311, 3.134375000341423245, 1.214306433183764966E-14 ) ) ;
#47434=CARTESIAN_POINT ( 'NONE',  ( -6.073689629242151611, 10.02979563418376685, -0.7216878364870278340 ) ) ;
#47440=CARTESIAN_POINT ( 'NONE',  ( 2.679707916995359263, 6.278076336469897711, -0.7998128361456291469 ) ) ;
#47442=ORIENTED_EDGE ( 'NONE', *, *, #53608, .F. ) ;
#47443=CARTESIAN_POINT ( 'NONE',  ( 9.459838494033030898, 12.05956421450382088, 1.599625672291281386 ) ) ;
#47450=CARTESIAN_POINT ( 'NONE',  ( -2.137381772448751605, 5.645362501165475777, -0.7998128361456281477 ) ) ;
#47451=CARTESIAN_POINT ( 'NONE',  ( 6.988338112840064120, 10.24047933403371502, 1.199719254218460707 ) ) ;
#47453=CARTESIAN_POINT ( 'NONE',  ( 3.131570294632282092, 5.636953862837537521, -1.082531754730543971 ) ) ;
#47463=CARTESIAN_POINT ( 'NONE',  ( -1.420000000000021911, 6.200000000000045475, 2.900000000000013678 ) ) ;
#47465=CARTESIAN_POINT ( 'NONE',  ( -6.412643469583822586, 6.583764924043652655, 1.040834085586084257E-14 ) ) ;
#47466=CARTESIAN_POINT ( 'NONE',  ( 4.039439701867726384, 6.800097854565950506, 1.199719254218462483 ) ) ;
#47469=CARTESIAN_POINT ( 'NONE',  ( -9.508345801885592863, 9.987491611821676329, 0.7998128361456462443 ) ) ;
#47476=CARTESIAN_POINT ( 'NONE',  ( -8.839026081105473054, 12.39961529701003684, -1.199719254218446718 ) ) ;
#47481=CARTESIAN_POINT ( 'NONE',  ( 9.206149998879153529, 10.69926207256923689, 1.199719254218453823 ) ) ;
#47482=CARTESIAN_POINT ( 'NONE',  ( 5.636439174979242850, 7.598931675607687453, -1.599625672291262513 ) ) ;
#47494=CARTESIAN_POINT ( 'NONE',  ( -9.671043645249580933, 10.17730576241299900, 0.7998128361456462443 ) ) ;
#47498=CARTESIAN_POINT ( 'NONE',  ( 6.426201623197458801, 9.480690412830290015, -1.082531754730537088 ) ) ;
#47500=CARTESIAN_POINT ( 'NONE',  ( 2.686486993802192913, 6.285985259411197568, 0.7998128361456362523 ) ) ;
#47502=CARTESIAN_POINT ( 'NONE',  ( 5.840865249388943248, 5.708764300575555062, 0.7998128361456341429 ) ) ;
#47504=CARTESIAN_POINT ( 'NONE',  ( -7.386494761346872551, 7.511998731193139989, -0.7998128361456291469 ) ) ;
#47512=CARTESIAN_POINT ( 'NONE',  ( -1.364683531249997417, 3.821875000341416584, 1.214306433183764966E-14 ) ) ;
#47513=CARTESIAN_POINT ( 'NONE',  ( 2.060660350337685465, 8.500464906089362671, 2.499999999999998668 ) ) ;
#47514=CARTESIAN_POINT ( 'NONE',  ( 8.565000355531088516, 11.01558638625153286, -1.599625672291257406 ) ) ;
#47516=CARTESIAN_POINT ( 'NONE',  ( -4.663641653420935285, 5.503632019488245319, 1.082531754730560403 ) ) ;
#47518=CARTESIAN_POINT ( 'NONE',  ( -3.755245360860925086, 6.364574773437617239, -1.082531754730548412 ) ) ;
#47523=ORIENTED_EDGE ( 'NONE', *, *, #131672, .F. ) ;
#47525=CARTESIAN_POINT ( 'NONE',  ( 2.347533153460546806, 5.890539112345938300, 0.000000000000000000 ) ) ;
#47533=CARTESIAN_POINT ( 'NONE',  ( 4.976006071415387311, 5.764094157194782575, 1.199719254218462483 ) ) ;
#47539=CARTESIAN_POINT ( 'NONE',  ( -1.364683531250012516, 3.592708333674750509, 0.7879004041258379498 ) ) ;
#47545=CARTESIAN_POINT ( 'NONE',  ( 6.043183783389218355, 8.073467052085995022, 1.599625672291267398 ) ) ;
#47547=CARTESIAN_POINT ( 'NONE',  ( -3.425406365747000859, 7.148057860013469877, 1.040834085586084257E-14 ) ) ;
#47549=CARTESIAN_POINT ( 'NONE',  ( 4.948362878863507675, 8.716914425408678113, -0.7216878364870267237 ) ) ;
#47550=CARTESIAN_POINT ( 'NONE',  ( -1.499999999999997780, 2.650000000000020339, 1.214306433183764966E-14 ) ) ;
#47553=CARTESIAN_POINT ( 'NONE',  ( -4.894657149733403045, 5.669187081899118574, -1.199719254218446718 ) ) ;
#47554=CARTESIAN_POINT ( 'NONE',  ( 0.4933182949324292355, 7.812106778932951023, -1.990607459109241972 ) ) ;
#47556=CARTESIAN_POINT ( 'NONE',  ( -1.364683531249997417, 3.759375000341423689, 1.214306433183764966E-14 ) ) ;
#47557=EDGE_CURVE ( 'NONE', #186824, #171443, #181433, .T. ) ;
#47559=CARTESIAN_POINT ( 'NONE',  ( -4.663641653420935285, 5.503632019488245319, 1.082531754730560403 ) ) ;
#47564=CARTESIAN_POINT ( 'NONE',  ( 4.493637847925535667, 7.329995691633395261, -1.199719254218452047 ) ) ;
#47566=CARTESIAN_POINT ( 'NONE',  ( -4.168895032367330167, 3.976329666238523242, -0.6109567437776577403 ) ) ;
#47567=CARTESIAN_POINT ( 'NONE',  ( 0.4856440469271376958, 6.671526543591629554, -3.376304580250021559 ) ) ;
#47568=CARTESIAN_POINT ( 'NONE',  ( -1.364683531249997417, 4.071875000341417028, 1.214306433183764966E-14 ) ) ;
#47572=CARTESIAN_POINT ( 'NONE',  ( 0.6823417656249882723, -0.09479166632524876901, 1.181850606188755259 ) ) ;
#47574=CARTESIAN_POINT ( 'NONE',  ( -8.109748439268576803, 12.61312361245537517, 0.7998128361456481317 ) ) ;
#47575=CARTESIAN_POINT ( 'NONE',  ( -5.653386866774179786, 8.579073197003079798, 1.082531754730548412 ) ) ;
#47578=DIRECTION ( 'NONE',  ( -1.000000000000000000, 5.578564026256504688E-16, 0.000000000000000000 ) ) ;
#47580=CARTESIAN_POINT ( 'NONE',  ( -1.364683531250012516, 3.738541667008087099, -0.7879004041258300672 ) ) ;
#47588=CARTESIAN_POINT ( 'NONE',  ( -5.626270559546828309, 7.587068290936515247, 1.443375672974064550 ) ) ;
#47593=CARTESIAN_POINT ( 'NONE',  ( -5.056828107772848746, 8.843457192469559303, -0.7216878364870207285 ) ) ;
#47596=CARTESIAN_POINT ( 'NONE',  ( -4.688236331909272359, 5.260680481867119340, 1.129709447323426152 ) ) ;
#47602=CARTESIAN_POINT ( 'NONE',  ( 0.03686668447251651576, 7.053483931691109099, 3.954540522192132812 ) ) ;
#47607=CARTESIAN_POINT ( 'NONE',  ( -3.581325132304157943, 7.329963087663487364, -0.7998128361456281477 ) ) ;
#47610=CARTESIAN_POINT ( 'NONE',  ( -1.500000000000001332, 1.150000000000019007, 0.000000000000000000 ) ) ;
#47611=CARTESIAN_POINT ( 'NONE',  ( 8.581948047770334043, 12.95609712246668899, 0.000000000000000000 ) ) ;
#47612=CARTESIAN_POINT ( 'NONE',  ( 7.657657833620182153, 7.828355648845348291, -0.7998128361456281477 ) ) ;
#47615=CARTESIAN_POINT ( 'NONE',  ( 5.087333953625774008, 6.958308917361963886, 1.599625672291267398 ) ) ;
#47623=CARTESIAN_POINT ( 'NONE',  ( -5.111060722671894929, 5.065251719313053513, 0.000000000000000000 ) ) ;
#47629=CARTESIAN_POINT ( 'NONE',  ( -0.5158641071528082822, 6.759906959843508645, 3.511243559023642824 ) ) ;
#47632=CARTESIAN_POINT ( 'NONE',  ( 0.6823417656249899377, 3.176041667008085323, -1.181850606188754593 ) ) ;
#47633=CARTESIAN_POINT ( 'NONE',  ( 10.01911233037458260, 10.79131192829960462, 0.7216878364870438212 ) ) ;
#47634=CARTESIAN_POINT ( 'NONE',  ( -7.711890448074853133, 7.891627032375787998, -0.7998128361456291469 ) ) ;
#47637=CARTESIAN_POINT ( 'NONE',  ( 7.156006149914539982, 7.243095351188763686, 1.040834085586084257E-14 ) ) ;
#47638=CARTESIAN_POINT ( 'NONE',  ( -7.400052914960538963, 7.527816577075747695, 1.040834085586084257E-14 ) ) ;
#47643=CARTESIAN_POINT ( 'NONE',  ( 1.499999999999989120, 0.8062500006828163812, 0.000000000000000000 ) ) ;
#47646=CARTESIAN_POINT ( 'NONE',  ( 6.141480397310468575, 10.10888486359680982, 1.040834085586084257E-14 ) ) ;
#47650=CARTESIAN_POINT ( 'NONE',  ( -1.364683531250000748, 1.571875000341421691, 0.000000000000000000 ) ) ;
#47652=CARTESIAN_POINT ( 'NONE',  ( 5.938108092661121162, 9.871617174839238729, 1.040834085586084257E-14 ) ) ;
#47654=CARTESIAN_POINT ( 'NONE',  ( -3.129460678718345878, 6.444905630999884671, -0.7687999843507524744 ) ) ;
#47655=CARTESIAN_POINT ( 'NONE',  ( -3.795919822146289313, 5.451659097302528068, -1.443375672974053447 ) ) ;
#47657=CARTESIAN_POINT ( 'NONE',  ( 0.6823417656249917140, 5.342708333674749177, 1.181850606188765695 ) ) ;
#47661=CARTESIAN_POINT ( 'NONE',  ( -4.957984823605727343, 6.829280066411827832, -1.450623857674667283 ) ) ;
#47668=CARTESIAN_POINT ( 'NONE',  ( 5.361359679200154105, 8.342337828120466980, 1.199719254218462483 ) ) ;
#47671=CARTESIAN_POINT ( 'NONE',  ( 5.196852952739813070, 4.957416621151553571, -0.7998128361456221525 ) ) ;
#47677=VERTEX_POINT ( 'NONE', #39424 ) ;
#47679=CARTESIAN_POINT ( 'NONE',  ( 5.124618876285529367, 7.962177208099690873, -1.082531754730549078 ) ) ;
#47680=CARTESIAN_POINT ( 'NONE',  ( -0.6823417656250003738, 1.030208333674752286, -1.181850606188749264 ) ) ;
#47681=CARTESIAN_POINT ( 'NONE',  ( 1.419999999999987272, 2.244000000000016648, 2.508000000000020435 ) ) ;
#47682=CARTESIAN_POINT ( 'NONE',  ( 0.2082862990473907383, 7.047992147687566877, -4.030656196916692302 ) ) ;
#47686=CARTESIAN_POINT ( 'NONE',  ( -0.7500000000000006661, 1.608333333333357373, -1.299038105676652011 ) ) ;
#47687=CARTESIAN_POINT ( 'NONE',  ( 5.425234023762710578, 9.481190127698507553, -0.7998128361456291469 ) ) ;
#47688=CARTESIAN_POINT ( 'NONE',  ( -7.446452682403657874, 9.710614100936176385, -1.599625672291263179 ) ) ;
#47692=CARTESIAN_POINT ( 'NONE',  ( -1.364683531250000748, 1.759375000341421913, 0.000000000000000000 ) ) ;
#47693=CARTESIAN_POINT ( 'NONE',  ( -1.201851678989727383E-14, 1.962500000000020783, 1.732050807568877637 ) ) ;
#47695=CARTESIAN_POINT ( 'NONE',  ( 8.581948047770334043, 12.95609712246668899, 0.000000000000000000 ) ) ;
#47703=CARTESIAN_POINT ( 'NONE',  ( -0.7500000000000249800, 0.2229166673494847872, 1.299038105676659116 ) ) ;
#47704=CARTESIAN_POINT ( 'NONE',  ( -5.693534442735004752, 8.729875052244421951, 1.199719254218452047 ) ) ;
#47705=CARTESIAN_POINT ( 'NONE',  ( -5.287316719649550301, 5.270883715786984780, 0.7216878364870317197 ) ) ;
#47712=CARTESIAN_POINT ( 'NONE',  ( 7.461064606222022277, 7.598996883547496139, 1.040834085586084257E-14 ) ) ;
#47716=CARTESIAN_POINT ( 'NONE',  ( 5.635385404774530649, 9.726366738878972740, 0.7998128361456462443 ) ) ;
#47717=CARTESIAN_POINT ( 'NONE',  ( 9.381879110532285182, 10.04787317181692075, 0.000000000000000000 ) ) ;
#47718=ORIENTED_EDGE ( 'NONE', *, *, #160495, .T. ) ;
#47723=CARTESIAN_POINT ( 'NONE',  ( -7.854251061018346469, 8.057714414143200443, -0.7998128361456291469 ) ) ;
#47725=CARTESIAN_POINT ( 'NONE',  ( 5.515469562660962666, 5.329135999392899947, 0.7998128361456341429 ) ) ;
#47728=CARTESIAN_POINT ( 'NONE',  ( 4.707534831891463156, 6.823246043637223757, 1.233988984638714426 ) ) ;
#47729=CARTESIAN_POINT ( 'NONE',  ( 8.270110514656016321, 12.59228666716665401, 0.7216878364870438212 ) ) ;
#47730=ORIENTED_EDGE ( 'NONE', *, *, #96602, .T. ) ;
#47735=CYLINDRICAL_SURFACE ( 'NONE', #26116, 1.250000000000000000 ) ;
#47740=CARTESIAN_POINT ( 'NONE',  ( -4.473827502829599290, 4.321812962830357208, 0.7216878364870317197 ) ) ;
#47741=CARTESIAN_POINT ( 'NONE',  ( 6.616015773788773480, 10.66250946948817813, -0.7216878364870267237 ) ) ;
#47744=CARTESIAN_POINT ( 'NONE',  ( -5.555090253297260361, 7.504024600312024340, 1.599625672291269396 ) ) ;
#47746=CYLINDRICAL_SURFACE ( 'NONE', #139260, 1.500000000000000222 ) ;
#47750=CARTESIAN_POINT ( 'NONE',  ( -5.343885102080728977, 9.386283052402845328, 0.7998128361456481317 ) ) ;
#47756=VERTEX_POINT ( 'NONE', #14374 ) ;
#47768=CARTESIAN_POINT ( 'NONE',  ( -4.720210035852093533, 8.658662141802762946, -0.7998128361456281477 ) ) ;
#47771=CARTESIAN_POINT ( 'NONE',  ( 2.887523530030648988, 6.312601851770308414, 0.000000000000000000 ) ) ;
#47775=CARTESIAN_POINT ( 'NONE',  ( -2.123823618835070537, 5.629544655282869847, 1.040834085586084257E-14 ) ) ;
#47779=CARTESIAN_POINT ( 'NONE',  ( 8.890396042259068210, 11.39521468743417998, -1.599625672291257406 ) ) ;
#47783=CARTESIAN_POINT ( 'NONE',  ( -8.040148788103921973, 9.338927326664741457, 1.199719254218462483 ) ) ;
#47784=CARTESIAN_POINT ( 'NONE',  ( 4.638861114170084399, 8.563755066507100722, 0.7998128361456462443 ) ) ;
#47789=CARTESIAN_POINT ( 'NONE',  ( -0.6823417656250003738, 1.030208333674752286, -1.181850606188749264 ) ) ;
#47792=CARTESIAN_POINT ( 'NONE',  ( 8.161645285746708112, 9.584636257201740506, -1.082531754730543083 ) ) ;
#47800=CARTESIAN_POINT ( 'NONE',  ( 8.527715432871318058, 12.89282573841782664, -0.7216878364870338292 ) ) ;
#47802=CARTESIAN_POINT ( 'NONE',  ( 4.763909876611899463, 5.178992836847385206, -0.8608806284969447997 ) ) ;
#47808=CARTESIAN_POINT ( 'NONE',  ( -8.618179199781044630, 13.20629283305325963, 0.7998128361456341429 ) ) ;
#47815=CARTESIAN_POINT ( 'NONE',  ( 0.000000000000000000, 2.800000000000024691, 1.214306433183764966E-14 ) ) ;
#47822=CARTESIAN_POINT ( 'NONE',  ( 1.499999999999987121, 0.5354166673494816786, 0.8660254037844524744 ) ) ;
#47826=ORIENTED_EDGE ( 'NONE', *, *, #159504, .F. ) ;
#47828=CARTESIAN_POINT ( 'NONE',  ( -0.7500000000000006661, -0.3916666666666443475, -1.299038105676652011 ) ) ;
#47829=CARTESIAN_POINT ( 'NONE',  ( 9.589694723567584234, 10.08239868711733855, -0.7998128361456281477 ) ) ;
#47835=CARTESIAN_POINT ( 'NONE',  ( 9.571693261567954636, 12.19006144329456731, 1.443375672974076540 ) ) ;
#47836=CARTESIAN_POINT ( 'NONE',  ( -6.046573322014817897, 9.998159942418544333, 0.7216878364870458196 ) ) ;
#47840=CARTESIAN_POINT ( 'NONE',  ( -6.693975156845199059, 8.832723654451292816, 1.599625672291283607 ) ) ;
#47843=CARTESIAN_POINT ( 'NONE',  ( 0.7499999999999902300, 1.764583334016148086, 1.299038105676657340 ) ) ;
#47850=CARTESIAN_POINT ( 'NONE',  ( -9.022061154889962964, 12.61315621642528129, -1.199719254218446718 ) ) ;
#47853=CARTESIAN_POINT ( 'NONE',  ( 4.171261675657679469, 7.370687464442305270, 0.7961138118306176903 ) ) ;
#47858=CARTESIAN_POINT ( 'NONE',  ( -9.642873567817536795, 12.27310513391906532, 1.599625672291281386 ) ) ;
#47859=CARTESIAN_POINT ( 'NONE',  ( 8.015895134177609904, 10.37496362800581018, 1.599625672291281386 ) ) ;
#47868=CARTESIAN_POINT ( 'NONE',  ( -9.429859533504656000, 10.96025652963230534, -1.199719254218441611 ) ) ;
#47873=CARTESIAN_POINT ( 'NONE',  ( 3.785751206713845018, 5.439795712631356750, 1.599625672291267398 ) ) ;
#47877=CARTESIAN_POINT ( 'NONE',  ( -9.755255220232635693, 11.33988483081495957, -1.199719254218441611 ) ) ;
#47891=CARTESIAN_POINT ( 'NONE',  ( 7.121056995675668411, 9.330985799753529264, -1.599625672291262513 ) ) ;
#47893=CARTESIAN_POINT ( 'NONE',  ( -2.923754682041362241, 6.562797562356882608, 0.7998128361456341429 ) ) ;
#47897=FACE_OUTER_BOUND ( 'NONE', #110527, .T. ) ;
#47903=CARTESIAN_POINT ( 'NONE',  ( -0.7500000000000006661, -0.3604166659838467512, -1.299038105676652011 ) ) ;
#47906=CARTESIAN_POINT ( 'NONE',  ( -1.536019160937945438, 8.701056780447583350, -2.509677374736781985 ) ) ;
#47907=CARTESIAN_POINT ( 'NONE',  ( 5.138177029454882749, 5.096887410559832965, 0.7216878364870096263 ) ) ;
#47909=CARTESIAN_POINT ( 'NONE',  ( -2.625475302540713152, 6.214804952939456228, -0.7998128361456281477 ) ) ;
#47915=CARTESIAN_POINT ( 'NONE',  ( 4.907688418466886304, 5.788353245375237321, -1.082531754730548412 ) ) ;
#47920=CARTESIAN_POINT ( 'NONE',  ( 3.836594282542914236, 5.499112634431936542, 1.443375672974062551 ) ) ;
#47928=CARTESIAN_POINT ( 'NONE',  ( -5.544970132138452357, 6.385306161890050625, 1.248999107086716798 ) ) ;
#47930=CARTESIAN_POINT ( 'NONE',  ( -0.6823417656250003738, -0.7822916663252423852, -1.181850606188749264 ) ) ;
#47937=CARTESIAN_POINT ( 'NONE',  ( 0.7499999999999902300, 5.066666666666684193, -1.299038105676658228 ) ) ;
#47942=ORIENTED_EDGE ( 'NONE', *, *, #201935, .F. ) ;
#47944=CARTESIAN_POINT ( 'NONE',  ( -1.499999999999982903, 4.379166666666687746, -0.8660254037844477004 ) ) ;
#47945=CARTESIAN_POINT ( 'NONE',  ( -0.6823417656250212460, 5.613541667008087543, 1.181850606188767472 ) ) ;
#47947=CARTESIAN_POINT ( 'NONE',  ( 6.636879889089462026, 7.701780277814560982, -1.199719254218446718 ) ) ;
#47948=CARTESIAN_POINT ( 'NONE',  ( -9.365985188942097750, 9.821404230054264772, 0.7998128361456462443 ) ) ;
#47950=CARTESIAN_POINT ( 'NONE',  ( 10.37606763316019531, 10.99983374830873650, 0.7998128361456462443 ) ) ;
#47955=CARTESIAN_POINT ( 'NONE',  ( 0.7499999999999920064, 5.733333333333353821, 1.299038105676669330 ) ) ;
#47962=CARTESIAN_POINT ( 'NONE',  ( 8.595506201384020883, 9.130438111143927671, 0.7216878364870438212 ) ) ;
#47967=CARTESIAN_POINT ( 'NONE',  ( -1.500000000000011324, 4.660416667349484676, -0.8660254037844313801 ) ) ;
#47969=CARTESIAN_POINT ( 'NONE',  ( -4.711622075948912247, 5.455646162483875017, -1.199719254218446718 ) ) ;
#47970=CARTESIAN_POINT ( 'NONE',  ( 4.785665035499516051, 8.527100274817353665, -0.7216878364870207285 ) ) ;
#47978=CARTESIAN_POINT ( 'NONE',  ( 4.844340958784499662, 4.546152628203684820, 0.7998128361456341429 ) ) ;
#47991=CYLINDRICAL_SURFACE ( 'NONE', #34932, 0.08000000000000004330 ) ;
#47994=CARTESIAN_POINT ( 'NONE',  ( 8.809047120577066181, 11.30030761213851953, 1.599625672291281386 ) ) ;
#47997=CARTESIAN_POINT ( 'NONE',  ( -0.6823417656250246877, 0.3010416670080895418, 1.181850606188755259 ) ) ;
#47998=CARTESIAN_POINT ( 'NONE',  ( 5.992340707560163793, 6.093411701682730275, 0.7216878364870317197 ) ) ;
#47999=CARTESIAN_POINT ( 'NONE',  ( -9.490344339885977476, 11.13478515369756217, -1.082531754730539753 ) ) ;
#48004=CARTESIAN_POINT ( 'NONE',  ( -3.079673448598517549, 6.744702790006905424, 1.040834085586084257E-14 ) ) ;
#48017=ADVANCED_FACE ( 'NONE', ( #77254 ), #128637, .T. ) ;
#48019=CARTESIAN_POINT ( 'NONE',  ( 5.603691946294323323, 6.350013490765915591, -1.172630952486140243 ) ) ;
#48027=CARTESIAN_POINT ( 'NONE',  ( -7.754900677336769022, 9.110100880723427608, 1.082531754730558626 ) ) ;
#48033=CARTESIAN_POINT ( 'NONE',  ( 5.991813822235618758, 9.077867661661846554, 1.199719254218462483 ) ) ;
#48035=CARTESIAN_POINT ( 'NONE',  ( 3.541704441667858472, 5.155074486744371853, -1.599625672291262513 ) ) ;
#48037=CARTESIAN_POINT ( 'NONE',  ( -4.466521540698216164, 7.298359999868178960, -1.199719254218452047 ) ) ;
#48040=CARTESIAN_POINT ( 'NONE',  ( -4.554649539187067830, 7.401175998105142817, 1.199719254218464037 ) ) ;
#48043=ADVANCED_FACE ( 'NONE', ( #127170 ), #203551, .T. ) ;
#48045=CARTESIAN_POINT ( 'NONE',  ( 7.892817981449907982, 12.36003807833360391, 0.7998128361456462443 ) ) ;
#48046=CARTESIAN_POINT ( 'NONE',  ( -1.500000000000043299, 3.452083334016150751, 0.8660254037844216102 ) ) ;
#48048=CARTESIAN_POINT ( 'NONE',  ( 4.314144046604536875, 7.442532859859907646, 1.092782195075291396 ) ) ;
#48049=CARTESIAN_POINT ( 'NONE',  ( 5.016153647376205171, 6.875265226737464985, 1.443375672974062551 ) ) ;
#48056=CARTESIAN_POINT ( 'NONE',  ( 6.426201622753093368, 10.44105962661321563, 1.040834085586084257E-14 ) ) ;
#48059=CARTESIAN_POINT ( 'NONE',  ( -8.727698198895085469, 11.20540053684285553, -1.599625672291263179 ) ) ;
#48060=CARTESIAN_POINT ( 'NONE',  ( -6.340409392685171674, 10.54889472477470846, 0.7998128361456481317 ) ) ;
#48064=B_SPLINE_CURVE_WITH_KNOTS ( 'NONE', 3,
 ( #139223, #204169, #74221, #191145 ),
 .UNSPECIFIED., .F., .F.,
 ( 4, 4 ),
 ( 0.000000000000000000, 7.241384396099075972E-05 ),
 .UNSPECIFIED. ) ;
#48069=CARTESIAN_POINT ( 'NONE',  ( 10.05067194643221207, 10.62020544712608938, 0.7998128361456462443 ) ) ;
#48073=CARTESIAN_POINT ( 'NONE',  ( 3.551346171775753735, 6.230655402791975384, 1.199719254218462483 ) ) ;
#48076=CARTESIAN_POINT ( 'NONE',  ( 0.7499999999999902300, 4.847916667349482012, -1.299038105676658228 ) ) ;
#48080=VERTEX_POINT ( 'NONE', #63149 ) ;
#48082=CARTESIAN_POINT ( 'NONE',  ( 1.499999999999987121, 3.545833333333356041, -0.8660254037844262731 ) ) ;
#48083=CARTESIAN_POINT ( 'NONE',  ( 5.769158057814842699, 6.689438141327490150, 1.199719254218462483 ) ) ;
#48086=CARTESIAN_POINT ( 'NONE',  ( 8.459924665247367415, 8.972259652317825740, -0.7216878364870267237 ) ) ;
#48088=CARTESIAN_POINT ( 'NONE',  ( -8.459924664802993988, 12.81373650900478189, 1.040834085586084257E-14 ) ) ;
#48093=CARTESIAN_POINT ( 'NONE',  ( -3.632695093457760649, 6.325562478087638496, -1.199719254218452047 ) ) ;
#48094=CARTESIAN_POINT ( 'NONE',  ( -1.499999999999997780, 4.681250000682819490, 1.214306433183764966E-14 ) ) ;
#48095=CARTESIAN_POINT ( 'NONE',  ( 0.6823417656249882723, -0.4072916663252490466, 1.181850606188755259 ) ) ;
#48099=CARTESIAN_POINT ( 'NONE',  ( 3.928111819657337911, 5.605883094398769195, 1.599625672291267398 ) ) ;
#48101=CARTESIAN_POINT ( 'NONE',  ( 0.6823417656249917140, 4.905208333674755394, 1.181850606188765695 ) ) ;
#48103=LINE ( 'NONE', #114215, #18947 ) ;
#48109=CARTESIAN_POINT ( 'NONE',  ( -5.554036483092550824, 9.631459663583308739, -0.7998128361456231517 ) ) ;
#48112=CARTESIAN_POINT ( 'NONE',  ( 5.867981556616276073, 5.740399992340775803, -0.7998128361456281477 ) ) ;
#48115=CARTESIAN_POINT ( 'NONE',  ( -1.364683531250014514, 0.7385416670080887647, -0.7879004041258289570 ) ) ;
#48119=CARTESIAN_POINT ( 'NONE',  ( 10.08456733046637765, 10.65975006183261087, 0.000000000000000000 ) ) ;
#48122=CARTESIAN_POINT ( 'NONE',  ( -6.205881626753225966, 8.263281202677319470, 1.599625672291283607 ) ) ;
#48126=CARTESIAN_POINT ( 'NONE',  ( 8.402302512167096893, 10.82577223566020841, -1.599625672291268286 ) ) ;
#48128=CARTESIAN_POINT ( 'NONE',  ( 8.426556166093362776, 9.789735934319136135, -1.199719254218446718 ) ) ;
#48130=CARTESIAN_POINT ( 'NONE',  ( -10.00555417720528872, 10.77549408293541866, 0.7216878364870438212 ) ) ;
#48131=CARTESIAN_POINT ( 'NONE',  ( -7.531718027591449705, 8.745758106066849891, 1.199719254218462483 ) ) ;
#48134=CARTESIAN_POINT ( 'NONE',  ( -4.313069242314466756, 7.435226253386592710, 1.131090909019900614 ) ) ;
#48135=CARTESIAN_POINT ( 'NONE',  ( -0.6823417656250246877, 0.3010416670080895418, 1.181850606188755259 ) ) ;
#48140=CARTESIAN_POINT ( 'NONE',  ( 8.297226821883377568, 8.782445501726501291, -0.7216878364870267237 ) ) ;
#48160=CARTESIAN_POINT ( 'NONE',  ( 10.72180055030867329, 11.40318881831530540, 0.7998128361456341429 ) ) ;
#48164=CARTESIAN_POINT ( 'NONE',  ( -3.815730167242251003, 6.539103397502874948, -1.199719254218452047 ) ) ;
#48165=CARTESIAN_POINT ( 'NONE',  ( -6.347188469492005325, 10.55680364771601809, -0.7998128361456291469 ) ) ;
#48171=CARTESIAN_POINT ( 'NONE',  ( -1.500000000000013101, 3.160416667349486008, -0.8660254037844313801 ) ) ;
#48172=CARTESIAN_POINT ( 'NONE',  ( 8.914649696185335870, 10.35917838609310593, -1.199719254218446718 ) ) ;
#48175=CARTESIAN_POINT ( 'NONE',  ( -8.690940161559884913, 10.09818392903003748, 1.199719254218462483 ) ) ;
#48177=CARTESIAN_POINT ( 'NONE',  ( -0.6823417656250212460, 3.301041667008085323, 1.181850606188767472 ) ) ;
#48183=CARTESIAN_POINT ( 'NONE',  ( -9.653042183249972652, 10.36423008998754192, -0.7216878364870267237 ) ) ;
#48188=CARTESIAN_POINT ( 'NONE',  ( 0.6823417656249882723, 1.738541667008083991, -1.181850606188749264 ) ) ;
#48193=CARTESIAN_POINT ( 'NONE',  ( 1.364683531249986537, 2.655208333674754062, -0.7879004041258239610 ) ) ;
#48195=CARTESIAN_POINT ( 'NONE',  ( -5.599681137644054729, 6.491715067794862293, 1.199719254218450271 ) ) ;
#48198=EDGE_CURVE ( 'NONE', #192556, #6976, #17801, .T. ) ;
#48199=CARTESIAN_POINT ( 'NONE',  ( -1.364683531250000748, 2.071875000341422357, 1.214306433183764966E-14 ) ) ;
#48203=CARTESIAN_POINT ( 'NONE',  ( -4.446711195602239819, 8.131654128270509929, -0.7216878364870267237 ) ) ;
#48207=CARTESIAN_POINT ( 'NONE',  ( 4.690757960648224589, 6.495636925554817864, 1.443375672974062551 ) ) ;
#48210=CARTESIAN_POINT ( 'NONE',  ( -7.069687034522070590, 10.33538640932937724, -1.199719254218440723 ) ) ;
#48211=CARTESIAN_POINT ( 'NONE',  ( -10.49364770729726359, 11.34493653470939023, 0.7216878364870438212 ) ) ;
#48213=CARTESIAN_POINT ( 'NONE',  ( 0.6823417656249899377, 5.676041667008087543, -1.181850606188754593 ) ) ;
#48218=CARTESIAN_POINT ( 'NONE',  ( -6.114364089638801403, 8.156510742710487705, 1.443375672974078761 ) ) ;
#48220=CARTESIAN_POINT ( 'NONE',  ( -0.6823417656250246877, -1.136458332991911790, 1.181850606188755259 ) ) ;
#48223=CARTESIAN_POINT ( 'NONE',  ( 7.809133291791403586, 8.213003049952529722, -0.7216878364870257245 ) ) ;
#48239=CARTESIAN_POINT ( 'NONE',  ( 5.276094334012385367, 9.307193822989793475, 1.040834085586084257E-14 ) ) ;
#48240=CARTESIAN_POINT ( 'NONE',  ( -4.172158584703340445, 5.890604320285754980, -1.599625672291256295 ) ) ;
#48244=CARTESIAN_POINT ( 'NONE',  ( 5.788968402910812827, 6.816513227226497662, 1.082531754730558626 ) ) ;
#48245=CARTESIAN_POINT ( 'NONE',  ( 1.364683531249988757, 0.4468750003414206917, 0.000000000000000000 ) ) ;
#48247=CARTESIAN_POINT ( 'NONE',  ( -9.321394304595349567, 10.83371376257142416, 1.199719254218462483 ) ) ;
#48256=CARTESIAN_POINT ( 'NONE',  ( 1.499999999999990896, 4.525000000000021672, 1.214306433183764966E-14 ) ) ;
#48264=CARTESIAN_POINT ( 'NONE',  ( 6.283314124929436417, 9.417951348137970413, -1.199719254218440723 ) ) ;
#48265=CARTESIAN_POINT ( 'NONE',  ( 6.608709811657416999, 9.797579649320619311, -1.199719254218440723 ) ) ;
#48269=EDGE_LOOP ( 'NONE', ( #34584, #62627, #52058, #114449, #140160, #198144, #31716, #133505, #160013, #141663, #63975, #91937, #209362 ) ) ;
#48277=CARTESIAN_POINT ( 'NONE',  ( -4.451154503988200339, 4.087435097607984957, 1.214306433183764966E-14 ) ) ;
#48282=CARTESIAN_POINT ( 'NONE',  ( -0.5500358407890207912, 7.827628757559874195, 1.923053904898951005 ) ) ;
#48287=CARTESIAN_POINT ( 'NONE',  ( -9.164948653157990677, 11.71552606681625619, -1.443375672974059665 ) ) ;
#48291=CARTESIAN_POINT ( 'NONE',  ( 6.010342169559767633, 5.906487374108181143, -0.7998128361456281477 ) ) ;
#48292=CARTESIAN_POINT ( 'NONE',  ( -1.201851678989727383E-14, 5.446875000341422357, -1.575800808251660134 ) ) ;
#48298=CARTESIAN_POINT ( 'NONE',  ( 5.788968402910816380, 5.856144012925152076, 0.7216878364870317197 ) ) ;
#48305=CARTESIAN_POINT ( 'NONE',  ( -6.663996196316808174, 7.733415969579778171, -1.199719254218446718 ) ) ;
#48306=CARTESIAN_POINT ( 'NONE',  ( -4.517891501851816649, 6.293959390292322986, -1.599625672291256295 ) ) ;
#48315=CARTESIAN_POINT ( 'NONE',  ( 6.257251587906815793, 7.258880593101466161, 1.199719254218462483 ) ) ;
#48322=CARTESIAN_POINT ( 'NONE',  ( 4.161989969715272686, 4.726297878971393196, 2.420000000000010587 ) ) ;
#48328=CARTESIAN_POINT ( 'NONE',  ( -1.364683531250000748, -0.4281249996585800854, 0.000000000000000000 ) ) ;
#48330=CARTESIAN_POINT ( 'NONE',  ( 5.542585869888291938, 5.360771691158120689, -0.7998128361456211532 ) ) ;
#48332=CARTESIAN_POINT ( 'NONE',  ( -7.104109303880803417, 8.350844278358124484, 1.082531754730549967 ) ) ;
#48334=CARTESIAN_POINT ( 'NONE',  ( -6.520158902582610772, 5.290451655907115303, -2.438235897557448961 ) ) ;
#48335=CARTESIAN_POINT ( 'NONE',  ( 4.772106882330221289, 6.590544000850479200, -1.443375672974051449 ) ) ;
#48336=CARTESIAN_POINT ( 'NONE',  ( -7.090551149822745813, 9.295395646258437949, 1.443375672974078761 ) ) ;
#48338=ORIENTED_EDGE ( 'NONE', *, *, #138645, .F. ) ;
#48340=CARTESIAN_POINT ( 'NONE',  ( 7.786460292950004636, 7.978625184730144149, 1.040834085586084257E-14 ) ) ;
#48344=CARTESIAN_POINT ( 'NONE',  ( -4.609409038966246541, 6.400729850259146758, -1.443375672974053892 ) ) ;
#48345=CARTESIAN_POINT ( 'NONE',  ( 0.6823417656249917140, 4.092708333674755394, 1.181850606188765695 ) ) ;
#48349=CARTESIAN_POINT ( 'NONE',  ( 7.283754839039659146, 9.520799950344851936, -1.599625672291262513 ) ) ;
#48353=CARTESIAN_POINT ( 'NONE',  ( -7.853197290813634268, 10.18514947741448573, 1.599625672291295375 ) ) ;
#48359=CARTESIAN_POINT ( 'NONE',  ( 9.023114925094663619, 10.48572115315399245, 1.199719254218453823 ) ) ;
#48361=CARTESIAN_POINT ( 'NONE',  ( -7.720478407978036195, 11.09464301169468037, -1.199719254218446718 ) ) ;
#48365=CARTESIAN_POINT ( 'NONE',  ( 4.809732914444119878, 6.735689552132856583, -1.248430568442916888 ) ) ;
#48366=CARTESIAN_POINT ( 'NONE',  ( -8.500599126088349777, 12.86119004717103209, 1.040834085586084257E-14 ) ) ;
#48372=CARTESIAN_POINT ( 'NONE',  ( 6.972971076130050072, 7.029554431773520129, 1.040834085586084257E-14 ) ) ;
#48374=CARTESIAN_POINT ( 'NONE',  ( 5.473741331615251227, 7.409117525016355010, -1.599625672291262513 ) ) ;
#48375=CARTESIAN_POINT ( 'NONE',  ( -4.099290701344459720, 7.507401141727952698, 0.5799236987427489609 ) ) ;
#48376=CARTESIAN_POINT ( 'NONE',  ( 3.871016551901614200, 4.474939717762034697, -1.199719254218446718 ) ) ;
#48378=CARTESIAN_POINT ( 'NONE',  ( -6.887178846062116833, 9.058127958537705027, -1.443375672974059665 ) ) ;
#48384=CARTESIAN_POINT ( 'NONE',  ( -5.296940370067747317, 6.395615756200102808, 1.134431874056667233 ) ) ;
#48385=CARTESIAN_POINT ( 'NONE',  ( -1.364683531250000748, -0.4281249996585800854, 0.000000000000000000 ) ) ;
#48389=CARTESIAN_POINT ( 'NONE',  ( 3.660338286009610975, 6.253849852777763729, -1.082531754730543083 ) ) ;
#48394=CARTESIAN_POINT ( 'NONE',  ( -9.178506806327330736, 10.77097469787910455, 1.082531754730558626 ) ) ;
#48397=DIRECTION ( 'NONE',  ( -0.000000000000000000, -8.546850786086437571E-32, -1.000000000000000000 ) ) ;
#48400=CARTESIAN_POINT ( 'NONE',  ( -8.310784975052669665, 12.63974020429606249, -0.7216878364870267237 ) ) ;
#48408=CARTESIAN_POINT ( 'NONE',  ( -8.527715432871366019, 10.01171809551380143, 1.082531754730558626 ) ) ;
#48412=CARTESIAN_POINT ( 'NONE',  ( -0.6823417656250212460, 5.363541667008087543, 1.181850606188767472 ) ) ;
#48413=CARTESIAN_POINT ( 'NONE',  ( -0.7500000000000215383, 2.972916667349487341, 1.299038105676671107 ) ) ;
#48417=CARTESIAN_POINT ( 'NONE',  ( -6.561256274009600986, 9.742217188731485678, -1.199719254218440723 ) ) ;
#48421=CARTESIAN_POINT ( 'NONE',  ( 6.986529229743720926, 7.045372277656132276, -0.7998128361456281477 ) ) ;
#48423=CARTESIAN_POINT ( 'NONE',  ( -4.168895032367330167, 3.976329666238523242, -0.6109567437776577403 ) ) ;
#48426=CARTESIAN_POINT ( 'NONE',  ( 7.639129486296027061, 10.99973593639901814, 1.199719254218460707 ) ) ;
#48427=CARTESIAN_POINT ( 'NONE',  ( -6.959052028702998882, 5.167241622962444936, 1.214306433183764966E-14 ) ) ;
#48429=CARTESIAN_POINT ( 'NONE',  ( 4.638229190868996987, 5.411267389347211854, 2.420000000000010587 ) ) ;
#48432=CARTESIAN_POINT ( 'NONE',  ( -6.561783159334137139, 8.678499657355050800, -1.443375672974059665 ) ) ;
#48435=CARTESIAN_POINT ( 'NONE',  ( 1.364683531249988535, 4.967708333674756283, -0.7879004041258300672 ) ) ;
#48439=CARTESIAN_POINT ( 'NONE',  ( -5.883875478206491927, 5.966868934103426447, 0.000000000000000000 ) ) ;
#48442=CARTESIAN_POINT ( 'NONE',  ( -8.696665468161981494, 12.23352791524263239, -1.199719254218446718 ) ) ;
#48445=CARTESIAN_POINT ( 'NONE',  ( 7.248805684800777804, 11.60869039890961218, 1.040834085586084257E-14 ) ) ;
#48447=CARTESIAN_POINT ( 'NONE',  ( -8.992082194361570302, 11.51384853155376220, 1.599625672291269396 ) ) ;
#48448=CARTESIAN_POINT ( 'NONE',  ( 1.499999999999989120, 6.280000000000042881, -2.579999999999995630 ) ) ;
#48450=CARTESIAN_POINT ( 'NONE',  ( -1.201851678989727383E-14, 2.571875000341417472, 1.575800808251672791 ) ) ;
#48451=EDGE_CURVE ( 'NONE', #106888, #5398, #40254, .T. ) ;
#48452=CARTESIAN_POINT ( 'NONE',  ( 4.546061579283848353, 4.198160018786257552, -0.7998128361456211532 ) ) ;
#48456=CARTESIAN_POINT ( 'NONE',  ( -4.222669843016471525, 3.519858668466405494, -2.499999999999995559 ) ) ;
#48457=DIRECTION ( 'NONE',  ( 0.7592566023653005702, -0.6507913734559640506, 0.000000000000000000 ) ) ;
#48458=CARTESIAN_POINT ( 'NONE',  ( 8.215877899756996783, 12.52901528311778989, 1.040834085586084257E-14 ) ) ;
#48459=CARTESIAN_POINT ( 'NONE',  ( -7.700668062882078502, 9.046829497192987901, -1.082531754730543971 ) ) ;
#48460=CARTESIAN_POINT ( 'NONE',  ( 0.6823417656249882723, 0.3427083336747516196, 1.181850606188755259 ) ) ;
#48462=CARTESIAN_POINT ( 'NONE',  ( 0.5473748313345295768, 7.493086169160064536, 1.923660786605030149 ) ) ;
#48464=CARTESIAN_POINT ( 'NONE',  ( -8.518600588087975822, 8.832788862391110385, 1.040834085586084257E-14 ) ) ;
#48465=CARTESIAN_POINT ( 'NONE',  ( -3.592547517496935683, 6.174760622846296343, -1.082531754730548412 ) ) ;
#48466=CARTESIAN_POINT ( 'NONE',  ( -1.201851678989727383E-14, 2.884375000341418804, 1.575800808251672791 ) ) ;
#48483=CARTESIAN_POINT ( 'NONE',  ( -1.364683531250012516, 4.301041667008089320, -0.7879004041258300672 ) ) ;
#48488=CARTESIAN_POINT ( 'NONE',  ( 8.609591239877852686, 10.00327685373437347, -1.199719254218445830 ) ) ;
#48491=CARTESIAN_POINT ( 'NONE',  ( -0.6823417656250212460, 2.801041667008084879, 1.181850606188767472 ) ) ;
#48493=CARTESIAN_POINT ( 'NONE',  ( -6.046573322014817897, 9.998159942418544333, 0.7216878364870458196 ) ) ;
#48498=CARTESIAN_POINT ( 'NONE',  ( 5.366329872910639232, 5.155139694684188534, 1.040834085586084257E-14 ) ) ;
#48501=CARTESIAN_POINT ( 'NONE',  ( 9.511208455186636712, 11.05516360492796935, 1.199719254218453823 ) ) ;
#48506=ORIENTED_EDGE ( 'NONE', *, *, #80530, .F. ) ;
#48508=CARTESIAN_POINT ( 'NONE',  ( -3.297657676621885692, 4.870353260857385180, 1.599625672291267398 ) ) ;
#48509=CARTESIAN_POINT ( 'NONE',  ( 6.662942426112080874, 9.860851032851066122, 1.199719254218460707 ) ) ;
#48511=CARTESIAN_POINT ( 'NONE',  ( 3.497640442201256139, 7.024404915969360452, 1.040834085586084257E-14 ) ) ;
#48522=CARTESIAN_POINT ( 'NONE',  ( -7.266807147244793263, 8.540658428949452485, 1.082531754730549967 ) ) ;
#48523=CARTESIAN_POINT ( 'NONE',  ( 4.660252114795294887, 6.460046772059735432, -1.599625672291256295 ) ) ;
#48526=CARTESIAN_POINT ( 'NONE',  ( -7.483210719738908168, 10.81783070874899799, 1.199719254218453823 ) ) ;
#48531=CARTESIAN_POINT ( 'NONE',  ( -10.45741655484220267, 11.09474082360439873, -0.7998128361456221525 ) ) ;
#48534=EDGE_CURVE ( 'NONE', #72912, #31219, #138922, .T. ) ;
#48536=CARTESIAN_POINT ( 'NONE',  ( 7.801827329660018684, 11.18955008699033726, 1.199719254218460707 ) ) ;
#48537=DIRECTION ( 'NONE',  ( -0.8079921913829680724, -5.171644362755859381E-12, -0.5891931929886402575 ) ) ;
#48547=CARTESIAN_POINT ( 'NONE',  ( -4.038971567461725698, 3.986455684509185193, -0.5169845646830102392 ) ) ;
#48549=CARTESIAN_POINT ( 'NONE',  ( -7.700141177557535244, 11.07091624287075859, -1.199719254218446718 ) ) ;
#48553=CARTESIAN_POINT ( 'NONE',  ( 7.998947442382716488, 9.394822106610419610, -1.082531754730543083 ) ) ;
#48555=CARTESIAN_POINT ( 'NONE',  ( 4.467575310902914154, 5.170924936596891008, 1.199719254218464037 ) ) ;
#48556=FACE_BOUND ( 'NONE', #152390, .T. ) ;
#48558=CARTESIAN_POINT ( 'NONE',  ( -5.716734326456539783, 9.821273814174633188, -0.7998128361456231517 ) ) ;
#48568=CARTESIAN_POINT ( 'NONE',  ( 1.364683531249988535, 3.967708333674751842, -0.7879004041258239610 ) ) ;
#48569=CARTESIAN_POINT ( 'NONE',  ( 4.957044826792370351, 6.512741263613364140, 2.499999999999778399 ) ) ;
#48570=CARTESIAN_POINT ( 'NONE',  ( 7.865701674222579598, 12.32840238656838139, -0.7998128361456352531 ) ) ;
#48573=CARTESIAN_POINT ( 'NONE',  ( -2.643476764984671767, 6.027880625883323518, 1.040834085586084257E-14 ) ) ;
#48576=CARTESIAN_POINT ( 'NONE',  ( -3.863710589770277259, 6.491117540498504646, 1.082531754730560403 ) ) ;
#48581=ORIENTED_EDGE ( 'NONE', *, *, #71920, .T. ) ;
#48583=CARTESIAN_POINT ( 'NONE',  ( 3.323720213644492993, 7.029424015893889433, 1.040834085586084257E-14 ) ) ;
#48591=CARTESIAN_POINT ( 'NONE',  ( 4.547870462380197765, 7.393267075163835855, 1.199719254218462483 ) ) ;
#48595=CARTESIAN_POINT ( 'NONE',  ( 0.6823417656249917140, 4.405208333674755394, 1.181850606188765695 ) ) ;
#48600=CARTESIAN_POINT ( 'NONE',  ( 7.070740804726770357, 8.207951346058097286, 1.199719254218462483 ) ) ;
#48602=CARTESIAN_POINT ( 'NONE',  ( -6.087774667736030487, 7.061157519568837415, 1.199719254218450271 ) ) ;
#48603=CARTESIAN_POINT ( 'NONE',  ( -1.500000000000011324, 2.670833333333352044, 0.8660254037844403729 ) ) ;
#48606=CARTESIAN_POINT ( 'NONE',  ( -5.111587607552082524, 5.922272616020886282, 1.199719254218450271 ) ) ;
#48607=CARTESIAN_POINT ( 'NONE',  ( 0.004619473214107315887, 7.151453204069587066, -1.999995854215781410 ) ) ;
#48609=( BOUNDED_CURVE ( )  B_SPLINE_CURVE ( 2, ( #198, #146526, #130325, #66267, #198417, #183247, #50061 ),
 .UNSPECIFIED., .F., .T. ) 
 B_SPLINE_CURVE_WITH_KNOTS ( ( 3, 2, 2, 3 ),
 ( 0.2375000000000003775, 0.2416666666666668351, 0.2458333333333332926, 0.2499999999999997502 ),
 .UNSPECIFIED. ) 
 CURVE ( )  GEOMETRIC_REPRESENTATION_ITEM ( )  RATIONAL_B_SPLINE_CURVE ( ( 0.9999999999999874545, 0.8660254037844512531, 1.000000000000000000, 0.8660254037844387076, 1.000000000000000000, 0.8660254037844467012, 0.9999999999999920064 ) ) 
 REPRESENTATION_ITEM ( '' )  );
#48611=CARTESIAN_POINT ( 'NONE',  ( 1.364683531249990311, 2.884375000341422801, 1.214306433183764966E-14 ) ) ;
#48613=CARTESIAN_POINT ( 'NONE',  ( -5.260200412422220140, 5.239248024021764039, -0.7216878364870207285 ) ) ;
#48619=CARTESIAN_POINT ( 'NONE',  ( 4.306686350635271054, 8.176217842383143974, -0.7998128361456221525 ) ) ;
#48622=CARTESIAN_POINT ( 'NONE',  ( -1.364683531250010295, 4.092708333674751842, 0.7879004041258379498 ) ) ;
#48624=CARTESIAN_POINT ( 'NONE',  ( 3.979481780810941949, 4.601482484822914998, 1.199719254218464037 ) ) ;
#48625=CARTESIAN_POINT ( 'NONE',  ( -1.402160292154681736E-14, -0.4906249996585810846, -1.575800808251665908 ) ) ;
#48628=CARTESIAN_POINT ( 'NONE',  ( -2.788173145904702555, 6.404619103530779789, -0.7998128361456281477 ) ) ;
#48629=CARTESIAN_POINT ( 'NONE',  ( -7.199016378732087773, 7.501199984716642177, 0.7216878364870317197 ) ) ;
#48633=CARTESIAN_POINT ( 'NONE',  ( -1.364683531250012516, 2.780208333674754506, 0.7879004041258379498 ) ) ;
#48641=CARTESIAN_POINT ( 'NONE',  ( -6.277061933002790362, 8.346324893301817482, 1.443375672974078761 ) ) ;
#48648=CARTESIAN_POINT ( 'NONE',  ( -5.043269954159181445, 8.827639346586952485, 1.214306433183764966E-14 ) ) ;
#48660=CARTESIAN_POINT ( 'NONE',  ( -4.554649539187067830, 7.401175998105142817, 1.199719254218464037 ) ) ;
#48662=CARTESIAN_POINT ( 'NONE',  ( -0.7500000000000249800, -0.05833333333331303105, 1.299038105676659116 ) ) ;
#48663=CARTESIAN_POINT ( 'NONE',  ( 10.41229878561526512, 11.25002945941372623, -0.7216878364870257245 ) ) ;
#48664=CARTESIAN_POINT ( 'NONE',  ( 6.259060471003163428, 10.45398764947904624, -0.7998128361456291469 ) ) ;
#48667=CARTESIAN_POINT ( 'NONE',  ( 5.789495288235341874, 6.713164910151406595, 1.199719254218462483 ) ) ;
#48673=CARTESIAN_POINT ( 'NONE',  ( -2.982430605326328532, 5.462957558647244305, -1.082531754730543971 ) ) ;
#48679=CIRCLE ( 'NONE', #31517, 0.07999999999999975187 ) ;
#48682=CARTESIAN_POINT ( 'NONE',  ( -1.364683531250000748, 2.009375000341421913, 1.214306433183764966E-14 ) ) ;
#48683=CARTESIAN_POINT ( 'NONE',  ( 9.693716643646590470, 12.33242205571964512, 1.443375672974076540 ) ) ;
#48684=CARTESIAN_POINT ( 'NONE',  ( -5.876569516519495551, 8.943415971659659292, 1.199719254218452047 ) ) ;
#48688=CARTESIAN_POINT ( 'NONE',  ( 4.971035877704902184, 8.951292290631053916, 1.040834085586084257E-14 ) ) ;
#48689=CARTESIAN_POINT ( 'NONE',  ( -5.391338639728555648, 9.441645512991978961, -0.7998128361456231517 ) ) ;
#48692=CARTESIAN_POINT ( 'NONE',  ( -1.402160292154681736E-14, -0.006249999317184824418, 1.732050807568877637 ) ) ;
#48696=CARTESIAN_POINT ( 'NONE',  ( 7.944714827928050838, 9.331550723079971021, 1.082531754730558626 ) ) ;
#48699=CARTESIAN_POINT ( 'NONE',  ( -1.402160292154681736E-14, 0.3843750003414230232, 1.575800808251672791 ) ) ;
#48701=CARTESIAN_POINT ( 'NONE',  ( 5.612712405933139692, 9.491988873656591608, 1.040834085586084257E-14 ) ) ;
#48704=CARTESIAN_POINT ( 'NONE',  ( -4.663641653420935285, 5.503632019488245319, 1.082531754730560403 ) ) ;
#48706=CARTESIAN_POINT ( 'NONE',  ( -1.201851678989727383E-14, 4.446875000341417916, -1.575800808251660134 ) ) ;
#48710=CARTESIAN_POINT ( 'NONE',  ( -5.927203485463973465, 6.129067544638190590, -0.8144944673919730649 ) ) ;
#48717=CARTESIAN_POINT ( 'NONE',  ( 6.958359152311676787, 9.141171649162195934, -1.599625672291262513 ) ) ;
#48720=CARTESIAN_POINT ( 'NONE',  ( 3.225950485047770933, 5.851027101609320269, 1.199719254218450271 ) ) ;
#48726=EDGE_LOOP ( 'NONE', ( #100794, #43159, #173613, #134539, #53544 ) ) ;
#48727=CARTESIAN_POINT ( 'NONE',  ( 4.202664430556241726, 7.846932902383524144, 0.7216878364870298324 ) ) ;
#48728=VECTOR ( 'NONE', #166049, 1000.000000000000000 ) ;
#48729=CARTESIAN_POINT ( 'NONE',  ( 0.6823417656249882723, 0.1552083336747514530, 1.181850606188755259 ) ) ;
#48731=CARTESIAN_POINT ( 'NONE',  ( 4.376584659113025744, 4.000436945253625254, 0.7998128361456341429 ) ) ;
#48734=CARTESIAN_POINT ( 'NONE',  ( 0.7499999999999902300, 3.764583334016149863, 1.299038105676669330 ) ) ;
#48736=CARTESIAN_POINT ( 'NONE',  ( 0.7499999999999902300, 1.233333333333357151, 1.299038105676657340 ) ) ;
#48737=CARTESIAN_POINT ( 'NONE',  ( 7.019370843573166319, 9.212351955633947043, 1.599625672291281386 ) ) ;
#48738=CARTESIAN_POINT ( 'NONE',  ( -7.340850106795412167, 10.65174332698158643, 1.199719254218453823 ) ) ;
#48742=CARTESIAN_POINT ( 'NONE',  ( -1.364683531250000748, 0.7593750003414210248, 0.000000000000000000 ) ) ;
#48743=EDGE_LOOP ( 'NONE', ( #180060, #21988, #85250 ) ) ;
#48744=CARTESIAN_POINT ( 'NONE',  ( -1.500000000000013101, 1.920833333333356263, 0.8660254037844403729 ) ) ;
#48746=CARTESIAN_POINT ( 'NONE',  ( 4.684505768721569652, 5.424010470718658716, -1.199719254218452047 ) ) ;
#48751=SPHERICAL_SURFACE ( 'NONE', #83893, 0.08000000000000000167 ) ;
#48753=CARTESIAN_POINT ( 'NONE',  ( -1.500000000000015099, -1.089583332650509773, -0.8660254037844383745 ) ) ;
#48754=CARTESIAN_POINT ( 'NONE',  ( -5.357443255694392725, 9.402100898285455699, 0.000000000000000000 ) ) ;
#48755=CARTESIAN_POINT ( 'NONE',  ( -4.500943810056945438, 5.313817868896925312, 1.082531754730560403 ) ) ;
#48762=ORIENTED_EDGE ( 'NONE', *, *, #86749, .F. ) ;
#48763=CARTESIAN_POINT ( 'NONE',  ( 6.612626235163189925, 8.737816579155630592, -1.599625672291262513 ) ) ;
#48766=CARTESIAN_POINT ( 'NONE',  ( 6.440286661691305703, 7.472421512516709718, 1.199719254218462483 ) ) ;
#48767=CARTESIAN_POINT ( 'NONE',  ( 10.01911233037458260, 10.79131192829960462, 0.7216878364870438212 ) ) ;
#48771=CARTESIAN_POINT ( 'NONE',  ( -7.531718027591449705, 8.745758106066849891, 1.199719254218462483 ) ) ;
#48773=CARTESIAN_POINT ( 'NONE',  ( 3.655894977179307226, 7.416961240017848844, -0.7998128361456291469 ) ) ;
#48777=CARTESIAN_POINT ( 'NONE',  ( 4.055251984284337752, 7.519160923078652026, -0.4935718261673445184 ) ) ;
#48778=CARTESIAN_POINT ( 'NONE',  ( 9.300530189294644146, 10.91333531134101165, -1.082531754730543083 ) ) ;
#48784=CARTESIAN_POINT ( 'NONE',  ( -7.334597915313094241, 9.580116872663850813, 1.040834085586084257E-14 ) ) ;
#48787=CARTESIAN_POINT ( 'NONE',  ( 8.107412671292031803, 11.44210330227398487, 1.082531754730557072 ) ) ;
#48790=CARTESIAN_POINT ( 'NONE',  ( -4.232116505760120440, 8.089219690028791376, -0.7998128361456281477 ) ) ;
#48796=CARTESIAN_POINT ( 'NONE',  ( -6.938021921891187382, 9.117444880338284818, -1.599625672291263179 ) ) ;
#48798=DIRECTION ( 'NONE',  ( 0.7592566023653010143, -0.6507913734559633845, -5.900213523162838665E-32 ) ) ;
#48811=CARTESIAN_POINT ( 'NONE',  ( -6.878064000834399394, 6.918829510595249310, -0.7998128361456291469 ) ) ;
#48814=CARTESIAN_POINT ( 'NONE',  ( 4.202664430556247055, 6.886563688082179446, 1.082531754730558626 ) ) ;
#48819=CARTESIAN_POINT ( 'NONE',  ( 1.408489644581676137, 7.311701683604759694, 4.382268911472973372 ) ) ;
#48822=CARTESIAN_POINT ( 'NONE',  ( 9.836604141914616406, 11.43479190611061647, 1.199719254218452047 ) ) ;
#48826=CARTESIAN_POINT ( 'NONE',  ( -8.853638004923878313, 10.28799807962136548, 1.199719254218462483 ) ) ;
#48827=CARTESIAN_POINT ( 'NONE',  ( 5.178324605415663306, 8.128796908705222535, 1.199719254218462483 ) ) ;
#48831=CARTESIAN_POINT ( 'NONE',  ( 3.811813743736467419, 7.598866467667865443, 1.040834085586084257E-14 ) ) ;
#48834=CARTESIAN_POINT ( 'NONE',  ( -0.6823417656250246877, -0.1364583329919108468, 1.181850606188755259 ) ) ;
#48837=CARTESIAN_POINT ( 'NONE',  ( 8.270110514656026979, 10.67154823856396817, 1.443375672974076540 ) ) ;
#48844=LINE ( 'NONE', #160453, #198090 ) ;
#48865=CARTESIAN_POINT ( 'NONE',  ( -1.500000000000013101, 0.7020833340161545255, 0.8660254037844403729 ) ) ;
#48869=ORIENTED_EDGE ( 'NONE', *, *, #1922, .F. ) ;
#48871=CARTESIAN_POINT ( 'NONE',  ( 9.185812768458653466, 10.67553530374532045, 1.199719254218453823 ) ) ;
#48876=CARTESIAN_POINT ( 'NONE',  ( 5.495132332240461714, 5.305409230568988832, 0.7998128361456341429 ) ) ;
#48877=CARTESIAN_POINT ( 'NONE',  ( -5.883875478650828050, 9.808345791827219884, 0.7216878364870458196 ) ) ;
#48878=CARTESIAN_POINT ( 'NONE',  ( -5.910622443071302357, 6.001017179288033354, 0.07212419881679615896 ) ) ;
#48881=CARTESIAN_POINT ( 'NONE',  ( -6.008234629150358330, 10.16135750065076060, 0.000000000000000000 ) ) ;
#48882=CARTESIAN_POINT ( 'NONE',  ( -4.406036734316900905, 5.203092947200234519, -1.082531754730543971 ) ) ;
#48885=CARTESIAN_POINT ( 'NONE',  ( 0.7499999999999902300, 1.264583334016147642, 1.299038105676657340 ) ) ;
#48892=CARTESIAN_POINT ( 'NONE',  ( -3.212919216314315207, 5.731860938133201522, 1.082531754730560403 ) ) ;
#48895=CARTESIAN_POINT ( 'NONE',  ( 4.071134731106788252, 7.497899514862828241, -0.5496474101556632075 ) ) ;
#48901=CARTESIAN_POINT ( 'NONE',  ( -4.406036734316906234, 4.242723732898890709, -0.7216878364870207285 ) ) ;
#48902=CARTESIAN_POINT ( 'NONE',  ( 6.448874621594486989, 10.67543749183559143, 0.7998128361456462443 ) ) ;
#48911=CARTESIAN_POINT ( 'NONE',  ( -9.508345801885592863, 9.987491611821676329, 0.7998128361456462443 ) ) ;
#48916=CARTESIAN_POINT ( 'NONE',  ( 4.005544317833563461, 6.760553239859419250, -1.199719254218452047 ) ) ;
#48922=CARTESIAN_POINT ( 'NONE',  ( -9.484092147959342967, 11.02352791316275216, 1.199719254218462483 ) ) ;
#48926=CARTESIAN_POINT ( 'NONE',  ( 4.650083499807220910, 5.295740330745369207, -2.420000000000000373 ) ) ;
#48936=CARTESIAN_POINT ( 'NONE',  ( 8.281332899848809603, 8.555976559445431562, 0.7998128361456481317 ) ) ;
#48938=CARTESIAN_POINT ( 'NONE',  ( -3.113568832632681360, 6.784247404713427798, -0.7998128361456281477 ) ) ;
#48939=ORIENTED_EDGE ( 'NONE', *, *, #197116, .F. ) ;
#48945=CARTESIAN_POINT ( 'NONE',  ( -0.7500000000000006661, 0.6395833340161540814, -1.299038105676652011 ) ) ;
#48951=CARTESIAN_POINT ( 'NONE',  ( 4.390142812726693045, 4.016254791136236513, 1.214306433183764966E-14 ) ) ;
#48953=CARTESIAN_POINT ( 'NONE',  ( -4.406563619641430840, 5.099744630125142564, -1.199719254218446718 ) ) ;
#48959=CARTESIAN_POINT ( 'NONE',  ( 4.311129659465574804, 7.013106455143060636, -1.082531754730548412 ) ) ;
#48962=CARTESIAN_POINT ( 'NONE',  ( -1.364683531250010295, 4.342708333674753618, 0.7879004041258379498 ) ) ;
#48964=CARTESIAN_POINT ( 'NONE',  ( 3.511198595814926993, 6.079853547550633230, 1.082531754730558626 ) ) ;
#48973=CARTESIAN_POINT ( 'NONE',  ( -6.063230027062802563, 6.042581475280591086, 0.5001817740485012820 ) ) ;
#48975=CARTESIAN_POINT ( 'NONE',  ( -0.6823417656250246877, -0.6989583329919113464, 1.181850606188755259 ) ) ;
#48981=CARTESIAN_POINT ( 'NONE',  ( 1.499999999999987121, -0.9958333333333134751, 0.8660254037844524744 ) ) ;
#48983=CARTESIAN_POINT ( 'NONE',  ( -0.7499999999999972244, 4.858333333333353821, -1.299038105676652011 ) ) ;
#48990=CARTESIAN_POINT ( 'NONE',  ( -1.499999999999997780, 4.400000000000021672, 1.214306433183764966E-14 ) ) ;
#48991=CARTESIAN_POINT ( 'NONE',  ( -1.201851678989727383E-14, 5.259375000341421469, -1.575800808251660134 ) ) ;
#48993=CARTESIAN_POINT ( 'NONE',  ( 6.124532705071213279, 8.168374127381657246, -1.599625672291262513 ) ) ;
#48994=CARTESIAN_POINT ( 'NONE',  ( -8.877891658850122880, 9.251961778280284321, 0.7998128361456462443 ) ) ;
#49001=CARTESIAN_POINT ( 'NONE',  ( 0.7499999999999920064, 5.233333333333353821, 1.299038105676669330 ) ) ;
#49006=ORIENTED_EDGE ( 'NONE', *, *, #123570, .T. ) ;
#49008=CARTESIAN_POINT ( 'NONE',  ( 8.934460041725669655, 9.525884258209195821, 1.040834085586084257E-14 ) ) ;
#49012=CARTESIAN_POINT ( 'NONE',  ( -1.201851678989727383E-14, 3.368750000682815049, -1.732050807568863648 ) ) ;
#49014=CARTESIAN_POINT ( 'NONE',  ( -4.115063316947640715, 4.759660943649018705, 1.199719254218462483 ) ) ;
#49015=CARTESIAN_POINT ( 'NONE',  ( 7.117667457050084856, 7.406292909420979953, -0.7216878364870257245 ) ) ;
#49016=CARTESIAN_POINT ( 'NONE',  ( -8.446366511189330240, 12.79791866312216442, 0.7216878364870317197 ) ) ;
#49023=CARTESIAN_POINT ( 'NONE',  ( 3.225950485047770933, 5.851027101609320269, 1.199719254218450271 ) ) ;
#49025=DIRECTION ( 'NONE',  ( 3.451266460341927524E-31, -0.6000000000000035305, -0.7999999999999974909 ) ) ;
#49026=CARTESIAN_POINT ( 'NONE',  ( 5.027376032568989572, 4.759693547618927489, 0.7998128361456341429 ) ) ;
#49039=CIRCLE ( 'NONE', #7406, 1.000000000000000000 ) ;
#49041=CARTESIAN_POINT ( 'NONE',  ( 7.553864141108259211, 11.96459193126834464, 1.040834085586084257E-14 ) ) ;
#49045=CARTESIAN_POINT ( 'NONE',  ( 1.364683531249988757, -0.1156249996585798079, 0.000000000000000000 ) ) ;
#49046=CARTESIAN_POINT ( 'NONE',  ( 4.826339496784873617, 8.574553812983598533, -0.7216878364870257245 ) ) ;
#49047=CARTESIAN_POINT ( 'NONE',  ( -10.31739171031960822, 11.13930453823545186, 1.040834085586084257E-14 ) ) ;
#49053=CARTESIAN_POINT ( 'NONE',  ( -5.115504031057831469, 4.862509545855891346, 0.7998128361456341429 ) ) ;
#49057=ORIENTED_EDGE ( 'NONE', *, *, #36946, .T. ) ;
#49066=CARTESIAN_POINT ( 'NONE',  ( 5.841900715481964212, 6.189949835993628469, -0.9061318016433889122 ) ) ;
#49067=CARTESIAN_POINT ( 'NONE',  ( -1.123270288250315163, 3.047697346350006331, -0.7749999999993613109 ) ) ;
#49070=CARTESIAN_POINT ( 'NONE',  ( 5.495132332240461714, 5.305409230568988832, 0.7998128361456341429 ) ) ;
#49075=CARTESIAN_POINT ( 'NONE',  ( -8.432808358020034589, 10.86136238915529084, 1.443375672974064550 ) ) ;
#49079=CARTESIAN_POINT ( 'NONE',  ( 6.962275575817444384, 8.081408578997208991, -1.199719254218446718 ) ) ;
#49081=CARTESIAN_POINT ( 'NONE',  ( -3.750802052474980108, 7.527686161196117887, 1.040834085586084257E-14 ) ) ;
#49082=EDGE_CURVE ( 'NONE', #185972, #210868, #98594, .T. ) ;
#49084=CARTESIAN_POINT ( 'NONE',  ( -4.415151579544611238, 8.302760609444034046, -0.7998128361456281477 ) ) ;
#49085=CARTESIAN_POINT ( 'NONE',  ( 4.546061579283848353, 4.198160018786257552, -0.7998128361456211532 ) ) ;
#49087=CARTESIAN_POINT ( 'NONE',  ( -4.543954038874438162, 8.453030145328826350, 1.040834085586084257E-14 ) ) ;
#49090=CARTESIAN_POINT ( 'NONE',  ( 9.725276259704228821, 10.24057714594344048, 0.7998128361456462443 ) ) ;
#49091=CARTESIAN_POINT ( 'NONE',  ( -0.1263102688159843945, 6.363441598446243574, 3.117922131261606999 ) ) ;
#49093=CARTESIAN_POINT ( 'NONE',  ( 4.715454802112915011, 7.044561259014620269, 1.385117731104364536 ) ) ;
#49094=CARTESIAN_POINT ( 'NONE',  ( 4.175548123328908900, 7.815297210618305179, -0.7216878364870197293 ) ) ;
#49102=CARTESIAN_POINT ( 'NONE',  ( 6.263503779389103521, 10.25124547602188763, 1.040834085586084257E-14 ) ) ;
#49106=CARTESIAN_POINT ( 'NONE',  ( -10.29471871147821282, 10.90492667301307605, -0.7998128361456291469 ) ) ;
#49108=CARTESIAN_POINT ( 'NONE',  ( -7.202405917357668663, 9.425892875049191488, 1.599625672291295375 ) ) ;
#49117=CARTESIAN_POINT ( 'NONE',  ( 7.944187942603509356, 11.35563746875774882, 1.199719254218460707 ) ) ;
#49122=CARTESIAN_POINT ( 'NONE',  ( 4.708759422647839976, 4.387974169377582001, -0.7998128361456211532 ) ) ;
#49125=CARTESIAN_POINT ( 'NONE',  ( 1.499999999999989120, 4.035416667349482012, 0.8660254037844524744 ) ) ;
#49129=EDGE_LOOP ( 'NONE', ( #210367, #46278, #97091, #158149 ) ) ;
#49131=CARTESIAN_POINT ( 'NONE',  ( -0.7500000000000215383, 2.691666666666689522, 1.299038105676671107 ) ) ;
#49132=CARTESIAN_POINT ( 'NONE',  ( 7.284808609244363353, 7.393364887073558656, 0.7998128361456341429 ) ) ;
#49135=CARTESIAN_POINT ( 'NONE',  ( 8.107412671292035355, 10.48173408797264194, 1.443375672974076540 ) ) ;
#49136=CARTESIAN_POINT ( 'NONE',  ( 0.006768871532346317291, 8.210909518262139883, 2.038649385027042626 ) ) ;
#49142=CARTESIAN_POINT ( 'NONE',  ( -3.405069135326500351, 7.124331091189553433, 1.040834085586084257E-14 ) ) ;
#49143=CARTESIAN_POINT ( 'NONE',  ( 1.499999999999989120, 5.327083334016152527, -0.8660254037844323793 ) ) ;
#49144=CARTESIAN_POINT ( 'NONE',  ( 0.6823417656249882723, -0.1572916663252488245, 1.181850606188755259 ) ) ;
#49148=CARTESIAN_POINT ( 'NONE',  ( 3.337278367258157630, 7.045241861776501580, 0.7998128361456341429 ) ) ;
#49150=CARTESIAN_POINT ( 'NONE',  ( 1.364683531249984538, -1.094791666325247936, -0.7879004041258309554 ) ) ;
#49153=CARTESIAN_POINT ( 'NONE',  ( 4.264541082807580707, 7.493297298796540495, 1.068285269651513936 ) ) ;
#49158=CARTESIAN_POINT ( 'NONE',  ( -8.213542131780492639, 8.476887330032372603, 1.040834085586084257E-14 ) ) ;
#49160=CARTESIAN_POINT ( 'NONE',  ( 5.678167406024951624, 5.518950149984223508, 0.7998128361456341429 ) ) ;
#49163=CARTESIAN_POINT ( 'NONE',  ( 1.364683531249984538, -1.094791666325247936, -0.7879004041258309554 ) ) ;
#49167=CARTESIAN_POINT ( 'NONE',  ( 8.387690588348714726, 12.93738945304888333, 1.040834085586084257E-14 ) ) ;
#49170=CARTESIAN_POINT ( 'NONE',  ( -4.693093728624763372, 8.627026450037540428, 0.7998128361456481317 ) ) ;
#49175=CARTESIAN_POINT ( 'NONE',  ( 7.716561984472250835, 12.15440608185967086, 1.040834085586084257E-14 ) ) ;
#49177=CARTESIAN_POINT ( 'NONE',  ( 9.088043039861931405, 9.497138389460751284, 1.040834085586084257E-14 ) ) ;
#49179=CARTESIAN_POINT ( 'NONE',  ( -3.093231602212184850, 6.760520635889515795, -0.7998128361456281477 ) ) ;
#49180=CARTESIAN_POINT ( 'NONE',  ( -7.854251061018346469, 8.057714414143200443, -0.7998128361456291469 ) ) ;
#49183=CARTESIAN_POINT ( 'NONE',  ( -5.301779071304492774, 6.560601962741976045, 1.383466813282836716 ) ) ;
#49184=CARTESIAN_POINT ( 'NONE',  ( -1.364683531250014514, -0.01145833299191483488, -0.7879004041258359514 ) ) ;
#49188=CARTESIAN_POINT ( 'NONE',  ( 5.965224400332808763, 9.903252867122883885, -0.7216878364870267237 ) ) ;
#49208=CARTESIAN_POINT ( 'NONE',  ( 10.42352117080803708, 11.05519620889787724, -0.7998128361456281477 ) ) ;
#49212=CARTESIAN_POINT ( 'NONE',  ( -5.057354993097396445, 5.859001232490445688, -1.199719254218446718 ) ) ;
#49213=CARTESIAN_POINT ( 'NONE',  ( -7.296259222448620463, 11.66405285949874759, 0.7998128361456481317 ) ) ;
#49215=VERTEX_POINT ( 'NONE', #169205 ) ;
#49219=EDGE_CURVE ( 'NONE', #14088, #197822, #70595, .T. ) ;
#49220=CARTESIAN_POINT ( 'NONE',  ( -1.201851678989727383E-14, 2.743750000682820378, 1.732050807568877637 ) ) ;
#49221=CARTESIAN_POINT ( 'NONE',  ( 8.535021395002688749, 9.916278701380017324, 1.199719254218462483 ) ) ;
#49224=CARTESIAN_POINT ( 'NONE',  ( -8.962103233833181193, 10.41454084668224489, -1.199719254218446718 ) ) ;
#49225=CARTESIAN_POINT ( 'NONE',  ( 1.364683531249990311, 3.384375000341416140, 1.214306433183764966E-14 ) ) ;
#49228=CARTESIAN_POINT ( 'NONE',  ( 6.938893903907228378E-15, 10.64264068711930733, 1.214306433183764966E-14 ) ) ;
#49233=CARTESIAN_POINT ( 'NONE',  ( -9.327646496521984076, 11.90534021740758064, -1.443375672974059665 ) ) ;
#49237=CARTESIAN_POINT ( 'NONE',  ( -1.364683531250014514, 1.301041667008083325, -0.7879004041258289570 ) ) ;
#49242=CARTESIAN_POINT ( 'NONE',  ( -0.6823417656250003738, 0.9677083336747521747, -1.181850606188749264 ) ) ;
#49244=CARTESIAN_POINT ( 'NONE',  ( -5.656776405399756236, 7.622658444431597680, -1.599625672291256295 ) ) ;
#49245=CARTESIAN_POINT ( 'NONE',  ( 0.000000000000000000, 9.200000000000020606, -0.3999999999999941380 ) ) ;
#49246=EDGE_CURVE ( 'NONE', #16779, #55454, #182242, .T. ) ;
#49248=CARTESIAN_POINT ( 'NONE',  ( 1.499999999999989120, 5.504166666666685970, 0.8660254037844524744 ) ) ;
#49249=CARTESIAN_POINT ( 'NONE',  ( 1.364683531249988535, 3.176041667008084435, 0.7879004041258500513 ) ) ;
#49253=CARTESIAN_POINT ( 'NONE',  ( -4.555176424511596878, 7.297827681030051750, 1.082531754730560403 ) ) ;
#49256=CARTESIAN_POINT ( 'NONE',  ( 3.823036129373602154, 6.443664003369091731, -1.082531754730548412 ) ) ;
#49259=CARTESIAN_POINT ( 'NONE',  ( -8.040148788103921973, 9.338927326664741457, 1.199719254218462483 ) ) ;
#49260=CARTESIAN_POINT ( 'NONE',  ( -3.440018289565379028, 5.036440642624797626, 1.599625672291267398 ) ) ;
#49262=CARTESIAN_POINT ( 'NONE',  ( 1.364683531249990311, 4.863541667008084879, 0.7879004041258500513 ) ) ;
#49267=CARTESIAN_POINT ( 'NONE',  ( -8.337901282280023807, 8.829899038855916871, 0.7216878364870438212 ) ) ;
#49269=CARTESIAN_POINT ( 'NONE',  ( 0.6823417656249882723, -0.01145833299191073573, -1.181850606188749264 ) ) ;
#49273=CARTESIAN_POINT ( 'NONE',  ( 7.782016984564054773, 10.10210578678999482, 1.443375672974076540 ) ) ;
#49279=CARTESIAN_POINT ( 'NONE',  ( 2.968872451268290913, 5.447139712246216625, -1.082531754730543971 ) ) ;
#49284=CARTESIAN_POINT ( 'NONE',  ( 7.741342523278686549, 11.97539067722642869, 0.7216878364870438212 ) ) ;
#49292=CARTESIAN_POINT ( 'NONE',  ( 4.937140493670735708, 8.911747675924535983, -0.7998128361456281477 ) ) ;
#49294=CARTESIAN_POINT ( 'NONE',  ( -6.013204822860843457, 6.974159367214481264, -1.199719254218446718 ) ) ;
#49299=CARTESIAN_POINT ( 'NONE',  ( 6.616015773344440021, 6.821032611764393572, 1.040834085586084257E-14 ) ) ;
#49300=CARTESIAN_POINT ( 'NONE',  ( 1.364683531249986537, -0.3239583329919163424, 0.7879004041258500513 ) ) ;
#49301=CARTESIAN_POINT ( 'NONE',  ( -10.47097470845587175, 11.11055866948701443, 1.040834085586084257E-14 ) ) ;
#49316=CARTESIAN_POINT ( 'NONE',  ( 7.416473721875251890, 8.611306416064660851, 1.199719254218462483 ) ) ;
#49317=CARTESIAN_POINT ( 'NONE',  ( 6.337546739384100292, 9.481222731668410120, 1.199719254218460707 ) ) ;
#49327=CARTESIAN_POINT ( 'NONE',  ( 9.398826802771546696, 11.98838390803207865, -1.599625672291262513 ) ) ;
#49333=DIRECTION ( 'NONE',  ( 5.578564026256504688E-16, 1.000000000000000000, 9.066213480720158442E-32 ) ) ;
#49334=CARTESIAN_POINT ( 'NONE',  ( 1.419999999067301788, 7.203691543881689086, 4.238255391842193909 ) ) ;
#49339=CARTESIAN_POINT ( 'NONE',  ( -10.31739171031960822, 11.13930453823545186, 1.040834085586084257E-14 ) ) ;
#49342=CARTESIAN_POINT ( 'NONE',  ( 6.257251587906815793, 7.258880593101466161, 1.199719254218462483 ) ) ;
#49348=CARTESIAN_POINT ( 'NONE',  ( 5.355107487273504496, 6.310342158982962246, -1.082531754730543083 ) ) ;
#49349=CARTESIAN_POINT ( 'NONE',  ( -5.831978632172702071, 9.955725504176825780, 0.7998128361456481317 ) ) ;
#49355=CARTESIAN_POINT ( 'NONE',  ( -6.856673000209188906, 9.022537805042615489, 1.599625672291283607 ) ) ;
#49356=CARTESIAN_POINT ( 'NONE',  ( -5.623934791570306402, 5.455678766453782913, 0.7998128361456341429 ) ) ;
#49362=CARTESIAN_POINT ( 'NONE',  ( 5.991813822235618758, 9.077867661661846554, 1.199719254218462483 ) ) ;
#49369=CARTESIAN_POINT ( 'NONE',  ( -1.203907071533411699, 2.993479746939697872, 0.7750000000000152323 ) ) ;
#49375=CARTESIAN_POINT ( 'NONE',  ( -1.364683531250014514, -0.1572916663252435232, 0.7879004041258379498 ) ) ;
#49376=CARTESIAN_POINT ( 'NONE',  ( 3.344057444064992168, 7.053150784717805877, 1.040834085586084257E-14 ) ) ;
#49378=CARTESIAN_POINT ( 'NONE',  ( -7.700668062882078502, 9.046829497192987901, -1.082531754730543971 ) ) ;
#49380=CARTESIAN_POINT ( 'NONE',  ( 4.202664430556247055, 6.886563688082179446, 1.082531754730558626 ) ) ;
#49381=CARTESIAN_POINT ( 'NONE',  ( -5.856759170979136897, 9.776710099543576504, 0.000000000000000000 ) ) ;
#49385=CARTESIAN_POINT ( 'NONE',  ( 7.775764792637399836, 9.030479331953833011, -1.199719254218441611 ) ) ;
#49391=CARTESIAN_POINT ( 'NONE',  ( -1.364683531249997417, 4.259375000341424133, 1.214306433183764966E-14 ) ) ;
#49395=CARTESIAN_POINT ( 'NONE',  ( 6.608709811657416999, 9.797579649320619311, -1.199719254218440723 ) ) ;
#49398=CARTESIAN_POINT ( 'NONE',  ( -9.016335848287868160, 10.47781223021269170, 1.199719254218462483 ) ) ;
#49404=CARTESIAN_POINT ( 'NONE',  ( 9.738834413317897898, 10.25639499182604730, 0.000000000000000000 ) ) ;
#49406=CARTESIAN_POINT ( 'NONE',  ( -7.503547950159405566, 10.84155747757291266, 1.199719254218453823 ) ) ;
#49409=CARTESIAN_POINT ( 'NONE',  ( 5.737025562671778545, 6.072208551910874164, -0.6475843906825241580 ) ) ;
#49410=CARTESIAN_POINT ( 'NONE',  ( -9.571693261567968847, 12.19006144329456731, 1.443375672974076540 ) ) ;
#49413=CIRCLE ( 'NONE', #153302, 0.08000000000000041800 ) ;
#49416=CARTESIAN_POINT ( 'NONE',  ( 6.799577732453452761, 7.891594428405881878, -1.199719254218446718 ) ) ;
#49418=CARTESIAN_POINT ( 'NONE',  ( 6.823831386379729302, 6.855558127064808716, -0.7998128361456281477 ) ) ;
#49419=CARTESIAN_POINT ( 'NONE',  ( -4.014161209245137307, 7.626991082632122776, -0.01188119308113272377 ) ) ;
#49420=CARTESIAN_POINT ( 'NONE',  ( 3.063252641683779753, 5.661212951017999373, 1.199719254218450271 ) ) ;
#49422=CARTESIAN_POINT ( 'NONE',  ( -6.697364695470783502, 10.75741654478384035, 0.7216878364870458196 ) ) ;
#49428=CARTESIAN_POINT ( 'NONE',  ( -4.117634752470962667, 7.483002602015099924, 0.6335975934644126895 ) ) ;
#49429=CARTESIAN_POINT ( 'NONE',  ( 0.6823417656249882723, -1.094791666325249713, 1.181850606188755259 ) ) ;
#49432=CARTESIAN_POINT ( 'NONE',  ( 4.690757960648231695, 5.535267711253469614, 1.082531754730560403 ) ) ;
#49437=CARTESIAN_POINT ( 'NONE',  ( -9.205623113554631587, 11.76297960394566466, 1.443375672974076540 ) ) ;
#49443=DIRECTION ( 'NONE',  ( 0.6507913734559640506, -0.7592566023653004592, 0.000000000000000000 ) ) ;
#49449=CARTESIAN_POINT ( 'NONE',  ( -8.609064354553318310, 12.98773281371349775, 0.7216878364870317197 ) ) ;
#49454=ORIENTED_EDGE ( 'NONE', *, *, #170571, .F. ) ;
#49456=CARTESIAN_POINT ( 'NONE',  ( 0.7499999999999902300, 3.014583334016149418, 1.299038105676669330 ) ) ;
#49459=EDGE_LOOP ( 'NONE', ( #58883, #254, #173662, #47826 ) ) ;
#49460=CARTESIAN_POINT ( 'NONE',  ( -8.670602931139386627, 10.07445716020612103, 1.199719254218462483 ) ) ;
#49461=CARTESIAN_POINT ( 'NONE',  ( 0.001128590447023392540, 8.210952333604110365, 2.038660652713624177 ) ) ;
#49465=CARTESIAN_POINT ( 'NONE',  ( 5.986088515633498197, 6.942523675449257858, -1.199719254218446718 ) ) ;
#49470=CARTESIAN_POINT ( 'NONE',  ( 6.774270308322468459, 11.05506579301824743, 0.7998128361456462443 ) ) ;
#49472=CARTESIAN_POINT ( 'NONE',  ( -4.846024844760177253, 5.033942040585545286, -0.8809814305317772432 ) ) ;
#49476=CARTESIAN_POINT ( 'NONE',  ( -6.236387472606145010, 9.259240570473746601, -1.082531754730538864 ) ) ;
#49485=CARTESIAN_POINT ( 'NONE',  ( -3.972175818679615222, 4.696921878956699103, 1.082531754730558626 ) ) ;
#49487=CARTESIAN_POINT ( 'NONE',  ( 10.39640486358069360, 11.02356051713265650, 0.7998128361456462443 ) ) ;
#49489=CARTESIAN_POINT ( 'NONE',  ( -7.641992139597101108, 12.06740792950531649, 0.7998128361456481317 ) ) ;
#49492=CARTESIAN_POINT ( 'NONE',  ( 0.6823417656249899377, 1.842708333674752952, 1.181850606188755259 ) ) ;
#49493=CARTESIAN_POINT ( 'NONE',  ( 4.090809663021327758, 5.795697244990093644, 1.599625672291267398 ) ) ;
#49499=CARTESIAN_POINT ( 'NONE',  ( 8.880227426826630577, 12.34372051706435869, 1.082531754730546636 ) ) ;
#49501=CARTESIAN_POINT ( 'NONE',  ( -7.456621297836087514, 9.722477485607340597, 1.443375672974090751 ) ) ;
#49502=CARTESIAN_POINT ( 'NONE',  ( -0.6823417656250003738, 0.4677083336747517306, -1.181850606188749264 ) ) ;
#49504=CARTESIAN_POINT ( 'NONE',  ( 0.4545350412507122573, 7.933623023433559851, 1.993241281637238460 ) ) ;
#49506=CARTESIAN_POINT ( 'NONE',  ( -9.155833807930273238, 9.576227618873799585, -0.7998128361456291469 ) ) ;
#49507=CARTESIAN_POINT ( 'NONE',  ( -5.544921637864841379, 5.571422787038166291, -0.7216878364870197293 ) ) ;
#49508=CARTESIAN_POINT ( 'NONE',  ( -1.364683531250012516, 2.842708333674754506, 0.7879004041258379498 ) ) ;
#49526=CARTESIAN_POINT ( 'NONE',  ( 1.364683531249988535, 4.426041667008082214, 0.7879004041258500513 ) ) ;
#49532=CARTESIAN_POINT ( 'NONE',  ( 8.048736748007069508, 12.54194330598362406, -0.7998128361456352531 ) ) ;
#49534=CARTESIAN_POINT ( 'NONE',  ( 1.364683531249988535, 2.905208333674754506, -0.7879004041258239610 ) ) ;
#49536=CARTESIAN_POINT ( 'NONE',  ( -8.053180056837398126, 8.497724275839514618, 0.7216878364870578100 ) ) ;
#49542=CARTESIAN_POINT ( 'NONE',  ( 3.493197133815315603, 7.227147089426516402, -0.7998128361456291469 ) ) ;
#49545=CARTESIAN_POINT ( 'NONE',  ( 7.703003830858588863, 12.13858823597705872, -0.7998128361456291469 ) ) ;
#49552=CARTESIAN_POINT ( 'NONE',  ( -10.63367255181986160, 11.30037282007833532, 1.040834085586084257E-14 ) ) ;
#49553=CARTESIAN_POINT ( 'NONE',  ( 7.820355676984174664, 8.018169799436671852, -0.7998128361456281477 ) ) ;
#49555=CARTESIAN_POINT ( 'NONE',  ( 4.161989969270892153, 6.839110149915929249, 1.082531754730558626 ) ) ;
#49567=VECTOR ( 'NONE', #14960, 1000.000000000000000 ) ;
#49568=CARTESIAN_POINT ( 'NONE',  ( -8.053180056837398126, 8.497724275839514618, 0.7216878364870578100 ) ) ;
#49569=CARTESIAN_POINT ( 'NONE',  ( 5.118366684358879759, 5.930181538962194132, 1.199719254218462483 ) ) ;
#49572=CARTESIAN_POINT ( 'NONE',  ( -8.670602931139386627, 10.07445716020612103, 1.199719254218462483 ) ) ;
#49577=CARTESIAN_POINT ( 'NONE',  ( -9.297140650669053485, 11.86975006391249643, 1.599625672291281386 ) ) ;
#49582=CARTESIAN_POINT ( 'NONE',  ( 8.015895134177609904, 10.37496362800581018, 1.599625672291281386 ) ) ;
#49584=CARTESIAN_POINT ( 'NONE',  ( 2.191614386903386613, 5.708633884695917260, -0.7998128361456281477 ) ) ;
#49586=ORIENTED_EDGE ( 'NONE', *, *, #162125, .F. ) ;
#49590=CARTESIAN_POINT ( 'NONE',  ( 2.738383840280328663, 5.178236332760252303, 1.082531754730548412 ) ) ;
#49593=CARTESIAN_POINT ( 'NONE',  ( -4.060830702492950195, 4.696389560118578999, -1.199719254218452047 ) ) ;
#49596=CARTESIAN_POINT ( 'NONE',  ( -8.993135964566285168, 9.386413468282476913, -0.7998128361456291469 ) ) ;
#49600=CARTESIAN_POINT ( 'NONE',  ( 6.317736394288122170, 10.31451686007074997, 0.7216878364870438212 ) ) ;
#49601=CARTESIAN_POINT ( 'NONE',  ( -1.001543065824772872E-14, 4.884375000341420581, 1.575800808251672791 ) ) ;
#49603=CARTESIAN_POINT ( 'NONE',  ( 2.198393463710220264, 5.716542807637226886, 0.7998128361456462443 ) ) ;
#49606=CARTESIAN_POINT ( 'NONE',  ( -5.689618019229208734, 9.789638122409414223, 0.7998128361456481317 ) ) ;
#49615=CARTESIAN_POINT ( 'NONE',  ( 1.364683531249990311, 3.446875000341416584, 1.214306433183764966E-14 ) ) ;
#49616=CARTESIAN_POINT ( 'NONE',  ( 1.608462485350607762, 8.735270501766764895, 2.463594439587639240 ) ) ;
#49617=CARTESIAN_POINT ( 'NONE',  ( 8.646349277213076334, 11.11049346154719508, 1.599625672291281386 ) ) ;
#49619=CARTESIAN_POINT ( 'NONE',  ( -5.924549939491850381, 6.014322472269677533, 0.000000000000000000 ) ) ;
#49621=CARTESIAN_POINT ( 'NONE',  ( -5.233084104750526322, 5.207612331738130429, 0.000000000000000000 ) ) ;
#49628=CARTESIAN_POINT ( 'NONE',  ( 5.007038802148489509, 4.735966778795008381, 0.7998128361456341429 ) ) ;
#49635=B_SPLINE_CURVE_WITH_KNOTS ( 'NONE', 3,
 ( #100917, #18596, #173416, #24997, #39130, #91099 ),
 .UNSPECIFIED., .F., .F.,
 ( 4, 2, 4 ),
 ( 0.000000000000000000, 0.0001363166885564072721, 0.0002726333771128145443 ),
 .UNSPECIFIED. ) ;
#49638=EDGE_CURVE ( 'NONE', #80984, #146527, #98579, .T. ) ;
#49639=CARTESIAN_POINT ( 'NONE',  ( 4.710568305744190276, 7.583081225755162968, 1.199719254218462483 ) ) ;
#49644=CARTESIAN_POINT ( 'NONE',  ( -1.001543065824772872E-14, 4.384375000341417916, 1.575800808251672791 ) ) ;
#49649=CARTESIAN_POINT ( 'NONE',  ( 5.937581207780954884, 9.014596278131406848, -1.199719254218440723 ) ) ;
#49651=CARTESIAN_POINT ( 'NONE',  ( -4.564291269294938225, 8.476756914152748124, 1.040834085586084257E-14 ) ) ;
#49653=CARTESIAN_POINT ( 'NONE',  ( 5.788968402910805722, 7.776882441527838807, 1.443375672974062551 ) ) ;
#49654=CARTESIAN_POINT ( 'NONE',  ( -1.201851678989727383E-14, 2.212500000000021672, 1.732050807568877637 ) ) ;
#49655=CARTESIAN_POINT ( 'NONE',  ( -4.948889764188092677, 5.732458465429559169, 1.199719254218462483 ) ) ;
#49658=CARTESIAN_POINT ( 'NONE',  ( -4.076197739202962467, 7.907314462378773001, 1.040834085586084257E-14 ) ) ;
#49662=CARTESIAN_POINT ( 'NONE',  ( -1.201851678989727383E-14, 3.071875000341420137, 1.575800808251672791 ) ) ;
#49664=CARTESIAN_POINT ( 'NONE',  ( -3.606105671554953318, 7.150947683548662503, 0.7216878364870317197 ) ) ;
#49669=CARTESIAN_POINT ( 'NONE',  ( -1.483456582844936422, 7.293967155396054558, 4.258619948151441292 ) ) ;
#49670=CARTESIAN_POINT ( 'NONE',  ( 6.003563092752934871, 5.898578451166879510, 0.7998128361456341429 ) ) ;
#49672=CARTESIAN_POINT ( 'NONE',  ( 1.364683531249988535, 3.176041667008084435, 0.7879004041258500513 ) ) ;
#49674=CARTESIAN_POINT ( 'NONE',  ( 3.521367211247359741, 5.131347717920458962, -1.599625672291262513 ) ) ;
#49676=CARTESIAN_POINT ( 'NONE',  ( -1.364683531250014514, 0.3427083336747508424, 0.7879004041258379498 ) ) ;
#49679=CARTESIAN_POINT ( 'NONE',  ( -2.286521462199063492, 5.819358805874190743, 1.040834085586084257E-14 ) ) ;
#49680=CARTESIAN_POINT ( 'NONE',  ( -5.544921637864820951, 9.412899644243539754, -0.7216878364870207285 ) ) ;
#49684=CARTESIAN_POINT ( 'NONE',  ( -1.201851678989727383E-14, 2.821875000341418804, 1.575800808251672791 ) ) ;
#49692=CARTESIAN_POINT ( 'NONE',  ( -7.836249598574384301, 8.244638741199329601, 1.040834085586084257E-14 ) ) ;
#49698=CARTESIAN_POINT ( 'NONE',  ( -7.361714222096077620, 7.691014135307965738, 0.7216878364870317197 ) ) ;
#49710=CARTESIAN_POINT ( 'NONE',  ( -4.543954038874438162, 8.453030145328826350, 1.040834085586084257E-14 ) ) ;
#49712=CARTESIAN_POINT ( 'NONE',  ( -0.7500000000000249800, -0.5583333333333134751, 1.299038105676659116 ) ) ;
#49713=CARTESIAN_POINT ( 'NONE',  ( 2.347533153460546806, 5.890539112345938300, 0.000000000000000000 ) ) ;
#49715=CARTESIAN_POINT ( 'NONE',  ( 3.734320285776532078, 4.105063559066064016, 0.9403128211546033510 ) ) ;
#49716=CARTESIAN_POINT ( 'NONE',  ( 5.952193131599331721, 6.902979060742733708, 1.199719254218462483 ) ) ;
#49723=CARTESIAN_POINT ( 'NONE',  ( -4.175548123328963079, 4.934189567714277302, 1.082531754730560403 ) ) ;
#49732=CARTESIAN_POINT ( 'NONE',  ( 0.6823417656249899377, 1.842708333674752952, 1.181850606188755259 ) ) ;
#49733=CARTESIAN_POINT ( 'NONE',  ( 10.66990370383054731, 11.55056853066490952, 0.7216878364870317197 ) ) ;
#49734=CARTESIAN_POINT ( 'NONE',  ( -6.042130013184518589, 10.20090211535728031, -0.7998128361456291469 ) ) ;
#49738=CARTESIAN_POINT ( 'NONE',  ( 7.630541526392844887, 7.796719957080126662, 0.7998128361456341429 ) ) ;
#49739=CARTESIAN_POINT ( 'NONE',  ( -6.898401231254901234, 6.942556279419168419, -0.7998128361456291469 ) ) ;
#49740=CARTESIAN_POINT ( 'NONE',  ( -1.458514304043844634, 8.731595392684152301, 2.560210433951525033 ) ) ;
#49742=CARTESIAN_POINT ( 'NONE',  ( -1.602468905319636405E-14, -1.131249999317182064, -1.732050807568870754 ) ) ;
#49744=EDGE_CURVE ( 'NONE', #78710, #182393, #139068, .T. ) ;
#49746=CARTESIAN_POINT ( 'NONE',  ( 6.968527767744088663, 11.07377346243604599, 0.7216878364870438212 ) ) ;
#49749=CARTESIAN_POINT ( 'NONE',  ( -0.6823417656250003738, 0.5302083336747518416, -1.181850606188749264 ) ) ;
#49751=CARTESIAN_POINT ( 'NONE',  ( 7.266807146800403849, 7.580289214129690478, 1.040834085586084257E-14 ) ) ;
#49755=CARTESIAN_POINT ( 'NONE',  ( -5.151735183512911043, 6.073074471262228435, 1.082531754730548412 ) ) ;
#49758=CARTESIAN_POINT ( 'NONE',  ( 1.364683531249988535, 4.905208333674756283, -0.7879004041258300672 ) ) ;
#49762=CARTESIAN_POINT ( 'NONE',  ( -5.904496024515287544, 6.143719773163115683, -0.8530293227379917020 ) ) ;
#49768=CARTESIAN_POINT ( 'NONE',  ( 7.955937213120826357, 8.176348258262782664, 0.7998128361456481317 ) ) ;
#49771=CARTESIAN_POINT ( 'NONE',  ( 3.063252641683779753, 5.661212951017999373, 1.199719254218450271 ) ) ;
#49777=CARTESIAN_POINT ( 'NONE',  ( 6.344852701515477200, 6.504675694630598137, -0.7216878364870257245 ) ) ;
#49778=CARTESIAN_POINT ( 'NONE',  ( -1.364683531250014514, 0.8010416670080889867, -0.7879004041258289570 ) ) ;
#49781=CARTESIAN_POINT ( 'NONE',  ( -1.580000000000022276, 8.674529973577531194, 2.420000000000010587 ) ) ;
#49786=CARTESIAN_POINT ( 'NONE',  ( -1.499999999999997780, 1.900000000000019673, 0.000000000000000000 ) ) ;
#49787=CARTESIAN_POINT ( 'NONE',  ( 7.637320603199683866, 7.804628880021436288, -0.7998128361456281477 ) ) ;
#49788=CARTESIAN_POINT ( 'NONE',  ( -6.530223543276495235, 10.77034456713125188, -0.7998128361456291469 ) ) ;
#49792=CARTESIAN_POINT ( 'NONE',  ( -1.201851678989727383E-14, 1.071875000341418138, 1.575800808251672791 ) ) ;
#49794=CARTESIAN_POINT ( 'NONE',  ( 1.499999999999989120, 2.525000000000020339, 1.214306433183764966E-14 ) ) ;
#49796=CARTESIAN_POINT ( 'NONE',  ( 4.416205349749311004, 6.175325546172740765, 1.599625672291267398 ) ) ;
#49803=CARTESIAN_POINT ( 'NONE',  ( -1.500000000000015099, -1.047916665983845919, 0.8660254037844403729 ) ) ;
#49804=CARTESIAN_POINT ( 'NONE',  ( -6.021792782764022078, 10.17717534653336209, -0.7998128361456291469 ) ) ;
#49805=CARTESIAN_POINT ( 'NONE',  ( -5.450014563013544588, 5.460697866378308341, 0.7216878364870317197 ) ) ;
#49808=CARTESIAN_POINT ( 'NONE',  ( -1.500000000000053957, 7.176846818246210624, -4.202462424328210489 ) ) ;
#49814=CARTESIAN_POINT ( 'NONE',  ( 5.452350330990040739, 9.512825819463730070, 0.7998128361456462443 ) ) ;
#49818=CARTESIAN_POINT ( 'NONE',  ( 6.877010230629674759, 9.046264573866535486, 1.599625672291281386 ) ) ;
#49819=CARTESIAN_POINT ( 'NONE',  ( 8.392133896734662812, 10.81390885098904420, 1.443375672974076540 ) ) ;
#49823=CARTESIAN_POINT ( 'NONE',  ( -7.314787569772770226, 8.492672571945082183, -1.199719254218452935 ) ) ;
#49824=CARTESIAN_POINT ( 'NONE',  ( 3.181359600701000989, 6.863336634126477875, 0.000000000000000000 ) ) ;
#49829=CARTESIAN_POINT ( 'NONE',  ( 4.001984418394623155, 7.593073144423666321, -0.1798963839820325039 ) ) ;
#49830=CARTESIAN_POINT ( 'NONE',  ( 9.490344339885973923, 12.09515436799890331, -1.443375672974057666 ) ) ;
#49838=CARTESIAN_POINT ( 'NONE',  ( -4.772106882330241717, 5.630174786549132726, -1.082531754730544860 ) ) ;
#49839=CARTESIAN_POINT ( 'NONE',  ( 7.931156674314368438, 12.19684052010138586, 1.040834085586084257E-14 ) ) ;
#49842=CARTESIAN_POINT ( 'NONE',  ( -5.205440912643032547, 8.160432600470439723, 1.199719254218452047 ) ) ;
#49848=CARTESIAN_POINT ( 'NONE',  ( -7.043624497499477499, 8.176315654292865887, 1.199719254218450271 ) ) ;
#49852=CARTESIAN_POINT ( 'NONE',  ( 3.469446951953614189E-15, 5.900000000000023448, 1.214306433183764966E-14 ) ) ;
#49853=ORIENTED_EDGE ( 'NONE', *, *, #71271, .T. ) ;
#49855=ORIENTED_EDGE ( 'NONE', *, *, #18560, .T. ) ;
#49863=CARTESIAN_POINT ( 'NONE',  ( 1.492390896412032708, 7.408229809041984915, -4.235510822234025419 ) ) ;
#49864=CARTESIAN_POINT ( 'NONE',  ( -5.205440912643032547, 8.160432600470439723, 1.199719254218452047 ) ) ;
#49867=CARTESIAN_POINT ( 'NONE',  ( 4.311129659465574804, 7.013106455143060636, -1.082531754730548412 ) ) ;
#49869=CARTESIAN_POINT ( 'NONE',  ( 1.579999999999991189, 8.674529973577531194, 2.500000000000000444 ) ) ;
#49872=ADVANCED_FACE ( 'NONE', ( #125882 ), #18207, .T. ) ;
#49873=CARTESIAN_POINT ( 'NONE',  ( -3.249150368769345043, 6.942425863539538611, 0.7998128361456341429 ) ) ;
#49878=CARTESIAN_POINT ( 'NONE',  ( 4.151089105449103478, 2.978104760819428432, -0.7749999999999935829 ) ) ;
#49881=CARTESIAN_POINT ( 'NONE',  ( -9.176171038350775078, 9.599954387697719582, -0.7998128361456291469 ) ) ;
#49882=CARTESIAN_POINT ( 'NONE',  ( 4.950698647284403009, 8.927565521807144577, 1.040834085586084257E-14 ) ) ;
#49885=CARTESIAN_POINT ( 'NONE',  ( -7.147119532698295252, 11.49005655479003174, 0.000000000000000000 ) ) ;
#49888=CARTESIAN_POINT ( 'NONE',  ( 4.951779652976496138, 6.537757797665411985, -2.442612065051301684 ) ) ;
#49889=CARTESIAN_POINT ( 'NONE',  ( -1.402160292154681736E-14, -0.6156249996585817508, 1.575800808251672791 ) ) ;
#49893=CARTESIAN_POINT ( 'NONE',  ( 8.432808358020016826, 10.86136238915529084, 1.443375672974076540 ) ) ;
#49900=CARTESIAN_POINT ( 'NONE',  ( 9.042925270190622200, 12.53353466765568669, 1.082531754730546636 ) ) ;
#49901=ADVANCED_FACE ( 'NONE', ( #29368 ), #23906, .T. ) ;
#49921=CARTESIAN_POINT ( 'NONE',  ( -1.500000000000015099, -0.08958333265051321437, -0.8660254037844383745 ) ) ;
#49928=CARTESIAN_POINT ( 'NONE',  ( 9.459838494033030898, 12.05956421450382088, 1.599625672291281386 ) ) ;
#49932=CARTESIAN_POINT ( 'NONE',  ( 4.955668840994886359, 5.740367388370866131, 1.199719254218462483 ) ) ;
#49933=CARTESIAN_POINT ( 'NONE',  ( -7.890482213473404727, 8.307910125248191946, 0.7216878364870578100 ) ) ;
#49937=CARTESIAN_POINT ( 'NONE',  ( -6.347188469492005325, 10.55680364771601809, -0.7998128361456291469 ) ) ;
#49938=CARTESIAN_POINT ( 'NONE',  ( -3.267151830768952880, 5.795132321663641228, -1.082531754730549078 ) ) ;
#49940=ORIENTED_EDGE ( 'NONE', *, *, #81974, .F. ) ;
#49941=CARTESIAN_POINT ( 'NONE',  ( -0.7500000000000249800, -0.02708333265051543481, 1.299038105676659116 ) ) ;
#49948=CARTESIAN_POINT ( 'NONE',  ( -4.460269348771590536, 5.266364330730674226, 1.082531754730558626 ) ) ;
#49957=CARTESIAN_POINT ( 'NONE',  ( -10.10098813738111545, 11.74323990082152491, -1.199719254218441611 ) ) ;
#49958=CARTESIAN_POINT ( 'NONE',  ( 6.760712154708803823, 11.03924794713562818, 1.040834085586084257E-14 ) ) ;
#49967=CARTESIAN_POINT ( 'NONE',  ( -8.025536864285518490, 11.45054454405341282, -1.199719254218446718 ) ) ;
#49970=ORIENTED_EDGE ( 'NONE', *, *, #207366, .T. ) ;
#49972=CARTESIAN_POINT ( 'NONE',  ( 5.691725559638619814, 5.534767995866836543, 1.040834085586084257E-14 ) ) ;
#49978=CARTESIAN_POINT ( 'NONE',  ( -7.334597915313094241, 9.580116872663850813, 1.040834085586084257E-14 ) ) ;
#49981=CARTESIAN_POINT ( 'NONE',  ( -1.270916165646597928, 3.166024509562812561, -0.7749999999999953593 ) ) ;
#49990=CARTESIAN_POINT ( 'NONE',  ( 6.096362627639171805, 10.26417349888772179, -0.7998128361456291469 ) ) ;
#49992=CARTESIAN_POINT ( 'NONE',  ( -4.355193658487827690, 6.104145239700998538, -1.599625672291256295 ) ) ;
#49998=CARTESIAN_POINT ( 'NONE',  ( 0.6823417656249899377, 5.676041667008087543, -1.181850606188754593 ) ) ;
#50002=CARTESIAN_POINT ( 'NONE',  ( 4.566398809704347528, 4.221886787610169556, -0.7998128361456211532 ) ) ;
#50004=CARTESIAN_POINT ( 'NONE',  ( -2.923754682041362241, 6.562797562356882608, 0.7998128361456341429 ) ) ;
#50010=CARTESIAN_POINT ( 'NONE',  ( 5.233084105194869551, 6.167981546557892436, -1.082531754730548412 ) ) ;
#50013=CARTESIAN_POINT ( 'NONE',  ( 7.904040366642689719, 10.24446639921506552, 1.443375672974076540 ) ) ;
#50014=CARTESIAN_POINT ( 'NONE',  ( 0.6823417656249899377, 4.988541667008086655, -1.181850606188754593 ) ) ;
#50016=CARTESIAN_POINT ( 'NONE',  ( 4.324687812634887329, 6.068555086205916105, 1.443375672974062551 ) ) ;
#50024=CARTESIAN_POINT ( 'NONE',  ( -6.126391799051042142, 6.003160260013642890, 0.2011063304240209848 ) ) ;
#50028=CARTESIAN_POINT ( 'NONE',  ( 1.364683531249988535, 5.217708333674750065, -0.7879004041258300672 ) ) ;
#50034=CARTESIAN_POINT ( 'NONE',  ( -1.500000000000001332, -0.8499999999999757749, 0.000000000000000000 ) ) ;
#50036=CARTESIAN_POINT ( 'NONE',  ( 0.7499999999999920064, 4.233333333333352932, 1.299038105676669330 ) ) ;
#50045=CARTESIAN_POINT ( 'NONE',  ( -1.001543065824772872E-14, 4.384375000341417916, 1.575800808251672791 ) ) ;
#50047=CARTESIAN_POINT ( 'NONE',  ( 5.449487677688982679, 8.445153826357429949, -1.199719254218446718 ) ) ;
#50050=CARTESIAN_POINT ( 'NONE',  ( -9.664264568442742842, 10.16939683947169115, -0.7998128361456291469 ) ) ;
#50051=CARTESIAN_POINT ( 'NONE',  ( 6.938893903907228378E-15, 10.64264068711930733, 1.214306433183764966E-14 ) ) ;
#50057=CARTESIAN_POINT ( 'NONE',  ( -0.7500000000000215383, 5.691666666666685082, 1.299038105676671107 ) ) ;
#50061=CARTESIAN_POINT ( 'NONE',  ( 5.802526556524483681, 5.871961858807763335, 1.040834085586084257E-14 ) ) ;
#50064=CARTESIAN_POINT ( 'NONE',  ( 6.941411460516762943, 11.04213777067082702, -0.7216878364870267237 ) ) ;
#50069=( BOUNDED_CURVE ( )  B_SPLINE_CURVE ( 2, ( #106534, #205025, #89186, #173648, #124953, #25222, #157385 ),
 .UNSPECIFIED., .F., .T. ) 
 B_SPLINE_CURVE_WITH_KNOTS ( ( 3, 2, 2, 3 ),
 ( 0.2321428571428570953, 0.2380952380952381098, 0.2440476190476191798, 0.2500000000000002220 ),
 .UNSPECIFIED. ) 
 CURVE ( )  GEOMETRIC_REPRESENTATION_ITEM ( )  RATIONAL_B_SPLINE_CURVE ( ( 1.000000000000001332, 0.8660254037844374864, 1.000000000000000000, 0.8660254037844387076, 1.000000000000000000, 0.8660254037844337116, 1.000000000000005107 ) ) 
 REPRESENTATION_ITEM ( '' )  );
#50071=CARTESIAN_POINT ( 'NONE',  ( -0.7499999999999972244, 3.639583334016149863, -1.299038105676652011 ) ) ;
#50073=CARTESIAN_POINT ( 'NONE',  ( -4.120788623549732854, 6.895004929861607401, -1.199719254218452047 ) ) ;
#50074=CARTESIAN_POINT ( 'NONE',  ( 4.650083499362880346, 4.527444958785877382, 0.7216878364870317197 ) ) ;
#50075=CARTESIAN_POINT ( 'NONE',  ( -9.612367721964606204, 12.23751498042398289, -1.443375672974058777 ) ) ;
#50082=CARTESIAN_POINT ( 'NONE',  ( 4.630273154266905777, 5.360739087188218122, 1.199719254218464037 ) ) ;
#50083=CARTESIAN_POINT ( 'NONE',  ( -1.284279953904132077, 2.909610286488902187, -0.7749999999999935829 ) ) ;
#50088=FACE_OUTER_BOUND ( 'NONE', #117600, .T. ) ;
#50097=CARTESIAN_POINT ( 'NONE',  ( 2.280903940472752467, 5.594607745005274246, -0.6109567437776646237 ) ) ;
#50098=CARTESIAN_POINT ( 'NONE',  ( 5.718470792885002041, 6.083800970187063228, -0.6820517675651931455 ) ) ;
#50100=CARTESIAN_POINT ( 'NONE',  ( 10.56588178375152864, 11.22128359066528169, -0.7998128361456281477 ) ) ;
#50105=CARTESIAN_POINT ( 'NONE',  ( 6.317736394288140822, 7.433409217166723870, 1.082531754730558626 ) ) ;
#50106=CARTESIAN_POINT ( 'NONE',  ( -2.103486388414573138, 5.605817886458954291, 1.040834085586084257E-14 ) ) ;
#50113=CARTESIAN_POINT ( 'NONE',  ( -5.278201874421821316, 5.052323696447222900, 0.7998128361456341429 ) ) ;
#50125=CARTESIAN_POINT ( 'NONE',  ( 6.115260013507548109, 6.015528159276049891, -0.005231617032384894284 ) ) ;
#50129=CARTESIAN_POINT ( 'NONE',  ( 4.497554271431305040, 6.270232621468402989, -1.599625672291256295 ) ) ;
#50133=CARTESIAN_POINT ( 'NONE',  ( -9.192064960385334160, 9.826423329978791088, 0.7216878364870438212 ) ) ;
#50136=CARTESIAN_POINT ( 'NONE',  ( 8.101160479365381306, 9.410107633136481908, -1.199719254218446718 ) ) ;
#50137=CARTESIAN_POINT ( 'NONE',  ( -4.086893239515592136, 6.855460315155083251, 1.199719254218464037 ) ) ;
#50140=CARTESIAN_POINT ( 'NONE',  ( -6.573005544526917099, 6.562927978236513304, -0.7998128361456291469 ) ) ;
#50141=CARTESIAN_POINT ( 'NONE',  ( 2.737856954955798727, 5.281584649835344258, 1.199719254218452047 ) ) ;
#50143=CARTESIAN_POINT ( 'NONE',  ( -5.880485940025243607, 7.883652901494672349, 1.599625672291269396 ) ) ;
#50146=CARTESIAN_POINT ( 'NONE',  ( 7.730120138085914583, 12.17022392774227768, 0.7998128361456462443 ) ) ;
#50149=CARTESIAN_POINT ( 'NONE',  ( 4.075930520424391190, 7.726065465775651120, -0.5982635945973235891 ) ) ;
#50150=CARTESIAN_POINT ( 'NONE',  ( 5.585596099150174965, 7.539614753807099667, -1.443375672974057666 ) ) ;
#50158=VERTEX_POINT ( 'NONE', #165951 ) ;
#50159=CARTESIAN_POINT ( 'NONE',  ( 6.548225005276093746, 9.623051025255367819, -1.082531754730537976 ) ) ;
#50160=ADVANCED_FACE ( 'NONE', ( #149707 ), #200555, .T. ) ;
#50163=CARTESIAN_POINT ( 'NONE',  ( 4.322138105957547438, 3.567377917394175313, -2.444429911049615711 ) ) ;
#50164=CARTESIAN_POINT ( 'NONE',  ( -6.692921386640485082, 10.96015871772258521, -0.7998128361456291469 ) ) ;
#50170=LINE ( 'NONE', #32851, #48728 ) ;
#50173=CARTESIAN_POINT ( 'NONE',  ( 8.866142388332804103, 12.43125098877526113, -1.199719254218446718 ) ) ;
#50177=CARTESIAN_POINT ( 'NONE',  ( 5.495132332240461714, 5.305409230568988832, 0.7998128361456341429 ) ) ;
#50180=CARTESIAN_POINT ( 'NONE',  ( 0.7499999999999902300, 3.597916667349487785, -1.299038105676658228 ) ) ;
#50184=ORIENTED_EDGE ( 'NONE', *, *, #140381, .T. ) ;
#50186=CARTESIAN_POINT ( 'NONE',  ( -1.499999999999997780, 2.400000000000020339, 1.214306433183764966E-14 ) ) ;
#50187=CARTESIAN_POINT ( 'NONE',  ( 5.764187864104357573, 9.876636274763768597, 1.040834085586084257E-14 ) ) ;
#50188=CARTESIAN_POINT ( 'NONE',  ( 5.138177029454847222, 6.057256624861201644, 1.082531754730560403 ) ) ;
#50190=CARTESIAN_POINT ( 'NONE',  ( -1.201851678989727383E-14, 4.837500000000018119, -1.732050807568863648 ) ) ;
#50191=CARTESIAN_POINT ( 'NONE',  ( 6.954969614130424027, 11.05795561655343384, 1.040834085586084257E-14 ) ) ;
#50198=CARTESIAN_POINT ( 'NONE',  ( -5.603597561149804562, 5.431951997629870910, 0.7998128361456341429 ) ) ;
#50200=CARTESIAN_POINT ( 'NONE',  ( -1.499999999999997780, 3.931250000682819046, 1.214306433183764966E-14 ) ) ;
#50201=CARTESIAN_POINT ( 'NONE',  ( -1.402160292154681736E-14, -0.8031249996585825279, -1.575800808251665908 ) ) ;
#50205=CARTESIAN_POINT ( 'NONE',  ( 3.876741858503734761, 6.610283703974623393, 1.199719254218462483 ) ) ;
#50207=CARTESIAN_POINT ( 'NONE',  ( -1.201851678989727383E-14, 5.259375000341421469, -1.575800808251660134 ) ) ;
#50215=CARTESIAN_POINT ( 'NONE',  ( -8.050844288416501016, 8.287073179441051707, 1.040834085586084257E-14 ) ) ;
#50216=CARTESIAN_POINT ( 'NONE',  ( 5.168682875307768931, 7.053215992657626110, -1.599625672291256295 ) ) ;
#50219=CARTESIAN_POINT ( 'NONE',  ( -1.364683531250000748, -0.2406249996585799189, 0.000000000000000000 ) ) ;
#50225=CARTESIAN_POINT ( 'NONE',  ( -6.287230548435221777, 8.358188277972981695, -1.599625672291263179 ) ) ;
#50228=CARTESIAN_POINT ( 'NONE',  ( 8.055515824813896941, 12.54985222892493368, 0.7998128361456462443 ) ) ;
#50230=CARTESIAN_POINT ( 'NONE',  ( 9.915090410295563927, 10.46202698829998567, -0.7998128361456281477 ) ) ;
#50231=CARTESIAN_POINT ( 'NONE',  ( -4.848826244296223109, 5.027555131033083491, -0.8732430475888955934 ) ) ;
#50232=CARTESIAN_POINT ( 'NONE',  ( -4.762992037102518950, 4.451245552908022596, -0.7998128361456221525 ) ) ;
#50233=CARTESIAN_POINT ( 'NONE',  ( -8.345207244411405156, 9.694828859023472134, 1.199719254218462483 ) ) ;
#50235=CIRCLE ( 'NONE', #8622, 0.07999999999999997391 ) ;
#50237=CARTESIAN_POINT ( 'NONE',  ( -4.762889583212370326, 6.995502248939536649, 1.426468515190159714 ) ) ;
#50238=CARTESIAN_POINT ( 'NONE',  ( 0.6823417656249882723, -0.07395833299191079124, -1.181850606188749264 ) ) ;
#50242=CARTESIAN_POINT ( 'NONE',  ( 9.246297574839983824, 9.889694713509232571, 0.7216878364870438212 ) ) ;
#50245=CARTESIAN_POINT ( 'NONE',  ( 6.017121246366603060, 5.914396297049491658, 1.040834085586084257E-14 ) ) ;
#50263=EDGE_CURVE ( 'NONE', #140339, #97926, #142782, .T. ) ;
#50265=CARTESIAN_POINT ( 'NONE',  ( 10.39640486358069360, 11.02356051713265650, 0.7998128361456462443 ) ) ;
#50267=EDGE_LOOP ( 'NONE', ( #120311, #125979, #66186 ) ) ;
#50269=CARTESIAN_POINT ( 'NONE',  ( -5.623934791570306402, 5.455678766453782913, 0.7998128361456341429 ) ) ;
#50274=CARTESIAN_POINT ( 'NONE',  ( -1.500000000000011324, 2.952083334016149418, 0.8660254037844403729 ) ) ;
#50275=CARTESIAN_POINT ( 'NONE',  ( 8.158255747121103241, 10.54105100977322174, 1.599625672291281386 ) ) ;
#50280=CARTESIAN_POINT ( 'NONE',  ( -9.341731535015849630, 10.85744053139533349, 1.199719254218462483 ) ) ;
#50282=CARTESIAN_POINT ( 'NONE',  ( 1.364683531249988535, 1.613541667008084879, 0.7879004041258500513 ) ) ;
#50285=ORIENTED_EDGE ( 'NONE', *, *, #47557, .F. ) ;
#50289=CARTESIAN_POINT ( 'NONE',  ( -2.591579918506545344, 6.175260338232929413, 1.040834085586084257E-14 ) ) ;
#50293=CARTESIAN_POINT ( 'NONE',  ( -1.364683531250012516, 1.592708333674756727, 0.7879004041258379498 ) ) ;
#50294=EDGE_CURVE ( 'NONE', #17249, #135745, #101151, .T. ) ;
#50299=CARTESIAN_POINT ( 'NONE',  ( -1.364683531250014514, 1.988541667008086655, -0.7879004041258289570 ) ) ;
#50301=CARTESIAN_POINT ( 'NONE',  ( -4.740547266272593596, 8.682388910626682943, -0.7998128361456281477 ) ) ;
#50302=CARTESIAN_POINT ( 'NONE',  ( 8.938903350111612411, 9.323142084752035430, -0.7998128361456221525 ) ) ;
#50303=CARTESIAN_POINT ( 'NONE',  ( 0.9999999999999833467, 9.200000000000018829, -0.3999999999999961919 ) ) ;
#50305=CARTESIAN_POINT ( 'NONE',  ( 0.7499999999999902300, 3.816666666666690411, -1.299038105676658228 ) ) ;
#50306=CARTESIAN_POINT ( 'NONE',  ( 1.364683531249990311, 2.946875000341416140, 1.214306433183764966E-14 ) ) ;
#50310=EDGE_CURVE ( 'NONE', #79803, #21610, #186451, .T. ) ;
#50313=CARTESIAN_POINT ( 'NONE',  ( 4.839897650398541806, 8.590371658866210680, 1.040834085586084257E-14 ) ) ;
#50316=CARTESIAN_POINT ( 'NONE',  ( -8.962103233833181193, 10.41454084668224489, -1.199719254218446718 ) ) ;
#50317=CARTESIAN_POINT ( 'NONE',  ( -2.266184231778562541, 5.795632037050281404, 1.040834085586084257E-14 ) ) ;
#50318=CARTESIAN_POINT ( 'NONE',  ( 0.6823417656249899377, 4.926041667008086655, -1.181850606188754593 ) ) ;
#50323=CARTESIAN_POINT ( 'NONE',  ( -6.182154857707119255, 10.15633840072622363, 0.000000000000000000 ) ) ;
#50325=CARTESIAN_POINT ( 'NONE',  ( 1.499999999999989120, 4.754166666666689522, 0.8660254037844524744 ) ) ;
#50328=CARTESIAN_POINT ( 'NONE',  ( 7.293923454472077239, 10.49303254931736262, 1.082531754730558626 ) ) ;
#50336=CARTESIAN_POINT ( 'NONE',  ( 10.04622863760192963, 10.82294762006482713, -0.7216878364870257245 ) ) ;
#50343=CARTESIAN_POINT ( 'NONE',  ( 5.926885707468349196, 10.06645042535509660, 1.040834085586084257E-14 ) ) ;
#50344=CARTESIAN_POINT ( 'NONE',  ( -4.822949958159302497, 6.649860922651058992, -1.599625672291256295 ) ) ;
#50349=CARTESIAN_POINT ( 'NONE',  ( 6.602457619730771832, 6.805214765881779648, 0.7216878364870317197 ) ) ;
#50350=CARTESIAN_POINT ( 'NONE',  ( -1.364683531250014514, 0.09270833367475767028, 0.7879004041258379498 ) ) ;
#50351=CARTESIAN_POINT ( 'NONE',  ( 4.067082894419602468, 3.847277586352047862, -0.7216878364870188411 ) ) ;
#50352=CARTESIAN_POINT ( 'NONE',  ( -8.350932551013499960, 11.83017284523606172, -1.199719254218446718 ) ) ;
#50368=CARTESIAN_POINT ( 'NONE',  ( 7.308008492965924141, 8.484763649003774333, -1.199719254218451159 ) ) ;
#50369=CARTESIAN_POINT ( 'NONE',  ( 6.012151052656117933, 9.101594430485762999, 1.199719254218460707 ) ) ;
#50380=CARTESIAN_POINT ( 'NONE',  ( -4.924636110261798372, 6.768494766770632332, 1.599625672291267398 ) ) ;
#50382=CARTESIAN_POINT ( 'NONE',  ( -4.762992037102518950, 4.451245552908022596, -0.7998128361456221525 ) ) ;
#50385=CYLINDRICAL_SURFACE ( 'NONE', #136, 1.500000000000000222 ) ;
#50393=CARTESIAN_POINT ( 'NONE',  ( -3.195971524519394702, 4.751719416737803847, -1.599625672291262513 ) ) ;
#50396=CARTESIAN_POINT ( 'NONE',  ( 5.961834861707224320, 7.978559976790334574, -1.599625672291262513 ) ) ;
#50397=CARTESIAN_POINT ( 'NONE',  ( -1.364683531249997417, 4.509375000341424133, 1.214306433183764966E-14 ) ) ;
#50404=CARTESIAN_POINT ( 'NONE',  ( 4.731432421044862835, 6.543090462684225450, -1.443375672974051449 ) ) ;
#50405=CARTESIAN_POINT ( 'NONE',  ( -7.477485413136760073, 8.682486722536401302, -1.199719254218446718 ) ) ;
#50407=EDGE_LOOP ( 'NONE', ( #42542, #144393, #103443, #5182, #170024 ) ) ;
#50410=CARTESIAN_POINT ( 'NONE',  ( -7.426115451983156923, 9.686887332112256388, -1.599625672291263179 ) ) ;
#50411=CARTESIAN_POINT ( 'NONE',  ( -5.220052836461385404, 6.048815383081766583, -1.199719254218446718 ) ) ;
#50412=CARTESIAN_POINT ( 'NONE',  ( 3.023105066167310895, 5.702484939155337607, -7.499999999999997335 ) ) ;
#50419=CARTESIAN_POINT ( 'NONE',  ( 6.962275575817444384, 8.081408578997208991, -1.199719254218446718 ) ) ;
#50432=CARTESIAN_POINT ( 'NONE',  ( -1.499999999999997780, 5.400000000000022560, 1.214306433183764966E-14 ) ) ;
#50433=CARTESIAN_POINT ( 'NONE',  ( 4.532503425670185493, 4.182342172903648070, 1.214306433183764966E-14 ) ) ;
#50434=CARTESIAN_POINT ( 'NONE',  ( 4.924636110261782385, 6.768494766770632332, 1.599625672291267398 ) ) ;
#50436=CARTESIAN_POINT ( 'NONE',  ( -7.212574532790100079, 9.437756259720353924, -1.443375672974059665 ) ) ;
#50438=CARTESIAN_POINT ( 'NONE',  ( 5.504247177468175600, 8.405076892812779477, 1.082531754730558626 ) ) ;
#50439=CARTESIAN_POINT ( 'NONE',  ( -7.307481607641392429, 11.46921960898288972, 0.7216878364870458196 ) ) ;
#50440=EDGE_CURVE ( 'NONE', #53793, #6901, #201323, .T. ) ;
#50444=CARTESIAN_POINT ( 'NONE',  ( 7.800018446563675489, 7.994443030612759848, -0.7998128361456281477 ) ) ;
#50448=CARTESIAN_POINT ( 'NONE',  ( -4.121315508874262790, 6.791656612786516334, -1.082531754730549967 ) ) ;
#50449=CARTESIAN_POINT ( 'NONE',  ( -1.364683531250012516, 3.488541667008085767, -0.7879004041258300672 ) ) ;
#50455=CARTESIAN_POINT ( 'NONE',  ( 7.446452682403650769, 9.710614100936176385, -1.599625672291262513 ) ) ;
#50458=CARTESIAN_POINT ( 'NONE',  ( -8.474009703741204547, 9.845098394908269768, -1.199719254218446718 ) ) ;
#50464=CARTESIAN_POINT ( 'NONE',  ( 7.730120138085914583, 12.17022392774227768, 0.7998128361456462443 ) ) ;
#50467=CARTESIAN_POINT ( 'NONE',  ( -6.828502922777144768, 11.11833717654868892, 0.7998128361456481317 ) ) ;
#50471=CARTESIAN_POINT ( 'NONE',  ( 5.794097129154974546, 6.036864960932135205, -0.5213279746436976225 ) ) ;
#50472=CARTESIAN_POINT ( 'NONE',  ( -3.090368948911150770, 5.692848642783215674, 1.199719254218462483 ) ) ;
#50477=CARTESIAN_POINT ( 'NONE',  ( 5.615048174354031474, 9.702639970055050966, 0.7998128361456462443 ) ) ;
#50479=CARTESIAN_POINT ( 'NONE',  ( 5.606460214450851964, 6.499623990736163037, 1.199719254218462483 ) ) ;
#50480=CARTESIAN_POINT ( 'NONE',  ( -4.022721148277657477, 7.614442113290216696, -0.1953124528039917873 ) ) ;
#50482=CARTESIAN_POINT ( 'NONE',  ( 5.332434488876471868, 5.115595079977664383, 0.7998128361456341429 ) ) ;
#50484=CARTESIAN_POINT ( 'NONE',  ( -8.215877900201387973, 8.687538426430837291, 0.7216878364870578100 ) ) ;
#50491=CARTESIAN_POINT ( 'NONE',  ( -4.082753340799282427, 7.529786358835235838, 0.5248769202933333267 ) ) ;
#50492=CARTESIAN_POINT ( 'NONE',  ( -1.402160292154681736E-14, -0.8656249996585829720, 1.575800808251672791 ) ) ;
#50495=CARTESIAN_POINT ( 'NONE',  ( 5.558479791922850133, 6.547609847740540445, -1.082531754730542195 ) ) ;
#50505=CARTESIAN_POINT ( 'NONE',  ( -8.283668667825340393, 12.60810451253083997, 0.7216878364870458196 ) ) ;
#50511=CARTESIAN_POINT ( 'NONE',  ( -9.368320956918621434, 11.95279375453699622, 1.443375672974076540 ) ) ;
#50518=CARTESIAN_POINT ( 'NONE',  ( 1.499999999999990896, 3.306250000682818602, 1.214306433183764966E-14 ) ) ;
#50520=CARTESIAN_POINT ( 'NONE',  ( -7.067878151425722955, 7.140279352951794500, 0.7998128361456341429 ) ) ;
#50523=CARTESIAN_POINT ( 'NONE',  ( -9.494787648271923786, 9.971673765939062406, 1.040834085586084257E-14 ) ) ;
#50526=CARTESIAN_POINT ( 'NONE',  ( 5.178324605415663306, 8.128796908705222535, 1.199719254218462483 ) ) ;
#50528=DIRECTION ( 'NONE',  ( 0.6507913734559627184, 0.7592566023653016805, 0.000000000000000000 ) ) ;
#50531=CARTESIAN_POINT ( 'NONE',  ( 9.596473800374404561, 10.09030761005864285, 0.000000000000000000 ) ) ;
#50533=CYLINDRICAL_SURFACE ( 'NONE', #84416, 1.250000000000000000 ) ;
#50537=CARTESIAN_POINT ( 'NONE',  ( -5.883875478650828050, 9.808345791827219884, 0.7216878364870458196 ) ) ;
#50540=CARTESIAN_POINT ( 'NONE',  ( 1.364683531249990311, 5.426041667008086655, 0.7879004041258500513 ) ) ;
#50544=CARTESIAN_POINT ( 'NONE',  ( -0.6823417656249969321, 4.967708333674755394, -1.181850606188749264 ) ) ;
#50547=CARTESIAN_POINT ( 'NONE',  ( -9.561524646135538319, 12.17819805862340310, -1.599625672291263179 ) ) ;
#50549=CARTESIAN_POINT ( 'NONE',  ( 10.42352117080803708, 11.05519620889787724, -0.7998128361456281477 ) ) ;
#50551=CARTESIAN_POINT ( 'NONE',  ( -8.618179199781044630, 13.20629283305325963, 0.7998128361456341429 ) ) ;
#50554=CARTESIAN_POINT ( 'NONE',  ( -1.364683531250000748, 2.009375000341421913, 1.214306433183764966E-14 ) ) ;
#50557=CARTESIAN_POINT ( 'NONE',  ( 3.323720213644492993, 7.029424015893889433, 1.040834085586084257E-14 ) ) ;
#50558=ORIENTED_EDGE ( 'NONE', *, *, #18068, .F. ) ;
#50564=CARTESIAN_POINT ( 'NONE',  ( 9.747949258101261449, 11.43532422494874368, -1.082531754730537088 ) ) ;
#50566=CARTESIAN_POINT ( 'NONE',  ( -6.968527767744110868, 9.153035033833367251, 1.443375672974078761 ) ) ;
#50568=CARTESIAN_POINT ( 'NONE',  ( -3.652727762210548068, 6.150616677256791398, 1.207173405259515775 ) ) ;
#50570=CARTESIAN_POINT ( 'NONE',  ( -8.993135964566285168, 9.386413468282476913, -0.7998128361456291469 ) ) ;
#50571=CARTESIAN_POINT ( 'NONE',  ( -4.080641047588907888, 6.744203074620265248, -1.082531754730548412 ) ) ;
#50572=CARTESIAN_POINT ( 'NONE',  ( -1.364683531250012516, 3.301041667008084879, -0.7879004041258289570 ) ) ;
#50580=EDGE_LOOP ( 'NONE', ( #103997, #140075, #155489, #84478 ) ) ;
#50590=CARTESIAN_POINT ( 'NONE',  ( -1.201851678989727383E-14, 3.884375000341423689, 1.575800808251672791 ) ) ;
#50597=CARTESIAN_POINT ( 'NONE',  ( 9.748476143425788720, 11.33197590787365172, -1.199719254218440723 ) ) ;
#50600=CARTESIAN_POINT ( 'NONE',  ( -1.364683531250012516, 2.988541667008091096, -0.7879004041258289570 ) ) ;
#50602=CARTESIAN_POINT ( 'NONE',  ( -7.754900677336769022, 9.110100880723427608, 1.082531754730558626 ) ) ;
#50609=ORIENTED_EDGE ( 'NONE', *, *, #153621, .F. ) ;
#50611=CARTESIAN_POINT ( 'NONE',  ( 4.436542580169809291, 6.199052314996659874, 1.599625672291267398 ) ) ;
#50615=CARTESIAN_POINT ( 'NONE',  ( 8.269583629331492602, 11.73526576994040482, 1.199719254218450271 ) ) ;
#50620=ORIENTED_EDGE ( 'NONE', *, *, #49638, .F. ) ;
#50622=CARTESIAN_POINT ( 'NONE',  ( -4.959585264500673496, 4.680604318205876524, 1.214306433183764966E-14 ) ) ;
#50623=CARTESIAN_POINT ( 'NONE',  ( 5.798083248138522272, 9.916180889470295412, 0.7998128361456462443 ) ) ;
#50625=CARTESIAN_POINT ( 'NONE',  ( 5.639828713160493834, 5.682147708216442439, 1.040834085586084257E-14 ) ) ;
#50635=CARTESIAN_POINT ( 'NONE',  ( -6.643132081016132062, 8.773406732650713025, 1.443375672974078761 ) ) ;
#50637=CARTESIAN_POINT ( 'NONE',  ( 5.684946482831785275, 5.526859072925533134, -0.7998128361456231517 ) ) ;
#50640=CARTESIAN_POINT ( 'NONE',  ( -8.833300774503376473, 10.26427131079744193, 1.199719254218462483 ) ) ;
#50645=CARTESIAN_POINT ( 'NONE',  ( -2.137381772448751605, 5.645362501165475777, -0.7998128361456281477 ) ) ;
#50648=CARTESIAN_POINT ( 'NONE',  ( 7.723341061279088038, 12.16231500480096983, -0.7998128361456291469 ) ) ;
#50650=CARTESIAN_POINT ( 'NONE',  ( 3.018661757337009810, 6.673522483535157868, 0.000000000000000000 ) ) ;
#50656=CARTESIAN_POINT ( 'NONE',  ( -3.054546515950523400, 6.451825606165701998, 0.6676900015689657408 ) ) ;
#50659=CARTESIAN_POINT ( 'NONE',  ( -3.952365473583647315, 4.569846793057691592, 1.199719254218462483 ) ) ;
#50660=CARTESIAN_POINT ( 'NONE',  ( 6.938893903907228378E-15, 10.64264068711930733, 1.214306433183764966E-14 ) ) ;
#50662=CARTESIAN_POINT ( 'NONE',  ( -9.820183334999905256, 10.35130206712171130, 1.040834085586084257E-14 ) ) ;
#50667=CARTESIAN_POINT ( 'NONE',  ( 8.120970824905713314, 8.576813505252564696, 1.040834085586084257E-14 ) ) ;
#50668=CARTESIAN_POINT ( 'NONE',  ( 1.364683531249990311, 5.176041667008085767, 0.7879004041258499402 ) ) ;
#50670=CARTESIAN_POINT ( 'NONE',  ( 4.708759422647839976, 4.387974169377582001, -0.7998128361456211532 ) ) ;
#50673=CARTESIAN_POINT ( 'NONE',  ( -5.879432169820529630, 10.01108796476595764, -0.7998128361456221525 ) ) ;
#50684=CARTESIAN_POINT ( 'NONE',  ( -1.201851678989727383E-14, 3.384375000341421469, 1.575800808251672791 ) ) ;
#50685=CARTESIAN_POINT ( 'NONE',  ( 10.07778825365955733, 10.65184113889131012, -0.7998128361456281477 ) ) ;
#50687=CARTESIAN_POINT ( 'NONE',  ( -3.782361668532609134, 7.356579680022602652, 1.040834085586084257E-14 ) ) ;
#50689=CARTESIAN_POINT ( 'NONE',  ( -4.568734577680894304, 5.392907097791561633, -1.082531754730543971 ) ) ;
#50690=EDGE_CURVE ( 'NONE', #33202, #84740, #25085, .T. ) ;
#50697=CARTESIAN_POINT ( 'NONE',  ( 5.495132332240461714, 5.305409230568988832, 0.7998128361456341429 ) ) ;
#50707=CARTESIAN_POINT ( 'NONE',  ( 5.840865249388943248, 5.708764300575555062, 0.7998128361456341429 ) ) ;
#50711=CARTESIAN_POINT ( 'NONE',  ( -5.982172092127739482, 8.002286745614243912, -1.599625672291263179 ) ) ;
#50715=CARTESIAN_POINT ( 'NONE',  ( 6.124532705071213279, 8.168374127381657246, -1.599625672291262513 ) ) ;
#50719=CARTESIAN_POINT ( 'NONE',  ( -5.494078562035765501, 7.432844293840273231, -1.599625672291256295 ) ) ;
#50720=CARTESIAN_POINT ( 'NONE',  ( -1.201851678989727383E-14, 1.712500000000019229, 1.732050807568877637 ) ) ;
#50721=CARTESIAN_POINT ( 'NONE',  ( -4.273844736805832767, 6.009238164405336313, 1.599625672291267398 ) ) ;
#50724=CARTESIAN_POINT ( 'NONE',  ( -5.168682875307782254, 7.053215992657626110, -1.599625672291256295 ) ) ;
#50726=CARTESIAN_POINT ( 'NONE',  ( -1.201851678989727383E-14, 3.321875000341421025, 1.575800808251672791 ) ) ;
#50728=CARTESIAN_POINT ( 'NONE',  ( -4.121315508874262790, 6.791656612786516334, -1.082531754730549967 ) ) ;
#50734=CARTESIAN_POINT ( 'NONE',  ( 4.547870462380197765, 7.393267075163835855, 1.199719254218462483 ) ) ;
#50737=CARTESIAN_POINT ( 'NONE',  ( -0.6823417656250212460, 2.613541667008084879, 1.181850606188767472 ) ) ;
#50739=CARTESIAN_POINT ( 'NONE',  ( 2.198393463710220264, 5.716542807637226886, 0.7998128361456462443 ) ) ;
#50741=CARTESIAN_POINT ( 'NONE',  ( 1.364683531249988757, 0.1968750003414204697, 0.000000000000000000 ) ) ;
#50744=CARTESIAN_POINT ( 'NONE',  ( -3.297657676621885692, 4.870353260857385180, 1.599625672291267398 ) ) ;
#50745=CARTESIAN_POINT ( 'NONE',  ( -6.304178240230145391, 9.338329799368375816, 1.082531754730548412 ) ) ;
#50748=CARTESIAN_POINT ( 'NONE',  ( -0.6823417656250003738, 2.967708333674754062, -1.181850606188749264 ) ) ;
#50756=CARTESIAN_POINT ( 'NONE',  ( -7.849807752188049825, 8.260456587081938196, 0.7216878364870578100 ) ) ;
#50761=CARTESIAN_POINT ( 'NONE',  ( -5.368665640887164692, 9.207267647769599606, 0.000000000000000000 ) ) ;
#50771=CIRCLE ( 'NONE', #99170, 0.08000000000000025147 ) ;
#50772=CARTESIAN_POINT ( 'NONE',  ( 1.446373960595475516, 8.704174803020480411, -2.603708784378553354 ) ) ;
#50776=CARTESIAN_POINT ( 'NONE',  ( -4.557512192488103686, 8.468847991211438497, -0.7998128361456281477 ) ) ;
#50778=CARTESIAN_POINT ( 'NONE',  ( -1.500000000000013101, -0.3291666666666463459, 0.8660254037844403729 ) ) ;
#50779=CARTESIAN_POINT ( 'NONE',  ( 4.356247428692526569, 3.976710176429713250, 0.7998128361456341429 ) ) ;
#50783=CARTESIAN_POINT ( 'NONE',  ( 4.482942347612929979, 8.381849838857084123, 1.040834085586084257E-14 ) ) ;
#50789=CARTESIAN_POINT ( 'NONE',  ( -3.253593677599670109, 5.779314476299451719, 1.082531754730560403 ) ) ;
#50794=CARTESIAN_POINT ( 'NONE',  ( -0.4421197159228375528, 6.952754122461416664, 3.903672163281833640 ) ) ;
#50799=CARTESIAN_POINT ( 'NONE',  ( -0.6823417656250212460, 1.801041667008083991, 1.181850606188755259 ) ) ;
#50800=CARTESIAN_POINT ( 'NONE',  ( 9.449669878600614581, 12.04770082983265844, -1.443375672974058777 ) ) ;
#50801=CARTESIAN_POINT ( 'NONE',  ( -7.497822643557261024, 8.706213491360317747, -1.199719254218446718 ) ) ;
#50804=CARTESIAN_POINT ( 'NONE',  ( 5.957918438201454059, 9.038323046955323292, -1.199719254218440723 ) ) ;
#50805=CARTESIAN_POINT ( 'NONE',  ( -7.335124800193271177, 8.516399340768996851, -1.199719254218452935 ) ) ;
#50808=CARTESIAN_POINT ( 'NONE',  ( 1.499999999999987121, -0.7145833326505161009, 0.8660254037844524744 ) ) ;
#50809=ADVANCED_FACE ( 'NONE', ( #142018 ), #4281, .T. ) ;
#50811=CARTESIAN_POINT ( 'NONE',  ( 9.422553571817644524, 10.09532670998316384, 0.000000000000000000 ) ) ;
#50814=CARTESIAN_POINT ( 'NONE',  ( -0.6823417656250246877, 0.6135416670080897639, 1.181850606188755259 ) ) ;
#50817=CARTESIAN_POINT ( 'NONE',  ( 7.280365300414074703, 7.596107060012304402, -0.7216878364870257245 ) ) ;
#50821=CARTESIAN_POINT ( 'NONE',  ( -4.284013352238262407, 6.021101549076499637, -1.443375672974053447 ) ) ;
#50823=CARTESIAN_POINT ( 'NONE',  ( -1.001543065824772872E-14, 5.321875000341422357, 1.575800808251672791 ) ) ;
#50827=CARTESIAN_POINT ( 'NONE',  ( -4.069418662396130593, 7.899405539437467816, -0.7998128361456281477 ) ) ;
#50828=CARTESIAN_POINT ( 'NONE',  ( -5.703190497605960196, 6.276721696052339539, -1.111643793752248754 ) ) ;
#50835=CARTESIAN_POINT ( 'NONE',  ( 8.281332899848809603, 8.555976559445431562, 0.7998128361456481317 ) ) ;
#50839=CARTESIAN_POINT ( 'NONE',  ( -0.7500000000000215383, 2.691666666666689522, 1.299038105676671107 ) ) ;
#50840=EDGE_CURVE ( 'NONE', #97926, #7066, #13441, .T. ) ;
#50846=CARTESIAN_POINT ( 'NONE',  ( 4.189106276942576201, 7.831115056500907556, 1.040834085586084257E-14 ) ) ;
#50848=CARTESIAN_POINT ( 'NONE',  ( 1.364683531249988757, 0.1968750003414204697, 0.000000000000000000 ) ) ;
#50850=CARTESIAN_POINT ( 'NONE',  ( 10.16199982864259788, 11.81442020729326536, 1.199719254218452047 ) ) ;
#50855=CARTESIAN_POINT ( 'NONE',  ( -0.7500000000000215383, 0.9416666666666878571, 1.299038105676659116 ) ) ;
#50856=CARTESIAN_POINT ( 'NONE',  ( 5.913327553854682783, 10.05063257947248800, -0.7998128361456291469 ) ) ;
#50857=CARTESIAN_POINT ( 'NONE',  ( -6.665805079413154921, 10.92852302595736447, 0.7998128361456481317 ) ) ;
#50860=CARTESIAN_POINT ( 'NONE',  ( 1.364683531249988757, 0.8843750003414210248, 0.000000000000000000 ) ) ;
#50863=CARTESIAN_POINT ( 'NONE',  ( -1.499999999999997780, 2.150000000000019895, 1.214306433183764966E-14 ) ) ;
#50865=CARTESIAN_POINT ( 'NONE',  ( 4.090809663021327758, 5.795697244990093644, 1.599625672291267398 ) ) ;
#50872=CARTESIAN_POINT ( 'NONE',  ( -0.7500000000000006661, -0.8604166659838472508, -1.299038105676652011 ) ) ;
#50873=CARTESIAN_POINT ( 'NONE',  ( -8.667740277838301921, 9.006785167099828016, -0.7998128361456291469 ) ) ;
#50874=CARTESIAN_POINT ( 'NONE',  ( -3.470524135418300737, 6.032400010421219427, -1.082531754730549967 ) ) ;
#50881=ORIENTED_EDGE ( 'NONE', *, *, #87068, .T. ) ;
#50882=CARTESIAN_POINT ( 'NONE',  ( 5.777746017718023097, 9.892454120646377191, 0.7998128361456462443 ) ) ;
#50883=DIRECTION ( 'NONE',  ( 0.000000000000000000, 0.7766560405359869135, 0.6299249119529750640 ) ) ;
#50886=CARTESIAN_POINT ( 'NONE',  ( 7.983053520348166288, 8.207983950027992748, -0.7998128361456281477 ) ) ;
#50887=CARTESIAN_POINT ( 'NONE',  ( 7.754900676892376055, 8.149731665903665601, 1.040834085586084257E-14 ) ) ;
#50888=CARTESIAN_POINT ( 'NONE',  ( -0.4735722981419963062, 7.464727232010883284, -4.424040350390532339 ) ) ;
#50891=CARTESIAN_POINT ( 'NONE',  ( -5.506582945444718824, 9.576097202994168001, 0.7998128361456481317 ) ) ;
#50892=CARTESIAN_POINT ( 'NONE',  ( 5.030238685870051185, 5.827365540725222282, -1.199719254218452047 ) ) ;
#50897=CARTESIAN_POINT ( 'NONE',  ( 4.073938026035560434, 7.494178044256873505, -0.5588469191320240004 ) ) ;
#50898=CARTESIAN_POINT ( 'NONE',  ( 9.897088948295943212, 11.60932053017587506, 1.082531754730548412 ) ) ;
#50899=ORIENTED_EDGE ( 'NONE', *, *, #60938, .F. ) ;
#50905=CARTESIAN_POINT ( 'NONE',  ( -1.555203039002693188, 8.692270211428450466, -2.503634413632307876 ) ) ;
#50906=CARTESIAN_POINT ( 'NONE',  ( -3.456965981804629884, 6.976951378839947537, 1.040834085586084257E-14 ) ) ;
#50907=CARTESIAN_POINT ( 'NONE',  ( 9.761507412159302177, 10.49077285704843199, -0.7216878364870257245 ) ) ;
#50910=CARTESIAN_POINT ( 'NONE',  ( -6.254388934605767503, 6.191208599995166040, 0.7998128361456341429 ) ) ;
#50912=CARTESIAN_POINT ( 'NONE',  ( -3.116716552580018451, 6.446646959060242210, -0.7524088503868963107 ) ) ;
#50916=CARTESIAN_POINT ( 'NONE',  ( -8.182509401047415309, 9.505014708432145909, 1.199719254218462483 ) ) ;
#50919=CARTESIAN_POINT ( 'NONE',  ( -0.2802162696003129283, 8.153957901067540703, 2.020850277443522192 ) ) ;
#50920=ORIENTED_EDGE ( 'NONE', *, *, #4614, .F. ) ;
#50932=CARTESIAN_POINT ( 'NONE',  ( -6.230135280679522936, 7.227244901336242755, 1.199719254218450271 ) ) ;
#50936=CARTESIAN_POINT ( 'NONE',  ( 5.680503174445848735, 5.729601246382692636, 1.040834085586084257E-14 ) ) ;
#50940=CARTESIAN_POINT ( 'NONE',  ( -3.438964519360665051, 7.163875705896082913, -0.7998128361456281477 ) ) ;
#50947=CARTESIAN_POINT ( 'NONE',  ( -6.665805079413154921, 10.92852302595736447, 0.7998128361456481317 ) ) ;
#50948=CARTESIAN_POINT ( 'NONE',  ( 7.447506452608354088, 7.583179037664891098, 0.7998128361456341429 ) ) ;
#50952=CARTESIAN_POINT ( 'NONE',  ( -8.616370316684697883, 10.01118577667568132, -1.199719254218446718 ) ) ;
#50955=CARTESIAN_POINT ( 'NONE',  ( 3.741289556128908345, 7.428763123923395106, -2.448390356388091327 ) ) ;
#50956=CARTESIAN_POINT ( 'NONE',  ( -1.364683531250012516, 0.5927083336747520637, 0.7879004041258379498 ) ) ;
#50957=EDGE_LOOP ( 'NONE', ( #168384, #154276, #152456, #13846, #28642 ) ) ;
#50959=CARTESIAN_POINT ( 'NONE',  ( 7.592202833972727660, 11.80139437303613015, -0.7216878364870267237 ) ) ;
#50980=CARTESIAN_POINT ( 'NONE',  ( -2.272963308585411735, 5.803540959991587478, 0.7998128361456341429 ) ) ;
#50987=CIRCLE ( 'NONE', #5962, 0.07999999999999971023 ) ;
#50988=CARTESIAN_POINT ( 'NONE',  ( -0.7500000000000006661, -0.1104166659838465292, -1.299038105676652011 ) ) ;
#50994=DIRECTION ( 'NONE',  ( 0.6507913734559640506, -0.7592566023653004592, 0.000000000000000000 ) ) ;
#50996=CARTESIAN_POINT ( 'NONE',  ( 8.646349277213076334, 11.11049346154719508, 1.599625672291281386 ) ) ;
#50998=DIRECTION ( 'NONE',  ( 0.7592566023652990159, -0.6507913734559659380, 1.175982368226361624E-15 ) ) ;
#51002=CARTESIAN_POINT ( 'NONE',  ( 3.928111819657337911, 5.605883094398769195, 1.599625672291267398 ) ) ;
#51003=CARTESIAN_POINT ( 'NONE',  ( -6.060131475628484310, 10.01397778830115470, 0.000000000000000000 ) ) ;
#51004=EDGE_CURVE ( 'NONE', #138703, #170885, #106855, .T. ) ;
#51007=CARTESIAN_POINT ( 'NONE',  ( -7.670162217029145246, 9.971608557999250166, 1.599625672291295375 ) ) ;
#51008=CARTESIAN_POINT ( 'NONE',  ( -4.568734577680899633, 4.432537883490215158, -0.7216878364870207285 ) ) ;
#51011=CARTESIAN_POINT ( 'NONE',  ( -1.500000000000001332, -0.06874999931718445145, 0.000000000000000000 ) ) ;
#51018=CARTESIAN_POINT ( 'NONE',  ( -3.240035523541616502, 6.723865844199768738, 0.7216878364870317197 ) ) ;
#51026=CARTESIAN_POINT ( 'NONE',  ( -2.589244150085650009, 5.964609241834465614, 0.7216878364870317197 ) ) ;
#51027=CARTESIAN_POINT ( 'NONE',  ( 7.560643217915098191, 11.97250085420964716, -0.7998128361456291469 ) ) ;
#51036=CARTESIAN_POINT ( 'NONE',  ( -9.806625181386236179, 10.33548422123910449, -0.7998128361456291469 ) ) ;
#51041=CARTESIAN_POINT ( 'NONE',  ( 6.030679399980265920, 5.930214142932100252, -0.7998128361456281477 ) ) ;
#51045=ORIENTED_EDGE ( 'NONE', *, *, #58523, .F. ) ;
#51046=CARTESIAN_POINT ( 'NONE',  ( -3.022498986271275001, 2.800000000000024691, 2.500000000000011102 ) ) ;
#51058=CARTESIAN_POINT ( 'NONE',  ( 7.969495366734495434, 8.192166104145387706, 1.040834085586084257E-14 ) ) ;
#51060=CARTESIAN_POINT ( 'NONE',  ( -5.596818484342970912, 5.424043074688562172, -0.7998128361456221525 ) ) ;
#51067=CARTESIAN_POINT ( 'NONE',  ( -1.364683531249997417, 5.509375000341417916, 1.214306433183764966E-14 ) ) ;
#51070=CARTESIAN_POINT ( 'NONE',  ( 2.706824224222692088, 6.309712028235118453, 0.7998128361456362523 ) ) ;
#51072=CARTESIAN_POINT ( 'NONE',  ( -2.785310492603665367, 5.336947110424484109, 1.199719254218462483 ) ) ;
#51079=CARTESIAN_POINT ( 'NONE',  ( 4.636525346193557162, 7.392734756325715750, -1.082531754730549078 ) ) ;
#51082=CARTESIAN_POINT ( 'NONE',  ( 6.738039155867407537, 10.80487008191325771, -0.7216878364870267237 ) ) ;
#51083=CARTESIAN_POINT ( 'NONE',  ( -1.364683531249997417, 4.321875000341417028, 1.214306433183764966E-14 ) ) ;
#51085=CARTESIAN_POINT ( 'NONE',  ( 4.812781342726866640, 5.677628323678546529, 1.082531754730560403 ) ) ;
#51092=CARTESIAN_POINT ( 'NONE',  ( -6.126358594793636314, 6.003181085514223803, -0.2003443317756918585 ) ) ;
#51094=CARTESIAN_POINT ( 'NONE',  ( -0.6823417656250212460, 4.863541667008086655, 1.181850606188767472 ) ) ;
#51100=CARTESIAN_POINT ( 'NONE',  ( 1.499999999999985123, -0.9541666666666493990, -0.8660254037844323793 ) ) ;
#51109=CARTESIAN_POINT ( 'NONE',  ( -1.364683531250010295, 4.592708333674755394, 0.7879004041258379498 ) ) ;
#51111=CARTESIAN_POINT ( 'NONE',  ( 7.962716289927667113, 8.184257181204083409, -0.7998128361456291469 ) ) ;
#51112=CARTESIAN_POINT ( 'NONE',  ( -10.01677656239806247, 10.58066083241955901, 0.7998128361456462443 ) ) ;
#51120=CARTESIAN_POINT ( 'NONE',  ( -1.500000000000013101, 4.129166666666687746, -0.8660254037844313801 ) ) ;
#51124=EDGE_CURVE ( 'NONE', #159043, #10129, #28785, .T. ) ;
#51125=CARTESIAN_POINT ( 'NONE',  ( 4.881142843665459807, 6.718083573547731113, -1.292325262782492823 ) ) ;
#51129=CARTESIAN_POINT ( 'NONE',  ( 7.266807147244743526, 11.42176607185347414, -0.7216878364870267237 ) ) ;
#51134=CARTESIAN_POINT ( 'NONE',  ( -0.7499999999999972244, 3.889583334016149863, -1.299038105676652011 ) ) ;
#51136=CARTESIAN_POINT ( 'NONE',  ( -3.391510981712833939, 7.108513245306943062, 0.7998128361456341429 ) ) ;
#51137=CARTESIAN_POINT ( 'NONE',  ( 3.782361668088245921, 6.396210465202840645, -1.082531754730548412 ) ) ;
#51144=CARTESIAN_POINT ( 'NONE',  ( 4.253507506385319381, 5.985511395581417204, 1.599625672291267398 ) ) ;
#51148=CARTESIAN_POINT ( 'NONE',  ( 3.181359600701000989, 6.863336634126477875, 0.000000000000000000 ) ) ;
#51150=ADVANCED_FACE ( 'NONE', ( #41523 ), #166254, .T. ) ;
#51162=CARTESIAN_POINT ( 'NONE',  ( 4.872649465673598357, 6.683545894502381124, -1.250567445346082218 ) ) ;
#51166=CARTESIAN_POINT ( 'NONE',  ( 8.028399517586572998, 12.51821653715971472, -0.7998128361456352531 ) ) ;
#51170=CARTESIAN_POINT ( 'NONE',  ( 1.364683531249986537, -0.8864583329919110133, 0.7879004041258500513 ) ) ;
#51171=CARTESIAN_POINT ( 'NONE',  ( 6.643132081016125845, 6.852668304048034287, 0.7216878364870317197 ) ) ;
#51172=CARTESIAN_POINT ( 'NONE',  ( -10.48008955368359629, 11.32911868882677986, 1.040834085586084257E-14 ) ) ;
#51177=CARTESIAN_POINT ( 'NONE',  ( -4.253507506385335368, 5.985511395581417204, 1.599625672291267398 ) ) ;
#51188=CARTESIAN_POINT ( 'NONE',  ( 9.531545685607134999, 11.07889037375188401, 1.199719254218450271 ) ) ;
#51189=CARTESIAN_POINT ( 'NONE',  ( 5.769745475479523655, 6.237591007168648005, 1.002400605009654111 ) ) ;
#51195=CARTESIAN_POINT ( 'NONE',  ( 4.416205349749311004, 6.175325546172740765, 1.599625672291267398 ) ) ;
#51199=CARTESIAN_POINT ( 'NONE',  ( -4.322138105957580301, 3.567377917394196629, 2.444429911049618820 ) ) ;
#51200=CARTESIAN_POINT ( 'NONE',  ( -7.510853912290736289, 11.70648729774046792, 0.7216878364870458196 ) ) ;
#51204=CARTESIAN_POINT ( 'NONE',  ( 5.926885707468349196, 10.06645042535509660, 1.040834085586084257E-14 ) ) ;
#51205=CARTESIAN_POINT ( 'NONE',  ( -3.601662362724658895, 7.353689856487406473, -0.7998128361456282587 ) ) ;
#51207=CARTESIAN_POINT ( 'NONE',  ( 3.897079088924235712, 6.634010472798538949, 1.199719254218462483 ) ) ;
#51209=CARTESIAN_POINT ( 'NONE',  ( -5.494078562035765501, 7.432844293840273231, -1.599625672291256295 ) ) ;
#51210=CARTESIAN_POINT ( 'NONE',  ( 2.900554798319789906, 5.471398800426671372, 1.199719254218452047 ) ) ;
#51214=CARTESIAN_POINT ( 'NONE',  ( 7.567422294721922960, 11.98040977715095323, 0.7998128361456462443 ) ) ;
#51215=CARTESIAN_POINT ( 'NONE',  ( 0.1100172516615150753, 7.047065462482141385, 3.945011421259202677 ) ) ;
#51218=CARTESIAN_POINT ( 'NONE',  ( 4.250508905105749413, 7.277302409985156650, -0.9232175757047023090 ) ) ;
#51219=CARTESIAN_POINT ( 'NONE',  ( 6.168596704537822717, 6.299043698156668647, 1.040834085586084257E-14 ) ) ;
#51226=CARTESIAN_POINT ( 'NONE',  ( 7.199016378732056687, 10.38230762762066384, -1.082531754730537976 ) ) ;
#51230=CARTESIAN_POINT ( 'NONE',  ( -7.557780564614042795, 10.90482886110335414, -1.199719254218446718 ) ) ;
#51239=CARTESIAN_POINT ( 'NONE',  ( 3.728655938958122196, 4.308852335994623139, -1.199719254218446718 ) ) ;
#51243=CARTESIAN_POINT ( 'NONE',  ( 4.660252114795294887, 6.460046772059735432, -1.599625672291256295 ) ) ;
#51246=AXIS2_PLACEMENT_3D ( 'NONE', #163638, #14146, #196134 ) ;
#51247=CARTESIAN_POINT ( 'NONE',  ( -1.500000000000011324, 4.660416667349484676, -0.8660254037844313801 ) ) ;
#51253=CARTESIAN_POINT ( 'NONE',  ( 1.499999999999987121, 1.295833333333353377, -0.8660254037844253849 ) ) ;
#51254=CARTESIAN_POINT ( 'NONE',  ( 7.135668919494039031, 7.219368582364847242, 1.040834085586084257E-14 ) ) ;
#51255=CARTESIAN_POINT ( 'NONE',  ( 4.487385655998878953, 6.258369236797239665, 1.443375672974062551 ) ) ;
#51257=ADVANCED_FACE ( 'NONE', ( #170425 ), #4691, .F. ) ;
#51260=CARTESIAN_POINT ( 'NONE',  ( 8.107412671292031803, 11.44210330227398487, 1.082531754730557072 ) ) ;
#51267=CARTESIAN_POINT ( 'NONE',  ( -3.716906668440817185, 7.488141546489591072, 0.7998128361456341429 ) ) ;
#51268=CARTESIAN_POINT ( 'NONE',  ( 0.7499999999999920064, 4.264583334016150751, 1.299038105676669330 ) ) ;
#51269=CARTESIAN_POINT ( 'NONE',  ( -1.402160292154681736E-14, -0.1781249996585796136, 1.575800808251672791 ) ) ;
#51273=CARTESIAN_POINT ( 'NONE',  ( 2.984766373302843778, 6.633977868828633717, -0.7998128361456291469 ) ) ;
#51275=CARTESIAN_POINT ( 'NONE',  ( 1.364683531249990311, 4.696875000341417916, 1.214306433183764966E-14 ) ) ;
#51283=CARTESIAN_POINT ( 'NONE',  ( -6.855619230004478482, 11.14997286831390788, -0.7998128361456291469 ) ) ;
#51284=CARTESIAN_POINT ( 'NONE',  ( 5.494078562035752178, 7.432844293840273231, -1.599625672291262513 ) ) ;
#51286=CARTESIAN_POINT ( 'NONE',  ( 0.6823417656249882723, -0.9072916663252494907, 1.181850606188755259 ) ) ;
#51293=CARTESIAN_POINT ( 'NONE',  ( -6.718228810771495141, 7.796687353110217877, 1.199719254218450271 ) ) ;
#51296=CARTESIAN_POINT ( 'NONE',  ( 8.516493047678546091, 13.08765898893368629, -0.7998128361456352531 ) ) ;
#51298=CARTESIAN_POINT ( 'NONE',  ( 10.38962578677386084, 11.01565159419135043, 0.000000000000000000 ) ) ;
#51301=CARTESIAN_POINT ( 'NONE',  ( -2.591579918506545344, 6.175260338232929413, 1.040834085586084257E-14 ) ) ;
#51302=CARTESIAN_POINT ( 'NONE',  ( -7.802881099864745984, 9.062115023719057305, -1.199719254218446718 ) ) ;
#51304=CARTESIAN_POINT ( 'NONE',  ( -4.418103850092305329, 7.323797853316306394, 1.240345400901581296 ) ) ;
#51305=CARTESIAN_POINT ( 'NONE',  ( 1.364683531249986537, -0.3864583329919166199, 0.7879004041258500513 ) ) ;
#51309=CARTESIAN_POINT ( 'NONE',  ( 7.239690840017413365, 10.42976116578691403, -1.082531754730537976 ) ) ;
#51330=CARTESIAN_POINT ( 'NONE',  ( 3.768803514918948938, 4.459654191235965293, -1.082531754730543083 ) ) ;
#51331=LINE ( 'NONE', #400, #67768 ) ;
#51335=CARTESIAN_POINT ( 'NONE',  ( -4.436542580169821726, 6.199052314996659874, 1.599625672291267398 ) ) ;
#51336=CARTESIAN_POINT ( 'NONE',  ( -7.700141177557535244, 11.07091624287075859, -1.199719254218446718 ) ) ;
#51337=DIRECTION ( 'NONE',  ( 0.7592566023653005702, 0.6507913734559639396, 0.000000000000000000 ) ) ;
#51341=CARTESIAN_POINT ( 'NONE',  ( 1.499999999999989120, 2.806250000682818158, 1.214306433183764966E-14 ) ) ;
#51342=CARTESIAN_POINT ( 'NONE',  ( 10.24048609702354717, 10.84165528948263457, -0.7998128361456281477 ) ) ;
#51348=CARTESIAN_POINT ( 'NONE',  ( -7.804689982961090955, 12.25722208009664094, 0.7998128361456481317 ) ) ;
#51350=CARTESIAN_POINT ( 'NONE',  ( 1.364683531249988535, 2.113541667008087099, 0.7879004041258500513 ) ) ;
#51353=CARTESIAN_POINT ( 'NONE',  ( -5.736990052169587351, 5.898621588803449001, 2.499999999999785061 ) ) ;
#51354=ORIENTED_EDGE ( 'NONE', *, *, #85850, .F. ) ;
#51358=CARTESIAN_POINT ( 'NONE',  ( -3.952365473583647315, 4.569846793057691592, 1.199719254218462483 ) ) ;
#51363=CARTESIAN_POINT ( 'NONE',  ( 0.6823417656249899377, 1.155208333674752286, 1.181850606188755259 ) ) ;
#51368=CARTESIAN_POINT ( 'NONE',  ( -1.364683531250012516, 2.030208333674750953, 0.7879004041258379498 ) ) ;
#51370=CARTESIAN_POINT ( 'NONE',  ( -5.768104287610143821, 8.816873204598778102, -1.199719254218440723 ) ) ;
#51371=CARTESIAN_POINT ( 'NONE',  ( 6.913768267964901071, 10.15348118167935709, -1.199719254218441611 ) ) ;
#51372=CARTESIAN_POINT ( 'NONE',  ( 3.167801447087334132, 6.847518788243869281, -0.7998128361456291469 ) ) ;
#51373=CARTESIAN_POINT ( 'NONE',  ( 6.006425746053997372, 6.966250444273174303, -1.199719254218445830 ) ) ;
#51375=CARTESIAN_POINT ( 'NONE',  ( -1.500000000000013101, 3.379166666666691299, -0.8660254037844313801 ) ) ;
#51377=CARTESIAN_POINT ( 'NONE',  ( 1.364683531249988535, 2.676041667008082214, 0.7879004041258500513 ) ) ;
#51381=CARTESIAN_POINT ( 'NONE',  ( -1.364683531250000748, -1.240624999658580752, 0.000000000000000000 ) ) ;
#51385=CARTESIAN_POINT ( 'NONE',  ( 4.338245966692901412, 8.005111361209628740, -0.7216878364870197293 ) ) ;
#51388=CARTESIAN_POINT ( 'NONE',  ( -7.991641480251377772, 11.41099992934688956, 1.199719254218453823 ) ) ;
#51389=CARTESIAN_POINT ( 'NONE',  ( -2.279742385392243165, 5.811449882932888222, -0.7998128361456281477 ) ) ;
#51394=CARTESIAN_POINT ( 'NONE',  ( 3.469446951953614189E-15, 3.300000000000018030, 1.214306433183764966E-14 ) ) ;
#51395=CARTESIAN_POINT ( 'NONE',  ( -7.985389288324703294, 9.379004260209384825, -1.082531754730543083 ) ) ;
#51397=CARTESIAN_POINT ( 'NONE',  ( -1.500000000000011324, 5.379166666666692187, -0.8660254037844313801 ) ) ;
#51400=CARTESIAN_POINT ( 'NONE',  ( 6.643132081016105417, 10.69414516125339887, 0.7216878364870438212 ) ) ;
#51405=CARTESIAN_POINT ( 'NONE',  ( -4.252937622776048698, 3.981816863952433838, 0.4689809815191707809 ) ) ;
#51406=VECTOR ( 'NONE', #161231, 1000.000000000000000 ) ;
#51414=CARTESIAN_POINT ( 'NONE',  ( 6.425674737872927089, 9.584038729905381970, -1.199719254218440723 ) ) ;
#51415=CARTESIAN_POINT ( 'NONE',  ( -6.403528624356093601, 6.365204904703887223, 1.040834085586084257E-14 ) ) ;
#51420=CARTESIAN_POINT ( 'NONE',  ( 4.812781342726855982, 7.598366752281232372, 1.082531754730558626 ) ) ;
#51422=CARTESIAN_POINT ( 'NONE',  ( 4.378920427533921078, 4.211088041652093494, 1.214306433183764966E-14 ) ) ;
#51423=CARTESIAN_POINT ( 'NONE',  ( -2.300079615812729905, 5.835176651756807331, -0.7998128361456281477 ) ) ;
#51432=ORIENTED_EDGE ( 'NONE', *, *, #165043, .T. ) ;
#51440=CARTESIAN_POINT ( 'NONE',  ( 5.635385404774530649, 9.726366738878972740, 0.7998128361456462443 ) ) ;
#51441=CARTESIAN_POINT ( 'NONE',  ( 7.983053520348166288, 8.207983950027992748, -0.7998128361456281477 ) ) ;
#51449=CARTESIAN_POINT ( 'NONE',  ( -2.429488990373097845, 5.239623814575174343, 0.8733349908450799282 ) ) ;
#51452=CARTESIAN_POINT ( 'NONE',  ( -5.494078562035765501, 7.432844293840273231, -1.599625672291256295 ) ) ;
#51454=CARTESIAN_POINT ( 'NONE',  ( -2.754277761870538299, 6.365074488824250309, 1.040834085586084257E-14 ) ) ;
#51463=CARTESIAN_POINT ( 'NONE',  ( -3.789667630219657912, 4.380032642466370696, 1.199719254218462483 ) ) ;
#51466=CARTESIAN_POINT ( 'NONE',  ( 4.950698647284403009, 8.927565521807144577, 1.040834085586084257E-14 ) ) ;
#51467=CARTESIAN_POINT ( 'NONE',  ( 1.364683531249990311, 4.384375000341417028, 1.214306433183764966E-14 ) ) ;
#51473=CARTESIAN_POINT ( 'NONE',  ( 4.650083499362864359, 7.408552601689905259, 1.082531754730558626 ) ) ;
#51474=CARTESIAN_POINT ( 'NONE',  ( -5.856232286098998152, 8.919689202835742847, 1.199719254218452047 ) ) ;
#51480=CARTESIAN_POINT ( 'NONE',  ( -7.640183256500752584, 8.872300873127729304, -1.199719254218446718 ) ) ;
#51481=CARTESIAN_POINT ( 'NONE',  ( -4.388035272317281077, 8.271124917678806199, 0.7998128361456481317 ) ) ;
#51489=CARTESIAN_POINT ( 'NONE',  ( 5.926885707468349196, 10.06645042535509660, 1.040834085586084257E-14 ) ) ;
#51502=CARTESIAN_POINT ( 'NONE',  ( -1.499999999999997780, 5.900000000000023448, 1.214306433183764966E-14 ) ) ;
#51503=CARTESIAN_POINT ( 'NONE',  ( 2.822068529938852155, 6.444163718237301275, -0.7998128361456291469 ) ) ;
#51504=CARTESIAN_POINT ( 'NONE',  ( 6.342516933094585418, 6.294024598232139667, 1.040834085586084257E-14 ) ) ;
#51507=CARTESIAN_POINT ( 'NONE',  ( -7.375272376154093479, 9.627570410311676596, -1.443375672974059665 ) ) ;
#51508=CARTESIAN_POINT ( 'NONE',  ( -5.738313685646318163, 5.917571446856342732, -2.440166996132832722 ) ) ;
#51509=CARTESIAN_POINT ( 'NONE',  ( 5.341549334104188418, 7.254893527920112994, 1.443375672974062551 ) ) ;
#51510=CARTESIAN_POINT ( 'NONE',  ( -8.202319746143382773, 9.632089794331152532, 1.082531754730558626 ) ) ;
#51514=CARTESIAN_POINT ( 'NONE',  ( 6.693975156845185737, 8.832723654451292816, 1.599625672291281386 ) ) ;
#51519=CARTESIAN_POINT ( 'NONE',  ( 1.364683531249988535, 3.613541667008086211, 0.7879004041258500513 ) ) ;
#51525=CARTESIAN_POINT ( 'NONE',  ( 7.587759525142423911, 12.00413654597487501, 0.7998128361456462443 ) ) ;
#51530=CARTESIAN_POINT ( 'NONE',  ( -8.341290820905609138, 10.75459192918846618, 1.599625672291269396 ) ) ;
#51536=CARTESIAN_POINT ( 'NONE',  ( 3.541704441667858472, 5.155074486744371853, -1.599625672291262513 ) ) ;
#51539=CARTESIAN_POINT ( 'NONE',  ( -7.771848369131641121, 10.09024240211882351, -1.599625672291263179 ) ) ;
#51545=CARTESIAN_POINT ( 'NONE',  ( 5.881923755780003482, 5.983360633994940336, 0.1790317558759656202 ) ) ;
#51546=CARTESIAN_POINT ( 'NONE',  ( -10.03267048443264109, 11.76749898900197877, 1.082531754730558626 ) ) ;
#51551=CARTESIAN_POINT ( 'NONE',  ( 6.856673000209174695, 9.022537805042615489, 1.599625672291281386 ) ) ;
#51553=CARTESIAN_POINT ( 'NONE',  ( 5.503720292143644777, 8.508425209887878538, 1.199719254218462483 ) ) ;
#51554=CARTESIAN_POINT ( 'NONE',  ( -4.275059339850010076, 7.289437269727999436, -0.9335736327708322735 ) ) ;
#51555=CARTESIAN_POINT ( 'NONE',  ( 5.983225862332436584, 5.874851682342960402, 0.7998128361456341429 ) ) ;
#51557=CARTESIAN_POINT ( 'NONE',  ( -7.158341918335454857, 10.33485409049125003, 1.082531754730549967 ) ) ;
#51558=AXIS2_PLACEMENT_3D ( 'NONE', #171897, #58147, #75464 ) ;
#51565=CARTESIAN_POINT ( 'NONE',  ( -4.099542569701578820, 7.506983624740954930, -0.5818660602148464367 ) ) ;
#51566=CARTESIAN_POINT ( 'NONE',  ( 4.184706906298553797, 7.590773377710720915, -0.8858016571234141878 ) ) ;
#51569=CARTESIAN_POINT ( 'NONE',  ( 5.829642864196168617, 6.863966765392747860, 1.082531754730558626 ) ) ;
#51573=CARTESIAN_POINT ( 'NONE',  ( -8.636180661780651135, 13.01936850547871138, -0.7216878364870257245 ) ) ;
#51579=CARTESIAN_POINT ( 'NONE',  ( -8.120970824461345217, 12.41829036193951730, 0.7216878364870458196 ) ) ;
#51587=CARTESIAN_POINT ( 'NONE',  ( -9.937763408692600109, 10.69640485300394417, -0.7216878364870267237 ) ) ;
#51595=CARTESIAN_POINT ( 'NONE',  ( -1.499999999999997780, 2.931250000682818158, 1.214306433183764966E-14 ) ) ;
#51597=CARTESIAN_POINT ( 'NONE',  ( -6.579784621333750749, 6.570836901177822931, 0.7998128361456341429 ) ) ;
#51600=CARTESIAN_POINT ( 'NONE',  ( -8.727698198895085469, 11.20540053684285553, -1.599625672291263179 ) ) ;
#51603=CARTESIAN_POINT ( 'NONE',  ( -0.7499999999999972244, 4.389583334016150751, -1.299038105676652899 ) ) ;
#51604=CARTESIAN_POINT ( 'NONE',  ( 7.461064606222022277, 7.598996883547496139, 1.040834085586084257E-14 ) ) ;
#51606=AXIS2_PLACEMENT_3D ( 'NONE', #176277, #27879, #46282 ) ;
#51610=CARTESIAN_POINT ( 'NONE',  ( 8.398386088661320414, 11.88553530582519357, -1.199719254218446718 ) ) ;
#51616=CARTESIAN_POINT ( 'NONE',  ( -8.202319746587722449, 8.671720580548228696, 1.040834085586084257E-14 ) ) ;
#51626=CARTESIAN_POINT ( 'NONE',  ( -2.290964770585000920, 5.616616632417037458, -0.7216878364870257245 ) ) ;
#51628=CARTESIAN_POINT ( 'NONE',  ( 10.57266086055835075, 11.22919251360659310, 0.000000000000000000 ) ) ;
#51630=CARTESIAN_POINT ( 'NONE',  ( -10.64045162862669081, 11.30828174301964140, -0.7998128361456221525 ) ) ;
#51635=CARTESIAN_POINT ( 'NONE',  ( 0.6823417656249899377, 2.092708333674753174, 1.181850606188767472 ) ) ;
#51637=CARTESIAN_POINT ( 'NONE',  ( 3.147464216666835402, 6.823792019419957278, -0.7998128361456291469 ) ) ;
#51643=CARTESIAN_POINT ( 'NONE',  ( 4.067082894419602468, 3.847277586352047862, -0.7216878364870188411 ) ) ;
#51646=CARTESIAN_POINT ( 'NONE',  ( -6.724481002698120768, 9.828683022247721723, -1.082531754730538864 ) ) ;
#51647=EDGE_CURVE ( 'NONE', #152273, #93282, #29526, .T. ) ;
#51652=CARTESIAN_POINT ( 'NONE',  ( -7.635213062790267458, 12.05949900656400686, 0.000000000000000000 ) ) ;
#51653=CARTESIAN_POINT ( 'NONE',  ( -5.395781948114519722, 5.397426482329451325, 0.000000000000000000 ) ) ;
#51654=CARTESIAN_POINT ( 'NONE',  ( -0.6823417656250003738, 2.280208333674753174, -1.181850606188749264 ) ) ;
#51676=CARTESIAN_POINT ( 'NONE',  ( 0.6823417656249899377, 4.488541667008086655, -1.181850606188754593 ) ) ;
#51683=CARTESIAN_POINT ( 'NONE',  ( 7.560643217915098191, 11.97250085420964716, -0.7998128361456291469 ) ) ;
#51686=CARTESIAN_POINT ( 'NONE',  ( 0.6823417656249882723, 1.926041667008083991, -1.181850606188749264 ) ) ;
#51689=CARTESIAN_POINT ( 'NONE',  ( -7.700668062882072284, 10.00719871149432549, -1.443375672974059665 ) ) ;
#51697=CARTESIAN_POINT ( 'NONE',  ( 3.408985558832261731, 6.064568021024562938, 1.199719254218462483 ) ) ;
#51708=CARTESIAN_POINT ( 'NONE',  ( -4.973143418114339021, 4.696422164088486895, 0.7998128361456341429 ) ) ;
#51710=CARTESIAN_POINT ( 'NONE',  ( 7.958799866421889746, 9.244020251369077457, -1.199719254218441611 ) ) ;
#51713=CARTESIAN_POINT ( 'NONE',  ( 3.823036128929238942, 7.404033217152015567, 1.040834085586084257E-14 ) ) ;
#51715=DIRECTION ( 'NONE',  ( -5.578564026256490882E-16, -1.000000000000000000, -9.066213480720158442E-32 ) ) ;
#51720=CARTESIAN_POINT ( 'NONE',  ( -6.236387472606141458, 10.21960978477508952, -0.7216878364870278340 ) ) ;
#51721=CARTESIAN_POINT ( 'NONE',  ( 5.335297142177534369, 6.183267073083954735, -1.199719254218452047 ) ) ;
#51724=CARTESIAN_POINT ( 'NONE',  ( -7.914208982075130905, 10.25632978388623684, -1.599625672291263179 ) ) ;
#51726=CARTESIAN_POINT ( 'NONE',  ( -6.520158902582635640, 5.290451655907115303, 2.438235897557452514 ) ) ;
#51728=CARTESIAN_POINT ( 'NONE',  ( -2.950870989268691957, 6.594433254122103349, -0.7998128361456281477 ) ) ;
#51730=CARTESIAN_POINT ( 'NONE',  ( 9.596473800374404561, 10.09030761005864285, 0.000000000000000000 ) ) ;
#51731=CARTESIAN_POINT ( 'NONE',  ( 3.704402285031850539, 5.344888637335695414, -1.599625672291262513 ) ) ;
#51737=CARTESIAN_POINT ( 'NONE',  ( -5.000000000000024869, 0.2350621082554960051, 0.7750000000000117906 ) ) ;
#51740=CARTESIAN_POINT ( 'NONE',  ( -4.055860508782465068, 7.883587693554856557, 1.040834085586084257E-14 ) ) ;
#51743=CARTESIAN_POINT ( 'NONE',  ( -7.811469059767924605, 12.26513100303794168, -0.7998128361456281477 ) ) ;
#51748=CARTESIAN_POINT ( 'NONE',  ( 5.965224400332808763, 9.903252867122883885, -0.7216878364870267237 ) ) ;
#51749=CARTESIAN_POINT ( 'NONE',  ( 1.364683531249990311, 5.676041667008088432, 0.7879004041258499402 ) ) ;
#51752=CARTESIAN_POINT ( 'NONE',  ( 5.671388329218120639, 5.511041227042920099, 1.040834085586084257E-14 ) ) ;
#51754=CARTESIAN_POINT ( 'NONE',  ( 4.517891501851804215, 6.293959390292322986, -1.599625672291255185 ) ) ;
#51756=CARTESIAN_POINT ( 'NONE',  ( -6.015013705957189316, 10.16926642359206134, 0.7998128361456481317 ) ) ;
#51767=CARTESIAN_POINT ( 'NONE',  ( 0.6823417656249882723, 1.988541667008083991, -1.181850606188749264 ) ) ;
#51768=CARTESIAN_POINT ( 'NONE',  ( 9.725276259704228821, 10.24057714594344048, 0.7998128361456462443 ) ) ;
#51772=CARTESIAN_POINT ( 'NONE',  ( -5.422898255786203769, 6.389431388914436738, -1.082531754730544860 ) ) ;
#51774=CARTESIAN_POINT ( 'NONE',  ( 2.223174002961016082, 5.537527403522402025, -0.7216878364870267237 ) ) ;
#51775=CARTESIAN_POINT ( 'NONE',  ( -6.249945625775490399, 7.354319987235250267, 1.082531754730549967 ) ) ;
#51782=CARTESIAN_POINT ( 'NONE',  ( 3.876741858503734761, 6.610283703974623393, 1.199719254218462483 ) ) ;
#51792=CARTESIAN_POINT ( 'NONE',  ( 3.655894977179307226, 7.416961240017848844, -0.7998128361456291469 ) ) ;
#51796=CARTESIAN_POINT ( 'NONE',  ( -4.713430959045263435, 8.650753218861462202, 0.7998128361456481317 ) ) ;
#51800=CARTESIAN_POINT ( 'NONE',  ( 5.774883364416965037, 8.824782127540085952, -1.199719254218440723 ) ) ;
#51803=CARTESIAN_POINT ( 'NONE',  ( -4.238895582566952314, 8.097128612970093897, 1.040834085586084257E-14 ) ) ;
#51804=CARTESIAN_POINT ( 'NONE',  ( 5.626270559546810546, 8.547437505237857280, 1.082531754730558626 ) ) ;
#51805=CARTESIAN_POINT ( 'NONE',  ( -0.7500000000000006661, 2.608333333333358262, -1.299038105676652011 ) ) ;
#51806=CARTESIAN_POINT ( 'NONE',  ( -5.122283107864663343, 4.870418468797203637, 0.000000000000000000 ) ) ;
#51809=CARTESIAN_POINT ( 'NONE',  ( -5.870844209917351009, 6.808071985447069707, -1.199719254218446718 ) ) ;
#51812=CARTESIAN_POINT ( 'NONE',  ( -1.201851678989727383E-14, 2.696875000341417916, -1.575800808251660134 ) ) ;
#51813=CARTESIAN_POINT ( 'NONE',  ( -2.279984679289828176, 5.601133616484927025, -0.06592222766762731445 ) ) ;
#51814=CARTESIAN_POINT ( 'NONE',  ( -6.249945626219832739, 6.393950773452325542, 1.040834085586084257E-14 ) ) ;
#51820=CARTESIAN_POINT ( 'NONE',  ( 6.166260936116925606, 6.088392601758203071, 0.7998128361456341429 ) ) ;
#51823=CARTESIAN_POINT ( 'NONE',  ( -1.364683531250012516, 3.342708333674756727, 0.7879004041258379498 ) ) ;
#51825=CARTESIAN_POINT ( 'NONE',  ( -0.3584499564876342803, 8.158857887134011833, 1.968348077346307790 ) ) ;
#51829=CARTESIAN_POINT ( 'NONE',  ( -4.959585264500673496, 4.680604318205876524, 1.214306433183764966E-14 ) ) ;
#51830=CARTESIAN_POINT ( 'NONE',  ( -6.765155463094763455, 8.915767345075790828, 1.443375672974078761 ) ) ;
#51832=CARTESIAN_POINT ( 'NONE',  ( 0.6823417656249882723, 2.426041667008084435, -1.181850606188749264 ) ) ;
#51839=CARTESIAN_POINT ( 'NONE',  ( -5.680503174001480637, 9.571078103069643461, 0.7216878364870458196 ) ) ;
#51844=CARTESIAN_POINT ( 'NONE',  ( -7.334597914868743018, 7.659378443542744996, -0.7216878364870267237 ) ) ;
#51857=CARTESIAN_POINT ( 'NONE',  ( -6.566226467720086113, 6.555019055295208119, 1.040834085586084257E-14 ) ) ;
#51859=CARTESIAN_POINT ( 'NONE',  ( 1.499999999999987121, -0.7458333333333122539, 0.8660254037844524744 ) ) ;
#51860=CARTESIAN_POINT ( 'NONE',  ( 3.009020027229115879, 5.597941567487558778, -1.199719254218446718 ) ) ;
#51862=CARTESIAN_POINT ( 'NONE',  ( -3.755245360860925086, 6.364574773437617239, -1.082531754730548412 ) ) ;
#51864=CARTESIAN_POINT ( 'NONE',  ( 4.971035877704902184, 8.951292290631053916, 1.040834085586084257E-14 ) ) ;
#51870=CARTESIAN_POINT ( 'NONE',  ( -3.782361668532609134, 7.356579680022602652, 1.040834085586084257E-14 ) ) ;
#51874=LINE ( 'NONE', #83278, #115205 ) ;
#51878=CARTESIAN_POINT ( 'NONE',  ( 0.6823417656249882723, 2.676041667008084879, -1.181850606188749264 ) ) ;
#51880=CARTESIAN_POINT ( 'NONE',  ( -6.530223543276495235, 10.77034456713125188, -0.7998128361456291469 ) ) ;
#51882=CARTESIAN_POINT ( 'NONE',  ( 7.820355676984174664, 8.018169799436671852, -0.7998128361456281477 ) ) ;
#51883=CARTESIAN_POINT ( 'NONE',  ( -5.689618019229208734, 9.789638122409414223, 0.7998128361456481317 ) ) ;
#51886=CARTESIAN_POINT ( 'NONE',  ( -1.500000000000001332, -1.318749999317178734, 0.000000000000000000 ) ) ;
#51888=CARTESIAN_POINT ( 'NONE',  ( 8.758204044748010730, 9.320252261735261001, 0.7216878364870438212 ) ) ;
#51891=CARTESIAN_POINT ( 'NONE',  ( 1.364683531249986537, 1.176041667008082658, 0.7879004041258500513 ) ) ;
#51893=CARTESIAN_POINT ( 'NONE',  ( 6.546325832964379643, 5.229711127717882491, 2.448021111374941938 ) ) ;
#51894=CARTESIAN_POINT ( 'NONE',  ( 5.626270559546810546, 8.547437505237857280, 1.082531754730558626 ) ) ;
#51897=CARTESIAN_POINT ( 'NONE',  ( -4.989037340148921196, 5.883260320670900434, 1.082531754730560403 ) ) ;
#51900=CARTESIAN_POINT ( 'NONE',  ( 0.6823417656249899377, 3.176041667008085323, -1.181850606188754593 ) ) ;
#51904=CARTESIAN_POINT ( 'NONE',  ( -5.042743069279040036, 7.970618449879118828, 1.199719254218464037 ) ) ;
#51905=CARTESIAN_POINT ( 'NONE',  ( 1.364683531249990311, 5.676041667008088432, 0.7879004041258500513 ) ) ;
#51911=CARTESIAN_POINT ( 'NONE',  ( 6.123478934866503742, 10.29580919065294431, 0.7998128361456462443 ) ) ;
#51915=CARTESIAN_POINT ( 'NONE',  ( -1.201851678989727383E-14, 2.962500000000025224, 1.732050807568877637 ) ) ;
#51921=ORIENTED_EDGE ( 'NONE', *, *, #19236, .T. ) ;
#51922=CARTESIAN_POINT ( 'NONE',  ( 5.151735183512854199, 8.954182114166247430, -0.7216878364870257245 ) ) ;
#51923=CARTESIAN_POINT ( 'NONE',  ( -1.364683531250014514, 0.3010416670080866552, -0.7879004041258359514 ) ) ;
#51925=CARTESIAN_POINT ( 'NONE',  ( -0.6992639221309246977, 2.800524997876915112, 1.172080594574814727 ) ) ;
#51927=FACE_OUTER_BOUND ( 'NONE', #34372, .T. ) ;
#51931=CARTESIAN_POINT ( 'NONE',  ( -0.7500000000000006661, 0.3583333333333563187, -1.299038105676652011 ) ) ;
#51932=CARTESIAN_POINT ( 'NONE',  ( 6.753933077901968396, 11.03133902419432566, 0.7998128361456462443 ) ) ;
#51933=CARTESIAN_POINT ( 'NONE',  ( -7.828943636887387925, 11.22118577875556156, 1.199719254218453823 ) ) ;
#51935=CARTESIAN_POINT ( 'NONE',  ( 0.6823417656249899377, 1.092708333674752286, 1.181850606188755259 ) ) ;
#51936=CARTESIAN_POINT ( 'NONE',  ( -1.500000000000011324, 3.170833333333354265, 0.8660254037844403729 ) ) ;
#51938=CARTESIAN_POINT ( 'NONE',  ( 3.486418057008484617, 7.219238166485217434, 1.040834085586084257E-14 ) ) ;
#51946=CARTESIAN_POINT ( 'NONE',  ( -1.500000000000015099, -0.5895833326505155458, -0.8660254037844383745 ) ) ;
#51947=APPLICATION_CONTEXT ( 'automotive_design' ) ;
#51948=CARTESIAN_POINT ( 'NONE',  ( -8.518600588087975822, 8.832788862391110385, 1.040834085586084257E-14 ) ) ;
#51949=CARTESIAN_POINT ( 'NONE',  ( -3.145128448690310830, 6.613140923539910787, -0.7216878364870267237 ) ) ;
#51951=CARTESIAN_POINT ( 'NONE',  ( 1.249999999999820588, 10.00000000000000178, -4.154462424328206893 ) ) ;
#51957=CARTESIAN_POINT ( 'NONE',  ( 5.262536180398716290, 9.291375977107183104, -0.7998128361456291469 ) ) ;
#51961=CARTESIAN_POINT ( 'NONE',  ( 6.765155463094751909, 8.915767345075790828, 1.443375672974076540 ) ) ;
#51965=CARTESIAN_POINT ( 'NONE',  ( -6.723954117373590833, 9.932031339322813679, -1.199719254218440723 ) ) ;
#51966=CARTESIAN_POINT ( 'NONE',  ( 4.168242161197552420, 6.950367390450747251, -1.199719254218452047 ) ) ;
#51970=CARTESIAN_POINT ( 'NONE',  ( 3.995022045461748217, 7.603044914155053569, 0.06581304817247432548 ) ) ;
#51971=CARTESIAN_POINT ( 'NONE',  ( 9.924205255523292024, 10.68058700763975466, -0.7216878364870257245 ) ) ;
#51976=CARTESIAN_POINT ( 'NONE',  ( 2.275020158240702361, 5.648663482265439129, 0.5226904017501784461 ) ) ;
#51977=FACE_BOUND ( 'NONE', #44743, .T. ) ;
#51978=CARTESIAN_POINT ( 'NONE',  ( -5.450014563013544588, 5.460697866378308341, 0.7216878364870317197 ) ) ;
#51979=CARTESIAN_POINT ( 'NONE',  ( 8.541273586929342798, 11.94827437051752206, -1.082531754730543083 ) ) ;
#51982=CARTESIAN_POINT ( 'NONE',  ( -6.501298352952815662, 7.543601818988450169, -1.199719254218446718 ) ) ;
#51988=CARTESIAN_POINT ( 'NONE',  ( -7.320512876374914768, 10.62801655815766999, 1.199719254218453823 ) ) ;
#51992=ORIENTED_EDGE ( 'NONE', *, *, #119054, .F. ) ;
#52001=CARTESIAN_POINT ( 'NONE',  ( -5.045605722580076780, 9.038290442985410067, -0.7998128361456231517 ) ) ;
#52004=CARTESIAN_POINT ( 'NONE',  ( 3.524756749872944628, 7.056040608253000279, -0.7216878364870267237 ) ) ;
#52009=CARTESIAN_POINT ( 'NONE',  ( -5.057354993097396445, 5.859001232490445688, -1.199719254218446718 ) ) ;
#52017=CARTESIAN_POINT ( 'NONE',  ( -8.910733272679575379, 11.41894145625809820, -1.599625672291263179 ) ) ;
#52018=CARTESIAN_POINT ( 'NONE',  ( 6.257251587906815793, 7.258880593101466161, 1.199719254218462483 ) ) ;
#52022=CARTESIAN_POINT ( 'NONE',  ( -8.462260433223891098, 13.02438760540324481, -0.7998128361456281477 ) ) ;
#52025=CARTESIAN_POINT ( 'NONE',  ( -0.6823417656250003738, 0.5302083336747518416, -1.181850606188749264 ) ) ;
#52029=CARTESIAN_POINT ( 'NONE',  ( 6.968527767744088663, 11.07377346243604599, 0.7216878364870438212 ) ) ;
#52033=CARTESIAN_POINT ( 'NONE',  ( -5.462143695033999435, 6.282726080954706305, -1.018839928044611653 ) ) ;
#52036=DIRECTION ( 'NONE',  ( 0.000000000000000000, 0.000000000000000000, 1.000000000000000000 ) ) ;
#52054=CARTESIAN_POINT ( 'NONE',  ( 0.7499999999999867883, -0.4020833326505157679, -1.299038105676652899 ) ) ;
#52058=ORIENTED_EDGE ( 'NONE', *, *, #149015, .F. ) ;
#52060=CARTESIAN_POINT ( 'NONE',  ( 0.006158830626129541130, 7.078243236992583398, -2.121324627965408993 ) ) ;
#52062=CARTESIAN_POINT ( 'NONE',  ( 10.37606763316019531, 10.99983374830873650, 0.7998128361456462443 ) ) ;
#52065=SPHERICAL_SURFACE ( 'NONE', #80287, 0.08000000000000000167 ) ;
#52068=CARTESIAN_POINT ( 'NONE',  ( 3.714044015139744914, 6.420469553383295391, 1.199719254218462483 ) ) ;
#52069=CARTESIAN_POINT ( 'NONE',  ( 1.364683531249988535, 2.426041667008088432, 0.7879004041258500513 ) ) ;
#52070=CARTESIAN_POINT ( 'NONE',  ( 4.369805582306193870, 3.992528022312320957, 1.214306433183764966E-14 ) ) ;
#52072=CARTESIAN_POINT ( 'NONE',  ( -7.857113714319432063, 9.125386407249497012, 1.199719254218462483 ) ) ;
#52073=CARTESIAN_POINT ( 'NONE',  ( -5.111060722227552588, 6.025620933095978238, 1.082531754730546636 ) ) ;
#52076=CARTESIAN_POINT ( 'NONE',  ( -1.500000000000013101, -0.2979166659838501929, 0.8660254037844403729 ) ) ;
#52084=CARTESIAN_POINT ( 'NONE',  ( -4.894130264408873110, 5.772535398974209642, -1.082531754730543971 ) ) ;
#52091=CARTESIAN_POINT ( 'NONE',  ( -3.050221372950322252, 5.542046787541873520, 1.082531754730560403 ) ) ;
#52092=CARTESIAN_POINT ( 'NONE',  ( 8.503988664269582998, 10.94440607977979063, 1.599625672291281386 ) ) ;
#52095=CARTESIAN_POINT ( 'NONE',  ( -1.203941962966186052, 3.133481847795091646, 0.7750000000000083489 ) ) ;
#52102=CARTESIAN_POINT ( 'NONE',  ( -9.494787648271923786, 9.971673765939062406, 1.040834085586084257E-14 ) ) ;
#52107=CARTESIAN_POINT ( 'NONE',  ( 6.328958779480917229, 6.278206752349526631, 0.7998128361456341429 ) ) ;
#52115=CARTESIAN_POINT ( 'NONE',  ( 3.029357257649615054, 5.621668336311468117, -1.199719254218446718 ) ) ;
#52125=CARTESIAN_POINT ( 'NONE',  ( 7.235247531187115833, 11.59287255302699648, -0.7998128361456291469 ) ) ;
#52127=CARTESIAN_POINT ( 'NONE',  ( -5.412729640353771465, 7.337937218544611895, 1.599625672291269396 ) ) ;
#52132=CARTESIAN_POINT ( 'NONE',  ( -1.201851678989727383E-14, 5.446875000341422357, -1.575800808251660134 ) ) ;
#52136=CARTESIAN_POINT ( 'NONE',  ( 3.897079088924235712, 6.634010472798538949, 1.199719254218462483 ) ) ;
#52137=CARTESIAN_POINT ( 'NONE',  ( -5.298539104842322267, 5.076050465271134016, 0.7998128361456341429 ) ) ;
#52143=CARTESIAN_POINT ( 'NONE',  ( 5.910991785878156435, 7.919243054989755670, -1.443375672974057666 ) ) ;
#52145=ORIENTED_EDGE ( 'NONE', *, *, #156739, .F. ) ;
#52146=CARTESIAN_POINT ( 'NONE',  ( 8.066738210006679566, 10.43428054980638997, 1.443375672974076540 ) ) ;
#52147=CARTESIAN_POINT ( 'NONE',  ( -1.201851678989727383E-14, 5.009375000341421469, -1.575800808251660134 ) ) ;
#52149=CARTESIAN_POINT ( 'NONE',  ( 5.002595493318194642, 4.938708951733754127, -0.7216878364870197293 ) ) ;
#52157=CARTESIAN_POINT ( 'NONE',  ( -5.829309506874599478, 6.192769411583809003, 0.9639237645304669089 ) ) ;
#52160=CARTESIAN_POINT ( 'NONE',  ( -1.001543065824772872E-14, 5.134375000341421469, 1.575800808251672791 ) ) ;
#52164=CARTESIAN_POINT ( 'NONE',  ( -9.398826802771548472, 11.98838390803207865, -1.599625672291263179 ) ) ;
#52173=ORIENTED_EDGE ( 'NONE', *, *, #5514, .T. ) ;
#52175=FACE_OUTER_BOUND ( 'NONE', #106350, .T. ) ;
#52176=CARTESIAN_POINT ( 'NONE',  ( -1.001543065824772872E-14, 4.634375000341418804, 1.575800808251672791 ) ) ;
#52179=CARTESIAN_POINT ( 'NONE',  ( 6.076025397218672630, 10.24044673006381245, -0.7998128361456291469 ) ) ;
#52180=CARTESIAN_POINT ( 'NONE',  ( -7.831806290188425557, 12.28885777186185990, -0.7998128361456281477 ) ) ;
#52186=CARTESIAN_POINT ( 'NONE',  ( -1.201851678989727383E-14, 5.087500000000019007, -1.732050807568863648 ) ) ;
#52193=CARTESIAN_POINT ( 'NONE',  ( 8.975134502566660899, 10.53370701015836275, -1.082531754730543083 ) ) ;
#52198=CARTESIAN_POINT ( 'NONE',  ( 1.499999999999987121, 2.827083334016148530, -0.8660254037844262731 ) ) ;
#52200=CARTESIAN_POINT ( 'NONE',  ( -4.416205349749324327, 6.175325546172740765, 1.599625672291267398 ) ) ;
#52202=CARTESIAN_POINT ( 'NONE',  ( 4.243338890952890630, 5.973648010910253880, -1.443375672974051449 ) ) ;
#52210=CARTESIAN_POINT ( 'NONE',  ( 6.435316467980822353, 10.65961964595298817, 1.040834085586084257E-14 ) ) ;
#52211=CARTESIAN_POINT ( 'NONE',  ( 5.034155109375821446, 4.767602470560229122, -0.7998128361456221525 ) ) ;
#52213=CARTESIAN_POINT ( 'NONE',  ( 5.005985031943777308, 6.863401842066294556, -1.599625672291256295 ) ) ;
#52221=CARTESIAN_POINT ( 'NONE',  ( -5.000000000000024869, 3.300000000000025135, 0.7750000000000238920 ) ) ;
#52226=CARTESIAN_POINT ( 'NONE',  ( 5.575284262857175044, 6.175169341367511500, -0.8878447928483481633 ) ) ;
#52229=CARTESIAN_POINT ( 'NONE',  ( 8.353795204314554468, 12.89784483834236184, -0.7998128361456352531 ) ) ;
#52235=CARTESIAN_POINT ( 'NONE',  ( 6.805829924380118356, 7.042482454639357847, 0.7216878364870317197 ) ) ;
#52236=CARTESIAN_POINT ( 'NONE',  ( -9.408995418203979000, 12.00024729270324286, 1.443375672974076540 ) ) ;
#52241=CARTESIAN_POINT ( 'NONE',  ( -5.229694566569281555, 7.124396299129368337, 1.599625672291267398 ) ) ;
#52252=CARTESIAN_POINT ( 'NONE',  ( 7.747594715205354809, 11.12627870345989756, -1.199719254218446718 ) ) ;
#52253=CARTESIAN_POINT ( 'NONE',  ( 6.089152713731276201, 6.031799978164165132, 0.2946234760112295126 ) ) ;
#52254=DIRECTION ( 'NONE',  ( -0.6507913734559640506, -0.7592566023653004592, 0.000000000000000000 ) ) ;
#52256=CARTESIAN_POINT ( 'NONE',  ( 3.337278367258157630, 7.045241861776501580, 0.7998128361456341429 ) ) ;
#52262=CARTESIAN_POINT ( 'NONE',  ( -9.829298180227631576, 10.56986208646148384, 1.040834085586084257E-14 ) ) ;
#52266=CARTESIAN_POINT ( 'NONE',  ( 6.428537391173986038, 10.65171072301167854, 0.7998128361456462443 ) ) ;
#52268=CARTESIAN_POINT ( 'NONE',  ( -4.249591082879585535, 7.045274465746411252, 1.199719254218464037 ) ) ;
#52269=EDGE_CURVE ( 'NONE', #12495, #164712, #132448, .T. ) ;
#52271=CARTESIAN_POINT ( 'NONE',  ( 5.190073875932979419, 4.949507698210251938, 0.7998128361456341429 ) ) ;
#52273=CARTESIAN_POINT ( 'NONE',  ( -5.364222332501225488, 9.410009821226765325, 0.7998128361456481317 ) ) ;
#52274=CARTESIAN_POINT ( 'NONE',  ( 3.334415713957098681, 5.977569868670206787, -1.199719254218446718 ) ) ;
#52278=CARTESIAN_POINT ( 'NONE',  ( 8.028399517586572998, 12.51821653715971472, -0.7998128361456352531 ) ) ;
#52282=CARTESIAN_POINT ( 'NONE',  ( 4.149696378627680815, 7.633013953984455036, -0.8115063166676712569 ) ) ;
#52283=CARTESIAN_POINT ( 'NONE',  ( 6.819388077993785657, 7.058300300521964665, 1.040834085586084257E-14 ) ) ;
#52287=CARTESIAN_POINT ( 'NONE',  ( -1.233356347899354111, 3.300000000000025135, -0.5988873898902316029 ) ) ;
#52290=CARTESIAN_POINT ( 'NONE',  ( 7.904040366642684390, 11.20483561351640844, 1.082531754730558626 ) ) ;
#52291=ADVANCED_FACE ( 'NONE', ( #24395 ), #158052, .F. ) ;
#52293=CARTESIAN_POINT ( 'NONE',  ( 6.518203450479811423, 5.167241622962441383, -2.437504649502886256 ) ) ;
#52294=CARTESIAN_POINT ( 'NONE',  ( -6.679363233026820446, 10.94434087183997129, 0.000000000000000000 ) ) ;
#52299=DIRECTION ( 'NONE',  ( 0.000000000000000000, -1.000000000000000000, 0.000000000000000000 ) ) ;
#52303=CARTESIAN_POINT ( 'NONE',  ( 9.890836756369282057, 11.49806328964105617, -1.199719254218440723 ) ) ;
#52307=CARTESIAN_POINT ( 'NONE',  ( 3.811813743736467419, 7.598866467667865443, 1.040834085586084257E-14 ) ) ;
#52310=CARTESIAN_POINT ( 'NONE',  ( 1.499999999999989120, 3.785416667349481123, 0.8660254037844524744 ) ) ;
#52314=EDGE_LOOP ( 'NONE', ( #192375, #92719, #194481, #94415 ) ) ;
#52317=CARTESIAN_POINT ( 'NONE',  ( -1.500000000000013101, 1.420833333333354043, 0.8660254037844403729 ) ) ;
#52318=CARTESIAN_POINT ( 'NONE',  ( 6.612626235163189925, 8.737816579155630592, -1.599625672291262513 ) ) ;
#52319=CARTESIAN_POINT ( 'NONE',  ( 3.619663824724254741, 6.206396314611513532, -1.082531754730543971 ) ) ;
#52323=CARTESIAN_POINT ( 'NONE',  ( 6.968527767744088663, 11.07377346243604599, 0.7216878364870438212 ) ) ;
#52329=CARTESIAN_POINT ( 'NONE',  ( -4.055860508782465068, 7.883587693554856557, 1.040834085586084257E-14 ) ) ;
#52331=CARTESIAN_POINT ( 'NONE',  ( 0.7499999999999920064, 4.514583334016150751, 1.299038105676669330 ) ) ;
#52332=EDGE_CURVE ( 'NONE', #78570, #93560, #40397, .T. ) ;
#52333=CARTESIAN_POINT ( 'NONE',  ( 1.364683531249990311, 5.196875000341417916, 1.214306433183764966E-14 ) ) ;
#52339=CARTESIAN_POINT ( 'NONE',  ( 1.364683531249990311, 4.196875000341417028, 1.214306433183764966E-14 ) ) ;
#52342=EDGE_CURVE ( 'NONE', #17744, #60775, #94393, .T. ) ;
#52343=LINE ( 'NONE', #117403, #170794 ) ;
#52347=CARTESIAN_POINT ( 'NONE',  ( -7.446452682403657874, 9.710614100936176385, -1.599625672291263179 ) ) ;
#52349=CARTESIAN_POINT ( 'NONE',  ( 4.971035877704902184, 8.951292290631053916, 1.040834085586084257E-14 ) ) ;
#52351=CARTESIAN_POINT ( 'NONE',  ( -1.364683531250014514, -1.219791666325248602, 0.7879004041258379498 ) ) ;
#52355=CARTESIAN_POINT ( 'NONE',  ( 2.273349394227877074, 5.683342515206170731, 0.4597581080974435519 ) ) ;
#52357=CARTESIAN_POINT ( 'NONE',  ( -6.880926654135487652, 7.986501503701545879, 1.199719254218450271 ) ) ;
#52362=CARTESIAN_POINT ( 'NONE',  ( 8.106885785967500979, 11.54545161934907682, 1.199719254218460707 ) ) ;
#52364=CARTESIAN_POINT ( 'NONE',  ( 3.404766800216717737, 6.348112014766642552, 1.069586989871921467 ) ) ;
#52366=CARTESIAN_POINT ( 'NONE',  ( -2.764973262183167968, 5.313220341600567664, 1.199719254218462483 ) ) ;
#52367=CARTESIAN_POINT ( 'NONE',  ( -7.374745490829552885, 10.69128794168811680, -1.199719254218446718 ) ) ;
#52369=CARTESIAN_POINT ( 'NONE',  ( -4.127447729399665199, 7.650344214561823009, 0.8192481249636590634 ) ) ;
#52370=CARTESIAN_POINT ( 'NONE',  ( 1.364683531249986537, -0.8864583329919110133, 0.7879004041258500513 ) ) ;
#52374=CARTESIAN_POINT ( 'NONE',  ( 7.266807147244743526, 11.42176607185347414, -0.7216878364870267237 ) ) ;
#52377=CARTESIAN_POINT ( 'NONE',  ( 6.166260936116925606, 6.088392601758203071, 0.7998128361456341429 ) ) ;
#52398=CARTESIAN_POINT ( 'NONE',  ( -5.331380718671772101, 7.243030143248949670, -1.599625672291256295 ) ) ;
#52399=CARTESIAN_POINT ( 'NONE',  ( -8.239604668803112375, 10.63595808506888396, -1.599625672291263179 ) ) ;
#52400=DIRECTION ( 'NONE',  ( 0.000000000000000000, 8.546850786086437571E-32, 1.000000000000000000 ) ) ;
#52404=CARTESIAN_POINT ( 'NONE',  ( -1.500000000000013101, 1.452083334016150085, 0.8660254037844403729 ) ) ;
#52405=CARTESIAN_POINT ( 'NONE',  ( 8.041957671200231417, 12.53403438304231976, 1.040834085586084257E-14 ) ) ;
#52410=CARTESIAN_POINT ( 'NONE',  ( -8.157201976916404362, 12.66848607304450702, -0.7998128361456281477 ) ) ;
#52412=CARTESIAN_POINT ( 'NONE',  ( -0.6823417656250212460, 1.801041667008083991, 1.181850606188755259 ) ) ;
#52413=CARTESIAN_POINT ( 'NONE',  ( 1.499999999999990896, 5.525000000000022560, 1.214306433183764966E-14 ) ) ;
#52420=CARTESIAN_POINT ( 'NONE',  ( -2.981903720001798597, 5.566305875722335372, -1.199719254218446718 ) ) ;
#52424=CARTESIAN_POINT ( 'NONE',  ( -1.364683531250014514, 0.3427083336747508424, 0.7879004041258379498 ) ) ;
#52430=CARTESIAN_POINT ( 'NONE',  ( -0.6823417656250212460, 1.051041667008083325, 1.181850606188755259 ) ) ;
#52432=CARTESIAN_POINT ( 'NONE',  ( -5.540478329478883524, 9.615641817700700145, 0.000000000000000000 ) ) ;
#52433=CARTESIAN_POINT ( 'NONE',  ( 8.697719238366680372, 10.10609285197134533, 1.199719254218462483 ) ) ;
#52434=CARTESIAN_POINT ( 'NONE',  ( 4.704842999142070603, 5.447737239542574272, -1.199719254218452047 ) ) ;
#52435=CARTESIAN_POINT ( 'NONE',  ( 4.171104814498611368, 8.018039383557042044, 0.7998128361456321445 ) ) ;
#52437=CARTESIAN_POINT ( 'NONE',  ( -1.500000000000011324, 4.420833333333352044, 0.8660254037844403729 ) ) ;
#52439=CARTESIAN_POINT ( 'NONE',  ( -1.402160292154681736E-14, 0.7593750003414168059, -1.575800808251659024 ) ) ;
#52445=CARTESIAN_POINT ( 'NONE',  ( 6.832946231607457399, 7.074118146404578589, -0.7216878364870257245 ) ) ;
#52448=CARTESIAN_POINT ( 'NONE',  ( -8.666686507633592385, 11.13422023037111330, 1.599625672291269396 ) ) ;
#52449=CARTESIAN_POINT ( 'NONE',  ( -4.765854690403601879, 5.518917546014321829, 1.199719254218462483 ) ) ;
#52453=CARTESIAN_POINT ( 'NONE',  ( -6.521108698048767138, 10.55178454779148289, -0.7216878364870267237 ) ) ;
#52455=CARTESIAN_POINT ( 'NONE',  ( 1.499999999999991118, 5.754166666666685970, 0.8660254037844524744 ) ) ;
#52458=CARTESIAN_POINT ( 'NONE',  ( 7.076992996653421741, 10.23994701519558781, -1.082531754730537976 ) ) ;
#52463=VECTOR ( 'NONE', #193767, 1000.000000000000227 ) ;
#52472=CARTESIAN_POINT ( 'NONE',  ( 7.610204295972345712, 7.772993188256215547, 0.7998128361456341429 ) ) ;
#52473=CARTESIAN_POINT ( 'NONE',  ( -5.752737250900127997, 5.605948302338584099, 0.000000000000000000 ) ) ;
#52476=CARTESIAN_POINT ( 'NONE',  ( 5.138177029454829459, 8.938364267765221527, 0.7216878364870438212 ) ) ;
#52477=CARTESIAN_POINT ( 'NONE',  ( -1.402160292154681736E-14, -0.4906249996585810846, -1.575800808251665908 ) ) ;
#52478=CARTESIAN_POINT ( 'NONE',  ( 4.094199201646931741, 4.839282492418613302, -1.082531754730543083 ) ) ;
#52479=CARTESIAN_POINT ( 'NONE',  ( -2.123823618835070537, 5.629544655282869847, 1.040834085586084257E-14 ) ) ;
#52484=CARTESIAN_POINT ( 'NONE',  ( -3.621833129746846680, 4.096114899008192367, 2.500000000000011102 ) ) ;
#52495=CARTESIAN_POINT ( 'NONE',  ( 7.121056995675668411, 9.330985799753529264, -1.599625672291262513 ) ) ;
#52497=VERTEX_POINT ( 'NONE', #213839 ) ;
#52506=CARTESIAN_POINT ( 'NONE',  ( -3.764360206088648297, 7.543504007078730922, -0.7998128361456281477 ) ) ;
#52508=CARTESIAN_POINT ( 'NONE',  ( -3.846762897975357198, 5.510976019103107859, -1.599625672291256295 ) ) ;
#52518=CARTESIAN_POINT ( 'NONE',  ( -8.839552966430002101, 12.29626697993494666, -1.082531754730543971 ) ) ;
#52521=CARTESIAN_POINT ( 'NONE',  ( 6.962275575817444384, 8.081408578997208991, -1.199719254218446718 ) ) ;
#52522=CARTESIAN_POINT ( 'NONE',  ( -0.6823417656250212460, 5.051041667008086655, 1.181850606188767472 ) ) ;
#52528=CARTESIAN_POINT ( 'NONE',  ( 6.127922243252466039, 6.251590159990418449, 1.040834085586084257E-14 ) ) ;
#52530=CARTESIAN_POINT ( 'NONE',  ( -7.152089726408780379, 8.302858421353754181, -1.199719254218446718 ) ) ;
#52533=CARTESIAN_POINT ( 'NONE',  ( -7.477485413136760073, 8.682486722536401302, -1.199719254218446718 ) ) ;
#52534=CARTESIAN_POINT ( 'NONE',  ( -4.629219384062206011, 7.488174150459498968, -1.199719254218452047 ) ) ;
#52542=CARTESIAN_POINT ( 'NONE',  ( 6.479907352327590964, 9.647310113435821677, 1.199719254218462483 ) ) ;
#52557=CARTESIAN_POINT ( 'NONE',  ( 1.364683531249988757, -0.8031249996585804185, 0.000000000000000000 ) ) ;
#52558=CARTESIAN_POINT ( 'NONE',  ( 5.020596955762157698, 4.751784624677624080, 1.040834085586084257E-14 ) ) ;
#52559=CARTESIAN_POINT ( 'NONE',  ( 6.491656622844908853, 6.468020902940851968, 0.7998128361456341429 ) ) ;
#52561=CARTESIAN_POINT ( 'NONE',  ( -6.724481002698120768, 9.828683022247721723, -1.082531754730538864 ) ) ;
#52563=CARTESIAN_POINT ( 'NONE',  ( 5.178851490740196795, 7.065079377328788546, 1.443375672974062551 ) ) ;
#52564=CARTESIAN_POINT ( 'NONE',  ( -7.985389288324697965, 10.33937347451072775, -1.443375672974058777 ) ) ;
#52568=CARTESIAN_POINT ( 'NONE',  ( 8.613507663383630941, 8.943513783569379427, -0.7998128361456221525 ) ) ;
#52572=EDGE_CURVE ( 'NONE', #23747, #166540, #80586, .T. ) ;
#52573=CARTESIAN_POINT ( 'NONE',  ( -1.201851678989727383E-14, 3.946875000341423689, -1.575800808251660134 ) ) ;
#52580=CARTESIAN_POINT ( 'NONE',  ( 9.121938423896107651, 9.536683004167278099, -0.7998128361456221525 ) ) ;
#52583=CARTESIAN_POINT ( 'NONE',  ( -7.492852449846775897, 11.89341162479659531, 0.000000000000000000 ) ) ;
#52588=( BOUNDED_SURFACE ( )  B_SPLINE_SURFACE ( 1, 2, ( 
 ( #105439, #167214, #35055, #154168, #137923, #184506, #83812, #67539, #70742, #203944, #101126, #18802, #55591, #2538, #51330, #134738, #174705, #25216, #7891, #76108, #206097, #190910, #11093, #205020, #208226, #122830, #89181, #56666, #123888, #73979, #189854, #140073, #138998, #108677, #155233, #26281, #142212, #91320, #110811, #6814, #126010, #191971, #209282, #41499, #141161, #188791, #107612, #8972, #157378, #173643, #59858, #109752, #57731, #43637, #24139, #207169, #75046, #23065, #58793, #124948, #90241, #42574, #143291, #156307, #92395, #158433, #10034, #40426, #175762, #27355, #93457, #159494, #77170, #60929, #106529, #127086, #193049, #172555, #44703, #72892, #14285, #78242, #178964, #154, #97719, #63062, #112953, #62005, #82498, #28431, #148585, #144364, #180021, #129229, #80380, #30579, #46839, #13242, #47915, #98772, #96660, #79315, #146476, #195202, #114025, #164828, #162713, #212495, #31642, #210365, #45772, #81449, #64136, #130280, #196268, #163777, #128161, #15356, #145431, #211431, #65170, #16418, #50010, #147526, #48959, #213547, #131325, #66220, #197318, #115077, #181073, #161647, #32691, #132368, #198370, #177893, #176816, #94524, #111889, #194122, #160562, #12170, #29506, #95599, #33752, #69431, #68363, #135536, #51079, #83564, #35882, #149646, #99829, #119337, #53206, #201560, #54279, #137673, #104099, #21735, #199436, #20682, #182123, #1228, #203695, #120417, #86773, #71566, #185324, #186391, #36948, #100882, #165895, #166969, #152844, #200500, #153915, #103028, #184255, #67290, #169083, #4418, #38028, #19628, #70489, #3361, #34807, #85699, #116134, #18559, #17480, #133429, #118271, #151787, #117204, #183201, #136605, #101957, #202629, #170149, #87844, #84636, #168024, #5485, #150727, #2287, #134497, #52143, #141959, #39094, #9780, #191717, #73717, #138740, #156044, #190650, #76905, #55341, #143029, #105180, #121493, #108426, #74795, #43374, #10831, #8710, #207971, #158188, #93199, #174447, #206906, #92133, #140896, #189599, #124692, #159230, #125754, #139815, #41245, #109495, #122571, #205844, #88925, #107352, #157121, #187465, #175502, #57477, #75852, #172298, #171216, #7632, #59597, #123636, #58537, #42310, #173374, #27092, #26023, #24959, #23886, #56409, #89992, #154978, #22810, #6563, #72644, #204758, #188533, #91060, #40163, #106277, #64920, #79044, #194930, #131069, #61738, #145160, #28168, #46568, #96397, #60661, #197057, #211165, #97454, #111622, #32435, #161383, #163509, #12968, #162447, #80109, #62790, #81184, #47646, #178697, #177634, #210098, #29243, #94264, #82235, #98503, #77980, #160303, #179762, #113757, #95334, #209025, #126824, #14023, #128952, #146214, #144104, #176558, #112687, #11907, #192781, #212231, #63865, #130020, #147262, #16150, #48696, #114810, #127905, #31378, #44439, #193857, #110557, #213294, #15094, #164565, #196011, #180809, #45506, #30311, #198115, #133165, #119075, #18290, #186130, #167763, #2025, #33494, #151525, #3094, #152575, #51888, #102769, #35614, #67028, #118011, #169886, #199165, #21475, #49746, #150464, #184000, #148326, #214325, #69164, #68094, #185056, #19360, #36682, #115873, #134229, #101692, #132107, #202365, #168824, #182937, #20428, #181858, #86511, #70232, #166699, #17219, #34553, #135284, #65957, #99567, #165631, #83295, #149380, #201298, #85440, #136344, #103837, #52939, #4162, #54014, #37765, #120154, #963, #100624, #50811, #84377, #116937, #200238, #173117, #153656, #24699, #206652, #89740, #175252, #5225, #190398, #42055, #59346, #39910, #205582, #55085, #106019, #73453, #7374, #172040, #124440, #174195, #72379, #108169, #88662, #57219, #155790, #87584, #139555, #23633, #154722, #123379, #207722, #6304, #138478, #189344, #40984, #121234, #204500, #58284, #122312, #107095, #90801, #125499, #104916, #188269, #25768, #203431, #170957, #187204, #156865, #38833, #8451, #191463, #74539, #140639, #91880, #22557, #43128, #71299, #109244, #56150, #157935, #9528, #75601, #141712, #137411, #77725, #112431, #163257, #28986, #143848, #78784, #193608, #178444, #14839, #45250, #144906, #30051, #142771, #110302, #145964, #210913, #62540 ),
 ( #209840, #27914, #61479, #126568, #114565, #130818, #176310, #60407, #211974, #79855, #127644, #26838, #158986, #194671, #111368, #46315, #94010, #208776, #161120, #192528, #10582, #96142, #162193, #13780, #179510, #48452, #80929, #63614, #128702, #129769, #195752, #47389, #44182, #113501, #177372, #95072, #31130, #147020, #92941, #97205, #213043, #12708, #64672, #196808, #76656, #160049, #11653, #165370, #167510, #69974, #183751, #181609, #35361, #180557, #131854, #65705, #184801, #197861, #182677, #34298, #117761, #100371, #16963, #19107, #149118, #133981, #168569, #148073, #151269, #49493, #32179, #214079, #66765, #83044, #132906, #701, #81985, #51637, #98255, #101436, #85185, #166441, #53761, #164312, #68910, #135030, #152326, #198911, #84120, #115614, #50557, #18032, #150206, #116678, #2841, #52686, #1778, #201043, #33238, #67835, #199989, #15903, #118816, #36431, #99320, #102507, #86256, #20169, #3904, #136085, #202102, #153394, #186947, #90546, #154469, #171775, #39640, #157676, #137158, #6046, #58024, #21222, #203183, #4965, #23371, #87327, #122048, #9274, #40727, #72118, #55891, #71043, #25517, #185870, #91625, #54829, #123136, #138226, #89480, #188012, #204239, #170703, #205324, #41805, #105748, #22288, #155536, #7115, #56961, #107919, #73188, #139294, #189094, #120979, #38580, #106833, #104655, #169639, #88401, #156610, #172863, #75345, #24435, #8200, #74285, #140379, #206399, #124188, #190151, #173944, #141461, #207468, #119895, #37505, #103581, #149682, #177925, #64170, #97753, #59087, #128195, #65204, #130313, #32724, #81482, #98806, #111925, #196301, #163812, #45804, #116170, #164859, #96701, #148619, #29540, #16452, #198405, #80414, #145466, #162748, #197351, #83600, #194156, #95631, #161681, #13275, #115111, #147559, #50047, #17513, #15388, #187, #82533, #99865, #181108, #213581, #66255, #131356, #47947, #48993, #165928, #132403, #146512, #114062, #182156, #129265, #212529, #79349, #180054, #33786, #211461, #63096, #31676, #195235, #178997, #46873, #14321, #112987, #30612, #169118, #86808, #168060, #87876, #54313, #185359, #118304, #2323, #184291, #100915, #88959, #105211, #84672, #34840, #186425, #120451, #101991, #1263, #133465, #20715, #19662, #152874, #150761, #183236, #135570, #167003, #199469, #4452, #70522, #136638, #153948, #22844, #203726, #121528, #68399, #38064, #67321, #18594, #51111, #5517, #104134, #171248, #202663, #71597, #117236, #3396, #36981, #134527, #200533, #170180, #69465, #21768, #137706, #55374, #52179, #201594, #103064, #35916, #187498, #39128, #85737, #151822, #53242, #119371, #76941, #173414, #23921, #41283, #75888, #176595, #155012, #28206, #204792, #6597, #208010, #174483, #143066, #110592, #108463, #93234, #43409, #192818, #59634, #92173, #191754, #26059, #74832, #9813, #44476, #10867, #24995, #140931, #209060, #7669, #91098, #188567, #206945, #42348, #72678, #60696, #157158, #109533, #57513, #138774, #107392, #175538, #8750, #158224, #141996, #58574, #27128, #125792, #124730, #123671, #156083, #189634, #40199, #56445, #122604, #90027, #106310, #159267, #126861, #190689, #172333, #73754, #139849, #205878, #145197, #210133, #11944, #95369, #78016, #160341, #211204, #62829, #128989, #112724, #80146, #96434, #162485, #61775, #194968, #94300, #127943, #144141, #193896, #45543, #111657, #177669, #29278, #161420, #46604, #79079, #178735, #13003, #30349, #14058, #92859, #141629, #173033, #76575, #142687, #77645, #191380, #27833, #175171, #206573, #43046, #94993, #124359, #161039, #75517, #190316, #125414, #25687, #158906, #61402, #91795, #109159, #208697, #189264, #156786, #192448, #26758, #10502, #60324, #126484, #107009, #44103, #41974, #108085, #176231, #127565, #73367, #110223, #159970, #9446, #174114, #193534, #93929, #11575, #143767, #58200, #209761, #177294, #45176, #74455, #111288, #139472, #24615, #90724, #28908, #8372, #207638, #59256, #205501, #57134, #157852, #123301, #40903, #140559, #3285, #165820, #149570, #104024, #21658, #199357, #20608, #182045, #1153, #137601, #54201, #86696, #71488, #53127, #120341, #135462, #100806, #17403, #166892, #152765 ) ),
 .UNSPECIFIED., .F., .F., .F. ) 
 B_SPLINE_SURFACE_WITH_KNOTS ( ( 2, 2 ),
 ( 3, 2, 2, 2, 2, 2, 2, 2, 2, 2, 2, 2, 2, 2, 2, 2, 2, 2, 2, 2, 2, 2, 2, 2, 2, 2, 2, 2, 2, 2, 2, 2, 2, 2, 2, 2, 2, 2, 2, 2, 2, 2, 2, 2, 2, 2, 2, 2, 2, 2, 2, 2, 2, 2, 2, 2, 2, 2, 2, 2, 2, 2, 2, 2, 2, 2, 2, 2, 2, 2, 2, 2, 2, 2, 2, 2, 2, 2, 2, 2, 2, 2, 2, 2, 2, 2, 2, 2, 2, 2, 2, 2, 2, 2, 2, 2, 2, 2, 2, 2, 2, 2, 2, 2, 2, 2, 2, 2, 2, 2, 2, 2, 2, 2, 2, 2, 2, 2, 2, 2, 2, 2, 2, 2, 2, 2, 2, 2, 2, 2, 2, 2, 2, 2, 2, 2, 2, 2, 2, 2, 2, 2, 2, 2, 2, 2, 2, 2, 2, 2, 2, 2, 2, 2, 2, 2, 2, 2, 2, 2, 2, 2, 2, 2, 2, 2, 2, 2, 2, 2, 2, 2, 2, 2, 2, 2, 2, 2, 2, 2, 2, 2, 2, 2, 2, 2, 2, 2, 2, 2, 2, 2, 2, 2, 2, 2, 2, 2, 2, 2, 2, 2, 2, 2, 2, 2, 2, 2, 2, 2, 2, 2, 2, 2, 2, 2, 2, 2, 2, 2, 2, 2, 2, 2, 2, 2, 2, 2, 2, 2, 2, 2, 2, 2, 2, 2, 2, 2, 2, 2, 3 ),
 ( 0.000000000000000000, 1.000000000000000000 ),
 ( 0.000000000000000000, 0.004166666666666666609, 0.008333333333333333218, 0.01250000000000000069, 0.01666666666666666644, 0.02083333333333333218, 0.02500000000000000139, 0.02916666666666666713, 0.03333333333333333287, 0.03749999999999999861, 0.04166666666666666435, 0.04583333333333333010, 0.05000000000000000278, 0.05416666666666666852, 0.05833333333333333426, 0.06250000000000000000, 0.06666666666666666574, 0.07083333333333333148, 0.07499999999999999722, 0.07916666666666666297, 0.08333333333333332871, 0.08749999999999999445, 0.09166666666666666019, 0.09583333333333333981, 0.1000000000000000056, 0.1041666666666666713, 0.1083333333333333370, 0.1125000000000000028, 0.1166666666666666685, 0.1208333333333333343, 0.1250000000000000000, 0.1291666666666666796, 0.1333333333333333315, 0.1375000000000000111, 0.1416666666666666630, 0.1458333333333333426, 0.1499999999999999944, 0.1541666666666666741, 0.1583333333333333259, 0.1625000000000000056, 0.1666666666666666574, 0.1708333333333333370, 0.1749999999999999889, 0.1791666666666666685, 0.1833333333333333204, 0.1875000000000000000, 0.1916666666666666796, 0.1958333333333333315, 0.2000000000000000111, 0.2041666666666666630, 0.2083333333333333426, 0.2124999999999999944, 0.2166666666666666741, 0.2208333333333333259, 0.2250000000000000056, 0.2291666666666666574, 0.2333333333333333370, 0.2374999999999999889, 0.2416666666666666685, 0.2458333333333333204, 0.2500000000000000000, 0.2541666666666666519, 0.2583333333333333592, 0.2625000000000000111, 0.2666666666666666630, 0.2708333333333333148, 0.2750000000000000222, 0.2791666666666666741, 0.2833333333333333259, 0.2874999999999999778, 0.2916666666666666852, 0.2958333333333333370, 0.2999999999999999889, 0.3041666666666666408, 0.3083333333333333481, 0.3125000000000000000, 0.3166666666666666519, 0.3208333333333333592, 0.3250000000000000111, 0.3291666666666666630, 0.3333333333333333148, 0.3375000000000000222, 0.3416666666666666741, 0.3458333333333333259, 0.3499999999999999778, 0.3541666666666666852, 0.3583333333333333370, 0.3624999999999999889, 0.3666666666666666408, 0.3708333333333333481, 0.3750000000000000000, 0.3791666666666666519, 0.3833333333333333592, 0.3875000000000000111, 0.3916666666666666630, 0.3958333333333333148, 0.4000000000000000222, 0.4041666666666666741, 0.4083333333333333259, 0.4124999999999999778, 0.4166666666666666852, 0.4208333333333333370, 0.4249999999999999889, 0.4291666666666666408, 0.4333333333333333481, 0.4375000000000000000, 0.4416666666666666519, 0.4458333333333333592, 0.4500000000000000111, 0.4541666666666666630, 0.4583333333333333148, 0.4625000000000000222, 0.4666666666666666741, 0.4708333333333333259, 0.4749999999999999778, 0.4791666666666666852, 0.4833333333333333370, 0.4874999999999999889, 0.4916666666666666408, 0.4958333333333333481, 0.5000000000000000000, 0.5041666666666666519, 0.5083333333333333037, 0.5124999999999999556, 0.5166666666666667185, 0.5208333333333333703, 0.5250000000000000222, 0.5291666666666666741, 0.5333333333333333259, 0.5374999999999999778, 0.5416666666666666297, 0.5458333333333332815, 0.5500000000000000444, 0.5541666666666666963, 0.5583333333333333481, 0.5625000000000000000, 0.5666666666666666519, 0.5708333333333333037, 0.5749999999999999556, 0.5791666666666667185, 0.5833333333333333703, 0.5875000000000000222, 0.5916666666666666741, 0.5958333333333333259, 0.5999999999999999778, 0.6041666666666666297, 0.6083333333333332815, 0.6125000000000000444, 0.6166666666666666963, 0.6208333333333333481, 0.6250000000000000000, 0.6291666666666666519, 0.6333333333333333037, 0.6374999999999999556, 0.6416666666666667185, 0.6458333333333333703, 0.6500000000000000222, 0.6541666666666666741, 0.6583333333333333259, 0.6624999999999999778, 0.6666666666666666297, 0.6708333333333332815, 0.6750000000000000444, 0.6791666666666666963, 0.6833333333333333481, 0.6875000000000000000, 0.6916666666666666519, 0.6958333333333333037, 0.6999999999999999556, 0.7041666666666667185, 0.7083333333333333703, 0.7125000000000000222, 0.7166666666666666741, 0.7208333333333333259, 0.7249999999999999778, 0.7291666666666666297, 0.7333333333333332815, 0.7375000000000000444, 0.7416666666666666963, 0.7458333333333333481, 0.7500000000000000000, 0.7541666666666666519, 0.7583333333333333037, 0.7624999999999999556, 0.7666666666666667185, 0.7708333333333333703, 0.7750000000000000222, 0.7791666666666666741, 0.7833333333333333259, 0.7874999999999999778, 0.7916666666666666297, 0.7958333333333332815, 0.8000000000000000444, 0.8041666666666666963, 0.8083333333333333481, 0.8125000000000000000, 0.8166666666666666519, 0.8208333333333333037, 0.8249999999999999556, 0.8291666666666667185, 0.8333333333333333703, 0.8375000000000000222, 0.8416666666666666741, 0.8458333333333333259, 0.8499999999999999778, 0.8541666666666666297, 0.8583333333333332815, 0.8625000000000000444, 0.8666666666666666963, 0.8708333333333333481, 0.8750000000000000000, 0.8791666666666666519, 0.8833333333333333037, 0.8874999999999999556, 0.8916666666666667185, 0.8958333333333333703, 0.9000000000000000222, 0.9041666666666666741, 0.9083333333333333259, 0.9124999999999999778, 0.9166666666666666297, 0.9208333333333332815, 0.9250000000000000444, 0.9291666666666666963, 0.9333333333333333481, 0.9375000000000000000, 0.9416666666666666519, 0.9458333333333333037, 0.9499999999999999556, 0.9541666666666667185, 0.9583333333333333703, 0.9625000000000000222, 0.9666666666666666741, 0.9708333333333333259, 0.9749999999999999778, 0.9791666666666666297, 0.9833333333333332815, 0.9875000000000000444, 0.9916666666666666963, 0.9958333333333333481, 1.000000000000000000 ),
 .UNSPECIFIED. ) 
 GEOMETRIC_REPRESENTATION_ITEM ( )  RATIONAL_B_SPLINE_SURFACE ( (
 ( 1.000000000000000000, 0.8660254037844387076, 1.000000000000000000, 0.8660254037844387076, 1.000000000000000000, 0.8660254037844387076, 1.000000000000000000, 0.8660254037844387076, 1.000000000000000000, 0.8660254037844387076, 1.000000000000000000, 0.8660254037844387076, 1.000000000000000000, 0.8660254037844387076, 1.000000000000000000, 0.8660254037844387076, 1.000000000000000000, 0.8660254037844387076, 1.000000000000000000, 0.8660254037844387076, 1.000000000000000000, 0.8660254037844387076, 1.000000000000000000, 0.8660254037844387076, 1.000000000000000000, 0.8660254037844387076, 1.000000000000000000, 0.8660254037844387076, 1.000000000000000000, 0.8660254037844387076, 1.000000000000000000, 0.8660254037844387076, 1.000000000000000000, 0.8660254037844387076, 1.000000000000000000, 0.8660254037844387076, 1.000000000000000000, 0.8660254037844387076, 1.000000000000000000, 0.8660254037844387076, 1.000000000000000000, 0.8660254037844387076, 1.000000000000000000, 0.8660254037844387076, 1.000000000000000000, 0.8660254037844387076, 1.000000000000000000, 0.8660254037844387076, 1.000000000000000000, 0.8660254037844387076, 1.000000000000000000, 0.8660254037844387076, 1.000000000000000000, 0.8660254037844387076, 1.000000000000000000, 0.8660254037844387076, 1.000000000000000000, 0.8660254037844387076, 1.000000000000000000, 0.8660254037844387076, 1.000000000000000000, 0.8660254037844387076, 1.000000000000000000, 0.8660254037844387076, 1.000000000000000000, 0.8660254037844387076, 1.000000000000000000, 0.8660254037844387076, 1.000000000000000000, 0.8660254037844387076, 1.000000000000000000, 0.8660254037844387076, 1.000000000000000000, 0.8660254037844387076, 1.000000000000000000, 0.8660254037844387076, 1.000000000000000000, 0.8660254037844387076, 1.000000000000000000, 0.8660254037844387076, 1.000000000000000000, 0.8660254037844387076, 1.000000000000000000, 0.8660254037844387076, 1.000000000000000000, 0.8660254037844387076, 1.000000000000000000, 0.8660254037844387076, 1.000000000000000000, 0.8660254037844387076, 1.000000000000000000, 0.8660254037844387076, 1.000000000000000000, 0.8660254037844387076, 1.000000000000000000, 0.8660254037844387076, 1.000000000000000000, 0.8660254037844387076, 1.000000000000000000, 0.8660254037844387076, 1.000000000000000000, 0.8660254037844387076, 1.000000000000000000, 0.8660254037844387076, 1.000000000000000000, 0.8660254037844387076, 1.000000000000000000, 0.8660254037844387076, 1.000000000000000000, 0.8660254037844387076, 1.000000000000000000, 0.8660254037844387076, 1.000000000000000000, 0.8660254037844387076, 1.000000000000000000, 0.8660254037844387076, 1.000000000000000000, 0.8660254037844387076, 1.000000000000000000, 0.8660254037844387076, 1.000000000000000000, 0.8660254037844387076, 1.000000000000000000, 0.8660254037844387076, 1.000000000000000000, 0.8660254037844387076, 1.000000000000000000, 0.8660254037844387076, 1.000000000000000000, 0.8660254037844387076, 1.000000000000000000, 0.8660254037844387076, 1.000000000000000000, 0.8660254037844387076, 1.000000000000000000, 0.8660254037844387076, 1.000000000000000000, 0.8660254037844387076, 1.000000000000000000, 0.8660254037844387076, 1.000000000000000000, 0.8660254037844387076, 1.000000000000000000, 0.8660254037844387076, 1.000000000000000000, 0.8660254037844387076, 1.000000000000000000, 0.8660254037844387076, 1.000000000000000000, 0.8660254037844387076, 1.000000000000000000, 0.8660254037844387076, 1.000000000000000000, 0.8660254037844387076, 1.000000000000000000, 0.8660254037844387076, 1.000000000000000000, 0.8660254037844387076, 1.000000000000000000, 0.8660254037844387076, 1.000000000000000000, 0.8660254037844387076, 1.000000000000000000, 0.8660254037844387076, 1.000000000000000000, 0.8660254037844387076, 1.000000000000000000, 0.8660254037844387076, 1.000000000000000000, 0.8660254037844387076, 1.000000000000000000, 0.8660254037844387076, 1.000000000000000000, 0.8660254037844387076, 1.000000000000000000, 0.8660254037844387076, 1.000000000000000000, 0.8660254037844387076, 1.000000000000000000, 0.8660254037844387076, 1.000000000000000000, 0.8660254037844387076, 1.000000000000000000, 0.8660254037844387076, 1.000000000000000000, 0.8660254037844387076, 1.000000000000000000, 0.8660254037844387076, 1.000000000000000000, 0.8660254037844387076, 1.000000000000000000, 0.8660254037844387076, 1.000000000000000000, 0.8660254037844387076, 1.000000000000000000, 0.8660254037844387076, 1.000000000000000000, 0.8660254037844387076, 1.000000000000000000, 0.8660254037844387076, 1.000000000000000000, 0.8660254037844387076, 1.000000000000000000, 0.8660254037844387076, 1.000000000000000000, 0.8660254037844387076, 1.000000000000000000, 0.8660254037844387076, 1.000000000000000000, 0.8660254037844387076, 1.000000000000000000, 0.8660254037844387076, 1.000000000000000000, 0.8660254037844387076, 1.000000000000000000, 0.8660254037844387076, 1.000000000000000000, 0.8660254037844387076, 1.000000000000000000, 0.8660254037844387076, 1.000000000000000000, 0.8660254037844387076, 1.000000000000000000, 0.8660254037844387076, 1.000000000000000000, 0.8660254037844387076, 1.000000000000000000, 0.8660254037844387076, 1.000000000000000000, 0.8660254037844387076, 1.000000000000000000, 0.8660254037844387076, 1.000000000000000000, 0.8660254037844387076, 1.000000000000000000, 0.8660254037844387076, 1.000000000000000000, 0.8660254037844387076, 1.000000000000000000, 0.8660254037844387076, 1.000000000000000000, 0.8660254037844387076, 1.000000000000000000, 0.8660254037844387076, 1.000000000000000000, 0.8660254037844387076, 1.000000000000000000, 0.8660254037844387076, 1.000000000000000000, 0.8660254037844387076, 1.000000000000000000, 0.8660254037844387076, 1.000000000000000000, 0.8660254037844387076, 1.000000000000000000, 0.8660254037844387076, 1.000000000000000000, 0.8660254037844387076, 1.000000000000000000, 0.8660254037844387076, 1.000000000000000000, 0.8660254037844387076, 1.000000000000000000, 0.8660254037844387076, 1.000000000000000000, 0.8660254037844387076, 1.000000000000000000, 0.8660254037844387076, 1.000000000000000000, 0.8660254037844387076, 1.000000000000000000, 0.8660254037844387076, 1.000000000000000000, 0.8660254037844387076, 1.000000000000000000, 0.8660254037844387076, 1.000000000000000000, 0.8660254037844387076, 1.000000000000000000, 0.8660254037844387076, 1.000000000000000000, 0.8660254037844387076, 1.000000000000000000, 0.8660254037844387076, 1.000000000000000000, 0.8660254037844387076, 1.000000000000000000, 0.8660254037844387076, 1.000000000000000000, 0.8660254037844387076, 1.000000000000000000, 0.8660254037844387076, 1.000000000000000000, 0.8660254037844387076, 1.000000000000000000, 0.8660254037844387076, 1.000000000000000000, 0.8660254037844387076, 1.000000000000000000, 0.8660254037844387076, 1.000000000000000000, 0.8660254037844387076, 1.000000000000000000, 0.8660254037844387076, 1.000000000000000000, 0.8660254037844387076, 1.000000000000000000, 0.8660254037844387076, 1.000000000000000000, 0.8660254037844387076, 1.000000000000000000, 0.8660254037844387076, 1.000000000000000000, 0.8660254037844387076, 1.000000000000000000, 0.8660254037844387076, 1.000000000000000000, 0.8660254037844387076, 1.000000000000000000, 0.8660254037844387076, 1.000000000000000000, 0.8660254037844387076, 1.000000000000000000, 0.8660254037844387076, 1.000000000000000000, 0.8660254037844387076, 1.000000000000000000, 0.8660254037844387076, 1.000000000000000000, 0.8660254037844387076, 1.000000000000000000, 0.8660254037844387076, 1.000000000000000000, 0.8660254037844387076, 1.000000000000000000, 0.8660254037844387076, 1.000000000000000000, 0.8660254037844387076, 1.000000000000000000, 0.8660254037844387076, 1.000000000000000000, 0.8660254037844387076, 1.000000000000000000, 0.8660254037844387076, 1.000000000000000000, 0.8660254037844387076, 1.000000000000000000, 0.8660254037844387076, 1.000000000000000000, 0.8660254037844387076, 1.000000000000000000, 0.8660254037844387076, 1.000000000000000000, 0.8660254037844387076, 1.000000000000000000, 0.8660254037844387076, 1.000000000000000000, 0.8660254037844387076, 1.000000000000000000, 0.8660254037844387076, 1.000000000000000000, 0.8660254037844387076, 1.000000000000000000, 0.8660254037844387076, 1.000000000000000000, 0.8660254037844387076, 1.000000000000000000, 0.8660254037844387076, 1.000000000000000000, 0.8660254037844387076, 1.000000000000000000, 0.8660254037844387076, 1.000000000000000000, 0.8660254037844387076, 1.000000000000000000, 0.8660254037844387076, 1.000000000000000000, 0.8660254037844387076, 1.000000000000000000, 0.8660254037844387076, 1.000000000000000000, 0.8660254037844387076, 1.000000000000000000, 0.8660254037844387076, 1.000000000000000000, 0.8660254037844387076, 1.000000000000000000, 0.8660254037844387076, 1.000000000000000000, 0.8660254037844387076, 1.000000000000000000, 0.8660254037844387076, 1.000000000000000000, 0.8660254037844387076, 1.000000000000000000, 0.8660254037844387076, 1.000000000000000000, 0.8660254037844387076, 1.000000000000000000, 0.8660254037844387076, 1.000000000000000000, 0.8660254037844387076, 1.000000000000000000, 0.8660254037844387076, 1.000000000000000000, 0.8660254037844387076, 1.000000000000000000, 0.8660254037844387076, 1.000000000000000000, 0.8660254037844387076, 1.000000000000000000, 0.8660254037844387076, 1.000000000000000000, 0.8660254037844387076, 1.000000000000000000, 0.8660254037844387076, 1.000000000000000000, 0.8660254037844387076, 1.000000000000000000, 0.8660254037844387076, 1.000000000000000000, 0.8660254037844387076, 1.000000000000000000, 0.8660254037844387076, 1.000000000000000000, 0.8660254037844387076, 1.000000000000000000, 0.8660254037844387076, 1.000000000000000000, 0.8660254037844387076, 1.000000000000000000, 0.8660254037844387076, 1.000000000000000000, 0.8660254037844387076, 1.000000000000000000, 0.8660254037844387076, 1.000000000000000000, 0.8660254037844387076, 1.000000000000000000, 0.8660254037844387076, 1.000000000000000000, 0.8660254037844387076, 1.000000000000000000, 0.8660254037844387076, 1.000000000000000000, 0.8660254037844387076, 1.000000000000000000, 0.8660254037844387076, 1.000000000000000000, 0.8660254037844387076, 1.000000000000000000, 0.8660254037844387076, 1.000000000000000000, 0.8660254037844387076, 1.000000000000000000, 0.8660254037844387076, 1.000000000000000000, 0.8660254037844387076, 1.000000000000000000, 0.8660254037844387076, 1.000000000000000000, 0.8660254037844387076, 1.000000000000000000, 0.8660254037844387076, 1.000000000000000000, 0.8660254037844387076, 1.000000000000000000, 0.8660254037844387076, 1.000000000000000000, 0.8660254037844387076, 1.000000000000000000, 0.8660254037844387076, 1.000000000000000000, 0.8660254037844387076, 1.000000000000000000, 0.8660254037844387076, 1.000000000000000000, 0.8660254037844387076, 1.000000000000000000, 0.8660254037844387076, 1.000000000000000000),
 ( 1.000000000000000000, 0.8660254037844387076, 1.000000000000000000, 0.8660254037844387076, 1.000000000000000000, 0.8660254037844387076, 1.000000000000000000, 0.8660254037844387076, 1.000000000000000000, 0.8660254037844387076, 1.000000000000000000, 0.8660254037844387076, 1.000000000000000000, 0.8660254037844387076, 1.000000000000000000, 0.8660254037844387076, 1.000000000000000000, 0.8660254037844387076, 1.000000000000000000, 0.8660254037844387076, 1.000000000000000000, 0.8660254037844387076, 1.000000000000000000, 0.8660254037844387076, 1.000000000000000000, 0.8660254037844387076, 1.000000000000000000, 0.8660254037844387076, 1.000000000000000000, 0.8660254037844387076, 1.000000000000000000, 0.8660254037844387076, 1.000000000000000000, 0.8660254037844387076, 1.000000000000000000, 0.8660254037844387076, 1.000000000000000000, 0.8660254037844387076, 1.000000000000000000, 0.8660254037844387076, 1.000000000000000000, 0.8660254037844387076, 1.000000000000000000, 0.8660254037844387076, 1.000000000000000000, 0.8660254037844387076, 1.000000000000000000, 0.8660254037844387076, 1.000000000000000000, 0.8660254037844387076, 1.000000000000000000, 0.8660254037844387076, 1.000000000000000000, 0.8660254037844387076, 1.000000000000000000, 0.8660254037844387076, 1.000000000000000000, 0.8660254037844387076, 1.000000000000000000, 0.8660254037844387076, 1.000000000000000000, 0.8660254037844387076, 1.000000000000000000, 0.8660254037844387076, 1.000000000000000000, 0.8660254037844387076, 1.000000000000000000, 0.8660254037844387076, 1.000000000000000000, 0.8660254037844387076, 1.000000000000000000, 0.8660254037844387076, 1.000000000000000000, 0.8660254037844387076, 1.000000000000000000, 0.8660254037844387076, 1.000000000000000000, 0.8660254037844387076, 1.000000000000000000, 0.8660254037844387076, 1.000000000000000000, 0.8660254037844387076, 1.000000000000000000, 0.8660254037844387076, 1.000000000000000000, 0.8660254037844387076, 1.000000000000000000, 0.8660254037844387076, 1.000000000000000000, 0.8660254037844387076, 1.000000000000000000, 0.8660254037844387076, 1.000000000000000000, 0.8660254037844387076, 1.000000000000000000, 0.8660254037844387076, 1.000000000000000000, 0.8660254037844387076, 1.000000000000000000, 0.8660254037844387076, 1.000000000000000000, 0.8660254037844387076, 1.000000000000000000, 0.8660254037844387076, 1.000000000000000000, 0.8660254037844387076, 1.000000000000000000, 0.8660254037844387076, 1.000000000000000000, 0.8660254037844387076, 1.000000000000000000, 0.8660254037844387076, 1.000000000000000000, 0.8660254037844387076, 1.000000000000000000, 0.8660254037844387076, 1.000000000000000000, 0.8660254037844387076, 1.000000000000000000, 0.8660254037844387076, 1.000000000000000000, 0.8660254037844387076, 1.000000000000000000, 0.8660254037844387076, 1.000000000000000000, 0.8660254037844387076, 1.000000000000000000, 0.8660254037844387076, 1.000000000000000000, 0.8660254037844387076, 1.000000000000000000, 0.8660254037844387076, 1.000000000000000000, 0.8660254037844387076, 1.000000000000000000, 0.8660254037844387076, 1.000000000000000000, 0.8660254037844387076, 1.000000000000000000, 0.8660254037844387076, 1.000000000000000000, 0.8660254037844387076, 1.000000000000000000, 0.8660254037844387076, 1.000000000000000000, 0.8660254037844387076, 1.000000000000000000, 0.8660254037844387076, 1.000000000000000000, 0.8660254037844387076, 1.000000000000000000, 0.8660254037844387076, 1.000000000000000000, 0.8660254037844387076, 1.000000000000000000, 0.8660254037844387076, 1.000000000000000000, 0.8660254037844387076, 1.000000000000000000, 0.8660254037844387076, 1.000000000000000000, 0.8660254037844387076, 1.000000000000000000, 0.8660254037844387076, 1.000000000000000000, 0.8660254037844387076, 1.000000000000000000, 0.8660254037844387076, 1.000000000000000000, 0.8660254037844387076, 1.000000000000000000, 0.8660254037844387076, 1.000000000000000000, 0.8660254037844387076, 1.000000000000000000, 0.8660254037844387076, 1.000000000000000000, 0.8660254037844387076, 1.000000000000000000, 0.8660254037844387076, 1.000000000000000000, 0.8660254037844387076, 1.000000000000000000, 0.8660254037844387076, 1.000000000000000000, 0.8660254037844387076, 1.000000000000000000, 0.8660254037844387076, 1.000000000000000000, 0.8660254037844387076, 1.000000000000000000, 0.8660254037844387076, 1.000000000000000000, 0.8660254037844387076, 1.000000000000000000, 0.8660254037844387076, 1.000000000000000000, 0.8660254037844387076, 1.000000000000000000, 0.8660254037844387076, 1.000000000000000000, 0.8660254037844387076, 1.000000000000000000, 0.8660254037844387076, 1.000000000000000000, 0.8660254037844387076, 1.000000000000000000, 0.8660254037844387076, 1.000000000000000000, 0.8660254037844387076, 1.000000000000000000, 0.8660254037844387076, 1.000000000000000000, 0.8660254037844387076, 1.000000000000000000, 0.8660254037844387076, 1.000000000000000000, 0.8660254037844387076, 1.000000000000000000, 0.8660254037844387076, 1.000000000000000000, 0.8660254037844387076, 1.000000000000000000, 0.8660254037844387076, 1.000000000000000000, 0.8660254037844387076, 1.000000000000000000, 0.8660254037844387076, 1.000000000000000000, 0.8660254037844387076, 1.000000000000000000, 0.8660254037844387076, 1.000000000000000000, 0.8660254037844387076, 1.000000000000000000, 0.8660254037844387076, 1.000000000000000000, 0.8660254037844387076, 1.000000000000000000, 0.8660254037844387076, 1.000000000000000000, 0.8660254037844387076, 1.000000000000000000, 0.8660254037844387076, 1.000000000000000000, 0.8660254037844387076, 1.000000000000000000, 0.8660254037844387076, 1.000000000000000000, 0.8660254037844387076, 1.000000000000000000, 0.8660254037844387076, 1.000000000000000000, 0.8660254037844387076, 1.000000000000000000, 0.8660254037844387076, 1.000000000000000000, 0.8660254037844387076, 1.000000000000000000, 0.8660254037844387076, 1.000000000000000000, 0.8660254037844387076, 1.000000000000000000, 0.8660254037844387076, 1.000000000000000000, 0.8660254037844387076, 1.000000000000000000, 0.8660254037844387076, 1.000000000000000000, 0.8660254037844387076, 1.000000000000000000, 0.8660254037844387076, 1.000000000000000000, 0.8660254037844387076, 1.000000000000000000, 0.8660254037844387076, 1.000000000000000000, 0.8660254037844387076, 1.000000000000000000, 0.8660254037844387076, 1.000000000000000000, 0.8660254037844387076, 1.000000000000000000, 0.8660254037844387076, 1.000000000000000000, 0.8660254037844387076, 1.000000000000000000, 0.8660254037844387076, 1.000000000000000000, 0.8660254037844387076, 1.000000000000000000, 0.8660254037844387076, 1.000000000000000000, 0.8660254037844387076, 1.000000000000000000, 0.8660254037844387076, 1.000000000000000000, 0.8660254037844387076, 1.000000000000000000, 0.8660254037844387076, 1.000000000000000000, 0.8660254037844387076, 1.000000000000000000, 0.8660254037844387076, 1.000000000000000000, 0.8660254037844387076, 1.000000000000000000, 0.8660254037844387076, 1.000000000000000000, 0.8660254037844387076, 1.000000000000000000, 0.8660254037844387076, 1.000000000000000000, 0.8660254037844387076, 1.000000000000000000, 0.8660254037844387076, 1.000000000000000000, 0.8660254037844387076, 1.000000000000000000, 0.8660254037844387076, 1.000000000000000000, 0.8660254037844387076, 1.000000000000000000, 0.8660254037844387076, 1.000000000000000000, 0.8660254037844387076, 1.000000000000000000, 0.8660254037844387076, 1.000000000000000000, 0.8660254037844387076, 1.000000000000000000, 0.8660254037844387076, 1.000000000000000000, 0.8660254037844387076, 1.000000000000000000, 0.8660254037844387076, 1.000000000000000000, 0.8660254037844387076, 1.000000000000000000, 0.8660254037844387076, 1.000000000000000000, 0.8660254037844387076, 1.000000000000000000, 0.8660254037844387076, 1.000000000000000000, 0.8660254037844387076, 1.000000000000000000, 0.8660254037844387076, 1.000000000000000000, 0.8660254037844387076, 1.000000000000000000, 0.8660254037844387076, 1.000000000000000000, 0.8660254037844387076, 1.000000000000000000, 0.8660254037844387076, 1.000000000000000000, 0.8660254037844387076, 1.000000000000000000, 0.8660254037844387076, 1.000000000000000000, 0.8660254037844387076, 1.000000000000000000, 0.8660254037844387076, 1.000000000000000000, 0.8660254037844387076, 1.000000000000000000, 0.8660254037844387076, 1.000000000000000000, 0.8660254037844387076, 1.000000000000000000, 0.8660254037844387076, 1.000000000000000000, 0.8660254037844387076, 1.000000000000000000, 0.8660254037844387076, 1.000000000000000000, 0.8660254037844387076, 1.000000000000000000, 0.8660254037844387076, 1.000000000000000000, 0.8660254037844387076, 1.000000000000000000, 0.8660254037844387076, 1.000000000000000000, 0.8660254037844387076, 1.000000000000000000, 0.8660254037844387076, 1.000000000000000000, 0.8660254037844387076, 1.000000000000000000, 0.8660254037844387076, 1.000000000000000000, 0.8660254037844387076, 1.000000000000000000, 0.8660254037844387076, 1.000000000000000000, 0.8660254037844387076, 1.000000000000000000, 0.8660254037844387076, 1.000000000000000000, 0.8660254037844387076, 1.000000000000000000, 0.8660254037844387076, 1.000000000000000000, 0.8660254037844387076, 1.000000000000000000, 0.8660254037844387076, 1.000000000000000000, 0.8660254037844387076, 1.000000000000000000, 0.8660254037844387076, 1.000000000000000000, 0.8660254037844387076, 1.000000000000000000, 0.8660254037844387076, 1.000000000000000000, 0.8660254037844387076, 1.000000000000000000, 0.8660254037844387076, 1.000000000000000000, 0.8660254037844387076, 1.000000000000000000, 0.8660254037844387076, 1.000000000000000000, 0.8660254037844387076, 1.000000000000000000, 0.8660254037844387076, 1.000000000000000000, 0.8660254037844387076, 1.000000000000000000, 0.8660254037844387076, 1.000000000000000000, 0.8660254037844387076, 1.000000000000000000, 0.8660254037844387076, 1.000000000000000000, 0.8660254037844387076, 1.000000000000000000, 0.8660254037844387076, 1.000000000000000000, 0.8660254037844387076, 1.000000000000000000, 0.8660254037844387076, 1.000000000000000000, 0.8660254037844387076, 1.000000000000000000, 0.8660254037844387076, 1.000000000000000000, 0.8660254037844387076, 1.000000000000000000, 0.8660254037844387076, 1.000000000000000000, 0.8660254037844387076, 1.000000000000000000, 0.8660254037844387076, 1.000000000000000000, 0.8660254037844387076, 1.000000000000000000, 0.8660254037844387076, 1.000000000000000000, 0.8660254037844387076, 1.000000000000000000, 0.8660254037844387076, 1.000000000000000000, 0.8660254037844387076, 1.000000000000000000, 0.8660254037844387076, 1.000000000000000000, 0.8660254037844387076, 1.000000000000000000, 0.8660254037844387076, 1.000000000000000000, 0.8660254037844387076, 1.000000000000000000, 0.8660254037844387076, 1.000000000000000000, 0.8660254037844387076, 1.000000000000000000, 0.8660254037844387076, 1.000000000000000000) ) ) 
 REPRESENTATION_ITEM ( '' )  SURFACE ( )  );
#52590=CARTESIAN_POINT ( 'NONE',  ( 4.227444969362701421, 3.826440640544909400, 1.214306433183764966E-14 ) ) ;
#52593=CARTESIAN_POINT ( 'NONE',  ( -7.669108446824431269, 12.09904362127053545, -0.7998128361456291469 ) ) ;
#52598=CARTESIAN_POINT ( 'NONE',  ( 5.744750223003346257, 6.067414509003485001, 0.6312745094601609486 ) ) ;
#52600=CARTESIAN_POINT ( 'NONE',  ( -2.754277761870538299, 6.365074488824250309, 1.040834085586084257E-14 ) ) ;
#52604=CARTESIAN_POINT ( 'NONE',  ( 7.019370843573166319, 9.212351955633947043, 1.599625672291281386 ) ) ;
#52606=CARTESIAN_POINT ( 'NONE',  ( 7.122110765880372618, 7.203550736482235095, 0.7998128361456341429 ) ) ;
#52607=CARTESIAN_POINT ( 'NONE',  ( 5.443762371086860341, 6.309809840144842141, 1.199719254218462483 ) ) ;
#52609=CARTESIAN_POINT ( 'NONE',  ( -7.944714827928056167, 10.29191993738131927, 1.443375672974090751 ) ) ;
#52616=AXIS2_PLACEMENT_3D ( 'NONE', #201616, #120478, #23946 ) ;
#52617=CARTESIAN_POINT ( 'NONE',  ( -4.124570878694319376, 7.473888947179561981, -0.6522657496016289747 ) ) ;
#52621=CARTESIAN_POINT ( 'NONE',  ( 4.528060117284229413, 7.266191989264828344, 1.082531754730558626 ) ) ;
#52630=CARTESIAN_POINT ( 'NONE',  ( -10.43941509239824228, 11.28166515066052966, 1.040834085586084257E-14 ) ) ;
#52632=ORIENTED_EDGE ( 'NONE', *, *, #88440, .T. ) ;
#52638=CARTESIAN_POINT ( 'NONE',  ( -8.120970824461345217, 12.41829036193951730, 0.7216878364870458196 ) ) ;
#52642=CARTESIAN_POINT ( 'NONE',  ( 8.067265095331215718, 9.370563018429956870, 1.199719254218462483 ) ) ;
#52646=CARTESIAN_POINT ( 'NONE',  ( 1.499999999999987121, 1.577083334016150751, -0.8660254037844253849 ) ) ;
#52647=CARTESIAN_POINT ( 'NONE',  ( 5.021104450059825197, 4.960302734598949215, 0.4581612399162004468 ) ) ;
#52648=CARTESIAN_POINT ( 'NONE',  ( -5.259673527097670664, 8.223703984000886535, -1.199719254218446718 ) ) ;
#52651=CARTESIAN_POINT ( 'NONE',  ( -8.809047120577080392, 11.30030761213851953, 1.599625672291269396 ) ) ;
#52652=CARTESIAN_POINT ( 'NONE',  ( 0.005641171162447556654, 8.210923785195014091, 2.038653139403750369 ) ) ;
#52655=CARTESIAN_POINT ( 'NONE',  ( 6.531277313481192337, 8.642909503859968368, 1.599625672291281386 ) ) ;
#52661=CARTESIAN_POINT ( 'NONE',  ( 9.772729797352075920, 10.29593960653257234, -0.7998128361456281477 ) ) ;
#52666=CARTESIAN_POINT ( 'NONE',  ( -7.537970219518089543, 8.857015346601659900, -1.082531754730543971 ) ) ;
#52669=CARTESIAN_POINT ( 'NONE',  ( 0.6823417656249917140, 3.905208333674754950, 1.181850606188765695 ) ) ;
#52673=CARTESIAN_POINT ( 'NONE',  ( 1.364683531249988535, 5.405208333674750953, -0.7879004041258300672 ) ) ;
#52676=CARTESIAN_POINT ( 'NONE',  ( -4.568734577680899633, 4.432537883490215158, -0.7216878364870207285 ) ) ;
#52678=CARTESIAN_POINT ( 'NONE',  ( 10.72180055030867329, 11.40318881831530540, 0.7998128361456341429 ) ) ;
#52680=CARTESIAN_POINT ( 'NONE',  ( -10.10098813738111545, 11.74323990082152491, -1.199719254218441611 ) ) ;
#52684=CARTESIAN_POINT ( 'NONE',  ( -1.364683531250012516, 1.530208333674756505, 0.7879004041258379498 ) ) ;
#52685=CARTESIAN_POINT ( 'NONE',  ( -2.155383234892699562, 5.458438174109348395, 1.040834085586084257E-14 ) ) ;
#52686=CARTESIAN_POINT ( 'NONE',  ( 5.495132332240461714, 5.305409230568988832, 0.7998128361456341429 ) ) ;
#52692=CARTESIAN_POINT ( 'NONE',  ( 4.586165880992507660, 5.350526861157986147, -7.499999999999997335 ) ) ;
#52693=CARTESIAN_POINT ( 'NONE',  ( 0.1263921867887893569, 7.114106634750518410, 3.985475513000639847 ) ) ;
#52694=CARTESIAN_POINT ( 'NONE',  ( -8.676855123066030018, 9.225345186439589895, -0.7216878364870267237 ) ) ;
#52699=CARTESIAN_POINT ( 'NONE',  ( -8.779068160048691283, 10.20099992726700933, -1.199719254218446718 ) ) ;
#52700=CARTESIAN_POINT ( 'NONE',  ( -5.707619481228834779, 5.761236937629489852, -0.7216878364870197293 ) ) ;
#52701=CARTESIAN_POINT ( 'NONE',  ( -0.6823417656250212460, 2.363541667008084435, 1.181850606188767472 ) ) ;
#52709=CARTESIAN_POINT ( 'NONE',  ( 8.940712233207955606, 12.51824914112961729, 1.199719254218450271 ) ) ;
#52711=ORIENTED_EDGE ( 'NONE', *, *, #109929, .T. ) ;
#52716=EDGE_CURVE ( 'NONE', #49215, #20719, #133728, .T. ) ;
#52723=CARTESIAN_POINT ( 'NONE',  ( 1.364683531249990311, 2.696875000341415696, 1.214306433183764966E-14 ) ) ;
#52730=CARTESIAN_POINT ( 'NONE',  ( 7.574201371528760163, 11.98831870009225931, 1.040834085586084257E-14 ) ) ;
#52733=CARTESIAN_POINT ( 'NONE',  ( 1.364683531249986537, 1.113541667008082658, 0.7879004041258500513 ) ) ;
#52735=ORIENTED_EDGE ( 'NONE', *, *, #50294, .T. ) ;
#52743=CARTESIAN_POINT ( 'NONE',  ( 2.855963913973019963, 6.483708332943829866, 0.000000000000000000 ) ) ;
#52748=CARTESIAN_POINT ( 'NONE',  ( 4.514586370236258084, 5.411880727520489209, 1.219673154775415824 ) ) ;
#52754=CARTESIAN_POINT ( 'NONE',  ( -4.081167932913447594, 4.720116328942494555, -1.199719254218452047 ) ) ;
#52756=CARTESIAN_POINT ( 'NONE',  ( 8.121497709785879593, 9.433834401960398353, -1.199719254218445830 ) ) ;
#52760=CARTESIAN_POINT ( 'NONE',  ( 4.867013957181530515, 5.740899707208986236, -1.082531754730548412 ) ) ;
#52767=CARTESIAN_POINT ( 'NONE',  ( -5.558479791922849245, 9.428717490644563881, 0.7216878364870458196 ) ) ;
#52769=CARTESIAN_POINT ( 'NONE',  ( 5.311043488251262268, 7.219303374425030562, -1.599625672291256295 ) ) ;
#52772=CARTESIAN_POINT ( 'NONE',  ( -7.635213062790267458, 12.05949900656400686, 0.000000000000000000 ) ) ;
#52774=CARTESIAN_POINT ( 'NONE',  ( -4.702146809683744877, 5.356480858934594025, 2.420000000000010587 ) ) ;
#52777=CARTESIAN_POINT ( 'NONE',  ( -2.300079615812729905, 5.835176651756807331, -0.7998128361456281477 ) ) ;
#52779=CARTESIAN_POINT ( 'NONE',  ( 9.049177462117294013, 12.64479190819049670, -1.199719254218446718 ) ) ;
#52781=CARTESIAN_POINT ( 'NONE',  ( 4.715538499454675403, 4.395883092318884522, 1.214306433183764966E-14 ) ) ;
#52787=CARTESIAN_POINT ( 'NONE',  ( 5.016153647376217606, 4.954526798134778254, 0.7216878364870317197 ) ) ;
#52790=CARTESIAN_POINT ( 'NONE',  ( -3.255929445576174697, 6.950334786480840243, -0.7998128361456281477 ) ) ;
#52793=CARTESIAN_POINT ( 'NONE',  ( -9.321394304595349567, 10.83371376257142416, 1.199719254218462483 ) ) ;
#52798=CARTESIAN_POINT ( 'NONE',  ( 7.456621297836067086, 10.68284669990868174, 1.082531754730558626 ) ) ;
#52799=CARTESIAN_POINT ( 'NONE',  ( -0.6823417656249969321, 5.530208333674756283, -1.181850606188749264 ) ) ;
#52802=CARTESIAN_POINT ( 'NONE',  ( 3.662674053986138656, 7.424870162959149589, 0.7998128361456321445 ) ) ;
#52806=CARTESIAN_POINT ( 'NONE',  ( -6.795661308947694934, 8.951357498570873261, -1.599625672291263179 ) ) ;
#52816=CARTESIAN_POINT ( 'NONE',  ( -1.201851678989727383E-14, 3.009375000341419248, -1.575800808251660134 ) ) ;
#52818=CARTESIAN_POINT ( 'NONE',  ( 8.703444544968814256, 12.24143683818393313, -1.199719254218446718 ) ) ;
#52820=CARTESIAN_POINT ( 'NONE',  ( -5.097502569058221411, 6.009803087731781623, -1.082531754730544860 ) ) ;
#52821=CARTESIAN_POINT ( 'NONE',  ( 4.365362273920252889, 4.195270195769483124, 0.7216878364870317197 ) ) ;
#52823=CARTESIAN_POINT ( 'NONE',  ( -4.839897649954225223, 7.630002444046455778, 1.082531754730560403 ) ) ;
#52828=CARTESIAN_POINT ( 'NONE',  ( 4.147904930777053245, 6.926640621626830807, -1.199719254218452047 ) ) ;
#52839=CARTESIAN_POINT ( 'NONE',  ( 6.331821432781979730, 7.345878745455822312, -1.199719254218445830 ) ) ;
#52844=CARTESIAN_POINT ( 'NONE',  ( -4.876128802409253282, 8.840567369452784874, 0.7998128361456481317 ) ) ;
#52848=CARTESIAN_POINT ( 'NONE',  ( 8.288111976655649471, 8.563885482386732306, -0.7998128361456291469 ) ) ;
#52853=CARTESIAN_POINT ( 'NONE',  ( -5.708146366553361162, 6.618257834855742594, -1.199719254218446718 ) ) ;
#52854=CARTESIAN_POINT ( 'NONE',  ( 7.443063143778065438, 7.785921210603627962, -0.7216878364870257245 ) ) ;
#52855=CARTESIAN_POINT ( 'NONE',  ( 5.008269389056229315, 6.794162766424465261, 1.424127363233711252 ) ) ;
#52857=CARTESIAN_POINT ( 'NONE',  ( -4.460796234096120472, 5.163016013655583158, 1.199719254218462483 ) ) ;
#52860=CARTESIAN_POINT ( 'NONE',  ( -6.274726165026268454, 6.214935368819085149, 0.7998128361456341429 ) ) ;
#52863=CARTESIAN_POINT ( 'NONE',  ( 0.6823417656249882723, 1.426041667008083547, -1.181850606188749264 ) ) ;
#52865=CARTESIAN_POINT ( 'NONE',  ( -3.768803514918943609, 7.340761834139994058, 0.7216878364870317197 ) ) ;
#52868=ORIENTED_EDGE ( 'NONE', *, *, #205893, .F. ) ;
#52871=CARTESIAN_POINT ( 'NONE',  ( 5.120175567455225618, 9.125288595339771547, -0.7998128361456281477 ) ) ;
#52873=CARTESIAN_POINT ( 'NONE',  ( 1.364683531249988535, 2.426041667008088432, 0.7879004041258500513 ) ) ;
#52876=CARTESIAN_POINT ( 'NONE',  ( -0.6823417656250003738, -0.9697916663252494907, -1.181850606188749264 ) ) ;
#52879=CARTESIAN_POINT ( 'NONE',  ( -4.973143418114339021, 4.696422164088486895, 0.7998128361456341429 ) ) ;
#52881=CARTESIAN_POINT ( 'NONE',  ( -8.161645285302366659, 8.624267042381978499, 1.040834085586084257E-14 ) ) ;
#52883=CARTESIAN_POINT ( 'NONE',  ( -1.364683531249997417, 3.509375000341423245, 1.214306433183764966E-14 ) ) ;
#52890=CARTESIAN_POINT ( 'NONE',  ( -7.388830529323428209, 8.683019041374528513, 1.082531754730549967 ) ) ;
#52894=CARTESIAN_POINT ( 'NONE',  ( -6.466876083594135238, 9.528143949959703818, 1.082531754730548412 ) ) ;
#52899=CARTESIAN_POINT ( 'NONE',  ( 1.499999999999990896, 4.806250000682819490, 1.214306433183765124E-14 ) ) ;
#52908=CARTESIAN_POINT ( 'NONE',  ( -7.230575994789712801, 7.330093503543126054, 0.7998128361456341429 ) ) ;
#52910=CARTESIAN_POINT ( 'NONE',  ( 0.7499999999999867883, -0.4333333333333133641, -1.299038105676652899 ) ) ;
#52911=CARTESIAN_POINT ( 'NONE',  ( 3.225950485047770933, 5.851027101609320269, 1.199719254218450271 ) ) ;
#52915=CARTESIAN_POINT ( 'NONE',  ( 6.169123589417988995, 7.156064594864501416, -1.199719254218445830 ) ) ;
#52918=AXIS2_PLACEMENT_3D ( 'NONE', #170193, #105222, #21778 ) ;
#52921=CARTESIAN_POINT ( 'NONE',  ( -4.284013352238255301, 6.981470763377843447, -1.082531754730549967 ) ) ;
#52926=CARTESIAN_POINT ( 'NONE',  ( 3.109879841324575622, 6.447534329559368338, -0.5062228152068328768 ) ) ;
#52929=CARTESIAN_POINT ( 'NONE',  ( -1.364683531250014514, 1.738541667008085545, -0.7879004041258289570 ) ) ;
#52930=DIRECTION ( 'NONE',  ( 1.000000000000000000, 0.000000000000000000, 0.000000000000000000 ) ) ;
#52931=CARTESIAN_POINT ( 'NONE',  ( -7.202405917357668663, 9.425892875049191488, 1.599625672291295375 ) ) ;
#52933=CARTESIAN_POINT ( 'NONE',  ( 5.960781091502512119, 10.10599504006161986, 0.7998128361456462443 ) ) ;
#52934=CARTESIAN_POINT ( 'NONE',  ( -6.367525699912501835, 10.58053041653993098, -0.7998128361456291469 ) ) ;
#52937=CARTESIAN_POINT ( 'NONE',  ( -1.500000000000013101, -0.2979166659838501929, 0.8660254037844403729 ) ) ;
#52939=CARTESIAN_POINT ( 'NONE',  ( 7.429504990608736037, 11.61158022244479682, -0.7216878364870267237 ) ) ;
#52941=CARTESIAN_POINT ( 'NONE',  ( -0.6823417656250246877, -0.3864583329919110688, 1.181850606188755259 ) ) ;
#52944=CARTESIAN_POINT ( 'NONE',  ( 7.470179451005385829, 8.777926116670192513, -1.082531754730537976 ) ) ;
#52947=CARTESIAN_POINT ( 'NONE',  ( -5.748293942514189681, 5.808690475795744490, -0.7216878364870207285 ) ) ;
#52949=CARTESIAN_POINT ( 'NONE',  ( -1.364683531249997417, 3.509375000341423245, 1.214306433183764966E-14 ) ) ;
#52953=CARTESIAN_POINT ( 'NONE',  ( -4.706651882238427120, 8.642844295920152575, 1.040834085586084257E-14 ) ) ;
#52960=CARTESIAN_POINT ( 'NONE',  ( 6.446011968293428041, 9.607765498729298415, -1.199719254218440723 ) ) ;
#52963=CARTESIAN_POINT ( 'NONE',  ( 1.499999999999989120, 3.025000000000020783, 1.214306433183764966E-14 ) ) ;
#52969=CARTESIAN_POINT ( 'NONE',  ( 7.158341918335438869, 7.453746447587225710, -0.7216878364870257245 ) ) ;
#52971=CARTESIAN_POINT ( 'NONE',  ( 1.364683531249988757, -0.8031249996585804185, 0.000000000000000000 ) ) ;
#52980=CARTESIAN_POINT ( 'NONE',  ( -1.402160292154681736E-14, 0.8375000000000232259, -1.732050807568863648 ) ) ;
#52981=CARTESIAN_POINT ( 'NONE',  ( 6.265839547809997079, 10.46189657242035587, 0.7998128361456462443 ) ) ;
#52982=CARTESIAN_POINT ( 'NONE',  ( -7.330154606482786050, 11.70359747420527619, 0.000000000000000000 ) ) ;
#52984=CARTESIAN_POINT ( 'NONE',  ( -1.364683531250014514, -0.4697916663252449943, 0.7879004041258379498 ) ) ;
#52985=CARTESIAN_POINT ( 'NONE',  ( -1.500000000000001332, 0.6500000000000255573, 0.000000000000000000 ) ) ;
#52987=CARTESIAN_POINT ( 'NONE',  ( 4.147904930777053245, 6.926640621626830807, -1.199719254218452047 ) ) ;
#52995=CARTESIAN_POINT ( 'NONE',  ( 1.499999999999987121, -0.7145833326505161009, 0.8660254037844524744 ) ) ;
#52997=CARTESIAN_POINT ( 'NONE',  ( -6.995117189646935962, 10.24838825697502109, 1.199719254218453823 ) ) ;
#52998=CARTESIAN_POINT ( 'NONE',  ( -6.100805936469506641, 6.219954468743612352, 0.7216878364870317197 ) ) ;
#53000=LINE ( 'NONE', #166763, #4230 ) ;
#53003=CARTESIAN_POINT ( 'NONE',  ( 3.992368507422526136, 7.606667543653665042, 0.1043914665942706627 ) ) ;
#53006=CARTESIAN_POINT ( 'NONE',  ( 6.428537391173986038, 10.65171072301167854, 0.7998128361456462443 ) ) ;
#53010=CARTESIAN_POINT ( 'NONE',  ( 5.897433631820129918, 8.863794422890064695, -1.082531754730537976 ) ) ;
#53015=CARTESIAN_POINT ( 'NONE',  ( -8.128276786592724790, 9.441743324901704426, -1.199719254218446718 ) ) ;
#53016=CARTESIAN_POINT ( 'NONE',  ( 4.656335691289526402, 7.519809842224722374, -1.199719254218452047 ) ) ;
#53017=DIRECTION ( 'NONE',  ( -1.000000000000000000, 5.578564026256490882E-16, -1.264049978315544409E-61 ) ) ;
#53019=CARTESIAN_POINT ( 'NONE',  ( 3.928111819657337911, 5.605883094398769195, 1.599625672291267398 ) ) ;
#53020=ORIENTED_EDGE ( 'NONE', *, *, #129464, .T. ) ;
#53025=DIRECTION ( 'NONE',  ( 6.314299915563594049E-62, 8.546850786086437571E-32, 1.000000000000000000 ) ) ;
#53026=CARTESIAN_POINT ( 'NONE',  ( -4.067082894419624672, 6.728385229256075739, 1.082531754730560403 ) ) ;
#53027=CARTESIAN_POINT ( 'NONE',  ( 8.595506201384004896, 12.01154575404795466, 1.082531754730546636 ) ) ;
#53030=CARTESIAN_POINT ( 'NONE',  ( -5.910464900553636269, 8.982960586366182554, -1.199719254218440723 ) ) ;
#53035=CARTESIAN_POINT ( 'NONE',  ( -8.694856585065634746, 9.038420858865048757, 0.7998128361456462443 ) ) ;
#53052=CARTESIAN_POINT ( 'NONE',  ( -5.194745412330402878, 9.212286747694129474, 0.000000000000000000 ) ) ;
#53055=CARTESIAN_POINT ( 'NONE',  ( 6.371969008742804697, 7.496680600697164465, -1.082531754730543083 ) ) ;
#53059=CARTESIAN_POINT ( 'NONE',  ( -5.284980951228653190, 5.060232619388524533, 0.000000000000000000 ) ) ;
#53069=CARTESIAN_POINT ( 'NONE',  ( -8.422639742587602285, 10.84949900448412841, -1.599625672291263179 ) ) ;
#53070=CARTESIAN_POINT ( 'NONE',  ( 7.558834334818744338, 8.777393797832065303, 1.199719254218462483 ) ) ;
#53073=CARTESIAN_POINT ( 'NONE',  ( -10.48453286206953727, 11.12637651536962125, 0.7998128361456462443 ) ) ;
#53074=CIRCLE ( 'NONE', #87714, 0.07999999999999993228 ) ;
#53076=CARTESIAN_POINT ( 'NONE',  ( 1.364683531249986537, 0.4260416670080872659, 0.7879004041258500513 ) ) ;
#53077=B_SPLINE_CURVE_WITH_KNOTS ( 'NONE', 3,
 ( #73815, #173478, #140995, #157212, #207003, #9872, #124787, #13061, #29336, #159329 ),
 .UNSPECIFIED., .F., .F.,
 ( 4, 3, 3, 4 ),
 ( 3.907308343762969252E-16, 8.899070015639609047E-05, 0.0001343825223669382267, 0.0001804666533476734377 ),
 .UNSPECIFIED. ) ;
#53081=CARTESIAN_POINT ( 'NONE',  ( 7.619319141200051604, 11.83303006480134911, 0.7216878364870438212 ) ) ;
#53088=CARTESIAN_POINT ( 'NONE',  ( -5.520955638564554846, 6.243838396700211568, -0.9653654033580265637 ) ) ;
#53097=ORIENTED_EDGE ( 'NONE', *, *, #209714, .F. ) ;
#53110=CARTESIAN_POINT ( 'NONE',  ( 1.364683531249990311, 5.613541667008087543, 0.7879004041258500513 ) ) ;
#53114=CARTESIAN_POINT ( 'NONE',  ( 8.380911511541880188, 12.92948053010758258, 0.7998128361456462443 ) ) ;
#53116=CARTESIAN_POINT ( 'NONE',  ( 1.217358635584784965, 3.014784080462326266, -0.7749999999999840350 ) ) ;
#53119=CARTESIAN_POINT ( 'NONE',  ( 9.134442807305049428, 11.67993591332117376, 1.599625672291281386 ) ) ;
#53120=CARTESIAN_POINT ( 'NONE',  ( -5.395781948114519722, 5.397426482329451325, 0.000000000000000000 ) ) ;
#53124=CARTESIAN_POINT ( 'NONE',  ( 3.388648328411762556, 6.040841252200647382, 1.199719254218462483 ) ) ;
#53125=CARTESIAN_POINT ( 'NONE',  ( -0.6823417656250003738, 3.030208333674754062, -1.181850606188749264 ) ) ;
#53126=CARTESIAN_POINT ( 'NONE',  ( -5.852179643265606579, 6.035944939585320412, -0.4116468081218557784 ) ) ;
#53127=CARTESIAN_POINT ( 'NONE',  ( 8.530051201292206287, 13.10347683481629488, 0.000000000000000000 ) ) ;
#53131=CARTESIAN_POINT ( 'NONE',  ( -7.588813295347149435, 9.876701482703580837, -1.599625672291263179 ) ) ;
#53132=EDGE_CURVE ( 'NONE', #21505, #62722, #147729, .T. ) ;
#53133=CARTESIAN_POINT ( 'NONE',  ( -3.253593677155282471, 6.739683690082376444, 1.040834085586084257E-14 ) ) ;
#53135=CARTESIAN_POINT ( 'NONE',  ( -5.904739593951539689, 6.847616600153594746, 1.199719254218450271 ) ) ;
#53137=CARTESIAN_POINT ( 'NONE',  ( -0.7500000000000006661, 0.3895833340161539149, -1.299038105676652011 ) ) ;
#53140=VECTOR ( 'NONE', #42323, 1000.000000000000114 ) ;
#53145=CARTESIAN_POINT ( 'NONE',  ( -4.406036734316900905, 5.203092947200234519, -1.082531754730543971 ) ) ;
#53147=CARTESIAN_POINT ( 'NONE',  ( 4.001984418394623155, 7.593073144423666321, -0.1798963839820325039 ) ) ;
#53153=CARTESIAN_POINT ( 'NONE',  ( -4.758548728272219641, 4.653987725846768342, 0.7216878364870317197 ) ) ;
#53155=CARTESIAN_POINT ( 'NONE',  ( 8.259941899223605333, 10.65968485389279508, -1.599625672291268286 ) ) ;
#53157=CARTESIAN_POINT ( 'NONE',  ( -1.230761180058579152, 3.146116465842661025, 0.7750000000000100142 ) ) ;
#53164=CARTESIAN_POINT ( 'NONE',  ( -3.898132859128961236, 4.506575409527250997, -1.199719254218452047 ) ) ;
#53165=CARTESIAN_POINT ( 'NONE',  ( -10.63367255181986160, 11.30037282007833532, 1.040834085586084257E-14 ) ) ;
#53170=CARTESIAN_POINT ( 'NONE',  ( 6.166260936116925606, 6.088392601758203071, 0.7998128361456341429 ) ) ;
#53186=CARTESIAN_POINT ( 'NONE',  ( 7.086107841436786181, 11.41887624831828418, 1.040834085586084257E-14 ) ) ;
#53189=CARTESIAN_POINT ( 'NONE',  ( -6.084912014434944894, 5.993485526462540847, -0.7998128361456291469 ) ) ;
#53191=CARTESIAN_POINT ( 'NONE',  ( -3.578989363883261277, 7.119311991265024453, 1.040834085586084257E-14 ) ) ;
#53194=CARTESIAN_POINT ( 'NONE',  ( -0.7500000000000249800, -1.277083332650516656, 1.299038105676659116 ) ) ;
#53199=CARTESIAN_POINT ( 'NONE',  ( 3.181359600701000989, 6.863336634126477875, 0.000000000000000000 ) ) ;
#53200=CARTESIAN_POINT ( 'NONE',  ( -3.411848212133334446, 7.132240014130862171, 0.7998128361456341429 ) ) ;
#53206=CARTESIAN_POINT ( 'NONE',  ( 5.666945020832177882, 6.674152614801420746, 1.082531754730558626 ) ) ;
#53208=ORIENTED_EDGE ( 'NONE', *, *, #198981, .F. ) ;
#53210=CARTESIAN_POINT ( 'NONE',  ( 7.795575137733369075, 9.157554417852841411, -1.082531754730537976 ) ) ;
#53211=CARTESIAN_POINT ( 'NONE',  ( 1.364683531249990311, 5.196875000341417916, 1.214306433183764966E-14 ) ) ;
#53213=CARTESIAN_POINT ( 'NONE',  ( 4.731432421044862835, 6.543090462684225450, -1.443375672974051449 ) ) ;
#53220=CARTESIAN_POINT ( 'NONE',  ( -4.357679483485834560, 7.387146062586773532, 1.181458644690215998 ) ) ;
#53223=CARTESIAN_POINT ( 'NONE',  ( -0.6823417656249969321, 5.280208333674756283, -1.181850606188749264 ) ) ;
#53227=CARTESIAN_POINT ( 'NONE',  ( -8.292783513053063160, 12.82666453187061073, 0.7998128361456481317 ) ) ;
#53229=DIRECTION ( 'NONE',  ( -7.387867266669436732E-31, -1.000000000000000000, 8.546850786086437571E-32 ) ) ;
#53230=B_SPLINE_CURVE_WITH_KNOTS ( 'NONE', 3,
 ( #167611, #84221, #129865, #115714 ),
 .UNSPECIFIED., .F., .F.,
 ( 4, 4 ),
 ( -1.944647862007489213E-06, 0.0001035599091551129175 ),
 .UNSPECIFIED. ) ;
#53240=CARTESIAN_POINT ( 'NONE',  ( -0.6823417656250212460, 4.113541667008085767, 1.181850606188767472 ) ) ;
#53242=CARTESIAN_POINT ( 'NONE',  ( 8.288111976655649471, 8.563885482386732306, -0.7998128361456291469 ) ) ;
#53243=CARTESIAN_POINT ( 'NONE',  ( -7.492852449846775897, 11.89341162479659531, 0.000000000000000000 ) ) ;
#53245=CARTESIAN_POINT ( 'NONE',  ( -4.416205349749324327, 6.175325546172741653, 1.599625672291267175 ) ) ;
#53249=CARTESIAN_POINT ( 'NONE',  ( 1.499999999999990896, 4.275000000000021672, 1.214306433183764966E-14 ) ) ;
#53250=CARTESIAN_POINT ( 'NONE',  ( 5.335297142177534369, 6.183267073083954735, -1.199719254218452047 ) ) ;
#53254=EDGE_LOOP ( 'NONE', ( #74761, #81117, #9415, #66185, #149490 ) ) ;
#53256=CARTESIAN_POINT ( 'NONE',  ( 7.890482213473377193, 11.18901776815221716, -1.082531754730543083 ) ) ;
#53261=CARTESIAN_POINT ( 'NONE',  ( -1.499999999999997780, 3.931250000682819046, 1.214306433183764966E-14 ) ) ;
#53263=CARTESIAN_POINT ( 'NONE',  ( -4.055860508782465068, 7.883587693554856557, 1.040834085586084257E-14 ) ) ;
#53264=CARTESIAN_POINT ( 'NONE',  ( 3.755245360860917536, 5.404205559136275205, -1.443375672974051449 ) ) ;
#53273=CARTESIAN_POINT ( 'NONE',  ( 6.771407655021410399, 9.987393799911945536, -1.199719254218441611 ) ) ;
#53274=CARTESIAN_POINT ( 'NONE',  ( 5.660692828905515839, 6.562895374266609849, -1.199719254218445830 ) ) ;
#53277=CARTESIAN_POINT ( 'NONE',  ( 3.734381245560244089, 6.444196322207211836, 1.199719254218462483 ) ) ;
#53284=CARTESIAN_POINT ( 'NONE',  ( 9.348510611822643313, 10.86534945433664134, 1.199719254218453823 ) ) ;
#53289=CARTESIAN_POINT ( 'NONE',  ( 5.387724311900628393, 6.300193624175450147, -1.063853923354351361 ) ) ;
#53299=CARTESIAN_POINT ( 'NONE',  ( 6.697364695470787943, 7.876308901879812474, -1.082531754730543083 ) ) ;
#53300=CARTESIAN_POINT ( 'NONE',  ( -8.351459436338023679, 12.68719374246231624, -0.7216878364870267237 ) ) ;
#53306=CARTESIAN_POINT ( 'NONE',  ( -5.091250377131585125, 5.898545847196970726, 1.199719254218450271 ) ) ;
#53308=CARTESIAN_POINT ( 'NONE',  ( -5.378281411895281749, 4.339595938922590435, 2.499999999999998668 ) ) ;
#53316=CARTESIAN_POINT ( 'NONE',  ( 9.206149998879153529, 10.69926207256923689, 1.199719254218453823 ) ) ;
#53317=CARTESIAN_POINT ( 'NONE',  ( 6.067817914410090552, 6.045155426100865981, -0.3955105627355664510 ) ) ;
#53324=CARTESIAN_POINT ( 'NONE',  ( -9.341204650135658483, 10.00041963468749984, 1.040834085586084257E-14 ) ) ;
#53326=CARTESIAN_POINT ( 'NONE',  ( 3.680326755797796778, 6.126960397039161066, -1.194586299139585694 ) ) ;
#53328=CARTESIAN_POINT ( 'NONE',  ( 6.577677080924314801, 10.82570702772039262, 1.040834085586084257E-14 ) ) ;
#53331=CARTESIAN_POINT ( 'NONE',  ( 3.785751206713845018, 5.439795712631356750, 1.599625672291267398 ) ) ;
#53333=CARTESIAN_POINT ( 'NONE',  ( -6.226218857173722476, 8.287007971501239467, 1.599625672291283607 ) ) ;
#53334=CARTESIAN_POINT ( 'NONE',  ( 2.171277156482887882, 5.684907115872006145, -0.7998128361456291469 ) ) ;
#53342=CARTESIAN_POINT ( 'NONE',  ( 4.176068722599148408, 7.364853391560295393, -0.8050483301465498620 ) ) ;
#53344=CARTESIAN_POINT ( 'NONE',  ( 5.504247177468175600, 8.405076892812779477, 1.082531754730558626 ) ) ;
#53352=CARTESIAN_POINT ( 'NONE',  ( 8.880227426826646564, 9.462612874160329923, 0.7216878364870458196 ) ) ;
#53354=CARTESIAN_POINT ( 'NONE',  ( -7.181014916732457287, 11.52960116949655678, -0.7998128361456291469 ) ) ;
#53364=CARTESIAN_POINT ( 'NONE',  ( 10.40318394038753702, 11.03146944007395724, -0.7998128361456281477 ) ) ;
#53368=CARTESIAN_POINT ( 'NONE',  ( 3.714044015139744914, 6.420469553383295391, 1.199719254218462483 ) ) ;
#53371=CARTESIAN_POINT ( 'NONE',  ( -1.201851678989727383E-14, 4.118750000682818602, -1.732050807568863648 ) ) ;
#53375=EDGE_LOOP ( 'NONE', ( #7160, #91801, #165974, #75771 ) ) ;
#53377=CARTESIAN_POINT ( 'NONE',  ( -1.500000000000013101, 1.629166666666691077, -0.8660254037844313801 ) ) ;
#53378=CARTESIAN_POINT ( 'NONE',  ( 6.582647274634798151, 7.638508894284114170, 1.199719254218462483 ) ) ;
#53379=CARTESIAN_POINT ( 'NONE',  ( 3.321384445223597659, 6.818772919495430074, -0.7216878364870267237 ) ) ;
#53383=CARTESIAN_POINT ( 'NONE',  ( 8.514157279702022407, 10.95626946445095307, -1.443375672974063439 ) ) ;
#53388=CARTESIAN_POINT ( 'NONE',  ( -5.590039407536138150, 5.416134151747256986, 0.000000000000000000 ) ) ;
#53389=CARTESIAN_POINT ( 'NONE',  ( -1.500000000000011324, 3.452083334016151639, 0.8660254037844403729 ) ) ;
#53390=CARTESIAN_POINT ( 'NONE',  ( -0.6823417656249969321, 5.280208333674756283, -1.181850606188749264 ) ) ;
#53395=CARTESIAN_POINT ( 'NONE',  ( 1.364683531249988535, 3.926041667008087543, 0.7879004041258500513 ) ) ;
#53398=DIRECTION ( 'NONE',  ( 0.000000000000000000, 0.000000000000000000, 1.000000000000000000 ) ) ;
#53403=CARTESIAN_POINT ( 'NONE',  ( -7.004758919754800139, 11.32396917302262018, 0.000000000000000000 ) ) ;
#53404=CARTESIAN_POINT ( 'NONE',  ( 5.133733721068893807, 9.141106441222381918, 1.040834085586084257E-14 ) ) ;
#53413=CARTESIAN_POINT ( 'NONE',  ( -6.938021921891187382, 9.117444880338284818, -1.599625672291263179 ) ) ;
#53416=CARTESIAN_POINT ( 'NONE',  ( 10.71502147350184231, 11.39527989537399755, 0.000000000000000000 ) ) ;
#53418=CARTESIAN_POINT ( 'NONE',  ( 9.725276259704228821, 10.24057714594344048, 0.7998128361456462443 ) ) ;
#53421=CARTESIAN_POINT ( 'NONE',  ( -5.115504031057831469, 4.862509545855891346, 0.7998128361456341429 ) ) ;
#53422=CARTESIAN_POINT ( 'NONE',  ( -7.832860060393135093, 10.16142270859057462, 1.599625672291295375 ) ) ;
#53425=CARTESIAN_POINT ( 'NONE',  ( -3.985474048508588663, 7.835680043367737824, -0.2278754907324483936 ) ) ;
#53426=CARTESIAN_POINT ( 'NONE',  ( -1.402160292154681736E-14, -1.178124999658576311, 1.575800808251672791 ) ) ;
#53430=CARTESIAN_POINT ( 'NONE',  ( 7.280365300858406385, 11.43758391773608984, 1.040834085586084257E-14 ) ) ;
#53433=CARTESIAN_POINT ( 'NONE',  ( 5.575427483717746213, 7.527751369135936343, 1.599625672291267398 ) ) ;
#53453=CARTESIAN_POINT ( 'NONE',  ( 1.387358672531703974, 7.315968950352358391, 4.254625267140708544 ) ) ;
#53456=ORIENTED_EDGE ( 'NONE', *, *, #113684, .F. ) ;
#53458=CARTESIAN_POINT ( 'NONE',  ( -7.971304249830880373, 11.38727316052296601, 1.199719254218453823 ) ) ;
#53459=CIRCLE ( 'NONE', #126215, 1.250000000000000222 ) ;
#53464=CARTESIAN_POINT ( 'NONE',  ( 1.499999999999989120, 2.285416667349482012, 0.8660254037844524744 ) ) ;
#53465=CARTESIAN_POINT ( 'NONE',  ( 10.55232363013785246, 11.20546574478267132, 0.000000000000000000 ) ) ;
#53469=CARTESIAN_POINT ( 'NONE',  ( -10.47775378526269918, 11.11846759242831872, -0.7998128361456221525 ) ) ;
#53470=DIRECTION ( 'NONE',  ( -0.7592566023653017915, -0.6507913734559624963, 9.298211678181604981E-17 ) ) ;
#53471=CARTESIAN_POINT ( 'NONE',  ( -1.364683531250000748, 2.259375000341422357, 1.214306433183764966E-14 ) ) ;
#53477=CARTESIAN_POINT ( 'NONE',  ( -2.266184231778562541, 5.795632037050281404, 1.040834085586084257E-14 ) ) ;
#53482=CARTESIAN_POINT ( 'NONE',  ( 0.6823417656249882723, 0.4052083336747516751, 1.181850606188755259 ) ) ;
#53488=CARTESIAN_POINT ( 'NONE',  ( -0.6823417656250212460, 2.051041667008083991, 1.181850606188767472 ) ) ;
#53490=CARTESIAN_POINT ( 'NONE',  ( -6.388916700537716764, 8.476822122092563916, 1.599625672291283607 ) ) ;
#53491=CARTESIAN_POINT ( 'NONE',  ( 7.588813295347141441, 9.876701482703580837, -1.599625672291262513 ) ) ;
#53493=CARTESIAN_POINT ( 'NONE',  ( 4.008406971134620633, 7.828225232965717595, 0.7998128361456321445 ) ) ;
#53496=CARTESIAN_POINT ( 'NONE',  ( 0.7499999999999885647, 3.566666666666690411, -1.299038105676658228 ) ) ;
#53498=CARTESIAN_POINT ( 'NONE',  ( -0.6823417656250003738, 2.030208333674753174, -1.181850606188749264 ) ) ;
#53506=CARTESIAN_POINT ( 'NONE',  ( 5.178851490740196795, 7.065079377328788546, 1.443375672974062551 ) ) ;
#53509=CARTESIAN_POINT ( 'NONE',  ( -8.422639742587602285, 10.84949900448412841, -1.599625672291263179 ) ) ;
#53510=CARTESIAN_POINT ( 'NONE',  ( -5.264643720808155791, 5.036505850564608089, 0.000000000000000000 ) ) ;
#53511=CARTESIAN_POINT ( 'NONE',  ( -4.292360784660903761, 7.401453155497748959, -1.060140167543128564 ) ) ;
#53515=CARTESIAN_POINT ( 'NONE',  ( -7.415946836550729948, 9.675023947441092176, 1.443375672974090751 ) ) ;
#53517=CARTESIAN_POINT ( 'NONE',  ( 1.499999999999987121, 4.795833333333353821, -0.8660254037844323793 ) ) ;
#53520=CARTESIAN_POINT ( 'NONE',  ( 7.619319141200051604, 11.83303006480134911, 0.7216878364870438212 ) ) ;
#53522=CARTESIAN_POINT ( 'NONE',  ( 1.284279953904126748, 10.64264068711930733, -0.7749999999999874767 ) ) ;
#53528=CARTESIAN_POINT ( 'NONE',  ( 10.53432216769390095, 11.39239007183880581, -0.7216878364870257245 ) ) ;
#53530=ADVANCED_FACE ( 'NONE', ( #82544 ), #18606, .F. ) ;
#53534=CARTESIAN_POINT ( 'NONE',  ( 7.226132685959389512, 11.37431253368722750, -0.7216878364870267237 ) ) ;
#53535=CARTESIAN_POINT ( 'NONE',  ( 6.938021921891177612, 9.117444880338284818, -1.599625672291262513 ) ) ;
#53536=CARTESIAN_POINT ( 'NONE',  ( -5.199715606040888005, 6.025088614257851027, -1.199719254218446718 ) ) ;
#53540=CARTESIAN_POINT ( 'NONE',  ( 7.090551149822744925, 7.374657217655760100, 0.7216878364870317197 ) ) ;
#53542=CARTESIAN_POINT ( 'NONE',  ( 1.419999999999999485, 7.176846818246214177, 4.202462424328220258 ) ) ;
#53543=CARTESIAN_POINT ( 'NONE',  ( 3.009546912553647147, 5.494593250412460606, -1.082531754730543083 ) ) ;
#53544=ORIENTED_EDGE ( 'NONE', *, *, #137732, .F. ) ;
#53545=CARTESIAN_POINT ( 'NONE',  ( -3.460355519985875983, 5.060167411448709629, 1.599625672291267398 ) ) ;
#53562=CARTESIAN_POINT ( 'NONE',  ( 6.421758314367153275, 10.64380180007036891, -0.7998128361456291469 ) ) ;
#53565=ORIENTED_EDGE ( 'NONE', *, *, #72633, .F. ) ;
#53567=CARTESIAN_POINT ( 'NONE',  ( 1.506334365903699402, 8.679455619938613253, 2.541882285198393987 ) ) ;
#53574=CARTESIAN_POINT ( 'NONE',  ( -5.412729640353771465, 7.337937218544611895, 1.599625672291269396 ) ) ;
#53576=CARTESIAN_POINT ( 'NONE',  ( -3.578462479003122976, 6.262291094557191684, 1.199719254218464037 ) ) ;
#53586=CARTESIAN_POINT ( 'NONE',  ( -4.613852347352193739, 4.277249248199312071, 1.214306433183764966E-14 ) ) ;
#53590=CARTESIAN_POINT ( 'NONE',  ( 5.615048174354031474, 9.702639970055050966, 0.7998128361456462443 ) ) ;
#53591=CARTESIAN_POINT ( 'NONE',  ( 1.364683531249988535, 4.655208333674755394, -0.7879004041258300672 ) ) ;
#53597=CARTESIAN_POINT ( 'NONE',  ( 5.056828107772846082, 6.922718763866881453, -1.443375672974051449 ) ) ;
#53598=CARTESIAN_POINT ( 'NONE',  ( -5.208303565944065738, 9.228104593576741621, -0.7998128361456231517 ) ) ;
#53602=CARTESIAN_POINT ( 'NONE',  ( -6.170932472514347289, 10.35117165124207972, 0.000000000000000000 ) ) ;
#53603=CARTESIAN_POINT ( 'NONE',  ( -6.586563698140583512, 6.578745824119123675, 1.040834085586084257E-14 ) ) ;
#53607=FACE_OUTER_BOUND ( 'NONE', #84567, .T. ) ;
#53608=EDGE_CURVE ( 'NONE', #44957, #121448, #111559, .T. ) ;
#53611=CARTESIAN_POINT ( 'NONE',  ( 6.252281394196331554, 10.44607872653774372, 1.040834085586084257E-14 ) ) ;
#53621=AXIS2_PLACEMENT_3D ( 'NONE', #100947, #37015, #152910 ) ;
#53626=CARTESIAN_POINT ( 'NONE',  ( -0.7500000000000215383, 5.441666666666685082, 1.299038105676671107 ) ) ;
#53627=CARTESIAN_POINT ( 'NONE',  ( 3.551346171775753735, 6.230655402791975384, 1.199719254218462483 ) ) ;
#53628=CARTESIAN_POINT ( 'NONE',  ( 4.819033534653518025, 7.709623992816043270, -1.199719254218452047 ) ) ;
#53630=CARTESIAN_POINT ( 'NONE',  ( -6.385527162356466668, 10.39360608948380182, 0.000000000000000000 ) ) ;
#53631=CARTESIAN_POINT ( 'NONE',  ( 6.805829924380118356, 7.042482454639357847, 0.7216878364870317197 ) ) ;
#53632=CARTESIAN_POINT ( 'NONE',  ( -7.171900071504729191, 11.31104115015678779, -0.7216878364870267237 ) ) ;
#53635=CARTESIAN_POINT ( 'NONE',  ( 6.913768267964901071, 10.15348118167935709, -1.199719254218441611 ) ) ;
#53641=CARTESIAN_POINT ( 'NONE',  ( -1.364683531249997417, 2.509375000341422357, 1.214306433183764966E-14 ) ) ;
#53648=CARTESIAN_POINT ( 'NONE',  ( 7.072549687823125097, 11.40305840243567381, -0.7998128361456291469 ) ) ;
#53651=CARTESIAN_POINT ( 'NONE',  ( -7.655550293210764856, 12.08322577538792331, 0.000000000000000000 ) ) ;
#53657=CARTESIAN_POINT ( 'NONE',  ( 8.353795204314554468, 12.89784483834236184, -0.7998128361456352531 ) ) ;
#53661=CARTESIAN_POINT ( 'NONE',  ( -9.317477881089553549, 11.89347683273641820, 1.599625672291281386 ) ) ;
#53668=CARTESIAN_POINT ( 'NONE',  ( 5.888650760256147088, 5.979308965038350188, -0.1076000636002025918 ) ) ;
#53669=CARTESIAN_POINT ( 'NONE',  ( -2.442440228756222353, 6.001264033524212671, -0.7998128361456281477 ) ) ;
#53673=CARTESIAN_POINT ( 'NONE',  ( 7.344766530301147789, 9.591980256816594164, 1.599625672291281386 ) ) ;
#53675=CARTESIAN_POINT ( 'NONE',  ( 5.991813822235618758, 9.077867661661846554, 1.199719254218462483 ) ) ;
#53676=CARTESIAN_POINT ( 'NONE',  ( 5.172599298813543633, 5.993452922492633839, -1.199719254218452047 ) ) ;
#53678=CARTESIAN_POINT ( 'NONE',  ( -6.548225005720456515, 10.58342024007512983, 0.000000000000000000 ) ) ;
#53687=CARTESIAN_POINT ( 'NONE',  ( -5.513283157632952403, 6.248865724650796594, -0.9728955443181900309 ) ) ;
#53690=CARTESIAN_POINT ( 'NONE',  ( 5.721177635286841756, 6.737423998331861341, -1.082531754730543083 ) ) ;
#53693=EDGE_CURVE ( 'NONE', #160642, #11923, #48609, .T. ) ;
#53694=CIRCLE ( 'NONE', #192054, 1.219999999999999751 ) ;
#53709=CARTESIAN_POINT ( 'NONE',  ( -9.937763408692596556, 11.65677406730528887, -1.082531754730537976 ) ) ;
#53713=CARTESIAN_POINT ( 'NONE',  ( 6.923409998072794558, 11.22906209772695618, 1.040834085586084257E-14 ) ) ;
#53717=CARTESIAN_POINT ( 'NONE',  ( 1.499999999999989120, 2.056250000682817269, 1.214306433183764966E-14 ) ) ;
#53719=CARTESIAN_POINT ( 'NONE',  ( -4.771579997005698459, 7.654261532226910525, -1.199719254218452047 ) ) ;
#53721=ORIENTED_EDGE ( 'NONE', *, *, #156347, .F. ) ;
#53722=CARTESIAN_POINT ( 'NONE',  ( -8.833300774503376473, 10.26427131079744193, 1.199719254218462483 ) ) ;
#53726=CARTESIAN_POINT ( 'NONE',  ( 7.610204295972345712, 7.772993188256215547, 0.7998128361456341429 ) ) ;
#53729=CARTESIAN_POINT ( 'NONE',  ( -7.172426956829277778, 8.326585190177668849, -1.199719254218452935 ) ) ;
#53731=CARTESIAN_POINT ( 'NONE',  ( 8.289920859751990889, 11.75899253876431416, 1.199719254218450271 ) ) ;
#53732=CARTESIAN_POINT ( 'NONE',  ( -1.001543065824772872E-14, 5.571875000341416140, 1.575800808251672791 ) ) ;
#53738=CARTESIAN_POINT ( 'NONE',  ( -8.026063749610061748, 9.426457798375635022, -1.082531754730543971 ) ) ;
#53741=CARTESIAN_POINT ( 'NONE',  ( -1.364683531249997417, 4.571875000341417028, 1.214306433183764966E-14 ) ) ;
#53746=CARTESIAN_POINT ( 'NONE',  ( 1.364683531249990311, 5.134375000341417916, 1.214306433183764966E-14 ) ) ;
#53748=CARTESIAN_POINT ( 'NONE',  ( -6.471393748265563239, 5.229711127717889596, 2.419999999999998597 ) ) ;
#53749=CARTESIAN_POINT ( 'NONE',  ( -4.406036734316900905, 5.203092947200234519, -1.082531754730543971 ) ) ;
#53752=CARTESIAN_POINT ( 'NONE',  ( 2.806174607904299734, 5.257325561654889512, -1.082531754730543083 ) ) ;
#53753=CARTESIAN_POINT ( 'NONE',  ( -0.6823417656249969321, 4.780208333674755394, -1.181850606188749264 ) ) ;
#53754=CARTESIAN_POINT ( 'NONE',  ( -9.938290294017125603, 11.55342575023019691, -1.199719254218441611 ) ) ;
#53759=CARTESIAN_POINT ( 'NONE',  ( -1.364683531250012516, 0.7802083336747528408, 0.7879004041258379498 ) ) ;
#53760=CARTESIAN_POINT ( 'NONE',  ( -3.253593677599670109, 5.779314476299451719, 1.082531754730560403 ) ) ;
#53761=CARTESIAN_POINT ( 'NONE',  ( 4.792970997630896512, 5.550553237779539018, 1.199719254218464037 ) ) ;
#53763=ADVANCED_FACE ( 'NONE', ( #99876 ), #165939, .F. ) ;
#53768=DIRECTION ( 'NONE',  ( 3.451266460341927524E-31, -0.6000000000000035305, 0.7999999999999974909 ) ) ;
#53771=CARTESIAN_POINT ( 'NONE',  ( -9.192064960385334160, 9.826423329978791088, 0.7216878364870438212 ) ) ;
#53776=CARTESIAN_POINT ( 'NONE',  ( -8.025536864285518490, 11.45054454405341282, -1.199719254218446718 ) ) ;
#53777=CARTESIAN_POINT ( 'NONE',  ( -4.568734577680887199, 6.353276312092901890, -1.443375672974051449 ) ) ;
#53778=CARTESIAN_POINT ( 'NONE',  ( 0.6823417656249882723, 1.738541667008083991, -1.181850606188749264 ) ) ;
#53785=CARTESIAN_POINT ( 'NONE',  ( 9.398826802771546696, 11.98838390803207865, -1.599625672291262513 ) ) ;
#53793=VERTEX_POINT ( 'NONE', #169131 ) ;
#53794=EDGE_LOOP ( 'NONE', ( #89421, #88183, #132044, #199946, #26203, #51432, #141597, #139329, #175578, #137751, #46600, #165333, #201812, #65987, #206476, #133507, #7549, #204912, #140151, #148727 ) ) ;
#53798=DIRECTION ( 'NONE',  ( 0.000000000000000000, -1.000000000000000000, 0.000000000000000000 ) ) ;
#53803=CARTESIAN_POINT ( 'NONE',  ( -0.6823417656249969321, 3.280208333674754062, -1.181850606188749264 ) ) ;
#53805=CIRCLE ( 'NONE', #195597, 0.07999999999999984901 ) ;
#53809=CYLINDRICAL_SURFACE ( 'NONE', #172026, 1.250000000000000000 ) ;
#53812=CARTESIAN_POINT ( 'NONE',  ( 10.39640486358069360, 11.02356051713265650, 0.7998128361456462443 ) ) ;
#53814=CARTESIAN_POINT ( 'NONE',  ( 1.364683531249988757, 1.384375000341421469, 0.000000000000000000 ) ) ;
#53824=CARTESIAN_POINT ( 'NONE',  ( 3.845709127770629010, 7.638411082374393146, 0.7998128361456321445 ) ) ;
#53828=CARTESIAN_POINT ( 'NONE',  ( 9.622536337397022521, 12.24937836509514710, 1.599625672291281386 ) ) ;
#53833=EDGE_LOOP ( 'NONE', ( #182161, #121566, #70842, #84516 ) ) ;
#53835=CARTESIAN_POINT ( 'NONE',  ( -2.839543107058306592, 5.400218493954923815, -1.199719254218446718 ) ) ;
#53836=CARTESIAN_POINT ( 'NONE',  ( 9.121938423896107651, 9.536683004167278099, -0.7998128361456221525 ) ) ;
#53837=DIRECTION ( 'NONE',  ( 0.7592566023652994600, 0.6507913734559651608, 0.000000000000000000 ) ) ;
#53847=CARTESIAN_POINT ( 'NONE',  ( -7.782016984564068096, 10.10210578678999482, 1.443375672974090751 ) ) ;
#53849=CARTESIAN_POINT ( 'NONE',  ( 6.986529229743720926, 7.045372277656132276, -0.7998128361456281477 ) ) ;
#53852=CARTESIAN_POINT ( 'NONE',  ( -8.299562589859897699, 12.83457345481192036, -0.7998128361456281477 ) ) ;
#53857=CARTESIAN_POINT ( 'NONE',  ( -3.972702704004144714, 4.593573561881607148, 1.199719254218462483 ) ) ;
#53859=CARTESIAN_POINT ( 'NONE',  ( 9.561524646135536543, 12.17819805862340310, -1.599625672291262513 ) ) ;
#53860=CARTESIAN_POINT ( 'NONE',  ( 4.552840656090682891, 4.206068941727564514, 1.214306433183764966E-14 ) ) ;
#53866=CARTESIAN_POINT ( 'NONE',  ( 4.853455804012228647, 4.764712647543454693, 0.7216878364870317197 ) ) ;
#53869=CARTESIAN_POINT ( 'NONE',  ( -5.915435094264120508, 5.795762452929912101, 0.000000000000000000 ) ) ;
#53872=CARTESIAN_POINT ( 'NONE',  ( -8.123306592882240551, 12.62894145833798376, 0.000000000000000000 ) ) ;
#53877=CARTESIAN_POINT ( 'NONE',  ( 7.782016984564054773, 10.10210578678999482, 1.443375672974076540 ) ) ;
#53878=CARTESIAN_POINT ( 'NONE',  ( 0.6823417656249899377, 5.238541667008086655, -1.181850606188754593 ) ) ;
#53880=CARTESIAN_POINT ( 'NONE',  ( 5.522248639467795428, 5.337044922334209573, -0.7998128361456231517 ) ) ;
#53885=CARTESIAN_POINT ( 'NONE',  ( 1.426686711745578151, 7.396164654317697540, 4.272688476054470996 ) ) ;
#53892=CARTESIAN_POINT ( 'NONE',  ( 0.6823417656249899377, 3.155208333674754062, 1.181850606188765695 ) ) ;
#53894=CARTESIAN_POINT ( 'NONE',  ( 8.543609354905870035, 13.11929468069890525, 0.7998128361456462443 ) ) ;
#53896=CARTESIAN_POINT ( 'NONE',  ( -5.585596099150193616, 6.579245539505756746, -1.082531754730544860 ) ) ;
#53899=CARTESIAN_POINT ( 'NONE',  ( -6.060131475184148186, 6.172500930577367484, 0.7216878364870317197 ) ) ;
#53903=ORIENTED_EDGE ( 'NONE', *, *, #123570, .F. ) ;
#53905=CARTESIAN_POINT ( 'NONE',  ( 4.313465427442102929, 8.184126765324453601, 0.7998128361456462443 ) ) ;
#53914=CARTESIAN_POINT ( 'NONE',  ( 7.142447996300871793, 7.227277505306155092, 0.7998128361456341429 ) ) ;
#53919=CARTESIAN_POINT ( 'NONE',  ( -5.605406444246153974, 8.627059054007450101, -1.199719254218440723 ) ) ;
#53923=CARTESIAN_POINT ( 'NONE',  ( 7.558834334818744338, 8.777393797832065303, 1.199719254218462483 ) ) ;
#53926=CARTESIAN_POINT ( 'NONE',  ( -7.711890448074853133, 7.891627032375787998, -0.7998128361456291469 ) ) ;
#53927=CARTESIAN_POINT ( 'NONE',  ( 6.683806541412754321, 8.820860269780128604, -1.443375672974058777 ) ) ;
#53928=CARTESIAN_POINT ( 'NONE',  ( 4.137223920935246824, 7.648466568186386816, 0.7801199165378830402 ) ) ;
#53929=ADVANCED_FACE ( 'NONE', ( #135583 ), #127764, .T. ) ;
#53930=CARTESIAN_POINT ( 'NONE',  ( -4.894657149733403045, 5.669187081899118574, -1.199719254218446718 ) ) ;
#53934=CARTESIAN_POINT ( 'NONE',  ( -6.098470168048611306, 6.009303372345148553, 1.040834085586084257E-14 ) ) ;
#53937=CARTESIAN_POINT ( 'NONE',  ( -1.201851678989727383E-14, 2.071875000341422801, 1.575800808251672791 ) ) ;
#53939=CARTESIAN_POINT ( 'NONE',  ( -4.934804725694220906, 7.740727365743146571, -1.082531754730549967 ) ) ;
#53945=CARTESIAN_POINT ( 'NONE',  ( 7.318703993278529829, 7.432909501780090800, 1.040834085586084257E-14 ) ) ;
#53947=CARTESIAN_POINT ( 'NONE',  ( -1.402160292154681736E-14, 2.509375000341417028, -1.575800808251660134 ) ) ;
#53954=CARTESIAN_POINT ( 'NONE',  ( -3.438964519360665051, 7.163875705896082913, -0.7998128361456281477 ) ) ;
#53955=CARTESIAN_POINT ( 'NONE',  ( -6.195713011320783892, 10.17215624660883577, -0.7216878364870267237 ) ) ;
#53963=CARTESIAN_POINT ( 'NONE',  ( -7.985389288324703294, 9.379004260209384825, -1.082531754730543083 ) ) ;
#53969=CARTESIAN_POINT ( 'NONE',  ( -6.033015167956800262, 9.021972881716168402, -1.082531754730537976 ) ) ;
#53972=ORIENTED_EDGE ( 'NONE', *, *, #56788, .F. ) ;
#53983=CARTESIAN_POINT ( 'NONE',  ( -4.720210035852093533, 8.658662141802762946, -0.7998128361456281477 ) ) ;
#53985=CARTESIAN_POINT ( 'NONE',  ( 4.334856428067313416, 6.080418470877079429, -1.599625672291256295 ) ) ;
#53989=CARTESIAN_POINT ( 'NONE',  ( 6.388916700537700777, 8.476822122092563916, 1.599625672291281386 ) ) ;
#53994=CARTESIAN_POINT ( 'NONE',  ( -5.612712406377534435, 5.650512016969639895, 0.7216878364870317197 ) ) ;
#54003=CARTESIAN_POINT ( 'NONE',  ( -0.6823417656250003738, 0.9677083336747521747, -1.181850606188749264 ) ) ;
#54005=CARTESIAN_POINT ( 'NONE',  ( -8.311311860377216476, 9.655284244316948872, -1.199719254218446718 ) ) ;
#54007=CARTESIAN_POINT ( 'NONE',  ( 6.714312387265682247, 8.856450423275211037, 1.599625672291281386 ) ) ;
#54009=CARTESIAN_POINT ( 'NONE',  ( -6.028571859570855729, 10.18508426947466816, 0.000000000000000000 ) ) ;
#54012=CARTESIAN_POINT ( 'NONE',  ( 1.499999999999987566, -0.6937499993171849511, 0.000000000000000000 ) ) ;
#54014=CARTESIAN_POINT ( 'NONE',  ( 7.456621297836061757, 11.64321591421002644, 0.7216878364870438212 ) ) ;
#54015=EDGE_CURVE ( 'NONE', #67678, #153088, #156682, .T. ) ;
#54018=CARTESIAN_POINT ( 'NONE',  ( -1.402160292154681736E-14, -0.7406249996585823059, -1.575800808251665908 ) ) ;
#54021=CARTESIAN_POINT ( 'NONE',  ( 6.602457619730756733, 9.686322408785807525, 1.082531754730558626 ) ) ;
#54024=CARTESIAN_POINT ( 'NONE',  ( -6.100805936469506641, 6.219954468743612352, 0.7216878364870317197 ) ) ;
#54027=CARTESIAN_POINT ( 'NONE',  ( -1.364683531250012516, 3.530208333674758059, 0.7879004041258379498 ) ) ;
#54029=CARTESIAN_POINT ( 'NONE',  ( 3.146123468421266001, 6.442327133617253843, 0.5169845646841256803 ) ) ;
#54031=CARTESIAN_POINT ( 'NONE',  ( -5.368138756007025947, 8.350246751061767725, 1.199719254218452047 ) ) ;
#54032=CARTESIAN_POINT ( 'NONE',  ( -1.364683531250010295, 5.801041667008088432, -0.7879004041258300672 ) ) ;
#54037=EDGE_CURVE ( 'NONE', #57355, #80549, #92917, .T. ) ;
#54040=CARTESIAN_POINT ( 'NONE',  ( 7.747594715205354809, 11.12627870345989756, -1.199719254218446718 ) ) ;
#54043=CARTESIAN_POINT ( 'NONE',  ( -0.7499999999999972244, 3.108333333333358706, -1.299038105676652011 ) ) ;
#54049=CARTESIAN_POINT ( 'NONE',  ( 5.775410249741494972, 8.721433810464993996, -1.082531754730537088 ) ) ;
#54053=CARTESIAN_POINT ( 'NONE',  ( 2.530568227245037605, 6.104080031761181857, 0.000000000000000000 ) ) ;
#54058=CONICAL_SURFACE ( 'NONE', #164755, 4.000000000000000000, 0.8960553845713404852 ) ;
#54059=CARTESIAN_POINT ( 'NONE',  ( -1.500000000000001332, 0.9000000000000187850, 0.000000000000000000 ) ) ;
#54060=CARTESIAN_POINT ( 'NONE',  ( 6.903072767652295383, 11.20533532890304684, 1.040834085586084257E-14 ) ) ;
#54061=CARTESIAN_POINT ( 'NONE',  ( -7.669108446824431269, 12.09904362127053545, -0.7998128361456291469 ) ) ;
#54063=EDGE_CURVE ( 'NONE', #69090, #183003, #46087, .T. ) ;
#54064=CARTESIAN_POINT ( 'NONE',  ( -0.6823417656250246877, 0.5510416670080897639, 1.181850606188755259 ) ) ;
#54065=CARTESIAN_POINT ( 'NONE',  ( 1.499999999999987121, 1.795833333333355819, -0.8660254037844253849 ) ) ;
#54067=CARTESIAN_POINT ( 'NONE',  ( 4.741601036477289810, 6.554953847355395880, 1.599625672291267398 ) ) ;
#54074=CARTESIAN_POINT ( 'NONE',  ( -1.001543065824772872E-14, 4.821875000341419693, 1.575800808251672791 ) ) ;
#54076=CARTESIAN_POINT ( 'NONE',  ( -8.453672473320708036, 9.821371626084353323, -1.199719254218446718 ) ) ;
#54077=CARTESIAN_POINT ( 'NONE',  ( -6.087247782855839340, 6.204136622861004646, 0.000000000000000000 ) ) ;
#54079=DIRECTION ( 'NONE',  ( 1.000000000000000000, 0.000000000000000000, 0.000000000000000000 ) ) ;
#54082=CARTESIAN_POINT ( 'NONE',  ( 4.015551651036665781, 7.573759128756977432, -0.3041731733383628566 ) ) ;
#54085=CARTESIAN_POINT ( 'NONE',  ( 5.940443861082012944, 10.08226827123770697, 0.7998128361456462443 ) ) ;
#54088=CARTESIAN_POINT ( 'NONE',  ( 6.114364089638782751, 9.116879957011832403, 1.082531754730558626 ) ) ;
#54092=VECTOR ( 'NONE', #152908, 1000.000000000000000 ) ;
#54093=CARTESIAN_POINT ( 'NONE',  ( -8.453672473320708036, 9.821371626084353323, -1.199719254218446718 ) ) ;
#54094=CARTESIAN_POINT ( 'NONE',  ( 5.005985031943777308, 6.863401842066294556, -1.599625672291256295 ) ) ;
#54097=CARTESIAN_POINT ( 'NONE',  ( 2.347533153460546806, 5.890539112345938300, 0.000000000000000000 ) ) ;
#54103=CARTESIAN_POINT ( 'NONE',  ( 2.273922426215241099, 5.667243959216540006, 0.4897358640176532329 ) ) ;
#54104=CARTESIAN_POINT ( 'NONE',  ( -1.561525566895192618, 8.688907412369037075, -2.501944002935404310 ) ) ;
#54105=CARTESIAN_POINT ( 'NONE',  ( -5.260200412422213923, 6.199617238323108737, -1.082531754730544860 ) ) ;
#54106=CARTESIAN_POINT ( 'NONE',  ( 8.256552361042350796, 12.57646882128404187, 1.040834085586084257E-14 ) ) ;
#54109=CARTESIAN_POINT ( 'NONE',  ( -6.287230548435221777, 8.358188277972981695, -1.599625672291263179 ) ) ;
#54114=CARTESIAN_POINT ( 'NONE',  ( 6.518203450479836292, 5.167241622962441383, 2.437504649502901355 ) ) ;
#54116=CARTESIAN_POINT ( 'NONE',  ( -6.157374318900681764, 10.33535380535947290, 0.7998128361456481317 ) ) ;
#54130=EDGE_CURVE ( 'NONE', #107270, #179291, #137181, .T. ) ;
#54132=CARTESIAN_POINT ( 'NONE',  ( -6.181627972826976958, 9.299317504018391745, 1.199719254218452047 ) ) ;
#54135=CARTESIAN_POINT ( 'NONE',  ( 5.341549334104188418, 7.254893527920112994, 1.443375672974062551 ) ) ;
#54139=CARTESIAN_POINT ( 'NONE',  ( -3.262708522383007903, 6.958243709422141876, 1.040834085586084257E-14 ) ) ;
#54143=CARTESIAN_POINT ( 'NONE',  ( -4.855791571988752331, 8.816840600628864877, 0.7998128361456481317 ) ) ;
#54144=CARTESIAN_POINT ( 'NONE',  ( -5.903988413730030693, 6.004926949446717011, -0.1838238861417510472 ) ) ;
#54148=CARTESIAN_POINT ( 'NONE',  ( -9.341731535015849630, 10.85744053139533349, 1.199719254218462483 ) ) ;
#54149=CARTESIAN_POINT ( 'NONE',  ( 7.263417608619159083, 9.497073181520933716, -1.599625672291262513 ) ) ;
#54152=CARTESIAN_POINT ( 'NONE',  ( -9.053093885623068715, 11.58502883802551153, -1.599625672291263179 ) ) ;
#54159=CARTESIAN_POINT ( 'NONE',  ( 9.571693261567965294, 10.26932301469188857, 0.7216878364870438212 ) ) ;
#54164=CARTESIAN_POINT ( 'NONE',  ( -5.426287360647527258, 6.306760859481674864, -1.047964138152550406 ) ) ;
#54166=CARTESIAN_POINT ( 'NONE',  ( -0.1822957779078477336, 6.496859778797933416, -3.113708315861777098 ) ) ;
#54176=CARTESIAN_POINT ( 'NONE',  ( -4.029797971759847997, 5.724516938518342535, -1.599625672291256295 ) ) ;
#54183=CARTESIAN_POINT ( 'NONE',  ( 1.499999999999987566, -1.193749999317185395, 0.000000000000000000 ) ) ;
#54187=CARTESIAN_POINT ( 'NONE',  ( 10.55232363013785246, 11.20546574478267132, 0.000000000000000000 ) ) ;
#54189=CARTESIAN_POINT ( 'NONE',  ( 1.123270288250309834, 2.971052654332832610, -0.7749999999993620881 ) ) ;
#54190=CARTESIAN_POINT ( 'NONE',  ( 0.07727525906045540349, 7.079397053215386038, -2.120984693056187531 ) ) ;
#54192=CARTESIAN_POINT ( 'NONE',  ( 2.544126380858701797, 6.119897877643793116, 0.7998128361456462443 ) ) ;
#54198=CARTESIAN_POINT ( 'NONE',  ( 6.094553744542824170, 7.069066442510145265, 1.199719254218462483 ) ) ;
#54199=CARTESIAN_POINT ( 'NONE',  ( -1.364683531249997417, 3.071875000341423245, 1.214306433183764966E-14 ) ) ;
#54200=CARTESIAN_POINT ( 'NONE',  ( -4.836546220603817225, 6.746162335969787094, 1.249072166269946216 ) ) ;
#54201=CARTESIAN_POINT ( 'NONE',  ( 9.541187415715040032, 12.15447128979948310, -1.599625672291262513 ) ) ;
#54204=CARTESIAN_POINT ( 'NONE',  ( -7.157815033010924921, 10.43820240756634199, 1.199719254218453823 ) ) ;
#54206=CARTESIAN_POINT ( 'NONE',  ( -5.056828107772866510, 5.962349549565537643, -1.082531754730543971 ) ) ;
#54209=CARTESIAN_POINT ( 'NONE',  ( -5.392392409933270514, 7.314210449720692786, 1.599625672291269396 ) ) ;
#54211=CARTESIAN_POINT ( 'NONE',  ( -0.7500000000000215383, 0.4729166673494850093, 1.299038105676659116 ) ) ;
#54219=CARTESIAN_POINT ( 'NONE',  ( -4.894130264408878439, 4.812166184672871161, -0.7216878364870197293 ) ) ;
#54220=CARTESIAN_POINT ( 'NONE',  ( 0.4702634422546589366, 7.494255424137728383, -4.464191613399470349 ) ) ;
#54225=CARTESIAN_POINT ( 'NONE',  ( -4.595850884908229794, 4.464173575255435011, 0.7216878364870317197 ) ) ;
#54227=CARTESIAN_POINT ( 'NONE',  ( 9.433775957010412938, 9.900493459467314850, 0.000000000000000000 ) ) ;
#54237=CARTESIAN_POINT ( 'NONE',  ( -9.592557376868645846, 11.15007068022363157, -1.199719254218441611 ) ) ;
#54242=CARTESIAN_POINT ( 'NONE',  ( 5.867981556616276073, 5.740399992340775803, -0.7998128361456281477 ) ) ;
#54247=FACE_OUTER_BOUND ( 'NONE', #42829, .T. ) ;
#54248=CARTESIAN_POINT ( 'NONE',  ( 3.541704441667858472, 5.155074486744371853, -1.599625672291262513 ) ) ;
#54251=ORIENTED_EDGE ( 'NONE', *, *, #34448, .T. ) ;
#54259=CARTESIAN_POINT ( 'NONE',  ( 8.932124273304774320, 9.315233161810734686, 0.7998128361456462443 ) ) ;
#54261=CARTESIAN_POINT ( 'NONE',  ( -5.005985031943793295, 6.863401842066301661, -1.599625672291256295 ) ) ;
#54267=CARTESIAN_POINT ( 'NONE',  ( -1.364683531250010295, 5.738541667008088432, -0.7879004041258300672 ) ) ;
#54272=CARTESIAN_POINT ( 'NONE',  ( 4.111146893441827821, 5.819424013814004759, 1.599625672291267398 ) ) ;
#54273=CARTESIAN_POINT ( 'NONE',  ( -5.759516327706961647, 5.613857225279885732, -0.7998128361456221525 ) ) ;
#54279=CARTESIAN_POINT ( 'NONE',  ( 6.168596704537822717, 6.299043698156668647, 1.040834085586084257E-14 ) ) ;
#54283=CARTESIAN_POINT ( 'NONE',  ( 8.554831740098659765, 10.04335378727902395, 1.082531754730558626 ) ) ;
#54284=CARTESIAN_POINT ( 'NONE',  ( -1.201851678989727383E-14, 3.009375000341419248, -1.575800808251660134 ) ) ;
#54286=CARTESIAN_POINT ( 'NONE',  ( 5.626270559546826533, 5.666329862333828515, 0.7216878364870317197 ) ) ;
#54290=CARTESIAN_POINT ( 'NONE',  ( 5.530578433931943927, 6.204385438716983003, -0.9373897679112530579 ) ) ;
#54293=CARTESIAN_POINT ( 'NONE',  ( -5.301779071304492774, 6.560601962741976045, 1.383466813282836716 ) ) ;
#54300=CARTESIAN_POINT ( 'NONE',  ( -9.317477881089553549, 11.89347683273641820, 1.599625672291281386 ) ) ;
#54305=CARTESIAN_POINT ( 'NONE',  ( -4.081167932913447594, 4.720116328942494555, -1.199719254218452047 ) ) ;
#54310=CARTESIAN_POINT ( 'NONE',  ( 4.229780737783593203, 4.037091736943370535, -0.7216878364870188411 ) ) ;
#54311=CARTESIAN_POINT ( 'NONE',  ( -1.201851678989727383E-14, 3.384375000341421469, 1.575800808251672791 ) ) ;
#54313=CARTESIAN_POINT ( 'NONE',  ( 6.449928391799196525, 8.548002428564306143, -1.599625672291262513 ) ) ;
#54314=CARTESIAN_POINT ( 'NONE',  ( -8.479735010343349089, 11.98044238112085758, 1.199719254218453823 ) ) ;
#54316=CARTESIAN_POINT ( 'NONE',  ( -5.264643720808155791, 5.036505850564608089, 0.000000000000000000 ) ) ;
#54320=CARTESIAN_POINT ( 'NONE',  ( 1.499999999999989120, 4.504166666666688634, 0.8660254037844524744 ) ) ;
#54321=CARTESIAN_POINT ( 'NONE',  ( 4.473300617505036492, 7.306268922809479704, -1.199719254218452047 ) ) ;
#54325=CARTESIAN_POINT ( 'NONE',  ( 1.499999999999990674, 8.226475397238271370, 3.114076396431860960 ) ) ;
#54327=CARTESIAN_POINT ( 'NONE',  ( -1.364683531249997417, 4.509375000341424133, 1.214306433183764966E-14 ) ) ;
#54330=CARTESIAN_POINT ( 'NONE',  ( 9.408995418203971894, 11.03987807840189816, 1.082531754730549967 ) ) ;
#54335=CARTESIAN_POINT ( 'NONE',  ( 0.7499999999999885647, 1.847916667349486231, -1.299038105676652899 ) ) ;
#54337=CARTESIAN_POINT ( 'NONE',  ( -5.148345644887285744, 7.029489223833707001, -1.599625672291256295 ) ) ;
#54339=CARTESIAN_POINT ( 'NONE',  ( 3.348500752450937590, 5.890039396959305229, 1.082531754730558626 ) ) ;
#54348=CARTESIAN_POINT ( 'NONE',  ( 6.795661308947685164, 8.951357498570873261, -1.599625672291262513 ) ) ;
#54349=CARTESIAN_POINT ( 'NONE',  ( 5.172599298813543633, 5.993452922492633839, -1.199719254218452047 ) ) ;
#54352=SURFACE_STYLE_USAGE ( .BOTH. , #134564 ) ;
#54353=CARTESIAN_POINT ( 'NONE',  ( 3.655894977179307226, 7.416961240017848844, -0.7998128361456291469 ) ) ;
#54357=ORIENTED_EDGE ( 'NONE', *, *, #96785, .T. ) ;
#54359=ORIENTED_EDGE ( 'NONE', *, *, #138422, .T. ) ;
#54360=CARTESIAN_POINT ( 'NONE',  ( 8.432281472695482449, 11.92507992053172572, 1.199719254218450271 ) ) ;
#54361=FACE_OUTER_BOUND ( 'NONE', #28249, .T. ) ;
#54365=CARTESIAN_POINT ( 'NONE',  ( 5.064587263324675348, 6.532718652379178259, -1.222898410871699593 ) ) ;
#54369=CARTESIAN_POINT ( 'NONE',  ( 3.469446951953614189E-15, 5.290451655907108197, 1.214306433183764966E-14 ) ) ;
#54370=CARTESIAN_POINT ( 'NONE',  ( -4.853455804012230423, 6.685451076146141425, 1.443375672974064550 ) ) ;
#54373=DIRECTION ( 'NONE',  ( 6.314299915563594049E-62, 8.546850786086437571E-32, 1.000000000000000000 ) ) ;
#54374=CARTESIAN_POINT ( 'NONE',  ( 1.364683531249986537, -1.136458332991912235, 0.7879004041258500513 ) ) ;
#54375=CARTESIAN_POINT ( 'NONE',  ( 8.270110514656037637, 8.750809809961280550, 0.7216878364870458196 ) ) ;
#54376=CARTESIAN_POINT ( 'NONE',  ( -4.939248034080176097, 4.656877549381960080, 1.214306433183764966E-14 ) ) ;
#54380=CARTESIAN_POINT ( 'NONE',  ( -5.901876940650454095, 5.779944607047298177, -0.7998128361456291469 ) ) ;
#54392=CARTESIAN_POINT ( 'NONE',  ( 8.127223016387999266, 11.56917838817298616, 1.199719254218460707 ) ) ;
#54393=CARTESIAN_POINT ( 'NONE',  ( 6.067506501917478090, 6.045351875519452634, 0.3962785553160239616 ) ) ;
#54395=ORIENTED_EDGE ( 'NONE', *, *, #123006, .T. ) ;
#54397=DIRECTION ( 'NONE',  ( -0.6507913734559640506, -0.7592566023653004592, 0.000000000000000000 ) ) ;
#54399=CARTESIAN_POINT ( 'NONE',  ( -3.763657168278658816, 3.180244510940675173, 2.446973152615721236 ) ) ;
#54400=CARTESIAN_POINT ( 'NONE',  ( -10.03267048443264109, 11.76749898900197877, 1.082531754730558626 ) ) ;
#54405=CARTESIAN_POINT ( 'NONE',  ( 7.751511138711133064, 10.06651563329490529, -1.599625672291262513 ) ) ;
#54409=CARTESIAN_POINT ( 'NONE',  ( -7.009729113465285266, 8.136771039586342624, -1.199719254218446718 ) ) ;
#54410=CARTESIAN_POINT ( 'NONE',  ( 4.039439701867726384, 6.800097854565950506, 1.199719254218462483 ) ) ;
#54413=CARTESIAN_POINT ( 'NONE',  ( 0.2412978493891524412, 7.030157881589111035, 3.919897618274023277 ) ) ;
#54416=CARTESIAN_POINT ( 'NONE',  ( 4.459584003380381745, 7.054591843250856975, -1.127873490090089748 ) ) ;
#54417=VERTEX_POINT ( 'NONE', #29288 ) ;
#54419=CARTESIAN_POINT ( 'NONE',  ( 5.260200412422194383, 7.159986452624450770, -1.443375672974051449 ) ) ;
#54428=CARTESIAN_POINT ( 'NONE',  ( 8.120970824461352322, 9.537182719035495637, -1.082531754730543083 ) ) ;
#54431=CARTESIAN_POINT ( 'NONE',  ( -8.947491310014823895, 12.52615806407091803, 1.199719254218462483 ) ) ;
#54432=CARTESIAN_POINT ( 'NONE',  ( -7.690499447449645309, 9.995335326823163058, 1.599625672291295375 ) ) ;
#54441=CARTESIAN_POINT ( 'NONE',  ( 4.054051625686104998, 4.688480637177271149, -1.199719254218446718 ) ) ;
#54445=CARTESIAN_POINT ( 'NONE',  ( 3.649115900372475796, 7.409052317076538330, 1.040834085586084257E-14 ) ) ;
#54448=CARTESIAN_POINT ( 'NONE',  ( -0.7500000000000215383, 2.222916667349486453, 1.299038105676671107 ) ) ;
#54454=CARTESIAN_POINT ( 'NONE',  ( -1.500000000000001332, 1.150000000000019007, 0.000000000000000000 ) ) ;
#54455=CARTESIAN_POINT ( 'NONE',  ( 7.344766530301147789, 9.591980256816594164, 1.599625672291281386 ) ) ;
#54456=CARTESIAN_POINT ( 'NONE',  ( 5.327991180046175224, 5.318337252916401248, -0.7216878364870207285 ) ) ;
#54460=CARTESIAN_POINT ( 'NONE',  ( 9.761507412159302177, 10.49077285704843199, -0.7216878364870257245 ) ) ;
#54465=CARTESIAN_POINT ( 'NONE',  ( -6.403528624356093601, 6.365204904703887223, 1.040834085586084257E-14 ) ) ;
#54466=CARTESIAN_POINT ( 'NONE',  ( 1.499999999999990896, 4.306250000682819490, 1.214306433183764966E-14 ) ) ;
#54467=CARTESIAN_POINT ( 'NONE',  ( 1.364683531249992088, 5.696875000341418804, 1.214306433183764966E-14 ) ) ;
#54472=CARTESIAN_POINT ( 'NONE',  ( -0.6823417656249969321, 4.530208333674755394, -1.181850606188749264 ) ) ;
#54479=CARTESIAN_POINT ( 'NONE',  ( -6.353967546298838087, 10.56471257065732416, 0.000000000000000000 ) ) ;
#54481=CARTESIAN_POINT ( 'NONE',  ( 5.575427483717746213, 7.527751369135936343, 1.599625672291267398 ) ) ;
#54487=CARTESIAN_POINT ( 'NONE',  ( 2.273217432877753463, 5.716990842764664293, 0.1274701612217898072 ) ) ;
#54490=CARTESIAN_POINT ( 'NONE',  ( -7.854251061018346469, 8.057714414143200443, -0.7998128361456291469 ) ) ;
#54493=CARTESIAN_POINT ( 'NONE',  ( 8.204655514564224816, 12.72384853363364066, 1.040834085586084257E-14 ) ) ;
#54495=CARTESIAN_POINT ( 'NONE',  ( 8.757677159423465696, 12.30470822171437284, 1.199719254218450271 ) ) ;
#54497=CARTESIAN_POINT ( 'NONE',  ( -3.242371291962510504, 6.934516940598226320, 1.040834085586084257E-14 ) ) ;
#54498=CARTESIAN_POINT ( 'NONE',  ( -6.347188469492005325, 10.55680364771601809, -0.7998128361456291469 ) ) ;
#54501=CARTESIAN_POINT ( 'NONE',  ( -4.044288467547167976, 7.756266588949179308, -0.5710662792986564984 ) ) ;
#54502=CARTESIAN_POINT ( 'NONE',  ( 1.364683531249986537, -1.136458332991912235, 0.7879004041258500513 ) ) ;
#54508=CARTESIAN_POINT ( 'NONE',  ( 5.819474248763732760, 7.812472595022922128, -1.599625672291262513 ) ) ;
#54531=CARTESIAN_POINT ( 'NONE',  ( -8.296699936558862731, 11.76690146170562201, 1.199719254218453823 ) ) ;
#54532=CARTESIAN_POINT ( 'NONE',  ( -4.080641063585716211, 5.783833847506671511, -1.249999999999999334 ) ) ;
#54535=CARTESIAN_POINT ( 'NONE',  ( -1.500000000000013101, 1.952083334016152527, 0.8660254037844403729 ) ) ;
#54536=CARTESIAN_POINT ( 'NONE',  ( 9.673906298550626559, 11.24497775551929557, 1.199719254218452047 ) ) ;
#54540=CARTESIAN_POINT ( 'NONE',  ( -8.533967624797991647, 12.04371376465130439, -1.199719254218446718 ) ) ;
#54542=CARTESIAN_POINT ( 'NONE',  ( 1.364683531249988757, 1.884375000341421913, 0.000000000000000000 ) ) ;
#54549=CARTESIAN_POINT ( 'NONE',  ( -3.253066792275140173, 5.882662793374543675, 1.199719254218462483 ) ) ;
#54551=CARTESIAN_POINT ( 'NONE',  ( -0.3247179164460003986, 6.996819380137557332, -3.870394258462603432 ) ) ;
#54554=CARTESIAN_POINT ( 'NONE',  ( 0.6823417656249882723, 0.4885416670080827695, -1.181850606188749264 ) ) ;
#54560=CARTESIAN_POINT ( 'NONE',  ( -1.402160292154681736E-14, 0.07187500034142156602, 1.575800808251672791 ) ) ;
#54562=CARTESIAN_POINT ( 'NONE',  ( -6.144869935491728441, 8.192100896205577243, -1.599625672291263179 ) ) ;
#54563=CARTESIAN_POINT ( 'NONE',  ( 7.401861798056875053, 10.72292363345333399, -1.199719254218441611 ) ) ;
#54564=CARTESIAN_POINT ( 'NONE',  ( 3.842846474469570062, 6.570739089268092137, -1.199719254218452047 ) ) ;
#54565=CARTESIAN_POINT ( 'NONE',  ( 6.667912619822566000, 6.673652899414787676, 1.040834085586084257E-14 ) ) ;
#54567=CARTESIAN_POINT ( 'NONE',  ( -1.201851678989727383E-14, 3.212500000000018119, 1.732050807568877637 ) ) ;
#54569=CARTESIAN_POINT ( 'NONE',  ( -1.201851678989727383E-14, 1.884375000341422135, 1.575800808251672791 ) ) ;
#54575=CARTESIAN_POINT ( 'NONE',  ( 5.002595493762530765, 8.780185809457538681, 1.040834085586084257E-14 ) ) ;
#54578=CARTESIAN_POINT ( 'NONE',  ( -8.259941899223614215, 10.65968485389279508, -1.599625672291263179 ) ) ;
#54579=CARTESIAN_POINT ( 'NONE',  ( -5.278201874421821316, 5.052323696447222900, 0.7998128361456341429 ) ) ;
#54583=DIRECTION ( 'NONE',  ( 1.000000000000000000, 0.000000000000000000, 0.000000000000000000 ) ) ;
#54585=CARTESIAN_POINT ( 'NONE',  ( -8.365017589507372620, 9.821903944922480534, 1.082531754730558626 ) ) ;
#54587=CARTESIAN_POINT ( 'NONE',  ( -1.500000000000011324, 5.629166666666693963, -0.8660254037844313801 ) ) ;
#54591=CARTESIAN_POINT ( 'NONE',  ( 8.920901888111989919, 11.43080484092926241, 1.443375672974076540 ) ) ;
#54593=CARTESIAN_POINT ( 'NONE',  ( -4.324687812634898876, 6.068555086205916105, 1.443375672974064550 ) ) ;
#54599=CARTESIAN_POINT ( 'NONE',  ( 8.880227426826630577, 12.34372051706435869, 1.082531754730546636 ) ) ;
#54603=CARTESIAN_POINT ( 'NONE',  ( 7.076992996209058973, 11.20031622897851165, 1.040834085586084257E-14 ) ) ;
#54604=CARTESIAN_POINT ( 'NONE',  ( 6.076025397218672630, 10.24044673006381245, -0.7998128361456291469 ) ) ;
#54605=CARTESIAN_POINT ( 'NONE',  ( -5.747767057189642870, 8.793146435774861658, -1.199719254218440723 ) ) ;
#54608=CARTESIAN_POINT ( 'NONE',  ( -4.113984376790197572, 3.977835813768412887, -0.5576404437566493399 ) ) ;
#54611=CARTESIAN_POINT ( 'NONE',  ( 3.877268743828270470, 5.546566172598190292, 1.443375672974062551 ) ) ;
#54613=CARTESIAN_POINT ( 'NONE',  ( -3.918470089549458635, 4.530302178351167441, -1.199719254218452047 ) ) ;
#54628=CARTESIAN_POINT ( 'NONE',  ( 6.771407655021410399, 9.987393799911945536, -1.199719254218441611 ) ) ;
#54639=CARTESIAN_POINT ( 'NONE',  ( -5.713871673155502151, 8.753601821068331290, 1.199719254218452047 ) ) ;
#54640=AXIS2_PLACEMENT_3D ( 'NONE', #108542, #9900, #124812 ) ;
#54642=CARTESIAN_POINT ( 'NONE',  ( -3.066115294984855133, 6.728884944124295053, 0.7998128361456341429 ) ) ;
#54651=CARTESIAN_POINT ( 'NONE',  ( -5.101945877444165944, 4.846691699973280976, 0.000000000000000000 ) ) ;
#54656=CARTESIAN_POINT ( 'NONE',  ( 6.775324078527185989, 8.927630729746953264, -1.599625672291262513 ) ) ;
#54657=CARTESIAN_POINT ( 'NONE',  ( -1.201851678989727383E-14, 4.196875000341417028, -1.575800808251660134 ) ) ;
#54663=CARTESIAN_POINT ( 'NONE',  ( 5.788968402910805722, 7.776882441527838807, 1.443375672974062551 ) ) ;
#54664=CARTESIAN_POINT ( 'NONE',  ( -7.588813295347149435, 9.876701482703580837, -1.599625672291263179 ) ) ;
#54667=CARTESIAN_POINT ( 'NONE',  ( -5.859094939400033120, 9.987361195942037639, -0.7998128361456231517 ) ) ;
#54668=CARTESIAN_POINT ( 'NONE',  ( -6.112028321662274166, 6.025121218227761588, 0.7998128361456341429 ) ) ;
#54675=CARTESIAN_POINT ( 'NONE',  ( 6.265839547809997079, 10.46189657242035587, 0.7998128361456462443 ) ) ;
#54687=VERTEX_POINT ( 'NONE', #172381 ) ;
#54689=CARTESIAN_POINT ( 'NONE',  ( -0.7500000000000215383, 5.191666666666685082, 1.299038105676671107 ) ) ;
#54690=CARTESIAN_POINT ( 'NONE',  ( 5.007038802148489509, 4.735966778795008381, 0.7998128361456341429 ) ) ;
#54691=CARTESIAN_POINT ( 'NONE',  ( 5.361359679200154105, 8.342337828120466980, 1.199719254218462483 ) ) ;
#54694=CARTESIAN_POINT ( 'NONE',  ( -7.646435448427427062, 10.90429654226522693, 1.082531754730549967 ) ) ;
#54697=CARTESIAN_POINT ( 'NONE',  ( 4.989037340148863464, 8.764367963574922982, -0.7216878364870257245 ) ) ;
#54698=CARTESIAN_POINT ( 'NONE',  ( -7.443063143778079649, 10.66702885350765584, 1.082531754730549967 ) ) ;
#54702=CARTESIAN_POINT ( 'NONE',  ( 8.209625708274705502, 9.536650400197368427, 1.199719254218462483 ) ) ;
#54707=CARTESIAN_POINT ( 'NONE',  ( -1.201851678989727383E-14, 2.071875000341422801, 1.575800808251672791 ) ) ;
#54714=CARTESIAN_POINT ( 'NONE',  ( 7.910292558569346433, 11.31609285405122556, -1.199719254218446718 ) ) ;
#54718=CARTESIAN_POINT ( 'NONE',  ( -7.804689982961090955, 12.25722208009664094, 0.7998128361456481317 ) ) ;
#54724=CARTESIAN_POINT ( 'NONE',  ( 9.378489572351044856, 11.96465713920816043, -1.599625672291262513 ) ) ;
#54727=CARTESIAN_POINT ( 'NONE',  ( -9.154780037725563702, 11.70366268214508487, 1.599625672291281386 ) ) ;
#54732=CARTESIAN_POINT ( 'NONE',  ( 5.874728247277303694, 5.987702652136856152, -0.2291304890473921385 ) ) ;
#54735=CARTESIAN_POINT ( 'NONE',  ( -5.199715606040888005, 6.025088614257851027, -1.199719254218446718 ) ) ;
#54739=CARTESIAN_POINT ( 'NONE',  ( 7.182068686937156166, 9.402166106225269715, 1.599625672291281386 ) ) ;
#54741=CARTESIAN_POINT ( 'NONE',  ( 7.284808609244363353, 7.393364887073558656, 0.7998128361456341429 ) ) ;
#54742=CARTESIAN_POINT ( 'NONE',  ( 5.834086172582112262, 5.700855377634248100, 1.040834085586084257E-14 ) ) ;
#54744=CARTESIAN_POINT ( 'NONE',  ( -7.971831135155409420, 11.28392484344787405, 1.082531754730549967 ) ) ;
#54752=CARTESIAN_POINT ( 'NONE',  ( -5.125485847170801357, 6.519186964134095597, -1.210412105186658094 ) ) ;
#54755=CARTESIAN_POINT ( 'NONE',  ( 0.000000000000000000, 9.200000000000020606, 0.4000000000000166755 ) ) ;
#54756=CARTESIAN_POINT ( 'NONE',  ( 6.507550544879468823, 6.694489845221929691, -0.7216878364870257245 ) ) ;
#54760=CARTESIAN_POINT ( 'NONE',  ( -9.612367721964606204, 12.23751498042398289, -1.443375672974058777 ) ) ;
#54763=EDGE_CURVE ( 'NONE', #211245, #213399, #57410, .T. ) ;
#54764=CARTESIAN_POINT ( 'NONE',  ( 1.499999999999989120, 6.280000000000042881, 2.580000000000000515 ) ) ;
#54779=CARTESIAN_POINT ( 'NONE',  ( 7.446452682403650769, 9.710614100936176385, -1.599625672291262513 ) ) ;
#54783=CARTESIAN_POINT ( 'NONE',  ( 0.7499999999999902300, 2.014583334016148530, 1.299038105676669330 ) ) ;
#54784=CARTESIAN_POINT ( 'NONE',  ( -4.295235737431041478, 3.905529869957963029, -0.7998128361456221525 ) ) ;
#54785=CARTESIAN_POINT ( 'NONE',  ( -6.067437437315529536, 7.037430750744921859, 1.199719254218450271 ) ) ;
#54789=CARTESIAN_POINT ( 'NONE',  ( -9.996439331977562404, 10.55693406359564790, 0.7998128361456462443 ) ) ;
#54794=CARTESIAN_POINT ( 'NONE',  ( 5.926885707468349196, 10.06645042535509660, 1.040834085586084257E-14 ) ) ;
#54796=CARTESIAN_POINT ( 'NONE',  ( -6.028571859570855729, 10.18508426947466816, 0.000000000000000000 ) ) ;
#54798=CARTESIAN_POINT ( 'NONE',  ( 7.801827329660018684, 11.18955008699033726, 1.199719254218460707 ) ) ;
#54799=CARTESIAN_POINT ( 'NONE',  ( -6.471393748265538370, 5.229711127717889596, -2.419999999999995044 ) ) ;
#54801=CARTESIAN_POINT ( 'NONE',  ( -1.580000000000021165, 8.674529973577531194, 2.500000000000011102 ) ) ;
#54806=CARTESIAN_POINT ( 'NONE',  ( -6.697364695470783502, 10.75741654478384035, 0.7216878364870458196 ) ) ;
#54810=CARTESIAN_POINT ( 'NONE',  ( -1.364683531250010295, 4.092708333674751842, 0.7879004041258379498 ) ) ;
#54820=CARTESIAN_POINT ( 'NONE',  ( 2.697709378994964879, 6.091152008895348580, 0.7216878364870338292 ) ) ;
#54821=CARTESIAN_POINT ( 'NONE',  ( -1.201851678989727383E-14, 5.759375000341417028, -1.575800808251660801 ) ) ;
#54822=CARTESIAN_POINT ( 'NONE',  ( -10.31505594189871111, 10.92865344183699428, -0.7998128361456291469 ) ) ;
#54827=CARTESIAN_POINT ( 'NONE',  ( -1.402160292154681736E-14, 0.4468750003414233563, -1.575800808251665908 ) ) ;
#54828=CARTESIAN_POINT ( 'NONE',  ( -4.134873662487946966, 3.926366815765101936, 1.214306433183764966E-14 ) ) ;
#54829=CARTESIAN_POINT ( 'NONE',  ( 4.985647801523278133, 6.839675073242382553, -1.599625672291256295 ) ) ;
#54838=CARTESIAN_POINT ( 'NONE',  ( -7.700668062882072284, 10.00719871149432549, -1.443375672974059665 ) ) ;
#54843=CARTESIAN_POINT ( 'NONE',  ( -8.890396042259075315, 11.39521468743417998, -1.599625672291263179 ) ) ;
#54845=CARTESIAN_POINT ( 'NONE',  ( -4.216222583725562245, 7.862750747747711877, 0.7216878364870317197 ) ) ;
#54846=CARTESIAN_POINT ( 'NONE',  ( -1.364683531250012516, 1.592708333674756727, 0.7879004041258379498 ) ) ;
#54853=VERTEX_POINT ( 'NONE', #75936 ) ;
#54868=CARTESIAN_POINT ( 'NONE',  ( -1.364683531249997417, 2.821875000341422801, 1.214306433183764966E-14 ) ) ;
#54878=CARTESIAN_POINT ( 'NONE',  ( 1.364683531249988757, 1.634375000341421691, 0.000000000000000000 ) ) ;
#54888=CARTESIAN_POINT ( 'NONE',  ( 4.222474775652216294, 7.013638773981186958, 1.199719254218462483 ) ) ;
#54898=CARTESIAN_POINT ( 'NONE',  ( -4.634189577772691138, 4.300976017023221409, 1.214306433183764966E-14 ) ) ;
#54899=CARTESIAN_POINT ( 'NONE',  ( 9.271078113646423091, 9.710679308875986848, 1.040834085586084257E-14 ) ) ;
#54906=VERTEX_POINT ( 'NONE', #82315 ) ;
#54913=CARTESIAN_POINT ( 'NONE',  ( -6.832946231607472498, 9.955225789308602913, 1.082531754730549967 ) ) ;
#54917=CARTESIAN_POINT ( 'NONE',  ( -9.972185678051314284, 11.59297036493672017, 1.199719254218462483 ) ) ;
#54919=DIRECTION ( 'NONE',  ( -0.7592566023652990159, -0.6507913734559659380, 1.175982368226361821E-15 ) ) ;
#54922=CARTESIAN_POINT ( 'NONE',  ( -2.598358995313378550, 6.183169261174235487, 0.7998128361456341429 ) ) ;
#54924=CARTESIAN_POINT ( 'NONE',  ( 8.401248741962376698, 12.95320729893149370, 0.7998128361456462443 ) ) ;
#54926=CARTESIAN_POINT ( 'NONE',  ( 4.029797971759831121, 5.724516938518342535, -1.599625672291255185 ) ) ;
#54932=CARTESIAN_POINT ( 'NONE',  ( 4.867013957625893283, 4.780530493426062399, 1.040834085586084257E-14 ) ) ;
#54934=CARTESIAN_POINT ( 'NONE',  ( -3.418627288940168096, 7.140148937072163804, -0.7998128361456281477 ) ) ;
#54937=CARTESIAN_POINT ( 'NONE',  ( -9.484092147959342967, 11.02352791316275216, 1.199719254218462483 ) ) ;
#54943=CARTESIAN_POINT ( 'NONE',  ( 8.771762198361678031, 9.336070107617867819, 1.040834085586084257E-14 ) ) ;
#54944=CARTESIAN_POINT ( 'NONE',  ( 1.364683531249988535, 4.176041667008080438, 0.7879004041258499402 ) ) ;
#54946=CARTESIAN_POINT ( 'NONE',  ( 4.039439701867726384, 6.800097854565950506, 1.199719254218462483 ) ) ;
#54952=( BOUNDED_CURVE ( )  B_SPLINE_CURVE ( 2, ( #158226, #9816, #60700, #175541, #110596 ),
 .UNSPECIFIED., .F., .T. ) 
 B_SPLINE_CURVE_WITH_KNOTS ( ( 3, 2, 3 ),
 ( 0.000000000000000000, 0.3063186054016480142, 1.000000000000000000 ),
 .UNSPECIFIED. ) 
 CURVE ( )  GEOMETRIC_REPRESENTATION_ITEM ( )  RATIONAL_B_SPLINE_CURVE ( ( 0.9866942343795712667, 0.9929791993688333873, 1.000000000000000000, 0.9841008718140421552, 0.9719753288332495522 ) ) 
 REPRESENTATION_ITEM ( '' )  );
#54956=CARTESIAN_POINT ( 'NONE',  ( -3.511198596259295535, 6.271927390929313617, -1.000000000000001776 ) ) ;
#54960=ORIENTED_EDGE ( 'NONE', *, *, #128510, .T. ) ;
#54962=CARTESIAN_POINT ( 'NONE',  ( -0.6823417656250212460, 3.113541667008084879, 1.181850606188767472 ) ) ;
#54964=CARTESIAN_POINT ( 'NONE',  ( 8.367353357928214663, 12.91366268422496688, 1.040834085586084257E-14 ) ) ;
#54966=CARTESIAN_POINT ( 'NONE',  ( -6.073689629242165822, 7.148687991279732756, -1.082531754730544860 ) ) ;
#54967=CARTESIAN_POINT ( 'NONE',  ( 4.053524740805938720, 3.831459740469437936, 1.214306433183764966E-14 ) ) ;
#54968=CARTESIAN_POINT ( 'NONE',  ( -6.209271164934474285, 6.346497235286081562, 1.040834085586084257E-14 ) ) ;
#54971=VERTEX_POINT ( 'NONE', #115952 ) ;
#54973=CARTESIAN_POINT ( 'NONE',  ( 3.811813743736467419, 7.598866467667865443, 1.040834085586084257E-14 ) ) ;
#54984=CARTESIAN_POINT ( 'NONE',  ( 4.873266149108180123, 7.772895376346490970, 1.199719254218462483 ) ) ;
#54988=CARTESIAN_POINT ( 'NONE',  ( -5.870844209917351009, 6.808071985447069707, -1.199719254218446718 ) ) ;
#54992=CARTESIAN_POINT ( 'NONE',  ( 6.805303039055573322, 10.02693841461847057, 1.199719254218460707 ) ) ;
#54995=CARTESIAN_POINT ( 'NONE',  ( -6.714312387265696458, 8.856450423275211037, 1.599625672291283607 ) ) ;
#54996=CARTESIAN_POINT ( 'NONE',  ( 5.599154252319471503, 9.476171027773981237, -0.7216878364870267237 ) ) ;
#54997=CARTESIAN_POINT ( 'NONE',  ( 5.168313817042160530, 6.667327647676385638, 1.400930397336812572 ) ) ;
#54998=CARTESIAN_POINT ( 'NONE',  ( -3.750802052474980108, 7.527686161196117887, 1.040834085586084257E-14 ) ) ;
#55002=CARTESIAN_POINT ( 'NONE',  ( -6.847031270101295419, 7.946956888995021728, -1.199719254218446718 ) ) ;
#55006=CARTESIAN_POINT ( 'NONE',  ( 1.364683531249986537, 2.405208333674752286, -0.7879004041258239610 ) ) ;
#55008=CARTESIAN_POINT ( 'NONE',  ( -6.087247782855839340, 6.204136622861004646, 0.000000000000000000 ) ) ;
#55012=ORIENTED_EDGE ( 'NONE', *, *, #132223, .F. ) ;
#55014=CARTESIAN_POINT ( 'NONE',  ( 6.654354466208897811, 6.657835053532175529, 0.7998128361456341429 ) ) ;
#55016=CARTESIAN_POINT ( 'NONE',  ( -5.863297782511878609, 6.029266553239049919, -0.3729355709888391157 ) ) ;
#55017=CARTESIAN_POINT ( 'NONE',  ( -0.6823417656250212460, 1.613541667008083769, 1.181850606188755259 ) ) ;
#55019=SPHERICAL_SURFACE ( 'NONE', #167184, 0.08000000000000000167 ) ;
#55024=CARTESIAN_POINT ( 'NONE',  ( -4.086893239515592136, 6.855460315155083251, 1.199719254218464037 ) ) ;
#55025=CARTESIAN_POINT ( 'NONE',  ( -6.493992390821436977, 10.52014885602626393, 0.7216878364870458196 ) ) ;
#55029=EDGE_CURVE ( 'NONE', #138277, #160319, #111910, .T. ) ;
#55034=CARTESIAN_POINT ( 'NONE',  ( -7.497295758232724872, 9.769931022736756177, -1.443375672974058777 ) ) ;
#55038=CARTESIAN_POINT ( 'NONE',  ( -6.792271770322117597, 9.907772251142352715, 1.082531754730549967 ) ) ;
#55044=CARTESIAN_POINT ( 'NONE',  ( 4.222827212797172436, 7.545785358913557950, -0.9571512059609885714 ) ) ;
#55046=CARTESIAN_POINT ( 'NONE',  ( -3.673896439623299148, 4.156855427197417185, -2.420000000000000373 ) ) ;
#55051=CARTESIAN_POINT ( 'NONE',  ( -8.044065211609668253, 8.279164256499745633, 0.7998128361456602331 ) ) ;
#55052=CARTESIAN_POINT ( 'NONE',  ( -1.177110729581203774, 3.210371626218858410, -0.7749999999999883649 ) ) ;
#55054=CARTESIAN_POINT ( 'NONE',  ( 5.332434488876471868, 5.115595079977664383, 0.7998128361456341429 ) ) ;
#55058=CARTESIAN_POINT ( 'NONE',  ( 7.332262146892202459, 7.448727347662698506, -0.7998128361456281477 ) ) ;
#55063=CARTESIAN_POINT ( 'NONE',  ( -5.422898255786203769, 6.389431388914436738, -1.082531754730544860 ) ) ;
#55074=CARTESIAN_POINT ( 'NONE',  ( 1.364683531249986537, 0.9052083336747533959, -0.7879004041258239610 ) ) ;
#55076=CARTESIAN_POINT ( 'NONE',  ( -8.585337585951595685, 11.03931315507545108, -1.599625672291263179 ) ) ;
#55078=CARTESIAN_POINT ( 'NONE',  ( 7.365103760721646076, 9.615707025640515937, 1.599625672291281386 ) ) ;
#55080=CARTESIAN_POINT ( 'NONE',  ( -7.888146445052511169, 8.097259028849730811, 1.040834085586084257E-14 ) ) ;
#55083=CARTESIAN_POINT ( 'NONE',  ( -1.364683531250012516, 4.488541667008090208, -0.7879004041258300672 ) ) ;
#55085=CARTESIAN_POINT ( 'NONE',  ( 8.215877900201359552, 11.56864606933486606, -1.082531754730543083 ) ) ;
#55088=CARTESIAN_POINT ( 'NONE',  ( 1.364683531249984538, -1.032291666325247714, -0.7879004041258309554 ) ) ;
#55091=CARTESIAN_POINT ( 'NONE',  ( 7.904040366642695048, 9.284097184913720824, 1.082531754730558626 ) ) ;
#55094=CARTESIAN_POINT ( 'NONE',  ( -6.738039156311804945, 6.963393225226301553, 1.040834085586084257E-14 ) ) ;
#55096=CARTESIAN_POINT ( 'NONE',  ( 1.364683531249988535, 3.655208333674750509, -0.7879004041258239610 ) ) ;
#55100=CARTESIAN_POINT ( 'NONE',  ( -5.636439174979254396, 7.598931675607687453, -1.599625672291256295 ) ) ;
#55108=CARTESIAN_POINT ( 'NONE',  ( 8.633844893804129228, 8.967240552393299424, -0.7998128361456211532 ) ) ;
#55111=CARTESIAN_POINT ( 'NONE',  ( -1.201851678989727383E-14, 2.462500000000023004, 1.732050807568877637 ) ) ;
#55113=CARTESIAN_POINT ( 'NONE',  ( -4.092446641025072829, 3.979529022206003575, 0.4031905389056175126 ) ) ;
#55116=ORIENTED_EDGE ( 'NONE', *, *, #105176, .T. ) ;
#55117=CARTESIAN_POINT ( 'NONE',  ( 7.131225611108100715, 7.422110755822004968, 0.7216878364870317197 ) ) ;
#55118=CARTESIAN_POINT ( 'NONE',  ( -1.364683531250000748, -0.9281249996585805295, 0.000000000000000000 ) ) ;
#55120=CARTESIAN_POINT ( 'NONE',  ( 4.054051625686104998, 4.688480637177271149, -1.199719254218446718 ) ) ;
#55125=CARTESIAN_POINT ( 'NONE',  ( -1.500000000000015099, 0.3791666666666850261, -0.8660254037844383745 ) ) ;
#55126=CARTESIAN_POINT ( 'NONE',  ( 7.263417608619159083, 9.497073181520933716, -1.599625672291262513 ) ) ;
#55127=CARTESIAN_POINT ( 'NONE',  ( -8.585337585951595685, 11.03931315507545108, -1.599625672291263179 ) ) ;
#55129=CARTESIAN_POINT ( 'NONE',  ( 0.6823417656249882723, 0.09270833367475139752, 1.181850606188755259 ) ) ;
#55130=CARTESIAN_POINT ( 'NONE',  ( -1.500000000000001332, 0.9000000000000187850, 0.000000000000000000 ) ) ;
#55132=CARTESIAN_POINT ( 'NONE',  ( 5.834086172582112262, 5.700855377634248100, 1.040834085586084257E-14 ) ) ;
#55138=CARTESIAN_POINT ( 'NONE',  ( 0.6823417656249899377, 5.176041667008086655, -1.181850606188754593 ) ) ;
#55140=CARTESIAN_POINT ( 'NONE',  ( -6.821723845970312894, 11.11042825360738284, 0.000000000000000000 ) ) ;
#55141=CARTESIAN_POINT ( 'NONE',  ( -5.504247177468192476, 7.444707678511436555, 1.443375672974064550 ) ) ;
#55149=CARTESIAN_POINT ( 'NONE',  ( 7.751511138711133064, 10.06651563329490529, -1.599625672291262513 ) ) ;
#55153=CARTESIAN_POINT ( 'NONE',  ( 7.795575137733369075, 9.157554417852841411, -1.082531754730537976 ) ) ;
#55156=CARTESIAN_POINT ( 'NONE',  ( -6.320072162264675164, 10.52516795595079557, 0.7998128361456481317 ) ) ;
#55157=CARTESIAN_POINT ( 'NONE',  ( 5.168682875307768931, 7.053215992657626110, -1.599625672291256295 ) ) ;
#55158=DIRECTION ( 'NONE',  ( -0.6507913734559640506, -0.7592566023653004592, 0.000000000000000000 ) ) ;
#55159=CARTESIAN_POINT ( 'NONE',  ( 3.429849674132933846, 5.024577257953626308, -1.443375672974058777 ) ) ;
#55160=DIRECTION ( 'NONE',  ( 0.000000000000000000, -0.7766560405359869135, 0.6299249119529750640 ) ) ;
#55161=CARTESIAN_POINT ( 'NONE',  ( 2.496672843210871129, 6.064535417054653266, -0.7998128361456291469 ) ) ;
#55162=VERTEX_POINT ( 'NONE', #178411 ) ;
#55170=CARTESIAN_POINT ( 'NONE',  ( -4.270455198624581783, 7.926022131796578662, 1.040834085586084257E-14 ) ) ;
#55171=CARTESIAN_POINT ( 'NONE',  ( 9.408995418203963013, 12.00024729270324286, 1.443375672974076540 ) ) ;
#55174=CARTESIAN_POINT ( 'NONE',  ( -6.235860587281615075, 9.362588887548838557, -1.199719254218440723 ) ) ;
#55177=CARTESIAN_POINT ( 'NONE',  ( 3.946537740505224878, 2.817530495244566335, 0.7750000000000135669 ) ) ;
#55179=CARTESIAN_POINT ( 'NONE',  ( -7.802881099864745984, 9.062115023719057305, -1.199719254218446718 ) ) ;
#55195=CARTESIAN_POINT ( 'NONE',  ( -7.393273838153706201, 7.519907654134449615, 0.7998128361456341429 ) ) ;
#55198=CARTESIAN_POINT ( 'NONE',  ( 4.189106276942576201, 7.831115056500907556, 1.040834085586084257E-14 ) ) ;
#55201=CARTESIAN_POINT ( 'NONE',  ( -0.05544532671888474651, 6.488672696939749684, 3.101758036159037335 ) ) ;
#55204=CARTESIAN_POINT ( 'NONE',  ( -5.870844209917351009, 6.808071985447069707, -1.199719254218446718 ) ) ;
#55207=CARTESIAN_POINT ( 'NONE',  ( -6.082770849258695378, 6.030316128467411829, -0.4441228188259391252 ) ) ;
#55208=CARTESIAN_POINT ( 'NONE',  ( -5.585069213825653023, 8.603332285183535433, -1.199719254218440723 ) ) ;
#55209=CARTESIAN_POINT ( 'NONE',  ( -5.815587556173210437, 6.058072081512762885, -0.5160206335057929694 ) ) ;
#55214=CARTESIAN_POINT ( 'NONE',  ( -7.804689982961090955, 12.25722208009664094, 0.7998128361456481317 ) ) ;
#55215=CARTESIAN_POINT ( 'NONE',  ( 8.098297826064319693, 8.342435640030188893, 0.7998128361456481317 ) ) ;
#55219=CARTESIAN_POINT ( 'NONE',  ( -9.001723924469462901, 12.58942944760136484, -1.199719254218446718 ) ) ;
#55225=CARTESIAN_POINT ( 'NONE',  ( 10.23604278863759909, 11.04439746293979496, 0.000000000000000000 ) ) ;
#55230=CARTESIAN_POINT ( 'NONE',  ( 4.161989969715272686, 4.726297878971393196, 2.500000000000011102 ) ) ;
#55234=CARTESIAN_POINT ( 'NONE',  ( -0.5973881975621483376, 6.735339005392440903, -3.613785340523188339 ) ) ;
#55241=ORIENTED_EDGE ( 'NONE', *, *, #177361, .T. ) ;
#55246=CARTESIAN_POINT ( 'NONE',  ( -4.406563619641430840, 5.099744630125142564, -1.199719254218446718 ) ) ;
#55249=CARTESIAN_POINT ( 'NONE',  ( -4.081167932913447594, 4.720116328942494555, -1.199719254218452047 ) ) ;
#55254=CARTESIAN_POINT ( 'NONE',  ( 1.364683531249988535, 5.655208333674751842, -0.7879004041258300672 ) ) ;
#55260=CARTESIAN_POINT ( 'NONE',  ( 1.387358672530661030, 7.251968950356647348, -4.302625267142129672 ) ) ;
#55262=CARTESIAN_POINT ( 'NONE',  ( 4.227444969362701421, 3.826440640544909400, 1.214306433183764966E-14 ) ) ;
#55263=CARTESIAN_POINT ( 'NONE',  ( -4.586165880992542299, 5.350526861157986147, 2.420000000000010587 ) ) ;
#55267=CARTESIAN_POINT ( 'NONE',  ( 6.159481859310094620, 6.080483678816896109, 1.040834085586084257E-14 ) ) ;
#55268=CARTESIAN_POINT ( 'NONE',  ( 1.364683531249988757, 2.196875000341415252, 1.214306433183764966E-14 ) ) ;
#55271=CARTESIAN_POINT ( 'NONE',  ( -7.808606406466886973, 11.19745900993164511, 1.199719254218453823 ) ) ;
#55272=CARTESIAN_POINT ( 'NONE',  ( -4.785665035499573783, 5.645992631913323123, 1.082531754730558626 ) ) ;
#55274=CARTESIAN_POINT ( 'NONE',  ( -5.259673527097670664, 8.223703984000886535, -1.199719254218446718 ) ) ;
#55276=CARTESIAN_POINT ( 'NONE',  ( 1.364683531249988535, 5.655208333674751842, -0.7879004041258300672 ) ) ;
#55285=CARTESIAN_POINT ( 'NONE',  ( -4.677199806590235376, 7.440188293455128665, 1.082531754730560403 ) ) ;
#55290=CARTESIAN_POINT ( 'NONE',  ( -3.592547517496935683, 6.174760622846296343, -1.082531754730548412 ) ) ;
#55302=CARTESIAN_POINT ( 'NONE',  ( -3.277320446201389181, 4.846626492033466072, 1.599625672291267398 ) ) ;
#55303=CARTESIAN_POINT ( 'NONE',  ( -10.64723070543352712, 11.31619066596094392, 0.7998128361456462443 ) ) ;
#55306=ORIENTED_EDGE ( 'NONE', *, *, #42375, .T. ) ;
#55308=CARTESIAN_POINT ( 'NONE',  ( 6.979750152936881058, 7.037463354714830643, 0.7998128361456341429 ) ) ;
#55314=CARTESIAN_POINT ( 'NONE',  ( 2.517010073631369860, 6.088262185878572375, -0.7998128361456281477 ) ) ;
#55323=CARTESIAN_POINT ( 'NONE',  ( 7.853197290813620945, 10.18514947741448573, 1.599625672291281386 ) ) ;
#55324=CARTESIAN_POINT ( 'NONE',  ( -4.761938266897808525, 6.578680616179308771, 1.599625672291267398 ) ) ;
#55330=CARTESIAN_POINT ( 'NONE',  ( 1.364683531249988535, 4.405208333674754506, -0.7879004041258300672 ) ) ;
#55333=ORIENTED_EDGE ( 'NONE', *, *, #69490, .T. ) ;
#55334=CARTESIAN_POINT ( 'NONE',  ( 5.217190183160311356, 4.981143389975473568, -0.7998128361456211532 ) ) ;
#55335=CARTESIAN_POINT ( 'NONE',  ( -3.086452525405351643, 6.752611712948207057, 0.7998128361456341429 ) ) ;
#55341=CARTESIAN_POINT ( 'NONE',  ( 6.995644074971448134, 7.263932296995902149, -0.7216878364870257245 ) ) ;
#55343=CARTESIAN_POINT ( 'NONE',  ( 7.632877294369377452, 8.967740267261513409, -1.082531754730537976 ) ) ;
#55344=CARTESIAN_POINT ( 'NONE',  ( -1.201851678989727383E-14, 3.759375000341422801, -1.575800808251660134 ) ) ;
#55346=CARTESIAN_POINT ( 'NONE',  ( 4.650083499362867911, 6.448183387388563226, 1.443375672974062551 ) ) ;
#55354=CARTESIAN_POINT ( 'NONE',  ( -4.153558989372251986, 7.618438364782146976, 0.8772435784342603737 ) ) ;
#55361=CARTESIAN_POINT ( 'NONE',  ( -9.504429378379839477, 11.04725468198666150, 1.199719254218462483 ) ) ;
#55363=CARTESIAN_POINT ( 'NONE',  ( -2.193105066167322370, 5.702484939155337607, -2.420000000000000373 ) ) ;
#55371=CARTESIAN_POINT ( 'NONE',  ( 2.724825686666657809, 6.122787701178987518, 0.000000000000000000 ) ) ;
#55372=CARTESIAN_POINT ( 'NONE',  ( -1.201851678989727383E-14, 4.009375000341416140, -1.575800808251660134 ) ) ;
#55374=CARTESIAN_POINT ( 'NONE',  ( 6.588372581236919601, 9.773852880496709972, -1.199719254218440723 ) ) ;
#55375=CARTESIAN_POINT ( 'NONE',  ( -10.66756793585402363, 11.33991743478486391, 0.7998128361456462443 ) ) ;
#55377=CARTESIAN_POINT ( 'NONE',  ( -3.066115294984855133, 6.728884944124295053, 0.7998128361456341429 ) ) ;
#55378=CARTESIAN_POINT ( 'NONE',  ( 0.000000000000000000, 2.800000000000024691, -2.499999999999995115 ) ) ;
#55381=CARTESIAN_POINT ( 'NONE',  ( -1.001543065824772872E-14, 4.712500000000017231, 1.732050807568877637 ) ) ;
#55382=CARTESIAN_POINT ( 'NONE',  ( 4.527533231959700366, 7.369540306339926516, 1.199719254218462483 ) ) ;
#55385=CARTESIAN_POINT ( 'NONE',  ( -1.364683531250012516, 3.280208333674756727, 0.7879004041258379498 ) ) ;
#55388=CARTESIAN_POINT ( 'NONE',  ( 8.432808358020015049, 11.82173160345663376, 1.082531754730546636 ) ) ;
#55393=CARTESIAN_POINT ( 'NONE',  ( -1.500000000000013101, 2.202083334016153859, 0.8660254037844403729 ) ) ;
#55395=CARTESIAN_POINT ( 'NONE',  ( -6.566226467720086113, 6.555019055295208119, 1.040834085586084257E-14 ) ) ;
#55396=CARTESIAN_POINT ( 'NONE',  ( 5.639828713160493834, 5.682147708216442439, 1.040834085586084257E-14 ) ) ;
#55405=CARTESIAN_POINT ( 'NONE',  ( 6.662942426112080874, 9.860851032851066122, 1.199719254218460707 ) ) ;
#55406=CARTESIAN_POINT ( 'NONE',  ( 4.985647801523278133, 6.839675073242382553, -1.599625672291256295 ) ) ;
#55410=CARTESIAN_POINT ( 'NONE',  ( 4.469384193999260901, 8.366031992974468423, -0.7998128361456231517 ) ) ;
#55413=CARTESIAN_POINT ( 'NONE',  ( -1.284279953904152949, 3.171639714193937198, 0.7750000000000152323 ) ) ;
#55417=CARTESIAN_POINT ( 'NONE',  ( 8.041957671200231417, 12.53403438304231976, 1.040834085586084257E-14 ) ) ;
#55422=CARTESIAN_POINT ( 'NONE',  ( 5.757945239960298167, 6.059206896687658883, 0.6045188873357760784 ) ) ;
#55423=EDGE_CURVE ( 'NONE', #32719, #153422, #69447, .T. ) ;
#55432=CARTESIAN_POINT ( 'NONE',  ( 6.127922243696800386, 10.09306701771420656, -0.7216878364870267237 ) ) ;
#55433=CARTESIAN_POINT ( 'NONE',  ( -3.765413976293358278, 5.416068943807445635, 1.599625672291267398 ) ) ;
#55438=CARTESIAN_POINT ( 'NONE',  ( -5.066996723205291708, 6.934582148538044777, 1.599625672291267398 ) ) ;
#55440=CARTESIAN_POINT ( 'NONE',  ( -4.226925616482887449, 3.500738074553344070, 2.444828727306146199 ) ) ;
#55445=CARTESIAN_POINT ( 'NONE',  ( -1.284279953904156280, 3.202889714876734573, 0.7750000000000117906 ) ) ;
#55451=CARTESIAN_POINT ( 'NONE',  ( 8.062294901620731480, 12.55776115186623620, 1.040834085586084257E-14 ) ) ;
#55453=CARTESIAN_POINT ( 'NONE',  ( 3.226477370372305753, 4.787309570232886280, 1.443375672974062551 ) ) ;
#55454=VERTEX_POINT ( 'NONE', #6018 ) ;
#55459=CARTESIAN_POINT ( 'NONE',  ( -9.978437869977959451, 10.74385839117019614, -0.7216878364870267237 ) ) ;
#55461=CARTESIAN_POINT ( 'NONE',  ( 4.080641032480825103, 5.783833874167997102, -1.249999999999999334 ) ) ;
#55463=CARTESIAN_POINT ( 'NONE',  ( 8.751951852821344247, 10.16936423550178503, -1.199719254218446718 ) ) ;
#55465=CARTESIAN_POINT ( 'NONE',  ( 1.010509813927327416, 2.800000000000067768, 1.061904942541237462 ) ) ;
#55467=CARTESIAN_POINT ( 'NONE',  ( -5.228640796364566690, 9.251831362400652736, -0.7998128361456231517 ) ) ;
#55468=CARTESIAN_POINT ( 'NONE',  ( 4.334856428067313416, 6.080418470877079429, -1.599625672291256295 ) ) ;
#55472=CARTESIAN_POINT ( 'NONE',  ( 10.05353459973327368, 11.68787744023238417, -1.199719254218440723 ) ) ;
#55473=CARTESIAN_POINT ( 'NONE',  ( -3.633221978782304351, 4.301475732409860697, -1.082531754730549967 ) ) ;
#55477=CARTESIAN_POINT ( 'NONE',  ( -1.364683531250012516, 2.342708333674752286, 0.7879004041258379498 ) ) ;
#55478=ORIENTED_EDGE ( 'NONE', *, *, #12460, .F. ) ;
#55480=CARTESIAN_POINT ( 'NONE',  ( 6.805829924380114804, 8.002851668940699881, 1.082531754730558626 ) ) ;
#55488=CARTESIAN_POINT ( 'NONE',  ( 6.765155463094740362, 10.83650577367847667, 0.7216878364870438212 ) ) ;
#55493=CARTESIAN_POINT ( 'NONE',  ( -10.01677656239806247, 10.58066083241955901, 0.7998128361456462443 ) ) ;
#55502=CARTESIAN_POINT ( 'NONE',  ( 2.530568227245037605, 6.104080031761181857, 0.000000000000000000 ) ) ;
#55503=CIRCLE ( 'NONE', #20992, 0.08000000000000020983 ) ;
#55507=CARTESIAN_POINT ( 'NONE',  ( 5.606460214450851964, 6.499623990736163037, 1.199719254218462483 ) ) ;
#55510=CARTESIAN_POINT ( 'NONE',  ( -0.7500000000000215383, 3.472916667349487785, 1.299038105676671107 ) ) ;
#55516=CARTESIAN_POINT ( 'NONE',  ( 1.499999999999985123, 0.2958333333333566517, -0.8660254037844323793 ) ) ;
#55517=CARTESIAN_POINT ( 'NONE',  ( 8.125414133291656071, 8.374071331795406081, -0.7998128361456291469 ) ) ;
#55518=CARTESIAN_POINT ( 'NONE',  ( 4.785665035499516051, 8.527100274817353665, -0.7216878364870207285 ) ) ;
#55521=AXIS2_PLACEMENT_3D ( 'NONE', #109874, #45891, #46959 ) ;
#55523=CARTESIAN_POINT ( 'NONE',  ( 9.490344339885973923, 12.09515436799890331, -1.443375672974057666 ) ) ;
#55528=CARTESIAN_POINT ( 'NONE',  ( -6.175902666224832416, 7.163973517805802160, -1.199719254218446718 ) ) ;
#55529=CARTESIAN_POINT ( 'NONE',  ( -0.7500000000000215383, 3.222916667349487341, 1.299038105676671107 ) ) ;
#55530=CARTESIAN_POINT ( 'NONE',  ( -0.6823417656250212460, 5.113541667008086655, 1.181850606188767472 ) ) ;
#55536=CARTESIAN_POINT ( 'NONE',  ( 0.6823417656249917140, 3.905208333674754950, 1.181850606188765695 ) ) ;
#55546=CARTESIAN_POINT ( 'NONE',  ( -6.367525699912501835, 10.58053041653993098, -0.7998128361456291469 ) ) ;
#55547=CARTESIAN_POINT ( 'NONE',  ( 6.277588818327314080, 7.282607361925381717, 1.199719254218462483 ) ) ;
#55556=CARTESIAN_POINT ( 'NONE',  ( -7.531718027591449705, 8.745758106066849891, 1.199719254218462483 ) ) ;
#55561=CARTESIAN_POINT ( 'NONE',  ( 3.216308754939877446, 4.775446185561722956, -1.599625672291262513 ) ) ;
#55562=FACE_OUTER_BOUND ( 'NONE', #148433, .T. ) ;
#55563=CARTESIAN_POINT ( 'NONE',  ( -4.334856428067329404, 6.080418470877079429, -1.599625672291256295 ) ) ;
#55565=CARTESIAN_POINT ( 'NONE',  ( -9.982881178363895103, 10.54111621771303753, 1.040834085586084257E-14 ) ) ;
#55568=CARTESIAN_POINT ( 'NONE',  ( -4.144866890078757748, 7.628995377423835045, -0.8586628004631415845 ) ) ;
#55575=CARTESIAN_POINT ( 'NONE',  ( 6.494519276145969577, 7.535692896047149425, -1.199719254218446718 ) ) ;
#55578=EDGE_CURVE ( 'NONE', #66472, #187417, #145313, .T. ) ;
#55591=CARTESIAN_POINT ( 'NONE',  ( 4.216222584169931231, 4.021273891060765493, 1.214306433183764966E-14 ) ) ;
#55595=CARTESIAN_POINT ( 'NONE',  ( -8.809047120577080392, 11.30030761213851953, 1.599625672291269396 ) ) ;
#55596=DIRECTION ( 'NONE',  ( 0.6507913734559640506, -0.7592566023653004592, 0.000000000000000000 ) ) ;
#55601=CARTESIAN_POINT ( 'NONE',  ( 0.7499999999999885647, 1.097916667349485564, -1.299038105676652899 ) ) ;
#55602=CARTESIAN_POINT ( 'NONE',  ( 9.622536337397022521, 12.24937836509514710, 1.599625672291281386 ) ) ;
#55603=CARTESIAN_POINT ( 'NONE',  ( -3.128199800776549466, 2.800000000000122835, 2.480560084996058734 ) ) ;
#55606=CARTESIAN_POINT ( 'NONE',  ( -10.16591625214838679, 10.75465713712827487, 1.040834085586084257E-14 ) ) ;
#55608=CARTESIAN_POINT ( 'NONE',  ( 0.6823417656249899377, 1.092708333674752286, 1.181850606188755259 ) ) ;
#55610=ORIENTED_EDGE ( 'NONE', *, *, #3649, .T. ) ;
#55614=CARTESIAN_POINT ( 'NONE',  ( -5.037017762676898158, 5.835274463666530131, -1.199719254218446718 ) ) ;
#55616=CARTESIAN_POINT ( 'NONE',  ( 1.445103857048099405, 8.688264192037886247, -2.625611233228245300 ) ) ;
#55619=CARTESIAN_POINT ( 'NONE',  ( -1.364683531250014514, -0.4072916663252447167, 0.7879004041258379498 ) ) ;
#55624=CARTESIAN_POINT ( 'NONE',  ( 0.6823417656249899377, 0.8427083336747520637, 1.181850606188755259 ) ) ;
#55626=CARTESIAN_POINT ( 'NONE',  ( -6.958359152311683893, 9.141171649162195934, -1.599625672291263179 ) ) ;
#55627=CARTESIAN_POINT ( 'NONE',  ( 8.378048858240820351, 11.86180853700128601, -1.199719254218446718 ) ) ;
#55628=CARTESIAN_POINT ( 'NONE',  ( 5.854423403002611437, 5.724582146458163656, 1.040834085586084257E-14 ) ) ;
#55632=CARTESIAN_POINT ( 'NONE',  ( -1.364683531250014514, 1.301041667008083325, -0.7879004041258289570 ) ) ;
#55638=CARTESIAN_POINT ( 'NONE',  ( 5.612712406377503349, 8.531619659873665995, -1.082531754730543083 ) ) ;
#55641=CARTESIAN_POINT ( 'NONE',  ( -7.711890448074853133, 7.891627032375787998, -0.7998128361456291469 ) ) ;
#55642=CARTESIAN_POINT ( 'NONE',  ( -5.088387723830502196, 4.830873854090670605, -0.7998128361456221525 ) ) ;
#55646=CARTESIAN_POINT ( 'NONE',  ( -2.927671105547157371, 5.503034492191895666, 1.199719254218462483 ) ) ;
#55647=CARTESIAN_POINT ( 'NONE',  ( 5.056828107772846082, 6.922718763866881453, -1.443375672974051449 ) ) ;
#55648=CARTESIAN_POINT ( 'NONE',  ( -8.798878505144665851, 9.367705798864669475, -0.7216878364870267237 ) ) ;
#55650=CARTESIAN_POINT ( 'NONE',  ( 0.7499999999999902300, 3.983333333333352488, 1.299038105676669330 ) ) ;
#55654=CARTESIAN_POINT ( 'NONE',  ( 7.280365300858406385, 11.43758391773608984, 1.040834085586084257E-14 ) ) ;
#55666=CARTESIAN_POINT ( 'NONE',  ( 7.822691444960700125, 10.14955932391940330, -1.443375672974058777 ) ) ;
#55667=CARTESIAN_POINT ( 'NONE',  ( 7.588813295347141441, 9.876701482703580837, -1.599625672291262513 ) ) ;
#55668=CARTESIAN_POINT ( 'NONE',  ( -5.693534442735004752, 8.729875052244421951, 1.199719254218452047 ) ) ;
#55671=CARTESIAN_POINT ( 'NONE',  ( -4.052968920965120958, 3.984128252961195216, -0.5207863488562065601 ) ) ;
#55672=CARTESIAN_POINT ( 'NONE',  ( -0.6823417656250246877, -0.6364583329919113464, 1.181850606188755259 ) ) ;
#55673=CARTESIAN_POINT ( 'NONE',  ( 3.063779527008304360, 6.518233848244248563, 0.7216878364870317197 ) ) ;
#55675=CARTESIAN_POINT ( 'NONE',  ( -7.944714827928056167, 10.29191993738131927, 1.443375672974090751 ) ) ;
#55692=CARTESIAN_POINT ( 'NONE',  ( 6.123478934866503742, 10.29580919065294431, 0.7998128361456462443 ) ) ;
#55695=VERTEX_POINT ( 'NONE', #38550 ) ;
#55704=CARTESIAN_POINT ( 'NONE',  ( -4.740547266272593596, 8.682388910626682943, -0.7998128361456281477 ) ) ;
#55707=CARTESIAN_POINT ( 'NONE',  ( -5.148345644887285744, 7.029489223833707001, -1.599625672291256295 ) ) ;
#55717=CARTESIAN_POINT ( 'NONE',  ( -2.740719608256871442, 6.349256642941639051, 0.7998128361456341429 ) ) ;
#55720=CARTESIAN_POINT ( 'NONE',  ( 7.772902139336337335, 7.962807338847539107, 0.7998128361456341429 ) ) ;
#55721=CARTESIAN_POINT ( 'NONE',  ( -0.9486429539237333231, 3.292910930033766892, 1.028101543438982635 ) ) ;
#55723=CARTESIAN_POINT ( 'NONE',  ( 6.093061176370408560, 6.029359313278345844, 0.2718797729955486631 ) ) ;
#55728=CARTESIAN_POINT ( 'NONE',  ( 6.290620086616457662, 6.441404310581745563, 1.040834085586084257E-14 ) ) ;
#55729=CARTESIAN_POINT ( 'NONE',  ( -9.006694118179950692, 9.402231314165087284, 1.040834085586084257E-14 ) ) ;
#55733=CARTESIAN_POINT ( 'NONE',  ( -9.332089804907933939, 9.781859615347734405, 1.040834085586084257E-14 ) ) ;
#55734=CARTESIAN_POINT ( 'NONE',  ( -6.087774667736030487, 7.061157519568837415, 1.199719254218450271 ) ) ;
#55738=CARTESIAN_POINT ( 'NONE',  ( -0.7499999999999972244, 3.389583334016149863, -1.299038105676652011 ) ) ;
#55741=CARTESIAN_POINT ( 'NONE',  ( 6.425674737872927089, 9.584038729905381970, -1.199719254218440723 ) ) ;
#55756=CARTESIAN_POINT ( 'NONE',  ( 1.499999999999989120, 5.004166666666691299, 0.8660254037844524744 ) ) ;
#55757=CARTESIAN_POINT ( 'NONE',  ( 4.955668840994886359, 5.740367388370866131, 1.199719254218462483 ) ) ;
#55758=CARTESIAN_POINT ( 'NONE',  ( 4.659198344590585350, 8.587481835331020719, 0.7998128361456462443 ) ) ;
#55760=CARTESIAN_POINT ( 'NONE',  ( -7.212574532790087645, 11.35849468832304154, -0.7216878364870267237 ) ) ;
#55762=CARTESIAN_POINT ( 'NONE',  ( 5.314433026876846711, 9.143996264757578984, -0.7216878364870267237 ) ) ;
#55763=CARTESIAN_POINT ( 'NONE',  ( -9.951321562306267410, 10.71222269888655987, 1.040834085586084257E-14 ) ) ;
#55766=CARTESIAN_POINT ( 'NONE',  ( 8.076906825439115423, 10.44614393447756129, -1.599625672291262513 ) ) ;
#55771=CARTESIAN_POINT ( 'NONE',  ( -2.298420387838187473, 5.509269730139584986, -0.7346435760097105305 ) ) ;
#55772=CARTESIAN_POINT ( 'NONE',  ( -1.201851678989727383E-14, 2.946875000341419248, -1.575800808251660134 ) ) ;
#55778=CARTESIAN_POINT ( 'NONE',  ( 6.909851844459134362, 11.21324425184434936, -0.7998128361456291469 ) ) ;
#55782=CARTESIAN_POINT ( 'NONE',  ( -9.775592450653132204, 11.36361159963886891, -1.199719254218441611 ) ) ;
#55788=CARTESIAN_POINT ( 'NONE',  ( 10.71502147350184231, 11.39527989537399755, 0.000000000000000000 ) ) ;
#55792=CARTESIAN_POINT ( 'NONE',  ( -8.317037166979361018, 11.79062823052953668, 1.199719254218453823 ) ) ;
#55796=CARTESIAN_POINT ( 'NONE',  ( 8.289920859751990889, 11.75899253876431416, 1.199719254218450271 ) ) ;
#55798=CARTESIAN_POINT ( 'NONE',  ( 5.530423754462008290, 6.204488192500752675, 0.9375459734879583173 ) ) ;
#55799=CARTESIAN_POINT ( 'NONE',  ( -1.127943160727153060, 2.800000000000024691, -0.7749999999999935829 ) ) ;
#55800=CARTESIAN_POINT ( 'NONE',  ( -2.916975605234527702, 6.554888639415577423, 1.040834085586084257E-14 ) ) ;
#55805=CARTESIAN_POINT ( 'NONE',  ( 6.916630921265960019, 11.22115317478565188, 0.7998128361456462443 ) ) ;
#55807=CARTESIAN_POINT ( 'NONE',  ( 7.772902139336337335, 7.962807338847539107, 0.7998128361456341429 ) ) ;
#55810=CARTESIAN_POINT ( 'NONE',  ( -9.164948653158003111, 9.794787638213568570, -0.7216878364870267237 ) ) ;
#55818=CARTESIAN_POINT ( 'NONE',  ( -4.567562471335953944, 6.984949105684680859, -1.180336305634868577 ) ) ;
#55820=CARTESIAN_POINT ( 'NONE',  ( 7.321039761699430493, 7.643560598178549270, -0.7216878364870257245 ) ) ;
#55843=CARTESIAN_POINT ( 'NONE',  ( 7.609150525767641504, 9.900428251527500834, -1.599625672291262513 ) ) ;
#55847=CARTESIAN_POINT ( 'NONE',  ( -1.402160292154681736E-14, 1.368750000682821710, -1.732050807568863648 ) ) ;
#55848=CARTESIAN_POINT ( 'NONE',  ( -6.693975156845199059, 8.832723654451292816, 1.599625672291283607 ) ) ;
#55851=CARTESIAN_POINT ( 'NONE',  ( -8.350932551013499960, 11.83017284523606172, -1.199719254218446718 ) ) ;
#55856=CARTESIAN_POINT ( 'NONE',  ( 6.908042961362778733, 8.018137195466769285, 1.199719254218462483 ) ) ;
#55859=CARTESIAN_POINT ( 'NONE',  ( -5.716734326456539783, 9.821273814174633188, -0.7998128361456231517 ) ) ;
#55861=CARTESIAN_POINT ( 'NONE',  ( 5.549815083142378924, 6.383051840172381475, -1.247766374558601399 ) ) ;
#55868=CARTESIAN_POINT ( 'NONE',  ( -8.690413276679693766, 9.241163032322203819, 1.040834085586084257E-14 ) ) ;
#55872=CARTESIAN_POINT ( 'NONE',  ( -0.6823417656249969321, 3.780208333674754506, -1.181850606188749264 ) ) ;
#55878=CARTESIAN_POINT ( 'NONE',  ( -0.6823417656250212460, 4.301041667008085767, 1.181850606188767472 ) ) ;
#55882=CARTESIAN_POINT ( 'NONE',  ( 2.968872451268290913, 5.447139712246216625, -1.082531754730543971 ) ) ;
#55883=CARTESIAN_POINT ( 'NONE',  ( -0.6823417656249969321, 5.530208333674756283, -1.181850606188749264 ) ) ;
#55889=CARTESIAN_POINT ( 'NONE',  ( 1.364683531249986537, 1.155208333674754728, -0.7879004041258239610 ) ) ;
#55890=CARTESIAN_POINT ( 'NONE',  ( -3.551873057100300990, 5.166937871415542283, 1.443375672974064550 ) ) ;
#55891=CARTESIAN_POINT ( 'NONE',  ( 5.443762371086860341, 6.309809840144842141, 1.199719254218462483 ) ) ;
#55897=CARTESIAN_POINT ( 'NONE',  ( 4.121315508874254796, 5.831287398485176077, -1.443375672974051449 ) ) ;
#55900=CARTESIAN_POINT ( 'NONE',  ( -8.703971430293361067, 9.256980878204810637, 0.7216878364870438212 ) ) ;
#55905=CARTESIAN_POINT ( 'NONE',  ( -7.160677686311960777, 11.50587440067263678, -0.7998128361456291469 ) ) ;
#55906=CARTESIAN_POINT ( 'NONE',  ( -4.731432421044873493, 7.503459676985569260, -1.082531754730548412 ) ) ;
#55908=CARTESIAN_POINT ( 'NONE',  ( -0.6823417656250212460, 2.613541667008084879, 1.181850606188767472 ) ) ;
#55909=CARTESIAN_POINT ( 'NONE',  ( 0.7499999999999920064, 4.483333333333352932, 1.299038105676669330 ) ) ;
#55915=CARTESIAN_POINT ( 'NONE',  ( 10.58621901417202515, 11.24501035948919991, -0.7998128361456281477 ) ) ;
#55926=EDGE_LOOP ( 'NONE', ( #139321, #78127, #71442, #3600 ) ) ;
#55932=CARTESIAN_POINT ( 'NONE',  ( -3.440018289565379028, 5.036440642624797626, 1.599625672291267398 ) ) ;
#55935=CARTESIAN_POINT ( 'NONE',  ( 1.364683531249986537, 2.467708333674753174, -0.7879004041258239610 ) ) ;
#55946=CARTESIAN_POINT ( 'NONE',  ( 1.364683531249988757, 0.6343750003414208027, 0.000000000000000000 ) ) ;
#55956=CARTESIAN_POINT ( 'NONE',  ( 5.087333953625774008, 6.958308917361963886, 1.599625672291267398 ) ) ;
#55961=CARTESIAN_POINT ( 'NONE',  ( 10.70146331988817323, 11.37946204949139251, 0.7998128361456341429 ) ) ;
#55965=CARTESIAN_POINT ( 'NONE',  ( 7.609150525767641504, 9.900428251527500834, -1.599625672291262513 ) ) ;
#55968=CARTESIAN_POINT ( 'NONE',  ( 8.932124273304774320, 9.315233161810734686, 0.7998128361456462443 ) ) ;
#55980=CARTESIAN_POINT ( 'NONE',  ( -7.212574532790100079, 9.437756259720353924, -1.443375672974059665 ) ) ;
#55985=CARTESIAN_POINT ( 'NONE',  ( -9.134442807305063639, 11.67993591332117376, 1.599625672291281386 ) ) ;
#55987=CARTESIAN_POINT ( 'NONE',  ( 2.231648340698067834, 5.547414130882294181, -0.2706067644340047207 ) ) ;
#55990=CARTESIAN_POINT ( 'NONE',  ( -3.750802052474980108, 7.527686161196117887, 1.040834085586084257E-14 ) ) ;
#55992=CARTESIAN_POINT ( 'NONE',  ( 9.748476143425788720, 11.33197590787365172, -1.199719254218440723 ) ) ;
#55994=CARTESIAN_POINT ( 'NONE',  ( 3.832150974156964818, 7.622593236491780999, 1.040834085586084257E-14 ) ) ;
#56000=CARTESIAN_POINT ( 'NONE',  ( 4.039966587192259873, 5.736380323189513852, 1.443375672974062551 ) ) ;
#56002=CARTESIAN_POINT ( 'NONE',  ( -4.985647801523292344, 6.839675073242382553, -1.599625672291256295 ) ) ;
#56005=CARTESIAN_POINT ( 'NONE',  ( -9.134442807305063639, 11.67993591332117376, 1.599625672291281386 ) ) ;
#56011=CARTESIAN_POINT ( 'NONE',  ( 8.270110514656026979, 10.67154823856396817, 1.443375672974076540 ) ) ;
#56012=CARTESIAN_POINT ( 'NONE',  ( -0.6823417656250212460, 4.363541667008085767, 1.181850606188767472 ) ) ;
#56014=CARTESIAN_POINT ( 'NONE',  ( 4.955668840994886359, 5.740367388370866131, 1.199719254218462483 ) ) ;
#56030=CARTESIAN_POINT ( 'NONE',  ( -1.364683531250014514, 2.051041667008086655, -0.7879004041258289570 ) ) ;
#56032=CARTESIAN_POINT ( 'NONE',  ( 8.757677159423465696, 12.30470822171437284, 1.199719254218450271 ) ) ;
#56034=CARTESIAN_POINT ( 'NONE',  ( -5.097502569058210753, 7.930541516334467467, -1.082531754730549967 ) ) ;
#56035=CARTESIAN_POINT ( 'NONE',  ( 4.867013957625893283, 4.780530493426062399, 1.040834085586084257E-14 ) ) ;
#56036=CARTESIAN_POINT ( 'NONE',  ( -6.683806541412780078, 6.900121841177441873, -0.7216878364870267237 ) ) ;
#56040=CARTESIAN_POINT ( 'NONE',  ( 5.335297142177534369, 6.183267073083954735, -1.199719254218452047 ) ) ;
#56050=CARTESIAN_POINT ( 'NONE',  ( 6.494519276145969577, 7.535692896047149425, -1.199719254218446718 ) ) ;
#56054=CARTESIAN_POINT ( 'NONE',  ( -6.795661308947694934, 8.951357498570873261, -1.599625672291263179 ) ) ;
#56058=CARTESIAN_POINT ( 'NONE',  ( 8.599949509769960088, 8.927695937686774386, 1.040834085586084257E-14 ) ) ;
#56060=CARTESIAN_POINT ( 'NONE',  ( -5.201524489137236529, 9.220195670635433771, 0.7998128361456481317 ) ) ;
#56062=CARTESIAN_POINT ( 'NONE',  ( 6.358410854684775515, 8.441231968597481483, -1.443375672974058777 ) ) ;
#56063=CARTESIAN_POINT ( 'NONE',  ( 5.274334856052985465, 6.586744271544701768, 1.367809967355391398 ) ) ;
#56064=CARTESIAN_POINT ( 'NONE',  ( -3.978428010606240850, 6.728917548094202949, -1.199719254218452047 ) ) ;
#56068=CARTESIAN_POINT ( 'NONE',  ( -5.930802130974132780, 9.006687355190106103, -1.199719254218440723 ) ) ;
#56073=CARTESIAN_POINT ( 'NONE',  ( 4.081882008079450230, 3.980588341361369853, -0.7346435760097060896 ) ) ;
#56074=CARTESIAN_POINT ( 'NONE',  ( -1.364683531250012516, 1.280208333674755172, 0.7879004041258379498 ) ) ;
#56076=CARTESIAN_POINT ( 'NONE',  ( -5.260200412422196159, 9.080724881227137502, -0.7216878364870207285 ) ) ;
#56081=CARTESIAN_POINT ( 'NONE',  ( 6.667912619822566000, 6.673652899414787676, 1.040834085586084257E-14 ) ) ;
#56083=CARTESIAN_POINT ( 'NONE',  ( -5.910693218230258061, 6.000975156485434781, -0.07073762994192281384 ) ) ;
#56084=CARTESIAN_POINT ( 'NONE',  ( -0.6823417656250003738, 1.780208333674752952, -1.181850606188749264 ) ) ;
#56087=CARTESIAN_POINT ( 'NONE',  ( -0.5631007116328591300, 7.823254984196720940, 1.919102855466193303 ) ) ;
#56090=CARTESIAN_POINT ( 'NONE',  ( -3.924195396151603177, 6.665646164563756138, 1.199719254218464037 ) ) ;
#56092=CARTESIAN_POINT ( 'NONE',  ( -8.663296969008007054, 9.209527340038563992, 0.7216878364870438212 ) ) ;
#56100=CARTESIAN_POINT ( 'NONE',  ( -8.310784975052685652, 9.758632561392040827, -1.082531754730543083 ) ) ;
#56104=EDGE_LOOP ( 'NONE', ( #124913, #213896, #180129, #23233 ) ) ;
#56105=CARTESIAN_POINT ( 'NONE',  ( -6.033015167956794933, 9.982342096017511324, -0.7216878364870267237 ) ) ;
#56111=CARTESIAN_POINT ( 'NONE',  ( -1.500000000000011324, 5.202083334016151639, 0.8660254037844403729 ) ) ;
#56112=CARTESIAN_POINT ( 'NONE',  ( 4.470816497852414528, 7.277750640693428252, -1.251308411505752671 ) ) ;
#56113=DIRECTION ( 'NONE',  ( 1.000000000000000000, 0.000000000000000000, 0.000000000000000000 ) ) ;
#56116=VERTEX_POINT ( 'NONE', #141432 ) ;
#56119=CARTESIAN_POINT ( 'NONE',  ( -5.910464900553636269, 8.982960586366182554, -1.199719254218440723 ) ) ;
#56121=CARTESIAN_POINT ( 'NONE',  ( 3.876741858503734761, 6.610283703974623393, 1.199719254218462483 ) ) ;
#56125=CARTESIAN_POINT ( 'NONE',  ( 4.957477724091233995, 8.935474444748447098, -0.7998128361456281477 ) ) ;
#56130=CARTESIAN_POINT ( 'NONE',  ( -3.606105671554953318, 7.150947683548662503, 0.7216878364870317197 ) ) ;
#56139=CARTESIAN_POINT ( 'NONE',  ( 1.364683531249986537, 0.4052083336747511200, -0.7879004041258309554 ) ) ;
#56141=CARTESIAN_POINT ( 'NONE',  ( -9.677822722056413696, 10.18521468535430685, 1.040834085586084257E-14 ) ) ;
#56143=CARTESIAN_POINT ( 'NONE',  ( 7.313733799568044702, 10.62010763521636214, 1.199719254218460707 ) ) ;
#56145=CARTESIAN_POINT ( 'NONE',  ( -8.148614017013223076, 9.465470093725620870, -1.199719254218446718 ) ) ;
#56148=CARTESIAN_POINT ( 'NONE',  ( -1.364683531250010295, 4.780208333674755394, 0.7879004041258379498 ) ) ;
#56150=CARTESIAN_POINT ( 'NONE',  ( 9.788623719386617239, 11.48277776311499387, -1.082531754730537088 ) ) ;
#56153=CARTESIAN_POINT ( 'NONE',  ( -1.402160292154681736E-14, -1.115624999658584082, 1.575800808251672791 ) ) ;
#56155=CARTESIAN_POINT ( 'NONE',  ( 7.090551149822735155, 9.295395646258437949, 1.443375672974076540 ) ) ;
#56157=CARTESIAN_POINT ( 'NONE',  ( 1.123270288250308280, 2.922697346350005887, 0.7749999999993786304 ) ) ;
#56158=CARTESIAN_POINT ( 'NONE',  ( -5.585596099150193616, 6.579245539505756746, -1.082531754730544860 ) ) ;
#56160=CARTESIAN_POINT ( 'NONE',  ( -0.6823417656250212460, 2.801041667008084879, 1.181850606188767472 ) ) ;
#56163=CARTESIAN_POINT ( 'NONE',  ( -6.905180308061733996, 6.950465202360470052, 0.7998128361456341429 ) ) ;
#56170=AXIS2_PLACEMENT_3D ( 'NONE', #90539, #188006, #41799 ) ;
#56172=CARTESIAN_POINT ( 'NONE',  ( 9.094822116668764167, 9.505047312402055582, 0.7998128361456462443 ) ) ;
#56181=ORIENTED_EDGE ( 'NONE', *, *, #198981, .T. ) ;
#56182=CARTESIAN_POINT ( 'NONE',  ( 6.480434237652132445, 7.623223367758051872, 1.082531754730558626 ) ) ;
#56183=CARTESIAN_POINT ( 'NONE',  ( -1.364683531250014514, -0.1572916663252435232, 0.7879004041258379498 ) ) ;
#56190=CARTESIAN_POINT ( 'NONE',  ( 7.130698725783555680, 10.40656671580112658, 1.199719254218460707 ) ) ;
#56191=CARTESIAN_POINT ( 'NONE',  ( -9.612894607289142357, 11.17379744904754801, -1.199719254218441611 ) ) ;
#56193=CARTESIAN_POINT ( 'NONE',  ( 0.6823417656249882723, -0.1572916663252488245, 1.181850606188755259 ) ) ;
#56194=CARTESIAN_POINT ( 'NONE',  ( 1.499999999999989120, 1.275000000000019229, 0.000000000000000000 ) ) ;
#56197=CARTESIAN_POINT ( 'NONE',  ( 4.123651276850781144, 7.962676922967908411, -0.7998128361456221525 ) ) ;
#56203=CARTESIAN_POINT ( 'NONE',  ( 1.364683531249990311, 4.634375000341417916, 1.214306433183764966E-14 ) ) ;
#56204=CARTESIAN_POINT ( 'NONE',  ( -7.147119532698295252, 11.49005655479003174, 0.000000000000000000 ) ) ;
#56205=CARTESIAN_POINT ( 'NONE',  ( -3.782361668532609134, 7.356579680022602652, 1.040834085586084257E-14 ) ) ;
#56214=CARTESIAN_POINT ( 'NONE',  ( 7.130698725783555680, 10.40656671580112658, 1.199719254218460707 ) ) ;
#56215=CARTESIAN_POINT ( 'NONE',  ( -3.958617665510272943, 6.601842462195195438, -1.082531754730549967 ) ) ;
#56216=CARTESIAN_POINT ( 'NONE',  ( 5.355107487273504496, 6.310342158982962246, -1.082531754730543083 ) ) ;
#56219=CARTESIAN_POINT ( 'NONE',  ( 7.171900071504736296, 9.390302721554109056, -1.443375672974058777 ) ) ;
#56222=CARTESIAN_POINT ( 'NONE',  ( -6.835281999583978418, 11.12624609948998966, -0.7998128361456291469 ) ) ;
#56223=( BOUNDED_SURFACE ( )  B_SPLINE_SURFACE ( 1, 2, ( 
 ( #109520, #27117, #74821, #93223, #159255, #210123, #156072, #40187, #7658, #205867, #91087, #76929, #143055, #172321, #192807, #58564, #44466, #123660, #196037, #12993, #96423, #63889, #114835, #178723, #81208, #33519, #113782, #97478, #95359, #112711, #128978, #163534, #49771, #197083, #62817, #45533, #46593, #211192, #131094, #161409, #14047, #99591, #193884, #181882, #48720, #165657, #989, #180833, #17244, #32458, #98528, #162474, #80135, #115897, #83320, #111647, #149408, #177659, #145186, #194957, #179784, #31404, #65981, #214351, #164589, #127932, #132132, #30338, #146238, #29267, #212255, #79068, #130044, #47671, #15119, #16175, #82259, #213319, #147287, #148351, #31757, #197428, #182239, #16529, #200609, #150839, #148696, #83675, #33864, #17591, #133544, #52256, #163893, #51195, #117317, #49070, #66336, #15469, #183313, #50129, #115189, #116251, #100992, #18673, #84752, #2400, #118383, #30692, #14401, #64248, #130390, #196381, #32809, #98884, #40006, #108266, #88763, #8552, #125596, #172138, #188366, #74631, #109337, #42151, #122408, #105014, #106116, #56251, #190493, #6404, #73556, #159077, #38931, #26927, #174287, #10674, #60498, #25862, #93035, #91972, #158030, #155886, #7474, #175347, #76745, #171054, #142867, #22651, #204599, #23732, #173217, #24796, #191556, #59439, #9618, #184371, #43220, #89837, #139658, #208868, #205678, #154819, #57315, #123479, #90900, #75694, #141807, #58380, #189442, #72476, #41085, #107192, #124536, #156960, #138576, #140738, #206750, #207811, #13868, #79946, #129858, #130905, #127740, #47482, #163348, #45341, #211001, #193697, #126657, #44276, #160145, #77817, #209934, #177466, #29080, #95164, #161213, #12800, #78873, #144996, #207458, #56951, #59077, #156598, #172850, #26574, #7103, #125237, #43924, #158723, #61218, #91615, #193347, #174989, #155522, #143580, #127375, #189082, #191196, #25506, #74275, #108970, #157665, #209573, #73175, #77462, #139283, #205313, #8190, #10320, #9263, #105734, #92678, #140368, #42862, #76394, #173934, #123123, #206386, #41794, #142503, #58012, #208511, #11384, #75334, #60145, #40715, #124177, #126303, #171763, #192262, #110039, #24421, #90534, #190140, #176051, #27644, #93744, #107907, #23359, #89469, #194413, #114308, #78527, #145717, #16705, #111100, #99058, #180306, #148864, #44991, #31928, #165113, #98009, #15643, #13526, #79598, #181356, #438, #177106, #28722, #94808, #112176, #178181, #30870, #96948, #32982, #131600, #164064, #160857, #12449, #29796, #95880, #144644, #161935, #210660, #211715, #63352, #130563, #81731, #147813, #213832, #129510, #195491, #47126, #113242, #65450, #179246, #154204, #104389, #184543, #37244, #201847, #119628, #135822, #22024, #51371, #169377, #20961, #167252, #36163, #117494, #87059, #102242, #151011, #168314, #153131, #53491, #4704, #70778, #118559, #88133, #5773, #19911, #85996, #149941, #152070, #35094, #183485, #185613, #100113, #3640, #136892, #103315, #71852, #69719, #198653, #202919, #34040, #50302, #116420, #67575, #54563, #120709, #18838, #186684, #38312, #182411, #166174, #170436, #17763, #83851, #101165, #1509, #133720, #199725, #84923, #2580, #68650, #134773, #52433, #200781, #106567, #74018, #124984, #189894, #76145, #10069, #207206, #137960, #142248, #72929, #205059, #175798, #122868, #93490, #188829, #90276, #41536, #190944, #141195, #9007, #155270, #208261, #139035, #24173, #75082, #123926, #159529, #43672, #107647, #42608, #58830, #108716, #174743, #27390, #56701, #26317, #92429, #172595, #173679, #40464, #158469, #25254, #156345, #91355, #59894, #126045, #192007, #109790, #57765, #11128, #203980, #157416, #55627, #89218, #121784, #7930, #140108, #187751, #39380, #105476, #171509, #23102, #6851, #206135, #209317, #146514, #193090, #115114, #32728, #160599, #162752, #14324, #45806, #80416, #212533, #110846, #144400, #210401, #128198, #145469, #64173, #130316, #196304, #47950, #114064, #15392, #200273, #2061, #116976, #148363, #17255, #199203, #101729, #999, #68133, #20463, #34589, #18329, #16186, #67063, #133200, #150500, #36717, #118049, #198148, #98538, #50850, #132141, #167800 ),
 ( #102803, #86547, #114844, #152612, #164600, #65992, #182973, #19396, #85476, #151563, #3130, #48731, #69200, #119110, #4197, #214362, #39942, #137450, #170991, #138512, #189378, #22590, #155823, #108204, #73489, #57253, #55120, #187240, #6340, #123414, #54053, #41021, #107129, #173152, #24734, #90836, #206687, #207505, #63132, #148654, #25551, #16487, #15424, #221, #173978, #81514, #82567, #131388, #197384, #145499, #211496, #98843, #66293, #91661, #132439, #9310, #194191, #45835, #162780, #49026, #115144, #181141, #32763, #157713, #164893, #177958, #29572, #198440, #161715, #75383, #13307, #129295, #141497, #59125, #125282, #95663, #79380, #113020, #51148, #2360, #53277, #102030, #71634, #21805, #168100, #169157, #119409, #103098, #185398, #153984, #183270, #86845, #152911, #84709, #19699, #34874, #4488, #85777, #68436, #3434, #70559, #20750, #136678, #202703, #35952, #5552, #137747, #69501, #135609, #67356, #201629, #167035, #100948, #54353, #17547, #120492, #186465, #38101, #203766, #104173, #116208, #170221, #165962, #182194, #99901, #199505, #87911, #149718, #150796, #1297, #133501, #117272, #18630, #134565, #200567, #52213, #118343, #184327, #206981, #27167, #23960, #92212, #142030, #39165, #25032, #105249, #122642, #121564, #57549, #156125, #173452, #58611, #208044, #158263, #9852, #75927, #10903, #123707, #90063, #93272, #7707, #40237, #59672, #188605, #125830, #205915, #191791, #73790, #204830, #108498, #189668, #107427, #124766, #55410, #6636, #41318, #43449, #91132, #56482, #139885, #157190, #8786, #74867, #140972, #190725, #109572, #42389, #106348, #174522, #175576, #172370, #159305, #26098, #138811, #88997, #76980, #72715, #143106, #187536, #171290, #22881, #155050, #48766, #193932, #13038, #210171, #209099, #192855, #62864, #64984, #131140, #44514, #197128, #79118, #11980, #14094, #61811, #114881, #147334, #129030, #126898, #195005, #45579, #78054, #180881, #111695, #211238, #97528, #127979, #160378, #213363, #177702, #161459, #110631, #176632, #29313, #32502, #98576, #60734, #196084, #95407, #145233, #144178, #46639, #94337, #179830, #112761, #178774, #30386, #164638, #130089, #80184, #82305, #28243, #96473, #162521, #146289, #212301, #63934, #47716, #113832, #31450, #16222, #163585, #15167, #81255, #119144, #4231, #120225, #37833, #103910, #148400, #67098, #49818, #17291, #117009, #199239, #50886, #68170, #105820, #204308, #171846, #90619, #123200, #156676, #206468, #39711, #9344, #75417, #23439, #7186, #71113, #73258, #170774, #38648, #40800, #21293, #155601, #58095, #172931, #119962, #89550, #185937, #189161, #169703, #157747, #37572, #203251, #57033, #106906, #88475, #24508, #8269, #87398, #137230, #91694, #121048, #104726, #22363, #124256, #190214, #154534, #41874, #6114, #107985, #174012, #188082, #55965, #122117, #25583, #46135, #110118, #144725, #179329, #45073, #28801, #92756, #176130, #192341, #160938, #47207, #128523, #208588, #191274, #27729, #93824, #194492, #158801, #159865, #30950, #125315, #113322, #112251, #97024, #146841, #178262, #163078, #29875, #95959, #11467, #77540, #14660, #59157, #42940, #109049, #10398, #143662, #209656, #210737, #162013, #211795, #63432, #79676, #61297, #127458, #193429, #52252, #22923, #184367, #155094, #35990, #151895, #103138, #186509, #202742, #70602, #2397, #71673, #134603, #85816, #136716, #185436, #37056, #89038, #100986, #171328, #34913, #167076, #102070, #38140, #119449, #72756, #104212, #168135, #54392, #152952, #53316, #84747, #19737, #135646, #170259, #3470, #4527, #105292, #169197, #20790, #18667, #69539, #200605, #86885, #121603, #120530, #118379, #117311, #201669, #68476, #21844, #150835, #87952, #6679, #51188, #39200, #154026, #199546, #183307, #5593, #137786, #203805, #55451, #187575, #107474, #60784, #192900, #204870, #44556, #188648, #156168, #7749, #124808, #190769, #77021, #10947, #208087, #138853, #143151, #73836, #205959, #176672, #123749, #94379, #189710, #91177, #42431, #125874, #142073, #9893, #139932, #209145, #57592, #25074, #75970, #108537, #160419, #110672, #174567, #191833, #59715, #43496, #109616, #28284, #41363 ) ),
 .UNSPECIFIED., .F., .F., .T. ) 
 B_SPLINE_SURFACE_WITH_KNOTS ( ( 2, 2 ),
 ( 3, 2, 2, 2, 2, 2, 2, 2, 2, 2, 2, 2, 2, 2, 2, 2, 2, 2, 2, 2, 2, 2, 2, 2, 2, 2, 2, 2, 2, 2, 2, 2, 2, 2, 2, 2, 2, 2, 2, 2, 2, 2, 2, 2, 2, 2, 2, 2, 2, 2, 2, 2, 2, 2, 2, 2, 2, 2, 2, 2, 2, 2, 2, 2, 2, 2, 2, 2, 2, 2, 2, 2, 2, 2, 2, 2, 2, 2, 2, 2, 2, 2, 2, 2, 2, 2, 2, 2, 2, 2, 2, 2, 2, 2, 2, 2, 2, 2, 2, 2, 2, 2, 2, 2, 2, 2, 2, 2, 2, 2, 2, 2, 2, 2, 2, 2, 2, 2, 2, 2, 2, 2, 2, 2, 2, 2, 2, 2, 2, 2, 2, 2, 2, 2, 2, 2, 2, 2, 2, 2, 2, 2, 2, 2, 2, 2, 2, 2, 2, 2, 2, 2, 2, 2, 2, 2, 2, 2, 2, 2, 2, 2, 2, 2, 2, 2, 2, 2, 2, 2, 2, 2, 2, 2, 2, 2, 2, 2, 2, 2, 2, 2, 2, 2, 2, 2, 2, 2, 2, 2, 2, 2, 2, 2, 2, 2, 2, 2, 2, 2, 2, 2, 2, 2, 2, 2, 2, 2, 2, 2, 2, 2, 2, 2, 2, 2, 2, 2, 2, 2, 2, 2, 2, 2, 2, 2, 2, 2, 2, 2, 2, 2, 2, 2, 2, 2, 2, 2, 2, 2, 3 ),
 ( 0.000000000000000000, 1.000000000000000000 ),
 ( 0.000000000000000000, 0.004166666666666666609, 0.008333333333333333218, 0.01250000000000000069, 0.01666666666666666644, 0.02083333333333333218, 0.02500000000000000139, 0.02916666666666666713, 0.03333333333333333287, 0.03749999999999999861, 0.04166666666666666435, 0.04583333333333333010, 0.05000000000000000278, 0.05416666666666666852, 0.05833333333333333426, 0.06250000000000000000, 0.06666666666666666574, 0.07083333333333333148, 0.07499999999999999722, 0.07916666666666666297, 0.08333333333333332871, 0.08749999999999999445, 0.09166666666666666019, 0.09583333333333333981, 0.1000000000000000056, 0.1041666666666666713, 0.1083333333333333370, 0.1125000000000000028, 0.1166666666666666685, 0.1208333333333333343, 0.1250000000000000000, 0.1291666666666666796, 0.1333333333333333315, 0.1375000000000000111, 0.1416666666666666630, 0.1458333333333333426, 0.1499999999999999944, 0.1541666666666666741, 0.1583333333333333259, 0.1625000000000000056, 0.1666666666666666574, 0.1708333333333333370, 0.1749999999999999889, 0.1791666666666666685, 0.1833333333333333204, 0.1875000000000000000, 0.1916666666666666796, 0.1958333333333333315, 0.2000000000000000111, 0.2041666666666666630, 0.2083333333333333426, 0.2124999999999999944, 0.2166666666666666741, 0.2208333333333333259, 0.2250000000000000056, 0.2291666666666666574, 0.2333333333333333370, 0.2374999999999999889, 0.2416666666666666685, 0.2458333333333333204, 0.2500000000000000000, 0.2541666666666666519, 0.2583333333333333592, 0.2625000000000000111, 0.2666666666666666630, 0.2708333333333333148, 0.2750000000000000222, 0.2791666666666666741, 0.2833333333333333259, 0.2874999999999999778, 0.2916666666666666852, 0.2958333333333333370, 0.2999999999999999889, 0.3041666666666666408, 0.3083333333333333481, 0.3125000000000000000, 0.3166666666666666519, 0.3208333333333333592, 0.3250000000000000111, 0.3291666666666666630, 0.3333333333333333148, 0.3375000000000000222, 0.3416666666666666741, 0.3458333333333333259, 0.3499999999999999778, 0.3541666666666666852, 0.3583333333333333370, 0.3624999999999999889, 0.3666666666666666408, 0.3708333333333333481, 0.3750000000000000000, 0.3791666666666666519, 0.3833333333333333592, 0.3875000000000000111, 0.3916666666666666630, 0.3958333333333333148, 0.4000000000000000222, 0.4041666666666666741, 0.4083333333333333259, 0.4124999999999999778, 0.4166666666666666852, 0.4208333333333333370, 0.4249999999999999889, 0.4291666666666666408, 0.4333333333333333481, 0.4375000000000000000, 0.4416666666666666519, 0.4458333333333333592, 0.4500000000000000111, 0.4541666666666666630, 0.4583333333333333148, 0.4625000000000000222, 0.4666666666666666741, 0.4708333333333333259, 0.4749999999999999778, 0.4791666666666666852, 0.4833333333333333370, 0.4874999999999999889, 0.4916666666666666408, 0.4958333333333333481, 0.5000000000000000000, 0.5041666666666666519, 0.5083333333333333037, 0.5124999999999999556, 0.5166666666666667185, 0.5208333333333333703, 0.5250000000000000222, 0.5291666666666666741, 0.5333333333333333259, 0.5374999999999999778, 0.5416666666666666297, 0.5458333333333332815, 0.5500000000000000444, 0.5541666666666666963, 0.5583333333333333481, 0.5625000000000000000, 0.5666666666666666519, 0.5708333333333333037, 0.5749999999999999556, 0.5791666666666667185, 0.5833333333333333703, 0.5875000000000000222, 0.5916666666666666741, 0.5958333333333333259, 0.5999999999999999778, 0.6041666666666666297, 0.6083333333333332815, 0.6125000000000000444, 0.6166666666666666963, 0.6208333333333333481, 0.6250000000000000000, 0.6291666666666666519, 0.6333333333333333037, 0.6374999999999999556, 0.6416666666666667185, 0.6458333333333333703, 0.6500000000000000222, 0.6541666666666666741, 0.6583333333333333259, 0.6624999999999999778, 0.6666666666666666297, 0.6708333333333332815, 0.6750000000000000444, 0.6791666666666666963, 0.6833333333333333481, 0.6875000000000000000, 0.6916666666666666519, 0.6958333333333333037, 0.6999999999999999556, 0.7041666666666667185, 0.7083333333333333703, 0.7125000000000000222, 0.7166666666666666741, 0.7208333333333333259, 0.7249999999999999778, 0.7291666666666666297, 0.7333333333333332815, 0.7375000000000000444, 0.7416666666666666963, 0.7458333333333333481, 0.7500000000000000000, 0.7541666666666666519, 0.7583333333333333037, 0.7624999999999999556, 0.7666666666666667185, 0.7708333333333333703, 0.7750000000000000222, 0.7791666666666666741, 0.7833333333333333259, 0.7874999999999999778, 0.7916666666666666297, 0.7958333333333332815, 0.8000000000000000444, 0.8041666666666666963, 0.8083333333333333481, 0.8125000000000000000, 0.8166666666666666519, 0.8208333333333333037, 0.8249999999999999556, 0.8291666666666667185, 0.8333333333333333703, 0.8375000000000000222, 0.8416666666666666741, 0.8458333333333333259, 0.8499999999999999778, 0.8541666666666666297, 0.8583333333333332815, 0.8625000000000000444, 0.8666666666666666963, 0.8708333333333333481, 0.8750000000000000000, 0.8791666666666666519, 0.8833333333333333037, 0.8874999999999999556, 0.8916666666666667185, 0.8958333333333333703, 0.9000000000000000222, 0.9041666666666666741, 0.9083333333333333259, 0.9124999999999999778, 0.9166666666666666297, 0.9208333333333332815, 0.9250000000000000444, 0.9291666666666666963, 0.9333333333333333481, 0.9375000000000000000, 0.9416666666666666519, 0.9458333333333333037, 0.9499999999999999556, 0.9541666666666667185, 0.9583333333333333703, 0.9625000000000000222, 0.9666666666666666741, 0.9708333333333333259, 0.9749999999999999778, 0.9791666666666666297, 0.9833333333333332815, 0.9875000000000000444, 0.9916666666666666963, 0.9958333333333333481, 1.000000000000000000 ),
 .UNSPECIFIED. ) 
 GEOMETRIC_REPRESENTATION_ITEM ( )  RATIONAL_B_SPLINE_SURFACE ( (
 ( 1.000000000000000000, 0.8660254037844387076, 1.000000000000000000, 0.8660254037844387076, 1.000000000000000000, 0.8660254037844387076, 1.000000000000000000, 0.8660254037844387076, 1.000000000000000000, 0.8660254037844387076, 1.000000000000000000, 0.8660254037844387076, 1.000000000000000000, 0.8660254037844387076, 1.000000000000000000, 0.8660254037844387076, 1.000000000000000000, 0.8660254037844387076, 1.000000000000000000, 0.8660254037844387076, 1.000000000000000000, 0.8660254037844387076, 1.000000000000000000, 0.8660254037844387076, 1.000000000000000000, 0.8660254037844387076, 1.000000000000000000, 0.8660254037844387076, 1.000000000000000000, 0.8660254037844387076, 1.000000000000000000, 0.8660254037844387076, 1.000000000000000000, 0.8660254037844387076, 1.000000000000000000, 0.8660254037844387076, 1.000000000000000000, 0.8660254037844387076, 1.000000000000000000, 0.8660254037844387076, 1.000000000000000000, 0.8660254037844387076, 1.000000000000000000, 0.8660254037844387076, 1.000000000000000000, 0.8660254037844387076, 1.000000000000000000, 0.8660254037844387076, 1.000000000000000000, 0.8660254037844387076, 1.000000000000000000, 0.8660254037844387076, 1.000000000000000000, 0.8660254037844387076, 1.000000000000000000, 0.8660254037844387076, 1.000000000000000000, 0.8660254037844387076, 1.000000000000000000, 0.8660254037844387076, 1.000000000000000000, 0.8660254037844387076, 1.000000000000000000, 0.8660254037844387076, 1.000000000000000000, 0.8660254037844387076, 1.000000000000000000, 0.8660254037844387076, 1.000000000000000000, 0.8660254037844387076, 1.000000000000000000, 0.8660254037844387076, 1.000000000000000000, 0.8660254037844387076, 1.000000000000000000, 0.8660254037844387076, 1.000000000000000000, 0.8660254037844387076, 1.000000000000000000, 0.8660254037844387076, 1.000000000000000000, 0.8660254037844387076, 1.000000000000000000, 0.8660254037844387076, 1.000000000000000000, 0.8660254037844387076, 1.000000000000000000, 0.8660254037844387076, 1.000000000000000000, 0.8660254037844387076, 1.000000000000000000, 0.8660254037844387076, 1.000000000000000000, 0.8660254037844387076, 1.000000000000000000, 0.8660254037844387076, 1.000000000000000000, 0.8660254037844387076, 1.000000000000000000, 0.8660254037844387076, 1.000000000000000000, 0.8660254037844387076, 1.000000000000000000, 0.8660254037844387076, 1.000000000000000000, 0.8660254037844387076, 1.000000000000000000, 0.8660254037844387076, 1.000000000000000000, 0.8660254037844387076, 1.000000000000000000, 0.8660254037844387076, 1.000000000000000000, 0.8660254037844387076, 1.000000000000000000, 0.8660254037844387076, 1.000000000000000000, 0.8660254037844387076, 1.000000000000000000, 0.8660254037844387076, 1.000000000000000000, 0.8660254037844387076, 1.000000000000000000, 0.8660254037844387076, 1.000000000000000000, 0.8660254037844387076, 1.000000000000000000, 0.8660254037844387076, 1.000000000000000000, 0.8660254037844387076, 1.000000000000000000, 0.8660254037844387076, 1.000000000000000000, 0.8660254037844387076, 1.000000000000000000, 0.8660254037844387076, 1.000000000000000000, 0.8660254037844387076, 1.000000000000000000, 0.8660254037844387076, 1.000000000000000000, 0.8660254037844387076, 1.000000000000000000, 0.8660254037844387076, 1.000000000000000000, 0.8660254037844387076, 1.000000000000000000, 0.8660254037844387076, 1.000000000000000000, 0.8660254037844387076, 1.000000000000000000, 0.8660254037844387076, 1.000000000000000000, 0.8660254037844387076, 1.000000000000000000, 0.8660254037844387076, 1.000000000000000000, 0.8660254037844387076, 1.000000000000000000, 0.8660254037844387076, 1.000000000000000000, 0.8660254037844387076, 1.000000000000000000, 0.8660254037844387076, 1.000000000000000000, 0.8660254037844387076, 1.000000000000000000, 0.8660254037844387076, 1.000000000000000000, 0.8660254037844387076, 1.000000000000000000, 0.8660254037844387076, 1.000000000000000000, 0.8660254037844387076, 1.000000000000000000, 0.8660254037844387076, 1.000000000000000000, 0.8660254037844387076, 1.000000000000000000, 0.8660254037844387076, 1.000000000000000000, 0.8660254037844387076, 1.000000000000000000, 0.8660254037844387076, 1.000000000000000000, 0.8660254037844387076, 1.000000000000000000, 0.8660254037844387076, 1.000000000000000000, 0.8660254037844387076, 1.000000000000000000, 0.8660254037844387076, 1.000000000000000000, 0.8660254037844387076, 1.000000000000000000, 0.8660254037844387076, 1.000000000000000000, 0.8660254037844387076, 1.000000000000000000, 0.8660254037844387076, 1.000000000000000000, 0.8660254037844387076, 1.000000000000000000, 0.8660254037844387076, 1.000000000000000000, 0.8660254037844387076, 1.000000000000000000, 0.8660254037844387076, 1.000000000000000000, 0.8660254037844387076, 1.000000000000000000, 0.8660254037844387076, 1.000000000000000000, 0.8660254037844387076, 1.000000000000000000, 0.8660254037844387076, 1.000000000000000000, 0.8660254037844387076, 1.000000000000000000, 0.8660254037844387076, 1.000000000000000000, 0.8660254037844387076, 1.000000000000000000, 0.8660254037844387076, 1.000000000000000000, 0.8660254037844387076, 1.000000000000000000, 0.8660254037844387076, 1.000000000000000000, 0.8660254037844387076, 1.000000000000000000, 0.8660254037844387076, 1.000000000000000000, 0.8660254037844387076, 1.000000000000000000, 0.8660254037844387076, 1.000000000000000000, 0.8660254037844387076, 1.000000000000000000, 0.8660254037844387076, 1.000000000000000000, 0.8660254037844387076, 1.000000000000000000, 0.8660254037844387076, 1.000000000000000000, 0.8660254037844387076, 1.000000000000000000, 0.8660254037844387076, 1.000000000000000000, 0.8660254037844387076, 1.000000000000000000, 0.8660254037844387076, 1.000000000000000000, 0.8660254037844387076, 1.000000000000000000, 0.8660254037844387076, 1.000000000000000000, 0.8660254037844387076, 1.000000000000000000, 0.8660254037844387076, 1.000000000000000000, 0.8660254037844387076, 1.000000000000000000, 0.8660254037844387076, 1.000000000000000000, 0.8660254037844387076, 1.000000000000000000, 0.8660254037844387076, 1.000000000000000000, 0.8660254037844387076, 1.000000000000000000, 0.8660254037844387076, 1.000000000000000000, 0.8660254037844387076, 1.000000000000000000, 0.8660254037844387076, 1.000000000000000000, 0.8660254037844387076, 1.000000000000000000, 0.8660254037844387076, 1.000000000000000000, 0.8660254037844387076, 1.000000000000000000, 0.8660254037844387076, 1.000000000000000000, 0.8660254037844387076, 1.000000000000000000, 0.8660254037844387076, 1.000000000000000000, 0.8660254037844387076, 1.000000000000000000, 0.8660254037844387076, 1.000000000000000000, 0.8660254037844387076, 1.000000000000000000, 0.8660254037844387076, 1.000000000000000000, 0.8660254037844387076, 1.000000000000000000, 0.8660254037844387076, 1.000000000000000000, 0.8660254037844387076, 1.000000000000000000, 0.8660254037844387076, 1.000000000000000000, 0.8660254037844387076, 1.000000000000000000, 0.8660254037844387076, 1.000000000000000000, 0.8660254037844387076, 1.000000000000000000, 0.8660254037844387076, 1.000000000000000000, 0.8660254037844387076, 1.000000000000000000, 0.8660254037844387076, 1.000000000000000000, 0.8660254037844387076, 1.000000000000000000, 0.8660254037844387076, 1.000000000000000000, 0.8660254037844387076, 1.000000000000000000, 0.8660254037844387076, 1.000000000000000000, 0.8660254037844387076, 1.000000000000000000, 0.8660254037844387076, 1.000000000000000000, 0.8660254037844387076, 1.000000000000000000, 0.8660254037844387076, 1.000000000000000000, 0.8660254037844387076, 1.000000000000000000, 0.8660254037844387076, 1.000000000000000000, 0.8660254037844387076, 1.000000000000000000, 0.8660254037844387076, 1.000000000000000000, 0.8660254037844387076, 1.000000000000000000, 0.8660254037844387076, 1.000000000000000000, 0.8660254037844387076, 1.000000000000000000, 0.8660254037844387076, 1.000000000000000000, 0.8660254037844387076, 1.000000000000000000, 0.8660254037844387076, 1.000000000000000000, 0.8660254037844387076, 1.000000000000000000, 0.8660254037844387076, 1.000000000000000000, 0.8660254037844387076, 1.000000000000000000, 0.8660254037844387076, 1.000000000000000000, 0.8660254037844387076, 1.000000000000000000, 0.8660254037844387076, 1.000000000000000000, 0.8660254037844387076, 1.000000000000000000, 0.8660254037844387076, 1.000000000000000000, 0.8660254037844387076, 1.000000000000000000, 0.8660254037844387076, 1.000000000000000000, 0.8660254037844387076, 1.000000000000000000, 0.8660254037844387076, 1.000000000000000000, 0.8660254037844387076, 1.000000000000000000, 0.8660254037844387076, 1.000000000000000000, 0.8660254037844387076, 1.000000000000000000, 0.8660254037844387076, 1.000000000000000000, 0.8660254037844387076, 1.000000000000000000, 0.8660254037844387076, 1.000000000000000000, 0.8660254037844387076, 1.000000000000000000, 0.8660254037844387076, 1.000000000000000000, 0.8660254037844387076, 1.000000000000000000, 0.8660254037844387076, 1.000000000000000000, 0.8660254037844387076, 1.000000000000000000, 0.8660254037844387076, 1.000000000000000000, 0.8660254037844387076, 1.000000000000000000, 0.8660254037844387076, 1.000000000000000000, 0.8660254037844387076, 1.000000000000000000, 0.8660254037844387076, 1.000000000000000000, 0.8660254037844387076, 1.000000000000000000, 0.8660254037844387076, 1.000000000000000000, 0.8660254037844387076, 1.000000000000000000, 0.8660254037844387076, 1.000000000000000000, 0.8660254037844387076, 1.000000000000000000, 0.8660254037844387076, 1.000000000000000000, 0.8660254037844387076, 1.000000000000000000, 0.8660254037844387076, 1.000000000000000000, 0.8660254037844387076, 1.000000000000000000, 0.8660254037844387076, 1.000000000000000000, 0.8660254037844387076, 1.000000000000000000, 0.8660254037844387076, 1.000000000000000000, 0.8660254037844387076, 1.000000000000000000, 0.8660254037844387076, 1.000000000000000000, 0.8660254037844387076, 1.000000000000000000, 0.8660254037844387076, 1.000000000000000000, 0.8660254037844387076, 1.000000000000000000, 0.8660254037844387076, 1.000000000000000000, 0.8660254037844387076, 1.000000000000000000, 0.8660254037844387076, 1.000000000000000000, 0.8660254037844387076, 1.000000000000000000, 0.8660254037844387076, 1.000000000000000000, 0.8660254037844387076, 1.000000000000000000, 0.8660254037844387076, 1.000000000000000000, 0.8660254037844387076, 1.000000000000000000, 0.8660254037844387076, 1.000000000000000000, 0.8660254037844387076, 1.000000000000000000, 0.8660254037844387076, 1.000000000000000000, 0.8660254037844387076, 1.000000000000000000, 0.8660254037844387076, 1.000000000000000000, 0.8660254037844387076, 1.000000000000000000, 0.8660254037844387076, 1.000000000000000000, 0.8660254037844387076, 1.000000000000000000, 0.8660254037844387076, 1.000000000000000000, 0.8660254037844387076, 1.000000000000000000, 0.8660254037844387076, 1.000000000000000000),
 ( 1.000000000000000000, 0.8660254037844387076, 1.000000000000000000, 0.8660254037844387076, 1.000000000000000000, 0.8660254037844387076, 1.000000000000000000, 0.8660254037844387076, 1.000000000000000000, 0.8660254037844387076, 1.000000000000000000, 0.8660254037844387076, 1.000000000000000000, 0.8660254037844387076, 1.000000000000000000, 0.8660254037844387076, 1.000000000000000000, 0.8660254037844387076, 1.000000000000000000, 0.8660254037844387076, 1.000000000000000000, 0.8660254037844387076, 1.000000000000000000, 0.8660254037844387076, 1.000000000000000000, 0.8660254037844387076, 1.000000000000000000, 0.8660254037844387076, 1.000000000000000000, 0.8660254037844387076, 1.000000000000000000, 0.8660254037844387076, 1.000000000000000000, 0.8660254037844387076, 1.000000000000000000, 0.8660254037844387076, 1.000000000000000000, 0.8660254037844387076, 1.000000000000000000, 0.8660254037844387076, 1.000000000000000000, 0.8660254037844387076, 1.000000000000000000, 0.8660254037844387076, 1.000000000000000000, 0.8660254037844387076, 1.000000000000000000, 0.8660254037844387076, 1.000000000000000000, 0.8660254037844387076, 1.000000000000000000, 0.8660254037844387076, 1.000000000000000000, 0.8660254037844387076, 1.000000000000000000, 0.8660254037844387076, 1.000000000000000000, 0.8660254037844387076, 1.000000000000000000, 0.8660254037844387076, 1.000000000000000000, 0.8660254037844387076, 1.000000000000000000, 0.8660254037844387076, 1.000000000000000000, 0.8660254037844387076, 1.000000000000000000, 0.8660254037844387076, 1.000000000000000000, 0.8660254037844387076, 1.000000000000000000, 0.8660254037844387076, 1.000000000000000000, 0.8660254037844387076, 1.000000000000000000, 0.8660254037844387076, 1.000000000000000000, 0.8660254037844387076, 1.000000000000000000, 0.8660254037844387076, 1.000000000000000000, 0.8660254037844387076, 1.000000000000000000, 0.8660254037844387076, 1.000000000000000000, 0.8660254037844387076, 1.000000000000000000, 0.8660254037844387076, 1.000000000000000000, 0.8660254037844387076, 1.000000000000000000, 0.8660254037844387076, 1.000000000000000000, 0.8660254037844387076, 1.000000000000000000, 0.8660254037844387076, 1.000000000000000000, 0.8660254037844387076, 1.000000000000000000, 0.8660254037844387076, 1.000000000000000000, 0.8660254037844387076, 1.000000000000000000, 0.8660254037844387076, 1.000000000000000000, 0.8660254037844387076, 1.000000000000000000, 0.8660254037844387076, 1.000000000000000000, 0.8660254037844387076, 1.000000000000000000, 0.8660254037844387076, 1.000000000000000000, 0.8660254037844387076, 1.000000000000000000, 0.8660254037844387076, 1.000000000000000000, 0.8660254037844387076, 1.000000000000000000, 0.8660254037844387076, 1.000000000000000000, 0.8660254037844387076, 1.000000000000000000, 0.8660254037844387076, 1.000000000000000000, 0.8660254037844387076, 1.000000000000000000, 0.8660254037844387076, 1.000000000000000000, 0.8660254037844387076, 1.000000000000000000, 0.8660254037844387076, 1.000000000000000000, 0.8660254037844387076, 1.000000000000000000, 0.8660254037844387076, 1.000000000000000000, 0.8660254037844387076, 1.000000000000000000, 0.8660254037844387076, 1.000000000000000000, 0.8660254037844387076, 1.000000000000000000, 0.8660254037844387076, 1.000000000000000000, 0.8660254037844387076, 1.000000000000000000, 0.8660254037844387076, 1.000000000000000000, 0.8660254037844387076, 1.000000000000000000, 0.8660254037844387076, 1.000000000000000000, 0.8660254037844387076, 1.000000000000000000, 0.8660254037844387076, 1.000000000000000000, 0.8660254037844387076, 1.000000000000000000, 0.8660254037844387076, 1.000000000000000000, 0.8660254037844387076, 1.000000000000000000, 0.8660254037844387076, 1.000000000000000000, 0.8660254037844387076, 1.000000000000000000, 0.8660254037844387076, 1.000000000000000000, 0.8660254037844387076, 1.000000000000000000, 0.8660254037844387076, 1.000000000000000000, 0.8660254037844387076, 1.000000000000000000, 0.8660254037844387076, 1.000000000000000000, 0.8660254037844387076, 1.000000000000000000, 0.8660254037844387076, 1.000000000000000000, 0.8660254037844387076, 1.000000000000000000, 0.8660254037844387076, 1.000000000000000000, 0.8660254037844387076, 1.000000000000000000, 0.8660254037844387076, 1.000000000000000000, 0.8660254037844387076, 1.000000000000000000, 0.8660254037844387076, 1.000000000000000000, 0.8660254037844387076, 1.000000000000000000, 0.8660254037844387076, 1.000000000000000000, 0.8660254037844387076, 1.000000000000000000, 0.8660254037844387076, 1.000000000000000000, 0.8660254037844387076, 1.000000000000000000, 0.8660254037844387076, 1.000000000000000000, 0.8660254037844387076, 1.000000000000000000, 0.8660254037844387076, 1.000000000000000000, 0.8660254037844387076, 1.000000000000000000, 0.8660254037844387076, 1.000000000000000000, 0.8660254037844387076, 1.000000000000000000, 0.8660254037844387076, 1.000000000000000000, 0.8660254037844387076, 1.000000000000000000, 0.8660254037844387076, 1.000000000000000000, 0.8660254037844387076, 1.000000000000000000, 0.8660254037844387076, 1.000000000000000000, 0.8660254037844387076, 1.000000000000000000, 0.8660254037844387076, 1.000000000000000000, 0.8660254037844387076, 1.000000000000000000, 0.8660254037844387076, 1.000000000000000000, 0.8660254037844387076, 1.000000000000000000, 0.8660254037844387076, 1.000000000000000000, 0.8660254037844387076, 1.000000000000000000, 0.8660254037844387076, 1.000000000000000000, 0.8660254037844387076, 1.000000000000000000, 0.8660254037844387076, 1.000000000000000000, 0.8660254037844387076, 1.000000000000000000, 0.8660254037844387076, 1.000000000000000000, 0.8660254037844387076, 1.000000000000000000, 0.8660254037844387076, 1.000000000000000000, 0.8660254037844387076, 1.000000000000000000, 0.8660254037844387076, 1.000000000000000000, 0.8660254037844387076, 1.000000000000000000, 0.8660254037844387076, 1.000000000000000000, 0.8660254037844387076, 1.000000000000000000, 0.8660254037844387076, 1.000000000000000000, 0.8660254037844387076, 1.000000000000000000, 0.8660254037844387076, 1.000000000000000000, 0.8660254037844387076, 1.000000000000000000, 0.8660254037844387076, 1.000000000000000000, 0.8660254037844387076, 1.000000000000000000, 0.8660254037844387076, 1.000000000000000000, 0.8660254037844387076, 1.000000000000000000, 0.8660254037844387076, 1.000000000000000000, 0.8660254037844387076, 1.000000000000000000, 0.8660254037844387076, 1.000000000000000000, 0.8660254037844387076, 1.000000000000000000, 0.8660254037844387076, 1.000000000000000000, 0.8660254037844387076, 1.000000000000000000, 0.8660254037844387076, 1.000000000000000000, 0.8660254037844387076, 1.000000000000000000, 0.8660254037844387076, 1.000000000000000000, 0.8660254037844387076, 1.000000000000000000, 0.8660254037844387076, 1.000000000000000000, 0.8660254037844387076, 1.000000000000000000, 0.8660254037844387076, 1.000000000000000000, 0.8660254037844387076, 1.000000000000000000, 0.8660254037844387076, 1.000000000000000000, 0.8660254037844387076, 1.000000000000000000, 0.8660254037844387076, 1.000000000000000000, 0.8660254037844387076, 1.000000000000000000, 0.8660254037844387076, 1.000000000000000000, 0.8660254037844387076, 1.000000000000000000, 0.8660254037844387076, 1.000000000000000000, 0.8660254037844387076, 1.000000000000000000, 0.8660254037844387076, 1.000000000000000000, 0.8660254037844387076, 1.000000000000000000, 0.8660254037844387076, 1.000000000000000000, 0.8660254037844387076, 1.000000000000000000, 0.8660254037844387076, 1.000000000000000000, 0.8660254037844387076, 1.000000000000000000, 0.8660254037844387076, 1.000000000000000000, 0.8660254037844387076, 1.000000000000000000, 0.8660254037844387076, 1.000000000000000000, 0.8660254037844387076, 1.000000000000000000, 0.8660254037844387076, 1.000000000000000000, 0.8660254037844387076, 1.000000000000000000, 0.8660254037844387076, 1.000000000000000000, 0.8660254037844387076, 1.000000000000000000, 0.8660254037844387076, 1.000000000000000000, 0.8660254037844387076, 1.000000000000000000, 0.8660254037844387076, 1.000000000000000000, 0.8660254037844387076, 1.000000000000000000, 0.8660254037844387076, 1.000000000000000000, 0.8660254037844387076, 1.000000000000000000, 0.8660254037844387076, 1.000000000000000000, 0.8660254037844387076, 1.000000000000000000, 0.8660254037844387076, 1.000000000000000000, 0.8660254037844387076, 1.000000000000000000, 0.8660254037844387076, 1.000000000000000000, 0.8660254037844387076, 1.000000000000000000, 0.8660254037844387076, 1.000000000000000000, 0.8660254037844387076, 1.000000000000000000, 0.8660254037844387076, 1.000000000000000000, 0.8660254037844387076, 1.000000000000000000, 0.8660254037844387076, 1.000000000000000000, 0.8660254037844387076, 1.000000000000000000, 0.8660254037844387076, 1.000000000000000000, 0.8660254037844387076, 1.000000000000000000, 0.8660254037844387076, 1.000000000000000000, 0.8660254037844387076, 1.000000000000000000, 0.8660254037844387076, 1.000000000000000000, 0.8660254037844387076, 1.000000000000000000, 0.8660254037844387076, 1.000000000000000000, 0.8660254037844387076, 1.000000000000000000, 0.8660254037844387076, 1.000000000000000000, 0.8660254037844387076, 1.000000000000000000, 0.8660254037844387076, 1.000000000000000000, 0.8660254037844387076, 1.000000000000000000, 0.8660254037844387076, 1.000000000000000000, 0.8660254037844387076, 1.000000000000000000, 0.8660254037844387076, 1.000000000000000000, 0.8660254037844387076, 1.000000000000000000, 0.8660254037844387076, 1.000000000000000000, 0.8660254037844387076, 1.000000000000000000, 0.8660254037844387076, 1.000000000000000000, 0.8660254037844387076, 1.000000000000000000, 0.8660254037844387076, 1.000000000000000000, 0.8660254037844387076, 1.000000000000000000, 0.8660254037844387076, 1.000000000000000000, 0.8660254037844387076, 1.000000000000000000, 0.8660254037844387076, 1.000000000000000000, 0.8660254037844387076, 1.000000000000000000, 0.8660254037844387076, 1.000000000000000000, 0.8660254037844387076, 1.000000000000000000, 0.8660254037844387076, 1.000000000000000000, 0.8660254037844387076, 1.000000000000000000, 0.8660254037844387076, 1.000000000000000000, 0.8660254037844387076, 1.000000000000000000, 0.8660254037844387076, 1.000000000000000000, 0.8660254037844387076, 1.000000000000000000, 0.8660254037844387076, 1.000000000000000000, 0.8660254037844387076, 1.000000000000000000, 0.8660254037844387076, 1.000000000000000000, 0.8660254037844387076, 1.000000000000000000, 0.8660254037844387076, 1.000000000000000000, 0.8660254037844387076, 1.000000000000000000, 0.8660254037844387076, 1.000000000000000000, 0.8660254037844387076, 1.000000000000000000, 0.8660254037844387076, 1.000000000000000000, 0.8660254037844387076, 1.000000000000000000, 0.8660254037844387076, 1.000000000000000000, 0.8660254037844387076, 1.000000000000000000, 0.8660254037844387076, 1.000000000000000000) ) ) 
 REPRESENTATION_ITEM ( '' )  SURFACE ( )  );
#56224=CARTESIAN_POINT ( 'NONE',  ( 6.030679399980265920, 5.930214142932100252, -0.7998128361456281477 ) ) ;
#56228=CARTESIAN_POINT ( 'NONE',  ( 3.979481780810941949, 4.601482484822914998, 1.199719254218464037 ) ) ;
#56235=CARTESIAN_POINT ( 'NONE',  ( -3.768803514918943609, 7.340761834139994058, 0.7216878364870317197 ) ) ;
#56236=CARTESIAN_POINT ( 'NONE',  ( 3.871016551901614200, 4.474939717762034697, -1.199719254218446718 ) ) ;
#56240=CARTESIAN_POINT ( 'NONE',  ( -6.663996196316808174, 7.733415969579778171, -1.199719254218446718 ) ) ;
#56241=CARTESIAN_POINT ( 'NONE',  ( -3.076612070176407698, 6.450603142078709773, -0.6987248798898172408 ) ) ;
#56245=CARTESIAN_POINT ( 'NONE',  ( -9.657485491635913633, 10.16148791653038330, 1.040834085586084257E-14 ) ) ;
#56251=CARTESIAN_POINT ( 'NONE',  ( 3.825371897350130723, 7.614684313550482031, 0.7998128361456321445 ) ) ;
#56263=CARTESIAN_POINT ( 'NONE',  ( -7.152089726408780379, 8.302858421353754181, -1.199719254218446718 ) ) ;
#56266=CARTESIAN_POINT ( 'NONE',  ( 4.636525346193557162, 7.392734756325715750, -1.082531754730549078 ) ) ;
#56272=CARTESIAN_POINT ( 'NONE',  ( -5.949330478298285207, 5.835307067636438028, 0.7998128361456341429 ) ) ;
#56275=CARTESIAN_POINT ( 'NONE',  ( -7.217017841176048165, 7.314275657660511243, 1.040834085586084257E-14 ) ) ;
#56281=CARTESIAN_POINT ( 'NONE',  ( -7.655550293210764856, 12.08322577538792331, 0.000000000000000000 ) ) ;
#56282=CARTESIAN_POINT ( 'NONE',  ( 7.786460292950004636, 7.978625184730144149, 1.040834085586084257E-14 ) ) ;
#56284=CARTESIAN_POINT ( 'NONE',  ( -3.470524135418306511, 5.072030796119872953, -1.443375672974053447 ) ) ;
#56285=CARTESIAN_POINT ( 'NONE',  ( -8.622095623286845978, 12.14652976288826913, 1.199719254218462483 ) ) ;
#56292=CARTESIAN_POINT ( 'NONE',  ( 8.419250204406344196, 12.76628297187536809, 1.040834085586084257E-14 ) ) ;
#56312=CARTESIAN_POINT ( 'NONE',  ( -2.948008335967658322, 5.526761261015804116, 1.199719254218462483 ) ) ;
#56314=CARTESIAN_POINT ( 'NONE',  ( -4.647747731386360215, 4.316793862905830892, 0.7998128361456341429 ) ) ;
#56319=CARTESIAN_POINT ( 'NONE',  ( -1.402160292154681736E-14, -1.006249999317181620, 1.732050807568877637 ) ) ;
#56322=CARTESIAN_POINT ( 'NONE',  ( -3.307826292054316664, 4.882216645528547616, -1.443375672974059665 ) ) ;
#56329=CARTESIAN_POINT ( 'NONE',  ( 10.55232363013785246, 11.20546574478267132, 0.000000000000000000 ) ) ;
#56333=CARTESIAN_POINT ( 'NONE',  ( 9.205623113554615600, 11.76297960394566466, 1.443375672974076540 ) ) ;
#56335=CARTESIAN_POINT ( 'NONE',  ( -0.6823417656250212460, 2.113541667008083991, 1.181850606188767472 ) ) ;
#56336=FACE_OUTER_BOUND ( 'NONE', #145384, .T. ) ;
#56338=CARTESIAN_POINT ( 'NONE',  ( -7.133561379084627063, 11.47423870890741782, 0.7998128361456481317 ) ) ;
#56339=CARTESIAN_POINT ( 'NONE',  ( -3.402733366905605905, 6.913679994791092298, 0.7216878364870317197 ) ) ;
#56341=CARTESIAN_POINT ( 'NONE',  ( -7.040761844198392794, 7.108643661186573759, -0.7998128361456291469 ) ) ;
#56343=CARTESIAN_POINT ( 'NONE',  ( 1.364683531249990311, 5.613541667008087543, 0.7879004041258500513 ) ) ;
#56351=CARTESIAN_POINT ( 'NONE',  ( -4.731432421044873493, 7.503459676985569260, -1.082531754730548412 ) ) ;
#56355=CARTESIAN_POINT ( 'NONE',  ( -5.219525951136856357, 6.152163700156858539, -1.082531754730543971 ) ) ;
#56357=CARTESIAN_POINT ( 'NONE',  ( 10.42352117080803708, 11.05519620889787724, -0.7998128361456281477 ) ) ;
#56362=VERTEX_POINT ( 'NONE', #134754 ) ;
#56365=CARTESIAN_POINT ( 'NONE',  ( 3.199361063144932960, 6.676412307070378915, -0.7216878364870045193 ) ) ;
#56366=CARTESIAN_POINT ( 'NONE',  ( -3.228813138348844536, 6.918699094715619502, 0.7998128361456341429 ) ) ;
#56368=CARTESIAN_POINT ( 'NONE',  ( -10.62011439820619429, 11.28455497419572318, -0.7998128361456221525 ) ) ;
#56373=CARTESIAN_POINT ( 'NONE',  ( 4.821896187954575197, 8.777295985922343391, 0.7998128361456462443 ) ) ;
#56377=CARTESIAN_POINT ( 'NONE',  ( 6.471393748265540147, 5.229711127717882491, 2.420000000000010587 ) ) ;
#56378=CARTESIAN_POINT ( 'NONE',  ( 2.218730694130720771, 5.740269576461138890, 0.7998128361456462443 ) ) ;
#56388=CARTESIAN_POINT ( 'NONE',  ( 9.447334110624092673, 9.916311305349925220, -0.7998128361456281477 ) ) ;
#56389=CARTESIAN_POINT ( 'NONE',  ( -4.401593425930945713, 8.286942763561420122, 1.040834085586084257E-14 ) ) ;
#56397=CARTESIAN_POINT ( 'NONE',  ( -1.364683531250012516, 4.238541667008090208, -0.7879004041258300672 ) ) ;
#56399=CARTESIAN_POINT ( 'NONE',  ( -4.388035272317281077, 8.271124917678806199, 0.7998128361456481317 ) ) ;
#56402=CARTESIAN_POINT ( 'NONE',  ( 5.840865249388943248, 5.708764300575555062, 0.7998128361456341429 ) ) ;
#56403=CARTESIAN_POINT ( 'NONE',  ( -4.252453736180621391, 8.112946458852704268, -0.7998128361456281477 ) ) ;
#56409=CARTESIAN_POINT ( 'NONE',  ( 6.643132081016117851, 8.773406732650713025, 1.443375672974076540 ) ) ;
#56412=CARTESIAN_POINT ( 'NONE',  ( 6.602457619730756733, 9.686322408785807525, 1.082531754730558626 ) ) ;
#56413=CARTESIAN_POINT ( 'NONE',  ( -1.364683531249997417, 3.321875000341423245, 1.214306433183764966E-14 ) ) ;
#56415=CARTESIAN_POINT ( 'NONE',  ( 3.484082288587588838, 7.008587070086755411, -0.7216878364870267237 ) ) ;
#56417=FACE_OUTER_BOUND ( 'NONE', #142024, .T. ) ;
#56420=B_SPLINE_CURVE_WITH_KNOTS ( 'NONE', 3,
 ( #8175, #108953, #142484, #172832, #197326, #112960, #174973, #26554, #46846, #41777 ),
 .UNSPECIFIED., .F., .F.,
 ( 4, 3, 3, 4 ),
 ( 8.603168645141783524E-16, 3.125222853364259014E-05, 6.323671013787866575E-05, 9.524404753373414908E-05 ),
 .UNSPECIFIED. ) ;
#56426=CARTESIAN_POINT ( 'NONE',  ( -4.095724654357025152, 7.689947244493171574, 0.7385042830605083042 ) ) ;
#56432=CARTESIAN_POINT ( 'NONE',  ( -7.967387826325084355, 12.44703623068796361, 0.7998128361456481317 ) ) ;
#56440=EDGE_LOOP ( 'NONE', ( #27689, #115790, #199539, #92442, #96911 ) ) ;
#56442=CARTESIAN_POINT ( 'NONE',  ( 2.901081683644312736, 6.328419697652925002, 0.7216878364870338292 ) ) ;
#56443=CARTESIAN_POINT ( 'NONE',  ( 1.364683531249990311, 3.696875000341416584, 1.214306433183764966E-14 ) ) ;
#56445=CARTESIAN_POINT ( 'NONE',  ( 7.456094412511537151, 10.78619501698377370, 1.199719254218460707 ) ) ;
#56452=CARTESIAN_POINT ( 'NONE',  ( 1.499999999999987121, 3.795833333333356929, -0.8660254037844262731 ) ) ;
#56453=CARTESIAN_POINT ( 'NONE',  ( 5.660692828905515839, 6.562895374266609849, -1.199719254218445830 ) ) ;
#56456=CARTESIAN_POINT ( 'NONE',  ( 1.445103857048099627, 8.688264192037895128, 2.625611233228258179 ) ) ;
#56457=CARTESIAN_POINT ( 'NONE',  ( -1.364683531250010295, 4.530208333674754506, 0.7879004041258379498 ) ) ;
#56459=CARTESIAN_POINT ( 'NONE',  ( 8.839552966430002101, 11.33589776563360019, -1.443375672974052559 ) ) ;
#56464=CARTESIAN_POINT ( 'NONE',  ( -0.7500000000000215383, 1.972916667349486453, 1.299038105676659116 ) ) ;
#56466=CARTESIAN_POINT ( 'NONE',  ( -6.403528624356093601, 6.365204904703887223, 1.040834085586084257E-14 ) ) ;
#56467=CARTESIAN_POINT ( 'NONE',  ( 5.477130869796502211, 5.492333557625114437, 1.040834085586084257E-14 ) ) ;
#56476=CARTESIAN_POINT ( 'NONE',  ( 5.960781091502512119, 10.10599504006161986, 0.7998128361456462443 ) ) ;
#56477=CARTESIAN_POINT ( 'NONE',  ( 6.173040012923759257, 6.096301524699504704, -0.7998128361456281477 ) ) ;
#56478=LINE ( 'NONE', #155047, #147494 ) ;
#56482=CARTESIAN_POINT ( 'NONE',  ( 6.114890974963323345, 7.092793211334054604, 1.199719254218462483 ) ) ;
#56487=ORIENTED_EDGE ( 'NONE', *, *, #46380, .F. ) ;
#56490=CARTESIAN_POINT ( 'NONE',  ( 9.028840231696797503, 12.62106513936658203, -1.199719254218446718 ) ) ;
#56496=CARTESIAN_POINT ( 'NONE',  ( 5.086710258240730198, 6.515995995190169587, 1.216687342998038934 ) ) ;
#56505=CARTESIAN_POINT ( 'NONE',  ( 7.809133291791403586, 8.213003049952529722, -0.7216878364870257245 ) ) ;
#56507=CARTESIAN_POINT ( 'NONE',  ( -3.079673448598517549, 6.744702790006905424, 1.040834085586084257E-14 ) ) ;
#56511=CARTESIAN_POINT ( 'NONE',  ( -4.069418662396130593, 7.899405539437467816, -0.7998128361456281477 ) ) ;
#56520=DIRECTION ( 'NONE',  ( 0.000000000000000000, 8.546850786086437571E-32, 1.000000000000000000 ) ) ;
#56528=CARTESIAN_POINT ( 'NONE',  ( 2.738383840280328663, 5.178236332760252303, 1.082531754730548412 ) ) ;
#56533=CARTESIAN_POINT ( 'NONE',  ( -10.16825202056928390, 10.96530823352674133, 0.7216878364870438212 ) ) ;
#56537=CARTESIAN_POINT ( 'NONE',  ( 9.576136569953906275, 10.06658084123472641, 0.000000000000000000 ) ) ;
#56541=CARTESIAN_POINT ( 'NONE',  ( -6.358937740009323214, 7.377514437221045718, -1.199719254218446718 ) ) ;
#56542=CARTESIAN_POINT ( 'NONE',  ( 4.578903193113299963, 6.365139696764064325, 1.599625672291267398 ) ) ;
#56551=CARTESIAN_POINT ( 'NONE',  ( 0.6823417656249882723, 2.238541667008084435, -1.181850606188749264 ) ) ;
#56555=CARTESIAN_POINT ( 'NONE',  ( 6.643132081016117851, 8.773406732650713025, 1.443375672974076540 ) ) ;
#56563=CARTESIAN_POINT ( 'NONE',  ( 8.229436053370658755, 12.54483312900040026, 0.7216878364870438212 ) ) ;
#56567=B_SPLINE_CURVE_WITH_KNOTS ( 'NONE', 3,
 ( #75548, #9475, #203643, #52095, #26783, #53157, #119286, #92888, #102977, #158933 ),
 .UNSPECIFIED., .F., .F.,
 ( 4, 3, 3, 4 ),
 ( 0.000000000000000000, 8.893179197954857176E-05, 0.0001334007970840202239, 0.0001778705873658964021 ),
 .UNSPECIFIED. ) ;
#56569=CARTESIAN_POINT ( 'NONE',  ( -8.157201976916404362, 12.66848607304450702, -0.7998128361456281477 ) ) ;
#56577=CARTESIAN_POINT ( 'NONE',  ( 5.190073875932979419, 4.949507698210251938, 0.7998128361456341429 ) ) ;
#56583=CARTESIAN_POINT ( 'NONE',  ( 4.299907273828439180, 8.168308919441841454, 1.040834085586084257E-14 ) ) ;
#56586=CARTESIAN_POINT ( 'NONE',  ( 1.499999999999987121, 3.327083334016150751, -0.8660254037844262731 ) ) ;
#56591=CARTESIAN_POINT ( 'NONE',  ( 1.499999999999989120, 0.5250000000000185629, 0.000000000000000000 ) ) ;
#56592=CARTESIAN_POINT ( 'NONE',  ( 8.423693512792301163, 8.722063941212843119, 0.7998128361456481317 ) ) ;
#56593=CARTESIAN_POINT ( 'NONE',  ( -1.402160292154681736E-14, -0.05312499965857903073, -1.575800808251665908 ) ) ;
#56596=CARTESIAN_POINT ( 'NONE',  ( 9.910647101909615841, 10.66476916175714607, 0.000000000000000000 ) ) ;
#56601=CARTESIAN_POINT ( 'NONE',  ( -6.067437437315529536, 7.037430750744921859, 1.199719254218450271 ) ) ;
#56602=CARTESIAN_POINT ( 'NONE',  ( -1.201851678989727383E-14, 2.243750000682818158, 1.732050807568877637 ) ) ;
#56603=CARTESIAN_POINT ( 'NONE',  ( 1.364683531249990311, 5.176041667008085767, 0.7879004041258500513 ) ) ;
#56608=CARTESIAN_POINT ( 'NONE',  ( 0.6823417656249899377, 4.238541667008085767, -1.181850606188754593 ) ) ;
#56616=CARTESIAN_POINT ( 'NONE',  ( -8.208571938070008400, 11.66408546346865016, -1.199719254218446718 ) ) ;
#56617=CARTESIAN_POINT ( 'NONE',  ( 7.630541526392844887, 7.796719957080126662, 0.7998128361456341429 ) ) ;
#56624=CARTESIAN_POINT ( 'NONE',  ( -6.008234629150358330, 10.16135750065076060, 0.000000000000000000 ) ) ;
#56630=CARTESIAN_POINT ( 'NONE',  ( 4.539282502477016479, 4.190251095844947926, 0.7998128361456341429 ) ) ;
#56632=CARTESIAN_POINT ( 'NONE',  ( -5.416646063859567484, 6.278174148379618735, 1.199719254218450271 ) ) ;
#56634=CARTESIAN_POINT ( 'NONE',  ( -8.941766003412679353, 10.39081407785832845, -1.199719254218446718 ) ) ;
#56638=CARTESIAN_POINT ( 'NONE',  ( -4.074744958279661766, 7.716589449174610316, -0.6783282581392232613 ) ) ;
#56645=CARTESIAN_POINT ( 'NONE',  ( 4.496500501226593727, 8.397667684739696270, 0.7998128361456462443 ) ) ;
#56646=EDGE_CURVE ( 'NONE', #109221, #197571, #113836, .T. ) ;
#56649=CARTESIAN_POINT ( 'NONE',  ( 5.381422217466650615, 4.322449550048924394, 2.440471613107408011 ) ) ;
#56666=CARTESIAN_POINT ( 'NONE',  ( 3.470524135418292300, 5.072030796119872953, -1.443375672974057666 ) ) ;
#56670=CARTESIAN_POINT ( 'NONE',  ( -7.784352752540590004, 12.23349531127272094, 0.7998128361456481317 ) ) ;
#56676=CARTESIAN_POINT ( 'NONE',  ( -0.7500000000000006661, 1.389583334016154748, -1.299038105676652011 ) ) ;
#56680=DIRECTION ( 'NONE',  ( 0.000000000000000000, 1.000000000000000000, 0.000000000000000000 ) ) ;
#56682=CARTESIAN_POINT ( 'NONE',  ( 1.364683531249986537, 0.8635416670080893198, 0.7879004041258500513 ) ) ;
#56688=CARTESIAN_POINT ( 'NONE',  ( -3.307299406729781399, 5.945934176904983381, -1.199719254218452935 ) ) ;
#56690=CARTESIAN_POINT ( 'NONE',  ( 0.000000000000000000, 6.487495393664096888, -3.100011470320000573 ) ) ;
#56693=CARTESIAN_POINT ( 'NONE',  ( -1.364683531250000748, 0.5718750003414208027, 0.000000000000000000 ) ) ;
#56698=CARTESIAN_POINT ( 'NONE',  ( 1.364683531249986537, 0.8635416670080893198, 0.7879004041258500513 ) ) ;
#56700=CARTESIAN_POINT ( 'NONE',  ( -8.064402442030170093, 8.302891025323665630, 0.7998128361456602331 ) ) ;
#56701=CARTESIAN_POINT ( 'NONE',  ( 9.185812768458653466, 10.67553530374532045, 1.199719254218453823 ) ) ;
#56705=CARTESIAN_POINT ( 'NONE',  ( -1.402160292154681736E-14, 1.259375000341419248, -1.575800808251659024 ) ) ;
#56713=CARTESIAN_POINT ( 'NONE',  ( 6.317736394288135493, 8.393778431468064127, 1.443375672974076540 ) ) ;
#56716=CARTESIAN_POINT ( 'NONE',  ( -4.172158584703340445, 5.890604320285754980, -1.599625672291256295 ) ) ;
#56721=CARTESIAN_POINT ( 'NONE',  ( 4.487385655998873624, 7.218738451098584363, 1.082531754730558626 ) ) ;
#56722=CARTESIAN_POINT ( 'NONE',  ( -8.148087131688692253, 9.568818410800712826, -1.082531754730543083 ) ) ;
#56724=CARTESIAN_POINT ( 'NONE',  ( 1.499999999999990896, 4.025000000000021672, 1.214306433183764966E-14 ) ) ;
#56728=CARTESIAN_POINT ( 'NONE',  ( 8.107412671292022921, 12.40247251657532956, 0.7216878364870438212 ) ) ;
#56739=CARTESIAN_POINT ( 'NONE',  ( -2.476786429007699297, 5.182949722010740778, -0.9424847539492169357 ) ) ;
#56740=CARTESIAN_POINT ( 'NONE',  ( 7.741342523278698096, 10.05465224862374285, 1.443375672974076540 ) ) ;
#56741=CARTESIAN_POINT ( 'NONE',  ( 6.740374924288304648, 11.01552117831172062, 1.040834085586084257E-14 ) ) ;
#56742=CARTESIAN_POINT ( 'NONE',  ( -4.693093728624763372, 8.627026450037540428, 0.7998128361456481317 ) ) ;
#56749=CARTESIAN_POINT ( 'NONE',  ( 4.039966587192257208, 6.696749537490852333, 1.082531754730558626 ) ) ;
#56752=CARTESIAN_POINT ( 'NONE',  ( -8.866669273657352690, 9.446795028796142191, 0.7216878364870438212 ) ) ;
#56778=CARTESIAN_POINT ( 'NONE',  ( -5.551173829791513192, 8.563787670477010394, 1.199719254218452047 ) ) ;
#56788=EDGE_CURVE ( 'NONE', #179865, #15325, #195015, .T. ) ;
#56789=CARTESIAN_POINT ( 'NONE',  ( -2.927671105547157371, 5.503034492191895666, 1.199719254218462483 ) ) ;
#56792=CARTESIAN_POINT ( 'NONE',  ( 7.287671262545424966, 8.461036880179857889, -1.199719254218451159 ) ) ;
#56793=CARTESIAN_POINT ( 'NONE',  ( -1.201851678989727383E-14, 3.696875000341422801, -1.575800808251660134 ) ) ;
#56795=CARTESIAN_POINT ( 'NONE',  ( 6.082781304119575516, 6.035783188292461077, -0.3281998023207943760 ) ) ;
#56800=CARTESIAN_POINT ( 'NONE',  ( 5.788968402910802169, 8.737251655829183505, 1.082531754730558626 ) ) ;
#56801=CARTESIAN_POINT ( 'NONE',  ( -8.857554428429624593, 9.228235009456373206, 0.7998128361456462443 ) ) ;
#56804=CARTESIAN_POINT ( 'NONE',  ( -9.155833807930273238, 9.576227618873799585, -0.7998128361456291469 ) ) ;
#56805=CARTESIAN_POINT ( 'NONE',  ( -5.605406444246153974, 8.627059054007450101, -1.199719254218440723 ) ) ;
#56809=CARTESIAN_POINT ( 'NONE',  ( 0.7499999999999885647, 3.347916667349487341, -1.299038105676658228 ) ) ;
#56813=CARTESIAN_POINT ( 'NONE',  ( 7.564559641420864899, 10.91273778404466199, -1.199719254218446718 ) ) ;
#56828=CARTESIAN_POINT ( 'NONE',  ( 0.7499999999999902300, 4.566666666666691299, -1.299038105676658228 ) ) ;
#56829=CARTESIAN_POINT ( 'NONE',  ( 4.416205349749311004, 6.175325546172740765, 1.599625672291267398 ) ) ;
#56830=CARTESIAN_POINT ( 'NONE',  ( 5.309989718046547402, 9.346738437696316737, 0.7998128361456462443 ) ) ;
#56832=CARTESIAN_POINT ( 'NONE',  ( -8.351459436338037889, 10.76645531385962862, -1.443375672974059665 ) ) ;
#56834=CARTESIAN_POINT ( 'NONE',  ( 5.666945020832167224, 8.594891043404107478, 1.082531754730558626 ) ) ;
#56835=CARTESIAN_POINT ( 'NONE',  ( -9.449669878600623463, 11.08733161553131197, -1.082531754730537976 ) ) ;
#56836=AXIS2_PLACEMENT_3D ( 'NONE', #189972, #12280, #42695 ) ;
#56839=CARTESIAN_POINT ( 'NONE',  ( 7.401861798056875053, 10.72292363345333399, -1.199719254218441611 ) ) ;
#56846=CARTESIAN_POINT ( 'NONE',  ( 1.364683531249990311, 2.884375000341422801, 1.214306433183764966E-14 ) ) ;
#56852=CARTESIAN_POINT ( 'NONE',  ( 7.899597058256738968, 12.36794700127490820, 1.040834085586084257E-14 ) ) ;
#56855=CARTESIAN_POINT ( 'NONE',  ( -9.073431116043565225, 11.60875560684942265, -1.599625672291263179 ) ) ;
#56861=CARTESIAN_POINT ( 'NONE',  ( 2.693266070609028784, 6.293894182352508970, 0.000000000000000000 ) ) ;
#56864=CARTESIAN_POINT ( 'NONE',  ( -8.045874094706015001, 11.47427131287732927, -1.199719254218446718 ) ) ;
#56867=CARTESIAN_POINT ( 'NONE',  ( 7.099665995050449041, 11.43469409420089455, 0.7998128361456462443 ) ) ;
#56869=CARTESIAN_POINT ( 'NONE',  ( 4.215071147998584955, 7.318223152490296535, 0.8720340548805920466 ) ) ;
#56871=CARTESIAN_POINT ( 'NONE',  ( -3.632695093457760649, 6.325562478087638496, -1.199719254218452047 ) ) ;
#56875=CARTESIAN_POINT ( 'NONE',  ( 8.046927864910717432, 9.346836249606042202, 1.199719254218462483 ) ) ;
#56877=CARTESIAN_POINT ( 'NONE',  ( 5.777746017718023097, 9.892454120646377191, 0.7998128361456462443 ) ) ;
#56880=CARTESIAN_POINT ( 'NONE',  ( -7.687109909268394325, 11.91211929421440097, 0.000000000000000000 ) ) ;
#56888=CARTESIAN_POINT ( 'NONE',  ( -4.512490679940424521, 7.037946173918820492, -1.151410311177623935 ) ) ;
#56889=CARTESIAN_POINT ( 'NONE',  ( 1.364683531249986537, 1.655208333674748955, -0.7879004041258239610 ) ) ;
#56891=CARTESIAN_POINT ( 'NONE',  ( 6.697364695470787943, 7.876308901879812474, -1.082531754730543083 ) ) ;
#56913=CARTESIAN_POINT ( 'NONE',  ( 8.880754312151170282, 10.31963377138658089, 1.199719254218453823 ) ) ;
#56917=CARTESIAN_POINT ( 'NONE',  ( -2.300079615812729905, 5.835176651756807331, -0.7998128361456281477 ) ) ;
#56918=CARTESIAN_POINT ( 'NONE',  ( -7.691553217654356622, 7.867900263551875994, -0.7998128361456291469 ) ) ;
#56921=CARTESIAN_POINT ( 'NONE',  ( -9.297140650669053485, 11.86975006391249643, 1.599625672291281386 ) ) ;
#56925=CARTESIAN_POINT ( 'NONE',  ( 0.7499999999999920064, 5.264583334016151639, 1.299038105676669330 ) ) ;
#56926=CARTESIAN_POINT ( 'NONE',  ( 7.401861798056875053, 10.72292363345333399, -1.199719254218441611 ) ) ;
#56929=CARTESIAN_POINT ( 'NONE',  ( -5.930802130974132780, 9.006687355190106103, -1.199719254218440723 ) ) ;
#56931=CARTESIAN_POINT ( 'NONE',  ( 1.364683531249990311, 5.113541667008084879, 0.7879004041258500513 ) ) ;
#56938=CARTESIAN_POINT ( 'NONE',  ( -8.188761592974051595, 9.616271948966963024, -1.082531754730543971 ) ) ;
#56942=CARTESIAN_POINT ( 'NONE',  ( 0.6823417656249917140, 3.655208333674754506, 1.181850606188765695 ) ) ;
#56948=CARTESIAN_POINT ( 'NONE',  ( -1.201851678989727383E-14, 3.821875000341423689, 1.575800808251672791 ) ) ;
#56950=CARTESIAN_POINT ( 'NONE',  ( -3.815730167242251003, 6.539103397502874948, -1.199719254218452047 ) ) ;
#56951=CARTESIAN_POINT ( 'NONE',  ( 5.880485940025228508, 7.883652901494672349, 1.599625672291267398 ) ) ;
#56954=CARTESIAN_POINT ( 'NONE',  ( 4.812781342726870193, 4.717259109377208048, 0.7216878364870317197 ) ) ;
#56955=CARTESIAN_POINT ( 'NONE',  ( 1.364683531249990311, 5.196875000341417916, 1.214306433183764966E-14 ) ) ;
#56960=CARTESIAN_POINT ( 'NONE',  ( -1.364683531250012516, 1.280208333674755172, 0.7879004041258379498 ) ) ;
#56961=CARTESIAN_POINT ( 'NONE',  ( 4.635998460869027227, 7.496083073400806818, -1.199719254218452047 ) ) ;
#56967=CARTESIAN_POINT ( 'NONE',  ( 3.334942599281629949, 5.874221551595115720, -1.082531754730543083 ) ) ;
#56970=CARTESIAN_POINT ( 'NONE',  ( -7.375272376154077492, 11.54830883891436422, -0.7216878364870267237 ) ) ;
#56972=CARTESIAN_POINT ( 'NONE',  ( 1.500000000000009104, 5.004166666666691299, 0.8660254037844407060 ) ) ;
#56975=CARTESIAN_POINT ( 'NONE',  ( -8.676328237741483207, 12.20980114641871062, -1.199719254218446718 ) ) ;
#56976=CARTESIAN_POINT ( 'NONE',  ( -6.209271164934474285, 6.346497235286081562, 1.040834085586084257E-14 ) ) ;
#56978=CARTESIAN_POINT ( 'NONE',  ( -1.402160292154681736E-14, 1.259375000341419248, -1.575800808251659024 ) ) ;
#56980=DIRECTION ( 'NONE',  ( 0.6507913734559640506, 0.7592566023653005702, 0.000000000000000000 ) ) ;
#56987=CARTESIAN_POINT ( 'NONE',  ( 8.609064354553323639, 10.10662517080946543, -1.082531754730543083 ) ) ;
#56996=CARTESIAN_POINT ( 'NONE',  ( 6.471393748265519719, 5.229711127717882491, -2.499999999999995115 ) ) ;
#56997=CARTESIAN_POINT ( 'NONE',  ( -2.266184231778562541, 5.795632037050281404, 1.040834085586084257E-14 ) ) ;
#56999=CARTESIAN_POINT ( 'NONE',  ( -3.914243274428899966, 2.801588762746444417, 0.7750000000000135669 ) ) ;
#57001=CARTESIAN_POINT ( 'NONE',  ( 1.364683531249988535, 2.926041667008082658, 0.7879004041258500513 ) ) ;
#57013=CARTESIAN_POINT ( 'NONE',  ( 0.6823417656249882723, 1.676041667008083769, -1.181850606188749264 ) ) ;
#57016=VERTEX_POINT ( 'NONE', #115880 ) ;
#57018=SPHERICAL_SURFACE ( 'NONE', #59617, 0.08000000000000000167 ) ;
#57021=ORIENTED_EDGE ( 'NONE', *, *, #159108, .T. ) ;
#57025=CARTESIAN_POINT ( 'NONE',  ( 5.952193131599331721, 6.902979060742733708, 1.199719254218462483 ) ) ;
#57033=CARTESIAN_POINT ( 'NONE',  ( 6.825640269476072497, 10.05066518344239412, 1.199719254218460707 ) ) ;
#57036=CARTESIAN_POINT ( 'NONE',  ( 9.596473800374404561, 10.09030761005864285, 0.000000000000000000 ) ) ;
#57049=CARTESIAN_POINT ( 'NONE',  ( -7.944714827928056167, 10.29191993738131927, 1.443375672974090751 ) ) ;
#57054=CARTESIAN_POINT ( 'NONE',  ( -7.784352752540590004, 12.23349531127272094, 0.7998128361456481317 ) ) ;
#57060=CARTESIAN_POINT ( 'NONE',  ( 9.236128959407556849, 11.79856975744075598, -1.599625672291262513 ) ) ;
#57062=CARTESIAN_POINT ( 'NONE',  ( 5.352771719296971042, 5.139321848801576387, 0.7998128361456341429 ) ) ;
#57069=CARTESIAN_POINT ( 'NONE',  ( -6.392833124043511894, 7.417059051927569868, 1.199719254218450271 ) ) ;
#57071=CARTESIAN_POINT ( 'NONE',  ( -2.785310492603665367, 5.336947110424484109, 1.199719254218462483 ) ) ;
#57077=CARTESIAN_POINT ( 'NONE',  ( 7.944714827928043732, 10.29191993738131927, 1.443375672974076540 ) ) ;
#57079=CARTESIAN_POINT ( 'NONE',  ( 0.6823417656249917140, 4.155208333674755394, 1.181850606188765695 ) ) ;
#57081=CARTESIAN_POINT ( 'NONE',  ( 3.960953433486789521, 7.772862772376584850, -0.7998128361456221525 ) ) ;
#57092=ORIENTED_EDGE ( 'NONE', *, *, #127934, .F. ) ;
#57094=CARTESIAN_POINT ( 'NONE',  ( 1.364683531249988757, 1.196875000341421469, 0.000000000000000000 ) ) ;
#57096=CARTESIAN_POINT ( 'NONE',  ( 3.216308754939877446, 4.775446185561722956, -1.599625672291262513 ) ) ;
#57098=CARTESIAN_POINT ( 'NONE',  ( -6.399085315970155285, 6.567947078161039620, -0.7216878364870278340 ) ) ;
#57099=CARTESIAN_POINT ( 'NONE',  ( 4.202664430556254160, 5.926194473780837413, 1.443375672974062551 ) ) ;
#57100=CARTESIAN_POINT ( 'NONE',  ( -7.185458225118419584, 7.485382138834033583, 1.040834085586084257E-14 ) ) ;
#57104=CARTESIAN_POINT ( 'NONE',  ( 6.647575389402066826, 6.649926130590872120, 1.040834085586084257E-14 ) ) ;
#57114=CARTESIAN_POINT ( 'NONE',  ( 6.277588818327314080, 7.282607361925381717, 1.199719254218462483 ) ) ;
#57118=CARTESIAN_POINT ( 'NONE',  ( -5.526920175865215334, 9.599823971818089774, 0.7998128361456481317 ) ) ;
#57122=CARTESIAN_POINT ( 'NONE',  ( 8.586391356156291010, 8.911878091804165791, 0.7998128361456481317 ) ) ;
#57125=CARTESIAN_POINT ( 'NONE',  ( -6.901263884555985051, 8.010228272525461435, 1.199719254218450271 ) ) ;
#57126=CARTESIAN_POINT ( 'NONE',  ( 6.602457619730756733, 9.686322408785807525, 1.082531754730558626 ) ) ;
#57127=CARTESIAN_POINT ( 'NONE',  ( 4.001130546182508851, 7.826233022050814725, 0.1222016466962717873 ) ) ;
#57128=CARTESIAN_POINT ( 'NONE',  ( -6.247609857798938293, 6.183299677053865295, -0.7998128361456291469 ) ) ;
#57134=CARTESIAN_POINT ( 'NONE',  ( 10.38962578677386084, 11.01565159419135043, 0.000000000000000000 ) ) ;
#57135=CARTESIAN_POINT ( 'NONE',  ( 0.6823417656249882723, 2.426041667008084435, -1.181850606188749264 ) ) ;
#57137=CARTESIAN_POINT ( 'NONE',  ( -6.724481002698130538, 7.907944593645035880, -1.082531754730544860 ) ) ;
#57144=CARTESIAN_POINT ( 'NONE',  ( -5.796211742468360129, 6.069872997065163922, -0.5622600474686073602 ) ) ;
#57145=CARTESIAN_POINT ( 'NONE',  ( -0.6823417656250212460, 1.363541667008083547, 1.181850606188755259 ) ) ;
#57148=CARTESIAN_POINT ( 'NONE',  ( 3.050221373394638835, 6.502416002361635528, 0.000000000000000000 ) ) ;
#57153=CARTESIAN_POINT ( 'NONE',  ( -4.623494077460110319, 5.352830164246910272, 1.199719254218462483 ) ) ;
#57155=CARTESIAN_POINT ( 'NONE',  ( -6.995644074527074707, 11.10540915368285475, 0.000000000000000000 ) ) ;
#57164=CARTESIAN_POINT ( 'NONE',  ( -7.822691444960713447, 9.189190109618056823, -1.082531754730543083 ) ) ;
#57165=ORIENTED_EDGE ( 'NONE', *, *, #33313, .F. ) ;
#57170=CARTESIAN_POINT ( 'NONE',  ( -7.659993601596713830, 9.959745173328078849, -1.443375672974058777 ) ) ;
#57176=CARTESIAN_POINT ( 'NONE',  ( 0.7499999999999920064, 5.014583334016150751, 1.299038105676669330 ) ) ;
#57184=CARTESIAN_POINT ( 'NONE',  ( -5.747767057189642870, 8.793146435774861658, -1.199719254218440723 ) ) ;
#57188=CARTESIAN_POINT ( 'NONE',  ( 5.118366684358879759, 5.930181538962194132, 1.199719254218462483 ) ) ;
#57192=CARTESIAN_POINT ( 'NONE',  ( 5.472687561410540802, 9.536552588287639409, 0.7998128361456462443 ) ) ;
#57195=ORIENTED_EDGE ( 'NONE', *, *, #195841, .F. ) ;
#57199=CARTESIAN_POINT ( 'NONE',  ( -6.561783159334145132, 6.757761228752363181, -0.7216878364870278340 ) ) ;
#57208=CARTESIAN_POINT ( 'NONE',  ( 1.364683531249986537, 1.155208333674754728, -0.7879004041258239610 ) ) ;
#57210=CARTESIAN_POINT ( 'NONE',  ( -6.991200766141138168, 11.30815132714001159, 0.7998128361456481317 ) ) ;
#57212=CARTESIAN_POINT ( 'NONE',  ( 6.988338112840064120, 10.24047933403371502, 1.199719254218460707 ) ) ;
#57214=CARTESIAN_POINT ( 'NONE',  ( -8.178592977541617515, 10.56477777859713463, 1.599625672291295375 ) ) ;
#57217=CARTESIAN_POINT ( 'NONE',  ( -1.001543065824772872E-14, 4.321875000341417916, 1.575800808251672791 ) ) ;
#57219=CARTESIAN_POINT ( 'NONE',  ( 9.300530189294644146, 10.91333531134101165, -1.082531754730543083 ) ) ;
#57222=CARTESIAN_POINT ( 'NONE',  ( -1.364683531250014514, -0.4072916663252447167, 0.7879004041258379498 ) ) ;
#57225=CARTESIAN_POINT ( 'NONE',  ( 9.097157884645296733, 10.67606762258344055, -1.082531754730543083 ) ) ;
#57228=CARTESIAN_POINT ( 'NONE',  ( -5.097502569058210753, 7.930541516334467467, -1.082531754730549967 ) ) ;
#57230=CARTESIAN_POINT ( 'NONE',  ( -1.402160292154681736E-14, 2.446875000341416584, -1.575800808251660134 ) ) ;
#57234=CARTESIAN_POINT ( 'NONE',  ( -8.030507057996002729, 8.263346410617135263, 1.040834085586084257E-14 ) ) ;
#57236=CARTESIAN_POINT ( 'NONE',  ( -1.364683531250012516, 5.051041667008085767, -0.7879004041258300672 ) ) ;
#57241=CARTESIAN_POINT ( 'NONE',  ( 9.121938423896107651, 9.536683004167278099, -0.7998128361456221525 ) ) ;
#57244=CARTESIAN_POINT ( 'NONE',  ( 1.499999999999987121, 1.004166666666687968, 0.8660254037844524744 ) ) ;
#57247=CARTESIAN_POINT ( 'NONE',  ( -1.201851678989727383E-14, 5.368750000682816825, -1.732050807568863648 ) ) ;
#57250=CARTESIAN_POINT ( 'NONE',  ( 8.283668668269706714, 8.766627655843892697, 1.040834085586084257E-14 ) ) ;
#57251=CARTESIAN_POINT ( 'NONE',  ( 8.992082194361556091, 11.51384853155376220, 1.599625672291279388 ) ) ;
#57253=CARTESIAN_POINT ( 'NONE',  ( 4.566398809704347528, 4.221886787610169556, -0.7998128361456211532 ) ) ;
#57259=CARTESIAN_POINT ( 'NONE',  ( 9.240045382913317340, 10.73880668727576015, -1.199719254218446718 ) ) ;
#57260=CARTESIAN_POINT ( 'NONE',  ( -8.967828540435322182, 12.54988483289483980, 1.199719254218462483 ) ) ;
#57262=DIRECTION ( 'NONE',  ( 0.7592566023653005702, -0.6507913734559639396, 0.000000000000000000 ) ) ;
#57263=CARTESIAN_POINT ( 'NONE',  ( -0.6823417656250003738, -0.03229166632524871350, -1.181850606188749264 ) ) ;
#57264=CARTESIAN_POINT ( 'NONE',  ( -1.500000000000013101, 0.6708333333333583726, 0.8660254037844403729 ) ) ;
#57267=CARTESIAN_POINT ( 'NONE',  ( -1.284279953904132077, 2.909610286488902187, -0.7749999999999936939 ) ) ;
#57271=CARTESIAN_POINT ( 'NONE',  ( 1.364683531249988535, 5.405208333674750953, -0.7879004041258300672 ) ) ;
#57273=CARTESIAN_POINT ( 'NONE',  ( -8.483651433849100698, 10.92067931095586886, 1.599625672291269396 ) ) ;
#57274=CARTESIAN_POINT ( 'NONE',  ( -5.910991785878183080, 5.998504626387068051, -0.7216878364870278340 ) ) ;
#57283=CARTESIAN_POINT ( 'NONE',  ( 7.944187942603509356, 11.35563746875774882, 1.199719254218460707 ) ) ;
#57286=CARTESIAN_POINT ( 'NONE',  ( 8.392133896734671694, 8.893170422386358354, 0.7216878364870458196 ) ) ;
#57289=CARTESIAN_POINT ( 'NONE',  ( -7.797910906154257304, 12.24931315715533486, 0.000000000000000000 ) ) ;
#57290=CARTESIAN_POINT ( 'NONE',  ( 6.328958779480917229, 6.278206752349526631, 0.7998128361456341429 ) ) ;
#57291=CARTESIAN_POINT ( 'NONE',  ( 2.358755538653318773, 5.695705861830088423, 1.040834085586084257E-14 ) ) ;
#57293=CARTESIAN_POINT ( 'NONE',  ( 2.822068529938852155, 6.444163718237301275, -0.7998128361456291469 ) ) ;
#57302=CARTESIAN_POINT ( 'NONE',  ( -6.100805936469506641, 6.219954468743612352, 0.7216878364870317197 ) ) ;
#57303=CARTESIAN_POINT ( 'NONE',  ( 3.979481780810941949, 4.601482484822914998, 1.199719254218464037 ) ) ;
#57306=CARTESIAN_POINT ( 'NONE',  ( -5.831978632172702071, 9.955725504176825780, 0.7998128361456481317 ) ) ;
#57310=CARTESIAN_POINT ( 'NONE',  ( -9.508345801885592863, 9.987491611821676329, 0.7998128361456462443 ) ) ;
#57315=CARTESIAN_POINT ( 'NONE',  ( 4.299907273828439180, 8.168308919441841454, 1.040834085586084257E-14 ) ) ;
#57326=CARTESIAN_POINT ( 'NONE',  ( -6.612626235163205024, 8.737816579155630592, -1.599625672291263179 ) ) ;
#57329=CARTESIAN_POINT ( 'NONE',  ( 6.005898861173831094, 6.109229547565340646, 1.040834085586084257E-14 ) ) ;
#57333=CARTESIAN_POINT ( 'NONE',  ( 3.167801447087334576, 6.847518788243868393, -0.7998128361456291469 ) ) ;
#57335=CARTESIAN_POINT ( 'NONE',  ( -4.225337428953291230, 8.081310767087481750, 0.7998128361456341429 ) ) ;
#57345=CARTESIAN_POINT ( 'NONE',  ( 6.100279051144945619, 9.204410428722734849, -1.199719254218440723 ) ) ;
#57350=CARTESIAN_POINT ( 'NONE',  ( -4.379705010876359772, 7.173806194452361673, -1.050513582990858064 ) ) ;
#57352=DIRECTION ( 'NONE',  ( -5.578564026256490882E-16, -1.000000000000000000, -9.066213480720158442E-32 ) ) ;
#57353=CARTESIAN_POINT ( 'NONE',  ( 1.364683531249986981, -1.053124999658580752, 0.000000000000000000 ) ) ;
#57355=VERTEX_POINT ( 'NONE', #56157 ) ;
#57357=CARTESIAN_POINT ( 'NONE',  ( 9.463228032658635769, 11.10314946193233965, -1.082531754730543083 ) ) ;
#57375=CARTESIAN_POINT ( 'NONE',  ( -4.111146893441842920, 5.819424013814012753, 1.599625672291267398 ) ) ;
#57377=CARTESIAN_POINT ( 'NONE',  ( -3.110706179331648169, 5.716575411607132118, 1.199719254218462483 ) ) ;
#57381=CARTESIAN_POINT ( 'NONE',  ( -1.500000000000015099, -0.7979166659838445863, 0.8660254037844403729 ) ) ;
#57390=CARTESIAN_POINT ( 'NONE',  ( 4.729096653068339151, 4.411700938201493116, -0.7998128361456211532 ) ) ;
#57393=CARTESIAN_POINT ( 'NONE',  ( 10.35806617071623315, 11.18675807536486566, 0.000000000000000000 ) ) ;
#57395=CARTESIAN_POINT ( 'NONE',  ( -1.364683531250012516, 1.342708333674755616, 0.7879004041258379498 ) ) ;
#57396=EDGE_CURVE ( 'NONE', #94342, #54853, #149845, .T. ) ;
#57397=CARTESIAN_POINT ( 'NONE',  ( -0.7500000000000215383, 3.691666666666690411, 1.299038105676671107 ) ) ;
#57399=CARTESIAN_POINT ( 'NONE',  ( -7.296259222448620463, 11.66405285949874759, 0.7998128361456481317 ) ) ;
#57400=CARTESIAN_POINT ( 'NONE',  ( -4.406036734316882253, 8.084200590104265061, -0.7216878364870257245 ) ) ;
#57402=CARTESIAN_POINT ( 'NONE',  ( -6.878064000834399394, 6.918829510595249310, -0.7998128361456291469 ) ) ;
#57404=CARTESIAN_POINT ( 'NONE',  ( 0.7499999999999885647, -0.9854166659838472508, 1.299038105676657340 ) ) ;
#57410=B_SPLINE_CURVE_WITH_KNOTS ( 'NONE', 3,
 ( #92220, #140981, #13050, #10914 ),
 .UNSPECIFIED., .F., .F.,
 ( 4, 4 ),
 ( 4.159586391574946371E-16, 0.0002852080176109775202 ),
 .UNSPECIFIED. ) ;
#57413=CARTESIAN_POINT ( 'NONE',  ( -6.033015167956818026, 6.140865238812146742, -0.7216878364870267237 ) ) ;
#57420=CARTESIAN_POINT ( 'NONE',  ( -4.650083499362882122, 6.448183387388563226, 1.443375672974064550 ) ) ;
#57422=CARTESIAN_POINT ( 'NONE',  ( 8.062294901620731480, 12.55776115186623620, 1.040834085586084257E-14 ) ) ;
#57432=CARTESIAN_POINT ( 'NONE',  ( -4.603156847039612920, 5.329103395422994716, 1.199719254218462483 ) ) ;
#57433=CARTESIAN_POINT ( 'NONE',  ( -8.839026081105473054, 12.39961529701003684, -1.199719254218446718 ) ) ;
#57436=ORIENTED_EDGE ( 'NONE', *, *, #692, .T. ) ;
#57438=CARTESIAN_POINT ( 'NONE',  ( 7.076992996653421741, 10.23994701519558781, -1.082531754730537976 ) ) ;
#57439=CARTESIAN_POINT ( 'NONE',  ( 6.494519276145969577, 7.535692896047149425, -1.199719254218446718 ) ) ;
#57442=VERTEX_POINT ( 'NONE', #39917 ) ;
#57445=CARTESIAN_POINT ( 'NONE',  ( 3.680148631105580215, 6.380924938676771241, -1.199719254218446718 ) ) ;
#57456=CARTESIAN_POINT ( 'NONE',  ( -6.196239896645333367, 7.187700286629718605, -1.199719254218446718 ) ) ;
#57458=AXIS2_PLACEMENT_3D ( 'NONE', #39643, #175797, #204242 ) ;
#57463=CARTESIAN_POINT ( 'NONE',  ( 1.364683531249988535, 4.363541667008090208, 0.7879004041258500513 ) ) ;
#57466=CARTESIAN_POINT ( 'NONE',  ( -4.740547266272593596, 8.682388910626682943, -0.7998128361456281477 ) ) ;
#57469=CARTESIAN_POINT ( 'NONE',  ( 4.819033534653518025, 7.709623992816043270, -1.199719254218452047 ) ) ;
#57470=CARTESIAN_POINT ( 'NONE',  ( -5.063080299699540987, 7.994345218703034384, 1.199719254218464037 ) ) ;
#57477=CARTESIAN_POINT ( 'NONE',  ( 5.504247177468168495, 9.365446107114122398, 0.7216878364870438212 ) ) ;
#57479=CARTESIAN_POINT ( 'NONE',  ( 5.775410249297131315, 9.681803024247919609, 1.040834085586084257E-14 ) ) ;
#57480=CARTESIAN_POINT ( 'NONE',  ( -1.364683531250012516, 3.051041667008083547, -0.7879004041258289570 ) ) ;
#57482=CARTESIAN_POINT ( 'NONE',  ( 4.148431815657221300, 7.783661518334664464, 1.040834085586084257E-14 ) ) ;
#57490=CARTESIAN_POINT ( 'NONE',  ( -5.337630915675663168, 6.534101986612459001, 1.368282111488251074 ) ) ;
#57491=DIRECTION ( 'NONE',  ( 0.7592566023653005702, 0.6507913734559640506, 0.000000000000000000 ) ) ;
#57499=CARTESIAN_POINT ( 'NONE',  ( -2.453662613948990323, 5.806430783008362795, -0.7216878364870257245 ) ) ;
#57504=CARTESIAN_POINT ( 'NONE',  ( -3.972702704004144714, 4.593573561881607148, 1.199719254218462483 ) ) ;
#57507=VERTEX_POINT ( 'NONE', #170965 ) ;
#57509=CARTESIAN_POINT ( 'NONE',  ( 3.375617060122621194, 6.882044303544283537, 1.040834085586084257E-14 ) ) ;
#57511=CARTESIAN_POINT ( 'NONE',  ( -0.6823417656250003738, 3.030208333674754062, -1.181850606188749264 ) ) ;
#57513=CARTESIAN_POINT ( 'NONE',  ( 6.726816770674637347, 10.99970333242910669, -0.7998128361456291469 ) ) ;
#57514=CARTESIAN_POINT ( 'NONE',  ( -8.455481356417053007, 13.01647868246193518, 0.7998128361456341429 ) ) ;
#57516=CARTESIAN_POINT ( 'NONE',  ( -5.603597561149804562, 5.431951997629870910, 0.7998128361456341429 ) ) ;
#57520=CARTESIAN_POINT ( 'NONE',  ( -0.7499999999999972244, 3.108333333333358706, -1.299038105676652011 ) ) ;
#57521=CARTESIAN_POINT ( 'NONE',  ( 5.281064527722868718, 6.119995689553514140, 1.199719254218462483 ) ) ;
#57525=CARTESIAN_POINT ( 'NONE',  ( 0.6823417656249917140, 3.842708333674754506, 1.181850606188765695 ) ) ;
#57529=CARTESIAN_POINT ( 'NONE',  ( 8.758204044747998296, 11.24099069033793974, 1.443375672974076540 ) ) ;
#57534=CARTESIAN_POINT ( 'NONE',  ( -0.7500000000000215383, 2.472916667349486897, 1.299038105676671107 ) ) ;
#57536=CARTESIAN_POINT ( 'NONE',  ( -6.389970470742427189, 6.349387058821269747, -0.7998128361456291469 ) ) ;
#57537=CARTESIAN_POINT ( 'NONE',  ( 1.500000000000007105, 10.64264068711930733, 1.214306433183764966E-14 ) ) ;
#57546=CARTESIAN_POINT ( 'NONE',  ( 4.364835388595708743, 7.179726155748598515, 1.199719254218462483 ) ) ;
#57549=CARTESIAN_POINT ( 'NONE',  ( 4.656335691289526402, 7.519809842224722374, -1.199719254218452047 ) ) ;
#57551=ORIENTED_EDGE ( 'NONE', *, *, #84582, .T. ) ;
#57556=CARTESIAN_POINT ( 'NONE',  ( 9.673906298550626559, 11.24497775551929557, 1.199719254218452047 ) ) ;
#57561=CARTESIAN_POINT ( 'NONE',  ( 5.841717777309253457, 6.007722996832359996, 0.3783690319567531435 ) ) ;
#57572=CARTESIAN_POINT ( 'NONE',  ( 5.639828713604826405, 9.523624565940227882, -0.7216878364870267237 ) ) ;
#57574=CARTESIAN_POINT ( 'NONE',  ( -4.253507506385335368, 5.985511395581417204, 1.599625672291267398 ) ) ;
#57577=CARTESIAN_POINT ( 'NONE',  ( -6.579784621333750749, 6.570836901177822931, 0.7998128361456341429 ) ) ;
#57587=CARTESIAN_POINT ( 'NONE',  ( 3.094265954482837255, 2.800000000000017586, 2.490342512183689294 ) ) ;
#57592=CARTESIAN_POINT ( 'NONE',  ( 10.57266086055835075, 11.22919251360659310, 0.000000000000000000 ) ) ;
#57599=CARTESIAN_POINT ( 'NONE',  ( -2.103486388414573138, 5.605817886458954291, 1.040834085586084257E-14 ) ) ;
#57602=CARTESIAN_POINT ( 'NONE',  ( 8.239604668803105270, 10.63595808506888396, -1.599625672291268286 ) ) ;
#57604=CARTESIAN_POINT ( 'NONE',  ( 0.5281409364047099375, 2.800000000000018030, 1.340854145587128787 ) ) ;
#57606=CARTESIAN_POINT ( 'NONE',  ( -8.213542131780492639, 8.476887330032372603, 1.040834085586084257E-14 ) ) ;
#57607=CARTESIAN_POINT ( 'NONE',  ( 5.009901455449552010, 5.803638771901306725, -1.199719254218452047 ) ) ;
#57612=CARTESIAN_POINT ( 'NONE',  ( 10.37606763316019531, 10.99983374830873650, 0.7998128361456462443 ) ) ;
#57616=CARTESIAN_POINT ( 'NONE',  ( -1.364683531250012516, 3.051041667008083547, -0.7879004041258289570 ) ) ;
#57619=CARTESIAN_POINT ( 'NONE',  ( 5.639828713604826405, 9.523624565940227882, -0.7216878364870267237 ) ) ;
#57627=CARTESIAN_POINT ( 'NONE',  ( 9.531018800282609504, 10.22186947652563305, 0.7216878364870458196 ) ) ;
#57632=CARTESIAN_POINT ( 'NONE',  ( -8.585337585951595685, 11.03931315507545108, -1.599625672291263179 ) ) ;
#57640=CARTESIAN_POINT ( 'NONE',  ( 3.344057444064992168, 7.053150784717805877, 1.040834085586084257E-14 ) ) ;
#57646=CARTESIAN_POINT ( 'NONE',  ( 4.961394147597008697, 7.875711374583454827, -1.199719254218452047 ) ) ;
#57649=CIRCLE ( 'NONE', #113071, 0.08000000000000023759 ) ;
#57650=CARTESIAN_POINT ( 'NONE',  ( 1.499999999999987121, 2.827083334016148530, -0.8660254037844262731 ) ) ;
#57654=ORIENTED_EDGE ( 'NONE', *, *, #148115, .F. ) ;
#57656=CARTESIAN_POINT ( 'NONE',  ( 1.499999999999989120, 0.2750000000000182854, 0.000000000000000000 ) ) ;
#57657=CARTESIAN_POINT ( 'NONE',  ( 8.101160479365381306, 9.410107633136481908, -1.199719254218446718 ) ) ;
#57659=CARTESIAN_POINT ( 'NONE',  ( 1.364683531249988757, -0.3656249996585800299, 0.000000000000000000 ) ) ;
#57661=VECTOR ( 'NONE', #158972, 1000.000000000000000 ) ;
#57663=CARTESIAN_POINT ( 'NONE',  ( 8.432808358020004391, 12.78210081775797669, 0.7216878364870438212 ) ) ;
#57667=CARTESIAN_POINT ( 'NONE',  ( -4.693093728624763372, 8.627026450037540428, 0.7998128361456481317 ) ) ;
#57669=CARTESIAN_POINT ( 'NONE',  ( -1.500000000000013101, 2.160416667349489561, -0.8660254037844313801 ) ) ;
#57670=CARTESIAN_POINT ( 'NONE',  ( 1.364683531249988535, 4.467708333674754506, -0.7879004041258300672 ) ) ;
#57685=CARTESIAN_POINT ( 'NONE',  ( -7.991641480251377772, 11.41099992934688956, 1.199719254218453823 ) ) ;
#57686=CARTESIAN_POINT ( 'NONE',  ( 5.784525094524856748, 9.900363043587685041, 1.040834085586084257E-14 ) ) ;
#57693=CARTESIAN_POINT ( 'NONE',  ( -8.342344591110322227, 8.627156865917170236, -0.7998128361456291469 ) ) ;
#57697=CARTESIAN_POINT ( 'NONE',  ( 3.297657676621871925, 4.870353260857385180, 1.599625672291267398 ) ) ;
#57700=CARTESIAN_POINT ( 'NONE',  ( -3.879604511804807032, 7.677955697080923514, 0.7998128361456341429 ) ) ;
#57701=CARTESIAN_POINT ( 'NONE',  ( -7.784352752540590004, 12.23349531127272094, 0.7998128361456481317 ) ) ;
#57704=CARTESIAN_POINT ( 'NONE',  ( -3.985535776513723150, 7.835598525918981316, 0.2247789072947203870 ) ) ;
#57711=CARTESIAN_POINT ( 'NONE',  ( 7.142447996300871793, 7.227277505306155092, 0.7998128361456341429 ) ) ;
#57726=EDGE_CURVE ( 'NONE', #73290, #4315, #180904, .T. ) ;
#57731=CARTESIAN_POINT ( 'NONE',  ( 3.334942599281629949, 5.874221551595115720, -1.082531754730543083 ) ) ;
#57733=ORIENTED_EDGE ( 'NONE', *, *, #59313, .F. ) ;
#57735=CARTESIAN_POINT ( 'NONE',  ( -8.134002093194872884, 11.57708731111429401, 1.199719254218453823 ) ) ;
#57740=CARTESIAN_POINT ( 'NONE',  ( -1.402160292154681736E-14, 0.2437500006828163535, 1.732050807568877637 ) ) ;
#57746=CARTESIAN_POINT ( 'NONE',  ( -0.6823417656250246877, 0.3010416670080895418, 1.181850606188755259 ) ) ;
#57748=ORIENTED_EDGE ( 'NONE', *, *, #89709, .T. ) ;
#57752=CARTESIAN_POINT ( 'NONE',  ( -3.391510981712833939, 7.108513245306943062, 0.7998128361456341429 ) ) ;
#57753=CARTESIAN_POINT ( 'NONE',  ( -0.1263493754108893363, 6.487495393664095111, -3.100011470320000573 ) ) ;
#57755=CARTESIAN_POINT ( 'NONE',  ( -0.7500000000000249800, -0.5583333333333134751, 1.299038105676659116 ) ) ;
#57757=CARTESIAN_POINT ( 'NONE',  ( -1.402160292154681736E-14, -1.115624999658584082, 1.575800808251672791 ) ) ;
#57762=CARTESIAN_POINT ( 'NONE',  ( -0.6823417656250003738, 0.7177083336747519526, -1.181850606188749264 ) ) ;
#57764=CARTESIAN_POINT ( 'NONE',  ( -6.201965203247477909, 9.323044272842313518, 1.199719254218452047 ) ) ;
#57765=CARTESIAN_POINT ( 'NONE',  ( 9.901532256681887745, 10.44620914241737530, 0.000000000000000000 ) ) ;
#57766=CARTESIAN_POINT ( 'NONE',  ( 5.678167406024951624, 5.518950149984223508, 0.7998128361456341429 ) ) ;
#57770=CARTESIAN_POINT ( 'NONE',  ( 0.6823417656249882723, 0.4885416670080827695, -1.181850606188749264 ) ) ;
#57777=CARTESIAN_POINT ( 'NONE',  ( 7.158341918335438869, 7.453746447587225710, -0.7216878364870257245 ) ) ;
#57780=CARTESIAN_POINT ( 'NONE',  ( -3.879604511804807032, 7.677955697080923514, 0.7998128361456341429 ) ) ;
#57782=CARTESIAN_POINT ( 'NONE',  ( -1.500000000000011324, 5.410416667349489117, -0.8660254037844313801 ) ) ;
#57785=CARTESIAN_POINT ( 'NONE',  ( 5.219525951136835928, 7.112532914458205013, -1.443375672974051449 ) ) ;
#57786=CARTESIAN_POINT ( 'NONE',  ( -8.812436658758329600, 9.383523644747281622, 1.040834085586084257E-14 ) ) ;
#57788=CARTESIAN_POINT ( 'NONE',  ( 1.499999999999987121, 3.545833333333356041, -0.8660254037844262731 ) ) ;
#57792=CARTESIAN_POINT ( 'NONE',  ( 8.812436659202669276, 10.34389285956704363, -1.082531754730543083 ) ) ;
#57803=B_SPLINE_CURVE_WITH_KNOTS ( 'NONE', 3,
 ( #38616, #85218, #83075, #732 ),
 .UNSPECIFIED., .F., .F.,
 ( 4, 4 ),
 ( 0.000000000000000000, 0.002006572499523629795 ),
 .UNSPECIFIED. ) ;
#57807=CARTESIAN_POINT ( 'NONE',  ( 9.101601193475611140, 9.512956235343358102, -0.7998128361456221525 ) ) ;
#57810=CARTESIAN_POINT ( 'NONE',  ( 3.551873057100274789, 7.087676300018221021, 0.7216878364870298324 ) ) ;
#57812=CARTESIAN_POINT ( 'NONE',  ( -7.293923454472094114, 9.532663335016016148, 1.443375672974090751 ) ) ;
#57838=CARTESIAN_POINT ( 'NONE',  ( -1.420000000000001039, 7.176846818246207960, -4.202462424328208712 ) ) ;
#57840=CARTESIAN_POINT ( 'NONE',  ( -5.065942953000576843, 9.062017211809330064, -0.7998128361456231517 ) ) ;
#57843=CARTESIAN_POINT ( 'NONE',  ( 6.148786358997489820, 7.132337826040578754, -1.199719254218446718 ) ) ;
#57854=CARTESIAN_POINT ( 'NONE',  ( -6.064574784014443942, 5.969758757638621738, -0.7998128361456291469 ) ) ;
#57857=CARTESIAN_POINT ( 'NONE',  ( 6.100279051144945619, 9.204410428722734849, -1.199719254218440723 ) ) ;
#57860=CARTESIAN_POINT ( 'NONE',  ( 5.714115171586898079, 6.274818061858235652, 1.066218439657661721 ) ) ;
#57862=DIRECTION ( 'NONE',  ( -0.9782075119097244364, 0.1245777785627091433, -0.1661037047502772757 ) ) ;
#57866=CARTESIAN_POINT ( 'NONE',  ( 6.954969613686092345, 7.216478758829655504, -0.7216878364870257245 ) ) ;
#57867=CARTESIAN_POINT ( 'NONE',  ( -8.342344591110322227, 8.627156865917170236, -0.7998128361456291469 ) ) ;
#57870=CARTESIAN_POINT ( 'NONE',  ( -8.076906825439122528, 10.44614393447756129, -1.599625672291263179 ) ) ;
#57872=CARTESIAN_POINT ( 'NONE',  ( -6.925517538482230506, 6.974191971184389160, 0.7998128361456341429 ) ) ;
#57879=CARTESIAN_POINT ( 'NONE',  ( 6.968000882419564945, 10.21675256520979858, 1.199719254218460707 ) ) ;
#57893=CARTESIAN_POINT ( 'NONE',  ( -0.7500000000000215383, 3.941666666666690411, 1.299038105676671107 ) ) ;
#57894=CARTESIAN_POINT ( 'NONE',  ( 5.118366684358879759, 5.930181538962194132, 1.199719254218462483 ) ) ;
#57895=CARTESIAN_POINT ( 'NONE',  ( 6.657217119509961201, 7.725507046638470321, -1.199719254218446718 ) ) ;
#57897=CARTESIAN_POINT ( 'NONE',  ( -7.510853912290736289, 11.70648729774046792, 0.7216878364870458196 ) ) ;
#57898=CARTESIAN_POINT ( 'NONE',  ( 7.022760382198770301, 8.255937203062467589, -1.082531754730543083 ) ) ;
#57899=CARTESIAN_POINT ( 'NONE',  ( -8.581948047326017459, 11.99572790764693409, 1.082531754730558626 ) ) ;
#57903=CARTESIAN_POINT ( 'NONE',  ( 9.426996880203592610, 9.892584536526015881, -0.7998128361456281477 ) ) ;
#57908=CARTESIAN_POINT ( 'NONE',  ( -0.6823417656250212460, 2.551041667008084435, 1.181850606188767472 ) ) ;
#57913=CARTESIAN_POINT ( 'NONE',  ( 1.364683531249988757, -0.6156249996585803075, 0.000000000000000000 ) ) ;
#57916=CARTESIAN_POINT ( 'NONE',  ( 9.694243528971124846, 11.26870452434320491, 1.199719254218450271 ) ) ;
#57920=CARTESIAN_POINT ( 'NONE',  ( -8.469039510030723861, 13.03229652834454733, 1.040834085586084257E-14 ) ) ;
#57926=CARTESIAN_POINT ( 'NONE',  ( 3.246287715468270108, 5.874753870433235825, 1.199719254218450271 ) ) ;
#57930=CARTESIAN_POINT ( 'NONE',  ( -8.631737353394710155, 13.22211067893587533, 1.040834085586084257E-14 ) ) ;
#57933=CARTESIAN_POINT ( 'NONE',  ( 7.574201371528760163, 11.98831870009225931, 1.040834085586084257E-14 ) ) ;
#57935=CARTESIAN_POINT ( 'NONE',  ( 4.301718403444327876, 7.219878030919558043, 0.9872997725082887088 ) ) ;
#57937=CARTESIAN_POINT ( 'NONE',  ( -4.416205349749324327, 6.175325546172740765, 1.599625672291267398 ) ) ;
#57941=CARTESIAN_POINT ( 'NONE',  ( 8.938903350111612411, 9.323142084752035430, -0.7998128361456221525 ) ) ;
#57943=CARTESIAN_POINT ( 'NONE',  ( 8.111855979677986994, 8.358253485912799263, 1.040834085586084257E-14 ) ) ;
#57944=EDGE_CURVE ( 'NONE', #154674, #123959, #111142, .T. ) ;
#57946=CARTESIAN_POINT ( 'NONE',  ( -8.893785580884703279, 10.43879993486270585, 1.082531754730558626 ) ) ;
#57953=CARTESIAN_POINT ( 'NONE',  ( -5.565591498217608013, 6.214750235347503704, -0.9194985501971261188 ) ) ;
#57954=CARTESIAN_POINT ( 'NONE',  ( -0.6823417656250212460, 1.551041667008083769, 1.181850606188755259 ) ) ;
#57956=CARTESIAN_POINT ( 'NONE',  ( 7.470179451449751262, 7.817556902887268677, 1.040834085586084257E-14 ) ) ;
#57959=ORIENTED_EDGE ( 'NONE', *, *, #183332, .F. ) ;
#57965=EDGE_CURVE ( 'NONE', #170226, #159704, #10002, .T. ) ;
#57977=CARTESIAN_POINT ( 'NONE',  ( 9.759171643738394408, 10.28012176064996197, 0.000000000000000000 ) ) ;
#57981=CARTESIAN_POINT ( 'NONE',  ( -4.485049888022365927, 4.126979712314507331, 0.7998128361456341429 ) ) ;
#57982=CARTESIAN_POINT ( 'NONE',  ( -6.775324078527193983, 8.927630729746953264, -1.599625672291263179 ) ) ;
#57985=CARTESIAN_POINT ( 'NONE',  ( -8.462260433223891098, 13.02438760540324481, -0.7998128361456281477 ) ) ;
#57989=CARTESIAN_POINT ( 'NONE',  ( -1.500000000000011324, 5.660416667349481123, -0.8660254037844313801 ) ) ;
#57990=CARTESIAN_POINT ( 'NONE',  ( 8.288111976655649471, 8.563885482386732306, -0.7998128361456291469 ) ) ;
#57993=CARTESIAN_POINT ( 'NONE',  ( -6.204827856548512877, 10.39071626594860476, -0.7998128361456291469 ) ) ;
#57995=CARTESIAN_POINT ( 'NONE',  ( -1.001543065824772872E-14, 4.821875000341419693, 1.575800808251672791 ) ) ;
#58000=CARTESIAN_POINT ( 'NONE',  ( -7.212574532790087645, 11.35849468832304154, -0.7216878364870267237 ) ) ;
#58004=CARTESIAN_POINT ( 'NONE',  ( 1.364683531249990311, 2.696875000341415696, 1.214306433183764966E-14 ) ) ;
#58010=CARTESIAN_POINT ( 'NONE',  ( -1.201851678989727383E-14, 4.946875000341420581, -1.575800808251660134 ) ) ;
#58011=CARTESIAN_POINT ( 'NONE',  ( -5.271422797614987665, 5.044414773505913274, -0.7998128361456221525 ) ) ;
#58012=CARTESIAN_POINT ( 'NONE',  ( 7.474622759835693131, 7.614814729430110951, -0.7998128361456281477 ) ) ;
#58014=( BOUNDED_CURVE ( )  B_SPLINE_CURVE ( 2, ( #201396, #167861, #105007, #136443, #185153, #103936, #151624 ),
 .UNSPECIFIED., .F., .T. ) 
 B_SPLINE_CURVE_WITH_KNOTS ( ( 3, 2, 2, 3 ),
 ( 0.3962798098108560874, 0.3988095238095238360, 0.4047619047619047672, 0.4072916187605725158 ),
 .UNSPECIFIED. ) 
 CURVE ( )  GEOMETRIC_REPRESENTATION_ITEM ( )  RATIONAL_B_SPLINE_CURVE ( ( 0.9345202395942615592, 0.9430618748659230777, 1.000000000000000000, 0.8660254037844387076, 1.000000000000000000, 0.9430618748659225226, 0.9345202395942613371 ) ) 
 REPRESENTATION_ITEM ( '' )  );
#58016=CARTESIAN_POINT ( 'NONE',  ( 3.348500752450937590, 5.890039396959305229, 1.082531754730558626 ) ) ;
#58017=CARTESIAN_POINT ( 'NONE',  ( -0.6823417656249969321, 3.530208333674754506, -1.181850606188749264 ) ) ;
#58022=CARTESIAN_POINT ( 'NONE',  ( -1.201851678989727383E-14, 1.321875000341419248, 1.575800808251672791 ) ) ;
#58023=CARTESIAN_POINT ( 'NONE',  ( -4.528060117284246289, 6.305822774963486310, 1.443375672974064550 ) ) ;
#58024=CARTESIAN_POINT ( 'NONE',  ( 5.834086172582112262, 5.700855377634248100, 1.040834085586084257E-14 ) ) ;
#58028=CARTESIAN_POINT ( 'NONE',  ( 3.172244755917638770, 5.684407401003788607, -1.082531754730543083 ) ) ;
#58031=CARTESIAN_POINT ( 'NONE',  ( -8.324343129110692630, 12.65555805069709550, 0.7216878364870338292 ) ) ;
#58037=CARTESIAN_POINT ( 'NONE',  ( -5.138177029454855216, 7.017625839162543677, 1.443375672974064550 ) ) ;
#58039=CARTESIAN_POINT ( 'NONE',  ( -0.6823417656250212460, 0.8635416670080899859, 1.181850606188755259 ) ) ;
#58041=CARTESIAN_POINT ( 'NONE',  ( 1.438722679664439452, 7.870294296420976110, 3.684004759497596204 ) ) ;
#58051=CARTESIAN_POINT ( 'NONE',  ( 7.822691444960700125, 10.14955932391940330, -1.443375672974058777 ) ) ;
#58065=CARTESIAN_POINT ( 'NONE',  ( 1.270904146967303028, 3.246556430829583118, 0.7750000000000135669 ) ) ;
#58067=CARTESIAN_POINT ( 'NONE',  ( 1.364683531249988757, 1.696875000341414808, 0.000000000000000000 ) ) ;
#58087=CARTESIAN_POINT ( 'NONE',  ( 5.854423403002611437, 5.724582146458163656, 1.040834085586084257E-14 ) ) ;
#58095=CARTESIAN_POINT ( 'NONE',  ( 7.741869408603235136, 8.990934717247309749, 1.199719254218462483 ) ) ;
#58099=( BOUNDED_CURVE ( )  B_SPLINE_CURVE ( 2, ( #23700, #108233, #174258, #203498, #186197 ),
 .UNSPECIFIED., .F., .T. ) 
 B_SPLINE_CURVE_WITH_KNOTS ( ( 3, 2, 3 ),
 ( 0.1113702160535958441, 0.1125000000000000028, 0.1138193015819520398 ),
 .UNSPECIFIED. ) 
 CURVE ( )  GEOMETRIC_REPRESENTATION_ITEM ( )  RATIONAL_B_SPLINE_CURVE ( ( 0.9470460506485149921, 0.9636730364727230658, 1.000000000000000000, 0.9575793047851419715, 0.9420221409164282189 ) ) 
 REPRESENTATION_ITEM ( '' )  );
#58100=CARTESIAN_POINT ( 'NONE',  ( 8.075853055234393452, 12.57357899774884658, 0.7998128361456462443 ) ) ;
#58102=CARTESIAN_POINT ( 'NONE',  ( 1.523896559881090074, 8.692074762372739016, -2.522933744808672163 ) ) ;
#58113=CARTESIAN_POINT ( 'NONE',  ( -8.080296364064746939, 9.489729181906076505, 1.082531754730558626 ) ) ;
#58120=CARTESIAN_POINT ( 'NONE',  ( -5.426287360647527258, 6.306760859481674864, -1.047964138152550406 ) ) ;
#58124=CARTESIAN_POINT ( 'NONE',  ( 4.989037339704528229, 4.922891105851139315, 1.040834085586084257E-14 ) ) ;
#58133=CARTESIAN_POINT ( 'NONE',  ( -4.530395885260773525, 8.437212299446219532, 0.7998128361456481317 ) ) ;
#58135=CARTESIAN_POINT ( 'NONE',  ( -4.457933580795036654, 4.095344020549286590, -0.7998128361456221525 ) ) ;
#58141=CARTESIAN_POINT ( 'NONE',  ( 7.605760987586388744, 11.81721221891873697, 1.040834085586084257E-14 ) ) ;
#58142=ORIENTED_EDGE ( 'NONE', *, *, #80217, .F. ) ;
#58143=CARTESIAN_POINT ( 'NONE',  ( 1.364683531249990311, 4.676041667008083103, 0.7879004041258499402 ) ) ;
#58146=CARTESIAN_POINT ( 'NONE',  ( 4.313465427442102929, 8.184126765324453601, 0.7998128361456462443 ) ) ;
#58147=DIRECTION ( 'NONE',  ( -7.387867266669436732E-31, 1.000000000000000000, 8.546850786086424434E-32 ) ) ;
#58148=CARTESIAN_POINT ( 'NONE',  ( 1.561525566895185957, 8.688907412369037075, 2.501944002935413192 ) ) ;
#58160=CARTESIAN_POINT ( 'NONE',  ( -1.201851678989727383E-14, 1.134375000341418582, 1.575800808251672791 ) ) ;
#58162=CARTESIAN_POINT ( 'NONE',  ( 5.190073875932979419, 4.949507698210251938, 0.7998128361456341429 ) ) ;
#58164=CARTESIAN_POINT ( 'NONE',  ( -5.992340707560165569, 8.014150130285418783, 1.443375672974064550 ) ) ;
#58165=CARTESIAN_POINT ( 'NONE',  ( 3.334942599281629949, 5.874221551595115720, -1.082531754730543083 ) ) ;
#58166=CARTESIAN_POINT ( 'NONE',  ( -5.056828107772848746, 8.843457192469559303, -0.7216878364870207285 ) ) ;
#58170=CARTESIAN_POINT ( 'NONE',  ( 4.690231075323689325, 7.559354456931247412, 1.199719254218462483 ) ) ;
#58178=EDGE_CURVE ( 'NONE', #93128, #169987, #94173, .T. ) ;
#58179=CARTESIAN_POINT ( 'NONE',  ( 7.494959990256193194, 7.638541498254023843, -0.7998128361456281477 ) ) ;
#58183=CARTESIAN_POINT ( 'NONE',  ( -5.852315862593199469, 9.979452273000736895, 0.7998128361456481317 ) ) ;
#58187=CARTESIAN_POINT ( 'NONE',  ( 6.591235234537977661, 10.84152487360300299, 0.7998128361456462443 ) ) ;
#58189=CARTESIAN_POINT ( 'NONE',  ( -6.470265622219711688, 8.571729197388226140, -1.599625672291263179 ) ) ;
#58190=CARTESIAN_POINT ( 'NONE',  ( -4.121315508874269007, 5.831287398485175189, -1.443375672974053892 ) ) ;
#58191=CARTESIAN_POINT ( 'NONE',  ( 7.415946836550714849, 9.675023947441092176, 1.443375672974076540 ) ) ;
#58192=CARTESIAN_POINT ( 'NONE',  ( 4.159596813995052322, 7.384974941181836172, -0.7733407813514819873 ) ) ;
#58193=CARTESIAN_POINT ( 'NONE',  ( -6.112028321662274166, 6.025121218227761588, 0.7998128361456341429 ) ) ;
#58200=CARTESIAN_POINT ( 'NONE',  ( 9.673906298550626559, 11.24497775551929557, 1.199719254218452047 ) ) ;
#58201=CARTESIAN_POINT ( 'NONE',  ( -5.219248474292968787, 6.450796296714536915, 1.173595342525960206 ) ) ;
#58202=CARTESIAN_POINT ( 'NONE',  ( -1.402160292154681736E-14, -0.05312499965857903073, -1.575800808251665908 ) ) ;
#58204=CARTESIAN_POINT ( 'NONE',  ( -5.422898255786193111, 8.310169817517122581, -1.082531754730544860 ) ) ;
#58211=CARTESIAN_POINT ( 'NONE',  ( -5.845765802024414981, 6.039811503853035113, 0.4322504083978280232 ) ) ;
#58212=CARTESIAN_POINT ( 'NONE',  ( -0.6823417656250003738, 0.7802083336747520637, -1.181850606188749264 ) ) ;
#58216=CARTESIAN_POINT ( 'NONE',  ( 3.768803514918948938, 4.459654191235965293, -1.082531754730543083 ) ) ;
#58220=CARTESIAN_POINT ( 'NONE',  ( -7.280365300414089802, 10.47721470291632784, 1.082531754730549967 ) ) ;
#58228=CARTESIAN_POINT ( 'NONE',  ( -8.473482818416675499, 9.948446711983361723, -1.082531754730543083 ) ) ;
#58234=ORIENTED_EDGE ( 'NONE', *, *, #87487, .F. ) ;
#58235=CARTESIAN_POINT ( 'NONE',  ( -8.148087131688699358, 8.608449196499371681, -0.7216878364870267237 ) ) ;
#58241=CARTESIAN_POINT ( 'NONE',  ( -1.499999999999997780, 5.431250000682820378, 1.214306433183764966E-14 ) ) ;
#58242=FACE_OUTER_BOUND ( 'NONE', #6638, .T. ) ;
#58243=DIRECTION ( 'NONE',  ( 0.6507913734559627184, -0.7592566023653016805, 0.000000000000000000 ) ) ;
#58248=EDGE_CURVE ( 'NONE', #92214, #183003, #112595, .T. ) ;
#58249=CARTESIAN_POINT ( 'NONE',  ( -5.181187258716735577, 9.196468901811520880, 0.7998128361456481317 ) ) ;
#58250=B_SPLINE_CURVE_WITH_KNOTS ( 'NONE', 3,
 ( #185451, #137801, #55465, #86900, #57604, #168151, #38155, #135662, #119463, #24016, #39215, #121620 ),
 .UNSPECIFIED., .F., .F.,
 ( 4, 2, 2, 2, 2, 4 ),
 ( 0.000000000000000000, 0.0005575204076271189505, 0.001115040815254237901, 0.001672561222881356960, 0.001951321426694916164, 0.002230081630508475368 ),
 .UNSPECIFIED. ) ;
#58253=CARTESIAN_POINT ( 'NONE',  ( 4.578903193113299963, 6.365139696764064325, 1.599625672291267398 ) ) ;
#58257=CARTESIAN_POINT ( 'NONE',  ( 6.109920781252839994, 10.27999134477033216, 1.040834085586084257E-14 ) ) ;
#58264=CARTESIAN_POINT ( 'NONE',  ( -5.341549334104202629, 7.254893527920112994, 1.443375672974064550 ) ) ;
#58276=CARTESIAN_POINT ( 'NONE',  ( -9.515124878692420296, 9.995400534762978850, 1.040834085586084257E-14 ) ) ;
#58278=CARTESIAN_POINT ( 'NONE',  ( 8.796542737168120851, 9.157054702984622097, -0.7998128361456211532 ) ) ;
#58279=CARTESIAN_POINT ( 'NONE',  ( -1.402160292154681736E-14, 0.2125000000000202283, 1.732050807568877637 ) ) ;
#58280=CARTESIAN_POINT ( 'NONE',  ( -8.341290820905609138, 10.75459192918846618, 1.599625672291269396 ) ) ;
#58283=CARTESIAN_POINT ( 'NONE',  ( 1.364683531249988535, 4.905208333674756283, -0.7879004041258300672 ) ) ;
#58284=CARTESIAN_POINT ( 'NONE',  ( 8.541273586929342798, 11.94827437051752206, -1.082531754730543083 ) ) ;
#58287=CARTESIAN_POINT ( 'NONE',  ( 1.499999999999989120, 4.754166666666689522, 0.8660254037844524744 ) ) ;
#58289=( BOUNDED_SURFACE ( )  B_SPLINE_SURFACE ( 3, 2, ( 
 ( #199706, #31913, #81714 ),
 ( #2558, #51353, #419 ),
 ( #165096, #84906, #150993 ),
 ( #68632, #200764, #131583 ),
 ( #181339, #13128, #61896 ),
 ( #177786, #96556, #213444 ),
 ( #129118, #14179, #126984 ),
 ( #130173, #195095, #111780 ) ),
 .UNSPECIFIED., .F., .F., .F. ) 
 B_SPLINE_SURFACE_WITH_KNOTS ( ( 4, 2, 2, 4 ),
 ( 3, 3 ),
 ( 0.000000000000000000, 0.003001918495469456383, 0.004502877743204184574, 0.006003836990938912765 ),
 ( 0.000000000000000000, 1.000000000000000000 ),
 .UNSPECIFIED. ) 
 GEOMETRIC_REPRESENTATION_ITEM ( )  RATIONAL_B_SPLINE_SURFACE ( (
 ( 1.000000000000000000, 0.7835651598521267136, 1.000000000000000000),
 ( 1.000000000000000000, 0.7913519369917237922, 1.000000000000000000),
 ( 1.000000000000000000, 0.8009496234828819006, 1.000000000000000000),
 ( 1.000000000000000000, 0.8230981486291126803, 1.000000000000000000),
 ( 1.000000000000000000, 0.8318333311017226395, 1.000000000000000000),
 ( 1.000000000000000000, 0.8529518727575166048, 1.000000000000000000),
 ( 1.000000000000000000, 0.8654984584225899891, 1.000000000000000000),
 ( 1.000000000000000000, 0.8789000212895413666, 1.000000000000000000) ) ) 
 REPRESENTATION_ITEM ( '' )  SURFACE ( )  );
#58290=CARTESIAN_POINT ( 'NONE',  ( 8.717529583462649612, 10.23316793787035195, 1.082531754730558626 ) ) ;
#58292=CARTESIAN_POINT ( 'NONE',  ( 3.740297717422798041, 7.429476292658457659, 2.448395595369510680 ) ) ;
#58293=CARTESIAN_POINT ( 'NONE',  ( -6.561783159334145132, 6.757761228752363181, -0.7216878364870278340 ) ) ;
#58295=CARTESIAN_POINT ( 'NONE',  ( -0.6823417656250212460, 2.301041667008084435, 1.181850606188767472 ) ) ;
#58299=CARTESIAN_POINT ( 'NONE',  ( -6.531277313481209212, 8.642909503859968368, 1.599625672291283607 ) ) ;
#58300=CARTESIAN_POINT ( 'NONE',  ( 0.6823417656249899377, 5.238541667008086655, -1.181850606188754593 ) ) ;
#58306=CARTESIAN_POINT ( 'NONE',  ( 6.760712154708803823, 11.03924794713562818, 1.040834085586084257E-14 ) ) ;
#58309=CARTESIAN_POINT ( 'NONE',  ( 1.499999999999989120, 1.775000000000019673, 0.000000000000000000 ) ) ;
#58311=AXIS2_PLACEMENT_3D ( 'NONE', #184807, #36436, #86261 ) ;
#58315=CARTESIAN_POINT ( 'NONE',  ( 6.317736394288131052, 9.354147645769410602, 1.082531754730558626 ) ) ;
#58322=CARTESIAN_POINT ( 'NONE',  ( 8.239604668803105270, 10.63595808506888396, -1.599625672291268286 ) ) ;
#58323=CARTESIAN_POINT ( 'NONE',  ( -10.66756793585402363, 11.33991743478486391, 0.7998128361456462443 ) ) ;
#58326=CARTESIAN_POINT ( 'NONE',  ( 1.364683531249986537, -0.8864583329919110133, 0.7879004041258500513 ) ) ;
#58327=CARTESIAN_POINT ( 'NONE',  ( -0.7500000000000006661, 0.3583333333333563187, -1.299038105676652011 ) ) ;
#58330=CARTESIAN_POINT ( 'NONE',  ( -3.975497760493641675, 7.849573349659754840, -7.471960471057975262E-11 ) ) ;
#58334=CARTESIAN_POINT ( 'NONE',  ( -0.6823417656249969321, 5.717708333674756283, -1.181850606188749264 ) ) ;
#58336=CARTESIAN_POINT ( 'NONE',  ( -4.609409038966229666, 8.321468278861834378, -0.7216878364870267237 ) ) ;
#58345=CARTESIAN_POINT ( 'NONE',  ( 9.264299036839600987, 9.702770385934682551, -0.7998128361456281477 ) ) ;
#58351=CARTESIAN_POINT ( 'NONE',  ( -9.982881178363895103, 10.54111621771303753, 1.040834085586084257E-14 ) ) ;
#58353=CARTESIAN_POINT ( 'NONE',  ( 4.971035877704902184, 8.951292290631053916, 1.040834085586084257E-14 ) ) ;
#58355=CARTESIAN_POINT ( 'NONE',  ( 4.500943809612556024, 4.353448654077163305, 1.214306433183764966E-14 ) ) ;
#58356=CARTESIAN_POINT ( 'NONE',  ( -2.081668171172168513E-14, 6.468705557303652931, 4.925226524755076163 ) ) ;
#58357=CARTESIAN_POINT ( 'NONE',  ( 3.649115900372475796, 7.409052317076538330, 1.040834085586084257E-14 ) ) ;
#58367=CARTESIAN_POINT ( 'NONE',  ( -4.934804725694220906, 7.740727365743146571, -1.082531754730549967 ) ) ;
#58368=CARTESIAN_POINT ( 'NONE',  ( 9.164948653157988900, 11.71552606681625619, -1.443375672974057666 ) ) ;
#58371=CARTESIAN_POINT ( 'NONE',  ( -6.723954117373590833, 9.932031339322813679, -1.199719254218440723 ) ) ;
#58375=CARTESIAN_POINT ( 'NONE',  ( -9.494787648271923786, 9.971673765939062406, 1.040834085586084257E-14 ) ) ;
#58378=CARTESIAN_POINT ( 'NONE',  ( 6.096362627639171805, 10.26417349888772179, -0.7998128361456291469 ) ) ;
#58380=CARTESIAN_POINT ( 'NONE',  ( 6.471319392424407901, 6.444294134116939077, 0.7998128361456341429 ) ) ;
#58392=CARTESIAN_POINT ( 'NONE',  ( -6.347188469492005325, 10.55680364771601809, -0.7998128361456291469 ) ) ;
#58395=CARTESIAN_POINT ( 'NONE',  ( 7.646435448427411963, 8.023188899361205273, -0.7216878364870257245 ) ) ;
#58400=CARTESIAN_POINT ( 'NONE',  ( 4.867540842506059562, 5.637551390133895168, -1.199719254218452047 ) ) ;
#58402=CARTESIAN_POINT ( 'NONE',  ( -3.899941742225307539, 7.701682465904834629, 0.7998128361456341429 ) ) ;
#58406=CARTESIAN_POINT ( 'NONE',  ( -5.874320061489284761, 6.022657918099090679, -0.3309714775648956997 ) ) ;
#58412=CARTESIAN_POINT ( 'NONE',  ( 9.250740883225924804, 9.686952540052077509, 1.040834085586084257E-14 ) ) ;
#58414=CARTESIAN_POINT ( 'NONE',  ( -4.148431816101615155, 3.942184661647709198, 0.7216878364870317197 ) ) ;
#58417=CARTESIAN_POINT ( 'NONE',  ( -4.916882227542496153, 6.680427897100001289, -1.249109758411016236 ) ) ;
#58420=CARTESIAN_POINT ( 'NONE',  ( -1.364683531250014514, -0.9489583329919112353, -0.7879004041258359514 ) ) ;
#58424=CARTESIAN_POINT ( 'NONE',  ( 8.093854517678360949, 12.38665467069271386, 1.040834085586084257E-14 ) ) ;
#58442=CARTESIAN_POINT ( 'NONE',  ( -5.122283107864663343, 4.870418468797203637, 0.000000000000000000 ) ) ;
#58444=CARTESIAN_POINT ( 'NONE',  ( 1.499999999999989120, 4.004166666666685970, 0.8660254037844524744 ) ) ;
#58446=CARTESIAN_POINT ( 'NONE',  ( -2.948008335967658322, 5.526761261015804116, 1.199719254218462483 ) ) ;
#58451=CARTESIAN_POINT ( 'NONE',  ( -1.201851678989727383E-14, 4.446875000341417916, -1.575800808251660134 ) ) ;
#58454=CARTESIAN_POINT ( 'NONE',  ( -3.795919822146293754, 4.491289883001181593, -1.082531754730549967 ) ) ;
#58460=CARTESIAN_POINT ( 'NONE',  ( 10.05353459973327368, 11.68787744023238417, -1.199719254218440723 ) ) ;
#58466=CARTESIAN_POINT ( 'NONE',  ( -1.364683531250000748, 1.321875000341421469, 0.000000000000000000 ) ) ;
#58469=CARTESIAN_POINT ( 'NONE',  ( -7.700141177557535244, 11.07091624287075859, -1.199719254218446718 ) ) ;
#58470=CARTESIAN_POINT ( 'NONE',  ( -4.541618270453545492, 8.242379048930368768, 0.7216878364870458196 ) ) ;
#58474=CARTESIAN_POINT ( 'NONE',  ( -1.500000000000015099, -1.297916665983847029, 0.8660254037844403729 ) ) ;
#58482=CARTESIAN_POINT ( 'NONE',  ( -4.406036734316890247, 7.123831375802920363, -1.082531754730548412 ) ) ;
#58483=CARTESIAN_POINT ( 'NONE',  ( 1.408489644590610990, 7.311701683603665458, -4.382268911471478567 ) ) ;
#58487=CARTESIAN_POINT ( 'NONE',  ( -4.487385655998893164, 6.258369236797239665, 1.443375672974064550 ) ) ;
#58489=CARTESIAN_POINT ( 'NONE',  ( 10.23370702021670020, 10.83374636654133383, 0.7998128361456462443 ) ) ;
#58494=VERTEX_POINT ( 'NONE', #147179 ) ;
#58498=CARTESIAN_POINT ( 'NONE',  ( -3.242371291962510504, 6.934516940598226320, 1.040834085586084257E-14 ) ) ;
#58504=CARTESIAN_POINT ( 'NONE',  ( 9.083599731475988648, 10.66024977721925104, 1.082531754730549967 ) ) ;
#58505=CARTESIAN_POINT ( 'NONE',  ( 6.819914962873951936, 7.915321197229798322, -1.199719254218446718 ) ) ;
#58510=CARTESIAN_POINT ( 'NONE',  ( 3.842846474469570062, 6.570739089268092137, -1.199719254218452047 ) ) ;
#58519=CARTESIAN_POINT ( 'NONE',  ( -4.550733115681270036, 8.460939068270139529, 0.7998128361456481317 ) ) ;
#58523=EDGE_CURVE ( 'NONE', #147848, #108613, #210004, .T. ) ;
#58525=CARTESIAN_POINT ( 'NONE',  ( -1.001543065824772872E-14, 5.321875000341422357, 1.575800808251672791 ) ) ;
#58526=CARTESIAN_POINT ( 'NONE',  ( 8.392133896734655707, 11.77427806529038357, 1.082531754730546636 ) ) ;
#58527=CARTESIAN_POINT ( 'NONE',  ( -6.762819695118240659, 6.784377820593065600, 0.7998128361456341429 ) ) ;
#58530=CARTESIAN_POINT ( 'NONE',  ( 4.493637847925535667, 7.329995691633395261, -1.199719254218452047 ) ) ;
#58531=CARTESIAN_POINT ( 'NONE',  ( -5.575427483717760424, 7.527751369135936343, 1.599625672291269396 ) ) ;
#58537=CARTESIAN_POINT ( 'NONE',  ( 7.022760382198770301, 8.255937203062467589, -1.082531754730543083 ) ) ;
#58539=CARTESIAN_POINT ( 'NONE',  ( 7.904040366642699489, 8.323727970612377902, 0.7216878364870458196 ) ) ;
#58540=CARTESIAN_POINT ( 'NONE',  ( -1.201851678989727383E-14, 2.759375000341417916, -1.575800808251660134 ) ) ;
#58542=CARTESIAN_POINT ( 'NONE',  ( 4.948362878863507675, 8.716914425408678113, -0.7216878364870267237 ) ) ;
#58544=LINE ( 'NONE', #141966, #161983 ) ;
#58545=CARTESIAN_POINT ( 'NONE',  ( -2.304522924643024773, 5.632434478818063361, 0.7216878364870317197 ) ) ;
#58552=CARTESIAN_POINT ( 'NONE',  ( -4.009952404978103679, 7.802135278885950598, 0.4104602055842437314 ) ) ;
#58560=CARTESIAN_POINT ( 'NONE',  ( 6.328958779480917229, 6.278206752349526631, 0.7998128361456341429 ) ) ;
#58562=CARTESIAN_POINT ( 'NONE',  ( -3.348500752450953577, 4.929670182657964084, 1.443375672974062551 ) ) ;
#58564=CARTESIAN_POINT ( 'NONE',  ( 3.358669367883368118, 4.941533567329135401, -1.599625672291262513 ) ) ;
#58571=CARTESIAN_POINT ( 'NONE',  ( 3.823036129373602154, 6.443664003369091731, -1.082531754730548412 ) ) ;
#58572=CARTESIAN_POINT ( 'NONE',  ( -0.6823417656250212460, 3.863541667008085767, 1.181850606188767472 ) ) ;
#58574=CARTESIAN_POINT ( 'NONE',  ( 8.925345196497941558, 9.307324238869423283, 1.040834085586084257E-14 ) ) ;
#58576=CARTESIAN_POINT ( 'NONE',  ( -9.398826802771548472, 11.98838390803207865, -1.599625672291263179 ) ) ;
#58578=CARTESIAN_POINT ( 'NONE',  ( -5.766295404513793521, 5.621766148221195358, 0.7998128361456341429 ) ) ;
#58582=CARTESIAN_POINT ( 'NONE',  ( -1.201851678989727383E-14, 3.712500000000020339, 1.732050807568877637 ) ) ;
#58583=CARTESIAN_POINT ( 'NONE',  ( 6.745345117998789775, 7.828323044875442172, 1.199719254218462483 ) ) ;
#58587=CARTESIAN_POINT ( 'NONE',  ( -1.364683531250012516, 3.488541667008085767, -0.7879004041258300672 ) ) ;
#58589=CARTESIAN_POINT ( 'NONE',  ( 10.23604278863759909, 11.04439746293979496, 0.000000000000000000 ) ) ;
#58595=CARTESIAN_POINT ( 'NONE',  ( -0.7500000000000215383, 1.722916667349486008, 1.299038105676659116 ) ) ;
#58598=CARTESIAN_POINT ( 'NONE',  ( -4.693093728624763372, 8.627026450037540428, 0.7998128361456481317 ) ) ;
#58599=CARTESIAN_POINT ( 'NONE',  ( -3.551873057100300990, 5.166937871415542283, 1.443375672974064550 ) ) ;
#58608=CARTESIAN_POINT ( 'NONE',  ( 4.788000803920411386, 8.737751371215816576, 1.040834085586084257E-14 ) ) ;
#58611=CARTESIAN_POINT ( 'NONE',  ( 4.171104814498611368, 8.018039383557042044, 0.7998128361456321445 ) ) ;
#58616=CARTESIAN_POINT ( 'NONE',  ( 3.460355519985863548, 5.060167411448709629, 1.599625672291267398 ) ) ;
#58621=DIRECTION ( 'NONE',  ( 0.7592566023653005702, 0.6507913734559639396, 0.000000000000000000 ) ) ;
#58622=CARTESIAN_POINT ( 'NONE',  ( 5.861148881710747993, 5.995921596292371092, 0.2991943293650864422 ) ) ;
#58623=VECTOR ( 'NONE', #81752, 1000.000000000000114 ) ;
#58635=CARTESIAN_POINT ( 'NONE',  ( 6.751597309925441159, 9.860318714012938912, -1.082531754730537088 ) ) ;
#58637=CARTESIAN_POINT ( 'NONE',  ( -2.578021764892882040, 6.159442492350315490, 0.7998128361456341429 ) ) ;
#58641=CARTESIAN_POINT ( 'NONE',  ( -6.230135280679522936, 7.227244901336242755, 1.199719254218450271 ) ) ;
#58654=DIRECTION ( 'NONE',  ( -0.4243160830846619547, -0.9055141421511264666, 5.421010862427548676E-14 ) ) ;
#58655=CARTESIAN_POINT ( 'NONE',  ( 4.035228272797701798, 3.987058170690799042, -0.7945584926636685141 ) ) ;
#58662=CARTESIAN_POINT ( 'NONE',  ( -9.110716038703348119, 12.61262389758715408, 1.082531754730560403 ) ) ;
#58666=CARTESIAN_POINT ( 'NONE',  ( 7.540305987494599016, 11.94877408538573427, -0.7998128361456291469 ) ) ;
#58671=CARTESIAN_POINT ( 'NONE',  ( -7.552055258011950656, 8.769484874890757453, 1.199719254218462483 ) ) ;
#58672=CARTESIAN_POINT ( 'NONE',  ( 5.497994985541524215, 6.373081223675282736, -1.199719254218445830 ) ) ;
#58675=CARTESIAN_POINT ( 'NONE',  ( -4.134873662487946966, 3.926366815765101936, 1.214306433183764966E-14 ) ) ;
#58679=CARTESIAN_POINT ( 'NONE',  ( -1.364683531250012516, 2.801041667008090652, -0.7879004041258289570 ) ) ;
#58682=CARTESIAN_POINT ( 'NONE',  ( 7.470179451449751262, 7.817556902887268677, 1.040834085586084257E-14 ) ) ;
#58688=VERTEX_POINT ( 'NONE', #71384 ) ;
#58689=CARTESIAN_POINT ( 'NONE',  ( 9.585251414737269826, 11.24551007435741568, -1.082531754730537088 ) ) ;
#58694=CARTESIAN_POINT ( 'NONE',  ( -7.655550293210764856, 12.08322577538792331, 0.000000000000000000 ) ) ;
#58712=CARTESIAN_POINT ( 'NONE',  ( 1.499999999999987121, 2.327083334016154303, -0.8660254037844262731 ) ) ;
#58717=CARTESIAN_POINT ( 'NONE',  ( 0.7499999999999885647, 0.4833333333333564297, 1.299038105676657340 ) ) ;
#58718=CARTESIAN_POINT ( 'NONE',  ( 6.968000882419564945, 10.21675256520979858, 1.199719254218460707 ) ) ;
#58719=CARTESIAN_POINT ( 'NONE',  ( 0.6823417656249882723, -0.4072916663252490466, 1.181850606188755259 ) ) ;
#58722=CARTESIAN_POINT ( 'NONE',  ( 8.758204044747998296, 11.24099069033793974, 1.443375672974076540 ) ) ;
#58723=CARTESIAN_POINT ( 'NONE',  ( -6.073689629242165822, 7.148687991279732756, -1.082531754730544860 ) ) ;
#58729=CARTESIAN_POINT ( 'NONE',  ( -4.880045225915050189, 7.780804299287790826, 1.199719254218464037 ) ) ;
#58731=CARTESIAN_POINT ( 'NONE',  ( -0.7500000000000215383, 2.222916667349486453, 1.299038105676671107 ) ) ;
#58732=CARTESIAN_POINT ( 'NONE',  ( -0.6823417656249969321, 3.780208333674754506, -1.181850606188749264 ) ) ;
#58745=CARTESIAN_POINT ( 'NONE',  ( -8.341290820905609138, 10.75459192918846618, 1.599625672291269396 ) ) ;
#58746=CARTESIAN_POINT ( 'NONE',  ( 6.500244582748090139, 9.671036882259738121, 1.199719254218460707 ) ) ;
#58754=CARTESIAN_POINT ( 'NONE',  ( -6.984421689334302741, 11.30024240419870374, 0.000000000000000000 ) ) ;
#58759=CARTESIAN_POINT ( 'NONE',  ( 4.552840656090682891, 4.206068941727564514, 1.214306433183764966E-14 ) ) ;
#58762=CARTESIAN_POINT ( 'NONE',  ( -6.064574784014443942, 5.969758757638621738, -0.7998128361456291469 ) ) ;
#58763=CARTESIAN_POINT ( 'NONE',  ( -8.833300774503376473, 10.26427131079744193, 1.199719254218462483 ) ) ;
#58773=CARTESIAN_POINT ( 'NONE',  ( 5.635385404774530649, 9.726366738878972740, 0.7998128361456462443 ) ) ;
#58793=CARTESIAN_POINT ( 'NONE',  ( 4.365362273920250225, 5.155639410070820716, 1.082531754730560403 ) ) ;
#58797=CARTESIAN_POINT ( 'NONE',  ( -9.053093885623068715, 11.58502883802551153, -1.599625672291263179 ) ) ;
#58800=CARTESIAN_POINT ( 'NONE',  ( 4.324687812634897988, 4.147816657603229373, 0.7216878364870317197 ) ) ;
#58803=B_SPLINE_CURVE_WITH_KNOTS ( 'NONE', 3,
 ( #104058, #151746, #170104, #24916, #109457, #128911, #95294, #161343, #91020, #94226, #158146, #76868, #25984, #108382, #125714, #107312, #28130, #11866, #9738, #8670, #93156, #157082 ),
 .UNSPECIFIED., .F., .F.,
 ( 4, 2, 2, 2, 2, 2, 2, 2, 2, 2, 4 ),
 ( 0.5001299408125404744, 0.5533639344558343165, 0.5799809312774814041, 0.6065979280991283806, 0.6598319217424222227, 0.6864489185640691993, 0.7130659153857161758, 0.7662999090290101289, 0.8195339026723040821, 0.8727678963155980352, 0.9260018899588919883 ),
 .UNSPECIFIED. ) ;
#58805=CARTESIAN_POINT ( 'NONE',  ( 4.515632184204340760, 7.124593881049110955, 1.261186505319204398 ) ) ;
#58810=CARTESIAN_POINT ( 'NONE',  ( -1.201851678989727383E-14, 1.071875000341418138, 1.575800808251672791 ) ) ;
#58817=CARTESIAN_POINT ( 'NONE',  ( -4.928552533767591726, 5.708731696605642725, 1.199719254218462483 ) ) ;
#58820=CARTESIAN_POINT ( 'NONE',  ( 1.499999999999989120, 0.2750000000000182854, 0.000000000000000000 ) ) ;
#58822=CARTESIAN_POINT ( 'NONE',  ( -1.499999999999997780, 5.650000000000023448, 1.214306433183764966E-14 ) ) ;
#58827=CARTESIAN_POINT ( 'NONE',  ( 1.364683531249986537, 0.9052083336747533959, -0.7879004041258239610 ) ) ;
#58829=CARTESIAN_POINT ( 'NONE',  ( -6.364663046611467756, 9.512858423433634414, 1.199719254218452047 ) ) ;
#58830=CARTESIAN_POINT ( 'NONE',  ( 7.553864141108259211, 11.96459193126834464, 1.040834085586084257E-14 ) ) ;
#58831=CARTESIAN_POINT ( 'NONE',  ( 5.515469562660962666, 5.329135999392899947, 0.7998128361456341429 ) ) ;
#58835=CARTESIAN_POINT ( 'NONE',  ( 0.6823417656249882723, -0.01145833299191073573, -1.181850606188749264 ) ) ;
#58842=CARTESIAN_POINT ( 'NONE',  ( 5.829642864196151741, 9.745074408296771296, 0.7216878364870438212 ) ) ;
#58846=CARTESIAN_POINT ( 'NONE',  ( -6.227272627378437342, 6.159572908229946187, -0.7998128361456291469 ) ) ;
#58850=CARTESIAN_POINT ( 'NONE',  ( -2.252626078164912560, 5.779814191167667481, 0.7998128361456341429 ) ) ;
#58851=CARTESIAN_POINT ( 'NONE',  ( 6.304178240230120522, 6.457222156464352381, -0.7216878364870257245 ) ) ;
#58852=CARTESIAN_POINT ( 'NONE',  ( -8.473482818416664841, 11.86918514058604757, -1.082531754730543083 ) ) ;
#58854=CARTESIAN_POINT ( 'NONE',  ( -1.500000000000013101, 3.379166666666691299, -0.8660254037844313801 ) ) ;
#58858=CARTESIAN_POINT ( 'NONE',  ( 9.246297574839974942, 11.81043314211192019, 1.443375672974076540 ) ) ;
#58872=CARTESIAN_POINT ( 'NONE',  ( 8.473482818416664841, 10.90881592628469932, -1.443375672974063439 ) ) ;
#58875=CARTESIAN_POINT ( 'NONE',  ( 8.450809820019639318, 8.753699632978056755, -0.7998128361456291469 ) ) ;
#58879=CARTESIAN_POINT ( 'NONE',  ( 10.72180055030867329, 11.40318881831530540, 0.7998128361456341429 ) ) ;
#58882=CARTESIAN_POINT ( 'NONE',  ( 3.714570900464269076, 7.277490450609545469, 0.7216878364870298324 ) ) ;
#58883=ORIENTED_EDGE ( 'NONE', *, *, #76553, .F. ) ;
#58884=CARTESIAN_POINT ( 'NONE',  ( -8.365017589951714072, 8.861534731139549592, 1.040834085586084257E-14 ) ) ;
#58891=( BOUNDED_SURFACE ( )  B_SPLINE_SURFACE ( 1, 2, ( 
 ( #166559, #211019, #179614, #33347, #100484, #14943, #147125, #49603, #32292, #99429, #112537, #62643, #163368, #34412, #83157, #18148, #149237, #148186, #133024, #17080, #213151, #165483, #31235, #812, #66880, #199023, #63719, #46420, #84235, #129877, #128802, #195860, #194784, #178549, #30159, #96247, #13885, #50670, #79964, #98358, #214188, #65815, #164423, #47500, #146068, #212081, #113609, #97308, #16007, #81039, #182793, #64781, #82093, #130922, #115727, #116796, #196915, #131962, #48555, #114674, #197974, #181718, #101556, #137279, #85302, #167625, #121099, #153518, #19224, #151388, #72233, #188134, #21342, #2958, #69030, #70093, #170825, #6164, #35479, #169755, #154587, #138341, #118940, #150323, #88525, #86377, #204358, #152445, #4024, #183864, #203299, #67949, #39765, #105870, #56014, #122168, #135146, #53880, #87451, #104777, #171896, #23493, #168687, #1889, #54946, #134094, #187066, #200102, #51752, #136208, #117875, #202227, #22416, #103703, #201162, #52802, #184920, #36544, #38698, #5087, #102631, #120013, #71162, #185989, #37623, #20291, #109101, #159911, #92804, #156728, #59202, #140503, #125359, #10445, #73309, #108032, #90665, #57081, #176176, #111232, #190263, #174058, #61347, #124304, #9391, #139412, #44046, #75463, #175115, #155650, #25630, #208639, #77588, #76518, #91742, #206514, #11518, #127507, #42989, #141575, #74403, #172980, #60271, #58146, #8318, #191323, #40848, #143711, #189209, #7233, #123245, #26702, #110166, #41922, #157795, #205445, #126428, #207582, #158848, #142629, #192391, #27776, #93874, #209703, #106955, #193477, #45121, #177234, #89599, #24559, #48315, #195618, #130686, #115482, #16823, #94935, #64542, #162057, #148980, #160984, #181474, #99178, #13646, #555, #97070, #163123, #14705, #113368, #33104, #198769, #196676, #80799, #114426, #146889, #82907, #178311, #194534, #81852, #212909, #180427, #78647, #129631, #66619, #179374, #112295, #131718, #116538, #79718, #165230, #145835, #132766, #29920, #32044, #98131, #96003, #164182, #15767, #30995, #213950, #147934, #211839, #63477, #50419, #28847, #65571, #47254, #46181, #197722, #49362, #12575, #128570, #144774, #210783, #62406, #151129, #182528, #120824, #118675, #170553, #184659, #36279, #1630, #169492, #100227, #71965, #138075, #104509, #186800, #35212, #86114, #201954, #137007, #5893, #204088, #200895, #22136, #21074, #88249, #87176, #154319, #55741, #168428, #51489, #2696, #52542, #18957, #152184, #83969, #34158, #153242, #69828, #203034, #102356, #20024, #17885, #166295, #117611, #70896, #150058, #3754, #67689, #133835, #68769, #4815, #199846, #135936, #53611, #54675, #119744, #38429, #183603, #101287, #134888, #167369, #85041, #185723, #37356, #103431, #43797, #142374, #57879, #10191, #156463, #208384, #76265, #60015, #188941, #171624, #77333, #40580, #121897, #106686, #11255, #105590, #187865, #155379, #143446, #126168, #209443, #91474, #58949, #191065, #75206, #172711, #139143, #205171, #23218, #90393, #157535, #89331, #93612, #24287, #207329, #140232, #174863, #175921, #8049, #9130, #192132, #74139, #206254, #108837, #73044, #26442, #56813, #122983, #141316, #109910, #125107, #124041, #42729, #190008, #92552, #158592, #6963, #41658, #107771, #173797, #27513, #39493, #25373, #159657, #32854, #95750, #195360, #110969, #15513, #46992, #146634, #127247, #79469, #180175, #49117, #196424, #211583, #178049, #197473, #98929, #14447, #113109, #45928, #144518, #31801, #112048, #194284, #30736, #12317, #115237, #160724, #193217, #28594, #80538, #81598, #13392, #29666, #44864, #97877, #179114, #161802, #212650, #145586, #63219, #129381, #96818, #176976, #62162, #162867, #148741, #64291, #82657, #130437, #48069, #114181, #147683, #181226, #94681, #163937, #213700, #164983, #78398, #65323, #131471, #16574, #61088, #210526, #128320, #68522, #84797, #153002, #170306, #168186, #134649, #19785, #200654, #202791, #149813, #166052, #53364, #52303, #118432, #50173, #101037, #120583, #150885, #83722, #103188, #88005, #133592, #4579, #199596, #186560, #1386, #184420, #36037, #67447, #102117, #85867, #2448, #21895, #151943, #86936 ),
 ( #309, #3516, #51239, #183362, #18713, #117364, #69587, #116293, #38189, #201723, #135697, #169249, #119498, #185484, #182284, #104260, #34966, #20837, #33909, #37110, #66380, #132529, #167128, #70653, #198526, #136763, #54441, #99985, #17637, #45393, #55502, #154076, #106440, #194817, #29128, #46453, #95215, #94154, #78926, #177515, #90153, #111509, #188699, #161265, #12851, #145049, #6726, #203857, #112575, #72804, #5643, #138906, #178586, #137836, #71724, #187623, #30194, #211050, #121656, #123800, #160193, #11794, #110447, #204924, #171381, #22972, #39251, #122736, #189758, #105344, #128835, #56577, #28061, #172463, #209984, #62676, #40334, #44325, #89090, #24050, #156221, #143992, #155144, #61625, #7797, #73890, #127792, #77869, #139983, #206005, #57640, #176449, #193746, #97347, #47533, #16046, #116831, #166597, #195897, #115762, #100523, #18186, #64815, #96283, #34449, #32326, #84272, #98394, #164458, #129912, #83191, #13919, #200139, #51792, #150359, #1929, #163403, #214223, #181752, #50707, #134130, #117910, #114708, #67988, #149274, #183902, #854, #79999, #66920, #82129, #147160, #33384, #81074, #213187, #196951, #130961, #212115, #14978, #148222, #162334, #48591, #146104, #99464, #180703, #198011, #182833, #63752, #113646, #132001, #65852, #179651, #31272, #49639, #165522, #17114, #133061, #199061, #103738, #169789, #120051, #188168, #205482, #203330, #21378, #54984, #87486, #23527, #184953, #201200, #88562, #153553, #5123, #85342, #136244, #155686, #186025, #118975, #138378, #123283, #168725, #39801, #20327, #7269, #36580, #71198, #137315, #102668, #121137, #187099, #37662, #57114, #38733, #122206, #104814, #52839, #105909, #19260, #89634, #154621, #170859, #151423, #22450, #6200, #72269, #204396, #86413, #56050, #171935, #73346, #152480, #139447, #4060, #35513, #101591, #2996, #53914, #70131, #69064, #167659, #135184, #202264, #59234, #161015, #9427, #109137, #24595, #143745, #175150, #60304, #40885, #207617, #93909, #177269, #110199, #125392, #91773, #111265, #12610, #142663, #26737, #174093, #58179, #159949, #25665, #108066, #158882, #140537, #28885, #74437, #106989, #156765, #208673, #209740, #141609, #157830, #124339, #77623, #62440, #75496, #193512, #191358, #94968, #190296, #43024, #92838, #41954, #76554, #126463, #10479, #210815, #192426, #61383, #44081, #206550, #45153, #173014, #78684, #11552, #176209, #90703, #27810, #127540, #144809, #189246, #8352, #147971, #198808, #131751, #195654, #98165, #179408, #164212, #49395, #112333, #146922, #129668, #96040, #591, #150098, #14740, #212940, #100265, #163156, #48349, #178345, #82942, #114461, #213982, #194569, #64577, #33137, #116573, #115514, #130718, #31029, #50455, #166331, #81886, #180460, #113402, #211875, #99217, #97104, #47288, #15799, #79752, #182567, #13681, #46216, #162092, #65602, #149016, #80832, #196709, #29954, #165267, #32077, #197757, #181508, #16862, #66658, #132804, #34191, #145868, #17922, #84007, #1669, #128603, #63514, #87214, #20060, #169530, #154354, #55778, #133875, #103468, #200932, #187902, #199882, #5932, #138116, #52580, #39532, #135975, #201990, #53648, #152221, #72004, #23256, #21110, #119780, #153279, #185761, #121935, #2733, #18998, #120864, #37393, #4856, #117651, #168462, #105632, #3790, #86150, #118708, #70934, #183644, #171660, #54714, #137044, #22176, #69866, #203070, #35249, #89369, #68805, #170590, #101324, #186837, #155417, #67724, #36317, #104545, #51525, #38469, #88292, #204126, #167406, #85078, #151163, #134925, #184696, #102395, #93646, #44899, #159689, #158630, #143482, #27550, #157573, #109945, #41696, #11289, #175954, #77368, #74179, #56852, #177011, #140272, #7001, #206291, #111006, #205210, #73078, #40620, #28628, #209479, #94715, #191100, #10228, #76302, #174899, #57916, #24325, #90433, #123025, #190044, #42768, #188976, #193252, #124081, #92588, #25409, #60051, #61120, #107807, #108875, #127281, #173832, #91513, #208417, #172750, #126206, #156501, #8091, #192168, #142409, #9165, #75241, #139179, #106723, #43829, #141352, #207367, #58986, #125143, #26478, #45962, #180213, #165018, #16613 ) ),
 .UNSPECIFIED., .F., .F., .T. ) 
 B_SPLINE_SURFACE_WITH_KNOTS ( ( 2, 2 ),
 ( 3, 2, 2, 2, 2, 2, 2, 2, 2, 2, 2, 2, 2, 2, 2, 2, 2, 2, 2, 2, 2, 2, 2, 2, 2, 2, 2, 2, 2, 2, 2, 2, 2, 2, 2, 2, 2, 2, 2, 2, 2, 2, 2, 2, 2, 2, 2, 2, 2, 2, 2, 2, 2, 2, 2, 2, 2, 2, 2, 2, 2, 2, 2, 2, 2, 2, 2, 2, 2, 2, 2, 2, 2, 2, 2, 2, 2, 2, 2, 2, 2, 2, 2, 2, 2, 2, 2, 2, 2, 2, 2, 2, 2, 2, 2, 2, 2, 2, 2, 2, 2, 2, 2, 2, 2, 2, 2, 2, 2, 2, 2, 2, 2, 2, 2, 2, 2, 2, 2, 2, 2, 2, 2, 2, 2, 2, 2, 2, 2, 2, 2, 2, 2, 2, 2, 2, 2, 2, 2, 2, 2, 2, 2, 2, 2, 2, 2, 2, 2, 2, 2, 2, 2, 2, 2, 2, 2, 2, 2, 2, 2, 2, 2, 2, 2, 2, 2, 2, 2, 2, 2, 2, 2, 2, 2, 2, 2, 2, 2, 2, 2, 2, 2, 2, 2, 2, 2, 2, 2, 2, 2, 2, 2, 2, 2, 2, 2, 2, 2, 2, 2, 2, 2, 2, 2, 2, 2, 2, 2, 2, 2, 2, 2, 2, 2, 2, 2, 2, 2, 2, 2, 2, 2, 2, 2, 2, 2, 2, 2, 2, 2, 2, 2, 2, 2, 2, 2, 2, 2, 2, 3 ),
 ( 0.000000000000000000, 1.000000000000000000 ),
 ( 0.000000000000000000, 0.004166666666666666609, 0.008333333333333333218, 0.01250000000000000069, 0.01666666666666666644, 0.02083333333333333218, 0.02500000000000000139, 0.02916666666666666713, 0.03333333333333333287, 0.03749999999999999861, 0.04166666666666666435, 0.04583333333333333010, 0.05000000000000000278, 0.05416666666666666852, 0.05833333333333333426, 0.06250000000000000000, 0.06666666666666666574, 0.07083333333333333148, 0.07499999999999999722, 0.07916666666666666297, 0.08333333333333332871, 0.08749999999999999445, 0.09166666666666666019, 0.09583333333333333981, 0.1000000000000000056, 0.1041666666666666713, 0.1083333333333333370, 0.1125000000000000028, 0.1166666666666666685, 0.1208333333333333343, 0.1250000000000000000, 0.1291666666666666796, 0.1333333333333333315, 0.1375000000000000111, 0.1416666666666666630, 0.1458333333333333426, 0.1499999999999999944, 0.1541666666666666741, 0.1583333333333333259, 0.1625000000000000056, 0.1666666666666666574, 0.1708333333333333370, 0.1749999999999999889, 0.1791666666666666685, 0.1833333333333333204, 0.1875000000000000000, 0.1916666666666666796, 0.1958333333333333315, 0.2000000000000000111, 0.2041666666666666630, 0.2083333333333333426, 0.2124999999999999944, 0.2166666666666666741, 0.2208333333333333259, 0.2250000000000000056, 0.2291666666666666574, 0.2333333333333333370, 0.2374999999999999889, 0.2416666666666666685, 0.2458333333333333204, 0.2500000000000000000, 0.2541666666666666519, 0.2583333333333333592, 0.2625000000000000111, 0.2666666666666666630, 0.2708333333333333148, 0.2750000000000000222, 0.2791666666666666741, 0.2833333333333333259, 0.2874999999999999778, 0.2916666666666666852, 0.2958333333333333370, 0.2999999999999999889, 0.3041666666666666408, 0.3083333333333333481, 0.3125000000000000000, 0.3166666666666666519, 0.3208333333333333592, 0.3250000000000000111, 0.3291666666666666630, 0.3333333333333333148, 0.3375000000000000222, 0.3416666666666666741, 0.3458333333333333259, 0.3499999999999999778, 0.3541666666666666852, 0.3583333333333333370, 0.3624999999999999889, 0.3666666666666666408, 0.3708333333333333481, 0.3750000000000000000, 0.3791666666666666519, 0.3833333333333333592, 0.3875000000000000111, 0.3916666666666666630, 0.3958333333333333148, 0.4000000000000000222, 0.4041666666666666741, 0.4083333333333333259, 0.4124999999999999778, 0.4166666666666666852, 0.4208333333333333370, 0.4249999999999999889, 0.4291666666666666408, 0.4333333333333333481, 0.4375000000000000000, 0.4416666666666666519, 0.4458333333333333592, 0.4500000000000000111, 0.4541666666666666630, 0.4583333333333333148, 0.4625000000000000222, 0.4666666666666666741, 0.4708333333333333259, 0.4749999999999999778, 0.4791666666666666852, 0.4833333333333333370, 0.4874999999999999889, 0.4916666666666666408, 0.4958333333333333481, 0.5000000000000000000, 0.5041666666666666519, 0.5083333333333333037, 0.5124999999999999556, 0.5166666666666667185, 0.5208333333333333703, 0.5250000000000000222, 0.5291666666666666741, 0.5333333333333333259, 0.5374999999999999778, 0.5416666666666666297, 0.5458333333333332815, 0.5500000000000000444, 0.5541666666666666963, 0.5583333333333333481, 0.5625000000000000000, 0.5666666666666666519, 0.5708333333333333037, 0.5749999999999999556, 0.5791666666666667185, 0.5833333333333333703, 0.5875000000000000222, 0.5916666666666666741, 0.5958333333333333259, 0.5999999999999999778, 0.6041666666666666297, 0.6083333333333332815, 0.6125000000000000444, 0.6166666666666666963, 0.6208333333333333481, 0.6250000000000000000, 0.6291666666666666519, 0.6333333333333333037, 0.6374999999999999556, 0.6416666666666667185, 0.6458333333333333703, 0.6500000000000000222, 0.6541666666666666741, 0.6583333333333333259, 0.6624999999999999778, 0.6666666666666666297, 0.6708333333333332815, 0.6750000000000000444, 0.6791666666666666963, 0.6833333333333333481, 0.6875000000000000000, 0.6916666666666666519, 0.6958333333333333037, 0.6999999999999999556, 0.7041666666666667185, 0.7083333333333333703, 0.7125000000000000222, 0.7166666666666666741, 0.7208333333333333259, 0.7249999999999999778, 0.7291666666666666297, 0.7333333333333332815, 0.7375000000000000444, 0.7416666666666666963, 0.7458333333333333481, 0.7500000000000000000, 0.7541666666666666519, 0.7583333333333333037, 0.7624999999999999556, 0.7666666666666667185, 0.7708333333333333703, 0.7750000000000000222, 0.7791666666666666741, 0.7833333333333333259, 0.7874999999999999778, 0.7916666666666666297, 0.7958333333333332815, 0.8000000000000000444, 0.8041666666666666963, 0.8083333333333333481, 0.8125000000000000000, 0.8166666666666666519, 0.8208333333333333037, 0.8249999999999999556, 0.8291666666666667185, 0.8333333333333333703, 0.8375000000000000222, 0.8416666666666666741, 0.8458333333333333259, 0.8499999999999999778, 0.8541666666666666297, 0.8583333333333332815, 0.8625000000000000444, 0.8666666666666666963, 0.8708333333333333481, 0.8750000000000000000, 0.8791666666666666519, 0.8833333333333333037, 0.8874999999999999556, 0.8916666666666667185, 0.8958333333333333703, 0.9000000000000000222, 0.9041666666666666741, 0.9083333333333333259, 0.9124999999999999778, 0.9166666666666666297, 0.9208333333333332815, 0.9250000000000000444, 0.9291666666666666963, 0.9333333333333333481, 0.9375000000000000000, 0.9416666666666666519, 0.9458333333333333037, 0.9499999999999999556, 0.9541666666666667185, 0.9583333333333333703, 0.9625000000000000222, 0.9666666666666666741, 0.9708333333333333259, 0.9749999999999999778, 0.9791666666666666297, 0.9833333333333332815, 0.9875000000000000444, 0.9916666666666666963, 0.9958333333333333481, 1.000000000000000000 ),
 .UNSPECIFIED. ) 
 GEOMETRIC_REPRESENTATION_ITEM ( )  RATIONAL_B_SPLINE_SURFACE ( (
 ( 1.000000000000000000, 0.8660254037844387076, 1.000000000000000000, 0.8660254037844387076, 1.000000000000000000, 0.8660254037844387076, 1.000000000000000000, 0.8660254037844387076, 1.000000000000000000, 0.8660254037844387076, 1.000000000000000000, 0.8660254037844387076, 1.000000000000000000, 0.8660254037844387076, 1.000000000000000000, 0.8660254037844387076, 1.000000000000000000, 0.8660254037844387076, 1.000000000000000000, 0.8660254037844387076, 1.000000000000000000, 0.8660254037844387076, 1.000000000000000000, 0.8660254037844387076, 1.000000000000000000, 0.8660254037844387076, 1.000000000000000000, 0.8660254037844387076, 1.000000000000000000, 0.8660254037844387076, 1.000000000000000000, 0.8660254037844387076, 1.000000000000000000, 0.8660254037844387076, 1.000000000000000000, 0.8660254037844387076, 1.000000000000000000, 0.8660254037844387076, 1.000000000000000000, 0.8660254037844387076, 1.000000000000000000, 0.8660254037844387076, 1.000000000000000000, 0.8660254037844387076, 1.000000000000000000, 0.8660254037844387076, 1.000000000000000000, 0.8660254037844387076, 1.000000000000000000, 0.8660254037844387076, 1.000000000000000000, 0.8660254037844387076, 1.000000000000000000, 0.8660254037844387076, 1.000000000000000000, 0.8660254037844387076, 1.000000000000000000, 0.8660254037844387076, 1.000000000000000000, 0.8660254037844387076, 1.000000000000000000, 0.8660254037844387076, 1.000000000000000000, 0.8660254037844387076, 1.000000000000000000, 0.8660254037844387076, 1.000000000000000000, 0.8660254037844387076, 1.000000000000000000, 0.8660254037844387076, 1.000000000000000000, 0.8660254037844387076, 1.000000000000000000, 0.8660254037844387076, 1.000000000000000000, 0.8660254037844387076, 1.000000000000000000, 0.8660254037844387076, 1.000000000000000000, 0.8660254037844387076, 1.000000000000000000, 0.8660254037844387076, 1.000000000000000000, 0.8660254037844387076, 1.000000000000000000, 0.8660254037844387076, 1.000000000000000000, 0.8660254037844387076, 1.000000000000000000, 0.8660254037844387076, 1.000000000000000000, 0.8660254037844387076, 1.000000000000000000, 0.8660254037844387076, 1.000000000000000000, 0.8660254037844387076, 1.000000000000000000, 0.8660254037844387076, 1.000000000000000000, 0.8660254037844387076, 1.000000000000000000, 0.8660254037844387076, 1.000000000000000000, 0.8660254037844387076, 1.000000000000000000, 0.8660254037844387076, 1.000000000000000000, 0.8660254037844387076, 1.000000000000000000, 0.8660254037844387076, 1.000000000000000000, 0.8660254037844387076, 1.000000000000000000, 0.8660254037844387076, 1.000000000000000000, 0.8660254037844387076, 1.000000000000000000, 0.8660254037844387076, 1.000000000000000000, 0.8660254037844387076, 1.000000000000000000, 0.8660254037844387076, 1.000000000000000000, 0.8660254037844387076, 1.000000000000000000, 0.8660254037844387076, 1.000000000000000000, 0.8660254037844387076, 1.000000000000000000, 0.8660254037844387076, 1.000000000000000000, 0.8660254037844387076, 1.000000000000000000, 0.8660254037844387076, 1.000000000000000000, 0.8660254037844387076, 1.000000000000000000, 0.8660254037844387076, 1.000000000000000000, 0.8660254037844387076, 1.000000000000000000, 0.8660254037844387076, 1.000000000000000000, 0.8660254037844387076, 1.000000000000000000, 0.8660254037844387076, 1.000000000000000000, 0.8660254037844387076, 1.000000000000000000, 0.8660254037844387076, 1.000000000000000000, 0.8660254037844387076, 1.000000000000000000, 0.8660254037844387076, 1.000000000000000000, 0.8660254037844387076, 1.000000000000000000, 0.8660254037844387076, 1.000000000000000000, 0.8660254037844387076, 1.000000000000000000, 0.8660254037844387076, 1.000000000000000000, 0.8660254037844387076, 1.000000000000000000, 0.8660254037844387076, 1.000000000000000000, 0.8660254037844387076, 1.000000000000000000, 0.8660254037844387076, 1.000000000000000000, 0.8660254037844387076, 1.000000000000000000, 0.8660254037844387076, 1.000000000000000000, 0.8660254037844387076, 1.000000000000000000, 0.8660254037844387076, 1.000000000000000000, 0.8660254037844387076, 1.000000000000000000, 0.8660254037844387076, 1.000000000000000000, 0.8660254037844387076, 1.000000000000000000, 0.8660254037844387076, 1.000000000000000000, 0.8660254037844387076, 1.000000000000000000, 0.8660254037844387076, 1.000000000000000000, 0.8660254037844387076, 1.000000000000000000, 0.8660254037844387076, 1.000000000000000000, 0.8660254037844387076, 1.000000000000000000, 0.8660254037844387076, 1.000000000000000000, 0.8660254037844387076, 1.000000000000000000, 0.8660254037844387076, 1.000000000000000000, 0.8660254037844387076, 1.000000000000000000, 0.8660254037844387076, 1.000000000000000000, 0.8660254037844387076, 1.000000000000000000, 0.8660254037844387076, 1.000000000000000000, 0.8660254037844387076, 1.000000000000000000, 0.8660254037844387076, 1.000000000000000000, 0.8660254037844387076, 1.000000000000000000, 0.8660254037844387076, 1.000000000000000000, 0.8660254037844387076, 1.000000000000000000, 0.8660254037844387076, 1.000000000000000000, 0.8660254037844387076, 1.000000000000000000, 0.8660254037844387076, 1.000000000000000000, 0.8660254037844387076, 1.000000000000000000, 0.8660254037844387076, 1.000000000000000000, 0.8660254037844387076, 1.000000000000000000, 0.8660254037844387076, 1.000000000000000000, 0.8660254037844387076, 1.000000000000000000, 0.8660254037844387076, 1.000000000000000000, 0.8660254037844387076, 1.000000000000000000, 0.8660254037844387076, 1.000000000000000000, 0.8660254037844387076, 1.000000000000000000, 0.8660254037844387076, 1.000000000000000000, 0.8660254037844387076, 1.000000000000000000, 0.8660254037844387076, 1.000000000000000000, 0.8660254037844387076, 1.000000000000000000, 0.8660254037844387076, 1.000000000000000000, 0.8660254037844387076, 1.000000000000000000, 0.8660254037844387076, 1.000000000000000000, 0.8660254037844387076, 1.000000000000000000, 0.8660254037844387076, 1.000000000000000000, 0.8660254037844387076, 1.000000000000000000, 0.8660254037844387076, 1.000000000000000000, 0.8660254037844387076, 1.000000000000000000, 0.8660254037844387076, 1.000000000000000000, 0.8660254037844387076, 1.000000000000000000, 0.8660254037844387076, 1.000000000000000000, 0.8660254037844387076, 1.000000000000000000, 0.8660254037844387076, 1.000000000000000000, 0.8660254037844387076, 1.000000000000000000, 0.8660254037844387076, 1.000000000000000000, 0.8660254037844387076, 1.000000000000000000, 0.8660254037844387076, 1.000000000000000000, 0.8660254037844387076, 1.000000000000000000, 0.8660254037844387076, 1.000000000000000000, 0.8660254037844387076, 1.000000000000000000, 0.8660254037844387076, 1.000000000000000000, 0.8660254037844387076, 1.000000000000000000, 0.8660254037844387076, 1.000000000000000000, 0.8660254037844387076, 1.000000000000000000, 0.8660254037844387076, 1.000000000000000000, 0.8660254037844387076, 1.000000000000000000, 0.8660254037844387076, 1.000000000000000000, 0.8660254037844387076, 1.000000000000000000, 0.8660254037844387076, 1.000000000000000000, 0.8660254037844387076, 1.000000000000000000, 0.8660254037844387076, 1.000000000000000000, 0.8660254037844387076, 1.000000000000000000, 0.8660254037844387076, 1.000000000000000000, 0.8660254037844387076, 1.000000000000000000, 0.8660254037844387076, 1.000000000000000000, 0.8660254037844387076, 1.000000000000000000, 0.8660254037844387076, 1.000000000000000000, 0.8660254037844387076, 1.000000000000000000, 0.8660254037844387076, 1.000000000000000000, 0.8660254037844387076, 1.000000000000000000, 0.8660254037844387076, 1.000000000000000000, 0.8660254037844387076, 1.000000000000000000, 0.8660254037844387076, 1.000000000000000000, 0.8660254037844387076, 1.000000000000000000, 0.8660254037844387076, 1.000000000000000000, 0.8660254037844387076, 1.000000000000000000, 0.8660254037844387076, 1.000000000000000000, 0.8660254037844387076, 1.000000000000000000, 0.8660254037844387076, 1.000000000000000000, 0.8660254037844387076, 1.000000000000000000, 0.8660254037844387076, 1.000000000000000000, 0.8660254037844387076, 1.000000000000000000, 0.8660254037844387076, 1.000000000000000000, 0.8660254037844387076, 1.000000000000000000, 0.8660254037844387076, 1.000000000000000000, 0.8660254037844387076, 1.000000000000000000, 0.8660254037844387076, 1.000000000000000000, 0.8660254037844387076, 1.000000000000000000, 0.8660254037844387076, 1.000000000000000000, 0.8660254037844387076, 1.000000000000000000, 0.8660254037844387076, 1.000000000000000000, 0.8660254037844387076, 1.000000000000000000, 0.8660254037844387076, 1.000000000000000000, 0.8660254037844387076, 1.000000000000000000, 0.8660254037844387076, 1.000000000000000000, 0.8660254037844387076, 1.000000000000000000, 0.8660254037844387076, 1.000000000000000000, 0.8660254037844387076, 1.000000000000000000, 0.8660254037844387076, 1.000000000000000000, 0.8660254037844387076, 1.000000000000000000, 0.8660254037844387076, 1.000000000000000000, 0.8660254037844387076, 1.000000000000000000, 0.8660254037844387076, 1.000000000000000000, 0.8660254037844387076, 1.000000000000000000, 0.8660254037844387076, 1.000000000000000000, 0.8660254037844387076, 1.000000000000000000, 0.8660254037844387076, 1.000000000000000000, 0.8660254037844387076, 1.000000000000000000, 0.8660254037844387076, 1.000000000000000000, 0.8660254037844387076, 1.000000000000000000, 0.8660254037844387076, 1.000000000000000000, 0.8660254037844387076, 1.000000000000000000, 0.8660254037844387076, 1.000000000000000000, 0.8660254037844387076, 1.000000000000000000, 0.8660254037844387076, 1.000000000000000000, 0.8660254037844387076, 1.000000000000000000, 0.8660254037844387076, 1.000000000000000000, 0.8660254037844387076, 1.000000000000000000, 0.8660254037844387076, 1.000000000000000000, 0.8660254037844387076, 1.000000000000000000, 0.8660254037844387076, 1.000000000000000000, 0.8660254037844387076, 1.000000000000000000, 0.8660254037844387076, 1.000000000000000000, 0.8660254037844387076, 1.000000000000000000, 0.8660254037844387076, 1.000000000000000000, 0.8660254037844387076, 1.000000000000000000, 0.8660254037844387076, 1.000000000000000000, 0.8660254037844387076, 1.000000000000000000, 0.8660254037844387076, 1.000000000000000000, 0.8660254037844387076, 1.000000000000000000, 0.8660254037844387076, 1.000000000000000000, 0.8660254037844387076, 1.000000000000000000, 0.8660254037844387076, 1.000000000000000000, 0.8660254037844387076, 1.000000000000000000, 0.8660254037844387076, 1.000000000000000000, 0.8660254037844387076, 1.000000000000000000, 0.8660254037844387076, 1.000000000000000000, 0.8660254037844387076, 1.000000000000000000, 0.8660254037844387076, 1.000000000000000000, 0.8660254037844387076, 1.000000000000000000, 0.8660254037844387076, 1.000000000000000000, 0.8660254037844387076, 1.000000000000000000, 0.8660254037844387076, 1.000000000000000000, 0.8660254037844387076, 1.000000000000000000),
 ( 1.000000000000000000, 0.8660254037844387076, 1.000000000000000000, 0.8660254037844387076, 1.000000000000000000, 0.8660254037844387076, 1.000000000000000000, 0.8660254037844387076, 1.000000000000000000, 0.8660254037844387076, 1.000000000000000000, 0.8660254037844387076, 1.000000000000000000, 0.8660254037844387076, 1.000000000000000000, 0.8660254037844387076, 1.000000000000000000, 0.8660254037844387076, 1.000000000000000000, 0.8660254037844387076, 1.000000000000000000, 0.8660254037844387076, 1.000000000000000000, 0.8660254037844387076, 1.000000000000000000, 0.8660254037844387076, 1.000000000000000000, 0.8660254037844387076, 1.000000000000000000, 0.8660254037844387076, 1.000000000000000000, 0.8660254037844387076, 1.000000000000000000, 0.8660254037844387076, 1.000000000000000000, 0.8660254037844387076, 1.000000000000000000, 0.8660254037844387076, 1.000000000000000000, 0.8660254037844387076, 1.000000000000000000, 0.8660254037844387076, 1.000000000000000000, 0.8660254037844387076, 1.000000000000000000, 0.8660254037844387076, 1.000000000000000000, 0.8660254037844387076, 1.000000000000000000, 0.8660254037844387076, 1.000000000000000000, 0.8660254037844387076, 1.000000000000000000, 0.8660254037844387076, 1.000000000000000000, 0.8660254037844387076, 1.000000000000000000, 0.8660254037844387076, 1.000000000000000000, 0.8660254037844387076, 1.000000000000000000, 0.8660254037844387076, 1.000000000000000000, 0.8660254037844387076, 1.000000000000000000, 0.8660254037844387076, 1.000000000000000000, 0.8660254037844387076, 1.000000000000000000, 0.8660254037844387076, 1.000000000000000000, 0.8660254037844387076, 1.000000000000000000, 0.8660254037844387076, 1.000000000000000000, 0.8660254037844387076, 1.000000000000000000, 0.8660254037844387076, 1.000000000000000000, 0.8660254037844387076, 1.000000000000000000, 0.8660254037844387076, 1.000000000000000000, 0.8660254037844387076, 1.000000000000000000, 0.8660254037844387076, 1.000000000000000000, 0.8660254037844387076, 1.000000000000000000, 0.8660254037844387076, 1.000000000000000000, 0.8660254037844387076, 1.000000000000000000, 0.8660254037844387076, 1.000000000000000000, 0.8660254037844387076, 1.000000000000000000, 0.8660254037844387076, 1.000000000000000000, 0.8660254037844387076, 1.000000000000000000, 0.8660254037844387076, 1.000000000000000000, 0.8660254037844387076, 1.000000000000000000, 0.8660254037844387076, 1.000000000000000000, 0.8660254037844387076, 1.000000000000000000, 0.8660254037844387076, 1.000000000000000000, 0.8660254037844387076, 1.000000000000000000, 0.8660254037844387076, 1.000000000000000000, 0.8660254037844387076, 1.000000000000000000, 0.8660254037844387076, 1.000000000000000000, 0.8660254037844387076, 1.000000000000000000, 0.8660254037844387076, 1.000000000000000000, 0.8660254037844387076, 1.000000000000000000, 0.8660254037844387076, 1.000000000000000000, 0.8660254037844387076, 1.000000000000000000, 0.8660254037844387076, 1.000000000000000000, 0.8660254037844387076, 1.000000000000000000, 0.8660254037844387076, 1.000000000000000000, 0.8660254037844387076, 1.000000000000000000, 0.8660254037844387076, 1.000000000000000000, 0.8660254037844387076, 1.000000000000000000, 0.8660254037844387076, 1.000000000000000000, 0.8660254037844387076, 1.000000000000000000, 0.8660254037844387076, 1.000000000000000000, 0.8660254037844387076, 1.000000000000000000, 0.8660254037844387076, 1.000000000000000000, 0.8660254037844387076, 1.000000000000000000, 0.8660254037844387076, 1.000000000000000000, 0.8660254037844387076, 1.000000000000000000, 0.8660254037844387076, 1.000000000000000000, 0.8660254037844387076, 1.000000000000000000, 0.8660254037844387076, 1.000000000000000000, 0.8660254037844387076, 1.000000000000000000, 0.8660254037844387076, 1.000000000000000000, 0.8660254037844387076, 1.000000000000000000, 0.8660254037844387076, 1.000000000000000000, 0.8660254037844387076, 1.000000000000000000, 0.8660254037844387076, 1.000000000000000000, 0.8660254037844387076, 1.000000000000000000, 0.8660254037844387076, 1.000000000000000000, 0.8660254037844387076, 1.000000000000000000, 0.8660254037844387076, 1.000000000000000000, 0.8660254037844387076, 1.000000000000000000, 0.8660254037844387076, 1.000000000000000000, 0.8660254037844387076, 1.000000000000000000, 0.8660254037844387076, 1.000000000000000000, 0.8660254037844387076, 1.000000000000000000, 0.8660254037844387076, 1.000000000000000000, 0.8660254037844387076, 1.000000000000000000, 0.8660254037844387076, 1.000000000000000000, 0.8660254037844387076, 1.000000000000000000, 0.8660254037844387076, 1.000000000000000000, 0.8660254037844387076, 1.000000000000000000, 0.8660254037844387076, 1.000000000000000000, 0.8660254037844387076, 1.000000000000000000, 0.8660254037844387076, 1.000000000000000000, 0.8660254037844387076, 1.000000000000000000, 0.8660254037844387076, 1.000000000000000000, 0.8660254037844387076, 1.000000000000000000, 0.8660254037844387076, 1.000000000000000000, 0.8660254037844387076, 1.000000000000000000, 0.8660254037844387076, 1.000000000000000000, 0.8660254037844387076, 1.000000000000000000, 0.8660254037844387076, 1.000000000000000000, 0.8660254037844387076, 1.000000000000000000, 0.8660254037844387076, 1.000000000000000000, 0.8660254037844387076, 1.000000000000000000, 0.8660254037844387076, 1.000000000000000000, 0.8660254037844387076, 1.000000000000000000, 0.8660254037844387076, 1.000000000000000000, 0.8660254037844387076, 1.000000000000000000, 0.8660254037844387076, 1.000000000000000000, 0.8660254037844387076, 1.000000000000000000, 0.8660254037844387076, 1.000000000000000000, 0.8660254037844387076, 1.000000000000000000, 0.8660254037844387076, 1.000000000000000000, 0.8660254037844387076, 1.000000000000000000, 0.8660254037844387076, 1.000000000000000000, 0.8660254037844387076, 1.000000000000000000, 0.8660254037844387076, 1.000000000000000000, 0.8660254037844387076, 1.000000000000000000, 0.8660254037844387076, 1.000000000000000000, 0.8660254037844387076, 1.000000000000000000, 0.8660254037844387076, 1.000000000000000000, 0.8660254037844387076, 1.000000000000000000, 0.8660254037844387076, 1.000000000000000000, 0.8660254037844387076, 1.000000000000000000, 0.8660254037844387076, 1.000000000000000000, 0.8660254037844387076, 1.000000000000000000, 0.8660254037844387076, 1.000000000000000000, 0.8660254037844387076, 1.000000000000000000, 0.8660254037844387076, 1.000000000000000000, 0.8660254037844387076, 1.000000000000000000, 0.8660254037844387076, 1.000000000000000000, 0.8660254037844387076, 1.000000000000000000, 0.8660254037844387076, 1.000000000000000000, 0.8660254037844387076, 1.000000000000000000, 0.8660254037844387076, 1.000000000000000000, 0.8660254037844387076, 1.000000000000000000, 0.8660254037844387076, 1.000000000000000000, 0.8660254037844387076, 1.000000000000000000, 0.8660254037844387076, 1.000000000000000000, 0.8660254037844387076, 1.000000000000000000, 0.8660254037844387076, 1.000000000000000000, 0.8660254037844387076, 1.000000000000000000, 0.8660254037844387076, 1.000000000000000000, 0.8660254037844387076, 1.000000000000000000, 0.8660254037844387076, 1.000000000000000000, 0.8660254037844387076, 1.000000000000000000, 0.8660254037844387076, 1.000000000000000000, 0.8660254037844387076, 1.000000000000000000, 0.8660254037844387076, 1.000000000000000000, 0.8660254037844387076, 1.000000000000000000, 0.8660254037844387076, 1.000000000000000000, 0.8660254037844387076, 1.000000000000000000, 0.8660254037844387076, 1.000000000000000000, 0.8660254037844387076, 1.000000000000000000, 0.8660254037844387076, 1.000000000000000000, 0.8660254037844387076, 1.000000000000000000, 0.8660254037844387076, 1.000000000000000000, 0.8660254037844387076, 1.000000000000000000, 0.8660254037844387076, 1.000000000000000000, 0.8660254037844387076, 1.000000000000000000, 0.8660254037844387076, 1.000000000000000000, 0.8660254037844387076, 1.000000000000000000, 0.8660254037844387076, 1.000000000000000000, 0.8660254037844387076, 1.000000000000000000, 0.8660254037844387076, 1.000000000000000000, 0.8660254037844387076, 1.000000000000000000, 0.8660254037844387076, 1.000000000000000000, 0.8660254037844387076, 1.000000000000000000, 0.8660254037844387076, 1.000000000000000000, 0.8660254037844387076, 1.000000000000000000, 0.8660254037844387076, 1.000000000000000000, 0.8660254037844387076, 1.000000000000000000, 0.8660254037844387076, 1.000000000000000000, 0.8660254037844387076, 1.000000000000000000, 0.8660254037844387076, 1.000000000000000000, 0.8660254037844387076, 1.000000000000000000, 0.8660254037844387076, 1.000000000000000000, 0.8660254037844387076, 1.000000000000000000, 0.8660254037844387076, 1.000000000000000000, 0.8660254037844387076, 1.000000000000000000, 0.8660254037844387076, 1.000000000000000000, 0.8660254037844387076, 1.000000000000000000, 0.8660254037844387076, 1.000000000000000000, 0.8660254037844387076, 1.000000000000000000, 0.8660254037844387076, 1.000000000000000000, 0.8660254037844387076, 1.000000000000000000, 0.8660254037844387076, 1.000000000000000000, 0.8660254037844387076, 1.000000000000000000, 0.8660254037844387076, 1.000000000000000000, 0.8660254037844387076, 1.000000000000000000, 0.8660254037844387076, 1.000000000000000000, 0.8660254037844387076, 1.000000000000000000, 0.8660254037844387076, 1.000000000000000000, 0.8660254037844387076, 1.000000000000000000, 0.8660254037844387076, 1.000000000000000000, 0.8660254037844387076, 1.000000000000000000, 0.8660254037844387076, 1.000000000000000000, 0.8660254037844387076, 1.000000000000000000, 0.8660254037844387076, 1.000000000000000000, 0.8660254037844387076, 1.000000000000000000, 0.8660254037844387076, 1.000000000000000000, 0.8660254037844387076, 1.000000000000000000, 0.8660254037844387076, 1.000000000000000000, 0.8660254037844387076, 1.000000000000000000, 0.8660254037844387076, 1.000000000000000000, 0.8660254037844387076, 1.000000000000000000, 0.8660254037844387076, 1.000000000000000000, 0.8660254037844387076, 1.000000000000000000, 0.8660254037844387076, 1.000000000000000000, 0.8660254037844387076, 1.000000000000000000, 0.8660254037844387076, 1.000000000000000000, 0.8660254037844387076, 1.000000000000000000, 0.8660254037844387076, 1.000000000000000000, 0.8660254037844387076, 1.000000000000000000, 0.8660254037844387076, 1.000000000000000000, 0.8660254037844387076, 1.000000000000000000, 0.8660254037844387076, 1.000000000000000000, 0.8660254037844387076, 1.000000000000000000, 0.8660254037844387076, 1.000000000000000000, 0.8660254037844387076, 1.000000000000000000, 0.8660254037844387076, 1.000000000000000000, 0.8660254037844387076, 1.000000000000000000, 0.8660254037844387076, 1.000000000000000000, 0.8660254037844387076, 1.000000000000000000, 0.8660254037844387076, 1.000000000000000000, 0.8660254037844387076, 1.000000000000000000, 0.8660254037844387076, 1.000000000000000000, 0.8660254037844387076, 1.000000000000000000) ) ) 
 REPRESENTATION_ITEM ( '' )  SURFACE ( )  );
#58895=ORIENTED_EDGE ( 'NONE', *, *, #171975, .F. ) ;
#58901=ORIENTED_EDGE ( 'NONE', *, *, #22449, .T. ) ;
#58913=CARTESIAN_POINT ( 'NONE',  ( -7.074657228232555717, 7.148188275893099686, 1.040834085586084257E-14 ) ) ;
#58916=CARTESIAN_POINT ( 'NONE',  ( 6.972971076130050072, 7.029554431773520129, 1.040834085586084257E-14 ) ) ;
#58923=CARTESIAN_POINT ( 'NONE',  ( -5.251085567194491155, 5.020688004682002159, -0.7998128361456221525 ) ) ;
#58926=CARTESIAN_POINT ( 'NONE',  ( 8.263858322729371153, 9.599921783727809910, -1.199719254218446718 ) ) ;
#58928=EDGE_CURVE ( 'NONE', #178928, #48080, #36260, .T. ) ;
#58930=CARTESIAN_POINT ( 'NONE',  ( 6.095406204355903412, 6.027892130464396203, -0.2603320317973931153 ) ) ;
#58937=CARTESIAN_POINT ( 'NONE',  ( 6.819388077549422889, 8.018669514304889390, -1.082531754730543971 ) ) ;
#58938=CARTESIAN_POINT ( 'NONE',  ( -7.049349804101573191, 10.31165964050546258, -1.199719254218440723 ) ) ;
#58941=CARTESIAN_POINT ( 'NONE',  ( -7.472515219426274946, 11.86968485597268064, 0.000000000000000000 ) ) ;
#58942=CARTESIAN_POINT ( 'NONE',  ( -5.982172092127739482, 8.002286745614243912, -1.599625672291263179 ) ) ;
#58949=CARTESIAN_POINT ( 'NONE',  ( 7.239163954692881653, 10.53310948286200599, -1.199719254218441611 ) ) ;
#58960=CARTESIAN_POINT ( 'NONE',  ( -0.1505076982584017398, 7.030243935902841912, -1.995512553310450521 ) ) ;
#58965=CARTESIAN_POINT ( 'NONE',  ( -0.7499999999999972244, 4.858333333333353821, -1.299038105676652011 ) ) ;
#58966=CARTESIAN_POINT ( 'NONE',  ( 5.172599298813543633, 5.993452922492633839, -1.199719254218452047 ) ) ;
#58967=CARTESIAN_POINT ( 'NONE',  ( 6.714312387265682247, 8.856450423275211037, 1.599625672291281386 ) ) ;
#58970=CARTESIAN_POINT ( 'NONE',  ( 7.646435448427411963, 8.023188899361205273, -0.7216878364870257245 ) ) ;
#58971=CARTESIAN_POINT ( 'NONE',  ( -10.12757755928392456, 10.91785469536048758, 0.7216878364870438212 ) ) ;
#58974=CARTESIAN_POINT ( 'NONE',  ( 7.781490099239519509, 11.16582331816642260, 1.199719254218460707 ) ) ;
#58979=CARTESIAN_POINT ( 'NONE',  ( -0.6823417656250246877, 0.5510416670080897639, 1.181850606188755259 ) ) ;
#58984=CARTESIAN_POINT ( 'NONE',  ( -1.402160292154681736E-14, -0.05312499965857903073, -1.575800808251665908 ) ) ;
#58986=CARTESIAN_POINT ( 'NONE',  ( 8.550388431712704573, 13.12720360364021133, 0.000000000000000000 ) ) ;
#58990=CARTESIAN_POINT ( 'NONE',  ( -9.130526383799315582, 12.73969898348616070, 1.199719254218462483 ) ) ;
#58996=CARTESIAN_POINT ( 'NONE',  ( 3.493197133815315603, 7.227147089426516402, -0.7998128361456291469 ) ) ;
#59002=CARTESIAN_POINT ( 'NONE',  ( 9.043452155515161905, 10.50944792197790889, 1.199719254218453823 ) ) ;
#59005=CARTESIAN_POINT ( 'NONE',  ( -5.088387723830502196, 4.830873854090670605, -0.7998128361456221525 ) ) ;
#59009=CARTESIAN_POINT ( 'NONE',  ( 8.911787042884274257, 9.291506392986812912, 0.7998128361456462443 ) ) ;
#59011=CARTESIAN_POINT ( 'NONE',  ( 6.938021921891177612, 9.117444880338284818, -1.599625672291262513 ) ) ;
#59013=CARTESIAN_POINT ( 'NONE',  ( -9.490344339885981029, 10.17441593939621924, -0.7216878364870267237 ) ) ;
#59020=CARTESIAN_POINT ( 'NONE',  ( -5.732528328060045197, 6.256990841418501148, 1.080875701640615638 ) ) ;
#59021=CARTESIAN_POINT ( 'NONE',  ( -1.364683531250014514, 1.988541667008086655, -0.7879004041258289570 ) ) ;
#59023=CARTESIAN_POINT ( 'NONE',  ( 5.165293337126522388, 8.969999960048859577, 1.040834085586084257E-14 ) ) ;
#59039=CARTESIAN_POINT ( 'NONE',  ( 9.772729797352075920, 10.29593960653257234, -0.7998128361456281477 ) ) ;
#59041=ORIENTED_EDGE ( 'NONE', *, *, #95883, .T. ) ;
#59043=CARTESIAN_POINT ( 'NONE',  ( -2.625475302540713152, 6.214804952939456228, -0.7998128361456281477 ) ) ;
#59044=CARTESIAN_POINT ( 'NONE',  ( -6.989391883044787868, 8.113044270762433285, -1.199719254218446718 ) ) ;
#59050=CARTESIAN_POINT ( 'NONE',  ( -0.7500000000000215383, 4.972916667349482012, 1.299038105676671107 ) ) ;
#59051=CARTESIAN_POINT ( 'NONE',  ( 7.344766530301147789, 9.591980256816594164, 1.599625672291281386 ) ) ;
#59055=CARTESIAN_POINT ( 'NONE',  ( -8.376239975144482486, 8.666701480623698828, 1.040834085586084257E-14 ) ) ;
#59057=CARTESIAN_POINT ( 'NONE',  ( -1.001543065824772872E-14, 5.071875000341421469, 1.575800808251672791 ) ) ;
#59063=CARTESIAN_POINT ( 'NONE',  ( -8.853111120043687166, 9.430977182913531820, 1.040834085586084257E-14 ) ) ;
#59067=CARTESIAN_POINT ( 'NONE',  ( -1.364683531249997417, 2.571875000341422357, 1.214306433183764966E-14 ) ) ;
#59075=CARTESIAN_POINT ( 'NONE',  ( -1.364683531250012516, 4.238541667008090208, -0.7879004041258300672 ) ) ;
#59076=CARTESIAN_POINT ( 'NONE',  ( -5.596818484342970912, 5.424043074688562172, -0.7998128361456221525 ) ) ;
#59077=CARTESIAN_POINT ( 'NONE',  ( 6.419949431270806528, 7.448694743692793274, 1.199719254218462483 ) ) ;
#59080=CARTESIAN_POINT ( 'NONE',  ( 0.6823417656249899377, 4.488541667008086655, -1.181850606188754593 ) ) ;
#59085=CARTESIAN_POINT ( 'NONE',  ( 1.364683531249986537, 0.1135416670080857532, 0.7879004041258500513 ) ) ;
#59086=CARTESIAN_POINT ( 'NONE',  ( -3.443407828190963915, 6.961133532957338943, 0.7216878364870317197 ) ) ;
#59087=CARTESIAN_POINT ( 'NONE',  ( 6.634017235788401301, 6.634108284708264414, 0.7998128361456341429 ) ) ;
#59091=CARTESIAN_POINT ( 'NONE',  ( 3.931501358282940117, 4.649468341827285300, -1.082531754730543083 ) ) ;
#59094=CARTESIAN_POINT ( 'NONE',  ( -9.327646496521989405, 10.94497100310623594, -1.082531754730539753 ) ) ;
#59099=CARTESIAN_POINT ( 'NONE',  ( -10.62011439820619429, 11.28455497419572318, -0.7998128361456221525 ) ) ;
#59100=CARTESIAN_POINT ( 'NONE',  ( -5.300874872818844175, 7.207439989753867238, 1.443375672974064550 ) ) ;
#59102=CARTESIAN_POINT ( 'NONE',  ( 0.6823417656249882723, 0.4052083336747516751, 1.181850606188755259 ) ) ;
#59115=CARTESIAN_POINT ( 'NONE',  ( 0.7499999999999867883, -0.6833333333333135862, -1.299038105676652899 ) ) ;
#59117=CARTESIAN_POINT ( 'NONE',  ( 8.893785580440313865, 9.478430720042945623, 1.040834085586084257E-14 ) ) ;
#59123=VERTEX_POINT ( 'NONE', #72459 ) ;
#59125=CARTESIAN_POINT ( 'NONE',  ( 5.217190183160311356, 4.981143389975473568, -0.7998128361456211532 ) ) ;
#59130=CARTESIAN_POINT ( 'NONE',  ( 1.364683531249986537, 2.217708333674751398, -0.7879004041258239610 ) ) ;
#59141=VERTEX_POINT ( 'NONE', #23714 ) ;
#59150=CARTESIAN_POINT ( 'NONE',  ( 5.361359679200154105, 8.342337828120466980, 1.199719254218462483 ) ) ;
#59157=CARTESIAN_POINT ( 'NONE',  ( 8.609591239877852686, 10.00327685373437347, -1.199719254218445830 ) ) ;
#59160=CARTESIAN_POINT ( 'NONE',  ( 9.908311333488716954, 10.45411806535867782, 0.7998128361456462443 ) ) ;
#59162=CARTESIAN_POINT ( 'NONE',  ( -3.015033485013444370, 6.452462698123035523, 0.6092158896764710008 ) ) ;
#59170=CARTESIAN_POINT ( 'NONE',  ( -8.676855123066019360, 11.14608361504227574, -1.443375672974059665 ) ) ;
#59177=EDGE_CURVE ( 'NONE', #110911, #67678, #10851, .T. ) ;
#59185=CARTESIAN_POINT ( 'NONE',  ( 4.216222583725566686, 4.981643104843690217, -1.082531754730548412 ) ) ;
#59193=CARTESIAN_POINT ( 'NONE',  ( -4.394814349124112951, 8.279033840620114049, -0.7998128361456281477 ) ) ;
#59194=CARTESIAN_POINT ( 'NONE',  ( -3.972702704004144714, 4.593573561881607148, 1.199719254218462483 ) ) ;
#59195=DIRECTION ( 'NONE',  ( -5.578564026256490882E-16, -1.000000000000000000, -9.066213480720158442E-32 ) ) ;
#59200=CARTESIAN_POINT ( 'NONE',  ( 1.364683531249988535, 4.426041667008082214, 0.7879004041258499402 ) ) ;
#59202=CARTESIAN_POINT ( 'NONE',  ( 5.443762371086860341, 6.309809840144842141, 1.199719254218462483 ) ) ;
#59204=CARTESIAN_POINT ( 'NONE',  ( 1.507330767849599962, 8.672482115169971806, 2.545833800658963142 ) ) ;
#59215=CARTESIAN_POINT ( 'NONE',  ( -0.6823417656250212460, 1.363541667008083547, 1.181850606188755259 ) ) ;
#59216=CARTESIAN_POINT ( 'NONE',  ( 6.518203450479836292, 5.167241622962441383, 2.437504649502901355 ) ) ;
#59217=CARTESIAN_POINT ( 'NONE',  ( 2.869522067586683711, 6.499526178826442013, 0.7998128361456362523 ) ) ;
#59219=CARTESIAN_POINT ( 'NONE',  ( -5.585596099150182958, 8.499983968108443477, -1.082531754730544860 ) ) ;
#59220=CARTESIAN_POINT ( 'NONE',  ( 3.226477370372293763, 6.708047998835573900, 0.7216878364870317197 ) ) ;
#59221=CARTESIAN_POINT ( 'NONE',  ( -7.009202228140755331, 8.240119356661432803, -1.082531754730543083 ) ) ;
#59225=CARTESIAN_POINT ( 'NONE',  ( 6.986529229743720926, 7.045372277656132276, -0.7998128361456281477 ) ) ;
#59230=CARTESIAN_POINT ( 'NONE',  ( -1.364683531250010295, 5.280208333674758059, 0.7879004041258379498 ) ) ;
#59234=CARTESIAN_POINT ( 'NONE',  ( 5.120175567455225618, 9.125288595339771547, -0.7998128361456281477 ) ) ;
#59237=CARTESIAN_POINT ( 'NONE',  ( -8.064402442030170093, 8.302891025323665630, 0.7998128361456602331 ) ) ;
#59243=CARTESIAN_POINT ( 'NONE',  ( 9.426996880203592610, 9.892584536526015881, -0.7998128361456281477 ) ) ;
#59245=CARTESIAN_POINT ( 'NONE',  ( -8.148614017013223076, 9.465470093725620870, -1.199719254218446718 ) ) ;
#59247=CARTESIAN_POINT ( 'NONE',  ( 7.659993601596707613, 9.959745173328078849, -1.443375672974058777 ) ) ;
#59248=CARTESIAN_POINT ( 'NONE',  ( 4.035592002476674267, 7.779268892024251869, 0.4218195438757850191 ) ) ;
#59249=CARTESIAN_POINT ( 'NONE',  ( -6.261168011412601153, 6.199117522936475666, 1.040834085586084257E-14 ) ) ;
#59254=CARTESIAN_POINT ( 'NONE',  ( 5.443762371086860341, 6.309809840144842141, 1.199719254218462483 ) ) ;
#59256=CARTESIAN_POINT ( 'NONE',  ( 9.836604141914616406, 11.43479190611061647, 1.199719254218452047 ) ) ;
#59257=CARTESIAN_POINT ( 'NONE',  ( -4.868194452378435955, 6.719997196398590056, 1.250117667640719077 ) ) ;
#59259=CARTESIAN_POINT ( 'NONE',  ( -1.402160292154681736E-14, 0.4468750003414233563, -1.575800808251665908 ) ) ;
#59262=CARTESIAN_POINT ( 'NONE',  ( -6.738039156311804945, 6.963393225226301553, 1.040834085586084257E-14 ) ) ;
#59271=CARTESIAN_POINT ( 'NONE',  ( -5.901816349531303629, 6.006251404816039141, -0.1731548415426099052 ) ) ;
#59272=CARTESIAN_POINT ( 'NONE',  ( -1.364683531250012516, 0.8427083336747532849, 0.7879004041258379498 ) ) ;
#59275=CARTESIAN_POINT ( 'NONE',  ( 4.690757960648234359, 4.574898496952131133, 0.7216878364870317197 ) ) ;
#59279=CARTESIAN_POINT ( 'NONE',  ( -7.334597914868722590, 11.50085530074811935, -0.7216878364870267237 ) ) ;
#59287=CARTESIAN_POINT ( 'NONE',  ( -7.971831134711019118, 12.24429405723079967, 0.000000000000000000 ) ) ;
#59289=EDGE_LOOP ( 'NONE', ( #129581, #211528, #175477 ) ) ;
#59294=CARTESIAN_POINT ( 'NONE',  ( -8.039621902779392926, 9.442275643739831636, 1.082531754730558626 ) ) ;
#59300=CARTESIAN_POINT ( 'NONE',  ( -1.201851678989727383E-14, 4.618750000682821266, -1.732050807568863648 ) ) ;
#59301=CARTESIAN_POINT ( 'NONE',  ( 4.254006295369892499, 7.509857431501010261, -1.008242097476583554 ) ) ;
#59303=CARTESIAN_POINT ( 'NONE',  ( -1.436838838544729491, 7.449283400311743186, -4.203727439823575551 ) ) ;
#59308=CARTESIAN_POINT ( 'NONE',  ( -6.181627972826976958, 9.299317504018391745, 1.199719254218452047 ) ) ;
#59312=CARTESIAN_POINT ( 'NONE',  ( 4.527533231959700366, 7.369540306339926516, 1.199719254218462483 ) ) ;
#59313=EDGE_CURVE ( 'NONE', #42674, #177025, #33585, .T. ) ;
#59319=CARTESIAN_POINT ( 'NONE',  ( 6.877010230629674759, 9.046264573866535486, 1.599625672291281386 ) ) ;
#59323=ORIENTED_EDGE ( 'NONE', *, *, #1599, .F. ) ;
#59326=CARTESIAN_POINT ( 'NONE',  ( -5.260200412422208593, 7.159986452624450770, -1.443375672974053447 ) ) ;
#59334=CARTESIAN_POINT ( 'NONE',  ( 4.017000712418451691, 7.784014420058316119, -0.3037147205706329789 ) ) ;
#59338=CARTESIAN_POINT ( 'NONE',  ( -7.991641480251377772, 11.41099992934688956, 1.199719254218453823 ) ) ;
#59340=CARTESIAN_POINT ( 'NONE',  ( 9.108380270282433244, 9.520865158284665952, 1.040834085586084257E-14 ) ) ;
#59341=CARTESIAN_POINT ( 'NONE',  ( -1.402160292154681736E-14, 0.08750000000001964540, -1.732050807568870754 ) ) ;
#59342=CARTESIAN_POINT ( 'NONE',  ( -8.474009703741204547, 9.845098394908269768, -1.199719254218446718 ) ) ;
#59345=CARTESIAN_POINT ( 'NONE',  ( 1.364683531249990311, 5.363541667008086655, 0.7879004041258500513 ) ) ;
#59346=CARTESIAN_POINT ( 'NONE',  ( 9.598809568795314107, 10.30095870645710754, -0.7216878364870257245 ) ) ;
#59348=CARTESIAN_POINT ( 'NONE',  ( -1.001543065824772872E-14, 5.712500000000021672, 1.732050807568877637 ) ) ;
#59350=CARTESIAN_POINT ( 'NONE',  ( 7.226132685959389512, 11.37431253368722750, -0.7216878364870267237 ) ) ;
#59353=CARTESIAN_POINT ( 'NONE',  ( -5.910991785878170646, 7.919243054989755670, -1.443375672974059665 ) ) ;
#59355=CARTESIAN_POINT ( 'NONE',  ( 1.364683531249986537, 1.405208333674755838, -0.7879004041258239610 ) ) ;
#59359=CARTESIAN_POINT ( 'NONE',  ( -5.910464900553636269, 8.982960586366182554, -1.199719254218440723 ) ) ;
#59361=CARTESIAN_POINT ( 'NONE',  ( -1.364683531249997417, 5.071875000341417916, 1.214306433183764966E-14 ) ) ;
#59363=CIRCLE ( 'NONE', #190772, 0.08000000000000012657 ) ;
#59368=CARTESIAN_POINT ( 'NONE',  ( 10.23370702021670020, 10.83374636654133383, 0.7998128361456462443 ) ) ;
#59371=CARTESIAN_POINT ( 'NONE',  ( 1.499999999999987121, 1.754166666666691521, 0.8660254037844524744 ) ) ;
#59376=CARTESIAN_POINT ( 'NONE',  ( 7.456621297836078632, 8.762108271306003004, 1.082531754730558626 ) ) ;
#59378=CARTESIAN_POINT ( 'NONE',  ( 10.09812548408005384, 10.67556790771522124, -0.7998128361456281477 ) ) ;
#59383=CARTESIAN_POINT ( 'NONE',  ( 8.860417081730671995, 10.29590700256267155, 1.199719254218453823 ) ) ;
#59384=CARTESIAN_POINT ( 'NONE',  ( -9.236128959407555072, 11.79856975744075598, -1.599625672291263179 ) ) ;
#59387=CARTESIAN_POINT ( 'NONE',  ( -0.6823417656249969321, 5.780208333674756283, -1.181850606188749264 ) ) ;
#59391=CARTESIAN_POINT ( 'NONE',  ( -3.975492009593180942, 7.849578277493553635, 0.1138384667214070584 ) ) ;
#59394=CARTESIAN_POINT ( 'NONE',  ( -0.6823417656250212460, 4.301041667008085767, 1.181850606188767472 ) ) ;
#59396=CARTESIAN_POINT ( 'NONE',  ( -5.748293942514172805, 8.689798118699771479, -1.082531754730538864 ) ) ;
#59402=CARTESIAN_POINT ( 'NONE',  ( 3.083589872104280705, 5.684939719841914929, 1.199719254218450271 ) ) ;
#59405=CARTESIAN_POINT ( 'NONE',  ( 7.404724451357931336, 11.79059562655963056, 0.7998128361456462443 ) ) ;
#59406=CARTESIAN_POINT ( 'NONE',  ( 2.065088895208815334, 8.523968132013772347, -2.459875961809442124 ) ) ;
#59411=CARTESIAN_POINT ( 'NONE',  ( -7.309817376062285099, 11.67987070538135264, 0.000000000000000000 ) ) ;
#59412=CARTESIAN_POINT ( 'NONE',  ( 6.440286661691305703, 7.472421512516709718, 1.199719254218462483 ) ) ;
#59415=CARTESIAN_POINT ( 'NONE',  ( 5.002595493318194642, 4.938708951733754127, -0.7216878364870197293 ) ) ;
#59417=CARTESIAN_POINT ( 'NONE',  ( 4.416205349749311004, 6.175325546172740765, 1.599625672291267398 ) ) ;
#59424=CARTESIAN_POINT ( 'NONE',  ( -6.399085315970151733, 7.528316292462387871, -1.082531754730544860 ) ) ;
#59425=CARTESIAN_POINT ( 'NONE',  ( 2.523789150438203510, 6.096171108819874007, 0.7998128361456462443 ) ) ;
#59428=CARTESIAN_POINT ( 'NONE',  ( -8.030507057996002729, 8.263346410617135263, 1.040834085586084257E-14 ) ) ;
#59430=EDGE_CURVE ( 'NONE', #123166, #193490, #76423, .T. ) ;
#59434=CARTESIAN_POINT ( 'NONE',  ( -8.134002093194872884, 11.57708731111429401, 1.199719254218453823 ) ) ;
#59435=CARTESIAN_POINT ( 'NONE',  ( 1.451998047843343409, 7.315968950353815892, -4.301760722578415574 ) ) ;
#59438=CARTESIAN_POINT ( 'NONE',  ( 6.421758314367153275, 10.64380180007036891, -0.7998128361456291469 ) ) ;
#59439=CARTESIAN_POINT ( 'NONE',  ( 5.229694566569264680, 7.124396299129368337, 1.599625672291267398 ) ) ;
#59442=EDGE_LOOP ( 'NONE', ( #112457, #105785, #62102, #71886 ) ) ;
#59449=FACE_OUTER_BOUND ( 'NONE', #75379, .T. ) ;
#59452=CARTESIAN_POINT ( 'NONE',  ( -6.561256274009600986, 9.742217188731485678, -1.199719254218440723 ) ) ;
#59455=CARTESIAN_POINT ( 'NONE',  ( 6.982085921357777281, 7.248114451113292667, 1.040834085586084257E-14 ) ) ;
#59459=CARTESIAN_POINT ( 'NONE',  ( -3.913499895838973508, 7.717500311787445000, 1.040834085586084257E-14 ) ) ;
#59468=CARTESIAN_POINT ( 'NONE',  ( -1.499999999999997780, 5.650000000000023448, 1.214306433183764966E-14 ) ) ;
#59469=CARTESIAN_POINT ( 'NONE',  ( 6.577677080924314801, 10.82570702772039262, 1.040834085586084257E-14 ) ) ;
#59471=CARTESIAN_POINT ( 'NONE',  ( -3.145128448690323264, 4.692402494937224056, -1.443375672974059665 ) ) ;
#59474=CARTESIAN_POINT ( 'NONE',  ( -5.609265928939476176, 6.186647267178685183, -0.8691123025580966832 ) ) ;
#59481=CARTESIAN_POINT ( 'NONE',  ( 8.568389894156670294, 12.94027927658408217, -0.7216878364870257245 ) ) ;
#59498=CARTESIAN_POINT ( 'NONE',  ( -5.382750679825375251, 6.238629533673094585, -1.199719254218446718 ) ) ;
#59499=CARTESIAN_POINT ( 'NONE',  ( 5.965224399888476192, 6.061776009399090448, 1.040834085586084257E-14 ) ) ;
#59500=CARTESIAN_POINT ( 'NONE',  ( 1.499999999999987121, 3.545833333333356041, -0.8660254037844262731 ) ) ;
#59502=FACE_OUTER_BOUND ( 'NONE', #11025, .T. ) ;
#59506=CARTESIAN_POINT ( 'NONE',  ( -0.6823417656250212460, 4.301041667008085767, 1.181850606188767472 ) ) ;
#59509=CARTESIAN_POINT ( 'NONE',  ( -4.473827502829599290, 4.321812962830357208, 0.7216878364870317197 ) ) ;
#59512=CARTESIAN_POINT ( 'NONE',  ( 1.499999999999990896, 8.627523663848661428, -2.579999999999989413 ) ) ;
#59514=CARTESIAN_POINT ( 'NONE',  ( 5.352771719296971042, 5.139321848801576387, 0.7998128361456341429 ) ) ;
#59516=CARTESIAN_POINT ( 'NONE',  ( -5.181758602633715682, 4.945385036406048762, 2.419999999999998597 ) ) ;
#59517=CARTESIAN_POINT ( 'NONE',  ( 1.284279953904121641, 3.034610286488902187, 0.7750000000000117906 ) ) ;
#59518=CARTESIAN_POINT ( 'NONE',  ( 8.229436053370658755, 12.54483312900040026, 0.7216878364870438212 ) ) ;
#59520=CARTESIAN_POINT ( 'NONE',  ( -0.6823417656250212460, 1.363541667008083547, 1.181850606188755259 ) ) ;
#59521=CARTESIAN_POINT ( 'NONE',  ( 0.7499999999999902300, 3.733333333333352488, 1.299038105676669330 ) ) ;
#59523=CARTESIAN_POINT ( 'NONE',  ( -9.169391961543940539, 9.592045464756413509, 1.040834085586084257E-14 ) ) ;
#59524=CARTESIAN_POINT ( 'NONE',  ( -5.761852095683518193, 6.784877535461274256, 1.082531754730546636 ) ) ;
#59528=CARTESIAN_POINT ( 'NONE',  ( -1.364683531250010295, 5.280208333674758059, 0.7879004041258379498 ) ) ;
#59536=CARTESIAN_POINT ( 'NONE',  ( -5.721177634842498527, 5.777054783512106440, 0.000000000000000000 ) ) ;
#59541=CARTESIAN_POINT ( 'NONE',  ( -5.599154252319524794, 6.595063384869953360, 1.082531754730546636 ) ) ;
#59544=CARTESIAN_POINT ( 'NONE',  ( 9.856941372335116469, 11.45851867493453291, 1.199719254218450271 ) ) ;
#59554=CARTESIAN_POINT ( 'NONE',  ( -4.172158584703340445, 5.890604320285754980, -1.599625672291256295 ) ) ;
#59557=CARTESIAN_POINT ( 'NONE',  ( 1.499999999999987121, 1.504166666666690411, 0.8660254037844524744 ) ) ;
#59560=CARTESIAN_POINT ( 'NONE',  ( 9.571693261567961741, 11.22969222899322617, 1.082531754730548412 ) ) ;
#59561=CARTESIAN_POINT ( 'NONE',  ( 5.982172092127724383, 8.002286745614243912, -1.599625672291262513 ) ) ;
#59565=DIRECTION ( 'NONE',  ( 1.000000000000000000, 0.000000000000000000, 0.000000000000000000 ) ) ;
#59566=CARTESIAN_POINT ( 'NONE',  ( 4.436542580169809291, 6.199052314996659874, 1.599625672291267398 ) ) ;
#59568=VECTOR ( 'NONE', #206828, 1000.000000000000000 ) ;
#59569=CARTESIAN_POINT ( 'NONE',  ( 0.004619473214107315887, 7.151453204069587066, -1.999995854215781410 ) ) ;
#59577=CARTESIAN_POINT ( 'NONE',  ( 9.610031953988080744, 10.10612545594124967, -0.7998128361456281477 ) ) ;
#59578=CARTESIAN_POINT ( 'NONE',  ( -6.575868197828002693, 7.630599971342813426, 1.199719254218450271 ) ) ;
#59585=CARTESIAN_POINT ( 'NONE',  ( -1.364683531249997417, 4.759375000341424133, 1.214306433183764966E-14 ) ) ;
#59586=CARTESIAN_POINT ( 'NONE',  ( 7.904040366642684390, 11.20483561351640844, 1.082531754730558626 ) ) ;
#59587=CARTESIAN_POINT ( 'NONE',  ( -6.033542053281340856, 6.997886136038390603, -1.199719254218446718 ) ) ;
#59590=CARTESIAN_POINT ( 'NONE',  ( 4.873266149108180123, 7.772895376346490970, 1.199719254218462483 ) ) ;
#59591=CARTESIAN_POINT ( 'NONE',  ( -6.410307701162927252, 6.373113827645189744, -0.7998128361456291469 ) ) ;
#59597=CARTESIAN_POINT ( 'NONE',  ( 7.470179451449751262, 7.817556902887268677, 1.040834085586084257E-14 ) ) ;
#59601=CARTESIAN_POINT ( 'NONE',  ( 0.6823417656249899377, 1.405208333674752508, 1.181850606188755259 ) ) ;
#59603=CARTESIAN_POINT ( 'NONE',  ( 6.941411460072420603, 7.200660912947041581, 1.040834085586084257E-14 ) ) ;
#59607=CARTESIAN_POINT ( 'NONE',  ( -3.551873057100300990, 5.166937871415542283, 1.443375672974064550 ) ) ;
#59609=CARTESIAN_POINT ( 'NONE',  ( -1.364683531249997417, 5.759375000341418804, 1.214306433183764966E-14 ) ) ;
#59614=CARTESIAN_POINT ( 'NONE',  ( -4.061770719603903679, 7.733366158448967909, -0.6361108440643822304 ) ) ;
#59615=DIRECTION ( 'NONE',  ( -0.6507913734559658270, 0.7592566023652989049, 0.000000000000000000 ) ) ;
#59617=AXIS2_PLACEMENT_3D ( 'NONE', #76459, #123187, #189148 ) ;
#59622=CARTESIAN_POINT ( 'NONE',  ( 7.318703993278529829, 7.432909501780090800, 1.040834085586084257E-14 ) ) ;
#59631=CARTESIAN_POINT ( 'NONE',  ( 3.958617665510264949, 5.641473247893851628, -1.443375672974051449 ) ) ;
#59632=CARTESIAN_POINT ( 'NONE',  ( -0.6823417656250212460, 2.613541667008084879, 1.181850606188767472 ) ) ;
#59634=CARTESIAN_POINT ( 'NONE',  ( 7.507464373665139412, 9.781794407407920389, 1.599625672291281386 ) ) ;
#59637=CARTESIAN_POINT ( 'NONE',  ( -4.741601036477307574, 6.554953847355395880, 1.599625672291267175 ) ) ;
#59639=AXIS2_PLACEMENT_3D ( 'NONE', #98850, #29579, #80456 ) ;
#59640=EDGE_LOOP ( 'NONE', ( #203963, #35157, #96208 ) ) ;
#59642=CARTESIAN_POINT ( 'NONE',  ( -1.500000000000013101, 2.879166666666688634, -0.8660254037844313801 ) ) ;
#59643=CARTESIAN_POINT ( 'NONE',  ( 4.625302960556422427, 8.547937220624488575, 1.040834085586084257E-14 ) ) ;
#59644=CARTESIAN_POINT ( 'NONE',  ( -8.037286134802835491, 8.271255333558444889, -0.7998128361456291469 ) ) ;
#59648=CARTESIAN_POINT ( 'NONE',  ( -0.6823417656250003738, 1.967708333674753174, -1.181850606188749264 ) ) ;
#59650=CARTESIAN_POINT ( 'NONE',  ( 4.532503425670185493, 4.182342172903648070, 1.214306433183764966E-14 ) ) ;
#59657=CARTESIAN_POINT ( 'NONE',  ( 1.499999999999987121, 0.5354166673494816786, 0.8660254037844524744 ) ) ;
#59660=CARTESIAN_POINT ( 'NONE',  ( -4.232116505760120440, 8.089219690028791376, -0.7998128361456281477 ) ) ;
#59667=CARTESIAN_POINT ( 'NONE',  ( 5.555090253297246150, 7.504024600312024340, 1.599625672291267398 ) ) ;
#59672=CARTESIAN_POINT ( 'NONE',  ( 4.320244504248938355, 8.192035688265757898, 1.040834085586084257E-14 ) ) ;
#59677=CARTESIAN_POINT ( 'NONE',  ( 4.216749469050096621, 4.878294787768598262, -1.199719254218452047 ) ) ;
#59682=CARTESIAN_POINT ( 'NONE',  ( 5.580611138136594818, 6.171711880978127063, 0.8815597724760818599 ) ) ;
#59691=CARTESIAN_POINT ( 'NONE',  ( 7.131225611108079399, 11.26358761302737754, 0.7216878364870438212 ) ) ;
#59693=CARTESIAN_POINT ( 'NONE',  ( -6.078132937628113908, 5.985576603521232109, 1.040834085586084257E-14 ) ) ;
#59697=CARTESIAN_POINT ( 'NONE',  ( 7.853197290813620945, 10.18514947741448573, 1.599625672291281386 ) ) ;
#59699=CARTESIAN_POINT ( 'NONE',  ( -5.422371370461663176, 8.413518134592214537, -1.199719254218446718 ) ) ;
#59705=ORIENTED_EDGE ( 'NONE', *, *, #122310, .T. ) ;
#59708=ORIENTED_EDGE ( 'NONE', *, *, #154260, .F. ) ;
#59715=CARTESIAN_POINT ( 'NONE',  ( 9.103410076571945453, 12.70806329172093818, 1.199719254218450271 ) ) ;
#59716=CARTESIAN_POINT ( 'NONE',  ( -5.915435094264120508, 5.795762452929912101, 0.000000000000000000 ) ) ;
#59719=CARTESIAN_POINT ( 'NONE',  ( 2.548569689688999329, 5.917155704705049146, -0.7216878364870267237 ) ) ;
#59724=CARTESIAN_POINT ( 'NONE',  ( -4.172158584703340445, 5.890604320285754980, -1.599625672291256295 ) ) ;
#59728=CARTESIAN_POINT ( 'NONE',  ( 9.725276259704228821, 10.24057714594344048, 0.7998128361456462443 ) ) ;
#59733=CARTESIAN_POINT ( 'NONE',  ( -6.028571859570855729, 10.18508426947466816, 0.000000000000000000 ) ) ;
#59734=CARTESIAN_POINT ( 'NONE',  ( 4.473300617505036492, 7.306268922809479704, -1.199719254218452047 ) ) ;
#59736=EDGE_CURVE ( 'NONE', #163352, #44633, #142889, .T. ) ;
#59737=CARTESIAN_POINT ( 'NONE',  ( 3.659811400685081040, 6.357198169852855685, -1.199719254218446718 ) ) ;
#59740=CARTESIAN_POINT ( 'NONE',  ( -0.6823417656250003738, 2.780208333674753618, -1.181850606188749264 ) ) ;
#59743=CARTESIAN_POINT ( 'NONE',  ( 8.134528978519385944, 8.592631351135175066, -0.7216878364870267237 ) ) ;
#59750=CARTESIAN_POINT ( 'NONE',  ( 9.883530794237934458, 10.63313346947350269, -0.7216878364870257245 ) ) ;
#59751=ORIENTED_EDGE ( 'NONE', *, *, #34448, .F. ) ;
#59755=CARTESIAN_POINT ( 'NONE',  ( -9.287498920561160887, 10.79416914786490089, -1.199719254218441611 ) ) ;
#59773=CARTESIAN_POINT ( 'NONE',  ( -0.7500000000000215383, 1.972916667349486453, 1.299038105676659116 ) ) ;
#59779=ORIENTED_EDGE ( 'NONE', *, *, #155510, .F. ) ;
#59781=CARTESIAN_POINT ( 'NONE',  ( -0.7500000000000006661, 0.3583333333333563187, -1.299038105676652011 ) ) ;
#59782=CARTESIAN_POINT ( 'NONE',  ( 8.925345196497941558, 9.307324238869423283, 1.040834085586084257E-14 ) ) ;
#59783=CARTESIAN_POINT ( 'NONE',  ( 1.364683531249986537, -0.8447916663252468261, -0.7879004041258309554 ) ) ;
#59786=CARTESIAN_POINT ( 'NONE',  ( 4.518945272056516416, 4.166524327021037699, 0.7998128361456341429 ) ) ;
#59787=CARTESIAN_POINT ( 'NONE',  ( -4.921246572080546500, 8.685278734161874681, 1.214306433183764966E-14 ) ) ;
#59793=CARTESIAN_POINT ( 'NONE',  ( -5.018489415352746619, 9.006654751220198207, 0.7998128361456481317 ) ) ;
#59795=CARTESIAN_POINT ( 'NONE',  ( -0.7500000000000215383, 2.472916667349486897, 1.299038105676671107 ) ) ;
#59809=CARTESIAN_POINT ( 'NONE',  ( -10.00321840878439339, 10.56484298653695397, 1.040834085586084257E-14 ) ) ;
#59810=CARTESIAN_POINT ( 'NONE',  ( 6.608709811657416999, 9.797579649320619311, -1.199719254218440723 ) ) ;
#59818=CARTESIAN_POINT ( 'NONE',  ( -6.347188469492005325, 10.55680364771601809, -0.7998128361456291469 ) ) ;
#59821=CARTESIAN_POINT ( 'NONE',  ( 0.000000000000000000, 8.600000000000017408, -0.3999999999999819811 ) ) ;
#59824=CARTESIAN_POINT ( 'NONE',  ( 9.459838494033030898, 12.05956421450382088, 1.599625672291281386 ) ) ;
#59828=CARTESIAN_POINT ( 'NONE',  ( -9.671043645249580933, 10.17730576241299900, 0.7998128361456462443 ) ) ;
#59831=CARTESIAN_POINT ( 'NONE',  ( -4.816275411463948330, 6.948951914485960835, -1.437501944199247372 ) ) ;
#59846=CARTESIAN_POINT ( 'NONE',  ( 1.499999999999987121, 1.327083334016149641, -0.8660254037844253849 ) ) ;
#59858=CARTESIAN_POINT ( 'NONE',  ( 4.256897045010922476, 5.029096643009940415, -1.082531754730548412 ) ) ;
#59861=ORIENTED_EDGE ( 'NONE', *, *, #11172, .T. ) ;
#59863=CARTESIAN_POINT ( 'NONE',  ( -1.001543065824772872E-14, 5.384375000341415252, 1.575800808251672791 ) ) ;
#59866=CARTESIAN_POINT ( 'NONE',  ( 8.048736748007069508, 12.54194330598362406, -0.7998128361456352531 ) ) ;
#59869=CARTESIAN_POINT ( 'NONE',  ( 4.008199524592567897, 7.584238231759597326, 0.2402771892247856922 ) ) ;
#59874=CARTESIAN_POINT ( 'NONE',  ( -1.201851678989727383E-14, 1.321875000341419248, 1.575800808251672791 ) ) ;
#59881=CARTESIAN_POINT ( 'NONE',  ( -3.554208825076827782, 7.298327395898266623, 0.7998128361456341429 ) ) ;
#59884=CARTESIAN_POINT ( 'NONE',  ( -1.500000000000013101, -0.3291666666666463459, 0.8660254037844403729 ) ) ;
#59886=CARTESIAN_POINT ( 'NONE',  ( -1.364683531250014514, -1.157291666325248158, 0.7879004041258379498 ) ) ;
#59891=CARTESIAN_POINT ( 'NONE',  ( -1.364683531249997417, 5.571875000341417916, 1.214306433183764966E-14 ) ) ;
#59893=CARTESIAN_POINT ( 'NONE',  ( -6.191269702934848240, 10.37489842006599616, 0.000000000000000000 ) ) ;
#59894=CARTESIAN_POINT ( 'NONE',  ( 8.269583629331492602, 11.73526576994040482, 1.199719254218450271 ) ) ;
#59900=CARTESIAN_POINT ( 'NONE',  ( -1.364683531250014514, 0.05104166700808546175, -0.7879004041258359514 ) ) ;
#59906=CARTESIAN_POINT ( 'NONE',  ( 5.504247177468168495, 9.365446107114122398, 0.7216878364870438212 ) ) ;
#59909=CARTESIAN_POINT ( 'NONE',  ( -5.253948220495577637, 6.088359997788290734, 1.199719254218450271 ) ) ;
#59913=CARTESIAN_POINT ( 'NONE',  ( 5.978782553502139940, 6.077593855281705260, -0.7216878364870257245 ) ) ;
#59914=CARTESIAN_POINT ( 'NONE',  ( -10.26315909542058336, 11.07603315418659840, -0.7216878364870267237 ) ) ;
#59917=B_SPLINE_CURVE_WITH_KNOTS ( 'NONE', 3,
 ( #135269, #3080, #34538, #947, #182923, #35601, #153637, #52926, #20414, #168809 ),
 .UNSPECIFIED., .F., .F.,
 ( 4, 3, 3, 4 ),
 ( 0.000000000000000000, 0.0001748898611877313010, 0.0003306773789565961162, 0.0004872651007806716407 ),
 .UNSPECIFIED. ) ;
#59921=CARTESIAN_POINT ( 'NONE',  ( 10.08690309888728187, 10.87040115823107911, -0.7216878364870257245 ) ) ;
#59935=CARTESIAN_POINT ( 'NONE',  ( 7.578644679914694926, 11.78557652663510424, 0.7216878364870438212 ) ) ;
#59937=CARTESIAN_POINT ( 'NONE',  ( 7.914208982075123799, 10.25632978388623684, -1.599625672291262513 ) ) ;
#59943=CARTESIAN_POINT ( 'NONE',  ( 5.680503174445848735, 5.729601246382692636, 1.040834085586084257E-14 ) ) ;
#59945=CARTESIAN_POINT ( 'NONE',  ( -8.839552966430007430, 11.33589776563360019, -1.443375672974059665 ) ) ;
#59956=DIRECTION ( 'NONE',  ( 1.000000000000000000, 0.000000000000000000, 0.000000000000000000 ) ) ;
#59965=ADVANCED_FACE ( 'NONE', ( #160254 ), #11855, .F. ) ;
#59972=( BOUNDED_CURVE ( )  B_SPLINE_CURVE ( 3, ( #119046, #20403, #102741, #168796 ),
 .UNSPECIFIED., .F., .T. ) 
 B_SPLINE_CURVE_WITH_KNOTS ( ( 4, 4 ),
 ( 4.082329036743725936, 4.712388980384688786 ),
 .UNSPECIFIED. ) 
 CURVE ( )  GEOMETRIC_REPRESENTATION_ITEM ( )  RATIONAL_B_SPLINE_CURVE ( ( 1.000000000000000000, 0.9671913951488946282, 0.9671913951488946282, 1.000000000000000000 ) ) 
 REPRESENTATION_ITEM ( '' )  );
#59975=CARTESIAN_POINT ( 'NONE',  ( -6.399085315970132193, 10.40942393536641397, -0.7216878364870278340 ) ) ;
#59979=CARTESIAN_POINT ( 'NONE',  ( 4.798696304233017074, 7.685897223992134819, -1.199719254218452047 ) ) ;
#59980=CARTESIAN_POINT ( 'NONE',  ( -4.623494077460110319, 5.352830164246910272, 1.199719254218462483 ) ) ;
#59982=CARTESIAN_POINT ( 'NONE',  ( 3.216308754939877446, 4.775446185561722956, -1.599625672291262513 ) ) ;
#59984=CARTESIAN_POINT ( 'NONE',  ( -4.731959306369413198, 5.479372931307791461, -1.199719254218446718 ) ) ;
#59988=CARTESIAN_POINT ( 'NONE',  ( -4.391951695823077984, 7.211361847513815704, 1.199719254218464037 ) ) ;
#59992=CARTESIAN_POINT ( 'NONE',  ( 8.046927864910717432, 9.346836249606042202, 1.199719254218462483 ) ) ;
#59993=CARTESIAN_POINT ( 'NONE',  ( 0.6823417656249917140, 3.342708333674754506, 1.181850606188765695 ) ) ;
#59995=CARTESIAN_POINT ( 'NONE',  ( 6.112956004491900686, 6.016961049888108981, 0.08799760576284378077 ) ) ;
#59996=CARTESIAN_POINT ( 'NONE',  ( 3.334942599281629949, 5.874221551595115720, -1.082531754730543083 ) ) ;
#60003=CARTESIAN_POINT ( 'NONE',  ( 6.602457619730760285, 8.725953194484466380, 1.443375672974076540 ) ) ;
#60004=CARTESIAN_POINT ( 'NONE',  ( -9.020252271793614440, 9.418049160047695878, 0.7998128361456462443 ) ) ;
#60007=CARTESIAN_POINT ( 'NONE',  ( -8.779068160048691283, 10.20099992726700933, -1.199719254218446718 ) ) ;
#60008=CARTESIAN_POINT ( 'NONE',  ( -4.876128802409253282, 8.840567369452784874, 0.7998128361456481317 ) ) ;
#60015=CARTESIAN_POINT ( 'NONE',  ( 8.613507663383630941, 8.943513783569379427, -0.7998128361456221525 ) ) ;
#60030=CARTESIAN_POINT ( 'NONE',  ( 0.7499999999999902300, 5.066666666666684193, -1.299038105676658228 ) ) ;
#60031=CARTESIAN_POINT ( 'NONE',  ( 5.508690485854129903, 5.321227076451600091, 1.040834085586084257E-14 ) ) ;
#60032=CARTESIAN_POINT ( 'NONE',  ( 7.820355676984174664, 8.018169799436671852, -0.7998128361456281477 ) ) ;
#60034=CARTESIAN_POINT ( 'NONE',  ( 5.504247177468168495, 9.365446107114122398, 0.7216878364870438212 ) ) ;
#60035=CARTESIAN_POINT ( 'NONE',  ( -9.463228032214294316, 10.14278024711257764, 1.040834085586084257E-14 ) ) ;
#60039=CARTESIAN_POINT ( 'NONE',  ( 9.915090410295563927, 10.46202698829998567, -0.7998128361456281477 ) ) ;
#60042=CARTESIAN_POINT ( 'NONE',  ( -2.252626078164912560, 5.779814191167667481, 0.7998128361456341429 ) ) ;
#60044=CARTESIAN_POINT ( 'NONE',  ( -1.364683531250014514, 1.238541667008091096, -0.7879004041258289570 ) ) ;
#60049=CARTESIAN_POINT ( 'NONE',  ( 0.6823417656249864960, -0.5739583329919112353, -1.181850606188749264 ) ) ;
#60051=CARTESIAN_POINT ( 'NONE',  ( 9.317477881089539338, 11.89347683273640932, 1.599625672291279388 ) ) ;
#60055=CARTESIAN_POINT ( 'NONE',  ( -2.616360457312984167, 5.996244933599686355, -0.7216878364870257245 ) ) ;
#60058=CARTESIAN_POINT ( 'NONE',  ( -5.225778143063529946, 8.184159369294361497, 1.199719254218452047 ) ) ;
#60061=CARTESIAN_POINT ( 'NONE',  ( 3.785751206713845018, 5.439795712631356750, 1.599625672291267398 ) ) ;
#60065=ORIENTED_EDGE ( 'NONE', *, *, #154260, .T. ) ;
#60067=CARTESIAN_POINT ( 'NONE',  ( 9.582915646760733708, 10.07448976417602893, 0.7998128361456462443 ) ) ;
#60070=CARTESIAN_POINT ( 'NONE',  ( -3.893162665418476109, 7.693773542963529444, 1.040834085586084257E-14 ) ) ;
#60074=CARTESIAN_POINT ( 'NONE',  ( 8.589254009457354400, 9.979550084910457031, -1.199719254218446718 ) ) ;
#60076=CARTESIAN_POINT ( 'NONE',  ( 8.260995669428309540, 8.532249790621511565, 0.7998128361456481317 ) ) ;
#60078=CARTESIAN_POINT ( 'NONE',  ( -9.978437869977950569, 11.70422760547153906, -1.082531754730539753 ) ) ;
#60080=FACE_OUTER_BOUND ( 'NONE', #105441, .T. ) ;
#60085=CARTESIAN_POINT ( 'NONE',  ( -5.926191280687664431, 6.129739482751896062, 0.8152664440823562675 ) ) ;
#60086=CARTESIAN_POINT ( 'NONE',  ( -1.402160292154681736E-14, 1.196875000341419026, -1.575800808251659024 ) ) ;
#60088=CARTESIAN_POINT ( 'NONE',  ( 6.968527767744104651, 8.192665819532020777, 1.082531754730558626 ) ) ;
#60109=CARTESIAN_POINT ( 'NONE',  ( 8.072990401933337168, 11.50590700464255356, -1.199719254218446718 ) ) ;
#60113=CARTESIAN_POINT ( 'NONE',  ( -3.623053363349869382, 5.249981562040033189, 1.599625672291267398 ) ) ;
#60114=CARTESIAN_POINT ( 'NONE',  ( -6.073162743917628781, 9.172774736957510555, -1.199719254218440723 ) ) ;
#60119=CARTESIAN_POINT ( 'NONE',  ( -0.7500000000000215383, 4.472916667349482012, 1.299038105676671107 ) ) ;
#60120=CARTESIAN_POINT ( 'NONE',  ( 8.209625708274705502, 9.536650400197368427, 1.199719254218462483 ) ) ;
#60123=CARTESIAN_POINT ( 'NONE',  ( -8.864333505236459132, 9.236143932397675727, 1.040834085586084257E-14 ) ) ;
#60125=CARTESIAN_POINT ( 'NONE',  ( -1.364683531250010295, 4.280208333674753618, 0.7879004041258379498 ) ) ;
#60130=CARTESIAN_POINT ( 'NONE',  ( -9.164948653158003111, 9.794787638213568570, -0.7216878364870267237 ) ) ;
#60135=CARTESIAN_POINT ( 'NONE',  ( -1.364683531250000748, 2.321875000341422357, 1.214306433183764966E-14 ) ) ;
#60142=CARTESIAN_POINT ( 'NONE',  ( -0.6823417656249969321, 3.467708333674754506, -1.181850606188749264 ) ) ;
#60144=CARTESIAN_POINT ( 'NONE',  ( -4.517891501851816649, 6.293959390292322986, -1.599625672291256295 ) ) ;
#60145=CARTESIAN_POINT ( 'NONE',  ( 5.425234023762710578, 9.481190127698507553, -0.7998128361456291469 ) ) ;
#60149=CARTESIAN_POINT ( 'NONE',  ( 0.6823417656249899377, 3.738541667008085767, -1.181850606188754593 ) ) ;
#60152=CARTESIAN_POINT ( 'NONE',  ( -0.6823417656250003738, -0.2822916663252489355, -1.181850606188749264 ) ) ;
#60153=CARTESIAN_POINT ( 'NONE',  ( -4.961921032921567054, 4.891255414604337659, 0.7216878364870317197 ) ) ;
#60157=CARTESIAN_POINT ( 'NONE',  ( 3.050221373394638835, 6.502416002361635528, 0.000000000000000000 ) ) ;
#60161=CARTESIAN_POINT ( 'NONE',  ( -9.246297574839990929, 11.81043314211192019, 1.443375672974076540 ) ) ;
#60166=CARTESIAN_POINT ( 'NONE',  ( -8.109748439268576803, 12.61312361245537517, 0.7998128361456481317 ) ) ;
#60167=CARTESIAN_POINT ( 'NONE',  ( -5.951666246274811556, 7.966696592119163256, 1.443375672974064550 ) ) ;
#60169=CARTESIAN_POINT ( 'NONE',  ( 1.364683531249986537, 0.4677083336747514530, -0.7879004041258309554 ) ) ;
#60171=FACE_OUTER_BOUND ( 'NONE', #162743, .T. ) ;
#60175=CARTESIAN_POINT ( 'NONE',  ( -1.364683531250000748, -0.6781249996585803075, 0.000000000000000000 ) ) ;
#60181=CARTESIAN_POINT ( 'NONE',  ( -1.500000000000013101, -0.3291666666666463459, 0.8660254037844403729 ) ) ;
#60189=CARTESIAN_POINT ( 'NONE',  ( 6.173040012923759257, 6.096301524699504704, -0.7998128361456281477 ) ) ;
#60191=CARTESIAN_POINT ( 'NONE',  ( -4.274898507010545856, 3.881803101134051470, -0.7998128361456221525 ) ) ;
#60195=CARTESIAN_POINT ( 'NONE',  ( -1.364683531250000748, 1.821875000341421913, 0.000000000000000000 ) ) ;
#60214=CARTESIAN_POINT ( 'NONE',  ( 6.654354466208897811, 6.657835053532175529, 0.7998128361456341429 ) ) ;
#60217=EDGE_CURVE ( 'NONE', #73782, #110797, #209250, .T. ) ;
#60223=CARTESIAN_POINT ( 'NONE',  ( -6.138157471807708987, 5.995865026538652387, 1.148737437293850421E-12 ) ) ;
#60225=CARTESIAN_POINT ( 'NONE',  ( 9.772729797352075920, 10.29593960653257234, -0.7998128361456281477 ) ) ;
#60227=CARTESIAN_POINT ( 'NONE',  ( 1.517589660447897781, 8.687973171320628296, -2.529458313501610434 ) ) ;
#60233=CARTESIAN_POINT ( 'NONE',  ( -0.006800380015323652903, 7.009756401597622144, 1.999988438675414759 ) ) ;
#60236=EDGE_CURVE ( 'NONE', #157004, #24729, #172853, .T. ) ;
#60238=CARTESIAN_POINT ( 'NONE',  ( -9.164948653157999559, 10.75515685251491504, -1.082531754730539753 ) ) ;
#60245=CARTESIAN_POINT ( 'NONE',  ( 6.308621549060418054, 6.254479983525607523, 0.7998128361456341429 ) ) ;
#60252=CARTESIAN_POINT ( 'NONE',  ( 2.697709378994964879, 6.091152008895348580, 0.7216878364870338292 ) ) ;
#60260=CARTESIAN_POINT ( 'NONE',  ( -6.579784621333750749, 6.570836901177822931, 0.7998128361456341429 ) ) ;
#60262=CARTESIAN_POINT ( 'NONE',  ( -4.406563619641430840, 5.099744630125142564, -1.199719254218446718 ) ) ;
#60271=CARTESIAN_POINT ( 'NONE',  ( 4.299907273828439180, 8.168308919441841454, 1.040834085586084257E-14 ) ) ;
#60273=CARTESIAN_POINT ( 'NONE',  ( 1.545144449789729091, 8.695096949162934408, 2.507961912884413280 ) ) ;
#60284=CARTESIAN_POINT ( 'NONE',  ( -0.6823417656250212460, 1.113541667008083325, 1.181850606188755259 ) ) ;
#60285=CARTESIAN_POINT ( 'NONE',  ( 4.867540842506059562, 5.637551390133895168, -1.199719254218452047 ) ) ;
#60287=CARTESIAN_POINT ( 'NONE',  ( -6.480434237652138663, 8.583592582059388576, 1.443375672974078761 ) ) ;
#60289=CARTESIAN_POINT ( 'NONE',  ( 5.016153647376217606, 4.954526798134778254, 0.7216878364870317197 ) ) ;
#60290=CARTESIAN_POINT ( 'NONE',  ( -5.680503174001480637, 9.571078103069643461, 0.7216878364870458196 ) ) ;
#60295=CARTESIAN_POINT ( 'NONE',  ( 6.810273232766058449, 6.839740281182199233, 1.040834085586084257E-14 ) ) ;
#60297=CARTESIAN_POINT ( 'NONE',  ( -3.004347502343385212, 6.455130793263525568, -0.4817541042819983854 ) ) ;
#60300=CARTESIAN_POINT ( 'NONE',  ( 1.364683531249990311, 4.613541667008083103, 0.7879004041258500513 ) ) ;
#60304=CARTESIAN_POINT ( 'NONE',  ( 7.318703993278529829, 7.432909501780090800, 1.040834085586084257E-14 ) ) ;
#60306=CARTESIAN_POINT ( 'NONE',  ( -6.226218857173722476, 8.287007971501239467, 1.599625672291283607 ) ) ;
#60311=CARTESIAN_POINT ( 'NONE',  ( 8.158255747121103241, 10.54105100977322174, 1.599625672291281386 ) ) ;
#60313=CARTESIAN_POINT ( 'NONE',  ( -8.213542131780492639, 8.476887330032372603, 1.040834085586084257E-14 ) ) ;
#60314=CARTESIAN_POINT ( 'NONE',  ( 3.215772567386471437, 6.427315425527130088, -0.8732430475888957044 ) ) ;
#60316=CARTESIAN_POINT ( 'NONE',  ( 7.904040366642699489, 8.323727970612377902, 0.7216878364870458196 ) ) ;
#60317=CARTESIAN_POINT ( 'NONE',  ( 4.202513864555980305, 7.333163887849894813, -0.8510647575735978965 ) ) ;
#60318=CARTESIAN_POINT ( 'NONE',  ( -8.188761592974040937, 11.53701037756964887, -1.082531754730543971 ) ) ;
#60322=CARTESIAN_POINT ( 'NONE',  ( 6.148786358997489820, 7.132337826040578754, -1.199719254218446718 ) ) ;
#60324=CARTESIAN_POINT ( 'NONE',  ( 7.865701674222579598, 12.32840238656838139, -0.7998128361456352531 ) ) ;
#60325=CARTESIAN_POINT ( 'NONE',  ( -4.511607644515479798, 7.038970647229928268, 1.150300019105324978 ) ) ;
#60326=CARTESIAN_POINT ( 'NONE',  ( 2.198393463710220264, 5.716542807637226886, 0.7998128361456462443 ) ) ;
#60327=CARTESIAN_POINT ( 'NONE',  ( 0.6823417656249899377, 0.8427083336747520637, 1.181850606188755259 ) ) ;
#60329=CARTESIAN_POINT ( 'NONE',  ( -5.368665641331555882, 8.246898433986675769, 1.082531754730548412 ) ) ;
#60330=ORIENTED_EDGE ( 'NONE', *, *, #19714, .T. ) ;
#60335=CARTESIAN_POINT ( 'NONE',  ( -5.227141986104622440, 6.445127484965264664, 1.169998774669118946 ) ) ;
#60336=CARTESIAN_POINT ( 'NONE',  ( 1.364683531249988757, 0.4468750003414206917, 0.000000000000000000 ) ) ;
#60340=CARTESIAN_POINT ( 'NONE',  ( 2.901081683644319842, 5.368050483351580304, 1.082531754730548412 ) ) ;
#60344=CARTESIAN_POINT ( 'NONE',  ( -9.314088342463968218, 9.968783942403868892, 0.7216878364870438212 ) ) ;
#60350=CARTESIAN_POINT ( 'NONE',  ( -9.137832345486311070, 9.763151945929928743, 1.040834085586084257E-14 ) ) ;
#60358=CARTESIAN_POINT ( 'NONE',  ( -8.988692655735990300, 9.589155641221221771, 0.7216878364870438212 ) ) ;
#60362=CARTESIAN_POINT ( 'NONE',  ( 1.364683531249988535, 4.967708333674756283, -0.7879004041258300672 ) ) ;
#60363=CARTESIAN_POINT ( 'NONE',  ( 1.499999999999990896, 3.806250000682819046, 1.214306433183764966E-14 ) ) ;
#60364=CARTESIAN_POINT ( 'NONE',  ( 4.877963630130927264, 6.902327454639943127, -1.420620101560632342 ) ) ;
#60370=CARTESIAN_POINT ( 'NONE',  ( -6.509886312855995172, 10.74661779830734254, -0.7998128361456291469 ) ) ;
#60374=CARTESIAN_POINT ( 'NONE',  ( 6.010342169559767633, 5.906487374108181143, -0.7998128361456281477 ) ) ;
#60379=CARTESIAN_POINT ( 'NONE',  ( 7.983053520348166288, 8.207983950027992748, -0.7998128361456281477 ) ) ;
#60380=CARTESIAN_POINT ( 'NONE',  ( -4.911709678547487634, 4.704967246051090513, 0.3769511059573752432 ) ) ;
#60386=CARTESIAN_POINT ( 'NONE',  ( -4.921246572080546500, 8.685278734161874681, 1.214306433183764966E-14 ) ) ;
#60396=CARTESIAN_POINT ( 'NONE',  ( -8.455481356417053007, 13.01647868246193518, 0.7998128361456341429 ) ) ;
#60399=EDGE_CURVE ( 'NONE', #127447, #93714, #138915, .T. ) ;
#60400=CARTESIAN_POINT ( 'NONE',  ( 9.935427640716063991, 10.48575375712389679, -0.7998128361456281477 ) ) ;
#60401=CARTESIAN_POINT ( 'NONE',  ( 1.499999999999987566, -0.7249999999999825473, 0.000000000000000000 ) ) ;
#60402=CARTESIAN_POINT ( 'NONE',  ( -7.395082721250053837, 10.71501471051202614, -1.199719254218446718 ) ) ;
#60404=B_SPLINE_CURVE_WITH_KNOTS ( 'NONE', 1,
 ( #2326, #104136 ),
 .UNSPECIFIED., .F., .F.,
 ( 2, 2 ),
 ( 0.2143153648627418029, 0.6378831769527100182 ),
 .UNSPECIFIED. ) ;
#60405=CARTESIAN_POINT ( 'NONE',  ( -1.364683531250012516, 2.988541667008091096, -0.7879004041258289570 ) ) ;
#60407=CARTESIAN_POINT ( 'NONE',  ( 2.198393463710220264, 5.716542807637226886, 0.7998128361456462443 ) ) ;
#60410=CARTESIAN_POINT ( 'NONE',  ( -1.500000000000011324, 5.379166666666692187, -0.8660254037844313801 ) ) ;
#60412=CARTESIAN_POINT ( 'NONE',  ( 3.469446951953614189E-15, 5.227586206896610577, 1.214306433183764966E-14 ) ) ;
#60413=CARTESIAN_POINT ( 'NONE',  ( 8.148087131688683371, 10.52918762510205042, -1.443375672974063439 ) ) ;
#60417=CARTESIAN_POINT ( 'NONE',  ( -7.239690840017442675, 7.548653522882887934, 0.7216878364870317197 ) ) ;
#60419=CARTESIAN_POINT ( 'NONE',  ( -1.201851678989727383E-14, 2.071875000341422801, 1.575800808251672791 ) ) ;
#60423=CARTESIAN_POINT ( 'NONE',  ( -6.073162743917628781, 9.172774736957510555, -1.199719254218440723 ) ) ;
#60424=CARTESIAN_POINT ( 'NONE',  ( -0.6823417656249969321, 4.530208333674755394, -1.181850606188749264 ) ) ;
#60429=CARTESIAN_POINT ( 'NONE',  ( 7.886038904643079661, 12.35212915539230139, -0.7998128361456352531 ) ) ;
#60432=CARTESIAN_POINT ( 'NONE',  ( 1.499999999999987121, 0.7958333333333510451, -0.8660254037844253849 ) ) ;
#60437=CARTESIAN_POINT ( 'NONE',  ( 10.23370702021670020, 10.83374636654133383, 0.7998128361456462443 ) ) ;
#60443=CARTESIAN_POINT ( 'NONE',  ( 9.413438726589914651, 9.876766690643398405, 0.000000000000000000 ) ) ;
#60444=CARTESIAN_POINT ( 'NONE',  ( -1.517589660447928868, 8.687973171320628296, 2.529458313501630418 ) ) ;
#60447=CARTESIAN_POINT ( 'NONE',  ( 1.364683531249986537, -0.8447916663252468261, -0.7879004041258309554 ) ) ;
#60452=CARTESIAN_POINT ( 'NONE',  ( 7.425061681778431399, 11.81432239538354345, 0.7998128361456462443 ) ) ;
#60455=CARTESIAN_POINT ( 'NONE',  ( -1.001543065824772872E-14, 4.321875000341417916, 1.575800808251672791 ) ) ;
#60457=CARTESIAN_POINT ( 'NONE',  ( -5.585596099150191840, 7.539614753807099667, -1.443375672974052559 ) ) ;
#60459=CARTESIAN_POINT ( 'NONE',  ( 5.639828713160493834, 5.682147708216442439, 1.040834085586084257E-14 ) ) ;
#60463=CARTESIAN_POINT ( 'NONE',  ( 3.029357257649615054, 5.621668336311468117, -1.199719254218446718 ) ) ;
#60465=ORIENTED_EDGE ( 'NONE', *, *, #204199, .T. ) ;
#60466=CARTESIAN_POINT ( 'NONE',  ( 7.065770611016287006, 11.39514947949436774, 1.040834085586084257E-14 ) ) ;
#60472=CARTESIAN_POINT ( 'NONE',  ( -7.862839020921525091, 11.26073039346208660, -1.199719254218446718 ) ) ;
#60473=CARTESIAN_POINT ( 'NONE',  ( 5.307127064745490230, 8.279066444590018392, -1.199719254218452935 ) ) ;
#60476=CARTESIAN_POINT ( 'NONE',  ( 5.332434488876471868, 5.115595079977664383, 0.7998128361456341429 ) ) ;
#60481=CARTESIAN_POINT ( 'NONE',  ( 3.050221373394638835, 6.502416002361635528, 0.000000000000000000 ) ) ;
#60484=CARTESIAN_POINT ( 'NONE',  ( -4.744990575102892905, 8.479646737687938085, 0.7216878364870458196 ) ) ;
#60485=CARTESIAN_POINT ( 'NONE',  ( 3.551346171775753735, 6.230655402791975384, 1.199719254218462483 ) ) ;
#60488=CARTESIAN_POINT ( 'NONE',  ( -7.477485413136760073, 8.682486722536401302, -1.199719254218446718 ) ) ;
#60493=CARTESIAN_POINT ( 'NONE',  ( -8.779068160048691283, 10.20099992726700933, -1.199719254218446718 ) ) ;
#60497=CARTESIAN_POINT ( 'NONE',  ( 8.633844893804129228, 8.967240552393299424, -0.7998128361456211532 ) ) ;
#60498=CARTESIAN_POINT ( 'NONE',  ( 4.473300617505036492, 7.306268922809479704, -1.199719254218452047 ) ) ;
#60510=CARTESIAN_POINT ( 'NONE',  ( -7.857113714319432063, 9.125386407249497012, 1.199719254218462483 ) ) ;
#60514=CARTESIAN_POINT ( 'NONE',  ( 7.470179451449751262, 7.817556902887268677, 1.040834085586084257E-14 ) ) ;
#60515=VERTEX_POINT ( 'NONE', #68049 ) ;
#60518=CARTESIAN_POINT ( 'NONE',  ( -3.782361668532609134, 7.356579680022602652, 1.040834085586084257E-14 ) ) ;
#60520=CARTESIAN_POINT ( 'NONE',  ( -4.550733115681270036, 8.460939068270139529, 0.7998128361456481317 ) ) ;
#60531=CARTESIAN_POINT ( 'NONE',  ( -8.482597663644387609, 13.04811437422715414, -0.7998128361456281477 ) ) ;
#60532=CARTESIAN_POINT ( 'NONE',  ( 6.916630921265960019, 11.22115317478565188, 0.7998128361456462443 ) ) ;
#60536=CARTESIAN_POINT ( 'NONE',  ( -4.567562471335953944, 6.984949105684680859, -1.180336305634868577 ) ) ;
#60545=CARTESIAN_POINT ( 'NONE',  ( 3.521367211247359741, 5.131347717920458962, -1.599625672291262513 ) ) ;
#60556=( BOUNDED_CURVE ( )  B_SPLINE_CURVE ( 2, ( #19222, #99427, #82091, #150321, #166557, #83155, #85300, #51749, #84233, #809, #165481, #151386, #185987, #36542, #52799, #116794, #134092, #67947, #37621, #17077, #182791, #65813, #102629, #4022, #100481, #149235, #2956, #135144, #53878, #201160, #118938, #50668, #86374, #214185, #33345, #103701, #133022, #152443, #70091, #34409, #131960, #136206, #202224, #169752, #148184, #49601, #115725, #199021, #24556, #90663, #39763, #105868, #171894, #123243, #91740, #58143, #156725, #139409, #109098, #137277, #23491, #189207, #205443, #89597, #154585, #38696, #106953, #59200, #190261, #206512, #56012, #73307, #155647, #125357, #104774, #122165, #174055, #203297, #170823, #54944, #57079, #7230, #40845, #207580, #172977, #8316, #204355, #74401, #153516, #187063, #191320, #88523, #140501, #124302, #188132, #71160, #41919, #108030, #121096, #22414, #25628, #157793, #9389, #75460, #141573, #42987, #21340, #87448, #5085, #6162, #72231, #138338, #210781, #128567, #194532, #208636, #158846, #176174, #97068, #26700, #80797, #145832, #76515 ),
 .UNSPECIFIED., .F., .T. ) 
 B_SPLINE_CURVE_WITH_KNOTS ( ( 3, 2, 2, 2, 2, 2, 2, 2, 2, 2, 2, 2, 2, 2, 2, 2, 2, 2, 2, 2, 2, 2, 2, 2, 2, 2, 2, 2, 2, 2, 2, 2, 2, 2, 2, 2, 2, 2, 2, 2, 2, 2, 2, 2, 2, 2, 2, 2, 2, 2, 2, 2, 2, 2, 2, 2, 2, 2, 2, 2, 2, 3 ),
 ( 0.000000000000000000, 0.005952380952380951183, 0.01190476190476190237, 0.01785714285714285615, 0.02380952380952380473, 0.02976190476190476372, 0.03571428571428571230, 0.04166666666666666435, 0.04761904761904760947, 0.05357142857142857539, 0.05952380952380952744, 0.06547619047619047949, 0.07142857142857142461, 0.07738095238095238360, 0.08333333333333332871, 0.08928571428571428770, 0.09523809523809521893, 0.1011904761904761918, 0.1071428571428571508, 0.1130952380952380959, 0.1190476190476190549, 0.1250000000000000000, 0.1309523809523809590, 0.1369047619047619180, 0.1428571428571428492, 0.1488095238095238082, 0.1547619047619047672, 0.1607142857142857262, 0.1666666666666666574, 0.1726190476190476164, 0.1785714285714285754, 0.1845238095238095621, 0.1904761904761904379, 0.1964285714285714246, 0.2023809523809523836, 0.2083333333333333703, 0.2142857142857143016, 0.2202380952380952328, 0.2261904761904761918, 0.2321428571428571785, 0.2380952380952381098, 0.2440476190476190410, 0.2500000000000000000, 0.2559523809523809312, 0.2619047619047619180, 0.2678571428571428492, 0.2738095238095238360, 0.2797619047619047672, 0.2857142857142856984, 0.2916666666666666852, 0.2976190476190476164, 0.3035714285714285476, 0.3095238095238095344, 0.3154761904761904656, 0.3214285714285714524, 0.3273809523809523836, 0.3333333333333333148, 0.3392857142857143016, 0.3452380952380952328, 0.3511904761904762196, 0.3571428571428571508, 0.3602579105411656268 ),
 .UNSPECIFIED. ) 
 CURVE ( )  GEOMETRIC_REPRESENTATION_ITEM ( )  RATIONAL_B_SPLINE_CURVE ( ( 1.000000000000000000, 0.8660254037844387076, 1.000000000000000000, 0.8660254037844387076, 1.000000000000000000, 0.8660254037844387076, 1.000000000000000000, 0.8660254037844387076, 1.000000000000000000, 0.8660254037844387076, 1.000000000000000000, 0.8660254037844387076, 1.000000000000000000, 0.8660254037844387076, 1.000000000000000000, 0.8660254037844387076, 1.000000000000000000, 0.8660254037844387076, 1.000000000000000000, 0.8660254037844387076, 1.000000000000000000, 0.8660254037844387076, 1.000000000000000000, 0.8660254037844387076, 1.000000000000000000, 0.8660254037844387076, 1.000000000000000000, 0.8660254037844387076, 1.000000000000000000, 0.8660254037844387076, 1.000000000000000000, 0.8660254037844387076, 1.000000000000000000, 0.8660254037844387076, 1.000000000000000000, 0.8660254037844387076, 1.000000000000000000, 0.8660254037844387076, 1.000000000000000000, 0.8660254037844387076, 1.000000000000000000, 0.8660254037844387076, 1.000000000000000000, 0.8660254037844387076, 1.000000000000000000, 0.8660254037844387076, 1.000000000000000000, 0.8660254037844387076, 1.000000000000000000, 0.8660254037844387076, 1.000000000000000000, 0.8660254037844387076, 1.000000000000000000, 0.8660254037844387076, 1.000000000000000000, 0.8660254037844387076, 1.000000000000000000, 0.8660254037844387076, 1.000000000000000000, 0.8660254037844387076, 1.000000000000000000, 0.8660254037844387076, 1.000000000000000000, 0.8660254037844387076, 1.000000000000000000, 0.8660254037844387076, 1.000000000000000000, 0.8660254037844387076, 1.000000000000000000, 0.8660254037844387076, 1.000000000000000000, 0.8660254037844387076, 1.000000000000000000, 0.8660254037844387076, 1.000000000000000000, 0.8660254037844387076, 1.000000000000000000, 0.8660254037844387076, 1.000000000000000000, 0.8660254037844387076, 1.000000000000000000, 0.8660254037844387076, 1.000000000000000000, 0.8660254037844387076, 1.000000000000000000, 0.8660254037844387076, 1.000000000000000000, 0.8660254037844387076, 1.000000000000000000, 0.8660254037844387076, 1.000000000000000000, 0.8660254037844387076, 1.000000000000000000, 0.8660254037844387076, 1.000000000000000000, 0.8660254037844387076, 1.000000000000000000, 0.8660254037844387076, 1.000000000000000000, 0.8660254037844387076, 1.000000000000000000, 0.8660254037844387076, 1.000000000000000000, 0.8660254037844387076, 1.000000000000000000, 0.8660254037844387076, 1.000000000000000000, 0.8660254037844387076, 1.000000000000000000, 0.8660254037844387076, 1.000000000000000000, 0.8660254037844387076, 1.000000000000000000, 0.8660254037844387076, 1.000000000000000000, 0.8660254037844387076, 1.000000000000000000, 0.8660254037844387076, 1.000000000000000000, 0.8660254037844387076, 1.000000000000000000, 0.9298872124336470257, 0.9331585307975728272 ) ) 
 REPRESENTATION_ITEM ( '' )  );
#60564=CARTESIAN_POINT ( 'NONE',  ( -5.461236948206312114, 5.265864615862458464, 0.7998128361456341429 ) ) ;
#60565=CARTESIAN_POINT ( 'NONE',  ( 6.277061933002788585, 6.425586464699131639, 0.7216878364870317197 ) ) ;
#60566=CARTESIAN_POINT ( 'NONE',  ( 0.7499999999999902300, 3.733333333333352488, 1.299038105676669330 ) ) ;
#60568=CARTESIAN_POINT ( 'NONE',  ( -5.759516327706961647, 5.613857225279885732, -0.7998128361456221525 ) ) ;
#60569=CARTESIAN_POINT ( 'NONE',  ( 0.1479172090190853939, 8.281400213891396689, -2.000566733410582554 ) ) ;
#60570=( BOUNDED_CURVE ( )  B_SPLINE_CURVE ( 2, ( #102835, #20494, #56215, #173184, #156930, #136415, #72442 ),
 .UNSPECIFIED., .F., .T. ) 
 B_SPLINE_CURVE_WITH_KNOTS ( ( 3, 2, 2, 3 ),
 ( 0.2000000000000000944, 0.2041666666666667185, 0.2083333333333333981, 0.2125000000000000222 ),
 .UNSPECIFIED. ) 
 CURVE ( )  GEOMETRIC_REPRESENTATION_ITEM ( )  RATIONAL_B_SPLINE_CURVE ( ( 0.9999999999999973355, 0.8660254037844413721, 1.000000000000000000, 0.8660254037844387076, 1.000000000000000000, 0.8660254037844378194, 1.000000000000000888 ) ) 
 REPRESENTATION_ITEM ( '' )  );
#60573=CARTESIAN_POINT ( 'NONE',  ( 0.6823417656249917140, 4.592708333674755394, 1.181850606188765695 ) ) ;
#60576=MECHANICAL_DESIGN_GEOMETRIC_PRESENTATION_REPRESENTATION('',(#153990),#12036);
#60577=CARTESIAN_POINT ( 'NONE',  ( -2.765500147507697459, 5.209872024525476597, 1.082531754730560403 ) ) ;
#60582=CARTESIAN_POINT ( 'NONE',  ( 4.813308228051395687, 5.574280006603454574, 1.199719254218462483 ) ) ;
#60585=CARTESIAN_POINT ( 'NONE',  ( 4.905139262582266291, 4.827437033166341429, 0.6004564335717228474 ) ) ;
#60588=CARTESIAN_POINT ( 'NONE',  ( -0.6823417656250003738, 0.7802083336747520637, -1.181850606188749264 ) ) ;
#60591=CARTESIAN_POINT ( 'NONE',  ( -10.29471871147821282, 10.90492667301307605, -0.7998128361456291469 ) ) ;
#60592=CARTESIAN_POINT ( 'NONE',  ( -6.683806541412780078, 6.900121841177441873, -0.7216878364870267237 ) ) ;
#60595=VERTEX_POINT ( 'NONE', #100585 ) ;
#60596=CARTESIAN_POINT ( 'NONE',  ( -0.6823417656250212460, 4.051041667008085767, 1.181850606188767472 ) ) ;
#60604=CARTESIAN_POINT ( 'NONE',  ( -6.033015167956805591, 8.061603667414825480, -1.443375672974058777 ) ) ;
#60611=CARTESIAN_POINT ( 'NONE',  ( -4.731432421044873493, 7.503459676985569260, -1.082531754730548412 ) ) ;
#60621=DIRECTION ( 'NONE',  ( 3.347138415753903010E-16, 0.6000000000000018652, -0.7999999999999984901 ) ) ;
#60623=CARTESIAN_POINT ( 'NONE',  ( -2.578021764892882040, 6.159442492350315490, 0.7998128361456341429 ) ) ;
#60626=CARTESIAN_POINT ( 'NONE',  ( -0.7500000000000006661, 1.108333333333356929, -1.299038105676652011 ) ) ;
#60628=CARTESIAN_POINT ( 'NONE',  ( 8.107412671292022921, 12.40247251657532956, 0.7216878364870438212 ) ) ;
#60629=CARTESIAN_POINT ( 'NONE',  ( 7.253775878511261155, 8.421492265473332850, 1.199719254218462483 ) ) ;
#60634=CARTESIAN_POINT ( 'NONE',  ( 3.897079088924235712, 6.634010472798538949, 1.199719254218462483 ) ) ;
#60635=( BOUNDED_SURFACE ( )  B_SPLINE_SURFACE ( 1, 2, ( 
 ( #28943, #129727, #93966, #192486, #179465, #11608, #45211, #10539, #76613, #61436, #146981, #97162, #26793, #79812, #209800, #111326, #176268, #44138, #126525, #145924, #177329, #210873, #48412, #31090, #211936, #46273, #114524, #92898, #62498, #110259, #128663, #95027, #112389, #194631, #208735, #160007, #158944, #96097, #178401, #161077, #78742, #60362, #63571, #143803, #195711, #47346, #127602, #27870, #163217, #113460, #14800, #142726, #80891, #212998, #64635, #130774, #196769, #213163, #46433, #129889, #97325, #148200, #116809, #162312, #33361, #114688, #130937, #128814, #146082, #13897, #196930, #83170, #16021, #96260, #78904, #79979, #30171, #164435, #195873, #17092, #12830, #145026, #113624, #179628, #212094, #149254, #197987, #99443, #211030, #48568, #62656, #63730, #65830, #64793, #199036, #214200, #47512, #133037, #31249, #180680, #115740, #165499, #131979, #194796, #112551, #181730, #178562, #827, #14955, #163381, #81053, #66897, #147137, #32305, #49615, #98372, #82107, #50684, #161243, #182809, #34426, #137294, #136220, #117887, #134107, #103716, #202240, #102645, #53892, #168701, #54962, #21357, #85319, #121114, #187079, #52816, #38712, #169767, #183880, #200116, #151402, #35492, #101570, #4038, #138356, #2974, #87463, #154601, #69042, #118954, #167637, #100499, #84250, #20305, #19239, #135159, #150336, #122183, #184933, #201178, #120027, #36557, #86390, #152458, #166575, #153531, #71176, #70107, #186003, #104792, #37638, #5100, #67963, #203312, #170838, #22429, #88539, #6180, #72248, #18162, #204373, #56030, #188149, #1904, #51767, #11531, #108047, #43002, #125373, #10459, #7247, #175129, #93888, #92818, #76532, #127521, #171911, #190277, #89613, #207596, #26716, #75477, #74417, #110180, #209717, #105886, #141589, #140516, #124318, #189224, #109115, #8332, #156742, #158862, #59215, #61362, #90681, #206528, #157808, #142645, #208653, #191336, #57094, #126442, #40864, #58160, #60284, #41934, #192405, #39780, #44060, #176190, #27790, #159928, #77601, #174072, #143724, #155664, #106969, #23508, #172993, #139426, #24574, #25644, #91755, #9406, #73324, #205461, #123259, #213962, #113381, #82920, #148993, #179388, #80810, #144789, #146900, #29934, #46193, #65582, #47266, #131729, #31008, #32055, #568, #97083, #66635, #15778, #96018, #165244, #181487, #197734, #62419, #130697, #193492, #196689, #163135, #16838, #94948, #45134, #28861, #160996, #162071, #98143, #14719, #111244, #180438, #49375, #115492, #177249, #212920, #78661, #13660, #129647, #164192, #12588, #81864, #210796, #33116, #147948, #48328, #114438, #99193, #64554, #128583, #194549, #112311, #178326, #79732, #145848, #211855, #63491, #195632, #118689, #103446, #135953, #169506, #153256, #52557, #22150, #88265, #184673, #20040, #83984, #86127, #183619, #199859, #4831, #200908, #70911, #36295, #185737, #154333, #102371, #5908, #21088, #35226 ),
 ( #51502, #150072, #137021, #117628, #85056, #116551, #182543, #167382, #38443, #1644, #152200, #170568, #198783, #2709, #67702, #133849, #17898, #119758, #68783, #168441, #132780, #203048, #53626, #3767, #50432, #34169, #69842, #101302, #201968, #151142, #37370, #87191, #100241, #18972, #54689, #166309, #134902, #120840, #186815, #104523, #60030, #108850, #158605, #55756, #41674, #138091, #139157, #191078, #124056, #109922, #58965, #205187, #43809, #73058, #190022, #26456, #10204, #125120, #204104, #187881, #92565, #39508, #76279, #140247, #56828, #8067, #142387, #90408, #6977, #42745, #74153, #107785, #9145, #71981, #23235, #206268, #174876, #173810, #25389, #106700, #208396, #27526, #121912, #91488, #172725, #156478, #122998, #141330, #40595, #188955, #207344, #157549, #93625, #24303, #57893, #75219, #126181, #192145, #175933, #89346, #159667, #105607, #171638, #155395, #194297, #196438, #32867, #97890, #64305, #14460, #146648, #162881, #145601, #48082, #61101, #160737, #212663, #144532, #110983, #12331, #211596, #178061, #63232, #114193, #80551, #180193, #31814, #129395, #115249, #181239, #195374, #113122, #176989, #179128, #62175, #78411, #163951, #79482, #15526, #47006, #130450, #98943, #30750, #11269, #81612, #128334, #197489, #213714, #147696, #94696, #65337, #77347, #131484, #96831, #49131, #127260, #143459, #193231, #44878, #45942, #209457, #28607, #210541, #112061, #29679, #95763, #161816, #13406, #50186, #133605, #101052, #151958, #120597, #166066, #37123, #118446, #134664, #132542, #149828, #17653, #200667, #86948, #19798, #99999, #82670, #83736, #33925, #168199, #1398, #164997, #136776, #18726, #85882, #36050, #135710, #198540, #3528, #4592, #69603, #201736, #38202, #148754, #167141, #324, #184433, #53377, #70666, #119512, #185498, #16588, #66394, #84810, #116307, #102130, #103202, #52317, #199610, #20850, #186574, #182297, #169264, #51253, #34981, #67459, #153016, #117378, #183375, #202805, #54454, #150899, #2460, #68536, #7813, #91240, #107535, #189776, #121672, #190833, #39265, #204940, #41427, #72819, #74969, #125938, #42492, #157300, #173567, #25138, #8890, #24067, #141079, #154089, #105359, #207088, #22987, #203872, #171396, #90170, #56591, #156236, #58717, #124867, #108601, #174629, #73906, #208151, #59781, #139999, #206020, #55516, #57656, #155159, #89105, #26205, #172480, #92322, #123815, #158364, #191896, #9956, #104276, #76033, #6741, #142136, #170320, #21908, #187638, #88018, #5657, #71737, #137851, #138923, #122752, #188714, #40350, #106456, #94444, #96578, #177810, #131244, #30494, #113940, #47828, #15273, #95517, #143217, #12090, #194037, #162625, #213464, #44620, #130193, #211348, #13153, #11014, #28348, #110735, #79230, #179935, #112867, #192967, #175681, #176735, #127009, #46756, #160483, #43558, #81360, #111804, #178882, #129142, #14201, #77090, #80295, #78157, #128081, #144288 ) ),
 .UNSPECIFIED., .F., .F., .T. ) 
 B_SPLINE_SURFACE_WITH_KNOTS ( ( 2, 2 ),
 ( 3, 2, 2, 2, 2, 2, 2, 2, 2, 2, 2, 2, 2, 2, 2, 2, 2, 2, 2, 2, 2, 2, 2, 2, 2, 2, 2, 2, 2, 2, 2, 2, 2, 2, 2, 2, 2, 2, 2, 2, 2, 2, 2, 2, 2, 2, 2, 2, 2, 2, 2, 2, 2, 2, 2, 2, 2, 2, 2, 2, 2, 2, 2, 2, 2, 2, 2, 2, 2, 2, 2, 2, 2, 2, 2, 2, 2, 2, 2, 2, 2, 2, 2, 2, 2, 2, 2, 2, 2, 2, 2, 2, 2, 2, 2, 2, 2, 2, 2, 2, 2, 2, 2, 2, 2, 2, 2, 2, 2, 2, 2, 2, 2, 2, 2, 2, 2, 2, 2, 2, 2, 2, 2, 2, 2, 2, 2, 2, 2, 2, 2, 2, 2, 2, 2, 2, 2, 2, 2, 2, 2, 2, 2, 2, 2, 2, 2, 2, 2, 2, 2, 2, 2, 2, 2, 2, 2, 2, 2, 2, 2, 2, 2, 2, 2, 2, 2, 2, 3 ),
 ( 0.000000000000000000, 1.000000000000000000 ),
 ( 0.000000000000000000, 0.005952380952380952051, 0.01190476190476190410, 0.01785714285714285615, 0.02380952380952380820, 0.02976190476190476025, 0.03571428571428571230, 0.04166666666666666435, 0.04761904761904761640, 0.05357142857142856845, 0.05952380952380952051, 0.06547619047619047949, 0.07142857142857142461, 0.07738095238095238360, 0.08333333333333332871, 0.08928571428571428770, 0.09523809523809523281, 0.1011904761904761918, 0.1071428571428571369, 0.1130952380952380959, 0.1190476190476190410, 0.1250000000000000000, 0.1309523809523809590, 0.1369047619047619180, 0.1428571428571428492, 0.1488095238095238082, 0.1547619047619047672, 0.1607142857142857262, 0.1666666666666666574, 0.1726190476190476164, 0.1785714285714285754, 0.1845238095238095344, 0.1904761904761904656, 0.1964285714285714246, 0.2023809523809523836, 0.2083333333333333426, 0.2142857142857142738, 0.2202380952380952328, 0.2261904761904761918, 0.2321428571428571508, 0.2380952380952380820, 0.2440476190476190410, 0.2500000000000000000, 0.2559523809523809312, 0.2619047619047619180, 0.2678571428571428492, 0.2738095238095238360, 0.2797619047619047672, 0.2857142857142856984, 0.2916666666666666852, 0.2976190476190476164, 0.3035714285714285476, 0.3095238095238095344, 0.3154761904761904656, 0.3214285714285714524, 0.3273809523809523836, 0.3333333333333333148, 0.3392857142857143016, 0.3452380952380952328, 0.3511904761904761640, 0.3571428571428571508, 0.3630952380952380820, 0.3690476190476190688, 0.3750000000000000000, 0.3809523809523809312, 0.3869047619047619180, 0.3928571428571428492, 0.3988095238095238360, 0.4047619047619047672, 0.4107142857142856984, 0.4166666666666666852, 0.4226190476190476164, 0.4285714285714285476, 0.4345238095238095344, 0.4404761904761904656, 0.4464285714285714524, 0.4523809523809523836, 0.4583333333333333148, 0.4642857142857143016, 0.4702380952380952328, 0.4761904761904761640, 0.4821428571428571508, 0.4880952380952380820, 0.4940476190476190688, 0.5000000000000000000, 0.5059523809523809312, 0.5119047619047618625, 0.5178571428571429047, 0.5238095238095238360, 0.5297619047619047672, 0.5357142857142856984, 0.5416666666666666297, 0.5476190476190476719, 0.5535714285714286031, 0.5595238095238095344, 0.5654761904761904656, 0.5714285714285713969, 0.5773809523809523281, 0.5833333333333333703, 0.5892857142857143016, 0.5952380952380952328, 0.6011904761904761640, 0.6071428571428570953, 0.6130952380952381375, 0.6190476190476190688, 0.6250000000000000000, 0.6309523809523809312, 0.6369047619047618625, 0.6428571428571429047, 0.6488095238095238360, 0.6547619047619047672, 0.6607142857142856984, 0.6666666666666666297, 0.6726190476190476719, 0.6785714285714286031, 0.6845238095238095344, 0.6904761904761904656, 0.6964285714285713969, 0.7023809523809523281, 0.7083333333333333703, 0.7142857142857143016, 0.7202380952380952328, 0.7261904761904761640, 0.7321428571428570953, 0.7380952380952381375, 0.7440476190476190688, 0.7500000000000000000, 0.7559523809523809312, 0.7619047619047618625, 0.7678571428571429047, 0.7738095238095238360, 0.7797619047619047672, 0.7857142857142856984, 0.7916666666666666297, 0.7976190476190476719, 0.8035714285714286031, 0.8095238095238095344, 0.8154761904761904656, 0.8214285714285713969, 0.8273809523809523281, 0.8333333333333333703, 0.8392857142857143016, 0.8452380952380952328, 0.8511904761904761640, 0.8571428571428570953, 0.8630952380952381375, 0.8690476190476190688, 0.8750000000000000000, 0.8809523809523809312, 0.8869047619047618625, 0.8928571428571429047, 0.8988095238095238360, 0.9047619047619047672, 0.9107142857142856984, 0.9166666666666666297, 0.9226190476190476719, 0.9285714285714286031, 0.9345238095238095344, 0.9404761904761904656, 0.9464285714285713969, 0.9523809523809523281, 0.9583333333333333703, 0.9642857142857143016, 0.9702380952380952328, 0.9761904761904761640, 0.9821428571428570953, 0.9880952380952381375, 0.9940476190476190688, 1.000000000000000000 ),
 .UNSPECIFIED. ) 
 GEOMETRIC_REPRESENTATION_ITEM ( )  RATIONAL_B_SPLINE_SURFACE ( (
 ( 1.000000000000000000, 0.8660254037844387076, 1.000000000000000000, 0.8660254037844387076, 1.000000000000000000, 0.8660254037844387076, 1.000000000000000000, 0.8660254037844387076, 1.000000000000000000, 0.8660254037844387076, 1.000000000000000000, 0.8660254037844387076, 1.000000000000000000, 0.8660254037844387076, 1.000000000000000000, 0.8660254037844387076, 1.000000000000000000, 0.8660254037844387076, 1.000000000000000000, 0.8660254037844387076, 1.000000000000000000, 0.8660254037844387076, 1.000000000000000000, 0.8660254037844387076, 1.000000000000000000, 0.8660254037844387076, 1.000000000000000000, 0.8660254037844387076, 1.000000000000000000, 0.8660254037844387076, 1.000000000000000000, 0.8660254037844387076, 1.000000000000000000, 0.8660254037844387076, 1.000000000000000000, 0.8660254037844387076, 1.000000000000000000, 0.8660254037844387076, 1.000000000000000000, 0.8660254037844387076, 1.000000000000000000, 0.8660254037844387076, 1.000000000000000000, 0.8660254037844387076, 1.000000000000000000, 0.8660254037844387076, 1.000000000000000000, 0.8660254037844387076, 1.000000000000000000, 0.8660254037844387076, 1.000000000000000000, 0.8660254037844387076, 1.000000000000000000, 0.8660254037844387076, 1.000000000000000000, 0.8660254037844387076, 1.000000000000000000, 0.8660254037844387076, 1.000000000000000000, 0.8660254037844387076, 1.000000000000000000, 0.8660254037844387076, 1.000000000000000000, 0.8660254037844387076, 1.000000000000000000, 0.8660254037844387076, 1.000000000000000000, 0.8660254037844387076, 1.000000000000000000, 0.8660254037844387076, 1.000000000000000000, 0.8660254037844387076, 1.000000000000000000, 0.8660254037844387076, 1.000000000000000000, 0.8660254037844387076, 1.000000000000000000, 0.8660254037844387076, 1.000000000000000000, 0.8660254037844387076, 1.000000000000000000, 0.8660254037844387076, 1.000000000000000000, 0.8660254037844387076, 1.000000000000000000, 0.8660254037844387076, 1.000000000000000000, 0.8660254037844387076, 1.000000000000000000, 0.8660254037844387076, 1.000000000000000000, 0.8660254037844387076, 1.000000000000000000, 0.8660254037844387076, 1.000000000000000000, 0.8660254037844387076, 1.000000000000000000, 0.8660254037844387076, 1.000000000000000000, 0.8660254037844387076, 1.000000000000000000, 0.8660254037844387076, 1.000000000000000000, 0.8660254037844387076, 1.000000000000000000, 0.8660254037844387076, 1.000000000000000000, 0.8660254037844387076, 1.000000000000000000, 0.8660254037844387076, 1.000000000000000000, 0.8660254037844387076, 1.000000000000000000, 0.8660254037844387076, 1.000000000000000000, 0.8660254037844387076, 1.000000000000000000, 0.8660254037844387076, 1.000000000000000000, 0.8660254037844387076, 1.000000000000000000, 0.8660254037844387076, 1.000000000000000000, 0.8660254037844387076, 1.000000000000000000, 0.8660254037844387076, 1.000000000000000000, 0.8660254037844387076, 1.000000000000000000, 0.8660254037844387076, 1.000000000000000000, 0.8660254037844387076, 1.000000000000000000, 0.8660254037844387076, 1.000000000000000000, 0.8660254037844387076, 1.000000000000000000, 0.8660254037844387076, 1.000000000000000000, 0.8660254037844387076, 1.000000000000000000, 0.8660254037844387076, 1.000000000000000000, 0.8660254037844387076, 1.000000000000000000, 0.8660254037844387076, 1.000000000000000000, 0.8660254037844387076, 1.000000000000000000, 0.8660254037844387076, 1.000000000000000000, 0.8660254037844387076, 1.000000000000000000, 0.8660254037844387076, 1.000000000000000000, 0.8660254037844387076, 1.000000000000000000, 0.8660254037844387076, 1.000000000000000000, 0.8660254037844387076, 1.000000000000000000, 0.8660254037844387076, 1.000000000000000000, 0.8660254037844387076, 1.000000000000000000, 0.8660254037844387076, 1.000000000000000000, 0.8660254037844387076, 1.000000000000000000, 0.8660254037844387076, 1.000000000000000000, 0.8660254037844387076, 1.000000000000000000, 0.8660254037844387076, 1.000000000000000000, 0.8660254037844387076, 1.000000000000000000, 0.8660254037844387076, 1.000000000000000000, 0.8660254037844387076, 1.000000000000000000, 0.8660254037844387076, 1.000000000000000000, 0.8660254037844387076, 1.000000000000000000, 0.8660254037844387076, 1.000000000000000000, 0.8660254037844387076, 1.000000000000000000, 0.8660254037844387076, 1.000000000000000000, 0.8660254037844387076, 1.000000000000000000, 0.8660254037844387076, 1.000000000000000000, 0.8660254037844387076, 1.000000000000000000, 0.8660254037844387076, 1.000000000000000000, 0.8660254037844387076, 1.000000000000000000, 0.8660254037844387076, 1.000000000000000000, 0.8660254037844387076, 1.000000000000000000, 0.8660254037844387076, 1.000000000000000000, 0.8660254037844387076, 1.000000000000000000, 0.8660254037844387076, 1.000000000000000000, 0.8660254037844387076, 1.000000000000000000, 0.8660254037844387076, 1.000000000000000000, 0.8660254037844387076, 1.000000000000000000, 0.8660254037844387076, 1.000000000000000000, 0.8660254037844387076, 1.000000000000000000, 0.8660254037844387076, 1.000000000000000000, 0.8660254037844387076, 1.000000000000000000, 0.8660254037844387076, 1.000000000000000000, 0.8660254037844387076, 1.000000000000000000, 0.8660254037844387076, 1.000000000000000000, 0.8660254037844387076, 1.000000000000000000, 0.8660254037844387076, 1.000000000000000000, 0.8660254037844387076, 1.000000000000000000, 0.8660254037844387076, 1.000000000000000000, 0.8660254037844387076, 1.000000000000000000, 0.8660254037844387076, 1.000000000000000000, 0.8660254037844387076, 1.000000000000000000, 0.8660254037844387076, 1.000000000000000000, 0.8660254037844387076, 1.000000000000000000, 0.8660254037844387076, 1.000000000000000000, 0.8660254037844387076, 1.000000000000000000, 0.8660254037844387076, 1.000000000000000000, 0.8660254037844387076, 1.000000000000000000, 0.8660254037844387076, 1.000000000000000000, 0.8660254037844387076, 1.000000000000000000, 0.8660254037844387076, 1.000000000000000000, 0.8660254037844387076, 1.000000000000000000, 0.8660254037844387076, 1.000000000000000000, 0.8660254037844387076, 1.000000000000000000, 0.8660254037844387076, 1.000000000000000000, 0.8660254037844387076, 1.000000000000000000, 0.8660254037844387076, 1.000000000000000000, 0.8660254037844387076, 1.000000000000000000, 0.8660254037844387076, 1.000000000000000000, 0.8660254037844387076, 1.000000000000000000, 0.8660254037844387076, 1.000000000000000000, 0.8660254037844387076, 1.000000000000000000, 0.8660254037844387076, 1.000000000000000000, 0.8660254037844387076, 1.000000000000000000, 0.8660254037844387076, 1.000000000000000000, 0.8660254037844387076, 1.000000000000000000, 0.8660254037844387076, 1.000000000000000000, 0.8660254037844387076, 1.000000000000000000, 0.8660254037844387076, 1.000000000000000000, 0.8660254037844387076, 1.000000000000000000, 0.8660254037844387076, 1.000000000000000000, 0.8660254037844387076, 1.000000000000000000, 0.8660254037844387076, 1.000000000000000000, 0.8660254037844387076, 1.000000000000000000, 0.8660254037844387076, 1.000000000000000000, 0.8660254037844387076, 1.000000000000000000, 0.8660254037844387076, 1.000000000000000000, 0.8660254037844387076, 1.000000000000000000, 0.8660254037844387076, 1.000000000000000000, 0.8660254037844387076, 1.000000000000000000, 0.8660254037844387076, 1.000000000000000000, 0.8660254037844387076, 1.000000000000000000, 0.8660254037844387076, 1.000000000000000000, 0.8660254037844387076, 1.000000000000000000, 0.8660254037844387076, 1.000000000000000000, 0.8660254037844387076, 1.000000000000000000, 0.8660254037844387076, 1.000000000000000000, 0.8660254037844387076, 1.000000000000000000),
 ( 1.000000000000000000, 0.8660254037844387076, 1.000000000000000000, 0.8660254037844387076, 1.000000000000000000, 0.8660254037844387076, 1.000000000000000000, 0.8660254037844387076, 1.000000000000000000, 0.8660254037844387076, 1.000000000000000000, 0.8660254037844387076, 1.000000000000000000, 0.8660254037844387076, 1.000000000000000000, 0.8660254037844387076, 1.000000000000000000, 0.8660254037844387076, 1.000000000000000000, 0.8660254037844387076, 1.000000000000000000, 0.8660254037844387076, 1.000000000000000000, 0.8660254037844387076, 1.000000000000000000, 0.8660254037844387076, 1.000000000000000000, 0.8660254037844387076, 1.000000000000000000, 0.8660254037844387076, 1.000000000000000000, 0.8660254037844387076, 1.000000000000000000, 0.8660254037844387076, 1.000000000000000000, 0.8660254037844387076, 1.000000000000000000, 0.8660254037844387076, 1.000000000000000000, 0.8660254037844387076, 1.000000000000000000, 0.8660254037844387076, 1.000000000000000000, 0.8660254037844387076, 1.000000000000000000, 0.8660254037844387076, 1.000000000000000000, 0.8660254037844387076, 1.000000000000000000, 0.8660254037844387076, 1.000000000000000000, 0.8660254037844387076, 1.000000000000000000, 0.8660254037844387076, 1.000000000000000000, 0.8660254037844387076, 1.000000000000000000, 0.8660254037844387076, 1.000000000000000000, 0.8660254037844387076, 1.000000000000000000, 0.8660254037844387076, 1.000000000000000000, 0.8660254037844387076, 1.000000000000000000, 0.8660254037844387076, 1.000000000000000000, 0.8660254037844387076, 1.000000000000000000, 0.8660254037844387076, 1.000000000000000000, 0.8660254037844387076, 1.000000000000000000, 0.8660254037844387076, 1.000000000000000000, 0.8660254037844387076, 1.000000000000000000, 0.8660254037844387076, 1.000000000000000000, 0.8660254037844387076, 1.000000000000000000, 0.8660254037844387076, 1.000000000000000000, 0.8660254037844387076, 1.000000000000000000, 0.8660254037844387076, 1.000000000000000000, 0.8660254037844387076, 1.000000000000000000, 0.8660254037844387076, 1.000000000000000000, 0.8660254037844387076, 1.000000000000000000, 0.8660254037844387076, 1.000000000000000000, 0.8660254037844387076, 1.000000000000000000, 0.8660254037844387076, 1.000000000000000000, 0.8660254037844387076, 1.000000000000000000, 0.8660254037844387076, 1.000000000000000000, 0.8660254037844387076, 1.000000000000000000, 0.8660254037844387076, 1.000000000000000000, 0.8660254037844387076, 1.000000000000000000, 0.8660254037844387076, 1.000000000000000000, 0.8660254037844387076, 1.000000000000000000, 0.8660254037844387076, 1.000000000000000000, 0.8660254037844387076, 1.000000000000000000, 0.8660254037844387076, 1.000000000000000000, 0.8660254037844387076, 1.000000000000000000, 0.8660254037844387076, 1.000000000000000000, 0.8660254037844387076, 1.000000000000000000, 0.8660254037844387076, 1.000000000000000000, 0.8660254037844387076, 1.000000000000000000, 0.8660254037844387076, 1.000000000000000000, 0.8660254037844387076, 1.000000000000000000, 0.8660254037844387076, 1.000000000000000000, 0.8660254037844387076, 1.000000000000000000, 0.8660254037844387076, 1.000000000000000000, 0.8660254037844387076, 1.000000000000000000, 0.8660254037844387076, 1.000000000000000000, 0.8660254037844387076, 1.000000000000000000, 0.8660254037844387076, 1.000000000000000000, 0.8660254037844387076, 1.000000000000000000, 0.8660254037844387076, 1.000000000000000000, 0.8660254037844387076, 1.000000000000000000, 0.8660254037844387076, 1.000000000000000000, 0.8660254037844387076, 1.000000000000000000, 0.8660254037844387076, 1.000000000000000000, 0.8660254037844387076, 1.000000000000000000, 0.8660254037844387076, 1.000000000000000000, 0.8660254037844387076, 1.000000000000000000, 0.8660254037844387076, 1.000000000000000000, 0.8660254037844387076, 1.000000000000000000, 0.8660254037844387076, 1.000000000000000000, 0.8660254037844387076, 1.000000000000000000, 0.8660254037844387076, 1.000000000000000000, 0.8660254037844387076, 1.000000000000000000, 0.8660254037844387076, 1.000000000000000000, 0.8660254037844387076, 1.000000000000000000, 0.8660254037844387076, 1.000000000000000000, 0.8660254037844387076, 1.000000000000000000, 0.8660254037844387076, 1.000000000000000000, 0.8660254037844387076, 1.000000000000000000, 0.8660254037844387076, 1.000000000000000000, 0.8660254037844387076, 1.000000000000000000, 0.8660254037844387076, 1.000000000000000000, 0.8660254037844387076, 1.000000000000000000, 0.8660254037844387076, 1.000000000000000000, 0.8660254037844387076, 1.000000000000000000, 0.8660254037844387076, 1.000000000000000000, 0.8660254037844387076, 1.000000000000000000, 0.8660254037844387076, 1.000000000000000000, 0.8660254037844387076, 1.000000000000000000, 0.8660254037844387076, 1.000000000000000000, 0.8660254037844387076, 1.000000000000000000, 0.8660254037844387076, 1.000000000000000000, 0.8660254037844387076, 1.000000000000000000, 0.8660254037844387076, 1.000000000000000000, 0.8660254037844387076, 1.000000000000000000, 0.8660254037844387076, 1.000000000000000000, 0.8660254037844387076, 1.000000000000000000, 0.8660254037844387076, 1.000000000000000000, 0.8660254037844387076, 1.000000000000000000, 0.8660254037844387076, 1.000000000000000000, 0.8660254037844387076, 1.000000000000000000, 0.8660254037844387076, 1.000000000000000000, 0.8660254037844387076, 1.000000000000000000, 0.8660254037844387076, 1.000000000000000000, 0.8660254037844387076, 1.000000000000000000, 0.8660254037844387076, 1.000000000000000000, 0.8660254037844387076, 1.000000000000000000, 0.8660254037844387076, 1.000000000000000000, 0.8660254037844387076, 1.000000000000000000, 0.8660254037844387076, 1.000000000000000000, 0.8660254037844387076, 1.000000000000000000, 0.8660254037844387076, 1.000000000000000000, 0.8660254037844387076, 1.000000000000000000, 0.8660254037844387076, 1.000000000000000000, 0.8660254037844387076, 1.000000000000000000, 0.8660254037844387076, 1.000000000000000000, 0.8660254037844387076, 1.000000000000000000, 0.8660254037844387076, 1.000000000000000000, 0.8660254037844387076, 1.000000000000000000, 0.8660254037844387076, 1.000000000000000000, 0.8660254037844387076, 1.000000000000000000, 0.8660254037844387076, 1.000000000000000000, 0.8660254037844387076, 1.000000000000000000, 0.8660254037844387076, 1.000000000000000000, 0.8660254037844387076, 1.000000000000000000, 0.8660254037844387076, 1.000000000000000000, 0.8660254037844387076, 1.000000000000000000, 0.8660254037844387076, 1.000000000000000000, 0.8660254037844387076, 1.000000000000000000, 0.8660254037844387076, 1.000000000000000000, 0.8660254037844387076, 1.000000000000000000, 0.8660254037844387076, 1.000000000000000000, 0.8660254037844387076, 1.000000000000000000, 0.8660254037844387076, 1.000000000000000000, 0.8660254037844387076, 1.000000000000000000, 0.8660254037844387076, 1.000000000000000000, 0.8660254037844387076, 1.000000000000000000, 0.8660254037844387076, 1.000000000000000000, 0.8660254037844387076, 1.000000000000000000, 0.8660254037844387076, 1.000000000000000000, 0.8660254037844387076, 1.000000000000000000, 0.8660254037844387076, 1.000000000000000000, 0.8660254037844387076, 1.000000000000000000, 0.8660254037844387076, 1.000000000000000000, 0.8660254037844387076, 1.000000000000000000, 0.8660254037844387076, 1.000000000000000000, 0.8660254037844387076, 1.000000000000000000, 0.8660254037844387076, 1.000000000000000000, 0.8660254037844387076, 1.000000000000000000, 0.8660254037844387076, 1.000000000000000000, 0.8660254037844387076, 1.000000000000000000, 0.8660254037844387076, 1.000000000000000000, 0.8660254037844387076, 1.000000000000000000) ) ) 
 REPRESENTATION_ITEM ( '' )  SURFACE ( )  );
#60636=CARTESIAN_POINT ( 'NONE',  ( -0.5050423914800155067, 7.726475908227449452, -1.936073478083378596 ) ) ;
#60643=CARTESIAN_POINT ( 'NONE',  ( -6.762819695118240659, 6.784377820593065600, 0.7998128361456341429 ) ) ;
#60648=CARTESIAN_POINT ( 'NONE',  ( 1.364683531249990311, 3.634375000341416584, 1.214306433183764966E-14 ) ) ;
#60649=CARTESIAN_POINT ( 'NONE',  ( 9.097157884645296733, 10.67606762258344055, -1.082531754730543083 ) ) ;
#60650=CARTESIAN_POINT ( 'NONE',  ( -7.874588291438845644, 8.081441182967111558, -0.7998128361456291469 ) ) ;
#60653=CARTESIAN_POINT ( 'NONE',  ( 3.669453130792974971, 7.432779085900453886, 1.040834085586084257E-14 ) ) ;
#60654=CARTESIAN_POINT ( 'NONE',  ( -5.117312914154178216, 8.057616602233474978, -1.199719254218452047 ) ) ;
#60659=ADVANCED_FACE ( 'NONE', ( #22512 ), #159308, .F. ) ;
#60661=CARTESIAN_POINT ( 'NONE',  ( 5.965224400332808763, 9.903252867122883885, -0.7216878364870267237 ) ) ;
#60664=CARTESIAN_POINT ( 'NONE',  ( 1.364683531249988757, 1.946875000341415030, 0.000000000000000000 ) ) ;
#60666=CARTESIAN_POINT ( 'NONE',  ( 5.544921637864819175, 7.492161215640853023, -1.443375672974057666 ) ) ;
#60668=CARTESIAN_POINT ( 'NONE',  ( -3.145128448690310830, 6.613140923539910787, -0.7216878364870267237 ) ) ;
#60670=B_SPLINE_CURVE_WITH_KNOTS ( 'NONE', 3,
 ( #100346, #167485, #201015, #150182, #6017, #55861, #138198, #204208, #68885, #22262, #203155, #184776, #71013, #135004 ),
 .UNSPECIFIED., .F., .F.,
 ( 4, 2, 2, 2, 2, 2, 4 ),
 ( 0.0002398601398896809181, 0.09869445199344967223, 0.1971490438470096807, 0.2956036357005696891, 0.3202172836639597397, 0.3448309316273497904, 0.3940582275541297808 ),
 .UNSPECIFIED. ) ;
#60676=CARTESIAN_POINT ( 'NONE',  ( -3.980123661693549142, 7.843117270353603843, 0.1539385989055529202 ) ) ;
#60683=CARTESIAN_POINT ( 'NONE',  ( 4.971035877704902184, 8.951292290631053916, 1.040834085586084257E-14 ) ) ;
#60694=CARTESIAN_POINT ( 'NONE',  ( 3.551873057100274789, 7.087676300018221021, 0.7216878364870298324 ) ) ;
#60695=CARTESIAN_POINT ( 'NONE',  ( -1.364683531250012516, 1.592708333674756727, 0.7879004041258379498 ) ) ;
#60696=CARTESIAN_POINT ( 'NONE',  ( 8.263858322729371153, 9.599921783727809910, -1.199719254218446718 ) ) ;
#60699=CARTESIAN_POINT ( 'NONE',  ( 0.4588732745636386334, 6.941177932071661338, -3.888237242762151435 ) ) ;
#60700=CARTESIAN_POINT ( 'NONE',  ( 3.009546912109283934, 6.454962464195385330, 0.000000000000000000 ) ) ;
#60704=CARTESIAN_POINT ( 'NONE',  ( 1.499999999999989120, 2.504166666666687302, 0.8660254037844524744 ) ) ;
#60705=CARTESIAN_POINT ( 'NONE',  ( 5.503720292143644777, 8.508425209887878538, 1.199719254218462483 ) ) ;
#60706=CARTESIAN_POINT ( 'NONE',  ( -7.877450944739929461, 9.149113176073413456, 1.199719254218462483 ) ) ;
#60709=CARTESIAN_POINT ( 'NONE',  ( 1.499999999999956257, 5.795833333333352044, -0.8660254037844512531 ) ) ;
#60710=CARTESIAN_POINT ( 'NONE',  ( 0.6823417656249882723, 2.676041667008084879, -1.181850606188749264 ) ) ;
#60713=CARTESIAN_POINT ( 'NONE',  ( 3.521367211247359741, 5.131347717920458962, -1.599625672291262513 ) ) ;
#60719=CARTESIAN_POINT ( 'NONE',  ( 1.499999999999987121, 1.077083334016148308, -0.8660254037844253849 ) ) ;
#60721=CARTESIAN_POINT ( 'NONE',  ( -5.696397096036042385, 9.797547045350714967, -0.7998128361456231517 ) ) ;
#60722=CARTESIAN_POINT ( 'NONE',  ( -2.155383234892699562, 5.458438174109348395, 1.040834085586084257E-14 ) ) ;
#60730=CARTESIAN_POINT ( 'NONE',  ( 6.823831386379729302, 6.855558127064808716, -0.7998128361456281477 ) ) ;
#60734=CARTESIAN_POINT ( 'NONE',  ( 6.928380191783277908, 8.041863964290678624, 1.199719254218462483 ) ) ;
#60740=CARTESIAN_POINT ( 'NONE',  ( -7.067878151425722955, 7.140279352951794500, 0.7998128361456341429 ) ) ;
#60742=CARTESIAN_POINT ( 'NONE',  ( 5.027376032568989572, 4.759693547618927489, 0.7998128361456341429 ) ) ;
#60743=ORIENTED_EDGE ( 'NONE', *, *, #44167, .T. ) ;
#60748=CARTESIAN_POINT ( 'NONE',  ( 4.171261675657679469, 7.370687464442305270, 0.7961138118306176903 ) ) ;
#60759=CARTESIAN_POINT ( 'NONE',  ( -3.946537740505278613, 2.817530495244580102, 0.7750000000000135669 ) ) ;
#60760=CARTESIAN_POINT ( 'NONE',  ( -4.121315508874276112, 4.870918184183829602, -1.082531754730549967 ) ) ;
#60761=CARTESIAN_POINT ( 'NONE',  ( 7.537970219518073556, 9.817384560903001045, -1.443375672974057666 ) ) ;
#60763=CARTESIAN_POINT ( 'NONE',  ( -5.427341564172148303, 5.226320001155936090, 0.000000000000000000 ) ) ;
#60767=CARTESIAN_POINT ( 'NONE',  ( 6.923409998072794558, 11.22906209772695618, 1.040834085586084257E-14 ) ) ;
#60769=CARTESIAN_POINT ( 'NONE',  ( -5.717788096661253761, 7.693838750903348789, 1.599625672291269396 ) ) ;
#60775=VERTEX_POINT ( 'NONE', #211351 ) ;
#60784=CARTESIAN_POINT ( 'NONE',  ( 9.154780037725547714, 11.70366268214508487, 1.599625672291279388 ) ) ;
#60785=CARTESIAN_POINT ( 'NONE',  ( -3.581325132304157943, 7.329963087663487364, -0.7998128361456281477 ) ) ;
#60788=CARTESIAN_POINT ( 'NONE',  ( 3.497640442645619796, 6.064035702186436616, -1.082531754730543083 ) ) ;
#60792=CARTESIAN_POINT ( 'NONE',  ( -2.449219305563052895, 6.009172956465517856, 1.040834085586084257E-14 ) ) ;
#60793=CARTESIAN_POINT ( 'NONE',  ( -4.627410500965859264, 4.293067094081919777, 0.7998128361456341429 ) ) ;
#60796=CARTESIAN_POINT ( 'NONE',  ( 9.215791728987056786, 11.77484298861683598, -1.599625672291262513 ) ) ;
#60801=CARTESIAN_POINT ( 'NONE',  ( -7.888146445052511169, 8.097259028849730811, 1.040834085586084257E-14 ) ) ;
#60802=CARTESIAN_POINT ( 'NONE',  ( 6.173040012923759257, 6.096301524699504704, -0.7998128361456281477 ) ) ;
#60806=CARTESIAN_POINT ( 'NONE',  ( -1.201851678989727383E-14, 0.8843750003414173610, 1.575800808251672791 ) ) ;
#60807=ORIENTED_EDGE ( 'NONE', *, *, #59736, .F. ) ;
#60809=CARTESIAN_POINT ( 'NONE',  ( 5.992340707560141588, 9.934888558888093968, 0.7216878364870438212 ) ) ;
#60817=CARTESIAN_POINT ( 'NONE',  ( 9.042925270190625753, 11.57316545335434199, 1.443375672974076540 ) ) ;
#60819=EDGE_LOOP ( 'NONE', ( #26352, #46444, #198613, #158604 ) ) ;
#60825=CARTESIAN_POINT ( 'NONE',  ( -9.317477881089553549, 11.89347683273641820, 1.599625672291281386 ) ) ;
#60826=DIRECTION ( 'NONE',  ( -5.578564026256490882E-16, -1.000000000000000000, -9.066213480720158442E-32 ) ) ;
#60841=CARTESIAN_POINT ( 'NONE',  ( -1.402160292154681736E-14, 1.618750000682814827, -1.732050807568863648 ) ) ;
#60847=CARTESIAN_POINT ( 'NONE',  ( 7.832860060393120882, 10.16142270859057462, 1.599625672291281386 ) ) ;
#60848=CARTESIAN_POINT ( 'NONE',  ( 1.364683531249988757, -0.8656249996585805295, 0.000000000000000000 ) ) ;
#60851=CARTESIAN_POINT ( 'NONE',  ( 9.029367117021314115, 12.51771682229149008, -1.082531754730543083 ) ) ;
#60852=CARTESIAN_POINT ( 'NONE',  ( -6.561783159334145132, 6.757761228752363181, -0.7216878364870278340 ) ) ;
#60857=CARTESIAN_POINT ( 'NONE',  ( -6.507023659554960204, 9.678945805201045971, 1.199719254218452047 ) ) ;
#60859=ORIENTED_EDGE ( 'NONE', *, *, #213533, .F. ) ;
#60860=CARTESIAN_POINT ( 'NONE',  ( -1.201851678989727383E-14, 1.743750000682815493, 1.732050807568877637 ) ) ;
#60875=CARTESIAN_POINT ( 'NONE',  ( -7.330154606482786050, 11.70359747420527619, 0.000000000000000000 ) ) ;
#60876=CARTESIAN_POINT ( 'NONE',  ( 7.579171565239241737, 8.801120566655981747, 1.199719254218462483 ) ) ;
#60883=CARTESIAN_POINT ( 'NONE',  ( -8.843996274815957293, 9.212417163573759282, 1.040834085586084257E-14 ) ) ;
#60886=CARTESIAN_POINT ( 'NONE',  ( 0.9999999999999833467, 9.200000000000018829, 0.4000000000000144551 ) ) ;
#60889=CARTESIAN_POINT ( 'NONE',  ( 4.192495815123822744, 5.914331089109666983, -1.599625672291255185 ) ) ;
#60893=CARTESIAN_POINT ( 'NONE',  ( -4.608882153641705059, 7.464447381635583412, -1.199719254218452047 ) ) ;
#60898=CARTESIAN_POINT ( 'NONE',  ( -4.798872725802947770, 6.964071866812478362, -1.434128239971976138 ) ) ;
#60907=CARTESIAN_POINT ( 'NONE',  ( 7.305145839664861640, 7.417091655897478653, 0.7998128361456341429 ) ) ;
#60916=CARTESIAN_POINT ( 'NONE',  ( -1.500000000000015099, 0.1604166673494879791, -0.8660254037844383745 ) ) ;
#60929=CARTESIAN_POINT ( 'NONE',  ( 5.043269954603547767, 4.986162489899998995, -0.7216878364870197293 ) ) ;
#60933=CARTESIAN_POINT ( 'NONE',  ( -10.48453286206953727, 11.12637651536962125, 0.7998128361456462443 ) ) ;
#60935=CARTESIAN_POINT ( 'NONE',  ( 8.387690588348714726, 12.93738945304888333, 1.040834085586084257E-14 ) ) ;
#60938=EDGE_CURVE ( 'NONE', #21699, #12172, #94074, .T. ) ;
#60945=CARTESIAN_POINT ( 'NONE',  ( 1.364683531249986537, -0.6364583329919177856, 0.7879004041258500513 ) ) ;
#60950=CARTESIAN_POINT ( 'NONE',  ( -6.417086777969760902, 6.381022750586497594, 0.7998128361456341429 ) ) ;
#60953=CARTESIAN_POINT ( 'NONE',  ( 1.499999999999987566, -0.7249999999999825473, 0.000000000000000000 ) ) ;
#60955=CARTESIAN_POINT ( 'NONE',  ( -1.500000000000011324, 5.379166666666692187, -0.8660254037844313801 ) ) ;
#60961=CARTESIAN_POINT ( 'NONE',  ( -1.364683531250000748, -0.4906249996585801409, 0.000000000000000000 ) ) ;
#60963=CARTESIAN_POINT ( 'NONE',  ( -7.690499447449645309, 9.995335326823163058, 1.599625672291295375 ) ) ;
#60966=ADVANCED_FACE ( 'NONE', ( #67210 ), #52065, .T. ) ;
#60970=CARTESIAN_POINT ( 'NONE',  ( -1.402160292154681736E-14, 0.6343750003414162508, 1.575800808251672791 ) ) ;
#60977=CARTESIAN_POINT ( 'NONE',  ( -1.499999999999997780, 3.681250000682819046, 1.214306433183764966E-14 ) ) ;
#60979=CARTESIAN_POINT ( 'NONE',  ( 8.107412671292042461, 9.521364873671299023, 1.082531754730558626 ) ) ;
#60982=CARTESIAN_POINT ( 'NONE',  ( -5.229694566569281555, 7.124396299129368337, 1.599625672291267398 ) ) ;
#60984=CARTESIAN_POINT ( 'NONE',  ( -1.201851678989727383E-14, 5.368750000682816825, -1.732050807568863648 ) ) ;
#60987=CARTESIAN_POINT ( 'NONE',  ( -4.253507506385335368, 5.985511395581417204, 1.599625672291267398 ) ) ;
#60988=CARTESIAN_POINT ( 'NONE',  ( 5.951666246274792016, 8.927065806420504401, 1.082531754730558626 ) ) ;
#60989=CARTESIAN_POINT ( 'NONE',  ( -9.964879715919934711, 10.72804054476916313, 0.7216878364870438212 ) ) ;
#60995=CARTESIAN_POINT ( 'NONE',  ( 8.419250204406344196, 12.76628297187536809, 1.040834085586084257E-14 ) ) ;
#61010=CARTESIAN_POINT ( 'NONE',  ( 9.077347539549325717, 10.54899253668443393, -1.199719254218446718 ) ) ;
#61015=CARTESIAN_POINT ( 'NONE',  ( -0.6823417656250246877, 0.05104166700808931978, 1.181850606188755259 ) ) ;
#61016=CARTESIAN_POINT ( 'NONE',  ( 6.005898861173831094, 6.109229547565340646, 1.040834085586084257E-14 ) ) ;
#61017=ORIENTED_EDGE ( 'NONE', *, *, #172073, .T. ) ;
#61018=CARTESIAN_POINT ( 'NONE',  ( -7.361714222540411967, 11.53249099303175385, 0.000000000000000000 ) ) ;
#61022=CARTESIAN_POINT ( 'NONE',  ( -4.613852347352193739, 4.277249248199312071, 1.214306433183764966E-14 ) ) ;
#61037=CARTESIAN_POINT ( 'NONE',  ( 4.628062896017484995, 7.124942365035781933, -1.349859865738218145 ) ) ;
#61045=CARTESIAN_POINT ( 'NONE',  ( -8.703971430293361067, 9.256980878204810637, 0.7216878364870438212 ) ) ;
#61050=CARTESIAN_POINT ( 'NONE',  ( 5.666418135507635512, 8.698239360479199433, 1.199719254218462483 ) ) ;
#61053=CARTESIAN_POINT ( 'NONE',  ( 3.379006598303866848, 4.965260336153046516, -1.599625672291262513 ) ) ;
#61055=CARTESIAN_POINT ( 'NONE',  ( -4.569261463005423352, 5.289558780716470565, -1.199719254218446718 ) ) ;
#61059=CARTESIAN_POINT ( 'NONE',  ( -3.418627288940168096, 7.140148937072163804, -0.7998128361456281477 ) ) ;
#61062=CARTESIAN_POINT ( 'NONE',  ( 4.355193658487811703, 6.104145239700998538, -1.599625672291255185 ) ) ;
#61063=CARTESIAN_POINT ( 'NONE',  ( 8.589254009457354400, 9.979550084910457031, -1.199719254218446718 ) ) ;
#61064=CARTESIAN_POINT ( 'NONE',  ( 0.1851009548687417572, 6.360931694699415218, 3.114575592932423476 ) ) ;
#61066=CARTESIAN_POINT ( 'NONE',  ( 4.901917485988815493, 6.882077164048857831, 1.422854466155202502 ) ) ;
#61067=CARTESIAN_POINT ( 'NONE',  ( 4.744990575102895569, 5.598539094783909320, -1.082531754730548412 ) ) ;
#61069=CARTESIAN_POINT ( 'NONE',  ( 5.626270559546852290, 5.666329862333807199, 0.7216878364870122908 ) ) ;
#61074=CARTESIAN_POINT ( 'NONE',  ( 7.592202833528386208, 7.959917515312338487, 1.040834085586084257E-14 ) ) ;
#61075=CARTESIAN_POINT ( 'NONE',  ( -9.820183334999905256, 10.35130206712171130, 1.040834085586084257E-14 ) ) ;
#61078=CARTESIAN_POINT ( 'NONE',  ( -8.839026081105473054, 12.39961529701003684, -1.199719254218446718 ) ) ;
#61079=CARTESIAN_POINT ( 'NONE',  ( -5.554036483092550824, 9.631459663583308739, -0.7998128361456231517 ) ) ;
#61088=CARTESIAN_POINT ( 'NONE',  ( 10.21336978979620191, 10.81001959771741205, 0.7998128361456462443 ) ) ;
#61092=CARTESIAN_POINT ( 'NONE',  ( 4.220665892555866883, 3.818531717603609987, -0.7998128361456211532 ) ) ;
#61101=CARTESIAN_POINT ( 'NONE',  ( 1.499999999999989120, 3.525000000000021227, 1.214306433183764966E-14 ) ) ;
#61102=CARTESIAN_POINT ( 'NONE',  ( 6.647575389402066826, 6.649926130590872120, 1.040834085586084257E-14 ) ) ;
#61105=CARTESIAN_POINT ( 'NONE',  ( 8.134528978519385944, 8.592631351135175066, -0.7216878364870267237 ) ) ;
#61106=CARTESIAN_POINT ( 'NONE',  ( -10.27671724903424888, 11.09185100006920877, 1.040834085586084257E-14 ) ) ;
#61109=CARTESIAN_POINT ( 'NONE',  ( 9.053093885623066939, 11.58502883802551153, -1.599625672291262513 ) ) ;
#61111=CARTESIAN_POINT ( 'NONE',  ( -4.627410500965859264, 4.293067094081919777, 0.7998128361456341429 ) ) ;
#61113=CARTESIAN_POINT ( 'NONE',  ( 0.6823417656249899377, 0.5927083336747518416, 1.181850606188755259 ) ) ;
#61118=CARTESIAN_POINT ( 'NONE',  ( -1.364683531250014514, -0.7197916663252461600, 0.7879004041258379498 ) ) ;
#61120=CARTESIAN_POINT ( 'NONE',  ( 9.856941372335116469, 11.45851867493453291, 1.199719254218450271 ) ) ;
#61124=CARTESIAN_POINT ( 'NONE',  ( -3.212919216314315207, 5.731860938133201522, 1.082531754730560403 ) ) ;
#61127=CARTESIAN_POINT ( 'NONE',  ( -7.400052914960538963, 7.527816577075747695, 1.040834085586084257E-14 ) ) ;
#61130=CARTESIAN_POINT ( 'NONE',  ( 4.976006071415387311, 5.764094157194782575, 1.199719254218462483 ) ) ;
#61136=CARTESIAN_POINT ( 'NONE',  ( 10.39640486358069360, 11.02356051713265650, 0.7998128361456462443 ) ) ;
#61139=CARTESIAN_POINT ( 'NONE',  ( -4.934277840369690971, 7.844075682818238526, -1.199719254218452047 ) ) ;
#61143=CARTESIAN_POINT ( 'NONE',  ( 7.242026607993941489, 11.60078147596829901, 0.7998128361456462443 ) ) ;
#61145=CARTESIAN_POINT ( 'NONE',  ( 6.577677080924314801, 10.82570702772039262, 1.040834085586084257E-14 ) ) ;
#61148=CARTESIAN_POINT ( 'NONE',  ( -10.30383355670593737, 11.12348669235284504, -0.7216878364870267237 ) ) ;
#61152=CARTESIAN_POINT ( 'NONE',  ( -5.994676475536691029, 10.14553965476814845, 0.7998128361456481317 ) ) ;
#61156=CARTESIAN_POINT ( 'NONE',  ( -6.121777486219434294, 6.006025806897081765, -0.2357381234046468377 ) ) ;
#61157=CARTESIAN_POINT ( 'NONE',  ( 1.364683531249988535, 2.113541667008087099, 0.7879004041258500513 ) ) ;
#61160=CARTESIAN_POINT ( 'NONE',  ( 7.673551755654734130, 9.015193805427763607, -1.082531754730537976 ) ) ;
#61179=CARTESIAN_POINT ( 'NONE',  ( 7.736899214892750010, 12.17813285068358020, 1.040834085586084257E-14 ) ) ;
#61183=CARTESIAN_POINT ( 'NONE',  ( -4.973143418114339021, 4.696422164088486895, 0.7998128361456341429 ) ) ;
#61184=CARTESIAN_POINT ( 'NONE',  ( -8.019811557683421910, 9.315200557840817908, 1.199719254218462483 ) ) ;
#61186=ORIENTED_EDGE ( 'NONE', *, *, #64812, .F. ) ;
#61191=CARTESIAN_POINT ( 'NONE',  ( -1.001543065824772872E-14, 4.743750000682822154, 1.732050807568877637 ) ) ;
#61192=CARTESIAN_POINT ( 'NONE',  ( 6.740374924288304648, 11.01552117831172062, 1.040834085586084257E-14 ) ) ;
#61195=CARTESIAN_POINT ( 'NONE',  ( -6.828502922777144768, 11.11833717654868892, 0.7998128361456481317 ) ) ;
#61197=CARTESIAN_POINT ( 'NONE',  ( -0.6823417656250003738, 2.717708333674753618, -1.181850606188749264 ) ) ;
#61201=CARTESIAN_POINT ( 'NONE',  ( -7.285838599102589797E-14, 7.078193277237590841, -2.121339347286493648 ) ) ;
#61203=CARTESIAN_POINT ( 'NONE',  ( -9.815740026613960723, 11.51441345488021106, -1.082531754730539753 ) ) ;
#61207=CARTESIAN_POINT ( 'NONE',  ( -0.6823417656250003738, 3.030208333674754062, -1.181850606188749264 ) ) ;
#61208=AXIS2_PLACEMENT_3D ( 'NONE', #78769, #62526, #128688 ) ;
#61215=CARTESIAN_POINT ( 'NONE',  ( -0.6823417656250212460, 2.801041667008084879, 1.181850606188767472 ) ) ;
#61217=CARTESIAN_POINT ( 'NONE',  ( -3.764360206088648297, 7.543504007078730922, -0.7998128361456281477 ) ) ;
#61218=CARTESIAN_POINT ( 'NONE',  ( 4.950698647284403009, 8.927565521807144577, 1.040834085586084257E-14 ) ) ;
#61222=CARTESIAN_POINT ( 'NONE',  ( -0.6823417656250212460, 4.613541667008086655, 1.181850606188767472 ) ) ;
#61225=CARTESIAN_POINT ( 'NONE',  ( -1.364683531250000748, -0.2406249996585799189, 0.000000000000000000 ) ) ;
#61227=CARTESIAN_POINT ( 'NONE',  ( -5.422898255786209099, 5.429062174613087599, -0.7216878364870207285 ) ) ;
#61230=CARTESIAN_POINT ( 'NONE',  ( 6.005898861173831094, 6.109229547565340646, 1.040834085586084257E-14 ) ) ;
#61233=CARTESIAN_POINT ( 'NONE',  ( -9.013473194986783454, 9.410140237106395134, -0.7998128361456291469 ) ) ;
#61234=CARTESIAN_POINT ( 'NONE',  ( -8.514157279702027736, 10.95626946445095307, -1.443375672974059665 ) ) ;
#61240=CARTESIAN_POINT ( 'NONE',  ( -7.524412065460066579, 7.880828285899290186, 0.7216878364870317197 ) ) ;
#61242=CARTESIAN_POINT ( 'NONE',  ( -1.402160292154681736E-14, 0.2593750003414224681, -1.575800808251665908 ) ) ;
#61254=CARTESIAN_POINT ( 'NONE',  ( -1.500000000000015099, -0.8291666666666407393, 0.8660254037844403729 ) ) ;
#61255=CARTESIAN_POINT ( 'NONE',  ( 8.229436053370669413, 10.62409470039771442, 1.443375672974076540 ) ) ;
#61263=CARTESIAN_POINT ( 'NONE',  ( 6.094553744542824170, 7.069066442510145265, 1.199719254218462483 ) ) ;
#61265=CARTESIAN_POINT ( 'NONE',  ( -5.427341564172148303, 5.226320001155936090, 0.000000000000000000 ) ) ;
#61267=CARTESIAN_POINT ( 'NONE',  ( 0.000000000000000000, -2.856854249492362996, 0.000000000000000000 ) ) ;
#61268=CARTESIAN_POINT ( 'NONE',  ( -4.884430620531565737, 4.928167907039282980, -0.5181559072752897066 ) ) ;
#61269=CARTESIAN_POINT ( 'NONE',  ( 1.364683531249986537, 1.176041667008082658, 0.7879004041258500513 ) ) ;
#61271=CARTESIAN_POINT ( 'NONE',  ( -7.808606406466886973, 11.19745900993164511, 1.199719254218453823 ) ) ;
#61281=VECTOR ( 'NONE', #7501, 1000.000000000000000 ) ;
#61286=EDGE_LOOP ( 'NONE', ( #86923, #45849, #99932, #96170, #67074, #54357, #202881, #200163, #117822, #83923, #7709, #119452, #174808, #148625, #195022, #140453, #137494, #164137 ) ) ;
#61290=CARTESIAN_POINT ( 'NONE',  ( 5.795220594837462436, 8.848508896363995291, -1.199719254218440723 ) ) ;
#61297=CARTESIAN_POINT ( 'NONE',  ( 9.284636267260101050, 9.726497154758602548, -0.7998128361456281477 ) ) ;
#61300=CARTESIAN_POINT ( 'NONE',  ( 7.964525173024008531, 11.37936423758166526, 1.199719254218460707 ) ) ;
#61302=CARTESIAN_POINT ( 'NONE',  ( 1.554911173149762016, 8.692115300649543741, -2.503913477513633357 ) ) ;
#61305=ORIENTED_EDGE ( 'NONE', *, *, #65262, .T. ) ;
#61309=CARTESIAN_POINT ( 'NONE',  ( -0.4998684179605343281, 7.978338306495868615, 1.936700108954719335 ) ) ;
#61315=CARTESIAN_POINT ( 'NONE',  ( -7.849807752632384172, 12.10193344480572897, 0.000000000000000000 ) ) ;
#61322=CARTESIAN_POINT ( 'NONE',  ( 3.974511587100456822, 7.788680618259193444, 1.040834085586084257E-14 ) ) ;
#61329=CARTESIAN_POINT ( 'NONE',  ( 3.158686601859607368, 6.628958768904106513, -0.7216878364870267237 ) ) ;
#61332=ORIENTED_EDGE ( 'NONE', *, *, #49246, .T. ) ;
#61337=CARTESIAN_POINT ( 'NONE',  ( -5.856232286098998152, 8.919689202835742847, 1.199719254218452047 ) ) ;
#61338=CARTESIAN_POINT ( 'NONE',  ( 4.800089777832203808, 5.120415418395356077, -0.7784788408505428636 ) ) ;
#61339=CARTESIAN_POINT ( 'NONE',  ( -3.436101866059630527, 6.096203712789787232, 1.199719254218462483 ) ) ;
#61344=CARTESIAN_POINT ( 'NONE',  ( -0.005132432257077002187, 7.078226584369338603, 2.121329534126264349 ) ) ;
#61347=CARTESIAN_POINT ( 'NONE',  ( 5.606460214450851964, 6.499623990736163037, 1.199719254218462483 ) ) ;
#61349=CARTESIAN_POINT ( 'NONE',  ( 4.161989969715248705, 4.726297878971393196, -2.420000000000000373 ) ) ;
#61362=CARTESIAN_POINT ( 'NONE',  ( -1.364683531250012516, 1.342708333674755616, 0.7879004041258379498 ) ) ;
#61364=CARTESIAN_POINT ( 'NONE',  ( 3.194917754314666514, 6.879154480009089134, 0.7998128361456321445 ) ) ;
#61365=AXIS2_PLACEMENT_3D ( 'NONE', #86812, #69469, #106314 ) ;
#61367=CARTESIAN_POINT ( 'NONE',  ( -7.375272376154101472, 7.706831981708990753, -0.7216878364870278340 ) ) ;
#61368=CARTESIAN_POINT ( 'NONE',  ( 4.026408433578586354, 7.641300905909586660, 1.040834085586084257E-14 ) ) ;
#61369=CARTESIAN_POINT ( 'NONE',  ( -5.192409643909507544, 9.001635651295671892, 0.7216878364870458196 ) ) ;
#61371=ORIENTED_EDGE ( 'NONE', *, *, #140986, .F. ) ;
#61373=CARTESIAN_POINT ( 'NONE',  ( 7.447506452608354088, 7.583179037664891098, 0.7998128361456341429 ) ) ;
#61375=CARTESIAN_POINT ( 'NONE',  ( -2.964627556058684554, 6.451541201391447267, 0.3872157855231770918 ) ) ;
#61379=CARTESIAN_POINT ( 'NONE',  ( -1.201851678989727383E-14, 4.446875000341417916, -1.575800808251660134 ) ) ;
#61383=CARTESIAN_POINT ( 'NONE',  ( 5.798083248138522272, 9.916180889470295412, 0.7998128361456462443 ) ) ;
#61385=CARTESIAN_POINT ( 'NONE',  ( -6.581593504430098385, 9.765943957555402122, -1.199719254218440723 ) ) ;
#61390=CARTESIAN_POINT ( 'NONE',  ( 7.944187942603509356, 11.35563746875774882, 1.199719254218460707 ) ) ;
#61392=CARTESIAN_POINT ( 'NONE',  ( -8.050844288416501016, 8.287073179441051707, 1.040834085586084257E-14 ) ) ;
#61394=CARTESIAN_POINT ( 'NONE',  ( 8.256552360598020002, 8.734991963560254646, -0.7216878364870267237 ) ) ;
#61395=CARTESIAN_POINT ( 'NONE',  ( 4.359152798643180837, 7.157646611464889119, -1.047953017514296370 ) ) ;
#61396=CARTESIAN_POINT ( 'NONE',  ( -9.991996023591624976, 10.75967623705280296, 1.040834085586084257E-14 ) ) ;
#61400=CARTESIAN_POINT ( 'NONE',  ( 6.145923705696426431, 6.064665832934283962, 0.7998128361456341429 ) ) ;
#61402=CARTESIAN_POINT ( 'NONE',  ( 8.269583629331492602, 11.73526576994040482, 1.199719254218450271 ) ) ;
#61403=CARTESIAN_POINT ( 'NONE',  ( -5.250693970737303928, 6.428279158139240224, 1.158874695820178324 ) ) ;
#61404=CARTESIAN_POINT ( 'NONE',  ( 2.900554798319789906, 5.471398800426671372, 1.199719254218452047 ) ) ;
#61405=CARTESIAN_POINT ( 'NONE',  ( -1.364683531250000748, 0.5093750003414208027, 0.000000000000000000 ) ) ;
#61407=CARTESIAN_POINT ( 'NONE',  ( -6.222829318992474157, 10.20379193889247382, 0.000000000000000000 ) ) ;
#61413=CARTESIAN_POINT ( 'NONE',  ( -4.327620591935813721, 7.230343590456815406, 0.9971501367836959062 ) ) ;
#61414=CARTESIAN_POINT ( 'NONE',  ( -1.402160292154681736E-14, -0.3656249996585805295, 1.575800808251672791 ) ) ;
#61417=CARTESIAN_POINT ( 'NONE',  ( 4.853455804012228647, 4.764712647543454693, 0.7216878364870317197 ) ) ;
#61420=CARTESIAN_POINT ( 'NONE',  ( -8.120970824461345217, 12.41829036193951730, 0.7216878364870458196 ) ) ;
#61425=CARTESIAN_POINT ( 'NONE',  ( -9.314088342463968218, 9.968783942403868892, 0.7216878364870438212 ) ) ;
#61428=CARTESIAN_POINT ( 'NONE',  ( -6.385527162356468445, 10.39360608948380538, 1.040834085586084257E-14 ) ) ;
#61431=CARTESIAN_POINT ( 'NONE',  ( -7.171900071504729191, 11.31104115015678779, -0.7216878364870267237 ) ) ;
#61436=CARTESIAN_POINT ( 'NONE',  ( -1.001543065824772872E-14, 5.634375000341415252, 1.575800808251672791 ) ) ;
#61437=CARTESIAN_POINT ( 'NONE',  ( -1.500000000000011324, 4.452083334016148086, 0.8660254037844403729 ) ) ;
#61438=CARTESIAN_POINT ( 'NONE',  ( 5.603691946294323323, 6.350013490765915591, -1.172630952486140243 ) ) ;
#61443=CARTESIAN_POINT ( 'NONE',  ( -8.518600588087975822, 8.832788862391110385, 1.040834085586084257E-14 ) ) ;
#61445=EDGE_CURVE ( 'NONE', #123984, #106888, #137593, .T. ) ;
#61447=CARTESIAN_POINT ( 'NONE',  ( 6.335737856287750880, 6.286115675290828264, -0.7998128361456281477 ) ) ;
#61452=CARTESIAN_POINT ( 'NONE',  ( 7.969495366734495434, 8.192166104145387706, 1.040834085586084257E-14 ) ) ;
#61455=LINE ( 'NONE', #62519, #29063 ) ;
#61456=ORIENTED_EDGE ( 'NONE', *, *, #122971, .F. ) ;
#61460=CARTESIAN_POINT ( 'NONE',  ( -5.748293942514186128, 6.769059690097084747, -1.082531754730544860 ) ) ;
#61466=CARTESIAN_POINT ( 'NONE',  ( 5.504247177468215568, 5.523969249908735613, 0.7216878364870122908 ) ) ;
#61470=CARTESIAN_POINT ( 'NONE',  ( -7.655550293210764856, 12.08322577538792331, 0.000000000000000000 ) ) ;
#61472=CARTESIAN_POINT ( 'NONE',  ( 8.127223016387999266, 11.56917838817298616, 1.199719254218460707 ) ) ;
#61473=CARTESIAN_POINT ( 'NONE',  ( -0.7500000000000249800, -0.05833333333331303105, 1.299038105676659116 ) ) ;
#61474=CARTESIAN_POINT ( 'NONE',  ( -9.450196763925152510, 10.98398329845622001, -1.199719254218441611 ) ) ;
#61477=CARTESIAN_POINT ( 'NONE',  ( -1.201851678989727383E-14, 3.071875000341420137, 1.575800808251672791 ) ) ;
#61478=EDGE_CURVE ( 'NONE', #158010, #68875, #188452, .T. ) ;
#61479=CARTESIAN_POINT ( 'NONE',  ( 3.708318708537623021, 4.285125567170706695, -1.199719254218446718 ) ) ;
#61482=CARTESIAN_POINT ( 'NONE',  ( 1.499999999999990896, 5.525000000000022560, 1.214306433183764966E-14 ) ) ;
#61485=CARTESIAN_POINT ( 'NONE',  ( 7.524412065460039933, 10.76193592880331984, -1.082531754730537976 ) ) ;
#61488=CARTESIAN_POINT ( 'NONE',  ( -5.992340707560165569, 8.014150130285418783, 1.443375672974064550 ) ) ;
#61489=CARTESIAN_POINT ( 'NONE',  ( 1.364683531249986537, 2.405208333674752286, -0.7879004041258239610 ) ) ;
#61493=CARTESIAN_POINT ( 'NONE',  ( -7.718669524881690336, 7.899535955317097624, 0.7998128361456462443 ) ) ;
#61494=CARTESIAN_POINT ( 'NONE',  ( -0.6823417656250212460, 4.113541667008085767, 1.181850606188767472 ) ) ;
#61500=CARTESIAN_POINT ( 'NONE',  ( 7.425061681778431399, 11.81432239538354345, 0.7998128361456462443 ) ) ;
#61503=CARTESIAN_POINT ( 'NONE',  ( -1.402160292154681736E-14, 0.5875000000000220046, -1.732050807568863648 ) ) ;
#61509=CARTESIAN_POINT ( 'NONE',  ( 7.886038904643079661, 12.35212915539230139, -0.7998128361456352531 ) ) ;
#61514=CARTESIAN_POINT ( 'NONE',  ( 9.576136569953906275, 10.06658084123472641, 0.000000000000000000 ) ) ;
#61515=CARTESIAN_POINT ( 'NONE',  ( -9.561524646135538319, 12.17819805862340310, -1.599625672291263179 ) ) ;
#61518=CARTESIAN_POINT ( 'NONE',  ( -0.6823417656250003738, -0.7822916663252423852, -1.181850606188749264 ) ) ;
#61522=CARTESIAN_POINT ( 'NONE',  ( 9.108380270282433244, 9.520865158284665952, 1.040834085586084257E-14 ) ) ;
#61525=CARTESIAN_POINT ( 'NONE',  ( -1.364683531250010295, 4.280208333674753618, 0.7879004041258379498 ) ) ;
#61527=CARTESIAN_POINT ( 'NONE',  ( -6.236387472606153892, 8.298871356172400127, -1.443375672974059665 ) ) ;
#61536=CARTESIAN_POINT ( 'NONE',  ( 7.377608144130607393, 11.75895993479440982, -0.7998128361456291469 ) ) ;
#61537=CARTESIAN_POINT ( 'NONE',  ( 2.493739017040997208, 8.265916556960590356, -2.456386464945223835 ) ) ;
#61542=CARTESIAN_POINT ( 'NONE',  ( -9.345647958521597687, 9.797677461230342999, 0.7998128361456462443 ) ) ;
#61543=CARTESIAN_POINT ( 'NONE',  ( 5.459129407796876166, 9.520734742405036144, 1.040834085586084257E-14 ) ) ;
#61545=CARTESIAN_POINT ( 'NONE',  ( 3.836594282542914236, 5.499112634431936542, 1.443375672974062551 ) ) ;
#61548=CARTESIAN_POINT ( 'NONE',  ( 5.169736645512481132, 4.925780929386339935, 0.7998128361456341429 ) ) ;
#61550=AXIS2_PLACEMENT_3D ( 'NONE', #157718, #74323, #109020 ) ;
#61557=CARTESIAN_POINT ( 'NONE',  ( -5.097502569058210753, 7.930541516334467467, -1.082531754730549967 ) ) ;
#61558=CARTESIAN_POINT ( 'NONE',  ( 3.161022370280501814, 6.839609865302569425, 0.000000000000000000 ) ) ;
#61562=CARTESIAN_POINT ( 'NONE',  ( -6.496328159242330536, 10.73079995242472862, 0.000000000000000000 ) ) ;
#61568=CARTESIAN_POINT ( 'NONE',  ( -8.136864746495904299, 12.64475930422059768, -0.7998128361456281477 ) ) ;
#61572=CARTESIAN_POINT ( 'NONE',  ( 8.620286740190458374, 8.951422706510690830, 1.040834085586084257E-14 ) ) ;
#61584=CARTESIAN_POINT ( 'NONE',  ( -8.830438121202295321, 9.196599317691152464, -0.7998128361456291469 ) ) ;
#61588=CARTESIAN_POINT ( 'NONE',  ( 6.561783159334121152, 8.678499657355050800, -1.443375672974057666 ) ) ;
#61592=CARTESIAN_POINT ( 'NONE',  ( -7.223796917982883592, 7.322184580601816428, -0.7998128361456291469 ) ) ;
#61595=CARTESIAN_POINT ( 'NONE',  ( -1.284279953904128524, 10.64264068711930733, -0.7749999999999892530 ) ) ;
#61603=CARTESIAN_POINT ( 'NONE',  ( -9.022061154889962964, 12.61315621642528129, -1.199719254218446718 ) ) ;
#61604=CARTESIAN_POINT ( 'NONE',  ( 7.052212457402625922, 11.37933163361175382, -0.7998128361456291469 ) ) ;
#61606=CARTESIAN_POINT ( 'NONE',  ( -2.968872451712654126, 6.407508927065978632, 1.040834085586084257E-14 ) ) ;
#61607=CARTESIAN_POINT ( 'NONE',  ( -4.595871994550918771, 6.958256438637705266, -1.193191807407071536 ) ) ;
#61616=CARTESIAN_POINT ( 'NONE',  ( 2.198393463710220264, 5.716542807637226886, 0.7998128361456462443 ) ) ;
#61625=CARTESIAN_POINT ( 'NONE',  ( 5.352771719296971042, 5.139321848801576387, 0.7998128361456341429 ) ) ;
#61626=CARTESIAN_POINT ( 'NONE',  ( -4.911285141672522059, 4.693790260148114513, 0.3511878651327460243 ) ) ;
#61630=CARTESIAN_POINT ( 'NONE',  ( -0.6823417656249969321, 3.530208333674754506, -1.181850606188749264 ) ) ;
#61635=CARTESIAN_POINT ( 'NONE',  ( 4.690231075323689325, 7.559354456931247412, 1.199719254218462483 ) ) ;
#61639=CARTESIAN_POINT ( 'NONE',  ( -4.249591082879585535, 7.045274465746411252, 1.199719254218464037 ) ) ;
#61640=CARTESIAN_POINT ( 'NONE',  ( 4.311129659021211147, 7.973475668925984472, 1.040834085586084257E-14 ) ) ;
#61641=CARTESIAN_POINT ( 'NONE',  ( -1.201851678989727383E-14, 3.212500000000018119, 1.732050807568877637 ) ) ;
#61643=CARTESIAN_POINT ( 'NONE',  ( -4.192495815123836955, 5.914331089109674089, -1.599625672291256295 ) ) ;
#61644=CARTESIAN_POINT ( 'NONE',  ( 0.2652791711382319617, 7.171141847836379313, -2.094821536884158508 ) ) ;
#61647=CARTESIAN_POINT ( 'NONE',  ( 1.364683531249988535, 4.113541667008088432, 0.7879004041258500513 ) ) ;
#61650=CARTESIAN_POINT ( 'NONE',  ( -4.202664430556263930, 5.926194473780837413, 1.443375672974064550 ) ) ;
#61655=CARTESIAN_POINT ( 'NONE',  ( 5.190073875932979419, 4.949507698210251938, 0.7998128361456341429 ) ) ;
#61658=CARTESIAN_POINT ( 'NONE',  ( 4.911177513620411439, 4.783069230954930084, 0.3872126393177600101 ) ) ;
#61663=CARTESIAN_POINT ( 'NONE',  ( 0.6823417656249882723, 0.7385416670080829915, -1.181850606188749264 ) ) ;
#61665=CARTESIAN_POINT ( 'NONE',  ( -8.272446282632566650, 12.80293776304669962, 0.7998128361456481317 ) ) ;
#61666=CARTESIAN_POINT ( 'NONE',  ( -5.219525951136845698, 8.072902128759544382, -1.082531754730543971 ) ) ;
#61670=CARTESIAN_POINT ( 'NONE',  ( 1.364683531249990311, 4.384375000341417028, 1.214306433183764966E-14 ) ) ;
#61678=CARTESIAN_POINT ( 'NONE',  ( -6.412643469139482910, 7.544134137826577380, 1.082531754730549967 ) ) ;
#61684=CARTESIAN_POINT ( 'NONE',  ( -5.788968402910818156, 7.776882441527838807, 1.443375672974064550 ) ) ;
#61691=CARTESIAN_POINT ( 'NONE',  ( 3.877268743828242936, 7.467304601200888570, 0.7216878364870187301 ) ) ;
#61696=CARTESIAN_POINT ( 'NONE',  ( 0.4734109229373711925, 6.656475628599715755, -3.353491478376180890 ) ) ;
#61697=CARTESIAN_POINT ( 'NONE',  ( -5.037017762676898158, 5.835274463666530131, -1.199719254218446718 ) ) ;
#61700=CARTESIAN_POINT ( 'NONE',  ( -0.7500000000000215383, 0.9416666666666878571, 1.299038105676659116 ) ) ;
#61703=CARTESIAN_POINT ( 'NONE',  ( 8.839552966430002101, 11.33589776563360019, -1.443375672974052559 ) ) ;
#61704=CARTESIAN_POINT ( 'NONE',  ( 7.039708073993665494, 9.236078724457858158, 1.599625672291281386 ) ) ;
#61709=CARTESIAN_POINT ( 'NONE',  ( 3.018661757337009810, 6.673522483535157868, 0.000000000000000000 ) ) ;
#61710=CARTESIAN_POINT ( 'NONE',  ( -0.4636475088197898886, 7.942422027498800219, -1.946104516853415678 ) ) ;
#61718=CARTESIAN_POINT ( 'NONE',  ( -6.738566041191992539, 7.820414121934134322, 1.199719254218450271 ) ) ;
#61724=CARTESIAN_POINT ( 'NONE',  ( -1.201851678989727383E-14, 3.321875000341421025, 1.575800808251672791 ) ) ;
#61725=CARTESIAN_POINT ( 'NONE',  ( 8.554831740098654436, 11.00372300158037042, 1.443375672974076540 ) ) ;
#61726=CARTESIAN_POINT ( 'NONE',  ( -6.388916700537716764, 8.476822122092563916, 1.599625672291283607 ) ) ;
#61729=CARTESIAN_POINT ( 'NONE',  ( 4.659198344590585350, 8.587481835331020719, 0.7998128361456462443 ) ) ;
#61730=CARTESIAN_POINT ( 'NONE',  ( -4.740547266272593596, 8.682388910626682943, -0.7998128361456281477 ) ) ;
#61734=CARTESIAN_POINT ( 'NONE',  ( -1.500000000000001332, 0.6812500006828161592, 0.000000000000000000 ) ) ;
#61736=ADVANCED_FACE ( 'NONE', ( #109418 ), #9699, .T. ) ;
#61738=CARTESIAN_POINT ( 'NONE',  ( 7.795575138177731844, 8.197185204069915798, 1.040834085586084257E-14 ) ) ;
#61741=CARTESIAN_POINT ( 'NONE',  ( 1.364683531249986537, 2.217708333674751398, -0.7879004041258239610 ) ) ;
#61743=CARTESIAN_POINT ( 'NONE',  ( 5.707619481228810798, 7.681975366232176583, -1.443375672974057666 ) ) ;
#61745=CARTESIAN_POINT ( 'NONE',  ( -2.819732761962335577, 5.273143408055916304, -1.082531754730543971 ) ) ;
#61750=CARTESIAN_POINT ( 'NONE',  ( -3.609978820808566802, 4.211641957610042120, -2.420000000000000373 ) ) ;
#61753=CARTESIAN_POINT ( 'NONE',  ( -4.432925279414208219, 7.308574008990986748, -1.253226476263115341 ) ) ;
#61754=CYLINDRICAL_SURFACE ( 'NONE', #72044, 0.08000000000000041800 ) ;
#61761=CARTESIAN_POINT ( 'NONE',  ( 7.467843683028853263, 7.606905806488803101, 0.7998128361456341429 ) ) ;
#61773=CARTESIAN_POINT ( 'NONE',  ( 3.877268743828266029, 6.506935386899531437, 1.082531754730558626 ) ) ;
#61774=CARTESIAN_POINT ( 'NONE',  ( 1.364683531249986537, 2.467708333674753174, -0.7879004041258239610 ) ) ;
#61775=CARTESIAN_POINT ( 'NONE',  ( 7.781490099239519509, 11.16582331816642260, 1.199719254218460707 ) ) ;
#61776=EDGE_CURVE ( 'NONE', #23582, #73840, #166722, .T. ) ;
#61779=CARTESIAN_POINT ( 'NONE',  ( -4.229253852459088137, 7.021547696922494808, 1.199719254218464037 ) ) ;
#61781=CIRCLE ( 'NONE', #179449, 0.07999999999999969635 ) ;
#61783=CARTESIAN_POINT ( 'NONE',  ( -1.500000000000013101, 2.170833333333357373, 0.8660254037844403729 ) ) ;
#61784=CARTESIAN_POINT ( 'NONE',  ( 5.961834861707224320, 7.978559976790334574, -1.599625672291262513 ) ) ;
#61785=CARTESIAN_POINT ( 'NONE',  ( -8.050844288416501016, 8.287073179441051707, 1.040834085586084257E-14 ) ) ;
#61788=CARTESIAN_POINT ( 'NONE',  ( 0.6823417656249882723, 2.926041667008084879, -1.181850606188754593 ) ) ;
#61791=CARTESIAN_POINT ( 'NONE',  ( 10.54788032175191326, 11.40820791823982994, 0.7216878364870317197 ) ) ;
#61796=CARTESIAN_POINT ( 'NONE',  ( -1.500000000000015099, 0.6604166673494823447, -0.8660254037844313801 ) ) ;
#61798=CARTESIAN_POINT ( 'NONE',  ( -6.531277313481209212, 8.642909503859968368, 1.599625672291283607 ) ) ;
#61799=CARTESIAN_POINT ( 'NONE',  ( -3.145128448690317935, 5.652771709238564313, -1.082531754730549967 ) ) ;
#61807=CARTESIAN_POINT ( 'NONE',  ( 6.986529229743720926, 7.045372277656132276, -0.7998128361456281477 ) ) ;
#61811=CARTESIAN_POINT ( 'NONE',  ( 7.156006149914539982, 7.243095351188763686, 1.040834085586084257E-14 ) ) ;
#61816=CARTESIAN_POINT ( 'NONE',  ( -4.882907879216086933, 8.848476292394087395, -0.7998128361456281477 ) ) ;
#61818=CARTESIAN_POINT ( 'NONE',  ( 4.390142812726693045, 4.016254791136236513, 1.214306433183764966E-14 ) ) ;
#61824=CARTESIAN_POINT ( 'NONE',  ( 4.546345379095670047, 6.970243970676179401, 1.177900817425497904 ) ) ;
#61833=CARTESIAN_POINT ( 'NONE',  ( 7.402388683381404988, 10.61957531637824204, -1.082531754730537976 ) ) ;
#61835=CARTESIAN_POINT ( 'NONE',  ( -5.066996723205291708, 6.934582148538044777, 1.599625672291267398 ) ) ;
#61836=CARTESIAN_POINT ( 'NONE',  ( -0.5100041365948099203, 6.733978373159967390, 3.471634244333542618 ) ) ;
#61840=CARTESIAN_POINT ( 'NONE',  ( -5.392392409933270514, 7.314210449720692786, 1.599625672291269396 ) ) ;
#61844=CARTESIAN_POINT ( 'NONE',  ( -0.006158830626153827259, 7.078243236992583398, 2.121324627965421872 ) ) ;
#61853=CARTESIAN_POINT ( 'NONE',  ( 1.474248253919626883, 7.378028154546084849, -4.279201940601814691 ) ) ;
#61854=CARTESIAN_POINT ( 'NONE',  ( -4.042302355168801320, 7.867769847672247074, 0.7998128361456341429 ) ) ;
#61857=CARTESIAN_POINT ( 'NONE',  ( 4.039966587192259873, 5.736380323189513852, 1.443375672974062551 ) ) ;
#61864=CARTESIAN_POINT ( 'NONE',  ( -3.066115294984855133, 6.728884944124295053, 0.7998128361456341429 ) ) ;
#61867=CARTESIAN_POINT ( 'NONE',  ( 10.21336978979620191, 10.81001959771741205, 0.7998128361456462443 ) ) ;
#61870=CARTESIAN_POINT ( 'NONE',  ( -7.226659571283968297, 8.389856573708110332, 1.199719254218450271 ) ) ;
#61871=CARTESIAN_POINT ( 'NONE',  ( 4.123651276850781144, 7.962676922967908411, -0.7998128361456221525 ) ) ;
#61873=CARTESIAN_POINT ( 'NONE',  ( 3.876741858503734761, 6.610283703974623393, 1.199719254218462483 ) ) ;
#61876=CARTESIAN_POINT ( 'NONE',  ( 0.6823417656249882723, 0.7385416670080829915, -1.181850606188749264 ) ) ;
#61877=VERTEX_POINT ( 'NONE', #47566 ) ;
#61879=CARTESIAN_POINT ( 'NONE',  ( 6.141480397310468575, 10.10888486359680982, 1.040834085586084257E-14 ) ) ;
#61882=CARTESIAN_POINT ( 'NONE',  ( -5.436456409399874623, 5.444880020495701523, 0.000000000000000000 ) ) ;
#61885=B_SPLINE_CURVE_WITH_KNOTS ( 'NONE', 3,
 ( #172632, #110885, #42645, #209357 ),
 .UNSPECIFIED., .F., .F.,
 ( 4, 4 ),
 ( 0.002911097519902588939, 0.003691190409735757919 ),
 .UNSPECIFIED. ) ;
#61889=CARTESIAN_POINT ( 'NONE',  ( 10.52076401408022299, 11.37657222595619189, 0.000000000000000000 ) ) ;
#61896=CARTESIAN_POINT ( 'NONE',  ( -3.332168893502611251, 7.719402352560151392, 2.450693629706233168 ) ) ;
#61898=CARTESIAN_POINT ( 'NONE',  ( -10.47775378526269918, 11.11846759242831872, -0.7998128361456221525 ) ) ;
#61913=( BOUNDED_SURFACE ( )  B_SPLINE_SURFACE ( 3, 2, ( 
 ( #212345, #96518, #181978 ),
 ( #65029, #49863, #195050 ),
 ( #14139, #61853, #193974 ),
 ( #80232, #146330, #45622 ) ),
 .UNSPECIFIED., .F., .F., .T. ) 
 B_SPLINE_SURFACE_WITH_KNOTS ( ( 4, 4 ),
 ( 3, 3 ),
 ( 0.000000000000000000, 0.0001288481725889855669 ),
 ( 0.000000000000000000, 1.000000000000000000 ),
 .UNSPECIFIED. ) 
 GEOMETRIC_REPRESENTATION_ITEM ( )  RATIONAL_B_SPLINE_SURFACE ( (
 ( 1.000000000000000000, 0.7779734834199504290, 1.000000000000000000),
 ( 1.000000000000000000, 0.8164436902898472015, 1.000000000000000000),
 ( 1.000000000000000000, 0.8496999780352315623, 1.000000000000000000),
 ( 1.000000000000000000, 0.8739472344198672138, 1.000000000000000000) ) ) 
 REPRESENTATION_ITEM ( '' )  SURFACE ( )  );
#61915=CARTESIAN_POINT ( 'NONE',  ( 1.499999999999989120, 1.556250000682817047, 0.000000000000000000 ) ) ;
#61921=DIRECTION ( 'NONE',  ( 5.578564026256490882E-16, 1.000000000000000000, 9.066213480720158442E-32 ) ) ;
#61922=CARTESIAN_POINT ( 'NONE',  ( 7.564559641420864899, 10.91273778404466199, -1.199719254218446718 ) ) ;
#61926=CARTESIAN_POINT ( 'NONE',  ( 2.737856954955798727, 5.281584649835344258, 1.199719254218452047 ) ) ;
#61927=CARTESIAN_POINT ( 'NONE',  ( -4.758548728716557541, 8.495464583570553785, 1.040834085586084257E-14 ) ) ;
#61932=CARTESIAN_POINT ( 'NONE',  ( -5.856232286098998152, 8.919689202835742847, 1.199719254218452047 ) ) ;
#61934=CARTESIAN_POINT ( 'NONE',  ( 0.7499999999999885647, 1.097916667349485564, -1.299038105676652899 ) ) ;
#61941=CARTESIAN_POINT ( 'NONE',  ( -4.731432421044888592, 4.622352034081546712, -0.7216878364870207285 ) ) ;
#61943=CARTESIAN_POINT ( 'NONE',  ( 4.196871964084724738, 7.339766560697110975, 0.8424661700066529146 ) ) ;
#61948=CARTESIAN_POINT ( 'NONE',  ( -9.667127221743832877, 11.23706883257798772, 1.199719254218462483 ) ) ;
#61949=CARTESIAN_POINT ( 'NONE',  ( 8.782984583554449998, 9.141236857102018831, 1.040834085586084257E-14 ) ) ;
#61957=CARTESIAN_POINT ( 'NONE',  ( -8.128276786592724790, 9.441743324901704426, -1.199719254218446718 ) ) ;
#61963=CARTESIAN_POINT ( 'NONE',  ( 3.246287715468270108, 5.874753870433235825, 1.199719254218450271 ) ) ;
#61969=ORIENTED_EDGE ( 'NONE', *, *, #98928, .F. ) ;
#61970=CARTESIAN_POINT ( 'NONE',  ( -9.110189153378817295, 12.71597221466224603, 1.199719254218462483 ) ) ;
#61973=CARTESIAN_POINT ( 'NONE',  ( -5.562564655730993124, 6.373022183664215135, -1.235959600235781330 ) ) ;
#61982=CARTESIAN_POINT ( 'NONE',  ( 5.282873410819217241, 9.315102745931094219, -0.7998128361456281477 ) ) ;
#61985=CIRCLE ( 'NONE', #189835, 6.961139734775127152 ) ;
#61992=CARTESIAN_POINT ( 'NONE',  ( -1.500000000000013101, 0.7020833340161545255, 0.8660254037844403729 ) ) ;
#61996=CARTESIAN_POINT ( 'NONE',  ( 4.376584659113025744, 4.000436945253625254, 0.7998128361456341429 ) ) ;
#61998=CARTESIAN_POINT ( 'NONE',  ( -8.109748439268576803, 12.61312361245537517, 0.7998128361456481317 ) ) ;
#62003=DIRECTION ( 'NONE',  ( 0.9782075119096202975, 0.1245777785630026030, 0.1661037047506698505 ) ) ;
#62005=CARTESIAN_POINT ( 'NONE',  ( 4.284013352238246419, 6.021101549076499637, -1.443375672974051449 ) ) ;
#62008=CARTESIAN_POINT ( 'NONE',  ( -4.903732577545095950, 4.837283930932079201, 0.1501914610188368471 ) ) ;
#62010=CARTESIAN_POINT ( 'NONE',  ( 4.175548122884573665, 3.973820352894515295, 1.214306433183764966E-14 ) ) ;
#62021=CARTESIAN_POINT ( 'NONE',  ( 0.6823417656249882723, -0.4072916663252490466, 1.181850606188755259 ) ) ;
#62025=CARTESIAN_POINT ( 'NONE',  ( -5.473741331615264549, 7.409117525016355010, -1.599625672291256295 ) ) ;
#62029=CARTESIAN_POINT ( 'NONE',  ( 1.499999999999985123, 0.04583333333335545129, -0.8660254037844323793 ) ) ;
#62031=CARTESIAN_POINT ( 'NONE',  ( 1.499999999999989120, 5.295833333333356485, -0.8660254037844323793 ) ) ;
#62040=CARTESIAN_POINT ( 'NONE',  ( -1.364683531250000748, -1.240624999658580752, 0.000000000000000000 ) ) ;
#62043=CARTESIAN_POINT ( 'NONE',  ( -9.027031348600448979, 9.425958082989001952, 1.040834085586084257E-14 ) ) ;
#62049=CARTESIAN_POINT ( 'NONE',  ( -0.6823417656250246877, -1.136458332991911790, 1.181850606188755259 ) ) ;
#62057=CARTESIAN_POINT ( 'NONE',  ( 6.588899466561449536, 9.670504563421618016, -1.082531754730537088 ) ) ;
#62061=CARTESIAN_POINT ( 'NONE',  ( -1.499999999999997780, 4.181250000682819490, 1.214306433183764966E-14 ) ) ;
#62063=CARTESIAN_POINT ( 'NONE',  ( -2.767835915484202047, 6.380892334706859792, -0.7998128361456281477 ) ) ;
#62064=CARTESIAN_POINT ( 'NONE',  ( 4.961921032477176752, 8.732732271291288484, 1.040834085586084257E-14 ) ) ;
#62065=CARTESIAN_POINT ( 'NONE',  ( -8.283668667825340393, 12.60810451253083997, 0.7216878364870458196 ) ) ;
#62071=CARTESIAN_POINT ( 'NONE',  ( 3.440018289565364817, 5.036440642624797626, 1.599625672291267398 ) ) ;
#62084=CARTESIAN_POINT ( 'NONE',  ( 7.404724451357931336, 11.79059562655963056, 0.7998128361456462443 ) ) ;
#62089=CARTESIAN_POINT ( 'NONE',  ( -1.402160292154681736E-14, 0.1968750003414221628, -1.575800808251665908 ) ) ;
#62090=CARTESIAN_POINT ( 'NONE',  ( 4.853455804012216213, 6.685451076146141425, 1.443375672974062551 ) ) ;
#62092=CARTESIAN_POINT ( 'NONE',  ( -8.026063749610047537, 11.34719622697832264, -1.082531754730543971 ) ) ;
#62097=CARTESIAN_POINT ( 'NONE',  ( -2.279742385392243165, 5.811449882932888222, -0.7998128361456281477 ) ) ;
#62099=EDGE_CURVE ( 'NONE', #85030, #84121, #198505, .T. ) ;
#62102=ORIENTED_EDGE ( 'NONE', *, *, #191462, .T. ) ;
#62113=CARTESIAN_POINT ( 'NONE',  ( 4.612443543746578278, 7.139628114692022187, -1.342220757880496995 ) ) ;
#62117=DIRECTION ( 'NONE',  ( -1.000000000000000000, 5.578564026256504688E-16, 0.000000000000000000 ) ) ;
#62120=CARTESIAN_POINT ( 'NONE',  ( -7.863365906246068349, 9.236643647784308797, -1.082531754730543971 ) ) ;
#62124=CARTESIAN_POINT ( 'NONE',  ( 7.935599982700328958, 8.152621489438862667, 0.7998128361456481317 ) ) ;
#62125=CARTESIAN_POINT ( 'NONE',  ( -3.113568832632681360, 6.784247404713426910, -0.7998128361456282587 ) ) ;
#62127=CARTESIAN_POINT ( 'NONE',  ( -3.601662362724658895, 7.353689856487406473, -0.7998128361456281477 ) ) ;
#62128=DIRECTION ( 'NONE',  ( -6.314299915563594049E-62, -8.546850786086437571E-32, -1.000000000000000000 ) ) ;
#62130=AXIS2_PLACEMENT_3D ( 'NONE', #33804, #199486, #68418 ) ;
#62132=CARTESIAN_POINT ( 'NONE',  ( -6.078132937628113908, 5.985576603521232109, 1.040834085586084257E-14 ) ) ;
#62135=CARTESIAN_POINT ( 'NONE',  ( 3.655894977179307226, 7.416961240017848844, -0.7998128361456291469 ) ) ;
#62136=CARTESIAN_POINT ( 'NONE',  ( 7.832860060393120882, 10.16142270859057462, 1.599625672291281386 ) ) ;
#62139=CARTESIAN_POINT ( 'NONE',  ( 4.666586266758273815, 7.089143983547513628, 1.366926838653566012 ) ) ;
#62140=CARTESIAN_POINT ( 'NONE',  ( 4.934804725694211136, 6.780358151441803649, -1.443375672974051449 ) ) ;
#62148=CARTESIAN_POINT ( 'NONE',  ( 7.632877294369377452, 8.967740267261513409, -1.082531754730537976 ) ) ;
#62149=CARTESIAN_POINT ( 'NONE',  ( -6.970863535720637216, 11.28442455831609337, 0.7998128361456481317 ) ) ;
#62152=CARTESIAN_POINT ( 'NONE',  ( -9.671043645249580933, 10.17730576241299900, 0.7998128361456462443 ) ) ;
#62153=CARTESIAN_POINT ( 'NONE',  ( -7.985916173649233230, 9.275655943134292869, -1.199719254218446718 ) ) ;
#62162=CARTESIAN_POINT ( 'NONE',  ( 7.865701674222579598, 12.32840238656838139, -0.7998128361456352531 ) ) ;
#62163=CARTESIAN_POINT ( 'NONE',  ( -1.499999999999997780, 4.150000000000021672, 1.214306433183764966E-14 ) ) ;
#62166=CARTESIAN_POINT ( 'NONE',  ( 3.816783937446950770, 4.411668334231586996, 1.199719254218464037 ) ) ;
#62169=CARTESIAN_POINT ( 'NONE',  ( -3.360966176420824070, 6.372552851524760698, 0.8599059493307342761 ) ) ;
#62175=CARTESIAN_POINT ( 'NONE',  ( -0.7499999999999972244, 3.108333333333358706, -1.299038105676652011 ) ) ;
#62176=CARTESIAN_POINT ( 'NONE',  ( 4.690231075323689325, 7.559354456931247412, 1.199719254218462483 ) ) ;
#62180=CARTESIAN_POINT ( 'NONE',  ( 6.792271770766432404, 10.86814146596211472, 1.040834085586084257E-14 ) ) ;
#62181=CARTESIAN_POINT ( 'NONE',  ( -9.449669878600616357, 12.04770082983265844, -1.443375672974058777 ) ) ;
#62185=CARTESIAN_POINT ( 'NONE',  ( 8.727698198895078363, 11.20540053684285553, -1.599625672291257406 ) ) ;
#62188=CARTESIAN_POINT ( 'NONE',  ( -3.391510981712833939, 7.108513245306943062, 0.7998128361456341429 ) ) ;
#62189=CARTESIAN_POINT ( 'NONE',  ( -1.499999999999997780, 5.181250000682820378, 1.214306433183764966E-14 ) ) ;
#62190=CARTESIAN_POINT ( 'NONE',  ( 1.364683531249986537, 1.155208333674754728, -0.7879004041258239610 ) ) ;
#62195=CARTESIAN_POINT ( 'NONE',  ( 1.364683531249988757, -0.3656249996585800299, 0.000000000000000000 ) ) ;
#62203=CARTESIAN_POINT ( 'NONE',  ( -5.391338639728555648, 9.441645512991978961, -0.7998128361456231517 ) ) ;
#62206=CARTESIAN_POINT ( 'NONE',  ( 4.493637847925535667, 7.329995691633395261, -1.199719254218452047 ) ) ;
#62212=CARTESIAN_POINT ( 'NONE',  ( 8.550388431712704573, 13.12720360364021133, 0.000000000000000000 ) ) ;
#62215=CARTESIAN_POINT ( 'NONE',  ( -4.530395885260773525, 8.437212299446219532, 0.7998128361456481317 ) ) ;
#62219=CARTESIAN_POINT ( 'NONE',  ( 7.879259827836241570, 12.34422023245099176, 1.040834085586084257E-14 ) ) ;
#62221=CARTESIAN_POINT ( 'NONE',  ( 8.762647353133951711, 9.117510088278095282, 1.040834085586084257E-14 ) ) ;
#62224=CARTESIAN_POINT ( 'NONE',  ( -8.514157279702020631, 11.91663867875229776, -1.082531754730543971 ) ) ;
#62226=CARTESIAN_POINT ( 'NONE',  ( -6.938021921891187382, 9.117444880338284818, -1.599625672291263179 ) ) ;
#62230=CARTESIAN_POINT ( 'NONE',  ( -5.702738293170157569, 6.277038442308466415, 1.111922112425635989 ) ) ;
#62231=CARTESIAN_POINT ( 'NONE',  ( -1.364683531250014514, 0.2802083336747505649, 0.7879004041258379498 ) ) ;
#62234=CARTESIAN_POINT ( 'NONE',  ( 6.263503779833467178, 9.290876262238963790, -1.082531754730537088 ) ) ;
#62249=CARTESIAN_POINT ( 'NONE',  ( 8.615316546479974136, 12.13862083994696839, 1.199719254218450271 ) ) ;
#62253=CARTESIAN_POINT ( 'NONE',  ( -5.284980951228653190, 5.060232619388524533, 0.000000000000000000 ) ) ;
#62254=CARTESIAN_POINT ( 'NONE',  ( -8.030507057996002729, 8.263346410617135263, 1.040834085586084257E-14 ) ) ;
#62256=VERTEX_POINT ( 'NONE', #105652 ) ;
#62259=CARTESIAN_POINT ( 'NONE',  ( -1.500000000000011324, 4.452083334016148086, 0.8660254037844403729 ) ) ;
#62260=CARTESIAN_POINT ( 'NONE',  ( 6.916630921265960019, 11.22115317478565188, 0.7998128361456462443 ) ) ;
#62264=CARTESIAN_POINT ( 'NONE',  ( -8.015895134177625891, 10.37496362800581018, 1.599625672291295375 ) ) ;
#62266=CARTESIAN_POINT ( 'NONE',  ( -1.364683531250012516, 3.738541667008087099, -0.7879004041258300672 ) ) ;
#62271=CARTESIAN_POINT ( 'NONE',  ( -8.026063749610043985, 12.30756544127966912, -0.7216878364870267237 ) ) ;
#62275=CARTESIAN_POINT ( 'NONE',  ( -1.364683531250012516, 2.342708333674752286, 0.7879004041258379498 ) ) ;
#62284=CARTESIAN_POINT ( 'NONE',  ( 1.364683531249988535, 2.613541667008089764, 0.7879004041258500513 ) ) ;
#62286=CARTESIAN_POINT ( 'NONE',  ( -4.954615070790188369, 7.867802451642154082, -1.199719254218452047 ) ) ;
#62289=CARTESIAN_POINT ( 'NONE',  ( 1.364683531249988535, 4.717708333674756283, -0.7879004041258300672 ) ) ;
#62293=CARTESIAN_POINT ( 'NONE',  ( 0.6823417656249882723, -1.157291666325249713, 1.181850606188755259 ) ) ;
#62294=CARTESIAN_POINT ( 'NONE',  ( -3.294268138440636928, 6.787137228248626641, 1.040834085586084257E-14 ) ) ;
#62298=CARTESIAN_POINT ( 'NONE',  ( 3.985733972737593778, 6.633478153960411738, -1.082531754730548412 ) ) ;
#62301=CARTESIAN_POINT ( 'NONE',  ( -8.376239975144482486, 8.666701480623698828, 1.040834085586084257E-14 ) ) ;
#62302=CARTESIAN_POINT ( 'NONE',  ( -8.175203439360366531, 12.48156174598837787, 1.040834085586084257E-14 ) ) ;
#62304=CARTESIAN_POINT ( 'NONE',  ( 1.364683531249988535, 4.655208333674755394, -0.7879004041258300672 ) ) ;
#62309=CARTESIAN_POINT ( 'NONE',  ( -5.382223794500835545, 8.262716279350872384, -1.082531754730543971 ) ) ;
#62311=CARTESIAN_POINT ( 'NONE',  ( 1.364683531249986537, -0.3239583329919163424, 0.7879004041258500513 ) ) ;
#62324=CARTESIAN_POINT ( 'NONE',  ( 8.663296969007976855, 12.09063498294259809, -1.082531754730543083 ) ) ;
#62333=CARTESIAN_POINT ( 'NONE',  ( 6.972971076130050072, 7.029554431773520129, 1.040834085586084257E-14 ) ) ;
#62334=CARTESIAN_POINT ( 'NONE',  ( -3.228813138348844536, 6.918699094715619502, 0.7998128361456341429 ) ) ;
#62338=CARTESIAN_POINT ( 'NONE',  ( -1.364683531250012516, 1.842708333674749843, 0.7879004041258379498 ) ) ;
#62339=CARTESIAN_POINT ( 'NONE',  ( -8.283668668269720925, 8.766627655843896250, 1.056142170575426150E-14 ) ) ;
#62340=CARTESIAN_POINT ( 'NONE',  ( -9.541187415715041809, 12.15447128979948310, -1.599625672291263179 ) ) ;
#62356=CARTESIAN_POINT ( 'NONE',  ( 4.808338034340912337, 8.761478140039733020, 1.040834085586084257E-14 ) ) ;
#62366=CARTESIAN_POINT ( 'NONE',  ( -3.735435015764967837, 4.316761258935923884, -1.199719254218452047 ) ) ;
#62371=CARTESIAN_POINT ( 'NONE',  ( -0.3520457843950398069, 7.165311474886403076, 1.969365997876477037 ) ) ;
#62376=CARTESIAN_POINT ( 'NONE',  ( -8.731087737520713432, 10.24898578427137963, 1.082531754730558626 ) ) ;
#62380=CARTESIAN_POINT ( 'NONE',  ( 4.635998460869027227, 7.496083073400806818, -1.199719254218452047 ) ) ;
#62381=CARTESIAN_POINT ( 'NONE',  ( -1.364683531250010740, 5.738541667008088432, -0.7879004041258300672 ) ) ;
#62386=CARTESIAN_POINT ( 'NONE',  ( 4.338245966248566177, 4.163634503485842409, 1.214306433183764966E-14 ) ) ;
#62394=CARTESIAN_POINT ( 'NONE',  ( -6.043183783389232566, 8.073467052085995022, 1.599625672291269396 ) ) ;
#62395=DIRECTION ( 'NONE',  ( -1.000000000000000000, 0.000000000000000000, 0.000000000000000000 ) ) ;
#62397=CARTESIAN_POINT ( 'NONE',  ( -4.086893239515592136, 6.855460315155083251, 1.199719254218464037 ) ) ;
#62403=CARTESIAN_POINT ( 'NONE',  ( 0.2981862293453664825, 7.114787932596398079, -1.978802099905859535 ) ) ;
#62406=CARTESIAN_POINT ( 'NONE',  ( 7.637320603199683866, 7.804628880021436288, -0.7998128361456281477 ) ) ;
#62417=VERTEX_POINT ( 'NONE', #86169 ) ;
#62419=CARTESIAN_POINT ( 'NONE',  ( 0.6823417656249882723, 0.1552083336747514530, 1.181850606188755259 ) ) ;
#62421=CARTESIAN_POINT ( 'NONE',  ( 4.680589345215795838, 6.483773540883647435, -1.599625672291256295 ) ) ;
#62423=CARTESIAN_POINT ( 'NONE',  ( -7.049876689426113785, 8.287572894827684777, -1.082531754730544860 ) ) ;
#62424=CARTESIAN_POINT ( 'NONE',  ( 4.853455804012222430, 5.725081861844796727, 1.082531754730560403 ) ) ;
#62425=CARTESIAN_POINT ( 'NONE',  ( -6.466876083594135238, 9.528143949959703818, 1.082531754730548412 ) ) ;
#62431=CARTESIAN_POINT ( 'NONE',  ( 5.717788096661236885, 7.693838750903348789, 1.599625672291267398 ) ) ;
#62436=CARTESIAN_POINT ( 'NONE',  ( 1.364683531249988535, 4.655208333674755394, -0.7879004041258300672 ) ) ;
#62440=CARTESIAN_POINT ( 'NONE',  ( 5.608269097547198712, 9.694731047113750222, -0.7998128361456281477 ) ) ;
#62444=CARTESIAN_POINT ( 'NONE',  ( -8.688077508258798431, 9.030511935923748013, -0.7998128361456291469 ) ) ;
#62449=CARTESIAN_POINT ( 'NONE',  ( 8.076906825439115423, 10.44614393447756129, -1.599625672291262513 ) ) ;
#62452=CARTESIAN_POINT ( 'NONE',  ( -7.039708073993679704, 9.236078724457858158, 1.599625672291283607 ) ) ;
#62456=CARTESIAN_POINT ( 'NONE',  ( 5.048403365090235795, 6.545034038527520082, -1.227034678662905609 ) ) ;
#62457=CARTESIAN_POINT ( 'NONE',  ( -9.707274797704657843, 11.38787068781932987, 1.082531754730558626 ) ) ;
#62463=CARTESIAN_POINT ( 'NONE',  ( 5.341022448779654930, 8.318611059296550536, 1.199719254218462483 ) ) ;
#62465=CARTESIAN_POINT ( 'NONE',  ( 4.798696304233017074, 7.685897223992134819, -1.199719254218452047 ) ) ;
#62466=CARTESIAN_POINT ( 'NONE',  ( -4.026842413655439046, 7.608452276161581374, 0.2328349793435397497 ) ) ;
#62467=CARTESIAN_POINT ( 'NONE',  ( 5.196852952739813070, 4.957416621151553571, -0.7998128361456221525 ) ) ;
#62469=CARTESIAN_POINT ( 'NONE',  ( -7.876924059859742755, 8.292092279365579799, 1.040834085586084257E-14 ) ) ;
#62475=CARTESIAN_POINT ( 'NONE',  ( -5.171837412746745244, 6.485142596490002909, 1.193510785747232905 ) ) ;
#62476=CARTESIAN_POINT ( 'NONE',  ( 1.364683531249986537, 0.2177083336747502595, -0.7879004041258309554 ) ) ;
#62479=CARTESIAN_POINT ( 'NONE',  ( 5.016153647376212277, 5.914896012436124728, 1.082531754730558626 ) ) ;
#62483=CARTESIAN_POINT ( 'NONE',  ( -8.148087131688683371, 11.48955683940339867, -1.082531754730543083 ) ) ;
#62488=CARTESIAN_POINT ( 'NONE',  ( -9.639484029191951464, 10.34841224358651601, 0.7216878364870438212 ) ) ;
#62494=CARTESIAN_POINT ( 'NONE',  ( -8.825994812371996900, 9.399341490629888440, 0.7216878364870438212 ) ) ;
#62498=CARTESIAN_POINT ( 'NONE',  ( 0.6823417656249899377, 5.238541667008086655, -1.181850606188754593 ) ) ;
#62499=CARTESIAN_POINT ( 'NONE',  ( -1.500000000000011324, 3.952083334016153415, 0.8660254037844403729 ) ) ;
#62500=CARTESIAN_POINT ( 'NONE',  ( 5.693912546396379781, 6.288398852508453096, -1.088204328156989087 ) ) ;
#62505=CARTESIAN_POINT ( 'NONE',  ( -6.496328159242330536, 10.73079995242472862, 0.000000000000000000 ) ) ;
#62507=LINE ( 'NONE', #25735, #209912 ) ;
#62509=CARTESIAN_POINT ( 'NONE',  ( 4.476163270806094552, 8.373940915915776273, 0.7998128361456462443 ) ) ;
#62514=CARTESIAN_POINT ( 'NONE',  ( 8.284195553149872993, 9.623648552551724578, -1.199719254218445830 ) ) ;
#62519=CARTESIAN_POINT ( 'NONE',  ( 1.284279953904126748, 10.64264068711930733, -0.7749999999999874767 ) ) ;
#62523=CARTESIAN_POINT ( 'NONE',  ( -6.941411460516810017, 8.161030127766803588, 1.082531754730549967 ) ) ;
#62526=DIRECTION ( 'NONE',  ( -5.578564026256491869E-16, -1.000000000000000000, -9.066213480720160632E-32 ) ) ;
#62529=DIRECTION ( 'NONE',  ( 1.000000000000000000, -5.578564026256504688E-16, 1.972152263052529514E-31 ) ) ;
#62532=CARTESIAN_POINT ( 'NONE',  ( -10.17947440576205054, 10.77047498301088346, 0.7998128361456462443 ) ) ;
#62534=CARTESIAN_POINT ( 'NONE',  ( 7.801827329660018684, 11.18955008699033726, 1.199719254218460707 ) ) ;
#62535=CARTESIAN_POINT ( 'NONE',  ( 1.499999999999987121, -0.9958333333333134751, 0.8660254037844524744 ) ) ;
#62536=CARTESIAN_POINT ( 'NONE',  ( -9.124801077197171040, 10.60435499727357289, -1.199719254218441611 ) ) ;
#62539=CARTESIAN_POINT ( 'NONE',  ( -1.364683531249997417, 4.009375000341424133, 1.214306433183764966E-14 ) ) ;
#62540=CARTESIAN_POINT ( 'NONE',  ( 10.56143847536557878, 11.42402576412244386, 0.000000000000000000 ) ) ;
#62544=CARTESIAN_POINT ( 'NONE',  ( 8.717529583462646059, 11.19353715217169309, 1.443375672974076540 ) ) ;
#62547=CARTESIAN_POINT ( 'NONE',  ( -6.019457014787517046, 9.006155036351978893, 1.082531754730548412 ) ) ;
#62548=CARTESIAN_POINT ( 'NONE',  ( 1.364683531249988757, 0.3843750003414206362, 0.000000000000000000 ) ) ;
#62552=CARTESIAN_POINT ( 'NONE',  ( -8.505042434474312074, 8.816971016508505343, -0.7998128361456291469 ) ) ;
#62553=CARTESIAN_POINT ( 'NONE',  ( -4.270455198180246548, 4.084545274072787890, 0.7216878364870317197 ) ) ;
#62554=CARTESIAN_POINT ( 'NONE',  ( -0.6823417656250003738, 2.780208333674753618, -1.181850606188749264 ) ) ;
#62559=CARTESIAN_POINT ( 'NONE',  ( 8.048736748007069508, 12.54194330598362406, -0.7998128361456352531 ) ) ;
#62562=EDGE_CURVE ( 'NONE', #116082, #148658, #15141, .T. ) ;
#62564=CARTESIAN_POINT ( 'NONE',  ( -7.285838599102589797E-14, 7.078193277237590841, -2.121339347286493648 ) ) ;
#62568=AXIS2_PLACEMENT_3D ( 'NONE', #133331, #97621, #99727 ) ;
#62574=CARTESIAN_POINT ( 'NONE',  ( -1.402160292154681736E-14, -0.8031249996585825279, -1.575800808251665908 ) ) ;
#62578=CARTESIAN_POINT ( 'NONE',  ( 7.801827329660018684, 11.18955008699033726, 1.199719254218460707 ) ) ;
#62579=CARTESIAN_POINT ( 'NONE',  ( 6.385527162356455122, 10.39360608948380538, 1.056142170575426150E-14 ) ) ;
#62581=CARTESIAN_POINT ( 'NONE',  ( 0.6823417656249917140, 4.092708333674755394, 1.181850606188765695 ) ) ;
#62583=CARTESIAN_POINT ( 'NONE',  ( -6.561783159334130922, 9.638868871656395498, -1.082531754730538864 ) ) ;
#62589=CARTESIAN_POINT ( 'NONE',  ( 4.227444969362701421, 3.826440640544909400, 1.214306433183764966E-14 ) ) ;
#62592=CARTESIAN_POINT ( 'NONE',  ( 8.041957671200231417, 12.53403438304231976, 1.040834085586084257E-14 ) ) ;
#62593=CARTESIAN_POINT ( 'NONE',  ( 1.598423149420349354, 8.713846000021359117, -2.499999999999995115 ) ) ;
#62599=CARTESIAN_POINT ( 'NONE',  ( -8.947491310014823895, 12.52615806407091803, 1.199719254218462483 ) ) ;
#62600=CARTESIAN_POINT ( 'NONE',  ( 7.142447996300871793, 7.227277505306155092, 0.7998128361456341429 ) ) ;
#62602=CARTESIAN_POINT ( 'NONE',  ( 4.039439701867726384, 6.800097854565950506, 1.199719254218462483 ) ) ;
#62612=CARTESIAN_POINT ( 'NONE',  ( -7.226132686403777150, 7.532835677000276675, 1.040834085586084257E-14 ) ) ;
#62613=CARTESIAN_POINT ( 'NONE',  ( 5.332434488876471868, 5.115595079977664383, 0.7998128361456341429 ) ) ;
#62616=CARTESIAN_POINT ( 'NONE',  ( -8.016948904382338981, 8.247528564734524892, -0.7998128361456291469 ) ) ;
#62618=DIRECTION ( 'NONE',  ( 3.451266460341927524E-31, -0.6000000000000035305, -0.7999999999999974909 ) ) ;
#62620=CARTESIAN_POINT ( 'NONE',  ( -10.08065090696061716, 11.71951313199760136, -1.199719254218441611 ) ) ;
#62624=CARTESIAN_POINT ( 'NONE',  ( 8.457588896826466751, 8.761608555919362828, 1.040834085586084257E-14 ) ) ;
#62625=CARTESIAN_POINT ( 'NONE',  ( 4.403700966340357681, 4.032072637018845107, -0.7998128361456211532 ) ) ;
#62627=ORIENTED_EDGE ( 'NONE', *, *, #189117, .T. ) ;
#62636=CARTESIAN_POINT ( 'NONE',  ( -8.355902744723985975, 8.642974711799791265, 1.040834085586084257E-14 ) ) ;
#62641=CARTESIAN_POINT ( 'NONE',  ( 5.178851490740187913, 8.985817805931475277, 0.7216878364870438212 ) ) ;
#62643=CARTESIAN_POINT ( 'NONE',  ( 4.356247428692526569, 3.976710176429713250, 0.7998128361456341429 ) ) ;
#62646=CARTESIAN_POINT ( 'NONE',  ( -6.144869935491728441, 8.192100896205577243, -1.599625672291263179 ) ) ;
#62656=CARTESIAN_POINT ( 'NONE',  ( 1.364683531249990311, 3.946875000341417028, 1.214306433183764966E-14 ) ) ;
#62657=CARTESIAN_POINT ( 'NONE',  ( 3.998178221199472748, 7.810824081292446763, -0.04219917931748625589 ) ) ;
#62658=CARTESIAN_POINT ( 'NONE',  ( 8.101160479365381306, 9.410107633136481908, -1.199719254218446718 ) ) ;
#62660=CARTESIAN_POINT ( 'NONE',  ( -4.338245966692955591, 5.124003718305597310, 1.082531754730560403 ) ) ;
#62662=CARTESIAN_POINT ( 'NONE',  ( -5.544921637864841379, 5.571422787038166291, -0.7216878364870197293 ) ) ;
#62667=EDGE_LOOP ( 'NONE', ( #5630, #37582, #14338, #131946 ) ) ;
#62669=CARTESIAN_POINT ( 'NONE',  ( 4.695201269034174452, 4.372156323494968966, 1.214306433183764966E-14 ) ) ;
#62676=CARTESIAN_POINT ( 'NONE',  ( 4.192495815123822744, 5.914331089109666983, -1.599625672291255185 ) ) ;
#62681=CARTESIAN_POINT ( 'NONE',  ( -1.364683531249997417, 4.571875000341417028, 1.214306433183764966E-14 ) ) ;
#62686=CARTESIAN_POINT ( 'NONE',  ( 5.066996723205273057, 6.934582148538044777, 1.599625672291267398 ) ) ;
#62690=CARTESIAN_POINT ( 'NONE',  ( -5.274285450916075035, 6.112086766612214284, 1.199719254218450271 ) ) ;
#62691=CARTESIAN_POINT ( 'NONE',  ( 4.622967192135525316, 8.337286124226029216, -0.7216878364870207285 ) ) ;
#62692=CARTESIAN_POINT ( 'NONE',  ( -1.500000000000011324, 2.920833333333352932, 0.8660254037844403729 ) ) ;
#62694=CARTESIAN_POINT ( 'NONE',  ( -4.086893239515592136, 6.855460315155083251, 1.199719254218464037 ) ) ;
#62695=CARTESIAN_POINT ( 'NONE',  ( 0.1081551476993989624, 7.159877756659379422, -1.998460492244654274 ) ) ;
#62697=CARTESIAN_POINT ( 'NONE',  ( -0.6823417656250212460, 4.801041667008086655, 1.181850606188767472 ) ) ;
#62700=CARTESIAN_POINT ( 'NONE',  ( -4.446711195602252253, 6.210915699667823198, -1.443375672974053447 ) ) ;
#62706=CARTESIAN_POINT ( 'NONE',  ( 4.487912541323413329, 5.194651705420806564, 1.199719254218462483 ) ) ;
#62709=CARTESIAN_POINT ( 'NONE',  ( 0.3387147352624392815, 6.550290604319550347, -3.193285863367457900 ) ) ;
#62710=CARTESIAN_POINT ( 'NONE',  ( 0.6823417656249899377, 4.238541667008085767, -1.181850606188754593 ) ) ;
#62714=CARTESIAN_POINT ( 'NONE',  ( 1.364683531249986537, -0.2822916663252520997, -0.7879004041258309554 ) ) ;
#62715=CARTESIAN_POINT ( 'NONE',  ( 1.579999999999989413, 6.280000000000042881, 2.580000000000000515 ) ) ;
#62717=CARTESIAN_POINT ( 'NONE',  ( -9.429859533504656000, 10.96025652963230534, -1.199719254218441611 ) ) ;
#62719=CARTESIAN_POINT ( 'NONE',  ( -6.873620692004104527, 7.121571683533994168, 0.7216878364870317197 ) ) ;
#62722=VERTEX_POINT ( 'NONE', #195159 ) ;
#62723=CARTESIAN_POINT ( 'NONE',  ( 1.364683531249988535, 4.155208333674753618, -0.7879004041258239610 ) ) ;
#62731=CARTESIAN_POINT ( 'NONE',  ( -7.361714222096077620, 7.691014135307965738, 0.7216878364870317197 ) ) ;
#62737=CARTESIAN_POINT ( 'NONE',  ( -5.165293336682207581, 8.009630745229104676, 1.082531754730548412 ) ) ;
#62739=CARTESIAN_POINT ( 'NONE',  ( -4.650083499807267984, 5.295740330745369207, 1.164732466530402855 ) ) ;
#62750=CARTESIAN_POINT ( 'NONE',  ( -5.739179097286464248, 5.590130456455974617, -0.7998128361456221525 ) ) ;
#62753=CARTESIAN_POINT ( 'NONE',  ( -0.7500000000000006661, 0.3583333333333563187, -1.299038105676652011 ) ) ;
#62755=CARTESIAN_POINT ( 'NONE',  ( 7.429504990608736037, 11.61158022244479682, -0.7216878364870267237 ) ) ;
#62756=CARTESIAN_POINT ( 'NONE',  ( 6.928380191783277908, 8.041863964290678624, 1.199719254218462483 ) ) ;
#62760=CARTESIAN_POINT ( 'NONE',  ( 4.330940004561544043, 7.140181541042074365, -1.199719254218452047 ) ) ;
#62761=CARTESIAN_POINT ( 'NONE',  ( -0.04711431077965874681, 7.150937050891459812, -2.000088718515178776 ) ) ;
#62762=ORIENTED_EDGE ( 'NONE', *, *, #175809, .F. ) ;
#62768=CARTESIAN_POINT ( 'NONE',  ( -4.785665035943912571, 4.685623418130398399, 1.214306433183764966E-14 ) ) ;
#62770=VECTOR ( 'NONE', #66041, 1000.000000000000000 ) ;
#62774=( BOUNDED_SURFACE ( )  B_SPLINE_SURFACE ( 3, 2, ( 
 ( #110397, #172140, #28007 ),
 ( #208869, #126659, #209935 ),
 ( #188367, #40007, #106117 ),
 ( #89838, #7475, #139659 ),
 ( #129859, #15990, #146050 ),
 ( #97291, #95165, #78874 ),
 ( #131944, #45342, #177467 ),
 ( #99410, #96231, #164406 ) ),
 .UNSPECIFIED., .F., .F., .T. ) 
 B_SPLINE_SURFACE_WITH_KNOTS ( ( 4, 2, 2, 4 ),
 ( 3, 3 ),
 ( -2.253405795293872416E-15, 0.003001918495467197773, 0.004502877743201923362, 0.006003836990936648951 ),
 ( 0.000000000000000000, 1.000000000000000000 ),
 .UNSPECIFIED. ) 
 GEOMETRIC_REPRESENTATION_ITEM ( )  RATIONAL_B_SPLINE_SURFACE ( (
 ( 1.000000000000000000, 0.7835651598521441441, 1.000000000000000000),
 ( 1.000000000000000000, 0.7913519369914218116, 1.000000000000000000),
 ( 1.000000000000000000, 0.8009496234832708117, 1.000000000000000000),
 ( 1.000000000000000000, 0.8230981486289181692, 1.000000000000000000),
 ( 1.000000000000000000, 0.8318333311020545962, 1.000000000000000000),
 ( 1.000000000000000000, 0.8529518727571846481, 1.000000000000000000),
 ( 1.000000000000000000, 0.8654984584228418987, 1.000000000000000000),
 ( 1.000000000000000000, 0.8789000212895415887, 1.000000000000000000) ) ) 
 REPRESENTATION_ITEM ( '' )  SURFACE ( )  );
#62776=CARTESIAN_POINT ( 'NONE',  ( -1.364683531250012516, 3.238541667008084879, -0.7879004041258289570 ) ) ;
#62777=CARTESIAN_POINT ( 'NONE',  ( 7.565086526301031178, 11.76975868075249387, 1.040834085586084257E-14 ) ) ;
#62778=CARTESIAN_POINT ( 'NONE',  ( -7.223796917982883592, 7.322184580601816428, -0.7998128361456291469 ) ) ;
#62781=CARTESIAN_POINT ( 'NONE',  ( 4.469384193999260901, 8.366031992974468423, -0.7998128361456231517 ) ) ;
#62782=CARTESIAN_POINT ( 'NONE',  ( -6.226218857173722476, 8.287007971501239467, 1.599625672291283607 ) ) ;
#62786=CARTESIAN_POINT ( 'NONE',  ( -0.7500000000000006661, 0.6395833340161540814, -1.299038105676652011 ) ) ;
#62790=CARTESIAN_POINT ( 'NONE',  ( 6.588899466561449536, 9.670504563421618016, -1.082531754730537088 ) ) ;
#62793=CARTESIAN_POINT ( 'NONE',  ( -1.364683531250000748, 2.321875000341422357, 1.214306433183764966E-14 ) ) ;
#62795=CARTESIAN_POINT ( 'NONE',  ( 4.297571505407542958, 7.957657823043374989, -0.7216878364870197293 ) ) ;
#62798=CARTESIAN_POINT ( 'NONE',  ( -4.338245966692955591, 5.124003718305597310, 1.082531754730560403 ) ) ;
#62800=B_SPLINE_CURVE_WITH_KNOTS ( 'NONE', 3,
 ( #143885, #44221, #90844, #175291, #107138, #110344, #42098, #207759, #156908, #140682 ),
 .UNSPECIFIED., .F., .F.,
 ( 4, 3, 3, 4 ),
 ( 5.423634105407616645E-16, 3.125291908127631347E-05, 6.323748278266503285E-05, 9.524284239289069348E-05 ),
 .UNSPECIFIED. ) ;
#62801=CARTESIAN_POINT ( 'NONE',  ( -0.6823417656250212460, 4.551041667008086655, 1.181850606188767472 ) ) ;
#62807=CARTESIAN_POINT ( 'NONE',  ( -4.398207409718558836, 7.344456035913847103, -1.221965942340837552 ) ) ;
#62814=CARTESIAN_POINT ( 'NONE',  ( 6.602984505055297326, 7.662235663108029726, 1.199719254218462483 ) ) ;
#62817=CARTESIAN_POINT ( 'NONE',  ( 4.142179624174931796, 4.791296635414242111, 1.199719254218464037 ) ) ;
#62825=VERTEX_POINT ( 'NONE', #33707 ) ;
#62827=CARTESIAN_POINT ( 'NONE',  ( 4.934804725694211136, 6.780358151441803649, -1.443375672974051449 ) ) ;
#62828=CARTESIAN_POINT ( 'NONE',  ( -1.201851678989727383E-14, 1.884375000341422135, 1.575800808251672791 ) ) ;
#62829=CARTESIAN_POINT ( 'NONE',  ( 8.751951852821344247, 10.16936423550178503, -1.199719254218446718 ) ) ;
#62831=CARTESIAN_POINT ( 'NONE',  ( -6.471393748265563239, 5.229711127717889596, 2.419999999999998597 ) ) ;
#62835=CARTESIAN_POINT ( 'NONE',  ( -1.402160292154681736E-14, 1.587500000000018785, -1.732050807568863648 ) ) ;
#62836=CARTESIAN_POINT ( 'NONE',  ( 5.124091990960999432, 8.065525525174782828, -1.199719254218452047 ) ) ;
#62837=CARTESIAN_POINT ( 'NONE',  ( -7.771848369131641121, 10.09024240211882351, -1.599625672291263179 ) ) ;
#62842=CARTESIAN_POINT ( 'NONE',  ( -1.364683531250014514, 1.988541667008086655, -0.7879004041258289570 ) ) ;
#62844=CARTESIAN_POINT ( 'NONE',  ( 0.7499999999999902300, 3.233333333333352044, 1.299038105676669330 ) ) ;
#62846=CARTESIAN_POINT ( 'NONE',  ( 8.595506201383999567, 12.97191496834930113, 0.7216878364870438212 ) ) ;
#62851=CARTESIAN_POINT ( 'NONE',  ( -0.7500000000000006661, 0.6395833340161540814, -1.299038105676652011 ) ) ;
#62853=CARTESIAN_POINT ( 'NONE',  ( -7.867809214632013770, 8.073532260025807261, 1.040834085586084257E-14 ) ) ;
#62860=CARTESIAN_POINT ( 'NONE',  ( 5.015626762051672571, 7.938982758113895422, 1.199719254218462483 ) ) ;
#62864=CARTESIAN_POINT ( 'NONE',  ( 5.469824908109481854, 8.468880595181346393, -1.199719254218446718 ) ) ;
#62865=ORIENTED_EDGE ( 'NONE', *, *, #98111, .T. ) ;
#62869=CARTESIAN_POINT ( 'NONE',  ( -6.073162743917628781, 9.172774736957510555, -1.199719254218440723 ) ) ;
#62871=CARTESIAN_POINT ( 'NONE',  ( 4.487912541323413329, 5.194651705420806564, 1.199719254218462483 ) ) ;
#62877=CARTESIAN_POINT ( 'NONE',  ( 4.113906668039927439, 7.442175195026684342, 0.6721147198667943856 ) ) ;
#62886=CARTESIAN_POINT ( 'NONE',  ( -4.446711195602264688, 4.290177271065136466, -0.7216878364870207285 ) ) ;
#62887=CARTESIAN_POINT ( 'NONE',  ( 6.914295153289432783, 10.05013286460426691, -1.082531754730537976 ) ) ;
#62890=CARTESIAN_POINT ( 'NONE',  ( -5.590039407536138150, 5.416134151747256986, 0.000000000000000000 ) ) ;
#62895=CARTESIAN_POINT ( 'NONE',  ( -7.019370843573183194, 9.212351955633947043, 1.599625672291283607 ) ) ;
#62900=EDGE_LOOP ( 'NONE', ( #184608, #74311, #47718, #142983 ) ) ;
#62910=CARTESIAN_POINT ( 'NONE',  ( -5.739179097286464248, 5.590130456455974617, -0.7998128361456221525 ) ) ;
#62911=ADVANCED_FACE ( 'NONE', ( #113978 ), #28498, .T. ) ;
#62914=CARTESIAN_POINT ( 'NONE',  ( 3.660338286009610975, 6.253849852777763729, -1.082531754730543083 ) ) ;
#62919=CARTESIAN_POINT ( 'NONE',  ( -4.647747731386360215, 4.316793862905830892, 0.7998128361456341429 ) ) ;
#62920=CARTESIAN_POINT ( 'NONE',  ( -2.578021764892882040, 6.159442492350315490, 0.7998128361456341429 ) ) ;
#62923=CARTESIAN_POINT ( 'NONE',  ( 10.40318394038753702, 11.03146944007395724, -0.7998128361456281477 ) ) ;
#62927=CARTESIAN_POINT ( 'NONE',  ( -7.934546212495630968, 10.28005655271014795, -1.599625672291263179 ) ) ;
#62928=CARTESIAN_POINT ( 'NONE',  ( 6.010342169559767633, 5.906487374108181143, -0.7998128361456281477 ) ) ;
#62931=CARTESIAN_POINT ( 'NONE',  ( 4.847203612085560387, 5.613824621309978724, -1.199719254218452047 ) ) ;
#62934=CARTESIAN_POINT ( 'NONE',  ( 0.6823417656249882723, 1.738541667008083991, -1.181850606188749264 ) ) ;
#62937=CARTESIAN_POINT ( 'NONE',  ( 8.107412671292042461, 9.521364873671299023, 1.082531754730558626 ) ) ;
#62951=CARTESIAN_POINT ( 'NONE',  ( -8.455481356417053007, 13.01647868246193518, 0.7998128361456341429 ) ) ;
#62967=CARTESIAN_POINT ( 'NONE',  ( -0.7500000000000215383, 0.9729166673494854534, 1.299038105676659116 ) ) ;
#62974=CARTESIAN_POINT ( 'NONE',  ( 7.404724451357931336, 11.79059562655963056, 0.7998128361456462443 ) ) ;
#62979=CARTESIAN_POINT ( 'NONE',  ( 3.708318708537623021, 4.285125567170706695, -1.199719254218446718 ) ) ;
#62980=CARTESIAN_POINT ( 'NONE',  ( -6.738039156311804945, 6.963393225226301553, 1.040834085586084257E-14 ) ) ;
#62985=CARTESIAN_POINT ( 'NONE',  ( -6.856673000209188906, 9.022537805042615489, 1.599625672291283607 ) ) ;
#62988=CARTESIAN_POINT ( 'NONE',  ( 1.499999999999987121, 0.7854166673494828999, 0.8660254037844524744 ) ) ;
#62995=CARTESIAN_POINT ( 'NONE',  ( -4.406036734316906234, 4.242723732898890709, -0.7216878364870207285 ) ) ;
#62998=CARTESIAN_POINT ( 'NONE',  ( 4.052428274714076295, 7.522979123003127988, 0.4826459875755910733 ) ) ;
#63003=CARTESIAN_POINT ( 'NONE',  ( -10.47775378526269918, 11.11846759242831872, -0.7998128361456221525 ) ) ;
#63004=CARTESIAN_POINT ( 'NONE',  ( 7.934546212495622086, 10.28005655271014795, -1.599625672291262513 ) ) ;
#63012=CARTESIAN_POINT ( 'NONE',  ( -7.751511138711140170, 10.06651563329490529, -1.599625672291263179 ) ) ;
#63020=CARTESIAN_POINT ( 'NONE',  ( 5.217190183160311356, 4.981143389975473568, -0.7998128361456211532 ) ) ;
#63024=ORIENTED_EDGE ( 'NONE', *, *, #120212, .F. ) ;
#63026=CARTESIAN_POINT ( 'NONE',  ( -5.579343907223557331, 6.467988298970945849, 1.199719254218450271 ) ) ;
#63027=CARTESIAN_POINT ( 'NONE',  ( -7.974166903131914452, 12.45494515362926435, -0.7998128361456281477 ) ) ;
#63039=CARTESIAN_POINT ( 'NONE',  ( 7.202405917357655341, 9.425892875049191488, 1.599625672291281386 ) ) ;
#63050=CARTESIAN_POINT ( 'NONE',  ( -1.500000000000001332, -0.06874999931718445145, 0.000000000000000000 ) ) ;
#63055=CARTESIAN_POINT ( 'NONE',  ( -4.783329267523015460, 4.474972321731942593, -0.7998128361456221525 ) ) ;
#63062=CARTESIAN_POINT ( 'NONE',  ( 5.205967797967541166, 5.175976640491323444, -0.7216878364870197293 ) ) ;
#63065=CARTESIAN_POINT ( 'NONE',  ( -1.364683531249997417, 5.571875000341417916, 1.214306433183764966E-14 ) ) ;
#63066=CARTESIAN_POINT ( 'NONE',  ( 1.579999999999991189, 8.758163473637745611, -2.499999999999989342 ) ) ;
#63067=CARTESIAN_POINT ( 'NONE',  ( 10.58621901417202515, 11.24501035948919991, -0.7998128361456281477 ) ) ;
#63069=CARTESIAN_POINT ( 'NONE',  ( -1.123270288254055060, 3.033552654332631437, 0.7749999999939940487 ) ) ;
#63072=DIRECTION ( 'NONE',  ( -0.7592566023652994600, 0.6507913734559651608, 0.000000000000000000 ) ) ;
#63077=CARTESIAN_POINT ( 'NONE',  ( -1.364683531250014514, -0.9697916663252473812, 0.7879004041258379498 ) ) ;
#63082=CARTESIAN_POINT ( 'NONE',  ( -5.555090253297260361, 7.504024600312024340, 1.599625672291269396 ) ) ;
#63086=CARTESIAN_POINT ( 'NONE',  ( -0.7499999999999972244, 4.608333333333352932, -1.299038105676652011 ) ) ;
#63094=CARTESIAN_POINT ( 'NONE',  ( -1.364683531250014514, -0.5114583329919092369, -0.7879004041258359514 ) ) ;
#63096=CARTESIAN_POINT ( 'NONE',  ( 6.287230548435207567, 8.358188277972981695, -1.599625672291262513 ) ) ;
#63097=CARTESIAN_POINT ( 'NONE',  ( -8.715193815486133033, 9.062147627688959872, 0.7998128361456462443 ) ) ;
#63104=CARTESIAN_POINT ( 'NONE',  ( -1.364683531250014514, -0.6989583329919100141, -0.7879004041258359514 ) ) ;
#63111=VERTEX_POINT ( 'NONE', #201516 ) ;
#63112=ADVANCED_FACE ( 'NONE', ( #187422 ), #87811, .T. ) ;
#63114=CARTESIAN_POINT ( 'NONE',  ( 6.968527767744093993, 10.11340424813470662, 1.082531754730558626 ) ) ;
#63118=CARTESIAN_POINT ( 'NONE',  ( -1.500000000000013101, 4.160416667349482900, -0.8660254037844313801 ) ) ;
#63120=CARTESIAN_POINT ( 'NONE',  ( -2.605138072120212200, 6.191078184115536232, -0.7998128361456281477 ) ) ;
#63122=CARTESIAN_POINT ( 'NONE',  ( 5.897433631820129918, 8.863794422890064695, -1.082531754730537976 ) ) ;
#63123=CARTESIAN_POINT ( 'NONE',  ( -9.802181872555943087, 10.53822639417784046, 0.7216878364870438212 ) ) ;
#63129=CARTESIAN_POINT ( 'NONE',  ( 8.568389894156670294, 12.94027927658408217, -0.7216878364870257245 ) ) ;
#63130=CARTESIAN_POINT ( 'NONE',  ( 1.499999999999990896, 4.775000000000022560, 1.214306433183764966E-14 ) ) ;
#63132=CARTESIAN_POINT ( 'NONE',  ( 4.216749469050096621, 4.878294787768598262, -1.199719254218452047 ) ) ;
#63136=EDGE_LOOP ( 'NONE', ( #97153, #184030, #97293, #166927 ) ) ;
#63145=ORIENTED_EDGE ( 'NONE', *, *, #80091, .F. ) ;
#63147=CARTESIAN_POINT ( 'NONE',  ( 8.565000355531088516, 11.01558638625153286, -1.599625672291257406 ) ) ;
#63149=CARTESIAN_POINT ( 'NONE',  ( -4.083708824282378913, 7.596498746673441715, 0.5977277219625460880 ) ) ;
#63151=CARTESIAN_POINT ( 'NONE',  ( 1.364683531249986537, -0.3447916663252443836, -0.7879004041258309554 ) ) ;
#63152=CARTESIAN_POINT ( 'NONE',  ( 5.341549334104188418, 7.254893527920112994, 1.443375672974062551 ) ) ;
#63153=CARTESIAN_POINT ( 'NONE',  ( -8.297226821883391779, 11.66355314463053006, 1.082531754730549967 ) ) ;
#63158=CARTESIAN_POINT ( 'NONE',  ( -3.415764635639130020, 6.072476943965863683, 1.199719254218462483 ) ) ;
#63171=CARTESIAN_POINT ( 'NONE',  ( 5.232446707518059625, 6.618332276934084213, -1.382299536160000120 ) ) ;
#63176=CARTESIAN_POINT ( 'NONE',  ( -4.307832228787286333, 7.438438422310007958, -1.137755099753708254 ) ) ;
#63179=CARTESIAN_POINT ( 'NONE',  ( -7.944714827928056167, 10.29191993738131927, 1.443375672974090751 ) ) ;
#63183=CARTESIAN_POINT ( 'NONE',  ( 6.154511665599609493, 9.267681812253174556, 1.199719254218462483 ) ) ;
#63186=CARTESIAN_POINT ( 'NONE',  ( -4.761938266897808525, 6.578680616179308771, 1.599625672291267398 ) ) ;
#63190=CARTESIAN_POINT ( 'NONE',  ( -5.392392409933270514, 7.314210449720692786, 1.599625672291269396 ) ) ;
#63194=CARTESIAN_POINT ( 'NONE',  ( 7.079328764629950754, 11.41096732537697633, 0.7998128361456462443 ) ) ;
#63195=CARTESIAN_POINT ( 'NONE',  ( 0.7499999999999902300, 3.514583334016149863, 1.299038105676669330 ) ) ;
#63197=CARTESIAN_POINT ( 'NONE',  ( 4.945911955618520928, 6.845357471522081738, 1.424928946000488583 ) ) ;
#63198=CARTESIAN_POINT ( 'NONE',  ( 5.341549334104200852, 5.334155099317434257, 0.7216878364870317197 ) ) ;
#63205=CARTESIAN_POINT ( 'NONE',  ( 6.846504384776753049, 9.010674420371453053, -1.443375672974058777 ) ) ;
#63208=CARTESIAN_POINT ( 'NONE',  ( -7.784352752540590004, 12.23349531127272094, 0.7998128361456481317 ) ) ;
#63209=CARTESIAN_POINT ( 'NONE',  ( -6.418895661066105873, 9.576129806964074120, -1.199719254218440723 ) ) ;
#63210=CARTESIAN_POINT ( 'NONE',  ( -5.734735788456140959, 5.792872629394733686, 0.7216878364870513707 ) ) ;
#63218=EDGE_CURVE ( 'NONE', #2895, #54417, #101431, .T. ) ;
#63219=CARTESIAN_POINT ( 'NONE',  ( 9.915090410295563927, 10.46202698829998567, -0.7998128361456281477 ) ) ;
#63220=CARTESIAN_POINT ( 'NONE',  ( -0.7499999999999972244, 4.108333333333360038, -1.299038105676652011 ) ) ;
#63223=CARTESIAN_POINT ( 'NONE',  ( 5.007038802148489509, 4.735966778795008381, 0.7998128361456341429 ) ) ;
#63226=CARTESIAN_POINT ( 'NONE',  ( -1.499999999999997780, 5.681250000682820378, 1.214306433183764966E-14 ) ) ;
#63232=CARTESIAN_POINT ( 'NONE',  ( -0.7499999999999972244, 3.358333333333359150, -1.299038105676652011 ) ) ;
#63233=CARTESIAN_POINT ( 'NONE',  ( 4.449046963578762615, 8.342305224150557308, -0.7998128361456231517 ) ) ;
#63234=EDGE_CURVE ( 'NONE', #60595, #119323, #11161, .T. ) ;
#63236=CARTESIAN_POINT ( 'NONE',  ( 8.622622508611357262, 9.162073802909148412, -0.7216878364870197293 ) ) ;
#63237=EDGE_CURVE ( 'NONE', #159976, #116082, #203475, .T. ) ;
#63238=CARTESIAN_POINT ( 'NONE',  ( -8.907343734053998929, 12.37535620882957588, 1.082531754730558626 ) ) ;
#63241=CARTESIAN_POINT ( 'NONE',  ( 9.890836756369282057, 11.49806328964105617, -1.199719254218440723 ) ) ;
#63244=CARTESIAN_POINT ( 'NONE',  ( -3.578462479003122976, 6.262291094557191684, 1.199719254218464037 ) ) ;
#63245=CARTESIAN_POINT ( 'NONE',  ( 1.499999999999990896, 5.556250000682820378, 1.214306433183764966E-14 ) ) ;
#63246=CARTESIAN_POINT ( 'NONE',  ( -1.364683531250014514, 0.9885416670080898749, -0.7879004041258289570 ) ) ;
#63250=CARTESIAN_POINT ( 'NONE',  ( 4.847203612085560387, 5.613824621309978724, -1.199719254218452047 ) ) ;
#63252=CARTESIAN_POINT ( 'NONE',  ( 1.364683531249990311, 5.426041667008086655, 0.7879004041258500513 ) ) ;
#63261=CARTESIAN_POINT ( 'NONE',  ( -6.744291347794091784, 9.955758108146730123, -1.199719254218440723 ) ) ;
#63264=CARTESIAN_POINT ( 'NONE',  ( 3.669453130792974971, 7.432779085900453886, 1.040834085586084257E-14 ) ) ;
#63269=ORIENTED_EDGE ( 'NONE', *, *, #163343, .F. ) ;
#63271=CARTESIAN_POINT ( 'NONE',  ( 10.40996301719436090, 11.03937836301526687, 0.000000000000000000 ) ) ;
#63274=CARTESIAN_POINT ( 'NONE',  ( -3.879604511804807032, 7.677955697080923514, 0.7998128361456341429 ) ) ;
#63278=CARTESIAN_POINT ( 'NONE',  ( 7.214910300766615769, 11.56914578420308715, -0.7998128361456291469 ) ) ;
#63280=CARTESIAN_POINT ( 'NONE',  ( 7.564559641420864899, 10.91273778404466199, -1.199719254218446718 ) ) ;
#63284=CARTESIAN_POINT ( 'NONE',  ( -9.002250809794000830, 11.52571191622492464, -1.443375672974059665 ) ) ;
#63286=CARTESIAN_POINT ( 'NONE',  ( -7.152089726408780379, 8.302858421353754181, -1.199719254218446718 ) ) ;
#63291=CARTESIAN_POINT ( 'NONE',  ( -5.988731108142371085, 6.089685199429741402, 0.6933981374793452002 ) ) ;
#63292=CARTESIAN_POINT ( 'NONE',  ( -0.6823417656250212460, 0.8010416670080899859, 1.181850606188755259 ) ) ;
#63295=CARTESIAN_POINT ( 'NONE',  ( 7.293923454472080792, 9.532663335016016148, 1.443375672974076540 ) ) ;
#63308=CARTESIAN_POINT ( 'NONE',  ( -2.000000000000000000, -2.856854249492362108, 0.000000000000000000 ) ) ;
#63313=CARTESIAN_POINT ( 'NONE',  ( 8.563946585326370098, 13.14302144952281814, 0.7998128361456462443 ) ) ;
#63317=CARTESIAN_POINT ( 'NONE',  ( -3.460355519985875983, 5.060167411448709629, 1.599625672291267398 ) ) ;
#63318=CARTESIAN_POINT ( 'NONE',  ( -8.518600588087975822, 8.832788862391110385, 1.040834085586084257E-14 ) ) ;
#63324=CARTESIAN_POINT ( 'NONE',  ( 1.499999999999990896, 3.556250000682818602, 1.214306433183764966E-14 ) ) ;
#63325=CARTESIAN_POINT ( 'NONE',  ( 8.483651433849084711, 10.92067931095586886, 1.599625672291281386 ) ) ;
#63329=CARTESIAN_POINT ( 'NONE',  ( -7.503547950159405566, 10.84155747757291266, 1.199719254218453823 ) ) ;
#63331=CARTESIAN_POINT ( 'NONE',  ( 1.364683531249988535, 3.863541667008087543, 0.7879004041258500513 ) ) ;
#63337=CARTESIAN_POINT ( 'NONE',  ( -8.514157279702020631, 11.91663867875229776, -1.082531754730543971 ) ) ;
#63341=CARTESIAN_POINT ( 'NONE',  ( 1.364683531249986537, 1.967708333674750731, -0.7879004041258239610 ) ) ;
#63348=CARTESIAN_POINT ( 'NONE',  ( -1.201851678989727383E-14, 2.946875000341419248, -1.575800808251660134 ) ) ;
#63351=CARTESIAN_POINT ( 'NONE',  ( -6.573005544526917099, 6.562927978236513304, -0.7998128361456291469 ) ) ;
#63352=CARTESIAN_POINT ( 'NONE',  ( 7.182068686937156166, 9.402166106225269715, 1.599625672291281386 ) ) ;
#63355=CARTESIAN_POINT ( 'NONE',  ( 1.364683531249986537, 2.467708333674753174, -0.7879004041258239610 ) ) ;
#63358=EDGE_CURVE ( 'NONE', #44776, #162623, #119887, .T. ) ;
#63359=CARTESIAN_POINT ( 'NONE',  ( -1.364683531250014514, -0.2614583329919080157, -0.7879004041258359514 ) ) ;
#63360=CARTESIAN_POINT ( 'NONE',  ( -5.965224400332865606, 7.022145224218852455, 1.082531754730549967 ) ) ;
#63365=CARTESIAN_POINT ( 'NONE',  ( 5.504247177468186258, 6.484338464210099851, 1.082531754730558626 ) ) ;
#63368=CARTESIAN_POINT ( 'NONE',  ( -6.692921386640485082, 10.96015871772258521, -0.7998128361456291469 ) ) ;
#63369=CARTESIAN_POINT ( 'NONE',  ( -3.195971524519394702, 4.751719416737803847, -1.599625672291262513 ) ) ;
#63371=CARTESIAN_POINT ( 'NONE',  ( -1.364683531250010295, 5.030208333674757171, 0.7879004041258379498 ) ) ;
#63376=CARTESIAN_POINT ( 'NONE',  ( -7.022760381754429737, 7.295567988242705582, 1.040834085586084257E-14 ) ) ;
#63378=CARTESIAN_POINT ( 'NONE',  ( -1.402160292154681736E-14, -0.3656249996585805295, 1.575800808251672791 ) ) ;
#63382=CARTESIAN_POINT ( 'NONE',  ( 7.795575138177731844, 8.197185204069915798, 1.040834085586084257E-14 ) ) ;
#63391=CARTESIAN_POINT ( 'NONE',  ( 1.499999999999987566, -0.7249999999999825473, 0.000000000000000000 ) ) ;
#63392=CARTESIAN_POINT ( 'NONE',  ( 8.500599125643985232, 11.90082083235127008, -1.082531754730543083 ) ) ;
#63398=CARTESIAN_POINT ( 'NONE',  ( 5.341022448779654930, 8.318611059296550536, 1.199719254218462483 ) ) ;
#63400=CARTESIAN_POINT ( 'NONE',  ( -3.405069135326500351, 7.124331091189553433, 1.040834085586084257E-14 ) ) ;
#63404=CARTESIAN_POINT ( 'NONE',  ( 4.975479186090839612, 8.748550117173898855, 0.7216878364870438212 ) ) ;
#63405=CARTESIAN_POINT ( 'NONE',  ( 1.364683531249988757, -0.05312499965857975237, 0.000000000000000000 ) ) ;
#63407=CARTESIAN_POINT ( 'NONE',  ( -8.971744963941075568, 11.49012176272984931, 1.599625672291269396 ) ) ;
#63413=CARTESIAN_POINT ( 'NONE',  ( -1.001543065824772872E-14, 5.712500000000022560, 1.732050807568877637 ) ) ;
#63417=ORIENTED_EDGE ( 'NONE', *, *, #76005, .F. ) ;
#63422=CARTESIAN_POINT ( 'NONE',  ( 2.284651335525438309, 5.570284631188780367, 0.4445386711868243856 ) ) ;
#63426=CARTESIAN_POINT ( 'NONE',  ( 6.817052309572890323, 6.847649204123507083, 0.7998128361456341429 ) ) ;
#63432=CARTESIAN_POINT ( 'NONE',  ( 9.257519960032755790, 9.694861462993381807, 0.7998128361456462443 ) ) ;
#63434=CARTESIAN_POINT ( 'NONE',  ( -4.083708824282378913, 7.596498746673441715, 0.5977277219625460880 ) ) ;
#63435=CARTESIAN_POINT ( 'NONE',  ( 9.911173986789782120, 11.52179005846497972, -1.199719254218440723 ) ) ;
#63436=B_SPLINE_CURVE_WITH_KNOTS ( 'NONE', 3,
 ( #182537, #130693, #114433, #98137, #131724, #34164, #49369, #165238, #100235, #12583 ),
 .UNSPECIFIED., .F., .F.,
 ( 4, 3, 3, 4 ),
 ( 0.000000000000000000, 4.502046072369050747E-05, 9.004093402560574516E-05, 0.0001800865003196817178 ),
 .UNSPECIFIED. ) ;
#63439=CARTESIAN_POINT ( 'NONE',  ( -3.358669367883384105, 4.941533567329135401, -1.599625672291262513 ) ) ;
#63449=CARTESIAN_POINT ( 'NONE',  ( -9.354762803749327560, 10.01623748057011376, 0.7216878364870438212 ) ) ;
#63453=CARTESIAN_POINT ( 'NONE',  ( 6.661133543015731462, 6.665743976473484267, -0.7998128361456281477 ) ) ;
#63454=CARTESIAN_POINT ( 'NONE',  ( -1.364683531249997417, 5.759375000341418804, 1.214306433183764966E-14 ) ) ;
#63459=CARTESIAN_POINT ( 'NONE',  ( 3.321384445223597659, 6.818772919495430074, -0.7216878364870267237 ) ) ;
#63467=CARTESIAN_POINT ( 'NONE',  ( -5.032047568966410367, 9.022472597102808578, 1.214306433183764966E-14 ) ) ;
#63468=CARTESIAN_POINT ( 'NONE',  ( -5.786632634934295361, 5.645492917045106473, 0.7998128361456341429 ) ) ;
#63473=CARTESIAN_POINT ( 'NONE',  ( 0.4963857527935924274, 7.354535952643626473, -1.939768365030055897 ) ) ;
#63477=CARTESIAN_POINT ( 'NONE',  ( 7.474622759835693131, 7.614814729430110951, -0.7998128361456281477 ) ) ;
#63486=CARTESIAN_POINT ( 'NONE',  ( 1.257518954444996062, 3.091479010054028809, -0.7749999999999926947 ) ) ;
#63488=CARTESIAN_POINT ( 'NONE',  ( 5.477130869796502211, 5.492333557625114437, 1.040834085586084257E-14 ) ) ;
#63489=ORIENTED_EDGE ( 'NONE', *, *, #27948, .F. ) ;
#63491=CARTESIAN_POINT ( 'NONE',  ( -1.364683531250014514, -0.6572916663252459379, 0.7879004041258379498 ) ) ;
#63493=CARTESIAN_POINT ( 'NONE',  ( 3.981290663907289140, 7.796589541200495965, -0.7998128361456221525 ) ) ;
#63496=CARTESIAN_POINT ( 'NONE',  ( -5.897433632264490910, 9.824163637709826702, 0.000000000000000000 ) ) ;
#63497=CARTESIAN_POINT ( 'NONE',  ( 3.389175213736285386, 6.897862149426897460, 0.7216878364870317197 ) ) ;
#63499=CARTESIAN_POINT ( 'NONE',  ( -7.876924059415400414, 9.252461493148505411, 1.082531754730558626 ) ) ;
#63502=ORIENTED_EDGE ( 'NONE', *, *, #132223, .T. ) ;
#63504=CARTESIAN_POINT ( 'NONE',  ( 5.764187864104357573, 9.876636274763768597, 1.040834085586084257E-14 ) ) ;
#63510=CARTESIAN_POINT ( 'NONE',  ( -1.001543065824772872E-14, 5.571875000341416140, 1.575800808251672791 ) ) ;
#63514=CARTESIAN_POINT ( 'NONE',  ( 8.945682426918439845, 9.331051007693339727, 1.040834085586084257E-14 ) ) ;
#63520=CARTESIAN_POINT ( 'NONE',  ( -7.714753101375940503, 8.959299025482085455, 1.199719254218462483 ) ) ;
#63525=CARTESIAN_POINT ( 'NONE',  ( 8.215351014876830504, 11.67199438640995801, -1.199719254218446718 ) ) ;
#63527=CARTESIAN_POINT ( 'NONE',  ( -8.199983978166823562, 8.461069484149769337, -0.7998128361456291469 ) ) ;
#63528=CARTESIAN_POINT ( 'NONE',  ( 0.5341120678215394157, 6.541965215396897904, 3.355953620529147141 ) ) ;
#63530=CARTESIAN_POINT ( 'NONE',  ( 5.298667053604809496, 6.361919491657284986, -1.123377533431538566 ) ) ;
#63531=CARTESIAN_POINT ( 'NONE',  ( -8.351459436338023679, 12.68719374246231624, -0.7216878364870267237 ) ) ;
#63533=CARTESIAN_POINT ( 'NONE',  ( 3.257290338497324633, 6.415022595892624580, -0.9198371423531578328 ) ) ;
#63535=CARTESIAN_POINT ( 'NONE',  ( 5.880485940025228508, 7.883652901494672349, 1.599625672291267398 ) ) ;
#63537=CARTESIAN_POINT ( 'NONE',  ( 6.322179702674084467, 6.270297829408224111, 1.040834085586084257E-14 ) ) ;
#63538=CARTESIAN_POINT ( 'NONE',  ( -4.099542569701578820, 7.506983624740954930, -0.5818660602148464367 ) ) ;
#63539=CARTESIAN_POINT ( 'NONE',  ( 4.871457266011829823, 4.577788319968905562, -0.7998128361456221525 ) ) ;
#63541=CARTESIAN_POINT ( 'NONE',  ( -5.856759171423528088, 8.816340885760650892, 1.082531754730548412 ) ) ;
#63546=CARTESIAN_POINT ( 'NONE',  ( -4.373253022481784491, 7.180661499490419430, 1.044565980707335529 ) ) ;
#63547=CARTESIAN_POINT ( 'NONE',  ( -1.402160292154681736E-14, 0.2593750003414224681, -1.575800808251665908 ) ) ;
#63550=CARTESIAN_POINT ( 'NONE',  ( 5.341549334104200852, 5.334155099317434257, 0.7216878364870317197 ) ) ;
#63551=CARTESIAN_POINT ( 'NONE',  ( 0.7499999999999902300, 3.597916667349487785, -1.299038105676658228 ) ) ;
#63554=CARTESIAN_POINT ( 'NONE',  ( -9.476786185827959841, 10.15859809299519334, 0.7216878364870438212 ) ) ;
#63559=CARTESIAN_POINT ( 'NONE',  ( -7.321039761255057066, 11.48503745486550365, 0.000000000000000000 ) ) ;
#63566=CARTESIAN_POINT ( 'NONE',  ( -9.476786185827959841, 10.15859809299519334, 0.7216878364870438212 ) ) ;
#63571=CARTESIAN_POINT ( 'NONE',  ( 1.364683531249990311, 4.946875000341417916, 1.214306433183764966E-14 ) ) ;
#63572=CARTESIAN_POINT ( 'NONE',  ( -1.499999999999997780, 4.431250000682819490, 1.214306433183764966E-14 ) ) ;
#63573=CARTESIAN_POINT ( 'NONE',  ( 5.142929413680796813, 6.687119857356774055, -1.406168165883972421 ) ) ;
#63578=CARTESIAN_POINT ( 'NONE',  ( -6.832419346282942563, 10.05857410638369487, 1.199719254218453823 ) ) ;
#63579=DIRECTION ( 'NONE',  ( -1.207943261119674327E-30, -2.168404344971008079E-15, 1.000000000000000000 ) ) ;
#63582=CARTESIAN_POINT ( 'NONE',  ( 6.972971076130050072, 7.029554431773520129, 1.040834085586084257E-14 ) ) ;
#63587=CARTESIAN_POINT ( 'NONE',  ( 8.606728586576791074, 8.935604860628076906, 0.7998128361456462443 ) ) ;
#63591=CARTESIAN_POINT ( 'NONE',  ( 1.499999999999990896, 5.525000000000022560, 1.214306433183764966E-14 ) ) ;
#63595=CARTESIAN_POINT ( 'NONE',  ( -5.748293942514172805, 8.689798118699771479, -1.082531754730538864 ) ) ;
#63605=CARTESIAN_POINT ( 'NONE',  ( -7.994504133552415404, 12.47867192245318435, -0.7998128361456281477 ) ) ;
#63607=CARTESIAN_POINT ( 'NONE',  ( 9.284636267260101050, 9.726497154758602548, -0.7998128361456281477 ) ) ;
#63609=CARTESIAN_POINT ( 'NONE',  ( -8.371269781434001800, 11.85389961405997816, -1.199719254218446718 ) ) ;
#63612=EDGE_CURVE ( 'NONE', #210868, #133229, #187583, .T. ) ;
#63613=CARTESIAN_POINT ( 'NONE',  ( -1.201851678989727383E-14, 3.696875000341422801, -1.575800808251660134 ) ) ;
#63614=CARTESIAN_POINT ( 'NONE',  ( 3.521367211247359741, 5.131347717920458962, -1.599625672291262513 ) ) ;
#63619=CARTESIAN_POINT ( 'NONE',  ( 8.229436053370658755, 12.54483312900040026, 0.7216878364870438212 ) ) ;
#63623=CARTESIAN_POINT ( 'NONE',  ( -6.182154858151506893, 9.195969186943299789, 1.082531754730548412 ) ) ;
#63625=CARTESIAN_POINT ( 'NONE',  ( -1.364683531250000748, 1.259375000341421469, 0.000000000000000000 ) ) ;
#63627=CARTESIAN_POINT ( 'NONE',  ( 0.09868764650533826122, 7.157731444430377898, 1.998865700660830358 ) ) ;
#63629=CARTESIAN_POINT ( 'NONE',  ( -6.995117189646935962, 10.24838825697502109, 1.199719254218453823 ) ) ;
#63630=CARTESIAN_POINT ( 'NONE',  ( -3.755245360860931303, 5.404205559136275205, -1.443375672974051449 ) ) ;
#63631=CARTESIAN_POINT ( 'NONE',  ( -0.6823417656249969321, 3.280208333674754062, -1.181850606188749264 ) ) ;
#63636=CARTESIAN_POINT ( 'NONE',  ( 9.260382613333817403, 10.76253345609967660, -1.199719254218446718 ) ) ;
#63651=CARTESIAN_POINT ( 'NONE',  ( -1.201851678989727383E-14, 3.759375000341422801, -1.575800808251660134 ) ) ;
#63656=CARTESIAN_POINT ( 'NONE',  ( 8.959240580532112475, 9.346868853575953651, -0.7998128361456221525 ) ) ;
#63659=CARTESIAN_POINT ( 'NONE',  ( 0.6823417656249899377, 4.176041667008085767, -1.181850606188754593 ) ) ;
#63661=CARTESIAN_POINT ( 'NONE',  ( -7.049876689426113785, 8.287572894827684777, -1.082531754730544860 ) ) ;
#63667=CARTESIAN_POINT ( 'NONE',  ( 4.216749469050096621, 4.878294787768598262, -1.199719254218452047 ) ) ;
#63670=CARTESIAN_POINT ( 'NONE',  ( 8.367353357928214663, 12.91366268422496688, 1.040834085586084257E-14 ) ) ;
#63676=CARTESIAN_POINT ( 'NONE',  ( -8.462260433223891098, 13.02438760540324481, -0.7998128361456281477 ) ) ;
#63677=CARTESIAN_POINT ( 'NONE',  ( 6.435316467980822353, 10.65961964595298817, 1.040834085586084257E-14 ) ) ;
#63679=CARTESIAN_POINT ( 'NONE',  ( 2.995988758495615745, 6.439144618312774959, -0.7216878364870267237 ) ) ;
#63682=ORIENTED_EDGE ( 'NONE', *, *, #181883, .T. ) ;
#63686=CARTESIAN_POINT ( 'NONE',  ( -1.499999999999996003, 8.226475397236011844, -3.114076396431513682 ) ) ;
#63690=CARTESIAN_POINT ( 'NONE',  ( -5.748293942514172805, 8.689798118699771479, -1.082531754730538864 ) ) ;
#63691=CARTESIAN_POINT ( 'NONE',  ( 3.310162060030825248, 7.013606170011280838, -0.7998128361456291469 ) ) ;
#63694=CARTESIAN_POINT ( 'NONE',  ( -8.830438121202295321, 9.196599317691152464, -0.7998128361456291469 ) ) ;
#63698=CARTESIAN_POINT ( 'NONE',  ( -9.053093885623068715, 11.58502883802551153, -1.599625672291263179 ) ) ;
#63702=CARTESIAN_POINT ( 'NONE',  ( 8.341290820905593151, 10.75459192918846618, 1.599625672291281386 ) ) ;
#63704=VERTEX_POINT ( 'NONE', #25511 ) ;
#63708=DIRECTION ( 'NONE',  ( -0.7592566023653004592, -0.6507913734559641616, 0.000000000000000000 ) ) ;
#63713=CARTESIAN_POINT ( 'NONE',  ( -9.006694118179950692, 9.402231314165087284, 1.040834085586084257E-14 ) ) ;
#63717=CARTESIAN_POINT ( 'NONE',  ( 7.456621297836072415, 9.722477485607340597, 1.443375672974076540 ) ) ;
#63719=CARTESIAN_POINT ( 'NONE',  ( 4.033714395265605823, 4.664753868353354704, -1.199719254218446718 ) ) ;
#63720=CARTESIAN_POINT ( 'NONE',  ( -1.500000000000022204, 6.200000000000045475, 2.580000000000011173 ) ) ;
#63722=CARTESIAN_POINT ( 'NONE',  ( -4.903245109636583443, 8.872203061218007392, -0.7998128361456281477 ) ) ;
#63724=CARTESIAN_POINT ( 'NONE',  ( -3.621833129746822255, 4.096114899008192367, -2.420000000000000373 ) ) ;
#63730=CARTESIAN_POINT ( 'NONE',  ( 1.364683531249988535, 3.926041667008087543, 0.7879004041258500513 ) ) ;
#63731=CARTESIAN_POINT ( 'NONE',  ( 3.332168893502837737, 7.719402352559943559, 2.450693629706348631 ) ) ;
#63732=CARTESIAN_POINT ( 'NONE',  ( 7.540305987494599016, 11.94877408538573427, -0.7998128361456291469 ) ) ;
#63735=CARTESIAN_POINT ( 'NONE',  ( -3.741687207691642314, 6.348756928073427730, 1.082531754730560403 ) ) ;
#63737=CARTESIAN_POINT ( 'NONE',  ( -5.707619481228834779, 5.761236937629489852, -0.7216878364870197293 ) ) ;
#63744=CARTESIAN_POINT ( 'NONE',  ( 4.304877467538922531, 4.981110786005563007, 1.199719254218464037 ) ) ;
#63752=CARTESIAN_POINT ( 'NONE',  ( 5.681030059326015014, 6.586622143090519188, -1.199719254218445830 ) ) ;
#63757=CARTESIAN_POINT ( 'NONE',  ( -1.201851678989727383E-14, 4.009375000341416140, -1.575800808251660134 ) ) ;
#63762=CARTESIAN_POINT ( 'NONE',  ( 7.311924916471702396, 7.425000578838787391, -0.7998128361456281477 ) ) ;
#63765=CARTESIAN_POINT ( 'NONE',  ( -5.284980951228653190, 5.060232619388524533, 0.000000000000000000 ) ) ;
#63766=CARTESIAN_POINT ( 'NONE',  ( -1.500000000000013101, 2.170833333333357373, 0.8660254037844403729 ) ) ;
#63769=CARTESIAN_POINT ( 'NONE',  ( -4.569261463005423352, 5.289558780716470565, -1.199719254218446718 ) ) ;
#63770=CARTESIAN_POINT ( 'NONE',  ( 0.4942023283146224633, 7.349555083877798545, -1.940391385854344897 ) ) ;
#63773=CARTESIAN_POINT ( 'NONE',  ( -1.364683531249997417, 3.509375000341423245, 1.214306433183764966E-14 ) ) ;
#63775=CARTESIAN_POINT ( 'NONE',  ( -3.470524135418300737, 6.032400010421219427, -1.082531754730549967 ) ) ;
#63781=CARTESIAN_POINT ( 'NONE',  ( 3.354752944377597856, 6.001296637494123232, -1.199719254218446718 ) ) ;
#63785=CARTESIAN_POINT ( 'NONE',  ( 1.364683531249988535, 4.176041667008081326, 0.7879004041258500513 ) ) ;
#63789=CARTESIAN_POINT ( 'NONE',  ( 0.6823417656249882723, -0.01145833299191073573, -1.181850606188749264 ) ) ;
#63793=CARTESIAN_POINT ( 'NONE',  ( -2.123823618835070537, 5.629544655282869847, 1.040834085586084257E-14 ) ) ;
#63794=CARTESIAN_POINT ( 'NONE',  ( -6.033015167956805591, 8.061603667414825480, -1.443375672974058777 ) ) ;
#63796=CARTESIAN_POINT ( 'NONE',  ( -1.499999999999997780, 6.200000000000045475, -2.579999999999995630 ) ) ;
#63798=CARTESIAN_POINT ( 'NONE',  ( 1.364683531249988535, 3.905208333674751842, -0.7879004041258239610 ) ) ;
#63806=CARTESIAN_POINT ( 'NONE',  ( -6.683806541412776525, 7.860491055478785682, -1.082531754730543083 ) ) ;
#63812=CARTESIAN_POINT ( 'NONE',  ( -6.358410854684793279, 7.480862754296137673, -1.082531754730543083 ) ) ;
#63818=CARTESIAN_POINT ( 'NONE',  ( -1.499999999999997780, 4.931250000682820378, 1.214306433183764808E-14 ) ) ;
#63822=CARTESIAN_POINT ( 'NONE',  ( -3.023105066167347310, 5.702484939155337607, 2.420000000000010587 ) ) ;
#63828=CARTESIAN_POINT ( 'NONE',  ( -4.232116505760120440, 8.089219690028791376, -0.7998128361456281477 ) ) ;
#63831=CARTESIAN_POINT ( 'NONE',  ( -0.7500000000000006661, 1.358333333333357151, -1.299038105676652011 ) ) ;
#63832=CARTESIAN_POINT ( 'NONE',  ( 3.602716132929354664, 5.226254793216122074, 1.599625672291267398 ) ) ;
#63833=CARTESIAN_POINT ( 'NONE',  ( 5.947222937888848371, 10.09017719417900416, 1.040834085586084257E-14 ) ) ;
#63836=CARTESIAN_POINT ( 'NONE',  ( 5.518332215962025167, 6.396807992499198292, -1.199719254218445830 ) ) ;
#63837=CARTESIAN_POINT ( 'NONE',  ( -0.1616376092239741047, 8.277406474725948371, -1.999409923707612391 ) ) ;
#63843=CARTESIAN_POINT ( 'NONE',  ( -2.480778921620681921, 5.838066475291996404, 1.040834085586084257E-14 ) ) ;
#63846=DIRECTION ( 'NONE',  ( -0.7071067811865457964, 0.7071067811865492381, 6.410781031902129473E-32 ) ) ;
#63851=CARTESIAN_POINT ( 'NONE',  ( 1.364683531249988535, 3.113541667008083991, 0.7879004041258500513 ) ) ;
#63852=SPHERICAL_SURFACE ( 'NONE', #88176, 0.08000000000000000167 ) ;
#63853=CARTESIAN_POINT ( 'NONE',  ( -5.554036483092550824, 9.631459663583308739, -0.7998128361456231517 ) ) ;
#63856=CARTESIAN_POINT ( 'NONE',  ( 6.440286661691305703, 7.472421512516709718, 1.199719254218462483 ) ) ;
#63857=CARTESIAN_POINT ( 'NONE',  ( -4.876128802409253282, 8.840567369452784874, 0.7998128361456481317 ) ) ;
#63861=CARTESIAN_POINT ( 'NONE',  ( -1.402160292154681736E-14, -0.2562499993171780122, 1.732050807568877637 ) ) ;
#63865=CARTESIAN_POINT ( 'NONE',  ( 6.466876084038451822, 10.48851316477946582, 1.040834085586084257E-14 ) ) ;
#63868=CARTESIAN_POINT ( 'NONE',  ( -1.201851678989727383E-14, 1.634375000341421025, 1.575800808251672791 ) ) ;
#63870=CARTESIAN_POINT ( 'NONE',  ( 6.683806541412754321, 8.820860269780128604, -1.443375672974058777 ) ) ;
#63873=CARTESIAN_POINT ( 'NONE',  ( -2.467220768007014176, 5.822248629409386922, 0.7216878364870317197 ) ) ;
#63876=CARTESIAN_POINT ( 'NONE',  ( 1.364683531249990311, 4.134375000341417028, 1.214306433183764966E-14 ) ) ;
#63880=CARTESIAN_POINT ( 'NONE',  ( -5.775737613422593952, 6.228167737865282660, -1.031624843267029190 ) ) ;
#63886=CARTESIAN_POINT ( 'NONE',  ( 7.305145839664861640, 7.417091655897478653, 0.7998128361456341429 ) ) ;
#63889=CARTESIAN_POINT ( 'NONE',  ( 3.440018289565364817, 5.036440642624797626, 1.599625672291267398 ) ) ;
#63897=CARTESIAN_POINT ( 'NONE',  ( 6.480434237652135998, 6.662854153456708950, 0.7216878364870317197 ) ) ;
#63898=CARTESIAN_POINT ( 'NONE',  ( -0.6823417656250212460, 1.113541667008083325, 1.181850606188755259 ) ) ;
#63900=CARTESIAN_POINT ( 'NONE',  ( 1.123270288254022198, 3.158552654332631882, -0.7749999999939810591 ) ) ;
#63905=CARTESIAN_POINT ( 'NONE',  ( 0.7499999999999885647, 2.316666666666689078, -1.299038105676652899 ) ) ;
#63906=CARTESIAN_POINT ( 'NONE',  ( 6.856673000209174695, 9.022537805042615489, 1.599625672291281386 ) ) ;
#63907=CARTESIAN_POINT ( 'NONE',  ( -7.167456763118792651, 11.51378332361394818, 0.000000000000000000 ) ) ;
#63911=CARTESIAN_POINT ( 'NONE',  ( -1.201851678989727383E-14, 2.946875000341419248, -1.575800808251660134 ) ) ;
#63912=CARTESIAN_POINT ( 'NONE',  ( 1.499999999999987121, 2.795833333333352488, -0.8660254037844262731 ) ) ;
#63914=CARTESIAN_POINT ( 'NONE',  ( 3.009020027229115879, 5.597941567487558778, -1.199719254218446718 ) ) ;
#63917=DIRECTION ( 'NONE',  ( -0.6507913734559640506, -0.7592566023653004592, 0.000000000000000000 ) ) ;
#63920=CARTESIAN_POINT ( 'NONE',  ( 1.499999999999987121, 0.8270833340161471980, -0.8660254037844253849 ) ) ;
#63922=CARTESIAN_POINT ( 'NONE',  ( -6.989391883044787868, 8.113044270762433285, -1.199719254218446718 ) ) ;
#63923=CARTESIAN_POINT ( 'NONE',  ( -2.955314298098991266, 6.391691081183366485, 0.7216878364870317197 ) ) ;
#63930=CARTESIAN_POINT ( 'NONE',  ( 6.856673000209174695, 9.022537805042615489, 1.599625672291281386 ) ) ;
#63934=CARTESIAN_POINT ( 'NONE',  ( 5.621827251160867789, 9.710548892996357040, 1.040834085586084257E-14 ) ) ;
#63935=CARTESIAN_POINT ( 'NONE',  ( 8.053180056393003383, 12.33920113252646367, 1.040834085586084257E-14 ) ) ;
#63937=ORIENTED_EDGE ( 'NONE', *, *, #71089, .F. ) ;
#63938=CARTESIAN_POINT ( 'NONE',  ( 1.403499169903295263, 7.376709478543810761, -4.304123474983216902 ) ) ;
#63942=CARTESIAN_POINT ( 'NONE',  ( -5.357443255694392725, 9.402100898285455699, 0.000000000000000000 ) ) ;
#63943=CARTESIAN_POINT ( 'NONE',  ( 4.330940004561544043, 7.140181541042074365, -1.199719254218452047 ) ) ;
#63946=CARTESIAN_POINT ( 'NONE',  ( 2.359223927328457648E-13, 7.078193277237625480, 2.121339347286388843 ) ) ;
#63947=CARTESIAN_POINT ( 'NONE',  ( 4.052428274714076295, 7.522979123003127988, 0.4826459875755910733 ) ) ;
#63948=CARTESIAN_POINT ( 'NONE',  ( 10.38518247838791986, 11.21839376764850726, 0.7216878364870438212 ) ) ;
#63949=VERTEX_POINT ( 'NONE', #124182 ) ;
#63958=CARTESIAN_POINT ( 'NONE',  ( -4.134873662487946966, 3.926366815765101936, 1.214306433183764966E-14 ) ) ;
#63959=AXIS2_PLACEMENT_3D ( 'NONE', #180909, #198211, #131167 ) ;
#63960=CARTESIAN_POINT ( 'NONE',  ( 8.446366511633696561, 8.956441806435218922, 1.040834085586084257E-14 ) ) ;
#63963=CARTESIAN_POINT ( 'NONE',  ( -4.229253852459088137, 7.021547696922494808, 1.199719254218464037 ) ) ;
#63965=CARTESIAN_POINT ( 'NONE',  ( -3.103560622218558329, 6.448189014018472776, -0.7351483804875698080 ) ) ;
#63969=CARTESIAN_POINT ( 'NONE',  ( -6.287230548435221777, 8.358188277972981695, -1.599625672291263179 ) ) ;
#63974=( BOUNDED_CURVE ( )  B_SPLINE_CURVE ( 2, ( #78422, #1143, #110995, #142399, #208407, #13417, #175944 ),
 .UNSPECIFIED., .F., .T. ) 
 B_SPLINE_CURVE_WITH_KNOTS ( ( 3, 2, 2, 3 ),
 ( 0.07142857142857149400, 0.07738095238095236972, 0.08333333333333324544, 0.08928571428571412116 ),
 .UNSPECIFIED. ) 
 CURVE ( )  GEOMETRIC_REPRESENTATION_ITEM ( )  RATIONAL_B_SPLINE_CURVE ( ( 0.9999999999999984457, 0.8660254037844402619, 1.000000000000000000, 0.8660254037844387076, 1.000000000000000000, 0.8660254037844424824, 0.9999999999999962252 ) ) 
 REPRESENTATION_ITEM ( '' )  );
#63975=ORIENTED_EDGE ( 'NONE', *, *, #179709, .T. ) ;
#63977=VERTEX_POINT ( 'NONE', #70669 ) ;
#63980=ORIENTED_EDGE ( 'NONE', *, *, #24241, .F. ) ;
#63986=CARTESIAN_POINT ( 'NONE',  ( 4.081882008079450230, 3.980588341361369853, -0.7346435760097062007 ) ) ;
#63987=CARTESIAN_POINT ( 'NONE',  ( -6.013204822860843457, 6.974159367214481264, -1.199719254218446718 ) ) ;
#63990=CARTESIAN_POINT ( 'NONE',  ( 4.202664430556257713, 4.965825259479493603, 1.082531754730560403 ) ) ;
#63991=CARTESIAN_POINT ( 'NONE',  ( -1.123270288249905713, 3.300000000000025135, 0.7750000000000117906 ) ) ;
#63994=CARTESIAN_POINT ( 'NONE',  ( -2.611917148927046295, 6.198987107056845858, 1.040834085586084257E-14 ) ) ;
#63998=CARTESIAN_POINT ( 'NONE',  ( 8.028399517586572998, 12.51821653715971472, -0.7998128361456352531 ) ) ;
#64001=CARTESIAN_POINT ( 'NONE',  ( -7.720478407978036195, 11.09464301169468037, -1.199719254218446718 ) ) ;
#64002=CARTESIAN_POINT ( 'NONE',  ( 6.311484202361478779, 7.322151976631905868, -1.199719254218446718 ) ) ;
#64009=CARTESIAN_POINT ( 'NONE',  ( -0.6823417656250212460, 1.113541667008083325, 1.181850606188755259 ) ) ;
#64012=CARTESIAN_POINT ( 'NONE',  ( 7.782016984564060103, 9.141736572488651902, 1.082531754730558626 ) ) ;
#64029=CARTESIAN_POINT ( 'NONE',  ( -9.236128959407555072, 11.79856975744075598, -1.599625672291263179 ) ) ;
#64035=B_SPLINE_CURVE_WITH_KNOTS ( 'NONE', 3,
 ( #46109, #212836, #77514, #29850, #163053, #112227 ),
 .UNSPECIFIED., .F., .F.,
 ( 4, 2, 4 ),
 ( 0.3940582275541298363, 0.4471490536060385157, 0.5002398796579472506 ),
 .UNSPECIFIED. ) ;
#64042=CARTESIAN_POINT ( 'NONE',  ( 1.499999999999987121, 0.2854166673494805684, 0.8660254037844524744 ) ) ;
#64048=DIRECTION ( 'NONE',  ( -7.387867266669436732E-31, 1.000000000000000000, 8.546850786086424434E-32 ) ) ;
#64049=CARTESIAN_POINT ( 'NONE',  ( 8.914649696185335870, 10.35917838609310593, -1.199719254218446718 ) ) ;
#64055=CARTESIAN_POINT ( 'NONE',  ( 3.334415713957098681, 5.977569868670206787, -1.199719254218446718 ) ) ;
#64056=CARTESIAN_POINT ( 'NONE',  ( -7.049876689426106680, 9.247942109129029475, -1.443375672974059665 ) ) ;
#64060=CARTESIAN_POINT ( 'NONE',  ( -6.073162743917628781, 9.172774736957510555, -1.199719254218440723 ) ) ;
#64062=ORIENTED_EDGE ( 'NONE', *, *, #14091, .T. ) ;
#64063=CARTESIAN_POINT ( 'NONE',  ( -1.402160292154681736E-14, 1.868750000682816381, -1.732050807568863648 ) ) ;
#64071=CARTESIAN_POINT ( 'NONE',  ( -9.480175724453545172, 12.08329098332774265, 1.599625672291281386 ) ) ;
#64073=CARTESIAN_POINT ( 'NONE',  ( 1.436838838544733044, 7.449283400311756509, -4.203727439823553347 ) ) ;
#64075=CARTESIAN_POINT ( 'NONE',  ( 4.589221341884758942, 6.929947237659640713, 1.197292633685101748 ) ) ;
#64080=CARTESIAN_POINT ( 'NONE',  ( -9.317477881089553549, 11.89347683273641820, 1.599625672291281386 ) ) ;
#64081=CARTESIAN_POINT ( 'NONE',  ( 8.620286740190458374, 8.951422706510690830, 1.040834085586084257E-14 ) ) ;
#64082=CARTESIAN_POINT ( 'NONE',  ( -2.535011536075351124, 5.133042487381361596, -2.419999999999995044 ) ) ;
#64088=CIRCLE ( 'NONE', #185117, 1.250000000000000222 ) ;
#64091=CARTESIAN_POINT ( 'NONE',  ( -8.350932551013499960, 11.83017284523606172, -1.199719254218446718 ) ) ;
#64094=ORIENTED_EDGE ( 'NONE', *, *, #81974, .T. ) ;
#64096=CARTESIAN_POINT ( 'NONE',  ( 4.867540842506059562, 5.637551390133895168, -1.199719254218452047 ) ) ;
#64101=CARTESIAN_POINT ( 'NONE',  ( -5.148345644887285744, 7.029489223833707001, -1.599625672291256295 ) ) ;
#64102=CARTESIAN_POINT ( 'NONE',  ( -10.15913717534155047, 10.74674821418697057, 0.7998128361456462443 ) ) ;
#64105=CARTESIAN_POINT ( 'NONE',  ( -1.230761180058556281, 3.185133534840179248, -0.7749999999999918066 ) ) ;
#64114=CARTESIAN_POINT ( 'NONE',  ( 5.770966940911189447, 9.884545197705074671, -0.7998128361456291469 ) ) ;
#64116=CARTESIAN_POINT ( 'NONE',  ( -3.761497552787613330, 6.475832013972435242, 1.199719254218464037 ) ) ;
#64117=VERTEX_POINT ( 'NONE', #55113 ) ;
#64124=CARTESIAN_POINT ( 'NONE',  ( -1.402160292154681736E-14, 0.4937500006828175469, 1.732050807568877637 ) ) ;
#64128=CARTESIAN_POINT ( 'NONE',  ( 3.704402285031850539, 5.344888637335695414, -1.599625672291262513 ) ) ;
#64130=CARTESIAN_POINT ( 'NONE',  ( -4.081167932913447594, 4.720116328942494555, -1.199719254218452047 ) ) ;
#64136=CARTESIAN_POINT ( 'NONE',  ( 4.148431816101584957, 6.823292304551739740, -1.082531754730548412 ) ) ;
#64138=ORIENTED_EDGE ( 'NONE', *, *, #4855, .T. ) ;
#64139=CARTESIAN_POINT ( 'NONE',  ( -8.611400122974211868, 13.19838391011195888, 1.040834085586084257E-14 ) ) ;
#64141=CARTESIAN_POINT ( 'NONE',  ( 3.999292125906911188, 4.728557570721922509, 1.082531754730560403 ) ) ;
#64150=CARTESIAN_POINT ( 'NONE',  ( -6.007394967034264788, 6.077829431587280062, -0.6506939886842719734 ) ) ;
#64152=CARTESIAN_POINT ( 'NONE',  ( -1.402160292154681736E-14, -0.4281249996585808071, 1.575800808251672791 ) ) ;
#64157=CARTESIAN_POINT ( 'NONE',  ( -4.367698041896780126, 8.247398148854895084, 0.7998128361456481317 ) ) ;
#64161=CARTESIAN_POINT ( 'NONE',  ( -1.201851678989727383E-14, 4.837500000000018119, -1.732050807568863648 ) ) ;
#64168=CARTESIAN_POINT ( 'NONE',  ( -1.364683531250014514, -1.219791666325248602, 0.7879004041258379498 ) ) ;
#64170=CARTESIAN_POINT ( 'NONE',  ( 5.555090253297246150, 7.504024600312024340, 1.599625672291267398 ) ) ;
#64171=CARTESIAN_POINT ( 'NONE',  ( -7.232384877886063990, 10.52520055992070525, -1.199719254218446718 ) ) ;
#64173=CARTESIAN_POINT ( 'NONE',  ( 8.757677159423465696, 12.30470822171437284, 1.199719254218450271 ) ) ;
#64180=CARTESIAN_POINT ( 'NONE',  ( -1.500000000000011324, 5.379166666666692187, -0.8660254037844313801 ) ) ;
#64184=CARTESIAN_POINT ( 'NONE',  ( 4.219703575591028155, 7.337867620521338452, -0.8994424175318147530 ) ) ;
#64188=CARTESIAN_POINT ( 'NONE',  ( 7.131225611108085616, 10.30321839872603462, 1.082531754730558626 ) ) ;
#64193=CARTESIAN_POINT ( 'NONE',  ( -1.499999999999997780, 4.681250000682819490, 1.214306433183764966E-14 ) ) ;
#64195=CARTESIAN_POINT ( 'NONE',  ( -4.172158584703340445, 5.890604320285754980, -1.599625672291256295 ) ) ;
#64196=CARTESIAN_POINT ( 'NONE',  ( 5.273758565591489145, 9.096542726591325234, -0.7216878364870267237 ) ) ;
#64204=CARTESIAN_POINT ( 'NONE',  ( 3.521367211247359741, 5.131347717920458962, -1.599625672291262513 ) ) ;
#64205=CARTESIAN_POINT ( 'NONE',  ( 0.7499999999999902300, 3.847916667349481123, -1.299038105676658228 ) ) ;
#64208=ORIENTED_EDGE ( 'NONE', *, *, #45988, .T. ) ;
#64221=CARTESIAN_POINT ( 'NONE',  ( 8.269583629331492602, 11.73526576994040482, 1.199719254218450271 ) ) ;
#64224=CARTESIAN_POINT ( 'NONE',  ( -1.364683531250000748, -0.7406249996585803075, 0.000000000000000000 ) ) ;
#64225=CARTESIAN_POINT ( 'NONE',  ( 5.016153647376201619, 7.835634441038803466, 1.082531754730558626 ) ) ;
#64226=CARTESIAN_POINT ( 'NONE',  ( -9.354762803749327560, 10.01623748057011376, 0.7216878364870438212 ) ) ;
#64231=CARTESIAN_POINT ( 'NONE',  ( -3.928111819657352566, 5.605883094398769195, 1.599625672291267398 ) ) ;
#64244=CARTESIAN_POINT ( 'NONE',  ( 5.089368577813358385, 6.729159871965151751, -1.415889853396500975 ) ) ;
#64248=CARTESIAN_POINT ( 'NONE',  ( 5.684946482831785275, 5.526859072925533134, -0.7998128361456231517 ) ) ;
#64253=CARTESIAN_POINT ( 'NONE',  ( -8.514157279702033065, 9.995900250149611921, -1.082531754730543971 ) ) ;
#64257=CARTESIAN_POINT ( 'NONE',  ( 7.461064606222022277, 7.598996883547496139, 1.040834085586084257E-14 ) ) ;
#64258=CARTESIAN_POINT ( 'NONE',  ( -5.610376637956639101, 5.439860920571172542, 0.000000000000000000 ) ) ;
#64261=CARTESIAN_POINT ( 'NONE',  ( -5.870844209917351009, 6.808071985447069707, -1.199719254218446718 ) ) ;
#64265=CARTESIAN_POINT ( 'NONE',  ( -5.687809136132860210, 6.594531066031826150, -1.199719254218446718 ) ) ;
#64269=CARTESIAN_POINT ( 'NONE',  ( 9.915090410295563927, 10.46202698829998567, -0.7998128361456281477 ) ) ;
#64271=CARTESIAN_POINT ( 'NONE',  ( 4.344452866495080556, 7.409550296852231099, 1.129427019999120985 ) ) ;
#64272=CARTESIAN_POINT ( 'NONE',  ( 5.829642864196171281, 5.903597551091405826, 0.7216878364870317197 ) ) ;
#64274=CARTESIAN_POINT ( 'NONE',  ( 3.660338285565247762, 7.214219066560688454, 1.040834085586084257E-14 ) ) ;
#64279=CARTESIAN_POINT ( 'NONE',  ( 5.924549939047454750, 9.855799328956630134, -0.7216878364870267237 ) ) ;
#64283=CARTESIAN_POINT ( 'NONE',  ( -10.15913717534155047, 10.74674821418697057, 0.7998128361456462443 ) ) ;
#64284=CARTESIAN_POINT ( 'NONE',  ( -5.689618019229208734, 9.789638122409414223, 0.7998128361456481317 ) ) ;
#64285=CARTESIAN_POINT ( 'NONE',  ( -4.351804119862249465, 7.060559992272473551, 1.082531754730560403 ) ) ;
#64291=CARTESIAN_POINT ( 'NONE',  ( 8.432281472695482449, 11.92507992053172572, 1.199719254218450271 ) ) ;
#64295=CARTESIAN_POINT ( 'NONE',  ( 2.998324526916512411, 6.649795714711241423, 0.000000000000000000 ) ) ;
#64299=CARTESIAN_POINT ( 'NONE',  ( -1.500000000000011324, 4.952083334016150751, 0.8660254037844403729 ) ) ;
#64305=CARTESIAN_POINT ( 'NONE',  ( -1.499999999999997780, 3.650000000000021227, 1.214306433183764966E-14 ) ) ;
#64306=CARTESIAN_POINT ( 'NONE',  ( 5.717788096661236885, 7.693838750903348789, 1.599625672291267398 ) ) ;
#64307=DIRECTION ( 'NONE',  ( 0.000000000000000000, 1.000000000000000000, -8.546850786086437571E-32 ) ) ;
#64308=CARTESIAN_POINT ( 'NONE',  ( 8.107412671292047790, 8.560995659369956101, 0.7216878364870458196 ) ) ;
#64309=CARTESIAN_POINT ( 'NONE',  ( -10.60211293576223213, 11.47147930125185589, 1.040834085586084257E-14 ) ) ;
#64313=CARTESIAN_POINT ( 'NONE',  ( 8.543609354905870035, 13.11929468069890525, 0.7998128361456462443 ) ) ;
#64315=CARTESIAN_POINT ( 'NONE',  ( -3.958090780185743451, 6.705190779270287393, -1.199719254218452047 ) ) ;
#64316=CARTESIAN_POINT ( 'NONE',  ( -1.001543065824772872E-14, 4.743750000682822154, 1.732050807568877637 ) ) ;
#64318=CARTESIAN_POINT ( 'NONE',  ( 1.364683531249986537, -0.3864583329919166199, 0.7879004041258500513 ) ) ;
#64322=CARTESIAN_POINT ( 'NONE',  ( 5.345992642490140057, 5.131412925860272090, 1.040834085586084257E-14 ) ) ;
#64324=CARTESIAN_POINT ( 'NONE',  ( -1.201851678989727383E-14, 5.009375000341421469, -1.575800808251660134 ) ) ;
#64328=CARTESIAN_POINT ( 'NONE',  ( 3.998552357014331982, 7.829812261164016185, 1.248643980066187585E-14 ) ) ;
#64335=CARTESIAN_POINT ( 'NONE',  ( -6.204827856548512877, 10.39071626594860476, -0.7998128361456291469 ) ) ;
#64338=CARTESIAN_POINT ( 'NONE',  ( 6.003563092752934871, 5.898578451166879510, 0.7998128361456341429 ) ) ;
#64344=CARTESIAN_POINT ( 'NONE',  ( 10.55910270694468345, 11.21337466772398095, 0.7998128361456462443 ) ) ;
#64347=CARTESIAN_POINT ( 'NONE',  ( -5.579343907223557331, 6.467988298970945849, 1.199719254218450271 ) ) ;
#64351=CARTESIAN_POINT ( 'NONE',  ( 8.727698198895078363, 11.20540053684285553, -1.599625672291257406 ) ) ;
#64353=CARTESIAN_POINT ( 'NONE',  ( 9.264299036839600987, 9.702770385934682551, -0.7998128361456281477 ) ) ;
#64354=CARTESIAN_POINT ( 'NONE',  ( 4.891850447398502943, 4.899046648864193720, -0.7063863167381065900 ) ) ;
#64355=CARTESIAN_POINT ( 'NONE',  ( -10.03267048443264109, 11.76749898900197877, 1.082531754730558626 ) ) ;
#64356=CARTESIAN_POINT ( 'NONE',  ( -7.182068686937172153, 9.402166106225269715, 1.599625672291283607 ) ) ;
#64359=CARTESIAN_POINT ( 'NONE',  ( -4.038103646828244742, 7.764432012698684105, 0.5462726908427618655 ) ) ;
#64360=CARTESIAN_POINT ( 'NONE',  ( 1.364683531249986537, 0.9052083336747533959, -0.7879004041258239610 ) ) ;
#64364=CARTESIAN_POINT ( 'NONE',  ( 8.134528978519385944, 8.592631351135175066, -0.7216878364870267237 ) ) ;
#64381=CARTESIAN_POINT ( 'NONE',  ( 9.748476143425788720, 11.33197590787365172, -1.199719254218440723 ) ) ;
#64383=ORIENTED_EDGE ( 'NONE', *, *, #148663, .F. ) ;
#64385=CARTESIAN_POINT ( 'NONE',  ( -6.112028321662274166, 6.025121218227761588, 0.7998128361456341429 ) ) ;
#64386=CARTESIAN_POINT ( 'NONE',  ( -6.320072162264675164, 10.52516795595079557, 0.7998128361456481317 ) ) ;
#64388=EDGE_LOOP ( 'NONE', ( #34779, #6125, #157274, #157193, #47730, #202466, #16259, #52868, #15308, #36838, #23667, #119973, #13567 ) ) ;
#64393=CARTESIAN_POINT ( 'NONE',  ( -1.201851678989727383E-14, 3.493750000682815493, 1.732050807568877637 ) ) ;
#64394=CARTESIAN_POINT ( 'NONE',  ( 9.738834413317897898, 10.25639499182604730, 0.000000000000000000 ) ) ;
#64397=CARTESIAN_POINT ( 'NONE',  ( -9.450196763925152510, 10.98398329845622001, -1.199719254218441611 ) ) ;
#64399=CARTESIAN_POINT ( 'NONE',  ( -1.364683531250012516, 3.030208333674755394, 0.7879004041258379498 ) ) ;
#64405=CARTESIAN_POINT ( 'NONE',  ( -8.839552966430002101, 12.29626697993494666, -1.082531754730543971 ) ) ;
#64409=CARTESIAN_POINT ( 'NONE',  ( 0.6823417656249899377, 0.9052083336747520637, 1.181850606188755259 ) ) ;
#64415=CARTESIAN_POINT ( 'NONE',  ( 0.6823417656249882723, 2.426041667008084435, -1.181850606188749264 ) ) ;
#64418=CARTESIAN_POINT ( 'NONE',  ( -4.577849422908604637, 8.492574760035358494, -0.7998128361456281477 ) ) ;
#64422=CARTESIAN_POINT ( 'NONE',  ( 0.6823417656249882723, 2.238541667008084435, -1.181850606188749264 ) ) ;
#64427=CARTESIAN_POINT ( 'NONE',  ( -5.924549939491850381, 6.014322472269677533, 0.000000000000000000 ) ) ;
#64431=CARTESIAN_POINT ( 'NONE',  ( 4.772106882330221289, 6.590544000850479200, -1.443375672974051449 ) ) ;
#64434=CARTESIAN_POINT ( 'NONE',  ( -8.688077508258798431, 9.030511935923748013, -0.7998128361456291469 ) ) ;
#64435=CARTESIAN_POINT ( 'NONE',  ( -3.090368948911150770, 5.692848642783215674, 1.199719254218462483 ) ) ;
#64437=CARTESIAN_POINT ( 'NONE',  ( -1.364683531250010295, 5.280208333674758059, 0.7879004041258379498 ) ) ;
#64442=CARTESIAN_POINT ( 'NONE',  ( -7.171900071504754060, 7.469564292951421436, -0.7216878364870267237 ) ) ;
#64444=CARTESIAN_POINT ( 'NONE',  ( 1.364683531249986537, -1.073958332991911790, 0.7879004041258500513 ) ) ;
#64447=CARTESIAN_POINT ( 'NONE',  ( 6.643132081016111634, 9.733775946952057723, 1.082531754730558626 ) ) ;
#64457=CARTESIAN_POINT ( 'NONE',  ( 8.554831740098654436, 11.00372300158037042, 1.443375672974076540 ) ) ;
#64461=ORIENTED_EDGE ( 'NONE', *, *, #104706, .T. ) ;
#64466=CARTESIAN_POINT ( 'NONE',  ( 4.964256800898067645, 8.943383367689749619, 0.7998128361456462443 ) ) ;
#64467=CARTESIAN_POINT ( 'NONE',  ( -3.581325132304157943, 7.329963087663487364, -0.7998128361456281477 ) ) ;
#64470=CARTESIAN_POINT ( 'NONE',  ( 4.894543267554960053, 4.887125941896303338, -0.6895117023006970269 ) ) ;
#64471=CARTESIAN_POINT ( 'NONE',  ( 5.138177029454836564, 7.977995053463880382, 1.082531754730558626 ) ) ;
#64472=CARTESIAN_POINT ( 'NONE',  ( -1.364683531250012516, 0.5927083336747520637, 0.7879004041258379498 ) ) ;
#64474=CARTESIAN_POINT ( 'NONE',  ( -9.297140650669053485, 11.86975006391249643, 1.599625672291281386 ) ) ;
#64486=ORIENTED_EDGE ( 'NONE', *, *, #155922, .T. ) ;
#64487=LINE ( 'NONE', #179318, #116328 ) ;
#64491=CARTESIAN_POINT ( 'NONE',  ( 7.793239369756836510, 7.986534107671458216, 0.7998128361456341429 ) ) ;
#64499=CARTESIAN_POINT ( 'NONE',  ( 4.991989969715272757, 4.726297878971393196, 2.420000000000010587 ) ) ;
#64500=CARTESIAN_POINT ( 'NONE',  ( 8.723781775389312543, 12.26516360700784958, -1.199719254218446718 ) ) ;
#64502=CARTESIAN_POINT ( 'NONE',  ( -4.437596350374534815, 4.071617251725375475, -0.7998128361456221525 ) ) ;
#64510=B_SPLINE_CURVE_WITH_KNOTS ( 'NONE', 3,
 ( #192739, #110515, #79002, #213256, #160261, #15052, #111579, #210056, #80070, #176515, #27044, #159190, #12922 ),
 .UNSPECIFIED., .F., .F.,
 ( 4, 3, 3, 3, 4 ),
 ( 0.000000000000000000, 6.251649345123172139E-05, 0.0001877439649095022150, 0.0003000588009599786999, 0.0004131109743063360296 ),
 .UNSPECIFIED. ) ;
#64512=CARTESIAN_POINT ( 'NONE',  ( -4.302014814237876017, 3.913438792899272212, 0.7998128361456341429 ) ) ;
#64516=CARTESIAN_POINT ( 'NONE',  ( 4.611744806942754238, 8.532119374741881757, -0.7998128361456231517 ) ) ;
#64517=CARTESIAN_POINT ( 'NONE',  ( -1.364683531250010740, 5.488541667008087543, -0.7879004041258300672 ) ) ;
#64523=CARTESIAN_POINT ( 'NONE',  ( 3.497640442201256139, 7.024404915969360452, 1.040834085586084257E-14 ) ) ;
#64531=CARTESIAN_POINT ( 'NONE',  ( -6.693975156845199059, 8.832723654451292816, 1.599625672291283607 ) ) ;
#64533=CARTESIAN_POINT ( 'NONE',  ( -3.249150368769345043, 6.942425863539538611, 0.7998128361456341429 ) ) ;
#64534=FACE_OUTER_BOUND ( 'NONE', #198324, .T. ) ;
#64538=CARTESIAN_POINT ( 'NONE',  ( 4.879410147971470657, 4.944948943068641967, -0.7687999843507594688 ) ) ;
#64542=CARTESIAN_POINT ( 'NONE',  ( 5.286789834324991055, 8.255339675766103724, -1.199719254218452935 ) ) ;
#64554=CARTESIAN_POINT ( 'NONE',  ( -1.402160292154681736E-14, -0.4906249996585810846, -1.575800808251665908 ) ) ;
#64555=CARTESIAN_POINT ( 'NONE',  ( 2.846322183865124700, 5.408127416896231665, -1.199719254218446718 ) ) ;
#64556=CARTESIAN_POINT ( 'NONE',  ( 4.059776932288224671, 6.823824623389866950, 1.199719254218462483 ) ) ;
#64558=CARTESIAN_POINT ( 'NONE',  ( -7.429504990608782222, 8.730472579540773381, 1.082531754730549967 ) ) ;
#64560=CARTESIAN_POINT ( 'NONE',  ( 3.985733972737593778, 6.633478153960411738, -1.082531754730548412 ) ) ;
#64561=CARTESIAN_POINT ( 'NONE',  ( -7.673551755210395342, 8.054824590608001600, 1.040834085586084257E-14 ) ) ;
#64566=CARTESIAN_POINT ( 'NONE',  ( 6.479907352327590964, 9.647310113435821677, 1.199719254218462483 ) ) ;
#64571=EDGE_CURVE ( 'NONE', #137371, #201176, #14734, .T. ) ;
#64572=CARTESIAN_POINT ( 'NONE',  ( 0.6823417656249917140, 3.592708333674754506, 1.181850606188765695 ) ) ;
#64577=CARTESIAN_POINT ( 'NONE',  ( 7.365103760721646076, 9.615707025640515937, 1.599625672291281386 ) ) ;
#64580=CARTESIAN_POINT ( 'NONE',  ( -6.503107236049161521, 10.73870887536603291, 0.7998128361456481317 ) ) ;
#64586=CARTESIAN_POINT ( 'NONE',  ( 7.865701674222579598, 12.32840238656838139, -0.7998128361456352531 ) ) ;
#64589=CARTESIAN_POINT ( 'NONE',  ( -9.338868881714763148, 9.789768538289042255, -0.7998128361456291469 ) ) ;
#64593=CARTESIAN_POINT ( 'NONE',  ( 4.513260471453858003, 7.001907027245110271, -1.160773635454902530 ) ) ;
#64594=CARTESIAN_POINT ( 'NONE',  ( -9.869972641068651242, 11.57768483841065787, 1.082531754730558626 ) ) ;
#64597=CARTESIAN_POINT ( 'NONE',  ( 7.135668919494039031, 7.219368582364847242, 1.040834085586084257E-14 ) ) ;
#64599=CARTESIAN_POINT ( 'NONE',  ( 6.148786358997489820, 7.132337826040578754, -1.199719254218446718 ) ) ;
#64600=CARTESIAN_POINT ( 'NONE',  ( -4.327620591935813721, 7.230343590456815406, 0.9971501367836959062 ) ) ;
#64601=CARTESIAN_POINT ( 'NONE',  ( 4.009460741339333723, 5.700790169694431420, -1.599625672291256295 ) ) ;
#64604=CARTESIAN_POINT ( 'NONE',  ( -7.537970219518091319, 7.896646132300314314, -0.7216878364870278340 ) ) ;
#64611=CARTESIAN_POINT ( 'NONE',  ( -4.137838753588869878, 7.456630865025390520, 0.6858938789830407723 ) ) ;
#64612=CARTESIAN_POINT ( 'NONE',  ( -1.402160292154681736E-14, 0.3843750003414230232, 1.575800808251672791 ) ) ;
#64615=CARTESIAN_POINT ( 'NONE',  ( 4.311129659465574804, 7.013106455143060636, -1.082531754730548412 ) ) ;
#64616=AXIS2_PLACEMENT_3D ( 'NONE', #25718, #124389, #9478 ) ;
#64619=CARTESIAN_POINT ( 'NONE',  ( -7.470179451005382276, 11.65903375957422128, 0.7216878364870458196 ) ) ;
#64624=CARTESIAN_POINT ( 'NONE',  ( -8.446366511189330240, 12.79791866312216442, 0.7216878364870317197 ) ) ;
#64626=EDGE_LOOP ( 'NONE', ( #60330, #145788, #34876, #187504 ) ) ;
#64631=CARTESIAN_POINT ( 'NONE',  ( -8.554831740098665094, 11.00372300158037042, 1.443375672974064550 ) ) ;
#64635=CARTESIAN_POINT ( 'NONE',  ( 1.364683531249990311, 4.696875000341417916, 1.214306433183764966E-14 ) ) ;
#64636=CARTESIAN_POINT ( 'NONE',  ( -1.402160292154681736E-14, 2.618750000682819490, -1.732050807568863648 ) ) ;
#64641=CARTESIAN_POINT ( 'NONE',  ( -7.832860060393135093, 10.16142270859057462, 1.599625672291295375 ) ) ;
#64644=CARTESIAN_POINT ( 'NONE',  ( 1.499999999999976907, 4.327083334016148086, -0.8660254037844394848 ) ) ;
#64645=CARTESIAN_POINT ( 'NONE',  ( 6.094553744542824170, 7.069066442510145265, 1.199719254218462483 ) ) ;
#64650=CARTESIAN_POINT ( 'NONE',  ( 6.611572464958476836, 10.86525164242692298, 0.7998128361456462443 ) ) ;
#64656=CARTESIAN_POINT ( 'NONE',  ( -5.585596099150174965, 9.460353182409786399, -0.7216878364870207285 ) ) ;
#64661=CARTESIAN_POINT ( 'NONE',  ( 0.4634916963840204351, 7.369626292149082936, 4.459501722865414131 ) ) ;
#64664=CARTESIAN_POINT ( 'NONE',  ( -10.50487009249003378, 11.15010328419353947, 0.7998128361456462443 ) ) ;
#64666=CARTESIAN_POINT ( 'NONE',  ( 7.750457368506414646, 12.19395069656619945, 0.7998128361456462443 ) ) ;
#64668=CARTESIAN_POINT ( 'NONE',  ( -8.154339323615371171, 11.60081407993821045, 1.199719254218453823 ) ) ;
#64669=DIRECTION ( 'NONE',  ( -0.6507913734559658270, -0.7592566023652989049, 0.000000000000000000 ) ) ;
#64671=CARTESIAN_POINT ( 'NONE',  ( 1.364683531249988535, 3.905208333674751842, -0.7879004041258239610 ) ) ;
#64672=CARTESIAN_POINT ( 'NONE',  ( 2.672928840188529609, 6.270167413528593414, 0.000000000000000000 ) ) ;
#64676=CARTESIAN_POINT ( 'NONE',  ( 10.35806617071623315, 11.18675807536486566, 0.000000000000000000 ) ) ;
#64678=CARTESIAN_POINT ( 'NONE',  ( -6.548225005720456515, 10.58342024007512983, 0.000000000000000000 ) ) ;
#64680=CARTESIAN_POINT ( 'NONE',  ( -1.402160292154681736E-14, 0.4468750003414233563, -1.575800808251665908 ) ) ;
#64682=CARTESIAN_POINT ( 'NONE',  ( 0.2555917649597919117, 7.163498069673003066, 2.096924645512464824 ) ) ;
#64684=CARTESIAN_POINT ( 'NONE',  ( -8.453672473320708036, 9.821371626084353323, -1.199719254218446718 ) ) ;
#64686=CARTESIAN_POINT ( 'NONE',  ( -4.080641047588914994, 5.783833860318930320, -1.443375672974051449 ) ) ;
#64687=CARTESIAN_POINT ( 'NONE',  ( -1.201851678989727383E-14, 3.259375000341420581, -1.575800808251660134 ) ) ;
#64692=CARTESIAN_POINT ( 'NONE',  ( 10.26082332744404368, 10.86538205830655279, -0.7998128361456281477 ) ) ;
#64705=CARTESIAN_POINT ( 'NONE',  ( -0.6823417656250212460, 4.363541667008085767, 1.181850606188767472 ) ) ;
#64711=CARTESIAN_POINT ( 'NONE',  ( 8.015895134177609904, 10.37496362800581018, 1.599625672291281386 ) ) ;
#64714=CARTESIAN_POINT ( 'NONE',  ( -1.364683531250012516, 2.780208333674754506, 0.7879004041258379498 ) ) ;
#64716=CARTESIAN_POINT ( 'NONE',  ( -6.887178846062116833, 9.058127958537705027, -1.443375672974059665 ) ) ;
#64722=CARTESIAN_POINT ( 'NONE',  ( 3.571683402196252910, 6.254382171615883834, 1.199719254218462483 ) ) ;
#64725=CARTESIAN_POINT ( 'NONE',  ( 10.21336978979620191, 10.81001959771741205, 0.7998128361456462443 ) ) ;
#64730=EDGE_LOOP ( 'NONE', ( #26538, #37224, #14690, #196184 ) ) ;
#64733=CARTESIAN_POINT ( 'NONE',  ( -10.08065090696061716, 11.71951313199760136, -1.199719254218441611 ) ) ;
#64734=CARTESIAN_POINT ( 'NONE',  ( 7.470706336329915764, 8.674577799595093452, -1.199719254218441611 ) ) ;
#64735=B_SPLINE_CURVE_WITH_KNOTS ( 'NONE', 3,
 ( #39354, #124959, #55603, #27365 ),
 .UNSPECIFIED., .F., .F.,
 ( 4, 4 ),
 ( -1.944647862008625085E-06, 0.0001035599091551142457 ),
 .UNSPECIFIED. ) ;
#64737=CARTESIAN_POINT ( 'NONE',  ( 4.161989969270895706, 5.878740935614591656, 1.443375672974062551 ) ) ;
#64741=ORIENTED_EDGE ( 'NONE', *, *, #84646, .F. ) ;
#64748=CARTESIAN_POINT ( 'NONE',  ( -6.236387472606145010, 9.259240570473746601, -1.082531754730538864 ) ) ;
#64749=CARTESIAN_POINT ( 'NONE',  ( 3.960953433486789521, 7.772862772376584850, -0.7998128361456221525 ) ) ;
#64752=CARTESIAN_POINT ( 'NONE',  ( -7.458957065812611198, 11.85386701009007204, 0.7998128361456481317 ) ) ;
#64758=CARTESIAN_POINT ( 'NONE',  ( -8.971744963941075568, 11.49012176272984931, 1.599625672291269396 ) ) ;
#64762=CARTESIAN_POINT ( 'NONE',  ( 9.108380270282433244, 9.520865158284665952, 1.040834085586084257E-14 ) ) ;
#64763=ADVANCED_FACE ( 'NONE', ( #96193 ), #75163, .T. ) ;
#64770=CARTESIAN_POINT ( 'NONE',  ( 2.684151225825664788, 5.114964949229812596, -1.082531754730543083 ) ) ;
#64773=DIRECTION ( 'NONE',  ( 0.7592566023652994600, 0.6507913734559651608, 0.000000000000000000 ) ) ;
#64775=CARTESIAN_POINT ( 'NONE',  ( -6.997979842947967377, 11.31606025008131233, -0.7998128361456291469 ) ) ;
#64779=CARTESIAN_POINT ( 'NONE',  ( 6.968527767744093993, 10.11340424813470662, 1.082531754730558626 ) ) ;
#64781=CARTESIAN_POINT ( 'NONE',  ( 3.846762897975340767, 5.510976019103107859, -1.599625672291256295 ) ) ;
#64784=CARTESIAN_POINT ( 'NONE',  ( -5.900823170445743671, 7.907379670318584353, 1.599625672291269396 ) ) ;
#64786=CARTESIAN_POINT ( 'NONE',  ( -3.563261906135775536, 6.332667919118538435, -2.500000000000000444 ) ) ;
#64793=CARTESIAN_POINT ( 'NONE',  ( -1.201851678989727383E-14, 3.884375000341423689, 1.575800808251672791 ) ) ;
#64794=CARTESIAN_POINT ( 'NONE',  ( -4.218512253981382187, 3.978430757497701364, -0.5307291018261834914 ) ) ;
#64795=CARTESIAN_POINT ( 'NONE',  ( 8.890396042259068210, 11.39521468743417998, -1.599625672291257406 ) ) ;
#64797=CARTESIAN_POINT ( 'NONE',  ( -5.287316719649550301, 5.270883715786984780, 0.7216878364870317197 ) ) ;
#64799=CARTESIAN_POINT ( 'NONE',  ( -3.253593677155282471, 6.739683690082376444, 1.040834085586084257E-14 ) ) ;
#64806=CARTESIAN_POINT ( 'NONE',  ( 3.472859903394816872, 7.203420320602605287, -0.7998128361456291469 ) ) ;
#64812=EDGE_CURVE ( 'NONE', #109653, #116176, #110019, .T. ) ;
#64815=CARTESIAN_POINT ( 'NONE',  ( 3.506755287428983792, 7.242964935309132990, 1.040834085586084257E-14 ) ) ;
#64819=CARTESIAN_POINT ( 'NONE',  ( 1.364683531249988535, 4.217708333674752730, -0.7879004041258239610 ) ) ;
#64825=CARTESIAN_POINT ( 'NONE',  ( 7.122110765880372618, 7.203550736482235095, 0.7998128361456341429 ) ) ;
#64828=CARTESIAN_POINT ( 'NONE',  ( -5.412729640353771465, 7.337937218544611895, 1.599625672291269396 ) ) ;
#64829=CARTESIAN_POINT ( 'NONE',  ( -1.201851678989727383E-14, 2.712500000000023892, 1.732050807568877637 ) ) ;
#64832=CARTESIAN_POINT ( 'NONE',  ( -5.284980951228653190, 5.060232619388524533, 0.000000000000000000 ) ) ;
#64833=CARTESIAN_POINT ( 'NONE',  ( 0.4138605925102775140, 8.005950907165225061, -1.999879544075613191 ) ) ;
#64835=CARTESIAN_POINT ( 'NONE',  ( -1.201851678989727383E-14, 2.946875000341419248, -1.575800808251660134 ) ) ;
#64837=CARTESIAN_POINT ( 'NONE',  ( -4.528060117284246289, 6.305822774963486310, 1.443375672974064550 ) ) ;
#64842=CARTESIAN_POINT ( 'NONE',  ( -4.365362273920257330, 6.116008624372161862, 1.443375672974064550 ) ) ;
#64843=CARTESIAN_POINT ( 'NONE',  ( 5.035963992472171746, 7.962709526937818083, 1.199719254218462483 ) ) ;
#64846=CARTESIAN_POINT ( 'NONE',  ( 0.4705731923490074631, 6.890484253938548243, -3.710072764477224005 ) ) ;
#64847=CARTESIAN_POINT ( 'NONE',  ( 0.6823417656249899377, 4.738541667008086655, -1.181850606188754593 ) ) ;
#64851=CARTESIAN_POINT ( 'NONE',  ( 0.6823417656249882723, 0.4052083336747516751, 1.181850606188755259 ) ) ;
#64854=CARTESIAN_POINT ( 'NONE',  ( -8.611400122974211868, 13.19838391011195888, 1.040834085586084257E-14 ) ) ;
#64856=CARTESIAN_POINT ( 'NONE',  ( -7.348156068482412095, 7.675196289425353591, 1.040834085586084257E-14 ) ) ;
#64861=CARTESIAN_POINT ( 'NONE',  ( -0.6823417656249969321, 4.217708333674755394, -1.181850606188749264 ) ) ;
#64869=CARTESIAN_POINT ( 'NONE',  ( -5.707619481228817904, 8.642344580533519505, -1.082531754730537976 ) ) ;
#64874=CARTESIAN_POINT ( 'NONE',  ( -5.219525951136845698, 8.072902128759544382, -1.082531754730543971 ) ) ;
#64882=CARTESIAN_POINT ( 'NONE',  ( 1.445184293213131577, 8.696352241143832984, -2.614796098495196119 ) ) ;
#64887=CARTESIAN_POINT ( 'NONE',  ( -4.283486466913726254, 7.084819080452935403, -1.199719254218452047 ) ) ;
#64889=CARTESIAN_POINT ( 'NONE',  ( -1.402160292154681736E-14, -0.2874999999999741096, 1.732050807568877637 ) ) ;
#64890=CARTESIAN_POINT ( 'NONE',  ( 8.920901888111986366, 12.39117405523060889, 1.082531754730546636 ) ) ;
#64891=CARTESIAN_POINT ( 'NONE',  ( 5.784525094524856748, 9.900363043587685041, 1.040834085586084257E-14 ) ) ;
#64894=CARTESIAN_POINT ( 'NONE',  ( 6.030679399980265920, 5.930214142932100252, -0.7998128361456281477 ) ) ;
#64901=CARTESIAN_POINT ( 'NONE',  ( -2.792616454734997866, 6.201876930592042925, 0.7216878364870317197 ) ) ;
#64908=CARTESIAN_POINT ( 'NONE',  ( 0.6823417656249917140, 3.842708333674754506, 1.181850606188765695 ) ) ;
#64909=CARTESIAN_POINT ( 'NONE',  ( 10.53432216769390095, 11.39239007183880581, -0.7216878364870257245 ) ) ;
#64910=CARTESIAN_POINT ( 'NONE',  ( -5.052384799386910430, 9.046199365926717917, 1.214306433183764966E-14 ) ) ;
#64913=CARTESIAN_POINT ( 'NONE',  ( 4.645640190976921602, 8.571663989448405019, 1.040834085586084257E-14 ) ) ;
#64914=CARTESIAN_POINT ( 'NONE',  ( -5.442708600882160574, 8.437244903416123876, -1.199719254218446718 ) ) ;
#64917=CARTESIAN_POINT ( 'NONE',  ( 0.7499999999999885647, 0.7645833340161543035, 1.299038105676657340 ) ) ;
#64920=CARTESIAN_POINT ( 'NONE',  ( 6.317736394288131052, 9.354147645769410602, 1.082531754730558626 ) ) ;
#64923=EDGE_CURVE ( 'NONE', #84740, #116525, #48844, .T. ) ;
#64924=CARTESIAN_POINT ( 'NONE',  ( -1.364683531250000748, 1.321875000341421469, 0.000000000000000000 ) ) ;
#64926=CARTESIAN_POINT ( 'NONE',  ( 5.951666246274792016, 8.927065806420504401, 1.082531754730558626 ) ) ;
#64928=CARTESIAN_POINT ( 'NONE',  ( -4.446711195602245148, 7.171284913969171448, -1.082531754730549967 ) ) ;
#64930=CARTESIAN_POINT ( 'NONE',  ( -1.364683531249997417, 5.259375000341425022, 1.214306433183764966E-14 ) ) ;
#64934=CARTESIAN_POINT ( 'NONE',  ( -4.747088307715054967, 7.009658186011790804, -1.421664413759090806 ) ) ;
#64940=CARTESIAN_POINT ( 'NONE',  ( 6.435316467980822353, 10.65961964595298817, 1.040834085586084257E-14 ) ) ;
#64948=CARTESIAN_POINT ( 'NONE',  ( 4.311129659465574804, 7.013106455143060636, -1.082531754730548412 ) ) ;
#64950=CARTESIAN_POINT ( 'NONE',  ( 1.364683531249988757, 0.4468750003414206917, 0.000000000000000000 ) ) ;
#64956=CARTESIAN_POINT ( 'NONE',  ( 1.499999999999987121, 2.004166666666684637, 0.8660254037844524744 ) ) ;
#64957=CARTESIAN_POINT ( 'NONE',  ( 5.926885707468349196, 10.06645042535509660, 1.040834085586084257E-14 ) ) ;
#64958=CARTESIAN_POINT ( 'NONE',  ( -7.503547950159405566, 10.84155747757291266, 1.199719254218453823 ) ) ;
#64962=CARTESIAN_POINT ( 'NONE',  ( -0.6823417656250003738, 0.7177083336747519526, -1.181850606188749264 ) ) ;
#64963=CARTESIAN_POINT ( 'NONE',  ( -0.7500000000000215383, 2.441666666666689078, 1.299038105676671107 ) ) ;
#64965=CARTESIAN_POINT ( 'NONE',  ( 3.662674053986138656, 7.424870162959149589, 0.7998128361456321445 ) ) ;
#64972=CARTESIAN_POINT ( 'NONE',  ( -1.402160292154681736E-14, -0.7562499993171803991, 1.732050807568877637 ) ) ;
#64973=CARTESIAN_POINT ( 'NONE',  ( -7.379715684540041565, 7.504089808251839244, 1.040834085586084257E-14 ) ) ;
#64974=CARTESIAN_POINT ( 'NONE',  ( -3.578989364327652467, 6.158942777482099729, 1.082531754730560403 ) ) ;
#64980=CARTESIAN_POINT ( 'NONE',  ( 7.610204295972345712, 7.772993188256215547, 0.7998128361456341429 ) ) ;
#64984=CARTESIAN_POINT ( 'NONE',  ( 4.957477724091233995, 8.935474444748447098, -0.7998128361456281477 ) ) ;
#64985=CARTESIAN_POINT ( 'NONE',  ( 9.368320956918614328, 10.99242454023565507, 1.082531754730549967 ) ) ;
#64989=CARTESIAN_POINT ( 'NONE',  ( -6.856673000209188906, 9.022537805042615489, 1.599625672291283607 ) ) ;
#64991=CARTESIAN_POINT ( 'NONE',  ( 3.680148631105580215, 6.380924938676771241, -1.199719254218446718 ) ) ;
#64995=CARTESIAN_POINT ( 'NONE',  ( 4.753338833179075351, 6.783512570024928579, 1.242321799368527380 ) ) ;
#64996=CARTESIAN_POINT ( 'NONE',  ( 8.541273586929342798, 11.94827437051752206, -1.082531754730543083 ) ) ;
#65006=CARTESIAN_POINT ( 'NONE',  ( -4.148431816101615155, 3.942184661647709198, 0.7216878364870317197 ) ) ;
#65007=CARTESIAN_POINT ( 'NONE',  ( 7.944714827928039291, 11.25228915168265864, 1.082531754730557072 ) ) ;
#65010=CARTESIAN_POINT ( 'NONE',  ( -6.905180308061733996, 6.950465202360470052, 0.7998128361456341429 ) ) ;
#65014=CARTESIAN_POINT ( 'NONE',  ( 0.1021010164683408550, 6.360493866598974755, -3.113991822131910059 ) ) ;
#65016=CARTESIAN_POINT ( 'NONE',  ( -6.073162743917628781, 9.172774736957510555, -1.199719254218440723 ) ) ;
#65028=DIRECTION ( 'NONE',  ( 1.000000000000000000, -8.673617379884035472E-16, 0.000000000000000000 ) ) ;
#65029=CARTESIAN_POINT ( 'NONE',  ( 1.499999999999819034, 7.361486028692880268, -4.203520246202064214 ) ) ;
#65030=CARTESIAN_POINT ( 'NONE',  ( -4.934277840369690971, 7.844075682818238526, -1.199719254218452047 ) ) ;
#65033=CARTESIAN_POINT ( 'NONE',  ( 4.690757960648224589, 6.495636925554817864, 1.443375672974062551 ) ) ;
#65037=CARTESIAN_POINT ( 'NONE',  ( -4.620631424159025613, 4.285158171140619032, -0.7998128361456221525 ) ) ;
#65041=CARTESIAN_POINT ( 'NONE',  ( 8.540746701604824409, 12.05162268759261224, -1.199719254218446718 ) ) ;
#65044=CARTESIAN_POINT ( 'NONE',  ( -7.666245793523398078, 11.03137162816423356, 1.199719254218453823 ) ) ;
#65045=CARTESIAN_POINT ( 'NONE',  ( 5.717788096661236885, 7.693838750903348789, 1.599625672291267398 ) ) ;
#65050=CARTESIAN_POINT ( 'NONE',  ( 2.492951620383182298, 8.266420250602603659, -2.456391984604371359 ) ) ;
#65051=CARTESIAN_POINT ( 'NONE',  ( -1.364683531250012516, 1.092708333674754506, 0.7879004041258379498 ) ) ;
#65054=CARTESIAN_POINT ( 'NONE',  ( 7.293923454472077239, 10.49303254931736262, 1.082531754730558626 ) ) ;
#65061=CARTESIAN_POINT ( 'NONE',  ( 10.18181017373857067, 11.94149529319227909, 1.082531754730548412 ) ) ;
#65067=DIRECTION ( 'NONE',  ( -0.6507913734559640506, -0.7592566023653004592, 0.000000000000000000 ) ) ;
#65075=CARTESIAN_POINT ( 'NONE',  ( 1.123270288250309834, 3.221052654332833054, -0.7749999999993620881 ) ) ;
#65078=AXIS2_PLACEMENT_3D ( 'NONE', #168380, #170505, #70845 ) ;
#65082=CARTESIAN_POINT ( 'NONE',  ( 1.499999999999987121, 0.3270833340161527492, -0.8660254037844323793 ) ) ;
#65089=CARTESIAN_POINT ( 'NONE',  ( 8.353795204314554468, 12.89784483834236184, -0.7998128361456352531 ) ) ;
#65093=CARTESIAN_POINT ( 'NONE',  ( 4.090809663021327758, 5.795697244990093644, 1.599625672291267398 ) ) ;
#65094=CARTESIAN_POINT ( 'NONE',  ( -7.700668062882084719, 8.086460282891644979, -0.7216878364870278340 ) ) ;
#65098=CARTESIAN_POINT ( 'NONE',  ( -7.854251061018346469, 8.057714414143200443, -0.7998128361456291469 ) ) ;
#65100=CARTESIAN_POINT ( 'NONE',  ( -3.429849674132942727, 5.984946472254969230, -1.082531754730549078 ) ) ;
#65103=CARTESIAN_POINT ( 'NONE',  ( 1.499999999999987121, 1.827083334016151861, -0.8660254037844253849 ) ) ;
#65110=CARTESIAN_POINT ( 'NONE',  ( -4.582292731294565158, 4.448355729372827305, 1.214306433183764966E-14 ) ) ;
#65113=CARTESIAN_POINT ( 'NONE',  ( 4.027228449831594226, 7.557535101434955216, 0.3677212997342318990 ) ) ;
#65117=CARTESIAN_POINT ( 'NONE',  ( -3.917943204224928699, 4.633650495426258509, -1.082531754730548412 ) ) ;
#65118=CARTESIAN_POINT ( 'NONE',  ( 6.988338112840064120, 10.24047933403371502, 1.199719254218460707 ) ) ;
#65121=DIRECTION ( 'NONE',  ( 0.000000000000000000, 8.546850786086437571E-32, 1.000000000000000000 ) ) ;
#65126=CARTESIAN_POINT ( 'NONE',  ( -9.332089804907933939, 9.781859615347734405, 1.040834085586084257E-14 ) ) ;
#65131=CARTESIAN_POINT ( 'NONE',  ( 4.976006071415387311, 5.764094157194782575, 1.199719254218462483 ) ) ;
#65134=ORIENTED_EDGE ( 'NONE', *, *, #92482, .F. ) ;
#65136=CARTESIAN_POINT ( 'NONE',  ( -10.08065090696061716, 11.71951313199760136, -1.199719254218441611 ) ) ;
#65140=FACE_OUTER_BOUND ( 'NONE', #85732, .T. ) ;
#65148=CARTESIAN_POINT ( 'NONE',  ( 6.877010230629674759, 9.046264573866535486, 1.599625672291281386 ) ) ;
#65150=CARTESIAN_POINT ( 'NONE',  ( -3.100010679019018500, 6.768429558830820980, 1.040834085586084257E-14 ) ) ;
#65151=ORIENTED_EDGE ( 'NONE', *, *, #43730, .T. ) ;
#65158=CARTESIAN_POINT ( 'NONE',  ( 0.7499999999999867883, -0.4020833326505157679, -1.299038105676652899 ) ) ;
#65164=CARTESIAN_POINT ( 'NONE',  ( -2.948008335967658322, 5.526761261015804116, 1.199719254218462483 ) ) ;
#65170=CARTESIAN_POINT ( 'NONE',  ( 5.680503174445848735, 5.729601246382692636, 1.040834085586084257E-14 ) ) ;
#65173=CARTESIAN_POINT ( 'NONE',  ( 0.6823417656249917140, 4.905208333674755394, 1.181850606188765695 ) ) ;
#65175=CARTESIAN_POINT ( 'NONE',  ( 3.348500752450937590, 5.890039396959305229, 1.082531754730558626 ) ) ;
#65183=CARTESIAN_POINT ( 'NONE',  ( -6.087928554039494067, 6.027116558704463500, 0.4103310871990673014 ) ) ;
#65185=CARTESIAN_POINT ( 'NONE',  ( -1.402160292154681736E-14, -0.05312499965857903073, -1.575800808251665908 ) ) ;
#65192=CARTESIAN_POINT ( 'NONE',  ( 1.499999999999989120, 4.754166666666689522, 0.8660254037844524744 ) ) ;
#65202=CARTESIAN_POINT ( 'NONE',  ( -1.364683531249997417, 5.321875000341417916, 1.214306433183764966E-14 ) ) ;
#65204=CARTESIAN_POINT ( 'NONE',  ( 6.661133543015731462, 6.665743976473484267, -0.7998128361456281477 ) ) ;
#65205=CARTESIAN_POINT ( 'NONE',  ( -9.040589502214116280, 9.441775928871617651, 0.7998128361456462443 ) ) ;
#65212=CARTESIAN_POINT ( 'NONE',  ( 0.6823417656249882723, -0.8447916663252494907, 1.181850606188755259 ) ) ;
#65218=CARTESIAN_POINT ( 'NONE',  ( 5.992340707560141588, 9.934888558888093968, 0.7216878364870438212 ) ) ;
#65224=CARTESIAN_POINT ( 'NONE',  ( -0.7499999999999972244, 5.139583334016151639, -1.299038105676652899 ) ) ;
#65226=CARTESIAN_POINT ( 'NONE',  ( -3.242371291962510504, 6.934516940598226320, 1.040834085586084257E-14 ) ) ;
#65227=CARTESIAN_POINT ( 'NONE',  ( 6.765155463094761679, 6.995028916473103209, 0.7216878364870317197 ) ) ;
#65228=CARTESIAN_POINT ( 'NONE',  ( -8.785320351530977234, 13.19336481018743079, 1.040834085586084257E-14 ) ) ;
#65236=CARTESIAN_POINT ( 'NONE',  ( 4.708759422647839976, 4.387974169377582001, -0.7998128361456211532 ) ) ;
#65252=CARTESIAN_POINT ( 'NONE',  ( 9.511208455186636712, 11.05516360492796935, 1.199719254218453823 ) ) ;
#65257=CARTESIAN_POINT ( 'NONE',  ( 1.364683531249986537, -0.09479166632524321789, -0.7879004041258309554 ) ) ;
#65258=CARTESIAN_POINT ( 'NONE',  ( 5.124618876285529367, 7.962177208099690873, -1.082531754730549078 ) ) ;
#65259=CARTESIAN_POINT ( 'NONE',  ( -9.978437869977959451, 10.74385839117019614, -0.7216878364870267237 ) ) ;
#65262=EDGE_CURVE ( 'NONE', #201912, #62417, #84569, .T. ) ;
#65266=CARTESIAN_POINT ( 'NONE',  ( -3.846762897975357198, 5.510976019103107859, -1.599625672291256295 ) ) ;
#65278=CARTESIAN_POINT ( 'NONE',  ( 5.539635733611046220, 6.394625955944754914, -1.222580188273769908 ) ) ;
#65279=CARTESIAN_POINT ( 'NONE',  ( -1.217323170181705771, 3.094494316908636744, -0.7749999999999918066 ) ) ;
#65282=CARTESIAN_POINT ( 'NONE',  ( -5.210200771661759767, 6.624310050620605850, -1.450205880198666364 ) ) ;
#65285=CARTESIAN_POINT ( 'NONE',  ( -9.219181267612684749, 10.81842823604534765, 1.082531754730558626 ) ) ;
#65289=CARTESIAN_POINT ( 'NONE',  ( 7.949158136313996259, 8.168439335321471262, 1.040834085586084257E-14 ) ) ;
#65290=CARTESIAN_POINT ( 'NONE',  ( -5.623934791570304625, 5.455678766453782913, 0.7998128361456341429 ) ) ;
#65292=CARTESIAN_POINT ( 'NONE',  ( -5.005985031943793295, 6.863401842066301661, -1.599625672291256295 ) ) ;
#65293=CARTESIAN_POINT ( 'NONE',  ( 2.672928840188529609, 6.270167413528593414, 0.000000000000000000 ) ) ;
#65296=CARTESIAN_POINT ( 'NONE',  ( -4.381256195510448315, 8.263215994737505454, 1.040834085586084257E-14 ) ) ;
#65297=AXIS2_PLACEMENT_3D ( 'NONE', #48322, #198777, #115487 ) ;
#65300=CARTESIAN_POINT ( 'NONE',  ( 7.879259827836241570, 12.34422023245099176, 1.040834085586084257E-14 ) ) ;
#65302=CARTESIAN_POINT ( 'NONE',  ( 4.114373074986557910, 7.676947195153840831, 0.7202382532921544067 ) ) ;
#65303=CARTESIAN_POINT ( 'NONE',  ( 5.097502569058200983, 6.970172302033127210, -1.443375672974051449 ) ) ;
#65309=ORIENTED_EDGE ( 'NONE', *, *, #190382, .T. ) ;
#65310=CARTESIAN_POINT ( 'NONE',  ( 8.242994206984347372, 8.719174117677642499, 1.040834085586084257E-14 ) ) ;
#65313=CARTESIAN_POINT ( 'NONE',  ( -10.47097470845587175, 11.11055866948701443, 1.040834085586084257E-14 ) ) ;
#65314=CARTESIAN_POINT ( 'NONE',  ( -6.364663046611467756, 9.512858423433634414, 1.199719254218452047 ) ) ;
#65323=CARTESIAN_POINT ( 'NONE',  ( 8.594979316059474073, 12.11489407112305372, 1.199719254218450271 ) ) ;
#65328=CARTESIAN_POINT ( 'NONE',  ( 4.196412238629597447, 4.854568018944682706, -1.199719254218452047 ) ) ;
#65331=CARTESIAN_POINT ( 'NONE',  ( 1.499999999999990896, 3.556250000682818602, 1.214306433183764966E-14 ) ) ;
#65337=CARTESIAN_POINT ( 'NONE',  ( 1.499999999999989120, 2.775000000000020339, 1.214306433183764966E-14 ) ) ;
#65338=CARTESIAN_POINT ( 'NONE',  ( 7.800018446563675489, 7.994443030612759848, -0.7998128361456281477 ) ) ;
#65341=CARTESIAN_POINT ( 'NONE',  ( 8.934460041725669655, 9.525884258209195821, 1.040834085586084257E-14 ) ) ;
#65343=CARTESIAN_POINT ( 'NONE',  ( -9.531018800282611281, 12.14260790512831889, 1.443375672974076540 ) ) ;
#65346=CARTESIAN_POINT ( 'NONE',  ( 10.70146331988817323, 11.37946204949139251, 0.7998128361456341429 ) ) ;
#65348=CARTESIAN_POINT ( 'NONE',  ( -4.952806187693842510, 4.672695395264567786, 0.7998128361456341429 ) ) ;
#65349=CARTESIAN_POINT ( 'NONE',  ( -1.499999999999997780, 5.431250000682820378, 1.214306433183764966E-14 ) ) ;
#65350=CARTESIAN_POINT ( 'NONE',  ( -1.364683531250014514, -0.2197916663252438285, 0.7879004041258379498 ) ) ;
#65354=CARTESIAN_POINT ( 'NONE',  ( 3.161022370280501814, 6.839609865302569425, 0.000000000000000000 ) ) ;
#65356=CARTESIAN_POINT ( 'NONE',  ( 1.364683531249988535, 4.717708333674756283, -0.7879004041258300672 ) ) ;
#65364=CARTESIAN_POINT ( 'NONE',  ( -5.540478329478883524, 9.615641817700700145, 0.000000000000000000 ) ) ;
#65366=CARTESIAN_POINT ( 'NONE',  ( 6.328958779480917229, 6.278206752349526631, 0.7998128361456341429 ) ) ;
#65369=CARTESIAN_POINT ( 'NONE',  ( -1.364683531250014514, 0.4885416670080875434, -0.7879004041258289570 ) ) ;
#65373=CARTESIAN_POINT ( 'NONE',  ( 8.886479618753304166, 12.45497775759917758, -1.199719254218446718 ) ) ;
#65377=CARTESIAN_POINT ( 'NONE',  ( -5.045605722580076780, 9.038290442985410067, -0.7998128361456231517 ) ) ;
#65381=CARTESIAN_POINT ( 'NONE',  ( 7.703003830858588863, 12.13858823597705872, -0.7998128361456291469 ) ) ;
#65383=CARTESIAN_POINT ( 'NONE',  ( 9.562578416340237197, 10.05076299535211781, 0.7998128361456462443 ) ) ;
#65385=CARTESIAN_POINT ( 'NONE',  ( -3.066115294984855133, 6.728884944124295053, 0.7998128361456341429 ) ) ;
#65386=CARTESIAN_POINT ( 'NONE',  ( -7.043624497499477499, 8.176315654292865887, 1.199719254218450271 ) ) ;
#65389=CARTESIAN_POINT ( 'NONE',  ( -4.331906098249381110, 7.414796467324478613, 1.153063172049747065 ) ) ;
#65390=CARTESIAN_POINT ( 'NONE',  ( 1.364683531249988757, 0.1343750003414204142, 0.000000000000000000 ) ) ;
#65395=CARTESIAN_POINT ( 'NONE',  ( 6.304178240674458422, 10.29869901418813782, 1.040834085586084257E-14 ) ) ;
#65398=CARTESIAN_POINT ( 'NONE',  ( 4.385172619016207918, 7.203452924572514959, 1.199719254218462483 ) ) ;
#65400=CARTESIAN_POINT ( 'NONE',  ( -7.285838599102589797E-14, 7.078193277237590841, -2.121339347286493648 ) ) ;
#65414=CARTESIAN_POINT ( 'NONE',  ( 10.01963921569910632, 11.64833282552586091, 1.199719254218450271 ) ) ;
#65418=CARTESIAN_POINT ( 'NONE',  ( -5.786632634934295361, 5.645492917045106473, 0.7998128361456341429 ) ) ;
#65419=CARTESIAN_POINT ( 'NONE',  ( -8.179646747746328828, 8.437342715325849341, -0.7998128361456291469 ) ) ;
#65425=CARTESIAN_POINT ( 'NONE',  ( -0.7500000000000006661, 2.639583334016156080, -1.299038105676652011 ) ) ;
#65426=CARTESIAN_POINT ( 'NONE',  ( 9.264299036839600987, 9.702770385934682551, -0.7998128361456281477 ) ) ;
#65429=CARTESIAN_POINT ( 'NONE',  ( -8.259941899223614215, 10.65968485389279508, -1.599625672291263179 ) ) ;
#65431=CARTESIAN_POINT ( 'NONE',  ( -0.6823417656250212460, 2.801041667008084879, 1.181850606188767472 ) ) ;
#65434=CARTESIAN_POINT ( 'NONE',  ( -3.728129053633564283, 7.293308295973763400, 0.7216878364870122908 ) ) ;
#65436=CARTESIAN_POINT ( 'NONE',  ( -9.869972641068651242, 11.57768483841065787, 1.082531754730558626 ) ) ;
#65441=CARTESIAN_POINT ( 'NONE',  ( -0.6823417656250212460, 1.363541667008083547, 1.181850606188755259 ) ) ;
#65447=CARTESIAN_POINT ( 'NONE',  ( 1.364683531249986537, 1.405208333674755838, -0.7879004041258239610 ) ) ;
#65449=CARTESIAN_POINT ( 'NONE',  ( -6.033542053281340856, 6.997886136038390603, -1.199719254218446718 ) ) ;
#65450=CARTESIAN_POINT ( 'NONE',  ( 6.252281394196331554, 10.44607872653774372, 1.040834085586084257E-14 ) ) ;
#65451=CARTESIAN_POINT ( 'NONE',  ( -1.000000000000017097, 8.600000000000013856, 0.4000000000000026867 ) ) ;
#65453=CARTESIAN_POINT ( 'NONE',  ( 0.7499999999999920064, 5.733333333333353821, 1.299038105676669330 ) ) ;
#65454=CARTESIAN_POINT ( 'NONE',  ( 1.364683531249986537, 2.217708333674751398, -0.7879004041258239610 ) ) ;
#65458=CARTESIAN_POINT ( 'NONE',  ( -6.236387472606166327, 6.378132927569716060, -0.7216878364870278340 ) ) ;
#65462=CARTESIAN_POINT ( 'NONE',  ( 4.744990575102895569, 5.598539094783909320, -1.082531754730548412 ) ) ;
#65465=CARTESIAN_POINT ( 'NONE',  ( -8.474009703741204547, 9.845098394908269768, -1.199719254218446718 ) ) ;
#65466=CARTESIAN_POINT ( 'NONE',  ( -4.223528545856940042, 4.886203710709899006, -1.199719254218446718 ) ) ;
#65468=CARTESIAN_POINT ( 'NONE',  ( -0.6823417656249969321, 4.967708333674755394, -1.181850606188749264 ) ) ;
#65474=CARTESIAN_POINT ( 'NONE',  ( -7.497295758232724872, 9.769931022736756177, -1.443375672974058777 ) ) ;
#65476=CARTESIAN_POINT ( 'NONE',  ( -1.499999999999997780, 5.900000000000023448, 1.214306433183764966E-14 ) ) ;
#65479=CARTESIAN_POINT ( 'NONE',  ( 6.941411460516762943, 11.04213777067082702, -0.7216878364870267237 ) ) ;
#65486=CARTESIAN_POINT ( 'NONE',  ( 4.324687812634897988, 4.147816657603229373, 0.7216878364870317197 ) ) ;
#65489=VERTEX_POINT ( 'NONE', #40054 ) ;
#65490=CARTESIAN_POINT ( 'NONE',  ( 8.053180056393003383, 12.33920113252646367, 1.040834085586084257E-14 ) ) ;
#65496=CARTESIAN_POINT ( 'NONE',  ( 5.262536180398716290, 9.291375977107183104, -0.7998128361456291469 ) ) ;
#65497=CARTESIAN_POINT ( 'NONE',  ( -5.590039407536138150, 5.416134151747256986, 0.000000000000000000 ) ) ;
#65500=CARTESIAN_POINT ( 'NONE',  ( 1.500000000000007105, 10.64264068711930733, 1.214306433183764966E-14 ) ) ;
#65501=CARTESIAN_POINT ( 'NONE',  ( 4.975479186090847605, 7.788180902872553268, 1.082531754730558626 ) ) ;
#65503=CARTESIAN_POINT ( 'NONE',  ( -1.402160292154681736E-14, -0.2406249996585799189, -1.575800808251665908 ) ) ;
#65504=CARTESIAN_POINT ( 'NONE',  ( 3.469446951953614189E-15, 8.900000000000019895, 1.214306433183764966E-14 ) ) ;
#65505=CARTESIAN_POINT ( 'NONE',  ( -8.676328237741483207, 12.20980114641871062, -1.199719254218446718 ) ) ;
#65524=CARTESIAN_POINT ( 'NONE',  ( 7.983053520348166288, 8.207983950027992748, -0.7998128361456281477 ) ) ;
#65525=CARTESIAN_POINT ( 'NONE',  ( 5.947222937888848371, 10.09017719417900416, 1.040834085586084257E-14 ) ) ;
#65528=ORIENTED_EDGE ( 'NONE', *, *, #2128, .T. ) ;
#65531=FACE_OUTER_BOUND ( 'NONE', #2985, .T. ) ;
#65536=CARTESIAN_POINT ( 'NONE',  ( -2.981903720001798597, 5.566305875722335372, -1.199719254218446718 ) ) ;
#65539=CARTESIAN_POINT ( 'NONE',  ( -5.886439722289627419, 6.118937485343679761, -0.7679415244158314113 ) ) ;
#65546=CARTESIAN_POINT ( 'NONE',  ( -9.246297574839990929, 11.81043314211192019, 1.443375672974076540 ) ) ;
#65549=CARTESIAN_POINT ( 'NONE',  ( 4.788000803920411386, 8.737751371215816576, 1.040834085586084257E-14 ) ) ;
#65555=CARTESIAN_POINT ( 'NONE',  ( 4.568734577680873876, 6.353276312092901890, -1.443375672974051449 ) ) ;
#65556=CARTESIAN_POINT ( 'NONE',  ( -7.867809214632013770, 8.073532260025807261, 1.040834085586084257E-14 ) ) ;
#65562=CARTESIAN_POINT ( 'NONE',  ( -6.555530967407501741, 7.606873202518897870, 1.199719254218450271 ) ) ;
#65563=CARTESIAN_POINT ( 'NONE',  ( -3.086452525405351643, 6.752611712948207057, 0.7998128361456341429 ) ) ;
#65568=CARTESIAN_POINT ( 'NONE',  ( 1.400751299550835549, 7.315968950352074174, -4.333496285527503211 ) ) ;
#65571=CARTESIAN_POINT ( 'NONE',  ( 5.937581207780954884, 9.014596278131406848, -1.199719254218440723 ) ) ;
#65572=CARTESIAN_POINT ( 'NONE',  ( -3.314994193297896796, 6.393354490853021765, -0.7784788408506218005 ) ) ;
#65582=CARTESIAN_POINT ( 'NONE',  ( 1.364683531249986537, 0.4260416670080872659, 0.7879004041258500513 ) ) ;
#65584=CARTESIAN_POINT ( 'NONE',  ( 6.003563092752934871, 5.898578451166879510, 0.7998128361456341429 ) ) ;
#65586=CARTESIAN_POINT ( 'NONE',  ( -6.060131475628484310, 10.01397778830115470, 0.000000000000000000 ) ) ;
#65588=CARTESIAN_POINT ( 'NONE',  ( 5.666945020832181434, 5.713783400500082266, 0.7216878364870317197 ) ) ;
#65589=CARTESIAN_POINT ( 'NONE',  ( -8.310784975052689205, 8.798263347090697906, -0.7216878364870267237 ) ) ;
#65593=CARTESIAN_POINT ( 'NONE',  ( 6.938021921891177612, 9.117444880338284818, -1.599625672291262513 ) ) ;
#65598=CARTESIAN_POINT ( 'NONE',  ( 1.364683531249988535, 3.363541667008084879, 0.7879004041258500513 ) ) ;
#65602=CARTESIAN_POINT ( 'NONE',  ( 6.598014311344812199, 10.84943379654430906, 1.040834085586084257E-14 ) ) ;
#65605=CARTESIAN_POINT ( 'NONE',  ( -7.121056995675673740, 9.330985799753529264, -1.599625672291263179 ) ) ;
#65611=CARTESIAN_POINT ( 'NONE',  ( 10.22692794340986921, 10.82583744360002243, 0.000000000000000000 ) ) ;
#65615=CARTESIAN_POINT ( 'NONE',  ( -7.018317073368468328, 11.33978701890523233, -0.7998128361456291469 ) ) ;
#65618=CARTESIAN_POINT ( 'NONE',  ( 4.439983357641082762, 7.074277023141499754, -1.114066652139956926 ) ) ;
#65620=CARTESIAN_POINT ( 'NONE',  ( -9.978437869977950569, 11.70422760547153906, -1.082531754730539753 ) ) ;
#65626=CARTESIAN_POINT ( 'NONE',  ( 5.799137018343234473, 7.788745826199009237, -1.599625672291262513 ) ) ;
#65628=CARTESIAN_POINT ( 'NONE',  ( 4.638861114170084399, 8.563755066507100722, 0.7998128361456462443 ) ) ;
#65629=CARTESIAN_POINT ( 'NONE',  ( -4.014146127519945928, 7.627013291057631150, 0.008764090477326666462 ) ) ;
#65631=CARTESIAN_POINT ( 'NONE',  ( 3.684065054611349144, 5.321161868511784299, -1.599625672291262513 ) ) ;
#65633=CARTESIAN_POINT ( 'NONE',  ( -8.053180056837398126, 8.497724275839514618, 0.7216878364870578100 ) ) ;
#65639=CARTESIAN_POINT ( 'NONE',  ( -4.029167574269930441, 7.605081013511371779, 0.2528308249854539502 ) ) ;
#65640=CARTESIAN_POINT ( 'NONE',  ( 1.364683531249986981, -1.053124999658580752, 0.000000000000000000 ) ) ;
#65642=CYLINDRICAL_SURFACE ( 'NONE', #70352, 0.08000000000000020983 ) ;
#65643=CARTESIAN_POINT ( 'NONE',  ( 5.178851490740205676, 6.104710163027444736, 1.082531754730558626 ) ) ;
#65647=EDGE_CURVE ( 'NONE', #107270, #6713, #68797, .T. ) ;
#65649=CARTESIAN_POINT ( 'NONE',  ( -7.809133291347029271, 12.05447990663947877, 0.000000000000000000 ) ) ;
#65656=ORIENTED_EDGE ( 'NONE', *, *, #211661, .F. ) ;
#65661=CARTESIAN_POINT ( 'NONE',  ( -9.991996023147281747, 11.72004545083573568, 1.082531754730558626 ) ) ;
#65665=ORIENTED_EDGE ( 'NONE', *, *, #156299, .F. ) ;
#65667=CARTESIAN_POINT ( 'NONE',  ( -1.500000000000011324, 3.452083334016151639, 0.8660254037844403729 ) ) ;
#65672=CARTESIAN_POINT ( 'NONE',  ( -7.472515219426274946, 11.86968485597268064, 0.000000000000000000 ) ) ;
#65676=CARTESIAN_POINT ( 'NONE',  ( 5.612185521052973414, 8.634967976948757951, -1.199719254218440723 ) ) ;
#65682=CARTESIAN_POINT ( 'NONE',  ( 7.934546212495622086, 10.28005655271014795, -1.599625672291262513 ) ) ;
#65688=CARTESIAN_POINT ( 'NONE',  ( -7.565086526745425033, 7.928281824065535055, 0.7216878364870317197 ) ) ;
#65691=FACE_OUTER_BOUND ( 'NONE', #34476, .T. ) ;
#65694=CARTESIAN_POINT ( 'NONE',  ( 2.535011536075336913, 5.133042487381361596, 0.9999999999999991118 ) ) ;
#65697=CARTESIAN_POINT ( 'NONE',  ( -2.928197990427299668, 6.360055388899728435, 1.040834085586084257E-14 ) ) ;
#65699=CARTESIAN_POINT ( 'NONE',  ( 2.358755538653318773, 5.695705861830088423, 1.040834085586084257E-14 ) ) ;
#65701=CARTESIAN_POINT ( 'NONE',  ( -8.642432853707342488, 12.17025653171218558, 1.199719254218462483 ) ) ;
#65704=CARTESIAN_POINT ( 'NONE',  ( -1.201851678989727383E-14, 2.321875000341416584, 1.575800808251672791 ) ) ;
#65705=CARTESIAN_POINT ( 'NONE',  ( 2.849184837166184536, 6.475799410002530898, 0.7998128361456362523 ) ) ;
#65712=CARTESIAN_POINT ( 'NONE',  ( 9.205623113554624481, 10.80261038964432707, 1.082531754730549967 ) ) ;
#65713=CARTESIAN_POINT ( 'NONE',  ( -0.7500000000000215383, 3.972916667349481123, 1.299038105676671107 ) ) ;
#65714=CARTESIAN_POINT ( 'NONE',  ( -8.202319746587722449, 8.671720580548228696, 1.040834085586084257E-14 ) ) ;
#65715=CARTESIAN_POINT ( 'NONE',  ( -1.402160292154681736E-14, 0.9468750003414176941, -1.575800808251659024 ) ) ;
#65717=CARTESIAN_POINT ( 'NONE',  ( 0.1616376092238826501, 8.277406474726792140, 1.999409923707613945 ) ) ;
#65719=CARTESIAN_POINT ( 'NONE',  ( -8.369460898337653276, 8.658792557682392754, 0.7998128361456462443 ) ) ;
#65720=CARTESIAN_POINT ( 'NONE',  ( -4.731432421044883263, 5.582721248382882528, -1.082531754730543971 ) ) ;
#65721=CARTESIAN_POINT ( 'NONE',  ( 0.6823417656249899377, 3.238541667008085323, -1.181850606188754593 ) ) ;
#65741=EDGE_CURVE ( 'NONE', #62417, #66472, #74225, .T. ) ;
#65742=CARTESIAN_POINT ( 'NONE',  ( 1.364683531249988535, 4.717708333674756283, -0.7879004041258300672 ) ) ;
#65748=CARTESIAN_POINT ( 'NONE',  ( 7.886038904643079661, 12.35212915539230139, -0.7998128361456352531 ) ) ;
#65749=CARTESIAN_POINT ( 'NONE',  ( -2.279776052174470546, 5.602663296202901932, -0.04407265314621480051 ) ) ;
#65751=CARTESIAN_POINT ( 'NONE',  ( -0.6823417656250003738, 1.967708333674753174, -1.181850606188749264 ) ) ;
#65753=CARTESIAN_POINT ( 'NONE',  ( -8.188761592974058701, 8.655902734665618325, -0.7216878364870278340 ) ) ;
#65755=CARTESIAN_POINT ( 'NONE',  ( 1.436717785781294943, 7.422226822640119792, 4.237127798884887220 ) ) ;
#65759=CARTESIAN_POINT ( 'NONE',  ( 5.515469562660962666, 5.329135999392899947, 0.7998128361456341429 ) ) ;
#65762=CARTESIAN_POINT ( 'NONE',  ( 9.836604141914616406, 11.43479190611061647, 1.199719254218452047 ) ) ;
#65768=CARTESIAN_POINT ( 'NONE',  ( -10.64723070543352712, 11.31619066596094392, 0.7998128361456462443 ) ) ;
#65769=CARTESIAN_POINT ( 'NONE',  ( 6.877010230629674759, 9.046264573866535486, 1.599625672291281386 ) ) ;
#65771=CARTESIAN_POINT ( 'NONE',  ( 5.477130869796502211, 5.492333557625114437, 1.040834085586084257E-14 ) ) ;
#65772=DIRECTION ( 'NONE',  ( 5.057645237790724994E-47, 9.066213480720158442E-32, -1.000000000000000000 ) ) ;
#65779=CARTESIAN_POINT ( 'NONE',  ( -1.499999999999997335, 7.809254910130847271, -3.635752117226044522 ) ) ;
#65780=CARTESIAN_POINT ( 'NONE',  ( -5.910991785878158211, 9.839981483592442402, -0.7216878364870278340 ) ) ;
#65781=CARTESIAN_POINT ( 'NONE',  ( 6.159481859310094620, 6.080483678816896109, 1.040834085586084257E-14 ) ) ;
#65784=CARTESIAN_POINT ( 'NONE',  ( -8.941766003412679353, 10.39081407785832845, -1.199719254218446718 ) ) ;
#65789=CARTESIAN_POINT ( 'NONE',  ( -7.960608749518247151, 12.43912730774665576, 0.000000000000000000 ) ) ;
#65794=CARTESIAN_POINT ( 'NONE',  ( 8.259941899223605333, 10.65968485389279508, -1.599625672291268286 ) ) ;
#65795=( BOUNDED_CURVE ( )  B_SPLINE_CURVE ( 2, ( #189730, #120553, #89060 ),
 .UNSPECIFIED., .F., .T. ) 
 B_SPLINE_CURVE_WITH_KNOTS ( ( 3, 3 ),
 ( 0.1249999999999998751, 0.1276624645066402886 ),
 .UNSPECIFIED. ) 
 CURVE ( )  GEOMETRIC_REPRESENTATION_ITEM ( )  RATIONAL_B_SPLINE_CURVE ( ( 1.000000000000003997, 0.9143913742683040802, 0.9381891137235958134 ) ) 
 REPRESENTATION_ITEM ( '' )  );
#65808=CARTESIAN_POINT ( 'NONE',  ( -9.267161690140662600, 10.77044237904097734, -1.199719254218441611 ) ) ;
#65812=CARTESIAN_POINT ( 'NONE',  ( 7.836249599018724865, 9.205007956019091608, -1.082531754730537976 ) ) ;
#65813=CARTESIAN_POINT ( 'NONE',  ( -1.001543065824772872E-14, 5.384375000341413475, 1.575800808251672791 ) ) ;
#65815=CARTESIAN_POINT ( 'NONE',  ( 2.659370686574860976, 6.254349567645977714, -0.7998128361456291469 ) ) ;
#65818=CARTESIAN_POINT ( 'NONE',  ( -6.632963465583701534, 8.761543347979550589, -1.599625672291263179 ) ) ;
#65830=CARTESIAN_POINT ( 'NONE',  ( 0.6823417656249917140, 3.905208333674754950, 1.181850606188765695 ) ) ;
#65831=CARTESIAN_POINT ( 'NONE',  ( 5.314433026432511475, 5.302519407033794430, 1.040834085586084257E-14 ) ) ;
#65832=CARTESIAN_POINT ( 'NONE',  ( 9.348510611822643313, 10.86534945433664134, 1.199719254218453823 ) ) ;
#65833=VECTOR ( 'NONE', #167338, 1000.000000000000000 ) ;
#65835=CARTESIAN_POINT ( 'NONE',  ( -4.039966587192274083, 5.736380323189513852, 1.443375672974064550 ) ) ;
#65837=CARTESIAN_POINT ( 'NONE',  ( -4.568734577680887199, 6.353276312092901890, -1.443375672974051449 ) ) ;
#65844=CARTESIAN_POINT ( 'NONE',  ( 3.659811400685081040, 6.357198169852855685, -1.199719254218446718 ) ) ;
#65852=CARTESIAN_POINT ( 'NONE',  ( 4.143988507271280319, 7.986403691791820414, -0.7998128361456221525 ) ) ;
#65856=CARTESIAN_POINT ( 'NONE',  ( 1.364683531249990311, 3.446875000341416584, 1.214306433183764966E-14 ) ) ;
#65861=CARTESIAN_POINT ( 'NONE',  ( 5.615048174354031474, 9.702639970055050966, 0.7998128361456462443 ) ) ;
#65863=CARTESIAN_POINT ( 'NONE',  ( -4.889686956022917919, 8.856385215335397021, 1.214306433183764966E-14 ) ) ;
#65864=CARTESIAN_POINT ( 'NONE',  ( 5.870317324592803310, 7.871789516823500144, -1.443375672974057666 ) ) ;
#65865=CARTESIAN_POINT ( 'NONE',  ( -1.500000000000013101, 1.629166666666691077, -0.8660254037844313801 ) ) ;
#65867=CARTESIAN_POINT ( 'NONE',  ( -3.761497552787613330, 6.475832013972435242, 1.199719254218464037 ) ) ;
#65870=CARTESIAN_POINT ( 'NONE',  ( -4.924636110261798372, 6.768494766770632332, 1.599625672291267398 ) ) ;
#65874=CARTESIAN_POINT ( 'NONE',  ( 1.364683531249988535, 3.655208333674750509, -0.7879004041258239610 ) ) ;
#65876=CARTESIAN_POINT ( 'NONE',  ( -4.067082894419624672, 6.728385229256075739, 1.082531754730560403 ) ) ;
#65882=CARTESIAN_POINT ( 'NONE',  ( 4.385172619016207918, 7.203452924572514959, 1.199719254218462483 ) ) ;
#65885=CARTESIAN_POINT ( 'NONE',  ( 1.364683531249988535, 2.967708333674755394, -0.7879004041258239610 ) ) ;
#65887=CARTESIAN_POINT ( 'NONE',  ( 2.361091307074211887, 5.906356958228550447, 0.7998128361456462443 ) ) ;
#65890=CARTESIAN_POINT ( 'NONE',  ( 1.364683531249988757, -0.5531249996585801965, 0.000000000000000000 ) ) ;
#65894=CARTESIAN_POINT ( 'NONE',  ( -3.623053363349869382, 5.249981562040033189, 1.599625672291267398 ) ) ;
#65895=CARTESIAN_POINT ( 'NONE',  ( -6.358410854684793279, 7.480862754296137673, -1.082531754730543083 ) ) ;
#65899=CARTESIAN_POINT ( 'NONE',  ( -1.201851678989727383E-14, 3.446875000341421469, -1.575800808251660134 ) ) ;
#65907=CARTESIAN_POINT ( 'NONE',  ( -6.439759776366783761, 8.536139043893143707, 1.443375672974078761 ) ) ;
#65913=CARTESIAN_POINT ( 'NONE',  ( -4.555176424067209240, 8.258196894812975586, 1.040834085586084257E-14 ) ) ;
#65925=CARTESIAN_POINT ( 'NONE',  ( -4.229253852459088137, 7.021547696922494808, 1.199719254218464037 ) ) ;
#65927=CARTESIAN_POINT ( 'NONE',  ( 0.7499999999999885647, -0.5166666666666444030, 1.299038105676657340 ) ) ;
#65928=CARTESIAN_POINT ( 'NONE',  ( 3.358669367883368118, 4.941533567329135401, -1.599625672291262513 ) ) ;
#65930=CARTESIAN_POINT ( 'NONE',  ( 3.912411256987575303, 4.016135269252925077, 0.7252027155559813698 ) ) ;
#65931=CARTESIAN_POINT ( 'NONE',  ( 4.306686350635271054, 8.176217842383143974, -0.7998128361456221525 ) ) ;
#65937=CARTESIAN_POINT ( 'NONE',  ( -4.636525346193588248, 4.511627113421689650, 0.7216878364870317197 ) ) ;
#65945=CARTESIAN_POINT ( 'NONE',  ( 0.6823417656249899377, 2.092708333674753174, 1.181850606188767472 ) ) ;
#65946=CARTESIAN_POINT ( 'NONE',  ( 10.68346185744421462, 11.56638637654751989, 0.000000000000000000 ) ) ;
#65947=CARTESIAN_POINT ( 'NONE',  ( -6.744291347794091784, 9.955758108146730123, -1.199719254218440723 ) ) ;
#65950=CARTESIAN_POINT ( 'NONE',  ( 7.091078035147269532, 8.231678114882006625, 1.199719254218462483 ) ) ;
#65951=CARTESIAN_POINT ( 'NONE',  ( -7.172426956829277778, 8.326585190177668849, -1.199719254218452935 ) ) ;
#65954=CARTESIAN_POINT ( 'NONE',  ( -0.7500000000000249800, -1.277083332650516656, 1.299038105676659116 ) ) ;
#65957=CARTESIAN_POINT ( 'NONE',  ( 7.782016984564049444, 11.06247500109133064, 1.082531754730557072 ) ) ;
#65958=EDGE_CURVE ( 'NONE', #56116, #192556, #79189, .T. ) ;
#65961=CARTESIAN_POINT ( 'NONE',  ( 0.6823417656249882723, 0.4885416670080827695, -1.181850606188749264 ) ) ;
#65963=CARTESIAN_POINT ( 'NONE',  ( 7.754900676892376055, 8.149731665903665601, 1.040834085586084257E-14 ) ) ;
#65965=CARTESIAN_POINT ( 'NONE',  ( -5.585596099150199834, 5.618876325204420930, -0.7216878364870207285 ) ) ;
#65967=CARTESIAN_POINT ( 'NONE',  ( 0.6823417656249917140, 4.842708333674755394, 1.181850606188765695 ) ) ;
#65971=CARTESIAN_POINT ( 'NONE',  ( -5.194998520284300980, 6.641152480062820551, -1.419077516013200313 ) ) ;
#65978=CARTESIAN_POINT ( 'NONE',  ( 7.796102023057898123, 9.054206100777749455, -1.199719254218441611 ) ) ;
#65981=CARTESIAN_POINT ( 'NONE',  ( 4.521807925357579805, 5.234196320127330715, -1.199719254218452047 ) ) ;
#65987=ORIENTED_EDGE ( 'NONE', *, *, #125678, .T. ) ;
#65988=CARTESIAN_POINT ( 'NONE',  ( 5.829642864196168617, 6.863966765392747860, 1.082531754730558626 ) ) ;
#65990=CARTESIAN_POINT ( 'NONE',  ( -0.6823417656250003738, 1.280208333674752508, -1.181850606188749264 ) ) ;
#65992=CARTESIAN_POINT ( 'NONE',  ( 2.191614386903386613, 5.708633884695917260, -0.7998128361456281477 ) ) ;
#65997=CARTESIAN_POINT ( 'NONE',  ( -0.7500000000000215383, 1.441666666666688190, 1.299038105676659116 ) ) ;
#65998=CARTESIAN_POINT ( 'NONE',  ( 7.447506452608354088, 7.583179037664891098, 0.7998128361456341429 ) ) ;
#65999=CARTESIAN_POINT ( 'NONE',  ( -7.720478407978036195, 11.09464301169468037, -1.199719254218446718 ) ) ;
#66004=CARTESIAN_POINT ( 'NONE',  ( -0.6823417656250212460, 1.301041667008083547, 1.181850606188755259 ) ) ;
#66005=CARTESIAN_POINT ( 'NONE',  ( -0.7500000000000215383, 2.941666666666689522, 1.299038105676671107 ) ) ;
#66007=CARTESIAN_POINT ( 'NONE',  ( 5.359550796103802028, 5.147230771742885125, -0.7998128361456231517 ) ) ;
#66008=EDGE_CURVE ( 'NONE', #116455, #161726, #141400, .T. ) ;
#66011=CARTESIAN_POINT ( 'NONE',  ( -0.7500000000000215383, 4.472916667349482012, 1.299038105676671107 ) ) ;
#66015=CARTESIAN_POINT ( 'NONE',  ( -1.500000000000001332, -0.5687499993171779566, 0.000000000000000000 ) ) ;
#66016=CARTESIAN_POINT ( 'NONE',  ( -7.507464373665155399, 9.781794407407920389, 1.599625672291295375 ) ) ;
#66017=CARTESIAN_POINT ( 'NONE',  ( -3.307826292054304673, 6.802955074131234348, -0.7216878364870267237 ) ) ;
#66025=CARTESIAN_POINT ( 'NONE',  ( 6.262976894508937242, 9.394224579314053969, -1.199719254218440723 ) ) ;
#66029=CARTESIAN_POINT ( 'NONE',  ( 9.720832950873944611, 10.44331931888218001, -0.7216878364870257245 ) ) ;
#66030=CARTESIAN_POINT ( 'NONE',  ( 1.499999999999990896, 4.306250000682819490, 1.214306433183764966E-14 ) ) ;
#66031=CARTESIAN_POINT ( 'NONE',  ( -6.338600509588822263, 7.353787668397130162, -1.199719254218446718 ) ) ;
#66034=CARTESIAN_POINT ( 'NONE',  ( -6.938021921891187382, 9.117444880338284818, -1.599625672291263179 ) ) ;
#66036=CARTESIAN_POINT ( 'NONE',  ( 5.379888026524302980, 5.170957540566797128, -0.7998128361456211532 ) ) ;
#66041=DIRECTION ( 'NONE',  ( 0.000000000000000000, 8.546850786086437571E-32, 1.000000000000000000 ) ) ;
#66043=CARTESIAN_POINT ( 'NONE',  ( 9.951321562750607086, 11.67259191370631477, -1.082531754730537088 ) ) ;
#66049=EDGE_CURVE ( 'NONE', #78570, #22516, #38448, .T. ) ;
#66052=CARTESIAN_POINT ( 'NONE',  ( -2.806174608348664723, 6.217694776474651519, 1.040834085586084257E-14 ) ) ;
#66053=CARTESIAN_POINT ( 'NONE',  ( 9.598809568795314107, 10.30095870645710754, -0.7216878364870257245 ) ) ;
#66056=CARTESIAN_POINT ( 'NONE',  ( -6.579784621333750749, 6.570836901177822931, 0.7998128361456341429 ) ) ;
#66062=CARTESIAN_POINT ( 'NONE',  ( -6.235860587281615075, 9.362588887548838557, -1.199719254218440723 ) ) ;
#66067=DIRECTION ( 'NONE',  ( -1.000000000000000000, 5.578564026256503701E-16, -1.972152263052529514E-31 ) ) ;
#66077=CARTESIAN_POINT ( 'NONE',  ( -6.728924311084075960, 6.744833205886536120, 1.040834085586084257E-14 ) ) ;
#66080=CARTESIAN_POINT ( 'NONE',  ( 3.877268743828266029, 6.506935386899531437, 1.082531754730558626 ) ) ;
#66081=CARTESIAN_POINT ( 'NONE',  ( 3.294945724223604877, 7.655198976062517424, 2.499999999999998668 ) ) ;
#66084=CARTESIAN_POINT ( 'NONE',  ( -4.355193658487827690, 6.104145239700998538, -1.599625672291256295 ) ) ;
#66089=CARTESIAN_POINT ( 'NONE',  ( 10.71502147350184231, 11.39527989537399755, 0.000000000000000000 ) ) ;
#66092=CARTESIAN_POINT ( 'NONE',  ( -9.013473194986783454, 9.410140237106395134, -0.7998128361456291469 ) ) ;
#66093=CARTESIAN_POINT ( 'NONE',  ( 5.452350330990040739, 9.512825819463730070, 0.7998128361456462443 ) ) ;
#66095=CARTESIAN_POINT ( 'NONE',  ( -8.076906825439122528, 10.44614393447756129, -1.599625672291263179 ) ) ;
#66097=CARTESIAN_POINT ( 'NONE',  ( 4.660252114795294887, 6.460046772059735432, -1.599625672291256517 ) ) ;
#66100=CARTESIAN_POINT ( 'NONE',  ( 0.6823417656249899377, 0.6552083336747518416, 1.181850606188755259 ) ) ;
#66103=CARTESIAN_POINT ( 'NONE',  ( 8.920901888111997025, 10.47043562662792304, 1.082531754730549967 ) ) ;
#66109=CARTESIAN_POINT ( 'NONE',  ( 9.856414487010587422, 11.56186699200962487, 1.082531754730548412 ) ) ;
#66128=CARTESIAN_POINT ( 'NONE',  ( 1.499999999999989120, 0.3062500006828158816, 0.000000000000000000 ) ) ;
#66134=CARTESIAN_POINT ( 'NONE',  ( 9.378489572351044856, 11.96465713920816043, -1.599625672291262513 ) ) ;
#66140=CARTESIAN_POINT ( 'NONE',  ( 5.345992642490140057, 5.131412925860272090, 1.040834085586084257E-14 ) ) ;
#66141=CARTESIAN_POINT ( 'NONE',  ( -6.968527767744110868, 9.153035033833367251, 1.443375672974078761 ) ) ;
#66142=CARTESIAN_POINT ( 'NONE',  ( -5.752954180755987856, 6.096397935365156506, 0.6526304460669953844 ) ) ;
#66145=CARTESIAN_POINT ( 'NONE',  ( -8.843996274815957293, 9.212417163573759282, 1.040834085586084257E-14 ) ) ;
#66146=CARTESIAN_POINT ( 'NONE',  ( -8.631737353394710155, 13.22211067893587533, 1.040834085586084257E-14 ) ) ;
#66149=CARTESIAN_POINT ( 'NONE',  ( 1.499999999999985123, -0.6729166659838520248, -0.8660254037844323793 ) ) ;
#66156=CARTESIAN_POINT ( 'NONE',  ( -5.395781948114519722, 5.397426482329451325, 0.000000000000000000 ) ) ;
#66159=CARTESIAN_POINT ( 'NONE',  ( 4.055251984284337752, 7.519160923078652026, -0.4935718261673445184 ) ) ;
#66165=CARTESIAN_POINT ( 'NONE',  ( -10.50487009249003378, 11.15010328419353947, 0.7998128361456462443 ) ) ;
#66166=CARTESIAN_POINT ( 'NONE',  ( 7.151035956204054855, 10.43029348462504124, 1.199719254218460707 ) ) ;
#66176=CARTESIAN_POINT ( 'NONE',  ( -8.320953590485107298, 10.73086516036454618, 1.599625672291269396 ) ) ;
#66181=CARTESIAN_POINT ( 'NONE',  ( 4.333802657862601215, 8.207853534148366492, 0.7998128361456462443 ) ) ;
#66184=VERTEX_POINT ( 'NONE', #87197 ) ;
#66185=ORIENTED_EDGE ( 'NONE', *, *, #150826, .T. ) ;
#66186=ORIENTED_EDGE ( 'NONE', *, *, #32339, .F. ) ;
#66191=CARTESIAN_POINT ( 'NONE',  ( -1.244150428499003036, 3.178773246564667421, -0.7749999999999918066 ) ) ;
#66196=CARTESIAN_POINT ( 'NONE',  ( -3.741289556128929661, 7.428763123923387113, 2.448390356388095768 ) ) ;
#66200=CARTESIAN_POINT ( 'NONE',  ( 8.457588896826466751, 8.761608555919362828, 1.040834085586084257E-14 ) ) ;
#66202=CARTESIAN_POINT ( 'NONE',  ( -3.262708522383007903, 6.958243709422141876, 1.040834085586084257E-14 ) ) ;
#66203=CARTESIAN_POINT ( 'NONE',  ( 0.6823417656249882723, 2.926041667008084879, -1.181850606188754593 ) ) ;
#66208=CARTESIAN_POINT ( 'NONE',  ( 1.499999999999987121, -1.214583332650518432, 0.8660254037844524744 ) ) ;
#66212=DIRECTION ( 'NONE',  ( -0.6507913734559640506, -0.7592566023653004592, 0.000000000000000000 ) ) ;
#66214=CARTESIAN_POINT ( 'NONE',  ( -4.647747731386360215, 4.316793862905830892, 0.7998128361456341429 ) ) ;
#66220=CARTESIAN_POINT ( 'NONE',  ( 3.877268743828258479, 7.467304601200877023, 0.7216878364870298324 ) ) ;
#66224=CARTESIAN_POINT ( 'NONE',  ( 0.6823417656249917140, 4.655208333674755394, 1.181850606188765695 ) ) ;
#66226=CARTESIAN_POINT ( 'NONE',  ( 3.836594282542909795, 6.459481848733281240, 1.082531754730558626 ) ) ;
#66234=CARTESIAN_POINT ( 'NONE',  ( -6.110283559904478246, 6.013173453705326743, 0.3066926896367061506 ) ) ;
#66237=CARTESIAN_POINT ( 'NONE',  ( 0.6823417656249917140, 5.405208333674749177, 1.181850606188765695 ) ) ;
#66245=CARTESIAN_POINT ( 'NONE',  ( -0.7500000000000215383, 4.441666666666691299, 1.299038105676671107 ) ) ;
#66253=CARTESIAN_POINT ( 'NONE',  ( 0.6823417656249917140, 5.155208333674749177, 1.181850606188765695 ) ) ;
#66255=CARTESIAN_POINT ( 'NONE',  ( 7.135668919494039031, 7.219368582364847242, 1.040834085586084257E-14 ) ) ;
#66256=CARTESIAN_POINT ( 'NONE',  ( -9.154780037725563702, 11.70366268214508487, 1.599625672291281386 ) ) ;
#66263=CARTESIAN_POINT ( 'NONE',  ( -0.7499999999999972244, 5.858333333333353821, -1.299038105676652011 ) ) ;
#66267=CARTESIAN_POINT ( 'NONE',  ( 4.812781342726857758, 6.637997537979888563, 1.443375672974062551 ) ) ;
#66271=CARTESIAN_POINT ( 'NONE',  ( 8.595506201384013778, 10.09080732544527592, 1.082531754730558626 ) ) ;
#66276=CARTESIAN_POINT ( 'NONE',  ( 0.7499999999999902300, 3.597916667349487785, -1.299038105676658228 ) ) ;
#66278=CARTESIAN_POINT ( 'NONE',  ( -4.928552533767591726, 5.708731696605642725, 1.199719254218462483 ) ) ;
#66280=CARTESIAN_POINT ( 'NONE',  ( 5.327991180046175224, 5.318337252916401248, -0.7216878364870207285 ) ) ;
#66281=CARTESIAN_POINT ( 'NONE',  ( -10.10046125205658463, 11.84658821789661509, -1.082531754730537976 ) ) ;
#66288=CARTESIAN_POINT ( 'NONE',  ( 3.551346171775753735, 6.230655402791975384, 1.199719254218462483 ) ) ;
#66290=CARTESIAN_POINT ( 'NONE',  ( -1.257539916218605169, 2.922412844624491246, -0.7749999999999988010 ) ) ;
#66293=CARTESIAN_POINT ( 'NONE',  ( 3.354752944377597856, 6.001296637494123232, -1.199719254218446718 ) ) ;
#66305=CARTESIAN_POINT ( 'NONE',  ( 5.394965581569445057, 6.295244270701876310, -1.058425382943289028 ) ) ;
#66306=ORIENTED_EDGE ( 'NONE', *, *, #97869, .F. ) ;
#66309=CARTESIAN_POINT ( 'NONE',  ( 9.215791728987056786, 11.77484298861683598, -1.599625672291262513 ) ) ;
#66313=CARTESIAN_POINT ( 'NONE',  ( 3.019342412789784547, 6.452475500722323787, 0.1501914610189964416 ) ) ;
#66315=CARTESIAN_POINT ( 'NONE',  ( 6.643132081016124069, 7.813037518349371879, 1.082531754730558626 ) ) ;
#66316=CARTESIAN_POINT ( 'NONE',  ( -10.03267048443264109, 11.76749898900197877, 1.082531754730558626 ) ) ;
#66322=CARTESIAN_POINT ( 'NONE',  ( -3.469997250093771246, 6.135748327496311383, -1.199719254218452935 ) ) ;
#66333=CARTESIAN_POINT ( 'NONE',  ( 6.021928883684827483, 6.074059740061504620, -0.5497475987105825412 ) ) ;
#66334=CARTESIAN_POINT ( 'NONE',  ( -4.080641063585716211, 5.783833847506671511, -1.249999999999999334 ) ) ;
#66336=CARTESIAN_POINT ( 'NONE',  ( 5.508690485854129903, 5.321227076451600091, 1.040834085586084257E-14 ) ) ;
#66340=CARTESIAN_POINT ( 'NONE',  ( -7.673551755654729689, 11.89630144833179060, 0.7216878364870458196 ) ) ;
#66344=EDGE_CURVE ( 'NONE', #155158, #77611, #102601, .T. ) ;
#66346=CARTESIAN_POINT ( 'NONE',  ( 6.564118927310645724, 10.80988918183778225, -0.7998128361456291469 ) ) ;
#66348=CARTESIAN_POINT ( 'NONE',  ( -5.382750679825375251, 6.238629533673094585, -1.199719254218446718 ) ) ;
#66349=CARTESIAN_POINT ( 'NONE',  ( 2.530568227245037605, 6.104080031761181857, 0.000000000000000000 ) ) ;
#66351=CARTESIAN_POINT ( 'NONE',  ( -5.087333953625788219, 6.958308917361963886, 1.599625672291267398 ) ) ;
#66352=CARTESIAN_POINT ( 'NONE',  ( 3.979481780810941949, 4.601482484822914998, 1.199719254218464037 ) ) ;
#66354=CARTESIAN_POINT ( 'NONE',  ( -6.878064000834399394, 6.918829510595249310, -0.7998128361456291469 ) ) ;
#66357=CARTESIAN_POINT ( 'NONE',  ( 9.576136569953906275, 10.06658084123472641, 0.000000000000000000 ) ) ;
#66358=CARTESIAN_POINT ( 'NONE',  ( 0.5159288176862960595, 6.781431689740628599, 3.543831299045886229 ) ) ;
#66360=CARTESIAN_POINT ( 'NONE',  ( 4.026354976812863917, 7.791716866330316904, -0.3671166487079768892 ) ) ;
#66361=CARTESIAN_POINT ( 'NONE',  ( 5.721177635286841756, 6.737423998331861341, -1.082531754730543083 ) ) ;
#66364=CARTESIAN_POINT ( 'NONE',  ( -4.161989969715274462, 4.726297878971393196, -2.420000000000000373 ) ) ;
#66368=CARTESIAN_POINT ( 'NONE',  ( 6.588899466117086767, 10.63087377720454363, 1.040834085586084257E-14 ) ) ;
#66371=CARTESIAN_POINT ( 'NONE',  ( 3.763657168278617959, 3.180244510940670288, -2.446973152615704361 ) ) ;
#66372=CARTESIAN_POINT ( 'NONE',  ( -6.367525699912501835, 10.58053041653993098, -0.7998128361456291469 ) ) ;
#66376=CARTESIAN_POINT ( 'NONE',  ( 3.985733972293228344, 7.593847367743336463, 1.040834085586084257E-14 ) ) ;
#66380=CARTESIAN_POINT ( 'NONE',  ( 2.920892028740289081, 5.495125569250587816, 1.199719254218452047 ) ) ;
#66385=CARTESIAN_POINT ( 'NONE',  ( 2.846322183865124700, 5.408127416896231665, -1.199719254218446718 ) ) ;
#66388=CARTESIAN_POINT ( 'NONE',  ( -1.499999999999997780, 3.681250000682819046, 1.214306433183764966E-14 ) ) ;
#66394=CARTESIAN_POINT ( 'NONE',  ( 1.499999999999989120, 1.525000000000019451, 0.000000000000000000 ) ) ;
#66395=CARTESIAN_POINT ( 'NONE',  ( 7.461064606222022277, 7.598996883547496139, 1.040834085586084257E-14 ) ) ;
#66396=CARTESIAN_POINT ( 'NONE',  ( 5.165293336682183600, 5.128523102325077687, -0.7216878364870197293 ) ) ;
#66400=CARTESIAN_POINT ( 'NONE',  ( 8.432808358020025707, 9.900993174853955026, 1.082531754730558626 ) ) ;
#66406=CARTESIAN_POINT ( 'NONE',  ( -3.079673448598517549, 6.744702790006905424, 1.040834085586084257E-14 ) ) ;
#66407=CARTESIAN_POINT ( 'NONE',  ( 0.7499999999999902300, 4.097916667349481123, -1.299038105676658228 ) ) ;
#66408=CARTESIAN_POINT ( 'NONE',  ( -0.6823417656250246877, 0.3010416670080895418, 1.181850606188755259 ) ) ;
#66412=CARTESIAN_POINT ( 'NONE',  ( 2.998324526916512411, 6.649795714711241423, 0.000000000000000000 ) ) ;
#66414=CARTESIAN_POINT ( 'NONE',  ( -1.001543065824772872E-14, 5.634375000341415252, 1.575800808251672791 ) ) ;
#66422=CARTESIAN_POINT ( 'NONE',  ( -7.497822643557261024, 8.706213491360317747, -1.199719254218446718 ) ) ;
#66423=CARTESIAN_POINT ( 'NONE',  ( 4.171104814498611368, 8.018039383557042044, 0.7998128361456321445 ) ) ;
#66426=CARTESIAN_POINT ( 'NONE',  ( -0.6823417656250003738, -0.7822916663252423852, -1.181850606188749264 ) ) ;
#66432=CARTESIAN_POINT ( 'NONE',  ( -5.693534442735004752, 8.729875052244421951, 1.199719254218452047 ) ) ;
#66439=CARTESIAN_POINT ( 'NONE',  ( 9.101601193475611140, 9.512956235343358102, -0.7998128361456221525 ) ) ;
#66442=CARTESIAN_POINT ( 'NONE',  ( -2.740719608256871442, 6.349256642941639051, 0.7998128361456341429 ) ) ;
#66443=CARTESIAN_POINT ( 'NONE',  ( -7.344766530301162000, 9.591980256816594164, 1.599625672291295375 ) ) ;
#66446=CARTESIAN_POINT ( 'NONE',  ( -4.357679483485834560, 7.387146062586773532, 1.181458644690215998 ) ) ;
#66447=CARTESIAN_POINT ( 'NONE',  ( -1.402160292154681736E-14, 0.3218750003414227456, 1.575800808251672791 ) ) ;
#66451=CARTESIAN_POINT ( 'NONE',  ( 8.595506201384020883, 9.130438111143927671, 0.7216878364870438212 ) ) ;
#66454=CARTESIAN_POINT ( 'NONE',  ( 3.981290663907289140, 7.796589541200495965, -0.7998128361456221525 ) ) ;
#66470=CARTESIAN_POINT ( 'NONE',  ( 10.18233705906309972, 11.83814697611718714, 1.199719254218450271 ) ) ;
#66471=CARTESIAN_POINT ( 'NONE',  ( 1.436838838544731267, 7.449283400311756509, 4.203727439823562229 ) ) ;
#66472=VERTEX_POINT ( 'NONE', #93628 ) ;
#66475=CARTESIAN_POINT ( 'NONE',  ( -4.948889764188092677, 5.732458465429559169, 1.199719254218462483 ) ) ;
#66476=CARTESIAN_POINT ( 'NONE',  ( -8.779068160048691283, 10.20099992726700933, -1.199719254218446718 ) ) ;
#66481=CARTESIAN_POINT ( 'NONE',  ( -0.7500000000000215383, 2.472916667349486897, 1.299038105676671107 ) ) ;
#66482=CARTESIAN_POINT ( 'NONE',  ( 9.562578416340237197, 10.05076299535211781, 0.7998128361456462443 ) ) ;
#66486=CARTESIAN_POINT ( 'NONE',  ( -9.840520565420403543, 10.37502883594562597, 1.040834085586084257E-14 ) ) ;
#66487=CARTESIAN_POINT ( 'NONE',  ( 1.252085211431714251, 3.300000000000025135, 0.7750000000000100142 ) ) ;
#66488=CARTESIAN_POINT ( 'NONE',  ( 1.364683531249986537, 2.155208333674751398, -0.7879004041258239610 ) ) ;
#66496=CARTESIAN_POINT ( 'NONE',  ( -3.521367211247373508, 5.131347717920458962, -1.599625672291256295 ) ) ;
#66500=CARTESIAN_POINT ( 'NONE',  ( 0.6823417656249899377, 2.155208333674753174, 1.181850606188767472 ) ) ;
#66505=CARTESIAN_POINT ( 'NONE',  ( 1.364683531249986537, 1.655208333674748955, -0.7879004041258239610 ) ) ;
#66507=CARTESIAN_POINT ( 'NONE',  ( -5.005985031943793295, 6.863401842066301661, -1.599625672291256295 ) ) ;
#66508=CARTESIAN_POINT ( 'NONE',  ( -0.9999999999999988898, 6.468705557303653819, -4.925226524755048629 ) ) ;
#66510=CARTESIAN_POINT ( 'NONE',  ( -0.7500000000000215383, 3.691666666666690411, 1.299038105676671107 ) ) ;
#66511=CARTESIAN_POINT ( 'NONE',  ( 1.364683531249988757, 2.196875000341415252, 1.214306433183764966E-14 ) ) ;
#66515=CARTESIAN_POINT ( 'NONE',  ( -5.422898255786203769, 6.389431388914436738, -1.082531754730544860 ) ) ;
#66518=CARTESIAN_POINT ( 'NONE',  ( 6.046573322014824114, 7.117052299514516456, -1.082531754730543083 ) ) ;
#66521=CARTESIAN_POINT ( 'NONE',  ( -9.124801077197171040, 10.60435499727357289, -1.199719254218441611 ) ) ;
#66522=CARTESIAN_POINT ( 'NONE',  ( -9.002250809793991948, 12.48608113052627289, -1.082531754730543971 ) ) ;
#66524=CARTESIAN_POINT ( 'NONE',  ( -0.6823417656250212460, 5.551041667008087543, 1.181850606188767472 ) ) ;
#66530=CARTESIAN_POINT ( 'NONE',  ( -6.846504384776758378, 9.010674420371453053, -1.443375672974058777 ) ) ;
#66532=CARTESIAN_POINT ( 'NONE',  ( -1.364683531250014514, -0.6989583329919100141, -0.7879004041258359514 ) ) ;
#66536=CARTESIAN_POINT ( 'NONE',  ( 8.324343129110697959, 9.774450407793066731, -1.082531754730543083 ) ) ;
#66542=EDGE_LOOP ( 'NONE', ( #129616, #62762, #54359, #139000 ) ) ;
#66548=ORIENTED_EDGE ( 'NONE', *, *, #124471, .F. ) ;
#66549=CARTESIAN_POINT ( 'NONE',  ( 5.449487677688982679, 8.445153826357429949, -1.199719254218446718 ) ) ;
#66551=CARTESIAN_POINT ( 'NONE',  ( -3.893162665418476109, 7.693773542963529444, 1.040834085586084257E-14 ) ) ;
#66556=CARTESIAN_POINT ( 'NONE',  ( 5.544921637864819175, 7.492161215640853023, -1.443375672974057666 ) ) ;
#66557=CARTESIAN_POINT ( 'NONE',  ( -1.402160292154681736E-14, 0.3843750003414230232, 1.575800808251672791 ) ) ;
#66558=CARTESIAN_POINT ( 'NONE',  ( 2.724825686666657809, 6.122787701178987518, 0.000000000000000000 ) ) ;
#66559=CARTESIAN_POINT ( 'NONE',  ( -8.947491310014823895, 12.52615806407091803, 1.199719254218462483 ) ) ;
#66575=CARTESIAN_POINT ( 'NONE',  ( 8.145751363712157911, 8.397798100619326078, -0.7998128361456281477 ) ) ;
#66576=CARTESIAN_POINT ( 'NONE',  ( 6.388916700537700777, 8.476822122092563916, 1.599625672291281386 ) ) ;
#66585=CARTESIAN_POINT ( 'NONE',  ( 8.387690588348714726, 12.93738945304888333, 1.040834085586084257E-14 ) ) ;
#66587=CARTESIAN_POINT ( 'NONE',  ( -6.247609857798938293, 6.183299677053865295, -0.7998128361456291469 ) ) ;
#66588=CARTESIAN_POINT ( 'NONE',  ( 1.499999999999990896, 3.775000000000021227, 1.214306433183764966E-14 ) ) ;
#66591=CARTESIAN_POINT ( 'NONE',  ( 2.000000000000000000, -2.856854249492364328, 2.449293598294706414E-16 ) ) ;
#66597=CARTESIAN_POINT ( 'NONE',  ( -10.49364770729726359, 11.34493653470939023, 0.7216878364870438212 ) ) ;
#66600=CARTESIAN_POINT ( 'NONE',  ( 5.829115978871627135, 8.888053511070525659, 1.199719254218462483 ) ) ;
#66601=CARTESIAN_POINT ( 'NONE',  ( 0.6823417656249917140, 5.342708333674749177, 1.181850606188765695 ) ) ;
#66606=CARTESIAN_POINT ( 'NONE',  ( 4.161989969270895706, 5.878740935614591656, 1.443375672974062551 ) ) ;
#66607=CARTESIAN_POINT ( 'NONE',  ( -5.669280788808708671, 9.765911353585494226, 0.7998128361456481317 ) ) ;
#66611=CARTESIAN_POINT ( 'NONE',  ( -7.344766530301162000, 9.591980256816594164, 1.599625672291295375 ) ) ;
#66612=CARTESIAN_POINT ( 'NONE',  ( -3.653032323878261600, 6.349289246911547835, -1.199719254218452047 ) ) ;
#66619=CARTESIAN_POINT ( 'NONE',  ( 5.113396490648394632, 9.117379672398465473, 1.040834085586084257E-14 ) ) ;
#66633=ORIENTED_EDGE ( 'NONE', *, *, #142863, .T. ) ;
#66635=CARTESIAN_POINT ( 'NONE',  ( -0.6823417656250003738, 0.2802083336747515641, -1.181850606188749264 ) ) ;
#66636=CARTESIAN_POINT ( 'NONE',  ( 2.659370686574860976, 6.254349567645977714, -0.7998128361456291469 ) ) ;
#66637=CARTESIAN_POINT ( 'NONE',  ( 5.168682875307768931, 7.053215992657626110, -1.599625672291256295 ) ) ;
#66639=CARTESIAN_POINT ( 'NONE',  ( -7.131225611108100715, 9.342849184424693476, 1.443375672974078761 ) ) ;
#66640=CARTESIAN_POINT ( 'NONE',  ( -1.608462485350604876, 8.735270501766756013, -2.463594439587629914 ) ) ;
#66642=CARTESIAN_POINT ( 'NONE',  ( 6.819388077993785657, 7.058300300521964665, 1.040834085586084257E-14 ) ) ;
#66643=CARTESIAN_POINT ( 'NONE',  ( -6.792271770322117597, 9.907772251142352715, 1.082531754730549967 ) ) ;
#66647=CARTESIAN_POINT ( 'NONE',  ( 5.940443861082012944, 10.08226827123770697, 0.7998128361456462443 ) ) ;
#66652=CARTESIAN_POINT ( 'NONE',  ( -0.6823417656249969321, 3.967708333674754950, -1.181850606188749264 ) ) ;
#66657=ADVANCED_FACE ( 'NONE', ( #94699 ), #96834, .T. ) ;
#66658=CARTESIAN_POINT ( 'NONE',  ( 7.259501185113382604, 10.55683625168592243, -1.199719254218441611 ) ) ;
#66661=CARTESIAN_POINT ( 'NONE',  ( -7.018317073368468328, 11.33978701890523233, -0.7998128361456291469 ) ) ;
#66667=CARTESIAN_POINT ( 'NONE',  ( 8.432281472695482449, 11.92507992053172572, 1.199719254218450271 ) ) ;
#66669=CARTESIAN_POINT ( 'NONE',  ( -8.178592977541617515, 10.56477777859713463, 1.599625672291295375 ) ) ;
#66672=CARTESIAN_POINT ( 'NONE',  ( 5.342823980928582905, 4.390142039796938178, -2.499999999999995115 ) ) ;
#66674=CARTESIAN_POINT ( 'NONE',  ( 5.096651299933133039, 6.508523278119453082, -1.213691435513279293 ) ) ;
#66675=CARTESIAN_POINT ( 'NONE',  ( -2.428882075142555497, 5.985446187641602300, 1.040834085586084257E-14 ) ) ;
#66681=CARTESIAN_POINT ( 'NONE',  ( 7.474622759835693131, 7.614814729430110951, -0.7998128361456281477 ) ) ;
#66683=CARTESIAN_POINT ( 'NONE',  ( 6.647575389402066826, 6.649926130590872120, 1.040834085586084257E-14 ) ) ;
#66684=CARTESIAN_POINT ( 'NONE',  ( -4.322081814030608982, 7.236479734952984799, 0.9908985150933833363 ) ) ;
#66685=CARTESIAN_POINT ( 'NONE',  ( 5.671388329218120639, 5.511041227042920099, 1.040834085586084257E-14 ) ) ;
#66687=CARTESIAN_POINT ( 'NONE',  ( -6.385527162356466668, 10.39360608948380182, 0.000000000000000000 ) ) ;
#66693=CARTESIAN_POINT ( 'NONE',  ( -4.014161209245137307, 7.626991082632122776, -0.01188119308113272377 ) ) ;
#66697=CARTESIAN_POINT ( 'NONE',  ( 4.039966587192257208, 6.696749537490852333, 1.082531754730558626 ) ) ;
#66701=CARTESIAN_POINT ( 'NONE',  ( -8.798878505144648088, 12.24881344176869469, -1.082531754730543083 ) ) ;
#66705=EDGE_CURVE ( 'NONE', #10073, #23962, #147281, .T. ) ;
#66708=CARTESIAN_POINT ( 'NONE',  ( -8.798878505144648088, 12.24881344176869469, -1.082531754730543083 ) ) ;
#66716=CARTESIAN_POINT ( 'NONE',  ( -8.744645890690007306, 12.18554205823825498, 1.082531754730558626 ) ) ;
#66724=CARTESIAN_POINT ( 'NONE',  ( 0.7499999999999885647, 2.347916667349486453, -1.299038105676652899 ) ) ;
#66726=CARTESIAN_POINT ( 'NONE',  ( -4.717347382551060342, 7.590990148696470818, 1.199719254218464037 ) ) ;
#66729=CARTESIAN_POINT ( 'NONE',  ( -9.318531651294266638, 9.766041769465124034, -0.7998128361456291469 ) ) ;
#66733=CARTESIAN_POINT ( 'NONE',  ( 6.124532705071213279, 8.168374127381657246, -1.599625672291262513 ) ) ;
#66734=AXIS2_PLACEMENT_3D ( 'NONE', #74414, #72245, #125370 ) ;
#66740=CARTESIAN_POINT ( 'NONE',  ( 8.555358625423188812, 9.940005470203933768, 1.199719254218462483 ) ) ;
#66742=CARTESIAN_POINT ( 'NONE',  ( -4.833902094211216749, 5.059593709313742416, -0.9115025817279830411 ) ) ;
#66747=CARTESIAN_POINT ( 'NONE',  ( -6.805829924380121909, 8.963220883242035697, 1.443375672974078761 ) ) ;
#66750=CARTESIAN_POINT ( 'NONE',  ( -1.201851678989727383E-14, 3.118750000682814161, -1.732050807568863648 ) ) ;
#66753=CARTESIAN_POINT ( 'NONE',  ( -1.364683531250010295, 5.530208333674751842, 0.7879004041258379498 ) ) ;
#66756=CARTESIAN_POINT ( 'NONE',  ( -3.104453987404963478, 5.605318171072321221, -1.082531754730549078 ) ) ;
#66758=CARTESIAN_POINT ( 'NONE',  ( 8.723781775389312543, 12.26516360700784958, -1.199719254218446718 ) ) ;
#66759=CARTESIAN_POINT ( 'NONE',  ( 1.436838838544733044, 7.449283400311756509, -4.203727439823553347 ) ) ;
#66760=CARTESIAN_POINT ( 'NONE',  ( -8.805130697071332335, 12.36007068230351358, 1.199719254218462483 ) ) ;
#66763=CARTESIAN_POINT ( 'NONE',  ( 1.364683531249988757, 2.384375000341422357, 1.214306433183764966E-14 ) ) ;
#66765=CARTESIAN_POINT ( 'NONE',  ( 5.183294799126148433, 4.941598775268944976, 1.040834085586084257E-14 ) ) ;
#66770=CARTESIAN_POINT ( 'NONE',  ( -3.642287698956971020, 3.120124397464318022, -2.499999999999528821 ) ) ;
#66772=CARTESIAN_POINT ( 'NONE',  ( 9.869972640624258275, 10.61731562359089587, 0.000000000000000000 ) ) ;
#66774=CARTESIAN_POINT ( 'NONE',  ( -7.876924059859742755, 8.292092279365579799, 1.040834085586084257E-14 ) ) ;
#66776=CARTESIAN_POINT ( 'NONE',  ( -4.313792511808268060, 5.583989749030219052, 1.358440613521926910 ) ) ;
#66778=CARTESIAN_POINT ( 'NONE',  ( -7.049349804101573191, 10.31165964050546258, -1.199719254218440723 ) ) ;
#66780=CARTESIAN_POINT ( 'NONE',  ( -4.731432421044877934, 6.543090462684225450, -1.443375672974051449 ) ) ;
#66781=CARTESIAN_POINT ( 'NONE',  ( -1.364683531249997417, 3.321875000341423245, 1.214306433183764966E-14 ) ) ;
#66799=CARTESIAN_POINT ( 'NONE',  ( -1.559074708514275542, 8.689926414953912825, 2.502785155726149569 ) ) ;
#66801=CARTESIAN_POINT ( 'NONE',  ( 1.364683531249988535, 3.967708333674751842, -0.7879004041258239610 ) ) ;
#66805=CARTESIAN_POINT ( 'NONE',  ( -5.427887300360803913, 4.356806483369918048, -2.440341253675376798 ) ) ;
#66808=CARTESIAN_POINT ( 'NONE',  ( 8.561083932025322696, 12.07534945641652158, -1.199719254218446718 ) ) ;
#66811=CARTESIAN_POINT ( 'NONE',  ( 1.364683531249988757, 1.884375000341421913, 0.000000000000000000 ) ) ;
#66813=CARTESIAN_POINT ( 'NONE',  ( -8.215877900201387973, 8.687538426430837291, 0.7216878364870578100 ) ) ;
#66819=ORIENTED_EDGE ( 'NONE', *, *, #187111, .F. ) ;
#66821=CARTESIAN_POINT ( 'NONE',  ( 4.878236342818665250, 4.585697242910212523, 1.040834085586084257E-14 ) ) ;
#66825=CARTESIAN_POINT ( 'NONE',  ( 9.890836756369282057, 11.49806328964105617, -1.199719254218440723 ) ) ;
#66832=CARTESIAN_POINT ( 'NONE',  ( -2.785310492603665367, 5.336947110424484109, 1.199719254218462483 ) ) ;
#66833=CARTESIAN_POINT ( 'NONE',  ( 5.947222937888848371, 10.09017719417900416, 1.040834085586084257E-14 ) ) ;
#66835=CARTESIAN_POINT ( 'NONE',  ( 4.487385655998878953, 6.258369236797239665, 1.443375672974062551 ) ) ;
#66844=CIRCLE ( 'NONE', #94604, 0.08000000000000025147 ) ;
#66845=CARTESIAN_POINT ( 'NONE',  ( -6.724481002698126098, 8.868313807946373473, -1.443375672974059665 ) ) ;
#66846=CARTESIAN_POINT ( 'NONE',  ( 5.847644326195776010, 5.716673223516856694, -0.7998128361456281477 ) ) ;
#66849=CARTESIAN_POINT ( 'NONE',  ( -8.076906825439122528, 10.44614393447756129, -1.599625672291263179 ) ) ;
#66854=CARTESIAN_POINT ( 'NONE',  ( -4.796887421136680985, 4.490790167614548523, 1.214306433183764966E-14 ) ) ;
#66858=CARTESIAN_POINT ( 'NONE',  ( 7.747594715205354809, 11.12627870345989756, -1.199719254218446718 ) ) ;
#66860=CARTESIAN_POINT ( 'NONE',  ( 3.408985558832261731, 6.064568021024562938, 1.199719254218462483 ) ) ;
#66869=CARTESIAN_POINT ( 'NONE',  ( -4.115063316947640715, 4.759660943649018705, 1.199719254218462483 ) ) ;
#66870=CARTESIAN_POINT ( 'NONE',  ( 7.334597915313080918, 9.580116872663850813, 1.040834085586084257E-14 ) ) ;
#66872=CARTESIAN_POINT ( 'NONE',  ( -8.507905087775398556, 9.884643009614800135, 1.199719254218462483 ) ) ;
#66876=CARTESIAN_POINT ( 'NONE',  ( 7.619319141200063150, 9.912291636198670375, 1.443375672974076540 ) ) ;
#66880=CARTESIAN_POINT ( 'NONE',  ( 4.532503425670185493, 4.182342172903648070, 1.214306433183764966E-14 ) ) ;
#66881=CARTESIAN_POINT ( 'NONE',  ( 5.998049851660174348, 5.987234766784138351, -0.01316317710055334329 ) ) ;
#66883=CARTESIAN_POINT ( 'NONE',  ( -7.901704598666176693, 8.113076874732334076, 0.7998128361456602331 ) ) ;
#66897=CARTESIAN_POINT ( 'NONE',  ( -1.201851678989727383E-14, 3.509375000341421469, -1.575800808251660134 ) ) ;
#66898=CARTESIAN_POINT ( 'NONE',  ( 10.05067194643221207, 10.62020544712608938, 0.7998128361456462443 ) ) ;
#66900=CARTESIAN_POINT ( 'NONE',  ( -6.100805936469506641, 6.219954468743612352, 0.7216878364870317197 ) ) ;
#66902=CARTESIAN_POINT ( 'NONE',  ( -4.243338890952904841, 5.973648010910253880, -1.443375672974051449 ) ) ;
#66909=CARTESIAN_POINT ( 'NONE',  ( 5.183294799126148433, 4.941598775268944976, 1.040834085586084257E-14 ) ) ;
#66920=CARTESIAN_POINT ( 'NONE',  ( 4.385172619016207918, 7.203452924572514959, 1.199719254218462483 ) ) ;
#66925=CARTESIAN_POINT ( 'NONE',  ( -5.656776405399756236, 7.622658444431597680, -1.599625672291256295 ) ) ;
#66929=CARTESIAN_POINT ( 'NONE',  ( 5.601490020740366838, 9.686822124172440596, 1.040834085586084257E-14 ) ) ;
#66932=CARTESIAN_POINT ( 'NONE',  ( -5.900823170445743671, 7.907379670318584353, 1.599625672291269396 ) ) ;
#66933=UNCERTAINTY_MEASURE_WITH_UNIT (LENGTH_MEASURE( 1.000000000000000082E-05 ), #170220, 'distance_accuracy_value', 'NONE');
#66934=CARTESIAN_POINT ( 'NONE',  ( -1.500000000000013101, 2.629166666666687746, -0.8660254037844313801 ) ) ;
#66935=CARTESIAN_POINT ( 'NONE',  ( -3.436101866059630527, 6.096203712789787232, 1.199719254218462483 ) ) ;
#66938=CARTESIAN_POINT ( 'NONE',  ( -6.112028321662274166, 6.025121218227761588, 0.7998128361456341429 ) ) ;
#66942=CARTESIAN_POINT ( 'NONE',  ( -0.6823417656249969321, 3.217708333674754062, -1.181850606188749264 ) ) ;
#66944=CARTESIAN_POINT ( 'NONE',  ( -4.284013352238255301, 6.981470763377843447, -1.082531754730549967 ) ) ;
#66951=CARTESIAN_POINT ( 'NONE',  ( 4.710568305744190276, 7.583081225755162968, 1.199719254218462483 ) ) ;
#66954=CARTESIAN_POINT ( 'NONE',  ( -1.201851678989727383E-14, 2.134375000341423689, 1.575800808251672791 ) ) ;
#66956=CARTESIAN_POINT ( 'NONE',  ( 2.900554798319789906, 5.471398800426671372, 1.199719254218452047 ) ) ;
#66958=CARTESIAN_POINT ( 'NONE',  ( -1.364683531250014514, -0.1572916663252435232, 0.7879004041258379498 ) ) ;
#66961=CARTESIAN_POINT ( 'NONE',  ( -4.647747731386360215, 4.316793862905830892, 0.7998128361456341429 ) ) ;
#66962=AXIS2_PLACEMENT_3D ( 'NONE', #47335, #31078, #97152 ) ;
#66963=CARTESIAN_POINT ( 'NONE',  ( -6.602457619730773608, 8.725953194484466380, 1.443375672974078761 ) ) ;
#66965=ORIENTED_EDGE ( 'NONE', *, *, #160465, .T. ) ;
#66966=CARTESIAN_POINT ( 'NONE',  ( -1.364683531250012516, 3.030208333674755394, 0.7879004041258379498 ) ) ;
#66975=CARTESIAN_POINT ( 'NONE',  ( -7.659993601596726265, 8.039006744725394782, -0.7216878364870267237 ) ) ;
#66978=CARTESIAN_POINT ( 'NONE',  ( 4.786522169170392971, 5.141580351323886688, 0.8077998227834035649 ) ) ;
#66981=CARTESIAN_POINT ( 'NONE',  ( -6.019457014343129408, 9.966524250134902729, 0.000000000000000000 ) ) ;
#66991=EDGE_LOOP ( 'NONE', ( #55012, #129550, #168619, #106939 ) ) ;
#66994=CARTESIAN_POINT ( 'NONE',  ( -5.717788096661253761, 7.693838750903348789, 1.599625672291269396 ) ) ;
#66996=CARTESIAN_POINT ( 'NONE',  ( -0.7500000000000006661, 0.1083333333333560966, -1.299038105676652011 ) ) ;
#66997=CARTESIAN_POINT ( 'NONE',  ( 8.419250204406344196, 12.76628297187536809, 1.040834085586084257E-14 ) ) ;
#67001=ADVANCED_FACE ( 'NONE', ( #150391 ), #55019, .T. ) ;
#67002=CARTESIAN_POINT ( 'NONE',  ( 4.171104814498611368, 8.018039383557042044, 0.7998128361456321445 ) ) ;
#67008=CARTESIAN_POINT ( 'NONE',  ( -3.958617665510279160, 5.641473247893851628, -1.443375672974053447 ) ) ;
#67010=CARTESIAN_POINT ( 'NONE',  ( -4.257741265285667431, 3.982435197156672491, 0.4597581080974452727 ) ) ;
#67011=CARTESIAN_POINT ( 'NONE',  ( -0.1841593485105972039, 7.053066371975295290, 4.037421829300336995 ) ) ;
#67016=CARTESIAN_POINT ( 'NONE',  ( -1.364683531250014514, 1.988541667008086655, -0.7879004041258289570 ) ) ;
#67017=CARTESIAN_POINT ( 'NONE',  ( 8.690413276235306128, 13.08263988900915109, -0.7216878364870267237 ) ) ;
#67018=CARTESIAN_POINT ( 'NONE',  ( -7.823218330285243383, 9.085841792542966644, -1.199719254218446718 ) ) ;
#67022=CARTESIAN_POINT ( 'NONE',  ( 6.551614543901692400, 8.666636272683888365, 1.599625672291281386 ) ) ;
#67023=CARTESIAN_POINT ( 'NONE',  ( -6.581593504430098385, 9.765943957555402122, -1.199719254218440723 ) ) ;
#67026=CARTESIAN_POINT ( 'NONE',  ( -1.500000000000015099, -0.5479166659838513587, 0.8660254037844403729 ) ) ;
#67028=CARTESIAN_POINT ( 'NONE',  ( 8.324343129110697959, 9.774450407793066731, -1.082531754730543083 ) ) ;
#67031=CARTESIAN_POINT ( 'NONE',  ( -1.364683531250014514, 1.301041667008083325, -0.7879004041258289570 ) ) ;
#67034=CARTESIAN_POINT ( 'NONE',  ( 6.982085920913413624, 8.208483664896217391, -1.082531754730543971 ) ) ;
#67038=CARTESIAN_POINT ( 'NONE',  ( -3.741687207691642314, 6.348756928073427730, 1.082531754730560403 ) ) ;
#67040=CARTESIAN_POINT ( 'NONE',  ( 0.6823417656249899377, 5.176041667008086655, -1.181850606188754593 ) ) ;
#67044=CARTESIAN_POINT ( 'NONE',  ( -5.122186659821378996, 6.697499048860120041, -1.435703471572645551 ) ) ;
#67050=CARTESIAN_POINT ( 'NONE',  ( 7.308008492965924141, 8.484763649003774333, -1.199719254218451159 ) ) ;
#67054=CARTESIAN_POINT ( 'NONE',  ( -1.201851678989727383E-14, 2.212500000000021672, 1.732050807568877637 ) ) ;
#67060=CARTESIAN_POINT ( 'NONE',  ( 5.422898255786183341, 7.349800603215774331, -1.443375672974051449 ) ) ;
#67061=CARTESIAN_POINT ( 'NONE',  ( -1.364683531250012516, 0.5927083336747520637, 0.7879004041258379498 ) ) ;
#67063=CARTESIAN_POINT ( 'NONE',  ( 9.541187415715040032, 12.15447128979948310, -1.599625672291262513 ) ) ;
#67064=DIRECTION ( 'NONE',  ( -0.4243160830846685605, 0.9055141421511231359, 0.000000000000000000 ) ) ;
#67068=CARTESIAN_POINT ( 'NONE',  ( -1.500000000000015099, 0.6291666666666863028, -0.8660254037844313801 ) ) ;
#67069=CARTESIAN_POINT ( 'NONE',  ( 8.125414133291656071, 8.374071331795406081, -0.7998128361456291469 ) ) ;
#67070=CARTESIAN_POINT ( 'NONE',  ( -8.525379664894808585, 8.840697785332414682, -0.7998128361456291469 ) ) ;
#67073=CARTESIAN_POINT ( 'NONE',  ( -0.6823417656250003738, 0.9677083336747521747, -1.181850606188749264 ) ) ;
#67074=ORIENTED_EDGE ( 'NONE', *, *, #71139, .T. ) ;
#67075=CARTESIAN_POINT ( 'NONE',  ( -0.7500000000000006661, 2.858333333333358706, -1.299038105676652011 ) ) ;
#67077=CARTESIAN_POINT ( 'NONE',  ( 4.847203612085560387, 5.613824621309978724, -1.199719254218452047 ) ) ;
#67085=CARTESIAN_POINT ( 'NONE',  ( 1.499999999999985123, -1.172916665983846363, -0.8660254037844323793 ) ) ;
#67086=CARTESIAN_POINT ( 'NONE',  ( -6.496328159242330536, 10.73079995242472862, 0.000000000000000000 ) ) ;
#67087=CARTESIAN_POINT ( 'NONE',  ( -5.097502569058225852, 5.049433873430440478, -0.7216878364870207285 ) ) ;
#67092=CARTESIAN_POINT ( 'NONE',  ( 4.055646997469144033, 7.518606479810191701, -0.4957702256945207830 ) ) ;
#67095=CARTESIAN_POINT ( 'NONE',  ( 7.786460292950004636, 7.978625184730144149, 1.040834085586084257E-14 ) ) ;
#67098=CARTESIAN_POINT ( 'NONE',  ( 6.337546739384100292, 9.481222731668410120, 1.199719254218460707 ) ) ;
#67099=CARTESIAN_POINT ( 'NONE',  ( 5.938108092661121162, 9.871617174839238729, 1.040834085586084257E-14 ) ) ;
#67103=CARTESIAN_POINT ( 'NONE',  ( -6.669721502918952716, 9.868759955792373972, 1.199719254218452047 ) ) ;
#67104=CARTESIAN_POINT ( 'NONE',  ( 3.571683402196252910, 6.254382171615883834, 1.199719254218462483 ) ) ;
#67109=DIRECTION ( 'NONE',  ( -0.7808688094430278337, 0.6246950475544273962, 5.663618661477066041E-32 ) ) ;
#67110=CARTESIAN_POINT ( 'NONE',  ( 8.270110514656021650, 11.63191745286530576, 1.082531754730557072 ) ) ;
#67121=CARTESIAN_POINT ( 'NONE',  ( -1.567286081490176786, 8.684911043814580012, -2.501016734198262981 ) ) ;
#67122=CARTESIAN_POINT ( 'NONE',  ( -3.118012141462980669, 6.581505231774690046, 0.7216878364870317197 ) ) ;
#67123=CARTESIAN_POINT ( 'NONE',  ( 7.443063144222396232, 11.62739806832741785, 1.040834085586084257E-14 ) ) ;
#67126=CARTESIAN_POINT ( 'NONE',  ( -6.013204822860843457, 6.974159367214481264, -1.199719254218446718 ) ) ;
#67132=CARTESIAN_POINT ( 'NONE',  ( -8.667740277838301921, 9.006785167099828016, -0.7998128361456291469 ) ) ;
#67136=ORIENTED_EDGE ( 'NONE', *, *, #92074, .T. ) ;
#67146=CARTESIAN_POINT ( 'NONE',  ( -5.636439174979254396, 7.598931675607687453, -1.599625672291256295 ) ) ;
#67149=CARTESIAN_POINT ( 'NONE',  ( 4.609409038966229666, 6.400729850259146758, -1.443375672974051449 ) ) ;
#67153=CARTESIAN_POINT ( 'NONE',  ( -3.436101866059630527, 6.096203712789787232, 1.199719254218462483 ) ) ;
#67160=CARTESIAN_POINT ( 'NONE',  ( -8.715193815486133033, 9.062147627688959872, 0.7998128361456462443 ) ) ;
#67161=CARTESIAN_POINT ( 'NONE',  ( 5.880485940025228508, 7.883652901494672349, 1.599625672291267398 ) ) ;
#67164=B_SPLINE_CURVE_WITH_KNOTS ( 'NONE', 3,
 ( #86165, #85093, #151178, #133889, #39547, #102410 ),
 .UNSPECIFIED., .F., .F.,
 ( 4, 2, 4 ),
 ( 1.347205729526718589E-17, 9.978364048176284397E-05, 0.0001995672809635122167 ),
 .UNSPECIFIED. ) ;
#67166=CARTESIAN_POINT ( 'NONE',  ( -8.239604668803112375, 10.63595808506888396, -1.599625672291263179 ) ) ;
#67167=CARTESIAN_POINT ( 'NONE',  ( 5.281064527722868718, 6.119995689553514140, 1.199719254218462483 ) ) ;
#67170=CARTESIAN_POINT ( 'NONE',  ( 0.6823417656249882723, 0.4885416670080827695, -1.181850606188749264 ) ) ;
#67173=CARTESIAN_POINT ( 'NONE',  ( 7.944714827928043732, 10.29191993738131927, 1.443375672974076540 ) ) ;
#67200=CARTESIAN_POINT ( 'NONE',  ( 0.7499999999999885647, -0.2354166659838466402, 1.299038105676657340 ) ) ;
#67205=CARTESIAN_POINT ( 'NONE',  ( 0.000000000000000000, 2.817530495244580102, 1.214306433183764966E-14 ) ) ;
#67208=CARTESIAN_POINT ( 'NONE',  ( 10.06423010004587759, 10.63602329300870153, 0.000000000000000000 ) ) ;
#67210=FACE_OUTER_BOUND ( 'NONE', #16088, .T. ) ;
#67213=CARTESIAN_POINT ( 'NONE',  ( 3.337278367258157630, 7.045241861776501580, 0.7998128361456341429 ) ) ;
#67214=CARTESIAN_POINT ( 'NONE',  ( -7.714226216495749355, 8.102278128774251797, 1.040834085586084257E-14 ) ) ;
#67215=CARTESIAN_POINT ( 'NONE',  ( -5.903030530102264528, 6.005529115149156993, -0.1628943571830038795 ) ) ;
#67218=CARTESIAN_POINT ( 'NONE',  ( -8.342344591110322227, 8.627156865917170236, -0.7998128361456291469 ) ) ;
#67219=CARTESIAN_POINT ( 'NONE',  ( -4.433153041544240835, 4.274359424664112339, 0.7216878364870317197 ) ) ;
#67223=CARTESIAN_POINT ( 'NONE',  ( -1.500000000000001332, -0.3187499993171846735, 0.000000000000000000 ) ) ;
#67231=CARTESIAN_POINT ( 'NONE',  ( -4.189106276498259618, 6.870745841681152655, 1.082531754730560403 ) ) ;
#67235=EDGE_CURVE ( 'NONE', #53793, #34146, #86447, .T. ) ;
#67236=CARTESIAN_POINT ( 'NONE',  ( 4.063008298707909027, 7.508743736771079647, -0.5217633019904341918 ) ) ;
#67240=CARTESIAN_POINT ( 'NONE',  ( -5.219525951136862574, 5.191794485855519170, -0.7216878364870197293 ) ) ;
#67241=CARTESIAN_POINT ( 'NONE',  ( 8.097244055859613709, 10.46987070330147063, -1.599625672291262513 ) ) ;
#67249=CARTESIAN_POINT ( 'NONE',  ( -4.437596350374534815, 4.071617251725375475, -0.7998128361456221525 ) ) ;
#67250=CARTESIAN_POINT ( 'NONE',  ( -8.188234707649510113, 11.64035869464474082, -1.199719254218446718 ) ) ;
#67254=CARTESIAN_POINT ( 'NONE',  ( 5.250031796989762967, 7.148123067953287446, 1.599625672291267398 ) ) ;
#67259=CARTESIAN_POINT ( 'NONE',  ( 2.888709804529736136, 6.440345301045965698, 0.3798094595594287415 ) ) ;
#67270=CARTESIAN_POINT ( 'NONE',  ( 6.446011968293428041, 9.607765498729298415, -1.199719254218440723 ) ) ;
#67272=CARTESIAN_POINT ( 'NONE',  ( -3.490334480514268645, 6.159475096320226939, -1.199719254218452935 ) ) ;
#67274=CARTESIAN_POINT ( 'NONE',  ( -0.6823417656250003738, 2.967708333674754062, -1.181850606188749264 ) ) ;
#67278=CARTESIAN_POINT ( 'NONE',  ( 1.499999999999987566, -0.4437499993171847845, 0.000000000000000000 ) ) ;
#67282=CARTESIAN_POINT ( 'NONE',  ( 5.515469562660962666, 5.329135999392899947, 0.7998128361456341429 ) ) ;
#67284=CARTESIAN_POINT ( 'NONE',  ( -2.449219305563052895, 6.009172956465517856, 1.040834085586084257E-14 ) ) ;
#67290=CARTESIAN_POINT ( 'NONE',  ( 6.480434237652135998, 6.662854153456708950, 0.7216878364870317197 ) ) ;
#67293=CARTESIAN_POINT ( 'NONE',  ( 7.090551149822722721, 11.21613407486112379, 0.7216878364870438212 ) ) ;
#67294=CARTESIAN_POINT ( 'NONE',  ( -1.364683531250012516, 4.801041667008083991, -0.7879004041258300672 ) ) ;
#67296=CARTESIAN_POINT ( 'NONE',  ( 4.812781342726870193, 4.717259109377208048, 0.7216878364870317197 ) ) ;
#67302=CARTESIAN_POINT ( 'NONE',  ( -6.112394247781385737, 6.011859825068855301, 0.2949881747824866229 ) ) ;
#67305=CARTESIAN_POINT ( 'NONE',  ( 1.364683531249990311, 4.946875000341417916, 1.214306433183764966E-14 ) ) ;
#67313=CARTESIAN_POINT ( 'NONE',  ( 4.184706906422049677, 7.590773377626947038, -0.8858016570119742195 ) ) ;
#67319=CARTESIAN_POINT ( 'NONE',  ( -1.364683531250012516, 4.301041667008089320, -0.7879004041258300672 ) ) ;
#67321=CARTESIAN_POINT ( 'NONE',  ( 7.935599982700328958, 8.152621489438862667, 0.7998128361456481317 ) ) ;
#67323=CARTESIAN_POINT ( 'NONE',  ( -7.804689982961090955, 12.25722208009664094, 0.7998128361456481317 ) ) ;
#67330=CARTESIAN_POINT ( 'NONE',  ( 1.499999999999987121, 4.295833333333352044, -0.8660254037844323793 ) ) ;
#67336=CARTESIAN_POINT ( 'NONE',  ( 7.131225611108079399, 11.26358761302737754, 0.7216878364870438212 ) ) ;
#67341=CARTESIAN_POINT ( 'NONE',  ( 1.499999999999989120, 3.285416667349486897, 0.8660254037844524744 ) ) ;
#67343=CARTESIAN_POINT ( 'NONE',  ( -3.418627288940168096, 7.140148937072163804, -0.7998128361456281477 ) ) ;
#67344=CARTESIAN_POINT ( 'NONE',  ( 3.673896439178918172, 6.269667698141953238, 1.082531754730558626 ) ) ;
#67345=DIRECTION ( 'NONE',  ( -1.207943261119674327E-30, -2.168404344971008079E-15, 1.000000000000000000 ) ) ;
#67352=CARTESIAN_POINT ( 'NONE',  ( 3.659811400685081040, 6.357198169852855685, -1.199719254218446718 ) ) ;
#67355=CARTESIAN_POINT ( 'NONE',  ( -1.499999999999997780, 4.681250000682819490, 1.214306433183764966E-14 ) ) ;
#67356=CARTESIAN_POINT ( 'NONE',  ( 5.705283713252285338, 5.550585841749444249, -0.7998128361456211532 ) ) ;
#67369=CARTESIAN_POINT ( 'NONE',  ( 5.833718835943604297, 6.012594516355426855, -0.4067158398524447493 ) ) ;
#67373=CARTESIAN_POINT ( 'NONE',  ( 8.516493047678546091, 13.08765898893368629, -0.7998128361456352531 ) ) ;
#67380=CARTESIAN_POINT ( 'NONE',  ( 4.989037340148863464, 8.764367963574922982, -0.7216878364870257245 ) ) ;
#67381=CARTESIAN_POINT ( 'NONE',  ( -2.656508033273816238, 5.186677574539687363, -1.199719254218446718 ) ) ;
#67387=CARTESIAN_POINT ( 'NONE',  ( -4.765854690403601879, 5.518917546014321829, 1.199719254218462483 ) ) ;
#67399=CARTESIAN_POINT ( 'NONE',  ( 5.915399107357110609, 6.142141269072955545, 0.7871259410536131096 ) ) ;
#67400=DIRECTION ( 'NONE',  ( 0.7592566023653005702, -0.6507913734559639396, 0.000000000000000000 ) ) ;
#67407=CARTESIAN_POINT ( 'NONE',  ( -9.680158490477310806, 10.39586578175276266, 0.7216878364870438212 ) ) ;
#67409=CARTESIAN_POINT ( 'NONE',  ( 1.150196859685074235, 2.895291321728038714, -0.7750000000000022427 ) ) ;
#67411=CARTESIAN_POINT ( 'NONE',  ( 8.098297826064319693, 8.342435640030188893, 0.7998128361456481317 ) ) ;
#67412=CARTESIAN_POINT ( 'NONE',  ( -3.913499895838973508, 7.717500311787445000, 1.040834085586084257E-14 ) ) ;
#67413=CARTESIAN_POINT ( 'NONE',  ( 3.246287715468270108, 5.874753870433235825, 1.199719254218450271 ) ) ;
#67415=CARTESIAN_POINT ( 'NONE',  ( -5.117312914154178216, 8.057616602233474978, -1.199719254218452047 ) ) ;
#67416=CARTESIAN_POINT ( 'NONE',  ( 3.871016551901614200, 4.474939717762034697, -1.199719254218446718 ) ) ;
#67418=CARTESIAN_POINT ( 'NONE',  ( -5.259673527097670664, 8.223703984000886535, -1.199719254218446718 ) ) ;
#67421=CARTESIAN_POINT ( 'NONE',  ( 9.426996880203592610, 9.892584536526015881, -0.7998128361456281477 ) ) ;
#67422=CARTESIAN_POINT ( 'NONE',  ( 0.1263921867887890238, 7.050106634750518353, 4.033475513000639445 ) ) ;
#67425=CARTESIAN_POINT ( 'NONE',  ( 4.670798236633449285, 6.855725761985807409, -1.225018586207384352 ) ) ;
#67426=CARTESIAN_POINT ( 'NONE',  ( 5.341549334104188418, 7.254893527920112994, 1.443375672974062551 ) ) ;
#67430=CARTESIAN_POINT ( 'NONE',  ( -1.360600954992994938, 3.300000000000193445, 0.1676728910578147713 ) ) ;
#67433=CARTESIAN_POINT ( 'NONE',  ( 7.849807752188022292, 11.14156422998596696, -1.082531754730543083 ) ) ;
#67438=CARTESIAN_POINT ( 'NONE',  ( -9.189729191964438826, 9.615772233580322848, 1.040834085586084257E-14 ) ) ;
#67447=CARTESIAN_POINT ( 'NONE',  ( 8.530051201292206287, 13.10347683481629488, 0.000000000000000000 ) ) ;
#67450=CARTESIAN_POINT ( 'NONE',  ( 3.472859903394816872, 7.203420320602605287, -0.7998128361456291469 ) ) ;
#67453=CARTESIAN_POINT ( 'NONE',  ( 0.7499999999999920064, 4.514583334016150751, 1.299038105676669330 ) ) ;
#67459=CARTESIAN_POINT ( 'NONE',  ( 1.499999999999987121, 1.254166666666689300, 0.8660254037844524744 ) ) ;
#67460=CARTESIAN_POINT ( 'NONE',  ( 5.113396490648394632, 9.117379672398465473, 1.040834085586084257E-14 ) ) ;
#67461=CARTESIAN_POINT ( 'NONE',  ( 5.626270559546826533, 5.666329862333828515, 0.7216878364870317197 ) ) ;
#67465=CARTESIAN_POINT ( 'NONE',  ( 9.422553571817644524, 10.09532670998316384, 0.000000000000000000 ) ) ;
#67471=CARTESIAN_POINT ( 'NONE',  ( -4.608882153641705059, 7.464447381635583412, -1.199719254218452047 ) ) ;
#67472=( BOUNDED_CURVE ( )  B_SPLINE_CURVE ( 2, ( #27007, #93113, #182862, #46483, #16074, #113676, #100552 ),
 .UNSPECIFIED., .F., .T. ) 
 B_SPLINE_CURVE_WITH_KNOTS ( ( 3, 2, 2, 3 ),
 ( 0.3959408239114771133, 0.3988095238095238360, 0.4047619047619047672, 0.4076306046599514343 ),
 .UNSPECIFIED. ) 
 CURVE ( )  GEOMETRIC_REPRESENTATION_ITEM ( )  RATIONAL_B_SPLINE_CURVE ( ( 0.9331000818465633451, 0.9354320710352559409, 1.000000000000000000, 0.8660254037844387076, 1.000000000000000000, 0.9354320710352564960, 0.9331000818465632340 ) ) 
 REPRESENTATION_ITEM ( '' )  );
#67473=VECTOR ( 'NONE', #155665, 1000.000000000000227 ) ;
#67474=CARTESIAN_POINT ( 'NONE',  ( -0.7500000000000215383, 4.472916667349482012, 1.299038105676671107 ) ) ;
#67475=CARTESIAN_POINT ( 'NONE',  ( 1.364683531249988757, 0.1343750003414204142, 0.000000000000000000 ) ) ;
#67479=CARTESIAN_POINT ( 'NONE',  ( 2.672928840188529609, 6.270167413528593414, 0.000000000000000000 ) ) ;
#67482=CARTESIAN_POINT ( 'NONE',  ( -1.364683531250010295, 4.842708333674756283, 0.7879004041258379498 ) ) ;
#67489=CARTESIAN_POINT ( 'NONE',  ( -8.040148788103921973, 9.338927326664741457, 1.199719254218462483 ) ) ;
#67490=( BOUNDED_SURFACE ( )  B_SPLINE_SURFACE ( 3, 2, ( 
 ( #158159, #59569, #125727 ),
 ( #27063, #62761, #77954 ),
 ( #128923, #174419, #79016 ),
 ( #112661, #191688, #176530 ),
 ( #109468, #29215, #146186 ),
 ( #145133, #144075, #212200 ),
 ( #28142, #178670, #44411 ),
 ( #30284, #60636, #160276 ),
 ( #194902, #192754, #11878 ),
 ( #210071, #61710, #127878 ),
 ( #25995, #43348, #13999 ),
 ( #193828, #12937, #9750 ),
 ( #95305, #175476, #63837 ),
 ( #45478, #93169, #161354 ) ),
 .UNSPECIFIED., .F., .F., .F. ) 
 B_SPLINE_SURFACE_WITH_KNOTS ( ( 4, 2, 2, 2, 2, 2, 4 ),
 ( 3, 3 ),
 ( 0.000000000000000000, 0.0002390010041311327435, 0.0004780020082622654870, 0.0009560040165245309741, 0.001195005020655663663, 0.001434006024786796570, 0.001912008033049061948 ),
 ( 0.000000000000000000, 1.000000000000000000 ),
 .UNSPECIFIED. ) 
 GEOMETRIC_REPRESENTATION_ITEM ( )  RATIONAL_B_SPLINE_SURFACE ( (
 ( 1.000000000000000000, 0.4915962107220928079, 1.000000000000000000),
 ( 1.000000000000000000, 0.4903111309377012894, 1.000000000000000000),
 ( 1.000000000000000000, 0.5057854813392914650, 1.000000000000000000),
 ( 1.000000000000000000, 0.5532305778937092189, 1.000000000000000000),
 ( 1.000000000000000000, 0.5846576190777243998, 1.000000000000000000),
 ( 1.000000000000000000, 0.6796638612361862730, 1.000000000000000000),
 ( 1.000000000000000000, 0.7435379557940324791, 1.000000000000000000),
 ( 1.000000000000000000, 0.8106661767825003029, 1.000000000000000000),
 ( 1.000000000000000000, 0.8285023559306291530, 1.000000000000000000),
 ( 1.000000000000000000, 0.8541358093761527437, 1.000000000000000000),
 ( 1.000000000000000000, 0.8615977546920583485, 1.000000000000000000),
 ( 1.000000000000000000, 0.8740883989871980342, 1.000000000000000000),
 ( 1.000000000000000000, 0.8700938199805592355, 1.000000000000000000),
 ( 1.000000000000000000, 0.8708456909032173954, 1.000000000000000000) ) ) 
 REPRESENTATION_ITEM ( '' )  SURFACE ( )  );
#67491=CARTESIAN_POINT ( 'NONE',  ( 4.659198344590585350, 8.587481835331020719, 0.7998128361456462443 ) ) ;
#67495=CARTESIAN_POINT ( 'NONE',  ( -1.402160292154681736E-14, -0.5531249996585814177, -1.575800808251665908 ) ) ;
#67501=CARTESIAN_POINT ( 'NONE',  ( -6.728924311084075960, 6.744833205886536120, 1.040834085586084257E-14 ) ) ;
#67505=CARTESIAN_POINT ( 'NONE',  ( 8.055515824813896941, 12.54985222892493368, 0.7998128361456462443 ) ) ;
#67508=CARTESIAN_POINT ( 'NONE',  ( -2.605138072120212200, 6.191078184115536232, -0.7998128361456281477 ) ) ;
#67509=CARTESIAN_POINT ( 'NONE',  ( -6.645467848992654858, 10.90479625713344625, 0.7998128361456481317 ) ) ;
#67512=CARTESIAN_POINT ( 'NONE',  ( -4.920796802804098924, 6.860114910817498135, 1.449587651302047364 ) ) ;
#67517=CARTESIAN_POINT ( 'NONE',  ( 8.459924665247367415, 8.972259652317825740, -0.7216878364870267237 ) ) ;
#67520=CARTESIAN_POINT ( 'NONE',  ( 4.157546660884947620, 8.002221537674429896, 1.040834085586084257E-14 ) ) ;
#67524=EDGE_CURVE ( 'NONE', #204725, #52497, #80857, .T. ) ;
#67539=CARTESIAN_POINT ( 'NONE',  ( 2.250290310188348464, 5.569163095287620990, 0.7216878364870438212 ) ) ;
#67543=CARTESIAN_POINT ( 'NONE',  ( -5.434120640978981065, 5.234228924097238611, -0.7998128361456221525 ) ) ;
#67548=CARTESIAN_POINT ( 'NONE',  ( -1.201851678989727383E-14, 3.618750000682816381, -1.732050807568863648 ) ) ;
#67553=CARTESIAN_POINT ( 'NONE',  ( -8.853638004923878313, 10.28799807962136548, 1.199719254218462483 ) ) ;
#67554=CARTESIAN_POINT ( 'NONE',  ( 1.361729690220290223, 3.300000000000025135, 0.6158276295007287793 ) ) ;
#67555=CARTESIAN_POINT ( 'NONE',  ( -1.364683531249997417, 2.509375000341422357, 1.214306433183764966E-14 ) ) ;
#67563=CARTESIAN_POINT ( 'NONE',  ( -4.302014814237876017, 3.913438792899272212, 0.7998128361456341429 ) ) ;
#67567=CARTESIAN_POINT ( 'NONE',  ( 1.364683531249988535, 1.426041667008083991, 0.7879004041258500513 ) ) ;
#67572=CARTESIAN_POINT ( 'NONE',  ( -0.6823417656250003738, 2.217708333674753174, -1.181850606188749264 ) ) ;
#67574=CARTESIAN_POINT ( 'NONE',  ( -7.061099074618889304, 7.132370430010492868, -0.7998128361456291469 ) ) ;
#67575=CARTESIAN_POINT ( 'NONE',  ( 7.914208982075123799, 10.25632978388623684, -1.599625672291262513 ) ) ;
#67576=CARTESIAN_POINT ( 'NONE',  ( 4.192495815123822744, 5.914331089109666983, -1.599625672291255185 ) ) ;
#67578=CARTESIAN_POINT ( 'NONE',  ( 1.499999999999990896, 4.275000000000021672, 1.214306433183764966E-14 ) ) ;
#67580=CARTESIAN_POINT ( 'NONE',  ( 1.364683531249988535, 2.176041667008087543, 0.7879004041258500513 ) ) ;
#67583=CARTESIAN_POINT ( 'NONE',  ( -0.7158994178059416846, 2.800000000000024691, 1.161830092591057184 ) ) ;
#67587=CARTESIAN_POINT ( 'NONE',  ( 4.189106276942576201, 7.831115056500907556, 1.040834085586084257E-14 ) ) ;
#67590=CARTESIAN_POINT ( 'NONE',  ( -8.853638004923878313, 10.28799807962136548, 1.199719254218462483 ) ) ;
#67591=CARTESIAN_POINT ( 'NONE',  ( -9.408995418203979000, 12.00024729270324286, 1.443375672974076540 ) ) ;
#67596=CARTESIAN_POINT ( 'NONE',  ( -7.985389288324710400, 8.418635045908049008, -0.7216878364870267237 ) ) ;
#67598=CARTESIAN_POINT ( 'NONE',  ( -1.499999999999997780, 4.900000000000022560, 1.214306433183764966E-14 ) ) ;
#67601=CARTESIAN_POINT ( 'NONE',  ( 7.619319141200063150, 9.912291636198670375, 1.443375672974076540 ) ) ;
#67607=CARTESIAN_POINT ( 'NONE',  ( 3.999292125906911188, 4.728557570721922509, 1.082531754730560403 ) ) ;
#67617=CARTESIAN_POINT ( 'NONE',  ( 7.396136491454752715, 8.587579647240744407, 1.199719254218462483 ) ) ;
#67618=CARTESIAN_POINT ( 'NONE',  ( -4.120788623549732854, 6.895004929861607401, -1.199719254218452047 ) ) ;
#67620=CARTESIAN_POINT ( 'NONE',  ( 4.044555541517573793, 7.746237447724527492, 0.4662041258270445132 ) ) ;
#67622=CARTESIAN_POINT ( 'NONE',  ( 5.788968402910805722, 7.776882441527838807, 1.443375672974062551 ) ) ;
#67623=CARTESIAN_POINT ( 'NONE',  ( 0.6823417656249882723, 0.9885416670080832136, -1.181850606188749264 ) ) ;
#67624=CARTESIAN_POINT ( 'NONE',  ( 2.562127843302666186, 5.932973550587659517, 0.000000000000000000 ) ) ;
#67625=CARTESIAN_POINT ( 'NONE',  ( -4.783329267523015460, 4.474972321731942593, -0.7998128361456221525 ) ) ;
#67640=CARTESIAN_POINT ( 'NONE',  ( 7.253775878511261155, 8.421492265473332850, 1.199719254218462483 ) ) ;
#67641=CARTESIAN_POINT ( 'NONE',  ( 5.621827251160867789, 9.710548892996357040, 1.040834085586084257E-14 ) ) ;
#67652=CARTESIAN_POINT ( 'NONE',  ( -6.098470168048611306, 6.009303372345148553, 1.040834085586084257E-14 ) ) ;
#67654=CARTESIAN_POINT ( 'NONE',  ( -5.101945877444165944, 4.846691699973280976, 0.000000000000000000 ) ) ;
#67659=CARTESIAN_POINT ( 'NONE',  ( -1.500000000000031530, 4.702083334016148974, 0.8660254037844287156 ) ) ;
#67664=CARTESIAN_POINT ( 'NONE',  ( -3.735435015764967837, 4.316761258935923884, -1.199719254218452047 ) ) ;
#67667=CARTESIAN_POINT ( 'NONE',  ( 4.774442650306744085, 8.721933525333202653, -0.7998128361456281477 ) ) ;
#67668=CARTESIAN_POINT ( 'NONE',  ( -1.364683531249997417, 4.259375000341424133, 1.214306433183764966E-14 ) ) ;
#67675=CARTESIAN_POINT ( 'NONE',  ( 5.463572716182834910, 5.476515711742504067, 0.7216878364870317197 ) ) ;
#67676=CARTESIAN_POINT ( 'NONE',  ( -7.531718027591449705, 8.745758106066849891, 1.199719254218462483 ) ) ;
#67677=ORIENTED_EDGE ( 'NONE', *, *, #157331, .T. ) ;
#67678=VERTEX_POINT ( 'NONE', #80868 ) ;
#67681=CARTESIAN_POINT ( 'NONE',  ( -5.831978632172702071, 9.955725504176825780, 0.7998128361456481317 ) ) ;
#67682=CARTESIAN_POINT ( 'NONE',  ( -5.575427483717760424, 7.527751369135936343, 1.599625672291269396 ) ) ;
#67689=CARTESIAN_POINT ( 'NONE',  ( 8.274553823041976841, 8.548067636504127265, 1.040834085586084257E-14 ) ) ;
#67702=CARTESIAN_POINT ( 'NONE',  ( -0.7499999999999972244, 5.608333333333353821, -1.299038105676652011 ) ) ;
#67703=CARTESIAN_POINT ( 'NONE',  ( 4.359110081993588182, 5.044382169536003602, -1.199719254218452047 ) ) ;
#67704=CARTESIAN_POINT ( 'NONE',  ( 6.440286661691305703, 7.472421512516709718, 1.199719254218462483 ) ) ;
#67706=CARTESIAN_POINT ( 'NONE',  ( -6.995644074971465010, 10.14503993989993091, 1.082531754730549967 ) ) ;
#67707=CARTESIAN_POINT ( 'NONE',  ( -1.164422670175135899, 3.300000000000025135, -0.7116747751938151678 ) ) ;
#67708=CARTESIAN_POINT ( 'NONE',  ( 6.155038550924150087, 7.243595066575396757, 1.082531754730558626 ) ) ;
#67709=CARTESIAN_POINT ( 'NONE',  ( -7.117667457050096402, 10.28740055232499984, 1.082531754730549967 ) ) ;
#67713=CARTESIAN_POINT ( 'NONE',  ( 6.856673000209174695, 9.022537805042615489, 1.599625672291281386 ) ) ;
#67717=CARTESIAN_POINT ( 'NONE',  ( -2.306848205364723903, 5.479977701987478689, -0.7739106563221284096 ) ) ;
#67718=CARTESIAN_POINT ( 'NONE',  ( 1.364683531249990311, 3.884375000341417028, 1.214306433183764966E-14 ) ) ;
#67724=CARTESIAN_POINT ( 'NONE',  ( 8.072990401933337168, 11.50590700464255356, -1.199719254218446718 ) ) ;
#67727=CARTESIAN_POINT ( 'NONE',  ( -8.690940161559884913, 10.09818392903003748, 1.199719254218462483 ) ) ;
#67729=DIRECTION ( 'NONE',  ( 5.578564026256490882E-16, 1.000000000000000000, 9.066213480720158442E-32 ) ) ;
#67731=( BOUNDED_CURVE ( )  B_SPLINE_CURVE ( 1, ( #295, #1369 ),
 .UNSPECIFIED., .F., .T. ) 
 B_SPLINE_CURVE_WITH_KNOTS ( ( 2, 2 ),
 ( 0.000000000000000000, 6.249999999999918815E-05 ),
 .UNSPECIFIED. ) 
 CURVE ( )  GEOMETRIC_REPRESENTATION_ITEM ( )  RATIONAL_B_SPLINE_CURVE ( ( 0.9345202395942815432, 0.9345202395942815432 ) ) 
 REPRESENTATION_ITEM ( '' )  );
#67733=CARTESIAN_POINT ( 'NONE',  ( 9.240045382913317340, 10.73880668727576015, -1.199719254218446718 ) ) ;
#67736=CARTESIAN_POINT ( 'NONE',  ( -6.991200766141138168, 11.30815132714001159, 0.7998128361456481317 ) ) ;
#67742=CARTESIAN_POINT ( 'NONE',  ( 5.782412516234797017, 6.044064802175099338, 0.5499171889626064402 ) ) ;
#67743=CARTESIAN_POINT ( 'NONE',  ( -2.740719608256871442, 6.349256642941639051, 0.7998128361456341429 ) ) ;
#67748=CARTESIAN_POINT ( 'NONE',  ( 7.772902139336337335, 7.962807338847539107, 0.7998128361456341429 ) ) ;
#67750=CARTESIAN_POINT ( 'NONE',  ( 6.124532705071213279, 8.168374127381657246, -1.599625672291262513 ) ) ;
#67751=CARTESIAN_POINT ( 'NONE',  ( -4.183908731771626144, 7.398323783528643283, -0.7858605482065593728 ) ) ;
#67752=CARTESIAN_POINT ( 'NONE',  ( 4.741601036477289810, 6.554953847355395880, 1.599625672291267398 ) ) ;
#67754=CARTESIAN_POINT ( 'NONE',  ( -6.724481002698115439, 10.78905223654906109, -0.7216878364870267237 ) ) ;
#67761=CARTESIAN_POINT ( 'NONE',  ( -4.037710856648669022, 7.592775851288043221, -0.3149755216912339395 ) ) ;
#67762=FACE_BOUND ( 'NONE', #64626, .T. ) ;
#67765=CARTESIAN_POINT ( 'NONE',  ( 6.643132081016125845, 6.852668304048034287, 0.7216878364870317197 ) ) ;
#67768=VECTOR ( 'NONE', #117458, 1000.000000000000000 ) ;
#67770=CARTESIAN_POINT ( 'NONE',  ( -8.473482818416657736, 12.82955435488738516, -0.7216878364870267237 ) ) ;
#67777=CARTESIAN_POINT ( 'NONE',  ( -8.744645890690007306, 12.18554205823825498, 1.082531754730558626 ) ) ;
#67784=CARTESIAN_POINT ( 'NONE',  ( -9.802181872555943087, 10.53822639417784046, 0.7216878364870438212 ) ) ;
#67791=CARTESIAN_POINT ( 'NONE',  ( -1.201851678989727383E-14, 3.118750000682814161, -1.732050807568863648 ) ) ;
#67793=CARTESIAN_POINT ( 'NONE',  ( -4.869349725602420520, 8.832658446511480577, 1.040834085586084257E-14 ) ) ;
#67797=CARTESIAN_POINT ( 'NONE',  ( -8.646349277213090545, 11.11049346154719508, 1.599625672291269396 ) ) ;
#67801=CARTESIAN_POINT ( 'NONE',  ( 8.098297826064319693, 8.342435640030188893, 0.7998128361456481317 ) ) ;
#67803=CARTESIAN_POINT ( 'NONE',  ( -4.282998556134152146, 3.891253158444922811, -0.3219805702579207063 ) ) ;
#67806=CARTESIAN_POINT ( 'NONE',  ( 7.560643217915098191, 11.97250085420964716, -0.7998128361456291469 ) ) ;
#67807=FACE_OUTER_BOUND ( 'NONE', #214140, .T. ) ;
#67813=CARTESIAN_POINT ( 'NONE',  ( -6.968527767744110868, 9.153035033833367251, 1.443375672974078761 ) ) ;
#67816=CARTESIAN_POINT ( 'NONE',  ( -0.6823417656250212460, 5.363541667008087543, 1.181850606188767472 ) ) ;
#67824=CARTESIAN_POINT ( 'NONE',  ( -2.426546306721660606, 5.774795091243142053, 0.7216878364870317197 ) ) ;
#67826=CARTESIAN_POINT ( 'NONE',  ( 8.401248741962376698, 12.95320729893149370, 0.7998128361456462443 ) ) ;
#67828=CARTESIAN_POINT ( 'NONE',  ( -9.130526383799315582, 12.73969898348616070, 1.199719254218462483 ) ) ;
#67832=CARTESIAN_POINT ( 'NONE',  ( 1.364683531249986537, 2.655208333674754062, -0.7879004041258239610 ) ) ;
#67835=CARTESIAN_POINT ( 'NONE',  ( 4.497554271431305040, 6.270232621468402989, -1.599625672291256295 ) ) ;
#67842=CARTESIAN_POINT ( 'NONE',  ( 8.703971429848968100, 13.09845773489176679, 0.000000000000000000 ) ) ;
#67843=CARTESIAN_POINT ( 'NONE',  ( -1.499999999999997780, 3.931250000682819046, 1.214306433183764966E-14 ) ) ;
#67844=CARTESIAN_POINT ( 'NONE',  ( -7.293923454472094114, 9.532663335016016148, 1.443375672974090751 ) ) ;
#67849=CARTESIAN_POINT ( 'NONE',  ( -7.862839020921525091, 11.26073039346208660, -1.199719254218446718 ) ) ;
#67850=CARTESIAN_POINT ( 'NONE',  ( -5.572037945092175981, 5.603058478803387032, 0.7216878364870317197 ) ) ;
#67851=CARTESIAN_POINT ( 'NONE',  ( 0.6823417656249899377, 2.405208333674753618, 1.181850606188767472 ) ) ;
#67870=CARTESIAN_POINT ( 'NONE',  ( 0.6823417656249917140, 4.405208333674755394, 1.181850606188765695 ) ) ;
#67878=CARTESIAN_POINT ( 'NONE',  ( 8.748035429315576650, 11.22912730566677553, -1.599625672291255185 ) ) ;
#67881=CARTESIAN_POINT ( 'NONE',  ( 0.6823417656249899377, 2.342708333674753618, 1.181850606188767472 ) ) ;
#67885=CARTESIAN_POINT ( 'NONE',  ( -6.887178846062109727, 10.01849717283904262, -1.082531754730537976 ) ) ;
#67893=CARTESIAN_POINT ( 'NONE',  ( 4.273844736805816780, 6.009238164405336313, 1.599625672291267398 ) ) ;
#67904=CARTESIAN_POINT ( 'NONE',  ( -3.110706179331648169, 5.716575411607132118, 1.199719254218462483 ) ) ;
#67905=CARTESIAN_POINT ( 'NONE',  ( 8.471147050440139381, 8.777426401801974976, -0.7998128361456281477 ) ) ;
#67907=CARTESIAN_POINT ( 'NONE',  ( 3.999292125906899198, 6.649295999324608353, 1.082531754730558626 ) ) ;
#67910=DIRECTION ( 'NONE',  ( 0.000000000000000000, 0.7999999999999947153, -0.6000000000000068612 ) ) ;
#67916=CARTESIAN_POINT ( 'NONE',  ( -6.222829318992474157, 10.20379193889247382, 0.000000000000000000 ) ) ;
#67917=AXIS2_PLACEMENT_3D ( 'NONE', #50412, #148974, #101280 ) ;
#67918=CARTESIAN_POINT ( 'NONE',  ( 5.281064527722868718, 6.119995689553514140, 1.199719254218462483 ) ) ;
#67922=CARTESIAN_POINT ( 'NONE',  ( -9.332089804907933939, 9.781859615347734405, 1.040834085586084257E-14 ) ) ;
#67926=CARTESIAN_POINT ( 'NONE',  ( -4.298098390732130625, 4.973201863064262263, 1.199719254218462483 ) ) ;
#67928=CARTESIAN_POINT ( 'NONE',  ( 9.368847842243145152, 10.88907622316056312, 1.199719254218453823 ) ) ;
#67929=CARTESIAN_POINT ( 'NONE',  ( 3.192055101013606233, 5.811482486902795230, -1.199719254218446718 ) ) ;
#67935=FACE_OUTER_BOUND ( 'NONE', #48269, .T. ) ;
#67938=CARTESIAN_POINT ( 'NONE',  ( -6.064574784014443942, 5.969758757638621738, -0.7998128361456291469 ) ) ;
#67941=CARTESIAN_POINT ( 'NONE',  ( -7.472515219426274946, 11.86968485597268064, 0.000000000000000000 ) ) ;
#67946=CARTESIAN_POINT ( 'NONE',  ( 6.629573927402440781, 10.67832731537079383, 1.040834085586084257E-14 ) ) ;
#67947=CARTESIAN_POINT ( 'NONE',  ( 1.364683531249988535, 5.467708333674750953, -0.7879004041258300672 ) ) ;
#67949=CARTESIAN_POINT ( 'NONE',  ( 3.337278367258157630, 7.045241861776501580, 0.7998128361456341429 ) ) ;
#67950=CARTESIAN_POINT ( 'NONE',  ( 5.800636919132594826, 6.158450155783071978, -0.8617315278892097030 ) ) ;
#67952=CARTESIAN_POINT ( 'NONE',  ( -7.226659571283968297, 8.389856573708110332, 1.199719254218450271 ) ) ;
#67963=CARTESIAN_POINT ( 'NONE',  ( 0.6823417656249882723, 2.238541667008084435, -1.181850606188749264 ) ) ;
#67964=CARTESIAN_POINT ( 'NONE',  ( 8.028399517586572998, 12.51821653715971472, -0.7998128361456352531 ) ) ;
#67967=CARTESIAN_POINT ( 'NONE',  ( -4.528060117284246289, 6.305822774963486310, 1.443375672974064550 ) ) ;
#67968=CARTESIAN_POINT ( 'NONE',  ( 2.385871846325007706, 5.727341554113725586, -0.7216878364870267237 ) ) ;
#67969=CARTESIAN_POINT ( 'NONE',  ( -4.717874267431199087, 8.448011045404303587, 1.040834085586084257E-14 ) ) ;
#67975=VERTEX_POINT ( 'NONE', #131791 ) ;
#67977=CARTESIAN_POINT ( 'NONE',  ( 5.345992642490140057, 5.131412925860272090, 1.040834085586084257E-14 ) ) ;
#67988=CARTESIAN_POINT ( 'NONE',  ( 4.843287188579786573, 6.673587691474970107, -1.599625672291256295 ) ) ;
#67993=CARTESIAN_POINT ( 'NONE',  ( -6.573005544526917099, 6.562927978236513304, -0.7998128361456291469 ) ) ;
#67997=CARTESIAN_POINT ( 'NONE',  ( 5.438792177376376991, 9.497007973581119700, 1.040834085586084257E-14 ) ) ;
#68000=CARTESIAN_POINT ( 'NONE',  ( -5.063080299699540987, 7.994345218703034384, 1.199719254218464037 ) ) ;
#68001=ADVANCED_FACE ( 'NONE', ( #185801 ), #65642, .T. ) ;
#68002=CARTESIAN_POINT ( 'NONE',  ( 6.765155463094761679, 6.995028916473103209, 0.7216878364870317197 ) ) ;
#68003=CARTESIAN_POINT ( 'NONE',  ( -1.201851678989727383E-14, 2.462500000000023004, 1.732050807568877637 ) ) ;
#68004=CARTESIAN_POINT ( 'NONE',  ( -4.135400547368138113, 4.783387712472935149, 1.199719254218462483 ) ) ;
#68007=CARTESIAN_POINT ( 'NONE',  ( -5.250031796989778066, 7.148123067953287446, 1.599625672291267398 ) ) ;
#68009=CARTESIAN_POINT ( 'NONE',  ( 1.364683531249988535, 3.405208333674749621, -0.7879004041258239610 ) ) ;
#68011=CARTESIAN_POINT ( 'NONE',  ( -4.121315508874255684, 7.752025827087861920, -0.7216878364870267237 ) ) ;
#68017=CARTESIAN_POINT ( 'NONE',  ( 5.331380718671758778, 7.243030143248949670, -1.599625672291256295 ) ) ;
#68021=CARTESIAN_POINT ( 'NONE',  ( 0.6823417656249917140, 3.405208333674754506, 1.181850606188765695 ) ) ;
#68023=CARTESIAN_POINT ( 'NONE',  ( -1.387358672536802340, 7.315968950354509559, 4.254625267136455058 ) ) ;
#68027=EDGE_CURVE ( 'NONE', #170885, #177299, #3944, .T. ) ;
#68028=CARTESIAN_POINT ( 'NONE',  ( -4.946027110887008860, 4.664786472323266153, -0.7998128361456221525 ) ) ;
#68029=CARTESIAN_POINT ( 'NONE',  ( -6.344852701071109102, 10.34615255131755163, 0.000000000000000000 ) ) ;
#68031=CARTESIAN_POINT ( 'NONE',  ( -0.6823417656250003738, 2.467708333674753618, -1.181850606188749264 ) ) ;
#68038=CARTESIAN_POINT ( 'NONE',  ( -6.683806541412762314, 9.781229484081471526, -1.082531754730537976 ) ) ;
#68045=CARTESIAN_POINT ( 'NONE',  ( -6.683806541412768532, 8.820860269780128604, -1.443375672974058777 ) ) ;
#68049=CARTESIAN_POINT ( 'NONE',  ( 1.931788062848141441E-13, 7.054063922337705073, -3.955400951015614730 ) ) ;
#68050=DIRECTION ( 'NONE',  ( 1.000000000000000000, -5.391474854832587087E-16, 0.000000000000000000 ) ) ;
#68053=AXIS2_PLACEMENT_3D ( 'NONE', #163691, #61921, #145347 ) ;
#68059=CARTESIAN_POINT ( 'NONE',  ( -5.032047568966410367, 9.022472597102808578, 1.214306433183764966E-14 ) ) ;
#68061=CARTESIAN_POINT ( 'NONE',  ( -1.500000000000015099, -1.079166666666641961, 0.8660254037844403729 ) ) ;
#68062=CARTESIAN_POINT ( 'NONE',  ( 3.063252641683779753, 5.661212951017999373, 1.199719254218450271 ) ) ;
#68066=CARTESIAN_POINT ( 'NONE',  ( 4.659198344590585350, 8.587481835331020719, 0.7998128361456462443 ) ) ;
#68073=CARTESIAN_POINT ( 'NONE',  ( -3.958617665510272943, 6.601842462195195438, -1.082531754730549967 ) ) ;
#68078=LINE ( 'NONE', #151510, #94140 ) ;
#68083=CARTESIAN_POINT ( 'NONE',  ( -1.201851678989727383E-14, 2.071875000341422801, 1.575800808251672791 ) ) ;
#68084=CARTESIAN_POINT ( 'NONE',  ( 10.01911233037457905, 11.75168114260095109, 1.082531754730548412 ) ) ;
#68085=CARTESIAN_POINT ( 'NONE',  ( -6.503107236049161521, 10.73870887536603291, 0.7998128361456481317 ) ) ;
#68088=CARTESIAN_POINT ( 'NONE',  ( 6.795661308947685164, 8.951357498570873261, -1.599625672291262513 ) ) ;
#68089=CARTESIAN_POINT ( 'NONE',  ( -5.852315862593199469, 9.979452273000736895, 0.7998128361456481317 ) ) ;
#68090=CARTESIAN_POINT ( 'NONE',  ( -1.608462485350629301, 8.735270501766756013, 2.463594439587650342 ) ) ;
#68092=CARTESIAN_POINT ( 'NONE',  ( -1.402160292154681736E-14, -0.6312499993171797330, -1.732050807568870754 ) ) ;
#68094=CARTESIAN_POINT ( 'NONE',  ( 8.948018195339340508, 9.541702104091804415, -0.7216878364870197293 ) ) ;
#68097=CARTESIAN_POINT ( 'NONE',  ( 0.6823417656249882723, 0.4052083336747516751, 1.181850606188755259 ) ) ;
#68100=CARTESIAN_POINT ( 'NONE',  ( 6.927853306458743532, 9.105581495667113501, 1.443375672974076540 ) ) ;
#68103=CARTESIAN_POINT ( 'NONE',  ( -4.853455804012230423, 6.685451076146141425, 1.443375672974064550 ) ) ;
#68105=CARTESIAN_POINT ( 'NONE',  ( -0.6823417656249969321, 3.967708333674754950, -1.181850606188749264 ) ) ;
#68109=CARTESIAN_POINT ( 'NONE',  ( -3.716906668440817185, 7.488141546489591072, 0.7998128361456341429 ) ) ;
#68110=CARTESIAN_POINT ( 'NONE',  ( -6.471393748265563239, 5.229711127717889596, 2.420000000000002149 ) ) ;
#68117=CARTESIAN_POINT ( 'NONE',  ( 8.118635056484817980, 8.366162408854107113, 0.7998128361456481317 ) ) ;
#68121=CARTESIAN_POINT ( 'NONE',  ( -0.7500000000000215383, 2.941666666666689522, 1.299038105676671107 ) ) ;
#68129=CARTESIAN_POINT ( 'NONE',  ( 6.968527767744109980, 7.232296605230681408, 0.7216878364870317197 ) ) ;
#68130=TOROIDAL_SURFACE ( 'NONE', #26719, 6.909076424898650259, 0.08000000000000000167 ) ;
#68131=CARTESIAN_POINT ( 'NONE',  ( -0.6823417656250246877, 0.1135416670080893753, 1.181850606188755259 ) ) ;
#68133=CARTESIAN_POINT ( 'NONE',  ( 9.999301985278609806, 11.62460605670194447, 1.199719254218452047 ) ) ;
#68134=CARTESIAN_POINT ( 'NONE',  ( -0.6823417656250212460, 2.801041667008084879, 1.181850606188767472 ) ) ;
#68139=CARTESIAN_POINT ( 'NONE',  ( -1.500000000000015099, 0.1291666666666918539, -0.8660254037844383745 ) ) ;
#68140=CARTESIAN_POINT ( 'NONE',  ( 5.777746017718023097, 9.892454120646377191, 0.7998128361456462443 ) ) ;
#68141=CARTESIAN_POINT ( 'NONE',  ( -7.506410603460441422, 11.90922947067921278, -0.7998128361456291469 ) ) ;
#68143=CARTESIAN_POINT ( 'NONE',  ( -1.364683531250000748, 1.259375000341421469, 0.000000000000000000 ) ) ;
#68146=CARTESIAN_POINT ( 'NONE',  ( 1.499999999999989120, 2.275000000000019895, 1.214306433183764966E-14 ) ) ;
#68149=CARTESIAN_POINT ( 'NONE',  ( 3.174580523894166006, 6.855427711185178019, 0.7998128361456341429 ) ) ;
#68155=CARTESIAN_POINT ( 'NONE',  ( 1.499999999999985123, -0.1729166659838496101, -0.8660254037844323793 ) ) ;
#68156=CARTESIAN_POINT ( 'NONE',  ( -8.016948904382338981, 8.247528564734524892, -0.7998128361456291469 ) ) ;
#68157=CARTESIAN_POINT ( 'NONE',  ( -4.446711195602252253, 6.210915699667823198, -1.443375672974053447 ) ) ;
#68160=CARTESIAN_POINT ( 'NONE',  ( 4.227444969362701421, 3.826440640544909400, 1.214306433183764966E-14 ) ) ;
#68166=CARTESIAN_POINT ( 'NONE',  ( 7.284808609244363353, 7.393364887073558656, 0.7998128361456341429 ) ) ;
#68170=CARTESIAN_POINT ( 'NONE',  ( 7.470706336329915764, 8.674577799595093452, -1.199719254218441611 ) ) ;
#68171=CARTESIAN_POINT ( 'NONE',  ( 6.222829318548112276, 9.243422724072711816, -1.082531754730537976 ) ) ;
#68176=CARTESIAN_POINT ( 'NONE',  ( -7.588813295347149435, 9.876701482703580837, -1.599625672291263179 ) ) ;
#68177=CARTESIAN_POINT ( 'NONE',  ( 5.691725559638619814, 5.534767995866836543, 1.040834085586084257E-14 ) ) ;
#68181=CARTESIAN_POINT ( 'NONE',  ( 4.143432174609324115, 7.404820066527033617, -0.7413545030366501809 ) ) ;
#68182=CARTESIAN_POINT ( 'NONE',  ( 8.758204044747998296, 11.24099069033793974, 1.443375672974076540 ) ) ;
#68188=CARTESIAN_POINT ( 'NONE',  ( -1.507330767849605069, 8.672482115169964700, -2.545833800658952484 ) ) ;
#68189=CARTESIAN_POINT ( 'NONE',  ( -3.958617665510272943, 6.601842462195195438, -1.082531754730549967 ) ) ;
#68190=CARTESIAN_POINT ( 'NONE',  ( 7.429504990608736037, 11.61158022244479682, -0.7216878364870267237 ) ) ;
#68192=ADVANCED_FACE ( 'NONE', ( #203110 ), #14404, .T. ) ;
#68194=CARTESIAN_POINT ( 'NONE',  ( -5.229694566569281555, 7.124396299129368337, 1.599625672291267398 ) ) ;
#68200=CARTESIAN_POINT ( 'NONE',  ( -7.965578943228732278, 9.251929174310385307, -1.199719254218446718 ) ) ;
#68205=EDGE_LOOP ( 'NONE', ( #147491, #142626, #170758, #105531 ) ) ;
#68217=CARTESIAN_POINT ( 'NONE',  ( -4.855791571988752331, 8.816840600628864877, 0.7998128361456481317 ) ) ;
#68220=CARTESIAN_POINT ( 'NONE',  ( 5.016153647376205171, 6.875265226737464985, 1.443375672974062551 ) ) ;
#68225=CARTESIAN_POINT ( 'NONE',  ( -3.276266675996675204, 6.974061555304760240, -0.7998128361456281477 ) ) ;
#68232=CARTESIAN_POINT ( 'NONE',  ( -8.208571938070008400, 11.66408546346865016, -1.199719254218446718 ) ) ;
#68233=CARTESIAN_POINT ( 'NONE',  ( 6.636879889089462026, 7.701780277814560982, -1.199719254218446718 ) ) ;
#68236=CARTESIAN_POINT ( 'NONE',  ( -8.971744963941075568, 11.49012176272984931, 1.599625672291269396 ) ) ;
#68239=CARTESIAN_POINT ( 'NONE',  ( 1.364683531249986537, 0.1760416670080860446, 0.7879004041258500513 ) ) ;
#68243=CARTESIAN_POINT ( 'NONE',  ( 7.293923454472069245, 11.45340176361870199, 0.7216878364870438212 ) ) ;
#68246=B_SPLINE_CURVE_WITH_KNOTS ( 'NONE', 3,
 ( #183344, #1368, #85849, #117347, #67430, #133573, #34948, #150868, #52287, #151926 ),
 .UNSPECIFIED., .F., .F.,
 ( 4, 2, 2, 2, 4 ),
 ( 1.563658610346539661E-18, 0.0003961377057362423597, 0.0007922754114724830932, 0.001188413117208723989, 0.001584550822944964668 ),
 .UNSPECIFIED. ) ;
#68264=CARTESIAN_POINT ( 'NONE',  ( -4.295235737431041478, 3.905529869957963029, -0.7998128361456221525 ) ) ;
#68272=CARTESIAN_POINT ( 'NONE',  ( -1.402160292154681736E-14, -0.3812499993171785673, -1.732050807568870754 ) ) ;
#68279=CARTESIAN_POINT ( 'NONE',  ( 9.728138913005292210, 11.30824913904973705, -1.199719254218440723 ) ) ;
#68280=CARTESIAN_POINT ( 'NONE',  ( -1.001543065824772872E-14, 5.243750000682815937, 1.732050807568877637 ) ) ;
#68285=CARTESIAN_POINT ( 'NONE',  ( 2.984766373302843778, 6.633977868828633717, -0.7998128361456291469 ) ) ;
#68286=CARTESIAN_POINT ( 'NONE',  ( -6.182154858151506893, 9.195969186943299789, 1.082531754730548412 ) ) ;
#68287=CARTESIAN_POINT ( 'NONE',  ( -5.911504460181634002, 6.000493611234613667, 0.05175081109743372154 ) ) ;
#68290=CARTESIAN_POINT ( 'NONE',  ( -7.182068686937172153, 9.402166106225269715, 1.599625672291283607 ) ) ;
#68291=CARTESIAN_POINT ( 'NONE',  ( -3.890826896997578999, 7.483122446565064756, 0.7216878364870317197 ) ) ;
#68293=ORIENTED_EDGE ( 'NONE', *, *, #93285, .F. ) ;
#68294=CARTESIAN_POINT ( 'NONE',  ( -0.7500000000000006661, -0.1104166659838465292, -1.299038105676652011 ) ) ;
#68302=CARTESIAN_POINT ( 'NONE',  ( -3.999292125906916073, 5.688926785023260102, 1.443375672974064550 ) ) ;
#68311=CARTESIAN_POINT ( 'NONE',  ( -3.673896439178936824, 5.309298483840612093, 1.443375672974064550 ) ) ;
#68312=CARTESIAN_POINT ( 'NONE',  ( 7.747594715205354809, 11.12627870345989756, -1.199719254218446718 ) ) ;
#68322=CARTESIAN_POINT ( 'NONE',  ( -8.941766003412679353, 10.39081407785832845, -1.199719254218446718 ) ) ;
#68327=CARTESIAN_POINT ( 'NONE',  ( 3.669453130792974971, 7.432779085900453886, 1.040834085586084257E-14 ) ) ;
#68332=CARTESIAN_POINT ( 'NONE',  ( 2.913866314233864774, 6.444514562149673331, 0.4333858203510139173 ) ) ;
#68343=CARTESIAN_POINT ( 'NONE',  ( 8.880754312151170282, 10.31963377138658089, 1.199719254218453823 ) ) ;
#68345=CARTESIAN_POINT ( 'NONE',  ( -3.927058049452637700, 7.733318157670055371, -0.7998128361456281477 ) ) ;
#68351=CARTESIAN_POINT ( 'NONE',  ( -1.402160292154681736E-14, -0.5062499993171791779, 1.732050807568877637 ) ) ;
#68355=CARTESIAN_POINT ( 'NONE',  ( 4.355193658487811703, 6.104145239700998538, -1.599625672291255185 ) ) ;
#68357=CARTESIAN_POINT ( 'NONE',  ( -4.111146893441842920, 5.819424013814012753, 1.599625672291267398 ) ) ;
#68363=CARTESIAN_POINT ( 'NONE',  ( 5.558479791922850133, 6.547609847740540445, -1.082531754730542195 ) ) ;
#68367=CARTESIAN_POINT ( 'NONE',  ( 7.985389288324691748, 10.33937347451072775, -1.443375672974058777 ) ) ;
#68368=CARTESIAN_POINT ( 'NONE',  ( -1.364683531249997417, 5.071875000341417916, 1.214306433183764966E-14 ) ) ;
#68370=CARTESIAN_POINT ( 'NONE',  ( 4.677199806590210507, 4.559080650551097236, -0.7216878364870197293 ) ) ;
#68374=CARTESIAN_POINT ( 'NONE',  ( 5.329058858627603534, 6.340665403613130913, -1.104591990443883454 ) ) ;
#68377=CARTESIAN_POINT ( 'NONE',  ( -6.104320841615721527, 6.016881168963393200, -0.3405398961462170471 ) ) ;
#68381=CARTESIAN_POINT ( 'NONE',  ( 1.364683531249988535, 4.717708333674756283, -0.7879004041258300672 ) ) ;
#68397=CARTESIAN_POINT ( 'NONE',  ( -0.6823417656249969321, 5.030208333674755394, -1.181850606188749264 ) ) ;
#68399=CARTESIAN_POINT ( 'NONE',  ( 6.856673000209174695, 9.022537805042615489, 1.599625672291281386 ) ) ;
#68400=CARTESIAN_POINT ( 'NONE',  ( -9.515124878692420296, 9.995400534762978850, 1.040834085586084257E-14 ) ) ;
#68407=CARTESIAN_POINT ( 'NONE',  ( 0.7499999999999920064, 4.733333333333352932, 1.299038105676669330 ) ) ;
#68415=CARTESIAN_POINT ( 'NONE',  ( 8.649738815838679429, 10.15407870897571563, -1.082531754730543083 ) ) ;
#68418=DIRECTION ( 'NONE',  ( 0.7592566023653005702, -0.6507913734559639396, 0.000000000000000000 ) ) ;
#68420=CARTESIAN_POINT ( 'NONE',  ( -1.201851678989727383E-14, 2.868750000682821266, -1.732050807568863648 ) ) ;
#68422=CARTESIAN_POINT ( 'NONE',  ( -5.362413449404877852, 6.214902764849178141, -1.199719254218446718 ) ) ;
#68423=CARTESIAN_POINT ( 'NONE',  ( 4.216222583725566686, 4.981643104843690217, -1.082531754730548412 ) ) ;
#68424=CARTESIAN_POINT ( 'NONE',  ( -8.636180661780651135, 13.01936850547871138, -0.7216878364870257245 ) ) ;
#68431=CARTESIAN_POINT ( 'NONE',  ( 2.510230996824538430, 6.080353262937265413, 0.000000000000000000 ) ) ;
#68432=CARTESIAN_POINT ( 'NONE',  ( -1.244150428498999705, 2.928773246564666977, -0.7749999999999988010 ) ) ;
#68436=CARTESIAN_POINT ( 'NONE',  ( 5.030238685870051185, 5.827365540725222282, -1.199719254218452047 ) ) ;
#68449=CARTESIAN_POINT ( 'NONE',  ( 5.365762136054953224, 6.315268812753259020, -1.079746804988683806 ) ) ;
#68452=CARTESIAN_POINT ( 'NONE',  ( 8.191097360950562845, 12.70803068775103739, -0.7998128361456352531 ) ) ;
#68458=CARTESIAN_POINT ( 'NONE',  ( 5.612712406377503349, 8.531619659873665995, -1.082531754730543083 ) ) ;
#68460=CARTESIAN_POINT ( 'NONE',  ( -3.358669367883384105, 4.941533567329135401, -1.599625672291262513 ) ) ;
#68465=CARTESIAN_POINT ( 'NONE',  ( -3.405069135326500351, 7.124331091189553433, 1.040834085586084257E-14 ) ) ;
#68476=CARTESIAN_POINT ( 'NONE',  ( 7.886038904643079661, 12.35212915539230139, -0.7998128361456352531 ) ) ;
#68477=CARTESIAN_POINT ( 'NONE',  ( 6.103366240126457676, 6.022929404904433071, 0.2034074856576886248 ) ) ;
#68485=CARTESIAN_POINT ( 'NONE',  ( -9.666600336863641729, 10.38004793587015584, 1.040834085586084257E-14 ) ) ;
#68489=CARTESIAN_POINT ( 'NONE',  ( 6.751070424600909448, 9.963667031088037973, -1.199719254218441611 ) ) ;
#68491=CARTESIAN_POINT ( 'NONE',  ( -5.057354993097396445, 5.859001232490445688, -1.199719254218446718 ) ) ;
#68494=CARTESIAN_POINT ( 'NONE',  ( -6.261168011412601153, 6.199117522936475666, 1.040834085586084257E-14 ) ) ;
#68495=CARTESIAN_POINT ( 'NONE',  ( 4.033714395265605823, 4.664753868353354704, -1.199719254218446718 ) ) ;
#68498=CARTESIAN_POINT ( 'NONE',  ( 9.738834413317897898, 10.25639499182604730, 0.000000000000000000 ) ) ;
#68502=CARTESIAN_POINT ( 'NONE',  ( 3.998507505471064594, 7.829874410826325182, -0.01819030738507872169 ) ) ;
#68503=CARTESIAN_POINT ( 'NONE',  ( 5.992340707560160240, 7.053780915984068756, 1.082531754730558626 ) ) ;
#68510=CARTESIAN_POINT ( 'NONE',  ( 9.042925270190638187, 9.652427024751663254, 0.7216878364870458196 ) ) ;
#68513=CARTESIAN_POINT ( 'NONE',  ( -9.338868881714763148, 9.789768538289042255, -0.7998128361456291469 ) ) ;
#68514=FACE_OUTER_BOUND ( 'NONE', #139958, .T. ) ;
#68522=CARTESIAN_POINT ( 'NONE',  ( 9.728138913005292210, 11.30824913904973705, -1.199719254218440723 ) ) ;
#68526=CARTESIAN_POINT ( 'NONE',  ( 4.334856428067313416, 6.080418470877079429, -1.599625672291256295 ) ) ;
#68530=CARTESIAN_POINT ( 'NONE',  ( 0.7499999999999902300, 3.847916667349481123, -1.299038105676658228 ) ) ;
#68536=CARTESIAN_POINT ( 'NONE',  ( -1.402160292154681736E-14, 1.087500000000024336, -1.732050807568863648 ) ) ;
#68537=CARTESIAN_POINT ( 'NONE',  ( 6.799577732453452761, 7.891594428405881878, -1.199719254218446718 ) ) ;
#68538=CARTESIAN_POINT ( 'NONE',  ( 5.314433026432511475, 5.302519407033794430, 1.040834085586084257E-14 ) ) ;
#68542=CARTESIAN_POINT ( 'NONE',  ( 7.944714827928043732, 10.29191993738131927, 1.443375672974076540 ) ) ;
#68546=AXIS2_PLACEMENT_3D ( 'NONE', #79187, #45644, #198249 ) ;
#68550=CARTESIAN_POINT ( 'NONE',  ( -4.904298879841297421, 6.744767997946721216, 1.599625672291267398 ) ) ;
#68551=CARTESIAN_POINT ( 'NONE',  ( -0.7500000000000215383, 3.972916667349481123, 1.299038105676671107 ) ) ;
#68552=CARTESIAN_POINT ( 'NONE',  ( -1.364683531250014514, 0.2385416670080863499, -0.7879004041258359514 ) ) ;
#68556=CARTESIAN_POINT ( 'NONE',  ( 8.988692655735958326, 12.47026328412523988, -1.082531754730543083 ) ) ;
#68558=CARTESIAN_POINT ( 'NONE',  ( -1.201851678989727383E-14, 4.259375000341417028, -1.575800808251660134 ) ) ;
#68565=CARTESIAN_POINT ( 'NONE',  ( -8.538937818508475885, 8.856515631215026829, 1.040834085586084257E-14 ) ) ;
#68566=CARTESIAN_POINT ( 'NONE',  ( 4.469384193999260901, 8.366031992974468423, -0.7998128361456231517 ) ) ;
#68568=CARTESIAN_POINT ( 'NONE',  ( 1.364683531249986537, -0.3447916663252443836, -0.7879004041258309554 ) ) ;
#68574=CARTESIAN_POINT ( 'NONE',  ( -4.706651882238427120, 8.642844295920152575, 1.040834085586084257E-14 ) ) ;
#68578=CARTESIAN_POINT ( 'NONE',  ( 9.215791728987056786, 11.77484298861683598, -1.599625672291262513 ) ) ;
#68580=CARTESIAN_POINT ( 'NONE',  ( 7.540305987494599016, 11.94877408538573427, -0.7998128361456291469 ) ) ;
#68581=CARTESIAN_POINT ( 'NONE',  ( 3.208946231067535848, 6.430484326561804131, 0.7152403155292674786 ) ) ;
#68582=ORIENTED_EDGE ( 'NONE', *, *, #138558, .F. ) ;
#68583=CARTESIAN_POINT ( 'NONE',  ( -4.790108344329849110, 4.482881244673243337, 0.7998128361456341429 ) ) ;
#68584=CARTESIAN_POINT ( 'NONE',  ( -6.886651960737580680, 10.12184548991413457, -1.199719254218440723 ) ) ;
#68586=CARTESIAN_POINT ( 'NONE',  ( -4.181557753866925964, 7.584876391898649928, 0.9328056193420256603 ) ) ;
#68587=CARTESIAN_POINT ( 'NONE',  ( -1.364683531250014514, -0.5114583329919092369, -0.7879004041258359514 ) ) ;
#68591=CARTESIAN_POINT ( 'NONE',  ( 7.727784370109387346, 10.99920361756089093, -1.082531754730543083 ) ) ;
#68594=CARTESIAN_POINT ( 'NONE',  ( 4.320244504248938355, 8.192035688265757898, 1.040834085586084257E-14 ) ) ;
#68597=EDGE_CURVE ( 'NONE', #5398, #138555, #37754, .T. ) ;
#68615=ORIENTED_EDGE ( 'NONE', *, *, #31584, .F. ) ;
#68617=CARTESIAN_POINT ( 'NONE',  ( -4.249591082879585535, 7.045274465746411252, 1.199719254218464037 ) ) ;
#68618=CARTESIAN_POINT ( 'NONE',  ( -6.997979842947967377, 11.31606025008131233, -0.7998128361456291469 ) ) ;
#68623=CARTESIAN_POINT ( 'NONE',  ( 1.499999999999987121, 1.577083334016150751, -0.8660254037844253849 ) ) ;
#68624=CARTESIAN_POINT ( 'NONE',  ( 8.540746701604824409, 12.05162268759261224, -1.199719254218446718 ) ) ;
#68629=CARTESIAN_POINT ( 'NONE',  ( -8.992082194361570302, 11.51384853155376220, 1.599625672291269396 ) ) ;
#68631=CARTESIAN_POINT ( 'NONE',  ( 0.6823417656249899377, 2.092708333674753174, 1.181850606188767472 ) ) ;
#68632=CARTESIAN_POINT ( 'NONE',  ( -3.697672731464882734, 7.367968498737599958, 2.499999999999998668 ) ) ;
#68637=CARTESIAN_POINT ( 'NONE',  ( -9.110716038703348119, 12.61262389758715408, 1.082531754730560403 ) ) ;
#68642=CARTESIAN_POINT ( 'NONE',  ( -1.402160292154681736E-14, 0.7593750003414168059, -1.575800808251659024 ) ) ;
#68647=CARTESIAN_POINT ( 'NONE',  ( 0.6823417656249882723, 1.176041667008083325, -1.181850606188749264 ) ) ;
#68649=CARTESIAN_POINT ( 'NONE',  ( -7.009729113465285266, 8.136771039586342624, -1.199719254218446718 ) ) ;
#68650=CARTESIAN_POINT ( 'NONE',  ( 7.618792255875527886, 10.97600916757510170, 1.199719254218460707 ) ) ;
#68651=DIRECTION ( 'NONE',  ( 0.000000000000000000, 0.7996470168499997255, 0.6004703560067694568 ) ) ;
#68652=CARTESIAN_POINT ( 'NONE',  ( 6.356075086708249167, 6.309842444114747373, -0.7998128361456281477 ) ) ;
#68654=CARTESIAN_POINT ( 'NONE',  ( 1.499999999999990896, 4.025000000000021672, 1.214306433183764966E-14 ) ) ;
#68656=CARTESIAN_POINT ( 'NONE',  ( -1.364683531250000748, 0.8218750003414210248, 0.000000000000000000 ) ) ;
#68663=CARTESIAN_POINT ( 'NONE',  ( 4.175548123328908900, 7.815297210618305179, -0.7216878364870197293 ) ) ;
#68666=CARTESIAN_POINT ( 'NONE',  ( -9.826962411806732689, 10.35921099006301382, -0.7998128361456291469 ) ) ;
#68667=CARTESIAN_POINT ( 'NONE',  ( -4.009460741339347045, 5.700790169694431420, -1.599625672291256295 ) ) ;
#68673=CARTESIAN_POINT ( 'NONE',  ( -8.148087131688699358, 8.608449196499371681, -0.7216878364870267237 ) ) ;
#68675=CARTESIAN_POINT ( 'NONE',  ( -0.7499999999999972244, 5.608333333333353821, -1.299038105676652011 ) ) ;
#68678=CARTESIAN_POINT ( 'NONE',  ( 8.459924665247367415, 8.972259652317825740, -0.7216878364870267237 ) ) ;
#68684=ORIENTED_EDGE ( 'NONE', *, *, #198992, .F. ) ;
#68688=CARTESIAN_POINT ( 'NONE',  ( 9.368320956918608999, 11.95279375453699622, 1.443375672974076540 ) ) ;
#68693=CARTESIAN_POINT ( 'NONE',  ( 5.913327553854682783, 10.05063257947248800, -0.7998128361456291469 ) ) ;
#68694=CARTESIAN_POINT ( 'NONE',  ( -5.904739593951539689, 6.847616600153594746, 1.199719254218450271 ) ) ;
#68697=DIRECTION ( 'NONE',  ( 1.000000000000000000, 0.000000000000000000, 0.000000000000000000 ) ) ;
#68699=CARTESIAN_POINT ( 'NONE',  ( -1.402160292154681736E-14, -0.3656249996585805295, 1.575800808251672791 ) ) ;
#68700=CARTESIAN_POINT ( 'NONE',  ( 3.389175213736297820, 4.977123720824209840, 1.443375672974062551 ) ) ;
#68701=CARTESIAN_POINT ( 'NONE',  ( -3.216308754939891212, 4.775446185561722956, -1.599625672291262513 ) ) ;
#68719=CARTESIAN_POINT ( 'NONE',  ( 5.635385404774530649, 9.726366738878972740, 0.7998128361456462443 ) ) ;
#68726=CARTESIAN_POINT ( 'NONE',  ( 1.580000000000019389, 8.674529973577556063, 2.499999999999961364 ) ) ;
#68730=CARTESIAN_POINT ( 'NONE',  ( -0.5987734146285321746, 6.693217038951044806, 3.557622718601344047 ) ) ;
#68732=CARTESIAN_POINT ( 'NONE',  ( -6.261168011412601153, 6.199117522936475666, 1.040834085586084257E-14 ) ) ;
#68734=CARTESIAN_POINT ( 'NONE',  ( -4.223528545856940042, 4.886203710709899006, -1.199719254218446718 ) ) ;
#68744=CARTESIAN_POINT ( 'NONE',  ( -8.785320351975364872, 12.23299559640450518, 1.082531754730560403 ) ) ;
#68747=CARTESIAN_POINT ( 'NONE',  ( 7.461064606222022277, 7.598996883547496139, 1.040834085586084257E-14 ) ) ;
#68748=CARTESIAN_POINT ( 'NONE',  ( 1.364683531249988535, 4.363541667008089320, 0.7879004041258499402 ) ) ;
#68754=CARTESIAN_POINT ( 'NONE',  ( 4.812781342726855982, 7.598366752281232372, 1.082531754730558626 ) ) ;
#68755=CARTESIAN_POINT ( 'NONE',  ( -6.612626235163205024, 8.737816579155630592, -1.599625672291263179 ) ) ;
#68760=CARTESIAN_POINT ( 'NONE',  ( -8.518600588087975822, 8.832788862391110385, 1.040834085586084257E-14 ) ) ;
#68761=CARTESIAN_POINT ( 'NONE',  ( -6.098470168048611306, 6.009303372345148553, 1.040834085586084257E-14 ) ) ;
#68768=VECTOR ( 'NONE', #23304, 1000.000000000000000 ) ;
#68769=CARTESIAN_POINT ( 'NONE',  ( 7.775764792637399836, 9.030479331953833011, -1.199719254218441611 ) ) ;
#68783=CARTESIAN_POINT ( 'NONE',  ( 1.499999999999990896, 5.525000000000022560, 1.214306433183764966E-14 ) ) ;
#68784=CARTESIAN_POINT ( 'NONE',  ( 3.009020027229115879, 5.597941567487558778, -1.199719254218446718 ) ) ;
#68785=CARTESIAN_POINT ( 'NONE',  ( 5.656776405399742025, 7.622658444431597680, -1.599625672291262513 ) ) ;
#68787=CARTESIAN_POINT ( 'NONE',  ( -6.236387472606141458, 10.21960978477508952, -0.7216878364870278340 ) ) ;
#68789=CARTESIAN_POINT ( 'NONE',  ( 5.016153647376201619, 7.835634441038803466, 1.082531754730558626 ) ) ;
#68790=CARTESIAN_POINT ( 'NONE',  ( -8.636180661780668899, 10.13826086257468795, -1.082531754730543083 ) ) ;
#68793=CARTESIAN_POINT ( 'NONE',  ( 6.577677080924314801, 10.82570702772039262, 1.040834085586084257E-14 ) ) ;
#68797=B_SPLINE_CURVE_WITH_KNOTS ( 'NONE', 3,
 ( #106163, #23779, #89885, #189491 ),
 .UNSPECIFIED., .F., .F.,
 ( 4, 4 ),
 ( 0.001812203442042607240, 0.002059939351771563048 ),
 .UNSPECIFIED. ) ;
#68799=CARTESIAN_POINT ( 'NONE',  ( 1.364683531249988535, 3.905208333674751842, -0.7879004041258239610 ) ) ;
#68805=CARTESIAN_POINT ( 'NONE',  ( 9.582915646760733708, 10.07448976417602893, 0.7998128361456462443 ) ) ;
#68808=CARTESIAN_POINT ( 'NONE',  ( -7.479294296233107708, 11.87759377891399204, 0.7998128361456481317 ) ) ;
#68813=CARTESIAN_POINT ( 'NONE',  ( 4.376584659113025744, 4.000436945253625254, 0.7998128361456341429 ) ) ;
#68816=CARTESIAN_POINT ( 'NONE',  ( -8.877891658850122880, 9.251961778280284321, 0.7998128361456462443 ) ) ;
#68821=CARTESIAN_POINT ( 'NONE',  ( 5.228900738148710481, 6.411469580122314049, 1.161126877744517838 ) ) ;
#68822=CARTESIAN_POINT ( 'NONE',  ( 1.270916165646588603, 3.290225491120026380, -0.7749999999999910294 ) ) ;
#68823=CARTESIAN_POINT ( 'NONE',  ( -2.279742385392243165, 5.811449882932888222, -0.7998128361456281477 ) ) ;
#68827=CARTESIAN_POINT ( 'NONE',  ( 5.940443861082012944, 10.08226827123770697, 0.7998128361456462443 ) ) ;
#68829=CARTESIAN_POINT ( 'NONE',  ( 6.636879889089462026, 7.701780277814560982, -1.199719254218446718 ) ) ;
#68830=CARTESIAN_POINT ( 'NONE',  ( 3.960953433486789521, 7.772862772376584850, -0.7998128361456221525 ) ) ;
#68832=CARTESIAN_POINT ( 'NONE',  ( -8.866669273657352690, 9.446795028796142191, 0.7216878364870438212 ) ) ;
#68841=CARTESIAN_POINT ( 'NONE',  ( -4.118090981180881016, 7.482401814132296103, -0.6348448669579254133 ) ) ;
#68842=CARTESIAN_POINT ( 'NONE',  ( -0.6823417656250003738, -0.9697916663252494907, -1.181850606188749264 ) ) ;
#68845=CARTESIAN_POINT ( 'NONE',  ( 5.829642864196171281, 5.903597551091405826, 0.7216878364870317197 ) ) ;
#68855=CARTESIAN_POINT ( 'NONE',  ( -7.334597915313094241, 9.580116872663850813, 1.040834085586084257E-14 ) ) ;
#68863=CARTESIAN_POINT ( 'NONE',  ( -8.419250203962027612, 11.80591375705560608, 1.082531754730549967 ) ) ;
#68867=CARTESIAN_POINT ( 'NONE',  ( 6.747154001095143627, 11.02343010125301959, -0.7998128361456291469 ) ) ;
#68871=CARTESIAN_POINT ( 'NONE',  ( -1.201851678989727383E-14, 2.868750000682821266, -1.732050807568863648 ) ) ;
#68873=CARTESIAN_POINT ( 'NONE',  ( -6.230135280679522936, 7.227244901336242755, 1.199719254218450271 ) ) ;
#68875=VERTEX_POINT ( 'NONE', #155286 ) ;
#68876=CARTESIAN_POINT ( 'NONE',  ( -8.134002093194872884, 11.57708731111429401, 1.199719254218453823 ) ) ;
#68879=CARTESIAN_POINT ( 'NONE',  ( 7.124973419181436007, 8.271222729588529887, -1.199719254218446718 ) ) ;
#68884=CARTESIAN_POINT ( 'NONE',  ( 8.561083932025322696, 12.07534945641652158, -1.199719254218446718 ) ) ;
#68885=CARTESIAN_POINT ( 'NONE',  ( 5.960673519960956845, 6.112995148063339101, -0.7021749152587808407 ) ) ;
#68890=CARTESIAN_POINT ( 'NONE',  ( -7.876924059859742755, 8.292092279365579799, 1.040834085586084257E-14 ) ) ;
#68900=CARTESIAN_POINT ( 'NONE',  ( -4.419594887930571758, 4.258541578781506409, 1.214306433183764966E-14 ) ) ;
#68902=CARTESIAN_POINT ( 'NONE',  ( 10.73535870392234237, 11.41900666419791399, 0.000000000000000000 ) ) ;
#68903=CARTESIAN_POINT ( 'NONE',  ( 1.364683531249990311, 5.676041667008088432, 0.7879004041258500513 ) ) ;
#68904=CARTESIAN_POINT ( 'NONE',  ( -8.319899820280397762, 12.85830022363583147, -0.7998128361456281477 ) ) ;
#68908=CARTESIAN_POINT ( 'NONE',  ( 1.364683531249988535, 2.363541667008088432, 0.7879004041258500513 ) ) ;
#68909=CARTESIAN_POINT ( 'NONE',  ( -3.470524135418306511, 5.072030796119872953, -1.443375672974053447 ) ) ;
#68910=CARTESIAN_POINT ( 'NONE',  ( 5.345992642490140057, 5.131412925860272090, 1.040834085586084257E-14 ) ) ;
#68916=CARTESIAN_POINT ( 'NONE',  ( 3.145128448690309053, 4.692402494937224056, -1.443375672974057666 ) ) ;
#68917=CARTESIAN_POINT ( 'NONE',  ( 9.205623113554612047, 12.72334881824701469, 1.082531754730546636 ) ) ;
#68919=CARTESIAN_POINT ( 'NONE',  ( -8.026063749610063525, 8.466088584074293877, -0.7216878364870278340 ) ) ;
#68924=CARTESIAN_POINT ( 'NONE',  ( -8.646349277213090545, 11.11049346154719508, 1.599625672291269396 ) ) ;
#68925=CARTESIAN_POINT ( 'NONE',  ( -5.382223794500845315, 6.341977850748185652, -1.082531754730543971 ) ) ;
#68926=CARTESIAN_POINT ( 'NONE',  ( -1.364683531249997417, 2.571875000341422357, 1.214306433183764966E-14 ) ) ;
#68927=AXIS2_PLACEMENT_3D ( 'NONE', #54799, #102480, #168546 ) ;
#68944=LINE ( 'NONE', #21260, #36289 ) ;
#68947=CARTESIAN_POINT ( 'NONE',  ( -0.6823417656250003738, 2.780208333674753618, -1.181850606188749264 ) ) ;
#68955=CARTESIAN_POINT ( 'NONE',  ( 9.423080456697809026, 10.95234760669099749, -1.199719254218446718 ) ) ;
#68958=EDGE_CURVE ( 'NONE', #27161, #160642, #178930, .T. ) ;
#68959=CARTESIAN_POINT ( 'NONE',  ( 1.364683531249986537, 2.155208333674751398, -0.7879004041258239610 ) ) ;
#68970=CARTESIAN_POINT ( 'NONE',  ( 5.192936529234042808, 6.017179691316550283, -1.199719254218452047 ) ) ;
#68974=CARTESIAN_POINT ( 'NONE',  ( 8.543609354905870035, 13.11929468069890525, 0.7998128361456462443 ) ) ;
#68981=CARTESIAN_POINT ( 'NONE',  ( -2.300079615812729905, 5.835176651756807331, -0.7998128361456281477 ) ) ;
#68983=CARTESIAN_POINT ( 'NONE',  ( 8.555358625423188812, 9.940005470203933768, 1.199719254218462483 ) ) ;
#68986=CARTESIAN_POINT ( 'NONE',  ( 5.138177029454847222, 6.057256624861201644, 1.082531754730560403 ) ) ;
#68990=ORIENTED_EDGE ( 'NONE', *, *, #182079, .T. ) ;
#68996=CARTESIAN_POINT ( 'NONE',  ( -6.561783159334137139, 8.678499657355050800, -1.443375672974059665 ) ) ;
#68998=CARTESIAN_POINT ( 'NONE',  ( 5.497994985541524215, 6.373081223675282736, -1.199719254218445830 ) ) ;
#69001=CARTESIAN_POINT ( 'NONE',  ( -10.15913717534155047, 10.74674821418697057, 0.7998128361456462443 ) ) ;
#69003=CARTESIAN_POINT ( 'NONE',  ( 2.310781476690497271, 5.467761476598782089, -0.5169845646830224517 ) ) ;
#69006=CARTESIAN_POINT ( 'NONE',  ( -4.295235737431041478, 3.905529869957963029, -0.7998128361456221525 ) ) ;
#69008=CARTESIAN_POINT ( 'NONE',  ( 8.940712233207955606, 12.51824914112961729, 1.199719254218450271 ) ) ;
#69009=CARTESIAN_POINT ( 'NONE',  ( 3.680148631105580215, 6.380924938676771241, -1.199719254218446718 ) ) ;
#69015=CARTESIAN_POINT ( 'NONE',  ( 3.389175213736292047, 5.937492935125556315, 1.082531754730558626 ) ) ;
#69018=CARTESIAN_POINT ( 'NONE',  ( -4.497554271431319250, 6.270232621468402989, -1.599625672291256295 ) ) ;
#69021=CARTESIAN_POINT ( 'NONE',  ( -10.48453286206953727, 11.12637651536962125, 0.7998128361456462443 ) ) ;
#69026=CARTESIAN_POINT ( 'NONE',  ( 8.920901888111997025, 10.47043562662792304, 1.082531754730549967 ) ) ;
#69030=CARTESIAN_POINT ( 'NONE',  ( 4.684505768721569652, 5.424010470718658716, -1.199719254218452047 ) ) ;
#69033=CARTESIAN_POINT ( 'NONE',  ( -6.581593504430098385, 9.765943957555402122, -1.199719254218440723 ) ) ;
#69042=CARTESIAN_POINT ( 'NONE',  ( 0.6823417656249882723, 2.738541667008084879, -1.181850606188749264 ) ) ;
#69044=CARTESIAN_POINT ( 'NONE',  ( 3.728655938958122196, 4.308852335994623139, -1.199719254218446718 ) ) ;
#69046=CARTESIAN_POINT ( 'NONE',  ( -4.446711195602252253, 6.210915699667823198, -1.443375672974053447 ) ) ;
#69047=CIRCLE ( 'NONE', #20663, 6.961139734775127152 ) ;
#69049=CARTESIAN_POINT ( 'NONE',  ( -5.219525951136850139, 7.112532914458205013, -1.443375672974051449 ) ) ;
#69054=CARTESIAN_POINT ( 'NONE',  ( 3.649115900372475796, 7.409052317076538330, 1.040834085586084257E-14 ) ) ;
#69064=CARTESIAN_POINT ( 'NONE',  ( 7.169564303528210836, 7.258913197071374945, -0.7998128361456281477 ) ) ;
#69069=CARTESIAN_POINT ( 'NONE',  ( -4.726989112658928072, 8.666571064744069020, 1.040834085586084257E-14 ) ) ;
#69073=CARTESIAN_POINT ( 'NONE',  ( 6.089583550832340819, 10.25626457594641749, 1.040834085586084257E-14 ) ) ;
#69076=CARTESIAN_POINT ( 'NONE',  ( -6.437424008390261854, 6.404749519410410485, 0.7998128361456341429 ) ) ;
#69077=CARTESIAN_POINT ( 'NONE',  ( 7.117667457050084856, 7.406292909420979953, -0.7216878364870257245 ) ) ;
#69078=CARTESIAN_POINT ( 'NONE',  ( 4.618624277135228162, 7.133842259902017702, 1.345135577604664512 ) ) ;
#69079=CARTESIAN_POINT ( 'NONE',  ( -3.327636637150278798, 5.969660945728899826, -1.199719254218452935 ) ) ;
#69082=CARTESIAN_POINT ( 'NONE',  ( -6.084912014434944894, 5.993485526462540847, -0.7998128361456291469 ) ) ;
#69085=CARTESIAN_POINT ( 'NONE',  ( 0.6823417656249899377, 1.592708333674752730, 1.181850606188755259 ) ) ;
#69087=CARTESIAN_POINT ( 'NONE',  ( -3.795919822146277767, 7.372397525905215687, -0.7216878364870267237 ) ) ;
#69090=VERTEX_POINT ( 'NONE', #125004 ) ;
#69092=CARTESIAN_POINT ( 'NONE',  ( -1.500000000000079936, 7.268077025657370349, 4.207854987879517950 ) ) ;
#69093=CARTESIAN_POINT ( 'NONE',  ( 7.169564303528210836, 7.258913197071374945, -0.7998128361456281477 ) ) ;
#69096=CARTESIAN_POINT ( 'NONE',  ( -1.201851678989727383E-14, 2.759375000341417916, -1.575800808251660134 ) ) ;
#69099=CARTESIAN_POINT ( 'NONE',  ( 1.364683531249988757, -0.8031249996585804185, 0.000000000000000000 ) ) ;
#69102=ADVANCED_FACE ( 'NONE', ( #39398 ), #37836, .F. ) ;
#69104=CARTESIAN_POINT ( 'NONE',  ( -4.243865776277440993, 4.909930479533815451, -1.199719254218446718 ) ) ;
#69105=CARTESIAN_POINT ( 'NONE',  ( -7.659993601596720936, 8.999375959026737704, -1.082531754730543083 ) ) ;
#69107=CARTESIAN_POINT ( 'NONE',  ( -1.201851678989727383E-14, 2.696875000341417916, -1.575800808251660134 ) ) ;
#69114=CARTESIAN_POINT ( 'NONE',  ( -5.856759170979136897, 9.776710099543576504, 0.000000000000000000 ) ) ;
#69119=CARTESIAN_POINT ( 'NONE',  ( -7.334597914868741242, 8.619747657844088806, -1.082531754730543083 ) ) ;
#69129=ORIENTED_EDGE ( 'NONE', *, *, #77767, .F. ) ;
#69132=CARTESIAN_POINT ( 'NONE',  ( -7.067878151425722955, 7.140279352951794500, 0.7998128361456341429 ) ) ;
#69134=CARTESIAN_POINT ( 'NONE',  ( -1.500000000000013101, 0.1708333333333560411, 0.8660254037844403729 ) ) ;
#69135=CARTESIAN_POINT ( 'NONE',  ( 4.196412238629597447, 4.854568018944682706, -1.199719254218452047 ) ) ;
#69139=CARTESIAN_POINT ( 'NONE',  ( 5.296431564432884542, 9.330920591813708143, 1.040834085586084257E-14 ) ) ;
#69145=CARTESIAN_POINT ( 'NONE',  ( -3.633221978782283923, 7.182583375313884133, -0.7216878364870267237 ) ) ;
#69149=CARTESIAN_POINT ( 'NONE',  ( -0.02081124878883705218, 7.037281880797342737, 4.016375841068750674 ) ) ;
#69153=CARTESIAN_POINT ( 'NONE',  ( 1.364683531249988757, 1.634375000341421691, 0.000000000000000000 ) ) ;
#69154=CARTESIAN_POINT ( 'NONE',  ( 3.469446951953614189E-15, 6.400000000000023448, 1.214306433183764966E-14 ) ) ;
#69156=CARTESIAN_POINT ( 'NONE',  ( -6.665805079413154921, 10.92852302595736447, 0.7998128361456481317 ) ) ;
#69158=CARTESIAN_POINT ( 'NONE',  ( 7.039708073993665494, 9.236078724457858158, 1.599625672291281386 ) ) ;
#69159=CARTESIAN_POINT ( 'NONE',  ( -6.958359152311683893, 9.141171649162195934, -1.599625672291263179 ) ) ;
#69162=CARTESIAN_POINT ( 'NONE',  ( 0.7499999999999867883, -0.4020833326505157679, -1.299038105676652899 ) ) ;
#69164=CARTESIAN_POINT ( 'NONE',  ( 8.934460041725669655, 9.525884258209195821, 1.040834085586084257E-14 ) ) ;
#69167=CARTESIAN_POINT ( 'NONE',  ( -1.201851678989727383E-14, 1.134375000341418582, 1.575800808251672791 ) ) ;
#69169=DIRECTION ( 'NONE',  ( 1.000000000000000000, -5.578564026256504688E-16, 0.000000000000000000 ) ) ;
#69170=CARTESIAN_POINT ( 'NONE',  ( 6.548225005276093746, 9.623051025255367819, -1.082531754730537976 ) ) ;
#69173=CARTESIAN_POINT ( 'NONE',  ( -3.795919822146283540, 6.412028311603867436, -1.082531754730549967 ) ) ;
#69175=CARTESIAN_POINT ( 'NONE',  ( -1.201851678989727383E-14, 3.946875000341423689, -1.575800808251660134 ) ) ;
#69179=CARTESIAN_POINT ( 'NONE',  ( -6.878064000834399394, 6.918829510595249310, -0.7998128361456291469 ) ) ;
#69187=CARTESIAN_POINT ( 'NONE',  ( 7.446452682403650769, 9.710614100936176385, -1.599625672291262513 ) ) ;
#69190=CARTESIAN_POINT ( 'NONE',  ( 1.499999999999987121, 2.045833333333356929, -0.8660254037844262731 ) ) ;
#69196=CARTESIAN_POINT ( 'NONE',  ( 4.826339496784873617, 8.574553812983598533, -0.7216878364870257245 ) ) ;
#69197=CARTESIAN_POINT ( 'NONE',  ( 0.6823417656249864960, -1.011458332991911568, -1.181850606188749264 ) ) ;
#69200=CARTESIAN_POINT ( 'NONE',  ( 4.390142812726693045, 4.016254791136236513, 1.214306433183764966E-14 ) ) ;
#69206=CARTESIAN_POINT ( 'NONE',  ( 0.7499999999999885647, -0.01666666666664401442, 1.299038105676657340 ) ) ;
#69207=CARTESIAN_POINT ( 'NONE',  ( 6.740374924288304648, 11.01552117831172062, 1.040834085586084257E-14 ) ) ;
#69208=CARTESIAN_POINT ( 'NONE',  ( -9.352427035328430449, 9.805586384171650849, 1.040834085586084257E-14 ) ) ;
#69210=CARTESIAN_POINT ( 'NONE',  ( 1.364683531249988757, 1.384375000341421469, 0.000000000000000000 ) ) ;
#69212=CARTESIAN_POINT ( 'NONE',  ( -1.500000000000015099, 0.8791666666666874130, -0.8660254037844313801 ) ) ;
#69214=CARTESIAN_POINT ( 'NONE',  ( 4.172158584703322681, 5.890604320285754980, -1.599625672291256295 ) ) ;
#69221=CARTESIAN_POINT ( 'NONE',  ( -0.7500000000000249800, -1.027083332650516212, 1.299038105676659116 ) ) ;
#69223=CARTESIAN_POINT ( 'NONE',  ( -6.645467848992654858, 10.90479625713344625, 0.7998128361456481317 ) ) ;
#69224=CARTESIAN_POINT ( 'NONE',  ( -4.270455198624581783, 7.926022131796578662, 1.040834085586084257E-14 ) ) ;
#69233=CARTESIAN_POINT ( 'NONE',  ( 7.507464373665139412, 9.781794407407920389, 1.599625672291281386 ) ) ;
#69236=CARTESIAN_POINT ( 'NONE',  ( 5.612712405933139692, 9.491988873656591608, 1.040834085586084257E-14 ) ) ;
#69240=CARTESIAN_POINT ( 'NONE',  ( -6.659026002606323047, 10.92061410301605662, 0.000000000000000000 ) ) ;
#69241=CARTESIAN_POINT ( 'NONE',  ( 5.331380718671758778, 7.243030143248949670, -1.599625672291256295 ) ) ;
#69245=CARTESIAN_POINT ( 'NONE',  ( 9.083599731475976213, 12.58098820582193689, 1.082531754730546636 ) ) ;
#69253=CARTESIAN_POINT ( 'NONE',  ( -3.253593677599670109, 5.779314476299451719, 1.082531754730560403 ) ) ;
#69254=CARTESIAN_POINT ( 'NONE',  ( 7.782016984564043227, 12.02284421539267356, 0.7216878364870438212 ) ) ;
#69257=CARTESIAN_POINT ( 'NONE',  ( -5.018489415352746619, 9.006654751220198207, 0.7998128361456481317 ) ) ;
#69261=CARTESIAN_POINT ( 'NONE',  ( 3.930962900855079489, 2.807348321460013452, 0.7750000000000135669 ) ) ;
#69263=CARTESIAN_POINT ( 'NONE',  ( -8.193204901359996128, 8.453160561208463264, 1.040834085586084257E-14 ) ) ;
#69278=CARTESIAN_POINT ( 'NONE',  ( -5.669280788808708671, 9.765911353585494226, 0.7998128361456481317 ) ) ;
#69281=CARTESIAN_POINT ( 'NONE',  ( 3.226477370372293763, 6.708047998835573900, 0.7216878364870317197 ) ) ;
#69286=CARTESIAN_POINT ( 'NONE',  ( -5.111587607552082524, 5.922272616020886282, 1.199719254218450271 ) ) ;
#69291=CARTESIAN_POINT ( 'NONE',  ( 6.938893903907228378E-15, 10.64264068711930733, 1.214306433183764966E-14 ) ) ;
#69295=CARTESIAN_POINT ( 'NONE',  ( -9.840520565420403543, 10.37502883594562597, 1.040834085586084257E-14 ) ) ;
#69296=CARTESIAN_POINT ( 'NONE',  ( 7.962716289927667113, 8.184257181204083409, -0.7998128361456291469 ) ) ;
#69299=CARTESIAN_POINT ( 'NONE',  ( -7.960608749518247151, 12.43912730774665576, 0.000000000000000000 ) ) ;
#69302=CARTESIAN_POINT ( 'NONE',  ( 0.6823417656249882723, -0.3447916663252489911, 1.181850606188755259 ) ) ;
#69303=ORIENTED_EDGE ( 'NONE', *, *, #62099, .T. ) ;
#69307=CARTESIAN_POINT ( 'NONE',  ( 7.944714827928039291, 11.25228915168265864, 1.082531754730557072 ) ) ;
#69334=CARTESIAN_POINT ( 'NONE',  ( -1.402160292154681736E-14, -1.256249999317182953, 1.732050807568877637 ) ) ;
#69338=CARTESIAN_POINT ( 'NONE',  ( 10.05353459973327368, 11.68787744023238417, -1.199719254218440723 ) ) ;
#69341=CARTESIAN_POINT ( 'NONE',  ( -1.123270288250339366, 3.283552654332833054, 0.7749999999993804067 ) ) ;
#69343=CARTESIAN_POINT ( 'NONE',  ( 8.890396042259068210, 11.39521468743417998, -1.599625672291257406 ) ) ;
#69348=CARTESIAN_POINT ( 'NONE',  ( 2.998324526916512411, 6.649795714711241423, 0.000000000000000000 ) ) ;
#69349=CARTESIAN_POINT ( 'NONE',  ( 1.364683531249986537, 2.467708333674753174, -0.7879004041258239610 ) ) ;
#69351=CARTESIAN_POINT ( 'NONE',  ( -5.897748123441601820, 6.008673066555767051, -0.2037434952626964724 ) ) ;
#69354=CARTESIAN_POINT ( 'NONE',  ( -8.993135964566285168, 9.386413468282476913, -0.7998128361456291469 ) ) ;
#69355=( BOUNDED_CURVE ( )  B_SPLINE_CURVE ( 2, ( #14944, #29098, #114675, #111477, #180667, #208887, #60518 ),
 .UNSPECIFIED., .F., .T. ) 
 B_SPLINE_CURVE_WITH_KNOTS ( ( 3, 2, 2, 3 ),
 ( 0.2375000000000004052, 0.2416666666666670293, 0.2458333333333336534, 0.2500000000000002776 ),
 .UNSPECIFIED. ) 
 CURVE ( )  GEOMETRIC_REPRESENTATION_ITEM ( )  RATIONAL_B_SPLINE_CURVE ( ( 0.9999999999999865663, 0.8660254037844521413, 1.000000000000000000, 0.8660254037844387076, 1.000000000000000000, 0.8660254037844298258, 1.000000000000008882 ) ) 
 REPRESENTATION_ITEM ( '' )  );
#69356=CARTESIAN_POINT ( 'NONE',  ( -5.395781948114519722, 5.397426482329451325, 0.000000000000000000 ) ) ;
#69359=CARTESIAN_POINT ( 'NONE',  ( -6.742482464697739708, 6.760651051769146491, 0.7998128361456341429 ) ) ;
#69361=CARTESIAN_POINT ( 'NONE',  ( 1.499999999999989120, 0.5562500006828161592, 0.000000000000000000 ) ) ;
#69368=CARTESIAN_POINT ( 'NONE',  ( -4.080641047588914994, 5.783833860318930320, -1.443375672974051449 ) ) ;
#69371=CARTESIAN_POINT ( 'NONE',  ( 3.994299746785815231, 7.604083813490793098, 0.004591788735710394809 ) ) ;
#69376=CARTESIAN_POINT ( 'NONE',  ( -3.429849674132942727, 5.984946472254969230, -1.082531754730549078 ) ) ;
#69377=CARTESIAN_POINT ( 'NONE',  ( 9.596473800374404561, 10.09030761005864285, 0.000000000000000000 ) ) ;
#69385=CARTESIAN_POINT ( 'NONE',  ( -4.451154503988200339, 4.087435097607984957, 1.214306433183764966E-14 ) ) ;
#69386=CARTESIAN_POINT ( 'NONE',  ( -10.14557902172788495, 10.73093036830436553, 1.040834085586084257E-14 ) ) ;
#69391=CARTESIAN_POINT ( 'NONE',  ( 4.924636110261782385, 6.768494766770632332, 1.599625672291267398 ) ) ;
#69395=ORIENTED_EDGE ( 'NONE', *, *, #63218, .T. ) ;
#69400=VERTEX_POINT ( 'NONE', #158282 ) ;
#69409=CARTESIAN_POINT ( 'NONE',  ( 7.771848369131631351, 10.09024240211882351, -1.599625672291262513 ) ) ;
#69411=CARTESIAN_POINT ( 'NONE',  ( -5.759516327706961647, 5.613857225279885732, -0.7998128361456221525 ) ) ;
#69417=CARTESIAN_POINT ( 'NONE',  ( -1.500000000000015099, -1.297916665983847029, 0.8660254037844403729 ) ) ;
#69423=CARTESIAN_POINT ( 'NONE',  ( 3.018661757337009810, 6.673522483535157868, 0.000000000000000000 ) ) ;
#69424=CARTESIAN_POINT ( 'NONE',  ( -3.262708522383007903, 6.958243709422141876, 1.040834085586084257E-14 ) ) ;
#69425=CARTESIAN_POINT ( 'NONE',  ( 3.511198596259283544, 6.271927390929313617, -2.420000000000000373 ) ) ;
#69427=ADVANCED_FACE ( 'NONE', ( #142050 ), #105270, .T. ) ;
#69431=CARTESIAN_POINT ( 'NONE',  ( 6.019457014787495730, 6.125047393447951016, -0.7216878364870257245 ) ) ;
#69434=CARTESIAN_POINT ( 'NONE',  ( 8.229436053370683624, 8.703356271795033905, 0.7216878364870458196 ) ) ;
#69435=CARTESIAN_POINT ( 'NONE',  ( -1.364683531250012516, 4.301041667008089320, -0.7879004041258300672 ) ) ;
#69436=CARTESIAN_POINT ( 'NONE',  ( 5.788968402910816380, 5.856144012925152076, 0.7216878364870317197 ) ) ;
#69442=CARTESIAN_POINT ( 'NONE',  ( -4.503925953283787642, 7.237052973511334919, 1.308369160636771333 ) ) ;
#69445=CARTESIAN_POINT ( 'NONE',  ( -1.364683531250010295, 5.592708333674750953, 0.7879004041258379498 ) ) ;
#69447=( BOUNDED_CURVE ( )  B_SPLINE_CURVE ( 2, ( #163227, #34265, #51603, #117728, #151238, #64644, #183717 ),
 .UNSPECIFIED., .F., .T. ) 
 B_SPLINE_CURVE_WITH_KNOTS ( ( 3, 2, 2, 3 ),
 ( 0.1785714285714287142, 0.1845238095238095899, 0.1904761904761904656, 0.1964285714285713413 ),
 .UNSPECIFIED. ) 
 CURVE ( )  GEOMETRIC_REPRESENTATION_ITEM ( )  RATIONAL_B_SPLINE_CURVE ( ( 0.9999999999999968914, 0.8660254037844418162, 1.000000000000000000, 0.8660254037844387076, 1.000000000000000000, 0.8660254037844405950, 0.9999999999999981126 ) ) 
 REPRESENTATION_ITEM ( '' )  );
#69451=CARTESIAN_POINT ( 'NONE',  ( -8.130085669689073313, 12.63685038127928806, 0.7998128361456481317 ) ) ;
#69460=ORIENTED_EDGE ( 'NONE', *, *, #193595, .F. ) ;
#69462=CARTESIAN_POINT ( 'NONE',  ( 3.795919822146273326, 5.451659097302528068, -1.443375672974051449 ) ) ;
#69463=CARTESIAN_POINT ( 'NONE',  ( -1.201851678989727383E-14, 4.134375000341417028, 1.575800808251672791 ) ) ;
#69465=CARTESIAN_POINT ( 'NONE',  ( 8.125414133291656071, 8.374071331795406081, -0.7998128361456291469 ) ) ;
#69466=CARTESIAN_POINT ( 'NONE',  ( -9.840520565420403543, 10.37502883594562597, 1.040834085586084257E-14 ) ) ;
#69468=CARTESIAN_POINT ( 'NONE',  ( -4.928552533767591726, 5.708731696605642725, 1.199719254218462483 ) ) ;
#69469=DIRECTION ( 'NONE',  ( -7.387867266669436732E-31, 1.000000000000000000, 8.546850786086424434E-32 ) ) ;
#69470=EDGE_LOOP ( 'NONE', ( #205022, #115670, #13319 ) ) ;
#69472=CARTESIAN_POINT ( 'NONE',  ( -0.7499999999999972244, 4.858333333333353821, -1.299038105676652011 ) ) ;
#69473=CARTESIAN_POINT ( 'NONE',  ( 3.472859903394816872, 7.203420320602605287, -0.7998128361456291469 ) ) ;
#69478=CARTESIAN_POINT ( 'NONE',  ( 8.432808358020025707, 9.900993174853955026, 1.082531754730558626 ) ) ;
#69483=CARTESIAN_POINT ( 'NONE',  ( 0.7499999999999902300, 2.764583334016148974, 1.299038105676669330 ) ) ;
#69485=CARTESIAN_POINT ( 'NONE',  ( -3.903858165731105778, 6.641919395739846799, 1.199719254218464037 ) ) ;
#69486=CARTESIAN_POINT ( 'NONE',  ( 5.165293336682183600, 5.128523102325077687, -0.7216878364870197293 ) ) ;
#69490=EDGE_CURVE ( 'NONE', #161364, #66472, #84156, .T. ) ;
#69496=CARTESIAN_POINT ( 'NONE',  ( 7.609150525767641504, 9.900428251527500834, -1.599625672291262513 ) ) ;
#69497=CARTESIAN_POINT ( 'NONE',  ( 5.996784015946103885, 5.890669528225568996, 1.040834085586084257E-14 ) ) ;
#69501=CARTESIAN_POINT ( 'NONE',  ( 5.678167406024951624, 5.518950149984223508, 0.7998128361456341429 ) ) ;
#69505=ORIENTED_EDGE ( 'NONE', *, *, #206116, .T. ) ;
#69507=VERTEX_POINT ( 'NONE', #155071 ) ;
#69512=CARTESIAN_POINT ( 'NONE',  ( 5.859090863903361424, 5.997168572722006097, -0.3086645125121977862 ) ) ;
#69514=CARTESIAN_POINT ( 'NONE',  ( 10.71502147350184231, 11.39527989537399755, 0.000000000000000000 ) ) ;
#69520=CARTESIAN_POINT ( 'NONE',  ( 1.499999999999990896, 5.556250000682820378, 1.214306433183764966E-14 ) ) ;
#69521=CARTESIAN_POINT ( 'NONE',  ( -1.364683531250000748, -0.9906249996585805295, 0.000000000000000000 ) ) ;
#69522=CARTESIAN_POINT ( 'NONE',  ( 5.748293942514166588, 7.729428904398431222, -1.443375672974057666 ) ) ;
#69523=CARTESIAN_POINT ( 'NONE',  ( -9.164948653157990677, 11.71552606681625619, -1.443375672974059665 ) ) ;
#69529=CARTESIAN_POINT ( 'NONE',  ( -4.205000198532790279, 8.057583998263570635, 0.7998128361456341429 ) ) ;
#69539=CARTESIAN_POINT ( 'NONE',  ( 8.829384350997564468, 11.32403438096243775, 1.599625672291281386 ) ) ;
#69540=CARTESIAN_POINT ( 'NONE',  ( 6.112872195911107198, 6.017013290715023111, -0.08730524813132384265 ) ) ;
#69545=CARTESIAN_POINT ( 'NONE',  ( -8.514157279702020631, 11.91663867875229776, -1.082531754730543971 ) ) ;
#69549=CARTESIAN_POINT ( 'NONE',  ( 8.613507663383630941, 8.943513783569379427, -0.7998128361456221525 ) ) ;
#69553=CARTESIAN_POINT ( 'NONE',  ( 3.354752944377597856, 6.001296637494123232, -1.199719254218446718 ) ) ;
#69555=CARTESIAN_POINT ( 'NONE',  ( -7.413611068574208041, 7.543634422958360730, 0.7998128361456341429 ) ) ;
#69556=CARTESIAN_POINT ( 'NONE',  ( 2.835626683552519012, 6.459981564119914310, 0.000000000000000000 ) ) ;
#69564=CARTESIAN_POINT ( 'NONE',  ( 3.998447120444656555, 7.829958269474884602, 0.005269623924535754567 ) ) ;
#69566=CARTESIAN_POINT ( 'NONE',  ( 5.910991785878156435, 7.919243054989755670, -1.443375672974057666 ) ) ;
#69574=CARTESIAN_POINT ( 'NONE',  ( 7.415946836550703303, 11.59576237604377091, 0.7216878364870438212 ) ) ;
#69576=CARTESIAN_POINT ( 'NONE',  ( -9.001723924469462901, 12.58942944760136484, -1.199719254218446718 ) ) ;
#69577=CARTESIAN_POINT ( 'NONE',  ( -8.097244055859620815, 10.46987070330147063, -1.599625672291263179 ) ) ;
#69583=DIRECTION ( 'NONE',  ( 1.000000000000000000, -5.578564026256490882E-16, -5.570868214615546318E-48 ) ) ;
#69587=CARTESIAN_POINT ( 'NONE',  ( 2.205172540517054802, 5.724451730578533848, 1.040834085586084257E-14 ) ) ;
#69591=CARTESIAN_POINT ( 'NONE',  ( 5.118366684358879759, 5.930181538962194132, 1.199719254218462483 ) ) ;
#69596=CARTESIAN_POINT ( 'NONE',  ( -1.500000000000011324, 3.702083334016152971, 0.8660254037844403729 ) ) ;
#69602=CIRCLE ( 'NONE', #211549, 0.07999999999999998779 ) ;
#69603=CARTESIAN_POINT ( 'NONE',  ( 1.499999999999989120, 1.775000000000019673, 0.000000000000000000 ) ) ;
#69604=CARTESIAN_POINT ( 'NONE',  ( 4.964256800898067645, 8.943383367689749619, 0.7998128361456462443 ) ) ;
#69605=CARTESIAN_POINT ( 'NONE',  ( 4.107757354816228279, 6.775838766385488654, -1.082531754730548412 ) ) ;
#69609=CARTESIAN_POINT ( 'NONE',  ( 8.026063749610047537, 10.38682701267698150, -1.443375672974057666 ) ) ;
#69610=CARTESIAN_POINT ( 'NONE',  ( 2.359223927328457648E-13, 7.078193277237625480, 2.121339347286388843 ) ) ;
#69615=CARTESIAN_POINT ( 'NONE',  ( -5.766295404513795297, 5.621766148221195358, 0.7998128361456341429 ) ) ;
#69616=CARTESIAN_POINT ( 'NONE',  ( 1.499999999999990896, 3.556250000682818602, 1.214306433183764966E-14 ) ) ;
#69617=CARTESIAN_POINT ( 'NONE',  ( -1.364683531249997417, 5.571875000341417916, 1.214306433183764966E-14 ) ) ;
#69622=CARTESIAN_POINT ( 'NONE',  ( -0.6823417656250212460, 4.113541667008085767, 1.181850606188767472 ) ) ;
#69626=DIRECTION ( 'NONE',  ( 1.000000000000000000, -4.985516615831701596E-16, 0.000000000000000000 ) ) ;
#69631=CARTESIAN_POINT ( 'NONE',  ( -6.679363233026820446, 10.94434087183997129, 0.000000000000000000 ) ) ;
#69632=( BOUNDED_CURVE ( )  B_SPLINE_CURVE ( 2, ( #46116, #112233, #79657, #63413, #195551, #92735, #10377 ),
 .UNSPECIFIED., .F., .T. ) 
 B_SPLINE_CURVE_WITH_KNOTS ( ( 3, 2, 2, 3 ),
 ( 0.01785714285714263064, 0.02380952380952366942, 0.02976190476190470821, 0.03571428571428574700 ),
 .UNSPECIFIED. ) 
 CURVE ( )  GEOMETRIC_REPRESENTATION_ITEM ( )  RATIONAL_B_SPLINE_CURVE ( ( 1.000000000000005107, 0.8660254037844337116, 1.000000000000000000, 0.8660254037844387076, 1.000000000000000000, 0.8660254037844379305, 1.000000000000000666 ) ) 
 REPRESENTATION_ITEM ( '' )  );
#69633=CARTESIAN_POINT ( 'NONE',  ( 5.120175567455225618, 9.125288595339771547, -0.7998128361456281477 ) ) ;
#69635=CARTESIAN_POINT ( 'NONE',  ( -1.364683531250000748, -1.240624999658580752, 0.000000000000000000 ) ) ;
#69639=CARTESIAN_POINT ( 'NONE',  ( -6.520158902582610772, 5.290451655907115303, -2.438235897557448961 ) ) ;
#69641=CARTESIAN_POINT ( 'NONE',  ( -7.152089726408780379, 8.302858421353754181, -1.199719254218446718 ) ) ;
#69644=CARTESIAN_POINT ( 'NONE',  ( 9.459838494033030898, 12.05956421450382088, 1.599625672291281386 ) ) ;
#69646=CARTESIAN_POINT ( 'NONE',  ( 7.865701674222579598, 12.32840238656838139, -0.7998128361456352531 ) ) ;
#69650=CARTESIAN_POINT ( 'NONE',  ( -5.088387723830502196, 4.830873854090670605, -0.7998128361456221525 ) ) ;
#69651=CARTESIAN_POINT ( 'NONE',  ( -7.588813295347149435, 9.876701482703580837, -1.599625672291263179 ) ) ;
#69654=CARTESIAN_POINT ( 'NONE',  ( -4.096253560606756494, 7.689279582349398012, -0.7399548657811344521 ) ) ;
#69659=CARTESIAN_POINT ( 'NONE',  ( 7.782016984564054773, 10.10210578678999482, 1.443375672974076540 ) ) ;
#69662=CARTESIAN_POINT ( 'NONE',  ( 5.982172092127724383, 8.002286745614243912, -1.599625672291262513 ) ) ;
#69670=EDGE_CURVE ( 'NONE', #76077, #64117, #53077, .T. ) ;
#69686=CARTESIAN_POINT ( 'NONE',  ( -8.402302512167102222, 10.82577223566020841, -1.599625672291263179 ) ) ;
#69691=CARTESIAN_POINT ( 'NONE',  ( 0.7499999999999902300, 1.764583334016148086, 1.299038105676657340 ) ) ;
#69692=CARTESIAN_POINT ( 'NONE',  ( 9.999301985278609806, 11.62460605670194447, 1.199719254218452047 ) ) ;
#69698=CARTESIAN_POINT ( 'NONE',  ( 1.419999999999990603, 6.280000000000042881, 2.900000000000001688 ) ) ;
#69700=CARTESIAN_POINT ( 'NONE',  ( -1.201851678989727383E-14, 1.571875000341420581, 1.575800808251672791 ) ) ;
#69705=CARTESIAN_POINT ( 'NONE',  ( -4.613852347352193739, 4.277249248199312071, 1.214306433183764966E-14 ) ) ;
#69707=CARTESIAN_POINT ( 'NONE',  ( 3.967483781714987057, 7.780481511976146791, -0.4145792352998460273 ) ) ;
#69710=CARTESIAN_POINT ( 'NONE',  ( 1.364683531249986537, -0.3239583329919163424, 0.7879004041258500513 ) ) ;
#69716=CARTESIAN_POINT ( 'NONE',  ( -1.364683531250012516, 1.030208333674754062, 0.7879004041258379498 ) ) ;
#69718=CARTESIAN_POINT ( 'NONE',  ( -5.038826645773246682, 9.030381520044109322, 0.7998128361456481317 ) ) ;
#69719=CARTESIAN_POINT ( 'NONE',  ( 7.832860060393120882, 10.16142270859057462, 1.599625672291281386 ) ) ;
#69720=CARTESIAN_POINT ( 'NONE',  ( 3.032219910950674890, 6.689340329417765574, 0.7998128361456321445 ) ) ;
#69721=CARTESIAN_POINT ( 'NONE',  ( 6.166260936116925606, 6.088392601758203071, 0.7998128361456341429 ) ) ;
#69723=CARTESIAN_POINT ( 'NONE',  ( -1.201851678989727383E-14, 3.837500000000021227, -1.732050807568863648 ) ) ;
#69725=CARTESIAN_POINT ( 'NONE',  ( -1.364683531250014514, 2.051041667008086655, -0.7879004041258289570 ) ) ;
#69731=CARTESIAN_POINT ( 'NONE',  ( 6.670248388243460447, 6.884303995813253252, -0.7216878364870257245 ) ) ;
#69734=CARTESIAN_POINT ( 'NONE',  ( -9.840520565420403543, 10.37502883594562597, 1.040834085586084257E-14 ) ) ;
#69735=CARTESIAN_POINT ( 'NONE',  ( -5.091250377131585125, 5.898545847196970726, 1.199719254218450271 ) ) ;
#69736=CARTESIAN_POINT ( 'NONE',  ( -0.9486429539237359876, 3.105410930033766448, 1.028101543438980858 ) ) ;
#69739=CARTESIAN_POINT ( 'NONE',  ( -7.849807752188049825, 8.260456587081938196, 0.7216878364870578100 ) ) ;
#69741=CARTESIAN_POINT ( 'NONE',  ( 0.7499999999999902300, 5.566666666666685082, -1.299038105676658228 ) ) ;
#69744=CARTESIAN_POINT ( 'NONE',  ( 8.188761592974039161, 10.57664116326830595, -1.443375672974063439 ) ) ;
#69752=ORIENTED_EDGE ( 'NONE', *, *, #213928, .F. ) ;
#69754=CARTESIAN_POINT ( 'NONE',  ( 9.042925270190622200, 12.53353466765568669, 1.082531754730546636 ) ) ;
#69759=CARTESIAN_POINT ( 'NONE',  ( 7.687109908824030668, 10.95175007939464606, -1.082531754730543083 ) ) ;
#69760=CARTESIAN_POINT ( 'NONE',  ( 7.450369105909416589, 8.650851030771185890, -1.199719254218441611 ) ) ;
#69761=CARTESIAN_POINT ( 'NONE',  ( -5.066996723205291708, 6.934582148538044777, 1.599625672291267398 ) ) ;
#69764=CARTESIAN_POINT ( 'NONE',  ( 6.927853306458752414, 7.184843067064434763, 0.7216878364870317197 ) ) ;
#69765=CARTESIAN_POINT ( 'NONE',  ( 0.6823417656249864960, -1.011458332991911568, -1.181850606188749264 ) ) ;
#69766=CARTESIAN_POINT ( 'NONE',  ( 4.256897045010922476, 5.029096643009940415, -1.082531754730548412 ) ) ;
#69768=CARTESIAN_POINT ( 'NONE',  ( -2.948008335967658322, 5.526761261015804116, 1.199719254218462483 ) ) ;
#69775=ORIENTED_EDGE ( 'NONE', *, *, #5833, .T. ) ;
#69783=CARTESIAN_POINT ( 'NONE',  ( 7.969495366734495434, 8.192166104145387706, 1.040834085586084257E-14 ) ) ;
#69794=CARTESIAN_POINT ( 'NONE',  ( -5.087333953625788219, 6.958308917361963886, 1.599625672291267398 ) ) ;
#69796=CARTESIAN_POINT ( 'NONE',  ( -2.903417451620861289, 6.539070793532962611, 0.7998128361456341429 ) ) ;
#69799=CYLINDRICAL_SURFACE ( 'NONE', #90024, 1.500000000000000222 ) ;
#69803=ADVANCED_FACE ( 'NONE', ( #79140 ), #185843, .T. ) ;
#69806=CARTESIAN_POINT ( 'NONE',  ( -3.952365473583647315, 4.569846793057691592, 1.199719254218462483 ) ) ;
#69809=CARTESIAN_POINT ( 'NONE',  ( 5.425234023762710578, 9.481190127698507553, -0.7998128361456291469 ) ) ;
#69810=CARTESIAN_POINT ( 'NONE',  ( 1.364683531249990311, 4.613541667008083103, 0.7879004041258499402 ) ) ;
#69816=CARTESIAN_POINT ( 'NONE',  ( 6.765155463094761679, 6.995028916473103209, 0.7216878364870317197 ) ) ;
#69817=CARTESIAN_POINT ( 'NONE',  ( -5.845536785786364931, 9.971543350059432598, 0.000000000000000000 ) ) ;
#69820=CARTESIAN_POINT ( 'NONE',  ( -6.672584156219988571, 10.93643194889866521, -0.7998128361456291469 ) ) ;
#69821=CARTESIAN_POINT ( 'NONE',  ( -6.084912014434944894, 5.993485526462540847, -0.7998128361456291469 ) ) ;
#69828=CARTESIAN_POINT ( 'NONE',  ( 7.613066949273408213, 8.840665181362512115, -1.199719254218441611 ) ) ;
#69842=CARTESIAN_POINT ( 'NONE',  ( -0.7499999999999972244, 5.358333333333353821, -1.299038105676652011 ) ) ;
#69843=CARTESIAN_POINT ( 'NONE',  ( 3.171717870593107058, 5.787755718078879674, -1.199719254218446718 ) ) ;
#69844=CARTESIAN_POINT ( 'NONE',  ( 5.982172092127724383, 8.002286745614243912, -1.599625672291262513 ) ) ;
#69846=CARTESIAN_POINT ( 'NONE',  ( -7.321039761699444703, 10.52466824108257804, 1.082531754730549967 ) ) ;
#69847=DIRECTION ( 'NONE',  ( 0.6507913734559640506, -0.7592566023653004592, 0.000000000000000000 ) ) ;
#69848=CARTESIAN_POINT ( 'NONE',  ( 5.883875478650832491, 6.927238148923188454, -1.082531754730543083 ) ) ;
#69850=CARTESIAN_POINT ( 'NONE',  ( -6.995644074527074707, 11.10540915368285475, 0.000000000000000000 ) ) ;
#69853=CARTESIAN_POINT ( 'NONE',  ( 8.925345196497941558, 9.307324238869423283, 1.040834085586084257E-14 ) ) ;
#69859=CARTESIAN_POINT ( 'NONE',  ( 0.6823417656249882723, 2.926041667008084879, -1.181850606188754593 ) ) ;
#69865=EDGE_CURVE ( 'NONE', #145094, #159043, #76095, .T. ) ;
#69866=CARTESIAN_POINT ( 'NONE',  ( 7.425061681778431399, 11.81432239538354345, 0.7998128361456462443 ) ) ;
#69869=CARTESIAN_POINT ( 'NONE',  ( -9.691380875670077444, 10.20103253123691189, 0.7998128361456462443 ) ) ;
#69875=CARTESIAN_POINT ( 'NONE',  ( 8.367353357928214663, 12.91366268422496688, 1.040834085586084257E-14 ) ) ;
#69878=CARTESIAN_POINT ( 'NONE',  ( -8.292783513053063160, 12.82666453187061073, 0.7998128361456481317 ) ) ;
#69883=CARTESIAN_POINT ( 'NONE',  ( 5.844719547729445353, 6.005894922780862899, -0.3676955087418033452 ) ) ;
#69884=CARTESIAN_POINT ( 'NONE',  ( -3.195971524519394702, 4.751719416737803847, -1.599625672291262513 ) ) ;
#69888=CARTESIAN_POINT ( 'NONE',  ( 6.425674737872927089, 9.584038729905381970, -1.199719254218440723 ) ) ;
#69890=CARTESIAN_POINT ( 'NONE',  ( 6.287230548435207567, 8.358188277972981695, -1.599625672291262513 ) ) ;
#69892=CARTESIAN_POINT ( 'NONE',  ( 5.359550796103802028, 5.147230771742885125, -0.7998128361456231517 ) ) ;
#69894=CARTESIAN_POINT ( 'NONE',  ( -7.619319141200077361, 9.912291636198670375, 1.443375672974090751 ) ) ;
#69895=AXIS2_PLACEMENT_3D ( 'NONE', #59516, #175423, #27008 ) ;
#69904=CARTESIAN_POINT ( 'NONE',  ( -4.409912583257236562, 7.141888050452717351, -1.077592642408040424 ) ) ;
#69907=CARTESIAN_POINT ( 'NONE',  ( 5.124618876285529367, 7.962177208099690873, -1.082531754730549078 ) ) ;
#69911=CARTESIAN_POINT ( 'NONE',  ( -8.459924664802993988, 12.81373650900478189, 1.040834085586084257E-14 ) ) ;
#69924=CARTESIAN_POINT ( 'NONE',  ( -10.11401940567025548, 10.90203684947788076, 1.040834085586084257E-14 ) ) ;
#69929=CARTESIAN_POINT ( 'NONE',  ( 8.015895134177609904, 10.37496362800581018, 1.599625672291281386 ) ) ;
#69931=VERTEX_POINT ( 'NONE', #1195 ) ;
#69933=CARTESIAN_POINT ( 'NONE',  ( 1.499999999999989120, 2.035416667349480679, 0.8660254037844524744 ) ) ;
#69935=CARTESIAN_POINT ( 'NONE',  ( -6.728924311084075960, 6.744833205886536120, 1.040834085586084257E-14 ) ) ;
#69939=CARTESIAN_POINT ( 'NONE',  ( -7.323375529675950624, 11.69568855126397011, -0.7998128361456291469 ) ) ;
#69942=CARTESIAN_POINT ( 'NONE',  ( 6.262976894508937242, 9.394224579314053969, -1.199719254218440723 ) ) ;
#69944=CARTESIAN_POINT ( 'NONE',  ( -6.470265622219711688, 8.571729197388226140, -1.599625672291263179 ) ) ;
#69946=CARTESIAN_POINT ( 'NONE',  ( 9.097684769969825780, 10.57271930550834860, -1.199719254218446718 ) ) ;
#69947=CARTESIAN_POINT ( 'NONE',  ( 1.364683531249988535, 5.655208333674751842, -0.7879004041258300672 ) ) ;
#69948=CARTESIAN_POINT ( 'NONE',  ( -6.056815632531343141, 6.015240258500212711, 0.3115616189311651296 ) ) ;
#69953=CARTESIAN_POINT ( 'NONE',  ( -6.534666852106790103, 10.56760239419251590, 0.7216878364870458196 ) ) ;
#69956=CARTESIAN_POINT ( 'NONE',  ( -1.364683531250010295, 3.842708333674751398, 0.7879004041258379498 ) ) ;
#69965=CARTESIAN_POINT ( 'NONE',  ( -3.836594282542926226, 5.499112634431936542, 1.443375672974064550 ) ) ;
#69967=CARTESIAN_POINT ( 'NONE',  ( 8.387690588348714726, 12.93738945304888333, 1.040834085586084257E-14 ) ) ;
#69968=CARTESIAN_POINT ( 'NONE',  ( -1.364683531250010295, 5.301041667008085767, -0.7879004041258300672 ) ) ;
#69969=CARTESIAN_POINT ( 'NONE',  ( -10.50487009249003378, 11.15010328419353947, 0.7998128361456462443 ) ) ;
#69972=CARTESIAN_POINT ( 'NONE',  ( 1.364683531249986537, 0.9052083336747533959, -0.7879004041258239610 ) ) ;
#69973=CARTESIAN_POINT ( 'NONE',  ( -2.643476764984671767, 6.027880625883323518, 1.040834085586084257E-14 ) ) ;
#69974=CARTESIAN_POINT ( 'NONE',  ( 4.871457266011829823, 4.577788319968905562, -0.7998128361456221525 ) ) ;
#69979=CARTESIAN_POINT ( 'NONE',  ( -5.946383829929366094, 4.757679660040812664, -2.499999999999995559 ) ) ;
#69980=CARTESIAN_POINT ( 'NONE',  ( 1.419999999999820739, 7.240846818246208905, -4.154462424328212222 ) ) ;
#69983=CARTESIAN_POINT ( 'NONE',  ( -9.341204650135658483, 10.00041963468749984, 1.040834085586084257E-14 ) ) ;
#69988=CARTESIAN_POINT ( 'NONE',  ( -8.941766003412679353, 10.39081407785832845, -1.199719254218446718 ) ) ;
#69989=CARTESIAN_POINT ( 'NONE',  ( -5.436456408955534947, 6.405249234278626247, 1.082531754730546636 ) ) ;
#69990=CARTESIAN_POINT ( 'NONE',  ( -1.364683531250000748, 1.821875000341421913, 0.000000000000000000 ) ) ;
#69998=VERTEX_POINT ( 'NONE', #202595 ) ;
#70007=CARTESIAN_POINT ( 'NONE',  ( 5.692136587293062711, 5.855332880448197663, -2.499999999999994671 ) ) ;
#70012=CARTESIAN_POINT ( 'NONE',  ( 1.364683531249988535, 2.967708333674755394, -0.7879004041258239610 ) ) ;
#70016=DIRECTION ( 'NONE',  ( -0.6507913734559640506, -0.7592566023653004592, 0.000000000000000000 ) ) ;
#70019=CARTESIAN_POINT ( 'NONE',  ( 9.908311333488716954, 10.45411806535867782, 0.7998128361456462443 ) ) ;
#70022=CARTESIAN_POINT ( 'NONE',  ( 0.6823417656249899377, 1.342708333674752508, 1.181850606188755259 ) ) ;
#70033=CARTESIAN_POINT ( 'NONE',  ( 6.356075086708249167, 6.309842444114747373, -0.7998128361456281477 ) ) ;
#70038=CARTESIAN_POINT ( 'NONE',  ( 3.850147086611925396, 5.981400113484194314, 1.344841084984424562 ) ) ;
#70042=( BOUNDED_SURFACE ( )  B_SPLINE_SURFACE ( 3, 2, ( 
 ( #162265, #214153, #196883 ),
 ( #65779, #113578, #46385 ),
 ( #63686, #181683, #197939 ),
 ( #116759, #166522, #99395 ) ),
 .UNSPECIFIED., .F., .F., .T. ) 
 B_SPLINE_SURFACE_WITH_KNOTS ( ( 4, 4 ),
 ( 3, 3 ),
 ( -6.071532165918824830E-18, 0.002003486994853880768 ),
 ( 0.000000000000000000, 1.000000000000000000 ),
 .UNSPECIFIED. ) 
 GEOMETRIC_REPRESENTATION_ITEM ( )  RATIONAL_B_SPLINE_SURFACE ( (
 ( 1.000000000000000000, 0.7779734834199515392, 1.000000000000000000),
 ( 1.000000000000000000, 0.7856061901475719367, 1.000000000000000000),
 ( 1.000000000000000000, 0.7951961705782245593, 1.000000000000000000),
 ( 1.000000000000000000, 0.8104931255419017821, 1.000000000000000000) ) ) 
 REPRESENTATION_ITEM ( '' )  SURFACE ( )  );
#70043=ORIENTED_EDGE ( 'NONE', *, *, #166950, .T. ) ;
#70045=CARTESIAN_POINT ( 'NONE',  ( -4.620631424159025613, 4.285158171140619032, -0.7998128361456221525 ) ) ;
#70047=CARTESIAN_POINT ( 'NONE',  ( 8.015895134177609904, 10.37496362800581018, 1.599625672291281386 ) ) ;
#70060=CARTESIAN_POINT ( 'NONE',  ( -6.371969008742801144, 10.37778824360119145, 0.7216878364870458196 ) ) ;
#70062=CARTESIAN_POINT ( 'NONE',  ( 5.880485940025228508, 7.883652901494672349, 1.599625672291267398 ) ) ;
#70065=CARTESIAN_POINT ( 'NONE',  ( -9.297140650669053485, 11.86975006391249643, 1.599625672291281386 ) ) ;
#70070=CARTESIAN_POINT ( 'NONE',  ( -2.761056838677368397, 6.372983411765559048, 0.7998128361456341429 ) ) ;
#70072=CARTESIAN_POINT ( 'NONE',  ( 8.211434591371064684, 12.73175745657494851, -0.7998128361456352531 ) ) ;
#70073=EDGE_CURVE ( 'NONE', #24729, #70347, #96843, .T. ) ;
#70074=CARTESIAN_POINT ( 'NONE',  ( 4.878236342818665250, 4.585697242910212523, 1.040834085586084257E-14 ) ) ;
#70080=CARTESIAN_POINT ( 'NONE',  ( 5.178851490740207453, 5.144340948726102702, 0.7216878364870317197 ) ) ;
#70083=CARTESIAN_POINT ( 'NONE',  ( -3.405069135326500351, 7.124331091189553433, 1.040834085586084257E-14 ) ) ;
#70085=CARTESIAN_POINT ( 'NONE',  ( -8.676328237741483207, 12.20980114641871062, -1.199719254218446718 ) ) ;
#70090=CARTESIAN_POINT ( 'NONE',  ( 7.293923454472069245, 11.45340176361870199, 0.7216878364870438212 ) ) ;
#70091=CARTESIAN_POINT ( 'NONE',  ( -0.6823417656249969321, 5.030208333674755394, -1.181850606188749264 ) ) ;
#70093=CARTESIAN_POINT ( 'NONE',  ( 4.172158584703322681, 5.890604320285754980, -1.599625672291256295 ) ) ;
#70107=CARTESIAN_POINT ( 'NONE',  ( -1.364683531250012516, 2.342708333674752286, 0.7879004041258379498 ) ) ;
#70109=CARTESIAN_POINT ( 'NONE',  ( 9.836604141914616406, 11.43479190611061647, 1.199719254218452047 ) ) ;
#70111=CARTESIAN_POINT ( 'NONE',  ( -3.931501358282937009, 7.530575984731317618, 0.7216878364870317197 ) ) ;
#70114=CARTESIAN_POINT ( 'NONE',  ( -4.229780737339226881, 7.878568593630327577, 1.040834085586084257E-14 ) ) ;
#70120=CARTESIAN_POINT ( 'NONE',  ( 4.150767584078112193, 7.994312614733129152, 0.7998128361456321445 ) ) ;
#70130=EDGE_CURVE ( 'NONE', #62722, #205506, #202670, .T. ) ;
#70131=CARTESIAN_POINT ( 'NONE',  ( 7.156006149914539982, 7.243095351188763686, 1.040834085586084257E-14 ) ) ;
#70134=CARTESIAN_POINT ( 'NONE',  ( -4.288456660624211381, 3.897620947016656956, 1.214306433183764966E-14 ) ) ;
#70136=CARTESIAN_POINT ( 'NONE',  ( -5.052384799386910430, 9.046199365926717917, 1.214306433183764966E-14 ) ) ;
#70140=CARTESIAN_POINT ( 'NONE',  ( 7.396136491454752715, 8.587579647240744407, 1.199719254218462483 ) ) ;
#70143=CARTESIAN_POINT ( 'NONE',  ( -5.377780486114890124, 9.425827667109372143, 0.000000000000000000 ) ) ;
#70144=CARTESIAN_POINT ( 'NONE',  ( 7.578644679914718019, 7.944099669429731669, 0.7216878364870317197 ) ) ;
#70145=CARTESIAN_POINT ( 'NONE',  ( 5.497327176576959573, 6.424397595302826502, 1.252573174869066941 ) ) ;
#70146=CIRCLE ( 'NONE', #66734, 0.07999999999999969635 ) ;
#70147=CARTESIAN_POINT ( 'NONE',  ( -4.192495815123836955, 5.914331089109674089, -1.599625672291256295 ) ) ;
#70150=CARTESIAN_POINT ( 'NONE',  ( -4.577849422908604637, 8.492574760035358494, -0.7998128361456281477 ) ) ;
#70153=CARTESIAN_POINT ( 'NONE',  ( -1.402160292154681736E-14, 1.946875000341422579, -1.575800808251660134 ) ) ;
#70155=CARTESIAN_POINT ( 'NONE',  ( -4.107757355260591936, 7.736207981205250661, 1.040834085586084257E-14 ) ) ;
#70162=CARTESIAN_POINT ( 'NONE',  ( 6.226218857173709154, 8.287007971501239467, 1.599625672291281386 ) ) ;
#70165=CARTESIAN_POINT ( 'NONE',  ( -1.201851678989727383E-14, 2.884375000341418804, 1.575800808251672791 ) ) ;
#70167=CARTESIAN_POINT ( 'NONE',  ( -0.9999999999999965583, 6.400000000000024336, 1.226552901175238481E-14 ) ) ;
#70171=CARTESIAN_POINT ( 'NONE',  ( -2.785310492603665367, 5.336947110424484109, 1.199719254218462483 ) ) ;
#70172=CARTESIAN_POINT ( 'NONE',  ( -7.673551755210395342, 8.054824590608001600, 1.040834085586084257E-14 ) ) ;
#70174=CARTESIAN_POINT ( 'NONE',  ( -1.201851678989727383E-14, 1.071875000341418138, 1.575800808251672791 ) ) ;
#70181=CARTESIAN_POINT ( 'NONE',  ( -7.822691444960716112, 8.228820895316715678, -0.7216878364870267237 ) ) ;
#70185=CARTESIAN_POINT ( 'NONE',  ( -5.544921637864820951, 9.412899644243539754, -0.7216878364870207285 ) ) ;
#70191=CARTESIAN_POINT ( 'NONE',  ( 0.7499999999999902300, 5.347916667349482012, -1.299038105676658228 ) ) ;
#70199=CARTESIAN_POINT ( 'NONE',  ( -6.742482464697739708, 6.760651051769146491, 0.7998128361456341429 ) ) ;
#70202=CARTESIAN_POINT ( 'NONE',  ( 5.359550796103802028, 5.147230771742885125, -0.7998128361456231517 ) ) ;
#70206=CARTESIAN_POINT ( 'NONE',  ( 6.470265622219697477, 8.571729197388226140, -1.599625672291262513 ) ) ;
#70212=CARTESIAN_POINT ( 'NONE',  ( -4.107757355260591936, 7.736207981205250661, 1.040834085586084257E-14 ) ) ;
#70222=CARTESIAN_POINT ( 'NONE',  ( 1.364683531249988535, 1.613541667008084879, 0.7879004041258500513 ) ) ;
#70224=CARTESIAN_POINT ( 'NONE',  ( -7.178152263431422320, 10.46192917639026554, 1.199719254218453823 ) ) ;
#70226=CARTESIAN_POINT ( 'NONE',  ( 5.282873410819217241, 9.315102745931094219, -0.7998128361456281477 ) ) ;
#70228=CARTESIAN_POINT ( 'NONE',  ( -7.901704598666176693, 8.113076874732334076, 0.7998128361456602331 ) ) ;
#70230=CARTESIAN_POINT ( 'NONE',  ( -1.402160292154681736E-14, -1.006249999317181620, 1.732050807568877637 ) ) ;
#70232=CARTESIAN_POINT ( 'NONE',  ( 8.188761592974039161, 10.57664116326830595, -1.443375672974063439 ) ) ;
#70235=CARTESIAN_POINT ( 'NONE',  ( -1.402160292154681736E-14, -0.2406249996585799189, -1.575800808251665908 ) ) ;
#70237=CARTESIAN_POINT ( 'NONE',  ( 8.229436053370676518, 9.663725486096376827, 1.082531754730558626 ) ) ;
#70240=CARTESIAN_POINT ( 'NONE',  ( -5.504247177468192476, 7.444707678511436555, 1.443375672974064550 ) ) ;
#70242=CARTESIAN_POINT ( 'NONE',  ( -1.364683531249997417, 3.259375000341423245, 1.214306433183764966E-14 ) ) ;
#70246=CARTESIAN_POINT ( 'NONE',  ( -4.557512192488103686, 8.468847991211438497, -0.7998128361456281477 ) ) ;
#70255=CARTESIAN_POINT ( 'NONE',  ( 6.598014311344812199, 10.84943379654430906, 1.040834085586084257E-14 ) ) ;
#70258=CARTESIAN_POINT ( 'NONE',  ( 1.499999999999989120, 2.775000000000020339, 1.214306433183764966E-14 ) ) ;
#70264=CARTESIAN_POINT ( 'NONE',  ( 5.002595493762530765, 8.780185809457538681, 1.040834085586084257E-14 ) ) ;
#70265=CARTESIAN_POINT ( 'NONE',  ( -1.402160292154681736E-14, -0.1156249996585793222, 1.575800808251672791 ) ) ;
#70272=CARTESIAN_POINT ( 'NONE',  ( -1.500000000000001332, -0.09999999999997510880, 0.000000000000000000 ) ) ;
#70273=CARTESIAN_POINT ( 'NONE',  ( 8.613507663383630941, 8.943513783569379427, -0.7998128361456221525 ) ) ;
#70274=CARTESIAN_POINT ( 'NONE',  ( -8.208571938070008400, 11.66408546346865016, -1.199719254218446718 ) ) ;
#70276=CARTESIAN_POINT ( 'NONE',  ( 1.364683531249986537, 0.4052083336747511200, -0.7879004041258309554 ) ) ;
#70277=CARTESIAN_POINT ( 'NONE',  ( 1.499999999999987121, 1.295833333333353377, -0.8660254037844253849 ) ) ;
#70279=CARTESIAN_POINT ( 'NONE',  ( 6.471319392424407901, 6.444294134116939077, 0.7998128361456341429 ) ) ;
#70287=CARTESIAN_POINT ( 'NONE',  ( 1.364683531249990311, 5.363541667008086655, 0.7879004041258500513 ) ) ;
#70289=CARTESIAN_POINT ( 'NONE',  ( -8.857554428429624593, 9.228235009456373206, 0.7998128361456462443 ) ) ;
#70290=CARTESIAN_POINT ( 'NONE',  ( -5.097502569058215194, 6.970172302033127210, -1.443375672974053447 ) ) ;
#70292=FACE_OUTER_BOUND ( 'NONE', #93832, .T. ) ;
#70295=CARTESIAN_POINT ( 'NONE',  ( 4.064230490221667935, 7.507048082629879104, -0.5272979928686331030 ) ) ;
#70298=CARTESIAN_POINT ( 'NONE',  ( 8.749089199520284410, 9.101692242395490240, 0.7998128361456481317 ) ) ;
#70302=CARTESIAN_POINT ( 'NONE',  ( 7.090551149822739596, 8.335026431957096804, 1.082531754730558626 ) ) ;
#70306=CARTESIAN_POINT ( 'NONE',  ( -7.995557903757128493, 10.35123685918189729, 1.599625672291295375 ) ) ;
#70307=CARTESIAN_POINT ( 'NONE',  ( 4.143988507271280319, 7.986403691791820414, -0.7998128361456221525 ) ) ;
#70310=CARTESIAN_POINT ( 'NONE',  ( 8.595506201383999567, 12.97191496834930113, 0.7216878364870438212 ) ) ;
#70316=CARTESIAN_POINT ( 'NONE',  ( 2.275435306267621804, 5.643409308550367598, 0.5316758947214432762 ) ) ;
#70318=CARTESIAN_POINT ( 'NONE',  ( -4.500943810056945438, 5.313817868896925312, 1.082531754730560403 ) ) ;
#70319=CARTESIAN_POINT ( 'NONE',  ( 9.246297574839974942, 11.81043314211192019, 1.443375672974076540 ) ) ;
#70322=CARTESIAN_POINT ( 'NONE',  ( -5.506582945444718824, 9.576097202994168001, 0.7998128361456481317 ) ) ;
#70323=CARTESIAN_POINT ( 'NONE',  ( -3.253593677155282471, 6.739683690082376444, 1.040834085586084257E-14 ) ) ;
#70326=FACE_OUTER_BOUND ( 'NONE', #127608, .T. ) ;
#70328=CARTESIAN_POINT ( 'NONE',  ( -8.369460898337653276, 8.658792557682392754, 0.7998128361456462443 ) ) ;
#70330=CARTESIAN_POINT ( 'NONE',  ( 7.334597915313080918, 9.580116872663850813, 1.040834085586084257E-14 ) ) ;
#70332=ORIENTED_EDGE ( 'NONE', *, *, #158186, .F. ) ;
#70343=CARTESIAN_POINT ( 'NONE',  ( -6.775324078527193983, 8.927630729746953264, -1.599625672291263179 ) ) ;
#70346=CARTESIAN_POINT ( 'NONE',  ( 5.666945020832177882, 6.674152614801420746, 1.082531754730558626 ) ) ;
#70347=VERTEX_POINT ( 'NONE', #122540 ) ;
#70351=CARTESIAN_POINT ( 'NONE',  ( -2.788173145904702555, 6.404619103530779789, -0.7998128361456281477 ) ) ;
#70352=AXIS2_PLACEMENT_3D ( 'NONE', #34232, #632, #181547 ) ;
#70356=CARTESIAN_POINT ( 'NONE',  ( -0.7499999999999972244, 3.358333333333359150, -1.299038105676652011 ) ) ;
#70361=CARTESIAN_POINT ( 'NONE',  ( -9.179033691651859783, 10.66762638080401260, 1.199719254218462483 ) ) ;
#70362=CARTESIAN_POINT ( 'NONE',  ( 6.252281394196331554, 10.44607872653774372, 1.040834085586084257E-14 ) ) ;
#70365=CARTESIAN_POINT ( 'NONE',  ( -10.13488352141530768, 11.78278451552804817, 1.199719254218462483 ) ) ;
#70368=CARTESIAN_POINT ( 'NONE',  ( -1.364683531250014514, 0.3427083336747508424, 0.7879004041258379498 ) ) ;
#70372=CARTESIAN_POINT ( 'NONE',  ( 9.585251415181632595, 10.28514086057449184, 0.000000000000000000 ) ) ;
#70397=CARTESIAN_POINT ( 'NONE',  ( -0.7500000000000249800, -0.7770833326505161009, 1.299038105676659116 ) ) ;
#70401=CARTESIAN_POINT ( 'NONE',  ( 8.204655514564224816, 12.72384853363364066, 1.040834085586084257E-14 ) ) ;
#70404=CARTESIAN_POINT ( 'NONE',  ( -1.230728480726522411, 3.230010058876359835, 0.7750000000000100142 ) ) ;
#70405=CARTESIAN_POINT ( 'NONE',  ( 4.162516854595432747, 4.815023404238158555, 1.199719254218464037 ) ) ;
#70410=CARTESIAN_POINT ( 'NONE',  ( 5.311043488251262268, 7.219303374425030562, -1.599625672291256295 ) ) ;
#70411=CARTESIAN_POINT ( 'NONE',  ( 0.6823417656249899377, 2.405208333674753618, 1.181850606188767472 ) ) ;
#70412=CARTESIAN_POINT ( 'NONE',  ( -5.845765802024414981, 6.039811503853035113, 0.4322504083978280232 ) ) ;
#70415=CIRCLE ( 'NONE', #122497, 1.500000000000000222 ) ;
#70417=CARTESIAN_POINT ( 'NONE',  ( -8.355902744723985975, 8.642974711799791265, 1.040834085586084257E-14 ) ) ;
#70418=CARTESIAN_POINT ( 'NONE',  ( -5.572037945092175981, 5.603058478803387032, 0.7216878364870317197 ) ) ;
#70420=CARTESIAN_POINT ( 'NONE',  ( -6.718228810771495141, 7.796687353110217877, 1.199719254218450271 ) ) ;
#70422=CARTESIAN_POINT ( 'NONE',  ( -1.402160292154681736E-14, -0.1312499993171854229, -1.732050807568870754 ) ) ;
#70423=ADVANCED_FACE ( 'NONE', ( #171187 ), #21700, .T. ) ;
#70431=CARTESIAN_POINT ( 'NONE',  ( -3.592547517496935683, 6.174760622846296343, -1.082531754730548412 ) ) ;
#70433=LINE ( 'NONE', #170088, #74829 ) ;
#70436=CARTESIAN_POINT ( 'NONE',  ( -3.267151830768952880, 5.795132321663641228, -1.082531754730549078 ) ) ;
#70438=CARTESIAN_POINT ( 'NONE',  ( 9.610031953988080744, 10.10612545594124967, -0.7998128361456281477 ) ) ;
#70454=CARTESIAN_POINT ( 'NONE',  ( 5.412729640353754590, 7.337937218544611895, 1.599625672291267398 ) ) ;
#70459=CARTESIAN_POINT ( 'NONE',  ( 4.715538499454675403, 4.395883092318884522, 1.214306433183764966E-14 ) ) ;
#70469=CARTESIAN_POINT ( 'NONE',  ( 7.690499447449630210, 9.995335326823163058, 1.599625672291281386 ) ) ;
#70472=CARTESIAN_POINT ( 'NONE',  ( -3.899941742225307539, 7.701682465904834629, 0.7998128361456341429 ) ) ;
#70474=CARTESIAN_POINT ( 'NONE',  ( -4.568734577680888087, 6.353276312092901890, -1.443375672974051449 ) ) ;
#70478=CARTESIAN_POINT ( 'NONE',  ( -1.500000000000001332, -1.068749999317178290, 0.000000000000000000 ) ) ;
#70482=CARTESIAN_POINT ( 'NONE',  ( 5.027376032568989572, 4.759693547618927489, 0.7998128361456341429 ) ) ;
#70483=CARTESIAN_POINT ( 'NONE',  ( -4.843287188579803448, 6.673587691474970107, -1.599625672291256295 ) ) ;
#70489=CARTESIAN_POINT ( 'NONE',  ( 5.124618876285529367, 7.962177208099690873, -1.082531754730549078 ) ) ;
#70492=CARTESIAN_POINT ( 'NONE',  ( 8.283668667825342169, 9.726996869626816533, -1.082531754730543083 ) ) ;
#70493=CARTESIAN_POINT ( 'NONE',  ( -0.6823417656249969321, 3.780208333674754506, -1.181850606188749264 ) ) ;
#70495=CARTESIAN_POINT ( 'NONE',  ( 3.673896439178911066, 7.230036912443299713, 0.7216878364870317197 ) ) ;
#70502=CARTESIAN_POINT ( 'NONE',  ( -4.612682051294048513, 7.132468998681293471, 1.371008595254997964 ) ) ;
#70509=CARTESIAN_POINT ( 'NONE',  ( -8.642432853707342488, 12.17025653171218558, 1.199719254218462483 ) ) ;
#70514=CARTESIAN_POINT ( 'NONE',  ( -4.295235737431041478, 3.905529869957963029, -0.7998128361456221525 ) ) ;
#70519=CARTESIAN_POINT ( 'NONE',  ( 3.768803514918948938, 4.459654191235965293, -1.082531754730543083 ) ) ;
#70520=CARTESIAN_POINT ( 'NONE',  ( -1.364683531249997417, 3.071875000341423245, 1.214306433183764966E-14 ) ) ;
#70522=CARTESIAN_POINT ( 'NONE',  ( 6.775324078527185989, 8.927630729746953264, -1.599625672291262513 ) ) ;
#70523=CARTESIAN_POINT ( 'NONE',  ( -9.287498920561160887, 10.79416914786490089, -1.199719254218441611 ) ) ;
#70529=CARTESIAN_POINT ( 'NONE',  ( -1.499999999999997780, 4.900000000000022560, 1.214306433183764966E-14 ) ) ;
#70530=CARTESIAN_POINT ( 'NONE',  ( 4.364835388595708743, 7.179726155748598515, 1.199719254218462483 ) ) ;
#70533=CARTESIAN_POINT ( 'NONE',  ( 1.436838838544731267, 7.449283400311756509, 4.203727439823562229 ) ) ;
#70534=CARTESIAN_POINT ( 'NONE',  ( -1.364683531250010295, 4.030208333674751842, 0.7879004041258379498 ) ) ;
#70537=CARTESIAN_POINT ( 'NONE',  ( 8.242994207428692377, 12.56065097540143327, -0.7216878364870328300 ) ) ;
#70542=CARTESIAN_POINT ( 'NONE',  ( -1.500000000000013101, 3.410416667349487785, -0.8660254037844313801 ) ) ;
#70544=CARTESIAN_POINT ( 'NONE',  ( -5.413783410558481002, 5.210502155273325720, -0.7998128361456221525 ) ) ;
#70545=CARTESIAN_POINT ( 'NONE',  ( 3.009546912109283934, 6.454962464195385330, 0.000000000000000000 ) ) ;
#70554=CARTESIAN_POINT ( 'NONE',  ( 8.308449207076147758, 8.587612251210650527, -0.7998128361456281477 ) ) ;
#70555=CARTESIAN_POINT ( 'NONE',  ( 5.847644326195776010, 5.716673223516856694, -0.7998128361456281477 ) ) ;
#70559=CARTESIAN_POINT ( 'NONE',  ( 4.005544317833563461, 6.760553239859419250, -1.199719254218452047 ) ) ;
#70565=CARTESIAN_POINT ( 'NONE',  ( 7.879259827836241570, 12.34422023245099176, 1.040834085586084257E-14 ) ) ;
#70570=CARTESIAN_POINT ( 'NONE',  ( 5.048403365090235795, 6.545034038527520082, -1.227034678662905609 ) ) ;
#70571=EDGE_CURVE ( 'NONE', #92214, #69090, #3719, .T. ) ;
#70573=CARTESIAN_POINT ( 'NONE',  ( 10.24048609702354717, 10.84165528948263457, -0.7998128361456281477 ) ) ;
#70575=AXIS2_PLACEMENT_3D ( 'NONE', #126739, #12881, #46481 ) ;
#70577=CARTESIAN_POINT ( 'NONE',  ( -5.761852096127856981, 5.824508321678349532, 0.000000000000000000 ) ) ;
#70578=CARTESIAN_POINT ( 'NONE',  ( 0.7499999999999902300, 3.233333333333352044, 1.299038105676669330 ) ) ;
#70581=CARTESIAN_POINT ( 'NONE',  ( 5.666945020832170776, 7.634521829102760115, 1.443375672974062551 ) ) ;
#70582=CARTESIAN_POINT ( 'NONE',  ( -2.930533758848195447, 6.570706485298192234, -0.7998128361456281477 ) ) ;
#70589=CARTESIAN_POINT ( 'NONE',  ( -5.766295404513795297, 5.621766148221195358, 0.7998128361456341429 ) ) ;
#70595=B_SPLINE_CURVE_WITH_KNOTS ( 'NONE', 3,
 ( #86893, #54399, #51199, #167086, #183319, #200614 ),
 .UNSPECIFIED., .F., .F.,
 ( 4, 2, 4 ),
 ( 1.052505139324892547E-16, 0.002037829324722971718, 0.004075658649445837618 ),
 .UNSPECIFIED. ) ;
#70597=CARTESIAN_POINT ( 'NONE',  ( 1.284279953904121641, 3.284610286488902187, 0.7750000000000135669 ) ) ;
#70602=CARTESIAN_POINT ( 'NONE',  ( 9.447334110624092673, 9.916311305349925220, -0.7998128361456281477 ) ) ;
#70603=CARTESIAN_POINT ( 'NONE',  ( 6.108949960370312127, 6.019453914259918825, -0.1454340903971618193 ) ) ;
#70606=CARTESIAN_POINT ( 'NONE',  ( -4.161989969715274462, 4.726297878971393196, -2.500000000000000444 ) ) ;
#70608=DIRECTION ( 'NONE',  ( 0.6507913734559640506, -0.7592566023653004592, 0.000000000000000000 ) ) ;
#70609=CARTESIAN_POINT ( 'NONE',  ( -8.487040972474682476, 12.84537220128841817, 0.7216878364870338292 ) ) ;
#70613=CARTESIAN_POINT ( 'NONE',  ( 6.265839547809997079, 10.46189657242035587, 0.7998128361456462443 ) ) ;
#70615=ADVANCED_FACE ( 'NONE', ( #54247 ), #39061, .T. ) ;
#70618=CARTESIAN_POINT ( 'NONE',  ( -5.713871673155502151, 8.753601821068331290, 1.199719254218452047 ) ) ;
#70619=CARTESIAN_POINT ( 'NONE',  ( 5.281064527722868718, 6.119995689553514140, 1.199719254218462483 ) ) ;
#70621=( BOUNDED_CURVE ( )  B_SPLINE_CURVE ( 2, ( #135946, #200902, #18965, #85049, #88257, #2703, #102365 ),
 .UNSPECIFIED., .F., .T. ) 
 B_SPLINE_CURVE_WITH_KNOTS ( ( 3, 2, 2, 3 ),
 ( 0.2678571428571428492, 0.2738095238095239470, 0.2797619047619049337, 0.2857142857142859760 ),
 .UNSPECIFIED. ) 
 CURVE ( )  GEOMETRIC_REPRESENTATION_ITEM ( )  RATIONAL_B_SPLINE_CURVE ( ( 1.000000000000000000, 0.8660254037844387076, 1.000000000000000000, 0.8660254037844387076, 1.000000000000000000, 0.8660254037844324904, 1.000000000000006217 ) ) 
 REPRESENTATION_ITEM ( '' )  );
#70624=CARTESIAN_POINT ( 'NONE',  ( 9.836604141914616406, 11.43479190611061647, 1.199719254218452047 ) ) ;
#70629=CARTESIAN_POINT ( 'NONE',  ( 4.001130546182508851, 7.826233022050814725, 0.1222016466962717873 ) ) ;
#70631=CARTESIAN_POINT ( 'NONE',  ( 6.155038550924155416, 6.283225852274053835, 0.7216878364870317197 ) ) ;
#70638=ORIENTED_EDGE ( 'NONE', *, *, #73270, .F. ) ;
#70639=CARTESIAN_POINT ( 'NONE',  ( 8.473482818416664841, 10.90881592628469932, -1.443375672974063439 ) ) ;
#70643=CARTESIAN_POINT ( 'NONE',  ( -8.259941899223614215, 10.65968485389279508, -1.599625672291263179 ) ) ;
#70653=CARTESIAN_POINT ( 'NONE',  ( 4.539282502477016479, 4.190251095844947926, 0.7998128361456341429 ) ) ;
#70657=CARTESIAN_POINT ( 'NONE',  ( 4.253507506385319381, 5.985511395581417204, 1.599625672291267398 ) ) ;
#70660=CARTESIAN_POINT ( 'NONE',  ( 0.7499999999999902300, 2.264583334016148530, 1.299038105676669330 ) ) ;
#70666=CARTESIAN_POINT ( 'NONE',  ( -0.7500000000000006661, 1.608333333333357373, -1.299038105676652011 ) ) ;
#70667=CARTESIAN_POINT ( 'NONE',  ( 6.425674737872927089, 9.584038729905381970, -1.199719254218440723 ) ) ;
#70668=CARTESIAN_POINT ( 'NONE',  ( 3.836594282542902246, 7.419851063034623273, 0.7216878364870317197 ) ) ;
#70669=CARTESIAN_POINT ( 'NONE',  ( 5.355107487717867265, 5.349972945200037522, 1.040834085586084257E-14 ) ) ;
#70672=CARTESIAN_POINT ( 'NONE',  ( 10.38518247838791986, 11.21839376764850726, 0.7216878364870438212 ) ) ;
#70678=CARTESIAN_POINT ( 'NONE',  ( -4.554649539187067830, 7.401175998105142817, 1.199719254218464037 ) ) ;
#70679=CARTESIAN_POINT ( 'NONE',  ( 1.499999999999989120, 4.535416667349484676, 0.8660254037844524744 ) ) ;
#70680=CARTESIAN_POINT ( 'NONE',  ( 1.364683531249988535, 4.967708333674756283, -0.7879004041258300672 ) ) ;
#70685=CARTESIAN_POINT ( 'NONE',  ( -1.364683531250012516, 3.342708333674756727, 0.7879004041258379498 ) ) ;
#70692=CARTESIAN_POINT ( 'NONE',  ( -8.525379664894808585, 8.840697785332414682, -0.7998128361456291469 ) ) ;
#70693=CARTESIAN_POINT ( 'NONE',  ( 6.226218857173709154, 8.287007971501239467, 1.599625672291281386 ) ) ;
#70699=CARTESIAN_POINT ( 'NONE',  ( -4.907068755522976389, 4.827261090972641000, -0.03298405530800324614 ) ) ;
#70701=CARTESIAN_POINT ( 'NONE',  ( -8.355902744723985975, 8.642974711799791265, 1.040834085586084257E-14 ) ) ;
#70704=CARTESIAN_POINT ( 'NONE',  ( 8.866142388332804103, 12.43125098877526113, -1.199719254218446718 ) ) ;
#70706=CARTESIAN_POINT ( 'NONE',  ( 9.565441069641300587, 11.11843498845840905, -1.199719254218440723 ) ) ;
#70709=CARTESIAN_POINT ( 'NONE',  ( -5.766295404513795297, 5.621766148221195358, 0.7998128361456341429 ) ) ;
#70711=CARTESIAN_POINT ( 'NONE',  ( -6.997979842947967377, 11.31606025008131233, -0.7998128361456291469 ) ) ;
#70714=CARTESIAN_POINT ( 'NONE',  ( -4.172464037091858202, 7.595707080679858336, -0.9154354581521230161 ) ) ;
#70721=CARTESIAN_POINT ( 'NONE',  ( 6.331821432781979730, 7.345878745455822312, -1.199719254218445830 ) ) ;
#70742=CARTESIAN_POINT ( 'NONE',  ( 2.738383840280328663, 5.178236332760252303, 1.082531754730548412 ) ) ;
#70746=CARTESIAN_POINT ( 'NONE',  ( -8.483651433849100698, 10.92067931095586886, 1.599625672291269396 ) ) ;
#70752=CARTESIAN_POINT ( 'NONE',  ( -1.499999999999997780, 1.931250000682817269, 0.000000000000000000 ) ) ;
#70753=CARTESIAN_POINT ( 'NONE',  ( 10.22692794340986921, 10.82583744360002243, 0.000000000000000000 ) ) ;
#70757=CARTESIAN_POINT ( 'NONE',  ( -10.15522075183580419, 11.80651128435196462, 1.199719254218462483 ) ) ;
#70759=CARTESIAN_POINT ( 'NONE',  ( -1.402160292154681736E-14, 1.446875000341420137, -1.575800808251659024 ) ) ;
#70764=CARTESIAN_POINT ( 'NONE',  ( -8.487040972474682476, 12.84537220128841817, 0.7216878364870338292 ) ) ;
#70769=CARTESIAN_POINT ( 'NONE',  ( -1.402160292154681736E-14, 0.5093750003414236893, -1.575800808251659024 ) ) ;
#70772=EDGE_CURVE ( 'NONE', #123959, #166540, #207944, .T. ) ;
#70775=CARTESIAN_POINT ( 'NONE',  ( 1.364683531249986537, 0.6552083336747522857, -0.7879004041258239610 ) ) ;
#70777=CARTESIAN_POINT ( 'NONE',  ( -5.713871673155502151, 8.753601821068331290, 1.199719254218452047 ) ) ;
#70778=CARTESIAN_POINT ( 'NONE',  ( 6.564118927310645724, 10.80988918183778225, -0.7998128361456291469 ) ) ;
#70779=CARTESIAN_POINT ( 'NONE',  ( 5.192936529234042808, 6.017179691316550283, -1.199719254218452047 ) ) ;
#70780=CARTESIAN_POINT ( 'NONE',  ( 5.575427483717746213, 7.527751369135936343, 1.599625672291267398 ) ) ;
#70783=CARTESIAN_POINT ( 'NONE',  ( 0.7499999999999885647, 3.316666666666689967, -1.299038105676658228 ) ) ;
#70785=CARTESIAN_POINT ( 'NONE',  ( 0.6823417656249899377, 1.155208333674752286, 1.181850606188755259 ) ) ;
#70792=CARTESIAN_POINT ( 'NONE',  ( 5.016153647376201619, 7.835634441038803466, 1.082531754730558626 ) ) ;
#70795=CARTESIAN_POINT ( 'NONE',  ( -9.176171038350775078, 9.599954387697719582, -0.7998128361456291469 ) ) ;
#70796=CARTESIAN_POINT ( 'NONE',  ( -2.930533758848195447, 6.570706485298192234, -0.7998128361456281477 ) ) ;
#70798=CARTESIAN_POINT ( 'NONE',  ( 1.499999999999990896, 8.627523663848661428, 2.580000000000000515 ) ) ;
#70801=CARTESIAN_POINT ( 'NONE',  ( -7.497295758232720431, 10.73030023703809555, -1.082531754730543083 ) ) ;
#70803=CARTESIAN_POINT ( 'NONE',  ( 1.499999999999987121, 4.545833333333352932, -0.8660254037844323793 ) ) ;
#70807=CARTESIAN_POINT ( 'NONE',  ( 9.747949258545622442, 10.47495501116581984, 0.000000000000000000 ) ) ;
#70820=CARTESIAN_POINT ( 'NONE',  ( 7.063434842595398777, 11.18449838309590483, -0.7216878364870267237 ) ) ;
#70821=CARTESIAN_POINT ( 'NONE',  ( 5.937581207780954884, 9.014596278131406848, -1.199719254218440723 ) ) ;
#70822=CARTESIAN_POINT ( 'NONE',  ( -5.253948220495577637, 6.088359997788290734, 1.199719254218450271 ) ) ;
#70826=CARTESIAN_POINT ( 'NONE',  ( 0.6823417656249864960, -0.5114583329919111243, -1.181850606188749264 ) ) ;
#70827=CARTESIAN_POINT ( 'NONE',  ( 4.392478581147586603, 4.226905887534702977, -0.7216878364870188411 ) ) ;
#70828=ORIENTED_EDGE ( 'NONE', *, *, #95161, .T. ) ;
#70829=CARTESIAN_POINT ( 'NONE',  ( -3.297657676621885692, 4.870353260857385180, 1.599625672291267398 ) ) ;
#70832=ADVANCED_FACE ( 'NONE', ( #11876 ), #30280, .T. ) ;
#70842=ORIENTED_EDGE ( 'NONE', *, *, #208497, .T. ) ;
#70845=DIRECTION ( 'NONE',  ( 1.000000000000000000, 0.000000000000000000, 0.000000000000000000 ) ) ;
#70846=CARTESIAN_POINT ( 'NONE',  ( 8.444030743212801227, 8.745790710036752458, 0.7998128361456462443 ) ) ;
#70850=ORIENTED_EDGE ( 'NONE', *, *, #77409, .F. ) ;
#70858=CARTESIAN_POINT ( 'NONE',  ( -3.927058049452637700, 7.733318157670055371, -0.7998128361456281477 ) ) ;
#70860=CARTESIAN_POINT ( 'NONE',  ( -4.440459003675619520, 5.139289244831666714, 1.199719254218462483 ) ) ;
#70869=CARTESIAN_POINT ( 'NONE',  ( -2.605138072120212200, 6.191078184115536232, -0.7998128361456281477 ) ) ;
#70873=CARTESIAN_POINT ( 'NONE',  ( 6.751070424600909448, 9.963667031088037973, -1.199719254218441611 ) ) ;
#70874=CARTESIAN_POINT ( 'NONE',  ( -0.6823417656250212460, 4.301041667008085767, 1.181850606188767472 ) ) ;
#70882=CARTESIAN_POINT ( 'NONE',  ( 4.636525345749193505, 8.353103970108639587, 1.040834085586084257E-14 ) ) ;
#70883=CARTESIAN_POINT ( 'NONE',  ( -7.832860060393135093, 10.16142270859057462, 1.599625672291295375 ) ) ;
#70884=( BOUNDED_CURVE ( )  B_SPLINE_CURVE ( 2, ( #39857, #102719, #152529, #4114, #72323, #7323, #170908 ),
 .UNSPECIFIED., .F., .T. ) 
 B_SPLINE_CURVE_WITH_KNOTS ( ( 3, 2, 2, 3 ),
 ( 0.3780836810543342641, 0.3809523809523809312, 0.3869047619047619180, 0.3897734618028085851 ),
 .UNSPECIFIED. ) 
 CURVE ( )  GEOMETRIC_REPRESENTATION_ITEM ( )  RATIONAL_B_SPLINE_CURVE ( ( 0.9331000818465633451, 0.9354320710352566071, 1.000000000000000000, 0.8660254037844387076, 1.000000000000000000, 0.9354320710352564960, 0.9331000818465632340 ) ) 
 REPRESENTATION_ITEM ( '' )  );
#70887=CARTESIAN_POINT ( 'NONE',  ( -8.505042434474312074, 8.816971016508505343, -0.7998128361456291469 ) ) ;
#70889=CARTESIAN_POINT ( 'NONE',  ( -6.735703387890906946, 6.752742128827836865, -0.7998128361456291469 ) ) ;
#70896=CARTESIAN_POINT ( 'NONE',  ( 7.182068686937156166, 9.402166106225269715, 1.599625672291281386 ) ) ;
#70909=ORIENTED_EDGE ( 'NONE', *, *, #129470, .T. ) ;
#70911=CARTESIAN_POINT ( 'NONE',  ( 1.364683531249984538, -1.032291666325247714, -0.7879004041258309554 ) ) ;
#70912=CARTESIAN_POINT ( 'NONE',  ( 2.510230996824538430, 6.080353262937265413, 0.000000000000000000 ) ) ;
#70913=CARTESIAN_POINT ( 'NONE',  ( 4.171104814498611368, 8.018039383557042044, 0.7998128361456321445 ) ) ;
#70915=CARTESIAN_POINT ( 'NONE',  ( -9.327646496521992958, 9.984601788804893019, -0.7216878364870267237 ) ) ;
#70916=CARTESIAN_POINT ( 'NONE',  ( 6.371969008742804697, 7.496680600697164465, -1.082531754730543083 ) ) ;
#70917=CARTESIAN_POINT ( 'NONE',  ( -8.853111119599343937, 10.39134639669645566, 1.082531754730558626 ) ) ;
#70919=ORIENTED_EDGE ( 'NONE', *, *, #175809, .T. ) ;
#70921=CARTESIAN_POINT ( 'NONE',  ( 6.740374924288304648, 11.01552117831172062, 1.040834085586084257E-14 ) ) ;
#70928=CARTESIAN_POINT ( 'NONE',  ( 0.6823417656249882723, 2.426041667008084435, -1.181850606188749264 ) ) ;
#70934=CARTESIAN_POINT ( 'NONE',  ( 9.447334110624092673, 9.916311305349925220, -0.7998128361456281477 ) ) ;
#70938=CARTESIAN_POINT ( 'NONE',  ( -9.287498920561160887, 10.79416914786490089, -1.199719254218441611 ) ) ;
#70943=CARTESIAN_POINT ( 'NONE',  ( 3.083589872104280705, 5.684939719841914929, 1.199719254218450271 ) ) ;
#70947=CARTESIAN_POINT ( 'NONE',  ( -10.15235809853472126, 10.73883929124566983, -0.7998128361456291469 ) ) ;
#70953=CARTESIAN_POINT ( 'NONE',  ( 5.463439706979909438, 6.248932391672394893, 1.002290858133829010 ) ) ;
#70955=CARTESIAN_POINT ( 'NONE',  ( -5.278201874421821316, 5.052323696447222900, 0.7998128361456341429 ) ) ;
#70959=CARTESIAN_POINT ( 'NONE',  ( 6.693975156845185737, 8.832723654451292816, 1.599625672291281386 ) ) ;
#70961=CARTESIAN_POINT ( 'NONE',  ( 5.126954644262057492, 9.133197518281081173, 0.7998128361456462443 ) ) ;
#70962=CARTESIAN_POINT ( 'NONE',  ( 5.996784015946103885, 5.890669528225568996, 1.040834085586084257E-14 ) ) ;
#70964=CARTESIAN_POINT ( 'NONE',  ( -8.568389894156720032, 10.05917163368005163, 1.082531754730558626 ) ) ;
#70972=CARTESIAN_POINT ( 'NONE',  ( -4.447391987980185313, 7.103198448885253313, -1.107391122544647333 ) ) ;
#70975=CARTESIAN_POINT ( 'NONE',  ( 5.504247177468179153, 7.444707678511436555, 1.443375672974062551 ) ) ;
#70995=CARTESIAN_POINT ( 'NONE',  ( 7.365103760721646076, 9.615707025640515937, 1.599625672291281386 ) ) ;
#70999=CARTESIAN_POINT ( 'NONE',  ( -1.402160292154681736E-14, 1.618750000682814827, -1.732050807568863648 ) ) ;
#71000=CARTESIAN_POINT ( 'NONE',  ( -3.297657676621885692, 4.870353260857385180, 1.599625672291267398 ) ) ;
#71001=CARTESIAN_POINT ( 'NONE',  ( -5.368138756007025947, 8.350246751061767725, 1.199719254218452047 ) ) ;
#71004=CARTESIAN_POINT ( 'NONE',  ( -9.134442807305063639, 11.67993591332117376, 1.599625672291281386 ) ) ;
#71008=CARTESIAN_POINT ( 'NONE',  ( 6.856673000209174695, 9.022537805042615489, 1.599625672291281386 ) ) ;
#71010=CARTESIAN_POINT ( 'NONE',  ( -5.526920175865215334, 9.599823971818089774, 0.7998128361456481317 ) ) ;
#71012=CARTESIAN_POINT ( 'NONE',  ( 9.420217803396747414, 9.884675613584706255, 0.7998128361456462443 ) ) ;
#71013=CARTESIAN_POINT ( 'NONE',  ( 6.115102234889607580, 6.015626655811740164, -0.1465594925542352267 ) ) ;
#71015=CARTESIAN_POINT ( 'NONE',  ( -1.499999999998296696, 8.673756432004703143, 2.614717076620993730 ) ) ;
#71019=CARTESIAN_POINT ( 'NONE',  ( -7.619319141200077361, 9.912291636198670375, 1.443375672974090751 ) ) ;
#71023=CARTESIAN_POINT ( 'NONE',  ( -1.001543065824772872E-14, 4.634375000341418804, 1.575800808251672791 ) ) ;
#71030=CARTESIAN_POINT ( 'NONE',  ( 1.364683531249990311, 5.613541667008087543, 0.7879004041258500513 ) ) ;
#71031=AXIS2_PLACEMENT_3D ( 'NONE', #207065, #60826, #190809 ) ;
#71033=CARTESIAN_POINT ( 'NONE',  ( -4.894130264408878439, 4.812166184672871161, -0.7216878364870197293 ) ) ;
#71036=CARTESIAN_POINT ( 'NONE',  ( 2.846849068745292755, 6.265148313604064434, 0.000000000000000000 ) ) ;
#71041=CARTESIAN_POINT ( 'NONE',  ( -1.364683531250014514, 0.4885416670080875434, -0.7879004041258289570 ) ) ;
#71042=CARTESIAN_POINT ( 'NONE',  ( -4.297571505851936813, 4.116180966356429494, 1.214306433183764966E-14 ) ) ;
#71043=CARTESIAN_POINT ( 'NONE',  ( 5.983225862332436584, 5.874851682342960402, 0.7998128361456341429 ) ) ;
#71044=ORIENTED_EDGE ( 'NONE', *, *, #126447, .T. ) ;
#71052=CARTESIAN_POINT ( 'NONE',  ( -7.022760382198764084, 11.13704484596649635, 0.7216878364870458196 ) ) ;
#71057=CARTESIAN_POINT ( 'NONE',  ( -7.784352752540590004, 12.23349531127272094, 0.7998128361456481317 ) ) ;
#71058=CARTESIAN_POINT ( 'NONE',  ( -6.534666851662457532, 6.726125536468730459, 1.040834085586084257E-14 ) ) ;
#71059=CARTESIAN_POINT ( 'NONE',  ( -1.201851678989727383E-14, 2.134375000341423689, 1.575800808251672791 ) ) ;
#71066=CARTESIAN_POINT ( 'NONE',  ( 10.57266086055835075, 11.22919251360659310, 0.000000000000000000 ) ) ;
#71069=VERTEX_POINT ( 'NONE', #129993 ) ;
#71083=CARTESIAN_POINT ( 'NONE',  ( -0.6823417656250212460, 3.613541667008085767, 1.181850606188767472 ) ) ;
#71089=EDGE_CURVE ( 'NONE', #17872, #77955, #93779, .T. ) ;
#71095=CARTESIAN_POINT ( 'NONE',  ( -1.364683531250012516, 1.030208333674754062, 0.7879004041258379498 ) ) ;
#71106=CARTESIAN_POINT ( 'NONE',  ( 4.008406971134620633, 7.828225232965717595, 0.7998128361456321445 ) ) ;
#71113=CARTESIAN_POINT ( 'NONE',  ( 7.121056995675668411, 9.330985799753529264, -1.599625672291262513 ) ) ;
#71117=CARTESIAN_POINT ( 'NONE',  ( -3.918470089549458635, 4.530302178351167441, -1.199719254218452047 ) ) ;
#71118=CARTESIAN_POINT ( 'NONE',  ( 8.178592977541601527, 10.56477777859713463, 1.599625672291281386 ) ) ;
#71129=CARTESIAN_POINT ( 'NONE',  ( -8.351459436338048548, 8.845716885256940998, -0.7216878364870278340 ) ) ;
#71133=CARTESIAN_POINT ( 'NONE',  ( -8.676328237741483207, 12.20980114641871062, -1.199719254218446718 ) ) ;
#71138=CARTESIAN_POINT ( 'NONE',  ( -3.541704441667874903, 5.155074486744371853, -1.599625672291256295 ) ) ;
#71139=EDGE_CURVE ( 'NONE', #193812, #178469, #118240, .T. ) ;
#71141=CARTESIAN_POINT ( 'NONE',  ( 10.72180055030867329, 11.40318881831530540, 0.7998128361456341429 ) ) ;
#71142=CARTESIAN_POINT ( 'NONE',  ( 5.217190183160311356, 4.981143389975473568, -0.7998128361456211532 ) ) ;
#71144=ORIENTED_EDGE ( 'NONE', *, *, #4772, .T. ) ;
#71148=CARTESIAN_POINT ( 'NONE',  ( 4.541618270897912701, 4.400902192243413502, 1.214306433183764966E-14 ) ) ;
#71150=CARTESIAN_POINT ( 'NONE',  ( -3.242371291962510504, 6.934516940598226320, 1.040834085586084257E-14 ) ) ;
#71153=CARTESIAN_POINT ( 'NONE',  ( -10.62011439820619429, 11.28455497419572318, -0.7998128361456221525 ) ) ;
#71159=CARTESIAN_POINT ( 'NONE',  ( 6.805829924380097040, 10.88395931184472154, 0.7216878364870438212 ) ) ;
#71160=CARTESIAN_POINT ( 'NONE',  ( -1.364683531250010740, 3.842708333674751398, 0.7879004041258379498 ) ) ;
#71162=CARTESIAN_POINT ( 'NONE',  ( 5.335297142177534369, 6.183267073083954735, -1.199719254218452047 ) ) ;
#71163=CARTESIAN_POINT ( 'NONE',  ( 1.499999999999990896, 3.775000000000021227, 1.214306433183764966E-14 ) ) ;
#71173=CARTESIAN_POINT ( 'NONE',  ( 3.798255590122798342, 7.583048621785260401, -0.7998128361456221525 ) ) ;
#71176=CARTESIAN_POINT ( 'NONE',  ( -0.6823417656250212460, 2.363541667008084435, 1.181850606188767472 ) ) ;
#71178=CARTESIAN_POINT ( 'NONE',  ( 3.379006598303866848, 4.965260336153046516, -1.599625672291262513 ) ) ;
#71180=CARTESIAN_POINT ( 'NONE',  ( -5.260200412422213923, 6.199617238323108737, -1.082531754730544860 ) ) ;
#71183=CARTESIAN_POINT ( 'NONE',  ( -4.216222583725562245, 7.862750747747711877, 0.7216878364870317197 ) ) ;
#71184=CARTESIAN_POINT ( 'NONE',  ( -1.387358672527355008, 7.251968950354660493, 4.302625267139497112 ) ) ;
#71188=CARTESIAN_POINT ( 'NONE',  ( 4.364835388595708743, 7.179726155748598515, 1.199719254218462483 ) ) ;
#71194=CARTESIAN_POINT ( 'NONE',  ( 8.500000000000000000, 6.120000000000034746, -2.580000000000001403 ) ) ;
#71198=CARTESIAN_POINT ( 'NONE',  ( 5.144429221381498607, 8.089252293998699272, -1.199719254218452047 ) ) ;
#71201=CARTESIAN_POINT ( 'NONE',  ( -2.656508033273816238, 5.186677574539687363, -1.199719254218446718 ) ) ;
#71203=CARTESIAN_POINT ( 'NONE',  ( -5.900823170445743671, 7.907379670318584353, 1.599625672291269396 ) ) ;
#71207=CARTESIAN_POINT ( 'NONE',  ( 5.750629710490689384, 9.860818428881154674, -0.7998128361456291469 ) ) ;
#71210=CARTESIAN_POINT ( 'NONE',  ( -7.725448601688521322, 7.907444878258402809, 1.040834085586084257E-14 ) ) ;
#71211=CARTESIAN_POINT ( 'NONE',  ( 6.982085920913413624, 8.208483664896217391, -1.082531754730543971 ) ) ;
#71212=CARTESIAN_POINT ( 'NONE',  ( 4.556571072163061231, 7.192851904033680910, 1.311937382574361877 ) ) ;
#71213=CARTESIAN_POINT ( 'NONE',  ( -5.382750679825375251, 6.238629533673094585, -1.199719254218446718 ) ) ;
#71216=CARTESIAN_POINT ( 'NONE',  ( -4.903245109636583443, 8.872203061218007392, -0.7998128361456281477 ) ) ;
#71219=CARTESIAN_POINT ( 'NONE',  ( -1.364683531250012516, 2.280208333674751842, 0.7879004041258379498 ) ) ;
#71223=CARTESIAN_POINT ( 'NONE',  ( -4.934804725694224459, 6.780358151441803649, -1.443375672974053447 ) ) ;
#71229=CARTESIAN_POINT ( 'NONE',  ( 4.659198344590585350, 8.587481835331020719, 0.7998128361456462443 ) ) ;
#71231=CARTESIAN_POINT ( 'NONE',  ( -5.901845825571131243, 6.006233656505717278, 0.1738135011533047114 ) ) ;
#71232=CARTESIAN_POINT ( 'NONE',  ( 0.6823417656249882723, 1.488541667008083547, -1.181850606188749264 ) ) ;
#71235=CARTESIAN_POINT ( 'NONE',  ( 0.6823417656249864960, -0.7614583329919113464, -1.181850606188749264 ) ) ;
#71238=CARTESIAN_POINT ( 'NONE',  ( -5.111587607552082524, 5.922272616020886282, 1.199719254218450271 ) ) ;
#71240=CARTESIAN_POINT ( 'NONE',  ( -7.090551149822745813, 9.295395646258437949, 1.443375672974078761 ) ) ;
#71248=CARTESIAN_POINT ( 'NONE',  ( -7.659993601596710278, 10.92011438762942355, -1.082531754730543083 ) ) ;
#71254=CARTESIAN_POINT ( 'NONE',  ( -7.998947441938374148, 8.434452891790657603, 1.040834085586084257E-14 ) ) ;
#71268=CARTESIAN_POINT ( 'NONE',  ( -4.934277840369690971, 7.844075682818238526, -1.199719254218452047 ) ) ;
#71270=CARTESIAN_POINT ( 'NONE',  ( 4.253507506385319381, 5.985511395581417204, 1.599625672291267398 ) ) ;
#71271=EDGE_CURVE ( 'NONE', #170224, #172377, #59972, .T. ) ;
#71275=CARTESIAN_POINT ( 'NONE',  ( 7.467843683028853263, 7.606905806488803101, 0.7998128361456341429 ) ) ;
#71279=CARTESIAN_POINT ( 'NONE',  ( -4.446711195602245148, 7.171284913969171448, -1.082531754730549967 ) ) ;
#71283=EDGE_CURVE ( 'NONE', #128332, #96549, #29692, .T. ) ;
#71288=CARTESIAN_POINT ( 'NONE',  ( 1.364683531249988757, 0.6343750003414208027, 0.000000000000000000 ) ) ;
#71289=CARTESIAN_POINT ( 'NONE',  ( 2.286103771890017011, 5.558832614202657396, -0.5700755669254429225 ) ) ;
#71290=CARTESIAN_POINT ( 'NONE',  ( -7.004758919754800139, 11.32396917302262018, 0.000000000000000000 ) ) ;
#71292=CARTESIAN_POINT ( 'NONE',  ( 6.421758314367153275, 10.64380180007036891, -0.7998128361456291469 ) ) ;
#71294=CARTESIAN_POINT ( 'NONE',  ( -7.739006755302186846, 7.923262724141010516, 0.7998128361456462443 ) ) ;
#71297=CARTESIAN_POINT ( 'NONE',  ( -0.6823417656249969321, 4.967708333674755394, -1.181850606188749264 ) ) ;
#71299=CARTESIAN_POINT ( 'NONE',  ( 10.23604278863759909, 11.04439746293979496, 0.000000000000000000 ) ) ;
#71302=CARTESIAN_POINT ( 'NONE',  ( -1.364683531250014514, -0.9489583329919112353, -0.7879004041258359514 ) ) ;
#71305=CARTESIAN_POINT ( 'NONE',  ( 8.283668667825342169, 9.726996869626816533, -1.082531754730543083 ) ) ;
#71307=CARTESIAN_POINT ( 'NONE',  ( 2.065456695249153540, 8.523797939977239224, 2.459872958007392807 ) ) ;
#71308=CARTESIAN_POINT ( 'NONE',  ( -6.127922243696855453, 7.211959374810172463, 1.082531754730549967 ) ) ;
#71311=CARTESIAN_POINT ( 'NONE',  ( -0.6823417656250003738, 2.967708333674754062, -1.181850606188749264 ) ) ;
#71315=CARTESIAN_POINT ( 'NONE',  ( -5.961834861707238531, 7.978559976790334574, -1.599625672291263179 ) ) ;
#71322=CARTESIAN_POINT ( 'NONE',  ( 7.853197290813620945, 10.18514947741448573, 1.599625672291281386 ) ) ;
#71325=CARTESIAN_POINT ( 'NONE',  ( 1.499999999999989120, 2.275000000000019895, 1.214306433183764966E-14 ) ) ;
#71331=CARTESIAN_POINT ( 'NONE',  ( 7.293923454472091450, 7.611924906413328529, 0.7216878364870317197 ) ) ;
#71339=CIRCLE ( 'NONE', #33315, 0.08000000000000020983 ) ;
#71340=CARTESIAN_POINT ( 'NONE',  ( 1.499999999999987121, 1.004166666666687968, 0.8660254037844524744 ) ) ;
#71341=CARTESIAN_POINT ( 'NONE',  ( 6.588372581236919601, 9.773852880496709972, -1.199719254218440723 ) ) ;
#71342=CARTESIAN_POINT ( 'NONE',  ( -7.980945979938748103, 12.46285407657057220, 0.000000000000000000 ) ) ;
#71344=CARTESIAN_POINT ( 'NONE',  ( 0.6823417656249882723, 0.3427083336747516196, 1.181850606188755259 ) ) ;
#71345=CARTESIAN_POINT ( 'NONE',  ( 1.499999999999987121, 1.504166666666690411, 0.8660254037844524744 ) ) ;
#71347=CARTESIAN_POINT ( 'NONE',  ( 3.798255590122797898, 7.583048621785260401, -0.7998128361456221525 ) ) ;
#71351=CARTESIAN_POINT ( 'NONE',  ( -1.084637062511542016, 2.898878807974804239, -1.105835307554790647 ) ) ;
#71355=CARTESIAN_POINT ( 'NONE',  ( -0.6823417656249969321, 5.467708333674756283, -1.181850606188749264 ) ) ;
#71357=CARTESIAN_POINT ( 'NONE',  ( -9.020252271793614440, 9.418049160047695878, 0.7998128361456462443 ) ) ;
#71358=CARTESIAN_POINT ( 'NONE',  ( -6.412643469583822586, 6.583764924043652655, 1.040834085586084257E-14 ) ) ;
#71366=CARTESIAN_POINT ( 'NONE',  ( 6.564118927310645724, 10.80988918183778225, -0.7998128361456291469 ) ) ;
#71367=CARTESIAN_POINT ( 'NONE',  ( -6.056815632531343141, 6.015240258500212711, 0.3115616189311651296 ) ) ;
#71370=CARTESIAN_POINT ( 'NONE',  ( 7.592202833528386208, 7.959917515312338487, 1.040834085586084257E-14 ) ) ;
#71374=CARTESIAN_POINT ( 'NONE',  ( -7.802881099864745984, 9.062115023719057305, -1.199719254218446718 ) ) ;
#71376=CARTESIAN_POINT ( 'NONE',  ( 5.656776405399742025, 7.622658444431597680, -1.599625672291262513 ) ) ;
#71378=CARTESIAN_POINT ( 'NONE',  ( 3.890826896997583884, 4.602014803661035103, -1.082531754730543083 ) ) ;
#71380=CARTESIAN_POINT ( 'NONE',  ( 3.816783937446950770, 4.411668334231586996, 1.199719254218464037 ) ) ;
#71384=CARTESIAN_POINT ( 'NONE',  ( 3.009610312849396951, 6.452363523749469643, -0.06592220986071165023 ) ) ;
#71386=CARTESIAN_POINT ( 'NONE',  ( 2.274666334179356930, 5.653847144074187980, 0.5136602295931251838 ) ) ;
#71387=CARTESIAN_POINT ( 'NONE',  ( -5.585596099150193616, 6.579245539505756746, -1.082531754730544860 ) ) ;
#71388=CARTESIAN_POINT ( 'NONE',  ( 9.788623719386617239, 11.48277776311499387, -1.082531754730537088 ) ) ;
#71391=CARTESIAN_POINT ( 'NONE',  ( -5.520141099058386125, 9.591915048876776595, 0.000000000000000000 ) ) ;
#71395=CARTESIAN_POINT ( 'NONE',  ( 5.974410882859532812, 4.760127796209649098, 2.438793965253449159 ) ) ;
#71397=CARTESIAN_POINT ( 'NONE',  ( -6.008234629150358330, 10.16135750065076060, 0.000000000000000000 ) ) ;
#71411=CARTESIAN_POINT ( 'NONE',  ( 6.938893903907228378E-15, 10.64264068711930733, 1.214306433183764966E-14 ) ) ;
#71414=CARTESIAN_POINT ( 'NONE',  ( -7.379715684540041565, 7.504089808251839244, 1.040834085586084257E-14 ) ) ;
#71417=CARTESIAN_POINT ( 'NONE',  ( 4.853455804012212660, 7.645820290447483458, 1.082531754730558626 ) ) ;
#71418=EDGE_LOOP ( 'NONE', ( #9061, #111989, #131824, #27172 ) ) ;
#71419=CARTESIAN_POINT ( 'NONE',  ( -2.081668171172168513E-14, 6.487495393664096888, 3.100011470320013451 ) ) ;
#71422=CARTESIAN_POINT ( 'NONE',  ( -5.599681137644054729, 6.491715067794862293, 1.199719254218450271 ) ) ;
#71426=CARTESIAN_POINT ( 'NONE',  ( -6.718228810771495141, 7.796687353110217877, 1.199719254218450271 ) ) ;
#71427=CARTESIAN_POINT ( 'NONE',  ( -5.911302602197302747, 6.000609024624352195, 0.1125370128407701259 ) ) ;
#71432=CARTESIAN_POINT ( 'NONE',  ( -8.157201976916404362, 12.66848607304450702, -0.7998128361456281477 ) ) ;
#71433=CARTESIAN_POINT ( 'NONE',  ( 7.287671262545424966, 8.461036880179857889, -1.199719254218451159 ) ) ;
#71436=CARTESIAN_POINT ( 'NONE',  ( -8.123306592882240551, 12.62894145833798376, 0.000000000000000000 ) ) ;
#71442=ORIENTED_EDGE ( 'NONE', *, *, #95883, .F. ) ;
#71444=CARTESIAN_POINT ( 'NONE',  ( 8.758204044747994743, 12.20135990463928266, 1.082531754730546636 ) ) ;
#71450=CARTESIAN_POINT ( 'NONE',  ( -5.558128722462742033, 6.219596756869237630, -0.9274318607392477709 ) ) ;
#71452=CARTESIAN_POINT ( 'NONE',  ( -0.4997071982806468582, 6.813474644879237374, -3.717966193172169920 ) ) ;
#71463=CARTESIAN_POINT ( 'NONE',  ( -2.774614992291035698, 6.388801257648172971, 1.040834085586084257E-14 ) ) ;
#71466=CARTESIAN_POINT ( 'NONE',  ( -3.810004860640155311, 4.403759411290286252, 1.199719254218462483 ) ) ;
#71471=CARTESIAN_POINT ( 'NONE',  ( 1.499999999999985123, -0.6729166659838520248, -0.8660254037844323793 ) ) ;
#71481=CARTESIAN_POINT ( 'NONE',  ( 2.758194185376297902, 5.305311418659259814, 1.199719254218452047 ) ) ;
#71485=CARTESIAN_POINT ( 'NONE',  ( 3.798255590122797898, 7.583048621785260401, -0.7998128361456221525 ) ) ;
#71486=CARTESIAN_POINT ( 'NONE',  ( 1.364683531249986537, 2.217708333674751398, -0.7879004041258239610 ) ) ;
#71487=CARTESIAN_POINT ( 'NONE',  ( -5.386593377506219582, 6.333579893170925068, 1.078181536478119762 ) ) ;
#71488=CARTESIAN_POINT ( 'NONE',  ( 8.516493047678546091, 13.08765898893368629, -0.7998128361456352531 ) ) ;
#71491=CARTESIAN_POINT ( 'NONE',  ( -8.670602931139386627, 10.07445716020612103, 1.199719254218462483 ) ) ;
#71492=CARTESIAN_POINT ( 'NONE',  ( -4.894130264408873110, 5.772535398974209642, -1.082531754730543971 ) ) ;
#71496=CARTESIAN_POINT ( 'NONE',  ( -4.934277840369690971, 7.844075682818238526, -1.199719254218452047 ) ) ;
#71497=VERTEX_POINT ( 'NONE', #200210 ) ;
#71498=CARTESIAN_POINT ( 'NONE',  ( 1.499999999999987121, -0.9645833326505173222, 0.8660254037844524744 ) ) ;
#71506=CARTESIAN_POINT ( 'NONE',  ( -4.053524740361572398, 7.672936597156388316, 0.7216878364870317197 ) ) ;
#71507=CARTESIAN_POINT ( 'NONE',  ( -1.408489644583400535, 7.311701683604569624, -4.382268911472688266 ) ) ;
#71510=CARTESIAN_POINT ( 'NONE',  ( -4.894130264408878439, 4.812166184672871161, -0.7216878364870197293 ) ) ;
#71512=CARTESIAN_POINT ( 'NONE',  ( 9.121938423896107651, 9.536683004167278099, -0.7998128361456221525 ) ) ;
#71522=CARTESIAN_POINT ( 'NONE',  ( -2.428882075142555497, 5.985446187641602300, 1.040834085586084257E-14 ) ) ;
#71523=CARTESIAN_POINT ( 'NONE',  ( -10.29471871147821282, 10.90492667301307605, -0.7998128361456291469 ) ) ;
#71528=CARTESIAN_POINT ( 'NONE',  ( 5.900823170445728572, 7.907379670318584353, 1.599625672291267398 ) ) ;
#71544=CARTESIAN_POINT ( 'NONE',  ( 7.262363838414439776, 11.62450824479221900, 0.7998128361456462443 ) ) ;
#71545=CARTESIAN_POINT ( 'NONE',  ( -6.274726165026268454, 6.214935368819085149, 0.7998128361456341429 ) ) ;
#71550=CARTESIAN_POINT ( 'NONE',  ( 1.144815873399098738, 2.850330900256261568, 0.7749999999993786304 ) ) ;
#71553=CARTESIAN_POINT ( 'NONE',  ( -1.364683531249997417, 5.009375000341425022, 1.214306433183764966E-14 ) ) ;
#71557=CARTESIAN_POINT ( 'NONE',  ( -1.485618637124742625, 7.335443175656797266, -4.255655007286210711 ) ) ;
#71558=CARTESIAN_POINT ( 'NONE',  ( 3.408985558832261731, 6.064568021024562938, 1.199719254218462483 ) ) ;
#71559=CARTESIAN_POINT ( 'NONE',  ( -4.761938266897808525, 6.578680616179308771, 1.599625672291267398 ) ) ;
#71566=CARTESIAN_POINT ( 'NONE',  ( 6.317736394288147039, 6.473040002865377396, 0.7216878364870317197 ) ) ;
#71568=CARTESIAN_POINT ( 'NONE',  ( 8.880227426826646564, 9.462612874160329923, 0.7216878364870458196 ) ) ;
#71569=CARTESIAN_POINT ( 'NONE',  ( -1.364683531250010295, 3.842708333674751398, 0.7879004041258379498 ) ) ;
#71571=CARTESIAN_POINT ( 'NONE',  ( 4.161989969270892153, 6.839110149915929249, 1.082531754730558626 ) ) ;
#71578=CARTESIAN_POINT ( 'NONE',  ( -4.181557753866925964, 7.584876391898649928, 0.9328056193420256603 ) ) ;
#71584=CARTESIAN_POINT ( 'NONE',  ( -10.64045162862669081, 11.30828174301964140, -0.7998128361456221525 ) ) ;
#71594=CARTESIAN_POINT ( 'NONE',  ( 4.053524740805938720, 3.831459740469437936, 1.214306433183764966E-14 ) ) ;
#71595=CARTESIAN_POINT ( 'NONE',  ( 1.364683531249990311, 2.946875000341416140, 1.214306433183764966E-14 ) ) ;
#71597=CARTESIAN_POINT ( 'NONE',  ( 5.926885707468349196, 10.06645042535509660, 1.040834085586084257E-14 ) ) ;
#71600=CARTESIAN_POINT ( 'NONE',  ( -4.497554271431319250, 6.270232621468402989, -1.599625672291256517 ) ) ;
#71604=CARTESIAN_POINT ( 'NONE',  ( 0.7499999999999920064, 4.983333333333353821, 1.299038105676669330 ) ) ;
#71605=CARTESIAN_POINT ( 'NONE',  ( 3.798255590122797898, 7.583048621785260401, -0.7998128361456221525 ) ) ;
#71608=CARTESIAN_POINT ( 'NONE',  ( -1.364683531249997417, 3.259375000341423245, 1.214306433183764966E-14 ) ) ;
#71611=CARTESIAN_POINT ( 'NONE',  ( 9.246297574839974942, 11.81043314211192019, 1.443375672974076540 ) ) ;
#71614=SPHERICAL_SURFACE ( 'NONE', #186581, 0.08000000000000000167 ) ;
#71616=CARTESIAN_POINT ( 'NONE',  ( -1.402160292154681736E-14, 2.618750000682819490, -1.732050807568863648 ) ) ;
#71619=CARTESIAN_POINT ( 'NONE',  ( -5.018489415352746619, 9.006654751220198207, 0.7998128361456481317 ) ) ;
#71620=CARTESIAN_POINT ( 'NONE',  ( 4.731432421044862835, 6.543090462684225450, -1.443375672974051449 ) ) ;
#71629=CARTESIAN_POINT ( 'NONE',  ( 8.620286740190458374, 8.951422706510690830, 1.040834085586084257E-14 ) ) ;
#71630=CARTESIAN_POINT ( 'NONE',  ( 4.741601036477289810, 6.554953847355395880, 1.599625672291267398 ) ) ;
#71633=CARTESIAN_POINT ( 'NONE',  ( -4.229020061460118107, 7.343517960532633282, -0.8650006913940473385 ) ) ;
#71634=CARTESIAN_POINT ( 'NONE',  ( 4.813308228051395687, 5.574280006603454574, 1.199719254218462483 ) ) ;
#71636=VERTEX_POINT ( 'NONE', #73424 ) ;
#71641=CARTESIAN_POINT ( 'NONE',  ( 9.378489572351044856, 11.96465713920816043, -1.599625672291262513 ) ) ;
#71645=CARTESIAN_POINT ( 'NONE',  ( 5.320181785876097358, 6.346852008952179602, 1.110229221197155169 ) ) ;
#71652=CARTESIAN_POINT ( 'NONE',  ( -1.201851678989727383E-14, 3.212500000000018119, 1.732050807568877637 ) ) ;
#71654=CARTESIAN_POINT ( 'NONE',  ( 6.304178240674458422, 10.29869901418813782, 1.040834085586084257E-14 ) ) ;
#71655=CARTESIAN_POINT ( 'NONE',  ( -4.627410500965859264, 4.293067094081919777, 0.7998128361456341429 ) ) ;
#71660=CARTESIAN_POINT ( 'NONE',  ( -3.581325132304157943, 7.329963087663487364, -0.7998128361456281477 ) ) ;
#71666=ORIENTED_EDGE ( 'NONE', *, *, #76499, .T. ) ;
#71667=CARTESIAN_POINT ( 'NONE',  ( -0.7500000000000215383, 3.222916667349487341, 1.299038105676671107 ) ) ;
#71673=CARTESIAN_POINT ( 'NONE',  ( 8.422639742587595180, 10.84949900448412130, -1.599625672291268286 ) ) ;
#71675=CARTESIAN_POINT ( 'NONE',  ( 2.236732156574683827, 5.553345249405011508, 1.040834085586084257E-14 ) ) ;
#71676=EDGE_LOOP ( 'NONE', ( #49855, #61456, #136671, #159206 ) ) ;
#71681=CARTESIAN_POINT ( 'NONE',  ( -8.337901282724359930, 12.67137589657970409, 1.040834085586084257E-14 ) ) ;
#71686=CARTESIAN_POINT ( 'NONE',  ( 8.589254009457354400, 9.979550084910457031, -1.199719254218446718 ) ) ;
#71691=CARTESIAN_POINT ( 'NONE',  ( -5.388475986427523345, 8.373973519885682393, 1.199719254218452047 ) ) ;
#71692=CARTESIAN_POINT ( 'NONE',  ( 4.253507506385319381, 5.985511395581417204, 1.599625672291267398 ) ) ;
#71696=CARTESIAN_POINT ( 'NONE',  ( 9.890836756369282057, 11.49806328964105617, -1.199719254218440723 ) ) ;
#71697=CARTESIAN_POINT ( 'NONE',  ( -3.145128448690323264, 4.692402494937224056, -1.443375672974059665 ) ) ;
#71698=ORIENTED_EDGE ( 'NONE', *, *, #57396, .F. ) ;
#71701=CARTESIAN_POINT ( 'NONE',  ( 0.6823417656249899377, 2.155208333674753174, 1.181850606188767472 ) ) ;
#71703=CARTESIAN_POINT ( 'NONE',  ( 6.155038550924144758, 8.203964280876741455, 1.443375672974076540 ) ) ;
#71704=CARTESIAN_POINT ( 'NONE',  ( -0.7499999999999972244, 4.639583334016150751, -1.299038105676652899 ) ) ;
#71710=CARTESIAN_POINT ( 'NONE',  ( 7.090551149822722721, 11.21613407486112379, 0.7216878364870438212 ) ) ;
#71714=CARTESIAN_POINT ( 'NONE',  ( -7.828943636887387925, 11.22118577875556156, 1.199719254218453823 ) ) ;
#71724=CARTESIAN_POINT ( 'NONE',  ( 2.855963913973019963, 6.483708332943829866, 0.000000000000000000 ) ) ;
#71728=CARTESIAN_POINT ( 'NONE',  ( 3.310162060030825248, 7.013606170011280838, -0.7998128361456291469 ) ) ;
#71731=CARTESIAN_POINT ( 'NONE',  ( -1.201851678989727383E-14, 3.493750000682815493, 1.732050807568877637 ) ) ;
#71737=CARTESIAN_POINT ( 'NONE',  ( -1.500000000000015099, -0.1208333333333093396, -0.8660254037844383745 ) ) ;
#71738=CARTESIAN_POINT ( 'NONE',  ( 7.130698725783555680, 10.40656671580112658, 1.199719254218460707 ) ) ;
#71739=CARTESIAN_POINT ( 'NONE',  ( 5.707619481228810798, 7.681975366232176583, -1.443375672974057666 ) ) ;
#71743=CARTESIAN_POINT ( 'NONE',  ( 8.758204044747994743, 12.20135990463928266, 1.082531754730546636 ) ) ;
#71748=CARTESIAN_POINT ( 'NONE',  ( -6.715366157470410435, 6.729015360003925750, -0.7998128361456291469 ) ) ;
#71749=CARTESIAN_POINT ( 'NONE',  ( -1.499999999999997780, 2.931250000682818158, 1.214306433183764966E-14 ) ) ;
#71750=CARTESIAN_POINT ( 'NONE',  ( 0.6823417656249882723, -1.157291666325249713, 1.181850606188755259 ) ) ;
#71755=CARTESIAN_POINT ( 'NONE',  ( -1.364683531249997417, 4.571875000341417028, 1.214306433183764966E-14 ) ) ;
#71764=CARTESIAN_POINT ( 'NONE',  ( -8.701635661872465732, 9.046329781806354831, 1.040834085586084257E-14 ) ) ;
#71765=CARTESIAN_POINT ( 'NONE',  ( 6.993308306550549247, 7.053281200597435685, 1.040834085586084257E-14 ) ) ;
#71774=CARTESIAN_POINT ( 'NONE',  ( -6.018930129462987999, 9.109503353427070849, 1.199719254218452047 ) ) ;
#71779=CARTESIAN_POINT ( 'NONE',  ( 8.269583629331492602, 11.73526576994040482, 1.199719254218450271 ) ) ;
#71782=CARTESIAN_POINT ( 'NONE',  ( -3.391510981712833939, 7.108513245306943062, 0.7998128361456341429 ) ) ;
#71783=CARTESIAN_POINT ( 'NONE',  ( -8.565000355531095622, 11.01558638625153286, -1.599625672291263179 ) ) ;
#71786=CARTESIAN_POINT ( 'NONE',  ( -4.002466101043451019, 7.812316210466456745, 0.3644823170804913914 ) ) ;
#71787=CARTESIAN_POINT ( 'NONE',  ( -1.364683531250014514, -0.7197916663252461600, 0.7879004041258379498 ) ) ;
#71793=CARTESIAN_POINT ( 'NONE',  ( 7.006866460164219212, 7.069099046480051385, -0.7998128361456281477 ) ) ;
#71796=CARTESIAN_POINT ( 'NONE',  ( 5.946383829931009224, 4.757679660038602876, 2.499999999987512656 ) ) ;
#71822=CARTESIAN_POINT ( 'NONE',  ( -0.7500000000000006661, 1.139583334016154526, -1.299038105676652011 ) ) ;
#71823=CARTESIAN_POINT ( 'NONE',  ( 10.40318394038753702, 11.03146944007395724, -0.7998128361456281477 ) ) ;
#71826=EDGE_LOOP ( 'NONE', ( #153450, #168788, #18589 ) ) ;
#71828=CARTESIAN_POINT ( 'NONE',  ( -8.319899820280397762, 12.85830022363583147, -0.7998128361456281477 ) ) ;
#71830=CARTESIAN_POINT ( 'NONE',  ( -1.364683531250012516, 0.7802083336747528408, 0.7879004041258379498 ) ) ;
#71831=CARTESIAN_POINT ( 'NONE',  ( -1.500000000000021316, 5.420833333333356485, 0.8660254037844343777 ) ) ;
#71837=CARTESIAN_POINT ( 'NONE',  ( -4.548924232584923288, 5.265832011892554121, -1.199719254218446718 ) ) ;
#71843=CARTESIAN_POINT ( 'NONE',  ( -1.402160292154681736E-14, -0.2406249996585799189, -1.575800808251665908 ) ) ;
#71844=TOROIDAL_SURFACE ( 'NONE', #109988, 0.1600000000000000033, 0.08000000000000000167 ) ;
#71849=CARTESIAN_POINT ( 'NONE',  ( -1.402160292154681736E-14, -0.3031249996585801965, -1.575800808251665908 ) ) ;
#71851=CARTESIAN_POINT ( 'NONE',  ( -6.039267359883488950, 9.133230122250985517, 1.199719254218452047 ) ) ;
#71852=CARTESIAN_POINT ( 'NONE',  ( 7.293396569147545527, 10.59638086639245280, 1.199719254218460707 ) ) ;
#71853=CARTESIAN_POINT ( 'NONE',  ( 5.867981556616276073, 5.740399992340776691, -0.7998128361456282587 ) ) ;
#71857=CARTESIAN_POINT ( 'NONE',  ( -0.6823417656250003738, 1.530208333674752730, -1.181850606188749264 ) ) ;
#71862=CARTESIAN_POINT ( 'NONE',  ( 6.534666852106798096, 7.686494751288491578, -1.082531754730543083 ) ) ;
#71865=CARTESIAN_POINT ( 'NONE',  ( -6.581593504430098385, 9.765943957555402122, -1.199719254218440723 ) ) ;
#71866=CARTESIAN_POINT ( 'NONE',  ( -3.255929445576174697, 6.950334786480840243, -0.7998128361456281477 ) ) ;
#71867=CARTESIAN_POINT ( 'NONE',  ( -1.201851678989727383E-14, 3.134375000341420137, 1.575800808251672791 ) ) ;
#71870=LINE ( 'NONE', #136913, #167082 ) ;
#71871=CARTESIAN_POINT ( 'NONE',  ( 6.629573926958101993, 6.836850457647000390, -0.7216878364870257245 ) ) ;
#71872=CARTESIAN_POINT ( 'NONE',  ( -7.741342523278709642, 10.05465224862374285, 1.443375672974090751 ) ) ;
#71874=CARTESIAN_POINT ( 'NONE',  ( -1.500000000000011324, 4.420833333333352044, 0.8660254037844403729 ) ) ;
#71878=CARTESIAN_POINT ( 'NONE',  ( 8.432808358020016826, 10.86136238915529084, 1.443375672974076540 ) ) ;
#71886=ORIENTED_EDGE ( 'NONE', *, *, #165463, .F. ) ;
#71893=CARTESIAN_POINT ( 'NONE',  ( 8.120970824461352322, 9.537182719035495637, -1.082531754730543083 ) ) ;
#71894=CARTESIAN_POINT ( 'NONE',  ( 6.265839547809997079, 10.46189657242035587, 0.7998128361456462443 ) ) ;
#71895=CARTESIAN_POINT ( 'NONE',  ( -5.530836599371015794, 8.540060901653093950, 1.199719254218452047 ) ) ;
#71900=CARTESIAN_POINT ( 'NONE',  ( 1.419999999999822737, 7.204077025658621736, 4.238769367544763966 ) ) ;
#71901=CARTESIAN_POINT ( 'NONE',  ( 4.907688418466886304, 5.788353245375237321, -1.082531754730548412 ) ) ;
#71903=CARTESIAN_POINT ( 'NONE',  ( -6.697364695470783502, 10.75741654478384035, 0.7216878364870458196 ) ) ;
#71915=VERTEX_POINT ( 'NONE', #189317 ) ;
#71918=CARTESIAN_POINT ( 'NONE',  ( 7.904567251967224095, 9.180748867838630645, 1.199719254218462483 ) ) ;
#71920=EDGE_CURVE ( 'NONE', #100909, #19519, #213034, .T. ) ;
#71922=ORIENTED_EDGE ( 'NONE', *, *, #86821, .T. ) ;
#71929=CARTESIAN_POINT ( 'NONE',  ( -5.052384799386910430, 9.046199365926717917, 1.214306433183764966E-14 ) ) ;
#71932=CARTESIAN_POINT ( 'NONE',  ( -3.567766978690493307, 7.314145241780881435, 1.040834085586084257E-14 ) ) ;
#71941=CARTESIAN_POINT ( 'NONE',  ( -3.079673448598517549, 6.744702790006905424, 1.040834085586084257E-14 ) ) ;
#71945=CARTESIAN_POINT ( 'NONE',  ( 7.450369105909416589, 8.650851030771185890, -1.199719254218441611 ) ) ;
#71946=CARTESIAN_POINT ( 'NONE',  ( -1.364683531249997417, 3.509375000341423245, 1.214306433183764966E-14 ) ) ;
#71948=CARTESIAN_POINT ( 'NONE',  ( 6.113440106766272031, 6.016660024919275429, -0.07562458862005703997 ) ) ;
#71953=CARTESIAN_POINT ( 'NONE',  ( 4.975479186090847605, 7.788180902872553268, 1.082531754730558626 ) ) ;
#71954=CARTESIAN_POINT ( 'NONE',  ( -8.505042434474312074, 8.816971016508505343, -0.7998128361456291469 ) ) ;
#71957=CARTESIAN_POINT ( 'NONE',  ( -7.323375529675950624, 11.69568855126397011, -0.7998128361456291469 ) ) ;
#71958=CARTESIAN_POINT ( 'NONE',  ( -5.708146366553361162, 6.618257834855742594, -1.199719254218446718 ) ) ;
#71959=CARTESIAN_POINT ( 'NONE',  ( -1.499999999999997780, 5.681250000682820378, 1.214306433183764966E-14 ) ) ;
#71965=CARTESIAN_POINT ( 'NONE',  ( 7.786460292950004636, 7.978625184730144149, 1.040834085586084257E-14 ) ) ;
#71976=CARTESIAN_POINT ( 'NONE',  ( -0.07278863622987721826, 7.008482404162161394, -2.000259058016610414 ) ) ;
#71981=CARTESIAN_POINT ( 'NONE',  ( -1.500000000000011324, 4.379166666666688634, -0.8660254037844313801 ) ) ;
#71982=CARTESIAN_POINT ( 'NONE',  ( 6.173040012923759257, 6.096301524699504704, -0.7998128361456281477 ) ) ;
#71983=CARTESIAN_POINT ( 'NONE',  ( 6.505214776458575265, 6.483838748823460563, 1.040834085586084257E-14 ) ) ;
#71986=CARTESIAN_POINT ( 'NONE',  ( -7.036318535812428721, 11.15286269184909784, 0.000000000000000000 ) ) ;
#71988=CARTESIAN_POINT ( 'NONE',  ( 5.490689023854504747, 9.349628261231513804, 1.040834085586084257E-14 ) ) ;
#71989=CARTESIAN_POINT ( 'NONE',  ( -8.717529583462656717, 11.19353715217169309, 1.443375672974064550 ) ) ;
#71992=CARTESIAN_POINT ( 'NONE',  ( 7.456094412511537151, 10.78619501698377370, 1.199719254218460707 ) ) ;
#71997=CARTESIAN_POINT ( 'NONE',  ( -3.009396220815599321, 6.452359640394901952, 0.6004564335717228474 ) ) ;
#71998=CARTESIAN_POINT ( 'NONE',  ( -1.364683531250012516, 2.530208333674753174, 0.7879004041258379498 ) ) ;
#72004=CARTESIAN_POINT ( 'NONE',  ( 7.099665995050449041, 11.43469409420089455, 0.7998128361456462443 ) ) ;
#72007=CARTESIAN_POINT ( 'NONE',  ( -9.504429378379839477, 11.04725468198666150, 1.199719254218462483 ) ) ;
#72013=CARTESIAN_POINT ( 'NONE',  ( 2.920892028740289081, 5.495125569250587816, 1.199719254218452047 ) ) ;
#72016=CARTESIAN_POINT ( 'NONE',  ( -9.840520565420403543, 10.37502883594562597, 1.040834085586084257E-14 ) ) ;
#72021=CARTESIAN_POINT ( 'NONE',  ( 5.364345920411571100, 6.316227854031381206, 1.080878399565273540 ) ) ;
#72024=CARTESIAN_POINT ( 'NONE',  ( -4.874319919312905647, 5.645460313075203018, -1.199719254218446718 ) ) ;
#72028=CARTESIAN_POINT ( 'NONE',  ( 7.832860060393120882, 10.16142270859057462, 1.599625672291281386 ) ) ;
#72030=CARTESIAN_POINT ( 'NONE',  ( 6.531277313481192337, 8.642909503859968368, 1.599625672291281386 ) ) ;
#72033=CARTESIAN_POINT ( 'NONE',  ( -9.178506806771670412, 9.810605484096178941, 1.040834085586084257E-14 ) ) ;
#72041=CARTESIAN_POINT ( 'NONE',  ( -6.007394967034264788, 6.077829431587280062, -0.6506939886842719734 ) ) ;
#72044=AXIS2_PLACEMENT_3D ( 'NONE', #172312, #57491, #59615 ) ;
#72045=CARTESIAN_POINT ( 'NONE',  ( 4.473827502829567315, 7.202920605734387749, -1.082531754730548412 ) ) ;
#72067=CARTESIAN_POINT ( 'NONE',  ( 6.774270308322468459, 11.05506579301824743, 0.7998128361456462443 ) ) ;
#72071=CARTESIAN_POINT ( 'NONE',  ( -1.402160292154681736E-14, 1.118750000682820378, -1.732050807568863648 ) ) ;
#72073=CARTESIAN_POINT ( 'NONE',  ( -6.018930129462987999, 9.109503353427070849, 1.199719254218452047 ) ) ;
#72076=CARTESIAN_POINT ( 'NONE',  ( -10.48453286206953727, 11.12637651536962125, 0.7998128361456462443 ) ) ;
#72077=CARTESIAN_POINT ( 'NONE',  ( -1.500000000000079936, 7.267697830503743184, 4.207111467970349850 ) ) ;
#72080=CARTESIAN_POINT ( 'NONE',  ( -1.500000000000011324, 5.452083334016153415, 0.8660254037844403729 ) ) ;
#72081=CARTESIAN_POINT ( 'NONE',  ( 7.558834334818744338, 8.777393797832065303, 1.199719254218462483 ) ) ;
#72084=CARTESIAN_POINT ( 'NONE',  ( -7.497822643557261024, 8.706213491360317747, -1.199719254218446718 ) ) ;
#72088=CARTESIAN_POINT ( 'NONE',  ( -1.492665153618444762, 8.694790292835948620, 2.590406265390401419 ) ) ;
#72093=CARTESIAN_POINT ( 'NONE',  ( -8.107412671292051343, 10.48173408797264194, 1.443375672974090751 ) ) ;
#72097=CARTESIAN_POINT ( 'NONE',  ( -1.201851678989727383E-14, 3.884375000341423689, 1.575800808251672791 ) ) ;
#72103=CARTESIAN_POINT ( 'NONE',  ( 0.6823417656249899377, 4.176041667008085767, -1.181850606188754593 ) ) ;
#72105=CARTESIAN_POINT ( 'NONE',  ( -2.398572866711294438, 5.287202466803544887, -0.8077998227820496480 ) ) ;
#72108=CARTESIAN_POINT ( 'NONE',  ( 4.663641652976547647, 4.543262804668490418, 1.214306433183764966E-14 ) ) ;
#72109=CARTESIAN_POINT ( 'NONE',  ( 1.364683531249992088, 5.446875000341417916, 1.214306433183764966E-14 ) ) ;
#72115=CARTESIAN_POINT ( 'NONE',  ( -0.6823417656250003738, 0.4677083336747517306, -1.181850606188749264 ) ) ;
#72116=CARTESIAN_POINT ( 'NONE',  ( -3.633221978782304351, 4.301475732409860697, -1.082531754730549967 ) ) ;
#72118=CARTESIAN_POINT ( 'NONE',  ( 4.904298879841284098, 6.744767997946721216, 1.599625672291267398 ) ) ;
#72124=CARTESIAN_POINT ( 'NONE',  ( 4.582292731738905722, 5.408724944192588424, -1.082531754730548412 ) ) ;
#72127=CARTESIAN_POINT ( 'NONE',  ( -9.029367117021344313, 9.636609179387466639, 0.7216878364870438212 ) ) ;
#72132=CARTESIAN_POINT ( 'NONE',  ( -7.309817376062285099, 11.67987070538135264, 0.000000000000000000 ) ) ;
#72133=CARTESIAN_POINT ( 'NONE',  ( -4.894130264408862452, 7.693273827576896373, -1.082531754730548412 ) ) ;
#72135=CARTESIAN_POINT ( 'NONE',  ( -1.364683531250000748, 1.571875000341421691, 0.000000000000000000 ) ) ;
#72136=CARTESIAN_POINT ( 'NONE',  ( 1.500000000000001332, 4.504166666666688634, 0.8660254037844450359 ) ) ;
#72154=CARTESIAN_POINT ( 'NONE',  ( -4.762992037102518950, 4.451245552908022596, -0.7998128361456221525 ) ) ;
#72157=CARTESIAN_POINT ( 'NONE',  ( -1.364683531250012516, 3.051041667008083547, -0.7879004041258289570 ) ) ;
#72165=( BOUNDED_SURFACE ( )  B_SPLINE_SURFACE ( 1, 2, ( 
 ( #7264, #206545, #73341, #41950, #110195, #26732, #14736, #31024, #109133, #63510, #143741, #79748, #46211, #210811, #127536, #113396, #175146, #129662, #128599, #193508, #176205, #195649, #47284, #59230, #78678, #28880, #191354, #92834, #179404, #97100, #10474, #112327, #207612, #158878, #163152, #145864, #141604, #125388, #43019, #94963, #76549, #178341, #159944, #211870, #11548, #142659, #194565, #208669, #12606, #126458, #161011, #144805, #77618, #62436, #27806, #60300, #192422, #45149, #29950, #44076, #93904, #209735, #96035, #61379, #111261, #177264, #162087, #13677, #196705, #99212, #36310, #80828, #49391, #117644, #184690, #165261, #115510, #180456, #168457, #102389, #48345, #2726, #82937, #18990, #199876, #150091, #66652, #52573, #114456, #68799, #67718, #132798, #181503, #134918, #200925, #212935, #17915, #182561, #130714, #32073, #118702, #146917, #164208, #51519, #64572, #98161, #15795, #85072, #81881, #50449, #84001, #1662, #147966, #213978, #167400, #65598, #131747, #33132, #116567, #197752, #16856, #133869, #586, #166325, #198801, #34184, #100258, #149010, #151157, #183637, #35243, #101318, #107800, #135968, #22169, #55772, #69859, #206284, #56846, #3784, #188969, #86144, #201984, #152215, #185754, #154348, #40613, #90425, #119774, #39526, #24319, #156494, #121929, #155411, #57908, #71998, #53641, #37387, #88284, #103462, #70928, #169524, #204120, #8083, #105624, #203064, #170584, #38462, #187896, #123018, #171653, #21104, #87208, #153272, #4849, #137037, #120858, #54707, #186831, #104539, #5926, #138109, #23250, #20055, #89363, #6994, #73072, #139173, #205204, #106717, #74172, #172743, #140264, #124073, #190037, #41689, #78425, #28620, #178076, #127273, #47020, #27543, #93638, #43821, #112075, #173825, #159681, #109938, #174891, #42761, #45954, #211610, #126199, #76294, #11282, #194313, #128346, #60044, #79495, #175947, #108867, #62190, #25402, #92581, #29694, #91504, #125135, #191092, #207359, #63246, #94708, #145614, #157565, #160750, #208410, #144547, #77361, #9158, #129407, #141344, #177003, #75234, #26471, #12345, #95775, #143475, #193245, #209471, #61113, #195390, #58979, #210554, #158623, #10220, #44892, #142402, #192161, #110998, #161832, #13420, #82684, #148766, #66408, #132553, #146663, #68552, #133621, #163963, #100014, #162892, #67475, #32880, #198552, #179142, #131497, #17666, #101067, #199623, #16603, #97902, #166078, #15539, #196452, #212677, #49144, #51269, #1413, #65350, #14475, #130462, #2475, #117393, #167154, #183390, #200682, #64318, #48095, #114207, #150914, #33939, #18741, #30765, #83752, #147709, #149843, #115260, #96845, #84826, #80564, #116319, #113135, #180205, #34995, #134679, #181253, #50201, #98957, #335, #31827, #81624, #213727, #197501, #165008, #182310, #19812, #169278, #168213, #135727, #171412, #21922, #88031, #5672, #71750, #85899, #7826, #72831, #103218 ),
 ( #20864, #151973, #140011, #156248, #3547, #188727, #54467, #204955, #23000, #121685, #38216, #24080, #69617, #40365, #39278, #104289, #86963, #106467, #172494, #184447, #203886, #154103, #102147, #201749, #90185, #73918, #53390, #89118, #118461, #119527, #52333, #56603, #36065, #137866, #55530, #187652, #185513, #37137, #138934, #153032, #4606, #70680, #105373, #136792, #202818, #155172, #186588, #6756, #170337, #122767, #120611, #42509, #64847, #174642, #29160, #195930, #82160, #107549, #211087, #30230, #41441, #180735, #31303, #189790, #163435, #57670, #173583, #123828, #157314, #128871, #15015, #130993, #91254, #13950, #213217, #196983, #62710, #147192, #113679, #63785, #194854, #32362, #25153, #48622, #47568, #46486, #95251, #114737, #98426, #8905, #146136, #96315, #74985, #141093, #164491, #16077, #207105, #179683, #58732, #124884, #206036, #190848, #108615, #178620, #212149, #129943, #161300, #12885, #81104, #78962, #145084, #112609, #162370, #80033, #97378, #85374, #68021, #19292, #134160, #51823, #183934, #199091, #4094, #116863, #182865, #135220, #21411, #49672, #150389, #35546, #198043, #120086, #184987, #132033, #102700, #214254, #115797, #65885, #99497, #200169, #168757, #70165, #33419, #167691, #152510, #136276, #101624, #69096, #186061, #117941, #181785, #165554, #1958, #17147, #50737, #83223, #151456, #202296, #3028, #53947, #103773, #201232, #37697, #52873, #166626, #86445, #18218, #169825, #119009, #148253, #36613, #133093, #20361, #149306, #84304, #887, #34481, #66954, #100555, #73379, #189275, #153586, #157866, #89667, #190329, #204431, #23559, #5156, #122242, #108098, #203365, #105944, #43058, #87521, #56084, #124371, #191393, #171968, #188200, #187135, #175184, #109171, #55017, #155718, #206584, #156797, #91808, #40914, #71232, #7303, #139485, #205513, #25700, #137347, #57145, #123311, #88594, #170891, #174127, #125427, #39837, #107020, #173044, #9459, #41990, #24627, #207651, #90734, #22483, #75531, #121166, #6233, #141642, #38764, #104845, #154651, #72305, #138410, #8384, #59272, #74466, #140571, #58212, #145901, #28919, #92872, #146956, #208709, #29987, #26771, #27845, #13714, #195685, #95004, #46248, #177305, #144844, #212971, #60336, #211910, #126497, #64612, #112365, #192460, #143779, #142700, #110235, #63547, #210850, #62476, #194604, #178378, #44114, #196745, #47322, #77657, #79787, #76589, #113435, #161050, #96072, #158918, #45187, #129703, #14775, #179442, #128639, #11585, #31063, #209774, #176243, #93943, #12646, #97138, #163192, #193545, #159983, #61414, #130751, #80866, #48385, #127577, #78718, #111302, #162126, #114499, #10514, #197794, #98198, #148007, #180496, #214018, #82978, #33173, #149051, #165302, #81920, #115549, #132841, #32113, #16897, #50492, #84047, #116613, #182607, #19035, #68842, #15834, #17961, #199919, #65640, #131788, #49429, #34230, #150136, #181545, #2771 ) ),
 .UNSPECIFIED., .F., .F., .F. ) 
 B_SPLINE_SURFACE_WITH_KNOTS ( ( 2, 2 ),
 ( 3, 2, 2, 2, 2, 2, 2, 2, 2, 2, 2, 2, 2, 2, 2, 2, 2, 2, 2, 2, 2, 2, 2, 2, 2, 2, 2, 2, 2, 2, 2, 2, 2, 2, 2, 2, 2, 2, 2, 2, 2, 2, 2, 2, 2, 2, 2, 2, 2, 2, 2, 2, 2, 2, 2, 2, 2, 2, 2, 2, 2, 2, 2, 2, 2, 2, 2, 2, 2, 2, 2, 2, 2, 2, 2, 2, 2, 2, 2, 2, 2, 2, 2, 2, 2, 2, 2, 2, 2, 2, 2, 2, 2, 2, 2, 2, 2, 2, 2, 2, 2, 2, 2, 2, 2, 2, 2, 2, 2, 2, 2, 2, 2, 2, 2, 2, 2, 2, 2, 2, 2, 2, 2, 2, 2, 2, 2, 2, 2, 2, 2, 2, 2, 2, 2, 2, 2, 2, 2, 2, 2, 2, 2, 2, 2, 2, 2, 2, 2, 2, 2, 2, 2, 2, 2, 2, 2, 2, 2, 2, 2, 2, 2, 2, 2, 2, 2, 2, 3 ),
 ( 0.000000000000000000, 1.000000000000000000 ),
 ( 0.000000000000000000, 0.005952380952380952051, 0.01190476190476190410, 0.01785714285714285615, 0.02380952380952380820, 0.02976190476190476025, 0.03571428571428571230, 0.04166666666666666435, 0.04761904761904761640, 0.05357142857142856845, 0.05952380952380952051, 0.06547619047619047949, 0.07142857142857142461, 0.07738095238095238360, 0.08333333333333332871, 0.08928571428571428770, 0.09523809523809523281, 0.1011904761904761918, 0.1071428571428571369, 0.1130952380952380959, 0.1190476190476190410, 0.1250000000000000000, 0.1309523809523809590, 0.1369047619047619180, 0.1428571428571428492, 0.1488095238095238082, 0.1547619047619047672, 0.1607142857142857262, 0.1666666666666666574, 0.1726190476190476164, 0.1785714285714285754, 0.1845238095238095344, 0.1904761904761904656, 0.1964285714285714246, 0.2023809523809523836, 0.2083333333333333426, 0.2142857142857142738, 0.2202380952380952328, 0.2261904761904761918, 0.2321428571428571508, 0.2380952380952380820, 0.2440476190476190410, 0.2500000000000000000, 0.2559523809523809312, 0.2619047619047619180, 0.2678571428571428492, 0.2738095238095238360, 0.2797619047619047672, 0.2857142857142856984, 0.2916666666666666852, 0.2976190476190476164, 0.3035714285714285476, 0.3095238095238095344, 0.3154761904761904656, 0.3214285714285714524, 0.3273809523809523836, 0.3333333333333333148, 0.3392857142857143016, 0.3452380952380952328, 0.3511904761904761640, 0.3571428571428571508, 0.3630952380952380820, 0.3690476190476190688, 0.3750000000000000000, 0.3809523809523809312, 0.3869047619047619180, 0.3928571428571428492, 0.3988095238095238360, 0.4047619047619047672, 0.4107142857142856984, 0.4166666666666666852, 0.4226190476190476164, 0.4285714285714285476, 0.4345238095238095344, 0.4404761904761904656, 0.4464285714285714524, 0.4523809523809523836, 0.4583333333333333148, 0.4642857142857143016, 0.4702380952380952328, 0.4761904761904761640, 0.4821428571428571508, 0.4880952380952380820, 0.4940476190476190688, 0.5000000000000000000, 0.5059523809523809312, 0.5119047619047618625, 0.5178571428571429047, 0.5238095238095238360, 0.5297619047619047672, 0.5357142857142856984, 0.5416666666666666297, 0.5476190476190476719, 0.5535714285714286031, 0.5595238095238095344, 0.5654761904761904656, 0.5714285714285713969, 0.5773809523809523281, 0.5833333333333333703, 0.5892857142857143016, 0.5952380952380952328, 0.6011904761904761640, 0.6071428571428570953, 0.6130952380952381375, 0.6190476190476190688, 0.6250000000000000000, 0.6309523809523809312, 0.6369047619047618625, 0.6428571428571429047, 0.6488095238095238360, 0.6547619047619047672, 0.6607142857142856984, 0.6666666666666666297, 0.6726190476190476719, 0.6785714285714286031, 0.6845238095238095344, 0.6904761904761904656, 0.6964285714285713969, 0.7023809523809523281, 0.7083333333333333703, 0.7142857142857143016, 0.7202380952380952328, 0.7261904761904761640, 0.7321428571428570953, 0.7380952380952381375, 0.7440476190476190688, 0.7500000000000000000, 0.7559523809523809312, 0.7619047619047618625, 0.7678571428571429047, 0.7738095238095238360, 0.7797619047619047672, 0.7857142857142856984, 0.7916666666666666297, 0.7976190476190476719, 0.8035714285714286031, 0.8095238095238095344, 0.8154761904761904656, 0.8214285714285713969, 0.8273809523809523281, 0.8333333333333333703, 0.8392857142857143016, 0.8452380952380952328, 0.8511904761904761640, 0.8571428571428570953, 0.8630952380952381375, 0.8690476190476190688, 0.8750000000000000000, 0.8809523809523809312, 0.8869047619047618625, 0.8928571428571429047, 0.8988095238095238360, 0.9047619047619047672, 0.9107142857142856984, 0.9166666666666666297, 0.9226190476190476719, 0.9285714285714286031, 0.9345238095238095344, 0.9404761904761904656, 0.9464285714285713969, 0.9523809523809523281, 0.9583333333333333703, 0.9642857142857143016, 0.9702380952380952328, 0.9761904761904761640, 0.9821428571428570953, 0.9880952380952381375, 0.9940476190476190688, 1.000000000000000000 ),
 .UNSPECIFIED. ) 
 GEOMETRIC_REPRESENTATION_ITEM ( )  RATIONAL_B_SPLINE_SURFACE ( (
 ( 1.000000000000000000, 0.8660254037844387076, 1.000000000000000000, 0.8660254037844387076, 1.000000000000000000, 0.8660254037844387076, 1.000000000000000000, 0.8660254037844387076, 1.000000000000000000, 0.8660254037844387076, 1.000000000000000000, 0.8660254037844387076, 1.000000000000000000, 0.8660254037844387076, 1.000000000000000000, 0.8660254037844387076, 1.000000000000000000, 0.8660254037844387076, 1.000000000000000000, 0.8660254037844387076, 1.000000000000000000, 0.8660254037844387076, 1.000000000000000000, 0.8660254037844387076, 1.000000000000000000, 0.8660254037844387076, 1.000000000000000000, 0.8660254037844387076, 1.000000000000000000, 0.8660254037844387076, 1.000000000000000000, 0.8660254037844387076, 1.000000000000000000, 0.8660254037844387076, 1.000000000000000000, 0.8660254037844387076, 1.000000000000000000, 0.8660254037844387076, 1.000000000000000000, 0.8660254037844387076, 1.000000000000000000, 0.8660254037844387076, 1.000000000000000000, 0.8660254037844387076, 1.000000000000000000, 0.8660254037844387076, 1.000000000000000000, 0.8660254037844387076, 1.000000000000000000, 0.8660254037844387076, 1.000000000000000000, 0.8660254037844387076, 1.000000000000000000, 0.8660254037844387076, 1.000000000000000000, 0.8660254037844387076, 1.000000000000000000, 0.8660254037844387076, 1.000000000000000000, 0.8660254037844387076, 1.000000000000000000, 0.8660254037844387076, 1.000000000000000000, 0.8660254037844387076, 1.000000000000000000, 0.8660254037844387076, 1.000000000000000000, 0.8660254037844387076, 1.000000000000000000, 0.8660254037844387076, 1.000000000000000000, 0.8660254037844387076, 1.000000000000000000, 0.8660254037844387076, 1.000000000000000000, 0.8660254037844387076, 1.000000000000000000, 0.8660254037844387076, 1.000000000000000000, 0.8660254037844387076, 1.000000000000000000, 0.8660254037844387076, 1.000000000000000000, 0.8660254037844387076, 1.000000000000000000, 0.8660254037844387076, 1.000000000000000000, 0.8660254037844387076, 1.000000000000000000, 0.8660254037844387076, 1.000000000000000000, 0.8660254037844387076, 1.000000000000000000, 0.8660254037844387076, 1.000000000000000000, 0.8660254037844387076, 1.000000000000000000, 0.8660254037844387076, 1.000000000000000000, 0.8660254037844387076, 1.000000000000000000, 0.8660254037844387076, 1.000000000000000000, 0.8660254037844387076, 1.000000000000000000, 0.8660254037844387076, 1.000000000000000000, 0.8660254037844387076, 1.000000000000000000, 0.8660254037844387076, 1.000000000000000000, 0.8660254037844387076, 1.000000000000000000, 0.8660254037844387076, 1.000000000000000000, 0.8660254037844387076, 1.000000000000000000, 0.8660254037844387076, 1.000000000000000000, 0.8660254037844387076, 1.000000000000000000, 0.8660254037844387076, 1.000000000000000000, 0.8660254037844387076, 1.000000000000000000, 0.8660254037844387076, 1.000000000000000000, 0.8660254037844387076, 1.000000000000000000, 0.8660254037844387076, 1.000000000000000000, 0.8660254037844387076, 1.000000000000000000, 0.8660254037844387076, 1.000000000000000000, 0.8660254037844387076, 1.000000000000000000, 0.8660254037844387076, 1.000000000000000000, 0.8660254037844387076, 1.000000000000000000, 0.8660254037844387076, 1.000000000000000000, 0.8660254037844387076, 1.000000000000000000, 0.8660254037844387076, 1.000000000000000000, 0.8660254037844387076, 1.000000000000000000, 0.8660254037844387076, 1.000000000000000000, 0.8660254037844387076, 1.000000000000000000, 0.8660254037844387076, 1.000000000000000000, 0.8660254037844387076, 1.000000000000000000, 0.8660254037844387076, 1.000000000000000000, 0.8660254037844387076, 1.000000000000000000, 0.8660254037844387076, 1.000000000000000000, 0.8660254037844387076, 1.000000000000000000, 0.8660254037844387076, 1.000000000000000000, 0.8660254037844387076, 1.000000000000000000, 0.8660254037844387076, 1.000000000000000000, 0.8660254037844387076, 1.000000000000000000, 0.8660254037844387076, 1.000000000000000000, 0.8660254037844387076, 1.000000000000000000, 0.8660254037844387076, 1.000000000000000000, 0.8660254037844387076, 1.000000000000000000, 0.8660254037844387076, 1.000000000000000000, 0.8660254037844387076, 1.000000000000000000, 0.8660254037844387076, 1.000000000000000000, 0.8660254037844387076, 1.000000000000000000, 0.8660254037844387076, 1.000000000000000000, 0.8660254037844387076, 1.000000000000000000, 0.8660254037844387076, 1.000000000000000000, 0.8660254037844387076, 1.000000000000000000, 0.8660254037844387076, 1.000000000000000000, 0.8660254037844387076, 1.000000000000000000, 0.8660254037844387076, 1.000000000000000000, 0.8660254037844387076, 1.000000000000000000, 0.8660254037844387076, 1.000000000000000000, 0.8660254037844387076, 1.000000000000000000, 0.8660254037844387076, 1.000000000000000000, 0.8660254037844387076, 1.000000000000000000, 0.8660254037844387076, 1.000000000000000000, 0.8660254037844387076, 1.000000000000000000, 0.8660254037844387076, 1.000000000000000000, 0.8660254037844387076, 1.000000000000000000, 0.8660254037844387076, 1.000000000000000000, 0.8660254037844387076, 1.000000000000000000, 0.8660254037844387076, 1.000000000000000000, 0.8660254037844387076, 1.000000000000000000, 0.8660254037844387076, 1.000000000000000000, 0.8660254037844387076, 1.000000000000000000, 0.8660254037844387076, 1.000000000000000000, 0.8660254037844387076, 1.000000000000000000, 0.8660254037844387076, 1.000000000000000000, 0.8660254037844387076, 1.000000000000000000, 0.8660254037844387076, 1.000000000000000000, 0.8660254037844387076, 1.000000000000000000, 0.8660254037844387076, 1.000000000000000000, 0.8660254037844387076, 1.000000000000000000, 0.8660254037844387076, 1.000000000000000000, 0.8660254037844387076, 1.000000000000000000, 0.8660254037844387076, 1.000000000000000000, 0.8660254037844387076, 1.000000000000000000, 0.8660254037844387076, 1.000000000000000000, 0.8660254037844387076, 1.000000000000000000, 0.8660254037844387076, 1.000000000000000000, 0.8660254037844387076, 1.000000000000000000, 0.8660254037844387076, 1.000000000000000000, 0.8660254037844387076, 1.000000000000000000, 0.8660254037844387076, 1.000000000000000000, 0.8660254037844387076, 1.000000000000000000, 0.8660254037844387076, 1.000000000000000000, 0.8660254037844387076, 1.000000000000000000, 0.8660254037844387076, 1.000000000000000000, 0.8660254037844387076, 1.000000000000000000, 0.8660254037844387076, 1.000000000000000000, 0.8660254037844387076, 1.000000000000000000, 0.8660254037844387076, 1.000000000000000000, 0.8660254037844387076, 1.000000000000000000, 0.8660254037844387076, 1.000000000000000000, 0.8660254037844387076, 1.000000000000000000, 0.8660254037844387076, 1.000000000000000000, 0.8660254037844387076, 1.000000000000000000, 0.8660254037844387076, 1.000000000000000000, 0.8660254037844387076, 1.000000000000000000, 0.8660254037844387076, 1.000000000000000000, 0.8660254037844387076, 1.000000000000000000, 0.8660254037844387076, 1.000000000000000000, 0.8660254037844387076, 1.000000000000000000, 0.8660254037844387076, 1.000000000000000000, 0.8660254037844387076, 1.000000000000000000, 0.8660254037844387076, 1.000000000000000000, 0.8660254037844387076, 1.000000000000000000, 0.8660254037844387076, 1.000000000000000000, 0.8660254037844387076, 1.000000000000000000, 0.8660254037844387076, 1.000000000000000000, 0.8660254037844387076, 1.000000000000000000, 0.8660254037844387076, 1.000000000000000000, 0.8660254037844387076, 1.000000000000000000, 0.8660254037844387076, 1.000000000000000000, 0.8660254037844387076, 1.000000000000000000, 0.8660254037844387076, 1.000000000000000000, 0.8660254037844387076, 1.000000000000000000),
 ( 1.000000000000000000, 0.8660254037844387076, 1.000000000000000000, 0.8660254037844387076, 1.000000000000000000, 0.8660254037844387076, 1.000000000000000000, 0.8660254037844387076, 1.000000000000000000, 0.8660254037844387076, 1.000000000000000000, 0.8660254037844387076, 1.000000000000000000, 0.8660254037844387076, 1.000000000000000000, 0.8660254037844387076, 1.000000000000000000, 0.8660254037844387076, 1.000000000000000000, 0.8660254037844387076, 1.000000000000000000, 0.8660254037844387076, 1.000000000000000000, 0.8660254037844387076, 1.000000000000000000, 0.8660254037844387076, 1.000000000000000000, 0.8660254037844387076, 1.000000000000000000, 0.8660254037844387076, 1.000000000000000000, 0.8660254037844387076, 1.000000000000000000, 0.8660254037844387076, 1.000000000000000000, 0.8660254037844387076, 1.000000000000000000, 0.8660254037844387076, 1.000000000000000000, 0.8660254037844387076, 1.000000000000000000, 0.8660254037844387076, 1.000000000000000000, 0.8660254037844387076, 1.000000000000000000, 0.8660254037844387076, 1.000000000000000000, 0.8660254037844387076, 1.000000000000000000, 0.8660254037844387076, 1.000000000000000000, 0.8660254037844387076, 1.000000000000000000, 0.8660254037844387076, 1.000000000000000000, 0.8660254037844387076, 1.000000000000000000, 0.8660254037844387076, 1.000000000000000000, 0.8660254037844387076, 1.000000000000000000, 0.8660254037844387076, 1.000000000000000000, 0.8660254037844387076, 1.000000000000000000, 0.8660254037844387076, 1.000000000000000000, 0.8660254037844387076, 1.000000000000000000, 0.8660254037844387076, 1.000000000000000000, 0.8660254037844387076, 1.000000000000000000, 0.8660254037844387076, 1.000000000000000000, 0.8660254037844387076, 1.000000000000000000, 0.8660254037844387076, 1.000000000000000000, 0.8660254037844387076, 1.000000000000000000, 0.8660254037844387076, 1.000000000000000000, 0.8660254037844387076, 1.000000000000000000, 0.8660254037844387076, 1.000000000000000000, 0.8660254037844387076, 1.000000000000000000, 0.8660254037844387076, 1.000000000000000000, 0.8660254037844387076, 1.000000000000000000, 0.8660254037844387076, 1.000000000000000000, 0.8660254037844387076, 1.000000000000000000, 0.8660254037844387076, 1.000000000000000000, 0.8660254037844387076, 1.000000000000000000, 0.8660254037844387076, 1.000000000000000000, 0.8660254037844387076, 1.000000000000000000, 0.8660254037844387076, 1.000000000000000000, 0.8660254037844387076, 1.000000000000000000, 0.8660254037844387076, 1.000000000000000000, 0.8660254037844387076, 1.000000000000000000, 0.8660254037844387076, 1.000000000000000000, 0.8660254037844387076, 1.000000000000000000, 0.8660254037844387076, 1.000000000000000000, 0.8660254037844387076, 1.000000000000000000, 0.8660254037844387076, 1.000000000000000000, 0.8660254037844387076, 1.000000000000000000, 0.8660254037844387076, 1.000000000000000000, 0.8660254037844387076, 1.000000000000000000, 0.8660254037844387076, 1.000000000000000000, 0.8660254037844387076, 1.000000000000000000, 0.8660254037844387076, 1.000000000000000000, 0.8660254037844387076, 1.000000000000000000, 0.8660254037844387076, 1.000000000000000000, 0.8660254037844387076, 1.000000000000000000, 0.8660254037844387076, 1.000000000000000000, 0.8660254037844387076, 1.000000000000000000, 0.8660254037844387076, 1.000000000000000000, 0.8660254037844387076, 1.000000000000000000, 0.8660254037844387076, 1.000000000000000000, 0.8660254037844387076, 1.000000000000000000, 0.8660254037844387076, 1.000000000000000000, 0.8660254037844387076, 1.000000000000000000, 0.8660254037844387076, 1.000000000000000000, 0.8660254037844387076, 1.000000000000000000, 0.8660254037844387076, 1.000000000000000000, 0.8660254037844387076, 1.000000000000000000, 0.8660254037844387076, 1.000000000000000000, 0.8660254037844387076, 1.000000000000000000, 0.8660254037844387076, 1.000000000000000000, 0.8660254037844387076, 1.000000000000000000, 0.8660254037844387076, 1.000000000000000000, 0.8660254037844387076, 1.000000000000000000, 0.8660254037844387076, 1.000000000000000000, 0.8660254037844387076, 1.000000000000000000, 0.8660254037844387076, 1.000000000000000000, 0.8660254037844387076, 1.000000000000000000, 0.8660254037844387076, 1.000000000000000000, 0.8660254037844387076, 1.000000000000000000, 0.8660254037844387076, 1.000000000000000000, 0.8660254037844387076, 1.000000000000000000, 0.8660254037844387076, 1.000000000000000000, 0.8660254037844387076, 1.000000000000000000, 0.8660254037844387076, 1.000000000000000000, 0.8660254037844387076, 1.000000000000000000, 0.8660254037844387076, 1.000000000000000000, 0.8660254037844387076, 1.000000000000000000, 0.8660254037844387076, 1.000000000000000000, 0.8660254037844387076, 1.000000000000000000, 0.8660254037844387076, 1.000000000000000000, 0.8660254037844387076, 1.000000000000000000, 0.8660254037844387076, 1.000000000000000000, 0.8660254037844387076, 1.000000000000000000, 0.8660254037844387076, 1.000000000000000000, 0.8660254037844387076, 1.000000000000000000, 0.8660254037844387076, 1.000000000000000000, 0.8660254037844387076, 1.000000000000000000, 0.8660254037844387076, 1.000000000000000000, 0.8660254037844387076, 1.000000000000000000, 0.8660254037844387076, 1.000000000000000000, 0.8660254037844387076, 1.000000000000000000, 0.8660254037844387076, 1.000000000000000000, 0.8660254037844387076, 1.000000000000000000, 0.8660254037844387076, 1.000000000000000000, 0.8660254037844387076, 1.000000000000000000, 0.8660254037844387076, 1.000000000000000000, 0.8660254037844387076, 1.000000000000000000, 0.8660254037844387076, 1.000000000000000000, 0.8660254037844387076, 1.000000000000000000, 0.8660254037844387076, 1.000000000000000000, 0.8660254037844387076, 1.000000000000000000, 0.8660254037844387076, 1.000000000000000000, 0.8660254037844387076, 1.000000000000000000, 0.8660254037844387076, 1.000000000000000000, 0.8660254037844387076, 1.000000000000000000, 0.8660254037844387076, 1.000000000000000000, 0.8660254037844387076, 1.000000000000000000, 0.8660254037844387076, 1.000000000000000000, 0.8660254037844387076, 1.000000000000000000, 0.8660254037844387076, 1.000000000000000000, 0.8660254037844387076, 1.000000000000000000, 0.8660254037844387076, 1.000000000000000000, 0.8660254037844387076, 1.000000000000000000, 0.8660254037844387076, 1.000000000000000000, 0.8660254037844387076, 1.000000000000000000, 0.8660254037844387076, 1.000000000000000000, 0.8660254037844387076, 1.000000000000000000, 0.8660254037844387076, 1.000000000000000000, 0.8660254037844387076, 1.000000000000000000, 0.8660254037844387076, 1.000000000000000000, 0.8660254037844387076, 1.000000000000000000, 0.8660254037844387076, 1.000000000000000000, 0.8660254037844387076, 1.000000000000000000, 0.8660254037844387076, 1.000000000000000000, 0.8660254037844387076, 1.000000000000000000, 0.8660254037844387076, 1.000000000000000000, 0.8660254037844387076, 1.000000000000000000, 0.8660254037844387076, 1.000000000000000000, 0.8660254037844387076, 1.000000000000000000, 0.8660254037844387076, 1.000000000000000000, 0.8660254037844387076, 1.000000000000000000, 0.8660254037844387076, 1.000000000000000000, 0.8660254037844387076, 1.000000000000000000, 0.8660254037844387076, 1.000000000000000000, 0.8660254037844387076, 1.000000000000000000, 0.8660254037844387076, 1.000000000000000000, 0.8660254037844387076, 1.000000000000000000, 0.8660254037844387076, 1.000000000000000000, 0.8660254037844387076, 1.000000000000000000, 0.8660254037844387076, 1.000000000000000000, 0.8660254037844387076, 1.000000000000000000, 0.8660254037844387076, 1.000000000000000000, 0.8660254037844387076, 1.000000000000000000) ) ) 
 REPRESENTATION_ITEM ( '' )  SURFACE ( )  );
#72167=CARTESIAN_POINT ( 'NONE',  ( 1.364683531249986537, 0.6135416670080880985, 0.7879004041258500513 ) ) ;
#72171=CARTESIAN_POINT ( 'NONE',  ( -0.2103062557254962439, 6.366301347167508951, -3.121735129556555854 ) ) ;
#72177=CARTESIAN_POINT ( 'NONE',  ( 4.168242161197552420, 6.950367390450747251, -1.199719254218452047 ) ) ;
#72187=CARTESIAN_POINT ( 'NONE',  ( 8.718056468787178659, 10.12981962079525289, 1.199719254218462483 ) ) ;
#72195=CARTESIAN_POINT ( 'NONE',  ( 6.938893903907228378E-15, 10.64264068711930733, 1.214306433183764966E-14 ) ) ;
#72200=CARTESIAN_POINT ( 'NONE',  ( -7.375272376154093479, 9.627570410311676596, -1.443375672974059665 ) ) ;
#72204=CARTESIAN_POINT ( 'NONE',  ( -8.947491310014823895, 12.52615806407091803, 1.199719254218462483 ) ) ;
#72209=CARTESIAN_POINT ( 'NONE',  ( -4.623494077460110319, 5.352830164246910272, 1.199719254218462483 ) ) ;
#72211=CARTESIAN_POINT ( 'NONE',  ( 9.531545685607134999, 11.07889037375188401, 1.199719254218450271 ) ) ;
#72213=CARTESIAN_POINT ( 'NONE',  ( 5.355634372598031767, 6.206993841907870291, -1.199719254218445830 ) ) ;
#72219=CARTESIAN_POINT ( 'NONE',  ( 3.497640442645619796, 6.064035702186436616, -1.082531754730543083 ) ) ;
#72221=CARTESIAN_POINT ( 'NONE',  ( -6.078132937628113908, 5.985576603521232109, 1.040834085586084257E-14 ) ) ;
#72224=CARTESIAN_POINT ( 'NONE',  ( -10.64723070543352712, 11.31619066596094392, 0.7998128361456462443 ) ) ;
#72230=CARTESIAN_POINT ( 'NONE',  ( 7.239690840017413365, 10.42976116578691403, -1.082531754730537976 ) ) ;
#72231=CARTESIAN_POINT ( 'NONE',  ( -0.6823417656249969321, 3.530208333674754506, -1.181850606188749264 ) ) ;
#72233=CARTESIAN_POINT ( 'NONE',  ( 4.630273154266905777, 5.360739087188218122, 1.199719254218464037 ) ) ;
#72245=DIRECTION ( 'NONE',  ( -0.5038915848355121074, -0.5182601445832860643, -0.6910135261110795790 ) ) ;
#72248=CARTESIAN_POINT ( 'NONE',  ( -0.6823417656250212460, 2.113541667008083991, 1.181850606188767472 ) ) ;
#72250=CARTESIAN_POINT ( 'NONE',  ( 4.227444969362701421, 3.826440640544909400, 1.214306433183764966E-14 ) ) ;
#72252=CARTESIAN_POINT ( 'NONE',  ( -6.887178846062128379, 7.137389529935019183, -0.7216878364870278340 ) ) ;
#72254=CARTESIAN_POINT ( 'NONE',  ( 2.873965376416980355, 6.296784005887697155, -0.7216878364870267237 ) ) ;
#72255=CARTESIAN_POINT ( 'NONE',  ( -6.046573321570485327, 6.156683084694754449, 0.000000000000000000 ) ) ;
#72259=CARTESIAN_POINT ( 'NONE',  ( 4.310602774141044868, 7.116454772218158809, -1.199719254218452047 ) ) ;
#72265=CARTESIAN_POINT ( 'NONE',  ( 0.006800380015298257419, 7.009756401597622144, -1.999988438674496383 ) ) ;
#72269=CARTESIAN_POINT ( 'NONE',  ( 6.979750152936881058, 7.037463354714830643, 0.7998128361456341429 ) ) ;
#72270=( NAMED_UNIT ( * ) PLANE_ANGLE_UNIT ( ) SI_UNIT ( $, .RADIAN. ) );
#72272=CARTESIAN_POINT ( 'NONE',  ( -4.437596350374534815, 4.071617251725375475, -0.7998128361456221525 ) ) ;
#72274=CARTESIAN_POINT ( 'NONE',  ( -6.632963465583701534, 8.761543347979550589, -1.599625672291263179 ) ) ;
#72278=CARTESIAN_POINT ( 'NONE',  ( 6.425674737872927089, 9.584038729905381970, -1.199719254218440723 ) ) ;
#72281=CARTESIAN_POINT ( 'NONE',  ( -7.576308911938196999, 7.733448573549685179, 0.7998128361456462443 ) ) ;
#72283=CARTESIAN_POINT ( 'NONE',  ( 7.280365300414074703, 7.596107060012304402, -0.7216878364870257245 ) ) ;
#72284=CARTESIAN_POINT ( 'NONE',  ( 4.161918892217930654, 7.618187422415517496, 0.8381857273355892701 ) ) ;
#72285=CARTESIAN_POINT ( 'NONE',  ( -5.057354993097396445, 5.859001232490445688, -1.199719254218446718 ) ) ;
#72288=CARTESIAN_POINT ( 'NONE',  ( -6.521635583373313061, 7.567328587812373719, -1.199719254218446718 ) ) ;
#72292=CARTESIAN_POINT ( 'NONE',  ( -1.201851678989727383E-14, 1.321875000341419248, 1.575800808251672791 ) ) ;
#72294=CARTESIAN_POINT ( 'NONE',  ( -5.233084105194862445, 9.049089189461916760, 0.7216878364870458196 ) ) ;
#72299=B_SPLINE_CURVE_WITH_KNOTS ( 'NONE', 3,
 ( #145019, #87456, #19230, #182799 ),
 .UNSPECIFIED., .F., .F.,
 ( 4, 4 ),
 ( 1.127778740529212779E-17, 0.0001292189244442736897 ),
 .UNSPECIFIED. ) ;
#72301=CARTESIAN_POINT ( 'NONE',  ( 4.645640190976921602, 8.571663989448405019, 1.040834085586084257E-14 ) ) ;
#72304=CARTESIAN_POINT ( 'NONE',  ( -5.882246656098474524, 6.017915526194586917, -0.2943127404537674296 ) ) ;
#72305=CARTESIAN_POINT ( 'NONE',  ( 0.6823417656249899377, 0.9052083336747520637, 1.181850606188755259 ) ) ;
#72308=CARTESIAN_POINT ( 'NONE',  ( 1.364683531249986537, -0.7822916663252464931, -0.7879004041258309554 ) ) ;
#72312=CARTESIAN_POINT ( 'NONE',  ( -3.815730167242251003, 6.539103397502874948, -1.199719254218452047 ) ) ;
#72313=CARTESIAN_POINT ( 'NONE',  ( -8.473482818416682605, 8.988077497682020578, -0.7216878364870267237 ) ) ;
#72321=CARTESIAN_POINT ( 'NONE',  ( -6.846504384776755714, 9.971043634672792422, -1.082531754730537088 ) ) ;
#72323=CARTESIAN_POINT ( 'NONE',  ( -0.7500000000000215383, 2.972916667349487341, 1.299038105676671107 ) ) ;
#72327=CARTESIAN_POINT ( 'NONE',  ( -8.663296969008007054, 9.209527340038563992, 0.7216878364870438212 ) ) ;
#72341=CARTESIAN_POINT ( 'NONE',  ( -5.343885102080728977, 9.386283052402845328, 0.7998128361456481317 ) ) ;
#72344=CARTESIAN_POINT ( 'NONE',  ( 4.416205349749311004, 6.175325546172740765, 1.599625672291267398 ) ) ;
#72346=EDGE_CURVE ( 'NONE', #179068, #17744, #140583, .T. ) ;
#72349=CARTESIAN_POINT ( 'NONE',  ( 6.979750152936881058, 7.037463354714830643, 0.7998128361456341429 ) ) ;
#72355=CARTESIAN_POINT ( 'NONE',  ( -3.795919822146283540, 6.412028311603867436, -1.082531754730549967 ) ) ;
#72366=CARTESIAN_POINT ( 'NONE',  ( -0.6823417656250003738, 0.4677083336747517306, -1.181850606188749264 ) ) ;
#72368=CARTESIAN_POINT ( 'NONE',  ( -9.338868881714763148, 9.789768538289042255, -0.7998128361456291469 ) ) ;
#72371=CARTESIAN_POINT ( 'NONE',  ( 6.435316467980822353, 10.65961964595298817, 1.040834085586084257E-14 ) ) ;
#72373=CARTESIAN_POINT ( 'NONE',  ( -7.330154606482786050, 11.70359747420527619, 0.000000000000000000 ) ) ;
#72376=CARTESIAN_POINT ( 'NONE',  ( 0.6823417656249917140, 5.342708333674749177, 1.181850606188765695 ) ) ;
#72379=CARTESIAN_POINT ( 'NONE',  ( 9.734391104931955141, 10.45913716528321125, 0.7216878364870438212 ) ) ;
#72382=CARTESIAN_POINT ( 'NONE',  ( -1.500000000000011324, 5.879166666666686858, -0.8660254037844313801 ) ) ;
#72385=CARTESIAN_POINT ( 'NONE',  ( 6.765155463094746580, 9.876136559377135526, 1.082531754730558626 ) ) ;
#72388=CARTESIAN_POINT ( 'NONE',  ( -4.934804725694212912, 8.701096580044490381, -0.7216878364870207285 ) ) ;
#72390=CARTESIAN_POINT ( 'NONE',  ( -1.364683531250012516, 3.280208333674756727, 0.7879004041258379498 ) ) ;
#72394=CARTESIAN_POINT ( 'NONE',  ( -5.205440912643032547, 8.160432600470439723, 1.199719254218452047 ) ) ;
#72400=CARTESIAN_POINT ( 'NONE',  ( 8.229962938695207342, 9.560377169021284871, 1.199719254218462483 ) ) ;
#72403=CARTESIAN_POINT ( 'NONE',  ( -1.201851678989727383E-14, 0.7125000000000225597, 1.732050807568877637 ) ) ;
#72408=ORIENTED_EDGE ( 'NONE', *, *, #50440, .T. ) ;
#72409=CARTESIAN_POINT ( 'NONE',  ( 5.910991785878156435, 7.919243054989755670, -1.443375672974057666 ) ) ;
#72410=CARTESIAN_POINT ( 'NONE',  ( 0.6823417656249882723, -0.5947916663252492686, 1.181850606188755259 ) ) ;
#72417=CARTESIAN_POINT ( 'NONE',  ( 6.089583550832340819, 10.25626457594641749, 1.040834085586084257E-14 ) ) ;
#72418=CARTESIAN_POINT ( 'NONE',  ( -7.641992139597101108, 12.06740792950531649, 0.7998128361456481317 ) ) ;
#72420=CARTESIAN_POINT ( 'NONE',  ( -1.364683531250014514, -0.01145833299191483488, -0.7879004041258359514 ) ) ;
#72421=CARTESIAN_POINT ( 'NONE',  ( 0.7499999999999885647, 1.566666666666688412, -1.299038105676652899 ) ) ;
#72423=CARTESIAN_POINT ( 'NONE',  ( 5.066996723205273057, 6.934582148538044777, 1.599625672291267398 ) ) ;
#72429=CARTESIAN_POINT ( 'NONE',  ( -0.6823417656249969321, 4.717708333674755394, -1.181850606188749264 ) ) ;
#72431=CARTESIAN_POINT ( 'NONE',  ( -8.993135964566285168, 9.386413468282476913, -0.7998128361456291469 ) ) ;
#72432=CARTESIAN_POINT ( 'NONE',  ( -4.107757355260591936, 7.736207981205250661, 1.040834085586084257E-14 ) ) ;
#72441=CARTESIAN_POINT ( 'NONE',  ( 6.089583550832340819, 10.25626457594641749, 1.040834085586084257E-14 ) ) ;
#72442=CARTESIAN_POINT ( 'NONE',  ( -5.436456409399874623, 5.444880020495701523, 0.000000000000000000 ) ) ;
#72446=CARTESIAN_POINT ( 'NONE',  ( 6.100805936025112786, 10.06143132543056673, 1.040834085586084257E-14 ) ) ;
#72450=CARTESIAN_POINT ( 'NONE',  ( -8.532158741701643123, 8.848606708273724308, 0.7998128361456462443 ) ) ;
#72451=CARTESIAN_POINT ( 'NONE',  ( 6.491656622844908853, 6.468020902940851968, 0.7998128361456341429 ) ) ;
#72453=CARTESIAN_POINT ( 'NONE',  ( 2.968872451268290913, 5.447139712246216625, -1.082531754730543971 ) ) ;
#72455=CARTESIAN_POINT ( 'NONE',  ( 2.686486993802192913, 6.285985259411197568, 0.7998128361456362523 ) ) ;
#72456=ORIENTED_EDGE ( 'NONE', *, *, #63234, .T. ) ;
#72459=CARTESIAN_POINT ( 'NONE',  ( -1.500000000000022204, 6.280000000000042881, 2.873333333333347728 ) ) ;
#72463=CARTESIAN_POINT ( 'NONE',  ( -6.236387472606166327, 6.378132927569716060, -0.7216878364870278340 ) ) ;
#72464=CARTESIAN_POINT ( 'NONE',  ( 8.920901888111986366, 12.39117405523060889, 1.082531754730546636 ) ) ;
#72467=CARTESIAN_POINT ( 'NONE',  ( -6.826694039680798021, 7.923230120171105284, -1.199719254218446718 ) ) ;
#72472=CARTESIAN_POINT ( 'NONE',  ( -8.993135964566285168, 9.386413468282476913, -0.7998128361456291469 ) ) ;
#72473=DIRECTION ( 'NONE',  ( 0.7592566023653005702, -0.6507913734559639396, 0.000000000000000000 ) ) ;
#72476=CARTESIAN_POINT ( 'NONE',  ( 6.498435699651741615, 6.475929825882159818, -0.7998128361456281477 ) ) ;
#72479=ORIENTED_EDGE ( 'NONE', *, *, #68958, .T. ) ;
#72487=CARTESIAN_POINT ( 'NONE',  ( -6.471393748265538370, 5.229711127717889596, -2.419999999999995044 ) ) ;
#72488=CARTESIAN_POINT ( 'NONE',  ( -6.073162743917628781, 9.172774736957510555, -1.199719254218440723 ) ) ;
#72491=CARTESIAN_POINT ( 'NONE',  ( 4.202664430556241726, 7.846932902383524144, 0.7216878364870298324 ) ) ;
#72493=B_SPLINE_CURVE_WITH_KNOTS ( 'NONE', 3,
 ( #193593, #142756, #141696, #125486, #160035, #143831, #25751, #112416, #11638, #144892 ),
 .UNSPECIFIED., .F., .F.,
 ( 4, 3, 3, 4 ),
 ( 0.000000000000000000, 6.251591618973408526E-05, 0.0001610295297539614614, 0.0002600460447856825378 ),
 .UNSPECIFIED. ) ;
#72498=CARTESIAN_POINT ( 'NONE',  ( -4.761938266897808525, 6.578680616179308771, 1.599625672291267398 ) ) ;
#72502=CARTESIAN_POINT ( 'NONE',  ( -5.018489415352746619, 9.006654751220198207, 0.7998128361456481317 ) ) ;
#72509=CARTESIAN_POINT ( 'NONE',  ( -9.989660255170729641, 10.54902514065433827, -0.7998128361456291469 ) ) ;
#72510=CARTESIAN_POINT ( 'NONE',  ( 5.601490020740366838, 9.686822124172440596, 1.040834085586084257E-14 ) ) ;
#72513=CARTESIAN_POINT ( 'NONE',  ( -2.982430605326328532, 5.462957558647244305, -1.082531754730543971 ) ) ;
#72515=CARTESIAN_POINT ( 'NONE',  ( -8.947491310014823895, 12.52615806407091803, 1.199719254218462483 ) ) ;
#72522=CARTESIAN_POINT ( 'NONE',  ( 9.137832345930652522, 10.72352116074969075, -1.082531754730543083 ) ) ;
#72542=CARTESIAN_POINT ( 'NONE',  ( -4.298098390732130625, 4.973201863064262263, 1.199719254218462483 ) ) ;
#72545=CARTESIAN_POINT ( 'NONE',  ( -4.135400547368138113, 4.783387712472935149, 1.199719254218462483 ) ) ;
#72550=CARTESIAN_POINT ( 'NONE',  ( -0.6823417656250212460, 5.301041667008086655, 1.181850606188767472 ) ) ;
#72553=CARTESIAN_POINT ( 'NONE',  ( -4.175548123328963079, 4.934189567714277302, 1.082531754730560403 ) ) ;
#72555=FACE_OUTER_BOUND ( 'NONE', #150767, .T. ) ;
#72559=CARTESIAN_POINT ( 'NONE',  ( 4.054051625686104998, 4.688480637177271149, -1.199719254218446718 ) ) ;
#72560=CARTESIAN_POINT ( 'NONE',  ( -3.429849674132907200, 6.945315686556337909, -0.7216878364870036311 ) ) ;
#72563=CARTESIAN_POINT ( 'NONE',  ( 8.880227426826630577, 12.34372051706435869, 1.082531754730546636 ) ) ;
#72565=CARTESIAN_POINT ( 'NONE',  ( 0.6823417656249882723, 2.488541667008084435, -1.181850606188749264 ) ) ;
#72568=CARTESIAN_POINT ( 'NONE',  ( -7.458957065812611198, 11.85386701009007204, 0.7998128361456481317 ) ) ;
#72569=CARTESIAN_POINT ( 'NONE',  ( -4.189106276498259618, 6.870745841681152655, 1.082531754730560403 ) ) ;
#72571=CARTESIAN_POINT ( 'NONE',  ( -6.552668314106420588, 6.539201209412602189, -0.7998128361456291469 ) ) ;
#72573=CARTESIAN_POINT ( 'NONE',  ( 1.364683531249990311, 5.134375000341417916, 1.214306433183764966E-14 ) ) ;
#72581=CARTESIAN_POINT ( 'NONE',  ( -4.541618270453545492, 8.242379048930368768, 0.7216878364870458196 ) ) ;
#72582=CARTESIAN_POINT ( 'NONE',  ( 7.334597915313080918, 9.580116872663850813, 1.040834085586084257E-14 ) ) ;
#72583=EDGE_CURVE ( 'NONE', #61877, #76077, #162467, .T. ) ;
#72587=CARTESIAN_POINT ( 'NONE',  ( -3.592547517496929466, 7.135129837147637488, -0.7216878364870257245 ) ) ;
#72589=CARTESIAN_POINT ( 'NONE',  ( 9.748476143425788720, 11.33197590787365172, -1.199719254218440723 ) ) ;
#72599=CARTESIAN_POINT ( 'NONE',  ( -5.278201874421821316, 5.052323696447222900, 0.7998128361456341429 ) ) ;
#72600=CARTESIAN_POINT ( 'NONE',  ( -9.459838494033043332, 12.05956421450382088, 1.599625672291281386 ) ) ;
#72603=ORIENTED_EDGE ( 'NONE', *, *, #206842, .T. ) ;
#72605=CARTESIAN_POINT ( 'NONE',  ( 6.830610463186557624, 6.863467050006115677, 1.040834085586084257E-14 ) ) ;
#72611=CARTESIAN_POINT ( 'NONE',  ( 3.469446951953614189E-15, 5.900000000000023448, 1.214306433183764966E-14 ) ) ;
#72612=CARTESIAN_POINT ( 'NONE',  ( 2.191614386903386613, 5.708633884695917260, -0.7998128361456281477 ) ) ;
#72614=EDGE_LOOP ( 'NONE', ( #199952, #188334, #70043, #120916 ) ) ;
#72622=CARTESIAN_POINT ( 'NONE',  ( 7.072549687823125097, 11.40305840243567381, -0.7998128361456291469 ) ) ;
#72623=CARTESIAN_POINT ( 'NONE',  ( -5.935772324684618795, 5.819489221753827657, 0.000000000000000000 ) ) ;
#72629=CARTESIAN_POINT ( 'NONE',  ( -1.364683531250010295, 4.280208333674753618, 0.7879004041258379498 ) ) ;
#72631=CARTESIAN_POINT ( 'NONE',  ( -5.575427483717760424, 7.527751369135936343, 1.599625672291269396 ) ) ;
#72633=EDGE_CURVE ( 'NONE', #40394, #169854, #164285, .T. ) ;
#72636=CARTESIAN_POINT ( 'NONE',  ( 4.008406971134620633, 7.828225232965717595, 0.7998128361456321445 ) ) ;
#72637=CARTESIAN_POINT ( 'NONE',  ( -4.436542580169821726, 6.199052314996659874, 1.599625672291267398 ) ) ;
#72644=CARTESIAN_POINT ( 'NONE',  ( 7.185458225562760148, 8.445751353653788485, -1.082531754730543083 ) ) ;
#72646=CARTESIAN_POINT ( 'NONE',  ( 6.277061933002774374, 9.306694107603160404, 1.082531754730558626 ) ) ;
#72647=CARTESIAN_POINT ( 'NONE',  ( 1.364683531249990311, 2.946875000341416140, 1.214306433183764966E-14 ) ) ;
#72649=CARTESIAN_POINT ( 'NONE',  ( 6.127922243252466039, 6.251590159990418449, 1.040834085586084257E-14 ) ) ;
#72651=CARTESIAN_POINT ( 'NONE',  ( 4.991989969715272757, 4.726297878971393196, 2.500000000000011102 ) ) ;
#72657=CARTESIAN_POINT ( 'NONE',  ( -4.661943307450316709, 7.086702294391122869, 1.392663581761391267 ) ) ;
#72658=LINE ( 'NONE', #88940, #6332 ) ;
#72663=CARTESIAN_POINT ( 'NONE',  ( -8.479735010343349089, 11.98044238112085758, 1.199719254218453823 ) ) ;
#72668=CARTESIAN_POINT ( 'NONE',  ( -3.379006598303881059, 4.965260336153046516, -1.599625672291256295 ) ) ;
#72672=EDGE_CURVE ( 'NONE', #98551, #8852, #90416, .T. ) ;
#72674=CARTESIAN_POINT ( 'NONE',  ( 3.714570900464278846, 5.356752022006865843, 1.443375672974062551 ) ) ;
#72676=CARTESIAN_POINT ( 'NONE',  ( 1.364683531249988535, 3.967708333674751842, -0.7879004041258239610 ) ) ;
#72678=CARTESIAN_POINT ( 'NONE',  ( 8.776205506747620788, 9.133327934160710981, -0.7998128361456221525 ) ) ;
#72679=CARTESIAN_POINT ( 'NONE',  ( -8.482597663644387609, 13.04811437422715414, -0.7998128361456281477 ) ) ;
#72686=CARTESIAN_POINT ( 'NONE',  ( 1.499999999999987121, 3.545833333333356041, -0.8660254037844262731 ) ) ;
#72687=CARTESIAN_POINT ( 'NONE',  ( 4.310602774141044868, 7.116454772218158809, -1.199719254218452047 ) ) ;
#72690=CARTESIAN_POINT ( 'NONE',  ( -1.123270288250343141, 2.846052654332832610, 0.7749999999993751887 ) ) ;
#72691=CARTESIAN_POINT ( 'NONE',  ( -1.364683531249997417, 3.759375000341423689, 1.214306433183764966E-14 ) ) ;
#72693=CARTESIAN_POINT ( 'NONE',  ( 8.215877900201359552, 11.56864606933486606, -1.082531754730543083 ) ) ;
#72698=CARTESIAN_POINT ( 'NONE',  ( -1.500000000000001332, 1.431250000682816825, 0.000000000000000000 ) ) ;
#72700=CARTESIAN_POINT ( 'NONE',  ( -5.473741331615264549, 7.409117525016355010, -1.599625672291256295 ) ) ;
#72701=CARTESIAN_POINT ( 'NONE',  ( 5.192409643909512873, 6.120528008391641350, -1.082531754730549078 ) ) ;
#72710=CARTESIAN_POINT ( 'NONE',  ( 8.121497709785879593, 9.433834401960398353, -1.199719254218445830 ) ) ;
#72711=CARTESIAN_POINT ( 'NONE',  ( 5.066996723205273057, 6.934582148538044777, 1.599625672291267398 ) ) ;
#72715=CARTESIAN_POINT ( 'NONE',  ( 5.307127064745490230, 8.279066444590018392, -1.199719254218452935 ) ) ;
#72723=CARTESIAN_POINT ( 'NONE',  ( 7.892817981449907982, 12.36003807833360391, 0.7998128361456462443 ) ) ;
#72728=CARTESIAN_POINT ( 'NONE',  ( 5.181774431428755712, 6.445567486282277159, 1.182616053296376979 ) ) ;
#72736=CARTESIAN_POINT ( 'NONE',  ( -1.445103857048105844, 8.688264192037886247, -2.625611233228243968 ) ) ;
#72738=CARTESIAN_POINT ( 'NONE',  ( 7.483737605063422116, 7.833374748769873719, -0.7216878364870257245 ) ) ;
#72739=CARTESIAN_POINT ( 'NONE',  ( -3.578462479003122976, 6.262291094557191684, 1.199719254218464037 ) ) ;
#72742=CARTESIAN_POINT ( 'NONE',  ( -5.579343907223557331, 6.467988298970945849, 1.199719254218450271 ) ) ;
#72746=CARTESIAN_POINT ( 'NONE',  ( 1.387358672525637715, 7.251968950354889643, -4.302625267139783993 ) ) ;
#72750=ORIENTED_EDGE ( 'NONE', *, *, #96141, .F. ) ;
#72756=CARTESIAN_POINT ( 'NONE',  ( 7.560643217915098191, 11.97250085420964716, -0.7998128361456291469 ) ) ;
#72764=CARTESIAN_POINT ( 'NONE',  ( -8.649738815838677652, 13.03518635187974262, 0.7216878364870357165 ) ) ;
#72768=CARTESIAN_POINT ( 'NONE',  ( 7.242026607993941489, 11.60078147596829901, 0.7998128361456462443 ) ) ;
#72773=CARTESIAN_POINT ( 'NONE',  ( -5.551173829791513192, 8.563787670477010394, 1.199719254218452047 ) ) ;
#72774=CARTESIAN_POINT ( 'NONE',  ( 4.009460741339333723, 5.700790169694431420, -1.599625672291256295 ) ) ;
#72781=CARTESIAN_POINT ( 'NONE',  ( -1.201851678989727383E-14, 2.134375000341423689, 1.575800808251672791 ) ) ;
#72783=CARTESIAN_POINT ( 'NONE',  ( 6.317736394288131052, 9.354147645769410602, 1.082531754730558626 ) ) ;
#72790=CARTESIAN_POINT ( 'NONE',  ( 9.368320956918614328, 10.99242454023565507, 1.082531754730549967 ) ) ;
#72791=EDGE_CURVE ( 'NONE', #106888, #23582, #38451, .T. ) ;
#72792=( BOUNDED_CURVE ( )  B_SPLINE_CURVE ( 2, ( #184118, #36801, #106133 ),
 .UNSPECIFIED., .F., .T. ) 
 B_SPLINE_CURVE_WITH_KNOTS ( ( 3, 3 ),
 ( 0.1472187422488249742, 0.1500000000000002165 ),
 .UNSPECIFIED. ) 
 CURVE ( )  GEOMETRIC_REPRESENTATION_ITEM ( )  RATIONAL_B_SPLINE_CURVE ( ( 0.9405305184077480396, 0.9105717077955798322, 1.000000000000007105 ) ) 
 REPRESENTATION_ITEM ( '' )  );
#72796=CARTESIAN_POINT ( 'NONE',  ( -9.016335848287868160, 10.47781223021269170, 1.199719254218462483 ) ) ;
#72804=CARTESIAN_POINT ( 'NONE',  ( 4.891794496432329886, 4.601515088792824670, -0.7998128361456211532 ) ) ;
#72811=CARTESIAN_POINT ( 'NONE',  ( 4.286349120214771879, 8.152491073559232859, -0.7998128361456221525 ) ) ;
#72814=CARTESIAN_POINT ( 'NONE',  ( 0.7499999999999885647, 2.847916667349487341, -1.299038105676658228 ) ) ;
#72819=CARTESIAN_POINT ( 'NONE',  ( -1.500000000000015099, 0.8791666666666874130, -0.8660254037844313801 ) ) ;
#72820=CARTESIAN_POINT ( 'NONE',  ( 7.938462636001388795, 9.220293482545153907, -1.199719254218441611 ) ) ;
#72821=CARTESIAN_POINT ( 'NONE',  ( -0.6823417656250003738, -0.5322916663252491576, -1.181850606188749264 ) ) ;
#72825=CARTESIAN_POINT ( 'NONE',  ( 9.137832345930652522, 10.72352116074969075, -1.082531754730543083 ) ) ;
#72829=CARTESIAN_POINT ( 'NONE',  ( -4.869349725602420520, 8.832658446511480577, 1.040834085586084257E-14 ) ) ;
#72830=CARTESIAN_POINT ( 'NONE',  ( -1.499999999999997780, 3.181250000682818602, 1.214306433183764966E-14 ) ) ;
#72831=CARTESIAN_POINT ( 'NONE',  ( -1.364683531250014514, -1.219791666325248602, 0.7879004041258379498 ) ) ;
#72836=CARTESIAN_POINT ( 'NONE',  ( -1.001543065824772872E-14, 4.634375000341418804, 1.575800808251672791 ) ) ;
#72844=CARTESIAN_POINT ( 'NONE',  ( -9.179033691651859783, 10.66762638080401260, 1.199719254218462483 ) ) ;
#72845=CARTESIAN_POINT ( 'NONE',  ( 5.445571254183207088, 9.504916896522420444, -0.7998128361456281477 ) ) ;
#72846=CARTESIAN_POINT ( 'NONE',  ( 3.847109862837356786, 4.045599327266925727, -0.8077998227820462063 ) ) ;
#72851=CARTESIAN_POINT ( 'NONE',  ( -7.314787569772770226, 8.492672571945082183, -1.199719254218452935 ) ) ;
#72856=CARTESIAN_POINT ( 'NONE',  ( 2.218730694130720771, 5.740269576461138890, 0.7998128361456462443 ) ) ;
#72860=CARTESIAN_POINT ( 'NONE',  ( -5.752737250900127997, 5.605948302338584099, 0.000000000000000000 ) ) ;
#72862=CARTESIAN_POINT ( 'NONE',  ( -9.643927338022246332, 10.14567007064778004, -0.7998128361456291469 ) ) ;
#72865=CARTESIAN_POINT ( 'NONE',  ( -4.014602626671047503, 7.795841479962435372, -0.4363419845254731255 ) ) ;
#72872=CARTESIAN_POINT ( 'NONE',  ( 6.277588818327314080, 7.282607361925381717, 1.199719254218462483 ) ) ;
#72874=CARTESIAN_POINT ( 'NONE',  ( 6.509799877575638050, 5.178456542363086612, 2.500000000000010214 ) ) ;
#72892=CARTESIAN_POINT ( 'NONE',  ( 3.226477370372293763, 6.708047998835573900, 0.7216878364870317197 ) ) ;
#72894=ORIENTED_EDGE ( 'NONE', *, *, #2500, .F. ) ;
#72897=CARTESIAN_POINT ( 'NONE',  ( -8.513630394377489807, 12.01998699582738972, -1.199719254218446718 ) ) ;
#72904=CARTESIAN_POINT ( 'NONE',  ( -1.201851678989727383E-14, 1.993750000682816381, 1.732050807568877637 ) ) ;
#72910=CARTESIAN_POINT ( 'NONE',  ( 0.6823417656249899377, 0.8427083336747520637, 1.181850606188755259 ) ) ;
#72912=VERTEX_POINT ( 'NONE', #108684 ) ;
#72916=CARTESIAN_POINT ( 'NONE',  ( -2.903417451620861289, 6.539070793532962611, 0.7998128361456341429 ) ) ;
#72918=CARTESIAN_POINT ( 'NONE',  ( 1.500000000000001332, 7.809254910133564209, -3.635752117228656211 ) ) ;
#72921=CARTESIAN_POINT ( 'NONE',  ( 1.364683531249986537, -0.2822916663252520997, -0.7879004041258309554 ) ) ;
#72926=CARTESIAN_POINT ( 'NONE',  ( -0.6823417656250212460, 0.8010416670080899859, 1.181850606188755259 ) ) ;
#72928=CARTESIAN_POINT ( 'NONE',  ( -6.367525699912501835, 10.58053041653993098, -0.7998128361456291469 ) ) ;
#72929=CARTESIAN_POINT ( 'NONE',  ( 8.320953590485093088, 10.73086516036454618, 1.599625672291281386 ) ) ;
#72934=CARTESIAN_POINT ( 'NONE',  ( 1.364683531249986537, 0.9260416670080896528, 0.7879004041258500513 ) ) ;
#72939=B_SPLINE_SURFACE_WITH_KNOTS ( 'NONE', 1, 3, ( 
 ( #57144, #140570, #91807, #104844, #55016, #72304, #38763, #170890, #139484, #59271, #138409, #25699, #105943, #56083, #8383, #22482, #21410, #5155, #89666, #88593, #154650, #71231, #43057, #23558, #122241, #40913, #188199, #39836, #155717, #87520, #206583, #58211, #7302, #203364, #205512, #123310, #189274, #124370, #107019, #187134, #174126, #173043, #24626, #137346, #121165, #90733, #141641, #190328, #41989, #108097, #157865, #9458, #75530, #207650, #125426, #191392, #109170, #78716, #196744, #179441, #96071, #194603, #48384, #175183, #144843, #60335, #210849, #193544, #46247, #62475, #142699, #143778, #31061, #26770, #92871, #161049, #145900, #178377, #211909, #195684, #95003, #113434, #45186, #130750, #47321, #126496, #128638, #11584, #27844, #212970, #12645, #77656, #158917, #111301, #192459, #112364, #176242, #93942, #177304, #10513, #162124, #63546, #209773, #208708, #29986, #61413, #28918, #129702, #159982, #44113, #97137, #127576, #13713, #76588, #110234, #79786, #80865, #163191, #14774, #146955, #64611, #198844, #49428, #131787, #214017, #101363, #50491, #17960, #136014, #118745, #35288, #133912, #202027, #114497, #84046, #65639, #150134, #132840, #199918, #1707, #81919, #82977, #184729, #180495, #32112, #66693, #116612, #115548, #102431, #151199, #200969, #98197, #67761, #164245, #181544, #19033, #166368, #152256, #167441, #33172, #86187, #99253, #51565, #68841, #52617, #85113, #15833, #148006, #134961, #197792, #36354, #182606, #165301, #34229, #168500, #100302, #16896, #2770, #117690, #183682, #20099, #149050, #628, #3830, #69904, #89407, #70972, #87255, #56888, #155456, #55818, #7039, #121975, #8129, #189017, #38507, #74215, #73116, #139217, #106760, #124118, #137082, #172789, #187939, #141391, #40659, #186875, #75276, #90472, #91551, #153319, #22216, #204163, #24361, #9204, #54752, #140310, #205247, #23297, #21149, #104585, #120902, #123063, #190081, #156539, #203107, #185798, #170630, #88329, #206328, #154393, #53687, #25444, #39569, #57953, #41733, #107842, #4894, #173870, #157608, #119818, #37431, #103509, #169568, #105671, #5971 ),
 ( #72041, #138154, #171698, #108912, #161876, #174934, #79539, #61156, #208453, #143520, #13463, #11325, #142445, #45998, #209515, #44933, #144587, #207401, #158665, #127318, #29735, #28665, #10263, #26515, #210601, #94750, #193288, #160798, #111041, #145657, #128388, #192204, #211653, #12389, #78468, #112117, #63291, #76338, #92623, #43866, #60085, #126243, #177048, #30807, #109982, #129451, #77403, #27586, #194355, #175992, #59020, #191138, #62230, #96887, #178120, #93684, #80611, #95817, #159726, #195434, #47063, #113180, #179184, #125176, #162936, #14517, #42803, #114247, #198590, #49183, #148803, #35028, #213768, #97947, #84861, #131536, #98995, #81664, #1447, #115302, #181292, #67512, #166115, #102182, #197538, #165050, #50237, #133657, #149882, #17700, #164001, #18775, #147750, #32919, #83787, #16642, #117429, #168249, #150949, #199658, #51304, #183427, #101101, #66446, #167188, #196492, #65389, #48134, #31868, #82726, #372, #132588, #116357, #182347, #2513, #68586, #134711, #200718, #33976, #52369, #100051, #19848, #118498, #15577, #184480, #36097, #146704, #212720, #64359, #130505, #180244, #138971, #41475, #71786, #173618, #122802, #136827, #57704, #73953, #172530, #169314, #23038, #107585, #89154, #137901, #123861, #201785, #189826, #135762, #53425, #202853, #204994, #5709, #85935, #72865, #4644, #152007, #188761, #3579, #185549, #54501, #21960, #56638, #69654, #86994, #24114, #39316, #55568, #119562, #70714, #153067, #121722, #7865, #155207, #20898, #37178, #120645, #186624, #6788, #38251, #103253, #104325, #154141, #40401, #171449, #106503, #170373, #90217, #140045, #156281, #206070, #88068, #203920, #187687, #105411, #193019, #12138, #60898, #59831, #95567, #195174, #91294, #127057, #125983, #109723, #208198, #142183, #160533, #44671, #46808, #76082, #191941, #143264, #78211, #28400, #110783, #42547, #111859, #174679, #43606, #176785, #175730, #210335, #112922, #177864, #144335, #94495, #61973, #128128, #159465, #194091, #75021, #26252, #141132, #124920, #10006, #27324, #11064, #93426, #77143, #45740, #29476, #161617, #13209, #209254, #79283 ) ),
 .UNSPECIFIED., .F., .T., .F.,
 ( 2, 2 ),
 ( 4, 2, 2, 2, 2, 2, 2, 2, 2, 2, 2, 2, 2, 2, 2, 2, 2, 2, 2, 2, 2, 2, 2, 2, 2, 2, 2, 2, 2, 2, 2, 2, 2, 2, 2, 2, 2, 2, 2, 2, 2, 2, 2, 2, 2, 2, 2, 2, 2, 2, 2, 2, 2, 2, 2, 2, 2, 2, 2, 2, 2, 2, 2, 2, 2, 2, 2, 2, 2, 2, 2, 2, 2, 2, 2, 2, 2, 2, 2, 2, 2, 2, 2, 2, 2, 2, 2, 2, 2, 2, 2, 2, 2, 2, 2, 2, 2, 2, 2, 2, 2, 2, 2, 2, 2, 2, 2, 2, 2, 2, 2, 2, 2, 2, 2, 2, 2, 2, 2, 2, 2, 2, 4 ),
 ( 0.000000000000000000, 1.000000000000000000 ),
 ( -6.441036414471523752E-08, 0.0001394059631734492798, 0.0002788763367110432749, 0.0004183467102486372428, 0.0004532143036330357755, 0.0004880818970174342539, 0.0005578170837862312650, 0.0006275522705550282219, 0.0006972874573238252872, 0.0007670226440926222440, 0.0008367578308614192009, 0.0009064930176302162662, 0.0009413606110146147989, 0.0009762282043990132231, 0.001045963391167810180, 0.001115698577936607245, 0.001255168951474201159, 0.001324904138242998224, 0.001394639325011795290, 0.001464374511780592355, 0.001534109698549389203, 0.001603844885318186052, 0.001673580072086983117, 0.001743315258855780182, 0.001813050445624577248, 0.001882785632393374313, 0.001917653225777772846, 0.001952520819162171161, 0.002022256005930968010, 0.002091991192699765075, 0.002231461566237359206, 0.002301196753006155837, 0.002370931939774952903, 0.002405799533159351435, 0.002440667126543749968, 0.002510402313312547033, 0.002649872686850141164, 0.002719607873618938229, 0.002789343060387735294, 0.002859078247156532360, 0.002928813433925329425, 0.002998548620694126490, 0.003068283807462923122, 0.003207754181000516819, 0.003277489367769313884, 0.003312356961153712417, 0.003347224554538110949, 0.003416959741306908015, 0.003486694928075705080, 0.003626165301613299211, 0.003695900488382096276, 0.003765635675150893341, 0.003800503268535291874, 0.003835370861919690406, 0.003905106048688487038, 0.003974841235457283670, 0.004044576422226080735, 0.004114311608994877800, 0.004184046795763674866, 0.004253781982532471931, 0.004323517169301268996, 0.004393252356070066061, 0.004462987542838863127, 0.004532722729607660192, 0.004602457916376456390, 0.004672193103145253455, 0.004741928289914050521, 0.004811663476682847586, 0.004881398663451644651, 0.004951133850220441716, 0.005020869036989238782, 0.005090604223758035847, 0.005125471817142434813, 0.005160339410526832912, 0.005299809784064427043, 0.005439280157602021173, 0.005509015344370818239, 0.005578750531139615304, 0.005613618124524013403, 0.005648485717908412369, 0.005718220904677209435, 0.005857691278214803565, 0.005927426464983600631, 0.005997161651752397696, 0.006066896838521193894, 0.006136632025289990959, 0.006206367212058788024, 0.006276102398827584222, 0.006415572772365178353, 0.006485307959133975418, 0.006520175552518374384, 0.006555043145902772483, 0.006624778332671569549, 0.006694513519440366614, 0.006833983892977960745, 0.006903719079746757810, 0.006973454266515554875, 0.007043189453284351940, 0.007112924640053149006, 0.007182659826821946071, 0.007252395013590743136, 0.007322130200359540202, 0.007391865387128337267, 0.007461600573897134332, 0.007496468167281533299, 0.007531335760665931398, 0.007601070947434728463, 0.007670806134203525528, 0.007810276507741118791, 0.007880011694509915857, 0.007949746881278712055, 0.007984614474663111888, 0.008019482068047509987, 0.008089217254816306185, 0.008228687628353900316, 0.008298422815122698248, 0.008368158001891494446, 0.008437893188660290644, 0.008472760782044688743, 0.008507628375429088577, 0.008647098748966682707, 0.008786569122504276838, 0.008926039496041870969 ),
 .UNSPECIFIED. ) ;
#72942=CARTESIAN_POINT ( 'NONE',  ( 5.341549334104176872, 9.175631956522799726, 0.7216878364870438212 ) ) ;
#72945=CARTESIAN_POINT ( 'NONE',  ( -3.741160322367112379, 6.452105245148518797, 1.199719254218464037 ) ) ;
#72950=CARTESIAN_POINT ( 'NONE',  ( 4.650083499362856365, 8.368921815991249957, 0.7216878364870438212 ) ) ;
#72951=CARTESIAN_POINT ( 'NONE',  ( -9.124274191872645545, 9.747334100047323702, -0.7216878364870267237 ) ) ;
#72953=CARTESIAN_POINT ( 'NONE',  ( 1.499999999999987121, 4.295833333333352044, -0.8660254037844323793 ) ) ;
#72957=CARTESIAN_POINT ( 'NONE',  ( 7.429504990608736037, 11.61158022244479682, -0.7216878364870267237 ) ) ;
#72970=CARTESIAN_POINT ( 'NONE',  ( 7.659993601596707613, 9.959745173328078849, -1.443375672974058777 ) ) ;
#72971=CARTESIAN_POINT ( 'NONE',  ( 9.074484886248265880, 9.481320543578137361, 0.7998128361456462443 ) ) ;
#72972=CARTESIAN_POINT ( 'NONE',  ( -5.042743069279040036, 7.970618449879118828, 1.199719254218464037 ) ) ;
#72975=CARTESIAN_POINT ( 'NONE',  ( -4.066554876651188977, 3.982284276321724992, -0.5266960748315950847 ) ) ;
#72977=CARTESIAN_POINT ( 'NONE',  ( 5.368665641331531013, 5.365790791082654998, -0.7216878364870207285 ) ) ;
#72978=ORIENTED_EDGE ( 'NONE', *, *, #99196, .T. ) ;
#72979=CARTESIAN_POINT ( 'NONE',  ( -7.619319141200077361, 9.912291636198670375, 1.443375672974090751 ) ) ;
#73003=CARTESIAN_POINT ( 'NONE',  ( -1.420000000000055440, 7.204077025658374822, -4.238769367544433564 ) ) ;
#73007=CARTESIAN_POINT ( 'NONE',  ( -5.605406444246153974, 8.627059054007450101, -1.199719254218440723 ) ) ;
#73014=CARTESIAN_POINT ( 'NONE',  ( -4.853001412603734188, 5.021300470422864315, 0.7152689200764159594 ) ) ;
#73021=CARTESIAN_POINT ( 'NONE',  ( -3.358669367883384105, 4.941533567329135401, -1.599625672291262513 ) ) ;
#73024=CARTESIAN_POINT ( 'NONE',  ( 6.612626235163189925, 8.737816579155630592, -1.599625672291262513 ) ) ;
#73025=CARTESIAN_POINT ( 'NONE',  ( -0.6823417656250212460, 3.801041667008085767, 1.181850606188767472 ) ) ;
#73027=CARTESIAN_POINT ( 'NONE',  ( 6.110807642276722795, 6.018297815386236316, -0.1222484578899986352 ) ) ;
#73032=CARTESIAN_POINT ( 'NONE',  ( 5.978782553502139940, 6.077593855281705260, -0.7216878364870257245 ) ) ;
#73033=CARTESIAN_POINT ( 'NONE',  ( -6.672584156219988571, 10.93643194889866521, -0.7998128361456291469 ) ) ;
#73036=CARTESIAN_POINT ( 'NONE',  ( -7.537443334193545397, 10.88110209227943770, -1.199719254218446718 ) ) ;
#73037=CARTESIAN_POINT ( 'NONE',  ( -6.039267359883488950, 9.133230122250985517, 1.199719254218452047 ) ) ;
#73041=CARTESIAN_POINT ( 'NONE',  ( 4.897706171852771462, 4.871974472535213430, 0.6676900015689657408 ) ) ;
#73044=CARTESIAN_POINT ( 'NONE',  ( 8.589254009457354400, 9.979550084910457031, -1.199719254218446718 ) ) ;
#73051=CARTESIAN_POINT ( 'NONE',  ( 3.708318708537623021, 4.285125567170706695, -1.199719254218446718 ) ) ;
#73058=CARTESIAN_POINT ( 'NONE',  ( 1.499999999999987121, 4.795833333333353821, -0.8660254037844323793 ) ) ;
#73059=CARTESIAN_POINT ( 'NONE',  ( 3.337278367258157630, 7.045241861776501580, 0.7998128361456341429 ) ) ;
#73060=CARTESIAN_POINT ( 'NONE',  ( 6.928380191783277908, 8.041863964290678624, 1.199719254218462483 ) ) ;
#73062=CARTESIAN_POINT ( 'NONE',  ( -8.731087737520713432, 10.24898578427137963, 1.082531754730558626 ) ) ;
#73064=CARTESIAN_POINT ( 'NONE',  ( 5.477130870240836558, 9.333810415348903433, -0.7216878364870267237 ) ) ;
#73065=CARTESIAN_POINT ( 'NONE',  ( -9.124274191872640216, 10.70770331434866485, -1.082531754730537976 ) ) ;
#73068=CARTESIAN_POINT ( 'NONE',  ( 6.401421083946654100, 10.62007503124645957, -0.7998128361456291469 ) ) ;
#73072=CARTESIAN_POINT ( 'NONE',  ( 1.364683531249988757, 1.884375000341421913, 0.000000000000000000 ) ) ;
#73078=CARTESIAN_POINT ( 'NONE',  ( 10.09812548408005384, 10.67556790771522124, -0.7998128361456281477 ) ) ;
#73082=CARTESIAN_POINT ( 'NONE',  ( -9.989660255170729641, 10.54902514065433827, -0.7998128361456291469 ) ) ;
#73088=CARTESIAN_POINT ( 'NONE',  ( 3.460355519985863548, 5.060167411448709629, 1.599625672291267398 ) ) ;
#73092=CARTESIAN_POINT ( 'NONE',  ( -8.696665468161981494, 12.23352791524263239, -1.199719254218446718 ) ) ;
#73095=CARTESIAN_POINT ( 'NONE',  ( 8.178592977541601527, 10.56477777859713463, 1.599625672291281386 ) ) ;
#73097=CARTESIAN_POINT ( 'NONE',  ( 4.341180335511626964, 7.176948212357606494, 1.029809165597308063 ) ) ;
#73099=CARTESIAN_POINT ( 'NONE',  ( -4.578903193113314174, 6.365139696764064325, 1.599625672291267398 ) ) ;
#73103=CARTESIAN_POINT ( 'NONE',  ( 7.914208982075123799, 10.25632978388623684, -1.599625672291262513 ) ) ;
#73105=CARTESIAN_POINT ( 'NONE',  ( 5.913327553854682783, 10.05063257947248800, -0.7998128361456291469 ) ) ;
#73108=CARTESIAN_POINT ( 'NONE',  ( -7.836249599018719536, 12.08611559892311504, 0.7216878364870478180 ) ) ;
#73116=CARTESIAN_POINT ( 'NONE',  ( -4.729598638066518035, 6.837371794175130191, -1.235194855336968045 ) ) ;
#73118=CARTESIAN_POINT ( 'NONE',  ( 5.639828713604826405, 9.523624565940227882, -0.7216878364870267237 ) ) ;
#73120=AXIS2_PLACEMENT_3D ( 'NONE', #86589, #55158, #138552 ) ;
#73137=CARTESIAN_POINT ( 'NONE',  ( 6.448874621594486989, 10.67543749183559143, 0.7998128361456462443 ) ) ;
#73141=CARTESIAN_POINT ( 'NONE',  ( -1.201851678989727383E-14, 0.9937500006828198229, 1.732050807568877637 ) ) ;
#73142=CARTESIAN_POINT ( 'NONE',  ( -5.910464900553636269, 8.982960586366182554, -1.199719254218440723 ) ) ;
#73145=CARTESIAN_POINT ( 'NONE',  ( -8.947491310014823895, 12.52615806407091803, 1.199719254218462483 ) ) ;
#73148=EDGE_CURVE ( 'NONE', #133229, #16921, #145804, .T. ) ;
#73150=CARTESIAN_POINT ( 'NONE',  ( -0.7500000000000215383, 5.472916667349482900, 1.299038105676671107 ) ) ;
#73151=CARTESIAN_POINT ( 'NONE',  ( 7.938462636001388795, 9.220293482545153907, -1.199719254218441611 ) ) ;
#73154=CARTESIAN_POINT ( 'NONE',  ( -8.213542131780492639, 8.476887330032372603, 1.040834085586084257E-14 ) ) ;
#73156=CARTESIAN_POINT ( 'NONE',  ( -1.364683531250010295, 5.238541667008086655, -0.7879004041258300672 ) ) ;
#73163=CARTESIAN_POINT ( 'NONE',  ( -9.002250809794013264, 9.604973487622245898, -0.7216878364870267237 ) ) ;
#73167=CARTESIAN_POINT ( 'NONE',  ( 1.364683531249990311, 3.946875000341417028, 1.214306433183764966E-14 ) ) ;
#73173=CARTESIAN_POINT ( 'NONE',  ( 1.364683531249990311, 3.634375000341416584, 1.214306433183764966E-14 ) ) ;
#73174=CARTESIAN_POINT ( 'NONE',  ( -4.731959306369413198, 5.479372931307791461, -1.199719254218446718 ) ) ;
#73175=CARTESIAN_POINT ( 'NONE',  ( 5.666418135507635512, 8.698239360479199433, 1.199719254218462483 ) ) ;
#73180=CARTESIAN_POINT ( 'NONE',  ( 3.348500752450942031, 4.929670182657964084, 1.443375672974066548 ) ) ;
#73181=CARTESIAN_POINT ( 'NONE',  ( -1.364683531249997417, 5.821875000341418804, 1.214306433183764966E-14 ) ) ;
#73186=CARTESIAN_POINT ( 'NONE',  ( -0.6823417656250212460, 1.051041667008083325, 1.181850606188755259 ) ) ;
#73187=CARTESIAN_POINT ( 'NONE',  ( -3.850152436600983386, 4.554561266531622188, 1.082531754730560403 ) ) ;
#73188=CARTESIAN_POINT ( 'NONE',  ( 4.137209430464448445, 7.978494768850520558, 1.040834085586084257E-14 ) ) ;
#73194=CARTESIAN_POINT ( 'NONE',  ( 2.873965376416980355, 6.296784005887697155, -0.7216878364870267237 ) ) ;
#73197=CARTESIAN_POINT ( 'NONE',  ( -7.348156068926747331, 11.51667314714914347, 0.7216878364870458196 ) ) ;
#73199=CARTESIAN_POINT ( 'NONE',  ( 0.7499999999999920064, 4.983333333333353821, 1.299038105676669330 ) ) ;
#73203=CARTESIAN_POINT ( 'NONE',  ( -6.683806541412780078, 6.900121841177441873, -0.7216878364870267237 ) ) ;
#73205=CARTESIAN_POINT ( 'NONE',  ( -0.6823417656250246877, 0.1135416670080893753, 1.181850606188755259 ) ) ;
#73213=CARTESIAN_POINT ( 'NONE',  ( 8.536830278099042602, 13.11138575775759563, -0.7998128361456352531 ) ) ;
#73226=CARTESIAN_POINT ( 'NONE',  ( -4.302014814237876017, 3.913438792899272212, 0.7998128361456341429 ) ) ;
#73229=CARTESIAN_POINT ( 'NONE',  ( -1.201851678989727383E-14, 2.384375000341416584, 1.575800808251672791 ) ) ;
#73239=CARTESIAN_POINT ( 'NONE',  ( -1.364683531250000748, 0.5093750003414208027, 0.000000000000000000 ) ) ;
#73243=CARTESIAN_POINT ( 'NONE',  ( -0.1021852871783679312, 7.053056311350174745, -4.037408415133499240 ) ) ;
#73249=CARTESIAN_POINT ( 'NONE',  ( 6.505214776458575265, 6.483838748823460563, 1.040834085586084257E-14 ) ) ;
#73258=CARTESIAN_POINT ( 'NONE',  ( 6.608709811657416999, 9.797579649320619311, -1.199719254218440723 ) ) ;
#73259=CARTESIAN_POINT ( 'NONE',  ( 3.172244755473273781, 6.644776614786712443, 0.000000000000000000 ) ) ;
#73261=( BOUNDED_SURFACE ( )  B_SPLINE_SURFACE ( 1, 2, ( 
 ( #154654, #6237, #117944, #10517, #11588, #8387, #175187, #141645, #90737, #124374, #140574, #24630, #74469, #206587, #58216, #155721, #190332, #123314, #126500, #92875, #60340, #189278, #41994, #107023, #73382, #109174, #207654, #108101, #158921, #173048, #174130, #156800, #40917, #171971, #25703, #208713, #91811, #157869, #76592, #192464, #193548, #9462, #159986, #142703, #44117, #75534, #110238, #59275, #23562, #125432, #191396, #43061, #26773, #176246, #209777, #27848, #143782, #93946, #77661, #61417, #127580, #45190, #89671, #7306, #139488, #205516, #57148, #211913, #32116, #96076, #148010, #162129, #82981, #99257, #197797, #194607, #48389, #132844, #13717, #95007, #178381, #29990, #49432, #198848, #79790, #131792, #112369, #14778, #180499, #98201, #145904, #111305, #214021, #149054, #16900, #63550, #633, #129706, #114502, #177307, #130754, #164249, #195688, #115552, #66697, #47324, #62479, #46251, #113438, #181548, #212974, #163195, #179445, #161054, #15837, #28922, #31066, #196748, #65643, #33176, #97141, #80869, #81923, #146959, #64615, #165306, #12649, #78720, #144847, #210853, #128642, #68845, #17964, #88331, #138157, #5973, #72045, #183686, #104587, #4897, #52621, #153322, #134965, #170632, #21152, #34233, #50495, #101367, #2775, #168503, #84051, #200973, #184732, #152259, #137085, #199923, #151203, #202030, #53690, #35292, #22218, #20103, #103512, #119822, #185802, #37435, #51569, #87258, #166372, #186877, #116616, #117694, #150139, #154395, #36358, #118749, #102435, #70975, #203111, #182611, #100306, #54756, #86190, #3833, #69907, #169571, #120905, #136017, #1711, #167445, #38509, #67765, #133916, #19039, #85117, #159730, #123066, #43870, #158669, #206331, #92626, #74218, #109986, #174937, #187941, #11329, #40662, #156542, #107845, #171700, #8132, #124122, #91554, #76341, #139219, #90476, #141394, #207404, #189020, #175997, #173874, #42807, #59023, #125179, #191141, #205249, #26518, #105673, #126248, #77407, #56891, #23299, #27590, #190084, #140313, #41736, #10266, #142448, #204165, #93688, #106764, #55820, #208456, #121977, #108915, #155459, #157611, #172792, #24364, #39571, #60088, #89410, #57956, #192208, #25447, #7042, #9207, #73118, #75279, #115307, #131541, #15582, #12393, #80616, #165055, #194359, #127322, #210606, #62234, #81669, #16647, #46002, #164006, #144591, #47068, #212725, #130510, #128392, #143524, #180249, #181297, #49188, #112121, #32924, #29739, #146709, #209520, #162941, #196497, #178124, #147755, #99000, #95821, #94754, #78472, #161880, #213773, #30813, #195438, #211657, #193293, #64364, #61160, #13467, #14522, #31873, #65395, #79543, #145661, #63295, #44937, #197543, #111045, #48140, #160802, #96892, #129455, #113185, #177052, #114253, #28669, #179189, #97952, #183432, #3584, #67517, #119567, #133662, #57438, #73681, #169319, #166120, #19853, #107316, #199663, #66451, #149887, #1452, #20903, #173340, #51309, #103258, #83792, #200723, #152013, #69659, #117435, #82732, #185554, #123599, #205807, #35033, #189564, #101107, #85940, #148808, #102187, #135767, #167193, #86999, #41209, #18780, #33981, #17705, #84866, #156009, #184485, #134717, #150954, #132593, #201790, #377, #2518, #168254, #37183, #7597, #68591, #52374, #53430, #118503, #36102, #139780, #198595, #50242, #116362, #182352, #100056, #43341, #206873, #62755, #112655, #194896, #46534, #158151, #79009, #193821, #27054, #127871, #109461, #145125, #210063, #8675, #24920, #75818, #191680, #142993, #58504, #175468, #159198, #126791, #111586, #174412, #125719, #176523, #28134, #9744, #211131, #208992, #77947, #94230, #160268, #11870, #25989, #61703, #140859, #161347, #91024, #92097, #124659, #128915, #10799, #93161, #76873, #45469, #177596, #157086, #74757, #141926, #190616, #60628, #29208, #207938, #59560, #42274, #95298, #144068, #108387, #192746, #12928, #44403, #110523, #131037, #147235, #31348, #15058, #213263, #81150, #162416, #197026, #129990, #133135, #99537, #66997, #195978, #64890, #113725, #80077, #115842, #148297, #48663, #165599, #179729, #114779, #97422, #47611, #178664, #180777, #930, #163476, #32403, #17189 ),
 ( #98469, #164534, #214294, #134198, #30276, #16120, #212194, #96362, #18261, #199134, #181828, #50779, #13993, #82203, #116907, #65928, #132075, #198086, #49713, #33461, #200208, #146179, #83264, #149350, #182907, #34523, #100595, #84344, #51860, #166670, #150432, #1997, #68062, #63832, #3065, #23599, #119044, #5196, #69135, #151496, #204468, #201271, #135257, #168794, #52911, #169859, #172008, #20401, #154689, #105988, #137385, #73421, #203400, #185028, #117982, #101664, #186102, #205549, #89707, #155758, #167732, #19333, #153624, #21447, #7343, #36653, #202334, #183973, #104883, #88632, #87556, #120124, #139523, #35585, #102739, #37734, #6273, #86482, #152547, #85412, #4133, #71270, #103810, #55054, #121205, #70202, #136315, #53985, #187174, #38801, #170926, #22523, #56121, #72344, #138448, #122279, #188237, #39877, #111337, #108137, #93979, #45222, #76625, #12678, #142738, #58253, #57188, #40953, #125469, #144878, #177341, #28954, #107060, #173086, #92910, #109212, #95038, #124409, #141680, #123348, #44150, #27882, #174165, #24666, #175223, #11619, #25738, #190366, #8421, #77694, #110271, #161088, #91848, #60374, #26808, #42027, #9499, #157905, #75571, #207693, #59312, #191431, #90772, #43098, #74506, #143815, #192499, #160020, #140611, #158956, #206623, #156834, #208747, #10551, #126537, #176280, #209812, #61447, #127614, #193579, #189315, #78753, #33207, #13751, #163228, #197832, #99291, #17998, #31100, #198879, #49465, #83012, #211946, #115584, #179477, #62509, #195722, #47357, #64645, #113472, #129739, #97174, #180527, #166405, #128674, #14809, #30022, #194641, #50526, #16932, #214048, #149087, #46285, #146991, #667, #80901, #145935, #213009, #130784, #84088, #210884, #162163, #196778, #165338, #63582, #48421, #116649, #112402, #98228, #114533, #164282, #32149, #178412, #96108, #182646, #15871, #81955, #79824, #148040, #66733, #65676, #131823, #181578, #132878, #34266, #100340, #201010, #186913, #138192, #169607, #105709, #21189, #151239, #150176, #133950, #3869, #23334, #204202, #55856, #199958, #51604, #185837, #202066, #122012, #2808, #20138, #1744, #137120, #120942, #52655, #117729, #53726, #104622, #118784, #68879, #101404, #170670, #203150, #187979, #184770, #153361, #119859, #134999, #102474, #36397, #168541, #86224, #152296, #69942, #183718, #136054, #167479, #22257, #71008, #38545, #19075, #37469, #85156, #35326, #87292, #103546, #4932, #54794, #88367, #154433, #6011, #72081, #67801, #39605, #171737, #106796, #41768, #76369, #126279, #111074, #124153, #77437, #142476, #176026, #90508, #208484, #57990, #155495, #74251, #140345, #157641, #206363, #8167, #190114, #59051, #44966, #7078, #107881, #123099, #73151, #143554, #110013, #92655, #27618, #139257, #25483, #93718, #173907, #24396, #91589, #207432, #9238, #156573, #40693, #89443, #75310, #192237, #172824, #141426, #60120, #43899, #177080, #125209, #209548, #159759, #11356, #191171, #61192, #42838, #205288, #108945, #174965, #26547, #158697, #10295, #127351, #193320, #56926, #189056, #195468, #62260, #160830, #82765, #49221, #31905, #115340, #12422, #179220, #181331, #47099, #178155, #211689, #146741, #30845, #50275, #28696, #194388, #96923, #65426, #95854, #145691, #148838, #116394, #130538, #162973, #196529, #14553, #210634, #128421, #410, #29769, #48172, #46031, #112152, #32959, #161910, #13498, #79572, #63325, #80649, #66482, #129486, #131575, #16680, #114285, #198628, #180282, #113215, #94782, #78502, #212759, #144620, #132622, #64394, #97982, #164041, #15616, #81706, #147787, #213803, #197576, #99034, #165089, #153104, #84898, #149916, #19885, #136865, #150985, #35066, #133693, #202891, #20936, #21997, #18811, #185586, #152044, #101137, #134747, #2549, #167225, #68624, #200756, #52405, #166148, #118532, #199697, #54536, #103289, #70753, #51342, #184515, #117467, #83823, #119602, #3614, #36136, #169351, #183460, #5746, #88107, #102219, #71823, #168288, #37216, #34012, #201820, #87032, #85969, #120683, #154178, #69692, #135796, #53465, #4679, #38286, #186660, #104363, #170408, #17734, #137933, #203955, #55602, #182382, #100087, #1484 ) ),
 .UNSPECIFIED., .F., .F., .F. ) 
 B_SPLINE_SURFACE_WITH_KNOTS ( ( 2, 2 ),
 ( 3, 2, 2, 2, 2, 2, 2, 2, 2, 2, 2, 2, 2, 2, 2, 2, 2, 2, 2, 2, 2, 2, 2, 2, 2, 2, 2, 2, 2, 2, 2, 2, 2, 2, 2, 2, 2, 2, 2, 2, 2, 2, 2, 2, 2, 2, 2, 2, 2, 2, 2, 2, 2, 2, 2, 2, 2, 2, 2, 2, 2, 2, 2, 2, 2, 2, 2, 2, 2, 2, 2, 2, 2, 2, 2, 2, 2, 2, 2, 2, 2, 2, 2, 2, 2, 2, 2, 2, 2, 2, 2, 2, 2, 2, 2, 2, 2, 2, 2, 2, 2, 2, 2, 2, 2, 2, 2, 2, 2, 2, 2, 2, 2, 2, 2, 2, 2, 2, 2, 2, 2, 2, 2, 2, 2, 2, 2, 2, 2, 2, 2, 2, 2, 2, 2, 2, 2, 2, 2, 2, 2, 2, 2, 2, 2, 2, 2, 2, 2, 2, 2, 2, 2, 2, 2, 2, 2, 2, 2, 2, 2, 2, 2, 2, 2, 2, 2, 2, 2, 2, 2, 2, 2, 2, 2, 2, 2, 2, 2, 2, 2, 2, 2, 2, 2, 2, 2, 2, 2, 2, 2, 2, 2, 2, 2, 2, 2, 2, 2, 2, 2, 2, 2, 2, 2, 2, 2, 2, 2, 2, 2, 2, 2, 2, 2, 2, 2, 2, 2, 2, 2, 2, 2, 2, 2, 2, 2, 2, 2, 2, 2, 2, 2, 2, 2, 2, 2, 2, 2, 2, 3 ),
 ( 0.000000000000000000, 1.000000000000000000 ),
 ( 0.000000000000000000, 0.004166666666666666609, 0.008333333333333333218, 0.01250000000000000069, 0.01666666666666666644, 0.02083333333333333218, 0.02500000000000000139, 0.02916666666666666713, 0.03333333333333333287, 0.03749999999999999861, 0.04166666666666666435, 0.04583333333333333010, 0.05000000000000000278, 0.05416666666666666852, 0.05833333333333333426, 0.06250000000000000000, 0.06666666666666666574, 0.07083333333333333148, 0.07499999999999999722, 0.07916666666666666297, 0.08333333333333332871, 0.08749999999999999445, 0.09166666666666666019, 0.09583333333333333981, 0.1000000000000000056, 0.1041666666666666713, 0.1083333333333333370, 0.1125000000000000028, 0.1166666666666666685, 0.1208333333333333343, 0.1250000000000000000, 0.1291666666666666796, 0.1333333333333333315, 0.1375000000000000111, 0.1416666666666666630, 0.1458333333333333426, 0.1499999999999999944, 0.1541666666666666741, 0.1583333333333333259, 0.1625000000000000056, 0.1666666666666666574, 0.1708333333333333370, 0.1749999999999999889, 0.1791666666666666685, 0.1833333333333333204, 0.1875000000000000000, 0.1916666666666666796, 0.1958333333333333315, 0.2000000000000000111, 0.2041666666666666630, 0.2083333333333333426, 0.2124999999999999944, 0.2166666666666666741, 0.2208333333333333259, 0.2250000000000000056, 0.2291666666666666574, 0.2333333333333333370, 0.2374999999999999889, 0.2416666666666666685, 0.2458333333333333204, 0.2500000000000000000, 0.2541666666666666519, 0.2583333333333333592, 0.2625000000000000111, 0.2666666666666666630, 0.2708333333333333148, 0.2750000000000000222, 0.2791666666666666741, 0.2833333333333333259, 0.2874999999999999778, 0.2916666666666666852, 0.2958333333333333370, 0.2999999999999999889, 0.3041666666666666408, 0.3083333333333333481, 0.3125000000000000000, 0.3166666666666666519, 0.3208333333333333592, 0.3250000000000000111, 0.3291666666666666630, 0.3333333333333333148, 0.3375000000000000222, 0.3416666666666666741, 0.3458333333333333259, 0.3499999999999999778, 0.3541666666666666852, 0.3583333333333333370, 0.3624999999999999889, 0.3666666666666666408, 0.3708333333333333481, 0.3750000000000000000, 0.3791666666666666519, 0.3833333333333333592, 0.3875000000000000111, 0.3916666666666666630, 0.3958333333333333148, 0.4000000000000000222, 0.4041666666666666741, 0.4083333333333333259, 0.4124999999999999778, 0.4166666666666666852, 0.4208333333333333370, 0.4249999999999999889, 0.4291666666666666408, 0.4333333333333333481, 0.4375000000000000000, 0.4416666666666666519, 0.4458333333333333592, 0.4500000000000000111, 0.4541666666666666630, 0.4583333333333333148, 0.4625000000000000222, 0.4666666666666666741, 0.4708333333333333259, 0.4749999999999999778, 0.4791666666666666852, 0.4833333333333333370, 0.4874999999999999889, 0.4916666666666666408, 0.4958333333333333481, 0.5000000000000000000, 0.5041666666666666519, 0.5083333333333333037, 0.5124999999999999556, 0.5166666666666667185, 0.5208333333333333703, 0.5250000000000000222, 0.5291666666666666741, 0.5333333333333333259, 0.5374999999999999778, 0.5416666666666666297, 0.5458333333333332815, 0.5500000000000000444, 0.5541666666666666963, 0.5583333333333333481, 0.5625000000000000000, 0.5666666666666666519, 0.5708333333333333037, 0.5749999999999999556, 0.5791666666666667185, 0.5833333333333333703, 0.5875000000000000222, 0.5916666666666666741, 0.5958333333333333259, 0.5999999999999999778, 0.6041666666666666297, 0.6083333333333332815, 0.6125000000000000444, 0.6166666666666666963, 0.6208333333333333481, 0.6250000000000000000, 0.6291666666666666519, 0.6333333333333333037, 0.6374999999999999556, 0.6416666666666667185, 0.6458333333333333703, 0.6500000000000000222, 0.6541666666666666741, 0.6583333333333333259, 0.6624999999999999778, 0.6666666666666666297, 0.6708333333333332815, 0.6750000000000000444, 0.6791666666666666963, 0.6833333333333333481, 0.6875000000000000000, 0.6916666666666666519, 0.6958333333333333037, 0.6999999999999999556, 0.7041666666666667185, 0.7083333333333333703, 0.7125000000000000222, 0.7166666666666666741, 0.7208333333333333259, 0.7249999999999999778, 0.7291666666666666297, 0.7333333333333332815, 0.7375000000000000444, 0.7416666666666666963, 0.7458333333333333481, 0.7500000000000000000, 0.7541666666666666519, 0.7583333333333333037, 0.7624999999999999556, 0.7666666666666667185, 0.7708333333333333703, 0.7750000000000000222, 0.7791666666666666741, 0.7833333333333333259, 0.7874999999999999778, 0.7916666666666666297, 0.7958333333333332815, 0.8000000000000000444, 0.8041666666666666963, 0.8083333333333333481, 0.8125000000000000000, 0.8166666666666666519, 0.8208333333333333037, 0.8249999999999999556, 0.8291666666666667185, 0.8333333333333333703, 0.8375000000000000222, 0.8416666666666666741, 0.8458333333333333259, 0.8499999999999999778, 0.8541666666666666297, 0.8583333333333332815, 0.8625000000000000444, 0.8666666666666666963, 0.8708333333333333481, 0.8750000000000000000, 0.8791666666666666519, 0.8833333333333333037, 0.8874999999999999556, 0.8916666666666667185, 0.8958333333333333703, 0.9000000000000000222, 0.9041666666666666741, 0.9083333333333333259, 0.9124999999999999778, 0.9166666666666666297, 0.9208333333333332815, 0.9250000000000000444, 0.9291666666666666963, 0.9333333333333333481, 0.9375000000000000000, 0.9416666666666666519, 0.9458333333333333037, 0.9499999999999999556, 0.9541666666666667185, 0.9583333333333333703, 0.9625000000000000222, 0.9666666666666666741, 0.9708333333333333259, 0.9749999999999999778, 0.9791666666666666297, 0.9833333333333332815, 0.9875000000000000444, 0.9916666666666666963, 0.9958333333333333481, 1.000000000000000000 ),
 .UNSPECIFIED. ) 
 GEOMETRIC_REPRESENTATION_ITEM ( )  RATIONAL_B_SPLINE_SURFACE ( (
 ( 1.000000000000000000, 0.8660254037844387076, 1.000000000000000000, 0.8660254037844387076, 1.000000000000000000, 0.8660254037844387076, 1.000000000000000000, 0.8660254037844387076, 1.000000000000000000, 0.8660254037844387076, 1.000000000000000000, 0.8660254037844387076, 1.000000000000000000, 0.8660254037844387076, 1.000000000000000000, 0.8660254037844387076, 1.000000000000000000, 0.8660254037844387076, 1.000000000000000000, 0.8660254037844387076, 1.000000000000000000, 0.8660254037844387076, 1.000000000000000000, 0.8660254037844387076, 1.000000000000000000, 0.8660254037844387076, 1.000000000000000000, 0.8660254037844387076, 1.000000000000000000, 0.8660254037844387076, 1.000000000000000000, 0.8660254037844387076, 1.000000000000000000, 0.8660254037844387076, 1.000000000000000000, 0.8660254037844387076, 1.000000000000000000, 0.8660254037844387076, 1.000000000000000000, 0.8660254037844387076, 1.000000000000000000, 0.8660254037844387076, 1.000000000000000000, 0.8660254037844387076, 1.000000000000000000, 0.8660254037844387076, 1.000000000000000000, 0.8660254037844387076, 1.000000000000000000, 0.8660254037844387076, 1.000000000000000000, 0.8660254037844387076, 1.000000000000000000, 0.8660254037844387076, 1.000000000000000000, 0.8660254037844387076, 1.000000000000000000, 0.8660254037844387076, 1.000000000000000000, 0.8660254037844387076, 1.000000000000000000, 0.8660254037844387076, 1.000000000000000000, 0.8660254037844387076, 1.000000000000000000, 0.8660254037844387076, 1.000000000000000000, 0.8660254037844387076, 1.000000000000000000, 0.8660254037844387076, 1.000000000000000000, 0.8660254037844387076, 1.000000000000000000, 0.8660254037844387076, 1.000000000000000000, 0.8660254037844387076, 1.000000000000000000, 0.8660254037844387076, 1.000000000000000000, 0.8660254037844387076, 1.000000000000000000, 0.8660254037844387076, 1.000000000000000000, 0.8660254037844387076, 1.000000000000000000, 0.8660254037844387076, 1.000000000000000000, 0.8660254037844387076, 1.000000000000000000, 0.8660254037844387076, 1.000000000000000000, 0.8660254037844387076, 1.000000000000000000, 0.8660254037844387076, 1.000000000000000000, 0.8660254037844387076, 1.000000000000000000, 0.8660254037844387076, 1.000000000000000000, 0.8660254037844387076, 1.000000000000000000, 0.8660254037844387076, 1.000000000000000000, 0.8660254037844387076, 1.000000000000000000, 0.8660254037844387076, 1.000000000000000000, 0.8660254037844387076, 1.000000000000000000, 0.8660254037844387076, 1.000000000000000000, 0.8660254037844387076, 1.000000000000000000, 0.8660254037844387076, 1.000000000000000000, 0.8660254037844387076, 1.000000000000000000, 0.8660254037844387076, 1.000000000000000000, 0.8660254037844387076, 1.000000000000000000, 0.8660254037844387076, 1.000000000000000000, 0.8660254037844387076, 1.000000000000000000, 0.8660254037844387076, 1.000000000000000000, 0.8660254037844387076, 1.000000000000000000, 0.8660254037844387076, 1.000000000000000000, 0.8660254037844387076, 1.000000000000000000, 0.8660254037844387076, 1.000000000000000000, 0.8660254037844387076, 1.000000000000000000, 0.8660254037844387076, 1.000000000000000000, 0.8660254037844387076, 1.000000000000000000, 0.8660254037844387076, 1.000000000000000000, 0.8660254037844387076, 1.000000000000000000, 0.8660254037844387076, 1.000000000000000000, 0.8660254037844387076, 1.000000000000000000, 0.8660254037844387076, 1.000000000000000000, 0.8660254037844387076, 1.000000000000000000, 0.8660254037844387076, 1.000000000000000000, 0.8660254037844387076, 1.000000000000000000, 0.8660254037844387076, 1.000000000000000000, 0.8660254037844387076, 1.000000000000000000, 0.8660254037844387076, 1.000000000000000000, 0.8660254037844387076, 1.000000000000000000, 0.8660254037844387076, 1.000000000000000000, 0.8660254037844387076, 1.000000000000000000, 0.8660254037844387076, 1.000000000000000000, 0.8660254037844387076, 1.000000000000000000, 0.8660254037844387076, 1.000000000000000000, 0.8660254037844387076, 1.000000000000000000, 0.8660254037844387076, 1.000000000000000000, 0.8660254037844387076, 1.000000000000000000, 0.8660254037844387076, 1.000000000000000000, 0.8660254037844387076, 1.000000000000000000, 0.8660254037844387076, 1.000000000000000000, 0.8660254037844387076, 1.000000000000000000, 0.8660254037844387076, 1.000000000000000000, 0.8660254037844387076, 1.000000000000000000, 0.8660254037844387076, 1.000000000000000000, 0.8660254037844387076, 1.000000000000000000, 0.8660254037844387076, 1.000000000000000000, 0.8660254037844387076, 1.000000000000000000, 0.8660254037844387076, 1.000000000000000000, 0.8660254037844387076, 1.000000000000000000, 0.8660254037844387076, 1.000000000000000000, 0.8660254037844387076, 1.000000000000000000, 0.8660254037844387076, 1.000000000000000000, 0.8660254037844387076, 1.000000000000000000, 0.8660254037844387076, 1.000000000000000000, 0.8660254037844387076, 1.000000000000000000, 0.8660254037844387076, 1.000000000000000000, 0.8660254037844387076, 1.000000000000000000, 0.8660254037844387076, 1.000000000000000000, 0.8660254037844387076, 1.000000000000000000, 0.8660254037844387076, 1.000000000000000000, 0.8660254037844387076, 1.000000000000000000, 0.8660254037844387076, 1.000000000000000000, 0.8660254037844387076, 1.000000000000000000, 0.8660254037844387076, 1.000000000000000000, 0.8660254037844387076, 1.000000000000000000, 0.8660254037844387076, 1.000000000000000000, 0.8660254037844387076, 1.000000000000000000, 0.8660254037844387076, 1.000000000000000000, 0.8660254037844387076, 1.000000000000000000, 0.8660254037844387076, 1.000000000000000000, 0.8660254037844387076, 1.000000000000000000, 0.8660254037844387076, 1.000000000000000000, 0.8660254037844387076, 1.000000000000000000, 0.8660254037844387076, 1.000000000000000000, 0.8660254037844387076, 1.000000000000000000, 0.8660254037844387076, 1.000000000000000000, 0.8660254037844387076, 1.000000000000000000, 0.8660254037844387076, 1.000000000000000000, 0.8660254037844387076, 1.000000000000000000, 0.8660254037844387076, 1.000000000000000000, 0.8660254037844387076, 1.000000000000000000, 0.8660254037844387076, 1.000000000000000000, 0.8660254037844387076, 1.000000000000000000, 0.8660254037844387076, 1.000000000000000000, 0.8660254037844387076, 1.000000000000000000, 0.8660254037844387076, 1.000000000000000000, 0.8660254037844387076, 1.000000000000000000, 0.8660254037844387076, 1.000000000000000000, 0.8660254037844387076, 1.000000000000000000, 0.8660254037844387076, 1.000000000000000000, 0.8660254037844387076, 1.000000000000000000, 0.8660254037844387076, 1.000000000000000000, 0.8660254037844387076, 1.000000000000000000, 0.8660254037844387076, 1.000000000000000000, 0.8660254037844387076, 1.000000000000000000, 0.8660254037844387076, 1.000000000000000000, 0.8660254037844387076, 1.000000000000000000, 0.8660254037844387076, 1.000000000000000000, 0.8660254037844387076, 1.000000000000000000, 0.8660254037844387076, 1.000000000000000000, 0.8660254037844387076, 1.000000000000000000, 0.8660254037844387076, 1.000000000000000000, 0.8660254037844387076, 1.000000000000000000, 0.8660254037844387076, 1.000000000000000000, 0.8660254037844387076, 1.000000000000000000, 0.8660254037844387076, 1.000000000000000000, 0.8660254037844387076, 1.000000000000000000, 0.8660254037844387076, 1.000000000000000000, 0.8660254037844387076, 1.000000000000000000, 0.8660254037844387076, 1.000000000000000000, 0.8660254037844387076, 1.000000000000000000, 0.8660254037844387076, 1.000000000000000000, 0.8660254037844387076, 1.000000000000000000, 0.8660254037844387076, 1.000000000000000000, 0.8660254037844387076, 1.000000000000000000, 0.8660254037844387076, 1.000000000000000000, 0.8660254037844387076, 1.000000000000000000, 0.8660254037844387076, 1.000000000000000000, 0.8660254037844387076, 1.000000000000000000, 0.8660254037844387076, 1.000000000000000000, 0.8660254037844387076, 1.000000000000000000, 0.8660254037844387076, 1.000000000000000000, 0.8660254037844387076, 1.000000000000000000, 0.8660254037844387076, 1.000000000000000000, 0.8660254037844387076, 1.000000000000000000, 0.8660254037844387076, 1.000000000000000000, 0.8660254037844387076, 1.000000000000000000, 0.8660254037844387076, 1.000000000000000000, 0.8660254037844387076, 1.000000000000000000, 0.8660254037844387076, 1.000000000000000000, 0.8660254037844387076, 1.000000000000000000, 0.8660254037844387076, 1.000000000000000000, 0.8660254037844387076, 1.000000000000000000, 0.8660254037844387076, 1.000000000000000000, 0.8660254037844387076, 1.000000000000000000, 0.8660254037844387076, 1.000000000000000000, 0.8660254037844387076, 1.000000000000000000, 0.8660254037844387076, 1.000000000000000000, 0.8660254037844387076, 1.000000000000000000, 0.8660254037844387076, 1.000000000000000000, 0.8660254037844387076, 1.000000000000000000, 0.8660254037844387076, 1.000000000000000000, 0.8660254037844387076, 1.000000000000000000, 0.8660254037844387076, 1.000000000000000000, 0.8660254037844387076, 1.000000000000000000, 0.8660254037844387076, 1.000000000000000000, 0.8660254037844387076, 1.000000000000000000, 0.8660254037844387076, 1.000000000000000000, 0.8660254037844387076, 1.000000000000000000, 0.8660254037844387076, 1.000000000000000000, 0.8660254037844387076, 1.000000000000000000, 0.8660254037844387076, 1.000000000000000000, 0.8660254037844387076, 1.000000000000000000, 0.8660254037844387076, 1.000000000000000000, 0.8660254037844387076, 1.000000000000000000, 0.8660254037844387076, 1.000000000000000000, 0.8660254037844387076, 1.000000000000000000, 0.8660254037844387076, 1.000000000000000000, 0.8660254037844387076, 1.000000000000000000, 0.8660254037844387076, 1.000000000000000000, 0.8660254037844387076, 1.000000000000000000, 0.8660254037844387076, 1.000000000000000000, 0.8660254037844387076, 1.000000000000000000, 0.8660254037844387076, 1.000000000000000000, 0.8660254037844387076, 1.000000000000000000, 0.8660254037844387076, 1.000000000000000000, 0.8660254037844387076, 1.000000000000000000, 0.8660254037844387076, 1.000000000000000000, 0.8660254037844387076, 1.000000000000000000, 0.8660254037844387076, 1.000000000000000000, 0.8660254037844387076, 1.000000000000000000, 0.8660254037844387076, 1.000000000000000000, 0.8660254037844387076, 1.000000000000000000, 0.8660254037844387076, 1.000000000000000000, 0.8660254037844387076, 1.000000000000000000, 0.8660254037844387076, 1.000000000000000000, 0.8660254037844387076, 1.000000000000000000, 0.8660254037844387076, 1.000000000000000000, 0.8660254037844387076, 1.000000000000000000, 0.8660254037844387076, 1.000000000000000000, 0.8660254037844387076, 1.000000000000000000, 0.8660254037844387076, 1.000000000000000000, 0.8660254037844387076, 1.000000000000000000, 0.8660254037844387076, 1.000000000000000000, 0.8660254037844387076, 1.000000000000000000, 0.8660254037844387076, 1.000000000000000000, 0.8660254037844387076, 1.000000000000000000),
 ( 1.000000000000000000, 0.8660254037844387076, 1.000000000000000000, 0.8660254037844387076, 1.000000000000000000, 0.8660254037844387076, 1.000000000000000000, 0.8660254037844387076, 1.000000000000000000, 0.8660254037844387076, 1.000000000000000000, 0.8660254037844387076, 1.000000000000000000, 0.8660254037844387076, 1.000000000000000000, 0.8660254037844387076, 1.000000000000000000, 0.8660254037844387076, 1.000000000000000000, 0.8660254037844387076, 1.000000000000000000, 0.8660254037844387076, 1.000000000000000000, 0.8660254037844387076, 1.000000000000000000, 0.8660254037844387076, 1.000000000000000000, 0.8660254037844387076, 1.000000000000000000, 0.8660254037844387076, 1.000000000000000000, 0.8660254037844387076, 1.000000000000000000, 0.8660254037844387076, 1.000000000000000000, 0.8660254037844387076, 1.000000000000000000, 0.8660254037844387076, 1.000000000000000000, 0.8660254037844387076, 1.000000000000000000, 0.8660254037844387076, 1.000000000000000000, 0.8660254037844387076, 1.000000000000000000, 0.8660254037844387076, 1.000000000000000000, 0.8660254037844387076, 1.000000000000000000, 0.8660254037844387076, 1.000000000000000000, 0.8660254037844387076, 1.000000000000000000, 0.8660254037844387076, 1.000000000000000000, 0.8660254037844387076, 1.000000000000000000, 0.8660254037844387076, 1.000000000000000000, 0.8660254037844387076, 1.000000000000000000, 0.8660254037844387076, 1.000000000000000000, 0.8660254037844387076, 1.000000000000000000, 0.8660254037844387076, 1.000000000000000000, 0.8660254037844387076, 1.000000000000000000, 0.8660254037844387076, 1.000000000000000000, 0.8660254037844387076, 1.000000000000000000, 0.8660254037844387076, 1.000000000000000000, 0.8660254037844387076, 1.000000000000000000, 0.8660254037844387076, 1.000000000000000000, 0.8660254037844387076, 1.000000000000000000, 0.8660254037844387076, 1.000000000000000000, 0.8660254037844387076, 1.000000000000000000, 0.8660254037844387076, 1.000000000000000000, 0.8660254037844387076, 1.000000000000000000, 0.8660254037844387076, 1.000000000000000000, 0.8660254037844387076, 1.000000000000000000, 0.8660254037844387076, 1.000000000000000000, 0.8660254037844387076, 1.000000000000000000, 0.8660254037844387076, 1.000000000000000000, 0.8660254037844387076, 1.000000000000000000, 0.8660254037844387076, 1.000000000000000000, 0.8660254037844387076, 1.000000000000000000, 0.8660254037844387076, 1.000000000000000000, 0.8660254037844387076, 1.000000000000000000, 0.8660254037844387076, 1.000000000000000000, 0.8660254037844387076, 1.000000000000000000, 0.8660254037844387076, 1.000000000000000000, 0.8660254037844387076, 1.000000000000000000, 0.8660254037844387076, 1.000000000000000000, 0.8660254037844387076, 1.000000000000000000, 0.8660254037844387076, 1.000000000000000000, 0.8660254037844387076, 1.000000000000000000, 0.8660254037844387076, 1.000000000000000000, 0.8660254037844387076, 1.000000000000000000, 0.8660254037844387076, 1.000000000000000000, 0.8660254037844387076, 1.000000000000000000, 0.8660254037844387076, 1.000000000000000000, 0.8660254037844387076, 1.000000000000000000, 0.8660254037844387076, 1.000000000000000000, 0.8660254037844387076, 1.000000000000000000, 0.8660254037844387076, 1.000000000000000000, 0.8660254037844387076, 1.000000000000000000, 0.8660254037844387076, 1.000000000000000000, 0.8660254037844387076, 1.000000000000000000, 0.8660254037844387076, 1.000000000000000000, 0.8660254037844387076, 1.000000000000000000, 0.8660254037844387076, 1.000000000000000000, 0.8660254037844387076, 1.000000000000000000, 0.8660254037844387076, 1.000000000000000000, 0.8660254037844387076, 1.000000000000000000, 0.8660254037844387076, 1.000000000000000000, 0.8660254037844387076, 1.000000000000000000, 0.8660254037844387076, 1.000000000000000000, 0.8660254037844387076, 1.000000000000000000, 0.8660254037844387076, 1.000000000000000000, 0.8660254037844387076, 1.000000000000000000, 0.8660254037844387076, 1.000000000000000000, 0.8660254037844387076, 1.000000000000000000, 0.8660254037844387076, 1.000000000000000000, 0.8660254037844387076, 1.000000000000000000, 0.8660254037844387076, 1.000000000000000000, 0.8660254037844387076, 1.000000000000000000, 0.8660254037844387076, 1.000000000000000000, 0.8660254037844387076, 1.000000000000000000, 0.8660254037844387076, 1.000000000000000000, 0.8660254037844387076, 1.000000000000000000, 0.8660254037844387076, 1.000000000000000000, 0.8660254037844387076, 1.000000000000000000, 0.8660254037844387076, 1.000000000000000000, 0.8660254037844387076, 1.000000000000000000, 0.8660254037844387076, 1.000000000000000000, 0.8660254037844387076, 1.000000000000000000, 0.8660254037844387076, 1.000000000000000000, 0.8660254037844387076, 1.000000000000000000, 0.8660254037844387076, 1.000000000000000000, 0.8660254037844387076, 1.000000000000000000, 0.8660254037844387076, 1.000000000000000000, 0.8660254037844387076, 1.000000000000000000, 0.8660254037844387076, 1.000000000000000000, 0.8660254037844387076, 1.000000000000000000, 0.8660254037844387076, 1.000000000000000000, 0.8660254037844387076, 1.000000000000000000, 0.8660254037844387076, 1.000000000000000000, 0.8660254037844387076, 1.000000000000000000, 0.8660254037844387076, 1.000000000000000000, 0.8660254037844387076, 1.000000000000000000, 0.8660254037844387076, 1.000000000000000000, 0.8660254037844387076, 1.000000000000000000, 0.8660254037844387076, 1.000000000000000000, 0.8660254037844387076, 1.000000000000000000, 0.8660254037844387076, 1.000000000000000000, 0.8660254037844387076, 1.000000000000000000, 0.8660254037844387076, 1.000000000000000000, 0.8660254037844387076, 1.000000000000000000, 0.8660254037844387076, 1.000000000000000000, 0.8660254037844387076, 1.000000000000000000, 0.8660254037844387076, 1.000000000000000000, 0.8660254037844387076, 1.000000000000000000, 0.8660254037844387076, 1.000000000000000000, 0.8660254037844387076, 1.000000000000000000, 0.8660254037844387076, 1.000000000000000000, 0.8660254037844387076, 1.000000000000000000, 0.8660254037844387076, 1.000000000000000000, 0.8660254037844387076, 1.000000000000000000, 0.8660254037844387076, 1.000000000000000000, 0.8660254037844387076, 1.000000000000000000, 0.8660254037844387076, 1.000000000000000000, 0.8660254037844387076, 1.000000000000000000, 0.8660254037844387076, 1.000000000000000000, 0.8660254037844387076, 1.000000000000000000, 0.8660254037844387076, 1.000000000000000000, 0.8660254037844387076, 1.000000000000000000, 0.8660254037844387076, 1.000000000000000000, 0.8660254037844387076, 1.000000000000000000, 0.8660254037844387076, 1.000000000000000000, 0.8660254037844387076, 1.000000000000000000, 0.8660254037844387076, 1.000000000000000000, 0.8660254037844387076, 1.000000000000000000, 0.8660254037844387076, 1.000000000000000000, 0.8660254037844387076, 1.000000000000000000, 0.8660254037844387076, 1.000000000000000000, 0.8660254037844387076, 1.000000000000000000, 0.8660254037844387076, 1.000000000000000000, 0.8660254037844387076, 1.000000000000000000, 0.8660254037844387076, 1.000000000000000000, 0.8660254037844387076, 1.000000000000000000, 0.8660254037844387076, 1.000000000000000000, 0.8660254037844387076, 1.000000000000000000, 0.8660254037844387076, 1.000000000000000000, 0.8660254037844387076, 1.000000000000000000, 0.8660254037844387076, 1.000000000000000000, 0.8660254037844387076, 1.000000000000000000, 0.8660254037844387076, 1.000000000000000000, 0.8660254037844387076, 1.000000000000000000, 0.8660254037844387076, 1.000000000000000000, 0.8660254037844387076, 1.000000000000000000, 0.8660254037844387076, 1.000000000000000000, 0.8660254037844387076, 1.000000000000000000, 0.8660254037844387076, 1.000000000000000000, 0.8660254037844387076, 1.000000000000000000, 0.8660254037844387076, 1.000000000000000000, 0.8660254037844387076, 1.000000000000000000, 0.8660254037844387076, 1.000000000000000000, 0.8660254037844387076, 1.000000000000000000, 0.8660254037844387076, 1.000000000000000000, 0.8660254037844387076, 1.000000000000000000, 0.8660254037844387076, 1.000000000000000000, 0.8660254037844387076, 1.000000000000000000, 0.8660254037844387076, 1.000000000000000000, 0.8660254037844387076, 1.000000000000000000, 0.8660254037844387076, 1.000000000000000000, 0.8660254037844387076, 1.000000000000000000, 0.8660254037844387076, 1.000000000000000000, 0.8660254037844387076, 1.000000000000000000, 0.8660254037844387076, 1.000000000000000000, 0.8660254037844387076, 1.000000000000000000, 0.8660254037844387076, 1.000000000000000000, 0.8660254037844387076, 1.000000000000000000, 0.8660254037844387076, 1.000000000000000000, 0.8660254037844387076, 1.000000000000000000, 0.8660254037844387076, 1.000000000000000000, 0.8660254037844387076, 1.000000000000000000, 0.8660254037844387076, 1.000000000000000000, 0.8660254037844387076, 1.000000000000000000, 0.8660254037844387076, 1.000000000000000000, 0.8660254037844387076, 1.000000000000000000, 0.8660254037844387076, 1.000000000000000000, 0.8660254037844387076, 1.000000000000000000, 0.8660254037844387076, 1.000000000000000000, 0.8660254037844387076, 1.000000000000000000, 0.8660254037844387076, 1.000000000000000000, 0.8660254037844387076, 1.000000000000000000, 0.8660254037844387076, 1.000000000000000000, 0.8660254037844387076, 1.000000000000000000, 0.8660254037844387076, 1.000000000000000000, 0.8660254037844387076, 1.000000000000000000, 0.8660254037844387076, 1.000000000000000000, 0.8660254037844387076, 1.000000000000000000, 0.8660254037844387076, 1.000000000000000000, 0.8660254037844387076, 1.000000000000000000, 0.8660254037844387076, 1.000000000000000000, 0.8660254037844387076, 1.000000000000000000, 0.8660254037844387076, 1.000000000000000000, 0.8660254037844387076, 1.000000000000000000, 0.8660254037844387076, 1.000000000000000000, 0.8660254037844387076, 1.000000000000000000, 0.8660254037844387076, 1.000000000000000000, 0.8660254037844387076, 1.000000000000000000, 0.8660254037844387076, 1.000000000000000000, 0.8660254037844387076, 1.000000000000000000, 0.8660254037844387076, 1.000000000000000000, 0.8660254037844387076, 1.000000000000000000, 0.8660254037844387076, 1.000000000000000000, 0.8660254037844387076, 1.000000000000000000, 0.8660254037844387076, 1.000000000000000000, 0.8660254037844387076, 1.000000000000000000, 0.8660254037844387076, 1.000000000000000000, 0.8660254037844387076, 1.000000000000000000, 0.8660254037844387076, 1.000000000000000000, 0.8660254037844387076, 1.000000000000000000, 0.8660254037844387076, 1.000000000000000000, 0.8660254037844387076, 1.000000000000000000, 0.8660254037844387076, 1.000000000000000000, 0.8660254037844387076, 1.000000000000000000, 0.8660254037844387076, 1.000000000000000000, 0.8660254037844387076, 1.000000000000000000, 0.8660254037844387076, 1.000000000000000000, 0.8660254037844387076, 1.000000000000000000, 0.8660254037844387076, 1.000000000000000000, 0.8660254037844387076, 1.000000000000000000) ) ) 
 REPRESENTATION_ITEM ( '' )  SURFACE ( )  );
#73262=CARTESIAN_POINT ( 'NONE',  ( 9.284636267260101050, 9.726497154758602548, -0.7998128361456281477 ) ) ;
#73267=EDGE_LOOP ( 'NONE', ( #201513, #31683, #107170, #137885 ) ) ;
#73270=EDGE_CURVE ( 'NONE', #104869, #104455, #210369, .T. ) ;
#73274=CARTESIAN_POINT ( 'NONE',  ( -8.202319746587722449, 8.671720580548228696, 1.040834085586084257E-14 ) ) ;
#73279=CARTESIAN_POINT ( 'NONE',  ( -9.982881178363895103, 10.54111621771303753, 1.040834085586084257E-14 ) ) ;
#73284=EDGE_CURVE ( 'NONE', #164674, #213687, #127588, .T. ) ;
#73286=CARTESIAN_POINT ( 'NONE',  ( 4.189106276498237413, 3.989638198777126110, -0.7216878364870188411 ) ) ;
#73288=CARTESIAN_POINT ( 'NONE',  ( 4.813308228051395687, 5.574280006603454574, 1.199719254218462483 ) ) ;
#73290=VERTEX_POINT ( 'NONE', #181077 ) ;
#73295=CARTESIAN_POINT ( 'NONE',  ( -6.254388934605767503, 6.191208599995166040, 0.7998128361456341429 ) ) ;
#73299=CARTESIAN_POINT ( 'NONE',  ( -9.969323024750229578, 10.52529837183042716, -0.7998128361456291469 ) ) ;
#73305=CARTESIAN_POINT ( 'NONE',  ( 6.778713617152772208, 10.85232362007950258, -0.7216878364870267237 ) ) ;
#73307=CARTESIAN_POINT ( 'NONE',  ( -1.364683531250010740, 4.342708333674753618, 0.7879004041258379498 ) ) ;
#73309=CARTESIAN_POINT ( 'NONE',  ( 5.497994985541524215, 6.373081223675282736, -1.199719254218445830 ) ) ;
#73318=CARTESIAN_POINT ( 'NONE',  ( 1.492665153618401241, 8.694790292836037437, -2.590406265390448048 ) ) ;
#73324=CARTESIAN_POINT ( 'NONE',  ( 1.364683531249988757, 0.6968750003414209138, 0.000000000000000000 ) ) ;
#73325=LINE ( 'NONE', #189225, #67473 ) ;
#73326=CARTESIAN_POINT ( 'NONE',  ( 10.71502147350184231, 11.39527989537399755, 0.000000000000000000 ) ) ;
#73328=CARTESIAN_POINT ( 'NONE',  ( -5.585596099150191840, 7.539614753807099667, -1.443375672974052559 ) ) ;
#73329=CARTESIAN_POINT ( 'NONE',  ( 4.690757960648231695, 5.535267711253469614, 1.082531754730560403 ) ) ;
#73330=CARTESIAN_POINT ( 'NONE',  ( -7.171900071504754060, 7.469564292951421436, -0.7216878364870267237 ) ) ;
#73334=CARTESIAN_POINT ( 'NONE',  ( 4.473300617505036492, 7.306268922809479704, -1.199719254218452047 ) ) ;
#73341=CARTESIAN_POINT ( 'NONE',  ( -0.6823417656249969321, 5.717708333674756283, -1.181850606188749264 ) ) ;
#73346=CARTESIAN_POINT ( 'NONE',  ( 5.469824908109481854, 8.468880595181346393, -1.199719254218446718 ) ) ;
#73349=CARTESIAN_POINT ( 'NONE',  ( -5.377780486114890124, 9.425827667109372143, 0.000000000000000000 ) ) ;
#73353=CARTESIAN_POINT ( 'NONE',  ( 7.775764792637399836, 9.030479331953833011, -1.199719254218441611 ) ) ;
#73356=CARTESIAN_POINT ( 'NONE',  ( -5.876569516519495551, 8.943415971659659292, 1.199719254218452047 ) ) ;
#73357=CARTESIAN_POINT ( 'NONE',  ( 5.450014562569148957, 9.302174723065263606, 1.040834085586084257E-14 ) ) ;
#73358=CARTESIAN_POINT ( 'NONE',  ( 4.919437264989244163, 6.867374270256937585, 1.424029350978267550 ) ) ;
#73359=CARTESIAN_POINT ( 'NONE',  ( -4.062639585589296942, 7.891496616496157301, 0.7998128361456341429 ) ) ;
#73362=CARTESIAN_POINT ( 'NONE',  ( -4.740547266272593596, 8.682388910626682943, -0.7998128361456281477 ) ) ;
#73367=CARTESIAN_POINT ( 'NONE',  ( 10.07778825365955733, 10.65184113889131012, -0.7998128361456281477 ) ) ;
#73369=CARTESIAN_POINT ( 'NONE',  ( -1.201851678989727383E-14, 1.821875000341421691, 1.575800808251672791 ) ) ;
#73371=CARTESIAN_POINT ( 'NONE',  ( -6.616015773788831211, 7.781401826584148473, 1.082531754730549967 ) ) ;
#73376=CARTESIAN_POINT ( 'NONE',  ( 4.794779880727245036, 8.745660294157122649, -0.7998128361456281477 ) ) ;
#73379=CARTESIAN_POINT ( 'NONE',  ( -1.364683531250012516, 2.092708333674750953, 0.7879004041258379498 ) ) ;
#73382=CARTESIAN_POINT ( 'NONE',  ( 4.378920427533921078, 4.211088041652093494, 1.214306433183764966E-14 ) ) ;
#73385=CARTESIAN_POINT ( 'NONE',  ( -5.773074481320628948, 5.629675071162500544, 0.000000000000000000 ) ) ;
#73388=CARTESIAN_POINT ( 'NONE',  ( -6.656690234185426824, 10.70996300661758660, 0.7216878364870458196 ) ) ;
#73398=CARTESIAN_POINT ( 'NONE',  ( -6.493992390821436977, 10.52014885602626393, 0.7216878364870458196 ) ) ;
#73403=CARTESIAN_POINT ( 'NONE',  ( -7.171900071504745178, 9.390302721554109056, -1.443375672974058777 ) ) ;
#73409=CARTESIAN_POINT ( 'NONE',  ( -1.001543065824772872E-14, 5.493750000682816825, 1.732050807568877637 ) ) ;
#73410=CARTESIAN_POINT ( 'NONE',  ( 4.757767692435503015, 7.006667324785019524, -1.397933448811568224 ) ) ;
#73411=CARTESIAN_POINT ( 'NONE',  ( -1.201851678989727383E-14, 5.118750000682815937, -1.732050807568863648 ) ) ;
#73417=CARTESIAN_POINT ( 'NONE',  ( -7.718669524881690336, 7.899535955317097624, 0.7998128361456462443 ) ) ;
#73421=CARTESIAN_POINT ( 'NONE',  ( 3.846762897975340767, 5.510976019103107859, -1.599625672291256295 ) ) ;
#73424=CARTESIAN_POINT ( 'NONE',  ( -3.022498986271247023, 2.800000000000024691, -2.500000000000000444 ) ) ;
#73426=CARTESIAN_POINT ( 'NONE',  ( 5.608269097547198712, 9.694731047113750222, -0.7998128361456281477 ) ) ;
#73431=CARTESIAN_POINT ( 'NONE',  ( -6.412643469583822586, 6.583764924043652655, 1.040834085586084257E-14 ) ) ;
#73436=CARTESIAN_POINT ( 'NONE',  ( -0.2753771601587257645, 6.383602266891855059, 3.144803022522423053 ) ) ;
#73437=CARTESIAN_POINT ( 'NONE',  ( 4.175548122884573665, 3.973820352894515295, 1.214306433183764966E-14 ) ) ;
#73440=CARTESIAN_POINT ( 'NONE',  ( 0.6823417656249882723, 0.6760416670080898749, -1.181850606188749264 ) ) ;
#73442=CARTESIAN_POINT ( 'NONE',  ( -7.395082721250053837, 10.71501471051202614, -1.199719254218446718 ) ) ;
#73444=CARTESIAN_POINT ( 'NONE',  ( 6.584456157731144899, 10.83361595066169514, -0.7998128361456291469 ) ) ;
#73446=CARTESIAN_POINT ( 'NONE',  ( -7.018317073368468328, 11.33978701890523233, -0.7998128361456291469 ) ) ;
#73450=CARTESIAN_POINT ( 'NONE',  ( 1.364683531249990311, 5.134375000341417916, 1.214306433183764966E-14 ) ) ;
#73453=CARTESIAN_POINT ( 'NONE',  ( 7.768458830950378591, 12.00702636951006497, 1.040834085586084257E-14 ) ) ;
#73456=CARTESIAN_POINT ( 'NONE',  ( 0.7499999999999902300, 5.816666666666685082, -1.299038105676658228 ) ) ;
#73460=CARTESIAN_POINT ( 'NONE',  ( 8.242994206984347372, 8.719174117677642499, 1.040834085586084257E-14 ) ) ;
#73463=CARTESIAN_POINT ( 'NONE',  ( -6.263503779833496488, 6.409768619334935913, 0.7216878364870317197 ) ) ;
#73465=CARTESIAN_POINT ( 'NONE',  ( 0.6823417656249899377, 2.592708333674753618, 1.181850606188767472 ) ) ;
#73469=CARTESIAN_POINT ( 'NONE',  ( -7.393273838153706201, 7.519907654134449615, 0.7998128361456341429 ) ) ;
#73470=CARTESIAN_POINT ( 'NONE',  ( 1.364683531249990311, 4.696875000341417916, 1.214306433183764966E-14 ) ) ;
#73476=CARTESIAN_POINT ( 'NONE',  ( 8.067265095331215718, 9.370563018429956870, 1.199719254218462483 ) ) ;
#73480=CARTESIAN_POINT ( 'NONE',  ( -1.499999999999997780, 1.650000000000019451, 0.000000000000000000 ) ) ;
#73486=CARTESIAN_POINT ( 'NONE',  ( 8.107412671292047790, 8.560995659369956101, 0.7216878364870458196 ) ) ;
#73489=CARTESIAN_POINT ( 'NONE',  ( 4.552840656090682891, 4.206068941727564514, 1.214306433183764966E-14 ) ) ;
#73495=CARTESIAN_POINT ( 'NONE',  ( 8.776205506747620788, 9.133327934160710981, -0.7998128361456221525 ) ) ;
#73496=CARTESIAN_POINT ( 'NONE',  ( -1.543624195544814226, 8.695410207106890610, 2.508689898543552399 ) ) ;
#73499=CARTESIAN_POINT ( 'NONE',  ( 0.6823417656249882723, -0.3239583329919110133, -1.181850606188749264 ) ) ;
#73500=CARTESIAN_POINT ( 'NONE',  ( -0.7500000000000215383, 0.6916666666666876351, 1.299038105676659116 ) ) ;
#73502=CARTESIAN_POINT ( 'NONE',  ( 5.392392409933256303, 7.314210449720692786, 1.599625672291267398 ) ) ;
#73508=CARTESIAN_POINT ( 'NONE',  ( 1.364683531249988535, 5.655208333674751842, -0.7879004041258300672 ) ) ;
#73510=CARTESIAN_POINT ( 'NONE',  ( -9.481229494658258261, 9.955855920056455588, -0.7998128361456291469 ) ) ;
#73511=CARTESIAN_POINT ( 'NONE',  ( -4.582292731738899505, 8.289832587096611860, 0.7216878364870458196 ) ) ;
#73519=ORIENTED_EDGE ( 'NONE', *, *, #193336, .F. ) ;
#73520=CARTESIAN_POINT ( 'NONE',  ( 8.111855979677986994, 8.358253485912799263, 1.040834085586084257E-14 ) ) ;
#73524=CARTESIAN_POINT ( 'NONE',  ( 7.741342523278705201, 9.094283034322399928, 1.082531754730558626 ) ) ;
#73527=CARTESIAN_POINT ( 'NONE',  ( -8.779068160048691283, 10.20099992726700933, -1.199719254218446718 ) ) ;
#73528=CARTESIAN_POINT ( 'NONE',  ( 6.169123589417988995, 7.156064594864501416, -1.199719254218445830 ) ) ;
#73532=CARTESIAN_POINT ( 'NONE',  ( 4.207107738942202246, 3.802713871720993399, 1.214306433183764966E-14 ) ) ;
#73540=CARTESIAN_POINT ( 'NONE',  ( -5.910991785878183080, 5.998504626387068051, -0.7216878364870278340 ) ) ;
#73541=CARTESIAN_POINT ( 'NONE',  ( 9.083599731475976213, 12.58098820582193689, 1.082531754730546636 ) ) ;
#73544=CARTESIAN_POINT ( 'NONE',  ( -6.856673000209188906, 9.022537805042615489, 1.599625672291283607 ) ) ;
#73549=CARTESIAN_POINT ( 'NONE',  ( -8.402302512167102222, 10.82577223566020841, -1.599625672291263179 ) ) ;
#73551=CYLINDRICAL_SURFACE ( 'NONE', #115965, 1.250000000000000000 ) ;
#73556=CARTESIAN_POINT ( 'NONE',  ( 5.443762371086860341, 6.309809840144842141, 1.199719254218462483 ) ) ;
#73559=ORIENTED_EDGE ( 'NONE', *, *, #113892, .F. ) ;
#73567=CARTESIAN_POINT ( 'NONE',  ( -7.542413527904030524, 7.693903958843159252, 1.040834085586084257E-14 ) ) ;
#73570=CARTESIAN_POINT ( 'NONE',  ( 6.209271165378815738, 7.306866450105836464, -1.082531754730543083 ) ) ;
#73573=DIRECTION ( 'NONE',  ( 0.000000000000000000, 8.546850786086437571E-32, 1.000000000000000000 ) ) ;
#73574=CARTESIAN_POINT ( 'NONE',  ( 4.379447312414087357, 5.068108938359919158, -1.199719254218452047 ) ) ;
#73576=CARTESIAN_POINT ( 'NONE',  ( -5.412729640353771465, 7.337937218544611895, 1.599625672291269396 ) ) ;
#73580=CARTESIAN_POINT ( 'NONE',  ( -5.961834861707238531, 7.978559976790334574, -1.599625672291263179 ) ) ;
#73581=CARTESIAN_POINT ( 'NONE',  ( -5.807007791129851881, 6.063258055044094874, 0.5391689476613946708 ) ) ;
#73586=CARTESIAN_POINT ( 'NONE',  ( 6.520158902582615212, 5.290451655907107309, 2.438235897557464948 ) ) ;
#73587=CARTESIAN_POINT ( 'NONE',  ( 7.772902139336337335, 7.962807338847539107, 0.7998128361456341429 ) ) ;
#73590=CARTESIAN_POINT ( 'NONE',  ( -5.603170282960403092, 6.190551086330195574, -0.8764620106105174280 ) ) ;
#73597=CARTESIAN_POINT ( 'NONE',  ( 8.270110514656016321, 12.59228666716665401, 0.7216878364870438212 ) ) ;
#73619=CARTESIAN_POINT ( 'NONE',  ( -4.620631424159025613, 4.285158171140619032, -0.7998128361456221525 ) ) ;
#73622=CARTESIAN_POINT ( 'NONE',  ( -2.611917148927046295, 6.198987107056845858, 1.040834085586084257E-14 ) ) ;
#73628=CARTESIAN_POINT ( 'NONE',  ( -0.7500000000000249800, -0.5270833326505158789, 1.299038105676659116 ) ) ;
#73638=CARTESIAN_POINT ( 'NONE',  ( 2.679707916995359263, 6.278076336469897711, -0.7998128361456291469 ) ) ;
#73642=CARTESIAN_POINT ( 'NONE',  ( 9.449669878600614581, 12.04770082983265844, -1.443375672974058777 ) ) ;
#73644=CARTESIAN_POINT ( 'NONE',  ( 1.364683531249988535, 2.967708333674755394, -0.7879004041258239610 ) ) ;
#73647=CARTESIAN_POINT ( 'NONE',  ( -8.134002093194872884, 11.57708731111429401, 1.199719254218453823 ) ) ;
#73648=CARTESIAN_POINT ( 'NONE',  ( -4.067082893975237035, 7.688754443039000464, 1.040834085586084257E-14 ) ) ;
#73650=CARTESIAN_POINT ( 'NONE',  ( -5.042743069279040036, 7.970618449879118828, 1.199719254218464037 ) ) ;
#73652=CARTESIAN_POINT ( 'NONE',  ( 0.6823417656249917140, 5.592708333674749177, 1.181850606188765695 ) ) ;
#73660=CARTESIAN_POINT ( 'NONE',  ( -4.568734577680875653, 8.274014740695587733, -0.7216878364870257245 ) ) ;
#73661=CARTESIAN_POINT ( 'NONE',  ( 1.387358672534392046, 7.251968950353694154, -4.302625267138185272 ) ) ;
#73665=CARTESIAN_POINT ( 'NONE',  ( -5.056828107772860292, 6.922718763866881453, -1.443375672974051449 ) ) ;
#73667=CARTESIAN_POINT ( 'NONE',  ( 8.075853055234393452, 12.57357899774884658, 0.7998128361456462443 ) ) ;
#73675=CARTESIAN_POINT ( 'NONE',  ( -3.415764635639130020, 6.072476943965863683, 1.199719254218462483 ) ) ;
#73676=CARTESIAN_POINT ( 'NONE',  ( -9.755255220232635693, 11.33988483081495957, -1.199719254218441611 ) ) ;
#73681=CARTESIAN_POINT ( 'NONE',  ( 6.616015773788773480, 10.66250946948817813, -0.7216878364870267237 ) ) ;
#73683=CARTESIAN_POINT ( 'NONE',  ( 6.654354466208897811, 6.657835053532175529, 0.7998128361456341429 ) ) ;
#73698=CARTESIAN_POINT ( 'NONE',  ( 9.596473800374404561, 10.09030761005864285, 0.000000000000000000 ) ) ;
#73699=CARTESIAN_POINT ( 'NONE',  ( -4.903245109636583443, 8.872203061218007392, -0.7998128361456281477 ) ) ;
#73706=CARTESIAN_POINT ( 'NONE',  ( -1.364683531250010295, 5.238541667008086655, -0.7879004041258300672 ) ) ;
#73708=CARTESIAN_POINT ( 'NONE',  ( -4.713430959045263435, 8.650753218861462202, 0.7998128361456481317 ) ) ;
#73710=CARTESIAN_POINT ( 'NONE',  ( 4.547870462380197765, 7.393267075163835855, 1.199719254218462483 ) ) ;
#73711=CARTESIAN_POINT ( 'NONE',  ( -5.250031796989778066, 7.148123067953287446, 1.599625672291267398 ) ) ;
#73717=CARTESIAN_POINT ( 'NONE',  ( 5.504247177468175600, 8.405076892812779477, 1.082531754730558626 ) ) ;
#73720=CARTESIAN_POINT ( 'NONE',  ( 6.683806541412754321, 8.820860269780128604, -1.443375672974058777 ) ) ;
#73721=CARTESIAN_POINT ( 'NONE',  ( -1.201851678989727383E-14, 2.884375000341418804, 1.575800808251672791 ) ) ;
#73723=CARTESIAN_POINT ( 'NONE',  ( 5.653386866774156694, 5.697965554099049257, -0.7216878364870207285 ) ) ;
#73725=CARTESIAN_POINT ( 'NONE',  ( -2.168941388506379742, 5.474256019991960542, -0.7216878364870267237 ) ) ;
#73733=CARTESIAN_POINT ( 'NONE',  ( -4.418103850092305329, 7.323797853316306394, 1.240345400901581296 ) ) ;
#73740=CARTESIAN_POINT ( 'NONE',  ( -8.967828540435322182, 12.54988483289483980, 1.199719254218462483 ) ) ;
#73751=CARTESIAN_POINT ( 'NONE',  ( 3.633221978782282147, 5.261844946711204507, -1.443375672974057666 ) ) ;
#73752=CARTESIAN_POINT ( 'NONE',  ( 1.364683531249988535, 3.467708333674749621, -0.7879004041258239610 ) ) ;
#73754=CARTESIAN_POINT ( 'NONE',  ( 7.564559641420864899, 10.91273778404466199, -1.199719254218446718 ) ) ;
#73756=CARTESIAN_POINT ( 'NONE',  ( -10.64045162862669081, 11.30828174301964140, -0.7998128361456221525 ) ) ;
#73761=CARTESIAN_POINT ( 'NONE',  ( -1.499999999999997780, 3.400000000000021227, 1.214306433183764966E-14 ) ) ;
#73762=CARTESIAN_POINT ( 'NONE',  ( 3.974511587100456822, 7.788680618259193444, 1.040834085586084257E-14 ) ) ;
#73766=CARTESIAN_POINT ( 'NONE',  ( -1.364683531250012516, 3.738541667008087099, -0.7879004041258300672 ) ) ;
#73768=CARTESIAN_POINT ( 'NONE',  ( 8.270110514656016321, 12.59228666716665401, 0.7216878364870438212 ) ) ;
#73773=CARTESIAN_POINT ( 'NONE',  ( -0.7500000000000006661, 1.389583334016154748, -1.299038105676652011 ) ) ;
#73775=CARTESIAN_POINT ( 'NONE',  ( -6.905180308061733996, 6.950465202360470052, 0.7998128361456341429 ) ) ;
#73776=DIRECTION ( 'NONE',  ( 0.000000000000000000, 0.000000000000000000, 1.000000000000000000 ) ) ;
#73782=VERTEX_POINT ( 'NONE', #85704 ) ;
#73784=CARTESIAN_POINT ( 'NONE',  ( 9.433775957010412938, 9.900493459467314850, 0.000000000000000000 ) ) ;
#73785=CARTESIAN_POINT ( 'NONE',  ( 3.985207087413062066, 6.736826471035503694, -1.199719254218452047 ) ) ;
#73790=CARTESIAN_POINT ( 'NONE',  ( 6.491656622844908853, 6.468020902940851968, 0.7998128361456341429 ) ) ;
#73792=ORIENTED_EDGE ( 'NONE', *, *, #80476, .T. ) ;
#73794=EDGE_LOOP ( 'NONE', ( #109038, #53020, #59708, #99794, #43556, #94413, #41231 ) ) ;
#73796=EDGE_LOOP ( 'NONE', ( #41320, #69303, #122411, #125420, #12521, #57092, #126968, #164386, #96016, #155567, #100425, #53208, #63489, #46583, #22850, #14621, #11132, #98845, #24005, #156196, #126971, #36488, #110625, #120485, #109540, #83771, #57021 ) ) ;
#73797=CARTESIAN_POINT ( 'NONE',  ( 10.70146331988817323, 11.37946204949139251, 0.7998128361456341429 ) ) ;
#73803=CARTESIAN_POINT ( 'NONE',  ( 5.872608658597049391, 5.988986745869715023, 0.2392922861021197500 ) ) ;
#73815=CARTESIAN_POINT ( 'NONE',  ( -4.217958839219735800, 3.978389137448586244, 0.5316758947214468289 ) ) ;
#73816=CARTESIAN_POINT ( 'NONE',  ( 5.802526556968819804, 9.713438716531550554, -0.7216878364870267237 ) ) ;
#73817=CARTESIAN_POINT ( 'NONE',  ( -4.223528545856940042, 4.886203710709899006, -1.199719254218446718 ) ) ;
#73821=CARTESIAN_POINT ( 'NONE',  ( -6.403528624356093601, 6.365204904703887223, 1.040834085586084257E-14 ) ) ;
#73831=CARTESIAN_POINT ( 'NONE',  ( -1.123270288254055060, 3.033552654332631437, 0.7749999999939940487 ) ) ;
#73836=CARTESIAN_POINT ( 'NONE',  ( 10.39640486358069360, 11.02356051713265650, 0.7998128361456462443 ) ) ;
#73840=VERTEX_POINT ( 'NONE', #38033 ) ;
#73846=CARTESIAN_POINT ( 'NONE',  ( -8.188761592974033832, 12.49737959187099179, -0.7216878364870267237 ) ) ;
#73848=CARTESIAN_POINT ( 'NONE',  ( -3.023105066167347310, 5.702484939155337607, 2.420000000000010587 ) ) ;
#73849=CARTESIAN_POINT ( 'NONE',  ( 6.916630921265960019, 11.22115317478565188, 0.7998128361456462443 ) ) ;
#73853=CARTESIAN_POINT ( 'NONE',  ( -7.172426956829277778, 8.326585190177668849, -1.199719254218452935 ) ) ;
#73854=CARTESIAN_POINT ( 'NONE',  ( 4.684505768721569652, 5.424010470718658716, -1.199719254218452047 ) ) ;
#73857=AXIS2_PLACEMENT_3D ( 'NONE', #176958, #180157, #195342 ) ;
#73858=CARTESIAN_POINT ( 'NONE',  ( 9.728138913005292210, 11.30824913904973705, -1.199719254218440723 ) ) ;
#73862=CARTESIAN_POINT ( 'NONE',  ( 0.6823417656249899377, 3.238541667008085323, -1.181850606188754593 ) ) ;
#73865=CARTESIAN_POINT ( 'NONE',  ( 5.992340707560147806, 8.974519344586754599, 1.082531754730558626 ) ) ;
#73874=CARTESIAN_POINT ( 'NONE',  ( 9.042925270190632858, 10.61279623905300085, 1.082531754730549967 ) ) ;
#73877=VERTEX_POINT ( 'NONE', #171220 ) ;
#73881=CARTESIAN_POINT ( 'NONE',  ( -8.143643823302737061, 12.65266822716189843, 0.000000000000000000 ) ) ;
#73882=LINE ( 'NONE', #29405, #209411 ) ;
#73890=CARTESIAN_POINT ( 'NONE',  ( 5.379888026524302980, 5.170957540566797128, -0.7998128361456211532 ) ) ;
#73897=CARTESIAN_POINT ( 'NONE',  ( 4.462605117192430804, 8.358123070033169455, 1.040834085586084257E-14 ) ) ;
#73900=CARTESIAN_POINT ( 'NONE',  ( -1.500000000000013101, 2.910416667349485120, -0.8660254037844313801 ) ) ;
#73904=VERTEX_POINT ( 'NONE', #75855 ) ;
#73906=CARTESIAN_POINT ( 'NONE',  ( -1.500000000000001332, 0.4000000000000253353, 0.000000000000000000 ) ) ;
#73907=CARTESIAN_POINT ( 'NONE',  ( 8.599949509769960088, 8.927695937686774386, 1.040834085586084257E-14 ) ) ;
#73908=CARTESIAN_POINT ( 'NONE',  ( -0.6823417656250003738, -0.2822916663252489355, -1.181850606188749264 ) ) ;
#73911=CARTESIAN_POINT ( 'NONE',  ( 8.920901888111989919, 11.43080484092926241, 1.443375672974076540 ) ) ;
#73916=CARTESIAN_POINT ( 'NONE',  ( -4.530395885260773525, 8.437212299446219532, 0.7998128361456481317 ) ) ;
#73917=CARTESIAN_POINT ( 'NONE',  ( 0.7499999999999885647, 3.097916667349487341, -1.299038105676658228 ) ) ;
#73918=CARTESIAN_POINT ( 'NONE',  ( -1.364683531250010295, 5.301041667008085767, -0.7879004041258300672 ) ) ;
#73931=CARTESIAN_POINT ( 'NONE',  ( -7.883176251342026042, 11.28445716228600126, -1.199719254218446718 ) ) ;
#73932=CARTESIAN_POINT ( 'NONE',  ( 7.416473721875251890, 8.611306416064660851, 1.199719254218462483 ) ) ;
#73939=CARTESIAN_POINT ( 'NONE',  ( -7.182068686937172153, 9.402166106225269715, 1.599625672291283607 ) ) ;
#73943=CARTESIAN_POINT ( 'NONE',  ( 10.70146331988817323, 11.37946204949139251, 0.7998128361456341429 ) ) ;
#73944=FACE_BOUND ( 'NONE', #143904, .T. ) ;
#73947=CARTESIAN_POINT ( 'NONE',  ( -5.037017762676898158, 5.835274463666530131, -1.199719254218446718 ) ) ;
#73949=CARTESIAN_POINT ( 'NONE',  ( -9.481229494658258261, 9.955855920056455588, -0.7998128361456291469 ) ) ;
#73953=CARTESIAN_POINT ( 'NONE',  ( -3.983506901647102083, 7.838413813543339437, 0.2012387096505599549 ) ) ;
#73960=CARTESIAN_POINT ( 'NONE',  ( 6.144869935491714230, 8.192100896205568361, -1.599625672291262513 ) ) ;
#73962=CARTESIAN_POINT ( 'NONE',  ( 3.001048869802148023, 2.786623193720112024, 2.499999999999998668 ) ) ;
#73979=CARTESIAN_POINT ( 'NONE',  ( 2.548569689688999329, 5.917155704705049146, -0.7216878364870267237 ) ) ;
#73983=CARTESIAN_POINT ( 'NONE',  ( -7.621654909176601045, 12.04368116068139472, 0.7998128361456481317 ) ) ;
#73988=CARTESIAN_POINT ( 'NONE',  ( -1.500000000000013101, 0.2020833340161521663, 0.8660254037844403729 ) ) ;
#73996=CARTESIAN_POINT ( 'NONE',  ( -1.402160292154681736E-14, 0.3218750003414227456, 1.575800808251672791 ) ) ;
#74002=CARTESIAN_POINT ( 'NONE',  ( -3.928111819657352566, 5.605883094398769195, 1.599625672291267398 ) ) ;
#74005=CARTESIAN_POINT ( 'NONE',  ( -1.500000000000015099, 0.3791666666666850261, -0.8660254037844383745 ) ) ;
#74007=CARTESIAN_POINT ( 'NONE',  ( -1.364683531250000748, -0.6781249996585803075, 0.000000000000000000 ) ) ;
#74013=CARTESIAN_POINT ( 'NONE',  ( -1.402160292154681736E-14, -0.05312499965857903073, -1.575800808251665908 ) ) ;
#74017=CARTESIAN_POINT ( 'NONE',  ( -7.527801604085656351, 9.805521176231838609, 1.599625672291295375 ) ) ;
#74018=CARTESIAN_POINT ( 'NONE',  ( 9.264299036839600987, 9.702770385934682551, -0.7998128361456281477 ) ) ;
#74019=CARTESIAN_POINT ( 'NONE',  ( 3.520313441042647984, 7.258782781191745137, 0.7998128361456321445 ) ) ;
#74023=CARTESIAN_POINT ( 'NONE',  ( 1.364683531249986537, 0.4677083336747514530, -0.7879004041258309554 ) ) ;
#74032=CARTESIAN_POINT ( 'NONE',  ( 6.480434237652132445, 7.623223367758051872, 1.082531754730558626 ) ) ;
#74035=CARTESIAN_POINT ( 'NONE',  ( -3.730464822054482710, 7.503959392372201442, 1.040834085586084257E-14 ) ) ;
#74037=CARTESIAN_POINT ( 'NONE',  ( 1.499999999999999778, 7.809273069926267574, 3.635729725621137387 ) ) ;
#74039=B_SPLINE_CURVE_WITH_KNOTS ( 'NONE', 3,
 ( #141272, #91432, #110925, #205131, #42688, #90348, #209397, #172670, #139104, #40539, #26397, #27468 ),
 .UNSPECIFIED., .F., .F.,
 ( 4, 2, 2, 2, 2, 4 ),
 ( 0.003750395023273722043, 0.003985267534258110644, 0.004220140045242499680, 0.004689885067211279485, 0.005159630089180061892, 0.005629375111148844299 ),
 .UNSPECIFIED. ) ;
#74040=CARTESIAN_POINT ( 'NONE',  ( -3.195971524519394702, 4.751719416737803847, -1.599625672291262513 ) ) ;
#74041=CARTESIAN_POINT ( 'NONE',  ( 3.999292125906894313, 7.609665213625947722, 0.7216878364870317197 ) ) ;
#74042=CARTESIAN_POINT ( 'NONE',  ( -8.798878505144658746, 10.32807501316600884, -1.082531754730543083 ) ) ;
#74044=CARTESIAN_POINT ( 'NONE',  ( -1.500000000000011324, 3.670833333333356485, 0.8660254037844403729 ) ) ;
#74048=CARTESIAN_POINT ( 'NONE',  ( 9.137832345930652522, 10.72352116074969075, -1.082531754730543083 ) ) ;
#74060=CARTESIAN_POINT ( 'NONE',  ( 7.090551149822728938, 10.25576486055978442, 1.082531754730558626 ) ) ;
#74061=CARTESIAN_POINT ( 'NONE',  ( 7.344766530301147789, 9.591980256816594164, 1.599625672291281386 ) ) ;
#74063=CARTESIAN_POINT ( 'NONE',  ( 5.192409644353875642, 5.160158794608717514, 1.040834085586084257E-14 ) ) ;
#74066=DIRECTION ( 'NONE',  ( 0.000000000000000000, 1.000000000000000000, -8.546850786086437571E-32 ) ) ;
#74067=CARTESIAN_POINT ( 'NONE',  ( 5.192409644353875642, 5.160158794608717514, 1.040834085586084257E-14 ) ) ;
#74069=CARTESIAN_POINT ( 'NONE',  ( -9.015808963407680565, 9.620791333504852716, 1.040834085586084257E-14 ) ) ;
#74080=EDGE_LOOP ( 'NONE', ( #157055, #146646, #99860, #143259, #118202 ) ) ;
#74084=ORIENTED_EDGE ( 'NONE', *, *, #139225, .T. ) ;
#74096=DIRECTION ( 'NONE',  ( 0.000000000000000000, 0.7999999999999973799, -0.6000000000000034195 ) ) ;
#74097=CARTESIAN_POINT ( 'NONE',  ( -1.408750476333751944, 7.229967155397921452, -4.273289540530492481 ) ) ;
#74098=CARTESIAN_POINT ( 'NONE',  ( -0.05958166578300463923, 7.052156984183643118, -3.952571211854608801 ) ) ;
#74100=CARTESIAN_POINT ( 'NONE',  ( -4.713430959045263435, 8.650753218861462202, 0.7998128361456481317 ) ) ;
#74103=CARTESIAN_POINT ( 'NONE',  ( 4.476163270806094552, 8.373940915915776273, 0.7998128361456462443 ) ) ;
#74112=CARTESIAN_POINT ( 'NONE',  ( -4.277761160311629673, 4.949475094240346706, 1.199719254218462483 ) ) ;
#74115=CARTESIAN_POINT ( 'NONE',  ( 7.623762449586013901, 7.788811034138823253, 1.040834085586084257E-14 ) ) ;
#74116=CARTESIAN_POINT ( 'NONE',  ( 1.364683531249988535, 3.363541667008085323, 0.7879004041258499402 ) ) ;
#74118=CARTESIAN_POINT ( 'NONE',  ( 5.931217288863120274, 6.131947776268360961, 0.7575795127007216578 ) ) ;
#74125=CARTESIAN_POINT ( 'NONE',  ( 6.033015167956792268, 8.061603667414825480, -1.443375672974057666 ) ) ;
#74126=CARTESIAN_POINT ( 'NONE',  ( -8.681298431451969222, 9.022603012982438386, 1.040834085586084257E-14 ) ) ;
#74129=CARTESIAN_POINT ( 'NONE',  ( -6.984421689334302741, 11.30024240419870374, 0.000000000000000000 ) ) ;
#74130=CARTESIAN_POINT ( 'NONE',  ( -6.388916700537716764, 8.476822122092563916, 1.599625672291283607 ) ) ;
#74139=CARTESIAN_POINT ( 'NONE',  ( 9.074484886248265880, 9.481320543578137361, 0.7998128361456462443 ) ) ;
#74153=CARTESIAN_POINT ( 'NONE',  ( -0.7500000000000215383, 4.441666666666691299, 1.299038105676671107 ) ) ;
#74154=CARTESIAN_POINT ( 'NONE',  ( 4.497554271431305040, 6.270232621468402989, -1.599625672291256295 ) ) ;
#74155=CARTESIAN_POINT ( 'NONE',  ( 7.142447996300871793, 7.227277505306155092, 0.7998128361456341429 ) ) ;
#74157=CARTESIAN_POINT ( 'NONE',  ( -7.971831135155409420, 11.28392484344787405, 1.082531754730549967 ) ) ;
#74159=CARTESIAN_POINT ( 'NONE',  ( 5.816084710582486217, 9.729256562414162701, 1.040834085586084257E-14 ) ) ;
#74160=CARTESIAN_POINT ( 'NONE',  ( -9.476786185827959841, 10.15859809299519334, 0.7216878364870438212 ) ) ;
#74161=CIRCLE ( 'NONE', #56836, 0.07999999999999994615 ) ;
#74165=CARTESIAN_POINT ( 'NONE',  ( 7.889955328148847258, 11.29236608522730911, -1.199719254218446718 ) ) ;
#74172=CARTESIAN_POINT ( 'NONE',  ( -0.6823417656250212460, 1.801041667008083991, 1.181850606188755259 ) ) ;
#74177=CARTESIAN_POINT ( 'NONE',  ( 1.364683531249988757, -0.1156249996585798079, 0.000000000000000000 ) ) ;
#74179=CARTESIAN_POINT ( 'NONE',  ( 7.886038904643079661, 12.35212915539230139, -0.7998128361456352531 ) ) ;
#74183=CARTESIAN_POINT ( 'NONE',  ( -9.992522908471816123, 11.61669713376064372, 1.199719254218462483 ) ) ;
#74190=CARTESIAN_POINT ( 'NONE',  ( 4.436542580169809291, 6.199052314996659874, 1.599625672291267398 ) ) ;
#74193=CARTESIAN_POINT ( 'NONE',  ( -7.831806290188425557, 12.28885777186185990, -0.7998128361456281477 ) ) ;
#74196=CARTESIAN_POINT ( 'NONE',  ( 8.748035429315576650, 11.22912730566677553, -1.599625672291255185 ) ) ;
#74198=CARTESIAN_POINT ( 'NONE',  ( 4.113906668039927439, 7.442175195026684342, 0.6721147198667943856 ) ) ;
#74200=CARTESIAN_POINT ( 'NONE',  ( -4.928552533767591726, 5.708731696605642725, 1.199719254218462483 ) ) ;
#74204=CARTESIAN_POINT ( 'NONE',  ( 6.753933077901968396, 11.03133902419432566, 0.7998128361456462443 ) ) ;
#74206=CARTESIAN_POINT ( 'NONE',  ( 7.450369105909416589, 8.650851030771185890, -1.199719254218441611 ) ) ;
#74208=CARTESIAN_POINT ( 'NONE',  ( -7.863365906246054138, 11.15738207638699464, -1.082531754730543971 ) ) ;
#74215=CARTESIAN_POINT ( 'NONE',  ( -4.699291399009611681, 6.864061528938182555, -1.228208583504811990 ) ) ;
#74216=CARTESIAN_POINT ( 'NONE',  ( -1.402160292154681736E-14, 1.946875000341422579, -1.575800808251660134 ) ) ;
#74218=CARTESIAN_POINT ( 'NONE',  ( 5.829642864196162400, 7.824335979694092558, 1.443375672974062551 ) ) ;
#74221=CARTESIAN_POINT ( 'NONE',  ( -3.070819976954469066, 2.800000000000024691, 2.497101503361902619 ) ) ;
#74225=B_SPLINE_CURVE_WITH_KNOTS ( 'NONE', 1,
 ( #32060, #34174 ),
 .UNSPECIFIED., .F., .F.,
 ( 2, 2 ),
 ( 0.000000000000000000, 0.5613011892072224951 ),
 .UNSPECIFIED. ) ;
#74234=CARTESIAN_POINT ( 'NONE',  ( -8.785320351530977234, 13.19336481018743079, 1.040834085586084257E-14 ) ) ;
#74238=CARTESIAN_POINT ( 'NONE',  ( 8.259941899223605333, 10.65968485389279508, -1.599625672291268286 ) ) ;
#74242=FACE_BOUND ( 'NONE', #97818, .T. ) ;
#74243=CARTESIAN_POINT ( 'NONE',  ( -5.669280788808708671, 9.765911353585494226, 0.7998128361456481317 ) ) ;
#74245=ORIENTED_EDGE ( 'NONE', *, *, #199925, .T. ) ;
#74246=CARTESIAN_POINT ( 'NONE',  ( -7.784352752540590004, 12.23349531127272094, 0.7998128361456481317 ) ) ;
#74250=CARTESIAN_POINT ( 'NONE',  ( -0.7499999999999972244, 5.139583334016151639, -1.299038105676652899 ) ) ;
#74251=CARTESIAN_POINT ( 'NONE',  ( 7.263417608619159083, 9.497073181520933716, -1.599625672291262513 ) ) ;
#74254=CARTESIAN_POINT ( 'NONE',  ( -7.874588291438845644, 8.081441182967111558, -0.7998128361456291469 ) ) ;
#74256=CARTESIAN_POINT ( 'NONE',  ( -1.364683531249997417, 5.259375000341425022, 1.214306433183764966E-14 ) ) ;
#74262=CARTESIAN_POINT ( 'NONE',  ( -8.026063749610056419, 10.38682701267698150, -1.443375672974059665 ) ) ;
#74266=CARTESIAN_POINT ( 'NONE',  ( 1.364683531249990311, 3.196875000341416140, 1.214306433183764966E-14 ) ) ;
#74273=CARTESIAN_POINT ( 'NONE',  ( 1.364683531249990311, 4.613541667008083103, 0.7879004041258500513 ) ) ;
#74274=CARTESIAN_POINT ( 'NONE',  ( -3.276266675996675204, 6.974061555304760240, -0.7998128361456281477 ) ) ;
#74275=CARTESIAN_POINT ( 'NONE',  ( 5.612185521052973414, 8.634967976948757951, -1.199719254218440723 ) ) ;
#74278=CARTESIAN_POINT ( 'NONE',  ( 3.836594282542920009, 4.538743420130594508, 1.082531754730560403 ) ) ;
#74279=CARTESIAN_POINT ( 'NONE',  ( -1.364683531250010295, 4.342708333674753618, 0.7879004041258379498 ) ) ;
#74283=CARTESIAN_POINT ( 'NONE',  ( -1.364683531250014514, 0.9885416670080898749, -0.7879004041258289570 ) ) ;
#74284=CARTESIAN_POINT ( 'NONE',  ( -4.284013352238255301, 6.981470763377843447, -1.082531754730549967 ) ) ;
#74285=CARTESIAN_POINT ( 'NONE',  ( 4.852928918687680948, 7.749168607522574526, 1.199719254218462483 ) ) ;
#74289=CARTESIAN_POINT ( 'NONE',  ( 4.202664430556254160, 5.926194473780837413, 1.443375672974062551 ) ) ;
#74292=CARTESIAN_POINT ( 'NONE',  ( -8.893785580884703279, 10.43879993486270585, 1.082531754730558626 ) ) ;
#74297=CARTESIAN_POINT ( 'NONE',  ( -9.459838494033043332, 12.05956421450382088, 1.599625672291281386 ) ) ;
#74298=CARTESIAN_POINT ( 'NONE',  ( -6.046573321570485327, 6.156683084694754449, 0.000000000000000000 ) ) ;
#74300=CARTESIAN_POINT ( 'NONE',  ( -0.6823417656250212460, 1.363541667008083547, 1.181850606188755259 ) ) ;
#74301=CARTESIAN_POINT ( 'NONE',  ( -1.499999999999997780, 4.400000000000021672, 1.214306433183764966E-14 ) ) ;
#74309=CARTESIAN_POINT ( 'NONE',  ( 10.18233705906309972, 11.83814697611718714, 1.199719254218450271 ) ) ;
#74311=ORIENTED_EDGE ( 'NONE', *, *, #120127, .T. ) ;
#74312=CARTESIAN_POINT ( 'NONE',  ( 7.388830529323379359, 11.56412668427855195, -0.7216878364870267237 ) ) ;
#74322=CARTESIAN_POINT ( 'NONE',  ( -2.252626078164912560, 5.779814191167667481, 0.7998128361456341429 ) ) ;
#74323=DIRECTION ( 'NONE',  ( -0.000000000000000000, -8.546850786086437571E-32, -1.000000000000000000 ) ) ;
#74324=CARTESIAN_POINT ( 'NONE',  ( -1.451998047845039830, 7.315968950354585942, -4.301760722576429607 ) ) ;
#74326=CARTESIAN_POINT ( 'NONE',  ( -1.364683531250014514, 1.301041667008083325, -0.7879004041258289570 ) ) ;
#74345=CARTESIAN_POINT ( 'NONE',  ( 4.981731378017507872, 7.899438143407371271, -1.199719254218452047 ) ) ;
#74355=CARTESIAN_POINT ( 'NONE',  ( 8.934986926605834157, 10.38290515491702770, -1.199719254218446718 ) ) ;
#74358=CARTESIAN_POINT ( 'NONE',  ( 1.513761821635687177, 8.683429030108589686, -2.534756493980068637 ) ) ;
#74359=CARTESIAN_POINT ( 'NONE',  ( -1.567404983201070801, 8.684828555514158666, -2.500997594616635844 ) ) ;
#74364=CARTESIAN_POINT ( 'NONE',  ( 4.008199524592567897, 7.584238231759597326, 0.2402771892247856922 ) ) ;
#74369=CARTESIAN_POINT ( 'NONE',  ( -8.514157279702033065, 9.995900250149611921, -1.082531754730543971 ) ) ;
#74381=CARTESIAN_POINT ( 'NONE',  ( 3.511198595814926993, 6.079853547550633230, 1.082531754730558626 ) ) ;
#74383=CARTESIAN_POINT ( 'NONE',  ( 5.705283713252285338, 5.550585841749444249, -0.7998128361456211532 ) ) ;
#74390=CARTESIAN_POINT ( 'NONE',  ( -5.473741331615264549, 7.409117525016355010, -1.599625672291256295 ) ) ;
#74392=CARTESIAN_POINT ( 'NONE',  ( -3.110706179331648169, 5.716575411607132118, 1.199719254218462483 ) ) ;
#74399=CARTESIAN_POINT ( 'NONE',  ( 9.598809568795314107, 10.30095870645710754, -0.7216878364870257245 ) ) ;
#74401=CARTESIAN_POINT ( 'NONE',  ( -1.201851678989727383E-14, 4.009375000341416140, -1.575800808251660134 ) ) ;
#74403=CARTESIAN_POINT ( 'NONE',  ( 4.798696304233017074, 7.685897223992134819, -1.199719254218452047 ) ) ;
#74412=CARTESIAN_POINT ( 'NONE',  ( 1.499999999998099076, 8.654187183607731981, -2.562246142702386376 ) ) ;
#74414=CARTESIAN_POINT ( 'NONE',  ( -1.387358672536882054, 7.315968950353378020, 4.254625267137783773 ) ) ;
#74417=CARTESIAN_POINT ( 'NONE',  ( -0.6823417656250212460, 1.613541667008083769, 1.181850606188755259 ) ) ;
#74419=CARTESIAN_POINT ( 'NONE',  ( 2.679707916995359263, 6.278076336469897711, -0.7998128361456291469 ) ) ;
#74421=CARTESIAN_POINT ( 'NONE',  ( -4.446711195602239819, 8.131654128270509929, -0.7216878364870267237 ) ) ;
#74422=CARTESIAN_POINT ( 'NONE',  ( 2.562127843302666186, 5.932973550587659517, 0.000000000000000000 ) ) ;
#74423=CARTESIAN_POINT ( 'NONE',  ( -6.575341312503472757, 7.733948288417905381, 1.082531754730549967 ) ) ;
#74428=CARTESIAN_POINT ( 'NONE',  ( 4.635998460869027227, 7.496083073400806818, -1.199719254218452047 ) ) ;
#74437=CARTESIAN_POINT ( 'NONE',  ( 6.012151052656117933, 9.101594430485762999, 1.199719254218460707 ) ) ;
#74439=CARTESIAN_POINT ( 'NONE',  ( -7.063961727919978451, 8.200042423116789436, 1.199719254218450271 ) ) ;
#74443=CARTESIAN_POINT ( 'NONE',  ( 6.889514614038635187, 11.18951748302043114, -0.7998128361456291469 ) ) ;
#74445=CARTESIAN_POINT ( 'NONE',  ( -7.063961727919978451, 8.200042423116789436, 1.199719254218450271 ) ) ;
#74446=VECTOR ( 'NONE', #166992, 1000.000000000000000 ) ;
#74447=CARTESIAN_POINT ( 'NONE',  ( 7.009202228140744673, 9.200488570962775725, -1.443375672974058777 ) ) ;
#74448=CARTESIAN_POINT ( 'NONE',  ( 4.176068722599148408, 7.364853391560295393, -0.8050483301465498620 ) ) ;
#74449=CARTESIAN_POINT ( 'NONE',  ( -4.924636110261798372, 6.768494766770632332, 1.599625672291267398 ) ) ;
#74455=CARTESIAN_POINT ( 'NONE',  ( 9.728138913005292210, 11.30824913904973705, -1.199719254218440723 ) ) ;
#74456=CARTESIAN_POINT ( 'NONE',  ( 3.708318708537623021, 4.285125567170706695, -1.199719254218446718 ) ) ;
#74457=CARTESIAN_POINT ( 'NONE',  ( -1.364683531250014514, -0.01145833299191483488, -0.7879004041258359514 ) ) ;
#74459=CARTESIAN_POINT ( 'NONE',  ( -5.748293942514180799, 7.729428904398431222, -1.443375672974052559 ) ) ;
#74466=CARTESIAN_POINT ( 'NONE',  ( -1.364683531250000748, 0.8218750003414210248, 0.000000000000000000 ) ) ;
#74469=CARTESIAN_POINT ( 'NONE',  ( 4.216222584169931231, 4.021273891060765493, 1.214306433183764966E-14 ) ) ;
#74472=CARTESIAN_POINT ( 'NONE',  ( -3.425406365747000859, 7.148057860013469877, 1.040834085586084257E-14 ) ) ;
#74474=CARTESIAN_POINT ( 'NONE',  ( -7.985389288324697965, 10.33937347451072775, -1.443375672974058777 ) ) ;
#74476=( BOUNDED_CURVE ( )  B_SPLINE_CURVE ( 2, ( #48990, #47944, #146509, #133462, #46870, #115108, #32721 ),
 .UNSPECIFIED., .F., .T. ) 
 B_SPLINE_CURVE_WITH_KNOTS ( ( 3, 2, 2, 3 ),
 ( 0.2142857142857144681, 0.2202380952380953438, 0.2261904761904762196, 0.2321428571428570953 ),
 .UNSPECIFIED. ) 
 CURVE ( )  GEOMETRIC_REPRESENTATION_ITEM ( )  RATIONAL_B_SPLINE_CURVE ( ( 0.9999999999999956701, 0.8660254037844430375, 1.000000000000000000, 0.8660254037844387076, 1.000000000000000000, 0.8660254037844399289, 0.9999999999999987788 ) ) 
 REPRESENTATION_ITEM ( '' )  );
#74484=CARTESIAN_POINT ( 'NONE',  ( -8.527715432871366019, 10.01171809551380143, 1.082531754730558626 ) ) ;
#74489=CARTESIAN_POINT ( 'NONE',  ( -7.822691444960713447, 9.189190109618056823, -1.082531754730543083 ) ) ;
#74498=CARTESIAN_POINT ( 'NONE',  ( -4.650083499807267984, 5.295740330745369207, 1.164732466530402855 ) ) ;
#74504=CARTESIAN_POINT ( 'NONE',  ( -5.859094939400033120, 9.987361195942037639, -0.7998128361456231517 ) ) ;
#74506=CARTESIAN_POINT ( 'NONE',  ( 6.159481859310094620, 6.080483678816896109, 1.040834085586084257E-14 ) ) ;
#74511=CARTESIAN_POINT ( 'NONE',  ( 6.608709811657416999, 9.797579649320619311, -1.199719254218440723 ) ) ;
#74518=CARTESIAN_POINT ( 'NONE',  ( -5.639828713604883248, 6.642516923036197340, 1.082531754730548412 ) ) ;
#74528=CARTESIAN_POINT ( 'NONE',  ( 0.6823417656249899377, 0.5927083336747518416, 1.181850606188755259 ) ) ;
#74530=CARTESIAN_POINT ( 'NONE',  ( -8.015895134177625891, 10.37496362800581018, 1.599625672291295375 ) ) ;
#74532=CARTESIAN_POINT ( 'NONE',  ( 6.286176778230493589, 10.48562334124426698, 0.7998128361456462443 ) ) ;
#74534=CARTESIAN_POINT ( 'NONE',  ( -9.203287345578106127, 9.631590079462940324, 0.7998128361456462443 ) ) ;
#74537=CARTESIAN_POINT ( 'NONE',  ( 1.364683531249992088, 5.384375000341417916, 1.214306433183764966E-14 ) ) ;
#74539=CARTESIAN_POINT ( 'NONE',  ( 8.270110514656016321, 12.59228666716665401, 0.7216878364870438212 ) ) ;
#74542=CARTESIAN_POINT ( 'NONE',  ( -1.364683531250014514, -0.6572916663252459379, 0.7879004041258379498 ) ) ;
#74545=CARTESIAN_POINT ( 'NONE',  ( 7.388830529323379359, 11.56412668427855195, -0.7216878364870267237 ) ) ;
#74548=CARTESIAN_POINT ( 'NONE',  ( -6.249945626219832739, 6.393950773452325542, 1.040834085586084257E-14 ) ) ;
#74550=CARTESIAN_POINT ( 'NONE',  ( 1.364683531249988757, 1.384375000341421469, 0.000000000000000000 ) ) ;
#74553=CARTESIAN_POINT ( 'NONE',  ( -7.528855374290365887, 7.678086112960552434, -0.7998128361456291469 ) ) ;
#74554=CARTESIAN_POINT ( 'NONE',  ( -1.364683531249997417, 4.571875000341417028, 1.214306433183764966E-14 ) ) ;
#74559=( BOUNDED_CURVE ( )  B_SPLINE_CURVE ( 2, ( #211560, #178024, #63195, #196401, #14423, #48046, #31778 ),
 .UNSPECIFIED., .F., .T. ) 
 B_SPLINE_CURVE_WITH_KNOTS ( ( 3, 2, 2, 3 ),
 ( 0.3035714285714285476, 0.3095238095238095899, 0.3154761904761906322, 0.3214285714285716744 ),
 .UNSPECIFIED. ) 
 CURVE ( )  GEOMETRIC_REPRESENTATION_ITEM ( )  RATIONAL_B_SPLINE_CURVE ( ( 1.000000000000000000, 0.8660254037844387076, 1.000000000000000000, 0.8660254037844387076, 1.000000000000000000, 0.8660254037844337116, 1.000000000000005107 ) ) 
 REPRESENTATION_ITEM ( '' )  );
#74560=CARTESIAN_POINT ( 'NONE',  ( 7.527801604085637699, 9.805521176231838609, 1.599625672291281386 ) ) ;
#74563=CARTESIAN_POINT ( 'NONE',  ( 0.7499999999999885647, 1.316666666666688190, -1.299038105676652899 ) ) ;
#74567=CARTESIAN_POINT ( 'NONE',  ( -0.4571195463272921256, 7.927888240403309084, -1.992899296338165982 ) ) ;
#74570=CARTESIAN_POINT ( 'NONE',  ( 6.561783159334121152, 8.678499657355050800, -1.443375672974057666 ) ) ;
#74575=CARTESIAN_POINT ( 'NONE',  ( 7.781490099239519509, 11.16582331816642260, 1.199719254218460707 ) ) ;
#74576=CARTESIAN_POINT ( 'NONE',  ( -8.319899820280397762, 12.85830022363583147, -0.7998128361456281477 ) ) ;
#74580=CARTESIAN_POINT ( 'NONE',  ( 1.364683531249988535, 5.217708333674750065, -0.7879004041258300672 ) ) ;
#74581=CARTESIAN_POINT ( 'NONE',  ( -0.7500000000000215383, 0.4416666666666874130, 1.299038105676659116 ) ) ;
#74588=CARTESIAN_POINT ( 'NONE',  ( -1.001543065824772872E-14, 5.321875000341422357, 1.575800808251672791 ) ) ;
#74590=CARTESIAN_POINT ( 'NONE',  ( -5.829642864196175722, 7.824335979694092558, 1.443375672974064550 ) ) ;
#74599=CARTESIAN_POINT ( 'NONE',  ( 6.889514614038635187, 11.18951748302043114, -0.7998128361456291469 ) ) ;
#74605=CARTESIAN_POINT ( 'NONE',  ( -8.025536864285518490, 11.45054454405341282, -1.199719254218446718 ) ) ;
#74606=CARTESIAN_POINT ( 'NONE',  ( 7.169564303528210836, 7.258913197071374945, -0.7998128361456281477 ) ) ;
#74608=CARTESIAN_POINT ( 'NONE',  ( 3.999292125906911188, 4.728557570721922509, 1.082531754730560403 ) ) ;
#74609=CARTESIAN_POINT ( 'NONE',  ( 4.521807925357579805, 5.234196320127330715, -1.199719254218452047 ) ) ;
#74615=DIRECTION ( 'NONE',  ( 1.735552045436534953E-14, 0.6004703560067730095, -0.7996470168499969500 ) ) ;
#74617=CARTESIAN_POINT ( 'NONE',  ( -4.419594888374909658, 8.100018436505289188, 0.7216878364870458196 ) ) ;
#74619=CARTESIAN_POINT ( 'NONE',  ( 8.568389894156670294, 12.94027927658408217, -0.7216878364870257245 ) ) ;
#74623=CARTESIAN_POINT ( 'NONE',  ( -6.157374318900681764, 10.33535380535947290, 0.7998128361456481317 ) ) ;
#74628=CARTESIAN_POINT ( 'NONE',  ( -7.914208982075130905, 10.25632978388623684, -1.599625672291263179 ) ) ;
#74631=CARTESIAN_POINT ( 'NONE',  ( 5.847644326195776010, 5.716673223516856694, -0.7998128361456281477 ) ) ;
#74641=CARTESIAN_POINT ( 'NONE',  ( -1.403499169903600574, 7.376709478543776122, 4.304123474983186703 ) ) ;
#74643=CARTESIAN_POINT ( 'NONE',  ( -8.179646747746328828, 8.437342715325849341, -0.7998128361456291469 ) ) ;
#74647=CARTESIAN_POINT ( 'NONE',  ( 6.331294547901813452, 6.488857848747989543, 1.040834085586084257E-14 ) ) ;
#74648=CARTESIAN_POINT ( 'NONE',  ( -1.426745631514137802, 7.396214564682365378, 4.272608017055013363 ) ) ;
#74650=CARTESIAN_POINT ( 'NONE',  ( 5.366329872910639232, 5.155139694684188534, 1.040834085586084257E-14 ) ) ;
#74652=CARTESIAN_POINT ( 'NONE',  ( -6.261168011412601153, 6.199117522936475666, 1.040834085586084257E-14 ) ) ;
#74661=CARTESIAN_POINT ( 'NONE',  ( 1.499999999999961586, 5.545833333333349380, -0.8660254037844482555 ) ) ;
#74662=CARTESIAN_POINT ( 'NONE',  ( 9.237182729612253951, 9.671134694169463586, 0.7998128361456462443 ) ) ;
#74667=CARTESIAN_POINT ( 'NONE',  ( -4.485938484121875902, 7.064193607440066636, -1.134896524841392473 ) ) ;
#74674=CARTESIAN_POINT ( 'NONE',  ( 8.270110514656021650, 11.63191745286530576, 1.082531754730557072 ) ) ;
#74694=CARTESIAN_POINT ( 'NONE',  ( -3.327636637150278798, 5.969660945728899826, -1.199719254218452935 ) ) ;
#74695=CARTESIAN_POINT ( 'NONE',  ( -1.201851678989727383E-14, 2.962500000000025224, 1.732050807568877637 ) ) ;
#74697=CARTESIAN_POINT ( 'NONE',  ( -3.704402285031864306, 5.344888637335695414, -1.599625672291256295 ) ) ;
#74701=CARTESIAN_POINT ( 'NONE',  ( -1.001543065824772872E-14, 4.321875000341417916, 1.575800808251672791 ) ) ;
#74707=ORIENTED_EDGE ( 'NONE', *, *, #103236, .T. ) ;
#74710=CARTESIAN_POINT ( 'NONE',  ( 3.999819011231439347, 4.625209253646830554, 1.199719254218464037 ) ) ;
#74714=CARTESIAN_POINT ( 'NONE',  ( 10.66990370383054731, 11.55056853066490952, 0.7216878364870317197 ) ) ;
#74716=CARTESIAN_POINT ( 'NONE',  ( -1.364683531250014514, 0.8010416670080889867, -0.7879004041258289570 ) ) ;
#74719=CARTESIAN_POINT ( 'NONE',  ( -7.160677686311960777, 11.50587440067263678, -0.7998128361456291469 ) ) ;
#74720=CARTESIAN_POINT ( 'NONE',  ( -6.195713011320807873, 6.330679389403470303, -0.7216878364870267237 ) ) ;
#74723=EDGE_LOOP ( 'NONE', ( #175076, #84856, #20194, #93988 ) ) ;
#74724=CARTESIAN_POINT ( 'NONE',  ( -1.364683531250010295, 5.530208333674751842, 0.7879004041258379498 ) ) ;
#74732=CARTESIAN_POINT ( 'NONE',  ( -4.229780737339226881, 7.878568593630327577, 1.040834085586084257E-14 ) ) ;
#74734=DIRECTION ( 'NONE',  ( -0.6507913734559640506, -0.7592566023653004592, 0.000000000000000000 ) ) ;
#74738=CARTESIAN_POINT ( 'NONE',  ( -5.273758565591545988, 6.215435083687305351, 1.082531754730546636 ) ) ;
#74740=CARTESIAN_POINT ( 'NONE',  ( 10.73535870392234237, 11.41900666419791399, 0.000000000000000000 ) ) ;
#74744=CARTESIAN_POINT ( 'NONE',  ( 5.829642864196179275, 5.903597551091400497, 0.7216878364870262796 ) ) ;
#74752=CARTESIAN_POINT ( 'NONE',  ( -4.334856428067329404, 6.080418470877079429, -1.599625672291256295 ) ) ;
#74757=CARTESIAN_POINT ( 'NONE',  ( 8.541273586929342798, 11.94827437051752206, -1.082531754730543083 ) ) ;
#74758=CARTESIAN_POINT ( 'NONE',  ( 5.686755365928134687, 8.721966129303114101, 1.199719254218462483 ) ) ;
#74761=ORIENTED_EDGE ( 'NONE', *, *, #163416, .F. ) ;
#74763=CARTESIAN_POINT ( 'NONE',  ( 3.005103603723342953, 6.657704637652544832, -0.7998128361456291469 ) ) ;
#74773=CARTESIAN_POINT ( 'NONE',  ( -4.577849422908604637, 8.492574760035358494, -0.7998128361456281477 ) ) ;
#74782=CARTESIAN_POINT ( 'NONE',  ( -0.6823417656250212460, 4.301041667008085767, 1.181850606188767472 ) ) ;
#74783=CARTESIAN_POINT ( 'NONE',  ( 7.741342523278686549, 11.97539067722642869, 0.7216878364870438212 ) ) ;
#74784=CARTESIAN_POINT ( 'NONE',  ( -6.911959384868566758, 6.958374125301778790, 1.040834085586084257E-14 ) ) ;
#74787=CARTESIAN_POINT ( 'NONE',  ( 5.681030059326015014, 6.586622143090519188, -1.199719254218445830 ) ) ;
#74788=CARTESIAN_POINT ( 'NONE',  ( -4.900382456335551140, 7.804531068111707270, 1.199719254218464037 ) ) ;
#74793=EDGE_CURVE ( 'NONE', #126491, #88615, #206722, .T. ) ;
#74795=CARTESIAN_POINT ( 'NONE',  ( 5.165293337126522388, 8.969999960048859577, 1.040834085586084257E-14 ) ) ;
#74797=CARTESIAN_POINT ( 'NONE',  ( 7.578644679914718019, 7.944099669429731669, 0.7216878364870317197 ) ) ;
#74798=CARTESIAN_POINT ( 'NONE',  ( -0.6823417656250003738, 2.780208333674753618, -1.181850606188749264 ) ) ;
#74800=CARTESIAN_POINT ( 'NONE',  ( 6.005898860729467437, 7.069598761348265370, -1.082531754730543083 ) ) ;
#74802=CARTESIAN_POINT ( 'NONE',  ( -3.687454593236990430, 4.364747115940301292, 1.082531754730560403 ) ) ;
#74809=CARTESIAN_POINT ( 'NONE',  ( -4.391370929004954959, 7.351591927832363815, -1.215465595245905250 ) ) ;
#74815=CIRCLE ( 'NONE', #182244, 0.08000000000000032085 ) ;
#74817=CARTESIAN_POINT ( 'NONE',  ( 5.738125327081736060, 7.717565519727259904, 1.599625672291267398 ) ) ;
#74819=CARTESIAN_POINT ( 'NONE',  ( -3.104453987404963478, 5.605318171072321221, -1.082531754730549078 ) ) ;
#74821=CARTESIAN_POINT ( 'NONE',  ( 3.708318708537623021, 4.285125567170706695, -1.199719254218446718 ) ) ;
#74828=CARTESIAN_POINT ( 'NONE',  ( 5.694061328059515148, 5.745419092265303007, -0.7216878364870207285 ) ) ;
#74829=VECTOR ( 'NONE', #74734, 1000.000000000000000 ) ;
#74830=CARTESIAN_POINT ( 'NONE',  ( 1.364683531249988535, 3.176041667008084435, 0.7879004041258500513 ) ) ;
#74832=CARTESIAN_POINT ( 'NONE',  ( 8.613507663383630941, 8.943513783569379427, -0.7998128361456221525 ) ) ;
#74833=CARTESIAN_POINT ( 'NONE',  ( -8.292783513053063160, 12.82666453187061073, 0.7998128361456481317 ) ) ;
#74839=CARTESIAN_POINT ( 'NONE',  ( 1.499999999999989120, 2.754166666666688190, 0.8660254037844524744 ) ) ;
#74840=CARTESIAN_POINT ( 'NONE',  ( 5.113396490648394632, 9.117379672398465473, 1.040834085586084257E-14 ) ) ;
#74844=CARTESIAN_POINT ( 'NONE',  ( 1.364683531249988535, 4.155208333674753618, -0.7879004041258239610 ) ) ;
#74848=CARTESIAN_POINT ( 'NONE',  ( 9.625925876022625616, 11.29296361252366765, -1.082531754730537088 ) ) ;
#74851=CARTESIAN_POINT ( 'NONE',  ( -1.387358672534890536, 7.315968950354793776, -4.254625267136668221 ) ) ;
#74853=CARTESIAN_POINT ( 'NONE',  ( 0.7499999999999902300, 1.764583334016148086, 1.299038105676657340 ) ) ;
#74855=CARTESIAN_POINT ( 'NONE',  ( -6.728924311084075960, 6.744833205886536120, 1.040834085586084257E-14 ) ) ;
#74856=CARTESIAN_POINT ( 'NONE',  ( -3.307826292054316664, 4.882216645528547616, -1.443375672974059665 ) ) ;
#74864=CARTESIAN_POINT ( 'NONE',  ( 6.634017235788401301, 6.634108284708264414, 0.7998128361456341429 ) ) ;
#74867=CARTESIAN_POINT ( 'NONE',  ( 6.169123589417988995, 7.156064594864501416, -1.199719254218445830 ) ) ;
#74871=ORIENTED_EDGE ( 'NONE', *, *, #30522, .T. ) ;
#74872=CARTESIAN_POINT ( 'NONE',  ( 8.530051201292206287, 13.10347683481629488, 0.000000000000000000 ) ) ;
#74877=CARTESIAN_POINT ( 'NONE',  ( 5.671489233189207724, 6.113434141373025099, 0.7590443732325997672 ) ) ;
#74883=CARTESIAN_POINT ( 'NONE',  ( 1.387358672531703974, 7.315968950352358391, 4.254625267140708544 ) ) ;
#74886=CARTESIAN_POINT ( 'NONE',  ( -1.566537053174817062, 8.754671357082440153, -2.463935854687004490 ) ) ;
#74888=CARTESIAN_POINT ( 'NONE',  ( 7.673551755654734130, 9.015193805427763607, -1.082531754730537976 ) ) ;
#74890=CARTESIAN_POINT ( 'NONE',  ( -2.605138072120212200, 6.191078184115536232, -0.7998128361456281477 ) ) ;
#74894=CARTESIAN_POINT ( 'NONE',  ( -4.530395885260773525, 8.437212299446219532, 0.7998128361456481317 ) ) ;
#74913=DIRECTION ( 'NONE',  ( -0.6260462619842731558, -0.7797859179643593652, 0.000000000000000000 ) ) ;
#74916=CARTESIAN_POINT ( 'NONE',  ( -3.898132859128961236, 4.506575409527250997, -1.199719254218452047 ) ) ;
#74918=CARTESIAN_POINT ( 'NONE',  ( 9.074484886248265880, 9.481320543578137361, 0.7998128361456462443 ) ) ;
#74922=CARTESIAN_POINT ( 'NONE',  ( -6.367525699912501835, 10.58053041653993098, -0.7998128361456291469 ) ) ;
#74923=CARTESIAN_POINT ( 'NONE',  ( 4.497554271431305040, 6.270232621468402989, -1.599625672291256295 ) ) ;
#74925=AXIS2_PLACEMENT_3D ( 'NONE', #62831, #111659, #126863 ) ;
#74927=CARTESIAN_POINT ( 'NONE',  ( -4.650083499807246668, 5.295740330745369207, -2.420000000000000373 ) ) ;
#74928=CARTESIAN_POINT ( 'NONE',  ( -2.331639231870358930, 5.664070170583284103, -0.7216878364870267237 ) ) ;
#74931=CARTESIAN_POINT ( 'NONE',  ( 1.364683531249988535, 2.967708333674755394, -0.7879004041258239610 ) ) ;
#74933=CARTESIAN_POINT ( 'NONE',  ( 5.151735183512854199, 8.954182114166247430, -0.7216878364870257245 ) ) ;
#74940=ORIENTED_EDGE ( 'NONE', *, *, #87487, .T. ) ;
#74941=CARTESIAN_POINT ( 'NONE',  ( 10.01911233037458260, 10.79131192829960462, 0.7216878364870438212 ) ) ;
#74946=CARTESIAN_POINT ( 'NONE',  ( -7.479294296233107708, 11.87759377891399204, 0.7998128361456481317 ) ) ;
#74963=CARTESIAN_POINT ( 'NONE',  ( -1.402160292154681736E-14, 2.618750000682819490, -1.732050807568863648 ) ) ;
#74969=CARTESIAN_POINT ( 'NONE',  ( -0.7500000000000006661, 0.8583333333333567072, -1.299038105676652011 ) ) ;
#74970=CARTESIAN_POINT ( 'NONE',  ( 8.762647353133951711, 9.117510088278095282, 1.040834085586084257E-14 ) ) ;
#74971=CARTESIAN_POINT ( 'NONE',  ( -0.6823417656250246877, -0.6989583329919113464, 1.181850606188755259 ) ) ;
#74973=AXIS2_PLACEMENT_3D ( 'NONE', #6254, #138430, #155737 ) ;
#74975=CARTESIAN_POINT ( 'NONE',  ( 10.22248463502393001, 11.02857961705718282, 0.7216878364870438212 ) ) ;
#74976=CARTESIAN_POINT ( 'NONE',  ( -5.233084105194862445, 9.049089189461916760, 0.7216878364870458196 ) ) ;
#74977=ADVANCED_FACE ( 'NONE', ( #51927 ), #186167, .T. ) ;
#74982=CARTESIAN_POINT ( 'NONE',  ( -6.338600509588822263, 7.353787668397130162, -1.199719254218446718 ) ) ;
#74984=CARTESIAN_POINT ( 'NONE',  ( -1.500000000000013101, 3.160416667349486008, -0.8660254037844313801 ) ) ;
#74985=CARTESIAN_POINT ( 'NONE',  ( 0.6823417656249917140, 3.905208333674754950, 1.181850606188765695 ) ) ;
#74994=CARTESIAN_POINT ( 'NONE',  ( -8.283668668269720925, 8.766627655843896250, 1.056142170575426150E-14 ) ) ;
#75000=CARTESIAN_POINT ( 'NONE',  ( -8.799405390469187793, 10.22472669609091689, -1.199719254218446718 ) ) ;
#75001=CARTESIAN_POINT ( 'NONE',  ( 6.470265622219697477, 8.571729197388226140, -1.599625672291262513 ) ) ;
#75008=CARTESIAN_POINT ( 'NONE',  ( -9.169391961543940539, 9.592045464756413509, 1.040834085586084257E-14 ) ) ;
#75013=CARTESIAN_POINT ( 'NONE',  ( 2.866659414285625651, 5.431854185720147221, -1.199719254218446718 ) ) ;
#75014=CARTESIAN_POINT ( 'NONE',  ( -4.903732577545095950, 4.837283930932079201, 0.1501914610188368471 ) ) ;
#75017=CARTESIAN_POINT ( 'NONE',  ( -4.283486466913726254, 7.084819080452935403, -1.199719254218452047 ) ) ;
#75018=CARTESIAN_POINT ( 'NONE',  ( -9.104463846776669200, 10.58062822844965645, -1.199719254218441611 ) ) ;
#75021=CARTESIAN_POINT ( 'NONE',  ( -5.688173390364544169, 6.286868445634342883, -1.126660468825124273 ) ) ;
#75046=CARTESIAN_POINT ( 'NONE',  ( 3.389175213736292047, 5.937492935125556315, 1.082531754730558626 ) ) ;
#75050=CARTESIAN_POINT ( 'NONE',  ( -9.806625181386236179, 10.33548422123910449, -0.7998128361456291469 ) ) ;
#75053=CARTESIAN_POINT ( 'NONE',  ( 9.935427640716063991, 10.48575375712389679, -0.7998128361456281477 ) ) ;
#75063=CARTESIAN_POINT ( 'NONE',  ( -0.6823417656250212460, 0.8010416670080899859, 1.181850606188755259 ) ) ;
#75069=CARTESIAN_POINT ( 'NONE',  ( -5.440899717785814715, 5.242137847038546461, 0.7998128361456341429 ) ) ;
#75072=CARTESIAN_POINT ( 'NONE',  ( -1.402160292154681736E-14, -0.1624999999999815481, -1.732050807568870754 ) ) ;
#75074=CARTESIAN_POINT ( 'NONE',  ( 1.364683531249986537, -0.7822916663252464931, -0.7879004041258309554 ) ) ;
#75079=CARTESIAN_POINT ( 'NONE',  ( -1.364683531250014514, -0.01145833299191483488, -0.7879004041258359514 ) ) ;
#75081=CARTESIAN_POINT ( 'NONE',  ( -7.888146445052511169, 8.097259028849730811, 1.040834085586084257E-14 ) ) ;
#75082=CARTESIAN_POINT ( 'NONE',  ( 9.576136569953906275, 10.06658084123472641, 0.000000000000000000 ) ) ;
#75083=CARTESIAN_POINT ( 'NONE',  ( 3.493197133815315603, 7.227147089426516402, -0.7998128361456291469 ) ) ;
#75088=CARTESIAN_POINT ( 'NONE',  ( 0.6823417656249882723, -0.5947916663252492686, 1.181850606188755259 ) ) ;
#75098=CARTESIAN_POINT ( 'NONE',  ( 7.307481608085759639, 7.627742752295940676, 1.040834085586084257E-14 ) ) ;
#75101=CARTESIAN_POINT ( 'NONE',  ( -5.915435094264120508, 5.795762452929912101, 0.000000000000000000 ) ) ;
#75103=CARTESIAN_POINT ( 'NONE',  ( -1.500000000000011324, 5.660416667349481123, -0.8660254037844313801 ) ) ;
#75105=CARTESIAN_POINT ( 'NONE',  ( -3.277320446201389181, 4.846626492033466072, 1.599625672291267398 ) ) ;
#75106=CARTESIAN_POINT ( 'NONE',  ( 4.650083499362864359, 7.408552601689905259, 1.082531754730558626 ) ) ;
#75107=CARTESIAN_POINT ( 'NONE',  ( -8.663296969008007054, 9.209527340038563992, 0.7216878364870438212 ) ) ;
#75109=CARTESIAN_POINT ( 'NONE',  ( -1.499999999999997780, 4.150000000000021672, 1.214306433183764966E-14 ) ) ;
#75113=CARTESIAN_POINT ( 'NONE',  ( 7.944714827928039291, 11.25228915168265864, 1.082531754730557072 ) ) ;
#75127=ORIENTED_EDGE ( 'NONE', *, *, #87363, .T. ) ;
#75128=AXIS2_PLACEMENT_3D ( 'NONE', #167220, #55596, #51337 ) ;
#75129=CARTESIAN_POINT ( 'NONE',  ( 8.771762197917315262, 10.29643932140079166, -1.082531754730543083 ) ) ;
#75131=CARTESIAN_POINT ( 'NONE',  ( 7.507464373665139412, 9.781794407407920389, 1.599625672291281386 ) ) ;
#75134=CARTESIAN_POINT ( 'NONE',  ( -5.395781948114519722, 5.397426482329451325, 0.000000000000000000 ) ) ;
#75136=CARTESIAN_POINT ( 'NONE',  ( 3.687454593236936251, 7.245854758844324728, -0.7216878364870267237 ) ) ;
#75138=CARTESIAN_POINT ( 'NONE',  ( -7.185458225562757484, 11.32685899655781903, 0.7216878364870458196 ) ) ;
#75163=( BOUNDED_SURFACE ( )  B_SPLINE_SURFACE ( 1, 2, ( 
 ( #62589, #30103, #94064, #92997, #212024, #13830, #195803, #175306, #45302, #79905, #160104, #44238, #142826, #146013, #26893, #159041, #125558, #179558, #194725, #111421, #147071, #11707, #77781, #143902, #209895, #177425, #208833, #95126, #60463, #12761, #31179, #161175, #59402, #78835, #144956, #210962, #128752, #46364, #63667, #191519, #129821, #47440, #113555, #97252, #163306, #14887, #80982, #213092, #66821, #200046, #35419, #20230, #33289, #148130, #52743, #182735, #51697, #98304, #184863, #118877, #99373, #755, #117819, #181662, #183809, #165425, #34354, #168627, #64722, #164369, #150266, #132964, #116736, #130864, #214131, #17023, #36490, #32233, #198967, #135089, #114617, #67893, #196860, #102567, #48498, #180608, #86315, #100427, #167567, #2897, #166498, #18089, #15953, #50611, #83099, #65759, #131906, #101497, #82036, #201103, #197914, #49542, #151329, #115668, #84177, #149179, #1834, #134038, #19167, #85241, #68970, #137224, #72177, #202166, #203244, #40792, #54888, #106897, #188074, #156669, #58087, #6107, #155593, #7178, #8261, #103645, #138285, #53824, #190207, #122109, #154528, #204300, #139356, #121042, #187009, #169697, #38640, #136149, #5031, #71106, #21285, #55956, #153458, #104719, #170767, #107976, #22356, #41867, #88468, #174005, #189153, #25576, #124249, #39703, #152387, #105812, #3965, #70033, #119954, #171838, #23431, #24499, #185929, #89542, #205386, #87391, #57025, #172923, #73249, #123192, #90610, #37565, #74345, #140449, #206460, #42932, #194485, #95952, #92749, #60214, #158793, #93816, #176122, #109042, #78598, #175061, #144718, #209649, #43993, #157740, #210730, #63426, #179322, #47201, #113316, #10390, #159857, #193422, #62356, #76465, #59150, #91687, #128517, #129578, #9337, #142574, #46128, #160931, #29869, #13596, #211788, #112245, #195565, #26648, #75410, #178256, #208581, #162007, #79670, #45066, #143654, #11460, #141523, #12525, #126375, #145785, #192334, #207531, #125308, #110111, #27722, #77533, #61290, #127451, #111177, #191266, #177179, #28795, #94879, #147885, #30943, #182480, #117559, #97018, #101237, #163072, #164133, #115433, #148935, #100180, #15717, #130633, #14653, #166245, #80747, #146835, #81802, #150009, #17835, #51440, #183554, #212854, #67640, #64491, #213901, #196625, #50368, #35161, #48264, #83918, #116491, #114378, #132717, #507, #49316, #197672, #180373, #65524, #31997, #181424, #98078, #131669, #34108, #33054, #198722, #99132, #165181, #16775, #82859, #66575, #1579, #133787, #199795, #58378, #109336, #10672, #208867, #112517, #77816, #111459, #26926, #174286, #28006, #91971, #30141, #207809, #143938, #45340, #175346, #25861, #78872, #177463, #62624, #190492, #126656, #95163, #43219, #59438, #158029, #29078, #108264, #42150, #206749, #46401, #61572, #60497, #13867, #93034, #125594, #191555, #159076, #76743, #124534, #142865, #9617, #94103, #178531, #192623, #140737, #44275, #75693, #141805, #209933, #128785, #110396, #194764, #144995, #176401, #160142, #11742, #127739, #193696, #161212, #96229, #162280, #12799, #211000, #49582, #114655, #131943, #64762, #34389, #115707, #84214, #200082, #148166, #83138, #149216, #150302, #31216, #214169, #129856, #117852, #181697, #82074, #65794, #66858, #130904, #196897, #97290, #48536, #63702, #147107, #213131, #163347, #197954, #81018, #180649, #32273, #35456, #98340, #183844, #164405, #101534, #116775, #167604, #51730, #15989, #79945, #33327, #146049, #212062, #195840, #99409, #165462, #166537, #47481, #17057, #133004, #14924, #199004, #100461, #791, #50648, #182772, #113592, #18125, #1868, #67928, #134073, #179595, #23470, #20269, #202205, #86353, #21321, #103683, #36523, #6141, #184899, #72211, #137258, #185969, #85281, #138318, #205422, #106935, #189188, #40825, #152424, #87428, #121076, #204334, #4003, #201141, #19202, #55992, #57060, #151367, #70072, #122143, #88502, #171873, #155627, #139389, #188111, #123224, #102610, #2936, #203278, #39742, #89578, #187043, #54924, #69008, #153495, #169732, #136185, #168665, #105846, #135125, #53859, #52779, #118918, #5065, #7212, #119992, #154565, #37602, #71141, #38675 ),
 ( #104754, #73286, #170803, #22393, #111213, #25611, #10426, #124283, #172958, #192371, #127488, #128551, #62386, #157774, #193459, #142610, #207562, #76498, #9372, #45103, #208618, #177215, #78630, #26683, #176158, #27758, #28828, #190243, #92785, #8296, #210766, #60252, #175096, #158830, #159891, #75443, #141555, #41901, #59185, #156706, #91723, #125340, #108012, #126409, #174038, #191303, #42971, #194516, #109081, #46164, #44027, #24537, #209685, #90645, #144755, #110145, #74381, #93854, #140482, #206494, #58124, #11499, #77570, #94917, #143693, #61329, #160966, #12556, #16806, #66606, #213934, #164164, #180409, #95986, #33089, #129613, #181459, #63459, #540, #116522, #113350, #80782, #179355, #114409, #196657, #195599, #99163, #47235, #165216, #15750, #64523, #178294, #82892, #83954, #199832, #67675, #133819, #30977, #32027, #65555, #148967, #97052, #79702, #112277, #163106, #132752, #198755, #131701, #81834, #98113, #162038, #50404, #14686, #182513, #146870, #34143, #100212, #212892, #130669, #48298, #147917, #197706, #49348, #166281, #115467, #17870, #150044, #1615, #29901, #13629, #145817, #211822, #6951, #73032, #184646, #53597, #153231, #22124, #36266, #18943, #51473, #104496, #23205, #139130, #52528, #88236, #120811, #204076, #187853, #171611, #154307, #89319, #68754, #117597, #169479, #5879, #55728, #4801, #21063, #183588, #119732, #135922, #118663, #200883, #71953, #167356, #39479, #134876, #105578, #121883, #102344, #103418, #2683, #35197, #70882, #138063, #101271, #155366, #168415, #85028, #87160, #86098, #136994, #20012, #151116, #203021, #152172, #3741, #185710, #54663, #186788, #69816, #201942, #37344, #38415, #170539, #174850, #207314, #125094, #192119, #41645, #107759, #8034, #173785, #188929, #57866, #124028, #74125, #191052, #206240, #189995, #25360, #160710, #91460, #28579, #157522, #12304, #27500, #94668, #110956, #9117, #78385, #75192, #205158, #56800, #176963, #26429, #141304, #77320, #122969, #58937, #43784, #42717, #156450, #40566, #10178, #159644, #106674, #172697, #108825, #11242, #92539, #158579, #76252, #142362, #143433, #208371, #209429, #24275, #60003, #126156, #109897, #61074, #140220, #175909, #90381, #93600, #127233, #193203, #44850, #131459, #195347, #46980, #161790, #113096, #128307, #211571, #63205, #13381, #64279, #145573, #129369, #179101, #99974, #30724, #182272, #96807, #166040, #181213, #33896, #50159, #162855, #17624, #14434, #144505, #210512, #116281, #114169, #80523, #16561, #62148, #146621, #197460, #79456, #49102, #98917, #31788, #196411, #212638, #194269, #65310, #130426, #213688, #95739, #32840, #148728, #48056, #180162, #97861, #163923, #15499, #81586, #115222, #147670, #164970, #82645, #297, #45915, #66368, #112033, #178036, #29653, #132515, #198513, #85854, #185473, #54428, #2435, #51226, #83709, #136750, #55488, #105330, #84783, #120569, #152990, #21882, #5629, #203842, #186546, #121642, #101023, #149798, #201709, #38176, #87989, #37095, #53352, #1372, #151929, #168173, #150871, #18701, #104248, #199583, #71710, #167114, #137823, #154064, #68510, #19772, #3504, #187610, #20824, #170294, #184405, #117350, #103173, #34952, #39237, #134637, #86922, #202777, #118419, #183347, #171366, #67433, #133577, #200642, #69574, #52290, #36025, #102103, #135684, #119486, #169235, #4564, #70639, #143187, #158336, #91210, #110705, #205991, #90139, #73874, #57627, #139969, #6714, #189744, #188685, #190803, #209178, #8862, #22960, #123785, #172449, #138891, #174600, #41396, #191868, #89075, #204910, #107506, #156206, #40320, #155132, #175654, #173535, #72790, #157272, #9930, #59750, #44591, #25108, #24036, #77057, #207058, #76004, #122723, #60817, #126978, #74941, #141052, #142108, #58689, #208121, #124837, #42463, #192937, #56563, #106426, #26176, #108572, #92292, #7782, #125910, #43528, #109651, #27241, #93348, #159384, #10983, #31531, #176705, #66109, #28317, #144258, #45, #113913, #97606, #210251, #47800, #179908, #12061, #49900, #78128, #178854, #212379, #61889, #128052, #82387, #177780, #194007, #45656, #163664, #15246, #81334, #111773, #65061, #132251, #14172 ) ),
 .UNSPECIFIED., .F., .F., .T. ) 
 B_SPLINE_SURFACE_WITH_KNOTS ( ( 2, 2 ),
 ( 3, 2, 2, 2, 2, 2, 2, 2, 2, 2, 2, 2, 2, 2, 2, 2, 2, 2, 2, 2, 2, 2, 2, 2, 2, 2, 2, 2, 2, 2, 2, 2, 2, 2, 2, 2, 2, 2, 2, 2, 2, 2, 2, 2, 2, 2, 2, 2, 2, 2, 2, 2, 2, 2, 2, 2, 2, 2, 2, 2, 2, 2, 2, 2, 2, 2, 2, 2, 2, 2, 2, 2, 2, 2, 2, 2, 2, 2, 2, 2, 2, 2, 2, 2, 2, 2, 2, 2, 2, 2, 2, 2, 2, 2, 2, 2, 2, 2, 2, 2, 2, 2, 2, 2, 2, 2, 2, 2, 2, 2, 2, 2, 2, 2, 2, 2, 2, 2, 2, 2, 2, 2, 2, 2, 2, 2, 2, 2, 2, 2, 2, 2, 2, 2, 2, 2, 2, 2, 2, 2, 2, 2, 2, 2, 2, 2, 2, 2, 2, 2, 2, 2, 2, 2, 2, 2, 2, 2, 2, 2, 2, 2, 2, 2, 2, 2, 2, 2, 2, 2, 2, 2, 2, 2, 2, 2, 2, 2, 2, 2, 2, 2, 2, 2, 2, 2, 2, 2, 2, 2, 2, 2, 2, 2, 2, 2, 2, 2, 2, 2, 2, 2, 2, 2, 2, 2, 2, 2, 2, 2, 2, 2, 2, 2, 2, 2, 2, 2, 2, 2, 2, 2, 2, 2, 2, 2, 2, 2, 2, 2, 2, 2, 2, 2, 2, 2, 2, 2, 2, 2, 3 ),
 ( 0.000000000000000000, 1.000000000000000000 ),
 ( 0.000000000000000000, 0.004166666666666666609, 0.008333333333333333218, 0.01250000000000000069, 0.01666666666666666644, 0.02083333333333333218, 0.02500000000000000139, 0.02916666666666666713, 0.03333333333333333287, 0.03749999999999999861, 0.04166666666666666435, 0.04583333333333333010, 0.05000000000000000278, 0.05416666666666666852, 0.05833333333333333426, 0.06250000000000000000, 0.06666666666666666574, 0.07083333333333333148, 0.07499999999999999722, 0.07916666666666666297, 0.08333333333333332871, 0.08749999999999999445, 0.09166666666666666019, 0.09583333333333333981, 0.1000000000000000056, 0.1041666666666666713, 0.1083333333333333370, 0.1125000000000000028, 0.1166666666666666685, 0.1208333333333333343, 0.1250000000000000000, 0.1291666666666666796, 0.1333333333333333315, 0.1375000000000000111, 0.1416666666666666630, 0.1458333333333333426, 0.1499999999999999944, 0.1541666666666666741, 0.1583333333333333259, 0.1625000000000000056, 0.1666666666666666574, 0.1708333333333333370, 0.1749999999999999889, 0.1791666666666666685, 0.1833333333333333204, 0.1875000000000000000, 0.1916666666666666796, 0.1958333333333333315, 0.2000000000000000111, 0.2041666666666666630, 0.2083333333333333426, 0.2124999999999999944, 0.2166666666666666741, 0.2208333333333333259, 0.2250000000000000056, 0.2291666666666666574, 0.2333333333333333370, 0.2374999999999999889, 0.2416666666666666685, 0.2458333333333333204, 0.2500000000000000000, 0.2541666666666666519, 0.2583333333333333592, 0.2625000000000000111, 0.2666666666666666630, 0.2708333333333333148, 0.2750000000000000222, 0.2791666666666666741, 0.2833333333333333259, 0.2874999999999999778, 0.2916666666666666852, 0.2958333333333333370, 0.2999999999999999889, 0.3041666666666666408, 0.3083333333333333481, 0.3125000000000000000, 0.3166666666666666519, 0.3208333333333333592, 0.3250000000000000111, 0.3291666666666666630, 0.3333333333333333148, 0.3375000000000000222, 0.3416666666666666741, 0.3458333333333333259, 0.3499999999999999778, 0.3541666666666666852, 0.3583333333333333370, 0.3624999999999999889, 0.3666666666666666408, 0.3708333333333333481, 0.3750000000000000000, 0.3791666666666666519, 0.3833333333333333592, 0.3875000000000000111, 0.3916666666666666630, 0.3958333333333333148, 0.4000000000000000222, 0.4041666666666666741, 0.4083333333333333259, 0.4124999999999999778, 0.4166666666666666852, 0.4208333333333333370, 0.4249999999999999889, 0.4291666666666666408, 0.4333333333333333481, 0.4375000000000000000, 0.4416666666666666519, 0.4458333333333333592, 0.4500000000000000111, 0.4541666666666666630, 0.4583333333333333148, 0.4625000000000000222, 0.4666666666666666741, 0.4708333333333333259, 0.4749999999999999778, 0.4791666666666666852, 0.4833333333333333370, 0.4874999999999999889, 0.4916666666666666408, 0.4958333333333333481, 0.5000000000000000000, 0.5041666666666666519, 0.5083333333333333037, 0.5124999999999999556, 0.5166666666666667185, 0.5208333333333333703, 0.5250000000000000222, 0.5291666666666666741, 0.5333333333333333259, 0.5374999999999999778, 0.5416666666666666297, 0.5458333333333332815, 0.5500000000000000444, 0.5541666666666666963, 0.5583333333333333481, 0.5625000000000000000, 0.5666666666666666519, 0.5708333333333333037, 0.5749999999999999556, 0.5791666666666667185, 0.5833333333333333703, 0.5875000000000000222, 0.5916666666666666741, 0.5958333333333333259, 0.5999999999999999778, 0.6041666666666666297, 0.6083333333333332815, 0.6125000000000000444, 0.6166666666666666963, 0.6208333333333333481, 0.6250000000000000000, 0.6291666666666666519, 0.6333333333333333037, 0.6374999999999999556, 0.6416666666666667185, 0.6458333333333333703, 0.6500000000000000222, 0.6541666666666666741, 0.6583333333333333259, 0.6624999999999999778, 0.6666666666666666297, 0.6708333333333332815, 0.6750000000000000444, 0.6791666666666666963, 0.6833333333333333481, 0.6875000000000000000, 0.6916666666666666519, 0.6958333333333333037, 0.6999999999999999556, 0.7041666666666667185, 0.7083333333333333703, 0.7125000000000000222, 0.7166666666666666741, 0.7208333333333333259, 0.7249999999999999778, 0.7291666666666666297, 0.7333333333333332815, 0.7375000000000000444, 0.7416666666666666963, 0.7458333333333333481, 0.7500000000000000000, 0.7541666666666666519, 0.7583333333333333037, 0.7624999999999999556, 0.7666666666666667185, 0.7708333333333333703, 0.7750000000000000222, 0.7791666666666666741, 0.7833333333333333259, 0.7874999999999999778, 0.7916666666666666297, 0.7958333333333332815, 0.8000000000000000444, 0.8041666666666666963, 0.8083333333333333481, 0.8125000000000000000, 0.8166666666666666519, 0.8208333333333333037, 0.8249999999999999556, 0.8291666666666667185, 0.8333333333333333703, 0.8375000000000000222, 0.8416666666666666741, 0.8458333333333333259, 0.8499999999999999778, 0.8541666666666666297, 0.8583333333333332815, 0.8625000000000000444, 0.8666666666666666963, 0.8708333333333333481, 0.8750000000000000000, 0.8791666666666666519, 0.8833333333333333037, 0.8874999999999999556, 0.8916666666666667185, 0.8958333333333333703, 0.9000000000000000222, 0.9041666666666666741, 0.9083333333333333259, 0.9124999999999999778, 0.9166666666666666297, 0.9208333333333332815, 0.9250000000000000444, 0.9291666666666666963, 0.9333333333333333481, 0.9375000000000000000, 0.9416666666666666519, 0.9458333333333333037, 0.9499999999999999556, 0.9541666666666667185, 0.9583333333333333703, 0.9625000000000000222, 0.9666666666666666741, 0.9708333333333333259, 0.9749999999999999778, 0.9791666666666666297, 0.9833333333333332815, 0.9875000000000000444, 0.9916666666666666963, 0.9958333333333333481, 1.000000000000000000 ),
 .UNSPECIFIED. ) 
 GEOMETRIC_REPRESENTATION_ITEM ( )  RATIONAL_B_SPLINE_SURFACE ( (
 ( 1.000000000000000000, 0.8660254037844387076, 1.000000000000000000, 0.8660254037844387076, 1.000000000000000000, 0.8660254037844387076, 1.000000000000000000, 0.8660254037844387076, 1.000000000000000000, 0.8660254037844387076, 1.000000000000000000, 0.8660254037844387076, 1.000000000000000000, 0.8660254037844387076, 1.000000000000000000, 0.8660254037844387076, 1.000000000000000000, 0.8660254037844387076, 1.000000000000000000, 0.8660254037844387076, 1.000000000000000000, 0.8660254037844387076, 1.000000000000000000, 0.8660254037844387076, 1.000000000000000000, 0.8660254037844387076, 1.000000000000000000, 0.8660254037844387076, 1.000000000000000000, 0.8660254037844387076, 1.000000000000000000, 0.8660254037844387076, 1.000000000000000000, 0.8660254037844387076, 1.000000000000000000, 0.8660254037844387076, 1.000000000000000000, 0.8660254037844387076, 1.000000000000000000, 0.8660254037844387076, 1.000000000000000000, 0.8660254037844387076, 1.000000000000000000, 0.8660254037844387076, 1.000000000000000000, 0.8660254037844387076, 1.000000000000000000, 0.8660254037844387076, 1.000000000000000000, 0.8660254037844387076, 1.000000000000000000, 0.8660254037844387076, 1.000000000000000000, 0.8660254037844387076, 1.000000000000000000, 0.8660254037844387076, 1.000000000000000000, 0.8660254037844387076, 1.000000000000000000, 0.8660254037844387076, 1.000000000000000000, 0.8660254037844387076, 1.000000000000000000, 0.8660254037844387076, 1.000000000000000000, 0.8660254037844387076, 1.000000000000000000, 0.8660254037844387076, 1.000000000000000000, 0.8660254037844387076, 1.000000000000000000, 0.8660254037844387076, 1.000000000000000000, 0.8660254037844387076, 1.000000000000000000, 0.8660254037844387076, 1.000000000000000000, 0.8660254037844387076, 1.000000000000000000, 0.8660254037844387076, 1.000000000000000000, 0.8660254037844387076, 1.000000000000000000, 0.8660254037844387076, 1.000000000000000000, 0.8660254037844387076, 1.000000000000000000, 0.8660254037844387076, 1.000000000000000000, 0.8660254037844387076, 1.000000000000000000, 0.8660254037844387076, 1.000000000000000000, 0.8660254037844387076, 1.000000000000000000, 0.8660254037844387076, 1.000000000000000000, 0.8660254037844387076, 1.000000000000000000, 0.8660254037844387076, 1.000000000000000000, 0.8660254037844387076, 1.000000000000000000, 0.8660254037844387076, 1.000000000000000000, 0.8660254037844387076, 1.000000000000000000, 0.8660254037844387076, 1.000000000000000000, 0.8660254037844387076, 1.000000000000000000, 0.8660254037844387076, 1.000000000000000000, 0.8660254037844387076, 1.000000000000000000, 0.8660254037844387076, 1.000000000000000000, 0.8660254037844387076, 1.000000000000000000, 0.8660254037844387076, 1.000000000000000000, 0.8660254037844387076, 1.000000000000000000, 0.8660254037844387076, 1.000000000000000000, 0.8660254037844387076, 1.000000000000000000, 0.8660254037844387076, 1.000000000000000000, 0.8660254037844387076, 1.000000000000000000, 0.8660254037844387076, 1.000000000000000000, 0.8660254037844387076, 1.000000000000000000, 0.8660254037844387076, 1.000000000000000000, 0.8660254037844387076, 1.000000000000000000, 0.8660254037844387076, 1.000000000000000000, 0.8660254037844387076, 1.000000000000000000, 0.8660254037844387076, 1.000000000000000000, 0.8660254037844387076, 1.000000000000000000, 0.8660254037844387076, 1.000000000000000000, 0.8660254037844387076, 1.000000000000000000, 0.8660254037844387076, 1.000000000000000000, 0.8660254037844387076, 1.000000000000000000, 0.8660254037844387076, 1.000000000000000000, 0.8660254037844387076, 1.000000000000000000, 0.8660254037844387076, 1.000000000000000000, 0.8660254037844387076, 1.000000000000000000, 0.8660254037844387076, 1.000000000000000000, 0.8660254037844387076, 1.000000000000000000, 0.8660254037844387076, 1.000000000000000000, 0.8660254037844387076, 1.000000000000000000, 0.8660254037844387076, 1.000000000000000000, 0.8660254037844387076, 1.000000000000000000, 0.8660254037844387076, 1.000000000000000000, 0.8660254037844387076, 1.000000000000000000, 0.8660254037844387076, 1.000000000000000000, 0.8660254037844387076, 1.000000000000000000, 0.8660254037844387076, 1.000000000000000000, 0.8660254037844387076, 1.000000000000000000, 0.8660254037844387076, 1.000000000000000000, 0.8660254037844387076, 1.000000000000000000, 0.8660254037844387076, 1.000000000000000000, 0.8660254037844387076, 1.000000000000000000, 0.8660254037844387076, 1.000000000000000000, 0.8660254037844387076, 1.000000000000000000, 0.8660254037844387076, 1.000000000000000000, 0.8660254037844387076, 1.000000000000000000, 0.8660254037844387076, 1.000000000000000000, 0.8660254037844387076, 1.000000000000000000, 0.8660254037844387076, 1.000000000000000000, 0.8660254037844387076, 1.000000000000000000, 0.8660254037844387076, 1.000000000000000000, 0.8660254037844387076, 1.000000000000000000, 0.8660254037844387076, 1.000000000000000000, 0.8660254037844387076, 1.000000000000000000, 0.8660254037844387076, 1.000000000000000000, 0.8660254037844387076, 1.000000000000000000, 0.8660254037844387076, 1.000000000000000000, 0.8660254037844387076, 1.000000000000000000, 0.8660254037844387076, 1.000000000000000000, 0.8660254037844387076, 1.000000000000000000, 0.8660254037844387076, 1.000000000000000000, 0.8660254037844387076, 1.000000000000000000, 0.8660254037844387076, 1.000000000000000000, 0.8660254037844387076, 1.000000000000000000, 0.8660254037844387076, 1.000000000000000000, 0.8660254037844387076, 1.000000000000000000, 0.8660254037844387076, 1.000000000000000000, 0.8660254037844387076, 1.000000000000000000, 0.8660254037844387076, 1.000000000000000000, 0.8660254037844387076, 1.000000000000000000, 0.8660254037844387076, 1.000000000000000000, 0.8660254037844387076, 1.000000000000000000, 0.8660254037844387076, 1.000000000000000000, 0.8660254037844387076, 1.000000000000000000, 0.8660254037844387076, 1.000000000000000000, 0.8660254037844387076, 1.000000000000000000, 0.8660254037844387076, 1.000000000000000000, 0.8660254037844387076, 1.000000000000000000, 0.8660254037844387076, 1.000000000000000000, 0.8660254037844387076, 1.000000000000000000, 0.8660254037844387076, 1.000000000000000000, 0.8660254037844387076, 1.000000000000000000, 0.8660254037844387076, 1.000000000000000000, 0.8660254037844387076, 1.000000000000000000, 0.8660254037844387076, 1.000000000000000000, 0.8660254037844387076, 1.000000000000000000, 0.8660254037844387076, 1.000000000000000000, 0.8660254037844387076, 1.000000000000000000, 0.8660254037844387076, 1.000000000000000000, 0.8660254037844387076, 1.000000000000000000, 0.8660254037844387076, 1.000000000000000000, 0.8660254037844387076, 1.000000000000000000, 0.8660254037844387076, 1.000000000000000000, 0.8660254037844387076, 1.000000000000000000, 0.8660254037844387076, 1.000000000000000000, 0.8660254037844387076, 1.000000000000000000, 0.8660254037844387076, 1.000000000000000000, 0.8660254037844387076, 1.000000000000000000, 0.8660254037844387076, 1.000000000000000000, 0.8660254037844387076, 1.000000000000000000, 0.8660254037844387076, 1.000000000000000000, 0.8660254037844387076, 1.000000000000000000, 0.8660254037844387076, 1.000000000000000000, 0.8660254037844387076, 1.000000000000000000, 0.8660254037844387076, 1.000000000000000000, 0.8660254037844387076, 1.000000000000000000, 0.8660254037844387076, 1.000000000000000000, 0.8660254037844387076, 1.000000000000000000, 0.8660254037844387076, 1.000000000000000000, 0.8660254037844387076, 1.000000000000000000, 0.8660254037844387076, 1.000000000000000000, 0.8660254037844387076, 1.000000000000000000, 0.8660254037844387076, 1.000000000000000000, 0.8660254037844387076, 1.000000000000000000, 0.8660254037844387076, 1.000000000000000000, 0.8660254037844387076, 1.000000000000000000, 0.8660254037844387076, 1.000000000000000000, 0.8660254037844387076, 1.000000000000000000, 0.8660254037844387076, 1.000000000000000000, 0.8660254037844387076, 1.000000000000000000, 0.8660254037844387076, 1.000000000000000000, 0.8660254037844387076, 1.000000000000000000, 0.8660254037844387076, 1.000000000000000000, 0.8660254037844387076, 1.000000000000000000, 0.8660254037844387076, 1.000000000000000000, 0.8660254037844387076, 1.000000000000000000, 0.8660254037844387076, 1.000000000000000000, 0.8660254037844387076, 1.000000000000000000, 0.8660254037844387076, 1.000000000000000000, 0.8660254037844387076, 1.000000000000000000, 0.8660254037844387076, 1.000000000000000000, 0.8660254037844387076, 1.000000000000000000, 0.8660254037844387076, 1.000000000000000000, 0.8660254037844387076, 1.000000000000000000, 0.8660254037844387076, 1.000000000000000000, 0.8660254037844387076, 1.000000000000000000, 0.8660254037844387076, 1.000000000000000000, 0.8660254037844387076, 1.000000000000000000, 0.8660254037844387076, 1.000000000000000000, 0.8660254037844387076, 1.000000000000000000, 0.8660254037844387076, 1.000000000000000000, 0.8660254037844387076, 1.000000000000000000, 0.8660254037844387076, 1.000000000000000000, 0.8660254037844387076, 1.000000000000000000, 0.8660254037844387076, 1.000000000000000000, 0.8660254037844387076, 1.000000000000000000, 0.8660254037844387076, 1.000000000000000000, 0.8660254037844387076, 1.000000000000000000, 0.8660254037844387076, 1.000000000000000000, 0.8660254037844387076, 1.000000000000000000, 0.8660254037844387076, 1.000000000000000000, 0.8660254037844387076, 1.000000000000000000, 0.8660254037844387076, 1.000000000000000000, 0.8660254037844387076, 1.000000000000000000, 0.8660254037844387076, 1.000000000000000000, 0.8660254037844387076, 1.000000000000000000, 0.8660254037844387076, 1.000000000000000000, 0.8660254037844387076, 1.000000000000000000, 0.8660254037844387076, 1.000000000000000000, 0.8660254037844387076, 1.000000000000000000, 0.8660254037844387076, 1.000000000000000000, 0.8660254037844387076, 1.000000000000000000, 0.8660254037844387076, 1.000000000000000000, 0.8660254037844387076, 1.000000000000000000, 0.8660254037844387076, 1.000000000000000000, 0.8660254037844387076, 1.000000000000000000, 0.8660254037844387076, 1.000000000000000000, 0.8660254037844387076, 1.000000000000000000, 0.8660254037844387076, 1.000000000000000000, 0.8660254037844387076, 1.000000000000000000, 0.8660254037844387076, 1.000000000000000000, 0.8660254037844387076, 1.000000000000000000, 0.8660254037844387076, 1.000000000000000000, 0.8660254037844387076, 1.000000000000000000, 0.8660254037844387076, 1.000000000000000000, 0.8660254037844387076, 1.000000000000000000, 0.8660254037844387076, 1.000000000000000000, 0.8660254037844387076, 1.000000000000000000, 0.8660254037844387076, 1.000000000000000000, 0.8660254037844387076, 1.000000000000000000, 0.8660254037844387076, 1.000000000000000000, 0.8660254037844387076, 1.000000000000000000, 0.8660254037844387076, 1.000000000000000000, 0.8660254037844387076, 1.000000000000000000, 0.8660254037844387076, 1.000000000000000000),
 ( 1.000000000000000000, 0.8660254037844387076, 1.000000000000000000, 0.8660254037844387076, 1.000000000000000000, 0.8660254037844387076, 1.000000000000000000, 0.8660254037844387076, 1.000000000000000000, 0.8660254037844387076, 1.000000000000000000, 0.8660254037844387076, 1.000000000000000000, 0.8660254037844387076, 1.000000000000000000, 0.8660254037844387076, 1.000000000000000000, 0.8660254037844387076, 1.000000000000000000, 0.8660254037844387076, 1.000000000000000000, 0.8660254037844387076, 1.000000000000000000, 0.8660254037844387076, 1.000000000000000000, 0.8660254037844387076, 1.000000000000000000, 0.8660254037844387076, 1.000000000000000000, 0.8660254037844387076, 1.000000000000000000, 0.8660254037844387076, 1.000000000000000000, 0.8660254037844387076, 1.000000000000000000, 0.8660254037844387076, 1.000000000000000000, 0.8660254037844387076, 1.000000000000000000, 0.8660254037844387076, 1.000000000000000000, 0.8660254037844387076, 1.000000000000000000, 0.8660254037844387076, 1.000000000000000000, 0.8660254037844387076, 1.000000000000000000, 0.8660254037844387076, 1.000000000000000000, 0.8660254037844387076, 1.000000000000000000, 0.8660254037844387076, 1.000000000000000000, 0.8660254037844387076, 1.000000000000000000, 0.8660254037844387076, 1.000000000000000000, 0.8660254037844387076, 1.000000000000000000, 0.8660254037844387076, 1.000000000000000000, 0.8660254037844387076, 1.000000000000000000, 0.8660254037844387076, 1.000000000000000000, 0.8660254037844387076, 1.000000000000000000, 0.8660254037844387076, 1.000000000000000000, 0.8660254037844387076, 1.000000000000000000, 0.8660254037844387076, 1.000000000000000000, 0.8660254037844387076, 1.000000000000000000, 0.8660254037844387076, 1.000000000000000000, 0.8660254037844387076, 1.000000000000000000, 0.8660254037844387076, 1.000000000000000000, 0.8660254037844387076, 1.000000000000000000, 0.8660254037844387076, 1.000000000000000000, 0.8660254037844387076, 1.000000000000000000, 0.8660254037844387076, 1.000000000000000000, 0.8660254037844387076, 1.000000000000000000, 0.8660254037844387076, 1.000000000000000000, 0.8660254037844387076, 1.000000000000000000, 0.8660254037844387076, 1.000000000000000000, 0.8660254037844387076, 1.000000000000000000, 0.8660254037844387076, 1.000000000000000000, 0.8660254037844387076, 1.000000000000000000, 0.8660254037844387076, 1.000000000000000000, 0.8660254037844387076, 1.000000000000000000, 0.8660254037844387076, 1.000000000000000000, 0.8660254037844387076, 1.000000000000000000, 0.8660254037844387076, 1.000000000000000000, 0.8660254037844387076, 1.000000000000000000, 0.8660254037844387076, 1.000000000000000000, 0.8660254037844387076, 1.000000000000000000, 0.8660254037844387076, 1.000000000000000000, 0.8660254037844387076, 1.000000000000000000, 0.8660254037844387076, 1.000000000000000000, 0.8660254037844387076, 1.000000000000000000, 0.8660254037844387076, 1.000000000000000000, 0.8660254037844387076, 1.000000000000000000, 0.8660254037844387076, 1.000000000000000000, 0.8660254037844387076, 1.000000000000000000, 0.8660254037844387076, 1.000000000000000000, 0.8660254037844387076, 1.000000000000000000, 0.8660254037844387076, 1.000000000000000000, 0.8660254037844387076, 1.000000000000000000, 0.8660254037844387076, 1.000000000000000000, 0.8660254037844387076, 1.000000000000000000, 0.8660254037844387076, 1.000000000000000000, 0.8660254037844387076, 1.000000000000000000, 0.8660254037844387076, 1.000000000000000000, 0.8660254037844387076, 1.000000000000000000, 0.8660254037844387076, 1.000000000000000000, 0.8660254037844387076, 1.000000000000000000, 0.8660254037844387076, 1.000000000000000000, 0.8660254037844387076, 1.000000000000000000, 0.8660254037844387076, 1.000000000000000000, 0.8660254037844387076, 1.000000000000000000, 0.8660254037844387076, 1.000000000000000000, 0.8660254037844387076, 1.000000000000000000, 0.8660254037844387076, 1.000000000000000000, 0.8660254037844387076, 1.000000000000000000, 0.8660254037844387076, 1.000000000000000000, 0.8660254037844387076, 1.000000000000000000, 0.8660254037844387076, 1.000000000000000000, 0.8660254037844387076, 1.000000000000000000, 0.8660254037844387076, 1.000000000000000000, 0.8660254037844387076, 1.000000000000000000, 0.8660254037844387076, 1.000000000000000000, 0.8660254037844387076, 1.000000000000000000, 0.8660254037844387076, 1.000000000000000000, 0.8660254037844387076, 1.000000000000000000, 0.8660254037844387076, 1.000000000000000000, 0.8660254037844387076, 1.000000000000000000, 0.8660254037844387076, 1.000000000000000000, 0.8660254037844387076, 1.000000000000000000, 0.8660254037844387076, 1.000000000000000000, 0.8660254037844387076, 1.000000000000000000, 0.8660254037844387076, 1.000000000000000000, 0.8660254037844387076, 1.000000000000000000, 0.8660254037844387076, 1.000000000000000000, 0.8660254037844387076, 1.000000000000000000, 0.8660254037844387076, 1.000000000000000000, 0.8660254037844387076, 1.000000000000000000, 0.8660254037844387076, 1.000000000000000000, 0.8660254037844387076, 1.000000000000000000, 0.8660254037844387076, 1.000000000000000000, 0.8660254037844387076, 1.000000000000000000, 0.8660254037844387076, 1.000000000000000000, 0.8660254037844387076, 1.000000000000000000, 0.8660254037844387076, 1.000000000000000000, 0.8660254037844387076, 1.000000000000000000, 0.8660254037844387076, 1.000000000000000000, 0.8660254037844387076, 1.000000000000000000, 0.8660254037844387076, 1.000000000000000000, 0.8660254037844387076, 1.000000000000000000, 0.8660254037844387076, 1.000000000000000000, 0.8660254037844387076, 1.000000000000000000, 0.8660254037844387076, 1.000000000000000000, 0.8660254037844387076, 1.000000000000000000, 0.8660254037844387076, 1.000000000000000000, 0.8660254037844387076, 1.000000000000000000, 0.8660254037844387076, 1.000000000000000000, 0.8660254037844387076, 1.000000000000000000, 0.8660254037844387076, 1.000000000000000000, 0.8660254037844387076, 1.000000000000000000, 0.8660254037844387076, 1.000000000000000000, 0.8660254037844387076, 1.000000000000000000, 0.8660254037844387076, 1.000000000000000000, 0.8660254037844387076, 1.000000000000000000, 0.8660254037844387076, 1.000000000000000000, 0.8660254037844387076, 1.000000000000000000, 0.8660254037844387076, 1.000000000000000000, 0.8660254037844387076, 1.000000000000000000, 0.8660254037844387076, 1.000000000000000000, 0.8660254037844387076, 1.000000000000000000, 0.8660254037844387076, 1.000000000000000000, 0.8660254037844387076, 1.000000000000000000, 0.8660254037844387076, 1.000000000000000000, 0.8660254037844387076, 1.000000000000000000, 0.8660254037844387076, 1.000000000000000000, 0.8660254037844387076, 1.000000000000000000, 0.8660254037844387076, 1.000000000000000000, 0.8660254037844387076, 1.000000000000000000, 0.8660254037844387076, 1.000000000000000000, 0.8660254037844387076, 1.000000000000000000, 0.8660254037844387076, 1.000000000000000000, 0.8660254037844387076, 1.000000000000000000, 0.8660254037844387076, 1.000000000000000000, 0.8660254037844387076, 1.000000000000000000, 0.8660254037844387076, 1.000000000000000000, 0.8660254037844387076, 1.000000000000000000, 0.8660254037844387076, 1.000000000000000000, 0.8660254037844387076, 1.000000000000000000, 0.8660254037844387076, 1.000000000000000000, 0.8660254037844387076, 1.000000000000000000, 0.8660254037844387076, 1.000000000000000000, 0.8660254037844387076, 1.000000000000000000, 0.8660254037844387076, 1.000000000000000000, 0.8660254037844387076, 1.000000000000000000, 0.8660254037844387076, 1.000000000000000000, 0.8660254037844387076, 1.000000000000000000, 0.8660254037844387076, 1.000000000000000000, 0.8660254037844387076, 1.000000000000000000, 0.8660254037844387076, 1.000000000000000000, 0.8660254037844387076, 1.000000000000000000, 0.8660254037844387076, 1.000000000000000000, 0.8660254037844387076, 1.000000000000000000, 0.8660254037844387076, 1.000000000000000000, 0.8660254037844387076, 1.000000000000000000, 0.8660254037844387076, 1.000000000000000000, 0.8660254037844387076, 1.000000000000000000, 0.8660254037844387076, 1.000000000000000000, 0.8660254037844387076, 1.000000000000000000, 0.8660254037844387076, 1.000000000000000000, 0.8660254037844387076, 1.000000000000000000, 0.8660254037844387076, 1.000000000000000000, 0.8660254037844387076, 1.000000000000000000, 0.8660254037844387076, 1.000000000000000000, 0.8660254037844387076, 1.000000000000000000, 0.8660254037844387076, 1.000000000000000000, 0.8660254037844387076, 1.000000000000000000, 0.8660254037844387076, 1.000000000000000000, 0.8660254037844387076, 1.000000000000000000, 0.8660254037844387076, 1.000000000000000000, 0.8660254037844387076, 1.000000000000000000, 0.8660254037844387076, 1.000000000000000000, 0.8660254037844387076, 1.000000000000000000, 0.8660254037844387076, 1.000000000000000000, 0.8660254037844387076, 1.000000000000000000, 0.8660254037844387076, 1.000000000000000000, 0.8660254037844387076, 1.000000000000000000, 0.8660254037844387076, 1.000000000000000000, 0.8660254037844387076, 1.000000000000000000, 0.8660254037844387076, 1.000000000000000000, 0.8660254037844387076, 1.000000000000000000, 0.8660254037844387076, 1.000000000000000000, 0.8660254037844387076, 1.000000000000000000, 0.8660254037844387076, 1.000000000000000000, 0.8660254037844387076, 1.000000000000000000, 0.8660254037844387076, 1.000000000000000000, 0.8660254037844387076, 1.000000000000000000, 0.8660254037844387076, 1.000000000000000000, 0.8660254037844387076, 1.000000000000000000, 0.8660254037844387076, 1.000000000000000000, 0.8660254037844387076, 1.000000000000000000, 0.8660254037844387076, 1.000000000000000000, 0.8660254037844387076, 1.000000000000000000, 0.8660254037844387076, 1.000000000000000000, 0.8660254037844387076, 1.000000000000000000, 0.8660254037844387076, 1.000000000000000000, 0.8660254037844387076, 1.000000000000000000, 0.8660254037844387076, 1.000000000000000000, 0.8660254037844387076, 1.000000000000000000, 0.8660254037844387076, 1.000000000000000000, 0.8660254037844387076, 1.000000000000000000, 0.8660254037844387076, 1.000000000000000000, 0.8660254037844387076, 1.000000000000000000, 0.8660254037844387076, 1.000000000000000000, 0.8660254037844387076, 1.000000000000000000, 0.8660254037844387076, 1.000000000000000000, 0.8660254037844387076, 1.000000000000000000, 0.8660254037844387076, 1.000000000000000000, 0.8660254037844387076, 1.000000000000000000, 0.8660254037844387076, 1.000000000000000000, 0.8660254037844387076, 1.000000000000000000, 0.8660254037844387076, 1.000000000000000000, 0.8660254037844387076, 1.000000000000000000, 0.8660254037844387076, 1.000000000000000000, 0.8660254037844387076, 1.000000000000000000, 0.8660254037844387076, 1.000000000000000000, 0.8660254037844387076, 1.000000000000000000, 0.8660254037844387076, 1.000000000000000000, 0.8660254037844387076, 1.000000000000000000, 0.8660254037844387076, 1.000000000000000000) ) ) 
 REPRESENTATION_ITEM ( '' )  SURFACE ( )  );
#75168=CARTESIAN_POINT ( 'NONE',  ( -7.562750758324527922, 7.717630727667075696, 1.040834085586084257E-14 ) ) ;
#75170=CARTESIAN_POINT ( 'NONE',  ( 1.244123718695673952, 2.848244533904600750, -0.7749999999999926947 ) ) ;
#75172=CARTESIAN_POINT ( 'NONE',  ( 5.286789834324991055, 8.255339675766103724, -1.199719254218452935 ) ) ;
#75180=CARTESIAN_POINT ( 'NONE',  ( -4.741601036477307574, 6.554953847355395880, 1.599625672291267398 ) ) ;
#75183=CARTESIAN_POINT ( 'NONE',  ( 5.913327553854682783, 10.05063257947248800, -0.7998128361456291469 ) ) ;
#75186=CARTESIAN_POINT ( 'NONE',  ( 6.108949960370312127, 6.019453914259918825, -0.1454340903971618193 ) ) ;
#75192=CARTESIAN_POINT ( 'NONE',  ( 5.287316719205157334, 9.112360572473935605, 1.040834085586084257E-14 ) ) ;
#75193=CARTESIAN_POINT ( 'NONE',  ( -8.290974629956718189, 9.631557475493025322, -1.199719254218446718 ) ) ;
#75196=CARTESIAN_POINT ( 'NONE',  ( -8.483651433849100698, 10.92067931095586886, 1.599625672291269396 ) ) ;
#75198=CARTESIAN_POINT ( 'NONE',  ( -6.898401231254901234, 6.942556279419168419, -0.7998128361456291469 ) ) ;
#75199=CARTESIAN_POINT ( 'NONE',  ( -3.578989363883261277, 7.119311991265024453, 1.040834085586084257E-14 ) ) ;
#75206=CARTESIAN_POINT ( 'NONE',  ( 6.740374924288304648, 11.01552117831172062, 1.040834085586084257E-14 ) ) ;
#75219=CARTESIAN_POINT ( 'NONE',  ( -1.500000000000011324, 3.920833333333357817, 0.8660254037844403729 ) ) ;
#75220=CARTESIAN_POINT ( 'NONE',  ( 5.495132332240461714, 5.305409230568988832, 0.7998128361456341429 ) ) ;
#75221=CARTESIAN_POINT ( 'NONE',  ( 5.957918438201454059, 9.038323046955323292, -1.199719254218440723 ) ) ;
#75224=CARTESIAN_POINT ( 'NONE',  ( 6.236387472606139681, 8.298871356172400127, -1.443375672974057666 ) ) ;
#75226=CARTESIAN_POINT ( 'NONE',  ( -9.503902493055310430, 11.15060299906175167, 1.082531754730558626 ) ) ;
#75230=CARTESIAN_POINT ( 'NONE',  ( 8.378048858240820351, 11.86180853700128601, -1.199719254218446718 ) ) ;
#75234=CARTESIAN_POINT ( 'NONE',  ( -1.364683531250014514, 0.7385416670080887647, -0.7879004041258289570 ) ) ;
#75239=CARTESIAN_POINT ( 'NONE',  ( 1.364683531249988757, -0.8656249996585805295, 0.000000000000000000 ) ) ;
#75241=CARTESIAN_POINT ( 'NONE',  ( 10.57266086055835075, 11.22919251360659310, 0.000000000000000000 ) ) ;
#75244=CARTESIAN_POINT ( 'NONE',  ( -9.829825065107822724, 11.42688298316931572, 1.199719254218462483 ) ) ;
#75250=CARTESIAN_POINT ( 'NONE',  ( 3.680148631105580215, 6.380924938676771241, -1.199719254218446718 ) ) ;
#75255=CARTESIAN_POINT ( 'NONE',  ( 8.934986926605834157, 10.38290515491702770, -1.199719254218446718 ) ) ;
#75257=CARTESIAN_POINT ( 'NONE',  ( 4.388421827844267042, 7.126904390760538277, 1.074283327121795528 ) ) ;
#75259=CARTESIAN_POINT ( 'NONE',  ( -3.469997250093771246, 6.135748327496311383, -1.199719254218452935 ) ) ;
#75263=CARTESIAN_POINT ( 'NONE',  ( 6.591235234537977661, 10.84152487360300299, 0.7998128361456462443 ) ) ;
#75265=CARTESIAN_POINT ( 'NONE',  ( 6.252281394196331554, 10.44607872653774372, 1.040834085586084257E-14 ) ) ;
#75269=CARTESIAN_POINT ( 'NONE',  ( -9.666600336863641729, 10.38004793587015584, 1.040834085586084257E-14 ) ) ;
#75276=CARTESIAN_POINT ( 'NONE',  ( -4.957065645985164970, 6.648394846229956023, -1.245809975726259067 ) ) ;
#75277=CARTESIAN_POINT ( 'NONE',  ( 0.6823417656249899377, 2.342708333674753618, 1.181850606188767472 ) ) ;
#75279=CARTESIAN_POINT ( 'NONE',  ( 5.653386867218496370, 9.539442411822841805, 1.040834085586084257E-14 ) ) ;
#75296=ADVANCED_FACE ( 'NONE', ( #59502 ), #30904, .T. ) ;
#75298=CARTESIAN_POINT ( 'NONE',  ( 9.596473800374404561, 10.09030761005864285, 0.000000000000000000 ) ) ;
#75302=CARTESIAN_POINT ( 'NONE',  ( -2.611917148927046295, 6.198987107056845858, 1.040834085586084257E-14 ) ) ;
#75303=CARTESIAN_POINT ( 'NONE',  ( -5.859094939400033120, 9.987361195942037639, -0.7998128361456231517 ) ) ;
#75306=CARTESIAN_POINT ( 'NONE',  ( -8.971744963941075568, 11.49012176272984931, 1.599625672291269396 ) ) ;
#75307=CARTESIAN_POINT ( 'NONE',  ( -1.483013432600015502, 7.294277089886564092, 4.259227663825926768 ) ) ;
#75309=CARTESIAN_POINT ( 'NONE',  ( 1.499999999999989120, 4.285416667349482900, 0.8660254037844524744 ) ) ;
#75310=CARTESIAN_POINT ( 'NONE',  ( 6.577677080924314801, 10.82570702772039262, 1.040834085586084257E-14 ) ) ;
#75313=CARTESIAN_POINT ( 'NONE',  ( -7.823218330285243383, 9.085841792542966644, -1.199719254218446718 ) ) ;
#75315=CARTESIAN_POINT ( 'NONE',  ( -1.201851678989727383E-14, 4.446875000341417916, -1.575800808251660134 ) ) ;
#75321=CARTESIAN_POINT ( 'NONE',  ( -7.863365906246054138, 11.15738207638699464, -1.082531754730543971 ) ) ;
#75325=CARTESIAN_POINT ( 'NONE',  ( 1.364683531249988535, 2.676041667008082214, 0.7879004041258500513 ) ) ;
#75332=CARTESIAN_POINT ( 'NONE',  ( 1.364683531249988535, 4.363541667008090208, 0.7879004041258500513 ) ) ;
#75333=CARTESIAN_POINT ( 'NONE',  ( -4.086893239515592136, 6.855460315155083251, 1.199719254218464037 ) ) ;
#75334=CARTESIAN_POINT ( 'NONE',  ( 5.937581207780954884, 9.014596278131406848, -1.199719254218440723 ) ) ;
#75337=CARTESIAN_POINT ( 'NONE',  ( 0.6823417656249917140, 4.655208333674755394, 1.181850606188765695 ) ) ;
#75343=CARTESIAN_POINT ( 'NONE',  ( -1.364683531250000748, -0.4906249996585801409, 0.000000000000000000 ) ) ;
#75344=CARTESIAN_POINT ( 'NONE',  ( -4.121315508874269007, 5.831287398485176077, -1.443375672974053447 ) ) ;
#75345=CARTESIAN_POINT ( 'NONE',  ( 4.286349120214771879, 8.152491073559232859, -0.7998128361456221525 ) ) ;
#75350=CARTESIAN_POINT ( 'NONE',  ( 2.548569689688999329, 5.917155704705049146, -0.7216878364870267237 ) ) ;
#75354=CARTESIAN_POINT ( 'NONE',  ( -9.653042183249972652, 10.36423008998754192, -0.7216878364870267237 ) ) ;
#75356=EDGE_CURVE ( 'NONE', #197889, #202349, #123081, .T. ) ;
#75360=CARTESIAN_POINT ( 'NONE',  ( -8.839026081105473054, 12.39961529701003684, -1.199719254218446718 ) ) ;
#75361=CARTESIAN_POINT ( 'NONE',  ( -5.544921637864838715, 6.531792001339513654, -1.082531754730543971 ) ) ;
#75363=CARTESIAN_POINT ( 'NONE',  ( 1.364683531249986537, 0.9677083336747538400, -0.7879004041258239610 ) ) ;
#75375=CARTESIAN_POINT ( 'NONE',  ( 8.148087131688683371, 10.52918762510205042, -1.443375672974063439 ) ) ;
#75379=EDGE_LOOP ( 'NONE', ( #46617, #72603, #160665, #173742, #107950 ) ) ;
#75383=CARTESIAN_POINT ( 'NONE',  ( 4.111146893441827821, 5.819424013814004759, 1.599625672291267398 ) ) ;
#75386=CARTESIAN_POINT ( 'NONE',  ( -2.103486388414573138, 5.605817886458954291, 1.040834085586084257E-14 ) ) ;
#75388=AXIS2_PLACEMENT_3D ( 'NONE', #55230, #108314, #207861 ) ;
#75390=CARTESIAN_POINT ( 'NONE',  ( 1.123270288250311610, 3.172697346350006331, 0.7749999999993734123 ) ) ;
#75392=CARTESIAN_POINT ( 'NONE',  ( -0.6823417656250003738, 1.530208333674752730, -1.181850606188749264 ) ) ;
#75406=EDGE_LOOP ( 'NONE', ( #176531, #20652, #168942, #204974 ) ) ;
#75410=CARTESIAN_POINT ( 'NONE',  ( 6.602984505055297326, 7.662235663108029726, 1.199719254218462483 ) ) ;
#75417=CARTESIAN_POINT ( 'NONE',  ( 8.132193210098487057, 8.381980254736715708, 1.040834085586084257E-14 ) ) ;
#75418=CARTESIAN_POINT ( 'NONE',  ( 3.619663824724254741, 6.206396314611513532, -1.082531754730543971 ) ) ;
#75420=CARTESIAN_POINT ( 'NONE',  ( 8.072990401933337168, 11.50590700464255356, -1.199719254218446718 ) ) ;
#75432=CARTESIAN_POINT ( 'NONE',  ( -8.432808358020034589, 10.86136238915529084, 1.443375672974064550 ) ) ;
#75438=CARTESIAN_POINT ( 'NONE',  ( -4.174586609897826150, 3.976382069392089047, -0.6022320305223278769 ) ) ;
#75443=CARTESIAN_POINT ( 'NONE',  ( 4.650083499362880346, 4.527444958785877382, 0.7216878364870317197 ) ) ;
#75446=ORIENTED_EDGE ( 'NONE', *, *, #190752, .T. ) ;
#75451=CARTESIAN_POINT ( 'NONE',  ( -5.742041750587549842, 6.657802449562273850, 1.199719254218450271 ) ) ;
#75453=CARTESIAN_POINT ( 'NONE',  ( -3.297657676621885692, 4.870353260857385180, 1.599625672291267398 ) ) ;
#75460=CARTESIAN_POINT ( 'NONE',  ( 1.364683531249988535, 3.676041667008087099, 0.7879004041258499402 ) ) ;
#75463=CARTESIAN_POINT ( 'NONE',  ( 5.148345644887269756, 7.029489223833707001, -1.599625672291256295 ) ) ;
#75464=DIRECTION ( 'NONE',  ( 0.000000000000000000, 0.000000000000000000, 1.000000000000000000 ) ) ;
#75477=CARTESIAN_POINT ( 'NONE',  ( -1.201851678989727383E-14, 1.634375000341421025, 1.575800808251672791 ) ) ;
#75479=CARTESIAN_POINT ( 'NONE',  ( 3.167801447087334576, 6.847518788243868393, -0.7998128361456291469 ) ) ;
#75482=CARTESIAN_POINT ( 'NONE',  ( -5.083944415444539899, 8.875092884753202682, 0.000000000000000000 ) ) ;
#75483=CARTESIAN_POINT ( 'NONE',  ( 4.880572111239557920, 4.796348339308675435, -0.7216878364870197293 ) ) ;
#75484=CARTESIAN_POINT ( 'NONE',  ( -5.531363484251157203, 9.397081798360927607, 0.000000000000000000 ) ) ;
#75486=ORIENTED_EDGE ( 'NONE', *, *, #211675, .T. ) ;
#75488=CARTESIAN_POINT ( 'NONE',  ( 7.461064606222022277, 7.598996883547496139, 1.040834085586084257E-14 ) ) ;
#75496=CARTESIAN_POINT ( 'NONE',  ( 5.621827251160867789, 9.710548892996357040, 1.040834085586084257E-14 ) ) ;
#75500=CARTESIAN_POINT ( 'NONE',  ( -7.497822643557261024, 8.706213491360317747, -1.199719254218446718 ) ) ;
#75504=CARTESIAN_POINT ( 'NONE',  ( 8.776205506747620788, 9.133327934160710981, -0.7998128361456221525 ) ) ;
#75506=CARTESIAN_POINT ( 'NONE',  ( -7.015454420067433361, 10.27211502579893754, 1.199719254218453823 ) ) ;
#75508=CARTESIAN_POINT ( 'NONE',  ( 8.554831740098663317, 9.082984572977682802, 0.7216878364870458196 ) ) ;
#75509=CARTESIAN_POINT ( 'NONE',  ( 4.114373074986557910, 7.676947195153840831, 0.7202382532921544067 ) ) ;
#75510=CARTESIAN_POINT ( 'NONE',  ( -5.935772324684618795, 5.819489221753827657, 0.000000000000000000 ) ) ;
#75515=CARTESIAN_POINT ( 'NONE',  ( 5.015626762051672571, 7.938982758113895422, 1.199719254218462483 ) ) ;
#75517=CARTESIAN_POINT ( 'NONE',  ( 8.727698198895078363, 11.20540053684285553, -1.599625672291257406 ) ) ;
#75518=CARTESIAN_POINT ( 'NONE',  ( -5.012544637203120601, 6.604931577287184830, 1.238112577840282169 ) ) ;
#75520=CARTESIAN_POINT ( 'NONE',  ( -0.6823417656250003738, 0.4677083336747517306, -1.181850606188749264 ) ) ;
#75522=CARTESIAN_POINT ( 'NONE',  ( -6.127922243696855453, 7.211959374810172463, 1.082531754730549967 ) ) ;
#75523=ORIENTED_EDGE ( 'NONE', *, *, #87121, .F. ) ;
#75530=CARTESIAN_POINT ( 'NONE',  ( -5.526177461252244960, 6.240421959547291841, 0.9601993850730760061 ) ) ;
#75531=CARTESIAN_POINT ( 'NONE',  ( -1.364683531250014514, 1.051041667008090208, -0.7879004041258289570 ) ) ;
#75534=CARTESIAN_POINT ( 'NONE',  ( 3.714570900464278846, 5.356752022006865843, 1.443375672974062551 ) ) ;
#75538=CARTESIAN_POINT ( 'NONE',  ( -8.690413276235355866, 10.20153224610512943, 1.082531754730558626 ) ) ;
#75539=CIRCLE ( 'NONE', #41068, 1.220000000000001750 ) ;
#75547=CARTESIAN_POINT ( 'NONE',  ( -7.009202228140739344, 11.12122699956546334, -0.7216878364870267237 ) ) ;
#75548=CARTESIAN_POINT ( 'NONE',  ( -1.123270288250342919, 3.096052654332833054, 0.7749999999993751887 ) ) ;
#75553=CARTESIAN_POINT ( 'NONE',  ( -7.497295758232731089, 8.809561808435409702, -1.082531754730543083 ) ) ;
#75559=CARTESIAN_POINT ( 'NONE',  ( -1.499999999999997780, 4.681250000682819490, 1.214306433183764966E-14 ) ) ;
#75561=CARTESIAN_POINT ( 'NONE',  ( 0.000000000000000000, 2.880000000000021210, 1.214306433183764966E-14 ) ) ;
#75564=EDGE_LOOP ( 'NONE', ( #120258, #76725, #143550, #126903 ) ) ;
#75567=CARTESIAN_POINT ( 'NONE',  ( -7.477485413136760073, 8.682486722536401302, -1.199719254218446718 ) ) ;
#75571=CARTESIAN_POINT ( 'NONE',  ( 3.974511587100456822, 7.788680618259193444, 1.040834085586084257E-14 ) ) ;
#75576=CARTESIAN_POINT ( 'NONE',  ( 6.500244582748090139, 9.671036882259738121, 1.199719254218460707 ) ) ;
#75583=CARTESIAN_POINT ( 'NONE',  ( -6.100805936469506641, 6.219954468743612352, 0.7216878364870317197 ) ) ;
#75592=CARTESIAN_POINT ( 'NONE',  ( -7.343712760096452463, 11.71941532008788833, -0.7998128361456291469 ) ) ;
#75594=CARTESIAN_POINT ( 'NONE',  ( 8.769426429940780920, 9.125419011219408461, 0.7998128361456462443 ) ) ;
#75595=CARTESIAN_POINT ( 'NONE',  ( -1.500000000000001332, -0.3499999999999753308, 0.000000000000000000 ) ) ;
#75596=CARTESIAN_POINT ( 'NONE',  ( -8.097244055859620815, 10.46987070330147063, -1.599625672291263179 ) ) ;
#75600=CARTESIAN_POINT ( 'NONE',  ( 0.6823417656249899377, 4.176041667008085767, -1.181850606188754593 ) ) ;
#75601=CARTESIAN_POINT ( 'NONE',  ( 8.405692050792682224, 12.75046512599275772, -0.7216878364870328300 ) ) ;
#75604=CARTESIAN_POINT ( 'NONE',  ( -0.7500000000000215383, 5.691666666666685082, 1.299038105676671107 ) ) ;
#75607=CARTESIAN_POINT ( 'NONE',  ( 8.012505595552012139, 11.33137838057728786, -1.082531754730543083 ) ) ;
#75610=CARTESIAN_POINT ( 'NONE',  ( -6.073689629242160493, 8.109057205581079231, -1.443375672974059665 ) ) ;
#75613=CARTESIAN_POINT ( 'NONE',  ( 1.364683531249988757, 1.884375000341421913, 0.000000000000000000 ) ) ;
#75617=CARTESIAN_POINT ( 'NONE',  ( -6.021792782764022078, 10.17717534653336209, -0.7998128361456291469 ) ) ;
#75619=CARTESIAN_POINT ( 'NONE',  ( -1.364683531250010295, 5.092708333674757171, 0.7879004041258379498 ) ) ;
#75625=CARTESIAN_POINT ( 'NONE',  ( 9.423080456697809026, 10.95234760669099749, -1.199719254218446718 ) ) ;
#75628=CARTESIAN_POINT ( 'NONE',  ( -0.7500000000000215383, 1.691666666666688634, 1.299038105676659116 ) ) ;
#75632=CARTESIAN_POINT ( 'NONE',  ( -0.4897149945007619465, 7.513091487862089579, -2.015070445391653475 ) ) ;
#75635=CARTESIAN_POINT ( 'NONE',  ( 5.829642864196151741, 9.745074408296771296, 0.7216878364870438212 ) ) ;
#75642=CARTESIAN_POINT ( 'NONE',  ( 7.214910300766615769, 11.56914578420308715, -0.7998128361456291469 ) ) ;
#75643=CARTESIAN_POINT ( 'NONE',  ( -10.32861409551237486, 10.94447128771960287, 1.040834085586084257E-14 ) ) ;
#75646=CARTESIAN_POINT ( 'NONE',  ( -1.201851678989727383E-14, 5.259375000341421469, -1.575800808251660134 ) ) ;
#75652=CARTESIAN_POINT ( 'NONE',  ( -0.6823417656249969321, 3.967708333674754950, -1.181850606188749264 ) ) ;
#75654=CARTESIAN_POINT ( 'NONE',  ( -7.049876689426121779, 7.327203680526343632, -0.7216878364870278340 ) ) ;
#75656=CARTESIAN_POINT ( 'NONE',  ( 1.500000000000013545, 5.035416667349488229, 0.8660254037844385966 ) ) ;
#75663=CARTESIAN_POINT ( 'NONE',  ( 8.589254009457354400, 9.979550084910457031, -1.199719254218446718 ) ) ;
#75669=CARTESIAN_POINT ( 'NONE',  ( -8.941766003412679353, 10.39081407785832845, -1.199719254218446718 ) ) ;
#75671=CARTESIAN_POINT ( 'NONE',  ( 6.494519276145969577, 7.535692896047149425, -1.199719254218446718 ) ) ;
#75673=FACE_OUTER_BOUND ( 'NONE', #99300, .T. ) ;
#75674=CARTESIAN_POINT ( 'NONE',  ( 3.337278367258157630, 7.045241861776501580, 0.7998128361456341429 ) ) ;
#75682=CARTESIAN_POINT ( 'NONE',  ( -4.690757960648240577, 6.495636925554817864, 1.443375672974064550 ) ) ;
#75683=CARTESIAN_POINT ( 'NONE',  ( 4.857899112398166075, 4.561970474086296079, 1.040834085586084257E-14 ) ) ;
#75686=CARTESIAN_POINT ( 'NONE',  ( -8.505042434474312074, 8.816971016508505343, -0.7998128361456291469 ) ) ;
#75691=CARTESIAN_POINT ( 'NONE',  ( -7.133561379084627063, 11.47423870890741782, 0.7998128361456481317 ) ) ;
#75693=CARTESIAN_POINT ( 'NONE',  ( 7.259501185113382604, 10.55683625168592243, -1.199719254218441611 ) ) ;
#75694=CARTESIAN_POINT ( 'NONE',  ( 5.392392409933256303, 7.314210449720692786, 1.599625672291267398 ) ) ;
#75706=CARTESIAN_POINT ( 'NONE',  ( -8.182509401047415309, 9.505014708432145909, 1.199719254218462483 ) ) ;
#75709=CARTESIAN_POINT ( 'NONE',  ( 6.697364695470787943, 7.876308901879812474, -1.082531754730543083 ) ) ;
#75715=CARTESIAN_POINT ( 'NONE',  ( -3.927058049452637700, 7.733318157670055371, -0.7998128361456281477 ) ) ;
#75718=CARTESIAN_POINT ( 'NONE',  ( 1.284279953904119864, 3.296639714193937198, -0.7749999999999910294 ) ) ;
#75723=CARTESIAN_POINT ( 'NONE',  ( -9.775592450653132204, 11.36361159963886891, -1.199719254218441611 ) ) ;
#75724=CARTESIAN_POINT ( 'NONE',  ( 8.599949509769960088, 8.927695937686774386, 1.040834085586084257E-14 ) ) ;
#75730=CARTESIAN_POINT ( 'NONE',  ( -5.472563271839127275, 6.275773694203630626, -1.010060153610029321 ) ) ;
#75735=ORIENTED_EDGE ( 'NONE', *, *, #101217, .F. ) ;
#75737=CARTESIAN_POINT ( 'NONE',  ( 2.184835310096557404, 5.700724961754617404, 1.040834085586084257E-14 ) ) ;
#75756=CARTESIAN_POINT ( 'NONE',  ( -5.773074481320628948, 5.629675071162500544, 0.000000000000000000 ) ) ;
#75758=CARTESIAN_POINT ( 'NONE',  ( 4.460269348771534581, 8.147471973634706544, -0.7216878364870207285 ) ) ;
#75759=CARTESIAN_POINT ( 'NONE',  ( 1.499999999999987121, 4.045833333333359150, -0.8660254037844323793 ) ) ;
#75761=CARTESIAN_POINT ( 'NONE',  ( -3.541704441667874903, 5.155074486744371853, -1.599625672291256295 ) ) ;
#75766=CARTESIAN_POINT ( 'NONE',  ( -1.364683531250010295, 5.238541667008086655, -0.7879004041258300672 ) ) ;
#75769=CARTESIAN_POINT ( 'NONE',  ( -3.226477370372317743, 4.787309570232886280, 1.443375672974064550 ) ) ;
#75771=ORIENTED_EDGE ( 'NONE', *, *, #54015, .F. ) ;
#75774=CARTESIAN_POINT ( 'NONE',  ( 4.680589345215795838, 6.483773540883647435, -1.599625672291256295 ) ) ;
#75779=CARTESIAN_POINT ( 'NONE',  ( 8.690413276235306128, 13.08263988900915109, -0.7216878364870267237 ) ) ;
#75781=CARTESIAN_POINT ( 'NONE',  ( 1.364683531249986537, 1.467708333674748289, -0.7879004041258239610 ) ) ;
#75784=CARTESIAN_POINT ( 'NONE',  ( -8.507905087775398556, 9.884643009614800135, 1.199719254218462483 ) ) ;
#75785=CARTESIAN_POINT ( 'NONE',  ( -5.138177029454855216, 7.017625839162543677, 1.443375672974064550 ) ) ;
#75789=CARTESIAN_POINT ( 'NONE',  ( 1.499999999999987121, -0.7145833326505161009, 0.8660254037844524744 ) ) ;
#75797=CARTESIAN_POINT ( 'NONE',  ( -4.975479186090865369, 6.827811688571220117, 1.443375672974064550 ) ) ;
#75801=CARTESIAN_POINT ( 'NONE',  ( -4.067082893975237035, 7.688754443039000464, 1.040834085586084257E-14 ) ) ;
#75803=CARTESIAN_POINT ( 'NONE',  ( 9.585778300061798873, 11.14216175728232550, -1.199719254218440723 ) ) ;
#75808=EDGE_LOOP ( 'NONE', ( #8156, #120746 ) ) ;
#75812=CARTESIAN_POINT ( 'NONE',  ( -5.413783410558481002, 5.210502155273325720, -0.7998128361456221525 ) ) ;
#75815=CARTESIAN_POINT ( 'NONE',  ( -1.500000000000001332, 0.6500000000000255573, 0.000000000000000000 ) ) ;
#75818=CARTESIAN_POINT ( 'NONE',  ( 7.619319141200051604, 11.83303006480134911, 0.7216878364870438212 ) ) ;
#75819=CARTESIAN_POINT ( 'NONE',  ( 4.645640190976921602, 8.571663989448405019, 1.040834085586084257E-14 ) ) ;
#75823=CARTESIAN_POINT ( 'NONE',  ( 2.855963913973019963, 6.483708332943829866, 0.000000000000000000 ) ) ;
#75834=CARTESIAN_POINT ( 'NONE',  ( -6.063521013809733518, 8.097193820909906137, 1.599625672291283607 ) ) ;
#75837=LINE ( 'NONE', #176540, #135719 ) ;
#75840=CARTESIAN_POINT ( 'NONE',  ( 0.6823417656249917140, 5.342708333674749177, 1.181850606188765695 ) ) ;
#75841=CARTESIAN_POINT ( 'NONE',  ( 9.544576953896278582, 10.23768732240824164, 0.000000000000000000 ) ) ;
#75842=CARTESIAN_POINT ( 'NONE',  ( -7.074657228232555717, 7.148188275893099686, 1.040834085586084257E-14 ) ) ;
#75845=CARTESIAN_POINT ( 'NONE',  ( 5.250031796989762967, 7.148123067953287446, 1.599625672291267398 ) ) ;
#75846=CARTESIAN_POINT ( 'NONE',  ( -5.599681137644054729, 6.491715067794862293, 1.199719254218450271 ) ) ;
#75852=CARTESIAN_POINT ( 'NONE',  ( 5.992340707560147806, 8.974519344586754599, 1.082531754730558626 ) ) ;
#75854=CARTESIAN_POINT ( 'NONE',  ( 1.364683531249986537, 1.467708333674748289, -0.7879004041258239610 ) ) ;
#75855=CARTESIAN_POINT ( 'NONE',  ( -0.006800380015319074101, 7.009756401597622144, 1.999988438674507485 ) ) ;
#75856=CARTESIAN_POINT ( 'NONE',  ( 5.951666246274797345, 7.966696592119163256, 1.443375672974062551 ) ) ;
#75858=CARTESIAN_POINT ( 'NONE',  ( -2.657034918598345730, 5.083329257464595408, -1.082531754730543971 ) ) ;
#75860=B_SPLINE_CURVE_WITH_KNOTS ( 'NONE', 3,
 ( #112343, #196719, #180472, #144818, #32087, #165278 ),
 .UNSPECIFIED., .F., .F.,
 ( 4, 2, 4 ),
 ( 0.8940582275390620559, 0.9471490438394758460, 1.000239860139889636 ),
 .UNSPECIFIED. ) ;
#75865=DIRECTION ( 'NONE',  ( -0.6507913734559640506, -0.7592566023653004592, 0.000000000000000000 ) ) ;
#75867=CARTESIAN_POINT ( 'NONE',  ( -3.976511113072466408, 7.848157239995420476, -0.08586869108932922157 ) ) ;
#75874=CARTESIAN_POINT ( 'NONE',  ( 6.505214776458575265, 6.483838748823460563, 1.040834085586084257E-14 ) ) ;
#75885=CARTESIAN_POINT ( 'NONE',  ( 3.050221373394638835, 6.502416002361635528, 0.000000000000000000 ) ) ;
#75886=CARTESIAN_POINT ( 'NONE',  ( -1.364683531250000748, 2.071875000341422357, 1.214306433183764966E-14 ) ) ;
#75888=CARTESIAN_POINT ( 'NONE',  ( 6.265839547809997079, 10.46189657242035587, 0.7998128361456462443 ) ) ;
#75890=CARTESIAN_POINT ( 'NONE',  ( -8.306341666666730461, 12.84248237775322643, 1.040834085586084257E-14 ) ) ;
#75894=EDGE_CURVE ( 'NONE', #5554, #180844, #119501, .T. ) ;
#75897=CARTESIAN_POINT ( 'NONE',  ( -0.7500000000000006661, 2.608333333333358262, -1.299038105676652011 ) ) ;
#75898=CARTESIAN_POINT ( 'NONE',  ( 4.852928918687680948, 7.749168607522574526, 1.199719254218462483 ) ) ;
#75899=CARTESIAN_POINT ( 'NONE',  ( -6.877010230629689858, 9.046264573866535486, 1.599625672291283607 ) ) ;
#75903=CARTESIAN_POINT ( 'NONE',  ( -1.364683531250000748, 2.259375000341422357, 1.214306433183764966E-14 ) ) ;
#75905=CARTESIAN_POINT ( 'NONE',  ( 9.029367117021314115, 12.51771682229149008, -1.082531754730543083 ) ) ;
#75911=CARTESIAN_POINT ( 'NONE',  ( -1.402160292154681736E-14, 0.8687500006828192678, -1.732050807568863648 ) ) ;
#75914=CARTESIAN_POINT ( 'NONE',  ( -5.422371370461663176, 8.413518134592214537, -1.199719254218446718 ) ) ;
#75915=CARTESIAN_POINT ( 'NONE',  ( -2.467220768007014176, 5.822248629409386922, 0.7216878364870317197 ) ) ;
#75923=CARTESIAN_POINT ( 'NONE',  ( 4.937140493670735708, 8.911747675924535983, -0.7998128361456281477 ) ) ;
#75927=CARTESIAN_POINT ( 'NONE',  ( 6.328958779480917229, 6.278206752349526631, 0.7998128361456341429 ) ) ;
#75930=ORIENTED_EDGE ( 'NONE', *, *, #63612, .F. ) ;
#75933=CARTESIAN_POINT ( 'NONE',  ( 2.866659414285625651, 5.431854185720147221, -1.199719254218446718 ) ) ;
#75936=CARTESIAN_POINT ( 'NONE',  ( 6.520158902582616101, 5.290451655907108197, 2.438235897557466281 ) ) ;
#75938=CARTESIAN_POINT ( 'NONE',  ( 5.766360146646302809, 6.053989883630594981, 0.5864573027323967125 ) ) ;
#75949=CARTESIAN_POINT ( 'NONE',  ( 7.727784370109387346, 10.99920361756089093, -1.082531754730543083 ) ) ;
#75951=CARTESIAN_POINT ( 'NONE',  ( -3.893162665418476109, 7.693773542963529444, 1.040834085586084257E-14 ) ) ;
#75954=CARTESIAN_POINT ( 'NONE',  ( 8.121497709785879593, 9.433834401960398353, -1.199719254218445830 ) ) ;
#75956=CARTESIAN_POINT ( 'NONE',  ( -6.728924311084075960, 6.744833205886536120, 1.040834085586084257E-14 ) ) ;
#75961=ORIENTED_EDGE ( 'NONE', *, *, #147857, .T. ) ;
#75970=CARTESIAN_POINT ( 'NONE',  ( 10.07387183015377197, 11.71160420905630062, -1.199719254218440723 ) ) ;
#75971=CARTESIAN_POINT ( 'NONE',  ( -4.497554271431319250, 6.270232621468402989, -1.599625672291256295 ) ) ;
#75974=CARTESIAN_POINT ( 'NONE',  ( 3.050221373394638835, 6.502416002361635528, 0.000000000000000000 ) ) ;
#75979=CARTESIAN_POINT ( 'NONE',  ( -4.440459003675619520, 5.139289244831666714, 1.199719254218462483 ) ) ;
#75982=CARTESIAN_POINT ( 'NONE',  ( 9.426996880203592610, 9.892584536526015881, -0.7998128361456281477 ) ) ;
#75986=CARTESIAN_POINT ( 'NONE',  ( -6.191269702934848240, 10.37489842006599616, 0.000000000000000000 ) ) ;
#75987=CARTESIAN_POINT ( 'NONE',  ( 4.985647801523278133, 6.839675073242382553, -1.599625672291256295 ) ) ;
#75990=LINE ( 'NONE', #91195, #80537 ) ;
#75993=CARTESIAN_POINT ( 'NONE',  ( 1.364683531249986537, 2.467708333674753174, -0.7879004041258239610 ) ) ;
#75996=CARTESIAN_POINT ( 'NONE',  ( 5.504247177468168495, 9.365446107114122398, 0.7216878364870438212 ) ) ;
#76004=CARTESIAN_POINT ( 'NONE',  ( 8.066738210006668908, 12.35501897840907581, 0.7216878364870438212 ) ) ;
#76005=EDGE_CURVE ( 'NONE', #177940, #33705, #108929, .T. ) ;
#76010=CARTESIAN_POINT ( 'NONE',  ( -9.341731535015849630, 10.85744053139533349, 1.199719254218462483 ) ) ;
#76011=CYLINDRICAL_SURFACE ( 'NONE', #71031, 1.500000000000000222 ) ;
#76027=CARTESIAN_POINT ( 'NONE',  ( 1.499999999999989120, 1.806250000682817269, 0.000000000000000000 ) ) ;
#76033=CARTESIAN_POINT ( 'NONE',  ( 1.499999999999985123, 0.04583333333335545129, -0.8660254037844323793 ) ) ;
#76034=CARTESIAN_POINT ( 'NONE',  ( 7.781490099239519509, 11.16582331816642260, 1.199719254218460707 ) ) ;
#76036=CARTESIAN_POINT ( 'NONE',  ( 0.6823417656249882723, 0.09270833367475139752, 1.181850606188755259 ) ) ;
#76039=CARTESIAN_POINT ( 'NONE',  ( 4.369805582306193870, 3.992528022312320957, 1.214306433183764966E-14 ) ) ;
#76040=CARTESIAN_POINT ( 'NONE',  ( -6.724481002698138532, 6.947575379343695623, -0.7216878364870278340 ) ) ;
#76045=CARTESIAN_POINT ( 'NONE',  ( -6.205881626753225966, 8.263281202677319470, 1.599625672291283607 ) ) ;
#76046=ORIENTED_EDGE ( 'NONE', *, *, #211660, .T. ) ;
#76047=CARTESIAN_POINT ( 'NONE',  ( -0.7500000000000006661, 2.139583334016155636, -1.299038105676652011 ) ) ;
#76055=DIRECTION ( 'NONE',  ( 0.6507913734559640506, -0.7592566023653004592, 0.000000000000000000 ) ) ;
#76061=CARTESIAN_POINT ( 'NONE',  ( -9.989660255170729641, 10.54902514065433827, -0.7998128361456291469 ) ) ;
#76062=CARTESIAN_POINT ( 'NONE',  ( 7.793239369756836510, 7.986534107671458216, 0.7998128361456341429 ) ) ;
#76069=CARTESIAN_POINT ( 'NONE',  ( -6.672584156219988571, 10.93643194889866521, -0.7998128361456291469 ) ) ;
#76071=B_SPLINE_CURVE_WITH_KNOTS ( 'NONE', 3,
 ( #148653, #116207, #182193, #209620 ),
 .UNSPECIFIED., .F., .F.,
 ( 4, 4 ),
 ( 1.226634733346700890E-18, 0.002003498272494348524 ),
 .UNSPECIFIED. ) ;
#76072=CARTESIAN_POINT ( 'NONE',  ( -1.000000000000014433, 6.468705557303653819, 4.925226524755080604 ) ) ;
#76075=CARTESIAN_POINT ( 'NONE',  ( 3.541704441667858472, 5.155074486744371853, -1.599625672291262513 ) ) ;
#76077=VERTEX_POINT ( 'NONE', #76354 ) ;
#76079=CARTESIAN_POINT ( 'NONE',  ( -7.309817376062285099, 11.67987070538135264, 0.000000000000000000 ) ) ;
#76082=CARTESIAN_POINT ( 'NONE',  ( -5.094707486240121597, 6.719114383638050469, -1.440239009331502062 ) ) ;
#76089=CARTESIAN_POINT ( 'NONE',  ( 6.551614543901692400, 8.666636272683888365, 1.599625672291281386 ) ) ;
#76095=B_SPLINE_CURVE_WITH_KNOTS ( 'NONE', 3,
 ( #112919, #162679, #194088, #111856, #193014 ),
 .UNSPECIFIED., .F., .F.,
 ( 4, 1, 4 ),
 ( 0.003112877374997422876, 0.003157543106160180107, 0.003202208837322937773 ),
 .UNSPECIFIED. ) ;
#76106=DIRECTION ( 'NONE',  ( 0.000000000000000000, 8.546850786086437571E-32, 1.000000000000000000 ) ) ;
#76108=CARTESIAN_POINT ( 'NONE',  ( 2.412988153552339643, 5.758977245878946327, 0.7216878364870438212 ) ) ;
#76113=CARTESIAN_POINT ( 'NONE',  ( -8.784793466650835825, 12.33634391347959713, 1.199719254218462483 ) ) ;
#76116=CARTESIAN_POINT ( 'NONE',  ( 8.401248741962376698, 12.95320729893149370, 0.7998128361456462443 ) ) ;
#76121=CARTESIAN_POINT ( 'NONE',  ( 5.756345505848640798, 6.148709499980903992, 0.8262799378709930753 ) ) ;
#76125=CARTESIAN_POINT ( 'NONE',  ( 3.511198596259283544, 6.271927390929319834, 1.164732466530402855 ) ) ;
#76126=CARTESIAN_POINT ( 'NONE',  ( -1.364683531250014514, 0.03020833367475737191, 0.7879004041258379498 ) ) ;
#76132=CARTESIAN_POINT ( 'NONE',  ( -3.632695093457760649, 6.325562478087638496, -1.199719254218452047 ) ) ;
#76135=CARTESIAN_POINT ( 'NONE',  ( -1.500000000000001332, 0.4000000000000253353, 0.000000000000000000 ) ) ;
#76137=CARTESIAN_POINT ( 'NONE',  ( -1.402160292154681736E-14, -0.6156249996585817508, 1.575800808251672791 ) ) ;
#76142=CARTESIAN_POINT ( 'NONE',  ( -0.6823417656250003738, -0.5322916663252491576, -1.181850606188749264 ) ) ;
#76144=CARTESIAN_POINT ( 'NONE',  ( -8.227100285394159940, 8.492705175914988303, 0.7998128361456602331 ) ) ;
#76145=CARTESIAN_POINT ( 'NONE',  ( 7.727257484784855635, 11.10255193463598111, -1.199719254218446718 ) ) ;
#76151=CARTESIAN_POINT ( 'NONE',  ( -1.364683531250012516, 0.5927083336747520637, 0.7879004041258379498 ) ) ;
#76158=CARTESIAN_POINT ( 'NONE',  ( 5.178851490740187913, 8.985817805931475277, 0.7216878364870438212 ) ) ;
#76161=CARTESIAN_POINT ( 'NONE',  ( -5.766295404513795297, 5.621766148221195358, 0.7998128361456341429 ) ) ;
#76163=CARTESIAN_POINT ( 'NONE',  ( -1.001543065824772872E-14, 5.493750000682816825, 1.732050807568877637 ) ) ;
#76165=CARTESIAN_POINT ( 'NONE',  ( -2.117044542028253318, 5.621635732341564662, -0.7998128361456281477 ) ) ;
#76166=CARTESIAN_POINT ( 'NONE',  ( 6.168596704093459060, 7.259412911939593371, -1.082531754730543083 ) ) ;
#76167=CARTESIAN_POINT ( 'NONE',  ( -8.297226821439000588, 12.62392235841345389, 1.040834085586084257E-14 ) ) ;
#76172=CARTESIAN_POINT ( 'NONE',  ( 9.734391104931951588, 11.41950637958454706, 1.082531754730548412 ) ) ;
#76186=CARTESIAN_POINT ( 'NONE',  ( 7.402388682937041331, 11.57994453016116587, 1.040834085586084257E-14 ) ) ;
#76189=CARTESIAN_POINT ( 'NONE',  ( 8.911787042884274257, 9.291506392986812912, 0.7998128361456462443 ) ) ;
#76191=CARTESIAN_POINT ( 'NONE',  ( -4.079286826253504472, 3.980871698815676041, -0.5338862410131425262 ) ) ;
#76193=CARTESIAN_POINT ( 'NONE',  ( 5.517805331081858888, 5.539787095791365523, 1.040834085586084257E-14 ) ) ;
#76195=CARTESIAN_POINT ( 'NONE',  ( -9.219181267612684749, 10.81842823604534765, 1.082531754730558626 ) ) ;
#76207=ORIENTED_EDGE ( 'NONE', *, *, #124997, .F. ) ;
#76223=CARTESIAN_POINT ( 'NONE',  ( -7.237355071596549116, 7.338002426484427687, 1.040834085586084257E-14 ) ) ;
#76227=CARTESIAN_POINT ( 'NONE',  ( 7.122110765880372618, 7.203550736482235095, 0.7998128361456341429 ) ) ;
#76232=CIRCLE ( 'NONE', #155723, 0.7500000000000011102 ) ;
#76233=CARTESIAN_POINT ( 'NONE',  ( 3.686212053427321056, 6.121915856213854923, 1.284222742053100941 ) ) ;
#76235=CARTESIAN_POINT ( 'NONE',  ( -5.610376637956639101, 5.439860920571172542, 0.000000000000000000 ) ) ;
#76239=CARTESIAN_POINT ( 'NONE',  ( -5.416646063859567484, 6.278174148379618735, 1.199719254218450271 ) ) ;
#76242=CARTESIAN_POINT ( 'NONE',  ( 8.938903350111612411, 9.323142084752035430, -0.7998128361456221525 ) ) ;
#76245=CARTESIAN_POINT ( 'NONE',  ( 6.115260013507548109, 6.015528159276049891, -0.005231617032384894284 ) ) ;
#76246=CARTESIAN_POINT ( 'NONE',  ( 4.419594888374914099, 5.218910793601261311, -1.082531754730548412 ) ) ;
#76252=CARTESIAN_POINT ( 'NONE',  ( 6.521108698048765362, 8.631046119188804155, -1.443375672974058777 ) ) ;
#76254=CARTESIAN_POINT ( 'NONE',  ( -7.635213062790267458, 12.05949900656400686, 0.000000000000000000 ) ) ;
#76257=CARTESIAN_POINT ( 'NONE',  ( -9.643927338022246332, 10.14567007064778004, -0.7998128361456291469 ) ) ;
#76258=CARTESIAN_POINT ( 'NONE',  ( -5.768104287610143821, 8.816873204598778102, -1.199719254218440723 ) ) ;
#76265=CARTESIAN_POINT ( 'NONE',  ( 8.599949509769960088, 8.927695937686774386, 1.040834085586084257E-14 ) ) ;
#76274=CARTESIAN_POINT ( 'NONE',  ( -0.7499999999999972244, 5.639583334016151639, -1.299038105676652899 ) ) ;
#76279=CARTESIAN_POINT ( 'NONE',  ( -0.7499999999999972244, 4.608333333333352932, -1.299038105676652011 ) ) ;
#76280=CARTESIAN_POINT ( 'NONE',  ( 4.527533231959700366, 7.369540306339926516, 1.199719254218462483 ) ) ;
#76281=CARTESIAN_POINT ( 'NONE',  ( 5.459129407796876166, 9.520734742405036144, 1.040834085586084257E-14 ) ) ;
#76284=CARTESIAN_POINT ( 'NONE',  ( 5.992340707560147806, 8.974519344586754599, 1.082531754730558626 ) ) ;
#76285=CARTESIAN_POINT ( 'NONE',  ( -8.297226821439000588, 12.62392235841345389, 1.040834085586084257E-14 ) ) ;
#76288=CARTESIAN_POINT ( 'NONE',  ( 9.901532256681887745, 10.44620914241737530, 0.000000000000000000 ) ) ;
#76291=CARTESIAN_POINT ( 'NONE',  ( -2.981903720001798597, 5.566305875722335372, -1.199719254218446718 ) ) ;
#76292=CARTESIAN_POINT ( 'NONE',  ( -2.312195109851927999, 5.463442068584685174, -0.7954731236790282267 ) ) ;
#76293=EDGE_CURVE ( 'NONE', #195170, #206877, #199759, .T. ) ;
#76294=CARTESIAN_POINT ( 'NONE',  ( -1.201851678989727383E-14, 1.321875000341419248, 1.575800808251672791 ) ) ;
#76299=CARTESIAN_POINT ( 'NONE',  ( -1.402160292154681736E-14, -0.8031249996585825279, -1.575800808251665908 ) ) ;
#76301=EDGE_CURVE ( 'NONE', #28244, #123589, #173519, .T. ) ;
#76302=CARTESIAN_POINT ( 'NONE',  ( 8.615316546479974136, 12.13862083994696839, 1.199719254218450271 ) ) ;
#76306=CARTESIAN_POINT ( 'NONE',  ( -2.602802303699316866, 5.980427087717073320, 1.040834085586084257E-14 ) ) ;
#76311=CARTESIAN_POINT ( 'NONE',  ( 3.842846474469570062, 6.570739089268092137, -1.199719254218452047 ) ) ;
#76319=CARTESIAN_POINT ( 'NONE',  ( 7.425061681778431399, 11.81432239538354345, 0.7998128361456462443 ) ) ;
#76322=CARTESIAN_POINT ( 'NONE',  ( -4.367698041896780126, 8.247398148854895084, 0.7998128361456481317 ) ) ;
#76326=CARTESIAN_POINT ( 'NONE',  ( 8.613507663383630941, 8.943513783569379427, -0.7998128361456221525 ) ) ;
#76328=CARTESIAN_POINT ( 'NONE',  ( 5.926885707468349196, 10.06645042535509660, 1.040834085586084257E-14 ) ) ;
#76331=CARTESIAN_POINT ( 'NONE',  ( -10.46653140006992899, 11.31330084294416771, -0.7216878364870267237 ) ) ;
#76338=CARTESIAN_POINT ( 'NONE',  ( -5.968994907891031154, 6.102274133640173126, 0.7348006213908353512 ) ) ;
#76339=CARTESIAN_POINT ( 'NONE',  ( -1.364683531250000748, 1.509375000341421691, 0.000000000000000000 ) ) ;
#76341=CARTESIAN_POINT ( 'NONE',  ( 5.992340707560151358, 8.014150130285418783, 1.443375672974062551 ) ) ;
#76354=CARTESIAN_POINT ( 'NONE',  ( -4.217958839219735800, 3.978389137448586244, 0.5316758947214468289 ) ) ;
#76358=CARTESIAN_POINT ( 'NONE',  ( 9.043452155515161905, 10.50944792197790889, 1.199719254218453823 ) ) ;
#76362=CARTESIAN_POINT ( 'NONE',  ( -2.435661151949389147, 5.993355110582911038, 0.7998128361456341429 ) ) ;
#76363=CARTESIAN_POINT ( 'NONE',  ( -7.379715684540041565, 7.504089808251839244, 1.040834085586084257E-14 ) ) ;
#76365=EDGE_LOOP ( 'NONE', ( #184802, #203798, #139967, #22478 ) ) ;
#76368=CARTESIAN_POINT ( 'NONE',  ( -0.7499999999999972244, 4.639583334016150751, -1.299038105676652899 ) ) ;
#76369=CARTESIAN_POINT ( 'NONE',  ( 6.588372581236919601, 9.773852880496709972, -1.199719254218440723 ) ) ;
#76372=CARTESIAN_POINT ( 'NONE',  ( -6.353967546298838087, 10.56471257065732416, 0.000000000000000000 ) ) ;
#76374=CARTESIAN_POINT ( 'NONE',  ( -0.6823417656249969321, 5.217708333674756283, -1.181850606188749264 ) ) ;
#76380=CARTESIAN_POINT ( 'NONE',  ( -8.432808358020034589, 10.86136238915529084, 1.443375672974064550 ) ) ;
#76384=CARTESIAN_POINT ( 'NONE',  ( 1.364683531249988535, 2.967708333674755394, -0.7879004041258239610 ) ) ;
#76392=CARTESIAN_POINT ( 'NONE',  ( -0.6823417656249969321, 3.717708333674754506, -1.181850606188749264 ) ) ;
#76393=CARTESIAN_POINT ( 'NONE',  ( -4.623494077460110319, 5.352830164246910272, 1.199719254218462483 ) ) ;
#76394=CARTESIAN_POINT ( 'NONE',  ( 5.289652487626049115, 9.323011668872403845, 0.7998128361456462443 ) ) ;
#76397=CARTESIAN_POINT ( 'NONE',  ( -0.6823417656249969321, 3.780208333674754506, -1.181850606188749264 ) ) ;
#76400=CARTESIAN_POINT ( 'NONE',  ( 0.6823417656249882723, -0.4072916663252490466, 1.181850606188755259 ) ) ;
#76401=CARTESIAN_POINT ( 'NONE',  ( -3.619663825168619731, 7.166765529431275539, 1.040834085586084257E-14 ) ) ;
#76404=CARTESIAN_POINT ( 'NONE',  ( 4.419594888374914099, 5.218910793601261311, -1.082531754730548412 ) ) ;
#76407=CARTESIAN_POINT ( 'NONE',  ( -9.829298180227631576, 10.56986208646148384, 1.040834085586084257E-14 ) ) ;
#76412=CARTESIAN_POINT ( 'NONE',  ( -7.185458225118419584, 7.485382138834033583, 1.040834085586084257E-14 ) ) ;
#76414=CARTESIAN_POINT ( 'NONE',  ( 1.364683531249988757, 0.6968750003414209138, 0.000000000000000000 ) ) ;
#76421=CARTESIAN_POINT ( 'NONE',  ( -1.364683531250000748, -0.4281249996585800854, 0.000000000000000000 ) ) ;
#76423=( BOUNDED_CURVE ( )  B_SPLINE_CURVE ( 2, ( #115443, #196634, #180382, #164141, #117569 ),
 .UNSPECIFIED., .F., .T. ) 
 B_SPLINE_CURVE_WITH_KNOTS ( ( 3, 2, 3 ),
 ( 0.1347995350948868465, 0.1375000000000000111, 0.1409922313975708053 ),
 .UNSPECIFIED. ) 
 CURVE ( )  GEOMETRIC_REPRESENTATION_ITEM ( )  RATIONAL_B_SPLINE_CURVE ( ( 0.9388907138593196589, 0.9131695131383610331, 1.000000000000000000, 0.8877111300685950335, 0.9636488443798445491 ) ) 
 REPRESENTATION_ITEM ( '' )  );
#76431=CARTESIAN_POINT ( 'NONE',  ( -1.500000000000015099, -0.6208333333333116988, -0.8660254037844383745 ) ) ;
#76433=CARTESIAN_POINT ( 'NONE',  ( 7.253248993186720561, 10.44557901115111065, 1.082531754730558626 ) ) ;
#76445=CARTESIAN_POINT ( 'NONE',  ( 1.203907071533382167, 3.212770253743141069, 0.7750000000000135669 ) ) ;
#76447=CARTESIAN_POINT ( 'NONE',  ( 1.364683531249986537, 1.467708333674748289, -0.7879004041258239610 ) ) ;
#76448=DIRECTION ( 'NONE',  ( 0.3502638921866460531, -1.953969548649011959E-16, -0.9366510587354619499 ) ) ;
#76459=CARTESIAN_POINT ( 'NONE',  ( 6.471393748265519719, 5.229711127717882491, -2.419999999999995044 ) ) ;
#76465=CARTESIAN_POINT ( 'NONE',  ( 4.821896187954575197, 8.777295985922343391, 0.7998128361456462443 ) ) ;
#76468=EDGE_LOOP ( 'NONE', ( #113353, #41324, #42649, #75446, #119610, #132447, #22780, #148828, #29508, #5320 ) ) ;
#76474=CARTESIAN_POINT ( 'NONE',  ( 9.043452155515161905, 10.50944792197790889, 1.199719254218453823 ) ) ;
#76476=CARTESIAN_POINT ( 'NONE',  ( 1.534377212605017915, 8.695787254938599276, -2.514108538948821359 ) ) ;
#76482=CARTESIAN_POINT ( 'NONE',  ( -0.4086240214900874745, 7.376738131363727469, 1.961326491624037160 ) ) ;
#76486=CARTESIAN_POINT ( 'NONE',  ( -9.503902493499651882, 10.19023378527882784, 1.040834085586084257E-14 ) ) ;
#76491=CARTESIAN_POINT ( 'NONE',  ( -4.905110356762790502, 4.827649200395154772, -0.06592220986076716138 ) ) ;
#76492=CARTESIAN_POINT ( 'NONE',  ( 4.527533231959700366, 7.369540306339926516, 1.199719254218462483 ) ) ;
#76498=CARTESIAN_POINT ( 'NONE',  ( 2.507895228403643539, 5.869702166538802501, -0.7216878364870267237 ) ) ;
#76499=EDGE_CURVE ( 'NONE', #153088, #68875, #42352, .T. ) ;
#76507=CARTESIAN_POINT ( 'NONE',  ( -5.311043488251275591, 7.219303374425030562, -1.599625672291256295 ) ) ;
#76509=CARTESIAN_POINT ( 'NONE',  ( -4.081167932913447594, 4.720116328942494555, -1.199719254218452047 ) ) ;
#76515=CARTESIAN_POINT ( 'NONE',  ( -1.164422670175135899, 3.300000000000025135, -0.7116747751938151678 ) ) ;
#76518=CARTESIAN_POINT ( 'NONE',  ( 5.229694566569264680, 7.124396299129368337, 1.599625672291267398 ) ) ;
#76520=CARTESIAN_POINT ( 'NONE',  ( 3.660338285565247762, 7.214219066560688454, 1.040834085586084257E-14 ) ) ;
#76532=CARTESIAN_POINT ( 'NONE',  ( -0.6823417656250003738, 1.780208333674752952, -1.181850606188749264 ) ) ;
#76534=CARTESIAN_POINT ( 'NONE',  ( 4.891794496432329886, 4.601515088792824670, -0.7998128361456211532 ) ) ;
#76537=CARTESIAN_POINT ( 'NONE',  ( -6.412643469583822586, 6.583764924043652655, 1.040834085586084257E-14 ) ) ;
#76538=CARTESIAN_POINT ( 'NONE',  ( 2.738383840280320669, 6.138605547061593448, 0.7216878364870338292 ) ) ;
#76539=CARTESIAN_POINT ( 'NONE',  ( -7.009202228140764213, 7.279750142360097875, -0.7216878364870267237 ) ) ;
#76543=CARTESIAN_POINT ( 'NONE',  ( 4.774442650306744085, 8.721933525333202653, -0.7998128361456281477 ) ) ;
#76549=CARTESIAN_POINT ( 'NONE',  ( 0.6823417656249899377, 4.926041667008086655, -1.181850606188754593 ) ) ;
#76553=EDGE_CURVE ( 'NONE', #56362, #170226, #126486, .T. ) ;
#76554=CARTESIAN_POINT ( 'NONE',  ( 7.308008492965924141, 8.484763649003774333, -1.199719254218451159 ) ) ;
#76556=CARTESIAN_POINT ( 'NONE',  ( -6.093499974338126179, 9.196501505781426999, -1.199719254218440723 ) ) ;
#76561=CARTESIAN_POINT ( 'NONE',  ( 6.740374924288304648, 11.01552117831172062, 1.040834085586084257E-14 ) ) ;
#76564=CARTESIAN_POINT ( 'NONE',  ( -7.901704598666176693, 8.113076874732334076, 0.7998128361456602331 ) ) ;
#76566=CARTESIAN_POINT ( 'NONE',  ( 6.873620692004076105, 10.00267932643801672, -1.082531754730537976 ) ) ;
#76567=CARTESIAN_POINT ( 'NONE',  ( 4.121712324234096059, 7.667736414601909800, 0.7403736254629582625 ) ) ;
#76568=CARTESIAN_POINT ( 'NONE',  ( -8.161645285746702783, 12.46574390010577105, 0.7216878364870478180 ) ) ;
#76573=CARTESIAN_POINT ( 'NONE',  ( 4.635998460869027227, 7.496083073400806818, -1.199719254218452047 ) ) ;
#76575=CARTESIAN_POINT ( 'NONE',  ( 8.052653171512838881, 11.48218023581863001, -1.199719254218446718 ) ) ;
#76576=CARTESIAN_POINT ( 'NONE',  ( -4.616994038156231106, 6.938643078242441753, 1.201688966319388374 ) ) ;
#76578=CARTESIAN_POINT ( 'NONE',  ( 1.364683531249986537, 1.155208333674754728, -0.7879004041258239610 ) ) ;
#76580=CARTESIAN_POINT ( 'NONE',  ( -6.561783159334145132, 6.757761228752363181, -0.7216878364870278340 ) ) ;
#76588=CARTESIAN_POINT ( 'NONE',  ( -4.217650912117239415, 7.357101779856191293, 0.8466403022913439047 ) ) ;
#76589=CARTESIAN_POINT ( 'NONE',  ( -1.364683531250014514, 0.05104166700808546175, -0.7879004041258359514 ) ) ;
#76592=CARTESIAN_POINT ( 'NONE',  ( 4.094199201646931741, 4.839282492418613302, -1.082531754730543083 ) ) ;
#76596=CARTESIAN_POINT ( 'NONE',  ( -7.659993601596713830, 9.959745173328078849, -1.443375672974058777 ) ) ;
#76602=CARTESIAN_POINT ( 'NONE',  ( -8.798878505144658746, 10.32807501316600884, -1.082531754730543083 ) ) ;
#76607=ORIENTED_EDGE ( 'NONE', *, *, #72791, .T. ) ;
#76608=CARTESIAN_POINT ( 'NONE',  ( -9.314088342463968218, 9.968783942403868892, 0.7216878364870438212 ) ) ;
#76613=CARTESIAN_POINT ( 'NONE',  ( 0.6823417656249917140, 5.655208333674749177, 1.181850606188765695 ) ) ;
#76614=CARTESIAN_POINT ( 'NONE',  ( -1.500000000000013101, 3.910416667349482012, -0.8660254037844313801 ) ) ;
#76615=CARTESIAN_POINT ( 'NONE',  ( 5.285422529909848066, 6.578444217690160301, -1.363614577128515082 ) ) ;
#76616=CARTESIAN_POINT ( 'NONE',  ( -1.499999999999997780, 7.240846818246208905, -4.154462424328208670 ) ) ;
#76621=CARTESIAN_POINT ( 'NONE',  ( -7.705111371268023923, 7.883718109434487253, 1.040834085586084257E-14 ) ) ;
#76625=CARTESIAN_POINT ( 'NONE',  ( 3.486418057008484617, 7.219238166485217434, 1.040834085586084257E-14 ) ) ;
#76630=CARTESIAN_POINT ( 'NONE',  ( 7.283754839039659146, 9.520799950344851936, -1.599625672291262513 ) ) ;
#76634=ORIENTED_EDGE ( 'NONE', *, *, #170328, .T. ) ;
#76638=CARTESIAN_POINT ( 'NONE',  ( -6.724481002698138532, 6.947575379343695623, -0.7216878364870278340 ) ) ;
#76642=CARTESIAN_POINT ( 'NONE',  ( -0.1099460098627005888, 6.494484681433106310, 3.110387376256865011 ) ) ;
#76648=CARTESIAN_POINT ( 'NONE',  ( -9.667127221743832877, 11.23706883257798772, 1.199719254218462483 ) ) ;
#76650=CARTESIAN_POINT ( 'NONE',  ( 9.368847842243145152, 10.88907622316056312, 1.199719254218453823 ) ) ;
#76651=CARTESIAN_POINT ( 'NONE',  ( -1.500000000000015099, -0.6208333333333116988, -0.8660254037844383745 ) ) ;
#76652=CARTESIAN_POINT ( 'NONE',  ( -8.365544474831901667, 9.718555627847388578, 1.199719254218462483 ) ) ;
#76655=CARTESIAN_POINT ( 'NONE',  ( 1.364683531249990311, 3.134375000341423245, 1.214306433183764966E-14 ) ) ;
#76656=CARTESIAN_POINT ( 'NONE',  ( 3.225950485047770933, 5.851027101609320269, 1.199719254218450271 ) ) ;
#76660=CARTESIAN_POINT ( 'NONE',  ( 1.499999999999990896, 5.275000000000022560, 1.214306433183764966E-14 ) ) ;
#76663=CARTESIAN_POINT ( 'NONE',  ( 7.985389288324691748, 10.33937347451072775, -1.443375672974058777 ) ) ;
#76666=CARTESIAN_POINT ( 'NONE',  ( -7.700668062882084719, 8.086460282891644979, -0.7216878364870278340 ) ) ;
#76668=CARTESIAN_POINT ( 'NONE',  ( -1.201851678989727383E-14, 2.321875000341416584, 1.575800808251672791 ) ) ;
#76672=CARTESIAN_POINT ( 'NONE',  ( -7.555971681517696936, 7.709721804725773175, 0.7998128361456462443 ) ) ;
#76673=CARTESIAN_POINT ( 'NONE',  ( 1.364683531249988535, 4.426041667008082214, 0.7879004041258500513 ) ) ;
#76679=CARTESIAN_POINT ( 'NONE',  ( 9.206149998879153529, 10.69926207256923689, 1.199719254218453823 ) ) ;
#76682=CARTESIAN_POINT ( 'NONE',  ( 0.7499999999999885647, 0.9833333333333569293, 1.299038105676657340 ) ) ;
#76684=CARTESIAN_POINT ( 'NONE',  ( -0.2607081404539076663, 7.167562920730330411, -2.095805658632995616 ) ) ;
#76687=CARTESIAN_POINT ( 'NONE',  ( 7.913155211870404493, 12.38376484715752213, 0.7998128361456462443 ) ) ;
#76692=CARTESIAN_POINT ( 'NONE',  ( -1.499999999922353666, 8.635424801869593381, 2.574739023100876878 ) ) ;
#76695=CARTESIAN_POINT ( 'NONE',  ( -1.201851678989727383E-14, 5.759375000341417028, -1.575800808251660801 ) ) ;
#76701=CARTESIAN_POINT ( 'NONE',  ( -1.201851678989727383E-14, 4.446875000341417916, -1.575800808251660134 ) ) ;
#76703=CARTESIAN_POINT ( 'NONE',  ( -5.992340707560165569, 8.014150130285418783, 1.443375672974064550 ) ) ;
#76713=CARTESIAN_POINT ( 'NONE',  ( 7.781490099239519509, 11.16582331816642260, 1.199719254218460707 ) ) ;
#76719=CARTESIAN_POINT ( 'NONE',  ( -9.321394304595349567, 10.83371376257142416, 1.199719254218462483 ) ) ;
#76720=CARTESIAN_POINT ( 'NONE',  ( 5.309989718046547402, 9.346738437696316737, 0.7998128361456462443 ) ) ;
#76723=CARTESIAN_POINT ( 'NONE',  ( 3.592547517496925913, 5.214391408544949869, -1.443375672974058777 ) ) ;
#76724=CARTESIAN_POINT ( 'NONE',  ( 3.499976210622149253, 7.235056012367825140, 0.7998128361456321445 ) ) ;
#76725=ORIENTED_EDGE ( 'NONE', *, *, #205691, .F. ) ;
#76731=CARTESIAN_POINT ( 'NONE',  ( -6.127922243696855453, 7.211959374810172463, 1.082531754730549967 ) ) ;
#76732=CARTESIAN_POINT ( 'NONE',  ( 5.034155109375821446, 4.767602470560229122, -0.7998128361456221525 ) ) ;
#76735=CARTESIAN_POINT ( 'NONE',  ( -6.669721502918952716, 9.868759955792373972, 1.199719254218452047 ) ) ;
#76739=CARTESIAN_POINT ( 'NONE',  ( -8.941766003412679353, 10.39081407785832845, -1.199719254218446718 ) ) ;
#76743=CARTESIAN_POINT ( 'NONE',  ( 6.611572464958476836, 10.86525164242692298, 0.7998128361456462443 ) ) ;
#76745=CARTESIAN_POINT ( 'NONE',  ( 6.159481859310094620, 6.080483678816896109, 1.040834085586084257E-14 ) ) ;
#76746=FACE_OUTER_BOUND ( 'NONE', #211500, .T. ) ;
#76756=CARTESIAN_POINT ( 'NONE',  ( -8.505042434474312074, 8.816971016508505343, -0.7998128361456291469 ) ) ;
#76760=CARTESIAN_POINT ( 'NONE',  ( 7.293923454472091450, 7.611924906413328529, 0.7216878364870317197 ) ) ;
#76764=FACE_OUTER_BOUND ( 'NONE', #144971, .T. ) ;
#76766=CARTESIAN_POINT ( 'NONE',  ( -5.225778143063529946, 8.184159369294361497, 1.199719254218452047 ) ) ;
#76776=CARTESIAN_POINT ( 'NONE',  ( -10.47775378526269918, 11.11846759242831872, -0.7998128361456221525 ) ) ;
#76777=CARTESIAN_POINT ( 'NONE',  ( 7.401861798056875053, 10.72292363345333399, -1.199719254218441611 ) ) ;
#76782=CARTESIAN_POINT ( 'NONE',  ( -5.357982633755392854, 6.353232995037386033, -1.097174801447881487 ) ) ;
#76789=CARTESIAN_POINT ( 'NONE',  ( 4.857899112398166075, 4.561970474086296079, 1.040834085586084257E-14 ) ) ;
#76809=CARTESIAN_POINT ( 'NONE',  ( -3.750802052474980108, 7.527686161196117887, 1.040834085586084257E-14 ) ) ;
#76810=CARTESIAN_POINT ( 'NONE',  ( 6.141480396866128899, 6.267408005873028820, -0.7216878364870257245 ) ) ;
#76811=CARTESIAN_POINT ( 'NONE',  ( -1.201851678989727383E-14, 3.337500000000019007, -1.732050807568863648 ) ) ;
#76814=CARTESIAN_POINT ( 'NONE',  ( -3.100010679019018500, 6.768429558830820980, 1.040834085586084257E-14 ) ) ;
#76815=CARTESIAN_POINT ( 'NONE',  ( 0.07580519709491868874, 7.079373232789521353, -2.120991669649995526 ) ) ;
#76818=CARTESIAN_POINT ( 'NONE',  ( -1.364683531249997417, 4.759375000341424133, 1.214306433183764966E-14 ) ) ;
#76821=CARTESIAN_POINT ( 'NONE',  ( -4.284013352238274841, 4.100363120473813794, -0.7216878364870207285 ) ) ;
#76826=CARTESIAN_POINT ( 'NONE',  ( 3.734381245560244089, 6.444196322207211836, 1.199719254218462483 ) ) ;
#76832=CARTESIAN_POINT ( 'NONE',  ( 0.6823417656249899377, 1.405208333674752508, 1.181850606188755259 ) ) ;
#76836=CARTESIAN_POINT ( 'NONE',  ( -9.917953063596627317, 11.52969898140628047, -1.199719254218441611 ) ) ;
#76838=CARTESIAN_POINT ( 'NONE',  ( -5.056828107772852299, 7.883087978168217269, -1.082531754730548412 ) ) ;
#76842=CARTESIAN_POINT ( 'NONE',  ( -1.364683531250012516, 4.488541667008090208, -0.7879004041258300672 ) ) ;
#76850=CARTESIAN_POINT ( 'NONE',  ( -6.697364695026446491, 6.915939687060050467, 1.040834085586084257E-14 ) ) ;
#76855=CARTESIAN_POINT ( 'NONE',  ( -5.138177029454855216, 7.017625839162543677, 1.443375672974064550 ) ) ;
#76863=CARTESIAN_POINT ( 'NONE',  ( 1.482143263342159623, 8.748906972890436506, -2.523193690251291699 ) ) ;
#76867=CARTESIAN_POINT ( 'NONE',  ( -3.765413976293358278, 5.416068943807445635, 1.599625672291267398 ) ) ;
#76868=CARTESIAN_POINT ( 'NONE',  ( -5.102699428007002602, 6.712334911283204697, 1.441218774086165721 ) ) ;
#76870=CARTESIAN_POINT ( 'NONE',  ( 1.499999999999989120, 0.2750000000000182854, 0.000000000000000000 ) ) ;
#76873=CARTESIAN_POINT ( 'NONE',  ( 9.910647101909615841, 10.66476916175714607, 0.000000000000000000 ) ) ;
#76874=CARTESIAN_POINT ( 'NONE',  ( 8.281332899848809603, 8.555976559445431562, 0.7998128361456481317 ) ) ;
#76879=CARTESIAN_POINT ( 'NONE',  ( 4.487912541323413329, 5.194651705420806564, 1.199719254218462483 ) ) ;
#76882=ORIENTED_EDGE ( 'NONE', *, *, #20455, .F. ) ;
#76888=CARTESIAN_POINT ( 'NONE',  ( -5.038826645773246682, 9.030381520044109322, 0.7998128361456481317 ) ) ;
#76890=DIRECTION ( 'NONE',  ( -0.6507913734559640506, -0.7592566023653004592, 0.000000000000000000 ) ) ;
#76893=CARTESIAN_POINT ( 'NONE',  ( 1.364683531249988535, 2.863541667008082658, 0.7879004041258500513 ) ) ;
#76894=CARTESIAN_POINT ( 'NONE',  ( 9.232739420781973294, 9.873876867108206667, -0.7216878364870257245 ) ) ;
#76895=CARTESIAN_POINT ( 'NONE',  ( -6.247609857798938293, 6.183299677053865295, -0.7998128361456291469 ) ) ;
#76898=CARTESIAN_POINT ( 'NONE',  ( 3.818592820543298405, 7.606775390609172405, -0.7998128361456221525 ) ) ;
#76899=CARTESIAN_POINT ( 'NONE',  ( -6.600121851754250812, 6.594563670001734046, 0.7998128361456341429 ) ) ;
#76905=CARTESIAN_POINT ( 'NONE',  ( 6.982085921357777281, 7.248114451113292667, 1.040834085586084257E-14 ) ) ;
#76908=CARTESIAN_POINT ( 'NONE',  ( -0.6823417656250212460, 1.613541667008083769, 1.181850606188755259 ) ) ;
#76910=CARTESIAN_POINT ( 'NONE',  ( 5.572037945092146671, 8.484166121707415797, -1.082531754730543971 ) ) ;
#76912=CARTESIAN_POINT ( 'NONE',  ( -4.121315508874269007, 5.831287398485176077, -1.443375672974053447 ) ) ;
#76919=CARTESIAN_POINT ( 'NONE',  ( -3.975490874141025088, 7.849583646728635955, 0.01022619435145193101 ) ) ;
#76926=CARTESIAN_POINT ( 'NONE',  ( 6.494519276145969577, 7.535692896047149425, -1.199719254218446718 ) ) ;
#76929=CARTESIAN_POINT ( 'NONE',  ( 4.356247428692526569, 3.976710176429713250, 0.7998128361456341429 ) ) ;
#76937=CARTESIAN_POINT ( 'NONE',  ( 4.528060117284240071, 5.345453560662148718, 1.082531754730560403 ) ) ;
#76938=EDGE_CURVE ( 'NONE', #102987, #47677, #188516, .T. ) ;
#76939=CARTESIAN_POINT ( 'NONE',  ( -1.364683531250012516, 1.842708333674749843, 0.7879004041258379498 ) ) ;
#76941=CARTESIAN_POINT ( 'NONE',  ( 7.263417608619159083, 9.497073181520933716, -1.599625672291262513 ) ) ;
#76944=CARTESIAN_POINT ( 'NONE',  ( -5.901876940650454095, 5.779944607047298177, -0.7998128361456291469 ) ) ;
#76949=CARTESIAN_POINT ( 'NONE',  ( 1.499999999999987121, 2.795833333333352488, -0.8660254037844262731 ) ) ;
#76950=CARTESIAN_POINT ( 'NONE',  ( 5.286789834324991055, 8.255339675766103724, -1.199719254218452935 ) ) ;
#76951=CARTESIAN_POINT ( 'NONE',  ( -6.177711549321182716, 10.35908057418338402, 0.7998128361456481317 ) ) ;
#76955=CARTESIAN_POINT ( 'NONE',  ( -0.6823417656250003738, 2.967708333674754062, -1.181850606188749264 ) ) ;
#76957=CARTESIAN_POINT ( 'NONE',  ( 2.347533153460546806, 5.890539112345938300, 0.000000000000000000 ) ) ;
#76963=CARTESIAN_POINT ( 'NONE',  ( -1.500000000000001332, 0.4312500006828159926, 0.000000000000000000 ) ) ;
#76966=CARTESIAN_POINT ( 'NONE',  ( -7.366157530926372488, 7.488271962369228874, -0.7998128361456291469 ) ) ;
#76967=CARTESIAN_POINT ( 'NONE',  ( -4.012850279964973232, 4.744375417122949301, 1.082531754730560403 ) ) ;
#76975=CARTESIAN_POINT ( 'NONE',  ( 5.124091990960999432, 8.065525525174782828, -1.199719254218452047 ) ) ;
#76976=VECTOR ( 'NONE', #39013, 1000.000000000000227 ) ;
#76980=CARTESIAN_POINT ( 'NONE',  ( 5.819474248763732760, 7.812472595022922128, -1.599625672291262513 ) ) ;
#76981=ORIENTED_EDGE ( 'NONE', *, *, #151476, .T. ) ;
#76984=CARTESIAN_POINT ( 'NONE',  ( -6.501298352952815662, 7.543601818988450169, -1.199719254218446718 ) ) ;
#76985=ORIENTED_EDGE ( 'NONE', *, *, #19052, .T. ) ;
#76986=CARTESIAN_POINT ( 'NONE',  ( 3.867100128395839942, 5.534702787927018974, -1.599625672291255185 ) ) ;
#76992=CARTESIAN_POINT ( 'NONE',  ( 4.274728378101444903, 7.249864702071729283, 0.9550516446962635797 ) ) ;
#77000=CARTESIAN_POINT ( 'NONE',  ( -4.355417078319587354, 3.138959145363762637, 0.7750000000000117906 ) ) ;
#77001=CARTESIAN_POINT ( 'NONE',  ( -3.389175213736311587, 4.977123720824209840, 1.443375672974064550 ) ) ;
#77002=CARTESIAN_POINT ( 'NONE',  ( 7.944714827928043732, 10.29191993738131927, 1.443375672974076540 ) ) ;
#77004=CARTESIAN_POINT ( 'NONE',  ( -5.091250377131585125, 5.898545847196970726, 1.199719254218450271 ) ) ;
#77007=CARTESIAN_POINT ( 'NONE',  ( 8.446893396513862839, 9.813462703143045474, -1.199719254218445830 ) ) ;
#77009=CARTESIAN_POINT ( 'NONE',  ( -4.720210035852093533, 8.658662141802762946, -0.7998128361456281477 ) ) ;
#77012=DIRECTION ( 'NONE',  ( -5.578564026256490882E-16, -1.000000000000000000, -9.066213480720158442E-32 ) ) ;
#77021=CARTESIAN_POINT ( 'NONE',  ( 8.224992744984721327, 12.74757530245756243, 1.040834085586084257E-14 ) ) ;
#77022=CARTESIAN_POINT ( 'NONE',  ( -4.283486466913726254, 7.084819080452935403, -1.199719254218452047 ) ) ;
#77025=CARTESIAN_POINT ( 'NONE',  ( 4.880572111239557920, 4.796348339308675435, -0.7216878364870197293 ) ) ;
#77028=( BOUNDED_CURVE ( )  B_SPLINE_CURVE ( 2, ( #15628, #193329, #128430, #29778, #213816, #65434, #28705 ),
 .UNSPECIFIED., .F., .T. ) 
 B_SPLINE_CURVE_WITH_KNOTS ( ( 3, 2, 2, 3 ),
 ( 0.2125000000000000222, 0.2166666666666667573, 0.2208333333333334647, 0.2250000000000001998 ),
 .UNSPECIFIED. ) 
 CURVE ( )  GEOMETRIC_REPRESENTATION_ITEM ( )  RATIONAL_B_SPLINE_CURVE ( ( 0.9999999999999991118, 0.8660254037844395958, 1.000000000000000000, 0.8660254037844387076, 1.000000000000000000, 0.8660254037844324904, 1.000000000000006217 ) ) 
 REPRESENTATION_ITEM ( '' )  );
#77030=CARTESIAN_POINT ( 'NONE',  ( -4.810445574750349174, 4.506608013497163334, 0.7998128361456341429 ) ) ;
#77031=CARTESIAN_POINT ( 'NONE',  ( -3.440018289565379028, 5.036440642624797626, 1.599625672291267398 ) ) ;
#77035=CARTESIAN_POINT ( 'NONE',  ( 10.05353459973327368, 11.68787744023238417, -1.199719254218440723 ) ) ;
#77040=CARTESIAN_POINT ( 'NONE',  ( -7.283754839039664475, 9.520799950344851936, -1.599625672291263179 ) ) ;
#77041=CARTESIAN_POINT ( 'NONE',  ( 4.852928918687680948, 7.749168607522574526, 1.199719254218462483 ) ) ;
#77043=CARTESIAN_POINT ( 'NONE',  ( 5.495132332240461714, 5.305409230568988832, 0.7998128361456341429 ) ) ;
#77045=FACE_OUTER_BOUND ( 'NONE', #139067, .T. ) ;
#77046=CARTESIAN_POINT ( 'NONE',  ( 0.6823417656249899377, 1.405208333674752508, 1.181850606188755259 ) ) ;
#77049=CARTESIAN_POINT ( 'NONE',  ( 6.453317930424781856, 10.47269531889685545, -0.7216878364870267237 ) ) ;
#77050=ORIENTED_EDGE ( 'NONE', *, *, #3407, .T. ) ;
#77057=CARTESIAN_POINT ( 'NONE',  ( 8.039621902779343188, 12.32338328664385507, -0.7216878364870328300 ) ) ;
#77064=CARTESIAN_POINT ( 'NONE',  ( -8.045874094706015001, 11.47427131287732927, -1.199719254218446718 ) ) ;
#77070=EDGE_CURVE ( 'NONE', #63977, #80984, #75837, .T. ) ;
#77074=AXIS2_PLACEMENT_3D ( 'NONE', #207046, #154048, #90125 ) ;
#77084=CARTESIAN_POINT ( 'NONE',  ( -1.500000000000013101, 0.9520833340161557468, 0.8660254037844403729 ) ) ;
#77090=CARTESIAN_POINT ( 'NONE',  ( 0.7499999999999885647, -1.016666666666644847, 1.299038105676657340 ) ) ;
#77091=CARTESIAN_POINT ( 'NONE',  ( 8.263858322729371153, 9.599921783727809910, -1.199719254218446718 ) ) ;
#77092=CARTESIAN_POINT ( 'NONE',  ( -1.364683531250014514, -1.011458332991911568, -0.7879004041258359514 ) ) ;
#77094=CARTESIAN_POINT ( 'NONE',  ( 2.659370686574860976, 6.254349567645977714, -0.7998128361456291469 ) ) ;
#77095=CARTESIAN_POINT ( 'NONE',  ( -7.212574532790110737, 7.517017831117667193, -0.7216878364870278340 ) ) ;
#77101=CARTESIAN_POINT ( 'NONE',  ( -6.344325816190970357, 9.489131654609717970, 1.199719254218452047 ) ) ;
#77104=CARTESIAN_POINT ( 'NONE',  ( 1.499999999999989120, 1.556250000682817047, 0.000000000000000000 ) ) ;
#77118=CARTESIAN_POINT ( 'NONE',  ( -9.677822722056413696, 10.18521468535430685, 1.040834085586084257E-14 ) ) ;
#77119=CARTESIAN_POINT ( 'NONE',  ( 6.877010230629674759, 9.046264573866535486, 1.599625672291281386 ) ) ;
#77127=CARTESIAN_POINT ( 'NONE',  ( -7.645908563102897126, 11.00764485934031889, 1.199719254218453823 ) ) ;
#77135=CARTESIAN_POINT ( 'NONE',  ( 3.005103603723342953, 6.657704637652544832, -0.7998128361456291469 ) ) ;
#77139=EDGE_LOOP ( 'NONE', ( #35199, #83606, #163598 ) ) ;
#77140=CARTESIAN_POINT ( 'NONE',  ( -10.47097470845587175, 11.11055866948701443, 1.040834085586084257E-14 ) ) ;
#77143=CARTESIAN_POINT ( 'NONE',  ( -5.830469385422084372, 6.191968629596825480, -0.9632026293319171373 ) ) ;
#77158=CARTESIAN_POINT ( 'NONE',  ( 1.499999999999989120, 0.8062500006828163812, 0.000000000000000000 ) ) ;
#77170=CARTESIAN_POINT ( 'NONE',  ( 5.029711800989886683, 4.970344644017389513, 1.040834085586084257E-14 ) ) ;
#77173=CARTESIAN_POINT ( 'NONE',  ( -8.448702279610222021, 13.00856975952063088, 1.040834085586084257E-14 ) ) ;
#77175=CARTESIAN_POINT ( 'NONE',  ( 10.55910270694468345, 11.21337466772398095, 0.7998128361456462443 ) ) ;
#77184=CARTESIAN_POINT ( 'NONE',  ( -1.364683531250000748, -0.2406249996585799189, 0.000000000000000000 ) ) ;
#77190=CARTESIAN_POINT ( 'NONE',  ( -4.205000198532790279, 8.057583998263570635, 0.7998128361456341429 ) ) ;
#77193=CARTESIAN_POINT ( 'NONE',  ( 1.499999999999987121, -0.2458333333333099502, 0.8660254037844524744 ) ) ;
#77195=CARTESIAN_POINT ( 'NONE',  ( -1.201851678989727383E-14, 5.587500000000021672, -1.732050807568863648 ) ) ;
#77202=CARTESIAN_POINT ( 'NONE',  ( 0.6823417656249882723, -0.9072916663252494907, 1.181850606188755259 ) ) ;
#77204=CARTESIAN_POINT ( 'NONE',  ( -6.340409392685171674, 10.54889472477470846, 0.7998128361456481317 ) ) ;
#77211=CARTESIAN_POINT ( 'NONE',  ( -1.402160292154681736E-14, 0.2593750003414224681, -1.575800808251665908 ) ) ;
#77218=CARTESIAN_POINT ( 'NONE',  ( 6.914295153289432783, 10.05013286460426691, -1.082531754730537976 ) ) ;
#77221=CARTESIAN_POINT ( 'NONE',  ( -4.055860508782465068, 7.883587693554856557, 1.040834085586084257E-14 ) ) ;
#77223=CARTESIAN_POINT ( 'NONE',  ( 0.7499999999999920064, 4.264583334016150751, 1.299038105676669330 ) ) ;
#77225=CARTESIAN_POINT ( 'NONE',  ( -3.952365473583647315, 4.569846793057691592, 1.199719254218462483 ) ) ;
#77226=CARTESIAN_POINT ( 'NONE',  ( 6.927853306458752414, 7.184843067064434763, 0.7216878364870317197 ) ) ;
#77227=CARTESIAN_POINT ( 'NONE',  ( -7.985389288324685531, 12.26011190311341537, -0.7216878364870267237 ) ) ;
#77234=CARTESIAN_POINT ( 'NONE',  ( 2.683624340501134853, 5.218313266304903664, -1.199719254218446718 ) ) ;
#77250=CARTESIAN_POINT ( 'NONE',  ( 9.589694723567584234, 10.08239868711733855, -0.7998128361456281477 ) ) ;
#77251=VECTOR ( 'NONE', #6826, 1000.000000000000000 ) ;
#77254=FACE_OUTER_BOUND ( 'NONE', #86044, .T. ) ;
#77258=CARTESIAN_POINT ( 'NONE',  ( 1.364683531249986537, 1.155208333674754728, -0.7879004041258239610 ) ) ;
#77259=CARTESIAN_POINT ( 'NONE',  ( 5.721177635286841756, 6.737423998331861341, -1.082531754730543083 ) ) ;
#77261=CARTESIAN_POINT ( 'NONE',  ( -7.524412065904404479, 11.72230514362308185, 0.000000000000000000 ) ) ;
#77263=EDGE_CURVE ( 'NONE', #119686, #201094, #210082, .T. ) ;
#77266=CARTESIAN_POINT ( 'NONE',  ( -4.274898507010545856, 3.881803101134051470, -0.7998128361456221525 ) ) ;
#77272=B_SPLINE_CURVE_WITH_KNOTS ( 'NONE', 3,
 ( #5214, #71289, #203419, #104905 ),
 .UNSPECIFIED., .F., .F.,
 ( 4, 4 ),
 ( 3.951020751517320303E-17, 0.0001635767864326787382 ),
 .UNSPECIFIED. ) ;
#77284=CARTESIAN_POINT ( 'NONE',  ( 4.477916600690244664, 7.270601638097409669, -1.256879854437189969 ) ) ;
#77285=CARTESIAN_POINT ( 'NONE',  ( -2.314109536355652530, 5.457892750589173225, -0.8025987720412944837 ) ) ;
#77293=CARTESIAN_POINT ( 'NONE',  ( -9.015808963407680565, 9.620791333504852716, 1.040834085586084257E-14 ) ) ;
#77297=CARTESIAN_POINT ( 'NONE',  ( 6.094553744542824170, 7.069066442510145265, 1.199719254218462483 ) ) ;
#77302=CARTESIAN_POINT ( 'NONE',  ( -4.355193658487827690, 6.104145239700998538, -1.599625672291256295 ) ) ;
#77306=CARTESIAN_POINT ( 'NONE',  ( -3.906720819032141190, 7.709591388846142479, -0.7998128361456281477 ) ) ;
#77309=CARTESIAN_POINT ( 'NONE',  ( 8.535021395002688749, 9.916278701380017324, 1.199719254218462483 ) ) ;
#77310=CARTESIAN_POINT ( 'NONE',  ( 0.01975730027497306709, 6.477791580114294234, 3.085592232244173339 ) ) ;
#77312=CARTESIAN_POINT ( 'NONE',  ( 5.026094266273638311, 6.779731885415203330, 1.422988838494985364 ) ) ;
#77313=CARTESIAN_POINT ( 'NONE',  ( 3.551873057100274789, 7.087676300018221021, 0.7216878364870298324 ) ) ;
#77320=CARTESIAN_POINT ( 'NONE',  ( 7.266807146800403849, 7.580289214129690478, 1.040834085586084257E-14 ) ) ;
#77321=CARTESIAN_POINT ( 'NONE',  ( -7.621654909176601045, 12.04368116068139472, 0.7998128361456481317 ) ) ;
#77324=CARTESIAN_POINT ( 'NONE',  ( -7.635213062790267458, 12.05949900656400686, 0.000000000000000000 ) ) ;
#77325=CARTESIAN_POINT ( 'NONE',  ( -6.413170354464012846, 7.440785820751486312, 1.199719254218450271 ) ) ;
#77333=CARTESIAN_POINT ( 'NONE',  ( 7.076466111328892694, 10.34329533227067799, -1.199719254218441611 ) ) ;
#77347=CARTESIAN_POINT ( 'NONE',  ( 1.499999999999989120, 2.754166666666688190, 0.8660254037844524744 ) ) ;
#77348=CARTESIAN_POINT ( 'NONE',  ( 4.852928918687680948, 7.749168607522574526, 1.199719254218462483 ) ) ;
#77351=CARTESIAN_POINT ( 'NONE',  ( 7.700668062882064291, 10.00719871149432549, -1.443375672974057666 ) ) ;
#77356=CARTESIAN_POINT ( 'NONE',  ( 10.06423010004587759, 10.63602329300870153, 0.000000000000000000 ) ) ;
#77361=CARTESIAN_POINT ( 'NONE',  ( 0.6823417656249899377, 0.8427083336747520637, 1.181850606188755259 ) ) ;
#77366=CARTESIAN_POINT ( 'NONE',  ( 0.6823417656249864960, -0.8239583329919114574, -1.181850606188749264 ) ) ;
#77368=CARTESIAN_POINT ( 'NONE',  ( 8.398386088661320414, 11.88553530582519357, -1.199719254218446718 ) ) ;
#77371=CARTESIAN_POINT ( 'NONE',  ( -4.256897044566581911, 4.068727428190179296, 1.214306433183764966E-14 ) ) ;
#77374=CARTESIAN_POINT ( 'NONE',  ( -6.575868197828002693, 7.630599971342813426, 1.199719254218450271 ) ) ;
#77377=CARTESIAN_POINT ( 'NONE',  ( 5.352771719296971042, 5.139321848801576387, 0.7998128361456341429 ) ) ;
#77383=CARTESIAN_POINT ( 'NONE',  ( 7.736899214892750010, 12.17813285068358020, 1.040834085586084257E-14 ) ) ;
#77386=CARTESIAN_POINT ( 'NONE',  ( -5.066996723205291708, 6.934582148538044777, 1.599625672291267398 ) ) ;
#77390=CARTESIAN_POINT ( 'NONE',  ( 9.185812768458653466, 10.67553530374532045, 1.199719254218453823 ) ) ;
#77392=CARTESIAN_POINT ( 'NONE',  ( 8.274553823041976841, 8.548067636504127265, 1.040834085586084257E-14 ) ) ;
#77396=CARTESIAN_POINT ( 'NONE',  ( -9.544576954340667996, 11.19805653722800365, 1.082531754730558626 ) ) ;
#77403=CARTESIAN_POINT ( 'NONE',  ( -5.816164686850935794, 6.201415483580719368, 0.9813818067917270405 ) ) ;
#77404=CARTESIAN_POINT ( 'NONE',  ( -1.364683531250000748, 2.009375000341421913, 1.214306433183764966E-14 ) ) ;
#77407=CARTESIAN_POINT ( 'NONE',  ( 7.158341918335438869, 7.453746447587225710, -0.7216878364870257245 ) ) ;
#77409=EDGE_CURVE ( 'NONE', #53793, #209728, #214309, .T. ) ;
#77415=AXIS2_PLACEMENT_3D ( 'NONE', #37145, #169286, #53398 ) ;
#77426=CARTESIAN_POINT ( 'NONE',  ( 8.718056468787178659, 10.12981962079525289, 1.199719254218462483 ) ) ;
#77430=CARTESIAN_POINT ( 'NONE',  ( -2.950870989268691957, 6.594433254122103349, -0.7998128361456281477 ) ) ;
#77431=CARTESIAN_POINT ( 'NONE',  ( -6.645467848992654858, 10.90479625713344625, 0.7998128361456481317 ) ) ;
#77436=CARTESIAN_POINT ( 'NONE',  ( 1.499999999999987121, 4.077083334016147198, -0.8660254037844323793 ) ) ;
#77437=CARTESIAN_POINT ( 'NONE',  ( 6.642605195691581699, 9.837124264027149678, 1.199719254218462483 ) ) ;
#77440=CARTESIAN_POINT ( 'NONE',  ( -7.178152263431422320, 10.46192917639026554, 1.199719254218453823 ) ) ;
#77442=CARTESIAN_POINT ( 'NONE',  ( 0.6823417656249899377, 4.426041667008086655, -1.181850606188754593 ) ) ;
#77447=CARTESIAN_POINT ( 'NONE',  ( -9.707274797704657843, 11.38787068781932987, 1.082531754730558626 ) ) ;
#77452=CARTESIAN_POINT ( 'NONE',  ( -1.201851678989727383E-14, 2.884375000341418804, 1.575800808251672791 ) ) ;
#77459=CARTESIAN_POINT ( 'NONE',  ( -1.364683531249997417, 3.009375000341422801, 1.214306433183764966E-14 ) ) ;
#77461=CARTESIAN_POINT ( 'NONE',  ( -4.761938266897808525, 6.578680616179308771, 1.599625672291267398 ) ) ;
#77462=CARTESIAN_POINT ( 'NONE',  ( 6.205881626753210867, 8.263281202677319470, 1.599625672291281386 ) ) ;
#77465=CARTESIAN_POINT ( 'NONE',  ( -1.364683531250012516, 3.592708333674750509, 0.7879004041258379498 ) ) ;
#77468=CARTESIAN_POINT ( 'NONE',  ( -1.364683531250014514, -0.4697916663252449943, 0.7879004041258379498 ) ) ;
#77469=CARTESIAN_POINT ( 'NONE',  ( -4.500943810056945438, 5.313817868896925312, 1.082531754730560403 ) ) ;
#77473=CARTESIAN_POINT ( 'NONE',  ( 4.365362273920238678, 7.076377838673507448, 1.082531754730558626 ) ) ;
#77476=CARTESIAN_POINT ( 'NONE',  ( -8.701635661872465732, 9.046329781806354831, 1.040834085586084257E-14 ) ) ;
#77477=CARTESIAN_POINT ( 'NONE',  ( -7.849807752632384172, 12.10193344480572897, 0.000000000000000000 ) ) ;
#77483=CARTESIAN_POINT ( 'NONE',  ( -9.215791728987058562, 11.77484298861683598, -1.599625672291263179 ) ) ;
#77484=CARTESIAN_POINT ( 'NONE',  ( -7.009202228140764213, 7.279750142360097875, -0.7216878364870267237 ) ) ;
#77486=CARTESIAN_POINT ( 'NONE',  ( 0.6823417656249882723, 0.4885416670080827695, -1.181850606188749264 ) ) ;
#77491=CARTESIAN_POINT ( 'NONE',  ( 4.177814833343409084, 3.976464848429826393, 1.040551764647542070E-14 ) ) ;
#77498=CARTESIAN_POINT ( 'NONE',  ( -1.402160292154681736E-14, -0.9124999999999769962, -1.732050807568870754 ) ) ;
#77499=CARTESIAN_POINT ( 'NONE',  ( 9.042925270190638187, 9.652427024751663254, 0.7216878364870458196 ) ) ;
#77507=CARTESIAN_POINT ( 'NONE',  ( 5.148345644887269756, 7.029489223833707001, -1.599625672291256295 ) ) ;
#77509=CARTESIAN_POINT ( 'NONE',  ( -5.088387723830502196, 4.830873854090670605, -0.7998128361456221525 ) ) ;
#77513=CARTESIAN_POINT ( 'NONE',  ( 1.364683531249988757, 1.196875000341421469, 0.000000000000000000 ) ) ;
#77514=CARTESIAN_POINT ( 'NONE',  ( 6.092610039548504552, 6.029531113932129038, 0.3159152987922431710 ) ) ;
#77515=CARTESIAN_POINT ( 'NONE',  ( -8.833300774503376473, 10.26427131079744193, 1.199719254218462483 ) ) ;
#77517=ADVANCED_FACE ( 'NONE', ( #111605 ), #44820, .T. ) ;
#77533=CARTESIAN_POINT ( 'NONE',  ( 6.307567778855705853, 8.381915046796901692, -1.599625672291262513 ) ) ;
#77540=CARTESIAN_POINT ( 'NONE',  ( 9.108380270282433244, 9.520865158284665952, 1.040834085586084257E-14 ) ) ;
#77543=CARTESIAN_POINT ( 'NONE',  ( 7.899597058256738968, 12.36794700127490820, 1.040834085586084257E-14 ) ) ;
#77557=CARTESIAN_POINT ( 'NONE',  ( -9.653042183249972652, 10.36423008998754192, -0.7216878364870267237 ) ) ;
#77563=CARTESIAN_POINT ( 'NONE',  ( -8.611400122974211868, 13.19838391011195888, 1.040834085586084257E-14 ) ) ;
#77564=CARTESIAN_POINT ( 'NONE',  ( 3.988069740714122791, 7.804498464141805592, 0.7998128361456321445 ) ) ;
#77570=CARTESIAN_POINT ( 'NONE',  ( 4.541618270453549044, 5.361271406026338227, -1.082531754730548412 ) ) ;
#77578=CARTESIAN_POINT ( 'NONE',  ( -5.392392409933270514, 7.314210449720692786, 1.599625672291269396 ) ) ;
#77580=CARTESIAN_POINT ( 'NONE',  ( -2.462777459176719308, 6.024990802348131780, -0.7998128361456281477 ) ) ;
#77585=CARTESIAN_POINT ( 'NONE',  ( -0.007473969438217894709, 8.279395425053857949, -1.999986034896452880 ) ) ;
#77588=CARTESIAN_POINT ( 'NONE',  ( 4.690231075323689325, 7.559354456931247412, 1.199719254218462483 ) ) ;
#77601=CARTESIAN_POINT ( 'NONE',  ( 1.364683531249988757, 0.9468750003414211358, 0.000000000000000000 ) ) ;
#77602=CARTESIAN_POINT ( 'NONE',  ( 4.383363735919856730, 4.008345868194933104, -0.7998128361456211532 ) ) ;
#77603=CARTESIAN_POINT ( 'NONE',  ( 3.680148631105580215, 6.380924938676771241, -1.199719254218446718 ) ) ;
#77605=CARTESIAN_POINT ( 'NONE',  ( -7.727784370109414880, 8.118095974656867497, 0.7216878364870578100 ) ) ;
#77606=CARTESIAN_POINT ( 'NONE',  ( 3.714570900464269076, 7.277490450609545469, 0.7216878364870298324 ) ) ;
#77607=CARTESIAN_POINT ( 'NONE',  ( -6.195713011320795438, 8.251417818006149929, -1.443375672974058777 ) ) ;
#77610=CIRCLE ( 'NONE', #184740, 0.8300000000000008482 ) ;
#77611=VERTEX_POINT ( 'NONE', #198098 ) ;
#77613=CARTESIAN_POINT ( 'NONE',  ( 5.124091990960999432, 8.065525525174782828, -1.199719254218452047 ) ) ;
#77618=CARTESIAN_POINT ( 'NONE',  ( 0.6823417656249899377, 4.676041667008086655, -1.181850606188754593 ) ) ;
#77623=CARTESIAN_POINT ( 'NONE',  ( 6.120616281565444794, 9.228137197546649517, -1.199719254218440723 ) ) ;
#77626=CARTESIAN_POINT ( 'NONE',  ( -6.028571859570855729, 10.18508426947466816, 0.000000000000000000 ) ) ;
#77631=CARTESIAN_POINT ( 'NONE',  ( 8.209625708274705502, 9.536650400197368427, 1.199719254218462483 ) ) ;
#77634=CARTESIAN_POINT ( 'NONE',  ( -7.552055258011950656, 8.769484874890757453, 1.199719254218462483 ) ) ;
#77636=CARTESIAN_POINT ( 'NONE',  ( 6.412643469139427843, 10.42524178073059993, -0.7216878364870267237 ) ) ;
#77637=CARTESIAN_POINT ( 'NONE',  ( 4.015052158831055706, 7.807088067957844046, 0.2846288760043579336 ) ) ;
#77638=CARTESIAN_POINT ( 'NONE',  ( -10.00555417720528872, 10.77549408293541866, 0.7216878364870438212 ) ) ;
#77643=CARTESIAN_POINT ( 'NONE',  ( 5.066996723205273057, 6.934582148538044777, 1.599625672291267398 ) ) ;
#77645=CARTESIAN_POINT ( 'NONE',  ( 7.553864141108259211, 11.96459193126834464, 1.040834085586084257E-14 ) ) ;
#77646=CARTESIAN_POINT ( 'NONE',  ( -4.728240158028945928, 6.838416746360681309, 1.235430216343525567 ) ) ;
#77647=CARTESIAN_POINT ( 'NONE',  ( 4.695201269034174452, 4.372156323494968966, 1.214306433183764966E-14 ) ) ;
#77648=CARTESIAN_POINT ( 'NONE',  ( -1.402160292154681736E-14, 0.1968750003414221628, -1.575800808251665908 ) ) ;
#77650=CARTESIAN_POINT ( 'NONE',  ( -5.422898255786186006, 9.270539031818461950, -0.7216878364870207285 ) ) ;
#77656=CARTESIAN_POINT ( 'NONE',  ( -4.595282798756362475, 6.958845989550745514, 1.192800718855389297 ) ) ;
#77657=CARTESIAN_POINT ( 'NONE',  ( -1.364683531250014514, 0.09270833367475767028, 0.7879004041258379498 ) ) ;
#77661=CARTESIAN_POINT ( 'NONE',  ( 4.365362273920250225, 5.155639410070820716, 1.082531754730560403 ) ) ;
#77666=CARTESIAN_POINT ( 'NONE',  ( -8.636180661780668899, 10.13826086257468795, -1.082531754730543083 ) ) ;
#77671=CARTESIAN_POINT ( 'NONE',  ( -9.151390499099978371, 9.778969791812544443, 0.7216878364870438212 ) ) ;
#77673=ORIENTED_EDGE ( 'NONE', *, *, #67235, .F. ) ;
#77677=ORIENTED_EDGE ( 'NONE', *, *, #192214, .F. ) ;
#77678=CARTESIAN_POINT ( 'NONE',  ( -9.137832345486311070, 9.763151945929928743, 1.040834085586084257E-14 ) ) ;
#77683=CARTESIAN_POINT ( 'NONE',  ( 1.499999999999989120, 4.827083334016149863, -0.8660254037844323793 ) ) ;
#77684=CARTESIAN_POINT ( 'NONE',  ( 6.021928883684827483, 6.074059740061504620, -0.5497475987105825412 ) ) ;
#77685=DIRECTION ( 'NONE',  ( -1.000000000000000000, 5.578564026256490882E-16, 2.058387550816952846E-48 ) ) ;
#77690=CARTESIAN_POINT ( 'NONE',  ( -7.263417608619167076, 9.497073181520933716, -1.599625672291263179 ) ) ;
#77694=CARTESIAN_POINT ( 'NONE',  ( 4.904298879841284098, 6.744767997946721216, 1.599625672291267398 ) ) ;
#77699=CARTESIAN_POINT ( 'NONE',  ( 7.630541526392844887, 7.796719957080126662, 0.7998128361456341429 ) ) ;
#77700=CARTESIAN_POINT ( 'NONE',  ( -4.911987184702322651, 4.724253982773818805, 0.4179318588051501027 ) ) ;
#77707=CARTESIAN_POINT ( 'NONE',  ( -6.127922243696855453, 7.211959374810172463, 1.082531754730549967 ) ) ;
#77710=CARTESIAN_POINT ( 'NONE',  ( 3.877268743828266029, 6.506935386899531437, 1.082531754730558626 ) ) ;
#77716=CARTESIAN_POINT ( 'NONE',  ( -7.980945979938748103, 12.46285407657057220, 0.000000000000000000 ) ) ;
#77719=CARTESIAN_POINT ( 'NONE',  ( 7.235247531187115833, 11.59287255302699648, -0.7998128361456291469 ) ) ;
#77720=CARTESIAN_POINT ( 'NONE',  ( 1.499999999999987121, -0.7458333333333122539, 0.8660254037844524744 ) ) ;
#77721=CARTESIAN_POINT ( 'NONE',  ( -9.854078719034067291, 10.39084668182823634, 0.7998128361456462443 ) ) ;
#77724=CARTESIAN_POINT ( 'NONE',  ( -1.364683531249997417, 3.259375000341423245, 1.214306433183764966E-14 ) ) ;
#77725=CARTESIAN_POINT ( 'NONE',  ( 8.920901888111986366, 12.39117405523060889, 1.082531754730546636 ) ) ;
#77726=EDGE_CURVE ( 'NONE', #96829, #108458, #186530, .T. ) ;
#77728=CARTESIAN_POINT ( 'NONE',  ( -1.499999999999993339, 10.64264068711930733, 1.232676135170975238E-14 ) ) ;
#77729=CARTESIAN_POINT ( 'NONE',  ( -0.7500000000000215383, 4.691666666666684193, 1.299038105676671107 ) ) ;
#77732=CARTESIAN_POINT ( 'NONE',  ( 9.544576953896278582, 10.23768732240824164, 0.000000000000000000 ) ) ;
#77736=CARTESIAN_POINT ( 'NONE',  ( -5.097502569058207200, 8.890910730635814829, -0.7216878364870207285 ) ) ;
#77737=CARTESIAN_POINT ( 'NONE',  ( -1.364683531249997417, 2.509375000341422357, 1.214306433183764966E-14 ) ) ;
#77741=CARTESIAN_POINT ( 'NONE',  ( -8.016948904382338981, 8.247528564734524892, -0.7998128361456291469 ) ) ;
#77742=CARTESIAN_POINT ( 'NONE',  ( -1.364683531250010295, 5.342708333674750953, 0.7879004041258379498 ) ) ;
#77748=CARTESIAN_POINT ( 'NONE',  ( 9.772729797352075920, 10.29593960653257234, -0.7998128361456281477 ) ) ;
#77751=CARTESIAN_POINT ( 'NONE',  ( 1.499999999999989120, 0.5250000000000185629, 0.000000000000000000 ) ) ;
#77755=CARTESIAN_POINT ( 'NONE',  ( 8.401248741962376698, 12.95320729893149370, 0.7998128361456462443 ) ) ;
#77760=CARTESIAN_POINT ( 'NONE',  ( 7.564559641420864899, 10.91273778404466199, -1.199719254218446718 ) ) ;
#77761=CARTESIAN_POINT ( 'NONE',  ( -8.455481356417053007, 13.01647868246193518, 0.7998128361456341429 ) ) ;
#77764=CARTESIAN_POINT ( 'NONE',  ( 1.364683531249990311, 5.196875000341417916, 1.214306433183764966E-14 ) ) ;
#77767=EDGE_CURVE ( 'NONE', #164652, #23582, #68078, .T. ) ;
#77770=CARTESIAN_POINT ( 'NONE',  ( 7.411503528164766763, 11.79850454950093841, 1.040834085586084257E-14 ) ) ;
#77773=CARTESIAN_POINT ( 'NONE',  ( -1.364683531250012516, 3.738541667008087099, -0.7879004041258300672 ) ) ;
#77775=CARTESIAN_POINT ( 'NONE',  ( -4.921246572080546500, 8.685278734161874681, 1.214306433183764966E-14 ) ) ;
#77781=CARTESIAN_POINT ( 'NONE',  ( 3.999819011231439347, 4.625209253646830554, 1.199719254218464037 ) ) ;
#77784=CARTESIAN_POINT ( 'NONE',  ( 9.426996880203592610, 9.892584536526015881, -0.7998128361456281477 ) ) ;
#77785=CARTESIAN_POINT ( 'NONE',  ( 3.741371894207385917, 7.428709027653158437, -2.448389769268734195 ) ) ;
#77790=CARTESIAN_POINT ( 'NONE',  ( -7.645908563102897126, 11.00764485934031889, 1.199719254218453823 ) ) ;
#77791=CARTESIAN_POINT ( 'NONE',  ( 6.993308306550549247, 7.053281200597435685, 1.040834085586084257E-14 ) ) ;
#77794=CARTESIAN_POINT ( 'NONE',  ( 3.511198595814926993, 6.079853547550633230, 1.082531754730558626 ) ) ;
#77796=CARTESIAN_POINT ( 'NONE',  ( 4.334856428067313416, 6.080418470877079429, -1.599625672291256295 ) ) ;
#77803=CARTESIAN_POINT ( 'NONE',  ( -4.609409038966229666, 8.321468278861834378, -0.7216878364870267237 ) ) ;
#77804=CARTESIAN_POINT ( 'NONE',  ( 2.984766373302843778, 6.633977868828633717, -0.7998128361456291469 ) ) ;
#77807=CARTESIAN_POINT ( 'NONE',  ( -6.320072162264675164, 10.52516795595079557, 0.7998128361456481317 ) ) ;
#77813=CARTESIAN_POINT ( 'NONE',  ( -8.809047120577080392, 11.30030761213851953, 1.599625672291269396 ) ) ;
#77816=CARTESIAN_POINT ( 'NONE',  ( 7.741869408603235136, 8.990934717247309749, 1.199719254218462483 ) ) ;
#77817=CARTESIAN_POINT ( 'NONE',  ( 6.796715079152391148, 6.823922435299587974, 0.7998128361456341429 ) ) ;
#77829=CARTESIAN_POINT ( 'NONE',  ( -6.184490626128011925, 10.36698949712469364, -0.7998128361456291469 ) ) ;
#77833=CARTESIAN_POINT ( 'NONE',  ( 6.995644074971448134, 7.263932296995902149, -0.7216878364870257245 ) ) ;
#77836=DIRECTION ( 'NONE',  ( -5.578564026256491869E-16, -1.000000000000000000, -9.066213480720160632E-32 ) ) ;
#77838=CARTESIAN_POINT ( 'NONE',  ( -6.586563698140583512, 6.578745824119123675, 1.040834085586084257E-14 ) ) ;
#77848=CARTESIAN_POINT ( 'NONE',  ( 8.450809820019639318, 8.753699632978056755, -0.7998128361456291469 ) ) ;
#77850=CARTESIAN_POINT ( 'NONE',  ( -3.795919822146283540, 6.412028311603867436, -1.082531754730549967 ) ) ;
#77853=CARTESIAN_POINT ( 'NONE',  ( -4.654334680973787108, 6.904393480334801048, -1.215188995478516221 ) ) ;
#77861=CARTESIAN_POINT ( 'NONE',  ( 2.900554798319789906, 5.471398800426671372, 1.199719254218452047 ) ) ;
#77867=CARTESIAN_POINT ( 'NONE',  ( -3.331659036430328236, 7.719744385808867015, -2.450696915730449454 ) ) ;
#77869=CARTESIAN_POINT ( 'NONE',  ( 4.355193658487811703, 6.104145239700998538, -1.599625672291255185 ) ) ;
#77874=CARTESIAN_POINT ( 'NONE',  ( -1.201851678989727383E-14, 4.259375000341417028, -1.575800808251660134 ) ) ;
#77879=CARTESIAN_POINT ( 'NONE',  ( 5.799137018343234473, 7.788745826199009237, -1.599625672291262513 ) ) ;
#77883=CARTESIAN_POINT ( 'NONE',  ( -5.220052836461385404, 6.048815383081766583, -1.199719254218446718 ) ) ;
#77884=CARTESIAN_POINT ( 'NONE',  ( 4.473827502385202770, 8.163289819517311585, 1.040834085586084257E-14 ) ) ;
#77885=CARTESIAN_POINT ( 'NONE',  ( 1.499999999999987121, 3.045833333333353377, -0.8660254037844262731 ) ) ;
#77888=CARTESIAN_POINT ( 'NONE',  ( -2.950870989268691957, 6.594433254122103349, -0.7998128361456281477 ) ) ;
#77889=CARTESIAN_POINT ( 'NONE',  ( 0.4599077567407924838, 8.047644787141630118, -1.947158400785528487 ) ) ;
#77891=CARTESIAN_POINT ( 'NONE',  ( 0.6823417656249899377, 4.176041667008085767, -1.181850606188754593 ) ) ;
#77894=CARTESIAN_POINT ( 'NONE',  ( -3.280709984826970516, 6.771319382366015383, 0.7216878364870317197 ) ) ;
#77898=CARTESIAN_POINT ( 'NONE',  ( -3.456965981804629884, 6.976951378839947537, 1.040834085586084257E-14 ) ) ;
#77899=CARTESIAN_POINT ( 'NONE',  ( 3.948449050077836642, 5.629609863222681199, 1.599625672291267398 ) ) ;
#77900=CARTESIAN_POINT ( 'NONE',  ( 4.908649743871434268, 4.822872567462811233, -0.4817574433751614094 ) ) ;
#77904=CARTESIAN_POINT ( 'NONE',  ( -1.364683531250000748, 0.8218750003414210248, 0.000000000000000000 ) ) ;
#77908=CARTESIAN_POINT ( 'NONE',  ( -8.299562589859897699, 12.83457345481192036, -0.7998128361456281477 ) ) ;
#77909=CARTESIAN_POINT ( 'NONE',  ( -6.209271164934474285, 6.346497235286081562, 1.040834085586084257E-14 ) ) ;
#77914=CARTESIAN_POINT ( 'NONE',  ( 1.364683531249990311, 4.884375000341417916, 1.214306433183764966E-14 ) ) ;
#77922=CARTESIAN_POINT ( 'NONE',  ( -7.009202228140764213, 7.279750142360097875, -0.7216878364870267237 ) ) ;
#77929=CARTESIAN_POINT ( 'NONE',  ( -4.704316113817535339, 8.432193199521691440, 0.7216878364870458196 ) ) ;
#77931=CARTESIAN_POINT ( 'NONE',  ( -4.676113526401191933, 5.272618711636657629, 1.141756068723397854 ) ) ;
#77942=CARTESIAN_POINT ( 'NONE',  ( -5.742041750587549842, 6.657802449562273850, 1.199719254218450271 ) ) ;
#77945=CARTESIAN_POINT ( 'NONE',  ( -0.7500000000000006661, 0.8583333333333567072, -1.299038105676652011 ) ) ;
#77947=CARTESIAN_POINT ( 'NONE',  ( 9.246297574839980271, 10.85006392781057905, 1.082531754730549967 ) ) ;
#77948=CARTESIAN_POINT ( 'NONE',  ( 7.091078035147269532, 8.231678114882006625, 1.199719254218462483 ) ) ;
#77953=CARTESIAN_POINT ( 'NONE',  ( 5.192936529234042808, 6.017179691316550283, -1.199719254218452047 ) ) ;
#77954=CARTESIAN_POINT ( 'NONE',  ( -0.07021666366558332317, 7.008523639392694626, -2.000250312771549854 ) ) ;
#77955=VERTEX_POINT ( 'NONE', #76642 ) ;
#77961=CARTESIAN_POINT ( 'NONE',  ( -7.074657228232555717, 7.148188275893099686, 1.040834085586084257E-14 ) ) ;
#77963=EDGE_LOOP ( 'NONE', ( #132293, #81324, #46938, #202483 ) ) ;
#77967=CARTESIAN_POINT ( 'NONE',  ( 1.364683531249988535, 3.655208333674750509, -0.7879004041258239610 ) ) ;
#77968=CARTESIAN_POINT ( 'NONE',  ( 8.012505595552012139, 11.33137838057728786, -1.082531754730543083 ) ) ;
#77969=CARTESIAN_POINT ( 'NONE',  ( -6.201965203247477909, 9.323044272842313518, 1.199719254218452047 ) ) ;
#77972=CARTESIAN_POINT ( 'NONE',  ( 6.657217119509961201, 7.725507046638470321, -1.199719254218446718 ) ) ;
#77973=CARTESIAN_POINT ( 'NONE',  ( -5.087333953625788219, 6.958308917361963886, 1.599625672291267398 ) ) ;
#77977=CARTESIAN_POINT ( 'NONE',  ( -0.7500000000000006661, 0.8895833340161543035, -1.299038105676652011 ) ) ;
#77980=CARTESIAN_POINT ( 'NONE',  ( 7.673551755654734130, 9.015193805427763607, -1.082531754730537976 ) ) ;
#77984=CARTESIAN_POINT ( 'NONE',  ( 0.6823417656249899377, 2.155208333674753174, 1.181850606188767472 ) ) ;
#77986=CARTESIAN_POINT ( 'NONE',  ( 6.466876083594112146, 6.647036307055676829, -0.7216878364870257245 ) ) ;
#77989=CARTESIAN_POINT ( 'NONE',  ( -4.772106882330247046, 4.669805572247793357, -0.7216878364870207285 ) ) ;
#77996=CARTESIAN_POINT ( 'NONE',  ( -4.201979666139121328, 7.560802217138083314, -0.9697280773930611053 ) ) ;
#78003=CARTESIAN_POINT ( 'NONE',  ( 7.006866460164219212, 7.069099046480051385, -0.7998128361456281477 ) ) ;
#78014=CARTESIAN_POINT ( 'NONE',  ( 4.867013957625893283, 4.780530493426062399, 1.040834085586084257E-14 ) ) ;
#78015=CARTESIAN_POINT ( 'NONE',  ( -0.6823417656250003738, 2.530208333674753618, -1.181850606188749264 ) ) ;
#78016=CARTESIAN_POINT ( 'NONE',  ( 9.237182729612253951, 9.671134694169463586, 0.7998128361456462443 ) ) ;
#78018=CARTESIAN_POINT ( 'NONE',  ( -1.123270288250318494, 3.235197346350006331, -0.7749999999993562039 ) ) ;
#78023=CARTESIAN_POINT ( 'NONE',  ( 0.7499999999999885647, 1.816666666666688634, -1.299038105676652899 ) ) ;
#78024=CARTESIAN_POINT ( 'NONE',  ( 4.313465427442102929, 8.184126765324453601, 0.7998128361456462443 ) ) ;
#78025=CARTESIAN_POINT ( 'NONE',  ( -5.526920175865215334, 9.599823971818089774, 0.7998128361456481317 ) ) ;
#78030=CARTESIAN_POINT ( 'NONE',  ( -0.6823417656250212460, 2.801041667008084879, 1.181850606188767472 ) ) ;
#78032=CARTESIAN_POINT ( 'NONE',  ( 2.171277156482887882, 5.684907115872006145, -0.7998128361456291469 ) ) ;
#78038=CARTESIAN_POINT ( 'NONE',  ( -1.500000000000001332, 0.6812500006828161592, 0.000000000000000000 ) ) ;
#78040=CARTESIAN_POINT ( 'NONE',  ( -6.368579470117215813, 8.453095353268645695, 1.599625672291283607 ) ) ;
#78050=CARTESIAN_POINT ( 'NONE',  ( 5.286789834324991055, 8.255339675766103724, -1.199719254218452935 ) ) ;
#78054=CARTESIAN_POINT ( 'NONE',  ( 5.147291874682557555, 9.156924287104992288, 0.7998128361456462443 ) ) ;
#78060=CARTESIAN_POINT ( 'NONE',  ( -7.230575994789712801, 7.330093503543126054, 0.7998128361456341429 ) ) ;
#78061=CARTESIAN_POINT ( 'NONE',  ( 3.408985558832261731, 6.064568021024562938, 1.199719254218462483 ) ) ;
#78066=CARTESIAN_POINT ( 'NONE',  ( 4.124567353486244592, 7.428622122647839277, 0.6979301818166357974 ) ) ;
#78071=CARTESIAN_POINT ( 'NONE',  ( 4.217276354152451390, 3.814577256132954730, 1.214306433183764966E-14 ) ) ;
#78076=CARTESIAN_POINT ( 'NONE',  ( 8.758204044748010730, 9.320252261735261001, 0.7216878364870438212 ) ) ;
#78078=CARTESIAN_POINT ( 'NONE',  ( -5.576481253922474401, 5.400316305864651056, -0.7998128361456221525 ) ) ;
#78082=CARTESIAN_POINT ( 'NONE',  ( 8.471147050440139381, 8.777426401801974976, -0.7998128361456281477 ) ) ;
#78084=CARTESIAN_POINT ( 'NONE',  ( -5.045605722580076780, 9.038290442985410067, -0.7998128361456231517 ) ) ;
#78087=LINE ( 'NONE', #81292, #117433 ) ;
#78096=CARTESIAN_POINT ( 'NONE',  ( 1.419999999999989049, 6.200000000000045475, -2.579999999999995630 ) ) ;
#78097=CARTESIAN_POINT ( 'NONE',  ( -6.091691091241777656, 6.001394449403842479, 0.7998128361456341429 ) ) ;
#78100=CARTESIAN_POINT ( 'NONE',  ( 4.704316114261903436, 4.590716342834741504, 1.214306433183764966E-14 ) ) ;
#78104=CARTESIAN_POINT ( 'NONE',  ( 0.4644214298828999166, 7.369507887686750358, 4.459343850248959740 ) ) ;
#78105=CARTESIAN_POINT ( 'NONE',  ( -4.939248034080176097, 4.656877549381960080, 1.214306433183764966E-14 ) ) ;
#78108=CARTESIAN_POINT ( 'NONE',  ( 9.511208455186636712, 11.05516360492796935, 1.199719254218453823 ) ) ;
#78111=CARTESIAN_POINT ( 'NONE',  ( -7.877450944739929461, 9.149113176073413456, 1.199719254218462483 ) ) ;
#78112=CARTESIAN_POINT ( 'NONE',  ( 5.066996723205273057, 6.934582148538044777, 1.599625672291267398 ) ) ;
#78114=CARTESIAN_POINT ( 'NONE',  ( 5.508690485854129903, 5.321227076451600091, 1.040834085586084257E-14 ) ) ;
#78117=CARTESIAN_POINT ( 'NONE',  ( 1.364683531249986537, 1.176041667008082658, 0.7879004041258500513 ) ) ;
#78120=CARTESIAN_POINT ( 'NONE',  ( 6.887178846062110615, 9.058127958537705027, -1.443375672974057666 ) ) ;
#78123=CARTESIAN_POINT ( 'NONE',  ( -3.606105671554928893, 7.150947683548683820, 0.7216878364870122908 ) ) ;
#78127=ORIENTED_EDGE ( 'NONE', *, *, #168064, .T. ) ;
#78128=CARTESIAN_POINT ( 'NONE',  ( 9.531018800282598846, 12.14260790512831889, 1.443375672974076540 ) ) ;
#78137=CARTESIAN_POINT ( 'NONE',  ( -9.829825065107822724, 11.42688298316931572, 1.199719254218462483 ) ) ;
#78151=CARTESIAN_POINT ( 'NONE',  ( 1.499999999999987121, 1.827083334016151861, -0.8660254037844253849 ) ) ;
#78157=CARTESIAN_POINT ( 'NONE',  ( -0.7500000000000249800, -1.058333333333314030, 1.299038105676659116 ) ) ;
#78158=CARTESIAN_POINT ( 'NONE',  ( 8.239604668803105270, 10.63595808506888396, -1.599625672291268286 ) ) ;
#78163=CARTESIAN_POINT ( 'NONE',  ( 2.510230996824538430, 6.080353262937265413, 0.000000000000000000 ) ) ;
#78164=CARTESIAN_POINT ( 'NONE',  ( -7.049876689426121779, 7.327203680526343632, -0.7216878364870278340 ) ) ;
#78169=CARTESIAN_POINT ( 'NONE',  ( -6.368579470117215813, 8.453095353268645695, 1.599625672291283607 ) ) ;
#78172=CARTESIAN_POINT ( 'NONE',  ( 0.7499999999999885647, 1.347916667349485786, -1.299038105676652899 ) ) ;
#78179=CARTESIAN_POINT ( 'NONE',  ( -4.433153041544240835, 4.274359424664112339, 0.7216878364870317197 ) ) ;
#78186=CARTESIAN_POINT ( 'NONE',  ( -3.189213936345670852, 2.817530495244580102, -2.450448857954567572 ) ) ;
#78188=CARTESIAN_POINT ( 'NONE',  ( -9.154780037725563702, 11.70366268214508487, 1.599625672291281386 ) ) ;
#78189=CARTESIAN_POINT ( 'NONE',  ( 8.229962938695207342, 9.560377169021284871, 1.199719254218462483 ) ) ;
#78195=CARTESIAN_POINT ( 'NONE',  ( -8.667740277838301921, 9.006785167099828016, -0.7998128361456291469 ) ) ;
#78202=CARTESIAN_POINT ( 'NONE',  ( 3.493197133815315603, 7.227147089426516402, -0.7998128361456291469 ) ) ;
#78207=CARTESIAN_POINT ( 'NONE',  ( -8.435144125996554720, 12.99275191363802229, 0.7998128361456341429 ) ) ;
#78211=CARTESIAN_POINT ( 'NONE',  ( -5.176859992674639699, 6.655076503622660233, -1.423794717725470171 ) ) ;
#78220=CARTESIAN_POINT ( 'NONE',  ( 5.445571254183207088, 9.504916896522420444, -0.7998128361456281477 ) ) ;
#78229=CARTESIAN_POINT ( 'NONE',  ( 0.7499999999999867883, 0.09791666734948467621, -1.299038105676652899 ) ) ;
#78232=CARTESIAN_POINT ( 'NONE',  ( -4.157718419935214627, 7.512196061762048238, 0.8120497619437796466 ) ) ;
#78233=CARTESIAN_POINT ( 'NONE',  ( 3.673896439178918172, 6.269667698141953238, 1.082531754730558626 ) ) ;
#78242=CARTESIAN_POINT ( 'NONE',  ( 4.202664430556254160, 5.926194473780837413, 1.443375672974062551 ) ) ;
#78246=DIRECTION ( 'NONE',  ( 1.000000000000000000, 0.000000000000000000, 0.000000000000000000 ) ) ;
#78247=CARTESIAN_POINT ( 'NONE',  ( 9.103410076571945453, 12.70806329172093818, 1.199719254218450271 ) ) ;
#78256=CARTESIAN_POINT ( 'NONE',  ( -1.364683531250000748, -0.7406249996585803075, 0.000000000000000000 ) ) ;
#78260=CARTESIAN_POINT ( 'NONE',  ( -6.240830780992103755, 6.175390754112560110, 1.040834085586084257E-14 ) ) ;
#78263=CARTESIAN_POINT ( 'NONE',  ( 1.499999999999987566, -0.2249999999999821587, 0.000000000000000000 ) ) ;
#78265=CARTESIAN_POINT ( 'NONE',  ( 1.499999999999990896, 5.525000000000022560, 1.214306433183764966E-14 ) ) ;
#78270=CARTESIAN_POINT ( 'NONE',  ( 1.364683531249986537, -0.6364583329919177856, 0.7879004041258500513 ) ) ;
#78272=CARTESIAN_POINT ( 'NONE',  ( -7.167456763118792651, 11.51378332361394818, 0.000000000000000000 ) ) ;
#78279=CARTESIAN_POINT ( 'NONE',  ( -0.6823417656250246877, 0.6135416670080897639, 1.181850606188755259 ) ) ;
#78286=CARTESIAN_POINT ( 'NONE',  ( 8.270110514656037637, 8.750809809961280550, 0.7216878364870458196 ) ) ;
#78290=CARTESIAN_POINT ( 'NONE',  ( 1.499999999999989120, 4.327083334016148086, -0.8660254037844323793 ) ) ;
#78293=CARTESIAN_POINT ( 'NONE',  ( -3.066115294984855133, 6.728884944124295053, 0.7998128361456341429 ) ) ;
#78295=CARTESIAN_POINT ( 'NONE',  ( 6.656690234185433042, 7.828855363713562276, -1.082531754730543971 ) ) ;
#78296=CARTESIAN_POINT ( 'NONE',  ( -9.205623113554631587, 11.76297960394566466, 1.443375672974076540 ) ) ;
#78302=CARTESIAN_POINT ( 'NONE',  ( 10.56143847536557878, 11.42402576412244386, 0.000000000000000000 ) ) ;
#78303=CARTESIAN_POINT ( 'NONE',  ( 1.500000000000005329, 4.754166666666690411, 0.8660254037844431485 ) ) ;
#78317=EDGE_CURVE ( 'NONE', #98551, #97523, #51874, .T. ) ;
#78319=CARTESIAN_POINT ( 'NONE',  ( 7.242026607993941489, 11.60078147596829901, 0.7998128361456462443 ) ) ;
#78323=ADVANCED_FACE ( 'NONE', ( #149364 ), #22624, .T. ) ;
#78326=CARTESIAN_POINT ( 'NONE',  ( -1.402160292154681736E-14, -0.5531249996585814177, -1.575800808251665908 ) ) ;
#78327=CARTESIAN_POINT ( 'NONE',  ( 4.690757960648221037, 7.456006139856155457, 1.082531754730558626 ) ) ;
#78329=CARTESIAN_POINT ( 'NONE',  ( -8.514157279702027736, 10.95626946445095307, -1.443375672974059665 ) ) ;
#78334=CARTESIAN_POINT ( 'NONE',  ( -3.195971524519394702, 4.751719416737803847, -1.599625672291262513 ) ) ;
#78337=ORIENTED_EDGE ( 'NONE', *, *, #10652, .F. ) ;
#78347=CARTESIAN_POINT ( 'NONE',  ( 5.302928268938337020, 6.565392180301311775, -1.356678214699511775 ) ) ;
#78354=CARTESIAN_POINT ( 'NONE',  ( -8.242994207428740339, 9.679543332497402730, 1.082531754730558626 ) ) ;
#78360=CARTESIAN_POINT ( 'NONE',  ( 6.124532705071213279, 8.168374127381657246, -1.599625672291262513 ) ) ;
#78361=CARTESIAN_POINT ( 'NONE',  ( -3.086452525405351643, 6.752611712948207057, 0.7998128361456341429 ) ) ;
#78363=CARTESIAN_POINT ( 'NONE',  ( 3.623053363349855172, 5.249981562040033189, 1.599625672291267398 ) ) ;
#78365=CARTESIAN_POINT ( 'NONE',  ( -4.273844736805832767, 6.009238164405336313, 1.599625672291267398 ) ) ;
#78369=CARTESIAN_POINT ( 'NONE',  ( -4.497554271431319250, 6.270232621468402989, -1.599625672291256295 ) ) ;
#78372=CARTESIAN_POINT ( 'NONE',  ( 5.691725559638619814, 5.534767995866836543, 1.040834085586084257E-14 ) ) ;
#78373=CARTESIAN_POINT ( 'NONE',  ( 7.456094412511537151, 10.78619501698377370, 1.199719254218460707 ) ) ;
#78376=CARTESIAN_POINT ( 'NONE',  ( 4.972575192752072937, 6.823350471033509557, 1.425105271486303282 ) ) ;
#78377=CARTESIAN_POINT ( 'NONE',  ( 3.714570900464269076, 7.277490450609545469, 0.7216878364870298324 ) ) ;
#78385=CARTESIAN_POINT ( 'NONE',  ( 5.273758565591489145, 9.096542726591325234, -0.7216878364870267237 ) ) ;
#78386=CARTESIAN_POINT ( 'NONE',  ( -8.507905087775398556, 9.884643009614800135, 1.199719254218462483 ) ) ;
#78389=CARTESIAN_POINT ( 'NONE',  ( -8.971744963941075568, 11.49012176272984931, 1.599625672291269396 ) ) ;
#78390=CARTESIAN_POINT ( 'NONE',  ( -8.227100285394159940, 8.492705175914988303, 0.7998128361456602331 ) ) ;
#78395=CARTESIAN_POINT ( 'NONE',  ( 1.499999999998266054, 8.673756432004708472, -2.614717076620979963 ) ) ;
#78398=CARTESIAN_POINT ( 'NONE',  ( 8.055515824813896941, 12.54985222892493368, 0.7998128361456462443 ) ) ;
#78402=CARTESIAN_POINT ( 'NONE',  ( 4.695201269034174452, 4.372156323494968966, 1.214306433183764966E-14 ) ) ;
#78405=CARTESIAN_POINT ( 'NONE',  ( 1.499999999999991118, 5.285416667349480235, 0.8660254037844524744 ) ) ;
#78411=CARTESIAN_POINT ( 'NONE',  ( -1.201851678989727383E-14, 3.087500000000026112, -1.732050807568863648 ) ) ;
#78412=CARTESIAN_POINT ( 'NONE',  ( 5.473741331615251227, 7.409117525016355010, -1.599625672291262513 ) ) ;
#78416=CARTESIAN_POINT ( 'NONE',  ( 6.480434237652121787, 9.543961796360731498, 1.082531754730558626 ) ) ;
#78420=CARTESIAN_POINT ( 'NONE',  ( 9.077347539549325717, 10.54899253668443393, -1.199719254218446718 ) ) ;
#78422=CARTESIAN_POINT ( 'NONE',  ( -1.499999999999997780, 5.400000000000022560, 1.214306433183764966E-14 ) ) ;
#78423=CARTESIAN_POINT ( 'NONE',  ( -3.228813138348844536, 6.918699094715619502, 0.7998128361456341429 ) ) ;
#78424=CARTESIAN_POINT ( 'NONE',  ( 0.7499999999999920064, 5.014583334016150751, 1.299038105676669330 ) ) ;
#78425=CARTESIAN_POINT ( 'NONE',  ( 0.6823417656249882723, 1.676041667008083769, -1.181850606188749264 ) ) ;
#78430=CARTESIAN_POINT ( 'NONE',  ( 1.364683531249986537, -0.8447916663252468261, -0.7879004041258309554 ) ) ;
#78435=CARTESIAN_POINT ( 'NONE',  ( -2.277406616971334508, 5.600798786534425311, 1.040834085586084257E-14 ) ) ;
#78439=CARTESIAN_POINT ( 'NONE',  ( -6.307567778855718288, 8.381915046796901692, -1.599625672291263179 ) ) ;
#78442=CARTESIAN_POINT ( 'NONE',  ( 5.529027716274630855, 5.344953845275508542, 1.040834085586084257E-14 ) ) ;
#78446=AXIS2_PLACEMENT_3D ( 'NONE', #121565, #155051, #187537 ) ;
#78450=CARTESIAN_POINT ( 'NONE',  ( 8.211434591371064684, 12.73175745657494851, -0.7998128361456352531 ) ) ;
#78453=CARTESIAN_POINT ( 'NONE',  ( -5.042743069279040036, 7.970618449879118828, 1.199719254218464037 ) ) ;
#78457=CARTESIAN_POINT ( 'NONE',  ( 7.404724451357931336, 11.79059562655963056, 0.7998128361456462443 ) ) ;
#78459=CARTESIAN_POINT ( 'NONE',  ( 8.776205506747620788, 9.133327934160710981, -0.7998128361456221525 ) ) ;
#78462=CARTESIAN_POINT ( 'NONE',  ( -3.277320446201389181, 4.846626492033466072, 1.599625672291267398 ) ) ;
#78464=CARTESIAN_POINT ( 'NONE',  ( -7.528855374290365887, 7.678086112960552434, -0.7998128361456291469 ) ) ;
#78468=CARTESIAN_POINT ( 'NONE',  ( -6.016097364521681534, 6.072308155256833651, 0.6301904134648171896 ) ) ;
#78469=CARTESIAN_POINT ( 'NONE',  ( 0.6823417656249882723, -0.1572916663252488245, 1.181850606188755259 ) ) ;
#78472=CARTESIAN_POINT ( 'NONE',  ( 6.141480397310468575, 10.10888486359680982, 1.040834085586084257E-14 ) ) ;
#78491=CARTESIAN_POINT ( 'NONE',  ( 7.801827329660018684, 11.18955008699033726, 1.199719254218460707 ) ) ;
#78495=CARTESIAN_POINT ( 'NONE',  ( -4.298098390732130625, 4.973201863064262263, 1.199719254218462483 ) ) ;
#78496=CARTESIAN_POINT ( 'NONE',  ( -7.802881099864745984, 9.062115023719057305, -1.199719254218446718 ) ) ;
#78498=ORIENTED_EDGE ( 'NONE', *, *, #27529, .T. ) ;
#78501=CARTESIAN_POINT ( 'NONE',  ( 0.7499999999999902300, 3.847916667349481123, -1.299038105676658228 ) ) ;
#78502=CARTESIAN_POINT ( 'NONE',  ( 8.106885785967500979, 11.54545161934907682, 1.199719254218460707 ) ) ;
#78505=CARTESIAN_POINT ( 'NONE',  ( -9.040589502214116280, 9.441775928871617651, 0.7998128361456462443 ) ) ;
#78507=CARTESIAN_POINT ( 'NONE',  ( 1.364683531249988535, 3.613541667008086211, 0.7879004041258500513 ) ) ;
#78513=CARTESIAN_POINT ( 'NONE',  ( -9.666600336863641729, 10.38004793587015584, 1.040834085586084257E-14 ) ) ;
#78517=CARTESIAN_POINT ( 'NONE',  ( 1.364683531249988535, 3.217708333674748289, -0.7879004041258239610 ) ) ;
#78524=CARTESIAN_POINT ( 'NONE',  ( -0.6823417656249969321, 3.217708333674754062, -1.181850606188749264 ) ) ;
#78526=CARTESIAN_POINT ( 'NONE',  ( -3.927058049452637700, 7.733318157670055371, -0.7998128361456281477 ) ) ;
#78527=CARTESIAN_POINT ( 'NONE',  ( 7.772902139336337335, 7.962807338847539107, 0.7998128361456341429 ) ) ;
#78530=CARTESIAN_POINT ( 'NONE',  ( 1.364683531249990311, 3.946875000341417028, 1.214306433183764966E-14 ) ) ;
#78533=CARTESIAN_POINT ( 'NONE',  ( 0.6823417656249882723, -0.9072916663252494907, 1.181850606188755259 ) ) ;
#78535=CARTESIAN_POINT ( 'NONE',  ( -3.280709984826970516, 6.771319382366015383, 0.7216878364870317197 ) ) ;
#78538=CARTESIAN_POINT ( 'NONE',  ( 5.395781948558860286, 6.357795697149212444, -1.082531754730542195 ) ) ;
#78541=CARTESIAN_POINT ( 'NONE',  ( -8.199983978166823562, 8.461069484149769337, -0.7998128361456291469 ) ) ;
#78542=CARTESIAN_POINT ( 'NONE',  ( -9.842856333841300653, 10.58567993234409421, 0.7216878364870438212 ) ) ;
#78544=CARTESIAN_POINT ( 'NONE',  ( -1.364683531250010295, 5.530208333674751842, 0.7879004041258379498 ) ) ;
#78550=CARTESIAN_POINT ( 'NONE',  ( -6.033015167956805591, 8.061603667414825480, -1.443375672974058777 ) ) ;
#78552=CARTESIAN_POINT ( 'NONE',  ( 0.6823417656249882723, -0.8447916663252494907, 1.181850606188755259 ) ) ;
#78563=CARTESIAN_POINT ( 'NONE',  ( 1.499999999999985123, -0.7041666666666481778, -0.8660254037844323793 ) ) ;
#78564=CARTESIAN_POINT ( 'NONE',  ( 9.531018800282605952, 11.18223869082697597, 1.082531754730548412 ) ) ;
#78570=VERTEX_POINT ( 'NONE', #120137 ) ;
#78572=CARTESIAN_POINT ( 'NONE',  ( 5.612185521052973414, 8.634967976948757951, -1.199719254218440723 ) ) ;
#78573=CARTESIAN_POINT ( 'NONE',  ( -3.253066792275140173, 5.882662793374543675, 1.199719254218462483 ) ) ;
#78577=CARTESIAN_POINT ( 'NONE',  ( 1.364683531249986537, 1.967708333674750731, -0.7879004041258239610 ) ) ;
#78579=CARTESIAN_POINT ( 'NONE',  ( -9.158696461231359720, 10.64389961198009615, 1.199719254218462483 ) ) ;
#78584=DIRECTION ( 'NONE',  ( -5.578564026256490882E-16, -1.000000000000000000, -9.066213480720158442E-32 ) ) ;
#78595=CARTESIAN_POINT ( 'NONE',  ( 2.280056242076713424, 5.600610285695403867, 0.4779128307904490502 ) ) ;
#78598=CARTESIAN_POINT ( 'NONE',  ( 5.144429221381498607, 8.089252293998699272, -1.199719254218452047 ) ) ;
#78607=CARTESIAN_POINT ( 'NONE',  ( 8.666686507633574621, 11.13422023037111330, 1.599625672291281386 ) ) ;
#78609=CARTESIAN_POINT ( 'NONE',  ( 5.908535366263007127, 4.807949608181236734, 2.500000000000011102 ) ) ;
#78612=CARTESIAN_POINT ( 'NONE',  ( 8.536830278099042602, 13.11138575775759563, -0.7998128361456352531 ) ) ;
#78613=CARTESIAN_POINT ( 'NONE',  ( -0.5021762176675858003, 7.740673110510177146, 1.993154341637425331 ) ) ;
#78618=CARTESIAN_POINT ( 'NONE',  ( -9.381879110976678149, 11.00824238663667565, 1.082531754730558626 ) ) ;
#78624=CARTESIAN_POINT ( 'NONE',  ( 6.471319392424407901, 6.444294134116939077, 0.7998128361456341429 ) ) ;
#78630=CARTESIAN_POINT ( 'NONE',  ( 3.999292125906911188, 4.728557570721922509, 1.082531754730560403 ) ) ;
#78638=CARTESIAN_POINT ( 'NONE',  ( -5.585069213825653023, 8.603332285183535433, -1.199719254218440723 ) ) ;
#78639=CARTESIAN_POINT ( 'NONE',  ( -4.761938266897808525, 6.578680616179308771, 1.599625672291267398 ) ) ;
#78647=CARTESIAN_POINT ( 'NONE',  ( 5.612185521052973414, 8.634967976948757951, -1.199719254218440723 ) ) ;
#78661=CARTESIAN_POINT ( 'NONE',  ( -1.402160292154681736E-14, -0.2406249996585799189, -1.575800808251665908 ) ) ;
#78663=CARTESIAN_POINT ( 'NONE',  ( 4.029797971759831121, 5.724516938518342535, -1.599625672291255185 ) ) ;
#78666=CARTESIAN_POINT ( 'NONE',  ( -7.551528373131759508, 7.912463978182924684, 1.040834085586084257E-14 ) ) ;
#78668=CARTESIAN_POINT ( 'NONE',  ( 5.829642864196171281, 5.903597551091405826, 0.7216878364870317197 ) ) ;
#78669=CARTESIAN_POINT ( 'NONE',  ( -7.551528372687420720, 8.872833191965849409, 1.082531754730558626 ) ) ;
#78673=CARTESIAN_POINT ( 'NONE',  ( 5.880485940025228508, 7.883652901494672349, 1.599625672291267398 ) ) ;
#78678=CARTESIAN_POINT ( 'NONE',  ( -1.364683531249997417, 5.259375000341425022, 1.214306433183764966E-14 ) ) ;
#78684=CARTESIAN_POINT ( 'NONE',  ( 7.969495366734495434, 8.192166104145387706, 1.040834085586084257E-14 ) ) ;
#78687=CARTESIAN_POINT ( 'NONE',  ( -8.040148788103921973, 9.338927326664741457, 1.199719254218462483 ) ) ;
#78692=CARTESIAN_POINT ( 'NONE',  ( 8.911787042884274257, 9.291506392986812912, 0.7998128361456462443 ) ) ;
#78694=CARTESIAN_POINT ( 'NONE',  ( -5.879432169820529630, 10.01108796476595764, -0.7998128361456221525 ) ) ;
#78695=CARTESIAN_POINT ( 'NONE',  ( 3.619250341049045527, 3.172667246362654847, -2.499999999999995115 ) ) ;
#78696=CARTESIAN_POINT ( 'NONE',  ( 8.080296363620359301, 8.529359967086321603, 1.040834085586084257E-14 ) ) ;
#78697=CARTESIAN_POINT ( 'NONE',  ( 4.007117460063951420, 7.817974094756804604, -0.2064290434495383852 ) ) ;
#78698=CARTESIAN_POINT ( 'NONE',  ( -8.175203439360366531, 12.48156174598837787, 1.040834085586084257E-14 ) ) ;
#78701=CARTESIAN_POINT ( 'NONE',  ( 3.243620375240426235, 6.419334294643912031, -0.9047145305212719313 ) ) ;
#78703=CARTESIAN_POINT ( 'NONE',  ( 5.774883364416965037, 8.824782127540085952, -1.199719254218440723 ) ) ;
#78705=CARTESIAN_POINT ( 'NONE',  ( 4.635998460869027227, 7.496083073400806818, -1.199719254218452047 ) ) ;
#78706=CARTESIAN_POINT ( 'NONE',  ( -4.068573627943592008, 7.549288226164498461, -0.4708643921484123585 ) ) ;
#78707=CARTESIAN_POINT ( 'NONE',  ( 5.169736645512481132, 4.925780929386339935, 0.7998128361456341429 ) ) ;
#78709=CARTESIAN_POINT ( 'NONE',  ( -5.734735788900501952, 9.634349487118505806, 0.000000000000000000 ) ) ;
#78710=VERTEX_POINT ( 'NONE', #42330 ) ;
#78716=CARTESIAN_POINT ( 'NONE',  ( -5.443780329924999606, 6.294985656096041993, 1.034245658874383578 ) ) ;
#78718=CARTESIAN_POINT ( 'NONE',  ( -0.6823417656250003738, -0.4697916663252491021, -1.181850606188749264 ) ) ;
#78720=CARTESIAN_POINT ( 'NONE',  ( 3.877268743828258479, 7.467304601200877023, 0.7216878364870298324 ) ) ;
#78724=CARTESIAN_POINT ( 'NONE',  ( -8.093854517234044366, 11.42628545587295186, 1.082531754730549967 ) ) ;
#78730=CARTESIAN_POINT ( 'NONE',  ( -9.449669878600623463, 11.08733161553131197, -1.082531754730537976 ) ) ;
#78732=VERTEX_POINT ( 'NONE', #162466 ) ;
#78738=CARTESIAN_POINT ( 'NONE',  ( -8.975134502122321223, 9.573337795338607847, 1.040834085586084257E-14 ) ) ;
#78742=CARTESIAN_POINT ( 'NONE',  ( 0.6823417656249899377, 4.988541667008086655, -1.181850606188754593 ) ) ;
#78743=CARTESIAN_POINT ( 'NONE',  ( -1.001543065824772872E-14, 4.493750000682820378, 1.732050807568877637 ) ) ;
#78744=CARTESIAN_POINT ( 'NONE',  ( 5.440174215215161979, 6.465126095745926449, -1.288585324421805511 ) ) ;
#78746=CARTESIAN_POINT ( 'NONE',  ( -6.227272627378437342, 6.159572908229946187, -0.7998128361456291469 ) ) ;
#78750=CARTESIAN_POINT ( 'NONE',  ( -7.212047647465563038, 10.50147379109678880, -1.199719254218446718 ) ) ;
#78753=CARTESIAN_POINT ( 'NONE',  ( 4.286349120214771879, 8.152491073559232859, -0.7998128361456221525 ) ) ;
#78759=CARTESIAN_POINT ( 'NONE',  ( 9.271078113646423091, 9.710679308875986848, 1.040834085586084257E-14 ) ) ;
#78766=CARTESIAN_POINT ( 'NONE',  ( -7.104109303880803417, 8.350844278358124484, 1.082531754730549967 ) ) ;
#78769=CARTESIAN_POINT ( 'NONE',  ( 3.469446951953614189E-15, 6.120000000000021423, 1.214306433183764966E-14 ) ) ;
#78776=CARTESIAN_POINT ( 'NONE',  ( -8.371269781434001800, 11.85389961405997816, -1.199719254218446718 ) ) ;
#78778=CARTESIAN_POINT ( 'NONE',  ( 7.560643217915098191, 11.97250085420964716, -0.7998128361456291469 ) ) ;
#78779=CARTESIAN_POINT ( 'NONE',  ( 1.499999999999985123, -0.9541666666666493990, -0.8660254037844323793 ) ) ;
#78780=CARTESIAN_POINT ( 'NONE',  ( -7.492852449846775897, 11.89341162479659531, 0.000000000000000000 ) ) ;
#78783=CARTESIAN_POINT ( 'NONE',  ( 0.6823417656249899377, 3.092708333674754062, 1.181850606188765695 ) ) ;
#78784=CARTESIAN_POINT ( 'NONE',  ( 10.41229878561526512, 11.25002945941372623, -0.7216878364870257245 ) ) ;
#78786=CARTESIAN_POINT ( 'NONE',  ( 1.445103857048098739, 8.688264192037886247, -2.625611233228243968 ) ) ;
#78788=CARTESIAN_POINT ( 'NONE',  ( 9.531018800282609504, 10.22186947652563305, 0.7216878364870458196 ) ) ;
#78791=CARTESIAN_POINT ( 'NONE',  ( -6.941411460516810017, 8.161030127766803588, 1.082531754730549967 ) ) ;
#78792=CARTESIAN_POINT ( 'NONE',  ( -0.6823417656250246877, 0.5510416670080897639, 1.181850606188755259 ) ) ;
#78796=CARTESIAN_POINT ( 'NONE',  ( -7.320512876374914768, 10.62801655815766999, 1.199719254218453823 ) ) ;
#78797=CARTESIAN_POINT ( 'NONE',  ( -3.375617059678305054, 5.921675088724528635, 1.082531754730560403 ) ) ;
#78798=CARTESIAN_POINT ( 'NONE',  ( -0.6823417656250003738, 3.030208333674754062, -1.181850606188749264 ) ) ;
#78804=CARTESIAN_POINT ( 'NONE',  ( 9.585778300061798873, 11.14216175728232550, -1.199719254218440723 ) ) ;
#78811=CARTESIAN_POINT ( 'NONE',  ( 8.778014389843965759, 12.32843499053828928, 1.199719254218450271 ) ) ;
#78816=CARTESIAN_POINT ( 'NONE',  ( -1.554911173149791992, 8.692115300649543741, 2.503913477513654673 ) ) ;
#78819=CARTESIAN_POINT ( 'NONE',  ( -0.6823417656249969321, 5.030208333674755394, -1.181850606188749264 ) ) ;
#78824=CARTESIAN_POINT ( 'NONE',  ( 7.248805684800777804, 11.60869039890961218, 1.040834085586084257E-14 ) ) ;
#78827=CARTESIAN_POINT ( 'NONE',  ( -0.6823417656250212460, 3.551041667008085323, 1.181850606188767472 ) ) ;
#78829=CARTESIAN_POINT ( 'NONE',  ( -6.236387472606158333, 7.338502141871059870, -1.082531754730544860 ) ) ;
#78835=CARTESIAN_POINT ( 'NONE',  ( 3.623053363349855172, 5.249981562040033189, 1.599625672291267398 ) ) ;
#78838=CARTESIAN_POINT ( 'NONE',  ( 7.832860060393120882, 10.16142270859057462, 1.599625672291281386 ) ) ;
#78840=CARTESIAN_POINT ( 'NONE',  ( 3.733524485140474969, 7.410126666105378845, -2.499999999999779288 ) ) ;
#78845=CARTESIAN_POINT ( 'NONE',  ( -8.784793466650835825, 12.33634391347959713, 1.199719254218462483 ) ) ;
#78846=CARTESIAN_POINT ( 'NONE',  ( 6.765682348419287173, 7.852049813699357728, 1.199719254218462483 ) ) ;
#78848=CARTESIAN_POINT ( 'NONE',  ( 4.663641652976547647, 4.543262804668490418, 1.214306433183764966E-14 ) ) ;
#78849=CARTESIAN_POINT ( 'NONE',  ( 3.011882680530176604, 6.665613560593854459, 0.7998128361456341429 ) ) ;
#78859=CARTESIAN_POINT ( 'NONE',  ( -7.212574532790110737, 7.517017831117667193, -0.7216878364870278340 ) ) ;
#78860=CARTESIAN_POINT ( 'NONE',  ( 4.172158584703322681, 5.890604320285754980, -1.599625672291256295 ) ) ;
#78863=CARTESIAN_POINT ( 'NONE',  ( -6.645467848992654858, 10.90479625713344625, 0.7998128361456481317 ) ) ;
#78869=CARTESIAN_POINT ( 'NONE',  ( -9.110189153378817295, 12.71597221466224603, 1.199719254218462483 ) ) ;
#78872=CARTESIAN_POINT ( 'NONE',  ( 7.904567251967224095, 9.180748867838630645, 1.199719254218462483 ) ) ;
#78873=CARTESIAN_POINT ( 'NONE',  ( 4.788000803920411386, 8.737751371215816576, 1.040834085586084257E-14 ) ) ;
#78874=CARTESIAN_POINT ( 'NONE',  ( -2.456316247939677400, 8.205176026796131339, -2.499999999999995115 ) ) ;
#78885=CARTESIAN_POINT ( 'NONE',  ( -7.914208982075130905, 10.25632978388623684, -1.599625672291263179 ) ) ;
#78889=CARTESIAN_POINT ( 'NONE',  ( 5.802526556968819804, 9.713438716531550554, -0.7216878364870267237 ) ) ;
#78891=LINE ( 'NONE', #189459, #112438 ) ;
#78892=CARTESIAN_POINT ( 'NONE',  ( -1.500000000000001332, -1.099999999999982991, -2.579999999999989413 ) ) ;
#78894=CARTESIAN_POINT ( 'NONE',  ( -6.684333426737305572, 7.757142738403693727, -1.199719254218446718 ) ) ;
#78904=CARTESIAN_POINT ( 'NONE',  ( -0.6823417656249969321, 4.280208333674755394, -1.181850606188749264 ) ) ;
#78906=CARTESIAN_POINT ( 'NONE',  ( 7.507464373665139412, 9.781794407407920389, 1.599625672291281386 ) ) ;
#78908=CARTESIAN_POINT ( 'NONE',  ( -2.819732761962332024, 6.233512622357263666, -0.7216878364870267237 ) ) ;
#78909=CARTESIAN_POINT ( 'NONE',  ( -4.948362878863562742, 5.835806782504650236, 1.082531754730558626 ) ) ;
#78918=CARTESIAN_POINT ( 'NONE',  ( 2.361091307074211887, 5.906356958228550447, 0.7998128361456462443 ) ) ;
#78926=CARTESIAN_POINT ( 'NONE',  ( 4.216749469050096621, 4.878294787768598262, -1.199719254218452047 ) ) ;
#78931=CARTESIAN_POINT ( 'NONE',  ( 1.364683531249990311, 4.196875000341417028, 1.214306433183764966E-14 ) ) ;
#78936=CARTESIAN_POINT ( 'NONE',  ( 4.476163270806094552, 8.373940915915776273, 0.7998128361456462443 ) ) ;
#78940=CARTESIAN_POINT ( 'NONE',  ( -5.057354993097396445, 5.859001232490445688, -1.199719254218446718 ) ) ;
#78941=CARTESIAN_POINT ( 'NONE',  ( 0.7499999999999902300, 3.816666666666690411, -1.299038105676658228 ) ) ;
#78943=CARTESIAN_POINT ( 'NONE',  ( -3.411848212133334446, 7.132240014130862171, 0.7998128361456341429 ) ) ;
#78949=CARTESIAN_POINT ( 'NONE',  ( -1.364683531250010295, 4.280208333674753618, 0.7879004041258379498 ) ) ;
#78952=CARTESIAN_POINT ( 'NONE',  ( -4.785665035943912571, 4.685623418130398399, 1.214306433183764966E-14 ) ) ;
#78958=CARTESIAN_POINT ( 'NONE',  ( 5.366329872910639232, 5.155139694684188534, 1.040834085586084257E-14 ) ) ;
#78961=CARTESIAN_POINT ( 'NONE',  ( 0.08113548435146850091, 6.430127061359857343, -3.206836081813071004 ) ) ;
#78962=CARTESIAN_POINT ( 'NONE',  ( -1.364683531250012516, 3.551041667008086211, -0.7879004041258300672 ) ) ;
#78967=CARTESIAN_POINT ( 'NONE',  ( 0.6823417656249882723, -0.2614583329919109578, -1.181850606188749264 ) ) ;
#78968=CARTESIAN_POINT ( 'NONE',  ( -4.270528892807586629, 7.372556535914950082, -0.9884938994864488349 ) ) ;
#78970=CARTESIAN_POINT ( 'NONE',  ( -8.448702279610222021, 13.00856975952063088, 1.040834085586084257E-14 ) ) ;
#78971=CARTESIAN_POINT ( 'NONE',  ( -5.382223794500835545, 8.262716279350872384, -1.082531754730543971 ) ) ;
#78975=CARTESIAN_POINT ( 'NONE',  ( -1.364683531250010295, 5.030208333674757171, 0.7879004041258379498 ) ) ;
#78984=CARTESIAN_POINT ( 'NONE',  ( -6.087247782411500552, 7.164505836643929371, 1.082531754730549967 ) ) ;
#78985=CARTESIAN_POINT ( 'NONE',  ( 2.200495758195375906, 5.718995484536574025, -0.2758893754505519214 ) ) ;
#78991=CARTESIAN_POINT ( 'NONE',  ( -6.033015167956810920, 7.101234453113482559, -1.082531754730543083 ) ) ;
#78993=CARTESIAN_POINT ( 'NONE',  ( -4.663391507278085157, 5.284333467198953471, 1.153445959906941320 ) ) ;
#79000=ORIENTED_EDGE ( 'NONE', *, *, #81687, .T. ) ;
#79002=CARTESIAN_POINT ( 'NONE',  ( 4.037162115432598064, 7.757183989314783368, -0.4293979441572001177 ) ) ;
#79003=CARTESIAN_POINT ( 'NONE',  ( -5.091250377131585125, 5.898545847196970726, 1.199719254218450271 ) ) ;
#79006=CARTESIAN_POINT ( 'NONE',  ( 1.499999999999989120, 1.025000000000019007, 0.000000000000000000 ) ) ;
#79009=CARTESIAN_POINT ( 'NONE',  ( 8.920901888111997025, 10.47043562662792304, 1.082531754730549967 ) ) ;
#79010=CARTESIAN_POINT ( 'NONE',  ( 5.849453209292126310, 8.911780279894442103, 1.199719254218462483 ) ) ;
#79014=DIRECTION ( 'NONE',  ( 0.1774649537764392826, 0.000000000000000000, 0.9841271209458288816 ) ) ;
#79015=CARTESIAN_POINT ( 'NONE',  ( 6.654354466208897811, 6.657835053532175529, 0.7998128361456341429 ) ) ;
#79016=CARTESIAN_POINT ( 'NONE',  ( -0.1471985351163795641, 7.029189141431414711, -1.995741298138918207 ) ) ;
#79024=CARTESIAN_POINT ( 'NONE',  ( -3.118012141462980669, 6.581505231774690046, 0.7216878364870317197 ) ) ;
#79027=CARTESIAN_POINT ( 'NONE',  ( 3.600749563572586798, 3.160087278257122989, -2.499999999999995115 ) ) ;
#79030=CARTESIAN_POINT ( 'NONE',  ( -1.364683531250012516, 3.738541667008087099, -0.7879004041258300672 ) ) ;
#79031=CARTESIAN_POINT ( 'NONE',  ( 9.381879110532285182, 10.04787317181692075, 0.000000000000000000 ) ) ;
#79032=CARTESIAN_POINT ( 'NONE',  ( -7.400052914960538963, 7.527816577075747695, 1.040834085586084257E-14 ) ) ;
#79036=CARTESIAN_POINT ( 'NONE',  ( 6.844168616800228477, 6.879284895888727824, -0.7998128361456281477 ) ) ;
#79037=CARTESIAN_POINT ( 'NONE',  ( -6.144869935491728441, 8.192100896205577243, -1.599625672291263179 ) ) ;
#79041=CARTESIAN_POINT ( 'NONE',  ( 1.499999999999987121, 0.5770833340161539704, -0.8660254037844253849 ) ) ;
#79044=CARTESIAN_POINT ( 'NONE',  ( 6.805829924380108586, 8.963220883242035697, 1.443375672974076540 ) ) ;
#79047=CARTESIAN_POINT ( 'NONE',  ( -1.364683531250012516, 1.842708333674749843, 0.7879004041258379498 ) ) ;
#79049=CARTESIAN_POINT ( 'NONE',  ( 4.785665035499516051, 8.527100274817353665, -0.7216878364870207285 ) ) ;
#79051=CARTESIAN_POINT ( 'NONE',  ( -4.446711195602264688, 4.290177271065136466, -0.7216878364870207285 ) ) ;
#79053=CARTESIAN_POINT ( 'NONE',  ( 1.364683531249988535, 5.155208333674749177, -0.7879004041258300672 ) ) ;
#79058=CARTESIAN_POINT ( 'NONE',  ( -4.351531800032816477, 7.393666969396889499, -1.175081553336376317 ) ) ;
#79063=VECTOR ( 'NONE', #145015, 1000.000000000000000 ) ;
#79065=CARTESIAN_POINT ( 'NONE',  ( 6.819914962873951936, 7.915321197229798322, -1.199719254218446718 ) ) ;
#79068=CARTESIAN_POINT ( 'NONE',  ( 5.169736645512481132, 4.925780929386339935, 0.7998128361456341429 ) ) ;
#79077=CARTESIAN_POINT ( 'NONE',  ( 6.493992391265805075, 6.678671999339316656, 1.040834085586084257E-14 ) ) ;
#79078=CARTESIAN_POINT ( 'NONE',  ( 0.6823417656249899377, 1.905208333674752952, 1.181850606188755259 ) ) ;
#79079=CARTESIAN_POINT ( 'NONE',  ( 7.944187942603509356, 11.35563746875774882, 1.199719254218460707 ) ) ;
#79086=CARTESIAN_POINT ( 'NONE',  ( -1.500000000000013101, 1.879166666666692187, -0.8660254037844313801 ) ) ;
#79087=CARTESIAN_POINT ( 'NONE',  ( 4.788000803920411386, 8.737751371215816576, 1.040834085586084257E-14 ) ) ;
#79088=CARTESIAN_POINT ( 'NONE',  ( -6.039267359883488950, 9.133230122250985517, 1.199719254218452047 ) ) ;
#79092=CARTESIAN_POINT ( 'NONE',  ( -1.201851678989727383E-14, 2.071875000341422801, 1.575800808251672791 ) ) ;
#79093=CARTESIAN_POINT ( 'NONE',  ( 1.499999999999989120, 3.254166666666690855, 0.8660254037844524744 ) ) ;
#79095=CARTESIAN_POINT ( 'NONE',  ( 4.844340958784499662, 4.546152628203684820, 0.7998128361456341429 ) ) ;
#79101=CARTESIAN_POINT ( 'NONE',  ( -1.500000000000001332, 0.1812500006828157706, 0.000000000000000000 ) ) ;
#79103=CARTESIAN_POINT ( 'NONE',  ( -6.181627972826976958, 9.299317504018391745, 1.199719254218452047 ) ) ;
#79104=CARTESIAN_POINT ( 'NONE',  ( -2.657034918598338180, 6.043698471765932112, -0.7216878364870267237 ) ) ;
#79112=CARTESIAN_POINT ( 'NONE',  ( 5.880485940025228508, 7.883652901494672349, 1.599625672291267398 ) ) ;
#79115=DIRECTION ( 'NONE',  ( 1.000000000000000000, 0.000000000000000000, 0.000000000000000000 ) ) ;
#79118=CARTESIAN_POINT ( 'NONE',  ( 6.063521013809720195, 8.097193820909906137, 1.599625672291281386 ) ) ;
#79119=EDGE_LOOP ( 'NONE', ( #137193, #210067, #130624, #30627, #136521, #190684 ) ) ;
#79123=CARTESIAN_POINT ( 'NONE',  ( -6.398558430645608475, 9.552403038140164782, -1.199719254218440723 ) ) ;
#79125=CARTESIAN_POINT ( 'NONE',  ( 2.693266070609028784, 6.293894182352508970, 0.000000000000000000 ) ) ;
#79130=CARTESIAN_POINT ( 'NONE',  ( 4.301718403444327876, 7.219878030919558043, 0.9872997725082887088 ) ) ;
#79140=FACE_OUTER_BOUND ( 'NONE', #139697, .T. ) ;
#79141=CARTESIAN_POINT ( 'NONE',  ( 8.934460041725669655, 9.525884258209195821, 1.040834085586084257E-14 ) ) ;
#79143=CARTESIAN_POINT ( 'NONE',  ( -5.413783410558481002, 5.210502155273325720, -0.7998128361456221525 ) ) ;
#79148=CARTESIAN_POINT ( 'NONE',  ( -7.718669524881690336, 7.899535955317097624, 0.7998128361456462443 ) ) ;
#79165=CARTESIAN_POINT ( 'NONE',  ( -5.576481253922474401, 5.400316305864651056, -0.7998128361456221525 ) ) ;
#79168=CARTESIAN_POINT ( 'NONE',  ( 3.551873057100283226, 6.127307085716883428, 1.082531754730558626 ) ) ;
#79171=DIRECTION ( 'NONE',  ( 0.000000000000000000, 8.546850786086437571E-32, 1.000000000000000000 ) ) ;
#79173=CARTESIAN_POINT ( 'NONE',  ( -4.081167932913447594, 4.720116328942494555, -1.199719254218452047 ) ) ;
#79174=CARTESIAN_POINT ( 'NONE',  ( -4.277761160311629673, 4.949475094240346706, 1.199719254218462483 ) ) ;
#79176=B_SPLINE_CURVE_WITH_KNOTS ( 'NONE', 3,
 ( #46189, #96013, #63486, #129641, #195627, #32049, #97077, #113376, #82914, #99187 ),
 .UNSPECIFIED., .F., .F.,
 ( 4, 3, 3, 4 ),
 ( 1.563658610346436624E-18, 4.502046072369090049E-05, 9.004093402560554187E-05, 0.0001800865003196811215 ),
 .UNSPECIFIED. ) ;
#79178=CARTESIAN_POINT ( 'NONE',  ( 8.378048858240820351, 11.86180853700128601, -1.199719254218446718 ) ) ;
#79182=CARTESIAN_POINT ( 'NONE',  ( -8.202846631467911820, 9.528741477256060577, 1.199719254218462483 ) ) ;
#79183=CARTESIAN_POINT ( 'NONE',  ( 4.476163270806094552, 8.373940915915776273, 0.7998128361456462443 ) ) ;
#79185=CARTESIAN_POINT ( 'NONE',  ( 4.172158584703322681, 5.890604320285754980, -1.599625672291256517 ) ) ;
#79187=CARTESIAN_POINT ( 'NONE',  ( -1.420000000000021911, 6.280000000000042881, 2.873333333333347728 ) ) ;
#79188=CARTESIAN_POINT ( 'NONE',  ( -0.6823417656250003738, 0.7802083336747520637, -1.181850606188749264 ) ) ;
#79189=B_SPLINE_CURVE_WITH_KNOTS ( 'NONE', 3,
 ( #66640, #132785, #1649, #77867, #131735, #115497, #51508, #48334 ),
 .UNSPECIFIED., .F., .F.,
 ( 4, 2, 2, 4 ),
 ( 0.000000000000000000, 0.001499836411158092650, 0.002999672822316185299, 0.005999345644632373201 ),
 .UNSPECIFIED. ) ;
#79192=CARTESIAN_POINT ( 'NONE',  ( 8.270110514656037637, 8.750809809961280550, 0.7216878364870458196 ) ) ;
#79200=DIRECTION ( 'NONE',  ( 1.000000000000000000, -7.387867266669436732E-31, 0.000000000000000000 ) ) ;
#79224=CARTESIAN_POINT ( 'NONE',  ( -0.7500000000000006661, 1.139583334016154526, -1.299038105676652011 ) ) ;
#79228=ORIENTED_EDGE ( 'NONE', *, *, #167641, .F. ) ;
#79230=CARTESIAN_POINT ( 'NONE',  ( 1.499999999999985123, -0.7041666666666481778, -0.8660254037844323793 ) ) ;
#79231=CARTESIAN_POINT ( 'NONE',  ( 9.426996880203592610, 9.892584536526015881, -0.7998128361456281477 ) ) ;
#79236=CARTESIAN_POINT ( 'NONE',  ( 3.009020027229115879, 5.597941567487558778, -1.199719254218446718 ) ) ;
#79237=CARTESIAN_POINT ( 'NONE',  ( -5.097502569058210753, 7.930541516334467467, -1.082531754730549967 ) ) ;
#79242=CARTESIAN_POINT ( 'NONE',  ( -7.379715684540041565, 7.504089808251839244, 1.040834085586084257E-14 ) ) ;
#79245=CARTESIAN_POINT ( 'NONE',  ( -1.499999999999997780, 1.931250000682817269, 0.000000000000000000 ) ) ;
#79248=EDGE_CURVE ( 'NONE', #187417, #164674, #163378, .T. ) ;
#79253=CARTESIAN_POINT ( 'NONE',  ( -3.267151830768959098, 4.834763107362302748, -1.443375672974058777 ) ) ;
#79257=CARTESIAN_POINT ( 'NONE',  ( 4.553433815925461481, 6.963525196941225737, 1.181321538200299281 ) ) ;
#79262=CARTESIAN_POINT ( 'NONE',  ( -9.398826802771548472, 11.98838390803207865, -1.599625672291263179 ) ) ;
#79263=CARTESIAN_POINT ( 'NONE',  ( 7.365103760721646076, 9.615707025640515937, 1.599625672291281386 ) ) ;
#79270=CARTESIAN_POINT ( 'NONE',  ( -7.995557903757128493, 10.35123685918189729, 1.599625672291295375 ) ) ;
#79275=CARTESIAN_POINT ( 'NONE',  ( 4.029797971759831121, 5.724516938518342535, -1.599625672291255185 ) ) ;
#79280=CARTESIAN_POINT ( 'NONE',  ( -8.272446282632566650, 12.80293776304669962, 0.7998128361456481317 ) ) ;
#79283=CARTESIAN_POINT ( 'NONE',  ( -6.007394967034264788, 6.077829431587280062, -0.6506939886842719734 ) ) ;
#79291=CARTESIAN_POINT ( 'NONE',  ( 5.472687561410540802, 9.536552588287639409, 0.7998128361456462443 ) ) ;
#79293=ORIENTED_EDGE ( 'NONE', *, *, #104706, .F. ) ;
#79298=EDGE_CURVE ( 'NONE', #16779, #178259, #27060, .T. ) ;
#79302=CARTESIAN_POINT ( 'NONE',  ( -0.7500000000000249800, -0.02708333265051543481, 1.299038105676659116 ) ) ;
#79306=CARTESIAN_POINT ( 'NONE',  ( 4.241003122976366058, 3.842258486427521103, -0.7998128361456211532 ) ) ;
#79308=CARTESIAN_POINT ( 'NONE',  ( -4.295235737431041478, 3.905529869957963029, -0.7998128361456221525 ) ) ;
#79315=CARTESIAN_POINT ( 'NONE',  ( 3.524756749872944628, 7.056040608253000279, -0.7216878364870267237 ) ) ;
#79318=CARTESIAN_POINT ( 'NONE',  ( -1.001543065824772872E-14, 5.634375000341415252, 1.575800808251672791 ) ) ;
#79320=CARTESIAN_POINT ( 'NONE',  ( 4.338245966248566177, 4.163634503485842409, 1.214306433183764966E-14 ) ) ;
#79329=CARTESIAN_POINT ( 'NONE',  ( -1.402160292154681736E-14, -0.8031249996585825279, -1.575800808251665908 ) ) ;
#79333=CARTESIAN_POINT ( 'NONE',  ( -6.067437437315529536, 7.037430750744921859, 1.199719254218450271 ) ) ;
#79338=CARTESIAN_POINT ( 'NONE',  ( -1.500000000000011324, 5.170833333333356485, 0.8660254037844403729 ) ) ;
#79347=CARTESIAN_POINT ( 'NONE',  ( 1.364683531249990311, 5.676041667008088432, 0.7879004041258500513 ) ) ;
#79349=CARTESIAN_POINT ( 'NONE',  ( 7.284808609244363353, 7.393364887073558656, 0.7998128361456341429 ) ) ;
#79350=CARTESIAN_POINT ( 'NONE',  ( -9.013473194986783454, 9.410140237106395134, -0.7998128361456291469 ) ) ;
#79353=CARTESIAN_POINT ( 'NONE',  ( 0.9999999999999833467, 9.200000000000018829, -0.3999999999999961919 ) ) ;
#79357=CARTESIAN_POINT ( 'NONE',  ( -1.500000000000011324, 5.670833333333358262, 0.8660254037844403729 ) ) ;
#79364=CARTESIAN_POINT ( 'NONE',  ( 7.944714827928056167, 8.371181508778631652, 0.7216878364870458196 ) ) ;
#79368=CARTESIAN_POINT ( 'NONE',  ( -1.201851678989727383E-14, 4.618750000682821266, -1.732050807568863648 ) ) ;
#79370=CARTESIAN_POINT ( 'NONE',  ( -2.930533758848195447, 6.570706485298192234, -0.7998128361456281477 ) ) ;
#79371=CARTESIAN_POINT ( 'NONE',  ( 6.033015167956792268, 8.061603667414825480, -1.443375672974057666 ) ) ;
#79372=CARTESIAN_POINT ( 'NONE',  ( -9.124274191872636663, 11.66807252865000244, -1.443375672974058777 ) ) ;
#79378=CARTESIAN_POINT ( 'NONE',  ( 9.951321562750607086, 11.67259191370631477, -1.082531754730537088 ) ) ;
#79380=CARTESIAN_POINT ( 'NONE',  ( 3.680148631105580215, 6.380924938676771241, -1.199719254218446718 ) ) ;
#79381=DIRECTION ( 'NONE',  ( 0.000000000000000000, 1.000000000000000000, 0.000000000000000000 ) ) ;
#79383=ORIENTED_EDGE ( 'NONE', *, *, #202081, .F. ) ;
#79394=CARTESIAN_POINT ( 'NONE',  ( 9.264299036839600987, 9.702770385934682551, -0.7998128361456281477 ) ) ;
#79398=CARTESIAN_POINT ( 'NONE',  ( 1.364683531249988757, -0.3656249996585800299, 0.000000000000000000 ) ) ;
#79399=CARTESIAN_POINT ( 'NONE',  ( 4.202664430556241726, 7.846932902383524144, 0.7216878364870298324 ) ) ;
#79401=CARTESIAN_POINT ( 'NONE',  ( -8.893785580884703279, 10.43879993486270585, 1.082531754730558626 ) ) ;
#79406=CARTESIAN_POINT ( 'NONE',  ( -4.416205349749324327, 6.175325546172740765, 1.599625672291267398 ) ) ;
#79421=CARTESIAN_POINT ( 'NONE',  ( 4.825890400613210396, 6.946991693042408045, -1.413043630229819048 ) ) ;
#79426=DIRECTION ( 'NONE',  ( 5.578564026256504688E-16, 1.000000000000000000, 9.066213480720158442E-32 ) ) ;
#79429=CARTESIAN_POINT ( 'NONE',  ( -7.863365906246061243, 10.19701286208565705, -1.443375672974059665 ) ) ;
#79433=CARTESIAN_POINT ( 'NONE',  ( 5.829115978871627135, 8.888053511070525659, 1.199719254218462483 ) ) ;
#79434=CARTESIAN_POINT ( 'NONE',  ( -5.271422797614988554, 5.044414773505913274, -0.7998128361456221525 ) ) ;
#79435=CARTESIAN_POINT ( 'NONE',  ( 2.920892028740289081, 5.495125569250587816, 1.199719254218452047 ) ) ;
#79437=CARTESIAN_POINT ( 'NONE',  ( -5.220052836461385404, 6.048815383081766583, -1.199719254218446718 ) ) ;
#79441=CARTESIAN_POINT ( 'NONE',  ( -4.985647801523292344, 6.839675073242382553, -1.599625672291256295 ) ) ;
#79444=CARTESIAN_POINT ( 'NONE',  ( 8.751951852821344247, 10.16936423550178503, -1.199719254218446718 ) ) ;
#79445=DIRECTION ( 'NONE',  ( 0.000000000000000000, 8.546850786086437571E-32, 1.000000000000000000 ) ) ;
#79447=CARTESIAN_POINT ( 'NONE',  ( 5.239055555121258756, 6.613325079961110298, 1.380154382352281495 ) ) ;
#79448=CARTESIAN_POINT ( 'NONE',  ( 4.039966587192250103, 7.657118751792200584, 0.7216878364870298324 ) ) ;
#79456=CARTESIAN_POINT ( 'NONE',  ( 6.249945625775433555, 10.23542763013927726, -0.7216878364870267237 ) ) ;
#79460=CARTESIAN_POINT ( 'NONE',  ( -9.646789991323334590, 11.21334206375407305, 1.199719254218462483 ) ) ;
#79461=CARTESIAN_POINT ( 'NONE',  ( -7.901704598666176693, 8.113076874732334076, 0.7998128361456602331 ) ) ;
#79466=CARTESIAN_POINT ( 'NONE',  ( 1.558973042058037439, 8.694236233170199668, -2.499999999999989786 ) ) ;
#79469=CARTESIAN_POINT ( 'NONE',  ( 7.391166297744269365, 11.77477778067701664, 1.040834085586084257E-14 ) ) ;
#79473=CARTESIAN_POINT ( 'NONE',  ( 2.672928840188529609, 6.270167413528593414, 0.000000000000000000 ) ) ;
#79476=CARTESIAN_POINT ( 'NONE',  ( -3.476130333331279854, 6.301985902010497576, 1.046962579147314498 ) ) ;
#79482=CARTESIAN_POINT ( 'NONE',  ( 1.499999999999987121, 3.045833333333353377, -0.8660254037844262731 ) ) ;
#79483=CARTESIAN_POINT ( 'NONE',  ( 6.322179702674084467, 6.270297829408224111, 1.040834085586084257E-14 ) ) ;
#79486=CARTESIAN_POINT ( 'NONE',  ( 8.595506201384020883, 9.130438111143927671, 0.7216878364870438212 ) ) ;
#79490=CARTESIAN_POINT ( 'NONE',  ( -3.023105066167326882, 5.702484939155337607, -7.499999999999997335 ) ) ;
#79493=CARTESIAN_POINT ( 'NONE',  ( -2.930533758848195447, 6.570706485298192234, -0.7998128361456281477 ) ) ;
#79494=CARTESIAN_POINT ( 'NONE',  ( -0.7500000000000215383, 4.972916667349482012, 1.299038105676671107 ) ) ;
#79495=CARTESIAN_POINT ( 'NONE',  ( -0.6823417656250003738, 1.217708333674752286, -1.181850606188749264 ) ) ;
#79499=CARTESIAN_POINT ( 'NONE',  ( 3.334415713957098681, 5.977569868670206787, -1.199719254218446718 ) ) ;
#79502=CARTESIAN_POINT ( 'NONE',  ( -1.001543065824772872E-14, 5.134375000341421469, 1.575800808251672791 ) ) ;
#79504=CARTESIAN_POINT ( 'NONE',  ( 4.108200496220536735, 7.684552599041165166, 0.7063325572433389876 ) ) ;
#79511=CARTESIAN_POINT ( 'NONE',  ( -6.877010230629689858, 9.046264573866535486, 1.599625672291283607 ) ) ;
#79513=ADVANCED_FACE ( 'NONE', ( #14078 ), #48751, .T. ) ;
#79515=CARTESIAN_POINT ( 'NONE',  ( 5.192936529234042808, 6.017179691316550283, -1.199719254218452047 ) ) ;
#79522=CARTESIAN_POINT ( 'NONE',  ( 9.694243528971124846, 11.26870452434320491, 1.199719254218450271 ) ) ;
#79525=CARTESIAN_POINT ( 'NONE',  ( -5.362413449404877852, 6.214902764849178141, -1.199719254218446718 ) ) ;
#79529=CARTESIAN_POINT ( 'NONE',  ( 8.041957671200231417, 12.53403438304231976, 1.040834085586084257E-14 ) ) ;
#79531=CARTESIAN_POINT ( 'NONE',  ( 7.670162217029129259, 9.971608557999250166, 1.599625672291281386 ) ) ;
#79532=CARTESIAN_POINT ( 'NONE',  ( 4.893239572183122554, 4.893064124118063241, -0.6979708156788643203 ) ) ;
#79534=CARTESIAN_POINT ( 'NONE',  ( -9.991996023591624976, 10.75967623705280296, 1.040834085586084257E-14 ) ) ;
#79535=CARTESIAN_POINT ( 'NONE',  ( -7.369020184227459858, 8.555943955475521889, 1.199719254218450271 ) ) ;
#79539=CARTESIAN_POINT ( 'NONE',  ( -6.113138475847556208, 6.011394290285472231, -0.2943476003282770037 ) ) ;
#79540=CARTESIAN_POINT ( 'NONE',  ( 1.364683531249988757, 0.8843750003414210248, 0.000000000000000000 ) ) ;
#79543=CARTESIAN_POINT ( 'NONE',  ( 6.317736394288122170, 10.31451686007074997, 0.7216878364870438212 ) ) ;
#79560=CARTESIAN_POINT ( 'NONE',  ( 10.24726517383036928, 10.84956421242393887, 0.000000000000000000 ) ) ;
#79564=CARTESIAN_POINT ( 'NONE',  ( -4.029797971759847997, 5.724516938518342535, -1.599625672291256295 ) ) ;
#79565=CARTESIAN_POINT ( 'NONE',  ( -8.342344591110322227, 8.627156865917170236, -0.7998128361456291469 ) ) ;
#79571=CARTESIAN_POINT ( 'NONE',  ( -1.499999999999997780, 4.681250000682819490, 1.214306433183764966E-14 ) ) ;
#79572=CARTESIAN_POINT ( 'NONE',  ( 7.944187942603509356, 11.35563746875774882, 1.199719254218460707 ) ) ;
#79575=CIRCLE ( 'NONE', #183314, 0.08000000000000004330 ) ;
#79576=CARTESIAN_POINT ( 'NONE',  ( -7.365103760721662951, 9.615707025640515937, 1.599625672291295375 ) ) ;
#79578=CARTESIAN_POINT ( 'NONE',  ( -0.6823417656250212460, 3.051041667008084879, 1.181850606188767472 ) ) ;
#79581=CARTESIAN_POINT ( 'NONE',  ( -3.046854503058780139, 2.800000000000024691, -2.500000000000000444 ) ) ;
#79583=CARTESIAN_POINT ( 'NONE',  ( -9.164948653157999559, 10.75515685251491504, -1.082531754730539753 ) ) ;
#79587=CARTESIAN_POINT ( 'NONE',  ( -1.201851678989727383E-14, 1.884375000341422135, 1.575800808251672791 ) ) ;
#79595=CARTESIAN_POINT ( 'NONE',  ( 0.6823417656249899377, 3.092708333674754062, 1.181850606188765695 ) ) ;
#79597=CARTESIAN_POINT ( 'NONE',  ( -5.087333953625788219, 6.958308917361963886, 1.599625672291267398 ) ) ;
#79598=CARTESIAN_POINT ( 'NONE',  ( 7.949158136313996259, 8.168439335321471262, 1.040834085586084257E-14 ) ) ;
#79601=CARTESIAN_POINT ( 'NONE',  ( -1.364683531250012516, 2.551041667008089320, -0.7879004041258289570 ) ) ;
#79604=CARTESIAN_POINT ( 'NONE',  ( -1.364683531250014514, -0.9697916663252473812, 0.7879004041258379498 ) ) ;
#79605=CARTESIAN_POINT ( 'NONE',  ( -5.585596099150193616, 6.579245539505756746, -1.082531754730544860 ) ) ;
#79608=CARTESIAN_POINT ( 'NONE',  ( 5.680503174445848735, 5.729601246382692636, 1.040834085586084257E-14 ) ) ;
#79611=CARTESIAN_POINT ( 'NONE',  ( -7.714753101375940503, 8.959299025482085455, 1.199719254218462483 ) ) ;
#79612=CARTESIAN_POINT ( 'NONE',  ( -8.676855123066019360, 11.14608361504227574, -1.443375672974059665 ) ) ;
#79614=CARTESIAN_POINT ( 'NONE',  ( -1.001543065824772872E-14, 5.571875000341416140, 1.575800808251672791 ) ) ;
#79619=CARTESIAN_POINT ( 'NONE',  ( -7.171900071504748730, 8.429933507252760805, -1.082531754730549078 ) ) ;
#79621=CARTESIAN_POINT ( 'NONE',  ( 1.364683531249986537, -0.8239583329919186738, 0.7879004041258500513 ) ) ;
#79624=CARTESIAN_POINT ( 'NONE',  ( 7.131225611108088280, 9.342849184424693476, 1.443375672974076540 ) ) ;
#79634=CARTESIAN_POINT ( 'NONE',  ( 0.7499999999999885647, -0.2666666666666442365, 1.299038105676657340 ) ) ;
#79635=CARTESIAN_POINT ( 'NONE',  ( 10.19536832735223975, 10.99694392477354477, 0.000000000000000000 ) ) ;
#79644=CARTESIAN_POINT ( 'NONE',  ( 5.799137018343234473, 7.788745826199009237, -1.599625672291262513 ) ) ;
#79645=CARTESIAN_POINT ( 'NONE',  ( -3.554208825076827782, 7.298327395898266623, 0.7998128361456341429 ) ) ;
#79648=CARTESIAN_POINT ( 'NONE',  ( -4.862871242741148237, 4.993698027119869209, -0.7753252576984640543 ) ) ;
#79649=CARTESIAN_POINT ( 'NONE',  ( 4.948362878863507675, 8.716914425408678113, -0.7216878364870267237 ) ) ;
#79650=CARTESIAN_POINT ( 'NONE',  ( -0.6823417656250246877, 0.3635416670080895973, 1.181850606188755259 ) ) ;
#79652=CARTESIAN_POINT ( 'NONE',  ( -8.109748439268576803, 12.61312361245537517, 0.7998128361456481317 ) ) ;
#79657=CARTESIAN_POINT ( 'NONE',  ( 0.7499999999999920064, 5.733333333333353821, 1.299038105676669330 ) ) ;
#79666=CARTESIAN_POINT ( 'NONE',  ( 2.295757763869426871, 5.519548059767960702, 0.4031905389056070765 ) ) ;
#79670=CARTESIAN_POINT ( 'NONE',  ( 6.657217119509961201, 7.725507046638470321, -1.199719254218446718 ) ) ;
#79676=CARTESIAN_POINT ( 'NONE',  ( 9.271078113646423091, 9.710679308875986848, 1.040834085586084257E-14 ) ) ;
#79680=CARTESIAN_POINT ( 'NONE',  ( 8.940712233207955606, 12.51824914112961729, 1.199719254218450271 ) ) ;
#79682=CARTESIAN_POINT ( 'NONE',  ( -3.195971524519394702, 4.751719416737803847, -1.599625672291262513 ) ) ;
#79687=CARTESIAN_POINT ( 'NONE',  ( -0.07580519709491854996, 7.079373232791049020, 2.120991669647492639 ) ) ;
#79692=CARTESIAN_POINT ( 'NONE',  ( -8.134528978519403708, 11.47373899403920205, 1.082531754730549967 ) ) ;
#79696=CARTESIAN_POINT ( 'NONE',  ( 4.310602774141044868, 7.116454772218158809, -1.199719254218452047 ) ) ;
#79702=CARTESIAN_POINT ( 'NONE',  ( 3.660338285565247762, 7.214219066560688454, 1.040834085586084257E-14 ) ) ;
#79710=CARTESIAN_POINT ( 'NONE',  ( -6.718228810771495141, 7.796687353110217877, 1.199719254218450271 ) ) ;
#79711=CARTESIAN_POINT ( 'NONE',  ( -5.298539104842322267, 5.076050465271134016, 0.7998128361456341429 ) ) ;
#79718=CARTESIAN_POINT ( 'NONE',  ( 7.284808609244363353, 7.393364887073558656, 0.7998128361456341429 ) ) ;
#79729=CARTESIAN_POINT ( 'NONE',  ( 3.511198595814909673, 7.040222761851984146, 0.7216878364870233931 ) ) ;
#79732=CARTESIAN_POINT ( 'NONE',  ( 0.6823417656249882723, -0.5947916663252492686, 1.181850606188755259 ) ) ;
#79734=CARTESIAN_POINT ( 'NONE',  ( 4.385172619016207918, 7.203452924572514959, 1.199719254218462483 ) ) ;
#79736=CARTESIAN_POINT ( 'NONE',  ( -7.714226216495749355, 8.102278128774251797, 1.040834085586084257E-14 ) ) ;
#79737=CARTESIAN_POINT ( 'NONE',  ( 5.992340707560163793, 6.093411701682730275, 0.7216878364870317197 ) ) ;
#79738=CARTESIAN_POINT ( 'NONE',  ( -6.846504384776755714, 9.971043634672792422, -1.082531754730537088 ) ) ;
#79742=CARTESIAN_POINT ( 'NONE',  ( 5.126954644262057492, 9.133197518281081173, 0.7998128361456462443 ) ) ;
#79748=CARTESIAN_POINT ( 'NONE',  ( -1.364683531250010295, 5.530208333674751842, 0.7879004041258379498 ) ) ;
#79752=CARTESIAN_POINT ( 'NONE',  ( 8.633844893804129228, 8.967240552393299424, -0.7998128361456211532 ) ) ;
#79755=CARTESIAN_POINT ( 'NONE',  ( -7.365103760721662951, 9.615707025640515937, 1.599625672291295375 ) ) ;
#79760=CARTESIAN_POINT ( 'NONE',  ( 10.37606763316019531, 10.99983374830873650, 0.7998128361456462443 ) ) ;
#79762=CARTESIAN_POINT ( 'NONE',  ( -7.714753101375940503, 8.959299025482085455, 1.199719254218462483 ) ) ;
#79768=CARTESIAN_POINT ( 'NONE',  ( 4.716373530444390560, 6.815548562371487762, -1.235710759775530798 ) ) ;
#79769=CARTESIAN_POINT ( 'NONE',  ( -8.595506201384022660, 11.05117653974661529, 1.443375672974064550 ) ) ;
#79775=CARTESIAN_POINT ( 'NONE',  ( 6.582647274634798151, 7.638508894284114170, 1.199719254218462483 ) ) ;
#79777=CARTESIAN_POINT ( 'NONE',  ( 6.959412922516382771, 7.013736585890911535, 0.7998128361456341429 ) ) ;
#79778=CARTESIAN_POINT ( 'NONE',  ( -4.082753340799282427, 7.529786358835235838, 0.5248769202933333267 ) ) ;
#79779=CARTESIAN_POINT ( 'NONE',  ( 4.383363735919856730, 4.008345868194933104, -0.7998128361456211532 ) ) ;
#79781=CARTESIAN_POINT ( 'NONE',  ( -6.507550544879489252, 9.575597488125954015, 1.082531754730548412 ) ) ;
#79786=CARTESIAN_POINT ( 'NONE',  ( -4.191772670604852813, 7.388608026231708870, 0.8008250379338277547 ) ) ;
#79787=CARTESIAN_POINT ( 'NONE',  ( -1.364683531250000748, 0.07187500034142035865, 0.000000000000000000 ) ) ;
#79790=CARTESIAN_POINT ( 'NONE',  ( 5.192409644353875642, 5.160158794608717514, 1.040834085586084257E-14 ) ) ;
#79795=CARTESIAN_POINT ( 'NONE',  ( -10.11401940567025548, 10.90203684947788076, 1.040834085586084257E-14 ) ) ;
#79801=CARTESIAN_POINT ( 'NONE',  ( -8.256552360598034213, 11.61609960646427986, 1.082531754730549967 ) ) ;
#79803=VERTEX_POINT ( 'NONE', #154774 ) ;
#79808=CARTESIAN_POINT ( 'NONE',  ( -7.768458830506062007, 11.04665715469030296, 1.082531754730549967 ) ) ;
#79812=CARTESIAN_POINT ( 'NONE',  ( -1.364683531250010295, 5.551041667008087543, -0.7879004041258300672 ) ) ;
#79813=CARTESIAN_POINT ( 'NONE',  ( 1.499999999999989120, 4.285416667349482900, 0.8660254037844524744 ) ) ;
#79814=CARTESIAN_POINT ( 'NONE',  ( 5.406339766261963220, 6.489514674222595758, -1.307707983115678152 ) ) ;
#79819=CARTESIAN_POINT ( 'NONE',  ( -6.995117189646935962, 10.24838825697502109, 1.199719254218453823 ) ) ;
#79820=CARTESIAN_POINT ( 'NONE',  ( -3.741687207247254676, 7.309126141856352454, 1.040834085586084257E-14 ) ) ;
#79824=CARTESIAN_POINT ( 'NONE',  ( 7.149227073107712549, 7.235186428247455837, -0.7998128361456281477 ) ) ;
#79830=CARTESIAN_POINT ( 'NONE',  ( 6.435316467980822353, 10.65961964595298817, 1.040834085586084257E-14 ) ) ;
#79838=CARTESIAN_POINT ( 'NONE',  ( -5.694061328059534688, 8.626526735169329996, 1.082531754730548412 ) ) ;
#79841=CARTESIAN_POINT ( 'NONE',  ( -1.284279953904132077, 3.159610286488902187, -0.7749999999999935829 ) ) ;
#79847=CARTESIAN_POINT ( 'NONE',  ( -7.804689982961090955, 12.25722208009664094, 0.7998128361456481317 ) ) ;
#79849=CARTESIAN_POINT ( 'NONE',  ( 9.772729797352075920, 10.29593960653257234, -0.7998128361456281477 ) ) ;
#79850=CARTESIAN_POINT ( 'NONE',  ( -0.7500000000000249800, -0.3083333333333132531, 1.299038105676659116 ) ) ;
#79851=CARTESIAN_POINT ( 'NONE',  ( -8.533967624797991647, 12.04371376465130439, -1.199719254218446718 ) ) ;
#79854=CARTESIAN_POINT ( 'NONE',  ( 1.364683531249988535, 3.655208333674750509, -0.7879004041258239610 ) ) ;
#79855=CARTESIAN_POINT ( 'NONE',  ( 3.277320446201373638, 4.846626492033466072, 1.599625672291267398 ) ) ;
#79859=CARTESIAN_POINT ( 'NONE',  ( 8.554831740098649107, 11.96409221588171157, 1.082531754730546636 ) ) ;
#79862=CARTESIAN_POINT ( 'NONE',  ( -7.551528373131759508, 7.912463978182924684, 1.040834085586084257E-14 ) ) ;
#79863=CARTESIAN_POINT ( 'NONE',  ( -1.402160292154681736E-14, 1.196875000341419026, -1.575800808251659024 ) ) ;
#79865=CARTESIAN_POINT ( 'NONE',  ( 0.2638905955352529031, 7.233311467405346029, 1.984662505942447419 ) ) ;
#79867=CARTESIAN_POINT ( 'NONE',  ( -7.588813295347149435, 9.876701482703580837, -1.599625672291263179 ) ) ;
#79868=CARTESIAN_POINT ( 'NONE',  ( -3.917943204224921150, 5.594019709727598766, -1.443375672974051449 ) ) ;
#79869=CARTESIAN_POINT ( 'NONE',  ( -0.6823417656250212460, 3.863541667008085767, 1.181850606188767472 ) ) ;
#79874=CARTESIAN_POINT ( 'NONE',  ( 8.910733272679570049, 11.41894145625809820, -1.599625672291255185 ) ) ;
#79888=CARTESIAN_POINT ( 'NONE',  ( 1.364683531249988535, 4.967708333674756283, -0.7879004041258300672 ) ) ;
#79893=CARTESIAN_POINT ( 'NONE',  ( 7.747594715205354809, 11.12627870345989756, -1.199719254218446718 ) ) ;
#79896=CARTESIAN_POINT ( 'NONE',  ( -1.364683531249997417, 4.259375000341424133, 1.214306433183764966E-14 ) ) ;
#79898=CARTESIAN_POINT ( 'NONE',  ( -6.344852701515500293, 9.385783337534627790, 1.082531754730548412 ) ) ;
#79905=CARTESIAN_POINT ( 'NONE',  ( 3.297657676621871925, 4.870353260857385180, 1.599625672291267398 ) ) ;
#79908=CARTESIAN_POINT ( 'NONE',  ( 8.866142388332804103, 12.43125098877526113, -1.199719254218446718 ) ) ;
#79909=CARTESIAN_POINT ( 'NONE',  ( 4.952636518945733535, 6.537114055553957748, -2.442608363190508669 ) ) ;
#79915=CARTESIAN_POINT ( 'NONE',  ( -7.974166903131914452, 12.45494515362926435, -0.7998128361456281477 ) ) ;
#79916=CARTESIAN_POINT ( 'NONE',  ( 7.416473721875251890, 8.611306416064660851, 1.199719254218462483 ) ) ;
#79918=CARTESIAN_POINT ( 'NONE',  ( 4.839897649954202130, 4.748894801142428790, -0.7216878364870197293 ) ) ;
#79930=CARTESIAN_POINT ( 'NONE',  ( -4.934804725694212912, 8.701096580044490381, -0.7216878364870207285 ) ) ;
#79931=CARTESIAN_POINT ( 'NONE',  ( 5.183294799126148433, 4.941598775268944976, 1.040834085586084257E-14 ) ) ;
#79935=CARTESIAN_POINT ( 'NONE',  ( -7.700141177557535244, 11.07091624287075859, -1.199719254218446718 ) ) ;
#79940=CARTESIAN_POINT ( 'NONE',  ( -9.484092147959342967, 11.02352791316275216, 1.199719254218462483 ) ) ;
#79945=CARTESIAN_POINT ( 'NONE',  ( 9.097684769969825780, 10.57271930550834860, -1.199719254218446718 ) ) ;
#79946=CARTESIAN_POINT ( 'NONE',  ( 6.634017235788401301, 6.634108284708264414, 0.7998128361456341429 ) ) ;
#79958=CARTESIAN_POINT ( 'NONE',  ( -7.323375529675950624, 11.69568855126397011, -0.7998128361456291469 ) ) ;
#79962=CARTESIAN_POINT ( 'NONE',  ( 6.155038550924139429, 9.164333495178082600, 1.082531754730558626 ) ) ;
#79964=CARTESIAN_POINT ( 'NONE',  ( 4.196412238629597447, 4.854568018944682706, -1.199719254218452047 ) ) ;
#79967=CARTESIAN_POINT ( 'NONE',  ( -5.713871673155502151, 8.753601821068331290, 1.199719254218452047 ) ) ;
#79979=CARTESIAN_POINT ( 'NONE',  ( -1.201851678989727383E-14, 4.259375000341417028, -1.575800808251660134 ) ) ;
#79980=CARTESIAN_POINT ( 'NONE',  ( 5.736990052184824940, 5.898621588824067175, 2.499999999981530330 ) ) ;
#79981=CARTESIAN_POINT ( 'NONE',  ( 7.377608144130607393, 11.75895993479440982, -0.7998128361456291469 ) ) ;
#79983=CARTESIAN_POINT ( 'NONE',  ( -4.772106882330247046, 4.669805572247793357, -0.7216878364870207285 ) ) ;
#79985=CARTESIAN_POINT ( 'NONE',  ( -4.785665035499573783, 5.645992631913323123, 1.082531754730558626 ) ) ;
#79992=CARTESIAN_POINT ( 'NONE',  ( 4.681643115420508039, 4.356338477612361260, 0.7998128361456341429 ) ) ;
#79999=CARTESIAN_POINT ( 'NONE',  ( 3.845709127770629010, 7.638411082374393146, 0.7998128361456321445 ) ) ;
#80003=CARTESIAN_POINT ( 'NONE',  ( 0.6823417656249899377, 3.988541667008085767, -1.181850606188754593 ) ) ;
#80008=CARTESIAN_POINT ( 'NONE',  ( 5.099838337034727331, 9.101561826515851550, -0.7998128361456281477 ) ) ;
#80011=CARTESIAN_POINT ( 'NONE',  ( -3.924195396151603177, 6.665646164563756138, 1.199719254218464037 ) ) ;
#80013=CARTESIAN_POINT ( 'NONE',  ( 5.951666246274797345, 7.966696592119163256, 1.443375672974062551 ) ) ;
#80014=CARTESIAN_POINT ( 'NONE',  ( -1.500000000000013101, 1.879166666666692187, -0.8660254037844313801 ) ) ;
#80017=CARTESIAN_POINT ( 'NONE',  ( -5.220052836461385404, 6.048815383081766583, -1.199719254218446718 ) ) ;
#80018=DIRECTION ( 'NONE',  ( 3.451266460341927524E-31, -0.6000000000000035305, 0.7999999999999974909 ) ) ;
#80020=CARTESIAN_POINT ( 'NONE',  ( -1.201851678989727383E-14, 3.571875000341422357, 1.575800808251672791 ) ) ;
#80023=CARTESIAN_POINT ( 'NONE',  ( -3.456965981804629884, 6.976951378839947537, 1.040834085586084257E-14 ) ) ;
#80026=ORIENTED_EDGE ( 'NONE', *, *, #55423, .F. ) ;
#80028=CARTESIAN_POINT ( 'NONE',  ( 3.903157637975605443, 4.019672535764859056, -0.7873708795828464613 ) ) ;
#80029=CARTESIAN_POINT ( 'NONE',  ( 4.059776932288224671, 6.823824623389866950, 1.199719254218462483 ) ) ;
#80032=CARTESIAN_POINT ( 'NONE',  ( 0.5137346906103140709, 6.676840427790344812, -3.535787237050524112 ) ) ;
#80033=CARTESIAN_POINT ( 'NONE',  ( 1.364683531249988535, 3.467708333674749621, -0.7879004041258239610 ) ) ;
#80035=CARTESIAN_POINT ( 'NONE',  ( 4.744990575102895569, 5.598539094783909320, -1.082531754730548412 ) ) ;
#80037=CARTESIAN_POINT ( 'NONE',  ( -0.6823417656250246877, 0.1135416670080893753, 1.181850606188755259 ) ) ;
#80039=CARTESIAN_POINT ( 'NONE',  ( -8.462260433223891098, 13.02438760540324481, -0.7998128361456281477 ) ) ;
#80040=AXIS2_PLACEMENT_3D ( 'NONE', #99293, #198882, #50528 ) ;
#80041=CARTESIAN_POINT ( 'NONE',  ( -6.846504384776774366, 7.089935991768773427, -0.7216878364870267237 ) ) ;
#80045=CARTESIAN_POINT ( 'NONE',  ( -1.364683531250010295, 3.780208333674750953, 0.7879004041258379498 ) ) ;
#80053=CARTESIAN_POINT ( 'NONE',  ( -6.548225005276122168, 6.741943382351338165, 0.7216878364870317197 ) ) ;
#80061=CARTESIAN_POINT ( 'NONE',  ( -6.710922848640111127, 6.931757532942661726, 0.7216878364870317197 ) ) ;
#80070=CARTESIAN_POINT ( 'NONE',  ( 4.086551013974742297, 7.685627118797787816, -0.6322510406990735632 ) ) ;
#80071=CARTESIAN_POINT ( 'NONE',  ( 0.2132228467416317219, 6.504871514021060896, -3.125808945088798474 ) ) ;
#80072=CARTESIAN_POINT ( 'NONE',  ( -4.985647801523292344, 6.839675073242382553, -1.599625672291256295 ) ) ;
#80075=CARTESIAN_POINT ( 'NONE',  ( 0.7499999999999885647, 0.2333333333333562076, 1.299038105676657340 ) ) ;
#80077=CARTESIAN_POINT ( 'NONE',  ( 9.897088948295943212, 11.60932053017587506, 1.082531754730548412 ) ) ;
#80078=CARTESIAN_POINT ( 'NONE',  ( 8.132193210098487057, 8.381980254736715708, 1.040834085586084257E-14 ) ) ;
#80079=AXIS2_PLACEMENT_3D ( 'NONE', #190106, #86216, #154423 ) ;
#80083=CARTESIAN_POINT ( 'NONE',  ( 4.143988507271280319, 7.986403691791820414, -0.7998128361456221525 ) ) ;
#80088=CARTESIAN_POINT ( 'NONE',  ( -3.714570900464290393, 5.356752022006865843, 1.443375672974064550 ) ) ;
#80091=EDGE_CURVE ( 'NONE', #71069, #148246, #97383, .T. ) ;
#80096=CARTESIAN_POINT ( 'NONE',  ( -0.6823417656250003738, 2.717708333674753618, -1.181850606188749264 ) ) ;
#80097=CARTESIAN_POINT ( 'NONE',  ( 8.039621902779343188, 12.32338328664385507, -0.7216878364870328300 ) ) ;
#80098=CARTESIAN_POINT ( 'NONE',  ( -7.009729113465285266, 8.136771039586342624, -1.199719254218446718 ) ) ;
#80101=CARTESIAN_POINT ( 'NONE',  ( 4.496500501226593727, 8.397667684739696270, 0.7998128361456462443 ) ) ;
#80102=CARTESIAN_POINT ( 'NONE',  ( -5.930802130974132780, 9.006687355190106103, -1.199719254218440723 ) ) ;
#80103=CARTESIAN_POINT ( 'NONE',  ( -1.580223361175689734, 8.746992034114509096, 2.465615386491402106 ) ) ;
#80106=CARTESIAN_POINT ( 'NONE',  ( -0.7500000000000006661, -0.1104166659838465292, -1.299038105676652011 ) ) ;
#80109=CARTESIAN_POINT ( 'NONE',  ( 7.049876689426101350, 9.247942109129029475, -1.443375672974057666 ) ) ;
#80112=CARTESIAN_POINT ( 'NONE',  ( -0.6823417656250212460, 1.863541667008083991, 1.181850606188755259 ) ) ;
#80114=CARTESIAN_POINT ( 'NONE',  ( 7.253248993186735660, 7.564471368247083660, 0.7216878364870317197 ) ) ;
#80117=CARTESIAN_POINT ( 'NONE',  ( -2.792616454734997866, 6.201876930592042925, 0.7216878364870317197 ) ) ;
#80119=CARTESIAN_POINT ( 'NONE',  ( 1.364683531249988535, 4.155208333674753618, -0.7879004041258239610 ) ) ;
#80124=CARTESIAN_POINT ( 'NONE',  ( -5.085529380082158823, 6.726364094520411285, -1.441608068093344741 ) ) ;
#80131=CARTESIAN_POINT ( 'NONE',  ( 6.331821432781979730, 7.345878745455822312, -1.199719254218445830 ) ) ;
#80135=CARTESIAN_POINT ( 'NONE',  ( 3.334415713957098681, 5.977569868670206787, -1.199719254218446718 ) ) ;
#80137=EDGE_CURVE ( 'NONE', #93347, #37648, #122022, .T. ) ;
#80144=CARTESIAN_POINT ( 'NONE',  ( 5.233084105194869551, 6.167981546557892436, -1.082531754730548412 ) ) ;
#80145=CARTESIAN_POINT ( 'NONE',  ( 1.364683531249988535, 1.426041667008083991, 0.7879004041258500513 ) ) ;
#80146=CARTESIAN_POINT ( 'NONE',  ( 7.214910300766615769, 11.56914578420308715, -0.7998128361456291469 ) ) ;
#80148=CARTESIAN_POINT ( 'NONE',  ( 2.404166168890689903, 5.245195659253913512, -0.8707498557368191783 ) ) ;
#80152=CARTESIAN_POINT ( 'NONE',  ( -1.500000000000013101, 1.379166666666689745, -0.8660254037844313801 ) ) ;
#80153=CARTESIAN_POINT ( 'NONE',  ( 7.124973419181436007, 8.271222729588529887, -1.199719254218446718 ) ) ;
#80154=CARTESIAN_POINT ( 'NONE',  ( -8.528242318195895066, 9.908369778438709474, 1.199719254218462483 ) ) ;
#80158=CARTESIAN_POINT ( 'NONE',  ( -1.201851678989727383E-14, 2.321875000341416584, 1.575800808251672791 ) ) ;
#80160=CARTESIAN_POINT ( 'NONE',  ( 1.499999999999987121, 2.004166666666684637, 0.8660254037844524744 ) ) ;
#80163=CARTESIAN_POINT ( 'NONE',  ( 3.979481780810941949, 4.601482484822914998, 1.199719254218464037 ) ) ;
#80169=CARTESIAN_POINT ( 'NONE',  ( -1.500000000000015099, 0.9104166673494835660, -0.8660254037844313801 ) ) ;
#80171=CARTESIAN_POINT ( 'NONE',  ( -5.831978632172702071, 9.955725504176825780, 0.7998128361456481317 ) ) ;
#80172=CARTESIAN_POINT ( 'NONE',  ( -3.741687207691642314, 6.348756928073427730, 1.082531754730560403 ) ) ;
#80180=CARTESIAN_POINT ( 'NONE',  ( 7.474622759835693131, 7.614814729430110951, -0.7998128361456281477 ) ) ;
#80184=CARTESIAN_POINT ( 'NONE',  ( 7.630541526392844887, 7.796719957080126662, 0.7998128361456341429 ) ) ;
#80185=CARTESIAN_POINT ( 'NONE',  ( 8.039621902779343188, 12.32338328664385507, -0.7216878364870328300 ) ) ;
#80190=CARTESIAN_POINT ( 'NONE',  ( -5.533699252672048985, 9.607732894759390518, -0.7998128361456231517 ) ) ;
#80191=CARTESIAN_POINT ( 'NONE',  ( 4.566398809704347528, 4.221886787610169556, -0.7998128361456211532 ) ) ;
#80195=CARTESIAN_POINT ( 'NONE',  ( 4.768780016659259324, 6.770301073365750710, 1.244442160714388068 ) ) ;
#80196=CARTESIAN_POINT ( 'NONE',  ( 8.419250204406344196, 12.76628297187536809, 1.040834085586084257E-14 ) ) ;
#80197=VERTEX_POINT ( 'NONE', #128876 ) ;
#80207=CARTESIAN_POINT ( 'NONE',  ( 8.609064354997688184, 9.146255957026539818, 1.040834085586084257E-14 ) ) ;
#80210=CARTESIAN_POINT ( 'NONE',  ( -5.416646063859567484, 6.278174148379618735, 1.199719254218450271 ) ) ;
#80211=CARTESIAN_POINT ( 'NONE',  ( -0.1231583423410937961, 7.054063922337696191, 3.955400951015612065 ) ) ;
#80212=CARTESIAN_POINT ( 'NONE',  ( -3.096762063222531225, 6.448889905702306358, -0.7260975201865252915 ) ) ;
#80216=CARTESIAN_POINT ( 'NONE',  ( -6.344325816190970357, 9.489131654609717970, 1.199719254218452047 ) ) ;
#80217=EDGE_CURVE ( 'NONE', #106888, #171296, #111814, .T. ) ;
#80218=CARTESIAN_POINT ( 'NONE',  ( -1.219999999999995977, 5.900000000000024336, 1.229247124133362667E-14 ) ) ;
#80223=ORIENTED_EDGE ( 'NONE', *, *, #170032, .F. ) ;
#80232=CARTESIAN_POINT ( 'NONE',  ( 1.451998047841835060, 7.315968950352750966, -4.301760722580861618 ) ) ;
#80233=CARTESIAN_POINT ( 'NONE',  ( -6.067437437315529536, 7.037430750744921859, 1.199719254218450271 ) ) ;
#80236=CARTESIAN_POINT ( 'NONE',  ( 2.738383840280320669, 6.138605547061593448, 0.7216878364870338292 ) ) ;
#80242=CARTESIAN_POINT ( 'NONE',  ( -3.810004860640155311, 4.403759411290286252, 1.199719254218462483 ) ) ;
#80246=CARTESIAN_POINT ( 'NONE',  ( 9.915090410295563927, 10.46202698829998567, -0.7998128361456281477 ) ) ;
#80249=CARTESIAN_POINT ( 'NONE',  ( -8.311311860377216476, 9.655284244316948872, -1.199719254218446718 ) ) ;
#80250=CARTESIAN_POINT ( 'NONE',  ( 6.145923705696426431, 6.064665832934283962, 0.7998128361456341429 ) ) ;
#80252=B_SPLINE_CURVE_WITH_KNOTS ( 'NONE', 3,
 ( #129682, #96052, #13694, #196723, #116589, #63528, #147986, #132820, #195666, #163170 ),
 .UNSPECIFIED., .F., .F.,
 ( 4, 2, 2, 2, 4 ),
 ( 0.001965249434206598270, 0.002424473194169422634, 0.002883696954132246131, 0.003342920714095069627, 0.003802144474057893558 ),
 .UNSPECIFIED. ) ;
#80253=CARTESIAN_POINT ( 'NONE',  ( 5.820528018968444961, 5.685037531751635953, 0.7998128361456341429 ) ) ;
#80256=CARTESIAN_POINT ( 'NONE',  ( -1.201851678989727383E-14, 1.384375000341419693, 1.575800808251672791 ) ) ;
#80259=CARTESIAN_POINT ( 'NONE',  ( 7.537970219518073556, 9.817384560903001045, -1.443375672974057666 ) ) ;
#80261=CARTESIAN_POINT ( 'NONE',  ( -3.619663825168619731, 7.166765529431275539, 1.040834085586084257E-14 ) ) ;
#80274=CARTESIAN_POINT ( 'NONE',  ( -8.805130697071332335, 12.36007068230351358, 1.199719254218462483 ) ) ;
#80287=AXIS2_PLACEMENT_3D ( 'NONE', #185238, #169004, #5404 ) ;
#80288=CARTESIAN_POINT ( 'NONE',  ( -0.7500000000000006661, 0.8895833340161543035, -1.299038105676652011 ) ) ;
#80295=CARTESIAN_POINT ( 'NONE',  ( -1.402160292154681736E-14, -1.037499999999977662, 1.732050807568877637 ) ) ;
#80296=CARTESIAN_POINT ( 'NONE',  ( 7.052212457402625922, 11.37933163361175382, -0.7998128361456291469 ) ) ;
#80301=CARTESIAN_POINT ( 'NONE',  ( 2.686486993802192913, 6.285985259411197568, 0.7998128361456362523 ) ) ;
#80302=CARTESIAN_POINT ( 'NONE',  ( -6.670248388243482651, 9.765411638717282017, 1.082531754730548412 ) ) ;
#80306=CARTESIAN_POINT ( 'NONE',  ( -6.938021921891187382, 9.117444880338284818, -1.599625672291263179 ) ) ;
#80308=ORIENTED_EDGE ( 'NONE', *, *, #1901, .F. ) ;
#80309=CARTESIAN_POINT ( 'NONE',  ( 1.499999999999987121, 1.285416667349485120, 0.8660254037844524744 ) ) ;
#80316=CARTESIAN_POINT ( 'NONE',  ( -8.618179199781044630, 13.20629283305325963, 0.7998128361456341429 ) ) ;
#80318=CARTESIAN_POINT ( 'NONE',  ( 4.078835981324096416, 7.487686104445945290, 0.5747339805607706298 ) ) ;
#80323=CARTESIAN_POINT ( 'NONE',  ( -8.482597663644387609, 13.04811437422715414, -0.7998128361456281477 ) ) ;
#80324=CARTESIAN_POINT ( 'NONE',  ( 6.936968151686458306, 11.24487994360957188, 0.7998128361456462443 ) ) ;
#80332=CARTESIAN_POINT ( 'NONE',  ( -8.809047120577080392, 11.30030761213851953, 1.599625672291269396 ) ) ;
#80339=CARTESIAN_POINT ( 'NONE',  ( 3.867100128395839942, 5.534702787927018974, -1.599625672291255185 ) ) ;
#80351=B_SPLINE_CURVE_WITH_KNOTS ( 'NONE', 3,
 ( #143471, #194310, #45951, #113132 ),
 .UNSPECIFIED., .F., .F.,
 ( 4, 4 ),
 ( 0.000000000000000000, 0.0002602974955195480741 ),
 .UNSPECIFIED. ) ;
#80356=CARTESIAN_POINT ( 'NONE',  ( 8.118635056484817980, 8.366162408854107113, 0.7998128361456481317 ) ) ;
#80359=CARTESIAN_POINT ( 'NONE',  ( -2.937312835655025101, 6.578615408239493867, 1.040834085586084257E-14 ) ) ;
#80361=EDGE_CURVE ( 'NONE', #108697, #71069, #211092, .T. ) ;
#80368=CARTESIAN_POINT ( 'NONE',  ( -1.500000000000013101, -0.2979166659838501929, 0.8660254037844403729 ) ) ;
#80372=CARTESIAN_POINT ( 'NONE',  ( 4.715538499454675403, 4.395883092318884522, 1.214306433183764966E-14 ) ) ;
#80374=CARTESIAN_POINT ( 'NONE',  ( -3.379006598303881059, 4.965260336153046516, -1.599625672291256295 ) ) ;
#80380=CARTESIAN_POINT ( 'NONE',  ( 4.853455804012222430, 5.725081861844796727, 1.082531754730560403 ) ) ;
#80383=CARTESIAN_POINT ( 'NONE',  ( 1.364683531249988535, 5.467708333674750953, -0.7879004041258300672 ) ) ;
#80385=CARTESIAN_POINT ( 'NONE',  ( 4.351804119862229037, 4.179452349368450115, -0.7216878364870188411 ) ) ;
#80393=CARTESIAN_POINT ( 'NONE',  ( -5.609631208091558463, 6.340496262503443781, 1.197921296376257994 ) ) ;
#80397=CARTESIAN_POINT ( 'NONE',  ( -0.6823417656250003738, -0.5322916663252491576, -1.181850606188749264 ) ) ;
#80401=CARTESIAN_POINT ( 'NONE',  ( -4.446184310277715213, 7.274633231044262516, -1.199719254218452047 ) ) ;
#80405=CARTESIAN_POINT ( 'NONE',  ( -1.001543065824772872E-14, 4.462500000000024336, 1.732050807568877637 ) ) ;
#80412=CARTESIAN_POINT ( 'NONE',  ( -1.364683531250014514, -0.4697916663252449943, 0.7879004041258379498 ) ) ;
#80414=CARTESIAN_POINT ( 'NONE',  ( 4.774442650306744085, 8.721933525333202653, -0.7998128361456281477 ) ) ;
#80415=CARTESIAN_POINT ( 'NONE',  ( -6.530223543276495235, 10.77034456713125188, -0.7998128361456291469 ) ) ;
#80416=CARTESIAN_POINT ( 'NONE',  ( 10.24048609702354717, 10.84165528948263457, -0.7998128361456281477 ) ) ;
#80422=CARTESIAN_POINT ( 'NONE',  ( 0.7499999999999902300, 5.316666666666685082, -1.299038105676658228 ) ) ;
#80426=CARTESIAN_POINT ( 'NONE',  ( 5.202472899321463728, 6.442273364155400195, -1.196158869778561673 ) ) ;
#80430=CARTESIAN_POINT ( 'NONE',  ( 8.134528978519385944, 8.592631351135175066, -0.7216878364870267237 ) ) ;
#80436=CARTESIAN_POINT ( 'NONE',  ( -0.7499999999999972244, 4.889583334016150751, -1.299038105676652899 ) ) ;
#80438=CARTESIAN_POINT ( 'NONE',  ( -3.578462479003122976, 6.262291094557191684, 1.199719254218464037 ) ) ;
#80439=CARTESIAN_POINT ( 'NONE',  ( 5.870317324592803310, 7.871789516823500144, -1.443375672974057666 ) ) ;
#80440=CARTESIAN_POINT ( 'NONE',  ( -7.822691444960696572, 12.07029775252209092, -0.7216878364870267237 ) ) ;
#80446=CARTESIAN_POINT ( 'NONE',  ( 10.23604278863759909, 11.04439746293979496, 0.000000000000000000 ) ) ;
#80449=CARTESIAN_POINT ( 'NONE',  ( -1.445103857048130047, 8.688264192037886247, 2.625611233228264840 ) ) ;
#80456=DIRECTION ( 'NONE',  ( 0.7592566023653005702, -0.6507913734559639396, 0.000000000000000000 ) ) ;
#80462=CARTESIAN_POINT ( 'NONE',  ( 9.240045382913317340, 10.73880668727576015, -1.199719254218446718 ) ) ;
#80464=CARTESIAN_POINT ( 'NONE',  ( -1.499999999999995559, 8.673756432004008587, 2.614717076620615810 ) ) ;
#80466=CARTESIAN_POINT ( 'NONE',  ( 1.364683531249986537, -0.8447916663252468261, -0.7879004041258309554 ) ) ;
#80467=CARTESIAN_POINT ( 'NONE',  ( 4.528060117284222308, 8.226561203566173930, 0.7216878364870438212 ) ) ;
#80470=CARTESIAN_POINT ( 'NONE',  ( -9.381879110976678149, 11.00824238663667565, 1.082531754730558626 ) ) ;
#80475=CARTESIAN_POINT ( 'NONE',  ( -4.223528545856940042, 4.886203710709899006, -1.199719254218446718 ) ) ;
#80476=EDGE_CURVE ( 'NONE', #21552, #39666, #166631, .T. ) ;
#80489=CARTESIAN_POINT ( 'NONE',  ( 5.125043568333415678, 6.701081866602433657, -1.409791652392645700 ) ) ;
#80490=PLANE ( 'NONE',  #211947 ) ;
#80498=CARTESIAN_POINT ( 'NONE',  ( -8.514157279702036618, 9.035531035848267223, -0.7216878364870278340 ) ) ;
#80502=CARTESIAN_POINT ( 'NONE',  ( 5.289652487626049115, 9.323011668872403845, 0.7998128361456462443 ) ) ;
#80505=CARTESIAN_POINT ( 'NONE',  ( -5.168682875307782254, 7.053215992657626110, -1.599625672291256295 ) ) ;
#80508=CARTESIAN_POINT ( 'NONE',  ( -4.069418662396130593, 7.899405539437467816, -0.7998128361456281477 ) ) ;
#80512=CARTESIAN_POINT ( 'NONE',  ( 6.740374924288304648, 11.01552117831172062, 1.040834085586084257E-14 ) ) ;
#80515=CARTESIAN_POINT ( 'NONE',  ( 4.363209728991265024, 7.389406413240373617, 1.150570763150955633 ) ) ;
#80516=CARTESIAN_POINT ( 'NONE',  ( 4.528060117284229413, 7.266191989264828344, 1.082531754730558626 ) ) ;
#80523=CARTESIAN_POINT ( 'NONE',  ( 8.080296363620359301, 8.529359967086321603, 1.040834085586084257E-14 ) ) ;
#80527=CARTESIAN_POINT ( 'NONE',  ( -7.811469059767924605, 12.26513100303794168, -0.7998128361456281477 ) ) ;
#80528=CARTESIAN_POINT ( 'NONE',  ( -7.335124800193271177, 8.516399340768996851, -1.199719254218452935 ) ) ;
#80530=EDGE_CURVE ( 'NONE', #167173, #50158, #152957, .T. ) ;
#80534=CARTESIAN_POINT ( 'NONE',  ( 1.499999999998155698, 8.627523663849286706, -2.580000000000244764 ) ) ;
#80537=VECTOR ( 'NONE', #142094, 1000.000000000000000 ) ;
#80538=CARTESIAN_POINT ( 'NONE',  ( 8.727698198895078363, 11.20540053684285553, -1.599625672291257406 ) ) ;
#80542=CARTESIAN_POINT ( 'NONE',  ( 4.009460741339333723, 5.700790169694431420, -1.599625672291256295 ) ) ;
#80545=CARTESIAN_POINT ( 'NONE',  ( 1.499999999999989120, 5.035416667349487341, 0.8660254037844524744 ) ) ;
#80549=VERTEX_POINT ( 'NONE', #86449 ) ;
#80551=CARTESIAN_POINT ( 'NONE',  ( 0.7499999999999885647, 3.316666666666689967, -1.299038105676658228 ) ) ;
#80552=CARTESIAN_POINT ( 'NONE',  ( 5.986088515633498197, 6.942523675449257858, -1.199719254218446718 ) ) ;
#80554=CARTESIAN_POINT ( 'NONE',  ( -1.420000000000001039, 6.280000000000042881, -2.873333333333329520 ) ) ;
#80555=CARTESIAN_POINT ( 'NONE',  ( 7.049876689426101350, 9.247942109129029475, -1.443375672974057666 ) ) ;
#80556=CARTESIAN_POINT ( 'NONE',  ( 0.3124725659141594503, 7.215207000027920259, 2.082817582596224515 ) ) ;
#80562=CARTESIAN_POINT ( 'NONE',  ( -4.334856428067329404, 6.080418470877079429, -1.599625672291256295 ) ) ;
#80563=CARTESIAN_POINT ( 'NONE',  ( 0.7499999999999902300, 4.847916667349482012, -1.299038105676658228 ) ) ;
#80564=CARTESIAN_POINT ( 'NONE',  ( 0.6823417656249882723, -0.6572916663252492686, 1.181850606188755259 ) ) ;
#80568=CARTESIAN_POINT ( 'NONE',  ( 2.822068529938852155, 6.444163718237301275, -0.7998128361456291469 ) ) ;
#80570=CARTESIAN_POINT ( 'NONE',  ( -1.201851678989727383E-14, 5.509375000341415252, -1.575800808251660134 ) ) ;
#80580=CARTESIAN_POINT ( 'NONE',  ( -6.177711549321182716, 10.35908057418338402, 0.7998128361456481317 ) ) ;
#80583=CARTESIAN_POINT ( 'NONE',  ( 5.705283713252285338, 5.550585841749444249, -0.7998128361456211532 ) ) ;
#80586=B_SPLINE_CURVE_WITH_KNOTS ( 'NONE', 3,
 ( #67583, #196560, #35103, #36174 ),
 .UNSPECIFIED., .F., .F.,
 ( 4, 4 ),
 ( 0.000000000000000000, 0.0005691741557773217965 ),
 .UNSPECIFIED. ) ;
#80591=CARTESIAN_POINT ( 'NONE',  ( 9.317477881089539338, 11.89347683273640932, 1.599625672291279388 ) ) ;
#80594=CARTESIAN_POINT ( 'NONE',  ( -4.554649539187067830, 7.401175998105142817, 1.199719254218464037 ) ) ;
#80598=CARTESIAN_POINT ( 'NONE',  ( 7.865701674222579598, 12.32840238656838139, -0.7998128361456352531 ) ) ;
#80600=CARTESIAN_POINT ( 'NONE',  ( 8.697719238366680372, 10.10609285197134533, 1.199719254218462483 ) ) ;
#80602=ORIENTED_EDGE ( 'NONE', *, *, #164742, .T. ) ;
#80604=CARTESIAN_POINT ( 'NONE',  ( -8.487040972474682476, 12.84537220128841817, 0.7216878364870338292 ) ) ;
#80606=CARTESIAN_POINT ( 'NONE',  ( -5.831978632172702071, 9.955725504176825780, 0.7998128361456481317 ) ) ;
#80611=CARTESIAN_POINT ( 'NONE',  ( -5.641245921709659328, 6.318796091258308323, 1.170641968482153850 ) ) ;
#80612=CARTESIAN_POINT ( 'NONE',  ( 1.364683531249986537, 0.3635416670080869328, 0.7879004041258500513 ) ) ;
#80616=CARTESIAN_POINT ( 'NONE',  ( 7.619319141200072920, 7.991553207595983643, 0.7216878364870317197 ) ) ;
#80619=CARTESIAN_POINT ( 'NONE',  ( 5.681030059326015014, 6.586622143090519188, -1.199719254218445830 ) ) ;
#80637=CARTESIAN_POINT ( 'NONE',  ( -4.959585264500673496, 4.680604318205876524, 1.214306433183764966E-14 ) ) ;
#80639=ORIENTED_EDGE ( 'NONE', *, *, #24646, .F. ) ;
#80641=CARTESIAN_POINT ( 'NONE',  ( -5.610376637956639101, 5.439860920571172542, 0.000000000000000000 ) ) ;
#80642=CARTESIAN_POINT ( 'NONE',  ( -6.723954117373590833, 9.932031339322813679, -1.199719254218440723 ) ) ;
#80644=VERTEX_POINT ( 'NONE', #202300 ) ;
#80648=CARTESIAN_POINT ( 'NONE',  ( 1.499999999999989120, 3.056250000682818158, 1.214306433183764966E-14 ) ) ;
#80649=CARTESIAN_POINT ( 'NONE',  ( 9.023114925094663619, 10.48572115315399245, 1.199719254218453823 ) ) ;
#80653=CARTESIAN_POINT ( 'NONE',  ( -8.910733272679575379, 11.41894145625809820, -1.599625672291263179 ) ) ;
#80655=CARTESIAN_POINT ( 'NONE',  ( -0.6823417656249969321, 3.717708333674754506, -1.181850606188749264 ) ) ;
#80660=CARTESIAN_POINT ( 'NONE',  ( -8.324343129110692630, 12.65555805069709550, 0.7216878364870338292 ) ) ;
#80664=CARTESIAN_POINT ( 'NONE',  ( 1.364683531249988757, 0.9468750003414211358, 0.000000000000000000 ) ) ;
#80671=CARTESIAN_POINT ( 'NONE',  ( 0.6823417656249899377, 2.842708333674753618, 1.181850606188765695 ) ) ;
#80674=CARTESIAN_POINT ( 'NONE',  ( -4.550733115681270036, 8.460939068270139529, 0.7998128361456481317 ) ) ;
#80677=CARTESIAN_POINT ( 'NONE',  ( -1.364683531250012516, 3.051041667008083547, -0.7879004041258289570 ) ) ;
#80682=CARTESIAN_POINT ( 'NONE',  ( -4.609409038966234995, 7.361099064560491456, -1.082531754730549967 ) ) ;
#80687=CARTESIAN_POINT ( 'NONE',  ( 3.701012746850603996, 7.261672604726938651, 1.040834085586084257E-14 ) ) ;
#80690=CARTESIAN_POINT ( 'NONE',  ( -7.340850106795412167, 10.65174332698158643, 1.199719254218453823 ) ) ;
#80691=CARTESIAN_POINT ( 'NONE',  ( -3.789667630219657912, 4.380032642466370696, 1.199719254218462483 ) ) ;
#80698=CARTESIAN_POINT ( 'NONE',  ( -6.521108698048783126, 7.670676904887464786, -1.082531754730543083 ) ) ;
#80700=CARTESIAN_POINT ( 'NONE',  ( -1.402160292154681736E-14, -0.4906249996585810846, -1.575800808251665908 ) ) ;
#80704=CARTESIAN_POINT ( 'NONE',  ( 6.805829924380108586, 8.963220883242035697, 1.443375672974076540 ) ) ;
#80719=CARTESIAN_POINT ( 'NONE',  ( 6.205881626753210867, 8.263281202677319470, 1.599625672291281386 ) ) ;
#80720=CARTESIAN_POINT ( 'NONE',  ( -3.632695093457760649, 6.325562478087638496, -1.199719254218452047 ) ) ;
#80723=CARTESIAN_POINT ( 'NONE',  ( -4.887223063278990587, 4.917640739834122421, -0.4608172110749644834 ) ) ;
#80724=CARTESIAN_POINT ( 'NONE',  ( 4.324687812634874895, 7.989293514808604613, 0.7216878364870317197 ) ) ;
#80725=CARTESIAN_POINT ( 'NONE',  ( -0.6823417656250246877, 0.1135416670080893753, 1.181850606188755259 ) ) ;
#80727=CARTESIAN_POINT ( 'NONE',  ( -9.806625181386236179, 10.33548422123910449, -0.7998128361456291469 ) ) ;
#80738=CARTESIAN_POINT ( 'NONE',  ( -1.201851678989727383E-14, 4.587500000000024336, -1.732050807568863648 ) ) ;
#80747=CARTESIAN_POINT ( 'NONE',  ( 7.145310649601935182, 8.294949498412453437, -1.199719254218446718 ) ) ;
#80759=CARTESIAN_POINT ( 'NONE',  ( -3.277320446201389181, 4.846626492033466072, 1.599625672291267398 ) ) ;
#80771=CIRCLE ( 'NONE', #66962, 0.07999999999999990452 ) ;
#80772=CARTESIAN_POINT ( 'NONE',  ( -8.487040972474682476, 12.84537220128841817, 0.7216878364870338292 ) ) ;
#80776=CARTESIAN_POINT ( 'NONE',  ( 5.769158057814842699, 6.689438141327490150, 1.199719254218462483 ) ) ;
#80782=CARTESIAN_POINT ( 'NONE',  ( 4.324687812634887329, 6.068555086205916105, 1.443375672974062551 ) ) ;
#80789=CARTESIAN_POINT ( 'NONE',  ( -7.867809214632013770, 8.073532260025807261, 1.040834085586084257E-14 ) ) ;
#80790=CARTESIAN_POINT ( 'NONE',  ( -4.192495815123836955, 5.914331089109674089, -1.599625672291256295 ) ) ;
#80797=CARTESIAN_POINT ( 'NONE',  ( -1.364683531249997417, 3.321875000341423245, 1.214306433183764966E-14 ) ) ;
#80799=CARTESIAN_POINT ( 'NONE',  ( 4.964256800898067645, 8.943383367689749619, 0.7998128361456462443 ) ) ;
#80810=CARTESIAN_POINT ( 'NONE',  ( -0.6823417656250003738, 0.5302083336747518416, -1.181850606188749264 ) ) ;
#80812=CARTESIAN_POINT ( 'NONE',  ( 3.897079088924235712, 6.634010472798538949, 1.199719254218462483 ) ) ;
#80814=CARTESIAN_POINT ( 'NONE',  ( -7.239690840017442675, 7.548653522882887934, 0.7216878364870317197 ) ) ;
#80815=CARTESIAN_POINT ( 'NONE',  ( 4.202664430556241726, 7.846932902383524144, 0.7216878364870298324 ) ) ;
#80817=CARTESIAN_POINT ( 'NONE',  ( -7.334597914868741242, 8.619747657844088806, -1.082531754730543083 ) ) ;
#80822=CARTESIAN_POINT ( 'NONE',  ( 6.317209508963599340, 9.457495962844502557, 1.199719254218462483 ) ) ;
#80828=CARTESIAN_POINT ( 'NONE',  ( -1.364683531250010295, 4.280208333674753618, 0.7879004041258379498 ) ) ;
#80832=CARTESIAN_POINT ( 'NONE',  ( 7.151035956204054855, 10.43029348462504124, 1.199719254218460707 ) ) ;
#80836=CARTESIAN_POINT ( 'NONE',  ( -6.516665389662827934, 10.75452672124865217, 0.000000000000000000 ) ) ;
#80842=CARTESIAN_POINT ( 'NONE',  ( 9.752392566931574081, 10.27221283770866300, -0.7998128361456281477 ) ) ;
#80845=CARTESIAN_POINT ( 'NONE',  ( -7.178152263431422320, 10.46192917639026554, 1.199719254218453823 ) ) ;
#80846=CARTESIAN_POINT ( 'NONE',  ( -4.609409038966248318, 5.440360635957812718, -1.082531754730544860 ) ) ;
#80848=CARTESIAN_POINT ( 'NONE',  ( 4.554780495368041748, 6.962214942802684270, -1.182099088617315497 ) ) ;
#80849=CARTESIAN_POINT ( 'NONE',  ( -10.31739171031960822, 11.13930453823545186, 1.040834085586084257E-14 ) ) ;
#80853=CARTESIAN_POINT ( 'NONE',  ( 6.986529229743720926, 7.045372277656132276, -0.7998128361456281477 ) ) ;
#80855=CARTESIAN_POINT ( 'NONE',  ( 5.769158057814842699, 6.689438141327490150, 1.199719254218462483 ) ) ;
#80856=CARTESIAN_POINT ( 'NONE',  ( -4.043761313400059620, 7.584134902449670257, 0.3518898875958225703 ) ) ;
#80857=( BOUNDED_CURVE ( )  B_SPLINE_CURVE ( 2, ( #210852, #143781, #113437 ),
 .UNSPECIFIED., .F., .T. ) 
 B_SPLINE_CURVE_WITH_KNOTS ( ( 3, 3 ),
 ( 0.3392857142857143571, 0.3402546486199640174 ),
 .UNSPECIFIED. ) 
 CURVE ( )  GEOMETRIC_REPRESENTATION_ITEM ( )  RATIONAL_B_SPLINE_CURVE ( ( 0.9999999999999987788, 0.9781914855199952408, 0.9634829932421007381 ) ) 
 REPRESENTATION_ITEM ( '' )  );
#80858=CARTESIAN_POINT ( 'NONE',  ( 4.304877467538922531, 4.981110786005563007, 1.199719254218464037 ) ) ;
#80860=CARTESIAN_POINT ( 'NONE',  ( -7.212574532790102744, 8.477387045419011002, -1.082531754730550855 ) ) ;
#80865=CARTESIAN_POINT ( 'NONE',  ( -4.183520347117292815, 7.398805986154902037, 0.7851016128354749712 ) ) ;
#80866=CARTESIAN_POINT ( 'NONE',  ( -1.364683531250014514, -0.4072916663252447167, 0.7879004041258379498 ) ) ;
#80868=CARTESIAN_POINT ( 'NONE',  ( 4.911989969715272686, 4.726297878971393196, 2.420000000000010587 ) ) ;
#80869=CARTESIAN_POINT ( 'NONE',  ( 5.694061328059515148, 5.745419092265303007, -0.7216878364870207285 ) ) ;
#80874=CARTESIAN_POINT ( 'NONE',  ( -7.646435447983039424, 11.86466575604815787, 0.000000000000000000 ) ) ;
#80879=CARTESIAN_POINT ( 'NONE',  ( -9.463228032214294316, 10.14278024711257764, 1.040834085586084257E-14 ) ) ;
#80886=CARTESIAN_POINT ( 'NONE',  ( -8.473482818416675499, 9.948446711983361723, -1.082531754730543083 ) ) ;
#80891=CARTESIAN_POINT ( 'NONE',  ( 0.6823417656249899377, 4.738541667008086655, -1.181850606188754593 ) ) ;
#80892=CARTESIAN_POINT ( 'NONE',  ( -1.500000000000013101, 2.660416667349483788, -0.8660254037844313801 ) ) ;
#80897=CARTESIAN_POINT ( 'NONE',  ( -6.672584156219988571, 10.93643194889866521, -0.7998128361456291469 ) ) ;
#80901=CARTESIAN_POINT ( 'NONE',  ( 5.799137018343234473, 7.788745826199009237, -1.599625672291262513 ) ) ;
#80906=CARTESIAN_POINT ( 'NONE',  ( 8.446893396513862839, 9.813462703143045474, -1.199719254218445830 ) ) ;
#80913=CARTESIAN_POINT ( 'NONE',  ( -7.402388683381436074, 7.738467673474211495, 0.7216878364870317197 ) ) ;
#80916=CARTESIAN_POINT ( 'NONE',  ( -1.001543065824772872E-14, 5.384375000341415252, 1.575800808251672791 ) ) ;
#80919=CARTESIAN_POINT ( 'NONE',  ( -0.4634916963857354522, 7.369626292149011881, 4.459501722865318207 ) ) ;
#80922=CARTESIAN_POINT ( 'NONE',  ( -8.642432853707342488, 12.17025653171218558, 1.199719254218462483 ) ) ;
#80924=CARTESIAN_POINT ( 'NONE',  ( 7.723341061279088038, 12.16231500480096983, -0.7998128361456291469 ) ) ;
#80925=CARTESIAN_POINT ( 'NONE',  ( -9.287498920561160887, 10.79416914786490089, -1.199719254218441611 ) ) ;
#80928=CARTESIAN_POINT ( 'NONE',  ( 1.364683531249988535, 3.405208333674749621, -0.7879004041258239610 ) ) ;
#80929=CARTESIAN_POINT ( 'NONE',  ( 4.033714395265605823, 4.664753868353354704, -1.199719254218446718 ) ) ;
#80934=CARTESIAN_POINT ( 'NONE',  ( 9.693716643646601128, 10.41168362711695750, 0.7216878364870438212 ) ) ;
#80936=CARTESIAN_POINT ( 'NONE',  ( -6.534666852106790103, 10.56760239419251590, 0.7216878364870458196 ) ) ;
#80937=CARTESIAN_POINT ( 'NONE',  ( -1.364683531250014514, 0.7385416670080887647, -0.7879004041258289570 ) ) ;
#80939=CARTESIAN_POINT ( 'NONE',  ( -4.140487720836006247, 5.732536712720713190, 1.378239279427504238 ) ) ;
#80941=CARTESIAN_POINT ( 'NONE',  ( -7.832860060393135093, 10.16142270859057462, 1.599625672291295375 ) ) ;
#80942=CARTESIAN_POINT ( 'NONE',  ( -2.602802303699316866, 5.980427087717073320, 1.040834085586084257E-14 ) ) ;
#80943=CARTESIAN_POINT ( 'NONE',  ( 1.364683531249988535, 3.717708333674750953, -0.7879004041258239610 ) ) ;
#80948=CARTESIAN_POINT ( 'NONE',  ( 10.24726517383036928, 10.84956421242393887, 0.000000000000000000 ) ) ;
#80963=CARTESIAN_POINT ( 'NONE',  ( -1.364683531250010295, 4.592708333674755394, 0.7879004041258379498 ) ) ;
#80968=CARTESIAN_POINT ( 'NONE',  ( 8.178592977541601527, 10.56477777859713463, 1.599625672291281386 ) ) ;
#80972=CARTESIAN_POINT ( 'NONE',  ( -1.364683531250012516, 3.030208333674755394, 0.7879004041258379498 ) ) ;
#80975=CARTESIAN_POINT ( 'NONE',  ( -7.714226216495749355, 8.102278128774251797, 1.040834085586084257E-14 ) ) ;
#80977=CARTESIAN_POINT ( 'NONE',  ( 1.499999999999822364, 7.388542872122566330, 4.154462424328215775 ) ) ;
#80982=CARTESIAN_POINT ( 'NONE',  ( 4.325214697959421706, 5.004837554829479451, 1.199719254218462483 ) ) ;
#80984=VERTEX_POINT ( 'NONE', #161055 ) ;
#80985=CARTESIAN_POINT ( 'NONE',  ( 8.540746701604824409, 12.05162268759261224, -1.199719254218446718 ) ) ;
#80990=ORIENTED_EDGE ( 'NONE', *, *, #179458, .T. ) ;
#80992=CARTESIAN_POINT ( 'NONE',  ( -10.45741655484220267, 11.09474082360439873, -0.7998128361456221525 ) ) ;
#80993=CARTESIAN_POINT ( 'NONE',  ( 6.934105498385400246, 10.17720795050327354, -1.199719254218441611 ) ) ;
#80995=CARTESIAN_POINT ( 'NONE',  ( 4.324687812634882000, 7.028924300507257250, 1.082531754730558626 ) ) ;
#81006=CARTESIAN_POINT ( 'NONE',  ( -6.453317930424837812, 7.591587675992828466, 1.082531754730549967 ) ) ;
#81007=CARTESIAN_POINT ( 'NONE',  ( 5.983225862332436584, 5.874851682342960402, 0.7998128361456341429 ) ) ;
#81010=CARTESIAN_POINT ( 'NONE',  ( -6.970863535720637216, 11.28442455831609337, 0.7998128361456481317 ) ) ;
#81015=CARTESIAN_POINT ( 'NONE',  ( -10.32183501870554387, 10.93656236477829502, 0.7998128361456462443 ) ) ;
#81016=CARTESIAN_POINT ( 'NONE',  ( 5.070386261830877928, 5.978167395966564435, -1.082531754730548412 ) ) ;
#81018=CARTESIAN_POINT ( 'NONE',  ( 8.934986926605834157, 10.38290515491702770, -1.199719254218446718 ) ) ;
#81026=CARTESIAN_POINT ( 'NONE',  ( 4.053524740805938720, 3.831459740469437936, 1.214306433183764966E-14 ) ) ;
#81032=CARTESIAN_POINT ( 'NONE',  ( -7.296259222448620463, 11.66405285949874759, 0.7998128361456481317 ) ) ;
#81036=CARTESIAN_POINT ( 'NONE',  ( 7.971831135155394321, 8.402817200543854170, -0.7216878364870267237 ) ) ;
#81039=CARTESIAN_POINT ( 'NONE',  ( 4.871457266011829823, 4.577788319968905562, -0.7998128361456221525 ) ) ;
#81041=CARTESIAN_POINT ( 'NONE',  ( 3.683011284406639607, 7.448596931783069586, 0.7998128361456321445 ) ) ;
#81043=CARTESIAN_POINT ( 'NONE',  ( -4.726989112658928072, 8.666571064744069020, 1.040834085586084257E-14 ) ) ;
#81050=EDGE_CURVE ( 'NONE', #88615, #43706, #198485, .T. ) ;
#81053=CARTESIAN_POINT ( 'NONE',  ( -0.6823417656249969321, 3.530208333674754506, -1.181850606188749264 ) ) ;
#81054=CARTESIAN_POINT ( 'NONE',  ( 4.905525160106620319, 6.476373528817379821, 2.499999999999998668 ) ) ;
#81055=CARTESIAN_POINT ( 'NONE',  ( 9.185812768458653466, 10.67553530374532045, 1.199719254218453823 ) ) ;
#81057=CARTESIAN_POINT ( 'NONE',  ( -5.124618876285560454, 5.081069565195661220, 0.7216878364870317197 ) ) ;
#81059=CARTESIAN_POINT ( 'NONE',  ( -5.273758565591545988, 6.215435083687305351, 1.082531754730546636 ) ) ;
#81066=CARTESIAN_POINT ( 'NONE',  ( 4.792970997630896512, 5.550553237779539018, 1.199719254218464037 ) ) ;
#81074=CARTESIAN_POINT ( 'NONE',  ( 6.017121246366603060, 5.914396297049491658, 1.040834085586084257E-14 ) ) ;
#81075=CARTESIAN_POINT ( 'NONE',  ( 6.471393748265519719, 5.229711127717882491, -2.499999999999995115 ) ) ;
#81078=CARTESIAN_POINT ( 'NONE',  ( 0.6823417656249899377, 4.488541667008086655, -1.181850606188754593 ) ) ;
#81083=CARTESIAN_POINT ( 'NONE',  ( 6.368579470117202490, 8.453095353268645695, 1.599625672291281386 ) ) ;
#81085=CARTESIAN_POINT ( 'NONE',  ( -6.925517538482230506, 6.974191971184389160, 0.7998128361456341429 ) ) ;
#81086=CARTESIAN_POINT ( 'NONE',  ( 1.499999999999987121, 2.795833333333352488, -0.8660254037844262731 ) ) ;
#81089=CARTESIAN_POINT ( 'NONE',  ( -5.773074481320628948, 5.629675071162500544, 0.000000000000000000 ) ) ;
#81092=CARTESIAN_POINT ( 'NONE',  ( -1.364683531250012516, 3.030208333674755394, 0.7879004041258379498 ) ) ;
#81094=CARTESIAN_POINT ( 'NONE',  ( -3.416291520963659512, 5.969128626890772615, 1.082531754730560403 ) ) ;
#81097=ORIENTED_EDGE ( 'NONE', *, *, #14168, .F. ) ;
#81099=CARTESIAN_POINT ( 'NONE',  ( -5.273758566035884776, 5.255065869904374409, 0.000000000000000000 ) ) ;
#81100=CARTESIAN_POINT ( 'NONE',  ( 5.250031796989762967, 7.148123067953287446, 1.599625672291267398 ) ) ;
#81103=CARTESIAN_POINT ( 'NONE',  ( -0.08896015505786540600, 7.049507384512283537, -3.948637857577287580 ) ) ;
#81104=CARTESIAN_POINT ( 'NONE',  ( -1.364683531249997417, 3.571875000341423245, 1.214306433183764966E-14 ) ) ;
#81108=CARTESIAN_POINT ( 'NONE',  ( -1.364683531250014514, -0.4072916663252447167, 0.7879004041258379498 ) ) ;
#81113=CARTESIAN_POINT ( 'NONE',  ( -10.15913717534155047, 10.74674821418697057, 0.7998128361456462443 ) ) ;
#81114=CARTESIAN_POINT ( 'NONE',  ( -5.056828107772848746, 8.843457192469559303, -0.7216878364870207285 ) ) ;
#81117=ORIENTED_EDGE ( 'NONE', *, *, #22766, .F. ) ;
#81118=CARTESIAN_POINT ( 'NONE',  ( -1.201851678989727383E-14, 4.946875000341420581, -1.575800808251660134 ) ) ;
#81127=CARTESIAN_POINT ( 'NONE',  ( -6.521108698048791119, 6.710307690586118312, -0.7216878364870267237 ) ) ;
#81133=CARTESIAN_POINT ( 'NONE',  ( -6.860062538390436337, 7.105753837651378468, 1.040834085586084257E-14 ) ) ;
#81138=DIRECTION ( 'NONE',  ( 0.000000000000000000, 0.7766560405360211083, 0.6299249119529329866 ) ) ;
#81147=CARTESIAN_POINT ( 'NONE',  ( -5.928993247877788697, 5.811580298812519807, 0.7998128361456341429 ) ) ;
#81149=CARTESIAN_POINT ( 'NONE',  ( -1.402160292154681736E-14, -0.03749999999998095135, 1.732050807568877637 ) ) ;
#81150=CARTESIAN_POINT ( 'NONE',  ( 10.23604278863759909, 11.04439746293979496, 0.000000000000000000 ) ) ;
#81151=CARTESIAN_POINT ( 'NONE',  ( 7.121056995675668411, 9.330985799753529264, -1.599625672291262513 ) ) ;
#81154=CARTESIAN_POINT ( 'NONE',  ( 4.710568305744190276, 7.583081225755162968, 1.199719254218462483 ) ) ;
#81162=CARTESIAN_POINT ( 'NONE',  ( -4.961921032921567054, 4.891255414604337659, 0.7216878364870317197 ) ) ;
#81165=CARTESIAN_POINT ( 'NONE',  ( 3.001048869802141805, 2.786623193720118685, -2.499999999999995115 ) ) ;
#81166=CARTESIAN_POINT ( 'NONE',  ( -0.4092328571444365237, 6.441158382021245465, 3.221544509361615738 ) ) ;
#81170=CARTESIAN_POINT ( 'NONE',  ( -1.364683531249997417, 3.759375000341423689, 1.214306433183764966E-14 ) ) ;
#81171=CARTESIAN_POINT ( 'NONE',  ( 8.825994812371966702, 12.28044913353391898, -1.082531754730543083 ) ) ;
#81173=CARTESIAN_POINT ( 'NONE',  ( -5.716734326456539783, 9.821273814174633188, -0.7998128361456231517 ) ) ;
#81176=CARTESIAN_POINT ( 'NONE',  ( 5.632522751473472589, 8.658694745772667289, -1.199719254218440723 ) ) ;
#81177=CARTESIAN_POINT ( 'NONE',  ( -5.038826645773246682, 9.030381520044109322, 0.7998128361456481317 ) ) ;
#81180=CARTESIAN_POINT ( 'NONE',  ( -0.7500000000000249800, 0.2229166673494847872, 1.299038105676659116 ) ) ;
#81184=CARTESIAN_POINT ( 'NONE',  ( 6.127922243696800386, 10.09306701771420656, -0.7216878364870267237 ) ) ;
#81187=CARTESIAN_POINT ( 'NONE',  ( -1.364683531250012516, 0.8427083336747532849, 0.7879004041258379498 ) ) ;
#81189=CARTESIAN_POINT ( 'NONE',  ( 6.656690234185433042, 7.828855363713562276, -1.082531754730543971 ) ) ;
#81193=CARTESIAN_POINT ( 'NONE',  ( -4.826339496784927796, 5.693446170079573321, 1.082531754730560403 ) ) ;
#81195=CARTESIAN_POINT ( 'NONE',  ( -1.001543065824772872E-14, 5.071875000341421469, 1.575800808251672791 ) ) ;
#81199=CARTESIAN_POINT ( 'NONE',  ( -5.732732414299474222, 6.256854150074313559, -1.080652830874342163 ) ) ;
#81205=CARTESIAN_POINT ( 'NONE',  ( 7.579171565239241737, 8.801120566655981747, 1.199719254218462483 ) ) ;
#81208=CARTESIAN_POINT ( 'NONE',  ( 4.532503425670185493, 4.182342172903648070, 1.214306433183764966E-14 ) ) ;
#81216=CARTESIAN_POINT ( 'NONE',  ( 5.341549334104194635, 6.294524313618772737, 1.082531754730558626 ) ) ;
#81217=CARTESIAN_POINT ( 'NONE',  ( 0.6823417656249899377, 0.6552083336747518416, 1.181850606188755259 ) ) ;
#81223=CARTESIAN_POINT ( 'NONE',  ( 1.499999999999987121, 1.254166666666689300, 0.8660254037844524744 ) ) ;
#81224=CARTESIAN_POINT ( 'NONE',  ( 7.287671262545424966, 8.461036880179857889, -1.199719254218451159 ) ) ;
#81225=CARTESIAN_POINT ( 'NONE',  ( -8.877891658850122880, 9.251961778280284321, 0.7998128361456462443 ) ) ;
#81229=CARTESIAN_POINT ( 'NONE',  ( -1.364683531250012516, 1.780208333674757615, 0.7879004041258379498 ) ) ;
#81231=CARTESIAN_POINT ( 'NONE',  ( 1.499999999999989120, 2.504166666666687302, 0.8660254037844524744 ) ) ;
#81233=CARTESIAN_POINT ( 'NONE',  ( 5.657830175604453338, 5.495223381160312393, 0.7998128361456341429 ) ) ;
#81240=CARTESIAN_POINT ( 'NONE',  ( 0.7499999999999885647, -0.2354166659838466402, 1.299038105676657340 ) ) ;
#81241=CARTESIAN_POINT ( 'NONE',  ( -7.542413527904030524, 7.693903958843159252, 1.040834085586084257E-14 ) ) ;
#81242=CARTESIAN_POINT ( 'NONE',  ( -4.934804725694231564, 5.819988937140460727, -1.082531754730544860 ) ) ;
#81251=CARTESIAN_POINT ( 'NONE',  ( 5.438792177376376991, 9.497007973581119700, 1.040834085586084257E-14 ) ) ;
#81255=CARTESIAN_POINT ( 'NONE',  ( 7.820355676984174664, 8.018169799436671852, -0.7998128361456281477 ) ) ;
#81256=CARTESIAN_POINT ( 'NONE',  ( 7.565086526301031178, 11.76975868075249387, 1.040834085586084257E-14 ) ) ;
#81261=CARTESIAN_POINT ( 'NONE',  ( -6.344325816190970357, 9.489131654609717970, 1.199719254218452047 ) ) ;
#81262=CARTESIAN_POINT ( 'NONE',  ( 3.845709127770629010, 7.638411082374393146, 0.7998128361456321445 ) ) ;
#81265=CARTESIAN_POINT ( 'NONE',  ( 1.499999999999989120, 6.280000000000035776, 2.775557561562891351E-14 ) ) ;
#81266=CARTESIAN_POINT ( 'NONE',  ( 4.553433815925461481, 6.963525196941225737, 1.181321538200299281 ) ) ;
#81267=CARTESIAN_POINT ( 'NONE',  ( 7.754900677336718395, 11.99120852362745460, -0.7216878364870267237 ) ) ;
#81278=CARTESIAN_POINT ( 'NONE',  ( -4.121315508874280553, 3.910548969882488901, -0.7216878364870207285 ) ) ;
#81280=CARTESIAN_POINT ( 'NONE',  ( 7.592202833972727660, 11.80139437303613015, -0.7216878364870267237 ) ) ;
#81283=CARTESIAN_POINT ( 'NONE',  ( -5.636439174979254396, 7.598931675607687453, -1.599625672291256295 ) ) ;
#81287=CARTESIAN_POINT ( 'NONE',  ( 1.419999999999999485, 7.176846818246214177, 4.202462424328220258 ) ) ;
#81289=CARTESIAN_POINT ( 'NONE',  ( -6.826694039680798021, 7.923230120171105284, -1.199719254218446718 ) ) ;
#81292=CARTESIAN_POINT ( 'NONE',  ( 7.034482758620714371, 5.227586206896606136, 1.214306433183764966E-14 ) ) ;
#81304=CARTESIAN_POINT ( 'NONE',  ( 4.076333666143569623, 3.981184372846183983, -0.7419984331740974159 ) ) ;
#81305=CARTESIAN_POINT ( 'NONE',  ( -7.217017841176048165, 7.314275657660511243, 1.040834085586084257E-14 ) ) ;
#81308=CARTESIAN_POINT ( 'NONE',  ( 3.877268743828258479, 7.467304601200877023, 0.7216878364870298324 ) ) ;
#81310=CARTESIAN_POINT ( 'NONE',  ( 5.692136587293079586, 5.855332880448198551, 2.500000000000010658 ) ) ;
#81312=CARTESIAN_POINT ( 'NONE',  ( -2.272963308585411735, 5.803540959991587478, 0.7998128361456341429 ) ) ;
#81315=CARTESIAN_POINT ( 'NONE',  ( 8.920375002787457319, 12.49452237230570084, 1.199719254218450271 ) ) ;
#81318=CARTESIAN_POINT ( 'NONE',  ( -8.015895134177625891, 10.37496362800581018, 1.599625672291295375 ) ) ;
#81319=CARTESIAN_POINT ( 'NONE',  ( 6.986529229743720926, 7.045372277656132276, -0.7998128361456281477 ) ) ;
#81323=CARTESIAN_POINT ( 'NONE',  ( -1.402160292154681736E-14, 1.009375000341417916, -1.575800808251659024 ) ) ;
#81324=ORIENTED_EDGE ( 'NONE', *, *, #98548, .F. ) ;
#81326=CARTESIAN_POINT ( 'NONE',  ( 6.778713617152772208, 10.85232362007950258, -0.7216878364870267237 ) ) ;
#81334=CARTESIAN_POINT ( 'NONE',  ( 9.205623113554612047, 12.72334881824701469, 1.082531754730546636 ) ) ;
#81340=CARTESIAN_POINT ( 'NONE',  ( 6.385527162356455122, 10.39360608948380538, 1.056142170575426150E-14 ) ) ;
#81354=CARTESIAN_POINT ( 'NONE',  ( -1.500000000000013101, 0.4520833340161533598, 0.8660254037844403729 ) ) ;
#81360=CARTESIAN_POINT ( 'NONE',  ( -1.402160292154681736E-14, -0.9124999999999769962, -1.732050807568870754 ) ) ;
#81361=CARTESIAN_POINT ( 'NONE',  ( 9.738834413317897898, 10.25639499182604730, 0.000000000000000000 ) ) ;
#81366=CARTESIAN_POINT ( 'NONE',  ( 3.649115900372475796, 7.409052317076538330, 1.040834085586084257E-14 ) ) ;
#81367=CARTESIAN_POINT ( 'NONE',  ( -6.019457014787517046, 9.006155036351978893, 1.082531754730548412 ) ) ;
#81371=CARTESIAN_POINT ( 'NONE',  ( -7.477485413136760073, 8.682486722536401302, -1.199719254218446718 ) ) ;
#81373=ORIENTED_EDGE ( 'NONE', *, *, #167443, .F. ) ;
#81374=CARTESIAN_POINT ( 'NONE',  ( -1.201851678989727383E-14, 1.493750000682814383, 1.732050807568877637 ) ) ;
#81381=CARTESIAN_POINT ( 'NONE',  ( -4.568734577680899633, 4.432537883490215158, -0.7216878364870207285 ) ) ;
#81382=B_SPLINE_SURFACE_WITH_KNOTS ( 'NONE', 1, 3, ( 
 ( #51566, #117691, #85114, #134962, #35289, #167442, #151200, #128272, #95701, #178001, #195314, #196377, #113063, #160675, #77284, #44815, #11203, #193165, #45878, #144470, #112000, #62113, #61037, #12271, #161756, #32806, #210475, #13346, #179069, #79421, #145538, #31753, #147634, #143396, #46945, #14398, #209393, #211536, #64244, #80489, #163890, #30689, #159605, #63171, #129337, #29615, #78347, #28541, #97825, #197424, #96771, #194234, #162822, #180127, #114135, #146588, #65278, #212605, #94632, #48019, #127198, #130387, #15465, #110920, #176925, #81551, #213652, #49066, #131424, #115186, #181181, #19738, #133540, #3471, #100987, #164934, #4528, #66333, #102071, #98881, #99939, #85817, #53317, #167077, #118380, #34914, #2398, #70603, #132478, #69540, #198479, #136717, #184368, #50125, #1338, #263, #182235, #135647, #68477, #134604, #52253, #35991, #116246, #54393, #119450, #149761, #151897, #148693, #185437, #18668, #168136, #16525, #117312, #201670, #86886, #37057, #200606, #83671, #103139, #67399, #33859, #166002, #84748, #169198, #20791, #51189, #17587, #199547, #202743, #152953, #120532, #183308, #150836, #186510, #82608, #105923, #169803, #70145, #88576, #171948, #23537, #201215, #22464, #183917, #151437, #139462, #56063, #205493, #87502, #54997, #187113, #85355, #19273, #204410, #52855, #167672, #86427, #153567, #3008, #73358, #121149, #37676, #203345, #103753, #21392, #5136, #168738, #188181, #152492, #4075, #104827, #117923, #69078, #38746, #155699, #71212, #135198, #35528, #120065, #118989, #20341, #184967, #137328, #39816, #170873, #89646, #101604, #154633, #7281, #6213, #136257, #122220, #202277, #36593, #72284, #102680, #138392, #53928, #186041, #76567, #75509, #208688, #157843, #107001, #90716, #43039, #158898, #123293, #127557, #59248, #159962, #174107, #207630, #189257, #91787, #77637, #173026, #141621, #12626, #57127, #25679, #93922, #161031, #125406, #9439, #156778, #144824, #78697, #24607, #193526, #191372, #209754, #176222, #126476, #109151, #28900, #8365, #45168, #44095, #175164, #26751, #111280, #177285, #40896, #94985, #92852, #10494, #27824 ),
 ( #58192, #142678, #74448, #108078, #60317, #192440, #110215, #11567, #143759, #140552, #206565, #61395, #124351, #190308, #41966, #115530, #65618, #607, #164227, #84025, #64593, #130732, #80848, #149031, #210831, #196725, #146939, #211891, #79768, #82958, #34209, #163172, #113417, #48365, #16877, #165283, #97120, #116592, #212954, #145882, #99234, #62456, #129684, #66674, #128619, #162107, #114478, #194585, #182586, #178360, #213998, #46231, #63530, #197772, #132822, #180476, #15815, #32093, #98179, #100282, #29968, #181525, #96054, #166348, #81900, #13696, #179424, #112348, #195668, #33153, #147988, #131768, #49409, #198826, #47303, #17939, #50471, #31044, #14757, #199898, #104565, #69883, #21130, #1688, #168481, #54732, #138134, #22197, #53668, #134943, #137063, #200949, #19016, #183662, #86168, #170610, #38488, #102413, #51545, #167424, #39550, #88310, #204143, #118726, #152238, #20079, #185778, #169549, #119799, #133892, #120883, #35266, #67742, #101343, #36335, #52598, #3810, #184711, #117669, #151181, #135994, #23276, #202008, #37412, #103488, #87234, #153298, #154374, #55798, #85096, #4874, #70953, #2751, #203088, #186857, #5951, #72021, #121953, #150115, #187919, #105651, #171679, #68821, #89387, #157591, #173850, #90453, #172769, #178905, #130218, #41715, #206311, #144309, #112894, #46780, #190063, #212433, #25426, #24343, #195146, #179961, #8110, #96600, #155436, #40639, #106741, #123045, #196212, #13179, #64075, #7021, #79257, #124099, #211372, #29449, #107825, #139198, #188996, #75257, #194060, #73097, #162652, #91533, #30519, #57935, #9186, #205228, #210307, #14223, #56869, #61943, #47853, #156519, #128102, #129168, #113964, #45713, #111831, #74198, #140292, #177835, #95540, #80318, #161590, #146420, #62998, #145374, #17421, #3302, #65113, #167964, #18501, #83504, #94, #19571, #85645, #163717, #151731, #149586, #198312, #2229, #69371, #135479, #115016, #150668, #97659, #131269, #53147, #184200, #119278, #1170, #183146, #100823, #213491, #147469, #118213, #181012, #81386, #66159, #67236, #197256, #48895, #32634, #98710, #166908, #35823, #199375, #31585 ) ),
 .UNSPECIFIED., .F., .T., .F.,
 ( 2, 2 ),
 ( 4, 2, 2, 2, 2, 2, 2, 2, 2, 2, 2, 2, 2, 2, 2, 2, 2, 2, 2, 2, 2, 2, 2, 2, 2, 2, 2, 2, 2, 2, 2, 2, 2, 2, 2, 2, 2, 2, 2, 2, 2, 2, 2, 2, 2, 2, 2, 2, 2, 2, 2, 2, 2, 2, 2, 2, 2, 2, 2, 2, 2, 2, 2, 2, 2, 2, 2, 2, 2, 2, 2, 2, 2, 2, 2, 2, 2, 2, 2, 2, 2, 2, 2, 2, 2, 2, 2, 2, 2, 2, 2, 2, 2, 2, 2, 2, 2, 2, 2, 2, 2, 2, 2, 2, 2, 2, 2, 2, 2, 2, 2, 2, 2, 2, 2, 2, 2, 2, 2, 2, 2, 2, 2, 4 ),
 ( 0.000000000000000000, 1.000000000000000000 ),
 ( 0.0003308050673979778117, 0.0003990699536394003003, 0.0004673348398808227890, 0.0005355997261222453319, 0.0006038646123636677663, 0.0007403943848465126352, 0.0008769241573293576125, 0.0009110566004500689381, 0.0009451890435707801554, 0.001013453929812202590, 0.001081718816053625024, 0.001149983702295047459, 0.001286513474777892328, 0.001354778361019314762, 0.001388910804140025979, 0.001423043247260737413, 0.001491308133502160065, 0.001559573019743582499, 0.001696102792226427368, 0.001764367678467849802, 0.001832632564709272237, 0.001900897450950694671, 0.001969162337192117106, 0.002037427223433539540, 0.002105692109674961975, 0.002173956995916384409, 0.002242221882157806843, 0.002310486768399229278, 0.002344619211519940495, 0.002378751654640651712, 0.002515281427123497015, 0.002651811199606342317, 0.002720076085847764752, 0.002788340972089187186, 0.002856605858330609621, 0.002924870744572032055, 0.003061400517054876924, 0.003129665403296299359, 0.003197930289537721793, 0.003266195175779144227, 0.003334460062020566662, 0.003402724948261989096, 0.003470989834503411531, 0.003607519606986256400, 0.003675784493227678834, 0.003709916936348390051, 0.003744049379469101269, 0.003812314265710523703, 0.003880579151951946137, 0.004017108924434791006, 0.004085373810676213441, 0.004153638696917635875, 0.004187771140038347092, 0.004221903583159058310, 0.004290168469400480744, 0.004358433355641903179, 0.004426698241883325613, 0.004494963128124748047, 0.004529095571245459265, 0.004563228014366170482, 0.004631492900607592916, 0.004699757786849016218, 0.004836287559331861954, 0.004904552445573284389, 0.004972817331814706823, 0.005041082218056129258, 0.005109347104297551692, 0.005177611990538974127, 0.005245876876780396561, 0.005314141763021818995, 0.005382406649263241430, 0.005450671535504663864, 0.005518936421746086299, 0.005587201307987508733, 0.005655466194228931168, 0.005791995966711776037, 0.005860260852953198471, 0.005928525739194620905, 0.005962658182315332123, 0.005996790625436043340, 0.006065055511677465774, 0.006133320397918888209, 0.006201585284160310643, 0.006269850170401733078, 0.006338115056643155512, 0.006406379942884577947, 0.006440512386005289164, 0.006474644829126000381, 0.006611174601608845250, 0.006747704374091690119, 0.006815969260333112553, 0.006850101703453823770, 0.006884234146574534988, 0.006952499032815957422, 0.007020763919057379857, 0.007157293691540224725, 0.007225558577781647160, 0.007293823464023069594, 0.007327955907143780812, 0.007362088350264492029, 0.007430353236505915331, 0.007498618122747338632, 0.007566883008988761067, 0.007635147895230183501, 0.007703412781471605936, 0.007771677667713028370, 0.007805810110833739587, 0.007839942553954450805, 0.007908207440195873239, 0.007976472326437295673, 0.008113002098920140542, 0.008181266985161562977, 0.008249531871402985411, 0.008317796757644407846, 0.008386061643885830280, 0.008454326530127252715, 0.008522591416368675149, 0.008590856302610097583, 0.008659121188851520018, 0.008727386075092942452, 0.008761518518213653670, 0.008795650961334364887, 0.008932180733817209756, 0.009068710506300054625 ),
 .UNSPECIFIED. ) ;
#81386=CARTESIAN_POINT ( 'NONE',  ( 4.050410598061423784, 7.525715715152009544, -0.4746587800704554772 ) ) ;
#81390=CARTESIAN_POINT ( 'NONE',  ( -2.453662613948990323, 5.806430783008362795, -0.7216878364870257245 ) ) ;
#81391=CARTESIAN_POINT ( 'NONE',  ( 7.958799866421889746, 9.244020251369077457, -1.199719254218441611 ) ) ;
#81399=DIRECTION ( 'NONE',  ( 1.000000000000000000, 0.000000000000000000, 0.000000000000000000 ) ) ;
#81400=CARTESIAN_POINT ( 'NONE',  ( -8.239604668803112375, 10.63595808506888396, -1.599625672291263179 ) ) ;
#81405=CARTESIAN_POINT ( 'NONE',  ( 2.842405760359353106, 6.467890487061221272, -0.7998128361456291469 ) ) ;
#81411=CARTESIAN_POINT ( 'NONE',  ( -8.676328237741483207, 12.20980114641871062, -1.199719254218446718 ) ) ;
#81415=EDGE_LOOP ( 'NONE', ( #55610, #74940, #2130, #63269 ) ) ;
#81423=CARTESIAN_POINT ( 'NONE',  ( 5.784525094524856748, 9.900363043587685041, 1.040834085586084257E-14 ) ) ;
#81425=CARTESIAN_POINT ( 'NONE',  ( -4.569261463005423352, 5.289558780716470565, -1.199719254218446718 ) ) ;
#81435=CARTESIAN_POINT ( 'NONE',  ( -1.500000000000015099, 0.6604166673494823447, -0.8660254037844313801 ) ) ;
#81440=CYLINDRICAL_SURFACE ( 'NONE', #85740, 1.250000000000000000 ) ;
#81442=CARTESIAN_POINT ( 'NONE',  ( -2.788173145904702555, 6.404619103530779789, -0.7998128361456281477 ) ) ;
#81449=CARTESIAN_POINT ( 'NONE',  ( 4.609409038966229666, 6.400729850259146758, -1.443375672974051449 ) ) ;
#81452=CARTESIAN_POINT ( 'NONE',  ( 1.364683531249990311, 4.446875000341417028, 1.214306433183764966E-14 ) ) ;
#81454=CARTESIAN_POINT ( 'NONE',  ( 3.023105065722954787, 5.510411095776657220, 1.082531754730546636 ) ) ;
#81462=CARTESIAN_POINT ( 'NONE',  ( -6.136274411746873270, 5.997031558969919018, 0.08344787587596068368 ) ) ;
#81464=CARTESIAN_POINT ( 'NONE',  ( -1.402160292154681736E-14, -1.178124999658576311, 1.575800808251672791 ) ) ;
#81472=CARTESIAN_POINT ( 'NONE',  ( 1.499999999999989120, 4.254166666666687746, 0.8660254037844524744 ) ) ;
#81480=CARTESIAN_POINT ( 'NONE',  ( 0.6823417656249917140, 4.405208333674755394, 1.181850606188765695 ) ) ;
#81482=CARTESIAN_POINT ( 'NONE',  ( 5.124091990960999432, 8.065525525174782828, -1.199719254218452047 ) ) ;
#81483=CARTESIAN_POINT ( 'NONE',  ( -7.557780564614042795, 10.90482886110335414, -1.199719254218446718 ) ) ;
#81489=CARTESIAN_POINT ( 'NONE',  ( -0.7499999999999972244, 5.608333333333353821, -1.299038105676652011 ) ) ;
#81493=CARTESIAN_POINT ( 'NONE',  ( 4.292412370785825715, 7.263935575258185118, -1.002239974148201762 ) ) ;
#81495=AXIS2_PLACEMENT_3D ( 'NONE', #50660, #116786, #182783 ) ;
#81497=CARTESIAN_POINT ( 'NONE',  ( 7.700668062882064291, 10.00719871149432549, -1.443375672974057666 ) ) ;
#81501=CARTESIAN_POINT ( 'NONE',  ( 0.7499999999999920064, 4.764583334016150751, 1.299038105676669330 ) ) ;
#81503=CARTESIAN_POINT ( 'NONE',  ( -3.846762897975357198, 5.510976019103107859, -1.599625672291256295 ) ) ;
#81504=CARTESIAN_POINT ( 'NONE',  ( 5.788968402910805722, 7.776882441527838807, 1.443375672974062551 ) ) ;
#81505=CARTESIAN_POINT ( 'NONE',  ( -8.609064354553318310, 12.98773281371349775, 0.7216878364870317197 ) ) ;
#81512=CARTESIAN_POINT ( 'NONE',  ( 3.822509244049070887, 6.547012320444182798, -1.199719254218452047 ) ) ;
#81514=CARTESIAN_POINT ( 'NONE',  ( 3.785751206713845018, 5.439795712631356750, 1.599625672291267398 ) ) ;
#81520=CARTESIAN_POINT ( 'NONE',  ( 8.269583629331492602, 11.73526576994040482, 1.199719254218450271 ) ) ;
#81528=CARTESIAN_POINT ( 'NONE',  ( 8.971744963941056028, 11.49012176272984931, 1.599625672291281386 ) ) ;
#81532=CARTESIAN_POINT ( 'NONE',  ( 0.6823417656249882723, -0.07395833299191079124, -1.181850606188749264 ) ) ;
#81533=CARTESIAN_POINT ( 'NONE',  ( 6.046573322014824114, 7.117052299514516456, -1.082531754730543083 ) ) ;
#81534=CARTESIAN_POINT ( 'NONE',  ( -8.649738815838677652, 13.03518635187974262, 0.7216878364870357165 ) ) ;
#81539=CARTESIAN_POINT ( 'NONE',  ( -4.115063316947640715, 4.759660943649018705, 1.199719254218462483 ) ) ;
#81542=ORIENTED_EDGE ( 'NONE', *, *, #6348, .F. ) ;
#81551=CARTESIAN_POINT ( 'NONE',  ( 5.803731464950218744, 6.215061796778338810, -0.9591748237987550718 ) ) ;
#81552=CARTESIAN_POINT ( 'NONE',  ( -4.480905194642735623, 5.440750306600657282, -1.194628488029887414 ) ) ;
#81555=FACE_OUTER_BOUND ( 'NONE', #2164, .T. ) ;
#81558=CARTESIAN_POINT ( 'NONE',  ( -8.351459436338041442, 9.806086099558291025, -1.082531754730543971 ) ) ;
#81562=CARTESIAN_POINT ( 'NONE',  ( 5.750629710490689384, 9.860818428881154674, -0.7998128361456291469 ) ) ;
#81563=CARTESIAN_POINT ( 'NONE',  ( -5.922214171070950606, 5.803671375871217286, -0.7998128361456291469 ) ) ;
#81564=CARTESIAN_POINT ( 'NONE',  ( 2.367870383881045981, 5.914265881169853856, 0.000000000000000000 ) ) ;
#81566=CARTESIAN_POINT ( 'NONE',  ( -4.252453736180621391, 8.112946458852704268, -0.7998128361456281477 ) ) ;
#81567=CARTESIAN_POINT ( 'NONE',  ( 4.871457266011829823, 4.577788319968905562, -0.7998128361456221525 ) ) ;
#81572=CARTESIAN_POINT ( 'NONE',  ( -6.067437437315529536, 7.037430750744921859, 1.199719254218450271 ) ) ;
#81576=CARTESIAN_POINT ( 'NONE',  ( 9.134442807305049428, 11.67993591332117376, 1.599625672291281386 ) ) ;
#81579=CARTESIAN_POINT ( 'NONE',  ( 4.441740843186996912, 7.307116142998927977, 1.228109861675081849 ) ) ;
#81580=CARTESIAN_POINT ( 'NONE',  ( 3.863710590214593399, 7.451486755318259547, 1.040834085586084257E-14 ) ) ;
#81586=CARTESIAN_POINT ( 'NONE',  ( 8.392133896734671694, 8.893170422386358354, 0.7216878364870458196 ) ) ;
#81589=CARTESIAN_POINT ( 'NONE',  ( -10.45741655484220267, 11.09474082360439873, -0.7998128361456221525 ) ) ;
#81590=CARTESIAN_POINT ( 'NONE',  ( -6.795661308947694934, 8.951357498570873261, -1.599625672291263179 ) ) ;
#81598=CARTESIAN_POINT ( 'NONE',  ( 8.215351014876830504, 11.67199438640995801, -1.199719254218446718 ) ) ;
#81602=CARTESIAN_POINT ( 'NONE',  ( 4.090809663021327758, 5.795697244990093644, 1.599625672291267398 ) ) ;
#81606=CARTESIAN_POINT ( 'NONE',  ( -1.001543065824772872E-14, 4.493750000682820378, 1.732050807568877637 ) ) ;
#81612=CARTESIAN_POINT ( 'NONE',  ( -1.499999999999997780, 2.900000000000020783, 1.214306433183764966E-14 ) ) ;
#81613=CARTESIAN_POINT ( 'NONE',  ( 4.611744806942754238, 8.532119374741881757, -0.7998128361456231517 ) ) ;
#81615=CARTESIAN_POINT ( 'NONE',  ( 1.499999999999990896, 4.775000000000022560, 1.214306433183764966E-14 ) ) ;
#81616=CARTESIAN_POINT ( 'NONE',  ( 6.466876084038451822, 10.48851316477946582, 1.040834085586084257E-14 ) ) ;
#81622=CARTESIAN_POINT ( 'NONE',  ( -5.264643720808155791, 5.036505850564608089, 0.000000000000000000 ) ) ;
#81623=CARTESIAN_POINT ( 'NONE',  ( -0.7499999999999972244, 5.639583334016151639, -1.299038105676652899 ) ) ;
#81624=CARTESIAN_POINT ( 'NONE',  ( 1.364683531249986537, -0.8864583329919110133, 0.7879004041258500513 ) ) ;
#81628=CARTESIAN_POINT ( 'NONE',  ( 3.323720213644492993, 7.029424015893889433, 1.040834085586084257E-14 ) ) ;
#81630=CARTESIAN_POINT ( 'NONE',  ( -0.6823417656249969321, 5.030208333674755394, -1.181850606188749264 ) ) ;
#81634=DIRECTION ( 'NONE',  ( -5.578564026256490882E-16, -1.000000000000000000, -9.066213480720158442E-32 ) ) ;
#81639=CARTESIAN_POINT ( 'NONE',  ( -7.562750758324527922, 7.717630727667075696, 1.040834085586084257E-14 ) ) ;
#81641=CARTESIAN_POINT ( 'NONE',  ( 4.843287188579786573, 6.673587691474970107, -1.599625672291256295 ) ) ;
#81644=CARTESIAN_POINT ( 'NONE',  ( -1.402160292154681736E-14, 0.07187500034142156602, 1.575800808251672791 ) ) ;
#81646=ORIENTED_EDGE ( 'NONE', *, *, #111378, .F. ) ;
#81648=CARTESIAN_POINT ( 'NONE',  ( 10.42352117080803708, 11.05519620889787724, -0.7998128361456281477 ) ) ;
#81651=CARTESIAN_POINT ( 'NONE',  ( -5.032047568966410367, 9.022472597102808578, 1.214306433183764966E-14 ) ) ;
#81655=CARTESIAN_POINT ( 'NONE',  ( 9.023114925094663619, 10.48572115315399245, 1.199719254218453823 ) ) ;
#81657=CARTESIAN_POINT ( 'NONE',  ( 7.944187942603509356, 11.35563746875774882, 1.199719254218460707 ) ) ;
#81659=DIRECTION ( 'NONE',  ( 0.1674078377056216482, 0.000000000000000000, 0.9858877298530133171 ) ) ;
#81660=CARTESIAN_POINT ( 'NONE',  ( -3.578462479003122976, 6.262291094557191684, 1.199719254218464037 ) ) ;
#81661=CARTESIAN_POINT ( 'NONE',  ( -5.506582945444718824, 9.576097202994168001, 0.7998128361456481317 ) ) ;
#81664=CARTESIAN_POINT ( 'NONE',  ( -5.029856876702963220, 6.770753873564038017, 1.447965164949674310 ) ) ;
#81665=CARTESIAN_POINT ( 'NONE',  ( -1.402160292154681736E-14, 0.07187500034142156602, 1.575800808251672791 ) ) ;
#81669=CARTESIAN_POINT ( 'NONE',  ( 5.802526556968819804, 9.713438716531550554, -0.7216878364870267237 ) ) ;
#81672=CARTESIAN_POINT ( 'NONE',  ( 5.626797444871351139, 6.523350759560078593, 1.199719254218462483 ) ) ;
#81686=DIRECTION ( 'NONE',  ( -0.7592566023652990159, 0.6507913734559659380, -1.175982368226361624E-15 ) ) ;
#81687=EDGE_CURVE ( 'NONE', #140589, #133576, #36353, .T. ) ;
#81691=CARTESIAN_POINT ( 'NONE',  ( 8.224992744984721327, 12.74757530245756243, 1.040834085586084257E-14 ) ) ;
#81696=CARTESIAN_POINT ( 'NONE',  ( -4.062639585589296942, 7.891496616496157301, 0.7998128361456341429 ) ) ;
#81697=CARTESIAN_POINT ( 'NONE',  ( -8.128276786592724790, 9.441743324901704426, -1.199719254218446718 ) ) ;
#81704=B_SPLINE_CURVE_WITH_KNOTS ( 'NONE', 3,
 ( #202292, #181781, #199087, #102695 ),
 .UNSPECIFIED., .F., .F.,
 ( 4, 4 ),
 ( 0.000000000000000000, 0.002006560693247981270 ),
 .UNSPECIFIED. ) ;
#81705=CARTESIAN_POINT ( 'NONE',  ( -1.500000000000013101, 2.702083334016155636, 0.8660254037844403729 ) ) ;
#81706=CARTESIAN_POINT ( 'NONE',  ( 8.215351014876830504, 11.67199438640995801, -1.199719254218446718 ) ) ;
#81710=CARTESIAN_POINT ( 'NONE',  ( -9.515124878692420296, 9.995400534762978850, 1.040834085586084257E-14 ) ) ;
#81711=CARTESIAN_POINT ( 'NONE',  ( 1.499999999999990896, 4.775000000000022560, 1.214306433183764966E-14 ) ) ;
#81712=CARTESIAN_POINT ( 'NONE',  ( 1.364683531249988535, 3.113541667008083991, 0.7879004041258500513 ) ) ;
#81714=CARTESIAN_POINT ( 'NONE',  ( -6.520158902582637417, 5.290451655907114414, 2.438235897557452958 ) ) ;
#81718=CARTESIAN_POINT ( 'NONE',  ( -8.676855123066012254, 12.10645282934361866, -1.082531754730543971 ) ) ;
#81722=CARTESIAN_POINT ( 'NONE',  ( -1.364683531250014514, 1.551041667008084435, -0.7879004041258289570 ) ) ;
#81727=CARTESIAN_POINT ( 'NONE',  ( -1.201851678989727383E-14, 2.571875000341417472, 1.575800808251672791 ) ) ;
#81730=CARTESIAN_POINT ( 'NONE',  ( -4.401593425930945713, 8.286942763561420122, 1.040834085586084257E-14 ) ) ;
#81731=CARTESIAN_POINT ( 'NONE',  ( 8.260995669428309540, 8.532249790621511565, 0.7998128361456481317 ) ) ;
#81732=CARTESIAN_POINT ( 'NONE',  ( 1.000000000000001554, 5.868705557303652398, -4.125226524755055024 ) ) ;
#81734=CARTESIAN_POINT ( 'NONE',  ( 0.7499999999999920064, 4.483333333333352932, 1.299038105676669330 ) ) ;
#81736=CARTESIAN_POINT ( 'NONE',  ( -0.6823417656250003738, 2.780208333674753618, -1.181850606188749264 ) ) ;
#81740=CARTESIAN_POINT ( 'NONE',  ( -5.748293942514189681, 5.808690475795744490, -0.7216878364870207285 ) ) ;
#81743=CARTESIAN_POINT ( 'NONE',  ( 3.863710590214593399, 7.451486755318259547, 1.040834085586084257E-14 ) ) ;
#81746=CARTESIAN_POINT ( 'NONE',  ( -6.503107236049161521, 10.73870887536603291, 0.7998128361456481317 ) ) ;
#81747=CARTESIAN_POINT ( 'NONE',  ( -2.764973262183167968, 5.313220341600567664, 1.199719254218462483 ) ) ;
#81749=CARTESIAN_POINT ( 'NONE',  ( 1.364683531249988535, 5.155208333674749177, -0.7879004041258300672 ) ) ;
#81752=DIRECTION ( 'NONE',  ( -3.347138415753902517E-16, -0.6000000000000018652, -0.7999999999999984901 ) ) ;
#81754=CARTESIAN_POINT ( 'NONE',  ( -6.765155463094763455, 8.915767345075790828, 1.443375672974078761 ) ) ;
#81756=CARTESIAN_POINT ( 'NONE',  ( -0.6823417656250246877, -0.6364583329919113464, 1.181850606188755259 ) ) ;
#81759=CARTESIAN_POINT ( 'NONE',  ( 6.914295153289432783, 10.05013286460426691, -1.082531754730537976 ) ) ;
#81769=CARTESIAN_POINT ( 'NONE',  ( 9.097157884645296733, 10.67606762258344055, -1.082531754730543083 ) ) ;
#81776=CARTESIAN_POINT ( 'NONE',  ( 7.311924916471702396, 7.425000578838787391, -0.7998128361456281477 ) ) ;
#81777=CARTESIAN_POINT ( 'NONE',  ( -4.253507506385335368, 5.985511395581417204, 1.599625672291267398 ) ) ;
#81779=CARTESIAN_POINT ( 'NONE',  ( -0.7500000000000215383, 3.441666666666689967, 1.299038105676671107 ) ) ;
#81781=CARTESIAN_POINT ( 'NONE',  ( 5.138177029454841893, 7.017625839162543677, 1.443375672974062551 ) ) ;
#81782=CARTESIAN_POINT ( 'NONE',  ( 0.6823417656249882723, 0.4052083336747516751, 1.181850606188755259 ) ) ;
#81784=CARTESIAN_POINT ( 'NONE',  ( -10.45741655484220267, 11.09474082360439873, -0.7998128361456221525 ) ) ;
#81790=CARTESIAN_POINT ( 'NONE',  ( 4.177814833343409084, 3.976464848429826393, 1.040551764647542070E-14 ) ) ;
#81794=CARTESIAN_POINT ( 'NONE',  ( -0.7499999999999972244, 4.608333333333352932, -1.299038105676652011 ) ) ;
#81802=CARTESIAN_POINT ( 'NONE',  ( 6.120616281565444794, 9.228137197546649517, -1.199719254218440723 ) ) ;
#81803=CARTESIAN_POINT ( 'NONE',  ( 5.798083248138522272, 9.916180889470295412, 0.7998128361456462443 ) ) ;
#81811=CARTESIAN_POINT ( 'NONE',  ( -2.285154342840974184, 5.536993397787091098, 0.3900462783498563901 ) ) ;
#81812=CARTESIAN_POINT ( 'NONE',  ( -1.500000000000022204, 6.280000000000042881, 2.580000000000011173 ) ) ;
#81814=CARTESIAN_POINT ( 'NONE',  ( -2.442440228756222353, 6.001264033524212671, -0.7998128361456281477 ) ) ;
#81819=PLANE ( 'NONE',  #193876 ) ;
#81825=CARTESIAN_POINT ( 'NONE',  ( -9.083599731475995753, 11.62061899152058686, 1.443375672974064550 ) ) ;
#81828=CARTESIAN_POINT ( 'NONE',  ( 5.099838337034727331, 9.101561826515851550, -0.7998128361456281477 ) ) ;
#81834=CARTESIAN_POINT ( 'NONE',  ( 5.639828713160493834, 5.682147708216442439, 1.040834085586084257E-14 ) ) ;
#81841=CARTESIAN_POINT ( 'NONE',  ( -7.379715684540041565, 7.504089808251839244, 1.040834085586084257E-14 ) ) ;
#81843=CARTESIAN_POINT ( 'NONE',  ( -5.284980951228653190, 5.060232619388524533, 0.000000000000000000 ) ) ;
#81852=CARTESIAN_POINT ( 'NONE',  ( 7.149227073107712549, 7.235186428247455837, -0.7998128361456281477 ) ) ;
#81861=CARTESIAN_POINT ( 'NONE',  ( 3.999292125906899198, 6.649295999324608353, 1.082531754730558626 ) ) ;
#81864=CARTESIAN_POINT ( 'NONE',  ( 0.6823417656249882723, -0.3447916663252489911, 1.181850606188755259 ) ) ;
#81865=CARTESIAN_POINT ( 'NONE',  ( 3.832150974156964818, 7.622593236491780999, 1.040834085586084257E-14 ) ) ;
#81867=CARTESIAN_POINT ( 'NONE',  ( -6.046573322014817897, 9.998159942418544333, 0.7216878364870458196 ) ) ;
#81868=CARTESIAN_POINT ( 'NONE',  ( -1.152833933277347844, 3.300000000000025135, -0.7331020405358537051 ) ) ;
#81870=CARTESIAN_POINT ( 'NONE',  ( 5.178851490740205676, 6.104710163027444736, 1.082531754730558626 ) ) ;
#81871=CARTESIAN_POINT ( 'NONE',  ( -6.954969613686107444, 10.09758640173367894, 1.082531754730549967 ) ) ;
#81876=CARTESIAN_POINT ( 'NONE',  ( 5.615048174354031474, 9.702639970055050966, 0.7998128361456462443 ) ) ;
#81881=CARTESIAN_POINT ( 'NONE',  ( -1.364683531249997417, 3.509375000341423245, 1.214306433183764966E-14 ) ) ;
#81886=CARTESIAN_POINT ( 'NONE',  ( 6.421758314367153275, 10.64380180007036891, -0.7998128361456291469 ) ) ;
#81889=CARTESIAN_POINT ( 'NONE',  ( -6.842061076390810292, 11.13415502243129218, 0.000000000000000000 ) ) ;
#81895=CARTESIAN_POINT ( 'NONE',  ( 9.511208455186636712, 11.05516360492796935, 1.199719254218453823 ) ) ;
#81897=CARTESIAN_POINT ( 'NONE',  ( -7.991641480251377772, 11.41099992934688956, 1.199719254218453823 ) ) ;
#81900=CARTESIAN_POINT ( 'NONE',  ( 5.587453275722374713, 6.167276584799368244, -0.8733612469495740660 ) ) ;
#81901=CARTESIAN_POINT ( 'NONE',  ( -4.776550190716183586, 4.467063398790632966, 1.214306433183764966E-14 ) ) ;
#81904=CARTESIAN_POINT ( 'NONE',  ( -1.484314741415495353, 7.334687650741205545, 4.257443109328100661 ) ) ;
#81906=CARTESIAN_POINT ( 'NONE',  ( 7.149227073107712549, 7.235186428247455837, -0.7998128361456281477 ) ) ;
#81908=CARTESIAN_POINT ( 'NONE',  ( 6.471319392424407901, 6.444294134116939077, 0.7998128361456341429 ) ) ;
#81909=CARTESIAN_POINT ( 'NONE',  ( -4.018125071768071876, 7.621166010707856486, 0.1319346992594405132 ) ) ;
#81910=CARTESIAN_POINT ( 'NONE',  ( 4.844340958784499662, 4.546152628203684820, 0.7998128361456341429 ) ) ;
#81913=CARTESIAN_POINT ( 'NONE',  ( -8.039621903223732602, 8.481906429956900695, 1.040834085586084257E-14 ) ) ;
#81919=CARTESIAN_POINT ( 'NONE',  ( -4.016961781477323079, 7.622873323794868483, 0.1115696107641880874 ) ) ;
#81920=CARTESIAN_POINT ( 'NONE',  ( 0.6823417656249864960, -0.7614583329919113464, -1.181850606188749264 ) ) ;
#81923=CARTESIAN_POINT ( 'NONE',  ( 5.233084105194869551, 6.167981546557892436, -1.082531754730548412 ) ) ;
#81928=CARTESIAN_POINT ( 'NONE',  ( -9.124274191872636663, 11.66807252865000244, -1.443375672974058777 ) ) ;
#81933=CARTESIAN_POINT ( 'NONE',  ( -8.907343734053998929, 12.37535620882957588, 1.082531754730558626 ) ) ;
#81936=VERTEX_POINT ( 'NONE', #24149 ) ;
#81942=CARTESIAN_POINT ( 'NONE',  ( -8.581948047326017459, 11.99572790764693409, 1.082531754730558626 ) ) ;
#81943=EDGE_CURVE ( 'NONE', #8852, #14053, #189867, .T. ) ;
#81948=CARTESIAN_POINT ( 'NONE',  ( 0.7499999999999902300, 2.514583334016148974, 1.299038105676669330 ) ) ;
#81952=CARTESIAN_POINT ( 'NONE',  ( -7.483210719738908168, 10.81783070874899799, 1.199719254218453823 ) ) ;
#81953=CARTESIAN_POINT ( 'NONE',  ( 6.938893903907228378E-15, 10.64264068711930733, 1.214306433183764966E-14 ) ) ;
#81955=CARTESIAN_POINT ( 'NONE',  ( 7.135668919494039031, 7.219368582364847242, 1.040834085586084257E-14 ) ) ;
#81961=CARTESIAN_POINT ( 'NONE',  ( 7.853197290813620945, 10.18514947741448573, 1.599625672291281386 ) ) ;
#81964=DIRECTION ( 'NONE',  ( -5.578564026256490882E-16, -1.000000000000000000, -9.066213480720158442E-32 ) ) ;
#81967=CARTESIAN_POINT ( 'NONE',  ( -5.083944415444539899, 8.875092884753202682, 0.000000000000000000 ) ) ;
#81970=CARTESIAN_POINT ( 'NONE',  ( 0.6823417656249917140, 4.905208333674755394, 1.181850606188765695 ) ) ;
#81973=DIRECTION ( 'NONE',  ( 0.6507913734559640506, -0.7592566023653004592, 0.000000000000000000 ) ) ;
#81974=EDGE_CURVE ( 'NONE', #14088, #154674, #64735, .T. ) ;
#81977=CARTESIAN_POINT ( 'NONE',  ( -8.618179199781044630, 13.20629283305325963, 0.7998128361456341429 ) ) ;
#81979=CARTESIAN_POINT ( 'NONE',  ( 10.09812548408005384, 10.67556790771522124, -0.7998128361456281477 ) ) ;
#81980=DIRECTION ( 'NONE',  ( 1.000000000000000000, -5.578564026256490882E-16, -5.570868214615546318E-48 ) ) ;
#81981=CARTESIAN_POINT ( 'NONE',  ( -8.208571938070008400, 11.66408546346865016, -1.199719254218446718 ) ) ;
#81982=CARTESIAN_POINT ( 'NONE',  ( 4.101444922696781070, 3.685019076479660427, 2.420000000000010587 ) ) ;
#81984=CARTESIAN_POINT ( 'NONE',  ( -1.402160292154681736E-14, 2.196875000341423689, -1.575800808251660134 ) ) ;
#81985=CARTESIAN_POINT ( 'NONE',  ( 3.659811400685081040, 6.357198169852855685, -1.199719254218446718 ) ) ;
#81991=CARTESIAN_POINT ( 'NONE',  ( 8.337901282279995385, 11.71100668175994386, -1.082531754730543083 ) ) ;
#81993=CARTESIAN_POINT ( 'NONE',  ( -6.060131475628484310, 10.01397778830115470, 0.000000000000000000 ) ) ;
#81995=CARTESIAN_POINT ( 'NONE',  ( -1.364683531250000748, 0.2593750003414205252, 0.000000000000000000 ) ) ;
#81997=CARTESIAN_POINT ( 'NONE',  ( 0.3088250840612624115, 7.211283896344578004, 2.083830622148073353 ) ) ;
#81999=CARTESIAN_POINT ( 'NONE',  ( -8.076906825439122528, 10.44614393447756129, -1.599625672291263179 ) ) ;
#82000=CARTESIAN_POINT ( 'NONE',  ( -2.440104460335327463, 5.790612937125752424, 1.040834085586084257E-14 ) ) ;
#82001=CARTESIAN_POINT ( 'NONE',  ( -0.6823417656249969321, 3.530208333674754506, -1.181850606188749264 ) ) ;
#82020=CARTESIAN_POINT ( 'NONE',  ( -0.6823417656250212460, 4.863541667008086655, 1.181850606188767472 ) ) ;
#82025=CARTESIAN_POINT ( 'NONE',  ( 8.072990401933337168, 11.50590700464255356, -1.199719254218446718 ) ) ;
#82026=DIRECTION ( 'NONE',  ( -0.6507913734559640506, -0.7592566023653004592, 0.000000000000000000 ) ) ;
#82028=CARTESIAN_POINT ( 'NONE',  ( 0.6823417656249882723, 2.176041667008084435, -1.181850606188749264 ) ) ;
#82030=CARTESIAN_POINT ( 'NONE',  ( -6.236387472606141458, 10.21960978477508952, -0.7216878364870278340 ) ) ;
#82036=CARTESIAN_POINT ( 'NONE',  ( 5.030238685870051185, 5.827365540725222282, -1.199719254218452047 ) ) ;
#82039=CARTESIAN_POINT ( 'NONE',  ( 10.56588178375152864, 11.22128359066528169, -0.7998128361456281477 ) ) ;
#82040=LINE ( 'NONE', #31183, #88895 ) ;
#82047=CARTESIAN_POINT ( 'NONE',  ( -7.960608749518247151, 12.43912730774665576, 0.000000000000000000 ) ) ;
#82048=CARTESIAN_POINT ( 'NONE',  ( 6.958359152311676787, 9.141171649162195934, -1.599625672291262513 ) ) ;
#82050=CARTESIAN_POINT ( 'NONE',  ( 4.812781342726858647, 6.637997537979888563, 1.443375672974062551 ) ) ;
#82061=CARTESIAN_POINT ( 'NONE',  ( -7.375272376154101472, 7.706831981708990753, -0.7216878364870278340 ) ) ;
#82062=CARTESIAN_POINT ( 'NONE',  ( 3.486418057008484617, 7.219238166485217434, 1.040834085586084257E-14 ) ) ;
#82065=CARTESIAN_POINT ( 'NONE',  ( -9.481229494658258261, 9.955855920056455588, -0.7998128361456291469 ) ) ;
#82070=CARTESIAN_POINT ( 'NONE',  ( -10.29471871147821282, 10.90492667301307605, -0.7998128361456291469 ) ) ;
#82071=CARTESIAN_POINT ( 'NONE',  ( -1.201851678989727383E-14, 3.071875000341419248, 1.575800808251672791 ) ) ;
#82074=CARTESIAN_POINT ( 'NONE',  ( 8.772289083241844310, 10.19309100432570148, -1.199719254218446718 ) ) ;
#82075=EDGE_CURVE ( 'NONE', #92250, #201176, #31400, .T. ) ;
#82084=CARTESIAN_POINT ( 'NONE',  ( -4.092446641025072829, 3.979529022206003575, 0.4031905389056175126 ) ) ;
#82086=CARTESIAN_POINT ( 'NONE',  ( -7.635213062790267458, 12.05949900656400686, 0.000000000000000000 ) ) ;
#82090=CARTESIAN_POINT ( 'NONE',  ( 6.968527767744098433, 9.153035033833367251, 1.443375672974076540 ) ) ;
#82091=CARTESIAN_POINT ( 'NONE',  ( -0.6823417656249969321, 5.780208333674756283, -1.181850606188749264 ) ) ;
#82093=CARTESIAN_POINT ( 'NONE',  ( 3.334415713957098681, 5.977569868670206787, -1.199719254218446718 ) ) ;
#82096=CARTESIAN_POINT ( 'NONE',  ( -6.551614543901706611, 8.666636272683888365, 1.599625672291283607 ) ) ;
#82101=DIRECTION ( 'NONE',  ( 5.578564026256491869E-16, 1.000000000000000000, 9.066213480720160632E-32 ) ) ;
#82107=CARTESIAN_POINT ( 'NONE',  ( 0.6823417656249917140, 3.405208333674754506, 1.181850606188765695 ) ) ;
#82108=CARTESIAN_POINT ( 'NONE',  ( 4.812781342726866640, 5.677628323678546529, 1.082531754730560403 ) ) ;
#82109=CARTESIAN_POINT ( 'NONE',  ( 8.402302512167096893, 10.82577223566020841, -1.599625672291268286 ) ) ;
#82111=CARTESIAN_POINT ( 'NONE',  ( -3.416291520963659512, 5.969128626890772615, 1.082531754730560403 ) ) ;
#82113=CARTESIAN_POINT ( 'NONE',  ( -5.056828107772866510, 5.962349549565537643, -1.082531754730543971 ) ) ;
#82120=CARTESIAN_POINT ( 'NONE',  ( 5.196852952739813070, 4.957416621151553571, -0.7998128361456221525 ) ) ;
#82126=CARTESIAN_POINT ( 'NONE',  ( -4.903732577545095950, 4.837283930932079201, 0.1501914610188368471 ) ) ;
#82128=EDGE_CURVE ( 'NONE', #1110, #10129, #4701, .T. ) ;
#82129=CARTESIAN_POINT ( 'NONE',  ( 4.924636110261782385, 6.768494766770632332, 1.599625672291267398 ) ) ;
#82130=CARTESIAN_POINT ( 'NONE',  ( -4.942274067367465662, 4.660407921550463684, 0.1785095769484911221 ) ) ;
#82134=CARTESIAN_POINT ( 'NONE',  ( -1.364683531250012516, 4.051041667008088432, -0.7879004041258300672 ) ) ;
#82139=CARTESIAN_POINT ( 'NONE',  ( 6.972971076130050072, 7.029554431773520129, 1.040834085586084257E-14 ) ) ;
#82141=CARTESIAN_POINT ( 'NONE',  ( -5.870844209917351009, 6.808071985447069707, -1.199719254218446718 ) ) ;
#82143=CARTESIAN_POINT ( 'NONE',  ( 0.7499999999999885647, 2.066666666666688634, -1.299038105676652899 ) ) ;
#82146=CARTESIAN_POINT ( 'NONE',  ( -6.423865854776591000, 6.388931673527803667, 1.040834085586084257E-14 ) ) ;
#82148=CARTESIAN_POINT ( 'NONE',  ( -2.113655003624821838, 5.617681270870908072, 1.040834085586084257E-14 ) ) ;
#82149=CARTESIAN_POINT ( 'NONE',  ( -0.6823417656250212460, 3.301041667008085323, 1.181850606188767472 ) ) ;
#82151=CARTESIAN_POINT ( 'NONE',  ( -3.958617665510272943, 6.601842462195195438, -1.082531754730549967 ) ) ;
#82157=CARTESIAN_POINT ( 'NONE',  ( 4.819033534653518025, 7.709623992816043270, -1.199719254218452047 ) ) ;
#82159=CARTESIAN_POINT ( 'NONE',  ( 1.217358635584784965, 3.264784080462327154, -0.7749999999999840350 ) ) ;
#82160=CARTESIAN_POINT ( 'NONE',  ( 0.6823417656249917140, 4.655208333674755394, 1.181850606188765695 ) ) ;
#82162=CARTESIAN_POINT ( 'NONE',  ( 4.518945272056516416, 4.166524327021037699, 0.7998128361456341429 ) ) ;
#82164=CARTESIAN_POINT ( 'NONE',  ( -1.402160292154681736E-14, 0.6343750003414162508, 1.575800808251672791 ) ) ;
#82165=CARTESIAN_POINT ( 'NONE',  ( -4.255544820792433569, 7.363048058395826878, -0.9459158008643682169 ) ) ;
#82167=CARTESIAN_POINT ( 'NONE',  ( -5.122283107864663343, 4.870418468797203637, 0.000000000000000000 ) ) ;
#82168=CARTESIAN_POINT ( 'NONE',  ( -4.880572110795192486, 8.637825195995631589, 1.214306433183764966E-14 ) ) ;
#82172=ORIENTED_EDGE ( 'NONE', *, *, #68597, .F. ) ;
#82173=CARTESIAN_POINT ( 'NONE',  ( -0.6823417656250212460, 3.551041667008085323, 1.181850606188767472 ) ) ;
#82181=CARTESIAN_POINT ( 'NONE',  ( -5.544921637864820951, 9.412899644243539754, -0.7216878364870207285 ) ) ;
#82188=CARTESIAN_POINT ( 'NONE',  ( -4.717874267431199087, 8.448011045404303587, 1.040834085586084257E-14 ) ) ;
#82191=CARTESIAN_POINT ( 'NONE',  ( -1.201851678989727383E-14, 4.868750000682822154, -1.732050807568863648 ) ) ;
#82200=CARTESIAN_POINT ( 'NONE',  ( -5.253948220495577637, 6.088359997788290734, 1.199719254218450271 ) ) ;
#82202=CARTESIAN_POINT ( 'NONE',  ( -0.7500000000000249800, -0.8083333333333136972, 1.299038105676659116 ) ) ;
#82203=CARTESIAN_POINT ( 'NONE',  ( 4.383363735919856730, 4.008345868194933104, -0.7998128361456211532 ) ) ;
#82204=CARTESIAN_POINT ( 'NONE',  ( 8.308449207076147758, 8.587612251210650527, -0.7998128361456281477 ) ) ;
#82207=CARTESIAN_POINT ( 'NONE',  ( 5.626797444871351139, 6.523350759560078593, 1.199719254218462483 ) ) ;
#82214=CARTESIAN_POINT ( 'NONE',  ( -3.145128448690317935, 5.652771709238564313, -1.082531754730549967 ) ) ;
#82216=AXIS2_PLACEMENT_3D ( 'NONE', #164603, #112729, #1002 ) ;
#82218=CARTESIAN_POINT ( 'NONE',  ( -4.702146809683723561, 5.356480858934594025, -2.500000000000000444 ) ) ;
#82223=CARTESIAN_POINT ( 'NONE',  ( -1.402160292154681736E-14, 1.946875000341422579, -1.575800808251660134 ) ) ;
#82224=CARTESIAN_POINT ( 'NONE',  ( 8.500599125643985232, 11.90082083235127008, -1.082531754730543083 ) ) ;
#82225=CARTESIAN_POINT ( 'NONE',  ( -7.039708073993679704, 9.236078724457858158, 1.599625672291283607 ) ) ;
#82228=CARTESIAN_POINT ( 'NONE',  ( 6.667912619822566000, 6.673652899414787676, 1.040834085586084257E-14 ) ) ;
#82229=CARTESIAN_POINT ( 'NONE',  ( -6.413170354464012846, 7.440785820751486312, 1.199719254218450271 ) ) ;
#82232=CARTESIAN_POINT ( 'NONE',  ( -1.500000000000001332, -0.5687499993171779566, 0.000000000000000000 ) ) ;
#82235=CARTESIAN_POINT ( 'NONE',  ( 8.120970824905713314, 8.576813505252564696, 1.040834085586084257E-14 ) ) ;
#82238=CARTESIAN_POINT ( 'NONE',  ( 1.364683531249986537, 0.9260416670080896528, 0.7879004041258500513 ) ) ;
#82240=CARTESIAN_POINT ( 'NONE',  ( 5.273758565591489145, 9.096542726591325234, -0.7216878364870267237 ) ) ;
#82244=CARTESIAN_POINT ( 'NONE',  ( -3.443407828190963915, 6.961133532957338943, 0.7216878364870317197 ) ) ;
#82246=CARTESIAN_POINT ( 'NONE',  ( -1.201851678989727383E-14, 4.946875000341420581, -1.575800808251660134 ) ) ;
#82250=CARTESIAN_POINT ( 'NONE',  ( -5.285102783734889620, 6.572932445422958736, -1.390504041276509062 ) ) ;
#82256=CARTESIAN_POINT ( 'NONE',  ( 7.283754839039659146, 9.520799950344851936, -1.599625672291262513 ) ) ;
#82259=CARTESIAN_POINT ( 'NONE',  ( 3.659811400685081040, 6.357198169852855685, -1.199719254218446718 ) ) ;
#82266=CARTESIAN_POINT ( 'NONE',  ( 4.026408433578586354, 7.641300905909586660, 1.040834085586084257E-14 ) ) ;
#82267=CARTESIAN_POINT ( 'NONE',  ( -0.6823417656250212460, 0.8635416670080899859, 1.181850606188755259 ) ) ;
#82269=CARTESIAN_POINT ( 'NONE',  ( -0.7158994178059416846, 2.800000000000024691, 1.161830092591057184 ) ) ;
#82273=CARTESIAN_POINT ( 'NONE',  ( 1.499999999999989120, 1.275000000000019229, 0.000000000000000000 ) ) ;
#82274=CARTESIAN_POINT ( 'NONE',  ( 5.438792177376376991, 9.497007973581119700, 1.040834085586084257E-14 ) ) ;
#82275=CARTESIAN_POINT ( 'NONE',  ( -8.015895134177625891, 10.37496362800581018, 1.599625672291295375 ) ) ;
#82279=CARTESIAN_POINT ( 'NONE',  ( -1.364683531250014514, 1.488541667008084435, -0.7879004041258289570 ) ) ;
#82281=CARTESIAN_POINT ( 'NONE',  ( -0.7499999999999972244, 3.108333333333358706, -1.299038105676652011 ) ) ;
#82283=CARTESIAN_POINT ( 'NONE',  ( 4.792970997630896512, 5.550553237779539018, 1.199719254218464037 ) ) ;
#82288=( BOUNDED_CURVE ( )  B_SPLINE_CURVE ( 2, ( #130119, #31479, #147360, #213387, #175078, #206478, #70323 ),
 .UNSPECIFIED., .F., .T. ) 
 B_SPLINE_CURVE_WITH_KNOTS ( ( 3, 2, 2, 3 ),
 ( 0.1375000000000000666, 0.1416666666666667740, 0.1458333333333335091, 0.1500000000000002165 ),
 .UNSPECIFIED. ) 
 CURVE ( )  GEOMETRIC_REPRESENTATION_ITEM ( )  RATIONAL_B_SPLINE_CURVE ( ( 0.9999999999999982236, 0.8660254037844404840, 1.000000000000000000, 0.8660254037844387076, 1.000000000000000000, 0.8660254037844316022, 1.000000000000007105 ) ) 
 REPRESENTATION_ITEM ( '' )  );
#82291=CARTESIAN_POINT ( 'NONE',  ( -1.500000000000013101, -0.04791666598384902026, 0.8660254037844403729 ) ) ;
#82293=CARTESIAN_POINT ( 'NONE',  ( -7.426115451983156923, 9.686887332112256388, -1.599625672291263179 ) ) ;
#82294=CARTESIAN_POINT ( 'NONE',  ( -3.958617665510272943, 6.601842462195195438, -1.082531754730549967 ) ) ;
#82302=CARTESIAN_POINT ( 'NONE',  ( 5.764187864104357573, 9.876636274763768597, 1.040834085586084257E-14 ) ) ;
#82305=CARTESIAN_POINT ( 'NONE',  ( 7.644099680006512187, 7.812537802962739697, 1.040834085586084257E-14 ) ) ;
#82306=CARTESIAN_POINT ( 'NONE',  ( 8.554831740098654436, 11.00372300158037042, 1.443375672974076540 ) ) ;
#82310=CARTESIAN_POINT ( 'NONE',  ( -7.206322340863467346, 8.366129804884193888, 1.199719254218450271 ) ) ;
#82312=CARTESIAN_POINT ( 'NONE',  ( 5.854423403002611437, 5.724582146458163656, 1.040834085586084257E-14 ) ) ;
#82315=CARTESIAN_POINT ( 'NONE',  ( 1.445103857048098739, 8.688264192037886247, -2.625611233228243968 ) ) ;
#82317=CARTESIAN_POINT ( 'NONE',  ( -4.000000000000000000, 2.800000000000026912, 1.214306433183764966E-14 ) ) ;
#82318=CARTESIAN_POINT ( 'NONE',  ( 8.256552361042350796, 12.57646882128404187, 1.040834085586084257E-14 ) ) ;
#82324=CARTESIAN_POINT ( 'NONE',  ( 4.897706171852771462, 4.871974472535213430, 0.6676900015689657408 ) ) ;
#82328=CARTESIAN_POINT ( 'NONE',  ( -3.795919822146283540, 6.412028311603867436, -1.082531754730549967 ) ) ;
#82329=CARTESIAN_POINT ( 'NONE',  ( 7.619319141200051604, 11.83303006480134911, 0.7216878364870438212 ) ) ;
#82332=CARTESIAN_POINT ( 'NONE',  ( -5.259673527097670664, 8.223703984000886535, -1.199719254218446718 ) ) ;
#82338=CARTESIAN_POINT ( 'NONE',  ( -7.555971681517696936, 7.709721804725773175, 0.7998128361456462443 ) ) ;
#82342=ORIENTED_EDGE ( 'NONE', *, *, #195841, .T. ) ;
#82353=CARTESIAN_POINT ( 'NONE',  ( -5.799137018343247796, 7.788745826199009237, -1.599625672291256295 ) ) ;
#82356=CARTESIAN_POINT ( 'NONE',  ( 4.202664430556254160, 5.926194473780837413, 1.443375672974062551 ) ) ;
#82359=CARTESIAN_POINT ( 'NONE',  ( 0.1263921868141488214, 7.050106634747087320, 4.033475512996062662 ) ) ;
#82361=CARTESIAN_POINT ( 'NONE',  ( -3.113568832632681360, 6.784247404713427798, -0.7998128361456281477 ) ) ;
#82370=CARTESIAN_POINT ( 'NONE',  ( -7.771848369131641121, 10.09024240211882351, -1.599625672291263179 ) ) ;
#82371=CARTESIAN_POINT ( 'NONE',  ( 6.908042961362778733, 8.018137195466769285, 1.199719254218462483 ) ) ;
#82373=CARTESIAN_POINT ( 'NONE',  ( -8.779068160048691283, 10.20099992726700933, -1.199719254218446718 ) ) ;
#82374=CARTESIAN_POINT ( 'NONE',  ( 5.996784015946103885, 5.890669528225568996, 1.040834085586084257E-14 ) ) ;
#82377=CARTESIAN_POINT ( 'NONE',  ( -1.364683531250000748, 0.5718750003414208027, 0.000000000000000000 ) ) ;
#82380=CARTESIAN_POINT ( 'NONE',  ( 8.595506201384013778, 10.09080732544527592, 1.082531754730558626 ) ) ;
#82386=ORIENTED_EDGE ( 'NONE', *, *, #106610, .T. ) ;
#82387=CARTESIAN_POINT ( 'NONE',  ( 10.07334494482924292, 11.81495252613139257, -1.082531754730537088 ) ) ;
#82407=CARTESIAN_POINT ( 'NONE',  ( -1.500000000000001332, 0.1812500006828157706, 0.000000000000000000 ) ) ;
#82414=CARTESIAN_POINT ( 'NONE',  ( 9.215791728987056786, 11.77484298861683598, -1.599625672291262513 ) ) ;
#82415=CARTESIAN_POINT ( 'NONE',  ( -1.500000000000021316, 5.202083334016151639, 0.8660254037844343777 ) ) ;
#82416=AXIS2_PLACEMENT_3D ( 'NONE', #195783, #212007, #144939 ) ;
#82419=CARTESIAN_POINT ( 'NONE',  ( 5.671388329218120639, 5.511041227042920099, 1.040834085586084257E-14 ) ) ;
#82420=CARTESIAN_POINT ( 'NONE',  ( -6.236387472606141458, 10.21960978477508952, -0.7216878364870278340 ) ) ;
#82421=CARTESIAN_POINT ( 'NONE',  ( -5.911556925646939575, 6.000462466000660022, -0.05029327469607651480 ) ) ;
#82424=CARTESIAN_POINT ( 'NONE',  ( -8.182509401047415309, 9.505014708432145909, 1.199719254218462483 ) ) ;
#82425=CARTESIAN_POINT ( 'NONE',  ( -3.917943204224921150, 5.594019709727598766, -1.443375672974051449 ) ) ;
#82428=CARTESIAN_POINT ( 'NONE',  ( 1.499999999999987121, -0.2145833326505137972, 0.8660254037844524744 ) ) ;
#82435=CARTESIAN_POINT ( 'NONE',  ( -4.785665035499573783, 5.645992631913323123, 1.082531754730558626 ) ) ;
#82442=CARTESIAN_POINT ( 'NONE',  ( -10.17947440576205054, 10.77047498301088346, 0.7998128361456462443 ) ) ;
#82443=CARTESIAN_POINT ( 'NONE',  ( 6.934105498385400246, 10.17720795050327354, -1.199719254218441611 ) ) ;
#82451=EDGE_CURVE ( 'NONE', #153088, #202349, #209292, .T. ) ;
#82454=CARTESIAN_POINT ( 'NONE',  ( -9.321394304595349567, 10.83371376257142416, 1.199719254218462483 ) ) ;
#82459=CARTESIAN_POINT ( 'NONE',  ( 4.222474775652216294, 7.013638773981186958, 1.199719254218462483 ) ) ;
#82476=CARTESIAN_POINT ( 'NONE',  ( 6.272618624616828953, 10.46980549536166016, 1.040834085586084257E-14 ) ) ;
#82478=CARTESIAN_POINT ( 'NONE',  ( -3.276266675996675204, 6.974061555304760240, -0.7998128361456281477 ) ) ;
#82486=CARTESIAN_POINT ( 'NONE',  ( -1.402160292154681736E-14, -0.8812499993171809543, -1.732050807568870754 ) ) ;
#82490=CARTESIAN_POINT ( 'NONE',  ( 2.544126380858701797, 6.119897877643793116, 0.7998128361456462443 ) ) ;
#82492=CARTESIAN_POINT ( 'NONE',  ( -3.948449050077848632, 5.629609863222681199, 1.599625672291267398 ) ) ;
#82498=CARTESIAN_POINT ( 'NONE',  ( 3.823036129373602154, 6.443664003369091731, -1.082531754730548412 ) ) ;
#82501=CARTESIAN_POINT ( 'NONE',  ( -1.364683531249997417, 4.821875000341417916, 1.214306433183764966E-14 ) ) ;
#82503=CARTESIAN_POINT ( 'NONE',  ( 3.511198595814932766, 5.119484333249288532, 1.443375672974066548 ) ) ;
#82511=CARTESIAN_POINT ( 'NONE',  ( -6.127725819454865608, 6.002332559294505820, -0.1884722350499398735 ) ) ;
#82514=CARTESIAN_POINT ( 'NONE',  ( 0.6823417656249917140, 5.655208333674749177, 1.181850606188765695 ) ) ;
#82521=CARTESIAN_POINT ( 'NONE',  ( 0.7499999999999902300, 4.316666666666691299, -1.299038105676658228 ) ) ;
#82522=AXIS2_PLACEMENT_3D ( 'NONE', #147372, #149489, #84479 ) ;
#82530=CARTESIAN_POINT ( 'NONE',  ( 1.364683531249990311, 4.946875000341417916, 1.214306433183764966E-14 ) ) ;
#82533=CARTESIAN_POINT ( 'NONE',  ( 5.503720292143644777, 8.508425209887878538, 1.199719254218462483 ) ) ;
#82534=CARTESIAN_POINT ( 'NONE',  ( -8.202846631467911820, 9.528741477256060577, 1.199719254218462483 ) ) ;
#82537=CARTESIAN_POINT ( 'NONE',  ( 1.499999999999822586, 10.00000000000000178, 4.154462424328221104 ) ) ;
#82540=CARTESIAN_POINT ( 'NONE',  ( -0.7500000000000215383, 5.191666666666685082, 1.299038105676671107 ) ) ;
#82544=FACE_OUTER_BOUND ( 'NONE', #189193, .T. ) ;
#82546=ORIENTED_EDGE ( 'NONE', *, *, #72791, .F. ) ;
#82548=CARTESIAN_POINT ( 'NONE',  ( 7.727784370109387346, 10.99920361756089093, -1.082531754730543083 ) ) ;
#82553=CARTESIAN_POINT ( 'NONE',  ( -1.201851678989727383E-14, 3.118750000682814161, -1.732050807568863648 ) ) ;
#82555=CARTESIAN_POINT ( 'NONE',  ( -4.283486466913726254, 7.084819080452935403, -1.199719254218452047 ) ) ;
#82556=CARTESIAN_POINT ( 'NONE',  ( 4.812781342726866640, 5.677628323678546529, 1.082531754730560403 ) ) ;
#82565=CARTESIAN_POINT ( 'NONE',  ( 5.020596955762157698, 4.751784624677624080, 1.040834085586084257E-14 ) ) ;
#82567=CARTESIAN_POINT ( 'NONE',  ( 4.325214697959421706, 5.004837554829479451, 1.199719254218462483 ) ) ;
#82569=ORIENTED_EDGE ( 'NONE', *, *, #149088, .F. ) ;
#82573=ORIENTED_EDGE ( 'NONE', *, *, #73148, .T. ) ;
#82578=CARTESIAN_POINT ( 'NONE',  ( 4.030162213014739869, 7.767662802593035209, -0.3896624696924297360 ) ) ;
#82579=CARTESIAN_POINT ( 'NONE',  ( 4.685856777024981490, 6.842343872427582241, -1.228950205364977899 ) ) ;
#82580=EDGE_LOOP ( 'NONE', ( #58895, #174142, #46497, #18700 ) ) ;
#82583=CARTESIAN_POINT ( 'NONE',  ( 9.836604141914616406, 11.43479190611061647, 1.199719254218452047 ) ) ;
#82588=CARTESIAN_POINT ( 'NONE',  ( 5.341549334104184865, 8.215262742221458581, 1.082531754730558626 ) ) ;
#82589=CARTESIAN_POINT ( 'NONE',  ( -8.839552966430002101, 12.29626697993494666, -1.082531754730543971 ) ) ;
#82596=CARTESIAN_POINT ( 'NONE',  ( -4.386226389220933441, 5.076017861301227008, -1.199719254218446718 ) ) ;
#82608=CARTESIAN_POINT ( 'NONE',  ( 5.577782935947014131, 6.368007920784547693, 1.193350709755973682 ) ) ;
#82610=ORIENTED_EDGE ( 'NONE', *, *, #182079, .F. ) ;
#82613=CARTESIAN_POINT ( 'NONE',  ( -4.600947939797212172, 7.141072520302401472, -1.375236645198579799 ) ) ;
#82616=CARTESIAN_POINT ( 'NONE',  ( -8.351459436338030784, 11.72682452816096976, -1.082531754730543971 ) ) ;
#82620=CARTESIAN_POINT ( 'NONE',  ( 6.401421083946654100, 10.62007503124645957, -0.7998128361456291469 ) ) ;
#82622=CARTESIAN_POINT ( 'NONE',  ( -4.599240423533815125, 6.388866465587985211, 1.599625672291267175 ) ) ;
#82624=CARTESIAN_POINT ( 'NONE',  ( -4.954615070790188369, 7.867802451642154082, -1.199719254218452047 ) ) ;
#82625=CARTESIAN_POINT ( 'NONE',  ( 3.063252641683779753, 5.661212951017999373, 1.199719254218450271 ) ) ;
#82627=CARTESIAN_POINT ( 'NONE',  ( -5.799137018343247796, 7.788745826199009237, -1.599625672291256295 ) ) ;
#82631=CARTESIAN_POINT ( 'NONE',  ( 7.553864141108259211, 11.96459193126834464, 1.040834085586084257E-14 ) ) ;
#82635=CARTESIAN_POINT ( 'NONE',  ( 4.554780495368041748, 6.962214942802684270, -1.182099088617315497 ) ) ;
#82636=CARTESIAN_POINT ( 'NONE',  ( 4.663641653420880218, 8.384739662392275861, -0.7216878364870207285 ) ) ;
#82644=ORIENTED_EDGE ( 'NONE', *, *, #134567, .F. ) ;
#82645=CARTESIAN_POINT ( 'NONE',  ( 7.497295758232718654, 9.769931022736756177, -1.443375672974058777 ) ) ;
#82649=CARTESIAN_POINT ( 'NONE',  ( -6.201965203247477909, 9.323044272842313518, 1.199719254218452047 ) ) ;
#82654=CARTESIAN_POINT ( 'NONE',  ( 2.179377205606497281, 5.694357173182881482, -0.3219805702579285889 ) ) ;
#82657=CARTESIAN_POINT ( 'NONE',  ( 8.971744963941056028, 11.49012176272984931, 1.599625672291281386 ) ) ;
#82661=CARTESIAN_POINT ( 'NONE',  ( 3.497113557321089861, 6.167384019261527683, -1.199719254218446718 ) ) ;
#82664=CARTESIAN_POINT ( 'NONE',  ( -0.7499999999999972244, 4.139583334016149863, -1.299038105676652899 ) ) ;
#82670=CARTESIAN_POINT ( 'NONE',  ( 0.7499999999999885647, 2.066666666666688634, -1.299038105676652899 ) ) ;
#82671=CARTESIAN_POINT ( 'NONE',  ( 5.829115978871627135, 8.888053511070525659, 1.199719254218462483 ) ) ;
#82672=CARTESIAN_POINT ( 'NONE',  ( 4.324687812634887329, 6.068555086205916105, 1.443375672974062551 ) ) ;
#82675=CARTESIAN_POINT ( 'NONE',  ( 8.487040972474689582, 9.964264558384387627, -1.082531754730543083 ) ) ;
#82676=AXIS2_PLACEMENT_3D ( 'NONE', #101166, #183486, #68651 ) ;
#82681=CARTESIAN_POINT ( 'NONE',  ( -5.440899717785814715, 5.242137847038546461, 0.7998128361456341429 ) ) ;
#82683=CARTESIAN_POINT ( 'NONE',  ( -1.499999999999997780, 5.681250000682820378, 1.214306433183764966E-14 ) ) ;
#82684=CARTESIAN_POINT ( 'NONE',  ( 0.6823417656249882723, 0.3427083336747516196, 1.181850606188755259 ) ) ;
#82688=CARTESIAN_POINT ( 'NONE',  ( 5.034155109375821446, 4.767602470560229122, -0.7998128361456221525 ) ) ;
#82690=CARTESIAN_POINT ( 'NONE',  ( -1.364683531250010295, 5.592708333674750953, 0.7879004041258379498 ) ) ;
#82696=CARTESIAN_POINT ( 'NONE',  ( -5.707619481228860536, 5.761236937629468535, -0.7216878364870003004 ) ) ;
#82698=CARTESIAN_POINT ( 'NONE',  ( -8.037286134802835491, 8.271255333558444889, -0.7998128361456291469 ) ) ;
#82701=CARTESIAN_POINT ( 'NONE',  ( 5.464099601507359516, 6.333536608968757697, 1.199719254218462483 ) ) ;
#82704=CARTESIAN_POINT ( 'NONE',  ( 0.6823417656249864960, -0.8239583329919114574, -1.181850606188749264 ) ) ;
#82709=CARTESIAN_POINT ( 'NONE',  ( 10.23370702021670020, 10.83374636654133383, 0.7998128361456462443 ) ) ;
#82713=CARTESIAN_POINT ( 'NONE',  ( -6.555530967407501741, 7.606873202518897870, 1.199719254218450271 ) ) ;
#82717=CARTESIAN_POINT ( 'NONE',  ( 10.70146331988817323, 11.37946204949139251, 0.7998128361456341429 ) ) ;
#82719=CARTESIAN_POINT ( 'NONE',  ( 6.726816770674637347, 10.99970333242910669, -0.7998128361456291469 ) ) ;
#82722=CARTESIAN_POINT ( 'NONE',  ( -4.776550190716183586, 4.467063398790632966, 1.214306433183764966E-14 ) ) ;
#82723=CARTESIAN_POINT ( 'NONE',  ( -7.426115451983156923, 9.686887332112256388, -1.599625672291263179 ) ) ;
#82726=CARTESIAN_POINT ( 'NONE',  ( -4.277165953568806245, 7.474871692096041187, 1.085114461911325101 ) ) ;
#82727=CARTESIAN_POINT ( 'NONE',  ( -1.201851678989727383E-14, 0.8218750003414171390, 1.575800808251672791 ) ) ;
#82732=CARTESIAN_POINT ( 'NONE',  ( 8.758204044748010730, 9.320252261735261001, 0.7216878364870438212 ) ) ;
#82735=CARTESIAN_POINT ( 'NONE',  ( 4.873266149108180123, 7.772895376346490970, 1.199719254218462483 ) ) ;
#82739=CARTESIAN_POINT ( 'NONE',  ( 0.005132432257108309609, 7.078226584369340380, -2.121329534126251470 ) ) ;
#82753=CARTESIAN_POINT ( 'NONE',  ( 8.778014389843965759, 12.32843499053828928, 1.199719254218450271 ) ) ;
#82757=CARTESIAN_POINT ( 'NONE',  ( -5.599681137644054729, 6.491715067794862293, 1.199719254218450271 ) ) ;
#82758=CARTESIAN_POINT ( 'NONE',  ( -9.155833807930273238, 9.576227618873799585, -0.7998128361456291469 ) ) ;
#82764=CARTESIAN_POINT ( 'NONE',  ( -1.201851678989727383E-14, 3.243750000682814161, 1.732050807568877637 ) ) ;
#82765=CARTESIAN_POINT ( 'NONE',  ( 7.995557903757111617, 10.35123685918189729, 1.599625672291281386 ) ) ;
#82768=CARTESIAN_POINT ( 'NONE',  ( -8.154339323615371171, 11.60081407993821045, 1.199719254218453823 ) ) ;
#82770=CARTESIAN_POINT ( 'NONE',  ( 1.364683531249988535, 3.905208333674751842, -0.7879004041258239610 ) ) ;
#82776=CARTESIAN_POINT ( 'NONE',  ( -3.022498986271247023, 2.800000000000024691, -2.500000000000000444 ) ) ;
#82778=CARTESIAN_POINT ( 'NONE',  ( -2.767835915484202047, 6.380892334706859792, -0.7998128361456281477 ) ) ;
#82782=CARTESIAN_POINT ( 'NONE',  ( 1.364683531249988757, 1.196875000341421469, 0.000000000000000000 ) ) ;
#82788=CARTESIAN_POINT ( 'NONE',  ( 1.364683531249988757, 1.884375000341421913, 0.000000000000000000 ) ) ;
#82790=CARTESIAN_POINT ( 'NONE',  ( -6.247609857798938293, 6.183299677053865295, -0.7998128361456291469 ) ) ;
#82791=CARTESIAN_POINT ( 'NONE',  ( -1.123270288250342919, 2.846052654332832610, 0.7749999999993751887 ) ) ;
#82793=CARTESIAN_POINT ( 'NONE',  ( 1.499999999999990896, 4.775000000000022560, 1.214306433183764966E-14 ) ) ;
#82794=CARTESIAN_POINT ( 'NONE',  ( -1.364683531250012516, 2.342708333674752286, 0.7879004041258379498 ) ) ;
#82798=CARTESIAN_POINT ( 'NONE',  ( -6.412643469583822586, 6.583764924043652655, 1.040834085586084257E-14 ) ) ;
#82801=CARTESIAN_POINT ( 'NONE',  ( 6.168596704537822717, 6.299043698156668647, 1.040834085586084257E-14 ) ) ;
#82804=CARTESIAN_POINT ( 'NONE',  ( -7.506410603460441422, 11.90922947067921278, -0.7998128361456291469 ) ) ;
#82805=CARTESIAN_POINT ( 'NONE',  ( -3.735435015764967837, 4.316761258935923884, -1.199719254218452047 ) ) ;
#82807=CARTESIAN_POINT ( 'NONE',  ( -0.6823417656250212460, 4.801041667008086655, 1.181850606188767472 ) ) ;
#82811=CARTESIAN_POINT ( 'NONE',  ( -6.195713011320783892, 10.17215624660883577, -0.7216878364870267237 ) ) ;
#82813=CARTESIAN_POINT ( 'NONE',  ( -0.6823417656250246877, -0.1364583329919108468, 1.181850606188755259 ) ) ;
#82817=CARTESIAN_POINT ( 'NONE',  ( 8.161645285746708112, 9.584636257201740506, -1.082531754730543083 ) ) ;
#82820=CARTESIAN_POINT ( 'NONE',  ( -3.416291520519271874, 6.929497840673697340, 1.040834085586084257E-14 ) ) ;
#82826=CARTESIAN_POINT ( 'NONE',  ( 8.066738210006668908, 12.35501897840907581, 0.7216878364870438212 ) ) ;
#82834=CARTESIAN_POINT ( 'NONE',  ( 6.368579470117202490, 8.453095353268645695, 1.599625672291281386 ) ) ;
#82835=CARTESIAN_POINT ( 'NONE',  ( -3.716906668440817185, 7.488141546489591072, 0.7998128361456341429 ) ) ;
#82838=CARTESIAN_POINT ( 'NONE',  ( 6.290620086616457662, 6.441404310581745563, 1.040834085586084257E-14 ) ) ;
#82839=CARTESIAN_POINT ( 'NONE',  ( -1.402160292154681736E-14, 0.5093750003414236893, -1.575800808251659024 ) ) ;
#82840=CARTESIAN_POINT ( 'NONE',  ( 2.548569689688999329, 5.917155704705049146, -0.7216878364870267237 ) ) ;
#82841=CARTESIAN_POINT ( 'NONE',  ( -8.622095623286845978, 12.14652976288826913, 1.199719254218462483 ) ) ;
#82859=CARTESIAN_POINT ( 'NONE',  ( 8.132193210098487057, 8.381980254736715708, 1.040834085586084257E-14 ) ) ;
#82860=CARTESIAN_POINT ( 'NONE',  ( 6.283314124929436417, 9.417951348137970413, -1.199719254218440723 ) ) ;
#82863=VERTEX_POINT ( 'NONE', #182133 ) ;
#82870=CARTESIAN_POINT ( 'NONE',  ( -5.005985031943793295, 6.863401842066301661, -1.599625672291256295 ) ) ;
#82871=CARTESIAN_POINT ( 'NONE',  ( 3.619250341048967812, 3.172667246362768534, 2.500000000000000444 ) ) ;
#82874=DIRECTION ( 'NONE',  ( 1.000000000000000000, 0.000000000000000000, 0.000000000000000000 ) ) ;
#82875=CARTESIAN_POINT ( 'NONE',  ( -0.7500000000000215383, 4.722916667349482012, 1.299038105676671107 ) ) ;
#82881=CARTESIAN_POINT ( 'NONE',  ( -9.571693261567968847, 12.19006144329456731, 1.443375672974076540 ) ) ;
#82884=CARTESIAN_POINT ( 'NONE',  ( 5.289652487626049115, 9.323011668872403845, 0.7998128361456462443 ) ) ;
#82885=CARTESIAN_POINT ( 'NONE',  ( -1.364683531249997417, 5.509375000341417916, 1.214306433183764966E-14 ) ) ;
#82892=CARTESIAN_POINT ( 'NONE',  ( 3.999292125906899198, 6.649295999324608353, 1.082531754730558626 ) ) ;
#82893=CARTESIAN_POINT ( 'NONE',  ( -6.826694039680798021, 7.923230120171105284, -1.199719254218446718 ) ) ;
#82896=ORIENTED_EDGE ( 'NONE', *, *, #105557, .F. ) ;
#82899=CARTESIAN_POINT ( 'NONE',  ( -5.208303565944065738, 9.228104593576741621, -0.7998128361456231517 ) ) ;
#82900=CARTESIAN_POINT ( 'NONE',  ( -4.623494077460110319, 5.352830164246910272, 1.199719254218462483 ) ) ;
#82907=CARTESIAN_POINT ( 'NONE',  ( 6.582647274634798151, 7.638508894284114170, 1.199719254218462483 ) ) ;
#82914=CARTESIAN_POINT ( 'NONE',  ( 1.150196859685074235, 3.145291321728038714, -0.7750000000000022427 ) ) ;
#82920=CARTESIAN_POINT ( 'NONE',  ( -1.364683531250012516, 0.5927083336747520637, 0.7879004041258379498 ) ) ;
#82921=CARTESIAN_POINT ( 'NONE',  ( 4.033714395265605823, 4.664753868353354704, -1.199719254218446718 ) ) ;
#82922=CARTESIAN_POINT ( 'NONE',  ( 5.678167406024951624, 5.518950149984223508, 0.7998128361456341429 ) ) ;
#82924=CARTESIAN_POINT ( 'NONE',  ( -6.724481002698115439, 10.78905223654906109, -0.7216878364870267237 ) ) ;
#82926=CARTESIAN_POINT ( 'NONE',  ( 6.155038550924155416, 6.283225852274053835, 0.7216878364870317197 ) ) ;
#82928=CARTESIAN_POINT ( 'NONE',  ( -7.836249598574384301, 8.244638741199329601, 1.040834085586084257E-14 ) ) ;
#82932=CARTESIAN_POINT ( 'NONE',  ( 5.991813822235618758, 9.077867661661846554, 1.199719254218462483 ) ) ;
#82937=CARTESIAN_POINT ( 'NONE',  ( -0.6823417656250212460, 4.051041667008085767, 1.181850606188767472 ) ) ;
#82942=CARTESIAN_POINT ( 'NONE',  ( 6.259060471003163428, 10.45398764947904624, -0.7998128361456291469 ) ) ;
#82946=CARTESIAN_POINT ( 'NONE',  ( -9.840520565420403543, 10.37502883594562597, 1.040834085586084257E-14 ) ) ;
#82950=CARTESIAN_POINT ( 'NONE',  ( 0.4634916963840206017, 7.369626292149110469, -4.459501722865408802 ) ) ;
#82952=CARTESIAN_POINT ( 'NONE',  ( 9.565441069641300587, 11.11843498845840905, -1.199719254218440723 ) ) ;
#82955=CARTESIAN_POINT ( 'NONE',  ( -7.232384877886063990, 10.52520055992070525, -1.199719254218446718 ) ) ;
#82958=CARTESIAN_POINT ( 'NONE',  ( 4.731797659388218946, 6.802130194288283249, -1.238660871931380303 ) ) ;
#82959=CARTESIAN_POINT ( 'NONE',  ( -3.789667630219657912, 4.380032642466370696, 1.199719254218462483 ) ) ;
#82965=CARTESIAN_POINT ( 'NONE',  ( 5.262536180398716290, 9.291375977107183104, -0.7998128361456291469 ) ) ;
#82967=CARTESIAN_POINT ( 'NONE',  ( 5.178324605415663306, 8.128796908705222535, 1.199719254218462483 ) ) ;
#82968=CARTESIAN_POINT ( 'NONE',  ( -4.137838753588869878, 7.456630865025390520, 0.6858938789830407723 ) ) ;
#82969=CARTESIAN_POINT ( 'NONE',  ( 5.118366684358879759, 5.930181538962194132, 1.199719254218462483 ) ) ;
#82971=CARTESIAN_POINT ( 'NONE',  ( -8.242994207428740339, 9.679543332497402730, 1.082531754730558626 ) ) ;
#82977=CARTESIAN_POINT ( 'NONE',  ( -4.015218494013213402, 7.625434522713817387, 0.07065147036973244699 ) ) ;
#82978=CARTESIAN_POINT ( 'NONE',  ( -1.364683531250000748, -0.6781249996585803075, 0.000000000000000000 ) ) ;
#82981=CARTESIAN_POINT ( 'NONE',  ( 5.029711800989886683, 4.970344644017389513, 1.040834085586084257E-14 ) ) ;
#82991=CARTESIAN_POINT ( 'NONE',  ( -9.042925270190641740, 11.57316545335434199, 1.443375672974064550 ) ) ;
#82997=CARTESIAN_POINT ( 'NONE',  ( -8.961576348508641487, 11.47825837805867799, -1.443375672974058777 ) ) ;
#83001=ORIENTED_EDGE ( 'NONE', *, *, #21559, .T. ) ;
#83003=CARTESIAN_POINT ( 'NONE',  ( -1.402160292154681736E-14, 2.368750000682818602, -1.732050807568863648 ) ) ;
#83005=CARTESIAN_POINT ( 'NONE',  ( -5.904739593951539689, 6.847616600153594746, 1.199719254218450271 ) ) ;
#83009=CARTESIAN_POINT ( 'NONE',  ( -6.997979842947967377, 11.31606025008131233, -0.7998128361456291469 ) ) ;
#83012=CARTESIAN_POINT ( 'NONE',  ( 5.473741331615251227, 7.409117525016355010, -1.599625672291262513 ) ) ;
#83019=CARTESIAN_POINT ( 'NONE',  ( 6.936968151686458306, 11.24487994360957188, 0.7998128361456462443 ) ) ;
#83024=CARTESIAN_POINT ( 'NONE',  ( -7.727784370109414880, 8.118095974656867497, 0.7216878364870578100 ) ) ;
#83028=CARTESIAN_POINT ( 'NONE',  ( 1.084637062511527361, 3.088621193390831632, -1.105835307554789759 ) ) ;
#83033=CARTESIAN_POINT ( 'NONE',  ( -1.364683531249997417, 5.009375000341425022, 1.214306433183764966E-14 ) ) ;
#83036=CARTESIAN_POINT ( 'NONE',  ( -4.406036734316906234, 4.242723732898890709, -0.7216878364870207285 ) ) ;
#83038=CARTESIAN_POINT ( 'NONE',  ( 7.899597058256738968, 12.36794700127490820, 1.040834085586084257E-14 ) ) ;
#83039=CARTESIAN_POINT ( 'NONE',  ( -0.7500000000000249800, -1.058333333333314030, 1.299038105676659116 ) ) ;
#83040=CARTESIAN_POINT ( 'NONE',  ( -10.32861409551237486, 10.94447128771960287, 1.040834085586084257E-14 ) ) ;
#83043=CARTESIAN_POINT ( 'NONE',  ( -0.6823417656250212460, 2.551041667008084435, 1.181850606188767472 ) ) ;
#83044=CARTESIAN_POINT ( 'NONE',  ( 5.196852952739813070, 4.957416621151553571, -0.7998128361456221525 ) ) ;
#83049=CARTESIAN_POINT ( 'NONE',  ( -5.951324661304710162, 4.742844146918499426, -2.438848701833497667 ) ) ;
#83050=FACE_OUTER_BOUND ( 'NONE', #161337, .T. ) ;
#83051=CARTESIAN_POINT ( 'NONE',  ( 8.554831740098642001, 12.92446143018304916, 0.7216878364870438212 ) ) ;
#83052=CARTESIAN_POINT ( 'NONE',  ( -2.279984679289828176, 5.601133616484927025, -0.06592222766762731445 ) ) ;
#83053=CARTESIAN_POINT ( 'NONE',  ( -6.046573322014817897, 9.998159942418544333, 0.7216878364870458196 ) ) ;
#83055=CARTESIAN_POINT ( 'NONE',  ( 0.1465803529717422671, 8.209140712741676893, 2.038183922479804178 ) ) ;
#83057=CARTESIAN_POINT ( 'NONE',  ( -8.290974629956718189, 9.631557475493025322, -1.199719254218446718 ) ) ;
#83058=CARTESIAN_POINT ( 'NONE',  ( -4.894130264408873110, 5.772535398974209642, -1.082531754730543971 ) ) ;
#83059=CARTESIAN_POINT ( 'NONE',  ( -1.364683531250012516, 3.592708333674750509, 0.7879004041258379498 ) ) ;
#83075=CARTESIAN_POINT ( 'NONE',  ( -1.438722645073123196, 7.870286565763556119, 3.684014302713788602 ) ) ;
#83078=CARTESIAN_POINT ( 'NONE',  ( -0.6823417656249969321, 4.030208333674754506, -1.181850606188749264 ) ) ;
#83086=CARTESIAN_POINT ( 'NONE',  ( 8.829384350997564468, 11.32403438096243775, 1.599625672291281386 ) ) ;
#83089=CARTESIAN_POINT ( 'NONE',  ( 1.364683531249990311, 2.884375000341422801, 1.214306433183764966E-14 ) ) ;
#83091=CARTESIAN_POINT ( 'NONE',  ( -8.026063749610063525, 8.466088584074293877, -0.7216878364870278340 ) ) ;
#83093=CARTESIAN_POINT ( 'NONE',  ( 1.492392680117907711, 7.408236896935762594, 4.235501437639942246 ) ) ;
#83099=CARTESIAN_POINT ( 'NONE',  ( 4.976006071415387311, 5.764094157194782575, 1.199719254218462483 ) ) ;
#83102=CARTESIAN_POINT ( 'NONE',  ( 8.218213668177886788, 12.73966637951625813, 0.7998128361456462443 ) ) ;
#83110=CARTESIAN_POINT ( 'NONE',  ( -8.513630394377489807, 12.01998699582738972, -1.199719254218446718 ) ) ;
#83111=CARTESIAN_POINT ( 'NONE',  ( 7.365103760721646076, 9.615707025640515937, 1.599625672291281386 ) ) ;
#83113=CARTESIAN_POINT ( 'NONE',  ( 4.812781342726866640, 5.677628323678546529, 1.082531754730560403 ) ) ;
#83123=CARTESIAN_POINT ( 'NONE',  ( -7.592202833972775622, 8.920286730132099606, 1.082531754730558626 ) ) ;
#83124=CARTESIAN_POINT ( 'NONE',  ( 5.009901455449552010, 5.803638771901306725, -1.199719254218452047 ) ) ;
#83127=CARTESIAN_POINT ( 'NONE',  ( -7.832860060393135093, 10.16142270859057462, 1.599625672291295375 ) ) ;
#83133=CARTESIAN_POINT ( 'NONE',  ( -3.273404022695637572, 5.906389562198459231, 1.199719254218462483 ) ) ;
#83134=CARTESIAN_POINT ( 'NONE',  ( 1.123270288250311610, 3.110197346350006331, 0.7749999999993734123 ) ) ;
#83138=CARTESIAN_POINT ( 'NONE',  ( 7.086107841436786181, 11.41887624831828418, 1.040834085586084257E-14 ) ) ;
#83145=CARTESIAN_POINT ( 'NONE',  ( 3.606105671554957759, 4.269840040644637291, -1.082531754730543083 ) ) ;
#83148=CARTESIAN_POINT ( 'NONE',  ( -4.253507506385335368, 5.985511395581417204, 1.599625672291267398 ) ) ;
#83150=CARTESIAN_POINT ( 'NONE',  ( -9.494787648271923786, 9.971673765939062406, 1.040834085586084257E-14 ) ) ;
#83154=CARTESIAN_POINT ( 'NONE',  ( 6.616015773788773480, 10.66250946948817813, -0.7216878364870267237 ) ) ;
#83155=CARTESIAN_POINT ( 'NONE',  ( 1.364683531249988535, 5.717708333674751842, -0.7879004041258300672 ) ) ;
#83157=CARTESIAN_POINT ( 'NONE',  ( 3.871016551901614200, 4.474939717762034697, -1.199719254218446718 ) ) ;
#83160=CARTESIAN_POINT ( 'NONE',  ( -7.739006755302186846, 7.923262724141010516, 0.7998128361456462443 ) ) ;
#83170=CARTESIAN_POINT ( 'NONE',  ( -1.364683531250010295, 4.342708333674753618, 0.7879004041258379498 ) ) ;
#83171=CARTESIAN_POINT ( 'NONE',  ( 8.914649696185335870, 10.35917838609310593, -1.199719254218446718 ) ) ;
#83174=CARTESIAN_POINT ( 'NONE',  ( -5.761852096127856981, 5.824508321678349532, 0.000000000000000000 ) ) ;
#83175=CARTESIAN_POINT ( 'NONE',  ( -5.734735788456164940, 5.792872629394710593, 0.7216878364870317197 ) ) ;
#83182=CARTESIAN_POINT ( 'NONE',  ( 4.630273154266905777, 5.360739087188218122, 1.199719254218464037 ) ) ;
#83191=CARTESIAN_POINT ( 'NONE',  ( 5.192936529234042808, 6.017179691316550283, -1.199719254218452047 ) ) ;
#83192=EDGE_LOOP ( 'NONE', ( #158505, #167312, #134263, #108015 ) ) ;
#83196=CARTESIAN_POINT ( 'NONE',  ( -5.063080299699540987, 7.994345218703034384, 1.199719254218464037 ) ) ;
#83200=CARTESIAN_POINT ( 'NONE',  ( 7.474622759835693131, 7.614814729430110951, -0.7998128361456281477 ) ) ;
#83204=CARTESIAN_POINT ( 'NONE',  ( -6.573005544526917099, 6.562927978236513304, -0.7998128361456291469 ) ) ;
#83205=CARTESIAN_POINT ( 'NONE',  ( -1.402160292154681736E-14, 2.337500000000022560, -1.732050807568863648 ) ) ;
#83206=CARTESIAN_POINT ( 'NONE',  ( -5.434120640978981065, 5.234228924097238611, -0.7998128361456221525 ) ) ;
#83209=CARTESIAN_POINT ( 'NONE',  ( -6.410307701162927252, 6.373113827645189744, -0.7998128361456291469 ) ) ;
#83212=CARTESIAN_POINT ( 'NONE',  ( 0.6823417656249899377, 3.176041667008085323, -1.181850606188754593 ) ) ;
#83215=CARTESIAN_POINT ( 'NONE',  ( -6.073689629242176480, 6.188318776978391611, -0.7216878364870278340 ) ) ;
#83221=CARTESIAN_POINT ( 'NONE',  ( 6.193377243344257543, 6.120028293523423812, -0.7998128361456281477 ) ) ;
#83223=CARTESIAN_POINT ( 'NONE',  ( -1.364683531250012516, 2.592708333674753174, 0.7879004041258379498 ) ) ;
#83225=CARTESIAN_POINT ( 'NONE',  ( 4.369805582306193870, 3.992528022312320957, 1.214306433183764966E-14 ) ) ;
#83227=CARTESIAN_POINT ( 'NONE',  ( 1.364683531249986537, 0.2177083336747502595, -0.7879004041258309554 ) ) ;
#83230=CARTESIAN_POINT ( 'NONE',  ( -2.435661151949389147, 5.993355110582911038, 0.7998128361456341429 ) ) ;
#83231=CARTESIAN_POINT ( 'NONE',  ( -7.063434842595444962, 8.303390740191881392, 1.082531754730549967 ) ) ;
#83235=CARTESIAN_POINT ( 'NONE',  ( 1.364683531249990311, 2.884375000341422801, 1.214306433183764966E-14 ) ) ;
#83243=CARTESIAN_POINT ( 'NONE',  ( -6.033015167956794933, 9.982342096017511324, -0.7216878364870267237 ) ) ;
#83249=CARTESIAN_POINT ( 'NONE',  ( -5.707619481228817904, 8.642344580533519505, -1.082531754730537976 ) ) ;
#83255=CARTESIAN_POINT ( 'NONE',  ( 0.000000000000000000, 2.817530495244580102, 1.214306433183764966E-14 ) ) ;
#83261=CARTESIAN_POINT ( 'NONE',  ( -4.869349725602420520, 8.832658446511480577, 1.040834085586084257E-14 ) ) ;
#83263=CARTESIAN_POINT ( 'NONE',  ( 1.499999999999985123, -0.9541666666666493990, -0.8660254037844323793 ) ) ;
#83264=CARTESIAN_POINT ( 'NONE',  ( 3.979481780810941949, 4.601482484822914998, 1.199719254218464037 ) ) ;
#83267=CARTESIAN_POINT ( 'NONE',  ( 5.005985031943777308, 6.863401842066294556, -1.599625672291256295 ) ) ;
#83273=CARTESIAN_POINT ( 'NONE',  ( -4.772106882330247046, 4.669805572247793357, -0.7216878364870207285 ) ) ;
#83278=CARTESIAN_POINT ( 'NONE',  ( 3.621833129746810265, 4.096114899008192367, -2.499999999999995115 ) ) ;
#83283=CARTESIAN_POINT ( 'NONE',  ( 0.6823417656249882723, 2.176041667008084435, -1.181850606188749264 ) ) ;
#83284=CARTESIAN_POINT ( 'NONE',  ( 9.286972035236624734, 11.85788667924133399, -1.443375672974058777 ) ) ;
#83285=CARTESIAN_POINT ( 'NONE',  ( -7.121056995675673740, 9.330985799753529264, -1.599625672291263179 ) ) ;
#83288=CARTESIAN_POINT ( 'NONE',  ( 7.481401836642521452, 7.622723652371411696, 1.040834085586084257E-14 ) ) ;
#83289=CARTESIAN_POINT ( 'NONE',  ( -5.605406444246153974, 8.627059054007450101, -1.199719254218440723 ) ) ;
#83292=CARTESIAN_POINT ( 'NONE',  ( -0.7500000000000006661, -0.3604166659838467512, -1.299038105676652011 ) ) ;
#83295=CARTESIAN_POINT ( 'NONE',  ( 9.246297574839983824, 9.889694713509232571, 0.7216878364870438212 ) ) ;
#83299=CARTESIAN_POINT ( 'NONE',  ( 1.364683531249986537, 0.7177083336747527298, -0.7879004041258239610 ) ) ;
#83301=CARTESIAN_POINT ( 'NONE',  ( 6.439759776366765998, 9.496508258194486629, 1.082531754730558626 ) ) ;
#83303=CARTESIAN_POINT ( 'NONE',  ( -5.314433026876900001, 6.262888621853549331, 1.082531754730548412 ) ) ;
#83305=CARTESIAN_POINT ( 'NONE',  ( -1.364683531250010295, 4.280208333674753618, 0.7879004041258379498 ) ) ;
#83316=CARTESIAN_POINT ( 'NONE',  ( 7.904567251967224095, 9.180748867838630645, 1.199719254218462483 ) ) ;
#83320=CARTESIAN_POINT ( 'NONE',  ( 2.835626683552519012, 6.459981564119914310, 0.000000000000000000 ) ) ;
#83327=CARTESIAN_POINT ( 'NONE',  ( 5.395781948558860286, 6.357795697149212444, -1.082531754730542195 ) ) ;
#83329=CARTESIAN_POINT ( 'NONE',  ( 0.6823417656249882723, 0.7385416670080829915, -1.181850606188749264 ) ) ;
#83336=CARTESIAN_POINT ( 'NONE',  ( -0.7500000000000249800, -0.05833333333331303105, 1.299038105676659116 ) ) ;
#83337=CARTESIAN_POINT ( 'NONE',  ( 7.800018446563675489, 7.994443030612759848, -0.7998128361456281477 ) ) ;
#83338=CARTESIAN_POINT ( 'NONE',  ( -6.842061076390810292, 11.13415502243129218, 0.000000000000000000 ) ) ;
#83341=CARTESIAN_POINT ( 'NONE',  ( -1.364683531250012516, 1.280208333674755172, 0.7879004041258379498 ) ) ;
#83343=CARTESIAN_POINT ( 'NONE',  ( -0.7500000000000006661, 2.358333333333358262, -1.299038105676652011 ) ) ;
#83345=CARTESIAN_POINT ( 'NONE',  ( 4.630273154266905777, 5.360739087188218122, 1.199719254218464037 ) ) ;
#83349=CARTESIAN_POINT ( 'NONE',  ( -1.500000000000031530, 4.452083334016148086, 0.8660254037844287156 ) ) ;
#83353=CARTESIAN_POINT ( 'NONE',  ( -1.402160292154681736E-14, -0.3812499993171785673, -1.732050807568870754 ) ) ;
#83354=CARTESIAN_POINT ( 'NONE',  ( -8.505042434474312074, 8.816971016508505343, -0.7998128361456291469 ) ) ;
#83355=CARTESIAN_POINT ( 'NONE',  ( -5.585596099150199834, 5.618876325204420930, -0.7216878364870207285 ) ) ;
#83363=CARTESIAN_POINT ( 'NONE',  ( 7.962716289927667113, 8.184257181204083409, -0.7998128361456291469 ) ) ;
#83367=CARTESIAN_POINT ( 'NONE',  ( 7.266807146800403849, 7.580289214129690478, 1.040834085586084257E-14 ) ) ;
#83368=CARTESIAN_POINT ( 'NONE',  ( -1.403499169902660437, 7.376709478543006071, -4.304123474984413278 ) ) ;
#83373=CARTESIAN_POINT ( 'NONE',  ( -5.994676475536691029, 10.14553965476814845, 0.7998128361456481317 ) ) ;
#83374=AXIS2_PLACEMENT_3D ( 'NONE', #56377, #188501, #40133 ) ;
#83375=CARTESIAN_POINT ( 'NONE',  ( 4.111146893441827821, 5.819424013814004759, 1.599625672291267398 ) ) ;
#83381=CARTESIAN_POINT ( 'NONE',  ( 3.994353263318512148, 7.604006752988897055, -0.01585061804776008443 ) ) ;
#83382=CARTESIAN_POINT ( 'NONE',  ( 8.758204044747994743, 12.20135990463928266, 1.082531754730546636 ) ) ;
#83390=CARTESIAN_POINT ( 'NONE',  ( -2.955314298098991266, 6.391691081183366485, 0.7216878364870317197 ) ) ;
#83391=CARTESIAN_POINT ( 'NONE',  ( 8.758204044748005401, 10.28062147603659504, 1.082531754730549967 ) ) ;
#83394=CARTESIAN_POINT ( 'NONE',  ( -4.869349725602420520, 8.832658446511480577, 1.040834085586084257E-14 ) ) ;
#83398=B_SPLINE_CURVE_WITH_KNOTS ( 'NONE', 3,
 ( #133653, #86989, #68581, #117425, #148797, #52364 ),
 .UNSPECIFIED., .F., .F.,
 ( 4, 2, 4 ),
 ( 2.337445424124602418E-15, 0.0003119544853778809289, 0.0006239089707534244264 ),
 .UNSPECIFIED. ) ;
#83402=CARTESIAN_POINT ( 'NONE',  ( -7.369020184227459858, 8.555943955475521889, 1.199719254218450271 ) ) ;
#83405=CARTESIAN_POINT ( 'NONE',  ( -0.4545465019492412884, 7.933486811681471629, 1.993247486878100494 ) ) ;
#83408=ORIENTED_EDGE ( 'NONE', *, *, #116484, .F. ) ;
#83418=CARTESIAN_POINT ( 'NONE',  ( -6.417086777969760902, 6.381022750586497594, 0.7998128361456341429 ) ) ;
#83421=CARTESIAN_POINT ( 'NONE',  ( 5.666945020832181434, 5.713783400500082266, 0.7216878364870317197 ) ) ;
#83426=CARTESIAN_POINT ( 'NONE',  ( -5.271422797614987665, 5.044414773505913274, -0.7998128361456221525 ) ) ;
#83433=CARTESIAN_POINT ( 'NONE',  ( -7.557780564614042795, 10.90482886110335414, -1.199719254218446718 ) ) ;
#83434=CARTESIAN_POINT ( 'NONE',  ( 5.774883364416965037, 8.824782127540085952, -1.199719254218440723 ) ) ;
#83437=CARTESIAN_POINT ( 'NONE',  ( -7.971304249830880373, 11.38727316052296601, 1.199719254218453823 ) ) ;
#83443=CARTESIAN_POINT ( 'NONE',  ( -1.364683531250014514, -0.1572916663252435232, 0.7879004041258379498 ) ) ;
#83444=ORIENTED_EDGE ( 'NONE', *, *, #154040, .T. ) ;
#83446=CARTESIAN_POINT ( 'NONE',  ( 7.782016984564049444, 11.06247500109133064, 1.082531754730557072 ) ) ;
#83451=ORIENTED_EDGE ( 'NONE', *, *, #188907, .T. ) ;
#83465=CARTESIAN_POINT ( 'NONE',  ( -2.676845263694313637, 5.210404343363602919, -1.199719254218446718 ) ) ;
#83472=CARTESIAN_POINT ( 'NONE',  ( -0.7500000000000249800, 0.2229166673494847872, 1.299038105676659116 ) ) ;
#83479=CARTESIAN_POINT ( 'NONE',  ( 8.594979316059474073, 12.11489407112305372, 1.199719254218450271 ) ) ;
#83484=CARTESIAN_POINT ( 'NONE',  ( 4.630273154266905777, 5.360739087188218122, 1.199719254218464037 ) ) ;
#83485=CARTESIAN_POINT ( 'NONE',  ( -6.561783159334137139, 8.678499657355050800, -1.443375672974059665 ) ) ;
#83486=CARTESIAN_POINT ( 'NONE',  ( -5.901816349531303629, 6.006251404816039141, -0.1731548415426099052 ) ) ;
#83489=CARTESIAN_POINT ( 'NONE',  ( -7.507464373665155399, 9.781794407407920389, 1.599625672291295375 ) ) ;
#83490=CARTESIAN_POINT ( 'NONE',  ( -3.538314903042294457, 6.111489239315849531, 1.082531754730560403 ) ) ;
#83494=CARTESIAN_POINT ( 'NONE',  ( -1.402160292154681736E-14, 0.4937500006828175469, 1.732050807568877637 ) ) ;
#83501=CARTESIAN_POINT ( 'NONE',  ( -3.917943204224921150, 5.594019709727598766, -1.443375672974051449 ) ) ;
#83504=CARTESIAN_POINT ( 'NONE',  ( 4.017310073039977780, 7.571390042887482963, 0.3083681156060176232 ) ) ;
#83509=CARTESIAN_POINT ( 'NONE',  ( -3.511198595814942980, 5.119484333249288532, 1.443375672974064550 ) ) ;
#83510=CARTESIAN_POINT ( 'NONE',  ( 8.829384350997564468, 11.32403438096243775, 1.599625672291281386 ) ) ;
#83516=ORIENTED_EDGE ( 'NONE', *, *, #190385, .T. ) ;
#83520=CARTESIAN_POINT ( 'NONE',  ( -9.657485491635913633, 10.16148791653038330, 1.040834085586084257E-14 ) ) ;
#83525=CARTESIAN_POINT ( 'NONE',  ( 4.680589345215795838, 6.483773540883647435, -1.599625672291256295 ) ) ;
#83528=EDGE_LOOP ( 'NONE', ( #98215, #83001, #45035, #169919 ) ) ;
#83544=CARTESIAN_POINT ( 'NONE',  ( 8.620286740190458374, 8.951422706510690830, 1.040834085586084257E-14 ) ) ;
#83546=CARTESIAN_POINT ( 'NONE',  ( -3.948449050077848632, 5.629609863222681199, 1.599625672291267398 ) ) ;
#83552=CARTESIAN_POINT ( 'NONE',  ( 0.7499999999999885647, -0.7354166659838470288, 1.299038105676657340 ) ) ;
#83556=CARTESIAN_POINT ( 'NONE',  ( 3.357615597678655917, 7.068968630600412695, 0.7998128361456321445 ) ) ;
#83558=CARTESIAN_POINT ( 'NONE',  ( -4.322352044658376968, 3.937165561723182883, 0.7998128361456341429 ) ) ;
#83564=CARTESIAN_POINT ( 'NONE',  ( 4.175548123328908900, 7.815297210618305179, -0.7216878364870197293 ) ) ;
#83568=CARTESIAN_POINT ( 'NONE',  ( 6.927853306458739979, 10.06595070996845642, 1.082531754730558626 ) ) ;
#83569=CARTESIAN_POINT ( 'NONE',  ( 0.6823417656249899377, 4.488541667008086655, -1.181850606188754593 ) ) ;
#83571=CARTESIAN_POINT ( 'NONE',  ( 4.500943809612556024, 4.353448654077163305, 1.214306433183764966E-14 ) ) ;
#83580=CARTESIAN_POINT ( 'NONE',  ( -6.133306371789854161, 5.998871118906519584, 0.1305517085098181207 ) ) ;
#83583=CARTESIAN_POINT ( 'NONE',  ( -1.201851678989727383E-14, 5.009375000341421469, -1.575800808251660134 ) ) ;
#83589=CARTESIAN_POINT ( 'NONE',  ( -1.500000000000015099, -0.8708333333333129200, -0.8660254037844383745 ) ) ;
#83598=CARTESIAN_POINT ( 'NONE',  ( 1.364683531249988535, 4.217708333674752730, -0.7879004041258239610 ) ) ;
#83600=CARTESIAN_POINT ( 'NONE',  ( 5.880485940025228508, 7.883652901494672349, 1.599625672291267398 ) ) ;
#83601=CARTESIAN_POINT ( 'NONE',  ( -7.818248136574758256, 12.27303992597924420, 0.000000000000000000 ) ) ;
#83606=ORIENTED_EDGE ( 'NONE', *, *, #178239, .F. ) ;
#83608=CARTESIAN_POINT ( 'NONE',  ( 0.6823417656249882723, -1.094791666325249713, 1.181850606188755259 ) ) ;
#83615=CARTESIAN_POINT ( 'NONE',  ( 9.436111725431318931, 10.11114455586577776, -0.7216878364870257245 ) ) ;
#83620=CARTESIAN_POINT ( 'NONE',  ( -0.7500000000000215383, 3.472916667349487785, 1.299038105676671107 ) ) ;
#83622=CARTESIAN_POINT ( 'NONE',  ( -5.590039407536138150, 5.416134151747256986, 0.000000000000000000 ) ) ;
#83623=CARTESIAN_POINT ( 'NONE',  ( 3.172244755473273781, 6.644776614786712443, 0.000000000000000000 ) ) ;
#83631=CARTESIAN_POINT ( 'NONE',  ( 2.672928840188529609, 6.270167413528593414, 0.000000000000000000 ) ) ;
#83633=CARTESIAN_POINT ( 'NONE',  ( -1.217358635584790738, 2.941465920220512231, -0.7749999999999944711 ) ) ;
#83643=CARTESIAN_POINT ( 'NONE',  ( -5.956409969451652131, 6.075908546082715134, -0.6293437877468227581 ) ) ;
#83644=CARTESIAN_POINT ( 'NONE',  ( 5.815065281910236195, 6.023992952839542170, -0.4647386070683479642 ) ) ;
#83647=CARTESIAN_POINT ( 'NONE',  ( 8.757677159423465696, 12.30470822171437284, 1.199719254218450271 ) ) ;
#83649=DIRECTION ( 'NONE',  ( -1.000000000000000000, 4.984021416236792516E-16, 0.000000000000000000 ) ) ;
#83651=CARTESIAN_POINT ( 'NONE',  ( 1.364683531249988757, -0.8656249996585805295, 0.000000000000000000 ) ) ;
#83652=CARTESIAN_POINT ( 'NONE',  ( 5.178851490740187913, 8.985817805931475277, 0.7216878364870438212 ) ) ;
#83653=CARTESIAN_POINT ( 'NONE',  ( -4.288456660624211381, 3.897620947016656956, 1.214306433183764966E-14 ) ) ;
#83659=CARTESIAN_POINT ( 'NONE',  ( -2.591579918506545344, 6.175260338232929413, 1.040834085586084257E-14 ) ) ;
#83671=CARTESIAN_POINT ( 'NONE',  ( 5.936406840065503232, 6.128608848081334770, 0.7476236741628620175 ) ) ;
#83672=CARTESIAN_POINT ( 'NONE',  ( -1.270904146967317017, 3.121556430829590223, -0.7749999999999892530 ) ) ;
#83675=CARTESIAN_POINT ( 'NONE',  ( 4.334856428067313416, 6.080418470877079429, -1.599625672291256295 ) ) ;
#83680=CARTESIAN_POINT ( 'NONE',  ( -7.849807752632384172, 12.10193344480572897, 0.000000000000000000 ) ) ;
#83683=CARTESIAN_POINT ( 'NONE',  ( -1.499999999999997780, 3.900000000000021672, 1.214306433183764966E-14 ) ) ;
#83685=CARTESIAN_POINT ( 'NONE',  ( 7.721532178182734185, 8.967207948423393304, 1.199719254218462483 ) ) ;
#83687=CARTESIAN_POINT ( 'NONE',  ( -3.978428010606240850, 6.728917548094202949, -1.199719254218452047 ) ) ;
#83688=CARTESIAN_POINT ( 'NONE',  ( 3.344057444064992168, 7.053150784717805877, 1.040834085586084257E-14 ) ) ;
#83690=CARTESIAN_POINT ( 'NONE',  ( -6.033542053281340856, 6.997886136038390603, -1.199719254218446718 ) ) ;
#83691=CARTESIAN_POINT ( 'NONE',  ( 2.198393463710220264, 5.716542807637226886, 0.7998128361456462443 ) ) ;
#83693=CARTESIAN_POINT ( 'NONE',  ( -5.096975683733680818, 8.033889833409558534, -1.199719254218452047 ) ) ;
#83697=CARTESIAN_POINT ( 'NONE',  ( 8.890396042259068210, 11.39521468743417998, -1.599625672291257406 ) ) ;
#83701=CARTESIAN_POINT ( 'NONE',  ( 4.167679133687917314, 7.375052378509237450, -0.7893339205088979460 ) ) ;
#83702=CARTESIAN_POINT ( 'NONE',  ( 5.992340707560151358, 8.014150130285418783, 1.443375672974062551 ) ) ;
#83705=CARTESIAN_POINT ( 'NONE',  ( 2.359223927328457648E-13, 7.078193277237625480, 2.121339347286388843 ) ) ;
#83709=CARTESIAN_POINT ( 'NONE',  ( 6.738039155867407537, 10.80487008191325771, -0.7216878364870267237 ) ) ;
#83713=CARTESIAN_POINT ( 'NONE',  ( -7.771848369131641121, 10.09024240211882351, -1.599625672291263179 ) ) ;
#83714=DIRECTION ( 'NONE',  ( -0.5996521035822321988, 0.8002608041566222630, 0.000000000000000000 ) ) ;
#83722=CARTESIAN_POINT ( 'NONE',  ( 8.920375002787457319, 12.49452237230570084, 1.199719254218450271 ) ) ;
#83727=CARTESIAN_POINT ( 'NONE',  ( 4.416205349749311004, 6.175325546172740765, 1.599625672291267398 ) ) ;
#83730=CARTESIAN_POINT ( 'NONE',  ( -1.499999999999997780, 4.681250000682819490, 1.214306433183764966E-14 ) ) ;
#83736=CARTESIAN_POINT ( 'NONE',  ( 1.499999999999987121, 2.045833333333356929, -0.8660254037844262731 ) ) ;
#83737=CARTESIAN_POINT ( 'NONE',  ( 5.438792177376376991, 9.497007973581119700, 1.040834085586084257E-14 ) ) ;
#83738=CARTESIAN_POINT ( 'NONE',  ( 4.812781342726866640, 5.677628323678546529, 1.082531754730560403 ) ) ;
#83742=CARTESIAN_POINT ( 'NONE',  ( 8.920901888111997025, 10.47043562662792304, 1.082531754730549967 ) ) ;
#83749=CARTESIAN_POINT ( 'NONE',  ( -4.069418662396130593, 7.899405539437467816, -0.7998128361456281477 ) ) ;
#83751=CARTESIAN_POINT ( 'NONE',  ( -1.201851678989727383E-14, 4.118750000682818602, -1.732050807568863648 ) ) ;
#83752=CARTESIAN_POINT ( 'NONE',  ( -0.6823417656250003738, -0.5322916663252491576, -1.181850606188749264 ) ) ;
#83756=CARTESIAN_POINT ( 'NONE',  ( 4.871457266011829823, 4.577788319968905562, -0.7998128361456221525 ) ) ;
#83758=CARTESIAN_POINT ( 'NONE',  ( 1.364683531249988535, 4.967708333674756283, -0.7879004041258300672 ) ) ;
#83765=CARTESIAN_POINT ( 'NONE',  ( -8.199983978166823562, 8.461069484149769337, -0.7998128361456291469 ) ) ;
#83766=CARTESIAN_POINT ( 'NONE',  ( 6.654354466208897811, 6.657835053532175529, 0.7998128361456341429 ) ) ;
#83769=CARTESIAN_POINT ( 'NONE',  ( -1.364683531250014514, -0.2197916663252438285, 0.7879004041258379498 ) ) ;
#83771=ORIENTED_EDGE ( 'NONE', *, *, #66008, .T. ) ;
#83773=DIRECTION ( 'NONE',  ( -7.387867266669436732E-31, 1.000000000000000000, 8.546850786086424434E-32 ) ) ;
#83775=CARTESIAN_POINT ( 'NONE',  ( -5.371001409308059138, 9.417918744168066070, -0.7998128361456231517 ) ) ;
#83779=CARTESIAN_POINT ( 'NONE',  ( 9.028840231696797503, 12.62106513936658203, -1.199719254218446718 ) ) ;
#83781=CARTESIAN_POINT ( 'NONE',  ( 8.646349277213076334, 11.11049346154719508, 1.599625672291281386 ) ) ;
#83783=CARTESIAN_POINT ( 'NONE',  ( -4.613852347352193739, 4.277249248199312071, 1.214306433183764966E-14 ) ) ;
#83784=CARTESIAN_POINT ( 'NONE',  ( -6.509886312855995172, 10.74661779830734254, -0.7998128361456291469 ) ) ;
#83787=CARTESIAN_POINT ( 'NONE',  ( -4.596643646408070438, 7.147595147647359148, 1.363028123281652793 ) ) ;
#83788=CARTESIAN_POINT ( 'NONE',  ( 0.6823417656249882723, -0.9072916663252494907, 1.181850606188755259 ) ) ;
#83792=CARTESIAN_POINT ( 'NONE',  ( 6.792271770766432404, 10.86814146596211472, 1.040834085586084257E-14 ) ) ;
#83795=CARTESIAN_POINT ( 'NONE',  ( 5.250031796989762967, 7.148123067953287446, 1.599625672291267398 ) ) ;
#83812=CARTESIAN_POINT ( 'NONE',  ( 2.236732156574683827, 5.553345249405011508, 1.040834085586084257E-14 ) ) ;
#83816=CARTESIAN_POINT ( 'NONE',  ( -4.076197739202962467, 7.907314462378773001, 1.040834085586084257E-14 ) ) ;
#83817=CARTESIAN_POINT ( 'NONE',  ( -7.995557903757128493, 10.35123685918189729, 1.599625672291295375 ) ) ;
#83822=CARTESIAN_POINT ( 'NONE',  ( -0.7500000000000215383, 3.222916667349487341, 1.299038105676671107 ) ) ;
#83823=CARTESIAN_POINT ( 'NONE',  ( 8.703444544968814256, 12.24143683818393313, -1.199719254218446718 ) ) ;
#83827=CARTESIAN_POINT ( 'NONE',  ( -9.365985188942097750, 9.821404230054264772, 0.7998128361456462443 ) ) ;
#83829=CARTESIAN_POINT ( 'NONE',  ( 0.6823417656249899377, 1.592708333674752730, 1.181850606188755259 ) ) ;
#83838=CARTESIAN_POINT ( 'NONE',  ( -2.279742385392243165, 5.811449882932888222, -0.7998128361456281477 ) ) ;
#83843=CARTESIAN_POINT ( 'NONE',  ( -0.6823417656250212460, 1.863541667008083991, 1.181850606188755259 ) ) ;
#83848=CARTESIAN_POINT ( 'NONE',  ( 1.364683531249988535, 1.863541667008086211, 0.7879004041258500513 ) ) ;
#83850=CARTESIAN_POINT ( 'NONE',  ( -6.898401231254901234, 6.942556279419168419, -0.7998128361456291469 ) ) ;
#83851=CARTESIAN_POINT ( 'NONE',  ( 9.101601193475611140, 9.512956235343358102, -0.7998128361456221525 ) ) ;
#83852=CARTESIAN_POINT ( 'NONE',  ( 3.284841267552055299, 6.405332120898776793, -0.9495590844852133117 ) ) ;
#83854=CARTESIAN_POINT ( 'NONE',  ( -0.7500000000000215383, 3.441666666666689967, 1.299038105676671107 ) ) ;
#83857=CARTESIAN_POINT ( 'NONE',  ( -0.6823417656250003738, 2.530208333674753618, -1.181850606188749264 ) ) ;
#83863=CARTESIAN_POINT ( 'NONE',  ( 4.961921032921539521, 7.772363057508363759, -1.082531754730549078 ) ) ;
#83866=CARTESIAN_POINT ( 'NONE',  ( -7.828943636887387925, 11.22118577875556156, 1.199719254218453823 ) ) ;
#83867=CARTESIAN_POINT ( 'NONE',  ( -4.274898507010545856, 3.881803101134051470, -0.7998128361456221525 ) ) ;
#83869=CARTESIAN_POINT ( 'NONE',  ( -0.6823417656249969321, 4.467708333674755394, -1.181850606188749264 ) ) ;
#83872=CYLINDRICAL_SURFACE ( 'NONE', #125720, 1.500000000000000222 ) ;
#83873=CARTESIAN_POINT ( 'NONE',  ( -8.324343128666356506, 8.814081192973304724, 1.040834085586084257E-14 ) ) ;
#83875=CARTESIAN_POINT ( 'NONE',  ( 1.499999999999990896, 5.775000000000023448, 1.040834085586084257E-14 ) ) ;
#83878=AXIS2_PLACEMENT_3D ( 'NONE', #91418, #90335, #59956 ) ;
#83879=CARTESIAN_POINT ( 'NONE',  ( 6.629573927402440781, 10.67832731537079383, 1.040834085586084257E-14 ) ) ;
#83892=CARTESIAN_POINT ( 'NONE',  ( 6.856673000209174695, 9.022537805042615489, 1.599625672291281386 ) ) ;
#83893=AXIS2_PLACEMENT_3D ( 'NONE', #130075, #197112, #147320 ) ;
#83894=CARTESIAN_POINT ( 'NONE',  ( -5.525111292768871252, 6.404716915440499037, -1.199719254218446718 ) ) ;
#83897=CARTESIAN_POINT ( 'NONE',  ( -1.499999999999996669, 5.129166666666691299, -0.8660254037844395958 ) ) ;
#83899=CARTESIAN_POINT ( 'NONE',  ( 4.785665035499516051, 8.527100274817353665, -0.7216878364870207285 ) ) ;
#83900=CARTESIAN_POINT ( 'NONE',  ( -1.364683531250014514, 0.3010416670080866552, -0.7879004041258359514 ) ) ;
#83901=CARTESIAN_POINT ( 'NONE',  ( 2.399429999938675007, 5.743159399996332404, 0.000000000000000000 ) ) ;
#83902=CARTESIAN_POINT ( 'NONE',  ( -8.462260433223891098, 13.02438760540324481, -0.7998128361456281477 ) ) ;
#83910=VERTEX_POINT ( 'NONE', #110970 ) ;
#83911=CARTESIAN_POINT ( 'NONE',  ( 3.511198596259283544, 6.271927390929313617, -7.499999999999997335 ) ) ;
#83918=CARTESIAN_POINT ( 'NONE',  ( 5.770966940911189447, 9.884545197705074671, -0.7998128361456291469 ) ) ;
#83919=CARTESIAN_POINT ( 'NONE',  ( 6.877010230629674759, 9.046264573866535486, 1.599625672291281386 ) ) ;
#83923=ORIENTED_EDGE ( 'NONE', *, *, #103873, .T. ) ;
#83930=CARTESIAN_POINT ( 'NONE',  ( 8.563946585326370098, 13.14302144952281814, 0.7998128361456462443 ) ) ;
#83932=CARTESIAN_POINT ( 'NONE',  ( -5.870844209917351009, 6.808071985447069707, -1.199719254218446718 ) ) ;
#83934=CARTESIAN_POINT ( 'NONE',  ( -4.939248034080176097, 4.656877549381960080, 1.214306433183764966E-14 ) ) ;
#83939=CARTESIAN_POINT ( 'NONE',  ( 1.499999999999822586, 7.176846818246208848, 4.202462424328222035 ) ) ;
#83943=CARTESIAN_POINT ( 'NONE',  ( -10.46653140006992899, 11.31330084294416771, -0.7216878364870267237 ) ) ;
#83946=CARTESIAN_POINT ( 'NONE',  ( 6.582647274634798151, 7.638508894284114170, 1.199719254218462483 ) ) ;
#83947=CARTESIAN_POINT ( 'NONE',  ( -1.364683531249997417, 5.259375000341425022, 1.214306433183764966E-14 ) ) ;
#83952=EDGE_CURVE ( 'NONE', #6371, #54971, #151695, .T. ) ;
#83954=CARTESIAN_POINT ( 'NONE',  ( 4.487385655998878953, 6.258369236797239665, 1.443375672974062551 ) ) ;
#83955=CARTESIAN_POINT ( 'NONE',  ( -7.366157530926372488, 7.488271962369228874, -0.7998128361456291469 ) ) ;
#83961=CARTESIAN_POINT ( 'NONE',  ( -8.369460898337653276, 8.658792557682392754, 0.7998128361456462443 ) ) ;
#83962=CARTESIAN_POINT ( 'NONE',  ( -5.949330478298285207, 5.835307067636438028, 0.7998128361456341429 ) ) ;
#83969=CARTESIAN_POINT ( 'NONE',  ( 8.098297826064319693, 8.342435640030188893, 0.7998128361456481317 ) ) ;
#83973=( BOUNDED_CURVE ( )  B_SPLINE_CURVE ( 2, ( #126777, #61691, #160257, #174399, #44390, #74744, #110511 ),
 .UNSPECIFIED., .F., .T. ) 
 B_SPLINE_CURVE_WITH_KNOTS ( ( 3, 2, 2, 3 ),
 ( 0.2624999999999999001, 0.2666666666666666075, 0.2708333333333333148, 0.2750000000000000777 ),
 .UNSPECIFIED. ) 
 CURVE ( )  GEOMETRIC_REPRESENTATION_ITEM ( )  RATIONAL_B_SPLINE_CURVE ( ( 1.000000000000003553, 0.8660254037844351549, 1.000000000000000000, 0.8660254037844387076, 1.000000000000000000, 0.8660254037844369313, 1.000000000000001776 ) ) 
 REPRESENTATION_ITEM ( '' )  );
#83984=CARTESIAN_POINT ( 'NONE',  ( -1.364683531250014514, -0.9072916663252470482, 0.7879004041258379498 ) ) ;
#83985=CARTESIAN_POINT ( 'NONE',  ( 2.523789150438203510, 6.096171108819874007, 0.7998128361456462443 ) ) ;
#83986=CARTESIAN_POINT ( 'NONE',  ( 5.840865249388943248, 5.708764300575555062, 0.7998128361456341429 ) ) ;
#83988=CARTESIAN_POINT ( 'NONE',  ( -7.917598520700757980, 9.299915031314755609, 1.082531754730558626 ) ) ;
#83991=CARTESIAN_POINT ( 'NONE',  ( 6.168596704537822717, 6.299043698156668647, 1.040834085586084257E-14 ) ) ;
#83992=CARTESIAN_POINT ( 'NONE',  ( -7.497295758232720431, 10.73030023703809555, -1.082531754730543083 ) ) ;
#83996=CARTESIAN_POINT ( 'NONE',  ( 8.274553823041976841, 8.548067636504127265, 1.040834085586084257E-14 ) ) ;
#84000=CARTESIAN_POINT ( 'NONE',  ( -2.303566469087102497, 5.490909403443315462, -0.7594041750639659583 ) ) ;
#84001=CARTESIAN_POINT ( 'NONE',  ( -0.6823417656249969321, 3.467708333674754506, -1.181850606188749264 ) ) ;
#84007=CARTESIAN_POINT ( 'NONE',  ( 7.853197290813620945, 10.18514947741448573, 1.599625672291281386 ) ) ;
#84010=CARTESIAN_POINT ( 'NONE',  ( -7.167456763118792651, 11.51378332361394818, 0.000000000000000000 ) ) ;
#84014=CARTESIAN_POINT ( 'NONE',  ( -0.7500000000000215383, 4.222916667349481123, 1.299038105676671107 ) ) ;
#84016=CARTESIAN_POINT ( 'NONE',  ( 9.053093885623066939, 11.58502883802551153, -1.599625672291262513 ) ) ;
#84019=CARTESIAN_POINT ( 'NONE',  ( -8.864333505236459132, 9.236143932397675727, 1.040834085586084257E-14 ) ) ;
#84025=CARTESIAN_POINT ( 'NONE',  ( 4.499659979152191625, 7.015106111828595559, -1.153029749421132566 ) ) ;
#84026=CARTESIAN_POINT ( 'NONE',  ( -4.762992037102518950, 4.451245552908022596, -0.7998128361456221525 ) ) ;
#84032=CARTESIAN_POINT ( 'NONE',  ( 7.558834334818744338, 8.777393797832065303, 1.199719254218462483 ) ) ;
#84034=CARTESIAN_POINT ( 'NONE',  ( 5.099838337034727331, 9.101561826515851550, -0.7998128361456281477 ) ) ;
#84035=CARTESIAN_POINT ( 'NONE',  ( -4.192242263785030509, 7.388029550104924681, -0.8017062249071702507 ) ) ;
#84036=CARTESIAN_POINT ( 'NONE',  ( 4.039439701867726384, 6.800097854565950506, 1.199719254218462483 ) ) ;
#84038=CARTESIAN_POINT ( 'NONE',  ( -8.541273586929371220, 9.067166727613487964, 0.7216878364870438212 ) ) ;
#84046=CARTESIAN_POINT ( 'NONE',  ( -4.034408581249735448, 7.597519823075112200, 0.2926387080343200164 ) ) ;
#84047=CARTESIAN_POINT ( 'NONE',  ( -0.6823417656250246877, -0.8864583329919115684, 1.181850606188755259 ) ) ;
#84051=CARTESIAN_POINT ( 'NONE',  ( 4.189106276942576201, 7.831115056500907556, 1.040834085586084257E-14 ) ) ;
#84056=CARTESIAN_POINT ( 'NONE',  ( -9.368320956918621434, 11.95279375453699622, 1.443375672974076540 ) ) ;
#84061=CARTESIAN_POINT ( 'NONE',  ( -9.368320956918621434, 11.95279375453699622, 1.443375672974076540 ) ) ;
#84070=CARTESIAN_POINT ( 'NONE',  ( -9.503902493055310430, 11.15060299906175167, 1.082531754730558626 ) ) ;
#84078=CARTESIAN_POINT ( 'NONE',  ( -0.7500000000000215383, 3.472916667349487785, 1.299038105676671107 ) ) ;
#84080=CARTESIAN_POINT ( 'NONE',  ( -6.417086777969760902, 6.381022750586497594, 0.7998128361456341429 ) ) ;
#84083=CARTESIAN_POINT ( 'NONE',  ( -8.188234707649510113, 11.64035869464474082, -1.199719254218446718 ) ) ;
#84088=CARTESIAN_POINT ( 'NONE',  ( 4.801558957534076022, 8.753569217098425170, 0.7998128361456462443 ) ) ;
#84094=CARTESIAN_POINT ( 'NONE',  ( 8.422639742587595180, 10.84949900448412130, -1.599625672291268286 ) ) ;
#84095=CARTESIAN_POINT ( 'NONE',  ( -1.364683531249997417, 5.759375000341418804, 1.214306433183764966E-14 ) ) ;
#84100=CARTESIAN_POINT ( 'NONE',  ( -7.049876689426106680, 9.247942109129029475, -1.443375672974059665 ) ) ;
#84103=CARTESIAN_POINT ( 'NONE',  ( -1.364683531250010295, 5.092708333674757171, 0.7879004041258379498 ) ) ;
#84108=CARTESIAN_POINT ( 'NONE',  ( -4.270455198180246548, 4.084545274072787890, 0.7216878364870317197 ) ) ;
#84111=CARTESIAN_POINT ( 'NONE',  ( 9.236128959407556849, 11.79856975744075598, -1.599625672291262513 ) ) ;
#84113=CARTESIAN_POINT ( 'NONE',  ( -1.284279953904132077, 2.878360285806111474, -0.7749999999999935829 ) ) ;
#84117=CARTESIAN_POINT ( 'NONE',  ( 1.364683531249988757, 1.884375000341421913, 0.000000000000000000 ) ) ;
#84120=CARTESIAN_POINT ( 'NONE',  ( 3.822509244049070887, 6.547012320444182798, -1.199719254218452047 ) ) ;
#84121=VERTEX_POINT ( 'NONE', #117366 ) ;
#84126=FACE_OUTER_BOUND ( 'NONE', #50957, .T. ) ;
#84127=CARTESIAN_POINT ( 'NONE',  ( 9.531018800282598846, 12.14260790512831889, 1.443375672974076540 ) ) ;
#84129=CARTESIAN_POINT ( 'NONE',  ( -7.890482213473404727, 8.307910125248191946, 0.7216878364870578100 ) ) ;
#84131=CARTESIAN_POINT ( 'NONE',  ( 1.451998047844732964, 7.315968950354620581, 4.301760722576522866 ) ) ;
#84134=CARTESIAN_POINT ( 'NONE',  ( -8.483651433849100698, 10.92067931095586886, 1.599625672291269396 ) ) ;
#84135=CARTESIAN_POINT ( 'NONE',  ( -3.429849674132936066, 6.945315686556313040, -0.7216878364870257245 ) ) ;
#84136=CARTESIAN_POINT ( 'NONE',  ( 0.6823417656249899377, 2.155208333674753174, 1.181850606188767472 ) ) ;
#84156=B_SPLINE_CURVE_WITH_KNOTS ( 'NONE', 3,
 ( #174544, #21824, #43474, #190747 ),
 .UNSPECIFIED., .F., .F.,
 ( 4, 4 ),
 ( 7.548539127806008953E-17, 0.0001647631253658502772 ),
 .UNSPECIFIED. ) ;
#84157=CARTESIAN_POINT ( 'NONE',  ( 1.364683531249990311, 4.926041667008083991, 0.7879004041258500513 ) ) ;
#84164=CARTESIAN_POINT ( 'NONE',  ( 9.596473800374404561, 10.09030761005864285, 0.000000000000000000 ) ) ;
#84167=CARTESIAN_POINT ( 'NONE',  ( -0.6823417656250212460, 2.551041667008084435, 1.181850606188767472 ) ) ;
#84169=CARTESIAN_POINT ( 'NONE',  ( -7.375272376154101472, 7.706831981708990753, -0.7216878364870278340 ) ) ;
#84177=CARTESIAN_POINT ( 'NONE',  ( 4.059776932288224671, 6.823824623389866950, 1.199719254218462483 ) ) ;
#84180=ORIENTED_EDGE ( 'NONE', *, *, #40172, .F. ) ;
#84181=CARTESIAN_POINT ( 'NONE',  ( 9.402743226277308963, 10.92862083786708816, -1.199719254218446718 ) ) ;
#84188=CARTESIAN_POINT ( 'NONE',  ( -2.923754682041362241, 6.562797562356882608, 0.7998128361456341429 ) ) ;
#84189=CARTESIAN_POINT ( 'NONE',  ( 8.457588896826466751, 8.761608555919362828, 1.040834085586084257E-14 ) ) ;
#84191=CARTESIAN_POINT ( 'NONE',  ( 3.673896439178918172, 6.269667698141953238, 1.082531754730558626 ) ) ;
#84193=CARTESIAN_POINT ( 'NONE',  ( 1.419999999999990603, 6.280000000000042881, 2.873333333333337070 ) ) ;
#84201=CARTESIAN_POINT ( 'NONE',  ( -7.131225611108100715, 9.342849184424693476, 1.443375672974078761 ) ) ;
#84202=CARTESIAN_POINT ( 'NONE',  ( 5.066996723205273057, 6.934582148538044777, 1.599625672291267398 ) ) ;
#84206=CARTESIAN_POINT ( 'NONE',  ( -9.006694118179950692, 9.402231314165087284, 1.040834085586084257E-14 ) ) ;
#84211=CARTESIAN_POINT ( 'NONE',  ( -3.948449050077848632, 5.629609863222681199, 1.599625672291267398 ) ) ;
#84214=CARTESIAN_POINT ( 'NONE',  ( 8.097244055859613709, 10.46987070330147063, -1.599625672291262513 ) ) ;
#84215=CARTESIAN_POINT ( 'NONE',  ( 3.571683402196252910, 6.254382171615883834, 1.199719254218462483 ) ) ;
#84221=CARTESIAN_POINT ( 'NONE',  ( 3.159872497350143750, 2.806782174840458666, -2.466584723216997510 ) ) ;
#84224=CARTESIAN_POINT ( 'NONE',  ( -3.906720819032141190, 7.709591388846142479, -0.7998128361456281477 ) ) ;
#84227=CARTESIAN_POINT ( 'NONE',  ( -9.104463846776669200, 10.58062822844965645, -1.199719254218441611 ) ) ;
#84232=CARTESIAN_POINT ( 'NONE',  ( 6.453317930424781856, 10.47269531889685545, -0.7216878364870267237 ) ) ;
#84233=CARTESIAN_POINT ( 'NONE',  ( 0.6823417656249917140, 5.655208333674749177, 1.181850606188765695 ) ) ;
#84235=CARTESIAN_POINT ( 'NONE',  ( 3.009020027229115879, 5.597941567487558778, -1.199719254218446718 ) ) ;
#84237=CARTESIAN_POINT ( 'NONE',  ( 4.222474775652216294, 7.013638773981186958, 1.199719254218462483 ) ) ;
#84239=CARTESIAN_POINT ( 'NONE',  ( -8.064402442030170093, 8.302891025323665630, 0.7998128361456602331 ) ) ;
#84248=ORIENTED_EDGE ( 'NONE', *, *, #210974, .T. ) ;
#84250=CARTESIAN_POINT ( 'NONE',  ( 0.6823417656249899377, 2.655208333674753618, 1.181850606188767472 ) ) ;
#84251=CARTESIAN_POINT ( 'NONE',  ( 8.215351014876830504, 11.67199438640995801, -1.199719254218446718 ) ) ;
#84253=CARTESIAN_POINT ( 'NONE',  ( -4.446711195602245148, 7.171284913969171448, -1.082531754730549967 ) ) ;
#84255=CARTESIAN_POINT ( 'NONE',  ( 2.250290310188348464, 5.569163095287620990, 0.7216878364870438212 ) ) ;
#84256=CARTESIAN_POINT ( 'NONE',  ( -4.392478580703220281, 8.068382744221649361, 1.040834085586084257E-14 ) ) ;
#84263=CARTESIAN_POINT ( 'NONE',  ( 3.147464216666835402, 6.823792019419957278, -0.7998128361456291469 ) ) ;
#84272=CARTESIAN_POINT ( 'NONE',  ( 5.138703914779377158, 5.953908307786102583, 1.199719254218462483 ) ) ;
#84276=CARTESIAN_POINT ( 'NONE',  ( -6.586563698140583512, 6.578745824119123675, 1.040834085586084257E-14 ) ) ;
#84280=CARTESIAN_POINT ( 'NONE',  ( 6.962275575817444384, 8.081408578997208991, -1.199719254218446718 ) ) ;
#84283=CARTESIAN_POINT ( 'NONE',  ( -5.225778143063529946, 8.184159369294361497, 1.199719254218452047 ) ) ;
#84285=CARTESIAN_POINT ( 'NONE',  ( -0.7500000000000215383, 2.691666666666689522, 1.299038105676671107 ) ) ;
#84286=CARTESIAN_POINT ( 'NONE',  ( -4.810445574750349174, 4.506608013497163334, 0.7998128361456341429 ) ) ;
#84289=CARTESIAN_POINT ( 'NONE',  ( -6.033542053281340856, 6.997886136038390603, -1.199719254218446718 ) ) ;
#84292=CARTESIAN_POINT ( 'NONE',  ( -1.201851678989727383E-14, 3.196875000341420137, -1.575800808251660134 ) ) ;
#84294=CARTESIAN_POINT ( 'NONE',  ( -4.772106882330234612, 6.590544000850479200, -1.443375672974053447 ) ) ;
#84301=CARTESIAN_POINT ( 'NONE',  ( 6.030679399980265920, 5.930214142932100252, -0.7998128361456281477 ) ) ;
#84304=CARTESIAN_POINT ( 'NONE',  ( 1.364683531249988757, 2.196875000341415252, 1.214306433183764966E-14 ) ) ;
#84307=CARTESIAN_POINT ( 'NONE',  ( -0.07074886611256257785, 8.280404612018088528, 2.000278354478734144 ) ) ;
#84308=CARTESIAN_POINT ( 'NONE',  ( 5.630352418794719149, 6.139657267270441920, -0.8181431533968346326 ) ) ;
#84310=CARTESIAN_POINT ( 'NONE',  ( -3.785751206713858785, 5.439795712631356750, 1.599625672291267398 ) ) ;
#84312=CARTESIAN_POINT ( 'NONE',  ( -6.792271770322117597, 9.907772251142352715, 1.082531754730549967 ) ) ;
#84314=CARTESIAN_POINT ( 'NONE',  ( -1.201851678989727383E-14, 3.696875000341422801, -1.575800808251660134 ) ) ;
#84322=CARTESIAN_POINT ( 'NONE',  ( -7.063434842595444962, 8.303390740191881392, 1.082531754730549967 ) ) ;
#84328=CARTESIAN_POINT ( 'NONE',  ( -7.171900071504754060, 7.469564292951421436, -0.7216878364870267237 ) ) ;
#84333=CARTESIAN_POINT ( 'NONE',  ( 2.836961834123311821, 6.429236568308559718, -0.07888921887194833005 ) ) ;
#84337=FACE_OUTER_BOUND ( 'NONE', #55926, .T. ) ;
#84341=CARTESIAN_POINT ( 'NONE',  ( -5.530836599371015794, 8.540060901653093950, 1.199719254218452047 ) ) ;
#84343=CARTESIAN_POINT ( 'NONE',  ( 0.7499999999999867883, -0.1833333333333131421, -1.299038105676652899 ) ) ;
#84344=CARTESIAN_POINT ( 'NONE',  ( 3.521367211247359741, 5.131347717920458962, -1.599625672291262513 ) ) ;
#84349=CARTESIAN_POINT ( 'NONE',  ( 5.133733721068893807, 9.141106441222381918, 1.040834085586084257E-14 ) ) ;
#84355=CARTESIAN_POINT ( 'NONE',  ( -4.229780737783618072, 6.918199379847403740, 1.082531754730560403 ) ) ;
#84358=CARTESIAN_POINT ( 'NONE',  ( -0.5341619149264997812, 6.871487518424857832, 3.795316691233094009 ) ) ;
#84362=CARTESIAN_POINT ( 'NONE',  ( 0.6823417656249882723, 1.676041667008083769, -1.181850606188749264 ) ) ;
#84363=CARTESIAN_POINT ( 'NONE',  ( 8.392133896734652154, 12.73464727959172293, 0.7216878364870438212 ) ) ;
#84364=CARTESIAN_POINT ( 'NONE',  ( -8.040148788103921973, 9.338927326664741457, 1.199719254218462483 ) ) ;
#84366=( BOUNDED_CURVE ( )  B_SPLINE_CURVE ( 1, ( #21348, #818 ),
 .UNSPECIFIED., .F., .T. ) 
 B_SPLINE_CURVE_WITH_KNOTS ( ( 2, 2 ),
 ( 0.000000000000000000, 6.249999999999788711E-05 ),
 .UNSPECIFIED. ) 
 CURVE ( )  GEOMETRIC_REPRESENTATION_ITEM ( )  RATIONAL_B_SPLINE_CURVE ( ( 0.9345202395942815432, 0.9345202395942815432 ) ) 
 REPRESENTATION_ITEM ( '' )  );
#84370=CARTESIAN_POINT ( 'NONE',  ( 6.012151052656117933, 9.101594430485762999, 1.199719254218460707 ) ) ;
#84371=CARTESIAN_POINT ( 'NONE',  ( -7.552055258011950656, 8.769484874890757453, 1.199719254218462483 ) ) ;
#84372=CARTESIAN_POINT ( 'NONE',  ( -1.446373960595505270, 8.704174803020482187, 2.603708784378574226 ) ) ;
#84374=CARTESIAN_POINT ( 'NONE',  ( 1.499999999999987566, -0.4437499993171847845, 0.000000000000000000 ) ) ;
#84377=CARTESIAN_POINT ( 'NONE',  ( 9.436111725431318931, 10.11114455586577776, -0.7216878364870257245 ) ) ;
#84380=CARTESIAN_POINT ( 'NONE',  ( -1.402160292154681736E-14, 0.5093750003414236893, -1.575800808251659024 ) ) ;
#84383=CARTESIAN_POINT ( 'NONE',  ( 6.277061933002774374, 9.306694107603160404, 1.082531754730558626 ) ) ;
#84386=CARTESIAN_POINT ( 'NONE',  ( -5.422898255786209099, 5.429062174613087599, -0.7216878364870207285 ) ) ;
#84388=CARTESIAN_POINT ( 'NONE',  ( -1.364683531250010295, 3.780208333674750953, 0.7879004041258379498 ) ) ;
#84392=CARTESIAN_POINT ( 'NONE',  ( -4.283486466913726254, 7.084819080452935403, -1.199719254218452047 ) ) ;
#84393=CARTESIAN_POINT ( 'NONE',  ( -4.922147708203060468, 6.858988491581952118, -1.449652397630277756 ) ) ;
#84399=CARTESIAN_POINT ( 'NONE',  ( 7.969495366734495434, 8.192166104145387706, 1.040834085586084257E-14 ) ) ;
#84403=CARTESIAN_POINT ( 'NONE',  ( -0.7500000000000006661, 2.358333333333358262, -1.299038105676652011 ) ) ;
#84409=CARTESIAN_POINT ( 'NONE',  ( 5.178851490740193242, 8.025448591630130579, 1.082531754730558626 ) ) ;
#84410=CARTESIAN_POINT ( 'NONE',  ( 0.6823417656249882723, 0.4885416670080827695, -1.181850606188749264 ) ) ;
#84412=DIRECTION ( 'NONE',  ( 0.9055141421511233579, 0.4243160830846685050, 2.454401000341482920E-15 ) ) ;
#84416=AXIS2_PLACEMENT_3D ( 'NONE', #117736, #166413, #116657 ) ;
#84418=CARTESIAN_POINT ( 'NONE',  ( 0.7499999999999885647, 0.4833333333333564297, 1.299038105676657340 ) ) ;
#84419=CARTESIAN_POINT ( 'NONE',  ( 6.154511665599609493, 9.267681812253174556, 1.199719254218462483 ) ) ;
#84420=CARTESIAN_POINT ( 'NONE',  ( -6.516665389662827934, 10.75452672124865217, 0.000000000000000000 ) ) ;
#84422=CARTESIAN_POINT ( 'NONE',  ( 1.364683531249988757, 0.6343750003414208027, 0.000000000000000000 ) ) ;
#84423=CARTESIAN_POINT ( 'NONE',  ( 0.7499999999999885647, 2.316666666666689078, -1.299038105676652899 ) ) ;
#84425=CARTESIAN_POINT ( 'NONE',  ( 3.876741858503734761, 6.610283703974623393, 1.199719254218462483 ) ) ;
#84432=CARTESIAN_POINT ( 'NONE',  ( -0.7500000000000006661, -0.6104166659838470288, -1.299038105676652011 ) ) ;
#84433=CARTESIAN_POINT ( 'NONE',  ( -8.179646747746328828, 8.437342715325849341, -0.7998128361456291469 ) ) ;
#84434=CARTESIAN_POINT ( 'NONE',  ( -2.982430605326321427, 6.423326772948587227, -0.7216878364870267237 ) ) ;
#84442=CARTESIAN_POINT ( 'NONE',  ( 7.949158136313996259, 8.168439335321471262, 1.040834085586084257E-14 ) ) ;
#84446=CARTESIAN_POINT ( 'NONE',  ( 5.951666246274792016, 8.927065806420504401, 1.082531754730558626 ) ) ;
#84447=CYLINDRICAL_SURFACE ( 'NONE', #103112, 0.08000000000000020983 ) ;
#84450=CARTESIAN_POINT ( 'NONE',  ( -8.843996274815957293, 9.212417163573759282, 1.040834085586084257E-14 ) ) ;
#84451=CARTESIAN_POINT ( 'NONE',  ( 5.542585869888291938, 5.360771691158120689, -0.7998128361456211532 ) ) ;
#84456=CARTESIAN_POINT ( 'NONE',  ( 9.747949258545622442, 10.47495501116581984, 0.000000000000000000 ) ) ;
#84461=CARTESIAN_POINT ( 'NONE',  ( 2.273584122437516175, 5.675375552130928369, 0.4747937928818931064 ) ) ;
#84462=CARTESIAN_POINT ( 'NONE',  ( -1.547033095191295171, 8.694673270357780481, -2.507079848779465436 ) ) ;
#84463=CARTESIAN_POINT ( 'NONE',  ( -4.284013352238265959, 5.060732334775157604, -1.082531754730544860 ) ) ;
#84464=CARTESIAN_POINT ( 'NONE',  ( 8.378575743565351175, 11.75846021992619406, -1.082531754730543083 ) ) ;
#84467=CARTESIAN_POINT ( 'NONE',  ( -4.543954038874438162, 8.453030145328826350, 1.040834085586084257E-14 ) ) ;
#84473=CARTESIAN_POINT ( 'NONE',  ( -6.672584156219988571, 10.93643194889866521, -0.7998128361456291469 ) ) ;
#84478=ORIENTED_EDGE ( 'NONE', *, *, #116366, .F. ) ;
#84479=DIRECTION ( 'NONE',  ( 0.7592566023653004592, -0.6507913734559641616, -1.725633230170963105E-31 ) ) ;
#84487=CARTESIAN_POINT ( 'NONE',  ( -6.389970470742427189, 6.349387058821269747, -0.7998128361456291469 ) ) ;
#84490=CARTESIAN_POINT ( 'NONE',  ( 4.026408433578586354, 7.641300905909586660, 1.040834085586084257E-14 ) ) ;
#84496=CARTESIAN_POINT ( 'NONE',  ( -3.653032323878261600, 6.349289246911547835, -1.199719254218452047 ) ) ;
#84504=CARTESIAN_POINT ( 'NONE',  ( -8.533967624797991647, 12.04371376465130439, -1.199719254218446718 ) ) ;
#84505=CARTESIAN_POINT ( 'NONE',  ( 6.972971076130050072, 7.029554431773520129, 1.040834085586084257E-14 ) ) ;
#84508=EDGE_CURVE ( 'NONE', #93339, #180365, #168141, .T. ) ;
#84510=CARTESIAN_POINT ( 'NONE',  ( -8.136864746495904299, 12.64475930422059768, -0.7998128361456281477 ) ) ;
#84511=CARTESIAN_POINT ( 'NONE',  ( 5.684946482831785275, 5.526859072925533134, -0.7998128361456231517 ) ) ;
#84513=CARTESIAN_POINT ( 'NONE',  ( 1.364683531249988757, 0.4468750003414206917, 0.000000000000000000 ) ) ;
#84516=ORIENTED_EDGE ( 'NONE', *, *, #151365, .T. ) ;
#84518=CARTESIAN_POINT ( 'NONE',  ( 7.117667457494414762, 11.24776976714476184, 1.040834085586084257E-14 ) ) ;
#84522=DIRECTION ( 'NONE',  ( -1.000000000000000000, 5.578564026256504688E-16, 0.000000000000000000 ) ) ;
#84526=CARTESIAN_POINT ( 'NONE',  ( -0.2091928449107274546, 6.366027919468703722, -3.121370559291495539 ) ) ;
#84544=CARTESIAN_POINT ( 'NONE',  ( 0.7499999999999867883, -0.1520833326505155458, -1.299038105676652899 ) ) ;
#84549=ORIENTED_EDGE ( 'NONE', *, *, #132737, .T. ) ;
#84550=CARTESIAN_POINT ( 'NONE',  ( 1.499999999999821032, 7.240846818246208905, -4.154462424328214887 ) ) ;
#84553=CARTESIAN_POINT ( 'NONE',  ( 10.24048609702354717, 10.84165528948263457, -0.7998128361456281477 ) ) ;
#84558=CARTESIAN_POINT ( 'NONE',  ( 3.659811400685081040, 6.357198169852855685, -1.199719254218446718 ) ) ;
#84559=CARTESIAN_POINT ( 'NONE',  ( -7.537970219518091319, 7.896646132300314314, -0.7216878364870278340 ) ) ;
#84562=CARTESIAN_POINT ( 'NONE',  ( -7.344766530301162000, 9.591980256816594164, 1.599625672291295375 ) ) ;
#84564=CARTESIAN_POINT ( 'NONE',  ( -4.487385655998893164, 6.258369236797239665, 1.443375672974064550 ) ) ;
#84567=EDGE_LOOP ( 'NONE', ( #99280, #39674, #106208, #27268 ) ) ;
#84568=CARTESIAN_POINT ( 'NONE',  ( 0.7499999999999867883, 0.09791666734948467621, -1.299038105676652899 ) ) ;
#84569=B_SPLINE_CURVE_WITH_KNOTS ( 'NONE', 3,
 ( #54164, #134383, #120302, #52033, #186276, #37913, #101843, #135423, #201445, #53088, #119221, #103988, #71450, #137563, #33639, #99712, #7521, #121378, #174335, #26978, #142917, #24847, #10726, #187352, #154868, #206797, #123526, #173266 ),
 .UNSPECIFIED., .F., .F.,
 ( 4, 2, 2, 2, 2, 2, 2, 1, 2, 2, 1, 2, 2, 2, 4 ),
 ( 0.9162434286749613355, 0.9214697481986482419, 0.9240829079604917506, 0.9266960677223353704, 0.9319223872460228320, 0.9371487067697102935, 0.9423750262933977551, 0.9476013458170851056, 0.9528276653407725671, 0.9554408251026164089, 0.9580539848644601397, 0.9685066239118349518, 0.9737329434355221913, 0.9789592629592095419, 0.9998645410539588330 ),
 .UNSPECIFIED. ) ;
#84576=CARTESIAN_POINT ( 'NONE',  ( -5.070386261386537363, 5.017798181146802428, 1.214306433183764966E-14 ) ) ;
#84582=EDGE_CURVE ( 'NONE', #58688, #112883, #201098, .T. ) ;
#84586=CARTESIAN_POINT ( 'NONE',  ( -2.751941993449643409, 6.154423392425789174, 0.7216878364870317197 ) ) ;
#84587=CARTESIAN_POINT ( 'NONE',  ( 9.582915646760733708, 10.07448976417602893, 0.7998128361456462443 ) ) ;
#84595=CARTESIAN_POINT ( 'NONE',  ( -2.103486388414573138, 5.605817886458954291, 1.040834085586084257E-14 ) ) ;
#84596=CARTESIAN_POINT ( 'NONE',  ( -7.947050595904583403, 12.42330946186405249, 0.7998128361456481317 ) ) ;
#84599=EDGE_LOOP ( 'NONE', ( #156978, #128271, #38175, #80308, #91739 ) ) ;
#84601=CARTESIAN_POINT ( 'NONE',  ( 5.087333953625774008, 6.958308917361963886, 1.599625672291267398 ) ) ;
#84616=CARTESIAN_POINT ( 'NONE',  ( 7.904567251967224095, 9.180748867838630645, 1.199719254218462483 ) ) ;
#84618=CARTESIAN_POINT ( 'NONE',  ( -3.588104209110990706, 7.337872010604796991, 1.040834085586084257E-14 ) ) ;
#84619=CARTESIAN_POINT ( 'NONE',  ( -1.123270288250315163, 2.985197346350006331, -0.7749999999993613109 ) ) ;
#84623=CARTESIAN_POINT ( 'NONE',  ( -0.7500000000000249800, -0.5270833326505158789, 1.299038105676659116 ) ) ;
#84626=ADVANCED_FACE ( 'NONE', ( #128068 ), #143204, .F. ) ;
#84627=CARTESIAN_POINT ( 'NONE',  ( -4.540505084823442949, 7.125209978135113253, 1.295423358617282972 ) ) ;
#84628=CARTESIAN_POINT ( 'NONE',  ( 3.330499290451326200, 7.037332938835193730, -0.7998128361456291469 ) ) ;
#84630=CARTESIAN_POINT ( 'NONE',  ( -3.438964519360665051, 7.163875705896082913, -0.7998128361456281477 ) ) ;
#84636=CARTESIAN_POINT ( 'NONE',  ( 5.829642864196162400, 7.824335979694092558, 1.443375672974062551 ) ) ;
#84639=CARTESIAN_POINT ( 'NONE',  ( 6.602457619730749627, 10.64669162308715222, 0.7216878364870438212 ) ) ;
#84640=CARTESIAN_POINT ( 'NONE',  ( -1.201851678989727383E-14, 5.259375000341421469, -1.575800808251660134 ) ) ;
#84642=CARTESIAN_POINT ( 'NONE',  ( 5.165293336682183600, 5.128523102325077687, -0.7216878364870197293 ) ) ;
#84646=EDGE_CURVE ( 'NONE', #195163, #170224, #124986, .T. ) ;
#84648=CARTESIAN_POINT ( 'NONE',  ( 5.503988762639142607, 6.221932061145267312, -0.9643604338056003256 ) ) ;
#84651=CARTESIAN_POINT ( 'NONE',  ( -6.138286310890375574, 5.995785266799176227, -0.01092221066891288506 ) ) ;
#84652=CARTESIAN_POINT ( 'NONE',  ( -2.535011536075354677, 5.133042487381361596, -7.499999999999997335 ) ) ;
#84654=CARTESIAN_POINT ( 'NONE',  ( -1.364683531249997417, 5.571875000341417916, 1.214306433183764966E-14 ) ) ;
#84670=CARTESIAN_POINT ( 'NONE',  ( -0.6823417656249969321, 4.280208333674755394, -1.181850606188749264 ) ) ;
#84672=CARTESIAN_POINT ( 'NONE',  ( 7.610204295972345712, 7.772993188256215547, 0.7998128361456341429 ) ) ;
#84674=CARTESIAN_POINT ( 'NONE',  ( -9.667127221743832877, 11.23706883257798772, 1.199719254218462483 ) ) ;
#84679=VERTEX_POINT ( 'NONE', #31546 ) ;
#84682=CARTESIAN_POINT ( 'NONE',  ( -1.500000000000011324, 4.379166666666688634, -0.8660254037844313801 ) ) ;
#84689=CARTESIAN_POINT ( 'NONE',  ( 9.273413882067330860, 9.921330405274451536, -0.7216878364870257245 ) ) ;
#84694=CARTESIAN_POINT ( 'NONE',  ( 0.7499999999999902300, 3.014583334016149418, 1.299038105676669330 ) ) ;
#84696=CARTESIAN_POINT ( 'NONE',  ( -3.730464822054482710, 7.503959392372201442, 1.040834085586084257E-14 ) ) ;
#84697=CARTESIAN_POINT ( 'NONE',  ( 5.151735183068521629, 5.112705256442466428, 1.040834085586084257E-14 ) ) ;
#84698=CARTESIAN_POINT ( 'NONE',  ( -10.45297324601190425, 11.29748299654313470, 0.7216878364870438212 ) ) ;
#84705=CARTESIAN_POINT ( 'NONE',  ( 4.009460741339333723, 5.700790169694431420, -1.599625672291256295 ) ) ;
#84708=FACE_OUTER_BOUND ( 'NONE', #150070, .T. ) ;
#84709=CARTESIAN_POINT ( 'NONE',  ( 4.436542580169809291, 6.199052314996659874, 1.599625672291267398 ) ) ;
#84720=CARTESIAN_POINT ( 'NONE',  ( 5.253083726123439767, 6.394172465367824465, -1.148862164228587890 ) ) ;
#84722=CARTESIAN_POINT ( 'NONE',  ( 10.21336978979620191, 10.81001959771741205, 0.7998128361456462443 ) ) ;
#84726=CIRCLE ( 'NONE', #18982, 0.08000000000000020983 ) ;
#84728=CARTESIAN_POINT ( 'NONE',  ( -1.402160292154681736E-14, -0.9281249996585830830, 1.575800808251672791 ) ) ;
#84729=CARTESIAN_POINT ( 'NONE',  ( 6.968527767744109980, 7.232296605230681408, 0.7216878364870317197 ) ) ;
#84730=CARTESIAN_POINT ( 'NONE',  ( -9.110716038703348119, 12.61262389758715408, 1.082531754730560403 ) ) ;
#84736=CARTESIAN_POINT ( 'NONE',  ( -6.254388934605767503, 6.191208599995166040, 0.7998128361456341429 ) ) ;
#84740=VERTEX_POINT ( 'NONE', #12077 ) ;
#84747=CARTESIAN_POINT ( 'NONE',  ( 9.745613490124728884, 10.26430391476735338, 0.7998128361456462443 ) ) ;
#84748=CARTESIAN_POINT ( 'NONE',  ( 5.870433092755101612, 6.171306251675328092, 0.8628692295504901688 ) ) ;
#84749=CARTESIAN_POINT ( 'NONE',  ( -1.150196859685088002, 3.060958678954801115, -0.7749999999999883649 ) ) ;
#84752=CARTESIAN_POINT ( 'NONE',  ( 4.039439701867726384, 6.800097854565950506, 1.199719254218462483 ) ) ;
#84757=CARTESIAN_POINT ( 'NONE',  ( -8.920901888112002354, 11.43080484092926241, 1.443375672974064550 ) ) ;
#84761=CARTESIAN_POINT ( 'NONE',  ( 8.260995669428309540, 8.532249790621511565, 0.7998128361456481317 ) ) ;
#84763=CARTESIAN_POINT ( 'NONE',  ( -3.276266675996675204, 6.974061555304760240, -0.7998128361456282587 ) ) ;
#84765=CARTESIAN_POINT ( 'NONE',  ( 2.693266070609028784, 6.293894182352508970, 0.000000000000000000 ) ) ;
#84767=CARTESIAN_POINT ( 'NONE',  ( -6.112028321662274166, 6.025121218227761588, 0.7998128361456341429 ) ) ;
#84768=CARTESIAN_POINT ( 'NONE',  ( 3.765413976293345844, 5.416068943807445635, 1.599625672291267398 ) ) ;
#84772=CARTESIAN_POINT ( 'NONE',  ( 8.432281472695482449, 11.92507992053172572, 1.199719254218450271 ) ) ;
#84773=CARTESIAN_POINT ( 'NONE',  ( 0.4084509640503868333, 6.973232988006186517, 3.930977317341532107 ) ) ;
#84776=CARTESIAN_POINT ( 'NONE',  ( 4.067188154045468629, 7.737431308562400467, -0.5659913801023385149 ) ) ;
#84777=CARTESIAN_POINT ( 'NONE',  ( 6.805829924380118356, 7.042482454639357847, 0.7216878364870317197 ) ) ;
#84779=CARTESIAN_POINT ( 'NONE',  ( 0.4784947886781562576, 6.877463695696398815, 3.690354617645239976 ) ) ;
#84783=CARTESIAN_POINT ( 'NONE',  ( 7.741342523278698096, 10.05465224862374285, 1.443375672974076540 ) ) ;
#84787=CARTESIAN_POINT ( 'NONE',  ( 3.189213936345663747, 2.817530495244580102, -2.450448857954562243 ) ) ;
#84788=CARTESIAN_POINT ( 'NONE',  ( -8.799405390469187793, 10.22472669609091689, -1.199719254218446718 ) ) ;
#84793=DIRECTION ( 'NONE',  ( 1.000000000000000000, 0.000000000000000000, 0.000000000000000000 ) ) ;
#84797=CARTESIAN_POINT ( 'NONE',  ( 9.215791728987056786, 11.77484298861683598, -1.599625672291262513 ) ) ;
#84801=CARTESIAN_POINT ( 'NONE',  ( 3.798255590122797898, 7.583048621785260401, -0.7998128361456221525 ) ) ;
#84804=CARTESIAN_POINT ( 'NONE',  ( 1.499999999999990896, 4.556250000682819490, 1.214306433183764966E-14 ) ) ;
#84810=CARTESIAN_POINT ( 'NONE',  ( 1.499999999999987121, 1.504166666666690411, 0.8660254037844524744 ) ) ;
#84811=CARTESIAN_POINT ( 'NONE',  ( 6.124532705071213279, 8.168374127381657246, -1.599625672291262513 ) ) ;
#84812=CARTESIAN_POINT ( 'NONE',  ( 5.355107487273504496, 6.310342158982962246, -1.082531754730543083 ) ) ;
#84816=CARTESIAN_POINT ( 'NONE',  ( 8.758204044748005401, 10.28062147603659504, 1.082531754730549967 ) ) ;
#84819=CIRCLE ( 'NONE', #212669, 0.08000000000000008493 ) ;
#84823=CARTESIAN_POINT ( 'NONE',  ( -4.283486466913726254, 7.084819080452935403, -1.199719254218452047 ) ) ;
#84825=CARTESIAN_POINT ( 'NONE',  ( -1.500000000000011324, 3.952083334016153415, 0.8660254037844403729 ) ) ;
#84826=CARTESIAN_POINT ( 'NONE',  ( 1.364683531249986537, -0.6364583329919177856, 0.7879004041258500513 ) ) ;
#84830=DIRECTION ( 'NONE',  ( 1.000000000000000000, 0.000000000000000000, 0.000000000000000000 ) ) ;
#84832=CARTESIAN_POINT ( 'NONE',  ( 0.6823417656249917140, 4.405208333674755394, 1.181850606188765695 ) ) ;
#84837=CARTESIAN_POINT ( 'NONE',  ( 4.559605246071184226, 3.300000000000025135, 0.7750000000000135669 ) ) ;
#84839=CARTESIAN_POINT ( 'NONE',  ( -7.015454420067433361, 10.27211502579893754, 1.199719254218453823 ) ) ;
#84841=CARTESIAN_POINT ( 'NONE',  ( 4.808338034340912337, 8.761478140039733020, 1.040834085586084257E-14 ) ) ;
#84843=CARTESIAN_POINT ( 'NONE',  ( -1.402160292154681736E-14, -0.1781249996585796136, 1.575800808251672791 ) ) ;
#84845=EDGE_LOOP ( 'NONE', ( #32660, #36462, #174532, #86200, #213211 ) ) ;
#84847=CARTESIAN_POINT ( 'NONE',  ( -0.001128590447031348198, 8.210952333604092601, -2.038660652713623733 ) ) ;
#84849=CARTESIAN_POINT ( 'NONE',  ( -7.393273838153706201, 7.519907654134449615, 0.7998128361456341429 ) ) ;
#84854=CARTESIAN_POINT ( 'NONE',  ( 8.594979316059474073, 12.11489407112305372, 1.199719254218450271 ) ) ;
#84856=ORIENTED_EDGE ( 'NONE', *, *, #124486, .F. ) ;
#84857=CARTESIAN_POINT ( 'NONE',  ( -3.415764635639130020, 6.072476943965863683, 1.199719254218462483 ) ) ;
#84858=CARTESIAN_POINT ( 'NONE',  ( -6.659026002606323047, 10.92061410301605662, 0.000000000000000000 ) ) ;
#84861=CARTESIAN_POINT ( 'NONE',  ( -5.120997767102647202, 6.698429628811411796, 1.435921996857256300 ) ) ;
#84862=CARTESIAN_POINT ( 'NONE',  ( 1.364683531249984538, -1.094791666325247936, -0.7879004041258309554 ) ) ;
#84866=CARTESIAN_POINT ( 'NONE',  ( 7.565086526745395723, 10.80938946696957004, -1.082531754730543083 ) ) ;
#84880=AXIS2_PLACEMENT_3D ( 'NONE', #17621, #12565, #62395 ) ;
#84886=DIRECTION ( 'NONE',  ( 1.000000000000000000, 0.000000000000000000, 0.000000000000000000 ) ) ;
#84890=CARTESIAN_POINT ( 'NONE',  ( -5.759516327706961647, 5.613857225279885732, -0.7998128361456221525 ) ) ;
#84891=CARTESIAN_POINT ( 'NONE',  ( -8.616370316684697883, 10.01118577667568132, -1.199719254218446718 ) ) ;
#84897=CARTESIAN_POINT ( 'NONE',  ( -1.500000000000011324, 3.202083334016150307, 0.8660254037844403729 ) ) ;
#84898=CARTESIAN_POINT ( 'NONE',  ( 9.887974103068218668, 10.43039129653476493, 0.7998128361456462443 ) ) ;
#84902=CARTESIAN_POINT ( 'NONE',  ( -10.01677656239806247, 10.58066083241955901, 0.7998128361456462443 ) ) ;
#84904=CARTESIAN_POINT ( 'NONE',  ( 0.6823417656249882723, 2.176041667008084435, -1.181850606188749264 ) ) ;
#84906=CARTESIAN_POINT ( 'NONE',  ( -4.957044826794427372, 6.512741263611735221, 2.499999999999999112 ) ) ;
#84910=CARTESIAN_POINT ( 'NONE',  ( -2.252626078164912560, 5.779814191167667481, 0.7998128361456341429 ) ) ;
#84914=CARTESIAN_POINT ( 'NONE',  ( -1.402160292154681736E-14, 0.1343750003414218575, 1.575800808251672791 ) ) ;
#84919=CARTESIAN_POINT ( 'NONE',  ( -1.402160292154681736E-14, 2.196875000341423689, -1.575800808251660134 ) ) ;
#84921=( BOUNDED_SURFACE ( )  B_SPLINE_SURFACE ( 1, 2, ( 
 ( #197955, #148168, #149217, #214170, #127741, #49584, #161214, #193698, #111461, #211002, #115708, #181698, #33328, #62625, #112519, #104756, #182773, #38677, #116776, #34391, #117854, #119993, #201143, #154567, #53860, #183846, #152425, #20270, #135126, #166538, #35458, #2937, #185970, #101536, #86354, #187045, #52781, #36524, #100463, #51731, #67929, #102611, #203279, #136188, #1869, #199005, #167605, #150303, #70074, #87429, #168666, #153497, #37603, #121078, #202206, #170805, #66860, #103684, #22396, #169733, #21322, #19203, #85282, #54926, #88505, #133005, #50650, #18126, #84215, #134074, #118920, #184900, #5067, #71142, #137259, #151368, #69009, #4004, #89580, #178022, #7214, #29640, #73288, #57062, #156708, #110944, #193190, #61062, #105849, #144492, #23472, #123226, #127221, #24539, #95726, #45903, #90647, #176951, #44838, #28567, #94654, #161778, #155629, #160698, #12292, #139391, #8298, #205424, #78372, #74383, #189191, #140484, #210500, #62135, #128295, #194257, #209416, #106937, #112021, #6143, #40828, #171876, #72213, #172960, #138320, #204336, #55994, #122145, #188113, #39744, #8736, #3642, #134775, #38315, #135825, #37247, #136894, #199727, #151014, #53493, #24980, #119630, #200783, #69721, #20964, #87061, #201849, #153133, #185614, #190673, #19913, #52435, #104391, #206931, #36165, #58560, #118561, #68652, #18840, #102244, #2582, #184545, #103317, #26044, #168317, #35096, #186686, #169379, #75874, #85998, #51373, #183487, #4706, #124714, #42334, #101167, #108449, #70780, #152072, #202921, #54565, #174468, #140917, #120713, #117496, #170438, #91083, #157143, #92157, #74817, #158210, #9799, #167254, #84926, #80131, #126847, #94287, #125778, #191740, #176581, #47668, #212252, #141981, #128975, #110579, #78003, #76926, #159252, #27114, #178720, #60683, #28192, #10853, #146235, #62814, #161406, #15116, #207995, #45529, #143052, #177656, #160327, #12990, #111644, #109517, #209047, #192804, #63886, #59622, #43395, #79065, #113779, #144127, #30335, #14044, #175524, #29264, #44463, #210120, #61761, #127929, #193881, #95356, #145183, #130041, #96420, #162471, #196034, #97475, #211189, #194954, #179781, #46590, #31401, #163531, #165654, #32455, #34575, #132128, #148348, #2046, #197080, #116962, #19383, #134253, #36704, #67050, #168847, #150487, #131091, #119098, #102791, #164586, #100647, #985, #49768, #84399, #133187, #185080, #48717, #52960, #114831, #180830, #198137, #200260, #199187, #81205, #68117, #115894, #166724, #18316, #149403, #98525, #181879, #17241, #51911, #33516, #118034, #201321, #50835, #182960, #16172, #65978, #82256, #184020, #3117, #35637, #214348, #213316, #99588, #83316, #101716, #167787, #85462, #151548, #69187, #135308, #147284, #64940, #108192, #155812, #74560, #73476, #205603, #203453, #55108, #156886, #140660, #86533, #206675, #70255, #37787, #103861, #6327, #72400, #173140, #107117, #89766, #20450, #24721, #169910, #87607, #58306, #5247, #190421, #71322, #187226, #138500, #7396, #23655, #106039, #21499, #90823, #153677, #38855, #172062, #204523, #152599, #124462, #56172, #139577, #57241, #123401, #189365, #4184, #137437, #41007, #8473, #104939, #122334, #170979, #136369, #188291, #22578, #39931, #202388, #54040, #120177, #186153, #154744, #88684, #209862, #11673, #111391, #174217, #125525, #27937, #210934, #94032, #175273, #192550, #61500, #127666, #176330, #193628, #160070, #162215, #208800, #26859, #12730, #178464, #10603, #30074, #92963, #43152, #207742, #76679, #191484, #109265, #77748, #63636, #159009, #9550, #161143, #143869, #47410, #142794, #25791, #157957, #45270, #96165, #13802, #75625, #79874, #44205, #60429, #177394, #126589, #145984, #112451, #29008, #91901, #95094, #110325, #78804, #129791, #144927, #62559, #128723, #194695, #46337, #195771, #141735, #59368, #80948, #64692, #148095, #135055, #114587, #98275, #117784, #131874, #132926, #198931, #116699, #152351, #7142, #103604, #21245, #53785, #40751, #171800, #138250, #140405, #52709, #22314, #169661, #88426, #71066, #55915, #122074, #87352, #137183, #73213, #106858, #102530, #168592, #8225, #74309, #118841, #144678 ),
 ( #206424, #176082, #26609, #178215, #158756, #92709, #46090, #10351, #142536, #147845, #166208, #65486, #212816, #198689, #197634, #165147, #49279, #33016, #116452, #182446, #149975, #1545, #67607, #183519, #101200, #18873, #148643, #165950, #182182, #2347, #103085, #35937, #116195, #98832, #99888, #50074, #184313, #201615, #68423, #53264, #168085, #20736, #102017, #4474, #54339, #19685, #86831, #85763, #151843, #149706, #1286, #169142, #152895, #32750, #70545, #16476, #198428, #33809, #167023, #18618, #119395, #185384, #3420, #181129, #37003, #17534, #83623, #136664, #67344, #202689, #133489, #199492, #84697, #69486, #135594, #52202, #51137, #164882, #117259, #183258, #118328, #150784, #82556, #209, #134551, #66280, #132427, #34862, #100936, #200554, #153972, #204816, #138796, #137733, #39153, #5539, #56467, #105234, #203752, #171275, #122629, #155036, #188591, #40223, #22868, #187522, #88984, #6622, #55396, #21790, #72701, #71620, #121551, #106334, #38087, #172356, #23945, #90050, #156109, #120477, #186450, #104158, #87899, #170206, #43694, #171528, #107672, #74041, #56721, #91378, #140131, #126070, #203998, #59913, #137981, #55647, #139052, #207227, #206157, #175820, #75106, #205079, #173701, #192031, #109811, #23121, #25276, #57785, #122889, #157438, #123945, #88154, #121803, #154222, #187770, #39402, #188848, #58851, #189914, #5794, #125007, #40484, #9032, #41559, #156365, #105496, #106588, #24192, #190964, #172616, #42630, #208282, #108739, #26341, #89238, #72950, #155289, #92454, #10092, #158493, #6872, #71871, #76166, #142271, #30638, #47970, #129286, #114087, #14349, #81504, #96722, #65227, #115134, #162771, #147583, #80439, #212557, #210422, #62064, #163835, #213601, #93511, #131378, #77226, #44762, #110870, #13298, #79371, #180077, #31700, #146538, #27413, #97775, #176875, #94578, #197374, #12222, #49015, #78295, #194181, #145490, #64196, #130337, #113011, #28487, #15414, #160621, #128219, #179020, #211485, #159552, #11149, #63122, #196326, #143345, #209340, #60988, #127141, #144420, #193113, #45826, #111947, #195262, #177949, #29563, #46896, #95655, #161706, #91063, #41247, #157123, #74797, #89995, #23889, #139817, #73720, #106279, #22813, #57479, #204760, #72646, #107355, #187467, #205846, #206909, #24961, #92135, #156046, #158190, #173377, #39097, #40165, #7635, #8712, #140898, #58539, #124694, #123638, #189601, #190652, #42313, #172300, #88927, #108429, #56412, #138742, #174449, #105182, #26025, #203697, #55343, #121495, #171218, #154981, #6566, #122573, #188535, #5487, #133432, #69434, #184259, #18563, #53210, #35885, #87846, #165898, #21737, #99832, #83568, #100885, #103031, #101961, #137676, #36951, #166972, #135539, #3364, #118274, #149650, #84639, #200503, #169086, #150730, #201564, #170151, #168027, #19631, #1231, #34810, #51082, #85702, #186394, #119341, #199439, #182126, #183204, #117207, #185328, #70492, #151790, #136608, #20685, #104101, #86776, #153917, #50013, #152847, #71568, #4422, #202633, #2290, #68367, #38031, #116137, #33755, #67293, #134500, #52146, #54283, #120420, #10820, #111610, #45493, #28156, #173363, #177621, #108413, #26012, #211153, #158175, #128939, #9767, #125743, #76894, #160291, #176545, #44427, #190639, #29230, #174436, #59586, #110544, #159220, #194917, #79031, #143018, #11894, #94252, #77968, #144090, #62777, #92123, #210086, #61725, #141948, #209013, #75841, #127893, #60649, #207960, #193844, #126812, #46555, #74783, #145147, #8699, #140882, #191704, #95322, #93187, #24945, #161371, #43363, #12953, #192768, #27080, #58526, #109485, #175493, #91049, #157110, #206895, #124681, #42299, #82224, #80097, #97442, #113744, #148315, #34543, #181846, #47633, #30298, #31366, #195999, #115861, #133153, #214314, #199155, #99555, #166689, #33482, #150454, #200228, #165620, #18280, #17208, #83284, #81171, #147251, #100613, #84363, #178685, #2015, #162435, #130008, #179748, #98490, #164553, #50800, #116927, #149369, #112675, #182927, #163498, #15081, #68084, #213283, #134219, #64909, #131058, #16139, #951, #67017, #198104, #197046, #96383, #48683, #114799, #49733, #65946 ) ),
 .UNSPECIFIED., .F., .F., .T. ) 
 B_SPLINE_SURFACE_WITH_KNOTS ( ( 2, 2 ),
 ( 3, 2, 2, 2, 2, 2, 2, 2, 2, 2, 2, 2, 2, 2, 2, 2, 2, 2, 2, 2, 2, 2, 2, 2, 2, 2, 2, 2, 2, 2, 2, 2, 2, 2, 2, 2, 2, 2, 2, 2, 2, 2, 2, 2, 2, 2, 2, 2, 2, 2, 2, 2, 2, 2, 2, 2, 2, 2, 2, 2, 2, 2, 2, 2, 2, 2, 2, 2, 2, 2, 2, 2, 2, 2, 2, 2, 2, 2, 2, 2, 2, 2, 2, 2, 2, 2, 2, 2, 2, 2, 2, 2, 2, 2, 2, 2, 2, 2, 2, 2, 2, 2, 2, 2, 2, 2, 2, 2, 2, 2, 2, 2, 2, 2, 2, 2, 2, 2, 2, 2, 2, 2, 2, 2, 2, 2, 2, 2, 2, 2, 2, 2, 2, 2, 2, 2, 2, 2, 2, 2, 2, 2, 2, 2, 2, 2, 2, 2, 2, 2, 2, 2, 2, 2, 2, 2, 2, 2, 2, 2, 2, 2, 2, 2, 2, 2, 2, 2, 2, 2, 2, 2, 2, 2, 2, 2, 2, 2, 2, 2, 2, 2, 2, 2, 2, 2, 2, 2, 2, 2, 2, 2, 2, 2, 2, 2, 2, 2, 2, 2, 2, 2, 2, 2, 2, 2, 2, 2, 2, 2, 2, 2, 2, 2, 2, 2, 2, 2, 2, 2, 2, 2, 2, 2, 2, 2, 2, 2, 2, 2, 2, 2, 2, 2, 2, 2, 2, 2, 2, 2, 3 ),
 ( 0.000000000000000000, 1.000000000000000000 ),
 ( 0.000000000000000000, 0.004166666666666666609, 0.008333333333333333218, 0.01250000000000000069, 0.01666666666666666644, 0.02083333333333333218, 0.02500000000000000139, 0.02916666666666666713, 0.03333333333333333287, 0.03749999999999999861, 0.04166666666666666435, 0.04583333333333333010, 0.05000000000000000278, 0.05416666666666666852, 0.05833333333333333426, 0.06250000000000000000, 0.06666666666666666574, 0.07083333333333333148, 0.07499999999999999722, 0.07916666666666666297, 0.08333333333333332871, 0.08749999999999999445, 0.09166666666666666019, 0.09583333333333333981, 0.1000000000000000056, 0.1041666666666666713, 0.1083333333333333370, 0.1125000000000000028, 0.1166666666666666685, 0.1208333333333333343, 0.1250000000000000000, 0.1291666666666666796, 0.1333333333333333315, 0.1375000000000000111, 0.1416666666666666630, 0.1458333333333333426, 0.1499999999999999944, 0.1541666666666666741, 0.1583333333333333259, 0.1625000000000000056, 0.1666666666666666574, 0.1708333333333333370, 0.1749999999999999889, 0.1791666666666666685, 0.1833333333333333204, 0.1875000000000000000, 0.1916666666666666796, 0.1958333333333333315, 0.2000000000000000111, 0.2041666666666666630, 0.2083333333333333426, 0.2124999999999999944, 0.2166666666666666741, 0.2208333333333333259, 0.2250000000000000056, 0.2291666666666666574, 0.2333333333333333370, 0.2374999999999999889, 0.2416666666666666685, 0.2458333333333333204, 0.2500000000000000000, 0.2541666666666666519, 0.2583333333333333592, 0.2625000000000000111, 0.2666666666666666630, 0.2708333333333333148, 0.2750000000000000222, 0.2791666666666666741, 0.2833333333333333259, 0.2874999999999999778, 0.2916666666666666852, 0.2958333333333333370, 0.2999999999999999889, 0.3041666666666666408, 0.3083333333333333481, 0.3125000000000000000, 0.3166666666666666519, 0.3208333333333333592, 0.3250000000000000111, 0.3291666666666666630, 0.3333333333333333148, 0.3375000000000000222, 0.3416666666666666741, 0.3458333333333333259, 0.3499999999999999778, 0.3541666666666666852, 0.3583333333333333370, 0.3624999999999999889, 0.3666666666666666408, 0.3708333333333333481, 0.3750000000000000000, 0.3791666666666666519, 0.3833333333333333592, 0.3875000000000000111, 0.3916666666666666630, 0.3958333333333333148, 0.4000000000000000222, 0.4041666666666666741, 0.4083333333333333259, 0.4124999999999999778, 0.4166666666666666852, 0.4208333333333333370, 0.4249999999999999889, 0.4291666666666666408, 0.4333333333333333481, 0.4375000000000000000, 0.4416666666666666519, 0.4458333333333333592, 0.4500000000000000111, 0.4541666666666666630, 0.4583333333333333148, 0.4625000000000000222, 0.4666666666666666741, 0.4708333333333333259, 0.4749999999999999778, 0.4791666666666666852, 0.4833333333333333370, 0.4874999999999999889, 0.4916666666666666408, 0.4958333333333333481, 0.5000000000000000000, 0.5041666666666666519, 0.5083333333333333037, 0.5124999999999999556, 0.5166666666666667185, 0.5208333333333333703, 0.5250000000000000222, 0.5291666666666666741, 0.5333333333333333259, 0.5374999999999999778, 0.5416666666666666297, 0.5458333333333332815, 0.5500000000000000444, 0.5541666666666666963, 0.5583333333333333481, 0.5625000000000000000, 0.5666666666666666519, 0.5708333333333333037, 0.5749999999999999556, 0.5791666666666667185, 0.5833333333333333703, 0.5875000000000000222, 0.5916666666666666741, 0.5958333333333333259, 0.5999999999999999778, 0.6041666666666666297, 0.6083333333333332815, 0.6125000000000000444, 0.6166666666666666963, 0.6208333333333333481, 0.6250000000000000000, 0.6291666666666666519, 0.6333333333333333037, 0.6374999999999999556, 0.6416666666666667185, 0.6458333333333333703, 0.6500000000000000222, 0.6541666666666666741, 0.6583333333333333259, 0.6624999999999999778, 0.6666666666666666297, 0.6708333333333332815, 0.6750000000000000444, 0.6791666666666666963, 0.6833333333333333481, 0.6875000000000000000, 0.6916666666666666519, 0.6958333333333333037, 0.6999999999999999556, 0.7041666666666667185, 0.7083333333333333703, 0.7125000000000000222, 0.7166666666666666741, 0.7208333333333333259, 0.7249999999999999778, 0.7291666666666666297, 0.7333333333333332815, 0.7375000000000000444, 0.7416666666666666963, 0.7458333333333333481, 0.7500000000000000000, 0.7541666666666666519, 0.7583333333333333037, 0.7624999999999999556, 0.7666666666666667185, 0.7708333333333333703, 0.7750000000000000222, 0.7791666666666666741, 0.7833333333333333259, 0.7874999999999999778, 0.7916666666666666297, 0.7958333333333332815, 0.8000000000000000444, 0.8041666666666666963, 0.8083333333333333481, 0.8125000000000000000, 0.8166666666666666519, 0.8208333333333333037, 0.8249999999999999556, 0.8291666666666667185, 0.8333333333333333703, 0.8375000000000000222, 0.8416666666666666741, 0.8458333333333333259, 0.8499999999999999778, 0.8541666666666666297, 0.8583333333333332815, 0.8625000000000000444, 0.8666666666666666963, 0.8708333333333333481, 0.8750000000000000000, 0.8791666666666666519, 0.8833333333333333037, 0.8874999999999999556, 0.8916666666666667185, 0.8958333333333333703, 0.9000000000000000222, 0.9041666666666666741, 0.9083333333333333259, 0.9124999999999999778, 0.9166666666666666297, 0.9208333333333332815, 0.9250000000000000444, 0.9291666666666666963, 0.9333333333333333481, 0.9375000000000000000, 0.9416666666666666519, 0.9458333333333333037, 0.9499999999999999556, 0.9541666666666667185, 0.9583333333333333703, 0.9625000000000000222, 0.9666666666666666741, 0.9708333333333333259, 0.9749999999999999778, 0.9791666666666666297, 0.9833333333333332815, 0.9875000000000000444, 0.9916666666666666963, 0.9958333333333333481, 1.000000000000000000 ),
 .UNSPECIFIED. ) 
 GEOMETRIC_REPRESENTATION_ITEM ( )  RATIONAL_B_SPLINE_SURFACE ( (
 ( 1.000000000000000000, 0.8660254037844387076, 1.000000000000000000, 0.8660254037844387076, 1.000000000000000000, 0.8660254037844387076, 1.000000000000000000, 0.8660254037844387076, 1.000000000000000000, 0.8660254037844387076, 1.000000000000000000, 0.8660254037844387076, 1.000000000000000000, 0.8660254037844387076, 1.000000000000000000, 0.8660254037844387076, 1.000000000000000000, 0.8660254037844387076, 1.000000000000000000, 0.8660254037844387076, 1.000000000000000000, 0.8660254037844387076, 1.000000000000000000, 0.8660254037844387076, 1.000000000000000000, 0.8660254037844387076, 1.000000000000000000, 0.8660254037844387076, 1.000000000000000000, 0.8660254037844387076, 1.000000000000000000, 0.8660254037844387076, 1.000000000000000000, 0.8660254037844387076, 1.000000000000000000, 0.8660254037844387076, 1.000000000000000000, 0.8660254037844387076, 1.000000000000000000, 0.8660254037844387076, 1.000000000000000000, 0.8660254037844387076, 1.000000000000000000, 0.8660254037844387076, 1.000000000000000000, 0.8660254037844387076, 1.000000000000000000, 0.8660254037844387076, 1.000000000000000000, 0.8660254037844387076, 1.000000000000000000, 0.8660254037844387076, 1.000000000000000000, 0.8660254037844387076, 1.000000000000000000, 0.8660254037844387076, 1.000000000000000000, 0.8660254037844387076, 1.000000000000000000, 0.8660254037844387076, 1.000000000000000000, 0.8660254037844387076, 1.000000000000000000, 0.8660254037844387076, 1.000000000000000000, 0.8660254037844387076, 1.000000000000000000, 0.8660254037844387076, 1.000000000000000000, 0.8660254037844387076, 1.000000000000000000, 0.8660254037844387076, 1.000000000000000000, 0.8660254037844387076, 1.000000000000000000, 0.8660254037844387076, 1.000000000000000000, 0.8660254037844387076, 1.000000000000000000, 0.8660254037844387076, 1.000000000000000000, 0.8660254037844387076, 1.000000000000000000, 0.8660254037844387076, 1.000000000000000000, 0.8660254037844387076, 1.000000000000000000, 0.8660254037844387076, 1.000000000000000000, 0.8660254037844387076, 1.000000000000000000, 0.8660254037844387076, 1.000000000000000000, 0.8660254037844387076, 1.000000000000000000, 0.8660254037844387076, 1.000000000000000000, 0.8660254037844387076, 1.000000000000000000, 0.8660254037844387076, 1.000000000000000000, 0.8660254037844387076, 1.000000000000000000, 0.8660254037844387076, 1.000000000000000000, 0.8660254037844387076, 1.000000000000000000, 0.8660254037844387076, 1.000000000000000000, 0.8660254037844387076, 1.000000000000000000, 0.8660254037844387076, 1.000000000000000000, 0.8660254037844387076, 1.000000000000000000, 0.8660254037844387076, 1.000000000000000000, 0.8660254037844387076, 1.000000000000000000, 0.8660254037844387076, 1.000000000000000000, 0.8660254037844387076, 1.000000000000000000, 0.8660254037844387076, 1.000000000000000000, 0.8660254037844387076, 1.000000000000000000, 0.8660254037844387076, 1.000000000000000000, 0.8660254037844387076, 1.000000000000000000, 0.8660254037844387076, 1.000000000000000000, 0.8660254037844387076, 1.000000000000000000, 0.8660254037844387076, 1.000000000000000000, 0.8660254037844387076, 1.000000000000000000, 0.8660254037844387076, 1.000000000000000000, 0.8660254037844387076, 1.000000000000000000, 0.8660254037844387076, 1.000000000000000000, 0.8660254037844387076, 1.000000000000000000, 0.8660254037844387076, 1.000000000000000000, 0.8660254037844387076, 1.000000000000000000, 0.8660254037844387076, 1.000000000000000000, 0.8660254037844387076, 1.000000000000000000, 0.8660254037844387076, 1.000000000000000000, 0.8660254037844387076, 1.000000000000000000, 0.8660254037844387076, 1.000000000000000000, 0.8660254037844387076, 1.000000000000000000, 0.8660254037844387076, 1.000000000000000000, 0.8660254037844387076, 1.000000000000000000, 0.8660254037844387076, 1.000000000000000000, 0.8660254037844387076, 1.000000000000000000, 0.8660254037844387076, 1.000000000000000000, 0.8660254037844387076, 1.000000000000000000, 0.8660254037844387076, 1.000000000000000000, 0.8660254037844387076, 1.000000000000000000, 0.8660254037844387076, 1.000000000000000000, 0.8660254037844387076, 1.000000000000000000, 0.8660254037844387076, 1.000000000000000000, 0.8660254037844387076, 1.000000000000000000, 0.8660254037844387076, 1.000000000000000000, 0.8660254037844387076, 1.000000000000000000, 0.8660254037844387076, 1.000000000000000000, 0.8660254037844387076, 1.000000000000000000, 0.8660254037844387076, 1.000000000000000000, 0.8660254037844387076, 1.000000000000000000, 0.8660254037844387076, 1.000000000000000000, 0.8660254037844387076, 1.000000000000000000, 0.8660254037844387076, 1.000000000000000000, 0.8660254037844387076, 1.000000000000000000, 0.8660254037844387076, 1.000000000000000000, 0.8660254037844387076, 1.000000000000000000, 0.8660254037844387076, 1.000000000000000000, 0.8660254037844387076, 1.000000000000000000, 0.8660254037844387076, 1.000000000000000000, 0.8660254037844387076, 1.000000000000000000, 0.8660254037844387076, 1.000000000000000000, 0.8660254037844387076, 1.000000000000000000, 0.8660254037844387076, 1.000000000000000000, 0.8660254037844387076, 1.000000000000000000, 0.8660254037844387076, 1.000000000000000000, 0.8660254037844387076, 1.000000000000000000, 0.8660254037844387076, 1.000000000000000000, 0.8660254037844387076, 1.000000000000000000, 0.8660254037844387076, 1.000000000000000000, 0.8660254037844387076, 1.000000000000000000, 0.8660254037844387076, 1.000000000000000000, 0.8660254037844387076, 1.000000000000000000, 0.8660254037844387076, 1.000000000000000000, 0.8660254037844387076, 1.000000000000000000, 0.8660254037844387076, 1.000000000000000000, 0.8660254037844387076, 1.000000000000000000, 0.8660254037844387076, 1.000000000000000000, 0.8660254037844387076, 1.000000000000000000, 0.8660254037844387076, 1.000000000000000000, 0.8660254037844387076, 1.000000000000000000, 0.8660254037844387076, 1.000000000000000000, 0.8660254037844387076, 1.000000000000000000, 0.8660254037844387076, 1.000000000000000000, 0.8660254037844387076, 1.000000000000000000, 0.8660254037844387076, 1.000000000000000000, 0.8660254037844387076, 1.000000000000000000, 0.8660254037844387076, 1.000000000000000000, 0.8660254037844387076, 1.000000000000000000, 0.8660254037844387076, 1.000000000000000000, 0.8660254037844387076, 1.000000000000000000, 0.8660254037844387076, 1.000000000000000000, 0.8660254037844387076, 1.000000000000000000, 0.8660254037844387076, 1.000000000000000000, 0.8660254037844387076, 1.000000000000000000, 0.8660254037844387076, 1.000000000000000000, 0.8660254037844387076, 1.000000000000000000, 0.8660254037844387076, 1.000000000000000000, 0.8660254037844387076, 1.000000000000000000, 0.8660254037844387076, 1.000000000000000000, 0.8660254037844387076, 1.000000000000000000, 0.8660254037844387076, 1.000000000000000000, 0.8660254037844387076, 1.000000000000000000, 0.8660254037844387076, 1.000000000000000000, 0.8660254037844387076, 1.000000000000000000, 0.8660254037844387076, 1.000000000000000000, 0.8660254037844387076, 1.000000000000000000, 0.8660254037844387076, 1.000000000000000000, 0.8660254037844387076, 1.000000000000000000, 0.8660254037844387076, 1.000000000000000000, 0.8660254037844387076, 1.000000000000000000, 0.8660254037844387076, 1.000000000000000000, 0.8660254037844387076, 1.000000000000000000, 0.8660254037844387076, 1.000000000000000000, 0.8660254037844387076, 1.000000000000000000, 0.8660254037844387076, 1.000000000000000000, 0.8660254037844387076, 1.000000000000000000, 0.8660254037844387076, 1.000000000000000000, 0.8660254037844387076, 1.000000000000000000, 0.8660254037844387076, 1.000000000000000000, 0.8660254037844387076, 1.000000000000000000, 0.8660254037844387076, 1.000000000000000000, 0.8660254037844387076, 1.000000000000000000, 0.8660254037844387076, 1.000000000000000000, 0.8660254037844387076, 1.000000000000000000, 0.8660254037844387076, 1.000000000000000000, 0.8660254037844387076, 1.000000000000000000, 0.8660254037844387076, 1.000000000000000000, 0.8660254037844387076, 1.000000000000000000, 0.8660254037844387076, 1.000000000000000000, 0.8660254037844387076, 1.000000000000000000, 0.8660254037844387076, 1.000000000000000000, 0.8660254037844387076, 1.000000000000000000, 0.8660254037844387076, 1.000000000000000000, 0.8660254037844387076, 1.000000000000000000, 0.8660254037844387076, 1.000000000000000000, 0.8660254037844387076, 1.000000000000000000, 0.8660254037844387076, 1.000000000000000000, 0.8660254037844387076, 1.000000000000000000, 0.8660254037844387076, 1.000000000000000000, 0.8660254037844387076, 1.000000000000000000, 0.8660254037844387076, 1.000000000000000000, 0.8660254037844387076, 1.000000000000000000, 0.8660254037844387076, 1.000000000000000000, 0.8660254037844387076, 1.000000000000000000, 0.8660254037844387076, 1.000000000000000000, 0.8660254037844387076, 1.000000000000000000, 0.8660254037844387076, 1.000000000000000000, 0.8660254037844387076, 1.000000000000000000, 0.8660254037844387076, 1.000000000000000000, 0.8660254037844387076, 1.000000000000000000, 0.8660254037844387076, 1.000000000000000000, 0.8660254037844387076, 1.000000000000000000, 0.8660254037844387076, 1.000000000000000000, 0.8660254037844387076, 1.000000000000000000, 0.8660254037844387076, 1.000000000000000000, 0.8660254037844387076, 1.000000000000000000, 0.8660254037844387076, 1.000000000000000000, 0.8660254037844387076, 1.000000000000000000, 0.8660254037844387076, 1.000000000000000000, 0.8660254037844387076, 1.000000000000000000, 0.8660254037844387076, 1.000000000000000000, 0.8660254037844387076, 1.000000000000000000, 0.8660254037844387076, 1.000000000000000000, 0.8660254037844387076, 1.000000000000000000, 0.8660254037844387076, 1.000000000000000000, 0.8660254037844387076, 1.000000000000000000, 0.8660254037844387076, 1.000000000000000000, 0.8660254037844387076, 1.000000000000000000, 0.8660254037844387076, 1.000000000000000000, 0.8660254037844387076, 1.000000000000000000, 0.8660254037844387076, 1.000000000000000000, 0.8660254037844387076, 1.000000000000000000, 0.8660254037844387076, 1.000000000000000000, 0.8660254037844387076, 1.000000000000000000, 0.8660254037844387076, 1.000000000000000000, 0.8660254037844387076, 1.000000000000000000, 0.8660254037844387076, 1.000000000000000000, 0.8660254037844387076, 1.000000000000000000, 0.8660254037844387076, 1.000000000000000000, 0.8660254037844387076, 1.000000000000000000, 0.8660254037844387076, 1.000000000000000000, 0.8660254037844387076, 1.000000000000000000, 0.8660254037844387076, 1.000000000000000000, 0.8660254037844387076, 1.000000000000000000, 0.8660254037844387076, 1.000000000000000000, 0.8660254037844387076, 1.000000000000000000, 0.8660254037844387076, 1.000000000000000000, 0.8660254037844387076, 1.000000000000000000, 0.8660254037844387076, 1.000000000000000000, 0.8660254037844387076, 1.000000000000000000, 0.8660254037844387076, 1.000000000000000000),
 ( 1.000000000000000000, 0.8660254037844387076, 1.000000000000000000, 0.8660254037844387076, 1.000000000000000000, 0.8660254037844387076, 1.000000000000000000, 0.8660254037844387076, 1.000000000000000000, 0.8660254037844387076, 1.000000000000000000, 0.8660254037844387076, 1.000000000000000000, 0.8660254037844387076, 1.000000000000000000, 0.8660254037844387076, 1.000000000000000000, 0.8660254037844387076, 1.000000000000000000, 0.8660254037844387076, 1.000000000000000000, 0.8660254037844387076, 1.000000000000000000, 0.8660254037844387076, 1.000000000000000000, 0.8660254037844387076, 1.000000000000000000, 0.8660254037844387076, 1.000000000000000000, 0.8660254037844387076, 1.000000000000000000, 0.8660254037844387076, 1.000000000000000000, 0.8660254037844387076, 1.000000000000000000, 0.8660254037844387076, 1.000000000000000000, 0.8660254037844387076, 1.000000000000000000, 0.8660254037844387076, 1.000000000000000000, 0.8660254037844387076, 1.000000000000000000, 0.8660254037844387076, 1.000000000000000000, 0.8660254037844387076, 1.000000000000000000, 0.8660254037844387076, 1.000000000000000000, 0.8660254037844387076, 1.000000000000000000, 0.8660254037844387076, 1.000000000000000000, 0.8660254037844387076, 1.000000000000000000, 0.8660254037844387076, 1.000000000000000000, 0.8660254037844387076, 1.000000000000000000, 0.8660254037844387076, 1.000000000000000000, 0.8660254037844387076, 1.000000000000000000, 0.8660254037844387076, 1.000000000000000000, 0.8660254037844387076, 1.000000000000000000, 0.8660254037844387076, 1.000000000000000000, 0.8660254037844387076, 1.000000000000000000, 0.8660254037844387076, 1.000000000000000000, 0.8660254037844387076, 1.000000000000000000, 0.8660254037844387076, 1.000000000000000000, 0.8660254037844387076, 1.000000000000000000, 0.8660254037844387076, 1.000000000000000000, 0.8660254037844387076, 1.000000000000000000, 0.8660254037844387076, 1.000000000000000000, 0.8660254037844387076, 1.000000000000000000, 0.8660254037844387076, 1.000000000000000000, 0.8660254037844387076, 1.000000000000000000, 0.8660254037844387076, 1.000000000000000000, 0.8660254037844387076, 1.000000000000000000, 0.8660254037844387076, 1.000000000000000000, 0.8660254037844387076, 1.000000000000000000, 0.8660254037844387076, 1.000000000000000000, 0.8660254037844387076, 1.000000000000000000, 0.8660254037844387076, 1.000000000000000000, 0.8660254037844387076, 1.000000000000000000, 0.8660254037844387076, 1.000000000000000000, 0.8660254037844387076, 1.000000000000000000, 0.8660254037844387076, 1.000000000000000000, 0.8660254037844387076, 1.000000000000000000, 0.8660254037844387076, 1.000000000000000000, 0.8660254037844387076, 1.000000000000000000, 0.8660254037844387076, 1.000000000000000000, 0.8660254037844387076, 1.000000000000000000, 0.8660254037844387076, 1.000000000000000000, 0.8660254037844387076, 1.000000000000000000, 0.8660254037844387076, 1.000000000000000000, 0.8660254037844387076, 1.000000000000000000, 0.8660254037844387076, 1.000000000000000000, 0.8660254037844387076, 1.000000000000000000, 0.8660254037844387076, 1.000000000000000000, 0.8660254037844387076, 1.000000000000000000, 0.8660254037844387076, 1.000000000000000000, 0.8660254037844387076, 1.000000000000000000, 0.8660254037844387076, 1.000000000000000000, 0.8660254037844387076, 1.000000000000000000, 0.8660254037844387076, 1.000000000000000000, 0.8660254037844387076, 1.000000000000000000, 0.8660254037844387076, 1.000000000000000000, 0.8660254037844387076, 1.000000000000000000, 0.8660254037844387076, 1.000000000000000000, 0.8660254037844387076, 1.000000000000000000, 0.8660254037844387076, 1.000000000000000000, 0.8660254037844387076, 1.000000000000000000, 0.8660254037844387076, 1.000000000000000000, 0.8660254037844387076, 1.000000000000000000, 0.8660254037844387076, 1.000000000000000000, 0.8660254037844387076, 1.000000000000000000, 0.8660254037844387076, 1.000000000000000000, 0.8660254037844387076, 1.000000000000000000, 0.8660254037844387076, 1.000000000000000000, 0.8660254037844387076, 1.000000000000000000, 0.8660254037844387076, 1.000000000000000000, 0.8660254037844387076, 1.000000000000000000, 0.8660254037844387076, 1.000000000000000000, 0.8660254037844387076, 1.000000000000000000, 0.8660254037844387076, 1.000000000000000000, 0.8660254037844387076, 1.000000000000000000, 0.8660254037844387076, 1.000000000000000000, 0.8660254037844387076, 1.000000000000000000, 0.8660254037844387076, 1.000000000000000000, 0.8660254037844387076, 1.000000000000000000, 0.8660254037844387076, 1.000000000000000000, 0.8660254037844387076, 1.000000000000000000, 0.8660254037844387076, 1.000000000000000000, 0.8660254037844387076, 1.000000000000000000, 0.8660254037844387076, 1.000000000000000000, 0.8660254037844387076, 1.000000000000000000, 0.8660254037844387076, 1.000000000000000000, 0.8660254037844387076, 1.000000000000000000, 0.8660254037844387076, 1.000000000000000000, 0.8660254037844387076, 1.000000000000000000, 0.8660254037844387076, 1.000000000000000000, 0.8660254037844387076, 1.000000000000000000, 0.8660254037844387076, 1.000000000000000000, 0.8660254037844387076, 1.000000000000000000, 0.8660254037844387076, 1.000000000000000000, 0.8660254037844387076, 1.000000000000000000, 0.8660254037844387076, 1.000000000000000000, 0.8660254037844387076, 1.000000000000000000, 0.8660254037844387076, 1.000000000000000000, 0.8660254037844387076, 1.000000000000000000, 0.8660254037844387076, 1.000000000000000000, 0.8660254037844387076, 1.000000000000000000, 0.8660254037844387076, 1.000000000000000000, 0.8660254037844387076, 1.000000000000000000, 0.8660254037844387076, 1.000000000000000000, 0.8660254037844387076, 1.000000000000000000, 0.8660254037844387076, 1.000000000000000000, 0.8660254037844387076, 1.000000000000000000, 0.8660254037844387076, 1.000000000000000000, 0.8660254037844387076, 1.000000000000000000, 0.8660254037844387076, 1.000000000000000000, 0.8660254037844387076, 1.000000000000000000, 0.8660254037844387076, 1.000000000000000000, 0.8660254037844387076, 1.000000000000000000, 0.8660254037844387076, 1.000000000000000000, 0.8660254037844387076, 1.000000000000000000, 0.8660254037844387076, 1.000000000000000000, 0.8660254037844387076, 1.000000000000000000, 0.8660254037844387076, 1.000000000000000000, 0.8660254037844387076, 1.000000000000000000, 0.8660254037844387076, 1.000000000000000000, 0.8660254037844387076, 1.000000000000000000, 0.8660254037844387076, 1.000000000000000000, 0.8660254037844387076, 1.000000000000000000, 0.8660254037844387076, 1.000000000000000000, 0.8660254037844387076, 1.000000000000000000, 0.8660254037844387076, 1.000000000000000000, 0.8660254037844387076, 1.000000000000000000, 0.8660254037844387076, 1.000000000000000000, 0.8660254037844387076, 1.000000000000000000, 0.8660254037844387076, 1.000000000000000000, 0.8660254037844387076, 1.000000000000000000, 0.8660254037844387076, 1.000000000000000000, 0.8660254037844387076, 1.000000000000000000, 0.8660254037844387076, 1.000000000000000000, 0.8660254037844387076, 1.000000000000000000, 0.8660254037844387076, 1.000000000000000000, 0.8660254037844387076, 1.000000000000000000, 0.8660254037844387076, 1.000000000000000000, 0.8660254037844387076, 1.000000000000000000, 0.8660254037844387076, 1.000000000000000000, 0.8660254037844387076, 1.000000000000000000, 0.8660254037844387076, 1.000000000000000000, 0.8660254037844387076, 1.000000000000000000, 0.8660254037844387076, 1.000000000000000000, 0.8660254037844387076, 1.000000000000000000, 0.8660254037844387076, 1.000000000000000000, 0.8660254037844387076, 1.000000000000000000, 0.8660254037844387076, 1.000000000000000000, 0.8660254037844387076, 1.000000000000000000, 0.8660254037844387076, 1.000000000000000000, 0.8660254037844387076, 1.000000000000000000, 0.8660254037844387076, 1.000000000000000000, 0.8660254037844387076, 1.000000000000000000, 0.8660254037844387076, 1.000000000000000000, 0.8660254037844387076, 1.000000000000000000, 0.8660254037844387076, 1.000000000000000000, 0.8660254037844387076, 1.000000000000000000, 0.8660254037844387076, 1.000000000000000000, 0.8660254037844387076, 1.000000000000000000, 0.8660254037844387076, 1.000000000000000000, 0.8660254037844387076, 1.000000000000000000, 0.8660254037844387076, 1.000000000000000000, 0.8660254037844387076, 1.000000000000000000, 0.8660254037844387076, 1.000000000000000000, 0.8660254037844387076, 1.000000000000000000, 0.8660254037844387076, 1.000000000000000000, 0.8660254037844387076, 1.000000000000000000, 0.8660254037844387076, 1.000000000000000000, 0.8660254037844387076, 1.000000000000000000, 0.8660254037844387076, 1.000000000000000000, 0.8660254037844387076, 1.000000000000000000, 0.8660254037844387076, 1.000000000000000000, 0.8660254037844387076, 1.000000000000000000, 0.8660254037844387076, 1.000000000000000000, 0.8660254037844387076, 1.000000000000000000, 0.8660254037844387076, 1.000000000000000000, 0.8660254037844387076, 1.000000000000000000, 0.8660254037844387076, 1.000000000000000000, 0.8660254037844387076, 1.000000000000000000, 0.8660254037844387076, 1.000000000000000000, 0.8660254037844387076, 1.000000000000000000, 0.8660254037844387076, 1.000000000000000000, 0.8660254037844387076, 1.000000000000000000, 0.8660254037844387076, 1.000000000000000000, 0.8660254037844387076, 1.000000000000000000, 0.8660254037844387076, 1.000000000000000000, 0.8660254037844387076, 1.000000000000000000, 0.8660254037844387076, 1.000000000000000000, 0.8660254037844387076, 1.000000000000000000, 0.8660254037844387076, 1.000000000000000000, 0.8660254037844387076, 1.000000000000000000, 0.8660254037844387076, 1.000000000000000000, 0.8660254037844387076, 1.000000000000000000, 0.8660254037844387076, 1.000000000000000000, 0.8660254037844387076, 1.000000000000000000, 0.8660254037844387076, 1.000000000000000000, 0.8660254037844387076, 1.000000000000000000, 0.8660254037844387076, 1.000000000000000000, 0.8660254037844387076, 1.000000000000000000, 0.8660254037844387076, 1.000000000000000000, 0.8660254037844387076, 1.000000000000000000, 0.8660254037844387076, 1.000000000000000000, 0.8660254037844387076, 1.000000000000000000, 0.8660254037844387076, 1.000000000000000000, 0.8660254037844387076, 1.000000000000000000, 0.8660254037844387076, 1.000000000000000000, 0.8660254037844387076, 1.000000000000000000, 0.8660254037844387076, 1.000000000000000000, 0.8660254037844387076, 1.000000000000000000, 0.8660254037844387076, 1.000000000000000000, 0.8660254037844387076, 1.000000000000000000, 0.8660254037844387076, 1.000000000000000000, 0.8660254037844387076, 1.000000000000000000, 0.8660254037844387076, 1.000000000000000000, 0.8660254037844387076, 1.000000000000000000, 0.8660254037844387076, 1.000000000000000000, 0.8660254037844387076, 1.000000000000000000, 0.8660254037844387076, 1.000000000000000000, 0.8660254037844387076, 1.000000000000000000, 0.8660254037844387076, 1.000000000000000000) ) ) 
 REPRESENTATION_ITEM ( '' )  SURFACE ( )  );
#84922=CARTESIAN_POINT ( 'NONE',  ( -6.684333426737305572, 7.757142738403693727, -1.199719254218446718 ) ) ;
#84923=CARTESIAN_POINT ( 'NONE',  ( 7.065770611016287006, 11.39514947949436774, 1.040834085586084257E-14 ) ) ;
#84926=CARTESIAN_POINT ( 'NONE',  ( 6.844168616800228477, 6.879284895888727824, -0.7998128361456281477 ) ) ;
#84928=CARTESIAN_POINT ( 'NONE',  ( -1.500000000000011324, 3.170833333333354265, 0.8660254037844403729 ) ) ;
#84930=CARTESIAN_POINT ( 'NONE',  ( -1.201851678989727383E-14, 1.134375000341418582, 1.575800808251672791 ) ) ;
#84936=CARTESIAN_POINT ( 'NONE',  ( 6.371969008742804697, 7.496680600697164465, -1.082531754730543083 ) ) ;
#84939=CARTESIAN_POINT ( 'NONE',  ( -8.208571938070008400, 11.66408546346865016, -1.199719254218446718 ) ) ;
#84940=CARTESIAN_POINT ( 'NONE',  ( -4.925689880466507908, 4.641059703499347044, -0.7998128361456221525 ) ) ;
#84944=CARTESIAN_POINT ( 'NONE',  ( -1.127943160727153060, 3.300000000000025135, -0.7749999999999935829 ) ) ;
#84946=CARTESIAN_POINT ( 'NONE',  ( -8.012505595552038784, 8.450270737673262644, 0.7216878364870578100 ) ) ;
#84948=CARTESIAN_POINT ( 'NONE',  ( -0.7499999999999972244, 4.608333333333352932, -1.299038105676652011 ) ) ;
#84951=CARTESIAN_POINT ( 'NONE',  ( 8.270110514656034084, 9.711179024262627024, 1.082531754730558626 ) ) ;
#84956=CARTESIAN_POINT ( 'NONE',  ( -4.226491779746760713, 3.979064867095216673, 0.5169678485880250252 ) ) ;
#84960=CARTESIAN_POINT ( 'NONE',  ( 10.52076401408022299, 11.37657222595619189, 0.000000000000000000 ) ) ;
#84967=CARTESIAN_POINT ( 'NONE',  ( 7.182068686937156166, 9.402166106225269715, 1.599625672291281386 ) ) ;
#84968=CARTESIAN_POINT ( 'NONE',  ( -4.660252114795309097, 6.460046772059735432, -1.599625672291256295 ) ) ;
#84972=VECTOR ( 'NONE', #21726, 1000.000000000000114 ) ;
#84974=CARTESIAN_POINT ( 'NONE',  ( 3.226477370372305753, 4.787309570232886280, 1.443375672974062551 ) ) ;
#84975=CARTESIAN_POINT ( 'NONE',  ( -8.597841969360544567, 13.18256606422934674, 0.7998128361456341429 ) ) ;
#84991=CARTESIAN_POINT ( 'NONE',  ( 7.039708073993665494, 9.236078724457858158, 1.599625672291281386 ) ) ;
#84994=ORIENTED_EDGE ( 'NONE', *, *, #88440, .F. ) ;
#84997=CARTESIAN_POINT ( 'NONE',  ( 1.608462485350656834, 8.735270501766779105, 2.463594439587601492 ) ) ;
#85003=CARTESIAN_POINT ( 'NONE',  ( -6.573005544526917099, 6.562927978236513304, -0.7998128361456291469 ) ) ;
#85006=CARTESIAN_POINT ( 'NONE',  ( -3.079673448598517549, 6.744702790006905424, 1.040834085586084257E-14 ) ) ;
#85017=CARTESIAN_POINT ( 'NONE',  ( -9.327646496521984076, 11.90534021740758064, -1.443375672974059665 ) ) ;
#85020=CARTESIAN_POINT ( 'NONE',  ( 5.262536180398716290, 9.291375977107183104, -0.7998128361456291469 ) ) ;
#85021=CARTESIAN_POINT ( 'NONE',  ( 1.364683531249990311, 4.863541667008084879, 0.7879004041258499402 ) ) ;
#85028=CARTESIAN_POINT ( 'NONE',  ( 6.602457619730771832, 6.805214765881779648, 0.7216878364870317197 ) ) ;
#85029=CARTESIAN_POINT ( 'NONE',  ( -7.854251061018346469, 8.057714414143200443, -0.7998128361456291469 ) ) ;
#85030=VERTEX_POINT ( 'NONE', #65075 ) ;
#85033=CARTESIAN_POINT ( 'NONE',  ( -6.333630315878337136, 10.54098580183340772, 0.000000000000000000 ) ) ;
#85034=CARTESIAN_POINT ( 'NONE',  ( -4.415151579544611238, 8.302760609444034046, -0.7998128361456281477 ) ) ;
#85041=CARTESIAN_POINT ( 'NONE',  ( 7.938462636001388795, 9.220293482545153907, -1.199719254218441611 ) ) ;
#85049=CARTESIAN_POINT ( 'NONE',  ( -1.201851678989727383E-14, 3.962500000000022560, 1.732050807568877637 ) ) ;
#85056=CARTESIAN_POINT ( 'NONE',  ( 0.7499999999999902300, 5.816666666666685082, -1.299038105676658228 ) ) ;
#85057=CARTESIAN_POINT ( 'NONE',  ( 4.684505768721569652, 5.424010470718658716, -1.199719254218452047 ) ) ;
#85058=CARTESIAN_POINT ( 'NONE',  ( 6.328958779480917229, 6.278206752349526631, 0.7998128361456341429 ) ) ;
#85060=CARTESIAN_POINT ( 'NONE',  ( -6.887178846062109727, 10.01849717283904262, -1.082531754730537976 ) ) ;
#85062=CARTESIAN_POINT ( 'NONE',  ( 4.663641653420880218, 8.384739662392275861, -0.7216878364870207285 ) ) ;
#85063=CARTESIAN_POINT ( 'NONE',  ( -7.321039761255057066, 11.48503745486550365, 0.000000000000000000 ) ) ;
#85066=CARTESIAN_POINT ( 'NONE',  ( 6.103141704446003679, 10.27208242182903142, 0.7998128361456462443 ) ) ;
#85072=CARTESIAN_POINT ( 'NONE',  ( -1.364683531250012516, 3.530208333674758059, 0.7879004041258379498 ) ) ;
#85078=CARTESIAN_POINT ( 'NONE',  ( 9.759171643738394408, 10.28012176064996197, 0.000000000000000000 ) ) ;
#85082=CARTESIAN_POINT ( 'NONE',  ( -9.515124878692420296, 9.995400534762978850, 1.040834085586084257E-14 ) ) ;
#85088=CARTESIAN_POINT ( 'NONE',  ( 4.162516854595432747, 4.815023404238158555, 1.199719254218464037 ) ) ;
#85091=CARTESIAN_POINT ( 'NONE',  ( -9.027031348600448979, 9.425958082989001952, 1.040834085586084257E-14 ) ) ;
#85093=CARTESIAN_POINT ( 'NONE',  ( 4.870353810550047235, 4.974663864576271521, -0.7564775847674284348 ) ) ;
#85096=CARTESIAN_POINT ( 'NONE',  ( 5.504159067553832330, 6.221818635116664886, 0.9641881782859774708 ) ) ;
#85097=CARTESIAN_POINT ( 'NONE',  ( -2.266184231778562541, 5.795632037050281404, 1.040834085586084257E-14 ) ) ;
#85101=CARTESIAN_POINT ( 'NONE',  ( 6.317209508963599340, 9.457495962844502557, 1.199719254218462483 ) ) ;
#85103=CARTESIAN_POINT ( 'NONE',  ( 7.070740804726770357, 8.207951346058097286, 1.199719254218462483 ) ) ;
#85104=CARTESIAN_POINT ( 'NONE',  ( 5.335297142177534369, 6.183267073083954735, -1.199719254218452047 ) ) ;
#85106=CARTESIAN_POINT ( 'NONE',  ( -6.860062538834774237, 10.94723069537516302, 0.7216878364870458196 ) ) ;
#85113=CARTESIAN_POINT ( 'NONE',  ( -4.138143308069708759, 7.456237844118314584, -0.6866288536411498944 ) ) ;
#85114=CARTESIAN_POINT ( 'NONE',  ( 4.203240766677102336, 7.568734712931471265, -0.9219714408205395006 ) ) ;
#85117=CARTESIAN_POINT ( 'NONE',  ( 6.209271165378815738, 7.306866450105836464, -1.082531754730543083 ) ) ;
#85128=FACE_OUTER_BOUND ( 'NONE', #121830, .T. ) ;
#85136=CARTESIAN_POINT ( 'NONE',  ( -10.45297324601190425, 11.29748299654313470, 0.7216878364870438212 ) ) ;
#85143=CARTESIAN_POINT ( 'NONE',  ( 1.499999999999989120, 2.806250000682818158, 1.214306433183764966E-14 ) ) ;
#85145=CARTESIAN_POINT ( 'NONE',  ( -6.566226467720086113, 6.555019055295208119, 1.040834085586084257E-14 ) ) ;
#85147=ORIENTED_EDGE ( 'NONE', *, *, #121295, .T. ) ;
#85150=CARTESIAN_POINT ( 'NONE',  ( -8.941766003412679353, 10.39081407785832845, -1.199719254218446718 ) ) ;
#85151=CARTESIAN_POINT ( 'NONE',  ( 0.003385325826184980898, 8.210945192570370921, 2.038658773260200174 ) ) ;
#85154=EDGE_CURVE ( 'NONE', #214357, #72912, #162948, .T. ) ;
#85156=CARTESIAN_POINT ( 'NONE',  ( 7.962716289927667113, 8.184257181204083409, -0.7998128361456291469 ) ) ;
#85160=CARTESIAN_POINT ( 'NONE',  ( 9.073431116043567002, 11.60875560684942265, -1.599625672291262513 ) ) ;
#85166=CARTESIAN_POINT ( 'NONE',  ( -7.049876689426103127, 10.20831132343037062, -1.082531754730537976 ) ) ;
#85169=CARTESIAN_POINT ( 'NONE',  ( 1.364683531249990311, 5.196875000341417916, 1.214306433183764966E-14 ) ) ;
#85175=CARTESIAN_POINT ( 'NONE',  ( -3.755245360860939297, 4.443836344834937613, -1.082531754730548412 ) ) ;
#85177=CARTESIAN_POINT ( 'NONE',  ( 9.642873567817520808, 12.27310513391906532, 1.599625672291279388 ) ) ;
#85183=CARTESIAN_POINT ( 'NONE',  ( 1.364683531249986537, 1.655208333674748955, -0.7879004041258239610 ) ) ;
#85184=CARTESIAN_POINT ( 'NONE',  ( -3.795919822146293754, 4.491289883001181593, -1.082531754730549967 ) ) ;
#85185=CARTESIAN_POINT ( 'NONE',  ( 3.714044015139744914, 6.420469553383295391, 1.199719254218462483 ) ) ;
#85190=CARTESIAN_POINT ( 'NONE',  ( -4.226925616482867909, 3.500738074553338741, -2.444828727306142646 ) ) ;
#85192=CARTESIAN_POINT ( 'NONE',  ( 8.690413276235306128, 13.08263988900915109, -0.7216878364870267237 ) ) ;
#85194=CARTESIAN_POINT ( 'NONE',  ( -7.375272376154093479, 9.627570410311676596, -1.443375672974059665 ) ) ;
#85199=CARTESIAN_POINT ( 'NONE',  ( -9.508345801885592863, 9.987491611821676329, 0.7998128361456462443 ) ) ;
#85201=CARTESIAN_POINT ( 'NONE',  ( -3.253593677155282471, 6.739683690082376444, 1.040834085586084257E-14 ) ) ;
#85202=CARTESIAN_POINT ( 'NONE',  ( -0.6823417656250003738, 2.030208333674753174, -1.181850606188749264 ) ) ;
#85218=CARTESIAN_POINT ( 'NONE',  ( -1.441120163477494165, 8.287694259231830785, 3.161243217722575327 ) ) ;
#85220=CARTESIAN_POINT ( 'NONE',  ( -1.364683531250012516, 3.092708333674755838, 0.7879004041258379498 ) ) ;
#85227=CARTESIAN_POINT ( 'NONE',  ( 9.206149998879153529, 10.69926207256923689, 1.199719254218453823 ) ) ;
#85230=CARTESIAN_POINT ( 'NONE',  ( 0.6823417656249899377, 3.092708333674754062, 1.181850606188765695 ) ) ;
#85241=CARTESIAN_POINT ( 'NONE',  ( 5.705283713252285338, 5.550585841749444249, -0.7998128361456211532 ) ) ;
#85250=ORIENTED_EDGE ( 'NONE', *, *, #99914, .F. ) ;
#85252=CARTESIAN_POINT ( 'NONE',  ( -4.471491734408701291, 4.111161866431900513, 1.214306433183764966E-14 ) ) ;
#85253=CARTESIAN_POINT ( 'NONE',  ( 8.959240580532112475, 9.346868853575953651, -0.7998128361456221525 ) ) ;
#85256=CARTESIAN_POINT ( 'NONE',  ( 3.809477975315569864, 7.388215371269402532, -0.7216878364870197293 ) ) ;
#85267=CARTESIAN_POINT ( 'NONE',  ( -6.073689629242158716, 9.069426419882418600, -1.082531754730538864 ) ) ;
#85270=CARTESIAN_POINT ( 'NONE',  ( 3.635557746758808495, 7.393234471193928847, -0.7998128361456291469 ) ) ;
#85273=CARTESIAN_POINT ( 'NONE',  ( -8.890396042259075315, 11.39521468743417998, -1.599625672291263179 ) ) ;
#85278=CARTESIAN_POINT ( 'NONE',  ( -3.785751206713858785, 5.439795712631356750, 1.599625672291267398 ) ) ;
#85279=EDGE_CURVE ( 'NONE', #158010, #202349, #48679, .T. ) ;
#85281=CARTESIAN_POINT ( 'NONE',  ( 10.09812548408005384, 10.67556790771522124, -0.7998128361456281477 ) ) ;
#85282=CARTESIAN_POINT ( 'NONE',  ( 4.542145155778077203, 5.257923088951247159, -1.199719254218452047 ) ) ;
#85288=CARTESIAN_POINT ( 'NONE',  ( 4.365362273920252889, 4.195270195769483124, 0.7216878364870317197 ) ) ;
#85291=CARTESIAN_POINT ( 'NONE',  ( -5.199715606040888005, 6.025088614257851027, -1.199719254218446718 ) ) ;
#85292=DIRECTION ( 'NONE',  ( 1.000000000000000000, -5.391474854832587087E-16, 0.000000000000000000 ) ) ;
#85294=CARTESIAN_POINT ( 'NONE',  ( -8.459397779922852578, 11.95671561229694824, 1.199719254218453823 ) ) ;
#85299=CARTESIAN_POINT ( 'NONE',  ( 8.026063749610047537, 10.38682701267698150, -1.443375672974057666 ) ) ;
#85300=CARTESIAN_POINT ( 'NONE',  ( 1.364683531249992088, 5.696875000341418804, 1.214306433183764966E-14 ) ) ;
#85302=CARTESIAN_POINT ( 'NONE',  ( 3.497113557321089861, 6.167384019261527683, -1.199719254218446718 ) ) ;
#85304=CARTESIAN_POINT ( 'NONE',  ( 4.761938266897790761, 6.578680616179308771, 1.599625672291267398 ) ) ;
#85306=CARTESIAN_POINT ( 'NONE',  ( -7.874588291438845644, 8.081441182967111558, -0.7998128361456291469 ) ) ;
#85310=( BOUNDED_CURVE ( )  B_SPLINE_CURVE ( 2, ( #151580, #98558, #135336, #16204, #66011, #83349, #18349 ),
 .UNSPECIFIED., .F., .T. ) 
 B_SPLINE_CURVE_WITH_KNOTS ( ( 3, 2, 2, 3 ),
 ( 0.1607142857142856152, 0.1666666666666666297, 0.1726190476190476719, 0.1785714285714287142 ),
 .UNSPECIFIED. ) 
 CURVE ( )  GEOMETRIC_REPRESENTATION_ITEM ( )  RATIONAL_B_SPLINE_CURVE ( ( 1.000000000000002442, 0.8660254037844361541, 1.000000000000000000, 0.8660254037844387076, 1.000000000000000000, 0.8660254037844355990, 1.000000000000003109 ) ) 
 REPRESENTATION_ITEM ( '' )  );
#85314=CARTESIAN_POINT ( 'NONE',  ( -1.420000000000021911, 6.216000000000048153, 2.921333333333346882 ) ) ;
#85319=CARTESIAN_POINT ( 'NONE',  ( -1.364683531249997417, 3.071875000341423245, 1.214306433183764966E-14 ) ) ;
#85320=CARTESIAN_POINT ( 'NONE',  ( 9.215791728987056786, 11.77484298861683598, -1.599625672291262513 ) ) ;
#85322=CARTESIAN_POINT ( 'NONE',  ( -4.934804725694224459, 6.780358151441803649, -1.443375672974053447 ) ) ;
#85323=CARTESIAN_POINT ( 'NONE',  ( 3.768803514918948938, 4.459654191235965293, -1.082531754730543083 ) ) ;
#85324=CARTESIAN_POINT ( 'NONE',  ( -5.544921637864838715, 6.531792001339513654, -1.082531754730543971 ) ) ;
#85330=CARTESIAN_POINT ( 'NONE',  ( 5.684946482831785275, 5.526859072925533134, -0.7998128361456231517 ) ) ;
#85341=EDGE_CURVE ( 'NONE', #22516, #3330, #6168, .T. ) ;
#85342=CARTESIAN_POINT ( 'NONE',  ( 4.981731378017507872, 7.899438143407371271, -1.199719254218452047 ) ) ;
#85346=CARTESIAN_POINT ( 'NONE',  ( -6.735703387890906946, 6.752742128827836865, -0.7998128361456291469 ) ) ;
#85350=CARTESIAN_POINT ( 'NONE',  ( 6.564118927310645724, 10.80988918183778225, -0.7998128361456291469 ) ) ;
#85353=CARTESIAN_POINT ( 'NONE',  ( -6.423865854776591000, 6.388931673527803667, 1.040834085586084257E-14 ) ) ;
#85354=CARTESIAN_POINT ( 'NONE',  ( 7.090551149822739596, 8.335026431957096804, 1.082531754730558626 ) ) ;
#85355=CARTESIAN_POINT ( 'NONE',  ( 5.079507498475252625, 6.736975590279616455, 1.417308049988776020 ) ) ;
#85356=CARTESIAN_POINT ( 'NONE',  ( -2.625475302540713152, 6.214804952939456228, -0.7998128361456281477 ) ) ;
#85359=CARTESIAN_POINT ( 'NONE',  ( -3.764360206088648297, 7.543504007078730922, -0.7998128361456281477 ) ) ;
#85362=CARTESIAN_POINT ( 'NONE',  ( -1.364683531250014514, 1.988541667008086655, -0.7879004041258289570 ) ) ;
#85364=CARTESIAN_POINT ( 'NONE',  ( -3.782361668532609134, 7.356579680022602652, 1.040834085586084257E-14 ) ) ;
#85365=VERTEX_POINT ( 'NONE', #84837 ) ;
#85368=VERTEX_POINT ( 'NONE', #2488 ) ;
#85371=CARTESIAN_POINT ( 'NONE',  ( 4.157546660884947620, 8.002221537674429896, 1.040834085586084257E-14 ) ) ;
#85374=CARTESIAN_POINT ( 'NONE',  ( 1.364683531249988535, 3.426041667008085323, 0.7879004041258500513 ) ) ;
#85377=CARTESIAN_POINT ( 'NONE',  ( -1.364683531250014514, -0.6989583329919100141, -0.7879004041258359514 ) ) ;
#85380=CARTESIAN_POINT ( 'NONE',  ( -3.460355519985875983, 5.060167411448709629, 1.599625672291267398 ) ) ;
#85381=CARTESIAN_POINT ( 'NONE',  ( -7.998947441938374148, 8.434452891790657603, 1.040834085586084257E-14 ) ) ;
#85383=CARTESIAN_POINT ( 'NONE',  ( 1.364683531249988535, 2.905208333674754506, -0.7879004041258239610 ) ) ;
#85390=CARTESIAN_POINT ( 'NONE',  ( -5.870317324592805086, 9.792527945426188651, -0.7216878364870197293 ) ) ;
#85394=CARTESIAN_POINT ( 'NONE',  ( -5.680503174001480637, 9.571078103069643461, 0.7216878364870458196 ) ) ;
#85408=CARTESIAN_POINT ( 'NONE',  ( -5.585069213825653023, 8.603332285183535433, -1.199719254218440723 ) ) ;
#85410=CARTESIAN_POINT ( 'NONE',  ( -1.402160292154681736E-14, -0.5374999999999753308, 1.732050807568877637 ) ) ;
#85412=CARTESIAN_POINT ( 'NONE',  ( 3.174580523894166006, 6.855427711185178019, 0.7998128361456341429 ) ) ;
#85414=CARTESIAN_POINT ( 'NONE',  ( -5.219525951136881226, 5.191794485855505847, -0.7216878364870058515 ) ) ;
#85416=CARTESIAN_POINT ( 'NONE',  ( 4.645640190976921602, 8.571663989448405019, 1.040834085586084257E-14 ) ) ;
#85421=CARTESIAN_POINT ( 'NONE',  ( -4.934804725694224459, 6.780358151441803649, -1.443375672974053447 ) ) ;
#85424=CARTESIAN_POINT ( 'NONE',  ( -4.281741921268227280, 3.985524603254129605, 0.2951291498071085262 ) ) ;
#85430=CARTESIAN_POINT ( 'NONE',  ( -1.201851678989727383E-14, 2.571875000341417472, 1.575800808251672791 ) ) ;
#85432=CARTESIAN_POINT ( 'NONE',  ( -6.690058733339450114, 9.892486724616283311, 1.199719254218452047 ) ) ;
#85434=CARTESIAN_POINT ( 'NONE',  ( 5.635385404774530649, 9.726366738878972740, 0.7998128361456462443 ) ) ;
#85435=CARTESIAN_POINT ( 'NONE',  ( -6.191269702934848240, 10.37489842006599616, 0.000000000000000000 ) ) ;
#85438=CARTESIAN_POINT ( 'NONE',  ( 1.499999999999987121, -0.4645833326505149907, 0.8660254037844524744 ) ) ;
#85440=CARTESIAN_POINT ( 'NONE',  ( 8.812436659202669276, 10.34389285956704363, -1.082531754730543083 ) ) ;
#85443=CARTESIAN_POINT ( 'NONE',  ( -1.364683531250000748, 0.8218750003414210248, 0.000000000000000000 ) ) ;
#85446=CARTESIAN_POINT ( 'NONE',  ( 8.554831740098663317, 9.082984572977682802, 0.7216878364870458196 ) ) ;
#85449=CARTESIAN_POINT ( 'NONE',  ( -3.768803514918943609, 7.340761834139994058, 0.7216878364870317197 ) ) ;
#85451=CARTESIAN_POINT ( 'NONE',  ( 0.6823417656249882723, 2.926041667008084879, -1.181850606188754593 ) ) ;
#85455=CARTESIAN_POINT ( 'NONE',  ( -5.357443255694392725, 9.402100898285455699, 0.000000000000000000 ) ) ;
#85456=CARTESIAN_POINT ( 'NONE',  ( -1.364683531250010295, 5.592708333674750953, 0.7879004041258379498 ) ) ;
#85462=CARTESIAN_POINT ( 'NONE',  ( 8.471147050440139381, 8.777426401801974976, -0.7998128361456281477 ) ) ;
#85465=CARTESIAN_POINT ( 'NONE',  ( -0.7500000000000006661, 2.108333333333357817, -1.299038105676652011 ) ) ;
#85470=ORIENTED_EDGE ( 'NONE', *, *, #140696, .T. ) ;
#85471=CARTESIAN_POINT ( 'NONE',  ( 5.490689023854504747, 9.349628261231513804, 1.040834085586084257E-14 ) ) ;
#85473=CARTESIAN_POINT ( 'NONE',  ( 1.364683531249986537, 0.1760416670080860446, 0.7879004041258500513 ) ) ;
#85476=CARTESIAN_POINT ( 'NONE',  ( 2.758194185376297902, 5.305311418659259814, 1.199719254218452047 ) ) ;
#85483=CARTESIAN_POINT ( 'NONE',  ( -1.402160292154681736E-14, 0.08750000000001964540, -1.732050807568870754 ) ) ;
#85484=CARTESIAN_POINT ( 'NONE',  ( 8.938903350111612411, 9.323142084752035430, -0.7998128361456221525 ) ) ;
#85485=CARTESIAN_POINT ( 'NONE',  ( -8.666686507633592385, 11.13422023037111330, 1.599625672291269396 ) ) ;
#85487=CARTESIAN_POINT ( 'NONE',  ( 1.364683531249986537, 0.6552083336747522857, -0.7879004041258239610 ) ) ;
#85488=CARTESIAN_POINT ( 'NONE',  ( 0.7499999999999885647, 0.8166666666666877461, -1.299038105676652899 ) ) ;
#85490=CARTESIAN_POINT ( 'NONE',  ( 5.172599298813543633, 5.993452922492633839, -1.199719254218452047 ) ) ;
#85497=CARTESIAN_POINT ( 'NONE',  ( -1.500000000000001332, -0.8187499993171781787, 0.000000000000000000 ) ) ;
#85498=CARTESIAN_POINT ( 'NONE',  ( -6.347188469492005325, 10.55680364771601809, -0.7998128361456291469 ) ) ;
#85499=CARTESIAN_POINT ( 'NONE',  ( -5.910991785878175975, 6.958873840688411860, -1.082531754730544860 ) ) ;
#85506=ORIENTED_EDGE ( 'NONE', *, *, #59177, .T. ) ;
#85508=CARTESIAN_POINT ( 'NONE',  ( 6.401421083946654100, 10.62007503124645957, -0.7998128361456291469 ) ) ;
#85509=DIRECTION ( 'NONE',  ( -5.578564026256490882E-16, -1.000000000000000000, -9.066213480720158442E-32 ) ) ;
#85511=CARTESIAN_POINT ( 'NONE',  ( 7.253248993186735660, 7.564471368247083660, 0.7216878364870317197 ) ) ;
#85515=CARTESIAN_POINT ( 'NONE',  ( -8.076906825439122528, 10.44614393447756129, -1.599625672291263179 ) ) ;
#85516=CARTESIAN_POINT ( 'NONE',  ( 5.087333953625774008, 6.958308917361963886, 1.599625672291267398 ) ) ;
#85520=CARTESIAN_POINT ( 'NONE',  ( 4.695201269034174452, 4.372156323494968966, 1.214306433183764966E-14 ) ) ;
#85526=CARTESIAN_POINT ( 'NONE',  ( -4.989037340148921196, 5.883260320670900434, 1.082531754730560403 ) ) ;
#85527=CARTESIAN_POINT ( 'NONE',  ( 9.924205255523292024, 10.68058700763975466, -0.7216878364870257245 ) ) ;
#85530=CARTESIAN_POINT ( 'NONE',  ( -4.771579997005698459, 7.654261532226910525, -1.199719254218452047 ) ) ;
#85536=CARTESIAN_POINT ( 'NONE',  ( -8.342344591110322227, 8.627156865917170236, -0.7998128361456291469 ) ) ;
#85550=CYLINDRICAL_SURFACE ( 'NONE', #174755, 1.500000000000000222 ) ;
#85551=CARTESIAN_POINT ( 'NONE',  ( -8.030507057996002729, 8.263346410617135263, 1.040834085586084257E-14 ) ) ;
#85554=CARTESIAN_POINT ( 'NONE',  ( 4.039966587192257208, 6.696749537490852333, 1.082531754730558626 ) ) ;
#85555=VERTEX_POINT ( 'NONE', #41452 ) ;
#85560=CARTESIAN_POINT ( 'NONE',  ( -5.623934791570306402, 5.455678766453782913, 0.7998128361456341429 ) ) ;
#85564=FACE_OUTER_BOUND ( 'NONE', #156710, .T. ) ;
#85568=CARTESIAN_POINT ( 'NONE',  ( -7.479294296233107708, 11.87759377891399204, 0.7998128361456481317 ) ) ;
#85569=CARTESIAN_POINT ( 'NONE',  ( 4.788000803920411386, 8.737751371215816576, 1.040834085586084257E-14 ) ) ;
#85572=CARTESIAN_POINT ( 'NONE',  ( -9.755255220232635693, 11.33988483081495957, -1.199719254218441611 ) ) ;
#85576=CARTESIAN_POINT ( 'NONE',  ( 1.364683531249988757, -0.05312499965857975237, 0.000000000000000000 ) ) ;
#85580=CARTESIAN_POINT ( 'NONE',  ( 9.259855728453651125, 9.905512559391842942, 1.040834085586084257E-14 ) ) ;
#85602=B_SPLINE_CURVE_WITH_KNOTS ( 'NONE', 3,
 ( #26653, #109047, #157745, #193427 ),
 .UNSPECIFIED., .F., .F.,
 ( 4, 4 ),
 ( 0.001235641190896560925, 0.001582017824277167153 ),
 .UNSPECIFIED. ) ;
#85610=CARTESIAN_POINT ( 'NONE',  ( -1.402160292154681736E-14, 0.2437500006828163535, 1.732050807568877637 ) ) ;
#85614=CARTESIAN_POINT ( 'NONE',  ( 8.757677159423465696, 12.30470822171437284, 1.199719254218450271 ) ) ;
#85617=CARTESIAN_POINT ( 'NONE',  ( -7.815970093360414158E-14, 8.210952333604092601, -2.038660652713623733 ) ) ;
#85619=CARTESIAN_POINT ( 'NONE',  ( 9.053093885623066939, 11.58502883802551153, -1.599625672291262513 ) ) ;
#85623=CIRCLE ( 'NONE', #61365, 0.08000000000000020983 ) ;
#85625=CARTESIAN_POINT ( 'NONE',  ( 5.169736645512481132, 4.925780929386339935, 0.7998128361456341429 ) ) ;
#85626=CARTESIAN_POINT ( 'NONE',  ( -0.6823417656250003738, 2.030208333674753174, -1.181850606188749264 ) ) ;
#85628=CARTESIAN_POINT ( 'NONE',  ( -1.500000000000022204, 7.388542872122518368, 4.154462424328226433 ) ) ;
#85630=CARTESIAN_POINT ( 'NONE',  ( -6.835281999583978418, 11.12624609948998966, -0.7998128361456291469 ) ) ;
#85631=CARTESIAN_POINT ( 'NONE',  ( -4.731432421044883263, 5.582721248382882528, -1.082531754730543971 ) ) ;
#85635=CARTESIAN_POINT ( 'NONE',  ( -1.402160292154681736E-14, -0.6312499993171797330, -1.732050807568870754 ) ) ;
#85643=CARTESIAN_POINT ( 'NONE',  ( -3.863710589770277259, 6.491117540498504646, 1.082531754730560403 ) ) ;
#85645=CARTESIAN_POINT ( 'NONE',  ( 4.009017875521604601, 7.583074288825860876, 0.2480677224083651655 ) ) ;
#85649=CARTESIAN_POINT ( 'NONE',  ( -3.538314903042294457, 6.111489239315849531, 1.082531754730560403 ) ) ;
#85650=CARTESIAN_POINT ( 'NONE',  ( 9.759171643738394408, 10.28012176064996197, 0.000000000000000000 ) ) ;
#85665=CARTESIAN_POINT ( 'NONE',  ( 4.306686350635271054, 8.176217842383143974, -0.7998128361456221525 ) ) ;
#85677=CARTESIAN_POINT ( 'NONE',  ( -3.332481584934697150, 7.719208080883564804, 2.450691333334236166 ) ) ;
#85681=CARTESIAN_POINT ( 'NONE',  ( 8.178592977541601527, 10.56477777859713463, 1.599625672291281386 ) ) ;
#85684=CARTESIAN_POINT ( 'NONE',  ( -5.331380718671772101, 7.243030143248949670, -1.599625672291256295 ) ) ;
#85688=CARTESIAN_POINT ( 'NONE',  ( -0.7500000000000006661, -0.6104166659838470288, -1.299038105676652011 ) ) ;
#85692=CARTESIAN_POINT ( 'NONE',  ( 3.867100128395839942, 5.534702787927018974, -1.599625672291255185 ) ) ;
#85693=CARTESIAN_POINT ( 'NONE',  ( -5.135841261478327979, 4.886236314679810455, 0.7998128361456341429 ) ) ;
#85699=CARTESIAN_POINT ( 'NONE',  ( 4.690757960648213931, 8.416375354157496602, 0.7216878364870438212 ) ) ;
#85702=CARTESIAN_POINT ( 'NONE',  ( 6.751597309481075726, 10.82068792779586985, 1.040834085586084257E-14 ) ) ;
#85703=CARTESIAN_POINT ( 'NONE',  ( 1.364683531249988535, 4.717708333674756283, -0.7879004041258300672 ) ) ;
#85704=CARTESIAN_POINT ( 'NONE',  ( -1.499999999999997780, 4.931250000682820378, 1.214306433183764966E-14 ) ) ;
#85705=CARTESIAN_POINT ( 'NONE',  ( 4.975479186090852046, 6.827811688571220117, 1.443375672974062551 ) ) ;
#85707=CARTESIAN_POINT ( 'NONE',  ( 1.931788062848141441E-13, 7.054063922337705073, -3.955400951015614730 ) ) ;
#85713=CARTESIAN_POINT ( 'NONE',  ( -5.193604695876673283, 6.642107527433549485, 1.420026453975403724 ) ) ;
#85717=CARTESIAN_POINT ( 'NONE',  ( 1.364683531249990311, 5.176041667008085767, 0.7879004041258500513 ) ) ;
#85722=CARTESIAN_POINT ( 'NONE',  ( -2.277406616971334508, 5.600798786534425311, 1.040834085586084257E-14 ) ) ;
#85732=EDGE_LOOP ( 'NONE', ( #125835, #154499, #84180, #49586 ) ) ;
#85734=CARTESIAN_POINT ( 'NONE',  ( 2.901081683644319842, 5.368050483351580304, 1.082531754730548412 ) ) ;
#85735=CARTESIAN_POINT ( 'NONE',  ( 0.6823417656249917140, 4.155208333674755394, 1.181850606188765695 ) ) ;
#85737=CARTESIAN_POINT ( 'NONE',  ( 8.260995669428309540, 8.532249790621511565, 0.7998128361456481317 ) ) ;
#85739=CARTESIAN_POINT ( 'NONE',  ( -9.775592450653132204, 11.36361159963886891, -1.199719254218441611 ) ) ;
#85740=AXIS2_PLACEMENT_3D ( 'NONE', #13233, #66212, #95589 ) ;
#85748=CARTESIAN_POINT ( 'NONE',  ( -1.201851678989727383E-14, 4.337500000000023448, -1.732050807568863648 ) ) ;
#85749=CARTESIAN_POINT ( 'NONE',  ( 4.635998460869027227, 7.496083073400806818, -1.199719254218452047 ) ) ;
#85753=EDGE_LOOP ( 'NONE', ( #114125, #14889, #172070, #104177 ) ) ;
#85755=CARTESIAN_POINT ( 'NONE',  ( 7.944714827928043732, 10.29191993738131927, 1.443375672974076540 ) ) ;
#85760=CARTESIAN_POINT ( 'NONE',  ( -1.499999999999997780, 2.931250000682818158, 1.214306433183764966E-14 ) ) ;
#85762=CARTESIAN_POINT ( 'NONE',  ( -5.066996723205291708, 6.934582148538044777, 1.599625672291267398 ) ) ;
#85763=CARTESIAN_POINT ( 'NONE',  ( 4.812781342726870193, 4.717259109377208048, 0.7216878364870317197 ) ) ;
#85764=CARTESIAN_POINT ( 'NONE',  ( -10.60211293576223213, 11.47147930125185589, 1.040834085586084257E-14 ) ) ;
#85772=CARTESIAN_POINT ( 'NONE',  ( 8.118635056484817980, 8.366162408854107113, 0.7998128361456481317 ) ) ;
#85773=CARTESIAN_POINT ( 'NONE',  ( 5.335297142177534369, 6.183267073083954735, -1.199719254218452047 ) ) ;
#85777=CARTESIAN_POINT ( 'NONE',  ( 5.542585869888291938, 5.360771691158120689, -0.7998128361456211532 ) ) ;
#85780=AXIS2_PLACEMENT_3D ( 'NONE', #196875, #65772, #167583 ) ;
#85784=ORIENTED_EDGE ( 'NONE', *, *, #50690, .F. ) ;
#85790=CARTESIAN_POINT ( 'NONE',  ( 5.430853319176391025, 6.270791292598644873, -1.030804022418196464 ) ) ;
#85797=CARTESIAN_POINT ( 'NONE',  ( 0.7499999999999902300, 5.597916667349482900, -1.299038105676658228 ) ) ;
#85799=CARTESIAN_POINT ( 'NONE',  ( 7.131225611108100715, 7.422110755822004968, 0.7216878364870317197 ) ) ;
#85800=CARTESIAN_POINT ( 'NONE',  ( -4.464712657601869417, 4.103252943490596216, 0.7998128361456341429 ) ) ;
#85805=CARTESIAN_POINT ( 'NONE',  ( -4.391951695823077984, 7.211361847513815704, 1.199719254218464037 ) ) ;
#85808=CARTESIAN_POINT ( 'NONE',  ( -3.028993686180034839, 2.741750000184234981, 2.499999999999998224 ) ) ;
#85816=CARTESIAN_POINT ( 'NONE',  ( 7.397945374551106568, 11.78268670361832093, -0.7998128361456291469 ) ) ;
#85817=CARTESIAN_POINT ( 'NONE',  ( 6.062205217752669739, 6.048677139763619870, -0.4177986087803304271 ) ) ;
#85818=CARTESIAN_POINT ( 'NONE',  ( -1.230728480726500429, 3.101239941806485767, -0.7749999999999918066 ) ) ;
#85825=CARTESIAN_POINT ( 'NONE',  ( -9.815740026613967828, 10.55404424057886636, -0.7216878364870267237 ) ) ;
#85829=CARTESIAN_POINT ( 'NONE',  ( 8.586391356156291010, 8.911878091804165791, 0.7998128361456481317 ) ) ;
#85833=CARTESIAN_POINT ( 'NONE',  ( 4.487912541323413329, 5.194651705420806564, 1.199719254218462483 ) ) ;
#85835=CARTESIAN_POINT ( 'NONE',  ( -5.982172092127739482, 8.002286745614243912, -1.599625672291263179 ) ) ;
#85836=CARTESIAN_POINT ( 'NONE',  ( 4.518945272056516416, 4.166524327021037699, 0.7998128361456341429 ) ) ;
#85838=( BOUNDED_CURVE ( )  B_SPLINE_CURVE ( 2, ( #89332, #6964, #22137 ),
 .UNSPECIFIED., .F., .T. ) 
 B_SPLINE_CURVE_WITH_KNOTS ( ( 3, 3 ),
 ( 0.000000000000000000, 0.002781257751169551561 ),
 .UNSPECIFIED. ) 
 CURVE ( )  GEOMETRIC_REPRESENTATION_ITEM ( )  RATIONAL_B_SPLINE_CURVE ( ( 1.000000000000000000, 0.9105717077957582450, 0.9405305184076298008 ) ) 
 REPRESENTATION_ITEM ( '' )  );
#85844=CARTESIAN_POINT ( 'NONE',  ( 4.202513864555980305, 7.333163887849894813, -0.8510647575735978965 ) ) ;
#85846=CARTESIAN_POINT ( 'NONE',  ( 5.124618876285529367, 7.962177208099690873, -1.082531754730549078 ) ) ;
#85849=CARTESIAN_POINT ( 'NONE',  ( -1.256902978990764641, 3.300000000000025580, 0.5473114391985675065 ) ) ;
#85850=EDGE_CURVE ( 'NONE', #97759, #141934, #183101, .T. ) ;
#85854=CARTESIAN_POINT ( 'NONE',  ( 8.568389893712330618, 9.098802418860289620, 1.040834085586084257E-14 ) ) ;
#85858=CARTESIAN_POINT ( 'NONE',  ( -7.340850106795412167, 10.65174332698158643, 1.199719254218453823 ) ) ;
#85867=CARTESIAN_POINT ( 'NONE',  ( 9.083072846151447166, 12.68433652289702884, 1.199719254218450271 ) ) ;
#85871=CARTESIAN_POINT ( 'NONE',  ( 4.039439701867726384, 6.800097854565950506, 1.199719254218462483 ) ) ;
#85875=CARTESIAN_POINT ( 'NONE',  ( -0.7500000000000215383, 3.972916667349481123, 1.299038105676671107 ) ) ;
#85882=CARTESIAN_POINT ( 'NONE',  ( -1.499999999999997780, 1.900000000000019673, 0.000000000000000000 ) ) ;
#85883=CARTESIAN_POINT ( 'NONE',  ( 5.937581207780954884, 9.014596278131406848, -1.199719254218440723 ) ) ;
#85884=CARTESIAN_POINT ( 'NONE',  ( 5.138177029454852551, 5.096887410559856946, 0.7216878364870317197 ) ) ;
#85888=CARTESIAN_POINT ( 'NONE',  ( 9.097157885089661278, 9.715698408800516717, 1.040834085586084257E-14 ) ) ;
#85893=AXIS2_PLACEMENT_3D ( 'NONE', #13280, #212535, #129268 ) ;
#85896=CARTESIAN_POINT ( 'NONE',  ( -5.311043488251275591, 7.219303374425030562, -1.599625672291256295 ) ) ;
#85898=CARTESIAN_POINT ( 'NONE',  ( -1.201851678989727383E-14, 3.618750000682816381, -1.732050807568863648 ) ) ;
#85899=CARTESIAN_POINT ( 'NONE',  ( -1.402160292154681736E-14, -1.178124999658576311, 1.575800808251672791 ) ) ;
#85904=CARTESIAN_POINT ( 'NONE',  ( -1.364683531250012516, 4.551041667008082214, -0.7879004041258300672 ) ) ;
#85911=CARTESIAN_POINT ( 'NONE',  ( -7.395082721250053837, 10.71501471051202614, -1.199719254218446718 ) ) ;
#85912=CARTESIAN_POINT ( 'NONE',  ( 6.063521013809720195, 8.097193820909906137, 1.599625672291281386 ) ) ;
#85914=CARTESIAN_POINT ( 'NONE',  ( -0.6823417656250246877, -0.1989583329919109023, 1.181850606188755259 ) ) ;
#85922=CARTESIAN_POINT ( 'NONE',  ( -5.530836599371015794, 8.540060901653093950, 1.199719254218452047 ) ) ;
#85925=CARTESIAN_POINT ( 'NONE',  ( 8.920375002787457319, 12.49452237230570084, 1.199719254218450271 ) ) ;
#85927=CARTESIAN_POINT ( 'NONE',  ( 8.727698198895078363, 11.20540053684285553, -1.599625672291257406 ) ) ;
#85930=CARTESIAN_POINT ( 'NONE',  ( -4.548924232584923288, 5.265832011892554121, -1.199719254218446718 ) ) ;
#85932=CARTESIAN_POINT ( 'NONE',  ( -7.049349804101573191, 10.31165964050546258, -1.199719254218440723 ) ) ;
#85935=CARTESIAN_POINT ( 'NONE',  ( -4.010472434439474654, 7.801430412234481082, -0.4134458547365611469 ) ) ;
#85936=CARTESIAN_POINT ( 'NONE',  ( 1.364683531249986981, -1.115624999658580752, 0.000000000000000000 ) ) ;
#85940=CARTESIAN_POINT ( 'NONE',  ( 6.954969614130424027, 11.05795561655343384, 1.040834085586084257E-14 ) ) ;
#85943=CARTESIAN_POINT ( 'NONE',  ( 5.120175567455225618, 9.125288595339771547, -0.7998128361456281477 ) ) ;
#85945=CARTESIAN_POINT ( 'NONE',  ( 0.001026545178762920067, 7.078193277237624592, -2.121339347286375965 ) ) ;
#85962=CARTESIAN_POINT ( 'NONE',  ( -7.309817376062285099, 11.67987070538135264, 0.000000000000000000 ) ) ;
#85968=CARTESIAN_POINT ( 'NONE',  ( 1.499999999999989120, 2.035416667349480679, 0.8660254037844524744 ) ) ;
#85969=CARTESIAN_POINT ( 'NONE',  ( 8.380911511541880188, 12.92948053010758258, 0.7998128361456462443 ) ) ;
#85974=CARTESIAN_POINT ( 'NONE',  ( -10.17947440576205054, 10.77047498301088346, 0.7998128361456462443 ) ) ;
#85976=CARTESIAN_POINT ( 'NONE',  ( 0.6823417656249882723, 1.676041667008083769, -1.181850606188749264 ) ) ;
#85981=CARTESIAN_POINT ( 'NONE',  ( -2.578021764892882040, 6.159442492350315490, 0.7998128361456341429 ) ) ;
#85983=CARTESIAN_POINT ( 'NONE',  ( 1.500000000000001110, 7.388542872122531691, -4.154462424328188241 ) ) ;
#85987=CARTESIAN_POINT ( 'NONE',  ( -1.364683531250014514, -0.1572916663252435232, 0.7879004041258379498 ) ) ;
#85993=CARTESIAN_POINT ( 'NONE',  ( -0.6823417656250003738, 1.467708333674752730, -1.181850606188749264 ) ) ;
#85995=CARTESIAN_POINT ( 'NONE',  ( -6.847031270101295419, 7.946956888995021728, -1.199719254218446718 ) ) ;
#85996=CARTESIAN_POINT ( 'NONE',  ( 8.209625708274705502, 9.536650400197368427, 1.199719254218462483 ) ) ;
#85997=CARTESIAN_POINT ( 'NONE',  ( 0.000000000000000000, 5.868705557303649734, -4.125226524755057689 ) ) ;
#85998=CARTESIAN_POINT ( 'NONE',  ( 6.518772930072240790, 6.499656594706071822, -0.7998128361456281477 ) ) ;
#86000=CARTESIAN_POINT ( 'NONE',  ( -1.500000000000011324, 4.170833333333359150, 0.8660254037844403729 ) ) ;
#86002=CARTESIAN_POINT ( 'NONE',  ( 0.6823417656249882723, 1.738541667008083991, -1.181850606188749264 ) ) ;
#86006=ADVANCED_FACE ( 'NONE', ( #21676 ), #106220, .T. ) ;
#86009=CARTESIAN_POINT ( 'NONE',  ( 6.344852701515477200, 6.504675694630598137, -0.7216878364870257245 ) ) ;
#86012=CARTESIAN_POINT ( 'NONE',  ( -9.691380875670077444, 10.20103253123691189, 0.7998128361456462443 ) ) ;
#86013=CARTESIAN_POINT ( 'NONE',  ( -5.440899717785814715, 5.242137847038546461, 0.7998128361456341429 ) ) ;
#86014=CARTESIAN_POINT ( 'NONE',  ( -4.281882426504885153, 7.413440659835691449, -1.046679656837728789 ) ) ;
#86018=CARTESIAN_POINT ( 'NONE',  ( -8.487040972030346353, 9.003895343564625620, 1.040834085586084257E-14 ) ) ;
#86020=CARTESIAN_POINT ( 'NONE',  ( 0.7499999999999902300, 4.816666666666684193, -1.299038105676658228 ) ) ;
#86023=CARTESIAN_POINT ( 'NONE',  ( 7.456621297836072415, 9.722477485607340597, 1.443375672974076540 ) ) ;
#86028=VECTOR ( 'NONE', #156729, 1000.000000000000114 ) ;
#86031=CARTESIAN_POINT ( 'NONE',  ( 10.35806617071623315, 11.18675807536486566, 0.000000000000000000 ) ) ;
#86034=DIRECTION ( 'NONE',  ( 5.578564026256490882E-16, 1.000000000000000000, 9.066213480720158442E-32 ) ) ;
#86035=CARTESIAN_POINT ( 'NONE',  ( 8.609064354553323639, 10.10662517080946543, -1.082531754730543083 ) ) ;
#86036=CARTESIAN_POINT ( 'NONE',  ( 5.750629710490689384, 9.860818428881154674, -0.7998128361456291469 ) ) ;
#86037=CARTESIAN_POINT ( 'NONE',  ( -4.554649539187067830, 7.401175998105142817, 1.199719254218464037 ) ) ;
#86042=CARTESIAN_POINT ( 'NONE',  ( -1.364683531250000748, -0.6781249996585803075, 0.000000000000000000 ) ) ;
#86043=CARTESIAN_POINT ( 'NONE',  ( 4.690757960648234359, 4.574898496952131133, 0.7216878364870317197 ) ) ;
#86044=EDGE_LOOP ( 'NONE', ( #41863, #183779, #156686, #68615 ) ) ;
#86045=CARTESIAN_POINT ( 'NONE',  ( -3.541704441667874903, 5.155074486744371853, -1.599625672291256295 ) ) ;
#86061=CARTESIAN_POINT ( 'NONE',  ( 7.091078035147269532, 8.231678114882006625, 1.199719254218462483 ) ) ;
#86072=CARTESIAN_POINT ( 'NONE',  ( -0.5707974126488067901, 6.595910036604164084, 3.427880048805499236 ) ) ;
#86074=CARTESIAN_POINT ( 'NONE',  ( -5.599681137644054729, 6.491715067794862293, 1.199719254218450271 ) ) ;
#86076=CARTESIAN_POINT ( 'NONE',  ( -2.767835915484202047, 6.380892334706859792, -0.7998128361456281477 ) ) ;
#86086=CARTESIAN_POINT ( 'NONE',  ( -3.928111819657352566, 5.605883094398769195, 1.599625672291267398 ) ) ;
#86089=CARTESIAN_POINT ( 'NONE',  ( 6.745345117998789775, 7.828323044875442172, 1.199719254218462483 ) ) ;
#86090=CARTESIAN_POINT ( 'NONE',  ( -1.001543065824772872E-14, 5.071875000341421469, 1.575800808251672791 ) ) ;
#86096=B_SPLINE_CURVE_WITH_KNOTS ( 'NONE', 3,
 ( #78786, #144908, #194673, #145966 ),
 .UNSPECIFIED., .F., .F.,
 ( 4, 4 ),
 ( 0.000000000000000000, 0.002006572499523605075 ),
 .UNSPECIFIED. ) ;
#86098=CARTESIAN_POINT ( 'NONE',  ( 6.629573926958101993, 6.836850457647000390, -0.7216878364870257245 ) ) ;
#86099=CARTESIAN_POINT ( 'NONE',  ( -7.691553217654356622, 7.867900263551875994, -0.7998128361456291469 ) ) ;
#86104=CARTESIAN_POINT ( 'NONE',  ( -6.659026002606323047, 10.92061410301605662, 0.000000000000000000 ) ) ;
#86105=CARTESIAN_POINT ( 'NONE',  ( -5.925076824372040640, 6.871343368977510302, 1.199719254218450271 ) ) ;
#86114=CARTESIAN_POINT ( 'NONE',  ( 5.750629710490689384, 9.860818428881154674, -0.7998128361456291469 ) ) ;
#86127=CARTESIAN_POINT ( 'NONE',  ( -1.364683531250000748, -0.9281249996585805295, 0.000000000000000000 ) ) ;
#86128=CARTESIAN_POINT ( 'NONE',  ( 2.998324526916512411, 6.649795714711241423, 0.000000000000000000 ) ) ;
#86129=CARTESIAN_POINT ( 'NONE',  ( 5.524057522564145728, 8.532151978711786100, 1.199719254218462483 ) ) ;
#86131=CARTESIAN_POINT ( 'NONE',  ( -8.026063749610061748, 9.426457798375635022, -1.082531754730543971 ) ) ;
#86133=CARTESIAN_POINT ( 'NONE',  ( 4.839897650398541806, 8.590371658866210680, 1.040834085586084257E-14 ) ) ;
#86134=CARTESIAN_POINT ( 'NONE',  ( -7.334597914868727919, 10.54048608644677465, -1.082531754730543083 ) ) ;
#86138=CARTESIAN_POINT ( 'NONE',  ( 7.832860060393120882, 10.16142270859057462, 1.599625672291281386 ) ) ;
#86144=CARTESIAN_POINT ( 'NONE',  ( -1.201851678989727383E-14, 2.821875000341418804, 1.575800808251672791 ) ) ;
#86150=CARTESIAN_POINT ( 'NONE',  ( 9.420217803396747414, 9.884675613584706255, 0.7998128361456462443 ) ) ;
#86153=CARTESIAN_POINT ( 'NONE',  ( -9.365985188942097750, 9.821404230054264772, 0.7998128361456462443 ) ) ;
#86157=CARTESIAN_POINT ( 'NONE',  ( -1.500000000000039524, 4.202083334016153415, 0.8660254037844240527 ) ) ;
#86159=CARTESIAN_POINT ( 'NONE',  ( 4.552840656090682891, 4.206068941727564514, 1.214306433183764966E-14 ) ) ;
#86162=CARTESIAN_POINT ( 'NONE',  ( -7.655550293210764856, 12.08322577538792331, 0.000000000000000000 ) ) ;
#86165=CARTESIAN_POINT ( 'NONE',  ( 4.879410147971470657, 4.944948943068641967, -0.7687999843507594688 ) ) ;
#86168=CARTESIAN_POINT ( 'NONE',  ( 5.892592298951464969, 5.976936425253049912, 0.01597356071081010298 ) ) ;
#86169=CARTESIAN_POINT ( 'NONE',  ( -5.796211742350026341, 6.069872996917573538, -0.5622600474562855499 ) ) ;
#86170=CARTESIAN_POINT ( 'NONE',  ( -3.846762897975357198, 5.510976019103107859, -1.599625672291256295 ) ) ;
#86174=CARTESIAN_POINT ( 'NONE',  ( 6.154511665599609493, 9.267681812253174556, 1.199719254218462483 ) ) ;
#86176=CARTESIAN_POINT ( 'NONE',  ( 5.289652487626049115, 9.323011668872403845, 0.7998128361456462443 ) ) ;
#86177=CARTESIAN_POINT ( 'NONE',  ( 4.147904930777053245, 6.926640621626830807, -1.199719254218452047 ) ) ;
#86179=CARTESIAN_POINT ( 'NONE',  ( -7.537970219518075332, 10.77775377520434574, -1.082531754730543971 ) ) ;
#86187=CARTESIAN_POINT ( 'NONE',  ( -4.073306942994160629, 7.542743630792291043, -0.4897309385070089394 ) ) ;
#86190=CARTESIAN_POINT ( 'NONE',  ( 6.046573322014824114, 7.117052299514516456, -1.082531754730543083 ) ) ;
#86200=ORIENTED_EDGE ( 'NONE', *, *, #149058, .T. ) ;
#86207=CARTESIAN_POINT ( 'NONE',  ( -10.10046125205659173, 10.88621900359527572, -0.7216878364870267237 ) ) ;
#86211=CARTESIAN_POINT ( 'NONE',  ( 7.476431642932036326, 10.80992178580769014, 1.199719254218460707 ) ) ;
#86213=EDGE_LOOP ( 'NONE', ( #209007, #14144, #105405, #70850 ) ) ;
#86215=CARTESIAN_POINT ( 'NONE',  ( 1.499999999999987121, 1.535416667349486453, 0.8660254037844524744 ) ) ;
#86216=DIRECTION ( 'NONE',  ( 5.578564026256504688E-16, 1.000000000000000000, 9.066213480720158442E-32 ) ) ;
#86217=CARTESIAN_POINT ( 'NONE',  ( -5.717788096661253761, 7.693838750903348789, 1.599625672291269396 ) ) ;
#86220=CARTESIAN_POINT ( 'NONE',  ( -9.020252271793614440, 9.418049160047695878, 0.7998128361456462443 ) ) ;
#86224=CARTESIAN_POINT ( 'NONE',  ( 7.287671262545424966, 8.461036880179857889, -1.199719254218451159 ) ) ;
#86227=CARTESIAN_POINT ( 'NONE',  ( -8.050844288416501016, 8.287073179441051707, 1.040834085586084257E-14 ) ) ;
#86229=CARTESIAN_POINT ( 'NONE',  ( 9.423080456697809026, 10.95234760669099749, -1.199719254218446718 ) ) ;
#86235=CARTESIAN_POINT ( 'NONE',  ( -6.399085315970132193, 10.40942393536641397, -0.7216878364870278340 ) ) ;
#86238=CARTESIAN_POINT ( 'NONE',  ( 0.6823417656249899377, 4.238541667008085767, -1.181850606188754593 ) ) ;
#86244=CARTESIAN_POINT ( 'NONE',  ( 0.6823417656249899377, 5.176041667008086655, -1.181850606188754593 ) ) ;
#86246=CARTESIAN_POINT ( 'NONE',  ( -2.887523529586332405, 5.352232636950553513, 1.082531754730560403 ) ) ;
#86248=CARTESIAN_POINT ( 'NONE',  ( 10.23370702021670020, 10.83374636654133383, 0.7998128361456462443 ) ) ;
#86249=CARTESIAN_POINT ( 'NONE',  ( -1.364683531250010295, 4.842708333674756283, 0.7879004041258379498 ) ) ;
#86250=CARTESIAN_POINT ( 'NONE',  ( -10.47775378526269918, 11.11846759242831872, -0.7998128361456221525 ) ) ;
#86252=CARTESIAN_POINT ( 'NONE',  ( 3.563261906135759993, 6.332667919118538435, -2.420000000000000373 ) ) ;
#86254=CARTESIAN_POINT ( 'NONE',  ( 0.6823417656249899377, 2.592708333674753618, 1.181850606188767472 ) ) ;
#86255=CARTESIAN_POINT ( 'NONE',  ( -3.145128448690323264, 4.692402494937224056, -1.443375672974059665 ) ) ;
#86256=CARTESIAN_POINT ( 'NONE',  ( 5.118366684358879759, 5.930181538962194132, 1.199719254218462483 ) ) ;
#86261=DIRECTION ( 'NONE',  ( 1.000000000000000000, 0.000000000000000000, 0.000000000000000000 ) ) ;
#86263=CARTESIAN_POINT ( 'NONE',  ( 10.66990370383054731, 11.55056853066490952, 0.7216878364870317197 ) ) ;
#86265=CARTESIAN_POINT ( 'NONE',  ( -8.188761592974046266, 10.57664116326830595, -1.443375672974059665 ) ) ;
#86270=CARTESIAN_POINT ( 'NONE',  ( -7.808606406466886973, 11.19745900993164511, 1.199719254218453823 ) ) ;
#86271=CARTESIAN_POINT ( 'NONE',  ( -3.917943204224914933, 6.554388924028945240, -1.082531754730548412 ) ) ;
#86272=CARTESIAN_POINT ( 'NONE',  ( -0.6823417656250212460, 1.863541667008083991, 1.181850606188755259 ) ) ;
#86274=CARTESIAN_POINT ( 'NONE',  ( -1.500000000000039524, 4.420833333333351156, 0.8660254037844240527 ) ) ;
#86293=CARTESIAN_POINT ( 'NONE',  ( 6.385527162356455122, 10.39360608948380538, 1.056142170575426150E-14 ) ) ;
#86297=CARTESIAN_POINT ( 'NONE',  ( -1.364683531249997417, 2.571875000341422357, 1.214306433183764966E-14 ) ) ;
#86304=CARTESIAN_POINT ( 'NONE',  ( 10.09812548408005384, 10.67556790771522124, -0.7998128361456281477 ) ) ;
#86306=CARTESIAN_POINT ( 'NONE',  ( 1.364683531249986537, 0.8635416670080893198, 0.7879004041258500513 ) ) ;
#86315=CARTESIAN_POINT ( 'NONE',  ( 4.867540842506059562, 5.637551390133895168, -1.199719254218452047 ) ) ;
#86320=DIRECTION ( 'NONE',  ( -0.9782075119097819460, 0.1245777785625464124, 0.1661037047500602826 ) ) ;
#86326=CARTESIAN_POINT ( 'NONE',  ( -2.948008335967658322, 5.526761261015804116, 1.199719254218462483 ) ) ;
#86328=CARTESIAN_POINT ( 'NONE',  ( 7.934546212495622086, 10.28005655271014795, -1.599625672291262513 ) ) ;
#86331=CARTESIAN_POINT ( 'NONE',  ( 4.595850884908202261, 7.345281218159464665, -1.082531754730549078 ) ) ;
#86339=DIRECTION ( 'NONE',  ( 0.7592566023653005702, -0.6507913734559639396, 0.000000000000000000 ) ) ;
#86340=CARTESIAN_POINT ( 'NONE',  ( -8.026063749610061748, 9.426457798375635022, -1.082531754730543971 ) ) ;
#86342=CARTESIAN_POINT ( 'NONE',  ( 5.555090253297246150, 7.504024600312024340, 1.599625672291267398 ) ) ;
#86346=CARTESIAN_POINT ( 'NONE',  ( -8.784793466650835825, 12.33634391347959713, 1.199719254218462483 ) ) ;
#86351=CARTESIAN_POINT ( 'NONE',  ( -2.272963308585411735, 5.803540959991587478, 0.7998128361456341429 ) ) ;
#86353=CARTESIAN_POINT ( 'NONE',  ( 8.398386088661320414, 11.88553530582519357, -1.199719254218446718 ) ) ;
#86354=CARTESIAN_POINT ( 'NONE',  ( 4.162516854595432747, 4.815023404238158555, 1.199719254218464037 ) ) ;
#86360=CARTESIAN_POINT ( 'NONE',  ( 2.724825686666657809, 6.122787701178987518, 0.000000000000000000 ) ) ;
#86363=CARTESIAN_POINT ( 'NONE',  ( -4.928552533767591726, 5.708731696605642725, 1.199719254218462483 ) ) ;
#86367=CARTESIAN_POINT ( 'NONE',  ( -8.435144125996554720, 12.99275191363802229, 0.7998128361456341429 ) ) ;
#86373=CARTESIAN_POINT ( 'NONE',  ( 8.432808358020025707, 9.900993174853955026, 1.082531754730558626 ) ) ;
#86374=CARTESIAN_POINT ( 'NONE',  ( 0.6823417656249917140, 5.155208333674749177, 1.181850606188765695 ) ) ;
#86377=CARTESIAN_POINT ( 'NONE',  ( 5.359550796103802028, 5.147230771742885125, -0.7998128361456231517 ) ) ;
#86378=CARTESIAN_POINT ( 'NONE',  ( 5.985929146193681660, 5.992403464881949304, 0.1705357982419167806 ) ) ;
#86379=CARTESIAN_POINT ( 'NONE',  ( 4.568734577680872988, 6.353276312092901890, -1.443375672974051449 ) ) ;
#86388=VERTEX_POINT ( 'NONE', #912 ) ;
#86390=CARTESIAN_POINT ( 'NONE',  ( 1.364683531249988757, 2.446875000341415696, 1.214306433183764966E-14 ) ) ;
#86392=CARTESIAN_POINT ( 'NONE',  ( 9.673906298550626559, 11.24497775551929557, 1.199719254218452047 ) ) ;
#86394=CARTESIAN_POINT ( 'NONE',  ( -3.795919822146277767, 7.372397525905215687, -0.7216878364870267237 ) ) ;
#86397=CARTESIAN_POINT ( 'NONE',  ( -4.568734577680875653, 8.274014740695587733, -0.7216878364870257245 ) ) ;
#86403=CARTESIAN_POINT ( 'NONE',  ( 5.606460214450851964, 6.499623990736163037, 1.199719254218462483 ) ) ;
#86409=CARTESIAN_POINT ( 'NONE',  ( 1.123270288250308280, 2.922697346350005887, 0.7749999999993786304 ) ) ;
#86413=CARTESIAN_POINT ( 'NONE',  ( 7.006866460164219212, 7.069099046480051385, -0.7998128361456281477 ) ) ;
#86417=CARTESIAN_POINT ( 'NONE',  ( -5.038826645773246682, 9.030381520044109322, 0.7998128361456481317 ) ) ;
#86422=CARTESIAN_POINT ( 'NONE',  ( 5.764187864104357573, 9.876636274763768597, 1.040834085586084257E-14 ) ) ;
#86425=CARTESIAN_POINT ( 'NONE',  ( -5.768104287610143821, 8.816873204598778102, -1.199719254218440723 ) ) ;
#86426=CARTESIAN_POINT ( 'NONE',  ( 5.111060722227499298, 8.906728576000002562, -0.7216878364870267237 ) ) ;
#86427=CARTESIAN_POINT ( 'NONE',  ( 4.972575192752072937, 6.823350471033509557, 1.425105271486303282 ) ) ;
#86428=CARTESIAN_POINT ( 'NONE',  ( -5.271422797614987665, 5.044414773505913274, -0.7998128361456221525 ) ) ;
#86431=CARTESIAN_POINT ( 'NONE',  ( -5.087333953625788219, 6.958308917361963886, 1.599625672291267398 ) ) ;
#86434=CARTESIAN_POINT ( 'NONE',  ( -1.402160292154681736E-14, 2.446875000341416584, -1.575800808251660134 ) ) ;
#86435=CARTESIAN_POINT ( 'NONE',  ( -2.278026279638522666, 5.601521726312811644, -0.03298406423010708660 ) ) ;
#86436=CARTESIAN_POINT ( 'NONE',  ( -5.016153647376219382, 6.875265226737464985, 1.443375672974064550 ) ) ;
#86442=CARTESIAN_POINT ( 'NONE',  ( 5.144429221381498607, 8.089252293998699272, -1.199719254218452047 ) ) ;
#86445=CARTESIAN_POINT ( 'NONE',  ( -1.201851678989727383E-14, 2.384375000341416584, 1.575800808251672791 ) ) ;
#86447=LINE ( 'NONE', #70167, #129247 ) ;
#86449=CARTESIAN_POINT ( 'NONE',  ( -1.123270288250342919, 2.846052654332832610, 0.7749999999993751887 ) ) ;
#86450=VECTOR ( 'NONE', #14922, 1000.000000000000227 ) ;
#86452=CARTESIAN_POINT ( 'NONE',  ( -4.569261463005423352, 5.289558780716470565, -1.199719254218446718 ) ) ;
#86453=CARTESIAN_POINT ( 'NONE',  ( -7.849807752188049825, 8.260456587081938196, 0.7216878364870578100 ) ) ;
#86456=CARTESIAN_POINT ( 'NONE',  ( 1.364683531249988535, 3.155208333674756283, -0.7879004041258239610 ) ) ;
#86463=CARTESIAN_POINT ( 'NONE',  ( -6.629573926958124197, 9.717958100551031819, 1.082531754730548412 ) ) ;
#86465=CARTESIAN_POINT ( 'NONE',  ( -2.103486388414573138, 5.605817886458954291, 1.040834085586084257E-14 ) ) ;
#86467=CARTESIAN_POINT ( 'NONE',  ( -7.009202228140755331, 8.240119356661432803, -1.082531754730543083 ) ) ;
#86480=CARTESIAN_POINT ( 'NONE',  ( -5.096975683733680818, 8.033889833409558534, -1.199719254218452047 ) ) ;
#86482=CARTESIAN_POINT ( 'NONE',  ( 3.147464216666835402, 6.823792019419957278, -0.7998128361456291469 ) ) ;
#86486=CARTESIAN_POINT ( 'NONE',  ( 7.006866460164219212, 7.069099046480051385, -0.7998128361456281477 ) ) ;
#86491=CARTESIAN_POINT ( 'NONE',  ( -4.365362273920257330, 6.116008624372160973, 1.443375672974064550 ) ) ;
#86495=CARTESIAN_POINT ( 'NONE',  ( -0.1004607481840987110, 6.432248552227529004, 3.209664736303321497 ) ) ;
#86499=CARTESIAN_POINT ( 'NONE',  ( 1.364683531249986537, 1.405208333674755838, -0.7879004041258239610 ) ) ;
#86501=CARTESIAN_POINT ( 'NONE',  ( -7.771848369131641121, 10.09024240211882351, -1.599625672291263179 ) ) ;
#86503=CARTESIAN_POINT ( 'NONE',  ( 6.109920781252839994, 10.27999134477033216, 1.040834085586084257E-14 ) ) ;
#86505=CARTESIAN_POINT ( 'NONE',  ( -8.538937818508475885, 8.856515631215026829, 1.040834085586084257E-14 ) ) ;
#86508=CARTESIAN_POINT ( 'NONE',  ( -1.364683531249997417, 5.509375000341417916, 1.214306433183764966E-14 ) ) ;
#86511=CARTESIAN_POINT ( 'NONE',  ( 8.649738815838679429, 10.15407870897571563, -1.082531754730543083 ) ) ;
#86513=CARTESIAN_POINT ( 'NONE',  ( -0.6823417656250246877, -0.8864583329919115684, 1.181850606188755259 ) ) ;
#86516=CARTESIAN_POINT ( 'NONE',  ( 6.765155463094740362, 10.83650577367847667, 0.7216878364870438212 ) ) ;
#86519=CARTESIAN_POINT ( 'NONE',  ( -4.256897045010916258, 7.910204285913967404, 0.7216878364870317197 ) ) ;
#86521=CARTESIAN_POINT ( 'NONE',  ( -1.364683531250012516, 3.488541667008085767, -0.7879004041258300672 ) ) ;
#86525=CARTESIAN_POINT ( 'NONE',  ( -6.891622154448065807, 6.934647356477856128, 1.040834085586084257E-14 ) ) ;
#86526=DIRECTION ( 'NONE',  ( 0.9840714016191985936, 0.1066641999242542993, -0.1422189332323393063 ) ) ;
#86533=CARTESIAN_POINT ( 'NONE',  ( 7.096803341749390981, 10.36702210109460154, -1.199719254218441611 ) ) ;
#86536=CARTESIAN_POINT ( 'NONE',  ( 1.499999999999989120, 2.025000000000019895, 1.214306433183764966E-14 ) ) ;
#86543=CARTESIAN_POINT ( 'NONE',  ( 5.666945020832167224, 8.594891043404107478, 1.082531754730558626 ) ) ;
#86544=CARTESIAN_POINT ( 'NONE',  ( 0.6823417656249882723, -0.2614583329919109578, -1.181850606188749264 ) ) ;
#86547=CARTESIAN_POINT ( 'NONE',  ( 4.241003122976366058, 3.842258486427521103, -0.7998128361456211532 ) ) ;
#86553=CARTESIAN_POINT ( 'NONE',  ( 0.7499999999999867883, 0.3166666666666873020, -1.299038105676652899 ) ) ;
#86554=CARTESIAN_POINT ( 'NONE',  ( 6.642605195691581699, 9.837124264027149678, 1.199719254218462483 ) ) ;
#86555=CARTESIAN_POINT ( 'NONE',  ( -9.826962411806732689, 10.35921099006301382, -0.7998128361456291469 ) ) ;
#86558=CARTESIAN_POINT ( 'NONE',  ( -1.364683531250014514, 0.2385416670080863499, -0.7879004041258359514 ) ) ;
#86560=CARTESIAN_POINT ( 'NONE',  ( -1.402160292154681736E-14, 1.087500000000024336, -1.732050807568863648 ) ) ;
#86562=CARTESIAN_POINT ( 'NONE',  ( 5.847644326195776010, 5.716673223516856694, -0.7998128361456281477 ) ) ;
#86569=CARTESIAN_POINT ( 'NONE',  ( -0.6823417656250212460, 4.551041667008086655, 1.181850606188767472 ) ) ;
#86570=CARTESIAN_POINT ( 'NONE',  ( -8.128276786592724790, 9.441743324901704426, -1.199719254218446718 ) ) ;
#86571=CARTESIAN_POINT ( 'NONE',  ( -5.775410249741523394, 5.840326167560965231, 0.7216878364870317197 ) ) ;
#86579=CARTESIAN_POINT ( 'NONE',  ( 8.613507663383630941, 8.943513783569379427, -0.7998128361456221525 ) ) ;
#86582=CARTESIAN_POINT ( 'NONE',  ( 6.927853306458743532, 9.105581495667113501, 1.443375672974076540 ) ) ;
#86586=CARTESIAN_POINT ( 'NONE',  ( -8.694856585065634746, 9.038420858865048757, 0.7998128361456462443 ) ) ;
#86588=CARTESIAN_POINT ( 'NONE',  ( 5.144429221381498607, 8.089252293998699272, -1.199719254218452047 ) ) ;
#86589=CARTESIAN_POINT ( 'NONE',  ( 7.334597915313080918, 9.580116872663850813, 1.040834085586084257E-14 ) ) ;
#86591=CARTESIAN_POINT ( 'NONE',  ( 4.532503425670185493, 4.182342172903648070, 1.214306433183764966E-14 ) ) ;
#86592=ORIENTED_EDGE ( 'NONE', *, *, #161158, .F. ) ;
#86598=FACE_OUTER_BOUND ( 'NONE', #76468, .T. ) ;
#86599=CARTESIAN_POINT ( 'NONE',  ( -4.202664430556263930, 5.926194473780837413, 1.443375672974064550 ) ) ;
#86600=CARTESIAN_POINT ( 'NONE',  ( 10.39874063200158893, 11.23421161353111586, 0.000000000000000000 ) ) ;
#86603=CARTESIAN_POINT ( 'NONE',  ( -7.691553217654356622, 7.867900263551875994, -0.7998128361456291469 ) ) ;
#86608=CARTESIAN_POINT ( 'NONE',  ( -7.263417608619167076, 9.497073181520933716, -1.599625672291263179 ) ) ;
#86611=CARTESIAN_POINT ( 'NONE',  ( -0.4914377447849399561, 7.519435632882157883, 2.014015809874911245 ) ) ;
#86623=CARTESIAN_POINT ( 'NONE',  ( -7.718669524881690336, 7.899535955317097624, 0.7998128361456462443 ) ) ;
#86627=CARTESIAN_POINT ( 'NONE',  ( 4.514501963670558560, 8.210743357683563559, 1.040834085586084257E-14 ) ) ;
#86628=VERTEX_POINT ( 'NONE', #182429 ) ;
#86632=CARTESIAN_POINT ( 'NONE',  ( -3.574546055497324737, 7.322054164722185732, 0.7998128361456341429 ) ) ;
#86636=CARTESIAN_POINT ( 'NONE',  ( -1.499999999999997780, 3.400000000000021227, 1.214306433183764966E-14 ) ) ;
#86640=CARTESIAN_POINT ( 'NONE',  ( -8.666686507633592385, 11.13422023037111330, 1.599625672291269396 ) ) ;
#86641=CARTESIAN_POINT ( 'NONE',  ( 8.260995669428309540, 8.532249790621511565, 0.7998128361456481317 ) ) ;
#86644=CARTESIAN_POINT ( 'NONE',  ( -8.513630394377489807, 12.01998699582738972, -1.199719254218446718 ) ) ;
#86647=CARTESIAN_POINT ( 'NONE',  ( 1.364683531249986537, -0.2822916663252520997, -0.7879004041258309554 ) ) ;
#86651=CARTESIAN_POINT ( 'NONE',  ( 8.595506201384008449, 11.05117653974661529, 1.443375672974076540 ) ) ;
#86670=B_SPLINE_CURVE_WITH_KNOTS ( 'NONE', 3,
 ( #52060, #54190, #134410, #86685, #170061, #200414, #101872, #135451, #152753, #116047, #184175, #132277, #167939, #85617 ),
 .UNSPECIFIED., .F., .F.,
 ( 4, 2, 2, 2, 2, 2, 4 ),
 ( 6.159050845453070644E-06, 0.0002195312228445668514, 0.0004329033948436806448, 0.0008596477388419082859, 0.001073019910841021890, 0.001286392082840135927, 0.001713136426838359665 ),
 .UNSPECIFIED. ) ;
#86679=CARTESIAN_POINT ( 'NONE',  ( -1.602468905319636405E-14, -1.131249999317182064, -1.732050807568870754 ) ) ;
#86685=CARTESIAN_POINT ( 'NONE',  ( 0.2656570211550720595, 7.171539594011578700, -2.094714161149643594 ) ) ;
#86687=CARTESIAN_POINT ( 'NONE',  ( 3.837121167867449945, 4.435395103055503441, 1.199719254218464037 ) ) ;
#86692=CARTESIAN_POINT ( 'NONE',  ( 4.310602774141044868, 7.116454772218158809, -1.199719254218452047 ) ) ;
#86693=CARTESIAN_POINT ( 'NONE',  ( -1.201851678989727383E-14, 2.634375000341417916, 1.575800808251672791 ) ) ;
#86695=CARTESIAN_POINT ( 'NONE',  ( -5.887541547804238995, 6.014758725225416214, 0.2650624260464862214 ) ) ;
#86696=CARTESIAN_POINT ( 'NONE',  ( 9.028840231696797503, 12.62106513936658203, -1.199719254218446718 ) ) ;
#86698=CARTESIAN_POINT ( 'NONE',  ( -9.020252271793614440, 9.418049160047695878, 0.7998128361456462443 ) ) ;
#86700=CARTESIAN_POINT ( 'NONE',  ( -3.578989363883261277, 7.119311991265024453, 1.040834085586084257E-14 ) ) ;
#86702=CARTESIAN_POINT ( 'NONE',  ( -4.367698041896780126, 8.247398148854895084, 0.7998128361456481317 ) ) ;
#86704=CARTESIAN_POINT ( 'NONE',  ( -1.500000000000015099, 0.1604166673494879791, -0.8660254037844383745 ) ) ;
#86711=CARTESIAN_POINT ( 'NONE',  ( -4.907688418022547516, 4.827984030555475314, 1.214306433183764966E-14 ) ) ;
#86717=CARTESIAN_POINT ( 'NONE',  ( -4.297571505407598025, 5.076550180139354218, 1.082531754730558626 ) ) ;
#86719=CARTESIAN_POINT ( 'NONE',  ( 9.447334110624092673, 9.916311305349925220, -0.7998128361456281477 ) ) ;
#86721=LINE ( 'NONE', #105129, #132742 ) ;
#86727=CARTESIAN_POINT ( 'NONE',  ( -4.627410500965859264, 4.293067094081919777, 0.7998128361456341429 ) ) ;
#86728=CARTESIAN_POINT ( 'NONE',  ( -9.622536337397040285, 12.24937836509514710, 1.599625672291281386 ) ) ;
#86733=CARTESIAN_POINT ( 'NONE',  ( 4.761938266897790761, 6.578680616179308771, 1.599625672291267398 ) ) ;
#86739=CARTESIAN_POINT ( 'NONE',  ( 2.920214025141053327, 6.445393704534057022, 0.4458799699700779495 ) ) ;
#86740=CARTESIAN_POINT ( 'NONE',  ( 4.701980345841006326, 4.380065246436280368, 0.7998128361456341429 ) ) ;
#86749=EDGE_CURVE ( 'NONE', #104869, #39666, #84726, .T. ) ;
#86752=CARTESIAN_POINT ( 'NONE',  ( 6.936968151686458306, 11.24487994360957188, 0.7998128361456462443 ) ) ;
#86754=CARTESIAN_POINT ( 'NONE',  ( -5.949330478298285207, 5.835307067636438028, 0.7998128361456341429 ) ) ;
#86760=CARTESIAN_POINT ( 'NONE',  ( 1.499999999999987121, -0.4645833326505149907, 0.8660254037844524744 ) ) ;
#86765=CARTESIAN_POINT ( 'NONE',  ( 3.354752944377597856, 6.001296637494123232, -1.199719254218446718 ) ) ;
#86766=CARTESIAN_POINT ( 'NONE',  ( -4.273844736805832767, 6.009238164405336313, 1.599625672291267398 ) ) ;
#86773=CARTESIAN_POINT ( 'NONE',  ( 5.829642864196168617, 6.863966765392747860, 1.082531754730558626 ) ) ;
#86776=CARTESIAN_POINT ( 'NONE',  ( 6.927853306458731986, 11.02631992426980112, 0.7216878364870438212 ) ) ;
#86777=CARTESIAN_POINT ( 'NONE',  ( -1.201851678989727383E-14, 3.384375000341421469, 1.575800808251672791 ) ) ;
#86779=CARTESIAN_POINT ( 'NONE',  ( 3.999292125906894313, 7.609665213625947722, 0.7216878364870317197 ) ) ;
#86786=CARTESIAN_POINT ( 'NONE',  ( -4.211465482254622472, 7.549728682704877514, 0.9859626088348661943 ) ) ;
#86794=CARTESIAN_POINT ( 'NONE',  ( -9.612894607289142357, 11.17379744904754801, -1.199719254218441611 ) ) ;
#86800=CARTESIAN_POINT ( 'NONE',  ( -3.460355519985875983, 5.060167411448709629, 1.599625672291267398 ) ) ;
#86805=CARTESIAN_POINT ( 'NONE',  ( 4.039966587192267866, 4.776011108888172707, 1.082531754730560403 ) ) ;
#86806=CARTESIAN_POINT ( 'NONE',  ( -1.364683531250010295, 3.842708333674751398, 0.7879004041258379498 ) ) ;
#86808=CARTESIAN_POINT ( 'NONE',  ( 7.461064606222022277, 7.598996883547496139, 1.040834085586084257E-14 ) ) ;
#86809=CARTESIAN_POINT ( 'NONE',  ( -8.585337585951595685, 11.03931315507545108, -1.599625672291263179 ) ) ;
#86812=CARTESIAN_POINT ( 'NONE',  ( -1.579999999999998073, 6.280000000000042881, -2.579999999999995630 ) ) ;
#86813=ORIENTED_EDGE ( 'NONE', *, *, #151561, .T. ) ;
#86815=CARTESIAN_POINT ( 'NONE',  ( -1.500000000000011324, 4.629166666666689522, -0.8660254037844313801 ) ) ;
#86816=CARTESIAN_POINT ( 'NONE',  ( 4.123651276850781144, 7.962676922967908411, -0.7998128361456221525 ) ) ;
#86821=EDGE_CURVE ( 'NONE', #166004, #26662, #18819, .T. ) ;
#86823=CARTESIAN_POINT ( 'NONE',  ( 7.592202833972727660, 11.80139437303613015, -0.7216878364870267237 ) ) ;
#86828=CARTESIAN_POINT ( 'NONE',  ( -1.500000000000011324, 3.452083334016151639, 0.8660254037844403729 ) ) ;
#86830=CARTESIAN_POINT ( 'NONE',  ( -4.660252114795309097, 6.460046772059735432, -1.599625672291256295 ) ) ;
#86831=CARTESIAN_POINT ( 'NONE',  ( 4.324687812634892659, 5.108185871904570519, 1.082531754730560403 ) ) ;
#86840=CARTESIAN_POINT ( 'NONE',  ( 6.584456157731144899, 10.83361595066169514, -0.7998128361456291469 ) ) ;
#86841=CARTESIAN_POINT ( 'NONE',  ( 3.337278367258157630, 7.045241861776501580, 0.7998128361456341429 ) ) ;
#86842=LINE ( 'NONE', #103095, #54092 ) ;
#86844=CARTESIAN_POINT ( 'NONE',  ( 3.673896439623286714, 4.156855427197417185, 2.420000000000023022 ) ) ;
#86845=CARTESIAN_POINT ( 'NONE',  ( 3.357615597678655917, 7.068968630600412695, 0.7998128361456321445 ) ) ;
#86853=CARTESIAN_POINT ( 'NONE',  ( 9.459838494033030898, 12.05956421450382088, 1.599625672291281386 ) ) ;
#86858=CARTESIAN_POINT ( 'NONE',  ( 5.827790676886797527, 6.016211147664318304, -0.4261259532085531765 ) ) ;
#86866=CARTESIAN_POINT ( 'NONE',  ( 6.480434237652124452, 8.583592582059388576, 1.443375672974076540 ) ) ;
#86867=CARTESIAN_POINT ( 'NONE',  ( -2.754277761870538299, 6.365074488824250309, 1.040834085586084257E-14 ) ) ;
#86873=CARTESIAN_POINT ( 'NONE',  ( -5.362413449404877852, 6.214902764849178141, -1.199719254218446718 ) ) ;
#86880=CARTESIAN_POINT ( 'NONE',  ( -3.804741806807946602, 4.044702255324862605, -0.8707498557368220649 ) ) ;
#86885=CARTESIAN_POINT ( 'NONE',  ( 9.908311333488716954, 10.45411806535867782, 0.7998128361456462443 ) ) ;
#86886=CARTESIAN_POINT ( 'NONE',  ( 5.966167892564917530, 6.109520806784549229, 0.6870465322655286977 ) ) ;
#86893=CARTESIAN_POINT ( 'NONE',  ( -3.189213936345698830, 2.817530495244580102, 2.450448857954578230 ) ) ;
#86894=CARTESIAN_POINT ( 'NONE',  ( -9.544576954340667996, 11.19805653722800365, 1.082531754730558626 ) ) ;
#86898=CARTESIAN_POINT ( 'NONE',  ( 7.426115451983150706, 9.686887332112256388, -1.599625672291262513 ) ) ;
#86900=CARTESIAN_POINT ( 'NONE',  ( 0.7035002141062960401, 2.800000000000067768, 1.266925154657448038 ) ) ;
#86902=CARTESIAN_POINT ( 'NONE',  ( 2.706824224222692088, 6.309712028235118453, 0.7998128361456362523 ) ) ;
#86904=CARTESIAN_POINT ( 'NONE',  ( -7.400052914960538963, 7.527816577075747695, 1.040834085586084257E-14 ) ) ;
#86905=CARTESIAN_POINT ( 'NONE',  ( 4.202137545231717120, 6.989912005157271402, 1.199719254218462483 ) ) ;
#86912=CARTESIAN_POINT ( 'NONE',  ( 4.221210552267129046, 7.311159377000789661, -0.8807526815687096722 ) ) ;
#86914=CARTESIAN_POINT ( 'NONE',  ( 4.528060117284222308, 8.226561203566173930, 0.7216878364870438212 ) ) ;
#86916=CARTESIAN_POINT ( 'NONE',  ( 0.1245482448182331087, 6.487495393664095111, 3.100011470320013895 ) ) ;
#86922=CARTESIAN_POINT ( 'NONE',  ( 9.205623113554628034, 9.842241175342985926, 0.7216878364870458196 ) ) ;
#86923=ORIENTED_EDGE ( 'NONE', *, *, #54763, .T. ) ;
#86926=CARTESIAN_POINT ( 'NONE',  ( -8.341290820905609138, 10.75459192918846618, 1.599625672291269396 ) ) ;
#86936=CARTESIAN_POINT ( 'NONE',  ( 10.71502147350184231, 11.39527989537399755, 0.000000000000000000 ) ) ;
#86940=CARTESIAN_POINT ( 'NONE',  ( 3.960953433486789521, 7.772862772376584850, -0.7998128361456221525 ) ) ;
#86943=CARTESIAN_POINT ( 'NONE',  ( -1.500000000000013101, 2.702083334016155636, 0.8660254037844403729 ) ) ;
#86947=ORIENTED_EDGE ( 'NONE', *, *, #171813, .F. ) ;
#86948=CARTESIAN_POINT ( 'NONE',  ( -1.500000000000013101, 2.129166666666693519, -0.8660254037844313801 ) ) ;
#86949=CARTESIAN_POINT ( 'NONE',  ( 5.099838337034727331, 9.101561826515851550, -0.7998128361456281477 ) ) ;
#86950=CARTESIAN_POINT ( 'NONE',  ( 5.653386866774156694, 5.697965554099049257, -0.7216878364870207285 ) ) ;
#86955=CARTESIAN_POINT ( 'NONE',  ( 8.649738815838679429, 10.15407870897571563, -1.082531754730543083 ) ) ;
#86961=CARTESIAN_POINT ( 'NONE',  ( -4.578903193113314174, 6.365139696764064325, 1.599625672291267398 ) ) ;
#86962=CARTESIAN_POINT ( 'NONE',  ( 1.499999999999989120, 4.577083334016148974, -0.8660254037844323793 ) ) ;
#86963=CARTESIAN_POINT ( 'NONE',  ( 0.6823417656249899377, 5.488541667008087543, -1.181850606188754593 ) ) ;
#86968=CARTESIAN_POINT ( 'NONE',  ( 1.364683531249990311, 3.696875000341416584, 1.214306433183764966E-14 ) ) ;
#86975=CARTESIAN_POINT ( 'NONE',  ( -8.690940161559884913, 10.09818392903003748, 1.199719254218462483 ) ) ;
#86976=CARTESIAN_POINT ( 'NONE',  ( 4.821896187954575197, 8.777295985922343391, 0.7998128361456462443 ) ) ;
#86978=CARTESIAN_POINT ( 'NONE',  ( 1.364683531249988757, -0.8656249996585805295, 0.000000000000000000 ) ) ;
#86983=CARTESIAN_POINT ( 'NONE',  ( -7.802881099864745984, 9.062115023719057305, -1.199719254218446718 ) ) ;
#86988=CARTESIAN_POINT ( 'NONE',  ( 7.879259827836241570, 12.34422023245099176, 1.040834085586084257E-14 ) ) ;
#86989=CARTESIAN_POINT ( 'NONE',  ( 3.173948600550551724, 6.437700466846534297, 0.6171826442077615882 ) ) ;
#86990=CARTESIAN_POINT ( 'NONE',  ( -4.874319919312905647, 5.645460313075203018, -1.199719254218446718 ) ) ;
#86991=CARTESIAN_POINT ( 'NONE',  ( -8.182509401047415309, 9.505014708432145909, 1.199719254218462483 ) ) ;
#86994=CARTESIAN_POINT ( 'NONE',  ( -4.103765016252827635, 7.679818082383993882, -0.7602138238151506799 ) ) ;
#86995=CARTESIAN_POINT ( 'NONE',  ( 1.364683531249988757, -0.8656249996585805295, 0.000000000000000000 ) ) ;
#86999=CARTESIAN_POINT ( 'NONE',  ( 8.920901888112002354, 9.510066412326583674, 0.7216878364870438212 ) ) ;
#87002=CARTESIAN_POINT ( 'NONE',  ( 5.198661835836162481, 8.152523677529138979, 1.199719254218462483 ) ) ;
#87019=EDGE_CURVE ( 'NONE', #37648, #178928, #193473, .T. ) ;
#87026=CARTESIAN_POINT ( 'NONE',  ( -7.808606406466886973, 11.19745900993164511, 1.199719254218453823 ) ) ;
#87029=CARTESIAN_POINT ( 'NONE',  ( 1.419999999999990603, 6.200000000000045475, 2.580000000000000515 ) ) ;
#87031=CARTESIAN_POINT ( 'NONE',  ( -1.499999999999997780, 1.681250000682817047, 0.000000000000000000 ) ) ;
#87032=CARTESIAN_POINT ( 'NONE',  ( 8.367353357928214663, 12.91366268422496688, 1.040834085586084257E-14 ) ) ;
#87037=CARTESIAN_POINT ( 'NONE',  ( -8.967828540435322182, 12.54988483289483980, 1.199719254218462483 ) ) ;
#87039=CARTESIAN_POINT ( 'NONE',  ( -1.364683531250012516, 2.238541667008087988, -0.7879004041258289570 ) ) ;
#87040=CARTESIAN_POINT ( 'NONE',  ( 1.500000000000016209, 5.504166666666685082, 0.8660254037844364872 ) ) ;
#87045=CARTESIAN_POINT ( 'NONE',  ( -4.776550190716183586, 4.467063398790632966, 1.214306433183764966E-14 ) ) ;
#87047=CARTESIAN_POINT ( 'NONE',  ( 1.499999999999990674, 8.226475397238111498, -3.114076396432628346 ) ) ;
#87050=CARTESIAN_POINT ( 'NONE',  ( -0.6823417656250003738, 0.5302083336747518416, -1.181850606188749264 ) ) ;
#87056=CARTESIAN_POINT ( 'NONE',  ( -1.364683531250000748, 1.009375000341421247, 0.000000000000000000 ) ) ;
#87058=CARTESIAN_POINT ( 'NONE',  ( -7.074657228232555717, 7.148188275893099686, 1.040834085586084257E-14 ) ) ;
#87059=CARTESIAN_POINT ( 'NONE',  ( 8.046927864910717432, 9.346836249606042202, 1.199719254218462483 ) ) ;
#87061=CARTESIAN_POINT ( 'NONE',  ( 6.193377243344257543, 6.120028293523423812, -0.7998128361456281477 ) ) ;
#87063=CARTESIAN_POINT ( 'NONE',  ( 1.499999999999990896, 3.775000000000021227, 1.214306433183764966E-14 ) ) ;
#87065=CARTESIAN_POINT ( 'NONE',  ( -1.364683531250000748, 1.571875000341421691, 0.000000000000000000 ) ) ;
#87068=EDGE_CURVE ( 'NONE', #32739, #176773, #173859, .T. ) ;
#87072=CARTESIAN_POINT ( 'NONE',  ( 6.155038550924155416, 6.283225852274053835, 0.7216878364870317197 ) ) ;
#87075=CARTESIAN_POINT ( 'NONE',  ( -8.317037166979361018, 11.79062823052953668, 1.199719254218453823 ) ) ;
#87076=CARTESIAN_POINT ( 'NONE',  ( -3.846762897975357198, 5.510976019103107859, -1.599625672291256295 ) ) ;
#87077=CARTESIAN_POINT ( 'NONE',  ( -1.123270288250315163, 3.047697346350006331, -0.7749999999993613109 ) ) ;
#87081=CARTESIAN_POINT ( 'NONE',  ( -7.605760987142072160, 10.85684300409898384, 1.082531754730549967 ) ) ;
#87083=CARTESIAN_POINT ( 'NONE',  ( 1.499999999999989120, 5.254166666666684193, 0.8660254037844524744 ) ) ;
#87087=CARTESIAN_POINT ( 'NONE',  ( 7.782016984564049444, 11.06247500109133064, 1.082531754730557072 ) ) ;
#87094=FACE_OUTER_BOUND ( 'NONE', #90649, .T. ) ;
#87100=CARTESIAN_POINT ( 'NONE',  ( 7.253248993186720561, 10.44557901115111065, 1.082531754730558626 ) ) ;
#87101=CARTESIAN_POINT ( 'NONE',  ( 8.125414133291656071, 8.374071331795406081, -0.7998128361456291469 ) ) ;
#87102=CARTESIAN_POINT ( 'NONE',  ( -4.934277840369690971, 7.844075682818238526, -1.199719254218452047 ) ) ;
#87108=FACE_OUTER_BOUND ( 'NONE', #167978, .T. ) ;
#87110=CARTESIAN_POINT ( 'NONE',  ( -3.110706179331648169, 5.716575411607132118, 1.199719254218462483 ) ) ;
#87121=EDGE_CURVE ( 'NONE', #137371, #44957, #141724, .T. ) ;
#87127=CARTESIAN_POINT ( 'NONE',  ( 8.782984583554449998, 9.141236857102018831, 1.040834085586084257E-14 ) ) ;
#87139=CARTESIAN_POINT ( 'NONE',  ( -4.843287188579803448, 6.673587691474970107, -1.599625672291256295 ) ) ;
#87141=CARTESIAN_POINT ( 'NONE',  ( -4.603156847039612920, 5.329103395422994716, 1.199719254218462483 ) ) ;
#87150=CARTESIAN_POINT ( 'NONE',  ( -4.451154503988200339, 4.087435097607984957, 1.214306433183764966E-14 ) ) ;
#87153=CARTESIAN_POINT ( 'NONE',  ( 7.800018446563675489, 7.994443030612759848, -0.7998128361456281477 ) ) ;
#87154=CARTESIAN_POINT ( 'NONE',  ( 1.364683531249988535, 4.405208333674754506, -0.7879004041258300672 ) ) ;
#87160=CARTESIAN_POINT ( 'NONE',  ( 6.616015773344440021, 6.821032611764393572, 1.040834085586084257E-14 ) ) ;
#87161=CARTESIAN_POINT ( 'NONE',  ( -8.179646747746328828, 8.437342715325849341, -0.7998128361456291469 ) ) ;
#87165=CARTESIAN_POINT ( 'NONE',  ( -8.355902744723985975, 8.642974711799791265, 1.040834085586084257E-14 ) ) ;
#87166=CARTESIAN_POINT ( 'NONE',  ( -4.238895582566952314, 8.097128612970093897, 1.040834085586084257E-14 ) ) ;
#87170=B_SPLINE_CURVE_WITH_KNOTS ( 'NONE', 3,
 ( #61844, #119173, #102867, #34658, #99668, #184101, #86611, #100728, #199277, #83405, #152678, #50919, #149487, #4261 ),
 .UNSPECIFIED., .F., .F.,
 ( 4, 2, 2, 2, 2, 2, 4 ),
 ( 6.159050845712786192E-06, 0.0002195312228448280628, 0.0004329033948439433470, 0.0008596477388421738071, 0.001073019910841287736, 0.001286392082840398954, 0.001713136426838625295 ),
 .UNSPECIFIED. ) ;
#87176=CARTESIAN_POINT ( 'NONE',  ( 7.450369105909416589, 8.650851030771185890, -1.199719254218441611 ) ) ;
#87191=CARTESIAN_POINT ( 'NONE',  ( 1.499999999999989120, 5.254166666666684193, 0.8660254037844524744 ) ) ;
#87192=CARTESIAN_POINT ( 'NONE',  ( 3.659811400685081040, 6.357198169852855685, -1.199719254218446718 ) ) ;
#87193=CARTESIAN_POINT ( 'NONE',  ( 6.169123589417988995, 7.156064594864501416, -1.199719254218445830 ) ) ;
#87196=CARTESIAN_POINT ( 'NONE',  ( -9.002250809794013264, 9.604973487622245898, -0.7216878364870267237 ) ) ;
#87197=CARTESIAN_POINT ( 'NONE',  ( -3.946537740501743219, 2.817530495241825417, -0.7749999999999944711 ) ) ;
#87198=CARTESIAN_POINT ( 'NONE',  ( 5.178851490740193242, 8.025448591630130579, 1.082531754730558626 ) ) ;
#87199=CARTESIAN_POINT ( 'NONE',  ( -7.605760987142072160, 10.85684300409898384, 1.082531754730549967 ) ) ;
#87202=CARTESIAN_POINT ( 'NONE',  ( 9.101601193475611140, 9.512956235343358102, -0.7998128361456221525 ) ) ;
#87208=CARTESIAN_POINT ( 'NONE',  ( 0.6823417656249882723, 2.176041667008084435, -1.181850606188749264 ) ) ;
#87214=CARTESIAN_POINT ( 'NONE',  ( 8.959240580532112475, 9.346868853575953651, -0.7998128361456221525 ) ) ;
#87219=CARTESIAN_POINT ( 'NONE',  ( -7.004758919754800139, 11.32396917302262018, 0.000000000000000000 ) ) ;
#87225=CARTESIAN_POINT ( 'NONE',  ( 3.216308754939877446, 4.775446185561722956, -1.599625672291262513 ) ) ;
#87228=SHAPE_DEFINITION_REPRESENTATION ( #90285, #113740 ) ;
#87229=CARTESIAN_POINT ( 'NONE',  ( -8.585337585951595685, 11.03931315507545108, -1.599625672291263179 ) ) ;
#87234=CARTESIAN_POINT ( 'NONE',  ( 5.580611138136594818, 6.171711880978127063, 0.8815597724760818599 ) ) ;
#87236=CARTESIAN_POINT ( 'NONE',  ( -3.581325132304157943, 7.329963087663487364, -0.7998128361456281477 ) ) ;
#87240=CARTESIAN_POINT ( 'NONE',  ( 5.913327553854682783, 10.05063257947248800, -0.7998128361456291469 ) ) ;
#87242=CARTESIAN_POINT ( 'NONE',  ( 6.100279051144945619, 9.204410428722734849, -1.199719254218440723 ) ) ;
#87243=CARTESIAN_POINT ( 'NONE',  ( 3.635557746758808495, 7.393234471193928847, -0.7998128361456291469 ) ) ;
#87245=CARTESIAN_POINT ( 'NONE',  ( -7.782016984564068096, 10.10210578678999482, 1.443375672974090751 ) ) ;
#87255=CARTESIAN_POINT ( 'NONE',  ( -4.485938484121875902, 7.064193607440066636, -1.134896524841392473 ) ) ;
#87257=CARTESIAN_POINT ( 'NONE',  ( 4.004543651933685666, 7.806729363262467913, 0.1824581366321497422 ) ) ;
#87258=CARTESIAN_POINT ( 'NONE',  ( 6.317736394288147039, 6.473040002865377396, 0.7216878364870317197 ) ) ;
#87274=CARTESIAN_POINT ( 'NONE',  ( -10.58855478214856660, 11.45566145536924552, -0.7216878364870217277 ) ) ;
#87279=CARTESIAN_POINT ( 'NONE',  ( 6.936968151686458306, 11.24487994360957188, 0.7998128361456462443 ) ) ;
#87283=CARTESIAN_POINT ( 'NONE',  ( -1.402160292154681736E-14, 1.868750000682816381, -1.732050807568863648 ) ) ;
#87284=CARTESIAN_POINT ( 'NONE',  ( -2.676845263694313637, 5.210404343363602919, -1.199719254218446718 ) ) ;
#87285=CARTESIAN_POINT ( 'NONE',  ( -4.557512192488103686, 8.468847991211438497, -0.7998128361456281477 ) ) ;
#87288=CARTESIAN_POINT ( 'NONE',  ( -9.969323024750229578, 10.52529837183042716, -0.7998128361456291469 ) ) ;
#87292=CARTESIAN_POINT ( 'NONE',  ( 6.938021921891177612, 9.117444880338284818, -1.599625672291262513 ) ) ;
#87294=CARTESIAN_POINT ( 'NONE',  ( -6.418895661066105873, 9.576129806964074120, -1.199719254218440723 ) ) ;
#87296=CARTESIAN_POINT ( 'NONE',  ( 9.206149998879153529, 10.69926207256923689, 1.199719254218453823 ) ) ;
#87297=CARTESIAN_POINT ( 'NONE',  ( -1.201851678989727383E-14, 5.446875000341422357, -1.575800808251660134 ) ) ;
#87299=CARTESIAN_POINT ( 'NONE',  ( -0.4652293495373896470, 7.465077128757534375, 4.424517295598821676 ) ) ;
#87303=CARTESIAN_POINT ( 'NONE',  ( -5.910991785878158211, 9.839981483592442402, -0.7216878364870278340 ) ) ;
#87306=CARTESIAN_POINT ( 'NONE',  ( 1.364683531249988535, 4.176041667008081326, 0.7879004041258500513 ) ) ;
#87312=CARTESIAN_POINT ( 'NONE',  ( -1.364683531250010295, 5.738541667008088432, -0.7879004041258300672 ) ) ;
#87316=CARTESIAN_POINT ( 'NONE',  ( -3.999292125906916073, 5.688926785023260102, 1.443375672974064550 ) ) ;
#87318=CARTESIAN_POINT ( 'NONE',  ( 2.535011535630975477, 5.901337858304024131, 0.7216878364870438212 ) ) ;
#87319=CARTESIAN_POINT ( 'NONE',  ( -8.292783513053063160, 12.82666453187061073, 0.7998128361456481317 ) ) ;
#87325=CARTESIAN_POINT ( 'NONE',  ( -1.364683531250014514, 0.7385416670080887647, -0.7879004041258289570 ) ) ;
#87326=CARTESIAN_POINT ( 'NONE',  ( -2.168941388506379742, 5.474256019991960542, -0.7216878364870267237 ) ) ;
#87327=CARTESIAN_POINT ( 'NONE',  ( 3.798255590122797898, 7.583048621785260401, -0.7998128361456221525 ) ) ;
#87333=CARTESIAN_POINT ( 'NONE',  ( 3.768803514918948938, 4.459654191235965293, -1.082531754730543083 ) ) ;
#87336=CARTESIAN_POINT ( 'NONE',  ( -8.853111120043687166, 9.430977182913531820, 1.040834085586084257E-14 ) ) ;
#87342=CARTESIAN_POINT ( 'NONE',  ( -8.809047120577080392, 11.30030761213851953, 1.599625672291269396 ) ) ;
#87344=CARTESIAN_POINT ( 'NONE',  ( -5.707619481228822345, 7.681975366232176583, -1.443375672974051449 ) ) ;
#87345=CARTESIAN_POINT ( 'NONE',  ( -1.201851678989727383E-14, 1.634375000341421025, 1.575800808251672791 ) ) ;
#87352=CARTESIAN_POINT ( 'NONE',  ( 9.561524646135536543, 12.17819805862340310, -1.599625672291262513 ) ) ;
#87354=ORIENTED_EDGE ( 'NONE', *, *, #1511, .F. ) ;
#87363=EDGE_CURVE ( 'NONE', #7066, #17518, #129635, .T. ) ;
#87369=CARTESIAN_POINT ( 'NONE',  ( 1.364683531249990311, 3.196875000341416140, 1.214306433183764966E-14 ) ) ;
#87380=CARTESIAN_POINT ( 'NONE',  ( -0.6823417656250003738, 1.217708333674752286, -1.181850606188749264 ) ) ;
#87391=CARTESIAN_POINT ( 'NONE',  ( 5.412729640353754590, 7.337937218544611895, 1.599625672291267398 ) ) ;
#87396=CARTESIAN_POINT ( 'NONE',  ( 4.104141037658032509, 5.763691012587534246, 1.360812383240009860 ) ) ;
#87398=CARTESIAN_POINT ( 'NONE',  ( 8.471147050440139381, 8.777426401801974976, -0.7998128361456281477 ) ) ;
#87402=CARTESIAN_POINT ( 'NONE',  ( -3.867100128395853709, 5.534702787927018974, -1.599625672291256295 ) ) ;
#87404=CARTESIAN_POINT ( 'NONE',  ( 7.151035956204054855, 10.43029348462504124, 1.199719254218460707 ) ) ;
#87413=CARTESIAN_POINT ( 'NONE',  ( 1.484314741415208694, 7.334687650741242848, -4.257443109328156616 ) ) ;
#87417=CARTESIAN_POINT ( 'NONE',  ( -7.863365906246068349, 9.236643647784308797, -1.082531754730543971 ) ) ;
#87421=CARTESIAN_POINT ( 'NONE',  ( -10.47097470845587175, 11.11055866948701443, 1.040834085586084257E-14 ) ) ;
#87426=CARTESIAN_POINT ( 'NONE',  ( -3.918470089549458635, 4.530302178351167441, -1.199719254218452047 ) ) ;
#87428=CARTESIAN_POINT ( 'NONE',  ( 8.615316546479974136, 12.13862083994696839, 1.199719254218450271 ) ) ;
#87429=CARTESIAN_POINT ( 'NONE',  ( 4.891794496432329886, 4.601515088792824670, -0.7998128361456211532 ) ) ;
#87435=CARTESIAN_POINT ( 'NONE',  ( 2.873965376416980355, 6.296784005887697155, -0.7216878364870267237 ) ) ;
#87437=CARTESIAN_POINT ( 'NONE',  ( -5.928993247877788697, 5.811580298812519807, 0.7998128361456341429 ) ) ;
#87440=CARTESIAN_POINT ( 'NONE',  ( -9.001723924469462901, 12.58942944760136484, -1.199719254218446718 ) ) ;
#87446=CARTESIAN_POINT ( 'NONE',  ( 7.131225611108079399, 11.26358761302737754, 0.7216878364870438212 ) ) ;
#87448=CARTESIAN_POINT ( 'NONE',  ( -1.364683531250012516, 3.592708333674750065, 0.7879004041258379498 ) ) ;
#87451=CARTESIAN_POINT ( 'NONE',  ( 5.009901455449552010, 5.803638771901306725, -1.199719254218452047 ) ) ;
#87456=CARTESIAN_POINT ( 'NONE',  ( -1.436715752608711538, 7.421775496532096561, 4.237684949271969259 ) ) ;
#87463=CARTESIAN_POINT ( 'NONE',  ( -0.6823417656250003738, 2.780208333674753618, -1.181850606188749264 ) ) ;
#87465=CARTESIAN_POINT ( 'NONE',  ( 10.55232363013785246, 11.20546574478267132, 0.000000000000000000 ) ) ;
#87468=CARTESIAN_POINT ( 'NONE',  ( -5.639828713604883248, 6.642516923036197340, 1.082531754730548412 ) ) ;
#87471=CARTESIAN_POINT ( 'NONE',  ( -6.033015167956818026, 6.140865238812146742, -0.7216878364870267237 ) ) ;
#87474=VERTEX_POINT ( 'NONE', #17011 ) ;
#87476=CARTESIAN_POINT ( 'NONE',  ( 3.960953433486789521, 7.772862772376584850, -0.7998128361456221525 ) ) ;
#87486=CARTESIAN_POINT ( 'NONE',  ( 5.412729640353754590, 7.337937218544611895, 1.599625672291267398 ) ) ;
#87487=EDGE_CURVE ( 'NONE', #25476, #180844, #113545, .T. ) ;
#87492=CARTESIAN_POINT ( 'NONE',  ( -7.237355071596549116, 7.338002426484427687, 1.040834085586084257E-14 ) ) ;
#87496=CARTESIAN_POINT ( 'NONE',  ( 6.588372581236919601, 9.773852880496709972, -1.199719254218440723 ) ) ;
#87499=CARTESIAN_POINT ( 'NONE',  ( -7.739006755302186846, 7.923262724141010516, 0.7998128361456462443 ) ) ;
#87501=CARTESIAN_POINT ( 'NONE',  ( 7.144783764277405247, 8.398297815487545392, -1.082531754730543971 ) ) ;
#87502=CARTESIAN_POINT ( 'NONE',  ( 5.221388208558932931, 6.626734370510860117, 1.385765457383714816 ) ) ;
#87504=CARTESIAN_POINT ( 'NONE',  ( -3.490334480514268645, 6.159475096320226939, -1.199719254218452935 ) ) ;
#87507=CARTESIAN_POINT ( 'NONE',  ( -7.250913225210214641, 7.353820272367037170, 0.7998128361456341429 ) ) ;
#87510=CARTESIAN_POINT ( 'NONE',  ( -1.364683531250000748, 1.759375000341421913, 0.000000000000000000 ) ) ;
#87512=CARTESIAN_POINT ( 'NONE',  ( -5.097502569058215194, 6.970172302033127210, -1.443375672974053447 ) ) ;
#87518=CARTESIAN_POINT ( 'NONE',  ( 5.469824908109481854, 8.468880595181346393, -1.199719254218446718 ) ) ;
#87520=CARTESIAN_POINT ( 'NONE',  ( -5.867692518273577740, 6.026634161543212187, 0.3546184694816056360 ) ) ;
#87521=CARTESIAN_POINT ( 'NONE',  ( -1.364683531250014514, 1.801041667008085767, -0.7879004041258289570 ) ) ;
#87523=DIRECTION ( 'NONE',  ( 1.000000000000000000, 0.000000000000000000, 0.000000000000000000 ) ) ;
#87524=CARTESIAN_POINT ( 'NONE',  ( -0.2939347205469681756, 8.204283511488997149, 1.979604457746021895 ) ) ;
#87525=DIRECTION ( 'NONE',  ( -5.578564026256490882E-16, -1.000000000000000000, -9.066213480720158442E-32 ) ) ;
#87527=CARTESIAN_POINT ( 'NONE',  ( -3.411848212133334446, 7.132240014130862171, 0.7998128361456341429 ) ) ;
#87528=CARTESIAN_POINT ( 'NONE',  ( -6.629573926958124197, 9.717958100551031819, 1.082531754730548412 ) ) ;
#87536=CARTESIAN_POINT ( 'NONE',  ( -6.507550544435101614, 10.53596670190887963, 0.000000000000000000 ) ) ;
#87539=CARTESIAN_POINT ( 'NONE',  ( -5.816084710138169633, 8.768887347594400694, 1.082531754730548412 ) ) ;
#87542=EDGE_LOOP ( 'NONE', ( #154519, #101122, #17827, #43081 ) ) ;
#87545=CARTESIAN_POINT ( 'NONE',  ( 1.499999999999989120, 5.577083334016153415, -0.8660254037844323793 ) ) ;
#87550=EDGE_LOOP ( 'NONE', ( #172575, #73519, #46027, #80223 ) ) ;
#87553=CARTESIAN_POINT ( 'NONE',  ( -6.728924311084075960, 6.744833205886536120, 1.040834085586084257E-14 ) ) ;
#87556=CARTESIAN_POINT ( 'NONE',  ( 4.630273154266905777, 5.360739087188218122, 1.199719254218464037 ) ) ;
#87560=CARTESIAN_POINT ( 'NONE',  ( 5.982172092127724383, 8.002286745614243912, -1.599625672291262513 ) ) ;
#87565=CARTESIAN_POINT ( 'NONE',  ( -5.450014563013544588, 5.460697866378308341, 0.7216878364870317197 ) ) ;
#87573=CARTESIAN_POINT ( 'NONE',  ( 0.6823417656249882723, 0.9260416670080831025, -1.181850606188749264 ) ) ;
#87575=CARTESIAN_POINT ( 'NONE',  ( -8.045874094706015001, 11.47427131287732927, -1.199719254218446718 ) ) ;
#87577=CARTESIAN_POINT ( 'NONE',  ( 6.120616281565444794, 9.228137197546649517, -1.199719254218440723 ) ) ;
#87579=CARTESIAN_POINT ( 'NONE',  ( -7.823218330285243383, 9.085841792542966644, -1.199719254218446718 ) ) ;
#87582=CARTESIAN_POINT ( 'NONE',  ( 0.6823417656249917140, 4.842708333674755394, 1.181850606188765695 ) ) ;
#87584=CARTESIAN_POINT ( 'NONE',  ( 8.378575743565351175, 11.75846021992619406, -1.082531754730543083 ) ) ;
#87587=CARTESIAN_POINT ( 'NONE',  ( -1.402160292154681736E-14, -0.1156249996585793222, 1.575800808251672791 ) ) ;
#87590=CARTESIAN_POINT ( 'NONE',  ( 7.415946836550714849, 9.675023947441092176, 1.443375672974076540 ) ) ;
#87593=CARTESIAN_POINT ( 'NONE',  ( -4.934804725694220906, 7.740727365743146571, -1.082531754730549967 ) ) ;
#87596=CARTESIAN_POINT ( 'NONE',  ( 0.6823417656249917140, 3.842708333674754506, 1.181850606188765695 ) ) ;
#87600=CARTESIAN_POINT ( 'NONE',  ( -6.392833124043511894, 7.417059051927569868, 1.199719254218450271 ) ) ;
#87607=CARTESIAN_POINT ( 'NONE',  ( 6.747154001095143627, 11.02343010125301959, -0.7998128361456291469 ) ) ;
#87615=CARTESIAN_POINT ( 'NONE',  ( 5.327991180490514012, 9.159814110640187579, 1.040834085586084257E-14 ) ) ;
#87616=CARTESIAN_POINT ( 'NONE',  ( 1.364683531249986537, -0.5322916663252452718, -0.7879004041258309554 ) ) ;
#87619=AXIS2_PLACEMENT_3D ( 'NONE', #120914, #205259, #41744 ) ;
#87623=CARTESIAN_POINT ( 'NONE',  ( -0.7500000000000215383, 0.6916666666666876351, 1.299038105676659116 ) ) ;
#87624=CARTESIAN_POINT ( 'NONE',  ( 8.586391356156291010, 8.911878091804165791, 0.7998128361456481317 ) ) ;
#87625=CARTESIAN_POINT ( 'NONE',  ( -8.992082194361570302, 11.51384853155376220, 1.599625672291269396 ) ) ;
#87627=CARTESIAN_POINT ( 'NONE',  ( -1.364683531250014514, -0.7197916663252461600, 0.7879004041258379498 ) ) ;
#87628=CARTESIAN_POINT ( 'NONE',  ( -1.201851678989727383E-14, 1.712500000000019229, 1.732050807568877637 ) ) ;
#87630=CARTESIAN_POINT ( 'NONE',  ( 5.820528018968444961, 5.685037531751635953, 0.7998128361456341429 ) ) ;
#87638=CARTESIAN_POINT ( 'NONE',  ( -1.201851678989727383E-14, 5.446875000341422357, -1.575800808251660134 ) ) ;
#87640=CARTESIAN_POINT ( 'NONE',  ( -9.494787648271923786, 9.971673765939062406, 1.040834085586084257E-14 ) ) ;
#87641=CARTESIAN_POINT ( 'NONE',  ( -4.433153041988574294, 8.115836282387899558, 1.040834085586084257E-14 ) ) ;
#87649=EDGE_LOOP ( 'NONE', ( #82610, #98648, #177860, #165242, #195985, #129179 ) ) ;
#87650=CARTESIAN_POINT ( 'NONE',  ( 7.344766530301147789, 9.591980256816594164, 1.599625672291281386 ) ) ;
#87654=DIRECTION ( 'NONE',  ( 1.000000000000000000, -5.391474854832587087E-16, 0.000000000000000000 ) ) ;
#87655=CARTESIAN_POINT ( 'NONE',  ( 5.463572716182812705, 9.317992568947877530, 0.7216878364870438212 ) ) ;
#87657=CARTESIAN_POINT ( 'NONE',  ( -8.830438121202295321, 9.196599317691152464, -0.7998128361456291469 ) ) ;
#87658=CARTESIAN_POINT ( 'NONE',  ( 4.873266149108180123, 7.772895376346490970, 1.199719254218462483 ) ) ;
#87660=DIRECTION ( 'NONE',  ( 3.209122457311483071E-14, 0.6299249119529743979, 0.7766560405359875796 ) ) ;
#87661=CARTESIAN_POINT ( 'NONE',  ( 3.708318708537623021, 4.285125567170706695, -1.199719254218446718 ) ) ;
#87666=CARTESIAN_POINT ( 'NONE',  ( -5.016153647376219382, 6.875265226737464985, 1.443375672974064550 ) ) ;
#87667=CARTESIAN_POINT ( 'NONE',  ( 3.816783937446950770, 4.411668334231586996, 1.199719254218464037 ) ) ;
#87670=CARTESIAN_POINT ( 'NONE',  ( -5.357443255694392725, 9.402100898285455699, 0.000000000000000000 ) ) ;
#87673=DIRECTION ( 'NONE',  ( -3.347138415753903010E-16, -0.6000000000000019762, 0.7999999999999986011 ) ) ;
#87675=CARTESIAN_POINT ( 'NONE',  ( -8.345207244411405156, 9.694828859023472134, 1.199719254218462483 ) ) ;
#87686=CARTESIAN_POINT ( 'NONE',  ( 2.310781476690497271, 5.467761476598782977, -0.5169845646830224517 ) ) ;
#87688=CARTESIAN_POINT ( 'NONE',  ( -6.205881626753225966, 8.263281202677319470, 1.599625672291283607 ) ) ;
#87691=CARTESIAN_POINT ( 'NONE',  ( 4.961921032921539521, 7.772363057508363759, -1.082531754730549078 ) ) ;
#87693=CARTESIAN_POINT ( 'NONE',  ( -0.09185872022810087634, 6.492156809554922248, 3.106929658804562067 ) ) ;
#87696=CARTESIAN_POINT ( 'NONE',  ( -6.112028321662274166, 6.025121218227761588, 0.7998128361456341429 ) ) ;
#87701=CARTESIAN_POINT ( 'NONE',  ( -4.394814349124112951, 8.279033840620114049, -0.7998128361456281477 ) ) ;
#87708=CARTESIAN_POINT ( 'NONE',  ( -10.01677656239806247, 10.58066083241955901, 0.7998128361456462443 ) ) ;
#87709=CARTESIAN_POINT ( 'NONE',  ( 5.991813822235618758, 9.077867661661846554, 1.199719254218462483 ) ) ;
#87710=EDGE_CURVE ( 'NONE', #177025, #73290, #197845, .T. ) ;
#87713=CARTESIAN_POINT ( 'NONE',  ( -9.484092147959342967, 11.02352791316275216, 1.199719254218462483 ) ) ;
#87714=AXIS2_PLACEMENT_3D ( 'NONE', #159997, #110249, #111315 ) ;
#87720=CARTESIAN_POINT ( 'NONE',  ( 8.703971430293332645, 12.13808852110884118, -1.082531754730543083 ) ) ;
#87728=CARTESIAN_POINT ( 'NONE',  ( -0.09252986280859777646, 7.021014873011406365, -3.994686497348480803 ) ) ;
#87739=CARTESIAN_POINT ( 'NONE',  ( -5.271422797614987665, 5.044414773505913274, -0.7998128361456221525 ) ) ;
#87746=CARTESIAN_POINT ( 'NONE',  ( 1.499999999999985123, -1.172916665983846363, -0.8660254037844323793 ) ) ;
#87752=CARTESIAN_POINT ( 'NONE',  ( 1.490514837427000527, 7.209629588552902035, -4.246172784737240136 ) ) ;
#87753=CARTESIAN_POINT ( 'NONE',  ( -1.150196859685111317, 3.270291321728038714, 0.7750000000000083489 ) ) ;
#87755=CARTESIAN_POINT ( 'NONE',  ( 2.706824224222692088, 6.309712028235118453, 0.7998128361456362523 ) ) ;
#87761=CARTESIAN_POINT ( 'NONE',  ( 6.010342169559767633, 5.906487374108181143, -0.7998128361456281477 ) ) ;
#87762=CARTESIAN_POINT ( 'NONE',  ( 1.364683531249990311, 2.946875000341416140, 1.214306433183764966E-14 ) ) ;
#87763=CARTESIAN_POINT ( 'NONE',  ( -4.397013243575890407, 7.155424720373004810, 1.066431095959238462 ) ) ;
#87766=CARTESIAN_POINT ( 'NONE',  ( -9.643927338022246332, 10.14567007064778004, -0.7998128361456291469 ) ) ;
#87767=CARTESIAN_POINT ( 'NONE',  ( -5.273758565591545988, 6.215435083687305351, 1.082531754730546636 ) ) ;
#87770=CARTESIAN_POINT ( 'NONE',  ( -6.579784621333750749, 6.570836901177822931, 0.7998128361456341429 ) ) ;
#87772=CARTESIAN_POINT ( 'NONE',  ( -1.364683531250010295, 5.738541667008088432, -0.7879004041258300672 ) ) ;
#87782=CARTESIAN_POINT ( 'NONE',  ( -4.406036734316882253, 8.084200590104265061, -0.7216878364870257245 ) ) ;
#87788=CARTESIAN_POINT ( 'NONE',  ( -3.402733366905605905, 6.913679994791092298, 0.7216878364870317197 ) ) ;
#87790=CARTESIAN_POINT ( 'NONE',  ( 9.097684769969825780, 10.57271930550834860, -1.199719254218446718 ) ) ;
#87796=ORIENTED_EDGE ( 'NONE', *, *, #98243, .T. ) ;
#87800=CARTESIAN_POINT ( 'NONE',  ( 4.582292731738905722, 5.408724944192588424, -1.082531754730548412 ) ) ;
#87801=CARTESIAN_POINT ( 'NONE',  ( -4.274898507010545856, 3.881803101134051470, -0.7998128361456221525 ) ) ;
#87802=CARTESIAN_POINT ( 'NONE',  ( -10.47097470845587175, 11.11055866948701443, 1.040834085586084257E-14 ) ) ;
#87807=CARTESIAN_POINT ( 'NONE',  ( 5.296431564432884542, 9.330920591813708143, 1.040834085586084257E-14 ) ) ;
#87811=( BOUNDED_SURFACE ( )  B_SPLINE_SURFACE ( 1, 2, ( 
 ( #84595, #166923, #149599, #170103, #118230, #87801, #153874, #203651, #186349, #55302, #150683, #1185, #135493, #37984, #5443, #36901, #53164, #67249, #69385, #101915, #2244, #35837, #104057, #133384, #71522, #199389, #167981, #117158, #19586, #119292, #102983, #86727, #136563, #202584, #126785, #60623, #156004, #208987, #175462, #142987, #92091, #7591, #125713, #206867, #27047, #76867, #24915, #174406, #25983, #93155, #122530, #91019, #6522, #9737, #140854, #207932, #188491, #158145, #73675, #139774, #40123, #205801, #154938, #23846, #89953, #106233, #157081, #172258, #57432, #123593, #192741, #189558, #44396, #41204, #171177, #59554, #22768, #88884, #107311, #72599, #173335, #138699, #204717, #56366, #58498, #8669, #43336, #74752, #124654, #75812, #190610, #141921, #191674, #42269, #108381, #109456, #159193, #10793, #127866, #179725, #61697, #213260, #114776, #111581, #79003, #177590, #112650, #194891, #193816, #47607, #97419, #30270, #176517, #62750, #28129, #15055, #82200, #198083, #65925, #132072, #29203, #164530, #64887, #178659, #131033, #46529, #16117, #81147, #94225, #110517, #95293, #147232, #31344, #160263, #148293, #80072, #161342, #197023, #214291, #12924, #163473, #45464, #48660, #180774, #212190, #162411, #96356, #11865, #32400, #145120, #98466, #211126, #77942, #144063, #128910, #13988, #146175, #63828, #129986, #195974, #113721, #210058, #183970, #115839, #1994, #181825, #168791, #21445, #137382, #5193, #71268, #182903, #103808, #4130, #51857, #152544, #134195, #169857, #20397, #33458, #49710, #50776, #86480, #119041, #202333, #186099, #87553, #70199, #153622, #66994, #99534, #167729, #136312, #53983, #3062, #19330, #165595, #117979, #200204, #116904, #199131, #120121, #17186, #37729, #83261, #34520, #149347, #927, #101661, #133132, #100592, #69132, #166667, #18258, #84341, #150429, #68059, #35582, #85408, #185025, #151493, #135254, #201268, #52908, #36650, #102736, #206620, #58249, #207689, #154686, #57184, #38799, #42025, #173082, #25733, #6270, #190363, #39874, #105984, #72341, #172006, #187171, #56119, #122276, #138447, #123346, #204465, #188234, #23596, #158952, #89705, #26804, #155755, #10547, #91844, #92906, #109207, #7340, #76621, #73417, #203398, #124405, #59308, #139520, #189312, #104880, #108134, #24663, #157901, #205546, #174162, #40950, #107057, #90770, #156831, #170923, #8418, #74504, #140608, #9495, #75567, #141677, #125465, #55051, #191427, #121201, #43094, #22520, #175219, #88630, #48417, #193575, #32145, #28950, #180523, #208743, #114529, #112397, #143811, #14806, #98225, #45218, #195718, #77690, #47353, #97169, #30019, #194638, #210880, #126533, #63578, #160016, #211943, #93975, #31097, #146987, #209808, #111333, #61443, #144873, #12674, #11616, #79819, #129735, #62505, #60370, #95034, #192494, #113468, #164277, #15867, #142734, #44146, #127610, #196774, #163224, #128670, #80897, #78750, #110267, #179473, #176276, #27878, #177337, #213005, #64641, #130781, #161084, #46281, #178408, #96104, #162159, #13746, #145931, #36392, #86220, #35322, #199954, #81952, #150172, #166402, #83009, #16929, #118780, #197828, #3865, #37464, #149084, #49460, #136050, #133946, #33204, #148037, #101400, #102470, #103542, #185833, #66729, #119855, #152291, #53722, #2804, #132873, #168536, #117725, #69939, #202062, #1739, #85150, #214045, #50523, #663, #115580, #19070, #198876, #20134, #65672, #181574, #116646, #182642, #99287, #131819, #169603, #34263, #165335, #67797, #68876, #184766, #100336, #17994, #84083, #51600, #183714, #134996, #201006, #167475, #151235, #52651, #23330, #74246, #204196, #8162, #55851, #205283, #194114, #87288, #187974, #54789, #153357, #75306, #41763, #24391, #107876, #4928, #120935, #89438, #157636, #137117, #90503, #21186, #128154, #71004, #203146, #61998, #172819, #156567, #186908, #106791, #140340, #38540, #111882, #104617, #155490, #56921, #170665, #22252, #141422, #88362, #123094, #154428, #6006, #173902, #206358, #72076, #124148, #45764, #73145, #207428, #138187, #57985, #9234, #40688, #122008, #190110, #105704, #7073, #39601, #25477, #91584, #171732, #139251 ),
 ( #189051, #30573, #129222, #148, #145424, #79308, #29499, #83558, #98765, #31636, #51072, #146469, #96654, #14279, #212488, #80374, #161640, #130273, #195196, #131319, #149640, #163771, #65164, #46833, #67284, #162707, #181067, #112946, #64130, #116128, #197312, #66214, #99823, #13235, #15349, #132362, #196262, #47909, #178958, #198364, #211425, #63055, #95591, #1222, #164821, #97713, #177886, #114019, #180015, #81442, #147520, #213541, #48953, #115071, #32685, #16412, #133423, #82492, #148579, #50004, #182115, #33745, #165889, #17474, #199429, #117197, #18553, #85693, #184249, #68357, #183195, #55335, #151781, #34801, #185318, #104093, #153909, #138734, #3354, #52137, #171210, #86766, #170142, #21728, #69424, #100876, #101951, #119331, #87838, #135530, #5479, #201554, #152837, #72637, #166963, #53200, #150721, #84630, #22804, #137667, #120410, #203689, #2281, #134490, #36940, #39087, #200493, #186385, #118265, #6557, #35876, #168018, #154972, #54273, #38022, #19621, #202623, #71559, #103022, #204752, #169077, #20676, #4412, #70483, #136599, #88918, #121487, #187459, #105173, #89986, #143023, #175497, #156037, #159224, #11899, #108419, #110549, #107346, #93193, #44432, #75846, #77973, #141953, #140888, #124686, #28161, #207965, #27085, #157115, #7626, #173368, #40157, #8704, #73711, #9773, #94257, #42304, #56403, #24952, #205837, #172292, #59591, #91054, #10825, #122564, #23880, #74788, #123629, #139809, #188526, #209018, #206900, #106270, #190644, #43368, #76899, #144096, #58531, #57470, #176551, #26017, #109490, #60654, #174441, #189593, #41239, #92128, #126817, #158180, #192773, #125748, #191710, #160296, #61730, #162440, #29235, #127898, #49739, #16144, #213288, #82229, #193849, #95327, #63857, #132100, #111615, #64914, #210091, #99560, #45499, #177627, #33488, #147256, #131063, #161376, #81177, #197051, #12959, #83289, #79037, #212222, #31371, #145152, #211158, #115866, #62782, #97447, #128945, #194923, #148320, #114804, #46560, #98495, #165625, #47638, #181851, #112680, #32429, #198109, #15087, #17213, #48689, #80102, #130013, #178690, #180803, #164559, #96389, #30303, #163503, #14016, #146206, #196004, #214319, #113750, #179754, #65951, #102764, #186125, #71294, #199160, #135279, #103832, #51883, #2020, #100619, #37759, #116933, #50805, #957, #55080, #70228, #3088, #22551, #118006, #68089, #200233, #183995, #149374, #69159, #136339, #169880, #170952, #35609, #84371, #203425, #119070, #202359, #54009, #101687, #67023, #134223, #151520, #120148, #167756, #21470, #19355, #185051, #104911, #133159, #85435, #182932, #34548, #121229, #87579, #152570, #153650, #166694, #18285, #201293, #137406, #150459, #4157, #52934, #38827, #36676, #168819, #187199, #86505, #5219, #20423, #174191, #91875, #138473, #176306, #204495, #90797, #124436, #56145, #188264, #208772, #89736, #190394, #39904, #122306, #175248, #207719, #106013, #191459, #44178, #140634, #142767, #139550, #125496, #76652, #108164, #110298, #25763, #173113, #156861, #60402, #157931, #59342, #189341, #172035, #42052, #23628, #192524, #155785, #9524, #7369, #73446, #26834, #75596, #43124, #10578, #205577, #74534, #109238, #57214, #123374, #40980, #92937, #107091, #24694, #154717, #126564, #141708, #8447, #88657, #206647, #58280, #158981, #6298, #72373, #11649, #194666, #193604, #195748, #214075, #13776, #27909, #210909, #177368, #143843, #179505, #78780, #196804, #94006, #209837, #62536, #95068, #45246, #160045, #180554, #128698, #64668, #49489, #46311, #28982, #81981, #211970, #80925, #14835, #112427, #77721, #12703, #30047, #147016, #178441, #213039, #96137, #63609, #197857, #61474, #162189, #127639, #111363, #148069, #48447, #31126, #114561, #161116, #144901, #79851, #164309, #145960, #97200, #129765, #131849, #47385, #113498, #65701, #163253, #130814, #32175, #98252, #15897, #115610, #54822, #83040, #183745, #2835, #149114, #66760, #87319, #182671, #68904, #132901, #695, #53754, #86250, #198906, #69969, #137150, #19101, #21216, #18026, #3897, #169633, #201037, #203177, #52680, #51630, #35355, #153387, #118811, #152320, #67828, #50551, #135023 ) ),
 .UNSPECIFIED., .F., .F., .T. ) 
 B_SPLINE_SURFACE_WITH_KNOTS ( ( 2, 2 ),
 ( 3, 2, 2, 2, 2, 2, 2, 2, 2, 2, 2, 2, 2, 2, 2, 2, 2, 2, 2, 2, 2, 2, 2, 2, 2, 2, 2, 2, 2, 2, 2, 2, 2, 2, 2, 2, 2, 2, 2, 2, 2, 2, 2, 2, 2, 2, 2, 2, 2, 2, 2, 2, 2, 2, 2, 2, 2, 2, 2, 2, 2, 2, 2, 2, 2, 2, 2, 2, 2, 2, 2, 2, 2, 2, 2, 2, 2, 2, 2, 2, 2, 2, 2, 2, 2, 2, 2, 2, 2, 2, 2, 2, 2, 2, 2, 2, 2, 2, 2, 2, 2, 2, 2, 2, 2, 2, 2, 2, 2, 2, 2, 2, 2, 2, 2, 2, 2, 2, 2, 2, 2, 2, 2, 2, 2, 2, 2, 2, 2, 2, 2, 2, 2, 2, 2, 2, 2, 2, 2, 2, 2, 2, 2, 2, 2, 2, 2, 2, 2, 2, 2, 2, 2, 2, 2, 2, 2, 2, 2, 2, 2, 2, 2, 2, 2, 2, 2, 2, 2, 2, 2, 2, 2, 2, 2, 2, 2, 2, 2, 2, 2, 2, 2, 2, 2, 2, 2, 2, 2, 2, 2, 2, 2, 2, 2, 2, 2, 2, 2, 2, 2, 2, 2, 2, 2, 2, 2, 2, 2, 2, 2, 2, 2, 2, 2, 2, 2, 2, 2, 2, 2, 2, 2, 2, 2, 2, 2, 2, 2, 2, 2, 2, 2, 2, 2, 2, 2, 2, 2, 2, 3 ),
 ( 0.000000000000000000, 1.000000000000000000 ),
 ( 0.000000000000000000, 0.004166666666666666609, 0.008333333333333333218, 0.01250000000000000069, 0.01666666666666666644, 0.02083333333333333218, 0.02500000000000000139, 0.02916666666666666713, 0.03333333333333333287, 0.03749999999999999861, 0.04166666666666666435, 0.04583333333333333010, 0.05000000000000000278, 0.05416666666666666852, 0.05833333333333333426, 0.06250000000000000000, 0.06666666666666666574, 0.07083333333333333148, 0.07499999999999999722, 0.07916666666666666297, 0.08333333333333332871, 0.08749999999999999445, 0.09166666666666666019, 0.09583333333333333981, 0.1000000000000000056, 0.1041666666666666713, 0.1083333333333333370, 0.1125000000000000028, 0.1166666666666666685, 0.1208333333333333343, 0.1250000000000000000, 0.1291666666666666796, 0.1333333333333333315, 0.1375000000000000111, 0.1416666666666666630, 0.1458333333333333426, 0.1499999999999999944, 0.1541666666666666741, 0.1583333333333333259, 0.1625000000000000056, 0.1666666666666666574, 0.1708333333333333370, 0.1749999999999999889, 0.1791666666666666685, 0.1833333333333333204, 0.1875000000000000000, 0.1916666666666666796, 0.1958333333333333315, 0.2000000000000000111, 0.2041666666666666630, 0.2083333333333333426, 0.2124999999999999944, 0.2166666666666666741, 0.2208333333333333259, 0.2250000000000000056, 0.2291666666666666574, 0.2333333333333333370, 0.2374999999999999889, 0.2416666666666666685, 0.2458333333333333204, 0.2500000000000000000, 0.2541666666666666519, 0.2583333333333333592, 0.2625000000000000111, 0.2666666666666666630, 0.2708333333333333148, 0.2750000000000000222, 0.2791666666666666741, 0.2833333333333333259, 0.2874999999999999778, 0.2916666666666666852, 0.2958333333333333370, 0.2999999999999999889, 0.3041666666666666408, 0.3083333333333333481, 0.3125000000000000000, 0.3166666666666666519, 0.3208333333333333592, 0.3250000000000000111, 0.3291666666666666630, 0.3333333333333333148, 0.3375000000000000222, 0.3416666666666666741, 0.3458333333333333259, 0.3499999999999999778, 0.3541666666666666852, 0.3583333333333333370, 0.3624999999999999889, 0.3666666666666666408, 0.3708333333333333481, 0.3750000000000000000, 0.3791666666666666519, 0.3833333333333333592, 0.3875000000000000111, 0.3916666666666666630, 0.3958333333333333148, 0.4000000000000000222, 0.4041666666666666741, 0.4083333333333333259, 0.4124999999999999778, 0.4166666666666666852, 0.4208333333333333370, 0.4249999999999999889, 0.4291666666666666408, 0.4333333333333333481, 0.4375000000000000000, 0.4416666666666666519, 0.4458333333333333592, 0.4500000000000000111, 0.4541666666666666630, 0.4583333333333333148, 0.4625000000000000222, 0.4666666666666666741, 0.4708333333333333259, 0.4749999999999999778, 0.4791666666666666852, 0.4833333333333333370, 0.4874999999999999889, 0.4916666666666666408, 0.4958333333333333481, 0.5000000000000000000, 0.5041666666666666519, 0.5083333333333333037, 0.5124999999999999556, 0.5166666666666667185, 0.5208333333333333703, 0.5250000000000000222, 0.5291666666666666741, 0.5333333333333333259, 0.5374999999999999778, 0.5416666666666666297, 0.5458333333333332815, 0.5500000000000000444, 0.5541666666666666963, 0.5583333333333333481, 0.5625000000000000000, 0.5666666666666666519, 0.5708333333333333037, 0.5749999999999999556, 0.5791666666666667185, 0.5833333333333333703, 0.5875000000000000222, 0.5916666666666666741, 0.5958333333333333259, 0.5999999999999999778, 0.6041666666666666297, 0.6083333333333332815, 0.6125000000000000444, 0.6166666666666666963, 0.6208333333333333481, 0.6250000000000000000, 0.6291666666666666519, 0.6333333333333333037, 0.6374999999999999556, 0.6416666666666667185, 0.6458333333333333703, 0.6500000000000000222, 0.6541666666666666741, 0.6583333333333333259, 0.6624999999999999778, 0.6666666666666666297, 0.6708333333333332815, 0.6750000000000000444, 0.6791666666666666963, 0.6833333333333333481, 0.6875000000000000000, 0.6916666666666666519, 0.6958333333333333037, 0.6999999999999999556, 0.7041666666666667185, 0.7083333333333333703, 0.7125000000000000222, 0.7166666666666666741, 0.7208333333333333259, 0.7249999999999999778, 0.7291666666666666297, 0.7333333333333332815, 0.7375000000000000444, 0.7416666666666666963, 0.7458333333333333481, 0.7500000000000000000, 0.7541666666666666519, 0.7583333333333333037, 0.7624999999999999556, 0.7666666666666667185, 0.7708333333333333703, 0.7750000000000000222, 0.7791666666666666741, 0.7833333333333333259, 0.7874999999999999778, 0.7916666666666666297, 0.7958333333333332815, 0.8000000000000000444, 0.8041666666666666963, 0.8083333333333333481, 0.8125000000000000000, 0.8166666666666666519, 0.8208333333333333037, 0.8249999999999999556, 0.8291666666666667185, 0.8333333333333333703, 0.8375000000000000222, 0.8416666666666666741, 0.8458333333333333259, 0.8499999999999999778, 0.8541666666666666297, 0.8583333333333332815, 0.8625000000000000444, 0.8666666666666666963, 0.8708333333333333481, 0.8750000000000000000, 0.8791666666666666519, 0.8833333333333333037, 0.8874999999999999556, 0.8916666666666667185, 0.8958333333333333703, 0.9000000000000000222, 0.9041666666666666741, 0.9083333333333333259, 0.9124999999999999778, 0.9166666666666666297, 0.9208333333333332815, 0.9250000000000000444, 0.9291666666666666963, 0.9333333333333333481, 0.9375000000000000000, 0.9416666666666666519, 0.9458333333333333037, 0.9499999999999999556, 0.9541666666666667185, 0.9583333333333333703, 0.9625000000000000222, 0.9666666666666666741, 0.9708333333333333259, 0.9749999999999999778, 0.9791666666666666297, 0.9833333333333332815, 0.9875000000000000444, 0.9916666666666666963, 0.9958333333333333481, 1.000000000000000000 ),
 .UNSPECIFIED. ) 
 GEOMETRIC_REPRESENTATION_ITEM ( )  RATIONAL_B_SPLINE_SURFACE ( (
 ( 1.000000000000000000, 0.8660254037844387076, 1.000000000000000000, 0.8660254037844387076, 1.000000000000000000, 0.8660254037844387076, 1.000000000000000000, 0.8660254037844387076, 1.000000000000000000, 0.8660254037844387076, 1.000000000000000000, 0.8660254037844387076, 1.000000000000000000, 0.8660254037844387076, 1.000000000000000000, 0.8660254037844387076, 1.000000000000000000, 0.8660254037844387076, 1.000000000000000000, 0.8660254037844387076, 1.000000000000000000, 0.8660254037844387076, 1.000000000000000000, 0.8660254037844387076, 1.000000000000000000, 0.8660254037844387076, 1.000000000000000000, 0.8660254037844387076, 1.000000000000000000, 0.8660254037844387076, 1.000000000000000000, 0.8660254037844387076, 1.000000000000000000, 0.8660254037844387076, 1.000000000000000000, 0.8660254037844387076, 1.000000000000000000, 0.8660254037844387076, 1.000000000000000000, 0.8660254037844387076, 1.000000000000000000, 0.8660254037844387076, 1.000000000000000000, 0.8660254037844387076, 1.000000000000000000, 0.8660254037844387076, 1.000000000000000000, 0.8660254037844387076, 1.000000000000000000, 0.8660254037844387076, 1.000000000000000000, 0.8660254037844387076, 1.000000000000000000, 0.8660254037844387076, 1.000000000000000000, 0.8660254037844387076, 1.000000000000000000, 0.8660254037844387076, 1.000000000000000000, 0.8660254037844387076, 1.000000000000000000, 0.8660254037844387076, 1.000000000000000000, 0.8660254037844387076, 1.000000000000000000, 0.8660254037844387076, 1.000000000000000000, 0.8660254037844387076, 1.000000000000000000, 0.8660254037844387076, 1.000000000000000000, 0.8660254037844387076, 1.000000000000000000, 0.8660254037844387076, 1.000000000000000000, 0.8660254037844387076, 1.000000000000000000, 0.8660254037844387076, 1.000000000000000000, 0.8660254037844387076, 1.000000000000000000, 0.8660254037844387076, 1.000000000000000000, 0.8660254037844387076, 1.000000000000000000, 0.8660254037844387076, 1.000000000000000000, 0.8660254037844387076, 1.000000000000000000, 0.8660254037844387076, 1.000000000000000000, 0.8660254037844387076, 1.000000000000000000, 0.8660254037844387076, 1.000000000000000000, 0.8660254037844387076, 1.000000000000000000, 0.8660254037844387076, 1.000000000000000000, 0.8660254037844387076, 1.000000000000000000, 0.8660254037844387076, 1.000000000000000000, 0.8660254037844387076, 1.000000000000000000, 0.8660254037844387076, 1.000000000000000000, 0.8660254037844387076, 1.000000000000000000, 0.8660254037844387076, 1.000000000000000000, 0.8660254037844387076, 1.000000000000000000, 0.8660254037844387076, 1.000000000000000000, 0.8660254037844387076, 1.000000000000000000, 0.8660254037844387076, 1.000000000000000000, 0.8660254037844387076, 1.000000000000000000, 0.8660254037844387076, 1.000000000000000000, 0.8660254037844387076, 1.000000000000000000, 0.8660254037844387076, 1.000000000000000000, 0.8660254037844387076, 1.000000000000000000, 0.8660254037844387076, 1.000000000000000000, 0.8660254037844387076, 1.000000000000000000, 0.8660254037844387076, 1.000000000000000000, 0.8660254037844387076, 1.000000000000000000, 0.8660254037844387076, 1.000000000000000000, 0.8660254037844387076, 1.000000000000000000, 0.8660254037844387076, 1.000000000000000000, 0.8660254037844387076, 1.000000000000000000, 0.8660254037844387076, 1.000000000000000000, 0.8660254037844387076, 1.000000000000000000, 0.8660254037844387076, 1.000000000000000000, 0.8660254037844387076, 1.000000000000000000, 0.8660254037844387076, 1.000000000000000000, 0.8660254037844387076, 1.000000000000000000, 0.8660254037844387076, 1.000000000000000000, 0.8660254037844387076, 1.000000000000000000, 0.8660254037844387076, 1.000000000000000000, 0.8660254037844387076, 1.000000000000000000, 0.8660254037844387076, 1.000000000000000000, 0.8660254037844387076, 1.000000000000000000, 0.8660254037844387076, 1.000000000000000000, 0.8660254037844387076, 1.000000000000000000, 0.8660254037844387076, 1.000000000000000000, 0.8660254037844387076, 1.000000000000000000, 0.8660254037844387076, 1.000000000000000000, 0.8660254037844387076, 1.000000000000000000, 0.8660254037844387076, 1.000000000000000000, 0.8660254037844387076, 1.000000000000000000, 0.8660254037844387076, 1.000000000000000000, 0.8660254037844387076, 1.000000000000000000, 0.8660254037844387076, 1.000000000000000000, 0.8660254037844387076, 1.000000000000000000, 0.8660254037844387076, 1.000000000000000000, 0.8660254037844387076, 1.000000000000000000, 0.8660254037844387076, 1.000000000000000000, 0.8660254037844387076, 1.000000000000000000, 0.8660254037844387076, 1.000000000000000000, 0.8660254037844387076, 1.000000000000000000, 0.8660254037844387076, 1.000000000000000000, 0.8660254037844387076, 1.000000000000000000, 0.8660254037844387076, 1.000000000000000000, 0.8660254037844387076, 1.000000000000000000, 0.8660254037844387076, 1.000000000000000000, 0.8660254037844387076, 1.000000000000000000, 0.8660254037844387076, 1.000000000000000000, 0.8660254037844387076, 1.000000000000000000, 0.8660254037844387076, 1.000000000000000000, 0.8660254037844387076, 1.000000000000000000, 0.8660254037844387076, 1.000000000000000000, 0.8660254037844387076, 1.000000000000000000, 0.8660254037844387076, 1.000000000000000000, 0.8660254037844387076, 1.000000000000000000, 0.8660254037844387076, 1.000000000000000000, 0.8660254037844387076, 1.000000000000000000, 0.8660254037844387076, 1.000000000000000000, 0.8660254037844387076, 1.000000000000000000, 0.8660254037844387076, 1.000000000000000000, 0.8660254037844387076, 1.000000000000000000, 0.8660254037844387076, 1.000000000000000000, 0.8660254037844387076, 1.000000000000000000, 0.8660254037844387076, 1.000000000000000000, 0.8660254037844387076, 1.000000000000000000, 0.8660254037844387076, 1.000000000000000000, 0.8660254037844387076, 1.000000000000000000, 0.8660254037844387076, 1.000000000000000000, 0.8660254037844387076, 1.000000000000000000, 0.8660254037844387076, 1.000000000000000000, 0.8660254037844387076, 1.000000000000000000, 0.8660254037844387076, 1.000000000000000000, 0.8660254037844387076, 1.000000000000000000, 0.8660254037844387076, 1.000000000000000000, 0.8660254037844387076, 1.000000000000000000, 0.8660254037844387076, 1.000000000000000000, 0.8660254037844387076, 1.000000000000000000, 0.8660254037844387076, 1.000000000000000000, 0.8660254037844387076, 1.000000000000000000, 0.8660254037844387076, 1.000000000000000000, 0.8660254037844387076, 1.000000000000000000, 0.8660254037844387076, 1.000000000000000000, 0.8660254037844387076, 1.000000000000000000, 0.8660254037844387076, 1.000000000000000000, 0.8660254037844387076, 1.000000000000000000, 0.8660254037844387076, 1.000000000000000000, 0.8660254037844387076, 1.000000000000000000, 0.8660254037844387076, 1.000000000000000000, 0.8660254037844387076, 1.000000000000000000, 0.8660254037844387076, 1.000000000000000000, 0.8660254037844387076, 1.000000000000000000, 0.8660254037844387076, 1.000000000000000000, 0.8660254037844387076, 1.000000000000000000, 0.8660254037844387076, 1.000000000000000000, 0.8660254037844387076, 1.000000000000000000, 0.8660254037844387076, 1.000000000000000000, 0.8660254037844387076, 1.000000000000000000, 0.8660254037844387076, 1.000000000000000000, 0.8660254037844387076, 1.000000000000000000, 0.8660254037844387076, 1.000000000000000000, 0.8660254037844387076, 1.000000000000000000, 0.8660254037844387076, 1.000000000000000000, 0.8660254037844387076, 1.000000000000000000, 0.8660254037844387076, 1.000000000000000000, 0.8660254037844387076, 1.000000000000000000, 0.8660254037844387076, 1.000000000000000000, 0.8660254037844387076, 1.000000000000000000, 0.8660254037844387076, 1.000000000000000000, 0.8660254037844387076, 1.000000000000000000, 0.8660254037844387076, 1.000000000000000000, 0.8660254037844387076, 1.000000000000000000, 0.8660254037844387076, 1.000000000000000000, 0.8660254037844387076, 1.000000000000000000, 0.8660254037844387076, 1.000000000000000000, 0.8660254037844387076, 1.000000000000000000, 0.8660254037844387076, 1.000000000000000000, 0.8660254037844387076, 1.000000000000000000, 0.8660254037844387076, 1.000000000000000000, 0.8660254037844387076, 1.000000000000000000, 0.8660254037844387076, 1.000000000000000000, 0.8660254037844387076, 1.000000000000000000, 0.8660254037844387076, 1.000000000000000000, 0.8660254037844387076, 1.000000000000000000, 0.8660254037844387076, 1.000000000000000000, 0.8660254037844387076, 1.000000000000000000, 0.8660254037844387076, 1.000000000000000000, 0.8660254037844387076, 1.000000000000000000, 0.8660254037844387076, 1.000000000000000000, 0.8660254037844387076, 1.000000000000000000, 0.8660254037844387076, 1.000000000000000000, 0.8660254037844387076, 1.000000000000000000, 0.8660254037844387076, 1.000000000000000000, 0.8660254037844387076, 1.000000000000000000, 0.8660254037844387076, 1.000000000000000000, 0.8660254037844387076, 1.000000000000000000, 0.8660254037844387076, 1.000000000000000000, 0.8660254037844387076, 1.000000000000000000, 0.8660254037844387076, 1.000000000000000000, 0.8660254037844387076, 1.000000000000000000, 0.8660254037844387076, 1.000000000000000000, 0.8660254037844387076, 1.000000000000000000, 0.8660254037844387076, 1.000000000000000000, 0.8660254037844387076, 1.000000000000000000, 0.8660254037844387076, 1.000000000000000000, 0.8660254037844387076, 1.000000000000000000, 0.8660254037844387076, 1.000000000000000000, 0.8660254037844387076, 1.000000000000000000, 0.8660254037844387076, 1.000000000000000000, 0.8660254037844387076, 1.000000000000000000, 0.8660254037844387076, 1.000000000000000000, 0.8660254037844387076, 1.000000000000000000, 0.8660254037844387076, 1.000000000000000000, 0.8660254037844387076, 1.000000000000000000, 0.8660254037844387076, 1.000000000000000000, 0.8660254037844387076, 1.000000000000000000, 0.8660254037844387076, 1.000000000000000000, 0.8660254037844387076, 1.000000000000000000, 0.8660254037844387076, 1.000000000000000000, 0.8660254037844387076, 1.000000000000000000, 0.8660254037844387076, 1.000000000000000000, 0.8660254037844387076, 1.000000000000000000, 0.8660254037844387076, 1.000000000000000000, 0.8660254037844387076, 1.000000000000000000, 0.8660254037844387076, 1.000000000000000000, 0.8660254037844387076, 1.000000000000000000, 0.8660254037844387076, 1.000000000000000000, 0.8660254037844387076, 1.000000000000000000, 0.8660254037844387076, 1.000000000000000000, 0.8660254037844387076, 1.000000000000000000, 0.8660254037844387076, 1.000000000000000000, 0.8660254037844387076, 1.000000000000000000, 0.8660254037844387076, 1.000000000000000000, 0.8660254037844387076, 1.000000000000000000, 0.8660254037844387076, 1.000000000000000000, 0.8660254037844387076, 1.000000000000000000, 0.8660254037844387076, 1.000000000000000000, 0.8660254037844387076, 1.000000000000000000, 0.8660254037844387076, 1.000000000000000000, 0.8660254037844387076, 1.000000000000000000),
 ( 1.000000000000000000, 0.8660254037844387076, 1.000000000000000000, 0.8660254037844387076, 1.000000000000000000, 0.8660254037844387076, 1.000000000000000000, 0.8660254037844387076, 1.000000000000000000, 0.8660254037844387076, 1.000000000000000000, 0.8660254037844387076, 1.000000000000000000, 0.8660254037844387076, 1.000000000000000000, 0.8660254037844387076, 1.000000000000000000, 0.8660254037844387076, 1.000000000000000000, 0.8660254037844387076, 1.000000000000000000, 0.8660254037844387076, 1.000000000000000000, 0.8660254037844387076, 1.000000000000000000, 0.8660254037844387076, 1.000000000000000000, 0.8660254037844387076, 1.000000000000000000, 0.8660254037844387076, 1.000000000000000000, 0.8660254037844387076, 1.000000000000000000, 0.8660254037844387076, 1.000000000000000000, 0.8660254037844387076, 1.000000000000000000, 0.8660254037844387076, 1.000000000000000000, 0.8660254037844387076, 1.000000000000000000, 0.8660254037844387076, 1.000000000000000000, 0.8660254037844387076, 1.000000000000000000, 0.8660254037844387076, 1.000000000000000000, 0.8660254037844387076, 1.000000000000000000, 0.8660254037844387076, 1.000000000000000000, 0.8660254037844387076, 1.000000000000000000, 0.8660254037844387076, 1.000000000000000000, 0.8660254037844387076, 1.000000000000000000, 0.8660254037844387076, 1.000000000000000000, 0.8660254037844387076, 1.000000000000000000, 0.8660254037844387076, 1.000000000000000000, 0.8660254037844387076, 1.000000000000000000, 0.8660254037844387076, 1.000000000000000000, 0.8660254037844387076, 1.000000000000000000, 0.8660254037844387076, 1.000000000000000000, 0.8660254037844387076, 1.000000000000000000, 0.8660254037844387076, 1.000000000000000000, 0.8660254037844387076, 1.000000000000000000, 0.8660254037844387076, 1.000000000000000000, 0.8660254037844387076, 1.000000000000000000, 0.8660254037844387076, 1.000000000000000000, 0.8660254037844387076, 1.000000000000000000, 0.8660254037844387076, 1.000000000000000000, 0.8660254037844387076, 1.000000000000000000, 0.8660254037844387076, 1.000000000000000000, 0.8660254037844387076, 1.000000000000000000, 0.8660254037844387076, 1.000000000000000000, 0.8660254037844387076, 1.000000000000000000, 0.8660254037844387076, 1.000000000000000000, 0.8660254037844387076, 1.000000000000000000, 0.8660254037844387076, 1.000000000000000000, 0.8660254037844387076, 1.000000000000000000, 0.8660254037844387076, 1.000000000000000000, 0.8660254037844387076, 1.000000000000000000, 0.8660254037844387076, 1.000000000000000000, 0.8660254037844387076, 1.000000000000000000, 0.8660254037844387076, 1.000000000000000000, 0.8660254037844387076, 1.000000000000000000, 0.8660254037844387076, 1.000000000000000000, 0.8660254037844387076, 1.000000000000000000, 0.8660254037844387076, 1.000000000000000000, 0.8660254037844387076, 1.000000000000000000, 0.8660254037844387076, 1.000000000000000000, 0.8660254037844387076, 1.000000000000000000, 0.8660254037844387076, 1.000000000000000000, 0.8660254037844387076, 1.000000000000000000, 0.8660254037844387076, 1.000000000000000000, 0.8660254037844387076, 1.000000000000000000, 0.8660254037844387076, 1.000000000000000000, 0.8660254037844387076, 1.000000000000000000, 0.8660254037844387076, 1.000000000000000000, 0.8660254037844387076, 1.000000000000000000, 0.8660254037844387076, 1.000000000000000000, 0.8660254037844387076, 1.000000000000000000, 0.8660254037844387076, 1.000000000000000000, 0.8660254037844387076, 1.000000000000000000, 0.8660254037844387076, 1.000000000000000000, 0.8660254037844387076, 1.000000000000000000, 0.8660254037844387076, 1.000000000000000000, 0.8660254037844387076, 1.000000000000000000, 0.8660254037844387076, 1.000000000000000000, 0.8660254037844387076, 1.000000000000000000, 0.8660254037844387076, 1.000000000000000000, 0.8660254037844387076, 1.000000000000000000, 0.8660254037844387076, 1.000000000000000000, 0.8660254037844387076, 1.000000000000000000, 0.8660254037844387076, 1.000000000000000000, 0.8660254037844387076, 1.000000000000000000, 0.8660254037844387076, 1.000000000000000000, 0.8660254037844387076, 1.000000000000000000, 0.8660254037844387076, 1.000000000000000000, 0.8660254037844387076, 1.000000000000000000, 0.8660254037844387076, 1.000000000000000000, 0.8660254037844387076, 1.000000000000000000, 0.8660254037844387076, 1.000000000000000000, 0.8660254037844387076, 1.000000000000000000, 0.8660254037844387076, 1.000000000000000000, 0.8660254037844387076, 1.000000000000000000, 0.8660254037844387076, 1.000000000000000000, 0.8660254037844387076, 1.000000000000000000, 0.8660254037844387076, 1.000000000000000000, 0.8660254037844387076, 1.000000000000000000, 0.8660254037844387076, 1.000000000000000000, 0.8660254037844387076, 1.000000000000000000, 0.8660254037844387076, 1.000000000000000000, 0.8660254037844387076, 1.000000000000000000, 0.8660254037844387076, 1.000000000000000000, 0.8660254037844387076, 1.000000000000000000, 0.8660254037844387076, 1.000000000000000000, 0.8660254037844387076, 1.000000000000000000, 0.8660254037844387076, 1.000000000000000000, 0.8660254037844387076, 1.000000000000000000, 0.8660254037844387076, 1.000000000000000000, 0.8660254037844387076, 1.000000000000000000, 0.8660254037844387076, 1.000000000000000000, 0.8660254037844387076, 1.000000000000000000, 0.8660254037844387076, 1.000000000000000000, 0.8660254037844387076, 1.000000000000000000, 0.8660254037844387076, 1.000000000000000000, 0.8660254037844387076, 1.000000000000000000, 0.8660254037844387076, 1.000000000000000000, 0.8660254037844387076, 1.000000000000000000, 0.8660254037844387076, 1.000000000000000000, 0.8660254037844387076, 1.000000000000000000, 0.8660254037844387076, 1.000000000000000000, 0.8660254037844387076, 1.000000000000000000, 0.8660254037844387076, 1.000000000000000000, 0.8660254037844387076, 1.000000000000000000, 0.8660254037844387076, 1.000000000000000000, 0.8660254037844387076, 1.000000000000000000, 0.8660254037844387076, 1.000000000000000000, 0.8660254037844387076, 1.000000000000000000, 0.8660254037844387076, 1.000000000000000000, 0.8660254037844387076, 1.000000000000000000, 0.8660254037844387076, 1.000000000000000000, 0.8660254037844387076, 1.000000000000000000, 0.8660254037844387076, 1.000000000000000000, 0.8660254037844387076, 1.000000000000000000, 0.8660254037844387076, 1.000000000000000000, 0.8660254037844387076, 1.000000000000000000, 0.8660254037844387076, 1.000000000000000000, 0.8660254037844387076, 1.000000000000000000, 0.8660254037844387076, 1.000000000000000000, 0.8660254037844387076, 1.000000000000000000, 0.8660254037844387076, 1.000000000000000000, 0.8660254037844387076, 1.000000000000000000, 0.8660254037844387076, 1.000000000000000000, 0.8660254037844387076, 1.000000000000000000, 0.8660254037844387076, 1.000000000000000000, 0.8660254037844387076, 1.000000000000000000, 0.8660254037844387076, 1.000000000000000000, 0.8660254037844387076, 1.000000000000000000, 0.8660254037844387076, 1.000000000000000000, 0.8660254037844387076, 1.000000000000000000, 0.8660254037844387076, 1.000000000000000000, 0.8660254037844387076, 1.000000000000000000, 0.8660254037844387076, 1.000000000000000000, 0.8660254037844387076, 1.000000000000000000, 0.8660254037844387076, 1.000000000000000000, 0.8660254037844387076, 1.000000000000000000, 0.8660254037844387076, 1.000000000000000000, 0.8660254037844387076, 1.000000000000000000, 0.8660254037844387076, 1.000000000000000000, 0.8660254037844387076, 1.000000000000000000, 0.8660254037844387076, 1.000000000000000000, 0.8660254037844387076, 1.000000000000000000, 0.8660254037844387076, 1.000000000000000000, 0.8660254037844387076, 1.000000000000000000, 0.8660254037844387076, 1.000000000000000000, 0.8660254037844387076, 1.000000000000000000, 0.8660254037844387076, 1.000000000000000000, 0.8660254037844387076, 1.000000000000000000, 0.8660254037844387076, 1.000000000000000000, 0.8660254037844387076, 1.000000000000000000, 0.8660254037844387076, 1.000000000000000000, 0.8660254037844387076, 1.000000000000000000, 0.8660254037844387076, 1.000000000000000000, 0.8660254037844387076, 1.000000000000000000, 0.8660254037844387076, 1.000000000000000000, 0.8660254037844387076, 1.000000000000000000, 0.8660254037844387076, 1.000000000000000000, 0.8660254037844387076, 1.000000000000000000, 0.8660254037844387076, 1.000000000000000000, 0.8660254037844387076, 1.000000000000000000, 0.8660254037844387076, 1.000000000000000000, 0.8660254037844387076, 1.000000000000000000, 0.8660254037844387076, 1.000000000000000000, 0.8660254037844387076, 1.000000000000000000, 0.8660254037844387076, 1.000000000000000000, 0.8660254037844387076, 1.000000000000000000, 0.8660254037844387076, 1.000000000000000000, 0.8660254037844387076, 1.000000000000000000, 0.8660254037844387076, 1.000000000000000000, 0.8660254037844387076, 1.000000000000000000, 0.8660254037844387076, 1.000000000000000000, 0.8660254037844387076, 1.000000000000000000, 0.8660254037844387076, 1.000000000000000000, 0.8660254037844387076, 1.000000000000000000, 0.8660254037844387076, 1.000000000000000000, 0.8660254037844387076, 1.000000000000000000, 0.8660254037844387076, 1.000000000000000000, 0.8660254037844387076, 1.000000000000000000, 0.8660254037844387076, 1.000000000000000000, 0.8660254037844387076, 1.000000000000000000, 0.8660254037844387076, 1.000000000000000000, 0.8660254037844387076, 1.000000000000000000, 0.8660254037844387076, 1.000000000000000000, 0.8660254037844387076, 1.000000000000000000, 0.8660254037844387076, 1.000000000000000000, 0.8660254037844387076, 1.000000000000000000, 0.8660254037844387076, 1.000000000000000000, 0.8660254037844387076, 1.000000000000000000, 0.8660254037844387076, 1.000000000000000000, 0.8660254037844387076, 1.000000000000000000, 0.8660254037844387076, 1.000000000000000000, 0.8660254037844387076, 1.000000000000000000, 0.8660254037844387076, 1.000000000000000000, 0.8660254037844387076, 1.000000000000000000, 0.8660254037844387076, 1.000000000000000000, 0.8660254037844387076, 1.000000000000000000, 0.8660254037844387076, 1.000000000000000000, 0.8660254037844387076, 1.000000000000000000, 0.8660254037844387076, 1.000000000000000000, 0.8660254037844387076, 1.000000000000000000, 0.8660254037844387076, 1.000000000000000000, 0.8660254037844387076, 1.000000000000000000, 0.8660254037844387076, 1.000000000000000000, 0.8660254037844387076, 1.000000000000000000, 0.8660254037844387076, 1.000000000000000000, 0.8660254037844387076, 1.000000000000000000, 0.8660254037844387076, 1.000000000000000000, 0.8660254037844387076, 1.000000000000000000, 0.8660254037844387076, 1.000000000000000000, 0.8660254037844387076, 1.000000000000000000, 0.8660254037844387076, 1.000000000000000000, 0.8660254037844387076, 1.000000000000000000, 0.8660254037844387076, 1.000000000000000000, 0.8660254037844387076, 1.000000000000000000, 0.8660254037844387076, 1.000000000000000000, 0.8660254037844387076, 1.000000000000000000) ) ) 
 REPRESENTATION_ITEM ( '' )  SURFACE ( )  );
#87812=DIRECTION ( 'NONE',  ( -0.7592566023652995710, 0.6507913734559652719, 0.000000000000000000 ) ) ;
#87813=CARTESIAN_POINT ( 'NONE',  ( 4.864678189204997949, 4.569879397027603929, 0.7998128361456341429 ) ) ;
#87823=CARTESIAN_POINT ( 'NONE',  ( 8.772289083241844310, 10.19309100432570148, -1.199719254218446718 ) ) ;
#87826=CARTESIAN_POINT ( 'NONE',  ( -6.247609857798938293, 6.183299677053865295, -0.7998128361456291469 ) ) ;
#87829=CARTESIAN_POINT ( 'NONE',  ( 1.123270288250308280, 2.860197346350005887, 0.7749999999993786304 ) ) ;
#87832=CARTESIAN_POINT ( 'NONE',  ( 0.6823417656249917140, 4.842708333674755394, 1.181850606188765695 ) ) ;
#87835=EDGE_LOOP ( 'NONE', ( #104802, #104689, #131660, #111604 ) ) ;
#87837=CARTESIAN_POINT ( 'NONE',  ( 5.379888026524302980, 5.170957540566797128, -0.7998128361456211532 ) ) ;
#87838=CARTESIAN_POINT ( 'NONE',  ( -4.894657149733403045, 5.669187081899118574, -1.199719254218446718 ) ) ;
#87844=CARTESIAN_POINT ( 'NONE',  ( 5.341549334104184865, 8.215262742221458581, 1.082531754730558626 ) ) ;
#87846=CARTESIAN_POINT ( 'NONE',  ( 6.873620692004076105, 10.00267932643801672, -1.082531754730537976 ) ) ;
#87847=CARTESIAN_POINT ( 'NONE',  ( 0.6823417656249917140, 3.905208333674754950, 1.181850606188765695 ) ) ;
#87849=CARTESIAN_POINT ( 'NONE',  ( 4.107757354816228279, 6.775838766385488654, -1.082531754730548412 ) ) ;
#87857=CARTESIAN_POINT ( 'NONE',  ( -4.956836104118029773, 6.830226236571708576, 1.450618959550575182 ) ) ;
#87863=CARTESIAN_POINT ( 'NONE',  ( -9.236128959407555072, 11.79856975744075598, -1.599625672291263179 ) ) ;
#87868=CARTESIAN_POINT ( 'NONE',  ( -2.300079615812729905, 5.835176651756807331, -0.7998128361456281477 ) ) ;
#87873=CARTESIAN_POINT ( 'NONE',  ( 4.094199201646931741, 4.839282492418613302, -1.082531754730543083 ) ) ;
#87874=CARTESIAN_POINT ( 'NONE',  ( 1.364683531249988535, 3.676041667008087099, 0.7879004041258500513 ) ) ;
#87876=CARTESIAN_POINT ( 'NONE',  ( 6.962275575817444384, 8.081408578997208991, -1.199719254218446718 ) ) ;
#87877=CARTESIAN_POINT ( 'NONE',  ( -9.642873567817536795, 12.27310513391906532, 1.599625672291281386 ) ) ;
#87879=CARTESIAN_POINT ( 'NONE',  ( -5.427341564172148303, 5.226320001155936090, 0.000000000000000000 ) ) ;
#87881=ORIENTED_EDGE ( 'NONE', *, *, #115314, .T. ) ;
#87883=CARTESIAN_POINT ( 'NONE',  ( -1.500000000000013101, 3.879166666666685970, -0.8660254037844313801 ) ) ;
#87884=CARTESIAN_POINT ( 'NONE',  ( 3.649115900372475796, 7.409052317076538330, 1.040834085586084257E-14 ) ) ;
#87887=CARTESIAN_POINT ( 'NONE',  ( 1.123270288250308280, 2.922697346350005887, 0.7749999999993786304 ) ) ;
#87888=CARTESIAN_POINT ( 'NONE',  ( -0.6823417656250212460, 3.551041667008085323, 1.181850606188767472 ) ) ;
#87891=CARTESIAN_POINT ( 'NONE',  ( 9.083599731475983319, 11.62061899152058686, 1.443375672974076540 ) ) ;
#87896=CARTESIAN_POINT ( 'NONE',  ( -1.500000000000013101, 2.410416667349482456, -0.8660254037844313801 ) ) ;
#87898=CARTESIAN_POINT ( 'NONE',  ( -5.229694566569281555, 7.124396299129368337, 1.599625672291267398 ) ) ;
#87899=CARTESIAN_POINT ( 'NONE',  ( 5.355107487273504496, 6.310342158982962246, -1.082531754730543083 ) ) ;
#87908=CARTESIAN_POINT ( 'NONE',  ( 6.123478934866503742, 10.29580919065294431, 0.7998128361456462443 ) ) ;
#87909=CARTESIAN_POINT ( 'NONE',  ( 3.876741858503734761, 6.610283703974623393, 1.199719254218462483 ) ) ;
#87911=CARTESIAN_POINT ( 'NONE',  ( 3.832150974156964818, 7.622593236491780999, 1.040834085586084257E-14 ) ) ;
#87918=CARTESIAN_POINT ( 'NONE',  ( 9.215791728987056786, 11.77484298861683598, -1.599625672291262513 ) ) ;
#87923=CARTESIAN_POINT ( 'NONE',  ( 5.712091369430416066, 6.087825614771766425, 0.6924918054137980672 ) ) ;
#87933=AXIS2_PLACEMENT_3D ( 'NONE', #97215, #211986, #98266 ) ;
#87934=CARTESIAN_POINT ( 'NONE',  ( 8.283668668269706714, 8.766627655843892697, 1.040834085586084257E-14 ) ) ;
#87935=CARTESIAN_POINT ( 'NONE',  ( -2.442440228756222353, 6.001264033524212671, -0.7998128361456281477 ) ) ;
#87940=CARTESIAN_POINT ( 'NONE',  ( -6.091691091241777656, 6.001394449403842479, 0.7998128361456341429 ) ) ;
#87942=CARTESIAN_POINT ( 'NONE',  ( -3.039951802757244526, 2.724153688964686904, 2.451370731312843443 ) ) ;
#87952=CARTESIAN_POINT ( 'NONE',  ( 8.452618703115982512, 11.94880668935564216, 1.199719254218450271 ) ) ;
#87954=CARTESIAN_POINT ( 'NONE',  ( 4.067082894419602468, 3.847277586352047862, -0.7216878364870188411 ) ) ;
#87957=CARTESIAN_POINT ( 'NONE',  ( 8.283668668269706714, 8.766627655843896250, 1.040834085586084257E-14 ) ) ;
#87960=CARTESIAN_POINT ( 'NONE',  ( -9.490344339885977476, 11.13478515369756217, -1.082531754730539753 ) ) ;
#87964=CARTESIAN_POINT ( 'NONE',  ( 7.618792255875527886, 10.97600916757510170, 1.199719254218460707 ) ) ;
#87969=CARTESIAN_POINT ( 'NONE',  ( -7.063961727919978451, 8.200042423116789436, 1.199719254218450271 ) ) ;
#87970=CARTESIAN_POINT ( 'NONE',  ( 3.161022370280501814, 6.839609865302569425, 0.000000000000000000 ) ) ;
#87971=EDGE_CURVE ( 'NONE', #119323, #1199, #102552, .T. ) ;
#87978=CARTESIAN_POINT ( 'NONE',  ( -1.364683531250014514, 2.051041667008086655, -0.7879004041258289570 ) ) ;
#87981=CARTESIAN_POINT ( 'NONE',  ( 5.178851490740187913, 8.985817805931475277, 0.7216878364870438212 ) ) ;
#87989=CARTESIAN_POINT ( 'NONE',  ( 7.904040366642689719, 10.24446639921506552, 1.443375672974076540 ) ) ;
#87991=( BOUNDED_SURFACE ( )  B_SPLINE_SURFACE ( 1, 2, ( 
 ( #73181, #155527, #3896, #54821, #88393, #105740, #172855, #68903, #4958, #104648, #102499, #7107, #135022, #205317, #55883, #6038, #118810, #137149, #72109, #186940, #38573, #168563, #138218, #139287, #204231, #69968, #122041, #202095, #188005, #39631, #56955, #171767, #23363, #184795, #89473, #24426, #37498, #21215, #123127, #185863, #189086, #201036, #40719, #106825, #151262, #36423, #20162, #86249, #152319, #136078, #53753, #119886, #103574, #62289, #43927, #142506, #75337, #127378, #61222, #208514, #141454, #193350, #207461, #25510, #59080, #44994, #144648, #93747, #12455, #42866, #9266, #74279, #111103, #112180, #178184, #143584, #191200, #125240, #108974, #174993, #206390, #91618, #92681, #90538, #26578, #156603, #110042, #158726, #192266, #177109, #78530, #8194, #126306, #10323, #210663, #140373, #28725, #160861, #76397, #128449, #60149, #176054, #27648, #159785, #94811, #46058, #11387, #77465, #209577, #194416, #58017, #157669, #41798, #124181, #190144, #107911, #173937, #130566, #149947, #114311, #113245, #132653, #117500, #163000, #34045, #198657, #29799, #49249, #145720, #15647, #179250, #131604, #115370, #80677, #196556, #1516, #180310, #30873, #50306, #95884, #14581, #100118, #116424, #161938, #181362, #211719, #81736, #96952, #197605, #32986, #146768, #51377, #13531, #31930, #99063, #195494, #166180, #79601, #83857, #148868, #165117, #63355, #98012, #16709, #164068, #147817, #47130, #82794, #17768, #443, #212785, #213836, #64422, #65454, #66511, #67580, #182415, #133725, #129514, #199731, #48199, #69725, #53498, #155275, #3646, #103321, #18845, #137964, #169383, #54569, #35100, #201854, #88138, #171513, #104394, #119635, #86002, #105480, #6855, #136898, #20968, #168322, #5778, #154208, #87065, #19917, #71857, #152076, #118565, #135829, #203985, #23107, #186690, #89222, #185619, #102248, #167260, #55632, #205063, #56705, #22029, #37251, #153137, #4711, #70785, #84930, #184550, #202927, #183491, #120717, #101171, #38318, #170441, #121788, #187755, #72934, #151019, #39384, #139038, #2586, #68656, #134779, #200788, #52439, #36171, #190949, #42613, #108723, #207211, #60970, #78279, #76151, #174749, #142255, #26322, #110851, #57770, #74023, #175804, #92436, #158475, #172599, #44745, #127126, #189899, #10075, #208267, #77211, #160606, #12208, #141200, #176858, #27396, #28471, #109797, #94563, #144407, #59900, #206139, #91361, #58835, #173684, #210407, #124990, #123931, #25260, #126053, #143330, #192015, #43678, #24178, #122872, #41541, #11134, #90281, #93496, #188833, #40469, #157421, #159536, #106572, #209323, #193096, #156350, #7934, #140113, #107655, #9012, #75088, #99872, #180062, #29547, #161690, #63104, #149689, #115119, #95639, #212540, #194165, #32734, #65212, #165935, #129272, #111932, #17520, #195245, #46881, #132411, #45812, #112993, #128204, #13284, #83608, #194, #62049, #31685, #213587 ),
 ( #182163, #177934, #66263, #198413, #179006, #33794, #130321, #196311, #47955, #146521, #50057, #79357, #15398, #114070, #81489, #97761, #116178, #211470, #145475, #181115, #163819, #147566, #30620, #162758, #96709, #64180, #14332, #164866, #80422, #131363, #197358, #16460, #49001, #98814, #82540, #148628, #150769, #103072, #20721, #52186, #22852, #133474, #3403, #5523, #71604, #151830, #185366, #152881, #70529, #203735, #69472, #135579, #34847, #4459, #2331, #137715, #68407, #55381, #121536, #134534, #119380, #86815, #170188, #39135, #105218, #19669, #187506, #54320, #171258, #202672, #88966, #1272, #201601, #84682, #184298, #85748, #118312, #67330, #53249, #200540, #35923, #169127, #21774, #36989, #136647, #51120, #199476, #102000, #104141, #117243, #120461, #183243, #100922, #168069, #38071, #167010, #186433, #87883, #153957, #18602, #43418, #56452, #155021, #107399, #192826, #58582, #122612, #40207, #156092, #28214, #208016, #188575, #91105, #72686, #125800, #158230, #44484, #7677, #204801, #110601, #73761, #139856, #10874, #138781, #205887, #6605, #106317, #176602, #93241, #172341, #124737, #92180, #9821, #108469, #57520, #23929, #90033, #123678, #189640, #190696, #41291, #126868, #173421, #26068, #25003, #59642, #209067, #157166, #42357, #76949, #8758, #74839, #142001, #140939, #191762, #206953, #174491, #109542, #75897, #175546, #27135, #143074, #159275, #60704, #95377, #45550, #14065, #114849, #164607, #193902, #113798, #147305, #63905, #197095, #210139, #94307, #46610, #132147, #212270, #61783, #111666, #161426, #181898, #213331, #127949, #30355, #11950, #64956, #97495, #198153, #13009, #144147, #49786, #79086, #145204, #16192, #78023, #211210, #160348, #177673, #115912, #32471, #29283, #130061, #31419, #163552, #47686, #62835, #128997, #194974, #112732, #178742, #196054, #96442, #65997, #162493, #179800, #80152, #131108, #148368, #146257, #15135, #82273, #81223, #48736, #180849, #98543, #214367, #182980, #199208, #4204, #36722, #116980, #34597, #169927, #71340, #119116, #100665, #50855, #167805, #54059, #103879, #133204, #52980, #37804, #21511, #184040, #3136, #185095, #102808, #87623, #35657, #101736, #67068, #168864, #166743, #153694, #18337, #5263, #137456, #84418, #151569, #20467, #202404, #203471, #55125, #51931, #121270, #86553, #33533, #152617, #99605, #165671, #19404, #150507, #2068, #118055, #68139, #17260, #85483, #134272, #200280, #135326, #120194, #69206, #201340, #83336, #149421, #70272, #136388, #1004, #186170, #145752, #187245, #158760, #12490, #79634, #208546, #126339, #60181, #128482, #211753, #143617, #43958, #209611, #176086, #178219, #125273, #141488, #28759, #27684, #93782, #22596, #76431, #95918, #192299, #59115, #78563, #63391, #109007, #194450, #144683, #38872, #61254, #88703, #159819, #191235, #77498, #127412, #26613, #104957, #170998, #110074, #193384, #207494, #46094, #154761 ) ),
 .UNSPECIFIED., .F., .F., .T. ) 
 B_SPLINE_SURFACE_WITH_KNOTS ( ( 2, 2 ),
 ( 3, 2, 2, 2, 2, 2, 2, 2, 2, 2, 2, 2, 2, 2, 2, 2, 2, 2, 2, 2, 2, 2, 2, 2, 2, 2, 2, 2, 2, 2, 2, 2, 2, 2, 2, 2, 2, 2, 2, 2, 2, 2, 2, 2, 2, 2, 2, 2, 2, 2, 2, 2, 2, 2, 2, 2, 2, 2, 2, 2, 2, 2, 2, 2, 2, 2, 2, 2, 2, 2, 2, 2, 2, 2, 2, 2, 2, 2, 2, 2, 2, 2, 2, 2, 2, 2, 2, 2, 2, 2, 2, 2, 2, 2, 2, 2, 2, 2, 2, 2, 2, 2, 2, 2, 2, 2, 2, 2, 2, 2, 2, 2, 2, 2, 2, 2, 2, 2, 2, 2, 2, 2, 2, 2, 2, 2, 2, 2, 2, 2, 2, 2, 2, 2, 2, 2, 2, 2, 2, 2, 2, 2, 2, 2, 2, 2, 2, 2, 2, 2, 2, 2, 2, 2, 2, 2, 2, 2, 2, 2, 2, 2, 2, 2, 2, 2, 2, 2, 3 ),
 ( 0.000000000000000000, 1.000000000000000000 ),
 ( 0.000000000000000000, 0.005952380952380952051, 0.01190476190476190410, 0.01785714285714285615, 0.02380952380952380820, 0.02976190476190476025, 0.03571428571428571230, 0.04166666666666666435, 0.04761904761904761640, 0.05357142857142856845, 0.05952380952380952051, 0.06547619047619047949, 0.07142857142857142461, 0.07738095238095238360, 0.08333333333333332871, 0.08928571428571428770, 0.09523809523809523281, 0.1011904761904761918, 0.1071428571428571369, 0.1130952380952380959, 0.1190476190476190410, 0.1250000000000000000, 0.1309523809523809590, 0.1369047619047619180, 0.1428571428571428492, 0.1488095238095238082, 0.1547619047619047672, 0.1607142857142857262, 0.1666666666666666574, 0.1726190476190476164, 0.1785714285714285754, 0.1845238095238095344, 0.1904761904761904656, 0.1964285714285714246, 0.2023809523809523836, 0.2083333333333333426, 0.2142857142857142738, 0.2202380952380952328, 0.2261904761904761918, 0.2321428571428571508, 0.2380952380952380820, 0.2440476190476190410, 0.2500000000000000000, 0.2559523809523809312, 0.2619047619047619180, 0.2678571428571428492, 0.2738095238095238360, 0.2797619047619047672, 0.2857142857142856984, 0.2916666666666666852, 0.2976190476190476164, 0.3035714285714285476, 0.3095238095238095344, 0.3154761904761904656, 0.3214285714285714524, 0.3273809523809523836, 0.3333333333333333148, 0.3392857142857143016, 0.3452380952380952328, 0.3511904761904761640, 0.3571428571428571508, 0.3630952380952380820, 0.3690476190476190688, 0.3750000000000000000, 0.3809523809523809312, 0.3869047619047619180, 0.3928571428571428492, 0.3988095238095238360, 0.4047619047619047672, 0.4107142857142856984, 0.4166666666666666852, 0.4226190476190476164, 0.4285714285714285476, 0.4345238095238095344, 0.4404761904761904656, 0.4464285714285714524, 0.4523809523809523836, 0.4583333333333333148, 0.4642857142857143016, 0.4702380952380952328, 0.4761904761904761640, 0.4821428571428571508, 0.4880952380952380820, 0.4940476190476190688, 0.5000000000000000000, 0.5059523809523809312, 0.5119047619047618625, 0.5178571428571429047, 0.5238095238095238360, 0.5297619047619047672, 0.5357142857142856984, 0.5416666666666666297, 0.5476190476190476719, 0.5535714285714286031, 0.5595238095238095344, 0.5654761904761904656, 0.5714285714285713969, 0.5773809523809523281, 0.5833333333333333703, 0.5892857142857143016, 0.5952380952380952328, 0.6011904761904761640, 0.6071428571428570953, 0.6130952380952381375, 0.6190476190476190688, 0.6250000000000000000, 0.6309523809523809312, 0.6369047619047618625, 0.6428571428571429047, 0.6488095238095238360, 0.6547619047619047672, 0.6607142857142856984, 0.6666666666666666297, 0.6726190476190476719, 0.6785714285714286031, 0.6845238095238095344, 0.6904761904761904656, 0.6964285714285713969, 0.7023809523809523281, 0.7083333333333333703, 0.7142857142857143016, 0.7202380952380952328, 0.7261904761904761640, 0.7321428571428570953, 0.7380952380952381375, 0.7440476190476190688, 0.7500000000000000000, 0.7559523809523809312, 0.7619047619047618625, 0.7678571428571429047, 0.7738095238095238360, 0.7797619047619047672, 0.7857142857142856984, 0.7916666666666666297, 0.7976190476190476719, 0.8035714285714286031, 0.8095238095238095344, 0.8154761904761904656, 0.8214285714285713969, 0.8273809523809523281, 0.8333333333333333703, 0.8392857142857143016, 0.8452380952380952328, 0.8511904761904761640, 0.8571428571428570953, 0.8630952380952381375, 0.8690476190476190688, 0.8750000000000000000, 0.8809523809523809312, 0.8869047619047618625, 0.8928571428571429047, 0.8988095238095238360, 0.9047619047619047672, 0.9107142857142856984, 0.9166666666666666297, 0.9226190476190476719, 0.9285714285714286031, 0.9345238095238095344, 0.9404761904761904656, 0.9464285714285713969, 0.9523809523809523281, 0.9583333333333333703, 0.9642857142857143016, 0.9702380952380952328, 0.9761904761904761640, 0.9821428571428570953, 0.9880952380952381375, 0.9940476190476190688, 1.000000000000000000 ),
 .UNSPECIFIED. ) 
 GEOMETRIC_REPRESENTATION_ITEM ( )  RATIONAL_B_SPLINE_SURFACE ( (
 ( 1.000000000000000000, 0.8660254037844387076, 1.000000000000000000, 0.8660254037844387076, 1.000000000000000000, 0.8660254037844387076, 1.000000000000000000, 0.8660254037844387076, 1.000000000000000000, 0.8660254037844387076, 1.000000000000000000, 0.8660254037844387076, 1.000000000000000000, 0.8660254037844387076, 1.000000000000000000, 0.8660254037844387076, 1.000000000000000000, 0.8660254037844387076, 1.000000000000000000, 0.8660254037844387076, 1.000000000000000000, 0.8660254037844387076, 1.000000000000000000, 0.8660254037844387076, 1.000000000000000000, 0.8660254037844387076, 1.000000000000000000, 0.8660254037844387076, 1.000000000000000000, 0.8660254037844387076, 1.000000000000000000, 0.8660254037844387076, 1.000000000000000000, 0.8660254037844387076, 1.000000000000000000, 0.8660254037844387076, 1.000000000000000000, 0.8660254037844387076, 1.000000000000000000, 0.8660254037844387076, 1.000000000000000000, 0.8660254037844387076, 1.000000000000000000, 0.8660254037844387076, 1.000000000000000000, 0.8660254037844387076, 1.000000000000000000, 0.8660254037844387076, 1.000000000000000000, 0.8660254037844387076, 1.000000000000000000, 0.8660254037844387076, 1.000000000000000000, 0.8660254037844387076, 1.000000000000000000, 0.8660254037844387076, 1.000000000000000000, 0.8660254037844387076, 1.000000000000000000, 0.8660254037844387076, 1.000000000000000000, 0.8660254037844387076, 1.000000000000000000, 0.8660254037844387076, 1.000000000000000000, 0.8660254037844387076, 1.000000000000000000, 0.8660254037844387076, 1.000000000000000000, 0.8660254037844387076, 1.000000000000000000, 0.8660254037844387076, 1.000000000000000000, 0.8660254037844387076, 1.000000000000000000, 0.8660254037844387076, 1.000000000000000000, 0.8660254037844387076, 1.000000000000000000, 0.8660254037844387076, 1.000000000000000000, 0.8660254037844387076, 1.000000000000000000, 0.8660254037844387076, 1.000000000000000000, 0.8660254037844387076, 1.000000000000000000, 0.8660254037844387076, 1.000000000000000000, 0.8660254037844387076, 1.000000000000000000, 0.8660254037844387076, 1.000000000000000000, 0.8660254037844387076, 1.000000000000000000, 0.8660254037844387076, 1.000000000000000000, 0.8660254037844387076, 1.000000000000000000, 0.8660254037844387076, 1.000000000000000000, 0.8660254037844387076, 1.000000000000000000, 0.8660254037844387076, 1.000000000000000000, 0.8660254037844387076, 1.000000000000000000, 0.8660254037844387076, 1.000000000000000000, 0.8660254037844387076, 1.000000000000000000, 0.8660254037844387076, 1.000000000000000000, 0.8660254037844387076, 1.000000000000000000, 0.8660254037844387076, 1.000000000000000000, 0.8660254037844387076, 1.000000000000000000, 0.8660254037844387076, 1.000000000000000000, 0.8660254037844387076, 1.000000000000000000, 0.8660254037844387076, 1.000000000000000000, 0.8660254037844387076, 1.000000000000000000, 0.8660254037844387076, 1.000000000000000000, 0.8660254037844387076, 1.000000000000000000, 0.8660254037844387076, 1.000000000000000000, 0.8660254037844387076, 1.000000000000000000, 0.8660254037844387076, 1.000000000000000000, 0.8660254037844387076, 1.000000000000000000, 0.8660254037844387076, 1.000000000000000000, 0.8660254037844387076, 1.000000000000000000, 0.8660254037844387076, 1.000000000000000000, 0.8660254037844387076, 1.000000000000000000, 0.8660254037844387076, 1.000000000000000000, 0.8660254037844387076, 1.000000000000000000, 0.8660254037844387076, 1.000000000000000000, 0.8660254037844387076, 1.000000000000000000, 0.8660254037844387076, 1.000000000000000000, 0.8660254037844387076, 1.000000000000000000, 0.8660254037844387076, 1.000000000000000000, 0.8660254037844387076, 1.000000000000000000, 0.8660254037844387076, 1.000000000000000000, 0.8660254037844387076, 1.000000000000000000, 0.8660254037844387076, 1.000000000000000000, 0.8660254037844387076, 1.000000000000000000, 0.8660254037844387076, 1.000000000000000000, 0.8660254037844387076, 1.000000000000000000, 0.8660254037844387076, 1.000000000000000000, 0.8660254037844387076, 1.000000000000000000, 0.8660254037844387076, 1.000000000000000000, 0.8660254037844387076, 1.000000000000000000, 0.8660254037844387076, 1.000000000000000000, 0.8660254037844387076, 1.000000000000000000, 0.8660254037844387076, 1.000000000000000000, 0.8660254037844387076, 1.000000000000000000, 0.8660254037844387076, 1.000000000000000000, 0.8660254037844387076, 1.000000000000000000, 0.8660254037844387076, 1.000000000000000000, 0.8660254037844387076, 1.000000000000000000, 0.8660254037844387076, 1.000000000000000000, 0.8660254037844387076, 1.000000000000000000, 0.8660254037844387076, 1.000000000000000000, 0.8660254037844387076, 1.000000000000000000, 0.8660254037844387076, 1.000000000000000000, 0.8660254037844387076, 1.000000000000000000, 0.8660254037844387076, 1.000000000000000000, 0.8660254037844387076, 1.000000000000000000, 0.8660254037844387076, 1.000000000000000000, 0.8660254037844387076, 1.000000000000000000, 0.8660254037844387076, 1.000000000000000000, 0.8660254037844387076, 1.000000000000000000, 0.8660254037844387076, 1.000000000000000000, 0.8660254037844387076, 1.000000000000000000, 0.8660254037844387076, 1.000000000000000000, 0.8660254037844387076, 1.000000000000000000, 0.8660254037844387076, 1.000000000000000000, 0.8660254037844387076, 1.000000000000000000, 0.8660254037844387076, 1.000000000000000000, 0.8660254037844387076, 1.000000000000000000, 0.8660254037844387076, 1.000000000000000000, 0.8660254037844387076, 1.000000000000000000, 0.8660254037844387076, 1.000000000000000000, 0.8660254037844387076, 1.000000000000000000, 0.8660254037844387076, 1.000000000000000000, 0.8660254037844387076, 1.000000000000000000, 0.8660254037844387076, 1.000000000000000000, 0.8660254037844387076, 1.000000000000000000, 0.8660254037844387076, 1.000000000000000000, 0.8660254037844387076, 1.000000000000000000, 0.8660254037844387076, 1.000000000000000000, 0.8660254037844387076, 1.000000000000000000, 0.8660254037844387076, 1.000000000000000000, 0.8660254037844387076, 1.000000000000000000, 0.8660254037844387076, 1.000000000000000000, 0.8660254037844387076, 1.000000000000000000, 0.8660254037844387076, 1.000000000000000000, 0.8660254037844387076, 1.000000000000000000, 0.8660254037844387076, 1.000000000000000000, 0.8660254037844387076, 1.000000000000000000, 0.8660254037844387076, 1.000000000000000000, 0.8660254037844387076, 1.000000000000000000, 0.8660254037844387076, 1.000000000000000000, 0.8660254037844387076, 1.000000000000000000, 0.8660254037844387076, 1.000000000000000000, 0.8660254037844387076, 1.000000000000000000, 0.8660254037844387076, 1.000000000000000000, 0.8660254037844387076, 1.000000000000000000, 0.8660254037844387076, 1.000000000000000000, 0.8660254037844387076, 1.000000000000000000, 0.8660254037844387076, 1.000000000000000000, 0.8660254037844387076, 1.000000000000000000, 0.8660254037844387076, 1.000000000000000000, 0.8660254037844387076, 1.000000000000000000, 0.8660254037844387076, 1.000000000000000000, 0.8660254037844387076, 1.000000000000000000, 0.8660254037844387076, 1.000000000000000000, 0.8660254037844387076, 1.000000000000000000, 0.8660254037844387076, 1.000000000000000000, 0.8660254037844387076, 1.000000000000000000, 0.8660254037844387076, 1.000000000000000000, 0.8660254037844387076, 1.000000000000000000, 0.8660254037844387076, 1.000000000000000000, 0.8660254037844387076, 1.000000000000000000, 0.8660254037844387076, 1.000000000000000000, 0.8660254037844387076, 1.000000000000000000, 0.8660254037844387076, 1.000000000000000000, 0.8660254037844387076, 1.000000000000000000, 0.8660254037844387076, 1.000000000000000000),
 ( 1.000000000000000000, 0.8660254037844387076, 1.000000000000000000, 0.8660254037844387076, 1.000000000000000000, 0.8660254037844387076, 1.000000000000000000, 0.8660254037844387076, 1.000000000000000000, 0.8660254037844387076, 1.000000000000000000, 0.8660254037844387076, 1.000000000000000000, 0.8660254037844387076, 1.000000000000000000, 0.8660254037844387076, 1.000000000000000000, 0.8660254037844387076, 1.000000000000000000, 0.8660254037844387076, 1.000000000000000000, 0.8660254037844387076, 1.000000000000000000, 0.8660254037844387076, 1.000000000000000000, 0.8660254037844387076, 1.000000000000000000, 0.8660254037844387076, 1.000000000000000000, 0.8660254037844387076, 1.000000000000000000, 0.8660254037844387076, 1.000000000000000000, 0.8660254037844387076, 1.000000000000000000, 0.8660254037844387076, 1.000000000000000000, 0.8660254037844387076, 1.000000000000000000, 0.8660254037844387076, 1.000000000000000000, 0.8660254037844387076, 1.000000000000000000, 0.8660254037844387076, 1.000000000000000000, 0.8660254037844387076, 1.000000000000000000, 0.8660254037844387076, 1.000000000000000000, 0.8660254037844387076, 1.000000000000000000, 0.8660254037844387076, 1.000000000000000000, 0.8660254037844387076, 1.000000000000000000, 0.8660254037844387076, 1.000000000000000000, 0.8660254037844387076, 1.000000000000000000, 0.8660254037844387076, 1.000000000000000000, 0.8660254037844387076, 1.000000000000000000, 0.8660254037844387076, 1.000000000000000000, 0.8660254037844387076, 1.000000000000000000, 0.8660254037844387076, 1.000000000000000000, 0.8660254037844387076, 1.000000000000000000, 0.8660254037844387076, 1.000000000000000000, 0.8660254037844387076, 1.000000000000000000, 0.8660254037844387076, 1.000000000000000000, 0.8660254037844387076, 1.000000000000000000, 0.8660254037844387076, 1.000000000000000000, 0.8660254037844387076, 1.000000000000000000, 0.8660254037844387076, 1.000000000000000000, 0.8660254037844387076, 1.000000000000000000, 0.8660254037844387076, 1.000000000000000000, 0.8660254037844387076, 1.000000000000000000, 0.8660254037844387076, 1.000000000000000000, 0.8660254037844387076, 1.000000000000000000, 0.8660254037844387076, 1.000000000000000000, 0.8660254037844387076, 1.000000000000000000, 0.8660254037844387076, 1.000000000000000000, 0.8660254037844387076, 1.000000000000000000, 0.8660254037844387076, 1.000000000000000000, 0.8660254037844387076, 1.000000000000000000, 0.8660254037844387076, 1.000000000000000000, 0.8660254037844387076, 1.000000000000000000, 0.8660254037844387076, 1.000000000000000000, 0.8660254037844387076, 1.000000000000000000, 0.8660254037844387076, 1.000000000000000000, 0.8660254037844387076, 1.000000000000000000, 0.8660254037844387076, 1.000000000000000000, 0.8660254037844387076, 1.000000000000000000, 0.8660254037844387076, 1.000000000000000000, 0.8660254037844387076, 1.000000000000000000, 0.8660254037844387076, 1.000000000000000000, 0.8660254037844387076, 1.000000000000000000, 0.8660254037844387076, 1.000000000000000000, 0.8660254037844387076, 1.000000000000000000, 0.8660254037844387076, 1.000000000000000000, 0.8660254037844387076, 1.000000000000000000, 0.8660254037844387076, 1.000000000000000000, 0.8660254037844387076, 1.000000000000000000, 0.8660254037844387076, 1.000000000000000000, 0.8660254037844387076, 1.000000000000000000, 0.8660254037844387076, 1.000000000000000000, 0.8660254037844387076, 1.000000000000000000, 0.8660254037844387076, 1.000000000000000000, 0.8660254037844387076, 1.000000000000000000, 0.8660254037844387076, 1.000000000000000000, 0.8660254037844387076, 1.000000000000000000, 0.8660254037844387076, 1.000000000000000000, 0.8660254037844387076, 1.000000000000000000, 0.8660254037844387076, 1.000000000000000000, 0.8660254037844387076, 1.000000000000000000, 0.8660254037844387076, 1.000000000000000000, 0.8660254037844387076, 1.000000000000000000, 0.8660254037844387076, 1.000000000000000000, 0.8660254037844387076, 1.000000000000000000, 0.8660254037844387076, 1.000000000000000000, 0.8660254037844387076, 1.000000000000000000, 0.8660254037844387076, 1.000000000000000000, 0.8660254037844387076, 1.000000000000000000, 0.8660254037844387076, 1.000000000000000000, 0.8660254037844387076, 1.000000000000000000, 0.8660254037844387076, 1.000000000000000000, 0.8660254037844387076, 1.000000000000000000, 0.8660254037844387076, 1.000000000000000000, 0.8660254037844387076, 1.000000000000000000, 0.8660254037844387076, 1.000000000000000000, 0.8660254037844387076, 1.000000000000000000, 0.8660254037844387076, 1.000000000000000000, 0.8660254037844387076, 1.000000000000000000, 0.8660254037844387076, 1.000000000000000000, 0.8660254037844387076, 1.000000000000000000, 0.8660254037844387076, 1.000000000000000000, 0.8660254037844387076, 1.000000000000000000, 0.8660254037844387076, 1.000000000000000000, 0.8660254037844387076, 1.000000000000000000, 0.8660254037844387076, 1.000000000000000000, 0.8660254037844387076, 1.000000000000000000, 0.8660254037844387076, 1.000000000000000000, 0.8660254037844387076, 1.000000000000000000, 0.8660254037844387076, 1.000000000000000000, 0.8660254037844387076, 1.000000000000000000, 0.8660254037844387076, 1.000000000000000000, 0.8660254037844387076, 1.000000000000000000, 0.8660254037844387076, 1.000000000000000000, 0.8660254037844387076, 1.000000000000000000, 0.8660254037844387076, 1.000000000000000000, 0.8660254037844387076, 1.000000000000000000, 0.8660254037844387076, 1.000000000000000000, 0.8660254037844387076, 1.000000000000000000, 0.8660254037844387076, 1.000000000000000000, 0.8660254037844387076, 1.000000000000000000, 0.8660254037844387076, 1.000000000000000000, 0.8660254037844387076, 1.000000000000000000, 0.8660254037844387076, 1.000000000000000000, 0.8660254037844387076, 1.000000000000000000, 0.8660254037844387076, 1.000000000000000000, 0.8660254037844387076, 1.000000000000000000, 0.8660254037844387076, 1.000000000000000000, 0.8660254037844387076, 1.000000000000000000, 0.8660254037844387076, 1.000000000000000000, 0.8660254037844387076, 1.000000000000000000, 0.8660254037844387076, 1.000000000000000000, 0.8660254037844387076, 1.000000000000000000, 0.8660254037844387076, 1.000000000000000000, 0.8660254037844387076, 1.000000000000000000, 0.8660254037844387076, 1.000000000000000000, 0.8660254037844387076, 1.000000000000000000, 0.8660254037844387076, 1.000000000000000000, 0.8660254037844387076, 1.000000000000000000, 0.8660254037844387076, 1.000000000000000000, 0.8660254037844387076, 1.000000000000000000, 0.8660254037844387076, 1.000000000000000000, 0.8660254037844387076, 1.000000000000000000, 0.8660254037844387076, 1.000000000000000000, 0.8660254037844387076, 1.000000000000000000, 0.8660254037844387076, 1.000000000000000000, 0.8660254037844387076, 1.000000000000000000, 0.8660254037844387076, 1.000000000000000000, 0.8660254037844387076, 1.000000000000000000, 0.8660254037844387076, 1.000000000000000000, 0.8660254037844387076, 1.000000000000000000, 0.8660254037844387076, 1.000000000000000000, 0.8660254037844387076, 1.000000000000000000, 0.8660254037844387076, 1.000000000000000000, 0.8660254037844387076, 1.000000000000000000, 0.8660254037844387076, 1.000000000000000000, 0.8660254037844387076, 1.000000000000000000, 0.8660254037844387076, 1.000000000000000000, 0.8660254037844387076, 1.000000000000000000, 0.8660254037844387076, 1.000000000000000000, 0.8660254037844387076, 1.000000000000000000, 0.8660254037844387076, 1.000000000000000000, 0.8660254037844387076, 1.000000000000000000, 0.8660254037844387076, 1.000000000000000000, 0.8660254037844387076, 1.000000000000000000, 0.8660254037844387076, 1.000000000000000000) ) ) 
 REPRESENTATION_ITEM ( '' )  SURFACE ( )  );
#87996=CARTESIAN_POINT ( 'NONE',  ( -8.636707547105197946, 10.03491254549959777, -1.199719254218446718 ) ) ;
#88005=CARTESIAN_POINT ( 'NONE',  ( 9.999301985278609806, 11.62460605670194447, 1.199719254218452047 ) ) ;
#88009=CARTESIAN_POINT ( 'NONE',  ( 5.009901455449552010, 5.803638771901306725, -1.199719254218452047 ) ) ;
#88012=CARTESIAN_POINT ( 'NONE',  ( -1.499999999999997780, 3.181250000682818602, 1.214306433183764966E-14 ) ) ;
#88016=ORIENTED_EDGE ( 'NONE', *, *, #164742, .F. ) ;
#88018=CARTESIAN_POINT ( 'NONE',  ( -1.500000000000013101, -0.07916666666664513852, 0.8660254037844403729 ) ) ;
#88019=CARTESIAN_POINT ( 'NONE',  ( 7.076466111328892694, 10.34329533227067799, -1.199719254218441611 ) ) ;
#88023=CARTESIAN_POINT ( 'NONE',  ( 7.917598520700710019, 12.18102267421877727, -0.7216878364870328300 ) ) ;
#88028=CARTESIAN_POINT ( 'NONE',  ( -5.362413449404877852, 6.214902764849178141, -1.199719254218446718 ) ) ;
#88029=CARTESIAN_POINT ( 'NONE',  ( -1.499999999999997780, 3.431250000682818602, 1.214306433183764966E-14 ) ) ;
#88030=EDGE_CURVE ( 'NONE', #93560, #155662, #115675, .T. ) ;
#88031=CARTESIAN_POINT ( 'NONE',  ( 1.364683531249986981, -1.115624999658580752, 0.000000000000000000 ) ) ;
#88036=CARTESIAN_POINT ( 'NONE',  ( -1.201851678989727383E-14, 4.134375000341417028, 1.575800808251672791 ) ) ;
#88046=CARTESIAN_POINT ( 'NONE',  ( -9.013473194986783454, 9.410140237106395134, -0.7998128361456291469 ) ) ;
#88047=CARTESIAN_POINT ( 'NONE',  ( 5.361359679200154105, 8.342337828120466980, 1.199719254218462483 ) ) ;
#88055=CARTESIAN_POINT ( 'NONE',  ( -6.693975156845199059, 8.832723654451292816, 1.599625672291283607 ) ) ;
#88060=CARTESIAN_POINT ( 'NONE',  ( 9.836604141914616406, 11.43479190611061647, 1.199719254218452047 ) ) ;
#88064=CARTESIAN_POINT ( 'NONE',  ( -5.251085567194491155, 5.020688004682002159, -0.7998128361456221525 ) ) ;
#88065=CARTESIAN_POINT ( 'NONE',  ( -9.806625181386236179, 10.33548422123910449, -0.7998128361456291469 ) ) ;
#88068=CARTESIAN_POINT ( 'NONE',  ( -4.646091124696241081, 7.101299429195864654, -1.386232413501260474 ) ) ;
#88075=CARTESIAN_POINT ( 'NONE',  ( 4.808338034340912337, 8.761478140039733020, 1.040834085586084257E-14 ) ) ;
#88081=VECTOR ( 'NONE', #123728, 1000.000000000000000 ) ;
#88099=CARTESIAN_POINT ( 'NONE',  ( -8.025536864285518490, 11.45054454405341282, -1.199719254218446718 ) ) ;
#88106=CARTESIAN_POINT ( 'NONE',  ( -1.500000000000015099, 1.160416667349484898, -0.8660254037844313801 ) ) ;
#88107=CARTESIAN_POINT ( 'NONE',  ( 10.37606763316019531, 10.99983374830873650, 0.7998128361456462443 ) ) ;
#88112=CARTESIAN_POINT ( 'NONE',  ( -9.667127221743832877, 11.23706883257798772, 1.199719254218462483 ) ) ;
#88114=CARTESIAN_POINT ( 'NONE',  ( 1.364683531249988757, 1.634375000341421691, 0.000000000000000000 ) ) ;
#88120=CARTESIAN_POINT ( 'NONE',  ( -4.440459003675619520, 5.139289244831666714, 1.199719254218462483 ) ) ;
#88122=CARTESIAN_POINT ( 'NONE',  ( 4.044555541517573793, 7.746237447724527492, 0.4662041258270445132 ) ) ;
#88125=CARTESIAN_POINT ( 'NONE',  ( 1.364683531249986537, -0.07395833299191513499, 0.7879004041258500513 ) ) ;
#88130=CARTESIAN_POINT ( 'NONE',  ( -1.402160292154681736E-14, 0.3218750003414227456, 1.575800808251672791 ) ) ;
#88132=CARTESIAN_POINT ( 'NONE',  ( -5.228640796364566690, 9.251831362400652736, -0.7998128361456231517 ) ) ;
#88133=CARTESIAN_POINT ( 'NONE',  ( 6.591235234537977661, 10.84152487360300299, 0.7998128361456462443 ) ) ;
#88134=CARTESIAN_POINT ( 'NONE',  ( 4.680589345215795838, 6.483773540883647435, -1.599625672291256517 ) ) ;
#88138=CARTESIAN_POINT ( 'NONE',  ( -1.364683531250000748, 1.821875000341421913, 0.000000000000000000 ) ) ;
#88146=CARTESIAN_POINT ( 'NONE',  ( 7.483737605063422116, 7.833374748769873719, -0.7216878364870257245 ) ) ;
#88149=CARTESIAN_POINT ( 'NONE',  ( -7.714753101375940503, 8.959299025482085455, 1.199719254218462483 ) ) ;
#88150=CARTESIAN_POINT ( 'NONE',  ( -4.952806187693842510, 4.672695395264567786, 0.7998128361456341429 ) ) ;
#88153=DIRECTION ( 'NONE',  ( 0.000000000000000000, 0.000000000000000000, 1.000000000000000000 ) ) ;
#88154=CARTESIAN_POINT ( 'NONE',  ( 4.324687812634874895, 7.989293514808604613, 0.7216878364870317197 ) ) ;
#88155=CARTESIAN_POINT ( 'NONE',  ( -7.117667457050096402, 10.28740055232499984, 1.082531754730549967 ) ) ;
#88157=CARTESIAN_POINT ( 'NONE',  ( -1.500000000000011324, 5.170833333333356485, 0.8660254037844403729 ) ) ;
#88161=CARTESIAN_POINT ( 'NONE',  ( 8.093854517678360949, 12.38665467069271386, 1.040834085586084257E-14 ) ) ;
#88167=CARTESIAN_POINT ( 'NONE',  ( -1.419999999067534713, 7.203691543881443948, -4.238255391841854625 ) ) ;
#88173=CARTESIAN_POINT ( 'NONE',  ( 6.575341312503417690, 10.61505593132193326, -0.7216878364870267237 ) ) ;
#88174=ADVANCED_FACE ( 'NONE', ( #8804 ), #92227, .T. ) ;
#88175=CARTESIAN_POINT ( 'NONE',  ( 6.751070424600909448, 9.963667031088037973, -1.199719254218441611 ) ) ;
#88176=AXIS2_PLACEMENT_3D ( 'NONE', #21465, #139545, #52930 ) ;
#88177=CARTESIAN_POINT ( 'NONE',  ( -5.032047568966410367, 9.022472597102808578, 1.214306433183764966E-14 ) ) ;
#88181=CARTESIAN_POINT ( 'NONE',  ( -0.6823417656250003738, -0.9697916663252494907, -1.181850606188749264 ) ) ;
#88182=CARTESIAN_POINT ( 'NONE',  ( 4.446711195602238931, 6.210915699667823198, -1.443375672974051449 ) ) ;
#88183=ORIENTED_EDGE ( 'NONE', *, *, #212623, .T. ) ;
#88184=CARTESIAN_POINT ( 'NONE',  ( -4.810445574750349174, 4.506608013497163334, 0.7998128361456341429 ) ) ;
#88185=CARTESIAN_POINT ( 'NONE',  ( -6.887178846062105286, 10.97886638714038554, -0.7216878364870267237 ) ) ;
#88200=CARTESIAN_POINT ( 'NONE',  ( 6.825640269476072497, 10.05066518344239412, 1.199719254218460707 ) ) ;
#88213=CARTESIAN_POINT ( 'NONE',  ( -7.400052914960538963, 7.527816577075747695, 1.040834085586084257E-14 ) ) ;
#88215=CARTESIAN_POINT ( 'NONE',  ( -2.740719608256871442, 6.349256642941639051, 0.7998128361456341429 ) ) ;
#88225=CARTESIAN_POINT ( 'NONE',  ( -4.115063316947640715, 4.759660943649018705, 1.199719254218462483 ) ) ;
#88229=CARTESIAN_POINT ( 'NONE',  ( 8.098297826064319693, 8.342435640030188893, 0.7998128361456481317 ) ) ;
#88230=CARTESIAN_POINT ( 'NONE',  ( -0.6823417656250212460, 4.051041667008085767, 1.181850606188767472 ) ) ;
#88236=CARTESIAN_POINT ( 'NONE',  ( 6.141480396866128899, 6.267408005873028820, -0.7216878364870257245 ) ) ;
#88238=CARTESIAN_POINT ( 'NONE',  ( -7.694415870955439551, 8.935572256658169010, 1.199719254218462483 ) ) ;
#88241=CARTESIAN_POINT ( 'NONE',  ( -8.193204901359996128, 8.453160561208463264, 1.040834085586084257E-14 ) ) ;
#88242=CARTESIAN_POINT ( 'NONE',  ( -5.063080299699540987, 7.994345218703034384, 1.199719254218464037 ) ) ;
#88249=CARTESIAN_POINT ( 'NONE',  ( 7.962716289927667113, 8.184257181204083409, -0.7998128361456291469 ) ) ;
#88257=CARTESIAN_POINT ( 'NONE',  ( -0.7500000000000215383, 3.941666666666690411, 1.299038105676671107 ) ) ;
#88260=VECTOR ( 'NONE', #189130, 1000.000000000000000 ) ;
#88261=CARTESIAN_POINT ( 'NONE',  ( -0.5475226324602718853, 7.495867147881379644, -1.923617955668145862 ) ) ;
#88265=CARTESIAN_POINT ( 'NONE',  ( 0.6823417656249882723, -0.8447916663252494907, 1.181850606188755259 ) ) ;
#88266=CARTESIAN_POINT ( 'NONE',  ( 5.281064527722868718, 6.119995689553514140, 1.199719254218462483 ) ) ;
#88267=CARTESIAN_POINT ( 'NONE',  ( 5.789495288235341874, 6.713164910151406595, 1.199719254218462483 ) ) ;
#88269=CARTESIAN_POINT ( 'NONE',  ( -7.944714827928056167, 10.29191993738131927, 1.443375672974090751 ) ) ;
#88270=CARTESIAN_POINT ( 'NONE',  ( -6.385527162356468445, 10.39360608948380538, 1.040834085586084257E-14 ) ) ;
#88271=CARTESIAN_POINT ( 'NONE',  ( 5.612712406377503349, 8.531619659873665995, -1.082531754730543083 ) ) ;
#88272=CARTESIAN_POINT ( 'NONE',  ( -8.961576348508655698, 9.557519949455999253, -0.7216878364870267237 ) ) ;
#88277=CARTESIAN_POINT ( 'NONE',  ( 8.437251666405968464, 8.737881787095446384, 1.040834085586084257E-14 ) ) ;
#88284=CARTESIAN_POINT ( 'NONE',  ( -0.6823417656250003738, 2.467708333674753618, -1.181850606188749264 ) ) ;
#88292=CARTESIAN_POINT ( 'NONE',  ( 8.666686507633574621, 11.13422023037111330, 1.599625672291281386 ) ) ;
#88296=CARTESIAN_POINT ( 'NONE',  ( -8.533967624797991647, 12.04371376465130439, -1.199719254218446718 ) ) ;
#88302=CARTESIAN_POINT ( 'NONE',  ( 3.728655938958122196, 4.308852335994623139, -1.199719254218446718 ) ) ;
#88305=CARTESIAN_POINT ( 'NONE',  ( -9.938290294017125603, 11.55342575023019691, -1.199719254218441611 ) ) ;
#88310=CARTESIAN_POINT ( 'NONE',  ( 5.861148881710747993, 5.995921596292371092, 0.2991943293650864422 ) ) ;
#88312=CARTESIAN_POINT ( 'NONE',  ( -4.711622075948912247, 5.455646162483875017, -1.199719254218446718 ) ) ;
#88316=CARTESIAN_POINT ( 'NONE',  ( 8.111855979677986994, 8.358253485912799263, 1.040834085586084257E-14 ) ) ;
#88318=CARTESIAN_POINT ( 'NONE',  ( 6.693975156845185737, 8.832723654451292816, 1.599625672291281386 ) ) ;
#88321=CARTESIAN_POINT ( 'NONE',  ( -8.134528978519403708, 11.47373899403920205, 1.082531754730549967 ) ) ;
#88329=CARTESIAN_POINT ( 'NONE',  ( -5.430810130430261395, 6.303639405459422917, -1.045180951442852946 ) ) ;
#88331=CARTESIAN_POINT ( 'NONE',  ( 5.856759171423504107, 5.935233242856626568, -0.7216878364870257245 ) ) ;
#88336=B_SPLINE_CURVE_WITH_KNOTS ( 'NONE', 3,
 ( #197092, #80148, #146251, #212267 ),
 .UNSPECIFIED., .F., .F.,
 ( 4, 4 ),
 ( 1.951563910473910678E-18, 0.0006335992342243210260 ),
 .UNSPECIFIED. ) ;
#88353=CARTESIAN_POINT ( 'NONE',  ( 7.096803341749390981, 10.36702210109460154, -1.199719254218441611 ) ) ;
#88357=CARTESIAN_POINT ( 'NONE',  ( -1.201851678989727383E-14, 1.243750000682821044, 1.732050807568877637 ) ) ;
#88359=CARTESIAN_POINT ( 'NONE',  ( -6.368579470117215813, 8.453095353268645695, 1.599625672291283607 ) ) ;
#88362=CARTESIAN_POINT ( 'NONE',  ( -8.299562589859897699, 12.83457345481192036, -0.7998128361456281477 ) ) ;
#88363=CARTESIAN_POINT ( 'NONE',  ( -1.408440994509118749, 7.230285460703087530, 4.273713947604063534 ) ) ;
#88366=CARTESIAN_POINT ( 'NONE',  ( 1.499999999999990896, 5.556250000682820378, 1.214306433183764966E-14 ) ) ;
#88367=CARTESIAN_POINT ( 'NONE',  ( 5.940443861082012944, 10.08226827123770697, 0.7998128361456462443 ) ) ;
#88369=CARTESIAN_POINT ( 'NONE',  ( -5.703176172842872482, 9.805455968292021041, 0.000000000000000000 ) ) ;
#88371=CARTESIAN_POINT ( 'NONE',  ( -1.364683531249997417, 5.509375000341417916, 1.214306433183764966E-14 ) ) ;
#88376=CARTESIAN_POINT ( 'NONE',  ( -7.212574532790092974, 10.39812547402169862, -1.082531754730543971 ) ) ;
#88380=CARTESIAN_POINT ( 'NONE',  ( -1.201851678989727383E-14, 4.009375000341416140, -1.575800808251660134 ) ) ;
#88386=CARTESIAN_POINT ( 'NONE',  ( -0.6823417656250212460, 4.801041667008086655, 1.181850606188767472 ) ) ;
#88392=CARTESIAN_POINT ( 'NONE',  ( 2.684151225381301575, 6.075334163012737321, 0.000000000000000000 ) ) ;
#88393=CARTESIAN_POINT ( 'NONE',  ( 0.6823417656249899377, 5.738541667008087543, -1.181850606188754593 ) ) ;
#88399=CARTESIAN_POINT ( 'NONE',  ( 1.364683531249988757, 0.6343750003414208027, 0.000000000000000000 ) ) ;
#88400=CARTESIAN_POINT ( 'NONE',  ( -3.090895834235680262, 5.589500325708124606, 1.082531754730560403 ) ) ;
#88401=CARTESIAN_POINT ( 'NONE',  ( 5.823390672269506574, 6.752709524857930745, -1.199719254218446718 ) ) ;
#88404=DIRECTION ( 'NONE',  ( 0.000000000000000000, -0.8000000000000623279, -0.5999999999999167111 ) ) ;
#88408=CARTESIAN_POINT ( 'NONE',  ( 10.68346185744421462, 11.56638637654751989, 0.000000000000000000 ) ) ;
#88410=CARTESIAN_POINT ( 'NONE',  ( -8.188761592974051595, 9.616271948966963024, -1.082531754730543971 ) ) ;
#88415=CARTESIAN_POINT ( 'NONE',  ( -9.484092147959342967, 11.02352791316275216, 1.199719254218462483 ) ) ;
#88417=CARTESIAN_POINT ( 'NONE',  ( -4.880572110795192486, 8.637825195995631589, 1.214306433183764966E-14 ) ) ;
#88419=CARTESIAN_POINT ( 'NONE',  ( 1.364683531249988757, 1.446875000341421469, 0.000000000000000000 ) ) ;
#88420=DIRECTION ( 'NONE',  ( 0.000000000000000000, 0.000000000000000000, -1.000000000000000000 ) ) ;
#88421=EDGE_CURVE ( 'NONE', #158934, #26788, #29333, .T. ) ;
#88426=CARTESIAN_POINT ( 'NONE',  ( 10.55910270694468345, 11.21337466772398095, 0.7998128361456462443 ) ) ;
#88440=EDGE_CURVE ( 'NONE', #19519, #137701, #182027, .T. ) ;
#88447=CARTESIAN_POINT ( 'NONE',  ( 1.364683531249988535, 3.426041667008085323, 0.7879004041258500513 ) ) ;
#88457=CARTESIAN_POINT ( 'NONE',  ( -1.402160292154681736E-14, 0.9468750003414176941, -1.575800808251659024 ) ) ;
#88468=CARTESIAN_POINT ( 'NONE',  ( 4.656335691289526402, 7.519809842224722374, -1.199719254218452047 ) ) ;
#88475=CARTESIAN_POINT ( 'NONE',  ( 7.904567251967224095, 9.180748867838630645, 1.199719254218462483 ) ) ;
#88479=CARTESIAN_POINT ( 'NONE',  ( 7.801827329660018684, 11.18955008699033726, 1.199719254218460707 ) ) ;
#88491=CARTESIAN_POINT ( 'NONE',  ( -7.700668062882078502, 9.046829497192987901, -1.082531754730543971 ) ) ;
#88495=CARTESIAN_POINT ( 'NONE',  ( -8.513630394377489807, 12.01998699582738972, -1.199719254218446718 ) ) ;
#88497=CARTESIAN_POINT ( 'NONE',  ( 2.236732156574683827, 5.553345249405011508, 1.040834085586084257E-14 ) ) ;
#88500=CARTESIAN_POINT ( 'NONE',  ( -5.122283107864663343, 4.870418468797203637, 0.000000000000000000 ) ) ;
#88502=CARTESIAN_POINT ( 'NONE',  ( 8.238550898598388628, 12.76339314834017102, 0.7998128361456462443 ) ) ;
#88503=ADVANCED_FACE ( 'NONE', ( #146305 ), #47735, .F. ) ;
#88505=CARTESIAN_POINT ( 'NONE',  ( 3.517450787741589036, 6.191110788085444128, -1.199719254218446718 ) ) ;
#88511=CARTESIAN_POINT ( 'NONE',  ( 4.582292731738905722, 5.408724944192588424, -1.082531754730548412 ) ) ;
#88513=CARTESIAN_POINT ( 'NONE',  ( -3.567766978690493307, 7.314145241780881435, 1.040834085586084257E-14 ) ) ;
#88516=CARTESIAN_POINT ( 'NONE',  ( -10.45741655484220267, 11.09474082360439873, -0.7998128361456221525 ) ) ;
#88522=CARTESIAN_POINT ( 'NONE',  ( 8.432808358020016826, 10.86136238915529084, 1.443375672974076540 ) ) ;
#88523=CARTESIAN_POINT ( 'NONE',  ( 1.364683531249988535, 3.926041667008087543, 0.7879004041258499402 ) ) ;
#88525=CARTESIAN_POINT ( 'NONE',  ( 5.345992642490140057, 5.131412925860272090, 1.040834085586084257E-14 ) ) ;
#88539=CARTESIAN_POINT ( 'NONE',  ( 0.6823417656249899377, 2.155208333674753174, 1.181850606188767472 ) ) ;
#88541=CARTESIAN_POINT ( 'NONE',  ( 8.191097360950562845, 12.70803068775103739, -0.7998128361456352531 ) ) ;
#88543=CARTESIAN_POINT ( 'NONE',  ( -6.900736999675794792, 7.153207375817628666, 1.040834085586084257E-14 ) ) ;
#88545=CARTESIAN_POINT ( 'NONE',  ( -4.080641047588902559, 7.704572288921609058, -0.7216878364870257245 ) ) ;
#88550=CARTESIAN_POINT ( 'NONE',  ( 4.449046963578762615, 8.342305224150557308, -0.7998128361456231517 ) ) ;
#88562=CARTESIAN_POINT ( 'NONE',  ( 6.518772930072240790, 6.499656594706071822, -0.7998128361456281477 ) ) ;
#88563=( LENGTH_UNIT ( ) NAMED_UNIT ( * ) SI_UNIT ( .MILLI., .METRE. ) );
#88565=CARTESIAN_POINT ( 'NONE',  ( -4.451154503988200339, 4.087435097607984957, 1.214306433183764966E-14 ) ) ;
#88567=CARTESIAN_POINT ( 'NONE',  ( -5.228640796364566690, 9.251831362400652736, -0.7998128361456231517 ) ) ;
#88571=CARTESIAN_POINT ( 'NONE',  ( 7.426115451983150706, 9.686887332112256388, -1.599625672291262513 ) ) ;
#88574=CARTESIAN_POINT ( 'NONE',  ( -7.088215381846223906, 7.164006121775713609, 0.7998128361456341429 ) ) ;
#88575=CARTESIAN_POINT ( 'NONE',  ( 6.222829318548112276, 9.243422724072711816, -1.082531754730537976 ) ) ;
#88576=CARTESIAN_POINT ( 'NONE',  ( 5.480859523967800406, 6.436073219340427976, 1.263442102793509880 ) ) ;
#88577=CARTESIAN_POINT ( 'NONE',  ( -3.411848212133334446, 7.132240014130862171, 0.7998128361456341429 ) ) ;
#88580=CARTESIAN_POINT ( 'NONE',  ( -5.377780486114890124, 9.425827667109372143, 0.000000000000000000 ) ) ;
#88583=CARTESIAN_POINT ( 'NONE',  ( -1.364683531250012516, 1.530208333674756505, 0.7879004041258379498 ) ) ;
#88586=CARTESIAN_POINT ( 'NONE',  ( -5.585596099150182958, 8.499983968108443477, -1.082531754730544860 ) ) ;
#88591=CARTESIAN_POINT ( 'NONE',  ( 4.957477724091233995, 8.935474444748447098, -0.7998128361456281477 ) ) ;
#88593=CARTESIAN_POINT ( 'NONE',  ( -5.907986510169434879, 6.002582827494773454, 0.1128355114666315662 ) ) ;
#88594=CARTESIAN_POINT ( 'NONE',  ( -1.364683531250000748, 1.321875000341421469, 0.000000000000000000 ) ) ;
#88597=FACE_OUTER_BOUND ( 'NONE', #173744, .T. ) ;
#88600=CARTESIAN_POINT ( 'NONE',  ( -3.113568832632681360, 6.784247404713427798, -0.7998128361456281477 ) ) ;
#88602=CARTESIAN_POINT ( 'NONE',  ( -7.009202228140744673, 10.16085778526412042, -1.082531754730537088 ) ) ;
#88606=B_SPLINE_CURVE_WITH_KNOTS ( 'NONE', 3,
 ( #185316, #36938, #116125, #103020 ),
 .UNSPECIFIED., .F., .F.,
 ( 4, 4 ),
 ( 0.000000000000000000, 3.568395612623403724E-05 ),
 .UNSPECIFIED. ) ;
#88611=CARTESIAN_POINT ( 'NONE',  ( -7.741342523278709642, 10.05465224862374285, 1.443375672974090751 ) ) ;
#88615=VERTEX_POINT ( 'NONE', #179848 ) ;
#88616=CARTESIAN_POINT ( 'NONE',  ( -7.714226216051410567, 9.062647342557177410, 1.082531754730558626 ) ) ;
#88619=ORIENTED_EDGE ( 'NONE', *, *, #6240, .T. ) ;
#88630=CARTESIAN_POINT ( 'NONE',  ( -6.021792782764022078, 10.17717534653336209, -0.7998128361456291469 ) ) ;
#88632=CARTESIAN_POINT ( 'NONE',  ( 4.090809663021327758, 5.795697244990093644, 1.599625672291267398 ) ) ;
#88636=CARTESIAN_POINT ( 'NONE',  ( 6.331821432781979730, 7.345878745455822312, -1.199719254218445830 ) ) ;
#88642=CARTESIAN_POINT ( 'NONE',  ( -4.284013352238262407, 6.021101549076499637, -1.443375672974053447 ) ) ;
#88651=CARTESIAN_POINT ( 'NONE',  ( -1.364683531250000748, 0.5093750003414208027, 0.000000000000000000 ) ) ;
#88653=CARTESIAN_POINT ( 'NONE',  ( -7.720478407978036195, 11.09464301169468037, -1.199719254218446718 ) ) ;
#88655=CARTESIAN_POINT ( 'NONE',  ( 8.392660782059197189, 9.750191319612612872, 1.199719254218462483 ) ) ;
#88657=CARTESIAN_POINT ( 'NONE',  ( -9.365985188942097750, 9.821404230054264772, 0.7998128361456462443 ) ) ;
#88660=CARTESIAN_POINT ( 'NONE',  ( 0.6823417656249917140, 4.342708333674755394, 1.181850606188765695 ) ) ;
#88662=CARTESIAN_POINT ( 'NONE',  ( 9.761507412159302177, 10.49077285704843199, -0.7216878364870257245 ) ) ;
#88665=CARTESIAN_POINT ( 'NONE',  ( 1.364683531249986537, -1.073958332991911790, 0.7879004041258500513 ) ) ;
#88669=CARTESIAN_POINT ( 'NONE',  ( 6.927853306458739979, 10.06595070996845642, 1.082531754730558626 ) ) ;
#88671=CARTESIAN_POINT ( 'NONE',  ( -5.368665641331555882, 8.246898433986675769, 1.082531754730548412 ) ) ;
#88674=CARTESIAN_POINT ( 'NONE',  ( 0.6823417656249899377, 3.676041667008085767, -1.181850606188754593 ) ) ;
#88676=CARTESIAN_POINT ( 'NONE',  ( 3.086313801757624820, 6.452272078211774620, 0.4027703449977940720 ) ) ;
#88678=CARTESIAN_POINT ( 'NONE',  ( -5.032047568966410367, 9.022472597102808578, 1.214306433183764966E-14 ) ) ;
#88679=CARTESIAN_POINT ( 'NONE',  ( 1.364683531249988535, 5.467708333674750953, -0.7879004041258300672 ) ) ;
#88684=CARTESIAN_POINT ( 'NONE',  ( 7.801827329660018684, 11.18955008699033726, 1.199719254218460707 ) ) ;
#88687=CARTESIAN_POINT ( 'NONE',  ( -1.499999999999997780, 2.400000000000020339, 1.214306433183764966E-14 ) ) ;
#88690=CYLINDRICAL_SURFACE ( 'NONE', #177635, 1.250000000000000000 ) ;
#88693=CARTESIAN_POINT ( 'NONE',  ( 5.504247177468168495, 9.365446107114122398, 0.7216878364870438212 ) ) ;
#88703=CARTESIAN_POINT ( 'NONE',  ( -1.500000000000001332, -0.8499999999999757749, 0.000000000000000000 ) ) ;
#88704=CARTESIAN_POINT ( 'NONE',  ( 8.450809820019639318, 8.753699632978056755, -0.7998128361456291469 ) ) ;
#88705=CARTESIAN_POINT ( 'NONE',  ( -9.664264568442742842, 10.16939683947169115, -0.7998128361456291469 ) ) ;
#88707=CARTESIAN_POINT ( 'NONE',  ( -1.364683531250000748, 0.2593750003414205252, 0.000000000000000000 ) ) ;
#88708=CARTESIAN_POINT ( 'NONE',  ( 0.7499999999999885647, 0.7333333333333567072, 1.299038105676657340 ) ) ;
#88710=CARTESIAN_POINT ( 'NONE',  ( 4.798696304233017074, 7.685897223992134819, -1.199719254218452047 ) ) ;
#88717=CARTESIAN_POINT ( 'NONE',  ( 0.6823417656249899377, 4.676041667008086655, -1.181850606188754593 ) ) ;
#88719=CARTESIAN_POINT ( 'NONE',  ( -6.835281999583978418, 11.12624609948998966, -0.7998128361456291469 ) ) ;
#88720=CARTESIAN_POINT ( 'NONE',  ( -4.284013352238250860, 7.941839977679187257, -0.7216878364870267237 ) ) ;
#88729=CARTESIAN_POINT ( 'NONE',  ( 8.437251666405968464, 8.737881787095446384, 1.040834085586084257E-14 ) ) ;
#88733=CARTESIAN_POINT ( 'NONE',  ( 6.114364089638775646, 10.07724917131317355, 0.7216878364870438212 ) ) ;
#88736=CARTESIAN_POINT ( 'NONE',  ( -7.049349804101573191, 10.31165964050546258, -1.199719254218440723 ) ) ;
#88737=CARTESIAN_POINT ( 'NONE',  ( 5.789495288235341874, 6.713164910151406595, 1.199719254218462483 ) ) ;
#88738=FACE_OUTER_BOUND ( 'NONE', #192755, .T. ) ;
#88740=CARTESIAN_POINT ( 'NONE',  ( 4.196412238629597447, 4.854568018944682706, -1.199719254218452047 ) ) ;
#88747=CARTESIAN_POINT ( 'NONE',  ( -4.853455804012230423, 6.685451076146141425, 1.443375672974064550 ) ) ;
#88748=CARTESIAN_POINT ( 'NONE',  ( 2.198393463710220264, 5.716542807637226886, 0.7998128361456462443 ) ) ;
#88751=CARTESIAN_POINT ( 'NONE',  ( -7.854251061018346469, 8.057714414143200443, -0.7998128361456291469 ) ) ;
#88757=CARTESIAN_POINT ( 'NONE',  ( -6.509886312855995172, 10.74661779830734254, -0.7998128361456291469 ) ) ;
#88760=DIRECTION ( 'NONE',  ( 0.000000000000000000, 8.546850786086437571E-32, 1.000000000000000000 ) ) ;
#88763=CARTESIAN_POINT ( 'NONE',  ( 4.202137545231717120, 6.989912005157271402, 1.199719254218462483 ) ) ;
#88774=CARTESIAN_POINT ( 'NONE',  ( -7.043624497499477499, 8.176315654292865887, 1.199719254218450271 ) ) ;
#88777=CARTESIAN_POINT ( 'NONE',  ( 4.338245966692901412, 8.005111361209628740, -0.7216878364870197293 ) ) ;
#88782=CARTESIAN_POINT ( 'NONE',  ( -3.750802052474980108, 7.527686161196117887, 1.040834085586084257E-14 ) ) ;
#88786=CARTESIAN_POINT ( 'NONE',  ( -7.054319997812058318, 7.124461507069184130, 1.040834085586084257E-14 ) ) ;
#88792=CARTESIAN_POINT ( 'NONE',  ( -8.371269781434001800, 11.85389961405997816, -1.199719254218446718 ) ) ;
#88793=CARTESIAN_POINT ( 'NONE',  ( 5.777746017718023097, 9.892454120646377191, 0.7998128361456462443 ) ) ;
#88795=CARTESIAN_POINT ( 'NONE',  ( -4.297571505851936813, 4.116180966356429494, 1.214306433183764966E-14 ) ) ;
#88796=CARTESIAN_POINT ( 'NONE',  ( -9.297140650669053485, 11.86975006391249643, 1.599625672291281386 ) ) ;
#88803=CARTESIAN_POINT ( 'NONE',  ( 10.08690309888728187, 10.87040115823107911, -0.7216878364870257245 ) ) ;
#88827=CARTESIAN_POINT ( 'NONE',  ( -2.598358995313378550, 6.183169261174235487, 0.7998128361456341429 ) ) ;
#88830=CARTESIAN_POINT ( 'NONE',  ( -3.623053363349869382, 5.249981562040033189, 1.599625672291267398 ) ) ;
#88834=CARTESIAN_POINT ( 'NONE',  ( -0.6823417656249969321, 5.467708333674756283, -1.181850606188749264 ) ) ;
#88842=CARTESIAN_POINT ( 'NONE',  ( 2.381428537494710618, 5.930083727052461562, 0.7998128361456462443 ) ) ;
#88846=CARTESIAN_POINT ( 'NONE',  ( 8.215877899756996783, 12.52901528311778989, 1.040834085586084257E-14 ) ) ;
#88848=CARTESIAN_POINT ( 'NONE',  ( 6.634017235788401301, 6.634108284708264414, 0.7998128361456341429 ) ) ;
#88849=CARTESIAN_POINT ( 'NONE',  ( -1.364683531249997417, 2.571875000341422357, 1.214306433183764966E-14 ) ) ;
#88853=CARTESIAN_POINT ( 'NONE',  ( -9.318531651294266638, 9.766041769465124034, -0.7998128361456291469 ) ) ;
#88855=CARTESIAN_POINT ( 'NONE',  ( -3.917943204224913156, 7.514758138330285497, -0.7216878364870257245 ) ) ;
#88857=CARTESIAN_POINT ( 'NONE',  ( -5.961834861707238531, 7.978559976790334574, -1.599625672291263179 ) ) ;
#88859=CARTESIAN_POINT ( 'NONE',  ( 1.364683531249990311, 5.363541667008086655, 0.7879004041258500513 ) ) ;
#88867=CARTESIAN_POINT ( 'NONE',  ( -5.883875478206491927, 5.966868934103426447, 0.000000000000000000 ) ) ;
#88872=CARTESIAN_POINT ( 'NONE',  ( -3.565431210269599749, 7.103494145382415859, 0.7216878364870317197 ) ) ;
#88880=ORIENTED_EDGE ( 'NONE', *, *, #167387, .F. ) ;
#88884=CARTESIAN_POINT ( 'NONE',  ( -5.251085567194491155, 5.020688004682002159, -0.7998128361456221525 ) ) ;
#88885=CARTESIAN_POINT ( 'NONE',  ( -9.297140650669053485, 11.86975006391249643, 1.599625672291281386 ) ) ;
#88888=ORIENTED_EDGE ( 'NONE', *, *, #71139, .F. ) ;
#88890=CARTESIAN_POINT ( 'NONE',  ( 4.659198344590585350, 8.587481835331020719, 0.7998128361456462443 ) ) ;
#88895=VECTOR ( 'NONE', #148134, 1000.000000000000000 ) ;
#88906=CARTESIAN_POINT ( 'NONE',  ( 7.259501185113382604, 10.55683625168592243, -1.199719254218441611 ) ) ;
#88907=CARTESIAN_POINT ( 'NONE',  ( -3.750802052474980108, 7.527686161196117887, 1.040834085586084257E-14 ) ) ;
#88912=CARTESIAN_POINT ( 'NONE',  ( -1.001543065824772872E-14, 4.321875000341417916, 1.575800808251672791 ) ) ;
#88914=CARTESIAN_POINT ( 'NONE',  ( -4.252453736180621391, 8.112946458852704268, -0.7998128361456281477 ) ) ;
#88917=CARTESIAN_POINT ( 'NONE',  ( 3.832150974156964818, 7.622593236491780999, 1.040834085586084257E-14 ) ) ;
#88918=CARTESIAN_POINT ( 'NONE',  ( -5.922214171070950606, 5.803671375871217286, -0.7998128361456291469 ) ) ;
#88920=CARTESIAN_POINT ( 'NONE',  ( 2.959812437696838661, 6.450877987504894051, 0.3496188560969323289 ) ) ;
#88925=CARTESIAN_POINT ( 'NONE',  ( 6.860062538834778678, 8.066123052471139587, -1.082531754730543083 ) ) ;
#88927=CARTESIAN_POINT ( 'NONE',  ( 6.100805936025112786, 10.06143132543056673, 1.040834085586084257E-14 ) ) ;
#88928=CARTESIAN_POINT ( 'NONE',  ( 1.364683531249988535, 3.217708333674748289, -0.7879004041258239610 ) ) ;
#88929=CARTESIAN_POINT ( 'NONE',  ( 5.355107487273504496, 6.310342158982962246, -1.082531754730543083 ) ) ;
#88939=CARTESIAN_POINT ( 'NONE',  ( -5.408724846006345288, 6.482216231307839749, 1.333832282565196925 ) ) ;
#88940=CARTESIAN_POINT ( 'NONE',  ( 1.500000000000007105, 10.64264068711930733, 1.214306433183764966E-14 ) ) ;
#88945=CARTESIAN_POINT ( 'NONE',  ( -9.480175724453545172, 12.08329098332774265, 1.599625672291281386 ) ) ;
#88950=CARTESIAN_POINT ( 'NONE',  ( -2.785310492603665367, 5.336947110424484109, 1.199719254218462483 ) ) ;
#88955=CARTESIAN_POINT ( 'NONE',  ( 4.717874267875568961, 4.606534188717351874, -0.7216878364870188411 ) ) ;
#88957=CARTESIAN_POINT ( 'NONE',  ( -1.201851678989727383E-14, 3.884375000341423689, 1.575800808251672791 ) ) ;
#88959=CARTESIAN_POINT ( 'NONE',  ( 6.531277313481192337, 8.642909503859968368, 1.599625672291281386 ) ) ;
#88964=EDGE_LOOP ( 'NONE', ( #154501, #213068, #11940, #41590, #38796 ) ) ;
#88966=CARTESIAN_POINT ( 'NONE',  ( -0.7500000000000215383, 4.441666666666691299, 1.299038105676671107 ) ) ;
#88967=CARTESIAN_POINT ( 'NONE',  ( 3.985207087413062066, 6.736826471035503694, -1.199719254218452047 ) ) ;
#88971=CARTESIAN_POINT ( 'NONE',  ( 1.364683531249990311, 3.884375000341417028, 1.214306433183764966E-14 ) ) ;
#88973=CARTESIAN_POINT ( 'NONE',  ( 8.541273586929342798, 11.94827437051752206, -1.082531754730543083 ) ) ;
#88978=CARTESIAN_POINT ( 'NONE',  ( -0.7500000000000006661, 2.139583334016155636, -1.299038105676652011 ) ) ;
#88982=CARTESIAN_POINT ( 'NONE',  ( -5.205440912643032547, 8.160432600470439723, 1.199719254218452047 ) ) ;
#88984=CARTESIAN_POINT ( 'NONE',  ( 5.138177029454847222, 6.057256624861201644, 1.082531754730560403 ) ) ;
#88992=CARTESIAN_POINT ( 'NONE',  ( 7.527801604085637699, 9.805521176231838609, 1.599625672291281386 ) ) ;
#88993=CARTESIAN_POINT ( 'NONE',  ( 3.960953433486789521, 7.772862772376584850, -0.7998128361456221525 ) ) ;
#88997=CARTESIAN_POINT ( 'NONE',  ( 6.331821432781979730, 7.345878745455822312, -1.199719254218445830 ) ) ;
#89004=CARTESIAN_POINT ( 'NONE',  ( 10.55232363013785246, 11.20546574478267132, 0.000000000000000000 ) ) ;
#89010=CARTESIAN_POINT ( 'NONE',  ( 5.407503677813131127, 6.286683671216334091, 1.048937882774292785 ) ) ;
#89016=CARTESIAN_POINT ( 'NONE',  ( -3.673896439623323129, 4.156855427197417185, 2.420000000000010587 ) ) ;
#89018=DIRECTION ( 'NONE',  ( 1.000000000000000000, 0.000000000000000000, 0.000000000000000000 ) ) ;
#89019=CARTESIAN_POINT ( 'NONE',  ( 7.510853912290742507, 8.825379654836435606, -1.082531754730537976 ) ) ;
#89021=CARTESIAN_POINT ( 'NONE',  ( -2.903417451620861289, 6.539070793532962611, 0.7998128361456341429 ) ) ;
#89026=CARTESIAN_POINT ( 'NONE',  ( -5.928993247877788697, 5.811580298812519807, 0.7998128361456341429 ) ) ;
#89038=CARTESIAN_POINT ( 'NONE',  ( 8.503988664269582998, 10.94440607977979063, 1.599625672291281386 ) ) ;
#89040=CARTESIAN_POINT ( 'NONE',  ( 4.001749955438753226, 7.811071542261023737, 0.1299566359906061952 ) ) ;
#89046=CARTESIAN_POINT ( 'NONE',  ( -10.46653140006992899, 11.31330084294416771, -0.7216878364870267237 ) ) ;
#89051=CARTESIAN_POINT ( 'NONE',  ( 9.264299036839600987, 9.702770385934682551, -0.7998128361456281477 ) ) ;
#89056=CARTESIAN_POINT ( 'NONE',  ( -5.819474248763749635, 7.812472595022922128, -1.599625672291256295 ) ) ;
#89057=CARTESIAN_POINT ( 'NONE',  ( 5.508690485854129903, 5.321227076451600091, 1.040834085586084257E-14 ) ) ;
#89060=CARTESIAN_POINT ( 'NONE',  ( -3.314994193297896796, 6.393354490853021765, -0.7784788408506219115 ) ) ;
#89064=CARTESIAN_POINT ( 'NONE',  ( 0.6823417656249882723, 2.738541667008084879, -1.181850606188749264 ) ) ;
#89066=CARTESIAN_POINT ( 'NONE',  ( 7.646435448427411963, 8.023188899361205273, -0.7216878364870257245 ) ) ;
#89075=CARTESIAN_POINT ( 'NONE',  ( 9.259855728009286580, 10.86588177317476855, -1.082531754730543083 ) ) ;
#89079=CARTESIAN_POINT ( 'NONE',  ( -9.528683032306089373, 10.01121838064558744, 0.7998128361456462443 ) ) ;
#89084=B_SPLINE_CURVE_WITH_KNOTS ( 'NONE', 3,
 ( #126543, #111343, #42032, #77700, #208754, #11626, #108144, #60380, #174170, #4401 ),
 .UNSPECIFIED., .F., .F.,
 ( 4, 3, 3, 4 ),
 ( 3.554236483114673897E-17, 3.125182663314470276E-05, 6.250390969754492131E-05, 0.0001046323561353133347 ),
 .UNSPECIFIED. ) ;
#89090=CARTESIAN_POINT ( 'NONE',  ( 3.181359600701000989, 6.863336634126477875, 0.000000000000000000 ) ) ;
#89097=CARTESIAN_POINT ( 'NONE',  ( 5.986088515633498197, 6.942523675449257858, -1.199719254218446718 ) ) ;
#89100=CARTESIAN_POINT ( 'NONE',  ( 0.7499999999999902300, 3.014583334016149418, 1.299038105676669330 ) ) ;
#89105=CARTESIAN_POINT ( 'NONE',  ( 0.7499999999999885647, 0.2333333333333562076, 1.299038105676657340 ) ) ;
#89106=CARTESIAN_POINT ( 'NONE',  ( 6.238723240582662477, 10.43026088065513513, -0.7998128361456291469 ) ) ;
#89107=CARTESIAN_POINT ( 'NONE',  ( -0.6823417656250246877, 0.05104166700808931978, 1.181850606188755259 ) ) ;
#89110=CARTESIAN_POINT ( 'NONE',  ( 7.931156674314368438, 12.19684052010138586, 1.040834085586084257E-14 ) ) ;
#89115=CARTESIAN_POINT ( 'NONE',  ( -5.904739593951539689, 6.847616600153594746, 1.199719254218450271 ) ) ;
#89117=CARTESIAN_POINT ( 'NONE',  ( 1.499999999999989120, 2.306250000682817713, 1.214306433183764966E-14 ) ) ;
#89118=CARTESIAN_POINT ( 'NONE',  ( -1.201851678989727383E-14, 5.259375000341421469, -1.575800808251660134 ) ) ;
#89123=CARTESIAN_POINT ( 'NONE',  ( -1.364683531249997417, 4.321875000341417028, 1.214306433183764966E-14 ) ) ;
#89132=CARTESIAN_POINT ( 'NONE',  ( -6.842061076390810292, 11.13415502243129218, 0.000000000000000000 ) ) ;
#89133=CARTESIAN_POINT ( 'NONE',  ( 7.470706336329915764, 8.674577799595093452, -1.199719254218441611 ) ) ;
#89135=DIRECTION ( 'NONE',  ( 0.5038915848600621361, -0.5182601445700819598, -0.6910135261030805331 ) ) ;
#89139=CARTESIAN_POINT ( 'NONE',  ( -3.070003471035267939, 6.451017196056028524, -0.6895117023006979151 ) ) ;
#89141=CARTESIAN_POINT ( 'NONE',  ( -6.612626235163205024, 8.737816579155630592, -1.599625672291263179 ) ) ;
#89146=CARTESIAN_POINT ( 'NONE',  ( 3.837121167867449945, 4.435395103055503441, 1.199719254218464037 ) ) ;
#89147=DIRECTION ( 'NONE',  ( 5.578564026256490882E-16, 1.000000000000000000, 9.066213480720158442E-32 ) ) ;
#89148=EDGE_LOOP ( 'NONE', ( #124838, #182969, #97788 ) ) ;
#89149=CARTESIAN_POINT ( 'NONE',  ( -5.253948220495577637, 6.088359997788290734, 1.199719254218450271 ) ) ;
#89150=CARTESIAN_POINT ( 'NONE',  ( -9.332089804907933939, 9.781859615347734405, 1.040834085586084257E-14 ) ) ;
#89154=CARTESIAN_POINT ( 'NONE',  ( -3.975569122714607495, 7.849474212055944200, 0.02231197147695325456 ) ) ;
#89161=CARTESIAN_POINT ( 'NONE',  ( 7.169564303528210836, 7.258913197071374945, -0.7998128361456281477 ) ) ;
#89181=CARTESIAN_POINT ( 'NONE',  ( 3.931501358282940117, 4.649468341827285300, -1.082531754730543083 ) ) ;
#89185=CARTESIAN_POINT ( 'NONE',  ( -7.797910906154257304, 12.24931315715533486, 0.000000000000000000 ) ) ;
#89186=CARTESIAN_POINT ( 'NONE',  ( 0.7499999999999920064, 4.233333333333352932, 1.299038105676669330 ) ) ;
#89191=CARTESIAN_POINT ( 'NONE',  ( -1.402160292154681736E-14, 2.118750000682816825, -1.732050807568863648 ) ) ;
#89193=CARTESIAN_POINT ( 'NONE',  ( 4.352673489508670279, 7.270661361071050877, 1.119103973195253232 ) ) ;
#89196=CARTESIAN_POINT ( 'NONE',  ( -10.64045162862669081, 11.30828174301964140, -0.7998128361456221525 ) ) ;
#89197=CARTESIAN_POINT ( 'NONE',  ( 1.364683531249988757, 1.134375000341421247, 0.000000000000000000 ) ) ;
#89203=CARTESIAN_POINT ( 'NONE',  ( -3.795392936821753604, 6.515376628678959392, -1.199719254218452047 ) ) ;
#89205=DIRECTION ( 'NONE',  ( -5.578564026256490882E-16, -1.000000000000000000, -9.066213480720158442E-32 ) ) ;
#89208=CARTESIAN_POINT ( 'NONE',  ( -1.364683531250014514, 0.05104166700808546175, -0.7879004041258359514 ) ) ;
#89215=CARTESIAN_POINT ( 'NONE',  ( -1.364683531250000748, -0.2406249996585799189, 0.000000000000000000 ) ) ;
#89217=CARTESIAN_POINT ( 'NONE',  ( -6.353967546298838087, 10.56471257065732416, 0.000000000000000000 ) ) ;
#89218=CARTESIAN_POINT ( 'NONE',  ( 7.865701674222579598, 12.32840238656838139, -0.7998128361456352531 ) ) ;
#89219=CARTESIAN_POINT ( 'NONE',  ( 5.464099601507359516, 6.333536608968757697, 1.199719254218462483 ) ) ;
#89222=CARTESIAN_POINT ( 'NONE',  ( -1.201851678989727383E-14, 1.384375000341419693, 1.575800808251672791 ) ) ;
#89226=B_SPLINE_CURVE_WITH_KNOTS ( 'NONE', 3,
 ( #7789, #173541, #107512, #12069 ),
 .UNSPECIFIED., .F., .F.,
 ( 4, 4 ),
 ( 1.062296840242581388E-18, 0.0002848003335318597751 ),
 .UNSPECIFIED. ) ;
#89227=EDGE_CURVE ( 'NONE', #80644, #25151, #195981, .T. ) ;
#89230=CARTESIAN_POINT ( 'NONE',  ( 6.073689629242148058, 8.109057205581079231, -1.443375672974057666 ) ) ;
#89233=CARTESIAN_POINT ( 'NONE',  ( -3.391510981712833939, 7.108513245306943062, 0.7998128361456341429 ) ) ;
#89235=CARTESIAN_POINT ( 'NONE',  ( -1.499999999999997780, 5.681250000682820378, 1.214306433183764966E-14 ) ) ;
#89238=CARTESIAN_POINT ( 'NONE',  ( 4.636525345749193505, 8.353103970108639587, 1.040834085586084257E-14 ) ) ;
#89239=CARTESIAN_POINT ( 'NONE',  ( -8.649738815394339753, 9.193709494155953621, 1.040834085586084257E-14 ) ) ;
#89241=CARTESIAN_POINT ( 'NONE',  ( -0.7500000000000215383, 3.941666666666690411, 1.299038105676671107 ) ) ;
#89245=CARTESIAN_POINT ( 'NONE',  ( 8.378575743565351175, 11.75846021992619406, -1.082531754730543083 ) ) ;
#89259=CARTESIAN_POINT ( 'NONE',  ( 6.751597309481075726, 10.82068792779586985, 1.040834085586084257E-14 ) ) ;
#89260=CARTESIAN_POINT ( 'NONE',  ( 7.052212457402625922, 11.37933163361175382, -0.7998128361456291469 ) ) ;
#89261=CARTESIAN_POINT ( 'NONE',  ( -6.287230548435221777, 8.358188277972981695, -1.599625672291263179 ) ) ;
#89265=CARTESIAN_POINT ( 'NONE',  ( -1.402160292154681736E-14, -1.115624999658584082, 1.575800808251672791 ) ) ;
#89266=CARTESIAN_POINT ( 'NONE',  ( 5.205967797967541166, 5.175976640491323444, -0.7216878364870197293 ) ) ;
#89268=CARTESIAN_POINT ( 'NONE',  ( -8.026063749610056419, 10.38682701267698150, -1.443375672974059665 ) ) ;
#89275=( BOUNDED_SURFACE ( )  B_SPLINE_SURFACE ( 1, 2, ( 
 ( #29880, #211801, #130645, #79682, #62366, #33067, #113328, #128528, #13607, #80759, #147897, #179335, #14666, #146848, #45079, #63439, #213913, #64502, #48277, #193435, #177191, #114390, #15729, #180385, #98092, #81814, #65536, #131682, #197684, #115448, #99145, #165195, #170520, #36243, #100193, #17849, #133800, #5860, #185692, #166259, #68734, #50382, #103397, #135905, #22102, #199810, #182494, #88215, #51454, #86076, #154286, #52508, #134855, #198735, #83934, #132732, #70860, #116503, #102322, #69796, #201923, #34122, #150024, #1593, #21044, #183569, #67654, #101252, #87141, #186767, #53576, #54642, #85006, #117574, #35175, #169457, #118641, #119710, #167335, #18921, #151097, #2661, #200861, #184626, #168395, #19992, #152151, #3721, #37322, #153212, #4782, #136975, #203002, #120790, #38393, #104473, #111740, #171589, #9894, #75971, #144224, #79165, #28285, #162567, #143152, #209146, #159351, #13085, #71932, #60785, #10948, #142074, #126944, #62910, #208088, #23182, #128021, #192901, #44557, #121861, #175622, #195051, #77022, #158303, #177746, #138042, #59716, #145281, #176673, #210218, #92257, #110673, #94380, #125875, #160420, #12026, #191834, #96519, #204055, #78097, #43497, #109617, #129080, #61854, #193975, #27209, #39459, #55707, #45623, #29361, #95456, #161505, #211287, #46690, #112807, #187832, #178821, #30433, #105554, #93315, #198228, #84487, #16268, #83418, #196128, #100738, #35733, #114928, #184112, #34668, #65030, #1082, #63987, #183054, #148443, #99680, #80233, #32547, #133281, #2140, #166818, #132218, #213408, #67146, #200351, #181979, #66077, #131186, #50932, #199288, #49864, #197175, #130139, #47768, #146331, #82353, #113881, #48811, #115990, #179876, #33610, #101808, #118127, #68217, #13, #165750, #17336, #180926, #150578, #98623, #164685, #117057, #14140, #31501, #149499, #18412, #134347, #52001, #97575, #15214, #212346, #163632, #81305, #147382, #119186, #87688, #188379, #23743, #53052, #187317, #172151, #89848, #122421, #154832, #71414, #55195, #155898, #169995, #103953, #201413, #171066, #168938, #7485, #20540, #22663, #185171, #73567, #40017, #88774, #6416, #139669, #135391, #186242, #205690, #72488, #57326, #56263, #138589, #3209, #86623, #37877, #105028, #54132, #69278, #123490, #21583, #102880, #70343, #121342, #106128, #153762, #5331, #137526, #19475, #202479, #189454, #36795, #203541, #41095, #167876, #136460, #204612, #85551, #38944, #120267, #152691, #151641, #4272, #8563, #107205, #59452, #145008, #10686, #74643, #206760, #108278, #194777, #160157, #140749, #43232, #24808, #77829, #110408, #211014, #174299, #156974, #62636, #25873, #60510, #128795, #26939, #109349, #173228, #58392, #90909, #45353, #124548, #76756, #44287, #176412, #94116, #190506, #42163, #175359, #142878, #143950, #28018, #91984, #158042, #29092, #9629, #192634, #75706, #141821, #93047, #127752, #177477, #207823, #126671, #111472, #95176, #61584, #11755, #208880, #209945, #161225, #159088, #193709, #125609, #12812, #191568, #78885, #113603, #49596, #63713, #166551, #66872, #115720, #99422, #34403, #13879, #64775, #182785, #165476, #100475, #149229, #181710, #96241, #179607, #130916, #197965, #147119, #162292, #18138, #48549, #195854, #163361, #148179, #804, #196909, #98351, #114667, #112530, #81032, #133017, #79958, #180661, #1881, #46414, #14936, #83150, #150315, #32286, #213145, #146060, #134085, #67941, #212074, #178543, #164417, #84227, #16001, #129870, #47494, #31228, #30153, #17072, #97302, #82086, #214180, #199016, #33340, #65808, #131955, #50662, #116788, #52793, #153509, #89590, #120005, #136200, #51743, #19215, #7223, #138331, #73299, #169745, #137270, #54937, #35470, #85294, #117866, #202218, #101548, #168679, #21334, #167617, #37615, #183857, #204347, #121089, #56005, #5078, #200094, #53872, #185981, #70085, #122156, #118932, #203290, #2949, #105860, #6155, #187056, #38688, #188124, #151380, #4016, #39755, #104767, #171886, #88516, #170816, #69021, #184912, #103695, #22407, #86367, #135138, #23483, #87440, #201154, #102623, #71153, #154578, #72224, #155639, #36536, #20282, #152437, #159902 ),
 ( #91733, #177226, #42981, #106946, #24548, #140494, #12567, #192383, #172969, #75453, #57071, #110155, #142620, #28839, #206504, #189200, #94927, #58135, #92795, #160976, #59194, #141566, #205434, #90655, #139401, #77580, #123235, #109091, #76509, #208629, #40837, #156717, #8308, #207574, #74392, #108022, #175107, #124294, #111223, #190253, #10437, #157785, #125350, #26693, #158840, #41911, #209696, #174048, #25621, #126419, #9382, #191313, #60262, #44037, #176168, #27768, #93864, #11509, #61339, #143703, #127498, #193469, #45113, #212900, #99171, #148973, #178303, #98121, #82900, #547, #33096, #65563, #196666, #180417, #66612, #80790, #14695, #112287, #81843, #79711, #147926, #95995, #130677, #64533, #13638, #32035, #164173, #129623, #100220, #210776, #146880, #29912, #162048, #132759, #213942, #15758, #145826, #46173, #166288, #48306, #131710, #114417, #197714, #49356, #115474, #181467, #62397, #198762, #165223, #211831, #195609, #16815, #50411, #116531, #182520, #63468, #34150, #78639, #179364, #144765, #128561, #47245, #194526, #113359, #30986, #97061, #163114, #83962, #36272, #136999, #5885, #104501, #135929, #2688, #4807, #204081, #185716, #69821, #68761, #54668, #203027, #201947, #134881, #120816, #200888, #167362, #52534, #186793, #71958, #21068, #154312, #184651, #151123, #1623, #38421, #152177, #87166, #118668, #117604, #102349, #168421, #20017, #133827, #18950, #86105, #105583, #3746, #51481, #199839, #85034, #170545, #22129, #138068, #150051, #53603, #119737, #55734, #67682, #88242, #153236, #121888, #37349, #17878, #103423, #169484, #70889, #187858, #183596, #39485, #35203, #101279, #157527, #159650, #106679, #122975, #10184, #9122, #75198, #6956, #57872, #77325, #41650, #40573, #60008, #44856, #90386, #175914, #58942, #188934, #141309, #207321, #172702, #125099, #191057, #8041, #193208, #89324, #173790, #56805, #24280, #11247, #174856, #42722, #156455, #139135, #171617, #25366, #108830, #107764, #26434, #76258, #92545, #142367, #155371, #143438, #158584, #205163, #74130, #208376, #27505, #91466, #126161, #140225, #43790, #23211, #124034, #127239, #192125, #206246, #109902, #73037, #93605, #209435, #61079, #190000, #129373, #15503, #98921, #197464, #14438, #95743, #97867, #82649, #64284, #162860, #161794, #147675, #81590, #80528, #13385, #213692, #79461, #45920, #145577, #65314, #164974, #114173, #32844, #63209, #29657, #94673, #131463, #30728, #180167, #211575, #210518, #195352, #46984, #113100, #12309, #112040, #179106, #198518, #96811, #144510, #78390, #178041, #49108, #115228, #16566, #176968, #146625, #212642, #148733, #28585, #181218, #31793, #301, #130430, #110961, #196416, #48060, #163928, #66372, #160715, #132520, #62153, #128312, #194275, #38180, #199587, #1377, #103180, #36028, #168177, #99979, #150876, #170298, #134640, #133583, #152994, #137827, #183352, #54432, #151932, #119489, #52294, #50164, #101027, #83713, #17628, #117354, #4570, #136754, #104252, #116285, #85858, #34956, #21886, #182276, #202782, #185476, #120574, #3507, #33900, #118423, #184409, #200645, #186551, #166043, #102106, #19776, #51230, #69577, #87996, #167118, #67438, #169240, #135688, #201713, #149803, #2439, #154068, #53354, #18705, #70643, #84788, #68513, #5633, #37100, #20828, #86926, #71714, #189749, #138896, #91217, #8867, #40326, #10989, #121647, #205996, #89079, #72796, #191874, #207064, #74946, #204915, #171371, #77064, #57632, #141057, #139974, #107511, #42468, #124842, #108578, #187614, #109657, #58694, #22964, #106431, #173540, #59755, #123791, #190808, #155136, #76010, #203848, #90144, #159390, #9935, #172454, #174606, #39242, #158341, #41401, #26182, #55493, #7788, #92297, #43534, #142113, #25114, #188690, #208126, #175659, #157278, #125915, #24041, #27247, #93353, #105334, #156212, #6718, #73881, #56569, #122727, #64029, #31539, #178862, #113921, #45665, #78137, #60825, #80274, #13130, #30473, #128059, #176712, #210260, #194015, #61898, #192945, #12068, #213446, #44597, #95496, #62951, #146372, #96558, #94421, #144267, #179917, #163672, #46734, #111782, #28325, #161543, #130175, #47808, #110712 ) ),
 .UNSPECIFIED., .F., .F., .T. ) 
 B_SPLINE_SURFACE_WITH_KNOTS ( ( 2, 2 ),
 ( 3, 2, 2, 2, 2, 2, 2, 2, 2, 2, 2, 2, 2, 2, 2, 2, 2, 2, 2, 2, 2, 2, 2, 2, 2, 2, 2, 2, 2, 2, 2, 2, 2, 2, 2, 2, 2, 2, 2, 2, 2, 2, 2, 2, 2, 2, 2, 2, 2, 2, 2, 2, 2, 2, 2, 2, 2, 2, 2, 2, 2, 2, 2, 2, 2, 2, 2, 2, 2, 2, 2, 2, 2, 2, 2, 2, 2, 2, 2, 2, 2, 2, 2, 2, 2, 2, 2, 2, 2, 2, 2, 2, 2, 2, 2, 2, 2, 2, 2, 2, 2, 2, 2, 2, 2, 2, 2, 2, 2, 2, 2, 2, 2, 2, 2, 2, 2, 2, 2, 2, 2, 2, 2, 2, 2, 2, 2, 2, 2, 2, 2, 2, 2, 2, 2, 2, 2, 2, 2, 2, 2, 2, 2, 2, 2, 2, 2, 2, 2, 2, 2, 2, 2, 2, 2, 2, 2, 2, 2, 2, 2, 2, 2, 2, 2, 2, 2, 2, 2, 2, 2, 2, 2, 2, 2, 2, 2, 2, 2, 2, 2, 2, 2, 2, 2, 2, 2, 2, 2, 2, 2, 2, 2, 2, 2, 2, 2, 2, 2, 2, 2, 2, 2, 2, 2, 2, 2, 2, 2, 2, 2, 2, 2, 2, 2, 2, 2, 2, 2, 2, 2, 2, 2, 2, 2, 2, 2, 2, 2, 2, 2, 2, 2, 2, 2, 2, 2, 2, 2, 2, 3 ),
 ( 0.000000000000000000, 1.000000000000000000 ),
 ( 0.000000000000000000, 0.004166666666666666609, 0.008333333333333333218, 0.01250000000000000069, 0.01666666666666666644, 0.02083333333333333218, 0.02500000000000000139, 0.02916666666666666713, 0.03333333333333333287, 0.03749999999999999861, 0.04166666666666666435, 0.04583333333333333010, 0.05000000000000000278, 0.05416666666666666852, 0.05833333333333333426, 0.06250000000000000000, 0.06666666666666666574, 0.07083333333333333148, 0.07499999999999999722, 0.07916666666666666297, 0.08333333333333332871, 0.08749999999999999445, 0.09166666666666666019, 0.09583333333333333981, 0.1000000000000000056, 0.1041666666666666713, 0.1083333333333333370, 0.1125000000000000028, 0.1166666666666666685, 0.1208333333333333343, 0.1250000000000000000, 0.1291666666666666796, 0.1333333333333333315, 0.1375000000000000111, 0.1416666666666666630, 0.1458333333333333426, 0.1499999999999999944, 0.1541666666666666741, 0.1583333333333333259, 0.1625000000000000056, 0.1666666666666666574, 0.1708333333333333370, 0.1749999999999999889, 0.1791666666666666685, 0.1833333333333333204, 0.1875000000000000000, 0.1916666666666666796, 0.1958333333333333315, 0.2000000000000000111, 0.2041666666666666630, 0.2083333333333333426, 0.2124999999999999944, 0.2166666666666666741, 0.2208333333333333259, 0.2250000000000000056, 0.2291666666666666574, 0.2333333333333333370, 0.2374999999999999889, 0.2416666666666666685, 0.2458333333333333204, 0.2500000000000000000, 0.2541666666666666519, 0.2583333333333333592, 0.2625000000000000111, 0.2666666666666666630, 0.2708333333333333148, 0.2750000000000000222, 0.2791666666666666741, 0.2833333333333333259, 0.2874999999999999778, 0.2916666666666666852, 0.2958333333333333370, 0.2999999999999999889, 0.3041666666666666408, 0.3083333333333333481, 0.3125000000000000000, 0.3166666666666666519, 0.3208333333333333592, 0.3250000000000000111, 0.3291666666666666630, 0.3333333333333333148, 0.3375000000000000222, 0.3416666666666666741, 0.3458333333333333259, 0.3499999999999999778, 0.3541666666666666852, 0.3583333333333333370, 0.3624999999999999889, 0.3666666666666666408, 0.3708333333333333481, 0.3750000000000000000, 0.3791666666666666519, 0.3833333333333333592, 0.3875000000000000111, 0.3916666666666666630, 0.3958333333333333148, 0.4000000000000000222, 0.4041666666666666741, 0.4083333333333333259, 0.4124999999999999778, 0.4166666666666666852, 0.4208333333333333370, 0.4249999999999999889, 0.4291666666666666408, 0.4333333333333333481, 0.4375000000000000000, 0.4416666666666666519, 0.4458333333333333592, 0.4500000000000000111, 0.4541666666666666630, 0.4583333333333333148, 0.4625000000000000222, 0.4666666666666666741, 0.4708333333333333259, 0.4749999999999999778, 0.4791666666666666852, 0.4833333333333333370, 0.4874999999999999889, 0.4916666666666666408, 0.4958333333333333481, 0.5000000000000000000, 0.5041666666666666519, 0.5083333333333333037, 0.5124999999999999556, 0.5166666666666667185, 0.5208333333333333703, 0.5250000000000000222, 0.5291666666666666741, 0.5333333333333333259, 0.5374999999999999778, 0.5416666666666666297, 0.5458333333333332815, 0.5500000000000000444, 0.5541666666666666963, 0.5583333333333333481, 0.5625000000000000000, 0.5666666666666666519, 0.5708333333333333037, 0.5749999999999999556, 0.5791666666666667185, 0.5833333333333333703, 0.5875000000000000222, 0.5916666666666666741, 0.5958333333333333259, 0.5999999999999999778, 0.6041666666666666297, 0.6083333333333332815, 0.6125000000000000444, 0.6166666666666666963, 0.6208333333333333481, 0.6250000000000000000, 0.6291666666666666519, 0.6333333333333333037, 0.6374999999999999556, 0.6416666666666667185, 0.6458333333333333703, 0.6500000000000000222, 0.6541666666666666741, 0.6583333333333333259, 0.6624999999999999778, 0.6666666666666666297, 0.6708333333333332815, 0.6750000000000000444, 0.6791666666666666963, 0.6833333333333333481, 0.6875000000000000000, 0.6916666666666666519, 0.6958333333333333037, 0.6999999999999999556, 0.7041666666666667185, 0.7083333333333333703, 0.7125000000000000222, 0.7166666666666666741, 0.7208333333333333259, 0.7249999999999999778, 0.7291666666666666297, 0.7333333333333332815, 0.7375000000000000444, 0.7416666666666666963, 0.7458333333333333481, 0.7500000000000000000, 0.7541666666666666519, 0.7583333333333333037, 0.7624999999999999556, 0.7666666666666667185, 0.7708333333333333703, 0.7750000000000000222, 0.7791666666666666741, 0.7833333333333333259, 0.7874999999999999778, 0.7916666666666666297, 0.7958333333333332815, 0.8000000000000000444, 0.8041666666666666963, 0.8083333333333333481, 0.8125000000000000000, 0.8166666666666666519, 0.8208333333333333037, 0.8249999999999999556, 0.8291666666666667185, 0.8333333333333333703, 0.8375000000000000222, 0.8416666666666666741, 0.8458333333333333259, 0.8499999999999999778, 0.8541666666666666297, 0.8583333333333332815, 0.8625000000000000444, 0.8666666666666666963, 0.8708333333333333481, 0.8750000000000000000, 0.8791666666666666519, 0.8833333333333333037, 0.8874999999999999556, 0.8916666666666667185, 0.8958333333333333703, 0.9000000000000000222, 0.9041666666666666741, 0.9083333333333333259, 0.9124999999999999778, 0.9166666666666666297, 0.9208333333333332815, 0.9250000000000000444, 0.9291666666666666963, 0.9333333333333333481, 0.9375000000000000000, 0.9416666666666666519, 0.9458333333333333037, 0.9499999999999999556, 0.9541666666666667185, 0.9583333333333333703, 0.9625000000000000222, 0.9666666666666666741, 0.9708333333333333259, 0.9749999999999999778, 0.9791666666666666297, 0.9833333333333332815, 0.9875000000000000444, 0.9916666666666666963, 0.9958333333333333481, 1.000000000000000000 ),
 .UNSPECIFIED. ) 
 GEOMETRIC_REPRESENTATION_ITEM ( )  RATIONAL_B_SPLINE_SURFACE ( (
 ( 1.000000000000000000, 0.8660254037844387076, 1.000000000000000000, 0.8660254037844387076, 1.000000000000000000, 0.8660254037844387076, 1.000000000000000000, 0.8660254037844387076, 1.000000000000000000, 0.8660254037844387076, 1.000000000000000000, 0.8660254037844387076, 1.000000000000000000, 0.8660254037844387076, 1.000000000000000000, 0.8660254037844387076, 1.000000000000000000, 0.8660254037844387076, 1.000000000000000000, 0.8660254037844387076, 1.000000000000000000, 0.8660254037844387076, 1.000000000000000000, 0.8660254037844387076, 1.000000000000000000, 0.8660254037844387076, 1.000000000000000000, 0.8660254037844387076, 1.000000000000000000, 0.8660254037844387076, 1.000000000000000000, 0.8660254037844387076, 1.000000000000000000, 0.8660254037844387076, 1.000000000000000000, 0.8660254037844387076, 1.000000000000000000, 0.8660254037844387076, 1.000000000000000000, 0.8660254037844387076, 1.000000000000000000, 0.8660254037844387076, 1.000000000000000000, 0.8660254037844387076, 1.000000000000000000, 0.8660254037844387076, 1.000000000000000000, 0.8660254037844387076, 1.000000000000000000, 0.8660254037844387076, 1.000000000000000000, 0.8660254037844387076, 1.000000000000000000, 0.8660254037844387076, 1.000000000000000000, 0.8660254037844387076, 1.000000000000000000, 0.8660254037844387076, 1.000000000000000000, 0.8660254037844387076, 1.000000000000000000, 0.8660254037844387076, 1.000000000000000000, 0.8660254037844387076, 1.000000000000000000, 0.8660254037844387076, 1.000000000000000000, 0.8660254037844387076, 1.000000000000000000, 0.8660254037844387076, 1.000000000000000000, 0.8660254037844387076, 1.000000000000000000, 0.8660254037844387076, 1.000000000000000000, 0.8660254037844387076, 1.000000000000000000, 0.8660254037844387076, 1.000000000000000000, 0.8660254037844387076, 1.000000000000000000, 0.8660254037844387076, 1.000000000000000000, 0.8660254037844387076, 1.000000000000000000, 0.8660254037844387076, 1.000000000000000000, 0.8660254037844387076, 1.000000000000000000, 0.8660254037844387076, 1.000000000000000000, 0.8660254037844387076, 1.000000000000000000, 0.8660254037844387076, 1.000000000000000000, 0.8660254037844387076, 1.000000000000000000, 0.8660254037844387076, 1.000000000000000000, 0.8660254037844387076, 1.000000000000000000, 0.8660254037844387076, 1.000000000000000000, 0.8660254037844387076, 1.000000000000000000, 0.8660254037844387076, 1.000000000000000000, 0.8660254037844387076, 1.000000000000000000, 0.8660254037844387076, 1.000000000000000000, 0.8660254037844387076, 1.000000000000000000, 0.8660254037844387076, 1.000000000000000000, 0.8660254037844387076, 1.000000000000000000, 0.8660254037844387076, 1.000000000000000000, 0.8660254037844387076, 1.000000000000000000, 0.8660254037844387076, 1.000000000000000000, 0.8660254037844387076, 1.000000000000000000, 0.8660254037844387076, 1.000000000000000000, 0.8660254037844387076, 1.000000000000000000, 0.8660254037844387076, 1.000000000000000000, 0.8660254037844387076, 1.000000000000000000, 0.8660254037844387076, 1.000000000000000000, 0.8660254037844387076, 1.000000000000000000, 0.8660254037844387076, 1.000000000000000000, 0.8660254037844387076, 1.000000000000000000, 0.8660254037844387076, 1.000000000000000000, 0.8660254037844387076, 1.000000000000000000, 0.8660254037844387076, 1.000000000000000000, 0.8660254037844387076, 1.000000000000000000, 0.8660254037844387076, 1.000000000000000000, 0.8660254037844387076, 1.000000000000000000, 0.8660254037844387076, 1.000000000000000000, 0.8660254037844387076, 1.000000000000000000, 0.8660254037844387076, 1.000000000000000000, 0.8660254037844387076, 1.000000000000000000, 0.8660254037844387076, 1.000000000000000000, 0.8660254037844387076, 1.000000000000000000, 0.8660254037844387076, 1.000000000000000000, 0.8660254037844387076, 1.000000000000000000, 0.8660254037844387076, 1.000000000000000000, 0.8660254037844387076, 1.000000000000000000, 0.8660254037844387076, 1.000000000000000000, 0.8660254037844387076, 1.000000000000000000, 0.8660254037844387076, 1.000000000000000000, 0.8660254037844387076, 1.000000000000000000, 0.8660254037844387076, 1.000000000000000000, 0.8660254037844387076, 1.000000000000000000, 0.8660254037844387076, 1.000000000000000000, 0.8660254037844387076, 1.000000000000000000, 0.8660254037844387076, 1.000000000000000000, 0.8660254037844387076, 1.000000000000000000, 0.8660254037844387076, 1.000000000000000000, 0.8660254037844387076, 1.000000000000000000, 0.8660254037844387076, 1.000000000000000000, 0.8660254037844387076, 1.000000000000000000, 0.8660254037844387076, 1.000000000000000000, 0.8660254037844387076, 1.000000000000000000, 0.8660254037844387076, 1.000000000000000000, 0.8660254037844387076, 1.000000000000000000, 0.8660254037844387076, 1.000000000000000000, 0.8660254037844387076, 1.000000000000000000, 0.8660254037844387076, 1.000000000000000000, 0.8660254037844387076, 1.000000000000000000, 0.8660254037844387076, 1.000000000000000000, 0.8660254037844387076, 1.000000000000000000, 0.8660254037844387076, 1.000000000000000000, 0.8660254037844387076, 1.000000000000000000, 0.8660254037844387076, 1.000000000000000000, 0.8660254037844387076, 1.000000000000000000, 0.8660254037844387076, 1.000000000000000000, 0.8660254037844387076, 1.000000000000000000, 0.8660254037844387076, 1.000000000000000000, 0.8660254037844387076, 1.000000000000000000, 0.8660254037844387076, 1.000000000000000000, 0.8660254037844387076, 1.000000000000000000, 0.8660254037844387076, 1.000000000000000000, 0.8660254037844387076, 1.000000000000000000, 0.8660254037844387076, 1.000000000000000000, 0.8660254037844387076, 1.000000000000000000, 0.8660254037844387076, 1.000000000000000000, 0.8660254037844387076, 1.000000000000000000, 0.8660254037844387076, 1.000000000000000000, 0.8660254037844387076, 1.000000000000000000, 0.8660254037844387076, 1.000000000000000000, 0.8660254037844387076, 1.000000000000000000, 0.8660254037844387076, 1.000000000000000000, 0.8660254037844387076, 1.000000000000000000, 0.8660254037844387076, 1.000000000000000000, 0.8660254037844387076, 1.000000000000000000, 0.8660254037844387076, 1.000000000000000000, 0.8660254037844387076, 1.000000000000000000, 0.8660254037844387076, 1.000000000000000000, 0.8660254037844387076, 1.000000000000000000, 0.8660254037844387076, 1.000000000000000000, 0.8660254037844387076, 1.000000000000000000, 0.8660254037844387076, 1.000000000000000000, 0.8660254037844387076, 1.000000000000000000, 0.8660254037844387076, 1.000000000000000000, 0.8660254037844387076, 1.000000000000000000, 0.8660254037844387076, 1.000000000000000000, 0.8660254037844387076, 1.000000000000000000, 0.8660254037844387076, 1.000000000000000000, 0.8660254037844387076, 1.000000000000000000, 0.8660254037844387076, 1.000000000000000000, 0.8660254037844387076, 1.000000000000000000, 0.8660254037844387076, 1.000000000000000000, 0.8660254037844387076, 1.000000000000000000, 0.8660254037844387076, 1.000000000000000000, 0.8660254037844387076, 1.000000000000000000, 0.8660254037844387076, 1.000000000000000000, 0.8660254037844387076, 1.000000000000000000, 0.8660254037844387076, 1.000000000000000000, 0.8660254037844387076, 1.000000000000000000, 0.8660254037844387076, 1.000000000000000000, 0.8660254037844387076, 1.000000000000000000, 0.8660254037844387076, 1.000000000000000000, 0.8660254037844387076, 1.000000000000000000, 0.8660254037844387076, 1.000000000000000000, 0.8660254037844387076, 1.000000000000000000, 0.8660254037844387076, 1.000000000000000000, 0.8660254037844387076, 1.000000000000000000, 0.8660254037844387076, 1.000000000000000000, 0.8660254037844387076, 1.000000000000000000, 0.8660254037844387076, 1.000000000000000000, 0.8660254037844387076, 1.000000000000000000, 0.8660254037844387076, 1.000000000000000000, 0.8660254037844387076, 1.000000000000000000, 0.8660254037844387076, 1.000000000000000000, 0.8660254037844387076, 1.000000000000000000, 0.8660254037844387076, 1.000000000000000000, 0.8660254037844387076, 1.000000000000000000, 0.8660254037844387076, 1.000000000000000000, 0.8660254037844387076, 1.000000000000000000, 0.8660254037844387076, 1.000000000000000000, 0.8660254037844387076, 1.000000000000000000, 0.8660254037844387076, 1.000000000000000000, 0.8660254037844387076, 1.000000000000000000, 0.8660254037844387076, 1.000000000000000000, 0.8660254037844387076, 1.000000000000000000, 0.8660254037844387076, 1.000000000000000000, 0.8660254037844387076, 1.000000000000000000, 0.8660254037844387076, 1.000000000000000000, 0.8660254037844387076, 1.000000000000000000, 0.8660254037844387076, 1.000000000000000000, 0.8660254037844387076, 1.000000000000000000, 0.8660254037844387076, 1.000000000000000000, 0.8660254037844387076, 1.000000000000000000, 0.8660254037844387076, 1.000000000000000000, 0.8660254037844387076, 1.000000000000000000, 0.8660254037844387076, 1.000000000000000000, 0.8660254037844387076, 1.000000000000000000, 0.8660254037844387076, 1.000000000000000000, 0.8660254037844387076, 1.000000000000000000, 0.8660254037844387076, 1.000000000000000000, 0.8660254037844387076, 1.000000000000000000, 0.8660254037844387076, 1.000000000000000000, 0.8660254037844387076, 1.000000000000000000, 0.8660254037844387076, 1.000000000000000000, 0.8660254037844387076, 1.000000000000000000, 0.8660254037844387076, 1.000000000000000000, 0.8660254037844387076, 1.000000000000000000, 0.8660254037844387076, 1.000000000000000000, 0.8660254037844387076, 1.000000000000000000, 0.8660254037844387076, 1.000000000000000000, 0.8660254037844387076, 1.000000000000000000, 0.8660254037844387076, 1.000000000000000000, 0.8660254037844387076, 1.000000000000000000, 0.8660254037844387076, 1.000000000000000000, 0.8660254037844387076, 1.000000000000000000, 0.8660254037844387076, 1.000000000000000000, 0.8660254037844387076, 1.000000000000000000, 0.8660254037844387076, 1.000000000000000000, 0.8660254037844387076, 1.000000000000000000, 0.8660254037844387076, 1.000000000000000000, 0.8660254037844387076, 1.000000000000000000, 0.8660254037844387076, 1.000000000000000000, 0.8660254037844387076, 1.000000000000000000, 0.8660254037844387076, 1.000000000000000000, 0.8660254037844387076, 1.000000000000000000, 0.8660254037844387076, 1.000000000000000000, 0.8660254037844387076, 1.000000000000000000, 0.8660254037844387076, 1.000000000000000000, 0.8660254037844387076, 1.000000000000000000, 0.8660254037844387076, 1.000000000000000000, 0.8660254037844387076, 1.000000000000000000, 0.8660254037844387076, 1.000000000000000000, 0.8660254037844387076, 1.000000000000000000, 0.8660254037844387076, 1.000000000000000000, 0.8660254037844387076, 1.000000000000000000, 0.8660254037844387076, 1.000000000000000000, 0.8660254037844387076, 1.000000000000000000, 0.8660254037844387076, 1.000000000000000000, 0.8660254037844387076, 1.000000000000000000, 0.8660254037844387076, 1.000000000000000000, 0.8660254037844387076, 1.000000000000000000),
 ( 1.000000000000000000, 0.8660254037844387076, 1.000000000000000000, 0.8660254037844387076, 1.000000000000000000, 0.8660254037844387076, 1.000000000000000000, 0.8660254037844387076, 1.000000000000000000, 0.8660254037844387076, 1.000000000000000000, 0.8660254037844387076, 1.000000000000000000, 0.8660254037844387076, 1.000000000000000000, 0.8660254037844387076, 1.000000000000000000, 0.8660254037844387076, 1.000000000000000000, 0.8660254037844387076, 1.000000000000000000, 0.8660254037844387076, 1.000000000000000000, 0.8660254037844387076, 1.000000000000000000, 0.8660254037844387076, 1.000000000000000000, 0.8660254037844387076, 1.000000000000000000, 0.8660254037844387076, 1.000000000000000000, 0.8660254037844387076, 1.000000000000000000, 0.8660254037844387076, 1.000000000000000000, 0.8660254037844387076, 1.000000000000000000, 0.8660254037844387076, 1.000000000000000000, 0.8660254037844387076, 1.000000000000000000, 0.8660254037844387076, 1.000000000000000000, 0.8660254037844387076, 1.000000000000000000, 0.8660254037844387076, 1.000000000000000000, 0.8660254037844387076, 1.000000000000000000, 0.8660254037844387076, 1.000000000000000000, 0.8660254037844387076, 1.000000000000000000, 0.8660254037844387076, 1.000000000000000000, 0.8660254037844387076, 1.000000000000000000, 0.8660254037844387076, 1.000000000000000000, 0.8660254037844387076, 1.000000000000000000, 0.8660254037844387076, 1.000000000000000000, 0.8660254037844387076, 1.000000000000000000, 0.8660254037844387076, 1.000000000000000000, 0.8660254037844387076, 1.000000000000000000, 0.8660254037844387076, 1.000000000000000000, 0.8660254037844387076, 1.000000000000000000, 0.8660254037844387076, 1.000000000000000000, 0.8660254037844387076, 1.000000000000000000, 0.8660254037844387076, 1.000000000000000000, 0.8660254037844387076, 1.000000000000000000, 0.8660254037844387076, 1.000000000000000000, 0.8660254037844387076, 1.000000000000000000, 0.8660254037844387076, 1.000000000000000000, 0.8660254037844387076, 1.000000000000000000, 0.8660254037844387076, 1.000000000000000000, 0.8660254037844387076, 1.000000000000000000, 0.8660254037844387076, 1.000000000000000000, 0.8660254037844387076, 1.000000000000000000, 0.8660254037844387076, 1.000000000000000000, 0.8660254037844387076, 1.000000000000000000, 0.8660254037844387076, 1.000000000000000000, 0.8660254037844387076, 1.000000000000000000, 0.8660254037844387076, 1.000000000000000000, 0.8660254037844387076, 1.000000000000000000, 0.8660254037844387076, 1.000000000000000000, 0.8660254037844387076, 1.000000000000000000, 0.8660254037844387076, 1.000000000000000000, 0.8660254037844387076, 1.000000000000000000, 0.8660254037844387076, 1.000000000000000000, 0.8660254037844387076, 1.000000000000000000, 0.8660254037844387076, 1.000000000000000000, 0.8660254037844387076, 1.000000000000000000, 0.8660254037844387076, 1.000000000000000000, 0.8660254037844387076, 1.000000000000000000, 0.8660254037844387076, 1.000000000000000000, 0.8660254037844387076, 1.000000000000000000, 0.8660254037844387076, 1.000000000000000000, 0.8660254037844387076, 1.000000000000000000, 0.8660254037844387076, 1.000000000000000000, 0.8660254037844387076, 1.000000000000000000, 0.8660254037844387076, 1.000000000000000000, 0.8660254037844387076, 1.000000000000000000, 0.8660254037844387076, 1.000000000000000000, 0.8660254037844387076, 1.000000000000000000, 0.8660254037844387076, 1.000000000000000000, 0.8660254037844387076, 1.000000000000000000, 0.8660254037844387076, 1.000000000000000000, 0.8660254037844387076, 1.000000000000000000, 0.8660254037844387076, 1.000000000000000000, 0.8660254037844387076, 1.000000000000000000, 0.8660254037844387076, 1.000000000000000000, 0.8660254037844387076, 1.000000000000000000, 0.8660254037844387076, 1.000000000000000000, 0.8660254037844387076, 1.000000000000000000, 0.8660254037844387076, 1.000000000000000000, 0.8660254037844387076, 1.000000000000000000, 0.8660254037844387076, 1.000000000000000000, 0.8660254037844387076, 1.000000000000000000, 0.8660254037844387076, 1.000000000000000000, 0.8660254037844387076, 1.000000000000000000, 0.8660254037844387076, 1.000000000000000000, 0.8660254037844387076, 1.000000000000000000, 0.8660254037844387076, 1.000000000000000000, 0.8660254037844387076, 1.000000000000000000, 0.8660254037844387076, 1.000000000000000000, 0.8660254037844387076, 1.000000000000000000, 0.8660254037844387076, 1.000000000000000000, 0.8660254037844387076, 1.000000000000000000, 0.8660254037844387076, 1.000000000000000000, 0.8660254037844387076, 1.000000000000000000, 0.8660254037844387076, 1.000000000000000000, 0.8660254037844387076, 1.000000000000000000, 0.8660254037844387076, 1.000000000000000000, 0.8660254037844387076, 1.000000000000000000, 0.8660254037844387076, 1.000000000000000000, 0.8660254037844387076, 1.000000000000000000, 0.8660254037844387076, 1.000000000000000000, 0.8660254037844387076, 1.000000000000000000, 0.8660254037844387076, 1.000000000000000000, 0.8660254037844387076, 1.000000000000000000, 0.8660254037844387076, 1.000000000000000000, 0.8660254037844387076, 1.000000000000000000, 0.8660254037844387076, 1.000000000000000000, 0.8660254037844387076, 1.000000000000000000, 0.8660254037844387076, 1.000000000000000000, 0.8660254037844387076, 1.000000000000000000, 0.8660254037844387076, 1.000000000000000000, 0.8660254037844387076, 1.000000000000000000, 0.8660254037844387076, 1.000000000000000000, 0.8660254037844387076, 1.000000000000000000, 0.8660254037844387076, 1.000000000000000000, 0.8660254037844387076, 1.000000000000000000, 0.8660254037844387076, 1.000000000000000000, 0.8660254037844387076, 1.000000000000000000, 0.8660254037844387076, 1.000000000000000000, 0.8660254037844387076, 1.000000000000000000, 0.8660254037844387076, 1.000000000000000000, 0.8660254037844387076, 1.000000000000000000, 0.8660254037844387076, 1.000000000000000000, 0.8660254037844387076, 1.000000000000000000, 0.8660254037844387076, 1.000000000000000000, 0.8660254037844387076, 1.000000000000000000, 0.8660254037844387076, 1.000000000000000000, 0.8660254037844387076, 1.000000000000000000, 0.8660254037844387076, 1.000000000000000000, 0.8660254037844387076, 1.000000000000000000, 0.8660254037844387076, 1.000000000000000000, 0.8660254037844387076, 1.000000000000000000, 0.8660254037844387076, 1.000000000000000000, 0.8660254037844387076, 1.000000000000000000, 0.8660254037844387076, 1.000000000000000000, 0.8660254037844387076, 1.000000000000000000, 0.8660254037844387076, 1.000000000000000000, 0.8660254037844387076, 1.000000000000000000, 0.8660254037844387076, 1.000000000000000000, 0.8660254037844387076, 1.000000000000000000, 0.8660254037844387076, 1.000000000000000000, 0.8660254037844387076, 1.000000000000000000, 0.8660254037844387076, 1.000000000000000000, 0.8660254037844387076, 1.000000000000000000, 0.8660254037844387076, 1.000000000000000000, 0.8660254037844387076, 1.000000000000000000, 0.8660254037844387076, 1.000000000000000000, 0.8660254037844387076, 1.000000000000000000, 0.8660254037844387076, 1.000000000000000000, 0.8660254037844387076, 1.000000000000000000, 0.8660254037844387076, 1.000000000000000000, 0.8660254037844387076, 1.000000000000000000, 0.8660254037844387076, 1.000000000000000000, 0.8660254037844387076, 1.000000000000000000, 0.8660254037844387076, 1.000000000000000000, 0.8660254037844387076, 1.000000000000000000, 0.8660254037844387076, 1.000000000000000000, 0.8660254037844387076, 1.000000000000000000, 0.8660254037844387076, 1.000000000000000000, 0.8660254037844387076, 1.000000000000000000, 0.8660254037844387076, 1.000000000000000000, 0.8660254037844387076, 1.000000000000000000, 0.8660254037844387076, 1.000000000000000000, 0.8660254037844387076, 1.000000000000000000, 0.8660254037844387076, 1.000000000000000000, 0.8660254037844387076, 1.000000000000000000, 0.8660254037844387076, 1.000000000000000000, 0.8660254037844387076, 1.000000000000000000, 0.8660254037844387076, 1.000000000000000000, 0.8660254037844387076, 1.000000000000000000, 0.8660254037844387076, 1.000000000000000000, 0.8660254037844387076, 1.000000000000000000, 0.8660254037844387076, 1.000000000000000000, 0.8660254037844387076, 1.000000000000000000, 0.8660254037844387076, 1.000000000000000000, 0.8660254037844387076, 1.000000000000000000, 0.8660254037844387076, 1.000000000000000000, 0.8660254037844387076, 1.000000000000000000, 0.8660254037844387076, 1.000000000000000000, 0.8660254037844387076, 1.000000000000000000, 0.8660254037844387076, 1.000000000000000000, 0.8660254037844387076, 1.000000000000000000, 0.8660254037844387076, 1.000000000000000000, 0.8660254037844387076, 1.000000000000000000, 0.8660254037844387076, 1.000000000000000000, 0.8660254037844387076, 1.000000000000000000, 0.8660254037844387076, 1.000000000000000000, 0.8660254037844387076, 1.000000000000000000, 0.8660254037844387076, 1.000000000000000000, 0.8660254037844387076, 1.000000000000000000, 0.8660254037844387076, 1.000000000000000000, 0.8660254037844387076, 1.000000000000000000, 0.8660254037844387076, 1.000000000000000000, 0.8660254037844387076, 1.000000000000000000, 0.8660254037844387076, 1.000000000000000000, 0.8660254037844387076, 1.000000000000000000, 0.8660254037844387076, 1.000000000000000000, 0.8660254037844387076, 1.000000000000000000, 0.8660254037844387076, 1.000000000000000000, 0.8660254037844387076, 1.000000000000000000, 0.8660254037844387076, 1.000000000000000000, 0.8660254037844387076, 1.000000000000000000, 0.8660254037844387076, 1.000000000000000000, 0.8660254037844387076, 1.000000000000000000, 0.8660254037844387076, 1.000000000000000000, 0.8660254037844387076, 1.000000000000000000, 0.8660254037844387076, 1.000000000000000000, 0.8660254037844387076, 1.000000000000000000, 0.8660254037844387076, 1.000000000000000000, 0.8660254037844387076, 1.000000000000000000, 0.8660254037844387076, 1.000000000000000000, 0.8660254037844387076, 1.000000000000000000, 0.8660254037844387076, 1.000000000000000000, 0.8660254037844387076, 1.000000000000000000, 0.8660254037844387076, 1.000000000000000000, 0.8660254037844387076, 1.000000000000000000, 0.8660254037844387076, 1.000000000000000000, 0.8660254037844387076, 1.000000000000000000, 0.8660254037844387076, 1.000000000000000000, 0.8660254037844387076, 1.000000000000000000, 0.8660254037844387076, 1.000000000000000000, 0.8660254037844387076, 1.000000000000000000, 0.8660254037844387076, 1.000000000000000000, 0.8660254037844387076, 1.000000000000000000, 0.8660254037844387076, 1.000000000000000000, 0.8660254037844387076, 1.000000000000000000, 0.8660254037844387076, 1.000000000000000000, 0.8660254037844387076, 1.000000000000000000, 0.8660254037844387076, 1.000000000000000000, 0.8660254037844387076, 1.000000000000000000, 0.8660254037844387076, 1.000000000000000000, 0.8660254037844387076, 1.000000000000000000, 0.8660254037844387076, 1.000000000000000000, 0.8660254037844387076, 1.000000000000000000) ) ) 
 REPRESENTATION_ITEM ( '' )  SURFACE ( )  );
#89295=CARTESIAN_POINT ( 'NONE',  ( -6.575868197828002693, 7.630599971342813426, 1.199719254218450271 ) ) ;
#89306=CARTESIAN_POINT ( 'NONE',  ( -4.762992037102518950, 4.451245552908022596, -0.7998128361456221525 ) ) ;
#89311=CARTESIAN_POINT ( 'NONE',  ( 7.182068686937156166, 9.402166106225269715, 1.599625672291281386 ) ) ;
#89312=CARTESIAN_POINT ( 'NONE',  ( -1.201851678989727383E-14, 3.446875000341421469, -1.575800808251660134 ) ) ;
#89314=CARTESIAN_POINT ( 'NONE',  ( 6.067506501917478090, 6.045351875519452634, 0.3962785553160239616 ) ) ;
#89319=CARTESIAN_POINT ( 'NONE',  ( 4.324687812634874895, 7.989293514808604613, 0.7216878364870317197 ) ) ;
#89320=CARTESIAN_POINT ( 'NONE',  ( -7.751511138711140170, 10.06651563329490529, -1.599625672291263179 ) ) ;
#89323=CARTESIAN_POINT ( 'NONE',  ( -7.971304249830880373, 11.38727316052296601, 1.199719254218453823 ) ) ;
#89324=CARTESIAN_POINT ( 'NONE',  ( -5.052384799386910430, 9.046199365926717917, 1.214306433183764966E-14 ) ) ;
#89331=CARTESIAN_POINT ( 'NONE',  ( 8.938903350111612411, 9.323142084752035430, -0.7998128361456221525 ) ) ;
#89332=CARTESIAN_POINT ( 'NONE',  ( -2.155383234892699562, 5.458438174109348395, 1.040834085586084257E-14 ) ) ;
#89339=CARTESIAN_POINT ( 'NONE',  ( -3.511198596259295535, 6.271927390929313617, -2.420000000000000373 ) ) ;
#89346=CARTESIAN_POINT ( 'NONE',  ( -1.201851678989727383E-14, 3.837500000000021227, -1.732050807568863648 ) ) ;
#89347=CARTESIAN_POINT ( 'NONE',  ( 4.822949958159288286, 6.649860922651058992, -1.599625672291256295 ) ) ;
#89348=CARTESIAN_POINT ( 'NONE',  ( 4.306686350635271054, 8.176217842383143974, -0.7998128361456221525 ) ) ;
#89351=CARTESIAN_POINT ( 'NONE',  ( -8.839552966430023417, 9.415159337030921449, -0.7216878364870267237 ) ) ;
#89352=CARTESIAN_POINT ( 'NONE',  ( 5.775410249741494972, 8.721433810464993996, -1.082531754730537088 ) ) ;
#89353=CARTESIAN_POINT ( 'NONE',  ( -7.958272981097355370, 12.22847621134819285, 0.7216878364870458196 ) ) ;
#89357=CARTESIAN_POINT ( 'NONE',  ( 8.697719238366680372, 10.10609285197134533, 1.199719254218462483 ) ) ;
#89363=CARTESIAN_POINT ( 'NONE',  ( 0.6823417656249882723, 1.926041667008083991, -1.181850606188749264 ) ) ;
#89369=CARTESIAN_POINT ( 'NONE',  ( 9.043452155515161905, 10.50944792197790889, 1.199719254218453823 ) ) ;
#89372=CARTESIAN_POINT ( 'NONE',  ( -8.829384350997580455, 11.32403438096243775, 1.599625672291269396 ) ) ;
#89378=CARTESIAN_POINT ( 'NONE',  ( 8.380911511541880188, 12.92948053010758258, 0.7998128361456462443 ) ) ;
#89382=CARTESIAN_POINT ( 'NONE',  ( -8.910733272679575379, 11.41894145625809820, -1.599625672291263179 ) ) ;
#89385=CARTESIAN_POINT ( 'NONE',  ( 7.747594715205354809, 11.12627870345989756, -1.199719254218446718 ) ) ;
#89387=CARTESIAN_POINT ( 'NONE',  ( 5.197613018050254219, 6.434050360596694773, 1.175743713691650871 ) ) ;
#89388=CARTESIAN_POINT ( 'NONE',  ( 1.257539916218596732, 3.283837156058347251, -0.7749999999999874767 ) ) ;
#89390=CARTESIAN_POINT ( 'NONE',  ( -5.603597561149804562, 5.431951997629870910, 0.7998128361456341429 ) ) ;
#89394=CARTESIAN_POINT ( 'NONE',  ( 9.250740883225924804, 9.686952540052077509, 1.040834085586084257E-14 ) ) ;
#89396=CARTESIAN_POINT ( 'NONE',  ( 7.182068686937156166, 9.402166106225269715, 1.599625672291281386 ) ) ;
#89399=CARTESIAN_POINT ( 'NONE',  ( -7.199016379176422120, 11.34267684244042584, 0.000000000000000000 ) ) ;
#89407=CARTESIAN_POINT ( 'NONE',  ( -4.434757016570429755, 7.116138787269118637, -1.097766128466563851 ) ) ;
#89410=CARTESIAN_POINT ( 'NONE',  ( 7.456621297836082185, 7.801739057004660971, 0.7216878364870317197 ) ) ;
#89421=ORIENTED_EDGE ( 'NONE', *, *, #213374, .F. ) ;
#89426=DIRECTION ( 'NONE',  ( 0.000000000000000000, 8.546850786086437571E-32, 1.000000000000000000 ) ) ;
#89430=CARTESIAN_POINT ( 'NONE',  ( 8.284195553149872993, 9.623648552551724578, -1.199719254218445830 ) ) ;
#89434=CARTESIAN_POINT ( 'NONE',  ( 1.499999999999987121, 1.285416667349485120, 0.8660254037844524744 ) ) ;
#89435=CARTESIAN_POINT ( 'NONE',  ( -7.528855374290365887, 7.678086112960552434, -0.7998128361456291469 ) ) ;
#89438=CARTESIAN_POINT ( 'NONE',  ( -9.053093885623068715, 11.58502883802551153, -1.599625672291263179 ) ) ;
#89442=CARTESIAN_POINT ( 'NONE',  ( 0.7499999999999902300, 5.347916667349482012, -1.299038105676658228 ) ) ;
#89443=CARTESIAN_POINT ( 'NONE',  ( 6.564118927310645724, 10.80988918183778225, -0.7998128361456291469 ) ) ;
#89447=CARTESIAN_POINT ( 'NONE',  ( -5.364222332501225488, 9.410009821226765325, 0.7998128361456481317 ) ) ;
#89449=CARTESIAN_POINT ( 'NONE',  ( -0.6823417656250212460, 4.301041667008085767, 1.181850606188767472 ) ) ;
#89450=CARTESIAN_POINT ( 'NONE',  ( -6.010528009390447401, 5.981201532351332339, 0.002814859141863571956 ) ) ;
#89453=AXIS2_PLACEMENT_3D ( 'NONE', #112538, #77836, #196916 ) ;
#89456=CARTESIAN_POINT ( 'NONE',  ( -8.568389894156720032, 10.05917163368005163, 1.082531754730558626 ) ) ;
#89460=CARTESIAN_POINT ( 'NONE',  ( 1.364683531249990311, 3.696875000341416584, 1.214306433183764966E-14 ) ) ;
#89466=CARTESIAN_POINT ( 'NONE',  ( -1.364683531249997417, 4.509375000341424133, 1.214306433183764966E-14 ) ) ;
#89468=CARTESIAN_POINT ( 'NONE',  ( -4.436542580169821726, 6.199052314996659874, 1.599625672291267398 ) ) ;
#89469=CARTESIAN_POINT ( 'NONE',  ( 6.154511665599609493, 9.267681812253174556, 1.199719254218462483 ) ) ;
#89470=DIRECTION ( 'NONE',  ( 5.578564026256490882E-16, 1.000000000000000000, 9.066213480720158442E-32 ) ) ;
#89472=CARTESIAN_POINT ( 'NONE',  ( 4.839897649954202130, 4.748894801142428790, -0.7216878364870197293 ) ) ;
#89473=CARTESIAN_POINT ( 'NONE',  ( -0.6823417656250212460, 5.113541667008086655, 1.181850606188767472 ) ) ;
#89478=CARTESIAN_POINT ( 'NONE',  ( 0.6823417656249882723, 0.3427083336747516196, 1.181850606188755259 ) ) ;
#89479=CARTESIAN_POINT ( 'NONE',  ( -2.657034918598345730, 5.083329257464595408, -1.082531754730543971 ) ) ;
#89480=CARTESIAN_POINT ( 'NONE',  ( 3.974511587100456822, 7.788680618259193444, 1.040834085586084257E-14 ) ) ;
#89481=EDGE_LOOP ( 'NONE', ( #193633, #190912, #27451, #140811, #144690, #49057 ) ) ;
#89482=EDGE_CURVE ( 'NONE', #145532, #5398, #195587, .T. ) ;
#89487=CARTESIAN_POINT ( 'NONE',  ( 3.063779527008304360, 6.518233848244248563, 0.7216878364870317197 ) ) ;
#89490=CARTESIAN_POINT ( 'NONE',  ( -8.731087737520713432, 10.24898578427137963, 1.082531754730558626 ) ) ;
#89496=CARTESIAN_POINT ( 'NONE',  ( -8.597841969360544567, 13.18256606422934674, 0.7998128361456341429 ) ) ;
#89497=CARTESIAN_POINT ( 'NONE',  ( -6.548225005276122168, 6.741943382351338165, 0.7216878364870317197 ) ) ;
#89499=CARTESIAN_POINT ( 'NONE',  ( -1.402160292154681736E-14, 1.009375000341417916, -1.575800808251659024 ) ) ;
#89517=CYLINDRICAL_SURFACE ( 'NONE', #172488, 1.250000000000000000 ) ;
#89519=CARTESIAN_POINT ( 'NONE',  ( 5.756345505848640798, 6.148709499980903992, 0.8262799378709930753 ) ) ;
#89523=CARTESIAN_POINT ( 'NONE',  ( 1.364683531249990311, 2.946875000341416140, 1.214306433183764966E-14 ) ) ;
#89532=CARTESIAN_POINT ( 'NONE',  ( 0.6823417656249899377, 0.5927083336747518416, 1.181850606188755259 ) ) ;
#89542=CARTESIAN_POINT ( 'NONE',  ( 4.333802657862601215, 8.207853534148366492, 0.7998128361456462443 ) ) ;
#89550=CARTESIAN_POINT ( 'NONE',  ( 8.308449207076147758, 8.587612251210650527, -0.7998128361456281477 ) ) ;
#89554=CARTESIAN_POINT ( 'NONE',  ( 7.072549687823125097, 11.40305840243567381, -0.7998128361456291469 ) ) ;
#89567=CARTESIAN_POINT ( 'NONE',  ( -6.697364695470783502, 10.75741654478384035, 0.7216878364870458196 ) ) ;
#89572=CARTESIAN_POINT ( 'NONE',  ( -8.809047120577080392, 11.30030761213851953, 1.599625672291269396 ) ) ;
#89578=CARTESIAN_POINT ( 'NONE',  ( 8.374132434735052755, 12.92157160716627295, -0.7998128361456352531 ) ) ;
#89580=CARTESIAN_POINT ( 'NONE',  ( 3.181359600701000989, 6.863336634126477875, 0.000000000000000000 ) ) ;
#89587=CARTESIAN_POINT ( 'NONE',  ( -5.717788096661253761, 7.693838750903348789, 1.599625672291269396 ) ) ;
#89590=CARTESIAN_POINT ( 'NONE',  ( -8.296699936558862731, 11.76690146170562201, 1.199719254218453823 ) ) ;
#89596=CARTESIAN_POINT ( 'NONE',  ( 8.351459436338029008, 10.76645531385962862, -1.443375672974063439 ) ) ;
#89597=CARTESIAN_POINT ( 'NONE',  ( -1.201851678989727383E-14, 4.509375000341417916, -1.575800808251660134 ) ) ;
#89599=CARTESIAN_POINT ( 'NONE',  ( 5.178324605415663306, 8.128796908705222535, 1.199719254218462483 ) ) ;
#89606=CIRCLE ( 'NONE', #51558, 4.624999999999993783 ) ;
#89613=CARTESIAN_POINT ( 'NONE',  ( 1.364683531249988757, 1.696875000341414808, 0.000000000000000000 ) ) ;
#89615=CARTESIAN_POINT ( 'NONE',  ( 10.21336978979620191, 10.81001959771741205, 0.7998128361456462443 ) ) ;
#89617=CARTESIAN_POINT ( 'NONE',  ( -4.744990575102892905, 8.479646737687938085, 0.7216878364870458196 ) ) ;
#89618=CARTESIAN_POINT ( 'NONE',  ( 3.063779527008311021, 5.557864633942907417, 1.082531754730546636 ) ) ;
#89619=CARTESIAN_POINT ( 'NONE',  ( -6.412643469139482910, 7.544134137826577380, 1.082531754730549967 ) ) ;
#89624=CARTESIAN_POINT ( 'NONE',  ( 5.555090253297246150, 7.504024600312024340, 1.599625672291267398 ) ) ;
#89634=CARTESIAN_POINT ( 'NONE',  ( 4.794779880727245036, 8.745660294157122649, -0.7998128361456281477 ) ) ;
#89637=CARTESIAN_POINT ( 'NONE',  ( -5.930802130974132780, 9.006687355190106103, -1.199719254218440723 ) ) ;
#89641=CARTESIAN_POINT ( 'NONE',  ( 5.926885707468349196, 10.06645042535509660, 1.040834085586084257E-14 ) ) ;
#89644=CARTESIAN_POINT ( 'NONE',  ( -5.689618019229208734, 9.789638122409414223, 0.7998128361456481317 ) ) ;
#89645=CARTESIAN_POINT ( 'NONE',  ( 7.415946836550727284, 7.754285518838408109, 0.7216878364870317197 ) ) ;
#89646=CARTESIAN_POINT ( 'NONE',  ( 4.326045746746942200, 7.429495238844160632, 1.107669923005821344 ) ) ;
#89647=CARTESIAN_POINT ( 'NONE',  ( -3.899941742225307539, 7.701682465904834629, 0.7998128361456341429 ) ) ;
#89650=CARTESIAN_POINT ( 'NONE',  ( -6.684333426737305572, 7.757142738403693727, -1.199719254218446718 ) ) ;
#89656=CARTESIAN_POINT ( 'NONE',  ( -1.364683531250000748, 2.009375000341421913, 1.214306433183764966E-14 ) ) ;
#89658=CARTESIAN_POINT ( 'NONE',  ( -5.910991785878170646, 7.919243054989755670, -1.443375672974059665 ) ) ;
#89663=CARTESIAN_POINT ( 'NONE',  ( 6.602984505055297326, 7.662235663108029726, 1.199719254218462483 ) ) ;
#89665=UNCERTAINTY_MEASURE_WITH_UNIT (LENGTH_MEASURE( 1.000000000000000082E-05 ), #88563, 'distance_accuracy_value', 'NONE');
#89666=CARTESIAN_POINT ( 'NONE',  ( -5.910622443071302357, 6.001017179288033354, 0.07212419881679615896 ) ) ;
#89667=CARTESIAN_POINT ( 'NONE',  ( -1.402160292154681736E-14, 2.009375000341422801, -1.575800808251660134 ) ) ;
#89671=CARTESIAN_POINT ( 'NONE',  ( 4.419594888374914099, 5.218910793601261311, -1.082531754730548412 ) ) ;
#89675=CARTESIAN_POINT ( 'NONE',  ( -4.599240423533815125, 6.388866465587984322, 1.599625672291267398 ) ) ;
#89677=CARTESIAN_POINT ( 'NONE',  ( -8.229436053370685400, 10.62409470039771442, 1.443375672974090751 ) ) ;
#89686=CARTESIAN_POINT ( 'NONE',  ( -7.415946836550729948, 9.675023947441092176, 1.443375672974090751 ) ) ;
#89689=EDGE_LOOP ( 'NONE', ( #63145, #82342, #125278, #74084 ) ) ;
#89690=CARTESIAN_POINT ( 'NONE',  ( -7.009202228140744673, 10.16085778526412042, -1.082531754730537088 ) ) ;
#89697=CARTESIAN_POINT ( 'NONE',  ( -0.7499999999999972244, 5.639583334016151639, -1.299038105676652899 ) ) ;
#89698=CARTESIAN_POINT ( 'NONE',  ( 4.628062896017484995, 7.124942365035781933, -1.349859865738218145 ) ) ;
#89699=CARTESIAN_POINT ( 'NONE',  ( -1.499999999999997780, 5.181250000682820378, 1.214306433183764966E-14 ) ) ;
#89705=CARTESIAN_POINT ( 'NONE',  ( -6.018930129462987999, 9.109503353427070849, 1.199719254218452047 ) ) ;
#89707=CARTESIAN_POINT ( 'NONE',  ( 4.467575310902914154, 5.170924936596891008, 1.199719254218464037 ) ) ;
#89709=EDGE_CURVE ( 'NONE', #6079, #164652, #15974, .T. ) ;
#89713=CARTESIAN_POINT ( 'NONE',  ( 6.174848896020108668, 9.291408581077091000, 1.199719254218460707 ) ) ;
#89718=CARTESIAN_POINT ( 'NONE',  ( -5.829642864196175722, 7.824335979694092558, 1.443375672974064550 ) ) ;
#89730=CARTESIAN_POINT ( 'NONE',  ( 0.6823417656249899377, 1.342708333674752508, 1.181850606188755259 ) ) ;
#89732=CARTESIAN_POINT ( 'NONE',  ( -8.365544474831901667, 9.718555627847388578, 1.199719254218462483 ) ) ;
#89734=CARTESIAN_POINT ( 'NONE',  ( 7.771848369131631351, 10.09024240211882351, -1.599625672291262513 ) ) ;
#89736=CARTESIAN_POINT ( 'NONE',  ( -8.715193815486133033, 9.062147627688959872, 0.7998128361456462443 ) ) ;
#89738=CARTESIAN_POINT ( 'NONE',  ( -0.6823417656249969321, 4.217708333674755394, -1.181850606188749264 ) ) ;
#89740=CARTESIAN_POINT ( 'NONE',  ( 8.107412671292031803, 11.44210330227398487, 1.082531754730557072 ) ) ;
#89741=ADVANCED_FACE ( 'NONE', ( #128771 ), #70042, .T. ) ;
#89744=CARTESIAN_POINT ( 'NONE',  ( 1.364683531249986537, -0.5739583329919174526, 0.7879004041258500513 ) ) ;
#89747=CARTESIAN_POINT ( 'NONE',  ( 8.405692050348340771, 8.908988268268968724, 1.040834085586084257E-14 ) ) ;
#89750=CARTESIAN_POINT ( 'NONE',  ( -4.446711195602239819, 8.131654128270509929, -0.7216878364870267237 ) ) ;
#89752=CARTESIAN_POINT ( 'NONE',  ( -1.364683531250000748, 2.259375000341422357, 1.214306433183764966E-14 ) ) ;
#89754=CARTESIAN_POINT ( 'NONE',  ( 3.039828102299942714, 6.452578276080809694, 0.2781515650015949914 ) ) ;
#89757=CARTESIAN_POINT ( 'NONE',  ( -7.379715684540041565, 7.504089808251839244, 1.040834085586084257E-14 ) ) ;
#89758=CARTESIAN_POINT ( 'NONE',  ( 4.894543267554960053, 4.887125941896303338, -0.6895117023006970269 ) ) ;
#89766=CARTESIAN_POINT ( 'NONE',  ( 8.796542737168120851, 9.157054702984622097, -0.7998128361456211532 ) ) ;
#89769=CARTESIAN_POINT ( 'NONE',  ( -0.7500000000000215383, 0.9416666666666878571, 1.299038105676659116 ) ) ;
#89772=CARTESIAN_POINT ( 'NONE',  ( -7.334597915313094241, 9.580116872663850813, 1.040834085586084257E-14 ) ) ;
#89775=CARTESIAN_POINT ( 'NONE',  ( 6.304178240674458422, 10.29869901418813782, 1.040834085586084257E-14 ) ) ;
#89777=ORIENTED_EDGE ( 'NONE', *, *, #54037, .T. ) ;
#89782=CARTESIAN_POINT ( 'NONE',  ( 7.239163954692881653, 10.53310948286200599, -1.199719254218441611 ) ) ;
#89783=CARTESIAN_POINT ( 'NONE',  ( -9.501566725078754772, 9.979582688880366703, -0.7998128361456291469 ) ) ;
#89787=CARTESIAN_POINT ( 'NONE',  ( 1.364683531249988757, -0.6156249996585803075, 0.000000000000000000 ) ) ;
#89788=CARTESIAN_POINT ( 'NONE',  ( -1.500000000000013101, 1.129166666666688634, -0.8660254037844313801 ) ) ;
#89790=CARTESIAN_POINT ( 'NONE',  ( 6.010342169559767633, 5.906487374108181143, -0.7998128361456281477 ) ) ;
#89796=CARTESIAN_POINT ( 'NONE',  ( -0.6823417656250212460, 5.301041667008086655, 1.181850606188767472 ) ) ;
#89798=CARTESIAN_POINT ( 'NONE',  ( -8.616370316684697883, 10.01118577667568132, -1.199719254218446718 ) ) ;
#89799=CARTESIAN_POINT ( 'NONE',  ( -4.446711195602245148, 7.171284913969171448, -1.082531754730549967 ) ) ;
#89801=CARTESIAN_POINT ( 'NONE',  ( -1.001543065824772872E-14, 4.993750000682815937, 1.732050807568877637 ) ) ;
#89808=CARTESIAN_POINT ( 'NONE',  ( 7.775764792637399836, 9.030479331953833011, -1.199719254218441611 ) ) ;
#89810=AXIS2_PLACEMENT_3D ( 'NONE', #167230, #118537, #36141 ) ;
#89812=CARTESIAN_POINT ( 'NONE',  ( 6.927853306458739979, 10.06595070996845642, 1.082531754730558626 ) ) ;
#89815=CARTESIAN_POINT ( 'NONE',  ( -8.565000355531095622, 11.01558638625153286, -1.599625672291263179 ) ) ;
#89816=CARTESIAN_POINT ( 'NONE',  ( 3.981290663907289140, 7.796589541200495965, -0.7998128361456221525 ) ) ;
#89819=CARTESIAN_POINT ( 'NONE',  ( 3.334415713957098681, 5.977569868670206787, -1.199719254218446718 ) ) ;
#89824=CARTESIAN_POINT ( 'NONE',  ( -5.422898255786203769, 6.389431388914436738, -1.082531754730544860 ) ) ;
#89825=CARTESIAN_POINT ( 'NONE',  ( 2.900554798319789906, 5.471398800426671372, 1.199719254218452047 ) ) ;
#89828=CARTESIAN_POINT ( 'NONE',  ( -6.989391883044787868, 8.113044270762433285, -1.199719254218446718 ) ) ;
#89833=CARTESIAN_POINT ( 'NONE',  ( -8.727698198895085469, 11.20540053684285553, -1.599625672291263179 ) ) ;
#89837=CARTESIAN_POINT ( 'NONE',  ( 6.335737856287750880, 6.286115675290828264, -0.7998128361456281477 ) ) ;
#89838=CARTESIAN_POINT ( 'NONE',  ( -3.741371894207415227, 7.428709027653175312, -2.448389769268637384 ) ) ;
#89848=CARTESIAN_POINT ( 'NONE',  ( -6.287230548435221777, 8.358188277972981695, -1.599625672291263179 ) ) ;
#89851=CARTESIAN_POINT ( 'NONE',  ( 6.155038550924150087, 7.243595066575396757, 1.082531754730558626 ) ) ;
#89856=CARTESIAN_POINT ( 'NONE',  ( -4.791917227426195858, 7.677988301050826969, -1.199719254218452047 ) ) ;
#89861=CARTESIAN_POINT ( 'NONE',  ( -7.379715684540041565, 7.504089808251839244, 1.040834085586084257E-14 ) ) ;
#89868=CARTESIAN_POINT ( 'NONE',  ( 6.265839547809997079, 10.46189657242035587, 0.7998128361456462443 ) ) ;
#89874=CARTESIAN_POINT ( 'NONE',  ( -1.402160292154681736E-14, -0.7406249996585823059, -1.575800808251665908 ) ) ;
#89878=CARTESIAN_POINT ( 'NONE',  ( 9.083599731475983319, 11.62061899152058686, 1.443375672974076540 ) ) ;
#89885=CARTESIAN_POINT ( 'NONE',  ( -3.288454681041543370, 6.406095492915408585, 0.7457829957396812093 ) ) ;
#89899=CARTESIAN_POINT ( 'NONE',  ( -3.490334480514268645, 6.159475096320226939, -1.199719254218452935 ) ) ;
#89901=CARTESIAN_POINT ( 'NONE',  ( -3.785751206713858785, 5.439795712631356750, 1.599625672291267398 ) ) ;
#89905=CARTESIAN_POINT ( 'NONE',  ( 1.364683531249990311, 5.363541667008086655, 0.7879004041258500513 ) ) ;
#89910=DIRECTION ( 'NONE',  ( 0.6507913734559640506, -0.7592566023653005702, 0.000000000000000000 ) ) ;
#89913=CARTESIAN_POINT ( 'NONE',  ( 4.715538499454675403, 4.395883092318884522, 1.214306433183764966E-14 ) ) ;
#89917=CARTESIAN_POINT ( 'NONE',  ( 9.910647101465253073, 11.62513837554007168, -1.082531754730537088 ) ) ;
#89920=CARTESIAN_POINT ( 'NONE',  ( -1.364683531250012516, 2.092708333674750953, 0.7879004041258379498 ) ) ;
#89923=CARTESIAN_POINT ( 'NONE',  ( -7.645908563102897126, 11.00764485934031889, 1.199719254218453823 ) ) ;
#89924=CARTESIAN_POINT ( 'NONE',  ( -4.514501963226242864, 7.250374142863800664, 1.082531754730560403 ) ) ;
#89926=CARTESIAN_POINT ( 'NONE',  ( -4.880045225915050189, 7.780804299287790826, 1.199719254218464037 ) ) ;
#89928=CARTESIAN_POINT ( 'NONE',  ( -1.500000000000001332, -0.8187499993171781787, 0.000000000000000000 ) ) ;
#89936=CARTESIAN_POINT ( 'NONE',  ( -6.060131475184148186, 6.172500930577367484, 0.7216878364870317197 ) ) ;
#89937=CARTESIAN_POINT ( 'NONE',  ( -1.403499169896182730, 7.376709478543820531, -4.304123474985523501 ) ) ;
#89942=CARTESIAN_POINT ( 'NONE',  ( -3.578989363883261277, 7.119311991265024453, 1.040834085586084257E-14 ) ) ;
#89944=CARTESIAN_POINT ( 'NONE',  ( 10.40996301719436090, 11.03937836301526687, 0.000000000000000000 ) ) ;
#89945=( BOUNDED_CURVE ( )  B_SPLINE_CURVE ( 2, ( #195613, #26699, #146885, #130682, #208634, #126424, #45118 ),
 .UNSPECIFIED., .F., .T. ) 
 B_SPLINE_CURVE_WITH_KNOTS ( ( 3, 2, 2, 3 ),
 ( 0.4137979667686199625, 0.4166666666666666852, 0.4226190476190476164, 0.4254877475170942835 ),
 .UNSPECIFIED. ) 
 CURVE ( )  GEOMETRIC_REPRESENTATION_ITEM ( )  RATIONAL_B_SPLINE_CURVE ( ( 0.9331000818465633451, 0.9354320710352559409, 1.000000000000000000, 0.8660254037844387076, 1.000000000000000000, 0.9354320710352564960, 0.9331000818465632340 ) ) 
 REPRESENTATION_ITEM ( '' )  );
#89953=CARTESIAN_POINT ( 'NONE',  ( -4.548924232584923288, 5.265832011892554121, -1.199719254218446718 ) ) ;
#89959=CARTESIAN_POINT ( 'NONE',  ( 4.981731378017507872, 7.899438143407371271, -1.199719254218452047 ) ) ;
#89964=CARTESIAN_POINT ( 'NONE',  ( 4.552840656090682891, 4.206068941727564514, 1.214306433183764966E-14 ) ) ;
#89966=ORIENTED_EDGE ( 'NONE', *, *, #26877, .T. ) ;
#89974=CARTESIAN_POINT ( 'NONE',  ( 7.801827329660018684, 11.18955008699033726, 1.199719254218460707 ) ) ;
#89975=CARTESIAN_POINT ( 'NONE',  ( -3.913499895838973508, 7.717500311787445000, 1.040834085586084257E-14 ) ) ;
#89980=CARTESIAN_POINT ( 'NONE',  ( 0.6823417656249899377, 4.426041667008086655, -1.181850606188754593 ) ) ;
#89982=CARTESIAN_POINT ( 'NONE',  ( -5.738125327081750271, 7.717565519727259904, 1.599625672291269396 ) ) ;
#89985=CARTESIAN_POINT ( 'NONE',  ( 5.464099601507359516, 6.333536608968757697, 1.199719254218462483 ) ) ;
#89986=CARTESIAN_POINT ( 'NONE',  ( -4.924636110261798372, 6.768494766770632332, 1.599625672291267398 ) ) ;
#89992=CARTESIAN_POINT ( 'NONE',  ( 7.131225611108096274, 8.382479970123348778, 1.082531754730558626 ) ) ;
#89995=CARTESIAN_POINT ( 'NONE',  ( 7.592202833528386208, 7.959917515312338487, 1.040834085586084257E-14 ) ) ;
#89996=CARTESIAN_POINT ( 'NONE',  ( 1.364683531249988535, 3.176041667008084435, 0.7879004041258500513 ) ) ;
#89998=CARTESIAN_POINT ( 'NONE',  ( 5.029711800545521250, 5.930713857800314237, -1.082531754730549078 ) ) ;
#90006=CARTESIAN_POINT ( 'NONE',  ( -5.355516094498059765, 6.520963868127283014, 1.360184235745926618 ) ) ;
#90013=CARTESIAN_POINT ( 'NONE',  ( -8.618179199781044630, 13.20629283305325963, 0.7998128361456341429 ) ) ;
#90015=CARTESIAN_POINT ( 'NONE',  ( 3.022498986271238586, 2.800000000000017586, -2.499999999999995115 ) ) ;
#90018=CARTESIAN_POINT ( 'NONE',  ( -4.471491734408701291, 4.111161866431900513, 1.214306433183764966E-14 ) ) ;
#90023=CARTESIAN_POINT ( 'NONE',  ( 4.256897045010922476, 5.029096643009940415, -1.082531754730548412 ) ) ;
#90024=AXIS2_PLACEMENT_3D ( 'NONE', #37324, #25340, #156427 ) ;
#90025=CARTESIAN_POINT ( 'NONE',  ( -0.6823417656250212460, 3.113541667008084879, 1.181850606188767472 ) ) ;
#90027=CARTESIAN_POINT ( 'NONE',  ( 8.535021395002688749, 9.916278701380017324, 1.199719254218462483 ) ) ;
#90030=CARTESIAN_POINT ( 'NONE',  ( -3.741160322367112379, 6.452105245148518797, 1.199719254218464037 ) ) ;
#90033=CARTESIAN_POINT ( 'NONE',  ( 0.7499999999999885647, 3.066666666666689522, -1.299038105676658228 ) ) ;
#90034=CARTESIAN_POINT ( 'NONE',  ( 6.173040012923759257, 6.096301524699504704, -0.7998128361456281477 ) ) ;
#90039=CARTESIAN_POINT ( 'NONE',  ( -1.201851678989727383E-14, 3.696875000341422801, -1.575800808251660134 ) ) ;
#90041=CARTESIAN_POINT ( 'NONE',  ( 10.07334494527360569, 10.85458331234846696, 0.000000000000000000 ) ) ;
#90046=CARTESIAN_POINT ( 'NONE',  ( -1.500000000000013101, 1.952083334016152527, 0.8660254037844403729 ) ) ;
#90048=CARTESIAN_POINT ( 'NONE',  ( -6.878064000834399394, 6.918829510595249310, -0.7998128361456291469 ) ) ;
#90050=CARTESIAN_POINT ( 'NONE',  ( 4.812781342726858647, 6.637997537979888563, 1.443375672974062551 ) ) ;
#90051=DIRECTION ( 'NONE',  ( -7.387867266669436732E-31, 1.000000000000000000, 8.546850786086424434E-32 ) ) ;
#90059=CARTESIAN_POINT ( 'NONE',  ( 6.259060471003163428, 10.45398764947904624, -0.7998128361456291469 ) ) ;
#90060=CARTESIAN_POINT ( 'NONE',  ( 3.649115900372475796, 7.409052317076538330, 1.040834085586084257E-14 ) ) ;
#90063=CARTESIAN_POINT ( 'NONE',  ( 5.843727902690005749, 6.776436293681846301, -1.199719254218445830 ) ) ;
#90069=CARTESIAN_POINT ( 'NONE',  ( 9.622536337397022521, 12.24937836509514710, 1.599625672291281386 ) ) ;
#90074=CARTESIAN_POINT ( 'NONE',  ( 4.959245870426344460, 6.614204113168008270, 1.243730795111185339 ) ) ;
#90086=CARTESIAN_POINT ( 'NONE',  ( 6.263503779833467178, 9.290876262238963790, -1.082531754730537088 ) ) ;
#90087=CARTESIAN_POINT ( 'NONE',  ( -5.278201874421821316, 5.052323696447222900, 0.7998128361456341429 ) ) ;
#90090=CARTESIAN_POINT ( 'NONE',  ( -7.040761844198392794, 7.108643661186573759, -0.7998128361456291469 ) ) ;
#90097=ORIENTED_EDGE ( 'NONE', *, *, #15281, .F. ) ;
#90103=CARTESIAN_POINT ( 'NONE',  ( 1.000000000000003553, 6.180000000000018368, 1.214306433183764966E-14 ) ) ;
#90109=CARTESIAN_POINT ( 'NONE',  ( -1.219999999999995977, 6.400000000000024336, 1.214306433183764966E-14 ) ) ;
#90112=CARTESIAN_POINT ( 'NONE',  ( -9.002250809793991948, 12.48608113052627289, -1.082531754730543971 ) ) ;
#90116=CARTESIAN_POINT ( 'NONE',  ( 8.911787042884274257, 9.291506392986812912, 0.7998128361456462443 ) ) ;
#90120=CARTESIAN_POINT ( 'NONE',  ( -6.738566041191992539, 7.820414121934134322, 1.199719254218450271 ) ) ;
#90121=CARTESIAN_POINT ( 'NONE',  ( 4.660252114795294887, 6.460046772059735432, -1.599625672291256295 ) ) ;
#90124=CARTESIAN_POINT ( 'NONE',  ( 8.866142388332804103, 12.43125098877526113, -1.199719254218446718 ) ) ;
#90125=DIRECTION ( 'NONE',  ( 1.000000000000000000, 0.000000000000000000, 0.000000000000000000 ) ) ;
#90128=CARTESIAN_POINT ( 'NONE',  ( -1.364683531249997417, 2.821875000341422801, 1.214306433183764966E-14 ) ) ;
#90129=ORIENTED_EDGE ( 'NONE', *, *, #117742, .T. ) ;
#90131=CARTESIAN_POINT ( 'NONE',  ( 6.399085315970131305, 8.488685506763726352, -1.443375672974057666 ) ) ;
#90139=CARTESIAN_POINT ( 'NONE',  ( 8.554831740098654436, 11.00372300158037042, 1.443375672974076540 ) ) ;
#90144=CARTESIAN_POINT ( 'NONE',  ( -8.317037166979361018, 11.79062823052953668, 1.199719254218453823 ) ) ;
#90153=CARTESIAN_POINT ( 'NONE',  ( 3.192055101013606233, 5.811482486902795230, -1.199719254218446718 ) ) ;
#90161=CARTESIAN_POINT ( 'NONE',  ( 6.308621549060418054, 6.254479983525607523, 0.7998128361456341429 ) ) ;
#90164=CARTESIAN_POINT ( 'NONE',  ( 0.7499999999999902300, 3.264583334016149418, 1.299038105676669330 ) ) ;
#90170=CARTESIAN_POINT ( 'NONE',  ( 1.499999999999985123, 0.5458333333333577064, -0.8660254037844253849 ) ) ;
#90171=CARTESIAN_POINT ( 'NONE',  ( 8.437251666405968464, 8.737881787095446384, 1.040834085586084257E-14 ) ) ;
#90172=CARTESIAN_POINT ( 'NONE',  ( -1.364683531250014514, -0.2614583329919080157, -0.7879004041258359514 ) ) ;
#90178=CARTESIAN_POINT ( 'NONE',  ( 9.083599731475983319, 11.62061899152058686, 1.443375672974076540 ) ) ;
#90183=CARTESIAN_POINT ( 'NONE',  ( -4.934277840369690971, 7.844075682818238526, -1.199719254218452047 ) ) ;
#90184=CARTESIAN_POINT ( 'NONE',  ( -1.201851678989727383E-14, 2.493750000682819046, 1.732050807568877637 ) ) ;
#90185=CARTESIAN_POINT ( 'NONE',  ( -1.364683531249997417, 5.321875000341417916, 1.214306433183764966E-14 ) ) ;
#90198=CARTESIAN_POINT ( 'NONE',  ( -7.316596452869116973, 11.68777962832266049, 0.7998128361456481317 ) ) ;
#90199=CARTESIAN_POINT ( 'NONE',  ( 7.145310649601935182, 8.294949498412453437, -1.199719254218446718 ) ) ;
#90206=CARTESIAN_POINT ( 'NONE',  ( -8.193204901359996128, 8.453160561208463264, 1.040834085586084257E-14 ) ) ;
#90210=CARTESIAN_POINT ( 'NONE',  ( 9.622536337397022521, 12.24937836509514710, 1.599625672291281386 ) ) ;
#90212=CARTESIAN_POINT ( 'NONE',  ( -3.903858165731105778, 6.641919395739846799, 1.199719254218464037 ) ) ;
#90214=CARTESIAN_POINT ( 'NONE',  ( -8.779068160048691283, 10.20099992726700933, -1.199719254218446718 ) ) ;
#90217=CARTESIAN_POINT ( 'NONE',  ( -4.520189846367452802, 7.221058948360024488, -1.319278014013465894 ) ) ;
#90224=CARTESIAN_POINT ( 'NONE',  ( 4.659198344590585350, 8.587481835331020719, 0.7998128361456462443 ) ) ;
#90226=CARTESIAN_POINT ( 'NONE',  ( 3.642287698956242714, 3.120124397465485533, 2.500000000001089795 ) ) ;
#90241=CARTESIAN_POINT ( 'NONE',  ( 4.867013957625893283, 4.780530493426062399, 1.040834085586084257E-14 ) ) ;
#90245=CARTESIAN_POINT ( 'NONE',  ( -9.833741488613570780, 10.36711991300432345, 0.7998128361456462443 ) ) ;
#90250=CARTESIAN_POINT ( 'NONE',  ( -0.7500000000000006661, 1.889583334016155192, -1.299038105676652011 ) ) ;
#90255=CARTESIAN_POINT ( 'NONE',  ( -10.65400978224035811, 11.32409958890225710, 1.040834085586084257E-14 ) ) ;
#90257=CARTESIAN_POINT ( 'NONE',  ( -1.402160292154681736E-14, 0.4468750003414233563, -1.575800808251665908 ) ) ;
#90263=CARTESIAN_POINT ( 'NONE',  ( -4.874319919312905647, 5.645460313075203018, -1.199719254218446718 ) ) ;
#90268=CARTESIAN_POINT ( 'NONE',  ( -0.7499999999999972244, 5.858333333333353821, -1.299038105676652011 ) ) ;
#90273=CARTESIAN_POINT ( 'NONE',  ( 0.6823417656249882723, 0.1760416670080894308, -1.181850606188749264 ) ) ;
#90275=CARTESIAN_POINT ( 'NONE',  ( -8.037286134802835491, 8.271255333558444889, -0.7998128361456291469 ) ) ;
#90276=CARTESIAN_POINT ( 'NONE',  ( 8.402302512167096893, 10.82577223566020841, -1.599625672291268286 ) ) ;
#90277=CARTESIAN_POINT ( 'NONE',  ( 5.542585869888291938, 5.360771691158120689, -0.7998128361456211532 ) ) ;
#90281=CARTESIAN_POINT ( 'NONE',  ( 1.364683531249988757, -0.3031249996585799744, 0.000000000000000000 ) ) ;
#90285=PRODUCT_DEFINITION_SHAPE ( 'NONE', 'NONE',  #128970 ) ;
#90288=CARTESIAN_POINT ( 'NONE',  ( 6.724481002698112775, 8.868313807946373473, -1.443375672974057666 ) ) ;
#90291=CARTESIAN_POINT ( 'NONE',  ( -6.254388934605767503, 6.191208599995166040, 0.7998128361456341429 ) ) ;
#90292=CARTESIAN_POINT ( 'NONE',  ( -1.499999999999997780, 5.431250000682820378, 1.214306433183764966E-14 ) ) ;
#90296=CARTESIAN_POINT ( 'NONE',  ( -7.931156673870055407, 11.23647130528163096, 1.082531754730549967 ) ) ;
#90298=CARTESIAN_POINT ( 'NONE',  ( -1.201851678989727383E-14, 3.712500000000020339, 1.732050807568877637 ) ) ;
#90302=CARTESIAN_POINT ( 'NONE',  ( 9.300530189294644146, 10.91333531134101165, -1.082531754730543083 ) ) ;
#90315=CARTESIAN_POINT ( 'NONE',  ( 7.090551149822722721, 11.21613407486112379, 0.7216878364870438212 ) ) ;
#90316=CARTESIAN_POINT ( 'NONE',  ( 7.076466111328892694, 10.34329533227067799, -1.199719254218441611 ) ) ;
#90317=CARTESIAN_POINT ( 'NONE',  ( -5.717788096661253761, 7.693838750903348789, 1.599625672291269396 ) ) ;
#90323=CARTESIAN_POINT ( 'NONE',  ( 3.497640442645619796, 6.064035702186436616, -1.082531754730543083 ) ) ;
#90325=CARTESIAN_POINT ( 'NONE',  ( -7.537970219518075332, 10.77775377520434574, -1.082531754730543971 ) ) ;
#90334=ORIENTED_EDGE ( 'NONE', *, *, #137350, .T. ) ;
#90335=DIRECTION ( 'NONE',  ( -0.000000000000000000, -8.546850786086437571E-32, -1.000000000000000000 ) ) ;
#90348=CARTESIAN_POINT ( 'NONE',  ( 0.4909899725976942797, 7.342450396234887044, 1.941297109531809006 ) ) ;
#90354=CARTESIAN_POINT ( 'NONE',  ( -5.377780486114890124, 9.425827667109372143, 0.000000000000000000 ) ) ;
#90357=B_SPLINE_CURVE_WITH_KNOTS ( 'NONE', 3,
 ( #13699, #194590, #178364, #147992, #63533, #12630, #78701, #144827, #163176, #112351 ),
 .UNSPECIFIED., .F., .F.,
 ( 4, 3, 3, 4 ),
 ( 1.474674387456768442E-18, 3.125271361792667814E-05, 6.250516575001786271E-05, 0.0001052821752614775306 ),
 .UNSPECIFIED. ) ;
#90359=CARTESIAN_POINT ( 'NONE',  ( 5.769158057814842699, 6.689438141327490150, 1.199719254218462483 ) ) ;
#90369=CARTESIAN_POINT ( 'NONE',  ( -2.578021764892882040, 6.159442492350315490, 0.7998128361456341429 ) ) ;
#90372=CARTESIAN_POINT ( 'NONE',  ( 6.265839547809997079, 10.46189657242035587, 0.7998128361456462443 ) ) ;
#90373=CARTESIAN_POINT ( 'NONE',  ( -1.364683531250012516, 3.488541667008085767, -0.7879004041258300672 ) ) ;
#90375=CARTESIAN_POINT ( 'NONE',  ( 5.728356146706021335, 6.265246534282280066, 1.050634566151719129 ) ) ;
#90381=CARTESIAN_POINT ( 'NONE',  ( 6.683806541412754321, 8.820860269780128604, -1.443375672974058777 ) ) ;
#90382=CARTESIAN_POINT ( 'NONE',  ( -8.128276786592724790, 9.441743324901704426, -1.199719254218446718 ) ) ;
#90385=CARTESIAN_POINT ( 'NONE',  ( -7.309817376062285099, 11.67987070538135264, 0.000000000000000000 ) ) ;
#90386=CARTESIAN_POINT ( 'NONE',  ( -4.903245109636583443, 8.872203061218007392, -0.7998128361456281477 ) ) ;
#90393=CARTESIAN_POINT ( 'NONE',  ( 8.911787042884274257, 9.291506392986812912, 0.7998128361456462443 ) ) ;
#90400=CARTESIAN_POINT ( 'NONE',  ( -3.563261906135775536, 6.332667919118538435, -2.420000000000000373 ) ) ;
#90403=CARTESIAN_POINT ( 'NONE',  ( -0.5221183067618221374, 7.970647359860968173, -1.933437843119017563 ) ) ;
#90408=CARTESIAN_POINT ( 'NONE',  ( 1.499999999999989120, 4.504166666666688634, 0.8660254037844524744 ) ) ;
#90409=CARTESIAN_POINT ( 'NONE',  ( 3.323720213644492993, 7.029424015893889433, 1.040834085586084257E-14 ) ) ;
#90410=CARTESIAN_POINT ( 'NONE',  ( 7.091078035147269532, 8.231678114882006625, 1.199719254218462483 ) ) ;
#90412=CARTESIAN_POINT ( 'NONE',  ( -9.490344339885981029, 10.17441593939621924, -0.7216878364870267237 ) ) ;
#90413=ADVANCED_FACE ( 'NONE', ( #20255 ), #36510, .F. ) ;
#90414=CARTESIAN_POINT ( 'NONE',  ( 7.483737605063422116, 7.833374748769873719, -0.7216878364870257245 ) ) ;
#90415=CARTESIAN_POINT ( 'NONE',  ( -7.985389288324692636, 11.29974268881207067, -1.082531754730543083 ) ) ;
#90416=CIRCLE ( 'NONE', #80040, 0.08000000000000012657 ) ;
#90419=CARTESIAN_POINT ( 'NONE',  ( 7.507464373665139412, 9.781794407407920389, 1.599625672291281386 ) ) ;
#90425=CARTESIAN_POINT ( 'NONE',  ( -1.201851678989727383E-14, 2.696875000341417916, -1.575800808251660134 ) ) ;
#90430=CARTESIAN_POINT ( 'NONE',  ( -0.6823417656250003738, -0.03229166632524871350, -1.181850606188749264 ) ) ;
#90433=CARTESIAN_POINT ( 'NONE',  ( 10.24726517383036928, 10.84956421242393887, 0.000000000000000000 ) ) ;
#90437=CARTESIAN_POINT ( 'NONE',  ( -8.130085669689073313, 12.63685038127928806, 0.7998128361456481317 ) ) ;
#90443=CARTESIAN_POINT ( 'NONE',  ( 2.869522067586683711, 6.499526178826442013, 0.7998128361456362523 ) ) ;
#90447=CARTESIAN_POINT ( 'NONE',  ( -10.34217224912604571, 10.96028913360221502, 0.7998128361456462443 ) ) ;
#90451=CARTESIAN_POINT ( 'NONE',  ( 9.097684769969825780, 10.57271930550834860, -1.199719254218446718 ) ) ;
#90453=CARTESIAN_POINT ( 'NONE',  ( 5.134314571617769829, 6.480444997182255307, 1.201143065674977528 ) ) ;
#90455=CARTESIAN_POINT ( 'NONE',  ( -4.925689880466507908, 4.641059703499347044, -0.7998128361456221525 ) ) ;
#90459=CARTESIAN_POINT ( 'NONE',  ( 7.670162217029129259, 9.971608557999250166, 1.599625672291281386 ) ) ;
#90461=CARTESIAN_POINT ( 'NONE',  ( 7.949158136313996259, 8.168439335321471262, 1.040834085586084257E-14 ) ) ;
#90463=CARTESIAN_POINT ( 'NONE',  ( -9.015808963407680565, 9.620791333504852716, 1.040834085586084257E-14 ) ) ;
#90464=ORIENTED_EDGE ( 'NONE', *, *, #170328, .F. ) ;
#90472=CARTESIAN_POINT ( 'NONE',  ( -4.965152591087599099, 6.642004417359813395, -1.244917454897740861 ) ) ;
#90473=CARTESIAN_POINT ( 'NONE',  ( 1.364683531249988535, 1.363541667008083769, 0.7879004041258500513 ) ) ;
#90476=CARTESIAN_POINT ( 'NONE',  ( 6.968527767744109980, 7.232296605230681408, 0.7216878364870317197 ) ) ;
#90496=CARTESIAN_POINT ( 'NONE',  ( 9.260382613333817403, 10.76253345609967660, -1.199719254218446718 ) ) ;
#90500=CARTESIAN_POINT ( 'NONE',  ( -6.880926654135487652, 7.986501503701545879, 1.199719254218450271 ) ) ;
#90502=ORIENTED_EDGE ( 'NONE', *, *, #187534, .T. ) ;
#90503=CARTESIAN_POINT ( 'NONE',  ( -10.14557902172788495, 10.73093036830436553, 1.040834085586084257E-14 ) ) ;
#90507=CARTESIAN_POINT ( 'NONE',  ( 1.499999999999989120, 5.077083334016151639, -0.8660254037844323793 ) ) ;
#90508=CARTESIAN_POINT ( 'NONE',  ( 8.260995669428309540, 8.532249790621511565, 0.7998128361456481317 ) ) ;
#90512=CARTESIAN_POINT ( 'NONE',  ( -6.177711549321182716, 10.35908057418338402, 0.7998128361456481317 ) ) ;
#90514=CARTESIAN_POINT ( 'NONE',  ( 1.364683531249990311, 5.134375000341417916, 1.214306433183764966E-14 ) ) ;
#90521=AXIS2_PLACEMENT_3D ( 'NONE', #201888, #17812, #19955 ) ;
#90522=CARTESIAN_POINT ( 'NONE',  ( -8.351459436338041442, 9.806086099558291025, -1.082531754730543971 ) ) ;
#90526=CARTESIAN_POINT ( 'NONE',  ( -1.364683531249997417, 3.571875000341423245, 1.214306433183764966E-14 ) ) ;
#90532=CARTESIAN_POINT ( 'NONE',  ( -1.364683531250010295, 4.530208333674754506, 0.7879004041258379498 ) ) ;
#90533=CARTESIAN_POINT ( 'NONE',  ( -5.949330478298285207, 5.835307067636438028, 0.7998128361456341429 ) ) ;
#90534=CARTESIAN_POINT ( 'NONE',  ( 7.637320603199683866, 7.804628880021436288, -0.7998128361456281477 ) ) ;
#90537=CARTESIAN_POINT ( 'NONE',  ( 4.053524740361575063, 4.791828954252362216, -1.082531754730543083 ) ) ;
#90538=CARTESIAN_POINT ( 'NONE',  ( -1.364683531250010295, 4.092708333674751842, 0.7879004041258379498 ) ) ;
#90539=CARTESIAN_POINT ( 'NONE',  ( -3.023105066167347310, 5.702484939155337607, 2.500000000000011102 ) ) ;
#90544=CARTESIAN_POINT ( 'NONE',  ( -1.364683531250000748, 1.009375000341421247, 0.000000000000000000 ) ) ;
#90545=CARTESIAN_POINT ( 'NONE',  ( -4.609409038966245653, 6.400729850259146758, -1.443375672974053447 ) ) ;
#90546=CARTESIAN_POINT ( 'NONE',  ( 3.635557746758808495, 7.393234471193928847, -0.7998128361456291469 ) ) ;
#90550=CARTESIAN_POINT ( 'NONE',  ( 4.555176424511575561, 4.416720038126027426, -0.7216878364870188411 ) ) ;
#90554=CARTESIAN_POINT ( 'NONE',  ( -8.270110514656041190, 10.67154823856396817, 1.443375672974090751 ) ) ;
#90560=CARTESIAN_POINT ( 'NONE',  ( -8.299562589859897699, 12.83457345481192036, -0.7998128361456281477 ) ) ;
#90562=CARTESIAN_POINT ( 'NONE',  ( -6.195713011320807873, 6.330679389403470303, -0.7216878364870267237 ) ) ;
#90564=CARTESIAN_POINT ( 'NONE',  ( 0.6823417656249899377, 0.9052083336747520637, 1.181850606188755259 ) ) ;
#90576=CARTESIAN_POINT ( 'NONE',  ( 8.392133896734662812, 10.81390885098904420, 1.443375672974076540 ) ) ;
#90587=CARTESIAN_POINT ( 'NONE',  ( -2.927671105547157371, 5.503034492191895666, 1.199719254218462483 ) ) ;
#90588=CARTESIAN_POINT ( 'NONE',  ( 1.284279953904121641, 3.253360285806104812, 0.7750000000000135669 ) ) ;
#90589=CARTESIAN_POINT ( 'NONE',  ( 1.364683531249988757, 1.446875000341421469, 0.000000000000000000 ) ) ;
#90599=CARTESIAN_POINT ( 'NONE',  ( -1.402160292154681736E-14, 1.196875000341419026, -1.575800808251659024 ) ) ;
#90610=CARTESIAN_POINT ( 'NONE',  ( 6.006425746053997372, 6.966250444273174303, -1.199719254218445830 ) ) ;
#90619=CARTESIAN_POINT ( 'NONE',  ( 5.947222937888848371, 10.09017719417900416, 1.040834085586084257E-14 ) ) ;
#90622=CARTESIAN_POINT ( 'NONE',  ( 9.236128959407556849, 11.79856975744075598, -1.599625672291262513 ) ) ;
#90629=CARTESIAN_POINT ( 'NONE',  ( 4.201496546123638431, 3.900130496719715456, 1.214306433183764966E-14 ) ) ;
#90634=CARTESIAN_POINT ( 'NONE',  ( -7.863365906246061243, 10.19701286208565705, -1.443375672974059665 ) ) ;
#90641=CARTESIAN_POINT ( 'NONE',  ( -4.207825419487694063, 3.977679809700697788, -0.5488412742886485951 ) ) ;
#90645=CARTESIAN_POINT ( 'NONE',  ( 2.995988758495615745, 6.439144618312774959, -0.7216878364870267237 ) ) ;
#90647=CARTESIAN_POINT ( 'NONE',  ( 5.529027716274630855, 5.344953845275508542, 1.040834085586084257E-14 ) ) ;
#90649=EDGE_LOOP ( 'NONE', ( #15611, #60807, #121045, #212895 ) ) ;
#90654=CARTESIAN_POINT ( 'NONE',  ( -5.904739593951539689, 6.847616600153594746, 1.199719254218450271 ) ) ;
#90655=CARTESIAN_POINT ( 'NONE',  ( -2.435661151949389147, 5.993355110582911038, 0.7998128361456341429 ) ) ;
#90661=CARTESIAN_POINT ( 'NONE',  ( 9.083599731475988648, 10.66024977721925104, 1.082531754730549967 ) ) ;
#90663=CARTESIAN_POINT ( 'NONE',  ( -1.364683531250012516, 4.801041667008083991, -0.7879004041258300672 ) ) ;
#90665=CARTESIAN_POINT ( 'NONE',  ( 4.473300617505036492, 7.306268922809479704, -1.199719254218452047 ) ) ;
#90667=CARTESIAN_POINT ( 'NONE',  ( 5.490689023410174840, 5.508151403507718591, -0.7216878364870152884 ) ) ;
#90681=CARTESIAN_POINT ( 'NONE',  ( -1.364683531250000748, 1.321875000341421469, 0.000000000000000000 ) ) ;
#90683=CARTESIAN_POINT ( 'NONE',  ( 3.571683402196252910, 6.254382171615883834, 1.199719254218462483 ) ) ;
#90685=CARTESIAN_POINT ( 'NONE',  ( -4.934804725694212912, 8.701096580044490381, -0.7216878364870207285 ) ) ;
#90687=CARTESIAN_POINT ( 'NONE',  ( 5.043269954603547767, 4.986162489899998995, -0.7216878364870197293 ) ) ;
#90688=CARTESIAN_POINT ( 'NONE',  ( -7.334597914868743018, 7.659378443542744996, -0.7216878364870267237 ) ) ;
#90692=CARTESIAN_POINT ( 'NONE',  ( 6.335737856287750880, 6.286115675290828264, -0.7998128361456281477 ) ) ;
#90702=EDGE_CURVE ( 'NONE', #171990, #11347, #103347, .T. ) ;
#90703=CARTESIAN_POINT ( 'NONE',  ( 6.958359152311676787, 9.141171649162195934, -1.599625672291262513 ) ) ;
#90707=CARTESIAN_POINT ( 'NONE',  ( -7.711890448074853133, 7.891627032375787998, -0.7998128361456291469 ) ) ;
#90711=CARTESIAN_POINT ( 'NONE',  ( 7.456094412511537151, 10.78619501698377370, 1.199719254218460707 ) ) ;
#90714=CARTESIAN_POINT ( 'NONE',  ( -6.684333426737305572, 7.757142738403693727, -1.199719254218446718 ) ) ;
#90715=CARTESIAN_POINT ( 'NONE',  ( 6.439759776366758892, 10.45687747249582955, 0.7216878364870438212 ) ) ;
#90716=CARTESIAN_POINT ( 'NONE',  ( 4.075236096247129680, 7.726954018008360237, 0.5961105570580684798 ) ) ;
#90717=CARTESIAN_POINT ( 'NONE',  ( -4.252453736180621391, 8.112946458852704268, -0.7998128361456281477 ) ) ;
#90724=CARTESIAN_POINT ( 'NONE',  ( 8.204655514564224816, 12.72384853363364066, 1.040834085586084257E-14 ) ) ;
#90725=CARTESIAN_POINT ( 'NONE',  ( 1.364683531249988757, 0.8843750003414210248, 0.000000000000000000 ) ) ;
#90727=CARTESIAN_POINT ( 'NONE',  ( -4.595850885352567694, 8.305650432979225783, 1.040834085586084257E-14 ) ) ;
#90733=CARTESIAN_POINT ( 'NONE',  ( -5.638288519115033814, 6.168138913823901781, 0.8326226707794943671 ) ) ;
#90734=CARTESIAN_POINT ( 'NONE',  ( -1.364683531250012516, 1.092708333674754506, 0.7879004041258379498 ) ) ;
#90737=CARTESIAN_POINT ( 'NONE',  ( 2.738383840280328663, 5.178236332760252303, 1.082531754730548412 ) ) ;
#90740=CARTESIAN_POINT ( 'NONE',  ( -3.750802052474980108, 7.527686161196117887, 1.040834085586084257E-14 ) ) ;
#90743=CARTESIAN_POINT ( 'NONE',  ( -8.961576348508655698, 9.557519949455999253, -0.7216878364870267237 ) ) ;
#90747=ADVANCED_FACE ( 'NONE', ( #87094 ), #161183, .T. ) ;
#90752=CARTESIAN_POINT ( 'NONE',  ( -8.988692655735990300, 9.589155641221221771, 0.7216878364870438212 ) ) ;
#90756=CARTESIAN_POINT ( 'NONE',  ( -7.334597914868727919, 10.54048608644677465, -1.082531754730543083 ) ) ;
#90762=CARTESIAN_POINT ( 'NONE',  ( -1.499999999999997780, 4.931250000682820378, 1.214306433183764966E-14 ) ) ;
#90764=CARTESIAN_POINT ( 'NONE',  ( 1.419999999999989049, 6.280000000000042881, -2.873333333333328632 ) ) ;
#90770=CARTESIAN_POINT ( 'NONE',  ( -6.856673000209188906, 9.022537805042615489, 1.599625672291283607 ) ) ;
#90772=CARTESIAN_POINT ( 'NONE',  ( 5.606460214450851964, 6.499623990736163037, 1.199719254218462483 ) ) ;
#90777=CARTESIAN_POINT ( 'NONE',  ( 8.145751363712157911, 8.397798100619326078, -0.7998128361456281477 ) ) ;
#90783=CARTESIAN_POINT ( 'NONE',  ( -6.236387472606166327, 6.378132927569716060, -0.7216878364870278340 ) ) ;
#90791=CARTESIAN_POINT ( 'NONE',  ( 1.364683531249986537, 0.6135416670080880985, 0.7879004041258500513 ) ) ;
#90793=CARTESIAN_POINT ( 'NONE',  ( -7.666245793523398078, 11.03137162816423356, 1.199719254218453823 ) ) ;
#90795=CARTESIAN_POINT ( 'NONE',  ( 6.825640269476072497, 10.05066518344239412, 1.199719254218460707 ) ) ;
#90797=CARTESIAN_POINT ( 'NONE',  ( -7.069687034522070590, 10.33538640932937724, -1.199719254218440723 ) ) ;
#90800=CARTESIAN_POINT ( 'NONE',  ( -1.364683531249997417, 5.259375000341425022, 1.214306433183764966E-14 ) ) ;
#90801=CARTESIAN_POINT ( 'NONE',  ( 8.107412671292022921, 12.40247251657532956, 0.7216878364870438212 ) ) ;
#90804=CARTESIAN_POINT ( 'NONE',  ( -0.6823417656250003738, 0.03020833367475134201, -1.181850606188749264 ) ) ;
#90807=CARTESIAN_POINT ( 'NONE',  ( 8.636180661780656465, 11.09863007687603087, -1.443375672974052559 ) ) ;
#90810=CARTESIAN_POINT ( 'NONE',  ( -4.758548728716557541, 8.495464583570553785, 1.040834085586084257E-14 ) ) ;
#90812=CARTESIAN_POINT ( 'NONE',  ( -1.364683531250014514, 1.488541667008084435, -0.7879004041258289570 ) ) ;
#90816=CARTESIAN_POINT ( 'NONE',  ( -5.845536785786364931, 9.971543350059432598, 0.000000000000000000 ) ) ;
#90818=CARTESIAN_POINT ( 'NONE',  ( -1.364683531250010295, 4.592708333674755394, 0.7879004041258379498 ) ) ;
#90823=CARTESIAN_POINT ( 'NONE',  ( 7.422199028477372451, 10.74665040227725044, -1.199719254218441611 ) ) ;
#90827=CARTESIAN_POINT ( 'NONE',  ( -1.500000000000001332, 0.9000000000000187850, 0.000000000000000000 ) ) ;
#90830=CARTESIAN_POINT ( 'NONE',  ( -0.1467296397388559992, 8.209138825498280667, -2.038183423090501378 ) ) ;
#90833=CARTESIAN_POINT ( 'NONE',  ( 5.802526556968819804, 9.713438716531550554, -0.7216878364870267237 ) ) ;
#90834=CARTESIAN_POINT ( 'NONE',  ( 8.387690588348714726, 12.93738945304888333, 1.040834085586084257E-14 ) ) ;
#90836=CARTESIAN_POINT ( 'NONE',  ( 4.701980345841006326, 4.380065246436280368, 0.7998128361456341429 ) ) ;
#90841=CARTESIAN_POINT ( 'NONE',  ( 8.914649696185335870, 10.35917838609310593, -1.199719254218446718 ) ) ;
#90842=CARTESIAN_POINT ( 'NONE',  ( -9.317477881089553549, 11.89347683273641820, 1.599625672291281386 ) ) ;
#90844=CARTESIAN_POINT ( 'NONE',  ( -4.910477722004077172, 4.678539768940303212, -0.3136693401591003072 ) ) ;
#90845=CARTESIAN_POINT ( 'NONE',  ( 1.364683531249988757, -0.3656249996585800299, 0.000000000000000000 ) ) ;
#90846=CARTESIAN_POINT ( 'NONE',  ( 0.7499999999999867883, 0.3166666666666873020, -1.299038105676652899 ) ) ;
#90854=CARTESIAN_POINT ( 'NONE',  ( -0.6823417656250212460, 5.551041667008087543, 1.181850606188767472 ) ) ;
#90856=CARTESIAN_POINT ( 'NONE',  ( -6.738039156311804945, 6.963393225226301553, 1.040834085586084257E-14 ) ) ;
#90865=CARTESIAN_POINT ( 'NONE',  ( 9.077347539549325717, 10.54899253668443393, -1.199719254218446718 ) ) ;
#90870=CARTESIAN_POINT ( 'NONE',  ( 8.242994206984347372, 8.719174117677642499, 1.040834085586084257E-14 ) ) ;
#90873=CARTESIAN_POINT ( 'NONE',  ( -9.996439331977562404, 10.55693406359564790, 0.7998128361456462443 ) ) ;
#90874=CARTESIAN_POINT ( 'NONE',  ( 7.657657833620182153, 7.828355648845348291, -0.7998128361456281477 ) ) ;
#90877=CARTESIAN_POINT ( 'NONE',  ( 5.007038802148489509, 4.735966778795008381, 0.7998128361456341429 ) ) ;
#90886=CARTESIAN_POINT ( 'NONE',  ( -4.256897045010916258, 7.910204285913967404, 0.7216878364870317197 ) ) ;
#90887=CARTESIAN_POINT ( 'NONE',  ( 8.419250204406344196, 12.76628297187536809, 1.040834085586084257E-14 ) ) ;
#90890=CARTESIAN_POINT ( 'NONE',  ( -7.217017841176048165, 7.314275657660511243, 1.040834085586084257E-14 ) ) ;
#90894=CARTESIAN_POINT ( 'NONE',  ( -7.862839020921525091, 11.26073039346208660, -1.199719254218446718 ) ) ;
#90895=CARTESIAN_POINT ( 'NONE',  ( 1.257539916218598286, 3.047412844624492134, 0.7750000000000100142 ) ) ;
#90900=CARTESIAN_POINT ( 'NONE',  ( 4.852928918687680948, 7.749168607522574526, 1.199719254218462483 ) ) ;
#90909=CARTESIAN_POINT ( 'NONE',  ( -6.886651960737580680, 10.12184548991413457, -1.199719254218440723 ) ) ;
#90912=CARTESIAN_POINT ( 'NONE',  ( 4.677199807034550183, 8.400557508274889784, 1.040834085586084257E-14 ) ) ;
#90917=CARTESIAN_POINT ( 'NONE',  ( 5.203632029546647608, 4.965325544092860532, 1.040834085586084257E-14 ) ) ;
#90919=CARTESIAN_POINT ( 'NONE',  ( -4.388035272317281077, 8.271124917678806199, 0.7998128361456481317 ) ) ;
#90928=CARTESIAN_POINT ( 'NONE',  ( -9.938290294017125603, 11.55342575023019691, -1.199719254218441611 ) ) ;
#90929=CARTESIAN_POINT ( 'NONE',  ( 7.456094412511537151, 10.78619501698377370, 1.199719254218460707 ) ) ;
#90933=CARTESIAN_POINT ( 'NONE',  ( -4.373759202716216876, 7.180157790548314267, -1.044885312346154782 ) ) ;
#90935=CARTESIAN_POINT ( 'NONE',  ( 3.469446951953614189E-15, 6.400000000000023448, 1.214306433183764966E-14 ) ) ;
#90936=CARTESIAN_POINT ( 'NONE',  ( -0.6823417656250246877, -1.136458332991911790, 1.181850606188755259 ) ) ;
#90940=CARTESIAN_POINT ( 'NONE',  ( 8.541273586929342798, 11.94827437051752206, -1.082531754730543083 ) ) ;
#90960=CARTESIAN_POINT ( 'NONE',  ( -4.796887421136680985, 4.490790167614548523, 1.214306433183764966E-14 ) ) ;
#90961=CARTESIAN_POINT ( 'NONE',  ( -0.7499999999999972244, 3.608333333333359150, -1.299038105676652011 ) ) ;
#90963=CARTESIAN_POINT ( 'NONE',  ( -2.300079615812729905, 5.835176651756807331, -0.7998128361456281477 ) ) ;
#90970=CARTESIAN_POINT ( 'NONE',  ( -1.500000000000015099, -1.089583332650509773, -0.8660254037844383745 ) ) ;
#90976=ORIENTED_EDGE ( 'NONE', *, *, #96602, .F. ) ;
#90980=CARTESIAN_POINT ( 'NONE',  ( 9.622536337397022521, 12.24937836509514710, 1.599625672291281386 ) ) ;
#90981=DIRECTION ( 'NONE',  ( -1.000000000000000000, 7.387867266669436732E-31, 0.000000000000000000 ) ) ;
#90982=CARTESIAN_POINT ( 'NONE',  ( 3.895595285070167169, 2.800000000000017586, -0.7749999999999935829 ) ) ;
#90983=CARTESIAN_POINT ( 'NONE',  ( 10.18181017373857600, 10.98112607889092907, 0.7216878364870438212 ) ) ;
#90985=CARTESIAN_POINT ( 'NONE',  ( -1.364683531250000748, 1.821875000341421913, 0.000000000000000000 ) ) ;
#90988=CARTESIAN_POINT ( 'NONE',  ( -8.320953590485107298, 10.73086516036454618, 1.599625672291269396 ) ) ;
#90989=CARTESIAN_POINT ( 'NONE',  ( -5.382223794500843539, 7.302347065049529462, -1.443375672974051449 ) ) ;
#90991=CARTESIAN_POINT ( 'NONE',  ( -5.096975683733680818, 8.033889833409558534, -1.199719254218452047 ) ) ;
#90993=CARTESIAN_POINT ( 'NONE',  ( 1.364683531249990311, 5.113541667008084879, 0.7879004041258500513 ) ) ;
#91002=CARTESIAN_POINT ( 'NONE',  ( -6.385527161912131433, 6.552129231760014605, 0.7216878364870317197 ) ) ;
#91004=CARTESIAN_POINT ( 'NONE',  ( -0.4702634422474149534, 7.494255424139877775, -4.464191613397623826 ) ) ;
#91008=CARTESIAN_POINT ( 'NONE',  ( -5.870317324592829067, 5.951051088220814300, -0.7216878364870197293 ) ) ;
#91010=CARTESIAN_POINT ( 'NONE',  ( 10.55910270694468345, 11.21337466772398095, 0.7998128361456462443 ) ) ;
#91019=CARTESIAN_POINT ( 'NONE',  ( -3.846762897975357198, 5.510976019103107859, -1.599625672291256295 ) ) ;
#91020=CARTESIAN_POINT ( 'NONE',  ( -4.735978408342542245, 7.017321386899737057, 1.427696578792345683 ) ) ;
#91024=CARTESIAN_POINT ( 'NONE',  ( 7.931156674314368438, 12.19684052010138586, 1.040834085586084257E-14 ) ) ;
#91026=CARTESIAN_POINT ( 'NONE',  ( 5.469824908109481854, 8.468880595181346393, -1.199719254218446718 ) ) ;
#91031=CARTESIAN_POINT ( 'NONE',  ( 4.111146893441827821, 5.819424013814004759, 1.599625672291267398 ) ) ;
#91041=CARTESIAN_POINT ( 'NONE',  ( -6.087774667736030487, 7.061157519568837415, 1.199719254218450271 ) ) ;
#91048=CARTESIAN_POINT ( 'NONE',  ( 1.364683531249988535, 4.655208333674755394, -0.7879004041258300672 ) ) ;
#91049=CARTESIAN_POINT ( 'NONE',  ( 9.856414487010592751, 10.60149777770828194, 0.7216878364870438212 ) ) ;
#91050=CARTESIAN_POINT ( 'NONE',  ( -5.280010757518168063, 8.247430752824802980, -1.199719254218446718 ) ) ;
#91053=CARTESIAN_POINT ( 'NONE',  ( 4.330940004561544043, 7.140181541042074365, -1.199719254218452047 ) ) ;
#91054=CARTESIAN_POINT ( 'NONE',  ( -6.423865854776591000, 6.388931673527803667, 1.040834085586084257E-14 ) ) ;
#91060=CARTESIAN_POINT ( 'NONE',  ( 5.802526556968819804, 9.713438716531550554, -0.7216878364870267237 ) ) ;
#91063=CARTESIAN_POINT ( 'NONE',  ( 6.114364089638782751, 9.116879957011832403, 1.082531754730558626 ) ) ;
#91064=CARTESIAN_POINT ( 'NONE',  ( 1.364683531249988535, 3.717708333674750953, -0.7879004041258239610 ) ) ;
#91066=CARTESIAN_POINT ( 'NONE',  ( 6.277061933002788585, 6.425586464699131639, 0.7216878364870317197 ) ) ;
#91075=VECTOR ( 'NONE', #30527, 1000.000000000000000 ) ;
#91076=CARTESIAN_POINT ( 'NONE',  ( -4.153809255294044434, 7.618134729639562508, -0.8777755718400248597 ) ) ;
#91083=CARTESIAN_POINT ( 'NONE',  ( 4.645640190976921602, 8.571663989448405019, 1.040834085586084257E-14 ) ) ;
#91085=CARTESIAN_POINT ( 'NONE',  ( -4.419594887930571758, 4.258541578781506409, 1.214306433183764966E-14 ) ) ;
#91087=CARTESIAN_POINT ( 'NONE',  ( 3.816783937446950770, 4.411668334231586996, 1.199719254218464037 ) ) ;
#91090=CARTESIAN_POINT ( 'NONE',  ( -2.462777459176719308, 6.024990802348131780, -0.7998128361456281477 ) ) ;
#91095=CARTESIAN_POINT ( 'NONE',  ( 5.070386261830877928, 5.978167395966564435, -1.082531754730548412 ) ) ;
#91096=CARTESIAN_POINT ( 'NONE',  ( -1.201851678989727383E-14, 3.509375000341421469, -1.575800808251660134 ) ) ;
#91098=CARTESIAN_POINT ( 'NONE',  ( 7.670162217029129259, 9.971608557999250166, 1.599625672291281386 ) ) ;
#91099=CARTESIAN_POINT ( 'NONE',  ( 1.608462485350599769, 8.735270501766756013, 2.463594439587641904 ) ) ;
#91103=ORIENTED_EDGE ( 'NONE', *, *, #88030, .F. ) ;
#91105=CARTESIAN_POINT ( 'NONE',  ( 0.7499999999999885647, 3.566666666666690411, -1.299038105676658228 ) ) ;
#91106=CARTESIAN_POINT ( 'NONE',  ( 6.636879889089462026, 7.701780277814560982, -1.199719254218446718 ) ) ;
#91110=CARTESIAN_POINT ( 'NONE',  ( -0.6823417656249969321, 3.717708333674754506, -1.181850606188749264 ) ) ;
#91111=CARTESIAN_POINT ( 'NONE',  ( 8.419250204406344196, 12.76628297187536809, 1.040834085586084257E-14 ) ) ;
#91117=CARTESIAN_POINT ( 'NONE',  ( 1.499999999999987121, 2.577083334016147198, -0.8660254037844262731 ) ) ;
#91119=CARTESIAN_POINT ( 'NONE',  ( -5.392392409933270514, 7.314210449720692786, 1.599625672291269396 ) ) ;
#91127=CARTESIAN_POINT ( 'NONE',  ( 4.852928918687680948, 7.749168607522574526, 1.199719254218462483 ) ) ;
#91129=FACE_BOUND ( 'NONE', #173153, .T. ) ;
#91132=CARTESIAN_POINT ( 'NONE',  ( 5.575427483717746213, 7.527751369135936343, 1.599625672291267398 ) ) ;
#91136=ORIENTED_EDGE ( 'NONE', *, *, #185057, .T. ) ;
#91139=CARTESIAN_POINT ( 'NONE',  ( 8.191097360950562845, 12.70803068775103739, -0.7998128361456352531 ) ) ;
#91145=CARTESIAN_POINT ( 'NONE',  ( 5.846986258851572416, 6.004518191619921730, 0.3586427151269864222 ) ) ;
#91158=CARTESIAN_POINT ( 'NONE',  ( 7.795575138177731844, 8.197185204069915798, 1.040834085586084257E-14 ) ) ;
#91160=CARTESIAN_POINT ( 'NONE',  ( -3.228813138348844536, 6.918699094715619502, 0.7998128361456341429 ) ) ;
#91164=CARTESIAN_POINT ( 'NONE',  ( -6.013204822860843457, 6.974159367214481264, -1.199719254218446718 ) ) ;
#91177=CARTESIAN_POINT ( 'NONE',  ( 8.374132434735052755, 12.92157160716627295, -0.7998128361456352531 ) ) ;
#91181=CARTESIAN_POINT ( 'NONE',  ( 4.028709946750490545, 3.988235255965033588, -0.8025987720412866011 ) ) ;
#91183=CARTESIAN_POINT ( 'NONE',  ( -2.252626078164912560, 5.779814191167667481, 0.7998128361456341429 ) ) ;
#91186=CARTESIAN_POINT ( 'NONE',  ( 7.944187942603509356, 11.35563746875774882, 1.199719254218460707 ) ) ;
#91190=CARTESIAN_POINT ( 'NONE',  ( -8.227100285394159940, 8.492705175914988303, 0.7998128361456602331 ) ) ;
#91191=CARTESIAN_POINT ( 'NONE',  ( 4.521807925357579805, 5.234196320127330715, -1.199719254218452047 ) ) ;
#91195=CARTESIAN_POINT ( 'NONE',  ( -2.129434811653636128, 5.532128030284154008, 1.040834085586084257E-14 ) ) ;
#91196=CARTESIAN_POINT ( 'NONE',  ( -2.765500147507697459, 5.209872024525476597, 1.082531754730560403 ) ) ;
#91199=CARTESIAN_POINT ( 'NONE',  ( 0.6823417656249899377, 2.405208333674753618, 1.181850606188767472 ) ) ;
#91200=AXIS2_PLACEMENT_3D ( 'NONE', #151981, #3555, #69626 ) ;
#91202=CARTESIAN_POINT ( 'NONE',  ( 7.809133291791403586, 8.213003049952529722, -0.7216878364870257245 ) ) ;
#91210=CARTESIAN_POINT ( 'NONE',  ( 7.565086526301031178, 11.76975868075249387, 1.040834085586084257E-14 ) ) ;
#91213=EDGE_LOOP ( 'NONE', ( #196628, #3709, #83516, #9751, #190866 ) ) ;
#91217=CARTESIAN_POINT ( 'NONE',  ( -7.343712760096452463, 11.71941532008788833, -0.7998128361456291469 ) ) ;
#91234=CARTESIAN_POINT ( 'NONE',  ( -0.7500000000000215383, 2.722916667349486897, 1.299038105676671107 ) ) ;
#91240=CARTESIAN_POINT ( 'NONE',  ( 1.499999999999987121, 1.045833333333352266, -0.8660254037844253849 ) ) ;
#91241=CARTESIAN_POINT ( 'NONE',  ( 7.775764792637399836, 9.030479331953833011, -1.199719254218441611 ) ) ;
#91242=CARTESIAN_POINT ( 'NONE',  ( -0.6823417656250246877, -0.4489583329919111243, 1.181850606188755259 ) ) ;
#91245=CARTESIAN_POINT ( 'NONE',  ( 9.747949258545622442, 10.47495501116581984, 0.000000000000000000 ) ) ;
#91246=CARTESIAN_POINT ( 'NONE',  ( -4.934804725694212912, 8.701096580044490381, -0.7216878364870207285 ) ) ;
#91251=CARTESIAN_POINT ( 'NONE',  ( -5.880485940025243607, 7.883652901494672349, 1.599625672291269396 ) ) ;
#91253=CARTESIAN_POINT ( 'NONE',  ( -1.402160292154681736E-14, 2.618750000682819490, -1.732050807568863648 ) ) ;
#91254=CARTESIAN_POINT ( 'NONE',  ( -1.364683531249997417, 4.321875000341417028, 1.214306433183764966E-14 ) ) ;
#91264=ORIENTED_EDGE ( 'NONE', *, *, #5833, .F. ) ;
#91270=CARTESIAN_POINT ( 'NONE',  ( -9.338868881714763148, 9.789768538289042255, -0.7998128361456291469 ) ) ;
#91271=CARTESIAN_POINT ( 'NONE',  ( 6.982612806237943559, 8.105135347821125436, -1.199719254218446718 ) ) ;
#91280=CARTESIAN_POINT ( 'NONE',  ( -7.542413527904030524, 7.693903958843159252, 1.040834085586084257E-14 ) ) ;
#91285=CARTESIAN_POINT ( 'NONE',  ( 10.71502147350184231, 11.39527989537399755, 0.000000000000000000 ) ) ;
#91287=VERTEX_POINT ( 'NONE', #39949 ) ;
#91289=CARTESIAN_POINT ( 'NONE',  ( -5.278201874421821316, 5.052323696447222900, 0.7998128361456341429 ) ) ;
#91291=CARTESIAN_POINT ( 'NONE',  ( -7.621654909176601045, 12.04368116068139472, 0.7998128361456481317 ) ) ;
#91294=CARTESIAN_POINT ( 'NONE',  ( -4.904330467487477918, 6.873893772473251396, -1.448588590679427801 ) ) ;
#91320=CARTESIAN_POINT ( 'NONE',  ( 4.555176424511575561, 4.416720038126027426, -0.7216878364870188411 ) ) ;
#91324=CARTESIAN_POINT ( 'NONE',  ( -9.429859533504656000, 10.96025652963230534, -1.199719254218441611 ) ) ;
#91327=CARTESIAN_POINT ( 'NONE',  ( 7.574201371528760163, 11.98831870009225931, 1.040834085586084257E-14 ) ) ;
#91336=CARTESIAN_POINT ( 'NONE',  ( -1.364683531250012516, 0.5302083336747518416, 0.7879004041258379498 ) ) ;
#91342=CARTESIAN_POINT ( 'NONE',  ( -3.415764635639130020, 6.072476943965863683, 1.199719254218462483 ) ) ;
#91344=CARTESIAN_POINT ( 'NONE',  ( -1.500000000000013101, -0.07916666666664513852, 0.8660254037844403729 ) ) ;
#91346=CARTESIAN_POINT ( 'NONE',  ( 1.499999999999991118, 5.754166666666685970, 0.8660254037844524744 ) ) ;
#91351=CARTESIAN_POINT ( 'NONE',  ( -1.364683531250000748, 0.2593750003414205252, 0.000000000000000000 ) ) ;
#91354=CARTESIAN_POINT ( 'NONE',  ( -5.689618019229208734, 9.789638122409414223, 0.7998128361456481317 ) ) ;
#91355=CARTESIAN_POINT ( 'NONE',  ( 7.730120138085914583, 12.17022392774227768, 0.7998128361456462443 ) ) ;
#91356=CARTESIAN_POINT ( 'NONE',  ( 5.301401758143367893, 6.143722458377430584, 1.199719254218462483 ) ) ;
#91361=CARTESIAN_POINT ( 'NONE',  ( -1.402160292154681736E-14, 0.009375000341421267647, -1.575800808251665908 ) ) ;
#91367=CARTESIAN_POINT ( 'NONE',  ( -1.500000000000051514, 3.702083334016151639, 0.8660254037844170583 ) ) ;
#91369=CARTESIAN_POINT ( 'NONE',  ( 6.968527767744109980, 7.232296605230681408, 0.7216878364870317197 ) ) ;
#91373=CARTESIAN_POINT ( 'NONE',  ( -5.742041750587549842, 6.657802449562273850, 1.199719254218450271 ) ) ;
#91375=CARTESIAN_POINT ( 'NONE',  ( 5.653386866774130937, 5.697965554099072349, -0.7216878364870402685 ) ) ;
#91378=CARTESIAN_POINT ( 'NONE',  ( 4.975479186090852046, 6.827811688571220117, 1.443375672974062551 ) ) ;
#91379=CARTESIAN_POINT ( 'NONE',  ( -8.148087131688692253, 10.52918762510205042, -1.443375672974058777 ) ) ;
#91381=CARTESIAN_POINT ( 'NONE',  ( -1.500000000000011324, 3.420833333333355597, 0.8660254037844403729 ) ) ;
#91385=CARTESIAN_POINT ( 'NONE',  ( 7.456621297836061757, 11.64321591421002644, 0.7216878364870438212 ) ) ;
#91391=ORIENTED_EDGE ( 'NONE', *, *, #54763, .F. ) ;
#91399=CARTESIAN_POINT ( 'NONE',  ( 7.741342523278686549, 11.97539067722642869, 0.7216878364870438212 ) ) ;
#91401=CARTESIAN_POINT ( 'NONE',  ( 7.618792255875527886, 10.97600916757510170, 1.199719254218460707 ) ) ;
#91404=CARTESIAN_POINT ( 'NONE',  ( 5.192409644353875642, 5.160158794608717514, 1.040834085586084257E-14 ) ) ;
#91405=CARTESIAN_POINT ( 'NONE',  ( 9.642873567817520808, 12.27310513391906532, 1.599625672291279388 ) ) ;
#91406=CARTESIAN_POINT ( 'NONE',  ( 5.070386261830877928, 5.978167395966564435, -1.082531754730548412 ) ) ;
#91408=CARTESIAN_POINT ( 'NONE',  ( -7.456621297836087514, 9.722477485607340597, 1.443375672974090751 ) ) ;
#91412=CARTESIAN_POINT ( 'NONE',  ( -2.442440228756222353, 6.001264033524212671, -0.7998128361456281477 ) ) ;
#91418=CARTESIAN_POINT ( 'NONE',  ( -3.023105066167323329, 5.702484939155337607, -2.420000000000000373 ) ) ;
#91432=CARTESIAN_POINT ( 'NONE',  ( 0.07278863622976063097, 7.008482404162149848, 2.000259058016622404 ) ) ;
#91436=CARTESIAN_POINT ( 'NONE',  ( -5.201524489137236529, 9.220195670635433771, 0.7998128361456481317 ) ) ;
#91440=CARTESIAN_POINT ( 'NONE',  ( 5.823390672269506574, 6.752709524857930745, -1.199719254218446718 ) ) ;
#91448=CARTESIAN_POINT ( 'NONE',  ( -3.567766978690493307, 7.314145241780881435, 1.040834085586084257E-14 ) ) ;
#91451=CARTESIAN_POINT ( 'NONE',  ( 7.949158136313996259, 8.168439335321471262, 1.040834085586084257E-14 ) ) ;
#91454=CARTESIAN_POINT ( 'NONE',  ( 5.975483201341563522, 6.103571115010600678, 0.6665044388154163224 ) ) ;
#91456=DIRECTION ( 'NONE',  ( -0.1674078377058430267, 0.000000000000000000, 0.9858877298529756805 ) ) ;
#91460=CARTESIAN_POINT ( 'NONE',  ( 6.114364089638786304, 8.156510742710487705, 1.443375672974076540 ) ) ;
#91461=CARTESIAN_POINT ( 'NONE',  ( -8.019811557683421910, 9.315200557840817908, 1.199719254218462483 ) ) ;
#91465=CARTESIAN_POINT ( 'NONE',  ( -7.483210719738908168, 10.81783070874899799, 1.199719254218453823 ) ) ;
#91466=CARTESIAN_POINT ( 'NONE',  ( -5.377780486114890124, 9.425827667109372143, 0.000000000000000000 ) ) ;
#91474=CARTESIAN_POINT ( 'NONE',  ( 7.751511138711133064, 10.06651563329490529, -1.599625672291262513 ) ) ;
#91480=CARTESIAN_POINT ( 'NONE',  ( 2.171277156482887882, 5.684907115872006145, -0.7998128361456291469 ) ) ;
#91488=CARTESIAN_POINT ( 'NONE',  ( -1.500000000000011324, 4.170833333333359150, 0.8660254037844403729 ) ) ;
#91489=CARTESIAN_POINT ( 'NONE',  ( 3.985207087413062066, 6.736826471035503694, -1.199719254218452047 ) ) ;
#91490=CARTESIAN_POINT ( 'NONE',  ( 7.305145839664861640, 7.417091655897478653, 0.7998128361456341429 ) ) ;
#91492=CARTESIAN_POINT ( 'NONE',  ( -9.056483424248693126, 10.62861408545402675, 1.082531754730558626 ) ) ;
#91494=CARTESIAN_POINT ( 'NONE',  ( 5.666945020832160118, 9.555260257705446847, 0.7216878364870438212 ) ) ;
#91495=CARTESIAN_POINT ( 'NONE',  ( -8.636180661780658241, 12.05899929117736846, -1.082531754730543083 ) ) ;
#91499=CARTESIAN_POINT ( 'NONE',  ( 8.269583629331492602, 11.73526576994040482, 1.199719254218450271 ) ) ;
#91504=CARTESIAN_POINT ( 'NONE',  ( -1.201851678989727383E-14, 1.071875000341418138, 1.575800808251672791 ) ) ;
#91510=CARTESIAN_POINT ( 'NONE',  ( 0.6823417656249882723, -0.4072916663252490466, 1.181850606188755259 ) ) ;
#91511=B_SPLINE_CURVE_WITH_KNOTS ( 'NONE', 3,
 ( #165489, #53885, #116801, #100490 ),
 .UNSPECIFIED., .F., .F.,
 ( 4, 4 ),
 ( 6.034005962831002237E-05, 0.0001895969026200594165 ),
 .UNSPECIFIED. ) ;
#91513=CARTESIAN_POINT ( 'NONE',  ( 9.398826802771546696, 11.98838390803207865, -1.599625672291262513 ) ) ;
#91517=CARTESIAN_POINT ( 'NONE',  ( -10.66756793585402363, 11.33991743478486391, 0.7998128361456462443 ) ) ;
#91524=CARTESIAN_POINT ( 'NONE',  ( 4.005544317833563461, 6.760553239859419250, -1.199719254218452047 ) ) ;
#91527=CARTESIAN_POINT ( 'NONE',  ( -2.589244150085650009, 5.964609241834465614, 0.7216878364870317197 ) ) ;
#91531=CARTESIAN_POINT ( 'NONE',  ( 8.772289083241844310, 10.19309100432570148, -1.199719254218446718 ) ) ;
#91533=CARTESIAN_POINT ( 'NONE',  ( 4.318426605249491068, 7.201576024430431211, 1.005918518748824875 ) ) ;
#91534=CARTESIAN_POINT ( 'NONE',  ( -4.386226389220933441, 5.076017861301227008, -1.199719254218446718 ) ) ;
#91538=CARTESIAN_POINT ( 'NONE',  ( 7.507464373665139412, 9.781794407407920389, 1.599625672291281386 ) ) ;
#91540=CARTESIAN_POINT ( 'NONE',  ( 6.103141704446003679, 10.27208242182903142, 0.7998128361456462443 ) ) ;
#91543=CARTESIAN_POINT ( 'NONE',  ( -9.815740026613967828, 10.55404424057886636, -0.7216878364870267237 ) ) ;
#91551=CARTESIAN_POINT ( 'NONE',  ( -4.981332701451811396, 6.629279788159643694, -1.242877772926734625 ) ) ;
#91552=CARTESIAN_POINT ( 'NONE',  ( -1.201851678989727383E-14, 2.321875000341416584, 1.575800808251672791 ) ) ;
#91554=CARTESIAN_POINT ( 'NONE',  ( 5.504247177468175600, 8.405076892812779477, 1.082531754730558626 ) ) ;
#91576=CARTESIAN_POINT ( 'NONE',  ( 7.747594715205354809, 11.12627870345989756, -1.199719254218446718 ) ) ;
#91580=CARTESIAN_POINT ( 'NONE',  ( -4.810445574750349174, 4.506608013497163334, 0.7998128361456341429 ) ) ;
#91581=CARTESIAN_POINT ( 'NONE',  ( -6.856673000209188906, 9.022537805042615489, 1.599625672291283607 ) ) ;
#91583=ORIENTED_EDGE ( 'NONE', *, *, #26877, .F. ) ;
#91584=CARTESIAN_POINT ( 'NONE',  ( -9.110189153378817295, 12.71597221466224603, 1.199719254218462483 ) ) ;
#91588=CARTESIAN_POINT ( 'NONE',  ( -0.7499999999999972244, 4.139583334016149863, -1.299038105676652899 ) ) ;
#91589=CARTESIAN_POINT ( 'NONE',  ( 8.599949509769960088, 8.927695937686774386, 1.040834085586084257E-14 ) ) ;
#91592=CARTESIAN_POINT ( 'NONE',  ( -7.015454420067433361, 10.27211502579893754, 1.199719254218453823 ) ) ;
#91594=CARTESIAN_POINT ( 'NONE',  ( -0.6823417656250212460, 5.051041667008086655, 1.181850606188767472 ) ) ;
#91596=CARTESIAN_POINT ( 'NONE',  ( -1.534012367094089946, 8.737164261768347373, 2.508166476568440828 ) ) ;
#91598=EDGE_CURVE ( 'NONE', #116549, #188383, #50235, .T. ) ;
#91601=CARTESIAN_POINT ( 'NONE',  ( -7.348156068926747331, 11.51667314714914347, 0.7216878364870458196 ) ) ;
#91606=CARTESIAN_POINT ( 'NONE',  ( 0.6823417656249899377, 3.155208333674754062, 1.181850606188765695 ) ) ;
#91612=CARTESIAN_POINT ( 'NONE',  ( -0.6823417656249969321, 4.717708333674755394, -1.181850606188749264 ) ) ;
#91614=CARTESIAN_POINT ( 'NONE',  ( -4.786191920824102830, 5.542644314838231168, 1.199719254218462483 ) ) ;
#91615=CARTESIAN_POINT ( 'NONE',  ( 4.964256800898067645, 8.943383367689749619, 0.7998128361456462443 ) ) ;
#91618=CARTESIAN_POINT ( 'NONE',  ( -1.201851678989727383E-14, 4.134375000341417028, 1.575800808251672791 ) ) ;
#91623=CARTESIAN_POINT ( 'NONE',  ( -1.364683531250014514, 0.2802083336747505649, 0.7879004041258379498 ) ) ;
#91624=CARTESIAN_POINT ( 'NONE',  ( -5.450014563013544588, 5.460697866378308341, 0.7216878364870317197 ) ) ;
#91625=CARTESIAN_POINT ( 'NONE',  ( 5.497994985541524215, 6.373081223675282736, -1.199719254218445830 ) ) ;
#91629=CARTESIAN_POINT ( 'NONE',  ( 5.192409644353875642, 5.160158794608717514, 1.040834085586084257E-14 ) ) ;
#91632=CARTESIAN_POINT ( 'NONE',  ( -8.188761592974040937, 11.53701037756964887, -1.082531754730543971 ) ) ;
#91637=CARTESIAN_POINT ( 'NONE',  ( -10.48453286206953727, 11.12637651536962125, 0.7998128361456462443 ) ) ;
#91638=CARTESIAN_POINT ( 'NONE',  ( -5.761852095683518193, 6.784877535461274256, 1.082531754730546636 ) ) ;
#91640=CARTESIAN_POINT ( 'NONE',  ( 1.364683531249988757, 0.4468750003414206917, 0.000000000000000000 ) ) ;
#91652=CARTESIAN_POINT ( 'NONE',  ( 6.914295152845067349, 11.01050207838719075, 1.040834085586084257E-14 ) ) ;
#91658=ORIENTED_EDGE ( 'NONE', *, *, #115804, .F. ) ;
#91661=CARTESIAN_POINT ( 'NONE',  ( 2.842405760359353106, 6.467890487061221272, -0.7998128361456291469 ) ) ;
#91666=CARTESIAN_POINT ( 'NONE',  ( 1.177073619093309986, 3.199321498342246883, 0.7750000000000135669 ) ) ;
#91668=CARTESIAN_POINT ( 'NONE',  ( 0.6823417656249882723, 1.988541667008083991, -1.181850606188749264 ) ) ;
#91669=CARTESIAN_POINT ( 'NONE',  ( 6.471393748265543699, 5.229711127717882491, 2.420000000000010587 ) ) ;
#91678=VECTOR ( 'NONE', #94276, 1000.000000000000000 ) ;
#91680=VERTEX_POINT ( 'NONE', #98286 ) ;
#91687=CARTESIAN_POINT ( 'NONE',  ( 5.900823170445728572, 7.907379670318584353, 1.599625672291267398 ) ) ;
#91694=CARTESIAN_POINT ( 'NONE',  ( 7.446452682403650769, 9.710614100936176385, -1.599625672291262513 ) ) ;
#91695=CARTESIAN_POINT ( 'NONE',  ( -5.956409969451652131, 6.075908546082715134, -0.6293437877468227581 ) ) ;
#91697=CARTESIAN_POINT ( 'NONE',  ( 8.748035429315576650, 11.22912730566677553, -1.599625672291255185 ) ) ;
#91700=CARTESIAN_POINT ( 'NONE',  ( 1.503277409322719471, 8.660639097433820766, -2.556074651073448667 ) ) ;
#91711=CARTESIAN_POINT ( 'NONE',  ( -8.676855123066022912, 10.18571440074093282, -1.082531754730543971 ) ) ;
#91716=CARTESIAN_POINT ( 'NONE',  ( -10.62011439820619429, 11.28455497419572318, -0.7998128361456221525 ) ) ;
#91723=CARTESIAN_POINT ( 'NONE',  ( 3.294268137996273715, 5.826768013428865522, -1.082531754730543971 ) ) ;
#91726=EDGE_LOOP ( 'NONE', ( #169700, #6110, #208651, #94626 ) ) ;
#91731=CARTESIAN_POINT ( 'NONE',  ( -4.869349725602420520, 8.832658446511480577, 1.040834085586084257E-14 ) ) ;
#91732=CARTESIAN_POINT ( 'NONE',  ( -3.954497087797542942, 7.557404335831681585, -0.5023533386407119661 ) ) ;
#91733=CARTESIAN_POINT ( 'NONE',  ( -2.123823618835070537, 5.629544655282869847, 1.040834085586084257E-14 ) ) ;
#91739=ORIENTED_EDGE ( 'NONE', *, *, #41655, .F. ) ;
#91740=CARTESIAN_POINT ( 'NONE',  ( 1.364683531249990311, 4.696875000341417916, 1.214306433183764966E-14 ) ) ;
#91742=CARTESIAN_POINT ( 'NONE',  ( 5.769158057814842699, 6.689438141327490150, 1.199719254218462483 ) ) ;
#91744=CARTESIAN_POINT ( 'NONE',  ( 1.525860493984659172, 8.693043820721578996, 2.521102513734321260 ) ) ;
#91755=CARTESIAN_POINT ( 'NONE',  ( 0.6823417656249882723, 0.7385416670080829915, -1.181850606188749264 ) ) ;
#91757=CARTESIAN_POINT ( 'NONE',  ( 4.054051625686104998, 4.688480637177271149, -1.199719254218446718 ) ) ;
#91759=CARTESIAN_POINT ( 'NONE',  ( -5.070386261830872598, 8.859275038870594088, 0.7216878364870458196 ) ) ;
#91760=CARTESIAN_POINT ( 'NONE',  ( 2.575685996916329046, 5.948791396470269888, 0.7216878364870438212 ) ) ;
#91761=CARTESIAN_POINT ( 'NONE',  ( -6.873620692004104527, 7.121571683533994168, 0.7216878364870317197 ) ) ;
#91765=CARTESIAN_POINT ( 'NONE',  ( 5.666418135507635512, 8.698239360479199433, 1.199719254218462483 ) ) ;
#91773=CARTESIAN_POINT ( 'NONE',  ( 5.309989718046547402, 9.346738437696316737, 0.7998128361456462443 ) ) ;
#91776=CARTESIAN_POINT ( 'NONE',  ( -6.901263884555985051, 8.010228272525461435, 1.199719254218450271 ) ) ;
#91780=CARTESIAN_POINT ( 'NONE',  ( 7.727257484784855635, 11.10255193463598111, -1.199719254218446718 ) ) ;
#91783=CARTESIAN_POINT ( 'NONE',  ( -7.660520486921249983, 8.896027641951645748, -1.199719254218446718 ) ) ;
#91786=CARTESIAN_POINT ( 'NONE',  ( 6.100805936025112786, 10.06143132543056673, 1.040834085586084257E-14 ) ) ;
#91787=CARTESIAN_POINT ( 'NONE',  ( 4.019508774049570299, 7.801013956325979493, 0.3192432753683968061 ) ) ;
#91788=CARTESIAN_POINT ( 'NONE',  ( -5.786632634934295361, 5.645492917045106473, 0.7998128361456341429 ) ) ;
#91795=CARTESIAN_POINT ( 'NONE',  ( 8.809047120577066181, 11.30030761213851953, 1.599625672291281386 ) ) ;
#91796=CARTESIAN_POINT ( 'NONE',  ( -5.227141986104622440, 6.445127484965264664, 1.169998774669118946 ) ) ;
#91797=CARTESIAN_POINT ( 'NONE',  ( -3.939296163840085629, 2.811845806437647699, -0.7749999999960115460 ) ) ;
#91798=CARTESIAN_POINT ( 'NONE',  ( 1.364683531249986537, 0.6552083336747522857, -0.7879004041258239610 ) ) ;
#91800=CARTESIAN_POINT ( 'NONE',  ( -4.609409038966229666, 8.321468278861834378, -0.7216878364870267237 ) ) ;
#91801=ORIENTED_EDGE ( 'NONE', *, *, #202366, .F. ) ;
#91807=CARTESIAN_POINT ( 'NONE',  ( -5.826669560333386677, 6.051347404617407832, -0.4878656478981869826 ) ) ;
#91808=CARTESIAN_POINT ( 'NONE',  ( -0.6823417656250003738, 1.530208333674752730, -1.181850606188749264 ) ) ;
#91811=CARTESIAN_POINT ( 'NONE',  ( 4.541618270897912701, 4.400902192243413502, 1.214306433183764966E-14 ) ) ;
#91816=CARTESIAN_POINT ( 'NONE',  ( -9.124274191872645545, 9.747334100047323702, -0.7216878364870267237 ) ) ;
#91824=CARTESIAN_POINT ( 'NONE',  ( -6.846504384776750385, 10.93141284897413890, -0.7216878364870267237 ) ) ;
#91830=CARTESIAN_POINT ( 'NONE',  ( -7.551528372687420720, 8.872833191965849409, 1.082531754730558626 ) ) ;
#91834=( BOUNDED_CURVE ( )  B_SPLINE_CURVE ( 2, ( #195577, #94891, #162018, #163085, #144731, #30956, #66588 ),
 .UNSPECIFIED., .F., .T. ) 
 B_SPLINE_CURVE_WITH_KNOTS ( ( 3, 2, 2, 3 ),
 ( 0.2857142857142859760, 0.2916666666666668517, 0.2976190476190477274, 0.3035714285714285476 ),
 .UNSPECIFIED. ) 
 CURVE ( )  GEOMETRIC_REPRESENTATION_ITEM ( )  RATIONAL_B_SPLINE_CURVE ( ( 0.9999999999999937828, 0.8660254037844449249, 1.000000000000000000, 0.8660254037844387076, 1.000000000000000000, 0.8660254037844387076, 1.000000000000000000 ) ) 
 REPRESENTATION_ITEM ( '' )  );
#91836=CARTESIAN_POINT ( 'NONE',  ( -1.500000000000011324, 4.910416667349486453, -0.8660254037844313801 ) ) ;
#91844=CARTESIAN_POINT ( 'NONE',  ( -6.073162743917628781, 9.172774736957510555, -1.199719254218440723 ) ) ;
#91848=CARTESIAN_POINT ( 'NONE',  ( 5.996784015946103885, 5.890669528225568996, 1.040834085586084257E-14 ) ) ;
#91852=CARTESIAN_POINT ( 'NONE',  ( 8.281332899848809603, 8.555976559445431562, 0.7998128361456481317 ) ) ;
#91861=CARTESIAN_POINT ( 'NONE',  ( -4.758548728716557541, 8.495464583570553785, 1.040834085586084257E-14 ) ) ;
#91871=CARTESIAN_POINT ( 'NONE',  ( -8.850775351622791831, 9.220326086515070685, -0.7998128361456291469 ) ) ;
#91873=CARTESIAN_POINT ( 'NONE',  ( 7.958799866421889746, 9.244020251369077457, -1.199719254218441611 ) ) ;
#91874=CARTESIAN_POINT ( 'NONE',  ( 1.499999999999987566, 0.02500000000001806333, 0.000000000000000000 ) ) ;
#91875=CARTESIAN_POINT ( 'NONE',  ( -7.015454420067433361, 10.27211502579893754, 1.199719254218453823 ) ) ;
#91878=CARTESIAN_POINT ( 'NONE',  ( -0.6823417656250212460, 5.301041667008086655, 1.181850606188767472 ) ) ;
#91880=CARTESIAN_POINT ( 'NONE',  ( 9.246297574839974942, 11.81043314211192019, 1.443375672974076540 ) ) ;
#91883=CARTESIAN_POINT ( 'NONE',  ( -1.500000000000011324, 4.629166666666689522, -0.8660254037844313801 ) ) ;
#91886=CARTESIAN_POINT ( 'NONE',  ( 8.934460041281305109, 10.48625347199211966, -1.082531754730543083 ) ) ;
#91888=CARTESIAN_POINT ( 'NONE',  ( 3.331659036430331344, 7.719744385808881226, 2.450696915730453007 ) ) ;
#91889=CARTESIAN_POINT ( 'NONE',  ( -5.260200412422196159, 9.080724881227137502, -0.7216878364870207285 ) ) ;
#91891=CARTESIAN_POINT ( 'NONE',  ( -1.402160292154681736E-14, 1.446875000341420137, -1.575800808251659024 ) ) ;
#91895=CARTESIAN_POINT ( 'NONE',  ( -5.696397096036042385, 9.797547045350714967, -0.7998128361456231517 ) ) ;
#91896=CARTESIAN_POINT ( 'NONE',  ( -1.364683531249997417, 4.821875000341417916, 1.214306433183764966E-14 ) ) ;
#91901=CARTESIAN_POINT ( 'NONE',  ( 10.07100917685271035, 10.64393221595000938, 0.7998128361456462443 ) ) ;
#91904=CARTESIAN_POINT ( 'NONE',  ( -1.500000000000001332, 1.150000000000019007, 0.000000000000000000 ) ) ;
#91909=CARTESIAN_POINT ( 'NONE',  ( 5.639828713604826405, 9.523624565940227882, -0.7216878364870267237 ) ) ;
#91916=CARTESIAN_POINT ( 'NONE',  ( 9.250740883225924804, 9.686952540052077509, 1.040834085586084257E-14 ) ) ;
#91917=CARTESIAN_POINT ( 'NONE',  ( -9.130526383799315582, 12.73969898348616070, 1.199719254218462483 ) ) ;
#91920=CARTESIAN_POINT ( 'NONE',  ( 1.364683531249988535, 5.467708333674750953, -0.7879004041258300672 ) ) ;
#91925=CARTESIAN_POINT ( 'NONE',  ( -4.944471571578556102, 4.870897709704155254, -0.2071306710573853627 ) ) ;
#91927=CARTESIAN_POINT ( 'NONE',  ( 0.6823417656249917140, 4.342708333674755394, 1.181850606188765695 ) ) ;
#91929=CARTESIAN_POINT ( 'NONE',  ( -5.070386261830872598, 8.859275038870594088, 0.7216878364870458196 ) ) ;
#91931=CARTESIAN_POINT ( 'NONE',  ( 0.7499999999999920064, 5.014583334016150751, 1.299038105676669330 ) ) ;
#91937=ORIENTED_EDGE ( 'NONE', *, *, #193834, .F. ) ;
#91938=CARTESIAN_POINT ( 'NONE',  ( 7.618792255875527886, 10.97600916757510170, 1.199719254218460707 ) ) ;
#91939=CARTESIAN_POINT ( 'NONE',  ( 3.289951133708762576, 7.658661826346122581, -2.499999999999995115 ) ) ;
#91943=CARTESIAN_POINT ( 'NONE',  ( -7.472515219426274946, 11.86968485597268064, 0.000000000000000000 ) ) ;
#91944=CARTESIAN_POINT ( 'NONE',  ( 6.979750152936881058, 7.037463354714830643, 0.7998128361456341429 ) ) ;
#91946=ADVANCED_FACE ( 'NONE', ( #183786 ), #200021, .T. ) ;
#91947=CARTESIAN_POINT ( 'NONE',  ( -2.081668171172168513E-14, 5.868705557303649734, 4.125226524755077229 ) ) ;
#91948=CARTESIAN_POINT ( 'NONE',  ( 5.359550796103802028, 5.147230771742885125, -0.7998128361456231517 ) ) ;
#91949=EDGE_LOOP ( 'NONE', ( #175323, #179358, #74871, #110229 ) ) ;
#91954=CARTESIAN_POINT ( 'NONE',  ( 3.146123468421266001, 6.442327133617253843, 0.5169845646841256803 ) ) ;
#91956=CARTESIAN_POINT ( 'NONE',  ( -6.087247782855839340, 6.204136622861004646, 0.000000000000000000 ) ) ;
#91958=CARTESIAN_POINT ( 'NONE',  ( 3.011882680530176604, 6.665613560593854459, 0.7998128361456341429 ) ) ;
#91962=CARTESIAN_POINT ( 'NONE',  ( -6.482770005628665011, 10.71498210654212002, 0.7998128361456481317 ) ) ;
#91967=CARTESIAN_POINT ( 'NONE',  ( -7.483210719738908168, 10.81783070874899799, 1.199719254218453823 ) ) ;
#91971=CARTESIAN_POINT ( 'NONE',  ( 7.283754839039659146, 9.520799950344851936, -1.599625672291262513 ) ) ;
#91972=CARTESIAN_POINT ( 'NONE',  ( 3.988069740714122791, 7.804498464141805592, 0.7998128361456321445 ) ) ;
#91984=CARTESIAN_POINT ( 'NONE',  ( -7.588813295347149435, 9.876701482703580837, -1.599625672291263179 ) ) ;
#91987=CARTESIAN_POINT ( 'NONE',  ( 6.399085315970131305, 8.488685506763726352, -1.443375672974057666 ) ) ;
#91992=CARTESIAN_POINT ( 'NONE',  ( -6.033542053281340856, 6.997886136038390603, -1.199719254218446718 ) ) ;
#92000=PLANE ( 'NONE',  #127094 ) ;
#92002=CARTESIAN_POINT ( 'NONE',  ( 6.903072767652295383, 11.20533532890304684, 1.040834085586084257E-14 ) ) ;
#92004=CARTESIAN_POINT ( 'NONE',  ( -2.304522924643024773, 5.632434478818063361, 0.7216878364870317197 ) ) ;
#92007=VECTOR ( 'NONE', #204012, 1000.000000000000000 ) ;
#92008=CARTESIAN_POINT ( 'NONE',  ( -5.402149754905330781, 6.322992007072439691, -1.066970298751448443 ) ) ;
#92015=CARTESIAN_POINT ( 'NONE',  ( 10.05978679165993483, 11.79913468076720306, 1.082531754730548412 ) ) ;
#92034=CARTESIAN_POINT ( 'NONE',  ( -2.761056838677368397, 6.372983411765559048, 0.7998128361456341429 ) ) ;
#92036=CARTESIAN_POINT ( 'NONE',  ( 3.972175818679561043, 7.578029521860726092, -0.7216878364870197293 ) ) ;
#92037=CARTESIAN_POINT ( 'NONE',  ( -0.7500000000000215383, 3.941666666666690411, 1.299038105676671107 ) ) ;
#92039=CARTESIAN_POINT ( 'NONE',  ( -2.462777459176719308, 6.024990802348131780, -0.7998128361456281477 ) ) ;
#92043=CARTESIAN_POINT ( 'NONE',  ( -0.6823417656250212460, 4.551041667008086655, 1.181850606188767472 ) ) ;
#92051=CARTESIAN_POINT ( 'NONE',  ( 4.891794496432329886, 4.601515088792824670, -0.7998128361456211532 ) ) ;
#92057=CARTESIAN_POINT ( 'NONE',  ( -0.6823417656250212460, 1.613541667008083769, 1.181850606188755259 ) ) ;
#92059=CARTESIAN_POINT ( 'NONE',  ( -7.486073373039941359, 11.88550270185529278, -0.7998128361456291469 ) ) ;
#92060=CARTESIAN_POINT ( 'NONE',  ( -4.731432421044873493, 7.503459676985569260, -1.082531754730548412 ) ) ;
#92064=CARTESIAN_POINT ( 'NONE',  ( -0.6823417656250212460, 5.551041667008087543, 1.181850606188767472 ) ) ;
#92072=CARTESIAN_POINT ( 'NONE',  ( -5.436456408955534947, 6.405249234278626247, 1.082531754730546636 ) ) ;
#92074=EDGE_CURVE ( 'NONE', #158436, #160642, #118853, .T. ) ;
#92078=CARTESIAN_POINT ( 'NONE',  ( -5.382223794500845315, 6.341977850748185652, -1.082531754730543971 ) ) ;
#92080=CARTESIAN_POINT ( 'NONE',  ( 8.048736748007069508, 12.54194330598362406, -0.7998128361456352531 ) ) ;
#92091=CARTESIAN_POINT ( 'NONE',  ( -4.223528545856940042, 4.886203710709899006, -1.199719254218446718 ) ) ;
#92095=ORIENTED_EDGE ( 'NONE', *, *, #171975, .T. ) ;
#92097=CARTESIAN_POINT ( 'NONE',  ( 7.944714827928033962, 12.21265836598400689, 0.7216878364870438212 ) ) ;
#92098=CARTESIAN_POINT ( 'NONE',  ( 5.147291874682557555, 9.156924287104992288, 0.7998128361456462443 ) ) ;
#92103=CARTESIAN_POINT ( 'NONE',  ( 3.194917754314666514, 6.879154480009089134, 0.7998128361456321445 ) ) ;
#92112=CARTESIAN_POINT ( 'NONE',  ( 7.560643217915098191, 11.97250085420964716, -0.7998128361456291469 ) ) ;
#92113=CARTESIAN_POINT ( 'NONE',  ( -5.065942953000576843, 9.062017211809330064, -0.7998128361456231517 ) ) ;
#92116=ORIENTED_EDGE ( 'NONE', *, *, #115314, .F. ) ;
#92122=CARTESIAN_POINT ( 'NONE',  ( -1.364683531250012516, 4.988541667008084879, -0.7879004041258300672 ) ) ;
#92123=CARTESIAN_POINT ( 'NONE',  ( 7.578644679914694926, 11.78557652663510424, 0.7216878364870438212 ) ) ;
#92124=CARTESIAN_POINT ( 'NONE',  ( -5.982172092127739482, 8.002286745614243912, -1.599625672291263179 ) ) ;
#92127=CARTESIAN_POINT ( 'NONE',  ( 6.003563092752934871, 5.898578451166879510, 0.7998128361456341429 ) ) ;
#92128=CARTESIAN_POINT ( 'NONE',  ( -6.749261541504576911, 6.768559974710451677, 1.040834085586084257E-14 ) ) ;
#92133=CARTESIAN_POINT ( 'NONE',  ( 6.236387472606139681, 8.298871356172400127, -1.443375672974057666 ) ) ;
#92135=CARTESIAN_POINT ( 'NONE',  ( 7.307481607641395094, 8.588111966078864512, -1.082531754730537976 ) ) ;
#92136=CARTESIAN_POINT ( 'NONE',  ( -0.6823417656250003738, 1.530208333674752730, -1.181850606188749264 ) ) ;
#92138=CARTESIAN_POINT ( 'NONE',  ( 5.300874872818828187, 8.167809204055208383, 1.082531754730558626 ) ) ;
#92142=CARTESIAN_POINT ( 'NONE',  ( -2.318081078256692518, 5.648252324700675508, 1.040834085586084257E-14 ) ) ;
#92144=CARTESIAN_POINT ( 'NONE',  ( 1.364683531249988535, 5.405208333674750953, -0.7879004041258300672 ) ) ;
#92149=EDGE_CURVE ( 'NONE', #207276, #8852, #68944, .T. ) ;
#92150=CARTESIAN_POINT ( 'NONE',  ( -4.023696502211203452, 7.783621949832661535, -0.4819376843918365960 ) ) ;
#92157=CARTESIAN_POINT ( 'NONE',  ( 5.198661835836162481, 8.152523677529138979, 1.199719254218462483 ) ) ;
#92169=CARTESIAN_POINT ( 'NONE',  ( 4.690757960648231695, 5.535267711253469614, 1.082531754730560403 ) ) ;
#92171=CARTESIAN_POINT ( 'NONE',  ( -1.364683531250000748, 2.321875000341422357, 1.214306433183764966E-14 ) ) ;
#92173=CARTESIAN_POINT ( 'NONE',  ( 8.046927864910717432, 9.346836249606042202, 1.199719254218462483 ) ) ;
#92175=CARTESIAN_POINT ( 'NONE',  ( -3.511198596259295535, 6.271927390929313617, -1.000000000000001776 ) ) ;
#92180=CARTESIAN_POINT ( 'NONE',  ( -1.500000000000011324, 3.170833333333354265, 0.8660254037844403729 ) ) ;
#92181=CARTESIAN_POINT ( 'NONE',  ( 5.636439174979242850, 7.598931675607687453, -1.599625672291262513 ) ) ;
#92182=CARTESIAN_POINT ( 'NONE',  ( -6.201965203247477909, 9.323044272842313518, 1.199719254218452047 ) ) ;
#92186=CARTESIAN_POINT ( 'NONE',  ( -1.364683531250012516, 2.488541667008088876, -0.7879004041258289570 ) ) ;
#92189=EDGE_CURVE ( 'NONE', #17090, #93714, #57803, .T. ) ;
#92191=CARTESIAN_POINT ( 'NONE',  ( 10.08690309888728187, 10.87040115823107911, -0.7216878364870257245 ) ) ;
#92194=FACE_OUTER_BOUND ( 'NONE', #68205, .T. ) ;
#92196=CARTESIAN_POINT ( 'NONE',  ( -3.741687207691642314, 6.348756928073427730, 1.082531754730560403 ) ) ;
#92197=CARTESIAN_POINT ( 'NONE',  ( 1.499999999999989120, 2.035416667349480679, 0.8660254037844524744 ) ) ;
#92200=CARTESIAN_POINT ( 'NONE',  ( -4.771579997005698459, 7.654261532226910525, -1.199719254218452047 ) ) ;
#92201=CARTESIAN_POINT ( 'NONE',  ( -3.145128448690323264, 4.692402494937224056, -1.443375672974059665 ) ) ;
#92208=CARTESIAN_POINT ( 'NONE',  ( 5.986088515633498197, 6.942523675449257858, -1.199719254218446718 ) ) ;
#92211=CARTESIAN_POINT ( 'NONE',  ( -5.761852096127856981, 5.824508321678349532, 0.000000000000000000 ) ) ;
#92212=CARTESIAN_POINT ( 'NONE',  ( 5.087333953625774008, 6.958308917361963886, 1.599625672291267398 ) ) ;
#92214=VERTEX_POINT ( 'NONE', #151304 ) ;
#92216=ORIENTED_EDGE ( 'NONE', *, *, #183234, .T. ) ;
#92217=CARTESIAN_POINT ( 'NONE',  ( 4.379447312414087357, 5.068108938359919158, -1.199719254218452047 ) ) ;
#92220=CARTESIAN_POINT ( 'NONE',  ( -4.816538118508267630, 5.092449105792602460, -0.9495590845017554127 ) ) ;
#92221=CARTESIAN_POINT ( 'NONE',  ( 5.790052644182137165, 6.039355072771209088, 0.5314338945540015846 ) ) ;
#92227=SPHERICAL_SURFACE ( 'NONE', #112618, 0.08000000000000000167 ) ;
#92232=CARTESIAN_POINT ( 'NONE',  ( 5.829642864196151741, 9.745074408296771296, 0.7216878364870438212 ) ) ;
#92235=CARTESIAN_POINT ( 'NONE',  ( -5.253948220495577637, 6.088359997788290734, 1.199719254218450271 ) ) ;
#92238=CARTESIAN_POINT ( 'NONE',  ( 6.934105498385400246, 10.17720795050327354, -1.199719254218441611 ) ) ;
#92240=CARTESIAN_POINT ( 'NONE',  ( -5.850506979496850057, 6.784345216623154151, -1.199719254218446718 ) ) ;
#92250=VERTEX_POINT ( 'NONE', #89519 ) ;
#92256=CARTESIAN_POINT ( 'NONE',  ( 4.048135823549415591, 3.984990093095080788, -0.7783338591275772433 ) ) ;
#92257=CARTESIAN_POINT ( 'NONE',  ( -4.391951695823077984, 7.211361847513815704, 1.199719254218464037 ) ) ;
#92260=CARTESIAN_POINT ( 'NONE',  ( 4.365362273920250225, 5.155639410070820716, 1.082531754730560403 ) ) ;
#92266=CARTESIAN_POINT ( 'NONE',  ( -3.684065054611367351, 5.321161868511784299, -1.599625672291256295 ) ) ;
#92269=CARTESIAN_POINT ( 'NONE',  ( 8.646349277213076334, 11.11049346154719508, 1.599625672291281386 ) ) ;
#92273=CARTESIAN_POINT ( 'NONE',  ( -6.340409392685171674, 10.54889472477470846, 0.7998128361456481317 ) ) ;
#92274=CARTESIAN_POINT ( 'NONE',  ( 3.960953433486789521, 7.772862772376584850, -0.7998128361456221525 ) ) ;
#92278=CARTESIAN_POINT ( 'NONE',  ( 4.062132091735995765, 3.841501649887839598, -0.4581612399152183990 ) ) ;
#92281=CARTESIAN_POINT ( 'NONE',  ( -1.201851678989727383E-14, 3.259375000341420581, -1.575800808251660134 ) ) ;
#92284=CARTESIAN_POINT ( 'NONE',  ( 6.534666852106798096, 7.686494751288491578, -1.082531754730543083 ) ) ;
#92292=CARTESIAN_POINT ( 'NONE',  ( 10.18181017373857600, 10.98112607889092907, 0.7216878364870438212 ) ) ;
#92297=CARTESIAN_POINT ( 'NONE',  ( -8.992082194361570302, 11.51384853155376220, 1.599625672291269396 ) ) ;
#92317=CARTESIAN_POINT ( 'NONE',  ( 1.499999999999987121, 1.327083334016149641, -0.8660254037844253849 ) ) ;
#92322=CARTESIAN_POINT ( 'NONE',  ( -1.500000000000013101, 0.1708333333333560411, 0.8660254037844403729 ) ) ;
#92323=CARTESIAN_POINT ( 'NONE',  ( 7.721532178182734185, 8.967207948423393304, 1.199719254218462483 ) ) ;
#92324=CARTESIAN_POINT ( 'NONE',  ( 0.6823417656249864960, -0.8239583329919114574, -1.181850606188749264 ) ) ;
#92328=CARTESIAN_POINT ( 'NONE',  ( 9.897088948295943212, 11.60932053017587506, 1.082531754730548412 ) ) ;
#92329=CARTESIAN_POINT ( 'NONE',  ( -4.582292731738899505, 8.289832587096611860, 0.7216878364870458196 ) ) ;
#92333=CARTESIAN_POINT ( 'NONE',  ( -7.230575994789712801, 7.330093503543126054, 0.7998128361456341429 ) ) ;
#92335=CARTESIAN_POINT ( 'NONE',  ( -1.402160292154681736E-14, 2.368750000682818602, -1.732050807568863648 ) ) ;
#92347=DIRECTION ( 'NONE',  ( 0.000000000000000000, 0.000000000000000000, -1.000000000000000000 ) ) ;
#92348=CARTESIAN_POINT ( 'NONE',  ( -9.840520565420403543, 10.37502883594562597, 1.040834085586084257E-14 ) ) ;
#92349=CARTESIAN_POINT ( 'NONE',  ( 7.820355676984174664, 8.018169799436671852, -0.7998128361456281477 ) ) ;
#92356=CARTESIAN_POINT ( 'NONE',  ( -8.158255747121117452, 10.54105100977322174, 1.599625672291295375 ) ) ;
#92359=EDGE_CURVE ( 'NONE', #32719, #111607, #123170, .T. ) ;
#92363=CARTESIAN_POINT ( 'NONE',  ( 10.16199982864259788, 11.81442020729326536, 1.199719254218452047 ) ) ;
#92367=CARTESIAN_POINT ( 'NONE',  ( -7.458957065812611198, 11.85386701009007204, 0.7998128361456481317 ) ) ;
#92376=CARTESIAN_POINT ( 'NONE',  ( 6.307567778855705853, 8.381915046796901692, -1.599625672291262513 ) ) ;
#92395=CARTESIAN_POINT ( 'NONE',  ( 3.497640442645619796, 6.064035702186436616, -1.082531754730543083 ) ) ;
#92400=CARTESIAN_POINT ( 'NONE',  ( -9.297140650669053485, 11.86975006391249643, 1.599625672291281386 ) ) ;
#92402=CARTESIAN_POINT ( 'NONE',  ( 2.535011535630975477, 5.901337858304024131, 0.7216878364870438212 ) ) ;
#92404=VECTOR ( 'NONE', #173295, 1000.000000000000000 ) ;
#92406=CARTESIAN_POINT ( 'NONE',  ( -0.1021852871539799257, 7.117056311352818909, -3.989408415137027042 ) ) ;
#92410=CARTESIAN_POINT ( 'NONE',  ( 3.468329555040600365, 6.306621445965236106, 1.127812995945943086 ) ) ;
#92411=CARTESIAN_POINT ( 'NONE',  ( -1.402160292154681736E-14, 0.5718750003414239114, 1.575800808251672791 ) ) ;
#92416=CARTESIAN_POINT ( 'NONE',  ( -4.925689880466507908, 4.641059703499347044, -0.7998128361456221525 ) ) ;
#92417=DIRECTION ( 'NONE',  ( 0.7592566023653004592, -0.6507913734559639396, -0.000000000000000000 ) ) ;
#92419=CARTESIAN_POINT ( 'NONE',  ( -1.500000000000001332, -0.3499999999999753308, 0.000000000000000000 ) ) ;
#92421=CARTESIAN_POINT ( 'NONE',  ( -0.7500000000000215383, 5.441666666666685082, 1.299038105676671107 ) ) ;
#92426=CARTESIAN_POINT ( 'NONE',  ( -1.402160292154681736E-14, -0.4281249996585808071, 1.575800808251672791 ) ) ;
#92428=CARTESIAN_POINT ( 'NONE',  ( -8.213542131780492639, 8.476887330032372603, 1.040834085586084257E-14 ) ) ;
#92429=CARTESIAN_POINT ( 'NONE',  ( 9.738834413317897898, 10.25639499182604730, 0.000000000000000000 ) ) ;
#92436=CARTESIAN_POINT ( 'NONE',  ( 1.364683531249986537, 0.4260416670080872659, 0.7879004041258500513 ) ) ;
#92442=ORIENTED_EDGE ( 'NONE', *, *, #8236, .F. ) ;
#92446=CARTESIAN_POINT ( 'NONE',  ( 7.293923454472087897, 8.572294120714675003, 1.082531754730558626 ) ) ;
#92449=CARTESIAN_POINT ( 'NONE',  ( -4.822949958159302497, 6.649860922651058992, -1.599625672291256295 ) ) ;
#92454=CARTESIAN_POINT ( 'NONE',  ( 5.626270559546814098, 7.587068290936515247, 1.443375672974062551 ) ) ;
#92455=CARTESIAN_POINT ( 'NONE',  ( -8.256552360598034213, 11.61609960646427986, 1.082531754730549967 ) ) ;
#92460=CARTESIAN_POINT ( 'NONE',  ( 2.737856954955798727, 5.281584649835344258, 1.199719254218452047 ) ) ;
#92463=ADVANCED_FACE ( 'NONE', ( #204276 ), #10601, .T. ) ;
#92476=CARTESIAN_POINT ( 'NONE',  ( 6.968000882419564945, 10.21675256520979858, 1.199719254218460707 ) ) ;
#92480=CARTESIAN_POINT ( 'NONE',  ( 3.036663219780971978, 6.486598156479028709, -0.7216878364870267237 ) ) ;
#92482=EDGE_CURVE ( 'NONE', #96549, #95577, #22845, .T. ) ;
#92483=CARTESIAN_POINT ( 'NONE',  ( -7.212574532790092974, 10.39812547402169862, -1.082531754730543971 ) ) ;
#92488=CARTESIAN_POINT ( 'NONE',  ( -2.252626078164912560, 5.779814191167667481, 0.7998128361456341429 ) ) ;
#92513=CARTESIAN_POINT ( 'NONE',  ( -5.442708600882160574, 8.437244903416123876, -1.199719254218446718 ) ) ;
#92517=CARTESIAN_POINT ( 'NONE',  ( 4.299907273828439180, 8.168308919441841454, 1.040834085586084257E-14 ) ) ;
#92522=CARTESIAN_POINT ( 'NONE',  ( -5.135841261478327979, 4.886236314679810455, 0.7998128361456341429 ) ) ;
#92526=CARTESIAN_POINT ( 'NONE',  ( -3.554208825076827782, 7.298327395898266623, 0.7998128361456341429 ) ) ;
#92529=CARTESIAN_POINT ( 'NONE',  ( 6.968000882419564945, 10.21675256520979858, 1.199719254218460707 ) ) ;
#92532=CARTESIAN_POINT ( 'NONE',  ( 5.834672162164848075, 6.194663582219344988, 0.9174233710642684114 ) ) ;
#92533=CARTESIAN_POINT ( 'NONE',  ( 3.063779527008311021, 5.557864633942907417, 1.082531754730546636 ) ) ;
#92539=CARTESIAN_POINT ( 'NONE',  ( 7.443063143778065438, 7.785921210603627962, -0.7216878364870257245 ) ) ;
#92540=CARTESIAN_POINT ( 'NONE',  ( -9.155833807930273238, 9.576227618873799585, -0.7998128361456291469 ) ) ;
#92543=CARTESIAN_POINT ( 'NONE',  ( -9.104463846776669200, 10.58062822844965645, -1.199719254218441611 ) ) ;
#92544=VECTOR ( 'NONE', #158110, 1000.000000000000000 ) ;
#92545=CARTESIAN_POINT ( 'NONE',  ( -6.307567778855718288, 8.381915046796901692, -1.599625672291263179 ) ) ;
#92552=CARTESIAN_POINT ( 'NONE',  ( 9.250740883225924804, 9.686952540052077509, 1.040834085586084257E-14 ) ) ;
#92557=CARTESIAN_POINT ( 'NONE',  ( 3.277320446201373638, 4.846626492033466072, 1.599625672291267398 ) ) ;
#92560=CARTESIAN_POINT ( 'NONE',  ( -0.7499999999999972244, 5.389583334016151639, -1.299038105676652899 ) ) ;
#92565=CARTESIAN_POINT ( 'NONE',  ( -1.499999999999997780, 4.650000000000022560, 1.214306433183764966E-14 ) ) ;
#92566=CARTESIAN_POINT ( 'NONE',  ( 3.876741858503734761, 6.610283703974623393, 1.199719254218462483 ) ) ;
#92567=CARTESIAN_POINT ( 'NONE',  ( 5.849453209292126310, 8.911780279894442103, 1.199719254218462483 ) ) ;
#92570=CARTESIAN_POINT ( 'NONE',  ( 6.317736394288131052, 9.354147645769410602, 1.082531754730558626 ) ) ;
#92571=CARTESIAN_POINT ( 'NONE',  ( -8.744645890690007306, 12.18554205823825498, 1.082531754730558626 ) ) ;
#92575=CARTESIAN_POINT ( 'NONE',  ( 9.402743226277308963, 10.92862083786708816, -1.199719254218446718 ) ) ;
#92578=CARTESIAN_POINT ( 'NONE',  ( -4.464712657601869417, 4.103252943490596216, 0.7998128361456341429 ) ) ;
#92580=CARTESIAN_POINT ( 'NONE',  ( 3.023105066167310895, 5.702484939155337607, -2.499999999999995115 ) ) ;
#92581=CARTESIAN_POINT ( 'NONE',  ( 1.364683531249986537, 1.113541667008082658, 0.7879004041258500513 ) ) ;
#92586=CARTESIAN_POINT ( 'NONE',  ( 1.364683531249988757, 0.1343750003414204142, 0.000000000000000000 ) ) ;
#92588=CARTESIAN_POINT ( 'NONE',  ( 8.238550898598388628, 12.76339314834017102, 0.7998128361456462443 ) ) ;
#92592=CARTESIAN_POINT ( 'NONE',  ( -9.854078719034067291, 10.39084668182823634, 0.7998128361456462443 ) ) ;
#92597=CARTESIAN_POINT ( 'NONE',  ( 5.379888026524302980, 5.170957540566797128, -0.7998128361456211532 ) ) ;
#92602=CARTESIAN_POINT ( 'NONE',  ( 8.259941899223605333, 10.65968485389279508, -1.599625672291268286 ) ) ;
#92605=CARTESIAN_POINT ( 'NONE',  ( -6.240830780992103755, 6.175390754112560110, 1.040834085586084257E-14 ) ) ;
#92609=CARTESIAN_POINT ( 'NONE',  ( 7.052212457402625922, 11.37933163361175382, -0.7998128361456291469 ) ) ;
#92611=CARTESIAN_POINT ( 'NONE',  ( 8.046927864910717432, 9.346836249606042202, 1.199719254218462483 ) ) ;
#92616=CARTESIAN_POINT ( 'NONE',  ( -8.758204044748012507, 11.24099069033793974, 1.443375672974064550 ) ) ;
#92618=DIRECTION ( 'NONE',  ( -5.578564026256490882E-16, -1.000000000000000000, -9.066213480720158442E-32 ) ) ;
#92623=CARTESIAN_POINT ( 'NONE',  ( -5.958637689794747949, 6.108898536480521280, 0.7553493914738591553 ) ) ;
#92624=CARTESIAN_POINT ( 'NONE',  ( -1.364683531250000748, 1.259375000341421469, 0.000000000000000000 ) ) ;
#92626=CARTESIAN_POINT ( 'NONE',  ( 5.341549334104184865, 8.215262742221458581, 1.082531754730558626 ) ) ;
#92644=CARTESIAN_POINT ( 'NONE',  ( 8.235688245297327015, 11.69572115523387268, -1.199719254218446718 ) ) ;
#92648=CARTESIAN_POINT ( 'NONE',  ( -3.867100128395853709, 5.534702787927018974, -1.599625672291256295 ) ) ;
#92649=CARTESIAN_POINT ( 'NONE',  ( -5.181187258716735577, 9.196468901811520880, 0.7998128361456481317 ) ) ;
#92654=CARTESIAN_POINT ( 'NONE',  ( -1.201851678989727383E-14, 4.868750000682822154, -1.732050807568863648 ) ) ;
#92655=CARTESIAN_POINT ( 'NONE',  ( 6.401421083946654100, 10.62007503124645957, -0.7998128361456291469 ) ) ;
#92658=CARTESIAN_POINT ( 'NONE',  ( -8.362681821530818738, 8.650883634741092010, -0.7998128361456291469 ) ) ;
#92660=CARTESIAN_POINT ( 'NONE',  ( 1.364683531249990311, 4.634375000341417916, 1.214306433183764966E-14 ) ) ;
#92665=CARTESIAN_POINT ( 'NONE',  ( -8.893785580884703279, 10.43879993486270585, 1.082531754730558626 ) ) ;
#92669=CARTESIAN_POINT ( 'NONE',  ( 1.364683531249988757, 2.446875000341415696, 1.214306433183764966E-14 ) ) ;
#92676=CARTESIAN_POINT ( 'NONE',  ( -1.001543065824772872E-14, 4.321875000341417916, 1.575800808251672791 ) ) ;
#92677=CARTESIAN_POINT ( 'NONE',  ( -5.122283107864663343, 4.870418468797203637, 0.000000000000000000 ) ) ;
#92678=CARTESIAN_POINT ( 'NONE',  ( 5.774883364416965037, 8.824782127540085952, -1.199719254218440723 ) ) ;
#92681=CARTESIAN_POINT ( 'NONE',  ( -0.6823417656250212460, 4.113541667008085767, 1.181850606188767472 ) ) ;
#92684=CARTESIAN_POINT ( 'NONE',  ( -1.402160292154681736E-14, -0.5531249996585814177, -1.575800808251665908 ) ) ;
#92685=CARTESIAN_POINT ( 'NONE',  ( -3.633221978782283923, 7.182583375313884133, -0.7216878364870267237 ) ) ;
#92689=CARTESIAN_POINT ( 'NONE',  ( 4.392478581147586603, 4.226905887534702977, -0.7216878364870188411 ) ) ;
#92692=CARTESIAN_POINT ( 'NONE',  ( -8.758204044748012507, 11.24099069033793974, 1.443375672974064550 ) ) ;
#92698=CARTESIAN_POINT ( 'NONE',  ( -6.521108698048779573, 8.631046119188804155, -1.443375672974058777 ) ) ;
#92700=CARTESIAN_POINT ( 'NONE',  ( -1.364683531250014514, 1.301041667008083325, -0.7879004041258289570 ) ) ;
#92706=CARTESIAN_POINT ( 'NONE',  ( 1.364683531249988757, -0.5531249996585801965, 0.000000000000000000 ) ) ;
#92709=CARTESIAN_POINT ( 'NONE',  ( 2.345197385039651472, 5.679888015947478941, -0.7216878364870267237 ) ) ;
#92715=CARTESIAN_POINT ( 'NONE',  ( 7.226132685959389512, 11.37431253368722750, -0.7216878364870267237 ) ) ;
#92719=ORIENTED_EDGE ( 'NONE', *, *, #185325, .F. ) ;
#92721=ORIENTED_EDGE ( 'NONE', *, *, #160495, .F. ) ;
#92728=CARTESIAN_POINT ( 'NONE',  ( 0.6823417656249899377, 1.905208333674752952, 1.181850606188755259 ) ) ;
#92730=ADVANCED_FACE ( 'NONE', ( #93236 ), #145199, .T. ) ;
#92735=CARTESIAN_POINT ( 'NONE',  ( -1.500000000000016209, 5.670833333333358262, 0.8660254037844375974 ) ) ;
#92741=FACE_OUTER_BOUND ( 'NONE', #187431, .T. ) ;
#92745=VERTEX_POINT ( 'NONE', #29279 ) ;
#92749=CARTESIAN_POINT ( 'NONE',  ( 6.114890974963323345, 7.092793211334054604, 1.199719254218462483 ) ) ;
#92752=ORIENTED_EDGE ( 'NONE', *, *, #29804, .T. ) ;
#92756=CARTESIAN_POINT ( 'NONE',  ( 8.782984583554449998, 9.141236857102018831, 1.040834085586084257E-14 ) ) ;
#92760=CARTESIAN_POINT ( 'NONE',  ( 8.585337585951586803, 11.03931315507545108, -1.599625672291255185 ) ) ;
#92769=DIRECTION ( 'NONE',  ( 1.000000000000000000, 0.000000000000000000, 0.000000000000000000 ) ) ;
#92774=CARTESIAN_POINT ( 'NONE',  ( -7.361714222540411967, 11.53249099303175385, 0.000000000000000000 ) ) ;
#92779=CARTESIAN_POINT ( 'NONE',  ( 4.150767584078112193, 7.994312614733129152, 0.7998128361456321445 ) ) ;
#92785=CARTESIAN_POINT ( 'NONE',  ( 3.131570294632282092, 5.636953862837537521, -1.082531754730543971 ) ) ;
#92793=CARTESIAN_POINT ( 'NONE',  ( -6.501298352952815662, 7.543601818988450169, -1.199719254218446718 ) ) ;
#92795=CARTESIAN_POINT ( 'NONE',  ( -4.471491734408701291, 4.111161866431900513, 1.214306433183764966E-14 ) ) ;
#92800=CARTESIAN_POINT ( 'NONE',  ( 0.3584499564876124644, 8.158857887133999398, -1.968348077346313341 ) ) ;
#92804=CARTESIAN_POINT ( 'NONE',  ( 4.364835388595708743, 7.179726155748598515, 1.199719254218462483 ) ) ;
#92806=CARTESIAN_POINT ( 'NONE',  ( 1.543281805264333117, 8.695372333414642441, 2.508924166024208979 ) ) ;
#92816=ORIENTED_EDGE ( 'NONE', *, *, #34246, .T. ) ;
#92818=CARTESIAN_POINT ( 'NONE',  ( -1.364683531250014514, 1.801041667008085767, -0.7879004041258289570 ) ) ;
#92820=CARTESIAN_POINT ( 'NONE',  ( 5.379888026524302980, 5.170957540566797128, -0.7998128361456211532 ) ) ;
#92822=CARTESIAN_POINT ( 'NONE',  ( -6.561783159334141580, 7.718130443053708767, -1.082531754730544860 ) ) ;
#92823=CARTESIAN_POINT ( 'NONE',  ( 3.063779527008304360, 6.518233848244248563, 0.7216878364870317197 ) ) ;
#92824=CARTESIAN_POINT ( 'NONE',  ( -6.277061933002790362, 8.346324893301817482, 1.443375672974078761 ) ) ;
#92829=CARTESIAN_POINT ( 'NONE',  ( 4.950698647284403009, 8.927565521807144577, 1.040834085586084257E-14 ) ) ;
#92834=CARTESIAN_POINT ( 'NONE',  ( -1.201851678989727383E-14, 5.196875000341422357, -1.575800808251660134 ) ) ;
#92838=CARTESIAN_POINT ( 'NONE',  ( 7.806797523370503811, 8.002351953554066810, 1.040834085586084257E-14 ) ) ;
#92842=CARTESIAN_POINT ( 'NONE',  ( -7.250913225210214641, 7.353820272367037170, 0.7998128361456341429 ) ) ;
#92847=CARTESIAN_POINT ( 'NONE',  ( 7.889955328148847258, 11.29236608522730911, -1.199719254218446718 ) ) ;
#92849=CARTESIAN_POINT ( 'NONE',  ( -7.877450944739929461, 9.149113176073413456, 1.199719254218462483 ) ) ;
#92851=CARTESIAN_POINT ( 'NONE',  ( 8.229436053370683624, 8.703356271795033905, 0.7216878364870458196 ) ) ;
#92852=CARTESIAN_POINT ( 'NONE',  ( 4.149696378627680815, 7.633013953984455036, -0.8115063166676712569 ) ) ;
#92853=CARTESIAN_POINT ( 'NONE',  ( -5.623934791570306402, 5.455678766453782913, 0.7998128361456341429 ) ) ;
#92857=CARTESIAN_POINT ( 'NONE',  ( 4.476163270806094552, 8.373940915915776273, 0.7998128361456462443 ) ) ;
#92859=CARTESIAN_POINT ( 'NONE',  ( 9.589694723567584234, 10.08239868711733855, -0.7998128361456281477 ) ) ;
#92860=CARTESIAN_POINT ( 'NONE',  ( -5.552553451737586521, 6.223206628393089801, 0.9334509375357492589 ) ) ;
#92862=CARTESIAN_POINT ( 'NONE',  ( -0.6823417656250212460, 0.8010416670080899859, 1.181850606188755259 ) ) ;
#92864=CARTESIAN_POINT ( 'NONE',  ( -7.063434843039784639, 7.343021526408956667, 1.040834085586084257E-14 ) ) ;
#92871=CARTESIAN_POINT ( 'NONE',  ( -5.012544637203120601, 6.604931577287184830, 1.238112577840282169 ) ) ;
#92872=CARTESIAN_POINT ( 'NONE',  ( 1.364683531249986537, 0.7177083336747527298, -0.7879004041258239610 ) ) ;
#92875=CARTESIAN_POINT ( 'NONE',  ( 2.412988153552339643, 5.758977245878946327, 0.7216878364870438212 ) ) ;
#92880=CARTESIAN_POINT ( 'NONE',  ( -7.158341917891067219, 11.29522330427417565, 0.000000000000000000 ) ) ;
#92887=CARTESIAN_POINT ( 'NONE',  ( -9.449669878600625239, 10.12696240122997082, -0.7216878364870267237 ) ) ;
#92888=CARTESIAN_POINT ( 'NONE',  ( -1.257539916218628262, 3.158837156058347695, 0.7750000000000100142 ) ) ;
#92894=CARTESIAN_POINT ( 'NONE',  ( -8.012505595552038784, 8.450270737673262644, 0.7216878364870578100 ) ) ;
#92898=CARTESIAN_POINT ( 'NONE',  ( -1.201851678989727383E-14, 5.259375000341421469, -1.575800808251660134 ) ) ;
#92899=CARTESIAN_POINT ( 'NONE',  ( 0.7499999999999920064, 4.514583334016150751, 1.299038105676669330 ) ) ;
#92900=CARTESIAN_POINT ( 'NONE',  ( 5.971451247601332391, 6.106144735068791185, -0.6754856502540294017 ) ) ;
#92906=CARTESIAN_POINT ( 'NONE',  ( -6.612626235163205024, 8.737816579155630592, -1.599625672291263179 ) ) ;
#92910=CARTESIAN_POINT ( 'NONE',  ( 3.649115900372475796, 7.409052317076538330, 1.040834085586084257E-14 ) ) ;
#92915=CARTESIAN_POINT ( 'NONE',  ( 6.096362627639171805, 10.26417349888772179, -0.7998128361456291469 ) ) ;
#92917=( BOUNDED_CURVE ( )  B_SPLINE_CURVE ( 2, ( #87887, #155025, #5527, #137719, #203739, #6609, #72690 ),
 .UNSPECIFIED., .F., .T. ) 
 B_SPLINE_CURVE_WITH_KNOTS ( ( 3, 2, 2, 3 ),
 ( 0.4141369526679988811, 0.4166666666666666852, 0.4226190476190476164, 0.4251487616177153650 ),
 .UNSPECIFIED. ) 
 CURVE ( )  GEOMETRIC_REPRESENTATION_ITEM ( )  RATIONAL_B_SPLINE_CURVE ( ( 0.9345202395942611151, 0.9430618748659218564, 1.000000000000000000, 0.8660254037844387076, 1.000000000000000000, 0.9430618748659225226, 0.9345202395942613371 ) ) 
 REPRESENTATION_ITEM ( '' )  );
#92923=CARTESIAN_POINT ( 'NONE',  ( -4.595850885352567694, 8.305650432979225783, 1.040834085586084257E-14 ) ) ;
#92927=FACE_OUTER_BOUND ( 'NONE', #188464, .T. ) ;
#92933=CARTESIAN_POINT ( 'NONE',  ( -9.398826802771548472, 11.98838390803207865, -1.599625672291263179 ) ) ;
#92935=CARTESIAN_POINT ( 'NONE',  ( 8.446893396513862839, 9.813462703143045474, -1.199719254218445830 ) ) ;
#92936=CARTESIAN_POINT ( 'NONE',  ( -1.402160292154681736E-14, -0.5374999999999753308, 1.732050807568877637 ) ) ;
#92937=CARTESIAN_POINT ( 'NONE',  ( -7.167456763118792651, 11.51378332361394818, 0.000000000000000000 ) ) ;
#92940=CARTESIAN_POINT ( 'NONE',  ( -1.201851678989727383E-14, 3.821875000341423689, 1.575800808251672791 ) ) ;
#92941=CARTESIAN_POINT ( 'NONE',  ( 4.196412238629597447, 4.854568018944682706, -1.199719254218452047 ) ) ;
#92944=CARTESIAN_POINT ( 'NONE',  ( -1.201851678989727383E-14, 5.087500000000019007, -1.732050807568863648 ) ) ;
#92946=DIRECTION ( 'NONE',  ( -5.578564026256490882E-16, -1.000000000000000000, -9.066213480720158442E-32 ) ) ;
#92947=CARTESIAN_POINT ( 'NONE',  ( 8.066738210006679566, 10.43428054980638997, 1.443375672974076540 ) ) ;
#92950=CARTESIAN_POINT ( 'NONE',  ( -6.236387472606145010, 9.259240570473746601, -1.082531754730538864 ) ) ;
#92952=CARTESIAN_POINT ( 'NONE',  ( -1.364683531250012516, 1.780208333674757615, 0.7879004041258379498 ) ) ;
#92956=CARTESIAN_POINT ( 'NONE',  ( -5.859094939400033120, 9.987361195942037639, -0.7998128361456231517 ) ) ;
#92957=CARTESIAN_POINT ( 'NONE',  ( -0.6823417656249969321, 5.280208333674756283, -1.181850606188749264 ) ) ;
#92963=CARTESIAN_POINT ( 'NONE',  ( 7.587759525142423911, 12.00413654597487501, 0.7998128361456462443 ) ) ;
#92966=CARTESIAN_POINT ( 'NONE',  ( -1.500000000000013101, 1.129166666666688634, -0.8660254037844313801 ) ) ;
#92971=CARTESIAN_POINT ( 'NONE',  ( 7.619319141200070256, 8.951922421897323900, 1.082531754730558626 ) ) ;
#92972=CARTESIAN_POINT ( 'NONE',  ( 10.08456733046637765, 10.65975006183261087, 0.000000000000000000 ) ) ;
#92977=CARTESIAN_POINT ( 'NONE',  ( 8.483651433849084711, 10.92067931095586886, 1.599625672291281386 ) ) ;
#92978=CARTESIAN_POINT ( 'NONE',  ( -8.292783513053063160, 12.82666453187061073, 0.7998128361456481317 ) ) ;
#92982=CARTESIAN_POINT ( 'NONE',  ( -1.364683531250014514, -1.219791666325248602, 0.7879004041258379498 ) ) ;
#92986=CARTESIAN_POINT ( 'NONE',  ( 4.127082626822145883, 7.435606486324357611, -0.7117951089531282527 ) ) ;
#92988=CARTESIAN_POINT ( 'NONE',  ( -1.201851678989727383E-14, 3.446875000341421469, -1.575800808251660134 ) ) ;
#92990=CARTESIAN_POINT ( 'NONE',  ( -7.239690840017442675, 7.548653522882887934, 0.7216878364870317197 ) ) ;
#92993=EDGE_CURVE ( 'NONE', #127447, #73877, #76071, .T. ) ;
#92997=CARTESIAN_POINT ( 'NONE',  ( 3.216308754939877446, 4.775446185561722956, -1.599625672291262513 ) ) ;
#93000=CARTESIAN_POINT ( 'NONE',  ( 7.995557903757111617, 10.35123685918189729, 1.599625672291281386 ) ) ;
#93001=CARTESIAN_POINT ( 'NONE',  ( 2.060660350336875002, 8.500464906087991324, -2.499999999999994671 ) ) ;
#93006=CARTESIAN_POINT ( 'NONE',  ( -8.402302512167102222, 10.82577223566020841, -1.599625672291263179 ) ) ;
#93008=CARTESIAN_POINT ( 'NONE',  ( 6.844168616800228477, 6.879284895888727824, -0.7998128361456281477 ) ) ;
#93010=CARTESIAN_POINT ( 'NONE',  ( 3.185802909086937973, 6.660594460669327255, 0.7216878364870317197 ) ) ;
#93012=CARTESIAN_POINT ( 'NONE',  ( 5.183294799126148433, 4.941598775268944976, 1.040834085586084257E-14 ) ) ;
#93022=CARTESIAN_POINT ( 'NONE',  ( -5.585596099150182958, 8.499983968108443477, -1.082531754730544860 ) ) ;
#93023=CARTESIAN_POINT ( 'NONE',  ( 4.009460741339333723, 5.700790169694431420, -1.599625672291256295 ) ) ;
#93026=CARTESIAN_POINT ( 'NONE',  ( -7.670162217029145246, 9.971608557999250166, 1.599625672291295375 ) ) ;
#93031=CARTESIAN_POINT ( 'NONE',  ( -7.458957065812611198, 11.85386701009007204, 0.7998128361456481317 ) ) ;
#93034=CARTESIAN_POINT ( 'NONE',  ( 7.609150525767641504, 9.900428251527500834, -1.599625672291262513 ) ) ;
#93035=CARTESIAN_POINT ( 'NONE',  ( 3.974511587100456822, 7.788680618259193444, 1.040834085586084257E-14 ) ) ;
#93047=CARTESIAN_POINT ( 'NONE',  ( -7.157815033010924921, 10.43820240756634199, 1.199719254218453823 ) ) ;
#93051=CARTESIAN_POINT ( 'NONE',  ( 5.016153647376196290, 8.796003655340152605, 0.7216878364870438212 ) ) ;
#93054=CARTESIAN_POINT ( 'NONE',  ( -1.492390896412726597, 7.408229809043063163, 4.235510822232345873 ) ) ;
#93057=CARTESIAN_POINT ( 'NONE',  ( -7.088215381846223906, 7.164006121775713609, 0.7998128361456341429 ) ) ;
#93060=DIRECTION ( 'NONE',  ( -0.7592566023653016805, -0.6507913734559627184, -7.055894209357776889E-15 ) ) ;
#93065=CARTESIAN_POINT ( 'NONE',  ( 8.426556166093362776, 9.789735934319136135, -1.199719254218446718 ) ) ;
#93067=CARTESIAN_POINT ( 'NONE',  ( -2.928197990871687306, 5.399686175116803710, 1.082531754730560403 ) ) ;
#93070=CARTESIAN_POINT ( 'NONE',  ( -4.512490679940424521, 7.037946173918820492, -1.151410311177623935 ) ) ;
#93077=CARTESIAN_POINT ( 'NONE',  ( 2.659370686574860976, 6.254349567645977714, -0.7998128361456291469 ) ) ;
#93096=CARTESIAN_POINT ( 'NONE',  ( -6.098470168048611306, 6.009303372345148553, 1.040834085586084257E-14 ) ) ;
#93097=CARTESIAN_POINT ( 'NONE',  ( 4.297571505407542958, 7.957657823043374989, -0.7216878364870197293 ) ) ;
#93098=CARTESIAN_POINT ( 'NONE',  ( -0.7500000000000215383, 3.441666666666689967, 1.299038105676671107 ) ) ;
#93100=CARTESIAN_POINT ( 'NONE',  ( -5.274285450916075035, 6.112086766612214284, 1.199719254218450271 ) ) ;
#93104=CARTESIAN_POINT ( 'NONE',  ( 1.364683531249990311, 4.384375000341417028, 1.214306433183764966E-14 ) ) ;
#93107=CARTESIAN_POINT ( 'NONE',  ( -4.622967192579922724, 4.495809267539077503, 1.214306433183764966E-14 ) ) ;
#93112=CARTESIAN_POINT ( 'NONE',  ( 4.029797971759831121, 5.724516938518342535, -1.599625672291255185 ) ) ;
#93113=CARTESIAN_POINT ( 'NONE',  ( -1.084637062511546901, 3.117628807292010862, -1.105835307554786429 ) ) ;
#93117=FACE_OUTER_BOUND ( 'NONE', #38973, .T. ) ;
#93119=CARTESIAN_POINT ( 'NONE',  ( -0.6823417656250212460, 0.8635416670080899859, 1.181850606188755259 ) ) ;
#93124=CARTESIAN_POINT ( 'NONE',  ( -10.13488352141530768, 11.78278451552804817, 1.199719254218462483 ) ) ;
#93125=CARTESIAN_POINT ( 'NONE',  ( -4.704316113817535339, 8.432193199521691440, 0.7216878364870458196 ) ) ;
#93128=VERTEX_POINT ( 'NONE', #67355 ) ;
#93129=CARTESIAN_POINT ( 'NONE',  ( 0.6823417656249899377, 4.926041667008086655, -1.181850606188754593 ) ) ;
#93137=CARTESIAN_POINT ( 'NONE',  ( -7.185458225118419584, 7.485382138834033583, 1.040834085586084257E-14 ) ) ;
#93142=CARTESIAN_POINT ( 'NONE',  ( -5.436456408955534947, 6.405249234278626247, 1.082531754730546636 ) ) ;
#93145=CARTESIAN_POINT ( 'NONE',  ( 10.57266086055835075, 11.22919251360659310, 0.000000000000000000 ) ) ;
#93150=CARTESIAN_POINT ( 'NONE',  ( 1.524175555628257905, 8.756493634679708649, -2.487619788734836135 ) ) ;
#93155=CARTESIAN_POINT ( 'NONE',  ( -2.767835915484202047, 6.380892334706859792, -0.7998128361456281477 ) ) ;
#93156=CARTESIAN_POINT ( 'NONE',  ( -6.138157188980746248, 5.995865266587975917, 0.1610769774899509232 ) ) ;
#93158=CARTESIAN_POINT ( 'NONE',  ( 0.7499999999999885647, 0.4833333333333564297, 1.299038105676657340 ) ) ;
#93159=ORIENTED_EDGE ( 'NONE', *, *, #78317, .T. ) ;
#93161=CARTESIAN_POINT ( 'NONE',  ( 9.897088948295946764, 10.64895131587453569, 0.7216878364870438212 ) ) ;
#93162=CARTESIAN_POINT ( 'NONE',  ( 6.662942426112080874, 9.860851032851066122, 1.199719254218460707 ) ) ;
#93167=CARTESIAN_POINT ( 'NONE',  ( 3.520313441042647540, 7.258782781191745137, 0.7998128361456321445 ) ) ;
#93169=CARTESIAN_POINT ( 'NONE',  ( -0.006913841192827608478, 8.234242197375163386, -1.999988128101763074 ) ) ;
#93178=CARTESIAN_POINT ( 'NONE',  ( 8.748035429315576650, 11.22912730566677553, -1.599625672291255185 ) ) ;
#93179=CARTESIAN_POINT ( 'NONE',  ( -5.605406444246153974, 8.627059054007450101, -1.199719254218440723 ) ) ;
#93186=CARTESIAN_POINT ( 'NONE',  ( -1.364683531250012516, 3.488541667008085767, -0.7879004041258300672 ) ) ;
#93187=CARTESIAN_POINT ( 'NONE',  ( 9.720832950873944611, 10.44331931888218001, -0.7216878364870257245 ) ) ;
#93188=ADVANCED_FACE ( 'NONE', ( #84708 ), #137746, .F. ) ;
#93189=CARTESIAN_POINT ( 'NONE',  ( -6.261168011412601153, 6.199117522936475666, 1.040834085586084257E-14 ) ) ;
#93192=CARTESIAN_POINT ( 'NONE',  ( 6.193377243344257543, 6.120028293523423812, -0.7998128361456281477 ) ) ;
#93193=CARTESIAN_POINT ( 'NONE',  ( -6.098470168048611306, 6.009303372345148553, 1.040834085586084257E-14 ) ) ;
#93199=CARTESIAN_POINT ( 'NONE',  ( 7.144783764721768904, 7.437928601704619780, 1.040834085586084257E-14 ) ) ;
#93202=CARTESIAN_POINT ( 'NONE',  ( 1.364683531249986537, 1.967708333674750731, -0.7879004041258239610 ) ) ;
#93204=CARTESIAN_POINT ( 'NONE',  ( 6.033015167956792268, 8.061603667414825480, -1.443375672974057666 ) ) ;
#93207=CARTESIAN_POINT ( 'NONE',  ( -3.578989364327652467, 6.158942777482099729, 1.082531754730560403 ) ) ;
#93213=CARTESIAN_POINT ( 'NONE',  ( -4.371234765837696656, 7.372762773471292164, -1.195546268109607846 ) ) ;
#93223=CARTESIAN_POINT ( 'NONE',  ( 3.195971524519376494, 4.751719416737803847, -1.599625672291262513 ) ) ;
#93231=CARTESIAN_POINT ( 'NONE',  ( 4.419594888374914099, 5.218910793601261311, -1.082531754730548412 ) ) ;
#93232=CARTESIAN_POINT ( 'NONE',  ( -0.6823417656250003738, 2.030208333674753174, -1.181850606188749264 ) ) ;
#93234=CARTESIAN_POINT ( 'NONE',  ( 6.414979237560321401, 10.63589287712906462, 1.040834085586084257E-14 ) ) ;
#93236=FACE_OUTER_BOUND ( 'NONE', #115149, .T. ) ;
#93241=CARTESIAN_POINT ( 'NONE',  ( 0.7499999999999902300, 3.233333333333352044, 1.299038105676669330 ) ) ;
#93242=CARTESIAN_POINT ( 'NONE',  ( 4.449046963578762615, 8.342305224150557308, -0.7998128361456231517 ) ) ;
#93243=CARTESIAN_POINT ( 'NONE',  ( -7.739006755302186846, 7.923262724141010516, 0.7998128361456462443 ) ) ;
#93247=CARTESIAN_POINT ( 'NONE',  ( 0.6823417656249899377, 3.176041667008085323, -1.181850606188754593 ) ) ;
#93249=CARTESIAN_POINT ( 'NONE',  ( 4.681643115420508039, 4.356338477612361260, 0.7998128361456341429 ) ) ;
#93255=CARTESIAN_POINT ( 'NONE',  ( 1.499999999999987121, 0.5770833340161539704, -0.8660254037844253849 ) ) ;
#93258=CARTESIAN_POINT ( 'NONE',  ( -6.018930129462987999, 9.109503353427070849, 1.199719254218452047 ) ) ;
#93259=CARTESIAN_POINT ( 'NONE',  ( -4.446711195602264688, 4.290177271065136466, -0.7216878364870207285 ) ) ;
#93268=CARTESIAN_POINT ( 'NONE',  ( 5.931855901178834323, 6.879252291918818152, 1.199719254218462483 ) ) ;
#93272=CARTESIAN_POINT ( 'NONE',  ( 5.331380718671758778, 7.243030143248949670, -1.599625672291256295 ) ) ;
#93275=CARTESIAN_POINT ( 'NONE',  ( 2.381428537494710618, 5.930083727052461562, 0.7998128361456462443 ) ) ;
#93281=CARTESIAN_POINT ( 'NONE',  ( 4.103641366189806128, 7.455328040159560743, 0.6459977421944228526 ) ) ;
#93282=VERTEX_POINT ( 'NONE', #86844 ) ;
#93285=EDGE_CURVE ( 'NONE', #152385, #121606, #2359, .T. ) ;
#93293=CARTESIAN_POINT ( 'NONE',  ( -3.307826292054316664, 4.882216645528547616, -1.443375672974059665 ) ) ;
#93294=CARTESIAN_POINT ( 'NONE',  ( 8.622622508611357262, 9.162073802909148412, -0.7216878364870197293 ) ) ;
#93296=CARTESIAN_POINT ( 'NONE',  ( -3.716906668440817185, 7.488141546489591072, 0.7998128361456341429 ) ) ;
#93299=CARTESIAN_POINT ( 'NONE',  ( 8.457588896826466751, 8.761608555919362828, 1.040834085586084257E-14 ) ) ;
#93301=CARTESIAN_POINT ( 'NONE',  ( -5.042743069279040036, 7.970618449879118828, 1.199719254218464037 ) ) ;
#93304=CARTESIAN_POINT ( 'NONE',  ( 1.419999999999820961, 7.204077025658620848, -4.238769367544755973 ) ) ;
#93306=ORIENTED_EDGE ( 'NONE', *, *, #158430, .T. ) ;
#93315=CARTESIAN_POINT ( 'NONE',  ( -5.311043488251275591, 7.219303374425030562, -1.599625672291256295 ) ) ;
#93318=CARTESIAN_POINT ( 'NONE',  ( 2.724825686666657809, 6.122787701178987518, 0.000000000000000000 ) ) ;
#93322=CARTESIAN_POINT ( 'NONE',  ( -2.415323921528888196, 5.969628341758991930, 0.7998128361456341429 ) ) ;
#93326=CARTESIAN_POINT ( 'NONE',  ( 8.703444544968814256, 12.24143683818393313, -1.199719254218446718 ) ) ;
#93330=CARTESIAN_POINT ( 'NONE',  ( -8.064402442030170093, 8.302891025323665630, 0.7998128361456602331 ) ) ;
#93331=CARTESIAN_POINT ( 'NONE',  ( 5.311043488251262268, 7.219303374425030562, -1.599625672291256295 ) ) ;
#93332=EDGE_CURVE ( 'NONE', #57355, #28244, #46696, .T. ) ;
#93335=CARTESIAN_POINT ( 'NONE',  ( 4.792970997630896512, 5.550553237779539018, 1.199719254218464037 ) ) ;
#93338=CARTESIAN_POINT ( 'NONE',  ( 1.364683531249988757, 0.9468750003414211358, 0.000000000000000000 ) ) ;
#93339=VERTEX_POINT ( 'NONE', #17546 ) ;
#93341=CARTESIAN_POINT ( 'NONE',  ( 7.944714827928056167, 8.371181508778631652, 0.7216878364870458196 ) ) ;
#93347=VERTEX_POINT ( 'NONE', #71633 ) ;
#93348=CARTESIAN_POINT ( 'NONE',  ( 8.365017589507326434, 12.70301158782650397, -0.7216878364870338292 ) ) ;
#93353=CARTESIAN_POINT ( 'NONE',  ( -9.667127221743832877, 11.23706883257798772, 1.199719254218462483 ) ) ;
#93359=MANIFOLD_SOLID_BREP ( 'Fillet4', #178018 ) ;
#93371=CARTESIAN_POINT ( 'NONE',  ( 0.7499999999999885647, 1.347916667349485786, -1.299038105676652899 ) ) ;
#93377=CARTESIAN_POINT ( 'NONE',  ( 9.101601193475611140, 9.512956235343358102, -0.7998128361456221525 ) ) ;
#93379=CARTESIAN_POINT ( 'NONE',  ( -1.402160292154681736E-14, -0.9281249996585830830, 1.575800808251672791 ) ) ;
#93382=CARTESIAN_POINT ( 'NONE',  ( 3.063252641683779753, 5.661212951017999373, 1.199719254218450271 ) ) ;
#93383=CARTESIAN_POINT ( 'NONE',  ( -6.236387472606153892, 8.298871356172400127, -1.443375672974059665 ) ) ;
#93388=CARTESIAN_POINT ( 'NONE',  ( -6.579784621333750749, 6.570836901177822931, 0.7998128361456341429 ) ) ;
#93390=CARTESIAN_POINT ( 'NONE',  ( 0.7499999999999885647, 2.347916667349486453, -1.299038105676652899 ) ) ;
#93404=CARTESIAN_POINT ( 'NONE',  ( -9.124801077197171040, 10.60435499727357289, -1.199719254218441611 ) ) ;
#93405=CARTESIAN_POINT ( 'NONE',  ( 5.798083248138522272, 9.916180889470295412, 0.7998128361456462443 ) ) ;
#93412=CARTESIAN_POINT ( 'NONE',  ( -8.830438121202295321, 9.196599317691152464, -0.7998128361456291469 ) ) ;
#93415=CARTESIAN_POINT ( 'NONE',  ( 0.000000000000000000, 8.600000000000017408, -0.3999999999999819811 ) ) ;
#93419=CARTESIAN_POINT ( 'NONE',  ( 4.216749469050096621, 4.878294787768598262, -1.199719254218452047 ) ) ;
#93423=CARTESIAN_POINT ( 'NONE',  ( -9.646789991323334590, 11.21334206375407305, 1.199719254218462483 ) ) ;
#93426=CARTESIAN_POINT ( 'NONE',  ( -5.796555320980813164, 6.214368590181693186, -1.006237437275556257 ) ) ;
#93434=CARTESIAN_POINT ( 'NONE',  ( 5.133733721068893807, 9.141106441222381918, 1.040834085586084257E-14 ) ) ;
#93443=CARTESIAN_POINT ( 'NONE',  ( -1.499999999999997780, 1.931250000682817269, 0.000000000000000000 ) ) ;
#93457=CARTESIAN_POINT ( 'NONE',  ( 4.528060117284240071, 5.345453560662148718, 1.082531754730560403 ) ) ;
#93462=CARTESIAN_POINT ( 'NONE',  ( 9.398826802771546696, 11.98838390803207865, -1.599625672291262513 ) ) ;
#93471=CARTESIAN_POINT ( 'NONE',  ( -1.402160292154681736E-14, -0.9281249996585830830, 1.575800808251672791 ) ) ;
#93477=CARTESIAN_POINT ( 'NONE',  ( -5.901876940650454095, 5.779944607047298177, -0.7998128361456291469 ) ) ;
#93479=CARTESIAN_POINT ( 'NONE',  ( -1.402160292154681736E-14, -0.4124999999999747202, -1.732050807568870754 ) ) ;
#93481=CARTESIAN_POINT ( 'NONE',  ( 1.364683531249986537, -1.073958332991911790, 0.7879004041258500513 ) ) ;
#93486=CARTESIAN_POINT ( 'NONE',  ( -0.6823417656250003738, -1.032291666325242607, -1.181850606188749264 ) ) ;
#93488=CARTESIAN_POINT ( 'NONE',  ( -5.716734326456539783, 9.821273814174633188, -0.7998128361456231517 ) ) ;
#93490=CARTESIAN_POINT ( 'NONE',  ( 9.426996880203592610, 9.892584536526015881, -0.7998128361456281477 ) ) ;
#93492=CARTESIAN_POINT ( 'NONE',  ( -0.9999999999999988898, 5.868705557303652398, -4.125226524755048807 ) ) ;
#93496=CARTESIAN_POINT ( 'NONE',  ( 1.364683531249986537, -0.3239583329919163424, 0.7879004041258500513 ) ) ;
#93503=CARTESIAN_POINT ( 'NONE',  ( 6.317736394288122170, 10.31451686007074997, 0.7216878364870438212 ) ) ;
#93506=CARTESIAN_POINT ( 'NONE',  ( -5.199715606040888005, 6.025088614257851027, -1.199719254218446718 ) ) ;
#93508=CARTESIAN_POINT ( 'NONE',  ( -0.7500000000000215383, 4.722916667349482012, 1.299038105676671107 ) ) ;
#93510=CARTESIAN_POINT ( 'NONE',  ( -3.789667630219657912, 4.380032642466370696, 1.199719254218462483 ) ) ;
#93511=CARTESIAN_POINT ( 'NONE',  ( 5.951666246274797345, 7.966696592119163256, 1.443375672974062551 ) ) ;
#93512=CARTESIAN_POINT ( 'NONE',  ( -8.717529583462656717, 11.19353715217169309, 1.443375672974064550 ) ) ;
#93517=CARTESIAN_POINT ( 'NONE',  ( 3.195971524519376494, 4.751719416737803847, -1.599625672291262513 ) ) ;
#93533=CARTESIAN_POINT ( 'NONE',  ( 9.088043039861931405, 9.497138389460751284, 1.040834085586084257E-14 ) ) ;
#93535=CARTESIAN_POINT ( 'NONE',  ( 5.178851490740248309, 5.144340948726068063, 0.7216878364870010776 ) ) ;
#93538=CARTESIAN_POINT ( 'NONE',  ( 4.311129659465574804, 7.013106455143060636, -1.082531754730548412 ) ) ;
#93540=CARTESIAN_POINT ( 'NONE',  ( -8.026063749610043985, 12.30756544127966912, -0.7216878364870267237 ) ) ;
#93560=VERTEX_POINT ( 'NONE', #92211 ) ;
#93563=AXIS2_PLACEMENT_3D ( 'NONE', #19455, #181959, #149479 ) ;
#93569=CARTESIAN_POINT ( 'NONE',  ( -9.002250809794013264, 9.604973487622245898, -0.7216878364870267237 ) ) ;
#93570=( BOUNDED_CURVE ( )  B_SPLINE_CURVE ( 2, ( #83852, #135823, #197602, #69720, #115367, #34041, #166175, #200782, #17764, #1510, #52434, #67576, #118560, #51372, #199726, #117495, #184544, #36164, #102243, #152071, #3641, #201848, #119629, #122869, #54564, #123927, #186685, #137961, #188830, #5774, #7931, #58831, #189895, #90277, #40465, #172596, #106568, #75083, #104390, #74019, #140109, #206136, #203981, #57766, #24174, #120710, #70779, #88134, #38313, #170437, #155271, #141196, #22025, #156346, #91356, #154205, #55628, #71853, #37245, #20962, #105477, #171510, #41537, #23103, #107648, #207207, #89219, #124985, #121785, #173680, #169378 ),
 .UNSPECIFIED., .F., .T. ) 
 B_SPLINE_CURVE_WITH_KNOTS ( ( 3, 2, 2, 2, 2, 2, 2, 2, 2, 2, 2, 2, 2, 2, 2, 2, 2, 2, 2, 2, 2, 2, 2, 2, 2, 2, 2, 2, 2, 2, 2, 2, 2, 2, 2, 3 ),
 ( 0.1345121972685508482, 0.1375000000000000111, 0.1416666666666666630, 0.1458333333333333426, 0.1499999999999999944, 0.1541666666666666741, 0.1583333333333333259, 0.1625000000000000056, 0.1666666666666666574, 0.1708333333333333370, 0.1749999999999999889, 0.1791666666666666685, 0.1833333333333333204, 0.1875000000000000000, 0.1916666666666666796, 0.1958333333333333315, 0.2000000000000000111, 0.2041666666666666630, 0.2083333333333333426, 0.2124999999999999944, 0.2166666666666666741, 0.2208333333333333259, 0.2250000000000000056, 0.2291666666666666574, 0.2333333333333333370, 0.2374999999999999889, 0.2416666666666666685, 0.2458333333333333204, 0.2500000000000000000, 0.2541666666666666519, 0.2583333333333333592, 0.2625000000000000111, 0.2666666666666666630, 0.2708333333333333148, 0.2750000000000000222, 0.2787508327459756741 ),
 .UNSPECIFIED. ) 
 CURVE ( )  GEOMETRIC_REPRESENTATION_ITEM ( )  RATIONAL_B_SPLINE_CURVE ( ( 0.9456386119390516320, 0.9039304805157636347, 1.000000000000000000, 0.8660254037844387076, 1.000000000000000000, 0.8660254037844387076, 1.000000000000000000, 0.8660254037844387076, 1.000000000000000000, 0.8660254037844387076, 1.000000000000000000, 0.8660254037844387076, 1.000000000000000000, 0.8660254037844387076, 1.000000000000000000, 0.8660254037844387076, 1.000000000000000000, 0.8660254037844387076, 1.000000000000000000, 0.8660254037844387076, 1.000000000000000000, 0.8660254037844387076, 1.000000000000000000, 0.8660254037844387076, 1.000000000000000000, 0.8660254037844387076, 1.000000000000000000, 0.8660254037844387076, 1.000000000000000000, 0.8660254037844387076, 1.000000000000000000, 0.8660254037844387076, 1.000000000000000000, 0.8660254037844387076, 1.000000000000000000, 0.8660254037844387076, 1.000000000000000000, 0.8660254037844387076, 1.000000000000000000, 0.8660254037844387076, 1.000000000000000000, 0.8660254037844387076, 1.000000000000000000, 0.8660254037844387076, 1.000000000000000000, 0.8660254037844387076, 1.000000000000000000, 0.8660254037844387076, 1.000000000000000000, 0.8660254037844387076, 1.000000000000000000, 0.8660254037844387076, 1.000000000000000000, 0.8660254037844387076, 1.000000000000000000, 0.8660254037844387076, 1.000000000000000000, 0.8660254037844387076, 1.000000000000000000, 0.8660254037844387076, 1.000000000000000000, 0.8660254037844387076, 1.000000000000000000, 0.8660254037844387076, 1.000000000000000000, 0.8660254037844387076, 1.000000000000000000, 0.8660254037844387076, 1.000000000000000000, 0.8793960873725932270, 0.9759274250375058468 ) ) 
 REPRESENTATION_ITEM ( '' )  );
#93574=CARTESIAN_POINT ( 'NONE',  ( 4.462605117192430804, 8.358123070033169455, 1.040834085586084257E-14 ) ) ;
#93576=ADVANCED_FACE ( 'NONE', ( #139884 ), #109571, .F. ) ;
#93579=CARTESIAN_POINT ( 'NONE',  ( 3.837121167867449945, 4.435395103055503441, 1.199719254218464037 ) ) ;
#93581=CARTESIAN_POINT ( 'NONE',  ( -5.461236948206312114, 5.265864615862458464, 0.7998128361456341429 ) ) ;
#93586=CARTESIAN_POINT ( 'NONE',  ( -3.228813138348844536, 6.918699094715619502, 0.7998128361456341429 ) ) ;
#93589=CARTESIAN_POINT ( 'NONE',  ( 6.916630921265960019, 11.22115317478565188, 0.7998128361456462443 ) ) ;
#93590=CARTESIAN_POINT ( 'NONE',  ( -0.6823417656249969321, 3.967708333674754950, -1.181850606188749264 ) ) ;
#93592=CARTESIAN_POINT ( 'NONE',  ( 5.291954866116698852, 6.573566887673666592, 1.361072633976003310 ) ) ;
#93593=CARTESIAN_POINT ( 'NONE',  ( 5.504247177468190699, 5.523969249908757817, 0.7216878364870317197 ) ) ;
#93600=CARTESIAN_POINT ( 'NONE',  ( 6.222829318548112276, 9.243422724072711816, -1.082531754730537976 ) ) ;
#93601=CARTESIAN_POINT ( 'NONE',  ( -8.158255747121117452, 10.54105100977322174, 1.599625672291295375 ) ) ;
#93604=CARTESIAN_POINT ( 'NONE',  ( -9.982881178363895103, 10.54111621771303753, 1.040834085586084257E-14 ) ) ;
#93605=CARTESIAN_POINT ( 'NONE',  ( -5.526920175865215334, 9.599823971818089774, 0.7998128361456481317 ) ) ;
#93612=CARTESIAN_POINT ( 'NONE',  ( 8.426556166093362776, 9.789735934319136135, -1.199719254218446718 ) ) ;
#93613=CARTESIAN_POINT ( 'NONE',  ( -1.499999999999981126, 4.129166666666685082, -0.8660254037844499209 ) ) ;
#93617=LINE ( 'NONE', #89339, #193345 ) ;
#93625=CARTESIAN_POINT ( 'NONE',  ( 0.7499999999999902300, 3.983333333333352488, 1.299038105676669330 ) ) ;
#93626=CARTESIAN_POINT ( 'NONE',  ( 6.484877546038077867, 6.460111979999551224, 1.040834085586084257E-14 ) ) ;
#93628=CARTESIAN_POINT ( 'NONE',  ( -5.914749137557818059, 6.074338953224275528, -0.6118981238392419142 ) ) ;
#93629=CARTESIAN_POINT ( 'NONE',  ( 7.836249599018724865, 9.205007956019091608, -1.082531754730537976 ) ) ;
#93630=CARTESIAN_POINT ( 'NONE',  ( -9.775065565328612038, 10.50659070241261794, -0.7216878364870267237 ) ) ;
#93633=CARTESIAN_POINT ( 'NONE',  ( 7.703003830858588863, 12.13858823597705872, -0.7998128361456291469 ) ) ;
#93638=CARTESIAN_POINT ( 'NONE',  ( -0.6823417656250212460, 1.551041667008083769, 1.181850606188755259 ) ) ;
#93643=CARTESIAN_POINT ( 'NONE',  ( -1.402160292154681736E-14, -0.5531249996585814177, -1.575800808251665908 ) ) ;
#93646=CARTESIAN_POINT ( 'NONE',  ( 7.723341061279088038, 12.16231500480096983, -0.7998128361456291469 ) ) ;
#93650=CARTESIAN_POINT ( 'NONE',  ( -2.440104460335327463, 5.790612937125752424, 1.040834085586084257E-14 ) ) ;
#93653=CARTESIAN_POINT ( 'NONE',  ( -7.074657228232555717, 7.148188275893099686, 1.040834085586084257E-14 ) ) ;
#93656=CARTESIAN_POINT ( 'NONE',  ( 5.366329872910639232, 5.155139694684188534, 1.040834085586084257E-14 ) ) ;
#93662=EDGE_LOOP ( 'NONE', ( #125599, #189515 ) ) ;
#93664=CARTESIAN_POINT ( 'NONE',  ( 7.072549687823125097, 11.40305840243567381, -0.7998128361456291469 ) ) ;
#93666=CARTESIAN_POINT ( 'NONE',  ( 1.064774733001451423, 2.800000000000024247, -1.047209855801954248 ) ) ;
#93667=CARTESIAN_POINT ( 'NONE',  ( -5.416646063859567484, 6.278174148379618735, 1.199719254218450271 ) ) ;
#93671=CARTESIAN_POINT ( 'NONE',  ( 8.158255747121103241, 10.54105100977322174, 1.599625672291281386 ) ) ;
#93673=CARTESIAN_POINT ( 'NONE',  ( 6.425674737872927089, 9.584038729905381970, -1.199719254218440723 ) ) ;
#93677=CARTESIAN_POINT ( 'NONE',  ( -10.49364770729726359, 11.34493653470939023, 0.7216878364870438212 ) ) ;
#93679=DIRECTION ( 'NONE',  ( 0.000000000000000000, 8.546850786086437571E-32, 1.000000000000000000 ) ) ;
#93684=CARTESIAN_POINT ( 'NONE',  ( -5.656850995454980158, 6.308143005704411443, 1.156498089891801140 ) ) ;
#93685=CARTESIAN_POINT ( 'NONE',  ( -0.6823417656250212460, 2.051041667008083991, 1.181850606188767472 ) ) ;
#93688=CARTESIAN_POINT ( 'NONE',  ( 7.293923454472091450, 7.611924906413328529, 0.7216878364870317197 ) ) ;
#93707=CARTESIAN_POINT ( 'NONE',  ( 7.397945374551106568, 11.78268670361832093, -0.7998128361456291469 ) ) ;
#93711=CARTESIAN_POINT ( 'NONE',  ( -4.111146893441842920, 5.819424013814012753, 1.599625672291267398 ) ) ;
#93712=CARTESIAN_POINT ( 'NONE',  ( -7.157815033010924921, 10.43820240756634199, 1.199719254218453823 ) ) ;
#93714=VERTEX_POINT ( 'NONE', #32501 ) ;
#93717=CARTESIAN_POINT ( 'NONE',  ( -1.499999999999997780, 4.931250000682820378, 1.214306433183764966E-14 ) ) ;
#93718=CARTESIAN_POINT ( 'NONE',  ( 7.507464373665139412, 9.781794407407920389, 1.599625672291281386 ) ) ;
#93722=CARTESIAN_POINT ( 'NONE',  ( -6.516665389662827934, 10.75452672124865217, 0.000000000000000000 ) ) ;
#93724=CARTESIAN_POINT ( 'NONE',  ( 1.364683531249988535, 4.113541667008088432, 0.7879004041258500513 ) ) ;
#93729=CARTESIAN_POINT ( 'NONE',  ( -7.944714827928056167, 10.29191993738131927, 1.443375672974090751 ) ) ;
#93733=CARTESIAN_POINT ( 'NONE',  ( -1.201851678989727383E-14, 2.759375000341417916, -1.575800808251660134 ) ) ;
#93741=CARTESIAN_POINT ( 'NONE',  ( -1.201851678989727383E-14, 3.071875000341420137, 1.575800808251672791 ) ) ;
#93743=CARTESIAN_POINT ( 'NONE',  ( -3.978428010606240850, 6.728917548094202949, -1.199719254218452047 ) ) ;
#93744=CARTESIAN_POINT ( 'NONE',  ( 5.587931867126699537, 9.671004278289832001, -0.7998128361456291469 ) ) ;
#93747=CARTESIAN_POINT ( 'NONE',  ( 1.364683531249988535, 4.426041667008082214, 0.7879004041258500513 ) ) ;
#93750=CARTESIAN_POINT ( 'NONE',  ( 1.364683531249986537, -1.136458332991912235, 0.7879004041258500513 ) ) ;
#93751=CARTESIAN_POINT ( 'NONE',  ( -5.612712406377534435, 5.650512016969639895, 0.7216878364870317197 ) ) ;
#93754=CARTESIAN_POINT ( 'NONE',  ( 4.039966587192259873, 5.736380323189513852, 1.443375672974062551 ) ) ;
#93756=CARTESIAN_POINT ( 'NONE',  ( -6.906989191158078079, 10.14557225873805812, -1.199719254218440723 ) ) ;
#93757=CARTESIAN_POINT ( 'NONE',  ( -9.815740026613960723, 11.51441345488021106, -1.082531754730539753 ) ) ;
#93764=CARTESIAN_POINT ( 'NONE',  ( -5.192409643909507544, 9.001635651295671892, 0.7216878364870458196 ) ) ;
#93766=CARTESIAN_POINT ( 'NONE',  ( -1.364683531250000748, 0.8218750003414210248, 0.000000000000000000 ) ) ;
#93772=CARTESIAN_POINT ( 'NONE',  ( -1.402160292154681736E-14, -0.9906249996585834161, -1.575800808251665908 ) ) ;
#93774=CARTESIAN_POINT ( 'NONE',  ( 9.083599731475988648, 10.66024977721925104, 1.082531754730549967 ) ) ;
#93779=CIRCLE ( 'NONE', #187127, 0.07999999999999994615 ) ;
#93782=CARTESIAN_POINT ( 'NONE',  ( -1.500000000000015099, -0.5791666666666476226, 0.8660254037844403729 ) ) ;
#93784=CARTESIAN_POINT ( 'NONE',  ( 7.415946836550712185, 10.63539316174243865, 1.082531754730558626 ) ) ;
#93792=CARTESIAN_POINT ( 'NONE',  ( 5.555090253297246150, 7.504024600312024340, 1.599625672291267398 ) ) ;
#93794=CARTESIAN_POINT ( 'NONE',  ( -4.386226389220933441, 5.076017861301227008, -1.199719254218446718 ) ) ;
#93796=LINE ( 'NONE', #65500, #27976 ) ;
#93797=CARTESIAN_POINT ( 'NONE',  ( 0.6823417656249899377, 1.405208333674752508, 1.181850606188755259 ) ) ;
#93799=CARTESIAN_POINT ( 'NONE',  ( -9.006694118179950692, 9.402231314165087284, 1.040834085586084257E-14 ) ) ;
#93816=CARTESIAN_POINT ( 'NONE',  ( 6.681470773436232413, 6.689470745297396270, -0.7998128361456281477 ) ) ;
#93824=CARTESIAN_POINT ( 'NONE',  ( 7.853197290813620945, 10.18514947741448573, 1.599625672291281386 ) ) ;
#93827=CARTESIAN_POINT ( 'NONE',  ( 8.235688245297327015, 11.69572115523387268, -1.199719254218446718 ) ) ;
#93832=EDGE_LOOP ( 'NONE', ( #66548, #113557, #37998, #109824, #19441 ) ) ;
#93835=CARTESIAN_POINT ( 'NONE',  ( 4.016103985132956744, 7.694334506561854248, -0.3640553937371555082 ) ) ;
#93842=CARTESIAN_POINT ( 'NONE',  ( -7.700668062882065179, 10.96756792579566664, -1.082531754730543971 ) ) ;
#93847=CARTESIAN_POINT ( 'NONE',  ( 5.443762371086860341, 6.309809840144842141, 1.199719254218462483 ) ) ;
#93854=CARTESIAN_POINT ( 'NONE',  ( 3.999292125906905859, 5.688926785023260102, 1.443375672974062551 ) ) ;
#93862=CARTESIAN_POINT ( 'NONE',  ( -6.227272627378437342, 6.159572908229946187, -0.7998128361456291469 ) ) ;
#93864=CARTESIAN_POINT ( 'NONE',  ( -4.460796234096120472, 5.163016013655583158, 1.199719254218462483 ) ) ;
#93874=CARTESIAN_POINT ( 'NONE',  ( 6.148786358997489820, 7.132337826040578754, -1.199719254218446718 ) ) ;
#93876=CARTESIAN_POINT ( 'NONE',  ( 1.576106191276486213, 8.678179183658462748, 2.499999999999318767 ) ) ;
#93888=CARTESIAN_POINT ( 'NONE',  ( -1.364683531250000748, 1.821875000341421913, 0.000000000000000000 ) ) ;
#93889=CARTESIAN_POINT ( 'NONE',  ( 3.816783937446950770, 4.411668334231586996, 1.199719254218464037 ) ) ;
#93890=CARTESIAN_POINT ( 'NONE',  ( 3.623053363349855172, 5.249981562040033189, 1.599625672291267398 ) ) ;
#93893=CARTESIAN_POINT ( 'NONE',  ( -6.616015773788831211, 7.781401826584148473, 1.082531754730549967 ) ) ;
#93894=CARTESIAN_POINT ( 'NONE',  ( 3.551873057100274789, 7.087676300018221021, 0.7216878364870298324 ) ) ;
#93895=CARTESIAN_POINT ( 'NONE',  ( -6.195713011320790109, 9.211787032307496403, -1.082531754730537976 ) ) ;
#93897=EDGE_LOOP ( 'NONE', ( #59705, #121406, #205426, #130842 ) ) ;
#93899=CARTESIAN_POINT ( 'NONE',  ( 5.099838337034727331, 9.101561826515851550, -0.7998128361456281477 ) ) ;
#93904=CARTESIAN_POINT ( 'NONE',  ( -1.364683531249997417, 4.509375000341424133, 1.214306433183764966E-14 ) ) ;
#93909=CARTESIAN_POINT ( 'NONE',  ( 6.307567778855705853, 8.381915046796901692, -1.599625672291262513 ) ) ;
#93911=CARTESIAN_POINT ( 'NONE',  ( -8.376239975144482486, 8.666701480623698828, 1.040834085586084257E-14 ) ) ;
#93916=CARTESIAN_POINT ( 'NONE',  ( 9.250740883225924804, 9.686952540052077509, 1.040834085586084257E-14 ) ) ;
#93918=B_SPLINE_CURVE_WITH_KNOTS ( 'NONE', 3,
 ( #95434, #80211, #125857, #211267, #94361, #61836, #9876, #44539, #192882, #142055 ),
 .UNSPECIFIED., .F., .F.,
 ( 4, 2, 2, 2, 4 ),
 ( 0.001603296788734610108, 0.001976506518550216057, 0.002349716248365820923, 0.002722925978181425788, 0.003096135707997031087 ),
 .UNSPECIFIED. ) ;
#93919=CARTESIAN_POINT ( 'NONE',  ( -7.609150525767646833, 9.900428251527500834, -1.599625672291263179 ) ) ;
#93921=CARTESIAN_POINT ( 'NONE',  ( 6.575341312503417690, 10.61505593132193326, -0.7216878364870267237 ) ) ;
#93922=CARTESIAN_POINT ( 'NONE',  ( 3.998447120444656555, 7.829958269474884602, 0.005269623924535754567 ) ) ;
#93923=CARTESIAN_POINT ( 'NONE',  ( -7.700668062882059850, 11.92793714009701311, -0.7216878364870267237 ) ) ;
#93927=CARTESIAN_POINT ( 'NONE',  ( 4.286349120214771879, 8.152491073559232859, -0.7998128361456221525 ) ) ;
#93929=CARTESIAN_POINT ( 'NONE',  ( 8.055515824813896941, 12.54985222892493368, 0.7998128361456462443 ) ) ;
#93930=CARTESIAN_POINT ( 'NONE',  ( -5.312135015290653683, 6.384990658495349081, 1.125702006352300000 ) ) ;
#93931=CARTESIAN_POINT ( 'NONE',  ( 4.369805582306193870, 3.992528022312320957, 1.214306433183764966E-14 ) ) ;
#93932=CARTESIAN_POINT ( 'NONE',  ( 0.6823417656249882723, 0.9260416670080831025, -1.181850606188749264 ) ) ;
#93934=CARTESIAN_POINT ( 'NONE',  ( -7.104109303880803417, 8.350844278358124484, 1.082531754730549967 ) ) ;
#93935=ORIENTED_EDGE ( 'NONE', *, *, #211621, .T. ) ;
#93942=CARTESIAN_POINT ( 'NONE',  ( -4.471757287801709779, 7.078374187635557924, 1.125421738336473299 ) ) ;
#93943=CARTESIAN_POINT ( 'NONE',  ( -1.402160292154681736E-14, -0.2406249996585799189, -1.575800808251665908 ) ) ;
#93946=CARTESIAN_POINT ( 'NONE',  ( 3.877268743828270470, 5.546566172598190292, 1.443375672974062551 ) ) ;
#93950=CARTESIAN_POINT ( 'NONE',  ( -7.117667457050096402, 10.28740055232499984, 1.082531754730549967 ) ) ;
#93955=CARTESIAN_POINT ( 'NONE',  ( -8.961576348508652146, 10.51788916375733685, -1.082531754730543083 ) ) ;
#93961=EDGE_LOOP ( 'NONE', ( #5369, #105032, #40808, #214213, #191258 ) ) ;
#93962=CARTESIAN_POINT ( 'NONE',  ( -9.463228032214294316, 10.14278024711257764, 1.040834085586084257E-14 ) ) ;
#93966=CARTESIAN_POINT ( 'NONE',  ( -0.6823417656249969321, 5.780208333674756283, -1.181850606188749264 ) ) ;
#93967=CARTESIAN_POINT ( 'NONE',  ( 1.499999999999990896, 4.556250000682819490, 1.214306433183764966E-14 ) ) ;
#93968=CARTESIAN_POINT ( 'NONE',  ( 4.930363510330384003, 6.858250545851714008, -1.424563464522425882 ) ) ;
#93970=CARTESIAN_POINT ( 'NONE',  ( -1.403499169902660437, 7.376709478543006071, -4.304123474984413278 ) ) ;
#93975=CARTESIAN_POINT ( 'NONE',  ( -6.347188469492005325, 10.55680364771601809, -0.7998128361456291469 ) ) ;
#93979=CARTESIAN_POINT ( 'NONE',  ( 3.985207087413062066, 6.736826471035503694, -1.199719254218452047 ) ) ;
#93984=CARTESIAN_POINT ( 'NONE',  ( 7.579171565239241737, 8.801120566655981747, 1.199719254218462483 ) ) ;
#93988=ORIENTED_EDGE ( 'NONE', *, *, #144354, .F. ) ;
#93991=CARTESIAN_POINT ( 'NONE',  ( -6.751597309925468693, 6.979211071108916364, 0.7216878364870317197 ) ) ;
#93994=CARTESIAN_POINT ( 'NONE',  ( -4.197870329852986693, 3.573279226090503080, -2.499999999999996003 ) ) ;
#94002=CARTESIAN_POINT ( 'NONE',  ( -9.236128959407555072, 11.79856975744075598, -1.599625672291263179 ) ) ;
#94004=CARTESIAN_POINT ( 'NONE',  ( 9.043452155515161905, 10.50944792197790889, 1.199719254218453823 ) ) ;
#94005=CARTESIAN_POINT ( 'NONE',  ( -1.500000000000015099, -0.3708333333333105331, -0.8660254037844383745 ) ) ;
#94006=CARTESIAN_POINT ( 'NONE',  ( -8.045874094706015001, 11.47427131287732927, -1.199719254218446718 ) ) ;
#94009=CARTESIAN_POINT ( 'NONE',  ( -0.6823417656250212460, 3.551041667008085323, 1.181850606188767472 ) ) ;
#94010=CARTESIAN_POINT ( 'NONE',  ( 2.846322183865124700, 5.408127416896231665, -1.199719254218446718 ) ) ;
#94012=LINE ( 'NONE', #77728, #26214 ) ;
#94013=CARTESIAN_POINT ( 'NONE',  ( 0.7499999999999902300, 4.816666666666684193, -1.299038105676658228 ) ) ;
#94016=CARTESIAN_POINT ( 'NONE',  ( 8.880227426826646564, 9.462612874160329923, 0.7216878364870458196 ) ) ;
#94019=CARTESIAN_POINT ( 'NONE',  ( -5.694061328059534688, 8.626526735169329996, 1.082531754730548412 ) ) ;
#94020=CARTESIAN_POINT ( 'NONE',  ( 1.364683531249988757, 1.634375000341421691, 0.000000000000000000 ) ) ;
#94024=CARTESIAN_POINT ( 'NONE',  ( -5.831978632172702071, 9.955725504176825780, 0.7998128361456481317 ) ) ;
#94025=CARTESIAN_POINT ( 'NONE',  ( 1.364683531249988535, 4.176041667008081326, 0.7879004041258500513 ) ) ;
#94032=CARTESIAN_POINT ( 'NONE',  ( 7.910292558569346433, 11.31609285405122556, -1.199719254218446718 ) ) ;
#94035=CARTESIAN_POINT ( 'NONE',  ( 0.7499999999999885647, 0.7333333333333567072, 1.299038105676657340 ) ) ;
#94039=AXIS2_PLACEMENT_3D ( 'NONE', #124481, #7416, #57262 ) ;
#94040=CARTESIAN_POINT ( 'NONE',  ( 9.856941372335116469, 11.45851867493453291, 1.199719254218450271 ) ) ;
#94044=CARTESIAN_POINT ( 'NONE',  ( 7.079328764629950754, 11.41096732537697633, 0.7998128361456462443 ) ) ;
#94045=CARTESIAN_POINT ( 'NONE',  ( -1.506030227042769010, 8.670273769332156988, 2.548074190919186410 ) ) ;
#94048=CARTESIAN_POINT ( 'NONE',  ( -1.364683531250010295, 5.551041667008087543, -0.7879004041258300672 ) ) ;
#94052=CARTESIAN_POINT ( 'NONE',  ( 8.718056468787178659, 10.12981962079525289, 1.199719254218462483 ) ) ;
#94055=CARTESIAN_POINT ( 'NONE',  ( -1.364683531250012516, 4.238541667008090208, -0.7879004041258300672 ) ) ;
#94057=CARTESIAN_POINT ( 'NONE',  ( -6.155038550924159857, 8.203964280876741455, 1.443375672974078761 ) ) ;
#94064=CARTESIAN_POINT ( 'NONE',  ( 3.728655938958122196, 4.308852335994623139, -1.199719254218446718 ) ) ;
#94067=CARTESIAN_POINT ( 'NONE',  ( 8.646349277213076334, 11.11049346154719508, 1.599625672291281386 ) ) ;
#94073=CARTESIAN_POINT ( 'NONE',  ( -7.700141177557535244, 11.07091624287075859, -1.199719254218446718 ) ) ;
#94074=CIRCLE ( 'NONE', #17952, 0.08000000000000041800 ) ;
#94075=CARTESIAN_POINT ( 'NONE',  ( 6.982612806237943559, 8.105135347821125436, -1.199719254218446718 ) ) ;
#94078=CARTESIAN_POINT ( 'NONE',  ( 3.917943204224906939, 5.594019709727598766, -1.443375672974051449 ) ) ;
#94080=CARTESIAN_POINT ( 'NONE',  ( 3.161022370280501814, 6.839609865302569425, 0.000000000000000000 ) ) ;
#94089=CARTESIAN_POINT ( 'NONE',  ( -5.992340707560165569, 8.014150130285418783, 1.443375672974064550 ) ) ;
#94090=CARTESIAN_POINT ( 'NONE',  ( 4.142179624174931796, 4.791296635414242111, 1.199719254218464037 ) ) ;
#94093=CARTESIAN_POINT ( 'NONE',  ( -7.640183256500752584, 8.872300873127729304, -1.199719254218446718 ) ) ;
#94097=LINE ( 'NONE', #31212, #171409 ) ;
#94099=CARTESIAN_POINT ( 'NONE',  ( -9.155833807930273238, 9.576227618873799585, -0.7998128361456291469 ) ) ;
#94103=CARTESIAN_POINT ( 'NONE',  ( 8.769426429940780920, 9.125419011219408461, 0.7998128361456462443 ) ) ;
#94104=EDGE_CURVE ( 'NONE', #113693, #190459, #105776, .T. ) ;
#94116=CARTESIAN_POINT ( 'NONE',  ( -8.019811557683421910, 9.315200557840817908, 1.199719254218462483 ) ) ;
#94120=CARTESIAN_POINT ( 'NONE',  ( 5.653386867218496370, 9.539442411822841805, 1.040834085586084257E-14 ) ) ;
#94126=CARTESIAN_POINT ( 'NONE',  ( -5.551173829791513192, 8.563787670477010394, 1.199719254218452047 ) ) ;
#94135=CARTESIAN_POINT ( 'NONE',  ( -9.236128959407555072, 11.79856975744075598, -1.599625672291263179 ) ) ;
#94136=CARTESIAN_POINT ( 'NONE',  ( 7.239163954692881653, 10.53310948286200599, -1.199719254218441611 ) ) ;
#94138=CARTESIAN_POINT ( 'NONE',  ( -3.551873057100300990, 5.166937871415542283, 1.443375672974064550 ) ) ;
#94140=VECTOR ( 'NONE', #134213, 1000.000000000000000 ) ;
#94141=CARTESIAN_POINT ( 'NONE',  ( -5.584559075236136039, 6.202510182859402477, -0.8982034194818852013 ) ) ;
#94147=CARTESIAN_POINT ( 'NONE',  ( 8.595506201383999567, 12.97191496834930113, 0.7216878364870438212 ) ) ;
#94154=CARTESIAN_POINT ( 'NONE',  ( 4.729096653068339151, 4.411700938201493116, -0.7998128361456211532 ) ) ;
#94162=CARTESIAN_POINT ( 'NONE',  ( 4.313465427442102929, 8.184126765324453601, 0.7998128361456462443 ) ) ;
#94166=CARTESIAN_POINT ( 'NONE',  ( -5.610376637956639101, 5.439860920571172542, 0.000000000000000000 ) ) ;
#94167=CARTESIAN_POINT ( 'NONE',  ( 5.544921637864819175, 7.492161215640853023, -1.443375672974057666 ) ) ;
#94168=CARTESIAN_POINT ( 'NONE',  ( -1.500000000000013101, 3.129166666666689967, -0.8660254037844313801 ) ) ;
#94171=CARTESIAN_POINT ( 'NONE',  ( -4.517891501851816649, 6.293959390292322986, -1.599625672291256295 ) ) ;
#94172=CARTESIAN_POINT ( 'NONE',  ( 0.4583599637079645572, 7.954360040268206866, -1.947354497276407415 ) ) ;
#94173=LINE ( 'NONE', #110467, #138763 ) ;
#94175=CARTESIAN_POINT ( 'NONE',  ( -0.6823417656249969321, 4.967708333674755394, -1.181850606188749264 ) ) ;
#94178=CARTESIAN_POINT ( 'NONE',  ( -4.636525346193588248, 4.511627113421689650, 0.7216878364870317197 ) ) ;
#94182=CARTESIAN_POINT ( 'NONE',  ( -1.164422670175135899, 3.300000000000025135, -0.7116747751938151678 ) ) ;
#94183=CARTESIAN_POINT ( 'NONE',  ( 3.194917754314666514, 6.879154480009089134, 0.7998128361456321445 ) ) ;
#94189=CARTESIAN_POINT ( 'NONE',  ( -1.201851678989727383E-14, 1.134375000341418582, 1.575800808251672791 ) ) ;
#94192=CARTESIAN_POINT ( 'NONE',  ( -8.971744963941075568, 11.49012176272984931, 1.599625672291269396 ) ) ;
#94193=CARTESIAN_POINT ( 'NONE',  ( -5.788968402910818156, 7.776882441527838807, 1.443375672974064550 ) ) ;
#94197=CARTESIAN_POINT ( 'NONE',  ( -0.6823417656250212460, 5.051041667008086655, 1.181850606188767472 ) ) ;
#94205=CARTESIAN_POINT ( 'NONE',  ( -7.022760381754429737, 7.295567988242705582, 1.040834085586084257E-14 ) ) ;
#94210=CARTESIAN_POINT ( 'NONE',  ( -7.036318535368094373, 7.311385834125318617, 0.7216878364870317197 ) ) ;
#94213=CARTESIAN_POINT ( 'NONE',  ( -2.298420387838187473, 5.509269730139584986, -0.7346435760097105305 ) ) ;
#94224=CARTESIAN_POINT ( 'NONE',  ( 0.3249880009247422818, 6.544903501124678336, -3.185264000678197149 ) ) ;
#94225=CARTESIAN_POINT ( 'NONE',  ( -5.416646063859567484, 6.278174148379618735, 1.199719254218450271 ) ) ;
#94226=CARTESIAN_POINT ( 'NONE',  ( -4.915125982297082530, 6.864361322996670012, 1.451325963391773888 ) ) ;
#94228=CARTESIAN_POINT ( 'NONE',  ( -1.201851678989727383E-14, 1.212500000000025002, 1.732050807568877637 ) ) ;
#94230=CARTESIAN_POINT ( 'NONE',  ( 9.734391104931955141, 10.45913716528321125, 0.7216878364870438212 ) ) ;
#94231=CARTESIAN_POINT ( 'NONE',  ( 6.632963465583686435, 8.761543347979550589, -1.599625672291262513 ) ) ;
#94236=CARTESIAN_POINT ( 'NONE',  ( 5.678167406024951624, 5.518950149984223508, 0.7998128361456341429 ) ) ;
#94244=CARTESIAN_POINT ( 'NONE',  ( -6.600121851754250812, 6.594563670001734046, 0.7998128361456341429 ) ) ;
#94251=CARTESIAN_POINT ( 'NONE',  ( -1.364683531249997417, 3.259375000341423245, 1.214306433183764966E-14 ) ) ;
#94252=CARTESIAN_POINT ( 'NONE',  ( 8.473482818416664841, 10.90881592628469932, -1.443375672974063439 ) ) ;
#94253=CARTESIAN_POINT ( 'NONE',  ( -6.684333426737305572, 7.757142738403693727, -1.199719254218446718 ) ) ;
#94256=CARTESIAN_POINT ( 'NONE',  ( 7.332262146892202459, 7.448727347662698506, -0.7998128361456281477 ) ) ;
#94257=CARTESIAN_POINT ( 'NONE',  ( -4.225337428953291230, 8.081310767087481750, 0.7998128361456341429 ) ) ;
#94261=CARTESIAN_POINT ( 'NONE',  ( 0.7499999999999885647, 0.5145833340161540814, 1.299038105676657340 ) ) ;
#94264=CARTESIAN_POINT ( 'NONE',  ( 8.107412671292047790, 8.560995659369956101, 0.7216878364870458196 ) ) ;
#94267=CARTESIAN_POINT ( 'NONE',  ( -1.364683531250012516, 2.301041667008087988, -0.7879004041258289570 ) ) ;
#94269=CARTESIAN_POINT ( 'NONE',  ( 4.487385655998867406, 8.179107665399927285, 0.7216878364870438212 ) ) ;
#94271=CARTESIAN_POINT ( 'NONE',  ( -3.131570295076647525, 6.597323077657299528, 1.040834085586084257E-14 ) ) ;
#94276=DIRECTION ( 'NONE',  ( -5.578564026256490882E-16, -1.000000000000000000, -9.066213480720158442E-32 ) ) ;
#94279=CARTESIAN_POINT ( 'NONE',  ( -3.990254785474510513, 7.829054500403880290, -0.2746884413801879976 ) ) ;
#94287=CARTESIAN_POINT ( 'NONE',  ( 5.307127064745490230, 8.279066444590018392, -1.199719254218452935 ) ) ;
#94298=CARTESIAN_POINT ( 'NONE',  ( 4.148431816101584957, 6.823292304551739740, -1.082531754730548412 ) ) ;
#94299=CARTESIAN_POINT ( 'NONE',  ( -0.6823417656250212460, 2.363541667008084435, 1.181850606188767472 ) ) ;
#94300=CARTESIAN_POINT ( 'NONE',  ( 8.860417081730671995, 10.29590700256267155, 1.199719254218453823 ) ) ;
#94303=CARTESIAN_POINT ( 'NONE',  ( -4.822949958159302497, 6.649860922651057216, -1.599625672291256517 ) ) ;
#94307=CARTESIAN_POINT ( 'NONE',  ( 1.499999999999989120, 2.254166666666685970, 0.8660254037844524744 ) ) ;
#94308=CARTESIAN_POINT ( 'NONE',  ( 5.178324605415663306, 8.128796908705222535, 1.199719254218462483 ) ) ;
#94309=CARTESIAN_POINT ( 'NONE',  ( -6.340409392685171674, 10.54889472477470846, 0.7998128361456481317 ) ) ;
#94312=CARTESIAN_POINT ( 'NONE',  ( 0.6823417656249899377, 2.592708333674753618, 1.181850606188767472 ) ) ;
#94315=CARTESIAN_POINT ( 'NONE',  ( 3.684065054611349144, 5.321161868511784299, -1.599625672291262513 ) ) ;
#94321=CARTESIAN_POINT ( 'NONE',  ( -1.402160292154681736E-14, 0.4937500006828175469, 1.732050807568877637 ) ) ;
#94323=CARTESIAN_POINT ( 'NONE',  ( -5.910464900553636269, 8.982960586366182554, -1.199719254218440723 ) ) ;
#94324=CARTESIAN_POINT ( 'NONE',  ( -2.494337075234348777, 5.853884321174607663, -0.7216878364870267237 ) ) ;
#94332=CARTESIAN_POINT ( 'NONE',  ( 4.299907273828439180, 8.168308919441841454, 1.040834085586084257E-14 ) ) ;
#94337=CARTESIAN_POINT ( 'NONE',  ( 5.957918438201454059, 9.038323046955323292, -1.199719254218440723 ) ) ;
#94339=CARTESIAN_POINT ( 'NONE',  ( 3.046854503058775254, 2.800000000000017586, 2.500000000000000444 ) ) ;
#94341=CARTESIAN_POINT ( 'NONE',  ( -4.869349725602420520, 8.832658446511480577, 1.040834085586084257E-14 ) ) ;
#94342=VERTEX_POINT ( 'NONE', #46948 ) ;
#94343=CARTESIAN_POINT ( 'NONE',  ( 2.842405760359353106, 6.467890487061221272, -0.7998128361456291469 ) ) ;
#94344=ORIENTED_EDGE ( 'NONE', *, *, #31584, .T. ) ;
#94348=CARTESIAN_POINT ( 'NONE',  ( 4.662511749779700843, 6.863130753939731932, 1.222702295491843616 ) ) ;
#94357=CARTESIAN_POINT ( 'NONE',  ( -2.982430605326328532, 5.462957558647244305, -1.082531754730543971 ) ) ;
#94358=CARTESIAN_POINT ( 'NONE',  ( 7.944714827928050838, 9.331550723079971021, 1.082531754730558626 ) ) ;
#94360=CARTESIAN_POINT ( 'NONE',  ( -3.418627288940168096, 7.140148937072163804, -0.7998128361456281477 ) ) ;
#94361=CARTESIAN_POINT ( 'NONE',  ( -0.4841690447253781393, 6.868374222573313759, 3.676448113726332068 ) ) ;
#94363=CARTESIAN_POINT ( 'NONE',  ( 7.476431642932036326, 10.80992178580769014, 1.199719254218460707 ) ) ;
#94365=CARTESIAN_POINT ( 'NONE',  ( -4.394814349124112951, 8.279033840620114049, -0.7998128361456281477 ) ) ;
#94379=CARTESIAN_POINT ( 'NONE',  ( 9.398826802771546696, 11.98838390803207865, -1.599625672291262513 ) ) ;
#94380=CARTESIAN_POINT ( 'NONE',  ( -3.893162665418476109, 7.693773542963529444, 1.040834085586084257E-14 ) ) ;
#94383=CARTESIAN_POINT ( 'NONE',  ( 3.931501358282940117, 4.649468341827285300, -1.082531754730543083 ) ) ;
#94387=CARTESIAN_POINT ( 'NONE',  ( -4.322352044658376968, 3.937165561723182883, 0.7998128361456341429 ) ) ;
#94388=CARTESIAN_POINT ( 'NONE',  ( -4.952806187693842510, 4.672695395264567786, 0.7998128361456341429 ) ) ;
#94391=FACE_OUTER_BOUND ( 'NONE', #211778, .T. ) ;
#94392=CARTESIAN_POINT ( 'NONE',  ( 10.07778825365955733, 10.65184113889131012, -0.7998128361456281477 ) ) ;
#94393=CIRCLE ( 'NONE', #174018, 1.250000000000000222 ) ;
#94396=CARTESIAN_POINT ( 'NONE',  ( -8.389798128758148010, 8.682519326506312751, 0.7998128361456462443 ) ) ;
#94397=CARTESIAN_POINT ( 'NONE',  ( 6.471319392424407901, 6.444294134116939077, 0.7998128361456341429 ) ) ;
#94399=CARTESIAN_POINT ( 'NONE',  ( 4.416205349749310116, 6.175325546172741653, 1.599625672291267175 ) ) ;
#94403=CARTESIAN_POINT ( 'NONE',  ( -1.402160292154681736E-14, 0.7593750003414168059, -1.575800808251659024 ) ) ;
#94406=CARTESIAN_POINT ( 'NONE',  ( 8.459924665247367415, 8.972259652317825740, -0.7216878364870267237 ) ) ;
#94407=ORIENTED_EDGE ( 'NONE', *, *, #97869, .T. ) ;
#94413=ORIENTED_EDGE ( 'NONE', *, *, #167966, .F. ) ;
#94414=CARTESIAN_POINT ( 'NONE',  ( 5.666945020832219626, 5.713783400500051179, 0.7216878364870037421 ) ) ;
#94415=ORIENTED_EDGE ( 'NONE', *, *, #174519, .F. ) ;
#94419=CARTESIAN_POINT ( 'NONE',  ( 3.524756749872931305, 7.056040608253012714, -0.7216878364870155105 ) ) ;
#94421=CARTESIAN_POINT ( 'NONE',  ( -9.022061154889962964, 12.61315621642528129, -1.199719254218446718 ) ) ;
#94438=CARTESIAN_POINT ( 'NONE',  ( -0.7500000000000215383, 1.472916667349486008, 1.299038105676659116 ) ) ;
#94444=CARTESIAN_POINT ( 'NONE',  ( 0.7499999999999885647, -0.2666666666666442365, 1.299038105676657340 ) ) ;
#94445=CARTESIAN_POINT ( 'NONE',  ( 7.228468454380276853, 11.58496363008569574, 1.040834085586084257E-14 ) ) ;
#94449=CARTESIAN_POINT ( 'NONE',  ( 2.846322183865124700, 5.408127416896231665, -1.199719254218446718 ) ) ;
#94450=CARTESIAN_POINT ( 'NONE',  ( -5.666945020832185875, 7.634521829102760115, 1.443375672974064550 ) ) ;
#94455=CARTESIAN_POINT ( 'NONE',  ( -7.705111371268023923, 7.883718109434487253, 1.040834085586084257E-14 ) ) ;
#94457=CARTESIAN_POINT ( 'NONE',  ( -1.500000000000001332, 0.9312500006828163812, 0.000000000000000000 ) ) ;
#94466=LINE ( 'NONE', #195147, #172998 ) ;
#94467=CARTESIAN_POINT ( 'NONE',  ( -3.128205532383699694, 2.800000000000122835, -2.480558432692051785 ) ) ;
#94470=CARTESIAN_POINT ( 'NONE',  ( -9.504429378379839477, 11.04725468198666150, 1.199719254218462483 ) ) ;
#94471=CARTESIAN_POINT ( 'NONE',  ( 8.932124273304774320, 9.315233161810734686, 0.7998128361456462443 ) ) ;
#94479=CARTESIAN_POINT ( 'NONE',  ( -7.133561379084627063, 11.47423870890741782, 0.7998128361456481317 ) ) ;
#94487=CARTESIAN_POINT ( 'NONE',  ( 3.344057444064992168, 7.053150784717805877, 1.040834085586084257E-14 ) ) ;
#94491=ORIENTED_EDGE ( 'NONE', *, *, #156739, .T. ) ;
#94492=CARTESIAN_POINT ( 'NONE',  ( -7.947050595904583403, 12.42330946186405249, 0.7998128361456481317 ) ) ;
#94495=CARTESIAN_POINT ( 'NONE',  ( -5.512600778122673795, 6.408089294489160537, -1.271103323116394845 ) ) ;
#94503=CARTESIAN_POINT ( 'NONE',  ( 7.793239369756836510, 7.986534107671458216, 0.7998128361456341429 ) ) ;
#94512=CARTESIAN_POINT ( 'NONE',  ( -1.500000000000015099, 0.4104166673494891726, -0.8660254037844383745 ) ) ;
#94515=CARTESIAN_POINT ( 'NONE',  ( -1.499999999999997558, 8.654128368560041196, -2.562285273914164829 ) ) ;
#94516=CARTESIAN_POINT ( 'NONE',  ( 3.185802909086937973, 6.660594460669328143, 0.7216878364870317197 ) ) ;
#94524=CARTESIAN_POINT ( 'NONE',  ( 4.012850279964918165, 7.625483060026979842, -0.7216878364870197293 ) ) ;
#94529=CARTESIAN_POINT ( 'NONE',  ( 2.806174607904299734, 5.257325561654889512, -1.082531754730543083 ) ) ;
#94536=CARTESIAN_POINT ( 'NONE',  ( 3.446398949047553728, 6.321615207124993141, 1.107993529894048645 ) ) ;
#94537=CARTESIAN_POINT ( 'NONE',  ( -1.364683531250014514, -0.01145833299191483488, -0.7879004041258359514 ) ) ;
#94544=CARTESIAN_POINT ( 'NONE',  ( -5.928993247877788697, 5.811580298812519807, 0.7998128361456341429 ) ) ;
#94547=CARTESIAN_POINT ( 'NONE',  ( -1.500000000000013101, 0.4208333333333572068, 0.8660254037844403729 ) ) ;
#94549=CARTESIAN_POINT ( 'NONE',  ( -1.364683531250014514, -0.9072916663252470482, 0.7879004041258379498 ) ) ;
#94555=CARTESIAN_POINT ( 'NONE',  ( 1.364683531249988757, -0.6156249996585803075, 0.000000000000000000 ) ) ;
#94557=CARTESIAN_POINT ( 'NONE',  ( -8.853638004923878313, 10.28799807962136548, 1.199719254218462483 ) ) ;
#94559=CARTESIAN_POINT ( 'NONE',  ( 1.499999999999990896, 8.627523663848661428, 2.580000000000000515 ) ) ;
#94563=CARTESIAN_POINT ( 'NONE',  ( -1.364683531250014514, 0.09270833367475767028, 0.7879004041258379498 ) ) ;
#94567=CARTESIAN_POINT ( 'NONE',  ( -3.294945724223623085, 7.655198976062502325, 2.499999999999998668 ) ) ;
#94570=CARTESIAN_POINT ( 'NONE',  ( 6.643132081016111634, 9.733775946952057723, 1.082531754730558626 ) ) ;
#94573=CARTESIAN_POINT ( 'NONE',  ( -5.416646063859567484, 6.278174148379618735, 1.199719254218450271 ) ) ;
#94575=CARTESIAN_POINT ( 'NONE',  ( -1.499999999999997780, 4.431250000682819490, 1.214306433183764966E-14 ) ) ;
#94577=CARTESIAN_POINT ( 'NONE',  ( -3.307299406729781399, 5.945934176904983381, -1.199719254218452935 ) ) ;
#94578=CARTESIAN_POINT ( 'NONE',  ( 6.602457619730767391, 7.765583980183128787, 1.082531754730558626 ) ) ;
#94579=CARTESIAN_POINT ( 'NONE',  ( -9.463228032214294316, 10.14278024711257764, 1.040834085586084257E-14 ) ) ;
#94586=CARTESIAN_POINT ( 'NONE',  ( 9.408995418203963013, 12.00024729270324286, 1.443375672974076540 ) ) ;
#94588=CARTESIAN_POINT ( 'NONE',  ( -5.111060722671894929, 5.065251719313053513, 0.000000000000000000 ) ) ;
#94591=ORIENTED_EDGE ( 'NONE', *, *, #52332, .T. ) ;
#94602=CARTESIAN_POINT ( 'NONE',  ( 8.402302512167096893, 10.82577223566020841, -1.599625672291268286 ) ) ;
#94604=AXIS2_PLACEMENT_3D ( 'NONE', #25356, #57862, #91456 ) ;
#94605=CARTESIAN_POINT ( 'NONE',  ( -1.441115678600793926, 8.287243072884518114, 3.161846531485497991 ) ) ;
#94608=CARTESIAN_POINT ( 'NONE',  ( 1.364683531249986537, 0.4052083336747511200, -0.7879004041258309554 ) ) ;
#94609=CARTESIAN_POINT ( 'NONE',  ( 4.039966587192250103, 7.657118751792200584, 0.7216878364870298324 ) ) ;
#94611=CARTESIAN_POINT ( 'NONE',  ( -9.178506806771670412, 9.810605484096178941, 1.040834085586084257E-14 ) ) ;
#94626=ORIENTED_EDGE ( 'NONE', *, *, #144102, .T. ) ;
#94632=CARTESIAN_POINT ( 'NONE',  ( 5.563869425686542414, 6.377698570463163463, -1.204193420357344557 ) ) ;
#94639=CARTESIAN_POINT ( 'NONE',  ( -6.697364695470783502, 10.75741654478384035, 0.7216878364870458196 ) ) ;
#94643=CARTESIAN_POINT ( 'NONE',  ( 7.637320603199683866, 7.804628880021436288, -0.7998128361456281477 ) ) ;
#94644=ADVANCED_FACE ( 'NONE', ( #181137, #177955, #165957 ), #212564, .F. ) ;
#94645=DIRECTION ( 'NONE',  ( 1.000000000000000000, 1.156482317317869753E-15, 0.000000000000000000 ) ) ;
#94647=CARTESIAN_POINT ( 'NONE',  ( -4.086893239515592136, 6.855460315155083251, 1.199719254218464037 ) ) ;
#94651=CARTESIAN_POINT ( 'NONE',  ( -5.413783410558481002, 5.210502155273325720, -0.7998128361456221525 ) ) ;
#94654=CARTESIAN_POINT ( 'NONE',  ( 4.005544317833563461, 6.760553239859419250, -1.199719254218452047 ) ) ;
#94655=CARTESIAN_POINT ( 'NONE',  ( 9.074484886248265880, 9.481320543578137361, 0.7998128361456462443 ) ) ;
#94656=CARTESIAN_POINT ( 'NONE',  ( 0.1613745041668577518, 6.492617261217120017, 3.107428622204797097 ) ) ;
#94659=CARTESIAN_POINT ( 'NONE',  ( 4.133273095458231516, 7.653358944556723387, 0.7702195724684970379 ) ) ;
#94660=CARTESIAN_POINT ( 'NONE',  ( 4.772106882330221289, 6.590544000850479200, -1.443375672974051449 ) ) ;
#94668=CARTESIAN_POINT ( 'NONE',  ( 6.656690234185433042, 7.828855363713562276, -1.082531754730543971 ) ) ;
#94669=CARTESIAN_POINT ( 'NONE',  ( -8.809047120577080392, 11.30030761213851953, 1.599625672291269396 ) ) ;
#94672=CARTESIAN_POINT ( 'NONE',  ( -8.350932551013499960, 11.83017284523606172, -1.199719254218446718 ) ) ;
#94673=CARTESIAN_POINT ( 'NONE',  ( -7.497822643557261024, 8.706213491360317747, -1.199719254218446718 ) ) ;
#94681=CARTESIAN_POINT ( 'NONE',  ( 9.053093885623066939, 11.58502883802551153, -1.599625672291262513 ) ) ;
#94686=CARTESIAN_POINT ( 'NONE',  ( 2.496672843210871129, 6.064535417054653266, -0.7998128361456291469 ) ) ;
#94690=CARTESIAN_POINT ( 'NONE',  ( -0.7500000000000215383, 5.472916667349482900, 1.299038105676671107 ) ) ;
#94696=CARTESIAN_POINT ( 'NONE',  ( 1.499999999999987121, 2.795833333333352488, -0.8660254037844262731 ) ) ;
#94697=CARTESIAN_POINT ( 'NONE',  ( 4.638861114170084399, 8.563755066507100722, 0.7998128361456462443 ) ) ;
#94699=FACE_OUTER_BOUND ( 'NONE', #169669, .T. ) ;
#94700=CARTESIAN_POINT ( 'NONE',  ( 7.239690840017413365, 10.42976116578691403, -1.082531754730537976 ) ) ;
#94701=CARTESIAN_POINT ( 'NONE',  ( -10.26315909542058336, 11.07603315418659840, -0.7216878364870267237 ) ) ;
#94704=CARTESIAN_POINT ( 'NONE',  ( 8.052653171512838881, 11.48218023581863001, -1.199719254218446718 ) ) ;
#94706=CARTESIAN_POINT ( 'NONE',  ( -5.278201874421821316, 5.052323696447222900, 0.7998128361456341429 ) ) ;
#94707=CARTESIAN_POINT ( 'NONE',  ( -1.001543065824772872E-14, 4.993750000682814161, 1.732050807568877637 ) ) ;
#94708=CARTESIAN_POINT ( 'NONE',  ( -0.6823417656250003738, 0.9677083336747521747, -1.181850606188749264 ) ) ;
#94713=CARTESIAN_POINT ( 'NONE',  ( -1.602468905319636405E-14, -1.053124999658583638, -1.575800808251665908 ) ) ;
#94715=CARTESIAN_POINT ( 'NONE',  ( 8.048736748007069508, 12.54194330598362406, -0.7998128361456352531 ) ) ;
#94719=CARTESIAN_POINT ( 'NONE',  ( -3.836594282542926226, 5.499112634431936542, 1.443375672974064550 ) ) ;
#94722=CARTESIAN_POINT ( 'NONE',  ( -5.982172092127739482, 8.002286745614243912, -1.599625672291263179 ) ) ;
#94725=CARTESIAN_POINT ( 'NONE',  ( 3.005103603723342953, 6.657704637652544832, -0.7998128361456291469 ) ) ;
#94731=CARTESIAN_POINT ( 'NONE',  ( 10.18233705906309972, 11.83814697611718714, 1.199719254218450271 ) ) ;
#94734=CARTESIAN_POINT ( 'NONE',  ( -4.042302355168801320, 7.867769847672247074, 0.7998128361456341429 ) ) ;
#94738=CARTESIAN_POINT ( 'NONE',  ( 8.432281472695482449, 11.92507992053172572, 1.199719254218450271 ) ) ;
#94740=CARTESIAN_POINT ( 'NONE',  ( 9.074484886248265880, 9.481320543578137361, 0.7998128361456462443 ) ) ;
#94743=CARTESIAN_POINT ( 'NONE',  ( -4.302014814237876017, 3.913438792899272212, 0.7998128361456341429 ) ) ;
#94746=CARTESIAN_POINT ( 'NONE',  ( -7.477485413136760073, 8.682486722536401302, -1.199719254218446718 ) ) ;
#94750=CARTESIAN_POINT ( 'NONE',  ( -6.112394247781385737, 6.011859825068855301, 0.2949881747824866229 ) ) ;
#94751=CARTESIAN_POINT ( 'NONE',  ( 1.364683531249986537, 1.113541667008082658, 0.7879004041258500513 ) ) ;
#94754=CARTESIAN_POINT ( 'NONE',  ( 6.127922243696800386, 10.09306701771420656, -0.7216878364870267237 ) ) ;
#94761=AXIS2_PLACEMENT_3D ( 'NONE', #123972, #25303, #41588 ) ;
#94771=CARTESIAN_POINT ( 'NONE',  ( 8.127223016387999266, 11.56917838817298616, 1.199719254218460707 ) ) ;
#94775=CARTESIAN_POINT ( 'NONE',  ( -3.653032323878261600, 6.349289246911547835, -1.199719254218452047 ) ) ;
#94776=CARTESIAN_POINT ( 'NONE',  ( -6.482770005628665011, 10.71498210654212002, 0.7998128361456481317 ) ) ;
#94781=CARTESIAN_POINT ( 'NONE',  ( -0.7499999999999972244, 3.889583334016149863, -1.299038105676652011 ) ) ;
#94782=CARTESIAN_POINT ( 'NONE',  ( 7.567422294721922960, 11.98040977715095323, 0.7998128361456462443 ) ) ;
#94785=CARTESIAN_POINT ( 'NONE',  ( -9.013473194986783454, 9.410140237106395134, -0.7998128361456291469 ) ) ;
#94787=CARTESIAN_POINT ( 'NONE',  ( 0.6823417656249899377, 3.676041667008085767, -1.181850606188754593 ) ) ;
#94793=CARTESIAN_POINT ( 'NONE',  ( -8.785320351975364872, 12.23299559640450518, 1.082531754730560403 ) ) ;
#94797=CARTESIAN_POINT ( 'NONE',  ( 0.6823417656249917140, 3.405208333674754506, 1.181850606188765695 ) ) ;
#94805=CARTESIAN_POINT ( 'NONE',  ( 1.364683531249988535, 2.905208333674754506, -0.7879004041258239610 ) ) ;
#94807=CARTESIAN_POINT ( 'NONE',  ( -6.735703387890906946, 6.752742128827836865, -0.7998128361456291469 ) ) ;
#94808=CARTESIAN_POINT ( 'NONE',  ( 5.913327553854682783, 10.05063257947248800, -0.7998128361456291469 ) ) ;
#94811=CARTESIAN_POINT ( 'NONE',  ( 0.6823417656249917140, 3.655208333674754506, 1.181850606188765695 ) ) ;
#94814=CARTESIAN_POINT ( 'NONE',  ( 1.364683531249986537, -0.3864583329919166199, 0.7879004041258500513 ) ) ;
#94815=CARTESIAN_POINT ( 'NONE',  ( -4.826339496784927796, 5.693446170079573321, 1.082531754730560403 ) ) ;
#94818=CARTESIAN_POINT ( 'NONE',  ( 5.016153647376212277, 5.914896012436124728, 1.082531754730558626 ) ) ;
#94821=CARTESIAN_POINT ( 'NONE',  ( -8.389798128758148010, 8.682519326506312751, 0.7998128361456462443 ) ) ;
#94822=CARTESIAN_POINT ( 'NONE',  ( -9.381879110976678149, 11.00824238663667565, 1.082531754730558626 ) ) ;
#94824=CARTESIAN_POINT ( 'NONE',  ( -1.499999999999997780, 4.900000000000022560, 1.214306433183764966E-14 ) ) ;
#94828=CARTESIAN_POINT ( 'NONE',  ( -5.707619481228817904, 8.642344580533519505, -1.082531754730537976 ) ) ;
#94830=CARTESIAN_POINT ( 'NONE',  ( -1.364683531250014514, -0.6572916663252459379, 0.7879004041258379498 ) ) ;
#94844=CARTESIAN_POINT ( 'NONE',  ( 8.717529583462649612, 10.23316793787035195, 1.082531754730558626 ) ) ;
#94852=CARTESIAN_POINT ( 'NONE',  ( 6.311484202361478779, 7.322151976631905868, -1.199719254218446718 ) ) ;
#94853=CARTESIAN_POINT ( 'NONE',  ( -4.497554271431319250, 6.270232621468402989, -1.599625672291256295 ) ) ;
#94857=CARTESIAN_POINT ( 'NONE',  ( 0.6823417656249899377, 2.155208333674753174, 1.181850606188767472 ) ) ;
#94859=CARTESIAN_POINT ( 'NONE',  ( -9.643927338022246332, 10.14567007064778004, -0.7998128361456291469 ) ) ;
#94879=CARTESIAN_POINT ( 'NONE',  ( 6.928380191783277908, 8.041863964290678624, 1.199719254218462483 ) ) ;
#94884=CARTESIAN_POINT ( 'NONE',  ( 4.856179778084614540, 5.010200168423447842, 0.6077543439236311462 ) ) ;
#94889=CARTESIAN_POINT ( 'NONE',  ( 9.531545685607134999, 11.07889037375188401, 1.199719254218450271 ) ) ;
#94891=CARTESIAN_POINT ( 'NONE',  ( -1.499999999999972689, 3.879166666666685082, -0.8660254037844548058 ) ) ;
#94897=CARTESIAN_POINT ( 'NONE',  ( -0.1479172090191771538, 8.281400213891689788, 2.000566733410582110 ) ) ;
#94903=CARTESIAN_POINT ( 'NONE',  ( -8.270110514656041190, 10.67154823856396817, 1.443375672974090751 ) ) ;
#94909=CARTESIAN_POINT ( 'NONE',  ( 4.286349120214771879, 8.152491073559232859, -0.7998128361456221525 ) ) ;
#94917=CARTESIAN_POINT ( 'NONE',  ( 4.080641047588898118, 5.783833860318930320, -1.443375672974051449 ) ) ;
#94925=CARTESIAN_POINT ( 'NONE',  ( -6.880926654135487652, 7.986501503701545879, 1.199719254218450271 ) ) ;
#94927=CARTESIAN_POINT ( 'NONE',  ( -3.918470089549458635, 4.530302178351167441, -1.199719254218452047 ) ) ;
#94932=CARTESIAN_POINT ( 'NONE',  ( -0.001026545178582605970, 7.078193277237621928, 2.121339347286388399 ) ) ;
#94935=CARTESIAN_POINT ( 'NONE',  ( 5.799137018343234473, 7.788745826199009237, -1.599625672291262513 ) ) ;
#94936=CARTESIAN_POINT ( 'NONE',  ( 4.080641032480825103, 5.783833874167997102, -1.249999999999999334 ) ) ;
#94937=CARTESIAN_POINT ( 'NONE',  ( 5.517805331081858888, 5.539787095791365523, 1.040834085586084257E-14 ) ) ;
#94948=CARTESIAN_POINT ( 'NONE',  ( -0.6823417656250003738, 0.03020833367475134201, -1.181850606188749264 ) ) ;
#94950=CARTESIAN_POINT ( 'NONE',  ( 5.027376032568989572, 4.759693547618927489, 0.7998128361456341429 ) ) ;
#94952=CARTESIAN_POINT ( 'NONE',  ( -5.260200412422196159, 9.080724881227137502, -0.7216878364870207285 ) ) ;
#94953=CARTESIAN_POINT ( 'NONE',  ( 4.365362273920244007, 6.116008624372160973, 1.443375672974062551 ) ) ;
#94954=CARTESIAN_POINT ( 'NONE',  ( -6.493992390821436977, 10.52014885602626393, 0.7216878364870458196 ) ) ;
#94958=CARTESIAN_POINT ( 'NONE',  ( 5.612185521052973414, 8.634967976948757951, -1.199719254218440723 ) ) ;
#94962=CARTESIAN_POINT ( 'NONE',  ( -3.619663825168619731, 7.166765529431275539, 1.040834085586084257E-14 ) ) ;
#94963=CARTESIAN_POINT ( 'NONE',  ( -1.201851678989727383E-14, 4.946875000341420581, -1.575800808251660134 ) ) ;
#94968=CARTESIAN_POINT ( 'NONE',  ( 6.714312387265682247, 8.856450423275211037, 1.599625672291281386 ) ) ;
#94973=CARTESIAN_POINT ( 'NONE',  ( -6.042130013184518589, 10.20090211535728031, -0.7998128361456291469 ) ) ;
#94978=CARTESIAN_POINT ( 'NONE',  ( 8.751951852821344247, 10.16936423550178503, -1.199719254218446718 ) ) ;
#94981=CARTESIAN_POINT ( 'NONE',  ( -7.690499447449645309, 9.995335326823163058, 1.599625672291295375 ) ) ;
#94984=CARTESIAN_POINT ( 'NONE',  ( 7.632877294369377452, 8.967740267261513409, -1.082531754730537976 ) ) ;
#94985=CARTESIAN_POINT ( 'NONE',  ( 4.118656133465138147, 7.671478758617087834, -0.7332979114653701558 ) ) ;
#94986=CARTESIAN_POINT ( 'NONE',  ( -8.026063749610043985, 12.30756544127966912, -0.7216878364870267237 ) ) ;
#94991=CARTESIAN_POINT ( 'NONE',  ( 7.122110765880372618, 7.203550736482235095, 0.7998128361456341429 ) ) ;
#94993=CARTESIAN_POINT ( 'NONE',  ( 9.738834413317897898, 10.25639499182604730, 0.000000000000000000 ) ) ;
#94994=CARTESIAN_POINT ( 'NONE',  ( -4.471757287801709779, 7.078374187635557924, 1.125421738336473299 ) ) ;
#94995=CARTESIAN_POINT ( 'NONE',  ( 4.090809663021327758, 5.795697244990093644, 1.599625672291267398 ) ) ;
#94997=CARTESIAN_POINT ( 'NONE',  ( -7.375272376154101472, 7.706831981708990753, -0.7216878364870278340 ) ) ;
#95003=CARTESIAN_POINT ( 'NONE',  ( -4.868194452378435955, 6.719997196398590056, 1.250117667640719077 ) ) ;
#95004=CARTESIAN_POINT ( 'NONE',  ( -1.364683531250014514, 0.5510416670080878765, -0.7879004041258289570 ) ) ;
#95007=CARTESIAN_POINT ( 'NONE',  ( 3.226477370372293763, 6.708047998835573900, 0.7216878364870317197 ) ) ;
#95008=CARTESIAN_POINT ( 'NONE',  ( -1.201851678989727383E-14, 3.618750000682816381, -1.732050807568863648 ) ) ;
#95011=CARTESIAN_POINT ( 'NONE',  ( -9.937763408692600109, 10.69640485300394417, -0.7216878364870267237 ) ) ;
#95016=CARTESIAN_POINT ( 'NONE',  ( -9.612367721964622191, 10.31677655182129527, -0.7216878364870267237 ) ) ;
#95018=ORIENTED_EDGE ( 'NONE', *, *, #77726, .F. ) ;
#95023=CARTESIAN_POINT ( 'NONE',  ( -8.229436053370685400, 10.62409470039771442, 1.443375672974090751 ) ) ;
#95027=CARTESIAN_POINT ( 'NONE',  ( 1.364683531249990311, 5.176041667008085767, 0.7879004041258500513 ) ) ;
#95028=CARTESIAN_POINT ( 'NONE',  ( -1.201851678989727383E-14, 3.618750000682816381, -1.732050807568863648 ) ) ;
#95029=CARTESIAN_POINT ( 'NONE',  ( 5.634486230560368902, 6.328851001874927107, -1.145628596103397623 ) ) ;
#95034=CARTESIAN_POINT ( 'NONE',  ( -7.049349804101573191, 10.31165964050546258, -1.199719254218440723 ) ) ;
#95038=CARTESIAN_POINT ( 'NONE',  ( 4.202137545231717120, 6.989912005157271402, 1.199719254218462483 ) ) ;
#95044=CARTESIAN_POINT ( 'NONE',  ( 6.421758314367153275, 10.64380180007036891, -0.7998128361456291469 ) ) ;
#95051=CARTESIAN_POINT ( 'NONE',  ( -6.236387472606153892, 8.298871356172400127, -1.443375672974059665 ) ) ;
#95059=CARTESIAN_POINT ( 'NONE',  ( 1.387358672525639269, 7.251968950354889643, 4.302625267139791987 ) ) ;
#95063=CARTESIAN_POINT ( 'NONE',  ( -9.287498920561160887, 10.79416914786490089, -1.199719254218441611 ) ) ;
#95066=CARTESIAN_POINT ( 'NONE',  ( 7.425061681778431399, 11.81432239538354345, 0.7998128361456462443 ) ) ;
#95067=CARTESIAN_POINT ( 'NONE',  ( -1.500000000000015099, -0.8708333333333129200, -0.8660254037844383745 ) ) ;
#95068=CARTESIAN_POINT ( 'NONE',  ( -9.664264568442742842, 10.16939683947169115, -0.7998128361456291469 ) ) ;
#95071=CARTESIAN_POINT ( 'NONE',  ( 1.364683531249990311, 2.884375000341422801, 1.214306433183764966E-14 ) ) ;
#95072=CARTESIAN_POINT ( 'NONE',  ( 4.681643115420508039, 4.356338477612361260, 0.7998128361456341429 ) ) ;
#95075=CARTESIAN_POINT ( 'NONE',  ( 0.7499999999999920064, 4.983333333333353821, 1.299038105676669330 ) ) ;
#95077=CARTESIAN_POINT ( 'NONE',  ( -2.482948226198895103, 5.072301959192136778, 2.420000000000010587 ) ) ;
#95078=CARTESIAN_POINT ( 'NONE',  ( 8.392133896734668141, 9.853539636687704828, 1.082531754730558626 ) ) ;
#95082=CARTESIAN_POINT ( 'NONE',  ( -5.083944415444539899, 8.875092884753202682, 0.000000000000000000 ) ) ;
#95083=CARTESIAN_POINT ( 'NONE',  ( 1.364683531249986537, 1.155208333674754728, -0.7879004041258239610 ) ) ;
#95087=CARTESIAN_POINT ( 'NONE',  ( -8.193204901359996128, 8.453160561208463264, 1.040834085586084257E-14 ) ) ;
#95088=CARTESIAN_POINT ( 'NONE',  ( -4.731432421044888592, 4.622352034081546712, -0.7216878364870207285 ) ) ;
#95089=CARTESIAN_POINT ( 'NONE',  ( -1.201851678989727383E-14, 4.759375000341419693, -1.575800808251660134 ) ) ;
#95094=CARTESIAN_POINT ( 'NONE',  ( 10.08456733046637765, 10.65975006183261087, 0.000000000000000000 ) ) ;
#95101=CARTESIAN_POINT ( 'NONE',  ( 8.238550898598388628, 12.76339314834017102, 0.7998128361456462443 ) ) ;
#95106=CARTESIAN_POINT ( 'NONE',  ( 7.618792255875527886, 10.97600916757510170, 1.199719254218460707 ) ) ;
#95107=CARTESIAN_POINT ( 'NONE',  ( -1.550536438491968427, 8.693843051952859113, 2.505472492508749038 ) ) ;
#95109=CARTESIAN_POINT ( 'NONE',  ( -0.6823417656249969321, 5.530208333674756283, -1.181850606188749264 ) ) ;
#95113=ADVANCED_FACE ( 'NONE', ( #176911 ), #180780, .T. ) ;
#95115=CARTESIAN_POINT ( 'NONE',  ( 6.936968151686458306, 11.24487994360957188, 0.7998128361456462443 ) ) ;
#95118=CARTESIAN_POINT ( 'NONE',  ( 1.364683531249988535, 3.863541667008087543, 0.7879004041258500513 ) ) ;
#95120=CARTESIAN_POINT ( 'NONE',  ( -6.575341312947811545, 6.773579074634973551, 1.040834085586084257E-14 ) ) ;
#95122=FACE_OUTER_BOUND ( 'NONE', #26784, .T. ) ;
#95126=CARTESIAN_POINT ( 'NONE',  ( 3.541704441667858472, 5.155074486744371853, -1.599625672291262513 ) ) ;
#95129=CARTESIAN_POINT ( 'NONE',  ( 9.562578416340237197, 10.05076299535211781, 0.7998128361456462443 ) ) ;
#95130=CARTESIAN_POINT ( 'NONE',  ( 5.736990052193561063, 5.898621588832019036, -2.499999999999135802 ) ) ;
#95135=CARTESIAN_POINT ( 'NONE',  ( -9.541187415715041809, 12.15447128979948310, -1.599625672291263179 ) ) ;
#95136=CARTESIAN_POINT ( 'NONE',  ( 5.982172092127724383, 8.002286745614243912, -1.599625672291262513 ) ) ;
#95139=CARTESIAN_POINT ( 'NONE',  ( 3.147464216666835402, 6.823792019419957278, -0.7998128361456291469 ) ) ;
#95147=CARTESIAN_POINT ( 'NONE',  ( -6.724481002698130538, 7.907944593645035880, -1.082531754730544860 ) ) ;
#95148=CARTESIAN_POINT ( 'NONE',  ( 3.714044015139744914, 6.420469553383295391, 1.199719254218462483 ) ) ;
#95151=CARTESIAN_POINT ( 'NONE',  ( -7.344766530301162000, 9.591980256816594164, 1.599625672291295375 ) ) ;
#95158=CARTESIAN_POINT ( 'NONE',  ( -10.62011439820619429, 11.28455497419572318, -0.7998128361456221525 ) ) ;
#95161=EDGE_CURVE ( 'NONE', #27525, #109221, #38432, .T. ) ;
#95163=CARTESIAN_POINT ( 'NONE',  ( 7.446452682403650769, 9.710614100936176385, -1.599625672291262513 ) ) ;
#95164=CARTESIAN_POINT ( 'NONE',  ( 5.799137018343234473, 7.788745826199009237, -1.599625672291262513 ) ) ;
#95165=CARTESIAN_POINT ( 'NONE',  ( -2.487170525094521079, 8.243531156566744400, -2.499999999999995559 ) ) ;
#95176=CARTESIAN_POINT ( 'NONE',  ( -8.290974629956718189, 9.631557475493025322, -1.199719254218446718 ) ) ;
#95180=CARTESIAN_POINT ( 'NONE',  ( 6.724481002698112775, 8.868313807946373473, -1.443375672974057666 ) ) ;
#95182=CARTESIAN_POINT ( 'NONE',  ( 4.161989969715261140, 4.726297878971393196, -7.499999999999991118 ) ) ;
#95184=CARTESIAN_POINT ( 'NONE',  ( -6.063521013809733518, 8.097193820909906137, 1.599625672291283607 ) ) ;
#95193=CARTESIAN_POINT ( 'NONE',  ( 3.733524485140252480, 7.410126666105652404, 2.500000000000107025 ) ) ;
#95194=CARTESIAN_POINT ( 'NONE',  ( 7.670162217029129259, 9.971608557999250166, 1.599625672291281386 ) ) ;
#95196=CARTESIAN_POINT ( 'NONE',  ( -4.175548123328963079, 4.934189567714277302, 1.082531754730560403 ) ) ;
#95200=CARTESIAN_POINT ( 'NONE',  ( -5.513283157632952403, 6.248865724650796594, -0.9728955443181900309 ) ) ;
#95208=CARTESIAN_POINT ( 'NONE',  ( 2.333974999846879061, 5.874721266463329705, -0.7998128361456291469 ) ) ;
#95215=CARTESIAN_POINT ( 'NONE',  ( 4.715538499454675403, 4.395883092318884522, 1.214306433183764966E-14 ) ) ;
#95216=CARTESIAN_POINT ( 'NONE',  ( 0.000000000000000000, 0.000000000000000000, 0.000000000000000000 ) ) ;
#95220=CARTESIAN_POINT ( 'NONE',  ( -1.364683531250010295, 4.092708333674751842, 0.7879004041258379498 ) ) ;
#95225=CARTESIAN_POINT ( 'NONE',  ( 4.625302960556422427, 8.547937220624488575, 1.040834085586084257E-14 ) ) ;
#95229=CARTESIAN_POINT ( 'NONE',  ( -5.447678794592645701, 5.250046769979851646, 0.000000000000000000 ) ) ;
#95232=CARTESIAN_POINT ( 'NONE',  ( 4.650083499362856365, 8.368921815991249957, 0.7216878364870438212 ) ) ;
#95233=CARTESIAN_POINT ( 'NONE',  ( -0.7499999999999972244, 3.108333333333358706, -1.299038105676652011 ) ) ;
#95235=CARTESIAN_POINT ( 'NONE',  ( -5.596818484342970912, 5.424043074688562172, -0.7998128361456221525 ) ) ;
#95236=CARTESIAN_POINT ( 'NONE',  ( 0.5049859354315242577, 7.739806959121696472, -1.936057643312006471 ) ) ;
#95238=CARTESIAN_POINT ( 'NONE',  ( -1.364683531250010295, 5.030208333674757171, 0.7879004041258379498 ) ) ;
#95242=CARTESIAN_POINT ( 'NONE',  ( -3.307826292054310890, 5.842585859829892314, -1.082531754730549967 ) ) ;
#95248=CARTESIAN_POINT ( 'NONE',  ( 3.330499290451326200, 7.037332938835193730, -0.7998128361456291469 ) ) ;
#95250=CARTESIAN_POINT ( 'NONE',  ( 0.4588732936604926760, 6.941177952499809400, -3.888237269999677004 ) ) ;
#95251=CARTESIAN_POINT ( 'NONE',  ( -0.6823417656249969321, 4.030208333674754506, -1.181850606188749264 ) ) ;
#95255=CARTESIAN_POINT ( 'NONE',  ( 1.364683531249986537, 1.217708333674754950, -0.7879004041258239610 ) ) ;
#95258=CARTESIAN_POINT ( 'NONE',  ( -9.053093885623068715, 11.58502883802551153, -1.599625672291263179 ) ) ;
#95259=CARTESIAN_POINT ( 'NONE',  ( -6.114364089638801403, 8.156510742710487705, 1.443375672974078761 ) ) ;
#95263=ORIENTED_EDGE ( 'NONE', *, *, #183348, .T. ) ;
#95264=CARTESIAN_POINT ( 'NONE',  ( -1.201851678989727383E-14, 3.821875000341423689, 1.575800808251672791 ) ) ;
#95272=CARTESIAN_POINT ( 'NONE',  ( -5.382223794500835545, 8.262716279350872384, -1.082531754730543971 ) ) ;
#95273=TOROIDAL_SURFACE ( 'NONE', #112631, 0.1600000000000000033, 0.08000000000000000167 ) ;
#95279=CARTESIAN_POINT ( 'NONE',  ( -4.894130264408862452, 7.693273827576896373, -1.082531754730548412 ) ) ;
#95292=CARTESIAN_POINT ( 'NONE',  ( 0.4875569042710574674, 6.863504106564645824, -3.669039421667600998 ) ) ;
#95293=CARTESIAN_POINT ( 'NONE',  ( -4.391951695823077984, 7.211361847513815704, 1.199719254218464037 ) ) ;
#95294=CARTESIAN_POINT ( 'NONE',  ( -4.465841460056652501, 7.274597540891426739, 1.282467851283217275 ) ) ;
#95296=CARTESIAN_POINT ( 'NONE',  ( -1.500000000000013101, 1.379166666666689745, -0.8660254037844313801 ) ) ;
#95298=CARTESIAN_POINT ( 'NONE',  ( 10.07334494527360569, 10.85458331234846696, 0.000000000000000000 ) ) ;
#95299=CARTESIAN_POINT ( 'NONE',  ( 6.337546739384100292, 9.481222731668410120, 1.199719254218460707 ) ) ;
#95304=CARTESIAN_POINT ( 'NONE',  ( 3.571683402196252910, 6.254382171615883834, 1.199719254218462483 ) ) ;
#95305=CARTESIAN_POINT ( 'NONE',  ( -0.1465803529718747722, 8.209140712741593404, -2.038183922479917420 ) ) ;
#95306=ORIENTED_EDGE ( 'NONE', *, *, #64923, .T. ) ;
#95312=CARTESIAN_POINT ( 'NONE',  ( -5.738125327081750271, 7.717565519727259904, 1.599625672291269396 ) ) ;
#95317=CARTESIAN_POINT ( 'NONE',  ( 5.381422217466640845, 4.322449550048925282, -2.440471613107405346 ) ) ;
#95321=CARTESIAN_POINT ( 'NONE',  ( -1.201851678989727383E-14, 2.821875000341418804, 1.575800808251672791 ) ) ;
#95322=CARTESIAN_POINT ( 'NONE',  ( 9.707274797260268429, 10.42750147299956964, 0.000000000000000000 ) ) ;
#95323=CARTESIAN_POINT ( 'NONE',  ( -6.364663046611467756, 9.512858423433634414, 1.199719254218452047 ) ) ;
#95326=CARTESIAN_POINT ( 'NONE',  ( 5.524057522564145728, 8.532151978711786100, 1.199719254218462483 ) ) ;
#95327=CARTESIAN_POINT ( 'NONE',  ( -5.388475986427523345, 8.373973519885682393, 1.199719254218452047 ) ) ;
#95331=CARTESIAN_POINT ( 'NONE',  ( -1.402160292154681736E-14, 0.4937500006828175469, 1.732050807568877637 ) ) ;
#95334=CARTESIAN_POINT ( 'NONE',  ( 6.304178240674458422, 10.29869901418813782, 1.040834085586084257E-14 ) ) ;
#95335=ADVANCED_FACE ( 'NONE', ( #23762 ), #135259, .T. ) ;
#95338=CARTESIAN_POINT ( 'NONE',  ( 0.6823417656249899377, 1.905208333674752952, 1.181850606188755259 ) ) ;
#95340=CARTESIAN_POINT ( 'NONE',  ( 6.792271770322100721, 7.026664608238323950, -0.7216878364870257245 ) ) ;
#95342=CARTESIAN_POINT ( 'NONE',  ( -2.657034918598338180, 6.043698471765932112, -0.7216878364870267237 ) ) ;
#95344=CARTESIAN_POINT ( 'NONE',  ( -0.6823417656249969321, 5.717708333674756283, -1.181850606188749264 ) ) ;
#95349=EDGE_LOOP ( 'NONE', ( #188042, #49853, #143188 ) ) ;
#95350=CARTESIAN_POINT ( 'NONE',  ( -4.172464037091858202, 7.595707080679858336, -0.9154354581521230161 ) ) ;
#95356=CARTESIAN_POINT ( 'NONE',  ( 6.982612806237943559, 8.105135347821125436, -1.199719254218446718 ) ) ;
#95359=CARTESIAN_POINT ( 'NONE',  ( 3.009020027229115879, 5.597941567487558778, -1.199719254218446718 ) ) ;
#95367=CARTESIAN_POINT ( 'NONE',  ( 4.880572111239557920, 4.796348339308675435, -0.7216878364870197293 ) ) ;
#95368=CARTESIAN_POINT ( 'NONE',  ( -1.402160292154681736E-14, 2.509375000341417028, -1.575800808251660134 ) ) ;
#95369=CARTESIAN_POINT ( 'NONE',  ( 8.697719238366680372, 10.10609285197134533, 1.199719254218462483 ) ) ;
#95374=( BOUNDED_SURFACE ( )  B_SPLINE_SURFACE ( 1, 2, ( 
 ( #82683, #31826, #81623, #144546, #147707, #162891, #63245, #112073, #148765, #47019, #177002, #213726, #65349, #13419, #98956, #211609, #210553, #49143, #334, #45953, #115259, #14474, #165007, #16601, #62189, #178075, #113134, #30764, #28618, #29693, #127272, #193244, #78424, #94707, #79494, #179141, #96844, #160749, #12344, #195388, #80563, #194312, #146662, #161831, #212676, #64316, #130461, #196451, #48094, #114206, #180204, #149842, #17665, #86962, #37136, #70679, #52331, #101066, #67474, #133620, #136791, #154102, #199622, #202817, #168212, #185512, #54466, #1412, #51268, #118460, #184446, #198551, #183388, #21921, #120610, #83751, #66407, #167153, #36064, #102146, #186587, #103217, #68551, #84825, #50200, #18740, #132552, #151972, #19811, #117392, #34994, #134678, #100012, #38215, #150913, #2474, #153031, #169277, #104288, #85898, #200681, #3546, #69616, #170336, #135725, #201748, #20863, #53389, #88029, #116318, #182309, #4604, #119526, #33938, #166077, #137865, #191908, #106466, #55529, #7825, #72830, #74984, #8904, #206035, #73917, #24079, #43571, #203885, #189789, #171410, #142149, #105372, #71749, #187651, #173582, #174641, #172493, #138933, #121684, #190847, #141092, #109690, #208164, #9970, #27284, #25152, #175694, #91253, #41440, #122766, #207103, #39277, #22999, #90184, #59795, #140010, #125952, #155171, #6755, #92335, #93390, #5671, #89117, #204954, #156247, #56602, #58731, #188726, #40363, #57669, #76047, #123826, #124883, #108614, #107548, #42508, #157313, #26219, #158377, #115004, #79245, #209218, #130208, #64063, #45702, #65103, #29440, #28361, #47843, #60860, #161580, #12102, #14214, #162640, #145364, #13167, #177823, #197246, #77104, #129157, #110749, #81374, #44634, #11026, #127021, #112884, #113954, #111820, #78172, #143228, #196201, #80309, #48885, #147457, #163707, #181002, #178896, #32622, #30510, #195133, #61934, #146409, #192980, #176747, #95531, #213479, #211363, #131259, #94457, #160497, #31573, #159426, #144300, #210293, #128092, #62988, #194050, #212422, #46770, #96591, #179950, #15289, #97648, #3293, #201491, #116062, #69361, #134427, #34740, #83494, #54211, #18490, #148518, #135469, #53137, #199365, #4354, #183134, #182052, #119268, #186325, #17410, #102959, #200430, #185253, #86704, #33682, #149576, #84568, #2219, #16347, #1160, #120349, #152773, #49941, #98699, #51011, #150656, #68294, #70422, #36877, #100813, #117132, #82428, #166898, #164758, #184191, #52076, #67223, #133358, #118203, #132294, #136540, #99757, #165826, #169018, #20616, #202559, #35813, #101890, #167955, #19559, #84, #85635, #151721, #66149, #198300, #75789, #141896, #153848, #190587, #138673, #89928, #157056, #170079, #9713, #204693, #21666, #37960, #71498, #57404, #8645, #106209, #39027, #23823, #121425, #105110, #172235, #140829, #158122, #139751, #188465, #123569, #203625, #155979, #58474, #108357 ),
 ( #7566, #87772, #154914, #207907, #25959, #55276, #104033, #56343, #73652, #205776, #92064, #74724, #40096, #122504, #5419, #189532, #137609, #41180, #107287, #88859, #171150, #173309, #187395, #59528, #22741, #6498, #124629, #206841, #42244, #24888, #72573, #90993, #174379, #125688, #94197, #78975, #96328, #46498, #15027, #81118, #93129, #129956, #77914, #29174, #162383, #109430, #163447, #144033, #27021, #193790, #44369, #112622, #194865, #177562, #45439, #210029, #147204, #175436, #161312, #142961, #113694, #76842, #43311, #159168, #145095, #146148, #61670, #110492, #10767, #13961, #178632, #213229, #179697, #195944, #64861, #211099, #191646, #62723, #12896, #160237, #30244, #208963, #60596, #127838, #31313, #111553, #97391, #126754, #192714, #63798, #176491, #28102, #11836, #95264, #128884, #80045, #212163, #47580, #184999, #84314, #168766, #150399, #100566, #33432, #200179, #196998, #82173, #898, #52883, #133105, #36624, #65899, #132045, #3038, #152520, #119018, #102708, #198054, #17161, #181799, #183945, #16089, #20371, #148267, #201242, #86456, #35555, #19303, #214266, #101635, #166638, #66966, #115811, #4105, #50748, #180748, #167701, #85383, #83235, #131006, #199103, #49684, #151467, #48633, #99509, #135229, #18230, #69107, #114750, #165566, #149320, #116877, #34492, #32375, #182876, #98440, #164505, #1967, #68031, #134171, #51832, #117950, #127319, #109983, #75277, #91552, #202306, #173871, #136286, #158666, #42804, #124119, #206329, #141392, #106761, #61157, #156540, #24362, #93685, #43867, #77404, #59021, #107843, #74216, #140311, #143521, #190082, #174935, #192205, #142446, #111042, #177049, #189018, #11326, #25445, #125177, #175993, #56889, #44934, #157609, #123064, #207402, #57954, #208454, #76339, #191139, #108913, #9205, #28666, #40660, #26516, #90473, #209516, #172790, #8130, #41734, #92624, #27587, #10264, #60086, #126244, #159727, #193289, #94751, #160799, #70174, #33977, #96888, #181293, #31869, #16643, #162937, #161877, #64360, #79540, #212721, #211654, #82727, #63292, #29736, #196493, #145658, #148804, #194356, #100052, #129452, #32920, #98996, #195435, #210602, #47064, #13464, #147751, #373, #14518, #179185, #113181, #30808, #165051, #80612, #130506, #66447, #48135, #62231, #146705, #131537, #114248, #178121, #180245, #97948, #65390, #164002, #15578, #81665, #213769, #132589, #197539, #49184, #115303, #198591, #50238, #116358, #182348, #12390, #78469, #144588, #128389, #45999, #112118, #95818, #121723, #18776, #35029, #170374, #102183, #51305, #133658, #166116, #2514, #137902, #103254, #68587, #120646, #186625, #134712, #200719, #38252, #187688, #104326, #20899, #21961, #71787, #183428, #118499, #199659, #150950, #184481, #201786, #86995, #52370, #83788, #17701, #117430, #185550, #136828, #19849, #167189, #152008, #101102, #84862, #85936, #54502, #203921, #53426, #168250, #37179, #36098 ) ),
 .UNSPECIFIED., .F., .F., .T. ) 
 B_SPLINE_SURFACE_WITH_KNOTS ( ( 2, 2 ),
 ( 3, 2, 2, 2, 2, 2, 2, 2, 2, 2, 2, 2, 2, 2, 2, 2, 2, 2, 2, 2, 2, 2, 2, 2, 2, 2, 2, 2, 2, 2, 2, 2, 2, 2, 2, 2, 2, 2, 2, 2, 2, 2, 2, 2, 2, 2, 2, 2, 2, 2, 2, 2, 2, 2, 2, 2, 2, 2, 2, 2, 2, 2, 2, 2, 2, 2, 2, 2, 2, 2, 2, 2, 2, 2, 2, 2, 2, 2, 2, 2, 2, 2, 2, 2, 2, 2, 2, 2, 2, 2, 2, 2, 2, 2, 2, 2, 2, 2, 2, 2, 2, 2, 2, 2, 2, 2, 2, 2, 2, 2, 2, 2, 2, 2, 2, 2, 2, 2, 2, 2, 2, 2, 2, 2, 2, 2, 2, 2, 2, 2, 2, 2, 2, 2, 2, 2, 2, 2, 2, 2, 2, 2, 2, 2, 2, 2, 2, 2, 2, 2, 2, 2, 2, 2, 2, 2, 2, 2, 2, 2, 2, 2, 2, 2, 2, 2, 2, 2, 3 ),
 ( 0.000000000000000000, 1.000000000000000000 ),
 ( 0.000000000000000000, 0.005952380952380952051, 0.01190476190476190410, 0.01785714285714285615, 0.02380952380952380820, 0.02976190476190476025, 0.03571428571428571230, 0.04166666666666666435, 0.04761904761904761640, 0.05357142857142856845, 0.05952380952380952051, 0.06547619047619047949, 0.07142857142857142461, 0.07738095238095238360, 0.08333333333333332871, 0.08928571428571428770, 0.09523809523809523281, 0.1011904761904761918, 0.1071428571428571369, 0.1130952380952380959, 0.1190476190476190410, 0.1250000000000000000, 0.1309523809523809590, 0.1369047619047619180, 0.1428571428571428492, 0.1488095238095238082, 0.1547619047619047672, 0.1607142857142857262, 0.1666666666666666574, 0.1726190476190476164, 0.1785714285714285754, 0.1845238095238095344, 0.1904761904761904656, 0.1964285714285714246, 0.2023809523809523836, 0.2083333333333333426, 0.2142857142857142738, 0.2202380952380952328, 0.2261904761904761918, 0.2321428571428571508, 0.2380952380952380820, 0.2440476190476190410, 0.2500000000000000000, 0.2559523809523809312, 0.2619047619047619180, 0.2678571428571428492, 0.2738095238095238360, 0.2797619047619047672, 0.2857142857142856984, 0.2916666666666666852, 0.2976190476190476164, 0.3035714285714285476, 0.3095238095238095344, 0.3154761904761904656, 0.3214285714285714524, 0.3273809523809523836, 0.3333333333333333148, 0.3392857142857143016, 0.3452380952380952328, 0.3511904761904761640, 0.3571428571428571508, 0.3630952380952380820, 0.3690476190476190688, 0.3750000000000000000, 0.3809523809523809312, 0.3869047619047619180, 0.3928571428571428492, 0.3988095238095238360, 0.4047619047619047672, 0.4107142857142856984, 0.4166666666666666852, 0.4226190476190476164, 0.4285714285714285476, 0.4345238095238095344, 0.4404761904761904656, 0.4464285714285714524, 0.4523809523809523836, 0.4583333333333333148, 0.4642857142857143016, 0.4702380952380952328, 0.4761904761904761640, 0.4821428571428571508, 0.4880952380952380820, 0.4940476190476190688, 0.5000000000000000000, 0.5059523809523809312, 0.5119047619047618625, 0.5178571428571429047, 0.5238095238095238360, 0.5297619047619047672, 0.5357142857142856984, 0.5416666666666666297, 0.5476190476190476719, 0.5535714285714286031, 0.5595238095238095344, 0.5654761904761904656, 0.5714285714285713969, 0.5773809523809523281, 0.5833333333333333703, 0.5892857142857143016, 0.5952380952380952328, 0.6011904761904761640, 0.6071428571428570953, 0.6130952380952381375, 0.6190476190476190688, 0.6250000000000000000, 0.6309523809523809312, 0.6369047619047618625, 0.6428571428571429047, 0.6488095238095238360, 0.6547619047619047672, 0.6607142857142856984, 0.6666666666666666297, 0.6726190476190476719, 0.6785714285714286031, 0.6845238095238095344, 0.6904761904761904656, 0.6964285714285713969, 0.7023809523809523281, 0.7083333333333333703, 0.7142857142857143016, 0.7202380952380952328, 0.7261904761904761640, 0.7321428571428570953, 0.7380952380952381375, 0.7440476190476190688, 0.7500000000000000000, 0.7559523809523809312, 0.7619047619047618625, 0.7678571428571429047, 0.7738095238095238360, 0.7797619047619047672, 0.7857142857142856984, 0.7916666666666666297, 0.7976190476190476719, 0.8035714285714286031, 0.8095238095238095344, 0.8154761904761904656, 0.8214285714285713969, 0.8273809523809523281, 0.8333333333333333703, 0.8392857142857143016, 0.8452380952380952328, 0.8511904761904761640, 0.8571428571428570953, 0.8630952380952381375, 0.8690476190476190688, 0.8750000000000000000, 0.8809523809523809312, 0.8869047619047618625, 0.8928571428571429047, 0.8988095238095238360, 0.9047619047619047672, 0.9107142857142856984, 0.9166666666666666297, 0.9226190476190476719, 0.9285714285714286031, 0.9345238095238095344, 0.9404761904761904656, 0.9464285714285713969, 0.9523809523809523281, 0.9583333333333333703, 0.9642857142857143016, 0.9702380952380952328, 0.9761904761904761640, 0.9821428571428570953, 0.9880952380952381375, 0.9940476190476190688, 1.000000000000000000 ),
 .UNSPECIFIED. ) 
 GEOMETRIC_REPRESENTATION_ITEM ( )  RATIONAL_B_SPLINE_SURFACE ( (
 ( 1.000000000000000000, 0.8660254037844387076, 1.000000000000000000, 0.8660254037844387076, 1.000000000000000000, 0.8660254037844387076, 1.000000000000000000, 0.8660254037844387076, 1.000000000000000000, 0.8660254037844387076, 1.000000000000000000, 0.8660254037844387076, 1.000000000000000000, 0.8660254037844387076, 1.000000000000000000, 0.8660254037844387076, 1.000000000000000000, 0.8660254037844387076, 1.000000000000000000, 0.8660254037844387076, 1.000000000000000000, 0.8660254037844387076, 1.000000000000000000, 0.8660254037844387076, 1.000000000000000000, 0.8660254037844387076, 1.000000000000000000, 0.8660254037844387076, 1.000000000000000000, 0.8660254037844387076, 1.000000000000000000, 0.8660254037844387076, 1.000000000000000000, 0.8660254037844387076, 1.000000000000000000, 0.8660254037844387076, 1.000000000000000000, 0.8660254037844387076, 1.000000000000000000, 0.8660254037844387076, 1.000000000000000000, 0.8660254037844387076, 1.000000000000000000, 0.8660254037844387076, 1.000000000000000000, 0.8660254037844387076, 1.000000000000000000, 0.8660254037844387076, 1.000000000000000000, 0.8660254037844387076, 1.000000000000000000, 0.8660254037844387076, 1.000000000000000000, 0.8660254037844387076, 1.000000000000000000, 0.8660254037844387076, 1.000000000000000000, 0.8660254037844387076, 1.000000000000000000, 0.8660254037844387076, 1.000000000000000000, 0.8660254037844387076, 1.000000000000000000, 0.8660254037844387076, 1.000000000000000000, 0.8660254037844387076, 1.000000000000000000, 0.8660254037844387076, 1.000000000000000000, 0.8660254037844387076, 1.000000000000000000, 0.8660254037844387076, 1.000000000000000000, 0.8660254037844387076, 1.000000000000000000, 0.8660254037844387076, 1.000000000000000000, 0.8660254037844387076, 1.000000000000000000, 0.8660254037844387076, 1.000000000000000000, 0.8660254037844387076, 1.000000000000000000, 0.8660254037844387076, 1.000000000000000000, 0.8660254037844387076, 1.000000000000000000, 0.8660254037844387076, 1.000000000000000000, 0.8660254037844387076, 1.000000000000000000, 0.8660254037844387076, 1.000000000000000000, 0.8660254037844387076, 1.000000000000000000, 0.8660254037844387076, 1.000000000000000000, 0.8660254037844387076, 1.000000000000000000, 0.8660254037844387076, 1.000000000000000000, 0.8660254037844387076, 1.000000000000000000, 0.8660254037844387076, 1.000000000000000000, 0.8660254037844387076, 1.000000000000000000, 0.8660254037844387076, 1.000000000000000000, 0.8660254037844387076, 1.000000000000000000, 0.8660254037844387076, 1.000000000000000000, 0.8660254037844387076, 1.000000000000000000, 0.8660254037844387076, 1.000000000000000000, 0.8660254037844387076, 1.000000000000000000, 0.8660254037844387076, 1.000000000000000000, 0.8660254037844387076, 1.000000000000000000, 0.8660254037844387076, 1.000000000000000000, 0.8660254037844387076, 1.000000000000000000, 0.8660254037844387076, 1.000000000000000000, 0.8660254037844387076, 1.000000000000000000, 0.8660254037844387076, 1.000000000000000000, 0.8660254037844387076, 1.000000000000000000, 0.8660254037844387076, 1.000000000000000000, 0.8660254037844387076, 1.000000000000000000, 0.8660254037844387076, 1.000000000000000000, 0.8660254037844387076, 1.000000000000000000, 0.8660254037844387076, 1.000000000000000000, 0.8660254037844387076, 1.000000000000000000, 0.8660254037844387076, 1.000000000000000000, 0.8660254037844387076, 1.000000000000000000, 0.8660254037844387076, 1.000000000000000000, 0.8660254037844387076, 1.000000000000000000, 0.8660254037844387076, 1.000000000000000000, 0.8660254037844387076, 1.000000000000000000, 0.8660254037844387076, 1.000000000000000000, 0.8660254037844387076, 1.000000000000000000, 0.8660254037844387076, 1.000000000000000000, 0.8660254037844387076, 1.000000000000000000, 0.8660254037844387076, 1.000000000000000000, 0.8660254037844387076, 1.000000000000000000, 0.8660254037844387076, 1.000000000000000000, 0.8660254037844387076, 1.000000000000000000, 0.8660254037844387076, 1.000000000000000000, 0.8660254037844387076, 1.000000000000000000, 0.8660254037844387076, 1.000000000000000000, 0.8660254037844387076, 1.000000000000000000, 0.8660254037844387076, 1.000000000000000000, 0.8660254037844387076, 1.000000000000000000, 0.8660254037844387076, 1.000000000000000000, 0.8660254037844387076, 1.000000000000000000, 0.8660254037844387076, 1.000000000000000000, 0.8660254037844387076, 1.000000000000000000, 0.8660254037844387076, 1.000000000000000000, 0.8660254037844387076, 1.000000000000000000, 0.8660254037844387076, 1.000000000000000000, 0.8660254037844387076, 1.000000000000000000, 0.8660254037844387076, 1.000000000000000000, 0.8660254037844387076, 1.000000000000000000, 0.8660254037844387076, 1.000000000000000000, 0.8660254037844387076, 1.000000000000000000, 0.8660254037844387076, 1.000000000000000000, 0.8660254037844387076, 1.000000000000000000, 0.8660254037844387076, 1.000000000000000000, 0.8660254037844387076, 1.000000000000000000, 0.8660254037844387076, 1.000000000000000000, 0.8660254037844387076, 1.000000000000000000, 0.8660254037844387076, 1.000000000000000000, 0.8660254037844387076, 1.000000000000000000, 0.8660254037844387076, 1.000000000000000000, 0.8660254037844387076, 1.000000000000000000, 0.8660254037844387076, 1.000000000000000000, 0.8660254037844387076, 1.000000000000000000, 0.8660254037844387076, 1.000000000000000000, 0.8660254037844387076, 1.000000000000000000, 0.8660254037844387076, 1.000000000000000000, 0.8660254037844387076, 1.000000000000000000, 0.8660254037844387076, 1.000000000000000000, 0.8660254037844387076, 1.000000000000000000, 0.8660254037844387076, 1.000000000000000000, 0.8660254037844387076, 1.000000000000000000, 0.8660254037844387076, 1.000000000000000000, 0.8660254037844387076, 1.000000000000000000, 0.8660254037844387076, 1.000000000000000000, 0.8660254037844387076, 1.000000000000000000, 0.8660254037844387076, 1.000000000000000000, 0.8660254037844387076, 1.000000000000000000, 0.8660254037844387076, 1.000000000000000000, 0.8660254037844387076, 1.000000000000000000, 0.8660254037844387076, 1.000000000000000000, 0.8660254037844387076, 1.000000000000000000, 0.8660254037844387076, 1.000000000000000000, 0.8660254037844387076, 1.000000000000000000, 0.8660254037844387076, 1.000000000000000000, 0.8660254037844387076, 1.000000000000000000, 0.8660254037844387076, 1.000000000000000000, 0.8660254037844387076, 1.000000000000000000, 0.8660254037844387076, 1.000000000000000000, 0.8660254037844387076, 1.000000000000000000, 0.8660254037844387076, 1.000000000000000000, 0.8660254037844387076, 1.000000000000000000, 0.8660254037844387076, 1.000000000000000000, 0.8660254037844387076, 1.000000000000000000, 0.8660254037844387076, 1.000000000000000000, 0.8660254037844387076, 1.000000000000000000, 0.8660254037844387076, 1.000000000000000000, 0.8660254037844387076, 1.000000000000000000, 0.8660254037844387076, 1.000000000000000000, 0.8660254037844387076, 1.000000000000000000, 0.8660254037844387076, 1.000000000000000000, 0.8660254037844387076, 1.000000000000000000, 0.8660254037844387076, 1.000000000000000000, 0.8660254037844387076, 1.000000000000000000, 0.8660254037844387076, 1.000000000000000000, 0.8660254037844387076, 1.000000000000000000, 0.8660254037844387076, 1.000000000000000000, 0.8660254037844387076, 1.000000000000000000, 0.8660254037844387076, 1.000000000000000000, 0.8660254037844387076, 1.000000000000000000, 0.8660254037844387076, 1.000000000000000000, 0.8660254037844387076, 1.000000000000000000, 0.8660254037844387076, 1.000000000000000000, 0.8660254037844387076, 1.000000000000000000, 0.8660254037844387076, 1.000000000000000000),
 ( 1.000000000000000000, 0.8660254037844387076, 1.000000000000000000, 0.8660254037844387076, 1.000000000000000000, 0.8660254037844387076, 1.000000000000000000, 0.8660254037844387076, 1.000000000000000000, 0.8660254037844387076, 1.000000000000000000, 0.8660254037844387076, 1.000000000000000000, 0.8660254037844387076, 1.000000000000000000, 0.8660254037844387076, 1.000000000000000000, 0.8660254037844387076, 1.000000000000000000, 0.8660254037844387076, 1.000000000000000000, 0.8660254037844387076, 1.000000000000000000, 0.8660254037844387076, 1.000000000000000000, 0.8660254037844387076, 1.000000000000000000, 0.8660254037844387076, 1.000000000000000000, 0.8660254037844387076, 1.000000000000000000, 0.8660254037844387076, 1.000000000000000000, 0.8660254037844387076, 1.000000000000000000, 0.8660254037844387076, 1.000000000000000000, 0.8660254037844387076, 1.000000000000000000, 0.8660254037844387076, 1.000000000000000000, 0.8660254037844387076, 1.000000000000000000, 0.8660254037844387076, 1.000000000000000000, 0.8660254037844387076, 1.000000000000000000, 0.8660254037844387076, 1.000000000000000000, 0.8660254037844387076, 1.000000000000000000, 0.8660254037844387076, 1.000000000000000000, 0.8660254037844387076, 1.000000000000000000, 0.8660254037844387076, 1.000000000000000000, 0.8660254037844387076, 1.000000000000000000, 0.8660254037844387076, 1.000000000000000000, 0.8660254037844387076, 1.000000000000000000, 0.8660254037844387076, 1.000000000000000000, 0.8660254037844387076, 1.000000000000000000, 0.8660254037844387076, 1.000000000000000000, 0.8660254037844387076, 1.000000000000000000, 0.8660254037844387076, 1.000000000000000000, 0.8660254037844387076, 1.000000000000000000, 0.8660254037844387076, 1.000000000000000000, 0.8660254037844387076, 1.000000000000000000, 0.8660254037844387076, 1.000000000000000000, 0.8660254037844387076, 1.000000000000000000, 0.8660254037844387076, 1.000000000000000000, 0.8660254037844387076, 1.000000000000000000, 0.8660254037844387076, 1.000000000000000000, 0.8660254037844387076, 1.000000000000000000, 0.8660254037844387076, 1.000000000000000000, 0.8660254037844387076, 1.000000000000000000, 0.8660254037844387076, 1.000000000000000000, 0.8660254037844387076, 1.000000000000000000, 0.8660254037844387076, 1.000000000000000000, 0.8660254037844387076, 1.000000000000000000, 0.8660254037844387076, 1.000000000000000000, 0.8660254037844387076, 1.000000000000000000, 0.8660254037844387076, 1.000000000000000000, 0.8660254037844387076, 1.000000000000000000, 0.8660254037844387076, 1.000000000000000000, 0.8660254037844387076, 1.000000000000000000, 0.8660254037844387076, 1.000000000000000000, 0.8660254037844387076, 1.000000000000000000, 0.8660254037844387076, 1.000000000000000000, 0.8660254037844387076, 1.000000000000000000, 0.8660254037844387076, 1.000000000000000000, 0.8660254037844387076, 1.000000000000000000, 0.8660254037844387076, 1.000000000000000000, 0.8660254037844387076, 1.000000000000000000, 0.8660254037844387076, 1.000000000000000000, 0.8660254037844387076, 1.000000000000000000, 0.8660254037844387076, 1.000000000000000000, 0.8660254037844387076, 1.000000000000000000, 0.8660254037844387076, 1.000000000000000000, 0.8660254037844387076, 1.000000000000000000, 0.8660254037844387076, 1.000000000000000000, 0.8660254037844387076, 1.000000000000000000, 0.8660254037844387076, 1.000000000000000000, 0.8660254037844387076, 1.000000000000000000, 0.8660254037844387076, 1.000000000000000000, 0.8660254037844387076, 1.000000000000000000, 0.8660254037844387076, 1.000000000000000000, 0.8660254037844387076, 1.000000000000000000, 0.8660254037844387076, 1.000000000000000000, 0.8660254037844387076, 1.000000000000000000, 0.8660254037844387076, 1.000000000000000000, 0.8660254037844387076, 1.000000000000000000, 0.8660254037844387076, 1.000000000000000000, 0.8660254037844387076, 1.000000000000000000, 0.8660254037844387076, 1.000000000000000000, 0.8660254037844387076, 1.000000000000000000, 0.8660254037844387076, 1.000000000000000000, 0.8660254037844387076, 1.000000000000000000, 0.8660254037844387076, 1.000000000000000000, 0.8660254037844387076, 1.000000000000000000, 0.8660254037844387076, 1.000000000000000000, 0.8660254037844387076, 1.000000000000000000, 0.8660254037844387076, 1.000000000000000000, 0.8660254037844387076, 1.000000000000000000, 0.8660254037844387076, 1.000000000000000000, 0.8660254037844387076, 1.000000000000000000, 0.8660254037844387076, 1.000000000000000000, 0.8660254037844387076, 1.000000000000000000, 0.8660254037844387076, 1.000000000000000000, 0.8660254037844387076, 1.000000000000000000, 0.8660254037844387076, 1.000000000000000000, 0.8660254037844387076, 1.000000000000000000, 0.8660254037844387076, 1.000000000000000000, 0.8660254037844387076, 1.000000000000000000, 0.8660254037844387076, 1.000000000000000000, 0.8660254037844387076, 1.000000000000000000, 0.8660254037844387076, 1.000000000000000000, 0.8660254037844387076, 1.000000000000000000, 0.8660254037844387076, 1.000000000000000000, 0.8660254037844387076, 1.000000000000000000, 0.8660254037844387076, 1.000000000000000000, 0.8660254037844387076, 1.000000000000000000, 0.8660254037844387076, 1.000000000000000000, 0.8660254037844387076, 1.000000000000000000, 0.8660254037844387076, 1.000000000000000000, 0.8660254037844387076, 1.000000000000000000, 0.8660254037844387076, 1.000000000000000000, 0.8660254037844387076, 1.000000000000000000, 0.8660254037844387076, 1.000000000000000000, 0.8660254037844387076, 1.000000000000000000, 0.8660254037844387076, 1.000000000000000000, 0.8660254037844387076, 1.000000000000000000, 0.8660254037844387076, 1.000000000000000000, 0.8660254037844387076, 1.000000000000000000, 0.8660254037844387076, 1.000000000000000000, 0.8660254037844387076, 1.000000000000000000, 0.8660254037844387076, 1.000000000000000000, 0.8660254037844387076, 1.000000000000000000, 0.8660254037844387076, 1.000000000000000000, 0.8660254037844387076, 1.000000000000000000, 0.8660254037844387076, 1.000000000000000000, 0.8660254037844387076, 1.000000000000000000, 0.8660254037844387076, 1.000000000000000000, 0.8660254037844387076, 1.000000000000000000, 0.8660254037844387076, 1.000000000000000000, 0.8660254037844387076, 1.000000000000000000, 0.8660254037844387076, 1.000000000000000000, 0.8660254037844387076, 1.000000000000000000, 0.8660254037844387076, 1.000000000000000000, 0.8660254037844387076, 1.000000000000000000, 0.8660254037844387076, 1.000000000000000000, 0.8660254037844387076, 1.000000000000000000, 0.8660254037844387076, 1.000000000000000000, 0.8660254037844387076, 1.000000000000000000, 0.8660254037844387076, 1.000000000000000000, 0.8660254037844387076, 1.000000000000000000, 0.8660254037844387076, 1.000000000000000000, 0.8660254037844387076, 1.000000000000000000, 0.8660254037844387076, 1.000000000000000000, 0.8660254037844387076, 1.000000000000000000, 0.8660254037844387076, 1.000000000000000000, 0.8660254037844387076, 1.000000000000000000, 0.8660254037844387076, 1.000000000000000000, 0.8660254037844387076, 1.000000000000000000, 0.8660254037844387076, 1.000000000000000000, 0.8660254037844387076, 1.000000000000000000, 0.8660254037844387076, 1.000000000000000000, 0.8660254037844387076, 1.000000000000000000, 0.8660254037844387076, 1.000000000000000000, 0.8660254037844387076, 1.000000000000000000, 0.8660254037844387076, 1.000000000000000000, 0.8660254037844387076, 1.000000000000000000, 0.8660254037844387076, 1.000000000000000000, 0.8660254037844387076, 1.000000000000000000, 0.8660254037844387076, 1.000000000000000000, 0.8660254037844387076, 1.000000000000000000, 0.8660254037844387076, 1.000000000000000000) ) ) 
 REPRESENTATION_ITEM ( '' )  SURFACE ( )  );
#95377=CARTESIAN_POINT ( 'NONE',  ( 0.7499999999999902300, 2.483333333333351156, 1.299038105676669330 ) ) ;
#95378=CARTESIAN_POINT ( 'NONE',  ( 7.122110765880372618, 7.203550736482235095, 0.7998128361456341429 ) ) ;
#95379=CARTESIAN_POINT ( 'NONE',  ( -8.227100285394159940, 8.492705175914988303, 0.7998128361456602331 ) ) ;
#95382=CARTESIAN_POINT ( 'NONE',  ( 0.6823417656249899377, 2.092708333674753174, 1.181850606188767472 ) ) ;
#95383=CARTESIAN_POINT ( 'NONE',  ( 1.499999999999987121, 3.295833333333354709, -0.8660254037844262731 ) ) ;
#95385=CARTESIAN_POINT ( 'NONE',  ( 2.672928840188529609, 6.270167413528593414, 0.000000000000000000 ) ) ;
#95392=CARTESIAN_POINT ( 'NONE',  ( 0.7499999999999885647, 0.3479166673494848983, -1.299038105676652899 ) ) ;
#95394=CARTESIAN_POINT ( 'NONE',  ( -5.343885102080728977, 9.386283052402845328, 0.7998128361456481317 ) ) ;
#95395=CARTESIAN_POINT ( 'NONE',  ( -3.307826292054310890, 5.842585859829892314, -1.082531754730549967 ) ) ;
#95403=CARTESIAN_POINT ( 'NONE',  ( 4.286349120214771879, 8.152491073559232859, -0.7998128361456221525 ) ) ;
#95407=CARTESIAN_POINT ( 'NONE',  ( 7.481401836642521452, 7.622723652371411696, 1.040834085586084257E-14 ) ) ;
#95413=CARTESIAN_POINT ( 'NONE',  ( -5.045605722580076780, 9.038290442985410067, -0.7998128361456231517 ) ) ;
#95414=CARTESIAN_POINT ( 'NONE',  ( 2.855963913973019963, 6.483708332943829866, 0.000000000000000000 ) ) ;
#95420=CARTESIAN_POINT ( 'NONE',  ( 4.117415066209698438, 7.437700365148243620, 0.6807796091479866307 ) ) ;
#95430=CARTESIAN_POINT ( 'NONE',  ( -3.795919822146293754, 4.491289883001181593, -1.082531754730549967 ) ) ;
#95431=CARTESIAN_POINT ( 'NONE',  ( 6.968527767744088663, 11.07377346243604599, 0.7216878364870438212 ) ) ;
#95433=CARTESIAN_POINT ( 'NONE',  ( -4.069418662396130593, 7.899405539437467816, -0.7998128361456281477 ) ) ;
#95434=CARTESIAN_POINT ( 'NONE',  ( -9.828980619278564011E-14, 7.054063922337708625, 3.955400951015630273 ) ) ;
#95435=EDGE_CURVE ( 'NONE', #73782, #10073, #179629, .T. ) ;
#95440=CARTESIAN_POINT ( 'NONE',  ( -7.314787569772770226, 8.492672571945082183, -1.199719254218452935 ) ) ;
#95445=EDGE_CURVE ( 'NONE', #96829, #108458, #104885, .T. ) ;
#95454=EDGE_CURVE ( 'NONE', #180844, #80984, #106183, .T. ) ;
#95456=CARTESIAN_POINT ( 'NONE',  ( -6.240830780992103755, 6.175390754112560110, 1.040834085586084257E-14 ) ) ;
#95459=CARTESIAN_POINT ( 'NONE',  ( 3.199361063144961825, 6.676412307070352270, -0.7216878364870267237 ) ) ;
#95463=CARTESIAN_POINT ( 'NONE',  ( -4.485049888022365927, 4.126979712314507331, 0.7998128361456341429 ) ) ;
#95464=CARTESIAN_POINT ( 'NONE',  ( -3.928111819657352566, 5.605883094398769195, 1.599625672291267398 ) ) ;
#95468=CARTESIAN_POINT ( 'NONE',  ( 8.809047120577066181, 11.30030761213851953, 1.599625672291281386 ) ) ;
#95471=CARTESIAN_POINT ( 'NONE',  ( -6.852756576703439961, 10.08230087520760954, 1.199719254218453823 ) ) ;
#95472=CARTESIAN_POINT ( 'NONE',  ( 5.015626762051672571, 7.938982758113895422, 1.199719254218462483 ) ) ;
#95474=EDGE_CURVE ( 'NONE', #177299, #164705, #202643, .T. ) ;
#95475=CARTESIAN_POINT ( 'NONE',  ( 5.169736645512481132, 4.925780929386340823, 0.7998128361456341429 ) ) ;
#95478=CARTESIAN_POINT ( 'NONE',  ( 1.364683531249988757, 0.6968750003414209138, 0.000000000000000000 ) ) ;
#95481=CARTESIAN_POINT ( 'NONE',  ( 6.426201623197458801, 9.480690412830290015, -1.082531754730537088 ) ) ;
#95489=CARTESIAN_POINT ( 'NONE',  ( 3.714570900464321479, 7.277490450609501949, 0.7216878364870685791 ) ) ;
#95496=CARTESIAN_POINT ( 'NONE',  ( -8.967828540435322182, 12.54988483289483980, 1.199719254218462483 ) ) ;
#95511=CARTESIAN_POINT ( 'NONE',  ( 1.499999999999989120, 1.056250000682816603, 0.000000000000000000 ) ) ;
#95515=ORIENTED_EDGE ( 'NONE', *, *, #72633, .T. ) ;
#95517=CARTESIAN_POINT ( 'NONE',  ( 0.7499999999999867883, -0.4333333333333133641, -1.299038105676652899 ) ) ;
#95518=CARTESIAN_POINT ( 'NONE',  ( 6.753933077901968396, 11.03133902419432566, 0.7998128361456462443 ) ) ;
#95522=CARTESIAN_POINT ( 'NONE',  ( 4.356247428692526569, 3.976710176429713250, 0.7998128361456341429 ) ) ;
#95523=CARTESIAN_POINT ( 'NONE',  ( -6.751597309925468693, 6.979211071108916364, 0.7216878364870317197 ) ) ;
#95527=CARTESIAN_POINT ( 'NONE',  ( -7.152089726408780379, 8.302858421353754181, -1.199719254218446718 ) ) ;
#95531=CARTESIAN_POINT ( 'NONE',  ( 0.7499999999999902300, 1.014583334016154526, 1.299038105676657340 ) ) ;
#95538=CARTESIAN_POINT ( 'NONE',  ( -10.65400978224035811, 11.32409958890225710, 1.040834085586084257E-14 ) ) ;
#95540=CARTESIAN_POINT ( 'NONE',  ( 4.084722907606431974, 7.479936734012107458, 0.5927516458891276541 ) ) ;
#95544=CARTESIAN_POINT ( 'NONE',  ( -3.972175818679615222, 4.696921878956699103, 1.082531754730558626 ) ) ;
#95545=CARTESIAN_POINT ( 'NONE',  ( 7.202405917357655341, 9.425892875049191488, 1.599625672291281386 ) ) ;
#95552=CARTESIAN_POINT ( 'NONE',  ( -8.019811557683421910, 9.315200557840817908, 1.199719254218462483 ) ) ;
#95558=CARTESIAN_POINT ( 'NONE',  ( 5.352771719296971042, 5.139321848801576387, 0.7998128361456341429 ) ) ;
#95563=CARTESIAN_POINT ( 'NONE',  ( -8.299562589859897699, 12.83457345481192036, -0.7998128361456281477 ) ) ;
#95565=AXIS2_PLACEMENT_3D ( 'NONE', #189665, #8782, #22878 ) ;
#95567=CARTESIAN_POINT ( 'NONE',  ( -4.851289806644571989, 6.918820993438449030, -1.443092038473028582 ) ) ;
#95575=CARTESIAN_POINT ( 'NONE',  ( 6.819914962873951936, 7.915321197229798322, -1.199719254218446718 ) ) ;
#95577=VERTEX_POINT ( 'NONE', #73437 ) ;
#95585=CARTESIAN_POINT ( 'NONE',  ( 1.499999999999989120, 0.05625000068281565957, 0.000000000000000000 ) ) ;
#95589=DIRECTION ( 'NONE',  ( 0.7592566023653005702, -0.6507913734559639396, 0.000000000000000000 ) ) ;
#95591=CARTESIAN_POINT ( 'NONE',  ( -4.796887421136680985, 4.490790167614548523, 1.214306433183764966E-14 ) ) ;
#95599=CARTESIAN_POINT ( 'NONE',  ( 5.992340707560163793, 6.093411701682730275, 0.7216878364870317197 ) ) ;
#95602=CARTESIAN_POINT ( 'NONE',  ( 1.364683531249992088, 5.696875000341418804, 1.214306433183764966E-14 ) ) ;
#95603=CARTESIAN_POINT ( 'NONE',  ( -6.007394966791244961, 6.077829431809393945, -0.6506939885215150543 ) ) ;
#95604=CARTESIAN_POINT ( 'NONE',  ( 8.211434591371064684, 12.73175745657494851, -0.7998128361456352531 ) ) ;
#95613=CARTESIAN_POINT ( 'NONE',  ( -1.364683531250014514, -0.4697916663252449943, 0.7879004041258379498 ) ) ;
#95617=CARTESIAN_POINT ( 'NONE',  ( -5.229694566569281555, 7.124396299129368337, 1.599625672291267398 ) ) ;
#95621=CARTESIAN_POINT ( 'NONE',  ( -1.500000000000011324, 5.129166666666691299, -0.8660254037844313801 ) ) ;
#95629=CARTESIAN_POINT ( 'NONE',  ( 0.6823417656249864960, -0.5739583329919112353, -1.181850606188749264 ) ) ;
#95631=CARTESIAN_POINT ( 'NONE',  ( 6.959412922516382771, 7.013736585890911535, 0.7998128361456341429 ) ) ;
#95633=CARTESIAN_POINT ( 'NONE',  ( -7.015454420067433361, 10.27211502579893754, 1.199719254218453823 ) ) ;
#95635=CARTESIAN_POINT ( 'NONE',  ( 1.000000000000001554, 6.468705557303653819, -4.925226524755053958 ) ) ;
#95639=CARTESIAN_POINT ( 'NONE',  ( 0.6823417656249864960, -0.7614583329919113464, -1.181850606188749264 ) ) ;
#95647=CARTESIAN_POINT ( 'NONE',  ( 7.619319141200070256, 8.951922421897323900, 1.082531754730558626 ) ) ;
#95652=CARTESIAN_POINT ( 'NONE',  ( 1.499999999999990896, 4.306250000682819490, 1.214306433183764966E-14 ) ) ;
#95654=CARTESIAN_POINT ( 'NONE',  ( -4.925689880466507908, 4.641059703499347044, -0.7998128361456221525 ) ) ;
#95655=CARTESIAN_POINT ( 'NONE',  ( 5.612712405933139692, 9.491988873656591608, 1.040834085586084257E-14 ) ) ;
#95656=CARTESIAN_POINT ( 'NONE',  ( -8.120970824461345217, 12.41829036193951730, 0.7216878364870458196 ) ) ;
#95662=CARTESIAN_POINT ( 'NONE',  ( 10.22248463502393001, 11.02857961705718282, 0.7216878364870438212 ) ) ;
#95663=CARTESIAN_POINT ( 'NONE',  ( 4.192495815123822744, 5.914331089109666983, -1.599625672291255185 ) ) ;
#95671=CARTESIAN_POINT ( 'NONE',  ( -0.6823417656249969321, 3.280208333674754062, -1.181850606188749264 ) ) ;
#95673=ORIENTED_EDGE ( 'NONE', *, *, #186210, .T. ) ;
#95675=CARTESIAN_POINT ( 'NONE',  ( 8.890396042259068210, 11.39521468743417998, -1.599625672291257406 ) ) ;
#95677=CARTESIAN_POINT ( 'NONE',  ( -1.499999999999996003, 8.226475397238283804, 3.114076396432755800 ) ) ;
#95679=CARTESIAN_POINT ( 'NONE',  ( 0.6823417656249882723, 0.3427083336747516196, 1.181850606188755259 ) ) ;
#95680=CARTESIAN_POINT ( 'NONE',  ( 4.026408433578586354, 7.641300905909586660, 1.040834085586084257E-14 ) ) ;
#95682=CARTESIAN_POINT ( 'NONE',  ( -8.188761592974046266, 10.57664116326830595, -1.443375672974059665 ) ) ;
#95687=CARTESIAN_POINT ( 'NONE',  ( -2.605138072120212200, 6.191078184115536232, -0.7998128361456281477 ) ) ;
#95701=CARTESIAN_POINT ( 'NONE',  ( 4.298292216229534723, 7.460037067547172107, -1.072071942351945584 ) ) ;
#95703=EDGE_LOOP ( 'NONE', ( #126596, #100548, #45869, #185252 ) ) ;
#95706=CARTESIAN_POINT ( 'NONE',  ( -5.681296809623264110, 6.286896183989623133, -1.175774015649774462 ) ) ;
#95709=CARTESIAN_POINT ( 'NONE',  ( -6.873620692448438874, 10.96304854125777695, 0.000000000000000000 ) ) ;
#95714=CARTESIAN_POINT ( 'NONE',  ( 6.100279051144945619, 9.204410428722734849, -1.199719254218440723 ) ) ;
#95718=CARTESIAN_POINT ( 'NONE',  ( -4.517891501851816649, 6.293959390292322986, -1.599625672291256295 ) ) ;
#95722=CARTESIAN_POINT ( 'NONE',  ( -3.958090780185743451, 6.705190779270287393, -1.199719254218452047 ) ) ;
#95726=CARTESIAN_POINT ( 'NONE',  ( 4.976006071415387311, 5.764094157194782575, 1.199719254218462483 ) ) ;
#95727=CARTESIAN_POINT ( 'NONE',  ( 9.264299036839600987, 9.702770385934682551, -0.7998128361456281477 ) ) ;
#95730=CARTESIAN_POINT ( 'NONE',  ( 5.274334856052985465, 6.586744271544701768, 1.367809967355391398 ) ) ;
#95731=CARTESIAN_POINT ( 'NONE',  ( 4.853455804012216213, 6.685451076146141425, 1.443375672974062551 ) ) ;
#95739=CARTESIAN_POINT ( 'NONE',  ( 7.334597914868727919, 9.580116872145431728, -1.443375672974058777 ) ) ;
#95742=CARTESIAN_POINT ( 'NONE',  ( -8.459397779922852578, 11.95671561229694824, 1.199719254218453823 ) ) ;
#95743=CARTESIAN_POINT ( 'NONE',  ( -7.226659571283968297, 8.389856573708110332, 1.199719254218450271 ) ) ;
#95750=CARTESIAN_POINT ( 'NONE',  ( 9.399880572976245574, 9.860948844760784482, 0.7998128361456462443 ) ) ;
#95754=CARTESIAN_POINT ( 'NONE',  ( 3.684065054611349144, 5.321161868511784299, -1.599625672291262513 ) ) ;
#95757=CARTESIAN_POINT ( 'NONE',  ( -1.500000000000011324, 5.202083334016151639, 0.8660254037844403729 ) ) ;
#95763=CARTESIAN_POINT ( 'NONE',  ( -1.201851678989727383E-14, 2.462500000000023004, 1.732050807568877637 ) ) ;
#95764=CARTESIAN_POINT ( 'NONE',  ( 4.313465427442102929, 8.184126765324453601, 0.7998128361456462443 ) ) ;
#95767=CARTESIAN_POINT ( 'NONE',  ( 6.629573927402440781, 10.67832731537079383, 1.040834085586084257E-14 ) ) ;
#95768=CARTESIAN_POINT ( 'NONE',  ( -9.693716643646601128, 12.33242205571964512, 1.443375672974076540 ) ) ;
#95771=CARTESIAN_POINT ( 'NONE',  ( 8.866142388332804103, 12.43125098877526113, -1.199719254218446718 ) ) ;
#95774=CARTESIAN_POINT ( 'NONE',  ( -4.790108344329849110, 4.482881244673243337, 0.7998128361456341429 ) ) ;
#95775=CARTESIAN_POINT ( 'NONE',  ( 0.6823417656249882723, 0.6760416670080898749, -1.181850606188749264 ) ) ;
#95781=CARTESIAN_POINT ( 'NONE',  ( 1.364683531249988535, 5.717708333674752730, -0.7879004041258300672 ) ) ;
#95790=CARTESIAN_POINT ( 'NONE',  ( -6.551614543901706611, 8.666636272683888365, 1.599625672291283607 ) ) ;
#95793=CARTESIAN_POINT ( 'NONE',  ( 3.845709127770629010, 7.638411082374393146, 0.7998128361456321445 ) ) ;
#95803=CARTESIAN_POINT ( 'NONE',  ( -4.608882153641705059, 7.464447381635583412, -1.199719254218452047 ) ) ;
#95807=CARTESIAN_POINT ( 'NONE',  ( 7.944187942603509356, 11.35563746875774882, 1.199719254218460707 ) ) ;
#95809=CARTESIAN_POINT ( 'NONE',  ( 6.916630921265960019, 11.22115317478565188, 0.7998128361456462443 ) ) ;
#95812=CARTESIAN_POINT ( 'NONE',  ( -9.408995418203979000, 12.00024729270324286, 1.443375672974076540 ) ) ;
#95813=CARTESIAN_POINT ( 'NONE',  ( -7.019370843573183194, 9.212351955633947043, 1.599625672291283607 ) ) ;
#95817=CARTESIAN_POINT ( 'NONE',  ( -5.609631208091558463, 6.340496262503443781, 1.197921296376257994 ) ) ;
#95818=CARTESIAN_POINT ( 'NONE',  ( -1.364683531250014514, -0.2614583329919080157, -0.7879004041258359514 ) ) ;
#95821=CARTESIAN_POINT ( 'NONE',  ( 6.588899466561449536, 9.670504563421618016, -1.082531754730537088 ) ) ;
#95825=AXIS2_PLACEMENT_3D ( 'NONE', #122496, #142954, #159161 ) ;
#95842=CARTESIAN_POINT ( 'NONE',  ( 9.236128959407556849, 11.79856975744075598, -1.599625672291262513 ) ) ;
#95846=CARTESIAN_POINT ( 'NONE',  ( -3.249150368769345043, 6.942425863539538611, 0.7998128361456341429 ) ) ;
#95847=CARTESIAN_POINT ( 'NONE',  ( -7.640183256500752584, 8.872300873127729304, -1.199719254218446718 ) ) ;
#95853=CARTESIAN_POINT ( 'NONE',  ( 0.7499999999999920064, 4.014583334016149863, 1.299038105676669330 ) ) ;
#95854=CARTESIAN_POINT ( 'NONE',  ( 8.751951852821344247, 10.16936423550178503, -1.199719254218446718 ) ) ;
#95857=CARTESIAN_POINT ( 'NONE',  ( -8.040148788103921973, 9.338927326664741457, 1.199719254218462483 ) ) ;
#95859=CARTESIAN_POINT ( 'NONE',  ( 0.6823417656249899377, 3.176041667008085323, -1.181850606188754593 ) ) ;
#95864=CARTESIAN_POINT ( 'NONE',  ( -9.164948653157990677, 11.71552606681625619, -1.443375672974059665 ) ) ;
#95866=EDGE_CURVE ( 'NONE', #207276, #17744, #6289, .T. ) ;
#95869=CARTESIAN_POINT ( 'NONE',  ( -1.364683531250012516, 2.801041667008090652, -0.7879004041258289570 ) ) ;
#95877=CARTESIAN_POINT ( 'NONE',  ( 1.364683531249988535, 3.613541667008086211, 0.7879004041258500513 ) ) ;
#95879=CARTESIAN_POINT ( 'NONE',  ( -6.423865854776591000, 6.388931673527803667, 1.040834085586084257E-14 ) ) ;
#95880=CARTESIAN_POINT ( 'NONE',  ( 6.588372581236919601, 9.773852880496709972, -1.199719254218440723 ) ) ;
#95883=EDGE_CURVE ( 'NONE', #112218, #115335, #15880, .T. ) ;
#95884=CARTESIAN_POINT ( 'NONE',  ( 1.364683531249988535, 2.926041667008082658, 0.7879004041258500513 ) ) ;
#95887=CARTESIAN_POINT ( 'NONE',  ( 1.364683531249986537, -0.1364583329919154264, 0.7879004041258500513 ) ) ;
#95889=CARTESIAN_POINT ( 'NONE',  ( -4.392478581147607031, 7.108013530438723748, 1.082531754730560403 ) ) ;
#95893=CARTESIAN_POINT ( 'NONE',  ( 4.012850279964918165, 7.625483060026979842, -0.7216878364870197293 ) ) ;
#95896=CARTESIAN_POINT ( 'NONE',  ( -7.202405917357668663, 9.425892875049191488, 1.599625672291295375 ) ) ;
#95897=CARTESIAN_POINT ( 'NONE',  ( -9.164948653157999559, 10.75515685251491504, -1.082531754730539753 ) ) ;
#95899=CARTESIAN_POINT ( 'NONE',  ( -1.201851678989727383E-14, 5.196875000341422357, -1.575800808251660134 ) ) ;
#95904=CARTESIAN_POINT ( 'NONE',  ( -5.531363484251157203, 9.397081798360927607, 0.000000000000000000 ) ) ;
#95906=CARTESIAN_POINT ( 'NONE',  ( -0.6823417656250003738, -0.4697916663252491021, -1.181850606188749264 ) ) ;
#95918=CARTESIAN_POINT ( 'NONE',  ( -0.7500000000000006661, -0.6416666666666446250, -1.299038105676652011 ) ) ;
#95919=CARTESIAN_POINT ( 'NONE',  ( 9.693716643646595799, 11.37205284141829686, 1.082531754730548412 ) ) ;
#95925=CARTESIAN_POINT ( 'NONE',  ( 4.801558957534076022, 8.753569217098425170, 0.7998128361456462443 ) ) ;
#95926=CARTESIAN_POINT ( 'NONE',  ( -4.578903193113314174, 6.365139696764064325, 1.599625672291267398 ) ) ;
#95930=CARTESIAN_POINT ( 'NONE',  ( 5.680503174001485078, 6.689970460165617361, -1.082531754730543083 ) ) ;
#95931=CARTESIAN_POINT ( 'NONE',  ( 1.364683531249988757, 0.6968750003414209138, 0.000000000000000000 ) ) ;
#95933=CARTESIAN_POINT ( 'NONE',  ( -8.727698198895085469, 11.20540053684285553, -1.599625672291263179 ) ) ;
#95948=CARTESIAN_POINT ( 'NONE',  ( -4.277974919820238142, 7.286213140905228869, -0.9367534487179690617 ) ) ;
#95952=CARTESIAN_POINT ( 'NONE',  ( 5.575427483717746213, 7.527751369135936343, 1.599625672291267398 ) ) ;
#95959=CARTESIAN_POINT ( 'NONE',  ( 8.555358625423188812, 9.940005470203933768, 1.199719254218462483 ) ) ;
#95964=FACE_OUTER_BOUND ( 'NONE', #59640, .T. ) ;
#95967=CARTESIAN_POINT ( 'NONE',  ( 9.398826802771546696, 11.98838390803207865, -1.599625672291262513 ) ) ;
#95969=CARTESIAN_POINT ( 'NONE',  ( -0.5049859354315073823, 7.739806959121713348, 1.936057643311939858 ) ) ;
#95975=CARTESIAN_POINT ( 'NONE',  ( -7.524412065904404479, 11.72230514362308185, 0.000000000000000000 ) ) ;
#95980=CARTESIAN_POINT ( 'NONE',  ( 5.555090253297246150, 7.504024600312024340, 1.599625672291267398 ) ) ;
#95986=CARTESIAN_POINT ( 'NONE',  ( 5.165293336682183600, 5.128523102325077687, -0.7216878364870197293 ) ) ;
#95994=CARTESIAN_POINT ( 'NONE',  ( -5.669280788808708671, 9.765911353585494226, 0.7998128361456481317 ) ) ;
#95995=CARTESIAN_POINT ( 'NONE',  ( -4.273844736805832767, 6.009238164405336313, 1.599625672291267398 ) ) ;
#96001=B_SPLINE_CURVE_WITH_KNOTS ( 'NONE', 3,
 ( #8267, #52748, #184868, #87396, #3970, #70038, #202171, #203249 ),
 .UNSPECIFIED., .F., .F.,
 ( 4, 2, 2, 4 ),
 ( 4.385326393719464467E-18, 0.0006692579211854246318, 0.001003886881778133641, 0.001338515842370842758 ),
 .UNSPECIFIED. ) ;
#96003=CARTESIAN_POINT ( 'NONE',  ( 5.276094334012385367, 9.307193822989793475, 1.040834085586084257E-14 ) ) ;
#96010=DIRECTION ( 'NONE',  ( 0.8002608041566210417, 0.5996521035822340862, 0.000000000000000000 ) ) ;
#96013=CARTESIAN_POINT ( 'NONE',  ( 1.270904146967301473, 3.084693569853256268, -0.7749999999999910294 ) ) ;
#96016=ORIENTED_EDGE ( 'NONE', *, *, #83952, .F. ) ;
#96018=CARTESIAN_POINT ( 'NONE',  ( 0.6823417656249882723, 0.2385416670080825474, -1.181850606188749264 ) ) ;
#96019=CARTESIAN_POINT ( 'NONE',  ( 5.529027716274630855, 5.344953845275508542, 1.040834085586084257E-14 ) ) ;
#96022=CARTESIAN_POINT ( 'NONE',  ( -7.402388683381436074, 7.738467673474211495, 0.7216878364870317197 ) ) ;
#96023=ADVANCED_FACE ( 'NONE', ( #112419 ), #180546, .F. ) ;
#96024=CARTESIAN_POINT ( 'NONE',  ( 5.395781948558860286, 6.357795697149212444, -1.082531754730542195 ) ) ;
#96026=CARTESIAN_POINT ( 'NONE',  ( -6.331294547457448019, 10.33033470543493770, 0.7216878364870458196 ) ) ;
#96030=CARTESIAN_POINT ( 'NONE',  ( 7.135668919494039031, 7.219368582364847242, 1.040834085586084257E-14 ) ) ;
#96034=DIRECTION ( 'NONE',  ( 0.000000000000000000, -1.000000000000000000, 0.000000000000000000 ) ) ;
#96035=CARTESIAN_POINT ( 'NONE',  ( -0.6823417656249969321, 4.467708333674755394, -1.181850606188749264 ) ) ;
#96040=CARTESIAN_POINT ( 'NONE',  ( 6.662942426112080874, 9.860851032851066122, 1.199719254218460707 ) ) ;
#96043=CARTESIAN_POINT ( 'NONE',  ( -8.538937818508475885, 8.856515631215026829, 1.040834085586084257E-14 ) ) ;
#96048=CARTESIAN_POINT ( 'NONE',  ( 8.757677159423465696, 12.30470822171437284, 1.199719254218450271 ) ) ;
#96051=CARTESIAN_POINT ( 'NONE',  ( -8.227100285394159940, 8.492705175914988303, 0.7998128361456602331 ) ) ;
#96052=CARTESIAN_POINT ( 'NONE',  ( 0.2756800312742226367, 7.029902384775073898, 4.006536513033384317 ) ) ;
#96054=CARTESIAN_POINT ( 'NONE',  ( 5.538030394937467626, 6.199453712711876285, -0.9301498999644899346 ) ) ;
#96055=CARTESIAN_POINT ( 'NONE',  ( -8.676855123066019360, 11.14608361504227574, -1.443375672974059665 ) ) ;
#96059=CARTESIAN_POINT ( 'NONE',  ( 5.829115978871627135, 8.888053511070525659, 1.199719254218462483 ) ) ;
#96061=CARTESIAN_POINT ( 'NONE',  ( 6.498435699651741615, 6.475929825882159818, -0.7998128361456281477 ) ) ;
#96062=CARTESIAN_POINT ( 'NONE',  ( -4.105200985651542567, 7.499488806860944656, 0.5979674706809139373 ) ) ;
#96064=CARTESIAN_POINT ( 'NONE',  ( 3.009020027229115879, 5.597941567487558778, -1.199719254218446718 ) ) ;
#96066=CARTESIAN_POINT ( 'NONE',  ( -5.748293942514169252, 9.650167333001109071, -0.7216878364870207285 ) ) ;
#96071=CARTESIAN_POINT ( 'NONE',  ( -5.357213605067637552, 6.353687308821166724, 1.098221101205157035 ) ) ;
#96072=CARTESIAN_POINT ( 'NONE',  ( 0.6823417656249882723, -0.01145833299191073573, -1.181850606188749264 ) ) ;
#96076=CARTESIAN_POINT ( 'NONE',  ( 4.039966587192259873, 5.736380323189513852, 1.443375672974062551 ) ) ;
#96080=CARTESIAN_POINT ( 'NONE',  ( -8.473482818416670170, 10.90881592628469932, -1.443375672974058777 ) ) ;
#96086=CARTESIAN_POINT ( 'NONE',  ( -7.822691444960700125, 11.10992853822074444, -1.082531754730543083 ) ) ;
#96087=ORIENTED_EDGE ( 'NONE', *, *, #2718, .T. ) ;
#96090=ADVANCED_FACE ( 'NONE', ( #15889 ), #27902, .F. ) ;
#96093=CARTESIAN_POINT ( 'NONE',  ( -9.612367721964622191, 10.31677655182129527, -0.7216878364870267237 ) ) ;
#96097=CARTESIAN_POINT ( 'NONE',  ( -1.364683531250012516, 5.051041667008085767, -0.7879004041258300672 ) ) ;
#96098=CARTESIAN_POINT ( 'NONE',  ( 1.499999999999989120, 4.535416667349484676, 0.8660254037844524744 ) ) ;
#96099=CARTESIAN_POINT ( 'NONE',  ( 5.722549628727856330, 6.269105753387675506, -1.057781258018471782 ) ) ;
#96104=CARTESIAN_POINT ( 'NONE',  ( -7.374745490829552885, 10.69128794168811680, -1.199719254218446718 ) ) ;
#96108=CARTESIAN_POINT ( 'NONE',  ( 6.043183783389218355, 8.073467052085995022, 1.599625672291267398 ) ) ;
#96110=CARTESIAN_POINT ( 'NONE',  ( 3.732121546690903457, 4.106948192567998035, -0.9424847539492161586 ) ) ;
#96113=CARTESIAN_POINT ( 'NONE',  ( 6.934105498385400246, 10.17720795050327354, -1.199719254218441611 ) ) ;
#96120=CARTESIAN_POINT ( 'NONE',  ( -6.914295153289458540, 7.169025221700239925, 0.7216878364870317197 ) ) ;
#96123=CARTESIAN_POINT ( 'NONE',  ( -6.471393748265538370, 5.229711127717889596, -2.499999999999995115 ) ) ;
#96126=CARTESIAN_POINT ( 'NONE',  ( 4.039966587192257208, 6.696749537490852333, 1.082531754730558626 ) ) ;
#96132=CARTESIAN_POINT ( 'NONE',  ( -8.292783513053063160, 12.82666453187061073, 0.7998128361456481317 ) ) ;
#96134=EDGE_CURVE ( 'NONE', #92745, #108467, #114554, .T. ) ;
#96135=CARTESIAN_POINT ( 'NONE',  ( 7.584896871841365851, 10.93646455286856956, -1.199719254218446718 ) ) ;
#96136=CARTESIAN_POINT ( 'NONE',  ( -1.500000000000013101, 0.1708333333333560411, 0.8660254037844403729 ) ) ;
#96137=CARTESIAN_POINT ( 'NONE',  ( -7.831806290188425557, 12.28885777186185990, -0.7998128361456281477 ) ) ;
#96140=CARTESIAN_POINT ( 'NONE',  ( 0.6823417656249899377, 2.842708333674753618, 1.181850606188765695 ) ) ;
#96141=EDGE_CURVE ( 'NONE', #32206, #164712, #97938, .T. ) ;
#96142=CARTESIAN_POINT ( 'NONE',  ( 3.440018289565364817, 5.036440642624797626, 1.599625672291267398 ) ) ;
#96147=CARTESIAN_POINT ( 'NONE',  ( 8.880227426826634129, 11.38335130276301754, 1.443375672974076540 ) ) ;
#96150=CARTESIAN_POINT ( 'NONE',  ( -5.395781948558855845, 9.238903340053241209, 0.7216878364870458196 ) ) ;
#96151=CARTESIAN_POINT ( 'NONE',  ( -0.6823417656250003738, 1.217708333674752286, -1.181850606188749264 ) ) ;
#96153=CARTESIAN_POINT ( 'NONE',  ( 0.4210486379898482623, 7.995128625469308581, 1.998698746375270341 ) ) ;
#96155=CARTESIAN_POINT ( 'NONE',  ( -6.509886312855995172, 10.74661779830734254, -0.7998128361456291469 ) ) ;
#96157=CARTESIAN_POINT ( 'NONE',  ( -3.511198595814942980, 5.119484333249288532, 1.443375672974064550 ) ) ;
#96158=CARTESIAN_POINT ( 'NONE',  ( 0.6823417656249882723, 2.988541667008084879, -1.181850606188754593 ) ) ;
#96162=EDGE_CURVE ( 'NONE', #69507, #2895, #45413, .T. ) ;
#96165=CARTESIAN_POINT ( 'NONE',  ( 9.921869487102386032, 10.46993591124128997, 0.000000000000000000 ) ) ;
#96170=ORIENTED_EDGE ( 'NONE', *, *, #168698, .T. ) ;
#96176=CARTESIAN_POINT ( 'NONE',  ( -1.546240757466864402, 8.694816975860053532, 2.507471980975723103 ) ) ;
#96178=CARTESIAN_POINT ( 'NONE',  ( 0.6823417656249864960, -0.8239583329919114574, -1.181850606188749264 ) ) ;
#96182=CARTESIAN_POINT ( 'NONE',  ( 8.769426429940780920, 9.125419011219408461, 0.7998128361456462443 ) ) ;
#96185=CARTESIAN_POINT ( 'NONE',  ( 0.6823417656249899377, 3.176041667008085323, -1.181850606188754593 ) ) ;
#96187=CARTESIAN_POINT ( 'NONE',  ( -7.537970219518089543, 8.857015346601659900, -1.082531754730543971 ) ) ;
#96189=CARTESIAN_POINT ( 'NONE',  ( 1.440240048130367878, 7.355731858843415516, 4.317885097515409498 ) ) ;
#96193=FACE_OUTER_BOUND ( 'NONE', #201526, .T. ) ;
#96196=CARTESIAN_POINT ( 'NONE',  ( 8.703444544968814256, 12.24143683818393313, -1.199719254218446718 ) ) ;
#96203=CARTESIAN_POINT ( 'NONE',  ( -8.136864746495904299, 12.64475930422059768, -0.7998128361456281477 ) ) ;
#96204=CARTESIAN_POINT ( 'NONE',  ( 7.446452682403650769, 9.710614100936176385, -1.599625672291262513 ) ) ;
#96206=CARTESIAN_POINT ( 'NONE',  ( 4.514501963226220660, 4.369266499959774563, -0.7216878364870197293 ) ) ;
#96208=ORIENTED_EDGE ( 'NONE', *, *, #79248, .F. ) ;
#96216=CARTESIAN_POINT ( 'NONE',  ( -6.724481002698138532, 6.947575379343695623, -0.7216878364870278340 ) ) ;
#96217=CARTESIAN_POINT ( 'NONE',  ( 3.225950485047770933, 5.851027101609320269, 1.199719254218450271 ) ) ;
#96220=CARTESIAN_POINT ( 'NONE',  ( -8.179646747746328828, 8.437342715325849341, -0.7998128361456291469 ) ) ;
#96225=CARTESIAN_POINT ( 'NONE',  ( -8.286004436246233951, 12.81875560892930466, 1.040834085586084257E-14 ) ) ;
#96229=CARTESIAN_POINT ( 'NONE',  ( 6.909851844459134362, 11.21324425184434936, -0.7998128361456291469 ) ) ;
#96230=( BOUNDED_SURFACE ( )  B_SPLINE_SURFACE ( 1, 2, ( 
 ( #170261, #87954, #154028, #7752, #22925, #139935, #71675, #203808, #56528, #55453, #138856, #188651, #205962, #123752, #173502, #109620, #125878, #145284, #177749, #43500, #175625, #96522, #212349, #45626, #27212, #191837, #94383, #195054, #30436, #59719, #193978, #178824, #162570, #143155, #174570, #112811, #110676, #14143, #176676, #28288, #208091, #29364, #93318, #80236, #159354, #146335, #63990, #10951, #78100, #111743, #129083, #130142, #196131, #192904, #47771, #13089, #26146, #161508, #92260, #158306, #160423, #77025, #209149, #44560, #60788, #144227, #75974, #9897, #79168, #61857, #46693, #12029, #210221, #142077, #126947, #128024, #62914, #95459, #211290, #69281, #113884, #82356, #150581, #3213, #16271, #15218, #114931, #115993, #201416, #164688, #135394, #133284, #66080, #1085, #200354, #101811, #179879, #149502, #32550, #19479, #31504, #52004, #184115, #98627, #85554, #181982, #33613, #99684, #198231, #118130, #97578, #67149, #165753, #199291, #17339, #167879, #48814, #65033, #166822, #83421, #50936, #163635, #16, #151644, #49867, #197178, #2143, #81308, #148446, #35736, #132221, #147385, #180929, #117060, #183057, #34671, #100741, #18416, #84490, #213411, #131189, #68220, #134351, #4275, #57329, #36798, #107208, #172154, #56266, #168941, #55198, #72491, #203544, #171069, #70346, #138592, #123493, #122425, #120270, #22666, #103956, #88777, #188382, #102883, #71417, #54135, #20543, #139672, #74647, #153766, #137529, #24811, #87691, #187320, #86627, #7488, #38948, #204615, #119189, #121345, #23746, #41099, #40020, #105031, #169999, #189457, #90912, #6419, #154835, #37880, #89851, #155901, #106131, #21586, #73570, #5334, #202482, #205694, #185174, #152694, #173231, #156977, #8566, #186245, #136463, #140752, #53055, #190509, #9632, #44291, #191571, #93051, #175362, #176416, #174302, #178547, #59455, #77833, #10690, #45357, #46418, #125612, #28023, #62641, #26944, #159092, #193714, #158046, #111476, #141824, #75709, #177481, #209949, #207826, #43235, #128799, #30157, #143954, #109352, #76760, #126675, #12816, #194781, #91987, #11759, #211018, #112535, #142882, #206763, #145012, #208884, #96245, #60514, #192638, #25877, #61588, #110413, #162296, #94120, #13883, #79962, #160161, #127757, #29096, #161229, #58395, #124551, #95180, #42166, #78889, #108281, #133021, #134091, #167622, #131959, #14941, #114671, #164421, #196913, #115724, #47498, #51748, #199020, #33344, #100480, #82090, #197969, #195858, #117871, #81036, #34408, #113607, #16005, #101553, #146065, #180665, #182790, #35475, #148183, #214184, #50667, #181715, #166556, #179611, #212078, #98356, #183862, #49600, #31232, #97306, #147123, #19221, #116793, #163365, #65812, #32290, #18144, #84232, #150320, #213149, #64779, #63717, #130920, #1886, #99426, #129875, #48553, #165480, #17076, #83154, #67946, #149234, #808, #66876, #200099, #38695, #152442, #102628, #168684, #135143, #72230, #73305, #106952, #71159, #20288, #53877, #103700, #136205, #54943, #201159, #205441, #138337, #187062, #39761, #21339, #137276, #52798, #57077, #86373, #188130, #118937, #169751, #40843, #85299, #120010, #122163, #189206, #87446, #153515, #204353, #121095, #105866, #184917, #151385, #37620, #123241, #203296, #36541, #4021, #70090, #172975, #56011, #202223, #5084, #185986, #171892, #23489, #89596, #104773, #170822, #2955, #22413, #155645, #88522, #69026, #154584, #6161, #7229, #139407, #190259, #108028, #206510, #58141, #124300, #41917, #156723, #90661, #8314, #24554, #74399, #140500, #196097, #200320, #81267, #99647, #32514, #67110, #68182, #147346, #198194, #84456, #197139, #48778, #1047, #179841, #133246, #163597, #31464, #199251, #17303, #97539, #15180, #150544, #51971, #165714, #213373, #64996, #148412, #34636, #2108, #113846, #33575, #18378, #134313, #114893, #14108, #166784, #164651, #118096, #16235, #82318, #47729, #83382, #131150, #184081, #180892, #35699, #101775, #98589, #132187, #149464, #183020, #80196, #146300, #197476, #212313, #50898, #63948, #117024, #130103, #66043, #49830, #115955, #181945, #100707, #70310, #69245, #168903, #169965, #41062, #4240 ),
 ( #73532, #21551, #87661, #153730, #37842, #106094, #123457, #121308, #5299, #187283, #71380, #155864, #102846, #119152, #6384, #137493, #203509, #3174, #54097, #139634, #103920, #36761, #56228, #167843, #86591, #172117, #152658, #205657, #20506, #55161, #38910, #136427, #104994, #171034, #202442, #189419, #85520, #22630, #88740, #185135, #23711, #151606, #7454, #72455, #154797, #135363, #138554, #204578, #122389, #188346, #120234, #39985, #89819, #57293, #186208, #19440, #201378, #53019, #27984, #90877, #125573, #108243, #74609, #193674, #128765, #207789, #191534, #78849, #141781, #26906, #156939, #61548, #93012, #192599, #173194, #43198, #11720, #95139, #94080, #109312, #9597, #29056, #144970, #60476, #159055, #91948, #143915, #77796, #10649, #158009, #209910, #75674, #42131, #59417, #24776, #140714, #126634, #127715, #175322, #25841, #8530, #45317, #206729, #76724, #62602, #107169, #142840, #111437, #210975, #208845, #44252, #160119, #110374, #177440, #58357, #124512, #176379, #194741, #161189, #190470, #174266, #12776, #142602, #159885, #79696, #26677, #208612, #128544, #129607, #127482, #93847, #158824, #145809, #48291, #10420, #192362, #12549, #11491, #61322, #77564, #76492, #176152, #177209, #175089, #143686, #196651, #194510, #193453, #62380, #47226, #163099, #92779, #210760, #209678, #80776, #60245, #113344, #30971, #45097, #146864, #28823, #94909, #160959, #111206, #179349, #130661, #46158, #78624, #112271, #144748, #14679, #110140, #126402, #13623, #178285, #29894, #44021, #95980, #212885, #162032, #27752, #63453, #211816, #195592, #97046, #64516, #20005, #115461, #182506, #100205, #49342, #1608, #133811, #165210, #135915, #32021, #116516, #67667, #65549, #118653, #98106, #168408, #18935, #117590, #15743, #34136, #199825, #50396, #17863, #131694, #51466, #184639, #183581, #181452, #83946, #16800, #150037, #35188, #164158, #132746, #33082, #81828, #200876, #201933, #533, #198749, #86089, #148961, #166271, #101264, #167348, #152165, #99157, #85020, #36257, #82884, #66600, #151109, #197700, #2675, #68747, #134869, #52521, #102336, #3734, #69809, #114403, #180402, #147911, #213926, #4794, #187845, #74115, #124019, #153224, #73024, #57857, #189984, #22117, #53590, #206230, #204068, #41636, #55720, #121874, #87153, #56792, #54656, #107750, #120804, #173776, #25351, #186781, #171602, #139122, #8025, #91451, #157512, #71945, #9107, #106664, #75183, #40558, #141295, #119724, #39471, #136987, #88229, #138055, #104489, #23195, #169471, #185703, #172689, #155358, #140211, #105570, #89311, #103410, #37337, #203014, #156441, #21056, #6943, #70873, #38407, #154297, #90372, #170532, #205149, #122961, #24267, #188920, #5872, #108816, #207304, #159633, #30712, #110945, #174840, #92529, #208361, #59992, #192108, #143422, #96795, #27489, #13370, #161779, #145561, #126145, #42708, #162844, #43772, #194258, #11229, #125085, #191043, #58926, #26417, #14422, #211559, #80512, #176952, #144493, #62136, #160699, #109885, #10168, #76242, #158569, #175898, #28568, #142351, #179090, #93589, #78373, #193191, #77309, #94655, #12293, #209418, #61063, #127222, #44839, #210501, #128296, #63194, #45904, #46968, #112022, #178023, #29642, #95727, #79444, #129358, #195336, #113084, #166026, #2421, #149785, #213675, #116270, #197449, #182259, #67421, #130412, #164957, #147659, #114158, #18690, #168160, #32828, #16549, #118404, #181200, #66357, #196400, #101012, #132503, #17611, #212627, #82631, #51214, #134626, #133564, #148716, #49090, #68498, #184391, #99962, #198501, #131448, #183335, #117338, #50146, #115210, #286, #180151, #98905, #34939, #64269, #31777, #83697, #167103, #33884, #65300, #48045, #84772, #19758, #97849, #163912, #1359, #199570, #150859, #200630, #15488, #52278, #36011, #146609, #102090, #81576, #105314, #38161, #187596, #172434, #73858, #151917, #121627, #4551, #205977, #3490, #24023, #156191, #70624, #57612, #154047, #5614, #71696, #170280, #90124, #41383, #39223, #137808, #171352, #203827, #139952, #20812, #37080, #138876, #55472, #22945, #135670, #186532, #123770, #21868, #169220, #188671, #173520, #136737, #7767 ) ),
 .UNSPECIFIED., .F., .F., .T. ) 
 B_SPLINE_SURFACE_WITH_KNOTS ( ( 2, 2 ),
 ( 3, 2, 2, 2, 2, 2, 2, 2, 2, 2, 2, 2, 2, 2, 2, 2, 2, 2, 2, 2, 2, 2, 2, 2, 2, 2, 2, 2, 2, 2, 2, 2, 2, 2, 2, 2, 2, 2, 2, 2, 2, 2, 2, 2, 2, 2, 2, 2, 2, 2, 2, 2, 2, 2, 2, 2, 2, 2, 2, 2, 2, 2, 2, 2, 2, 2, 2, 2, 2, 2, 2, 2, 2, 2, 2, 2, 2, 2, 2, 2, 2, 2, 2, 2, 2, 2, 2, 2, 2, 2, 2, 2, 2, 2, 2, 2, 2, 2, 2, 2, 2, 2, 2, 2, 2, 2, 2, 2, 2, 2, 2, 2, 2, 2, 2, 2, 2, 2, 2, 2, 2, 2, 2, 2, 2, 2, 2, 2, 2, 2, 2, 2, 2, 2, 2, 2, 2, 2, 2, 2, 2, 2, 2, 2, 2, 2, 2, 2, 2, 2, 2, 2, 2, 2, 2, 2, 2, 2, 2, 2, 2, 2, 2, 2, 2, 2, 2, 2, 2, 2, 2, 2, 2, 2, 2, 2, 2, 2, 2, 2, 2, 2, 2, 2, 2, 2, 2, 2, 2, 2, 2, 2, 2, 2, 2, 2, 2, 2, 2, 2, 2, 2, 2, 2, 2, 2, 2, 2, 2, 2, 2, 2, 2, 2, 2, 2, 2, 2, 2, 2, 2, 2, 2, 2, 2, 2, 2, 2, 2, 2, 2, 2, 2, 2, 2, 2, 2, 2, 2, 2, 3 ),
 ( 0.000000000000000000, 1.000000000000000000 ),
 ( 0.000000000000000000, 0.004166666666666666609, 0.008333333333333333218, 0.01250000000000000069, 0.01666666666666666644, 0.02083333333333333218, 0.02500000000000000139, 0.02916666666666666713, 0.03333333333333333287, 0.03749999999999999861, 0.04166666666666666435, 0.04583333333333333010, 0.05000000000000000278, 0.05416666666666666852, 0.05833333333333333426, 0.06250000000000000000, 0.06666666666666666574, 0.07083333333333333148, 0.07499999999999999722, 0.07916666666666666297, 0.08333333333333332871, 0.08749999999999999445, 0.09166666666666666019, 0.09583333333333333981, 0.1000000000000000056, 0.1041666666666666713, 0.1083333333333333370, 0.1125000000000000028, 0.1166666666666666685, 0.1208333333333333343, 0.1250000000000000000, 0.1291666666666666796, 0.1333333333333333315, 0.1375000000000000111, 0.1416666666666666630, 0.1458333333333333426, 0.1499999999999999944, 0.1541666666666666741, 0.1583333333333333259, 0.1625000000000000056, 0.1666666666666666574, 0.1708333333333333370, 0.1749999999999999889, 0.1791666666666666685, 0.1833333333333333204, 0.1875000000000000000, 0.1916666666666666796, 0.1958333333333333315, 0.2000000000000000111, 0.2041666666666666630, 0.2083333333333333426, 0.2124999999999999944, 0.2166666666666666741, 0.2208333333333333259, 0.2250000000000000056, 0.2291666666666666574, 0.2333333333333333370, 0.2374999999999999889, 0.2416666666666666685, 0.2458333333333333204, 0.2500000000000000000, 0.2541666666666666519, 0.2583333333333333592, 0.2625000000000000111, 0.2666666666666666630, 0.2708333333333333148, 0.2750000000000000222, 0.2791666666666666741, 0.2833333333333333259, 0.2874999999999999778, 0.2916666666666666852, 0.2958333333333333370, 0.2999999999999999889, 0.3041666666666666408, 0.3083333333333333481, 0.3125000000000000000, 0.3166666666666666519, 0.3208333333333333592, 0.3250000000000000111, 0.3291666666666666630, 0.3333333333333333148, 0.3375000000000000222, 0.3416666666666666741, 0.3458333333333333259, 0.3499999999999999778, 0.3541666666666666852, 0.3583333333333333370, 0.3624999999999999889, 0.3666666666666666408, 0.3708333333333333481, 0.3750000000000000000, 0.3791666666666666519, 0.3833333333333333592, 0.3875000000000000111, 0.3916666666666666630, 0.3958333333333333148, 0.4000000000000000222, 0.4041666666666666741, 0.4083333333333333259, 0.4124999999999999778, 0.4166666666666666852, 0.4208333333333333370, 0.4249999999999999889, 0.4291666666666666408, 0.4333333333333333481, 0.4375000000000000000, 0.4416666666666666519, 0.4458333333333333592, 0.4500000000000000111, 0.4541666666666666630, 0.4583333333333333148, 0.4625000000000000222, 0.4666666666666666741, 0.4708333333333333259, 0.4749999999999999778, 0.4791666666666666852, 0.4833333333333333370, 0.4874999999999999889, 0.4916666666666666408, 0.4958333333333333481, 0.5000000000000000000, 0.5041666666666666519, 0.5083333333333333037, 0.5124999999999999556, 0.5166666666666667185, 0.5208333333333333703, 0.5250000000000000222, 0.5291666666666666741, 0.5333333333333333259, 0.5374999999999999778, 0.5416666666666666297, 0.5458333333333332815, 0.5500000000000000444, 0.5541666666666666963, 0.5583333333333333481, 0.5625000000000000000, 0.5666666666666666519, 0.5708333333333333037, 0.5749999999999999556, 0.5791666666666667185, 0.5833333333333333703, 0.5875000000000000222, 0.5916666666666666741, 0.5958333333333333259, 0.5999999999999999778, 0.6041666666666666297, 0.6083333333333332815, 0.6125000000000000444, 0.6166666666666666963, 0.6208333333333333481, 0.6250000000000000000, 0.6291666666666666519, 0.6333333333333333037, 0.6374999999999999556, 0.6416666666666667185, 0.6458333333333333703, 0.6500000000000000222, 0.6541666666666666741, 0.6583333333333333259, 0.6624999999999999778, 0.6666666666666666297, 0.6708333333333332815, 0.6750000000000000444, 0.6791666666666666963, 0.6833333333333333481, 0.6875000000000000000, 0.6916666666666666519, 0.6958333333333333037, 0.6999999999999999556, 0.7041666666666667185, 0.7083333333333333703, 0.7125000000000000222, 0.7166666666666666741, 0.7208333333333333259, 0.7249999999999999778, 0.7291666666666666297, 0.7333333333333332815, 0.7375000000000000444, 0.7416666666666666963, 0.7458333333333333481, 0.7500000000000000000, 0.7541666666666666519, 0.7583333333333333037, 0.7624999999999999556, 0.7666666666666667185, 0.7708333333333333703, 0.7750000000000000222, 0.7791666666666666741, 0.7833333333333333259, 0.7874999999999999778, 0.7916666666666666297, 0.7958333333333332815, 0.8000000000000000444, 0.8041666666666666963, 0.8083333333333333481, 0.8125000000000000000, 0.8166666666666666519, 0.8208333333333333037, 0.8249999999999999556, 0.8291666666666667185, 0.8333333333333333703, 0.8375000000000000222, 0.8416666666666666741, 0.8458333333333333259, 0.8499999999999999778, 0.8541666666666666297, 0.8583333333333332815, 0.8625000000000000444, 0.8666666666666666963, 0.8708333333333333481, 0.8750000000000000000, 0.8791666666666666519, 0.8833333333333333037, 0.8874999999999999556, 0.8916666666666667185, 0.8958333333333333703, 0.9000000000000000222, 0.9041666666666666741, 0.9083333333333333259, 0.9124999999999999778, 0.9166666666666666297, 0.9208333333333332815, 0.9250000000000000444, 0.9291666666666666963, 0.9333333333333333481, 0.9375000000000000000, 0.9416666666666666519, 0.9458333333333333037, 0.9499999999999999556, 0.9541666666666667185, 0.9583333333333333703, 0.9625000000000000222, 0.9666666666666666741, 0.9708333333333333259, 0.9749999999999999778, 0.9791666666666666297, 0.9833333333333332815, 0.9875000000000000444, 0.9916666666666666963, 0.9958333333333333481, 1.000000000000000000 ),
 .UNSPECIFIED. ) 
 GEOMETRIC_REPRESENTATION_ITEM ( )  RATIONAL_B_SPLINE_SURFACE ( (
 ( 1.000000000000000000, 0.8660254037844387076, 1.000000000000000000, 0.8660254037844387076, 1.000000000000000000, 0.8660254037844387076, 1.000000000000000000, 0.8660254037844387076, 1.000000000000000000, 0.8660254037844387076, 1.000000000000000000, 0.8660254037844387076, 1.000000000000000000, 0.8660254037844387076, 1.000000000000000000, 0.8660254037844387076, 1.000000000000000000, 0.8660254037844387076, 1.000000000000000000, 0.8660254037844387076, 1.000000000000000000, 0.8660254037844387076, 1.000000000000000000, 0.8660254037844387076, 1.000000000000000000, 0.8660254037844387076, 1.000000000000000000, 0.8660254037844387076, 1.000000000000000000, 0.8660254037844387076, 1.000000000000000000, 0.8660254037844387076, 1.000000000000000000, 0.8660254037844387076, 1.000000000000000000, 0.8660254037844387076, 1.000000000000000000, 0.8660254037844387076, 1.000000000000000000, 0.8660254037844387076, 1.000000000000000000, 0.8660254037844387076, 1.000000000000000000, 0.8660254037844387076, 1.000000000000000000, 0.8660254037844387076, 1.000000000000000000, 0.8660254037844387076, 1.000000000000000000, 0.8660254037844387076, 1.000000000000000000, 0.8660254037844387076, 1.000000000000000000, 0.8660254037844387076, 1.000000000000000000, 0.8660254037844387076, 1.000000000000000000, 0.8660254037844387076, 1.000000000000000000, 0.8660254037844387076, 1.000000000000000000, 0.8660254037844387076, 1.000000000000000000, 0.8660254037844387076, 1.000000000000000000, 0.8660254037844387076, 1.000000000000000000, 0.8660254037844387076, 1.000000000000000000, 0.8660254037844387076, 1.000000000000000000, 0.8660254037844387076, 1.000000000000000000, 0.8660254037844387076, 1.000000000000000000, 0.8660254037844387076, 1.000000000000000000, 0.8660254037844387076, 1.000000000000000000, 0.8660254037844387076, 1.000000000000000000, 0.8660254037844387076, 1.000000000000000000, 0.8660254037844387076, 1.000000000000000000, 0.8660254037844387076, 1.000000000000000000, 0.8660254037844387076, 1.000000000000000000, 0.8660254037844387076, 1.000000000000000000, 0.8660254037844387076, 1.000000000000000000, 0.8660254037844387076, 1.000000000000000000, 0.8660254037844387076, 1.000000000000000000, 0.8660254037844387076, 1.000000000000000000, 0.8660254037844387076, 1.000000000000000000, 0.8660254037844387076, 1.000000000000000000, 0.8660254037844387076, 1.000000000000000000, 0.8660254037844387076, 1.000000000000000000, 0.8660254037844387076, 1.000000000000000000, 0.8660254037844387076, 1.000000000000000000, 0.8660254037844387076, 1.000000000000000000, 0.8660254037844387076, 1.000000000000000000, 0.8660254037844387076, 1.000000000000000000, 0.8660254037844387076, 1.000000000000000000, 0.8660254037844387076, 1.000000000000000000, 0.8660254037844387076, 1.000000000000000000, 0.8660254037844387076, 1.000000000000000000, 0.8660254037844387076, 1.000000000000000000, 0.8660254037844387076, 1.000000000000000000, 0.8660254037844387076, 1.000000000000000000, 0.8660254037844387076, 1.000000000000000000, 0.8660254037844387076, 1.000000000000000000, 0.8660254037844387076, 1.000000000000000000, 0.8660254037844387076, 1.000000000000000000, 0.8660254037844387076, 1.000000000000000000, 0.8660254037844387076, 1.000000000000000000, 0.8660254037844387076, 1.000000000000000000, 0.8660254037844387076, 1.000000000000000000, 0.8660254037844387076, 1.000000000000000000, 0.8660254037844387076, 1.000000000000000000, 0.8660254037844387076, 1.000000000000000000, 0.8660254037844387076, 1.000000000000000000, 0.8660254037844387076, 1.000000000000000000, 0.8660254037844387076, 1.000000000000000000, 0.8660254037844387076, 1.000000000000000000, 0.8660254037844387076, 1.000000000000000000, 0.8660254037844387076, 1.000000000000000000, 0.8660254037844387076, 1.000000000000000000, 0.8660254037844387076, 1.000000000000000000, 0.8660254037844387076, 1.000000000000000000, 0.8660254037844387076, 1.000000000000000000, 0.8660254037844387076, 1.000000000000000000, 0.8660254037844387076, 1.000000000000000000, 0.8660254037844387076, 1.000000000000000000, 0.8660254037844387076, 1.000000000000000000, 0.8660254037844387076, 1.000000000000000000, 0.8660254037844387076, 1.000000000000000000, 0.8660254037844387076, 1.000000000000000000, 0.8660254037844387076, 1.000000000000000000, 0.8660254037844387076, 1.000000000000000000, 0.8660254037844387076, 1.000000000000000000, 0.8660254037844387076, 1.000000000000000000, 0.8660254037844387076, 1.000000000000000000, 0.8660254037844387076, 1.000000000000000000, 0.8660254037844387076, 1.000000000000000000, 0.8660254037844387076, 1.000000000000000000, 0.8660254037844387076, 1.000000000000000000, 0.8660254037844387076, 1.000000000000000000, 0.8660254037844387076, 1.000000000000000000, 0.8660254037844387076, 1.000000000000000000, 0.8660254037844387076, 1.000000000000000000, 0.8660254037844387076, 1.000000000000000000, 0.8660254037844387076, 1.000000000000000000, 0.8660254037844387076, 1.000000000000000000, 0.8660254037844387076, 1.000000000000000000, 0.8660254037844387076, 1.000000000000000000, 0.8660254037844387076, 1.000000000000000000, 0.8660254037844387076, 1.000000000000000000, 0.8660254037844387076, 1.000000000000000000, 0.8660254037844387076, 1.000000000000000000, 0.8660254037844387076, 1.000000000000000000, 0.8660254037844387076, 1.000000000000000000, 0.8660254037844387076, 1.000000000000000000, 0.8660254037844387076, 1.000000000000000000, 0.8660254037844387076, 1.000000000000000000, 0.8660254037844387076, 1.000000000000000000, 0.8660254037844387076, 1.000000000000000000, 0.8660254037844387076, 1.000000000000000000, 0.8660254037844387076, 1.000000000000000000, 0.8660254037844387076, 1.000000000000000000, 0.8660254037844387076, 1.000000000000000000, 0.8660254037844387076, 1.000000000000000000, 0.8660254037844387076, 1.000000000000000000, 0.8660254037844387076, 1.000000000000000000, 0.8660254037844387076, 1.000000000000000000, 0.8660254037844387076, 1.000000000000000000, 0.8660254037844387076, 1.000000000000000000, 0.8660254037844387076, 1.000000000000000000, 0.8660254037844387076, 1.000000000000000000, 0.8660254037844387076, 1.000000000000000000, 0.8660254037844387076, 1.000000000000000000, 0.8660254037844387076, 1.000000000000000000, 0.8660254037844387076, 1.000000000000000000, 0.8660254037844387076, 1.000000000000000000, 0.8660254037844387076, 1.000000000000000000, 0.8660254037844387076, 1.000000000000000000, 0.8660254037844387076, 1.000000000000000000, 0.8660254037844387076, 1.000000000000000000, 0.8660254037844387076, 1.000000000000000000, 0.8660254037844387076, 1.000000000000000000, 0.8660254037844387076, 1.000000000000000000, 0.8660254037844387076, 1.000000000000000000, 0.8660254037844387076, 1.000000000000000000, 0.8660254037844387076, 1.000000000000000000, 0.8660254037844387076, 1.000000000000000000, 0.8660254037844387076, 1.000000000000000000, 0.8660254037844387076, 1.000000000000000000, 0.8660254037844387076, 1.000000000000000000, 0.8660254037844387076, 1.000000000000000000, 0.8660254037844387076, 1.000000000000000000, 0.8660254037844387076, 1.000000000000000000, 0.8660254037844387076, 1.000000000000000000, 0.8660254037844387076, 1.000000000000000000, 0.8660254037844387076, 1.000000000000000000, 0.8660254037844387076, 1.000000000000000000, 0.8660254037844387076, 1.000000000000000000, 0.8660254037844387076, 1.000000000000000000, 0.8660254037844387076, 1.000000000000000000, 0.8660254037844387076, 1.000000000000000000, 0.8660254037844387076, 1.000000000000000000, 0.8660254037844387076, 1.000000000000000000, 0.8660254037844387076, 1.000000000000000000, 0.8660254037844387076, 1.000000000000000000, 0.8660254037844387076, 1.000000000000000000, 0.8660254037844387076, 1.000000000000000000, 0.8660254037844387076, 1.000000000000000000, 0.8660254037844387076, 1.000000000000000000, 0.8660254037844387076, 1.000000000000000000, 0.8660254037844387076, 1.000000000000000000, 0.8660254037844387076, 1.000000000000000000, 0.8660254037844387076, 1.000000000000000000, 0.8660254037844387076, 1.000000000000000000, 0.8660254037844387076, 1.000000000000000000, 0.8660254037844387076, 1.000000000000000000, 0.8660254037844387076, 1.000000000000000000, 0.8660254037844387076, 1.000000000000000000, 0.8660254037844387076, 1.000000000000000000, 0.8660254037844387076, 1.000000000000000000, 0.8660254037844387076, 1.000000000000000000, 0.8660254037844387076, 1.000000000000000000, 0.8660254037844387076, 1.000000000000000000, 0.8660254037844387076, 1.000000000000000000, 0.8660254037844387076, 1.000000000000000000, 0.8660254037844387076, 1.000000000000000000, 0.8660254037844387076, 1.000000000000000000, 0.8660254037844387076, 1.000000000000000000, 0.8660254037844387076, 1.000000000000000000, 0.8660254037844387076, 1.000000000000000000, 0.8660254037844387076, 1.000000000000000000, 0.8660254037844387076, 1.000000000000000000, 0.8660254037844387076, 1.000000000000000000, 0.8660254037844387076, 1.000000000000000000, 0.8660254037844387076, 1.000000000000000000, 0.8660254037844387076, 1.000000000000000000, 0.8660254037844387076, 1.000000000000000000, 0.8660254037844387076, 1.000000000000000000, 0.8660254037844387076, 1.000000000000000000, 0.8660254037844387076, 1.000000000000000000, 0.8660254037844387076, 1.000000000000000000, 0.8660254037844387076, 1.000000000000000000, 0.8660254037844387076, 1.000000000000000000, 0.8660254037844387076, 1.000000000000000000, 0.8660254037844387076, 1.000000000000000000, 0.8660254037844387076, 1.000000000000000000, 0.8660254037844387076, 1.000000000000000000, 0.8660254037844387076, 1.000000000000000000, 0.8660254037844387076, 1.000000000000000000, 0.8660254037844387076, 1.000000000000000000, 0.8660254037844387076, 1.000000000000000000, 0.8660254037844387076, 1.000000000000000000, 0.8660254037844387076, 1.000000000000000000, 0.8660254037844387076, 1.000000000000000000, 0.8660254037844387076, 1.000000000000000000, 0.8660254037844387076, 1.000000000000000000, 0.8660254037844387076, 1.000000000000000000, 0.8660254037844387076, 1.000000000000000000, 0.8660254037844387076, 1.000000000000000000, 0.8660254037844387076, 1.000000000000000000, 0.8660254037844387076, 1.000000000000000000, 0.8660254037844387076, 1.000000000000000000, 0.8660254037844387076, 1.000000000000000000, 0.8660254037844387076, 1.000000000000000000, 0.8660254037844387076, 1.000000000000000000, 0.8660254037844387076, 1.000000000000000000, 0.8660254037844387076, 1.000000000000000000, 0.8660254037844387076, 1.000000000000000000, 0.8660254037844387076, 1.000000000000000000, 0.8660254037844387076, 1.000000000000000000, 0.8660254037844387076, 1.000000000000000000, 0.8660254037844387076, 1.000000000000000000, 0.8660254037844387076, 1.000000000000000000, 0.8660254037844387076, 1.000000000000000000, 0.8660254037844387076, 1.000000000000000000, 0.8660254037844387076, 1.000000000000000000, 0.8660254037844387076, 1.000000000000000000),
 ( 1.000000000000000000, 0.8660254037844387076, 1.000000000000000000, 0.8660254037844387076, 1.000000000000000000, 0.8660254037844387076, 1.000000000000000000, 0.8660254037844387076, 1.000000000000000000, 0.8660254037844387076, 1.000000000000000000, 0.8660254037844387076, 1.000000000000000000, 0.8660254037844387076, 1.000000000000000000, 0.8660254037844387076, 1.000000000000000000, 0.8660254037844387076, 1.000000000000000000, 0.8660254037844387076, 1.000000000000000000, 0.8660254037844387076, 1.000000000000000000, 0.8660254037844387076, 1.000000000000000000, 0.8660254037844387076, 1.000000000000000000, 0.8660254037844387076, 1.000000000000000000, 0.8660254037844387076, 1.000000000000000000, 0.8660254037844387076, 1.000000000000000000, 0.8660254037844387076, 1.000000000000000000, 0.8660254037844387076, 1.000000000000000000, 0.8660254037844387076, 1.000000000000000000, 0.8660254037844387076, 1.000000000000000000, 0.8660254037844387076, 1.000000000000000000, 0.8660254037844387076, 1.000000000000000000, 0.8660254037844387076, 1.000000000000000000, 0.8660254037844387076, 1.000000000000000000, 0.8660254037844387076, 1.000000000000000000, 0.8660254037844387076, 1.000000000000000000, 0.8660254037844387076, 1.000000000000000000, 0.8660254037844387076, 1.000000000000000000, 0.8660254037844387076, 1.000000000000000000, 0.8660254037844387076, 1.000000000000000000, 0.8660254037844387076, 1.000000000000000000, 0.8660254037844387076, 1.000000000000000000, 0.8660254037844387076, 1.000000000000000000, 0.8660254037844387076, 1.000000000000000000, 0.8660254037844387076, 1.000000000000000000, 0.8660254037844387076, 1.000000000000000000, 0.8660254037844387076, 1.000000000000000000, 0.8660254037844387076, 1.000000000000000000, 0.8660254037844387076, 1.000000000000000000, 0.8660254037844387076, 1.000000000000000000, 0.8660254037844387076, 1.000000000000000000, 0.8660254037844387076, 1.000000000000000000, 0.8660254037844387076, 1.000000000000000000, 0.8660254037844387076, 1.000000000000000000, 0.8660254037844387076, 1.000000000000000000, 0.8660254037844387076, 1.000000000000000000, 0.8660254037844387076, 1.000000000000000000, 0.8660254037844387076, 1.000000000000000000, 0.8660254037844387076, 1.000000000000000000, 0.8660254037844387076, 1.000000000000000000, 0.8660254037844387076, 1.000000000000000000, 0.8660254037844387076, 1.000000000000000000, 0.8660254037844387076, 1.000000000000000000, 0.8660254037844387076, 1.000000000000000000, 0.8660254037844387076, 1.000000000000000000, 0.8660254037844387076, 1.000000000000000000, 0.8660254037844387076, 1.000000000000000000, 0.8660254037844387076, 1.000000000000000000, 0.8660254037844387076, 1.000000000000000000, 0.8660254037844387076, 1.000000000000000000, 0.8660254037844387076, 1.000000000000000000, 0.8660254037844387076, 1.000000000000000000, 0.8660254037844387076, 1.000000000000000000, 0.8660254037844387076, 1.000000000000000000, 0.8660254037844387076, 1.000000000000000000, 0.8660254037844387076, 1.000000000000000000, 0.8660254037844387076, 1.000000000000000000, 0.8660254037844387076, 1.000000000000000000, 0.8660254037844387076, 1.000000000000000000, 0.8660254037844387076, 1.000000000000000000, 0.8660254037844387076, 1.000000000000000000, 0.8660254037844387076, 1.000000000000000000, 0.8660254037844387076, 1.000000000000000000, 0.8660254037844387076, 1.000000000000000000, 0.8660254037844387076, 1.000000000000000000, 0.8660254037844387076, 1.000000000000000000, 0.8660254037844387076, 1.000000000000000000, 0.8660254037844387076, 1.000000000000000000, 0.8660254037844387076, 1.000000000000000000, 0.8660254037844387076, 1.000000000000000000, 0.8660254037844387076, 1.000000000000000000, 0.8660254037844387076, 1.000000000000000000, 0.8660254037844387076, 1.000000000000000000, 0.8660254037844387076, 1.000000000000000000, 0.8660254037844387076, 1.000000000000000000, 0.8660254037844387076, 1.000000000000000000, 0.8660254037844387076, 1.000000000000000000, 0.8660254037844387076, 1.000000000000000000, 0.8660254037844387076, 1.000000000000000000, 0.8660254037844387076, 1.000000000000000000, 0.8660254037844387076, 1.000000000000000000, 0.8660254037844387076, 1.000000000000000000, 0.8660254037844387076, 1.000000000000000000, 0.8660254037844387076, 1.000000000000000000, 0.8660254037844387076, 1.000000000000000000, 0.8660254037844387076, 1.000000000000000000, 0.8660254037844387076, 1.000000000000000000, 0.8660254037844387076, 1.000000000000000000, 0.8660254037844387076, 1.000000000000000000, 0.8660254037844387076, 1.000000000000000000, 0.8660254037844387076, 1.000000000000000000, 0.8660254037844387076, 1.000000000000000000, 0.8660254037844387076, 1.000000000000000000, 0.8660254037844387076, 1.000000000000000000, 0.8660254037844387076, 1.000000000000000000, 0.8660254037844387076, 1.000000000000000000, 0.8660254037844387076, 1.000000000000000000, 0.8660254037844387076, 1.000000000000000000, 0.8660254037844387076, 1.000000000000000000, 0.8660254037844387076, 1.000000000000000000, 0.8660254037844387076, 1.000000000000000000, 0.8660254037844387076, 1.000000000000000000, 0.8660254037844387076, 1.000000000000000000, 0.8660254037844387076, 1.000000000000000000, 0.8660254037844387076, 1.000000000000000000, 0.8660254037844387076, 1.000000000000000000, 0.8660254037844387076, 1.000000000000000000, 0.8660254037844387076, 1.000000000000000000, 0.8660254037844387076, 1.000000000000000000, 0.8660254037844387076, 1.000000000000000000, 0.8660254037844387076, 1.000000000000000000, 0.8660254037844387076, 1.000000000000000000, 0.8660254037844387076, 1.000000000000000000, 0.8660254037844387076, 1.000000000000000000, 0.8660254037844387076, 1.000000000000000000, 0.8660254037844387076, 1.000000000000000000, 0.8660254037844387076, 1.000000000000000000, 0.8660254037844387076, 1.000000000000000000, 0.8660254037844387076, 1.000000000000000000, 0.8660254037844387076, 1.000000000000000000, 0.8660254037844387076, 1.000000000000000000, 0.8660254037844387076, 1.000000000000000000, 0.8660254037844387076, 1.000000000000000000, 0.8660254037844387076, 1.000000000000000000, 0.8660254037844387076, 1.000000000000000000, 0.8660254037844387076, 1.000000000000000000, 0.8660254037844387076, 1.000000000000000000, 0.8660254037844387076, 1.000000000000000000, 0.8660254037844387076, 1.000000000000000000, 0.8660254037844387076, 1.000000000000000000, 0.8660254037844387076, 1.000000000000000000, 0.8660254037844387076, 1.000000000000000000, 0.8660254037844387076, 1.000000000000000000, 0.8660254037844387076, 1.000000000000000000, 0.8660254037844387076, 1.000000000000000000, 0.8660254037844387076, 1.000000000000000000, 0.8660254037844387076, 1.000000000000000000, 0.8660254037844387076, 1.000000000000000000, 0.8660254037844387076, 1.000000000000000000, 0.8660254037844387076, 1.000000000000000000, 0.8660254037844387076, 1.000000000000000000, 0.8660254037844387076, 1.000000000000000000, 0.8660254037844387076, 1.000000000000000000, 0.8660254037844387076, 1.000000000000000000, 0.8660254037844387076, 1.000000000000000000, 0.8660254037844387076, 1.000000000000000000, 0.8660254037844387076, 1.000000000000000000, 0.8660254037844387076, 1.000000000000000000, 0.8660254037844387076, 1.000000000000000000, 0.8660254037844387076, 1.000000000000000000, 0.8660254037844387076, 1.000000000000000000, 0.8660254037844387076, 1.000000000000000000, 0.8660254037844387076, 1.000000000000000000, 0.8660254037844387076, 1.000000000000000000, 0.8660254037844387076, 1.000000000000000000, 0.8660254037844387076, 1.000000000000000000, 0.8660254037844387076, 1.000000000000000000, 0.8660254037844387076, 1.000000000000000000, 0.8660254037844387076, 1.000000000000000000, 0.8660254037844387076, 1.000000000000000000, 0.8660254037844387076, 1.000000000000000000, 0.8660254037844387076, 1.000000000000000000, 0.8660254037844387076, 1.000000000000000000, 0.8660254037844387076, 1.000000000000000000, 0.8660254037844387076, 1.000000000000000000, 0.8660254037844387076, 1.000000000000000000, 0.8660254037844387076, 1.000000000000000000, 0.8660254037844387076, 1.000000000000000000, 0.8660254037844387076, 1.000000000000000000, 0.8660254037844387076, 1.000000000000000000, 0.8660254037844387076, 1.000000000000000000, 0.8660254037844387076, 1.000000000000000000, 0.8660254037844387076, 1.000000000000000000, 0.8660254037844387076, 1.000000000000000000, 0.8660254037844387076, 1.000000000000000000, 0.8660254037844387076, 1.000000000000000000, 0.8660254037844387076, 1.000000000000000000, 0.8660254037844387076, 1.000000000000000000, 0.8660254037844387076, 1.000000000000000000, 0.8660254037844387076, 1.000000000000000000, 0.8660254037844387076, 1.000000000000000000, 0.8660254037844387076, 1.000000000000000000, 0.8660254037844387076, 1.000000000000000000, 0.8660254037844387076, 1.000000000000000000, 0.8660254037844387076, 1.000000000000000000, 0.8660254037844387076, 1.000000000000000000, 0.8660254037844387076, 1.000000000000000000, 0.8660254037844387076, 1.000000000000000000, 0.8660254037844387076, 1.000000000000000000, 0.8660254037844387076, 1.000000000000000000, 0.8660254037844387076, 1.000000000000000000, 0.8660254037844387076, 1.000000000000000000, 0.8660254037844387076, 1.000000000000000000, 0.8660254037844387076, 1.000000000000000000, 0.8660254037844387076, 1.000000000000000000, 0.8660254037844387076, 1.000000000000000000, 0.8660254037844387076, 1.000000000000000000, 0.8660254037844387076, 1.000000000000000000, 0.8660254037844387076, 1.000000000000000000, 0.8660254037844387076, 1.000000000000000000, 0.8660254037844387076, 1.000000000000000000, 0.8660254037844387076, 1.000000000000000000, 0.8660254037844387076, 1.000000000000000000, 0.8660254037844387076, 1.000000000000000000, 0.8660254037844387076, 1.000000000000000000, 0.8660254037844387076, 1.000000000000000000, 0.8660254037844387076, 1.000000000000000000, 0.8660254037844387076, 1.000000000000000000, 0.8660254037844387076, 1.000000000000000000, 0.8660254037844387076, 1.000000000000000000, 0.8660254037844387076, 1.000000000000000000, 0.8660254037844387076, 1.000000000000000000, 0.8660254037844387076, 1.000000000000000000, 0.8660254037844387076, 1.000000000000000000, 0.8660254037844387076, 1.000000000000000000, 0.8660254037844387076, 1.000000000000000000, 0.8660254037844387076, 1.000000000000000000, 0.8660254037844387076, 1.000000000000000000, 0.8660254037844387076, 1.000000000000000000, 0.8660254037844387076, 1.000000000000000000, 0.8660254037844387076, 1.000000000000000000, 0.8660254037844387076, 1.000000000000000000, 0.8660254037844387076, 1.000000000000000000, 0.8660254037844387076, 1.000000000000000000, 0.8660254037844387076, 1.000000000000000000, 0.8660254037844387076, 1.000000000000000000, 0.8660254037844387076, 1.000000000000000000, 0.8660254037844387076, 1.000000000000000000, 0.8660254037844387076, 1.000000000000000000, 0.8660254037844387076, 1.000000000000000000) ) ) 
 REPRESENTATION_ITEM ( '' )  SURFACE ( )  );
#96231=CARTESIAN_POINT ( 'NONE',  ( -1.598423149420354905, 8.713846000021355565, -2.499999999999995115 ) ) ;
#96241=CARTESIAN_POINT ( 'NONE',  ( -9.182950115157607840, 9.607863310639020327, 0.7998128361456462443 ) ) ;
#96245=CARTESIAN_POINT ( 'NONE',  ( 7.456621297836082185, 7.801739057004660971, 0.7216878364870317197 ) ) ;
#96247=CARTESIAN_POINT ( 'NONE',  ( 4.681643115420508039, 4.356338477612361260, 0.7998128361456341429 ) ) ;
#96248=DIRECTION ( 'NONE',  ( 5.578564026256490882E-16, 1.000000000000000000, 9.066213480720158442E-32 ) ) ;
#96250=CARTESIAN_POINT ( 'NONE',  ( -6.226218857173722476, 8.287007971501239467, 1.599625672291283607 ) ) ;
#96260=CARTESIAN_POINT ( 'NONE',  ( -1.364683531250012516, 4.301041667008089320, -0.7879004041258300672 ) ) ;
#96262=CARTESIAN_POINT ( 'NONE',  ( 9.077347539549325717, 10.54899253668443393, -1.199719254218446718 ) ) ;
#96264=CARTESIAN_POINT ( 'NONE',  ( -4.799223189557577207, 4.701441264013013210, 0.7216878364870317197 ) ) ;
#96265=EDGE_CURVE ( 'NONE', #201912, #200114, #136512, .T. ) ;
#96267=CARTESIAN_POINT ( 'NONE',  ( -5.219525951136862574, 5.191794485855519170, -0.7216878364870197293 ) ) ;
#96274=ORIENTED_EDGE ( 'NONE', *, *, #15120, .F. ) ;
#96276=CARTESIAN_POINT ( 'NONE',  ( 2.171277156482887882, 5.684907115872006145, -0.7998128361456291469 ) ) ;
#96283=CARTESIAN_POINT ( 'NONE',  ( 3.520313441042647540, 7.258782781191745137, 0.7998128361456321445 ) ) ;
#96288=CARTESIAN_POINT ( 'NONE',  ( -1.364683531250012516, 3.801041667008087099, -0.7879004041258300672 ) ) ;
#96293=CARTESIAN_POINT ( 'NONE',  ( 6.257251587906815793, 7.258880593101466161, 1.199719254218462483 ) ) ;
#96296=CARTESIAN_POINT ( 'NONE',  ( -4.466521540698216164, 7.298359999868178960, -1.199719254218452047 ) ) ;
#96297=CARTESIAN_POINT ( 'NONE',  ( 1.499999999999987121, 2.295833333333350268, -0.8660254037844262731 ) ) ;
#96299=CARTESIAN_POINT ( 'NONE',  ( -3.948449050077848632, 5.629609863222681199, 1.599625672291267398 ) ) ;
#96300=CARTESIAN_POINT ( 'NONE',  ( -0.006913841192830532355, 8.234242197375163386, -1.999988128101762186 ) ) ;
#96302=CARTESIAN_POINT ( 'NONE',  ( 1.364683531249986537, 2.655208333674754062, -0.7879004041258239610 ) ) ;
#96305=CARTESIAN_POINT ( 'NONE',  ( -3.904385051055635270, 6.538571078664754843, 1.082531754730560403 ) ) ;
#96311=CARTESIAN_POINT ( 'NONE',  ( 4.273844736805816780, 6.009238164405336313, 1.599625672291267398 ) ) ;
#96315=CARTESIAN_POINT ( 'NONE',  ( 1.364683531249988535, 3.926041667008087543, 0.7879004041258500513 ) ) ;
#96320=CARTESIAN_POINT ( 'NONE',  ( -1.364683531250014514, 0.05104166700808546175, -0.7879004041258359514 ) ) ;
#96321=CARTESIAN_POINT ( 'NONE',  ( -4.278446361140257892, 7.376938836250866771, -1.009706106759753030 ) ) ;
#96323=CARTESIAN_POINT ( 'NONE',  ( -9.969323024750229578, 10.52529837183042716, -0.7998128361456291469 ) ) ;
#96324=CARTESIAN_POINT ( 'NONE',  ( -7.009202228140764213, 7.279750142360097875, -0.7216878364870267237 ) ) ;
#96328=CARTESIAN_POINT ( 'NONE',  ( -1.364683531249997417, 5.009375000341425022, 1.214306433183764966E-14 ) ) ;
#96336=CARTESIAN_POINT ( 'NONE',  ( -5.192409643909507544, 9.001635651295671892, 0.7216878364870458196 ) ) ;
#96343=CARTESIAN_POINT ( 'NONE',  ( -4.731432421044865499, 8.463828891286912182, -0.7216878364870257245 ) ) ;
#96351=DIRECTION ( 'NONE',  ( 1.000000000000000000, -5.578564026256490882E-16, -5.570868214615546318E-48 ) ) ;
#96352=VERTEX_POINT ( 'NONE', #65694 ) ;
#96356=CARTESIAN_POINT ( 'NONE',  ( -4.608882153641705059, 7.464447381635583412, -1.199719254218452047 ) ) ;
#96359=CARTESIAN_POINT ( 'NONE',  ( 0.7499999999999885647, 0.7333333333333567072, 1.299038105676657340 ) ) ;
#96362=CARTESIAN_POINT ( 'NONE',  ( 2.198393463710220264, 5.716542807637226886, 0.7998128361456462443 ) ) ;
#96363=CARTESIAN_POINT ( 'NONE',  ( 6.120616281565444794, 9.228137197546649517, -1.199719254218440723 ) ) ;
#96368=CARTESIAN_POINT ( 'NONE',  ( 3.981290663907289140, 7.796589541200495965, -0.7998128361456221525 ) ) ;
#96376=CARTESIAN_POINT ( 'NONE',  ( -4.284013352238265959, 5.060732334775157604, -1.082531754730544860 ) ) ;
#96382=CARTESIAN_POINT ( 'NONE',  ( -1.364683531249997417, 2.759375000341422801, 1.214306433183764966E-14 ) ) ;
#96383=CARTESIAN_POINT ( 'NONE',  ( 9.205623113554612047, 12.72334881824701469, 1.082531754730546636 ) ) ;
#96384=CARTESIAN_POINT ( 'NONE',  ( -5.703176172842872482, 9.805455968292021041, 0.000000000000000000 ) ) ;
#96388=CARTESIAN_POINT ( 'NONE',  ( 5.120175567455225618, 9.125288595339771547, -0.7998128361456281477 ) ) ;
#96389=CARTESIAN_POINT ( 'NONE',  ( -7.576308911938196999, 7.733448573549685179, 0.7998128361456462443 ) ) ;
#96393=CARTESIAN_POINT ( 'NONE',  ( 0.7499999999999902300, 1.014583334016154526, 1.299038105676657340 ) ) ;
#96397=CARTESIAN_POINT ( 'NONE',  ( 6.426201623197458801, 9.480690412830290015, -1.082531754730537088 ) ) ;
#96400=CARTESIAN_POINT ( 'NONE',  ( 1.364683531249988757, 1.696875000341414808, 0.000000000000000000 ) ) ;
#96402=CARTESIAN_POINT ( 'NONE',  ( 5.287316719205157334, 9.112360572473935605, 1.040834085586084257E-14 ) ) ;
#96405=CARTESIAN_POINT ( 'NONE',  ( -2.928197990871687306, 5.399686175116803710, 1.082531754730560403 ) ) ;
#96407=CARTESIAN_POINT ( 'NONE',  ( -1.201851678989727383E-14, 4.196875000341417028, -1.575800808251660134 ) ) ;
#96413=CARTESIAN_POINT ( 'NONE',  ( -5.461413243215608837, 6.444398994036877326, -1.303746704243381238 ) ) ;
#96420=CARTESIAN_POINT ( 'NONE',  ( 5.445571254183207088, 9.504916896522420444, -0.7998128361456281477 ) ) ;
#96423=CARTESIAN_POINT ( 'NONE',  ( 2.900554798319789906, 5.471398800426671372, 1.199719254218452047 ) ) ;
#96432=CARTESIAN_POINT ( 'NONE',  ( 6.005898861173831094, 6.109229547565340646, 1.040834085586084257E-14 ) ) ;
#96433=CARTESIAN_POINT ( 'NONE',  ( 1.364683531249986537, 1.467708333674748289, -0.7879004041258239610 ) ) ;
#96434=CARTESIAN_POINT ( 'NONE',  ( 7.228468454380276853, 11.58496363008569574, 1.040834085586084257E-14 ) ) ;
#96436=CARTESIAN_POINT ( 'NONE',  ( 0.5625979714343026794, 6.581402773648894033, -3.408537031531792660 ) ) ;
#96437=CARTESIAN_POINT ( 'NONE',  ( -3.730464822054482710, 7.503959392372201442, 1.040834085586084257E-14 ) ) ;
#96442=CARTESIAN_POINT ( 'NONE',  ( -1.201851678989727383E-14, 1.462500000000018119, 1.732050807568877637 ) ) ;
#96443=CARTESIAN_POINT ( 'NONE',  ( 6.317209508963599340, 9.457495962844502557, 1.199719254218462483 ) ) ;
#96444=CARTESIAN_POINT ( 'NONE',  ( -7.004758919754800139, 11.32396917302262018, 0.000000000000000000 ) ) ;
#96448=CARTESIAN_POINT ( 'NONE',  ( 1.364683531249988535, 2.113541667008087099, 0.7879004041258500513 ) ) ;
#96450=CARTESIAN_POINT ( 'NONE',  ( 0.7499999999999902300, 4.066666666666690411, -1.299038105676658228 ) ) ;
#96452=CARTESIAN_POINT ( 'NONE',  ( 2.510230996824538430, 6.080353262937265413, 0.000000000000000000 ) ) ;
#96458=CARTESIAN_POINT ( 'NONE',  ( 1.499999999999989120, 1.056250000682816603, 0.000000000000000000 ) ) ;
#96460=CARTESIAN_POINT ( 'NONE',  ( -6.344325816190970357, 9.489131654609717970, 1.199719254218452047 ) ) ;
#96461=CARTESIAN_POINT ( 'NONE',  ( -3.877268743828284681, 5.546566172598190292, 1.443375672974064550 ) ) ;
#96468=CARTESIAN_POINT ( 'NONE',  ( 7.450369105909416589, 8.650851030771185890, -1.199719254218441611 ) ) ;
#96473=CARTESIAN_POINT ( 'NONE',  ( 7.145310649601935182, 8.294949498412453437, -1.199719254218446718 ) ) ;
#96474=CARTESIAN_POINT ( 'NONE',  ( 7.904040366642684390, 11.20483561351640844, 1.082531754730558626 ) ) ;
#96480=CARTESIAN_POINT ( 'NONE',  ( -6.561256274009600986, 9.742217188731485678, -1.199719254218440723 ) ) ;
#96481=CARTESIAN_POINT ( 'NONE',  ( 3.541704441667858472, 5.155074486744371853, -1.599625672291262513 ) ) ;
#96486=CARTESIAN_POINT ( 'NONE',  ( 4.038955833855768063, 7.541343398062151593, 0.4257906834902285276 ) ) ;
#96495=CARTESIAN_POINT ( 'NONE',  ( -4.609409038966253647, 4.479991421656468908, -0.7216878364870207285 ) ) ;
#96496=CARTESIAN_POINT ( 'NONE',  ( 7.619319141200057821, 10.87266085050000974, 1.082531754730557072 ) ) ;
#96498=CARTESIAN_POINT ( 'NONE',  ( -5.440899717785814715, 5.242137847038546461, 0.7998128361456341429 ) ) ;
#96499=DIRECTION ( 'NONE',  ( -5.578564026256490882E-16, -1.000000000000000000, -9.066213480720158442E-32 ) ) ;
#96503=CARTESIAN_POINT ( 'NONE',  ( -5.856232286098998152, 8.919689202835742847, 1.199719254218452047 ) ) ;
#96517=DIRECTION ( 'NONE',  ( -5.578564026256491869E-16, -1.000000000000000000, -9.066213480720160632E-32 ) ) ;
#96518=CARTESIAN_POINT ( 'NONE',  ( 1.499999999999819256, 7.438721522839173872, -4.195160983902622043 ) ) ;
#96519=CARTESIAN_POINT ( 'NONE',  ( -6.064574784014443942, 5.969758757638621738, -0.7998128361456291469 ) ) ;
#96522=CARTESIAN_POINT ( 'NONE',  ( 3.389175213736297820, 4.977123720824209840, 1.443375672974062551 ) ) ;
#96526=CARTESIAN_POINT ( 'NONE',  ( -3.623053363349869382, 5.249981562040033189, 1.599625672291267398 ) ) ;
#96529=CARTESIAN_POINT ( 'NONE',  ( 8.367353357928214663, 12.91366268422496688, 1.040834085586084257E-14 ) ) ;
#96533=ADVANCED_FACE ( 'NONE', ( #198897 ), #165601, .F. ) ;
#96534=CARTESIAN_POINT ( 'NONE',  ( -7.153898609505128015, 11.49796547773133604, 0.7998128361456481317 ) ) ;
#96535=CARTESIAN_POINT ( 'NONE',  ( 6.148786358997489820, 7.132337826040578754, -1.199719254218446718 ) ) ;
#96540=CARTESIAN_POINT ( 'NONE',  ( -0.6823417656250003738, 1.530208333674752730, -1.181850606188749264 ) ) ;
#96543=CARTESIAN_POINT ( 'NONE',  ( 5.965224400332808763, 9.903252867122883885, -0.7216878364870267237 ) ) ;
#96549=VERTEX_POINT ( 'NONE', #77491 ) ;
#96556=CARTESIAN_POINT ( 'NONE',  ( -2.487170525094696938, 8.243531156566643148, 2.499999999999999112 ) ) ;
#96558=CARTESIAN_POINT ( 'NONE',  ( -8.482597663644387609, 13.04811437422715414, -0.7998128361456281477 ) ) ;
#96572=CARTESIAN_POINT ( 'NONE',  ( -0.7500000000000215383, 1.222916667349485564, 1.299038105676659116 ) ) ;
#96578=CARTESIAN_POINT ( 'NONE',  ( -1.402160292154681736E-14, -0.2874999999999741096, 1.732050807568877637 ) ) ;
#96579=CARTESIAN_POINT ( 'NONE',  ( 8.697719238366680372, 10.10609285197134533, 1.199719254218462483 ) ) ;
#96583=CARTESIAN_POINT ( 'NONE',  ( 4.871457266011829823, 4.577788319968905562, -0.7998128361456221525 ) ) ;
#96584=CARTESIAN_POINT ( 'NONE',  ( -7.863365906246074566, 8.276274433482971205, -0.7216878364870278340 ) ) ;
#96588=CARTESIAN_POINT ( 'NONE',  ( -6.398558430645608475, 9.552403038140164782, -1.199719254218440723 ) ) ;
#96591=CARTESIAN_POINT ( 'NONE',  ( -1.500000000000013101, 0.7020833340161545255, 0.8660254037844403729 ) ) ;
#96598=CARTESIAN_POINT ( 'NONE',  ( -3.050221372950322252, 5.542046787541873520, 1.082531754730560403 ) ) ;
#96600=CARTESIAN_POINT ( 'NONE',  ( 4.753338833179075351, 6.783512570024928579, 1.242321799368527380 ) ) ;
#96602=EDGE_CURVE ( 'NONE', #84740, #84121, #102269, .T. ) ;
#96605=CARTESIAN_POINT ( 'NONE',  ( -4.243338890952916387, 4.052909582307567149, -0.7216878364870207285 ) ) ;
#96606=CARTESIAN_POINT ( 'NONE',  ( 7.259501185113382604, 10.55683625168592243, -1.199719254218441611 ) ) ;
#96614=CARTESIAN_POINT ( 'NONE',  ( -8.507905087775398556, 9.884643009614800135, 1.199719254218462483 ) ) ;
#96620=CARTESIAN_POINT ( 'NONE',  ( 4.878236342818665250, 4.585697242910212523, 1.040834085586084257E-14 ) ) ;
#96636=CARTESIAN_POINT ( 'NONE',  ( 7.039708073993665494, 9.236078724457858158, 1.599625672291281386 ) ) ;
#96638=CARTESIAN_POINT ( 'NONE',  ( -4.973143418114339021, 4.696422164088486895, 0.7998128361456341429 ) ) ;
#96639=ORIENTED_EDGE ( 'NONE', *, *, #63612, .T. ) ;
#96642=DIRECTION ( 'NONE',  ( 0.000000000000000000, 8.546850786086437571E-32, 1.000000000000000000 ) ) ;
#96647=CARTESIAN_POINT ( 'NONE',  ( 1.499999999999987121, 0.7854166673494828999, 0.8660254037844524744 ) ) ;
#96651=CARTESIAN_POINT ( 'NONE',  ( -1.499999999999997558, 8.627523663848661428, -2.579999999999989857 ) ) ;
#96652=CARTESIAN_POINT ( 'NONE',  ( 4.161989969270895706, 5.878740935614592544, 1.443375672974062551 ) ) ;
#96654=CARTESIAN_POINT ( 'NONE',  ( -2.286521462199063492, 5.819358805874190743, 1.040834085586084257E-14 ) ) ;
#96660=CARTESIAN_POINT ( 'NONE',  ( 3.985733972737593778, 6.633478153960411738, -1.082531754730548412 ) ) ;
#96663=CARTESIAN_POINT ( 'NONE',  ( -1.364683531250010295, 5.551041667008087543, -0.7879004041258300672 ) ) ;
#96666=CARTESIAN_POINT ( 'NONE',  ( 3.429849674132933846, 5.024577257953626308, -1.443375672974058777 ) ) ;
#96675=CIRCLE ( 'NONE', #183058, 0.8300000000000008482 ) ;
#96677=CARTESIAN_POINT ( 'NONE',  ( -5.687563394514326909, 6.287294490948974968, 1.127084646392717548 ) ) ;
#96680=CARTESIAN_POINT ( 'NONE',  ( -1.602468905319636405E-14, -1.053124999658583638, -1.575800808251665908 ) ) ;
#96685=CARTESIAN_POINT ( 'NONE',  ( -5.416646063859567484, 6.278174148379618735, 1.199719254218450271 ) ) ;
#96688=VECTOR ( 'NONE', #88760, 1000.000000000000000 ) ;
#96691=CARTESIAN_POINT ( 'NONE',  ( 1.499999999999987121, 4.545833333333352932, -0.8660254037844323793 ) ) ;
#96699=CARTESIAN_POINT ( 'NONE',  ( 0.6823417656249882723, -0.4072916663252490466, 1.181850606188755259 ) ) ;
#96701=CARTESIAN_POINT ( 'NONE',  ( 6.810273232766058449, 6.839740281182199233, 1.040834085586084257E-14 ) ) ;
#96702=CARTESIAN_POINT ( 'NONE',  ( -8.148614017013223076, 9.465470093725620870, -1.199719254218446718 ) ) ;
#96705=CARTESIAN_POINT ( 'NONE',  ( -1.000000000000017097, 9.200000000000018829, -0.3999999999999961919 ) ) ;
#96709=CARTESIAN_POINT ( 'NONE',  ( -1.499999999999997780, 5.400000000000022560, 1.214306433183764966E-14 ) ) ;
#96715=CARTESIAN_POINT ( 'NONE',  ( 7.076992996653421741, 10.23994701519558781, -1.082531754730537976 ) ) ;
#96719=CARTESIAN_POINT ( 'NONE',  ( 1.499999999999990896, 5.306250000682820378, 1.214306433183764966E-14 ) ) ;
#96721=CARTESIAN_POINT ( 'NONE',  ( -2.442440228756222353, 6.001264033524212671, -0.7998128361456281477 ) ) ;
#96722=CARTESIAN_POINT ( 'NONE',  ( 6.277061933002785032, 7.385955679000473673, 1.082531754730558626 ) ) ;
#96723=CARTESIAN_POINT ( 'NONE',  ( -8.798878505144649864, 11.28844422746735532, -1.443375672974058777 ) ) ;
#96729=CARTESIAN_POINT ( 'NONE',  ( 8.270110514656016321, 12.59228666716665401, 0.7216878364870438212 ) ) ;
#96731=DIRECTION ( 'NONE',  ( 0.3502638921866460531, -1.953969548649011959E-16, -0.9366510587354619499 ) ) ;
#96745=CARTESIAN_POINT ( 'NONE',  ( 7.781490099239519509, 11.16582331816642260, 1.199719254218460707 ) ) ;
#96749=CARTESIAN_POINT ( 'NONE',  ( -0.6823417656250003738, -0.2822916663252489355, -1.181850606188749264 ) ) ;
#96750=CARTESIAN_POINT ( 'NONE',  ( 4.934804725694211136, 6.780358151441803649, -1.443375672974051449 ) ) ;
#96751=CARTESIAN_POINT ( 'NONE',  ( -9.829298180227631576, 10.56986208646148384, 1.040834085586084257E-14 ) ) ;
#96756=CARTESIAN_POINT ( 'NONE',  ( -3.741160322367112379, 6.452105245148518797, 1.199719254218464037 ) ) ;
#96771=CARTESIAN_POINT ( 'NONE',  ( 5.406339766261963220, 6.489514674222595758, -1.307707983115678152 ) ) ;
#96779=CARTESIAN_POINT ( 'NONE',  ( -8.405692050792730186, 9.869357483088723626, 1.082531754730558626 ) ) ;
#96783=CARTESIAN_POINT ( 'NONE',  ( 7.610204295972345712, 7.772993188256215547, 0.7998128361456341429 ) ) ;
#96784=CARTESIAN_POINT ( 'NONE',  ( -3.737243898861318137, 7.511868315313509292, 0.7998128361456341429 ) ) ;
#96785=EDGE_CURVE ( 'NONE', #178469, #169262, #31506, .T. ) ;
#96786=CARTESIAN_POINT ( 'NONE',  ( 3.029357257649615054, 5.621668336311468117, -1.199719254218446718 ) ) ;
#96788=CARTESIAN_POINT ( 'NONE',  ( -6.087774667736030487, 7.061157519568837415, 1.199719254218450271 ) ) ;
#96792=CARTESIAN_POINT ( 'NONE',  ( -6.175902666224832416, 7.163973517805802160, -1.199719254218446718 ) ) ;
#96795=CARTESIAN_POINT ( 'NONE',  ( 8.613507663383630941, 8.943513783569379427, -0.7998128361456221525 ) ) ;
#96798=CARTESIAN_POINT ( 'NONE',  ( 4.867170269011318773, 6.911508770089412224, 1.419371323323643130 ) ) ;
#96799=CARTESIAN_POINT ( 'NONE',  ( 5.843201017809841247, 5.919415396974013532, 1.040834085586084257E-14 ) ) ;
#96807=CARTESIAN_POINT ( 'NONE',  ( 7.917598520256366790, 8.339545816494993602, 1.040834085586084257E-14 ) ) ;
#96810=CARTESIAN_POINT ( 'NONE',  ( -9.755255220232635693, 11.33988483081495957, -1.199719254218441611 ) ) ;
#96811=CARTESIAN_POINT ( 'NONE',  ( -8.199983978166823562, 8.461069484149769337, -0.7998128361456291469 ) ) ;
#96818=CARTESIAN_POINT ( 'NONE',  ( 8.890396042259068210, 11.39521468743417998, -1.599625672291257406 ) ) ;
#96822=CARTESIAN_POINT ( 'NONE',  ( 3.009020027229115879, 5.597941567487558778, -1.199719254218446718 ) ) ;
#96825=CARTESIAN_POINT ( 'NONE',  ( -0.7500000000000215383, 4.972916667349482012, 1.299038105676671107 ) ) ;
#96829=VERTEX_POINT ( 'NONE', #35124 ) ;
#96831=CARTESIAN_POINT ( 'NONE',  ( -1.201851678989727383E-14, 2.712500000000023892, 1.732050807568877637 ) ) ;
#96832=CARTESIAN_POINT ( 'NONE',  ( 5.286789834324991055, 8.255339675766103724, -1.199719254218452935 ) ) ;
#96834=SPHERICAL_SURFACE ( 'NONE', #42734, 0.08000000000000000167 ) ;
#96835=CARTESIAN_POINT ( 'NONE',  ( 6.588899466561449536, 9.670504563421618016, -1.082531754730537088 ) ) ;
#96836=CARTESIAN_POINT ( 'NONE',  ( 0.5031024701319273262, 7.721748688246023562, 1.994341720826588782 ) ) ;
#96840=CARTESIAN_POINT ( 'NONE',  ( 8.353795204314554468, 12.89784483834236184, -0.7998128361456352531 ) ) ;
#96842=CARTESIAN_POINT ( 'NONE',  ( -3.469997250093771246, 6.135748327496311383, -1.199719254218452935 ) ) ;
#96843=B_SPLINE_CURVE_WITH_KNOTS ( 'NONE', 3,
 ( #149613, #182086, #165861, #67259, #17447, #98735, #133395, #198338, #68332, #86739 ),
 .UNSPECIFIED., .F., .F.,
 ( 4, 3, 3, 4 ),
 ( 1.091119002910726144E-17, 3.125232789889730939E-05, 6.250428833270779022E-05, 0.0001046311988174829390 ),
 .UNSPECIFIED. ) ;
#96844=CARTESIAN_POINT ( 'NONE',  ( -1.499999999999997780, 4.931250000682820378, 1.214306433183764966E-14 ) ) ;
#96845=CARTESIAN_POINT ( 'NONE',  ( 1.364683531249988757, -0.6156249996585803075, 0.000000000000000000 ) ) ;
#96849=CARTESIAN_POINT ( 'NONE',  ( 3.846762897975340767, 5.510976019103107859, -1.599625672291256295 ) ) ;
#96851=CARTESIAN_POINT ( 'NONE',  ( -0.6823417656250212460, 5.113541667008086655, 1.181850606188767472 ) ) ;
#96860=CARTESIAN_POINT ( 'NONE',  ( -5.703176172842872482, 9.805455968292021041, 0.000000000000000000 ) ) ;
#96863=CARTESIAN_POINT ( 'NONE',  ( 4.547870462380197765, 7.393267075163835855, 1.199719254218462483 ) ) ;
#96869=CARTESIAN_POINT ( 'NONE',  ( 10.09812548408005384, 10.67556790771522124, -0.7998128361456281477 ) ) ;
#96872=CARTESIAN_POINT ( 'NONE',  ( -5.392392409933270514, 7.314210449720692786, 1.599625672291269396 ) ) ;
#96876=CARTESIAN_POINT ( 'NONE',  ( 8.971744963941056028, 11.49012176272984931, 1.599625672291281386 ) ) ;
#96878=CARTESIAN_POINT ( 'NONE',  ( 8.263858322729371153, 9.599921783727809910, -1.199719254218446718 ) ) ;
#96881=CARTESIAN_POINT ( 'NONE',  ( -9.842856333841300653, 10.58567993234409421, 0.7216878364870438212 ) ) ;
#96883=CARTESIAN_POINT ( 'NONE',  ( -5.343885102080728977, 9.386283052402845328, 0.7998128361456481317 ) ) ;
#96887=CARTESIAN_POINT ( 'NONE',  ( -5.687563394514326909, 6.287294490948974968, 1.127084646392717548 ) ) ;
#96888=CARTESIAN_POINT ( 'NONE',  ( -1.364683531250012516, 1.030208333674754062, 0.7879004041258379498 ) ) ;
#96892=CARTESIAN_POINT ( 'NONE',  ( 7.375272376154084597, 9.627570410311676596, -1.443375672974057666 ) ) ;
#96895=CARTESIAN_POINT ( 'NONE',  ( 5.518332215962025167, 6.396807992499198292, -1.199719254218445830 ) ) ;
#96909=CARTESIAN_POINT ( 'NONE',  ( 9.694243528971124846, 11.26870452434320491, 1.199719254218450271 ) ) ;
#96911=ORIENTED_EDGE ( 'NONE', *, *, #4772, .F. ) ;
#96914=CARTESIAN_POINT ( 'NONE',  ( -3.764360206088648297, 7.543504007078730922, -0.7998128361456281477 ) ) ;
#96915=CARTESIAN_POINT ( 'NONE',  ( -7.531718027591449705, 8.745758106066849891, 1.199719254218462483 ) ) ;
#96922=CARTESIAN_POINT ( 'NONE',  ( 0.7499999999999902300, 2.514583334016148974, 1.299038105676669330 ) ) ;
#96923=CARTESIAN_POINT ( 'NONE',  ( 9.250740883225924804, 9.686952540052077509, 1.040834085586084257E-14 ) ) ;
#96926=CARTESIAN_POINT ( 'NONE',  ( -7.506410603460441422, 11.90922947067921278, -0.7998128361456291469 ) ) ;
#96928=CARTESIAN_POINT ( 'NONE',  ( 0.6823417656249899377, 3.426041667008085323, -1.181850606188754593 ) ) ;
#96933=CARTESIAN_POINT ( 'NONE',  ( -10.14113571334194930, 10.93367254176152059, -0.7216878364870267237 ) ) ;
#96937=CARTESIAN_POINT ( 'NONE',  ( -0.6823417656250003738, 1.030208333674752286, -1.181850606188749264 ) ) ;
#96945=CARTESIAN_POINT ( 'NONE',  ( -1.364683531250012516, 3.280208333674756727, 0.7879004041258379498 ) ) ;
#96947=CARTESIAN_POINT ( 'NONE',  ( -4.076197739202962467, 7.907314462378773001, 1.040834085586084257E-14 ) ) ;
#96948=CARTESIAN_POINT ( 'NONE',  ( 7.019370843573166319, 9.212351955633947043, 1.599625672291281386 ) ) ;
#96952=CARTESIAN_POINT ( 'NONE',  ( -1.201851678989727383E-14, 2.759375000341417916, -1.575800808251660134 ) ) ;
#96956=CARTESIAN_POINT ( 'NONE',  ( 0.6823417656249882723, 0.09270833367475139752, 1.181850606188755259 ) ) ;
#96957=CARTESIAN_POINT ( 'NONE',  ( -4.934804725694220906, 7.740727365743146571, -1.082531754730549967 ) ) ;
#96960=CARTESIAN_POINT ( 'NONE',  ( 5.178851490740205676, 6.104710163027444736, 1.082531754730558626 ) ) ;
#96963=CARTESIAN_POINT ( 'NONE',  ( -8.864333505236459132, 9.236143932397675727, 1.040834085586084257E-14 ) ) ;
#96964=CARTESIAN_POINT ( 'NONE',  ( -3.144601563365788444, 5.756120026313656268, -1.199719254218452935 ) ) ;
#96966=CARTESIAN_POINT ( 'NONE',  ( 1.364683531249988535, 4.905208333674756283, -0.7879004041258300672 ) ) ;
#96971=CARTESIAN_POINT ( 'NONE',  ( -6.683806541412768532, 8.820860269780128604, -1.443375672974058777 ) ) ;
#96973=CARTESIAN_POINT ( 'NONE',  ( 1.364683531249988757, -0.05312499965857975237, 0.000000000000000000 ) ) ;
#96976=CARTESIAN_POINT ( 'NONE',  ( 7.470179451449751262, 7.817556902887268677, 1.040834085586084257E-14 ) ) ;
#96986=CARTESIAN_POINT ( 'NONE',  ( 9.259855728009286580, 10.86588177317476855, -1.082531754730543083 ) ) ;
#96990=VERTEX_POINT ( 'NONE', #173709 ) ;
#96992=VECTOR ( 'NONE', #200865, 1000.000000000000000 ) ;
#96993=CARTESIAN_POINT ( 'NONE',  ( 5.124091990960999432, 8.065525525174782828, -1.199719254218452047 ) ) ;
#96994=CARTESIAN_POINT ( 'NONE',  ( -5.115504031057831469, 4.862509545855891346, 0.7998128361456341429 ) ) ;
#96998=CARTESIAN_POINT ( 'NONE',  ( 5.382223794500827552, 7.302347065049529462, -1.443375672974051449 ) ) ;
#96999=CARTESIAN_POINT ( 'NONE',  ( -0.6823417656250246877, -0.1364583329919108468, 1.181850606188755259 ) ) ;
#97001=CARTESIAN_POINT ( 'NONE',  ( -9.215791728987058562, 11.77484298861683598, -1.599625672291263179 ) ) ;
#97010=ORIENTED_EDGE ( 'NONE', *, *, #142740, .F. ) ;
#97018=CARTESIAN_POINT ( 'NONE',  ( 6.470265622219697477, 8.571729197388226140, -1.599625672291262513 ) ) ;
#97024=CARTESIAN_POINT ( 'NONE',  ( 6.909851844459134362, 11.21324425184434936, -0.7998128361456291469 ) ) ;
#97028=CARTESIAN_POINT ( 'NONE',  ( -2.535011536075375105, 5.133042487381368701, 1.000000000000011324 ) ) ;
#97031=CARTESIAN_POINT ( 'NONE',  ( 4.197870329852989357, 3.573279226090490646, 2.499999999999999112 ) ) ;
#97036=CARTESIAN_POINT ( 'NONE',  ( 0.006768871532348800547, 8.210909518262138107, 2.038649385027043959 ) ) ;
#97042=CARTESIAN_POINT ( 'NONE',  ( -9.869972641068651242, 11.57768483841065787, 1.082531754730558626 ) ) ;
#97046=CARTESIAN_POINT ( 'NONE',  ( 5.124091990960999432, 8.065525525174782828, -1.199719254218452047 ) ) ;
#97047=CARTESIAN_POINT ( 'NONE',  ( 0.6823417656249899377, 5.676041667008087543, -1.181850606188754593 ) ) ;
#97052=CARTESIAN_POINT ( 'NONE',  ( 3.646780131951580461, 7.198401220678078971, -0.7216878364870267237 ) ) ;
#97060=CARTESIAN_POINT ( 'NONE',  ( -7.152089726408780379, 8.302858421353754181, -1.199719254218446718 ) ) ;
#97061=CARTESIAN_POINT ( 'NONE',  ( -5.922214171070950606, 5.803671375871217286, -0.7998128361456291469 ) ) ;
#97068=CARTESIAN_POINT ( 'NONE',  ( -0.6823417656250212460, 3.363541667008085323, 1.181850606188767472 ) ) ;
#97070=CARTESIAN_POINT ( 'NONE',  ( 6.972971076130050072, 7.029554431773520129, 1.040834085586084257E-14 ) ) ;
#97077=CARTESIAN_POINT ( 'NONE',  ( 1.203907071533380613, 3.118479746939697872, -0.7749999999999910294 ) ) ;
#97083=CARTESIAN_POINT ( 'NONE',  ( -1.364683531250014514, 0.3010416670080866552, -0.7879004041258359514 ) ) ;
#97085=CARTESIAN_POINT ( 'NONE',  ( 5.138703914779377158, 5.953908307786102583, 1.199719254218462483 ) ) ;
#97087=CARTESIAN_POINT ( 'NONE',  ( -7.537970219518091319, 7.896646132300314314, -0.7216878364870278340 ) ) ;
#97088=CARTESIAN_POINT ( 'NONE',  ( 4.636525346193557162, 7.392734756325715750, -1.082531754730549078 ) ) ;
#97089=CARTESIAN_POINT ( 'NONE',  ( -6.683806541412762314, 9.781229484081471526, -1.082531754730537976 ) ) ;
#97091=ORIENTED_EDGE ( 'NONE', *, *, #91598, .F. ) ;
#97093=CARTESIAN_POINT ( 'NONE',  ( 6.531277313481192337, 8.642909503859968368, 1.599625672291281386 ) ) ;
#97095=CARTESIAN_POINT ( 'NONE',  ( -3.009396220815599321, 6.452359640394901952, 0.6004564335717228474 ) ) ;
#97100=CARTESIAN_POINT ( 'NONE',  ( 1.364683531249988535, 5.155208333674749177, -0.7879004041258300672 ) ) ;
#97104=CARTESIAN_POINT ( 'NONE',  ( 8.067265095331215718, 9.370563018429956870, 1.199719254218462483 ) ) ;
#97107=CARTESIAN_POINT ( 'NONE',  ( -8.389798128758148010, 8.682519326506312751, 0.7998128361456462443 ) ) ;
#97113=CARTESIAN_POINT ( 'NONE',  ( 9.134442807305049428, 11.67993591332117376, 1.599625672291281386 ) ) ;
#97114=FACE_OUTER_BOUND ( 'NONE', #93897, .T. ) ;
#97116=CARTESIAN_POINT ( 'NONE',  ( -7.479294296233107708, 11.87759377891399204, 0.7998128361456481317 ) ) ;
#97120=CARTESIAN_POINT ( 'NONE',  ( 4.904330715672160501, 6.657863961833647259, -1.249385787368818113 ) ) ;
#97121=CARTESIAN_POINT ( 'NONE',  ( -8.920901888112002354, 11.43080484092926241, 1.443375672974064550 ) ) ;
#97126=CARTESIAN_POINT ( 'NONE',  ( 6.043183783389218355, 8.073467052085995022, 1.599625672291267398 ) ) ;
#97128=CARTESIAN_POINT ( 'NONE',  ( 6.308621549060418054, 6.254479983525607523, 0.7998128361456341429 ) ) ;
#97129=CARTESIAN_POINT ( 'NONE',  ( -4.145235801320589886, 7.447099624555288067, -0.7035710955675591460 ) ) ;
#97130=CARTESIAN_POINT ( 'NONE',  ( 3.358669367883368118, 4.941533567329135401, -1.599625672291262513 ) ) ;
#97132=CARTESIAN_POINT ( 'NONE',  ( -6.046573322014817897, 9.998159942418544333, 0.7216878364870458196 ) ) ;
#97137=CARTESIAN_POINT ( 'NONE',  ( -4.264599663924041550, 7.301641052403419430, 0.9184948912712449509 ) ) ;
#97138=CARTESIAN_POINT ( 'NONE',  ( 1.364683531249986537, -0.2822916663252520997, -0.7879004041258309554 ) ) ;
#97141=CARTESIAN_POINT ( 'NONE',  ( 5.680503174445848735, 5.729601246382692636, 1.040834085586084257E-14 ) ) ;
#97146=CARTESIAN_POINT ( 'NONE',  ( -9.951321562306267410, 10.71222269888655987, 1.040834085586084257E-14 ) ) ;
#97151=CARTESIAN_POINT ( 'NONE',  ( -9.476786185827959841, 10.15859809299519334, 0.7216878364870438212 ) ) ;
#97152=DIRECTION ( 'NONE',  ( -0.4243160830846685605, -0.9055141421511231359, 0.000000000000000000 ) ) ;
#97153=ORIENTED_EDGE ( 'NONE', *, *, #195936, .T. ) ;
#97158=CARTESIAN_POINT ( 'NONE',  ( -9.178506806327330736, 10.77097469787910455, 1.082531754730558626 ) ) ;
#97162=CARTESIAN_POINT ( 'NONE',  ( -1.364683531250010295, 5.592708333674750953, 0.7879004041258379498 ) ) ;
#97163=CARTESIAN_POINT ( 'NONE',  ( -1.500000000000013101, 2.910416667349485120, -0.8660254037844313801 ) ) ;
#97164=CARTESIAN_POINT ( 'NONE',  ( 5.943008360174058424, 6.124345481070006869, -0.7360307644482602107 ) ) ;
#97167=ORIENTED_EDGE ( 'NONE', *, *, #186498, .F. ) ;
#97169=CARTESIAN_POINT ( 'NONE',  ( -8.342344591110322227, 8.627156865917170236, -0.7998128361456291469 ) ) ;
#97174=CARTESIAN_POINT ( 'NONE',  ( 6.661133543015731462, 6.665743976473484267, -0.7998128361456281477 ) ) ;
#97179=CARTESIAN_POINT ( 'NONE',  ( 7.259501185113382604, 10.55683625168592243, -1.199719254218441611 ) ) ;
#97186=CARTESIAN_POINT ( 'NONE',  ( -6.778713617152821058, 7.971215977175476475, 1.082531754730549967 ) ) ;
#97196=CARTESIAN_POINT ( 'NONE',  ( -9.938290294017125603, 11.55342575023019691, -1.199719254218441611 ) ) ;
#97198=CARTESIAN_POINT ( 'NONE',  ( 8.880754312151170282, 10.31963377138658089, 1.199719254218453823 ) ) ;
#97200=CARTESIAN_POINT ( 'NONE',  ( -10.15235809853472126, 10.73883929124566983, -0.7998128361456291469 ) ) ;
#97203=CARTESIAN_POINT ( 'NONE',  ( 1.364683531249990311, 3.884375000341417028, 1.214306433183764966E-14 ) ) ;
#97205=CARTESIAN_POINT ( 'NONE',  ( 3.684065054611349144, 5.321161868511784299, -1.599625672291262513 ) ) ;
#97210=CARTESIAN_POINT ( 'NONE',  ( 9.585251414737269826, 11.24551007435741568, -1.082531754730537088 ) ) ;
#97212=CARTESIAN_POINT ( 'NONE',  ( -6.371969008742801144, 10.37778824360119145, 0.7216878364870458196 ) ) ;
#97213=CARTESIAN_POINT ( 'NONE',  ( -0.6823417656250003738, 0.9677083336747521747, -1.181850606188749264 ) ) ;
#97215=CARTESIAN_POINT ( 'NONE',  ( -3.023105066167323329, 5.702484939155337607, -2.420000000000000373 ) ) ;
#97217=CARTESIAN_POINT ( 'NONE',  ( -8.830438121202295321, 9.196599317691152464, -0.7998128361456291469 ) ) ;
#97218=CARTESIAN_POINT ( 'NONE',  ( -3.592547517496941900, 5.214391408544949869, -1.443375672974051449 ) ) ;
#97219=CARTESIAN_POINT ( 'NONE',  ( -1.364683531249997417, 3.571875000341423245, 1.214306433183764966E-14 ) ) ;
#97236=CARTESIAN_POINT ( 'NONE',  ( 1.364683531249990311, 4.446875000341417028, 1.214306433183764966E-14 ) ) ;
#97241=CARTESIAN_POINT ( 'NONE',  ( 8.932124273304774320, 9.315233161810734686, 0.7998128361456462443 ) ) ;
#97244=CARTESIAN_POINT ( 'NONE',  ( -0.6823417656250003738, 2.967708333674754062, -1.181850606188749264 ) ) ;
#97246=CARTESIAN_POINT ( 'NONE',  ( -5.585596099150174965, 9.460353182409786399, -0.7216878364870207285 ) ) ;
#97252=CARTESIAN_POINT ( 'NONE',  ( 2.706824224222692088, 6.309712028235118453, 0.7998128361456362523 ) ) ;
#97255=CARTESIAN_POINT ( 'NONE',  ( 10.53876547652418338, 11.18964789890005918, 0.7998128361456462443 ) ) ;
#97262=CARTESIAN_POINT ( 'NONE',  ( -10.13202086811422475, 10.71511252242175161, -0.7998128361456291469 ) ) ;
#97263=CARTESIAN_POINT ( 'NONE',  ( 7.253775878511261155, 8.421492265473332850, 1.199719254218462483 ) ) ;
#97265=CARTESIAN_POINT ( 'NONE',  ( 2.684151225381301575, 6.075334163012737321, 0.000000000000000000 ) ) ;
#97278=CARTESIAN_POINT ( 'NONE',  ( -5.205967797967562483, 8.057084283395347768, 1.082531754730548412 ) ) ;
#97279=CARTESIAN_POINT ( 'NONE',  ( 5.148345644887269756, 7.029489223833707001, -1.599625672291256295 ) ) ;
#97282=CARTESIAN_POINT ( 'NONE',  ( -8.290974629956718189, 9.631557475493025322, -1.199719254218446718 ) ) ;
#97284=CARTESIAN_POINT ( 'NONE',  ( 6.938893903907228378E-15, 10.64264068711930733, 1.214306433183764966E-14 ) ) ;
#97286=CARTESIAN_POINT ( 'NONE',  ( -9.646789991323334590, 11.21334206375407305, 1.199719254218462483 ) ) ;
#97290=CARTESIAN_POINT ( 'NONE',  ( 7.262363838414439776, 11.62450824479221900, 0.7998128361456462443 ) ) ;
#97291=CARTESIAN_POINT ( 'NONE',  ( -2.493739017041110895, 8.265916556960572592, -2.456386464945111481 ) ) ;
#97293=ORIENTED_EDGE ( 'NONE', *, *, #76293, .F. ) ;
#97302=CARTESIAN_POINT ( 'NONE',  ( -7.621654909176601045, 12.04368116068139472, 0.7998128361456481317 ) ) ;
#97306=CARTESIAN_POINT ( 'NONE',  ( 7.293923454472080792, 9.532663335016016148, 1.443375672974076540 ) ) ;
#97308=CARTESIAN_POINT ( 'NONE',  ( 4.844340958784499662, 4.546152628203684820, 0.7998128361456341429 ) ) ;
#97310=CARTESIAN_POINT ( 'NONE',  ( 3.669453130792974971, 7.432779085900453886, 1.040834085586084257E-14 ) ) ;
#97312=CARTESIAN_POINT ( 'NONE',  ( -5.442708600882160574, 8.437244903416123876, -1.199719254218446718 ) ) ;
#97317=VECTOR ( 'NONE', #142999, 1000.000000000000000 ) ;
#97325=CARTESIAN_POINT ( 'NONE',  ( -1.364683531249997417, 4.571875000341417028, 1.214306433183764966E-14 ) ) ;
#97326=CARTESIAN_POINT ( 'NONE',  ( 3.325722479477248861, 7.699077257575519972, 2.499999999999998224 ) ) ;
#97327=CARTESIAN_POINT ( 'NONE',  ( 8.052653171512838881, 11.48218023581863001, -1.199719254218446718 ) ) ;
#97329=CARTESIAN_POINT ( 'NONE',  ( -4.636525346193588248, 4.511627113421689650, 0.7216878364870317197 ) ) ;
#97330=CARTESIAN_POINT ( 'NONE',  ( -5.111060722227552588, 6.025620933095978238, 1.082531754730546636 ) ) ;
#97337=CARTESIAN_POINT ( 'NONE',  ( 4.334856428067313416, 6.080418470877079429, -1.599625672291256295 ) ) ;
#97341=EDGE_CURVE ( 'NONE', #23962, #169987, #2358, .T. ) ;
#97347=CARTESIAN_POINT ( 'NONE',  ( 4.436542580169809291, 6.199052314996659874, 1.599625672291267398 ) ) ;
#97351=CARTESIAN_POINT ( 'NONE',  ( -1.201851678989727383E-14, 3.884375000341423689, 1.575800808251672791 ) ) ;
#97356=CARTESIAN_POINT ( 'NONE',  ( 6.745345117998789775, 7.828323044875442172, 1.199719254218462483 ) ) ;
#97358=CARTESIAN_POINT ( 'NONE',  ( -5.545448523189368650, 6.428443684264421698, -1.199719254218446718 ) ) ;
#97360=CARTESIAN_POINT ( 'NONE',  ( -1.402160292154681736E-14, 2.587500000000023892, -1.732050807568863648 ) ) ;
#97363=CARTESIAN_POINT ( 'NONE',  ( -3.425406365747000859, 7.148057860013469877, 1.040834085586084257E-14 ) ) ;
#97366=CARTESIAN_POINT ( 'NONE',  ( -1.364683531250012516, 3.530208333674758059, 0.7879004041258379498 ) ) ;
#97368=CARTESIAN_POINT ( 'NONE',  ( -3.131570295076647525, 6.597323077657299528, 1.040834085586084257E-14 ) ) ;
#97374=CARTESIAN_POINT ( 'NONE',  ( 4.330940004561544043, 7.140181541042074365, -1.199719254218452047 ) ) ;
#97378=CARTESIAN_POINT ( 'NONE',  ( 1.364683531249990311, 3.446875000341416584, 1.214306433183764966E-14 ) ) ;
#97382=CARTESIAN_POINT ( 'NONE',  ( 0.6823417656249882723, -0.3447916663252489911, 1.181850606188755259 ) ) ;
#97383=LINE ( 'NONE', #164496, #146252 ) ;
#97385=CARTESIAN_POINT ( 'NONE',  ( -8.435144125996554720, 12.99275191363802229, 0.7998128361456341429 ) ) ;
#97387=CARTESIAN_POINT ( 'NONE',  ( -5.382223794500827552, 9.223085493652217082, -0.7216878364870207285 ) ) ;
#97391=CARTESIAN_POINT ( 'NONE',  ( -0.6823417656249969321, 3.967708333674754950, -1.181850606188749264 ) ) ;
#97399=CARTESIAN_POINT ( 'NONE',  ( -6.521108698048783126, 7.670676904887464786, -1.082531754730543083 ) ) ;
#97406=CARTESIAN_POINT ( 'NONE',  ( -6.195713011320807873, 6.330679389403470303, -0.7216878364870267237 ) ) ;
#97409=CARTESIAN_POINT ( 'NONE',  ( -2.123823618835070537, 5.629544655282869847, 1.040834085586084257E-14 ) ) ;
#97417=CARTESIAN_POINT ( 'NONE',  ( 1.499999999999987566, 2.244000000000016648, 2.508000000000020435 ) ) ;
#97419=CARTESIAN_POINT ( 'NONE',  ( -4.120788623549732854, 6.895004929861607401, -1.199719254218452047 ) ) ;
#97421=CARTESIAN_POINT ( 'NONE',  ( -1.500000000000013101, 0.6708333333333583726, 0.8660254037844403729 ) ) ;
#97422=CARTESIAN_POINT ( 'NONE',  ( 8.568389894156670294, 12.94027927658408217, -0.7216878364870257245 ) ) ;
#97423=CARTESIAN_POINT ( 'NONE',  ( 7.633404179693907388, 8.864391950186421454, -1.199719254218441611 ) ) ;
#97424=VECTOR ( 'NONE', #120757, 1000.000000000000000 ) ;
#97427=CARTESIAN_POINT ( 'NONE',  ( 4.656335691289526402, 7.519809842224722374, -1.199719254218452047 ) ) ;
#97433=CARTESIAN_POINT ( 'NONE',  ( -5.124618876285560454, 5.081069565195661220, 0.7216878364870317197 ) ) ;
#97438=CARTESIAN_POINT ( 'NONE',  ( -0.02103505235494400674, 7.063943641280277852, 3.970081552354725485 ) ) ;
#97441=CARTESIAN_POINT ( 'NONE',  ( -1.364683531250012516, 2.988541667008091096, -0.7879004041258289570 ) ) ;
#97442=CARTESIAN_POINT ( 'NONE',  ( 8.053180056393003383, 12.33920113252646367, 1.040834085586084257E-14 ) ) ;
#97443=CARTESIAN_POINT ( 'NONE',  ( -5.215082642750900277, 9.236013516518044142, 0.000000000000000000 ) ) ;
#97446=CARTESIAN_POINT ( 'NONE',  ( 6.006425746053997372, 6.966250444273174303, -1.199719254218445830 ) ) ;
#97447=CARTESIAN_POINT ( 'NONE',  ( -5.713871673155502151, 8.753601821068331290, 1.199719254218452047 ) ) ;
#97448=CARTESIAN_POINT ( 'NONE',  ( -1.482143263342189154, 8.748906972890436506, 2.523193690251313459 ) ) ;
#97451=CARTESIAN_POINT ( 'NONE',  ( 1.499999999999987121, 0.03541666734948738238, 0.8660254037844524744 ) ) ;
#97454=CARTESIAN_POINT ( 'NONE',  ( 6.480434237652121787, 9.543961796360731498, 1.082531754730558626 ) ) ;
#97457=CARTESIAN_POINT ( 'NONE',  ( -1.364683531250014514, 0.09270833367475767028, 0.7879004041258379498 ) ) ;
#97459=CARTESIAN_POINT ( 'NONE',  ( 6.114364089638786304, 8.156510742710487705, 1.443375672974076540 ) ) ;
#97461=CARTESIAN_POINT ( 'NONE',  ( -2.643476764984671767, 6.027880625883323518, 1.040834085586084257E-14 ) ) ;
#97463=CARTESIAN_POINT ( 'NONE',  ( 1.364683531249988535, 4.113541667008088432, 0.7879004041258500513 ) ) ;
#97467=CARTESIAN_POINT ( 'NONE',  ( -5.435328143874127882, 6.463069452080541843, -1.319038057358821403 ) ) ;
#97475=CARTESIAN_POINT ( 'NONE',  ( 6.012151052656117933, 9.101594430485762999, 1.199719254218460707 ) ) ;
#97478=CARTESIAN_POINT ( 'NONE',  ( 3.521367211247359741, 5.131347717920458962, -1.599625672291262513 ) ) ;
#97486=CARTESIAN_POINT ( 'NONE',  ( 5.666945020832177882, 6.674152614801420746, 1.082531754730558626 ) ) ;
#97487=CARTESIAN_POINT ( 'NONE',  ( 1.364683531249986537, 0.7177083336747527298, -0.7879004041258239610 ) ) ;
#97495=CARTESIAN_POINT ( 'NONE',  ( 0.7499999999999902300, 1.983333333333357817, 1.299038105676669330 ) ) ;
#97496=CARTESIAN_POINT ( 'NONE',  ( 6.799577732453452761, 7.891594428405881878, -1.199719254218446718 ) ) ;
#97497=CARTESIAN_POINT ( 'NONE',  ( -7.609150525767646833, 9.900428251527500834, -1.599625672291263179 ) ) ;
#97502=CARTESIAN_POINT ( 'NONE',  ( -1.402160292154681736E-14, 1.446875000341420137, -1.575800808251659024 ) ) ;
#97504=CARTESIAN_POINT ( 'NONE',  ( -1.201851678989727383E-14, 2.712500000000023892, 1.732050807568877637 ) ) ;
#97506=CARTESIAN_POINT ( 'NONE',  ( 3.846762897975340767, 5.510976019103107859, -1.599625672291256295 ) ) ;
#97514=CARTESIAN_POINT ( 'NONE',  ( 0.7499999999999885647, 0.8479166673494853423, -1.299038105676652899 ) ) ;
#97516=CARTESIAN_POINT ( 'NONE',  ( -6.938021921891187382, 9.117444880338284818, -1.599625672291263179 ) ) ;
#97517=CARTESIAN_POINT ( 'NONE',  ( -5.111060722671894929, 5.065251719313053513, 0.000000000000000000 ) ) ;
#97523=VERTEX_POINT ( 'NONE', #97784 ) ;
#97524=CARTESIAN_POINT ( 'NONE',  ( 5.666418135507635512, 8.698239360479199433, 1.199719254218462483 ) ) ;
#97528=CARTESIAN_POINT ( 'NONE',  ( 7.305145839664861640, 7.417091655897478653, 0.7998128361456341429 ) ) ;
#97529=CARTESIAN_POINT ( 'NONE',  ( 8.337901282279995385, 11.71100668175994386, -1.082531754730543083 ) ) ;
#97530=EDGE_LOOP ( 'NONE', ( #110265, #212988, #178534, #79228 ) ) ;
#97534=CARTESIAN_POINT ( 'NONE',  ( -7.555971681517696936, 7.709721804725773175, 0.7998128361456462443 ) ) ;
#97535=CARTESIAN_POINT ( 'NONE',  ( 3.344057444064992168, 7.053150784717805877, 1.040834085586084257E-14 ) ) ;
#97538=CARTESIAN_POINT ( 'NONE',  ( 4.047743032765107607, 7.529339606631276105, 0.4638284745723305624 ) ) ;
#97539=CARTESIAN_POINT ( 'NONE',  ( 9.408995418203971894, 11.03987807840189816, 1.082531754730549967 ) ) ;
#97549=CARTESIAN_POINT ( 'NONE',  ( -3.633221978782304351, 4.301475732409860697, -1.082531754730549967 ) ) ;
#97550=CARTESIAN_POINT ( 'NONE',  ( 8.188761592974039161, 10.57664116326830595, -1.443375672974063439 ) ) ;
#97553=CARTESIAN_POINT ( 'NONE',  ( -4.381256195510448315, 8.263215994737505454, 1.040834085586084257E-14 ) ) ;
#97559=CARTESIAN_POINT ( 'NONE',  ( -7.705111371268023923, 7.883718109434487253, 1.040834085586084257E-14 ) ) ;
#97560=LINE ( 'NONE', #131170, #193594 ) ;
#97567=ORIENTED_EDGE ( 'NONE', *, *, #37467, .F. ) ;
#97574=CARTESIAN_POINT ( 'NONE',  ( -4.889337272013151825, 4.909234758358784312, -0.4031905389056227307 ) ) ;
#97575=CARTESIAN_POINT ( 'NONE',  ( -5.585069213825653023, 8.603332285183535433, -1.199719254218440723 ) ) ;
#97578=CARTESIAN_POINT ( 'NONE',  ( 5.070386261830877928, 5.978167395966564435, -1.082531754730548412 ) ) ;
#97583=CARTESIAN_POINT ( 'NONE',  ( -2.785310492603665367, 5.336947110424484109, 1.199719254218462483 ) ) ;
#97586=CARTESIAN_POINT ( 'NONE',  ( 10.55232363013785246, 11.20546574478267132, 0.000000000000000000 ) ) ;
#97589=CARTESIAN_POINT ( 'NONE',  ( -6.692921386640485082, 10.96015871772258521, -0.7998128361456291469 ) ) ;
#97590=CARTESIAN_POINT ( 'NONE',  ( 6.419949431270806528, 7.448694743692793274, 1.199719254218462483 ) ) ;
#97595=CARTESIAN_POINT ( 'NONE',  ( -1.402160292154681736E-14, 1.259375000341419248, -1.575800808251659024 ) ) ;
#97598=CARTESIAN_POINT ( 'NONE',  ( 7.212574532790092974, 9.437756259720353924, -1.443375672974057666 ) ) ;
#97606=CARTESIAN_POINT ( 'NONE',  ( 9.449669878600614581, 12.04770082983265844, -1.443375672974058777 ) ) ;
#97607=EDGE_CURVE ( 'NONE', #159704, #126491, #150434, .T. ) ;
#97621=DIRECTION ( 'NONE',  ( -7.387867266669436732E-31, -1.000000000000000000, 8.546850786086437571E-32 ) ) ;
#97628=CARTESIAN_POINT ( 'NONE',  ( -0.7500000000000006661, 0.6395833340161540814, -1.299038105676652011 ) ) ;
#97635=CARTESIAN_POINT ( 'NONE',  ( 8.055515824813896941, 12.54985222892493368, 0.7998128361456462443 ) ) ;
#97640=CARTESIAN_POINT ( 'NONE',  ( 3.499976210622149253, 7.235056012367825140, 0.7998128361456321445 ) ) ;
#97641=CARTESIAN_POINT ( 'NONE',  ( -7.375272376154101472, 7.706831981708990753, -0.7216878364870278340 ) ) ;
#97645=CARTESIAN_POINT ( 'NONE',  ( -5.696397096036042385, 9.797547045350714967, -0.7998128361456231517 ) ) ;
#97648=CARTESIAN_POINT ( 'NONE',  ( -0.7500000000000006661, 0.6395833340161540814, -1.299038105676652011 ) ) ;
#97655=CARTESIAN_POINT ( 'NONE',  ( -2.616360457312984167, 5.996244933599686355, -0.7216878364870257245 ) ) ;
#97659=CARTESIAN_POINT ( 'NONE',  ( 3.997610708356745146, 7.599328567695712522, -0.1184163795967980992 ) ) ;
#97664=CARTESIAN_POINT ( 'NONE',  ( -3.348500752450953577, 4.929670182657964084, 1.443375672974062551 ) ) ;
#97665=CARTESIAN_POINT ( 'NONE',  ( 7.904567251967224095, 9.180748867838630645, 1.199719254218462483 ) ) ;
#97669=DIRECTION ( 'NONE',  ( -5.578564026256490882E-16, -1.000000000000000000, -9.066213480720158442E-32 ) ) ;
#97672=CARTESIAN_POINT ( 'NONE',  ( 4.161989969715272686, 4.726297878971393196, 2.420000000000010587 ) ) ;
#97673=CARTESIAN_POINT ( 'NONE',  ( -9.053093885623068715, 11.58502883802551153, -1.599625672291263179 ) ) ;
#97678=CARTESIAN_POINT ( 'NONE',  ( 3.167801447087334576, 6.847518788243868393, -0.7998128361456291469 ) ) ;
#97683=CARTESIAN_POINT ( 'NONE',  ( -8.136864746495904299, 12.64475930422059768, -0.7998128361456281477 ) ) ;
#97687=CARTESIAN_POINT ( 'NONE',  ( -1.580000000000022276, 8.674529973577531194, 2.500000000000011102 ) ) ;
#97696=CARTESIAN_POINT ( 'NONE',  ( 7.983053520348166288, 8.207983950027992748, -0.7998128361456281477 ) ) ;
#97698=CARTESIAN_POINT ( 'NONE',  ( -3.436101866059630527, 6.096203712789787232, 1.199719254218462483 ) ) ;
#97707=CARTESIAN_POINT ( 'NONE',  ( 1.499999999999987121, 0.5770833340161539704, -0.8660254037844253849 ) ) ;
#97710=CARTESIAN_POINT ( 'NONE',  ( -1.519204386771931148, 8.761797318405523782, -2.483775294098344411 ) ) ;
#97711=CARTESIAN_POINT ( 'NONE',  ( 3.216308754939877446, 4.775446185561722956, -1.599625672291262513 ) ) ;
#97713=CARTESIAN_POINT ( 'NONE',  ( -3.785751206713858785, 5.439795712631356750, 1.599625672291267398 ) ) ;
#97719=CARTESIAN_POINT ( 'NONE',  ( 5.192409644353875642, 5.160158794608717514, 1.040834085586084257E-14 ) ) ;
#97722=CARTESIAN_POINT ( 'NONE',  ( 1.364683531249990311, 5.426041667008086655, 0.7879004041258500513 ) ) ;
#97724=CARTESIAN_POINT ( 'NONE',  ( 4.663641652976547647, 4.543262804668490418, 1.214306433183764966E-14 ) ) ;
#97733=CARTESIAN_POINT ( 'NONE',  ( -5.732528328060045197, 6.256990841418501148, 1.080875701640615638 ) ) ;
#97736=CARTESIAN_POINT ( 'NONE',  ( 1.364683531249988757, -0.3656249996585800299, 0.000000000000000000 ) ) ;
#97743=CARTESIAN_POINT ( 'NONE',  ( 1.499999999999989120, 5.004166666666691299, 0.8660254037844524744 ) ) ;
#97748=ORIENTED_EDGE ( 'NONE', *, *, #71283, .T. ) ;
#97751=CARTESIAN_POINT ( 'NONE',  ( 1.364683531249988535, 4.967708333674756283, -0.7879004041258300672 ) ) ;
#97753=CARTESIAN_POINT ( 'NONE',  ( 6.094553744542824170, 7.069066442510145265, 1.199719254218462483 ) ) ;
#97755=CARTESIAN_POINT ( 'NONE',  ( -7.178152263431422320, 10.46192917639026554, 1.199719254218453823 ) ) ;
#97756=DIRECTION ( 'NONE',  ( 0.5265943820992835533, 0.4485553919786932076, -0.7221470882502503130 ) ) ;
#97759=VERTEX_POINT ( 'NONE', #3431 ) ;
#97761=CARTESIAN_POINT ( 'NONE',  ( -1.201851678989727383E-14, 5.587500000000021672, -1.732050807568863648 ) ) ;
#97768=CARTESIAN_POINT ( 'NONE',  ( 6.968527767744098433, 9.153035033833367251, 1.443375672974076540 ) ) ;
#97772=CARTESIAN_POINT ( 'NONE',  ( -1.500000000000011324, 4.410416667349484676, -0.8660254037844313801 ) ) ;
#97774=CARTESIAN_POINT ( 'NONE',  ( -5.264643720808155791, 5.036505850564608089, 0.000000000000000000 ) ) ;
#97775=CARTESIAN_POINT ( 'NONE',  ( 5.626270559546810546, 8.547437505237857280, 1.082531754730558626 ) ) ;
#97783=CARTESIAN_POINT ( 'NONE',  ( 2.496672843210871129, 6.064535417054653266, -0.7998128361456291469 ) ) ;
#97784=CARTESIAN_POINT ( 'NONE',  ( 3.621833129746810265, 4.096114899008192367, -2.499999999999995115 ) ) ;
#97788=ORIENTED_EDGE ( 'NONE', *, *, #72346, .T. ) ;
#97800=CARTESIAN_POINT ( 'NONE',  ( 8.378048858240820351, 11.86180853700128601, -1.199719254218446718 ) ) ;
#97804=CARTESIAN_POINT ( 'NONE',  ( 1.364683531249986537, -0.1364583329919154264, 0.7879004041258500513 ) ) ;
#97805=CARTESIAN_POINT ( 'NONE',  ( 5.097502569058200983, 6.970172302033127210, -1.443375672974051449 ) ) ;
#97806=CARTESIAN_POINT ( 'NONE',  ( -10.14113571334194930, 10.93367254176152059, -0.7216878364870267237 ) ) ;
#97811=CARTESIAN_POINT ( 'NONE',  ( -4.334856428067329404, 6.080418470877079429, -1.599625672291256295 ) ) ;
#97818=EDGE_LOOP ( 'NONE', ( #42022, #57436 ) ) ;
#97825=CARTESIAN_POINT ( 'NONE',  ( 5.354985324346148268, 6.526937442883553153, -1.333766491515418817 ) ) ;
#97833=CARTESIAN_POINT ( 'NONE',  ( -7.646435448427427062, 10.90429654226522693, 1.082531754730549967 ) ) ;
#97837=CARTESIAN_POINT ( 'NONE',  ( 5.615048174354031474, 9.702639970055050966, 0.7998128361456462443 ) ) ;
#97838=CARTESIAN_POINT ( 'NONE',  ( -5.447678794592645701, 5.250046769979851646, 0.000000000000000000 ) ) ;
#97840=CARTESIAN_POINT ( 'NONE',  ( -5.250031796989778066, 7.148123067953287446, 1.599625672291267398 ) ) ;
#97841=CARTESIAN_POINT ( 'NONE',  ( 2.510230996824538430, 6.080353262937265413, 0.000000000000000000 ) ) ;
#97845=CARTESIAN_POINT ( 'NONE',  ( -6.013204822860843457, 6.974159367214481264, -1.199719254218446718 ) ) ;
#97849=CARTESIAN_POINT ( 'NONE',  ( 9.511208455186636712, 11.05516360492796935, 1.199719254218453823 ) ) ;
#97852=CARTESIAN_POINT ( 'NONE',  ( 4.247106804623488330, 7.517614509530361033, 0.9983198370346995087 ) ) ;
#97853=CARTESIAN_POINT ( 'NONE',  ( 5.992340707560163793, 6.093411701682730275, 0.7216878364870317197 ) ) ;
#97860=VERTEX_POINT ( 'NONE', #164891 ) ;
#97861=CARTESIAN_POINT ( 'NONE',  ( 6.927853306458739979, 10.06595070996845642, 1.082531754730558626 ) ) ;
#97866=CARTESIAN_POINT ( 'NONE',  ( -8.299562589859897699, 12.83457345481192036, -0.7998128361456281477 ) ) ;
#97867=CARTESIAN_POINT ( 'NONE',  ( -6.714312387265696458, 8.856450423275211037, 1.599625672291283607 ) ) ;
#97869=EDGE_CURVE ( 'NONE', #91680, #6715, #185491, .T. ) ;
#97872=SPHERICAL_SURFACE ( 'NONE', #209478, 0.08000000000000000167 ) ;
#97873=DIRECTION ( 'NONE',  ( 0.01240427322300429423, 0.9999230640433337536, 0.000000000000000000 ) ) ;
#97877=CARTESIAN_POINT ( 'NONE',  ( 8.269583629331492602, 11.73526576994040482, 1.199719254218450271 ) ) ;
#97881=CARTESIAN_POINT ( 'NONE',  ( 3.358669367883368118, 4.941533567329135401, -1.599625672291262513 ) ) ;
#97884=CARTESIAN_POINT ( 'NONE',  ( 1.499999999999989120, 3.535416667349488229, 0.8660254037844524744 ) ) ;
#97890=CARTESIAN_POINT ( 'NONE',  ( -1.500000000000011324, 3.670833333333356485, 0.8660254037844403729 ) ) ;
#97891=CARTESIAN_POINT ( 'NONE',  ( 6.308621549060418054, 6.254479983525607523, 0.7998128361456341429 ) ) ;
#97894=CARTESIAN_POINT ( 'NONE',  ( 8.297226821883377568, 8.782445501726501291, -0.7216878364870267237 ) ) ;
#97899=CARTESIAN_POINT ( 'NONE',  ( 10.24048609702354717, 10.84165528948263457, -0.7998128361456281477 ) ) ;
#97901=CARTESIAN_POINT ( 'NONE',  ( -3.093231602212184850, 6.760520635889515795, -0.7998128361456281477 ) ) ;
#97902=CARTESIAN_POINT ( 'NONE',  ( -1.402160292154681736E-14, -0.05312499965857903073, -1.575800808251665908 ) ) ;
#97906=CARTESIAN_POINT ( 'NONE',  ( 4.196412238629597447, 4.854568018944682706, -1.199719254218452047 ) ) ;
#97909=CARTESIAN_POINT ( 'NONE',  ( 1.364683531249988535, 5.217708333674750065, -0.7879004041258300672 ) ) ;
#97911=DIRECTION ( 'NONE',  ( -1.000000000000000000, 7.109522442527899011E-16, 0.000000000000000000 ) ) ;
#97918=CARTESIAN_POINT ( 'NONE',  ( -6.042130013184518589, 10.20090211535728031, -0.7998128361456291469 ) ) ;
#97919=( BOUNDED_CURVE ( )  B_SPLINE_CURVE ( 2, ( #64274, #181206, #44845, #197455, #210507, #61069, #32834 ),
 .UNSPECIFIED., .F., .T. ) 
 B_SPLINE_CURVE_WITH_KNOTS ( ( 3, 2, 2, 3 ),
 ( 0.2125000000000001055, 0.2166666666666668128, 0.2208333333333334925, 0.2250000000000001998 ),
 .UNSPECIFIED. ) 
 CURVE ( )  GEOMETRIC_REPRESENTATION_ITEM ( )  RATIONAL_B_SPLINE_CURVE ( ( 0.9999999999999964473, 0.8660254037844422603, 1.000000000000000000, 0.8660254037844387076, 1.000000000000000000, 0.8660254037844324904, 1.000000000000006217 ) ) 
 REPRESENTATION_ITEM ( '' )  );
#97921=CARTESIAN_POINT ( 'NONE',  ( 6.356075086708249167, 6.309842444114747373, -0.7998128361456281477 ) ) ;
#97924=CARTESIAN_POINT ( 'NONE',  ( -1.364683531250000748, 1.259375000341421469, 0.000000000000000000 ) ) ;
#97926=VERTEX_POINT ( 'NONE', #165959 ) ;
#97928=CARTESIAN_POINT ( 'NONE',  ( 8.615316546479974136, 12.13862083994696839, 1.199719254218450271 ) ) ;
#97931=CARTESIAN_POINT ( 'NONE',  ( -6.368579470117215813, 8.453095353268645695, 1.599625672291283607 ) ) ;
#97935=CARTESIAN_POINT ( 'NONE',  ( 7.553864141108259211, 11.96459193126834464, 1.040834085586084257E-14 ) ) ;
#97937=CARTESIAN_POINT ( 'NONE',  ( 8.320953590485093088, 10.73086516036454618, 1.599625672291281386 ) ) ;
#97938=( BOUNDED_CURVE ( )  B_SPLINE_CURVE ( 3, ( #95059, #64661, #80919, #32168 ),
 .UNSPECIFIED., .F., .T. ) 
 B_SPLINE_CURVE_WITH_KNOTS ( ( 4, 4 ),
 ( 3.059570999471132424, 3.223614307708552840 ),
 .UNSPECIFIED. ) 
 CURVE ( )  GEOMETRIC_REPRESENTATION_ITEM ( )  RATIONAL_B_SPLINE_CURVE ( ( 1.000000000000000000, 0.9977587396908786932, 0.9977587396908786932, 1.000000000000000000 ) ) 
 REPRESENTATION_ITEM ( '' )  );
#97939=DIRECTION ( 'NONE',  ( -0.9782075119097819460, 0.1245777785625464124, 0.1661037047500602826 ) ) ;
#97940=CARTESIAN_POINT ( 'NONE',  ( -8.500599126088349777, 12.86119004717103209, 1.040834085586084257E-14 ) ) ;
#97942=CARTESIAN_POINT ( 'NONE',  ( -6.368579470117215813, 8.453095353268645695, 1.599625672291283607 ) ) ;
#97947=CARTESIAN_POINT ( 'NONE',  ( -5.139172151939493283, 6.684247474441955106, 1.432371535143169394 ) ) ;
#97948=CARTESIAN_POINT ( 'NONE',  ( 1.364683531249986537, 0.1552083336747499542, -0.7879004041258309554 ) ) ;
#97952=CARTESIAN_POINT ( 'NONE',  ( 7.944714827928050838, 9.331550723079971021, 1.082531754730558626 ) ) ;
#97970=CARTESIAN_POINT ( 'NONE',  ( 9.154780037725547714, 11.70366268214508487, 1.599625672291279388 ) ) ;
#97974=CARTESIAN_POINT ( 'NONE',  ( -4.303823697334223652, 7.108545849276850959, -1.199719254218452047 ) ) ;
#97975=CARTESIAN_POINT ( 'NONE',  ( -7.049349804101573191, 10.31165964050546258, -1.199719254218440723 ) ) ;
#97981=CARTESIAN_POINT ( 'NONE',  ( -1.500000000000013101, 2.910416667349485120, -0.8660254037844313801 ) ) ;
#97982=CARTESIAN_POINT ( 'NONE',  ( 9.752392566931574081, 10.27221283770866300, -0.7998128361456281477 ) ) ;
#97986=CARTESIAN_POINT ( 'NONE',  ( -9.501566725078754772, 9.979582688880366703, -0.7998128361456291469 ) ) ;
#97988=CARTESIAN_POINT ( 'NONE',  ( -1.364683531250012516, 3.988541667008088876, -0.7879004041258300672 ) ) ;
#97994=CARTESIAN_POINT ( 'NONE',  ( -9.490344339885977476, 11.13478515369756217, -1.082531754730539753 ) ) ;
#97998=CARTESIAN_POINT ( 'NONE',  ( 1.364683531249988535, 1.676041667008085101, 0.7879004041258500513 ) ) ;
#98004=CARTESIAN_POINT ( 'NONE',  ( -1.364683531250012516, 2.738541667008090208, -0.7879004041258289570 ) ) ;
#98008=CARTESIAN_POINT ( 'NONE',  ( -6.749261541504576911, 6.768559974710451677, 1.040834085586084257E-14 ) ) ;
#98009=CARTESIAN_POINT ( 'NONE',  ( 6.856673000209174695, 9.022537805042615489, 1.599625672291281386 ) ) ;
#98010=CARTESIAN_POINT ( 'NONE',  ( 2.535011536075338689, 5.133042487381368701, -0.9999999999999956701 ) ) ;
#98012=CARTESIAN_POINT ( 'NONE',  ( 1.364683531249988757, 2.446875000341415696, 1.214306433183764966E-14 ) ) ;
#98016=CARTESIAN_POINT ( 'NONE',  ( -6.399085315970155285, 6.567947078161039620, -0.7216878364870278340 ) ) ;
#98021=CARTESIAN_POINT ( 'NONE',  ( 5.558479791922850133, 6.547609847740540445, -1.082531754730542195 ) ) ;
#98024=CARTESIAN_POINT ( 'NONE',  ( -8.213542131780492639, 8.476887330032372603, 1.040834085586084257E-14 ) ) ;
#98025=CARTESIAN_POINT ( 'NONE',  ( -3.898132859128961236, 4.506575409527250997, -1.199719254218452047 ) ) ;
#98027=CARTESIAN_POINT ( 'NONE',  ( -0.6823417656250212460, 5.301041667008086655, 1.181850606188767472 ) ) ;
#98032=CARTESIAN_POINT ( 'NONE',  ( -7.876924059415400414, 9.252461493148505411, 1.082531754730558626 ) ) ;
#98034=CARTESIAN_POINT ( 'NONE',  ( 0.6823417656249882723, -1.094791666325249713, 1.181850606188755259 ) ) ;
#98038=CARTESIAN_POINT ( 'NONE',  ( 7.266807147244743526, 11.42176607185347414, -0.7216878364870267237 ) ) ;
#98046=CARTESIAN_POINT ( 'NONE',  ( 9.869972640624258275, 10.61731562359089587, 0.000000000000000000 ) ) ;
#98052=CARTESIAN_POINT ( 'NONE',  ( 6.986529229743720926, 7.045372277656132276, -0.7998128361456281477 ) ) ;
#98053=CARTESIAN_POINT ( 'NONE',  ( -2.930533758848195447, 6.570706485298192234, -0.7998128361456281477 ) ) ;
#98057=CARTESIAN_POINT ( 'NONE',  ( 5.300874872818828187, 8.167809204055208383, 1.082531754730558626 ) ) ;
#98058=CARTESIAN_POINT ( 'NONE',  ( 1.364683531249986537, 0.7177083336747527298, -0.7879004041258239610 ) ) ;
#98060=CARTESIAN_POINT ( 'NONE',  ( -9.378489572351046633, 11.96465713920816043, -1.599625672291263179 ) ) ;
#98066=EDGE_CURVE ( 'NONE', #176773, #205805, #186914, .T. ) ;
#98074=CARTESIAN_POINT ( 'NONE',  ( -4.454990830682073799, 7.094613310480975876, -1.116242305992283690 ) ) ;
#98078=CARTESIAN_POINT ( 'NONE',  ( 6.446011968293428041, 9.607765498729298415, -1.199719254218440723 ) ) ;
#98079=CARTESIAN_POINT ( 'NONE',  ( 5.795220594837462436, 8.848508896363995291, -1.199719254218440723 ) ) ;
#98089=CARTESIAN_POINT ( 'NONE',  ( 8.778014389843965759, 12.32843499053828928, 1.199719254218450271 ) ) ;
#98092=CARTESIAN_POINT ( 'NONE',  ( -2.428882075142555497, 5.985446187641602300, 1.040834085586084257E-14 ) ) ;
#98095=CARTESIAN_POINT ( 'NONE',  ( 4.911989969715260251, 4.726297878971393196, -7.499999999999991118 ) ) ;
#98097=CARTESIAN_POINT ( 'NONE',  ( -0.2718889520038957341, 8.158259021453911686, 2.022062967018402713 ) ) ;
#98103=CARTESIAN_POINT ( 'NONE',  ( -8.676855123066012254, 12.10645282934361866, -1.082531754730543971 ) ) ;
#98106=CARTESIAN_POINT ( 'NONE',  ( 5.341022448779654930, 8.318611059296550536, 1.199719254218462483 ) ) ;
#98107=CARTESIAN_POINT ( 'NONE',  ( 1.364683531249990311, 5.613541667008088432, 0.7879004041258499402 ) ) ;
#98111=EDGE_CURVE ( 'NONE', #104869, #169854, #9092, .T. ) ;
#98113=CARTESIAN_POINT ( 'NONE',  ( 5.653386866774156694, 5.697965554099049257, -0.7216878364870207285 ) ) ;
#98120=CARTESIAN_POINT ( 'NONE',  ( -7.854251061018346469, 8.057714414143200443, -0.7998128361456291469 ) ) ;
#98121=CARTESIAN_POINT ( 'NONE',  ( -5.135841261478327979, 4.886236314679810455, 0.7998128361456341429 ) ) ;
#98122=DIRECTION ( 'NONE',  ( -1.000000000000000000, 5.421010862427522170E-16, 0.000000000000000000 ) ) ;
#98131=CARTESIAN_POINT ( 'NONE',  ( 5.262536180398716290, 9.291375977107183104, -0.7998128361456291469 ) ) ;
#98137=CARTESIAN_POINT ( 'NONE',  ( -1.244123718695706815, 2.973244533904600750, 0.7750000000000170086 ) ) ;
#98141=ORIENTED_EDGE ( 'NONE', *, *, #32339, .T. ) ;
#98143=CARTESIAN_POINT ( 'NONE',  ( 1.364683531249986537, -0.07395833299191513499, 0.7879004041258500513 ) ) ;
#98144=CARTESIAN_POINT ( 'NONE',  ( 4.330940004561544043, 7.140181541042074365, -1.199719254218452047 ) ) ;
#98146=CARTESIAN_POINT ( 'NONE',  ( -6.941411460516810017, 8.161030127766803588, 1.082531754730549967 ) ) ;
#98148=CARTESIAN_POINT ( 'NONE',  ( 4.853455804012216213, 6.685451076146141425, 1.443375672974062551 ) ) ;
#98150=CARTESIAN_POINT ( 'NONE',  ( -6.195713011320783892, 10.17215624660883577, -0.7216878364870267237 ) ) ;
#98156=CARTESIAN_POINT ( 'NONE',  ( 7.100719765255169236, 9.307259030929609267, -1.599625672291262513 ) ) ;
#98158=CARTESIAN_POINT ( 'NONE',  ( -2.946110181334088196, 6.448586377034708050, 0.1685663139843082692 ) ) ;
#98161=CARTESIAN_POINT ( 'NONE',  ( -1.201851678989727383E-14, 3.571875000341422357, 1.575800808251672791 ) ) ;
#98165=CARTESIAN_POINT ( 'NONE',  ( 8.145751363712157911, 8.397798100619326078, -0.7998128361456281477 ) ) ;
#98168=CARTESIAN_POINT ( 'NONE',  ( -7.823218330285243383, 9.085841792542966644, -1.199719254218446718 ) ) ;
#98174=CARTESIAN_POINT ( 'NONE',  ( 9.887974103068218668, 10.43039129653476493, 0.7998128361456462443 ) ) ;
#98176=CARTESIAN_POINT ( 'NONE',  ( -8.636707547105197946, 10.03491254549959777, -1.199719254218446718 ) ) ;
#98179=CARTESIAN_POINT ( 'NONE',  ( 5.394965581569445057, 6.295244270701876310, -1.058425382943289028 ) ) ;
#98180=CARTESIAN_POINT ( 'NONE',  ( -3.602716132929368875, 5.226254793216122074, 1.599625672291267398 ) ) ;
#98185=CARTESIAN_POINT ( 'NONE',  ( 7.461064606222022277, 7.598996883547496139, 1.040834085586084257E-14 ) ) ;
#98187=CARTESIAN_POINT ( 'NONE',  ( 6.335737856287750880, 6.286115675290828264, -0.7998128361456281477 ) ) ;
#98188=CARTESIAN_POINT ( 'NONE',  ( -4.072711641797504001, 7.543564457389225986, 0.4874124537386469447 ) ) ;
#98189=CARTESIAN_POINT ( 'NONE',  ( 2.686486993802192913, 6.285985259411197568, 0.7998128361456362523 ) ) ;
#98191=CARTESIAN_POINT ( 'NONE',  ( -7.402388683381436074, 7.738467673474211495, 0.7216878364870317197 ) ) ;
#98197=CARTESIAN_POINT ( 'NONE',  ( -4.034767475943390025, 7.597003608976943489, -0.2951547658557127640 ) ) ;
#98198=CARTESIAN_POINT ( 'NONE',  ( 0.6823417656249882723, -0.5947916663252492686, 1.181850606188755259 ) ) ;
#98201=CARTESIAN_POINT ( 'NONE',  ( 3.362058906508953449, 6.866226457661676719, -0.7216878364870267237 ) ) ;
#98204=CARTESIAN_POINT ( 'NONE',  ( -8.581948047326017459, 11.99572790764693409, 1.082531754730558626 ) ) ;
#98215=ORIENTED_EDGE ( 'NONE', *, *, #126245, .F. ) ;
#98216=CARTESIAN_POINT ( 'NONE',  ( -9.286972035236635392, 9.937148250638648150, -0.7216878364870267237 ) ) ;
#98221=CARTESIAN_POINT ( 'NONE',  ( 0.7499999999999885647, 2.597916667349486897, -1.299038105676658228 ) ) ;
#98225=CARTESIAN_POINT ( 'NONE',  ( -6.170932472514347289, 10.35117165124207972, 0.000000000000000000 ) ) ;
#98228=CARTESIAN_POINT ( 'NONE',  ( 5.449487677688982679, 8.445153826357429949, -1.199719254218446718 ) ) ;
#98230=CARTESIAN_POINT ( 'NONE',  ( -4.217958839219735800, 3.978389137448586244, 0.5316758947214468289 ) ) ;
#98233=CARTESIAN_POINT ( 'NONE',  ( 7.072549687823125097, 11.40305840243567381, -0.7998128361456291469 ) ) ;
#98239=CARTESIAN_POINT ( 'NONE',  ( -6.643132081016132062, 8.773406732650713025, 1.443375672974078761 ) ) ;
#98242=CARTESIAN_POINT ( 'NONE',  ( 1.364683531249990311, 4.926041667008083991, 0.7879004041258500513 ) ) ;
#98243=EDGE_CURVE ( 'NONE', #69507, #146527, #86842, .T. ) ;
#98248=CARTESIAN_POINT ( 'NONE',  ( -10.15522075183580419, 11.80651128435196462, 1.199719254218462483 ) ) ;
#98250=CARTESIAN_POINT ( 'NONE',  ( 10.08456733046637765, 10.65975006183261087, 0.000000000000000000 ) ) ;
#98251=CARTESIAN_POINT ( 'NONE',  ( 3.469446951953614189E-15, 5.229711127717882491, 1.214306433183764966E-14 ) ) ;
#98252=CARTESIAN_POINT ( 'NONE',  ( -8.696665468161981494, 12.23352791524263239, -1.199719254218446718 ) ) ;
#98254=CARTESIAN_POINT ( 'NONE',  ( -1.364683531250012516, 2.030208333674750953, 0.7879004041258379498 ) ) ;
#98255=CARTESIAN_POINT ( 'NONE',  ( 3.161022370280501814, 6.839609865302569425, 0.000000000000000000 ) ) ;
#98260=DIRECTION ( 'NONE',  ( -1.000000000000000000, 6.308085367188389255E-16, 0.000000000000000000 ) ) ;
#98261=CARTESIAN_POINT ( 'NONE',  ( 9.259855728009286580, 10.86588177317476855, -1.082531754730543083 ) ) ;
#98263=CARTESIAN_POINT ( 'NONE',  ( -7.049876689426103127, 10.20831132343037062, -1.082531754730537976 ) ) ;
#98264=CARTESIAN_POINT ( 'NONE',  ( -1.364683531250000748, 0.5093750003414208027, 0.000000000000000000 ) ) ;
#98266=DIRECTION ( 'NONE',  ( 1.000000000000000000, 0.000000000000000000, 0.000000000000000000 ) ) ;
#98268=CARTESIAN_POINT ( 'NONE',  ( -7.483210719738908168, 10.81783070874899799, 1.199719254218453823 ) ) ;
#98269=CARTESIAN_POINT ( 'NONE',  ( -4.894130264408878439, 4.812166184672871161, -0.7216878364870197293 ) ) ;
#98270=CARTESIAN_POINT ( 'NONE',  ( -1.364683531250010295, 4.092708333674751842, 0.7879004041258379498 ) ) ;
#98275=CARTESIAN_POINT ( 'NONE',  ( 8.211434591371064684, 12.73175745657494851, -0.7998128361456352531 ) ) ;
#98286=CARTESIAN_POINT ( 'NONE',  ( -1.420000000000021911, 7.176846818246207960, 4.202462424328227364 ) ) ;
#98290=CARTESIAN_POINT ( 'NONE',  ( -1.364683531250012516, 4.801041667008083991, -0.7879004041258300672 ) ) ;
#98295=CARTESIAN_POINT ( 'NONE',  ( 7.313733799568044702, 10.62010763521636214, 1.199719254218460707 ) ) ;
#98297=CARTESIAN_POINT ( 'NONE',  ( -1.201851678989727383E-14, 2.571875000341417472, 1.575800808251672791 ) ) ;
#98299=CARTESIAN_POINT ( 'NONE',  ( -6.399085315970137522, 9.449054721065074602, -1.082531754730538864 ) ) ;
#98304=CARTESIAN_POINT ( 'NONE',  ( 3.948449050077836642, 5.629609863222681199, 1.599625672291267398 ) ) ;
#98306=ORIENTED_EDGE ( 'NONE', *, *, #195535, .F. ) ;
#98307=CARTESIAN_POINT ( 'NONE',  ( 7.892817981449907982, 12.36003807833360391, 0.7998128361456462443 ) ) ;
#98314=CARTESIAN_POINT ( 'NONE',  ( -9.297140650669053485, 11.86975006391249643, 1.599625672291281386 ) ) ;
#98315=CARTESIAN_POINT ( 'NONE',  ( 8.281332899848809603, 8.555976559445431562, 0.7998128361456481317 ) ) ;
#98317=CARTESIAN_POINT ( 'NONE',  ( 3.836594282542902246, 7.419851063034623273, 0.7216878364870317197 ) ) ;
#98319=DIRECTION ( 'NONE',  ( 0.1674078377060222722, 0.000000000000000000, 0.9858877298529452604 ) ) ;
#98327=CARTESIAN_POINT ( 'NONE',  ( -8.039621903223732602, 8.481906429956900695, 1.040834085586084257E-14 ) ) ;
#98328=CARTESIAN_POINT ( 'NONE',  ( 4.497554271431305040, 6.270232621468402989, -1.599625672291256295 ) ) ;
#98331=CARTESIAN_POINT ( 'NONE',  ( -7.296259222448620463, 11.66405285949874759, 0.7998128361456481317 ) ) ;
#98336=CARTESIAN_POINT ( 'NONE',  ( -9.592557376868645846, 11.15007068022363157, -1.199719254218441611 ) ) ;
#98340=CARTESIAN_POINT ( 'NONE',  ( 7.411503528164766763, 11.79850454950093841, 1.040834085586084257E-14 ) ) ;
#98351=CARTESIAN_POINT ( 'NONE',  ( -8.833300774503376473, 10.26427131079744193, 1.199719254218462483 ) ) ;
#98356=CARTESIAN_POINT ( 'NONE',  ( 6.290620087060792009, 10.28288116830553101, -0.7216878364870267237 ) ) ;
#98358=CARTESIAN_POINT ( 'NONE',  ( 3.684065054611349144, 5.321161868511784299, -1.599625672291262513 ) ) ;
#98360=CARTESIAN_POINT ( 'NONE',  ( 5.705283713252285338, 5.550585841749444249, -0.7998128361456211532 ) ) ;
#98362=CARTESIAN_POINT ( 'NONE',  ( -7.172426956829277778, 8.326585190177668849, -1.199719254218452935 ) ) ;
#98372=CARTESIAN_POINT ( 'NONE',  ( 1.364683531249988535, 3.426041667008085323, 0.7879004041258500513 ) ) ;
#98373=CARTESIAN_POINT ( 'NONE',  ( 4.324687812634887329, 6.068555086205916105, 1.443375672974062551 ) ) ;
#98374=CARTESIAN_POINT ( 'NONE',  ( 7.242026607993941489, 11.60078147596829901, 0.7998128361456462443 ) ) ;
#98376=CARTESIAN_POINT ( 'NONE',  ( -3.904385051055635270, 6.538571078664754843, 1.082531754730560403 ) ) ;
#98378=CARTESIAN_POINT ( 'NONE',  ( -5.572037945092175981, 5.603058478803387032, 0.7216878364870317197 ) ) ;
#98386=CARTESIAN_POINT ( 'NONE',  ( 3.486418057008484617, 7.219238166485217434, 1.040834085586084257E-14 ) ) ;
#98394=CARTESIAN_POINT ( 'NONE',  ( 5.678167406024951624, 5.518950149984223508, 0.7998128361456341429 ) ) ;
#98396=CARTESIAN_POINT ( 'NONE',  ( -4.939248034080176097, 4.656877549381960080, 1.214306433183764966E-14 ) ) ;
#98399=CARTESIAN_POINT ( 'NONE',  ( 1.364683531249988535, 4.176041667008081326, 0.7879004041258500513 ) ) ;
#98404=CARTESIAN_POINT ( 'NONE',  ( 6.100279051144945619, 9.204410428722734849, -1.199719254218440723 ) ) ;
#98406=CARTESIAN_POINT ( 'NONE',  ( -4.954615070790188369, 7.867802451642154082, -1.199719254218452047 ) ) ;
#98407=CARTESIAN_POINT ( 'NONE',  ( 6.277061933002785032, 7.385955679000473673, 1.082531754730558626 ) ) ;
#98408=CARTESIAN_POINT ( 'NONE',  ( -0.7500000000000215383, 1.691666666666688634, 1.299038105676659116 ) ) ;
#98411=CARTESIAN_POINT ( 'NONE',  ( -4.225337428953291230, 8.081310767087481750, 0.7998128361456341429 ) ) ;
#98412=CARTESIAN_POINT ( 'NONE',  ( 0.4998684179604583333, 7.978338306496072896, -1.936700108954743316 ) ) ;
#98414=CARTESIAN_POINT ( 'NONE',  ( 0.6823417656249917140, 3.842708333674754506, 1.181850606188765695 ) ) ;
#98416=CARTESIAN_POINT ( 'NONE',  ( -4.772106882330241717, 5.630174786549132726, -1.082531754730544860 ) ) ;
#98422=CARTESIAN_POINT ( 'NONE',  ( 6.491656622844908853, 6.468020902940851968, 0.7998128361456341429 ) ) ;
#98426=CARTESIAN_POINT ( 'NONE',  ( 0.6823417656249899377, 3.988541667008085767, -1.181850606188754593 ) ) ;
#98428=CARTESIAN_POINT ( 'NONE',  ( 2.510230996824538430, 6.080353262937265413, 0.000000000000000000 ) ) ;
#98430=CARTESIAN_POINT ( 'NONE',  ( -1.364683531250000748, -0.1781249996585798634, 0.000000000000000000 ) ) ;
#98435=CARTESIAN_POINT ( 'NONE',  ( -2.462777459176719308, 6.024990802348131780, -0.7998128361456281477 ) ) ;
#98436=CARTESIAN_POINT ( 'NONE',  ( -4.867013957181525186, 8.622007350113015889, 0.7216878364870458196 ) ) ;
#98440=CARTESIAN_POINT ( 'NONE',  ( -1.364683531250012516, 2.530208333674753174, 0.7879004041258379498 ) ) ;
#98449=CARTESIAN_POINT ( 'NONE',  ( -6.331294547457448019, 10.33033470543493770, 0.7216878364870458196 ) ) ;
#98454=CARTESIAN_POINT ( 'NONE',  ( -5.463572716182839351, 7.397254140345190798, 1.443375672974064550 ) ) ;
#98462=CARTESIAN_POINT ( 'NONE',  ( 1.445103857048098739, 8.688264192037886247, -2.625611233228243968 ) ) ;
#98466=CARTESIAN_POINT ( 'NONE',  ( -6.240830780992103755, 6.175390754112560110, 1.040834085586084257E-14 ) ) ;
#98468=CARTESIAN_POINT ( 'NONE',  ( 1.499999999999987121, 0.004166666666691258049, 0.8660254037844524744 ) ) ;
#98469=CARTESIAN_POINT ( 'NONE',  ( 4.207107738942202246, 3.802713871720993399, 1.214306433183764966E-14 ) ) ;
#98470=CARTESIAN_POINT ( 'NONE',  ( 8.229962938695207342, 9.560377169021284871, 1.199719254218462483 ) ) ;
#98473=CARTESIAN_POINT ( 'NONE',  ( 4.385172619016207918, 7.203452924572514959, 1.199719254218462483 ) ) ;
#98479=CARTESIAN_POINT ( 'NONE',  ( -2.629918611371007575, 6.012062780000711371, 0.7216878364870317197 ) ) ;
#98483=CARTESIAN_POINT ( 'NONE',  ( 6.518203450479811423, 5.167241622962440495, -2.437504649502885812 ) ) ;
#98489=CARTESIAN_POINT ( 'NONE',  ( -1.364683531250012516, 2.530208333674753174, 0.7879004041258379498 ) ) ;
#98490=CARTESIAN_POINT ( 'NONE',  ( 10.37162432432990755, 11.20257592124748136, -0.7216878364870257245 ) ) ;
#98491=CARTESIAN_POINT ( 'NONE',  ( -7.562750758324527922, 7.717630727667075696, 1.040834085586084257E-14 ) ) ;
#98494=CARTESIAN_POINT ( 'NONE',  ( 6.765682348419287173, 7.852049813699357728, 1.199719254218462483 ) ) ;
#98495=CARTESIAN_POINT ( 'NONE',  ( -6.847031270101295419, 7.946956888995021728, -1.199719254218446718 ) ) ;
#98498=CARTESIAN_POINT ( 'NONE',  ( -1.500000000000001332, -0.8187499993171781787, 0.000000000000000000 ) ) ;
#98501=ADVANCED_FACE ( 'NONE', ( #91129, #153982 ), #137744, .F. ) ;
#98503=CARTESIAN_POINT ( 'NONE',  ( 8.134528978519385944, 8.592631351135175066, -0.7216878364870267237 ) ) ;
#98506=CARTESIAN_POINT ( 'NONE',  ( -0.6823417656250246877, 0.3635416670080895973, 1.181850606188755259 ) ) ;
#98508=CARTESIAN_POINT ( 'NONE',  ( 6.819388077549422889, 8.018669514304889390, -1.082531754730543971 ) ) ;
#98512=CARTESIAN_POINT ( 'NONE',  ( -5.287316719649550301, 5.270883715786984780, 0.7216878364870317197 ) ) ;
#98514=CARTESIAN_POINT ( 'NONE',  ( -1.364683531250012516, 4.988541667008084879, -0.7879004041258300672 ) ) ;
#98518=CARTESIAN_POINT ( 'NONE',  ( -5.176859992674639699, 6.655076503622660233, -1.423794717725470171 ) ) ;
#98525=CARTESIAN_POINT ( 'NONE',  ( 6.608709811657416999, 9.797579649320619311, -1.199719254218440723 ) ) ;
#98528=CARTESIAN_POINT ( 'NONE',  ( 4.359110081993588182, 5.044382169536003602, -1.199719254218452047 ) ) ;
#98529=EDGE_CURVE ( 'NONE', #71497, #85365, #56478, .T. ) ;
#98535=CARTESIAN_POINT ( 'NONE',  ( 3.877268743828258479, 7.467304601200877023, 0.7216878364870298324 ) ) ;
#98536=CARTESIAN_POINT ( 'NONE',  ( -1.364683531250014514, 0.5510416670080878765, -0.7879004041258289570 ) ) ;
#98538=CARTESIAN_POINT ( 'NONE',  ( 9.622536337397022521, 12.24937836509514710, 1.599625672291281386 ) ) ;
#98543=CARTESIAN_POINT ( 'NONE',  ( -0.7500000000000215383, 1.191666666666688190, 1.299038105676659116 ) ) ;
#98544=CARTESIAN_POINT ( 'NONE',  ( 7.935599982700328958, 8.152621489438862667, 0.7998128361456481317 ) ) ;
#98545=CARTESIAN_POINT ( 'NONE',  ( -8.178592977541617515, 10.56477777859713463, 1.599625672291295375 ) ) ;
#98548=EDGE_CURVE ( 'NONE', #214172, #180436, #33355, .T. ) ;
#98550=CARTESIAN_POINT ( 'NONE',  ( -1.364683531250000748, 1.509375000341421691, 0.000000000000000000 ) ) ;
#98551=VERTEX_POINT ( 'NONE', #172367 ) ;
#98552=ADVANCED_FACE ( 'NONE', ( #190722, #156121 ), #138808, .F. ) ;
#98553=CARTESIAN_POINT ( 'NONE',  ( 0.7499999999999885647, 3.066666666666689522, -1.299038105676658228 ) ) ;
#98555=CARTESIAN_POINT ( 'NONE',  ( 3.388648328411762556, 6.040841252200647382, 1.199719254218462483 ) ) ;
#98558=CARTESIAN_POINT ( 'NONE',  ( 1.500000000000005329, 4.535416667349485564, 0.8660254037844431485 ) ) ;
#98562=CARTESIAN_POINT ( 'NONE',  ( 0.7499999999999885647, -0.7354166659838470288, 1.299038105676657340 ) ) ;
#98563=CARTESIAN_POINT ( 'NONE',  ( -6.157374318900681764, 10.33535380535947290, 0.7998128361456481317 ) ) ;
#98564=CARTESIAN_POINT ( 'NONE',  ( -4.609409038966248318, 5.440360635957812718, -1.082531754730544860 ) ) ;
#98572=CARTESIAN_POINT ( 'NONE',  ( 7.772902139336337335, 7.962807338847539107, 0.7998128361456341429 ) ) ;
#98576=CARTESIAN_POINT ( 'NONE',  ( 6.388916700537700777, 8.476822122092563916, 1.599625672291281386 ) ) ;
#98577=CARTESIAN_POINT ( 'NONE',  ( 8.175203438916005538, 11.52119253116861586, -1.082531754730543083 ) ) ;
#98579=( BOUNDED_CURVE ( )  B_SPLINE_CURVE ( 2, ( #187581, #205966, #10956, #109625, #175629, #39208, #105299 ),
 .UNSPECIFIED., .F., .T. ) 
 B_SPLINE_CURVE_WITH_KNOTS ( ( 3, 2, 2, 3 ),
 ( 0.1750000000000002942, 0.1791666666666668351, 0.1833333333333333759, 0.1874999999999999167 ),
 .UNSPECIFIED. ) 
 CURVE ( )  GEOMETRIC_REPRESENTATION_ITEM ( )  RATIONAL_B_SPLINE_CURVE ( ( 0.9999999999999902300, 0.8660254037844484776, 1.000000000000000000, 0.8660254037844387076, 1.000000000000000000, 0.8660254037844413721, 0.9999999999999973355 ) ) 
 REPRESENTATION_ITEM ( '' )  );
#98582=CARTESIAN_POINT ( 'NONE',  ( -8.193204901359996128, 8.453160561208463264, 1.040834085586084257E-14 ) ) ;
#98583=CARTESIAN_POINT ( 'NONE',  ( 3.194917754314666514, 6.879154480009089134, 0.7998128361456321445 ) ) ;
#98588=CARTESIAN_POINT ( 'NONE',  ( 3.995055777641403516, 7.602996552368006533, -0.05680687033517151097 ) ) ;
#98589=CARTESIAN_POINT ( 'NONE',  ( 9.788623719386617239, 11.48277776311499387, -1.082531754730537088 ) ) ;
#98594=LINE ( 'NONE', #102581, #187440 ) ;
#98595=DIRECTION ( 'NONE',  ( 0.6507913734559640506, -0.7592566023653004592, 0.000000000000000000 ) ) ;
#98598=CARTESIAN_POINT ( 'NONE',  ( -2.968872451712654126, 6.407508927065978632, 1.040834085586084257E-14 ) ) ;
#98600=CARTESIAN_POINT ( 'NONE',  ( 9.422553571817644524, 10.09532670998316384, 0.000000000000000000 ) ) ;
#98603=CARTESIAN_POINT ( 'NONE',  ( -5.096975683733680818, 8.033889833409558534, -1.199719254218452047 ) ) ;
#98609=CARTESIAN_POINT ( 'NONE',  ( -7.366157530926372488, 7.488271962369228874, -0.7998128361456291469 ) ) ;
#98623=CARTESIAN_POINT ( 'NONE',  ( -7.040761844198392794, 7.108643661186573759, -0.7998128361456291469 ) ) ;
#98627=CARTESIAN_POINT ( 'NONE',  ( 3.551873057100274789, 7.087676300018221021, 0.7216878364870298324 ) ) ;
#98631=CARTESIAN_POINT ( 'NONE',  ( -3.704402285031864306, 5.344888637335695414, -1.599625672291256295 ) ) ;
#98638=CARTESIAN_POINT ( 'NONE',  ( -7.690499447449645309, 9.995335326823163058, 1.599625672291295375 ) ) ;
#98639=CARTESIAN_POINT ( 'NONE',  ( 5.612185521052973414, 8.634967976948757951, -1.199719254218440723 ) ) ;
#98642=CARTESIAN_POINT ( 'NONE',  ( -7.309817376062285099, 11.67987070538135264, 0.000000000000000000 ) ) ;
#98647=CARTESIAN_POINT ( 'NONE',  ( -1.364683531250000748, 0.3218750003414205807, 0.000000000000000000 ) ) ;
#98648=ORIENTED_EDGE ( 'NONE', *, *, #173816, .T. ) ;
#98650=CARTESIAN_POINT ( 'NONE',  ( 7.565086526745395723, 10.80938946696957004, -1.082531754730543083 ) ) ;
#98677=CARTESIAN_POINT ( 'NONE',  ( 0.7499999999999885647, 0.2645833340161538039, 1.299038105676657340 ) ) ;
#98684=CARTESIAN_POINT ( 'NONE',  ( 9.915090410295563927, 10.46202698829998567, -0.7998128361456281477 ) ) ;
#98685=DIRECTION ( 'NONE',  ( 1.000000000000000000, -6.165071176878339540E-16, 0.000000000000000000 ) ) ;
#98689=CARTESIAN_POINT ( 'NONE',  ( 3.497113557321089861, 6.167384019261527683, -1.199719254218446718 ) ) ;
#98690=CARTESIAN_POINT ( 'NONE',  ( -8.026063749610063525, 8.466088584074293877, -0.7216878364870278340 ) ) ;
#98695=CARTESIAN_POINT ( 'NONE',  ( -7.393273838153706201, 7.519907654134449615, 0.7998128361456341429 ) ) ;
#98696=CARTESIAN_POINT ( 'NONE',  ( -3.972175818679615222, 4.696921878956699103, 1.082531754730558626 ) ) ;
#98699=CARTESIAN_POINT ( 'NONE',  ( -1.500000000000013101, -0.04791666598384902026, 0.8660254037844403729 ) ) ;
#98706=CARTESIAN_POINT ( 'NONE',  ( -2.779058300676974014, 6.186059084191009916, -0.7216878364870257245 ) ) ;
#98707=B_SPLINE_SURFACE_WITH_KNOTS ( 'NONE', 1, 3, ( 
 ( #164749, #99749, #18481, #53126, #117125, #118196, #16340, #69351, #4345, #83486, #67215, #169010, #17402, #150649, #82421, #151714, #2210, #68287, #48878, #1152, #101882, #36866, #135461, #134420, #33675, #184184, #86695, #19549, #3284, #165819, #102950, #70412, #197239, #149569, #114996, #133350, #148510, #77, #66142, #198292, #10503, #202550, #157853, #44104, #127566, #11576, #43047, #124360, #126485, #111289, #92860, #191381, #190317, #176232, #110224, #109160, #41975, #27834, #108086, #71487, #174115, #93930, #193535, #142688, #61403, #91796, #58201, #120340, #159971, #161040, #12635, #192449, #25688, #9447, #75518, #141630, #37951, #137600, #207639, #136530, #59257, #54200, #158907, #125415, #26759, #77646, #45177, #186316, #175172, #76576, #177295, #104023, #143768, #209762, #208698, #28909, #60325, #94994, #170071, #21657, #87763, #153839, #5409, #203617, #32103, #64600, #66684, #13705, #29977, #131778, #130741, #196734, #128628, #179432, #198835, #163181, #162115, #181534, #166358, #211901, #82968, #180484, #147997, #96062, #48375, #114487, #79778, #98188, #164236, #129693, #100291, #210840, #80856, #15824, #145890, #149041, #62466, #132831, #197781, #81909, #194595, #146947, #214007, #14766, #65629, #49419, #115539, #33162, #46239, #50480, #99243, #112356, #195676, #165292, #616, #212962, #16886, #178369, #116601, #78706, #31053, #182595, #63538, #47312, #34218, #113426, #97129, #144832, #17948, #67751, #84035, #1697, #150124, #133901, #199908, #51554, #117679, #183672, #35275, #101353, #24834, #90933, #57350, #190531, #191592, #189477, #193734, #74667, #93070, #25897, #60536, #61607, #140770, #43253, #77853, #42187, #108302, #208904, #173253, #126696, #156999, #8586, #192657, #10713, #206783, #58417, #143977, #45379, #159112, #124570, #174322, #141843, #28047, #209968, #107232, #26962, #11780, #127779, #176435, #44310, #125631, #109372, #111496, #9652, #158066, #41120, #76782, #92008, #177502, #75730, #29115, #95200, #207848, #175379, #142904, #94141, #7508, #73590, #59474, #139692, #110433, #205714, #160179, #123513, #99844, #2301 ),
 ( #64150, #183215, #118284, #197331, #181086, #68377, #131337, #16433, #146489, #51092, #82511, #182136, #162727, #115090, #1242, #84651, #34819, #167, #81462, #83580, #134508, #50024, #148598, #147540, #133442, #67302, #66234, #213561, #199449, #65183, #31656, #48973, #117216, #150740, #165909, #18573, #32704, #196281, #116148, #100895, #166983, #200512, #149662, #132383, #198383, #52157, #98786, #164841, #130292, #17493, #97733, #184270, #163790, #96677, #14298, #15369, #33766, #80393, #212509, #47928, #114041, #180034, #172311, #88939, #23900, #22824, #90006, #57490, #21749, #54293, #187478, #136618, #85713, #156060, #38042, #185338, #152855, #137686, #204771, #186405, #87857, #151800, #7648, #36962, #138753, #3375, #120430, #205858, #35894, #4433, #72657, #139830, #104112, #70502, #135550, #123651, #101971, #69442, #168039, #202644, #73733, #153929, #201575, #53220, #103042, #19642, #154992, #119351, #170160, #169096, #6577, #39108, #20695, #86786, #5497, #71578, #203707, #55354, #106291, #121505, #105192, #171229, #56426, #122585, #188547, #40177, #159245, #126839, #44455, #143045, #42325, #206923, #58552, #24973, #158203, #10845, #157136, #161400, #108441, #60676, #207986, #28184, #29258, #174461, #76919, #45522, #9792, #75867, #176573, #140910, #94279, #124706, #190665, #160320, #192796, #26037, #92150, #111638, #12984, #110571, #141974, #59614, #109509, #210113, #177649, #144119, #125771, #27106, #91076, #95350, #191732, #77996, #8728, #43388, #145176, #189613, #175517, #11924, #79058, #93213, #209040, #74809, #62807, #211181, #61753, #41259, #127921, #107369, #193873, #173390, #14038, #130034, #2040, #181873, #162462, #64934, #46584, #99582, #132120, #166717, #196025, #178713, #84393, #47661, #113772, #199181, #112703, #179775, #194948, #80124, #150480, #67044, #128968, #98518, #65971, #198130, #82250, #31392, #146229, #212246, #30329, #97467, #164580, #96413, #100640, #163523, #214341, #147277, #33509, #182954, #15110, #16165, #50828, #81199, #213309, #115888, #63880, #165646, #131084, #197073, #17234, #49762, #48710, #114824, #116955, #18307 ) ),
 .UNSPECIFIED., .F., .T., .F.,
 ( 2, 2 ),
 ( 4, 2, 2, 2, 2, 2, 2, 2, 2, 2, 2, 2, 2, 2, 2, 2, 2, 2, 2, 2, 2, 2, 2, 2, 2, 2, 2, 2, 2, 2, 2, 2, 2, 2, 2, 2, 2, 2, 2, 2, 2, 2, 2, 2, 2, 2, 2, 2, 2, 2, 2, 2, 2, 2, 2, 2, 2, 2, 2, 2, 2, 2, 2, 2, 2, 2, 2, 2, 2, 2, 2, 2, 2, 2, 2, 2, 2, 2, 2, 2, 2, 2, 2, 2, 2, 2, 2, 2, 2, 2, 2, 2, 2, 2, 2, 2, 2, 2, 2, 2, 2, 2, 2, 2, 2, 2, 2, 2, 2, 2, 2, 2, 2, 2, 2, 2, 2, 2, 2, 2, 2, 2, 4 ),
 ( 0.000000000000000000, 1.000000000000000000 ),
 ( -6.441036414471523752E-08, 0.0001394059631734492798, 0.0002788763367110432749, 0.0004183467102486372428, 0.0004532143036330357755, 0.0004880818970174342539, 0.0005578170837862312650, 0.0006275522705550282219, 0.0006972874573238252872, 0.0007670226440926222440, 0.0008367578308614192009, 0.0009064930176302162662, 0.0009413606110146147989, 0.0009762282043990132231, 0.001045963391167810180, 0.001115698577936607245, 0.001255168951474201159, 0.001324904138242998224, 0.001394639325011795290, 0.001464374511780592355, 0.001534109698549389203, 0.001603844885318186052, 0.001673580072086983117, 0.001743315258855780182, 0.001813050445624577248, 0.001882785632393374313, 0.001917653225777772846, 0.001952520819162171161, 0.002022256005930968010, 0.002091991192699765075, 0.002231461566237359206, 0.002301196753006155837, 0.002370931939774952903, 0.002405799533159351435, 0.002440667126543749968, 0.002510402313312547033, 0.002649872686850141164, 0.002719607873618938229, 0.002789343060387735294, 0.002859078247156532360, 0.002928813433925329425, 0.002998548620694126490, 0.003068283807462923122, 0.003207754181000516819, 0.003277489367769313884, 0.003312356961153712417, 0.003347224554538110949, 0.003416959741306908015, 0.003486694928075705080, 0.003626165301613299211, 0.003695900488382096276, 0.003765635675150893341, 0.003800503268535291874, 0.003835370861919690406, 0.003905106048688487038, 0.003974841235457283670, 0.004044576422226080735, 0.004114311608994877800, 0.004184046795763674866, 0.004253781982532471931, 0.004323517169301268996, 0.004393252356070066061, 0.004462987542838863127, 0.004532722729607660192, 0.004602457916376456390, 0.004672193103145253455, 0.004741928289914050521, 0.004811663476682847586, 0.004881398663451644651, 0.004951133850220441716, 0.005020869036989238782, 0.005090604223758035847, 0.005125471817142434813, 0.005160339410526832912, 0.005299809784064427043, 0.005439280157602021173, 0.005509015344370818239, 0.005578750531139615304, 0.005613618124524013403, 0.005648485717908412369, 0.005718220904677209435, 0.005857691278214803565, 0.005927426464983600631, 0.005997161651752397696, 0.006066896838521193894, 0.006136632025289990959, 0.006206367212058788024, 0.006276102398827584222, 0.006415572772365178353, 0.006485307959133975418, 0.006520175552518374384, 0.006555043145902772483, 0.006624778332671569549, 0.006694513519440366614, 0.006833983892977960745, 0.006903719079746757810, 0.006973454266515554875, 0.007043189453284351940, 0.007112924640053149006, 0.007182659826821946071, 0.007252395013590743136, 0.007322130200359540202, 0.007391865387128337267, 0.007461600573897134332, 0.007496468167281533299, 0.007531335760665931398, 0.007601070947434728463, 0.007670806134203525528, 0.007810276507741118791, 0.007880011694509915857, 0.007949746881278712055, 0.007984614474663111888, 0.008019482068047509987, 0.008089217254816306185, 0.008228687628353900316, 0.008298422815122698248, 0.008368158001891494446, 0.008437893188660290644, 0.008472760782044688743, 0.008507628375429088577, 0.008647098748966682707, 0.008786569122504276838, 0.008926039496041870969 ),
 .UNSPECIFIED. ) ;
#98710=CARTESIAN_POINT ( 'NONE',  ( 4.088303131848604721, 7.475188365022519932, -0.6044521916458069910 ) ) ;
#98715=CARTESIAN_POINT ( 'NONE',  ( -9.992522908471816123, 11.61669713376064372, 1.199719254218462483 ) ) ;
#98716=CARTESIAN_POINT ( 'NONE',  ( 7.796102023057898123, 9.054206100777749455, -1.199719254218441611 ) ) ;
#98724=CARTESIAN_POINT ( 'NONE',  ( -8.296699936558862731, 11.76690146170562201, 1.199719254218453823 ) ) ;
#98730=CARTESIAN_POINT ( 'NONE',  ( 5.027376032568989572, 4.759693547618927489, 0.7998128361456341429 ) ) ;
#98735=CARTESIAN_POINT ( 'NONE',  ( 2.897268479386962969, 6.441866702775564058, 0.3987452234321529065 ) ) ;
#98748=CARTESIAN_POINT ( 'NONE',  ( 5.798083248138522272, 9.916180889470295412, 0.7998128361456462443 ) ) ;
#98750=CARTESIAN_POINT ( 'NONE',  ( -5.284980951228653190, 5.060232619388524533, 0.000000000000000000 ) ) ;
#98758=CARTESIAN_POINT ( 'NONE',  ( 0.7499999999999885647, 0.5145833340161540814, 1.299038105676657340 ) ) ;
#98763=CARTESIAN_POINT ( 'NONE',  ( 3.029357257649615054, 5.621668336311468117, -1.199719254218446718 ) ) ;
#98765=CARTESIAN_POINT ( 'NONE',  ( -3.810004860640155311, 4.403759411290286252, 1.199719254218462483 ) ) ;
#98772=CARTESIAN_POINT ( 'NONE',  ( 4.446711195602238931, 6.210915699667823198, -1.443375672974051449 ) ) ;
#98776=CARTESIAN_POINT ( 'NONE',  ( -1.364683531250010295, 4.842708333674756283, 0.7879004041258379498 ) ) ;
#98778=CARTESIAN_POINT ( 'NONE',  ( 2.860407222358956503, 6.280966159486672140, 0.7216878364870338292 ) ) ;
#98786=CARTESIAN_POINT ( 'NONE',  ( -5.816164686850935794, 6.201415483580719368, 0.9813818067917270405 ) ) ;
#98788=CARTESIAN_POINT ( 'NONE',  ( -1.201851678989727383E-14, 5.259375000341421469, -1.575800808251660134 ) ) ;
#98796=CARTESIAN_POINT ( 'NONE',  ( 0.7499999999999920064, 4.483333333333352932, 1.299038105676669330 ) ) ;
#98804=CARTESIAN_POINT ( 'NONE',  ( 1.364683531249988535, 5.217708333674750065, -0.7879004041258300672 ) ) ;
#98806=CARTESIAN_POINT ( 'NONE',  ( 4.611744806942754238, 8.532119374741881757, -0.7998128361456231517 ) ) ;
#98807=CARTESIAN_POINT ( 'NONE',  ( -9.203287345578106127, 9.631590079462940324, 0.7998128361456462443 ) ) ;
#98812=ORIENTED_EDGE ( 'NONE', *, *, #6746, .T. ) ;
#98814=CARTESIAN_POINT ( 'NONE',  ( -1.001543065824772872E-14, 5.212500000000019895, 1.732050807568877637 ) ) ;
#98824=CARTESIAN_POINT ( 'NONE',  ( 8.026063749610047537, 10.38682701267698150, -1.443375672974057666 ) ) ;
#98825=CARTESIAN_POINT ( 'NONE',  ( -2.155383234892699562, 5.458438174109348395, 1.040834085586084257E-14 ) ) ;
#98829=CARTESIAN_POINT ( 'NONE',  ( 0.7499999999999902300, 3.264583334016149418, 1.299038105676669330 ) ) ;
#98831=CARTESIAN_POINT ( 'NONE',  ( -4.874319919312905647, 5.645460313075203018, -1.199719254218446718 ) ) ;
#98832=CARTESIAN_POINT ( 'NONE',  ( 3.673896439178923057, 5.309298483840612093, 1.443375672974066548 ) ) ;
#98833=CARTESIAN_POINT ( 'NONE',  ( -8.473482818416657736, 12.82955435488738516, -0.7216878364870267237 ) ) ;
#98840=CARTESIAN_POINT ( 'NONE',  ( 4.695201269034174452, 4.372156323494968966, 1.214306433183764966E-14 ) ) ;
#98843=CARTESIAN_POINT ( 'NONE',  ( 3.867100128395839942, 5.534702787927018974, -1.599625672291255185 ) ) ;
#98845=ORIENTED_EDGE ( 'NONE', *, *, #101958, .F. ) ;
#98848=ORIENTED_EDGE ( 'NONE', *, *, #16981, .T. ) ;
#98850=CARTESIAN_POINT ( 'NONE',  ( 7.334597915313080918, 9.580116872663850813, 1.040834085586084257E-14 ) ) ;
#98853=CARTESIAN_POINT ( 'NONE',  ( -1.387358672527355008, 7.251968950354660493, 4.302625267139497112 ) ) ;
#98856=CARTESIAN_POINT ( 'NONE',  ( 10.06423010004587759, 10.63602329300870153, 0.000000000000000000 ) ) ;
#98860=CARTESIAN_POINT ( 'NONE',  ( -1.364683531250014514, 0.2385416670080863499, -0.7879004041258359514 ) ) ;
#98861=CARTESIAN_POINT ( 'NONE',  ( 6.236387472606139681, 8.298871356172400127, -1.443375672974057666 ) ) ;
#98862=CARTESIAN_POINT ( 'NONE',  ( -9.707274797704657843, 11.38787068781932987, 1.082531754730558626 ) ) ;
#98868=CARTESIAN_POINT ( 'NONE',  ( -5.440899717785814715, 5.242137847038546461, 0.7998128361456341429 ) ) ;
#98873=ORIENTED_EDGE ( 'NONE', *, *, #152121, .F. ) ;
#98881=CARTESIAN_POINT ( 'NONE',  ( 6.043473040404234276, 6.060458613201341826, -0.4842117992061110154 ) ) ;
#98882=CARTESIAN_POINT ( 'NONE',  ( -1.244123718695689496, 3.108005466778244852, -0.7749999999999918066 ) ) ;
#98884=CARTESIAN_POINT ( 'NONE',  ( 3.635557746758808495, 7.393234471193928847, -0.7998128361456291469 ) ) ;
#98886=LINE ( 'NONE', #211541, #40753 ) ;
#98889=CARTESIAN_POINT ( 'NONE',  ( -7.687109909268394325, 11.91211929421440097, 0.000000000000000000 ) ) ;
#98893=CARTESIAN_POINT ( 'NONE',  ( 7.124973419181436007, 8.271222729588529887, -1.199719254218446718 ) ) ;
#98894=CARTESIAN_POINT ( 'NONE',  ( -3.815730167242251003, 6.539103397502874948, -1.199719254218452047 ) ) ;
#98895=CARTESIAN_POINT ( 'NONE',  ( 3.460355519985863548, 5.060167411448709629, 1.599625672291267398 ) ) ;
#98897=CARTESIAN_POINT ( 'NONE',  ( -4.089755892816631544, 7.923132308261379819, -0.7998128361456281477 ) ) ;
#98898=CARTESIAN_POINT ( 'NONE',  ( 4.383363735919856730, 4.008345868194933104, -0.7998128361456211532 ) ) ;
#98901=CARTESIAN_POINT ( 'NONE',  ( -4.720210035852093533, 8.658662141802762946, -0.7998128361456281477 ) ) ;
#98905=CARTESIAN_POINT ( 'NONE',  ( 9.887974103068218668, 10.43039129653476493, 0.7998128361456462443 ) ) ;
#98908=CARTESIAN_POINT ( 'NONE',  ( 4.145277420728366025, 7.638539262984231470, 0.7997124044470202975 ) ) ;
#98909=CARTESIAN_POINT ( 'NONE',  ( 6.317736394288147039, 6.473040002865377396, 0.7216878364870317197 ) ) ;
#98917=CARTESIAN_POINT ( 'NONE',  ( 6.277061933002769045, 10.26706332190449622, 0.7216878364870438212 ) ) ;
#98920=CARTESIAN_POINT ( 'NONE',  ( 5.427790276013049642, 4.356734706464521878, -2.440341524156855790 ) ) ;
#98921=CARTESIAN_POINT ( 'NONE',  ( -7.711890448074853133, 7.891627032375787998, -0.7998128361456291469 ) ) ;
#98928=EDGE_CURVE ( 'NONE', #86628, #92745, #116453, .T. ) ;
#98929=CARTESIAN_POINT ( 'NONE',  ( 9.589694723567584234, 10.08239868711733855, -0.7998128361456281477 ) ) ;
#98933=CARTESIAN_POINT ( 'NONE',  ( 3.846762897975340767, 5.510976019103107859, -1.599625672291256295 ) ) ;
#98937=CARTESIAN_POINT ( 'NONE',  ( -1.500000000000011324, 4.202083334016156080, 0.8660254037844403729 ) ) ;
#98941=EDGE_LOOP ( 'NONE', ( #98873, #46366, #45750, #110698 ) ) ;
#98943=CARTESIAN_POINT ( 'NONE',  ( -1.201851678989727383E-14, 2.962500000000025224, 1.732050807568877637 ) ) ;
#98944=CARTESIAN_POINT ( 'NONE',  ( 6.775324078527185989, 8.927630729746953264, -1.599625672291262513 ) ) ;
#98947=CARTESIAN_POINT ( 'NONE',  ( 7.131225611108079399, 11.26358761302737754, 0.7216878364870438212 ) ) ;
#98949=CARTESIAN_POINT ( 'NONE',  ( -10.58855478214856660, 11.45566145536924552, -0.7216878364870217277 ) ) ;
#98953=CARTESIAN_POINT ( 'NONE',  ( 9.378489572351044856, 11.96465713920816043, -1.599625672291262513 ) ) ;
#98955=CARTESIAN_POINT ( 'NONE',  ( -3.066115294984855133, 6.728884944124295053, 0.7998128361456341429 ) ) ;
#98956=CARTESIAN_POINT ( 'NONE',  ( -0.7499999999999972244, 5.389583334016151639, -1.299038105676652899 ) ) ;
#98957=CARTESIAN_POINT ( 'NONE',  ( 0.6823417656249864960, -0.8239583329919114574, -1.181850606188749264 ) ) ;
#98961=CARTESIAN_POINT ( 'NONE',  ( 5.508690485854129903, 5.321227076451600091, 1.040834085586084257E-14 ) ) ;
#98963=CARTESIAN_POINT ( 'NONE',  ( 1.364683531249986981, -1.115624999658580752, 0.000000000000000000 ) ) ;
#98971=CARTESIAN_POINT ( 'NONE',  ( -7.576308911938196999, 7.733448573549685179, 0.7998128361456462443 ) ) ;
#98973=CARTESIAN_POINT ( 'NONE',  ( 6.166260936116925606, 6.088392601758203071, 0.7998128361456341429 ) ) ;
#98976=CARTESIAN_POINT ( 'NONE',  ( 0.6823417656249882723, -0.07395833299191079124, -1.181850606188749264 ) ) ;
#98980=CARTESIAN_POINT ( 'NONE',  ( 7.913155211870404493, 12.38376484715752213, 0.7998128361456462443 ) ) ;
#98983=CARTESIAN_POINT ( 'NONE',  ( -5.259673527097670664, 8.223703984000886535, -1.199719254218446718 ) ) ;
#98987=CARTESIAN_POINT ( 'NONE',  ( 8.269583629331492602, 11.73526576994040482, 1.199719254218450271 ) ) ;
#98989=CARTESIAN_POINT ( 'NONE',  ( 7.242026607993941489, 11.60078147596829901, 0.7998128361456462443 ) ) ;
#98991=CARTESIAN_POINT ( 'NONE',  ( -2.415323921528888196, 5.969628341758991930, 0.7998128361456341429 ) ) ;
#98992=CARTESIAN_POINT ( 'NONE',  ( -7.705111371268023923, 7.883718109434487253, 1.040834085586084257E-14 ) ) ;
#98995=CARTESIAN_POINT ( 'NONE',  ( -5.066364649336571269, 6.741537443998309342, 1.444296757982476587 ) ) ;
#98996=CARTESIAN_POINT ( 'NONE',  ( 1.364683531249986537, 0.6135416670080880985, 0.7879004041258500513 ) ) ;
#99000=CARTESIAN_POINT ( 'NONE',  ( 7.049876689426101350, 9.247942109129029475, -1.443375672974057666 ) ) ;
#99003=CARTESIAN_POINT ( 'NONE',  ( 6.328958779480917229, 6.278206752349526631, 0.7998128361456341429 ) ) ;
#99021=CARTESIAN_POINT ( 'NONE',  ( 9.103410076571945453, 12.70806329172093818, 1.199719254218450271 ) ) ;
#99025=CARTESIAN_POINT ( 'NONE',  ( -4.466521540698216164, 7.298359999868178960, -1.199719254218452047 ) ) ;
#99026=CARTESIAN_POINT ( 'NONE',  ( -7.458957065812611198, 11.85386701009007204, 0.7998128361456481317 ) ) ;
#99028=ORIENTED_EDGE ( 'NONE', *, *, #92149, .F. ) ;
#99033=CARTESIAN_POINT ( 'NONE',  ( 1.499999999999989120, 2.556250000682817713, 1.214306433183764966E-14 ) ) ;
#99034=CARTESIAN_POINT ( 'NONE',  ( 8.269583629331492602, 11.73526576994040482, 1.199719254218450271 ) ) ;
#99037=CARTESIAN_POINT ( 'NONE',  ( -8.666686507633592385, 11.13422023037111330, 1.599625672291269396 ) ) ;
#99039=CARTESIAN_POINT ( 'NONE',  ( -1.364683531250012516, 3.488541667008085767, -0.7879004041258300672 ) ) ;
#99042=FACE_OUTER_BOUND ( 'NONE', #14316, .T. ) ;
#99046=CARTESIAN_POINT ( 'NONE',  ( -8.758204044748012507, 11.24099069033793974, 1.443375672974064550 ) ) ;
#99050=CARTESIAN_POINT ( 'NONE',  ( -0.6823417656250212460, 2.113541667008083991, 1.181850606188767472 ) ) ;
#99055=CARTESIAN_POINT ( 'NONE',  ( -1.201851678989727383E-14, 1.571875000341420581, 1.575800808251672791 ) ) ;
#99057=CARTESIAN_POINT ( 'NONE',  ( -5.250031796989778066, 7.148123067953287446, 1.599625672291267398 ) ) ;
#99058=CARTESIAN_POINT ( 'NONE',  ( 6.775324078527185989, 8.927630729746953264, -1.599625672291262513 ) ) ;
#99059=CARTESIAN_POINT ( 'NONE',  ( -1.150222622689996532, 2.858395032273045810, 0.7749999999993751887 ) ) ;
#99061=CARTESIAN_POINT ( 'NONE',  ( 1.499999999999989120, 5.045833333333354709, -0.8660254037844323793 ) ) ;
#99063=CARTESIAN_POINT ( 'NONE',  ( -0.6823417656250212460, 2.613541667008084879, 1.181850606188767472 ) ) ;
#99066=EDGE_CURVE ( 'NONE', #124240, #138555, #74815, .T. ) ;
#99068=CARTESIAN_POINT ( 'NONE',  ( -5.341549334104202629, 7.254893527920112994, 1.443375672974064550 ) ) ;
#99069=ADVANCED_FACE ( 'NONE', ( #34623 ), #180879, .F. ) ;
#99072=CARTESIAN_POINT ( 'NONE',  ( 4.826339496784873617, 8.574553812983598533, -0.7216878364870257245 ) ) ;
#99075=CARTESIAN_POINT ( 'NONE',  ( -9.338868881714763148, 9.789768538289042255, -0.7998128361456291469 ) ) ;
#99076=CARTESIAN_POINT ( 'NONE',  ( -8.663296969452339624, 13.05100419776235299, 1.040834085586084257E-14 ) ) ;
#99079=CARTESIAN_POINT ( 'NONE',  ( -1.364683531249997417, 5.509375000341417916, 1.214306433183764966E-14 ) ) ;
#99084=CARTESIAN_POINT ( 'NONE',  ( -7.009202228140751778, 9.200488570962775725, -1.443375672974058777 ) ) ;
#99086=CARTESIAN_POINT ( 'NONE',  ( 0.6823417656249882723, -0.2614583329919109578, -1.181850606188749264 ) ) ;
#99089=CARTESIAN_POINT ( 'NONE',  ( 8.758204044748010730, 9.320252261735261001, 0.7216878364870438212 ) ) ;
#99097=CARTESIAN_POINT ( 'NONE',  ( 7.890482213029013536, 12.14938698193514277, 1.040834085586084257E-14 ) ) ;
#99105=CARTESIAN_POINT ( 'NONE',  ( 7.298366762858032430, 7.409182732956175244, 1.040834085586084257E-14 ) ) ;
#99106=CARTESIAN_POINT ( 'NONE',  ( -4.741601036477307574, 6.554953847355395880, 1.599625672291267398 ) ) ;
#99110=CARTESIAN_POINT ( 'NONE',  ( 6.304178240230120522, 6.457222156464352381, -0.7216878364870257245 ) ) ;
#99111=CARTESIAN_POINT ( 'NONE',  ( 1.364683531249986537, 0.4260416670080872659, 0.7879004041258500513 ) ) ;
#99113=CARTESIAN_POINT ( 'NONE',  ( -10.14557902172788495, 10.73093036830436553, 1.040834085586084257E-14 ) ) ;
#99132=CARTESIAN_POINT ( 'NONE',  ( 7.039708073993665494, 9.236078724457858158, 1.599625672291281386 ) ) ;
#99133=CARTESIAN_POINT ( 'NONE',  ( 7.820355676984174664, 8.018169799436671852, -0.7998128361456281477 ) ) ;
#99144=CARTESIAN_POINT ( 'NONE',  ( -4.401593425930945713, 8.286942763561420122, 1.040834085586084257E-14 ) ) ;
#99145=CARTESIAN_POINT ( 'NONE',  ( -4.613852347352193739, 4.277249248199312071, 1.214306433183764966E-14 ) ) ;
#99150=CARTESIAN_POINT ( 'NONE',  ( 0.7499999999999920064, 4.764583334016150751, 1.299038105676669330 ) ) ;
#99154=CARTESIAN_POINT ( 'NONE',  ( -9.991996023591624976, 10.75967623705280296, 1.040834085586084257E-14 ) ) ;
#99157=CARTESIAN_POINT ( 'NONE',  ( 5.774883364416965037, 8.824782127540085952, -1.199719254218440723 ) ) ;
#99163=CARTESIAN_POINT ( 'NONE',  ( 4.867013957181530515, 5.740899707208986236, -1.082531754730548412 ) ) ;
#99164=CARTESIAN_POINT ( 'NONE',  ( -7.542413527904030524, 7.693903958843159252, 1.040834085586084257E-14 ) ) ;
#99166=ORIENTED_EDGE ( 'NONE', *, *, #36958, .F. ) ;
#99169=CARTESIAN_POINT ( 'NONE',  ( -5.693534442735004752, 8.729875052244421951, 1.199719254218452047 ) ) ;
#99170=AXIS2_PLACEMENT_3D ( 'NONE', #210431, #96731, #27422 ) ;
#99171=CARTESIAN_POINT ( 'NONE',  ( -4.569261463005423352, 5.289558780716470565, -1.199719254218446718 ) ) ;
#99178=CARTESIAN_POINT ( 'NONE',  ( 5.880485940025228508, 7.883652901494672349, 1.599625672291267398 ) ) ;
#99187=CARTESIAN_POINT ( 'NONE',  ( 1.123270288254022198, 3.158552654332631882, -0.7749999999939810591 ) ) ;
#99193=CARTESIAN_POINT ( 'NONE',  ( -0.6823417656250003738, -0.4697916663252491021, -1.181850606188749264 ) ) ;
#99194=CARTESIAN_POINT ( 'NONE',  ( 2.984766373302843778, 6.633977868828633717, -0.7998128361456291469 ) ) ;
#99195=CARTESIAN_POINT ( 'NONE',  ( 3.655894977179307226, 7.416961240017848844, -0.7998128361456291469 ) ) ;
#99196=EDGE_CURVE ( 'NONE', #58494, #87474, #60570, .T. ) ;
#99198=CARTESIAN_POINT ( 'NONE',  ( -6.561783159334121152, 10.59923808595773664, -0.7216878364870278340 ) ) ;
#99201=CARTESIAN_POINT ( 'NONE',  ( 5.992340707560160240, 7.053780915984068756, 1.082531754730558626 ) ) ;
#99202=CARTESIAN_POINT ( 'NONE',  ( -8.012505595552038784, 8.450270737673262644, 0.7216878364870578100 ) ) ;
#99207=CARTESIAN_POINT ( 'NONE',  ( 5.438792177376376991, 9.497007973581119700, 1.040834085586084257E-14 ) ) ;
#99212=CARTESIAN_POINT ( 'NONE',  ( -1.001543065824772872E-14, 4.321875000341417916, 1.575800808251672791 ) ) ;
#99217=CARTESIAN_POINT ( 'NONE',  ( 7.527801604085637699, 9.805521176231838609, 1.599625672291281386 ) ) ;
#99218=EDGE_CURVE ( 'NONE', #161364, #187417, #158655, .T. ) ;
#99221=CARTESIAN_POINT ( 'NONE',  ( -7.316596452869116973, 11.68777962832266049, 0.7998128361456481317 ) ) ;
#99227=CARTESIAN_POINT ( 'NONE',  ( 8.218213668177886788, 12.73966637951625813, 0.7998128361456462443 ) ) ;
#99228=DIRECTION ( 'NONE',  ( 5.578564026256490882E-16, 1.000000000000000000, 9.066213480720158442E-32 ) ) ;
#99230=CARTESIAN_POINT ( 'NONE',  ( -6.665805079413154921, 10.92852302595736447, 0.7998128361456481317 ) ) ;
#99234=CARTESIAN_POINT ( 'NONE',  ( 5.016205007133085481, 6.569753085731051989, -1.234251006731339917 ) ) ;
#99235=CARTESIAN_POINT ( 'NONE',  ( -10.49364770729726359, 11.34493653470939023, 0.7216878364870438212 ) ) ;
#99240=CARTESIAN_POINT ( 'NONE',  ( 6.745345117998789775, 7.828323044875442172, 1.199719254218462483 ) ) ;
#99242=CARTESIAN_POINT ( 'NONE',  ( 5.636439174979242850, 7.598931675607687453, -1.599625672291262513 ) ) ;
#99243=CARTESIAN_POINT ( 'NONE',  ( -4.026828402897194792, 7.608452879803509816, -0.2354461595876176927 ) ) ;
#99244=CARTESIAN_POINT ( 'NONE',  ( 3.497113557321089861, 6.167384019261527683, -1.199719254218446718 ) ) ;
#99246=CARTESIAN_POINT ( 'NONE',  ( -6.887178846062105286, 10.97886638714038554, -0.7216878364870267237 ) ) ;
#99253=CARTESIAN_POINT ( 'NONE',  ( -4.088362842241233253, 7.522098425605555860, -0.5455919966513862462 ) ) ;
#99254=CARTESIAN_POINT ( 'NONE',  ( 3.497640442201256139, 7.024404915969360452, 1.040834085586084257E-14 ) ) ;
#99257=CARTESIAN_POINT ( 'NONE',  ( 5.043269954603547767, 4.986162489899998995, -0.7216878364870197293 ) ) ;
#99262=CARTESIAN_POINT ( 'NONE',  ( -7.497295758232712437, 11.69066945133944380, -0.7216878364870267237 ) ) ;
#99268=CARTESIAN_POINT ( 'NONE',  ( -10.60211293576223213, 11.47147930125185589, 1.040834085586084257E-14 ) ) ;
#99275=CARTESIAN_POINT ( 'NONE',  ( -8.622622508166983835, 13.00355065959610279, 1.040834085586084257E-14 ) ) ;
#99280=ORIENTED_EDGE ( 'NONE', *, *, #192402, .T. ) ;
#99282=CARTESIAN_POINT ( 'NONE',  ( -0.7500000000000006661, 3.139583334016149418, -1.299038105676652011 ) ) ;
#99284=CARTESIAN_POINT ( 'NONE',  ( -6.254388934605767503, 6.191208599995166040, 0.7998128361456341429 ) ) ;
#99287=CARTESIAN_POINT ( 'NONE',  ( -9.104463846776669200, 10.58062822844965645, -1.199719254218441611 ) ) ;
#99291=CARTESIAN_POINT ( 'NONE',  ( 5.931855901178834323, 6.879252291918818152, 1.199719254218462483 ) ) ;
#99293=CARTESIAN_POINT ( 'NONE',  ( 2.482948226198858688, 5.072301959192136778, -2.419999999999995044 ) ) ;
#99296=CARTESIAN_POINT ( 'NONE',  ( 7.527801604085637699, 9.805521176231838609, 1.599625672291281386 ) ) ;
#99297=DIRECTION ( 'NONE',  ( 1.000000000000000000, 0.000000000000000000, 0.000000000000000000 ) ) ;
#99300=EDGE_LOOP ( 'NONE', ( #153577, #64138, #143327, #150158, #24812 ) ) ;
#99303=CARTESIAN_POINT ( 'NONE',  ( -6.155038550924159857, 8.203964280876741455, 1.443375672974078761 ) ) ;
#99306=CARTESIAN_POINT ( 'NONE',  ( 0.6823417656249899377, 5.238541667008086655, -1.181850606188754593 ) ) ;
#99309=CARTESIAN_POINT ( 'NONE',  ( -1.364683531250010295, 5.238541667008086655, -0.7879004041258300672 ) ) ;
#99312=CARTESIAN_POINT ( 'NONE',  ( -3.809477975315625375, 4.507107728365378208, 1.082531754730558626 ) ) ;
#99314=CARTESIAN_POINT ( 'NONE',  ( 10.07100917685271035, 10.64393221595000938, 0.7998128361456462443 ) ) ;
#99316=CARTESIAN_POINT ( 'NONE',  ( 7.034482758620714371, 5.227586206896606136, 1.214306433183764966E-14 ) ) ;
#99319=CARTESIAN_POINT ( 'NONE',  ( -1.364683531250012516, 2.780208333674754506, 0.7879004041258379498 ) ) ;
#99320=CARTESIAN_POINT ( 'NONE',  ( 4.039439701867726384, 6.800097854565950506, 1.199719254218462483 ) ) ;
#99326=CARTESIAN_POINT ( 'NONE',  ( 8.392133896734652154, 12.73464727959172293, 0.7216878364870438212 ) ) ;
#99328=CARTESIAN_POINT ( 'NONE',  ( -8.527715433315703919, 9.051348881730875817, 1.040834085586084257E-14 ) ) ;
#99332=CARTESIAN_POINT ( 'NONE',  ( 0.006913841192815062958, 8.234242197375175820, 1.999988128101762408 ) ) ;
#99334=CARTESIAN_POINT ( 'NONE',  ( -7.157815033010924921, 10.43820240756634199, 1.199719254218453823 ) ) ;
#99335=CARTESIAN_POINT ( 'NONE',  ( -4.026408433134269771, 6.680931691089825541, 1.082531754730560403 ) ) ;
#99336=CARTESIAN_POINT ( 'NONE',  ( -1.364683531250012516, 2.801041667008090652, -0.7879004041258289570 ) ) ;
#99356=CARTESIAN_POINT ( 'NONE',  ( -1.201851678989727383E-14, 4.134375000341417028, 1.575800808251672791 ) ) ;
#99360=DIRECTION ( 'NONE',  ( 0.7592566023653005702, 0.6507913734559639396, 0.000000000000000000 ) ) ;
#99363=CARTESIAN_POINT ( 'NONE',  ( 8.992082194361556091, 11.51384853155376220, 1.599625672291279388 ) ) ;
#99365=CARTESIAN_POINT ( 'NONE',  ( 1.364683531249988535, 2.613541667008089764, 0.7879004041258500513 ) ) ;
#99367=CARTESIAN_POINT ( 'NONE',  ( -7.388830529767770550, 7.722649827591604677, 1.040834085586084257E-14 ) ) ;
#99373=CARTESIAN_POINT ( 'NONE',  ( 5.040934186182656873, 4.775511393501539636, 1.040834085586084257E-14 ) ) ;
#99376=CARTESIAN_POINT ( 'NONE',  ( 9.565441069641300587, 11.11843498845840905, -1.199719254218440723 ) ) ;
#99384=CARTESIAN_POINT ( 'NONE',  ( -8.611400122974211868, 13.19838391011195888, 1.040834085586084257E-14 ) ) ;
#99385=CARTESIAN_POINT ( 'NONE',  ( 8.308449207076147758, 8.587612251210650527, -0.7998128361456281477 ) ) ;
#99387=CARTESIAN_POINT ( 'NONE',  ( 3.660338285565247762, 7.214219066560688454, 1.040834085586084257E-14 ) ) ;
#99395=CARTESIAN_POINT ( 'NONE',  ( -1.445103857048104512, 8.688264192037884470, -2.625611233228243524 ) ) ;
#99396=CARTESIAN_POINT ( 'NONE',  ( -6.887178846062116833, 9.058127958537705027, -1.443375672974059665 ) ) ;
#99397=CARTESIAN_POINT ( 'NONE',  ( 3.876741858503734761, 6.610283703974623393, 1.199719254218462483 ) ) ;
#99400=CARTESIAN_POINT ( 'NONE',  ( -8.843996274815957293, 9.212417163573759282, 1.040834085586084257E-14 ) ) ;
#99402=DIRECTION ( 'NONE',  ( 0.000000000000000000, 0.7999999999999973799, -0.6000000000000034195 ) ) ;
#99405=CARTESIAN_POINT ( 'NONE',  ( -4.783329267523015460, 4.474972321731942593, -0.7998128361456221525 ) ) ;
#99409=CARTESIAN_POINT ( 'NONE',  ( 7.587759525142423911, 12.00413654597487501, 0.7998128361456462443 ) ) ;
#99410=CARTESIAN_POINT ( 'NONE',  ( -1.608462485350604432, 8.735270501766748907, -2.463594439587635687 ) ) ;
#99416=CARTESIAN_POINT ( 'NONE',  ( 4.067082894419602468, 3.847277586352047862, -0.7216878364870188411 ) ) ;
#99419=CARTESIAN_POINT ( 'NONE',  ( -4.386226389220933441, 5.076017861301227008, -1.199719254218446718 ) ) ;
#99422=CARTESIAN_POINT ( 'NONE',  ( -7.483210719738908168, 10.81783070874899799, 1.199719254218453823 ) ) ;
#99426=CARTESIAN_POINT ( 'NONE',  ( 8.446366511633696561, 8.956441806435218922, 1.040834085586084257E-14 ) ) ;
#99427=CARTESIAN_POINT ( 'NONE',  ( -1.364683531250010740, 5.801041667008088432, -0.7879004041258300672 ) ) ;
#99429=CARTESIAN_POINT ( 'NONE',  ( 3.277320446201373638, 4.846626492033466072, 1.599625672291267398 ) ) ;
#99431=CARTESIAN_POINT ( 'NONE',  ( 4.005544317833563461, 6.760553239859419250, -1.199719254218452047 ) ) ;
#99433=CARTESIAN_POINT ( 'NONE',  ( -7.549192604710863286, 7.701812881784464437, -0.7998128361456291469 ) ) ;
#99443=CARTESIAN_POINT ( 'NONE',  ( -1.201851678989727383E-14, 4.009375000341416140, -1.575800808251660134 ) ) ;
#99444=CARTESIAN_POINT ( 'NONE',  ( 9.915090410295563927, 10.46202698829998567, -0.7998128361456281477 ) ) ;
#99447=CARTESIAN_POINT ( 'NONE',  ( -4.772106882330227506, 7.550913215151819458, -1.082531754730549967 ) ) ;
#99448=CARTESIAN_POINT ( 'NONE',  ( -4.812781342726871969, 6.637997537979888563, 1.443375672974064550 ) ) ;
#99455=CARTESIAN_POINT ( 'NONE',  ( 4.497554271431305040, 6.270232621468402989, -1.599625672291256295 ) ) ;
#99464=CARTESIAN_POINT ( 'NONE',  ( 5.626797444871351139, 6.523350759560078593, 1.199719254218462483 ) ) ;
#99468=CARTESIAN_POINT ( 'NONE',  ( 1.364683531249988535, 4.426041667008082214, 0.7879004041258500513 ) ) ;
#99473=CARTESIAN_POINT ( 'NONE',  ( 5.126954644262057492, 9.133197518281081173, 0.7998128361456462443 ) ) ;
#99476=CARTESIAN_POINT ( 'NONE',  ( -6.410307701162927252, 6.373113827645189744, -0.7998128361456291469 ) ) ;
#99478=CARTESIAN_POINT ( 'NONE',  ( -0.7500000000000215383, 2.441666666666689078, 1.299038105676671107 ) ) ;
#99479=CARTESIAN_POINT ( 'NONE',  ( -4.569261463005423352, 5.289558780716470565, -1.199719254218446718 ) ) ;
#99482=CARTESIAN_POINT ( 'NONE',  ( -5.382750679825375251, 6.238629533673094585, -1.199719254218446718 ) ) ;
#99485=CARTESIAN_POINT ( 'NONE',  ( 1.364683531249990311, 3.884375000341417028, 1.214306433183764966E-14 ) ) ;
#99487=CARTESIAN_POINT ( 'NONE',  ( -3.633221978782283923, 7.182583375313884133, -0.7216878364870267237 ) ) ;
#99491=VERTEX_POINT ( 'NONE', #206718 ) ;
#99494=CARTESIAN_POINT ( 'NONE',  ( 5.681030059326015014, 6.586622143090519188, -1.199719254218445830 ) ) ;
#99497=CARTESIAN_POINT ( 'NONE',  ( 1.364683531249990311, 2.946875000341416140, 1.214306433183764966E-14 ) ) ;
#99499=CARTESIAN_POINT ( 'NONE',  ( 4.220665892555866883, 3.818531717603609987, -0.7998128361456211532 ) ) ;
#99501=CARTESIAN_POINT ( 'NONE',  ( -0.6823417656250246877, -0.6364583329919113464, 1.181850606188755259 ) ) ;
#99502=CARTESIAN_POINT ( 'NONE',  ( -4.229020061460118107, 7.343517960532633282, -0.8650006913940473385 ) ) ;
#99504=CARTESIAN_POINT ( 'NONE',  ( -3.379006598303881059, 4.965260336153046516, -1.599625672291256295 ) ) ;
#99505=CARTESIAN_POINT ( 'NONE',  ( -5.531363484251157203, 9.397081798360927607, 0.000000000000000000 ) ) ;
#99509=CARTESIAN_POINT ( 'NONE',  ( -1.364683531249997417, 2.759375000341422801, 1.214306433183764966E-14 ) ) ;
#99517=CARTESIAN_POINT ( 'NONE',  ( -7.687109908824056426, 8.070642436490613747, 0.7216878364870438212 ) ) ;
#99522=CARTESIAN_POINT ( 'NONE',  ( -7.849807752188049825, 8.260456587081938196, 0.7216878364870578100 ) ) ;
#99525=CARTESIAN_POINT ( 'NONE',  ( -1.123270288250318494, 3.235197346350006331, -0.7749999999993560929 ) ) ;
#99530=CARTESIAN_POINT ( 'NONE',  ( 0.09201470549763642037, 7.049384003815710287, 3.948455284462528248 ) ) ;
#99534=CARTESIAN_POINT ( 'NONE',  ( -5.205440912643032547, 8.160432600470439723, 1.199719254218452047 ) ) ;
#99536=CARTESIAN_POINT ( 'NONE',  ( 1.499999999999987566, -0.9749999999999827693, 0.000000000000000000 ) ) ;
#99537=CARTESIAN_POINT ( 'NONE',  ( 8.405692050792682224, 12.75046512599275772, -0.7216878364870328300 ) ) ;
#99539=CARTESIAN_POINT ( 'NONE',  ( 5.412729640353754590, 7.337937218544611895, 1.599625672291267398 ) ) ;
#99546=CARTESIAN_POINT ( 'NONE',  ( -3.307826292054310890, 5.842585859829892314, -1.082531754730549967 ) ) ;
#99554=CARTESIAN_POINT ( 'NONE',  ( -1.402160292154681736E-14, 2.196875000341423689, -1.575800808251660134 ) ) ;
#99555=CARTESIAN_POINT ( 'NONE',  ( 8.229436053370658755, 12.54483312900040026, 0.7216878364870438212 ) ) ;
#99556=CARTESIAN_POINT ( 'NONE',  ( -8.376239975144482486, 8.666701480623698828, 1.040834085586084257E-14 ) ) ;
#99559=CARTESIAN_POINT ( 'NONE',  ( 6.928380191783277908, 8.041863964290678624, 1.199719254218462483 ) ) ;
#99560=CARTESIAN_POINT ( 'NONE',  ( -6.521635583373313061, 7.567328587812373719, -1.199719254218446718 ) ) ;
#99564=CARTESIAN_POINT ( 'NONE',  ( -1.500000000000015099, -1.047916665983845919, 0.8660254037844403729 ) ) ;
#99567=CARTESIAN_POINT ( 'NONE',  ( 8.270110514656026979, 10.67154823856396817, 1.443375672974076540 ) ) ;
#99570=CARTESIAN_POINT ( 'NONE',  ( -0.6823417656250212460, 1.363541667008083547, 1.181850606188755259 ) ) ;
#99572=CARTESIAN_POINT ( 'NONE',  ( 6.385527161912102123, 9.433236874664039817, -1.082531754730537976 ) ) ;
#99575=CARTESIAN_POINT ( 'NONE',  ( -4.202664430556263930, 5.926194473780837413, 1.443375672974064550 ) ) ;
#99577=EDGE_CURVE ( 'NONE', #97860, #84679, #16275, .T. ) ;
#99578=CARTESIAN_POINT ( 'NONE',  ( 1.364683531249988535, 4.363541667008090208, 0.7879004041258500513 ) ) ;
#99582=CARTESIAN_POINT ( 'NONE',  ( -4.798872725802947770, 6.964071866812478362, -1.434128239971976138 ) ) ;
#99588=CARTESIAN_POINT ( 'NONE',  ( 7.365103760721646076, 9.615707025640515937, 1.599625672291281386 ) ) ;
#99591=CARTESIAN_POINT ( 'NONE',  ( 2.659370686574860976, 6.254349567645977714, -0.7998128361456291469 ) ) ;
#99597=CARTESIAN_POINT ( 'NONE',  ( 4.500943810056890371, 8.194925511800951412, -0.7216878364870207285 ) ) ;
#99598=CARTESIAN_POINT ( 'NONE',  ( -1.402160292154681736E-14, 1.259375000341419248, -1.575800808251659024 ) ) ;
#99605=CARTESIAN_POINT ( 'NONE',  ( 1.499999999999987121, 0.2541666666666844154, 0.8660254037844524744 ) ) ;
#99606=CARTESIAN_POINT ( 'NONE',  ( 6.368579470117202490, 8.453095353268645695, 1.599625672291281386 ) ) ;
#99607=CARTESIAN_POINT ( 'NONE',  ( -8.202846631467911820, 9.528741477256060577, 1.199719254218462483 ) ) ;
#99611=CARTESIAN_POINT ( 'NONE',  ( -1.364683531250014514, 0.9885416670080898749, -0.7879004041258289570 ) ) ;
#99613=CARTESIAN_POINT ( 'NONE',  ( -1.499999999999997780, 3.150000000000020783, 1.214306433183764966E-14 ) ) ;
#99615=CARTESIAN_POINT ( 'NONE',  ( 2.822068529938852155, 6.444163718237301275, -0.7998128361456291469 ) ) ;
#99622=CARTESIAN_POINT ( 'NONE',  ( -1.500000000000015099, -0.08958333265051321437, -0.8660254037844383745 ) ) ;
#99623=CARTESIAN_POINT ( 'NONE',  ( -7.640183256500752584, 8.872300873127729304, -1.199719254218446718 ) ) ;
#99624=CARTESIAN_POINT ( 'NONE',  ( -3.633221978782283923, 7.182583375313884133, -0.7216878364870267237 ) ) ;
#99631=EDGE_LOOP ( 'NONE', ( #129070, #99166, #201768, #160564, #152406, #131296, #127039 ) ) ;
#99632=CARTESIAN_POINT ( 'NONE',  ( 7.396136491454752715, 8.587579647240744407, 1.199719254218462483 ) ) ;
#99635=CARTESIAN_POINT ( 'NONE',  ( 7.415946836550727284, 7.754285518838408109, 0.7216878364870317197 ) ) ;
#99639=CARTESIAN_POINT ( 'NONE',  ( -7.542413527904030524, 7.693903958843159252, 1.040834085586084257E-14 ) ) ;
#99640=CIRCLE ( 'NONE', #103049, 0.8299999999999999600 ) ;
#99641=CARTESIAN_POINT ( 'NONE',  ( 3.357615597678655917, 7.068968630600412695, 0.7998128361456321445 ) ) ;
#99646=CARTESIAN_POINT ( 'NONE',  ( 4.019038269249470829, 7.568960612331900428, -0.3200009682147019752 ) ) ;
#99647=CARTESIAN_POINT ( 'NONE',  ( 7.768458830950378591, 12.00702636951006497, 1.040834085586084257E-14 ) ) ;
#99648=ORIENTED_EDGE ( 'NONE', *, *, #100082, .F. ) ;
#99654=CARTESIAN_POINT ( 'NONE',  ( -1.528885273045263116, 8.694317336386671258, -2.518424357262861069 ) ) ;
#99655=CARTESIAN_POINT ( 'NONE',  ( -4.948362879307902418, 4.875437568721725512, 1.214306433183764966E-14 ) ) ;
#99656=CARTESIAN_POINT ( 'NONE',  ( 7.293923454472069245, 11.45340176361870199, 0.7216878364870438212 ) ) ;
#99659=CARTESIAN_POINT ( 'NONE',  ( -6.715366157470410435, 6.729015360003925750, -0.7998128361456291469 ) ) ;
#99660=DIRECTION ( 'NONE',  ( 0.000000000000000000, 1.000000000000000000, -8.546850786086437571E-32 ) ) ;
#99665=CARTESIAN_POINT ( 'NONE',  ( -5.533699252672048985, 9.607732894759390518, -0.7998128361456231517 ) ) ;
#99668=CARTESIAN_POINT ( 'NONE',  ( -0.3171178118501576382, 7.220087385434831972, 2.081545611384598704 ) ) ;
#99680=CARTESIAN_POINT ( 'NONE',  ( -6.579784621333750749, 6.570836901177822931, 0.7998128361456341429 ) ) ;
#99684=CARTESIAN_POINT ( 'NONE',  ( 5.504247177468190699, 5.523969249908757817, 0.7216878364870317197 ) ) ;
#99688=CARTESIAN_POINT ( 'NONE',  ( -3.411848212133334446, 7.132240014130862171, 0.7998128361456341429 ) ) ;
#99697=CARTESIAN_POINT ( 'NONE',  ( -9.338868881714763148, 9.789768538289042255, -0.7998128361456291469 ) ) ;
#99698=CARTESIAN_POINT ( 'NONE',  ( 7.135668919494039031, 7.219368582364847242, 1.040834085586084257E-14 ) ) ;
#99701=CARTESIAN_POINT ( 'NONE',  ( -7.323375529675950624, 11.69568855126397011, -0.7998128361456291469 ) ) ;
#99702=CARTESIAN_POINT ( 'NONE',  ( 5.657830175604453338, 5.495223381160312393, 0.7998128361456341429 ) ) ;
#99704=CARTESIAN_POINT ( 'NONE',  ( 0.6823417656249882723, 0.1552083336747514530, 1.181850606188755259 ) ) ;
#99707=CARTESIAN_POINT ( 'NONE',  ( 8.975134502566660899, 10.53370701015836275, -1.082531754730543083 ) ) ;
#99712=CARTESIAN_POINT ( 'NONE',  ( -5.607868592924734941, 6.187540734389447294, -0.8708238738269019619 ) ) ;
#99726=CARTESIAN_POINT ( 'NONE',  ( -3.810004860640155311, 4.403759411290286252, 1.199719254218462483 ) ) ;
#99727=DIRECTION ( 'NONE',  ( 1.000000000000000000, 0.000000000000000000, 0.000000000000000000 ) ) ;
#99733=CARTESIAN_POINT ( 'NONE',  ( -0.7500000000000249800, -0.02708333265051543481, 1.299038105676659116 ) ) ;
#99740=CARTESIAN_POINT ( 'NONE',  ( 7.703003830858588863, 12.13858823597705872, -0.7998128361456291469 ) ) ;
#99747=CARTESIAN_POINT ( 'NONE',  ( 3.174580523894166006, 6.855427711185178019, 0.7998128361456341429 ) ) ;
#99748=CARTESIAN_POINT ( 'NONE',  ( -6.507550544879489252, 9.575597488125954015, 1.082531754730548412 ) ) ;
#99749=CARTESIAN_POINT ( 'NONE',  ( -5.812277037385564782, 6.060071624232533871, -0.5253754717876522040 ) ) ;
#99752=CARTESIAN_POINT ( 'NONE',  ( -8.206763054973658100, 8.468978407091068306, 0.7998128361456602331 ) ) ;
#99754=CARTESIAN_POINT ( 'NONE',  ( -2.914639836813632812, 6.344237543017112735, 0.7216878364870317197 ) ) ;
#99757=CARTESIAN_POINT ( 'NONE',  ( 1.499999999999985123, -0.4229166659838508036, -0.8660254037844323793 ) ) ;
#99758=EDGE_CURVE ( 'NONE', #100909, #18401, #46900, .T. ) ;
#99766=CARTESIAN_POINT ( 'NONE',  ( -5.111060722227552588, 6.025620933095978238, 1.082531754730546636 ) ) ;
#99767=ADVANCED_FACE ( 'NONE', ( #160108 ), #156123, .T. ) ;
#99775=CARTESIAN_POINT ( 'NONE',  ( -4.731432421044888592, 4.622352034081546712, -0.7216878364870207285 ) ) ;
#99776=CARTESIAN_POINT ( 'NONE',  ( 7.587759525142423911, 12.00413654597487501, 0.7998128361456462443 ) ) ;
#99780=DIRECTION ( 'NONE',  ( 1.000000000000000000, 0.000000000000000000, 0.000000000000000000 ) ) ;
#99785=CARTESIAN_POINT ( 'NONE',  ( -8.995998617867369873, 10.45408546138876993, 1.199719254218462483 ) ) ;
#99790=CARTESIAN_POINT ( 'NONE',  ( 3.981290663907289140, 7.796589541200495965, -0.7998128361456221525 ) ) ;
#99794=ORIENTED_EDGE ( 'NONE', *, *, #185760, .F. ) ;
#99808=CARTESIAN_POINT ( 'NONE',  ( 6.795661308947685164, 8.951357498570873261, -1.599625672291262513 ) ) ;
#99810=CARTESIAN_POINT ( 'NONE',  ( -4.946027110887008860, 4.664786472323266153, -0.7998128361456221525 ) ) ;
#99817=CARTESIAN_POINT ( 'NONE',  ( 1.499999999999985123, -0.4229166659838508036, -0.8660254037844323793 ) ) ;
#99821=CARTESIAN_POINT ( 'NONE',  ( 4.867540842506059562, 5.637551390133895168, -1.199719254218452047 ) ) ;
#99823=CARTESIAN_POINT ( 'NONE',  ( -4.135400547368138113, 4.783387712472935149, 1.199719254218462483 ) ) ;
#99829=CARTESIAN_POINT ( 'NONE',  ( 4.690757960648221037, 7.456006139856155457, 1.082531754730558626 ) ) ;
#99831=EDGE_LOOP ( 'NONE', ( #167995, #188302, #211140, #167867 ) ) ;
#99832=CARTESIAN_POINT ( 'NONE',  ( 6.439759776366758892, 10.45687747249582955, 0.7216878364870438212 ) ) ;
#99833=CARTESIAN_POINT ( 'NONE',  ( -1.364683531250010295, 4.592708333674755394, 0.7879004041258379498 ) ) ;
#99835=CARTESIAN_POINT ( 'NONE',  ( 2.833290915131624566, 6.249330467721451399, -0.7216878364870267237 ) ) ;
#99844=CARTESIAN_POINT ( 'NONE',  ( -5.780146447551155475, 6.079674369897793085, -0.5991446231495625163 ) ) ;
#99847=CARTESIAN_POINT ( 'NONE',  ( 1.364683531249988535, 5.717708333674752730, -0.7879004041258300672 ) ) ;
#99860=ORIENTED_EDGE ( 'NONE', *, *, #207810, .F. ) ;
#99863=CARTESIAN_POINT ( 'NONE',  ( -1.364683531249997417, 4.321875000341417028, 1.214306433183764966E-14 ) ) ;
#99865=CARTESIAN_POINT ( 'NONE',  ( 6.043183783389218355, 8.073467052085995022, 1.599625672291267398 ) ) ;
#99866=CARTESIAN_POINT ( 'NONE',  ( -9.016335848287868160, 10.47781223021269170, 1.199719254218462483 ) ) ;
#99872=CARTESIAN_POINT ( 'NONE',  ( -1.402160292154681736E-14, -0.6156249996585817508, 1.575800808251672791 ) ) ;
#99876=FACE_OUTER_BOUND ( 'NONE', #6629, .T. ) ;
#99880=CARTESIAN_POINT ( 'NONE',  ( 8.771762198361678031, 9.336070107617867819, 1.040834085586084257E-14 ) ) ;
#99885=CARTESIAN_POINT ( 'NONE',  ( -0.7500000000000215383, 3.722916667349487785, 1.299038105676671107 ) ) ;
#99887=CARTESIAN_POINT ( 'NONE',  ( -6.254388934605767503, 6.191208599995166040, 0.7998128361456341429 ) ) ;
#99888=CARTESIAN_POINT ( 'NONE',  ( 4.161989969270902812, 4.918371721313249623, 1.082531754730560403 ) ) ;
#99889=CARTESIAN_POINT ( 'NONE',  ( -9.124274191872631334, 12.62844174295135069, -1.082531754730543083 ) ) ;
#99897=CARTESIAN_POINT ( 'NONE',  ( 4.142179624174931796, 4.791296635414242111, 1.199719254218464037 ) ) ;
#99901=CARTESIAN_POINT ( 'NONE',  ( 4.330940004561544043, 7.140181541042074365, -1.199719254218452047 ) ) ;
#99913=CARTESIAN_POINT ( 'NONE',  ( 5.622931663646434153, 6.144404617744410046, -0.8283694935172694063 ) ) ;
#99914=EDGE_CURVE ( 'NONE', #160319, #170502, #57649, .T. ) ;
#99920=CARTESIAN_POINT ( 'NONE',  ( -1.364683531250014514, -0.9697916663252473812, 0.7879004041258379498 ) ) ;
#99921=CARTESIAN_POINT ( 'NONE',  ( 7.158341918335438869, 7.453746447587225710, -0.7216878364870257245 ) ) ;
#99922=CARTESIAN_POINT ( 'NONE',  ( -3.195971524519394702, 4.751719416737803847, -1.599625672291262513 ) ) ;
#99928=CARTESIAN_POINT ( 'NONE',  ( -3.255929445576174697, 6.950334786480840243, -0.7998128361456281477 ) ) ;
#99932=ORIENTED_EDGE ( 'NONE', *, *, #45961, .T. ) ;
#99939=CARTESIAN_POINT ( 'NONE',  ( 6.050032868414796816, 6.056328681155354055, -0.4621489055621590403 ) ) ;
#99946=CARTESIAN_POINT ( 'NONE',  ( -8.758204044748012507, 11.24099069033793974, 1.443375672974064550 ) ) ;
#99951=CARTESIAN_POINT ( 'NONE',  ( 7.239163954692881653, 10.53310948286200599, -1.199719254218441611 ) ) ;
#99952=CARTESIAN_POINT ( 'NONE',  ( -5.434120640978981065, 5.234228924097237723, -0.7998128361456221525 ) ) ;
#99953=EDGE_CURVE ( 'NONE', #159976, #148658, #149139, .T. ) ;
#99955=CARTESIAN_POINT ( 'NONE',  ( -6.437424008390261854, 6.404749519410410485, 0.7998128361456341429 ) ) ;
#99956=CARTESIAN_POINT ( 'NONE',  ( 2.184835310096557404, 5.700724961754617404, 1.040834085586084257E-14 ) ) ;
#99958=CARTESIAN_POINT ( 'NONE',  ( -6.403528624356093601, 6.365204904703887223, 1.040834085586084257E-14 ) ) ;
#99962=CARTESIAN_POINT ( 'NONE',  ( 9.240045382913317340, 10.73880668727576015, -1.199719254218446718 ) ) ;
#99963=CARTESIAN_POINT ( 'NONE',  ( -1.201851678989727383E-14, 3.587500000000020339, -1.732050807568863648 ) ) ;
#99965=CARTESIAN_POINT ( 'NONE',  ( 4.046752668985390322, 7.764364035880440440, -0.4786816536347000550 ) ) ;
#99966=CARTESIAN_POINT ( 'NONE',  ( 4.853455804012203778, 8.606189504748821051, 0.7216878364870438212 ) ) ;
#99974=CARTESIAN_POINT ( 'NONE',  ( 6.927853306458743532, 9.105581495667113501, 1.443375672974076540 ) ) ;
#99978=CARTESIAN_POINT ( 'NONE',  ( -9.541187415715041809, 12.15447128979948310, -1.599625672291263179 ) ) ;
#99979=CARTESIAN_POINT ( 'NONE',  ( -6.530223543276495235, 10.77034456713125188, -0.7998128361456291469 ) ) ;
#99982=CARTESIAN_POINT ( 'NONE',  ( 2.275435306267621804, 5.643409308550367598, 0.5316758947214432762 ) ) ;
#99985=CARTESIAN_POINT ( 'NONE',  ( 3.541704441667858472, 5.155074486744371853, -1.599625672291262513 ) ) ;
#99990=CARTESIAN_POINT ( 'NONE',  ( 3.822509244049070887, 6.547012320444182798, -1.199719254218452047 ) ) ;
#99993=CARTESIAN_POINT ( 'NONE',  ( 1.499999999999989120, 4.827083334016149863, -0.8660254037844323793 ) ) ;
#99999=CARTESIAN_POINT ( 'NONE',  ( -1.402160292154681736E-14, 2.087500000000021227, -1.732050807568863648 ) ) ;
#100000=CARTESIAN_POINT ( 'NONE',  ( 7.124973419181436007, 8.271222729588529887, -1.199719254218446718 ) ) ;
#100001=CARTESIAN_POINT ( 'NONE',  ( 4.731432421044862835, 6.543090462684225450, -1.443375672974051449 ) ) ;
#100005=CARTESIAN_POINT ( 'NONE',  ( 8.351459436338029008, 10.76645531385962862, -1.443375672974063439 ) ) ;
#100011=CARTESIAN_POINT ( 'NONE',  ( -6.078132937628113908, 5.985576603521232109, 1.040834085586084257E-14 ) ) ;
#100012=CARTESIAN_POINT ( 'NONE',  ( 0.7499999999999902300, 3.764583334016149863, 1.299038105676669330 ) ) ;
#100014=CARTESIAN_POINT ( 'NONE',  ( 0.6823417656249882723, 0.1760416670080894308, -1.181850606188749264 ) ) ;
#100018=CARTESIAN_POINT ( 'NONE',  ( 3.174580523894166006, 6.855427711185178019, 0.7998128361456341429 ) ) ;
#100020=CARTESIAN_POINT ( 'NONE',  ( -1.001543065824772872E-14, 5.384375000341415252, 1.575800808251672791 ) ) ;
#100028=CARTESIAN_POINT ( 'NONE',  ( -6.795661308947694934, 8.951357498570873261, -1.599625672291263179 ) ) ;
#100030=CARTESIAN_POINT ( 'NONE',  ( 3.818592820543298405, 7.606775390609172405, -0.7998128361456221525 ) ) ;
#100033=CARTESIAN_POINT ( 'NONE',  ( 1.364683531249986537, -0.3864583329919166199, 0.7879004041258500513 ) ) ;
#100040=CARTESIAN_POINT ( 'NONE',  ( -5.357443255694392725, 9.402100898285455699, 0.000000000000000000 ) ) ;
#100043=CARTESIAN_POINT ( 'NONE',  ( 9.134442807305049428, 11.67993591332117376, 1.599625672291281386 ) ) ;
#100045=CARTESIAN_POINT ( 'NONE',  ( 8.809047120577066181, 11.30030761213851953, 1.599625672291281386 ) ) ;
#100047=CARTESIAN_POINT ( 'NONE',  ( -3.952365473583647315, 4.569846793057691592, 1.199719254218462483 ) ) ;
#100048=CARTESIAN_POINT ( 'NONE',  ( -8.128276786592724790, 9.441743324901704426, -1.199719254218446718 ) ) ;
#100051=CARTESIAN_POINT ( 'NONE',  ( -4.119138978170663989, 7.660627806941648466, 0.7993094217999627826 ) ) ;
#100052=CARTESIAN_POINT ( 'NONE',  ( 0.6823417656249882723, 0.6760416670080898749, -1.181850606188749264 ) ) ;
#100056=CARTESIAN_POINT ( 'NONE',  ( 8.812436659202669276, 10.34389285956704363, -1.082531754730543083 ) ) ;
#100059=CARTESIAN_POINT ( 'NONE',  ( 6.179819089730593795, 6.104210447640811665, 1.040834085586084257E-14 ) ) ;
#100075=CARTESIAN_POINT ( 'NONE',  ( 8.401248741962376698, 12.95320729893149370, 0.7998128361456462443 ) ) ;
#100079=CARTESIAN_POINT ( 'NONE',  ( -4.761938266897808525, 6.578680616179308771, 1.599625672291267398 ) ) ;
#100080=CARTESIAN_POINT ( 'NONE',  ( -6.808165692356648258, 11.09461040772476714, 0.7998128361456481317 ) ) ;
#100082=EDGE_CURVE ( 'NONE', #123409, #197571, #82040, .T. ) ;
#100086=CARTESIAN_POINT ( 'NONE',  ( -1.500000000000011324, 3.452083334016151639, 0.8660254037844403729 ) ) ;
#100087=CARTESIAN_POINT ( 'NONE',  ( 10.70146331988817323, 11.37946204949139251, 0.7998128361456341429 ) ) ;
#100091=CARTESIAN_POINT ( 'NONE',  ( -9.854078719034067291, 10.39084668182823634, 0.7998128361456462443 ) ) ;
#100093=CARTESIAN_POINT ( 'NONE',  ( -0.6823417656250003738, 1.467708333674752730, -1.181850606188749264 ) ) ;
#100101=CARTESIAN_POINT ( 'NONE',  ( -9.571693261567968847, 12.19006144329456731, 1.443375672974076540 ) ) ;
#100105=CARTESIAN_POINT ( 'NONE',  ( -0.6823417656250212460, 0.8635416670080899859, 1.181850606188755259 ) ) ;
#100110=CARTESIAN_POINT ( 'NONE',  ( -1.402160292154681736E-14, 1.446875000341420137, -1.575800808251659024 ) ) ;
#100112=CARTESIAN_POINT ( 'NONE',  ( -5.526920175865215334, 9.599823971818089774, 0.7998128361456481317 ) ) ;
#100113=CARTESIAN_POINT ( 'NONE',  ( 7.239163954692881653, 10.53310948286200599, -1.199719254218441611 ) ) ;
#100114=CARTESIAN_POINT ( 'NONE',  ( -1.000000000000017097, 9.200000000000018829, -0.3999999999999961919 ) ) ;
#100116=CARTESIAN_POINT ( 'NONE',  ( -1.500000000000011324, 3.920833333333357817, 0.8660254037844403729 ) ) ;
#100118=CARTESIAN_POINT ( 'NONE',  ( -1.201851678989727383E-14, 2.884375000341418804, 1.575800808251672791 ) ) ;
#100124=CARTESIAN_POINT ( 'NONE',  ( 4.690757960648221037, 7.456006139856155457, 1.082531754730558626 ) ) ;
#100127=CARTESIAN_POINT ( 'NONE',  ( -7.720478407978036195, 11.09464301169468037, -1.199719254218446718 ) ) ;
#100128=CARTESIAN_POINT ( 'NONE',  ( -2.442440228756222353, 6.001264033524212671, -0.7998128361456281477 ) ) ;
#100130=CARTESIAN_POINT ( 'NONE',  ( -0.6823417656250212460, 3.301041667008085323, 1.181850606188767472 ) ) ;
#100133=CARTESIAN_POINT ( 'NONE',  ( -6.846504384776755714, 9.971043634672792422, -1.082531754730537088 ) ) ;
#100135=CARTESIAN_POINT ( 'NONE',  ( -0.7500000000000215383, 4.691666666666684193, 1.299038105676671107 ) ) ;
#100138=CARTESIAN_POINT ( 'NONE',  ( 8.432808358020025707, 9.900993174853955026, 1.082531754730558626 ) ) ;
#100140=CARTESIAN_POINT ( 'NONE',  ( -5.246642258364174971, 5.223430177620755011, 0.7216878364870457085 ) ) ;
#100146=CARTESIAN_POINT ( 'NONE',  ( 9.368320956918614328, 10.99242454023565507, 1.082531754730549967 ) ) ;
#100156=CARTESIAN_POINT ( 'NONE',  ( 5.452350330990040739, 9.512825819463730070, 0.7998128361456462443 ) ) ;
#100157=CARTESIAN_POINT ( 'NONE',  ( -4.904298879841297421, 6.744767997946721216, 1.599625672291267398 ) ) ;
#100161=CARTESIAN_POINT ( 'NONE',  ( 5.219525951136835928, 7.112532914458205013, -1.443375672974051449 ) ) ;
#100162=CARTESIAN_POINT ( 'NONE',  ( -1.364683531250014514, -0.1989583329919157317, -0.7879004041258359514 ) ) ;
#100163=CARTESIAN_POINT ( 'NONE',  ( 3.606105671554957759, 4.269840040644637291, -1.082531754730543083 ) ) ;
#100164=CARTESIAN_POINT ( 'NONE',  ( -8.435144125996554720, 12.99275191363802229, 0.7998128361456341429 ) ) ;
#100180=CARTESIAN_POINT ( 'NONE',  ( 6.551614543901692400, 8.666636272683888365, 1.599625672291281386 ) ) ;
#100181=CARTESIAN_POINT ( 'NONE',  ( 5.459129407796876166, 9.520734742405036144, 1.040834085586084257E-14 ) ) ;
#100184=EDGE_LOOP ( 'NONE', ( #188504, #150207, #209715, #209111 ) ) ;
#100192=CARTESIAN_POINT ( 'NONE',  ( -4.076197739202962467, 7.907314462378773001, 1.040834085586084257E-14 ) ) ;
#100193=CARTESIAN_POINT ( 'NONE',  ( -3.090368948911150770, 5.692848642783215674, 1.199719254218462483 ) ) ;
#100198=CARTESIAN_POINT ( 'NONE',  ( 1.500000000000009104, 4.785416667349486453, 0.8660254037844407060 ) ) ;
#100202=CARTESIAN_POINT ( 'NONE',  ( -8.649738815838677652, 13.03518635187974262, 0.7216878364870357165 ) ) ;
#100205=CARTESIAN_POINT ( 'NONE',  ( 5.717788096661236885, 7.693838750903348789, 1.599625672291267398 ) ) ;
#100206=CARTESIAN_POINT ( 'NONE',  ( -1.364683531250010740, 5.030208333674756283, 0.7879004041258379498 ) ) ;
#100212=CARTESIAN_POINT ( 'NONE',  ( 4.324687812634882000, 7.028924300507257250, 1.082531754730558626 ) ) ;
#100214=CARTESIAN_POINT ( 'NONE',  ( -6.507023659554960204, 9.678945805201045971, 1.199719254218452047 ) ) ;
#100215=ORIENTED_EDGE ( 'NONE', *, *, #66008, .F. ) ;
#100219=CARTESIAN_POINT ( 'NONE',  ( -6.482770005628665011, 10.71498210654212002, 0.7998128361456481317 ) ) ;
#100220=CARTESIAN_POINT ( 'NONE',  ( -4.894657149733403045, 5.669187081899118574, -1.199719254218446718 ) ) ;
#100227=CARTESIAN_POINT ( 'NONE',  ( 7.772902139336337335, 7.962807338847539107, 0.7998128361456341429 ) ) ;
#100231=EDGE_CURVE ( 'NONE', #32206, #62256, #189064, .T. ) ;
#100235=CARTESIAN_POINT ( 'NONE',  ( -1.150196859685106876, 3.020291321728038714, 0.7750000000000152323 ) ) ;
#100241=CARTESIAN_POINT ( 'NONE',  ( 0.7499999999999920064, 5.233333333333353821, 1.299038105676669330 ) ) ;
#100242=CARTESIAN_POINT ( 'NONE',  ( 4.518945272056516416, 4.166524327021037699, 0.7998128361456341429 ) ) ;
#100243=CARTESIAN_POINT ( 'NONE',  ( 4.843287188579786573, 6.673587691474970107, -1.599625672291256295 ) ) ;
#100245=CARTESIAN_POINT ( 'NONE',  ( -8.365017589951714072, 8.861534731139549592, 1.040834085586084257E-14 ) ) ;
#100247=CARTESIAN_POINT ( 'NONE',  ( 5.992340707560151358, 8.014150130285418783, 1.443375672974062551 ) ) ;
#100248=CARTESIAN_POINT ( 'NONE',  ( -6.683806541412756985, 10.74159869838281622, -0.7216878364870267237 ) ) ;
#100252=CARTESIAN_POINT ( 'NONE',  ( 5.926885707468349196, 10.06645042535509660, 1.040834085586084257E-14 ) ) ;
#100258=CARTESIAN_POINT ( 'NONE',  ( 1.364683531249990311, 3.134375000341423245, 1.214306433183764966E-14 ) ) ;
#100265=CARTESIAN_POINT ( 'NONE',  ( 8.308449207076147758, 8.587612251210650527, -0.7998128361456281477 ) ) ;
#100269=CARTESIAN_POINT ( 'NONE',  ( -7.153898609505128015, 11.49796547773133604, 0.7998128361456481317 ) ) ;
#100274=CARTESIAN_POINT ( 'NONE',  ( 8.727698198895078363, 11.20540053684285553, -1.599625672291257406 ) ) ;
#100277=CARTESIAN_POINT ( 'NONE',  ( -7.316596452869116973, 11.68777962832266049, 0.7998128361456481317 ) ) ;
#100282=CARTESIAN_POINT ( 'NONE',  ( 5.430853319176391025, 6.270791292598644873, -1.030804022418196464 ) ) ;
#100283=CARTESIAN_POINT ( 'NONE',  ( -8.514157279702017078, 12.87700789305364069, -0.7216878364870267237 ) ) ;
#100288=CARTESIAN_POINT ( 'NONE',  ( 6.252281394196331554, 10.44607872653774372, 1.040834085586084257E-14 ) ) ;
#100290=CARTESIAN_POINT ( 'NONE',  ( 6.661133543015731462, 6.665743976473484267, -0.7998128361456281477 ) ) ;
#100291=CARTESIAN_POINT ( 'NONE',  ( -4.054949276293840832, 7.568305524423037056, 0.4105793130844727079 ) ) ;
#100292=CARTESIAN_POINT ( 'NONE',  ( 4.792970997630896512, 5.550553237779539018, 1.199719254218464037 ) ) ;
#100294=CARTESIAN_POINT ( 'NONE',  ( -8.365017589951714072, 8.861534731139549592, 1.040834085586084257E-14 ) ) ;
#100302=CARTESIAN_POINT ( 'NONE',  ( -4.275059339850010076, 7.289437269727999436, -0.9335736327708322735 ) ) ;
#100306=CARTESIAN_POINT ( 'NONE',  ( 6.493992391265805075, 6.678671999339316656, 1.040834085586084257E-14 ) ) ;
#100316=CARTESIAN_POINT ( 'NONE',  ( -8.473482818416657736, 12.82955435488738516, -0.7216878364870267237 ) ) ;
#100323=CARTESIAN_POINT ( 'NONE',  ( -10.27671724903424888, 11.09185100006920877, 1.040834085586084257E-14 ) ) ;
#100330=CARTESIAN_POINT ( 'NONE',  ( 0.7499999999999902300, 2.264583334016148530, 1.299038105676669330 ) ) ;
#100332=CARTESIAN_POINT ( 'NONE',  ( -7.054319997812058318, 7.124461507069184130, 1.040834085586084257E-14 ) ) ;
#100336=CARTESIAN_POINT ( 'NONE',  ( -7.635213062790267458, 12.05949900656400686, 0.000000000000000000 ) ) ;
#100340=CARTESIAN_POINT ( 'NONE',  ( 6.205881626753210867, 8.263281202677319470, 1.599625672291281386 ) ) ;
#100345=CARTESIAN_POINT ( 'NONE',  ( 8.072990401933337168, 11.50590700464255356, -1.199719254218446718 ) ) ;
#100346=CARTESIAN_POINT ( 'NONE',  ( 4.184706906422049677, 7.590773377626947038, -0.8858016570119742195 ) ) ;
#100347=CARTESIAN_POINT ( 'NONE',  ( -1.403499169903600574, 7.376709478543776122, 4.304123474983186703 ) ) ;
#100351=CARTESIAN_POINT ( 'NONE',  ( -6.399085315970137522, 9.449054721065074602, -1.082531754730538864 ) ) ;
#100354=CARTESIAN_POINT ( 'NONE',  ( -1.364683531250010295, 5.592708333674750953, 0.7879004041258379498 ) ) ;
#100358=CARTESIAN_POINT ( 'NONE',  ( -1.364683531249997417, 5.759375000341418804, 1.214306433183764966E-14 ) ) ;
#100361=CARTESIAN_POINT ( 'NONE',  ( -2.751941993449643409, 6.154423392425789174, 0.7216878364870317197 ) ) ;
#100363=CARTESIAN_POINT ( 'NONE',  ( 8.778014389843965759, 12.32843499053828928, 1.199719254218450271 ) ) ;
#100365=CARTESIAN_POINT ( 'NONE',  ( -1.206235080191141895, 2.838937307313431191, -0.7749999999999979128 ) ) ;
#100369=CARTESIAN_POINT ( 'NONE',  ( 1.364683531249988535, 2.613541667008089764, 0.7879004041258500513 ) ) ;
#100371=CARTESIAN_POINT ( 'NONE',  ( 5.034155109375821446, 4.767602470560229122, -0.7998128361456221525 ) ) ;
#100378=CARTESIAN_POINT ( 'NONE',  ( 7.876924059415351564, 12.13356913605253240, -0.7216878364870267237 ) ) ;
#100380=CARTESIAN_POINT ( 'NONE',  ( -6.236387472606141458, 10.21960978477508952, -0.7216878364870278340 ) ) ;
#100382=CARTESIAN_POINT ( 'NONE',  ( 0.5528008270654922729, 7.812676398891469809, 1.922238454054872037 ) ) ;
#100384=CARTESIAN_POINT ( 'NONE',  ( -7.344766530301162000, 9.591980256816594164, 1.599625672291295375 ) ) ;
#100386=CARTESIAN_POINT ( 'NONE',  ( -5.219525951136862574, 5.191794485855519170, -0.7216878364870197293 ) ) ;
#100387=CARTESIAN_POINT ( 'NONE',  ( -1.364683531250012516, 2.592708333674753174, 0.7879004041258379498 ) ) ;
#100398=ORIENTED_EDGE ( 'NONE', *, *, #119470, .T. ) ;
#100408=CARTESIAN_POINT ( 'NONE',  ( -0.6823417656250212460, 3.863541667008085767, 1.181850606188767472 ) ) ;
#100415=CARTESIAN_POINT ( 'NONE',  ( 8.235688245297327015, 11.69572115523387268, -1.199719254218446718 ) ) ;
#100417=CARTESIAN_POINT ( 'NONE',  ( 1.364683531249988757, 2.384375000341422357, 1.214306433183764966E-14 ) ) ;
#100419=CARTESIAN_POINT ( 'NONE',  ( -7.402388683381436074, 7.738467673474211495, 0.7216878364870317197 ) ) ;
#100425=ORIENTED_EDGE ( 'NONE', *, *, #187534, .F. ) ;
#100427=CARTESIAN_POINT ( 'NONE',  ( 4.355193658487811703, 6.104145239700998538, -1.599625672291255185 ) ) ;
#100431=CARTESIAN_POINT ( 'NONE',  ( 9.240045382913317340, 10.73880668727576015, -1.199719254218446718 ) ) ;
#100439=CARTESIAN_POINT ( 'NONE',  ( -2.598358995313378550, 6.183169261174235487, 0.7998128361456341429 ) ) ;
#100440=CARTESIAN_POINT ( 'NONE',  ( 6.123478934866503742, 10.29580919065294431, 0.7998128361456462443 ) ) ;
#100442=CARTESIAN_POINT ( 'NONE',  ( 4.650083499362867911, 6.448183387388563226, 1.443375672974062551 ) ) ;
#100450=CARTESIAN_POINT ( 'NONE',  ( -5.734735788900501952, 9.634349487118505806, 0.000000000000000000 ) ) ;
#100451=CARTESIAN_POINT ( 'NONE',  ( 4.473300617505036492, 7.306268922809479704, -1.199719254218452047 ) ) ;
#100454=CARTESIAN_POINT ( 'NONE',  ( -7.309817376062285099, 11.67987070538135264, 0.000000000000000000 ) ) ;
#100458=CARTESIAN_POINT ( 'NONE',  ( -4.081167932913447594, 4.720116328942494555, -1.199719254218452047 ) ) ;
#100461=CARTESIAN_POINT ( 'NONE',  ( 8.748035429315576650, 11.22912730566677553, -1.599625672291255185 ) ) ;
#100463=CARTESIAN_POINT ( 'NONE',  ( 4.216749469050096621, 4.878294787768598262, -1.199719254218452047 ) ) ;
#100472=CARTESIAN_POINT ( 'NONE',  ( -5.066996723205291708, 6.934582148538044777, 1.599625672291267398 ) ) ;
#100475=CARTESIAN_POINT ( 'NONE',  ( -8.616370316684697883, 10.01118577667568132, -1.199719254218446718 ) ) ;
#100480=CARTESIAN_POINT ( 'NONE',  ( 6.480434237652121787, 9.543961796360731498, 1.082531754730558626 ) ) ;
#100481=CARTESIAN_POINT ( 'NONE',  ( -1.364683531249997417, 5.321875000341417916, 1.214306433183764966E-14 ) ) ;
#100484=CARTESIAN_POINT ( 'NONE',  ( 2.683624340501134853, 5.218313266304903664, -1.199719254218446718 ) ) ;
#100486=CARTESIAN_POINT ( 'NONE',  ( 5.678167406024951624, 5.518950149984223508, 0.7998128361456341429 ) ) ;
#100488=CARTESIAN_POINT ( 'NONE',  ( -6.958359152311683893, 9.141171649162195934, -1.599625672291263179 ) ) ;
#100490=CARTESIAN_POINT ( 'NONE',  ( 1.436838838544731267, 7.449283400311756509, 4.203727439823562229 ) ) ;
#100492=CARTESIAN_POINT ( 'NONE',  ( 3.469446951953614189E-15, 6.180000000000019256, 1.214306433183764966E-14 ) ) ;
#100497=ORIENTED_EDGE ( 'NONE', *, *, #28211, .T. ) ;
#100499=CARTESIAN_POINT ( 'NONE',  ( 1.364683531249988535, 2.676041667008082214, 0.7879004041258500513 ) ) ;
#100500=CARTESIAN_POINT ( 'NONE',  ( 9.053093885623066939, 11.58502883802551153, -1.599625672291262513 ) ) ;
#100503=CARTESIAN_POINT ( 'NONE',  ( -5.422898255786209099, 5.429062174613087599, -0.7216878364870207285 ) ) ;
#100504=FACE_OUTER_BOUND ( 'NONE', #192814, .T. ) ;
#100505=CARTESIAN_POINT ( 'NONE',  ( -4.555176424067209240, 8.258196894812975586, 1.040834085586084257E-14 ) ) ;
#100507=CARTESIAN_POINT ( 'NONE',  ( -1.408750476333776369, 7.229967155397921452, 4.273289540530513797 ) ) ;
#100512=CARTESIAN_POINT ( 'NONE',  ( 3.928111819657337911, 5.605883094398769195, 1.599625672291267398 ) ) ;
#100519=CARTESIAN_POINT ( 'NONE',  ( 1.217323170181696002, 2.969494316908636300, 0.7750000000000100142 ) ) ;
#100523=CARTESIAN_POINT ( 'NONE',  ( 4.005544317833563461, 6.760553239859419250, -1.199719254218452047 ) ) ;
#100527=CARTESIAN_POINT ( 'NONE',  ( -5.225778143063529946, 8.184159369294361497, 1.199719254218452047 ) ) ;
#100531=CARTESIAN_POINT ( 'NONE',  ( 6.959412922516382771, 7.013736585890911535, 0.7998128361456341429 ) ) ;
#100535=CARTESIAN_POINT ( 'NONE',  ( -6.586563698140583512, 6.578745824119123675, 1.040834085586084257E-14 ) ) ;
#100536=CARTESIAN_POINT ( 'NONE',  ( 0.7499999999999885647, 1.566666666666688412, -1.299038105676652899 ) ) ;
#100537=CARTESIAN_POINT ( 'NONE',  ( -4.786191920824102830, 5.542644314838231168, 1.199719254218462483 ) ) ;
#100540=CARTESIAN_POINT ( 'NONE',  ( -4.791917227426195858, 7.677988301050826969, -1.199719254218452047 ) ) ;
#100543=CARTESIAN_POINT ( 'NONE',  ( -0.6823417656250212460, 2.801041667008084879, 1.181850606188767472 ) ) ;
#100545=CARTESIAN_POINT ( 'NONE',  ( -5.599154252763867134, 5.634694171087028636, 0.000000000000000000 ) ) ;
#100548=ORIENTED_EDGE ( 'NONE', *, *, #88421, .T. ) ;
#100551=CARTESIAN_POINT ( 'NONE',  ( 4.333802657862601215, 8.207853534148366492, 0.7998128361456462443 ) ) ;
#100552=CARTESIAN_POINT ( 'NONE',  ( 1.284279953904119864, 3.046639714193936754, -0.7749999999999910294 ) ) ;
#100555=CARTESIAN_POINT ( 'NONE',  ( -0.6823417656250212460, 2.113541667008083991, 1.181850606188767472 ) ) ;
#100557=CARTESIAN_POINT ( 'NONE',  ( 3.871016551901614200, 4.474939717762034697, -1.199719254218446718 ) ) ;
#100559=CARTESIAN_POINT ( 'NONE',  ( 1.364683531249986537, -0.07395833299191513499, 0.7879004041258500513 ) ) ;
#100562=CARTESIAN_POINT ( 'NONE',  ( -3.327636637150278798, 5.969660945728899826, -1.199719254218452935 ) ) ;
#100564=CARTESIAN_POINT ( 'NONE',  ( -7.334597914868741242, 8.619747657844088806, -1.082531754730543083 ) ) ;
#100566=CARTESIAN_POINT ( 'NONE',  ( 1.364683531249990311, 3.634375000341416584, 1.214306433183764966E-14 ) ) ;
#100574=CARTESIAN_POINT ( 'NONE',  ( -6.521108698048779573, 8.631046119188804155, -1.443375672974058777 ) ) ;
#100580=CARTESIAN_POINT ( 'NONE',  ( -7.673551755210395342, 8.054824590608001600, 1.040834085586084257E-14 ) ) ;
#100585=CARTESIAN_POINT ( 'NONE',  ( 3.094265954482833703, 2.800000000000017586, -2.490342512183683965 ) ) ;
#100592=CARTESIAN_POINT ( 'NONE',  ( -7.054319997812058318, 7.124461507069184130, 1.040834085586084257E-14 ) ) ;
#100594=CARTESIAN_POINT ( 'NONE',  ( 0.7499999999999885647, -1.016666666666644847, 1.299038105676657340 ) ) ;
#100595=CARTESIAN_POINT ( 'NONE',  ( 4.033714395265605823, 4.664753868353354704, -1.199719254218446718 ) ) ;
#100599=CARTESIAN_POINT ( 'NONE',  ( 6.328958779480917229, 6.278206752349526631, 0.7998128361456341429 ) ) ;
#100605=CARTESIAN_POINT ( 'NONE',  ( -4.528060117284246289, 6.305822774963486310, 1.443375672974064550 ) ) ;
#100608=CARTESIAN_POINT ( 'NONE',  ( -0.4768485052293973125, 6.608576083985783001, 3.444768111981479031 ) ) ;
#100612=CARTESIAN_POINT ( 'NONE',  ( -1.364683531250012516, 2.030208333674750953, 0.7879004041258379498 ) ) ;
#100613=CARTESIAN_POINT ( 'NONE',  ( 8.378575743120986630, 12.71882943370911789, 1.040834085586084257E-14 ) ) ;
#100614=CARTESIAN_POINT ( 'NONE',  ( -6.958359152311683893, 9.141171649162195934, -1.599625672291263179 ) ) ;
#100618=CARTESIAN_POINT ( 'NONE',  ( 7.145310649601935182, 8.294949498412453437, -1.199719254218446718 ) ) ;
#100619=CARTESIAN_POINT ( 'NONE',  ( -5.716734326456539783, 9.821273814174633188, -0.7998128361456231517 ) ) ;
#100620=CARTESIAN_POINT ( 'NONE',  ( -1.566031286093755304, 8.750666943143144749, 2.469538363634797840 ) ) ;
#100622=CARTESIAN_POINT ( 'NONE',  ( 1.499999999999987566, -0.9437499993171851731, 0.000000000000000000 ) ) ;
#100624=CARTESIAN_POINT ( 'NONE',  ( 9.408995418203975447, 10.07950886410055524, 0.7216878364870438212 ) ) ;
#100627=CARTESIAN_POINT ( 'NONE',  ( 1.364683531249986537, 0.6760416670080884316, 0.7879004041258500513 ) ) ;
#100629=CARTESIAN_POINT ( 'NONE',  ( 7.144783764277405247, 8.398297815487545392, -1.082531754730543971 ) ) ;
#100633=CARTESIAN_POINT ( 'NONE',  ( -5.422898255786203769, 6.389431388914436738, -1.082531754730544860 ) ) ;
#100635=CARTESIAN_POINT ( 'NONE',  ( 0.6823417656249917140, 4.342708333674755394, 1.181850606188765695 ) ) ;
#100639=CARTESIAN_POINT ( 'NONE',  ( -5.392392409933270514, 7.314210449720692786, 1.599625672291269396 ) ) ;
#100640=CARTESIAN_POINT ( 'NONE',  ( -5.470032677541931676, 6.438256155886466381, -1.298486150373518999 ) ) ;
#100647=CARTESIAN_POINT ( 'NONE',  ( 6.877010230629674759, 9.046264573866535486, 1.599625672291281386 ) ) ;
#100651=CARTESIAN_POINT ( 'NONE',  ( 1.499999999999989120, 2.754166666666688190, 0.8660254037844524744 ) ) ;
#100657=CARTESIAN_POINT ( 'NONE',  ( 4.853455804012216213, 6.685451076146141425, 1.443375672974062551 ) ) ;
#100660=CARTESIAN_POINT ( 'NONE',  ( 1.364683531249986537, 0.9260416670080896528, 0.7879004041258500513 ) ) ;
#100665=CARTESIAN_POINT ( 'NONE',  ( -1.201851678989727383E-14, 0.9625000000000237810, 1.732050807568877637 ) ) ;
#100666=CARTESIAN_POINT ( 'NONE',  ( 5.601490020740366838, 9.686822124172440596, 1.040834085586084257E-14 ) ) ;
#100667=CARTESIAN_POINT ( 'NONE',  ( -7.985916173649233230, 9.275655943134292869, -1.199719254218446718 ) ) ;
#100669=CARTESIAN_POINT ( 'NONE',  ( -1.402160292154681736E-14, 0.6968750003414164729, -1.575800808251659024 ) ) ;
#100670=CARTESIAN_POINT ( 'NONE',  ( -1.402160292154681736E-14, 2.087500000000021227, -1.732050807568863648 ) ) ;
#100672=CARTESIAN_POINT ( 'NONE',  ( 5.020596955762157698, 4.751784624677624080, 1.040834085586084257E-14 ) ) ;
#100675=EDGE_CURVE ( 'NONE', #24517, #3126, #96001, .T. ) ;
#100680=CARTESIAN_POINT ( 'NONE',  ( 1.499999999999987121, -1.214583332650518432, 0.8660254037844524744 ) ) ;
#100682=CARTESIAN_POINT ( 'NONE',  ( -7.857113714319432063, 9.125386407249497012, 1.199719254218462483 ) ) ;
#100683=CARTESIAN_POINT ( 'NONE',  ( -5.612712406377534435, 5.650512016969639895, 0.7216878364870317197 ) ) ;
#100685=FACE_OUTER_BOUND ( 'NONE', #69470, .T. ) ;
#100691=CARTESIAN_POINT ( 'NONE',  ( 7.800018446563675489, 7.994443030612759848, -0.7998128361456281477 ) ) ;
#100692=DIRECTION ( 'NONE',  ( 5.578564026256490882E-16, 1.000000000000000000, 9.066213480720158442E-32 ) ) ;
#100695=CARTESIAN_POINT ( 'NONE',  ( 5.761852095683461350, 9.665985178365305686, -0.7216878364870267237 ) ) ;
#100700=CARTESIAN_POINT ( 'NONE',  ( -7.477485413136760073, 8.682486722536401302, -1.199719254218446718 ) ) ;
#100702=CARTESIAN_POINT ( 'NONE',  ( 4.273844736805816780, 6.009238164405336313, 1.599625672291267398 ) ) ;
#100706=CARTESIAN_POINT ( 'NONE',  ( 3.994299746785815231, 7.604083813490793098, 0.004591788735710394809 ) ) ;
#100707=CARTESIAN_POINT ( 'NONE',  ( 8.581948047770334043, 12.95609712246668899, 0.000000000000000000 ) ) ;
#100713=CARTESIAN_POINT ( 'NONE',  ( 2.274126960250456797, 5.663124471396743687, 0.4971758506561237412 ) ) ;
#100714=CARTESIAN_POINT ( 'NONE',  ( -1.530509776559454860, 8.694755902745800569, -2.517145264428154672 ) ) ;
#100715=CARTESIAN_POINT ( 'NONE',  ( -4.446711195602255806, 5.250546485366484717, -1.082531754730544860 ) ) ;
#100716=CARTESIAN_POINT ( 'NONE',  ( 8.758204044747998296, 11.24099069033793974, 1.443375672974076540 ) ) ;
#100719=CARTESIAN_POINT ( 'NONE',  ( -6.240830780992103755, 6.175390754112560110, 1.040834085586084257E-14 ) ) ;
#100725=CARTESIAN_POINT ( 'NONE',  ( -8.290974629956718189, 9.631557475493025322, -1.199719254218446718 ) ) ;
#100728=CARTESIAN_POINT ( 'NONE',  ( -0.5028141819148801428, 7.728236690828136801, 1.993924427468481309 ) ) ;
#100729=ORIENTED_EDGE ( 'NONE', *, *, #28619, .T. ) ;
#100738=CARTESIAN_POINT ( 'NONE',  ( -5.392392409933270514, 7.314210449720692786, 1.599625672291269396 ) ) ;
#100741=CARTESIAN_POINT ( 'NONE',  ( 4.473827502829567315, 7.202920605734387749, -1.082531754730548412 ) ) ;
#100742=CARTESIAN_POINT ( 'NONE',  ( 6.471393748265540147, 5.229711127717882491, 2.500000000000011102 ) ) ;
#100745=CARTESIAN_POINT ( 'NONE',  ( -4.946027110887008860, 4.664786472323266153, -0.7998128361456221525 ) ) ;
#100748=CARTESIAN_POINT ( 'NONE',  ( -6.138157471807708987, 5.995865026538652387, 1.148737437293850421E-12 ) ) ;
#100749=CARTESIAN_POINT ( 'NONE',  ( 4.355419887332007356, 3.138961360799480627, -0.7749999999999935829 ) ) ;
#100752=CARTESIAN_POINT ( 'NONE',  ( -8.538937818508475885, 8.856515631215026829, 1.040834085586084257E-14 ) ) ;
#100753=CARTESIAN_POINT ( 'NONE',  ( 6.823831386379729302, 6.855558127064808716, -0.7998128361456281477 ) ) ;
#100756=CARTESIAN_POINT ( 'NONE',  ( -10.14557902172788495, 10.73093036830436553, 1.040834085586084257E-14 ) ) ;
#100758=CARTESIAN_POINT ( 'NONE',  ( 4.904298879841284098, 6.744767997946720328, 1.599625672291267175 ) ) ;
#100760=CARTESIAN_POINT ( 'NONE',  ( -0.6823417656250246877, 0.3635416670080895973, 1.181850606188755259 ) ) ;
#100763=CARTESIAN_POINT ( 'NONE',  ( 7.443063144222396232, 11.62739806832741785, 1.040834085586084257E-14 ) ) ;
#100766=CARTESIAN_POINT ( 'NONE',  ( 0.08888683327021307257, 6.492044364012829583, -3.106763327641859362 ) ) ;
#100779=EDGE_CURVE ( 'NONE', #58688, #80644, #85602, .T. ) ;
#100790=CARTESIAN_POINT ( 'NONE',  ( 1.499999999999987121, 0.8270833340161471980, -0.8660254037844253849 ) ) ;
#100794=ORIENTED_EDGE ( 'NONE', *, *, #166654, .F. ) ;
#100798=CARTESIAN_POINT ( 'NONE',  ( 8.727698198895078363, 11.20540053684285553, -1.599625672291257406 ) ) ;
#100799=CARTESIAN_POINT ( 'NONE',  ( 1.499999999999990896, 5.306250000682820378, 1.214306433183764966E-14 ) ) ;
#100801=AXIS2_PLACEMENT_3D ( 'NONE', #126387, #205399, #40805 ) ;
#100803=CARTESIAN_POINT ( 'NONE',  ( 4.578903193113299963, 6.365139696764064325, 1.599625672291267398 ) ) ;
#100804=CARTESIAN_POINT ( 'NONE',  ( -7.700668062882078502, 9.046829497192987901, -1.082531754730543971 ) ) ;
#100806=CARTESIAN_POINT ( 'NONE',  ( 9.622536337397022521, 12.24937836509514710, 1.599625672291281386 ) ) ;
#100808=CARTESIAN_POINT ( 'NONE',  ( -7.640183256500752584, 8.872300873127729304, -1.199719254218446718 ) ) ;
#100810=CARTESIAN_POINT ( 'NONE',  ( -3.429849674132948500, 5.024577257953626308, -1.443375672974051449 ) ) ;
#100813=CARTESIAN_POINT ( 'NONE',  ( 1.499999999999985123, -0.1729166659838496101, -0.8660254037844323793 ) ) ;
#100820=CARTESIAN_POINT ( 'NONE',  ( -4.080641047588907888, 6.744203074620265248, -1.082531754730548412 ) ) ;
#100823=CARTESIAN_POINT ( 'NONE',  ( 4.019038269249470829, 7.568960612331900428, -0.3200009682147019752 ) ) ;
#100828=CARTESIAN_POINT ( 'NONE',  ( -4.568734577680894304, 5.392907097791561633, -1.082531754730543971 ) ) ;
#100829=CARTESIAN_POINT ( 'NONE',  ( 7.736899214892750010, 12.17813285068358020, 1.040834085586084257E-14 ) ) ;
#100839=CARTESIAN_POINT ( 'NONE',  ( -8.779068160048691283, 10.20099992726700933, -1.199719254218446718 ) ) ;
#100844=CARTESIAN_POINT ( 'NONE',  ( 4.168242161197552420, 6.950367390450747251, -1.199719254218452047 ) ) ;
#100849=CARTESIAN_POINT ( 'NONE',  ( -5.908535366263027555, 4.807949608181242951, 2.499999999999999112 ) ) ;
#100862=CARTESIAN_POINT ( 'NONE',  ( 7.633404179693907388, 8.864391950186421454, -1.199719254218441611 ) ) ;
#100864=CARTESIAN_POINT ( 'NONE',  ( -5.111587607552082524, 5.922272616020886282, 1.199719254218450271 ) ) ;
#100870=CARTESIAN_POINT ( 'NONE',  ( -0.7500000000000249800, -0.7770833326505161009, 1.299038105676659116 ) ) ;
#100874=CARTESIAN_POINT ( 'NONE',  ( 3.948449050077836642, 5.629609863222681199, 1.599625672291267398 ) ) ;
#100876=CARTESIAN_POINT ( 'NONE',  ( -3.276266675996675204, 6.974061555304760240, -0.7998128361456281477 ) ) ;
#100882=CARTESIAN_POINT ( 'NONE',  ( 5.422898255786183341, 7.349800603215774331, -1.443375672974051449 ) ) ;
#100885=CARTESIAN_POINT ( 'NONE',  ( 7.415946836550714849, 9.675023947441092176, 1.443375672974076540 ) ) ;
#100886=CARTESIAN_POINT ( 'NONE',  ( 1.364683531249990311, 4.196875000341417028, 1.214306433183764966E-14 ) ) ;
#100888=CARTESIAN_POINT ( 'NONE',  ( 2.846849068745292755, 6.265148313604064434, 0.000000000000000000 ) ) ;
#100892=CARTESIAN_POINT ( 'NONE',  ( -1.387358672527334136, 7.251968950354660493, -4.302625267139479348 ) ) ;
#100895=CARTESIAN_POINT ( 'NONE',  ( -5.937252720508472414, 6.122620518184580973, 0.7955437839095025332 ) ) ;
#100897=CARTESIAN_POINT ( 'NONE',  ( -1.364683531250012516, 4.801041667008083991, -0.7879004041258300672 ) ) ;
#100903=CARTESIAN_POINT ( 'NONE',  ( -3.511198596259299087, 6.271927390929313617, -7.499999999999997335 ) ) ;
#100909=VERTEX_POINT ( 'NONE', #94884 ) ;
#100913=CARTESIAN_POINT ( 'NONE',  ( -0.6823417656249969321, 4.530208333674755394, -1.181850606188749264 ) ) ;
#100915=CARTESIAN_POINT ( 'NONE',  ( 5.991813822235618758, 9.077867661661846554, 1.199719254218462483 ) ) ;
#100916=CARTESIAN_POINT ( 'NONE',  ( -8.992082194361570302, 11.51384853155376220, 1.599625672291269396 ) ) ;
#100917=CARTESIAN_POINT ( 'NONE',  ( 1.445103857048100515, 8.688264192037886247, 2.625611233228254182 ) ) ;
#100922=CARTESIAN_POINT ( 'NONE',  ( 0.7499999999999902300, 3.983333333333352488, 1.299038105676669330 ) ) ;
#100926=CARTESIAN_POINT ( 'NONE',  ( 6.938893903907228378E-15, 10.64264068711930733, 1.214306433183764966E-14 ) ) ;
#100928=CARTESIAN_POINT ( 'NONE',  ( 8.270110514656034084, 9.711179024262627024, 1.082531754730558626 ) ) ;
#100933=CARTESIAN_POINT ( 'NONE',  ( -1.500000000000011324, 2.952083334016149418, 0.8660254037844403729 ) ) ;
#100935=CARTESIAN_POINT ( 'NONE',  ( -5.253948220495577637, 6.088359997788290734, 1.199719254218450271 ) ) ;
#100936=CARTESIAN_POINT ( 'NONE',  ( 3.945059511452237100, 6.586024615794168646, -1.082531754730548412 ) ) ;
#100937=CARTESIAN_POINT ( 'NONE',  ( -8.961576348508637935, 12.43862759236002269, -1.082531754730543083 ) ) ;
#100944=CARTESIAN_POINT ( 'NONE',  ( 4.681643115420508039, 4.356338477612361260, 0.7998128361456341429 ) ) ;
#100947=CARTESIAN_POINT ( 'NONE',  ( 3.469446951953614189E-15, 6.400000000000023448, 1.214306433183764966E-14 ) ) ;
#100948=CARTESIAN_POINT ( 'NONE',  ( 4.168242161197552420, 6.950367390450747251, -1.199719254218452047 ) ) ;
#100953=ORIENTED_EDGE ( 'NONE', *, *, #78317, .F. ) ;
#100958=CARTESIAN_POINT ( 'NONE',  ( 2.276274698451039580, 5.633392974947595278, -0.5486624834757477531 ) ) ;
#100959=CARTESIAN_POINT ( 'NONE',  ( 5.283544098290614777, 6.372568566219670494, -1.132182188465682859 ) ) ;
#100962=CARTESIAN_POINT ( 'NONE',  ( 9.297140650669039275, 11.86975006391249643, 1.599625672291281386 ) ) ;
#100967=FACE_OUTER_BOUND ( 'NONE', #105150, .T. ) ;
#100969=CARTESIAN_POINT ( 'NONE',  ( 5.450014563013511726, 8.341805509282339770, -1.082531754730543083 ) ) ;
#100970=CARTESIAN_POINT ( 'NONE',  ( -8.188761592974033832, 12.49737959187099179, -0.7216878364870267237 ) ) ;
#100975=CARTESIAN_POINT ( 'NONE',  ( -5.603597561149804562, 5.431951997629870910, 0.7998128361456341429 ) ) ;
#100979=ORIENTED_EDGE ( 'NONE', *, *, #193834, .T. ) ;
#100986=CARTESIAN_POINT ( 'NONE',  ( 9.043452155515161905, 10.50944792197790889, 1.199719254218453823 ) ) ;
#100987=CARTESIAN_POINT ( 'NONE',  ( 5.980536202102920917, 6.100347882654393317, -0.6550157475838751520 ) ) ;
#100992=CARTESIAN_POINT ( 'NONE',  ( 3.486418057008484617, 7.219238166485217434, 1.040834085586084257E-14 ) ) ;
#100997=CARTESIAN_POINT ( 'NONE',  ( -9.381879110976678149, 11.00824238663667565, 1.082531754730558626 ) ) ;
#100998=VECTOR ( 'NONE', #154901, 1000.000000000000227 ) ;
#101002=CARTESIAN_POINT ( 'NONE',  ( 6.479907352327590964, 9.647310113435821677, 1.199719254218462483 ) ) ;
#101004=CARTESIAN_POINT ( 'NONE',  ( -4.786191920824102830, 5.542644314838231168, 1.199719254218462483 ) ) ;
#101005=CARTESIAN_POINT ( 'NONE',  ( 4.891794496432329886, 4.601515088792824670, -0.7998128361456211532 ) ) ;
#101007=CARTESIAN_POINT ( 'NONE',  ( -4.737684612971557740, 7.614716917520386374, 1.199719254218464037 ) ) ;
#101008=CARTESIAN_POINT ( 'NONE',  ( 4.708759422647839976, 4.387974169377582001, -0.7998128361456211532 ) ) ;
#101012=CARTESIAN_POINT ( 'NONE',  ( 9.077347539549325717, 10.54899253668443393, -1.199719254218446718 ) ) ;
#101013=CARTESIAN_POINT ( 'NONE',  ( -0.7499999999999972244, 3.608333333333359150, -1.299038105676652011 ) ) ;
#101016=CARTESIAN_POINT ( 'NONE',  ( 4.012431654125413694, 7.810675627703163038, 0.2615036927465386740 ) ) ;
#101017=CARTESIAN_POINT ( 'NONE',  ( 4.826339496784873617, 8.574553812983598533, -0.7216878364870257245 ) ) ;
#101023=CARTESIAN_POINT ( 'NONE',  ( 6.900736999231407154, 10.99468423250458038, -0.7216878364870267237 ) ) ;
#101026=CARTESIAN_POINT ( 'NONE',  ( -8.462260433223891098, 13.02438760540324481, -0.7998128361456281477 ) ) ;
#101027=CARTESIAN_POINT ( 'NONE',  ( -7.232384877886063990, 10.52520055992070525, -1.199719254218446718 ) ) ;
#101037=CARTESIAN_POINT ( 'NONE',  ( 8.353795204314554468, 12.89784483834236184, -0.7998128361456352531 ) ) ;
#101042=CARTESIAN_POINT ( 'NONE',  ( 5.847644326195776010, 5.716673223516856694, -0.7998128361456281477 ) ) ;
#101045=CARTESIAN_POINT ( 'NONE',  ( 1.499999999999990896, 4.056250000682819490, 1.214306433183764966E-14 ) ) ;
#101049=ORIENTED_EDGE ( 'NONE', *, *, #125678, .F. ) ;
#101051=B_SPLINE_CURVE_WITH_KNOTS ( 'NONE', 3,
 ( #10753, #175420, #110474, #59512 ),
 .UNSPECIFIED., .F., .F.,
 ( 4, 4 ),
 ( 1.910166083080831124E-17, 0.002003498272494318600 ),
 .UNSPECIFIED. ) ;
#101052=CARTESIAN_POINT ( 'NONE',  ( -0.7500000000000006661, 2.358333333333358262, -1.299038105676652011 ) ) ;
#101053=CARTESIAN_POINT ( 'NONE',  ( 7.623762449586013901, 7.788811034138823253, 1.040834085586084257E-14 ) ) ;
#101054=CARTESIAN_POINT ( 'NONE',  ( 3.673896439178911066, 7.230036912443299713, 0.7216878364870317197 ) ) ;
#101057=CARTESIAN_POINT ( 'NONE',  ( 8.270110514656034084, 9.711179024262627024, 1.082531754730558626 ) ) ;
#101063=AXIS2_PLACEMENT_3D ( 'NONE', #160418, #7748, #10946 ) ;
#101065=CARTESIAN_POINT ( 'NONE',  ( -3.730464822054482710, 7.503959392372201442, 1.040834085586084257E-14 ) ) ;
#101066=CARTESIAN_POINT ( 'NONE',  ( -1.001543065824772872E-14, 4.493750000682820378, 1.732050807568877637 ) ) ;
#101067=CARTESIAN_POINT ( 'NONE',  ( -1.364683531250000748, 0.009375000341420303140, 0.000000000000000000 ) ) ;
#101071=DIRECTION ( 'NONE',  ( 0.000000000000000000, 8.546850786086437571E-32, 1.000000000000000000 ) ) ;
#101073=CARTESIAN_POINT ( 'NONE',  ( -1.364683531249997417, 4.071875000341417028, 1.214306433183764966E-14 ) ) ;
#101079=CARTESIAN_POINT ( 'NONE',  ( -9.189729191964438826, 9.615772233580322848, 1.040834085586084257E-14 ) ) ;
#101080=CARTESIAN_POINT ( 'NONE',  ( 5.144429221381498607, 8.089252293998699272, -1.199719254218452047 ) ) ;
#101082=CARTESIAN_POINT ( 'NONE',  ( 0.6823417656249864960, -0.5739583329919112353, -1.181850606188749264 ) ) ;
#101084=EDGE_LOOP ( 'NONE', ( #123482, #176091, #164128, #117173, #153395, #91103, #116210, #144172, #158966, #11044, #195630, #83408, #28308, #152946, #121010, #186382 ) ) ;
#101086=CARTESIAN_POINT ( 'NONE',  ( 2.272730219304121668, 5.707593880249651086, 0.2947169286177344638 ) ) ;
#101089=CARTESIAN_POINT ( 'NONE',  ( -7.379715684540041565, 7.504089808251839244, 1.040834085586084257E-14 ) ) ;
#101093=CARTESIAN_POINT ( 'NONE',  ( 9.673906298550626559, 11.24497775551929557, 1.199719254218452047 ) ) ;
#101095=CARTESIAN_POINT ( 'NONE',  ( 7.730120138085914583, 12.17022392774227768, 0.7998128361456462443 ) ) ;
#101097=CARTESIAN_POINT ( 'NONE',  ( -3.521367211247373508, 5.131347717920458962, -1.599625672291256295 ) ) ;
#101099=CARTESIAN_POINT ( 'NONE',  ( -6.496328159242330536, 10.73079995242472862, 0.000000000000000000 ) ) ;
#101101=CARTESIAN_POINT ( 'NONE',  ( -4.377387467589398007, 7.366231944554199274, 1.201952607213795821 ) ) ;
#101102=CARTESIAN_POINT ( 'NONE',  ( 0.6823417656249864960, -1.073958332991911568, -1.181850606188749264 ) ) ;
#101107=CARTESIAN_POINT ( 'NONE',  ( 6.941411460516762943, 11.04213777067082702, -0.7216878364870267237 ) ) ;
#101122=ORIENTED_EDGE ( 'NONE', *, *, #190752, .F. ) ;
#101126=CARTESIAN_POINT ( 'NONE',  ( 3.714570900464285064, 4.396382807705524698, 1.082531754730560403 ) ) ;
#101130=CARTESIAN_POINT ( 'NONE',  ( -4.599240423533815125, 6.388866465587984322, 1.599625672291267398 ) ) ;
#101131=CARTESIAN_POINT ( 'NONE',  ( -9.020252271793614440, 9.418049160047695878, 0.7998128361456462443 ) ) ;
#101136=CARTESIAN_POINT ( 'NONE',  ( -0.7500000000000006661, 3.139583334016149418, -1.299038105676652011 ) ) ;
#101137=CARTESIAN_POINT ( 'NONE',  ( 10.06423010004587759, 10.63602329300870153, 0.000000000000000000 ) ) ;
#101141=CARTESIAN_POINT ( 'NONE',  ( -9.989660255170729641, 10.54902514065433827, -0.7998128361456291469 ) ) ;
#101143=CARTESIAN_POINT ( 'NONE',  ( -0.6823417656250212460, 2.301041667008084435, 1.181850606188767472 ) ) ;
#101148=VECTOR ( 'NONE', #116673, 1000.000000000000000 ) ;
#101151=CIRCLE ( 'NONE', #132278, 0.08000000000000027922 ) ;
#101152=CARTESIAN_POINT ( 'NONE',  ( -2.415323921528888196, 5.969628341758991930, 0.7998128361456341429 ) ) ;
#101156=CARTESIAN_POINT ( 'NONE',  ( 0.6823417656249882723, 1.488541667008083547, -1.181850606188749264 ) ) ;
#101161=EDGE_CURVE ( 'NONE', #154836, #72912, #168492, .T. ) ;
#101162=CARTESIAN_POINT ( 'NONE',  ( 1.364683531249988757, 1.134375000341421247, 0.000000000000000000 ) ) ;
#101164=CARTESIAN_POINT ( 'NONE',  ( -5.391338639728555648, 9.441645512991978961, -0.7998128361456231517 ) ) ;
#101165=CARTESIAN_POINT ( 'NONE',  ( 8.589254009457354400, 9.979550084910457031, -1.199719254218446718 ) ) ;
#101166=CARTESIAN_POINT ( 'NONE',  ( -1.420000000000021911, 8.627523663848661428, 2.580000000000011173 ) ) ;
#101167=CARTESIAN_POINT ( 'NONE',  ( 4.496500501226593727, 8.397667684739696270, 0.7998128361456462443 ) ) ;
#101169=CARTESIAN_POINT ( 'NONE',  ( 1.499999999999987121, 3.295833333333354709, -0.8660254037844262731 ) ) ;
#101171=CARTESIAN_POINT ( 'NONE',  ( -0.6823417656250003738, 1.030208333674752286, -1.181850606188749264 ) ) ;
#101174=CARTESIAN_POINT ( 'NONE',  ( 1.284279953904126748, 10.64264068711930733, -0.7749999999999874767 ) ) ;
#101178=CARTESIAN_POINT ( 'NONE',  ( 6.209271165378815738, 7.306866450105836464, -1.082531754730543083 ) ) ;
#101181=CARTESIAN_POINT ( 'NONE',  ( -7.641992139597101108, 12.06740792950531649, 0.7998128361456481317 ) ) ;
#101182=CARTESIAN_POINT ( 'NONE',  ( -3.358669367883384105, 4.941533567329135401, -1.599625672291262513 ) ) ;
#101186=CARTESIAN_POINT ( 'NONE',  ( -1.123270288250318494, 3.297697346350006331, -0.7749999999993560929 ) ) ;
#101188=CARTESIAN_POINT ( 'NONE',  ( -5.870317324592805086, 9.792527945426188651, -0.7216878364870197293 ) ) ;
#101190=CARTESIAN_POINT ( 'NONE',  ( 1.499999999999989120, 5.004166666666691299, 0.8660254037844524744 ) ) ;
#101194=CARTESIAN_POINT ( 'NONE',  ( 7.402388683381404988, 10.61957531637824204, -1.082531754730537976 ) ) ;
#101196=DIRECTION ( 'NONE',  ( -5.578564026256490882E-16, -1.000000000000000000, -9.066213480720158442E-32 ) ) ;
#101200=CARTESIAN_POINT ( 'NONE',  ( 4.500943809612556024, 4.353448654077163305, 1.214306433183764966E-14 ) ) ;
#101203=CARTESIAN_POINT ( 'NONE',  ( 8.717529583462633624, 13.11427558077437894, 0.7216878364870438212 ) ) ;
#101209=CARTESIAN_POINT ( 'NONE',  ( 7.019370843573166319, 9.212351955633947043, 1.599625672291281386 ) ) ;
#101211=CARTESIAN_POINT ( 'NONE',  ( -5.766295404513795297, 5.621766148221195358, 0.7998128361456341429 ) ) ;
#101214=CARTESIAN_POINT ( 'NONE',  ( 0.7499999999999902300, 5.066666666666684193, -1.299038105676658228 ) ) ;
#101216=CARTESIAN_POINT ( 'NONE',  ( 6.493992390821439642, 7.639041213122241381, -1.082531754730543971 ) ) ;
#101217=EDGE_CURVE ( 'NONE', #135745, #12495, #50987, .T. ) ;
#101218=CARTESIAN_POINT ( 'NONE',  ( -1.364683531250014514, -0.9072916663252470482, 0.7879004041258379498 ) ) ;
#101219=CARTESIAN_POINT ( 'NONE',  ( 3.768803514918948938, 4.459654191235965293, -1.082531754730543083 ) ) ;
#101220=CARTESIAN_POINT ( 'NONE',  ( -4.081167932913447594, 4.720116328942494555, -1.199719254218452047 ) ) ;
#101231=DIRECTION ( 'NONE',  ( 0.000000000000000000, 8.546850786086437571E-32, 1.000000000000000000 ) ) ;
#101237=CARTESIAN_POINT ( 'NONE',  ( 5.957918438201454059, 9.038323046955323292, -1.199719254218440723 ) ) ;
#101238=CARTESIAN_POINT ( 'NONE',  ( 5.960781091502512119, 10.10599504006161986, 0.7998128361456462443 ) ) ;
#101247=CARTESIAN_POINT ( 'NONE',  ( -2.279673327430177476, 5.603443282069742182, 1.040551764627347231E-14 ) ) ;
#101250=CARTESIAN_POINT ( 'NONE',  ( -6.084912014434944894, 5.993485526462540847, -0.7998128361456291469 ) ) ;
#101252=CARTESIAN_POINT ( 'NONE',  ( -5.115504031057831469, 4.862509545855891346, 0.7998128361456341429 ) ) ;
#101257=CARTESIAN_POINT ( 'NONE',  ( 1.408440994508643129, 7.230285460703517408, 4.273713947604631080 ) ) ;
#101261=CARTESIAN_POINT ( 'NONE',  ( -2.252626078164912560, 5.779814191167667481, 0.7998128361456341429 ) ) ;
#101264=CARTESIAN_POINT ( 'NONE',  ( 7.311924916471702396, 7.425000578838787391, -0.7998128361456281477 ) ) ;
#101265=CARTESIAN_POINT ( 'NONE',  ( -1.364683531250010740, 4.280208333674753618, 0.7879004041258379498 ) ) ;
#101271=CARTESIAN_POINT ( 'NONE',  ( 5.138177029454836564, 7.977995053463880382, 1.082531754730558626 ) ) ;
#101272=CARTESIAN_POINT ( 'NONE',  ( -5.181187258716735577, 9.196468901811520880, 0.7998128361456481317 ) ) ;
#101277=CARTESIAN_POINT ( 'NONE',  ( -6.157374318900681764, 10.33535380535947290, 0.7998128361456481317 ) ) ;
#101279=CARTESIAN_POINT ( 'NONE',  ( -5.225778143063529946, 8.184159369294361497, 1.199719254218452047 ) ) ;
#101280=DIRECTION ( 'NONE',  ( 1.000000000000000000, 0.000000000000000000, 0.000000000000000000 ) ) ;
#101284=EDGE_CURVE ( 'NONE', #145502, #99491, #158431, .T. ) ;
#101287=CARTESIAN_POINT ( 'NONE',  ( 8.423693512792301163, 8.722063941212843119, 0.7998128361456481317 ) ) ;
#101302=CARTESIAN_POINT ( 'NONE',  ( -1.201851678989727383E-14, 5.337500000000020783, -1.732050807568863648 ) ) ;
#101303=CARTESIAN_POINT ( 'NONE',  ( 5.034155109375821446, 4.767602470560229122, -0.7998128361456221525 ) ) ;
#101304=CARTESIAN_POINT ( 'NONE',  ( 4.469384193999260901, 8.366031992974468423, -0.7998128361456231517 ) ) ;
#101306=CARTESIAN_POINT ( 'NONE',  ( -7.158341918335454857, 10.33485409049125003, 1.082531754730549967 ) ) ;
#101307=CARTESIAN_POINT ( 'NONE',  ( -1.140665321753059347, 3.300000000000025135, -0.7542256614604591070 ) ) ;
#101308=CARTESIAN_POINT ( 'NONE',  ( 4.338245966692901412, 8.005111361209628740, -0.7216878364870197293 ) ) ;
#101309=CARTESIAN_POINT ( 'NONE',  ( -6.819388077549415783, 10.89977715720891815, 0.7216878364870458196 ) ) ;
#101311=ORIENTED_EDGE ( 'NONE', *, *, #160649, .F. ) ;
#101313=CARTESIAN_POINT ( 'NONE',  ( 6.265839547809997079, 10.46189657242035587, 0.7998128361456462443 ) ) ;
#101318=CARTESIAN_POINT ( 'NONE',  ( -1.364683531250012516, 3.030208333674755394, 0.7879004041258379498 ) ) ;
#101324=CARTESIAN_POINT ( 'NONE',  ( 9.610031953988080744, 10.10612545594124967, -0.7998128361456281477 ) ) ;
#101328=CARTESIAN_POINT ( 'NONE',  ( -9.501566725078754772, 9.979582688880366703, -0.7998128361456291469 ) ) ;
#101334=CARTESIAN_POINT ( 'NONE',  ( 2.866659414285625651, 5.431854185720147221, -1.199719254218446718 ) ) ;
#101337=CARTESIAN_POINT ( 'NONE',  ( -9.189729191964438826, 9.615772233580322848, 1.040834085586084257E-14 ) ) ;
#101343=CARTESIAN_POINT ( 'NONE',  ( 5.766360146646302809, 6.053989883630594981, 0.5864573027323967125 ) ) ;
#101344=CARTESIAN_POINT ( 'NONE',  ( -3.253066792275140173, 5.882662793374543675, 1.199719254218462483 ) ) ;
#101350=CARTESIAN_POINT ( 'NONE',  ( 6.531277313481192337, 8.642909503859968368, 1.599625672291281386 ) ) ;
#101352=CARTESIAN_POINT ( 'NONE',  ( 6.262976894508937242, 9.394224579314053969, -1.199719254218440723 ) ) ;
#101353=CARTESIAN_POINT ( 'NONE',  ( -4.356251871828045630, 7.199010410547511007, -1.027643995846918790 ) ) ;
#101354=CARTESIAN_POINT ( 'NONE',  ( 5.820528018968444961, 5.685037531751635953, 0.7998128361456341429 ) ) ;
#101356=CARTESIAN_POINT ( 'NONE',  ( -8.676855123066030018, 9.225345186439589895, -0.7216878364870267237 ) ) ;
#101363=CARTESIAN_POINT ( 'NONE',  ( -4.088066877127150001, 7.522549914775793489, 0.5433784229755319606 ) ) ;
#101367=CARTESIAN_POINT ( 'NONE',  ( 5.097502569058200983, 6.970172302033127210, -1.443375672974051449 ) ) ;
#101379=CARTESIAN_POINT ( 'NONE',  ( -9.612367721964606204, 12.23751498042398289, -1.443375672974058777 ) ) ;
#101387=CARTESIAN_POINT ( 'NONE',  ( -10.42585693878457853, 11.26584730477792284, -0.7216878364870267237 ) ) ;
#101395=CARTESIAN_POINT ( 'NONE',  ( -1.499999999999997780, 3.431250000682818602, 1.214306433183764966E-14 ) ) ;
#101397=CARTESIAN_POINT ( 'NONE',  ( -6.338600509588822263, 7.353787668397130162, -1.199719254218446718 ) ) ;
#101400=CARTESIAN_POINT ( 'NONE',  ( -7.160677686311960777, 11.50587440067263678, -0.7998128361456291469 ) ) ;
#101404=CARTESIAN_POINT ( 'NONE',  ( 6.612626235163189925, 8.737816579155630592, -1.599625672291262513 ) ) ;
#101411=CARTESIAN_POINT ( 'NONE',  ( 8.992082194361556091, 11.51384853155376220, 1.599625672291279388 ) ) ;
#101414=DIRECTION ( 'NONE',  ( 5.578564026256287751E-16, 1.000000000000000000, 0.000000000000000000 ) ) ;
#101418=CARTESIAN_POINT ( 'NONE',  ( -6.507550544879489252, 9.575597488125954015, 1.082531754730548412 ) ) ;
#101421=CARTESIAN_POINT ( 'NONE',  ( 0.6823417656249917140, 5.655208333674749177, 1.181850606188765695 ) ) ;
#101425=CARTESIAN_POINT ( 'NONE',  ( 1.364683531249990311, 5.363541667008086655, 0.7879004041258500513 ) ) ;
#101427=CARTESIAN_POINT ( 'NONE',  ( -3.348500752450953577, 4.929670182657964084, 1.443375672974062551 ) ) ;
#101429=CARTESIAN_POINT ( 'NONE',  ( 8.550388431712704573, 13.12720360364021133, 0.000000000000000000 ) ) ;
#101431=LINE ( 'NONE', #4959, #101148 ) ;
#101434=CARTESIAN_POINT ( 'NONE',  ( -1.201851678989727383E-14, 1.571875000341420581, 1.575800808251672791 ) ) ;
#101435=CARTESIAN_POINT ( 'NONE',  ( -2.467220768007014176, 5.822248629409386922, 0.7216878364870317197 ) ) ;
#101436=CARTESIAN_POINT ( 'NONE',  ( 3.174580523894166006, 6.855427711185178019, 0.7998128361456341429 ) ) ;
#101437=ADVANCED_FACE ( 'NONE', ( #13240 ), #44053, .T. ) ;
#101441=CARTESIAN_POINT ( 'NONE',  ( -5.335766472694951190, 4.384919054141811046, -2.499999999999995115 ) ) ;
#101443=CARTESIAN_POINT ( 'NONE',  ( 8.717529583462633624, 13.11427558077437894, 0.7216878364870438212 ) ) ;
#101445=CARTESIAN_POINT ( 'NONE',  ( -6.887178846062109727, 10.01849717283904262, -1.082531754730537976 ) ) ;
#101450=CARTESIAN_POINT ( 'NONE',  ( -8.296699936558862731, 11.76690146170562201, 1.199719254218453823 ) ) ;
#101452=CARTESIAN_POINT ( 'NONE',  ( -3.755245360860919757, 7.324943987738961049, -0.7216878364870257245 ) ) ;
#101453=CARTESIAN_POINT ( 'NONE',  ( -1.402160292154681736E-14, 2.259375000341416140, -1.575800808251660134 ) ) ;
#101458=EDGE_CURVE ( 'NONE', #164652, #81936, #165098, .T. ) ;
#101462=AXIS2_PLACEMENT_3D ( 'NONE', #133243, #199248, #45221 ) ;
#101475=CARTESIAN_POINT ( 'NONE',  ( 0.6823417656249917140, 4.155208333674755394, 1.181850606188765695 ) ) ;
#101483=CARTESIAN_POINT ( 'NONE',  ( 8.398386088661320414, 11.88553530582519357, -1.199719254218446718 ) ) ;
#101486=CARTESIAN_POINT ( 'NONE',  ( 1.364683531249990311, 2.634375000341422801, 1.214306433183764966E-14 ) ) ;
#101489=CARTESIAN_POINT ( 'NONE',  ( -8.242994207428740339, 9.679543332497402730, 1.082531754730558626 ) ) ;
#101497=CARTESIAN_POINT ( 'NONE',  ( 5.542585869888291938, 5.360771691158120689, -0.7998128361456211532 ) ) ;
#101501=CARTESIAN_POINT ( 'NONE',  ( 9.083072846151447166, 12.68433652289702884, 1.199719254218450271 ) ) ;
#101506=ORIENTED_EDGE ( 'NONE', *, *, #140892, .F. ) ;
#101508=CARTESIAN_POINT ( 'NONE',  ( -4.783329267523015460, 4.474972321731942593, -0.7998128361456221525 ) ) ;
#101509=CARTESIAN_POINT ( 'NONE',  ( 8.782984583554449998, 9.141236857102018831, 1.040834085586084257E-14 ) ) ;
#101511=CARTESIAN_POINT ( 'NONE',  ( 5.138177029454852551, 5.096887410559856946, 0.7216878364870317197 ) ) ;
#101521=CARTESIAN_POINT ( 'NONE',  ( -6.182154858151506893, 9.195969186943299789, 1.082531754730548412 ) ) ;
#101523=CARTESIAN_POINT ( 'NONE',  ( 5.820528018968444961, 5.685037531751635953, 0.7998128361456341429 ) ) ;
#101527=CARTESIAN_POINT ( 'NONE',  ( -8.350932551013499960, 11.83017284523606172, -1.199719254218446718 ) ) ;
#101532=CARTESIAN_POINT ( 'NONE',  ( -4.308793891044708779, 3.921347715840572956, 1.214306433183764966E-14 ) ) ;
#101534=CARTESIAN_POINT ( 'NONE',  ( 8.503988664269582998, 10.94440607977979063, 1.599625672291281386 ) ) ;
#101536=CARTESIAN_POINT ( 'NONE',  ( 3.623053363349855172, 5.249981562040033189, 1.599625672291267398 ) ) ;
#101542=CARTESIAN_POINT ( 'NONE',  ( 4.216222584169931231, 4.021273891060765493, 1.214306433183764966E-14 ) ) ;
#101545=CARTESIAN_POINT ( 'NONE',  ( -5.590039407536138150, 5.416134151747256986, 0.000000000000000000 ) ) ;
#101548=CARTESIAN_POINT ( 'NONE',  ( -7.974166903131914452, 12.45494515362926435, -0.7998128361456281477 ) ) ;
#101553=CARTESIAN_POINT ( 'NONE',  ( 6.127922243696800386, 10.09306701771420656, -0.7216878364870267237 ) ) ;
#101556=CARTESIAN_POINT ( 'NONE',  ( 4.521807925357579805, 5.234196320127330715, -1.199719254218452047 ) ) ;
#101558=CARTESIAN_POINT ( 'NONE',  ( 4.599240423533799138, 6.388866465587984322, 1.599625672291267398 ) ) ;
#101560=CARTESIAN_POINT ( 'NONE',  ( -6.028571859570855729, 10.18508426947466816, 0.000000000000000000 ) ) ;
#101570=CARTESIAN_POINT ( 'NONE',  ( -0.6823417656250212460, 2.863541667008084879, 1.181850606188767472 ) ) ;
#101571=CARTESIAN_POINT ( 'NONE',  ( 4.241003122976366058, 3.842258486427521103, -0.7998128361456211532 ) ) ;
#101573=CARTESIAN_POINT ( 'NONE',  ( -4.555176424511596878, 7.297827681030051750, 1.082531754730560403 ) ) ;
#101574=CARTESIAN_POINT ( 'NONE',  ( 3.877268743828276243, 4.586196958296845594, 1.082531754730560403 ) ) ;
#101575=CARTESIAN_POINT ( 'NONE',  ( -5.002595493318215070, 7.819816594637776674, 1.082531754730560403 ) ) ;
#101581=CARTESIAN_POINT ( 'NONE',  ( 4.684505768721569652, 5.424010470718658716, -1.199719254218452047 ) ) ;
#101591=CARTESIAN_POINT ( 'NONE',  ( 6.063521013809720195, 8.097193820909906137, 1.599625672291281386 ) ) ;
#101595=CARTESIAN_POINT ( 'NONE',  ( -6.762819695118240659, 6.784377820593065600, 0.7998128361456341429 ) ) ;
#101599=CARTESIAN_POINT ( 'NONE',  ( 7.298366762858032430, 7.409182732956175244, 1.040834085586084257E-14 ) ) ;
#101602=CARTESIAN_POINT ( 'NONE',  ( -6.600121851754250812, 6.594563670001734046, 0.7998128361456341429 ) ) ;
#101603=CARTESIAN_POINT ( 'NONE',  ( 5.572037945092146671, 8.484166121707415797, -1.082531754730543971 ) ) ;
#101604=CARTESIAN_POINT ( 'NONE',  ( 4.314144046604536875, 7.442532859859907646, 1.092782195075291396 ) ) ;
#101605=EDGE_CURVE ( 'NONE', #18526, #80644, #59917, .T. ) ;
#101606=CARTESIAN_POINT ( 'NONE',  ( -4.436542580169821726, 6.199052314996659874, 1.599625672291267398 ) ) ;
#101609=CARTESIAN_POINT ( 'NONE',  ( -4.401593425930945713, 8.286942763561420122, 1.040834085586084257E-14 ) ) ;
#101613=CARTESIAN_POINT ( 'NONE',  ( -0.6823417656250212460, 2.301041667008084435, 1.181850606188767472 ) ) ;
#101615=CARTESIAN_POINT ( 'NONE',  ( -4.229780737783618072, 6.918199379847403740, 1.082531754730560403 ) ) ;
#101622=CARTESIAN_POINT ( 'NONE',  ( 5.301401758143367893, 6.143722458377430584, 1.199719254218462483 ) ) ;
#101624=CARTESIAN_POINT ( 'NONE',  ( -0.6823417656250003738, 2.780208333674753618, -1.181850606188749264 ) ) ;
#101628=CARTESIAN_POINT ( 'NONE',  ( -0.6823417656250246877, -1.136458332991911790, 1.181850606188755259 ) ) ;
#101632=CARTESIAN_POINT ( 'NONE',  ( -3.704402285031864306, 5.344888637335695414, -1.599625672291256295 ) ) ;
#101633=CARTESIAN_POINT ( 'NONE',  ( -6.182154857707119255, 10.15633840072622363, 0.000000000000000000 ) ) ;
#101635=CARTESIAN_POINT ( 'NONE',  ( -1.201851678989727383E-14, 3.071875000341420137, 1.575800808251672791 ) ) ;
#101643=CARTESIAN_POINT ( 'NONE',  ( -8.161645285302366659, 8.624267042381978499, 1.040834085586084257E-14 ) ) ;
#101648=CARTESIAN_POINT ( 'NONE',  ( -5.694061327615147050, 9.586895948952255608, 0.000000000000000000 ) ) ;
#101661=CARTESIAN_POINT ( 'NONE',  ( -6.501298352952815662, 7.543601818988450169, -1.199719254218446718 ) ) ;
#101663=CARTESIAN_POINT ( 'NONE',  ( 1.499999999999987121, -0.2458333333333099502, 0.8660254037844524744 ) ) ;
#101664=CARTESIAN_POINT ( 'NONE',  ( 2.849184837166184536, 6.475799410002530898, 0.7998128361456362523 ) ) ;
#101668=CARTESIAN_POINT ( 'NONE',  ( 6.277588818327314080, 7.282607361925381717, 1.199719254218462483 ) ) ;
#101673=CARTESIAN_POINT ( 'NONE',  ( -5.585596099150199834, 5.618876325204420930, -0.7216878364870207285 ) ) ;
#101676=CARTESIAN_POINT ( 'NONE',  ( -0.5987733972867143040, 6.693213315561105325, 3.557617754081424888 ) ) ;
#101681=CARTESIAN_POINT ( 'NONE',  ( 1.364683531249986537, 1.655208333674748955, -0.7879004041258239610 ) ) ;
#101683=CARTESIAN_POINT ( 'NONE',  ( -8.688077508258798431, 9.030511935923748013, -0.7998128361456291469 ) ) ;
#101686=CARTESIAN_POINT ( 'NONE',  ( 6.337546739384100292, 9.481222731668410120, 1.199719254218460707 ) ) ;
#101687=CARTESIAN_POINT ( 'NONE',  ( -6.042130013184518589, 10.20090211535728031, -0.7998128361456291469 ) ) ;
#101690=CARTESIAN_POINT ( 'NONE',  ( 0.6823417656249917140, 5.592708333674749177, 1.181850606188765695 ) ) ;
#101692=CARTESIAN_POINT ( 'NONE',  ( 7.131225611108079399, 11.26358761302737754, 0.7216878364870438212 ) ) ;
#101696=CARTESIAN_POINT ( 'NONE',  ( -1.364683531250014514, 0.05104166700808546175, -0.7879004041258359514 ) ) ;
#101699=CARTESIAN_POINT ( 'NONE',  ( 8.568389893712330618, 9.098802418860289620, 1.040834085586084257E-14 ) ) ;
#101701=CARTESIAN_POINT ( 'NONE',  ( -4.690757960648240577, 6.495636925554817864, 1.443375672974064550 ) ) ;
#101703=CARTESIAN_POINT ( 'NONE',  ( 1.364683531249988535, 3.905208333674751842, -0.7879004041258239610 ) ) ;
#101707=CARTESIAN_POINT ( 'NONE',  ( -5.856232286098998152, 8.919689202835742847, 1.199719254218452047 ) ) ;
#101716=CARTESIAN_POINT ( 'NONE',  ( 8.444030743212801227, 8.745790710036752458, 0.7998128361456462443 ) ) ;
#101720=CARTESIAN_POINT ( 'NONE',  ( 0.7499999999999902300, 2.483333333333351156, 1.299038105676669330 ) ) ;
#101726=CARTESIAN_POINT ( 'NONE',  ( 6.643132081016124069, 7.813037518349371879, 1.082531754730558626 ) ) ;
#101727=CARTESIAN_POINT ( 'NONE',  ( -1.402160292154681736E-14, 0.3843750003414230232, 1.575800808251672791 ) ) ;
#101729=CARTESIAN_POINT ( 'NONE',  ( 8.920375002787457319, 12.49452237230570084, 1.199719254218450271 ) ) ;
#101736=CARTESIAN_POINT ( 'NONE',  ( -1.500000000000001332, 0.6500000000000255573, 0.000000000000000000 ) ) ;
#101737=CARTESIAN_POINT ( 'NONE',  ( 6.591235234537977661, 10.84152487360300299, 0.7998128361456462443 ) ) ;
#101738=CARTESIAN_POINT ( 'NONE',  ( -7.967387826325084355, 12.44703623068796361, 0.7998128361456481317 ) ) ;
#101741=CARTESIAN_POINT ( 'NONE',  ( 1.364683531249986537, 1.155208333674754728, -0.7879004041258239610 ) ) ;
#101742=CARTESIAN_POINT ( 'NONE',  ( -1.500000000000011324, 2.670833333333352044, 0.8660254037844403729 ) ) ;
#101744=CARTESIAN_POINT ( 'NONE',  ( 5.671388329218120639, 5.511041227042920099, 1.040834085586084257E-14 ) ) ;
#101752=CARTESIAN_POINT ( 'NONE',  ( -1.500000000000015099, -0.7979166659838445863, 0.8660254037844403729 ) ) ;
#101753=CARTESIAN_POINT ( 'NONE',  ( -6.333630315878337136, 10.54098580183340772, 0.000000000000000000 ) ) ;
#101754=CARTESIAN_POINT ( 'NONE',  ( -4.256897045010916258, 7.910204285913967404, 0.7216878364870317197 ) ) ;
#101762=CARTESIAN_POINT ( 'NONE',  ( 6.252281394196331554, 10.44607872653774372, 1.040834085586084257E-14 ) ) ;
#101765=CARTESIAN_POINT ( 'NONE',  ( 5.951666246274784910, 9.887435020721849099, 0.7216878364870438212 ) ) ;
#101769=CARTESIAN_POINT ( 'NONE',  ( -6.482770005628665011, 10.71498210654212002, 0.7998128361456481317 ) ) ;
#101770=CARTESIAN_POINT ( 'NONE',  ( 4.517891501851804215, 6.293959390292322986, -1.599625672291255185 ) ) ;
#101775=CARTESIAN_POINT ( 'NONE',  ( 10.24960094225127172, 11.06021530882240356, -0.7216878364870257245 ) ) ;
#101780=EDGE_CURVE ( 'NONE', #212421, #191425, #123606, .T. ) ;
#101783=CARTESIAN_POINT ( 'NONE',  ( -1.501328131443588232, 8.653248444470658995, -2.562127481693517783 ) ) ;
#101784=CARTESIAN_POINT ( 'NONE',  ( -4.799223189557577207, 4.701441264013013210, 0.7216878364870317197 ) ) ;
#101785=CARTESIAN_POINT ( 'NONE',  ( 8.093854517678360949, 12.38665467069271386, 1.040834085586084257E-14 ) ) ;
#101788=CARTESIAN_POINT ( 'NONE',  ( -6.230135280679522936, 7.227244901336242755, 1.199719254218450271 ) ) ;
#101794=CARTESIAN_POINT ( 'NONE',  ( -6.886651960737580680, 10.12184548991413457, -1.199719254218440723 ) ) ;
#101808=CARTESIAN_POINT ( 'NONE',  ( -5.880485940025243607, 7.883652901494672349, 1.599625672291269396 ) ) ;
#101811=CARTESIAN_POINT ( 'NONE',  ( 5.341549334104200852, 5.334155099317434257, 0.7216878364870317197 ) ) ;
#101816=CARTESIAN_POINT ( 'NONE',  ( -5.596818484342970912, 5.424043074688562172, -0.7998128361456221525 ) ) ;
#101825=CARTESIAN_POINT ( 'NONE',  ( -8.642432853707342488, 12.17025653171218558, 1.199719254218462483 ) ) ;
#101826=CARTESIAN_POINT ( 'NONE',  ( 5.503720292143644777, 8.508425209887878538, 1.199719254218462483 ) ) ;
#101830=CARTESIAN_POINT ( 'NONE',  ( -9.110189153378817295, 12.71597221466224603, 1.199719254218462483 ) ) ;
#101833=CARTESIAN_POINT ( 'NONE',  ( -0.6823417656250246877, -0.3864583329919110688, 1.181850606188755259 ) ) ;
#101838=CARTESIAN_POINT ( 'NONE',  ( 7.280365300858406385, 11.43758391773608984, 1.040834085586084257E-14 ) ) ;
#101842=CARTESIAN_POINT ( 'NONE',  ( 0.000000000000000000, 2.800000000000024691, -0.7749999999999935829 ) ) ;
#101843=CARTESIAN_POINT ( 'NONE',  ( -5.478522506877910203, 6.271832789251446272, -1.004670684072657583 ) ) ;
#101845=CARTESIAN_POINT ( 'NONE',  ( 0.08888683327021046354, 6.492044364012832247, -3.106763327641855810 ) ) ;
#101865=CARTESIAN_POINT ( 'NONE',  ( -1.500000000000001332, -0.3187499993171846735, 0.000000000000000000 ) ) ;
#101871=CARTESIAN_POINT ( 'NONE',  ( 1.419999999067300234, 7.203691543881690862, -4.238255391842187692 ) ) ;
#101872=CARTESIAN_POINT ( 'NONE',  ( 0.4914377447849272440, 7.519435632882160547, -2.014015809874914797 ) ) ;
#101874=CARTESIAN_POINT ( 'NONE',  ( 9.725276259704228821, 10.24057714594344048, 0.7998128361456462443 ) ) ;
#101880=CARTESIAN_POINT ( 'NONE',  ( 4.684505768721569652, 5.424010470718658716, -1.199719254218452047 ) ) ;
#101881=CARTESIAN_POINT ( 'NONE',  ( -1.364683531250012516, 2.301041667008087988, -0.7879004041258289570 ) ) ;
#101882=CARTESIAN_POINT ( 'NONE',  ( -5.906232603126833958, 6.003624899985508634, 0.1331734367991978252 ) ) ;
#101885=CARTESIAN_POINT ( 'NONE',  ( -7.320512876374914768, 10.62801655815766999, 1.199719254218453823 ) ) ;
#101886=CARTESIAN_POINT ( 'NONE',  ( -5.219525951136862574, 5.191794485855519170, -0.7216878364870197293 ) ) ;
#101890=CARTESIAN_POINT ( 'NONE',  ( -1.500000000000015099, -0.5479166659838513587, 0.8660254037844403729 ) ) ;
#101897=CARTESIAN_POINT ( 'NONE',  ( -5.382223794500852421, 5.381608636446842731, -0.7216878364870197293 ) ) ;
#101905=CARTESIAN_POINT ( 'NONE',  ( -4.080641047588918546, 4.823464646017586510, -1.082531754730548412 ) ) ;
#101906=CARTESIAN_POINT ( 'NONE',  ( 8.422639742587595180, 10.84949900448412130, -1.599625672291268286 ) ) ;
#101915=CARTESIAN_POINT ( 'NONE',  ( -4.464712657601869417, 4.103252943490596216, 0.7998128361456341429 ) ) ;
#101921=CARTESIAN_POINT ( 'NONE',  ( 3.832150974156964818, 7.622593236491780999, 1.040834085586084257E-14 ) ) ;
#101927=CARTESIAN_POINT ( 'NONE',  ( 4.162516854595432747, 4.815023404238158555, 1.199719254218464037 ) ) ;
#101929=ORIENTED_EDGE ( 'NONE', *, *, #34246, .F. ) ;
#101933=CARTESIAN_POINT ( 'NONE',  ( -6.520158902582635640, 5.290451655907115303, 2.438235897557452514 ) ) ;
#101938=CARTESIAN_POINT ( 'NONE',  ( 7.964525173024008531, 11.37936423758166526, 1.199719254218460707 ) ) ;
#101940=CARTESIAN_POINT ( 'NONE',  ( -4.089755892816631544, 7.923132308261379819, -0.7998128361456281477 ) ) ;
#101946=CARTESIAN_POINT ( 'NONE',  ( 1.364683531249992088, 5.384375000341417916, 1.214306433183764966E-14 ) ) ;
#101950=CARTESIAN_POINT ( 'NONE',  ( 4.059776932288224671, 6.823824623389866950, 1.199719254218462483 ) ) ;
#101951=CARTESIAN_POINT ( 'NONE',  ( -3.815730167242251003, 6.539103397502874948, -1.199719254218452047 ) ) ;
#101957=CARTESIAN_POINT ( 'NONE',  ( 4.826339496784873617, 8.574553812983598533, -0.7216878364870257245 ) ) ;
#101958=EDGE_CURVE ( 'NONE', #21610, #86388, #193431, .T. ) ;
#101961=CARTESIAN_POINT ( 'NONE',  ( 8.392133896734671694, 8.893170422386358354, 0.7216878364870458196 ) ) ;
#101962=CARTESIAN_POINT ( 'NONE',  ( -1.364683531249997417, 4.071875000341417028, 1.214306433183764966E-14 ) ) ;
#101964=CARTESIAN_POINT ( 'NONE',  ( 4.161989969270895706, 5.878740935614591656, 1.443375672974062551 ) ) ;
#101968=CARTESIAN_POINT ( 'NONE',  ( 5.405874916910509143, 6.287787029864440491, -1.050246922354510559 ) ) ;
#101971=CARTESIAN_POINT ( 'NONE',  ( -4.549609453380520030, 7.192579769413725010, 1.336992641046318875 ) ) ;
#101974=CARTESIAN_POINT ( 'NONE',  ( 1.364683531249990311, 4.926041667008083991, 0.7879004041258500513 ) ) ;
#101978=CARTESIAN_POINT ( 'NONE',  ( -8.157201976916404362, 12.66848607304450702, -0.7998128361456281477 ) ) ;
#101988=CARTESIAN_POINT ( 'NONE',  ( 3.470524135418292300, 5.072030796119872953, -1.443375672974057666 ) ) ;
#101989=CARTESIAN_POINT ( 'NONE',  ( 1.364683531249988535, 4.176041667008081326, 0.7879004041258500513 ) ) ;
#101991=CARTESIAN_POINT ( 'NONE',  ( 6.612626235163189925, 8.737816579155630592, -1.599625672291262513 ) ) ;
#101993=CARTESIAN_POINT ( 'NONE',  ( -8.130085669689073313, 12.63685038127928806, 0.7998128361456481317 ) ) ;
#102000=CARTESIAN_POINT ( 'NONE',  ( -1.201851678989727383E-14, 4.087500000000022560, -1.732050807568863648 ) ) ;
#102005=EDGE_CURVE ( 'NONE', #115335, #199311, #137435, .T. ) ;
#102007=CARTESIAN_POINT ( 'NONE',  ( 9.083599731475992201, 9.699880562917908122, 0.7216878364870438212 ) ) ;
#102013=CARTESIAN_POINT ( 'NONE',  ( 1.499999999999989120, 3.056250000682818158, 1.214306433183764966E-14 ) ) ;
#102015=CARTESIAN_POINT ( 'NONE',  ( -4.446184310277715213, 7.274633231044262516, -1.199719254218452047 ) ) ;
#102017=CARTESIAN_POINT ( 'NONE',  ( 2.846849068745292755, 6.265148313604064434, 0.000000000000000000 ) ) ;
#102018=CARTESIAN_POINT ( 'NONE',  ( -8.459924664802993988, 12.81373650900478189, 1.040834085586084257E-14 ) ) ;
#102024=ORIENTED_EDGE ( 'NONE', *, *, #174354, .F. ) ;
#102026=CARTESIAN_POINT ( 'NONE',  ( 7.958799866421889746, 9.244020251369077457, -1.199719254218441611 ) ) ;
#102027=CARTESIAN_POINT ( 'NONE',  ( 5.183294799126148433, 4.941598775268944976, 1.040834085586084257E-14 ) ) ;
#102030=CARTESIAN_POINT ( 'NONE',  ( 4.273844736805816780, 6.009238164405336313, 1.599625672291267398 ) ) ;
#102032=ORIENTED_EDGE ( 'NONE', *, *, #121074, .T. ) ;
#102034=ORIENTED_EDGE ( 'NONE', *, *, #60236, .F. ) ;
#102036=AXIS2_PLACEMENT_3D ( 'NONE', #198944, #103620, #53798 ) ;
#102039=PLANE ( 'NONE',  #153028 ) ;
#102043=CARTESIAN_POINT ( 'NONE',  ( 4.708705726121224622, 6.822254573549790813, -1.234111767277449534 ) ) ;
#102045=CARTESIAN_POINT ( 'NONE',  ( 9.083072846151447166, 12.68433652289702884, 1.199719254218450271 ) ) ;
#102050=CARTESIAN_POINT ( 'NONE',  ( -1.499999999999997780, 5.681250000682820378, 1.214306433183764966E-14 ) ) ;
#102052=CARTESIAN_POINT ( 'NONE',  ( 6.805829924380114804, 8.002851668940699881, 1.082531754730558626 ) ) ;
#102054=CARTESIAN_POINT ( 'NONE',  ( -9.002250809793991948, 12.48608113052627289, -1.082531754730543971 ) ) ;
#102060=CARTESIAN_POINT ( 'NONE',  ( -4.608882153641705059, 7.464447381635583412, -1.199719254218452047 ) ) ;
#102070=CARTESIAN_POINT ( 'NONE',  ( 9.097684769969825780, 10.57271930550834860, -1.199719254218446718 ) ) ;
#102071=CARTESIAN_POINT ( 'NONE',  ( 6.029390871727402512, 6.069343164222702924, -0.5281050654588164139 ) ) ;
#102077=CARTESIAN_POINT ( 'NONE',  ( -8.595506201384022660, 11.05117653974661529, 1.443375672974064550 ) ) ;
#102081=CARTESIAN_POINT ( 'NONE',  ( 6.913768267964901071, 10.15348118167935709, -1.199719254218441611 ) ) ;
#102084=CARTESIAN_POINT ( 'NONE',  ( 3.867100128395839942, 5.534702787927018974, -1.599625672291255185 ) ) ;
#102086=CARTESIAN_POINT ( 'NONE',  ( -6.551614543901706611, 8.666636272683888365, 1.599625672291283607 ) ) ;
#102087=CARTESIAN_POINT ( 'NONE',  ( 2.822068529938852155, 6.444163718237301275, -0.7998128361456291469 ) ) ;
#102090=CARTESIAN_POINT ( 'NONE',  ( 8.594979316059474073, 12.11489407112305372, 1.199719254218450271 ) ) ;
#102091=CARTESIAN_POINT ( 'NONE',  ( 0.4426559099768930805, 6.562653563187502925, 3.383538084249848144 ) ) ;
#102094=CARTESIAN_POINT ( 'NONE',  ( 4.291716407524416077, 7.230775179981989709, -0.9765121647202840149 ) ) ;
#102096=CARTESIAN_POINT ( 'NONE',  ( 5.287316719649520991, 8.151991358691011769, -1.082531754730549078 ) ) ;
#102103=CARTESIAN_POINT ( 'NONE',  ( 8.880227426826641235, 10.42298208846167284, 1.082531754730549967 ) ) ;
#102106=CARTESIAN_POINT ( 'NONE',  ( -7.004758919754800139, 11.32396917302262018, 0.000000000000000000 ) ) ;
#102108=DIRECTION ( 'NONE',  ( -1.000000000000000000, 5.578564026256503701E-16, -1.972152263052529514E-31 ) ) ;
#102117=CARTESIAN_POINT ( 'NONE',  ( 8.543609354905870035, 13.11929468069890525, 0.7998128361456462443 ) ) ;
#102121=CARTESIAN_POINT ( 'NONE',  ( 3.147464216666835402, 6.823792019419957278, -0.7998128361456291469 ) ) ;
#102124=CARTESIAN_POINT ( 'NONE',  ( 0.7499999999999920064, 4.014583334016149863, 1.299038105676669330 ) ) ;
#102128=EDGE_LOOP ( 'NONE', ( #4409, #163429, #31444, #206205 ) ) ;
#102130=CARTESIAN_POINT ( 'NONE',  ( -1.201851678989727383E-14, 1.462500000000018119, 1.732050807568877637 ) ) ;
#102131=CARTESIAN_POINT ( 'NONE',  ( 5.615048174354031474, 9.702639970055050966, 0.7998128361456462443 ) ) ;
#102132=CARTESIAN_POINT ( 'NONE',  ( 5.151735183068521629, 5.112705256442466428, 1.040834085586084257E-14 ) ) ;
#102137=CARTESIAN_POINT ( 'NONE',  ( 8.188761592974039161, 10.57664116326830595, -1.443375672974063439 ) ) ;
#102140=AXIS2_PLACEMENT_3D ( 'NONE', #11999, #161482, #147354 ) ;
#102144=CARTESIAN_POINT ( 'NONE',  ( -3.744022975668147790, 7.519777238254810925, -0.7998128361456281477 ) ) ;
#102146=CARTESIAN_POINT ( 'NONE',  ( 1.499999999999989120, 4.035416667349482012, 0.8660254037844524744 ) ) ;
#102147=CARTESIAN_POINT ( 'NONE',  ( -0.6823417656250212460, 5.363541667008087543, 1.181850606188767472 ) ) ;
#102151=CARTESIAN_POINT ( 'NONE',  ( 8.825994812371966702, 12.28044913353391898, -1.082531754730543083 ) ) ;
#102153=CARTESIAN_POINT ( 'NONE',  ( 1.364683531249990311, 3.446875000341416584, 1.214306433183764966E-14 ) ) ;
#102159=DIRECTION ( 'NONE',  ( 0.7592566023652971285, -0.6507913734559680474, 0.000000000000000000 ) ) ;
#102161=CARTESIAN_POINT ( 'NONE',  ( -7.232384877886063990, 10.52520055992070525, -1.199719254218446718 ) ) ;
#102162=CARTESIAN_POINT ( 'NONE',  ( 7.169564303528210836, 7.258913197071374945, -0.7998128361456281477 ) ) ;
#102164=CARTESIAN_POINT ( 'NONE',  ( -0.6823417656250003738, -0.2822916663252489355, -1.181850606188749264 ) ) ;
#102168=CARTESIAN_POINT ( 'NONE',  ( -4.909104350095669034, 4.829635951307452046, 0.07536873999081075692 ) ) ;
#102170=CARTESIAN_POINT ( 'NONE',  ( -5.096975683733680818, 8.033889833409558534, -1.199719254218452047 ) ) ;
#102173=CARTESIAN_POINT ( 'NONE',  ( 10.16199982864259788, 11.81442020729326536, 1.199719254218452047 ) ) ;
#102175=CARTESIAN_POINT ( 'NONE',  ( 9.752392566931574081, 10.27221283770866300, -0.7998128361456281477 ) ) ;
#102178=CARTESIAN_POINT ( 'NONE',  ( -4.009460741339347045, 5.700790169694431420, -1.599625672291256295 ) ) ;
#102179=CARTESIAN_POINT ( 'NONE',  ( -9.006694118179950692, 9.402231314165087284, 1.040834085586084257E-14 ) ) ;
#102180=AXIS2_PLACEMENT_3D ( 'NONE', #187535, #108497, #209098 ) ;
#102182=CARTESIAN_POINT ( 'NONE',  ( -4.867404985860277478, 6.905081695904778272, 1.445136279841979121 ) ) ;
#102183=CARTESIAN_POINT ( 'NONE',  ( 1.364683531249988757, -0.3656249996585800299, 0.000000000000000000 ) ) ;
#102187=CARTESIAN_POINT ( 'NONE',  ( 7.456621297836067086, 10.68284669990868174, 1.082531754730558626 ) ) ;
#102190=CARTESIAN_POINT ( 'NONE',  ( 5.656776405399742025, 7.622658444431597680, -1.599625672291262513 ) ) ;
#102195=AXIS2_PLACEMENT_3D ( 'NONE', #192605, #74615, #161196 ) ;
#102213=CARTESIAN_POINT ( 'NONE',  ( -6.821723845970312894, 11.11042825360738284, 0.000000000000000000 ) ) ;
#102214=CARTESIAN_POINT ( 'NONE',  ( 1.419999999999989049, 6.280000000000042881, -2.579999999999995630 ) ) ;
#102218=CARTESIAN_POINT ( 'NONE',  ( 1.499999999999989120, 1.556250000682817047, 0.000000000000000000 ) ) ;
#102219=CARTESIAN_POINT ( 'NONE',  ( 10.38962578677386084, 11.01565159419135043, 0.000000000000000000 ) ) ;
#102220=CARTESIAN_POINT ( 'NONE',  ( -4.909853179035948756, 4.660783761091170874, 0.1377329554490049068 ) ) ;
#102223=CARTESIAN_POINT ( 'NONE',  ( -9.480175724453545172, 12.08329098332774265, 1.599625672291281386 ) ) ;
#102224=CARTESIAN_POINT ( 'NONE',  ( 4.650083499807235121, 5.295740330745369207, 1.082471891955963716 ) ) ;
#102225=CARTESIAN_POINT ( 'NONE',  ( -1.364683531250014514, 1.738541667008085545, -0.7879004041258289570 ) ) ;
#102230=CARTESIAN_POINT ( 'NONE',  ( -4.627410500965859264, 4.293067094081919777, 0.7998128361456341429 ) ) ;
#102234=CARTESIAN_POINT ( 'NONE',  ( -0.6823417656250246877, 0.1135416670080893753, 1.181850606188755259 ) ) ;
#102239=CARTESIAN_POINT ( 'NONE',  ( -0.6823417656250003738, 1.717708333674752730, -1.181850606188749264 ) ) ;
#102241=CARTESIAN_POINT ( 'NONE',  ( -6.226218857173722476, 8.287007971501239467, 1.599625672291283607 ) ) ;
#102242=CARTESIAN_POINT ( 'NONE',  ( 8.586391356156291010, 8.911878091804165791, 0.7998128361456481317 ) ) ;
#102243=CARTESIAN_POINT ( 'NONE',  ( 4.813308228051395687, 5.574280006603454574, 1.199719254218462483 ) ) ;
#102244=CARTESIAN_POINT ( 'NONE',  ( 5.331380718671758778, 7.243030143248949670, -1.599625672291256295 ) ) ;
#102246=CARTESIAN_POINT ( 'NONE',  ( -1.499999999999997780, 3.900000000000021672, 1.214306433183764966E-14 ) ) ;
#102248=CARTESIAN_POINT ( 'NONE',  ( -1.364683531250012516, 1.342708333674755616, 0.7879004041258379498 ) ) ;
#102254=CARTESIAN_POINT ( 'NONE',  ( 5.287316719649520991, 8.151991358691011769, -1.082531754730549078 ) ) ;
#102257=CARTESIAN_POINT ( 'NONE',  ( -7.666245793523398078, 11.03137162816423356, 1.199719254218453823 ) ) ;
#102258=CARTESIAN_POINT ( 'NONE',  ( -5.576481253922474401, 5.400316305864651056, -0.7998128361456221525 ) ) ;
#102262=CARTESIAN_POINT ( 'NONE',  ( -6.466876083594135238, 9.528143949959703818, 1.082531754730548412 ) ) ;
#102264=CARTESIAN_POINT ( 'NONE',  ( -1.201851678989727383E-14, 5.587500000000021672, -1.732050807568863648 ) ) ;
#102267=CARTESIAN_POINT ( 'NONE',  ( 7.619319141200057821, 10.87266085050000974, 1.082531754730557072 ) ) ;
#102269=LINE ( 'NONE', #53522, #171587 ) ;
#102273=ORIENTED_EDGE ( 'NONE', *, *, #82128, .T. ) ;
#102274=CARTESIAN_POINT ( 'NONE',  ( 8.703971429848968100, 13.09845773489176679, 0.000000000000000000 ) ) ;
#102280=CARTESIAN_POINT ( 'NONE',  ( 6.317209508963599340, 9.457495962844502557, 1.199719254218462483 ) ) ;
#102281=CARTESIAN_POINT ( 'NONE',  ( -4.985647801523292344, 6.839675073242382553, -1.599625672291256295 ) ) ;
#102285=( BOUNDED_CURVE ( )  B_SPLINE_CURVE ( 2, ( #117415, #70699, #120632, #102168, #200704 ),
 .UNSPECIFIED., .F., .T. ) 
 B_SPLINE_CURVE_WITH_KNOTS ( ( 3, 2, 3 ),
 ( 0.1122816501277887347, 0.1125000000000000028, 0.1129944696182164920 ),
 .UNSPECIFIED. ) 
 CURVE ( )  GEOMETRIC_REPRESENTATION_ITEM ( )  RATIONAL_B_SPLINE_CURVE ( ( 0.9866942343795583881, 0.9929791993688261709, 1.000000000000000000, 0.9841008718140600298, 0.9719753288332768637 ) ) 
 REPRESENTATION_ITEM ( '' )  );
#102288=CARTESIAN_POINT ( 'NONE',  ( 5.626270559546810546, 8.547437505237857280, 1.082531754730558626 ) ) ;
#102289=CARTESIAN_POINT ( 'NONE',  ( -1.364683531250014514, -0.9489583329919112353, -0.7879004041258359514 ) ) ;
#102290=CARTESIAN_POINT ( 'NONE',  ( 2.738383840280320669, 6.138605547061593448, 0.7216878364870338292 ) ) ;
#102292=CARTESIAN_POINT ( 'NONE',  ( -4.485049888022365927, 4.126979712314507331, 0.7998128361456341429 ) ) ;
#102307=CARTESIAN_POINT ( 'NONE',  ( 7.145310649601935182, 8.294949498412453437, -1.199719254218446718 ) ) ;
#102313=CARTESIAN_POINT ( 'NONE',  ( 6.518203450479811423, 5.167241622962441383, -2.437504649502886256 ) ) ;
#102319=CARTESIAN_POINT ( 'NONE',  ( -5.708146366553361162, 6.618257834855742594, -1.199719254218446718 ) ) ;
#102322=CARTESIAN_POINT ( 'NONE',  ( -3.415764635639130020, 6.072476943965863683, 1.199719254218462483 ) ) ;
#102333=CARTESIAN_POINT ( 'NONE',  ( -3.765413976293358278, 5.416068943807445635, 1.599625672291267398 ) ) ;
#102336=CARTESIAN_POINT ( 'NONE',  ( 6.449928391799196525, 8.548002428564306143, -1.599625672291262513 ) ) ;
#102337=CARTESIAN_POINT ( 'NONE',  ( -1.201851678989727383E-14, 4.446875000341417916, -1.575800808251660134 ) ) ;
#102344=CARTESIAN_POINT ( 'NONE',  ( 6.005898860729467437, 7.069598761348265370, -1.082531754730543083 ) ) ;
#102345=CARTESIAN_POINT ( 'NONE',  ( -7.369020184227459858, 8.555943955475521889, 1.199719254218450271 ) ) ;
#102348=CARTESIAN_POINT ( 'NONE',  ( -7.157815033010924921, 10.43820240756634199, 1.199719254218453823 ) ) ;
#102349=CARTESIAN_POINT ( 'NONE',  ( -5.331380718671772101, 7.243030143248949670, -1.599625672291256295 ) ) ;
#102353=DIRECTION ( 'NONE',  ( 0.000000000000000000, 8.546850786086437571E-32, 1.000000000000000000 ) ) ;
#102356=CARTESIAN_POINT ( 'NONE',  ( 6.588372581236919601, 9.773852880496709972, -1.199719254218440723 ) ) ;
#102363=( BOUNDED_SURFACE ( )  B_SPLINE_SURFACE ( 3, 2, ( 
 ( #165375, #32183, #33242 ),
 ( #201048, #69979, #83049 ),
 ( #101441, #182682, #136090 ),
 ( #149124, #48456, #85190 ),
 ( #20174, #66770, #152332 ),
 ( #3909, #132911, #135035 ) ),
 .UNSPECIFIED., .F., .F., .T. ) 
 B_SPLINE_SURFACE_WITH_KNOTS ( ( 4, 2, 4 ),
 ( 3, 3 ),
 ( 0.000000000000000000, 0.002122857551078454266, 0.004245715102156908533 ),
 ( 0.000000000000000000, 1.000000000000000000 ),
 .UNSPECIFIED. ) 
 GEOMETRIC_REPRESENTATION_ITEM ( )  RATIONAL_B_SPLINE_SURFACE ( (
 ( 1.000000000000000000, 0.7806433624857567199, 1.000000000000000000),
 ( 1.000000000000000000, 0.7860453980259759499, 1.000000000000000000),
 ( 1.000000000000000000, 0.7924770197564218188, 1.000000000000000000),
 ( 1.000000000000000000, 0.8094762427233131996, 1.000000000000000000),
 ( 1.000000000000000000, 0.8200718518785214961, 1.000000000000000000),
 ( 1.000000000000000000, 0.8343063410434347071, 1.000000000000000000) ) ) 
 REPRESENTATION_ITEM ( '' )  SURFACE ( )  );
#102365=CARTESIAN_POINT ( 'NONE',  ( -1.499999999999997780, 3.900000000000021672, 1.214306433183764966E-14 ) ) ;
#102371=CARTESIAN_POINT ( 'NONE',  ( -1.402160292154681736E-14, -1.115624999658584082, 1.575800808251672791 ) ) ;
#102372=CARTESIAN_POINT ( 'NONE',  ( 3.440018289565364817, 5.036440642624797626, 1.599625672291267398 ) ) ;
#102373=CARTESIAN_POINT ( 'NONE',  ( 6.006425746053997372, 6.966250444273174303, -1.199719254218445830 ) ) ;
#102375=CARTESIAN_POINT ( 'NONE',  ( -6.832946231607472498, 9.955225789308602913, 1.082531754730549967 ) ) ;
#102378=CARTESIAN_POINT ( 'NONE',  ( 4.853455804012212660, 7.645820290447483458, 1.082531754730558626 ) ) ;
#102379=CARTESIAN_POINT ( 'NONE',  ( -7.741342523278709642, 10.05465224862374285, 1.443375672974090751 ) ) ;
#102384=CARTESIAN_POINT ( 'NONE',  ( 8.776205506747620788, 9.133327934160710981, -0.7998128361456221525 ) ) ;
#102389=CARTESIAN_POINT ( 'NONE',  ( 1.364683531249988535, 4.113541667008088432, 0.7879004041258500513 ) ) ;
#102395=CARTESIAN_POINT ( 'NONE',  ( 8.235688245297327015, 11.69572115523387268, -1.199719254218446718 ) ) ;
#102398=CARTESIAN_POINT ( 'NONE',  ( -9.677822722056413696, 10.18521468535430685, 1.040834085586084257E-14 ) ) ;
#102404=CARTESIAN_POINT ( 'NONE',  ( 4.054051625686104998, 4.688480637177271149, -1.199719254218446718 ) ) ;
#102408=CARTESIAN_POINT ( 'NONE',  ( -9.450196763925152510, 10.98398329845622001, -1.199719254218441611 ) ) ;
#102410=CARTESIAN_POINT ( 'NONE',  ( 4.800089777832203808, 5.120415418395356077, -0.7784788408505428636 ) ) ;
#102413=CARTESIAN_POINT ( 'NONE',  ( 5.886424920137334205, 5.980649323864647648, 0.1385726864747312270 ) ) ;
#102415=CARTESIAN_POINT ( 'NONE',  ( -2.767835915484202047, 6.380892334706859792, -0.7998128361456281477 ) ) ;
#102419=CARTESIAN_POINT ( 'NONE',  ( 5.926885707468349196, 10.06645042535509660, 1.040834085586084257E-14 ) ) ;
#102421=CARTESIAN_POINT ( 'NONE',  ( 5.829115978871627135, 8.888053511070525659, 1.199719254218462483 ) ) ;
#102422=CARTESIAN_POINT ( 'NONE',  ( 4.497554271431305040, 6.270232621468402989, -1.599625672291256295 ) ) ;
#102424=CARTESIAN_POINT ( 'NONE',  ( -7.036318535812428721, 11.15286269184909784, 0.000000000000000000 ) ) ;
#102431=CARTESIAN_POINT ( 'NONE',  ( -4.016817522127867690, 7.623078265842172740, -0.1143880650965305862 ) ) ;
#102434=CARTESIAN_POINT ( 'NONE',  ( 4.044555541517573793, 7.746237447724527492, 0.4662041258270445132 ) ) ;
#102435=CARTESIAN_POINT ( 'NONE',  ( 5.016153647376201619, 7.835634441038803466, 1.082531754730558626 ) ) ;
#102440=CARTESIAN_POINT ( 'NONE',  ( -8.609064354553318310, 12.98773281371349775, 0.7216878364870317197 ) ) ;
#102447=CARTESIAN_POINT ( 'NONE',  ( -8.785320351530977234, 13.19336481018743079, 1.040834085586084257E-14 ) ) ;
#102457=CARTESIAN_POINT ( 'NONE',  ( -9.612367721964613310, 11.27714576612263997, -1.082531754730537976 ) ) ;
#102461=CARTESIAN_POINT ( 'NONE',  ( 8.769426429940780920, 9.125419011219408461, 0.7998128361456462443 ) ) ;
#102465=CARTESIAN_POINT ( 'NONE',  ( 0.7499999999999902300, 1.264583334016147642, 1.299038105676657340 ) ) ;
#102467=CARTESIAN_POINT ( 'NONE',  ( -6.392833124043511894, 7.417059051927569868, 1.199719254218450271 ) ) ;
#102470=CARTESIAN_POINT ( 'NONE',  ( -7.700141177557535244, 11.07091624287075859, -1.199719254218446718 ) ) ;
#102474=CARTESIAN_POINT ( 'NONE',  ( 7.772902139336337335, 7.962807338847539107, 0.7998128361456341429 ) ) ;
#102477=CARTESIAN_POINT ( 'NONE',  ( -6.632963465583701534, 8.761543347979550589, -1.599625672291263179 ) ) ;
#102479=CARTESIAN_POINT ( 'NONE',  ( 8.341290820905593151, 10.75459192918846618, 1.599625672291281386 ) ) ;
#102480=DIRECTION ( 'NONE',  ( -0.3502638921866464417, 1.953969548649013931E-16, 0.9366510587354618389 ) ) ;
#102482=CARTESIAN_POINT ( 'NONE',  ( -0.9398415344193471466, 7.435109595052176168, 4.383649807226260187 ) ) ;
#102487=CARTESIAN_POINT ( 'NONE',  ( -8.215877900201387973, 8.687538426430837291, 0.7216878364870578100 ) ) ;
#102490=CARTESIAN_POINT ( 'NONE',  ( -0.6823417656249969321, 3.530208333674754506, -1.181850606188749264 ) ) ;
#102494=CARTESIAN_POINT ( 'NONE',  ( 1.364683531249988535, 5.655208333674751842, -0.7879004041258300672 ) ) ;
#102496=CARTESIAN_POINT ( 'NONE',  ( -4.243338890952916387, 4.052909582307567149, -0.7216878364870207285 ) ) ;
#102498=CARTESIAN_POINT ( 'NONE',  ( 10.40996301719436090, 11.03937836301526687, 0.000000000000000000 ) ) ;
#102499=CARTESIAN_POINT ( 'NONE',  ( -0.6823417656250212460, 5.613541667008087543, 1.181850606188767472 ) ) ;
#102504=CARTESIAN_POINT ( 'NONE',  ( -1.402160292154681736E-14, 1.696875000341421469, -1.575800808251659024 ) ) ;
#102506=CARTESIAN_POINT ( 'NONE',  ( -3.389175213736311587, 4.977123720824209840, 1.443375672974064550 ) ) ;
#102507=CARTESIAN_POINT ( 'NONE',  ( 4.578903193113299963, 6.365139696764064325, 1.599625672291267398 ) ) ;
#102512=CARTESIAN_POINT ( 'NONE',  ( 4.216222584169931231, 4.021273891060765493, 1.214306433183764966E-14 ) ) ;
#102515=CARTESIAN_POINT ( 'NONE',  ( -8.405692050792730186, 9.869357483088723626, 1.082531754730558626 ) ) ;
#102520=CARTESIAN_POINT ( 'NONE',  ( -8.995998617867369873, 10.45408546138876993, 1.199719254218462483 ) ) ;
#102521=EDGE_CURVE ( 'NONE', #158436, #167173, #83973, .T. ) ;
#102522=CARTESIAN_POINT ( 'NONE',  ( -3.904385050611244079, 7.498940292447679568, 1.040834085586084257E-14 ) ) ;
#102523=CARTESIAN_POINT ( 'NONE',  ( 1.364683531249988535, 1.926041667008086211, 0.7879004041258500513 ) ) ;
#102530=CARTESIAN_POINT ( 'NONE',  ( 8.563946585326370098, 13.14302144952281814, 0.7998128361456462443 ) ) ;
#102532=ORIENTED_EDGE ( 'NONE', *, *, #65647, .F. ) ;
#102537=VERTEX_POINT ( 'NONE', #205795 ) ;
#102543=CARTESIAN_POINT ( 'NONE',  ( -1.364683531250012516, 2.551041667008089320, -0.7879004041258289570 ) ) ;
#102551=CARTESIAN_POINT ( 'NONE',  ( 9.097684769969825780, 10.57271930550834860, -1.199719254218446718 ) ) ;
#102552=LINE ( 'NONE', #21272, #164501 ) ;
#102553=B_SPLINE_CURVE_WITH_KNOTS ( 'NONE', 1,
 ( #189623, #188556 ),
 .UNSPECIFIED., .F., .F.,
 ( 2, 2 ),
 ( 0.000000000000000000, 0.5165575204427501621 ),
 .UNSPECIFIED. ) ;
#102556=CARTESIAN_POINT ( 'NONE',  ( -1.364683531250000748, 1.009375000341421247, 0.000000000000000000 ) ) ;
#102559=CIRCLE ( 'NONE', #40435, 0.08000000000000020983 ) ;
#102567=CARTESIAN_POINT ( 'NONE',  ( 5.352771719296971042, 5.139321848801576387, 0.7998128361456341429 ) ) ;
#102570=ORIENTED_EDGE ( 'NONE', *, *, #189072, .F. ) ;
#102578=CARTESIAN_POINT ( 'NONE',  ( -3.460355519985875983, 5.060167411448709629, 1.599625672291267398 ) ) ;
#102579=CARTESIAN_POINT ( 'NONE',  ( 6.584456157731144899, 10.83361595066169514, -0.7998128361456291469 ) ) ;
#102581=CARTESIAN_POINT ( 'NONE',  ( -5.181758602633715682, 4.945385036406048762, 2.499999999999998668 ) ) ;
#102583=CARTESIAN_POINT ( 'NONE',  ( 5.056828107772846082, 6.922718763866881453, -1.443375672974051449 ) ) ;
#102590=CARTESIAN_POINT ( 'NONE',  ( 1.499999999999821032, 7.360305807095781638, -4.205660139708353285 ) ) ;
#102595=CARTESIAN_POINT ( 'NONE',  ( 7.334597915313080918, 9.580116872663850813, 1.040834085586084257E-14 ) ) ;
#102596=CARTESIAN_POINT ( 'NONE',  ( -5.883875478650828050, 9.808345791827219884, 0.7216878364870458196 ) ) ;
#102599=CARTESIAN_POINT ( 'NONE',  ( 6.484877546038077867, 6.460111979999551224, 1.040834085586084257E-14 ) ) ;
#102601=B_SPLINE_CURVE_WITH_KNOTS ( 'NONE', 3,
 ( #43813, #41679, #140252, #109926, #110987, #112064 ),
 .UNSPECIFIED., .F., .F.,
 ( 4, 2, 4 ),
 ( 1.978668964786020170E-18, 0.0002104102383275119543, 0.0004208204766550219028 ),
 .UNSPECIFIED. ) ;
#102603=CARTESIAN_POINT ( 'NONE',  ( -8.134002093194872884, 11.57708731111429401, 1.199719254218453823 ) ) ;
#102608=CARTESIAN_POINT ( 'NONE',  ( -4.485049888022365927, 4.126979712314507331, 0.7998128361456341429 ) ) ;
#102610=CARTESIAN_POINT ( 'NONE',  ( 10.42352117080803708, 11.05519620889787724, -0.7998128361456281477 ) ) ;
#102611=CARTESIAN_POINT ( 'NONE',  ( 2.679707916995359263, 6.278076336469897711, -0.7998128361456291469 ) ) ;
#102617=CARTESIAN_POINT ( 'NONE',  ( 3.212919216758630014, 6.692230152952963529, 0.000000000000000000 ) ) ;
#102620=CARTESIAN_POINT ( 'NONE',  ( -3.391510981712833939, 7.108513245306943062, 0.7998128361456341429 ) ) ;
#102623=CARTESIAN_POINT ( 'NONE',  ( -10.08065090696061716, 11.71951313199760136, -1.199719254218441611 ) ) ;
#102628=CARTESIAN_POINT ( 'NONE',  ( 8.622622508611357262, 9.162073802909148412, -0.7216878364870197293 ) ) ;
#102629=CARTESIAN_POINT ( 'NONE',  ( -0.6823417656250212460, 5.363541667008087543, 1.181850606188767472 ) ) ;
#102631=CARTESIAN_POINT ( 'NONE',  ( 5.834086172582112262, 5.700855377634248100, 1.040834085586084257E-14 ) ) ;
#102645=CARTESIAN_POINT ( 'NONE',  ( 1.364683531249988535, 3.176041667008084435, 0.7879004041258500513 ) ) ;
#102647=CARTESIAN_POINT ( 'NONE',  ( 9.622536337397022521, 12.24937836509514710, 1.599625672291281386 ) ) ;
#102649=CARTESIAN_POINT ( 'NONE',  ( -5.151735183512911043, 6.073074471262228435, 1.082531754730548412 ) ) ;
#102651=CARTESIAN_POINT ( 'NONE',  ( -5.924549939047510705, 6.974691686052601369, 1.082531754730549967 ) ) ;
#102656=CARTESIAN_POINT ( 'NONE',  ( 6.173040012923759257, 6.096301524699504704, -0.7998128361456281477 ) ) ;
#102668=CARTESIAN_POINT ( 'NONE',  ( 4.645640190976921602, 8.571663989448405019, 1.040834085586084257E-14 ) ) ;
#102671=CARTESIAN_POINT ( 'NONE',  ( -7.088215381846223906, 7.164006121775713609, 0.7998128361456341429 ) ) ;
#102675=CARTESIAN_POINT ( 'NONE',  ( 6.642605195691581699, 9.837124264027149678, 1.199719254218462483 ) ) ;
#102678=CARTESIAN_POINT ( 'NONE',  ( -6.196239896645333367, 7.187700286629718605, -1.199719254218446718 ) ) ;
#102679=CARTESIAN_POINT ( 'NONE',  ( 7.253248993186735660, 7.564471368247083660, 0.7216878364870317197 ) ) ;
#102680=CARTESIAN_POINT ( 'NONE',  ( 4.149381719138396818, 7.633502232665817289, 0.8094099469760536181 ) ) ;
#102681=CARTESIAN_POINT ( 'NONE',  ( -2.923754682041362241, 6.562797562356882608, 0.7998128361456341429 ) ) ;
#102684=CARTESIAN_POINT ( 'NONE',  ( -4.550733115681270036, 8.460939068270139529, 0.7998128361456481317 ) ) ;
#102688=CARTESIAN_POINT ( 'NONE',  ( 0.6823417656249899377, 1.342708333674752508, 1.181850606188755259 ) ) ;
#102689=CARTESIAN_POINT ( 'NONE',  ( -3.945059511896602089, 7.546393830613923548, 1.040834085586084257E-14 ) ) ;
#102690=ORIENTED_EDGE ( 'NONE', *, *, #187111, .T. ) ;
#102695=CARTESIAN_POINT ( 'NONE',  ( -1.445103857048105844, 8.688264192037886247, -2.625611233228243968 ) ) ;
#102696=CARTESIAN_POINT ( 'NONE',  ( 5.524057522564145728, 8.532151978711786100, 1.199719254218462483 ) ) ;
#102700=CARTESIAN_POINT ( 'NONE',  ( -0.6823417656250003738, 3.030208333674754062, -1.181850606188749264 ) ) ;
#102702=CARTESIAN_POINT ( 'NONE',  ( -1.364683531250014514, -1.157291666325248158, 0.7879004041258379498 ) ) ;
#102705=CARTESIAN_POINT ( 'NONE',  ( -4.322352044658376968, 3.937165561723182883, 0.7998128361456341429 ) ) ;
#102706=CARTESIAN_POINT ( 'NONE',  ( -7.497295758232731089, 8.809561808435409702, -1.082531754730543083 ) ) ;
#102708=CARTESIAN_POINT ( 'NONE',  ( 0.6823417656249917140, 3.342708333674754506, 1.181850606188765695 ) ) ;
#102716=CARTESIAN_POINT ( 'NONE',  ( -7.524412065460066579, 7.880828285899290186, 0.7216878364870317197 ) ) ;
#102719=CARTESIAN_POINT ( 'NONE',  ( 1.084637062511528693, 3.023878807974804683, 1.105835307554807301 ) ) ;
#102721=CARTESIAN_POINT ( 'NONE',  ( -6.358410854684789726, 8.441231968597481483, -1.443375672974058777 ) ) ;
#102736=CARTESIAN_POINT ( 'NONE',  ( -6.205881626753225966, 8.263281202677319470, 1.599625672291283607 ) ) ;
#102738=CARTESIAN_POINT ( 'NONE',  ( -1.500000000000015099, -0.1208333333333093396, -0.8660254037844383745 ) ) ;
#102739=CARTESIAN_POINT ( 'NONE',  ( 4.684505768721569652, 5.424010470718658716, -1.199719254218452047 ) ) ;
#102741=CARTESIAN_POINT ( 'NONE',  ( -1.500000000000055511, 7.268077025657054158, -4.207854987878878461 ) ) ;
#102743=CARTESIAN_POINT ( 'NONE',  ( 6.602984505055297326, 7.662235663108029726, 1.199719254218462483 ) ) ;
#102747=CARTESIAN_POINT ( 'NONE',  ( -4.094199201646926412, 7.720390135322642067, 0.7216878364870317197 ) ) ;
#102748=B_SPLINE_CURVE_WITH_KNOTS ( 'NONE', 3,
 ( #77585, #110161, #192388, #177231, #92800, #44042, #176173, #30991, #63473, #162053, #62403, #158845, #209700, #28844 ),
 .UNSPECIFIED., .F., .F.,
 ( 4, 2, 2, 2, 2, 2, 4 ),
 ( 0.001872291076886156399, 0.002107054070185122602, 0.002341817063484089023, 0.002811343050082021865, 0.003280869036679954706, 0.003515632029978921561, 0.003750395023277889282 ),
 .UNSPECIFIED. ) ;
#102758=CARTESIAN_POINT ( 'NONE',  ( -0.6823417656250212460, 1.551041667008083769, 1.181850606188755259 ) ) ;
#102760=CARTESIAN_POINT ( 'NONE',  ( -6.679363233026820446, 10.94434087183997129, 0.000000000000000000 ) ) ;
#102762=CARTESIAN_POINT ( 'NONE',  ( 7.121056995675668411, 9.330985799753529264, -1.599625672291262513 ) ) ;
#102764=CARTESIAN_POINT ( 'NONE',  ( -7.711890448074853133, 7.891627032375787998, -0.7998128361456291469 ) ) ;
#102767=CARTESIAN_POINT ( 'NONE',  ( -1.364683531250010295, 5.530208333674751842, 0.7879004041258379498 ) ) ;
#102769=CARTESIAN_POINT ( 'NONE',  ( 8.771762198361678031, 9.336070107617867819, 1.040834085586084257E-14 ) ) ;
#102771=CARTESIAN_POINT ( 'NONE',  ( -0.6823417656250003738, -0.2197916663252488800, -1.181850606188749264 ) ) ;
#102773=CARTESIAN_POINT ( 'NONE',  ( 8.256552360598020002, 8.734991963560254646, -0.7216878364870267237 ) ) ;
#102776=CARTESIAN_POINT ( 'NONE',  ( -4.772106882330234612, 6.590544000850479200, -1.443375672974053447 ) ) ;
#102778=CARTESIAN_POINT ( 'NONE',  ( -1.364683531250012516, 3.738541667008087099, -0.7879004041258300672 ) ) ;
#102782=CARTESIAN_POINT ( 'NONE',  ( -6.715366157470410435, 6.729015360003925750, -0.7998128361456291469 ) ) ;
#102791=CARTESIAN_POINT ( 'NONE',  ( 5.798083248138522272, 9.916180889470295412, 0.7998128361456462443 ) ) ;
#102799=CARTESIAN_POINT ( 'NONE',  ( 5.992340707560151358, 8.014150130285418783, 1.443375672974062551 ) ) ;
#102801=CARTESIAN_POINT ( 'NONE',  ( -1.402160292154681736E-14, 0.009375000341421267647, -1.575800808251665908 ) ) ;
#102803=CARTESIAN_POINT ( 'NONE',  ( 4.227444969362701421, 3.826440640544909400, 1.214306433183764966E-14 ) ) ;
#102808=CARTESIAN_POINT ( 'NONE',  ( -1.201851678989727383E-14, 0.7125000000000225597, 1.732050807568877637 ) ) ;
#102809=CARTESIAN_POINT ( 'NONE',  ( 7.914208982075123799, 10.25632978388623684, -1.599625672291262513 ) ) ;
#102810=CARTESIAN_POINT ( 'NONE',  ( -7.479294296233107708, 11.87759377891399204, 0.7998128361456481317 ) ) ;
#102812=CARTESIAN_POINT ( 'NONE',  ( -1.364683531250014514, -0.5114583329919092369, -0.7879004041258359514 ) ) ;
#102813=AXIS2_PLACEMENT_3D ( 'NONE', #25911, #22694, #41133 ) ;
#102814=CARTESIAN_POINT ( 'NONE',  ( 0.7499999999999902300, 1.233333333333357151, 1.299038105676657340 ) ) ;
#102816=CARTESIAN_POINT ( 'NONE',  ( 5.931855901178834323, 6.879252291918818152, 1.199719254218462483 ) ) ;
#102823=CARTESIAN_POINT ( 'NONE',  ( -1.500000000000013101, -0.2979166659838501929, 0.8660254037844403729 ) ) ;
#102825=CARTESIAN_POINT ( 'NONE',  ( -8.830438121202295321, 9.196599317691152464, -0.7998128361456291469 ) ) ;
#102826=CARTESIAN_POINT ( 'NONE',  ( -5.938108093105513241, 6.030140318152288792, 0.7216878364870317197 ) ) ;
#102833=ORIENTED_EDGE ( 'NONE', *, *, #49246, .F. ) ;
#102834=CARTESIAN_POINT ( 'NONE',  ( 8.209625708274705502, 9.536650400197368427, 1.199719254218462483 ) ) ;
#102835=CARTESIAN_POINT ( 'NONE',  ( -3.456965981804629884, 6.976951378839947537, 1.040834085586084257E-14 ) ) ;
#102838=CARTESIAN_POINT ( 'NONE',  ( 5.626270559546804328, 9.507806719539201978, 0.7216878364870438212 ) ) ;
#102842=CARTESIAN_POINT ( 'NONE',  ( -6.886651960737580680, 10.12184548991413457, -1.199719254218440723 ) ) ;
#102843=CARTESIAN_POINT ( 'NONE',  ( 6.003563092752934871, 5.898578451166879510, 0.7998128361456341429 ) ) ;
#102844=FACE_OUTER_BOUND ( 'NONE', #146129, .T. ) ;
#102846=CARTESIAN_POINT ( 'NONE',  ( 4.369805582306193870, 3.992528022312320957, 1.214306433183764966E-14 ) ) ;
#102855=CARTESIAN_POINT ( 'NONE',  ( -3.619663825168619731, 7.166765529431275539, 1.040834085586084257E-14 ) ) ;
#102856=CARTESIAN_POINT ( 'NONE',  ( 8.975134502566660899, 10.53370701015836275, -1.082531754730543083 ) ) ;
#102859=CARTESIAN_POINT ( 'NONE',  ( -5.371001409308059138, 9.417918744168066070, -0.7998128361456231517 ) ) ;
#102862=CARTESIAN_POINT ( 'NONE',  ( -1.420000000000001039, 6.264000000000040203, -2.851999999999994984 ) ) ;
#102864=CARTESIAN_POINT ( 'NONE',  ( -7.182068686937172153, 9.402166106225269715, 1.599625672291283607 ) ) ;
#102867=CARTESIAN_POINT ( 'NONE',  ( -0.1460981902779853459, 7.101100029736113761, 2.114500818361210399 ) ) ;
#102880=CARTESIAN_POINT ( 'NONE',  ( -6.235860587281615075, 9.362588887548838557, -1.199719254218440723 ) ) ;
#102883=CARTESIAN_POINT ( 'NONE',  ( 4.365362273920230685, 8.036747052974847705, 0.7216878364870298324 ) ) ;
#102887=CARTESIAN_POINT ( 'NONE',  ( -5.108724954250998707, 4.854600622914589714, -0.7998128361456221525 ) ) ;
#102894=CARTESIAN_POINT ( 'NONE',  ( -8.143643823302737061, 12.65266822716189843, 0.000000000000000000 ) ) ;
#102895=CARTESIAN_POINT ( 'NONE',  ( 6.103141704446003679, 10.27208242182903142, 0.7998128361456462443 ) ) ;
#102898=CARTESIAN_POINT ( 'NONE',  ( -9.809487834687324437, 11.40315621434539395, 1.199719254218462483 ) ) ;
#102901=CARTESIAN_POINT ( 'NONE',  ( -1.402160292154681736E-14, 0.6343750003414162508, 1.575800808251672791 ) ) ;
#102905=CARTESIAN_POINT ( 'NONE',  ( 7.104109303880752790, 11.23195192126214970, -0.7216878364870267237 ) ) ;
#102934=CARTESIAN_POINT ( 'NONE',  ( 1.364683531249988535, 5.405208333674750953, -0.7879004041258300672 ) ) ;
#102938=CARTESIAN_POINT ( 'NONE',  ( 10.21336978979620191, 10.81001959771741205, 0.7998128361456462443 ) ) ;
#102940=FACE_OUTER_BOUND ( 'NONE', #75564, .T. ) ;
#102941=CARTESIAN_POINT ( 'NONE',  ( -1.177073619093346180, 3.256928502340592946, 0.7750000000000100142 ) ) ;
#102943=CARTESIAN_POINT ( 'NONE',  ( 3.891353782322113375, 4.498666486585943147, -1.199719254218446718 ) ) ;
#102948=CARTESIAN_POINT ( 'NONE',  ( 4.449046963578762615, 8.342305224150557308, -0.7998128361456231517 ) ) ;
#102949=CARTESIAN_POINT ( 'NONE',  ( -1.201851678989727383E-14, 3.009375000341419248, -1.575800808251660134 ) ) ;
#102950=CARTESIAN_POINT ( 'NONE',  ( -5.862510748852908016, 6.029743210627831473, 0.3741650707956689081 ) ) ;
#102953=CARTESIAN_POINT ( 'NONE',  ( -6.672584156219988571, 10.93643194889866521, -0.7998128361456291469 ) ) ;
#102954=CARTESIAN_POINT ( 'NONE',  ( -4.948362878863562742, 5.835806782504650236, 1.082531754730558626 ) ) ;
#102957=CARTESIAN_POINT ( 'NONE',  ( -5.473741331615264549, 7.409117525016355010, -1.599625672291256295 ) ) ;
#102959=CARTESIAN_POINT ( 'NONE',  ( -0.7500000000000249800, 0.2229166673494847872, 1.299038105676659116 ) ) ;
#102967=CARTESIAN_POINT ( 'NONE',  ( -5.083944415000202888, 5.033616027029415463, 0.7216878364870317197 ) ) ;
#102970=CARTESIAN_POINT ( 'NONE',  ( 0.4644214298860996903, 7.369507887687365866, -4.459343850249745778 ) ) ;
#102973=CARTESIAN_POINT ( 'NONE',  ( -3.267151830768946663, 6.755501535964989479, -0.7216878364870257245 ) ) ;
#102975=CARTESIAN_POINT ( 'NONE',  ( 8.398386088661320414, 11.88553530582519357, -1.199719254218446718 ) ) ;
#102977=CARTESIAN_POINT ( 'NONE',  ( -1.270916165646621243, 3.165225491120026380, 0.7750000000000152323 ) ) ;
#102983=CARTESIAN_POINT ( 'NONE',  ( -4.613852347352193739, 4.277249248199312071, 1.214306433183764966E-14 ) ) ;
#102984=CARTESIAN_POINT ( 'NONE',  ( -8.784793466650835825, 12.33634391347959713, 1.199719254218462483 ) ) ;
#102987=VERTEX_POINT ( 'NONE', #55046 ) ;
#102989=CARTESIAN_POINT ( 'NONE',  ( 4.385172619016207918, 7.203452924572514959, 1.199719254218462483 ) ) ;
#102996=FACE_OUTER_BOUND ( 'NONE', #209387, .T. ) ;
#103007=CARTESIAN_POINT ( 'NONE',  ( 8.609591239877852686, 10.00327685373437347, -1.199719254218445830 ) ) ;
#103009=CARTESIAN_POINT ( 'NONE',  ( -5.708146366553361162, 6.618257834855742594, -1.199719254218446718 ) ) ;
#103012=DIRECTION ( 'NONE',  ( -0.6507913734559658270, -0.7592566023652989049, 0.000000000000000000 ) ) ;
#103016=CARTESIAN_POINT ( 'NONE',  ( -1.364683531249997417, 5.759375000341418804, 1.214306433183764966E-14 ) ) ;
#103020=CARTESIAN_POINT ( 'NONE',  ( 1.284279953904121641, 3.284610286488902187, 0.7750000000000135669 ) ) ;
#103021=CARTESIAN_POINT ( 'NONE',  ( 2.842405760359353106, 6.467890487061221272, -0.7998128361456291469 ) ) ;
#103022=CARTESIAN_POINT ( 'NONE',  ( -4.249591082879585535, 7.045274465746411252, 1.199719254218464037 ) ) ;
#103028=CARTESIAN_POINT ( 'NONE',  ( 5.504247177468179153, 7.444707678511436555, 1.443375672974062551 ) ) ;
#103031=CARTESIAN_POINT ( 'NONE',  ( 7.904040366642695048, 9.284097184913720824, 1.082531754730558626 ) ) ;
#103032=CARTESIAN_POINT ( 'NONE',  ( -1.201851678989727383E-14, 4.509375000341417916, -1.575800808251660134 ) ) ;
#103034=CARTESIAN_POINT ( 'NONE',  ( 5.192409643909512873, 6.120528008391641350, -1.082531754730549078 ) ) ;
#103042=CARTESIAN_POINT ( 'NONE',  ( -4.351171265391168497, 7.394090626460979365, 1.174491979025530597 ) ) ;
#103045=CARTESIAN_POINT ( 'NONE',  ( 1.364683531249992088, 5.446875000341417916, 1.214306433183764966E-14 ) ) ;
#103049=AXIS2_PLACEMENT_3D ( 'NONE', #70606, #35993, #136720 ) ;
#103051=CARTESIAN_POINT ( 'NONE',  ( -10.16591625214838679, 10.75465713712827487, 1.040834085586084257E-14 ) ) ;
#103053=CARTESIAN_POINT ( 'NONE',  ( -3.104453987849326690, 4.644948957289396496, 1.040834085586084257E-14 ) ) ;
#103061=CARTESIAN_POINT ( 'NONE',  ( 2.250290310188348464, 5.569163095287620990, 0.7216878364870438212 ) ) ;
#103062=CARTESIAN_POINT ( 'NONE',  ( -0.6823417656250003738, 2.780208333674753618, -1.181850606188749264 ) ) ;
#103064=CARTESIAN_POINT ( 'NONE',  ( 6.103141704446003679, 10.27208242182903142, 0.7998128361456462443 ) ) ;
#103065=CARTESIAN_POINT ( 'NONE',  ( -9.124801077197171040, 10.60435499727357289, -1.199719254218441611 ) ) ;
#103070=ORIENTED_EDGE ( 'NONE', *, *, #141149, .T. ) ;
#103072=CARTESIAN_POINT ( 'NONE',  ( -1.500000000000011324, 5.129166666666691299, -0.8660254037844313801 ) ) ;
#103073=CARTESIAN_POINT ( 'NONE',  ( 5.148345644887269756, 7.029489223833707001, -1.599625672291256295 ) ) ;
#103076=CARTESIAN_POINT ( 'NONE',  ( -5.000000000000024869, 3.300000000000025135, 0.7750000000000238920 ) ) ;
#103078=CARTESIAN_POINT ( 'NONE',  ( 6.954969614130424027, 11.05795561655343384, 1.040834085586084257E-14 ) ) ;
#103082=CARTESIAN_POINT ( 'NONE',  ( 0.7499999999999885647, 3.347916667349487341, -1.299038105676658228 ) ) ;
#103084=CARTESIAN_POINT ( 'NONE',  ( -3.581325132304157943, 7.329963087663487364, -0.7998128361456281477 ) ) ;
#103085=CARTESIAN_POINT ( 'NONE',  ( 2.684151225381301575, 6.075334163012737321, 0.000000000000000000 ) ) ;
#103093=CARTESIAN_POINT ( 'NONE',  ( 6.337546739384100292, 9.481222731668410120, 1.199719254218460707 ) ) ;
#103094=CARTESIAN_POINT ( 'NONE',  ( 4.635998460869027227, 7.496083073400806818, -1.199719254218452047 ) ) ;
#103095=CARTESIAN_POINT ( 'NONE',  ( 6.385527162356455122, 10.39360608948380538, 1.056142170575426150E-14 ) ) ;
#103097=FILL_AREA_STYLE ('',( #135608 ) ) ;
#103098=CARTESIAN_POINT ( 'NONE',  ( 4.355193658487811703, 6.104145239700998538, -1.599625672291255185 ) ) ;
#103106=CARTESIAN_POINT ( 'NONE',  ( 8.890396042259068210, 11.39521468743417998, -1.599625672291257406 ) ) ;
#103111=CARTESIAN_POINT ( 'NONE',  ( 5.458613854904844409, 6.252117202148153474, -1.007154897844428687 ) ) ;
#103112=AXIS2_PLACEMENT_3D ( 'NONE', #149454, #112764, #178777 ) ;
#103120=CARTESIAN_POINT ( 'NONE',  ( 5.666945020832167224, 8.594891043404107478, 1.082531754730558626 ) ) ;
#103121=CARTESIAN_POINT ( 'NONE',  ( -4.277761160311629673, 4.949475094240346706, 1.199719254218462483 ) ) ;
#103127=CARTESIAN_POINT ( 'NONE',  ( -3.418627288940168096, 7.140148937072163804, -0.7998128361456281477 ) ) ;
#103138=CARTESIAN_POINT ( 'NONE',  ( 8.880754312151170282, 10.31963377138658089, 1.199719254218453823 ) ) ;
#103139=CARTESIAN_POINT ( 'NONE',  ( 5.931217288863120274, 6.131947776268360961, 0.7575795127007216578 ) ) ;
#103146=CARTESIAN_POINT ( 'NONE',  ( -7.348156068926747331, 11.51667314714914347, 0.7216878364870458196 ) ) ;
#103150=CARTESIAN_POINT ( 'NONE',  ( 7.670162217029129259, 9.971608557999250166, 1.599625672291281386 ) ) ;
#103155=CARTESIAN_POINT ( 'NONE',  ( -6.144869935491728441, 8.192100896205577243, -1.599625672291263179 ) ) ;
#103156=CARTESIAN_POINT ( 'NONE',  ( 3.649115900372475796, 7.409052317076538330, 1.040834085586084257E-14 ) ) ;
#103163=CARTESIAN_POINT ( 'NONE',  ( 3.999300167945916584, 7.828775037665852921, -0.06519116529766534607 ) ) ;
#103165=CARTESIAN_POINT ( 'NONE',  ( 4.351804120306567825, 8.020929207092235558, 1.040834085586084257E-14 ) ) ;
#103167=DIRECTION ( 'NONE',  ( 0.6260462619842731558, 0.7797859179643593652, 0.000000000000000000 ) ) ;
#103173=CARTESIAN_POINT ( 'NONE',  ( 7.253248993186713456, 11.40594822545244824, 0.7216878364870438212 ) ) ;
#103180=CARTESIAN_POINT ( 'NONE',  ( -7.015454420067433361, 10.27211502579893754, 1.199719254218453823 ) ) ;
#103181=CARTESIAN_POINT ( 'NONE',  ( -9.828980619278564011E-14, 7.054063922337708625, 3.955400951015630273 ) ) ;
#103188=CARTESIAN_POINT ( 'NONE',  ( 9.459838494033030898, 12.05956421450382088, 1.599625672291281386 ) ) ;
#103192=CARTESIAN_POINT ( 'NONE',  ( 4.985647801523278133, 6.839675073242382553, -1.599625672291256295 ) ) ;
#103196=CARTESIAN_POINT ( 'NONE',  ( -0.7500000000000006661, 2.889583334016148974, -1.299038105676652011 ) ) ;
#103202=CARTESIAN_POINT ( 'NONE',  ( -0.7500000000000215383, 1.441666666666688190, 1.299038105676659116 ) ) ;
#103203=CARTESIAN_POINT ( 'NONE',  ( 7.637320603199683866, 7.804628880021436288, -0.7998128361456281477 ) ) ;
#103204=CARTESIAN_POINT ( 'NONE',  ( 3.334942598837264960, 6.834590765378040444, 1.214306433183764966E-14 ) ) ;
#103208=CARTESIAN_POINT ( 'NONE',  ( 9.110716038703335684, 9.731516254683127087, -0.7216878364870197293 ) ) ;
#103213=VECTOR ( 'NONE', #109867, 1000.000000000000114 ) ;
#103216=CARTESIAN_POINT ( 'NONE',  ( -6.389970470742427189, 6.349387058821269747, -0.7998128361456291469 ) ) ;
#103217=CARTESIAN_POINT ( 'NONE',  ( -1.201851678989727383E-14, 3.993750000682817713, 1.732050807568877637 ) ) ;
#103218=CARTESIAN_POINT ( 'NONE',  ( -1.364683531250000748, -1.240624999658580752, 0.000000000000000000 ) ) ;
#103224=CARTESIAN_POINT ( 'NONE',  ( 0.6823417656249917140, 3.405208333674754506, 1.181850606188765695 ) ) ;
#103231=CARTESIAN_POINT ( 'NONE',  ( -7.666245793523398078, 11.03137162816423356, 1.199719254218453823 ) ) ;
#103232=CARTESIAN_POINT ( 'NONE',  ( 6.681470773436232413, 6.689470745297396270, -0.7998128361456281477 ) ) ;
#103234=CARTESIAN_POINT ( 'NONE',  ( -1.364683531250014514, -0.7614583329919104582, -0.7879004041258359514 ) ) ;
#103236=EDGE_CURVE ( 'NONE', #108282, #135381, #108689, .T. ) ;
#103239=CARTESIAN_POINT ( 'NONE',  ( 2.275391796764376640, 5.643962577969389827, -0.5307291018262025872 ) ) ;
#103242=CARTESIAN_POINT ( 'NONE',  ( -6.669721502918952716, 9.868759955792373972, 1.199719254218452047 ) ) ;
#103247=CARTESIAN_POINT ( 'NONE',  ( 8.218213668177886788, 12.73966637951625813, 0.7998128361456462443 ) ) ;
#103249=CARTESIAN_POINT ( 'NONE',  ( -4.416205349749324327, 6.175325546172740765, 1.599625672291267398 ) ) ;
#103250=CARTESIAN_POINT ( 'NONE',  ( -7.965578943228732278, 9.251929174310385307, -1.199719254218446718 ) ) ;
#103253=CARTESIAN_POINT ( 'NONE',  ( -4.377891688998395203, 7.365737962781053305, -1.202262209786943759 ) ) ;
#103254=CARTESIAN_POINT ( 'NONE',  ( -1.364683531250000748, -0.4906249996585801409, 0.000000000000000000 ) ) ;
#103258=CARTESIAN_POINT ( 'NONE',  ( 6.778713617152772208, 10.85232362007950258, -0.7216878364870267237 ) ) ;
#103261=CARTESIAN_POINT ( 'NONE',  ( 4.981731378017507872, 7.899438143407371271, -1.199719254218452047 ) ) ;
#103283=CARTESIAN_POINT ( 'NONE',  ( -8.833300774503376473, 10.26427131079744193, 1.199719254218462483 ) ) ;
#103288=CARTESIAN_POINT ( 'NONE',  ( -1.201851678989727383E-14, 2.243750000682818158, 1.732050807568877637 ) ) ;
#103289=CARTESIAN_POINT ( 'NONE',  ( 10.21336978979620191, 10.81001959771741205, 0.7998128361456462443 ) ) ;
#103294=CARTESIAN_POINT ( 'NONE',  ( -9.829825065107822724, 11.42688298316931572, 1.199719254218462483 ) ) ;
#103296=CARTESIAN_POINT ( 'NONE',  ( 0.6823417656249899377, 2.342708333674753618, 1.181850606188767472 ) ) ;
#103301=CARTESIAN_POINT ( 'NONE',  ( -3.358669367883384105, 4.941533567329135401, -1.599625672291262513 ) ) ;
#103303=CARTESIAN_POINT ( 'NONE',  ( 1.436838838544733044, 7.449283400311756509, -4.203727439823553347 ) ) ;
#103307=CARTESIAN_POINT ( 'NONE',  ( -1.364683531250014514, -0.4489583329919089039, -0.7879004041258359514 ) ) ;
#103312=CARTESIAN_POINT ( 'NONE',  ( 0.6823417656249882723, 1.676041667008083769, -1.181850606188749264 ) ) ;
#103314=CARTESIAN_POINT ( 'NONE',  ( -6.413170354464012846, 7.440785820751486312, 1.199719254218450271 ) ) ;
#103315=CARTESIAN_POINT ( 'NONE',  ( 6.753933077901968396, 11.03133902419432566, 0.7998128361456462443 ) ) ;
#103317=CARTESIAN_POINT ( 'NONE',  ( 4.320244504248938355, 8.192035688265757898, 1.040834085586084257E-14 ) ) ;
#103319=CARTESIAN_POINT ( 'NONE',  ( 1.499999999999989120, 3.504166666666683749, 0.8660254037844524744 ) ) ;
#103321=CARTESIAN_POINT ( 'NONE',  ( 1.364683531249986537, 1.967708333674750731, -0.7879004041258239610 ) ) ;
#103327=CARTESIAN_POINT ( 'NONE',  ( 5.124618876285529367, 7.962177208099690873, -1.082531754730549078 ) ) ;
#103330=CARTESIAN_POINT ( 'NONE',  ( -9.341731535015849630, 10.85744053139533349, 1.199719254218462483 ) ) ;
#103331=CARTESIAN_POINT ( 'NONE',  ( -3.066115294984855133, 6.728884944124295053, 0.7998128361456341429 ) ) ;
#103334=CARTESIAN_POINT ( 'NONE',  ( 4.207107738942202246, 3.802713871720993399, 1.214306433183764966E-14 ) ) ;
#103336=CARTESIAN_POINT ( 'NONE',  ( -6.819388077549415783, 10.89977715720891815, 0.7216878364870458196 ) ) ;
#103338=CARTESIAN_POINT ( 'NONE',  ( 0.7499999999999902300, 4.566666666666691299, -1.299038105676658228 ) ) ;
#103341=CARTESIAN_POINT ( 'NONE',  ( 7.754900677336718395, 11.99120852362745460, -0.7216878364870267237 ) ) ;
#103342=CARTESIAN_POINT ( 'NONE',  ( -6.056815632531343141, 6.015240258500212711, 0.3115616189311651296 ) ) ;
#103347=LINE ( 'NONE', #169412, #92007 ) ;
#103349=CARTESIAN_POINT ( 'NONE',  ( 9.856414487010587422, 11.56186699200962487, 1.082531754730548412 ) ) ;
#103357=CARTESIAN_POINT ( 'NONE',  ( 7.253248993186713456, 11.40594822545244824, 0.7216878364870438212 ) ) ;
#103358=CARTESIAN_POINT ( 'NONE',  ( 5.940443861082012944, 10.08226827123770697, 0.7998128361456462443 ) ) ;
#103359=CARTESIAN_POINT ( 'NONE',  ( -5.915435094264120508, 5.795762452929912101, 0.000000000000000000 ) ) ;
#103361=CARTESIAN_POINT ( 'NONE',  ( 1.499999999999968914, 5.045833333333356485, -0.8660254037844440367 ) ) ;
#103364=CARTESIAN_POINT ( 'NONE',  ( 4.202664430556261266, 4.005456045178151570, 0.7216878364870317197 ) ) ;
#103366=CARTESIAN_POINT ( 'NONE',  ( -10.13488352141530768, 11.78278451552804817, 1.199719254218462483 ) ) ;
#103375=ORIENTED_EDGE ( 'NONE', *, *, #133002, .T. ) ;
#103382=CARTESIAN_POINT ( 'NONE',  ( 7.422199028477372451, 10.74665040227725044, -1.199719254218441611 ) ) ;
#103388=CARTESIAN_POINT ( 'NONE',  ( 1.519204386771063398, 8.761797318405452728, 2.483775294098995889 ) ) ;
#103394=CARTESIAN_POINT ( 'NONE',  ( -5.925076824372040640, 6.871343368977510302, 1.199719254218450271 ) ) ;
#103397=CARTESIAN_POINT ( 'NONE',  ( -4.776550190716183586, 4.467063398790632966, 1.214306433183764966E-14 ) ) ;
#103407=CARTESIAN_POINT ( 'NONE',  ( -2.819205876637805641, 5.376491725131008259, -1.199719254218446718 ) ) ;
#103410=CARTESIAN_POINT ( 'NONE',  ( 7.721532178182734185, 8.967207948423393304, 1.199719254218462483 ) ) ;
#103411=CARTESIAN_POINT ( 'NONE',  ( -1.001543065824772872E-14, 4.821875000341421469, 1.575800808251672791 ) ) ;
#103418=CARTESIAN_POINT ( 'NONE',  ( 5.544921637864819175, 7.492161215640853023, -1.443375672974057666 ) ) ;
#103419=CARTESIAN_POINT ( 'NONE',  ( -7.019370843573183194, 9.212351955633947043, 1.599625672291283607 ) ) ;
#103422=CARTESIAN_POINT ( 'NONE',  ( -6.496328159242330536, 10.73079995242472862, 0.000000000000000000 ) ) ;
#103423=CARTESIAN_POINT ( 'NONE',  ( -5.656776405399756236, 7.622658444431597680, -1.599625672291256295 ) ) ;
#103427=CARTESIAN_POINT ( 'NONE',  ( -2.364368148460603614, 5.338642027447423999, -0.7873643464157237259 ) ) ;
#103431=CARTESIAN_POINT ( 'NONE',  ( 6.401421083946654100, 10.62007503124645957, -0.7998128361456291469 ) ) ;
#103443=ORIENTED_EDGE ( 'NONE', *, *, #15247, .T. ) ;
#103446=CARTESIAN_POINT ( 'NONE',  ( -0.6823417656250003738, -0.7197916663252492686, -1.181850606188749264 ) ) ;
#103447=CARTESIAN_POINT ( 'NONE',  ( 5.196852952739813070, 4.957416621151553571, -0.7998128361456221525 ) ) ;
#103448=CARTESIAN_POINT ( 'NONE',  ( 4.496500501226593727, 8.397667684739696270, 0.7998128361456462443 ) ) ;
#103450=CARTESIAN_POINT ( 'NONE',  ( -7.375272376154081932, 10.58793962461302485, -1.082531754730543971 ) ) ;
#103452=CARTESIAN_POINT ( 'NONE',  ( 6.344852701515477200, 6.504675694630598137, -0.7216878364870257245 ) ) ;
#103453=CARTESIAN_POINT ( 'NONE',  ( -8.812436658758329600, 9.383523644747281622, 1.040834085586084257E-14 ) ) ;
#103456=CARTESIAN_POINT ( 'NONE',  ( 9.237182729612253951, 9.671134694169463586, 0.7998128361456462443 ) ) ;
#103462=CARTESIAN_POINT ( 'NONE',  ( -1.402160292154681736E-14, 2.446875000341416584, -1.575800808251660134 ) ) ;
#103468=CARTESIAN_POINT ( 'NONE',  ( 6.936968151686458306, 11.24487994360957188, 0.7998128361456462443 ) ) ;
#103471=CARTESIAN_POINT ( 'NONE',  ( -8.208571938070008400, 11.66408546346865016, -1.199719254218446718 ) ) ;
#103477=CARTESIAN_POINT ( 'NONE',  ( 4.539282502477016479, 4.190251095844947926, 0.7998128361456341429 ) ) ;
#103481=CARTESIAN_POINT ( 'NONE',  ( -10.01677656239806247, 10.58066083241955901, 0.7998128361456462443 ) ) ;
#103488=CARTESIAN_POINT ( 'NONE',  ( 5.616475580598488726, 6.148514233939430973, 0.8375902553012237739 ) ) ;
#103490=CARTESIAN_POINT ( 'NONE',  ( -3.415764635639130020, 6.072476943965863683, 1.199719254218462483 ) ) ;
#103494=CARTESIAN_POINT ( 'NONE',  ( 6.612626235163189925, 8.737816579155630592, -1.599625672291262513 ) ) ;
#103496=CARTESIAN_POINT ( 'NONE',  ( 5.113396490648394632, 9.117379672398465473, 1.040834085586084257E-14 ) ) ;
#103497=CARTESIAN_POINT ( 'NONE',  ( 3.825371897350130723, 7.614684313550482031, 0.7998128361456321445 ) ) ;
#103499=CARTESIAN_POINT ( 'NONE',  ( -8.080296364064746939, 9.489729181906076505, 1.082531754730558626 ) ) ;
#103509=CARTESIAN_POINT ( 'NONE',  ( -5.725072791067139732, 6.113630025739863250, -0.7036897515925732982 ) ) ;
#103511=CARTESIAN_POINT ( 'NONE',  ( 4.040494898817784453, 7.752230779688214390, 0.4466632393476636098 ) ) ;
#103512=CARTESIAN_POINT ( 'NONE',  ( 4.351804120306567825, 8.020929207092235558, 1.040834085586084257E-14 ) ) ;
#103516=CARTESIAN_POINT ( 'NONE',  ( -9.829298179783291900, 11.53023130024440768, 1.082531754730558626 ) ) ;
#103534=CARTESIAN_POINT ( 'NONE',  ( 8.097244055859613709, 10.46987070330147063, -1.599625672291262513 ) ) ;
#103538=CARTESIAN_POINT ( 'NONE',  ( -1.402160292154681736E-14, 2.118750000682816825, -1.732050807568863648 ) ) ;
#103539=CARTESIAN_POINT ( 'NONE',  ( -5.311043488251275591, 7.219303374425030562, -1.599625672291256295 ) ) ;
#103542=CARTESIAN_POINT ( 'NONE',  ( -8.239604668803112375, 10.63595808506888396, -1.599625672291263179 ) ) ;
#103545=DIRECTION ( 'NONE',  ( 0.9782075119096202975, 0.1245777785630026030, 0.1661037047506698505 ) ) ;
#103546=CARTESIAN_POINT ( 'NONE',  ( 6.425674737872927089, 9.584038729905381970, -1.199719254218440723 ) ) ;
#103548=CIRCLE ( 'NONE', #51606, 0.7499999999999997780 ) ;
#103549=CARTESIAN_POINT ( 'NONE',  ( -7.562750758324527922, 7.717630727667075696, 1.040834085586084257E-14 ) ) ;
#103551=CARTESIAN_POINT ( 'NONE',  ( 8.452618703115982512, 11.94880668935564216, 1.199719254218450271 ) ) ;
#103552=CARTESIAN_POINT ( 'NONE',  ( -0.6823417656249969321, 5.467708333674756283, -1.181850606188749264 ) ) ;
#103558=CARTESIAN_POINT ( 'NONE',  ( -8.527715433315703919, 9.051348881730875817, 1.040834085586084257E-14 ) ) ;
#103561=CARTESIAN_POINT ( 'NONE',  ( 1.364683531249990311, 4.446875000341417028, 1.214306433183764966E-14 ) ) ;
#103571=CARTESIAN_POINT ( 'NONE',  ( -3.592547517496935683, 6.174760622846296343, -1.082531754730548412 ) ) ;
#103573=CARTESIAN_POINT ( 'NONE',  ( 4.324687812634892659, 5.108185871904570519, 1.082531754730560403 ) ) ;
#103574=CARTESIAN_POINT ( 'NONE',  ( 0.6823417656249899377, 4.738541667008086655, -1.181850606188754593 ) ) ;
#103575=DIRECTION ( 'NONE',  ( -5.578564026256490882E-16, -1.000000000000000000, -9.066213480720158442E-32 ) ) ;
#103579=CARTESIAN_POINT ( 'NONE',  ( -1.402160292154681736E-14, 0.6968750003414164729, -1.575800808251659024 ) ) ;
#103580=CARTESIAN_POINT ( 'NONE',  ( -2.318081078256692518, 5.648252324700675508, 1.040834085586084257E-14 ) ) ;
#103581=CARTESIAN_POINT ( 'NONE',  ( 4.462605117192430804, 8.358123070033169455, 1.040834085586084257E-14 ) ) ;
#103584=CARTESIAN_POINT ( 'NONE',  ( 3.863710590214593399, 7.451486755318259547, 1.040834085586084257E-14 ) ) ;
#103587=CARTESIAN_POINT ( 'NONE',  ( 2.223174002961016082, 5.537527403522402025, -0.7216878364870267237 ) ) ;
#103588=CARTESIAN_POINT ( 'NONE',  ( 10.52076401408022299, 11.37657222595619189, 0.000000000000000000 ) ) ;
#103590=CARTESIAN_POINT ( 'NONE',  ( -7.510853912290736289, 11.70648729774046792, 0.7216878364870458196 ) ) ;
#103595=CARTESIAN_POINT ( 'NONE',  ( -9.806625181386236179, 10.33548422123910449, -0.7998128361456291469 ) ) ;
#103596=CARTESIAN_POINT ( 'NONE',  ( -4.243338890952904841, 5.973648010910253880, -1.443375672974051449 ) ) ;
#103597=CARTESIAN_POINT ( 'NONE',  ( -0.6823417656250212460, 2.113541667008083991, 1.181850606188767472 ) ) ;
#103604=CARTESIAN_POINT ( 'NONE',  ( 10.42352117080803708, 11.05519620889787724, -0.7998128361456281477 ) ) ;
#103618=CARTESIAN_POINT ( 'NONE',  ( 3.701970883082863040, 7.364863713882357388, -2.499999999999995115 ) ) ;
#103620=DIRECTION ( 'NONE',  ( -1.000000000000000000, 5.578564026256503701E-16, 1.479114197289397135E-31 ) ) ;
#103624=CARTESIAN_POINT ( 'NONE',  ( -1.201851678989727383E-14, 3.634375000341422357, 1.575800808251672791 ) ) ;
#103631=CARTESIAN_POINT ( 'NONE',  ( 9.772729797352075920, 10.29593960653257234, -0.7998128361456281477 ) ) ;
#103634=CARTESIAN_POINT ( 'NONE',  ( -0.6823417656250003738, 1.467708333674752730, -1.181850606188749264 ) ) ;
#103645=CARTESIAN_POINT ( 'NONE',  ( 3.818592820543298405, 7.606775390609172405, -0.7998128361456221525 ) ) ;
#103656=CARTESIAN_POINT ( 'NONE',  ( -3.785751206713858785, 5.439795712631356750, 1.599625672291267398 ) ) ;
#103659=CARTESIAN_POINT ( 'NONE',  ( 8.446893396513862839, 9.813462703143045474, -1.199719254218445830 ) ) ;
#103672=CARTESIAN_POINT ( 'NONE',  ( -7.293923454472094114, 9.532663335016016148, 1.443375672974090751 ) ) ;
#103677=CARTESIAN_POINT ( 'NONE',  ( -9.917953063596627317, 11.52969898140628047, -1.199719254218441611 ) ) ;
#103681=CARTESIAN_POINT ( 'NONE',  ( -2.123823618835070537, 5.629544655282869847, 1.040834085586084257E-14 ) ) ;
#103683=CARTESIAN_POINT ( 'NONE',  ( 7.899597058256738968, 12.36794700127490820, 1.040834085586084257E-14 ) ) ;
#103684=CARTESIAN_POINT ( 'NONE',  ( 3.948449050077836642, 5.629609863222681199, 1.599625672291267398 ) ) ;
#103690=CARTESIAN_POINT ( 'NONE',  ( 5.205967797967541166, 5.175976640491323444, -0.7216878364870197293 ) ) ;
#103693=CARTESIAN_POINT ( 'NONE',  ( -4.283486466913726254, 7.084819080452935403, -1.199719254218452047 ) ) ;
#103695=CARTESIAN_POINT ( 'NONE',  ( -9.459838494033043332, 12.05956421450382088, 1.599625672291281386 ) ) ;
#103700=CARTESIAN_POINT ( 'NONE',  ( 8.270110514656034084, 9.711179024262627024, 1.082531754730558626 ) ) ;
#103701=CARTESIAN_POINT ( 'NONE',  ( -1.364683531250010740, 5.092708333674757171, 0.7879004041258379498 ) ) ;
#103703=CARTESIAN_POINT ( 'NONE',  ( 3.635557746758808495, 7.393234471193928847, -0.7998128361456291469 ) ) ;
#103709=CARTESIAN_POINT ( 'NONE',  ( 4.081882008079450230, 3.980588341361369853, -0.7346435760097062007 ) ) ;
#103716=CARTESIAN_POINT ( 'NONE',  ( 1.364683531249988535, 3.217708333674748289, -0.7879004041258239610 ) ) ;
#103718=CARTESIAN_POINT ( 'NONE',  ( 8.353795204314554468, 12.89784483834236184, -0.7998128361456352531 ) ) ;
#103720=CARTESIAN_POINT ( 'NONE',  ( -5.748293942514189681, 5.808690475795744490, -0.7216878364870207285 ) ) ;
#103723=CARTESIAN_POINT ( 'NONE',  ( -5.761852095683518193, 6.784877535461274256, 1.082531754730546636 ) ) ;
#103728=CARTESIAN_POINT ( 'NONE',  ( 5.473741331615251227, 7.409117525016355010, -1.599625672291262513 ) ) ;
#103738=CARTESIAN_POINT ( 'NONE',  ( 6.356075086708249167, 6.309842444114747373, -0.7998128361456281477 ) ) ;
#103743=CARTESIAN_POINT ( 'NONE',  ( -6.196239896645333367, 7.187700286629718605, -1.199719254218446718 ) ) ;
#103747=CARTESIAN_POINT ( 'NONE',  ( 7.721532178182734185, 8.967207948423393304, 1.199719254218462483 ) ) ;
#103750=CARTESIAN_POINT ( 'NONE',  ( -7.061099074618889304, 7.132370430010492868, -0.7998128361456291469 ) ) ;
#103752=CARTESIAN_POINT ( 'NONE',  ( 5.463572716182812705, 9.317992568947877530, 0.7216878364870438212 ) ) ;
#103753=CARTESIAN_POINT ( 'NONE',  ( 4.815752433886056671, 6.955745678547994970, 1.411323681429425880 ) ) ;
#103754=CARTESIAN_POINT ( 'NONE',  ( -3.598799709423620374, 6.286017863381107240, 1.199719254218464037 ) ) ;
#103758=CARTESIAN_POINT ( 'NONE',  ( -5.819474248763749635, 7.812472595022922128, -1.599625672291256295 ) ) ;
#103761=CARTESIAN_POINT ( 'NONE',  ( 0.6823417656249882723, 2.176041667008084435, -1.181850606188749264 ) ) ;
#103763=CARTESIAN_POINT ( 'NONE',  ( -5.748293942514186128, 6.769059690097084747, -1.082531754730544860 ) ) ;
#103764=EDGE_LOOP ( 'NONE', ( #128412, #2939, #156393, #28401 ) ) ;
#103770=CARTESIAN_POINT ( 'NONE',  ( 6.819914962873951936, 7.915321197229798322, -1.199719254218446718 ) ) ;
#103773=CARTESIAN_POINT ( 'NONE',  ( 0.6823417656249882723, 2.488541667008084435, -1.181850606188749264 ) ) ;
#103780=CARTESIAN_POINT ( 'NONE',  ( -4.355193658487827690, 6.104145239700998538, -1.599625672291256295 ) ) ;
#103781=CARTESIAN_POINT ( 'NONE',  ( -7.822691444960716112, 8.228820895316715678, -0.7216878364870267237 ) ) ;
#103789=CARTESIAN_POINT ( 'NONE',  ( -7.158341917891067219, 11.29522330427417565, 0.000000000000000000 ) ) ;
#103794=CARTESIAN_POINT ( 'NONE',  ( -6.738039155867462604, 7.923762439009225389, 1.082531754730549967 ) ) ;
#103797=VERTEX_POINT ( 'NONE', #180291 ) ;
#103805=VERTEX_POINT ( 'NONE', #61201 ) ;
#103808=CARTESIAN_POINT ( 'NONE',  ( -6.013204822860843457, 6.974159367214481264, -1.199719254218446718 ) ) ;
#103810=CARTESIAN_POINT ( 'NONE',  ( 4.792970997630896512, 5.550553237779539018, 1.199719254218464037 ) ) ;
#103814=CARTESIAN_POINT ( 'NONE',  ( 5.282873410819217241, 9.315102745931094219, -0.7998128361456281477 ) ) ;
#103819=CARTESIAN_POINT ( 'NONE',  ( -4.826339496784927796, 5.693446170079573321, 1.082531754730560403 ) ) ;
#103826=CARTESIAN_POINT ( 'NONE',  ( -1.402160292154681736E-14, 0.9468750003414176941, -1.575800808251659024 ) ) ;
#103828=CARTESIAN_POINT ( 'NONE',  ( -6.177711549321182716, 10.35908057418338402, 0.7998128361456481317 ) ) ;
#103830=CARTESIAN_POINT ( 'NONE',  ( 6.470265622219697477, 8.571729197388226140, -1.599625672291262513 ) ) ;
#103832=CARTESIAN_POINT ( 'NONE',  ( -6.201965203247477909, 9.323044272842313518, 1.199719254218452047 ) ) ;
#103835=CARTESIAN_POINT ( 'NONE',  ( -1.201851678989727383E-14, 5.196875000341422357, -1.575800808251660134 ) ) ;
#103837=CARTESIAN_POINT ( 'NONE',  ( 7.890482213473377193, 11.18901776815221716, -1.082531754730543083 ) ) ;
#103840=CARTESIAN_POINT ( 'NONE',  ( 1.364683531249986537, -0.5322916663252452718, -0.7879004041258309554 ) ) ;
#103844=CARTESIAN_POINT ( 'NONE',  ( 7.036318535368067728, 10.19249347702934294, -1.082531754730537976 ) ) ;
#103847=CARTESIAN_POINT ( 'NONE',  ( -5.965224400332865606, 7.022145224218852455, 1.082531754730549967 ) ) ;
#103849=CARTESIAN_POINT ( 'NONE',  ( 0.6823417656249899377, 3.426041667008085323, -1.181850606188754593 ) ) ;
#103853=CARTESIAN_POINT ( 'NONE',  ( -7.366157530926372488, 7.488271962369228874, -0.7998128361456291469 ) ) ;
#103854=CARTESIAN_POINT ( 'NONE',  ( 0.6823417656249899377, 5.488541667008087543, -1.181850606188754593 ) ) ;
#103861=CARTESIAN_POINT ( 'NONE',  ( 7.151035956204054855, 10.43029348462504124, 1.199719254218460707 ) ) ;
#103864=CARTESIAN_POINT ( 'NONE',  ( 0.7499999999999902300, 2.233333333333351156, 1.299038105676669330 ) ) ;
#103871=CARTESIAN_POINT ( 'NONE',  ( 4.853455804012203778, 8.606189504748821051, 0.7216878364870438212 ) ) ;
#103872=CARTESIAN_POINT ( 'NONE',  ( 0.6823417656249882723, -0.3447916663252489911, 1.181850606188755259 ) ) ;
#103873=EDGE_CURVE ( 'NONE', #206877, #22516, #77028, .T. ) ;
#103879=CARTESIAN_POINT ( 'NONE',  ( -1.500000000000015099, 0.8791666666666874130, -0.8660254037844313801 ) ) ;
#103880=CARTESIAN_POINT ( 'NONE',  ( 8.423693512792301163, 8.722063941212843119, 0.7998128361456481317 ) ) ;
#103881=CARTESIAN_POINT ( 'NONE',  ( -7.655550293210764856, 12.08322577538792331, 0.000000000000000000 ) ) ;
#103883=CARTESIAN_POINT ( 'NONE',  ( -0.6823417656250003738, -0.2822916663252489355, -1.181850606188749264 ) ) ;
#103884=CARTESIAN_POINT ( 'NONE',  ( -0.7500000000000006661, 1.108333333333356929, -1.299038105676652011 ) ) ;
#103885=EDGE_CURVE ( 'NONE', #97759, #71636, #13088, .T. ) ;
#103887=CARTESIAN_POINT ( 'NONE',  ( 6.159481859310094620, 6.080483678816896109, 1.040834085586084257E-14 ) ) ;
#103894=CARTESIAN_POINT ( 'NONE',  ( 0.6823417656249917140, 5.092708333674749177, 1.181850606188765695 ) ) ;
#103897=CARTESIAN_POINT ( 'NONE',  ( -8.134002093194872884, 11.57708731111429401, 1.199719254218453823 ) ) ;
#103898=CARTESIAN_POINT ( 'NONE',  ( -4.717874267875590277, 7.487641831621378863, 1.082531754730560403 ) ) ;
#103906=CARTESIAN_POINT ( 'NONE',  ( 6.751070424600909448, 9.963667031088037973, -1.199719254218441611 ) ) ;
#103910=CARTESIAN_POINT ( 'NONE',  ( 5.784525094524856748, 9.900363043587685041, 1.040834085586084257E-14 ) ) ;
#103911=CARTESIAN_POINT ( 'NONE',  ( 7.253248993186731219, 8.524840582548424806, 1.082531754730558626 ) ) ;
#103914=CARTESIAN_POINT ( 'NONE',  ( -8.507905087775398556, 9.884643009614800135, 1.199719254218462483 ) ) ;
#103915=CARTESIAN_POINT ( 'NONE',  ( 6.193377243344257543, 6.120028293523423812, -0.7998128361456281477 ) ) ;
#103918=CARTESIAN_POINT ( 'NONE',  ( 2.372313692266983853, 5.711523707712699682, 0.7216878364870438212 ) ) ;
#103920=CARTESIAN_POINT ( 'NONE',  ( 2.900554798319789906, 5.471398800426671372, 1.199719254218452047 ) ) ;
#103921=ORIENTED_EDGE ( 'NONE', *, *, #57944, .T. ) ;
#103927=CARTESIAN_POINT ( 'NONE',  ( -3.945059511896602089, 7.546393830613923548, 1.040834085586084257E-14 ) ) ;
#103928=CARTESIAN_POINT ( 'NONE',  ( 4.207107738942202246, 3.802713871720993399, 1.214306433183764966E-14 ) ) ;
#103932=CARTESIAN_POINT ( 'NONE',  ( -7.230575994789712801, 7.330093503543126054, 0.7998128361456341429 ) ) ;
#103936=CARTESIAN_POINT ( 'NONE',  ( 0.9486429539237064557, 2.980410930033766448, -1.028101543438967758 ) ) ;
#103938=CARTESIAN_POINT ( 'NONE',  ( -6.645467848992654858, 10.90479625713344625, 0.7998128361456481317 ) ) ;
#103953=CARTESIAN_POINT ( 'NONE',  ( -5.856232286098998152, 8.919689202835742847, 1.199719254218452047 ) ) ;
#103956=CARTESIAN_POINT ( 'NONE',  ( 4.799223189557548785, 7.582548906917042864, -1.082531754730549078 ) ) ;
#103961=CARTESIAN_POINT ( 'NONE',  ( -3.785751206713858785, 5.439795712631356750, 1.599625672291267398 ) ) ;
#103966=CARTESIAN_POINT ( 'NONE',  ( -5.148345644887285744, 7.029489223833707001, -1.599625672291256295 ) ) ;
#103972=CARTESIAN_POINT ( 'NONE',  ( -8.962103233833181193, 10.41454084668224489, -1.199719254218446718 ) ) ;
#103973=CARTESIAN_POINT ( 'NONE',  ( 7.613066949273408213, 8.840665181362512115, -1.199719254218441611 ) ) ;
#103976=CARTESIAN_POINT ( 'NONE',  ( -8.890396042259075315, 11.39521468743417998, -1.599625672291263179 ) ) ;
#103983=CARTESIAN_POINT ( 'NONE',  ( 9.598809568795314107, 10.30095870645710754, -0.7216878364870257245 ) ) ;
#103988=CARTESIAN_POINT ( 'NONE',  ( -5.547286221698657371, 6.226642220600762556, -0.9388435239387061815 ) ) ;
#103990=CARTESIAN_POINT ( 'NONE',  ( -0.3895070363647045175, 6.983478840415547673, -3.944638453887328922 ) ) ;
#103997=ORIENTED_EDGE ( 'NONE', *, *, #177848, .F. ) ;
#104002=CARTESIAN_POINT ( 'NONE',  ( -4.485049888022365927, 4.126979712314507331, 0.7998128361456341429 ) ) ;
#104009=CARTESIAN_POINT ( 'NONE',  ( -1.201851678989727383E-14, 5.446875000341422357, -1.575800808251660134 ) ) ;
#104014=CARTESIAN_POINT ( 'NONE',  ( 1.203941962966152968, 3.008481847795084541, -0.7749999999999840350 ) ) ;
#104015=CARTESIAN_POINT ( 'NONE',  ( -1.284279953904156280, 3.202889714876734573, 0.7750000000000117906 ) ) ;
#104017=CARTESIAN_POINT ( 'NONE',  ( 4.878236342818665250, 4.585697242910212523, 1.040834085586084257E-14 ) ) ;
#104021=CARTESIAN_POINT ( 'NONE',  ( 4.299907273828439180, 8.168308919441841454, 1.040834085586084257E-14 ) ) ;
#104022=CARTESIAN_POINT ( 'NONE',  ( 1.364683531249988535, 3.176041667008084435, 0.7879004041258500513 ) ) ;
#104023=CARTESIAN_POINT ( 'NONE',  ( -4.595282798756362475, 6.958845989550745514, 1.192800718855389297 ) ) ;
#104024=CARTESIAN_POINT ( 'NONE',  ( 8.920375002787457319, 12.49452237230570084, 1.199719254218450271 ) ) ;
#104026=CARTESIAN_POINT ( 'NONE',  ( -7.862839020921525091, 11.26073039346208660, -1.199719254218446718 ) ) ;
#104028=CARTESIAN_POINT ( 'NONE',  ( -5.721177634842498527, 5.777054783512106440, 0.000000000000000000 ) ) ;
#104031=CARTESIAN_POINT ( 'NONE',  ( -6.124532705071231931, 8.168374127381657246, -1.599625672291263179 ) ) ;
#104033=CARTESIAN_POINT ( 'NONE',  ( 1.364683531249992088, 5.634375000341417916, 1.214306433183764966E-14 ) ) ;
#104041=CARTESIAN_POINT ( 'NONE',  ( -3.578989363883261277, 7.119311991265024453, 1.040834085586084257E-14 ) ) ;
#104043=CARTESIAN_POINT ( 'NONE',  ( 1.403499169903363875, 7.376709478542918141, -4.304123474984290709 ) ) ;
#104046=CARTESIAN_POINT ( 'NONE',  ( -4.324687812634898876, 6.068555086205916105, 1.443375672974064550 ) ) ;
#104048=CARTESIAN_POINT ( 'NONE',  ( 8.609591239877852686, 10.00327685373437347, -1.199719254218445830 ) ) ;
#104057=CARTESIAN_POINT ( 'NONE',  ( -2.927671105547157371, 5.503034492191895666, 1.199719254218462483 ) ) ;
#104058=CARTESIAN_POINT ( 'NONE',  ( -4.067937748088393590, 7.725456827083305278, 0.6547958487484796253 ) ) ;
#104062=CARTESIAN_POINT ( 'NONE',  ( 5.005985031943777308, 6.863401842066294556, -1.599625672291256295 ) ) ;
#104066=ORIENTED_EDGE ( 'NONE', *, *, #50294, .F. ) ;
#104068=CARTESIAN_POINT ( 'NONE',  ( 3.785751206713845018, 5.439795712631356750, 1.599625672291267398 ) ) ;
#104078=CARTESIAN_POINT ( 'NONE',  ( 8.015895134177609904, 10.37496362800581018, 1.599625672291281386 ) ) ;
#104080=CARTESIAN_POINT ( 'NONE',  ( -4.076197739202962467, 7.907314462378773001, 1.040834085586084257E-14 ) ) ;
#104087=CARTESIAN_POINT ( 'NONE',  ( 0.7499999999999885647, -0.9854166659838472508, 1.299038105676657340 ) ) ;
#104091=CARTESIAN_POINT ( 'NONE',  ( -4.719485776398897769, 6.960464655427080594, 1.371982998767233175 ) ) ;
#104092=CARTESIAN_POINT ( 'NONE',  ( 3.734381245560244089, 6.444196322207211836, 1.199719254218462483 ) ) ;
#104093=CARTESIAN_POINT ( 'NONE',  ( -4.192495815123836955, 5.914331089109674089, -1.599625672291256295 ) ) ;
#104094=CARTESIAN_POINT ( 'NONE',  ( 2.920214025141053327, 6.445393704534057022, 0.4458799699700779495 ) ) ;
#104099=CARTESIAN_POINT ( 'NONE',  ( 5.721177635286841756, 6.737423998331861341, -1.082531754730543083 ) ) ;
#104101=CARTESIAN_POINT ( 'NONE',  ( 6.914295152845067349, 11.01050207838719075, 1.040834085586084257E-14 ) ) ;
#104102=CARTESIAN_POINT ( 'NONE',  ( -1.364683531250012516, 3.592708333674750509, 0.7879004041258379498 ) ) ;
#104104=CARTESIAN_POINT ( 'NONE',  ( 5.300874872818840622, 6.247070775452521652, 1.082531754730560403 ) ) ;
#104112=CARTESIAN_POINT ( 'NONE',  ( -4.637175514440688318, 7.109613026884349374, 1.382187809737724704 ) ) ;
#104120=CARTESIAN_POINT ( 'NONE',  ( -8.910733272679575379, 11.41894145625809820, -1.599625672291263179 ) ) ;
#104126=CARTESIAN_POINT ( 'NONE',  ( -2.449219305563052895, 6.009172956465517856, 1.040834085586084257E-14 ) ) ;
#104132=CARTESIAN_POINT ( 'NONE',  ( -1.364683531249997417, 2.821875000341422801, 1.214306433183764966E-14 ) ) ;
#104134=CARTESIAN_POINT ( 'NONE',  ( 6.938021921891177612, 9.117444880338284818, -1.599625672291262513 ) ) ;
#104135=CARTESIAN_POINT ( 'NONE',  ( -9.854078719034067291, 10.39084668182823634, 0.7998128361456462443 ) ) ;
#104136=CARTESIAN_POINT ( 'NONE',  ( -7.815970093360414158E-14, 8.210952333604092601, -2.038660652713623733 ) ) ;
#104137=CARTESIAN_POINT ( 'NONE',  ( -3.391510981712834383, 7.108513245306943062, 0.7998128361456341429 ) ) ;
#104139=VERTEX_POINT ( 'NONE', #199710 ) ;
#104141=CARTESIAN_POINT ( 'NONE',  ( 0.7499999999999902300, 4.066666666666690411, -1.299038105676658228 ) ) ;
#104142=CARTESIAN_POINT ( 'NONE',  ( 5.497994985541524215, 6.373081223675282736, -1.199719254218445830 ) ) ;
#104145=CARTESIAN_POINT ( 'NONE',  ( 1.499999999999999334, 7.388542872122531691, 4.154462424328197123 ) ) ;
#104146=CARTESIAN_POINT ( 'NONE',  ( -1.201851678989727383E-14, 4.196875000341417028, -1.575800808251660134 ) ) ;
#104150=CARTESIAN_POINT ( 'NONE',  ( 8.107412671292022921, 12.40247251657532956, 0.7216878364870438212 ) ) ;
#104155=CARTESIAN_POINT ( 'NONE',  ( 0.7499999999999885647, 1.597916667349486008, -1.299038105676652899 ) ) ;
#104157=CARTESIAN_POINT ( 'NONE',  ( -3.744022975668147790, 7.519777238254810925, -0.7998128361456281477 ) ) ;
#104158=CARTESIAN_POINT ( 'NONE',  ( 5.816084710138150093, 5.887779704690372817, -0.7216878364870257245 ) ) ;
#104167=CARTESIAN_POINT ( 'NONE',  ( 6.448874621594486989, 10.67543749183559143, 0.7998128361456462443 ) ) ;
#104168=CARTESIAN_POINT ( 'NONE',  ( 6.010342169559767633, 5.906487374108181143, -0.7998128361456281477 ) ) ;
#104172=SURFACE_STYLE_FILL_AREA ( #103097 ) ;
#104173=CARTESIAN_POINT ( 'NONE',  ( 5.840865249388943248, 5.708764300575555062, 0.7998128361456341429 ) ) ;
#104177=ORIENTED_EDGE ( 'NONE', *, *, #40619, .T. ) ;
#104180=CARTESIAN_POINT ( 'NONE',  ( 10.21336978979620191, 10.81001959771741205, 0.7998128361456462443 ) ) ;
#104184=CARTESIAN_POINT ( 'NONE',  ( 4.739561450132447007, 6.795411536013346243, -1.240012687728889951 ) ) ;
#104186=CARTESIAN_POINT ( 'NONE',  ( 10.22692794340986921, 10.82583744360002243, 0.000000000000000000 ) ) ;
#104192=CARTESIAN_POINT ( 'NONE',  ( -0.6823417656250246877, -1.198958332991911790, 1.181850606188755259 ) ) ;
#104193=CARTESIAN_POINT ( 'NONE',  ( 6.643132081016117851, 8.773406732650713025, 1.443375672974076540 ) ) ;
#104195=CARTESIAN_POINT ( 'NONE',  ( -3.307299406729781399, 5.945934176904983381, -1.199719254218452935 ) ) ;
#104200=CARTESIAN_POINT ( 'NONE',  ( -5.037017762676898158, 5.835274463666530131, -1.199719254218446718 ) ) ;
#104203=CARTESIAN_POINT ( 'NONE',  ( -6.471393748265563239, 5.229711127717889596, 2.499999999999998668 ) ) ;
#104206=ORIENTED_EDGE ( 'NONE', *, *, #178431, .T. ) ;
#104212=CARTESIAN_POINT ( 'NONE',  ( 7.574201371528760163, 11.98831870009225931, 1.040834085586084257E-14 ) ) ;
#104221=CARTESIAN_POINT ( 'NONE',  ( -8.161645285746702783, 12.46574390010577105, 0.7216878364870478180 ) ) ;
#104225=CARTESIAN_POINT ( 'NONE',  ( 7.293396569147545527, 10.59638086639245280, 1.199719254218460707 ) ) ;
#104228=AXIS2_PLACEMENT_3D ( 'NONE', #121575, #185408, #3444 ) ;
#104230=CARTESIAN_POINT ( 'NONE',  ( -5.442708600882160574, 8.437244903416123876, -1.199719254218446718 ) ) ;
#104231=CARTESIAN_POINT ( 'NONE',  ( 5.020596955762157698, 4.751784624677624080, 1.040834085586084257E-14 ) ) ;
#104238=CARTESIAN_POINT ( 'NONE',  ( -1.201851678989727383E-14, 3.134375000341420137, 1.575800808251672791 ) ) ;
#104240=CARTESIAN_POINT ( 'NONE',  ( 5.612712406377503349, 8.531619659873665995, -1.082531754730543083 ) ) ;
#104247=ORIENTED_EDGE ( 'NONE', *, *, #50690, .T. ) ;
#104248=CARTESIAN_POINT ( 'NONE',  ( 7.063434842595398777, 11.18449838309590483, -0.7216878364870267237 ) ) ;
#104252=CARTESIAN_POINT ( 'NONE',  ( -8.365544474831901667, 9.718555627847388578, 1.199719254218462483 ) ) ;
#104260=CARTESIAN_POINT ( 'NONE',  ( 3.379006598303866848, 4.965260336153046516, -1.599625672291262513 ) ) ;
#104265=CARTESIAN_POINT ( 'NONE',  ( 4.792970997630896512, 5.550553237779539018, 1.199719254218464037 ) ) ;
#104268=AXIS2_PLACEMENT_3D ( 'NONE', #64499, #2655, #148945 ) ;
#104269=CARTESIAN_POINT ( 'NONE',  ( -1.201851678989727383E-14, 2.743750000682820378, 1.732050807568877637 ) ) ;
#104273=ORIENTED_EDGE ( 'NONE', *, *, #149088, .T. ) ;
#104275=AXIS2_PLACEMENT_3D ( 'NONE', #54369, #202718, #83649 ) ;
#104276=CARTESIAN_POINT ( 'NONE',  ( 0.7499999999999867883, 0.06666666666668707997, -1.299038105676652899 ) ) ;
#104277=CARTESIAN_POINT ( 'NONE',  ( 6.938021921891177612, 9.117444880338284818, -1.599625672291262513 ) ) ;
#104278=CARTESIAN_POINT ( 'NONE',  ( 5.029711800545521250, 5.930713857800314237, -1.082531754730549078 ) ) ;
#104282=CARTESIAN_POINT ( 'NONE',  ( 10.24960094225127172, 11.06021530882240356, -0.7216878364870257245 ) ) ;
#104287=CARTESIAN_POINT ( 'NONE',  ( -5.576481253922474401, 5.400316305864651056, -0.7998128361456221525 ) ) ;
#104288=CARTESIAN_POINT ( 'NONE',  ( -0.7499999999999972244, 3.639583334016149863, -1.299038105676652011 ) ) ;
#104289=CARTESIAN_POINT ( 'NONE',  ( -1.201851678989727383E-14, 5.509375000341415252, -1.575800808251660134 ) ) ;
#104294=CARTESIAN_POINT ( 'NONE',  ( 0.6823417656249917140, 4.655208333674755394, 1.181850606188765695 ) ) ;
#104302=CARTESIAN_POINT ( 'NONE',  ( -8.850775351622791831, 9.220326086515070685, -0.7998128361456291469 ) ) ;
#104303=CARTESIAN_POINT ( 'NONE',  ( 6.494519276145969577, 7.535692896047149425, -1.199719254218446718 ) ) ;
#104311=CARTESIAN_POINT ( 'NONE',  ( -7.881367368245678406, 8.089350105908421185, 0.7998128361456602331 ) ) ;
#104317=CARTESIAN_POINT ( 'NONE',  ( 9.297140650669039275, 11.86975006391249643, 1.599625672291281386 ) ) ;
#104320=ORIENTED_EDGE ( 'NONE', *, *, #53608, .T. ) ;
#104321=CARTESIAN_POINT ( 'NONE',  ( -5.603597561149804562, 5.431951997629870910, 0.7998128361456341429 ) ) ;
#104322=CARTESIAN_POINT ( 'NONE',  ( -6.821723845970312894, 11.11042825360738284, 0.000000000000000000 ) ) ;
#104325=CARTESIAN_POINT ( 'NONE',  ( -4.391370929004954959, 7.351591927832363815, -1.215465595245905250 ) ) ;
#104326=CARTESIAN_POINT ( 'NONE',  ( 0.6823417656249882723, -0.6572916663252492686, 1.181850606188755259 ) ) ;
#104332=CARTESIAN_POINT ( 'NONE',  ( 6.169123589417988995, 7.156064594864501416, -1.199719254218445830 ) ) ;
#104338=VECTOR ( 'NONE', #89426, 1000.000000000000000 ) ;
#104357=CARTESIAN_POINT ( 'NONE',  ( -9.321394304595349567, 10.83371376257142416, 1.199719254218462483 ) ) ;
#104362=CARTESIAN_POINT ( 'NONE',  ( -0.7500000000000215383, 1.972916667349486453, 1.299038105676659116 ) ) ;
#104363=CARTESIAN_POINT ( 'NONE',  ( 9.028840231696797503, 12.62106513936658203, -1.199719254218446718 ) ) ;
#104370=CARTESIAN_POINT ( 'NONE',  ( 1.364683531249988535, 1.363541667008083769, 0.7879004041258500513 ) ) ;
#104376=CARTESIAN_POINT ( 'NONE',  ( -4.120788623549732854, 6.895004929861607401, -1.199719254218452047 ) ) ;
#104378=CARTESIAN_POINT ( 'NONE',  ( 1.499999999999990896, 8.266799604814712765, -3.162088779279259132 ) ) ;
#104381=CARTESIAN_POINT ( 'NONE',  ( -1.364683531250000748, 0.8218750003414210248, 0.000000000000000000 ) ) ;
#104386=CARTESIAN_POINT ( 'NONE',  ( -1.402160292154681736E-14, 0.1968750003414221628, -1.575800808251665908 ) ) ;
#104388=CARTESIAN_POINT ( 'NONE',  ( -5.215082642750900277, 9.236013516518044142, 0.000000000000000000 ) ) ;
#104389=CARTESIAN_POINT ( 'NONE',  ( 7.344766530301147789, 9.591980256816594164, 1.599625672291281386 ) ) ;
#104390=CARTESIAN_POINT ( 'NONE',  ( 3.506755287428983792, 7.242964935309132990, 1.040834085586084257E-14 ) ) ;
#104391=CARTESIAN_POINT ( 'NONE',  ( 4.710568305744190276, 7.583081225755162968, 1.199719254218462483 ) ) ;
#104392=CARTESIAN_POINT ( 'NONE',  ( 0.7499999999999902300, 3.983333333333352488, 1.299038105676669330 ) ) ;
#104394=CARTESIAN_POINT ( 'NONE',  ( -0.6823417656250003738, 1.780208333674752952, -1.181850606188749264 ) ) ;
#104401=CARTESIAN_POINT ( 'NONE',  ( 7.782016984564065432, 8.181367358187307204, 0.7216878364870458196 ) ) ;
#104404=CARTESIAN_POINT ( 'NONE',  ( -5.852315862593199469, 9.979452273000736895, 0.7998128361456481317 ) ) ;
#104405=CARTESIAN_POINT ( 'NONE',  ( -4.253507506385335368, 5.985511395581417204, 1.599625672291267398 ) ) ;
#104410=CARTESIAN_POINT ( 'NONE',  ( -6.670248387799091461, 10.72578085250020585, 0.000000000000000000 ) ) ;
#104412=CARTESIAN_POINT ( 'NONE',  ( -1.201851678989727383E-14, 5.337500000000020783, -1.732050807568863648 ) ) ;
#104416=CARTESIAN_POINT ( 'NONE',  ( 9.463228032658635769, 11.10314946193233965, -1.082531754730543083 ) ) ;
#104421=LINE ( 'NONE', #125018, #161498 ) ;
#104425=CARTESIAN_POINT ( 'NONE',  ( 10.66990370383054731, 11.55056853066490952, 0.7216878364870317197 ) ) ;
#104429=LINE ( 'NONE', #25295, #131925 ) ;
#104430=CARTESIAN_POINT ( 'NONE',  ( 8.446366511189332016, 9.916811020218137429, -1.082531754730543083 ) ) ;
#104431=CARTESIAN_POINT ( 'NONE',  ( 8.260995669428309540, 8.532249790621511565, 0.7998128361456481317 ) ) ;
#104432=CARTESIAN_POINT ( 'NONE',  ( -5.018489415352746619, 9.006654751220198207, 0.7998128361456481317 ) ) ;
#104434=CYLINDRICAL_SURFACE ( 'NONE', #90521, 1.250000000000000000 ) ;
#104435=CARTESIAN_POINT ( 'NONE',  ( -4.487385655998893164, 6.258369236797239665, 1.443375672974064550 ) ) ;
#104436=CARTESIAN_POINT ( 'NONE',  ( -1.402160292154681736E-14, -0.7406249996585823059, -1.575800808251665908 ) ) ;
#104437=CARTESIAN_POINT ( 'NONE',  ( 4.867013957625893283, 4.780530493426062399, 1.040834085586084257E-14 ) ) ;
#104439=CARTESIAN_POINT ( 'NONE',  ( -4.243865776277440993, 4.909930479533815451, -1.199719254218446718 ) ) ;
#104445=ADVANCED_FACE ( 'NONE', ( #111632 ), #128379, .F. ) ;
#104450=VERTEX_POINT ( 'NONE', #8588 ) ;
#104455=VERTEX_POINT ( 'NONE', #204637 ) ;
#104458=CYLINDRICAL_SURFACE ( 'NONE', #65078, 1.500000000000000222 ) ;
#104459=CARTESIAN_POINT ( 'NONE',  ( 8.606728586576791074, 8.935604860628076906, 0.7998128361456462443 ) ) ;
#104465=CARTESIAN_POINT ( 'NONE',  ( 1.445367865410934982, 8.714818166637854802, 2.590103969856952126 ) ) ;
#104471=CARTESIAN_POINT ( 'NONE',  ( -6.144869935491728441, 8.192100896205577243, -1.599625672291263179 ) ) ;
#104473=CARTESIAN_POINT ( 'NONE',  ( -3.391510981712833939, 7.108513245306943062, 0.7998128361456341429 ) ) ;
#104486=CARTESIAN_POINT ( 'NONE',  ( -4.952806187693842510, 4.672695395264567786, 0.7998128361456341429 ) ) ;
#104489=CARTESIAN_POINT ( 'NONE',  ( 8.125414133291656071, 8.374071331795406081, -0.7998128361456291469 ) ) ;
#104490=CARTESIAN_POINT ( 'NONE',  ( -0.6823417656250212460, 4.551041667008086655, 1.181850606188767472 ) ) ;
#104496=CARTESIAN_POINT ( 'NONE',  ( 5.138177029454841893, 7.017625839162543677, 1.443375672974062551 ) ) ;
#104497=CARTESIAN_POINT ( 'NONE',  ( -7.640183256500752584, 8.872300873127729304, -1.199719254218446718 ) ) ;
#104500=CARTESIAN_POINT ( 'NONE',  ( -7.531718027591449705, 8.745758106066849891, 1.199719254218462483 ) ) ;
#104501=CARTESIAN_POINT ( 'NONE',  ( -3.899941742225307539, 7.701682465904834629, 0.7998128361456341429 ) ) ;
#104509=CARTESIAN_POINT ( 'NONE',  ( 7.287671262545424966, 8.461036880179857889, -1.199719254218451159 ) ) ;
#104519=CARTESIAN_POINT ( 'NONE',  ( -0.007473969438217894709, 8.279395425053857949, -1.999986034896452880 ) ) ;
#104523=CARTESIAN_POINT ( 'NONE',  ( -1.201851678989727383E-14, 5.087500000000019007, -1.732050807568863648 ) ) ;
#104524=CARTESIAN_POINT ( 'NONE',  ( 5.606460214450851964, 6.499623990736163037, 1.199719254218462483 ) ) ;
#104525=CARTESIAN_POINT ( 'NONE',  ( 6.494519276145969577, 7.535692896047149425, -1.199719254218446718 ) ) ;
#104527=CARTESIAN_POINT ( 'NONE',  ( -9.002250809794006159, 10.56534270192358704, -1.082531754730543971 ) ) ;
#104529=CARTESIAN_POINT ( 'NONE',  ( 7.131225611108096274, 8.382479970123348778, 1.082531754730558626 ) ) ;
#104530=CARTESIAN_POINT ( 'NONE',  ( -7.171900071504738072, 10.35067193585544665, -1.082531754730543083 ) ) ;
#104533=CARTESIAN_POINT ( 'NONE',  ( 8.599949509769960088, 8.927695937686774386, 1.040834085586084257E-14 ) ) ;
#104539=CARTESIAN_POINT ( 'NONE',  ( -1.364683531250012516, 2.030208333674750953, 0.7879004041258379498 ) ) ;
#104545=CARTESIAN_POINT ( 'NONE',  ( 7.574201371528760163, 11.98831870009225931, 1.040834085586084257E-14 ) ) ;
#104548=EDGE_CURVE ( 'NONE', #205532, #73290, #194693, .T. ) ;
#104550=CARTESIAN_POINT ( 'NONE',  ( -8.157201976916404362, 12.66848607304450702, -0.7998128361456281477 ) ) ;
#104556=CARTESIAN_POINT ( 'NONE',  ( 2.530568227245037605, 6.104080031761181857, 0.000000000000000000 ) ) ;
#104560=CARTESIAN_POINT ( 'NONE',  ( -9.826962411806732689, 10.35921099006301382, -0.7998128361456291469 ) ) ;
#104565=CARTESIAN_POINT ( 'NONE',  ( 5.833718835943604297, 6.012594516355426855, -0.4067158398524447493 ) ) ;
#104566=CARTESIAN_POINT ( 'NONE',  ( -0.8368079278675620847, 2.800000000000018918, -1.135296483310510585 ) ) ;
#104567=CARTESIAN_POINT ( 'NONE',  ( -5.037017762676898158, 5.835274463666530131, -1.199719254218446718 ) ) ;
#104571=CARTESIAN_POINT ( 'NONE',  ( 6.751070424600909448, 9.963667031088037973, -1.199719254218441611 ) ) ;
#104573=CARTESIAN_POINT ( 'NONE',  ( 7.124973419181436007, 8.271222729588529887, -1.199719254218446718 ) ) ;
#104574=CARTESIAN_POINT ( 'NONE',  ( 3.714044015139744914, 6.420469553383295391, 1.199719254218462483 ) ) ;
#104576=CARTESIAN_POINT ( 'NONE',  ( -8.351459436338037889, 10.76645531385962862, -1.443375672974059665 ) ) ;
#104585=CARTESIAN_POINT ( 'NONE',  ( -5.266540691475234404, 6.417032612176464923, -1.150853802781536039 ) ) ;
#104587=CARTESIAN_POINT ( 'NONE',  ( 4.026408433578586354, 7.641300905909586660, 1.040834085586084257E-14 ) ) ;
#104592=CARTESIAN_POINT ( 'NONE',  ( -10.27671724903424888, 11.09185100006920877, 1.040834085586084257E-14 ) ) ;
#104599=EDGE_LOOP ( 'NONE', ( #185932, #61332, #44253, #176417, #23994, #214248, #209544 ) ) ;
#104606=LINE ( 'NONE', #204185, #25312 ) ;
#104609=CARTESIAN_POINT ( 'NONE',  ( 7.283754839039659146, 9.520799950344851936, -1.599625672291262513 ) ) ;
#104613=CARTESIAN_POINT ( 'NONE',  ( -0.7500000000000006661, 1.639583334016154970, -1.299038105676652011 ) ) ;
#104614=CARTESIAN_POINT ( 'NONE',  ( -5.530836599371015794, 8.540060901653093950, 1.199719254218452047 ) ) ;
#104617=CARTESIAN_POINT ( 'NONE',  ( -10.32183501870554387, 10.93656236477829502, 0.7998128361456462443 ) ) ;
#104618=FACE_OUTER_BOUND ( 'NONE', #204787, .T. ) ;
#104621=CARTESIAN_POINT ( 'NONE',  ( -1.201851678989727383E-14, 5.618750000682818602, -1.732050807568863648 ) ) ;
#104622=CARTESIAN_POINT ( 'NONE',  ( 7.623762449586013901, 7.788811034138823253, 1.040834085586084257E-14 ) ) ;
#104625=CARTESIAN_POINT ( 'NONE',  ( -5.554036483092550824, 9.631459663583308739, -0.7998128361456231517 ) ) ;
#104627=CARTESIAN_POINT ( 'NONE',  ( 1.364683531249988535, 5.405208333674750953, -0.7879004041258300672 ) ) ;
#104633=CARTESIAN_POINT ( 'NONE',  ( -7.917598520700757980, 9.299915031314755609, 1.082531754730558626 ) ) ;
#104637=CARTESIAN_POINT ( 'NONE',  ( -1.364683531250010295, 4.342708333674753618, 0.7879004041258379498 ) ) ;
#104643=CARTESIAN_POINT ( 'NONE',  ( 1.364683531249988535, 3.863541667008087543, 0.7879004041258500513 ) ) ;
#104647=CARTESIAN_POINT ( 'NONE',  ( 4.324687812634897988, 4.147816657603229373, 0.7216878364870317197 ) ) ;
#104648=CARTESIAN_POINT ( 'NONE',  ( -1.001543065824772872E-14, 5.634375000341415252, 1.575800808251672791 ) ) ;
#104653=CARTESIAN_POINT ( 'NONE',  ( -1.201851678989727383E-14, 0.8218750003414171390, 1.575800808251672791 ) ) ;
#104654=CARTESIAN_POINT ( 'NONE',  ( -3.307826292054310890, 5.842585859829892314, -1.082531754730549967 ) ) ;
#104655=CARTESIAN_POINT ( 'NONE',  ( 6.322179702674084467, 6.270297829408224111, 1.040834085586084257E-14 ) ) ;
#104656=ORIENTED_EDGE ( 'NONE', *, *, #193595, .T. ) ;
#104658=DIRECTION ( 'NONE',  ( 0.000000000000000000, -0.7999999999999973799, -0.6000000000000034195 ) ) ;
#104659=EDGE_CURVE ( 'NONE', #96352, #152273, #126775, .T. ) ;
#104662=DIRECTION ( 'NONE',  ( 0.6507913734559651608, 0.7592566023652994600, 1.725633230170963543E-31 ) ) ;
#104665=CARTESIAN_POINT ( 'NONE',  ( -6.887178846062105286, 10.97886638714038554, -0.7216878364870267237 ) ) ;
#104670=CARTESIAN_POINT ( 'NONE',  ( -9.982881178363895103, 10.54111621771303753, 1.040834085586084257E-14 ) ) ;
#104671=CARTESIAN_POINT ( 'NONE',  ( -6.195713011320804320, 7.291048603704809672, -1.082531754730543083 ) ) ;
#104672=CARTESIAN_POINT ( 'NONE',  ( -1.402160292154681736E-14, 1.509375000341420359, -1.575800808251659024 ) ) ;
#104689=ORIENTED_EDGE ( 'NONE', *, *, #100082, .T. ) ;
#104693=CARTESIAN_POINT ( 'NONE',  ( -4.437596350374534815, 4.071617251725375475, -0.7998128361456221525 ) ) ;
#104696=CARTESIAN_POINT ( 'NONE',  ( -0.6823417656250212460, 3.113541667008084879, 1.181850606188767472 ) ) ;
#104706=EDGE_CURVE ( 'NONE', #138593, #17304, #213613, .T. ) ;
#104707=CARTESIAN_POINT ( 'NONE',  ( -0.6823417656250003738, 0.7177083336747519526, -1.181850606188749264 ) ) ;
#104719=CARTESIAN_POINT ( 'NONE',  ( 6.166260936116925606, 6.088392601758203071, 0.7998128361456341429 ) ) ;
#104726=CARTESIAN_POINT ( 'NONE',  ( 6.421758314367153275, 10.64380180007036891, -0.7998128361456291469 ) ) ;
#104730=CARTESIAN_POINT ( 'NONE',  ( 6.611572464958476836, 10.86525164242692298, 0.7998128361456462443 ) ) ;
#104743=CARTESIAN_POINT ( 'NONE',  ( -7.537970219518083326, 9.817384560903001045, -1.443375672974059665 ) ) ;
#104747=CARTESIAN_POINT ( 'NONE',  ( -10.13202086811422475, 10.71511252242175161, -0.7998128361456291469 ) ) ;
#104752=CARTESIAN_POINT ( 'NONE',  ( -4.192495815123836955, 5.914331089109674089, -1.599625672291256295 ) ) ;
#104754=CARTESIAN_POINT ( 'NONE',  ( 4.175548122884573665, 3.973820352894515295, 1.214306433183764966E-14 ) ) ;
#104756=CARTESIAN_POINT ( 'NONE',  ( 3.379006598303866848, 4.965260336153046516, -1.599625672291262513 ) ) ;
#104762=CARTESIAN_POINT ( 'NONE',  ( 3.714570900464274850, 6.317121236308204324, 1.082531754730558626 ) ) ;
#104764=CARTESIAN_POINT ( 'NONE',  ( -3.893162665418476109, 7.693773542963529444, 1.040834085586084257E-14 ) ) ;
#104765=FACE_OUTER_BOUND ( 'NONE', #122081, .T. ) ;
#104767=CARTESIAN_POINT ( 'NONE',  ( -9.378489572351046633, 11.96465713920816043, -1.599625672291263179 ) ) ;
#104773=CARTESIAN_POINT ( 'NONE',  ( 7.890482213473377193, 11.18901776815221716, -1.082531754730543083 ) ) ;
#104774=CARTESIAN_POINT ( 'NONE',  ( -0.6823417656249969321, 4.280208333674755394, -1.181850606188749264 ) ) ;
#104777=CARTESIAN_POINT ( 'NONE',  ( 4.497554271431305040, 6.270232621468402989, -1.599625672291256295 ) ) ;
#104792=CARTESIAN_POINT ( 'NONE',  ( -1.364683531250012516, 2.301041667008087988, -0.7879004041258289570 ) ) ;
#104794=CARTESIAN_POINT ( 'NONE',  ( 9.134442807305049428, 11.67993591332117376, 1.599625672291281386 ) ) ;
#104796=CARTESIAN_POINT ( 'NONE',  ( -5.910991785878170646, 7.919243054989755670, -1.443375672974059665 ) ) ;
#104797=CARTESIAN_POINT ( 'NONE',  ( 2.236732156574683827, 5.553345249405011508, 1.040834085586084257E-14 ) ) ;
#104799=CARTESIAN_POINT ( 'NONE',  ( -4.731432421044865499, 8.463828891286912182, -0.7216878364870257245 ) ) ;
#104802=ORIENTED_EDGE ( 'NONE', *, *, #132407, .F. ) ;
#104804=CARTESIAN_POINT ( 'NONE',  ( 6.322179702674084467, 6.270297829408224111, 1.040834085586084257E-14 ) ) ;
#104814=CARTESIAN_POINT ( 'NONE',  ( 6.844168616800228477, 6.879284895888727824, -0.7998128361456281477 ) ) ;
#104817=CARTESIAN_POINT ( 'NONE',  ( -4.274898507010545856, 3.881803101134051470, -0.7998128361456221525 ) ) ;
#104819=CARTESIAN_POINT ( 'NONE',  ( -5.215082642750900277, 9.236013516518044142, 0.000000000000000000 ) ) ;
#104823=CARTESIAN_POINT ( 'NONE',  ( 7.344766530301147789, 9.591980256816594164, 1.599625672291281386 ) ) ;
#104825=CARTESIAN_POINT ( 'NONE',  ( -6.039267359883488950, 9.133230122250985517, 1.199719254218452047 ) ) ;
#104826=CARTESIAN_POINT ( 'NONE',  ( 5.436456408955479880, 9.286356877182658565, -0.7216878364870267237 ) ) ;
#104827=CARTESIAN_POINT ( 'NONE',  ( 4.650497622768338779, 7.104022005431295916, 1.360104839701151480 ) ) ;
#104829=CARTESIAN_POINT ( 'NONE',  ( -4.238895582566952314, 8.097128612970093897, 1.040834085586084257E-14 ) ) ;
#104832=CARTESIAN_POINT ( 'NONE',  ( -6.388916700537716764, 8.476822122092563916, 1.599625672291283607 ) ) ;
#104835=CARTESIAN_POINT ( 'NONE',  ( 1.364683531249988757, 1.634375000341421691, 0.000000000000000000 ) ) ;
#104837=CARTESIAN_POINT ( 'NONE',  ( -6.073689629242160493, 8.109057205581079231, -1.443375672974059665 ) ) ;
#104842=CARTESIAN_POINT ( 'NONE',  ( 5.819474248763732760, 7.812472595022922128, -1.599625672291262513 ) ) ;
#104844=CARTESIAN_POINT ( 'NONE',  ( -5.852179643265606579, 6.035944939585320412, -0.4116468081218557784 ) ) ;
#104845=CARTESIAN_POINT ( 'NONE',  ( 1.364683531249988757, 0.9468750003414211358, 0.000000000000000000 ) ) ;
#104848=CARTESIAN_POINT ( 'NONE',  ( -0.5512317429218814846, 7.510131493957778126, 1.922545642343826078 ) ) ;
#104849=CARTESIAN_POINT ( 'NONE',  ( 5.851953751776640900, 5.929626919935292229, -0.4658998429906337502 ) ) ;
#104852=CARTESIAN_POINT ( 'NONE',  ( -4.111146893441842920, 5.819424013814012753, 1.599625672291267398 ) ) ;
#104853=CARTESIAN_POINT ( 'NONE',  ( -6.358410854684783509, 9.401601182898824405, -1.082531754730537976 ) ) ;
#104855=( BOUNDED_SURFACE ( )  B_SPLINE_SURFACE ( 1, 2, ( 
 ( #211733, #182430, #31943, #113260, #48213, #33001, #148883, #12469, #114325, #79614, #66524, #78544, #99079, #16722, #145733, #132667, #14596, #146784, #212799, #30888, #165131, #116436, #98027, #64437, #15662, #130581, #456, #95899, #178198, #81749, #147831, #213849, #198673, #161952, #29815, #63371, #195507, #47144, #65468, #179265, #50318, #96966, #163014, #49262, #34057, #131619, #82807, #197618, #160875, #115383, #181377, #144662, #210676, #62304, #128463, #194431, #46072, #39141, #189645, #56457, #54327, #107404, #83869, #157170, #7682, #106322, #1529, #105223, #122618, #171263, #6611, #120466, #188580, #173427, #172345, #104146, #166191, #74844, #22856, #23935, #149960, #121540, #170194, #70534, #41296, #124742, #203740, #187510, #140944, #137721, #88971, #136653, #57525, #155026, #40212, #17781, #72691, #73766, #91110, #90039, #138786, #5528, #25008, #206958, #156097, #204805, #87888, #139861, #205892, #58587, #202677, #123684, #186438, #8763, #38075, #21779, #153962, #190701, #100130, #55385, #71608, #26074, #13015, #28220, #93247, #193909, #27142, #159281, #143080, #10880, #158237, #43424, #44490, #130067, #76955, #63911, #61788, #209074, #144153, #129003, #30362, #108474, #78030, #175552, #162499, #174497, #194980, #112738, #60710, #14070, #110608, #176608, #94312, #126874, #46616, #212276, #210145, #92186, #192832, #109548, #9827, #178748, #42363, #160353, #11956, #80158, #127954, #45556, #75903, #211216, #111672, #177678, #142007, #29289, #161433, #96448, #95382, #79092, #145210, #146264, #208022, #62842, #59648, #125807, #191769, #214373, #19408, #113805, #165677, #147311, #118059, #81229, #47692, #163558, #149427, #150511, #148373, #114855, #179806, #166747, #181905, #32477, #133209, #180855, #98550, #82279, #164613, #97502, #197102, #198159, #69210, #16198, #3141, #1009, #66004, #83341, #68143, #184044, #31425, #17266, #132153, #101741, #15143, #134277, #51935, #49792, #167809, #115918, #33539, #99611, #67073, #200284, #151573, #199213, #50860, #116984, #182984, #35661, #131114, #213337, #48742, #34601, #64962, #100669, #18342, #85487, #84422, #2072, #196060, #8497, #54064, #139601, #120198, #41029, #136392, #203476, #121274, #70276, #22600, #154765, #71344, #156909, #137461, #7417, #88707, #86558, #205624, #119120, #189387, #39954, #138522, #36726, #55129, #6349, #187249, #38877, #152621, #72420, #57263, #204545, #202408, #201344, #107139, #104961, #56193, #123425, #20471, #122356, #173165, #24744, #103883, #135330, #73499, #171002, #90845, #188312, #106061, #168868, #172083, #52984, #185100, #102812, #4208, #186174, #37808, #23676, #89787, #155833, #169932, #21515, #153698, #87627, #5267, #210948, #61518, #62574, #96178, #60447, #208817, #58326, #178477, #30088, #44222, #190440, #194710, #127683, #176348, #29027, #10620, #126605, #124482, #46350, #9569, #177410, #42100, #92982, #162229 ),
 ( #27955, #192568, #59387, #76695, #159027, #112467, #206698, #110345, #25810, #128736, #174238, #140683, #108214, #94048, #95109, #26879, #207760, #91920, #45286, #160088, #125543, #11691, #191505, #43170, #175292, #109283, #157981, #75646, #142811, #74580, #77764, #141753, #143886, #209879, #193644, #161159, #111406, #12746, #78819, #144941, #134017, #79888, #166477, #84157, #147054, #200024, #82020, #148111, #214115, #98290, #18069, #183789, #181644, #65742, #33271, #131889, #1812, #163289, #179542, #80963, #213075, #31163, #197897, #114601, #51676, #164351, #97236, #49526, #67870, #14871, #64705, #130848, #196845, #48483, #115649, #180592, #117797, #15936, #32216, #116715, #101475, #99356, #150244, #165406, #35397, #17003, #83078, #149157, #735, #66801, #132942, #198947, #13816, #50590, #100408, #182715, #34333, #145998, #212009, #63651, #129806, #195785, #47423, #113538, #186988, #103624, #71083, #118856, #38619, #23411, #170747, #168607, #19145, #139336, #169676, #88447, #151309, #185909, #20209, #135069, #39683, #189133, #53803, #37544, #205367, #202143, #87369, #2877, #122090, #153439, #104696, #85220, #21263, #72157, #155575, #154507, #5010, #70012, #89523, #57001, #121021, #137201, #152366, #203224, #54868, #123173, #68947, #22333, #184841, #7158, #52723, #201082, #36470, #6087, #188052, #119933, #86297, #102543, #138265, #204279, #3945, #55935, #136128, #105793, #171818, #73229, #40772, #167546, #109023, #194466, #157720, #128497, #126356, #59130, #208560, #193401, #94857, #172903, #142554, #25557, #12505, #24476, #45044, #177156, #91668, #78577, #175041, #26627, #92728, #191248, #111157, #62338, #60195, #158774, #192314, #43973, #42913, #110091, #58067, #10369, #127431, #28775, #206440, #176101, #160910, #144699, #75392, #106875, #210710, #76447, #90589, #27701, #93797, #140425, #159837, #156649, #8242, #74326, #124231, #190190, #173985, #11437, #77513, #61269, #41847, #107957, #125289, #9316, #143634, #141504, #209628, #207511, #67623, #31980, #180354, #29849, #149990, #1562, #15697, #161987, #166226, #33033, #147865, #489, #196605, #98058, #95931, #17816, #195544, #148915, #13577, #64472, #133767, #46108, #14631, #82839, #112226, #130613, #48245, #99111, #81782, #66557, #79650, #178234, #212835, #83900, #165161, #16756, #114359, #115415, #182462, #132699, #164112, #198705, #80725, #50350, #116470, #34091, #113294, #145766, #211767, #179302, #63405, #30923, #129558, #47180, #96999, #163052, #146816, #100162, #213881, #65503, #197653, #181407, #131650, #49300, #2627, #68699, #35142, #168362, #169425, #167302, #171554, #52477, #70826, #3688, #38358, #39427, #118604, #21008, #55672, #19957, #86042, #186736, #151064, #104436, #134821, #200826, #170485, #202969, #184592, #36210, #121828, #101218, #105520, #102289, #88181, #18889, #69765, #155315, #199775, #152117, #22069, #89265, #135871, #201890, #154253 ) ),
 .UNSPECIFIED., .F., .F., .T. ) 
 B_SPLINE_SURFACE_WITH_KNOTS ( ( 2, 2 ),
 ( 3, 2, 2, 2, 2, 2, 2, 2, 2, 2, 2, 2, 2, 2, 2, 2, 2, 2, 2, 2, 2, 2, 2, 2, 2, 2, 2, 2, 2, 2, 2, 2, 2, 2, 2, 2, 2, 2, 2, 2, 2, 2, 2, 2, 2, 2, 2, 2, 2, 2, 2, 2, 2, 2, 2, 2, 2, 2, 2, 2, 2, 2, 2, 2, 2, 2, 2, 2, 2, 2, 2, 2, 2, 2, 2, 2, 2, 2, 2, 2, 2, 2, 2, 2, 2, 2, 2, 2, 2, 2, 2, 2, 2, 2, 2, 2, 2, 2, 2, 2, 2, 2, 2, 2, 2, 2, 2, 2, 2, 2, 2, 2, 2, 2, 2, 2, 2, 2, 2, 2, 2, 2, 2, 2, 2, 2, 2, 2, 2, 2, 2, 2, 2, 2, 2, 2, 2, 2, 2, 2, 2, 2, 2, 2, 2, 2, 2, 2, 2, 2, 2, 2, 2, 2, 2, 2, 2, 2, 2, 2, 2, 2, 2, 2, 2, 2, 2, 2, 3 ),
 ( 0.000000000000000000, 1.000000000000000000 ),
 ( 0.000000000000000000, 0.005952380952380952051, 0.01190476190476190410, 0.01785714285714285615, 0.02380952380952380820, 0.02976190476190476025, 0.03571428571428571230, 0.04166666666666666435, 0.04761904761904761640, 0.05357142857142856845, 0.05952380952380952051, 0.06547619047619047949, 0.07142857142857142461, 0.07738095238095238360, 0.08333333333333332871, 0.08928571428571428770, 0.09523809523809523281, 0.1011904761904761918, 0.1071428571428571369, 0.1130952380952380959, 0.1190476190476190410, 0.1250000000000000000, 0.1309523809523809590, 0.1369047619047619180, 0.1428571428571428492, 0.1488095238095238082, 0.1547619047619047672, 0.1607142857142857262, 0.1666666666666666574, 0.1726190476190476164, 0.1785714285714285754, 0.1845238095238095344, 0.1904761904761904656, 0.1964285714285714246, 0.2023809523809523836, 0.2083333333333333426, 0.2142857142857142738, 0.2202380952380952328, 0.2261904761904761918, 0.2321428571428571508, 0.2380952380952380820, 0.2440476190476190410, 0.2500000000000000000, 0.2559523809523809312, 0.2619047619047619180, 0.2678571428571428492, 0.2738095238095238360, 0.2797619047619047672, 0.2857142857142856984, 0.2916666666666666852, 0.2976190476190476164, 0.3035714285714285476, 0.3095238095238095344, 0.3154761904761904656, 0.3214285714285714524, 0.3273809523809523836, 0.3333333333333333148, 0.3392857142857143016, 0.3452380952380952328, 0.3511904761904761640, 0.3571428571428571508, 0.3630952380952380820, 0.3690476190476190688, 0.3750000000000000000, 0.3809523809523809312, 0.3869047619047619180, 0.3928571428571428492, 0.3988095238095238360, 0.4047619047619047672, 0.4107142857142856984, 0.4166666666666666852, 0.4226190476190476164, 0.4285714285714285476, 0.4345238095238095344, 0.4404761904761904656, 0.4464285714285714524, 0.4523809523809523836, 0.4583333333333333148, 0.4642857142857143016, 0.4702380952380952328, 0.4761904761904761640, 0.4821428571428571508, 0.4880952380952380820, 0.4940476190476190688, 0.5000000000000000000, 0.5059523809523809312, 0.5119047619047618625, 0.5178571428571429047, 0.5238095238095238360, 0.5297619047619047672, 0.5357142857142856984, 0.5416666666666666297, 0.5476190476190476719, 0.5535714285714286031, 0.5595238095238095344, 0.5654761904761904656, 0.5714285714285713969, 0.5773809523809523281, 0.5833333333333333703, 0.5892857142857143016, 0.5952380952380952328, 0.6011904761904761640, 0.6071428571428570953, 0.6130952380952381375, 0.6190476190476190688, 0.6250000000000000000, 0.6309523809523809312, 0.6369047619047618625, 0.6428571428571429047, 0.6488095238095238360, 0.6547619047619047672, 0.6607142857142856984, 0.6666666666666666297, 0.6726190476190476719, 0.6785714285714286031, 0.6845238095238095344, 0.6904761904761904656, 0.6964285714285713969, 0.7023809523809523281, 0.7083333333333333703, 0.7142857142857143016, 0.7202380952380952328, 0.7261904761904761640, 0.7321428571428570953, 0.7380952380952381375, 0.7440476190476190688, 0.7500000000000000000, 0.7559523809523809312, 0.7619047619047618625, 0.7678571428571429047, 0.7738095238095238360, 0.7797619047619047672, 0.7857142857142856984, 0.7916666666666666297, 0.7976190476190476719, 0.8035714285714286031, 0.8095238095238095344, 0.8154761904761904656, 0.8214285714285713969, 0.8273809523809523281, 0.8333333333333333703, 0.8392857142857143016, 0.8452380952380952328, 0.8511904761904761640, 0.8571428571428570953, 0.8630952380952381375, 0.8690476190476190688, 0.8750000000000000000, 0.8809523809523809312, 0.8869047619047618625, 0.8928571428571429047, 0.8988095238095238360, 0.9047619047619047672, 0.9107142857142856984, 0.9166666666666666297, 0.9226190476190476719, 0.9285714285714286031, 0.9345238095238095344, 0.9404761904761904656, 0.9464285714285713969, 0.9523809523809523281, 0.9583333333333333703, 0.9642857142857143016, 0.9702380952380952328, 0.9761904761904761640, 0.9821428571428570953, 0.9880952380952381375, 0.9940476190476190688, 1.000000000000000000 ),
 .UNSPECIFIED. ) 
 GEOMETRIC_REPRESENTATION_ITEM ( )  RATIONAL_B_SPLINE_SURFACE ( (
 ( 1.000000000000000000, 0.8660254037844387076, 1.000000000000000000, 0.8660254037844387076, 1.000000000000000000, 0.8660254037844387076, 1.000000000000000000, 0.8660254037844387076, 1.000000000000000000, 0.8660254037844387076, 1.000000000000000000, 0.8660254037844387076, 1.000000000000000000, 0.8660254037844387076, 1.000000000000000000, 0.8660254037844387076, 1.000000000000000000, 0.8660254037844387076, 1.000000000000000000, 0.8660254037844387076, 1.000000000000000000, 0.8660254037844387076, 1.000000000000000000, 0.8660254037844387076, 1.000000000000000000, 0.8660254037844387076, 1.000000000000000000, 0.8660254037844387076, 1.000000000000000000, 0.8660254037844387076, 1.000000000000000000, 0.8660254037844387076, 1.000000000000000000, 0.8660254037844387076, 1.000000000000000000, 0.8660254037844387076, 1.000000000000000000, 0.8660254037844387076, 1.000000000000000000, 0.8660254037844387076, 1.000000000000000000, 0.8660254037844387076, 1.000000000000000000, 0.8660254037844387076, 1.000000000000000000, 0.8660254037844387076, 1.000000000000000000, 0.8660254037844387076, 1.000000000000000000, 0.8660254037844387076, 1.000000000000000000, 0.8660254037844387076, 1.000000000000000000, 0.8660254037844387076, 1.000000000000000000, 0.8660254037844387076, 1.000000000000000000, 0.8660254037844387076, 1.000000000000000000, 0.8660254037844387076, 1.000000000000000000, 0.8660254037844387076, 1.000000000000000000, 0.8660254037844387076, 1.000000000000000000, 0.8660254037844387076, 1.000000000000000000, 0.8660254037844387076, 1.000000000000000000, 0.8660254037844387076, 1.000000000000000000, 0.8660254037844387076, 1.000000000000000000, 0.8660254037844387076, 1.000000000000000000, 0.8660254037844387076, 1.000000000000000000, 0.8660254037844387076, 1.000000000000000000, 0.8660254037844387076, 1.000000000000000000, 0.8660254037844387076, 1.000000000000000000, 0.8660254037844387076, 1.000000000000000000, 0.8660254037844387076, 1.000000000000000000, 0.8660254037844387076, 1.000000000000000000, 0.8660254037844387076, 1.000000000000000000, 0.8660254037844387076, 1.000000000000000000, 0.8660254037844387076, 1.000000000000000000, 0.8660254037844387076, 1.000000000000000000, 0.8660254037844387076, 1.000000000000000000, 0.8660254037844387076, 1.000000000000000000, 0.8660254037844387076, 1.000000000000000000, 0.8660254037844387076, 1.000000000000000000, 0.8660254037844387076, 1.000000000000000000, 0.8660254037844387076, 1.000000000000000000, 0.8660254037844387076, 1.000000000000000000, 0.8660254037844387076, 1.000000000000000000, 0.8660254037844387076, 1.000000000000000000, 0.8660254037844387076, 1.000000000000000000, 0.8660254037844387076, 1.000000000000000000, 0.8660254037844387076, 1.000000000000000000, 0.8660254037844387076, 1.000000000000000000, 0.8660254037844387076, 1.000000000000000000, 0.8660254037844387076, 1.000000000000000000, 0.8660254037844387076, 1.000000000000000000, 0.8660254037844387076, 1.000000000000000000, 0.8660254037844387076, 1.000000000000000000, 0.8660254037844387076, 1.000000000000000000, 0.8660254037844387076, 1.000000000000000000, 0.8660254037844387076, 1.000000000000000000, 0.8660254037844387076, 1.000000000000000000, 0.8660254037844387076, 1.000000000000000000, 0.8660254037844387076, 1.000000000000000000, 0.8660254037844387076, 1.000000000000000000, 0.8660254037844387076, 1.000000000000000000, 0.8660254037844387076, 1.000000000000000000, 0.8660254037844387076, 1.000000000000000000, 0.8660254037844387076, 1.000000000000000000, 0.8660254037844387076, 1.000000000000000000, 0.8660254037844387076, 1.000000000000000000, 0.8660254037844387076, 1.000000000000000000, 0.8660254037844387076, 1.000000000000000000, 0.8660254037844387076, 1.000000000000000000, 0.8660254037844387076, 1.000000000000000000, 0.8660254037844387076, 1.000000000000000000, 0.8660254037844387076, 1.000000000000000000, 0.8660254037844387076, 1.000000000000000000, 0.8660254037844387076, 1.000000000000000000, 0.8660254037844387076, 1.000000000000000000, 0.8660254037844387076, 1.000000000000000000, 0.8660254037844387076, 1.000000000000000000, 0.8660254037844387076, 1.000000000000000000, 0.8660254037844387076, 1.000000000000000000, 0.8660254037844387076, 1.000000000000000000, 0.8660254037844387076, 1.000000000000000000, 0.8660254037844387076, 1.000000000000000000, 0.8660254037844387076, 1.000000000000000000, 0.8660254037844387076, 1.000000000000000000, 0.8660254037844387076, 1.000000000000000000, 0.8660254037844387076, 1.000000000000000000, 0.8660254037844387076, 1.000000000000000000, 0.8660254037844387076, 1.000000000000000000, 0.8660254037844387076, 1.000000000000000000, 0.8660254037844387076, 1.000000000000000000, 0.8660254037844387076, 1.000000000000000000, 0.8660254037844387076, 1.000000000000000000, 0.8660254037844387076, 1.000000000000000000, 0.8660254037844387076, 1.000000000000000000, 0.8660254037844387076, 1.000000000000000000, 0.8660254037844387076, 1.000000000000000000, 0.8660254037844387076, 1.000000000000000000, 0.8660254037844387076, 1.000000000000000000, 0.8660254037844387076, 1.000000000000000000, 0.8660254037844387076, 1.000000000000000000, 0.8660254037844387076, 1.000000000000000000, 0.8660254037844387076, 1.000000000000000000, 0.8660254037844387076, 1.000000000000000000, 0.8660254037844387076, 1.000000000000000000, 0.8660254037844387076, 1.000000000000000000, 0.8660254037844387076, 1.000000000000000000, 0.8660254037844387076, 1.000000000000000000, 0.8660254037844387076, 1.000000000000000000, 0.8660254037844387076, 1.000000000000000000, 0.8660254037844387076, 1.000000000000000000, 0.8660254037844387076, 1.000000000000000000, 0.8660254037844387076, 1.000000000000000000, 0.8660254037844387076, 1.000000000000000000, 0.8660254037844387076, 1.000000000000000000, 0.8660254037844387076, 1.000000000000000000, 0.8660254037844387076, 1.000000000000000000, 0.8660254037844387076, 1.000000000000000000, 0.8660254037844387076, 1.000000000000000000, 0.8660254037844387076, 1.000000000000000000, 0.8660254037844387076, 1.000000000000000000, 0.8660254037844387076, 1.000000000000000000, 0.8660254037844387076, 1.000000000000000000, 0.8660254037844387076, 1.000000000000000000, 0.8660254037844387076, 1.000000000000000000, 0.8660254037844387076, 1.000000000000000000, 0.8660254037844387076, 1.000000000000000000, 0.8660254037844387076, 1.000000000000000000, 0.8660254037844387076, 1.000000000000000000, 0.8660254037844387076, 1.000000000000000000, 0.8660254037844387076, 1.000000000000000000, 0.8660254037844387076, 1.000000000000000000, 0.8660254037844387076, 1.000000000000000000, 0.8660254037844387076, 1.000000000000000000, 0.8660254037844387076, 1.000000000000000000, 0.8660254037844387076, 1.000000000000000000, 0.8660254037844387076, 1.000000000000000000, 0.8660254037844387076, 1.000000000000000000, 0.8660254037844387076, 1.000000000000000000, 0.8660254037844387076, 1.000000000000000000, 0.8660254037844387076, 1.000000000000000000, 0.8660254037844387076, 1.000000000000000000, 0.8660254037844387076, 1.000000000000000000, 0.8660254037844387076, 1.000000000000000000, 0.8660254037844387076, 1.000000000000000000, 0.8660254037844387076, 1.000000000000000000, 0.8660254037844387076, 1.000000000000000000, 0.8660254037844387076, 1.000000000000000000, 0.8660254037844387076, 1.000000000000000000, 0.8660254037844387076, 1.000000000000000000, 0.8660254037844387076, 1.000000000000000000, 0.8660254037844387076, 1.000000000000000000, 0.8660254037844387076, 1.000000000000000000, 0.8660254037844387076, 1.000000000000000000, 0.8660254037844387076, 1.000000000000000000, 0.8660254037844387076, 1.000000000000000000),
 ( 1.000000000000000000, 0.8660254037844387076, 1.000000000000000000, 0.8660254037844387076, 1.000000000000000000, 0.8660254037844387076, 1.000000000000000000, 0.8660254037844387076, 1.000000000000000000, 0.8660254037844387076, 1.000000000000000000, 0.8660254037844387076, 1.000000000000000000, 0.8660254037844387076, 1.000000000000000000, 0.8660254037844387076, 1.000000000000000000, 0.8660254037844387076, 1.000000000000000000, 0.8660254037844387076, 1.000000000000000000, 0.8660254037844387076, 1.000000000000000000, 0.8660254037844387076, 1.000000000000000000, 0.8660254037844387076, 1.000000000000000000, 0.8660254037844387076, 1.000000000000000000, 0.8660254037844387076, 1.000000000000000000, 0.8660254037844387076, 1.000000000000000000, 0.8660254037844387076, 1.000000000000000000, 0.8660254037844387076, 1.000000000000000000, 0.8660254037844387076, 1.000000000000000000, 0.8660254037844387076, 1.000000000000000000, 0.8660254037844387076, 1.000000000000000000, 0.8660254037844387076, 1.000000000000000000, 0.8660254037844387076, 1.000000000000000000, 0.8660254037844387076, 1.000000000000000000, 0.8660254037844387076, 1.000000000000000000, 0.8660254037844387076, 1.000000000000000000, 0.8660254037844387076, 1.000000000000000000, 0.8660254037844387076, 1.000000000000000000, 0.8660254037844387076, 1.000000000000000000, 0.8660254037844387076, 1.000000000000000000, 0.8660254037844387076, 1.000000000000000000, 0.8660254037844387076, 1.000000000000000000, 0.8660254037844387076, 1.000000000000000000, 0.8660254037844387076, 1.000000000000000000, 0.8660254037844387076, 1.000000000000000000, 0.8660254037844387076, 1.000000000000000000, 0.8660254037844387076, 1.000000000000000000, 0.8660254037844387076, 1.000000000000000000, 0.8660254037844387076, 1.000000000000000000, 0.8660254037844387076, 1.000000000000000000, 0.8660254037844387076, 1.000000000000000000, 0.8660254037844387076, 1.000000000000000000, 0.8660254037844387076, 1.000000000000000000, 0.8660254037844387076, 1.000000000000000000, 0.8660254037844387076, 1.000000000000000000, 0.8660254037844387076, 1.000000000000000000, 0.8660254037844387076, 1.000000000000000000, 0.8660254037844387076, 1.000000000000000000, 0.8660254037844387076, 1.000000000000000000, 0.8660254037844387076, 1.000000000000000000, 0.8660254037844387076, 1.000000000000000000, 0.8660254037844387076, 1.000000000000000000, 0.8660254037844387076, 1.000000000000000000, 0.8660254037844387076, 1.000000000000000000, 0.8660254037844387076, 1.000000000000000000, 0.8660254037844387076, 1.000000000000000000, 0.8660254037844387076, 1.000000000000000000, 0.8660254037844387076, 1.000000000000000000, 0.8660254037844387076, 1.000000000000000000, 0.8660254037844387076, 1.000000000000000000, 0.8660254037844387076, 1.000000000000000000, 0.8660254037844387076, 1.000000000000000000, 0.8660254037844387076, 1.000000000000000000, 0.8660254037844387076, 1.000000000000000000, 0.8660254037844387076, 1.000000000000000000, 0.8660254037844387076, 1.000000000000000000, 0.8660254037844387076, 1.000000000000000000, 0.8660254037844387076, 1.000000000000000000, 0.8660254037844387076, 1.000000000000000000, 0.8660254037844387076, 1.000000000000000000, 0.8660254037844387076, 1.000000000000000000, 0.8660254037844387076, 1.000000000000000000, 0.8660254037844387076, 1.000000000000000000, 0.8660254037844387076, 1.000000000000000000, 0.8660254037844387076, 1.000000000000000000, 0.8660254037844387076, 1.000000000000000000, 0.8660254037844387076, 1.000000000000000000, 0.8660254037844387076, 1.000000000000000000, 0.8660254037844387076, 1.000000000000000000, 0.8660254037844387076, 1.000000000000000000, 0.8660254037844387076, 1.000000000000000000, 0.8660254037844387076, 1.000000000000000000, 0.8660254037844387076, 1.000000000000000000, 0.8660254037844387076, 1.000000000000000000, 0.8660254037844387076, 1.000000000000000000, 0.8660254037844387076, 1.000000000000000000, 0.8660254037844387076, 1.000000000000000000, 0.8660254037844387076, 1.000000000000000000, 0.8660254037844387076, 1.000000000000000000, 0.8660254037844387076, 1.000000000000000000, 0.8660254037844387076, 1.000000000000000000, 0.8660254037844387076, 1.000000000000000000, 0.8660254037844387076, 1.000000000000000000, 0.8660254037844387076, 1.000000000000000000, 0.8660254037844387076, 1.000000000000000000, 0.8660254037844387076, 1.000000000000000000, 0.8660254037844387076, 1.000000000000000000, 0.8660254037844387076, 1.000000000000000000, 0.8660254037844387076, 1.000000000000000000, 0.8660254037844387076, 1.000000000000000000, 0.8660254037844387076, 1.000000000000000000, 0.8660254037844387076, 1.000000000000000000, 0.8660254037844387076, 1.000000000000000000, 0.8660254037844387076, 1.000000000000000000, 0.8660254037844387076, 1.000000000000000000, 0.8660254037844387076, 1.000000000000000000, 0.8660254037844387076, 1.000000000000000000, 0.8660254037844387076, 1.000000000000000000, 0.8660254037844387076, 1.000000000000000000, 0.8660254037844387076, 1.000000000000000000, 0.8660254037844387076, 1.000000000000000000, 0.8660254037844387076, 1.000000000000000000, 0.8660254037844387076, 1.000000000000000000, 0.8660254037844387076, 1.000000000000000000, 0.8660254037844387076, 1.000000000000000000, 0.8660254037844387076, 1.000000000000000000, 0.8660254037844387076, 1.000000000000000000, 0.8660254037844387076, 1.000000000000000000, 0.8660254037844387076, 1.000000000000000000, 0.8660254037844387076, 1.000000000000000000, 0.8660254037844387076, 1.000000000000000000, 0.8660254037844387076, 1.000000000000000000, 0.8660254037844387076, 1.000000000000000000, 0.8660254037844387076, 1.000000000000000000, 0.8660254037844387076, 1.000000000000000000, 0.8660254037844387076, 1.000000000000000000, 0.8660254037844387076, 1.000000000000000000, 0.8660254037844387076, 1.000000000000000000, 0.8660254037844387076, 1.000000000000000000, 0.8660254037844387076, 1.000000000000000000, 0.8660254037844387076, 1.000000000000000000, 0.8660254037844387076, 1.000000000000000000, 0.8660254037844387076, 1.000000000000000000, 0.8660254037844387076, 1.000000000000000000, 0.8660254037844387076, 1.000000000000000000, 0.8660254037844387076, 1.000000000000000000, 0.8660254037844387076, 1.000000000000000000, 0.8660254037844387076, 1.000000000000000000, 0.8660254037844387076, 1.000000000000000000, 0.8660254037844387076, 1.000000000000000000, 0.8660254037844387076, 1.000000000000000000, 0.8660254037844387076, 1.000000000000000000, 0.8660254037844387076, 1.000000000000000000, 0.8660254037844387076, 1.000000000000000000, 0.8660254037844387076, 1.000000000000000000, 0.8660254037844387076, 1.000000000000000000, 0.8660254037844387076, 1.000000000000000000, 0.8660254037844387076, 1.000000000000000000, 0.8660254037844387076, 1.000000000000000000, 0.8660254037844387076, 1.000000000000000000, 0.8660254037844387076, 1.000000000000000000, 0.8660254037844387076, 1.000000000000000000, 0.8660254037844387076, 1.000000000000000000, 0.8660254037844387076, 1.000000000000000000, 0.8660254037844387076, 1.000000000000000000, 0.8660254037844387076, 1.000000000000000000, 0.8660254037844387076, 1.000000000000000000, 0.8660254037844387076, 1.000000000000000000, 0.8660254037844387076, 1.000000000000000000, 0.8660254037844387076, 1.000000000000000000, 0.8660254037844387076, 1.000000000000000000, 0.8660254037844387076, 1.000000000000000000, 0.8660254037844387076, 1.000000000000000000, 0.8660254037844387076, 1.000000000000000000, 0.8660254037844387076, 1.000000000000000000, 0.8660254037844387076, 1.000000000000000000, 0.8660254037844387076, 1.000000000000000000, 0.8660254037844387076, 1.000000000000000000) ) ) 
 REPRESENTATION_ITEM ( '' )  SURFACE ( )  );
#104862=CARTESIAN_POINT ( 'NONE',  ( -8.310784975052689205, 8.798263347090697906, -0.7216878364870267237 ) ) ;
#104864=CYLINDRICAL_SURFACE ( 'NONE', #74973, 1.250000000000000000 ) ;
#104866=CARTESIAN_POINT ( 'NONE',  ( -7.578644679914719795, 9.864838098032418401, 1.443375672974090751 ) ) ;
#104869=VERTEX_POINT ( 'NONE', #18250 ) ;
#104873=CARTESIAN_POINT ( 'NONE',  ( 1.499999999999990896, 5.556250000682820378, 1.214306433183764966E-14 ) ) ;
#104880=CARTESIAN_POINT ( 'NONE',  ( -5.696397096036042385, 9.797547045350714967, -0.7998128361456231517 ) ) ;
#104883=CARTESIAN_POINT ( 'NONE',  ( 3.551346171775753735, 6.230655402791975384, 1.199719254218462483 ) ) ;
#104885=( BOUNDED_CURVE ( )  B_SPLINE_CURVE ( 2, ( #64794, #148201, #32306, #16022, #130938 ),
 .UNSPECIFIED., .F., .T. ) 
 B_SPLINE_CURVE_WITH_KNOTS ( ( 3, 2, 3 ),
 ( 0.01092446968156914403, 0.01250000000000000069, 0.01386088777671200430 ),
 .UNSPECIFIED. ) 
 CURVE ( )  GEOMETRIC_REPRESENTATION_ITEM ( )  RATIONAL_B_SPLINE_CURVE ( ( 0.9369925407309227516, 0.9493405508230843282, 1.000000000000000000, 0.9562421463088759399, 0.9410680661649852841 ) ) 
 REPRESENTATION_ITEM ( '' )  );
#104886=CARTESIAN_POINT ( 'NONE',  ( 4.897706171852771462, 4.871974472535213430, 0.6676900015689657408 ) ) ;
#104888=CARTESIAN_POINT ( 'NONE',  ( 5.361359679200154105, 8.342337828120466980, 1.199719254218462483 ) ) ;
#104895=CARTESIAN_POINT ( 'NONE',  ( -4.690757960648240577, 6.495636925554817864, 1.443375672974064550 ) ) ;
#104904=CARTESIAN_POINT ( 'NONE',  ( -1.364683531250014514, 1.238541667008091096, -0.7879004041258289570 ) ) ;
#104905=CARTESIAN_POINT ( 'NONE',  ( 2.310781476690497271, 5.467761476598782977, -0.5169845646830224517 ) ) ;
#104907=CARTESIAN_POINT ( 'NONE',  ( -8.636707547105197946, 10.03491254549959777, -1.199719254218446718 ) ) ;
#104909=CARTESIAN_POINT ( 'NONE',  ( 8.281332899848809603, 8.555976559445431562, 0.7998128361456481317 ) ) ;
#104911=CARTESIAN_POINT ( 'NONE',  ( -6.690058733339450114, 9.892486724616283311, 1.199719254218452047 ) ) ;
#104914=CARTESIAN_POINT ( 'NONE',  ( 1.364683531249988535, 4.405208333674754506, -0.7879004041258300672 ) ) ;
#104916=CARTESIAN_POINT ( 'NONE',  ( 9.083599731475983319, 11.62061899152058686, 1.443375672974076540 ) ) ;
#104919=CARTESIAN_POINT ( 'NONE',  ( 1.364683531249988757, -0.3031249996585799744, 0.000000000000000000 ) ) ;
#104922=CARTESIAN_POINT ( 'NONE',  ( 7.822691444960700125, 10.14955932391940330, -1.443375672974058777 ) ) ;
#104925=CARTESIAN_POINT ( 'NONE',  ( -4.121315508874255684, 7.752025827087861920, -0.7216878364870267237 ) ) ;
#104927=CARTESIAN_POINT ( 'NONE',  ( 0.6823417656249899377, 3.926041667008085767, -1.181850606188754593 ) ) ;
#104931=CARTESIAN_POINT ( 'NONE',  ( -5.530836599371015794, 8.540060901653093950, 1.199719254218452047 ) ) ;
#104932=DIRECTION ( 'NONE',  ( -0.9366510587354612838, 0.000000000000000000, 0.3502638921866474409 ) ) ;
#104934=AXIS2_PLACEMENT_3D ( 'NONE', #69698, #203959, #56680 ) ;
#104939=CARTESIAN_POINT ( 'NONE',  ( 7.639129486296027061, 10.99973593639901814, 1.199719254218460707 ) ) ;
#104942=CARTESIAN_POINT ( 'NONE',  ( -1.500000000000013101, 2.629166666666687746, -0.8660254037844313801 ) ) ;
#104948=CARTESIAN_POINT ( 'NONE',  ( 6.860062538834778678, 8.066123052471139587, -1.082531754730543083 ) ) ;
#104949=CARTESIAN_POINT ( 'NONE',  ( 1.364683531249986537, -1.073958332991911790, 0.7879004041258500513 ) ) ;
#104951=AXIS2_PLACEMENT_3D ( 'NONE', #62715, #163440, #17152 ) ;
#104957=CARTESIAN_POINT ( 'NONE',  ( 1.499999999999987566, -0.9749999999999827693, 0.000000000000000000 ) ) ;
#104958=CARTESIAN_POINT ( 'NONE',  ( 6.414979237560321401, 10.63589287712906462, 1.040834085586084257E-14 ) ) ;
#104959=CARTESIAN_POINT ( 'NONE',  ( -9.341731535015849630, 10.85744053139533349, 1.199719254218462483 ) ) ;
#104961=CARTESIAN_POINT ( 'NONE',  ( 1.364683531249986537, -0.1364583329919154264, 0.7879004041258500513 ) ) ;
#104962=CARTESIAN_POINT ( 'NONE',  ( 1.499999999999987121, 0.7958333333333510451, -0.8660254037844253849 ) ) ;
#104964=CARTESIAN_POINT ( 'NONE',  ( 4.635998460869027227, 7.496083073400806818, -1.199719254218452047 ) ) ;
#104966=CARTESIAN_POINT ( 'NONE',  ( 1.084637062511527361, 2.838621193390831188, -1.105835307554789759 ) ) ;
#104971=CARTESIAN_POINT ( 'NONE',  ( 0.6823417656249917140, 4.842708333674755394, 1.181850606188765695 ) ) ;
#104973=CARTESIAN_POINT ( 'NONE',  ( -8.158255747121117452, 10.54105100977322174, 1.599625672291295375 ) ) ;
#104974=CARTESIAN_POINT ( 'NONE',  ( -4.934804725694224459, 6.780358151441803649, -1.443375672974053447 ) ) ;
#104983=CARTESIAN_POINT ( 'NONE',  ( 7.019370843573166319, 9.212351955633947043, 1.599625672291281386 ) ) ;
#104986=CARTESIAN_POINT ( 'NONE',  ( 7.334597914868727919, 9.580116872145431728, -1.443375672974058777 ) ) ;
#104989=CARTESIAN_POINT ( 'NONE',  ( -6.832419346282942563, 10.05857410638369487, 1.199719254218453823 ) ) ;
#104990=CARTESIAN_POINT ( 'NONE',  ( 4.008406971134620633, 7.828225232965717595, 0.7998128361456321445 ) ) ;
#104991=DIRECTION ( 'NONE',  ( -5.578564026256490882E-16, -1.000000000000000000, -9.066213480720158442E-32 ) ) ;
#104992=CARTESIAN_POINT ( 'NONE',  ( 3.836594282542920009, 4.538743420130594508, 1.082531754730560403 ) ) ;
#104994=CARTESIAN_POINT ( 'NONE',  ( 3.063252641683779753, 5.661212951017999373, 1.199719254218450271 ) ) ;
#105001=CARTESIAN_POINT ( 'NONE',  ( -5.924549939491850381, 6.014322472269677533, 0.000000000000000000 ) ) ;
#105002=CARTESIAN_POINT ( 'NONE',  ( 4.369805582306193870, 3.992528022312320957, 1.214306433183764966E-14 ) ) ;
#105005=CARTESIAN_POINT ( 'NONE',  ( -7.366157530926372488, 7.488271962369228874, -0.7998128361456291469 ) ) ;
#105007=CARTESIAN_POINT ( 'NONE',  ( -0.6823417656250003738, 3.030208333674754062, -1.181850606188749264 ) ) ;
#105009=CARTESIAN_POINT ( 'NONE',  ( -7.640183256500752584, 8.872300873127729304, -1.199719254218446718 ) ) ;
#105014=CARTESIAN_POINT ( 'NONE',  ( 3.798255590122797898, 7.583048621785260401, -0.7998128361456221525 ) ) ;
#105019=ORIENTED_EDGE ( 'NONE', *, *, #84508, .F. ) ;
#105028=CARTESIAN_POINT ( 'NONE',  ( -6.693975156845199059, 8.832723654451292816, 1.599625672291283607 ) ) ;
#105031=CARTESIAN_POINT ( 'NONE',  ( 5.585596099150174965, 7.539614753807099667, -1.443375672974057666 ) ) ;
#105032=ORIENTED_EDGE ( 'NONE', *, *, #105908, .T. ) ;
#105036=CARTESIAN_POINT ( 'NONE',  ( -4.629219384062206011, 7.488174150459498968, -1.199719254218452047 ) ) ;
#105041=CARTESIAN_POINT ( 'NONE',  ( -6.555530967407501741, 7.606873202518897870, 1.199719254218450271 ) ) ;
#105042=CARTESIAN_POINT ( 'NONE',  ( -5.786256696412555911, 6.075953140482280190, 0.5845640519336701146 ) ) ;
#105047=B_SPLINE_CURVE_WITH_KNOTS ( 'NONE', 3,
 ( #170254, #86880, #21839, #121597 ),
 .UNSPECIFIED., .F., .F.,
 ( 4, 4 ),
 ( 3.338216057386796243E-18, 0.0006335992342243239534 ),
 .UNSPECIFIED. ) ;
#105049=CARTESIAN_POINT ( 'NONE',  ( -7.967387826325084355, 12.44703623068796361, 0.7998128361456481317 ) ) ;
#105050=CARTESIAN_POINT ( 'NONE',  ( 7.450369105909416589, 8.650851030771185890, -1.199719254218441611 ) ) ;
#105054=CARTESIAN_POINT ( 'NONE',  ( -8.597841969360544567, 13.18256606422934674, 0.7998128361456341429 ) ) ;
#105057=CARTESIAN_POINT ( 'NONE',  ( 0.6823417656249882723, -0.8447916663252494907, 1.181850606188755259 ) ) ;
#105061=CARTESIAN_POINT ( 'NONE',  ( 8.920901888111986366, 12.39117405523060889, 1.082531754730546636 ) ) ;
#105081=CARTESIAN_POINT ( 'NONE',  ( -3.598799709423620374, 6.286017863381107240, 1.199719254218464037 ) ) ;
#105085=CARTESIAN_POINT ( 'NONE',  ( -7.334597915313094241, 9.580116872663850813, 1.040834085586084257E-14 ) ) ;
#105088=CARTESIAN_POINT ( 'NONE',  ( -1.500000000000015099, -1.297916665983847029, 0.8660254037844403729 ) ) ;
#105093=CARTESIAN_POINT ( 'NONE',  ( 1.435115314734431324, 7.268684689231784901, -4.324912918975645226 ) ) ;
#105094=CARTESIAN_POINT ( 'NONE',  ( 3.379006598303866848, 4.965260336153046516, -1.599625672291262513 ) ) ;
#105099=CARTESIAN_POINT ( 'NONE',  ( 3.974511587100456822, 7.788680618259193444, 1.040834085586084257E-14 ) ) ;
#105100=CARTESIAN_POINT ( 'NONE',  ( 1.364683531249988535, 2.176041667008087543, 0.7879004041258500513 ) ) ;
#105105=CARTESIAN_POINT ( 'NONE',  ( -9.806625181386236179, 10.33548422123910449, -0.7998128361456291469 ) ) ;
#105106=CARTESIAN_POINT ( 'NONE',  ( -5.382223794500852421, 5.381608636446842731, -0.7216878364870197293 ) ) ;
#105108=CARTESIAN_POINT ( 'NONE',  ( -5.555090253297260361, 7.504024600312024340, 1.599625672291269396 ) ) ;
#105110=CARTESIAN_POINT ( 'NONE',  ( -0.7500000000000006661, -1.110416665983847473, -1.299038105676652011 ) ) ;
#105119=CARTESIAN_POINT ( 'NONE',  ( -5.544921637864838715, 6.531792001339513654, -1.082531754730543971 ) ) ;
#105120=ADVANCED_FACE ( 'NONE', ( #58242 ), #114316, .T. ) ;
#105125=CARTESIAN_POINT ( 'NONE',  ( -4.894130264408873110, 5.772535398974209642, -1.082531754730543971 ) ) ;
#105127=CARTESIAN_POINT ( 'NONE',  ( 8.550388431712704573, 13.12720360364021133, 0.000000000000000000 ) ) ;
#105129=CARTESIAN_POINT ( 'NONE',  ( -1.499999999999993339, 10.64264068711930733, 1.232676135170975238E-14 ) ) ;
#105138=CARTESIAN_POINT ( 'NONE',  ( -8.676328237741483207, 12.20980114641871062, -1.199719254218446718 ) ) ;
#105141=ORIENTED_EDGE ( 'NONE', *, *, #142740, .T. ) ;
#105143=CARTESIAN_POINT ( 'NONE',  ( 7.142447996300871793, 7.227277505306155092, 0.7998128361456341429 ) ) ;
#105146=ORIENTED_EDGE ( 'NONE', *, *, #15931, .F. ) ;
#105148=CARTESIAN_POINT ( 'NONE',  ( 2.367870383881045981, 5.914265881169853856, 0.000000000000000000 ) ) ;
#105150=EDGE_LOOP ( 'NONE', ( #151990, #76634, #145780, #54395, #105019, #177993, #5335, #87354, #17446, #38638, #83444, #150729, #30681 ) ) ;
#105155=CARTESIAN_POINT ( 'NONE',  ( -3.023105066167323329, 5.702484939155337607, -2.500000000000000444 ) ) ;
#105159=CARTESIAN_POINT ( 'NONE',  ( 6.598014311344812199, 10.84943379654430906, 1.040834085586084257E-14 ) ) ;
#105160=CARTESIAN_POINT ( 'NONE',  ( -5.545448523189368650, 6.428443684264421698, -1.199719254218446718 ) ) ;
#105162=CARTESIAN_POINT ( 'NONE',  ( -0.7499999999999972244, 4.139583334016149863, -1.299038105676652899 ) ) ;
#105165=CARTESIAN_POINT ( 'NONE',  ( -0.6823417656250212460, 5.051041667008086655, 1.181850606188767472 ) ) ;
#105168=CARTESIAN_POINT ( 'NONE',  ( -6.274726165026268454, 6.214935368819085149, 0.7998128361456341429 ) ) ;
#105172=CARTESIAN_POINT ( 'NONE',  ( 6.328958779480917229, 6.278206752349526631, 0.7998128361456341429 ) ) ;
#105173=CARTESIAN_POINT ( 'NONE',  ( -5.436983294280064882, 6.301900917203534291, 1.199719254218450271 ) ) ;
#105176=EDGE_CURVE ( 'NONE', #202848, #43527, #136426, .T. ) ;
#105180=CARTESIAN_POINT ( 'NONE',  ( 6.073689629242148058, 8.109057205581079231, -1.443375672974057666 ) ) ;
#105182=CARTESIAN_POINT ( 'NONE',  ( 8.066738210006692000, 8.513542121203711233, 0.7216878364870458196 ) ) ;
#105183=CARTESIAN_POINT ( 'NONE',  ( -1.201851678989727383E-14, 3.634375000341422357, 1.575800808251672791 ) ) ;
#105185=CARTESIAN_POINT ( 'NONE',  ( 5.680503174001485078, 6.689970460165617361, -1.082531754730543083 ) ) ;
#105192=CARTESIAN_POINT ( 'NONE',  ( -4.119138978170663989, 7.660627806941648466, 0.7993094217999627826 ) ) ;
#105193=LINE ( 'NONE', #84652, #182754 ) ;
#105198=CARTESIAN_POINT ( 'NONE',  ( -9.992522908471816123, 11.61669713376064372, 1.199719254218462483 ) ) ;
#105200=LINE ( 'NONE', #100903, #74446 ) ;
#105203=CARTESIAN_POINT ( 'NONE',  ( -3.755772246185468788, 4.340488027759846545, -1.199719254218452047 ) ) ;
#105208=CARTESIAN_POINT ( 'NONE',  ( 3.145128448690309053, 4.692402494937224056, -1.443375672974057666 ) ) ;
#105209=CARTESIAN_POINT ( 'NONE',  ( 1.364683531249988535, 3.717708333674750953, -0.7879004041258239610 ) ) ;
#105211=CARTESIAN_POINT ( 'NONE',  ( 7.070740804726770357, 8.207951346058097286, 1.199719254218462483 ) ) ;
#105214=CARTESIAN_POINT ( 'NONE',  ( -3.795392936821753604, 6.515376628678959392, -1.199719254218452047 ) ) ;
#105218=CARTESIAN_POINT ( 'NONE',  ( 0.7499999999999902300, 4.566666666666691299, -1.299038105676658228 ) ) ;
#105219=CARTESIAN_POINT ( 'NONE',  ( 3.960953433486789521, 7.772862772376584850, -0.7998128361456221525 ) ) ;
#105222=DIRECTION ( 'NONE',  ( 0.000000000000000000, 8.546850786086437571E-32, 1.000000000000000000 ) ) ;
#105223=CARTESIAN_POINT ( 'NONE',  ( 1.364683531249988535, 4.363541667008090208, 0.7879004041258500513 ) ) ;
#105226=CARTESIAN_POINT ( 'NONE',  ( 9.910647101909615841, 10.66476916175714607, 0.000000000000000000 ) ) ;
#105229=FACE_OUTER_BOUND ( 'NONE', #181497, .T. ) ;
#105231=CARTESIAN_POINT ( 'NONE',  ( 1.499999999999987121, 2.327083334016154303, -0.8660254037844262731 ) ) ;
#105233=CARTESIAN_POINT ( 'NONE',  ( -5.032047568966410367, 9.022472597102808578, 1.214306433183764966E-14 ) ) ;
#105234=CARTESIAN_POINT ( 'NONE',  ( 5.490689023410166847, 5.508151403507724808, -0.7216878364870207285 ) ) ;
#105244=CARTESIAN_POINT ( 'NONE',  ( 6.958359152311676787, 9.141171649162195934, -1.599625672291262513 ) ) ;
#105245=CARTESIAN_POINT ( 'NONE',  ( 5.508690485854129903, 5.321227076451600091, 1.040834085586084257E-14 ) ) ;
#105249=CARTESIAN_POINT ( 'NONE',  ( 6.193377243344257543, 6.120028293523423812, -0.7998128361456281477 ) ) ;
#105252=CARTESIAN_POINT ( 'NONE',  ( -3.673896439623323129, 4.156855427197417185, 1.000000000000009548 ) ) ;
#105256=CARTESIAN_POINT ( 'NONE',  ( 8.866142388332804103, 12.43125098877526113, -1.199719254218446718 ) ) ;
#105261=CARTESIAN_POINT ( 'NONE',  ( 5.740253418993177981, 6.070215967746060315, 0.6401420356763661834 ) ) ;
#105270=SPHERICAL_SURFACE ( 'NONE', #108647, 0.08000000000000000167 ) ;
#105272=CARTESIAN_POINT ( 'NONE',  ( 7.131225611108096274, 8.382479970123348778, 1.082531754730558626 ) ) ;
#105273=CARTESIAN_POINT ( 'NONE',  ( -2.916975605234527702, 6.554888639415577423, 1.040834085586084257E-14 ) ) ;
#105278=CARTESIAN_POINT ( 'NONE',  ( -3.567766978690493307, 7.314145241780881435, 1.040834085586084257E-14 ) ) ;
#105286=CARTESIAN_POINT ( 'NONE',  ( 3.160134022698241729, 2.806877976488725501, 2.466440901444043377 ) ) ;
#105292=CARTESIAN_POINT ( 'NONE',  ( 7.723341061279088038, 12.16231500480096983, -0.7998128361456291469 ) ) ;
#105299=CARTESIAN_POINT ( 'NONE',  ( 3.497640442201256139, 7.024404915969360452, 1.040834085586084257E-14 ) ) ;
#105300=CARTESIAN_POINT ( 'NONE',  ( -9.083599731475995753, 11.62061899152058686, 1.443375672974064550 ) ) ;
#105304=CARTESIAN_POINT ( 'NONE',  ( 7.065770611016287006, 11.39514947949436774, 1.040834085586084257E-14 ) ) ;
#105308=CARTESIAN_POINT ( 'NONE',  ( -5.605406444246153974, 8.627059054007450101, -1.199719254218440723 ) ) ;
#105309=CARTESIAN_POINT ( 'NONE',  ( 4.955668840994886359, 5.740367388370866131, 1.199719254218462483 ) ) ;
#105314=CARTESIAN_POINT ( 'NONE',  ( 9.673906298550626559, 11.24497775551929557, 1.199719254218452047 ) ) ;
#105318=CARTESIAN_POINT ( 'NONE',  ( -1.364683531249997417, 3.071875000341423245, 1.214306433183764966E-14 ) ) ;
#105321=CARTESIAN_POINT ( 'NONE',  ( 5.653386867218496370, 9.539442411822841805, 1.040834085586084257E-14 ) ) ;
#105330=CARTESIAN_POINT ( 'NONE',  ( 7.253248993186720561, 10.44557901115111065, 1.082531754730558626 ) ) ;
#105334=CARTESIAN_POINT ( 'NONE',  ( -9.154780037725563702, 11.70366268214508487, 1.599625672291281386 ) ) ;
#105343=ADVANCED_FACE ( 'NONE', ( #139633 ), #37170, .T. ) ;
#105344=CARTESIAN_POINT ( 'NONE',  ( 4.111146893441827821, 5.819424013814004759, 1.599625672291267398 ) ) ;
#105350=CARTESIAN_POINT ( 'NONE',  ( 6.498435699651741615, 6.475929825882159818, -0.7998128361456281477 ) ) ;
#105353=CARTESIAN_POINT ( 'NONE',  ( -1.500000000000013101, 3.410416667349487785, -0.8660254037844313801 ) ) ;
#105359=CARTESIAN_POINT ( 'NONE',  ( -1.500000000000001332, 0.6500000000000255573, 0.000000000000000000 ) ) ;
#105360=CARTESIAN_POINT ( 'NONE',  ( 6.076025397218672630, 10.24044673006381245, -0.7998128361456291469 ) ) ;
#105362=CARTESIAN_POINT ( 'NONE',  ( 1.364683531249986537, -0.1364583329919154264, 0.7879004041258500513 ) ) ;
#105365=CARTESIAN_POINT ( 'NONE',  ( 8.107412671292022921, 12.40247251657532956, 0.7216878364870438212 ) ) ;
#105371=CARTESIAN_POINT ( 'NONE',  ( -5.717788096661253761, 7.693838750903348789, 1.599625672291269396 ) ) ;
#105372=CARTESIAN_POINT ( 'NONE',  ( -1.500000000000011324, 2.952083334016149418, 0.8660254037844403729 ) ) ;
#105373=CARTESIAN_POINT ( 'NONE',  ( 1.364683531249990311, 4.946875000341417916, 1.214306433183764966E-14 ) ) ;
#105378=CARTESIAN_POINT ( 'NONE',  ( -0.6823417656249969321, 4.030208333674754506, -1.181850606188749264 ) ) ;
#105388=CARTESIAN_POINT ( 'NONE',  ( -9.176171038350775078, 9.599954387697719582, -0.7998128361456291469 ) ) ;
#105389=CARTESIAN_POINT ( 'NONE',  ( 4.645640190976921602, 8.571663989448405019, 1.040834085586084257E-14 ) ) ;
#105398=CARTESIAN_POINT ( 'NONE',  ( -7.019370843573183194, 9.212351955633947043, 1.599625672291283607 ) ) ;
#105403=CARTESIAN_POINT ( 'NONE',  ( 2.758194185376297902, 5.305311418659259814, 1.199719254218452047 ) ) ;
#105405=ORIENTED_EDGE ( 'NONE', *, *, #24501, .F. ) ;
#105407=CARTESIAN_POINT ( 'NONE',  ( -4.253507506385335368, 5.985511395581417204, 1.599625672291267398 ) ) ;
#105408=CARTESIAN_POINT ( 'NONE',  ( -7.296259222448620463, 11.66405285949874759, 0.7998128361456481317 ) ) ;
#105411=CARTESIAN_POINT ( 'NONE',  ( -4.712932107567791462, 7.040231785572885315, -1.411385885297003373 ) ) ;
#105418=CARTESIAN_POINT ( 'NONE',  ( 6.063521013809720195, 8.097193820909906137, 1.599625672291281386 ) ) ;
#105439=CARTESIAN_POINT ( 'NONE',  ( 4.053524740805938720, 3.831459740469437936, 1.214306433183764966E-14 ) ) ;
#105441=EDGE_LOOP ( 'NONE', ( #133357, #157481, #146581, #17873, #145318, #102532, #199518, #31492, #134757, #203572, #107980, #131361, #177709 ) ) ;
#105448=CARTESIAN_POINT ( 'NONE',  ( -0.7500000000000215383, 2.222916667349486453, 1.299038105676671107 ) ) ;
#105453=CARTESIAN_POINT ( 'NONE',  ( -8.479735010343349089, 11.98044238112085758, 1.199719254218453823 ) ) ;
#105454=CARTESIAN_POINT ( 'NONE',  ( 2.876381804795541619, 6.437993120328354024, 0.3511878651327338674 ) ) ;
#105455=CARTESIAN_POINT ( 'NONE',  ( -1.364683531250000748, 1.259375000341421469, 0.000000000000000000 ) ) ;
#105458=ADVANCED_FACE ( 'NONE', ( #75673 ), #169964, .F. ) ;
#105463=CARTESIAN_POINT ( 'NONE',  ( -4.386226389220933441, 5.076017861301227008, -1.199719254218446718 ) ) ;
#105468=CARTESIAN_POINT ( 'NONE',  ( -0.6823417656250003738, -0.4697916663252491021, -1.181850606188749264 ) ) ;
#105473=CARTESIAN_POINT ( 'NONE',  ( -1.364683531250014514, -0.2197916663252438285, 0.7879004041258379498 ) ) ;
#105475=CARTESIAN_POINT ( 'NONE',  ( -6.015013705957189316, 10.16926642359206134, 0.7998128361456481317 ) ) ;
#105476=CARTESIAN_POINT ( 'NONE',  ( 10.05067194643221207, 10.62020544712608938, 0.7998128361456462443 ) ) ;
#105477=CARTESIAN_POINT ( 'NONE',  ( 4.330940004561544043, 7.140181541042074365, -1.199719254218452047 ) ) ;
#105480=CARTESIAN_POINT ( 'NONE',  ( 1.364683531249986537, 1.717708333674749399, -0.7879004041258239610 ) ) ;
#105487=CARTESIAN_POINT ( 'NONE',  ( 6.236387472606139681, 8.298871356172400127, -1.443375672974057666 ) ) ;
#105490=CARTESIAN_POINT ( 'NONE',  ( -5.703176172842872482, 9.805455968292021041, 0.000000000000000000 ) ) ;
#105491=CARTESIAN_POINT ( 'NONE',  ( -4.928552533767591726, 5.708731696605642725, 1.199719254218462483 ) ) ;
#105492=CARTESIAN_POINT ( 'NONE',  ( -4.241820592029106329, 7.460146341384830571, -0.9904578092340046158 ) ) ;
#105496=CARTESIAN_POINT ( 'NONE',  ( 5.463572716182824252, 7.397254140345190798, 1.443375672974062551 ) ) ;
#105497=CARTESIAN_POINT ( 'NONE',  ( -8.310784975052682100, 10.71900177569337487, -1.443375672974058777 ) ) ;
#105499=CARTESIAN_POINT ( 'NONE',  ( 0.7499999999999920064, 4.233333333333352932, 1.299038105676669330 ) ) ;
#105503=CARTESIAN_POINT ( 'NONE',  ( 8.215877900201359552, 11.56864606933486606, -1.082531754730543083 ) ) ;
#105514=CARTESIAN_POINT ( 'NONE',  ( 8.907343734053986495, 9.494248565925552441, -0.7216878364870197293 ) ) ;
#105515=CARTESIAN_POINT ( 'NONE',  ( 8.938903350111612411, 9.323142084752035430, -0.7998128361456221525 ) ) ;
#105516=CARTESIAN_POINT ( 'NONE',  ( -5.799137018343247796, 7.788745826199009237, -1.599625672291256295 ) ) ;
#105519=CARTESIAN_POINT ( 'NONE',  ( -4.168895032367330167, 3.976329666238523242, -0.6109567437776577403 ) ) ;
#105520=CARTESIAN_POINT ( 'NONE',  ( -1.364683531250000748, -0.9281249996585805295, 0.000000000000000000 ) ) ;
#105521=CARTESIAN_POINT ( 'NONE',  ( 3.958617665510264949, 5.641473247893851628, -1.443375672974051449 ) ) ;
#105522=ORIENTED_EDGE ( 'NONE', *, *, #89482, .F. ) ;
#105523=CARTESIAN_POINT ( 'NONE',  ( -7.049876689426097798, 11.16868053773170821, -0.7216878364870267237 ) ) ;
#105531=ORIENTED_EDGE ( 'NONE', *, *, #113401, .F. ) ;
#105539=CARTESIAN_POINT ( 'NONE',  ( 6.286176778230493589, 10.48562334124426698, 0.7998128361456462443 ) ) ;
#105552=CARTESIAN_POINT ( 'NONE',  ( -6.749261541504576911, 6.768559974710451677, 1.040834085586084257E-14 ) ) ;
#105554=CARTESIAN_POINT ( 'NONE',  ( -4.771579997005698459, 7.654261532226910525, -1.199719254218452047 ) ) ;
#105557=EDGE_CURVE ( 'NONE', #135381, #160603, #120495, .T. ) ;
#105566=CARTESIAN_POINT ( 'NONE',  ( -2.981903720001798597, 5.566305875722335372, -1.199719254218446718 ) ) ;
#105570=CARTESIAN_POINT ( 'NONE',  ( 6.642605195691581699, 9.837124264027149678, 1.199719254218462483 ) ) ;
#105573=CARTESIAN_POINT ( 'NONE',  ( 6.039686174407700392, 6.062845369715991417, 0.4964408002013191989 ) ) ;
#105578=CARTESIAN_POINT ( 'NONE',  ( 6.453317929980448397, 6.631218461173066459, 1.040834085586084257E-14 ) ) ;
#105579=CARTESIAN_POINT ( 'NONE',  ( -8.843996274815957293, 9.212417163573759282, 1.040834085586084257E-14 ) ) ;
#105582=CARTESIAN_POINT ( 'NONE',  ( -7.212047647465563038, 10.50147379109678880, -1.199719254218446718 ) ) ;
#105583=CARTESIAN_POINT ( 'NONE',  ( -5.412729640353771465, 7.337937218544611895, 1.599625672291269396 ) ) ;
#105587=CARTESIAN_POINT ( 'NONE',  ( -2.314109536355652530, 5.457892750589173225, -0.8025987720412944837 ) ) ;
#105590=CARTESIAN_POINT ( 'NONE',  ( 7.670162217029129259, 9.971608557999250166, 1.599625672291281386 ) ) ;
#105605=EDGE_LOOP ( 'NONE', ( #178000, #168138, #111819, #205720 ) ) ;
#105607=CARTESIAN_POINT ( 'NONE',  ( 1.499999999999987121, 3.795833333333356929, -0.8660254037844262731 ) ) ;
#105608=CARTESIAN_POINT ( 'NONE',  ( 3.822509244049070887, 6.547012320444182798, -1.199719254218452047 ) ) ;
#105609=CARTESIAN_POINT ( 'NONE',  ( 4.320244504248938355, 8.192035688265757898, 1.040834085586084257E-14 ) ) ;
#105611=CARTESIAN_POINT ( 'NONE',  ( -7.700668062882065179, 10.96756792579566664, -1.082531754730543971 ) ) ;
#105613=CARTESIAN_POINT ( 'NONE',  ( 7.809133291791403586, 8.213003049952529722, -0.7216878364870257245 ) ) ;
#105614=CARTESIAN_POINT ( 'NONE',  ( -9.625925875578284163, 10.33259439770390564, 1.040834085586084257E-14 ) ) ;
#105619=CARTESIAN_POINT ( 'NONE',  ( 7.618792255875527886, 10.97600916757510170, 1.199719254218460707 ) ) ;
#105624=CARTESIAN_POINT ( 'NONE',  ( 0.6823417656249899377, 2.342708333674753618, 1.181850606188767472 ) ) ;
#105632=CARTESIAN_POINT ( 'NONE',  ( 8.341290820905593151, 10.75459192918846618, 1.599625672291281386 ) ) ;
#105636=CARTESIAN_POINT ( 'NONE',  ( -8.992082194361570302, 11.51384853155376220, 1.599625672291269396 ) ) ;
#105638=CARTESIAN_POINT ( 'NONE',  ( 1.123270288250311610, 3.110197346350006331, 0.7749999999993734123 ) ) ;
#105642=CARTESIAN_POINT ( 'NONE',  ( 2.703961570921634028, 5.242040035128820108, -1.199719254218446718 ) ) ;
#105646=CARTESIAN_POINT ( 'NONE',  ( -7.641992139597101108, 12.06740792950531649, 0.7998128361456481317 ) ) ;
#105649=CARTESIAN_POINT ( 'NONE',  ( 9.121938423896107651, 9.536683004167278099, -0.7998128361456221525 ) ) ;
#105651=CARTESIAN_POINT ( 'NONE',  ( 5.275030131637754138, 6.378586025900190748, 1.136986337720545581 ) ) ;
#105652=CARTESIAN_POINT ( 'NONE',  ( 1.400751299547981610, 7.315968950352358391, 4.333496285527950853 ) ) ;
#105653=CARTESIAN_POINT ( 'NONE',  ( -5.752737250900127997, 5.605948302338584099, 0.000000000000000000 ) ) ;
#105657=CARTESIAN_POINT ( 'NONE',  ( 9.088043039861931405, 9.497138389460751284, 1.040834085586084257E-14 ) ) ;
#105659=CARTESIAN_POINT ( 'NONE',  ( 7.426115451983150706, 9.686887332112256388, -1.599625672291262513 ) ) ;
#105663=CARTESIAN_POINT ( 'NONE',  ( -9.002250809794006159, 10.56534270192358704, -1.082531754730543971 ) ) ;
#105671=CARTESIAN_POINT ( 'NONE',  ( -5.780146447551155475, 6.079674369897793085, -0.5991446231495625163 ) ) ;
#105673=CARTESIAN_POINT ( 'NONE',  ( 7.131225611108100715, 7.422110755822004968, 0.7216878364870317197 ) ) ;
#105675=CARTESIAN_POINT ( 'NONE',  ( 8.289920859751990889, 11.75899253876431416, 1.199719254218450271 ) ) ;
#105696=CARTESIAN_POINT ( 'NONE',  ( 8.555358625423188812, 9.940005470203933768, 1.199719254218462483 ) ) ;
#105700=CARTESIAN_POINT ( 'NONE',  ( -0.7500000000000215383, 0.9729166673494854534, 1.299038105676659116 ) ) ;
#105701=CARTESIAN_POINT ( 'NONE',  ( -7.718669524881690336, 7.899535955317097624, 0.7998128361456462443 ) ) ;
#105703=EDGE_LOOP ( 'NONE', ( #114619, #145638, #199197, #180448, #95673, #163851, #111423, #5616, #92095, #89966, #111536, #21295, #174255, #147777, #210769, #85147, #157635, #147371, #129798, #193136, #23664, #209179, #185403, #5736, #110909, #100979 ) ) ;
#105704=CARTESIAN_POINT ( 'NONE',  ( -10.63367255181986160, 11.30037282007833532, 1.040834085586084257E-14 ) ) ;
#105709=CARTESIAN_POINT ( 'NONE',  ( 6.799577732453452761, 7.891594428405881878, -1.199719254218446718 ) ) ;
#105712=CARTESIAN_POINT ( 'NONE',  ( -6.581593504430098385, 9.765943957555402122, -1.199719254218440723 ) ) ;
#105714=CARTESIAN_POINT ( 'NONE',  ( -1.364683531250010295, 5.280208333674758059, 0.7879004041258379498 ) ) ;
#105720=CARTESIAN_POINT ( 'NONE',  ( -8.731087737520713432, 10.24898578427137963, 1.082531754730558626 ) ) ;
#105725=CARTESIAN_POINT ( 'NONE',  ( -1.364683531250012516, 4.301041667008089320, -0.7879004041258300672 ) ) ;
#105731=CARTESIAN_POINT ( 'NONE',  ( -1.201851678989727383E-14, 4.071875000341425022, 1.575800808251672791 ) ) ;
#105734=CARTESIAN_POINT ( 'NONE',  ( 6.287230548435207567, 8.358188277972981695, -1.599625672291262513 ) ) ;
#105739=CARTESIAN_POINT ( 'NONE',  ( 3.294268137996273715, 5.826768013428865522, -1.082531754730543971 ) ) ;
#105740=CARTESIAN_POINT ( 'NONE',  ( 1.364683531249988535, 5.717708333674752730, -0.7879004041258300672 ) ) ;
#105746=CARTESIAN_POINT ( 'NONE',  ( 1.364683531249988535, 1.363541667008083769, 0.7879004041258500513 ) ) ;
#105747=CARTESIAN_POINT ( 'NONE',  ( -2.955314298098991266, 6.391691081183366485, 0.7216878364870317197 ) ) ;
#105748=CARTESIAN_POINT ( 'NONE',  ( 6.159481859310094620, 6.080483678816896109, 1.040834085586084257E-14 ) ) ;
#105754=CARTESIAN_POINT ( 'NONE',  ( 4.528060117284244512, 4.385084346360807572, 0.7216878364870317197 ) ) ;
#105758=CARTESIAN_POINT ( 'NONE',  ( -7.212574532790087645, 11.35849468832304154, -0.7216878364870267237 ) ) ;
#105764=CARTESIAN_POINT ( 'NONE',  ( -7.296259222448620463, 11.66405285949874759, 0.7998128361456481317 ) ) ;
#105765=CARTESIAN_POINT ( 'NONE',  ( -5.626270559546828309, 7.587068290936515247, 1.443375672974064550 ) ) ;
#105767=CARTESIAN_POINT ( 'NONE',  ( 1.364683531249988757, 0.1968750003414204697, 0.000000000000000000 ) ) ;
#105776=CIRCLE ( 'NONE', #112599, 4.021913119055696484 ) ;
#105785=ORIENTED_EDGE ( 'NONE', *, *, #148663, .T. ) ;
#105789=CARTESIAN_POINT ( 'NONE',  ( -4.277761160311629673, 4.949475094240346706, 1.199719254218462483 ) ) ;
#105793=CARTESIAN_POINT ( 'NONE',  ( 1.364683531249988535, 2.426041667008088432, 0.7879004041258500513 ) ) ;
#105803=CARTESIAN_POINT ( 'NONE',  ( -0.6823417656250212460, 0.8010416670080899859, 1.181850606188755259 ) ) ;
#105805=EDGE_LOOP ( 'NONE', ( #185308, #24555, #130951, #153943 ) ) ;
#105807=CARTESIAN_POINT ( 'NONE',  ( -0.04945587076000566851, 6.344066507677029065, -3.092088676902647659 ) ) ;
#105812=CARTESIAN_POINT ( 'NONE',  ( 6.328958779480917229, 6.278206752349526631, 0.7998128361456341429 ) ) ;
#105816=ORIENTED_EDGE ( 'NONE', *, *, #136635, .F. ) ;
#105817=CARTESIAN_POINT ( 'NONE',  ( 8.516493047678546091, 13.08765898893368629, -0.7998128361456352531 ) ) ;
#105820=CARTESIAN_POINT ( 'NONE',  ( 6.958359152311676787, 9.141171649162195934, -1.599625672291262513 ) ) ;
#105823=CARTESIAN_POINT ( 'NONE',  ( 6.747154001095143627, 11.02343010125301959, -0.7998128361456291469 ) ) ;
#105825=CARTESIAN_POINT ( 'NONE',  ( 1.510814038188205366, 8.678413394653590629, -2.539834060596333210 ) ) ;
#105834=CARTESIAN_POINT ( 'NONE',  ( -8.853111120043687166, 9.430977182913531820, 1.040834085586084257E-14 ) ) ;
#105839=CARTESIAN_POINT ( 'NONE',  ( -9.755255220232635693, 11.33988483081495957, -1.199719254218441611 ) ) ;
#105844=CARTESIAN_POINT ( 'NONE',  ( -4.249591082879585535, 7.045274465746411252, 1.199719254218464037 ) ) ;
#105846=CARTESIAN_POINT ( 'NONE',  ( 10.58621901417202515, 11.24501035948919991, -0.7998128361456281477 ) ) ;
#105849=CARTESIAN_POINT ( 'NONE',  ( 3.842846474469570062, 6.570739089268092137, -1.199719254218452047 ) ) ;
#105855=CARTESIAN_POINT ( 'NONE',  ( 4.717874267875568961, 4.606534188717351874, -0.7216878364870188411 ) ) ;
#105857=CARTESIAN_POINT ( 'NONE',  ( -6.013204822860843457, 6.974159367214481264, -1.199719254218446718 ) ) ;
#105860=CARTESIAN_POINT ( 'NONE',  ( -10.32183501870554387, 10.93656236477829502, 0.7998128361456462443 ) ) ;
#105866=CARTESIAN_POINT ( 'NONE',  ( 9.083599731475992201, 9.699880562917908122, 0.7216878364870438212 ) ) ;
#105868=CARTESIAN_POINT ( 'NONE',  ( -1.201851678989727383E-14, 4.759375000341420581, -1.575800808251660134 ) ) ;
#105870=CARTESIAN_POINT ( 'NONE',  ( 4.416205349749311004, 6.175325546172740765, 1.599625672291267398 ) ) ;
#105886=CARTESIAN_POINT ( 'NONE',  ( -1.364683531250014514, 1.551041667008084435, -0.7879004041258289570 ) ) ;
#105888=CARTESIAN_POINT ( 'NONE',  ( 4.376584659113025744, 4.000436945253625254, 0.7998128361456341429 ) ) ;
#105890=CARTESIAN_POINT ( 'NONE',  ( -4.582292731738899505, 8.289832587096611860, 0.7216878364870458196 ) ) ;
#105892=CARTESIAN_POINT ( 'NONE',  ( 5.178851490740207453, 5.144340948726102702, 0.7216878364870317197 ) ) ;
#105893=CARTESIAN_POINT ( 'NONE',  ( -5.219525951136837705, 9.033271343060892633, -0.7216878364870207285 ) ) ;
#105898=CARTESIAN_POINT ( 'NONE',  ( 5.986088515633498197, 6.942523675449257858, -1.199719254218446718 ) ) ;
#105908=EDGE_CURVE ( 'NONE', #69998, #212421, #130837, .T. ) ;
#105909=CARTESIAN_POINT ( 'NONE',  ( 5.819474248763732760, 7.812472595022922128, -1.599625672291262513 ) ) ;
#105913=CARTESIAN_POINT ( 'NONE',  ( -5.201524489137236529, 9.220195670635433771, 0.7998128361456481317 ) ) ;
#105917=CARTESIAN_POINT ( 'NONE',  ( 6.401421083946654100, 10.62007503124645957, -0.7998128361456291469 ) ) ;
#105920=CARTESIAN_POINT ( 'NONE',  ( -6.521635583373313061, 7.567328587812373719, -1.199719254218446718 ) ) ;
#105921=B_SPLINE_CURVE_WITH_KNOTS ( 'NONE', 3,
 ( #198079, #99530, #114771, #47602, #181821, #179720 ),
 .UNSPECIFIED., .F., .F.,
 ( 4, 2, 4 ),
 ( 0.001491904891164481895, 0.001547600839949546002, 0.001603296788734610108 ),
 .UNSPECIFIED. ) ;
#105922=CARTESIAN_POINT ( 'NONE',  ( 7.768458830506048685, 8.165549511786275971, -0.7216878364870267237 ) ) ;
#105923=CARTESIAN_POINT ( 'NONE',  ( 5.545980446453017798, 6.390169355917580951, 1.218016560845627483 ) ) ;
#105924=CARTESIAN_POINT ( 'NONE',  ( -4.303823697334223652, 7.108545849276850959, -1.199719254218452047 ) ) ;
#105928=CARTESIAN_POINT ( 'NONE',  ( -4.726989112658928072, 8.666571064744069020, 1.040834085586084257E-14 ) ) ;
#105933=CARTESIAN_POINT ( 'NONE',  ( 1.364683531249988757, 1.884375000341421913, 0.000000000000000000 ) ) ;
#105936=CARTESIAN_POINT ( 'NONE',  ( -6.575341312947811545, 6.773579074634973551, 1.040834085586084257E-14 ) ) ;
#105941=CARTESIAN_POINT ( 'NONE',  ( 6.681470773436232413, 6.689470745297396270, -0.7998128361456281477 ) ) ;
#105943=CARTESIAN_POINT ( 'NONE',  ( -5.908080316777766683, 6.002527095666024159, -0.1116623552285273685 ) ) ;
#105944=CARTESIAN_POINT ( 'NONE',  ( -1.364683531250012516, 1.842708333674749843, 0.7879004041258379498 ) ) ;
#105950=CARTESIAN_POINT ( 'NONE',  ( -4.680589345215810049, 6.483773540883647435, -1.599625672291256295 ) ) ;
#105953=CARTESIAN_POINT ( 'NONE',  ( -7.904040366642703930, 10.24446639921506552, 1.443375672974090751 ) ) ;
#105961=CARTESIAN_POINT ( 'NONE',  ( -8.636180661780668899, 10.13826086257468795, -1.082531754730543083 ) ) ;
#105963=VERTEX_POINT ( 'NONE', #214146 ) ;
#105969=CARTESIAN_POINT ( 'NONE',  ( -8.310784975052689205, 8.798263347090697906, -0.7216878364870267237 ) ) ;
#105975=CARTESIAN_POINT ( 'NONE',  ( 1.499999999999991118, 5.285416667349480235, 0.8660254037844524744 ) ) ;
#105976=CARTESIAN_POINT ( 'NONE',  ( 4.566373025097719029, 7.183545020864719355, -1.317121582780217404 ) ) ;
#105984=CARTESIAN_POINT ( 'NONE',  ( -5.856232286098998152, 8.919689202835742847, 1.199719254218452047 ) ) ;
#105988=CARTESIAN_POINT ( 'NONE',  ( 4.871457266011829823, 4.577788319968905562, -0.7998128361456221525 ) ) ;
#105992=CARTESIAN_POINT ( 'NONE',  ( 7.156006149914539982, 7.243095351188763686, 1.040834085586084257E-14 ) ) ;
#105997=CARTESIAN_POINT ( 'NONE',  ( -6.087247782855839340, 6.204136622861004646, 0.000000000000000000 ) ) ;
#106007=CARTESIAN_POINT ( 'NONE',  ( -1.402160292154681736E-14, 0.3218750003414227456, 1.575800808251672791 ) ) ;
#106009=CARTESIAN_POINT ( 'NONE',  ( -6.828502922777144768, 11.11833717654868892, 0.7998128361456481317 ) ) ;
#106011=CARTESIAN_POINT ( 'NONE',  ( 7.690499447449630210, 9.995335326823163058, 1.599625672291281386 ) ) ;
#106013=CARTESIAN_POINT ( 'NONE',  ( -6.692921386640485082, 10.96015871772258521, -0.7998128361456291469 ) ) ;
#106017=CARTESIAN_POINT ( 'NONE',  ( 1.364683531249990311, 4.613541667008083103, 0.7879004041258500513 ) ) ;
#106019=CARTESIAN_POINT ( 'NONE',  ( 7.754900677336718395, 11.99120852362745460, -0.7216878364870267237 ) ) ;
#106022=CARTESIAN_POINT ( 'NONE',  ( 1.364683531249988757, -0.05312499965857975237, 0.000000000000000000 ) ) ;
#106024=CARTESIAN_POINT ( 'NONE',  ( 7.253248993186724114, 9.485209796849769504, 1.443375672974076540 ) ) ;
#106027=CARTESIAN_POINT ( 'NONE',  ( -5.341549334104202629, 7.254893527920112994, 1.443375672974064550 ) ) ;
#106029=CARTESIAN_POINT ( 'NONE',  ( 0.6823417656249917140, 3.592708333674754506, 1.181850606188765695 ) ) ;
#106033=CARTESIAN_POINT ( 'NONE',  ( -6.287230548435221777, 8.358188277972981695, -1.599625672291263179 ) ) ;
#106039=CARTESIAN_POINT ( 'NONE',  ( 8.446893396513862839, 9.813462703143045474, -1.199719254218445830 ) ) ;
#106042=CARTESIAN_POINT ( 'NONE',  ( -1.500000000000015099, 0.6291666666666863028, -0.8660254037844313801 ) ) ;
#106048=CARTESIAN_POINT ( 'NONE',  ( 6.805829924380114804, 8.002851668940699881, 1.082531754730558626 ) ) ;
#106051=ORIENTED_EDGE ( 'NONE', *, *, #189072, .T. ) ;
#106057=CARTESIAN_POINT ( 'NONE',  ( 8.274553823041976841, 8.548067636504127265, 1.040834085586084257E-14 ) ) ;
#106058=CARTESIAN_POINT ( 'NONE',  ( -9.528683032306089373, 10.01121838064558744, 0.7998128361456462443 ) ) ;
#106061=CARTESIAN_POINT ( 'NONE',  ( 0.6823417656249882723, -0.4072916663252490466, 1.181850606188755259 ) ) ;
#106062=CARTESIAN_POINT ( 'NONE',  ( 1.499999999999989120, 1.525000000000019451, 0.000000000000000000 ) ) ;
#106064=CARTESIAN_POINT ( 'NONE',  ( 4.313465427442102929, 8.184126765324453601, 0.7998128361456462443 ) ) ;
#106066=CARTESIAN_POINT ( 'NONE',  ( -1.201851678989727383E-14, 2.868750000682821266, -1.732050807568863648 ) ) ;
#106070=CARTESIAN_POINT ( 'NONE',  ( -1.364683531250010295, 4.530208333674754506, 0.7879004041258379498 ) ) ;
#106072=CARTESIAN_POINT ( 'NONE',  ( -7.700141177557535244, 11.07091624287075859, -1.199719254218446718 ) ) ;
#106073=CARTESIAN_POINT ( 'NONE',  ( -4.419594888374909658, 8.100018436505289188, 0.7216878364870458196 ) ) ;
#106082=CARTESIAN_POINT ( 'NONE',  ( 5.913327553854682783, 10.05063257947248800, -0.7998128361456291469 ) ) ;
#106086=CARTESIAN_POINT ( 'NONE',  ( 8.229436053370683624, 8.703356271795033905, 0.7216878364870458196 ) ) ;
#106090=CARTESIAN_POINT ( 'NONE',  ( -8.993135964566285168, 9.386413468282476913, -0.7998128361456291469 ) ) ;
#106091=CARTESIAN_POINT ( 'NONE',  ( 5.494078562035752178, 7.432844293840273231, -1.599625672291262513 ) ) ;
#106094=CARTESIAN_POINT ( 'NONE',  ( 2.171277156482887882, 5.684907115872006145, -0.7998128361456291469 ) ) ;
#106098=CARTESIAN_POINT ( 'NONE',  ( -4.024564264787665380, 7.667365063520641399, 0.3471600818823785128 ) ) ;
#106101=CARTESIAN_POINT ( 'NONE',  ( -5.260200412422208593, 7.159986452624450770, -1.443375672974053447 ) ) ;
#106102=CARTESIAN_POINT ( 'NONE',  ( 2.333974999846879061, 5.874721266463329705, -0.7998128361456291469 ) ) ;
#106105=CARTESIAN_POINT ( 'NONE',  ( -7.203459687562382641, 7.298457811777897319, -0.7998128361456291469 ) ) ;
#106111=CARTESIAN_POINT ( 'NONE',  ( -8.453672473320708036, 9.821371626084353323, -1.199719254218446718 ) ) ;
#106116=CARTESIAN_POINT ( 'NONE',  ( 3.811813743736467419, 7.598866467667865443, 1.040834085586084257E-14 ) ) ;
#106117=CARTESIAN_POINT ( 'NONE',  ( -4.905525160107053750, 6.476373528817804370, -2.499999999999995115 ) ) ;
#106128=CARTESIAN_POINT ( 'NONE',  ( -7.854251061018346469, 8.057714414143200443, -0.7998128361456291469 ) ) ;
#106131=CARTESIAN_POINT ( 'NONE',  ( 6.656690234629796699, 6.868486149930637552, 1.040834085586084257E-14 ) ) ;
#106133=CARTESIAN_POINT ( 'NONE',  ( -3.131570295076647525, 6.597323077657299528, 1.040834085586084257E-14 ) ) ;
#106136=CARTESIAN_POINT ( 'NONE',  ( -4.089755892816631544, 7.923132308261379819, -0.7998128361456281477 ) ) ;
#106140=CARTESIAN_POINT ( 'NONE',  ( -6.043183783389232566, 8.073467052085995022, 1.599625672291269396 ) ) ;
#106146=CARTESIAN_POINT ( 'NONE',  ( -9.317477881089553549, 11.89347683273641820, 1.599625672291281386 ) ) ;
#106147=CARTESIAN_POINT ( 'NONE',  ( 6.938021921891177612, 9.117444880338284818, -1.599625672291262513 ) ) ;
#106149=CARTESIAN_POINT ( 'NONE',  ( -4.446711195602264688, 4.290177271065136466, -0.7216878364870207285 ) ) ;
#106155=VERTEX_POINT ( 'NONE', #183824 ) ;
#106157=CARTESIAN_POINT ( 'NONE',  ( 9.910647101909615841, 10.66476916175714607, 0.000000000000000000 ) ) ;
#106163=CARTESIAN_POINT ( 'NONE',  ( -3.197497122698730099, 6.431928158754200986, 0.6077543439236172684 ) ) ;
#106178=CARTESIAN_POINT ( 'NONE',  ( -3.002240950422295995, 5.590032644546251817, -1.199719254218452935 ) ) ;
#106181=CARTESIAN_POINT ( 'NONE',  ( -4.796887421136680985, 4.490790167614548523, 1.214306433183764966E-14 ) ) ;
#106183=( BOUNDED_CURVE ( )  B_SPLINE_CURVE ( 2, ( #145027, #111489, #211031, #98373, #82108, #214201, #65831 ),
 .UNSPECIFIED., .F., .T. ) 
 B_SPLINE_CURVE_WITH_KNOTS ( ( 3, 2, 2, 3 ),
 ( 0.1625000000000002276, 0.1666666666666669072, 0.1708333333333336146, 0.1750000000000002942 ),
 .UNSPECIFIED. ) 
 CURVE ( )  GEOMETRIC_REPRESENTATION_ITEM ( )  RATIONAL_B_SPLINE_CURVE ( ( 0.9999999999999928946, 0.8660254037844458130, 1.000000000000000000, 0.8660254037844387076, 1.000000000000000000, 0.8660254037844289376, 1.000000000000009770 ) ) 
 REPRESENTATION_ITEM ( '' )  );
#106186=CARTESIAN_POINT ( 'NONE',  ( -1.364683531250010295, 5.488541667008087543, -0.7879004041258300672 ) ) ;
#106189=CARTESIAN_POINT ( 'NONE',  ( -2.657034918598345730, 5.083329257464595408, -1.082531754730543971 ) ) ;
#106194=CARTESIAN_POINT ( 'NONE',  ( 3.541704441667858472, 5.155074486744371853, -1.599625672291262513 ) ) ;
#106197=CARTESIAN_POINT ( 'NONE',  ( 9.151390499099949949, 12.66007743471656788, -1.082531754730543971 ) ) ;
#106199=CARTESIAN_POINT ( 'NONE',  ( 0.6823417656249882723, 2.988541667008084879, -1.181850606188754593 ) ) ;
#106200=CARTESIAN_POINT ( 'NONE',  ( -1.201851678989727383E-14, 3.712500000000020339, 1.732050807568877637 ) ) ;
#106203=CARTESIAN_POINT ( 'NONE',  ( -7.621654909176601045, 12.04368116068139472, 0.7998128361456481317 ) ) ;
#106204=CARTESIAN_POINT ( 'NONE',  ( -5.870317324592829067, 5.951051088220814300, -0.7216878364870197293 ) ) ;
#106207=CARTESIAN_POINT ( 'NONE',  ( -6.555530967407501741, 7.606873202518897870, 1.199719254218450271 ) ) ;
#106208=ORIENTED_EDGE ( 'NONE', *, *, #101458, .F. ) ;
#106209=CARTESIAN_POINT ( 'NONE',  ( -0.7500000000000249800, -1.027083332650516212, 1.299038105676659116 ) ) ;
#106217=CARTESIAN_POINT ( 'NONE',  ( -5.897433631820158340, 5.982686779986042147, 0.7216878364870317197 ) ) ;
#106218=CARTESIAN_POINT ( 'NONE',  ( -0.4867935908771195419, 7.427453578134552536, -4.536604770845594992 ) ) ;
#106220=CYLINDRICAL_SURFACE ( 'NONE', #119263, 0.2500000000000002220 ) ;
#106222=CARTESIAN_POINT ( 'NONE',  ( -5.897433631820158340, 5.982686779986042147, 0.7216878364870317197 ) ) ;
#106233=CARTESIAN_POINT ( 'NONE',  ( -5.088387723830502196, 4.830873854090670605, -0.7998128361456221525 ) ) ;
#106234=CARTESIAN_POINT ( 'NONE',  ( -9.541187415715041809, 12.15447128979948310, -1.599625672291263179 ) ) ;
#106239=CARTESIAN_POINT ( 'NONE',  ( 5.656776405399742025, 7.622658444431597680, -1.599625672291262513 ) ) ;
#106244=CARTESIAN_POINT ( 'NONE',  ( 2.866659414285625651, 5.431854185720147221, -1.199719254218446718 ) ) ;
#106256=CARTESIAN_POINT ( 'NONE',  ( 7.910292558569346433, 11.31609285405122556, -1.199719254218446718 ) ) ;
#106257=CARTESIAN_POINT ( 'NONE',  ( -6.437424008390261854, 6.404749519410410485, 0.7998128361456341429 ) ) ;
#106264=CARTESIAN_POINT ( 'NONE',  ( 0.6823417656249899377, 4.176041667008085767, -1.181850606188754593 ) ) ;
#106266=CARTESIAN_POINT ( 'NONE',  ( -4.577849422908604637, 8.492574760035358494, -0.7998128361456281477 ) ) ;
#106269=CARTESIAN_POINT ( 'NONE',  ( 6.342516933094585418, 6.294024598232139667, 1.040834085586084257E-14 ) ) ;
#106270=CARTESIAN_POINT ( 'NONE',  ( -6.033542053281340856, 6.997886136038390603, -1.199719254218446718 ) ) ;
#106277=CARTESIAN_POINT ( 'NONE',  ( 5.829642864196151741, 9.745074408296771296, 0.7216878364870438212 ) ) ;
#106279=CARTESIAN_POINT ( 'NONE',  ( 6.222829318548112276, 9.243422724072711816, -1.082531754730537976 ) ) ;
#106280=CARTESIAN_POINT ( 'NONE',  ( -0.6823417656249969321, 3.280208333674754062, -1.181850606188749264 ) ) ;
#106282=CARTESIAN_POINT ( 'NONE',  ( 4.568734577680873876, 6.353276312092901890, -1.443375672974051449 ) ) ;
#106291=CARTESIAN_POINT ( 'NONE',  ( -4.144643181316929770, 7.629267798522465505, 0.8581763667485035052 ) ) ;
#106298=CARTESIAN_POINT ( 'NONE',  ( -8.482597663644387609, 13.04811437422715414, -0.7998128361456281477 ) ) ;
#106302=CARTESIAN_POINT ( 'NONE',  ( -4.457933580795036654, 4.095344020549286590, -0.7998128361456221525 ) ) ;
#106307=CARTESIAN_POINT ( 'NONE',  ( 4.202664430556257713, 4.965825259479493603, 1.082531754730560403 ) ) ;
#106308=CARTESIAN_POINT ( 'NONE',  ( -1.364683531250012516, 3.301041667008084879, -0.7879004041258289570 ) ) ;
#106310=CARTESIAN_POINT ( 'NONE',  ( 9.074484886248265880, 9.481320543578137361, 0.7998128361456462443 ) ) ;
#106311=CARTESIAN_POINT ( 'NONE',  ( -8.631737353394710155, 13.22211067893587533, 1.040834085586084257E-14 ) ) ;
#106313=CARTESIAN_POINT ( 'NONE',  ( -3.578462479003122976, 6.262291094557191684, 1.199719254218464037 ) ) ;
#106314=DIRECTION ( 'NONE',  ( 0.000000000000000000, 0.000000000000000000, 1.000000000000000000 ) ) ;
#106317=CARTESIAN_POINT ( 'NONE',  ( 1.499999999999989120, 3.275000000000020783, 1.214306433183764966E-14 ) ) ;
#106318=CARTESIAN_POINT ( 'NONE',  ( 3.499976210622149253, 7.235056012367825140, 0.7998128361456321445 ) ) ;
#106321=CARTESIAN_POINT ( 'NONE',  ( 1.499999999999990674, 8.673756432004019246, 2.614717076620609149 ) ) ;
#106322=CARTESIAN_POINT ( 'NONE',  ( 1.364683531249988535, 4.405208333674754506, -0.7879004041258300672 ) ) ;
#106324=CARTESIAN_POINT ( 'NONE',  ( 8.595506201384004896, 12.01154575404795466, 1.082531754730546636 ) ) ;
#106330=CARTESIAN_POINT ( 'NONE',  ( 1.499999999999987121, 1.577083334016150751, -0.8660254037844253849 ) ) ;
#106331=VECTOR ( 'NONE', #60621, 1000.000000000000114 ) ;
#106333=CARTESIAN_POINT ( 'NONE',  ( -6.417086777969760902, 6.381022750586497594, 0.7998128361456341429 ) ) ;
#106334=CARTESIAN_POINT ( 'NONE',  ( 3.809477975315569864, 7.388215371269402532, -0.7216878364870197293 ) ) ;
#106343=CARTESIAN_POINT ( 'NONE',  ( 8.281332899848809603, 8.555976559445431562, 0.7998128361456481317 ) ) ;
#106344=CARTESIAN_POINT ( 'NONE',  ( 4.690231075323689325, 7.559354456931247412, 1.199719254218462483 ) ) ;
#106345=DIRECTION ( 'NONE',  ( -5.578564026256504688E-16, -1.000000000000000000, -9.066213480720158442E-32 ) ) ;
#106348=CARTESIAN_POINT ( 'NONE',  ( 4.659198344590585350, 8.587481835331020719, 0.7998128361456462443 ) ) ;
#106350=EDGE_LOOP ( 'NONE', ( #197245, #22688 ) ) ;
#106355=CARTESIAN_POINT ( 'NONE',  ( 8.543609354905870035, 13.11929468069890525, 0.7998128361456462443 ) ) ;
#106359=CARTESIAN_POINT ( 'NONE',  ( 5.892675752748299800, 5.976886221469982274, -0.004604801460011270775 ) ) ;
#106372=CARTESIAN_POINT ( 'NONE',  ( 7.185458225562760148, 8.445751353653788485, -1.082531754730543083 ) ) ;
#106373=CARTESIAN_POINT ( 'NONE',  ( -5.251085567194491155, 5.020688004682002159, -0.7998128361456221525 ) ) ;
#106376=CARTESIAN_POINT ( 'NONE',  ( -4.557512192488103686, 8.468847991211438497, -0.7998128361456281477 ) ) ;
#106396=CARTESIAN_POINT ( 'NONE',  ( -2.656508033273816238, 5.186677574539687363, -1.199719254218446718 ) ) ;
#106401=CARTESIAN_POINT ( 'NONE',  ( 8.938903350111612411, 9.323142084752035430, -0.7998128361456221525 ) ) ;
#106407=CARTESIAN_POINT ( 'NONE',  ( -5.900823170445743671, 7.907379670318584353, 1.599625672291269396 ) ) ;
#106408=CARTESIAN_POINT ( 'NONE',  ( 5.034155109375821446, 4.767602470560229122, -0.7998128361456221525 ) ) ;
#106416=CARTESIAN_POINT ( 'NONE',  ( -1.201851678989727383E-14, 3.009375000341419248, -1.575800808251660134 ) ) ;
#106418=CARTESIAN_POINT ( 'NONE',  ( 7.293923454472091450, 7.611924906413328529, 0.7216878364870317197 ) ) ;
#106426=CARTESIAN_POINT ( 'NONE',  ( 8.717529583462638954, 12.15390636647303069, 1.082531754730546636 ) ) ;
#106427=ORIENTED_EDGE ( 'NONE', *, *, #149589, .T. ) ;
#106431=CARTESIAN_POINT ( 'NONE',  ( -8.208571938070008400, 11.66408546346865016, -1.199719254218446718 ) ) ;
#106432=CARTESIAN_POINT ( 'NONE',  ( -4.161989969715278015, 4.726297878971393196, -7.499999999999991118 ) ) ;
#106440=CARTESIAN_POINT ( 'NONE',  ( 3.083589872104280705, 5.684939719841914929, 1.199719254218450271 ) ) ;
#106447=CARTESIAN_POINT ( 'NONE',  ( 4.137209430464448445, 7.978494768850520558, 1.040834085586084257E-14 ) ) ;
#106450=CARTESIAN_POINT ( 'NONE',  ( -0.7500000000000215383, 3.222916667349487341, 1.299038105676671107 ) ) ;
#106456=CARTESIAN_POINT ( 'NONE',  ( 1.499999999999987121, -0.2458333333333099502, 0.8660254037844524744 ) ) ;
#106457=CARTESIAN_POINT ( 'NONE',  ( 6.428537391173986038, 10.65171072301167854, 0.7998128361456462443 ) ) ;
#106458=CARTESIAN_POINT ( 'NONE',  ( -0.6823417656250003738, 0.2177083336747515085, -1.181850606188749264 ) ) ;
#106461=CARTESIAN_POINT ( 'NONE',  ( 9.408995418203971894, 11.03987807840189816, 1.082531754730549967 ) ) ;
#106465=CARTESIAN_POINT ( 'NONE',  ( -5.585069213825653023, 8.603332285183535433, -1.199719254218440723 ) ) ;
#106466=CARTESIAN_POINT ( 'NONE',  ( -1.201851678989727383E-14, 3.243750000682814161, 1.732050807568877637 ) ) ;
#106467=CARTESIAN_POINT ( 'NONE',  ( 1.364683531249988535, 5.467708333674750953, -0.7879004041258300672 ) ) ;
#106481=CARTESIAN_POINT ( 'NONE',  ( -1.400751299551194151, 7.315968950354509559, 4.333496285525718861 ) ) ;
#106482=CARTESIAN_POINT ( 'NONE',  ( -9.612894607289142357, 11.17379744904754801, -1.199719254218441611 ) ) ;
#106483=CARTESIAN_POINT ( 'NONE',  ( 5.472687561410540802, 9.536552588287639409, 0.7998128361456462443 ) ) ;
#106491=CARTESIAN_POINT ( 'NONE',  ( -8.179646747746328828, 8.437342715325849341, -0.7998128361456291469 ) ) ;
#106496=CARTESIAN_POINT ( 'NONE',  ( 4.162516854595432747, 4.815023404238158555, 1.199719254218464037 ) ) ;
#106498=CARTESIAN_POINT ( 'NONE',  ( -3.744022975668147790, 7.519777238254810925, -0.7998128361456281477 ) ) ;
#106499=CARTESIAN_POINT ( 'NONE',  ( -9.318531651294266638, 9.766041769465124034, -0.7998128361456291469 ) ) ;
#106503=CARTESIAN_POINT ( 'NONE',  ( -4.461457896923207933, 7.279594253155052819, -1.276495073192641883 ) ) ;
#106510=CARTESIAN_POINT ( 'NONE',  ( 5.524057522564145728, 8.532151978711786100, 1.199719254218462483 ) ) ;
#106515=AXIS2_PLACEMENT_3D ( 'NONE', #23813, #101071, #84830 ) ;
#106529=CARTESIAN_POINT ( 'NONE',  ( 4.582292731738905722, 5.408724944192588424, -1.082531754730548412 ) ) ;
#106533=CARTESIAN_POINT ( 'NONE',  ( -7.811469059767924605, 12.26513100303794168, -0.7998128361456281477 ) ) ;
#106534=CARTESIAN_POINT ( 'NONE',  ( 1.499999999999990896, 4.275000000000021672, 1.214306433183764966E-14 ) ) ;
#106539=CARTESIAN_POINT ( 'NONE',  ( 0.7499999999999902300, 2.264583334016148530, 1.299038105676669330 ) ) ;
#106544=CARTESIAN_POINT ( 'NONE',  ( -8.130085669689073313, 12.63685038127928806, 0.7998128361456481317 ) ) ;
#106545=CARTESIAN_POINT ( 'NONE',  ( -0.6823417656250003738, 0.7177083336747519526, -1.181850606188749264 ) ) ;
#106552=CARTESIAN_POINT ( 'NONE',  ( -4.334856428067329404, 6.080418470877079429, -1.599625672291256295 ) ) ;
#106557=CARTESIAN_POINT ( 'NONE',  ( -1.402160292154681736E-14, -0.8656249996585829720, 1.575800808251672791 ) ) ;
#106564=CARTESIAN_POINT ( 'NONE',  ( 1.364683531249988757, 0.6343750003414208027, 0.000000000000000000 ) ) ;
#106566=CARTESIAN_POINT ( 'NONE',  ( -8.538937818508475885, 8.856515631215026829, 1.040834085586084257E-14 ) ) ;
#106567=CARTESIAN_POINT ( 'NONE',  ( 9.250740883225924804, 9.686952540052077509, 1.040834085586084257E-14 ) ) ;
#106568=CARTESIAN_POINT ( 'NONE',  ( 4.005544317833563461, 6.760553239859419250, -1.199719254218452047 ) ) ;
#106572=CARTESIAN_POINT ( 'NONE',  ( -1.364683531250000748, -0.4281249996585800854, 0.000000000000000000 ) ) ;
#106580=CARTESIAN_POINT ( 'NONE',  ( 7.131225611108096274, 8.382479970123348778, 1.082531754730558626 ) ) ;
#106583=CARTESIAN_POINT ( 'NONE',  ( -4.497554271431319250, 6.270232621468402989, -1.599625672291256295 ) ) ;
#106588=CARTESIAN_POINT ( 'NONE',  ( 5.951666246274803562, 7.006327377817825663, 1.082531754730558626 ) ) ;
#106589=CARTESIAN_POINT ( 'NONE',  ( -8.392133896734675247, 10.81390885098904420, 1.443375672974064550 ) ) ;
#106591=CARTESIAN_POINT ( 'NONE',  ( 1.499999999999989120, 3.754166666666685082, 0.8660254037844524744 ) ) ;
#106596=CARTESIAN_POINT ( 'NONE',  ( 9.408995418203975447, 10.07950886410055524, 0.7216878364870438212 ) ) ;
#106601=CARTESIAN_POINT ( 'NONE',  ( -1.387358672531441961, 7.251968950356099342, -4.302625267141395149 ) ) ;
#106608=FACE_OUTER_BOUND ( 'NONE', #87550, .T. ) ;
#106609=CARTESIAN_POINT ( 'NONE',  ( 7.415946836550712185, 10.63539316174243865, 1.082531754730558626 ) ) ;
#106610=EDGE_CURVE ( 'NONE', #12264, #207276, #1512, .T. ) ;
#106611=CARTESIAN_POINT ( 'NONE',  ( 6.401421083946654100, 10.62007503124645957, -0.7998128361456291469 ) ) ;
#106612=CARTESIAN_POINT ( 'NONE',  ( -5.422371370461663176, 8.413518134592214537, -1.199719254218446718 ) ) ;
#106616=CARTESIAN_POINT ( 'NONE',  ( 3.389175213736285386, 6.897862149426897460, 0.7216878364870317197 ) ) ;
#106618=CARTESIAN_POINT ( 'NONE',  ( -6.860062538834774237, 10.94723069537516302, 0.7216878364870458196 ) ) ;
#106644=CARTESIAN_POINT ( 'NONE',  ( -0.08896015503664694846, 7.049507384514476449, -3.948637857580539201 ) ) ;
#106646=CARTESIAN_POINT ( 'NONE',  ( -5.388475986427523345, 8.373973519885682393, 1.199719254218452047 ) ) ;
#106650=CARTESIAN_POINT ( 'NONE',  ( 4.313465427442102929, 8.184126765324453601, 0.7998128361456462443 ) ) ;
#106654=CARTESIAN_POINT ( 'NONE',  ( 4.403700966340357681, 4.032072637018845107, -0.7998128361456211532 ) ) ;
#106659=CARTESIAN_POINT ( 'NONE',  ( -4.711622075948912247, 5.455646162483875017, -1.199719254218446718 ) ) ;
#106664=CARTESIAN_POINT ( 'NONE',  ( 6.425674737872927089, 9.584038729905381970, -1.199719254218440723 ) ) ;
#106665=CARTESIAN_POINT ( 'NONE',  ( -1.201851678989727383E-14, 3.571875000341422357, 1.575800808251672791 ) ) ;
#106668=CARTESIAN_POINT ( 'NONE',  ( 5.809489818682099127, 6.211223759639540987, 0.9523037572534819306 ) ) ;
#106674=CARTESIAN_POINT ( 'NONE',  ( 6.439759776366769550, 8.536139043893143707, 1.443375672974076540 ) ) ;
#106675=CARTESIAN_POINT ( 'NONE',  ( -6.835281999583978418, 11.12624609948998966, -0.7998128361456291469 ) ) ;
#106678=CARTESIAN_POINT ( 'NONE',  ( -6.821723845970312894, 11.11042825360738284, 0.000000000000000000 ) ) ;
#106679=CARTESIAN_POINT ( 'NONE',  ( -4.740547266272593596, 8.682388910626682943, -0.7998128361456281477 ) ) ;
#106686=CARTESIAN_POINT ( 'NONE',  ( 6.591235234537977661, 10.84152487360300299, 0.7998128361456462443 ) ) ;
#106687=CARTESIAN_POINT ( 'NONE',  ( -4.650083499807243115, 5.295740330745369207, -1.052294140492322283 ) ) ;
#106700=CARTESIAN_POINT ( 'NONE',  ( 1.499999999999989120, 4.254166666666687746, 0.8660254037844524744 ) ) ;
#106701=CARTESIAN_POINT ( 'NONE',  ( 5.820528018968444961, 5.685037531751635953, 0.7998128361456341429 ) ) ;
#106702=CARTESIAN_POINT ( 'NONE',  ( 5.445571254183207088, 9.504916896522420444, -0.7998128361456281477 ) ) ;
#106705=CARTESIAN_POINT ( 'NONE',  ( -8.893785580884703279, 10.43879993486270585, 1.082531754730558626 ) ) ;
#106707=CARTESIAN_POINT ( 'NONE',  ( 6.155038550924139429, 9.164333495178082600, 1.082531754730558626 ) ) ;
#106708=CARTESIAN_POINT ( 'NONE',  ( -8.310784975052671442, 11.67937098999472667, -1.082531754730543083 ) ) ;
#106711=CARTESIAN_POINT ( 'NONE',  ( 8.589254009457354400, 9.979550084910457031, -1.199719254218446718 ) ) ;
#106717=CARTESIAN_POINT ( 'NONE',  ( -1.201851678989727383E-14, 1.821875000341421691, 1.575800808251672791 ) ) ;
#106723=CARTESIAN_POINT ( 'NONE',  ( 10.07387183015377197, 11.71160420905630062, -1.199719254218440723 ) ) ;
#106727=CARTESIAN_POINT ( 'NONE',  ( -9.938290294017125603, 11.55342575023019691, -1.199719254218441611 ) ) ;
#106733=CARTESIAN_POINT ( 'NONE',  ( 5.190073875932979419, 4.949507698210251938, 0.7998128361456341429 ) ) ;
#106736=CARTESIAN_POINT ( 'NONE',  ( -8.157201976916404362, 12.66848607304450702, -0.7998128361456281477 ) ) ;
#106739=CARTESIAN_POINT ( 'NONE',  ( 7.086107841436786181, 11.41887624831828418, 1.040834085586084257E-14 ) ) ;
#106741=CARTESIAN_POINT ( 'NONE',  ( 4.677432586336220055, 6.849818891840005364, 1.226792522213099979 ) ) ;
#106744=CARTESIAN_POINT ( 'NONE',  ( -4.334856428067329404, 6.080418470877079429, -1.599625672291256295 ) ) ;
#106748=CARTESIAN_POINT ( 'NONE',  ( 6.913768267964901071, 10.15348118167935709, -1.199719254218441611 ) ) ;
#106750=CARTESIAN_POINT ( 'NONE',  ( 8.437251666405968464, 8.737881787095446384, 1.040834085586084257E-14 ) ) ;
#106753=CARTESIAN_POINT ( 'NONE',  ( -7.185458225562757484, 11.32685899655781903, 0.7216878364870458196 ) ) ;
#106760=CARTESIAN_POINT ( 'NONE',  ( -4.775553520644376881, 6.797630844710244702, -1.243162211532616857 ) ) ;
#106761=CARTESIAN_POINT ( 'NONE',  ( 1.364683531249988757, 2.134375000341422357, 1.214306433183764966E-14 ) ) ;
#106764=CARTESIAN_POINT ( 'NONE',  ( 7.307481608085759639, 7.627742752295940676, 1.040834085586084257E-14 ) ) ;
#106783=CARTESIAN_POINT ( 'NONE',  ( 8.341290820905593151, 10.75459192918846618, 1.599625672291281386 ) ) ;
#106787=CARTESIAN_POINT ( 'NONE',  ( -2.286521462199063492, 5.819358805874190743, 1.040834085586084257E-14 ) ) ;
#106788=CARTESIAN_POINT ( 'NONE',  ( -7.705111371268023923, 7.883718109434487253, 1.040834085586084257E-14 ) ) ;
#106791=CARTESIAN_POINT ( 'NONE',  ( -9.215791728987058562, 11.77484298861683598, -1.599625672291263179 ) ) ;
#106795=CARTESIAN_POINT ( 'NONE',  ( -1.499999999999997780, 5.181250000682820378, 1.214306433183764966E-14 ) ) ;
#106796=CARTESIAN_POINT ( 'NONE',  ( 7.613066949273408213, 8.840665181362512115, -1.199719254218441611 ) ) ;
#106799=CARTESIAN_POINT ( 'NONE',  ( -7.714753101375940503, 8.959299025482085455, 1.199719254218462483 ) ) ;
#106801=CARTESIAN_POINT ( 'NONE',  ( 1.364683531249988535, 4.655208333674755394, -0.7879004041258300672 ) ) ;
#106802=CARTESIAN_POINT ( 'NONE',  ( -1.598423149420381106, 8.713846000021360894, 2.500000000000011102 ) ) ;
#106807=CARTESIAN_POINT ( 'NONE',  ( -8.242994207428740339, 9.679543332497402730, 1.082531754730558626 ) ) ;
#106811=CARTESIAN_POINT ( 'NONE',  ( -1.201851678989727383E-14, 3.634375000341422357, 1.575800808251672791 ) ) ;
#106818=CARTESIAN_POINT ( 'NONE',  ( 1.364683531249988535, 4.405208333674754506, -0.7879004041258300672 ) ) ;
#106819=CIRCLE ( 'NONE', #65297, 0.7499999999999997780 ) ;
#106820=CARTESIAN_POINT ( 'NONE',  ( -3.100010679019018500, 6.768429558830820980, 1.040834085586084257E-14 ) ) ;
#106824=CARTESIAN_POINT ( 'NONE',  ( 4.650083499362880346, 4.527444958785877382, 0.7216878364870317197 ) ) ;
#106825=CARTESIAN_POINT ( 'NONE',  ( 1.364683531249990311, 4.926041667008083991, 0.7879004041258500513 ) ) ;
#106831=CARTESIAN_POINT ( 'NONE',  ( -0.6823417656250003738, 1.217708333674752286, -1.181850606188749264 ) ) ;
#106832=CARTESIAN_POINT ( 'NONE',  ( -3.904385051055635270, 6.538571078664754843, 1.082531754730560403 ) ) ;
#106833=CARTESIAN_POINT ( 'NONE',  ( 6.308621549060418054, 6.254479983525607523, 0.7998128361456341429 ) ) ;
#106837=CARTESIAN_POINT ( 'NONE',  ( 3.199361063144961825, 6.676412307070352270, -0.7216878364870267237 ) ) ;
#106840=CARTESIAN_POINT ( 'NONE',  ( -8.351459436338041442, 9.806086099558291025, -1.082531754730543971 ) ) ;
#106845=CARTESIAN_POINT ( 'NONE',  ( -8.286004436246233951, 12.81875560892930466, 1.040834085586084257E-14 ) ) ;
#106846=CARTESIAN_POINT ( 'NONE',  ( -4.717874267431199087, 8.448011045404303587, 1.040834085586084257E-14 ) ) ;
#106848=CARTESIAN_POINT ( 'NONE',  ( -1.364683531250000748, 1.071875000341421247, 0.000000000000000000 ) ) ;
#106855=( BOUNDED_CURVE ( )  B_SPLINE_CURVE ( 2, ( #23090, #69707, #107635, #135811, #88122 ),
 .UNSPECIFIED., .F., .T. ) 
 B_SPLINE_CURVE_WITH_KNOTS ( ( 3, 2, 3 ),
 ( 0.2851912450777800423, 0.2874999999999999778, 0.2888802418687935192 ),
 .UNSPECIFIED. ) 
 CURVE ( )  GEOMETRIC_REPRESENTATION_ITEM ( )  RATIONAL_B_SPLINE_CURVE ( ( 0.9337969725178141278, 0.9257645179683744452, 1.000000000000000000, 0.9556198367076580436, 0.9406422459849084206 ) ) 
 REPRESENTATION_ITEM ( '' )  );
#106858=CARTESIAN_POINT ( 'NONE',  ( 8.550388431712704573, 13.12720360364021133, 0.000000000000000000 ) ) ;
#106860=EDGE_LOOP ( 'NONE', ( #41450, #131099, #109204, #69129 ) ) ;
#106861=CARTESIAN_POINT ( 'NONE',  ( 7.849807752188022292, 11.14156422998596696, -1.082531754730543083 ) ) ;
#106872=CARTESIAN_POINT ( 'NONE',  ( -4.451154503988200339, 4.087435097607984957, 1.214306433183764966E-14 ) ) ;
#106875=CARTESIAN_POINT ( 'NONE',  ( -1.402160292154681736E-14, 1.509375000341420359, -1.575800808251659024 ) ) ;
#106877=ORIENTED_EDGE ( 'NONE', *, *, #165849, .F. ) ;
#106887=CARTESIAN_POINT ( 'NONE',  ( 0.6823417656249899377, 1.092708333674752286, 1.181850606188755259 ) ) ;
#106888=VERTEX_POINT ( 'NONE', #54764 ) ;
#106897=CARTESIAN_POINT ( 'NONE',  ( 4.761938266897790761, 6.578680616179308771, 1.599625672291267398 ) ) ;
#106904=CARTESIAN_POINT ( 'NONE',  ( 1.387358672531572079, 7.315968950354051259, 4.254625267138675504 ) ) ;
#106906=CARTESIAN_POINT ( 'NONE',  ( 7.365103760721646076, 9.615707025640515937, 1.599625672291281386 ) ) ;
#106910=CARTESIAN_POINT ( 'NONE',  ( 9.759171643738394408, 10.28012176064996197, 0.000000000000000000 ) ) ;
#106917=AXIS2_PLACEMENT_3D ( 'NONE', #117007, #164636, #85509 ) ;
#106922=CARTESIAN_POINT ( 'NONE',  ( -7.483737605063437215, 10.71448239167390604, 1.082531754730549967 ) ) ;
#106927=CARTESIAN_POINT ( 'NONE',  ( -4.889337272013151825, 4.909234758358784312, -0.4031905389056227307 ) ) ;
#106935=CARTESIAN_POINT ( 'NONE',  ( 8.561083932025322696, 12.07534945641652158, -1.199719254218446718 ) ) ;
#106937=CARTESIAN_POINT ( 'NONE',  ( 4.761938266897790761, 6.578680616179308771, 1.599625672291267398 ) ) ;
#106939=ORIENTED_EDGE ( 'NONE', *, *, #171579, .F. ) ;
#106944=CARTESIAN_POINT ( 'NONE',  ( -4.608882153641705059, 7.464447381635583412, -1.199719254218452047 ) ) ;
#106946=CARTESIAN_POINT ( 'NONE',  ( -3.216308754939891212, 4.775446185561722956, -1.599625672291262513 ) ) ;
#106952=CARTESIAN_POINT ( 'NONE',  ( 6.792271770766432404, 10.86814146596211472, 1.040834085586084257E-14 ) ) ;
#106953=CARTESIAN_POINT ( 'NONE',  ( 1.364683531249990311, 4.446875000341417028, 1.214306433183764966E-14 ) ) ;
#106955=CARTESIAN_POINT ( 'NONE',  ( 5.124091990960999432, 8.065525525174782828, -1.199719254218452047 ) ) ;
#106956=LINE ( 'NONE', #172981, #86028 ) ;
#106969=CARTESIAN_POINT ( 'NONE',  ( -0.6823417656250212460, 0.8635416670080899859, 1.181850606188755259 ) ) ;
#106971=CARTESIAN_POINT ( 'NONE',  ( 4.273844736805816780, 6.009238164405336313, 1.599625672291267398 ) ) ;
#106973=CARTESIAN_POINT ( 'NONE',  ( -6.263503779833496488, 6.409768619334935913, 0.7216878364870317197 ) ) ;
#106974=CARTESIAN_POINT ( 'NONE',  ( 5.192409644353875642, 5.160158794608717514, 1.040834085586084257E-14 ) ) ;
#106975=CARTESIAN_POINT ( 'NONE',  ( -7.199016378732087773, 7.501199984716642177, 0.7216878364870317197 ) ) ;
#106977=EDGE_LOOP ( 'NONE', ( #37017, #138031, #132027, #57959 ) ) ;
#106979=CARTESIAN_POINT ( 'NONE',  ( 5.820528018968444961, 5.685037531751635953, 0.7998128361456341429 ) ) ;
#106989=CARTESIAN_POINT ( 'NONE',  ( 6.551614543901692400, 8.666636272683888365, 1.599625672291281386 ) ) ;
#106992=CARTESIAN_POINT ( 'NONE',  ( -5.716734326456539783, 9.821273814174633188, -0.7998128361456231517 ) ) ;
#106996=CARTESIAN_POINT ( 'NONE',  ( 5.940443861082012944, 10.08226827123770697, 0.7998128361456462443 ) ) ;
#106999=CARTESIAN_POINT ( 'NONE',  ( -7.413611068574208041, 7.543634422958360730, 0.7998128361456341429 ) ) ;
#107000=CARTESIAN_POINT ( 'NONE',  ( 7.334597914868727919, 9.580116872145431728, -1.443375672974058777 ) ) ;
#107001=CARTESIAN_POINT ( 'NONE',  ( 4.081185262901700028, 7.719248740676039056, 0.6171906885068592086 ) ) ;
#107002=CARTESIAN_POINT ( 'NONE',  ( -6.274726165026268454, 6.214935368819085149, 0.7998128361456341429 ) ) ;
#107009=CARTESIAN_POINT ( 'NONE',  ( 7.892817981449907982, 12.36003807833360391, 0.7998128361456462443 ) ) ;
#107011=CARTESIAN_POINT ( 'NONE',  ( -1.201851678989727383E-14, 1.071875000341418138, 1.575800808251672791 ) ) ;
#107013=CARTESIAN_POINT ( 'NONE',  ( -6.778713617152821058, 7.971215977175476475, 1.082531754730549967 ) ) ;
#107019=CARTESIAN_POINT ( 'NONE',  ( -5.752954180755987856, 6.096397935365156506, 0.6526304460669953844 ) ) ;
#107020=CARTESIAN_POINT ( 'NONE',  ( 1.364683531249986537, 1.217708333674754950, -0.7879004041258239610 ) ) ;
#107023=CARTESIAN_POINT ( 'NONE',  ( 4.365362273920252889, 4.195270195769483124, 0.7216878364870317197 ) ) ;
#107026=VECTOR ( 'NONE', #1000, 1000.000000000000000 ) ;
#107027=CARTESIAN_POINT ( 'NONE',  ( -4.249591082879585535, 7.045274465746411252, 1.199719254218464037 ) ) ;
#107029=CARTESIAN_POINT ( 'NONE',  ( -6.819388077549415783, 10.89977715720891815, 0.7216878364870458196 ) ) ;
#107036=CARTESIAN_POINT ( 'NONE',  ( -6.670248387799091461, 10.72578085250020585, 0.000000000000000000 ) ) ;
#107041=CARTESIAN_POINT ( 'NONE',  ( -7.009202228140751778, 9.200488570962775725, -1.443375672974058777 ) ) ;
#107046=( BOUNDED_CURVE ( )  B_SPLINE_CURVE ( 2, ( #7187, #189162, #75418, #109050, #73259 ),
 .UNSPECIFIED., .F., .T. ) 
 B_SPLINE_CURVE_WITH_KNOTS ( ( 3, 2, 3 ),
 ( 0.1312500000637053799, 0.1333333333333333315, 0.1375000000000000111 ),
 .UNSPECIFIED. ) 
 CURVE ( )  GEOMETRIC_REPRESENTATION_ITEM ( )  RATIONAL_B_SPLINE_CURVE ( ( 0.9330127018922194093, 0.9330127039405957667, 1.000000000000000000, 0.8660254037844387076, 1.000000000000000000 ) ) 
 REPRESENTATION_ITEM ( '' )  );
#107048=CARTESIAN_POINT ( 'NONE',  ( -0.7500000000000215383, 4.972916667349482012, 1.299038105676671107 ) ) ;
#107049=CARTESIAN_POINT ( 'NONE',  ( 4.184706906298553797, 7.590773377710720915, -0.8858016571234141878 ) ) ;
#107053=ORIENTED_EDGE ( 'NONE', *, *, #96162, .T. ) ;
#107057=CARTESIAN_POINT ( 'NONE',  ( -7.369020184227459858, 8.555943955475521889, 1.199719254218450271 ) ) ;
#107060=CARTESIAN_POINT ( 'NONE',  ( 4.147904930777053245, 6.926640621626830807, -1.199719254218452047 ) ) ;
#107065=CARTESIAN_POINT ( 'NONE',  ( 6.283314124929436417, 9.417951348137970413, -1.199719254218440723 ) ) ;
#107073=CARTESIAN_POINT ( 'NONE',  ( -5.504247177468192476, 7.444707678511436555, 1.443375672974064550 ) ) ;
#107085=CARTESIAN_POINT ( 'NONE',  ( -1.364683531250012516, 1.030208333674754062, 0.7879004041258379498 ) ) ;
#107087=CARTESIAN_POINT ( 'NONE',  ( -8.259941899223614215, 10.65968485389279508, -1.599625672291263179 ) ) ;
#107089=CARTESIAN_POINT ( 'NONE',  ( 6.934105498385400246, 10.17720795050327354, -1.199719254218441611 ) ) ;
#107091=CARTESIAN_POINT ( 'NONE',  ( -7.181014916732457287, 11.52960116949655678, -0.7998128361456291469 ) ) ;
#107094=CARTESIAN_POINT ( 'NONE',  ( 1.364683531249990311, 4.884375000341417916, 1.214306433183764966E-14 ) ) ;
#107095=CARTESIAN_POINT ( 'NONE',  ( 8.093854517678360949, 12.38665467069271386, 1.040834085586084257E-14 ) ) ;
#107098=CARTESIAN_POINT ( 'NONE',  ( 1.364683531249986537, -0.03229166632525094088, -0.7879004041258309554 ) ) ;
#107101=CARTESIAN_POINT ( 'NONE',  ( 7.904040366642684390, 11.20483561351640844, 1.082531754730558626 ) ) ;
#107104=CARTESIAN_POINT ( 'NONE',  ( -5.802526556968872207, 6.832331073627524454, 1.082531754730548412 ) ) ;
#107106=CARTESIAN_POINT ( 'NONE',  ( 0.6823417656249882723, 1.926041667008083991, -1.181850606188749264 ) ) ;
#107110=CARTESIAN_POINT ( 'NONE',  ( -7.206322340863467346, 8.366129804884193888, 1.199719254218450271 ) ) ;
#107111=CARTESIAN_POINT ( 'NONE',  ( -0.6823417656249969321, 4.780208333674755394, -1.181850606188749264 ) ) ;
#107117=CARTESIAN_POINT ( 'NONE',  ( 8.782984583554449998, 9.141236857102018831, 1.040834085586084257E-14 ) ) ;
#107120=CARTESIAN_POINT ( 'NONE',  ( -1.500000000000013101, 1.879166666666692187, -0.8660254037844313801 ) ) ;
#107123=DIRECTION ( 'NONE',  ( 0.6507913734559640506, -0.7592566023653004592, 0.000000000000000000 ) ) ;
#107126=CARTESIAN_POINT ( 'NONE',  ( 6.968527767744098433, 9.153035033833367251, 1.443375672974076540 ) ) ;
#107127=CARTESIAN_POINT ( 'NONE',  ( 8.224992744984721327, 12.74757530245756243, 1.040834085586084257E-14 ) ) ;
#107129=CARTESIAN_POINT ( 'NONE',  ( 3.083589872104280705, 5.684939719841914929, 1.199719254218450271 ) ) ;
#107135=CARTESIAN_POINT ( 'NONE',  ( 8.215351014876830504, 11.67199438640995801, -1.199719254218446718 ) ) ;
#107136=CARTESIAN_POINT ( 'NONE',  ( -1.501703635994465547, 8.650726486491324252, 2.563578082221948495 ) ) ;
#107138=CARTESIAN_POINT ( 'NONE',  ( -4.910932872253781944, 4.686298128553559650, -0.3332635495145727100 ) ) ;
#107139=CARTESIAN_POINT ( 'NONE',  ( 1.364683531249988757, -0.1156249996585798079, 0.000000000000000000 ) ) ;
#107140=CARTESIAN_POINT ( 'NONE',  ( -1.500000000000001332, 0.4000000000000253353, 0.000000000000000000 ) ) ;
#107147=CARTESIAN_POINT ( 'NONE',  ( 0.6823417656249917140, 5.592708333674749177, 1.181850606188765695 ) ) ;
#107149=CARTESIAN_POINT ( 'NONE',  ( -5.585596099150182958, 8.499983968108443477, -1.082531754730544860 ) ) ;
#107151=CARTESIAN_POINT ( 'NONE',  ( -0.7500000000000215383, 4.972916667349482012, 1.299038105676671107 ) ) ;
#107158=CARTESIAN_POINT ( 'NONE',  ( 6.916630921265960019, 11.22115317478565188, 0.7998128361456462443 ) ) ;
#107162=CARTESIAN_POINT ( 'NONE',  ( 8.066738210006692000, 8.513542121203711233, 0.7216878364870458196 ) ) ;
#107165=CARTESIAN_POINT ( 'NONE',  ( -7.784352752540590004, 12.23349531127272094, 0.7998128361456481317 ) ) ;
#107166=CARTESIAN_POINT ( 'NONE',  ( 4.157546660884947620, 8.002221537674429896, 1.040834085586084257E-14 ) ) ;
#107168=CARTESIAN_POINT ( 'NONE',  ( -1.000000000000017097, 8.600000000000013856, -0.3999999999999858113 ) ) ;
#107169=CARTESIAN_POINT ( 'NONE',  ( 4.578903193113299963, 6.365139696764064325, 1.599625672291267398 ) ) ;
#107170=ORIENTED_EDGE ( 'NONE', *, *, #76005, .T. ) ;
#107177=CARTESIAN_POINT ( 'NONE',  ( -5.761852096127856981, 5.824508321678349532, 0.000000000000000000 ) ) ;
#107178=CARTESIAN_POINT ( 'NONE',  ( 10.56143847536557878, 11.42402576412244386, 0.000000000000000000 ) ) ;
#107181=CARTESIAN_POINT ( 'NONE',  ( -7.867809214632013770, 8.073532260025807261, 1.040834085586084257E-14 ) ) ;
#107187=CARTESIAN_POINT ( 'NONE',  ( -9.020252271793614440, 9.418049160047695878, 0.7998128361456462443 ) ) ;
#107188=CARTESIAN_POINT ( 'NONE',  ( 1.270916165646590379, 3.041024509562812561, 0.7750000000000135669 ) ) ;
#107192=CARTESIAN_POINT ( 'NONE',  ( 5.473741331615251227, 7.409117525016355010, -1.599625672291262513 ) ) ;
#107203=EDGE_CURVE ( 'NONE', #30182, #62825, #183411, .T. ) ;
#107205=CARTESIAN_POINT ( 'NONE',  ( -6.021792782764022078, 10.17717534653336209, -0.7998128361456291469 ) ) ;
#107208=CARTESIAN_POINT ( 'NONE',  ( 5.558479791922850133, 6.547609847740540445, -1.082531754730542195 ) ) ;
#107212=CARTESIAN_POINT ( 'NONE',  ( -4.816538118508267630, 5.092449105792602460, -0.9495590845017554127 ) ) ;
#107213=CARTESIAN_POINT ( 'NONE',  ( 4.325214697959421706, 5.004837554829479451, 1.199719254218462483 ) ) ;
#107215=CARTESIAN_POINT ( 'NONE',  ( -5.786632634934295361, 5.645492917045106473, 0.7998128361456341429 ) ) ;
#107223=DIRECTION ( 'NONE',  ( 1.000000000000000000, -7.387867266669436732E-31, 0.000000000000000000 ) ) ;
#107224=CARTESIAN_POINT ( 'NONE',  ( -8.306341666666730461, 12.84248237775322643, 1.040834085586084257E-14 ) ) ;
#107225=CARTESIAN_POINT ( 'NONE',  ( 8.111855979677986994, 8.358253485912799263, 1.040834085586084257E-14 ) ) ;
#107231=B_SPLINE_CURVE_WITH_KNOTS ( 'NONE', 1,
 ( #157680, #120984 ),
 .UNSPECIFIED., .F., .F.,
 ( 2, 2 ),
 ( 0.3873181335520736179, 1.000000000000000000 ),
 .UNSPECIFIED. ) ;
#107232=CARTESIAN_POINT ( 'NONE',  ( -5.077710034904439951, 6.555083676148210081, -1.223860624452234980 ) ) ;
#107235=CARTESIAN_POINT ( 'NONE',  ( 1.364683531249986537, -0.8239583329919186738, 0.7879004041258500513 ) ) ;
#107239=CARTESIAN_POINT ( 'NONE',  ( 9.788623719386617239, 11.48277776311499387, -1.082531754730537088 ) ) ;
#107258=CARTESIAN_POINT ( 'NONE',  ( -3.918470089549458635, 4.530302178351167441, -1.199719254218452047 ) ) ;
#107260=CARTESIAN_POINT ( 'NONE',  ( -3.918470089549458635, 4.530302178351167441, -1.199719254218452047 ) ) ;
#107264=CARTESIAN_POINT ( 'NONE',  ( 1.499999999999987566, -0.9437499993171851731, 0.000000000000000000 ) ) ;
#107267=CARTESIAN_POINT ( 'NONE',  ( -3.145128448690323264, 4.692402494937224056, -1.443375672974059665 ) ) ;
#107270=VERTEX_POINT ( 'NONE', #188509 ) ;
#107273=CARTESIAN_POINT ( 'NONE',  ( 3.246287715468270108, 5.874753870433235825, 1.199719254218450271 ) ) ;
#107275=CARTESIAN_POINT ( 'NONE',  ( 1.419999999999990603, 6.120000000000041851, 2.580000000000000515 ) ) ;
#107277=CARTESIAN_POINT ( 'NONE',  ( 10.19536832735223975, 10.99694392477354477, 0.000000000000000000 ) ) ;
#107279=CARTESIAN_POINT ( 'NONE',  ( -0.6823417656250003738, 1.280208333674752508, -1.181850606188749264 ) ) ;
#107282=CARTESIAN_POINT ( 'NONE',  ( -6.970863535720637216, 11.28442455831609337, 0.7998128361456481317 ) ) ;
#107283=CARTESIAN_POINT ( 'NONE',  ( -6.060131475184148186, 6.172500930577367484, 0.7216878364870317197 ) ) ;
#107285=CARTESIAN_POINT ( 'NONE',  ( -7.203459687562382641, 7.298457811777897319, -0.7998128361456291469 ) ) ;
#107287=CARTESIAN_POINT ( 'NONE',  ( 1.364683531249992088, 5.384375000341417916, 1.214306433183764966E-14 ) ) ;
#107295=CARTESIAN_POINT ( 'NONE',  ( -5.382223794500843539, 7.302347065049529462, -1.443375672974051449 ) ) ;
#107300=CARTESIAN_POINT ( 'NONE',  ( -5.409340101728186134, 5.413244328212063472, 0.7216878364870317197 ) ) ;
#107302=CARTESIAN_POINT ( 'NONE',  ( 9.049177462117294013, 12.64479190819049670, -1.199719254218446718 ) ) ;
#107310=CARTESIAN_POINT ( 'NONE',  ( 3.660338286009610975, 6.253849852777763729, -1.082531754730543083 ) ) ;
#107311=CARTESIAN_POINT ( 'NONE',  ( -5.264643720808155791, 5.036505850564608089, 0.000000000000000000 ) ) ;
#107312=CARTESIAN_POINT ( 'NONE',  ( -5.691079914216616409, 6.283969663839313213, 1.134429477820863008 ) ) ;
#107316=CARTESIAN_POINT ( 'NONE',  ( 7.619319141200063150, 9.912291636198670375, 1.443375672974076540 ) ) ;
#107317=CARTESIAN_POINT ( 'NONE',  ( 6.657217119509961201, 7.725507046638470321, -1.199719254218446718 ) ) ;
#107322=CARTESIAN_POINT ( 'NONE',  ( 4.222474775652216294, 7.013638773981186958, 1.199719254218462483 ) ) ;
#107332=CARTESIAN_POINT ( 'NONE',  ( 8.666686507633574621, 11.13422023037111330, 1.599625672291281386 ) ) ;
#107333=CARTESIAN_POINT ( 'NONE',  ( -5.768104287610143821, 8.816873204598778102, -1.199719254218440723 ) ) ;
#107340=CARTESIAN_POINT ( 'NONE',  ( 0.6823417656249917140, 4.092708333674755394, 1.181850606188765695 ) ) ;
#107342=CARTESIAN_POINT ( 'NONE',  ( -4.225337428953291230, 8.081310767087481750, 0.7998128361456341429 ) ) ;
#107344=CARTESIAN_POINT ( 'NONE',  ( -1.436838838544789221, 7.449283400311735193, -4.203727439823564893 ) ) ;
#107345=CARTESIAN_POINT ( 'NONE',  ( 5.192936529234042808, 6.017179691316550283, -1.199719254218452047 ) ) ;
#107346=CARTESIAN_POINT ( 'NONE',  ( -6.084912014434944894, 5.993485526462540847, -0.7998128361456291469 ) ) ;
#107352=CARTESIAN_POINT ( 'NONE',  ( 6.399085315970131305, 8.488685506763726352, -1.443375672974057666 ) ) ;
#107353=EDGE_CURVE ( 'NONE', #15325, #147186, #77610, .T. ) ;
#107355=CARTESIAN_POINT ( 'NONE',  ( 6.765155463094751909, 8.915767345075790828, 1.443375672974076540 ) ) ;
#107356=CARTESIAN_POINT ( 'NONE',  ( -0.6823417656250003738, 3.030208333674754062, -1.181850606188749264 ) ) ;
#107358=CARTESIAN_POINT ( 'NONE',  ( 5.219525951136835928, 7.112532914458205013, -1.443375672974051449 ) ) ;
#107362=CARTESIAN_POINT ( 'NONE',  ( -3.633221978782304351, 4.301475732409860697, -1.082531754730549967 ) ) ;
#107364=CARTESIAN_POINT ( 'NONE',  ( -0.6823417656249969321, 5.467708333674756283, -1.181850606188749264 ) ) ;
#107369=CARTESIAN_POINT ( 'NONE',  ( -4.520189846367452802, 7.221058948360024488, -1.319278014013465894 ) ) ;
#107377=CARTESIAN_POINT ( 'NONE',  ( -2.941756144040970522, 5.415504020480993219, -1.082531754730543083 ) ) ;
#107388=CARTESIAN_POINT ( 'NONE',  ( 4.690757960648224589, 6.495636925554817864, 1.443375672974062551 ) ) ;
#107390=CARTESIAN_POINT ( 'NONE',  ( 1.364683531249988535, 3.426041667008085323, 0.7879004041258500513 ) ) ;
#107392=CARTESIAN_POINT ( 'NONE',  ( 6.753933077901968396, 11.03133902419432566, 0.7998128361456462443 ) ) ;
#107393=CARTESIAN_POINT ( 'NONE',  ( -8.469039510030723861, 13.03229652834454733, 1.040834085586084257E-14 ) ) ;
#107395=CARTESIAN_POINT ( 'NONE',  ( -3.567766978690493307, 7.314145241780881435, 1.040834085586084257E-14 ) ) ;
#107399=CARTESIAN_POINT ( 'NONE',  ( 1.499999999999989120, 3.754166666666685082, 0.8660254037844524744 ) ) ;
#107400=CARTESIAN_POINT ( 'NONE',  ( 6.094553744542824170, 7.069066442510145265, 1.199719254218462483 ) ) ;
#107404=CARTESIAN_POINT ( 'NONE',  ( -1.364683531250012516, 4.488541667008090208, -0.7879004041258300672 ) ) ;
#107405=ORIENTED_EDGE ( 'NONE', *, *, #99953, .F. ) ;
#107407=CARTESIAN_POINT ( 'NONE',  ( 9.788623719386617239, 11.48277776311499387, -1.082531754730537088 ) ) ;
#107412=CARTESIAN_POINT ( 'NONE',  ( -1.499999999999997780, 2.181250000682817713, 1.214306433183764966E-14 ) ) ;
#107414=CARTESIAN_POINT ( 'NONE',  ( -4.882907879216086933, 8.848476292394087395, -0.7998128361456281477 ) ) ;
#107415=CARTESIAN_POINT ( 'NONE',  ( -4.908906423376278028, 4.799815971864533459, -0.1755478183662619873 ) ) ;
#107423=CARTESIAN_POINT ( 'NONE',  ( 5.495132332240461714, 5.305409230568988832, 0.7998128361456341429 ) ) ;
#107427=CARTESIAN_POINT ( 'NONE',  ( 5.494078562035752178, 7.432844293840273231, -1.599625672291262513 ) ) ;
#107430=CARTESIAN_POINT ( 'NONE',  ( 3.022498986271242138, 2.800000000000017586, 2.500000000000000444 ) ) ;
#107435=CARTESIAN_POINT ( 'NONE',  ( 8.971744963941056028, 11.49012176272984931, 1.599625672291281386 ) ) ;
#107440=CARTESIAN_POINT ( 'NONE',  ( 5.830449476509543594, 6.014588727829297987, 0.4175459632603968352 ) ) ;
#107452=CARTESIAN_POINT ( 'NONE',  ( 5.965224400332808763, 9.903252867122883885, -0.7216878364870267237 ) ) ;
#107454=CARTESIAN_POINT ( 'NONE',  ( -4.600294193738529103, 4.261431402316699035, -0.7998128361456221525 ) ) ;
#107459=CARTESIAN_POINT ( 'NONE',  ( -7.067878151425722955, 7.140279352951794500, 0.7998128361456341429 ) ) ;
#107474=CARTESIAN_POINT ( 'NONE',  ( 8.615316546479974136, 12.13862083994696839, 1.199719254218450271 ) ) ;
#107479=DIRECTION ( 'NONE',  ( -0.7797859179643623628, 0.6260462619842697141, 0.000000000000000000 ) ) ;
#107483=CARTESIAN_POINT ( 'NONE',  ( -8.514157279702017078, 12.87700789305364069, -0.7216878364870267237 ) ) ;
#107486=CARTESIAN_POINT ( 'NONE',  ( 8.402302512167096893, 10.82577223566020841, -1.599625672291268286 ) ) ;
#107490=CARTESIAN_POINT ( 'NONE',  ( -6.015013705957189316, 10.16926642359206134, 0.7998128361456481317 ) ) ;
#107491=CARTESIAN_POINT ( 'NONE',  ( 3.928111819657337911, 5.605883094398769195, 1.599625672291267398 ) ) ;
#107497=CARTESIAN_POINT ( 'NONE',  ( -1.364683531250012516, 2.551041667008089320, -0.7879004041258289570 ) ) ;
#107499=CARTESIAN_POINT ( 'NONE',  ( 7.795575138177731844, 8.197185204069915798, 1.040834085586084257E-14 ) ) ;
#107506=CARTESIAN_POINT ( 'NONE',  ( 8.337901282279995385, 11.71100668175994386, -1.082531754730543083 ) ) ;
#107507=ORIENTED_EDGE ( 'NONE', *, *, #49082, .T. ) ;
#107511=CARTESIAN_POINT ( 'NONE',  ( -9.677822722056413696, 10.18521468535430685, 1.040834085586084257E-14 ) ) ;
#107512=CARTESIAN_POINT ( 'NONE',  ( 3.374996487695185010, 6.371758841431772957, -0.9566735593157035256 ) ) ;
#107525=CARTESIAN_POINT ( 'NONE',  ( 5.178324605415663306, 8.128796908705222535, 1.199719254218462483 ) ) ;
#107528=( BOUNDED_CURVE ( )  B_SPLINE_CURVE ( 2, ( #57267, #71351, #202415, #106066, #203481, #104966, #204550 ),
 .UNSPECIFIED., .F., .T. ) 
 B_SPLINE_CURVE_WITH_KNOTS ( ( 3, 2, 2, 3 ),
 ( 0.3959408239114771688, 0.3988095238095238360, 0.4047619047619047672, 0.4076306046599514343 ),
 .UNSPECIFIED. ) 
 CURVE ( )  GEOMETRIC_REPRESENTATION_ITEM ( )  RATIONAL_B_SPLINE_CURVE ( ( 0.9331000818465632340, 0.9354320710352570512, 1.000000000000000000, 0.8660254037844387076, 1.000000000000000000, 0.9354320710352564960, 0.9331000818465632340 ) ) 
 REPRESENTATION_ITEM ( '' )  );
#107529=CARTESIAN_POINT ( 'NONE',  ( -1.500000000000013101, 3.160416667349486008, -0.8660254037844313801 ) ) ;
#107535=CARTESIAN_POINT ( 'NONE',  ( 1.499999999999989120, 1.025000000000019007, 0.000000000000000000 ) ) ;
#107536=CARTESIAN_POINT ( 'NONE',  ( 7.670162217029129259, 9.971608557999250166, 1.599625672291281386 ) ) ;
#107537=CARTESIAN_POINT ( 'NONE',  ( -0.6823417656250246877, -0.1989583329919109023, 1.181850606188755259 ) ) ;
#107540=CARTESIAN_POINT ( 'NONE',  ( 9.571693261567961741, 11.22969222899322617, 1.082531754730548412 ) ) ;
#107541=CARTESIAN_POINT ( 'NONE',  ( -5.992340707560165569, 8.014150130285418783, 1.443375672974064550 ) ) ;
#107546=CARTESIAN_POINT ( 'NONE',  ( -6.043183783389232566, 8.073467052085995022, 1.599625672291269396 ) ) ;
#107548=CARTESIAN_POINT ( 'NONE',  ( 1.499999999999989120, 2.056250000682817269, 1.214306433183764966E-14 ) ) ;
#107549=CARTESIAN_POINT ( 'NONE',  ( -1.001543065824772872E-14, 4.634375000341418804, 1.575800808251672791 ) ) ;
#107562=CARTESIAN_POINT ( 'NONE',  ( -7.506410603460441422, 11.90922947067921278, -0.7998128361456291469 ) ) ;
#107563=CARTESIAN_POINT ( 'NONE',  ( 7.091078035147269532, 8.231678114882006625, 1.199719254218462483 ) ) ;
#107572=CARTESIAN_POINT ( 'NONE',  ( -8.016948904382338981, 8.247528564734524892, -0.7998128361456291469 ) ) ;
#107577=CARTESIAN_POINT ( 'NONE',  ( 2.354312230267378236, 5.898448035287240820, -0.7998128361456281477 ) ) ;
#107580=CARTESIAN_POINT ( 'NONE',  ( -5.091250377131585125, 5.898545847196970726, 1.199719254218450271 ) ) ;
#107582=CARTESIAN_POINT ( 'NONE',  ( -8.890396042259075315, 11.39521468743417998, -1.599625672291263179 ) ) ;
#107585=CARTESIAN_POINT ( 'NONE',  ( -3.976064435573588796, 7.848781721302746206, 0.05846302465613295585 ) ) ;
#107593=CARTESIAN_POINT ( 'NONE',  ( 5.296431564432884542, 9.330920591813708143, 1.040834085586084257E-14 ) ) ;
#107596=FACE_OUTER_BOUND ( 'NONE', #127837, .T. ) ;
#107612=CARTESIAN_POINT ( 'NONE',  ( 4.202664430556257713, 4.965825259479493603, 1.082531754730560403 ) ) ;
#107616=CARTESIAN_POINT ( 'NONE',  ( -9.755255220232635693, 11.33988483081495957, -1.199719254218441611 ) ) ;
#107619=CARTESIAN_POINT ( 'NONE',  ( 7.397945374551106568, 11.78268670361832093, -0.7998128361456291469 ) ) ;
#107628=CARTESIAN_POINT ( 'NONE',  ( 1.364683531249988757, 0.8843750003414210248, 0.000000000000000000 ) ) ;
#107634=CARTESIAN_POINT ( 'NONE',  ( -3.079673448598517549, 6.744702790006905424, 1.040834085586084257E-14 ) ) ;
#107635=CARTESIAN_POINT ( 'NONE',  ( 3.974511587100456822, 7.788680618259193444, 1.040834085586084257E-14 ) ) ;
#107637=CARTESIAN_POINT ( 'NONE',  ( -0.7500000000000215383, 0.1916666666666871910, 1.299038105676659116 ) ) ;
#107639=CARTESIAN_POINT ( 'NONE',  ( 1.499999999999989120, 5.795833333333350268, -0.8660254037844323793 ) ) ;
#107644=CARTESIAN_POINT ( 'NONE',  ( 1.364683531249988757, 0.3843750003414206362, 0.000000000000000000 ) ) ;
#107646=CARTESIAN_POINT ( 'NONE',  ( -7.985916173649233230, 9.275655943134292869, -1.199719254218446718 ) ) ;
#107647=CARTESIAN_POINT ( 'NONE',  ( 8.052653171512838881, 11.48218023581863001, -1.199719254218446718 ) ) ;
#107648=CARTESIAN_POINT ( 'NONE',  ( 4.385172619016207918, 7.203452924572514959, 1.199719254218462483 ) ) ;
#107655=CARTESIAN_POINT ( 'NONE',  ( 1.364683531249988757, -0.5531249996585801965, 0.000000000000000000 ) ) ;
#107664=CARTESIAN_POINT ( 'NONE',  ( 7.632877294813741109, 8.007371053478589573, 1.040834085586084257E-14 ) ) ;
#107667=CARTESIAN_POINT ( 'NONE',  ( -5.579343907223557331, 6.467988298970945849, 1.199719254218450271 ) ) ;
#107669=CARTESIAN_POINT ( 'NONE',  ( 5.639828713160493834, 5.682147708216442439, 1.040834085586084257E-14 ) ) ;
#107671=CARTESIAN_POINT ( 'NONE',  ( -4.274898507010545856, 3.881803101134051470, -0.7998128361456221525 ) ) ;
#107672=CARTESIAN_POINT ( 'NONE',  ( 3.985733972293228344, 7.593847367743336463, 1.040834085586084257E-14 ) ) ;
#107673=CARTESIAN_POINT ( 'NONE',  ( -9.286972035236635392, 9.937148250638648150, -0.7216878364870267237 ) ) ;
#107675=CARTESIAN_POINT ( 'NONE',  ( -1.499999999999997780, 3.650000000000021227, 1.214306433183764966E-14 ) ) ;
#107679=CARTESIAN_POINT ( 'NONE',  ( 9.422553571817644524, 10.09532670998316384, 0.000000000000000000 ) ) ;
#107694=CARTESIAN_POINT ( 'NONE',  ( 9.056483423804305488, 9.668244870634271848, 1.040834085586084257E-14 ) ) ;
#107696=CARTESIAN_POINT ( 'NONE',  ( 6.913768267964901071, 10.15348118167935709, -1.199719254218441611 ) ) ;
#107699=CARTESIAN_POINT ( 'NONE',  ( -4.091466733727974869, 3.979520368983120449, -0.5407646501769195480 ) ) ;
#107700=SPHERICAL_SURFACE ( 'NONE', #122507, 0.08000000000000000167 ) ;
#107701=CARTESIAN_POINT ( 'NONE',  ( 5.341549334104200852, 5.334155099317434257, 0.7216878364870317197 ) ) ;
#107703=CARTESIAN_POINT ( 'NONE',  ( -8.839552966430023417, 9.415159337030921449, -0.7216878364870267237 ) ) ;
#107707=CARTESIAN_POINT ( 'NONE',  ( -4.451154503988200339, 4.087435097607984957, 1.214306433183764966E-14 ) ) ;
#107715=ORIENTED_EDGE ( 'NONE', *, *, #102521, .F. ) ;
#107732=CARTESIAN_POINT ( 'NONE',  ( -4.726989112658928072, 8.666571064744069020, 1.040834085586084257E-14 ) ) ;
#107735=CARTESIAN_POINT ( 'NONE',  ( 1.284279953904119864, 2.827889714876734129, -0.7749999999999910294 ) ) ;
#107737=CARTESIAN_POINT ( 'NONE',  ( 4.625302960556422427, 8.547937220624488575, 1.040834085586084257E-14 ) ) ;
#107747=CARTESIAN_POINT ( 'NONE',  ( -5.278201874421821316, 5.052323696447222900, 0.7998128361456341429 ) ) ;
#107750=CARTESIAN_POINT ( 'NONE',  ( 6.262976894508937242, 9.394224579314053969, -1.199719254218440723 ) ) ;
#107751=CARTESIAN_POINT ( 'NONE',  ( 1.364683531249988535, 3.655208333674750509, -0.7879004041258239610 ) ) ;
#107753=CARTESIAN_POINT ( 'NONE',  ( 5.593492625449885125, 6.357122791843209164, 1.180528715873955692 ) ) ;
#107759=CARTESIAN_POINT ( 'NONE',  ( 5.951666246274797345, 7.966696592119163256, 1.443375672974062551 ) ) ;
#107760=CARTESIAN_POINT ( 'NONE',  ( -8.518600588087975822, 8.832788862391110385, 1.040834085586084257E-14 ) ) ;
#107763=CARTESIAN_POINT ( 'NONE',  ( -9.494787648271923786, 9.971673765939062406, 1.040834085586084257E-14 ) ) ;
#107764=CARTESIAN_POINT ( 'NONE',  ( -5.215082642750900277, 9.236013516518044142, 0.000000000000000000 ) ) ;
#107771=CARTESIAN_POINT ( 'NONE',  ( 7.727257484784855635, 11.10255193463598111, -1.199719254218446718 ) ) ;
#107785=CARTESIAN_POINT ( 'NONE',  ( -1.500000000000011324, 4.420833333333352044, 0.8660254037844403729 ) ) ;
#107786=CARTESIAN_POINT ( 'NONE',  ( 4.310602774141044868, 7.116454772218158809, -1.199719254218452047 ) ) ;
#107787=CARTESIAN_POINT ( 'NONE',  ( 7.644099680006512187, 7.812537802962739697, 1.040834085586084257E-14 ) ) ;
#107789=CARTESIAN_POINT ( 'NONE',  ( -8.107412671292051343, 10.48173408797264194, 1.443375672974090751 ) ) ;
#107791=CARTESIAN_POINT ( 'NONE',  ( 5.829642864196151741, 9.745074408296771296, 0.7216878364870438212 ) ) ;
#107792=CARTESIAN_POINT ( 'NONE',  ( -8.134528978075012517, 12.43410820782212767, 1.040834085586084257E-14 ) ) ;
#107796=CARTESIAN_POINT ( 'NONE',  ( 8.646349277213076334, 11.11049346154719508, 1.599625672291281386 ) ) ;
#107800=CARTESIAN_POINT ( 'NONE',  ( -1.364683531249997417, 3.009375000341422801, 1.214306433183764966E-14 ) ) ;
#107805=CARTESIAN_POINT ( 'NONE',  ( -1.364683531250000748, -0.4906249996585801409, 0.000000000000000000 ) ) ;
#107807=CARTESIAN_POINT ( 'NONE',  ( 10.39640486358069360, 11.02356051713265650, 0.7998128361456462443 ) ) ;
#107810=CARTESIAN_POINT ( 'NONE',  ( -10.64045162862669081, 11.30828174301964140, -0.7998128361456221525 ) ) ;
#107816=CARTESIAN_POINT ( 'NONE',  ( 5.217190183160311356, 4.981143389975473568, -0.7998128361456211532 ) ) ;
#107820=CARTESIAN_POINT ( 'NONE',  ( -3.972175818679615222, 4.696921878956699103, 1.082531754730558626 ) ) ;
#107823=CARTESIAN_POINT ( 'NONE',  ( 9.921869487102386032, 10.46993591124128997, 0.000000000000000000 ) ) ;
#107825=CARTESIAN_POINT ( 'NONE',  ( 4.490901714065265615, 7.023505696618186356, 1.148426366857359771 ) ) ;
#107827=CARTESIAN_POINT ( 'NONE',  ( -4.066556009095094737, 6.831733546331167695, 1.199719254218464037 ) ) ;
#107831=CARTESIAN_POINT ( 'NONE',  ( 7.293396569147545527, 10.59638086639245280, 1.199719254218460707 ) ) ;
#107833=CARTESIAN_POINT ( 'NONE',  ( 6.317209508963599340, 9.457495962844502557, 1.199719254218462483 ) ) ;
#107836=CARTESIAN_POINT ( 'NONE',  ( -9.164948653157999559, 10.75515685251491504, -1.082531754730539753 ) ) ;
#107842=CARTESIAN_POINT ( 'NONE',  ( -5.590823505525904125, 6.198478227408987351, -0.8910005059661347815 ) ) ;
#107843=CARTESIAN_POINT ( 'NONE',  ( -0.6823417656250003738, 1.967708333674753174, -1.181850606188749264 ) ) ;
#107845=CARTESIAN_POINT ( 'NONE',  ( 5.450014563013511726, 8.341805509282339770, -1.082531754730543083 ) ) ;
#107847=CARTESIAN_POINT ( 'NONE',  ( 9.921869487102386032, 10.46993591124128997, 0.000000000000000000 ) ) ;
#107867=CARTESIAN_POINT ( 'NONE',  ( 8.829384350997564468, 11.32403438096243775, 1.599625672291281386 ) ) ;
#107871=CARTESIAN_POINT ( 'NONE',  ( -2.948008335967658322, 5.526761261015804116, 1.199719254218462483 ) ) ;
#107872=CARTESIAN_POINT ( 'NONE',  ( -7.867809214632013770, 8.073532260025807261, 1.040834085586084257E-14 ) ) ;
#107876=CARTESIAN_POINT ( 'NONE',  ( -7.960608749518247151, 12.43912730774665576, 0.000000000000000000 ) ) ;
#107880=CARTESIAN_POINT ( 'NONE',  ( 0.7499999999999902300, 4.597916667349482012, -1.299038105676658228 ) ) ;
#107881=CARTESIAN_POINT ( 'NONE',  ( 8.437251666405968464, 8.737881787095446384, 1.040834085586084257E-14 ) ) ;
#107884=CARTESIAN_POINT ( 'NONE',  ( -8.688077508258798431, 9.030511935923748013, -0.7998128361456291469 ) ) ;
#107886=CARTESIAN_POINT ( 'NONE',  ( -0.6823417656250212460, 4.551041667008086655, 1.181850606188767472 ) ) ;
#107894=CARTESIAN_POINT ( 'NONE',  ( -8.188761592974046266, 10.57664116326830595, -1.443375672974059665 ) ) ;
#107896=EDGE_CURVE ( 'NONE', #47756, #116455, #60556, .T. ) ;
#107899=CARTESIAN_POINT ( 'NONE',  ( -1.201851678989727383E-14, 3.134375000341420137, 1.575800808251672791 ) ) ;
#107905=CARTESIAN_POINT ( 'NONE',  ( 0.6823417656249899377, 4.926041667008086655, -1.181850606188754593 ) ) ;
#107906=CARTESIAN_POINT ( 'NONE',  ( -3.411848212133334446, 7.132240014130862171, 0.7998128361456341429 ) ) ;
#107907=CARTESIAN_POINT ( 'NONE',  ( 5.601490020740366838, 9.686822124172440596, 1.040834085586084257E-14 ) ) ;
#107911=CARTESIAN_POINT ( 'NONE',  ( 1.364683531249988535, 3.426041667008085323, 0.7879004041258500513 ) ) ;
#107916=CARTESIAN_POINT ( 'NONE',  ( -1.402160292154681736E-14, 0.1968750003414221628, -1.575800808251665908 ) ) ;
#107917=CARTESIAN_POINT ( 'NONE',  ( -4.663641653420935285, 5.503632019488245319, 1.082531754730560403 ) ) ;
#107919=CARTESIAN_POINT ( 'NONE',  ( 4.123651276850781144, 7.962676922967908411, -0.7998128361456221525 ) ) ;
#107923=CARTESIAN_POINT ( 'NONE',  ( 4.690757960648231695, 5.535267711253469614, 1.082531754730560403 ) ) ;
#107926=CARTESIAN_POINT ( 'NONE',  ( -9.517460647113315630, 10.20605163116143821, 0.7216878364870438212 ) ) ;
#107931=CARTESIAN_POINT ( 'NONE',  ( -9.646789991323334590, 11.21334206375407305, 1.199719254218462483 ) ) ;
#107932=CARTESIAN_POINT ( 'NONE',  ( -6.222829318548141586, 6.362315081168691044, 0.7216878364870317197 ) ) ;
#107934=CARTESIAN_POINT ( 'NONE',  ( -0.6823417656250246877, 0.6135416670080897639, 1.181850606188755259 ) ) ;
#107944=CARTESIAN_POINT ( 'NONE',  ( 8.744645890689993095, 9.304434415334227992, -0.7216878364870197293 ) ) ;
#107950=ORIENTED_EDGE ( 'NONE', *, *, #177010, .T. ) ;
#107954=CARTESIAN_POINT ( 'NONE',  ( -4.600294193738529103, 4.261431402316699035, -0.7998128361456221525 ) ) ;
#107956=CARTESIAN_POINT ( 'NONE',  ( 1.244123718695675729, 3.233005466778238191, 0.7750000000000152323 ) ) ;
#107957=CARTESIAN_POINT ( 'NONE',  ( -1.201851678989727383E-14, 1.134375000341418582, 1.575800808251672791 ) ) ;
#107959=ORIENTED_EDGE ( 'NONE', *, *, #147857, .F. ) ;
#107976=CARTESIAN_POINT ( 'NONE',  ( 6.193377243344257543, 6.120028293523423812, -0.7998128361456281477 ) ) ;
#107980=ORIENTED_EDGE ( 'NONE', *, *, #5002, .F. ) ;
#107985=CARTESIAN_POINT ( 'NONE',  ( 8.620286740190458374, 8.951422706510690830, 1.040834085586084257E-14 ) ) ;
#107986=CARTESIAN_POINT ( 'NONE',  ( -5.935365280120787013, 6.088755149432644842, -0.6770708583819718962 ) ) ;
#107988=CARTESIAN_POINT ( 'NONE',  ( 10.08456733046637765, 10.65975006183261087, 0.000000000000000000 ) ) ;
#108000=CARTESIAN_POINT ( 'NONE',  ( -6.534666852106790103, 10.56760239419251590, 0.7216878364870458196 ) ) ;
#108012=CARTESIAN_POINT ( 'NONE',  ( 2.846849068745292755, 6.265148313604064434, 0.000000000000000000 ) ) ;
#108015=ORIENTED_EDGE ( 'NONE', *, *, #109929, .F. ) ;
#108020=CARTESIAN_POINT ( 'NONE',  ( -5.205440912643032547, 8.160432600470439723, 1.199719254218452047 ) ) ;
#108022=CARTESIAN_POINT ( 'NONE',  ( -2.598358995313378550, 6.183169261174235487, 0.7998128361456341429 ) ) ;
#108028=CARTESIAN_POINT ( 'NONE',  ( 8.053180056837369705, 11.37883191874353805, -1.082531754730543083 ) ) ;
#108030=CARTESIAN_POINT ( 'NONE',  ( -1.364683531250012516, 3.801041667008087099, -0.7879004041258300672 ) ) ;
#108032=CARTESIAN_POINT ( 'NONE',  ( 4.985647801523278133, 6.839675073242382553, -1.599625672291256295 ) ) ;
#108047=CARTESIAN_POINT ( 'NONE',  ( 1.364683531249988757, 1.946875000341415030, 0.000000000000000000 ) ) ;
#108049=CARTESIAN_POINT ( 'NONE',  ( 5.040934186182656873, 4.775511393501539636, 1.040834085586084257E-14 ) ) ;
#108051=CARTESIAN_POINT ( 'NONE',  ( -5.748293942514180799, 7.729428904398431222, -1.443375672974052559 ) ) ;
#108053=CARTESIAN_POINT ( 'NONE',  ( 4.256897045010922476, 5.029096643009940415, -1.082531754730548412 ) ) ;
#108054=CARTESIAN_POINT ( 'NONE',  ( -6.900736999231456004, 8.113576589600553390, 1.082531754730549967 ) ) ;
#108058=CARTESIAN_POINT ( 'NONE',  ( 5.113396490648394632, 9.117379672398465473, 1.040834085586084257E-14 ) ) ;
#108060=CARTESIAN_POINT ( 'NONE',  ( -4.092446641025072829, 3.979529022206003575, 0.4031905389056175126 ) ) ;
#108066=CARTESIAN_POINT ( 'NONE',  ( 5.957918438201454059, 9.038323046955323292, -1.199719254218440723 ) ) ;
#108068=CARTESIAN_POINT ( 'NONE',  ( -5.879432169820529630, 10.01108796476595764, -0.7998128361456221525 ) ) ;
#108072=CARTESIAN_POINT ( 'NONE',  ( 7.065770611016287006, 11.39514947949436774, 1.040834085586084257E-14 ) ) ;
#108074=CARTESIAN_POINT ( 'NONE',  ( -7.497822643557261024, 8.706213491360317747, -1.199719254218446718 ) ) ;
#108077=CARTESIAN_POINT ( 'NONE',  ( 8.405692050348340771, 8.908988268268968724, 1.040834085586084257E-14 ) ) ;
#108078=CARTESIAN_POINT ( 'NONE',  ( 4.193481561896174270, 7.343914482741291216, -0.8359065270147625348 ) ) ;
#108079=CARTESIAN_POINT ( 'NONE',  ( -3.588104209110990706, 7.337872010604796991, 1.040834085586084257E-14 ) ) ;
#108085=CARTESIAN_POINT ( 'NONE',  ( 9.511208455186636712, 11.05516360492796935, 1.199719254218453823 ) ) ;
#108086=CARTESIAN_POINT ( 'NONE',  ( -5.429614816329291216, 6.304498938506903016, 1.045551501023216368 ) ) ;
#108087=CARTESIAN_POINT ( 'NONE',  ( 3.195971524519376494, 4.751719416737803847, -1.599625672291262513 ) ) ;
#108088=CARTESIAN_POINT ( 'NONE',  ( -0.6823417656250246877, 0.5510416670080897639, 1.181850606188755259 ) ) ;
#108090=CARTESIAN_POINT ( 'NONE',  ( -6.073689629242165822, 7.148687991279732756, -1.082531754730544860 ) ) ;
#108097=CARTESIAN_POINT ( 'NONE',  ( -5.565401824202027115, 6.214873266482019432, 0.9197014482419992865 ) ) ;
#108098=CARTESIAN_POINT ( 'NONE',  ( -1.201851678989727383E-14, 1.884375000341422135, 1.575800808251672791 ) ) ;
#108101=CARTESIAN_POINT ( 'NONE',  ( 3.470524135418292300, 5.072030796119872953, -1.443375672974057666 ) ) ;
#108106=CARTESIAN_POINT ( 'NONE',  ( -8.975134502122321223, 9.573337795338607847, 1.040834085586084257E-14 ) ) ;
#108114=CARTESIAN_POINT ( 'NONE',  ( -8.337901282280023807, 8.829899038855916871, 0.7216878364870438212 ) ) ;
#108121=CARTESIAN_POINT ( 'NONE',  ( -6.493992390821436977, 10.52014885602626393, 0.7216878364870458196 ) ) ;
#108126=CARTESIAN_POINT ( 'NONE',  ( -1.500000000000011324, 4.202083334016156080, 0.8660254037844403729 ) ) ;
#108127=CARTESIAN_POINT ( 'NONE',  ( 4.536316240020330071, 7.212700717958764329, -1.298556639521078582 ) ) ;
#108131=ORIENTED_EDGE ( 'NONE', *, *, #120712, .T. ) ;
#108134=CARTESIAN_POINT ( 'NONE',  ( -6.235860587281615075, 9.362588887548838557, -1.199719254218440723 ) ) ;
#108137=CARTESIAN_POINT ( 'NONE',  ( 4.497554271431305040, 6.270232621468402989, -1.599625672291256295 ) ) ;
#108143=CARTESIAN_POINT ( 'NONE',  ( 5.784525094524856748, 9.900363043587685041, 1.040834085586084257E-14 ) ) ;
#108144=CARTESIAN_POINT ( 'NONE',  ( -4.911830889935877131, 4.710851378956548707, 0.3897001052374938213 ) ) ;
#108145=( BOUNDED_SURFACE ( )  B_SPLINE_SURFACE ( 1, 2, ( 
 ( #39120, #139841, #6589, #22836, #105203, #70514, #122596, #173406, #171240, #204784, #88950, #155004, #189626, #87868, #172324, #72668, #188559, #106302, #90018, #205870, #57504, #86800, #123663, #41274, #104126, #91090, #136629, #202656, #54305, #24987, #186417, #20342, #68004, #168739, #34466, #182847, #201216, #85356, #21393, #116846, #18202, #183918, #33400, #84286, #200152, #167673, #152493, #870, #166612, #3009, #69079, #199075, #37677, #35530, #118990, #135199, #52857, #184969, #66935, #102681, #181767, #202278, #87504, #133077, #99479, #120066, #51806, #150372, #117924, #36594, #103754, #132016, #115778, #149289, #169804, #70147, #153568, #86428, #17130, #19274, #100537, #50721, #65867, #4076, #198026, #1942, #165537, #136258, #53930, #83206, #186042, #134144, #49655, #101606, #151438, #88577, #156780, #26752, #56064, #203346, #72285, #138393, #157844, #92853, #122222, #25680, #6215, #123294, #108079, #140553, #187114, #41967, #188182, #191374, #207631, #91788, #154634, #8366, #5137, #39817, #54998, #204411, #105924, #9440, #71213, #171949, #75510, #23538, #189258, #74449, #206566, #89647, #137330, #174108, #43040, #125407, #155700, #109152, #7282, #58193, #121150, #24608, #124352, #73359, #141622, #175165, #139464, #170874, #205494, #57128, #59249, #107002, #40897, #173027, #38747, #190309, #104829, #90717, #22465, #203335, #54988, #182838, #133067, #153557, #152484, #37667, #166602, #4066, #134135, #17119, #150363, #1933, #19264, #67993, #84276, #200142, #135189, #121140, #83196, #117914, #199065, #149278, #5128, #66925, #103743, #85346, #18191, #101595, #186031, #183907, #100527, #51796, #69069, #167663, #187103, #165527, #116837, #151427, #202268, #35518, #3000, #71203, #38737, #52844, #201205, #118979, #184958, #50711, #34455, #137319, #36584, #102671, #168729, #20331, #169794, #86417, #70136, #136248, #53919, #859, #120056, #21383, #87492, #92842, #124341, #60306, #190299, #105913, #104819, #88567, #173017, #192428, #158886, #10482, #154625, #157833, #91776, #191361, #171938, #9430, #73349, #170865, #89637, #155689, #24598, #7272, #23529, #139452, #74439, #126465, #22455, #57118, #138383, #6205, #76556, #72274, #43028, #90707, #205484, #40887, #125396, #123285, #39807, #189248, #8355, #106992, #204401, #56054, #122211, #156769, #141611, #140541, #206555, #142666, #188173, #58183, #41956, #108068, #174096, #25669, #75500, #208677, #207620, #59237, #109140, #175153, #26739, #127544, #77626, #94973, #61385, #65605, #159952, #163159, #144812, #32080, #63520, #213985, #129672, #45156, #44083, #27814, #112337, #131755, #98168, #164216, #93911, #97107, #161019, #79755, #28889, #111270, #128607, #110202, #31033, #14744, #12614, #11556, #96043, #212943, #78687, #177273, #209743, #64580, #80836, #15803, #210819, #47291, #13685, #62444, #194574, #46220, #178349, #29957, #162096, #145871, #143748, #211879, #193515, #130721, #179412, #146926, #195657, #113406, #196712, #48353, #114464, #180464, #81889, #147975, #176212, #166334, #50458, #149020, #197760, #1673, #20064, #595, #150101, #21113, #87219, #66661, #165271, #185764, #34194, #200935, #167409, #116577, #67727, #17926, #182572, #100269, #84010, #133878, #181512, #199885, #132808, #152224, #118711, #86153, #198812, #51530, #117655, #99221, #134930, #19001, #183648, #184699, #35252, #101328, #85082, #151166, #49398, #2737, #3795, #68808, #52583, #153283, #4859, #36320, #16866, #37396, #102398, #69869, #168466, #135978, #201993, #115517, #53651, #119783, #103471, #169533, #70938, #33141, #82946, #92592, #203074, #89372, #170594, #54718, #191104, #38473, #9169, #205213, #138120, #73082, #157576, #155421, #72007, #105636, #40624, #139183, #158634, #137048, #88296, #56855, #173835, #204129, #39535, #42772, #10231, #24329, #123029, #90437, #188980, #104550, #22180, #108879, #55782, #156505, #154357, #5936, #75244, #121939, #187905, #171664, #23260, #120867, #7005, #41700, #106727, #125147, #8094, #186841, #74183, #172754, #140276, #206295, #57920, #124085, #174903, #26482, #190048, #107810, #25412, #91517, #141356, #207370, #58990, #142413, #66146 ),
 ( #78435, #180999, #147453, #43833, #175959, #199361, #77371, #32618, #27554, #109949, #165823, #159693, #93650, #127284, #11292, #100810, #192172, #198297, #177015, #67219, #98696, #34737, #164754, #143486, #76306, #60055, #213476, #166895, #133355, #51008, #126210, #132291, #193255, #115001, #61124, #209483, #160762, #208421, #49938, #116059, #44902, #111010, #131256, #33679, #28632, #94719, #12356, #99754, #182049, #117129, #65100, #82425, #48882, #197243, #16344, #148515, #81, #17407, #83490, #149573, #1157, #183131, #184188, #187391, #153843, #121420, #35809, #201487, #167951, #134424, #170075, #202554, #53133, #5414, #19554, #119262, #85631, #101886, #18487, #36871, #55272, #151718, #185248, #56339, #122500, #3288, #200427, #6494, #71492, #105106, #69356, #137604, #102954, #84564, #135465, #169013, #86700, #20611, #152768, #4349, #54206, #188461, #150653, #70418, #52073, #2215, #72569, #118200, #171145, #136535, #120344, #186320, #39023, #37955, #104028, #21661, #87767, #203621, #40092, #68291, #22737, #88855, #154910, #138668, #204689, #106204, #127834, #23819, #124625, #205771, #89924, #11832, #73648, #44365, #25954, #173305, #108353, #192709, #190583, #107283, #140824, #75785, #174375, #193786, #172231, #123565, #92060, #208959, #24884, #74720, #77909, #45435, #59524, #158117, #125684, #9709, #139747, #57400, #144029, #90989, #191642, #189528, #41176, #110488, #157052, #8640, #206837, #58470, #155975, #42240, #76838, #141892, #160233, #43306, #7562, #109426, #207903, #175431, #27017, #93125, #159164, #210024, #61666, #10763, #142957, #60592, #126750, #176487, #28098, #94193, #177558, #98436, #82168, #13957, #78971, #163443, #65895, #80041, #178628, #62719, #132041, #164500, #165562, #162379, #114746, #81114, #30240, #63794, #146144, #96324, #212159, #129951, #195940, #95259, #47575, #128880, #198051, #32371, #214262, #194861, #113690, #46494, #12892, #48629, #147199, #179692, #16085, #112617, #31309, #97387, #15023, #111549, #213225, #148263, #64856, #131002, #149316, #895, #196994, #145091, #99505, #49680, #115807, #180744, #181794, #33428, #29170, #17157, #83231, #66963, #133102, #199099, #161309, #211095, #166635, #169832, #151463, #38772, #70172, #6242, #136284, #51830, #50745, #34489, #119016, #138418, #104853, #170898, #100564, #103781, #167699, #86453, #35553, #117948, #135227, #116872, #37705, #21419, #19300, #18228, #102706, #5166, #85381, #183943, #1965, #71240, #87528, #22490, #101633, #53955, #20369, #3036, #69105, #201240, #52881, #184997, #36621, #168763, #84312, #152518, #68029, #137356, #186068, #153594, #134167, #4103, #200177, #150397, #202304, #120093, #203371, #55025, #121174, #187143, #88602, #154658, #182873, #72313, #26777, #7311, #156805, #27853, #93950, #73388, #171977, #192469, #191400, #76596, #205521, #43066, #173055, #56092, #189283, #40923, #58220, #107029, #123320, #24635, #174134, #159991, #122248, #8392, #23567, #188207, #44121, #105953, #142708, #124379, #57155, #140581, #10522, #74474, #139493, #90743, #108106, #206592, #11592, #204438, #155727, #190337, #92880, #41999, #25708, #110242, #77666, #91816, #157874, #9467, #75538, #89677, #141649, #176252, #207660, #59279, #125438, #109179, #208718, #175191, #158926, #60344, #126505, #39846, #46255, #64619, #163199, #99262, #194612, #96080, #47328, #111309, #162133, #63554, #31070, #15842, #78724, #29995, #80874, #146964, #62483, #115556, #113443, #196753, #212979, #130758, #48394, #144851, #180503, #45195, #65649, #165310, #210857, #177312, #197802, #129710, #13722, #195693, #114507, #181553, #209781, #193553, #12653, #33181, #148014, #16904, #32121, #95011, #97146, #112373, #128647, #143786, #98204, #61420, #178384, #28926, #164254, #81928, #161060, #214024, #79795, #127584, #131796, #49437, #145908, #211919, #179448, #14782, #66701, #150143, #1715, #21158, #104592, #133921, #103516, #84056, #200978, #152265, #69911, #67770, #170637, #119827, #120909, #203118, #199928, #186881, #183690, #20107, #149060, #102440, #136021, #51573, #169575, #54760, #117699, #34237, #166377, #35296, #153327, #184737, #134970, #151208, #132848 ) ),
 .UNSPECIFIED., .F., .F., .T. ) 
 B_SPLINE_SURFACE_WITH_KNOTS ( ( 2, 2 ),
 ( 3, 2, 2, 2, 2, 2, 2, 2, 2, 2, 2, 2, 2, 2, 2, 2, 2, 2, 2, 2, 2, 2, 2, 2, 2, 2, 2, 2, 2, 2, 2, 2, 2, 2, 2, 2, 2, 2, 2, 2, 2, 2, 2, 2, 2, 2, 2, 2, 2, 2, 2, 2, 2, 2, 2, 2, 2, 2, 2, 2, 2, 2, 2, 2, 2, 2, 2, 2, 2, 2, 2, 2, 2, 2, 2, 2, 2, 2, 2, 2, 2, 2, 2, 2, 2, 2, 2, 2, 2, 2, 2, 2, 2, 2, 2, 2, 2, 2, 2, 2, 2, 2, 2, 2, 2, 2, 2, 2, 2, 2, 2, 2, 2, 2, 2, 2, 2, 2, 2, 2, 2, 2, 2, 2, 2, 2, 2, 2, 2, 2, 2, 2, 2, 2, 2, 2, 2, 2, 2, 2, 2, 2, 2, 2, 2, 2, 2, 2, 2, 2, 2, 2, 2, 2, 2, 2, 2, 2, 2, 2, 2, 2, 2, 2, 2, 2, 2, 2, 2, 2, 2, 2, 2, 2, 2, 2, 2, 2, 2, 2, 2, 2, 2, 2, 2, 2, 2, 2, 2, 2, 2, 2, 2, 2, 2, 2, 2, 2, 2, 2, 2, 2, 2, 2, 2, 2, 2, 2, 2, 2, 2, 2, 2, 2, 2, 2, 2, 2, 2, 2, 2, 2, 2, 2, 2, 2, 2, 2, 2, 2, 2, 2, 2, 2, 2, 2, 2, 2, 2, 2, 3 ),
 ( 0.000000000000000000, 1.000000000000000000 ),
 ( 0.000000000000000000, 0.004166666666666666609, 0.008333333333333333218, 0.01250000000000000069, 0.01666666666666666644, 0.02083333333333333218, 0.02500000000000000139, 0.02916666666666666713, 0.03333333333333333287, 0.03749999999999999861, 0.04166666666666666435, 0.04583333333333333010, 0.05000000000000000278, 0.05416666666666666852, 0.05833333333333333426, 0.06250000000000000000, 0.06666666666666666574, 0.07083333333333333148, 0.07499999999999999722, 0.07916666666666666297, 0.08333333333333332871, 0.08749999999999999445, 0.09166666666666666019, 0.09583333333333333981, 0.1000000000000000056, 0.1041666666666666713, 0.1083333333333333370, 0.1125000000000000028, 0.1166666666666666685, 0.1208333333333333343, 0.1250000000000000000, 0.1291666666666666796, 0.1333333333333333315, 0.1375000000000000111, 0.1416666666666666630, 0.1458333333333333426, 0.1499999999999999944, 0.1541666666666666741, 0.1583333333333333259, 0.1625000000000000056, 0.1666666666666666574, 0.1708333333333333370, 0.1749999999999999889, 0.1791666666666666685, 0.1833333333333333204, 0.1875000000000000000, 0.1916666666666666796, 0.1958333333333333315, 0.2000000000000000111, 0.2041666666666666630, 0.2083333333333333426, 0.2124999999999999944, 0.2166666666666666741, 0.2208333333333333259, 0.2250000000000000056, 0.2291666666666666574, 0.2333333333333333370, 0.2374999999999999889, 0.2416666666666666685, 0.2458333333333333204, 0.2500000000000000000, 0.2541666666666666519, 0.2583333333333333592, 0.2625000000000000111, 0.2666666666666666630, 0.2708333333333333148, 0.2750000000000000222, 0.2791666666666666741, 0.2833333333333333259, 0.2874999999999999778, 0.2916666666666666852, 0.2958333333333333370, 0.2999999999999999889, 0.3041666666666666408, 0.3083333333333333481, 0.3125000000000000000, 0.3166666666666666519, 0.3208333333333333592, 0.3250000000000000111, 0.3291666666666666630, 0.3333333333333333148, 0.3375000000000000222, 0.3416666666666666741, 0.3458333333333333259, 0.3499999999999999778, 0.3541666666666666852, 0.3583333333333333370, 0.3624999999999999889, 0.3666666666666666408, 0.3708333333333333481, 0.3750000000000000000, 0.3791666666666666519, 0.3833333333333333592, 0.3875000000000000111, 0.3916666666666666630, 0.3958333333333333148, 0.4000000000000000222, 0.4041666666666666741, 0.4083333333333333259, 0.4124999999999999778, 0.4166666666666666852, 0.4208333333333333370, 0.4249999999999999889, 0.4291666666666666408, 0.4333333333333333481, 0.4375000000000000000, 0.4416666666666666519, 0.4458333333333333592, 0.4500000000000000111, 0.4541666666666666630, 0.4583333333333333148, 0.4625000000000000222, 0.4666666666666666741, 0.4708333333333333259, 0.4749999999999999778, 0.4791666666666666852, 0.4833333333333333370, 0.4874999999999999889, 0.4916666666666666408, 0.4958333333333333481, 0.5000000000000000000, 0.5041666666666666519, 0.5083333333333333037, 0.5124999999999999556, 0.5166666666666667185, 0.5208333333333333703, 0.5250000000000000222, 0.5291666666666666741, 0.5333333333333333259, 0.5374999999999999778, 0.5416666666666666297, 0.5458333333333332815, 0.5500000000000000444, 0.5541666666666666963, 0.5583333333333333481, 0.5625000000000000000, 0.5666666666666666519, 0.5708333333333333037, 0.5749999999999999556, 0.5791666666666667185, 0.5833333333333333703, 0.5875000000000000222, 0.5916666666666666741, 0.5958333333333333259, 0.5999999999999999778, 0.6041666666666666297, 0.6083333333333332815, 0.6125000000000000444, 0.6166666666666666963, 0.6208333333333333481, 0.6250000000000000000, 0.6291666666666666519, 0.6333333333333333037, 0.6374999999999999556, 0.6416666666666667185, 0.6458333333333333703, 0.6500000000000000222, 0.6541666666666666741, 0.6583333333333333259, 0.6624999999999999778, 0.6666666666666666297, 0.6708333333333332815, 0.6750000000000000444, 0.6791666666666666963, 0.6833333333333333481, 0.6875000000000000000, 0.6916666666666666519, 0.6958333333333333037, 0.6999999999999999556, 0.7041666666666667185, 0.7083333333333333703, 0.7125000000000000222, 0.7166666666666666741, 0.7208333333333333259, 0.7249999999999999778, 0.7291666666666666297, 0.7333333333333332815, 0.7375000000000000444, 0.7416666666666666963, 0.7458333333333333481, 0.7500000000000000000, 0.7541666666666666519, 0.7583333333333333037, 0.7624999999999999556, 0.7666666666666667185, 0.7708333333333333703, 0.7750000000000000222, 0.7791666666666666741, 0.7833333333333333259, 0.7874999999999999778, 0.7916666666666666297, 0.7958333333333332815, 0.8000000000000000444, 0.8041666666666666963, 0.8083333333333333481, 0.8125000000000000000, 0.8166666666666666519, 0.8208333333333333037, 0.8249999999999999556, 0.8291666666666667185, 0.8333333333333333703, 0.8375000000000000222, 0.8416666666666666741, 0.8458333333333333259, 0.8499999999999999778, 0.8541666666666666297, 0.8583333333333332815, 0.8625000000000000444, 0.8666666666666666963, 0.8708333333333333481, 0.8750000000000000000, 0.8791666666666666519, 0.8833333333333333037, 0.8874999999999999556, 0.8916666666666667185, 0.8958333333333333703, 0.9000000000000000222, 0.9041666666666666741, 0.9083333333333333259, 0.9124999999999999778, 0.9166666666666666297, 0.9208333333333332815, 0.9250000000000000444, 0.9291666666666666963, 0.9333333333333333481, 0.9375000000000000000, 0.9416666666666666519, 0.9458333333333333037, 0.9499999999999999556, 0.9541666666666667185, 0.9583333333333333703, 0.9625000000000000222, 0.9666666666666666741, 0.9708333333333333259, 0.9749999999999999778, 0.9791666666666666297, 0.9833333333333332815, 0.9875000000000000444, 0.9916666666666666963, 0.9958333333333333481, 1.000000000000000000 ),
 .UNSPECIFIED. ) 
 GEOMETRIC_REPRESENTATION_ITEM ( )  RATIONAL_B_SPLINE_SURFACE ( (
 ( 1.000000000000000000, 0.8660254037844387076, 1.000000000000000000, 0.8660254037844387076, 1.000000000000000000, 0.8660254037844387076, 1.000000000000000000, 0.8660254037844387076, 1.000000000000000000, 0.8660254037844387076, 1.000000000000000000, 0.8660254037844387076, 1.000000000000000000, 0.8660254037844387076, 1.000000000000000000, 0.8660254037844387076, 1.000000000000000000, 0.8660254037844387076, 1.000000000000000000, 0.8660254037844387076, 1.000000000000000000, 0.8660254037844387076, 1.000000000000000000, 0.8660254037844387076, 1.000000000000000000, 0.8660254037844387076, 1.000000000000000000, 0.8660254037844387076, 1.000000000000000000, 0.8660254037844387076, 1.000000000000000000, 0.8660254037844387076, 1.000000000000000000, 0.8660254037844387076, 1.000000000000000000, 0.8660254037844387076, 1.000000000000000000, 0.8660254037844387076, 1.000000000000000000, 0.8660254037844387076, 1.000000000000000000, 0.8660254037844387076, 1.000000000000000000, 0.8660254037844387076, 1.000000000000000000, 0.8660254037844387076, 1.000000000000000000, 0.8660254037844387076, 1.000000000000000000, 0.8660254037844387076, 1.000000000000000000, 0.8660254037844387076, 1.000000000000000000, 0.8660254037844387076, 1.000000000000000000, 0.8660254037844387076, 1.000000000000000000, 0.8660254037844387076, 1.000000000000000000, 0.8660254037844387076, 1.000000000000000000, 0.8660254037844387076, 1.000000000000000000, 0.8660254037844387076, 1.000000000000000000, 0.8660254037844387076, 1.000000000000000000, 0.8660254037844387076, 1.000000000000000000, 0.8660254037844387076, 1.000000000000000000, 0.8660254037844387076, 1.000000000000000000, 0.8660254037844387076, 1.000000000000000000, 0.8660254037844387076, 1.000000000000000000, 0.8660254037844387076, 1.000000000000000000, 0.8660254037844387076, 1.000000000000000000, 0.8660254037844387076, 1.000000000000000000, 0.8660254037844387076, 1.000000000000000000, 0.8660254037844387076, 1.000000000000000000, 0.8660254037844387076, 1.000000000000000000, 0.8660254037844387076, 1.000000000000000000, 0.8660254037844387076, 1.000000000000000000, 0.8660254037844387076, 1.000000000000000000, 0.8660254037844387076, 1.000000000000000000, 0.8660254037844387076, 1.000000000000000000, 0.8660254037844387076, 1.000000000000000000, 0.8660254037844387076, 1.000000000000000000, 0.8660254037844387076, 1.000000000000000000, 0.8660254037844387076, 1.000000000000000000, 0.8660254037844387076, 1.000000000000000000, 0.8660254037844387076, 1.000000000000000000, 0.8660254037844387076, 1.000000000000000000, 0.8660254037844387076, 1.000000000000000000, 0.8660254037844387076, 1.000000000000000000, 0.8660254037844387076, 1.000000000000000000, 0.8660254037844387076, 1.000000000000000000, 0.8660254037844387076, 1.000000000000000000, 0.8660254037844387076, 1.000000000000000000, 0.8660254037844387076, 1.000000000000000000, 0.8660254037844387076, 1.000000000000000000, 0.8660254037844387076, 1.000000000000000000, 0.8660254037844387076, 1.000000000000000000, 0.8660254037844387076, 1.000000000000000000, 0.8660254037844387076, 1.000000000000000000, 0.8660254037844387076, 1.000000000000000000, 0.8660254037844387076, 1.000000000000000000, 0.8660254037844387076, 1.000000000000000000, 0.8660254037844387076, 1.000000000000000000, 0.8660254037844387076, 1.000000000000000000, 0.8660254037844387076, 1.000000000000000000, 0.8660254037844387076, 1.000000000000000000, 0.8660254037844387076, 1.000000000000000000, 0.8660254037844387076, 1.000000000000000000, 0.8660254037844387076, 1.000000000000000000, 0.8660254037844387076, 1.000000000000000000, 0.8660254037844387076, 1.000000000000000000, 0.8660254037844387076, 1.000000000000000000, 0.8660254037844387076, 1.000000000000000000, 0.8660254037844387076, 1.000000000000000000, 0.8660254037844387076, 1.000000000000000000, 0.8660254037844387076, 1.000000000000000000, 0.8660254037844387076, 1.000000000000000000, 0.8660254037844387076, 1.000000000000000000, 0.8660254037844387076, 1.000000000000000000, 0.8660254037844387076, 1.000000000000000000, 0.8660254037844387076, 1.000000000000000000, 0.8660254037844387076, 1.000000000000000000, 0.8660254037844387076, 1.000000000000000000, 0.8660254037844387076, 1.000000000000000000, 0.8660254037844387076, 1.000000000000000000, 0.8660254037844387076, 1.000000000000000000, 0.8660254037844387076, 1.000000000000000000, 0.8660254037844387076, 1.000000000000000000, 0.8660254037844387076, 1.000000000000000000, 0.8660254037844387076, 1.000000000000000000, 0.8660254037844387076, 1.000000000000000000, 0.8660254037844387076, 1.000000000000000000, 0.8660254037844387076, 1.000000000000000000, 0.8660254037844387076, 1.000000000000000000, 0.8660254037844387076, 1.000000000000000000, 0.8660254037844387076, 1.000000000000000000, 0.8660254037844387076, 1.000000000000000000, 0.8660254037844387076, 1.000000000000000000, 0.8660254037844387076, 1.000000000000000000, 0.8660254037844387076, 1.000000000000000000, 0.8660254037844387076, 1.000000000000000000, 0.8660254037844387076, 1.000000000000000000, 0.8660254037844387076, 1.000000000000000000, 0.8660254037844387076, 1.000000000000000000, 0.8660254037844387076, 1.000000000000000000, 0.8660254037844387076, 1.000000000000000000, 0.8660254037844387076, 1.000000000000000000, 0.8660254037844387076, 1.000000000000000000, 0.8660254037844387076, 1.000000000000000000, 0.8660254037844387076, 1.000000000000000000, 0.8660254037844387076, 1.000000000000000000, 0.8660254037844387076, 1.000000000000000000, 0.8660254037844387076, 1.000000000000000000, 0.8660254037844387076, 1.000000000000000000, 0.8660254037844387076, 1.000000000000000000, 0.8660254037844387076, 1.000000000000000000, 0.8660254037844387076, 1.000000000000000000, 0.8660254037844387076, 1.000000000000000000, 0.8660254037844387076, 1.000000000000000000, 0.8660254037844387076, 1.000000000000000000, 0.8660254037844387076, 1.000000000000000000, 0.8660254037844387076, 1.000000000000000000, 0.8660254037844387076, 1.000000000000000000, 0.8660254037844387076, 1.000000000000000000, 0.8660254037844387076, 1.000000000000000000, 0.8660254037844387076, 1.000000000000000000, 0.8660254037844387076, 1.000000000000000000, 0.8660254037844387076, 1.000000000000000000, 0.8660254037844387076, 1.000000000000000000, 0.8660254037844387076, 1.000000000000000000, 0.8660254037844387076, 1.000000000000000000, 0.8660254037844387076, 1.000000000000000000, 0.8660254037844387076, 1.000000000000000000, 0.8660254037844387076, 1.000000000000000000, 0.8660254037844387076, 1.000000000000000000, 0.8660254037844387076, 1.000000000000000000, 0.8660254037844387076, 1.000000000000000000, 0.8660254037844387076, 1.000000000000000000, 0.8660254037844387076, 1.000000000000000000, 0.8660254037844387076, 1.000000000000000000, 0.8660254037844387076, 1.000000000000000000, 0.8660254037844387076, 1.000000000000000000, 0.8660254037844387076, 1.000000000000000000, 0.8660254037844387076, 1.000000000000000000, 0.8660254037844387076, 1.000000000000000000, 0.8660254037844387076, 1.000000000000000000, 0.8660254037844387076, 1.000000000000000000, 0.8660254037844387076, 1.000000000000000000, 0.8660254037844387076, 1.000000000000000000, 0.8660254037844387076, 1.000000000000000000, 0.8660254037844387076, 1.000000000000000000, 0.8660254037844387076, 1.000000000000000000, 0.8660254037844387076, 1.000000000000000000, 0.8660254037844387076, 1.000000000000000000, 0.8660254037844387076, 1.000000000000000000, 0.8660254037844387076, 1.000000000000000000, 0.8660254037844387076, 1.000000000000000000, 0.8660254037844387076, 1.000000000000000000, 0.8660254037844387076, 1.000000000000000000, 0.8660254037844387076, 1.000000000000000000, 0.8660254037844387076, 1.000000000000000000, 0.8660254037844387076, 1.000000000000000000, 0.8660254037844387076, 1.000000000000000000, 0.8660254037844387076, 1.000000000000000000, 0.8660254037844387076, 1.000000000000000000, 0.8660254037844387076, 1.000000000000000000, 0.8660254037844387076, 1.000000000000000000, 0.8660254037844387076, 1.000000000000000000, 0.8660254037844387076, 1.000000000000000000, 0.8660254037844387076, 1.000000000000000000, 0.8660254037844387076, 1.000000000000000000, 0.8660254037844387076, 1.000000000000000000, 0.8660254037844387076, 1.000000000000000000, 0.8660254037844387076, 1.000000000000000000, 0.8660254037844387076, 1.000000000000000000, 0.8660254037844387076, 1.000000000000000000, 0.8660254037844387076, 1.000000000000000000, 0.8660254037844387076, 1.000000000000000000, 0.8660254037844387076, 1.000000000000000000, 0.8660254037844387076, 1.000000000000000000, 0.8660254037844387076, 1.000000000000000000, 0.8660254037844387076, 1.000000000000000000, 0.8660254037844387076, 1.000000000000000000, 0.8660254037844387076, 1.000000000000000000, 0.8660254037844387076, 1.000000000000000000, 0.8660254037844387076, 1.000000000000000000, 0.8660254037844387076, 1.000000000000000000, 0.8660254037844387076, 1.000000000000000000, 0.8660254037844387076, 1.000000000000000000, 0.8660254037844387076, 1.000000000000000000, 0.8660254037844387076, 1.000000000000000000, 0.8660254037844387076, 1.000000000000000000, 0.8660254037844387076, 1.000000000000000000, 0.8660254037844387076, 1.000000000000000000, 0.8660254037844387076, 1.000000000000000000, 0.8660254037844387076, 1.000000000000000000, 0.8660254037844387076, 1.000000000000000000, 0.8660254037844387076, 1.000000000000000000, 0.8660254037844387076, 1.000000000000000000, 0.8660254037844387076, 1.000000000000000000, 0.8660254037844387076, 1.000000000000000000, 0.8660254037844387076, 1.000000000000000000, 0.8660254037844387076, 1.000000000000000000, 0.8660254037844387076, 1.000000000000000000, 0.8660254037844387076, 1.000000000000000000, 0.8660254037844387076, 1.000000000000000000, 0.8660254037844387076, 1.000000000000000000, 0.8660254037844387076, 1.000000000000000000, 0.8660254037844387076, 1.000000000000000000, 0.8660254037844387076, 1.000000000000000000, 0.8660254037844387076, 1.000000000000000000, 0.8660254037844387076, 1.000000000000000000, 0.8660254037844387076, 1.000000000000000000, 0.8660254037844387076, 1.000000000000000000, 0.8660254037844387076, 1.000000000000000000, 0.8660254037844387076, 1.000000000000000000, 0.8660254037844387076, 1.000000000000000000, 0.8660254037844387076, 1.000000000000000000, 0.8660254037844387076, 1.000000000000000000, 0.8660254037844387076, 1.000000000000000000, 0.8660254037844387076, 1.000000000000000000, 0.8660254037844387076, 1.000000000000000000, 0.8660254037844387076, 1.000000000000000000, 0.8660254037844387076, 1.000000000000000000, 0.8660254037844387076, 1.000000000000000000, 0.8660254037844387076, 1.000000000000000000, 0.8660254037844387076, 1.000000000000000000, 0.8660254037844387076, 1.000000000000000000, 0.8660254037844387076, 1.000000000000000000, 0.8660254037844387076, 1.000000000000000000, 0.8660254037844387076, 1.000000000000000000),
 ( 1.000000000000000000, 0.8660254037844387076, 1.000000000000000000, 0.8660254037844387076, 1.000000000000000000, 0.8660254037844387076, 1.000000000000000000, 0.8660254037844387076, 1.000000000000000000, 0.8660254037844387076, 1.000000000000000000, 0.8660254037844387076, 1.000000000000000000, 0.8660254037844387076, 1.000000000000000000, 0.8660254037844387076, 1.000000000000000000, 0.8660254037844387076, 1.000000000000000000, 0.8660254037844387076, 1.000000000000000000, 0.8660254037844387076, 1.000000000000000000, 0.8660254037844387076, 1.000000000000000000, 0.8660254037844387076, 1.000000000000000000, 0.8660254037844387076, 1.000000000000000000, 0.8660254037844387076, 1.000000000000000000, 0.8660254037844387076, 1.000000000000000000, 0.8660254037844387076, 1.000000000000000000, 0.8660254037844387076, 1.000000000000000000, 0.8660254037844387076, 1.000000000000000000, 0.8660254037844387076, 1.000000000000000000, 0.8660254037844387076, 1.000000000000000000, 0.8660254037844387076, 1.000000000000000000, 0.8660254037844387076, 1.000000000000000000, 0.8660254037844387076, 1.000000000000000000, 0.8660254037844387076, 1.000000000000000000, 0.8660254037844387076, 1.000000000000000000, 0.8660254037844387076, 1.000000000000000000, 0.8660254037844387076, 1.000000000000000000, 0.8660254037844387076, 1.000000000000000000, 0.8660254037844387076, 1.000000000000000000, 0.8660254037844387076, 1.000000000000000000, 0.8660254037844387076, 1.000000000000000000, 0.8660254037844387076, 1.000000000000000000, 0.8660254037844387076, 1.000000000000000000, 0.8660254037844387076, 1.000000000000000000, 0.8660254037844387076, 1.000000000000000000, 0.8660254037844387076, 1.000000000000000000, 0.8660254037844387076, 1.000000000000000000, 0.8660254037844387076, 1.000000000000000000, 0.8660254037844387076, 1.000000000000000000, 0.8660254037844387076, 1.000000000000000000, 0.8660254037844387076, 1.000000000000000000, 0.8660254037844387076, 1.000000000000000000, 0.8660254037844387076, 1.000000000000000000, 0.8660254037844387076, 1.000000000000000000, 0.8660254037844387076, 1.000000000000000000, 0.8660254037844387076, 1.000000000000000000, 0.8660254037844387076, 1.000000000000000000, 0.8660254037844387076, 1.000000000000000000, 0.8660254037844387076, 1.000000000000000000, 0.8660254037844387076, 1.000000000000000000, 0.8660254037844387076, 1.000000000000000000, 0.8660254037844387076, 1.000000000000000000, 0.8660254037844387076, 1.000000000000000000, 0.8660254037844387076, 1.000000000000000000, 0.8660254037844387076, 1.000000000000000000, 0.8660254037844387076, 1.000000000000000000, 0.8660254037844387076, 1.000000000000000000, 0.8660254037844387076, 1.000000000000000000, 0.8660254037844387076, 1.000000000000000000, 0.8660254037844387076, 1.000000000000000000, 0.8660254037844387076, 1.000000000000000000, 0.8660254037844387076, 1.000000000000000000, 0.8660254037844387076, 1.000000000000000000, 0.8660254037844387076, 1.000000000000000000, 0.8660254037844387076, 1.000000000000000000, 0.8660254037844387076, 1.000000000000000000, 0.8660254037844387076, 1.000000000000000000, 0.8660254037844387076, 1.000000000000000000, 0.8660254037844387076, 1.000000000000000000, 0.8660254037844387076, 1.000000000000000000, 0.8660254037844387076, 1.000000000000000000, 0.8660254037844387076, 1.000000000000000000, 0.8660254037844387076, 1.000000000000000000, 0.8660254037844387076, 1.000000000000000000, 0.8660254037844387076, 1.000000000000000000, 0.8660254037844387076, 1.000000000000000000, 0.8660254037844387076, 1.000000000000000000, 0.8660254037844387076, 1.000000000000000000, 0.8660254037844387076, 1.000000000000000000, 0.8660254037844387076, 1.000000000000000000, 0.8660254037844387076, 1.000000000000000000, 0.8660254037844387076, 1.000000000000000000, 0.8660254037844387076, 1.000000000000000000, 0.8660254037844387076, 1.000000000000000000, 0.8660254037844387076, 1.000000000000000000, 0.8660254037844387076, 1.000000000000000000, 0.8660254037844387076, 1.000000000000000000, 0.8660254037844387076, 1.000000000000000000, 0.8660254037844387076, 1.000000000000000000, 0.8660254037844387076, 1.000000000000000000, 0.8660254037844387076, 1.000000000000000000, 0.8660254037844387076, 1.000000000000000000, 0.8660254037844387076, 1.000000000000000000, 0.8660254037844387076, 1.000000000000000000, 0.8660254037844387076, 1.000000000000000000, 0.8660254037844387076, 1.000000000000000000, 0.8660254037844387076, 1.000000000000000000, 0.8660254037844387076, 1.000000000000000000, 0.8660254037844387076, 1.000000000000000000, 0.8660254037844387076, 1.000000000000000000, 0.8660254037844387076, 1.000000000000000000, 0.8660254037844387076, 1.000000000000000000, 0.8660254037844387076, 1.000000000000000000, 0.8660254037844387076, 1.000000000000000000, 0.8660254037844387076, 1.000000000000000000, 0.8660254037844387076, 1.000000000000000000, 0.8660254037844387076, 1.000000000000000000, 0.8660254037844387076, 1.000000000000000000, 0.8660254037844387076, 1.000000000000000000, 0.8660254037844387076, 1.000000000000000000, 0.8660254037844387076, 1.000000000000000000, 0.8660254037844387076, 1.000000000000000000, 0.8660254037844387076, 1.000000000000000000, 0.8660254037844387076, 1.000000000000000000, 0.8660254037844387076, 1.000000000000000000, 0.8660254037844387076, 1.000000000000000000, 0.8660254037844387076, 1.000000000000000000, 0.8660254037844387076, 1.000000000000000000, 0.8660254037844387076, 1.000000000000000000, 0.8660254037844387076, 1.000000000000000000, 0.8660254037844387076, 1.000000000000000000, 0.8660254037844387076, 1.000000000000000000, 0.8660254037844387076, 1.000000000000000000, 0.8660254037844387076, 1.000000000000000000, 0.8660254037844387076, 1.000000000000000000, 0.8660254037844387076, 1.000000000000000000, 0.8660254037844387076, 1.000000000000000000, 0.8660254037844387076, 1.000000000000000000, 0.8660254037844387076, 1.000000000000000000, 0.8660254037844387076, 1.000000000000000000, 0.8660254037844387076, 1.000000000000000000, 0.8660254037844387076, 1.000000000000000000, 0.8660254037844387076, 1.000000000000000000, 0.8660254037844387076, 1.000000000000000000, 0.8660254037844387076, 1.000000000000000000, 0.8660254037844387076, 1.000000000000000000, 0.8660254037844387076, 1.000000000000000000, 0.8660254037844387076, 1.000000000000000000, 0.8660254037844387076, 1.000000000000000000, 0.8660254037844387076, 1.000000000000000000, 0.8660254037844387076, 1.000000000000000000, 0.8660254037844387076, 1.000000000000000000, 0.8660254037844387076, 1.000000000000000000, 0.8660254037844387076, 1.000000000000000000, 0.8660254037844387076, 1.000000000000000000, 0.8660254037844387076, 1.000000000000000000, 0.8660254037844387076, 1.000000000000000000, 0.8660254037844387076, 1.000000000000000000, 0.8660254037844387076, 1.000000000000000000, 0.8660254037844387076, 1.000000000000000000, 0.8660254037844387076, 1.000000000000000000, 0.8660254037844387076, 1.000000000000000000, 0.8660254037844387076, 1.000000000000000000, 0.8660254037844387076, 1.000000000000000000, 0.8660254037844387076, 1.000000000000000000, 0.8660254037844387076, 1.000000000000000000, 0.8660254037844387076, 1.000000000000000000, 0.8660254037844387076, 1.000000000000000000, 0.8660254037844387076, 1.000000000000000000, 0.8660254037844387076, 1.000000000000000000, 0.8660254037844387076, 1.000000000000000000, 0.8660254037844387076, 1.000000000000000000, 0.8660254037844387076, 1.000000000000000000, 0.8660254037844387076, 1.000000000000000000, 0.8660254037844387076, 1.000000000000000000, 0.8660254037844387076, 1.000000000000000000, 0.8660254037844387076, 1.000000000000000000, 0.8660254037844387076, 1.000000000000000000, 0.8660254037844387076, 1.000000000000000000, 0.8660254037844387076, 1.000000000000000000, 0.8660254037844387076, 1.000000000000000000, 0.8660254037844387076, 1.000000000000000000, 0.8660254037844387076, 1.000000000000000000, 0.8660254037844387076, 1.000000000000000000, 0.8660254037844387076, 1.000000000000000000, 0.8660254037844387076, 1.000000000000000000, 0.8660254037844387076, 1.000000000000000000, 0.8660254037844387076, 1.000000000000000000, 0.8660254037844387076, 1.000000000000000000, 0.8660254037844387076, 1.000000000000000000, 0.8660254037844387076, 1.000000000000000000, 0.8660254037844387076, 1.000000000000000000, 0.8660254037844387076, 1.000000000000000000, 0.8660254037844387076, 1.000000000000000000, 0.8660254037844387076, 1.000000000000000000, 0.8660254037844387076, 1.000000000000000000, 0.8660254037844387076, 1.000000000000000000, 0.8660254037844387076, 1.000000000000000000, 0.8660254037844387076, 1.000000000000000000, 0.8660254037844387076, 1.000000000000000000, 0.8660254037844387076, 1.000000000000000000, 0.8660254037844387076, 1.000000000000000000, 0.8660254037844387076, 1.000000000000000000, 0.8660254037844387076, 1.000000000000000000, 0.8660254037844387076, 1.000000000000000000, 0.8660254037844387076, 1.000000000000000000, 0.8660254037844387076, 1.000000000000000000, 0.8660254037844387076, 1.000000000000000000, 0.8660254037844387076, 1.000000000000000000, 0.8660254037844387076, 1.000000000000000000, 0.8660254037844387076, 1.000000000000000000, 0.8660254037844387076, 1.000000000000000000, 0.8660254037844387076, 1.000000000000000000, 0.8660254037844387076, 1.000000000000000000, 0.8660254037844387076, 1.000000000000000000, 0.8660254037844387076, 1.000000000000000000, 0.8660254037844387076, 1.000000000000000000, 0.8660254037844387076, 1.000000000000000000, 0.8660254037844387076, 1.000000000000000000, 0.8660254037844387076, 1.000000000000000000, 0.8660254037844387076, 1.000000000000000000, 0.8660254037844387076, 1.000000000000000000, 0.8660254037844387076, 1.000000000000000000, 0.8660254037844387076, 1.000000000000000000, 0.8660254037844387076, 1.000000000000000000, 0.8660254037844387076, 1.000000000000000000, 0.8660254037844387076, 1.000000000000000000, 0.8660254037844387076, 1.000000000000000000, 0.8660254037844387076, 1.000000000000000000, 0.8660254037844387076, 1.000000000000000000, 0.8660254037844387076, 1.000000000000000000, 0.8660254037844387076, 1.000000000000000000, 0.8660254037844387076, 1.000000000000000000, 0.8660254037844387076, 1.000000000000000000, 0.8660254037844387076, 1.000000000000000000, 0.8660254037844387076, 1.000000000000000000, 0.8660254037844387076, 1.000000000000000000, 0.8660254037844387076, 1.000000000000000000, 0.8660254037844387076, 1.000000000000000000, 0.8660254037844387076, 1.000000000000000000, 0.8660254037844387076, 1.000000000000000000, 0.8660254037844387076, 1.000000000000000000, 0.8660254037844387076, 1.000000000000000000, 0.8660254037844387076, 1.000000000000000000, 0.8660254037844387076, 1.000000000000000000, 0.8660254037844387076, 1.000000000000000000, 0.8660254037844387076, 1.000000000000000000, 0.8660254037844387076, 1.000000000000000000, 0.8660254037844387076, 1.000000000000000000) ) ) 
 REPRESENTATION_ITEM ( '' )  SURFACE ( )  );
#108148=EDGE_LOOP ( 'NONE', ( #16991, #141260, #186748 ) ) ;
#108151=CARTESIAN_POINT ( 'NONE',  ( -5.666945020832185875, 7.634521829102760115, 1.443375672974064550 ) ) ;
#108159=CARTESIAN_POINT ( 'NONE',  ( -8.503988664269602538, 10.94440607977979063, 1.599625672291269396 ) ) ;
#108162=CARTESIAN_POINT ( 'NONE',  ( 7.422199028477372451, 10.74665040227725044, -1.199719254218441611 ) ) ;
#108163=CARTESIAN_POINT ( 'NONE',  ( -1.500000000000015099, -0.1208333333333093396, -0.8660254037844383745 ) ) ;
#108164=CARTESIAN_POINT ( 'NONE',  ( -7.853197290813634268, 10.18514947741448573, 1.599625672291295375 ) ) ;
#108167=CARTESIAN_POINT ( 'NONE',  ( -1.364683531250012516, 4.238541667008090208, -0.7879004041258300672 ) ) ;
#108169=CARTESIAN_POINT ( 'NONE',  ( 9.747949258545622442, 10.47495501116581984, 0.000000000000000000 ) ) ;
#108172=CARTESIAN_POINT ( 'NONE',  ( -0.7499999999999972244, 4.858333333333353821, -1.299038105676652011 ) ) ;
#108175=CARTESIAN_POINT ( 'NONE',  ( 7.849807752188022292, 11.14156422998596696, -1.082531754730543083 ) ) ;
#108178=CARTESIAN_POINT ( 'NONE',  ( -6.236387472606158333, 7.338502141871059870, -1.082531754730544860 ) ) ;
#108180=CARTESIAN_POINT ( 'NONE',  ( -1.364683531250000748, 2.009375000341421913, 1.214306433183764966E-14 ) ) ;
#108184=CARTESIAN_POINT ( 'NONE',  ( -6.507023659554960204, 9.678945805201045971, 1.199719254218452047 ) ) ;
#108186=CARTESIAN_POINT ( 'NONE',  ( -1.001543065824772872E-14, 4.384375000341417916, 1.575800808251672791 ) ) ;
#108192=CARTESIAN_POINT ( 'NONE',  ( 6.448874621594486989, 10.67543749183559143, 0.7998128361456462443 ) ) ;
#108196=CARTESIAN_POINT ( 'NONE',  ( -1.500000000000001332, 1.400000000000019229, 0.000000000000000000 ) ) ;
#108201=CARTESIAN_POINT ( 'NONE',  ( 7.646435448427411963, 8.023188899361205273, -0.7216878364870257245 ) ) ;
#108202=CARTESIAN_POINT ( 'NONE',  ( 8.075853055234393452, 12.57357899774884658, 0.7998128361456462443 ) ) ;
#108204=CARTESIAN_POINT ( 'NONE',  ( 4.539282502477016479, 4.190251095844947926, 0.7998128361456341429 ) ) ;
#108210=CARTESIAN_POINT ( 'NONE',  ( 8.106885785967500979, 11.54545161934907682, 1.199719254218460707 ) ) ;
#108211=CARTESIAN_POINT ( 'NONE',  ( -8.696665468161981494, 12.23352791524263239, -1.199719254218446718 ) ) ;
#108214=CARTESIAN_POINT ( 'NONE',  ( -1.364683531249997417, 5.571875000341417916, 1.214306433183764966E-14 ) ) ;
#108220=CARTESIAN_POINT ( 'NONE',  ( -0.6823417656249969321, 4.217708333674755394, -1.181850606188749264 ) ) ;
#108222=CARTESIAN_POINT ( 'NONE',  ( -6.724481002698138532, 6.947575379343695623, -0.7216878364870278340 ) ) ;
#108231=CARTESIAN_POINT ( 'NONE',  ( 8.751951852821344247, 10.16936423550178503, -1.199719254218446718 ) ) ;
#108232=DIRECTION ( 'NONE',  ( 0.5265943820948186804, 0.4485553919811647305, 0.7221470882519708256 ) ) ;
#108233=CARTESIAN_POINT ( 'NONE',  ( 2.852660156828608073, 6.479853949608683550, -0.1948928627674442193 ) ) ;
#108238=CARTESIAN_POINT ( 'NONE',  ( -7.296259222448620463, 11.66405285949874759, 0.7998128361456481317 ) ) ;
#108239=CARTESIAN_POINT ( 'NONE',  ( 4.957477724091233995, 8.935474444748447098, -0.7998128361456281477 ) ) ;
#108241=CARTESIAN_POINT ( 'NONE',  ( 2.806174607904299734, 5.257325561654889512, -1.082531754730543083 ) ) ;
#108243=CARTESIAN_POINT ( 'NONE',  ( 5.034155109375821446, 4.767602470560229122, -0.7998128361456221525 ) ) ;
#108252=CARTESIAN_POINT ( 'NONE',  ( -5.910991785878175975, 6.958873840688411860, -1.082531754730544860 ) ) ;
#108253=CARTESIAN_POINT ( 'NONE',  ( 2.510230996824538430, 6.080353262937265413, 0.000000000000000000 ) ) ;
#108256=CARTESIAN_POINT ( 'NONE',  ( -6.347188469492005325, 10.55680364771601809, -0.7998128361456291469 ) ) ;
#108259=CARTESIAN_POINT ( 'NONE',  ( -2.749999999999996447, 8.900000000000027001, 1.273770014145090163E-14 ) ) ;
#108261=CARTESIAN_POINT ( 'NONE',  ( -6.997979842947967377, 11.31606025008131233, -0.7998128361456291469 ) ) ;
#108264=CARTESIAN_POINT ( 'NONE',  ( 6.988338112840064120, 10.24047933403371502, 1.199719254218460707 ) ) ;
#108266=CARTESIAN_POINT ( 'NONE',  ( 3.662674053986138656, 7.424870162959149589, 0.7998128361456321445 ) ) ;
#108277=DIRECTION ( 'NONE',  ( 0.7797859179643623628, 0.6260462619842697141, 0.000000000000000000 ) ) ;
#108278=CARTESIAN_POINT ( 'NONE',  ( -8.206763054973658100, 8.468978407091068306, 0.7998128361456602331 ) ) ;
#108281=CARTESIAN_POINT ( 'NONE',  ( 5.816084710582486217, 9.729256562414162701, 1.040834085586084257E-14 ) ) ;
#108282=VERTEX_POINT ( 'NONE', #31311 ) ;
#108285=CARTESIAN_POINT ( 'NONE',  ( -1.403499169904654842, 7.376709478544411169, 4.304123474982140429 ) ) ;
#108288=CARTESIAN_POINT ( 'NONE',  ( -4.900382456335551140, 7.804531068111707270, 1.199719254218464037 ) ) ;
#108290=DIRECTION ( 'NONE',  ( -0.1674078377058430267, 0.000000000000000000, 0.9858877298529756805 ) ) ;
#108295=EDGE_CURVE ( 'NONE', #7144, #143545, #114748, .T. ) ;
#108297=CARTESIAN_POINT ( 'NONE',  ( 8.209625708274705502, 9.536650400197368427, 1.199719254218462483 ) ) ;
#108299=CARTESIAN_POINT ( 'NONE',  ( -3.307826292054316664, 4.882216645528547616, -1.443375672974059665 ) ) ;
#108302=CARTESIAN_POINT ( 'NONE',  ( -4.699291399009611681, 6.864061528938182555, -1.228208583504811990 ) ) ;
#108305=CARTESIAN_POINT ( 'NONE',  ( -1.402160292154681736E-14, -0.8656249996585829720, 1.575800808251672791 ) ) ;
#108307=ORIENTED_EDGE ( 'NONE', *, *, #72346, .F. ) ;
#108309=CARTESIAN_POINT ( 'NONE',  ( 9.897088948295946764, 10.64895131587453569, 0.7216878364870438212 ) ) ;
#108314=DIRECTION ( 'NONE',  ( -0.000000000000000000, -8.546850786086437571E-32, -1.000000000000000000 ) ) ;
#108328=CARTESIAN_POINT ( 'NONE',  ( -4.623494077460110319, 5.352830164246910272, 1.199719254218462483 ) ) ;
#108329=CARTESIAN_POINT ( 'NONE',  ( 5.626270559546821204, 6.626699076635176766, 1.082531754730560403 ) ) ;
#108330=CARTESIAN_POINT ( 'NONE',  ( 1.499999999999990896, 4.025000000000021672, 1.214306433183764966E-14 ) ) ;
#108332=CARTESIAN_POINT ( 'NONE',  ( -3.002240950422295995, 5.590032644546251817, -1.199719254218452935 ) ) ;
#108337=CARTESIAN_POINT ( 'NONE',  ( -1.364683531250010295, 4.530208333674754506, 0.7879004041258379498 ) ) ;
#108340=CARTESIAN_POINT ( 'NONE',  ( -2.928197990871687306, 5.399686175116803710, 1.082531754730560403 ) ) ;
#108345=CARTESIAN_POINT ( 'NONE',  ( 4.192495815123822744, 5.914331089109666983, -1.599625672291255185 ) ) ;
#108347=LINE ( 'NONE', #24877, #92544 ) ;
#108349=CARTESIAN_POINT ( 'NONE',  ( -1.402160292154681736E-14, 1.509375000341420359, -1.575800808251659024 ) ) ;
#108352=CARTESIAN_POINT ( 'NONE',  ( -9.345647958521597687, 9.797677461230342999, 0.7998128361456462443 ) ) ;
#108353=CARTESIAN_POINT ( 'NONE',  ( -5.544921637864838715, 6.531792001339513654, -1.082531754730543971 ) ) ;
#108357=CARTESIAN_POINT ( 'NONE',  ( -1.500000000000001332, -1.318749999317178734, 0.000000000000000000 ) ) ;
#108365=CARTESIAN_POINT ( 'NONE',  ( -5.138177029454855216, 7.017625839162543677, 1.443375672974064550 ) ) ;
#108371=CARTESIAN_POINT ( 'NONE',  ( -5.544921637864841379, 5.571422787038166291, -0.7216878364870197293 ) ) ;
#108373=CARTESIAN_POINT ( 'NONE',  ( 8.387690588348714726, 12.93738945304888333, 1.040834085586084257E-14 ) ) ;
#108381=CARTESIAN_POINT ( 'NONE',  ( -3.903858165731105778, 6.641919395739846799, 1.199719254218464037 ) ) ;
#108382=CARTESIAN_POINT ( 'NONE',  ( -5.348676671532174076, 6.524419919965190218, 1.372383455774844219 ) ) ;
#108387=CARTESIAN_POINT ( 'NONE',  ( 9.625925876022625616, 11.29296361252366765, -1.082531754730537088 ) ) ;
#108389=CARTESIAN_POINT ( 'NONE',  ( 5.361359679200154105, 8.342337828120466980, 1.199719254218462483 ) ) ;
#108392=ORIENTED_EDGE ( 'NONE', *, *, #69865, .F. ) ;
#108394=CARTESIAN_POINT ( 'NONE',  ( 4.650610384687404952, 5.384465856012134566, 1.199719254218462483 ) ) ;
#108403=CARTESIAN_POINT ( 'NONE',  ( 9.097684769969825780, 10.57271930550834860, -1.199719254218446718 ) ) ;
#108404=CARTESIAN_POINT ( 'NONE',  ( -6.911959384868566758, 6.958374125301778790, 1.040834085586084257E-14 ) ) ;
#108412=CARTESIAN_POINT ( 'NONE',  ( 0.6823417656249917140, 4.342708333674755394, 1.181850606188765695 ) ) ;
#108413=CARTESIAN_POINT ( 'NONE',  ( 7.239690839573049708, 11.39013037956983965, 1.040834085586084257E-14 ) ) ;
#108414=CARTESIAN_POINT ( 'NONE',  ( -6.413170354464012846, 7.440785820751486312, 1.199719254218450271 ) ) ;
#108417=CARTESIAN_POINT ( 'NONE',  ( -1.500000000000057065, 7.361490936992524325, -4.203511340218408776 ) ) ;
#108418=CARTESIAN_POINT ( 'NONE',  ( 5.168682875307768931, 7.053215992657626110, -1.599625672291256295 ) ) ;
#108419=CARTESIAN_POINT ( 'NONE',  ( -5.005985031943793295, 6.863401842066301661, -1.599625672291256295 ) ) ;
#108424=ADVANCED_FACE ( 'NONE', ( #162422 ), #67490, .T. ) ;
#108426=CARTESIAN_POINT ( 'NONE',  ( 5.151735183512854199, 8.954182114166247430, -0.7216878364870257245 ) ) ;
#108429=CARTESIAN_POINT ( 'NONE',  ( 6.114364089638775646, 10.07724917131317355, 0.7216878364870438212 ) ) ;
#108430=CARTESIAN_POINT ( 'NONE',  ( 0.6823417656249917140, 3.405208333674754506, 1.181850606188765695 ) ) ;
#108432=CARTESIAN_POINT ( 'NONE',  ( 6.778713616708431644, 7.010846762355714468, 1.040834085586084257E-14 ) ) ;
#108441=CARTESIAN_POINT ( 'NONE',  ( -3.983506901647102083, 7.838413813543339437, 0.2012387096505599549 ) ) ;
#108449=CARTESIAN_POINT ( 'NONE',  ( 5.035963992472171746, 7.962709526937818083, 1.199719254218462483 ) ) ;
#108458=VERTEX_POINT ( 'NONE', #129995 ) ;
#108460=CARTESIAN_POINT ( 'NONE',  ( 4.582292731738905722, 5.408724944192588424, -1.082531754730548412 ) ) ;
#108461=CARTESIAN_POINT ( 'NONE',  ( -1.402160292154681736E-14, 1.509375000341420359, -1.575800808251659024 ) ) ;
#108463=CARTESIAN_POINT ( 'NONE',  ( 6.401421083946654100, 10.62007503124645957, -0.7998128361456291469 ) ) ;
#108466=CARTESIAN_POINT ( 'NONE',  ( -5.915435094264120508, 5.795762452929912101, 0.000000000000000000 ) ) ;
#108467=VERTEX_POINT ( 'NONE', #42283 ) ;
#108469=CARTESIAN_POINT ( 'NONE',  ( -1.500000000000013101, 3.129166666666689967, -0.8660254037844313801 ) ) ;
#108470=CARTESIAN_POINT ( 'NONE',  ( 6.796715079152391148, 6.823922435299587974, 0.7998128361456341429 ) ) ;
#108474=CARTESIAN_POINT ( 'NONE',  ( -1.201851678989727383E-14, 2.821875000341418804, 1.575800808251672791 ) ) ;
#108476=CARTESIAN_POINT ( 'NONE',  ( 9.408995418203963013, 12.00024729270324286, 1.443375672974076540 ) ) ;
#108479=DIRECTION ( 'NONE',  ( 1.000000000000000000, 0.000000000000000000, 0.000000000000000000 ) ) ;
#108482=CARTESIAN_POINT ( 'NONE',  ( 1.499999999999987121, 2.077083334016153415, -0.8660254037844262731 ) ) ;
#108485=CARTESIAN_POINT ( 'NONE',  ( -5.042743069279040036, 7.970618449879118828, 1.199719254218464037 ) ) ;
#108492=ORIENTED_EDGE ( 'NONE', *, *, #116347, .T. ) ;
#108494=CARTESIAN_POINT ( 'NONE',  ( 6.959412922516382771, 7.013736585890911535, 0.7998128361456341429 ) ) ;
#108497=DIRECTION ( 'NONE',  ( -0.6507913734559640506, -0.7592566023653004592, 0.000000000000000000 ) ) ;
#108498=CARTESIAN_POINT ( 'NONE',  ( 6.518772930072240790, 6.499656594706071822, -0.7998128361456281477 ) ) ;
#108503=CARTESIAN_POINT ( 'NONE',  ( 4.878236342818665250, 4.585697242910212523, 1.040834085586084257E-14 ) ) ;
#108508=CARTESIAN_POINT ( 'NONE',  ( 5.731063993565963521, 6.075950606329157289, 0.6577720730673256577 ) ) ;
#108513=DIRECTION ( 'NONE',  ( 0.000000000000000000, 1.000000000000000000, -8.546850786086437571E-32 ) ) ;
#108516=CARTESIAN_POINT ( 'NONE',  ( -1.458833446111217569, 8.740432391875483376, -2.548463833528520794 ) ) ;
#108517=CARTESIAN_POINT ( 'NONE',  ( 7.944714827928056167, 8.371181508778631652, 0.7216878364870458196 ) ) ;
#108519=CARTESIAN_POINT ( 'NONE',  ( -5.928993247877788697, 5.811580298812519807, 0.7998128361456341429 ) ) ;
#108520=CARTESIAN_POINT ( 'NONE',  ( -2.193105066167346795, 5.702484939155337607, 2.420000000000010587 ) ) ;
#108523=CARTESIAN_POINT ( 'NONE',  ( -6.566226467720086113, 6.555019055295208119, 1.040834085586084257E-14 ) ) ;
#108536=FACE_OUTER_BOUND ( 'NONE', #45774, .T. ) ;
#108537=CARTESIAN_POINT ( 'NONE',  ( 9.561524646135536543, 12.17819805862340310, -1.599625672291262513 ) ) ;
#108542=CARTESIAN_POINT ( 'NONE',  ( 8.499999999999980460, 6.200000000000038369, 2.900000000000013678 ) ) ;
#108544=CARTESIAN_POINT ( 'NONE',  ( -9.164948653157990677, 11.71552606681625619, -1.443375672974059665 ) ) ;
#108547=CARTESIAN_POINT ( 'NONE',  ( 8.106885785967500979, 11.54545161934907682, 1.199719254218460707 ) ) ;
#108552=CARTESIAN_POINT ( 'NONE',  ( -6.418895661066105873, 9.576129806964074120, -1.199719254218440723 ) ) ;
#108553=CARTESIAN_POINT ( 'NONE',  ( 3.798255590122797898, 7.583048621785260401, -0.7998128361456221525 ) ) ;
#108557=CARTESIAN_POINT ( 'NONE',  ( 5.183294799126148433, 4.941598775268944976, 1.040834085586084257E-14 ) ) ;
#108561=CARTESIAN_POINT ( 'NONE',  ( -1.364683531249997417, 2.571875000341422357, 1.214306433183764966E-14 ) ) ;
#108564=CARTESIAN_POINT ( 'NONE',  ( 5.938108093105483931, 8.911247961056314892, -1.082531754730537088 ) ) ;
#108572=CARTESIAN_POINT ( 'NONE',  ( 9.693716643646595799, 11.37205284141829686, 1.082531754730548412 ) ) ;
#108578=CARTESIAN_POINT ( 'NONE',  ( -8.666686507633592385, 11.13422023037111330, 1.599625672291269396 ) ) ;
#108595=CARTESIAN_POINT ( 'NONE',  ( 0.7499999999999902300, 1.764583334016148086, 1.299038105676657340 ) ) ;
#108601=CARTESIAN_POINT ( 'NONE',  ( -0.7500000000000215383, 0.4416666666666874130, 1.299038105676659116 ) ) ;
#108602=CARTESIAN_POINT ( 'NONE',  ( 7.507464373665139412, 9.781794407407920389, 1.599625672291281386 ) ) ;
#108603=CARTESIAN_POINT ( 'NONE',  ( -1.402160292154681736E-14, -0.8031249996585825279, -1.575800808251665908 ) ) ;
#108606=CARTESIAN_POINT ( 'NONE',  ( 9.788623719386617239, 11.48277776311499387, -1.082531754730537088 ) ) ;
#108607=CARTESIAN_POINT ( 'NONE',  ( -5.395781948558855845, 9.238903340053241209, 0.7216878364870458196 ) ) ;
#108612=CARTESIAN_POINT ( 'NONE',  ( -6.663996196316808174, 7.733415969579778171, -1.199719254218446718 ) ) ;
#108613=VERTEX_POINT ( 'NONE', #164539 ) ;
#108614=CARTESIAN_POINT ( 'NONE',  ( 1.499999999999987121, 2.077083334016153415, -0.8660254037844262731 ) ) ;
#108615=CARTESIAN_POINT ( 'NONE',  ( 1.364683531249990311, 3.696875000341416584, 1.214306433183764966E-14 ) ) ;
#108629=CARTESIAN_POINT ( 'NONE',  ( -8.045874094706015001, 11.47427131287732927, -1.199719254218446718 ) ) ;
#108630=CARTESIAN_POINT ( 'NONE',  ( 5.635385404774530649, 9.726366738878972740, 0.7998128361456462443 ) ) ;
#108631=CARTESIAN_POINT ( 'NONE',  ( 1.387358672531703974, 7.315968950352358391, 4.254625267140708544 ) ) ;
#108634=ORIENTED_EDGE ( 'NONE', *, *, #197058, .T. ) ;
#108637=CARTESIAN_POINT ( 'NONE',  ( -8.076906825439122528, 10.44614393447756129, -1.599625672291263179 ) ) ;
#108643=CARTESIAN_POINT ( 'NONE',  ( 3.083589872104280705, 5.684939719841914929, 1.199719254218450271 ) ) ;
#108646=CARTESIAN_POINT ( 'NONE',  ( -5.066996723205291708, 6.934582148538044777, 1.599625672291267398 ) ) ;
#108647=AXIS2_PLACEMENT_3D ( 'NONE', #187554, #191809, #89018 ) ;
#108648=CARTESIAN_POINT ( 'NONE',  ( -9.182950115157607840, 9.607863310639020327, 0.7998128361456462443 ) ) ;
#108658=CARTESIAN_POINT ( 'NONE',  ( 7.644099680006512187, 7.812537802962739697, 1.040834085586084257E-14 ) ) ;
#108660=CARTESIAN_POINT ( 'NONE',  ( -1.432341765624997709, 5.720312500512116038, 1.214306433183764966E-14 ) ) ;
#108677=CARTESIAN_POINT ( 'NONE',  ( 3.551873057100287223, 5.166937871415542283, 1.443375672974062551 ) ) ;
#108682=CARTESIAN_POINT ( 'NONE',  ( -9.809487834687324437, 11.40315621434539395, 1.199719254218462483 ) ) ;
#108684=CARTESIAN_POINT ( 'NONE',  ( 6.546325832964355662, 5.229711127717882491, -2.448021111374927283 ) ) ;
#108685=CARTESIAN_POINT ( 'NONE',  ( 2.372313692266983853, 5.711523707712699682, 0.7216878364870438212 ) ) ;
#108689=B_SPLINE_CURVE_WITH_KNOTS ( 'NONE', 3,
 ( #93970, #207683, #139515, #59303 ),
 .UNSPECIFIED., .F., .F.,
 ( 4, 4 ),
 ( 6.034005962835825582E-05, 0.0001895969026200138800 ),
 .UNSPECIFIED. ) ;
#108695=CARTESIAN_POINT ( 'NONE',  ( -1.364683531250014514, 0.7385416670080887647, -0.7879004041258289570 ) ) ;
#108697=VERTEX_POINT ( 'NONE', #186107 ) ;
#108701=CARTESIAN_POINT ( 'NONE',  ( -3.903858165731105778, 6.641919395739846799, 1.199719254218464037 ) ) ;
#108704=CARTESIAN_POINT ( 'NONE',  ( -1.500000000000015099, 0.1291666666666918539, -0.8660254037844383745 ) ) ;
#108706=CARTESIAN_POINT ( 'NONE',  ( -0.6823417656250246877, -1.136458332991911790, 1.181850606188755259 ) ) ;
#108712=CARTESIAN_POINT ( 'NONE',  ( -1.364683531250014514, -0.2614583329919080157, -0.7879004041258359514 ) ) ;
#108715=CARTESIAN_POINT ( 'NONE',  ( -6.877010230629689858, 9.046264573866535486, 1.599625672291283607 ) ) ;
#108716=CARTESIAN_POINT ( 'NONE',  ( 7.567422294721922960, 11.98040977715095323, 0.7998128361456462443 ) ) ;
#108723=CARTESIAN_POINT ( 'NONE',  ( 1.364683531249986537, 0.6760416670080884316, 0.7879004041258500513 ) ) ;
#108731=CARTESIAN_POINT ( 'NONE',  ( 6.982085921357777281, 7.248114451113292667, 1.040834085586084257E-14 ) ) ;
#108734=CARTESIAN_POINT ( 'NONE',  ( -4.771579997005698459, 7.654261532226910525, -1.199719254218452047 ) ) ;
#108738=CARTESIAN_POINT ( 'NONE',  ( -2.266184231778562541, 5.795632037050281404, 1.040834085586084257E-14 ) ) ;
#108739=CARTESIAN_POINT ( 'NONE',  ( 5.083944415000174466, 7.914723669933440675, -1.082531754730549078 ) ) ;
#108740=CARTESIAN_POINT ( 'NONE',  ( -8.961576348508652146, 10.51788916375733685, -1.082531754730543083 ) ) ;
#108742=CARTESIAN_POINT ( 'NONE',  ( -0.7499999999999972244, 3.358333333333359150, -1.299038105676652011 ) ) ;
#108746=CARTESIAN_POINT ( 'NONE',  ( 8.581948047770334043, 12.95609712246668899, 0.000000000000000000 ) ) ;
#108753=VERTEX_POINT ( 'NONE', #112410 ) ;
#108759=ORIENTED_EDGE ( 'NONE', *, *, #4855, .F. ) ;
#108760=CARTESIAN_POINT ( 'NONE',  ( 7.727784369665023689, 11.95957283134381477, 1.040834085586084257E-14 ) ) ;
#108762=CARTESIAN_POINT ( 'NONE',  ( 6.726816770674637347, 10.99970333242910669, -0.7998128361456291469 ) ) ;
#108768=CARTESIAN_POINT ( 'NONE',  ( 3.226477370372293763, 6.708047998835573900, 0.7216878364870317197 ) ) ;
#108770=CARTESIAN_POINT ( 'NONE',  ( -8.568389894156720032, 10.05917163368005163, 1.082531754730558626 ) ) ;
#108774=CARTESIAN_POINT ( 'NONE',  ( -3.440018289565379028, 5.036440642624797626, 1.599625672291267398 ) ) ;
#108798=CARTESIAN_POINT ( 'NONE',  ( -7.063961727919978451, 8.200042423116789436, 1.199719254218450271 ) ) ;
#108803=CARTESIAN_POINT ( 'NONE',  ( 5.449487677688982679, 8.445153826357429949, -1.199719254218446718 ) ) ;
#108807=CARTESIAN_POINT ( 'NONE',  ( 4.227444969362701421, 3.826440640544909400, 1.214306433183764966E-14 ) ) ;
#108813=CARTESIAN_POINT ( 'NONE',  ( -4.874319919312905647, 5.645460313075203018, -1.199719254218446718 ) ) ;
#108816=CARTESIAN_POINT ( 'NONE',  ( 7.938462636001388795, 9.220293482545153907, -1.199719254218441611 ) ) ;
#108817=CARTESIAN_POINT ( 'NONE',  ( -1.201851678989727383E-14, 3.946875000341423689, -1.575800808251660134 ) ) ;
#108819=CARTESIAN_POINT ( 'NONE',  ( 5.951559787436734084, 6.118878616701469042, 0.7174803059855124898 ) ) ;
#108825=CARTESIAN_POINT ( 'NONE',  ( 7.415946836550727284, 7.754285518838408109, 0.7216878364870317197 ) ) ;
#108826=CARTESIAN_POINT ( 'NONE',  ( -6.496328159242330536, 10.73079995242472862, 0.000000000000000000 ) ) ;
#108829=CARTESIAN_POINT ( 'NONE',  ( -9.508345801885592863, 9.987491611821676329, 0.7998128361456462443 ) ) ;
#108830=CARTESIAN_POINT ( 'NONE',  ( -5.201524489137236529, 9.220195670635433771, 0.7998128361456481317 ) ) ;
#108837=CARTESIAN_POINT ( 'NONE',  ( 9.101601193475611140, 9.512956235343358102, -0.7998128361456221525 ) ) ;
#108842=DIRECTION ( 'NONE',  ( 0.6507913734559712671, -0.7592566023652943530, 0.000000000000000000 ) ) ;
#108850=CARTESIAN_POINT ( 'NONE',  ( 1.499999999999989120, 5.045833333333354709, -0.8660254037844323793 ) ) ;
#108851=CARTESIAN_POINT ( 'NONE',  ( 3.798255590122797898, 7.583048621785260401, -0.7998128361456221525 ) ) ;
#108852=CARTESIAN_POINT ( 'NONE',  ( 5.282873410819217241, 9.315102745931094219, -0.7998128361456281477 ) ) ;
#108855=CARTESIAN_POINT ( 'NONE',  ( 5.165293337126522388, 8.969999960048859577, 1.040834085586084257E-14 ) ) ;
#108856=CARTESIAN_POINT ( 'NONE',  ( -7.795575137733361970, 12.03866206075687018, 0.7216878364870458196 ) ) ;
#108860=CARTESIAN_POINT ( 'NONE',  ( 9.752392566931574081, 10.27221283770866300, -0.7998128361456281477 ) ) ;
#108863=CARTESIAN_POINT ( 'NONE',  ( -3.898132859128961236, 4.506575409527250997, -1.199719254218452047 ) ) ;
#108865=CIRCLE ( 'NONE', #205574, 0.08000000000000008493 ) ;
#108867=CARTESIAN_POINT ( 'NONE',  ( 0.6823417656249882723, 1.176041667008083325, -1.181850606188749264 ) ) ;
#108873=CARTESIAN_POINT ( 'NONE',  ( -1.402160292154681736E-14, 0.07187500034142156602, 1.575800808251672791 ) ) ;
#108875=CARTESIAN_POINT ( 'NONE',  ( 10.40996301719436090, 11.03937836301526687, 0.000000000000000000 ) ) ;
#108879=CARTESIAN_POINT ( 'NONE',  ( -9.236128959407555072, 11.79856975744075598, -1.599625672291263179 ) ) ;
#108886=CARTESIAN_POINT ( 'NONE',  ( 4.059776932288224671, 6.823824623389866950, 1.199719254218462483 ) ) ;
#108892=CARTESIAN_POINT ( 'NONE',  ( 9.108380270282433244, 9.520865158284665952, 1.040834085586084257E-14 ) ) ;
#108894=CARTESIAN_POINT ( 'NONE',  ( 0.2466033008277778715, 2.800000000000024691, -1.444539947226808341 ) ) ;
#108895=CARTESIAN_POINT ( 'NONE',  ( -3.744022975668147790, 7.519777238254810925, -0.7998128361456281477 ) ) ;
#108899=CARTESIAN_POINT ( 'NONE',  ( 8.263858322729371153, 9.599921783727809910, -1.199719254218446718 ) ) ;
#108901=CARTESIAN_POINT ( 'NONE',  ( 6.076025397218672630, 10.24044673006381245, -0.7998128361456291469 ) ) ;
#108904=CARTESIAN_POINT ( 'NONE',  ( -8.432808358020034589, 10.86136238915529084, 1.443375672974064550 ) ) ;
#108912=CARTESIAN_POINT ( 'NONE',  ( -6.070455375431035527, 6.038045056918933895, -0.4763334965118305453 ) ) ;
#108913=CARTESIAN_POINT ( 'NONE',  ( -0.6823417656250003738, 1.467708333674752730, -1.181850606188749264 ) ) ;
#108915=CARTESIAN_POINT ( 'NONE',  ( 5.938108093105483931, 8.911247961056314892, -1.082531754730537088 ) ) ;
#108929=LINE ( 'NONE', #63308, #4102 ) ;
#108933=CARTESIAN_POINT ( 'NONE',  ( 9.206149998879153529, 10.69926207256923689, 1.199719254218453823 ) ) ;
#108937=CARTESIAN_POINT ( 'NONE',  ( -3.164938793786285842, 5.779846795137578930, -1.199719254218452935 ) ) ;
#108938=CARTESIAN_POINT ( 'NONE',  ( -7.393273838153706201, 7.519907654134449615, 0.7998128361456341429 ) ) ;
#108944=CARTESIAN_POINT ( 'NONE',  ( 1.499999999999989120, 4.827083334016149863, -0.8660254037844323793 ) ) ;
#108945=CARTESIAN_POINT ( 'NONE',  ( 7.832860060393120882, 10.16142270859057462, 1.599625672291281386 ) ) ;
#108948=CARTESIAN_POINT ( 'NONE',  ( -7.609150525767646833, 9.900428251527500834, -1.599625672291263179 ) ) ;
#108950=CARTESIAN_POINT ( 'NONE',  ( -1.364683531249997417, 5.009375000341425022, 1.214306433183764966E-14 ) ) ;
#108952=CARTESIAN_POINT ( 'NONE',  ( -1.499999999998127498, 8.654187183607668032, 2.562246142702330864 ) ) ;
#108953=CARTESIAN_POINT ( 'NONE',  ( 2.885543303398817372, 6.439774126353135841, -0.3727371597862367270 ) ) ;
#108956=CARTESIAN_POINT ( 'NONE',  ( -7.185458225562757484, 11.32685899655781903, 0.7216878364870458196 ) ) ;
#108960=CARTESIAN_POINT ( 'NONE',  ( -1.201851678989727383E-14, 3.009375000341419248, -1.575800808251660134 ) ) ;
#108967=CARTESIAN_POINT ( 'NONE',  ( -1.001543065824772872E-14, 4.571875000341418804, 1.575800808251672791 ) ) ;
#108969=CARTESIAN_POINT ( 'NONE',  ( -3.574546055497324737, 7.322054164722185732, 0.7998128361456341429 ) ) ;
#108970=CARTESIAN_POINT ( 'NONE',  ( 5.099838337034727331, 9.101561826515851550, -0.7998128361456281477 ) ) ;
#108974=CARTESIAN_POINT ( 'NONE',  ( 1.364683531249990311, 4.196875000341417028, 1.214306433183764966E-14 ) ) ;
#108978=CARTESIAN_POINT ( 'NONE',  ( -1.364683531250014514, -0.01145833299191483488, -0.7879004041258359514 ) ) ;
#108979=CARTESIAN_POINT ( 'NONE',  ( -5.111060722671894929, 5.065251719313053513, 0.000000000000000000 ) ) ;
#108983=CARTESIAN_POINT ( 'NONE',  ( 2.711267533052988732, 6.106969855296372707, -0.7216878364870267237 ) ) ;
#108986=CARTESIAN_POINT ( 'NONE',  ( -7.673551755654729689, 11.89630144833179060, 0.7216878364870458196 ) ) ;
#108993=CARTESIAN_POINT ( 'NONE',  ( -5.219525951136845698, 8.072902128759544382, -1.082531754730543971 ) ) ;
#108995=CARTESIAN_POINT ( 'NONE',  ( -0.6823417656250212460, 1.113541667008083325, 1.181850606188755259 ) ) ;
#109001=CARTESIAN_POINT ( 'NONE',  ( 1.364683531249986537, -0.5739583329919174526, 0.7879004041258500513 ) ) ;
#109007=CARTESIAN_POINT ( 'NONE',  ( 1.499999999999987121, -0.7458333333333122539, 0.8660254037844524744 ) ) ;
#109008=CARTESIAN_POINT ( 'NONE',  ( 9.381879110532285182, 10.04787317181692075, 0.000000000000000000 ) ) ;
#109018=CARTESIAN_POINT ( 'NONE',  ( -3.358669367883384105, 4.941533567329135401, -1.599625672291262513 ) ) ;
#109020=DIRECTION ( 'NONE',  ( 1.000000000000000000, 1.156482317317871725E-15, 0.000000000000000000 ) ) ;
#109023=CARTESIAN_POINT ( 'NONE',  ( -1.364683531250000748, 2.321875000341422357, 1.214306433183764966E-14 ) ) ;
#109035=CARTESIAN_POINT ( 'NONE',  ( -0.5973138996857457750, 6.735707300253057639, -3.614276400337344874 ) ) ;
#109038=ORIENTED_EDGE ( 'NONE', *, *, #8106, .T. ) ;
#109042=CARTESIAN_POINT ( 'NONE',  ( 5.656776405399742025, 7.622658444431597680, -1.599625672291262513 ) ) ;
#109047=CARTESIAN_POINT ( 'NONE',  ( 3.017802228139008225, 6.452510944783090174, -0.1818790228878484905 ) ) ;
#109049=CARTESIAN_POINT ( 'NONE',  ( 7.584896871841365851, 10.93646455286856956, -1.199719254218446718 ) ) ;
#109050=CARTESIAN_POINT ( 'NONE',  ( 3.158686601859607812, 6.628958768904106513, -0.7216878364870269458 ) ) ;
#109052=CARTESIAN_POINT ( 'NONE',  ( 9.154780037725547714, 11.70366268214508487, 1.599625672291279388 ) ) ;
#109055=CARTESIAN_POINT ( 'NONE',  ( -3.054546515950523400, 6.451825606165701998, 0.6676900015689657408 ) ) ;
#109059=VERTEX_POINT ( 'NONE', #192507 ) ;
#109060=CARTESIAN_POINT ( 'NONE',  ( 9.911173986789782120, 11.52179005846497972, -1.199719254218440723 ) ) ;
#109067=CARTESIAN_POINT ( 'NONE',  ( -7.673551755654729689, 11.89630144833179060, 0.7216878364870458196 ) ) ;
#109072=CARTESIAN_POINT ( 'NONE',  ( -8.462260433223891098, 13.02438760540324481, -0.7998128361456281477 ) ) ;
#109074=CARTESIAN_POINT ( 'NONE',  ( -4.811125034100962594, 6.783301700437176507, -1.284903130169626539 ) ) ;
#109081=CARTESIAN_POINT ( 'NONE',  ( 4.826339496340538382, 4.733076955259818419, 1.040834085586084257E-14 ) ) ;
#109089=CARTESIAN_POINT ( 'NONE',  ( -4.218558352146454915, 8.073401844146177453, 1.040834085586084257E-14 ) ) ;
#109091=CARTESIAN_POINT ( 'NONE',  ( -3.541704441667874903, 5.155074486744371853, -1.599625672291256295 ) ) ;
#109098=CARTESIAN_POINT ( 'NONE',  ( -0.6823417656250212460, 4.613541667008086655, 1.181850606188767472 ) ) ;
#109101=CARTESIAN_POINT ( 'NONE',  ( 3.811813743736467419, 7.598866467667865443, 1.040834085586084257E-14 ) ) ;
#109103=CARTESIAN_POINT ( 'NONE',  ( 1.522028533774268277, 8.691231065131713507, 2.524624912498933504 ) ) ;
#109115=CARTESIAN_POINT ( 'NONE',  ( 1.364683531249988757, 1.446875000341421469, 0.000000000000000000 ) ) ;
#109117=CARTESIAN_POINT ( 'NONE',  ( 4.111146893441827821, 5.819424013814004759, 1.599625672291267398 ) ) ;
#109119=CARTESIAN_POINT ( 'NONE',  ( -5.965224400332865606, 7.022145224218852455, 1.082531754730549967 ) ) ;
#109120=CARTESIAN_POINT ( 'NONE',  ( 2.724825686666657809, 6.122787701178987518, 0.000000000000000000 ) ) ;
#109122=CARTESIAN_POINT ( 'NONE',  ( -7.524412065460066579, 7.880828285899290186, 0.7216878364870317197 ) ) ;
#109127=CARTESIAN_POINT ( 'NONE',  ( 6.449928391799196525, 8.548002428564306143, -1.599625672291262513 ) ) ;
#109129=CARTESIAN_POINT ( 'NONE',  ( -3.673896439623323129, 4.156855427197417185, 1.000000000000009548 ) ) ;
#109130=EDGE_CURVE ( 'NONE', #2289, #1199, #61455, .T. ) ;
#109133=CARTESIAN_POINT ( 'NONE',  ( 0.6823417656249917140, 5.592708333674749177, 1.181850606188765695 ) ) ;
#109137=CARTESIAN_POINT ( 'NONE',  ( 5.686755365928134687, 8.721966129303114101, 1.199719254218462483 ) ) ;
#109140=CARTESIAN_POINT ( 'NONE',  ( -7.552055258011950656, 8.769484874890757453, 1.199719254218462483 ) ) ;
#109145=CARTESIAN_POINT ( 'NONE',  ( 6.577677080924314801, 10.82570702772039262, 1.040834085586084257E-14 ) ) ;
#109148=CARTESIAN_POINT ( 'NONE',  ( -7.888146445052511169, 8.097259028849730811, 1.040834085586084257E-14 ) ) ;
#109150=CARTESIAN_POINT ( 'NONE',  ( 7.036318535368067728, 10.19249347702934294, -1.082531754730537976 ) ) ;
#109151=CARTESIAN_POINT ( 'NONE',  ( 4.037917249208685000, 7.776151245443112536, -0.4343759663945709892 ) ) ;
#109152=CARTESIAN_POINT ( 'NONE',  ( -6.084912014434944894, 5.993485526462540847, -0.7998128361456291469 ) ) ;
#109157=CARTESIAN_POINT ( 'NONE',  ( 6.308621549060418054, 6.254479983525607523, 0.7998128361456341429 ) ) ;
#109159=CARTESIAN_POINT ( 'NONE',  ( 9.348510611822643313, 10.86534945433664134, 1.199719254218453823 ) ) ;
#109160=CARTESIAN_POINT ( 'NONE',  ( -5.485560113408387117, 6.267152048184752466, 0.9985905309092910631 ) ) ;
#109162=CARTESIAN_POINT ( 'NONE',  ( 1.364683531249986537, 0.8635416670080893198, 0.7879004041258500513 ) ) ;
#109164=CARTESIAN_POINT ( 'NONE',  ( -5.992340707560165569, 8.014150130285418783, 1.443375672974064550 ) ) ;
#109170=CARTESIAN_POINT ( 'NONE',  ( -5.471750928372196121, 6.276313537582185909, 1.010767274114855008 ) ) ;
#109171=CARTESIAN_POINT ( 'NONE',  ( -1.201851678989727383E-14, 1.634375000341421025, 1.575800808251672791 ) ) ;
#109174=CARTESIAN_POINT ( 'NONE',  ( 4.392478581147586603, 4.226905887534702977, -0.7216878364870188411 ) ) ;
#109179=CARTESIAN_POINT ( 'NONE',  ( -8.310784975052682100, 10.71900177569337487, -1.443375672974058777 ) ) ;
#109187=CARTESIAN_POINT ( 'NONE',  ( -7.931156673870055407, 11.23647130528163096, 1.082531754730549967 ) ) ;
#109190=B_SPLINE_CURVE_WITH_KNOTS ( 'NONE', 3,
 ( #174116, #91797, #157854, #171957, #9448, #189265, #173034 ),
 .UNSPECIFIED., .F., .F.,
 ( 4, 3, 4 ),
 ( 5.085429910792683232E-15, 2.761892602843915009E-05, 5.460426739256992639E-05 ),
 .UNSPECIFIED. ) ;
#109192=DIRECTION ( 'NONE',  ( 0.6507913734559640506, -0.7592566023653004592, 0.000000000000000000 ) ) ;
#109195=CARTESIAN_POINT ( 'NONE',  ( -6.195713011320783892, 10.17215624660883577, -0.7216878364870267237 ) ) ;
#109200=CARTESIAN_POINT ( 'NONE',  ( -1.499999999999997780, 4.181250000682819490, 1.214306433183764966E-14 ) ) ;
#109204=ORIENTED_EDGE ( 'NONE', *, *, #61776, .F. ) ;
#109207=CARTESIAN_POINT ( 'NONE',  ( -7.152089726408780379, 8.302858421353754181, -1.199719254218446718 ) ) ;
#109210=EDGE_CURVE ( 'NONE', #108613, #205532, #47367, .T. ) ;
#109212=CARTESIAN_POINT ( 'NONE',  ( 3.662674053986138656, 7.424870162959149589, 0.7998128361456321445 ) ) ;
#109217=CARTESIAN_POINT ( 'NONE',  ( 7.470706336329915764, 8.674577799595093452, -1.199719254218441611 ) ) ;
#109221=VERTEX_POINT ( 'NONE', #63591 ) ;
#109225=CARTESIAN_POINT ( 'NONE',  ( -4.256897045010916258, 7.910204285913967404, 0.7216878364870317197 ) ) ;
#109228=CARTESIAN_POINT ( 'NONE',  ( 3.389175213736273840, 6.897862149426906342, 0.7216878364870233931 ) ) ;
#109234=CARTESIAN_POINT ( 'NONE',  ( -9.189729191964438826, 9.615772233580322848, 1.040834085586084257E-14 ) ) ;
#109236=CARTESIAN_POINT ( 'NONE',  ( 8.620286740190458374, 8.951422706510690830, 1.040834085586084257E-14 ) ) ;
#109237=CARTESIAN_POINT ( 'NONE',  ( 1.499999999999987121, -0.2458333333333099502, 0.8660254037844524744 ) ) ;
#109238=CARTESIAN_POINT ( 'NONE',  ( -8.690940161559884913, 10.09818392903003748, 1.199719254218462483 ) ) ;
#109241=CARTESIAN_POINT ( 'NONE',  ( -1.364683531250012516, 3.030208333674755394, 0.7879004041258379498 ) ) ;
#109244=CARTESIAN_POINT ( 'NONE',  ( 10.24960094225127172, 11.06021530882240356, -0.7216878364870257245 ) ) ;
#109247=CARTESIAN_POINT ( 'NONE',  ( -1.499999999999997780, 5.650000000000023448, 1.214306433183764966E-14 ) ) ;
#109250=CARTESIAN_POINT ( 'NONE',  ( 9.205623113554628034, 9.842241175342985926, 0.7216878364870458196 ) ) ;
#109253=CARTESIAN_POINT ( 'NONE',  ( -5.246642258808529746, 9.064907035344523578, 0.000000000000000000 ) ) ;
#109255=CARTESIAN_POINT ( 'NONE',  ( -1.201851678989727383E-14, 2.571875000341417472, 1.575800808251672791 ) ) ;
#109259=CARTESIAN_POINT ( 'NONE',  ( -7.881367368245678406, 8.089350105908421185, 0.7998128361456602331 ) ) ;
#109260=CARTESIAN_POINT ( 'NONE',  ( -1.001543065824772872E-14, 5.134375000341421469, 1.575800808251672791 ) ) ;
#109265=CARTESIAN_POINT ( 'NONE',  ( 9.759171643738394408, 10.28012176064996197, 0.000000000000000000 ) ) ;
#109268=CARTESIAN_POINT ( 'NONE',  ( 1.499999999999989120, 1.525000000000019451, 0.000000000000000000 ) ) ;
#109272=CARTESIAN_POINT ( 'NONE',  ( 7.958272981541723468, 8.386999354661243800, 1.040834085586084257E-14 ) ) ;
#109274=CARTESIAN_POINT ( 'NONE',  ( 10.40996301719436090, 11.03937836301526687, 0.000000000000000000 ) ) ;
#109279=CARTESIAN_POINT ( 'NONE',  ( 7.456094412511537151, 10.78619501698377370, 1.199719254218460707 ) ) ;
#109280=CARTESIAN_POINT ( 'NONE',  ( -4.342209589451060836, 5.574336833734898633, -1.249999994511378887 ) ) ;
#109283=CARTESIAN_POINT ( 'NONE',  ( -1.364683531250010295, 5.301041667008085767, -0.7879004041258300672 ) ) ;
#109287=CARTESIAN_POINT ( 'NONE',  ( -4.889337272013151825, 4.909234758358784312, -0.4031905389056227307 ) ) ;
#109289=CARTESIAN_POINT ( 'NONE',  ( -0.6823417656249969321, 3.467708333674754506, -1.181850606188749264 ) ) ;
#109291=CARTESIAN_POINT ( 'NONE',  ( -5.233084105194862445, 9.049089189461916760, 0.7216878364870458196 ) ) ;
#109299=VERTEX_POINT ( 'NONE', #133957 ) ;
#109300=CARTESIAN_POINT ( 'NONE',  ( 9.576136569953906275, 10.06658084123472641, 0.000000000000000000 ) ) ;
#109301=CARTESIAN_POINT ( 'NONE',  ( 4.816739869979735467, 5.096136759539821703, 0.7457829957396797660 ) ) ;
#109306=CARTESIAN_POINT ( 'NONE',  ( -9.657485491635913633, 10.16148791653038330, 1.040834085586084257E-14 ) ) ;
#109307=CARTESIAN_POINT ( 'NONE',  ( 7.332262146892202459, 7.448727347662698506, -0.7998128361456281477 ) ) ;
#109309=CARTESIAN_POINT ( 'NONE',  ( 3.158686601859607368, 6.628958768904106513, -0.7216878364870267237 ) ) ;
#109312=CARTESIAN_POINT ( 'NONE',  ( 3.174580523894166006, 6.855427711185178019, 0.7998128361456341429 ) ) ;
#109321=( BOUNDED_CURVE ( )  B_SPLINE_CURVE ( 2, ( #197952, #14923, #81016, #147105, #213129, #146047, #130901 ),
 .UNSPECIFIED., .F., .T. ) 
 B_SPLINE_CURVE_WITH_KNOTS ( ( 3, 2, 2, 3 ),
 ( 0.2250000000000001998, 0.2291666666666669072, 0.2333333333333336701, 0.2375000000000003775 ),
 .UNSPECIFIED. ) 
 CURVE ( )  GEOMETRIC_REPRESENTATION_ITEM ( )  RATIONAL_B_SPLINE_CURVE ( ( 0.9999999999999937828, 0.8660254037844449249, 1.000000000000000000, 0.8660254037844387076, 1.000000000000000000, 0.8660254037844261621, 1.000000000000012434 ) ) 
 REPRESENTATION_ITEM ( '' )  );
#109322=CARTESIAN_POINT ( 'NONE',  ( -5.910991785878170646, 7.919243054989755670, -1.443375672974059665 ) ) ;
#109324=CARTESIAN_POINT ( 'NONE',  ( 4.844340958784499662, 4.546152628203684820, 0.7998128361456341429 ) ) ;
#109327=CARTESIAN_POINT ( 'NONE',  ( -8.667740277838301921, 9.006785167099828016, -0.7998128361456291469 ) ) ;
#109332=CARTESIAN_POINT ( 'NONE',  ( -9.182950115157607840, 9.607863310639020327, 0.7998128361456462443 ) ) ;
#109335=ADVANCED_FACE ( 'NONE', ( #115592 ), #50533, .F. ) ;
#109336=CARTESIAN_POINT ( 'NONE',  ( 6.109920781252839994, 10.27999134477033216, 1.040834085586084257E-14 ) ) ;
#109337=CARTESIAN_POINT ( 'NONE',  ( 5.335297142177534369, 6.183267073083954735, -1.199719254218452047 ) ) ;
#109349=CARTESIAN_POINT ( 'NONE',  ( -6.320072162264675164, 10.52516795595079557, 0.7998128361456481317 ) ) ;
#109352=CARTESIAN_POINT ( 'NONE',  ( 6.805829924380114804, 8.002851668940699881, 1.082531754730558626 ) ) ;
#109356=CARTESIAN_POINT ( 'NONE',  ( -5.063080299699540987, 7.994345218703034384, 1.199719254218464037 ) ) ;
#109359=CARTESIAN_POINT ( 'NONE',  ( -1.001543065824772872E-14, 5.493750000682816825, 1.732050807568877637 ) ) ;
#109367=CARTESIAN_POINT ( 'NONE',  ( 6.428537391173986038, 10.65171072301167854, 0.7998128361456462443 ) ) ;
#109369=CARTESIAN_POINT ( 'NONE',  ( -3.389175213736311587, 4.977123720824209840, 1.443375672974064550 ) ) ;
#109372=CARTESIAN_POINT ( 'NONE',  ( -5.289711001425910553, 6.400709951683444920, -1.138330407662338617 ) ) ;
#109379=CARTESIAN_POINT ( 'NONE',  ( 4.142179624174931796, 4.791296635414242111, 1.199719254218464037 ) ) ;
#109383=ADVANCED_FACE ( 'NONE', ( #181586 ), #14818, .F. ) ;
#109400=CARTESIAN_POINT ( 'NONE',  ( -4.924636110261798372, 6.768494766770632332, 1.599625672291267398 ) ) ;
#109401=CARTESIAN_POINT ( 'NONE',  ( 4.161989969270883272, 7.799479364217271282, 0.7216878364870317197 ) ) ;
#109402=CARTESIAN_POINT ( 'NONE',  ( 1.499999999999989120, 3.504166666666683749, 0.8660254037844524744 ) ) ;
#109404=CARTESIAN_POINT ( 'NONE',  ( -4.485049888022365927, 4.126979712314507331, 0.7998128361456341429 ) ) ;
#109409=CARTESIAN_POINT ( 'NONE',  ( -1.364683531249997417, 5.259375000341425022, 1.214306433183764966E-14 ) ) ;
#109412=CARTESIAN_POINT ( 'NONE',  ( -2.629918611371007575, 6.012062780000711371, 0.7216878364870317197 ) ) ;
#109417=CARTESIAN_POINT ( 'NONE',  ( 3.167801447087334576, 6.847518788243868393, -0.7998128361456291469 ) ) ;
#109418=FACE_OUTER_BOUND ( 'NONE', #43983, .T. ) ;
#109419=CARTESIAN_POINT ( 'NONE',  ( 3.946537740505243974, 2.817530495244580102, -0.7749999999999935829 ) ) ;
#109422=CARTESIAN_POINT ( 'NONE',  ( 1.364683531249986537, 0.9260416670080896528, 0.7879004041258500513 ) ) ;
#109425=CARTESIAN_POINT ( 'NONE',  ( -8.890396042259075315, 11.39521468743417998, -1.599625672291263179 ) ) ;
#109426=CARTESIAN_POINT ( 'NONE',  ( -6.548225005276122168, 6.741943382351338165, 0.7216878364870317197 ) ) ;
#109430=CARTESIAN_POINT ( 'NONE',  ( -1.001543065824772872E-14, 4.821875000341419693, 1.575800808251672791 ) ) ;
#109438=CARTESIAN_POINT ( 'NONE',  ( -6.209271164934474285, 6.346497235286081562, 1.040834085586084257E-14 ) ) ;
#109443=CARTESIAN_POINT ( 'NONE',  ( -5.219525951136850139, 7.112532914458205013, -1.443375672974051449 ) ) ;
#109445=CARTESIAN_POINT ( 'NONE',  ( 8.561083932025322696, 12.07534945641652158, -1.199719254218446718 ) ) ;
#109456=CARTESIAN_POINT ( 'NONE',  ( -3.391510981712833939, 7.108513245306943062, 0.7998128361456341429 ) ) ;
#109457=CARTESIAN_POINT ( 'NONE',  ( -4.328202132483162323, 7.418225535201088405, 1.151854025577046636 ) ) ;
#109459=CARTESIAN_POINT ( 'NONE',  ( -0.7500000000000215383, 1.441666666666688190, 1.299038105676659116 ) ) ;
#109461=CARTESIAN_POINT ( 'NONE',  ( 8.975134502566660899, 10.53370701015836275, -1.082531754730543083 ) ) ;
#109462=CARTESIAN_POINT ( 'NONE',  ( 6.714312387265682247, 8.856450423275211037, 1.599625672291281386 ) ) ;
#109466=DIRECTION ( 'NONE',  ( 0.000000000000000000, 1.000000000000000000, -8.546850786086437571E-32 ) ) ;
#109467=CARTESIAN_POINT ( 'NONE',  ( 5.027376032568989572, 4.759693547618927489, 0.7998128361456341429 ) ) ;
#109468=CARTESIAN_POINT ( 'NONE',  ( -0.3088250840613139814, 7.211283896344582445, -2.083830622148103995 ) ) ;
#109475=CARTESIAN_POINT ( 'NONE',  ( 9.745613490124728884, 10.26430391476735338, 0.7998128361456462443 ) ) ;
#109476=CARTESIAN_POINT ( 'NONE',  ( -7.088215381846223906, 7.164006121775713609, 0.7998128361456341429 ) ) ;
#109483=AXIS2_PLACEMENT_3D ( 'NONE', #3509, #102108, #168179 ) ;
#109484=CARTESIAN_POINT ( 'NONE',  ( 0.6823417656249899377, 3.676041667008085767, -1.181850606188754593 ) ) ;
#109485=CARTESIAN_POINT ( 'NONE',  ( 8.880227426826634129, 11.38335130276301754, 1.443375672974076540 ) ) ;
#109486=CARTESIAN_POINT ( 'NONE',  ( -6.575868197828002693, 7.630599971342813426, 1.199719254218450271 ) ) ;
#109489=CARTESIAN_POINT ( 'NONE',  ( 4.710568305744190276, 7.583081225755162968, 1.199719254218462483 ) ) ;
#109490=CARTESIAN_POINT ( 'NONE',  ( -4.577849422908604637, 8.492574760035358494, -0.7998128361456281477 ) ) ;
#109495=CARTESIAN_POINT ( 'NONE',  ( 7.293923454472091450, 7.611924906413328529, 0.7216878364870317197 ) ) ;
#109498=CARTESIAN_POINT ( 'NONE',  ( 0.6823417656249882723, 2.488541667008084435, -1.181850606188749264 ) ) ;
#109500=CARTESIAN_POINT ( 'NONE',  ( 6.277061933002785032, 7.385955679000473673, 1.082531754730558626 ) ) ;
#109502=CARTESIAN_POINT ( 'NONE',  ( -4.636525346193588248, 4.511627113421689650, 0.7216878364870317197 ) ) ;
#109509=CARTESIAN_POINT ( 'NONE',  ( -4.074744958279661766, 7.716589449174610316, -0.6783282581392232613 ) ) ;
#109515=AXIS2_PLACEMENT_3D ( 'NONE', #4485, #49025, #19696 ) ;
#109517=CARTESIAN_POINT ( 'NONE',  ( 5.686755365928134687, 8.721966129303114101, 1.199719254218462483 ) ) ;
#109520=CARTESIAN_POINT ( 'NONE',  ( 4.207107738942202246, 3.802713871720993399, 1.214306433183764966E-14 ) ) ;
#109523=ADVANCED_FACE ( 'NONE', ( #33215 ), #179487, .T. ) ;
#109529=CARTESIAN_POINT ( 'NONE',  ( 3.538314903486612817, 7.071858454135611538, 1.040834085586084257E-14 ) ) ;
#109531=CARTESIAN_POINT ( 'NONE',  ( 1.364683531249990311, 2.696875000341415696, 1.214306433183764966E-14 ) ) ;
#109533=CARTESIAN_POINT ( 'NONE',  ( 7.239163954692881653, 10.53310948286200599, -1.199719254218441611 ) ) ;
#109540=ORIENTED_EDGE ( 'NONE', *, *, #107896, .T. ) ;
#109542=CARTESIAN_POINT ( 'NONE',  ( -1.500000000000013101, 2.629166666666687746, -0.8660254037844313801 ) ) ;
#109543=CARTESIAN_POINT ( 'NONE',  ( 5.612185521052973414, 8.634967976948757951, -1.199719254218440723 ) ) ;
#109544=CARTESIAN_POINT ( 'NONE',  ( -8.213542131780492639, 8.476887330032372603, 1.040834085586084257E-14 ) ) ;
#109547=CARTESIAN_POINT ( 'NONE',  ( -3.090895833791289071, 6.549869539491048442, 1.040834085586084257E-14 ) ) ;
#109548=CARTESIAN_POINT ( 'NONE',  ( -1.402160292154681736E-14, 2.446875000341416584, -1.575800808251660134 ) ) ;
#109550=CARTESIAN_POINT ( 'NONE',  ( 2.846322183865124700, 5.408127416896231665, -1.199719254218446718 ) ) ;
#109556=CARTESIAN_POINT ( 'NONE',  ( -0.7500000000000006661, 0.1395833340161536928, -1.299038105676652011 ) ) ;
#109559=CARTESIAN_POINT ( 'NONE',  ( -6.555530967407501741, 7.606873202518897870, 1.199719254218450271 ) ) ;
#109560=CARTESIAN_POINT ( 'NONE',  ( -3.795919822146293754, 4.491289883001181593, -1.082531754730549967 ) ) ;
#109568=CARTESIAN_POINT ( 'NONE',  ( 4.476163270806094552, 8.373940915915776273, 0.7998128361456462443 ) ) ;
#109571=CYLINDRICAL_SURFACE ( 'NONE', #102180, 1.250000000000000000 ) ;
#109572=CARTESIAN_POINT ( 'NONE',  ( 4.632082037363250748, 8.555846143565791095, -0.7998128361456231517 ) ) ;
#109573=CARTESIAN_POINT ( 'NONE',  ( 4.650083499807244891, 5.295740330745369207, 2.420000000000010587 ) ) ;
#109577=CARTESIAN_POINT ( 'NONE',  ( 4.325214697959421706, 5.004837554829479451, 1.199719254218462483 ) ) ;
#109583=CARTESIAN_POINT ( 'NONE',  ( 4.128212683569056018, 7.424016784313646866, 0.7064205832574363964 ) ) ;
#109593=CARTESIAN_POINT ( 'NONE',  ( 7.863365906246055914, 10.19701286208565705, -1.443375672974057666 ) ) ;
#109595=CARTESIAN_POINT ( 'NONE',  ( -3.255929445576174697, 6.950334786480840243, -0.7998128361456281477 ) ) ;
#109599=CARTESIAN_POINT ( 'NONE',  ( 6.448874621594486989, 10.67543749183559143, 0.7998128361456462443 ) ) ;
#109601=CARTESIAN_POINT ( 'NONE',  ( -5.018489415352746619, 9.006654751220198207, 0.7998128361456481317 ) ) ;
#109609=CIRCLE ( 'NONE', #9179, 4.624999999999993783 ) ;
#109616=CARTESIAN_POINT ( 'NONE',  ( 10.18233705906309972, 11.83814697611718714, 1.199719254218450271 ) ) ;
#109617=CARTESIAN_POINT ( 'NONE',  ( -5.066996723205291708, 6.934582148538044777, 1.599625672291267398 ) ) ;
#109620=CARTESIAN_POINT ( 'NONE',  ( 3.307826292054301121, 4.882216645528547616, -1.443375672974057666 ) ) ;
#109624=EDGE_CURVE ( 'NONE', #147312, #12172, #115207, .T. ) ;
#109625=CARTESIAN_POINT ( 'NONE',  ( 4.406036734316882253, 6.163462161501578329, -1.443375672974051449 ) ) ;
#109626=CARTESIAN_POINT ( 'NONE',  ( -4.451154503988200339, 4.087435097607984957, 1.214306433183764966E-14 ) ) ;
#109629=CARTESIAN_POINT ( 'NONE',  ( 8.372323551638698902, 9.726464550788689323, 1.199719254218462483 ) ) ;
#109633=CARTESIAN_POINT ( 'NONE',  ( -8.050844288416501016, 8.287073179441051707, 1.040834085586084257E-14 ) ) ;
#109634=CARTESIAN_POINT ( 'NONE',  ( 5.606460214450851964, 6.499623990736163037, 1.199719254218462483 ) ) ;
#109637=VECTOR ( 'NONE', #203515, 1000.000000000000000 ) ;
#109641=CARTESIAN_POINT ( 'NONE',  ( -1.364683531250000748, 1.321875000341421469, 0.000000000000000000 ) ) ;
#109644=CARTESIAN_POINT ( 'NONE',  ( 7.131225611108088280, 9.342849184424693476, 1.443375672974076540 ) ) ;
#109651=CARTESIAN_POINT ( 'NONE',  ( 9.286972035236624734, 11.85788667924133399, -1.443375672974058777 ) ) ;
#109653=VERTEX_POINT ( 'NONE', #151246 ) ;
#109657=CARTESIAN_POINT ( 'NONE',  ( -7.641992139597101108, 12.06740792950531649, 0.7998128361456481317 ) ) ;
#109666=DIRECTION ( 'NONE',  ( -1.000000000000000000, 0.000000000000000000, 0.000000000000000000 ) ) ;
#109673=CARTESIAN_POINT ( 'NONE',  ( 1.499999999999987121, 2.077083334016153415, -0.8660254037844262731 ) ) ;
#109679=CARTESIAN_POINT ( 'NONE',  ( 9.399880572976245574, 9.860948844760784482, 0.7998128361456462443 ) ) ;
#109680=CARTESIAN_POINT ( 'NONE',  ( -1.364683531250014514, -0.9697916663252473812, 0.7879004041258379498 ) ) ;
#109683=CARTESIAN_POINT ( 'NONE',  ( 3.195971524519376494, 4.751719416737803847, -1.599625672291262513 ) ) ;
#109684=CARTESIAN_POINT ( 'NONE',  ( -5.531363484695544841, 8.436712584578003771, 1.082531754730548412 ) ) ;
#109688=CARTESIAN_POINT ( 'NONE',  ( -6.013204822860843457, 6.974159367214481264, -1.199719254218446718 ) ) ;
#109690=CARTESIAN_POINT ( 'NONE',  ( -1.201851678989727383E-14, 2.743750000682820378, 1.732050807568877637 ) ) ;
#109701=CYLINDRICAL_SURFACE ( 'NONE', #145356, 0.2500000000000574540 ) ;
#109702=CARTESIAN_POINT ( 'NONE',  ( -7.967387826325084355, 12.44703623068796361, 0.7998128361456481317 ) ) ;
#109703=CARTESIAN_POINT ( 'NONE',  ( 6.795661308947685164, 8.951357498570873261, -1.599625672291262513 ) ) ;
#109711=CARTESIAN_POINT ( 'NONE',  ( -6.995117189646935962, 10.24838825697502109, 1.199719254218453823 ) ) ;
#109717=CARTESIAN_POINT ( 'NONE',  ( 2.706824224222692088, 6.309712028235118453, 0.7998128361456362523 ) ) ;
#109719=ORIENTED_EDGE ( 'NONE', *, *, #125104, .T. ) ;
#109720=CARTESIAN_POINT ( 'NONE',  ( -9.267161690140662600, 10.77044237904097734, -1.199719254218441611 ) ) ;
#109723=CARTESIAN_POINT ( 'NONE',  ( -4.976004696740268685, 6.814476922186354813, -1.450531527366223372 ) ) ;
#109732=CARTESIAN_POINT ( 'NONE',  ( 6.120616281565444794, 9.228137197546649517, -1.199719254218440723 ) ) ;
#109739=CARTESIAN_POINT ( 'NONE',  ( -1.500000000000013101, 1.660416667349487119, -0.8660254037844313801 ) ) ;
#109750=DIRECTION ( 'NONE',  ( -1.000000000000000000, 7.387867266669436732E-31, -0.000000000000000000 ) ) ;
#109752=CARTESIAN_POINT ( 'NONE',  ( 3.795919822146273326, 5.451659097302528068, -1.443375672974051449 ) ) ;
#109756=CARTESIAN_POINT ( 'NONE',  ( -4.874313559192080092, 4.961021341527962036, 0.5169845646830675268 ) ) ;
#109758=CARTESIAN_POINT ( 'NONE',  ( -3.023105066167347310, 5.702484939155337607, 2.500000000000011102 ) ) ;
#109759=CARTESIAN_POINT ( 'NONE',  ( 9.748476143425788720, 11.33197590787365172, -1.199719254218440723 ) ) ;
#109770=CARTESIAN_POINT ( 'NONE',  ( -1.364683531250014514, 0.9885416670080898749, -0.7879004041258289570 ) ) ;
#109775=CARTESIAN_POINT ( 'NONE',  ( -6.078132937628113908, 5.985576603521232109, 1.040834085586084257E-14 ) ) ;
#109777=CARTESIAN_POINT ( 'NONE',  ( 1.499999999999985123, -0.7041666666666481778, -0.8660254037844323793 ) ) ;
#109779=CARTESIAN_POINT ( 'NONE',  ( 0.7499999999999920064, 5.483333333333353821, 1.299038105676669330 ) ) ;
#109785=CARTESIAN_POINT ( 'NONE',  ( -0.6823417656249969321, 5.530208333674756283, -1.181850606188749264 ) ) ;
#109788=CARTESIAN_POINT ( 'NONE',  ( -8.389798128758148010, 8.682519326506312751, 0.7998128361456462443 ) ) ;
#109789=PLANE ( 'NONE',  #57458 ) ;
#109790=CARTESIAN_POINT ( 'NONE',  ( 9.887974103068218668, 10.43039129653476493, 0.7998128361456462443 ) ) ;
#109797=CARTESIAN_POINT ( 'NONE',  ( -0.6823417656250246877, 0.1135416670080893753, 1.181850606188755259 ) ) ;
#109803=CARTESIAN_POINT ( 'NONE',  ( 7.998947442382716488, 9.394822106610419610, -1.082531754730543083 ) ) ;
#109806=CARTESIAN_POINT ( 'NONE',  ( -3.716906668440817185, 7.488141546489591072, 0.7998128361456341429 ) ) ;
#109808=CARTESIAN_POINT ( 'NONE',  ( -1.001543065824772872E-14, 5.243750000682815937, 1.732050807568877637 ) ) ;
#109811=CARTESIAN_POINT ( 'NONE',  ( 6.127922243252466039, 6.251590159990418449, 1.040834085586084257E-14 ) ) ;
#109812=CARTESIAN_POINT ( 'NONE',  ( -9.124274191872640216, 10.70770331434866485, -1.082531754730537976 ) ) ;
#109817=CARTESIAN_POINT ( 'NONE',  ( 9.327646496521982300, 11.90534021740758064, -1.443375672974057666 ) ) ;
#109824=ORIENTED_EDGE ( 'NONE', *, *, #58248, .T. ) ;
#109832=TOROIDAL_SURFACE ( 'NONE', #33526, 0.8300000000000010703, 0.08000000000000000167 ) ;
#109834=CARTESIAN_POINT ( 'NONE',  ( 6.753933077901968396, 11.03133902419432566, 0.7998128361456462443 ) ) ;
#109837=CARTESIAN_POINT ( 'NONE',  ( 4.365362273920238678, 7.076377838673507448, 1.082531754730558626 ) ) ;
#109838=CARTESIAN_POINT ( 'NONE',  ( -7.863365906246054138, 11.15738207638699464, -1.082531754730543971 ) ) ;
#109843=CARTESIAN_POINT ( 'NONE',  ( -3.898132859128961236, 4.506575409527250997, -1.199719254218452047 ) ) ;
#109867=DIRECTION ( 'NONE',  ( 3.347138415753902517E-16, 0.6000000000000018652, 0.7999999999999984901 ) ) ;
#109869=CARTESIAN_POINT ( 'NONE',  ( -8.839552966430023417, 9.415159337030921449, -0.7216878364870267237 ) ) ;
#109873=CARTESIAN_POINT ( 'NONE',  ( 5.961834861707224320, 7.978559976790334574, -1.599625672291262513 ) ) ;
#109874=CARTESIAN_POINT ( 'NONE',  ( -7.334597915313094241, 9.580116872663850813, 1.040834085586084257E-14 ) ) ;
#109878=CARTESIAN_POINT ( 'NONE',  ( -3.490334480514268645, 6.159475096320226939, -1.199719254218452935 ) ) ;
#109882=CARTESIAN_POINT ( 'NONE',  ( -3.795392936821753604, 6.515376628678959392, -1.199719254218452047 ) ) ;
#109885=CARTESIAN_POINT ( 'NONE',  ( 8.911787042884274257, 9.291506392986812912, 0.7998128361456462443 ) ) ;
#109886=CARTESIAN_POINT ( 'NONE',  ( 0.6823417656249899377, 3.926041667008085767, -1.181850606188754593 ) ) ;
#109888=CARTESIAN_POINT ( 'NONE',  ( 5.639836874842681702, 6.325236607244836051, 1.140081021588116084 ) ) ;
#109889=CARTESIAN_POINT ( 'NONE',  ( 3.036663219780971978, 6.486598156479028709, -0.7216878364870267237 ) ) ;
#109897=CARTESIAN_POINT ( 'NONE',  ( 7.578644679914718019, 7.944099669429731669, 0.7216878364870317197 ) ) ;
#109898=CARTESIAN_POINT ( 'NONE',  ( -9.267161690140662600, 10.77044237904097734, -1.199719254218441611 ) ) ;
#109901=CARTESIAN_POINT ( 'NONE',  ( -8.158255747121117452, 10.54105100977322174, 1.599625672291295375 ) ) ;
#109902=CARTESIAN_POINT ( 'NONE',  ( -6.551614543901706611, 8.666636272683888365, 1.599625672291283607 ) ) ;
#109910=CARTESIAN_POINT ( 'NONE',  ( 7.079328764629950754, 11.41096732537697633, 0.7998128361456462443 ) ) ;
#109911=CARTESIAN_POINT ( 'NONE',  ( 1.499999999999990896, 4.025000000000021672, 1.214306433183764966E-14 ) ) ;
#109917=CARTESIAN_POINT ( 'NONE',  ( -1.201851678989727383E-14, 5.618750000682818602, -1.732050807568863648 ) ) ;
#109922=CARTESIAN_POINT ( 'NONE',  ( -1.500000000000011324, 4.879166666666690411, -0.8660254037844313801 ) ) ;
#109923=CARTESIAN_POINT ( 'NONE',  ( 6.471319392424407901, 6.444294134116939077, 0.7998128361456341429 ) ) ;
#109924=CARTESIAN_POINT ( 'NONE',  ( 7.169564303528210836, 7.258913197071374945, -0.7998128361456281477 ) ) ;
#109926=CARTESIAN_POINT ( 'NONE',  ( 4.382186172716248329, 4.009346271119131444, 0.09521571495261728357 ) ) ;
#109927=CARTESIAN_POINT ( 'NONE',  ( 8.107412671292042461, 9.521364873671299023, 1.082531754730558626 ) ) ;
#109928=CARTESIAN_POINT ( 'NONE',  ( -8.880227426826648340, 11.38335130276301754, 1.443375672974064550 ) ) ;
#109929=EDGE_CURVE ( 'NONE', #112883, #157004, #56420, .T. ) ;
#109933=CARTESIAN_POINT ( 'NONE',  ( 8.106885785967500979, 11.54545161934907682, 1.199719254218460707 ) ) ;
#109936=CARTESIAN_POINT ( 'NONE',  ( -4.613852347352193739, 4.277249248199312071, 1.214306433183764966E-14 ) ) ;
#109938=CARTESIAN_POINT ( 'NONE',  ( -1.402160292154681736E-14, 1.446875000341420137, -1.575800808251659024 ) ) ;
#109943=CARTESIAN_POINT ( 'NONE',  ( -0.6823417656250246877, -0.4489583329919111243, 1.181850606188755259 ) ) ;
#109945=CARTESIAN_POINT ( 'NONE',  ( 9.921869487102386032, 10.46993591124128997, 0.000000000000000000 ) ) ;
#109949=CARTESIAN_POINT ( 'NONE',  ( -3.348500752450953577, 4.929670182657964084, 1.443375672974062551 ) ) ;
#109952=CARTESIAN_POINT ( 'NONE',  ( -7.223796917982883592, 7.322184580601816428, -0.7998128361456291469 ) ) ;
#109955=CARTESIAN_POINT ( 'NONE',  ( 3.181359600701000989, 6.863336634126477875, 0.000000000000000000 ) ) ;
#109962=CARTESIAN_POINT ( 'NONE',  ( 7.560643217915098191, 11.97250085420964716, -0.7998128361456291469 ) ) ;
#109965=CARTESIAN_POINT ( 'NONE',  ( -6.064574784014443942, 5.969758757638621738, -0.7998128361456291469 ) ) ;
#109969=CARTESIAN_POINT ( 'NONE',  ( 7.079328764629950754, 11.41096732537697633, 0.7998128361456462443 ) ) ;
#109971=CARTESIAN_POINT ( 'NONE',  ( 5.764187864104357573, 9.876636274763768597, 1.040834085586084257E-14 ) ) ;
#109975=CARTESIAN_POINT ( 'NONE',  ( -2.103486388414573138, 5.605817886458954291, 1.040834085586084257E-14 ) ) ;
#109982=CARTESIAN_POINT ( 'NONE',  ( -5.854914268151548917, 6.175991412503675448, 0.9282606102084377531 ) ) ;
#109983=CARTESIAN_POINT ( 'NONE',  ( 1.364683531249988535, 2.363541667008088432, 0.7879004041258500513 ) ) ;
#109986=CARTESIAN_POINT ( 'NONE',  ( 6.317736394288140822, 7.433409217166723870, 1.082531754730558626 ) ) ;
#109988=AXIS2_PLACEMENT_3D ( 'NONE', #102214, #52400, #117462 ) ;
#110002=CARTESIAN_POINT ( 'NONE',  ( 7.425061681778431399, 11.81432239538354345, 0.7998128361456462443 ) ) ;
#110006=CARTESIAN_POINT ( 'NONE',  ( -3.490334480514268645, 6.159475096320226939, -1.199719254218452935 ) ) ;
#110007=CARTESIAN_POINT ( 'NONE',  ( -8.681298431451969222, 9.022603012982438386, 1.040834085586084257E-14 ) ) ;
#110012=CARTESIAN_POINT ( 'NONE',  ( -1.201851678989727383E-14, 3.868750000682817713, -1.732050807568863648 ) ) ;
#110013=CARTESIAN_POINT ( 'NONE',  ( 6.913768267964901071, 10.15348118167935709, -1.199719254218441611 ) ) ;
#110016=CARTESIAN_POINT ( 'NONE',  ( -8.538937818508475885, 8.856515631215026829, 1.040834085586084257E-14 ) ) ;
#110018=CARTESIAN_POINT ( 'NONE',  ( -0.6823417656249969321, 4.717708333674755394, -1.181850606188749264 ) ) ;
#110019=( BOUNDED_CURVE ( )  B_SPLINE_CURVE ( 2, ( #29396, #95489, #147412, #13121, #131217, #94414, #161535 ),
 .UNSPECIFIED., .F., .T. ) 
 B_SPLINE_CURVE_WITH_KNOTS ( ( 3, 2, 2, 3 ),
 ( 0.2375000000000003775, 0.2416666666666670293, 0.2458333333333336257, 0.2500000000000002776 ),
 .UNSPECIFIED. ) 
 CURVE ( )  GEOMETRIC_REPRESENTATION_ITEM ( )  RATIONAL_B_SPLINE_CURVE ( ( 0.9999999999999874545, 0.8660254037844512531, 1.000000000000000000, 0.8660254037844387076, 1.000000000000000000, 0.8660254037844298258, 1.000000000000008882 ) ) 
 REPRESENTATION_ITEM ( '' )  );
#110023=CARTESIAN_POINT ( 'NONE',  ( -8.514157279702027736, 10.95626946445095307, -1.443375672974059665 ) ) ;
#110027=CARTESIAN_POINT ( 'NONE',  ( 0.6823417656249899377, 2.405208333674753618, 1.181850606188767472 ) ) ;
#110036=CARTESIAN_POINT ( 'NONE',  ( 1.364683531249988535, 2.363541667008088432, 0.7879004041258500513 ) ) ;
#110038=CARTESIAN_POINT ( 'NONE',  ( -4.192495815123836955, 5.914331089109674089, -1.599625672291256295 ) ) ;
#110039=CARTESIAN_POINT ( 'NONE',  ( 7.610204295972345712, 7.772993188256215547, 0.7998128361456341429 ) ) ;
#110042=CARTESIAN_POINT ( 'NONE',  ( -0.6823417656249969321, 4.030208333674754506, -1.181850606188749264 ) ) ;
#110045=CARTESIAN_POINT ( 'NONE',  ( 0.6823417656249864960, -1.073958332991911568, -1.181850606188749264 ) ) ;
#110046=CARTESIAN_POINT ( 'NONE',  ( -5.097502569058221411, 6.009803087731781623, -1.082531754730544860 ) ) ;
#110049=CARTESIAN_POINT ( 'NONE',  ( 4.528060117284240071, 5.345453560662148718, 1.082531754730560403 ) ) ;
#110052=CARTESIAN_POINT ( 'NONE',  ( -9.978437869977959451, 10.74385839117019614, -0.7216878364870267237 ) ) ;
#110059=CARTESIAN_POINT ( 'NONE',  ( -7.334597914868743018, 7.659378443542744996, -0.7216878364870267237 ) ) ;
#110061=CARTESIAN_POINT ( 'NONE',  ( 0.6823417656249899377, 1.405208333674752508, 1.181850606188755259 ) ) ;
#110067=CARTESIAN_POINT ( 'NONE',  ( -0.6823417656250246877, -0.8864583329919115684, 1.181850606188755259 ) ) ;
#110074=CARTESIAN_POINT ( 'NONE',  ( 0.7499999999999885647, -1.016666666666644847, 1.299038105676657340 ) ) ;
#110075=CARTESIAN_POINT ( 'NONE',  ( 8.717529583462654941, 9.272798723569005475, 0.7216878364870458196 ) ) ;
#110081=ORIENTED_EDGE ( 'NONE', *, *, #153081, .F. ) ;
#110083=CARTESIAN_POINT ( 'NONE',  ( 3.960953433486789521, 7.772862772376584850, -0.7998128361456221525 ) ) ;
#110085=CARTESIAN_POINT ( 'NONE',  ( -3.415764635639130020, 6.072476943965863683, 1.199719254218462483 ) ) ;
#110089=CYLINDRICAL_SURFACE ( 'NONE', #2774, 2.000000000000000000 ) ;
#110091=CARTESIAN_POINT ( 'NONE',  ( 1.364683531249986537, 1.717708333674749399, -0.7879004041258239610 ) ) ;
#110093=CARTESIAN_POINT ( 'NONE',  ( -9.318531651294266638, 9.766041769465124034, -0.7998128361456291469 ) ) ;
#110111=CARTESIAN_POINT ( 'NONE',  ( 7.332262146892202459, 7.448727347662698506, -0.7998128361456281477 ) ) ;
#110118=CARTESIAN_POINT ( 'NONE',  ( 6.611572464958476836, 10.86525164242692298, 0.7998128361456462443 ) ) ;
#110121=CARTESIAN_POINT ( 'NONE',  ( 8.615316546479974136, 12.13862083994696839, 1.199719254218450271 ) ) ;
#110127=CARTESIAN_POINT ( 'NONE',  ( 8.940712233207955606, 12.51824914112961729, 1.199719254218450271 ) ) ;
#110130=CARTESIAN_POINT ( 'NONE',  ( -0.4138605925103633898, 8.005950907165120256, 1.999879544075660043 ) ) ;
#110134=CARTESIAN_POINT ( 'NONE',  ( -9.490344339885981029, 10.17441593939621924, -0.7216878364870267237 ) ) ;
#110140=CARTESIAN_POINT ( 'NONE',  ( 5.473741331615251227, 7.409117525016355010, -1.599625672291262513 ) ) ;
#110145=CARTESIAN_POINT ( 'NONE',  ( 3.023105065722948126, 6.470780310077995701, 0.7216878364870338292 ) ) ;
#110153=CARTESIAN_POINT ( 'NONE',  ( -4.880045225915050189, 7.780804299287790826, 1.199719254218464037 ) ) ;
#110155=CARTESIAN_POINT ( 'NONE',  ( -2.272963308585411735, 5.803540959991587478, 0.7998128361456341429 ) ) ;
#110161=CARTESIAN_POINT ( 'NONE',  ( 0.07074886611255049029, 8.280404612018074317, -2.000278354478734588 ) ) ;
#110166=CARTESIAN_POINT ( 'NONE',  ( 4.961394147597008697, 7.875711374583454827, -1.199719254218452047 ) ) ;
#110180=CARTESIAN_POINT ( 'NONE',  ( -1.364683531250012516, 1.592708333674756727, 0.7879004041258379498 ) ) ;
#110181=CARTESIAN_POINT ( 'NONE',  ( 3.029357257649615054, 5.621668336311468117, -1.199719254218446718 ) ) ;
#110183=CARTESIAN_POINT ( 'NONE',  ( -6.236387472606145010, 9.259240570473746601, -1.082531754730538864 ) ) ;
#110184=CARTESIAN_POINT ( 'NONE',  ( 3.389175213736292047, 5.937492935125556315, 1.082531754730558626 ) ) ;
#110185=CARTESIAN_POINT ( 'NONE',  ( -6.439759776366783761, 8.536139043893143707, 1.443375672974078761 ) ) ;
#110188=EDGE_LOOP ( 'NONE', ( #144450, #579, #88888, #91658 ) ) ;
#110190=CARTESIAN_POINT ( 'NONE',  ( 6.796715079152391148, 6.823922435299587974, 0.7998128361456341429 ) ) ;
#110195=CARTESIAN_POINT ( 'NONE',  ( 0.6823417656249899377, 5.676041667008087543, -1.181850606188754593 ) ) ;
#110199=CARTESIAN_POINT ( 'NONE',  ( 5.282873410819217241, 9.315102745931094219, -0.7998128361456281477 ) ) ;
#110202=CARTESIAN_POINT ( 'NONE',  ( -6.367525699912501835, 10.58053041653993098, -0.7998128361456291469 ) ) ;
#110208=CARTESIAN_POINT ( 'NONE',  ( 8.762647353133951711, 9.117510088278095282, 1.040834085586084257E-14 ) ) ;
#110211=CARTESIAN_POINT ( 'NONE',  ( -7.985916173649233230, 9.275655943134292869, -1.199719254218446718 ) ) ;
#110213=CARTESIAN_POINT ( 'NONE',  ( 3.009410498757215446, 6.662729348525398443, 0.6539756689588872574 ) ) ;
#110214=CARTESIAN_POINT ( 'NONE',  ( 7.741342523278705201, 9.094283034322399928, 1.082531754730558626 ) ) ;
#110215=CARTESIAN_POINT ( 'NONE',  ( 4.230803266364135951, 7.299989629454814555, -0.8951707687023923166 ) ) ;
#110216=CARTESIAN_POINT ( 'NONE',  ( -7.673551755654729689, 11.89630144833179060, 0.7216878364870458196 ) ) ;
#110221=CARTESIAN_POINT ( 'NONE',  ( 4.137209430464448445, 7.978494768850520558, 1.040834085586084257E-14 ) ) ;
#110223=CARTESIAN_POINT ( 'NONE',  ( 9.565441069641300587, 11.11843498845840905, -1.199719254218440723 ) ) ;
#110224=CARTESIAN_POINT ( 'NONE',  ( -5.505981461394960697, 6.253680794909101337, 0.9796770575781436063 ) ) ;
#110225=CARTESIAN_POINT ( 'NONE',  ( -2.081668171172168513E-14, 6.487495393664096888, 3.100011470320013451 ) ) ;
#110226=CARTESIAN_POINT ( 'NONE',  ( 1.364683531249986537, 0.6135416670080880985, 0.7879004041258500513 ) ) ;
#110228=CARTESIAN_POINT ( 'NONE',  ( -7.592202833972775622, 8.920286730132099606, 1.082531754730558626 ) ) ;
#110229=ORIENTED_EDGE ( 'NONE', *, *, #95445, .T. ) ;
#110234=CARTESIAN_POINT ( 'NONE',  ( -4.208837953572873047, 7.367755930811632936, 0.8315943877991900379 ) ) ;
#110235=CARTESIAN_POINT ( 'NONE',  ( -0.6823417656250003738, 0.2802083336747515641, -1.181850606188749264 ) ) ;
#110238=CARTESIAN_POINT ( 'NONE',  ( 4.202664430556257713, 4.965825259479493603, 1.082531754730560403 ) ) ;
#110242=CARTESIAN_POINT ( 'NONE',  ( -8.148087131688692253, 10.52918762510205042, -1.443375672974058777 ) ) ;
#110248=CARTESIAN_POINT ( 'NONE',  ( -8.310784975052682100, 10.71900177569337487, -1.443375672974058777 ) ) ;
#110249=DIRECTION ( 'NONE',  ( 0.9998757926790049488, 0.01538962834598772353, 0.003399787332178825280 ) ) ;
#110250=ORIENTED_EDGE ( 'NONE', *, *, #47118, .F. ) ;
#110254=ORIENTED_EDGE ( 'NONE', *, *, #5825, .F. ) ;
#110255=CARTESIAN_POINT ( 'NONE',  ( -9.449669878600625239, 10.12696240122997082, -0.7216878364870267237 ) ) ;
#110259=CARTESIAN_POINT ( 'NONE',  ( 1.364683531249988535, 5.217708333674750065, -0.7879004041258300672 ) ) ;
#110260=CARTESIAN_POINT ( 'NONE',  ( -1.201851678989727383E-14, 4.368750000682820378, -1.732050807568863648 ) ) ;
#110261=CARTESIAN_POINT ( 'NONE',  ( 5.178766244632133642, 6.659365504414815895, -1.397763381526682336 ) ) ;
#110265=ORIENTED_EDGE ( 'NONE', *, *, #194628, .F. ) ;
#110267=CARTESIAN_POINT ( 'NONE',  ( -7.751511138711140170, 10.06651563329490529, -1.599625672291263179 ) ) ;
#110271=CARTESIAN_POINT ( 'NONE',  ( 5.443762371086860341, 6.309809840144842141, 1.199719254218462483 ) ) ;
#110273=CARTESIAN_POINT ( 'NONE',  ( 3.847109862837356786, 4.045599327266925727, -0.8077998227820462063 ) ) ;
#110276=CARTESIAN_POINT ( 'NONE',  ( 6.825640269476072497, 10.05066518344239412, 1.199719254218460707 ) ) ;
#110280=VERTEX_POINT ( 'NONE', #63069 ) ;
#110283=CARTESIAN_POINT ( 'NONE',  ( -5.585596099150193616, 6.579245539505756746, -1.082531754730544860 ) ) ;
#110286=DIRECTION ( 'NONE',  ( -0.6507913734559640506, -0.7592566023653004592, 0.000000000000000000 ) ) ;
#110294=CARTESIAN_POINT ( 'NONE',  ( -9.073431116043565225, 11.60875560684942265, -1.599625672291263179 ) ) ;
#110296=CARTESIAN_POINT ( 'NONE',  ( 8.072990401933337168, 11.50590700464255356, -1.199719254218446718 ) ) ;
#110297=CARTESIAN_POINT ( 'NONE',  ( -0.7500000000000006661, -0.8916666666666448471, -1.299038105676652011 ) ) ;
#110298=CARTESIAN_POINT ( 'NONE',  ( -7.340850106795412167, 10.65174332698158643, 1.199719254218453823 ) ) ;
#110301=CARTESIAN_POINT ( 'NONE',  ( -0.6823417656250212460, 3.301041667008085323, 1.181850606188767472 ) ) ;
#110302=CARTESIAN_POINT ( 'NONE',  ( 9.571693261567954636, 12.19006144329456731, 1.443375672974076540 ) ) ;
#110305=CARTESIAN_POINT ( 'NONE',  ( -1.201851678989727383E-14, 5.587500000000021672, -1.732050807568863648 ) ) ;
#110308=CARTESIAN_POINT ( 'NONE',  ( 9.395437264145964917, 10.06369101769952934, -0.7216878364870257245 ) ) ;
#110311=CARTESIAN_POINT ( 'NONE',  ( -6.453317930424837812, 7.591587675992828466, 1.082531754730549967 ) ) ;
#110313=CARTESIAN_POINT ( 'NONE',  ( 1.364683531249988535, 1.863541667008086211, 0.7879004041258500513 ) ) ;
#110315=DIRECTION ( 'NONE',  ( 1.000000000000000000, 0.000000000000000000, 0.000000000000000000 ) ) ;
#110317=CARTESIAN_POINT ( 'NONE',  ( -6.775324078527193983, 8.927630729746953264, -1.599625672291263179 ) ) ;
#110318=CARTESIAN_POINT ( 'NONE',  ( 0.6823417656249899377, 4.988541667008086655, -1.181850606188754593 ) ) ;
#110325=CARTESIAN_POINT ( 'NONE',  ( 10.09812548408005384, 10.67556790771522124, -0.7998128361456281477 ) ) ;
#110328=CARTESIAN_POINT ( 'NONE',  ( 0.7499999999999885647, 0.8166666666666877461, -1.299038105676652899 ) ) ;
#110335=CARTESIAN_POINT ( 'NONE',  ( 10.26082332744404368, 10.86538205830655279, -0.7998128361456281477 ) ) ;
#110340=CARTESIAN_POINT ( 'NONE',  ( 8.320953590485093088, 10.73086516036454618, 1.599625672291281386 ) ) ;
#110341=CARTESIAN_POINT ( 'NONE',  ( -1.523896559881120938, 8.692074762372739016, 2.522933744808692147 ) ) ;
#110344=CARTESIAN_POINT ( 'NONE',  ( -4.911139836396910319, 4.690354089464431553, -0.3431232535803417916 ) ) ;
#110345=CARTESIAN_POINT ( 'NONE',  ( 1.364683531249990311, 5.676041667008088432, 0.7879004041258500513 ) ) ;
#110349=CARTESIAN_POINT ( 'NONE',  ( 6.760712154708803823, 11.03924794713562818, 1.040834085586084257E-14 ) ) ;
#110351=CARTESIAN_POINT ( 'NONE',  ( 1.364683531249990311, 3.634375000341416584, 1.214306433183764966E-14 ) ) ;
#110353=CARTESIAN_POINT ( 'NONE',  ( -5.097502569058207200, 8.890910730635814829, -0.7216878364870207285 ) ) ;
#110362=CARTESIAN_POINT ( 'NONE',  ( 9.250740883225924804, 9.686952540052077509, 1.040834085586084257E-14 ) ) ;
#110368=CARTESIAN_POINT ( 'NONE',  ( -9.429859533504656000, 10.96025652963230534, -1.199719254218441611 ) ) ;
#110370=CARTESIAN_POINT ( 'NONE',  ( 6.388916700537700777, 8.476822122092563916, 1.599625672291281386 ) ) ;
#110372=CARTESIAN_POINT ( 'NONE',  ( 3.294268137996273715, 5.826768013428865522, -1.082531754730543971 ) ) ;
#110374=CARTESIAN_POINT ( 'NONE',  ( 4.147904930777053245, 6.926640621626830807, -1.199719254218452047 ) ) ;
#110382=CARTESIAN_POINT ( 'NONE',  ( -5.368665641331555882, 8.246898433986675769, 1.082531754730548412 ) ) ;
#110383=CARTESIAN_POINT ( 'NONE',  ( 2.659370686574860976, 6.254349567645977714, -0.7998128361456291469 ) ) ;
#110386=CARTESIAN_POINT ( 'NONE',  ( -8.019811557683421910, 9.315200557840817908, 1.199719254218462483 ) ) ;
#110392=CARTESIAN_POINT ( 'NONE',  ( -9.104463846776669200, 10.58062822844965645, -1.199719254218441611 ) ) ;
#110396=CARTESIAN_POINT ( 'NONE',  ( 7.313733799568044702, 10.62010763521636214, 1.199719254218460707 ) ) ;
#110397=CARTESIAN_POINT ( 'NONE',  ( -6.520158902580853066, 5.290451655908523065, -2.438235897557453846 ) ) ;
#110408=CARTESIAN_POINT ( 'NONE',  ( -6.723954117373590833, 9.932031339322813679, -1.199719254218440723 ) ) ;
#110413=CARTESIAN_POINT ( 'NONE',  ( 6.100805936469477331, 9.101062111647635788, -1.082531754730537088 ) ) ;
#110418=CARTESIAN_POINT ( 'NONE',  ( -4.740547266272593596, 8.682388910626682943, -0.7998128361456281477 ) ) ;
#110427=CARTESIAN_POINT ( 'NONE',  ( -8.319899820280397762, 12.85830022363583147, -0.7998128361456281477 ) ) ;
#110428=CARTESIAN_POINT ( 'NONE',  ( 9.074484886248265880, 9.481320543578137361, 0.7998128361456462443 ) ) ;
#110430=CARTESIAN_POINT ( 'NONE',  ( -3.714570900464290393, 5.356752022006865843, 1.443375672974064550 ) ) ;
#110433=CARTESIAN_POINT ( 'NONE',  ( -5.662059632048889846, 6.153064387560178261, -0.8011038117717106388 ) ) ;
#110440=CARTESIAN_POINT ( 'NONE',  ( 4.356247428692526569, 3.976710176429713250, 0.7998128361456341429 ) ) ;
#110447=CARTESIAN_POINT ( 'NONE',  ( 4.542145155778077203, 5.257923088951247159, -1.199719254218452047 ) ) ;
#110459=CARTESIAN_POINT ( 'NONE',  ( -3.276266675996675204, 6.974061555304760240, -0.7998128361456281477 ) ) ;
#110461=CARTESIAN_POINT ( 'NONE',  ( 5.680503174001485078, 6.689970460165617361, -1.082531754730543083 ) ) ;
#110462=CARTESIAN_POINT ( 'NONE',  ( 0.7499999999999902300, 3.233333333333352044, 1.299038105676669330 ) ) ;
#110464=CARTESIAN_POINT ( 'NONE',  ( -5.447678794592645701, 5.250046769979851646, 0.000000000000000000 ) ) ;
#110465=FACE_OUTER_BOUND ( 'NONE', #48726, .T. ) ;
#110467=CARTESIAN_POINT ( 'NONE',  ( -1.499999999999993339, 10.64264068711930733, 1.232676135170975238E-14 ) ) ;
#110468=CARTESIAN_POINT ( 'NONE',  ( 0.6823417656249899377, 4.926041667008086655, -1.181850606188754593 ) ) ;
#110471=CARTESIAN_POINT ( 'NONE',  ( -2.494337075234348777, 5.853884321174607663, -0.7216878364870267237 ) ) ;
#110473=ORIENTED_EDGE ( 'NONE', *, *, #95445, .F. ) ;
#110474=CARTESIAN_POINT ( 'NONE',  ( 1.499999999999990674, 8.226407212580426176, -3.114167208185174118 ) ) ;
#110476=CARTESIAN_POINT ( 'NONE',  ( 4.650610384687404952, 5.384465856012134566, 1.199719254218462483 ) ) ;
#110477=CARTESIAN_POINT ( 'NONE',  ( -4.161989969715295778, 4.726297878971393196, 2.500000000000011102 ) ) ;
#110481=CARTESIAN_POINT ( 'NONE',  ( 5.192409644353875642, 5.160158794608717514, 1.040834085586084257E-14 ) ) ;
#110483=CARTESIAN_POINT ( 'NONE',  ( 0.6823417656249882723, 1.488541667008083547, -1.181850606188749264 ) ) ;
#110484=AXIS2_PLACEMENT_3D ( 'NONE', #63724, #93060, #12824 ) ;
#110487=CARTESIAN_POINT ( 'NONE',  ( -8.123306592882240551, 12.62894145833798376, 0.000000000000000000 ) ) ;
#110488=CARTESIAN_POINT ( 'NONE',  ( -6.385527161912131433, 6.552129231760014605, 0.7216878364870317197 ) ) ;
#110492=CARTESIAN_POINT ( 'NONE',  ( 1.364683531249988535, 4.363541667008090208, 0.7879004041258500513 ) ) ;
#110500=CARTESIAN_POINT ( 'NONE',  ( -7.171900071504754060, 7.469564292951421436, -0.7216878364870267237 ) ) ;
#110504=CARTESIAN_POINT ( 'NONE',  ( -5.870317324592812191, 7.871789516823500144, -1.443375672974051449 ) ) ;
#110511=CARTESIAN_POINT ( 'NONE',  ( 5.843201017809841247, 5.919415396974013532, 1.040834085586084257E-14 ) ) ;
#110513=ORIENTED_EDGE ( 'NONE', *, *, #15140, .T. ) ;
#110515=CARTESIAN_POINT ( 'NONE',  ( 4.033527471555918176, 7.762610268090422316, -0.4095974594184521034 ) ) ;
#110517=CARTESIAN_POINT ( 'NONE',  ( -4.904298879841297421, 6.744767997946721216, 1.599625672291267398 ) ) ;
#110520=CARTESIAN_POINT ( 'NONE',  ( 1.499999999999987121, 0.7541666666666868579, 0.8660254037844524744 ) ) ;
#110521=VERTEX_POINT ( 'NONE', #19636 ) ;
#110523=CARTESIAN_POINT ( 'NONE',  ( 8.256552361042350796, 12.57646882128404187, 1.040834085586084257E-14 ) ) ;
#110524=CARTESIAN_POINT ( 'NONE',  ( 5.635385404774530649, 9.726366738878972740, 0.7998128361456462443 ) ) ;
#110527=EDGE_LOOP ( 'NONE', ( #163041, #39203, #39600, #166467 ) ) ;
#110529=CARTESIAN_POINT ( 'NONE',  ( 3.948449050077836642, 5.629609863222681199, 1.599625672291267398 ) ) ;
#110538=CARTESIAN_POINT ( 'NONE',  ( -6.226218857173722476, 8.287007971501239467, 1.599625672291283607 ) ) ;
#110543=CARTESIAN_POINT ( 'NONE',  ( -0.6823417656249969321, 3.717708333674754506, -1.181850606188749264 ) ) ;
#110544=CARTESIAN_POINT ( 'NONE',  ( 8.392133896734662812, 10.81390885098904420, 1.443375672974076540 ) ) ;
#110545=CARTESIAN_POINT ( 'NONE',  ( -7.335124800193271177, 8.516399340768996851, -1.199719254218452935 ) ) ;
#110548=CARTESIAN_POINT ( 'NONE',  ( 7.169564303528210836, 7.258913197071374945, -0.7998128361456281477 ) ) ;
#110549=CARTESIAN_POINT ( 'NONE',  ( -5.545448523189368650, 6.428443684264421698, -1.199719254218446718 ) ) ;
#110553=CARTESIAN_POINT ( 'NONE',  ( 0.7499999999999867883, 0.09791666734948467621, -1.299038105676652899 ) ) ;
#110557=CARTESIAN_POINT ( 'NONE',  ( 7.076992996653421741, 10.23994701519558781, -1.082531754730537976 ) ) ;
#110560=CARTESIAN_POINT ( 'NONE',  ( -1.364683531250012516, 2.551041667008089320, -0.7879004041258289570 ) ) ;
#110562=CARTESIAN_POINT ( 'NONE',  ( 4.812781342726850653, 8.558735966582574406, 0.7216878364870438212 ) ) ;
#110564=CARTESIAN_POINT ( 'NONE',  ( -4.473827502829599290, 4.321812962830357208, 0.7216878364870317197 ) ) ;
#110571=CARTESIAN_POINT ( 'NONE',  ( -4.038790540952651220, 7.763523381248250033, -0.5490930765432913141 ) ) ;
#110579=CARTESIAN_POINT ( 'NONE',  ( 6.993308306550549247, 7.053281200597435685, 1.040834085586084257E-14 ) ) ;
#110582=FACE_OUTER_BOUND ( 'NONE', #170941, .T. ) ;
#110588=ORIENTED_EDGE ( 'NONE', *, *, #32218, .F. ) ;
#110590=CARTESIAN_POINT ( 'NONE',  ( 5.517805331081858888, 5.539787095791365523, 1.040834085586084257E-14 ) ) ;
#110591=CARTESIAN_POINT ( 'NONE',  ( 1.364683531249988535, 1.926041667008086211, 0.7879004041258500513 ) ) ;
#110592=CARTESIAN_POINT ( 'NONE',  ( 6.913768267964901071, 10.15348118167935709, -1.199719254218441611 ) ) ;
#110596=CARTESIAN_POINT ( 'NONE',  ( 3.019342412789784547, 6.452475500722323787, 0.1501914610189964416 ) ) ;
#110598=( BOUNDED_SURFACE ( )  B_SPLINE_SURFACE ( 3, 2, ( 
 ( #152156, #83939, #167340 ),
 ( #164148, #185695, #49334 ),
 ( #33072, #147902, #101257 ),
 ( #34128, #118646, #35180 ) ),
 .UNSPECIFIED., .F., .F., .T. ) 
 B_SPLINE_SURFACE_WITH_KNOTS ( ( 4, 4 ),
 ( 3, 3 ),
 ( 1.570796326794896114, 2.200856270471036158 ),
 ( 0.000000000000000000, 1.000000000000000000 ),
 .UNSPECIFIED. ) 
 GEOMETRIC_REPRESENTATION_ITEM ( )  RATIONAL_B_SPLINE_SURFACE ( (
 ( 1.000000000000000000, 0.7071067811865475727, 1.000000000000000000),
 ( 1.000000000000000000, 0.7517196685950601198, 1.000000000000000000),
 ( 1.000000000000000000, 0.7917671131335182189, 1.000000000000000000),
 ( 1.000000000000000000, 0.8226529996948372947, 1.000000000000000000) ) ) 
 REPRESENTATION_ITEM ( '' )  SURFACE ( )  );
#110601=CARTESIAN_POINT ( 'NONE',  ( -1.500000000000011324, 3.420833333333355597, 0.8660254037844403729 ) ) ;
#110602=CARTESIAN_POINT ( 'NONE',  ( 5.717788096661236885, 7.693838750903348789, 1.599625672291267398 ) ) ;
#110603=CARTESIAN_POINT ( 'NONE',  ( -5.554036483092550824, 9.631459663583308739, -0.7998128361456231517 ) ) ;
#110608=CARTESIAN_POINT ( 'NONE',  ( 1.364683531249990311, 2.634375000341422801, 1.214306433183764966E-14 ) ) ;
#110610=CARTESIAN_POINT ( 'NONE',  ( 4.142179624174931796, 4.791296635414242111, 1.199719254218464037 ) ) ;
#110616=CARTESIAN_POINT ( 'NONE',  ( -1.500000000000013101, 1.202083334016148974, 0.8660254037844403729 ) ) ;
#110618=CARTESIAN_POINT ( 'NONE',  ( -7.718669524881690336, 7.899535955317097624, 0.7998128361456462443 ) ) ;
#110619=CARTESIAN_POINT ( 'NONE',  ( -2.792616454734997866, 6.201876930592042925, 0.7216878364870317197 ) ) ;
#110625=ORIENTED_EDGE ( 'NONE', *, *, #54063, .F. ) ;
#110627=CARTESIAN_POINT ( 'NONE',  ( 4.798696304233017074, 7.685897223992134819, -1.199719254218452047 ) ) ;
#110628=DIRECTION ( 'NONE',  ( -1.207943261119674327E-30, -2.168404344971008079E-15, 1.000000000000000000 ) ) ;
#110631=CARTESIAN_POINT ( 'NONE',  ( 5.282873410819217241, 9.315102745931094219, -0.7998128361456281477 ) ) ;
#110632=LINE ( 'NONE', #176634, #158461 ) ;
#110634=CARTESIAN_POINT ( 'NONE',  ( -5.205440912643032547, 8.160432600470439723, 1.199719254218452047 ) ) ;
#110636=CARTESIAN_POINT ( 'NONE',  ( 3.192055101013606233, 5.811482486902795230, -1.199719254218446718 ) ) ;
#110642=CARTESIAN_POINT ( 'NONE',  ( 4.034853869772982549, 7.546986718285443985, 0.4065704115671017749 ) ) ;
#110651=CARTESIAN_POINT ( 'NONE',  ( -4.311129659465605002, 4.131998812239033647, 0.7216878364870317197 ) ) ;
#110652=CARTESIAN_POINT ( 'NONE',  ( 6.778713617152772208, 10.85232362007950258, -0.7216878364870267237 ) ) ;
#110654=CARTESIAN_POINT ( 'NONE',  ( -5.037017762676898158, 5.835274463666530131, -1.199719254218446718 ) ) ;
#110655=FACE_OUTER_BOUND ( 'NONE', #46342, .T. ) ;
#110657=CARTESIAN_POINT ( 'NONE',  ( 7.365103760721646076, 9.615707025640515937, 1.599625672291281386 ) ) ;
#110659=CARTESIAN_POINT ( 'NONE',  ( -6.043183783389232566, 8.073467052085995022, 1.599625672291269396 ) ) ;
#110672=CARTESIAN_POINT ( 'NONE',  ( 8.536830278099042602, 13.11138575775759563, -0.7998128361456352531 ) ) ;
#110673=CARTESIAN_POINT ( 'NONE',  ( -3.879604511804807032, 7.677955697080923514, 0.7998128361456341429 ) ) ;
#110676=CARTESIAN_POINT ( 'NONE',  ( 4.541618270897912701, 4.400902192243413502, 1.214306433183764966E-14 ) ) ;
#110680=CARTESIAN_POINT ( 'NONE',  ( -2.676845263694313637, 5.210404343363602919, -1.199719254218446718 ) ) ;
#110681=CARTESIAN_POINT ( 'NONE',  ( -3.846762897975357198, 5.510976019103107859, -1.599625672291256295 ) ) ;
#110686=CARTESIAN_POINT ( 'NONE',  ( 9.459838494033030898, 12.05956421450382088, 1.599625672291281386 ) ) ;
#110689=CARTESIAN_POINT ( 'NONE',  ( -6.364663046611467756, 9.512858423433634414, 1.199719254218452047 ) ) ;
#110690=CARTESIAN_POINT ( 'NONE',  ( 3.974511587100456822, 7.788680618259193444, 1.040834085586084257E-14 ) ) ;
#110694=CARTESIAN_POINT ( 'NONE',  ( 1.364683531249986537, 1.967708333674750731, -0.7879004041258239610 ) ) ;
#110695=ORIENTED_EDGE ( 'NONE', *, *, #87971, .T. ) ;
#110697=CARTESIAN_POINT ( 'NONE',  ( 6.643132081016111634, 9.733775946952057723, 1.082531754730558626 ) ) ;
#110698=ORIENTED_EDGE ( 'NONE', *, *, #51647, .F. ) ;
#110705=CARTESIAN_POINT ( 'NONE',  ( 7.578644679914694926, 11.78557652663510424, 0.7216878364870438212 ) ) ;
#110710=CARTESIAN_POINT ( 'NONE',  ( 4.446711195602238043, 6.210915699667824974, -1.443375672974051449 ) ) ;
#110712=CARTESIAN_POINT ( 'NONE',  ( -8.631737353394710155, 13.22211067893587533, 1.040834085586084257E-14 ) ) ;
#110729=CARTESIAN_POINT ( 'NONE',  ( -1.201851678989727383E-14, 1.993750000682816381, 1.732050807568877637 ) ) ;
#110735=CARTESIAN_POINT ( 'NONE',  ( 0.7499999999999867883, -0.6833333333333135862, -1.299038105676652899 ) ) ;
#110736=CARTESIAN_POINT ( 'NONE',  ( 6.916630921265960019, 11.22115317478565188, 0.7998128361456462443 ) ) ;
#110740=CARTESIAN_POINT ( 'NONE',  ( 3.846762897975340767, 5.510976019103107859, -1.599625672291256295 ) ) ;
#110741=CARTESIAN_POINT ( 'NONE',  ( -6.561783159334141580, 7.718130443053708767, -1.082531754730544860 ) ) ;
#110747=CARTESIAN_POINT ( 'NONE',  ( -7.100719765255177229, 9.307259030929609267, -1.599625672291263179 ) ) ;
#110748=ORIENTED_EDGE ( 'NONE', *, *, #2128, .F. ) ;
#110749=CARTESIAN_POINT ( 'NONE',  ( 0.7499999999999902300, 1.514583334016148086, 1.299038105676657340 ) ) ;
#110761=CARTESIAN_POINT ( 'NONE',  ( -8.503988664269602538, 10.94440607977979063, 1.599625672291269396 ) ) ;
#110762=CARTESIAN_POINT ( 'NONE',  ( 6.123478934866503742, 10.29580919065294431, 0.7998128361456462443 ) ) ;
#110763=DIRECTION ( 'NONE',  ( -7.387867266669436732E-31, -1.000000000000000000, 8.546850786086437571E-32 ) ) ;
#110766=ORIENTED_EDGE ( 'NONE', *, *, #196345, .F. ) ;
#110769=CARTESIAN_POINT ( 'NONE',  ( -8.532158741701643123, 8.848606708273724308, 0.7998128361456462443 ) ) ;
#110773=CARTESIAN_POINT ( 'NONE',  ( -1.000000000000017097, 8.600000000000013856, -0.3999999999999858113 ) ) ;
#110776=CARTESIAN_POINT ( 'NONE',  ( 3.842846474469570062, 6.570739089268092137, -1.199719254218452047 ) ) ;
#110780=CARTESIAN_POINT ( 'NONE',  ( -9.917953063596627317, 11.52969898140628047, -1.199719254218441611 ) ) ;
#110783=CARTESIAN_POINT ( 'NONE',  ( -5.249217764984337009, 6.599847349967512322, -1.403262209131036053 ) ) ;
#110792=CARTESIAN_POINT ( 'NONE',  ( 7.332262146892202459, 7.448727347662698506, -0.7998128361456281477 ) ) ;
#110797=VERTEX_POINT ( 'NONE', #184264 ) ;
#110799=CARTESIAN_POINT ( 'NONE',  ( -1.402160292154681736E-14, -0.1312499993171854229, -1.732050807568870754 ) ) ;
#110802=CARTESIAN_POINT ( 'NONE',  ( -1.608462485352074145, 8.735270501766109419, -2.463594439587580176 ) ) ;
#110811=CARTESIAN_POINT ( 'NONE',  ( 4.094199201646931741, 4.839282492418613302, -1.082531754730543083 ) ) ;
#110814=CARTESIAN_POINT ( 'NONE',  ( -10.63367255181986160, 11.30037282007833532, 1.040834085586084257E-14 ) ) ;
#110816=CARTESIAN_POINT ( 'NONE',  ( 8.550388431712704573, 13.12720360364021133, 0.000000000000000000 ) ) ;
#110824=CARTESIAN_POINT ( 'NONE',  ( -1.364683531249997417, 5.821875000341418804, 1.214306433183764966E-14 ) ) ;
#110832=CARTESIAN_POINT ( 'NONE',  ( -4.055860508782465068, 7.883587693554856557, 1.040834085586084257E-14 ) ) ;
#110835=CARTESIAN_POINT ( 'NONE',  ( 1.499999999999987121, -0.7458333333333122539, 0.8660254037844524744 ) ) ;
#110837=CARTESIAN_POINT ( 'NONE',  ( 0.7499999999999902300, 5.816666666666685082, -1.299038105676658228 ) ) ;
#110842=CARTESIAN_POINT ( 'NONE',  ( 1.364683531249988535, 5.467708333674750953, -0.7879004041258300672 ) ) ;
#110844=CARTESIAN_POINT ( 'NONE',  ( -7.153898609505128015, 11.49796547773133604, 0.7998128361456481317 ) ) ;
#110846=CARTESIAN_POINT ( 'NONE',  ( 9.215791728987056786, 11.77484298861683598, -1.599625672291262513 ) ) ;
#110851=CARTESIAN_POINT ( 'NONE',  ( -1.402160292154681736E-14, 0.5093750003414236893, -1.575800808251659024 ) ) ;
#110856=CARTESIAN_POINT ( 'NONE',  ( -2.460826785407703721, 8.202405370174460586, 2.499999999999999112 ) ) ;
#110861=CARTESIAN_POINT ( 'NONE',  ( 7.673551755654734130, 9.015193805427763607, -1.082531754730537976 ) ) ;
#110864=CARTESIAN_POINT ( 'NONE',  ( -3.581325132304157943, 7.329963087663487364, -0.7998128361456281477 ) ) ;
#110867=CARTESIAN_POINT ( 'NONE',  ( 1.499999999999989120, 4.535416667349484676, 0.8660254037844524744 ) ) ;
#110869=CARTESIAN_POINT ( 'NONE',  ( -4.277761160311629673, 4.949475094240346706, 1.199719254218462483 ) ) ;
#110870=CARTESIAN_POINT ( 'NONE',  ( 6.954969613686092345, 7.216478758829655504, -0.7216878364870257245 ) ) ;
#110871=CARTESIAN_POINT ( 'NONE',  ( -9.476786185827959841, 10.15859809299519334, 0.7216878364870438212 ) ) ;
#110877=CARTESIAN_POINT ( 'NONE',  ( 3.816783937446950770, 4.411668334231586996, 1.199719254218464037 ) ) ;
#110885=CARTESIAN_POINT ( 'NONE',  ( -4.151088913318013773, 2.978104609995165131, -0.7749999999999935829 ) ) ;
#110892=CARTESIAN_POINT ( 'NONE',  ( 9.426996880203592610, 9.892584536526015881, -0.7998128361456281477 ) ) ;
#110896=DIRECTION ( 'NONE',  ( 5.578564026256491869E-16, 1.000000000000000000, 9.066213480720160632E-32 ) ) ;
#110897=CARTESIAN_POINT ( 'NONE',  ( -1.402160292154681736E-14, -0.4281249996585808071, 1.575800808251672791 ) ) ;
#110898=CARTESIAN_POINT ( 'NONE',  ( 5.016153647376205171, 6.875265226737464985, 1.443375672974062551 ) ) ;
#110900=CARTESIAN_POINT ( 'NONE',  ( -7.836249599018719536, 12.08611559892311504, 0.7216878364870478180 ) ) ;
#110909=ORIENTED_EDGE ( 'NONE', *, *, #24241, .T. ) ;
#110911=VERTEX_POINT ( 'NONE', #72651 ) ;
#110913=EDGE_LOOP ( 'NONE', ( #107405, #118444, #161415 ) ) ;
#110920=CARTESIAN_POINT ( 'NONE',  ( 5.763841807162588537, 6.241519824923047466, -1.009562751112670576 ) ) ;
#110925=CARTESIAN_POINT ( 'NONE',  ( 0.1505076982582145839, 7.030243935902785957, 1.995512553310466952 ) ) ;
#110928=CARTESIAN_POINT ( 'NONE',  ( -8.351459436338048548, 8.845716885256940998, -0.7216878364870278340 ) ) ;
#110932=CARTESIAN_POINT ( 'NONE',  ( 5.774883364416965037, 8.824782127540085952, -1.199719254218440723 ) ) ;
#110937=CARTESIAN_POINT ( 'NONE',  ( -3.100010679019018500, 6.768429558830820980, 1.040834085586084257E-14 ) ) ;
#110941=CARTESIAN_POINT ( 'NONE',  ( -5.525111292768871252, 6.404716915440499037, -1.199719254218446718 ) ) ;
#110944=CARTESIAN_POINT ( 'NONE',  ( 5.379888026524302980, 5.170957540566797128, -0.7998128361456211532 ) ) ;
#110945=CARTESIAN_POINT ( 'NONE',  ( 6.414979237560321401, 10.63589287712906462, 1.040834085586084257E-14 ) ) ;
#110946=CARTESIAN_POINT ( 'NONE',  ( 0.3548561630248124876, 6.502427107676207463, 3.303236143568316407 ) ) ;
#110948=CARTESIAN_POINT ( 'NONE',  ( 4.149381719138396818, 7.633502232665817289, 0.8094099469760536181 ) ) ;
#110949=CARTESIAN_POINT ( 'NONE',  ( 3.877268743828266029, 6.506935386899531437, 1.082531754730558626 ) ) ;
#110956=CARTESIAN_POINT ( 'NONE',  ( 6.195713011320782115, 8.251417818006149929, -1.443375672974057666 ) ) ;
#110957=CARTESIAN_POINT ( 'NONE',  ( -7.862839020921525091, 11.26073039346208660, -1.199719254218446718 ) ) ;
#110960=CARTESIAN_POINT ( 'NONE',  ( -9.820183334999905256, 10.35130206712171130, 1.040834085586084257E-14 ) ) ;
#110961=CARTESIAN_POINT ( 'NONE',  ( -7.365103760721662951, 9.615707025640515937, 1.599625672291295375 ) ) ;
#110969=CARTESIAN_POINT ( 'NONE',  ( 9.426996880203592610, 9.892584536526015881, -0.7998128361456281477 ) ) ;
#110970=CARTESIAN_POINT ( 'NONE',  ( -4.067937748088393590, 7.725456827083305278, 0.6547958487484796253 ) ) ;
#110974=CARTESIAN_POINT ( 'NONE',  ( 5.196852952739813070, 4.957416621151553571, -0.7998128361456221525 ) ) ;
#110983=CARTESIAN_POINT ( 'NONE',  ( -0.7500000000000215383, 3.441666666666689967, 1.299038105676671107 ) ) ;
#110984=CARTESIAN_POINT ( 'NONE',  ( 5.823390672269506574, 6.752709524857930745, -1.199719254218446718 ) ) ;
#110987=CARTESIAN_POINT ( 'NONE',  ( 4.370186222871176085, 4.005496238621469196, 0.1648321253336959835 ) ) ;
#110988=CARTESIAN_POINT ( 'NONE',  ( 6.751597309925441159, 9.860318714012938912, -1.082531754730537088 ) ) ;
#110990=CARTESIAN_POINT ( 'NONE',  ( 0.4571195463272426651, 7.927888240403390796, 1.992899296338177306 ) ) ;
#110993=CARTESIAN_POINT ( 'NONE',  ( 8.860417081730671995, 10.29590700256267155, 1.199719254218453823 ) ) ;
#110995=CARTESIAN_POINT ( 'NONE',  ( -0.7499999999999972244, 5.358333333333353821, -1.299038105676652011 ) ) ;
#110996=CARTESIAN_POINT ( 'NONE',  ( -2.754277761870538299, 6.365074488824250309, 1.040834085586084257E-14 ) ) ;
#110997=FACE_OUTER_BOUND ( 'NONE', #105703, .T. ) ;
#110998=CARTESIAN_POINT ( 'NONE',  ( 1.364683531249986537, 0.4052083336747511200, -0.7879004041258309554 ) ) ;
#111004=CARTESIAN_POINT ( 'NONE',  ( 0.6823417656249882723, -0.6572916663252492686, 1.181850606188755259 ) ) ;
#111006=CARTESIAN_POINT ( 'NONE',  ( 10.07100917685271035, 10.64393221595000938, 0.7998128361456462443 ) ) ;
#111010=CARTESIAN_POINT ( 'NONE',  ( -4.731432421044888592, 4.622352034081546712, -0.7216878364870207285 ) ) ;
#111013=CARTESIAN_POINT ( 'NONE',  ( -5.201524489137236529, 9.220195670635433771, 0.7998128361456481317 ) ) ;
#111016=CARTESIAN_POINT ( 'NONE',  ( 3.734381245560244089, 6.444196322207211836, 1.199719254218462483 ) ) ;
#111022=CARTESIAN_POINT ( 'NONE',  ( 9.154780037725547714, 11.70366268214508487, 1.599625672291279388 ) ) ;
#111025=CARTESIAN_POINT ( 'NONE',  ( -6.417086777969760902, 6.381022750586497594, 0.7998128361456341429 ) ) ;
#111029=CARTESIAN_POINT ( 'NONE',  ( 9.738834413317897898, 10.25639499182604730, 0.000000000000000000 ) ) ;
#111031=CARTESIAN_POINT ( 'NONE',  ( 8.911787042884274257, 9.291506392986812912, 0.7998128361456462443 ) ) ;
#111034=CARTESIAN_POINT ( 'NONE',  ( -8.920901888112002354, 11.43080484092926241, 1.443375672974064550 ) ) ;
#111036=CARTESIAN_POINT ( 'NONE',  ( 6.938893903907228378E-15, 10.64264068711930733, 1.214306433183764966E-14 ) ) ;
#111037=CARTESIAN_POINT ( 'NONE',  ( -7.640183256500752584, 8.872300873127729304, -1.199719254218446718 ) ) ;
#111041=CARTESIAN_POINT ( 'NONE',  ( -6.098685391867989303, 6.020399689055939696, 0.3646554611961040360 ) ) ;
#111042=CARTESIAN_POINT ( 'NONE',  ( -0.6823417656250212460, 1.801041667008083991, 1.181850606188755259 ) ) ;
#111045=CARTESIAN_POINT ( 'NONE',  ( 8.283668668269706714, 8.766627655843892697, 1.040834085586084257E-14 ) ) ;
#111063=CARTESIAN_POINT ( 'NONE',  ( 9.745613490124728884, 10.26430391476735338, 0.7998128361456462443 ) ) ;
#111067=CARTESIAN_POINT ( 'NONE',  ( -3.785751206713858785, 5.439795712631356750, 1.599625672291267398 ) ) ;
#111068=CARTESIAN_POINT ( 'NONE',  ( -8.290974629956718189, 9.631557475493025322, -1.199719254218446718 ) ) ;
#111073=CARTESIAN_POINT ( 'NONE',  ( -0.7499999999999972244, 4.889583334016150751, -1.299038105676652899 ) ) ;
#111074=CARTESIAN_POINT ( 'NONE',  ( 6.089583550832340819, 10.25626457594641749, 1.040834085586084257E-14 ) ) ;
#111079=CARTESIAN_POINT ( 'NONE',  ( -7.934546212495630968, 10.28005655271014795, -1.599625672291263179 ) ) ;
#111081=CARTESIAN_POINT ( 'NONE',  ( -0.6823417656249969321, 3.467708333674754506, -1.181850606188749264 ) ) ;
#111085=CARTESIAN_POINT ( 'NONE',  ( -8.839552966430007430, 11.33589776563360019, -1.443375672974059665 ) ) ;
#111089=CARTESIAN_POINT ( 'NONE',  ( 0.6823417656249882723, 2.488541667008084435, -1.181850606188749264 ) ) ;
#111097=CARTESIAN_POINT ( 'NONE',  ( -0.6823417656250212460, 3.301041667008085323, 1.181850606188767472 ) ) ;
#111099=CARTESIAN_POINT ( 'NONE',  ( -5.610376637956639101, 5.439860920571172542, 0.000000000000000000 ) ) ;
#111100=CARTESIAN_POINT ( 'NONE',  ( 7.287671262545424966, 8.461036880179857889, -1.199719254218451159 ) ) ;
#111103=CARTESIAN_POINT ( 'NONE',  ( -1.364683531249997417, 4.321875000341417028, 1.214306433183764966E-14 ) ) ;
#111107=CARTESIAN_POINT ( 'NONE',  ( 0.6823417656249882723, -0.07395833299191079124, -1.181850606188749264 ) ) ;
#111108=CARTESIAN_POINT ( 'NONE',  ( -4.690757960648240577, 6.495636925554817864, 1.443375672974064550 ) ) ;
#111112=CARTESIAN_POINT ( 'NONE',  ( 4.907688418466886304, 5.788353245375237321, -1.082531754730548412 ) ) ;
#111116=CARTESIAN_POINT ( 'NONE',  ( -7.660520486921249983, 8.896027641951645748, -1.199719254218446718 ) ) ;
#111117=CARTESIAN_POINT ( 'NONE',  ( -9.219181267612684749, 10.81842823604534765, 1.082531754730558626 ) ) ;
#111119=CARTESIAN_POINT ( 'NONE',  ( 1.499999999999990896, 5.025000000000022560, 1.214306433183764966E-14 ) ) ;
#111124=CARTESIAN_POINT ( 'NONE',  ( -5.694061327615147050, 9.586895948952255608, 0.000000000000000000 ) ) ;
#111126=CARTESIAN_POINT ( 'NONE',  ( -1.402160292154681736E-14, -0.8656249996585829720, 1.575800808251672791 ) ) ;
#111133=CARTESIAN_POINT ( 'NONE',  ( -3.633221978782283923, 7.182583375313884133, -0.7216878364870267237 ) ) ;
#111138=B_SPLINE_CURVE_WITH_KNOTS ( 'NONE', 3,
 ( #210834, #81904, #16881, #131772 ),
 .UNSPECIFIED., .F., .F.,
 ( 4, 4 ),
 ( 8.516827915679375891E-05, 0.0002597075693986928267 ),
 .UNSPECIFIED. ) ;
#111142=CIRCLE ( 'NONE', #159469, 3.971937515251341644 ) ;
#111143=CARTESIAN_POINT ( 'NONE',  ( 7.985389288324691748, 10.33937347451072775, -1.443375672974058777 ) ) ;
#111151=CARTESIAN_POINT ( 'NONE',  ( 5.126954644262057492, 9.133197518281081173, 0.7998128361456462443 ) ) ;
#111153=CARTESIAN_POINT ( 'NONE',  ( -4.928552533767591726, 5.708731696605642725, 1.199719254218462483 ) ) ;
#111157=CARTESIAN_POINT ( 'NONE',  ( -0.6823417656250212460, 1.863541667008083991, 1.181850606188755259 ) ) ;
#111159=CARTESIAN_POINT ( 'NONE',  ( -8.025536864285518490, 11.45054454405341282, -1.199719254218446718 ) ) ;
#111168=ORIENTED_EDGE ( 'NONE', *, *, #24646, .T. ) ;
#111174=CARTESIAN_POINT ( 'NONE',  ( -4.253564693897453175, 7.314528304839084782, -0.9025151233474463242 ) ) ;
#111177=CARTESIAN_POINT ( 'NONE',  ( 5.296431564432884542, 9.330920591813708143, 1.040834085586084257E-14 ) ) ;
#111186=CARTESIAN_POINT ( 'NONE',  ( 10.23370702021670020, 10.83374636654133383, 0.7998128361456462443 ) ) ;
#111192=CARTESIAN_POINT ( 'NONE',  ( 8.563946585326370098, 13.14302144952281814, 0.7998128361456462443 ) ) ;
#111194=CARTESIAN_POINT ( 'NONE',  ( -0.05606965051303709063, 7.151966587341615167, 1.999903488156155262 ) ) ;
#111200=CARTESIAN_POINT ( 'NONE',  ( -9.327646496521989405, 10.94497100310623594, -1.082531754730539753 ) ) ;
#111205=CARTESIAN_POINT ( 'NONE',  ( -4.900252779738026199, 4.865835280224682258, -0.2959858980189531419 ) ) ;
#111206=CARTESIAN_POINT ( 'NONE',  ( 4.313465427442102929, 8.184126765324453601, 0.7998128361456462443 ) ) ;
#111213=CARTESIAN_POINT ( 'NONE',  ( 2.806174607904299734, 5.257325561654889512, -1.082531754730543083 ) ) ;
#111221=CARTESIAN_POINT ( 'NONE',  ( -6.531277313481209212, 8.642909503859968368, 1.599625672291283607 ) ) ;
#111222=CYLINDRICAL_SURFACE ( 'NONE', #22555, 1.500000000000000222 ) ;
#111223=CARTESIAN_POINT ( 'NONE',  ( -3.164938793786285842, 5.779846795137578930, -1.199719254218452935 ) ) ;
#111228=DIRECTION ( 'NONE',  ( 1.000000000000000000, 0.000000000000000000, 0.000000000000000000 ) ) ;
#111232=CARTESIAN_POINT ( 'NONE',  ( 3.988069740714122791, 7.804498464141805592, 0.7998128361456321445 ) ) ;
#111233=DIRECTION ( 'NONE',  ( 1.000000000000000000, 0.000000000000000000, 0.000000000000000000 ) ) ;
#111244=CARTESIAN_POINT ( 'NONE',  ( -1.402160292154681736E-14, -0.1156249996585793222, 1.575800808251672791 ) ) ;
#111246=CARTESIAN_POINT ( 'NONE',  ( 3.246287715468270108, 5.874753870433235825, 1.199719254218450271 ) ) ;
#111250=CARTESIAN_POINT ( 'NONE',  ( -5.395781948558855845, 9.238903340053241209, 0.7216878364870458196 ) ) ;
#111251=CARTESIAN_POINT ( 'NONE',  ( 5.016153647376205171, 6.875265226737464985, 1.443375672974062551 ) ) ;
#111252=CARTESIAN_POINT ( 'NONE',  ( -8.324343128666356506, 8.814081192973304724, 1.040834085586084257E-14 ) ) ;
#111256=CARTESIAN_POINT ( 'NONE',  ( 6.636879889089462026, 7.701780277814560982, -1.199719254218446718 ) ) ;
#111261=CARTESIAN_POINT ( 'NONE',  ( 0.6823417656249899377, 4.426041667008086655, -1.181850606188754593 ) ) ;
#111265=CARTESIAN_POINT ( 'NONE',  ( 5.849453209292126310, 8.911780279894442103, 1.199719254218462483 ) ) ;
#111267=ADVANCED_FACE ( 'NONE', ( #56417 ), #45398, .T. ) ;
#111270=CARTESIAN_POINT ( 'NONE',  ( -6.340409392685171674, 10.54889472477470846, 0.7998128361456481317 ) ) ;
#111275=CARTESIAN_POINT ( 'NONE',  ( 8.372323551638698902, 9.726464550788689323, 1.199719254218462483 ) ) ;
#111277=CARTESIAN_POINT ( 'NONE',  ( -8.715193815486133033, 9.062147627688959872, 0.7998128361456462443 ) ) ;
#111279=CARTESIAN_POINT ( 'NONE',  ( 6.846504384776753049, 9.010674420371453053, -1.443375672974058777 ) ) ;
#111280=CARTESIAN_POINT ( 'NONE',  ( 4.085089063302896228, 7.714230733137671159, -0.6301764584765887633 ) ) ;
#111281=CARTESIAN_POINT ( 'NONE',  ( -8.839552966430007430, 11.33589776563360019, -1.443375672974059665 ) ) ;
#111286=CARTESIAN_POINT ( 'NONE',  ( 5.449487677688982679, 8.445153826357429949, -1.199719254218446718 ) ) ;
#111288=CARTESIAN_POINT ( 'NONE',  ( 9.215791728987056786, 11.77484298861683598, -1.599625672291262513 ) ) ;
#111289=CARTESIAN_POINT ( 'NONE',  ( -5.565401824202027115, 6.214873266482019432, 0.9197014482419992865 ) ) ;
#111291=CARTESIAN_POINT ( 'NONE',  ( 2.822068529938852155, 6.444163718237301275, -0.7998128361456291469 ) ) ;
#111293=CARTESIAN_POINT ( 'NONE',  ( -6.399085315970137522, 9.449054721065074602, -1.082531754730538864 ) ) ;
#111301=CARTESIAN_POINT ( 'NONE',  ( -4.566676325625886435, 6.985790553628898003, 1.179912429979562249 ) ) ;
#111302=CARTESIAN_POINT ( 'NONE',  ( -1.402160292154681736E-14, -0.4906249996585810846, -1.575800808251665908 ) ) ;
#111305=CARTESIAN_POINT ( 'NONE',  ( 3.389175213736285386, 6.897862149426897460, 0.7216878364870317197 ) ) ;
#111309=CARTESIAN_POINT ( 'NONE',  ( -9.449669878600625239, 10.12696240122997082, -0.7216878364870267237 ) ) ;
#111314=CARTESIAN_POINT ( 'NONE',  ( -9.341204649691320583, 10.96078884847042545, 1.082531754730558626 ) ) ;
#111315=DIRECTION ( 'NONE',  ( -0.01538971728768316095, 0.9998815712882226370, 0.000000000000000000 ) ) ;
#111321=CARTESIAN_POINT ( 'NONE',  ( -7.321039761255057066, 11.48503745486550365, 0.000000000000000000 ) ) ;
#111326=CARTESIAN_POINT ( 'NONE',  ( -1.201851678989727383E-14, 5.509375000341415252, -1.575800808251660134 ) ) ;
#111327=CARTESIAN_POINT ( 'NONE',  ( -1.201851678989727383E-14, 3.993750000682817713, 1.732050807568877637 ) ) ;
#111328=CARTESIAN_POINT ( 'NONE',  ( 6.062205217752669739, 6.048677139763619870, -0.4177986087803304271 ) ) ;
#111331=ORIENTED_EDGE ( 'NONE', *, *, #99953, .T. ) ;
#111333=CARTESIAN_POINT ( 'NONE',  ( -8.505042434474312074, 8.816971016508505343, -0.7998128361456291469 ) ) ;
#111337=CARTESIAN_POINT ( 'NONE',  ( 5.009901455449552010, 5.803638771901306725, -1.199719254218452047 ) ) ;
#111342=CARTESIAN_POINT ( 'NONE',  ( 8.718056468787178659, 10.12981962079525289, 1.199719254218462483 ) ) ;
#111343=CARTESIAN_POINT ( 'NONE',  ( -4.911970600500787043, 4.733485073844196478, 0.4366108110982139801 ) ) ;
#111349=CARTESIAN_POINT ( 'NONE',  ( -6.344852701515500293, 9.385783337534627790, 1.082531754730548412 ) ) ;
#111352=CARTESIAN_POINT ( 'NONE',  ( 4.365362273920243119, 6.116008624372161862, 1.443375672974062551 ) ) ;
#111355=CARTESIAN_POINT ( 'NONE',  ( -5.786256696412555911, 6.075953140482280190, 0.5845640519336701146 ) ) ;
#111359=CARTESIAN_POINT ( 'NONE',  ( -9.154780037725563702, 11.70366268214508487, 1.599625672291281386 ) ) ;
#111361=CARTESIAN_POINT ( 'NONE',  ( 8.934986926605834157, 10.38290515491702770, -1.199719254218446718 ) ) ;
#111362=CARTESIAN_POINT ( 'NONE',  ( 1.499999999999985123, 0.04583333333335545129, -0.8660254037844323793 ) ) ;
#111363=CARTESIAN_POINT ( 'NONE',  ( -10.01677656239806247, 10.58066083241955901, 0.7998128361456462443 ) ) ;
#111367=CARTESIAN_POINT ( 'NONE',  ( 1.364683531249988535, 3.363541667008084879, 0.7879004041258500513 ) ) ;
#111368=CARTESIAN_POINT ( 'NONE',  ( 3.871016551901614200, 4.474939717762034697, -1.199719254218446718 ) ) ;
#111371=CARTESIAN_POINT ( 'NONE',  ( 0.7499999999999902300, 4.566666666666691299, -1.299038105676658228 ) ) ;
#111374=CARTESIAN_POINT ( 'NONE',  ( 7.415946836550703303, 11.59576237604377091, 0.7216878364870438212 ) ) ;
#111377=CARTESIAN_POINT ( 'NONE',  ( -5.233084105194862445, 9.049089189461916760, 0.7216878364870458196 ) ) ;
#111378=EDGE_CURVE ( 'NONE', #127447, #6715, #28046, .T. ) ;
#111379=CARTESIAN_POINT ( 'NONE',  ( 0.6823417656249899377, 1.092708333674752286, 1.181850606188755259 ) ) ;
#111383=CARTESIAN_POINT ( 'NONE',  ( -6.018930129462987999, 9.109503353427070849, 1.199719254218452047 ) ) ;
#111384=CARTESIAN_POINT ( 'NONE',  ( -2.887523529586332405, 5.352232636950553513, 1.082531754730560403 ) ) ;
#111385=CARTESIAN_POINT ( 'NONE',  ( -1.364683531250010295, 4.842708333674756283, 0.7879004041258379498 ) ) ;
#111391=CARTESIAN_POINT ( 'NONE',  ( 9.420217803396747414, 9.884675613584706255, 0.7998128361456462443 ) ) ;
#111397=CARTESIAN_POINT ( 'NONE',  ( 10.58621901417202515, 11.24501035948919991, -0.7998128361456281477 ) ) ;
#111403=CARTESIAN_POINT ( 'NONE',  ( 9.237182729612253951, 9.671134694169463586, 0.7998128361456462443 ) ) ;
#111404=CARTESIAN_POINT ( 'NONE',  ( -8.143643823302737061, 12.65266822716189843, 0.000000000000000000 ) ) ;
#111406=CARTESIAN_POINT ( 'NONE',  ( -1.364683531249997417, 5.071875000341417916, 1.214306433183764966E-14 ) ) ;
#111409=CARTESIAN_POINT ( 'NONE',  ( -3.983199035293045309, 7.838694717720641414, 0.2268021594909743477 ) ) ;
#111410=CARTESIAN_POINT ( 'NONE',  ( 6.611572464958476836, 10.86525164242692298, 0.7998128361456462443 ) ) ;
#111411=CARTESIAN_POINT ( 'NONE',  ( -2.279984679289828176, 5.601133616484927025, -0.06592222766762731445 ) ) ;
#111413=CARTESIAN_POINT ( 'NONE',  ( 0.6823417656249917140, 3.342708333674754506, 1.181850606188765695 ) ) ;
#111415=CARTESIAN_POINT ( 'NONE',  ( -6.399085315970142851, 8.488685506763726352, -1.443375672974059665 ) ) ;
#111421=CARTESIAN_POINT ( 'NONE',  ( 2.381428537494710618, 5.930083727052461562, 0.7998128361456462443 ) ) ;
#111423=ORIENTED_EDGE ( 'NONE', *, *, #132407, .T. ) ;
#111424=CARTESIAN_POINT ( 'NONE',  ( 7.391166297744269365, 11.77477778067701664, 1.040834085586084257E-14 ) ) ;
#111430=CARTESIAN_POINT ( 'NONE',  ( -8.622095623286845978, 12.14652976288826913, 1.199719254218462483 ) ) ;
#111432=CARTESIAN_POINT ( 'NONE',  ( 7.644099680006512187, 7.812537802962739697, 1.040834085586084257E-14 ) ) ;
#111435=CARTESIAN_POINT ( 'NONE',  ( 4.975479186090860928, 4.907073259968533385, 0.7216878364870317197 ) ) ;
#111437=CARTESIAN_POINT ( 'NONE',  ( 5.657830175604453338, 5.495223381160312393, 0.7998128361456341429 ) ) ;
#111438=ORIENTED_EDGE ( 'NONE', *, *, #173816, .F. ) ;
#111445=CARTESIAN_POINT ( 'NONE',  ( -5.246642258808529746, 9.064907035344523578, 0.000000000000000000 ) ) ;
#111446=CARTESIAN_POINT ( 'NONE',  ( 3.765413976293345844, 5.416068943807445635, 1.599625672291267398 ) ) ;
#111449=CARTESIAN_POINT ( 'NONE',  ( -6.398558430645608475, 9.552403038140164782, -1.199719254218440723 ) ) ;
#111456=CARTESIAN_POINT ( 'NONE',  ( -10.30827686509187835, 10.92074451889568643, 1.040834085586084257E-14 ) ) ;
#111459=CARTESIAN_POINT ( 'NONE',  ( 8.281332899848809603, 8.555976559445431562, 0.7998128361456481317 ) ) ;
#111461=CARTESIAN_POINT ( 'NONE',  ( 2.758194185376297902, 5.305311418659259814, 1.199719254218452047 ) ) ;
#111472=CARTESIAN_POINT ( 'NONE',  ( -7.751511138711140170, 10.06651563329490529, -1.599625672291263179 ) ) ;
#111476=CARTESIAN_POINT ( 'NONE',  ( 7.144783764721768904, 7.437928601704619780, 1.040834085586084257E-14 ) ) ;
#111477=CARTESIAN_POINT ( 'NONE',  ( -4.690757960648240577, 6.495636925554817864, 1.443375672974064550 ) ) ;
#111479=CARTESIAN_POINT ( 'NONE',  ( -6.087774667736030487, 7.061157519568837415, 1.199719254218450271 ) ) ;
#111482=CARTESIAN_POINT ( 'NONE',  ( -1.499999999999997558, 7.809273069926255140, -3.635729725621148489 ) ) ;
#111489=CARTESIAN_POINT ( 'NONE',  ( 3.348500752450959350, 6.850408611260626834, 0.7216878364870540352 ) ) ;
#111490=CARTESIAN_POINT ( 'NONE',  ( 8.263858322729371153, 9.599921783727809910, -1.199719254218446718 ) ) ;
#111493=CARTESIAN_POINT ( 'NONE',  ( -4.121315508874276112, 4.870918184183829602, -1.082531754730549967 ) ) ;
#111496=CARTESIAN_POINT ( 'NONE',  ( -5.297426666345223190, 6.395294968284933823, -1.134026229594787383 ) ) ;
#111503=CARTESIAN_POINT ( 'NONE',  ( 4.708759422647839976, 4.387974169377582001, -0.7998128361456211532 ) ) ;
#111509=CARTESIAN_POINT ( 'NONE',  ( 2.679707916995359263, 6.278076336469897711, -0.7998128361456291469 ) ) ;
#111514=CARTESIAN_POINT ( 'NONE',  ( -0.6823417656250212460, 3.363541667008085323, 1.181850606188767472 ) ) ;
#111519=CARTESIAN_POINT ( 'NONE',  ( 5.555090253297246150, 7.504024600312024340, 1.599625672291267398 ) ) ;
#111523=CARTESIAN_POINT ( 'NONE',  ( -5.759516327706961647, 5.613857225279885732, -0.7998128361456221525 ) ) ;
#111524=CARTESIAN_POINT ( 'NONE',  ( 4.650083499362864359, 7.408552601689905259, 1.082531754730558626 ) ) ;
#111525=CARTESIAN_POINT ( 'NONE',  ( -1.500000000000013101, 4.129166666666687746, -0.8660254037844313801 ) ) ;
#111528=CARTESIAN_POINT ( 'NONE',  ( -3.438964519360665051, 7.163875705896082913, -0.7998128361456281477 ) ) ;
#111531=CARTESIAN_POINT ( 'NONE',  ( -1.364683531249997417, 4.009375000341424133, 1.214306433183764966E-14 ) ) ;
#111534=CARTESIAN_POINT ( 'NONE',  ( -4.338245966692955591, 5.124003718305597310, 1.082531754730560403 ) ) ;
#111536=ORIENTED_EDGE ( 'NONE', *, *, #60217, .T. ) ;
#111539=CARTESIAN_POINT ( 'NONE',  ( 4.005544317833563461, 6.760553239859419250, -1.199719254218452047 ) ) ;
#111542=CARTESIAN_POINT ( 'NONE',  ( 0.5146009213643799596, 6.747837823239234645, -3.492810981166099005 ) ) ;
#111546=CARTESIAN_POINT ( 'NONE',  ( -0.6823417656250212460, 1.863541667008083991, 1.181850606188755259 ) ) ;
#111548=CARTESIAN_POINT ( 'NONE',  ( -9.592557376868645846, 11.15007068022363157, -1.199719254218441611 ) ) ;
#111549=CARTESIAN_POINT ( 'NONE',  ( -6.358410854684789726, 8.441231968597481483, -1.443375672974058777 ) ) ;
#111553=CARTESIAN_POINT ( 'NONE',  ( -1.364683531250012516, 3.988541667008088876, -0.7879004041258300672 ) ) ;
#111559=B_SPLINE_CURVE_WITH_KNOTS ( 'NONE', 3,
 ( #15403, #64184, #81493, #30624, #213591, #181119, #51125, #32738, #80426, #112997 ),
 .UNSPECIFIED., .F., .F.,
 ( 4, 2, 2, 2, 4 ),
 ( 0.0002564548269640155843, 0.0006929466575915253432, 0.001129438488219035265, 0.001565930318846545186, 0.002002422149474054891 ),
 .UNSPECIFIED. ) ;
#111562=CARTESIAN_POINT ( 'NONE',  ( -6.846504384776765484, 8.050305206070113684, -1.082531754730543083 ) ) ;
#111568=CARTESIAN_POINT ( 'NONE',  ( -5.056828107772852299, 7.883087978168217269, -1.082531754730548412 ) ) ;
#111579=CARTESIAN_POINT ( 'NONE',  ( 4.067759563269675915, 7.712442911444558291, -0.5649101002591673248 ) ) ;
#111581=CARTESIAN_POINT ( 'NONE',  ( -5.603597561149804562, 5.431951997629870910, 0.7998128361456341429 ) ) ;
#111584=CARTESIAN_POINT ( 'NONE',  ( -1.500000000000015099, 0.3791666666666850261, -0.8660254037844383745 ) ) ;
#111586=CARTESIAN_POINT ( 'NONE',  ( 9.137832345930652522, 10.72352116074969075, -1.082531754730543083 ) ) ;
#111587=CARTESIAN_POINT ( 'NONE',  ( 7.308008492965924141, 8.484763649003774333, -1.199719254218451159 ) ) ;
#111592=CARTESIAN_POINT ( 'NONE',  ( 4.680589345215795838, 6.483773540883647435, -1.599625672291256295 ) ) ;
#111602=CARTESIAN_POINT ( 'NONE',  ( -6.898401231254901234, 6.942556279419168419, -0.7998128361456291469 ) ) ;
#111604=ORIENTED_EDGE ( 'NONE', *, *, #50310, .F. ) ;
#111605=FACE_OUTER_BOUND ( 'NONE', #21763, .T. ) ;
#111607=VERTEX_POINT ( 'NONE', #122444 ) ;
#111609=CARTESIAN_POINT ( 'NONE',  ( 1.364683531249988535, 2.905208333674754506, -0.7879004041258239610 ) ) ;
#111610=CARTESIAN_POINT ( 'NONE',  ( 9.070041577417981671, 9.684062716516882219, -0.7216878364870197293 ) ) ;
#111611=CARTESIAN_POINT ( 'NONE',  ( -5.689618019229208734, 9.789638122409414223, 0.7998128361456481317 ) ) ;
#111614=CARTESIAN_POINT ( 'NONE',  ( 6.277588818327314080, 7.282607361925381717, 1.199719254218462483 ) ) ;
#111615=CARTESIAN_POINT ( 'NONE',  ( -4.903245109636583443, 8.872203061218007392, -0.7998128361456281477 ) ) ;
#111619=CARTESIAN_POINT ( 'NONE',  ( -1.500000000000015099, 0.6604166673494823447, -0.8660254037844313801 ) ) ;
#111622=CARTESIAN_POINT ( 'NONE',  ( 6.968527767744098433, 9.153035033833367251, 1.443375672974076540 ) ) ;
#111625=CARTESIAN_POINT ( 'NONE',  ( 0.6823417656249899377, 2.405208333674753618, 1.181850606188767472 ) ) ;
#111627=CARTESIAN_POINT ( 'NONE',  ( 6.168596704093459060, 7.259412911939593371, -1.082531754730543083 ) ) ;
#111629=CARTESIAN_POINT ( 'NONE',  ( -3.118012141462980669, 6.581505231774690046, 0.7216878364870317197 ) ) ;
#111632=FACE_OUTER_BOUND ( 'NONE', #5023, .T. ) ;
#111635=LINE ( 'NONE', #177646, #129316 ) ;
#111638=CARTESIAN_POINT ( 'NONE',  ( -4.028535363944735437, 7.777154369360758324, -0.5044922354892691363 ) ) ;
#111644=CARTESIAN_POINT ( 'NONE',  ( 5.147291874682557555, 9.156924287104992288, 0.7998128361456462443 ) ) ;
#111647=CARTESIAN_POINT ( 'NONE',  ( 2.849184837166184536, 6.475799410002530898, 0.7998128361456362523 ) ) ;
#111655=CARTESIAN_POINT ( 'NONE',  ( 3.687454593236936251, 7.245854758844324728, -0.7216878364870267237 ) ) ;
#111656=CARTESIAN_POINT ( 'NONE',  ( 1.364683531249988757, 2.446875000341415696, 1.214306433183764966E-14 ) ) ;
#111657=CARTESIAN_POINT ( 'NONE',  ( 8.402302512167096893, 10.82577223566020841, -1.599625672291268286 ) ) ;
#111659=DIRECTION ( 'NONE',  ( -0.8002608041566210417, 0.5996521035822340862, 0.000000000000000000 ) ) ;
#111666=CARTESIAN_POINT ( 'NONE',  ( -1.499999999999997780, 2.150000000000019895, 1.214306433183764966E-14 ) ) ;
#111667=CARTESIAN_POINT ( 'NONE',  ( 6.634017235788401301, 6.634108284708264414, 0.7998128361456341429 ) ) ;
#111668=CARTESIAN_POINT ( 'NONE',  ( -7.283754839039664475, 9.520799950344851936, -1.599625672291263179 ) ) ;
#111672=CARTESIAN_POINT ( 'NONE',  ( -0.6823417656250003738, 2.217708333674753174, -1.181850606188749264 ) ) ;
#111674=CARTESIAN_POINT ( 'NONE',  ( 4.356247428692526569, 3.976710176429713250, 0.7998128361456341429 ) ) ;
#111680=CARTESIAN_POINT ( 'NONE',  ( -1.500000000000001332, 0.9312500006828163812, 0.000000000000000000 ) ) ;
#111682=CARTESIAN_POINT ( 'NONE',  ( -6.693975156845199059, 8.832723654451292816, 1.599625672291283607 ) ) ;
#111683=CARTESIAN_POINT ( 'NONE',  ( -2.643476764984671767, 6.027880625883323518, 1.040834085586084257E-14 ) ) ;
#111691=CARTESIAN_POINT ( 'NONE',  ( 4.961394147597008697, 7.875711374583454827, -1.199719254218452047 ) ) ;
#111695=CARTESIAN_POINT ( 'NONE',  ( 6.226218857173709154, 8.287007971501239467, 1.599625672291281386 ) ) ;
#111698=ORIENTED_EDGE ( 'NONE', *, *, #210974, .F. ) ;
#111701=CARTESIAN_POINT ( 'NONE',  ( -7.054319997812058318, 7.124461507069184130, 1.040834085586084257E-14 ) ) ;
#111702=ORIENTED_EDGE ( 'NONE', *, *, #8106, .F. ) ;
#111703=CARTESIAN_POINT ( 'NONE',  ( 3.029357257649615054, 5.621668336311468117, -1.199719254218446718 ) ) ;
#111708=CARTESIAN_POINT ( 'NONE',  ( 4.254136489245101238, 7.273159757992218921, 0.9281648423343953347 ) ) ;
#111717=CARTESIAN_POINT ( 'NONE',  ( -4.622967192579922724, 4.495809267539077503, 1.214306433183764966E-14 ) ) ;
#111718=CARTESIAN_POINT ( 'NONE',  ( 7.293923454472077239, 10.49303254931736262, 1.082531754730558626 ) ) ;
#111720=CARTESIAN_POINT ( 'NONE',  ( -3.906720819032141190, 7.709591388846142479, -0.7998128361456281477 ) ) ;
#111724=CARTESIAN_POINT ( 'NONE',  ( -5.371001409308059138, 9.417918744168066070, -0.7998128361456231517 ) ) ;
#111740=CARTESIAN_POINT ( 'NONE',  ( -3.405069135326500351, 7.124331091189553433, 1.040834085586084257E-14 ) ) ;
#111743=CARTESIAN_POINT ( 'NONE',  ( 4.717874267875568961, 4.606534188717351874, -0.7216878364870188411 ) ) ;
#111747=CARTESIAN_POINT ( 'NONE',  ( -3.918470089549458635, 4.530302178351167441, -1.199719254218452047 ) ) ;
#111748=CARTESIAN_POINT ( 'NONE',  ( -2.916975605234527702, 6.554888639415577423, 1.040834085586084257E-14 ) ) ;
#111750=DIRECTION ( 'NONE',  ( 0.000000000000000000, 8.546850786086437571E-32, 1.000000000000000000 ) ) ;
#111751=CARTESIAN_POINT ( 'NONE',  ( 8.594979316059474073, 12.11489407112305372, 1.199719254218450271 ) ) ;
#111755=CARTESIAN_POINT ( 'NONE',  ( -6.690058733339450114, 9.892486724616283311, 1.199719254218452047 ) ) ;
#111756=CARTESIAN_POINT ( 'NONE',  ( 5.335297142177534369, 6.183267073083954735, -1.199719254218452047 ) ) ;
#111759=CARTESIAN_POINT ( 'NONE',  ( 3.486418057008484617, 7.219238166485217434, 1.040834085586084257E-14 ) ) ;
#111762=CARTESIAN_POINT ( 'NONE',  ( -1.364683531250014514, 1.051041667008090208, -0.7879004041258289570 ) ) ;
#111765=CARTESIAN_POINT ( 'NONE',  ( 6.466876084038451822, 10.48851316477946582, 1.040834085586084257E-14 ) ) ;
#111773=CARTESIAN_POINT ( 'NONE',  ( 9.693716643646590470, 12.33242205571964512, 1.443375672974076540 ) ) ;
#111780=CARTESIAN_POINT ( 'NONE',  ( -1.608462485350627524, 8.735270501766752460, 2.463594439587639240 ) ) ;
#111782=CARTESIAN_POINT ( 'NONE',  ( -10.66756793585402363, 11.33991743478486391, 0.7998128361456462443 ) ) ;
#111798=CARTESIAN_POINT ( 'NONE',  ( -1.402160292154681736E-14, 1.118750000682820378, -1.732050807568863648 ) ) ;
#111804=CARTESIAN_POINT ( 'NONE',  ( 0.7499999999999867883, -0.9333333333333138082, -1.299038105676652011 ) ) ;
#111805=CARTESIAN_POINT ( 'NONE',  ( 8.589254009457354400, 9.979550084910457031, -1.199719254218446718 ) ) ;
#111810=CARTESIAN_POINT ( 'NONE',  ( 4.681643115420508039, 4.356338477612361260, 0.7998128361456341429 ) ) ;
#111811=CARTESIAN_POINT ( 'NONE',  ( -4.609409038966229666, 8.321468278861834378, -0.7216878364870267237 ) ) ;
#111814=CIRCLE ( 'NONE', #104951, 0.08000000000000020983 ) ;
#111818=CARTESIAN_POINT ( 'NONE',  ( -7.043624497499477499, 8.176315654292865887, 1.199719254218450271 ) ) ;
#111819=ORIENTED_EDGE ( 'NONE', *, *, #13980, .F. ) ;
#111820=CARTESIAN_POINT ( 'NONE',  ( -1.402160292154681736E-14, 1.368750000682821710, -1.732050807568863648 ) ) ;
#111828=CARTESIAN_POINT ( 'NONE',  ( -3.267151830768952880, 5.795132321663641228, -1.082531754730549078 ) ) ;
#111831=CARTESIAN_POINT ( 'NONE',  ( 4.117415066209698438, 7.437700365148243620, 0.6807796091479866307 ) ) ;
#111837=CARTESIAN_POINT ( 'NONE',  ( -4.270455198180246548, 4.084545274072787890, 0.7216878364870317197 ) ) ;
#111838=CARTESIAN_POINT ( 'NONE',  ( 6.421758314367153275, 10.64380180007036891, -0.7998128361456291469 ) ) ;
#111845=CARTESIAN_POINT ( 'NONE',  ( -8.345207244411405156, 9.694828859023472134, 1.199719254218462483 ) ) ;
#111851=CARTESIAN_POINT ( 'NONE',  ( 3.181359600701000989, 6.863336634126477875, 0.000000000000000000 ) ) ;
#111856=CARTESIAN_POINT ( 'NONE',  ( 0.01493835450741834783, 6.487495393664098664, -3.100011470320001905 ) ) ;
#111859=CARTESIAN_POINT ( 'NONE',  ( -5.338497050760650176, 6.533440992188984886, -1.368045069562271010 ) ) ;
#111867=CARTESIAN_POINT ( 'NONE',  ( 7.657657833620182153, 7.828355648845348291, -0.7998128361456281477 ) ) ;
#111869=ORIENTED_EDGE ( 'NONE', *, *, #212623, .F. ) ;
#111871=CARTESIAN_POINT ( 'NONE',  ( -6.385527162356468445, 10.39360608948380538, 1.040834085586084257E-14 ) ) ;
#111874=( BOUNDED_CURVE ( )  B_SPLINE_CURVE ( 2, ( #111119, #56972, #73199, #40736, #28739, #209590, #94824 ),
 .UNSPECIFIED., .F., .T. ) 
 B_SPLINE_CURVE_WITH_KNOTS ( ( 3, 2, 2, 3 ),
 ( 0.1249999999999998612, 0.1309523809523809035, 0.1369047619047619735, 0.1428571428571429880 ),
 .UNSPECIFIED. ) 
 CURVE ( )  GEOMETRIC_REPRESENTATION_ITEM ( )  RATIONAL_B_SPLINE_CURVE ( ( 1.000000000000003109, 0.8660254037844355990, 1.000000000000000000, 0.8660254037844387076, 1.000000000000000000, 0.8660254037844355990, 1.000000000000003109 ) ) 
 REPRESENTATION_ITEM ( '' )  );
#111876=CARTESIAN_POINT ( 'NONE',  ( -1.500000000000013101, 0.4520833340161533598, 0.8660254037844403729 ) ) ;
#111880=CARTESIAN_POINT ( 'NONE',  ( 2.381428537494710618, 5.930083727052461562, 0.7998128361456462443 ) ) ;
#111882=CARTESIAN_POINT ( 'NONE',  ( -10.30827686509187835, 10.92074451889568643, 1.040834085586084257E-14 ) ) ;
#111889=CARTESIAN_POINT ( 'NONE',  ( 4.026408433578586354, 7.641300905909586660, 1.040834085586084257E-14 ) ) ;
#111893=DIRECTION ( 'NONE',  ( -0.000000000000000000, -8.546850786086437571E-32, -1.000000000000000000 ) ) ;
#111894=CARTESIAN_POINT ( 'NONE',  ( 10.72180055030867329, 11.40318881831530540, 0.7998128361456341429 ) ) ;
#111904=CARTESIAN_POINT ( 'NONE',  ( 1.364683531249988757, -0.6156249996585803075, 0.000000000000000000 ) ) ;
#111910=CIRCLE ( 'NONE', #101462, 0.07999999999999998779 ) ;
#111911=CARTESIAN_POINT ( 'NONE',  ( -4.717347382551060342, 7.590990148696470818, 1.199719254218464037 ) ) ;
#111914=CARTESIAN_POINT ( 'NONE',  ( -1.500000000000015099, -0.8291666666666407393, 0.8660254037844403729 ) ) ;
#111916=CARTESIAN_POINT ( 'NONE',  ( 1.499999999999987121, 4.795833333333353821, -0.8660254037844323793 ) ) ;
#111917=CARTESIAN_POINT ( 'NONE',  ( -1.420000000000001039, 6.120000000000041851, -2.499999999999995115 ) ) ;
#111923=CARTESIAN_POINT ( 'NONE',  ( 0.6823417656249864960, -0.8239583329919114574, -1.181850606188749264 ) ) ;
#111925=CARTESIAN_POINT ( 'NONE',  ( 4.625302960556422427, 8.547937220624488575, 1.040834085586084257E-14 ) ) ;
#111926=CARTESIAN_POINT ( 'NONE',  ( -7.666245793523398078, 11.03137162816423356, 1.199719254218453823 ) ) ;
#111932=CARTESIAN_POINT ( 'NONE',  ( -1.364683531250014514, -0.9072916663252470482, 0.7879004041258379498 ) ) ;
#111940=CARTESIAN_POINT ( 'NONE',  ( 7.809133291791403586, 8.213003049952529722, -0.7216878364870257245 ) ) ;
#111944=CARTESIAN_POINT ( 'NONE',  ( 0.7499999999999920064, 5.014583334016150751, 1.299038105676669330 ) ) ;
#111946=CARTESIAN_POINT ( 'NONE',  ( -3.253066792275140173, 5.882662793374543675, 1.199719254218462483 ) ) ;
#111947=CARTESIAN_POINT ( 'NONE',  ( 7.443063143778065438, 7.785921210603627962, -0.7216878364870257245 ) ) ;
#111948=CARTESIAN_POINT ( 'NONE',  ( -8.961576348508641487, 11.47825837805867799, -1.443375672974058777 ) ) ;
#111954=CARTESIAN_POINT ( 'NONE',  ( 9.083599731475976213, 12.58098820582193689, 1.082531754730546636 ) ) ;
#111963=FACE_OUTER_BOUND ( 'NONE', #81415, .T. ) ;
#111969=EDGE_CURVE ( 'NONE', #155662, #97860, #211035, .T. ) ;
#111971=CARTESIAN_POINT ( 'NONE',  ( 8.483651433849084711, 10.92067931095586886, 1.599625672291281386 ) ) ;
#111975=CARTESIAN_POINT ( 'NONE',  ( -1.500000000000021982, 7.438721522839123246, 4.195160983902633589 ) ) ;
#111977=CARTESIAN_POINT ( 'NONE',  ( -0.6823417656250003738, -0.7822916663252423852, -1.181850606188749264 ) ) ;
#111979=CARTESIAN_POINT ( 'NONE',  ( 5.260200412422194383, 7.159986452624450770, -1.443375672974051449 ) ) ;
#111980=CARTESIAN_POINT ( 'NONE',  ( -8.920901888112002354, 11.43080484092926241, 1.443375672974064550 ) ) ;
#111989=ORIENTED_EDGE ( 'NONE', *, *, #50440, .F. ) ;
#112000=CARTESIAN_POINT ( 'NONE',  ( 4.581598608702507569, 7.168929433314090716, -1.325851593340146461 ) ) ;
#112004=CARTESIAN_POINT ( 'NONE',  ( -4.946829630374642406, 6.829763058803005826, -1.486263735186076129 ) ) ;
#112007=CARTESIAN_POINT ( 'NONE',  ( -6.710922849084449915, 10.77323439066645783, 0.000000000000000000 ) ) ;
#112011=CARTESIAN_POINT ( 'NONE',  ( 5.425234023762710578, 9.481190127698507553, -0.7998128361456291469 ) ) ;
#112012=CARTESIAN_POINT ( 'NONE',  ( -4.731959306369413198, 5.479372931307791461, -1.199719254218446718 ) ) ;
#112014=CARTESIAN_POINT ( 'NONE',  ( -4.786191920824102830, 5.542644314838231168, 1.199719254218462483 ) ) ;
#112018=CARTESIAN_POINT ( 'NONE',  ( -3.255929445576174697, 6.950334786480840243, -0.7998128361456281477 ) ) ;
#112021=CARTESIAN_POINT ( 'NONE',  ( 5.301401758143367893, 6.143722458377430584, 1.199719254218462483 ) ) ;
#112022=CARTESIAN_POINT ( 'NONE',  ( 8.697719238366680372, 10.10609285197134533, 1.199719254218462483 ) ) ;
#112025=CARTESIAN_POINT ( 'NONE',  ( 4.197832665289490173, 7.575126408543901846, 0.9117821302269245587 ) ) ;
#112026=CARTESIAN_POINT ( 'NONE',  ( 3.538314903486612817, 7.071858454135611538, 1.040834085586084257E-14 ) ) ;
#112033=CARTESIAN_POINT ( 'NONE',  ( 6.602457619730749627, 10.64669162308715222, 0.7216878364870438212 ) ) ;
#112035=CARTESIAN_POINT ( 'NONE',  ( -9.508345801885592863, 9.987491611821676329, 0.7998128361456462443 ) ) ;
#112038=CARTESIAN_POINT ( 'NONE',  ( -7.797910906154257304, 12.24931315715533486, 0.000000000000000000 ) ) ;
#112040=CARTESIAN_POINT ( 'NONE',  ( -6.581593504430098385, 9.765943957555402122, -1.199719254218440723 ) ) ;
#112045=CARTESIAN_POINT ( 'NONE',  ( 1.458253848507185202, 8.740113170334296910, -2.549233421402206101 ) ) ;
#112048=CARTESIAN_POINT ( 'NONE',  ( 7.567422294721922960, 11.98040977715095323, 0.7998128361456462443 ) ) ;
#112052=CARTESIAN_POINT ( 'NONE',  ( 4.356247428692526569, 3.976710176429713250, 0.7998128361456341429 ) ) ;
#112055=CARTESIAN_POINT ( 'NONE',  ( 0.7499999999999920064, 5.264583334016151639, 1.299038105676669330 ) ) ;
#112061=CARTESIAN_POINT ( 'NONE',  ( 1.499999999999989120, 2.504166666666687302, 0.8660254037844524744 ) ) ;
#112062=CARTESIAN_POINT ( 'NONE',  ( 6.311484202361478779, 7.322151976631905868, -1.199719254218446718 ) ) ;
#112064=CARTESIAN_POINT ( 'NONE',  ( 4.350813900535696277, 4.000456626940672500, 0.2320863031703649382 ) ) ;
#112065=CARTESIAN_POINT ( 'NONE',  ( 8.446366511633696561, 8.956441806435218922, 1.040834085586084257E-14 ) ) ;
#112066=CARTESIAN_POINT ( 'NONE',  ( -10.61567108937589765, 11.48729714713446803, 0.7216878364870438212 ) ) ;
#112069=CARTESIAN_POINT ( 'NONE',  ( 8.402302512167096893, 10.82577223566020841, -1.599625672291268286 ) ) ;
#112072=CARTESIAN_POINT ( 'NONE',  ( -4.277761160311629673, 4.949475094240346706, 1.199719254218462483 ) ) ;
#112073=CARTESIAN_POINT ( 'NONE',  ( 1.499999999999991118, 5.535416667349481123, 0.8660254037844524744 ) ) ;
#112075=CARTESIAN_POINT ( 'NONE',  ( -1.364683531250000748, 1.509375000341421691, 0.000000000000000000 ) ) ;
#112080=CARTESIAN_POINT ( 'NONE',  ( -1.364683531250014514, -0.9697916663252473812, 0.7879004041258379498 ) ) ;
#112090=CARTESIAN_POINT ( 'NONE',  ( -6.632963465583701534, 8.761543347979550589, -1.599625672291263179 ) ) ;
#112093=CARTESIAN_POINT ( 'NONE',  ( 5.952193131599331721, 6.902979060742733708, 1.199719254218462483 ) ) ;
#112102=CARTESIAN_POINT ( 'NONE',  ( -3.730464822054482710, 7.503959392372201442, 1.040834085586084257E-14 ) ) ;
#112106=CARTESIAN_POINT ( 'NONE',  ( 9.053093885623066939, 11.58502883802551153, -1.599625672291262513 ) ) ;
#112108=CARTESIAN_POINT ( 'NONE',  ( 8.914649696185335870, 10.35917838609310593, -1.199719254218446718 ) ) ;
#112112=CARTESIAN_POINT ( 'NONE',  ( -8.351459436338023679, 12.68719374246231624, -0.7216878364870267237 ) ) ;
#112113=CARTESIAN_POINT ( 'NONE',  ( -7.881367368245678406, 8.089350105908421185, 0.7998128361456602331 ) ) ;
#112117=CARTESIAN_POINT ( 'NONE',  ( -5.998154408198820953, 6.083692137903044639, 0.6724663025347333845 ) ) ;
#112118=CARTESIAN_POINT ( 'NONE',  ( -1.364683531250000748, -0.2406249996585799189, 0.000000000000000000 ) ) ;
#112121=CARTESIAN_POINT ( 'NONE',  ( 5.978782553946477840, 9.919070713005490703, 1.040834085586084257E-14 ) ) ;
#112139=CARTESIAN_POINT ( 'NONE',  ( 10.26082332744404368, 10.86538205830655279, -0.7998128361456281477 ) ) ;
#112141=ORIENTED_EDGE ( 'NONE', *, *, #196828, .T. ) ;
#112144=CARTESIAN_POINT ( 'NONE',  ( -3.761497552787613330, 6.475832013972435242, 1.199719254218464037 ) ) ;
#112145=CARTESIAN_POINT ( 'NONE',  ( -8.345207244411405156, 9.694828859023472134, 1.199719254218462483 ) ) ;
#112151=CARTESIAN_POINT ( 'NONE',  ( -1.201851678989727383E-14, 3.743750000682817269, 1.732050807568877637 ) ) ;
#112152=CARTESIAN_POINT ( 'NONE',  ( 7.889955328148847258, 11.29236608522730911, -1.199719254218446718 ) ) ;
#112155=CARTESIAN_POINT ( 'NONE',  ( -6.744291347794091784, 9.955758108146730123, -1.199719254218440723 ) ) ;
#112157=CARTESIAN_POINT ( 'NONE',  ( 0.6823417656249917140, 3.592708333674754506, 1.181850606188765695 ) ) ;
#112162=CARTESIAN_POINT ( 'NONE',  ( -8.175203439360366531, 12.48156174598837787, 1.040834085586084257E-14 ) ) ;
#112166=CARTESIAN_POINT ( 'NONE',  ( 0.6823417656249899377, 3.488541667008085323, -1.181850606188754593 ) ) ;
#112173=CARTESIAN_POINT ( 'NONE',  ( 0.6823417656249917140, 3.342708333674754506, 1.181850606188765695 ) ) ;
#112175=CARTESIAN_POINT ( 'NONE',  ( -4.225337428953291230, 8.081310767087481750, 0.7998128361456341429 ) ) ;
#112176=CARTESIAN_POINT ( 'NONE',  ( 5.926885707468349196, 10.06645042535509660, 1.040834085586084257E-14 ) ) ;
#112180=CARTESIAN_POINT ( 'NONE',  ( -1.364683531250012516, 4.301041667008089320, -0.7879004041258300672 ) ) ;
#112183=CARTESIAN_POINT ( 'NONE',  ( -0.6823417656250246877, -0.1989583329919109023, 1.181850606188755259 ) ) ;
#112184=CARTESIAN_POINT ( 'NONE',  ( -4.107757355260591936, 7.736207981205250661, 1.040834085586084257E-14 ) ) ;
#112187=CARTESIAN_POINT ( 'NONE',  ( 5.829642864196171281, 5.903597551091405826, 0.7216878364870317197 ) ) ;
#112190=CARTESIAN_POINT ( 'NONE',  ( -7.365103760721662951, 9.615707025640515937, 1.599625672291295375 ) ) ;
#112191=CARTESIAN_POINT ( 'NONE',  ( -8.920901888112002354, 11.43080484092926241, 1.443375672974064550 ) ) ;
#112197=CARTESIAN_POINT ( 'NONE',  ( -5.653386866774179786, 8.579073197003079798, 1.082531754730548412 ) ) ;
#112199=CARTESIAN_POINT ( 'NONE',  ( 1.364683531249986537, -0.03229166632525094088, -0.7879004041258309554 ) ) ;
#112211=CARTESIAN_POINT ( 'NONE',  ( 8.229436053370658755, 12.54483312900040026, 0.7216878364870438212 ) ) ;
#112218=VERTEX_POINT ( 'NONE', #121120 ) ;
#112220=ADVANCED_FACE ( 'NONE', ( #100504 ), #832, .F. ) ;
#112221=CARTESIAN_POINT ( 'NONE',  ( 5.178324605415663306, 8.128796908705222535, 1.199719254218462483 ) ) ;
#112222=CARTESIAN_POINT ( 'NONE',  ( -3.903858165731105778, 6.641919395739846799, 1.199719254218464037 ) ) ;
#112225=CARTESIAN_POINT ( 'NONE',  ( -4.868066621355794155, 4.979192643662380569, -0.7254044385785942683 ) ) ;
#112226=CARTESIAN_POINT ( 'NONE',  ( 0.6823417656249882723, 0.4885416670080827695, -1.181850606188749264 ) ) ;
#112227=CARTESIAN_POINT ( 'NONE',  ( 5.858512798400357546, 6.179092012920288646, 0.8810539604525641222 ) ) ;
#112228=CARTESIAN_POINT ( 'NONE',  ( -8.188234707649510113, 11.64035869464474082, -1.199719254218446718 ) ) ;
#112233=CARTESIAN_POINT ( 'NONE',  ( 1.500000000000023981, 5.754166666666687746, 0.8660254037844334896 ) ) ;
#112245=CARTESIAN_POINT ( 'NONE',  ( 4.984594031318565932, 8.967110136513669616, 0.7998128361456462443 ) ) ;
#112251=CARTESIAN_POINT ( 'NONE',  ( 7.422199028477372451, 10.74665040227725044, -1.199719254218441611 ) ) ;
#112267=CARTESIAN_POINT ( 'NONE',  ( -9.341204650135658483, 10.00041963468749984, 1.040834085586084257E-14 ) ) ;
#112271=CARTESIAN_POINT ( 'NONE',  ( 6.484877546038077867, 6.460111979999551224, 1.040834085586084257E-14 ) ) ;
#112277=CARTESIAN_POINT ( 'NONE',  ( 3.673896439178911066, 7.230036912443299713, 0.7216878364870317197 ) ) ;
#112286=CARTESIAN_POINT ( 'NONE',  ( -5.371001409308059138, 9.417918744168066070, -0.7998128361456231517 ) ) ;
#112287=CARTESIAN_POINT ( 'NONE',  ( -5.271422797614987665, 5.044414773505913274, -0.7998128361456221525 ) ) ;
#112295=CARTESIAN_POINT ( 'NONE',  ( 5.666418135507635512, 8.698239360479199433, 1.199719254218462483 ) ) ;
#112311=CARTESIAN_POINT ( 'NONE',  ( 1.364683531249988757, -0.5531249996585801965, 0.000000000000000000 ) ) ;
#112312=CARTESIAN_POINT ( 'NONE',  ( 3.277320446201373638, 4.846626492033466072, 1.599625672291267398 ) ) ;
#112313=CARTESIAN_POINT ( 'NONE',  ( 5.515469562660962666, 5.329135999392899947, 0.7998128361456341429 ) ) ;
#112315=CARTESIAN_POINT ( 'NONE',  ( -6.317736394288148816, 8.393778431468064127, 1.443375672974078761 ) ) ;
#112316=CARTESIAN_POINT ( 'NONE',  ( 3.850152436600926542, 7.435668909435648288, -0.7216878364870197293 ) ) ;
#112317=CARTESIAN_POINT ( 'NONE',  ( -6.304178240230145391, 9.338329799368375816, 1.082531754730548412 ) ) ;
#112321=CARTESIAN_POINT ( 'NONE',  ( 7.311924916471702396, 7.425000578838787391, -0.7998128361456281477 ) ) ;
#112327=CARTESIAN_POINT ( 'NONE',  ( 1.364683531249990311, 5.113541667008084879, 0.7879004041258500513 ) ) ;
#112333=CARTESIAN_POINT ( 'NONE',  ( 6.096362627639171805, 10.26417349888772179, -0.7998128361456291469 ) ) ;
#112337=CARTESIAN_POINT ( 'NONE',  ( -6.744291347794091784, 9.955758108146730123, -1.199719254218440723 ) ) ;
#112342=CARTESIAN_POINT ( 'NONE',  ( 8.191097360950562845, 12.70803068775103739, -0.7998128361456352531 ) ) ;
#112343=CARTESIAN_POINT ( 'NONE',  ( 3.998552357014331982, 7.829812261164016185, 1.248643980066187585E-14 ) ) ;
#112345=CARTESIAN_POINT ( 'NONE',  ( -8.376239975144482486, 8.666701480623698828, 1.040834085586084257E-14 ) ) ;
#112348=CARTESIAN_POINT ( 'NONE',  ( 5.645731234294472323, 6.129814942853209381, -0.7970442531908157324 ) ) ;
#112349=CARTESIAN_POINT ( 'NONE',  ( -7.998947442382709383, 12.27592974951444660, 0.7216878364870478180 ) ) ;
#112351=CARTESIAN_POINT ( 'NONE',  ( 3.215772567386471437, 6.427315425527130088, -0.8732430475888955934 ) ) ;
#112353=CARTESIAN_POINT ( 'NONE',  ( 6.368579470117202490, 8.453095353268645695, 1.599625672291281386 ) ) ;
#112355=CARTESIAN_POINT ( 'NONE',  ( 5.660692828905515839, 6.562895374266609849, -1.199719254218445830 ) ) ;
#112356=CARTESIAN_POINT ( 'NONE',  ( -4.034767475943390025, 7.597003608976943489, -0.2951547658557127640 ) ) ;
#112357=CARTESIAN_POINT ( 'NONE',  ( 4.518945272056516416, 4.166524327021037699, 0.7998128361456341429 ) ) ;
#112359=CARTESIAN_POINT ( 'NONE',  ( -7.266807147244793263, 8.540658428949452485, 1.082531754730549967 ) ) ;
#112364=CARTESIAN_POINT ( 'NONE',  ( -4.525130642185515306, 7.025754810433701536, 1.158151338111103046 ) ) ;
#112365=CARTESIAN_POINT ( 'NONE',  ( -0.6823417656250246877, 0.3635416670080895973, 1.181850606188755259 ) ) ;
#112369=CARTESIAN_POINT ( 'NONE',  ( 4.744990575102895569, 5.598539094783909320, -1.082531754730548412 ) ) ;
#112373=CARTESIAN_POINT ( 'NONE',  ( -9.964879715919934711, 10.72804054476916313, 0.7216878364870438212 ) ) ;
#112378=CARTESIAN_POINT ( 'NONE',  ( -7.632877294369372123, 11.84884791016554573, 0.7216878364870458196 ) ) ;
#112382=LINE ( 'NONE', #27862, #164808 ) ;
#112385=CARTESIAN_POINT ( 'NONE',  ( -8.066738210006693777, 10.43428054980638997, 1.443375672974090751 ) ) ;
#112389=CARTESIAN_POINT ( 'NONE',  ( 0.6823417656249917140, 5.155208333674749177, 1.181850606188765695 ) ) ;
#112390=CARTESIAN_POINT ( 'NONE',  ( 0.7499999999999902300, 3.597916667349487785, -1.299038105676658228 ) ) ;
#112391=CARTESIAN_POINT ( 'NONE',  ( 5.337709665475443011, 6.539638787446115487, -1.341754179669167213 ) ) ;
#112397=CARTESIAN_POINT ( 'NONE',  ( -7.182068686937172153, 9.402166106225269715, 1.599625672291283607 ) ) ;
#112402=CARTESIAN_POINT ( 'NONE',  ( 5.961834861707224320, 7.978559976790334574, -1.599625672291262513 ) ) ;
#112407=CARTESIAN_POINT ( 'NONE',  ( 6.448874621594486989, 10.67543749183559143, 0.7998128361456462443 ) ) ;
#112410=CARTESIAN_POINT ( 'NONE',  ( 1.499999999999990896, 4.556250000682819490, 1.214306433183764966E-14 ) ) ;
#112413=CARTESIAN_POINT ( 'NONE',  ( -5.233084105194862445, 9.049089189461916760, 0.7216878364870458196 ) ) ;
#112416=CARTESIAN_POINT ( 'NONE',  ( -4.521192831603464413, 5.406218046348621797, 1.258376203098745316 ) ) ;
#112419=FACE_OUTER_BOUND ( 'NONE', #195272, .T. ) ;
#112423=CARTESIAN_POINT ( 'NONE',  ( -9.829825065107822724, 11.42688298316931572, 1.199719254218462483 ) ) ;
#112425=CARTESIAN_POINT ( 'NONE',  ( 9.745613490124728884, 10.26430391476735338, 0.7998128361456462443 ) ) ;
#112426=CARTESIAN_POINT ( 'NONE',  ( 1.499999999999985123, -0.7041666666666481778, -0.8660254037844323793 ) ) ;
#112427=CARTESIAN_POINT ( 'NONE',  ( -9.840520565420403543, 10.37502883594562597, 1.040834085586084257E-14 ) ) ;
#112430=CARTESIAN_POINT ( 'NONE',  ( 1.364683531249990311, 3.384375000341416140, 1.214306433183764966E-14 ) ) ;
#112431=CARTESIAN_POINT ( 'NONE',  ( 9.408995418203963013, 12.00024729270324286, 1.443375672974076540 ) ) ;
#112436=CARTESIAN_POINT ( 'NONE',  ( 9.286972035236624734, 11.85788667924133399, -1.443375672974058777 ) ) ;
#112438=VECTOR ( 'NONE', #143957, 1000.000000000000000 ) ;
#112439=CARTESIAN_POINT ( 'NONE',  ( -6.073689629242158716, 9.069426419882418600, -1.082531754730538864 ) ) ;
#112440=CARTESIAN_POINT ( 'NONE',  ( -1.364683531250014514, 0.4885416670080875434, -0.7879004041258289570 ) ) ;
#112442=CARTESIAN_POINT ( 'NONE',  ( 0.4636475088198339645, 7.942422027498646564, 1.946104516853490285 ) ) ;
#112444=CARTESIAN_POINT ( 'NONE',  ( -9.006694118179950692, 9.402231314165087284, 1.040834085586084257E-14 ) ) ;
#112445=CARTESIAN_POINT ( 'NONE',  ( -2.779058300676980675, 5.225689869889666106, -1.082531754730543083 ) ) ;
#112446=CARTESIAN_POINT ( 'NONE',  ( 0.6823417656249899377, 3.738541667008085767, -1.181850606188754593 ) ) ;
#112451=CARTESIAN_POINT ( 'NONE',  ( 8.992082194361556091, 11.51384853155376220, 1.599625672291279388 ) ) ;
#112457=ORIENTED_EDGE ( 'NONE', *, *, #59313, .T. ) ;
#112458=ADVANCED_FACE ( 'NONE', ( #34431 ), #127091, .T. ) ;
#112464=CARTESIAN_POINT ( 'NONE',  ( 2.482948226198860464, 5.072301959192136778, 2.500000000000000444 ) ) ;
#112466=CARTESIAN_POINT ( 'NONE',  ( 3.469446951953614189E-15, 5.900000000000023448, 1.214306433183764966E-14 ) ) ;
#112467=CARTESIAN_POINT ( 'NONE',  ( 1.364683531249988535, 5.717708333674752730, -0.7879004041258300672 ) ) ;
#112468=AXIS2_PLACEMENT_3D ( 'NONE', #141819, #190503, #123489 ) ;
#112473=CARTESIAN_POINT ( 'NONE',  ( 8.341290820905593151, 10.75459192918846618, 1.599625672291281386 ) ) ;
#112476=CARTESIAN_POINT ( 'NONE',  ( -0.6823417656249969321, 3.217708333674754062, -1.181850606188749264 ) ) ;
#112478=CARTESIAN_POINT ( 'NONE',  ( -7.266807147244793263, 8.540658428949452485, 1.082531754730549967 ) ) ;
#112480=CARTESIAN_POINT ( 'NONE',  ( 1.451998047843341633, 7.315968950353821221, 4.301760722578430673 ) ) ;
#112487=CARTESIAN_POINT ( 'NONE',  ( 8.378048858240820351, 11.86180853700128601, -1.199719254218446718 ) ) ;
#112492=CARTESIAN_POINT ( 'NONE',  ( -7.947050595904583403, 12.42330946186405249, 0.7998128361456481317 ) ) ;
#112493=CARTESIAN_POINT ( 'NONE',  ( 5.632522751473472589, 8.658694745772667289, -1.199719254218440723 ) ) ;
#112495=CARTESIAN_POINT ( 'NONE',  ( 4.324687812634892659, 5.108185871904570519, 1.082531754730560403 ) ) ;
#112505=CARTESIAN_POINT ( 'NONE',  ( -4.772106882330223954, 8.511282429453158827, -0.7216878364870267237 ) ) ;
#112506=CARTESIAN_POINT ( 'NONE',  ( 2.496672843210871129, 6.064535417054653266, -0.7998128361456291469 ) ) ;
#112509=CARTESIAN_POINT ( 'NONE',  ( -6.184490626128011925, 10.36698949712469364, -0.7998128361456291469 ) ) ;
#112513=CARTESIAN_POINT ( 'NONE',  ( -10.63367255181986160, 11.30037282007833532, 1.040834085586084257E-14 ) ) ;
#112517=CARTESIAN_POINT ( 'NONE',  ( 7.202405917357655341, 9.425892875049191488, 1.599625672291281386 ) ) ;
#112519=CARTESIAN_POINT ( 'NONE',  ( 3.891353782322113375, 4.498666486585943147, -1.199719254218446718 ) ) ;
#112530=CARTESIAN_POINT ( 'NONE',  ( -7.808606406466886973, 11.19745900993164511, 1.199719254218453823 ) ) ;
#112535=CARTESIAN_POINT ( 'NONE',  ( 5.490689023854504747, 9.349628261231513804, 1.040834085586084257E-14 ) ) ;
#112537=CARTESIAN_POINT ( 'NONE',  ( 3.816783937446950770, 4.411668334231586996, 1.199719254218464037 ) ) ;
#112538=CARTESIAN_POINT ( 'NONE',  ( 3.469446951953614189E-15, 6.120000000000021423, 1.214306433183764966E-14 ) ) ;
#112540=CARTESIAN_POINT ( 'NONE',  ( -5.215082642750900277, 9.236013516518044142, 0.000000000000000000 ) ) ;
#112545=CARTESIAN_POINT ( 'NONE',  ( -1.499999999999997780, 7.388542872122518368, -4.154462424328208670 ) ) ;
#112551=CARTESIAN_POINT ( 'NONE',  ( 0.6823417656249917140, 3.655208333674754506, 1.181850606188765695 ) ) ;
#112552=CARTESIAN_POINT ( 'NONE',  ( 1.579999999999999183, 8.674529973577541853, 2.499999999999998668 ) ) ;
#112553=CARTESIAN_POINT ( 'NONE',  ( 8.697719238366680372, 10.10609285197134533, 1.199719254218462483 ) ) ;
#112555=CARTESIAN_POINT ( 'NONE',  ( -3.131570295076647525, 6.597323077657299528, 1.040834085586084257E-14 ) ) ;
#112558=CARTESIAN_POINT ( 'NONE',  ( -4.161989969270909917, 5.878740935614591656, 1.443375672974064550 ) ) ;
#112567=CARTESIAN_POINT ( 'NONE',  ( 3.846762897975340767, 5.510976019103107859, -1.599625672291256295 ) ) ;
#112572=ADVANCED_FACE ( 'NONE', ( #166865 ), #195075, .T. ) ;
#112575=CARTESIAN_POINT ( 'NONE',  ( 4.878236342818665250, 4.585697242910212523, 1.040834085586084257E-14 ) ) ;
#112579=CARTESIAN_POINT ( 'NONE',  ( -1.364683531250012516, 4.301041667008089320, -0.7879004041258300672 ) ) ;
#112584=CARTESIAN_POINT ( 'NONE',  ( 4.638861114170084399, 8.563755066507100722, 0.7998128361456462443 ) ) ;
#112589=CARTESIAN_POINT ( 'NONE',  ( -3.574546055497324737, 7.322054164722185732, 0.7998128361456341429 ) ) ;
#112590=CARTESIAN_POINT ( 'NONE',  ( 6.778713616708431644, 7.010846762355714468, 1.040834085586084257E-14 ) ) ;
#112591=CARTESIAN_POINT ( 'NONE',  ( -1.500000000000011324, 3.420833333333355597, 0.8660254037844403729 ) ) ;
#112593=CARTESIAN_POINT ( 'NONE',  ( -4.141125853970233806, 6.918731698685530063, -1.199719254218452047 ) ) ;
#112594=CARTESIAN_POINT ( 'NONE',  ( 0.2734184563537064849, 7.240553437303591799, -1.983365796752657007 ) ) ;
#112595=LINE ( 'NONE', #212135, #7301 ) ;
#112596=CARTESIAN_POINT ( 'NONE',  ( 0.6823417656249899377, 4.676041667008086655, -1.181850606188754593 ) ) ;
#112599=AXIS2_PLACEMENT_3D ( 'NONE', #132177, #168893, #87654 ) ;
#112600=CARTESIAN_POINT ( 'NONE',  ( -3.307826292054304673, 6.802955074131234348, -0.7216878364870267237 ) ) ;
#112605=CARTESIAN_POINT ( 'NONE',  ( 4.517891501851804215, 6.293959390292322986, -1.599625672291255185 ) ) ;
#112609=CARTESIAN_POINT ( 'NONE',  ( -1.201851678989727383E-14, 3.509375000341421469, -1.575800808251660134 ) ) ;
#112612=CARTESIAN_POINT ( 'NONE',  ( 1.364683531249986537, 0.1760416670080860446, 0.7879004041258500513 ) ) ;
#112615=CARTESIAN_POINT ( 'NONE',  ( -10.14557902172788495, 10.73093036830436553, 1.040834085586084257E-14 ) ) ;
#112617=CARTESIAN_POINT ( 'NONE',  ( -5.355107487273497391, 9.191449801886996340, 0.7216878364870458196 ) ) ;
#112618=AXIS2_PLACEMENT_3D ( 'NONE', #74883, #108513, #140990 ) ;
#112622=CARTESIAN_POINT ( 'NONE',  ( -1.201851678989727383E-14, 4.696875000341419693, -1.575800808251660134 ) ) ;
#112630=CARTESIAN_POINT ( 'NONE',  ( -5.219525951136845698, 8.072902128759544382, -1.082531754730543971 ) ) ;
#112631=AXIS2_PLACEMENT_3D ( 'NONE', #199843, #102353, #135933 ) ;
#112637=CARTESIAN_POINT ( 'NONE',  ( -4.541618270453545492, 8.242379048930368768, 0.7216878364870458196 ) ) ;
#112642=CARTESIAN_POINT ( 'NONE',  ( 2.535011536075336913, 5.133042487381361596, -7.499999999999997335 ) ) ;
#112650=CARTESIAN_POINT ( 'NONE',  ( -4.066556009095094737, 6.831733546331167695, 1.199719254218464037 ) ) ;
#112653=CARTESIAN_POINT ( 'NONE',  ( -0.7500000000000006661, 0.6083333333333564852, -1.299038105676652011 ) ) ;
#112655=CARTESIAN_POINT ( 'NONE',  ( 7.443063144222396232, 11.62739806832741785, 1.040834085586084257E-14 ) ) ;
#112656=CARTESIAN_POINT ( 'NONE',  ( 5.621827251160867789, 9.710548892996357040, 1.040834085586084257E-14 ) ) ;
#112660=CARTESIAN_POINT ( 'NONE',  ( 4.333802657862601215, 8.207853534148366492, 0.7998128361456462443 ) ) ;
#112661=CARTESIAN_POINT ( 'NONE',  ( -0.2555917649598457575, 7.163498069672973756, -2.096924645512515895 ) ) ;
#112667=CARTESIAN_POINT ( 'NONE',  ( -2.928197990871687306, 5.399686175116803710, 1.082531754730560403 ) ) ;
#112674=CARTESIAN_POINT ( 'NONE',  ( -1.364683531250012516, 2.780208333674754506, 0.7879004041258379498 ) ) ;
#112675=CARTESIAN_POINT ( 'NONE',  ( 8.541273586484978253, 12.90864358430044589, 0.000000000000000000 ) ) ;
#112676=CARTESIAN_POINT ( 'NONE',  ( -6.470265622219711688, 8.571729197388226140, -1.599625672291263179 ) ) ;
#112679=CARTESIAN_POINT ( 'NONE',  ( 6.979750152936881058, 7.037463354714830643, 0.7998128361456341429 ) ) ;
#112680=CARTESIAN_POINT ( 'NONE',  ( -6.901263884555985051, 8.010228272525461435, 1.199719254218450271 ) ) ;
#112684=CARTESIAN_POINT ( 'NONE',  ( -1.500000000000015099, 0.4104166673494891726, -0.8660254037844383745 ) ) ;
#112687=CARTESIAN_POINT ( 'NONE',  ( 7.836249599018724865, 9.205007956019091608, -1.082531754730537976 ) ) ;
#112690=CARTESIAN_POINT ( 'NONE',  ( 0.6823417656249882723, 1.988541667008083991, -1.181850606188749264 ) ) ;
#112692=CARTESIAN_POINT ( 'NONE',  ( 5.870317324592803310, 7.871789516823500144, -1.443375672974057666 ) ) ;
#112695=CARTESIAN_POINT ( 'NONE',  ( -4.297571505851936813, 4.116180966356429494, 1.214306433183764966E-14 ) ) ;
#112697=CARTESIAN_POINT ( 'NONE',  ( 1.364683531249988535, 4.655208333674755394, -0.7879004041258300672 ) ) ;
#112703=CARTESIAN_POINT ( 'NONE',  ( -5.030466903028923298, 6.770262730772157234, -1.447917484242104758 ) ) ;
#112711=CARTESIAN_POINT ( 'NONE',  ( 2.496672843210871129, 6.064535417054653266, -0.7998128361456291469 ) ) ;
#112720=CARTESIAN_POINT ( 'NONE',  ( 4.853455804012212660, 7.645820290447483458, 1.082531754730558626 ) ) ;
#112721=ADVANCED_FACE ( 'NONE', ( #85128 ), #151214, .F. ) ;
#112722=CARTESIAN_POINT ( 'NONE',  ( -1.364683531250012516, 2.092708333674750953, 0.7879004041258379498 ) ) ;
#112724=CARTESIAN_POINT ( 'NONE',  ( 7.727257484784855635, 11.10255193463598111, -1.199719254218446718 ) ) ;
#112729=DIRECTION ( 'NONE',  ( -3.347138415753902517E-16, -0.6000000000000019762, -0.7999999999999986011 ) ) ;
#112731=CIRCLE ( 'NONE', #43570, 0.08000000000000020983 ) ;
#112732=CARTESIAN_POINT ( 'NONE',  ( 1.499999999999989120, 1.525000000000019451, 0.000000000000000000 ) ) ;
#112733=CARTESIAN_POINT ( 'NONE',  ( 5.587931867126699537, 9.671004278289832001, -0.7998128361456291469 ) ) ;
#112734=CARTESIAN_POINT ( 'NONE',  ( -7.395082721250053837, 10.71501471051202614, -1.199719254218446718 ) ) ;
#112738=CARTESIAN_POINT ( 'NONE',  ( -1.201851678989727383E-14, 2.696875000341417916, -1.575800808251660134 ) ) ;
#112739=CARTESIAN_POINT ( 'NONE',  ( -1.500000000000011324, 4.379166666666688634, -0.8660254037844313801 ) ) ;
#112741=CARTESIAN_POINT ( 'NONE',  ( 2.496672843210871129, 6.064535417054653266, -0.7998128361456291469 ) ) ;
#112747=CARTESIAN_POINT ( 'NONE',  ( -1.402160292154681736E-14, 1.368750000682821710, -1.732050807568863648 ) ) ;
#112749=CARTESIAN_POINT ( 'NONE',  ( -5.194745412330402878, 9.212286747694129474, 0.000000000000000000 ) ) ;
#112750=CARTESIAN_POINT ( 'NONE',  ( -3.090895834235680262, 5.589500325708124606, 1.082531754730560403 ) ) ;
#112758=CARTESIAN_POINT ( 'NONE',  ( 7.122110765880372618, 7.203550736482235095, 0.7998128361456341429 ) ) ;
#112761=CARTESIAN_POINT ( 'NONE',  ( 5.459129407796876166, 9.520734742405036144, 1.040834085586084257E-14 ) ) ;
#112762=CARTESIAN_POINT ( 'NONE',  ( 7.551528372687370094, 11.75394083486988528, -0.7216878364870267237 ) ) ;
#112764=DIRECTION ( 'NONE',  ( 1.207943261119674327E-30, 2.168404344971008079E-15, -1.000000000000000000 ) ) ;
#112768=CARTESIAN_POINT ( 'NONE',  ( -5.669280788808708671, 9.765911353585494226, 0.7998128361456481317 ) ) ;
#112770=CARTESIAN_POINT ( 'NONE',  ( 2.703961570921634028, 5.242040035128820108, -1.199719254218446718 ) ) ;
#112776=CARTESIAN_POINT ( 'NONE',  ( 4.490901714065265615, 7.023505696618186356, 1.148426366857359771 ) ) ;
#112784=CARTESIAN_POINT ( 'NONE',  ( -3.145128448690317935, 5.652771709238564313, -1.082531754730549967 ) ) ;
#112785=CARTESIAN_POINT ( 'NONE',  ( 7.565086526745395723, 10.80938946696957004, -1.082531754730543083 ) ) ;
#112787=CARTESIAN_POINT ( 'NONE',  ( -4.741601036477307574, 6.554953847355395880, 1.599625672291267398 ) ) ;
#112791=CARTESIAN_POINT ( 'NONE',  ( -7.477485413136760073, 8.682486722536401302, -1.199719254218446718 ) ) ;
#112807=CARTESIAN_POINT ( 'NONE',  ( -4.717347382551060342, 7.590990148696470818, 1.199719254218464037 ) ) ;
#112808=B_SPLINE_CURVE_WITH_KNOTS ( 'NONE', 3,
 ( #174312, #138602, #55209, #156988, #141832, #187330, #58406, #54144, #5345, #71427, #153775, #40029, #121355, #155912, #73581, #105042 ),
 .UNSPECIFIED., .F., .F.,
 ( 4, 2, 2, 2, 2, 2, 2, 4 ),
 ( 0.9998645410539588330, 1.009348164353689681, 1.018831787653420529, 1.037799034252882224, 1.075733527451805616, 1.113668020650729007, 1.132635267250190703, 1.151602513849652398 ),
 .UNSPECIFIED. ) ;
#112811=CARTESIAN_POINT ( 'NONE',  ( 4.528060117284244512, 4.385084346360807572, 0.7216878364870317197 ) ) ;
#112815=CARTESIAN_POINT ( 'NONE',  ( -2.948008335967658322, 5.526761261015804116, 1.199719254218462483 ) ) ;
#112818=CARTESIAN_POINT ( 'NONE',  ( 8.866142388332804103, 12.43125098877526113, -1.199719254218446718 ) ) ;
#112821=CARTESIAN_POINT ( 'NONE',  ( -8.365544474831901667, 9.718555627847388578, 1.199719254218462483 ) ) ;
#112822=CARTESIAN_POINT ( 'NONE',  ( 6.661133543015731462, 6.665743976473484267, -0.7998128361456281477 ) ) ;
#112824=CARTESIAN_POINT ( 'NONE',  ( 3.472859903394816872, 7.203420320602604399, -0.7998128361456291469 ) ) ;
#112827=CARTESIAN_POINT ( 'NONE',  ( 1.364683531249986537, 1.717708333674749399, -0.7879004041258239610 ) ) ;
#112830=CARTESIAN_POINT ( 'NONE',  ( 8.595506201384020883, 9.130438111143927671, 0.7216878364870438212 ) ) ;
#112861=CARTESIAN_POINT ( 'NONE',  ( 0.7499999999999902300, 1.014583334016154526, 1.299038105676657340 ) ) ;
#112867=CARTESIAN_POINT ( 'NONE',  ( 1.499999999999987121, -0.7458333333333122539, 0.8660254037844524744 ) ) ;
#112868=CARTESIAN_POINT ( 'NONE',  ( 7.377608144130607393, 11.75895993479440982, -0.7998128361456291469 ) ) ;
#112873=CARTESIAN_POINT ( 'NONE',  ( 2.672928840188529609, 6.270167413528593414, 0.000000000000000000 ) ) ;
#112874=CARTESIAN_POINT ( 'NONE',  ( -6.399085315970137522, 9.449054721065074602, -1.082531754730538864 ) ) ;
#112877=AXIS2_PLACEMENT_3D ( 'NONE', #207136, #89147, #138964 ) ;
#112879=CARTESIAN_POINT ( 'NONE',  ( -7.867809214632013770, 8.073532260025807261, 1.040834085586084257E-14 ) ) ;
#112883=VERTEX_POINT ( 'NONE', #187953 ) ;
#112884=CARTESIAN_POINT ( 'NONE',  ( -1.500000000000013101, 1.410416667349486008, -0.8660254037844313801 ) ) ;
#112891=CARTESIAN_POINT ( 'NONE',  ( -3.809477975315625375, 4.507107728365378208, 1.082531754730558626 ) ) ;
#112894=CARTESIAN_POINT ( 'NONE',  ( 4.911299649074239326, 6.652374229206746037, 1.248453844233877286 ) ) ;
#112895=DIRECTION ( 'NONE',  ( -0.6507913734559643837, -0.7592566023653002372, 0.000000000000000000 ) ) ;
#112899=CARTESIAN_POINT ( 'NONE',  ( -10.15522075183580419, 11.80651128435196462, 1.199719254218462483 ) ) ;
#112900=CARTESIAN_POINT ( 'NONE',  ( 7.313733799568044702, 10.62010763521636214, 1.199719254218460707 ) ) ;
#112908=CARTESIAN_POINT ( 'NONE',  ( -7.374745490829552885, 10.69128794168811680, -1.199719254218446718 ) ) ;
#112914=CARTESIAN_POINT ( 'NONE',  ( 3.517450787741589036, 6.191110788085444128, -1.199719254218446718 ) ) ;
#112918=CARTESIAN_POINT ( 'NONE',  ( -6.078132937628113908, 5.985576603521232109, 1.040834085586084257E-14 ) ) ;
#112919=CARTESIAN_POINT ( 'NONE',  ( 0.08888683327021307257, 6.492044364012829583, -3.106763327641859362 ) ) ;
#112920=FACE_OUTER_BOUND ( 'NONE', #75406, .T. ) ;
#112922=CARTESIAN_POINT ( 'NONE',  ( -5.461413243215608837, 6.444398994036877326, -1.303746704243381238 ) ) ;
#112930=CARTESIAN_POINT ( 'NONE',  ( 6.608709811657416999, 9.797579649320619311, -1.199719254218440723 ) ) ;
#112932=CARTESIAN_POINT ( 'NONE',  ( -5.108724954250998707, 4.854600622914589714, -0.7998128361456221525 ) ) ;
#112940=CARTESIAN_POINT ( 'NONE',  ( 1.499999999999989120, 0.5562500006828161592, 0.000000000000000000 ) ) ;
#112944=CARTESIAN_POINT ( 'NONE',  ( 4.701980345841006326, 4.380065246436280368, 0.7998128361456341429 ) ) ;
#112946=CARTESIAN_POINT ( 'NONE',  ( -3.541704441667874903, 5.155074486744371853, -1.599625672291256295 ) ) ;
#112953=CARTESIAN_POINT ( 'NONE',  ( 4.744990575102895569, 5.598539094783909320, -1.082531754730548412 ) ) ;
#112956=CARTESIAN_POINT ( 'NONE',  ( -1.364683531249997417, 5.821875000341418804, 1.214306433183764966E-14 ) ) ;
#112958=CARTESIAN_POINT ( 'NONE',  ( 3.267151830768944443, 4.834763107362302748, -1.443375672974058777 ) ) ;
#112960=CARTESIAN_POINT ( 'NONE',  ( 2.869309894402357841, 6.436557513332352265, -0.3339617207483085992 ) ) ;
#112968=CARTESIAN_POINT ( 'NONE',  ( 0.6823417656249882723, -0.9072916663252494907, 1.181850606188755259 ) ) ;
#112972=CARTESIAN_POINT ( 'NONE',  ( -4.218558352146454915, 8.073401844146177453, 1.040834085586084257E-14 ) ) ;
#112976=CARTESIAN_POINT ( 'NONE',  ( -1.500000000000011324, 4.920833333333354709, 0.8660254037844403729 ) ) ;
#112985=CARTESIAN_POINT ( 'NONE',  ( 0.6823417656249882723, -1.157291666325249713, 1.181850606188755259 ) ) ;
#112987=CARTESIAN_POINT ( 'NONE',  ( 6.368579470117202490, 8.453095353268645695, 1.599625672291281386 ) ) ;
#112988=CARTESIAN_POINT ( 'NONE',  ( -6.516665389662827934, 10.75452672124865217, 0.000000000000000000 ) ) ;
#112989=CARTESIAN_POINT ( 'NONE',  ( 0.000000000000000000, 8.600000000000017408, 0.4000000000000045186 ) ) ;
#112991=ORIENTED_EDGE ( 'NONE', *, *, #131672, .T. ) ;
#112993=CARTESIAN_POINT ( 'NONE',  ( 1.364683531249984538, -1.032291666325247714, -0.7879004041258309554 ) ) ;
#112997=CARTESIAN_POINT ( 'NONE',  ( 5.299301323368958094, 6.361497809228795930, -1.122821758042211959 ) ) ;
#112999=ORIENTED_EDGE ( 'NONE', *, *, #178570, .T. ) ;
#113000=ADVANCED_FACE ( 'NONE', ( #155468 ), #202040, .F. ) ;
#113002=CARTESIAN_POINT ( 'NONE',  ( 8.446366511633696561, 8.956441806435218922, 1.040834085586084257E-14 ) ) ;
#113007=CARTESIAN_POINT ( 'NONE',  ( -1.201851678989727383E-14, 4.868750000682822154, -1.732050807568863648 ) ) ;
#113010=CARTESIAN_POINT ( 'NONE',  ( -3.469997250093771246, 6.135748327496311383, -1.199719254218452935 ) ) ;
#113011=CARTESIAN_POINT ( 'NONE',  ( 5.300874872818821082, 9.128178418356554857, 0.7216878364870438212 ) ) ;
#113012=CARTESIAN_POINT ( 'NONE',  ( -7.985389288324692636, 11.29974268881207067, -1.082531754730543083 ) ) ;
#113018=CARTESIAN_POINT ( 'NONE',  ( 8.866669273657322492, 12.32790267170016207, -1.082531754730543083 ) ) ;
#113020=CARTESIAN_POINT ( 'NONE',  ( 3.167801447087334576, 6.847518788243868393, -0.7998128361456291469 ) ) ;
#113024=B_SPLINE_CURVE_WITH_KNOTS ( 'NONE', 3,
 ( #181999, #213427, #49888, #50955, #149522, #65050, #17358, #163653 ),
 .UNSPECIFIED., .F., .F.,
 ( 4, 2, 2, 4 ),
 ( 0.000000000000000000, 0.003005455498261387637, 0.004508183247392082323, 0.006010910996522775274 ),
 .UNSPECIFIED. ) ;
#113032=CARTESIAN_POINT ( 'NONE',  ( -1.420000000000021911, 6.200000000000045475, 2.580000000000011173 ) ) ;
#113037=CARTESIAN_POINT ( 'NONE',  ( 8.320953590485093088, 10.73086516036454618, 1.599625672291281386 ) ) ;
#113041=CARTESIAN_POINT ( 'NONE',  ( -1.364683531250014514, -0.2197916663252438285, 0.7879004041258379498 ) ) ;
#113042=CARTESIAN_POINT ( 'NONE',  ( 6.344852701515477200, 6.504675694630598137, -0.7216878364870257245 ) ) ;
#113043=CARTESIAN_POINT ( 'NONE',  ( -7.348156068926747331, 11.51667314714914347, 0.7216878364870458196 ) ) ;
#113048=CARTESIAN_POINT ( 'NONE',  ( -4.874319919312905647, 5.645460313075203018, -1.199719254218446718 ) ) ;
#113063=CARTESIAN_POINT ( 'NONE',  ( 4.435735274902380176, 7.313263296268260660, -1.222879399185505367 ) ) ;
#113070=CARTESIAN_POINT ( 'NONE',  ( -7.049876689426097798, 11.16868053773170821, -0.7216878364870267237 ) ) ;
#113071=AXIS2_PLACEMENT_3D ( 'NONE', #193663, #108232, #174257 ) ;
#113074=CARTESIAN_POINT ( 'NONE',  ( 6.531277313481192337, 8.642909503859968368, 1.599625672291281386 ) ) ;
#113077=CARTESIAN_POINT ( 'NONE',  ( 4.539282502477016479, 4.190251095844947926, 0.7998128361456341429 ) ) ;
#113079=CARTESIAN_POINT ( 'NONE',  ( -5.412729640353771465, 7.337937218544611895, 1.599625672291269396 ) ) ;
#113081=CARTESIAN_POINT ( 'NONE',  ( -5.904739593951539689, 6.847616600153594746, 1.199719254218450271 ) ) ;
#113084=CARTESIAN_POINT ( 'NONE',  ( 7.214910300766615769, 11.56914578420308715, -0.7998128361456291469 ) ) ;
#113087=CARTESIAN_POINT ( 'NONE',  ( 4.035592002476674267, 7.779268892024251869, 0.4218195438757850191 ) ) ;
#113088=CARTESIAN_POINT ( 'NONE',  ( 5.368665641331531013, 5.365790791082654998, -0.7216878364870207285 ) ) ;
#113096=CARTESIAN_POINT ( 'NONE',  ( 7.754900676892376055, 8.149731665903665601, 1.040834085586084257E-14 ) ) ;
#113099=CARTESIAN_POINT ( 'NONE',  ( -8.676328237741483207, 12.20980114641871062, -1.199719254218446718 ) ) ;
#113100=CARTESIAN_POINT ( 'NONE',  ( -6.028571859570855729, 10.18508426947466816, 0.000000000000000000 ) ) ;
#113106=FACE_OUTER_BOUND ( 'NONE', #127046, .T. ) ;
#113109=CARTESIAN_POINT ( 'NONE',  ( 8.565000355531088516, 11.01558638625153286, -1.599625672291257406 ) ) ;
#113113=CARTESIAN_POINT ( 'NONE',  ( 3.521367211247359741, 5.131347717920458962, -1.599625672291262513 ) ) ;
#113116=CARTESIAN_POINT ( 'NONE',  ( -1.001543065824772872E-14, 4.993750000682814161, 1.732050807568877637 ) ) ;
#113122=CARTESIAN_POINT ( 'NONE',  ( -1.500000000000011324, 3.170833333333354265, 0.8660254037844403729 ) ) ;
#113123=CARTESIAN_POINT ( 'NONE',  ( 5.799137018343234473, 7.788745826199009237, -1.599625672291262513 ) ) ;
#113126=CARTESIAN_POINT ( 'NONE',  ( 6.453317930424781856, 10.47269531889685545, -0.7216878364870267237 ) ) ;
#113130=CYLINDRICAL_SURFACE ( 'NONE', #178585, 0.7500000000000011102 ) ;
#113132=CARTESIAN_POINT ( 'NONE',  ( 3.511198596259283544, 6.271927390929319834, 1.164732466530402855 ) ) ;
#113133=CARTESIAN_POINT ( 'NONE',  ( -5.115504031057831469, 4.862509545855891346, 0.7998128361456341429 ) ) ;
#113134=CARTESIAN_POINT ( 'NONE',  ( -0.7499999999999972244, 5.139583334016151639, -1.299038105676652899 ) ) ;
#113135=CARTESIAN_POINT ( 'NONE',  ( -0.6823417656250246877, -0.6989583329919113464, 1.181850606188755259 ) ) ;
#113139=CARTESIAN_POINT ( 'NONE',  ( 3.822509244049070887, 6.547012320444182798, -1.199719254218452047 ) ) ;
#113141=CARTESIAN_POINT ( 'NONE',  ( 0.6823417656249899377, 5.488541667008087543, -1.181850606188754593 ) ) ;
#113143=EDGE_CURVE ( 'NONE', #138277, #65489, #66844, .T. ) ;
#113144=CARTESIAN_POINT ( 'NONE',  ( 4.131884898838331210, 7.654771682445123737, 0.7704574788214838543 ) ) ;
#113151=CARTESIAN_POINT ( 'NONE',  ( -6.690058733339450114, 9.892486724616283311, 1.199719254218452047 ) ) ;
#113155=CARTESIAN_POINT ( 'NONE',  ( 4.330940004561544043, 7.140181541042074365, -1.199719254218452047 ) ) ;
#113162=CARTESIAN_POINT ( 'NONE',  ( 8.561083932025322696, 12.07534945641652158, -1.199719254218446718 ) ) ;
#113165=CARTESIAN_POINT ( 'NONE',  ( -6.254388934605767503, 6.191208599995166040, 0.7998128361456341429 ) ) ;
#113169=CARTESIAN_POINT ( 'NONE',  ( 7.730120138085914583, 12.17022392774227768, 0.7998128361456462443 ) ) ;
#113171=CARTESIAN_POINT ( 'NONE',  ( 6.889514614038635187, 11.18951748302043114, -0.7998128361456291469 ) ) ;
#113175=CARTESIAN_POINT ( 'NONE',  ( -8.676855123066012254, 12.10645282934361866, -1.082531754730543971 ) ) ;
#113176=CARTESIAN_POINT ( 'NONE',  ( -6.181627972826976958, 9.299317504018391745, 1.199719254218452047 ) ) ;
#113180=CARTESIAN_POINT ( 'NONE',  ( -5.460715490240072079, 6.444878312648672392, 1.304320558087665782 ) ) ;
#113181=CARTESIAN_POINT ( 'NONE',  ( 0.6823417656249882723, 0.4260416670080896528, -1.181850606188749264 ) ) ;
#113185=CARTESIAN_POINT ( 'NONE',  ( 6.453317930424781856, 10.47269531889685545, -0.7216878364870267237 ) ) ;
#113203=CARTESIAN_POINT ( 'NONE',  ( 9.531545685607134999, 11.07889037375188401, 1.199719254218450271 ) ) ;
#113207=CARTESIAN_POINT ( 'NONE',  ( -6.098470168048611306, 6.009303372345148553, 1.040834085586084257E-14 ) ) ;
#113208=CARTESIAN_POINT ( 'NONE',  ( -7.019370843573183194, 9.212351955633947043, 1.599625672291283607 ) ) ;
#113210=ORIENTED_EDGE ( 'NONE', *, *, #182043, .T. ) ;
#113214=CARTESIAN_POINT ( 'NONE',  ( -1.402160292154681736E-14, 2.618750000682819490, -1.732050807568863648 ) ) ;
#113215=CARTESIAN_POINT ( 'NONE',  ( 7.553864141108259211, 11.96459193126834464, 1.040834085586084257E-14 ) ) ;
#113218=CARTESIAN_POINT ( 'NONE',  ( -7.991641480251377772, 11.41099992934688956, 1.199719254218453823 ) ) ;
#113220=CARTESIAN_POINT ( 'NONE',  ( 1.364683531249988535, 3.405208333674749621, -0.7879004041258239610 ) ) ;
#113223=( BOUNDED_SURFACE ( )  B_SPLINE_SURFACE ( 1, 2, ( 
 ( #38585, #51643, #167515, #68916, #135036, #103587, #201049, #118821, #169644, #21229, #22294, #36437, #102512, #20175, #87333, #4971, #120985, #170709, #154475, #166447, #18039, #157681, #189098, #191212, #27658, #92689, #59091, #9279, #141464, #75350, #155542, #42875, #122054, #142513, #188018, #105754, #205329, #90550, #206403, #172868, #58028, #108983, #207472, #175002, #26588, #140384, #158735, #156614, #176062, #10330, #171781, #173948, #56967, #73194, #192273, #125251, #138231, #40731, #41810, #24439, #7121, #23377, #76404, #123140, #43934, #208522, #60157, #89487, #126313, #93754, #110049, #124192, #6053, #39646, #72124, #55897, #139300, #106837, #204245, #190155, #8204, #74289, #107923, #25521, #91629, #197612, #65462, #210670, #49256, #46066, #115377, #160869, #31937, #113254, #129521, #127385, #144655, #12463, #111112, #28733, #62298, #15656, #179259, #177116, #145727, #196565, #94818, #159792, #131613, #13538, #163008, #30881, #130575, #193358, #80687, #213843, #212793, #48207, #96960, #146778, #79608, #11395, #14590, #64431, #195501, #194425, #81743, #181371, #77473, #47137, #143592, #112187, #32995, #128457, #78538, #178191, #29807, #95893, #209584, #161946, #211727, #114319, #63365, #180317, #61230, #164076, #98021, #147825, #45002, #68663, #67587, #19923, #100124, #53506, #36178, #87072, #82801, #133732, #169390, #165125, #16716, #51385, #117506, #166186, #153142, #135835, #185624, #148877, #134787, #86009, #199739, #450, #83863, #136905, #152083, #17775, #70792, #149954, #151025, #119641, #37257, #3653, #66518, #132661, #103327, #198665, #20975, #167267, #1523, #35107, #4717, #183498, #34051, #69731, #101178, #2594, #102254, #99072, #50313, #18852, #201860, #200794, #116431, #182424, #168328, #52445, #84936, #118571, #184557, #202932, #54575, #120723, #186696, #206149, #74032, #91369, #108731, #121794, #71862, #89230, #55638, #187762, #156357, #76158, #23113, #42621, #122882, #173692, #203990, #57777, #155282, #105487, #10084, #25268, #170450, #72942, #140123, #56713, #39392, #171520, #75098, #6863, #142263, #26332, #124999, #139045, #189906, #59906, #41551, #24184, #208274, #154213, #126060, #88146, #5785, #205071, #157430, #172608, #40476, #137971, #188840, #158485, #106580, #123938, #107664, #9023, #174758, #90288, #7942, #141208, #207219, #58842, #190956, #38325, #92446, #104401, #22035, #111940, #145482, #193104, #192023, #175812, #45819, #65218, #31693, #97768, #27405, #79364, #29556, #194174, #177942, #44754, #62057, #43685, #179013, #162764, #94570, #159544, #95647, #160614, #161698, #80430, #110861, #143337, #130329, #176867, #144413, #93503, #11141, #12215, #163828, #78286, #28479, #210415, #128212, #13291, #77218, #211478, #209331, #30629, #63114, #129279, #213594, #196318, #113002, #195253, #109803, #46889, #96715, #14341, #146530, #212547, #64188, #180069, #60979, #47962, #114078, #127133, #15406, #81497, #147575, #132419, #119386, #168077, #3412, #115126, #100928, #118319, #99880, #197367, #116187, #169133, #184305, #50064, #103078, #198420, #183250, #85755, #69478, #35929, #49008, #32742, #151836, #98824, #135586, #199483, #182172, #67336, #201607, #149697, #66271, #102007, #133481, #34853, #68415, #131370, #82548, #51129, #19675, #167016, #148635, #164873, #134542, #18609, #117251, #84689, #150776, #2338, #53256, #185374, #201, #16468, #33801, #165942, #17527, #200547, #20728, #83615, #52193, #1278, #36994, #86823, #152887, #181122, #4465, #138788, #158240, #124744, #190703, #120469, #172347, #122621, #72693, #204808, #137724, #155028, #136656, #57529, #41299, #187514, #38078, #188582, #39145, #56459, #173430, #203743, #21782, #8766, #55388, #22860, #54330, #186441, #105226, #42365, #171266, #121543, #88973, #6613, #40215, #104150, #106324, #87891, #123686, #23937, #90041, #92191, #74848, #205895, #156099, #70537, #7684, #73768, #189648, #71611, #25010, #139864, #58589, #170198, #107407, #140947, #202681, #153964, #91111, #157171, #206960, #108476, #174499, #26077, #5531, #193912, #211220, #192834, #75905, #209076, #47695, #62846, #143082, #196065, #10882, #61791, #178752 ),
 ( #160356, #127958, #161437, #9829, #175555, #78032, #46620, #45559, #27145, #43426, #13018, #111674, #11959, #177681, #144157, #191771, #109550, #130070, #76957, #212280, #208024, #44493, #80163, #142009, #59650, #176610, #28222, #60713, #63914, #112741, #96452, #125809, #29293, #129007, #110610, #93249, #126877, #113809, #194984, #94315, #179810, #210148, #95385, #30365, #162503, #14073, #159283, #79095, #146268, #145213, #31429, #97506, #164616, #99615, #184047, #181910, #98555, #2075, #165681, #1012, #100672, #163563, #114859, #17269, #200287, #199218, #180859, #197106, #166750, #50865, #83345, #116987, #149430, #131118, #48746, #69214, #16201, #182987, #34604, #68149, #19412, #32481, #82283, #214377, #148376, #66007, #67077, #201347, #132157, #133212, #198162, #18345, #84425, #49796, #15147, #147315, #150514, #36729, #3145, #135333, #213342, #134282, #51938, #118062, #35665, #115922, #33542, #81233, #101744, #167812, #85490, #151577, #52987, #119123, #185103, #64965, #169935, #54067, #43968, #87630, #55132, #86562, #152624, #137464, #11431, #71347, #21519, #153702, #203479, #5270, #4211, #121277, #120202, #89790, #38880, #6352, #127422, #110083, #23679, #122359, #193394, #72423, #187253, #155836, #103887, #60189, #39957, #77507, #104964, #56197, #138525, #7420, #176095, #186177, #136395, #171006, #37811, #22603, #204548, #143627, #88710, #188316, #154769, #106064, #172087, #73502, #102816, #70279, #139604, #168871, #159830, #209621, #202411, #205628, #126349, #192308, #27694, #93792, #61263, #20475, #31971, #15690, #161980, #12499, #96993, #13571, #47174, #147858, #112221, #210705, #197646, #29843, #211760, #28770, #94852, #79644, #165156, #145760, #178228, #95925, #63398, #129552, #160903, #195537, #62333, #98052, #113287, #163045, #66549, #49292, #180348, #64466, #132692, #14624, #179293, #164106, #46103, #213874, #196596, #33027, #78572, #30917, #115409, #111151, #177151, #80719, #146809, #212828, #99105, #81776, #131644, #144692, #130608, #65496, #48239, #128492, #114352, #82834, #181402, #16749, #148909, #483, #45038, #194458, #70821, #185654, #116464, #100156, #153170, #166219, #136937, #52472, #199769, #134816, #4746, #2622, #133761, #37285, #200821, #36204, #135865, #198699, #149983, #118597, #21004, #19952, #1555, #17809, #201885, #86036, #184586, #152112, #102280, #83892, #67617, #34084, #3683, #168357, #69760, #53535, #51414, #68693, #50343, #103358, #169421, #101209, #117535, #119667, #167296, #87101, #202964, #183530, #35136, #54604, #18882, #151059, #182456, #84967, #120752, #104431, #186730, #38353, #170478, #22064, #88175, #154247, #5819, #71894, #125031, #74061, #41581, #159577, #142297, #58875, #157461, #11174, #107696, #106611, #190988, #139076, #92476, #75131, #126092, #121823, #172638, #208307, #204019, #55667, #90316, #156387, #205099, #192053, #174787, #10114, #187792, #173722, #42652, #24214, #39421, #122909, #175844, #108762, #56741, #109834, #188867, #189936, #158516, #76189, #26362, #105515, #171549, #59937, #23144, #43718, #206178, #40507, #140153, #27435, #7971, #72971, #93533, #57807, #25299, #141240, #138002, #89260, #123968, #155310, #91401, #6893, #9056, #207249, #179043, #79394, #30661, #145512, #44786, #176899, #197398, #78319, #96745, #113037, #130362, #147608, #160644, #110892, #128242, #94602, #12244, #195287, #115161, #62084, #46919, #111971, #211511, #162795, #144443, #77250, #61010, #63147, #164907, #131401, #49041, #210446, #196351, #13321, #129309, #14372, #143367, #28512, #80462, #114109, #146561, #194206, #45851, #212581, #64221, #47994, #180101, #31727, #177974, #29587, #181155, #95675, #97800, #163859, #15439, #213627, #161729, #81528, #65252, #32778, #98856, #209364, #127167, #193138, #134581, #51166, #150810, #184344, #17561, #16502, #236, #84722, #104186, #70573, #136691, #66309, #118357, #68452, #18643, #2374, #83647, #100962, #82583, #3447, #201644, #133515, #198455, #200581, #199521, #52229, #119424, #149733, #182212, #169172, #1311, #183285, #132456, #50100, #117288, #202716, #34890, #67373, #167051, #35967, #102045, #116221, #168114, #33836, #69514 ) ),
 .UNSPECIFIED., .F., .F., .T. ) 
 B_SPLINE_SURFACE_WITH_KNOTS ( ( 2, 2 ),
 ( 3, 2, 2, 2, 2, 2, 2, 2, 2, 2, 2, 2, 2, 2, 2, 2, 2, 2, 2, 2, 2, 2, 2, 2, 2, 2, 2, 2, 2, 2, 2, 2, 2, 2, 2, 2, 2, 2, 2, 2, 2, 2, 2, 2, 2, 2, 2, 2, 2, 2, 2, 2, 2, 2, 2, 2, 2, 2, 2, 2, 2, 2, 2, 2, 2, 2, 2, 2, 2, 2, 2, 2, 2, 2, 2, 2, 2, 2, 2, 2, 2, 2, 2, 2, 2, 2, 2, 2, 2, 2, 2, 2, 2, 2, 2, 2, 2, 2, 2, 2, 2, 2, 2, 2, 2, 2, 2, 2, 2, 2, 2, 2, 2, 2, 2, 2, 2, 2, 2, 2, 2, 2, 2, 2, 2, 2, 2, 2, 2, 2, 2, 2, 2, 2, 2, 2, 2, 2, 2, 2, 2, 2, 2, 2, 2, 2, 2, 2, 2, 2, 2, 2, 2, 2, 2, 2, 2, 2, 2, 2, 2, 2, 2, 2, 2, 2, 2, 2, 2, 2, 2, 2, 2, 2, 2, 2, 2, 2, 2, 2, 2, 2, 2, 2, 2, 2, 2, 2, 2, 2, 2, 2, 2, 2, 2, 2, 2, 2, 2, 2, 2, 2, 2, 2, 2, 2, 2, 2, 2, 2, 2, 2, 2, 2, 2, 2, 2, 2, 2, 2, 2, 2, 2, 2, 2, 2, 2, 2, 2, 2, 2, 2, 2, 2, 2, 2, 2, 2, 2, 2, 3 ),
 ( 0.000000000000000000, 1.000000000000000000 ),
 ( 0.000000000000000000, 0.004166666666666666609, 0.008333333333333333218, 0.01250000000000000069, 0.01666666666666666644, 0.02083333333333333218, 0.02500000000000000139, 0.02916666666666666713, 0.03333333333333333287, 0.03749999999999999861, 0.04166666666666666435, 0.04583333333333333010, 0.05000000000000000278, 0.05416666666666666852, 0.05833333333333333426, 0.06250000000000000000, 0.06666666666666666574, 0.07083333333333333148, 0.07499999999999999722, 0.07916666666666666297, 0.08333333333333332871, 0.08749999999999999445, 0.09166666666666666019, 0.09583333333333333981, 0.1000000000000000056, 0.1041666666666666713, 0.1083333333333333370, 0.1125000000000000028, 0.1166666666666666685, 0.1208333333333333343, 0.1250000000000000000, 0.1291666666666666796, 0.1333333333333333315, 0.1375000000000000111, 0.1416666666666666630, 0.1458333333333333426, 0.1499999999999999944, 0.1541666666666666741, 0.1583333333333333259, 0.1625000000000000056, 0.1666666666666666574, 0.1708333333333333370, 0.1749999999999999889, 0.1791666666666666685, 0.1833333333333333204, 0.1875000000000000000, 0.1916666666666666796, 0.1958333333333333315, 0.2000000000000000111, 0.2041666666666666630, 0.2083333333333333426, 0.2124999999999999944, 0.2166666666666666741, 0.2208333333333333259, 0.2250000000000000056, 0.2291666666666666574, 0.2333333333333333370, 0.2374999999999999889, 0.2416666666666666685, 0.2458333333333333204, 0.2500000000000000000, 0.2541666666666666519, 0.2583333333333333592, 0.2625000000000000111, 0.2666666666666666630, 0.2708333333333333148, 0.2750000000000000222, 0.2791666666666666741, 0.2833333333333333259, 0.2874999999999999778, 0.2916666666666666852, 0.2958333333333333370, 0.2999999999999999889, 0.3041666666666666408, 0.3083333333333333481, 0.3125000000000000000, 0.3166666666666666519, 0.3208333333333333592, 0.3250000000000000111, 0.3291666666666666630, 0.3333333333333333148, 0.3375000000000000222, 0.3416666666666666741, 0.3458333333333333259, 0.3499999999999999778, 0.3541666666666666852, 0.3583333333333333370, 0.3624999999999999889, 0.3666666666666666408, 0.3708333333333333481, 0.3750000000000000000, 0.3791666666666666519, 0.3833333333333333592, 0.3875000000000000111, 0.3916666666666666630, 0.3958333333333333148, 0.4000000000000000222, 0.4041666666666666741, 0.4083333333333333259, 0.4124999999999999778, 0.4166666666666666852, 0.4208333333333333370, 0.4249999999999999889, 0.4291666666666666408, 0.4333333333333333481, 0.4375000000000000000, 0.4416666666666666519, 0.4458333333333333592, 0.4500000000000000111, 0.4541666666666666630, 0.4583333333333333148, 0.4625000000000000222, 0.4666666666666666741, 0.4708333333333333259, 0.4749999999999999778, 0.4791666666666666852, 0.4833333333333333370, 0.4874999999999999889, 0.4916666666666666408, 0.4958333333333333481, 0.5000000000000000000, 0.5041666666666666519, 0.5083333333333333037, 0.5124999999999999556, 0.5166666666666667185, 0.5208333333333333703, 0.5250000000000000222, 0.5291666666666666741, 0.5333333333333333259, 0.5374999999999999778, 0.5416666666666666297, 0.5458333333333332815, 0.5500000000000000444, 0.5541666666666666963, 0.5583333333333333481, 0.5625000000000000000, 0.5666666666666666519, 0.5708333333333333037, 0.5749999999999999556, 0.5791666666666667185, 0.5833333333333333703, 0.5875000000000000222, 0.5916666666666666741, 0.5958333333333333259, 0.5999999999999999778, 0.6041666666666666297, 0.6083333333333332815, 0.6125000000000000444, 0.6166666666666666963, 0.6208333333333333481, 0.6250000000000000000, 0.6291666666666666519, 0.6333333333333333037, 0.6374999999999999556, 0.6416666666666667185, 0.6458333333333333703, 0.6500000000000000222, 0.6541666666666666741, 0.6583333333333333259, 0.6624999999999999778, 0.6666666666666666297, 0.6708333333333332815, 0.6750000000000000444, 0.6791666666666666963, 0.6833333333333333481, 0.6875000000000000000, 0.6916666666666666519, 0.6958333333333333037, 0.6999999999999999556, 0.7041666666666667185, 0.7083333333333333703, 0.7125000000000000222, 0.7166666666666666741, 0.7208333333333333259, 0.7249999999999999778, 0.7291666666666666297, 0.7333333333333332815, 0.7375000000000000444, 0.7416666666666666963, 0.7458333333333333481, 0.7500000000000000000, 0.7541666666666666519, 0.7583333333333333037, 0.7624999999999999556, 0.7666666666666667185, 0.7708333333333333703, 0.7750000000000000222, 0.7791666666666666741, 0.7833333333333333259, 0.7874999999999999778, 0.7916666666666666297, 0.7958333333333332815, 0.8000000000000000444, 0.8041666666666666963, 0.8083333333333333481, 0.8125000000000000000, 0.8166666666666666519, 0.8208333333333333037, 0.8249999999999999556, 0.8291666666666667185, 0.8333333333333333703, 0.8375000000000000222, 0.8416666666666666741, 0.8458333333333333259, 0.8499999999999999778, 0.8541666666666666297, 0.8583333333333332815, 0.8625000000000000444, 0.8666666666666666963, 0.8708333333333333481, 0.8750000000000000000, 0.8791666666666666519, 0.8833333333333333037, 0.8874999999999999556, 0.8916666666666667185, 0.8958333333333333703, 0.9000000000000000222, 0.9041666666666666741, 0.9083333333333333259, 0.9124999999999999778, 0.9166666666666666297, 0.9208333333333332815, 0.9250000000000000444, 0.9291666666666666963, 0.9333333333333333481, 0.9375000000000000000, 0.9416666666666666519, 0.9458333333333333037, 0.9499999999999999556, 0.9541666666666667185, 0.9583333333333333703, 0.9625000000000000222, 0.9666666666666666741, 0.9708333333333333259, 0.9749999999999999778, 0.9791666666666666297, 0.9833333333333332815, 0.9875000000000000444, 0.9916666666666666963, 0.9958333333333333481, 1.000000000000000000 ),
 .UNSPECIFIED. ) 
 GEOMETRIC_REPRESENTATION_ITEM ( )  RATIONAL_B_SPLINE_SURFACE ( (
 ( 1.000000000000000000, 0.8660254037844387076, 1.000000000000000000, 0.8660254037844387076, 1.000000000000000000, 0.8660254037844387076, 1.000000000000000000, 0.8660254037844387076, 1.000000000000000000, 0.8660254037844387076, 1.000000000000000000, 0.8660254037844387076, 1.000000000000000000, 0.8660254037844387076, 1.000000000000000000, 0.8660254037844387076, 1.000000000000000000, 0.8660254037844387076, 1.000000000000000000, 0.8660254037844387076, 1.000000000000000000, 0.8660254037844387076, 1.000000000000000000, 0.8660254037844387076, 1.000000000000000000, 0.8660254037844387076, 1.000000000000000000, 0.8660254037844387076, 1.000000000000000000, 0.8660254037844387076, 1.000000000000000000, 0.8660254037844387076, 1.000000000000000000, 0.8660254037844387076, 1.000000000000000000, 0.8660254037844387076, 1.000000000000000000, 0.8660254037844387076, 1.000000000000000000, 0.8660254037844387076, 1.000000000000000000, 0.8660254037844387076, 1.000000000000000000, 0.8660254037844387076, 1.000000000000000000, 0.8660254037844387076, 1.000000000000000000, 0.8660254037844387076, 1.000000000000000000, 0.8660254037844387076, 1.000000000000000000, 0.8660254037844387076, 1.000000000000000000, 0.8660254037844387076, 1.000000000000000000, 0.8660254037844387076, 1.000000000000000000, 0.8660254037844387076, 1.000000000000000000, 0.8660254037844387076, 1.000000000000000000, 0.8660254037844387076, 1.000000000000000000, 0.8660254037844387076, 1.000000000000000000, 0.8660254037844387076, 1.000000000000000000, 0.8660254037844387076, 1.000000000000000000, 0.8660254037844387076, 1.000000000000000000, 0.8660254037844387076, 1.000000000000000000, 0.8660254037844387076, 1.000000000000000000, 0.8660254037844387076, 1.000000000000000000, 0.8660254037844387076, 1.000000000000000000, 0.8660254037844387076, 1.000000000000000000, 0.8660254037844387076, 1.000000000000000000, 0.8660254037844387076, 1.000000000000000000, 0.8660254037844387076, 1.000000000000000000, 0.8660254037844387076, 1.000000000000000000, 0.8660254037844387076, 1.000000000000000000, 0.8660254037844387076, 1.000000000000000000, 0.8660254037844387076, 1.000000000000000000, 0.8660254037844387076, 1.000000000000000000, 0.8660254037844387076, 1.000000000000000000, 0.8660254037844387076, 1.000000000000000000, 0.8660254037844387076, 1.000000000000000000, 0.8660254037844387076, 1.000000000000000000, 0.8660254037844387076, 1.000000000000000000, 0.8660254037844387076, 1.000000000000000000, 0.8660254037844387076, 1.000000000000000000, 0.8660254037844387076, 1.000000000000000000, 0.8660254037844387076, 1.000000000000000000, 0.8660254037844387076, 1.000000000000000000, 0.8660254037844387076, 1.000000000000000000, 0.8660254037844387076, 1.000000000000000000, 0.8660254037844387076, 1.000000000000000000, 0.8660254037844387076, 1.000000000000000000, 0.8660254037844387076, 1.000000000000000000, 0.8660254037844387076, 1.000000000000000000, 0.8660254037844387076, 1.000000000000000000, 0.8660254037844387076, 1.000000000000000000, 0.8660254037844387076, 1.000000000000000000, 0.8660254037844387076, 1.000000000000000000, 0.8660254037844387076, 1.000000000000000000, 0.8660254037844387076, 1.000000000000000000, 0.8660254037844387076, 1.000000000000000000, 0.8660254037844387076, 1.000000000000000000, 0.8660254037844387076, 1.000000000000000000, 0.8660254037844387076, 1.000000000000000000, 0.8660254037844387076, 1.000000000000000000, 0.8660254037844387076, 1.000000000000000000, 0.8660254037844387076, 1.000000000000000000, 0.8660254037844387076, 1.000000000000000000, 0.8660254037844387076, 1.000000000000000000, 0.8660254037844387076, 1.000000000000000000, 0.8660254037844387076, 1.000000000000000000, 0.8660254037844387076, 1.000000000000000000, 0.8660254037844387076, 1.000000000000000000, 0.8660254037844387076, 1.000000000000000000, 0.8660254037844387076, 1.000000000000000000, 0.8660254037844387076, 1.000000000000000000, 0.8660254037844387076, 1.000000000000000000, 0.8660254037844387076, 1.000000000000000000, 0.8660254037844387076, 1.000000000000000000, 0.8660254037844387076, 1.000000000000000000, 0.8660254037844387076, 1.000000000000000000, 0.8660254037844387076, 1.000000000000000000, 0.8660254037844387076, 1.000000000000000000, 0.8660254037844387076, 1.000000000000000000, 0.8660254037844387076, 1.000000000000000000, 0.8660254037844387076, 1.000000000000000000, 0.8660254037844387076, 1.000000000000000000, 0.8660254037844387076, 1.000000000000000000, 0.8660254037844387076, 1.000000000000000000, 0.8660254037844387076, 1.000000000000000000, 0.8660254037844387076, 1.000000000000000000, 0.8660254037844387076, 1.000000000000000000, 0.8660254037844387076, 1.000000000000000000, 0.8660254037844387076, 1.000000000000000000, 0.8660254037844387076, 1.000000000000000000, 0.8660254037844387076, 1.000000000000000000, 0.8660254037844387076, 1.000000000000000000, 0.8660254037844387076, 1.000000000000000000, 0.8660254037844387076, 1.000000000000000000, 0.8660254037844387076, 1.000000000000000000, 0.8660254037844387076, 1.000000000000000000, 0.8660254037844387076, 1.000000000000000000, 0.8660254037844387076, 1.000000000000000000, 0.8660254037844387076, 1.000000000000000000, 0.8660254037844387076, 1.000000000000000000, 0.8660254037844387076, 1.000000000000000000, 0.8660254037844387076, 1.000000000000000000, 0.8660254037844387076, 1.000000000000000000, 0.8660254037844387076, 1.000000000000000000, 0.8660254037844387076, 1.000000000000000000, 0.8660254037844387076, 1.000000000000000000, 0.8660254037844387076, 1.000000000000000000, 0.8660254037844387076, 1.000000000000000000, 0.8660254037844387076, 1.000000000000000000, 0.8660254037844387076, 1.000000000000000000, 0.8660254037844387076, 1.000000000000000000, 0.8660254037844387076, 1.000000000000000000, 0.8660254037844387076, 1.000000000000000000, 0.8660254037844387076, 1.000000000000000000, 0.8660254037844387076, 1.000000000000000000, 0.8660254037844387076, 1.000000000000000000, 0.8660254037844387076, 1.000000000000000000, 0.8660254037844387076, 1.000000000000000000, 0.8660254037844387076, 1.000000000000000000, 0.8660254037844387076, 1.000000000000000000, 0.8660254037844387076, 1.000000000000000000, 0.8660254037844387076, 1.000000000000000000, 0.8660254037844387076, 1.000000000000000000, 0.8660254037844387076, 1.000000000000000000, 0.8660254037844387076, 1.000000000000000000, 0.8660254037844387076, 1.000000000000000000, 0.8660254037844387076, 1.000000000000000000, 0.8660254037844387076, 1.000000000000000000, 0.8660254037844387076, 1.000000000000000000, 0.8660254037844387076, 1.000000000000000000, 0.8660254037844387076, 1.000000000000000000, 0.8660254037844387076, 1.000000000000000000, 0.8660254037844387076, 1.000000000000000000, 0.8660254037844387076, 1.000000000000000000, 0.8660254037844387076, 1.000000000000000000, 0.8660254037844387076, 1.000000000000000000, 0.8660254037844387076, 1.000000000000000000, 0.8660254037844387076, 1.000000000000000000, 0.8660254037844387076, 1.000000000000000000, 0.8660254037844387076, 1.000000000000000000, 0.8660254037844387076, 1.000000000000000000, 0.8660254037844387076, 1.000000000000000000, 0.8660254037844387076, 1.000000000000000000, 0.8660254037844387076, 1.000000000000000000, 0.8660254037844387076, 1.000000000000000000, 0.8660254037844387076, 1.000000000000000000, 0.8660254037844387076, 1.000000000000000000, 0.8660254037844387076, 1.000000000000000000, 0.8660254037844387076, 1.000000000000000000, 0.8660254037844387076, 1.000000000000000000, 0.8660254037844387076, 1.000000000000000000, 0.8660254037844387076, 1.000000000000000000, 0.8660254037844387076, 1.000000000000000000, 0.8660254037844387076, 1.000000000000000000, 0.8660254037844387076, 1.000000000000000000, 0.8660254037844387076, 1.000000000000000000, 0.8660254037844387076, 1.000000000000000000, 0.8660254037844387076, 1.000000000000000000, 0.8660254037844387076, 1.000000000000000000, 0.8660254037844387076, 1.000000000000000000, 0.8660254037844387076, 1.000000000000000000, 0.8660254037844387076, 1.000000000000000000, 0.8660254037844387076, 1.000000000000000000, 0.8660254037844387076, 1.000000000000000000, 0.8660254037844387076, 1.000000000000000000, 0.8660254037844387076, 1.000000000000000000, 0.8660254037844387076, 1.000000000000000000, 0.8660254037844387076, 1.000000000000000000, 0.8660254037844387076, 1.000000000000000000, 0.8660254037844387076, 1.000000000000000000, 0.8660254037844387076, 1.000000000000000000, 0.8660254037844387076, 1.000000000000000000, 0.8660254037844387076, 1.000000000000000000, 0.8660254037844387076, 1.000000000000000000, 0.8660254037844387076, 1.000000000000000000, 0.8660254037844387076, 1.000000000000000000, 0.8660254037844387076, 1.000000000000000000, 0.8660254037844387076, 1.000000000000000000, 0.8660254037844387076, 1.000000000000000000, 0.8660254037844387076, 1.000000000000000000, 0.8660254037844387076, 1.000000000000000000, 0.8660254037844387076, 1.000000000000000000, 0.8660254037844387076, 1.000000000000000000, 0.8660254037844387076, 1.000000000000000000, 0.8660254037844387076, 1.000000000000000000, 0.8660254037844387076, 1.000000000000000000, 0.8660254037844387076, 1.000000000000000000, 0.8660254037844387076, 1.000000000000000000, 0.8660254037844387076, 1.000000000000000000, 0.8660254037844387076, 1.000000000000000000, 0.8660254037844387076, 1.000000000000000000, 0.8660254037844387076, 1.000000000000000000, 0.8660254037844387076, 1.000000000000000000, 0.8660254037844387076, 1.000000000000000000, 0.8660254037844387076, 1.000000000000000000, 0.8660254037844387076, 1.000000000000000000, 0.8660254037844387076, 1.000000000000000000, 0.8660254037844387076, 1.000000000000000000, 0.8660254037844387076, 1.000000000000000000, 0.8660254037844387076, 1.000000000000000000, 0.8660254037844387076, 1.000000000000000000, 0.8660254037844387076, 1.000000000000000000, 0.8660254037844387076, 1.000000000000000000, 0.8660254037844387076, 1.000000000000000000, 0.8660254037844387076, 1.000000000000000000, 0.8660254037844387076, 1.000000000000000000, 0.8660254037844387076, 1.000000000000000000, 0.8660254037844387076, 1.000000000000000000, 0.8660254037844387076, 1.000000000000000000, 0.8660254037844387076, 1.000000000000000000, 0.8660254037844387076, 1.000000000000000000, 0.8660254037844387076, 1.000000000000000000, 0.8660254037844387076, 1.000000000000000000, 0.8660254037844387076, 1.000000000000000000, 0.8660254037844387076, 1.000000000000000000, 0.8660254037844387076, 1.000000000000000000, 0.8660254037844387076, 1.000000000000000000, 0.8660254037844387076, 1.000000000000000000, 0.8660254037844387076, 1.000000000000000000, 0.8660254037844387076, 1.000000000000000000, 0.8660254037844387076, 1.000000000000000000, 0.8660254037844387076, 1.000000000000000000, 0.8660254037844387076, 1.000000000000000000, 0.8660254037844387076, 1.000000000000000000, 0.8660254037844387076, 1.000000000000000000),
 ( 1.000000000000000000, 0.8660254037844387076, 1.000000000000000000, 0.8660254037844387076, 1.000000000000000000, 0.8660254037844387076, 1.000000000000000000, 0.8660254037844387076, 1.000000000000000000, 0.8660254037844387076, 1.000000000000000000, 0.8660254037844387076, 1.000000000000000000, 0.8660254037844387076, 1.000000000000000000, 0.8660254037844387076, 1.000000000000000000, 0.8660254037844387076, 1.000000000000000000, 0.8660254037844387076, 1.000000000000000000, 0.8660254037844387076, 1.000000000000000000, 0.8660254037844387076, 1.000000000000000000, 0.8660254037844387076, 1.000000000000000000, 0.8660254037844387076, 1.000000000000000000, 0.8660254037844387076, 1.000000000000000000, 0.8660254037844387076, 1.000000000000000000, 0.8660254037844387076, 1.000000000000000000, 0.8660254037844387076, 1.000000000000000000, 0.8660254037844387076, 1.000000000000000000, 0.8660254037844387076, 1.000000000000000000, 0.8660254037844387076, 1.000000000000000000, 0.8660254037844387076, 1.000000000000000000, 0.8660254037844387076, 1.000000000000000000, 0.8660254037844387076, 1.000000000000000000, 0.8660254037844387076, 1.000000000000000000, 0.8660254037844387076, 1.000000000000000000, 0.8660254037844387076, 1.000000000000000000, 0.8660254037844387076, 1.000000000000000000, 0.8660254037844387076, 1.000000000000000000, 0.8660254037844387076, 1.000000000000000000, 0.8660254037844387076, 1.000000000000000000, 0.8660254037844387076, 1.000000000000000000, 0.8660254037844387076, 1.000000000000000000, 0.8660254037844387076, 1.000000000000000000, 0.8660254037844387076, 1.000000000000000000, 0.8660254037844387076, 1.000000000000000000, 0.8660254037844387076, 1.000000000000000000, 0.8660254037844387076, 1.000000000000000000, 0.8660254037844387076, 1.000000000000000000, 0.8660254037844387076, 1.000000000000000000, 0.8660254037844387076, 1.000000000000000000, 0.8660254037844387076, 1.000000000000000000, 0.8660254037844387076, 1.000000000000000000, 0.8660254037844387076, 1.000000000000000000, 0.8660254037844387076, 1.000000000000000000, 0.8660254037844387076, 1.000000000000000000, 0.8660254037844387076, 1.000000000000000000, 0.8660254037844387076, 1.000000000000000000, 0.8660254037844387076, 1.000000000000000000, 0.8660254037844387076, 1.000000000000000000, 0.8660254037844387076, 1.000000000000000000, 0.8660254037844387076, 1.000000000000000000, 0.8660254037844387076, 1.000000000000000000, 0.8660254037844387076, 1.000000000000000000, 0.8660254037844387076, 1.000000000000000000, 0.8660254037844387076, 1.000000000000000000, 0.8660254037844387076, 1.000000000000000000, 0.8660254037844387076, 1.000000000000000000, 0.8660254037844387076, 1.000000000000000000, 0.8660254037844387076, 1.000000000000000000, 0.8660254037844387076, 1.000000000000000000, 0.8660254037844387076, 1.000000000000000000, 0.8660254037844387076, 1.000000000000000000, 0.8660254037844387076, 1.000000000000000000, 0.8660254037844387076, 1.000000000000000000, 0.8660254037844387076, 1.000000000000000000, 0.8660254037844387076, 1.000000000000000000, 0.8660254037844387076, 1.000000000000000000, 0.8660254037844387076, 1.000000000000000000, 0.8660254037844387076, 1.000000000000000000, 0.8660254037844387076, 1.000000000000000000, 0.8660254037844387076, 1.000000000000000000, 0.8660254037844387076, 1.000000000000000000, 0.8660254037844387076, 1.000000000000000000, 0.8660254037844387076, 1.000000000000000000, 0.8660254037844387076, 1.000000000000000000, 0.8660254037844387076, 1.000000000000000000, 0.8660254037844387076, 1.000000000000000000, 0.8660254037844387076, 1.000000000000000000, 0.8660254037844387076, 1.000000000000000000, 0.8660254037844387076, 1.000000000000000000, 0.8660254037844387076, 1.000000000000000000, 0.8660254037844387076, 1.000000000000000000, 0.8660254037844387076, 1.000000000000000000, 0.8660254037844387076, 1.000000000000000000, 0.8660254037844387076, 1.000000000000000000, 0.8660254037844387076, 1.000000000000000000, 0.8660254037844387076, 1.000000000000000000, 0.8660254037844387076, 1.000000000000000000, 0.8660254037844387076, 1.000000000000000000, 0.8660254037844387076, 1.000000000000000000, 0.8660254037844387076, 1.000000000000000000, 0.8660254037844387076, 1.000000000000000000, 0.8660254037844387076, 1.000000000000000000, 0.8660254037844387076, 1.000000000000000000, 0.8660254037844387076, 1.000000000000000000, 0.8660254037844387076, 1.000000000000000000, 0.8660254037844387076, 1.000000000000000000, 0.8660254037844387076, 1.000000000000000000, 0.8660254037844387076, 1.000000000000000000, 0.8660254037844387076, 1.000000000000000000, 0.8660254037844387076, 1.000000000000000000, 0.8660254037844387076, 1.000000000000000000, 0.8660254037844387076, 1.000000000000000000, 0.8660254037844387076, 1.000000000000000000, 0.8660254037844387076, 1.000000000000000000, 0.8660254037844387076, 1.000000000000000000, 0.8660254037844387076, 1.000000000000000000, 0.8660254037844387076, 1.000000000000000000, 0.8660254037844387076, 1.000000000000000000, 0.8660254037844387076, 1.000000000000000000, 0.8660254037844387076, 1.000000000000000000, 0.8660254037844387076, 1.000000000000000000, 0.8660254037844387076, 1.000000000000000000, 0.8660254037844387076, 1.000000000000000000, 0.8660254037844387076, 1.000000000000000000, 0.8660254037844387076, 1.000000000000000000, 0.8660254037844387076, 1.000000000000000000, 0.8660254037844387076, 1.000000000000000000, 0.8660254037844387076, 1.000000000000000000, 0.8660254037844387076, 1.000000000000000000, 0.8660254037844387076, 1.000000000000000000, 0.8660254037844387076, 1.000000000000000000, 0.8660254037844387076, 1.000000000000000000, 0.8660254037844387076, 1.000000000000000000, 0.8660254037844387076, 1.000000000000000000, 0.8660254037844387076, 1.000000000000000000, 0.8660254037844387076, 1.000000000000000000, 0.8660254037844387076, 1.000000000000000000, 0.8660254037844387076, 1.000000000000000000, 0.8660254037844387076, 1.000000000000000000, 0.8660254037844387076, 1.000000000000000000, 0.8660254037844387076, 1.000000000000000000, 0.8660254037844387076, 1.000000000000000000, 0.8660254037844387076, 1.000000000000000000, 0.8660254037844387076, 1.000000000000000000, 0.8660254037844387076, 1.000000000000000000, 0.8660254037844387076, 1.000000000000000000, 0.8660254037844387076, 1.000000000000000000, 0.8660254037844387076, 1.000000000000000000, 0.8660254037844387076, 1.000000000000000000, 0.8660254037844387076, 1.000000000000000000, 0.8660254037844387076, 1.000000000000000000, 0.8660254037844387076, 1.000000000000000000, 0.8660254037844387076, 1.000000000000000000, 0.8660254037844387076, 1.000000000000000000, 0.8660254037844387076, 1.000000000000000000, 0.8660254037844387076, 1.000000000000000000, 0.8660254037844387076, 1.000000000000000000, 0.8660254037844387076, 1.000000000000000000, 0.8660254037844387076, 1.000000000000000000, 0.8660254037844387076, 1.000000000000000000, 0.8660254037844387076, 1.000000000000000000, 0.8660254037844387076, 1.000000000000000000, 0.8660254037844387076, 1.000000000000000000, 0.8660254037844387076, 1.000000000000000000, 0.8660254037844387076, 1.000000000000000000, 0.8660254037844387076, 1.000000000000000000, 0.8660254037844387076, 1.000000000000000000, 0.8660254037844387076, 1.000000000000000000, 0.8660254037844387076, 1.000000000000000000, 0.8660254037844387076, 1.000000000000000000, 0.8660254037844387076, 1.000000000000000000, 0.8660254037844387076, 1.000000000000000000, 0.8660254037844387076, 1.000000000000000000, 0.8660254037844387076, 1.000000000000000000, 0.8660254037844387076, 1.000000000000000000, 0.8660254037844387076, 1.000000000000000000, 0.8660254037844387076, 1.000000000000000000, 0.8660254037844387076, 1.000000000000000000, 0.8660254037844387076, 1.000000000000000000, 0.8660254037844387076, 1.000000000000000000, 0.8660254037844387076, 1.000000000000000000, 0.8660254037844387076, 1.000000000000000000, 0.8660254037844387076, 1.000000000000000000, 0.8660254037844387076, 1.000000000000000000, 0.8660254037844387076, 1.000000000000000000, 0.8660254037844387076, 1.000000000000000000, 0.8660254037844387076, 1.000000000000000000, 0.8660254037844387076, 1.000000000000000000, 0.8660254037844387076, 1.000000000000000000, 0.8660254037844387076, 1.000000000000000000, 0.8660254037844387076, 1.000000000000000000, 0.8660254037844387076, 1.000000000000000000, 0.8660254037844387076, 1.000000000000000000, 0.8660254037844387076, 1.000000000000000000, 0.8660254037844387076, 1.000000000000000000, 0.8660254037844387076, 1.000000000000000000, 0.8660254037844387076, 1.000000000000000000, 0.8660254037844387076, 1.000000000000000000, 0.8660254037844387076, 1.000000000000000000, 0.8660254037844387076, 1.000000000000000000, 0.8660254037844387076, 1.000000000000000000, 0.8660254037844387076, 1.000000000000000000, 0.8660254037844387076, 1.000000000000000000, 0.8660254037844387076, 1.000000000000000000, 0.8660254037844387076, 1.000000000000000000, 0.8660254037844387076, 1.000000000000000000, 0.8660254037844387076, 1.000000000000000000, 0.8660254037844387076, 1.000000000000000000, 0.8660254037844387076, 1.000000000000000000, 0.8660254037844387076, 1.000000000000000000, 0.8660254037844387076, 1.000000000000000000, 0.8660254037844387076, 1.000000000000000000, 0.8660254037844387076, 1.000000000000000000, 0.8660254037844387076, 1.000000000000000000, 0.8660254037844387076, 1.000000000000000000, 0.8660254037844387076, 1.000000000000000000, 0.8660254037844387076, 1.000000000000000000, 0.8660254037844387076, 1.000000000000000000, 0.8660254037844387076, 1.000000000000000000, 0.8660254037844387076, 1.000000000000000000, 0.8660254037844387076, 1.000000000000000000, 0.8660254037844387076, 1.000000000000000000, 0.8660254037844387076, 1.000000000000000000, 0.8660254037844387076, 1.000000000000000000, 0.8660254037844387076, 1.000000000000000000, 0.8660254037844387076, 1.000000000000000000, 0.8660254037844387076, 1.000000000000000000, 0.8660254037844387076, 1.000000000000000000, 0.8660254037844387076, 1.000000000000000000, 0.8660254037844387076, 1.000000000000000000, 0.8660254037844387076, 1.000000000000000000, 0.8660254037844387076, 1.000000000000000000, 0.8660254037844387076, 1.000000000000000000, 0.8660254037844387076, 1.000000000000000000, 0.8660254037844387076, 1.000000000000000000, 0.8660254037844387076, 1.000000000000000000, 0.8660254037844387076, 1.000000000000000000, 0.8660254037844387076, 1.000000000000000000, 0.8660254037844387076, 1.000000000000000000, 0.8660254037844387076, 1.000000000000000000, 0.8660254037844387076, 1.000000000000000000, 0.8660254037844387076, 1.000000000000000000, 0.8660254037844387076, 1.000000000000000000, 0.8660254037844387076, 1.000000000000000000, 0.8660254037844387076, 1.000000000000000000, 0.8660254037844387076, 1.000000000000000000, 0.8660254037844387076, 1.000000000000000000, 0.8660254037844387076, 1.000000000000000000) ) ) 
 REPRESENTATION_ITEM ( '' )  SURFACE ( )  );
#113226=CARTESIAN_POINT ( 'NONE',  ( -8.297226821883391779, 11.66355314463053006, 1.082531754730549967 ) ) ;
#113231=CARTESIAN_POINT ( 'NONE',  ( -1.402160292154681736E-14, 1.509375000341420359, -1.575800808251659024 ) ) ;
#113239=CARTESIAN_POINT ( 'NONE',  ( 1.364683531249986537, 2.405208333674752286, -0.7879004041258239610 ) ) ;
#113241=CARTESIAN_POINT ( 'NONE',  ( -5.545448523189368650, 6.428443684264421698, -1.199719254218446718 ) ) ;
#113242=CARTESIAN_POINT ( 'NONE',  ( 6.238723240582662477, 10.43026088065513513, -0.7998128361456291469 ) ) ;
#113245=CARTESIAN_POINT ( 'NONE',  ( -1.364683531249997417, 3.321875000341423245, 1.214306433183764966E-14 ) ) ;
#113248=CARTESIAN_POINT ( 'NONE',  ( 1.364683531249986537, -0.6364583329919177856, 0.7879004041258500513 ) ) ;
#113250=CARTESIAN_POINT ( 'NONE',  ( -5.802526556968872207, 6.832331073627524454, 1.082531754730548412 ) ) ;
#113254=CARTESIAN_POINT ( 'NONE',  ( 4.365362273920244007, 6.116008624372160973, 1.443375672974062551 ) ) ;
#113257=CARTESIAN_POINT ( 'NONE',  ( -8.365544474831901667, 9.718555627847388578, 1.199719254218462483 ) ) ;
#113258=CARTESIAN_POINT ( 'NONE',  ( -4.627410500965859264, 4.293067094081919777, 0.7998128361456341429 ) ) ;
#113260=CARTESIAN_POINT ( 'NONE',  ( -1.201851678989727383E-14, 5.696875000341416140, -1.575800808251660134 ) ) ;
#113266=CARTESIAN_POINT ( 'NONE',  ( -5.490689023410187275, 8.389259046411751797, 1.082531754730548412 ) ) ;
#113268=CARTESIAN_POINT ( 'NONE',  ( 1.364683531249988757, -0.8031249996585804185, 0.000000000000000000 ) ) ;
#113271=CARTESIAN_POINT ( 'NONE',  ( 7.456621297836082185, 7.801739057004660971, 0.7216878364870317197 ) ) ;
#113281=CARTESIAN_POINT ( 'NONE',  ( 8.717529583462638954, 12.15390636647303069, 1.082531754730546636 ) ) ;
#113287=CARTESIAN_POINT ( 'NONE',  ( 6.474182045725470402, 7.511966127223233869, -1.199719254218446718 ) ) ;
#113288=CARTESIAN_POINT ( 'NONE',  ( -4.416205349749324327, 6.175325546172740765, 1.599625672291267398 ) ) ;
#113292=CARTESIAN_POINT ( 'NONE',  ( 4.161989969270883272, 7.799479364217271282, 0.7216878364870317197 ) ) ;
#113294=CARTESIAN_POINT ( 'NONE',  ( -0.6823417656250003738, 0.03020833367475134201, -1.181850606188749264 ) ) ;
#113296=CARTESIAN_POINT ( 'NONE',  ( -9.484092147959342967, 11.02352791316275216, 1.199719254218462483 ) ) ;
#113308=CARTESIAN_POINT ( 'NONE',  ( -1.499999999999997780, 4.650000000000022560, 1.214306433183765124E-14 ) ) ;
#113312=CARTESIAN_POINT ( 'NONE',  ( -4.267173273579143000, 7.298649460985302539, -0.9221393241729136658 ) ) ;
#113316=CARTESIAN_POINT ( 'NONE',  ( 6.331821432781979730, 7.345878745455822312, -1.199719254218445830 ) ) ;
#113322=CARTESIAN_POINT ( 'NONE',  ( 7.934546212495622086, 10.28005655271014795, -1.599625672291262513 ) ) ;
#113326=CARTESIAN_POINT ( 'NONE',  ( 10.01963921569910632, 11.64833282552586091, 1.199719254218450271 ) ) ;
#113328=CARTESIAN_POINT ( 'NONE',  ( -4.288456660624211381, 3.897620947016656956, 1.214306433183764966E-14 ) ) ;
#113331=CARTESIAN_POINT ( 'NONE',  ( 9.642873567817520808, 12.27310513391906532, 1.599625672291279388 ) ) ;
#113339=CARTESIAN_POINT ( 'NONE',  ( -9.015808963407680565, 9.620791333504852716, 1.040834085586084257E-14 ) ) ;
#113344=CARTESIAN_POINT ( 'NONE',  ( 6.322179702674084467, 6.270297829408224111, 1.040834085586084257E-14 ) ) ;
#113350=CARTESIAN_POINT ( 'NONE',  ( 3.836594282542909795, 6.459481848733281240, 1.082531754730558626 ) ) ;
#113353=ORIENTED_EDGE ( 'NONE', *, *, #24957, .T. ) ;
#113358=CARTESIAN_POINT ( 'NONE',  ( -7.542413527904030524, 7.693903958843159252, 1.040834085586084257E-14 ) ) ;
#113359=CARTESIAN_POINT ( 'NONE',  ( -4.843287188579803448, 6.673587691474970107, -1.599625672291256295 ) ) ;
#113368=CARTESIAN_POINT ( 'NONE',  ( 5.961834861707224320, 7.978559976790334574, -1.599625672291262513 ) ) ;
#113376=CARTESIAN_POINT ( 'NONE',  ( 1.177073619093308432, 3.131928502340592058, -0.7749999999999910294 ) ) ;
#113381=CARTESIAN_POINT ( 'NONE',  ( -0.6823417656250246877, 0.6135416670080897639, 1.181850606188755259 ) ) ;
#113382=CARTESIAN_POINT ( 'NONE',  ( 3.994848817520957773, 7.812407387083109001, 1.040834085586084257E-14 ) ) ;
#113384=CARTESIAN_POINT ( 'NONE',  ( -6.887178846062116833, 9.058127958537705027, -1.443375672974059665 ) ) ;
#113385=CARTESIAN_POINT ( 'NONE',  ( 4.365362273920238678, 7.076377838673507448, 1.082531754730558626 ) ) ;
#113386=CARTESIAN_POINT ( 'NONE',  ( -7.985389288324710400, 8.418635045908049008, -0.7216878364870267237 ) ) ;
#113390=CARTESIAN_POINT ( 'NONE',  ( 7.124973419181436007, 8.271222729588529887, -1.199719254218446718 ) ) ;
#113396=CARTESIAN_POINT ( 'NONE',  ( -1.201851678989727383E-14, 5.446875000341422357, -1.575800808251660134 ) ) ;
#113401=EDGE_CURVE ( 'NONE', #1642, #27161, #97919, .T. ) ;
#113402=CARTESIAN_POINT ( 'NONE',  ( 6.448874621594486989, 10.67543749183559143, 0.7998128361456462443 ) ) ;
#113406=CARTESIAN_POINT ( 'NONE',  ( -8.877891658850122880, 9.251961778280284321, 0.7998128361456462443 ) ) ;
#113411=CARTESIAN_POINT ( 'NONE',  ( 8.041957671200231417, 12.53403438304231976, 1.040834085586084257E-14 ) ) ;
#113414=CARTESIAN_POINT ( 'NONE',  ( -8.365544474831901667, 9.718555627847388578, 1.199719254218462483 ) ) ;
#113417=CARTESIAN_POINT ( 'NONE',  ( 4.778452461313970723, 6.762070782353614362, -1.245597109521460633 ) ) ;
#113418=CARTESIAN_POINT ( 'NONE',  ( -9.381879110976678149, 11.00824238663667565, 1.082531754730558626 ) ) ;
#113423=CARTESIAN_POINT ( 'NONE',  ( 5.717788096661236885, 7.693838750903348789, 1.599625672291267398 ) ) ;
#113425=CARTESIAN_POINT ( 'NONE',  ( 6.159481859310094620, 6.080483678816896109, 1.040834085586084257E-14 ) ) ;
#113426=CARTESIAN_POINT ( 'NONE',  ( -4.138143308069708759, 7.456237844118314584, -0.6866288536411498944 ) ) ;
#113427=CARTESIAN_POINT ( 'NONE',  ( 2.361091307074211887, 5.906356958228550447, 0.7998128361456462443 ) ) ;
#113429=CARTESIAN_POINT ( 'NONE',  ( -6.236387472606145010, 9.259240570473746601, -1.082531754730538864 ) ) ;
#113434=CARTESIAN_POINT ( 'NONE',  ( -4.836546220603817225, 6.746162335969787094, 1.249072166269946216 ) ) ;
#113435=CARTESIAN_POINT ( 'NONE',  ( -0.6823417656250003738, 0.03020833367475134201, -1.181850606188749264 ) ) ;
#113437=CARTESIAN_POINT ( 'NONE',  ( 1.479373551132449505, 3.300000000000025135, 0.2478989637125245671 ) ) ;
#113438=CARTESIAN_POINT ( 'NONE',  ( 5.517805331081858888, 5.539787095791365523, 1.040834085586084257E-14 ) ) ;
#113441=EDGE_CURVE ( 'NONE', #148246, #163352, #16555, .T. ) ;
#113443=CARTESIAN_POINT ( 'NONE',  ( -9.124274191872640216, 10.70770331434866485, -1.082531754730537976 ) ) ;
#113449=CARTESIAN_POINT ( 'NONE',  ( -7.809133291347029271, 12.05447990663947877, 0.000000000000000000 ) ) ;
#113451=ORIENTED_EDGE ( 'NONE', *, *, #22766, .T. ) ;
#113456=CARTESIAN_POINT ( 'NONE',  ( -8.636180661780660017, 11.09863007687603087, -1.443375672974058777 ) ) ;
#113460=CARTESIAN_POINT ( 'NONE',  ( -1.364683531250012516, 4.801041667008083991, -0.7879004041258300672 ) ) ;
#113461=CARTESIAN_POINT ( 'NONE',  ( -1.201851678989727383E-14, 2.743750000682820378, 1.732050807568877637 ) ) ;
#113462=CARTESIAN_POINT ( 'NONE',  ( 5.456969279648811622, 6.453098228331718644, -1.278498092073777626 ) ) ;
#113464=CARTESIAN_POINT ( 'NONE',  ( -6.240830780992103755, 6.175390754112560110, 1.040834085586084257E-14 ) ) ;
#113468=CARTESIAN_POINT ( 'NONE',  ( -8.128276786592724790, 9.441743324901704426, -1.199719254218446718 ) ) ;
#113472=CARTESIAN_POINT ( 'NONE',  ( 6.634017235788401301, 6.634108284708264414, 0.7998128361456341429 ) ) ;
#113477=CARTESIAN_POINT ( 'NONE',  ( 8.067265095331215718, 9.370563018429956870, 1.199719254218462483 ) ) ;
#113480=DIRECTION ( 'NONE',  ( 1.000000000000000000, -5.578564026256504688E-16, 0.000000000000000000 ) ) ;
#113483=CARTESIAN_POINT ( 'NONE',  ( -5.856759171423528088, 8.816340885760650892, 1.082531754730548412 ) ) ;
#113486=CARTESIAN_POINT ( 'NONE',  ( -1.201851678989727383E-14, 5.759375000341417028, -1.575800808251660801 ) ) ;
#113489=CARTESIAN_POINT ( 'NONE',  ( 8.500000000000000000, 6.200000000000038369, -2.873333333333334405 ) ) ;
#113494=CARTESIAN_POINT ( 'NONE',  ( -7.831806290188425557, 12.28885777186185990, -0.7998128361456281477 ) ) ;
#113496=CARTESIAN_POINT ( 'NONE',  ( 8.341290820905593151, 10.75459192918846618, 1.599625672291281386 ) ) ;
#113498=CARTESIAN_POINT ( 'NONE',  ( -9.154780037725563702, 11.70366268214508487, 1.599625672291281386 ) ) ;
#113500=CARTESIAN_POINT ( 'NONE',  ( 1.364683531249990311, 3.634375000341416584, 1.214306433183764966E-14 ) ) ;
#113501=CARTESIAN_POINT ( 'NONE',  ( 3.602716132929354664, 5.226254793216122074, 1.599625672291267398 ) ) ;
#113507=CARTESIAN_POINT ( 'NONE',  ( 8.825994812371966702, 12.28044913353391898, -1.082531754730543083 ) ) ;
#113510=CARTESIAN_POINT ( 'NONE',  ( -7.727784370109414880, 8.118095974656867497, 0.7216878364870578100 ) ) ;
#113511=CARTESIAN_POINT ( 'NONE',  ( -1.201851678989727383E-14, 1.321875000341419248, 1.575800808251672791 ) ) ;
#113513=CARTESIAN_POINT ( 'NONE',  ( 0.06360284778251625026, 7.077111424252135130, 2.121658048142260444 ) ) ;
#113515=CARTESIAN_POINT ( 'NONE',  ( -6.482770005628665011, 10.71498210654212002, 0.7998128361456481317 ) ) ;
#113516=CARTESIAN_POINT ( 'NONE',  ( -2.616360457312984167, 5.996244933599686355, -0.7216878364870257245 ) ) ;
#113517=CARTESIAN_POINT ( 'NONE',  ( -0.6823417656250212460, 2.863541667008084879, 1.181850606188767472 ) ) ;
#113538=CARTESIAN_POINT ( 'NONE',  ( 1.364683531249988535, 3.676041667008087099, 0.7879004041258500513 ) ) ;
#113544=CARTESIAN_POINT ( 'NONE',  ( 8.422639742587595180, 10.84949900448412130, -1.599625672291268286 ) ) ;
#113545=LINE ( 'NONE', #62579, #39896 ) ;
#113547=CARTESIAN_POINT ( 'NONE',  ( -1.364683531250014514, 1.988541667008086655, -0.7879004041258289570 ) ) ;
#113549=CARTESIAN_POINT ( 'NONE',  ( -6.480434237652138663, 8.583592582059388576, 1.443375672974078761 ) ) ;
#113551=CARTESIAN_POINT ( 'NONE',  ( 0.000000000000000000, 6.487495393664096888, -3.100011470320000573 ) ) ;
#113555=CARTESIAN_POINT ( 'NONE',  ( 2.693266070609028784, 6.293894182352508970, 0.000000000000000000 ) ) ;
#113557=ORIENTED_EDGE ( 'NONE', *, *, #180876, .F. ) ;
#113558=CARTESIAN_POINT ( 'NONE',  ( 9.999301985278609806, 11.62460605670194447, 1.199719254218452047 ) ) ;
#113565=CARTESIAN_POINT ( 'NONE',  ( -10.14557902172788495, 10.73093036830436553, 1.040834085586084257E-14 ) ) ;
#113566=CARTESIAN_POINT ( 'NONE',  ( 7.202405917357655341, 9.425892875049191488, 1.599625672291281386 ) ) ;
#113568=CARTESIAN_POINT ( 'NONE',  ( 4.378920427089557421, 5.171457255435017331, -1.082531754730548412 ) ) ;
#113573=TOROIDAL_SURFACE ( 'NONE', #210283, 0.8299999999999998490, 0.08000000000000000167 ) ;
#113578=CARTESIAN_POINT ( 'NONE',  ( -1.499999999998706812, 7.854386371690043056, -3.680172642286362983 ) ) ;
#113580=CARTESIAN_POINT ( 'NONE',  ( -6.561783159334145132, 6.757761228752363181, -0.7216878364870278340 ) ) ;
#113581=CARTESIAN_POINT ( 'NONE',  ( 3.974511587100456822, 7.788680618259193444, 1.040834085586084257E-14 ) ) ;
#113584=CARTESIAN_POINT ( 'NONE',  ( -6.835281999583978418, 11.12624609948998966, -0.7998128361456291469 ) ) ;
#113588=CARTESIAN_POINT ( 'NONE',  ( -8.296699936558862731, 11.76690146170562201, 1.199719254218453823 ) ) ;
#113589=CARTESIAN_POINT ( 'NONE',  ( 1.419999999999990603, 6.280000000000042881, 2.873333333333337070 ) ) ;
#113592=CARTESIAN_POINT ( 'NONE',  ( 7.750457368506414646, 12.19395069656619945, 0.7998128361456462443 ) ) ;
#113603=CARTESIAN_POINT ( 'NONE',  ( -8.453672473320708036, 9.821371626084353323, -1.199719254218446718 ) ) ;
#113607=CARTESIAN_POINT ( 'NONE',  ( 7.049876689426101350, 9.247942109129029475, -1.443375672974057666 ) ) ;
#113609=CARTESIAN_POINT ( 'NONE',  ( 4.304877467538922531, 4.981110786005563007, 1.199719254218464037 ) ) ;
#113611=CARTESIAN_POINT ( 'NONE',  ( 5.355634372598031767, 6.206993841907870291, -1.199719254218445830 ) ) ;
#113613=CARTESIAN_POINT ( 'NONE',  ( -7.400052914960538963, 7.527816577075747695, 1.040834085586084257E-14 ) ) ;
#113614=CARTESIAN_POINT ( 'NONE',  ( 3.511198596259283544, 6.271927390929319834, 1.164732466530402855 ) ) ;
#113624=CARTESIAN_POINT ( 'NONE',  ( -0.6823417656250212460, 4.113541667008085767, 1.181850606188767472 ) ) ;
#113626=CARTESIAN_POINT ( 'NONE',  ( 8.483651433849084711, 10.92067931095586886, 1.599625672291281386 ) ) ;
#113628=CARTESIAN_POINT ( 'NONE',  ( -3.307826292054304673, 6.802955074131234348, -0.7216878364870267237 ) ) ;
#113629=CARTESIAN_POINT ( 'NONE',  ( -3.917943204224913156, 7.514758138330285497, -0.7216878364870257245 ) ) ;
#113636=EDGE_LOOP ( 'NONE', ( #148394, #200840, #133982, #53565 ) ) ;
#113638=CARTESIAN_POINT ( 'NONE',  ( 2.683624340501134853, 5.218313266304903664, -1.199719254218446718 ) ) ;
#113646=CARTESIAN_POINT ( 'NONE',  ( 5.168682875307768931, 7.053215992657626110, -1.599625672291256295 ) ) ;
#113648=CARTESIAN_POINT ( 'NONE',  ( -4.909967638851771454, 4.671257834700952571, -0.2941531795261614346 ) ) ;
#113652=CARTESIAN_POINT ( 'NONE',  ( -0.6823417656249969321, 4.030208333674754506, -1.181850606188749264 ) ) ;
#113657=CARTESIAN_POINT ( 'NONE',  ( 5.503720292143644777, 8.508425209887878538, 1.199719254218462483 ) ) ;
#113659=CARTESIAN_POINT ( 'NONE',  ( -3.899941742225307539, 7.701682465904834629, 0.7998128361456341429 ) ) ;
#113660=CARTESIAN_POINT ( 'NONE',  ( -0.7500000000000215383, 2.191666666666689078, 1.299038105676671107 ) ) ;
#113664=CARTESIAN_POINT ( 'NONE',  ( -4.273844736805832767, 6.009238164405336313, 1.599625672291267398 ) ) ;
#113665=CARTESIAN_POINT ( 'NONE',  ( 0.1598595594940413200, 7.033953395470825321, -1.994736385849473104 ) ) ;
#113667=CARTESIAN_POINT ( 'NONE',  ( -0.6823417656250003738, 2.717708333674753618, -1.181850606188749264 ) ) ;
#113669=CARTESIAN_POINT ( 'NONE',  ( -3.795919822146283540, 6.412028311603867436, -1.082531754730549967 ) ) ;
#113674=CARTESIAN_POINT ( 'NONE',  ( -5.287316719649554742, 5.270883715786981227, 0.7216878364870288332 ) ) ;
#113675=CARTESIAN_POINT ( 'NONE',  ( 4.171104814498611368, 8.018039383557042044, 0.7998128361456321445 ) ) ;
#113676=CARTESIAN_POINT ( 'NONE',  ( 1.084637062511527361, 3.057371192708035146, -1.105835307554789759 ) ) ;
#113678=CARTESIAN_POINT ( 'NONE',  ( 0.3903331447352873518, 6.430882250648634724, -3.207843000864786465 ) ) ;
#113679=CARTESIAN_POINT ( 'NONE',  ( 1.364683531249990311, 4.196875000341417028, 1.214306433183764966E-14 ) ) ;
#113684=EDGE_CURVE ( 'NONE', #12264, #147312, #25454, .T. ) ;
#113685=CARTESIAN_POINT ( 'NONE',  ( -1.402160292154681736E-14, -0.2406249996585799189, -1.575800808251665908 ) ) ;
#113689=CARTESIAN_POINT ( 'NONE',  ( -7.974166903131914452, 12.45494515362926435, -0.7998128361456281477 ) ) ;
#113690=CARTESIAN_POINT ( 'NONE',  ( -6.683806541412776525, 7.860491055478785682, -1.082531754730543083 ) ) ;
#113693=VERTEX_POINT ( 'NONE', #144500 ) ;
#113694=CARTESIAN_POINT ( 'NONE',  ( -1.364683531249997417, 4.509375000341424133, 1.214306433183764966E-14 ) ) ;
#113702=CARTESIAN_POINT ( 'NONE',  ( -5.707619481228822345, 7.681975366232176583, -1.443375672974051449 ) ) ;
#113704=CARTESIAN_POINT ( 'NONE',  ( 4.991989969715248776, 4.726297878971393196, -2.500000000000000444 ) ) ;
#113708=CARTESIAN_POINT ( 'NONE',  ( -5.002595493318215070, 7.819816594637776674, 1.082531754730560403 ) ) ;
#113710=CARTESIAN_POINT ( 'NONE',  ( -4.725311769113643479, 5.222111817384738508, 1.090456963845821914 ) ) ;
#113721=CARTESIAN_POINT ( 'NONE',  ( -5.850506979496850057, 6.784345216623154151, -1.199719254218446718 ) ) ;
#113724=CARTESIAN_POINT ( 'NONE',  ( -0.7500000000000215383, 0.4416666666666874130, 1.299038105676659116 ) ) ;
#113725=CARTESIAN_POINT ( 'NONE',  ( 9.408995418203963013, 12.00024729270324286, 1.443375672974076540 ) ) ;
#113726=CARTESIAN_POINT ( 'NONE',  ( 7.806797523370503811, 8.002351953554066810, 1.040834085586084257E-14 ) ) ;
#113729=CARTESIAN_POINT ( 'NONE',  ( 5.681030059326015014, 6.586622143090519188, -1.199719254218445830 ) ) ;
#113735=CARTESIAN_POINT ( 'NONE',  ( -4.012850279964973232, 4.744375417122949301, 1.082531754730560403 ) ) ;
#113738=CARTESIAN_POINT ( 'NONE',  ( 6.509799877575611404, 5.178456542363087500, -2.499999999999995559 ) ) ;
#113739=CARTESIAN_POINT ( 'NONE',  ( 0.1263921868141482663, 7.050106634747087320, 4.033475512996064438 ) ) ;
#113740=SHAPE_REPRESENTATION ( 'positive coil', ( #200407 ), #124605 ) ;
#113743=CARTESIAN_POINT ( 'NONE',  ( 1.364683531249988535, 3.363541667008084879, 0.7879004041258500513 ) ) ;
#113744=CARTESIAN_POINT ( 'NONE',  ( 8.066738210006668908, 12.35501897840907581, 0.7216878364870438212 ) ) ;
#113745=CARTESIAN_POINT ( 'NONE',  ( -5.852315862593199469, 9.979452273000736895, 0.7998128361456481317 ) ) ;
#113747=B_SPLINE_CURVE_WITH_KNOTS ( 'NONE', 3,
 ( #121260, #90830, #187233, #8480, #74567, #140666, #206681, #75632, #42084, #9556, #76684, #30078, #29012, #62564 ),
 .UNSPECIFIED., .F., .F.,
 ( 4, 2, 2, 2, 2, 2, 4 ),
 ( 0.001720018798322440947, 0.002147110083253096074, 0.002360655725718421687, 0.002574201368183750335, 0.003001292653114406763, 0.003214838295579734977, 0.003428383938045063192 ),
 .UNSPECIFIED. ) ;
#113749=CARTESIAN_POINT ( 'NONE',  ( 5.035963992472171746, 7.962709526937818083, 1.199719254218462483 ) ) ;
#113750=CARTESIAN_POINT ( 'NONE',  ( -6.093499974338126179, 9.196501505781426999, -1.199719254218440723 ) ) ;
#113754=CARTESIAN_POINT ( 'NONE',  ( 0.7499999999999885647, 0.8479166673494853423, -1.299038105676652899 ) ) ;
#113757=CARTESIAN_POINT ( 'NONE',  ( 6.290620087060792009, 10.28288116830553101, -0.7216878364870267237 ) ) ;
#113761=CARTESIAN_POINT ( 'NONE',  ( 1.364683531249988757, 0.6968750003414209138, 0.000000000000000000 ) ) ;
#113763=CARTESIAN_POINT ( 'NONE',  ( 6.521108698048765362, 8.631046119188804155, -1.443375672974058777 ) ) ;
#113766=CARTESIAN_POINT ( 'NONE',  ( -3.958617665510283601, 4.681104033592509595, -1.082531754730549967 ) ) ;
#113768=CARTESIAN_POINT ( 'NONE',  ( -1.364683531249997417, 4.759375000341424133, 1.214306433183764966E-14 ) ) ;
#113772=CARTESIAN_POINT ( 'NONE',  ( -4.976004696740268685, 6.814476922186354813, -1.450531527366223372 ) ) ;
#113779=CARTESIAN_POINT ( 'NONE',  ( 6.307567778855705853, 8.381915046796901692, -1.599625672291262513 ) ) ;
#113782=CARTESIAN_POINT ( 'NONE',  ( 4.033714395265605823, 4.664753868353354704, -1.199719254218446718 ) ) ;
#113790=CARTESIAN_POINT ( 'NONE',  ( 4.351804120306567825, 8.020929207092235558, 1.040834085586084257E-14 ) ) ;
#113791=CARTESIAN_POINT ( 'NONE',  ( -1.364683531250014514, 0.05104166700808546175, -0.7879004041258359514 ) ) ;
#113793=CARTESIAN_POINT ( 'NONE',  ( -1.201851678989727383E-14, 3.196875000341421025, -1.575800808251660134 ) ) ;
#113795=FACE_OUTER_BOUND ( 'NONE', #196997, .T. ) ;
#113798=CARTESIAN_POINT ( 'NONE',  ( -0.7500000000000006661, 2.358333333333358262, -1.299038105676652011 ) ) ;
#113799=CARTESIAN_POINT ( 'NONE',  ( 7.396136491454752715, 8.587579647240744407, 1.199719254218462483 ) ) ;
#113800=CARTESIAN_POINT ( 'NONE',  ( -7.015454420067433361, 10.27211502579893754, 1.199719254218453823 ) ) ;
#113805=CARTESIAN_POINT ( 'NONE',  ( 1.364683531249988535, 1.863541667008086211, 0.7879004041258500513 ) ) ;
#113807=CARTESIAN_POINT ( 'NONE',  ( -0.7500000000000215383, 1.941666666666688634, 1.299038105676659116 ) ) ;
#113809=CARTESIAN_POINT ( 'NONE',  ( 4.708759422647839976, 4.387974169377582001, -0.7998128361456211532 ) ) ;
#113817=CARTESIAN_POINT ( 'NONE',  ( -0.7500000000000215383, 0.7229166673494852313, 1.299038105676659116 ) ) ;
#113818=CARTESIAN_POINT ( 'NONE',  ( -5.520141099058386125, 9.591915048876776595, 0.000000000000000000 ) ) ;
#113820=CARTESIAN_POINT ( 'NONE',  ( -4.826339496784927796, 5.693446170079573321, 1.082531754730560403 ) ) ;
#113827=CARTESIAN_POINT ( 'NONE',  ( 6.531277313481192337, 8.642909503859968368, 1.599625672291281386 ) ) ;
#113832=CARTESIAN_POINT ( 'NONE',  ( 6.174848896020108668, 9.291408581077091000, 1.199719254218460707 ) ) ;
#113833=CARTESIAN_POINT ( 'NONE',  ( 8.066738210006668908, 12.35501897840907581, 0.7216878364870438212 ) ) ;
#113834=ORIENTED_EDGE ( 'NONE', *, *, #81943, .F. ) ;
#113836=( BOUNDED_CURVE ( )  B_SPLINE_CURVE ( 2, ( #52413, #87040, #168296, #6832, #118539, #71831, #170415 ),
 .UNSPECIFIED., .F., .T. ) 
 B_SPLINE_CURVE_WITH_KNOTS ( ( 3, 2, 2, 3 ),
 ( 0.05357142857142838110, 0.05952380952380941642, 0.06547619047619046562, 0.07142857142857149400 ),
 .UNSPECIFIED. ) 
 CURVE ( )  GEOMETRIC_REPRESENTATION_ITEM ( )  RATIONAL_B_SPLINE_CURVE ( ( 1.000000000000004219, 0.8660254037844345998, 1.000000000000000000, 0.8660254037844387076, 1.000000000000000000, 0.8660254037844371533, 1.000000000000001554 ) ) 
 REPRESENTATION_ITEM ( '' )  );
#113840=CARTESIAN_POINT ( 'NONE',  ( -5.910464900553636269, 8.982960586366182554, -1.199719254218440723 ) ) ;
#113841=CARTESIAN_POINT ( 'NONE',  ( 5.355634372598031767, 6.206993841907870291, -1.199719254218445830 ) ) ;
#113844=LINE ( 'NONE', #81265, #10964 ) ;
#113845=CARTESIAN_POINT ( 'NONE',  ( 4.589221341884758942, 6.929947237659640713, 1.197292633685101748 ) ) ;
#113846=CARTESIAN_POINT ( 'NONE',  ( 8.595506201384004896, 12.01154575404795466, 1.082531754730546636 ) ) ;
#113856=CARTESIAN_POINT ( 'NONE',  ( -3.145128448690323264, 4.692402494937224056, -1.443375672974059665 ) ) ;
#113857=CARTESIAN_POINT ( 'NONE',  ( 9.110716038703335684, 9.731516254683127087, -0.7216878364870197293 ) ) ;
#113860=CARTESIAN_POINT ( 'NONE',  ( -4.205000198532790279, 8.057583998263570635, 0.7998128361456341429 ) ) ;
#113865=CARTESIAN_POINT ( 'NONE',  ( -5.520141099058386125, 9.591915048876776595, 0.000000000000000000 ) ) ;
#113881=CARTESIAN_POINT ( 'NONE',  ( -6.338600509588822263, 7.353787668397130162, -1.199719254218446718 ) ) ;
#113884=CARTESIAN_POINT ( 'NONE',  ( 3.714570900464274850, 6.317121236308204324, 1.082531754730558626 ) ) ;
#113885=CIRCLE ( 'NONE', #127661, 2.000000000000000000 ) ;
#113889=CARTESIAN_POINT ( 'NONE',  ( -0.4702634422557508409, 7.494255424136805566, 4.464191613400292802 ) ) ;
#113892=EDGE_CURVE ( 'NONE', #148658, #1199, #70415, .T. ) ;
#113893=CARTESIAN_POINT ( 'NONE',  ( 9.890836756369282057, 11.49806328964105617, -1.199719254218440723 ) ) ;
#113897=CARTESIAN_POINT ( 'NONE',  ( -6.855619230004478482, 11.14997286831390788, -0.7998128361456291469 ) ) ;
#113898=CARTESIAN_POINT ( 'NONE',  ( 6.959412922516382771, 7.013736585890911535, 0.7998128361456341429 ) ) ;
#113900=CARTESIAN_POINT ( 'NONE',  ( 4.741601036477289810, 6.554953847355395880, 1.599625672291267175 ) ) ;
#113903=CARTESIAN_POINT ( 'NONE',  ( -1.364683531250012516, 1.842708333674749843, 0.7879004041258379498 ) ) ;
#113906=CARTESIAN_POINT ( 'NONE',  ( 7.700668062882064291, 10.00719871149432549, -1.443375672974057666 ) ) ;
#113913=CARTESIAN_POINT ( 'NONE',  ( 9.910647101465253073, 11.62513837554007168, -1.082531754730537088 ) ) ;
#113919=CARTESIAN_POINT ( 'NONE',  ( 4.907688418466886304, 5.788353245375237321, -1.082531754730548412 ) ) ;
#113921=CARTESIAN_POINT ( 'NONE',  ( -10.32861409551237486, 10.94447128771960287, 1.040834085586084257E-14 ) ) ;
#113933=CARTESIAN_POINT ( 'NONE',  ( -0.7500000000000215383, 0.4729166673494850093, 1.299038105676659116 ) ) ;
#113940=CARTESIAN_POINT ( 'NONE',  ( -1.500000000000015099, -0.3708333333333105331, -0.8660254037844383745 ) ) ;
#113941=CARTESIAN_POINT ( 'NONE',  ( 9.264299036839600987, 9.702770385934682551, -0.7998128361456281477 ) ) ;
#113945=EDGE_CURVE ( 'NONE', #54853, #2091, #1154, .T. ) ;
#113946=CARTESIAN_POINT ( 'NONE',  ( 2.835626683552519012, 6.459981564119914310, 0.000000000000000000 ) ) ;
#113947=CARTESIAN_POINT ( 'NONE',  ( -7.388830529767770550, 7.722649827591604677, 1.040834085586084257E-14 ) ) ;
#113951=CARTESIAN_POINT ( 'NONE',  ( -7.542413527904030524, 7.693903958843159252, 1.040834085586084257E-14 ) ) ;
#113954=CARTESIAN_POINT ( 'NONE',  ( -0.7500000000000006661, 1.389583334016154748, -1.299038105676652011 ) ) ;
#113961=CARTESIAN_POINT ( 'NONE',  ( -10.50487009249003378, 11.15010328419353947, 0.7998128361456462443 ) ) ;
#113964=CARTESIAN_POINT ( 'NONE',  ( 4.128212683569056018, 7.424016784313646866, 0.7064205832574363964 ) ) ;
#113967=EDGE_CURVE ( 'NONE', #126795, #196229, #19931, .T. ) ;
#113970=CARTESIAN_POINT ( 'NONE',  ( -9.829825065107822724, 11.42688298316931572, 1.199719254218462483 ) ) ;
#113971=CARTESIAN_POINT ( 'NONE',  ( 8.555358625423188812, 9.940005470203933768, 1.199719254218462483 ) ) ;
#113978=FACE_OUTER_BOUND ( 'NONE', #158938, .T. ) ;
#113979=CARTESIAN_POINT ( 'NONE',  ( -9.982881178363895103, 10.54111621771303753, 1.040834085586084257E-14 ) ) ;
#113984=CARTESIAN_POINT ( 'NONE',  ( 4.111146893441827821, 5.819424013814004759, 1.599625672291267398 ) ) ;
#113991=CARTESIAN_POINT ( 'NONE',  ( -8.123306592882240551, 12.62894145833798376, 0.000000000000000000 ) ) ;
#114003=CARTESIAN_POINT ( 'NONE',  ( 5.933664784275179294, 10.07435934829639912, -0.7998128361456291469 ) ) ;
#114005=CARTESIAN_POINT ( 'NONE',  ( -4.029797971759847997, 5.724516938518342535, -1.599625672291256295 ) ) ;
#114013=CARTESIAN_POINT ( 'NONE',  ( 1.499999999999989120, 0.3062500006828158816, 0.000000000000000000 ) ) ;
#114016=CARTESIAN_POINT ( 'NONE',  ( -1.533805080507057772, 8.737074443703342297, -2.508413646267452890 ) ) ;
#114017=CARTESIAN_POINT ( 'NONE',  ( 2.920892028740289081, 5.495125569250587816, 1.199719254218452047 ) ) ;
#114019=CARTESIAN_POINT ( 'NONE',  ( -2.761056838677368397, 6.372983411765559048, 0.7998128361456341429 ) ) ;
#114025=CARTESIAN_POINT ( 'NONE',  ( 4.039966587192257208, 6.696749537490852333, 1.082531754730558626 ) ) ;
#114030=CARTESIAN_POINT ( 'NONE',  ( -0.6823417656249969321, 5.530208333674756283, -1.181850606188749264 ) ) ;
#114032=CARTESIAN_POINT ( 'NONE',  ( 3.294268137996273715, 5.826768013428865522, -1.082531754730543971 ) ) ;
#114041=CARTESIAN_POINT ( 'NONE',  ( -5.511734814698080243, 6.408623376260899285, 1.272316098655206229 ) ) ;
#114043=CARTESIAN_POINT ( 'NONE',  ( 0.6823417656249864960, -0.8239583329919114574, -1.181850606188749264 ) ) ;
#114051=CARTESIAN_POINT ( 'NONE',  ( 1.499999999999989120, 5.045833333333354709, -0.8660254037844323793 ) ) ;
#114060=CARTESIAN_POINT ( 'NONE',  ( -1.364683531250014514, -1.011458332991911568, -0.7879004041258359514 ) ) ;
#114062=CARTESIAN_POINT ( 'NONE',  ( 5.126954644262057492, 9.133197518281081173, 0.7998128361456462443 ) ) ;
#114063=CARTESIAN_POINT ( 'NONE',  ( -8.341290820905609138, 10.75459192918846618, 1.599625672291269396 ) ) ;
#114064=CARTESIAN_POINT ( 'NONE',  ( 10.38962578677386084, 11.01565159419135043, 0.000000000000000000 ) ) ;
#114070=CARTESIAN_POINT ( 'NONE',  ( -1.500000000000011324, 5.629166666666693963, -0.8660254037844313801 ) ) ;
#114078=CARTESIAN_POINT ( 'NONE',  ( 8.609064354997688184, 9.146255957026539818, 1.040834085586084257E-14 ) ) ;
#114083=CARTESIAN_POINT ( 'NONE',  ( -0.7499999999999972244, 4.389583334016150751, -1.299038105676652899 ) ) ;
#114085=CARTESIAN_POINT ( 'NONE',  ( -4.776550190716183586, 4.467063398790632966, 1.214306433183764966E-14 ) ) ;
#114087=CARTESIAN_POINT ( 'NONE',  ( 4.812781342726850653, 8.558735966582574406, 0.7216878364870438212 ) ) ;
#114094=CARTESIAN_POINT ( 'NONE',  ( 3.602716132929354664, 5.226254793216122074, 1.599625672291267398 ) ) ;
#114101=CARTESIAN_POINT ( 'NONE',  ( 7.716561984472250835, 12.15440608185967086, 1.040834085586084257E-14 ) ) ;
#114106=CARTESIAN_POINT ( 'NONE',  ( 2.277964293776285842, 5.617064315955532905, -0.5754907707892011892 ) ) ;
#114109=CARTESIAN_POINT ( 'NONE',  ( 8.727698198895078363, 11.20540053684285553, -1.599625672291257406 ) ) ;
#114114=CARTESIAN_POINT ( 'NONE',  ( 1.364683531249988757, 0.1343750003414204142, 0.000000000000000000 ) ) ;
#114115=CARTESIAN_POINT ( 'NONE',  ( 5.504247177468179153, 7.444707678511436555, 1.443375672974062551 ) ) ;
#114116=CARTESIAN_POINT ( 'NONE',  ( -9.490344339885981029, 10.17441593939621924, -0.7216878364870267237 ) ) ;
#114117=B_SPLINE_CURVE_WITH_KNOTS ( 'NONE', 3,
 ( #10116, #55671, #72975, #76191, #107699, #202968, #54608, #25302, #121827, #105519 ),
 .UNSPECIFIED., .F., .F.,
 ( 4, 3, 3, 4 ),
 ( 1.053630326498184013E-17, 4.407003120538926870E-05, 8.609159171476572650E-05, 0.0001625397904729946610 ),
 .UNSPECIFIED. ) ;
#114122=CARTESIAN_POINT ( 'NONE',  ( -2.767835915484202047, 6.380892334706859792, -0.7998128361456281477 ) ) ;
#114125=ORIENTED_EDGE ( 'NONE', *, *, #186592, .F. ) ;
#114135=CARTESIAN_POINT ( 'NONE',  ( 5.506841003474272966, 6.417672382999444203, -1.246111810019270738 ) ) ;
#114136=DIRECTION ( 'NONE',  ( -1.000000000000000000, 5.578564026256490882E-16, -1.264049978315544409E-61 ) ) ;
#114143=CARTESIAN_POINT ( 'NONE',  ( -7.049876689426103127, 10.20831132343037062, -1.082531754730537976 ) ) ;
#114147=CARTESIAN_POINT ( 'NONE',  ( 6.693975156845185737, 8.832723654451292816, 1.599625672291281386 ) ) ;
#114148=CARTESIAN_POINT ( 'NONE',  ( -3.249150368769345043, 6.942425863539538611, 0.7998128361456341429 ) ) ;
#114149=CARTESIAN_POINT ( 'NONE',  ( 2.517010073631369860, 6.088262185878572375, -0.7998128361456281477 ) ) ;
#114151=CARTESIAN_POINT ( 'NONE',  ( -4.062639585589296942, 7.891496616496157301, 0.7998128361456341429 ) ) ;
#114154=AXIS2_PLACEMENT_3D ( 'NONE', #176613, #63917, #130073 ) ;
#114155=CARTESIAN_POINT ( 'NONE',  ( -5.311043488251275591, 7.219303374425030562, -1.599625672291256295 ) ) ;
#114158=CARTESIAN_POINT ( 'NONE',  ( 7.377608144130607393, 11.75895993479440982, -0.7998128361456291469 ) ) ;
#114161=CARTESIAN_POINT ( 'NONE',  ( 4.849937260509308956, 6.926242028416789154, 1.417063245053858722 ) ) ;
#114162=CARTESIAN_POINT ( 'NONE',  ( 4.609409038966229666, 6.400729850259146758, -1.443375672974051449 ) ) ;
#114164=DIRECTION ( 'NONE',  ( 1.000000000000000000, -5.782411586589355667E-16, 0.000000000000000000 ) ) ;
#114169=CARTESIAN_POINT ( 'NONE',  ( 8.066738210006692000, 8.513542121203711233, 0.7216878364870458196 ) ) ;
#114172=CARTESIAN_POINT ( 'NONE',  ( -7.960608749518247151, 12.43912730774665576, 0.000000000000000000 ) ) ;
#114173=CARTESIAN_POINT ( 'NONE',  ( -5.865874016206865882, 9.995270118883347266, 0.000000000000000000 ) ) ;
#114177=CARTESIAN_POINT ( 'NONE',  ( -1.420000000000001039, 6.280000000000042881, -2.873333333333329520 ) ) ;
#114181=CARTESIAN_POINT ( 'NONE',  ( 10.06423010004587759, 10.63602329300870153, 0.000000000000000000 ) ) ;
#114184=CARTESIAN_POINT ( 'NONE',  ( 4.359110081993588182, 5.044382169536003602, -1.199719254218452047 ) ) ;
#114187=CARTESIAN_POINT ( 'NONE',  ( -0.7499999999999972244, 5.139583334016151639, -1.299038105676652899 ) ) ;
#114193=CARTESIAN_POINT ( 'NONE',  ( -1.201851678989727383E-14, 3.337500000000019007, -1.732050807568863648 ) ) ;
#114194=CARTESIAN_POINT ( 'NONE',  ( 4.137209430464448445, 7.978494768850520558, 1.040834085586084257E-14 ) ) ;
#114199=CARTESIAN_POINT ( 'NONE',  ( 7.537970219518073556, 9.817384560903001045, -1.443375672974057666 ) ) ;
#114200=CARTESIAN_POINT ( 'NONE',  ( -9.937763408692596556, 11.65677406730528887, -1.082531754730537976 ) ) ;
#114203=CARTESIAN_POINT ( 'NONE',  ( -3.189213936345670852, 2.817530495244580102, -2.450448857954567572 ) ) ;
#114205=CARTESIAN_POINT ( 'NONE',  ( -4.172158584703340445, 5.890604320285754980, -1.599625672291256295 ) ) ;
#114206=CARTESIAN_POINT ( 'NONE',  ( -1.500000000000011324, 4.660416667349484676, -0.8660254037844313801 ) ) ;
#114207=CARTESIAN_POINT ( 'NONE',  ( -1.402160292154681736E-14, -0.4281249996585808071, 1.575800808251672791 ) ) ;
#114211=CARTESIAN_POINT ( 'NONE',  ( 4.090809663021327758, 5.795697244990093644, 1.599625672291267398 ) ) ;
#114213=CARTESIAN_POINT ( 'NONE',  ( -0.6823417656250212460, 4.863541667008086655, 1.181850606188767472 ) ) ;
#114215=CARTESIAN_POINT ( 'NONE',  ( 1.500000000000007105, 10.64264068711930733, 1.214306433183764966E-14 ) ) ;
#114221=CARTESIAN_POINT ( 'NONE',  ( -6.256197817702116026, 9.386315656372753224, -1.199719254218440723 ) ) ;
#114224=CARTESIAN_POINT ( 'NONE',  ( 6.179819089730593795, 6.104210447640811665, 1.040834085586084257E-14 ) ) ;
#114227=CARTESIAN_POINT ( 'NONE',  ( 1.364683531249988757, 0.1343750003414204142, 0.000000000000000000 ) ) ;
#114231=CARTESIAN_POINT ( 'NONE',  ( 9.236128959407556849, 11.79856975744075598, -1.599625672291262513 ) ) ;
#114234=CARTESIAN_POINT ( 'NONE',  ( -5.717788096661253761, 7.693838750903348789, 1.599625672291269396 ) ) ;
#114238=CARTESIAN_POINT ( 'NONE',  ( 8.320953590485093088, 10.73086516036454618, 1.599625672291281386 ) ) ;
#114240=CARTESIAN_POINT ( 'NONE',  ( 7.065770611016287006, 11.39514947949436774, 1.040834085586084257E-14 ) ) ;
#114241=CARTESIAN_POINT ( 'NONE',  ( 4.894543267554960053, 4.887125941896303338, -0.6895117023006970269 ) ) ;
#114242=CARTESIAN_POINT ( 'NONE',  ( -8.324343129110692630, 12.65555805069709550, 0.7216878364870338292 ) ) ;
#114244=CARTESIAN_POINT ( 'NONE',  ( -5.533699252672048985, 9.607732894759390518, -0.7998128361456231517 ) ) ;
#114247=CARTESIAN_POINT ( 'NONE',  ( -5.337630915675663168, 6.534101986612459001, 1.368282111488251074 ) ) ;
#114248=CARTESIAN_POINT ( 'NONE',  ( -0.6823417656250003738, 0.2177083336747515085, -1.181850606188749264 ) ) ;
#114253=CARTESIAN_POINT ( 'NONE',  ( 6.480434237652115570, 10.50433101066207442, 0.7216878364870438212 ) ) ;
#114256=CARTESIAN_POINT ( 'NONE',  ( 4.330940004561544043, 7.140181541042074365, -1.199719254218452047 ) ) ;
#114272=CARTESIAN_POINT ( 'NONE',  ( -4.911752498546916534, 4.707425932596564166, -0.3822207396134598145 ) ) ;
#114276=CARTESIAN_POINT ( 'NONE',  ( -5.111587607552082524, 5.922272616020886282, 1.199719254218450271 ) ) ;
#114277=CARTESIAN_POINT ( 'NONE',  ( -6.886651960737580680, 10.12184548991413457, -1.199719254218440723 ) ) ;
#114284=CARTESIAN_POINT ( 'NONE',  ( 0.7499999999999902300, 3.014583334016149418, 1.299038105676669330 ) ) ;
#114285=CARTESIAN_POINT ( 'NONE',  ( 8.565000355531088516, 11.01558638625153286, -1.599625672291257406 ) ) ;
#114288=CARTESIAN_POINT ( 'NONE',  ( -9.338868881714763148, 9.789768538289042255, -0.7998128361456291469 ) ) ;
#114290=CARTESIAN_POINT ( 'NONE',  ( 0.6823417656249899377, 3.092708333674754062, 1.181850606188765695 ) ) ;
#114295=CARTESIAN_POINT ( 'NONE',  ( -8.337901282724359930, 12.67137589657970409, 1.040834085586084257E-14 ) ) ;
#114299=CARTESIAN_POINT ( 'NONE',  ( 0.6823417656249882723, 1.988541667008083991, -1.181850606188749264 ) ) ;
#114305=CARTESIAN_POINT ( 'NONE',  ( 1.364683531249988535, 3.363541667008084879, 0.7879004041258500513 ) ) ;
#114307=CARTESIAN_POINT ( 'NONE',  ( -5.331380718671772101, 7.243030143248949670, -1.599625672291256295 ) ) ;
#114308=CARTESIAN_POINT ( 'NONE',  ( 7.233438648090761980, 8.397765496649418182, 1.199719254218462483 ) ) ;
#114311=CARTESIAN_POINT ( 'NONE',  ( -1.364683531250012516, 3.342708333674756727, 0.7879004041258379498 ) ) ;
#114314=CARTESIAN_POINT ( 'NONE',  ( -1.364683531250014514, -1.219791666325248602, 0.7879004041258379498 ) ) ;
#114315=CARTESIAN_POINT ( 'NONE',  ( -5.504247177468192476, 7.444707678511436555, 1.443375672974064550 ) ) ;
#114316=B_SPLINE_SURFACE_WITH_KNOTS ( 'NONE', 1, 3, ( 
 ( #107049, #190356, #187163, #55044, #138440, #59301, #121194, #191421, #38792, #189303, #204458, #26795, #170916, #56112, #42018, #188227, #123339, #39867, #108127, #105976, #174154, #23590, #89698, #155748, #205540, #73410, #139513, #40943, #143805, #145926, #142728, #192488, #60364, #28945, #93968, #162154, #12669, #211938, #128665, #44140, #63573, #110261, #129729, #126527, #45213, #76615, #27872, #112391, #31092, #13741, #79814, #78744, #113462, #178403, #193570, #144868, #195713, #210875, #47348, #61438, #95029, #62500, #96099, #127604, #161079, #46275, #194633, #30015, #179467, #176270, #10541, #160009, #97164, #92900, #163219, #11610, #158946, #77684, #208737, #209802, #177331, #111328, #158572, #189988, #56795, #58930, #175901, #75186, #73027, #141298, #71948, #23199, #171605, #76245, #138058, #205152, #59995, #40561, #42711, #55723, #207307, #125088, #191046, #89314, #122964, #155361, #6946, #204071, #105573, #172692, #142354, #41639, #157515, #91454, #26420, #108819, #208364, #126148, #74118, #159636, #121877, #174843, #187848, #92532, #106668, #188923, #39474, #90375, #57860, #206233, #192111, #109888, #43775, #107753, #9110, #24270, #10171, #139125, #156444, #140214, #8028, #124022, #25354, #173779, #27492, #93592, #95730, #79447, #197452, #162847, #12296, #179093, #30715, #77312, #176955, #115213, #78376, #14425, #63197, #45907, #61066, #96798, #114161, #127225, #144496, #196403, #194261, #49093, #143425, #62139, #211562, #147662, #210504, #161782, #213679, #11233, #146612, #181203, #81579, #13373, #180154, #128299, #80515, #212630, #64271, #130416, #48048, #31780, #193194, #97852, #163915, #112025, #131451, #15491, #178027, #110948, #98908, #32831, #94659, #44842, #65302, #209421, #29645, #28571, #160702, #145564, #129361, #195339, #46971, #113087, #133568, #34944, #37084, #3494, #186536, #151921, #101016, #184395, #152980, #70629, #33887, #69564, #68502, #103163, #289, #199574, #183339, #18694, #150863, #135674, #36015, #149789, #66360, #1363, #169224, #99965, #136740, #117342, #84776, #50149, #168164, #19762, #167107, #2425, #134630, #52282, #20816, #201699 ),
 ( #200634, #83701, #53342, #16552, #85844, #86912, #119476, #51218, #118409, #102094, #202766, #182262, #185464, #4555, #132506, #166030, #198504, #54416, #120557, #38165, #17615, #164960, #82635, #148719, #116273, #67425, #82579, #102043, #135621, #18641, #104184, #148667, #119422, #233, #201641, #51162, #133513, #198452, #34886, #2371, #150807, #70570, #54365, #4501, #200579, #168112, #117285, #19711, #33833, #16498, #84720, #100959, #17559, #184342, #134579, #68449, #149731, #53289, #66305, #85790, #103111, #185409, #183281, #52226, #118354, #120505, #99913, #167049, #169170, #132454, #165973, #50098, #35965, #1309, #37027, #151871, #20764, #3445, #83644, #86858, #67369, #152923, #182207, #69512, #116219, #199517, #136689, #186478, #202714, #38113, #205928, #208055, #157201, #106359, #123718, #42399, #189680, #158273, #188617, #73803, #173464, #58622, #40249, #139897, #91145, #57561, #41331, #107440, #203778, #153997, #171302, #92221, #21818, #75938, #55422, #25044, #105261, #108508, #9861, #87923, #8798, #174531, #74877, #155062, #140983, #59682, #206992, #22893, #124777, #170234, #121576, #187547, #26110, #5566, #89010, #142039, #138822, #190736, #71645, #125842, #191799, #43462, #39177, #6650, #72728, #204843, #172383, #137758, #56496, #122654, #23972, #90074, #156137, #7719, #15179, #192869, #14107, #13052, #196096, #159319, #144192, #80195, #64995, #46653, #47728, #129045, #94348, #10915, #160390, #113845, #44525, #81266, #61824, #177717, #209110, #112776, #178787, #127990, #193945, #45591, #211254, #179840, #146299, #30401, #79130, #197138, #76992, #111708, #145247, #210184, #29326, #60748, #143119, #195021, #11991, #109583, #78066, #95420, #62877, #93281, #163596, #212312, #161472, #31463, #126910, #63947, #97538, #96486, #110642, #162534, #130102, #147345, #213372, #176644, #131149, #175587, #27177, #28256, #152657, #115954, #51970, #100706, #83381, #98588, #2107, #151605, #164650, #49829, #19439, #17302, #20505, #114892, #99646, #34635, #185134, #181944, #133245, #36760, #48777, #184080, #4239, #119151, #50897, #3173, #165713, #134312, #68181, #118095 ) ),
 .UNSPECIFIED., .F., .T., .F.,
 ( 2, 2 ),
 ( 4, 2, 2, 2, 2, 2, 2, 2, 2, 2, 2, 2, 2, 2, 2, 2, 2, 2, 2, 2, 2, 2, 2, 2, 2, 2, 2, 2, 2, 2, 2, 2, 2, 2, 2, 2, 2, 2, 2, 2, 2, 2, 2, 2, 2, 2, 2, 2, 2, 2, 2, 2, 2, 2, 2, 2, 2, 2, 2, 2, 2, 2, 2, 2, 2, 2, 2, 2, 2, 2, 2, 2, 2, 2, 2, 2, 2, 2, 2, 2, 2, 2, 2, 2, 2, 2, 2, 2, 2, 2, 2, 2, 2, 2, 2, 2, 2, 2, 2, 2, 2, 2, 2, 2, 2, 2, 2, 2, 2, 2, 2, 2, 2, 2, 2, 2, 2, 2, 2, 2, 2, 2, 2, 4 ),
 ( 0.000000000000000000, 1.000000000000000000 ),
 ( 0.0003308050673979778117, 0.0003990699536394003003, 0.0004673348398808227890, 0.0005355997261222453319, 0.0006038646123636677663, 0.0007403943848465126352, 0.0008769241573293576125, 0.0009110566004500689381, 0.0009451890435707801554, 0.001013453929812202590, 0.001081718816053625024, 0.001149983702295047459, 0.001286513474777892328, 0.001354778361019314762, 0.001388910804140025979, 0.001423043247260737413, 0.001491308133502160065, 0.001559573019743582499, 0.001696102792226427368, 0.001764367678467849802, 0.001832632564709272237, 0.001900897450950694671, 0.001969162337192117106, 0.002037427223433539540, 0.002105692109674961975, 0.002173956995916384409, 0.002242221882157806843, 0.002310486768399229278, 0.002344619211519940495, 0.002378751654640651712, 0.002515281427123497015, 0.002651811199606342317, 0.002720076085847764752, 0.002788340972089187186, 0.002856605858330609621, 0.002924870744572032055, 0.003061400517054876924, 0.003129665403296299359, 0.003197930289537721793, 0.003266195175779144227, 0.003334460062020566662, 0.003402724948261989096, 0.003470989834503411531, 0.003607519606986256400, 0.003675784493227678834, 0.003709916936348390051, 0.003744049379469101269, 0.003812314265710523703, 0.003880579151951946137, 0.004017108924434791006, 0.004085373810676213441, 0.004153638696917635875, 0.004187771140038347092, 0.004221903583159058310, 0.004290168469400480744, 0.004358433355641903179, 0.004426698241883325613, 0.004494963128124748047, 0.004529095571245459265, 0.004563228014366170482, 0.004631492900607592916, 0.004699757786849016218, 0.004836287559331861954, 0.004904552445573284389, 0.004972817331814706823, 0.005041082218056129258, 0.005109347104297551692, 0.005177611990538974127, 0.005245876876780396561, 0.005314141763021818995, 0.005382406649263241430, 0.005450671535504663864, 0.005518936421746086299, 0.005587201307987508733, 0.005655466194228931168, 0.005791995966711776037, 0.005860260852953198471, 0.005928525739194620905, 0.005962658182315332123, 0.005996790625436043340, 0.006065055511677465774, 0.006133320397918888209, 0.006201585284160310643, 0.006269850170401733078, 0.006338115056643155512, 0.006406379942884577947, 0.006440512386005289164, 0.006474644829126000381, 0.006611174601608845250, 0.006747704374091690119, 0.006815969260333112553, 0.006850101703453823770, 0.006884234146574534988, 0.006952499032815957422, 0.007020763919057379857, 0.007157293691540224725, 0.007225558577781647160, 0.007293823464023069594, 0.007327955907143780812, 0.007362088350264492029, 0.007430353236505915331, 0.007498618122747338632, 0.007566883008988761067, 0.007635147895230183501, 0.007703412781471605936, 0.007771677667713028370, 0.007805810110833739587, 0.007839942553954450805, 0.007908207440195873239, 0.007976472326437295673, 0.008113002098920140542, 0.008181266985161562977, 0.008249531871402985411, 0.008317796757644407846, 0.008386061643885830280, 0.008454326530127252715, 0.008522591416368675149, 0.008590856302610097583, 0.008659121188851520018, 0.008727386075092942452, 0.008761518518213653670, 0.008795650961334364887, 0.008932180733817209756, 0.009068710506300054625 ),
 .UNSPECIFIED. ) ;
#114319=CARTESIAN_POINT ( 'NONE',  ( 5.016153647376205171, 6.875265226737464985, 1.443375672974062551 ) ) ;
#114322=CARTESIAN_POINT ( 'NONE',  ( -7.771848369131641121, 10.09024240211882351, -1.599625672291263179 ) ) ;
#114323=CARTESIAN_POINT ( 'NONE',  ( -3.277320446201389181, 4.846626492033466072, 1.599625672291267398 ) ) ;
#114325=CARTESIAN_POINT ( 'NONE',  ( 0.6823417656249917140, 5.592708333674749177, 1.181850606188765695 ) ) ;
#114331=CARTESIAN_POINT ( 'NONE',  ( -6.195713011320795438, 8.251417818006149929, -1.443375672974058777 ) ) ;
#114333=CARTESIAN_POINT ( 'NONE',  ( -1.364683531250014514, -1.157291666325248158, 0.7879004041258379498 ) ) ;
#114336=CARTESIAN_POINT ( 'NONE',  ( 6.616015773788773480, 10.66250946948817813, -0.7216878364870267237 ) ) ;
#114345=CARTESIAN_POINT ( 'NONE',  ( 9.720832950873944611, 10.44331931888218001, -0.7216878364870257245 ) ) ;
#114352=CARTESIAN_POINT ( 'NONE',  ( 5.829115978871627135, 8.888053511070525659, 1.199719254218462483 ) ) ;
#114353=CARTESIAN_POINT ( 'NONE',  ( -5.264643720808155791, 5.036505850564608089, 0.000000000000000000 ) ) ;
#114358=CARTESIAN_POINT ( 'NONE',  ( 6.629573926958101993, 6.836850457647000390, -0.7216878364870257245 ) ) ;
#114359=CARTESIAN_POINT ( 'NONE',  ( 0.6823417656249882723, 0.2385416670080825474, -1.181850606188749264 ) ) ;
#114361=CARTESIAN_POINT ( 'NONE',  ( -8.286004436246233951, 12.81875560892930466, 1.040834085586084257E-14 ) ) ;
#114369=EDGE_LOOP ( 'NONE', ( #121112, #158257, #6479 ) ) ;
#114374=CARTESIAN_POINT ( 'NONE',  ( -4.233785845893567767, 7.337832232212887718, -0.8726355574809127047 ) ) ;
#114378=CARTESIAN_POINT ( 'NONE',  ( 5.798083248138522272, 9.916180889470295412, 0.7998128361456462443 ) ) ;
#114379=CARTESIAN_POINT ( 'NONE',  ( 5.849453209292126310, 8.911780279894442103, 1.199719254218462483 ) ) ;
#114388=CARTESIAN_POINT ( 'NONE',  ( 10.58621901417202515, 11.24501035948919991, -0.7998128361456281477 ) ) ;
#114390=CARTESIAN_POINT ( 'NONE',  ( -3.440018289565379028, 5.036440642624797626, 1.599625672291267398 ) ) ;
#114395=CARTESIAN_POINT ( 'NONE',  ( -0.5601741628962252362, 7.746630099212525877, 1.919951735362938505 ) ) ;
#114399=CARTESIAN_POINT ( 'NONE',  ( -9.978437869977950569, 11.70422760547153906, -1.082531754730539753 ) ) ;
#114403=CARTESIAN_POINT ( 'NONE',  ( 5.438792177376376991, 9.497007973581119700, 1.040834085586084257E-14 ) ) ;
#114404=CARTESIAN_POINT ( 'NONE',  ( 1.364683531249988535, 5.405208333674750953, -0.7879004041258300672 ) ) ;
#114409=CARTESIAN_POINT ( 'NONE',  ( 5.300874872818843286, 5.286701561151180506, 0.7216878364870317197 ) ) ;
#114416=CARTESIAN_POINT ( 'NONE',  ( -6.235860587281615075, 9.362588887548838557, -1.199719254218440723 ) ) ;
#114417=CARTESIAN_POINT ( 'NONE',  ( -5.596818484342970912, 5.424043074688562172, -0.7998128361456221525 ) ) ;
#114418=DIRECTION ( 'NONE',  ( -0.7071067811865497932, -0.7071067811865452413, 8.659560562354947649E-17 ) ) ;
#114426=CARTESIAN_POINT ( 'NONE',  ( 5.503720292143644777, 8.508425209887878538, 1.199719254218462483 ) ) ;
#114433=CARTESIAN_POINT ( 'NONE',  ( -1.257518954445029147, 2.966479010054028365, 0.7750000000000170086 ) ) ;
#114436=ORIENTED_EDGE ( 'NONE', *, *, #24579, .F. ) ;
#114438=CARTESIAN_POINT ( 'NONE',  ( -1.364683531250014514, -0.4489583329919089039, -0.7879004041258359514 ) ) ;
#114439=CARTESIAN_POINT ( 'NONE',  ( 3.195971524519376494, 4.751719416737803847, -1.599625672291262513 ) ) ;
#114440=CARTESIAN_POINT ( 'NONE',  ( 3.520313441042647540, 7.258782781191745137, 0.7998128361456321445 ) ) ;
#114442=CARTESIAN_POINT ( 'NONE',  ( -7.212574532790102744, 8.477387045419011002, -1.082531754730550855 ) ) ;
#114444=EDGE_CURVE ( 'NONE', #93128, #108753, #38418, .T. ) ;
#114445=CARTESIAN_POINT ( 'NONE',  ( 4.311129659465574804, 7.013106455143060636, -1.082531754730548412 ) ) ;
#114446=CARTESIAN_POINT ( 'NONE',  ( -7.714226216051410567, 9.062647342557177410, 1.082531754730558626 ) ) ;
#114449=ORIENTED_EDGE ( 'NONE', *, *, #76301, .F. ) ;
#114451=CARTESIAN_POINT ( 'NONE',  ( 7.287671262545424966, 8.461036880179857889, -1.199719254218451159 ) ) ;
#114455=CARTESIAN_POINT ( 'NONE',  ( -5.585596099150257565, 5.618876325204375632, -0.7216878364869792062 ) ) ;
#114456=CARTESIAN_POINT ( 'NONE',  ( 0.6823417656249899377, 3.926041667008085767, -1.181850606188754593 ) ) ;
#114461=CARTESIAN_POINT ( 'NONE',  ( 6.272618624616828953, 10.46980549536166016, 1.040834085586084257E-14 ) ) ;
#114464=CARTESIAN_POINT ( 'NONE',  ( -7.340850106795412167, 10.65174332698158643, 1.199719254218453823 ) ) ;
#114470=CARTESIAN_POINT ( 'NONE',  ( 7.553864141108259211, 11.96459193126834464, 1.040834085586084257E-14 ) ) ;
#114473=CARTESIAN_POINT ( 'NONE',  ( -9.365985188942097750, 9.821404230054264772, 0.7998128361456462443 ) ) ;
#114478=CARTESIAN_POINT ( 'NONE',  ( 5.160031065370225711, 6.461479299918838848, -1.191482946479218485 ) ) ;
#114479=CARTESIAN_POINT ( 'NONE',  ( -8.622622508611375025, 12.04318144581317895, 1.082531754730560403 ) ) ;
#114484=CARTESIAN_POINT ( 'NONE',  ( 5.276094334012385367, 9.307193822989793475, 1.040834085586084257E-14 ) ) ;
#114486=CARTESIAN_POINT ( 'NONE',  ( 4.961394147597008697, 7.875711374583454827, -1.199719254218452047 ) ) ;
#114487=CARTESIAN_POINT ( 'NONE',  ( -4.088066877127150001, 7.522549914775793489, 0.5433784229755319606 ) ) ;
#114488=CARTESIAN_POINT ( 'NONE',  ( 2.846322183865124700, 5.408127416896231665, -1.199719254218446718 ) ) ;
#114490=CARTESIAN_POINT ( 'NONE',  ( -7.863365906246074566, 8.276274433482971205, -0.7216878364870278340 ) ) ;
#114491=( BOUNDED_CURVE ( )  B_SPLINE_CURVE ( 1, ( #124547, #40016 ),
 .UNSPECIFIED., .F., .T. ) 
 B_SPLINE_CURVE_WITH_KNOTS ( ( 2, 2 ),
 ( 0.000000000000000000, 4.605265433281100981E-05 ),
 .UNSPECIFIED. ) 
 CURVE ( )  GEOMETRIC_REPRESENTATION_ITEM ( )  RATIONAL_B_SPLINE_CURVE ( ( 0.9345202395942924234, 0.9345202395942924234 ) ) 
 REPRESENTATION_ITEM ( '' )  );
#114497=CARTESIAN_POINT ( 'NONE',  ( -4.037324417950741484, 7.593329901778307800, 0.3124507474575183297 ) ) ;
#114499=CARTESIAN_POINT ( 'NONE',  ( 1.364683531249986537, -0.5322916663252452718, -0.7879004041258309554 ) ) ;
#114502=CARTESIAN_POINT ( 'NONE',  ( 4.907688418466886304, 5.788353245375237321, -1.082531754730548412 ) ) ;
#114504=AXIS2_PLACEMENT_3D ( 'NONE', #21352, #151398, #5096 ) ;
#114507=CARTESIAN_POINT ( 'NONE',  ( -9.341204649691320583, 10.96078884847042545, 1.082531754730558626 ) ) ;
#114516=EDGE_CURVE ( 'NONE', #97523, #207276, #198457, .T. ) ;
#114520=CARTESIAN_POINT ( 'NONE',  ( -8.310784975052682100, 10.71900177569337487, -1.443375672974058777 ) ) ;
#114524=CARTESIAN_POINT ( 'NONE',  ( -0.6823417656249969321, 5.280208333674756283, -1.181850606188749264 ) ) ;
#114525=CARTESIAN_POINT ( 'NONE',  ( 1.499999999999990896, 3.556250000682818602, 1.214306433183764966E-14 ) ) ;
#114529=CARTESIAN_POINT ( 'NONE',  ( -7.694415870955439551, 8.935572256658169010, 1.199719254218462483 ) ) ;
#114533=CARTESIAN_POINT ( 'NONE',  ( 4.937140493670735708, 8.911747675924535983, -0.7998128361456281477 ) ) ;
#114536=CARTESIAN_POINT ( 'NONE',  ( -4.288456660624211381, 3.897620947016656956, 1.214306433183764966E-14 ) ) ;
#114539=CARTESIAN_POINT ( 'NONE',  ( 8.457588896826466751, 8.761608555919362828, 1.040834085586084257E-14 ) ) ;
#114543=DIRECTION ( 'NONE',  ( 0.000000000000000000, 8.546850786086437571E-32, 1.000000000000000000 ) ) ;
#114548=CARTESIAN_POINT ( 'NONE',  ( -6.887178846062123938, 8.097758744236356776, -1.082531754730544860 ) ) ;
#114551=CARTESIAN_POINT ( 'NONE',  ( 1.364683531249990311, 4.946875000341417916, 1.214306433183764966E-14 ) ) ;
#114554=LINE ( 'NONE', #113489, #43604 ) ;
#114557=CARTESIAN_POINT ( 'NONE',  ( -4.243338890952911058, 5.013278796608906518, -1.082531754730543971 ) ) ;
#114559=CARTESIAN_POINT ( 'NONE',  ( 9.447334110624092673, 9.916311305349925220, -0.7998128361456281477 ) ) ;
#114561=CARTESIAN_POINT ( 'NONE',  ( -7.967387826325084355, 12.44703623068796361, 0.7998128361456481317 ) ) ;
#114564=CARTESIAN_POINT ( 'NONE',  ( -1.364683531249997417, 2.509375000341422357, 1.214306433183764966E-14 ) ) ;
#114565=CARTESIAN_POINT ( 'NONE',  ( 2.683624340501134853, 5.218313266304903664, -1.199719254218446718 ) ) ;
#114570=CARTESIAN_POINT ( 'NONE',  ( 3.375617060122621194, 6.882044303544283537, 1.040834085586084257E-14 ) ) ;
#114571=CARTESIAN_POINT ( 'NONE',  ( 9.883530794237934458, 10.63313346947350269, -0.7216878364870257245 ) ) ;
#114572=CARTESIAN_POINT ( 'NONE',  ( -2.298420387838187473, 5.509269730139584986, -0.7346435760097105305 ) ) ;
#114573=CARTESIAN_POINT ( 'NONE',  ( -6.073689629242151611, 10.02979563418376685, -0.7216878364870278340 ) ) ;
#114574=CARTESIAN_POINT ( 'NONE',  ( 1.364683531249986537, 0.9052083336747533959, -0.7879004041258239610 ) ) ;
#114576=CARTESIAN_POINT ( 'NONE',  ( 0.1332994001262571560, 7.096108761198728132, 2.115961662170631197 ) ) ;
#114578=CARTESIAN_POINT ( 'NONE',  ( -8.507905087775398556, 9.884643009614800135, 1.199719254218462483 ) ) ;
#114580=CARTESIAN_POINT ( 'NONE',  ( -2.426546306721660606, 5.774795091243142053, 0.7216878364870317197 ) ) ;
#114581=CARTESIAN_POINT ( 'NONE',  ( -1.364683531250012516, 4.051041667008088432, -0.7879004041258300672 ) ) ;
#114587=CARTESIAN_POINT ( 'NONE',  ( 8.723781775389312543, 12.26516360700784958, -1.199719254218446718 ) ) ;
#114601=CARTESIAN_POINT ( 'NONE',  ( -1.201851678989727383E-14, 4.509375000341417916, -1.575800808251660134 ) ) ;
#114606=CARTESIAN_POINT ( 'NONE',  ( 8.259941899223605333, 10.65968485389279508, -1.599625672291268286 ) ) ;
#114609=CARTESIAN_POINT ( 'NONE',  ( -0.6823417656250212460, 2.301041667008084435, 1.181850606188767472 ) ) ;
#114611=CARTESIAN_POINT ( 'NONE',  ( -5.748293942514169252, 9.650167333001109071, -0.7216878364870207285 ) ) ;
#114613=CARTESIAN_POINT ( 'NONE',  ( 1.426714497268818382, 7.396188545894305300, 4.272650097712511474 ) ) ;
#114617=CARTESIAN_POINT ( 'NONE',  ( 3.734381245560244089, 6.444196322207211836, 1.199719254218462483 ) ) ;
#114619=ORIENTED_EDGE ( 'NONE', *, *, #140892, .T. ) ;
#114620=CARTESIAN_POINT ( 'NONE',  ( 9.297140650669039275, 11.86975006391249643, 1.599625672291281386 ) ) ;
#114628=CARTESIAN_POINT ( 'NONE',  ( -2.272963308585411735, 5.803540959991587478, 0.7998128361456341429 ) ) ;
#114629=CARTESIAN_POINT ( 'NONE',  ( 6.109920781252839994, 10.27999134477033216, 1.040834085586084257E-14 ) ) ;
#114631=CARTESIAN_POINT ( 'NONE',  ( 4.107757354816228279, 6.775838766385488654, -1.082531754730548412 ) ) ;
#114642=CARTESIAN_POINT ( 'NONE',  ( -7.049876689426106680, 9.247942109129029475, -1.443375672974059665 ) ) ;
#114643=CARTESIAN_POINT ( 'NONE',  ( 3.662674053986138656, 7.424870162959149589, 0.7998128361456321445 ) ) ;
#114646=CARTESIAN_POINT ( 'NONE',  ( -8.616370316684697883, 10.01118577667568132, -1.199719254218446718 ) ) ;
#114651=CARTESIAN_POINT ( 'NONE',  ( -8.435144125996554720, 12.99275191363802229, 0.7998128361456341429 ) ) ;
#114652=CARTESIAN_POINT ( 'NONE',  ( 0.6823417656249899377, 3.092708333674754062, 1.181850606188765695 ) ) ;
#114655=CARTESIAN_POINT ( 'NONE',  ( 8.555358625423188812, 9.940005470203933768, 1.199719254218462483 ) ) ;
#114667=CARTESIAN_POINT ( 'NONE',  ( -8.320953590485107298, 10.73086516036454618, 1.599625672291269396 ) ) ;
#114671=CARTESIAN_POINT ( 'NONE',  ( 7.795575138177731844, 8.197185204069915798, 1.040834085586084257E-14 ) ) ;
#114672=EDGE_CURVE ( 'NONE', #87474, #185401, #9326, .T. ) ;
#114674=CARTESIAN_POINT ( 'NONE',  ( 5.007038802148489509, 4.735966778795008381, 0.7998128361456341429 ) ) ;
#114675=CARTESIAN_POINT ( 'NONE',  ( -5.151735183512911043, 6.073074471262228435, 1.082531754730548412 ) ) ;
#114677=CARTESIAN_POINT ( 'NONE',  ( -7.888146445052511169, 8.097259028849730811, 1.040834085586084257E-14 ) ) ;
#114688=CARTESIAN_POINT ( 'NONE',  ( 1.364683531249988535, 4.467708333674754506, -0.7879004041258300672 ) ) ;
#114689=CARTESIAN_POINT ( 'NONE',  ( 7.727257484784855635, 11.10255193463598111, -1.199719254218446718 ) ) ;
#114691=CARTESIAN_POINT ( 'NONE',  ( -4.365362273920257330, 6.116008624372160973, 1.443375672974064550 ) ) ;
#114692=CARTESIAN_POINT ( 'NONE',  ( -4.894130264408873110, 5.772535398974209642, -1.082531754730543971 ) ) ;
#114699=CARTESIAN_POINT ( 'NONE',  ( 5.009901455449552010, 5.803638771901306725, -1.199719254218452047 ) ) ;
#114705=CARTESIAN_POINT ( 'NONE',  ( 1.244123718695680836, 2.983005466778237746, 0.7750000000000100142 ) ) ;
#114708=CARTESIAN_POINT ( 'NONE',  ( 5.355634372598031767, 6.206993841907870291, -1.199719254218445830 ) ) ;
#114713=CARTESIAN_POINT ( 'NONE',  ( -0.6823417656250212460, 3.863541667008085767, 1.181850606188767472 ) ) ;
#114718=CARTESIAN_POINT ( 'NONE',  ( 7.610204295972345712, 7.772993188256215547, 0.7998128361456341429 ) ) ;
#114720=CARTESIAN_POINT ( 'NONE',  ( -5.656776405399756236, 7.622658444431597680, -1.599625672291256295 ) ) ;
#114721=CARTESIAN_POINT ( 'NONE',  ( -1.402160292154681736E-14, 2.087500000000021227, -1.732050807568863648 ) ) ;
#114724=CARTESIAN_POINT ( 'NONE',  ( -5.786632634934295361, 5.645492917045106473, 0.7998128361456341429 ) ) ;
#114726=CARTESIAN_POINT ( 'NONE',  ( -0.6823417656250212460, 3.551041667008085323, 1.181850606188767472 ) ) ;
#114728=CARTESIAN_POINT ( 'NONE',  ( -5.273758566035884776, 5.255065869904374409, 0.000000000000000000 ) ) ;
#114733=CARTESIAN_POINT ( 'NONE',  ( -3.904385051055635270, 6.538571078664754843, 1.082531754730560403 ) ) ;
#114734=CARTESIAN_POINT ( 'NONE',  ( 5.168682875307768931, 7.053215992657626110, -1.599625672291256295 ) ) ;
#114737=CARTESIAN_POINT ( 'NONE',  ( -1.201851678989727383E-14, 4.009375000341416140, -1.575800808251660134 ) ) ;
#114739=CARTESIAN_POINT ( 'NONE',  ( 2.171277156482887882, 5.684907115872006145, -0.7998128361456291469 ) ) ;
#114741=CARTESIAN_POINT ( 'NONE',  ( -1.364683531250000748, -0.4281249996585800854, 0.000000000000000000 ) ) ;
#114744=CARTESIAN_POINT ( 'NONE',  ( -3.436101866059630527, 6.096203712789787232, 1.199719254218462483 ) ) ;
#114746=CARTESIAN_POINT ( 'NONE',  ( -5.043269954159181445, 8.827639346586952485, 1.214306433183764966E-14 ) ) ;
#114748=LINE ( 'NONE', #63796, #146766 ) ;
#114750=CARTESIAN_POINT ( 'NONE',  ( 0.6823417656249882723, 2.676041667008084879, -1.181850606188749264 ) ) ;
#114759=CARTESIAN_POINT ( 'NONE',  ( -5.707619481228814351, 9.602713794834864203, -0.7216878364870207285 ) ) ;
#114765=CARTESIAN_POINT ( 'NONE',  ( -4.839897649954225223, 7.630002444046455778, 1.082531754730560403 ) ) ;
#114771=CARTESIAN_POINT ( 'NONE',  ( 0.07378579499363849270, 7.051136084633868428, 3.951055989447525896 ) ) ;
#114776=CARTESIAN_POINT ( 'NONE',  ( -5.590039407536138150, 5.416134151747256986, 0.000000000000000000 ) ) ;
#114778=CARTESIAN_POINT ( 'NONE',  ( -1.500000000000001332, -0.3499999999999753308, 0.000000000000000000 ) ) ;
#114779=CARTESIAN_POINT ( 'NONE',  ( 9.029367117021314115, 12.51771682229149008, -1.082531754730543083 ) ) ;
#114780=CARTESIAN_POINT ( 'NONE',  ( 8.620286740190458374, 8.951422706510690830, 1.040834085586084257E-14 ) ) ;
#114784=CARTESIAN_POINT ( 'NONE',  ( 6.342516933094585418, 6.294024598232139667, 1.040834085586084257E-14 ) ) ;
#114790=CARTESIAN_POINT ( 'NONE',  ( -3.145128448690310830, 6.613140923539910787, -0.7216878364870267237 ) ) ;
#114798=CARTESIAN_POINT ( 'NONE',  ( 0.6823417656249899377, 2.342708333674753618, 1.181850606188767472 ) ) ;
#114799=CARTESIAN_POINT ( 'NONE',  ( 10.18181017373857067, 11.94149529319227909, 1.082531754730548412 ) ) ;
#114800=CARTESIAN_POINT ( 'NONE',  ( -5.377780486114890124, 9.425827667109372143, 0.000000000000000000 ) ) ;
#114803=CARTESIAN_POINT ( 'NONE',  ( 5.147291874682557555, 9.156924287104992288, 0.7998128361456462443 ) ) ;
#114804=CARTESIAN_POINT ( 'NONE',  ( -5.768104287610143821, 8.816873204598778102, -1.199719254218440723 ) ) ;
#114807=CARTESIAN_POINT ( 'NONE',  ( -1.500000000000001332, 0.9312500006828163812, 0.000000000000000000 ) ) ;
#114810=CARTESIAN_POINT ( 'NONE',  ( 8.432808358020029260, 8.940623960552603222, 0.7216878364870438212 ) ) ;
#114813=CARTESIAN_POINT ( 'NONE',  ( -1.364683531250014514, 0.3427083336747508424, 0.7879004041258379498 ) ) ;
#114815=CARTESIAN_POINT ( 'NONE',  ( 6.222829318548112276, 9.243422724072711816, -1.082531754730537976 ) ) ;
#114818=CARTESIAN_POINT ( 'NONE',  ( -5.599154252763867134, 5.634694171087028636, 0.000000000000000000 ) ) ;
#114820=CARTESIAN_POINT ( 'NONE',  ( -0.6823417656250212460, 4.051041667008085767, 1.181850606188767472 ) ) ;
#114822=DIRECTION ( 'NONE',  ( -5.578564026256490882E-16, -1.000000000000000000, -9.066213480720158442E-32 ) ) ;
#114824=CARTESIAN_POINT ( 'NONE',  ( -5.969600656924041182, 6.101865228085409321, -0.7346798775042752139 ) ) ;
#114831=CARTESIAN_POINT ( 'NONE',  ( 5.933664784275179294, 10.07435934829639912, -0.7998128361456291469 ) ) ;
#114835=CARTESIAN_POINT ( 'NONE',  ( 3.979481780810941949, 4.601482484822914998, 1.199719254218464037 ) ) ;
#114841=CARTESIAN_POINT ( 'NONE',  ( 4.365362273920230685, 8.036747052974847705, 0.7216878364870298324 ) ) ;
#114842=CARTESIAN_POINT ( 'NONE',  ( 1.364683531249988757, 0.9468750003414211358, 0.000000000000000000 ) ) ;
#114844=CARTESIAN_POINT ( 'NONE',  ( 3.728655938958122196, 4.308852335994623139, -1.199719254218446718 ) ) ;
#114849=CARTESIAN_POINT ( 'NONE',  ( -1.500000000000013101, 2.420833333333359150, 0.8660254037844403729 ) ) ;
#114850=CARTESIAN_POINT ( 'NONE',  ( 5.262536180398716290, 9.291375977107183104, -0.7998128361456291469 ) ) ;
#114851=CARTESIAN_POINT ( 'NONE',  ( -9.176171038350775078, 9.599954387697719582, -0.7998128361456291469 ) ) ;
#114855=CARTESIAN_POINT ( 'NONE',  ( 1.364683531249986537, 1.655208333674748955, -0.7879004041258239610 ) ) ;
#114857=CARTESIAN_POINT ( 'NONE',  ( 1.499999999999989120, 2.775000000000020339, 1.214306433183764966E-14 ) ) ;
#114859=CARTESIAN_POINT ( 'NONE',  ( 4.521807925357579805, 5.234196320127330715, -1.199719254218452047 ) ) ;
#114866=CARTESIAN_POINT ( 'NONE',  ( -1.602468905319636405E-14, -1.131249999317182064, -1.732050807568870754 ) ) ;
#114867=CARTESIAN_POINT ( 'NONE',  ( -6.669721502918952716, 9.868759955792373972, 1.199719254218452047 ) ) ;
#114868=CARTESIAN_POINT ( 'NONE',  ( -4.067082894419624672, 6.728385229256075739, 1.082531754730560403 ) ) ;
#114875=CARTESIAN_POINT ( 'NONE',  ( 6.154511665599609493, 9.267681812253174556, 1.199719254218462483 ) ) ;
#114877=CARTESIAN_POINT ( 'NONE',  ( 1.579999999999985860, -1.099999999999976108, 2.579999999999999183 ) ) ;
#114881=CARTESIAN_POINT ( 'NONE',  ( 7.169564303528210836, 7.258913197071374945, -0.7998128361456281477 ) ) ;
#114882=CARTESIAN_POINT ( 'NONE',  ( 9.531018800282605952, 11.18223869082697597, 1.082531754730548412 ) ) ;
#114886=CARTESIAN_POINT ( 'NONE',  ( -7.019370843573183194, 9.212351955633947043, 1.599625672291283607 ) ) ;
#114887=CARTESIAN_POINT ( 'NONE',  ( 4.704842999142070603, 5.447737239542574272, -1.199719254218452047 ) ) ;
#114892=CARTESIAN_POINT ( 'NONE',  ( 4.016016189339381981, 7.573203028563332495, -0.3002613606930375489 ) ) ;
#114893=CARTESIAN_POINT ( 'NONE',  ( 10.07334494527360569, 10.85458331234846696, 0.000000000000000000 ) ) ;
#114903=CARTESIAN_POINT ( 'NONE',  ( -5.097502569058225852, 5.049433873430440478, -0.7216878364870207285 ) ) ;
#114904=CARTESIAN_POINT ( 'NONE',  ( 7.754900677336718395, 11.99120852362745460, -0.7216878364870267237 ) ) ;
#114907=CARTESIAN_POINT ( 'NONE',  ( -5.742041750587549842, 6.657802449562273850, 1.199719254218450271 ) ) ;
#114913=CARTESIAN_POINT ( 'NONE',  ( -8.030507057996002729, 8.263346410617135263, 1.040834085586084257E-14 ) ) ;
#114928=CARTESIAN_POINT ( 'NONE',  ( -4.367698041896780126, 8.247398148854895084, 0.7998128361456481317 ) ) ;
#114931=CARTESIAN_POINT ( 'NONE',  ( 4.744990575102895569, 5.598539094783909320, -1.082531754730548412 ) ) ;
#114935=CARTESIAN_POINT ( 'NONE',  ( -3.379006598303881059, 4.965260336153046516, -1.599625672291256295 ) ) ;
#114938=CARTESIAN_POINT ( 'NONE',  ( 10.70146331988817323, 11.37946204949139251, 0.7998128361456341429 ) ) ;
#114941=CARTESIAN_POINT ( 'NONE',  ( -9.203287345578106127, 9.631590079462940324, 0.7998128361456462443 ) ) ;
#114942=CARTESIAN_POINT ( 'NONE',  ( 7.149227073107712549, 7.235186428247455837, -0.7998128361456281477 ) ) ;
#114945=CARTESIAN_POINT ( 'NONE',  ( 3.635557746758808495, 7.393234471193928847, -0.7998128361456291469 ) ) ;
#114948=CARTESIAN_POINT ( 'NONE',  ( 1.364683531249988757, -0.5531249996585801965, 0.000000000000000000 ) ) ;
#114951=CARTESIAN_POINT ( 'NONE',  ( 8.107412671292035355, 10.48173408797264194, 1.443375672974076540 ) ) ;
#114981=CARTESIAN_POINT ( 'NONE',  ( 0.7499999999999885647, 0.7645833340161543035, 1.299038105676657340 ) ) ;
#114987=AXIS2_PLACEMENT_3D ( 'NONE', #169143, #90051, #73776 ) ;
#114989=CARTESIAN_POINT ( 'NONE',  ( 8.809047120577066181, 11.30030761213851953, 1.599625672291281386 ) ) ;
#114994=CARTESIAN_POINT ( 'NONE',  ( 4.497554271431305040, 6.270232621468402989, -1.599625672291256295 ) ) ;
#114995=CARTESIAN_POINT ( 'NONE',  ( -7.375272376154096143, 8.667201196010339004, -1.082531754730544860 ) ) ;
#114996=CARTESIAN_POINT ( 'NONE',  ( -5.803933766307007858, 6.065161521460068705, 0.5445525043519475750 ) ) ;
#114999=CARTESIAN_POINT ( 'NONE',  ( -6.021792782764022078, 10.17717534653336209, -0.7998128361456291469 ) ) ;
#115000=( BOUNDED_CURVE ( )  B_SPLINE_CURVE ( 3, ( #71184, #100507, #134115, #200124 ),
 .UNSPECIFIED., .F., .T. ) 
 B_SPLINE_CURVE_WITH_KNOTS ( ( 4, 4 ),
 ( 4.082329036714103410, 4.712388980384689674 ),
 .UNSPECIFIED. ) 
 CURVE ( )  GEOMETRIC_REPRESENTATION_ITEM ( )  RATIONAL_B_SPLINE_CURVE ( ( 1.000000000000000000, 0.9671913951458349645, 0.9671913951458349645, 1.000000000000000000 ) ) 
 REPRESENTATION_ITEM ( '' )  );
#115001=CARTESIAN_POINT ( 'NONE',  ( -3.673896439178936824, 5.309298483840612093, 1.443375672974064550 ) ) ;
#115004=CARTESIAN_POINT ( 'NONE',  ( -1.500000000000013101, 1.952083334016152527, 0.8660254037844403729 ) ) ;
#115012=CARTESIAN_POINT ( 'NONE',  ( -8.469039510030723861, 13.03229652834454733, 1.040834085586084257E-14 ) ) ;
#115016=CARTESIAN_POINT ( 'NONE',  ( 3.995055777641403516, 7.602996552368006533, -0.05680687033517151097 ) ) ;
#115021=CARTESIAN_POINT ( 'NONE',  ( -9.022061154889962964, 12.61315621642528129, -1.199719254218446718 ) ) ;
#115022=CARTESIAN_POINT ( 'NONE',  ( 8.121497709785879593, 9.433834401960398353, -1.199719254218445830 ) ) ;
#115028=ORIENTED_EDGE ( 'NONE', *, *, #144354, .T. ) ;
#115031=CARTESIAN_POINT ( 'NONE',  ( -9.158696461231359720, 10.64389961198009615, 1.199719254218462483 ) ) ;
#115037=CARTESIAN_POINT ( 'NONE',  ( 4.864678189204997949, 4.569879397027603929, 0.7998128361456341429 ) ) ;
#115041=ORIENTED_EDGE ( 'NONE', *, *, #203953, .F. ) ;
#115055=CARTESIAN_POINT ( 'NONE',  ( 6.448874621594486989, 10.67543749183559143, 0.7998128361456462443 ) ) ;
#115057=CARTESIAN_POINT ( 'NONE',  ( -4.192495815123836955, 5.914331089109674089, -1.599625672291256295 ) ) ;
#115065=CARTESIAN_POINT ( 'NONE',  ( -1.500000000000001332, 0.6812500006828161592, 0.000000000000000000 ) ) ;
#115069=CARTESIAN_POINT ( 'NONE',  ( 3.891353782322113375, 4.498666486585943147, -1.199719254218446718 ) ) ;
#115071=CARTESIAN_POINT ( 'NONE',  ( -4.946027110887008860, 4.664786472323266153, -0.7998128361456221525 ) ) ;
#115077=CARTESIAN_POINT ( 'NONE',  ( 4.853455804012216213, 6.685451076146141425, 1.443375672974062551 ) ) ;
#115080=CARTESIAN_POINT ( 'NONE',  ( 0.6823417656249899377, 5.238541667008086655, -1.181850606188754593 ) ) ;
#115081=CARTESIAN_POINT ( 'NONE',  ( -5.956409969451652131, 6.075908546082715134, -0.6293437877468227581 ) ) ;
#115082=CARTESIAN_POINT ( 'NONE',  ( 4.975479186090860928, 4.907073259968533385, 0.7216878364870317197 ) ) ;
#115090=CARTESIAN_POINT ( 'NONE',  ( -6.136354103119505687, 5.996982182489118962, -0.08184359936842452998 ) ) ;
#115092=CARTESIAN_POINT ( 'NONE',  ( -1.364683531250014514, -0.7197916663252461600, 0.7879004041258379498 ) ) ;
#115101=CARTESIAN_POINT ( 'NONE',  ( -0.7500000000000215383, 4.941666666666684193, 1.299038105676671107 ) ) ;
#115103=CARTESIAN_POINT ( 'NONE',  ( -1.579999999999998073, 8.674529973577531194, -2.419999999999989715 ) ) ;
#115108=CARTESIAN_POINT ( 'NONE',  ( 1.499999999999978906, 4.295833333333352044, -0.8660254037844369313 ) ) ;
#115109=CARTESIAN_POINT ( 'NONE',  ( -0.6823417656250212460, 4.613541667008086655, 1.181850606188767472 ) ) ;
#115111=CARTESIAN_POINT ( 'NONE',  ( 6.474182045725470402, 7.511966127223233869, -1.199719254218446718 ) ) ;
#115112=CARTESIAN_POINT ( 'NONE',  ( -8.850775351622791831, 9.220326086515070685, -0.7998128361456291469 ) ) ;
#115114=CARTESIAN_POINT ( 'NONE',  ( 8.055515824813896941, 12.54985222892493368, 0.7998128361456462443 ) ) ;
#115119=CARTESIAN_POINT ( 'NONE',  ( -1.402160292154681736E-14, -0.7406249996585823059, -1.575800808251665908 ) ) ;
#115126=CARTESIAN_POINT ( 'NONE',  ( 7.782016984564054773, 10.10210578678999482, 1.443375672974076540 ) ) ;
#115131=CARTESIAN_POINT ( 'NONE',  ( 1.499999999999990896, 3.306250000682818602, 1.214306433183764966E-14 ) ) ;
#115133=CARTESIAN_POINT ( 'NONE',  ( -3.928111819657352566, 5.605883094398769195, 1.599625672291267398 ) ) ;
#115134=CARTESIAN_POINT ( 'NONE',  ( 6.778713616708431644, 7.010846762355714468, 1.040834085586084257E-14 ) ) ;
#115135=CARTESIAN_POINT ( 'NONE',  ( -9.531018800282611281, 12.14260790512831889, 1.443375672974076540 ) ) ;
#115142=CARTESIAN_POINT ( 'NONE',  ( 4.304877467538922531, 4.981110786005563007, 1.199719254218464037 ) ) ;
#115144=CARTESIAN_POINT ( 'NONE',  ( 5.040934186182656873, 4.775511393501539636, 1.040834085586084257E-14 ) ) ;
#115149=EDGE_LOOP ( 'NONE', ( #76207, #145274, #186363, #169441 ) ) ;
#115161=CARTESIAN_POINT ( 'NONE',  ( 7.391166297744269365, 11.77477778067701664, 1.040834085586084257E-14 ) ) ;
#115165=CARTESIAN_POINT ( 'NONE',  ( -1.364683531250014514, 0.2802083336747505649, 0.7879004041258379498 ) ) ;
#115166=CARTESIAN_POINT ( 'NONE',  ( 5.016153647376196290, 8.796003655340152605, 0.7216878364870438212 ) ) ;
#115167=CARTESIAN_POINT ( 'NONE',  ( -10.46653140006992899, 11.31330084294416771, -0.7216878364870267237 ) ) ;
#115173=CARTESIAN_POINT ( 'NONE',  ( -3.242371291962510504, 6.934516940598226320, 1.040834085586084257E-14 ) ) ;
#115186=CARTESIAN_POINT ( 'NONE',  ( 5.877843389052785028, 6.166481636157870483, -0.8510708418205383818 ) ) ;
#115189=CARTESIAN_POINT ( 'NONE',  ( 3.985207087413062066, 6.736826471035503694, -1.199719254218452047 ) ) ;
#115195=CARTESIAN_POINT ( 'NONE',  ( -9.517460647113315630, 10.20605163116143821, 0.7216878364870438212 ) ) ;
#115199=CARTESIAN_POINT ( 'NONE',  ( 5.764187864104357573, 9.876636274763768597, 1.040834085586084257E-14 ) ) ;
#115200=CARTESIAN_POINT ( 'NONE',  ( -4.761938266897808525, 6.578680616179307883, 1.599625672291267175 ) ) ;
#115202=CARTESIAN_POINT ( 'NONE',  ( -5.331380718671772101, 7.243030143248949670, -1.599625672291256295 ) ) ;
#115203=CARTESIAN_POINT ( 'NONE',  ( 4.207107738942202246, 3.802713871720993399, 1.214306433183764966E-14 ) ) ;
#115205=VECTOR ( 'NONE', #151511, 1000.000000000000114 ) ;
#115206=CARTESIAN_POINT ( 'NONE',  ( -5.205440912643032547, 8.160432600470439723, 1.199719254218452047 ) ) ;
#115207=CIRCLE ( 'NONE', #135869, 0.8299999999999999600 ) ;
#115210=CARTESIAN_POINT ( 'NONE',  ( 8.269583629331492602, 11.73526576994040482, 1.199719254218450271 ) ) ;
#115213=CARTESIAN_POINT ( 'NONE',  ( 4.981510052282690282, 6.816019998287410786, 1.424969591591069396 ) ) ;
#115214=CARTESIAN_POINT ( 'NONE',  ( 6.019457014787495730, 6.125047393447951016, -0.7216878364870257245 ) ) ;
#115219=FACE_OUTER_BOUND ( 'NONE', #210344, .T. ) ;
#115222=CARTESIAN_POINT ( 'NONE',  ( 8.405692050348340771, 8.908988268268968724, 1.040834085586084257E-14 ) ) ;
#115227=CARTESIAN_POINT ( 'NONE',  ( -7.974166903131914452, 12.45494515362926435, -0.7998128361456281477 ) ) ;
#115228=CARTESIAN_POINT ( 'NONE',  ( -6.690058733339450114, 9.892486724616283311, 1.199719254218452047 ) ) ;
#115237=CARTESIAN_POINT ( 'NONE',  ( 9.725276259704228821, 10.24057714594344048, 0.7998128361456462443 ) ) ;
#115240=CARTESIAN_POINT ( 'NONE',  ( 2.333974999846879061, 5.874721266463329705, -0.7998128361456291469 ) ) ;
#115243=CARTESIAN_POINT ( 'NONE',  ( -1.500000000000011324, 4.410416667349484676, -0.8660254037844313801 ) ) ;
#115249=CARTESIAN_POINT ( 'NONE',  ( 0.7499999999999902300, 3.233333333333352044, 1.299038105676669330 ) ) ;
#115250=CARTESIAN_POINT ( 'NONE',  ( 6.100279051144945619, 9.204410428722734849, -1.199719254218440723 ) ) ;
#115252=CARTESIAN_POINT ( 'NONE',  ( 7.104109303880752790, 11.23195192126214970, -0.7216878364870267237 ) ) ;
#115256=CARTESIAN_POINT ( 'NONE',  ( 9.459838494033030898, 12.05956421450382088, 1.599625672291281386 ) ) ;
#115258=CARTESIAN_POINT ( 'NONE',  ( -4.765854690403601879, 5.518917546014321829, 1.199719254218462483 ) ) ;
#115259=CARTESIAN_POINT ( 'NONE',  ( 0.7499999999999920064, 5.264583334016151639, 1.299038105676669330 ) ) ;
#115260=CARTESIAN_POINT ( 'NONE',  ( 1.364683531249986537, -0.5947916663252456049, -0.7879004041258309554 ) ) ;
#115264=CARTESIAN_POINT ( 'NONE',  ( 2.659370686574860976, 6.254349567645977714, -0.7998128361456291469 ) ) ;
#115267=CARTESIAN_POINT ( 'NONE',  ( -1.364683531250010295, 5.342708333674750953, 0.7879004041258379498 ) ) ;
#115270=CARTESIAN_POINT ( 'NONE',  ( 4.068383102448127175, 7.735681852393593516, 0.5751369358401996479 ) ) ;
#115274=CARTESIAN_POINT ( 'NONE',  ( -8.227100285394159940, 8.492705175914988303, 0.7998128361456602331 ) ) ;
#115277=CARTESIAN_POINT ( 'NONE',  ( 5.138703914779377158, 5.953908307786102583, 1.199719254218462483 ) ) ;
#115280=CARTESIAN_POINT ( 'NONE',  ( -1.364683531250014514, -0.2614583329919080157, -0.7879004041258359514 ) ) ;
#115285=CARTESIAN_POINT ( 'NONE',  ( 8.062294901620731480, 12.55776115186623620, 1.040834085586084257E-14 ) ) ;
#115288=CARTESIAN_POINT ( 'NONE',  ( -6.392833124043511894, 7.417059051927569868, 1.199719254218450271 ) ) ;
#115292=CARTESIAN_POINT ( 'NONE',  ( 8.215351014876830504, 11.67199438640995801, -1.199719254218446718 ) ) ;
#115294=CARTESIAN_POINT ( 'NONE',  ( 8.589254009457354400, 9.979550084910457031, -1.199719254218446718 ) ) ;
#115296=CARTESIAN_POINT ( 'NONE',  ( -4.600294193738529103, 4.261431402316699035, -0.7998128361456221525 ) ) ;
#115298=CARTESIAN_POINT ( 'NONE',  ( -6.344325816190970357, 9.489131654609717970, 1.199719254218452047 ) ) ;
#115302=CARTESIAN_POINT ( 'NONE',  ( -4.974982779204009553, 6.815313220028144769, 1.450550931683711298 ) ) ;
#115303=CARTESIAN_POINT ( 'NONE',  ( -0.6823417656250003738, -0.03229166632524871350, -1.181850606188749264 ) ) ;
#115307=CARTESIAN_POINT ( 'NONE',  ( 5.666945020832160118, 9.555260257705446847, 0.7216878364870438212 ) ) ;
#115314=EDGE_CURVE ( 'NONE', #95577, #69400, #120111, .T. ) ;
#115328=CARTESIAN_POINT ( 'NONE',  ( 8.561083932025322696, 12.07534945641652158, -1.199719254218446718 ) ) ;
#115332=CARTESIAN_POINT ( 'NONE',  ( -5.436983294280064882, 6.301900917203534291, 1.199719254218450271 ) ) ;
#115333=CARTESIAN_POINT ( 'NONE',  ( -9.345647958521597687, 9.797677461230342999, 0.7998128361456462443 ) ) ;
#115335=VERTEX_POINT ( 'NONE', #166881 ) ;
#115339=CARTESIAN_POINT ( 'NONE',  ( 1.499999999999990896, 3.306250000682818602, 1.214306433183764966E-14 ) ) ;
#115340=CARTESIAN_POINT ( 'NONE',  ( 9.088043039861931405, 9.497138389460751284, 1.040834085586084257E-14 ) ) ;
#115344=CARTESIAN_POINT ( 'NONE',  ( -9.664264568442742842, 10.16939683947169115, -0.7998128361456291469 ) ) ;
#115346=CARTESIAN_POINT ( 'NONE',  ( -1.364683531249997417, 3.509375000341423245, 1.214306433183764966E-14 ) ) ;
#115352=CARTESIAN_POINT ( 'NONE',  ( -9.408995418203979000, 12.00024729270324286, 1.443375672974076540 ) ) ;
#115356=CARTESIAN_POINT ( 'NONE',  ( -1.364683531250000748, 2.071875000341422357, 1.214306433183764966E-14 ) ) ;
#115361=CARTESIAN_POINT ( 'NONE',  ( -1.364683531250000748, 1.509375000341421691, 0.000000000000000000 ) ) ;
#115366=CARTESIAN_POINT ( 'NONE',  ( -5.494078562035765501, 7.432844293840273231, -1.599625672291256295 ) ) ;
#115367=CARTESIAN_POINT ( 'NONE',  ( 3.571683402196252910, 6.254382171615883834, 1.199719254218462483 ) ) ;
#115369=CARTESIAN_POINT ( 'NONE',  ( 1.499999999999989120, 5.295833333333356485, -0.8660254037844323793 ) ) ;
#115370=CARTESIAN_POINT ( 'NONE',  ( -1.364683531249997417, 3.071875000341423245, 1.214306433183764966E-14 ) ) ;
#115373=CARTESIAN_POINT ( 'NONE',  ( -0.6823417656250246877, -1.198958332991911790, 1.181850606188755259 ) ) ;
#115374=CARTESIAN_POINT ( 'NONE',  ( -5.938108093105513241, 6.030140318152288792, 0.7216878364870317197 ) ) ;
#115377=CARTESIAN_POINT ( 'NONE',  ( 3.375617060122621194, 6.882044303544283537, 1.040834085586084257E-14 ) ) ;
#115380=CARTESIAN_POINT ( 'NONE',  ( -8.552495972122143186, 8.872333477097637200, 0.7998128361456462443 ) ) ;
#115381=CARTESIAN_POINT ( 'NONE',  ( -4.776550190716183586, 4.467063398790632966, 1.214306433183764966E-14 ) ) ;
#115383=CARTESIAN_POINT ( 'NONE',  ( -1.364683531250012516, 4.738541667008091096, -0.7879004041258300672 ) ) ;
#115388=CARTESIAN_POINT ( 'NONE',  ( -7.226132685959434809, 8.493204890783200511, 1.082531754730549967 ) ) ;
#115390=CARTESIAN_POINT ( 'NONE',  ( -1.402160292154681736E-14, 0.009375000341421267647, -1.575800808251665908 ) ) ;
#115394=CARTESIAN_POINT ( 'NONE',  ( 7.375272376154084597, 9.627570410311676596, -1.443375672974057666 ) ) ;
#115403=CARTESIAN_POINT ( 'NONE',  ( 8.229436053370667636, 11.58446391469906267, 1.082531754730558626 ) ) ;
#115408=EDGE_CURVE ( 'NONE', #63111, #93339, #143497, .T. ) ;
#115409=CARTESIAN_POINT ( 'NONE',  ( 5.113396490648394632, 9.117379672398465473, 1.040834085586084257E-14 ) ) ;
#115410=CARTESIAN_POINT ( 'NONE',  ( -6.078132937628113908, 5.985576603521232109, 1.040834085586084257E-14 ) ) ;
#115414=CARTESIAN_POINT ( 'NONE',  ( 6.168596704093459060, 7.259412911939593371, -1.082531754730543083 ) ) ;
#115415=CARTESIAN_POINT ( 'NONE',  ( 1.364683531249986537, 0.2177083336747502595, -0.7879004041258309554 ) ) ;
#115417=CARTESIAN_POINT ( 'NONE',  ( -9.972185678051314284, 11.59297036493672017, 1.199719254218462483 ) ) ;
#115428=ORIENTED_EDGE ( 'NONE', *, *, #101605, .T. ) ;
#115433=CARTESIAN_POINT ( 'NONE',  ( 5.472687561410540802, 9.536552588287639409, 0.7998128361456462443 ) ) ;
#115434=CARTESIAN_POINT ( 'NONE',  ( 6.109920781252839994, 10.27999134477033216, 1.040834085586084257E-14 ) ) ;
#115443=CARTESIAN_POINT ( 'NONE',  ( -4.848826244296223109, 5.027555131033083491, -0.8732430475888957044 ) ) ;
#115446=CARTESIAN_POINT ( 'NONE',  ( -5.250031796989778066, 7.148123067953287446, 1.599625672291267398 ) ) ;
#115448=CARTESIAN_POINT ( 'NONE',  ( -4.600294193738529103, 4.261431402316699035, -0.7998128361456221525 ) ) ;
#115458=CARTESIAN_POINT ( 'NONE',  ( -8.663296969452339624, 13.05100419776235299, 1.040834085586084257E-14 ) ) ;
#115461=CARTESIAN_POINT ( 'NONE',  ( 4.638861114170084399, 8.563755066507100722, 0.7998128361456462443 ) ) ;
#115462=CARTESIAN_POINT ( 'NONE',  ( 1.364683531249992088, 5.634375000341417916, 1.214306433183764966E-14 ) ) ;
#115467=CARTESIAN_POINT ( 'NONE',  ( 4.433153041544209749, 7.155467067568137551, -1.082531754730548412 ) ) ;
#115468=CARTESIAN_POINT ( 'NONE',  ( -5.859094939400033120, 9.987361195942037639, -0.7998128361456231517 ) ) ;
#115473=CARTESIAN_POINT ( 'NONE',  ( -6.287230548435221777, 8.358188277972981695, -1.599625672291263179 ) ) ;
#115474=CARTESIAN_POINT ( 'NONE',  ( -5.111587607552082524, 5.922272616020886282, 1.199719254218450271 ) ) ;
#115482=CARTESIAN_POINT ( 'NONE',  ( 6.823831386379729302, 6.855558127064808716, -0.7998128361456281477 ) ) ;
#115487=DIRECTION ( 'NONE',  ( 1.000000000000000000, 0.000000000000000000, 0.000000000000000000 ) ) ;
#115492=CARTESIAN_POINT ( 'NONE',  ( -1.364683531250000748, -0.1781249996585798634, 0.000000000000000000 ) ) ;
#115493=CARTESIAN_POINT ( 'NONE',  ( 2.737856954955798727, 5.281584649835344258, 1.199719254218452047 ) ) ;
#115494=CARTESIAN_POINT ( 'NONE',  ( 5.464099601507359516, 6.333536608968757697, 1.199719254218462483 ) ) ;
#115496=CARTESIAN_POINT ( 'NONE',  ( -7.049876689426103127, 10.20831132343037062, -1.082531754730537976 ) ) ;
#115497=CARTESIAN_POINT ( 'NONE',  ( -4.951116456853996262, 6.538279688806403200, -2.442614223628299719 ) ) ;
#115498=CARTESIAN_POINT ( 'NONE',  ( 4.012850279964918165, 7.625483060026979842, -0.7216878364870197293 ) ) ;
#115499=CARTESIAN_POINT ( 'NONE',  ( -6.019457014343129408, 9.966524250134902729, 0.000000000000000000 ) ) ;
#115504=CARTESIAN_POINT ( 'NONE',  ( 7.263417608619159083, 9.497073181520933716, -1.599625672291262513 ) ) ;
#115510=CARTESIAN_POINT ( 'NONE',  ( 0.6823417656249899377, 4.176041667008085767, -1.181850606188754593 ) ) ;
#115514=CARTESIAN_POINT ( 'NONE',  ( 8.457588896826466751, 8.761608555919362828, 1.040834085586084257E-14 ) ) ;
#115517=CARTESIAN_POINT ( 'NONE',  ( -7.641992139597101108, 12.06740792950531649, 0.7998128361456481317 ) ) ;
#115523=CARTESIAN_POINT ( 'NONE',  ( 8.378048858240820351, 11.86180853700128601, -1.199719254218446718 ) ) ;
#115526=CARTESIAN_POINT ( 'NONE',  ( -7.395082721250053837, 10.71501471051202614, -1.199719254218446718 ) ) ;
#115527=EDGE_CURVE ( 'NONE', #91287, #85555, #86670, .T. ) ;
#115530=CARTESIAN_POINT ( 'NONE',  ( 4.433499500630886381, 7.080826916883525612, -1.109343814354251112 ) ) ;
#115531=CARTESIAN_POINT ( 'NONE',  ( -2.578021764892882040, 6.159442492350315490, 0.7998128361456341429 ) ) ;
#115536=CARTESIAN_POINT ( 'NONE',  ( 4.788000803920411386, 8.737751371215816576, 1.040834085586084257E-14 ) ) ;
#115538=CARTESIAN_POINT ( 'NONE',  ( 6.634017235788401301, 6.634108284708264414, 0.7998128361456341429 ) ) ;
#115539=CARTESIAN_POINT ( 'NONE',  ( -4.014242769884851292, 7.626870978312306981, -0.02218799730280621163 ) ) ;
#115540=CARTESIAN_POINT ( 'NONE',  ( 3.225950485047770933, 5.851027101609320269, 1.199719254218450271 ) ) ;
#115542=CARTESIAN_POINT ( 'NONE',  ( -6.995644074971465010, 10.14503993989993091, 1.082531754730549967 ) ) ;
#115548=CARTESIAN_POINT ( 'NONE',  ( -4.015022313999534909, 7.625723350685065682, -0.07359193599470841007 ) ) ;
#115549=CARTESIAN_POINT ( 'NONE',  ( 1.364683531249986537, -0.7822916663252464931, -0.7879004041258309554 ) ) ;
#115552=CARTESIAN_POINT ( 'NONE',  ( 3.551873057100274789, 7.087676300018221021, 0.7216878364870298324 ) ) ;
#115556=CARTESIAN_POINT ( 'NONE',  ( -8.636180661780660017, 11.09863007687603087, -1.443375672974058777 ) ) ;
#115568=CARTESIAN_POINT ( 'NONE',  ( -9.775065565328612038, 10.50659070241261794, -0.7216878364870267237 ) ) ;
#115574=CARTESIAN_POINT ( 'NONE',  ( -1.500000000000013101, 2.410416667349482456, -0.8660254037844313801 ) ) ;
#115580=CARTESIAN_POINT ( 'NONE',  ( -8.995998617867369873, 10.45408546138876993, 1.199719254218462483 ) ) ;
#115584=CARTESIAN_POINT ( 'NONE',  ( 4.449046963578762615, 8.342305224150557308, -0.7998128361456231517 ) ) ;
#115589=CARTESIAN_POINT ( 'NONE',  ( 8.229962938695207342, 9.560377169021284871, 1.199719254218462483 ) ) ;
#115591=CARTESIAN_POINT ( 'NONE',  ( 0.4735722981416969346, 7.464727232010901048, 4.424040350390570531 ) ) ;
#115592=FACE_OUTER_BOUND ( 'NONE', #143215, .T. ) ;
#115596=CARTESIAN_POINT ( 'NONE',  ( -6.724481002698126098, 8.868313807946373473, -1.443375672974059665 ) ) ;
#115606=CARTESIAN_POINT ( 'NONE',  ( -3.267151830768952880, 5.795132321663641228, -1.082531754730549078 ) ) ;
#115608=CARTESIAN_POINT ( 'NONE',  ( 8.615316546479974136, 12.13862083994696839, 1.199719254218450271 ) ) ;
#115610=CARTESIAN_POINT ( 'NONE',  ( -9.775592450653132204, 11.36361159963886891, -1.199719254218441611 ) ) ;
#115611=CYLINDRICAL_SURFACE ( 'NONE', #23650, 0.08000000000000041800 ) ;
#115613=CARTESIAN_POINT ( 'NONE',  ( -1.364683531250012516, 2.738541667008090208, -0.7879004041258289570 ) ) ;
#115614=CARTESIAN_POINT ( 'NONE',  ( 3.310162060030825248, 7.013606170011280838, -0.7998128361456291469 ) ) ;
#115618=CYLINDRICAL_SURFACE ( 'NONE', #145333, 0.08000000000000012657 ) ;
#115619=CARTESIAN_POINT ( 'NONE',  ( 10.37162432432990755, 11.20257592124748136, -0.7216878364870257245 ) ) ;
#115621=CARTESIAN_POINT ( 'NONE',  ( -5.883875478650828050, 9.808345791827219884, 0.7216878364870458196 ) ) ;
#115622=CARTESIAN_POINT ( 'NONE',  ( -0.6823417656250212460, 1.301041667008083547, 1.181850606188755259 ) ) ;
#115626=CARTESIAN_POINT ( 'NONE',  ( -6.832419346282942563, 10.05857410638369487, 1.199719254218453823 ) ) ;
#115627=CARTESIAN_POINT ( 'NONE',  ( -5.558479791478509568, 5.587240632920778438, 0.000000000000000000 ) ) ;
#115628=CARTESIAN_POINT ( 'NONE',  ( 1.364683531249988535, 3.217708333674748289, -0.7879004041258239610 ) ) ;
#115649=CARTESIAN_POINT ( 'NONE',  ( -0.6823417656249969321, 4.280208333674755394, -1.181850606188749264 ) ) ;
#115656=CARTESIAN_POINT ( 'NONE',  ( 7.587759525142423911, 12.00413654597487501, 0.7998128361456462443 ) ) ;
#115660=CARTESIAN_POINT ( 'NONE',  ( 0.6823417656249882723, 2.426041667008084435, -1.181850606188749264 ) ) ;
#115662=CARTESIAN_POINT ( 'NONE',  ( -6.724481002698120768, 9.828683022247721723, -1.082531754730538864 ) ) ;
#115668=CARTESIAN_POINT ( 'NONE',  ( 3.520313441042647540, 7.258782781191745137, 0.7998128361456321445 ) ) ;
#115670=ORIENTED_EDGE ( 'NONE', *, *, #205691, .T. ) ;
#115671=CARTESIAN_POINT ( 'NONE',  ( 7.879259827836241570, 12.34422023245099176, 1.040834085586084257E-14 ) ) ;
#115675=( BOUNDED_CURVE ( )  B_SPLINE_CURVE ( 2, ( #70577, #20768, #202719, #54370, #38118, #11997, #174540 ),
 .UNSPECIFIED., .F., .T. ) 
 B_SPLINE_CURVE_WITH_KNOTS ( ( 3, 2, 2, 3 ),
 ( 0.2624999999999999001, 0.2666666666666666075, 0.2708333333333333148, 0.2750000000000000777 ),
 .UNSPECIFIED. ) 
 CURVE ( )  GEOMETRIC_REPRESENTATION_ITEM ( )  RATIONAL_B_SPLINE_CURVE ( ( 1.000000000000003553, 0.8660254037844351549, 1.000000000000000000, 0.8660254037844387076, 1.000000000000000000, 0.8660254037844369313, 1.000000000000001776 ) ) 
 REPRESENTATION_ITEM ( '' )  );
#115678=CARTESIAN_POINT ( 'NONE',  ( -10.13488352141530768, 11.78278451552804817, 1.199719254218462483 ) ) ;
#115679=CARTESIAN_POINT ( 'NONE',  ( 6.795661308947685164, 8.951357498570873261, -1.599625672291262513 ) ) ;
#115681=CARTESIAN_POINT ( 'NONE',  ( 5.802526556524483681, 5.871961858807763335, 1.040834085586084257E-14 ) ) ;
#115692=CARTESIAN_POINT ( 'NONE',  ( -5.856759171423528088, 8.816340885760650892, 1.082531754730548412 ) ) ;
#115693=CARTESIAN_POINT ( 'NONE',  ( 4.904298879841284098, 6.744767997946721216, 1.599625672291267398 ) ) ;
#115697=CARTESIAN_POINT ( 'NONE',  ( -7.147119532698295252, 11.49005655479003174, 0.000000000000000000 ) ) ;
#115699=CARTESIAN_POINT ( 'NONE',  ( 1.419999999999822515, 7.240846818246208905, 4.154462424328221104 ) ) ;
#115702=CARTESIAN_POINT ( 'NONE',  ( -9.541187415715041809, 12.15447128979948310, -1.599625672291263179 ) ) ;
#115707=CARTESIAN_POINT ( 'NONE',  ( 8.609591239877852686, 10.00327685373437347, -1.199719254218445830 ) ) ;
#115708=CARTESIAN_POINT ( 'NONE',  ( 3.837121167867449945, 4.435395103055503441, 1.199719254218464037 ) ) ;
#115714=CARTESIAN_POINT ( 'NONE',  ( 3.094265954482833703, 2.800000000000017586, -2.490342512183683965 ) ) ;
#115717=CARTESIAN_POINT ( 'NONE',  ( -3.253066792275140173, 5.882662793374543675, 1.199719254218462483 ) ) ;
#115720=CARTESIAN_POINT ( 'NONE',  ( -7.995557903757128493, 10.35123685918189729, 1.599625672291295375 ) ) ;
#115724=CARTESIAN_POINT ( 'NONE',  ( 6.887178846062110615, 9.058127958537705027, -1.443375672974057666 ) ) ;
#115725=CARTESIAN_POINT ( 'NONE',  ( -0.6823417656250212460, 4.863541667008086655, 1.181850606188767472 ) ) ;
#115727=CARTESIAN_POINT ( 'NONE',  ( 2.835626683552519012, 6.459981564119914310, 0.000000000000000000 ) ) ;
#115730=CARTESIAN_POINT ( 'NONE',  ( -7.009729113465285266, 8.136771039586342624, -1.199719254218446718 ) ) ;
#115740=CARTESIAN_POINT ( 'NONE',  ( 0.6823417656249899377, 3.738541667008085767, -1.181850606188754593 ) ) ;
#115741=CARTESIAN_POINT ( 'NONE',  ( 3.741371894207620397, 7.428709027653095376, 2.448389769268505933 ) ) ;
#115742=CARTESIAN_POINT ( 'NONE',  ( 7.716561984472250835, 12.15440608185967086, 1.040834085586084257E-14 ) ) ;
#115744=CARTESIAN_POINT ( 'NONE',  ( -4.121315508874255684, 7.752025827087861920, -0.7216878364870267237 ) ) ;
#115746=CARTESIAN_POINT ( 'NONE',  ( -3.741687207247254676, 7.309126141856352454, 1.040834085586084257E-14 ) ) ;
#115753=CARTESIAN_POINT ( 'NONE',  ( 5.657830175604453338, 5.495223381160312393, 0.7998128361456341429 ) ) ;
#115759=CARTESIAN_POINT ( 'NONE',  ( 1.203907071533389272, 2.962770253743141069, 0.7750000000000100142 ) ) ;
#115762=CARTESIAN_POINT ( 'NONE',  ( 4.517891501851804215, 6.293959390292322986, -1.599625672291255185 ) ) ;
#115767=CARTESIAN_POINT ( 'NONE',  ( -1.364683531249997417, 4.321875000341417028, 1.214306433183764966E-14 ) ) ;
#115772=CARTESIAN_POINT ( 'NONE',  ( 5.452350330990040739, 9.512825819463730070, 0.7998128361456462443 ) ) ;
#115774=CARTESIAN_POINT ( 'NONE',  ( -5.117312914154178216, 8.057616602233474978, -1.199719254218452047 ) ) ;
#115777=CARTESIAN_POINT ( 'NONE',  ( -0.7500000000000215383, 1.941666666666688634, 1.299038105676659116 ) ) ;
#115778=CARTESIAN_POINT ( 'NONE',  ( -3.100010679019018500, 6.768429558830820980, 1.040834085586084257E-14 ) ) ;
#115781=CARTESIAN_POINT ( 'NONE',  ( -5.436983294280064882, 6.301900917203534291, 1.199719254218450271 ) ) ;
#115784=B_SPLINE_CURVE_WITH_KNOTS ( 'NONE', 3,
 ( #73243, #126368, #155588, #206453, #109035, #26641, #207524, #72171, #105807, #175054 ),
 .UNSPECIFIED., .F., .F.,
 ( 4, 2, 2, 2, 4 ),
 ( 0.001944662270655115070, 0.002404849405959078121, 0.002865036541263041824, 0.003325223676567005959, 0.003785410811870969661 ),
 .UNSPECIFIED. ) ;
#115785=CARTESIAN_POINT ( 'NONE',  ( -1.201851678989727383E-14, 3.821875000341423689, 1.575800808251672791 ) ) ;
#115787=CARTESIAN_POINT ( 'NONE',  ( -4.826339496784927796, 5.693446170079573321, 1.082531754730560403 ) ) ;
#115790=ORIENTED_EDGE ( 'NONE', *, *, #126439, .F. ) ;
#115793=CARTESIAN_POINT ( 'NONE',  ( 5.518332215962025167, 6.396807992499198292, -1.199719254218445830 ) ) ;
#115797=CARTESIAN_POINT ( 'NONE',  ( 0.6823417656249882723, 2.988541667008084879, -1.181850606188754593 ) ) ;
#115799=CARTESIAN_POINT ( 'NONE',  ( 3.816783937446950770, 4.411668334231586996, 1.199719254218464037 ) ) ;
#115801=CARTESIAN_POINT ( 'NONE',  ( -1.364683531250014514, 0.5510416670080878765, -0.7879004041258289570 ) ) ;
#115804=EDGE_CURVE ( 'NONE', #178259, #193812, #199347, .T. ) ;
#115806=CARTESIAN_POINT ( 'NONE',  ( -4.135400547368138113, 4.783387712472935149, 1.199719254218462483 ) ) ;
#115807=CARTESIAN_POINT ( 'NONE',  ( -6.033015167956800262, 9.021972881716168402, -1.082531754730537976 ) ) ;
#115811=CARTESIAN_POINT ( 'NONE',  ( -1.364683531249997417, 3.009375000341422801, 1.214306433183764966E-14 ) ) ;
#115820=CARTESIAN_POINT ( 'NONE',  ( -5.517805330637490790, 9.381263952478319013, 0.7216878364870458196 ) ) ;
#115826=CARTESIAN_POINT ( 'NONE',  ( -6.439759776366783761, 8.536139043893143707, 1.443375672974078761 ) ) ;
#115831=DIRECTION ( 'NONE',  ( 2.526156499269438135E-14, 0.6299249119529302110, -0.7766560405360234398 ) ) ;
#115836=ORIENTED_EDGE ( 'NONE', *, *, #99758, .F. ) ;
#115839=CARTESIAN_POINT ( 'NONE',  ( -6.417086777969760902, 6.381022750586497594, 0.7998128361456341429 ) ) ;
#115841=CARTESIAN_POINT ( 'NONE',  ( -1.500000000000015099, -0.5791666666666476226, 0.8660254037844403729 ) ) ;
#115842=CARTESIAN_POINT ( 'NONE',  ( 10.38518247838791986, 11.21839376764850726, 0.7216878364870438212 ) ) ;
#115845=CARTESIAN_POINT ( 'NONE',  ( 6.505214776458575265, 6.483838748823460563, 1.040834085586084257E-14 ) ) ;
#115852=CARTESIAN_POINT ( 'NONE',  ( -2.806174608348664723, 6.217694776474651519, 1.040834085586084257E-14 ) ) ;
#115860=CARTESIAN_POINT ( 'NONE',  ( -1.402160292154681736E-14, 2.446875000341416584, -1.575800808251660134 ) ) ;
#115861=CARTESIAN_POINT ( 'NONE',  ( 9.124274191872634887, 11.66807252865000244, -1.443375672974058777 ) ) ;
#115862=CARTESIAN_POINT ( 'NONE',  ( -8.213542131780492639, 8.476887330032372603, 1.040834085586084257E-14 ) ) ;
#115865=CARTESIAN_POINT ( 'NONE',  ( 6.632963465583686435, 8.761543347979550589, -1.599625672291262513 ) ) ;
#115866=CARTESIAN_POINT ( 'NONE',  ( -6.738566041191992539, 7.820414121934134322, 1.199719254218450271 ) ) ;
#115869=CARTESIAN_POINT ( 'NONE',  ( -0.7500000000000249800, -0.5270833326505158789, 1.299038105676659116 ) ) ;
#115873=CARTESIAN_POINT ( 'NONE',  ( 7.104109303880752790, 11.23195192126214970, -0.7216878364870267237 ) ) ;
#115876=CARTESIAN_POINT ( 'NONE',  ( 0.6823417656249882723, 0.1552083336747514530, 1.181850606188755259 ) ) ;
#115878=CARTESIAN_POINT ( 'NONE',  ( 6.927853306458749749, 8.145212281365775908, 1.082531754730558626 ) ) ;
#115880=CARTESIAN_POINT ( 'NONE',  ( -4.475070042639309520, 5.445751865460756846, 1.284222742053057642 ) ) ;
#115882=CARTESIAN_POINT ( 'NONE',  ( -4.528060117284246289, 6.305822774963486310, 1.443375672974064550 ) ) ;
#115884=CARTESIAN_POINT ( 'NONE',  ( 1.364683531249990311, 4.634375000341417916, 1.214306433183764966E-14 ) ) ;
#115888=CARTESIAN_POINT ( 'NONE',  ( -5.768665591941109838, 6.232869020846472097, -1.039980349891131972 ) ) ;
#115894=CARTESIAN_POINT ( 'NONE',  ( 8.132193210098487057, 8.381980254736715708, 1.040834085586084257E-14 ) ) ;
#115897=CARTESIAN_POINT ( 'NONE',  ( 2.822068529938852155, 6.444163718237301275, -0.7998128361456291469 ) ) ;
#115904=CARTESIAN_POINT ( 'NONE',  ( 5.883875478650832491, 6.927238148923188454, -1.082531754730543083 ) ) ;
#115905=CARTESIAN_POINT ( 'NONE',  ( 0.6823417656249882723, 0.9885416670080832136, -1.181850606188749264 ) ) ;
#115909=CARTESIAN_POINT ( 'NONE',  ( 2.482948226198860464, 5.072301959192136778, 2.420000000000000373 ) ) ;
#115910=DIRECTION ( 'NONE',  ( 0.000000000000000000, 0.000000000000000000, -1.000000000000000000 ) ) ;
#115912=CARTESIAN_POINT ( 'NONE',  ( 0.7499999999999902300, 1.733333333333357595, 1.299038105676657340 ) ) ;
#115913=CARTESIAN_POINT ( 'NONE',  ( 5.991813822235618758, 9.077867661661846554, 1.199719254218462483 ) ) ;
#115914=CARTESIAN_POINT ( 'NONE',  ( -8.701635661872465732, 9.046329781806354831, 1.040834085586084257E-14 ) ) ;
#115918=CARTESIAN_POINT ( 'NONE',  ( -1.364683531250012516, 1.030208333674754062, 0.7879004041258379498 ) ) ;
#115919=CARTESIAN_POINT ( 'NONE',  ( 0.7499999999999902300, 2.483333333333351156, 1.299038105676669330 ) ) ;
#115922=CARTESIAN_POINT ( 'NONE',  ( 4.578903193113299963, 6.365139696764064325, 1.599625672291267398 ) ) ;
#115929=CARTESIAN_POINT ( 'NONE',  ( -0.7500000000000006661, -1.110416665983847473, -1.299038105676652011 ) ) ;
#115930=CARTESIAN_POINT ( 'NONE',  ( -7.182068686937172153, 9.402166106225269715, 1.599625672291283607 ) ) ;
#115931=CARTESIAN_POINT ( 'NONE',  ( -4.528060117284246289, 6.305822774963486310, 1.443375672974064550 ) ) ;
#115940=CARTESIAN_POINT ( 'NONE',  ( 5.289652487626049115, 9.323011668872403845, 0.7998128361456462443 ) ) ;
#115944=CARTESIAN_POINT ( 'NONE',  ( 5.273758565591489145, 9.096542726591325234, -0.7216878364870267237 ) ) ;
#115948=CARTESIAN_POINT ( 'NONE',  ( -8.179646747746328828, 8.437342715325849341, -0.7998128361456291469 ) ) ;
#115949=CARTESIAN_POINT ( 'NONE',  ( 3.734381245560244089, 6.444196322207211836, 1.199719254218462483 ) ) ;
#115952=CARTESIAN_POINT ( 'NONE',  ( 1.499999999999990896, 4.025000000000021672, 1.214306433183764966E-14 ) ) ;
#115954=CARTESIAN_POINT ( 'NONE',  ( 3.996677956334552029, 7.600660605679141035, 0.1064861495668877750 ) ) ;
#115955=CARTESIAN_POINT ( 'NONE',  ( 9.029367117021314115, 12.51771682229149008, -1.082531754730543083 ) ) ;
#115963=CARTESIAN_POINT ( 'NONE',  ( -1.534404370307023369, 8.695807324171010322, -2.514078760162028470 ) ) ;
#115964=CARTESIAN_POINT ( 'NONE',  ( -4.934804725694236893, 4.859619722839116918, -0.7216878364870207285 ) ) ;
#115965=AXIS2_PLACEMENT_3D ( 'NONE', #70330, #6401, #72473 ) ;
#115966=CARTESIAN_POINT ( 'NONE',  ( 8.432808358020016826, 10.86136238915529084, 1.443375672974076540 ) ) ;
#115970=CARTESIAN_POINT ( 'NONE',  ( -6.227272627378437342, 6.159572908229946187, -0.7998128361456291469 ) ) ;
#115975=CARTESIAN_POINT ( 'NONE',  ( -6.612626235163205024, 8.737816579155630592, -1.599625672291263179 ) ) ;
#115979=CARTESIAN_POINT ( 'NONE',  ( 5.551071401176296938, 6.352922844458268159, -1.167898382037794613 ) ) ;
#115990=CARTESIAN_POINT ( 'NONE',  ( -6.891622154448065807, 6.934647356477856128, 1.040834085586084257E-14 ) ) ;
#115993=CARTESIAN_POINT ( 'NONE',  ( 4.284013352238246419, 6.021101549076499637, -1.443375672974051449 ) ) ;
#115998=CARTESIAN_POINT ( 'NONE',  ( -5.447678794592645701, 5.250046769979851646, 0.000000000000000000 ) ) ;
#116002=COLOUR_RGB ( '', 0.72549020, 0.75294118, 0.79215686) ;
#116006=CARTESIAN_POINT ( 'NONE',  ( -8.690940161559884913, 10.09818392903003748, 1.199719254218462483 ) ) ;
#116007=CARTESIAN_POINT ( 'NONE',  ( 7.122110765880372618, 7.203550736482235095, 0.7998128361456341429 ) ) ;
#116009=CARTESIAN_POINT ( 'NONE',  ( -6.997979842947967377, 11.31606025008131233, -0.7998128361456291469 ) ) ;
#116014=CARTESIAN_POINT ( 'NONE',  ( -0.6823417656250246877, -0.6364583329919113464, 1.181850606188755259 ) ) ;
#116017=CARTESIAN_POINT ( 'NONE',  ( 7.619319141200057821, 10.87266085050000974, 1.082531754730557072 ) ) ;
#116035=CARTESIAN_POINT ( 'NONE',  ( -4.322352044658376968, 3.937165561723182883, 0.7998128361456341429 ) ) ;
#116042=CARTESIAN_POINT ( 'NONE',  ( 1.499999999999987121, 0.7854166673494828999, 0.8660254037844524744 ) ) ;
#116047=CARTESIAN_POINT ( 'NONE',  ( 0.4545465019492176406, 7.933486811681471629, -1.993247486878108266 ) ) ;
#116048=CARTESIAN_POINT ( 'NONE',  ( 3.023105066167310895, 5.702484939155337607, 2.500000000000000444 ) ) ;
#116049=CARTESIAN_POINT ( 'NONE',  ( 7.892817981449907982, 12.36003807833360391, 0.7998128361456462443 ) ) ;
#116053=CARTESIAN_POINT ( 'NONE',  ( 3.486418057008484617, 7.219238166485217434, 1.040834085586084257E-14 ) ) ;
#116054=CARTESIAN_POINT ( 'NONE',  ( -6.209271165378811297, 10.18797409300986878, 0.7216878364870458196 ) ) ;
#116058=CARTESIAN_POINT ( 'NONE',  ( -6.184490626128011925, 10.36698949712469364, -0.7998128361456291469 ) ) ;
#116059=CARTESIAN_POINT ( 'NONE',  ( -3.755245360860931303, 5.404205559136275205, -1.443375672974051449 ) ) ;
#116062=CARTESIAN_POINT ( 'NONE',  ( 1.499999999999987121, 0.5770833340161539704, -0.8660254037844253849 ) ) ;
#116069=CARTESIAN_POINT ( 'NONE',  ( -4.243338890952904841, 5.973648010910253880, -1.443375672974051449 ) ) ;
#116076=CARTESIAN_POINT ( 'NONE',  ( -9.561524646135538319, 12.17819805862340310, -1.599625672291263179 ) ) ;
#116077=CARTESIAN_POINT ( 'NONE',  ( 8.289920859751990889, 11.75899253876431416, 1.199719254218450271 ) ) ;
#116080=CARTESIAN_POINT ( 'NONE',  ( 1.500000000000013545, 5.254166666666685970, 0.8660254037844385966 ) ) ;
#116082=VERTEX_POINT ( 'NONE', #203608 ) ;
#116086=CARTESIAN_POINT ( 'NONE',  ( -8.459397779922852578, 11.95671561229694824, 1.199719254218453823 ) ) ;
#116091=CARTESIAN_POINT ( 'NONE',  ( 3.655894977179307226, 7.416961240017848844, -0.7998128361456291469 ) ) ;
#116109=CARTESIAN_POINT ( 'NONE',  ( 6.958359152311676787, 9.141171649162195934, -1.599625672291262513 ) ) ;
#116112=CARTESIAN_POINT ( 'NONE',  ( -4.406563619641430840, 5.099744630125142564, -1.199719254218446718 ) ) ;
#116121=CARTESIAN_POINT ( 'NONE',  ( -1.364683531250010295, 5.530208333674751842, 0.7879004041258379498 ) ) ;
#116125=CARTESIAN_POINT ( 'NONE',  ( 1.273556527089495960, 3.289757214169906074, 0.7750000000000135669 ) ) ;
#116126=CARTESIAN_POINT ( 'NONE',  ( 4.162516854595432747, 4.815023404238158555, 1.199719254218464037 ) ) ;
#116128=CARTESIAN_POINT ( 'NONE',  ( -4.620631424159025613, 4.285158171140619032, -0.7998128361456221525 ) ) ;
#116134=CARTESIAN_POINT ( 'NONE',  ( 5.178851490740193242, 8.025448591630130579, 1.082531754730558626 ) ) ;
#116137=CARTESIAN_POINT ( 'NONE',  ( 7.063434842595398777, 11.18449838309590483, -0.7216878364870267237 ) ) ;
#116138=CARTESIAN_POINT ( 'NONE',  ( 1.364683531249988535, 4.967708333674756283, -0.7879004041258300672 ) ) ;
#116140=CARTESIAN_POINT ( 'NONE',  ( 4.650083499362880346, 4.527444958785877382, 0.7216878364870317197 ) ) ;
#116148=CARTESIAN_POINT ( 'NONE',  ( -5.958637689794747949, 6.108898536480521280, 0.7553493914738591553 ) ) ;
#116152=CARTESIAN_POINT ( 'NONE',  ( -1.201851678989727383E-14, 5.509375000341415252, -1.575800808251660134 ) ) ;
#116159=CARTESIAN_POINT ( 'NONE',  ( -0.7500000000000006661, -0.8916666666666448471, -1.299038105676652011 ) ) ;
#116168=CARTESIAN_POINT ( 'NONE',  ( -0.6823417656250212460, 4.863541667008086655, 1.181850606188767472 ) ) ;
#116170=CARTESIAN_POINT ( 'NONE',  ( 6.257251587906815793, 7.258880593101466161, 1.199719254218462483 ) ) ;
#116171=CARTESIAN_POINT ( 'NONE',  ( -9.989660255170729641, 10.54902514065433827, -0.7998128361456291469 ) ) ;
#116175=CARTESIAN_POINT ( 'NONE',  ( -3.945059511896602089, 7.546393830613923548, 1.040834085586084257E-14 ) ) ;
#116176=VERTEX_POINT ( 'NONE', #122487 ) ;
#116178=CARTESIAN_POINT ( 'NONE',  ( 0.7499999999999902300, 5.566666666666685082, -1.299038105676658228 ) ) ;
#116187=CARTESIAN_POINT ( 'NONE',  ( 8.324343129110697959, 9.774450407793066731, -1.082531754730543083 ) ) ;
#116192=CARTESIAN_POINT ( 'NONE',  ( -1.201851678989727383E-14, 3.618750000682816381, -1.732050807568863648 ) ) ;
#116194=CARTESIAN_POINT ( 'NONE',  ( -4.069418662396130593, 7.899405539437467816, -0.7998128361456281477 ) ) ;
#116195=CARTESIAN_POINT ( 'NONE',  ( 3.185802909086945967, 5.700225246367978116, 1.082531754730546636 ) ) ;
#116203=CARTESIAN_POINT ( 'NONE',  ( 3.009020027229115879, 5.597941567487558778, -1.199719254218446718 ) ) ;
#116207=CARTESIAN_POINT ( 'NONE',  ( -1.500000000000021982, 7.809273069926255140, 3.635729725621167141 ) ) ;
#116208=CARTESIAN_POINT ( 'NONE',  ( 5.854423403002611437, 5.724582146458163656, 1.040834085586084257E-14 ) ) ;
#116210=ORIENTED_EDGE ( 'NONE', *, *, #52332, .F. ) ;
#116218=DIRECTION ( 'NONE',  ( 0.000000000000000000, -0.7999999999999973799, 0.6000000000000034195 ) ) ;
#116219=CARTESIAN_POINT ( 'NONE',  ( 5.863316726098953602, 5.994608360591326068, -0.2888550730815123702 ) ) ;
#116221=CARTESIAN_POINT ( 'NONE',  ( 9.622536337397022521, 12.24937836509514710, 1.599625672291281386 ) ) ;
#116225=CARTESIAN_POINT ( 'NONE',  ( 6.480434237652132445, 7.623223367758051872, 1.082531754730558626 ) ) ;
#116227=CARTESIAN_POINT ( 'NONE',  ( -9.991996023591624976, 10.75967623705280296, 1.040834085586084257E-14 ) ) ;
#116233=CARTESIAN_POINT ( 'NONE',  ( -3.253066792275140173, 5.882662793374543675, 1.199719254218462483 ) ) ;
#116237=ORIENTED_EDGE ( 'NONE', *, *, #66344, .F. ) ;
#116246=CARTESIAN_POINT ( 'NONE',  ( 6.075519867480115188, 6.040327746143013599, 0.3625371965378897388 ) ) ;
#116251=CARTESIAN_POINT ( 'NONE',  ( 3.472859903394816872, 7.203420320602605287, -0.7998128361456291469 ) ) ;
#116255=CARTESIAN_POINT ( 'NONE',  ( -9.503902493499651882, 10.19023378527882784, 1.040834085586084257E-14 ) ) ;
#116259=CARTESIAN_POINT ( 'NONE',  ( 6.588372581236919601, 9.773852880496709972, -1.199719254218440723 ) ) ;
#116260=CARTESIAN_POINT ( 'NONE',  ( -5.596818484342970912, 5.424043074688561283, -0.7998128361456221525 ) ) ;
#116262=CARTESIAN_POINT ( 'NONE',  ( -6.098470168048611306, 6.009303372345148553, 1.040834085586084257E-14 ) ) ;
#116263=CARTESIAN_POINT ( 'NONE',  ( 4.369805582306193870, 3.992528022312320957, 1.214306433183764966E-14 ) ) ;
#116265=CARTESIAN_POINT ( 'NONE',  ( -6.240830780992103755, 6.175390754112560110, 1.040834085586084257E-14 ) ) ;
#116270=CARTESIAN_POINT ( 'NONE',  ( 8.860417081730671995, 10.29590700256267155, 1.199719254218453823 ) ) ;
#116273=CARTESIAN_POINT ( 'NONE',  ( 4.626207451132414938, 6.895778996938287442, -1.211788453915439989 ) ) ;
#116274=CARTESIAN_POINT ( 'NONE',  ( 4.690757960648213931, 8.416375354157496602, 0.7216878364870438212 ) ) ;
#116278=DIRECTION ( 'NONE',  ( 5.176899690512889973E-31, -0.5999999999999999778, 0.8000000000000000444 ) ) ;
#116280=EDGE_LOOP ( 'NONE', ( #161293, #196342, #157722, #154065 ) ) ;
#116281=CARTESIAN_POINT ( 'NONE',  ( 7.578644679914713578, 8.904468883731073703, 1.082531754730558626 ) ) ;
#116285=CARTESIAN_POINT ( 'NONE',  ( -7.853197290813634268, 10.18514947741448573, 1.599625672291295375 ) ) ;
#116289=FACE_OUTER_BOUND ( 'NONE', #71826, .T. ) ;
#116290=CARTESIAN_POINT ( 'NONE',  ( 0.007772928215642942867, 8.279395425053875712, 2.079985476292312008 ) ) ;
#116293=CARTESIAN_POINT ( 'NONE',  ( 2.218730694130720771, 5.740269576461138890, 0.7998128361456462443 ) ) ;
#116297=CARTESIAN_POINT ( 'NONE',  ( 3.337278367258157630, 7.045241861776501580, 0.7998128361456341429 ) ) ;
#116300=AXIS2_PLACEMENT_3D ( 'NONE', #144894, #81973, #210902 ) ;
#116301=CARTESIAN_POINT ( 'NONE',  ( 0.7499999999999920064, 4.764583334016150751, 1.299038105676669330 ) ) ;
#116307=CARTESIAN_POINT ( 'NONE',  ( 0.7499999999999902300, 1.483333333333357373, 1.299038105676657340 ) ) ;
#116308=CARTESIAN_POINT ( 'NONE',  ( 5.777746017718023097, 9.892454120646377191, 0.7998128361456462443 ) ) ;
#116309=CARTESIAN_POINT ( 'NONE',  ( 4.080641047588898118, 5.783833860318930320, -1.443375672974051449 ) ) ;
#116311=CARTESIAN_POINT ( 'NONE',  ( 9.246297574839983824, 9.889694713509232571, 0.7216878364870438212 ) ) ;
#116317=CARTESIAN_POINT ( 'NONE',  ( -4.229253852459088137, 7.021547696922494808, 1.199719254218464037 ) ) ;
#116318=CARTESIAN_POINT ( 'NONE',  ( -1.500000000000013101, 3.410416667349487785, -0.8660254037844313801 ) ) ;
#116319=CARTESIAN_POINT ( 'NONE',  ( -1.402160292154681736E-14, -0.6781249996585819728, 1.575800808251672791 ) ) ;
#116323=CARTESIAN_POINT ( 'NONE',  ( 4.416205349749311004, 6.175325546172740765, 1.599625672291267398 ) ) ;
#116325=CARTESIAN_POINT ( 'NONE',  ( 1.364683531249990311, 5.176041667008085767, 0.7879004041258500513 ) ) ;
#116328=VECTOR ( 'NONE', #15713, 1000.000000000000000 ) ;
#116334=CARTESIAN_POINT ( 'NONE',  ( -8.376239975144482486, 8.666701480623698828, 1.040834085586084257E-14 ) ) ;
#116335=CARTESIAN_POINT ( 'NONE',  ( 5.789495288235341874, 6.713164910151406595, 1.199719254218462483 ) ) ;
#116338=CARTESIAN_POINT ( 'NONE',  ( 1.364683531249986537, -0.09479166632524321789, -0.7879004041258309554 ) ) ;
#116344=CARTESIAN_POINT ( 'NONE',  ( -5.856232286098998152, 8.919689202835742847, 1.199719254218452047 ) ) ;
#116347=EDGE_CURVE ( 'NONE', #30182, #62722, #150237, .T. ) ;
#116348=CARTESIAN_POINT ( 'NONE',  ( 10.37606763316019531, 10.99983374830873650, 0.7998128361456462443 ) ) ;
#116350=CARTESIAN_POINT ( 'NONE',  ( 9.673906298550626559, 11.24497775551929557, 1.199719254218452047 ) ) ;
#116352=CARTESIAN_POINT ( 'NONE',  ( -3.358669367883384105, 4.941533567329135401, -1.599625672291262513 ) ) ;
#116354=CARTESIAN_POINT ( 'NONE',  ( -6.808165692356648258, 11.09461040772476714, 0.7998128361456481317 ) ) ;
#116357=CARTESIAN_POINT ( 'NONE',  ( -4.232483270035822365, 7.525443216328503659, 1.020073867034466675 ) ) ;
#116358=CARTESIAN_POINT ( 'NONE',  ( 1.364683531249986537, -0.09479166632524321789, -0.7879004041258309554 ) ) ;
#116362=CARTESIAN_POINT ( 'NONE',  ( 9.259855728453651125, 9.905512559391842942, 1.040834085586084257E-14 ) ) ;
#116365=CARTESIAN_POINT ( 'NONE',  ( 4.008406971134620633, 7.828225232965717595, 0.7998128361456321445 ) ) ;
#116366=EDGE_CURVE ( 'NONE', #179068, #45871, #202889, .T. ) ;
#116383=DIRECTION ( 'NONE',  ( -0.7592566023652990159, -0.6507913734559659380, 0.000000000000000000 ) ) ;
#116387=CARTESIAN_POINT ( 'NONE',  ( -3.750802052474980108, 7.527686161196117887, 1.040834085586084257E-14 ) ) ;
#116393=CARTESIAN_POINT ( 'NONE',  ( 0.7499999999999885647, 2.847916667349487341, -1.299038105676658228 ) ) ;
#116394=CARTESIAN_POINT ( 'NONE',  ( 7.214910300766615769, 11.56914578420308715, -0.7998128361456291469 ) ) ;
#116399=CARTESIAN_POINT ( 'NONE',  ( -8.829384350997580455, 11.32403438096243775, 1.599625672291269396 ) ) ;
#116401=CARTESIAN_POINT ( 'NONE',  ( 1.364683531249986537, 2.655208333674754062, -0.7879004041258239610 ) ) ;
#116408=CARTESIAN_POINT ( 'NONE',  ( -2.819205876637805641, 5.376491725131008259, -1.199719254218446718 ) ) ;
#116412=CARTESIAN_POINT ( 'NONE',  ( -1.364683531250000748, 1.821875000341421913, 0.000000000000000000 ) ) ;
#116417=CARTESIAN_POINT ( 'NONE',  ( 0.6823417656249882723, 2.176041667008084435, -1.181850606188749264 ) ) ;
#116419=CARTESIAN_POINT ( 'NONE',  ( -6.063521013809733518, 8.097193820909906137, 1.599625672291283607 ) ) ;
#116420=CARTESIAN_POINT ( 'NONE',  ( 8.426556166093362776, 9.789735934319136135, -1.199719254218446718 ) ) ;
#116421=CARTESIAN_POINT ( 'NONE',  ( 0.000000000000000000, 8.600000000000017408, 0.4000000000000045186 ) ) ;
#116423=CARTESIAN_POINT ( 'NONE',  ( 1.499999999999987121, 4.295833333333352044, -0.8660254037844323793 ) ) ;
#116424=CARTESIAN_POINT ( 'NONE',  ( -0.6823417656250212460, 2.863541667008084879, 1.181850606188767472 ) ) ;
#116431=CARTESIAN_POINT ( 'NONE',  ( 6.317736394288140822, 7.433409217166723870, 1.082531754730558626 ) ) ;
#116434=CARTESIAN_POINT ( 'NONE',  ( -9.677822722056413696, 10.18521468535430685, 1.040834085586084257E-14 ) ) ;
#116435=CARTESIAN_POINT ( 'NONE',  ( -3.952365473583647315, 4.569846793057691592, 1.199719254218462483 ) ) ;
#116436=CARTESIAN_POINT ( 'NONE',  ( -1.001543065824772872E-14, 5.321875000341422357, 1.575800808251672791 ) ) ;
#116441=CARTESIAN_POINT ( 'NONE',  ( -7.171900071504745178, 9.390302721554109056, -1.443375672974058777 ) ) ;
#116443=CARTESIAN_POINT ( 'NONE',  ( -1.499999999999997780, 4.650000000000022560, 1.214306433183764966E-14 ) ) ;
#116446=CARTESIAN_POINT ( 'NONE',  ( 7.863365906246055914, 10.19701286208565705, -1.443375672974057666 ) ) ;
#116452=CARTESIAN_POINT ( 'NONE',  ( 2.521453382017309952, 5.885520012421409319, 0.000000000000000000 ) ) ;
#116453=CIRCLE ( 'NONE', #192453, 0.08000000000000020983 ) ;
#116455=VERTEX_POINT ( 'NONE', #94182 ) ;
#116456=CARTESIAN_POINT ( 'NONE',  ( 7.714226216051361718, 11.94375498546120795, -0.7216878364870267237 ) ) ;
#116462=EDGE_LOOP ( 'NONE', ( #5986, #48939, #101506, #127467 ) ) ;
#116464=CARTESIAN_POINT ( 'NONE',  ( 5.438792177376376991, 9.497007973581119700, 1.040834085586084257E-14 ) ) ;
#116465=CARTESIAN_POINT ( 'NONE',  ( -5.901876940650454095, 5.779944607047298177, -0.7998128361456291469 ) ) ;
#116469=CARTESIAN_POINT ( 'NONE',  ( 5.707619481228810798, 7.681975366232176583, -1.443375672974057666 ) ) ;
#116470=CARTESIAN_POINT ( 'NONE',  ( -1.364683531250000748, 0.07187500034142035865, 0.000000000000000000 ) ) ;
#116471=CARTESIAN_POINT ( 'NONE',  ( 2.412988153552339643, 5.758977245878946327, 0.7216878364870438212 ) ) ;
#116472=CARTESIAN_POINT ( 'NONE',  ( -8.299562589859897699, 12.83457345481192036, -0.7998128361456281477 ) ) ;
#116484=EDGE_CURVE ( 'NONE', #184579, #58494, #31491, .T. ) ;
#116487=ORIENTED_EDGE ( 'NONE', *, *, #60399, .F. ) ;
#116491=CARTESIAN_POINT ( 'NONE',  ( 5.784525094524856748, 9.900363043587685041, 1.040834085586084257E-14 ) ) ;
#116492=CARTESIAN_POINT ( 'NONE',  ( 5.784525094524856748, 9.900363043587685041, 1.040834085586084257E-14 ) ) ;
#116500=CARTESIAN_POINT ( 'NONE',  ( -2.474587689922123523, 5.184834355512716542, 0.9403128211546022408 ) ) ;
#116502=CARTESIAN_POINT ( 'NONE',  ( -4.564291269294938225, 8.476756914152748124, 1.040834085586084257E-14 ) ) ;
#116503=CARTESIAN_POINT ( 'NONE',  ( -3.928111819657352566, 5.605883094398769195, 1.599625672291267398 ) ) ;
#116513=CARTESIAN_POINT ( 'NONE',  ( -4.274898507010545856, 3.881803101134051470, -0.7998128361456221525 ) ) ;
#116516=CARTESIAN_POINT ( 'NONE',  ( 5.286789834324991055, 8.255339675766103724, -1.199719254218452935 ) ) ;
#116517=CARTESIAN_POINT ( 'NONE',  ( -1.364683531249997417, 4.009375000341424133, 1.214306433183764966E-14 ) ) ;
#116522=CARTESIAN_POINT ( 'NONE',  ( 3.348500752450929596, 6.850408611260650815, 0.7216878364870317197 ) ) ;
#116523=CARTESIAN_POINT ( 'NONE',  ( -7.379715684540041565, 7.504089808251839244, 1.040834085586084257E-14 ) ) ;
#116525=VERTEX_POINT ( 'NONE', #20356 ) ;
#116529=CARTESIAN_POINT ( 'NONE',  ( -8.532158741701643123, 8.848606708273724308, 0.7998128361456462443 ) ) ;
#116531=CARTESIAN_POINT ( 'NONE',  ( -5.759516327706961647, 5.613857225279885732, -0.7998128361456221525 ) ) ;
#116538=CARTESIAN_POINT ( 'NONE',  ( 6.745345117998789775, 7.828323044875442172, 1.199719254218462483 ) ) ;
#116549=VERTEX_POINT ( 'NONE', #164486 ) ;
#116551=CARTESIAN_POINT ( 'NONE',  ( 1.499999999999989120, 5.795833333333350268, -0.8660254037844323793 ) ) ;
#116552=CARTESIAN_POINT ( 'NONE',  ( 4.546061579283848353, 4.198160018786257552, -0.7998128361456211532 ) ) ;
#116553=CARTESIAN_POINT ( 'NONE',  ( 4.547870462380197765, 7.393267075163835855, 1.199719254218462483 ) ) ;
#116555=CARTESIAN_POINT ( 'NONE',  ( -8.215877900201387973, 8.687538426430837291, 0.7216878364870578100 ) ) ;
#116558=CARTESIAN_POINT ( 'NONE',  ( 5.721177635286841756, 6.737423998331861341, -1.082531754730543083 ) ) ;
#116559=CARTESIAN_POINT ( 'NONE',  ( -8.798878505144658746, 10.32807501316600884, -1.082531754730543083 ) ) ;
#116563=CARTESIAN_POINT ( 'NONE',  ( 8.260995669428309540, 8.532249790621511565, 0.7998128361456481317 ) ) ;
#116567=CARTESIAN_POINT ( 'NONE',  ( -0.6823417656250212460, 3.301041667008085323, 1.181850606188767472 ) ) ;
#116573=CARTESIAN_POINT ( 'NONE',  ( 8.444030743212801227, 8.745790710036752458, 0.7998128361456462443 ) ) ;
#116577=CARTESIAN_POINT ( 'NONE',  ( -9.203287345578106127, 9.631590079462940324, 0.7998128361456462443 ) ) ;
#116583=CARTESIAN_POINT ( 'NONE',  ( 8.052653171512838881, 11.48218023581863001, -1.199719254218446718 ) ) ;
#116586=CARTESIAN_POINT ( 'NONE',  ( -8.097244055859620815, 10.46987070330147063, -1.599625672291263179 ) ) ;
#116589=CARTESIAN_POINT ( 'NONE',  ( 0.5988051026822670542, 6.720402535194986982, 3.593870046926598061 ) ) ;
#116592=CARTESIAN_POINT ( 'NONE',  ( 4.952123820727618586, 6.619828698506379006, -1.244621138126526194 ) ) ;
#116593=CARTESIAN_POINT ( 'NONE',  ( -2.605138072120212200, 6.191078184115536232, -0.7998128361456281477 ) ) ;
#116598=CARTESIAN_POINT ( 'NONE',  ( 6.089583550832340819, 10.25626457594641749, 1.040834085586084257E-14 ) ) ;
#116600=CARTESIAN_POINT ( 'NONE',  ( 4.625302960556422427, 8.547937220624488575, 1.040834085586084257E-14 ) ) ;
#116601=CARTESIAN_POINT ( 'NONE',  ( -4.061901113999940804, 7.558576442610514867, -0.4421990992426305112 ) ) ;
#116602=CARTESIAN_POINT ( 'NONE',  ( 3.174580523894166006, 6.855427711185178019, 0.7998128361456341429 ) ) ;
#116605=CARTESIAN_POINT ( 'NONE',  ( -7.375272376154093479, 9.627570410311676596, -1.443375672974059665 ) ) ;
#116612=CARTESIAN_POINT ( 'NONE',  ( -4.014242769884851292, 7.626870978312306981, -0.02218799730280621163 ) ) ;
#116613=CARTESIAN_POINT ( 'NONE',  ( -1.364683531250014514, -0.9072916663252470482, 0.7879004041258379498 ) ) ;
#116615=CARTESIAN_POINT ( 'NONE',  ( 4.033180945112804672, 7.763139070050654844, 0.4071004073024475090 ) ) ;
#116616=CARTESIAN_POINT ( 'NONE',  ( 5.883875478650832491, 6.927238148923188454, -1.082531754730543083 ) ) ;
#116619=EDGE_CURVE ( 'NONE', #135381, #116549, #81704, .T. ) ;
#116627=CARTESIAN_POINT ( 'NONE',  ( -8.459924664802993988, 12.81373650900478189, 1.040834085586084257E-14 ) ) ;
#116633=CARTESIAN_POINT ( 'NONE',  ( -9.341204649691320583, 10.96078884847042545, 1.082531754730558626 ) ) ;
#116641=CARTESIAN_POINT ( 'NONE',  ( 1.499999999999989120, 2.556250000682817713, 1.214306433183764966E-14 ) ) ;
#116643=CARTESIAN_POINT ( 'NONE',  ( -5.045605722580076780, 9.038290442985410067, -0.7998128361456231517 ) ) ;
#116646=CARTESIAN_POINT ( 'NONE',  ( -8.025536864285518490, 11.45054454405341282, -1.199719254218446718 ) ) ;
#116649=CARTESIAN_POINT ( 'NONE',  ( 6.474182045725470402, 7.511966127223233869, -1.199719254218446718 ) ) ;
#116654=CARTESIAN_POINT ( 'NONE',  ( 8.585337585951586803, 11.03931315507545108, -1.599625672291255185 ) ) ;
#116656=CARTESIAN_POINT ( 'NONE',  ( 1.403499169902377552, 7.376709478543040710, 4.304123474984470121 ) ) ;
#116657=DIRECTION ( 'NONE',  ( 0.7592566023653005702, 0.6507913734559639396, 0.000000000000000000 ) ) ;
#116660=CARTESIAN_POINT ( 'NONE',  ( -7.863365906246068349, 9.236643647784308797, -1.082531754730543971 ) ) ;
#116663=CARTESIAN_POINT ( 'NONE',  ( -0.6823417656249969321, 5.280208333674756283, -1.181850606188749264 ) ) ;
#116669=CARTESIAN_POINT ( 'NONE',  ( -8.482597663644387609, 13.04811437422715414, -0.7998128361456281477 ) ) ;
#116671=CARTESIAN_POINT ( 'NONE',  ( 9.531545685607134999, 11.07889037375188401, 1.199719254218450271 ) ) ;
#116673=DIRECTION ( 'NONE',  ( -0.6507913734559640506, -0.7592566023653004592, 0.000000000000000000 ) ) ;
#116676=CARTESIAN_POINT ( 'NONE',  ( 0.6823417656249899377, 1.592708333674752730, 1.181850606188755259 ) ) ;
#116678=CARTESIAN_POINT ( 'NONE',  ( 4.416205349749311004, 6.175325546172740765, 1.599625672291267398 ) ) ;
#116684=DIRECTION ( 'NONE',  ( -5.578564026256490882E-16, -1.000000000000000000, -9.066213480720158442E-32 ) ) ;
#116685=CARTESIAN_POINT ( 'NONE',  ( 9.720832950873944611, 10.44331931888218001, -0.7216878364870257245 ) ) ;
#116687=CARTESIAN_POINT ( 'NONE',  ( -7.863365906246074566, 8.276274433482971205, -0.7216878364870278340 ) ) ;
#116690=CARTESIAN_POINT ( 'NONE',  ( 0.007473969438115558167, 8.279395425053873936, 1.999986034896453324 ) ) ;
#116692=CARTESIAN_POINT ( 'NONE',  ( -6.320072162264675164, 10.52516795595079557, 0.7998128361456481317 ) ) ;
#116693=CARTESIAN_POINT ( 'NONE',  ( -5.070386261386537363, 5.017798181146802428, 1.214306433183764966E-14 ) ) ;
#116694=CARTESIAN_POINT ( 'NONE',  ( 1.364683531249990311, 3.196875000341416140, 1.214306433183764966E-14 ) ) ;
#116699=CARTESIAN_POINT ( 'NONE',  ( 9.856941372335116469, 11.45851867493453291, 1.199719254218450271 ) ) ;
#116715=CARTESIAN_POINT ( 'NONE',  ( 1.364683531249988535, 4.176041667008081326, 0.7879004041258500513 ) ) ;
#116722=CARTESIAN_POINT ( 'NONE',  ( 7.899597058256738968, 12.36794700127490820, 1.040834085586084257E-14 ) ) ;
#116725=CARTESIAN_POINT ( 'NONE',  ( -0.6823417656250212460, 3.051041667008084879, 1.181850606188767472 ) ) ;
#116727=CARTESIAN_POINT ( 'NONE',  ( -6.222829318992474157, 10.20379193889247382, 0.000000000000000000 ) ) ;
#116730=EDGE_CURVE ( 'NONE', #6715, #17249, #150817, .T. ) ;
#116736=CARTESIAN_POINT ( 'NONE',  ( 5.203632029546647608, 4.965325544092860532, 1.040834085586084257E-14 ) ) ;
#116740=CARTESIAN_POINT ( 'NONE',  ( 7.865701674222579598, 12.32840238656838139, -0.7998128361456352531 ) ) ;
#116745=VERTEX_POINT ( 'NONE', #135214 ) ;
#116748=CARTESIAN_POINT ( 'NONE',  ( -2.625475302540713152, 6.214804952939456228, -0.7998128361456281477 ) ) ;
#116749=CARTESIAN_POINT ( 'NONE',  ( 5.933664784275179294, 10.07435934829639912, -0.7998128361456291469 ) ) ;
#116751=CARTESIAN_POINT ( 'NONE',  ( 5.029711800545521250, 5.930713857800314237, -1.082531754730549078 ) ) ;
#116759=CARTESIAN_POINT ( 'NONE',  ( -1.499999999999995781, 8.627523663848661428, -2.579999999999989413 ) ) ;
#116762=CARTESIAN_POINT ( 'NONE',  ( -7.402388683381436074, 7.738467673474211495, 0.7216878364870317197 ) ) ;
#116763=CARTESIAN_POINT ( 'NONE',  ( 5.996784015946103885, 5.890669528225568996, 1.040834085586084257E-14 ) ) ;
#116766=CARTESIAN_POINT ( 'NONE',  ( -8.993135964566285168, 9.386413468282476913, -0.7998128361456291469 ) ) ;
#116772=CARTESIAN_POINT ( 'NONE',  ( -4.406563619641430840, 5.099744630125142564, -1.199719254218446718 ) ) ;
#116773=DIRECTION ( 'NONE',  ( 1.000000000000000000, -8.673617379884035472E-16, 0.000000000000000000 ) ) ;
#116775=CARTESIAN_POINT ( 'NONE',  ( 9.043452155515161905, 10.50944792197790889, 1.199719254218453823 ) ) ;
#116776=CARTESIAN_POINT ( 'NONE',  ( 2.367870383881045981, 5.914265881169853856, 0.000000000000000000 ) ) ;
#116782=CARTESIAN_POINT ( 'NONE',  ( 4.202664430556261266, 4.005456045178151570, 0.7216878364870317197 ) ) ;
#116785=CARTESIAN_POINT ( 'NONE',  ( -2.981903720001798597, 5.566305875722335372, -1.199719254218446718 ) ) ;
#116786=DIRECTION ( 'NONE',  ( -5.578564026256490882E-16, -1.000000000000000000, -9.066213480720158442E-32 ) ) ;
#116788=CARTESIAN_POINT ( 'NONE',  ( -9.833741488613570780, 10.36711991300432345, 0.7998128361456462443 ) ) ;
#116793=CARTESIAN_POINT ( 'NONE',  ( 8.283668668269706714, 8.766627655843892697, 1.040834085586084257E-14 ) ) ;
#116794=CARTESIAN_POINT ( 'NONE',  ( -1.201851678989727383E-14, 5.509375000341415252, -1.575800808251660134 ) ) ;
#116796=CARTESIAN_POINT ( 'NONE',  ( 2.849184837166184536, 6.475799410002530898, 0.7998128361456362523 ) ) ;
#116797=CARTESIAN_POINT ( 'NONE',  ( 5.605114358992040913, 6.317488171369740613, -1.123711807521186490 ) ) ;
#116799=CARTESIAN_POINT ( 'NONE',  ( -7.725448601688521322, 7.907444878258402809, 1.040834085586084257E-14 ) ) ;
#116801=CARTESIAN_POINT ( 'NONE',  ( 1.436716030283395895, 7.421837552815621741, 4.237608343040937697 ) ) ;
#116809=CARTESIAN_POINT ( 'NONE',  ( -0.6823417656249969321, 4.530208333674755394, -1.181850606188749264 ) ) ;
#116810=CARTESIAN_POINT ( 'NONE',  ( 9.565441069641300587, 11.11843498845840905, -1.199719254218440723 ) ) ;
#116812=CARTESIAN_POINT ( 'NONE',  ( -4.853455804012230423, 6.685451076146141425, 1.443375672974064550 ) ) ;
#116813=CARTESIAN_POINT ( 'NONE',  ( 2.684151225825664788, 5.114964949229812596, -1.082531754730543083 ) ) ;
#116814=CARTESIAN_POINT ( 'NONE',  ( -4.406036734316890247, 7.123831375802920363, -1.082531754730548412 ) ) ;
#116821=CARTESIAN_POINT ( 'NONE',  ( 4.090809663021327758, 5.795697244990093644, 1.599625672291267398 ) ) ;
#116827=CARTESIAN_POINT ( 'NONE',  ( 1.284279953904125193, 3.003360285806104368, 0.7750000000000065725 ) ) ;
#116831=CARTESIAN_POINT ( 'NONE',  ( 5.529027716274630855, 5.344953845275508542, 1.040834085586084257E-14 ) ) ;
#116832=ORIENTED_EDGE ( 'NONE', *, *, #19052, .F. ) ;
#116837=CARTESIAN_POINT ( 'NONE',  ( -6.358937740009323214, 7.377514437221045718, -1.199719254218446718 ) ) ;
#116841=CARTESIAN_POINT ( 'NONE',  ( 7.786460292950004636, 7.978625184730144149, 1.040834085586084257E-14 ) ) ;
#116844=CARTESIAN_POINT ( 'NONE',  ( -5.280010757518168063, 8.247430752824802980, -1.199719254218446718 ) ) ;
#116845=CARTESIAN_POINT ( 'NONE',  ( -1.402160292154681736E-14, 1.587500000000018785, -1.732050807568863648 ) ) ;
#116846=CARTESIAN_POINT ( 'NONE',  ( -3.704402285031864306, 5.344888637335695414, -1.599625672291256295 ) ) ;
#116849=CARTESIAN_POINT ( 'NONE',  ( -5.762378981008047241, 6.681529218386182301, 1.199719254218450271 ) ) ;
#116851=CARTESIAN_POINT ( 'NONE',  ( 0.6823417656249882723, 2.926041667008084879, -1.181850606188754593 ) ) ;
#116853=CARTESIAN_POINT ( 'NONE',  ( -5.639828713604883248, 6.642516923036197340, 1.082531754730548412 ) ) ;
#116860=CARTESIAN_POINT ( 'NONE',  ( 4.873266149108180123, 7.772895376346490970, 1.199719254218462483 ) ) ;
#116863=CARTESIAN_POINT ( 'NONE',  ( -1.201851678989727383E-14, 3.259375000341420581, -1.575800808251660134 ) ) ;
#116865=CARTESIAN_POINT ( 'NONE',  ( 3.009020027229115879, 5.597941567487558778, -1.199719254218446718 ) ) ;
#116867=CARTESIAN_POINT ( 'NONE',  ( -1.364683531250000748, 0.3218750003414205807, 0.000000000000000000 ) ) ;
#116871=CARTESIAN_POINT ( 'NONE',  ( -4.796887421136680985, 4.490790167614548523, 1.214306433183764966E-14 ) ) ;
#116872=CARTESIAN_POINT ( 'NONE',  ( -6.005898860729463884, 9.950706404252290582, 0.7216878364870458196 ) ) ;
#116877=CARTESIAN_POINT ( 'NONE',  ( 1.364683531249988535, 2.613541667008089764, 0.7879004041258500513 ) ) ;
#116885=CARTESIAN_POINT ( 'NONE',  ( -6.195713011320783892, 10.17215624660883577, -0.7216878364870267237 ) ) ;
#116891=CARTESIAN_POINT ( 'NONE',  ( -6.846504384776765484, 8.050305206070113684, -1.082531754730543083 ) ) ;
#116904=CARTESIAN_POINT ( 'NONE',  ( -6.905180308061733996, 6.950465202360470052, 0.7998128361456341429 ) ) ;
#116906=CARTESIAN_POINT ( 'NONE',  ( 1.499999999999987566, -0.4749999999999823808, 0.000000000000000000 ) ) ;
#116907=CARTESIAN_POINT ( 'NONE',  ( 3.871016551901614200, 4.474939717762034697, -1.199719254218446718 ) ) ;
#116911=CARTESIAN_POINT ( 'NONE',  ( 4.496500501226593727, 8.397667684739696270, 0.7998128361456462443 ) ) ;
#116918=CARTESIAN_POINT ( 'NONE',  ( -4.446711195602255806, 5.250546485366484717, -1.082531754730544860 ) ) ;
#116926=CARTESIAN_POINT ( 'NONE',  ( -1.364683531250012516, 2.280208333674751842, 0.7879004041258379498 ) ) ;
#116927=CARTESIAN_POINT ( 'NONE',  ( 8.988692655735958326, 12.47026328412523988, -1.082531754730543083 ) ) ;
#116929=CARTESIAN_POINT ( 'NONE',  ( -8.525379664894808585, 8.840697785332414682, -0.7998128361456291469 ) ) ;
#116932=CARTESIAN_POINT ( 'NONE',  ( 5.296431564432884542, 9.330920591813708143, 1.040834085586084257E-14 ) ) ;
#116933=CARTESIAN_POINT ( 'NONE',  ( -6.795661308947694934, 8.951357498570873261, -1.599625672291263179 ) ) ;
#116935=CARTESIAN_POINT ( 'NONE',  ( -1.402160292154681736E-14, -0.7562499993171803991, 1.732050807568877637 ) ) ;
#116937=CARTESIAN_POINT ( 'NONE',  ( 8.975134502566660899, 10.53370701015836275, -1.082531754730543083 ) ) ;
#116940=CARTESIAN_POINT ( 'NONE',  ( 0.6823417656249899377, 0.9052083336747520637, 1.181850606188755259 ) ) ;
#116943=CARTESIAN_POINT ( 'NONE',  ( 5.626270559546804328, 9.507806719539201978, 0.7216878364870438212 ) ) ;
#116947=CARTESIAN_POINT ( 'NONE',  ( -5.612712406377534435, 5.650512016969639895, 0.7216878364870317197 ) ) ;
#116950=CARTESIAN_POINT ( 'NONE',  ( -1.364683531250012516, 4.488541667008090208, -0.7879004041258300672 ) ) ;
#116954=CARTESIAN_POINT ( 'NONE',  ( -6.254388934605767503, 6.191208599995166040, 0.7998128361456341429 ) ) ;
#116955=CARTESIAN_POINT ( 'NONE',  ( -5.989290089449875509, 6.089315518664643712, -0.6934025848366349720 ) ) ;
#116962=CARTESIAN_POINT ( 'NONE',  ( 7.253775878511261155, 8.421492265473332850, 1.199719254218462483 ) ) ;
#116966=CARTESIAN_POINT ( 'NONE',  ( -1.500000000000013101, 2.420833333333359150, 0.8660254037844403729 ) ) ;
#116973=CARTESIAN_POINT ( 'NONE',  ( 4.338245966692901412, 8.005111361209628740, -0.7216878364870197293 ) ) ;
#116974=CARTESIAN_POINT ( 'NONE',  ( -1.402160292154681736E-14, 0.1343750003414218575, 1.575800808251672791 ) ) ;
#116976=CARTESIAN_POINT ( 'NONE',  ( 8.866142388332804103, 12.43125098877526113, -1.199719254218446718 ) ) ;
#116980=CARTESIAN_POINT ( 'NONE',  ( 0.7499999999999885647, 1.066666666666687968, -1.299038105676652899 ) ) ;
#116981=CARTESIAN_POINT ( 'NONE',  ( 7.613066949273408213, 8.840665181362512115, -1.199719254218441611 ) ) ;
#116982=CARTESIAN_POINT ( 'NONE',  ( -8.690940161559884913, 10.09818392903003748, 1.199719254218462483 ) ) ;
#116984=CARTESIAN_POINT ( 'NONE',  ( 1.364683531249986537, 0.8635416670080893198, 0.7879004041258500513 ) ) ;
#116985=CARTESIAN_POINT ( 'NONE',  ( -0.7500000000000215383, 2.691666666666689522, 1.299038105676671107 ) ) ;
#116987=CARTESIAN_POINT ( 'NONE',  ( 5.169736645512481132, 4.925780929386339935, 0.7998128361456341429 ) ) ;
#116994=CARTESIAN_POINT ( 'NONE',  ( 0.7499999999999867883, -0.4020833326505157679, -1.299038105676652899 ) ) ;
#116995=CARTESIAN_POINT ( 'NONE',  ( -8.369460898337653276, 8.658792557682392754, 0.7998128361456462443 ) ) ;
#116996=CARTESIAN_POINT ( 'NONE',  ( -4.446711195602255806, 5.250546485366484717, -1.082531754730544860 ) ) ;
#117005=CARTESIAN_POINT ( 'NONE',  ( 5.612185521052973414, 8.634967976948757951, -1.199719254218440723 ) ) ;
#117007=CARTESIAN_POINT ( 'NONE',  ( 1.499999999999985789, -1.099999999999982991, 0.000000000000000000 ) ) ;
#117009=CARTESIAN_POINT ( 'NONE',  ( 7.955937213120826357, 8.176348258262782664, 0.7998128361456481317 ) ) ;
#117010=CARTESIAN_POINT ( 'NONE',  ( 7.415946836550722843, 8.714654733139752807, 1.082531754730558626 ) ) ;
#117014=CARTESIAN_POINT ( 'NONE',  ( -7.867809214632013770, 8.073532260025807261, 1.040834085586084257E-14 ) ) ;
#117017=CARTESIAN_POINT ( 'NONE',  ( 5.203632029546647608, 4.965325544092860532, 1.040834085586084257E-14 ) ) ;
#117024=CARTESIAN_POINT ( 'NONE',  ( 10.39874063200158893, 11.23421161353111586, 0.000000000000000000 ) ) ;
#117033=CARTESIAN_POINT ( 'NONE',  ( -1.522028533774275383, 8.691231065131706401, -2.524624912498922846 ) ) ;
#117034=CARTESIAN_POINT ( 'NONE',  ( -4.772106882330247046, 4.669805572247793357, -0.7216878364870207285 ) ) ;
#117035=CARTESIAN_POINT ( 'NONE',  ( 9.571693261567965294, 10.26932301469188857, 0.7216878364870438212 ) ) ;
#117038=CARTESIAN_POINT ( 'NONE',  ( -6.552668314106420588, 6.539201209412602189, -0.7998128361456291469 ) ) ;
#117039=FACE_OUTER_BOUND ( 'NONE', #152989, .T. ) ;
#117040=CARTESIAN_POINT ( 'NONE',  ( -3.110417573979663342, 6.447385285496729956, -0.7441446434824240397 ) ) ;
#117043=CARTESIAN_POINT ( 'NONE',  ( -7.100719765255177229, 9.307259030929609267, -1.599625672291263179 ) ) ;
#117057=CARTESIAN_POINT ( 'NONE',  ( -7.067878151425722955, 7.140279352951794500, 0.7998128361456341429 ) ) ;
#117060=CARTESIAN_POINT ( 'NONE',  ( 5.856759171423504107, 5.935233242856626568, -0.7216878364870257245 ) ) ;
#117064=CARTESIAN_POINT ( 'NONE',  ( -5.135841261478327979, 4.886236314679810455, 0.7998128361456341429 ) ) ;
#117072=CARTESIAN_POINT ( 'NONE',  ( -7.232384877886063990, 10.52520055992070525, -1.199719254218446718 ) ) ;
#117073=CARTESIAN_POINT ( 'NONE',  ( 6.962275575817444384, 8.081408578997208991, -1.199719254218446718 ) ) ;
#117076=CARTESIAN_POINT ( 'NONE',  ( -9.671043645249580933, 10.17730576241299900, 0.7998128361456462443 ) ) ;
#117080=CARTESIAN_POINT ( 'NONE',  ( 0.6823417656249882723, 0.2385416670080825474, -1.181850606188749264 ) ) ;
#117083=CARTESIAN_POINT ( 'NONE',  ( 8.934460041725669655, 9.525884258209195821, 1.040834085586084257E-14 ) ) ;
#117109=CARTESIAN_POINT ( 'NONE',  ( 1.499999999999987121, 0.03541666734948738238, 0.8660254037844524744 ) ) ;
#117116=CARTESIAN_POINT ( 'NONE',  ( 7.716561984472250835, 12.15440608185967086, 1.040834085586084257E-14 ) ) ;
#117122=CARTESIAN_POINT ( 'NONE',  ( 5.034155109375821446, 4.767602470560229122, -0.7998128361456221525 ) ) ;
#117123=CARTESIAN_POINT ( 'NONE',  ( -8.039621903223732602, 8.481906429956900695, 1.040834085586084257E-14 ) ) ;
#117124=EDGE_CURVE ( 'NONE', #179842, #13744, #74161, .T. ) ;
#117125=CARTESIAN_POINT ( 'NONE',  ( -5.863297782511878609, 6.029266553239049919, -0.3729355709888391157 ) ) ;
#117128=CARTESIAN_POINT ( 'NONE',  ( -8.857554428429624593, 9.228235009456373206, 0.7998128361456462443 ) ) ;
#117129=CARTESIAN_POINT ( 'NONE',  ( -2.941756144040963417, 6.375873234782333476, -0.7216878364870257245 ) ) ;
#117132=CARTESIAN_POINT ( 'NONE',  ( 1.499999999999989120, -0.1937499993171845625, 0.000000000000000000 ) ) ;
#117139=CARTESIAN_POINT ( 'NONE',  ( -4.487385655998893164, 6.258369236797239665, 1.443375672974064550 ) ) ;
#117147=CARTESIAN_POINT ( 'NONE',  ( -4.406036734316900905, 5.203092947200234519, -1.082531754730543971 ) ) ;
#117149=CARTESIAN_POINT ( 'NONE',  ( 7.397945374551106568, 11.78268670361832093, -0.7998128361456291469 ) ) ;
#117154=CARTESIAN_POINT ( 'NONE',  ( -1.499999999999997780, 5.150000000000022560, 1.214306433183764966E-14 ) ) ;
#117158=CARTESIAN_POINT ( 'NONE',  ( -3.521367211247373508, 5.131347717920458962, -1.599625672291256295 ) ) ;
#117159=CARTESIAN_POINT ( 'NONE',  ( -9.833741488613570780, 10.36711991300432345, 0.7998128361456462443 ) ) ;
#117164=CARTESIAN_POINT ( 'NONE',  ( 6.179819089730593795, 6.104210447640811665, 1.040834085586084257E-14 ) ) ;
#117173=ORIENTED_EDGE ( 'NONE', *, *, #80137, .F. ) ;
#117182=CARTESIAN_POINT ( 'NONE',  ( 8.308449207076147758, 8.587612251210650527, -0.7998128361456281477 ) ) ;
#117184=CARTESIAN_POINT ( 'NONE',  ( -5.057354993097396445, 5.859001232490445688, -1.199719254218446718 ) ) ;
#117190=CARTESIAN_POINT ( 'NONE',  ( -1.364683531250010295, 5.488541667008087543, -0.7879004041258300672 ) ) ;
#117194=LINE ( 'NONE', #135528, #84972 ) ;
#117195=CARTESIAN_POINT ( 'NONE',  ( 5.030238685870051185, 5.827365540725222282, -1.199719254218452047 ) ) ;
#117197=CARTESIAN_POINT ( 'NONE',  ( -5.108724954250998707, 4.854600622914589714, -0.7998128361456221525 ) ) ;
#117204=CARTESIAN_POINT ( 'NONE',  ( 6.209271165378815738, 7.306866450105836464, -1.082531754730543083 ) ) ;
#117206=ORIENTED_EDGE ( 'NONE', *, *, #202925, .F. ) ;
#117207=CARTESIAN_POINT ( 'NONE',  ( 8.731087737076324018, 9.288616569451617622, 1.040834085586084257E-14 ) ) ;
#117208=CARTESIAN_POINT ( 'NONE',  ( -1.201851678989727383E-14, 4.259375000341417028, -1.575800808251660134 ) ) ;
#117210=CARTESIAN_POINT ( 'NONE',  ( 4.324687812634892659, 5.108185871904570519, 1.082531754730560403 ) ) ;
#117216=CARTESIAN_POINT ( 'NONE',  ( -6.048854636777848626, 6.051613005247792998, 0.5441514604978964220 ) ) ;
#117219=CARTESIAN_POINT ( 'NONE',  ( -0.6823417656250212460, 5.363541667008087543, 1.181850606188767472 ) ) ;
#117234=CARTESIAN_POINT ( 'NONE',  ( 0.6823417656249899377, 4.738541667008086655, -1.181850606188754593 ) ) ;
#117236=CARTESIAN_POINT ( 'NONE',  ( 5.940443861082012944, 10.08226827123770697, 0.7998128361456462443 ) ) ;
#117237=CARTESIAN_POINT ( 'NONE',  ( -9.179033691651859783, 10.66762638080401260, 1.199719254218462483 ) ) ;
#117243=CARTESIAN_POINT ( 'NONE',  ( 1.499999999999987121, 4.045833333333359150, -0.8660254037844323793 ) ) ;
#117251=CARTESIAN_POINT ( 'NONE',  ( 9.259855728453651125, 9.905512559391842942, 1.040834085586084257E-14 ) ) ;
#117255=EDGE_CURVE ( 'NONE', #2289, #166897, #192540, .T. ) ;
#117256=CARTESIAN_POINT ( 'NONE',  ( 1.499999999999989120, 3.785416667349481123, 0.8660254037844524744 ) ) ;
#117258=CARTESIAN_POINT ( 'NONE',  ( -4.229253852459088137, 7.021547696922494808, 1.199719254218464037 ) ) ;
#117259=CARTESIAN_POINT ( 'NONE',  ( 3.334942598837264960, 6.834590765378040444, 1.214306433183764966E-14 ) ) ;
#117260=CARTESIAN_POINT ( 'NONE',  ( -1.387358672535449200, 7.315968950355252076, 4.254625267135948796 ) ) ;
#117268=CARTESIAN_POINT ( 'NONE',  ( 3.684065054611349144, 5.321161868511784299, -1.599625672291262513 ) ) ;
#117272=CARTESIAN_POINT ( 'NONE',  ( 6.003563092752934871, 5.898578451166879510, 0.7998128361456341429 ) ) ;
#117275=CARTESIAN_POINT ( 'NONE',  ( 2.535011536075336913, 5.133042487381361596, 2.420000000000000373 ) ) ;
#117285=CARTESIAN_POINT ( 'NONE',  ( 5.160031065370225711, 6.461479299918838848, -1.191482946479218485 ) ) ;
#117288=CARTESIAN_POINT ( 'NONE',  ( 10.05353459973327368, 11.68787744023238417, -1.199719254218440723 ) ) ;
#117294=CARTESIAN_POINT ( 'NONE',  ( 6.670248388243460447, 6.884303995813253252, -0.7216878364870257245 ) ) ;
#117295=CARTESIAN_POINT ( 'NONE',  ( -9.869972641068651242, 11.57768483841065787, 1.082531754730558626 ) ) ;
#117300=CARTESIAN_POINT ( 'NONE',  ( -4.928552533767591726, 5.708731696605642725, 1.199719254218462483 ) ) ;
#117302=CARTESIAN_POINT ( 'NONE',  ( -5.381422217466665714, 4.322449550048943046, 2.440471613107408011 ) ) ;
#117311=CARTESIAN_POINT ( 'NONE',  ( 8.910733272679570049, 11.41894145625809820, -1.599625672291255185 ) ) ;
#117312=CARTESIAN_POINT ( 'NONE',  ( 5.993251976321238850, 6.092249680885792884, 0.6249505139499841322 ) ) ;
#117317=CARTESIAN_POINT ( 'NONE',  ( 4.955668840994886359, 5.740367388370866131, 1.199719254218462483 ) ) ;
#117322=CARTESIAN_POINT ( 'NONE',  ( -9.056483424248693126, 10.62861408545402675, 1.082531754730558626 ) ) ;
#117326=CARTESIAN_POINT ( 'NONE',  ( 7.558834334818744338, 8.777393797832065303, 1.199719254218462483 ) ) ;
#117327=CARTESIAN_POINT ( 'NONE',  ( -3.425406365747000859, 7.148057860013469877, 1.040834085586084257E-14 ) ) ;
#117329=CARTESIAN_POINT ( 'NONE',  ( 3.704402285031850539, 5.344888637335695414, -1.599625672291262513 ) ) ;
#117331=CARTESIAN_POINT ( 'NONE',  ( -3.927058049452637700, 7.733318157670055371, -0.7998128361456281477 ) ) ;
#117332=CARTESIAN_POINT ( 'NONE',  ( 4.142179624174931796, 4.791296635414242111, 1.199719254218464037 ) ) ;
#117338=CARTESIAN_POINT ( 'NONE',  ( 7.716561984472250835, 12.15440608185967086, 1.040834085586084257E-14 ) ) ;
#117342=CARTESIAN_POINT ( 'NONE',  ( 4.061730550730160871, 7.744580798899280971, -0.5443347154160914636 ) ) ;
#117343=CARTESIAN_POINT ( 'NONE',  ( 6.209271165378815738, 7.306866450105836464, -1.082531754730543083 ) ) ;
#117347=CARTESIAN_POINT ( 'NONE',  ( -1.337789648166264334, 3.300000000000025135, 0.2994557852716039359 ) ) ;
#117348=CARTESIAN_POINT ( 'NONE',  ( -1.419999999999997708, 6.280000000000042881, -2.873333333333329520 ) ) ;
#117350=CARTESIAN_POINT ( 'NONE',  ( 7.239690839573049708, 11.39013037956983965, 1.040834085586084257E-14 ) ) ;
#117354=CARTESIAN_POINT ( 'NONE',  ( -8.850775351622791831, 9.220326086515070685, -0.7998128361456291469 ) ) ;
#117359=CARTESIAN_POINT ( 'NONE',  ( 3.895595285070167169, 2.800000000000017586, 0.7750000000000135669 ) ) ;
#117364=CARTESIAN_POINT ( 'NONE',  ( 2.191614386903386613, 5.708633884695917260, -0.7998128361456281477 ) ) ;
#117366=CARTESIAN_POINT ( 'NONE',  ( 1.284279953904119864, 3.296639714193937198, -0.7749999999999910294 ) ) ;
#117369=CARTESIAN_POINT ( 'NONE',  ( 4.202137545231717120, 6.989912005157271402, 1.199719254218462483 ) ) ;
#117372=CARTESIAN_POINT ( 'NONE',  ( -0.7500000000000215383, 4.222916667349481123, 1.299038105676671107 ) ) ;
#117378=CARTESIAN_POINT ( 'NONE',  ( -1.201851678989727383E-14, 1.212500000000025002, 1.732050807568877637 ) ) ;
#117379=CARTESIAN_POINT ( 'NONE',  ( 6.449928391799196525, 8.548002428564306143, -1.599625672291262513 ) ) ;
#117380=CARTESIAN_POINT ( 'NONE',  ( 3.823036128929238942, 7.404033217152015567, 1.040834085586084257E-14 ) ) ;
#117384=CARTESIAN_POINT ( 'NONE',  ( 9.083599731475988648, 10.66024977721925104, 1.082531754730549967 ) ) ;
#117391=CARTESIAN_POINT ( 'NONE',  ( -3.567766978690493307, 7.314145241780881435, 1.040834085586084257E-14 ) ) ;
#117392=CARTESIAN_POINT ( 'NONE',  ( 1.499999999999987121, 3.827083334016153415, -0.8660254037844323793 ) ) ;
#117393=CARTESIAN_POINT ( 'NONE',  ( -1.402160292154681736E-14, -0.3031249996585801965, -1.575800808251665908 ) ) ;
#117397=CARTESIAN_POINT ( 'NONE',  ( 5.169736645512481132, 4.925780929386339935, 0.7998128361456341429 ) ) ;
#117399=CARTESIAN_POINT ( 'NONE',  ( 1.364683531249990311, 4.676041667008083103, 0.7879004041258500513 ) ) ;
#117403=CARTESIAN_POINT ( 'NONE',  ( -1.420000000000021911, 6.200000000000045475, 2.900000000000013678 ) ) ;
#117408=CARTESIAN_POINT ( 'NONE',  ( -8.528242318195895066, 9.908369778438709474, 1.199719254218462483 ) ) ;
#117409=CARTESIAN_POINT ( 'NONE',  ( 6.006425746053997372, 6.966250444273174303, -1.199719254218445830 ) ) ;
#117411=CARTESIAN_POINT ( 'NONE',  ( -1.402160292154681736E-14, -0.3031249996585801965, -1.575800808251665908 ) ) ;
#117415=CARTESIAN_POINT ( 'NONE',  ( -4.905110356762790502, 4.827649200395154772, -0.06592220986076716138 ) ) ;
#117418=CARTESIAN_POINT ( 'NONE',  ( -6.905180308061733996, 6.950465202360470052, 0.7998128361456341429 ) ) ;
#117423=CARTESIAN_POINT ( 'NONE',  ( 8.215351014876830504, 11.67199438640995801, -1.199719254218446718 ) ) ;
#117425=CARTESIAN_POINT ( 'NONE',  ( 3.294557018017927330, 6.403080317724275439, 0.9028181842051991035 ) ) ;
#117426=CARTESIAN_POINT ( 'NONE',  ( -3.144601563365788444, 5.756120026313656268, -1.199719254218452935 ) ) ;
#117427=CARTESIAN_POINT ( 'NONE',  ( -8.369460898337653276, 8.658792557682392754, 0.7998128361456462443 ) ) ;
#117429=CARTESIAN_POINT ( 'NONE',  ( -4.549609453380520030, 7.192579769413725010, 1.336992641046318875 ) ) ;
#117430=CARTESIAN_POINT ( 'NONE',  ( -0.6823417656250246877, -0.9489583329919115684, 1.181850606188755259 ) ) ;
#117433=VECTOR ( 'NONE', #48798, 1000.000000000000000 ) ;
#117435=CARTESIAN_POINT ( 'NONE',  ( 8.270110514656034084, 9.711179024262627024, 1.082531754730558626 ) ) ;
#117438=CARTESIAN_POINT ( 'NONE',  ( 4.171104814498611368, 8.018039383557042044, 0.7998128361456321445 ) ) ;
#117458=DIRECTION ( 'NONE',  ( 0.000000000000000000, 8.546850786086437571E-32, 1.000000000000000000 ) ) ;
#117461=CARTESIAN_POINT ( 'NONE',  ( -5.447678794592645701, 5.250046769979851646, 0.000000000000000000 ) ) ;
#117462=DIRECTION ( 'NONE',  ( 1.000000000000000000, 0.000000000000000000, 0.000000000000000000 ) ) ;
#117466=CARTESIAN_POINT ( 'NONE',  ( 1.499999999999987121, 3.327083334016150751, -0.8660254037844262731 ) ) ;
#117467=CARTESIAN_POINT ( 'NONE',  ( 9.215791728987056786, 11.77484298861683598, -1.599625672291262513 ) ) ;
#117470=ORIENTED_EDGE ( 'NONE', *, *, #98066, .T. ) ;
#117472=CARTESIAN_POINT ( 'NONE',  ( -7.818248136574758256, 12.27303992597924420, 0.000000000000000000 ) ) ;
#117473=CARTESIAN_POINT ( 'NONE',  ( 1.479373551132449505, 3.300000000000025135, 0.2478989637125245671 ) ) ;
#117474=CARTESIAN_POINT ( 'NONE',  ( -1.201851678989727383E-14, 2.071875000341422801, 1.575800808251672791 ) ) ;
#117482=CARTESIAN_POINT ( 'NONE',  ( -4.437596350374534815, 4.071617251725375475, -0.7998128361456221525 ) ) ;
#117486=CARTESIAN_POINT ( 'NONE',  ( -1.364683531250000748, 1.571875000341421691, 0.000000000000000000 ) ) ;
#117491=CARTESIAN_POINT ( 'NONE',  ( 1.364683531249988535, 1.363541667008083769, 0.7879004041258500513 ) ) ;
#117493=CARTESIAN_POINT ( 'NONE',  ( -5.930802130974132780, 9.006687355190106103, -1.199719254218440723 ) ) ;
#117494=CARTESIAN_POINT ( 'NONE',  ( 7.507464373665139412, 9.781794407407920389, 1.599625672291281386 ) ) ;
#117495=CARTESIAN_POINT ( 'NONE',  ( 3.194917754314666514, 6.879154480009089134, 0.7998128361456321445 ) ) ;
#117496=CARTESIAN_POINT ( 'NONE',  ( 5.144429221381498607, 8.089252293998699272, -1.199719254218452047 ) ) ;
#117498=CARTESIAN_POINT ( 'NONE',  ( -1.500000000000013101, 4.129166666666687746, -0.8660254037844313801 ) ) ;
#117500=CARTESIAN_POINT ( 'NONE',  ( -0.6823417656249969321, 3.280208333674754062, -1.181850606188749264 ) ) ;
#117503=CARTESIAN_POINT ( 'NONE',  ( -5.748293942514174582, 5.808690475795755148, -0.7216878364870319418 ) ) ;
#117506=CARTESIAN_POINT ( 'NONE',  ( 4.351804120306567825, 8.020929207092235558, 1.040834085586084257E-14 ) ) ;
#117509=CARTESIAN_POINT ( 'NONE',  ( -7.492852449846775897, 11.89341162479659531, 0.000000000000000000 ) ) ;
#117510=CARTESIAN_POINT ( 'NONE',  ( -4.437596350374534815, 4.071617251725375475, -0.7998128361456221525 ) ) ;
#117515=CARTESIAN_POINT ( 'NONE',  ( -6.304178240230145391, 9.338329799368375816, 1.082531754730548412 ) ) ;
#117517=CARTESIAN_POINT ( 'NONE',  ( 0.7499999999999902300, 5.316666666666685082, -1.299038105676658228 ) ) ;
#117520=CARTESIAN_POINT ( 'NONE',  ( 8.771762198361678031, 9.336070107617867819, 1.040834085586084257E-14 ) ) ;
#117528=CARTESIAN_POINT ( 'NONE',  ( 10.37162432432990755, 11.20257592124748136, -0.7216878364870257245 ) ) ;
#117535=CARTESIAN_POINT ( 'NONE',  ( 7.558834334818744338, 8.777393797832065303, 1.199719254218462483 ) ) ;
#117536=CARTESIAN_POINT ( 'NONE',  ( -3.879604511804807032, 7.677955697080923514, 0.7998128361456341429 ) ) ;
#117538=CARTESIAN_POINT ( 'NONE',  ( -1.499999999999997780, 5.150000000000022560, 1.214306433183764808E-14 ) ) ;
#117541=CARTESIAN_POINT ( 'NONE',  ( 5.463572716182824252, 7.397254140345190798, 1.443375672974062551 ) ) ;
#117543=CARTESIAN_POINT ( 'NONE',  ( 3.172244755917638770, 5.684407401003788607, -1.082531754730543083 ) ) ;
#117544=CARTESIAN_POINT ( 'NONE',  ( -3.379006598303881059, 4.965260336153046516, -1.599625672291256295 ) ) ;
#117559=CARTESIAN_POINT ( 'NONE',  ( 6.982612806237943559, 8.105135347821125436, -1.199719254218446718 ) ) ;
#117560=CARTESIAN_POINT ( 'NONE',  ( 7.470706336329915764, 8.674577799595093452, -1.199719254218441611 ) ) ;
#117563=VERTEX_POINT ( 'NONE', #83683 ) ;
#117569=CARTESIAN_POINT ( 'NONE',  ( -4.741649638052999549, 5.202212439478444139, 1.069586989871945670 ) ) ;
#117572=CARTESIAN_POINT ( 'NONE',  ( -6.033542053281340856, 6.997886136038390603, -1.199719254218446718 ) ) ;
#117574=CARTESIAN_POINT ( 'NONE',  ( -3.093231602212184850, 6.760520635889515795, -0.7998128361456281477 ) ) ;
#117587=CARTESIAN_POINT ( 'NONE',  ( -3.277320446201389181, 4.846626492033466072, 1.599625672291267398 ) ) ;
#117590=CARTESIAN_POINT ( 'NONE',  ( 6.959412922516382771, 7.013736585890911535, 0.7998128361456341429 ) ) ;
#117591=CARTESIAN_POINT ( 'NONE',  ( 1.364683531249988535, 4.155208333674753618, -0.7879004041258239610 ) ) ;
#117597=CARTESIAN_POINT ( 'NONE',  ( 5.300874872818830852, 7.207439989753867238, 1.443375672974062551 ) ) ;
#117598=CARTESIAN_POINT ( 'NONE',  ( -6.235860587281615075, 9.362588887548838557, -1.199719254218440723 ) ) ;
#117600=EDGE_LOOP ( 'NONE', ( #70909, #87796, #50620, #10134 ) ) ;
#117603=CARTESIAN_POINT ( 'NONE',  ( -6.184490626128011925, 10.36698949712469364, -0.7998128361456291469 ) ) ;
#117604=CARTESIAN_POINT ( 'NONE',  ( -4.791917227426195858, 7.677988301050826969, -1.199719254218452047 ) ) ;
#117608=CARTESIAN_POINT ( 'NONE',  ( -3.621833129746846680, 4.096114899008192367, 2.420000000000010587 ) ) ;
#117611=CARTESIAN_POINT ( 'NONE',  ( 6.642605195691581699, 9.837124264027149678, 1.199719254218462483 ) ) ;
#117619=( BOUNDED_SURFACE ( )  B_SPLINE_SURFACE ( 1, 2, ( 
 ( #157256, #204895, #122709, #71697, #55473, #188672, #58675, #40305, #7768, #25095, #91196, #8848, #121628, #74928, #124824, #190790, #42452, #170281, #21869, #33472, #133145, #212207, #112667, #30290, #63843, #17199, #48673, #213272, #15070, #145140, #16130, #199145, #113735, #32413, #164545, #98479, #132086, #128932, #82214, #943, #214306, #198096, #148308, #65937, #49723, #80088, #50789, #64901, #115852, #181837, #99546, #165610, #96376, #83273, #62768, #149361, #194909, #46547, #146192, #31358, #147245, #179741, #131049, #67008, #116918, #182919, #34534, #81162, #161361, #12944, #130000, #79024, #178675, #114790, #195990, #14004, #211146, #162427, #47623, #97433, #197038, #163488, #180790, #117991, #137393, #151505, #72355, #88642, #187182, #183984, #37744, #122289, #103819, #86491, #138458, #2007, #204477, #150445, #68073, #3074, #153633, #20409, #188246, #87565, #19342, #100605, #203410, #56130, #6282, #69145, #166681, #201280, #18273, #101673, #38809, #53994, #167743, #104895, #84355, #135266, #51870, #35595, #52921, #170934, #202342, #152555, #168803, #134209, #169866, #200219, #119052, #186110, #21457, #5206, #71279, #85421, #55063, #154699, #121213, #22533, #185037, #36662, #4142, #102747, #70212, #136324, #120133, #173096, #110283, #209824, #105997, #75583, #74518, #124421, #189324, #109225, #8430, #156846, #175235, #59326, #61460, #90783, #206633, #157916, #7352, #58264, #174177, #141693, #126550, #40965, #140621, #191445, #207706, #42039, #73431, #139534, #160032, #107073, #125483, #43110, #92923, #176292, #123359, #205559, #190379, #57199, #24677, #9511, #77707, #108151, #26819, #25748, #91861, #158969, #10563, #39887, #23609, #76638, #127626, #93991, #11634, #89718, #142752, #208761, #60386, #192511, #44163, #27896, #172018, #143827, #155768, #96120, #161102, #31112, #162175, #195735, #81967, #46298, #144889, #131836, #178425, #145946, #177354, #28968, #13761, #99303, #79838, #112413, #30034, #211957, #63595, #95051, #129750, #210896, #180539, #47370, #97186, #680, #113483, #128685, #12690, #130797, #163239, #179490, #114548, #194654, #14821, #80913, #62523, #193590, #147003, #15883, #213021, #64656, #196791, #48432, #32162, #181590, #148054, #65688, #78766, #98239, #164294, #214060, #45234, #197843, #49476, #115596, #33219, #165351, #16945, #83024, #149101, #66747, #111349, #50537, #34278, #87303, #100351, #4943, #201023, #133960, #68890, #153372, #151250, #67813, #101418, #36408, #135009, #154443, #132888, #84100, #52666, #169617, #199968, #35338, #38557, #6023, #20150, #118795, #185849, #203161, #1756, #166419, #183732, #150187, #51616, #102487, #170680, #117739, #168551, #167490, #184782, #86235, #19086, #198891, #116660, #152306, #182658, #186925, #104633, #18011, #3883, #69953, #136065, #202078, #85166, #2819, #53738, #119870, #103558, #37481, #21201, #71019, #137132, #54806, #120954, #22267, #88376, #10306, #56938, #24407, #55868, #122024, #106807, #192247, #40703, #139269, #123110, #172836, #189068, #187991, #90522, #23345, #59063, #8178, #190126, #93729, #156584, #7090, #39616, #9250, #41780, #74262, #207444, #73163, #140355, #205299, #89456, #72093, #206373, #108956, #155508, #58000, #124164, #107894, #173921, #60130, #174976, #158709, #105720, #25494, #125223, #91601, #138203, #157652, #75321, #141438, #191181, #126288, #42849, #26558, #92665, #76380, #142489, #204215, #171749, #208495, #43909, #110023, #176037, #27629, #159769, #31916, #29780, #160841, #194399, #129496, #13511, #32970, #11368, #177092, #79583, #48183, #78513, #128432, #131587, #99046, #113226, #145701, #179230, #211701, #193331, #111085, #197589, #12433, #30856, #47110, #210645, #46041, #144630, #28707, #213818, #62271, #63337, #180293, #97994, #212769, #143565, #127361, #164052, #44977, #15631, #195477, #112162, #161920, #81718, #95864, #178165, #96933, #162983, #14564, #77447, #209558, #94793, #80660, #114295, #146751, #64405, #49233, #61203, #130549, #196540, #147800, #65436, #115352, #181343, #70764, #166161, #118546, #200769, #3627, #20948, #34027, #198641, #1497, #182398, #100101, #68637, #202904, #149928 ),
 ( #167237, #18826, #17748, #35080, #16692, #152057, #135809, #67563, #132635, #2566, #133706, #84910, #53477, #83838, #116408, #103301, #199712, #117482, #148850, #423, #51358, #136878, #183473, #101152, #150998, #134761, #52420, #66496, #184528, #36150, #69705, #102230, #168301, #186671, #19897, #85981, #50289, #201832, #119614, #185599, #37230, #169363, #87045, #153118, #4689, #165101, #54549, #120696, #38298, #82778, #56688, #122855, #105463, #92416, #141182, #190932, #88120, #74002, #91342, #72916, #170423, #155256, #188816, #7916, #71837, #40450, #24160, #206122, #42596, #39366, #205045, #41522, #107634, #23088, #76132, #140095, #157402, #173666, #25241, #8994, #171497, #207191, #5758, #26302, #137946, #203968, #89203, #106552, #90263, #172579, #156331, #75069, #58817, #124970, #108701, #57752, #158456, #174730, #6838, #10055, #55614, #123912, #139021, #189879, #142235, #208247, #22010, #59881, #126030, #191993, #104376, #121769, #154190, #187738, #18306, #34568, #130299, #127107, #195222, #68109, #46859, #29525, #84392, #159515, #150479, #93477, #11114, #94544, #96685, #177911, #134245, #30598, #176837, #43658, #80401, #2039, #166716, #160582, #109775, #144384, #175784, #44723, #196287, #211448, #110832, #50827, #27376, #12189, #209303, #193072, #78260, #116954, #145451, #95617, #111911, #77190, #112972, #143311, #210384, #129251, #178984, #162734, #14306, #60950, #146498, #100639, #212515, #64157, #182953, #28451, #161667, #62025, #128181, #194142, #45791, #13261, #79333, #63082, #51904, #21490, #20443, #70246, #135299, #55100, #168839, #102782, #121249, #5239, #155806, #201313, #72394, #153671, #52953, #138494, #172055, #36697, #151540, #69179, #86525, #56163, #87600, #37779, #54031, #184014, #187219, #23648, #152590, #71315, #203446, #137427, #170973, #167779, #38848, #39925, #104931, #22572, #88678, #154737, #120168, #118026, #119091, #204515, #6320, #185071, #122327, #7389, #35629, #188284, #4177, #136361, #202381, #106033, #186144, #103853, #89757, #73469, #200252, #169902, #101707, #19375, #85455, #3108, #59359, #26852, #11667, #74553, #25783, #76672, #142787, #58299, #111383, #43146, #192544, #208793, #60423, #126583, #140654, #176324, #40999, #61493, #107110, #24714, #124455, #9543, #125516, #91895, #191478, #110317, #44197, #27930, #160063, #109259, #193622, #143862, #190414, #94024, #90816, #92956, #42070, #206667, #177386, #77741, #57234, #174210, #175267, #157951, #108184, #156880, #209855, #75617, #29000, #127658, #45263, #8467, #95087, #161135, #12723, #159003, #139570, #173133, #205597, #189359, #141728, #207736, #123395, #10596, #166456, #65719, #211988, #100384, #115626, #116692, #198924, #129783, #182691, #179523, #34309, #62552, #48464, #131867, #47403, #144919, #63629, #113515, #145976, #96155, #66778, #79867, #130830, #33250, #165383, #197874, #210926, #194686, #99334, #46328, #16976, #147033, #195764, #14851, #83057, #97217, #13793, #31142, #196822, #80941, #78796, #128715, #30066, #213055, #181621, #163269, #64684, #50570, #112444, #180570, #114578, #32192, #98268, #178457, #162206, #164326, #15916, #81999, #148086, #49506, #149133, #214091, #714, #132919, #35376, #167523, #136100, #55905, #2855, #202116, #52699, #152341, #185884, #19120, #18047, #1792, #86270, #105764, #72132, #138239, #67849, #119909, #69988, #20183, #3919, #85199, #102520, #84134, #4979, #203197, #135045, #200002, #53776, #201058, #37519, #120994, #151284, #183766, #170718, #68924, #184816, #133996, #51652, #118830, #204253, #36446, #168583, #103595, #169652, #21237, #117775, #87342, #101450, #71057, #153410, #137173, #39655, #54843, #186961, #38593, #104670, #22304, #88415, #154483, #6061, #122062, #188026, #150220, #171789, #190164, #208530, #189106, #124200, #41818, #107931, #172876, #159802, #60166, #43942, #139308, #56975, #77483, #24448, #125259, #207479, #10337, #27668, #40739, #205337, #8212, #106845, #90560, #75360, #209594, #156622, #141472, #206412, #91637, #191219, #74297, #23384, #155550, #25529, #45013, #11406, #143602, #7129, #59099, #9287, #173955, #157689, #140393, #42882, #89496, #158743 ) ),
 .UNSPECIFIED., .F., .F., .T. ) 
 B_SPLINE_SURFACE_WITH_KNOTS ( ( 2, 2 ),
 ( 3, 2, 2, 2, 2, 2, 2, 2, 2, 2, 2, 2, 2, 2, 2, 2, 2, 2, 2, 2, 2, 2, 2, 2, 2, 2, 2, 2, 2, 2, 2, 2, 2, 2, 2, 2, 2, 2, 2, 2, 2, 2, 2, 2, 2, 2, 2, 2, 2, 2, 2, 2, 2, 2, 2, 2, 2, 2, 2, 2, 2, 2, 2, 2, 2, 2, 2, 2, 2, 2, 2, 2, 2, 2, 2, 2, 2, 2, 2, 2, 2, 2, 2, 2, 2, 2, 2, 2, 2, 2, 2, 2, 2, 2, 2, 2, 2, 2, 2, 2, 2, 2, 2, 2, 2, 2, 2, 2, 2, 2, 2, 2, 2, 2, 2, 2, 2, 2, 2, 2, 2, 2, 2, 2, 2, 2, 2, 2, 2, 2, 2, 2, 2, 2, 2, 2, 2, 2, 2, 2, 2, 2, 2, 2, 2, 2, 2, 2, 2, 2, 2, 2, 2, 2, 2, 2, 2, 2, 2, 2, 2, 2, 2, 2, 2, 2, 2, 2, 2, 2, 2, 2, 2, 2, 2, 2, 2, 2, 2, 2, 2, 2, 2, 2, 2, 2, 2, 2, 2, 2, 2, 2, 2, 2, 2, 2, 2, 2, 2, 2, 2, 2, 2, 2, 2, 2, 2, 2, 2, 2, 2, 2, 2, 2, 2, 2, 2, 2, 2, 2, 2, 2, 2, 2, 2, 2, 2, 2, 2, 2, 2, 2, 2, 2, 2, 2, 2, 2, 2, 2, 3 ),
 ( 0.000000000000000000, 1.000000000000000000 ),
 ( 0.000000000000000000, 0.004166666666666666609, 0.008333333333333333218, 0.01250000000000000069, 0.01666666666666666644, 0.02083333333333333218, 0.02500000000000000139, 0.02916666666666666713, 0.03333333333333333287, 0.03749999999999999861, 0.04166666666666666435, 0.04583333333333333010, 0.05000000000000000278, 0.05416666666666666852, 0.05833333333333333426, 0.06250000000000000000, 0.06666666666666666574, 0.07083333333333333148, 0.07499999999999999722, 0.07916666666666666297, 0.08333333333333332871, 0.08749999999999999445, 0.09166666666666666019, 0.09583333333333333981, 0.1000000000000000056, 0.1041666666666666713, 0.1083333333333333370, 0.1125000000000000028, 0.1166666666666666685, 0.1208333333333333343, 0.1250000000000000000, 0.1291666666666666796, 0.1333333333333333315, 0.1375000000000000111, 0.1416666666666666630, 0.1458333333333333426, 0.1499999999999999944, 0.1541666666666666741, 0.1583333333333333259, 0.1625000000000000056, 0.1666666666666666574, 0.1708333333333333370, 0.1749999999999999889, 0.1791666666666666685, 0.1833333333333333204, 0.1875000000000000000, 0.1916666666666666796, 0.1958333333333333315, 0.2000000000000000111, 0.2041666666666666630, 0.2083333333333333426, 0.2124999999999999944, 0.2166666666666666741, 0.2208333333333333259, 0.2250000000000000056, 0.2291666666666666574, 0.2333333333333333370, 0.2374999999999999889, 0.2416666666666666685, 0.2458333333333333204, 0.2500000000000000000, 0.2541666666666666519, 0.2583333333333333592, 0.2625000000000000111, 0.2666666666666666630, 0.2708333333333333148, 0.2750000000000000222, 0.2791666666666666741, 0.2833333333333333259, 0.2874999999999999778, 0.2916666666666666852, 0.2958333333333333370, 0.2999999999999999889, 0.3041666666666666408, 0.3083333333333333481, 0.3125000000000000000, 0.3166666666666666519, 0.3208333333333333592, 0.3250000000000000111, 0.3291666666666666630, 0.3333333333333333148, 0.3375000000000000222, 0.3416666666666666741, 0.3458333333333333259, 0.3499999999999999778, 0.3541666666666666852, 0.3583333333333333370, 0.3624999999999999889, 0.3666666666666666408, 0.3708333333333333481, 0.3750000000000000000, 0.3791666666666666519, 0.3833333333333333592, 0.3875000000000000111, 0.3916666666666666630, 0.3958333333333333148, 0.4000000000000000222, 0.4041666666666666741, 0.4083333333333333259, 0.4124999999999999778, 0.4166666666666666852, 0.4208333333333333370, 0.4249999999999999889, 0.4291666666666666408, 0.4333333333333333481, 0.4375000000000000000, 0.4416666666666666519, 0.4458333333333333592, 0.4500000000000000111, 0.4541666666666666630, 0.4583333333333333148, 0.4625000000000000222, 0.4666666666666666741, 0.4708333333333333259, 0.4749999999999999778, 0.4791666666666666852, 0.4833333333333333370, 0.4874999999999999889, 0.4916666666666666408, 0.4958333333333333481, 0.5000000000000000000, 0.5041666666666666519, 0.5083333333333333037, 0.5124999999999999556, 0.5166666666666667185, 0.5208333333333333703, 0.5250000000000000222, 0.5291666666666666741, 0.5333333333333333259, 0.5374999999999999778, 0.5416666666666666297, 0.5458333333333332815, 0.5500000000000000444, 0.5541666666666666963, 0.5583333333333333481, 0.5625000000000000000, 0.5666666666666666519, 0.5708333333333333037, 0.5749999999999999556, 0.5791666666666667185, 0.5833333333333333703, 0.5875000000000000222, 0.5916666666666666741, 0.5958333333333333259, 0.5999999999999999778, 0.6041666666666666297, 0.6083333333333332815, 0.6125000000000000444, 0.6166666666666666963, 0.6208333333333333481, 0.6250000000000000000, 0.6291666666666666519, 0.6333333333333333037, 0.6374999999999999556, 0.6416666666666667185, 0.6458333333333333703, 0.6500000000000000222, 0.6541666666666666741, 0.6583333333333333259, 0.6624999999999999778, 0.6666666666666666297, 0.6708333333333332815, 0.6750000000000000444, 0.6791666666666666963, 0.6833333333333333481, 0.6875000000000000000, 0.6916666666666666519, 0.6958333333333333037, 0.6999999999999999556, 0.7041666666666667185, 0.7083333333333333703, 0.7125000000000000222, 0.7166666666666666741, 0.7208333333333333259, 0.7249999999999999778, 0.7291666666666666297, 0.7333333333333332815, 0.7375000000000000444, 0.7416666666666666963, 0.7458333333333333481, 0.7500000000000000000, 0.7541666666666666519, 0.7583333333333333037, 0.7624999999999999556, 0.7666666666666667185, 0.7708333333333333703, 0.7750000000000000222, 0.7791666666666666741, 0.7833333333333333259, 0.7874999999999999778, 0.7916666666666666297, 0.7958333333333332815, 0.8000000000000000444, 0.8041666666666666963, 0.8083333333333333481, 0.8125000000000000000, 0.8166666666666666519, 0.8208333333333333037, 0.8249999999999999556, 0.8291666666666667185, 0.8333333333333333703, 0.8375000000000000222, 0.8416666666666666741, 0.8458333333333333259, 0.8499999999999999778, 0.8541666666666666297, 0.8583333333333332815, 0.8625000000000000444, 0.8666666666666666963, 0.8708333333333333481, 0.8750000000000000000, 0.8791666666666666519, 0.8833333333333333037, 0.8874999999999999556, 0.8916666666666667185, 0.8958333333333333703, 0.9000000000000000222, 0.9041666666666666741, 0.9083333333333333259, 0.9124999999999999778, 0.9166666666666666297, 0.9208333333333332815, 0.9250000000000000444, 0.9291666666666666963, 0.9333333333333333481, 0.9375000000000000000, 0.9416666666666666519, 0.9458333333333333037, 0.9499999999999999556, 0.9541666666666667185, 0.9583333333333333703, 0.9625000000000000222, 0.9666666666666666741, 0.9708333333333333259, 0.9749999999999999778, 0.9791666666666666297, 0.9833333333333332815, 0.9875000000000000444, 0.9916666666666666963, 0.9958333333333333481, 1.000000000000000000 ),
 .UNSPECIFIED. ) 
 GEOMETRIC_REPRESENTATION_ITEM ( )  RATIONAL_B_SPLINE_SURFACE ( (
 ( 1.000000000000000000, 0.8660254037844387076, 1.000000000000000000, 0.8660254037844387076, 1.000000000000000000, 0.8660254037844387076, 1.000000000000000000, 0.8660254037844387076, 1.000000000000000000, 0.8660254037844387076, 1.000000000000000000, 0.8660254037844387076, 1.000000000000000000, 0.8660254037844387076, 1.000000000000000000, 0.8660254037844387076, 1.000000000000000000, 0.8660254037844387076, 1.000000000000000000, 0.8660254037844387076, 1.000000000000000000, 0.8660254037844387076, 1.000000000000000000, 0.8660254037844387076, 1.000000000000000000, 0.8660254037844387076, 1.000000000000000000, 0.8660254037844387076, 1.000000000000000000, 0.8660254037844387076, 1.000000000000000000, 0.8660254037844387076, 1.000000000000000000, 0.8660254037844387076, 1.000000000000000000, 0.8660254037844387076, 1.000000000000000000, 0.8660254037844387076, 1.000000000000000000, 0.8660254037844387076, 1.000000000000000000, 0.8660254037844387076, 1.000000000000000000, 0.8660254037844387076, 1.000000000000000000, 0.8660254037844387076, 1.000000000000000000, 0.8660254037844387076, 1.000000000000000000, 0.8660254037844387076, 1.000000000000000000, 0.8660254037844387076, 1.000000000000000000, 0.8660254037844387076, 1.000000000000000000, 0.8660254037844387076, 1.000000000000000000, 0.8660254037844387076, 1.000000000000000000, 0.8660254037844387076, 1.000000000000000000, 0.8660254037844387076, 1.000000000000000000, 0.8660254037844387076, 1.000000000000000000, 0.8660254037844387076, 1.000000000000000000, 0.8660254037844387076, 1.000000000000000000, 0.8660254037844387076, 1.000000000000000000, 0.8660254037844387076, 1.000000000000000000, 0.8660254037844387076, 1.000000000000000000, 0.8660254037844387076, 1.000000000000000000, 0.8660254037844387076, 1.000000000000000000, 0.8660254037844387076, 1.000000000000000000, 0.8660254037844387076, 1.000000000000000000, 0.8660254037844387076, 1.000000000000000000, 0.8660254037844387076, 1.000000000000000000, 0.8660254037844387076, 1.000000000000000000, 0.8660254037844387076, 1.000000000000000000, 0.8660254037844387076, 1.000000000000000000, 0.8660254037844387076, 1.000000000000000000, 0.8660254037844387076, 1.000000000000000000, 0.8660254037844387076, 1.000000000000000000, 0.8660254037844387076, 1.000000000000000000, 0.8660254037844387076, 1.000000000000000000, 0.8660254037844387076, 1.000000000000000000, 0.8660254037844387076, 1.000000000000000000, 0.8660254037844387076, 1.000000000000000000, 0.8660254037844387076, 1.000000000000000000, 0.8660254037844387076, 1.000000000000000000, 0.8660254037844387076, 1.000000000000000000, 0.8660254037844387076, 1.000000000000000000, 0.8660254037844387076, 1.000000000000000000, 0.8660254037844387076, 1.000000000000000000, 0.8660254037844387076, 1.000000000000000000, 0.8660254037844387076, 1.000000000000000000, 0.8660254037844387076, 1.000000000000000000, 0.8660254037844387076, 1.000000000000000000, 0.8660254037844387076, 1.000000000000000000, 0.8660254037844387076, 1.000000000000000000, 0.8660254037844387076, 1.000000000000000000, 0.8660254037844387076, 1.000000000000000000, 0.8660254037844387076, 1.000000000000000000, 0.8660254037844387076, 1.000000000000000000, 0.8660254037844387076, 1.000000000000000000, 0.8660254037844387076, 1.000000000000000000, 0.8660254037844387076, 1.000000000000000000, 0.8660254037844387076, 1.000000000000000000, 0.8660254037844387076, 1.000000000000000000, 0.8660254037844387076, 1.000000000000000000, 0.8660254037844387076, 1.000000000000000000, 0.8660254037844387076, 1.000000000000000000, 0.8660254037844387076, 1.000000000000000000, 0.8660254037844387076, 1.000000000000000000, 0.8660254037844387076, 1.000000000000000000, 0.8660254037844387076, 1.000000000000000000, 0.8660254037844387076, 1.000000000000000000, 0.8660254037844387076, 1.000000000000000000, 0.8660254037844387076, 1.000000000000000000, 0.8660254037844387076, 1.000000000000000000, 0.8660254037844387076, 1.000000000000000000, 0.8660254037844387076, 1.000000000000000000, 0.8660254037844387076, 1.000000000000000000, 0.8660254037844387076, 1.000000000000000000, 0.8660254037844387076, 1.000000000000000000, 0.8660254037844387076, 1.000000000000000000, 0.8660254037844387076, 1.000000000000000000, 0.8660254037844387076, 1.000000000000000000, 0.8660254037844387076, 1.000000000000000000, 0.8660254037844387076, 1.000000000000000000, 0.8660254037844387076, 1.000000000000000000, 0.8660254037844387076, 1.000000000000000000, 0.8660254037844387076, 1.000000000000000000, 0.8660254037844387076, 1.000000000000000000, 0.8660254037844387076, 1.000000000000000000, 0.8660254037844387076, 1.000000000000000000, 0.8660254037844387076, 1.000000000000000000, 0.8660254037844387076, 1.000000000000000000, 0.8660254037844387076, 1.000000000000000000, 0.8660254037844387076, 1.000000000000000000, 0.8660254037844387076, 1.000000000000000000, 0.8660254037844387076, 1.000000000000000000, 0.8660254037844387076, 1.000000000000000000, 0.8660254037844387076, 1.000000000000000000, 0.8660254037844387076, 1.000000000000000000, 0.8660254037844387076, 1.000000000000000000, 0.8660254037844387076, 1.000000000000000000, 0.8660254037844387076, 1.000000000000000000, 0.8660254037844387076, 1.000000000000000000, 0.8660254037844387076, 1.000000000000000000, 0.8660254037844387076, 1.000000000000000000, 0.8660254037844387076, 1.000000000000000000, 0.8660254037844387076, 1.000000000000000000, 0.8660254037844387076, 1.000000000000000000, 0.8660254037844387076, 1.000000000000000000, 0.8660254037844387076, 1.000000000000000000, 0.8660254037844387076, 1.000000000000000000, 0.8660254037844387076, 1.000000000000000000, 0.8660254037844387076, 1.000000000000000000, 0.8660254037844387076, 1.000000000000000000, 0.8660254037844387076, 1.000000000000000000, 0.8660254037844387076, 1.000000000000000000, 0.8660254037844387076, 1.000000000000000000, 0.8660254037844387076, 1.000000000000000000, 0.8660254037844387076, 1.000000000000000000, 0.8660254037844387076, 1.000000000000000000, 0.8660254037844387076, 1.000000000000000000, 0.8660254037844387076, 1.000000000000000000, 0.8660254037844387076, 1.000000000000000000, 0.8660254037844387076, 1.000000000000000000, 0.8660254037844387076, 1.000000000000000000, 0.8660254037844387076, 1.000000000000000000, 0.8660254037844387076, 1.000000000000000000, 0.8660254037844387076, 1.000000000000000000, 0.8660254037844387076, 1.000000000000000000, 0.8660254037844387076, 1.000000000000000000, 0.8660254037844387076, 1.000000000000000000, 0.8660254037844387076, 1.000000000000000000, 0.8660254037844387076, 1.000000000000000000, 0.8660254037844387076, 1.000000000000000000, 0.8660254037844387076, 1.000000000000000000, 0.8660254037844387076, 1.000000000000000000, 0.8660254037844387076, 1.000000000000000000, 0.8660254037844387076, 1.000000000000000000, 0.8660254037844387076, 1.000000000000000000, 0.8660254037844387076, 1.000000000000000000, 0.8660254037844387076, 1.000000000000000000, 0.8660254037844387076, 1.000000000000000000, 0.8660254037844387076, 1.000000000000000000, 0.8660254037844387076, 1.000000000000000000, 0.8660254037844387076, 1.000000000000000000, 0.8660254037844387076, 1.000000000000000000, 0.8660254037844387076, 1.000000000000000000, 0.8660254037844387076, 1.000000000000000000, 0.8660254037844387076, 1.000000000000000000, 0.8660254037844387076, 1.000000000000000000, 0.8660254037844387076, 1.000000000000000000, 0.8660254037844387076, 1.000000000000000000, 0.8660254037844387076, 1.000000000000000000, 0.8660254037844387076, 1.000000000000000000, 0.8660254037844387076, 1.000000000000000000, 0.8660254037844387076, 1.000000000000000000, 0.8660254037844387076, 1.000000000000000000, 0.8660254037844387076, 1.000000000000000000, 0.8660254037844387076, 1.000000000000000000, 0.8660254037844387076, 1.000000000000000000, 0.8660254037844387076, 1.000000000000000000, 0.8660254037844387076, 1.000000000000000000, 0.8660254037844387076, 1.000000000000000000, 0.8660254037844387076, 1.000000000000000000, 0.8660254037844387076, 1.000000000000000000, 0.8660254037844387076, 1.000000000000000000, 0.8660254037844387076, 1.000000000000000000, 0.8660254037844387076, 1.000000000000000000, 0.8660254037844387076, 1.000000000000000000, 0.8660254037844387076, 1.000000000000000000, 0.8660254037844387076, 1.000000000000000000, 0.8660254037844387076, 1.000000000000000000, 0.8660254037844387076, 1.000000000000000000, 0.8660254037844387076, 1.000000000000000000, 0.8660254037844387076, 1.000000000000000000, 0.8660254037844387076, 1.000000000000000000, 0.8660254037844387076, 1.000000000000000000, 0.8660254037844387076, 1.000000000000000000, 0.8660254037844387076, 1.000000000000000000, 0.8660254037844387076, 1.000000000000000000, 0.8660254037844387076, 1.000000000000000000, 0.8660254037844387076, 1.000000000000000000, 0.8660254037844387076, 1.000000000000000000, 0.8660254037844387076, 1.000000000000000000, 0.8660254037844387076, 1.000000000000000000, 0.8660254037844387076, 1.000000000000000000, 0.8660254037844387076, 1.000000000000000000, 0.8660254037844387076, 1.000000000000000000, 0.8660254037844387076, 1.000000000000000000, 0.8660254037844387076, 1.000000000000000000, 0.8660254037844387076, 1.000000000000000000, 0.8660254037844387076, 1.000000000000000000, 0.8660254037844387076, 1.000000000000000000, 0.8660254037844387076, 1.000000000000000000, 0.8660254037844387076, 1.000000000000000000, 0.8660254037844387076, 1.000000000000000000, 0.8660254037844387076, 1.000000000000000000, 0.8660254037844387076, 1.000000000000000000, 0.8660254037844387076, 1.000000000000000000, 0.8660254037844387076, 1.000000000000000000, 0.8660254037844387076, 1.000000000000000000, 0.8660254037844387076, 1.000000000000000000, 0.8660254037844387076, 1.000000000000000000, 0.8660254037844387076, 1.000000000000000000, 0.8660254037844387076, 1.000000000000000000, 0.8660254037844387076, 1.000000000000000000, 0.8660254037844387076, 1.000000000000000000, 0.8660254037844387076, 1.000000000000000000, 0.8660254037844387076, 1.000000000000000000, 0.8660254037844387076, 1.000000000000000000, 0.8660254037844387076, 1.000000000000000000, 0.8660254037844387076, 1.000000000000000000, 0.8660254037844387076, 1.000000000000000000, 0.8660254037844387076, 1.000000000000000000, 0.8660254037844387076, 1.000000000000000000, 0.8660254037844387076, 1.000000000000000000, 0.8660254037844387076, 1.000000000000000000, 0.8660254037844387076, 1.000000000000000000, 0.8660254037844387076, 1.000000000000000000, 0.8660254037844387076, 1.000000000000000000, 0.8660254037844387076, 1.000000000000000000, 0.8660254037844387076, 1.000000000000000000, 0.8660254037844387076, 1.000000000000000000, 0.8660254037844387076, 1.000000000000000000, 0.8660254037844387076, 1.000000000000000000, 0.8660254037844387076, 1.000000000000000000, 0.8660254037844387076, 1.000000000000000000, 0.8660254037844387076, 1.000000000000000000),
 ( 1.000000000000000000, 0.8660254037844387076, 1.000000000000000000, 0.8660254037844387076, 1.000000000000000000, 0.8660254037844387076, 1.000000000000000000, 0.8660254037844387076, 1.000000000000000000, 0.8660254037844387076, 1.000000000000000000, 0.8660254037844387076, 1.000000000000000000, 0.8660254037844387076, 1.000000000000000000, 0.8660254037844387076, 1.000000000000000000, 0.8660254037844387076, 1.000000000000000000, 0.8660254037844387076, 1.000000000000000000, 0.8660254037844387076, 1.000000000000000000, 0.8660254037844387076, 1.000000000000000000, 0.8660254037844387076, 1.000000000000000000, 0.8660254037844387076, 1.000000000000000000, 0.8660254037844387076, 1.000000000000000000, 0.8660254037844387076, 1.000000000000000000, 0.8660254037844387076, 1.000000000000000000, 0.8660254037844387076, 1.000000000000000000, 0.8660254037844387076, 1.000000000000000000, 0.8660254037844387076, 1.000000000000000000, 0.8660254037844387076, 1.000000000000000000, 0.8660254037844387076, 1.000000000000000000, 0.8660254037844387076, 1.000000000000000000, 0.8660254037844387076, 1.000000000000000000, 0.8660254037844387076, 1.000000000000000000, 0.8660254037844387076, 1.000000000000000000, 0.8660254037844387076, 1.000000000000000000, 0.8660254037844387076, 1.000000000000000000, 0.8660254037844387076, 1.000000000000000000, 0.8660254037844387076, 1.000000000000000000, 0.8660254037844387076, 1.000000000000000000, 0.8660254037844387076, 1.000000000000000000, 0.8660254037844387076, 1.000000000000000000, 0.8660254037844387076, 1.000000000000000000, 0.8660254037844387076, 1.000000000000000000, 0.8660254037844387076, 1.000000000000000000, 0.8660254037844387076, 1.000000000000000000, 0.8660254037844387076, 1.000000000000000000, 0.8660254037844387076, 1.000000000000000000, 0.8660254037844387076, 1.000000000000000000, 0.8660254037844387076, 1.000000000000000000, 0.8660254037844387076, 1.000000000000000000, 0.8660254037844387076, 1.000000000000000000, 0.8660254037844387076, 1.000000000000000000, 0.8660254037844387076, 1.000000000000000000, 0.8660254037844387076, 1.000000000000000000, 0.8660254037844387076, 1.000000000000000000, 0.8660254037844387076, 1.000000000000000000, 0.8660254037844387076, 1.000000000000000000, 0.8660254037844387076, 1.000000000000000000, 0.8660254037844387076, 1.000000000000000000, 0.8660254037844387076, 1.000000000000000000, 0.8660254037844387076, 1.000000000000000000, 0.8660254037844387076, 1.000000000000000000, 0.8660254037844387076, 1.000000000000000000, 0.8660254037844387076, 1.000000000000000000, 0.8660254037844387076, 1.000000000000000000, 0.8660254037844387076, 1.000000000000000000, 0.8660254037844387076, 1.000000000000000000, 0.8660254037844387076, 1.000000000000000000, 0.8660254037844387076, 1.000000000000000000, 0.8660254037844387076, 1.000000000000000000, 0.8660254037844387076, 1.000000000000000000, 0.8660254037844387076, 1.000000000000000000, 0.8660254037844387076, 1.000000000000000000, 0.8660254037844387076, 1.000000000000000000, 0.8660254037844387076, 1.000000000000000000, 0.8660254037844387076, 1.000000000000000000, 0.8660254037844387076, 1.000000000000000000, 0.8660254037844387076, 1.000000000000000000, 0.8660254037844387076, 1.000000000000000000, 0.8660254037844387076, 1.000000000000000000, 0.8660254037844387076, 1.000000000000000000, 0.8660254037844387076, 1.000000000000000000, 0.8660254037844387076, 1.000000000000000000, 0.8660254037844387076, 1.000000000000000000, 0.8660254037844387076, 1.000000000000000000, 0.8660254037844387076, 1.000000000000000000, 0.8660254037844387076, 1.000000000000000000, 0.8660254037844387076, 1.000000000000000000, 0.8660254037844387076, 1.000000000000000000, 0.8660254037844387076, 1.000000000000000000, 0.8660254037844387076, 1.000000000000000000, 0.8660254037844387076, 1.000000000000000000, 0.8660254037844387076, 1.000000000000000000, 0.8660254037844387076, 1.000000000000000000, 0.8660254037844387076, 1.000000000000000000, 0.8660254037844387076, 1.000000000000000000, 0.8660254037844387076, 1.000000000000000000, 0.8660254037844387076, 1.000000000000000000, 0.8660254037844387076, 1.000000000000000000, 0.8660254037844387076, 1.000000000000000000, 0.8660254037844387076, 1.000000000000000000, 0.8660254037844387076, 1.000000000000000000, 0.8660254037844387076, 1.000000000000000000, 0.8660254037844387076, 1.000000000000000000, 0.8660254037844387076, 1.000000000000000000, 0.8660254037844387076, 1.000000000000000000, 0.8660254037844387076, 1.000000000000000000, 0.8660254037844387076, 1.000000000000000000, 0.8660254037844387076, 1.000000000000000000, 0.8660254037844387076, 1.000000000000000000, 0.8660254037844387076, 1.000000000000000000, 0.8660254037844387076, 1.000000000000000000, 0.8660254037844387076, 1.000000000000000000, 0.8660254037844387076, 1.000000000000000000, 0.8660254037844387076, 1.000000000000000000, 0.8660254037844387076, 1.000000000000000000, 0.8660254037844387076, 1.000000000000000000, 0.8660254037844387076, 1.000000000000000000, 0.8660254037844387076, 1.000000000000000000, 0.8660254037844387076, 1.000000000000000000, 0.8660254037844387076, 1.000000000000000000, 0.8660254037844387076, 1.000000000000000000, 0.8660254037844387076, 1.000000000000000000, 0.8660254037844387076, 1.000000000000000000, 0.8660254037844387076, 1.000000000000000000, 0.8660254037844387076, 1.000000000000000000, 0.8660254037844387076, 1.000000000000000000, 0.8660254037844387076, 1.000000000000000000, 0.8660254037844387076, 1.000000000000000000, 0.8660254037844387076, 1.000000000000000000, 0.8660254037844387076, 1.000000000000000000, 0.8660254037844387076, 1.000000000000000000, 0.8660254037844387076, 1.000000000000000000, 0.8660254037844387076, 1.000000000000000000, 0.8660254037844387076, 1.000000000000000000, 0.8660254037844387076, 1.000000000000000000, 0.8660254037844387076, 1.000000000000000000, 0.8660254037844387076, 1.000000000000000000, 0.8660254037844387076, 1.000000000000000000, 0.8660254037844387076, 1.000000000000000000, 0.8660254037844387076, 1.000000000000000000, 0.8660254037844387076, 1.000000000000000000, 0.8660254037844387076, 1.000000000000000000, 0.8660254037844387076, 1.000000000000000000, 0.8660254037844387076, 1.000000000000000000, 0.8660254037844387076, 1.000000000000000000, 0.8660254037844387076, 1.000000000000000000, 0.8660254037844387076, 1.000000000000000000, 0.8660254037844387076, 1.000000000000000000, 0.8660254037844387076, 1.000000000000000000, 0.8660254037844387076, 1.000000000000000000, 0.8660254037844387076, 1.000000000000000000, 0.8660254037844387076, 1.000000000000000000, 0.8660254037844387076, 1.000000000000000000, 0.8660254037844387076, 1.000000000000000000, 0.8660254037844387076, 1.000000000000000000, 0.8660254037844387076, 1.000000000000000000, 0.8660254037844387076, 1.000000000000000000, 0.8660254037844387076, 1.000000000000000000, 0.8660254037844387076, 1.000000000000000000, 0.8660254037844387076, 1.000000000000000000, 0.8660254037844387076, 1.000000000000000000, 0.8660254037844387076, 1.000000000000000000, 0.8660254037844387076, 1.000000000000000000, 0.8660254037844387076, 1.000000000000000000, 0.8660254037844387076, 1.000000000000000000, 0.8660254037844387076, 1.000000000000000000, 0.8660254037844387076, 1.000000000000000000, 0.8660254037844387076, 1.000000000000000000, 0.8660254037844387076, 1.000000000000000000, 0.8660254037844387076, 1.000000000000000000, 0.8660254037844387076, 1.000000000000000000, 0.8660254037844387076, 1.000000000000000000, 0.8660254037844387076, 1.000000000000000000, 0.8660254037844387076, 1.000000000000000000, 0.8660254037844387076, 1.000000000000000000, 0.8660254037844387076, 1.000000000000000000, 0.8660254037844387076, 1.000000000000000000, 0.8660254037844387076, 1.000000000000000000, 0.8660254037844387076, 1.000000000000000000, 0.8660254037844387076, 1.000000000000000000, 0.8660254037844387076, 1.000000000000000000, 0.8660254037844387076, 1.000000000000000000, 0.8660254037844387076, 1.000000000000000000, 0.8660254037844387076, 1.000000000000000000, 0.8660254037844387076, 1.000000000000000000, 0.8660254037844387076, 1.000000000000000000, 0.8660254037844387076, 1.000000000000000000, 0.8660254037844387076, 1.000000000000000000, 0.8660254037844387076, 1.000000000000000000, 0.8660254037844387076, 1.000000000000000000, 0.8660254037844387076, 1.000000000000000000, 0.8660254037844387076, 1.000000000000000000, 0.8660254037844387076, 1.000000000000000000, 0.8660254037844387076, 1.000000000000000000, 0.8660254037844387076, 1.000000000000000000, 0.8660254037844387076, 1.000000000000000000, 0.8660254037844387076, 1.000000000000000000, 0.8660254037844387076, 1.000000000000000000, 0.8660254037844387076, 1.000000000000000000, 0.8660254037844387076, 1.000000000000000000, 0.8660254037844387076, 1.000000000000000000, 0.8660254037844387076, 1.000000000000000000, 0.8660254037844387076, 1.000000000000000000, 0.8660254037844387076, 1.000000000000000000, 0.8660254037844387076, 1.000000000000000000, 0.8660254037844387076, 1.000000000000000000, 0.8660254037844387076, 1.000000000000000000, 0.8660254037844387076, 1.000000000000000000, 0.8660254037844387076, 1.000000000000000000, 0.8660254037844387076, 1.000000000000000000, 0.8660254037844387076, 1.000000000000000000, 0.8660254037844387076, 1.000000000000000000, 0.8660254037844387076, 1.000000000000000000, 0.8660254037844387076, 1.000000000000000000, 0.8660254037844387076, 1.000000000000000000, 0.8660254037844387076, 1.000000000000000000, 0.8660254037844387076, 1.000000000000000000, 0.8660254037844387076, 1.000000000000000000, 0.8660254037844387076, 1.000000000000000000, 0.8660254037844387076, 1.000000000000000000, 0.8660254037844387076, 1.000000000000000000, 0.8660254037844387076, 1.000000000000000000, 0.8660254037844387076, 1.000000000000000000, 0.8660254037844387076, 1.000000000000000000, 0.8660254037844387076, 1.000000000000000000, 0.8660254037844387076, 1.000000000000000000, 0.8660254037844387076, 1.000000000000000000, 0.8660254037844387076, 1.000000000000000000, 0.8660254037844387076, 1.000000000000000000, 0.8660254037844387076, 1.000000000000000000, 0.8660254037844387076, 1.000000000000000000, 0.8660254037844387076, 1.000000000000000000, 0.8660254037844387076, 1.000000000000000000, 0.8660254037844387076, 1.000000000000000000, 0.8660254037844387076, 1.000000000000000000, 0.8660254037844387076, 1.000000000000000000, 0.8660254037844387076, 1.000000000000000000, 0.8660254037844387076, 1.000000000000000000, 0.8660254037844387076, 1.000000000000000000, 0.8660254037844387076, 1.000000000000000000, 0.8660254037844387076, 1.000000000000000000, 0.8660254037844387076, 1.000000000000000000, 0.8660254037844387076, 1.000000000000000000, 0.8660254037844387076, 1.000000000000000000, 0.8660254037844387076, 1.000000000000000000, 0.8660254037844387076, 1.000000000000000000, 0.8660254037844387076, 1.000000000000000000) ) ) 
 REPRESENTATION_ITEM ( '' )  SURFACE ( )  );
#117628=CARTESIAN_POINT ( 'NONE',  ( -1.201851678989727383E-14, 5.837500000000023448, -1.732050807568863648 ) ) ;
#117629=CARTESIAN_POINT ( 'NONE',  ( 2.849184837166184536, 6.475799410002530898, 0.7998128361456362523 ) ) ;
#117630=CARTESIAN_POINT ( 'NONE',  ( 5.250031796989762967, 7.148123067953287446, 1.599625672291267398 ) ) ;
#117632=CARTESIAN_POINT ( 'NONE',  ( -7.592202833972775622, 8.920286730132099606, 1.082531754730558626 ) ) ;
#117634=CARTESIAN_POINT ( 'NONE',  ( 5.829642864196168617, 6.863966765392747860, 1.082531754730558626 ) ) ;
#117635=CARTESIAN_POINT ( 'NONE',  ( -7.009202228140739344, 11.12122699956546334, -0.7216878364870267237 ) ) ;
#117639=CARTESIAN_POINT ( 'NONE',  ( 7.962716289927667113, 8.184257181204083409, -0.7998128361456291469 ) ) ;
#117644=CARTESIAN_POINT ( 'NONE',  ( -1.364683531250012516, 4.238541667008090208, -0.7879004041258300672 ) ) ;
#117651=CARTESIAN_POINT ( 'NONE',  ( 7.262363838414439776, 11.62450824479221900, 0.7998128361456462443 ) ) ;
#117655=CARTESIAN_POINT ( 'NONE',  ( -7.828943636887387925, 11.22118577875556156, 1.199719254218453823 ) ) ;
#117657=CARTESIAN_POINT ( 'NONE',  ( 3.469446951953614189E-15, 5.290451655907108197, 1.214306433183764966E-14 ) ) ;
#117661=CARTESIAN_POINT ( 'NONE',  ( 10.56588178375152864, 11.22128359066528169, -0.7998128361456281477 ) ) ;
#117664=CARTESIAN_POINT ( 'NONE',  ( -9.528683032306089373, 10.01121838064558744, 0.7998128361456462443 ) ) ;
#117669=CARTESIAN_POINT ( 'NONE',  ( 5.726377019126981160, 6.078880280049443918, 0.6665230057388837892 ) ) ;
#117670=CARTESIAN_POINT ( 'NONE',  ( -4.600294193738529103, 4.261431402316699035, -0.7998128361456221525 ) ) ;
#117675=AXIS2_PLACEMENT_3D ( 'NONE', #52692, #104662, #182683 ) ;
#117676=CARTESIAN_POINT ( 'NONE',  ( 6.479907352327590964, 9.647310113435821677, 1.199719254218462483 ) ) ;
#117678=CARTESIAN_POINT ( 'NONE',  ( 5.774883364416965037, 8.824782127540085952, -1.199719254218440723 ) ) ;
#117679=CARTESIAN_POINT ( 'NONE',  ( -4.295541959788370612, 7.266047401097770475, -0.9601269197386901322 ) ) ;
#117681=CARTESIAN_POINT ( 'NONE',  ( 4.847203612085560387, 5.613824621309978724, -1.199719254218452047 ) ) ;
#117683=CARTESIAN_POINT ( 'NONE',  ( -6.710922849084449915, 10.77323439066645783, 0.000000000000000000 ) ) ;
#117690=CARTESIAN_POINT ( 'NONE',  ( -4.339127873110165901, 7.217636166161084610, -1.009937615098016606 ) ) ;
#117691=CARTESIAN_POINT ( 'NONE',  ( 4.193801852926431373, 7.579907728022624802, -0.9040490846396221913 ) ) ;
#117694=CARTESIAN_POINT ( 'NONE',  ( 5.422898255786183341, 7.349800603215774331, -1.443375672974051449 ) ) ;
#117699=CARTESIAN_POINT ( 'NONE',  ( -10.10046125205658463, 11.84658821789661509, -1.082531754730537976 ) ) ;
#117704=CARTESIAN_POINT ( 'NONE',  ( -9.937763408692596556, 11.65677406730528887, -1.082531754730537976 ) ) ;
#117711=CARTESIAN_POINT ( 'NONE',  ( -8.798878505144648088, 12.24881344176869469, -1.082531754730543083 ) ) ;
#117719=CARTESIAN_POINT ( 'NONE',  ( 0.7499999999999902300, 3.264583334016149418, 1.299038105676669330 ) ) ;
#117721=CARTESIAN_POINT ( 'NONE',  ( -4.880045225915050189, 7.780804299287790826, 1.199719254218464037 ) ) ;
#117725=CARTESIAN_POINT ( 'NONE',  ( -7.309817376062285099, 11.67987070538135264, 0.000000000000000000 ) ) ;
#117728=CARTESIAN_POINT ( 'NONE',  ( -1.201851678989727383E-14, 4.368750000682820378, -1.732050807568863648 ) ) ;
#117729=CARTESIAN_POINT ( 'NONE',  ( 7.070740804726770357, 8.207951346058097286, 1.199719254218462483 ) ) ;
#117734=CARTESIAN_POINT ( 'NONE',  ( 7.899597058256738968, 12.36794700127490820, 1.040834085586084257E-14 ) ) ;
#117736=CARTESIAN_POINT ( 'NONE',  ( -7.334597915313094241, 9.580116872663850813, 1.040834085586084257E-14 ) ) ;
#117739=CARTESIAN_POINT ( 'NONE',  ( -7.293923454472094114, 9.532663335016016148, 1.443375672974090751 ) ) ;
#117742=EDGE_CURVE ( 'NONE', #152353, #212749, #3748, .T. ) ;
#117743=CARTESIAN_POINT ( 'NONE',  ( -1.364683531250010295, 5.801041667008088432, -0.7879004041258300672 ) ) ;
#117751=CARTESIAN_POINT ( 'NONE',  ( -2.602802303699316866, 5.980427087717073320, 1.040834085586084257E-14 ) ) ;
#117753=CARTESIAN_POINT ( 'NONE',  ( 9.154780037725547714, 11.70366268214508487, 1.599625672291279388 ) ) ;
#117754=DIRECTION ( 'NONE',  ( -5.578564026256490882E-16, -1.000000000000000000, -9.066213480720158442E-32 ) ) ;
#117759=CARTESIAN_POINT ( 'NONE',  ( -0.6823417656250212460, 2.801041667008084879, 1.181850606188767472 ) ) ;
#117761=CARTESIAN_POINT ( 'NONE',  ( 5.020596955762157698, 4.751784624677624080, 1.040834085586084257E-14 ) ) ;
#117767=FACE_OUTER_BOUND ( 'NONE', #180918, .T. ) ;
#117770=CARTESIAN_POINT ( 'NONE',  ( -8.378575743565381373, 8.877352577022161739, 0.7216878364870438212 ) ) ;
#117775=CARTESIAN_POINT ( 'NONE',  ( -9.321394304595349567, 10.83371376257142416, 1.199719254218462483 ) ) ;
#117776=CARTESIAN_POINT ( 'NONE',  ( -3.755245360860925086, 6.364574773437617239, -1.082531754730548412 ) ) ;
#117777=CARTESIAN_POINT ( 'NONE',  ( 1.364683531249988757, 2.196875000341415252, 1.214306433183764966E-14 ) ) ;
#117784=CARTESIAN_POINT ( 'NONE',  ( 8.224992744984721327, 12.74757530245756243, 1.040834085586084257E-14 ) ) ;
#117797=CARTESIAN_POINT ( 'NONE',  ( 0.6823417656249899377, 4.238541667008085767, -1.181850606188754593 ) ) ;
#117801=CARTESIAN_POINT ( 'NONE',  ( 7.334597915313080918, 9.580116872663850813, 1.040834085586084257E-14 ) ) ;
#117804=CARTESIAN_POINT ( 'NONE',  ( 8.910733272679570049, 11.41894145625809820, -1.599625672291255185 ) ) ;
#117808=CARTESIAN_POINT ( 'NONE',  ( 0.6823417656249899377, 1.842708333674752952, 1.181850606188755259 ) ) ;
#117811=CARTESIAN_POINT ( 'NONE',  ( -8.188761592974051595, 9.616271948966963024, -1.082531754730543971 ) ) ;
#117819=CARTESIAN_POINT ( 'NONE',  ( 4.542145155778077203, 5.257923088951247159, -1.199719254218452047 ) ) ;
#117822=ORIENTED_EDGE ( 'NONE', *, *, #76293, .T. ) ;
#117829=CARTESIAN_POINT ( 'NONE',  ( -4.569261463005423352, 5.289558780716470565, -1.199719254218446718 ) ) ;
#117830=CARTESIAN_POINT ( 'NONE',  ( 8.769426429940780920, 9.125419011219408461, 0.7998128361456462443 ) ) ;
#117832=CARTESIAN_POINT ( 'NONE',  ( 5.788968402910816380, 5.856144012925152076, 0.7216878364870317197 ) ) ;
#117841=CARTESIAN_POINT ( 'NONE',  ( -6.399085315970137522, 9.449054721065074602, -1.082531754730538864 ) ) ;
#117843=CARTESIAN_POINT ( 'NONE',  ( 3.985207087413062066, 6.736826471035503694, -1.199719254218452047 ) ) ;
#117846=CARTESIAN_POINT ( 'NONE',  ( -8.453672473320708036, 9.821371626084353323, -1.199719254218446718 ) ) ;
#117850=CARTESIAN_POINT ( 'NONE',  ( -4.457933580795036654, 4.095344020549286590, -0.7998128361456221525 ) ) ;
#117852=CARTESIAN_POINT ( 'NONE',  ( 9.271078113646423091, 9.710679308875986848, 1.040834085586084257E-14 ) ) ;
#117854=CARTESIAN_POINT ( 'NONE',  ( 2.920892028740289081, 5.495125569250587816, 1.199719254218452047 ) ) ;
#117860=CARTESIAN_POINT ( 'NONE',  ( 2.412988153552339643, 5.758977245878946327, 0.7216878364870438212 ) ) ;
#117863=CARTESIAN_POINT ( 'NONE',  ( -3.958090780185743451, 6.705190779270287393, -1.199719254218452047 ) ) ;
#117866=CARTESIAN_POINT ( 'NONE',  ( -7.947050595904583403, 12.42330946186405249, 0.7998128361456481317 ) ) ;
#117871=CARTESIAN_POINT ( 'NONE',  ( 7.958272981541723468, 8.386999354661243800, 1.040834085586084257E-14 ) ) ;
#117875=CARTESIAN_POINT ( 'NONE',  ( 5.172599298813543633, 5.993452922492633839, -1.199719254218452047 ) ) ;
#117878=CARTESIAN_POINT ( 'NONE',  ( -6.039267359883488950, 9.133230122250985517, 1.199719254218452047 ) ) ;
#117883=FACE_OUTER_BOUND ( 'NONE', #53375, .T. ) ;
#117887=CARTESIAN_POINT ( 'NONE',  ( -1.201851678989727383E-14, 3.259375000341420581, -1.575800808251660134 ) ) ;
#117888=CARTESIAN_POINT ( 'NONE',  ( 9.562578416340237197, 10.05076299535211781, 0.7998128361456462443 ) ) ;
#117891=CARTESIAN_POINT ( 'NONE',  ( -5.314433026876900001, 6.262888621853549331, 1.082531754730548412 ) ) ;
#117892=CARTESIAN_POINT ( 'NONE',  ( 2.412988153552339643, 5.758977245878946327, 0.7216878364870438212 ) ) ;
#117893=CARTESIAN_POINT ( 'NONE',  ( -5.788968402910818156, 7.776882441527838807, 1.443375672974064550 ) ) ;
#117899=CARTESIAN_POINT ( 'NONE',  ( 3.635557746758808495, 7.393234471193928847, -0.7998128361456291469 ) ) ;
#117910=CARTESIAN_POINT ( 'NONE',  ( 5.867981556616276073, 5.740399992340775803, -0.7998128361456281477 ) ) ;
#117914=CARTESIAN_POINT ( 'NONE',  ( -4.550733115681270036, 8.460939068270139529, 0.7998128361456481317 ) ) ;
#117918=CARTESIAN_POINT ( 'NONE',  ( 5.961834861707224320, 7.978559976790334574, -1.599625672291262513 ) ) ;
#117921=CARTESIAN_POINT ( 'NONE',  ( -5.168682875307782254, 7.053215992657626110, -1.599625672291256295 ) ) ;
#117922=CARTESIAN_POINT ( 'NONE',  ( 7.429504990164394584, 7.770103364721017591, 1.040834085586084257E-14 ) ) ;
#117923=CARTESIAN_POINT ( 'NONE',  ( 4.626555186793138930, 7.126393038833472637, 1.348983236782254957 ) ) ;
#117924=CARTESIAN_POINT ( 'NONE',  ( -4.623494077460110319, 5.352830164246910272, 1.199719254218462483 ) ) ;
#117927=CARTESIAN_POINT ( 'NONE',  ( -6.600121851754250812, 6.594563670001734046, 0.7998128361456341429 ) ) ;
#117930=CARTESIAN_POINT ( 'NONE',  ( -0.6823417656249969321, 3.467708333674754506, -1.181850606188749264 ) ) ;
#117932=CARTESIAN_POINT ( 'NONE',  ( -5.612712406377534435, 5.650512016969639895, 0.7216878364870317197 ) ) ;
#117938=CARTESIAN_POINT ( 'NONE',  ( 4.008406971134620633, 7.828225232965717595, 0.7998128361456321445 ) ) ;
#117941=CARTESIAN_POINT ( 'NONE',  ( 1.364683531249986537, 2.717708333674754062, -0.7879004041258239610 ) ) ;
#117944=CARTESIAN_POINT ( 'NONE',  ( 3.606105671554957759, 4.269840040644637291, -1.082531754730543083 ) ) ;
#117947=CARTESIAN_POINT ( 'NONE',  ( -3.810004860640155311, 4.403759411290286252, 1.199719254218462483 ) ) ;
#117948=CARTESIAN_POINT ( 'NONE',  ( -6.927853306458756855, 9.105581495667113501, 1.443375672974078761 ) ) ;
#117950=CARTESIAN_POINT ( 'NONE',  ( 1.364683531249986537, 2.405208333674752286, -0.7879004041258239610 ) ) ;
#117957=CARTESIAN_POINT ( 'NONE',  ( -6.304178240230145391, 9.338329799368375816, 1.082531754730548412 ) ) ;
#117963=CARTESIAN_POINT ( 'NONE',  ( -7.063434842595444962, 8.303390740191881392, 1.082531754730549967 ) ) ;
#117973=DIRECTION ( 'NONE',  ( 1.000000000000000000, 0.000000000000000000, 0.000000000000000000 ) ) ;
#117979=CARTESIAN_POINT ( 'NONE',  ( -6.878064000834399394, 6.918829510595249310, -0.7998128361456291469 ) ) ;
#117981=CARTESIAN_POINT ( 'NONE',  ( 0.7499999999999867883, -0.9333333333333138082, -1.299038105676652011 ) ) ;
#117982=CARTESIAN_POINT ( 'NONE',  ( 2.835626683552519012, 6.459981564119914310, 0.000000000000000000 ) ) ;
#117986=CARTESIAN_POINT ( 'NONE',  ( 6.844168616800228477, 6.879284895888727824, -0.7998128361456281477 ) ) ;
#117991=CARTESIAN_POINT ( 'NONE',  ( -3.280709984826970516, 6.771319382366015383, 0.7216878364870317197 ) ) ;
#117996=AXIS2_PLACEMENT_3D ( 'NONE', #130181, #44606, #109666 ) ;
#118000=CARTESIAN_POINT ( 'NONE',  ( -1.364683531250012516, 1.530208333674756505, 0.7879004041258379498 ) ) ;
#118003=CARTESIAN_POINT ( 'NONE',  ( -7.069687034522070590, 10.33538640932937724, -1.199719254218440723 ) ) ;
#118005=CARTESIAN_POINT ( 'NONE',  ( 5.770966940911189447, 9.884545197705074671, -0.7998128361456291469 ) ) ;
#118006=CARTESIAN_POINT ( 'NONE',  ( -6.364663046611467756, 9.512858423433634414, 1.199719254218452047 ) ) ;
#118009=CARTESIAN_POINT ( 'NONE',  ( 1.364683531249988535, 5.655208333674751842, -0.7879004041258300672 ) ) ;
#118011=CARTESIAN_POINT ( 'NONE',  ( 7.863365906246055914, 10.19701286208565705, -1.443375672974057666 ) ) ;
#118014=CARTESIAN_POINT ( 'NONE',  ( 1.364683531249986537, 0.1760416670080860446, 0.7879004041258500513 ) ) ;
#118017=CARTESIAN_POINT ( 'NONE',  ( 7.090551149822728938, 10.25576486055978442, 1.082531754730558626 ) ) ;
#118020=CARTESIAN_POINT ( 'NONE',  ( -4.284013352238255301, 6.981470763377843447, -1.082531754730549967 ) ) ;
#118022=CARTESIAN_POINT ( 'NONE',  ( 1.364683531249988535, 3.113541667008083991, 0.7879004041258500513 ) ) ;
#118026=CARTESIAN_POINT ( 'NONE',  ( -6.124532705071231931, 8.168374127381657246, -1.599625672291263179 ) ) ;
#118034=CARTESIAN_POINT ( 'NONE',  ( 7.202405917357655341, 9.425892875049191488, 1.599625672291281386 ) ) ;
#118038=CARTESIAN_POINT ( 'NONE',  ( -1.201851678989727383E-14, 3.087500000000026112, -1.732050807568863648 ) ) ;
#118045=CARTESIAN_POINT ( 'NONE',  ( 4.690757960648213931, 8.416375354157496602, 0.7216878364870438212 ) ) ;
#118047=CARTESIAN_POINT ( 'NONE',  ( -1.402160292154681736E-14, 1.009375000341417916, -1.575800808251659024 ) ) ;
#118049=CARTESIAN_POINT ( 'NONE',  ( 8.543609354905870035, 13.11929468069890525, 0.7998128361456462443 ) ) ;
#118055=CARTESIAN_POINT ( 'NONE',  ( -1.500000000000001332, 0.1500000000000251132, 0.000000000000000000 ) ) ;
#118056=CARTESIAN_POINT ( 'NONE',  ( 7.293396569147545527, 10.59638086639245280, 1.199719254218460707 ) ) ;
#118057=CARTESIAN_POINT ( 'NONE',  ( -8.748035429315585532, 11.22912730566677553, -1.599625672291263179 ) ) ;
#118059=CARTESIAN_POINT ( 'NONE',  ( -0.6823417656250212460, 1.801041667008083991, 1.181850606188755259 ) ) ;
#118060=CARTESIAN_POINT ( 'NONE',  ( 1.499999999999987121, 2.045833333333356929, -0.8660254037844262731 ) ) ;
#118062=CARTESIAN_POINT ( 'NONE',  ( 3.499976210622149253, 7.235056012367825140, 0.7998128361456321445 ) ) ;
#118069=CARTESIAN_POINT ( 'NONE',  ( 1.499999999999987121, 0.03541666734948738238, 0.8660254037844524744 ) ) ;
#118070=CARTESIAN_POINT ( 'NONE',  ( -8.681298431451969222, 9.022603012982438386, 1.040834085586084257E-14 ) ) ;
#118071=CARTESIAN_POINT ( 'NONE',  ( -4.202664430556263930, 5.926194473780837413, 1.443375672974064550 ) ) ;
#118079=CARTESIAN_POINT ( 'NONE',  ( 6.265839547809997079, 10.46189657242035587, 0.7998128361456462443 ) ) ;
#118083=CARTESIAN_POINT ( 'NONE',  ( 6.060131475184119765, 9.053608573481392696, -1.082531754730537976 ) ) ;
#118088=CARTESIAN_POINT ( 'NONE',  ( -8.505042434474312074, 8.816971016508505343, -0.7998128361456291469 ) ) ;
#118090=CARTESIAN_POINT ( 'NONE',  ( 3.683011284406639607, 7.448596931783069586, 0.7998128361456321445 ) ) ;
#118095=CARTESIAN_POINT ( 'NONE',  ( 4.159596813995052322, 7.384974941181836172, -0.7733407813514819873 ) ) ;
#118096=CARTESIAN_POINT ( 'NONE',  ( 8.703971430293332645, 12.13808852110884118, -1.082531754730543083 ) ) ;
#118103=CARTESIAN_POINT ( 'NONE',  ( -3.294268138440636928, 6.787137228248626641, 1.040834085586084257E-14 ) ) ;
#118104=CARTESIAN_POINT ( 'NONE',  ( 9.436111725431318931, 10.11114455586577776, -0.7216878364870257245 ) ) ;
#118107=CARTESIAN_POINT ( 'NONE',  ( -5.473741331615264549, 7.409117525016355010, -1.599625672291256295 ) ) ;
#118108=CARTESIAN_POINT ( 'NONE',  ( 1.387358672533593129, 7.315968950352074174, -4.254625267140469624 ) ) ;
#118111=CARTESIAN_POINT ( 'NONE',  ( 3.939296163839981713, 2.811845806437661466, 0.7749999999965996311 ) ) ;
#118113=CARTESIAN_POINT ( 'NONE',  ( -6.808165692356648258, 11.09461040772476714, 0.7998128361456481317 ) ) ;
#118127=CARTESIAN_POINT ( 'NONE',  ( -5.368138756007025947, 8.350246751061767725, 1.199719254218452047 ) ) ;
#118130=CARTESIAN_POINT ( 'NONE',  ( 5.531363484695522637, 5.555604941673978558, -0.7216878364870207285 ) ) ;
#118131=ORIENTED_EDGE ( 'NONE', *, *, #11443, .T. ) ;
#118135=CARTESIAN_POINT ( 'NONE',  ( -4.569261463005423352, 5.289558780716470565, -1.199719254218446718 ) ) ;
#118143=CARTESIAN_POINT ( 'NONE',  ( -9.154780037725563702, 11.70366268214508487, 1.599625672291281386 ) ) ;
#118144=CARTESIAN_POINT ( 'NONE',  ( 6.368579470117202490, 8.453095353268645695, 1.599625672291281386 ) ) ;
#118147=CARTESIAN_POINT ( 'NONE',  ( -9.622536337397040285, 12.24937836509514710, 1.599625672291281386 ) ) ;
#118151=CARTESIAN_POINT ( 'NONE',  ( -1.402160292154681736E-14, 0.3843750003414230232, 1.575800808251672791 ) ) ;
#118155=CARTESIAN_POINT ( 'NONE',  ( 8.758204044748010730, 9.320252261735261001, 0.7216878364870438212 ) ) ;
#118174=CARTESIAN_POINT ( 'NONE',  ( -4.308793891044708779, 3.921347715840572956, 1.214306433183764966E-14 ) ) ;
#118181=CARTESIAN_POINT ( 'NONE',  ( 0.7499999999999885647, 0.01458333401615358182, 1.299038105676657340 ) ) ;
#118189=CARTESIAN_POINT ( 'NONE',  ( 7.865701674222579598, 12.32840238656838139, -0.7998128361456352531 ) ) ;
#118194=CARTESIAN_POINT ( 'NONE',  ( 4.334856428067313416, 6.080418470877079429, -1.599625672291256295 ) ) ;
#118195=CARTESIAN_POINT ( 'NONE',  ( -1.364683531250012516, 3.301041667008084879, -0.7879004041258289570 ) ) ;
#118196=CARTESIAN_POINT ( 'NONE',  ( -5.882246656098474524, 6.017915526194586917, -0.2943127404537674296 ) ) ;
#118199=CARTESIAN_POINT ( 'NONE',  ( -6.832419346282942563, 10.05857410638369487, 1.199719254218453823 ) ) ;
#118200=CARTESIAN_POINT ( 'NONE',  ( -3.728129053633589152, 7.293308295973741195, 0.7216878364870317197 ) ) ;
#118202=ORIENTED_EDGE ( 'NONE', *, *, #137857, .F. ) ;
#118203=CARTESIAN_POINT ( 'NONE',  ( -0.7500000000000006661, -0.3604166659838467512, -1.299038105676652011 ) ) ;
#118211=CARTESIAN_POINT ( 'NONE',  ( -3.701012746406287413, 6.301303389907177532, 1.082531754730560403 ) ) ;
#118213=CARTESIAN_POINT ( 'NONE',  ( 4.037125735401803084, 7.543859425723234757, -0.4173421496808590869 ) ) ;
#118218=CARTESIAN_POINT ( 'NONE',  ( -3.212919216314315207, 5.731860938133201522, 1.082531754730560403 ) ) ;
#118219=CARTESIAN_POINT ( 'NONE',  ( 8.718056468787178659, 10.12981962079525289, 1.199719254218462483 ) ) ;
#118230=CARTESIAN_POINT ( 'NONE',  ( -3.735435015764967837, 4.316761258935923884, -1.199719254218452047 ) ) ;
#118231=CARTESIAN_POINT ( 'NONE',  ( -9.671043645249580933, 10.17730576241299900, 0.7998128361456462443 ) ) ;
#118235=CARTESIAN_POINT ( 'NONE',  ( 3.683011284406639607, 7.448596931783069586, 0.7998128361456321445 ) ) ;
#118240=( BOUNDED_CURVE ( )  B_SPLINE_CURVE ( 2, ( #214297, #150435, #51862, #181830, #180781, #85414, #183976 ),
 .UNSPECIFIED., .F., .T. ) 
 B_SPLINE_CURVE_WITH_KNOTS ( ( 3, 2, 2, 3 ),
 ( 0.1500000000000002165, 0.1541666666666668684, 0.1583333333333334925, 0.1625000000000001443 ),
 .UNSPECIFIED. ) 
 CURVE ( )  GEOMETRIC_REPRESENTATION_ITEM ( )  RATIONAL_B_SPLINE_CURVE ( ( 0.9999999999999928946, 0.8660254037844458130, 1.000000000000000000, 0.8660254037844387076, 1.000000000000000000, 0.8660254037844342667, 1.000000000000004441 ) ) 
 REPRESENTATION_ITEM ( '' )  );
#118242=CARTESIAN_POINT ( 'NONE',  ( 2.530568227245037605, 6.104080031761181857, 0.000000000000000000 ) ) ;
#118254=CARTESIAN_POINT ( 'NONE',  ( 8.422639742587595180, 10.84949900448412130, -1.599625672291268286 ) ) ;
#118256=CARTESIAN_POINT ( 'NONE',  ( -6.573005544526917099, 6.562927978236513304, -0.7998128361456291469 ) ) ;
#118260=CARTESIAN_POINT ( 'NONE',  ( 0.7499999999999885647, -0.4854166659838468623, 1.299038105676657340 ) ) ;
#118264=CARTESIAN_POINT ( 'NONE',  ( 3.493197133815315603, 7.227147089426516402, -0.7998128361456291469 ) ) ;
#118265=CARTESIAN_POINT ( 'NONE',  ( -3.588104209110990706, 7.337872010604796991, 1.040834085586084257E-14 ) ) ;
#118271=CARTESIAN_POINT ( 'NONE',  ( 6.656690234629796699, 6.868486149930637552, 1.040834085586084257E-14 ) ) ;
#118274=CARTESIAN_POINT ( 'NONE',  ( 6.575341312503417690, 10.61505593132193326, -0.7216878364870267237 ) ) ;
#118275=CARTESIAN_POINT ( 'NONE',  ( 1.364683531249988535, 4.467708333674754506, -0.7879004041258300672 ) ) ;
#118277=CARTESIAN_POINT ( 'NONE',  ( 4.080641047588898118, 5.783833860318930320, -1.443375672974051449 ) ) ;
#118284=CARTESIAN_POINT ( 'NONE',  ( -6.041716223103725802, 6.056113169402001617, -0.5645603026655892087 ) ) ;
#118287=CARTESIAN_POINT ( 'NONE',  ( -1.001543065824772872E-14, 5.634375000341415252, 1.575800808251672791 ) ) ;
#118291=CARTESIAN_POINT ( 'NONE',  ( -10.65400978224035811, 11.32409958890225710, 1.040834085586084257E-14 ) ) ;
#118301=CARTESIAN_POINT ( 'NONE',  ( 4.067082894419602468, 3.847277586352047862, -0.7216878364870188411 ) ) ;
#118302=CARTESIAN_POINT ( 'NONE',  ( 1.364683531249988535, 4.467708333674754506, -0.7879004041258300672 ) ) ;
#118304=CARTESIAN_POINT ( 'NONE',  ( 5.425234023762710578, 9.481190127698507553, -0.7998128361456291469 ) ) ;
#118305=CARTESIAN_POINT ( 'NONE',  ( -8.962103233833181193, 10.41454084668224489, -1.199719254218446718 ) ) ;
#118312=CARTESIAN_POINT ( 'NONE',  ( 0.7499999999999902300, 4.316666666666691299, -1.299038105676658228 ) ) ;
#118319=CARTESIAN_POINT ( 'NONE',  ( 8.758204044748010730, 9.320252261735261001, 0.7216878364870438212 ) ) ;
#118324=CARTESIAN_POINT ( 'NONE',  ( 1.499999999999989120, 2.806250000682818158, 1.214306433183764966E-14 ) ) ;
#118326=CARTESIAN_POINT ( 'NONE',  ( -3.879604511804807032, 7.677955697080923514, 0.7998128361456341429 ) ) ;
#118328=CARTESIAN_POINT ( 'NONE',  ( 3.836594282542909795, 6.459481848733281240, 1.082531754730558626 ) ) ;
#118329=CARTESIAN_POINT ( 'NONE',  ( -8.907343734053998929, 12.37535620882957588, 1.082531754730558626 ) ) ;
#118337=CARTESIAN_POINT ( 'NONE',  ( 8.067265095331215718, 9.370563018429956870, 1.199719254218462483 ) ) ;
#118338=CARTESIAN_POINT ( 'NONE',  ( 5.359550796103802028, 5.147230771742885125, -0.7998128361456231517 ) ) ;
#118340=DIRECTION ( 'NONE',  ( 1.000000000000000000, 0.000000000000000000, 0.000000000000000000 ) ) ;
#118343=CARTESIAN_POINT ( 'NONE',  ( 4.493637847925535667, 7.329995691633395261, -1.199719254218452047 ) ) ;
#118354=CARTESIAN_POINT ( 'NONE',  ( 5.587453275722374713, 6.167276584799368244, -0.8733612469495740660 ) ) ;
#118357=CARTESIAN_POINT ( 'NONE',  ( 8.703444544968814256, 12.24143683818393313, -1.199719254218446718 ) ) ;
#118362=CARTESIAN_POINT ( 'NONE',  ( 5.341549334104176872, 9.175631956522799726, 0.7216878364870438212 ) ) ;
#118363=CARTESIAN_POINT ( 'NONE',  ( -3.898132859128961236, 4.506575409527250997, -1.199719254218452047 ) ) ;
#118369=CARTESIAN_POINT ( 'NONE',  ( -4.985647801523292344, 6.839675073242382553, -1.599625672291256295 ) ) ;
#118379=CARTESIAN_POINT ( 'NONE',  ( 9.423080456697809026, 10.95234760669099749, -1.199719254218446718 ) ) ;
#118380=CARTESIAN_POINT ( 'NONE',  ( 6.082781304119575516, 6.035783188292461077, -0.3281998023207943760 ) ) ;
#118383=CARTESIAN_POINT ( 'NONE',  ( 5.118366684358879759, 5.930181538962194132, 1.199719254218462483 ) ) ;
#118388=CARTESIAN_POINT ( 'NONE',  ( -9.490344339885981029, 10.17441593939621924, -0.7216878364870267237 ) ) ;
#118393=CARTESIAN_POINT ( 'NONE',  ( 7.019370843573166319, 9.212351955633947043, 1.599625672291281386 ) ) ;
#118398=CARTESIAN_POINT ( 'NONE',  ( 5.217190183160311356, 4.981143389975473568, -0.7998128361456211532 ) ) ;
#118400=CARTESIAN_POINT ( 'NONE',  ( -5.391338639728555648, 9.441645512991978961, -0.7998128361456231517 ) ) ;
#118401=CARTESIAN_POINT ( 'NONE',  ( 3.277320446201373638, 4.846626492033466072, 1.599625672291267398 ) ) ;
#118404=CARTESIAN_POINT ( 'NONE',  ( 9.023114925094663619, 10.48572115315399245, 1.199719254218453823 ) ) ;
#118405=CARTESIAN_POINT ( 'NONE',  ( -1.499999999999997780, 3.650000000000021227, 1.214306433183764966E-14 ) ) ;
#118409=CARTESIAN_POINT ( 'NONE',  ( 4.260617097460324132, 7.265790484119571957, -0.9368387426427534637 ) ) ;
#118412=CARTESIAN_POINT ( 'NONE',  ( 5.504247177468179153, 7.444707678511436555, 1.443375672974062551 ) ) ;
#118418=EDGE_LOOP ( 'NONE', ( #63682, #77050, #48762, #62865 ) ) ;
#118419=CARTESIAN_POINT ( 'NONE',  ( 9.232739420781973294, 9.873876867108206667, -0.7216878364870257245 ) ) ;
#118420=( BOUNDED_CURVE ( )  B_SPLINE_CURVE ( 2, ( #162067, #79729, #81861, #212917, #145845, #211852, #63488 ),
 .UNSPECIFIED., .F., .T. ) 
 B_SPLINE_CURVE_WITH_KNOTS ( ( 3, 2, 2, 3 ),
 ( 0.1874999999999999167, 0.1916666666666665964, 0.1958333333333332760, 0.1999999999999999556 ),
 .UNSPECIFIED. ) 
 CURVE ( )  GEOMETRIC_REPRESENTATION_ITEM ( )  RATIONAL_B_SPLINE_CURVE ( ( 1.000000000000002665, 0.8660254037844360431, 1.000000000000000000, 0.8660254037844387076, 1.000000000000000000, 0.8660254037844404840, 0.9999999999999982236 ) ) 
 REPRESENTATION_ITEM ( '' )  );
#118423=CARTESIAN_POINT ( 'NONE',  ( -9.040589502214116280, 9.441775928871617651, 0.7998128361456462443 ) ) ;
#118432=CARTESIAN_POINT ( 'NONE',  ( 9.378489572351044856, 11.96465713920816043, -1.599625672291262513 ) ) ;
#118437=CARTESIAN_POINT ( 'NONE',  ( 5.443762371086860341, 6.309809840144842141, 1.199719254218462483 ) ) ;
#118440=CARTESIAN_POINT ( 'NONE',  ( -1.201851678989727383E-14, 3.743750000682817269, 1.732050807568877637 ) ) ;
#118444=ORIENTED_EDGE ( 'NONE', *, *, #63237, .T. ) ;
#118446=CARTESIAN_POINT ( 'NONE',  ( 1.499999999999989120, 2.254166666666685970, 0.8660254037844524744 ) ) ;
#118447=CARTESIAN_POINT ( 'NONE',  ( 5.601490020740366838, 9.686822124172440596, 1.040834085586084257E-14 ) ) ;
#118448=CARTESIAN_POINT ( 'NONE',  ( 3.836594282542909795, 6.459481848733281240, 1.082531754730558626 ) ) ;
#118452=CARTESIAN_POINT ( 'NONE',  ( 7.863365906246055914, 10.19701286208565705, -1.443375672974057666 ) ) ;
#118459=CARTESIAN_POINT ( 'NONE',  ( -5.148345644887285744, 7.029489223833707001, -1.599625672291256295 ) ) ;
#118460=CARTESIAN_POINT ( 'NONE',  ( -1.001543065824772872E-14, 4.243750000682819490, 1.732050807568877637 ) ) ;
#118461=CARTESIAN_POINT ( 'NONE',  ( 0.6823417656249899377, 5.238541667008086655, -1.181850606188754593 ) ) ;
#118465=CARTESIAN_POINT ( 'NONE',  ( 9.747949258101261449, 11.43532422494874368, -1.082531754730537088 ) ) ;
#118467=CARTESIAN_POINT ( 'NONE',  ( 0.6823417656249899377, 3.738541667008085767, -1.181850606188754593 ) ) ;
#118475=CARTESIAN_POINT ( 'NONE',  ( -6.906989191158078079, 10.14557225873805812, -1.199719254218440723 ) ) ;
#118476=CARTESIAN_POINT ( 'NONE',  ( 5.524057522564145728, 8.532151978711786100, 1.199719254218462483 ) ) ;
#118478=CARTESIAN_POINT ( 'NONE',  ( 1.364683531249986537, -0.6364583329919177856, 0.7879004041258500513 ) ) ;
#118485=CARTESIAN_POINT ( 'NONE',  ( -5.636439174979254396, 7.598931675607687453, -1.599625672291256295 ) ) ;
#118491=CARTESIAN_POINT ( 'NONE',  ( 8.890396042259068210, 11.39521468743417998, -1.599625672291257406 ) ) ;
#118494=B_SPLINE_CURVE_WITH_KNOTS ( 'NONE', 3,
 ( #133261, #199268, #50912, #117040, #63965, #80212, #119165, #39998, #56241, #154809 ),
 .UNSPECIFIED., .F., .F.,
 ( 4, 3, 3, 4 ),
 ( 7.467508872541053688E-17, 3.125178967435692016E-05, 6.527220184319362914E-05, 9.930990297292533473E-05 ),
 .UNSPECIFIED. ) ;
#118495=CARTESIAN_POINT ( 'NONE',  ( -4.627410500965859264, 4.293067094081919777, 0.7998128361456341429 ) ) ;
#118496=CARTESIAN_POINT ( 'NONE',  ( -7.914208982075130905, 10.25632978388623684, -1.599625672291263179 ) ) ;
#118498=CARTESIAN_POINT ( 'NONE',  ( -4.095724654357025152, 7.689947244493171574, 0.7385042830605083042 ) ) ;
#118499=CARTESIAN_POINT ( 'NONE',  ( -1.364683531250014514, -0.7614583329919104582, -0.7879004041258359514 ) ) ;
#118503=CARTESIAN_POINT ( 'NONE',  ( 7.293923454472069245, 11.45340176361870199, 0.7216878364870438212 ) ) ;
#118525=CARTESIAN_POINT ( 'NONE',  ( -6.437424008390261854, 6.404749519410410485, 0.7998128361456341429 ) ) ;
#118526=CARTESIAN_POINT ( 'NONE',  ( -7.645908563102897126, 11.00764485934031889, 1.199719254218453823 ) ) ;
#118531=CARTESIAN_POINT ( 'NONE',  ( -1.500000000000001332, 1.431250000682816825, 0.000000000000000000 ) ) ;
#118532=CARTESIAN_POINT ( 'NONE',  ( 8.594979316059474073, 12.11489407112305372, 1.199719254218450271 ) ) ;
#118536=CARTESIAN_POINT ( 'NONE',  ( -9.938290294017125603, 11.55342575023019691, -1.199719254218441611 ) ) ;
#118537=DIRECTION ( 'NONE',  ( -5.578564026256490882E-16, -1.000000000000000000, -9.066213480720158442E-32 ) ) ;
#118538=CARTESIAN_POINT ( 'NONE',  ( -1.364683531250012516, 1.780208333674757615, 0.7879004041258379498 ) ) ;
#118539=CARTESIAN_POINT ( 'NONE',  ( -0.7500000000000215383, 5.441666666666685082, 1.299038105676671107 ) ) ;
#118546=CARTESIAN_POINT ( 'NONE',  ( -8.514157279702017078, 12.87700789305364069, -0.7216878364870267237 ) ) ;
#118550=CARTESIAN_POINT ( 'NONE',  ( -0.6823417656250003738, 0.2802083336747515641, -1.181850606188749264 ) ) ;
#118556=CARTESIAN_POINT ( 'NONE',  ( 1.364683531249988535, 1.613541667008084879, 0.7879004041258500513 ) ) ;
#118558=CARTESIAN_POINT ( 'NONE',  ( -5.554036483092550824, 9.631459663583308739, -0.7998128361456231517 ) ) ;
#118559=CARTESIAN_POINT ( 'NONE',  ( 6.577677080924314801, 10.82570702772039262, 1.040834085586084257E-14 ) ) ;
#118560=CARTESIAN_POINT ( 'NONE',  ( 3.680148631105580215, 6.380924938676771241, -1.199719254218446718 ) ) ;
#118561=CARTESIAN_POINT ( 'NONE',  ( 6.342516933094585418, 6.294024598232139667, 1.040834085586084257E-14 ) ) ;
#118563=CARTESIAN_POINT ( 'NONE',  ( 0.7499999999999902300, 4.316666666666691299, -1.299038105676658228 ) ) ;
#118565=CARTESIAN_POINT ( 'NONE',  ( 0.6823417656249882723, 1.488541667008083547, -1.181850606188749264 ) ) ;
#118568=CARTESIAN_POINT ( 'NONE',  ( -5.761852096127856981, 5.824508321678349532, 0.000000000000000000 ) ) ;
#118571=CARTESIAN_POINT ( 'NONE',  ( 5.910991785878156435, 7.919243054989755670, -1.443375672974057666 ) ) ;
#118574=CARTESIAN_POINT ( 'NONE',  ( -9.501566725078754772, 9.979582688880366703, -0.7998128361456291469 ) ) ;
#118575=CARTESIAN_POINT ( 'NONE',  ( -4.334856428067329404, 6.080418470877079429, -1.599625672291256295 ) ) ;
#118578=CARTESIAN_POINT ( 'NONE',  ( -7.009202228140744673, 10.16085778526412042, -1.082531754730537088 ) ) ;
#118580=CARTESIAN_POINT ( 'NONE',  ( 0.7499999999999920064, 5.483333333333353821, 1.299038105676669330 ) ) ;
#118583=AXIS2_PLACEMENT_3D ( 'NONE', #115699, #62618, #99402 ) ;
#118584=CARTESIAN_POINT ( 'NONE',  ( 8.595506201384013778, 10.09080732544527592, 1.082531754730558626 ) ) ;
#118585=CARTESIAN_POINT ( 'NONE',  ( -4.202664430556263042, 5.926194473780837413, 1.443375672974064550 ) ) ;
#118597=CARTESIAN_POINT ( 'NONE',  ( 7.772902139336337335, 7.962807338847539107, 0.7998128361456341429 ) ) ;
#118599=CARTESIAN_POINT ( 'NONE',  ( -3.730464822054482710, 7.503959392372201442, 1.040834085586084257E-14 ) ) ;
#118604=CARTESIAN_POINT ( 'NONE',  ( 0.6823417656249882723, -0.5947916663252492686, 1.181850606188755259 ) ) ;
#118607=CARTESIAN_POINT ( 'NONE',  ( -4.295235737431041478, 3.905529869957963029, -0.7998128361456221525 ) ) ;
#118610=ADVANCED_FACE ( 'NONE', ( #94391 ), #188402, .T. ) ;
#118625=CARTESIAN_POINT ( 'NONE',  ( 7.633404179693907388, 8.864391950186421454, -1.199719254218441611 ) ) ;
#118633=CARTESIAN_POINT ( 'NONE',  ( 1.558944071570338652, 8.694263516233171174, 2.499999999999954259 ) ) ;
#118636=CARTESIAN_POINT ( 'NONE',  ( -2.359468172627429805, 5.347229341561620330, 0.7252027155559838123 ) ) ;
#118637=CARTESIAN_POINT ( 'NONE',  ( -0.4092393038957372053, 6.441162235065689856, 3.221549646754199525 ) ) ;
#118639=CARTESIAN_POINT ( 'NONE',  ( -5.935772324684618795, 5.819489221753827657, 0.000000000000000000 ) ) ;
#118641=CARTESIAN_POINT ( 'NONE',  ( -4.711622075948912247, 5.455646162483875017, -1.199719254218446718 ) ) ;
#118646=CARTESIAN_POINT ( 'NONE',  ( 1.435115314734433989, 7.268684689231783125, 4.324912918975653220 ) ) ;
#118650=CARTESIAN_POINT ( 'NONE',  ( -3.898132859128961236, 4.506575409527250997, -1.199719254218452047 ) ) ;
#118653=CARTESIAN_POINT ( 'NONE',  ( 4.801558957534076022, 8.753569217098425170, 0.7998128361456462443 ) ) ;
#118654=CARTESIAN_POINT ( 'NONE',  ( 1.364683531249990311, 4.884375000341417916, 1.214306433183764966E-14 ) ) ;
#118658=B_SPLINE_CURVE_WITH_KNOTS ( 'NONE', 3,
 ( #157544, #71976, #58960, #5903, #6973, #188951, #88261, #40591, #90403, #155390, #174871, #104519 ),
 .UNSPECIFIED., .F., .F.,
 ( 4, 2, 2, 2, 2, 4 ),
 ( 0.003750395023277889282, 0.003985267534262568016, 0.004220140045247247618, 0.004689885067216603351, 0.005159630089185959952, 0.005629375111155316552 ),
 .UNSPECIFIED. ) ;
#118661=EDGE_CURVE ( 'NONE', #128332, #93282, #179886, .T. ) ;
#118663=CARTESIAN_POINT ( 'NONE',  ( 4.473827502385202770, 8.163289819517311585, 1.040834085586084257E-14 ) ) ;
#118664=CARTESIAN_POINT ( 'NONE',  ( -5.533699252672048985, 9.607732894759390518, -0.7998128361456231517 ) ) ;
#118667=CARTESIAN_POINT ( 'NONE',  ( -6.995117189646935962, 10.24838825697502109, 1.199719254218453823 ) ) ;
#118668=CARTESIAN_POINT ( 'NONE',  ( -4.252453736180621391, 8.112946458852704268, -0.7998128361456281477 ) ) ;
#118675=CARTESIAN_POINT ( 'NONE',  ( 5.587931867126699537, 9.671004278289832001, -0.7998128361456291469 ) ) ;
#118689=CARTESIAN_POINT ( 'NONE',  ( -1.364683531250014514, -0.6989583329919100141, -0.7879004041258359514 ) ) ;
#118690=CARTESIAN_POINT ( 'NONE',  ( 4.521807925357579805, 5.234196320127330715, -1.199719254218452047 ) ) ;
#118691=CARTESIAN_POINT ( 'NONE',  ( 4.984594031318565932, 8.967110136513669616, 0.7998128361456462443 ) ) ;
#118693=CARTESIAN_POINT ( 'NONE',  ( -7.537970219518083326, 9.817384560903001045, -1.443375672974059665 ) ) ;
#118694=CARTESIAN_POINT ( 'NONE',  ( 4.826339496784873617, 8.574553812983598533, -0.7216878364870257245 ) ) ;
#118695=CARTESIAN_POINT ( 'NONE',  ( -7.931156673870055407, 11.23647130528163096, 1.082531754730549967 ) ) ;
#118699=CARTESIAN_POINT ( 'NONE',  ( 8.046927864910717432, 9.346836249606042202, 1.199719254218462483 ) ) ;
#118702=CARTESIAN_POINT ( 'NONE',  ( 0.6823417656249899377, 3.676041667008085767, -1.181850606188754593 ) ) ;
#118708=CARTESIAN_POINT ( 'NONE',  ( 9.433775957010412938, 9.900493459467314850, 0.000000000000000000 ) ) ;
#118711=CARTESIAN_POINT ( 'NONE',  ( -9.352427035328430449, 9.805586384171650849, 1.040834085586084257E-14 ) ) ;
#118717=CARTESIAN_POINT ( 'NONE',  ( 2.218730694130720771, 5.740269576461138890, 0.7998128361456462443 ) ) ;
#118720=CARTESIAN_POINT ( 'NONE',  ( -8.829384350997580455, 11.32403438096243775, 1.599625672291269396 ) ) ;
#118726=CARTESIAN_POINT ( 'NONE',  ( 5.849510849484250485, 6.002983934024645585, 0.3487602046992159810 ) ) ;
#118728=CARTESIAN_POINT ( 'NONE',  ( -2.819205876637805641, 5.376491725131008259, -1.199719254218446718 ) ) ;
#118733=CARTESIAN_POINT ( 'NONE',  ( 6.076025397218672630, 10.24044673006381245, -0.7998128361456291469 ) ) ;
#118735=CARTESIAN_POINT ( 'NONE',  ( 7.149227073107712549, 7.235186428247455837, -0.7998128361456281477 ) ) ;
#118736=CARTESIAN_POINT ( 'NONE',  ( 4.527533231959700366, 7.369540306339926516, 1.199719254218462483 ) ) ;
#118738=CARTESIAN_POINT ( 'NONE',  ( -8.853111120043687166, 9.430977182913531820, 1.040834085586084257E-14 ) ) ;
#118745=CARTESIAN_POINT ( 'NONE',  ( -4.059107376188687333, 7.562469429224047524, 0.4300614504739261879 ) ) ;
#118749=CARTESIAN_POINT ( 'NONE',  ( 4.528060117284222308, 8.226561203566173930, 0.7216878364870438212 ) ) ;
#118758=CARTESIAN_POINT ( 'NONE',  ( -10.61567108937589765, 11.48729714713446803, 0.7216878364870438212 ) ) ;
#118766=CARTESIAN_POINT ( 'NONE',  ( -10.12757755928392456, 10.91785469536048758, 0.7216878364870438212 ) ) ;
#118772=CARTESIAN_POINT ( 'NONE',  ( 7.422199028477372451, 10.74665040227725044, -1.199719254218441611 ) ) ;
#118776=CARTESIAN_POINT ( 'NONE',  ( 0.7499999999999885647, 2.097916667349486453, -1.299038105676652899 ) ) ;
#118777=CARTESIAN_POINT ( 'NONE',  ( -6.878064000834399394, 6.918829510595249310, -0.7998128361456291469 ) ) ;
#118780=CARTESIAN_POINT ( 'NONE',  ( -8.076906825439122528, 10.44614393447756129, -1.599625672291263179 ) ) ;
#118784=CARTESIAN_POINT ( 'NONE',  ( 7.637320603199683866, 7.804628880021436288, -0.7998128361456281477 ) ) ;
#118789=CARTESIAN_POINT ( 'NONE',  ( 8.259941899223605333, 10.65968485389279508, -1.599625672291268286 ) ) ;
#118795=CARTESIAN_POINT ( 'NONE',  ( -6.209271165378811297, 10.18797409300986878, 0.7216878364870458196 ) ) ;
#118799=CARTESIAN_POINT ( 'NONE',  ( -1.364683531249997417, 4.321875000341417028, 1.214306433183764966E-14 ) ) ;
#118804=CARTESIAN_POINT ( 'NONE',  ( 1.364683531249992088, 5.384375000341417916, 1.214306433183764966E-14 ) ) ;
#118807=CARTESIAN_POINT ( 'NONE',  ( -4.134873662043608178, 4.886736029548026217, 1.082531754730558626 ) ) ;
#118809=CARTESIAN_POINT ( 'NONE',  ( 9.480175724453529185, 12.08329098332774265, 1.599625672291279388 ) ) ;
#118810=CARTESIAN_POINT ( 'NONE',  ( 0.6823417656249899377, 5.488541667008087543, -1.181850606188754593 ) ) ;
#118811=CARTESIAN_POINT ( 'NONE',  ( -10.15522075183580419, 11.80651128435196462, 1.199719254218462483 ) ) ;
#118814=CARTESIAN_POINT ( 'NONE',  ( 1.364683531249988757, 1.634375000341421691, 0.000000000000000000 ) ) ;
#118815=CARTESIAN_POINT ( 'NONE',  ( -4.636525346193588248, 4.511627113421689650, 0.7216878364870317197 ) ) ;
#118816=CARTESIAN_POINT ( 'NONE',  ( 3.486418057008484617, 7.219238166485217434, 1.040834085586084257E-14 ) ) ;
#118821=CARTESIAN_POINT ( 'NONE',  ( 2.250290310188348464, 5.569163095287620990, 0.7216878364870438212 ) ) ;
#118825=CARTESIAN_POINT ( 'NONE',  ( -8.690413276679693766, 9.241163032322203819, 1.040834085586084257E-14 ) ) ;
#118830=CARTESIAN_POINT ( 'NONE',  ( -7.648771216403934758, 12.07531685244661723, -0.7998128361456291469 ) ) ;
#118831=CARTESIAN_POINT ( 'NONE',  ( -5.883875478206491927, 5.966868934103426447, 0.000000000000000000 ) ) ;
#118832=CARTESIAN_POINT ( 'NONE',  ( -1.201851678989727383E-14, 2.634375000341417916, 1.575800808251672791 ) ) ;
#118841=CARTESIAN_POINT ( 'NONE',  ( 10.72180055030867329, 11.40318881831530540, 0.7998128361456341429 ) ) ;
#118853=LINE ( 'NONE', #86293, #167739 ) ;
#118856=CARTESIAN_POINT ( 'NONE',  ( -1.364683531250012516, 3.592708333674750509, 0.7879004041258379498 ) ) ;
#118861=EDGE_CURVE ( 'NONE', #154420, #213687, #187170, .T. ) ;
#118864=CARTESIAN_POINT ( 'NONE',  ( 9.531545685607134999, 11.07889037375188401, 1.199719254218450271 ) ) ;
#118867=CARTESIAN_POINT ( 'NONE',  ( -0.6823417656250212460, 1.051041667008083325, 1.181850606188755259 ) ) ;
#118877=CARTESIAN_POINT ( 'NONE',  ( 5.027376032568989572, 4.759693547618927489, 0.7998128361456341429 ) ) ;
#118889=CARTESIAN_POINT ( 'NONE',  ( -3.379006598303881059, 4.965260336153046516, -1.599625672291256295 ) ) ;
#118890=( BOUNDED_CURVE ( )  B_SPLINE_CURVE ( 1, ( #148284, #99525 ),
 .UNSPECIFIED., .F., .T. ) 
 B_SPLINE_CURVE_WITH_KNOTS ( ( 2, 2 ),
 ( 0.000000000000000000, 6.249999999999788711E-05 ),
 .UNSPECIFIED. ) 
 CURVE ( )  GEOMETRIC_REPRESENTATION_ITEM ( )  RATIONAL_B_SPLINE_CURVE ( ( 0.9345202395942819873, 0.9345202395942819873 ) ) 
 REPRESENTATION_ITEM ( '' )  );
#118891=CARTESIAN_POINT ( 'NONE',  ( 8.229962938695207342, 9.560377169021284871, 1.199719254218462483 ) ) ;
#118894=CARTESIAN_POINT ( 'NONE',  ( 5.165293336682183600, 5.128523102325077687, -0.7216878364870197293 ) ) ;
#118903=CARTESIAN_POINT ( 'NONE',  ( -6.019457014787517046, 9.006155036351978893, 1.082531754730548412 ) ) ;
#118905=CARTESIAN_POINT ( 'NONE',  ( 5.392392409933256303, 7.314210449720692786, 1.599625672291267398 ) ) ;
#118908=VECTOR ( 'NONE', #76055, 1000.000000000000000 ) ;
#118909=CARTESIAN_POINT ( 'NONE',  ( -9.267161690140662600, 10.77044237904097734, -1.199719254218441611 ) ) ;
#118911=DIRECTION ( 'NONE',  ( 0.6507913734559658270, -0.7592566023652989049, 0.000000000000000000 ) ) ;
#118915=CARTESIAN_POINT ( 'NONE',  ( -3.379006598303881059, 4.965260336153046516, -1.599625672291256295 ) ) ;
#118918=CARTESIAN_POINT ( 'NONE',  ( 8.536830278099042602, 13.11138575775759563, -0.7998128361456352531 ) ) ;
#118920=CARTESIAN_POINT ( 'NONE',  ( 4.650610384687404952, 5.384465856012134566, 1.199719254218462483 ) ) ;
#118926=CARTESIAN_POINT ( 'NONE',  ( 5.029711800989886683, 4.970344644017389513, 1.040834085586084257E-14 ) ) ;
#118929=CARTESIAN_POINT ( 'NONE',  ( -3.554208825076827782, 7.298327395898266623, 0.7998128361456341429 ) ) ;
#118932=CARTESIAN_POINT ( 'NONE',  ( -9.755255220232635693, 11.33988483081495957, -1.199719254218441611 ) ) ;
#118937=CARTESIAN_POINT ( 'NONE',  ( 8.934460041725669655, 9.525884258209195821, 1.040834085586084257E-14 ) ) ;
#118938=CARTESIAN_POINT ( 'NONE',  ( 1.364683531249990311, 5.196875000341417916, 1.214306433183764966E-14 ) ) ;
#118940=CARTESIAN_POINT ( 'NONE',  ( 4.792970997630896512, 5.550553237779539018, 1.199719254218464037 ) ) ;
#118944=CARTESIAN_POINT ( 'NONE',  ( -5.391338639728555648, 9.441645512991978961, -0.7998128361456231517 ) ) ;
#118954=CARTESIAN_POINT ( 'NONE',  ( 1.364683531249986537, 2.717708333674754062, -0.7879004041258239610 ) ) ;
#118956=CARTESIAN_POINT ( 'NONE',  ( 3.837121167867449945, 4.435395103055503441, 1.199719254218464037 ) ) ;
#118958=CARTESIAN_POINT ( 'NONE',  ( -4.690757960648240577, 6.495636925554817864, 1.443375672974064550 ) ) ;
#118960=CARTESIAN_POINT ( 'NONE',  ( -4.053524740361572398, 7.672936597156388316, 0.7216878364870317197 ) ) ;
#118965=CARTESIAN_POINT ( 'NONE',  ( 2.835626683552519012, 6.459981564119914310, 0.000000000000000000 ) ) ;
#118975=CARTESIAN_POINT ( 'NONE',  ( 5.035963992472171746, 7.962709526937818083, 1.199719254218462483 ) ) ;
#118979=CARTESIAN_POINT ( 'NONE',  ( -4.903245109636583443, 8.872203061218007392, -0.7998128361456281477 ) ) ;
#118983=CARTESIAN_POINT ( 'NONE',  ( 8.613507663383630941, 8.943513783569379427, -0.7998128361456221525 ) ) ;
#118987=CARTESIAN_POINT ( 'NONE',  ( -6.735703387890906946, 6.752742128827836865, -0.7998128361456291469 ) ) ;
#118988=CARTESIAN_POINT ( 'NONE',  ( 6.439759776366775768, 7.575769829591800786, 1.082531754730558626 ) ) ;
#118989=CARTESIAN_POINT ( 'NONE',  ( 4.401803827585060169, 7.348580664174646060, 1.190671039528957253 ) ) ;
#118990=CARTESIAN_POINT ( 'NONE',  ( -4.959585264500673496, 4.680604318205876524, 1.214306433183764966E-14 ) ) ;
#118993=CARTESIAN_POINT ( 'NONE',  ( -6.087774667736030487, 7.061157519568837415, 1.199719254218450271 ) ) ;
#118997=CARTESIAN_POINT ( 'NONE',  ( 1.364683531249988757, 1.384375000341421469, 0.000000000000000000 ) ) ;
#118999=CARTESIAN_POINT ( 'NONE',  ( -5.748293942514189681, 5.808690475795744490, -0.7216878364870207285 ) ) ;
#119006=CARTESIAN_POINT ( 'NONE',  ( 5.982172092127724383, 8.002286745614243912, -1.599625672291262513 ) ) ;
#119009=CARTESIAN_POINT ( 'NONE',  ( -1.364683531250000748, 2.321875000341422357, 1.214306433183764966E-14 ) ) ;
#119012=CARTESIAN_POINT ( 'NONE',  ( -1.402160292154681736E-14, -0.9906249996585834161, -1.575800808251665908 ) ) ;
#119015=CARTESIAN_POINT ( 'NONE',  ( -4.460796234096120472, 5.163016013655583158, 1.199719254218462483 ) ) ;
#119016=CARTESIAN_POINT ( 'NONE',  ( -5.856759170979136897, 9.776710099543576504, 0.000000000000000000 ) ) ;
#119018=CARTESIAN_POINT ( 'NONE',  ( 1.364683531249988535, 3.363541667008084879, 0.7879004041258500513 ) ) ;
#119025=CARTESIAN_POINT ( 'NONE',  ( -7.497295758232731089, 8.809561808435409702, -1.082531754730543083 ) ) ;
#119028=CARTESIAN_POINT ( 'NONE',  ( -5.219525951136837705, 9.033271343060892633, -0.7216878364870207285 ) ) ;
#119041=CARTESIAN_POINT ( 'NONE',  ( -5.636439174979254396, 7.598931675607687453, -1.599625672291256295 ) ) ;
#119043=CARTESIAN_POINT ( 'NONE',  ( -1.402160292154681736E-14, -0.4124999999999747202, -1.732050807568870754 ) ) ;
#119044=CARTESIAN_POINT ( 'NONE',  ( 4.695201269034174452, 4.372156323494968966, 1.214306433183764966E-14 ) ) ;
#119046=CARTESIAN_POINT ( 'NONE',  ( -1.451998047845039830, 7.315968950354585942, -4.301760722576429607 ) ) ;
#119048=CARTESIAN_POINT ( 'NONE',  ( 6.928380191783277908, 8.041863964290678624, 1.199719254218462483 ) ) ;
#119052=CARTESIAN_POINT ( 'NONE',  ( -4.392478581147607031, 7.108013530438723748, 1.082531754730560403 ) ) ;
#119054=EDGE_CURVE ( 'NONE', #171893, #123409, #171271, .T. ) ;
#119063=CARTESIAN_POINT ( 'NONE',  ( -1.402160292154681736E-14, 1.446875000341420137, -1.575800808251659024 ) ) ;
#119065=CARTESIAN_POINT ( 'NONE',  ( -5.879432169820529630, 10.01108796476595764, -0.7998128361456221525 ) ) ;
#119068=CARTESIAN_POINT ( 'NONE',  ( 8.118635056484817980, 8.366162408854107113, 0.7998128361456481317 ) ) ;
#119070=CARTESIAN_POINT ( 'NONE',  ( -6.527360889975461156, 9.702672574024962415, 1.199719254218452047 ) ) ;
#119073=CARTESIAN_POINT ( 'NONE',  ( 1.364683531249990311, 5.613541667008087543, 0.7879004041258500513 ) ) ;
#119075=CARTESIAN_POINT ( 'NONE',  ( 8.161645285746708112, 9.584636257201740506, -1.082531754730543083 ) ) ;
#119078=CARTESIAN_POINT ( 'NONE',  ( -1.364683531250000748, -0.1781249996585798634, 0.000000000000000000 ) ) ;
#119082=CARTESIAN_POINT ( 'NONE',  ( 6.751597309481075726, 10.82068792779586985, 1.040834085586084257E-14 ) ) ;
#119085=CARTESIAN_POINT ( 'NONE',  ( -3.307826292054304673, 6.802955074131234348, -0.7216878364870267237 ) ) ;
#119087=CARTESIAN_POINT ( 'NONE',  ( -1.201851678989727383E-14, 3.196875000341420137, -1.575800808251660134 ) ) ;
#119091=CARTESIAN_POINT ( 'NONE',  ( -6.663996196316808174, 7.733415969579778171, -1.199719254218446718 ) ) ;
#119098=CARTESIAN_POINT ( 'NONE',  ( 5.784525094524856748, 9.900363043587685041, 1.040834085586084257E-14 ) ) ;
#119101=CARTESIAN_POINT ( 'NONE',  ( 0.7499999999999885647, 2.316666666666689078, -1.299038105676652899 ) ) ;
#119107=CARTESIAN_POINT ( 'NONE',  ( 6.236387472606139681, 8.298871356172400127, -1.443375672974057666 ) ) ;
#119108=CARTESIAN_POINT ( 'NONE',  ( 1.364683531249988757, -0.05312499965857975237, 0.000000000000000000 ) ) ;
#119110=CARTESIAN_POINT ( 'NONE',  ( 4.403700966340357681, 4.032072637018845107, -0.7998128361456211532 ) ) ;
#119116=CARTESIAN_POINT ( 'NONE',  ( 0.7499999999999885647, 0.9833333333333569293, 1.299038105676657340 ) ) ;
#119117=CARTESIAN_POINT ( 'NONE',  ( 8.437251666405968464, 8.737881787095446384, 1.040834085586084257E-14 ) ) ;
#119118=CARTESIAN_POINT ( 'NONE',  ( -7.883176251342026042, 11.28445716228600126, -1.199719254218446718 ) ) ;
#119120=CARTESIAN_POINT ( 'NONE',  ( -1.402160292154681736E-14, 0.1968750003414221628, -1.575800808251665908 ) ) ;
#119121=CARTESIAN_POINT ( 'NONE',  ( -0.7500000000000006661, 0.6083333333333564852, -1.299038105676652011 ) ) ;
#119123=CARTESIAN_POINT ( 'NONE',  ( 3.635557746758808495, 7.393234471193928847, -0.7998128361456291469 ) ) ;
#119131=CARTESIAN_POINT ( 'NONE',  ( -1.500000000000001332, -1.068749999317178290, 0.000000000000000000 ) ) ;
#119133=CARTESIAN_POINT ( 'NONE',  ( -7.212047647465563038, 10.50147379109678880, -1.199719254218446718 ) ) ;
#119134=CARTESIAN_POINT ( 'NONE',  ( -4.595850885352567694, 8.305650432979225783, 1.040834085586084257E-14 ) ) ;
#119141=CARTESIAN_POINT ( 'NONE',  ( 7.588813295347141441, 9.876701482703580837, -1.599625672291262513 ) ) ;
#119144=CARTESIAN_POINT ( 'NONE',  ( 7.308008492965924141, 8.484763649003774333, -1.199719254218451159 ) ) ;
#119145=CARTESIAN_POINT ( 'NONE',  ( 5.450014562569148957, 9.302174723065263606, 1.040834085586084257E-14 ) ) ;
#119149=CARTESIAN_POINT ( 'NONE',  ( -8.342344591110322227, 8.627156865917170236, -0.7998128361456291469 ) ) ;
#119150=CARTESIAN_POINT ( 'NONE',  ( 6.830610463186557624, 6.863467050006115677, 1.040834085586084257E-14 ) ) ;
#119151=CARTESIAN_POINT ( 'NONE',  ( 4.071134731106788252, 7.497899514862828241, -0.5496474101556632075 ) ) ;
#119152=CARTESIAN_POINT ( 'NONE',  ( 4.383363735919856730, 4.008345868194933104, -0.7998128361456211532 ) ) ;
#119159=CARTESIAN_POINT ( 'NONE',  ( -2.792616454734997866, 6.201876930592042925, 0.7216878364870317197 ) ) ;
#119160=CARTESIAN_POINT ( 'NONE',  ( 9.083599731475983319, 11.62061899152058686, 1.443375672974076540 ) ) ;
#119163=CARTESIAN_POINT ( 'NONE',  ( -7.555971681517696936, 7.709721804725773175, 0.7998128361456462443 ) ) ;
#119165=CARTESIAN_POINT ( 'NONE',  ( -3.090026840240785777, 6.449493289948600605, -0.7169942672678782936 ) ) ;
#119170=CARTESIAN_POINT ( 'NONE',  ( -6.835281999583978418, 11.12624609948998966, -0.7998128361456291469 ) ) ;
#119173=CARTESIAN_POINT ( 'NONE',  ( -0.07727525906048532400, 7.079397053215386926, 2.120984693056199077 ) ) ;
#119186=CARTESIAN_POINT ( 'NONE',  ( -6.718228810771495141, 7.796687353110217877, 1.199719254218450271 ) ) ;
#119189=CARTESIAN_POINT ( 'NONE',  ( 5.992340707560160240, 7.053780915984068756, 1.082531754730558626 ) ) ;
#119194=CARTESIAN_POINT ( 'NONE',  ( -4.406563619641430840, 5.099744630125142564, -1.199719254218446718 ) ) ;
#119197=CARTESIAN_POINT ( 'NONE',  ( -6.050059093290697021, 6.050762344992199004, -0.5500513593517241118 ) ) ;
#119198=CARTESIAN_POINT ( 'NONE',  ( 10.16199982864259788, 11.81442020729326536, 1.199719254218452047 ) ) ;
#119202=CARTESIAN_POINT ( 'NONE',  ( -9.450196763925152510, 10.98398329845622001, -1.199719254218441611 ) ) ;
#119203=CARTESIAN_POINT ( 'NONE',  ( 6.693975156845185737, 8.832723654451292816, 1.599625672291281386 ) ) ;
#119207=CARTESIAN_POINT ( 'NONE',  ( -9.459838494033043332, 12.05956421450382088, 1.599625672291281386 ) ) ;
#119211=CARTESIAN_POINT ( 'NONE',  ( 0.6823417656249882723, -0.09479166632524876901, 1.181850606188755259 ) ) ;
#119216=CARTESIAN_POINT ( 'NONE',  ( 6.805829924380097040, 10.88395931184472154, 0.7216878364870438212 ) ) ;
#119220=ORIENTED_EDGE ( 'NONE', *, *, #137732, .T. ) ;
#119221=CARTESIAN_POINT ( 'NONE',  ( -5.529805931533524621, 6.238042758285092582, -0.9566377225056829081 ) ) ;
#119223=CARTESIAN_POINT ( 'NONE',  ( -0.3963168366282447952, 6.583269796083455638, -3.242944579665297145 ) ) ;
#119243=CARTESIAN_POINT ( 'NONE',  ( 0.7499999999999885647, -1.235416665983847473, 1.299038105676657340 ) ) ;
#119247=CARTESIAN_POINT ( 'NONE',  ( 9.215791728987056786, 11.77484298861683598, -1.599625672291262513 ) ) ;
#119252=CARTESIAN_POINT ( 'NONE',  ( 7.553864141108259211, 11.96459193126834464, 1.040834085586084257E-14 ) ) ;
#119257=CARTESIAN_POINT ( 'NONE',  ( 4.147904930777053245, 6.926640621626830807, -1.199719254218452047 ) ) ;
#119258=CARTESIAN_POINT ( 'NONE',  ( -1.201851678989727383E-14, 2.759375000341417916, -1.575800808251660134 ) ) ;
#119261=CARTESIAN_POINT ( 'NONE',  ( -6.645467848992654858, 10.90479625713344625, 0.7998128361456481317 ) ) ;
#119262=CARTESIAN_POINT ( 'NONE',  ( -4.243338890952904841, 5.973648010910253880, -1.443375672974051449 ) ) ;
#119263=AXIS2_PLACEMENT_3D ( 'NONE', #138686, #122516, #24900 ) ;
#119266=CARTESIAN_POINT ( 'NONE',  ( -5.636439174979254396, 7.598931675607687453, -1.599625672291256295 ) ) ;
#119268=CARTESIAN_POINT ( 'NONE',  ( 1.499999999999987121, 0.2854166673494805684, 0.8660254037844524744 ) ) ;
#119275=CARTESIAN_POINT ( 'NONE',  ( -4.921246571636213929, 4.843801876438091902, 0.7216878364870317197 ) ) ;
#119278=CARTESIAN_POINT ( 'NONE',  ( 4.008122245411202655, 7.584344604122328803, -0.2404964666735086298 ) ) ;
#119282=CARTESIAN_POINT ( 'NONE',  ( -4.622967192135580383, 5.456178481322002227, 1.082531754730558626 ) ) ;
#119284=CARTESIAN_POINT ( 'NONE',  ( 9.935427640716063991, 10.48575375712389679, -0.7998128361456281477 ) ) ;
#119286=CARTESIAN_POINT ( 'NONE',  ( -1.244150428499023908, 3.152476754118171964, 0.7750000000000100142 ) ) ;
#119292=CARTESIAN_POINT ( 'NONE',  ( -4.600294193738529103, 4.261431402316699035, -0.7998128361456221525 ) ) ;
#119298=CARTESIAN_POINT ( 'NONE',  ( 5.840865249388943248, 5.708764300575555062, 0.7998128361456341429 ) ) ;
#119310=CARTESIAN_POINT ( 'NONE',  ( -1.608462485350629301, 8.735270501766756013, 2.463594439587650342 ) ) ;
#119314=CARTESIAN_POINT ( 'NONE',  ( 7.639129486296027061, 10.99973593639901814, 1.199719254218460707 ) ) ;
#119317=CARTESIAN_POINT ( 'NONE',  ( -4.680589345215810049, 6.483773540883647435, -1.599625672291256295 ) ) ;
#119320=CARTESIAN_POINT ( 'NONE',  ( -5.544921637864844932, 5.571422787038162738, -0.7216878364870168427 ) ) ;
#119321=AXIS2_PLACEMENT_3D ( 'NONE', #212064, #163349, #14925 ) ;
#119323=VERTEX_POINT ( 'NONE', #23755 ) ;
#119325=CARTESIAN_POINT ( 'NONE',  ( 0.7499999999999867883, -0.6520833326505159899, -1.299038105676652899 ) ) ;
#119330=CARTESIAN_POINT ( 'NONE',  ( 2.693266070609028784, 6.293894182352508970, 0.000000000000000000 ) ) ;
#119331=CARTESIAN_POINT ( 'NONE',  ( -4.355193658487827690, 6.104145239700998538, -1.599625672291256295 ) ) ;
#119337=CARTESIAN_POINT ( 'NONE',  ( 5.178851490740196795, 7.065079377328788546, 1.443375672974062551 ) ) ;
#119341=CARTESIAN_POINT ( 'NONE',  ( 7.253248993186720561, 10.44557901115111065, 1.082531754730558626 ) ) ;
#119342=CARTESIAN_POINT ( 'NONE',  ( -0.6823417656250212460, 5.113541667008086655, 1.181850606188767472 ) ) ;
#119344=CARTESIAN_POINT ( 'NONE',  ( 5.138177029454841893, 7.017625839162543677, 1.443375672974062551 ) ) ;
#119351=CARTESIAN_POINT ( 'NONE',  ( -4.313069242314466756, 7.435226253386592710, 1.131090909019900614 ) ) ;
#119354=CARTESIAN_POINT ( 'NONE',  ( 1.364683531249990311, 5.196875000341417916, 1.214306433183764966E-14 ) ) ;
#119358=CARTESIAN_POINT ( 'NONE',  ( -10.00321840878439339, 10.56484298653695397, 1.040834085586084257E-14 ) ) ;
#119368=CARTESIAN_POINT ( 'NONE',  ( 3.931501358282940117, 4.649468341827285300, -1.082531754730543083 ) ) ;
#119369=CARTESIAN_POINT ( 'NONE',  ( -1.364683531249997417, 4.071875000341417028, 1.214306433183764966E-14 ) ) ;
#119371=CARTESIAN_POINT ( 'NONE',  ( 7.775764792637399836, 9.030479331953833011, -1.199719254218441611 ) ) ;
#119373=CARTESIAN_POINT ( 'NONE',  ( -9.691380875670077444, 10.20103253123691189, 0.7998128361456462443 ) ) ;
#119380=CARTESIAN_POINT ( 'NONE',  ( -1.499999999999997780, 4.650000000000022560, 1.214306433183764966E-14 ) ) ;
#119381=CARTESIAN_POINT ( 'NONE',  ( 5.996784015946103885, 5.890669528225568996, 1.040834085586084257E-14 ) ) ;
#119384=ORIENTED_EDGE ( 'NONE', *, *, #19510, .T. ) ;
#119386=CARTESIAN_POINT ( 'NONE',  ( 6.792271770766432404, 10.86814146596211472, 1.040834085586084257E-14 ) ) ;
#119392=CARTESIAN_POINT ( 'NONE',  ( -1.201851678989727383E-14, 2.743750000682820378, 1.732050807568877637 ) ) ;
#119394=CARTESIAN_POINT ( 'NONE',  ( -5.427341564172148303, 5.226320001155936090, 0.000000000000000000 ) ) ;
#119395=CARTESIAN_POINT ( 'NONE',  ( 4.989037339704528229, 4.922891105851139315, 1.040834085586084257E-14 ) ) ;
#119402=ORIENTED_EDGE ( 'NONE', *, *, #100779, .F. ) ;
#119404=CARTESIAN_POINT ( 'NONE',  ( 6.272618624616828953, 10.46980549536166016, 1.040834085586084257E-14 ) ) ;
#119405=CARTESIAN_POINT ( 'NONE',  ( 4.123651276850781144, 7.962676922967908411, -0.7998128361456221525 ) ) ;
#119409=CARTESIAN_POINT ( 'NONE',  ( 4.867540842506059562, 5.637551390133895168, -1.199719254218452047 ) ) ;
#119417=CARTESIAN_POINT ( 'NONE',  ( 8.204655514564224816, 12.72384853363364066, 1.040834085586084257E-14 ) ) ;
#119422=CARTESIAN_POINT ( 'NONE',  ( 4.778452461313970723, 6.762070782353614362, -1.245597109521460633 ) ) ;
#119424=CARTESIAN_POINT ( 'NONE',  ( 8.367353357928214663, 12.91366268422496688, 1.040834085586084257E-14 ) ) ;
#119431=CARTESIAN_POINT ( 'NONE',  ( 5.504247177468168495, 9.365446107114122398, 0.7216878364870438212 ) ) ;
#119432=CARTESIAN_POINT ( 'NONE',  ( -8.948018195339354719, 12.42280974699582607, 1.082531754730560403 ) ) ;
#119438=CARTESIAN_POINT ( 'NONE',  ( -4.578903193113314174, 6.365139696764064325, 1.599625672291267398 ) ) ;
#119449=CARTESIAN_POINT ( 'NONE',  ( 8.072990401933337168, 11.50590700464255356, -1.199719254218446718 ) ) ;
#119450=CARTESIAN_POINT ( 'NONE',  ( 6.064713176501767222, 6.047104440226040545, 0.4075101515045934097 ) ) ;
#119451=CARTESIAN_POINT ( 'NONE',  ( -1.123270288250315163, 2.985197346350006331, -0.7749999999993613109 ) ) ;
#119452=ORIENTED_EDGE ( 'NONE', *, *, #195535, .T. ) ;
#119457=CARTESIAN_POINT ( 'NONE',  ( -9.354762803749327560, 10.01623748057011376, 0.7216878364870438212 ) ) ;
#119461=CARTESIAN_POINT ( 'NONE',  ( 7.884230021546724920, 9.157022099014721306, 1.199719254218462483 ) ) ;
#119463=CARTESIAN_POINT ( 'NONE',  ( -0.3859971386777985569, 2.800000000000025580, 1.330683448905541022 ) ) ;
#119464=CARTESIAN_POINT ( 'NONE',  ( 3.192055101013606233, 5.811482486902795230, -1.199719254218446718 ) ) ;
#119466=CARTESIAN_POINT ( 'NONE',  ( -6.307567778855718288, 8.381915046796901692, -1.599625672291263179 ) ) ;
#119467=CARTESIAN_POINT ( 'NONE',  ( 3.876741858503734761, 6.610283703974623393, 1.199719254218462483 ) ) ;
#119470=EDGE_CURVE ( 'NONE', #170502, #138277, #209266, .T. ) ;
#119476=CARTESIAN_POINT ( 'NONE',  ( 4.230803266364135951, 7.299989629454814555, -0.8951707687023923166 ) ) ;
#119478=CARTESIAN_POINT ( 'NONE',  ( 4.853455804012212660, 7.645820290447483458, 1.082531754730558626 ) ) ;
#119486=CARTESIAN_POINT ( 'NONE',  ( 9.381879110532285182, 10.04787317181692075, 0.000000000000000000 ) ) ;
#119489=CARTESIAN_POINT ( 'NONE',  ( -6.665805079413154921, 10.92852302595736447, 0.7998128361456481317 ) ) ;
#119498=CARTESIAN_POINT ( 'NONE',  ( 4.390142812726693045, 4.016254791136236513, 1.214306433183764966E-14 ) ) ;
#119501=( BOUNDED_CURVE ( )  B_SPLINE_CURVE ( 2, ( #43884, #46015, #42823, #208469, #142461, #47081, #145675 ),
 .UNSPECIFIED., .F., .T. ) 
 B_SPLINE_CURVE_WITH_KNOTS ( ( 3, 2, 2, 3 ),
 ( 0.1500000000000002165, 0.1541666666666668961, 0.1583333333333335480, 0.1625000000000002276 ),
 .UNSPECIFIED. ) 
 CURVE ( )  GEOMETRIC_REPRESENTATION_ITEM ( )  RATIONAL_B_SPLINE_CURVE ( ( 0.9999999999999928946, 0.8660254037844458130, 1.000000000000000000, 0.8660254037844387076, 1.000000000000000000, 0.8660254037844316022, 1.000000000000007105 ) ) 
 REPRESENTATION_ITEM ( '' )  );
#119503=CARTESIAN_POINT ( 'NONE',  ( 4.310602774141044868, 7.116454772218158809, -1.199719254218452047 ) ) ;
#119506=CARTESIAN_POINT ( 'NONE',  ( -1.201851678989727383E-14, 4.368750000682820378, -1.732050807568863648 ) ) ;
#119510=VERTEX_POINT ( 'NONE', #141831 ) ;
#119512=CARTESIAN_POINT ( 'NONE',  ( -1.402160292154681736E-14, 1.587500000000018785, -1.732050807568863648 ) ) ;
#119513=CARTESIAN_POINT ( 'NONE',  ( 7.298366762858032430, 7.409182732956175244, 1.040834085586084257E-14 ) ) ;
#119514=CARTESIAN_POINT ( 'NONE',  ( 4.161989969270892153, 6.839110149915929249, 1.082531754730558626 ) ) ;
#119518=CARTESIAN_POINT ( 'NONE',  ( 8.324343129110697959, 9.774450407793066731, -1.082531754730543083 ) ) ;
#119524=CARTESIAN_POINT ( 'NONE',  ( -3.554208825076827782, 7.298327395898266623, 0.7998128361456341429 ) ) ;
#119526=CARTESIAN_POINT ( 'NONE',  ( 0.7499999999999885647, 3.347916667349487341, -1.299038105676658228 ) ) ;
#119527=CARTESIAN_POINT ( 'NONE',  ( 1.364683531249988535, 5.217708333674750065, -0.7879004041258300672 ) ) ;
#119532=CARTESIAN_POINT ( 'NONE',  ( -1.364683531249997417, 3.821875000341416584, 1.214306433183764966E-14 ) ) ;
#119541=CARTESIAN_POINT ( 'NONE',  ( -9.203287345578106127, 9.631590079462940324, 0.7998128361456462443 ) ) ;
#119542=CARTESIAN_POINT ( 'NONE',  ( 7.006866460164219212, 7.069099046480051385, -0.7998128361456281477 ) ) ;
#119550=CARTESIAN_POINT ( 'NONE',  ( -6.170932472514347289, 10.35117165124207972, 0.000000000000000000 ) ) ;
#119555=CARTESIAN_POINT ( 'NONE',  ( 9.402743226277308963, 10.92862083786708816, -1.199719254218446718 ) ) ;
#119557=CARTESIAN_POINT ( 'NONE',  ( -2.252626078164912560, 5.779814191167667481, 0.7998128361456341429 ) ) ;
#119558=CARTESIAN_POINT ( 'NONE',  ( -8.993135964566285168, 9.386413468282476913, -0.7998128361456291469 ) ) ;
#119562=CARTESIAN_POINT ( 'NONE',  ( -4.153809255294044434, 7.618134729639562508, -0.8777755718400248597 ) ) ;
#119567=CARTESIAN_POINT ( 'NONE',  ( 7.998947442382716488, 9.394822106610419610, -1.082531754730543083 ) ) ;
#119570=CARTESIAN_POINT ( 'NONE',  ( 4.645640190976921602, 8.571663989448405019, 1.040834085586084257E-14 ) ) ;
#119577=EDGE_CURVE ( 'NONE', #188383, #160603, #194830, .T. ) ;
#119584=TOROIDAL_SURFACE ( 'NONE', #26125, 3.971937515251341644, 0.08000000000000000167 ) ;
#119596=CARTESIAN_POINT ( 'NONE',  ( -7.486073373039941359, 11.88550270185529278, -0.7998128361456291469 ) ) ;
#119601=CARTESIAN_POINT ( 'NONE',  ( 1.499999999999987121, 2.077083334016153415, -0.8660254037844262731 ) ) ;
#119602=CARTESIAN_POINT ( 'NONE',  ( 8.191097360950562845, 12.70803068775103739, -0.7998128361456352531 ) ) ;
#119606=CARTESIAN_POINT ( 'NONE',  ( -10.49131193887636826, 11.13428543831092909, 1.040834085586084257E-14 ) ) ;
#119608=CARTESIAN_POINT ( 'NONE',  ( -1.402160292154681736E-14, 2.196875000341423689, -1.575800808251660134 ) ) ;
#119610=ORIENTED_EDGE ( 'NONE', *, *, #137765, .F. ) ;
#119614=CARTESIAN_POINT ( 'NONE',  ( -3.144601563365788444, 5.756120026313656268, -1.199719254218452935 ) ) ;
#119620=CARTESIAN_POINT ( 'NONE',  ( 0.6823417656249882723, -0.2614583329919109578, -1.181850606188749264 ) ) ;
#119625=CARTESIAN_POINT ( 'NONE',  ( -1.364683531250000748, 2.009375000341421913, 1.214306433183764966E-14 ) ) ;
#119627=CARTESIAN_POINT ( 'NONE',  ( -7.711890448074853133, 7.891627032375787998, -0.7998128361456291469 ) ) ;
#119628=CARTESIAN_POINT ( 'NONE',  ( 8.450809820019639318, 8.753699632978056755, -0.7998128361456291469 ) ) ;
#119629=CARTESIAN_POINT ( 'NONE',  ( 4.867540842506059562, 5.637551390133895168, -1.199719254218452047 ) ) ;
#119630=CARTESIAN_POINT ( 'NONE',  ( 5.087333953625774008, 6.958308917361963886, 1.599625672291267398 ) ) ;
#119632=CARTESIAN_POINT ( 'NONE',  ( 0.7499999999999902300, 4.066666666666690411, -1.299038105676658228 ) ) ;
#119635=CARTESIAN_POINT ( 'NONE',  ( -1.402160292154681736E-14, 1.759375000341421469, -1.575800808251659024 ) ) ;
#119641=CARTESIAN_POINT ( 'NONE',  ( 6.480434237652135998, 6.662854153456708950, 0.7216878364870317197 ) ) ;
#119644=CARTESIAN_POINT ( 'NONE',  ( -9.287498920561160887, 10.79416914786490089, -1.199719254218441611 ) ) ;
#119645=CARTESIAN_POINT ( 'NONE',  ( -5.101945877444165944, 4.846691699973280976, 0.000000000000000000 ) ) ;
#119649=CARTESIAN_POINT ( 'NONE',  ( -7.009202228140739344, 11.12122699956546334, -0.7216878364870267237 ) ) ;
#119651=CARTESIAN_POINT ( 'NONE',  ( -0.7499999999999972244, 5.108333333333353821, -1.299038105676652011 ) ) ;
#119654=CARTESIAN_POINT ( 'NONE',  ( 8.107412671292031803, 11.44210330227398487, 1.082531754730557072 ) ) ;
#119662=CARTESIAN_POINT ( 'NONE',  ( 10.68346185744421462, 11.56638637654751989, 0.000000000000000000 ) ) ;
#119666=CARTESIAN_POINT ( 'NONE',  ( 7.239690839573049708, 11.39013037956983965, 1.040834085586084257E-14 ) ) ;
#119667=CARTESIAN_POINT ( 'NONE',  ( 8.098297826064319693, 8.342435640030188893, 0.7998128361456481317 ) ) ;
#119668=CARTESIAN_POINT ( 'NONE',  ( -4.232116505760120440, 8.089219690028791376, -0.7998128361456281477 ) ) ;
#119673=CARTESIAN_POINT ( 'NONE',  ( 5.111060722227499298, 8.906728576000002562, -0.7216878364870267237 ) ) ;
#119674=CARTESIAN_POINT ( 'NONE',  ( 1.387358672525639269, 7.251968950354889643, 4.302625267139791987 ) ) ;
#119675=CARTESIAN_POINT ( 'NONE',  ( 4.704316114261903436, 4.590716342834741504, 1.214306433183764966E-14 ) ) ;
#119677=CARTESIAN_POINT ( 'NONE',  ( -10.62011439820619429, 11.28455497419572318, -0.7998128361456221525 ) ) ;
#119686=VERTEX_POINT ( 'NONE', #64786 ) ;
#119695=CARTESIAN_POINT ( 'NONE',  ( 7.151035956204054855, 10.43029348462504124, 1.199719254218460707 ) ) ;
#119707=CARTESIAN_POINT ( 'NONE',  ( -4.629219384062206011, 7.488174150459498968, -1.199719254218452047 ) ) ;
#119710=CARTESIAN_POINT ( 'NONE',  ( -5.251085567194491155, 5.020688004682002159, -0.7998128361456221525 ) ) ;
#119721=CARTESIAN_POINT ( 'NONE',  ( -2.930533758848195447, 6.570706485298192234, -0.7998128361456281477 ) ) ;
#119724=CARTESIAN_POINT ( 'NONE',  ( 6.479907352327590964, 9.647310113435821677, 1.199719254218462483 ) ) ;
#119725=CARTESIAN_POINT ( 'NONE',  ( -1.364683531250010740, 4.530208333674754506, 0.7879004041258379498 ) ) ;
#119732=CARTESIAN_POINT ( 'NONE',  ( 4.921246571636183731, 7.724909519342112674, -1.082531754730549078 ) ) ;
#119733=CARTESIAN_POINT ( 'NONE',  ( -5.506582945444718824, 9.576097202994168001, 0.7998128361456481317 ) ) ;
#119736=CARTESIAN_POINT ( 'NONE',  ( -7.670162217029145246, 9.971608557999250166, 1.599625672291295375 ) ) ;
#119737=CARTESIAN_POINT ( 'NONE',  ( -6.600121851754250812, 6.594563670001734046, 0.7998128361456341429 ) ) ;
#119741=CARTESIAN_POINT ( 'NONE',  ( 4.903184595771473475, 4.840886387581087469, 0.6212912700429285007 ) ) ;
#119744=CARTESIAN_POINT ( 'NONE',  ( 6.805303039055573322, 10.02693841461847057, 1.199719254218460707 ) ) ;
#119758=CARTESIAN_POINT ( 'NONE',  ( 1.499999999999989120, 5.545833333333350268, -0.8660254037844323793 ) ) ;
#119759=CARTESIAN_POINT ( 'NONE',  ( 4.009460741339333723, 5.700790169694431420, -1.599625672291256295 ) ) ;
#119760=CARTESIAN_POINT ( 'NONE',  ( 5.412729640353754590, 7.337937218544611895, 1.599625672291267398 ) ) ;
#119762=CARTESIAN_POINT ( 'NONE',  ( -6.860062538834774237, 10.94723069537516302, 0.7216878364870458196 ) ) ;
#119764=CARTESIAN_POINT ( 'NONE',  ( 6.182154858151487353, 6.314861544039274577, -0.7216878364870257245 ) ) ;
#119765=CARTESIAN_POINT ( 'NONE',  ( -6.846504384776750385, 10.93141284897413890, -0.7216878364870267237 ) ) ;
#119768=CARTESIAN_POINT ( 'NONE',  ( 8.938903350111612411, 9.323142084752035430, -0.7998128361456221525 ) ) ;
#119774=CARTESIAN_POINT ( 'NONE',  ( 0.6823417656249882723, 2.676041667008084879, -1.181850606188749264 ) ) ;
#119780=CARTESIAN_POINT ( 'NONE',  ( 8.718056468787178659, 10.12981962079525289, 1.199719254218462483 ) ) ;
#119783=CARTESIAN_POINT ( 'NONE',  ( -7.669108446824431269, 12.09904362127053545, -0.7998128361456291469 ) ) ;
#119789=CARTESIAN_POINT ( 'NONE',  ( 2.517010073631369860, 6.088262185878572375, -0.7998128361456281477 ) ) ;
#119794=CARTESIAN_POINT ( 'NONE',  ( -8.319899820280397762, 12.85830022363583147, -0.7998128361456281477 ) ) ;
#119799=CARTESIAN_POINT ( 'NONE',  ( 5.824368567101982030, 6.018301469053008113, 0.4368841385695241275 ) ) ;
#119801=CARTESIAN_POINT ( 'NONE',  ( -3.952365473583647315, 4.569846793057691592, 1.199719254218462483 ) ) ;
#119805=CARTESIAN_POINT ( 'NONE',  ( 7.884230021546724920, 9.157022099014721306, 1.199719254218462483 ) ) ;
#119807=CARTESIAN_POINT ( 'NONE',  ( 5.449487677688982679, 8.445153826357429949, -1.199719254218446718 ) ) ;
#119808=CARTESIAN_POINT ( 'NONE',  ( 5.281064527722868718, 6.119995689553514140, 1.199719254218462483 ) ) ;
#119810=CARTESIAN_POINT ( 'NONE',  ( -6.561783159334121152, 10.59923808595773664, -0.7216878364870278340 ) ) ;
#119818=CARTESIAN_POINT ( 'NONE',  ( -5.662059632048889846, 6.153064387560178261, -0.8011038117717106388 ) ) ;
#119822=CARTESIAN_POINT ( 'NONE',  ( 4.365362273920230685, 8.036747052974847705, 0.7216878364870298324 ) ) ;
#119827=CARTESIAN_POINT ( 'NONE',  ( -9.449669878600616357, 12.04770082983265844, -1.443375672974058777 ) ) ;
#119838=EDGE_CURVE ( 'NONE', #177712, #63704, #161235, .T. ) ;
#119842=CARTESIAN_POINT ( 'NONE',  ( -7.985389288324685531, 12.26011190311341537, -0.7216878364870267237 ) ) ;
#119846=CARTESIAN_POINT ( 'NONE',  ( 7.259501185113382604, 10.55683625168592243, -1.199719254218441611 ) ) ;
#119850=CARTESIAN_POINT ( 'NONE',  ( -0.7500000000000215383, 1.972916667349486453, 1.299038105676659116 ) ) ;
#119852=CARTESIAN_POINT ( 'NONE',  ( -4.934277840369690971, 7.844075682818238526, -1.199719254218452047 ) ) ;
#119855=CARTESIAN_POINT ( 'NONE',  ( -9.332089804907933939, 9.781859615347734405, 1.040834085586084257E-14 ) ) ;
#119859=CARTESIAN_POINT ( 'NONE',  ( 6.693975156845185737, 8.832723654451292816, 1.599625672291281386 ) ) ;
#119861=CARTESIAN_POINT ( 'NONE',  ( -5.865874016206865882, 9.995270118883347266, 0.000000000000000000 ) ) ;
#119863=CARTESIAN_POINT ( 'NONE',  ( 7.235247531187115833, 11.59287255302699648, -0.7998128361456291469 ) ) ;
#119870=CARTESIAN_POINT ( 'NONE',  ( -8.514157279702036618, 9.035531035848267223, -0.7216878364870278340 ) ) ;
#119873=CARTESIAN_POINT ( 'NONE',  ( 0.6823417656249899377, 4.738541667008086655, -1.181850606188754593 ) ) ;
#119880=CARTESIAN_POINT ( 'NONE',  ( 1.364683531249990311, 5.113541667008084879, 0.7879004041258500513 ) ) ;
#119881=DIRECTION ( 'NONE',  ( 1.000000000000000000, 0.000000000000000000, 0.000000000000000000 ) ) ;
#119882=CARTESIAN_POINT ( 'NONE',  ( -4.460269348771590536, 5.266364330730674226, 1.082531754730558626 ) ) ;
#119885=CARTESIAN_POINT ( 'NONE',  ( 8.062294901620731480, 12.55776115186623620, 1.040834085586084257E-14 ) ) ;
#119886=CARTESIAN_POINT ( 'NONE',  ( -1.201851678989727383E-14, 4.759375000341419693, -1.575800808251660134 ) ) ;
#119887=LINE ( 'NONE', #99316, #132271 ) ;
#119891=CARTESIAN_POINT ( 'NONE',  ( 1.364683531249986537, 1.405208333674755838, -0.7879004041258239610 ) ) ;
#119892=AXIS2_PLACEMENT_3D ( 'NONE', #51737, #14931, #149223 ) ;
#119893=CARTESIAN_POINT ( 'NONE',  ( -2.928197990871687306, 5.399686175116803710, 1.082531754730560403 ) ) ;
#119895=CARTESIAN_POINT ( 'NONE',  ( 4.961394147597008697, 7.875711374583454827, -1.199719254218452047 ) ) ;
#119898=CARTESIAN_POINT ( 'NONE',  ( 5.233084105194869551, 6.167981546557892436, -1.082531754730548412 ) ) ;
#119901=PLANE ( 'NONE',  #117675 ) ;
#119904=CARTESIAN_POINT ( 'NONE',  ( -8.351459436338037889, 10.76645531385962862, -1.443375672974059665 ) ) ;
#119909=CARTESIAN_POINT ( 'NONE',  ( -8.402302512167102222, 10.82577223566020841, -1.599625672291263179 ) ) ;
#119910=CARTESIAN_POINT ( 'NONE',  ( -3.728129053633589152, 7.293308295973741195, 0.7216878364870317197 ) ) ;
#119911=CARTESIAN_POINT ( 'NONE',  ( 1.364683531249988757, 1.696875000341414808, 0.000000000000000000 ) ) ;
#119919=ORIENTED_EDGE ( 'NONE', *, *, #114516, .T. ) ;
#119928=DIRECTION ( 'NONE',  ( 0.6507913734559640506, -0.7592566023653004592, 0.000000000000000000 ) ) ;
#119933=CARTESIAN_POINT ( 'NONE',  ( -1.364683531250012516, 2.592708333674753174, 0.7879004041258379498 ) ) ;
#119941=CARTESIAN_POINT ( 'NONE',  ( 10.40996301719436090, 11.03937836301526687, 0.000000000000000000 ) ) ;
#119943=CARTESIAN_POINT ( 'NONE',  ( 1.364683531249988535, 1.363541667008083769, 0.7879004041258500513 ) ) ;
#119952=ORIENTED_EDGE ( 'NONE', *, *, #18068, .T. ) ;
#119954=CARTESIAN_POINT ( 'NONE',  ( 5.843727902690005749, 6.776436293681846301, -1.199719254218445830 ) ) ;
#119962=CARTESIAN_POINT ( 'NONE',  ( 8.294891053462476904, 8.571794405328034827, 1.040834085586084257E-14 ) ) ;
#119966=CARTESIAN_POINT ( 'NONE',  ( -4.243865776277440993, 4.909930479533815451, -1.199719254218446718 ) ) ;
#119967=CARTESIAN_POINT ( 'NONE',  ( 6.936968151686458306, 11.24487994360957188, 0.7998128361456462443 ) ) ;
#119973=ORIENTED_EDGE ( 'NONE', *, *, #117255, .F. ) ;
#119980=CARTESIAN_POINT ( 'NONE',  ( -8.026063749610056419, 10.38682701267698150, -1.443375672974059665 ) ) ;
#119985=CARTESIAN_POINT ( 'NONE',  ( -8.839026081105473054, 12.39961529701003684, -1.199719254218446718 ) ) ;
#119990=CARTESIAN_POINT ( 'NONE',  ( -2.788173145904702555, 6.404619103530779789, -0.7998128361456281477 ) ) ;
#119992=CARTESIAN_POINT ( 'NONE',  ( 9.103410076571945453, 12.70806329172093818, 1.199719254218450271 ) ) ;
#119993=CARTESIAN_POINT ( 'NONE',  ( 3.460355519985863548, 5.060167411448709629, 1.599625672291267398 ) ) ;
#119999=CARTESIAN_POINT ( 'NONE',  ( 3.551873057100283226, 6.127307085716883428, 1.082531754730558626 ) ) ;
#120002=CARTESIAN_POINT ( 'NONE',  ( -5.037017762676898158, 5.835274463666530131, -1.199719254218446718 ) ) ;
#120005=CARTESIAN_POINT ( 'NONE',  ( -7.784352752540590004, 12.23349531127272094, 0.7998128361456481317 ) ) ;
#120010=CARTESIAN_POINT ( 'NONE',  ( 7.565086526745395723, 10.80938946696957004, -1.082531754730543083 ) ) ;
#120013=CARTESIAN_POINT ( 'NONE',  ( 5.847644326195776010, 5.716673223516856694, -0.7998128361456281477 ) ) ;
#120027=CARTESIAN_POINT ( 'NONE',  ( 0.6823417656249882723, 2.488541667008084435, -1.181850606188749264 ) ) ;
#120029=CARTESIAN_POINT ( 'NONE',  ( 4.403700966340357681, 4.032072637018845107, -0.7998128361456211532 ) ) ;
#120032=CARTESIAN_POINT ( 'NONE',  ( -6.073689629242176480, 6.188318776978391611, -0.7216878364870278340 ) ) ;
#120035=CARTESIAN_POINT ( 'NONE',  ( -5.544921637864833386, 7.492161215640853023, -1.443375672974051449 ) ) ;
#120040=CARTESIAN_POINT ( 'NONE',  ( 4.852928918687680948, 7.749168607522574526, 1.199719254218462483 ) ) ;
#120051=CARTESIAN_POINT ( 'NONE',  ( 5.331380718671758778, 7.243030143248949670, -1.599625672291256295 ) ) ;
#120054=CARTESIAN_POINT ( 'NONE',  ( -2.266184231778562541, 5.795632037050281404, 1.040834085586084257E-14 ) ) ;
#120056=CARTESIAN_POINT ( 'NONE',  ( -6.684333426737305572, 7.757142738403693727, -1.199719254218446718 ) ) ;
#120060=CARTESIAN_POINT ( 'NONE',  ( 6.775324078527185989, 8.927630729746953264, -1.599625672291262513 ) ) ;
#120063=CARTESIAN_POINT ( 'NONE',  ( -5.703176172842872482, 9.805455968292021041, 0.000000000000000000 ) ) ;
#120064=CARTESIAN_POINT ( 'NONE',  ( 6.819388077549422889, 8.018669514304889390, -1.082531754730543971 ) ) ;
#120065=CARTESIAN_POINT ( 'NONE',  ( 4.441740843186996912, 7.307116142998927977, 1.228109861675081849 ) ) ;
#120066=CARTESIAN_POINT ( 'NONE',  ( -5.108724954250998707, 4.854600622914589714, -0.7998128361456221525 ) ) ;
#120070=CARTESIAN_POINT ( 'NONE',  ( -4.954615070790188369, 7.867802451642154082, -1.199719254218452047 ) ) ;
#120073=CARTESIAN_POINT ( 'NONE',  ( 0.6823417656249899377, 1.842708333674752952, 1.181850606188755259 ) ) ;
#120075=CARTESIAN_POINT ( 'NONE',  ( -5.422898255786198440, 7.349800603215774331, -1.443375672974052559 ) ) ;
#120076=VERTEX_POINT ( 'NONE', #103709 ) ;
#120082=CARTESIAN_POINT ( 'NONE',  ( 7.332262146892202459, 7.448727347662698506, -0.7998128361456281477 ) ) ;
#120086=CARTESIAN_POINT ( 'NONE',  ( -1.364683531250012516, 3.092708333674755838, 0.7879004041258379498 ) ) ;
#120092=CARTESIAN_POINT ( 'NONE',  ( -3.978428010606240850, 6.728917548094202949, -1.199719254218452047 ) ) ;
#120093=CARTESIAN_POINT ( 'NONE',  ( -7.415946836550729948, 9.675023947441092176, 1.443375672974090751 ) ) ;
#120101=CARTESIAN_POINT ( 'NONE',  ( -8.975134502122321223, 9.573337795338607847, 1.040834085586084257E-14 ) ) ;
#120106=CARTESIAN_POINT ( 'NONE',  ( -5.843201017365469596, 9.760892253660966134, 0.7216878364870458196 ) ) ;
#120111=( BOUNDED_CURVE ( )  B_SPLINE_CURVE ( 2, ( #2201, #169000, #4334 ),
 .UNSPECIFIED., .F., .T. ) 
 B_SPLINE_CURVE_WITH_KNOTS ( ( 3, 3 ),
 ( 0.000000000000000000, 0.0002183499308599263643 ),
 .UNSPECIFIED. ) 
 CURVE ( )  GEOMETRIC_REPRESENTATION_ITEM ( )  RATIONAL_B_SPLINE_CURVE ( ( 1.000000000000000000, 0.9929791974830429746, 0.9866942310032822405 ) ) 
 REPRESENTATION_ITEM ( '' )  );
#120121=CARTESIAN_POINT ( 'NONE',  ( -5.880485940025243607, 7.883652901494672349, 1.599625672291269396 ) ) ;
#120122=DIRECTION ( 'NONE',  ( 1.000000000000000000, 0.000000000000000000, 0.000000000000000000 ) ) ;
#120124=CARTESIAN_POINT ( 'NONE',  ( 5.169736645512481132, 4.925780929386339935, 0.7998128361456341429 ) ) ;
#120127=EDGE_CURVE ( 'NONE', #166004, #12101, #84366, .T. ) ;
#120130=CARTESIAN_POINT ( 'NONE',  ( 6.307567778855705853, 8.381915046796901692, -1.599625672291262513 ) ) ;
#120133=CARTESIAN_POINT ( 'NONE',  ( -4.609409038966234995, 7.361099064560491456, -1.082531754730549967 ) ) ;
#120137=CARTESIAN_POINT ( 'NONE',  ( -3.782361668532609134, 7.356579680022602652, 1.040834085586084257E-14 ) ) ;
#120141=CARTESIAN_POINT ( 'NONE',  ( 0.6823417656249899377, 1.092708333674752286, 1.181850606188755259 ) ) ;
#120143=CARTESIAN_POINT ( 'NONE',  ( -6.015013705957189316, 10.16926642359206134, 0.7998128361456481317 ) ) ;
#120146=CARTESIAN_POINT ( 'NONE',  ( 5.459129407796876166, 9.520734742405036144, 1.040834085586084257E-14 ) ) ;
#120148=CARTESIAN_POINT ( 'NONE',  ( -8.199983978166823562, 8.461069484149769337, -0.7998128361456291469 ) ) ;
#120151=CARTESIAN_POINT ( 'NONE',  ( 0.7499999999999885647, -0.7354166659838470288, 1.299038105676657340 ) ) ;
#120152=EDGE_CURVE ( 'NONE', #44633, #195163, #84819, .T. ) ;
#120154=CARTESIAN_POINT ( 'NONE',  ( 8.432808358020016826, 10.86136238915529084, 1.443375672974076540 ) ) ;
#120157=CARTESIAN_POINT ( 'NONE',  ( -1.364683531250014514, -0.4489583329919089039, -0.7879004041258359514 ) ) ;
#120160=CARTESIAN_POINT ( 'NONE',  ( 6.710922848640084482, 9.812865175846695820, -1.082531754730537976 ) ) ;
#120162=CARTESIAN_POINT ( 'NONE',  ( -4.284013352238250860, 7.941839977679187257, -0.7216878364870267237 ) ) ;
#120164=CARTESIAN_POINT ( 'NONE',  ( -1.201851678989727383E-14, 3.696875000341422801, -1.575800808251660134 ) ) ;
#120168=CARTESIAN_POINT ( 'NONE',  ( -5.585069213825653023, 8.603332285183535433, -1.199719254218440723 ) ) ;
#120177=CARTESIAN_POINT ( 'NONE',  ( 7.235247531187115833, 11.59287255302699648, -0.7998128361456291469 ) ) ;
#120180=CARTESIAN_POINT ( 'NONE',  ( -1.402160292154681736E-14, 2.587500000000023892, -1.732050807568863648 ) ) ;
#120185=ORIENTED_EDGE ( 'NONE', *, *, #170416, .F. ) ;
#120186=CARTESIAN_POINT ( 'NONE',  ( 5.314433026876846711, 9.143996264757578984, -0.7216878364870267237 ) ) ;
#120188=CARTESIAN_POINT ( 'NONE',  ( -1.364683531250014514, -0.1989583329919157317, -0.7879004041258359514 ) ) ;
#120194=CARTESIAN_POINT ( 'NONE',  ( 1.499999999999987121, 0.004166666666691258049, 0.8660254037844524744 ) ) ;
#120195=CARTESIAN_POINT ( 'NONE',  ( 7.507464373665139412, 9.781794407407920389, 1.599625672291281386 ) ) ;
#120196=CARTESIAN_POINT ( 'NONE',  ( -8.371269781434001800, 11.85389961405997816, -1.199719254218446718 ) ) ;
#120198=CARTESIAN_POINT ( 'NONE',  ( -1.364683531250000748, 0.5093750003414208027, 0.000000000000000000 ) ) ;
#120200=CARTESIAN_POINT ( 'NONE',  ( -1.201851678989727383E-14, 1.212500000000025002, 1.732050807568877637 ) ) ;
#120202=CARTESIAN_POINT ( 'NONE',  ( 5.996784015946103885, 5.890669528225568996, 1.040834085586084257E-14 ) ) ;
#120209=CARTESIAN_POINT ( 'NONE',  ( -1.364683531250010295, 5.738541667008088432, -0.7879004041258300672 ) ) ;
#120211=CARTESIAN_POINT ( 'NONE',  ( -9.182950115157607840, 9.607863310639020327, 0.7998128361456462443 ) ) ;
#120212=EDGE_CURVE ( 'NONE', #63949, #124240, #91511, .T. ) ;
#120213=CARTESIAN_POINT ( 'NONE',  ( -3.795919822146277767, 7.372397525905215687, -0.7216878364870267237 ) ) ;
#120221=CARTESIAN_POINT ( 'NONE',  ( 5.926885707468349196, 10.06645042535509660, 1.040834085586084257E-14 ) ) ;
#120225=CARTESIAN_POINT ( 'NONE',  ( 6.283314124929436417, 9.417951348137970413, -1.199719254218440723 ) ) ;
#120226=CARTESIAN_POINT ( 'NONE',  ( 7.117667457050084856, 7.406292909420979953, -0.7216878364870257245 ) ) ;
#120227=LINE ( 'NONE', #172110, #37373 ) ;
#120230=CARTESIAN_POINT ( 'NONE',  ( -6.821723845970312894, 11.11042825360738284, 0.000000000000000000 ) ) ;
#120231=CARTESIAN_POINT ( 'NONE',  ( 6.342516933094585418, 6.294024598232139667, 1.040834085586084257E-14 ) ) ;
#120232=CARTESIAN_POINT ( 'NONE',  ( -1.500000000000001332, -1.099999999999982991, 0.000000000000000000 ) ) ;
#120233=CARTESIAN_POINT ( 'NONE',  ( 0.9999999999999833467, 9.200000000000018829, 0.4000000000000144551 ) ) ;
#120234=CARTESIAN_POINT ( 'NONE',  ( 4.359110081993588182, 5.044382169536003602, -1.199719254218452047 ) ) ;
#120240=CARTESIAN_POINT ( 'NONE',  ( -5.097502569058221411, 6.009803087731781623, -1.082531754730544860 ) ) ;
#120241=CARTESIAN_POINT ( 'NONE',  ( 10.05978679165993483, 11.79913468076720306, 1.082531754730548412 ) ) ;
#120244=CARTESIAN_POINT ( 'NONE',  ( -5.696397096036042385, 9.797547045350714967, -0.7998128361456231517 ) ) ;
#120250=CARTESIAN_POINT ( 'NONE',  ( -7.588813295347149435, 9.876701482703580837, -1.599625672291263179 ) ) ;
#120258=ORIENTED_EDGE ( 'NONE', *, *, #125125, .T. ) ;
#120267=CARTESIAN_POINT ( 'NONE',  ( -7.531718027591449705, 8.745758106066849891, 1.199719254218462483 ) ) ;
#120270=CARTESIAN_POINT ( 'NONE',  ( 5.721177635286841756, 6.737423998331861341, -1.082531754730543083 ) ) ;
#120275=CARTESIAN_POINT ( 'NONE',  ( -5.461236948206312114, 5.265864615862458464, 0.7998128361456341429 ) ) ;
#120279=CARTESIAN_POINT ( 'NONE',  ( -4.880045225915050189, 7.780804299287790826, 1.199719254218464037 ) ) ;
#120280=CARTESIAN_POINT ( 'NONE',  ( 1.123270288250309834, 2.971052654332832610, -0.7749999999993620881 ) ) ;
#120285=CARTESIAN_POINT ( 'NONE',  ( -10.00321840878439339, 10.56484298653695397, 1.040834085586084257E-14 ) ) ;
#120286=CARTESIAN_POINT ( 'NONE',  ( 6.775324078527185989, 8.927630729746953264, -1.599625672291262513 ) ) ;
#120290=CARTESIAN_POINT ( 'NONE',  ( -10.13202086811422475, 10.71511252242175161, -0.7998128361456291469 ) ) ;
#120298=CARTESIAN_POINT ( 'NONE',  ( 9.761507412159302177, 10.49077285704843199, -0.7216878364870257245 ) ) ;
#120302=CARTESIAN_POINT ( 'NONE',  ( -5.446377490701157065, 6.293253950424717580, -1.032046567709556273 ) ) ;
#120304=CARTESIAN_POINT ( 'NONE',  ( -0.5146802535525265565, 6.793498207845753534, -3.562260005870215629 ) ) ;
#120311=ORIENTED_EDGE ( 'NONE', *, *, #67524, .F. ) ;
#120316=CARTESIAN_POINT ( 'NONE',  ( -4.569261463005423352, 5.289558780716470565, -1.199719254218446718 ) ) ;
#120323=CARTESIAN_POINT ( 'NONE',  ( 1.364683531249992088, 5.634375000341417916, 1.214306433183764966E-14 ) ) ;
#120327=CARTESIAN_POINT ( 'NONE',  ( 9.028840231696797503, 12.62106513936658203, -1.199719254218446718 ) ) ;
#120329=CARTESIAN_POINT ( 'NONE',  ( 1.270916165646588603, 3.040225491120026380, -0.7749999999999910294 ) ) ;
#120332=CARTESIAN_POINT ( 'NONE',  ( 4.701980345841006326, 4.380065246436280368, 0.7998128361456341429 ) ) ;
#120338=CARTESIAN_POINT ( 'NONE',  ( 5.834086172582112262, 5.700855377634248100, 1.040834085586084257E-14 ) ) ;
#120339=CARTESIAN_POINT ( 'NONE',  ( 1.364683531249988535, 2.926041667008082658, 0.7879004041258500513 ) ) ;
#120340=CARTESIAN_POINT ( 'NONE',  ( -5.203466197636060997, 6.462176032175228180, 1.180525766716962410 ) ) ;
#120341=CARTESIAN_POINT ( 'NONE',  ( 8.543609354905870035, 13.11929468069890525, 0.7998128361456462443 ) ) ;
#120343=CARTESIAN_POINT ( 'NONE',  ( -8.694856585065634746, 9.038420858865048757, 0.7998128361456462443 ) ) ;
#120344=CARTESIAN_POINT ( 'NONE',  ( -4.243338890952901288, 6.934017225211593249, -1.082531754730548412 ) ) ;
#120347=CARTESIAN_POINT ( 'NONE',  ( -6.205881626753225966, 8.263281202677319470, 1.599625672291283607 ) ) ;
#120349=CARTESIAN_POINT ( 'NONE',  ( 0.7499999999999885647, 0.01458333401615358182, 1.299038105676657340 ) ) ;
#120357=CARTESIAN_POINT ( 'NONE',  ( -2.914639836813632812, 6.344237543017112735, 0.7216878364870317197 ) ) ;
#120363=CARTESIAN_POINT ( 'NONE',  ( -4.568734577680899633, 4.432537883490215158, -0.7216878364870207285 ) ) ;
#120365=CARTESIAN_POINT ( 'NONE',  ( 8.934986926605834157, 10.38290515491702770, -1.199719254218446718 ) ) ;
#120375=CARTESIAN_POINT ( 'NONE',  ( -10.15913717534155047, 10.74674821418697057, 0.7998128361456462443 ) ) ;
#120380=CARTESIAN_POINT ( 'NONE',  ( 4.493637847925535667, 7.329995691633395261, -1.199719254218452047 ) ) ;
#120386=CARTESIAN_POINT ( 'NONE',  ( 2.693266070609028784, 6.293894182352508970, 0.000000000000000000 ) ) ;
#120396=CARTESIAN_POINT ( 'NONE',  ( 8.555358625423188812, 9.940005470203933768, 1.199719254218462483 ) ) ;
#120398=CARTESIAN_POINT ( 'NONE',  ( -5.773074481320628948, 5.629675071162500544, 0.000000000000000000 ) ) ;
#120400=CARTESIAN_POINT ( 'NONE',  ( -1.499999999999997780, 4.181250000682819490, 1.214306433183764966E-14 ) ) ;
#120403=CARTESIAN_POINT ( 'NONE',  ( 1.364683531249992088, 5.634375000341417916, 1.214306433183764966E-14 ) ) ;
#120409=CARTESIAN_POINT ( 'NONE',  ( 3.246287715468270108, 5.874753870433235825, 1.199719254218450271 ) ) ;
#120410=CARTESIAN_POINT ( 'NONE',  ( -5.057354993097396445, 5.859001232490445688, -1.199719254218446718 ) ) ;
#120417=CARTESIAN_POINT ( 'NONE',  ( 5.341549334104188418, 7.254893527920112994, 1.443375672974062551 ) ) ;
#120420=CARTESIAN_POINT ( 'NONE',  ( 9.042925270190638187, 9.652427024751663254, 0.7216878364870458196 ) ) ;
#120421=CARTESIAN_POINT ( 'NONE',  ( -1.364683531249997417, 3.571875000341423245, 1.214306433183764966E-14 ) ) ;
#120423=CARTESIAN_POINT ( 'NONE',  ( 5.056828107772846082, 6.922718763866881453, -1.443375672974051449 ) ) ;
#120430=CARTESIAN_POINT ( 'NONE',  ( -4.762889583212370326, 6.995502248939536649, 1.426468515190159714 ) ) ;
#120431=DIRECTION ( 'NONE',  ( -5.578564026256490882E-16, -1.000000000000000000, -9.066213480720158442E-32 ) ) ;
#120432=EDGE_CURVE ( 'NONE', #154836, #214357, #32873, .T. ) ;
#120438=CARTESIAN_POINT ( 'NONE',  ( -8.533967624797991647, 12.04371376465130439, -1.199719254218446718 ) ) ;
#120440=DIRECTION ( 'NONE',  ( -0.6507913734559642727, 0.7592566023653003482, 2.775557561562893816E-17 ) ) ;
#120448=CARTESIAN_POINT ( 'NONE',  ( 4.528060117284244512, 4.385084346360807572, 0.7216878364870317197 ) ) ;
#120449=CARTESIAN_POINT ( 'NONE',  ( 0.6823417656249882723, 2.738541667008084879, -1.181850606188749264 ) ) ;
#120451=CARTESIAN_POINT ( 'NONE',  ( 7.124973419181436007, 8.271222729588529887, -1.199719254218446718 ) ) ;
#120452=CARTESIAN_POINT ( 'NONE',  ( -8.666686507633592385, 11.13422023037111330, 1.599625672291269396 ) ) ;
#120454=CARTESIAN_POINT ( 'NONE',  ( -5.413783410558481890, 5.210502155273325720, -0.7998128361456221525 ) ) ;
#120461=CARTESIAN_POINT ( 'NONE',  ( 1.499999999999990896, 4.025000000000021672, 1.214306433183764966E-14 ) ) ;
#120462=CARTESIAN_POINT ( 'NONE',  ( 4.137209430464448445, 7.978494768850520558, 1.040834085586084257E-14 ) ) ;
#120466=CARTESIAN_POINT ( 'NONE',  ( -1.364683531250010295, 4.280208333674753618, 0.7879004041258379498 ) ) ;
#120467=ORIENTED_EDGE ( 'NONE', *, *, #44771, .F. ) ;
#120469=CARTESIAN_POINT ( 'NONE',  ( 9.598809568795314107, 10.30095870645710754, -0.7216878364870257245 ) ) ;
#120474=CARTESIAN_POINT ( 'NONE',  ( -1.201851678989727383E-14, 2.493750000682819046, 1.732050807568877637 ) ) ;
#120476=CARTESIAN_POINT ( 'NONE',  ( -6.091691091241777656, 6.001394449403842479, 0.7998128361456341429 ) ) ;
#120477=CARTESIAN_POINT ( 'NONE',  ( 5.788968402910816380, 5.856144012925152076, 0.7216878364870317197 ) ) ;
#120478=DIRECTION ( 'NONE',  ( 5.578564026256491869E-16, 1.000000000000000000, 9.066213480720160632E-32 ) ) ;
#120480=B_SPLINE_CURVE_WITH_KNOTS ( 'NONE', 3,
 ( #84944, #20982, #131622, #101186 ),
 .UNSPECIFIED., .F., .F.,
 ( 4, 4 ),
 ( 3.104682540415231782E-18, 5.209409853017606958E-06 ),
 .UNSPECIFIED. ) ;
#120485=ORIENTED_EDGE ( 'NONE', *, *, #145044, .F. ) ;
#120487=CARTESIAN_POINT ( 'NONE',  ( 8.132193210098487057, 8.381980254736715708, 1.040834085586084257E-14 ) ) ;
#120488=CARTESIAN_POINT ( 'NONE',  ( 4.310602774141044868, 7.116454772218158809, -1.199719254218452047 ) ) ;
#120491=( NAMED_UNIT ( * ) PLANE_ANGLE_UNIT ( ) SI_UNIT ( $, .RADIAN. ) );
#120492=CARTESIAN_POINT ( 'NONE',  ( 3.683011284406639607, 7.448596931783069586, 0.7998128361456321445 ) ) ;
#120495=CIRCLE ( 'NONE', #16637, 0.08000000000000032085 ) ;
#120501=CARTESIAN_POINT ( 'NONE',  ( 8.594979316059474073, 12.11489407112305372, 1.199719254218450271 ) ) ;
#120505=CARTESIAN_POINT ( 'NONE',  ( 5.611280047485872835, 6.151892252731265387, -0.8436193503846599606 ) ) ;
#120511=DIRECTION ( 'NONE',  ( 1.000000000000000000, -7.387867266669436732E-31, 0.000000000000000000 ) ) ;
#120512=CARTESIAN_POINT ( 'NONE',  ( 8.297226821883377568, 8.782445501726501291, -0.7216878364870267237 ) ) ;
#120513=CARTESIAN_POINT ( 'NONE',  ( -3.521367211247373508, 5.131347717920458962, -1.599625672291256295 ) ) ;
#120518=CARTESIAN_POINT ( 'NONE',  ( -3.730464822054482710, 7.503959392372201442, 1.040834085586084257E-14 ) ) ;
#120530=CARTESIAN_POINT ( 'NONE',  ( 9.935427640716063991, 10.48575375712389679, -0.7998128361456281477 ) ) ;
#120532=CARTESIAN_POINT ( 'NONE',  ( 5.670051627282618689, 6.304626411287498122, 1.111461560052000586 ) ) ;
#120540=CARTESIAN_POINT ( 'NONE',  ( -8.948018195339354719, 12.42280974699582607, 1.082531754730560403 ) ) ;
#120544=CARTESIAN_POINT ( 'NONE',  ( 6.726816770674637347, 10.99970333242910669, -0.7998128361456291469 ) ) ;
#120549=CARTESIAN_POINT ( 'NONE',  ( -7.250913225210214641, 7.353820272367037170, 0.7998128361456341429 ) ) ;
#120550=CARTESIAN_POINT ( 'NONE',  ( 3.323720213644492993, 7.029424015893889433, 1.040834085586084257E-14 ) ) ;
#120553=CARTESIAN_POINT ( 'NONE',  ( -3.099101127474140682, 6.559442382121059900, -0.4367601086740290350 ) ) ;
#120554=CARTESIAN_POINT ( 'NONE',  ( 0.1144128442232072856, 7.018241394332943806, 3.990988525777207752 ) ) ;
#120557=CARTESIAN_POINT ( 'NONE',  ( 4.472818454536469090, 7.041451798021368447, -1.136577435397856384 ) ) ;
#120560=CARTESIAN_POINT ( 'NONE',  ( 6.805829924380108586, 8.963220883242035697, 1.443375672974076540 ) ) ;
#120565=LINE ( 'NONE', #204905, #202451 ) ;
#120569=CARTESIAN_POINT ( 'NONE',  ( 8.229436053370676518, 9.663725486096376827, 1.082531754730558626 ) ) ;
#120573=CARTESIAN_POINT ( 'NONE',  ( -10.63367255181986160, 11.30037282007833532, 1.040834085586084257E-14 ) ) ;
#120574=CARTESIAN_POINT ( 'NONE',  ( -8.474009703741204547, 9.845098394908269768, -1.199719254218446718 ) ) ;
#120575=CARTESIAN_POINT ( 'NONE',  ( 7.084367489069545069E-14, 8.210952333604106812, 2.038660652713624177 ) ) ;
#120583=CARTESIAN_POINT ( 'NONE',  ( 8.367353357928214663, 12.91366268422496688, 1.040834085586084257E-14 ) ) ;
#120587=CARTESIAN_POINT ( 'NONE',  ( 5.684946482831785275, 5.526859072925533134, -0.7998128361456231517 ) ) ;
#120591=CARTESIAN_POINT ( 'NONE',  ( -1.402160292154681736E-14, 2.368750000682818602, -1.732050807568863648 ) ) ;
#120597=CARTESIAN_POINT ( 'NONE',  ( 0.7499999999999885647, 2.316666666666689078, -1.299038105676652899 ) ) ;
#120598=CARTESIAN_POINT ( 'NONE',  ( 6.103141704446003679, 10.27208242182903142, 0.7998128361456462443 ) ) ;
#120599=CARTESIAN_POINT ( 'NONE',  ( 3.945059511452237100, 6.586024615794168646, -1.082531754730548412 ) ) ;
#120603=CARTESIAN_POINT ( 'NONE',  ( 8.595506201384004896, 12.01154575404795466, 1.082531754730546636 ) ) ;
#120609=CARTESIAN_POINT ( 'NONE',  ( -5.199715606040888005, 6.025088614257851027, -1.199719254218446718 ) ) ;
#120610=CARTESIAN_POINT ( 'NONE',  ( -0.7499999999999972244, 4.139583334016149863, -1.299038105676652899 ) ) ;
#120611=CARTESIAN_POINT ( 'NONE',  ( -0.6823417656249969321, 4.780208333674755394, -1.181850606188749264 ) ) ;
#120616=CARTESIAN_POINT ( 'NONE',  ( -1.001543065824772872E-14, 4.384375000341417916, 1.575800808251672791 ) ) ;
#120623=CARTESIAN_POINT ( 'NONE',  ( -4.731432421044877934, 6.543090462684225450, -1.443375672974051449 ) ) ;
#120625=CARTESIAN_POINT ( 'NONE',  ( -6.852756576703439961, 10.08230087520760954, 1.199719254218453823 ) ) ;
#120626=CARTESIAN_POINT ( 'NONE',  ( 7.318703993278529829, 7.432909501780090800, 1.040834085586084257E-14 ) ) ;
#120632=CARTESIAN_POINT ( 'NONE',  ( -4.907688418022547516, 4.827984030555475314, 1.214306433183764966E-14 ) ) ;
#120634=CARTESIAN_POINT ( 'NONE',  ( -7.691553217654356622, 7.867900263551875994, -0.7998128361456291469 ) ) ;
#120639=CARTESIAN_POINT ( 'NONE',  ( 8.028399517586572998, 12.51821653715971472, -0.7998128361456352531 ) ) ;
#120641=CARTESIAN_POINT ( 'NONE',  ( -5.264643720808155791, 5.036505850564608089, 0.000000000000000000 ) ) ;
#120642=CARTESIAN_POINT ( 'NONE',  ( -7.320512876374914768, 10.62801655815766999, 1.199719254218453823 ) ) ;
#120645=CARTESIAN_POINT ( 'NONE',  ( -4.301340604499551468, 7.447936736316801642, -1.117465989868490883 ) ) ;
#120646=CARTESIAN_POINT ( 'NONE',  ( -0.6823417656250003738, -0.5322916663252491576, -1.181850606188749264 ) ) ;
#120652=CARTESIAN_POINT ( 'NONE',  ( 4.482942347612929979, 8.381849838857084123, 1.040834085586084257E-14 ) ) ;
#120667=EDGE_LOOP ( 'NONE', ( #71666, #209868, #20945, #127419 ) ) ;
#120676=CARTESIAN_POINT ( 'NONE',  ( -8.272446282632566650, 12.80293776304669962, 0.7998128361456481317 ) ) ;
#120682=CARTESIAN_POINT ( 'NONE',  ( 0.7499999999999885647, 1.347916667349485786, -1.299038105676652899 ) ) ;
#120683=CARTESIAN_POINT ( 'NONE',  ( 8.920375002787457319, 12.49452237230570084, 1.199719254218450271 ) ) ;
#120687=CARTESIAN_POINT ( 'NONE',  ( -8.469039510030723861, 13.03229652834454733, 1.040834085586084257E-14 ) ) ;
#120689=CARTESIAN_POINT ( 'NONE',  ( -1.364683531250014514, 1.488541667008084435, -0.7879004041258289570 ) ) ;
#120696=CARTESIAN_POINT ( 'NONE',  ( -2.740719608256871442, 6.349256642941639051, 0.7998128361456341429 ) ) ;
#120698=CARTESIAN_POINT ( 'NONE',  ( -0.5087312005655101332, 6.815231585927279845, -3.595452205664221079 ) ) ;
#120701=CARTESIAN_POINT ( 'NONE',  ( -1.364683531250014514, 0.3010416670080866552, -0.7879004041258359514 ) ) ;
#120706=CARTESIAN_POINT ( 'NONE',  ( -1.201851678989727383E-14, 0.8218750003414171390, 1.575800808251672791 ) ) ;
#120708=CARTESIAN_POINT ( 'NONE',  ( -7.237355071596549116, 7.338002426484427687, 1.040834085586084257E-14 ) ) ;
#120709=CARTESIAN_POINT ( 'NONE',  ( 6.889514614038635187, 11.18951748302043114, -0.7998128361456291469 ) ) ;
#120710=CARTESIAN_POINT ( 'NONE',  ( 5.705283713252285338, 5.550585841749445137, -0.7998128361456211532 ) ) ;
#120712=EDGE_CURVE ( 'NONE', #78732, #121840, #210412, .T. ) ;
#120713=CARTESIAN_POINT ( 'NONE',  ( 5.656776405399742025, 7.622658444431597680, -1.599625672291262513 ) ) ;
#120715=CARTESIAN_POINT ( 'NONE',  ( -1.499999999999997780, 4.150000000000021672, 1.214306433183764966E-14 ) ) ;
#120717=CARTESIAN_POINT ( 'NONE',  ( -1.364683531250014514, 1.051041667008090208, -0.7879004041258289570 ) ) ;
#120723=CARTESIAN_POINT ( 'NONE',  ( 5.016153647376196290, 8.796003655340152605, 0.7216878364870438212 ) ) ;
#120726=CARTESIAN_POINT ( 'NONE',  ( -6.028571859570855729, 10.18508426947466816, 0.000000000000000000 ) ) ;
#120727=CARTESIAN_POINT ( 'NONE',  ( -4.386226389220933441, 5.076017861301227008, -1.199719254218446718 ) ) ;
#120728=CARTESIAN_POINT ( 'NONE',  ( -4.261456902168970551, 7.437061921213615534, -1.019078666317332349 ) ) ;
#120732=CARTESIAN_POINT ( 'NONE',  ( -8.636180661780668899, 10.13826086257468795, -1.082531754730543083 ) ) ;
#120734=CARTESIAN_POINT ( 'NONE',  ( 1.499999999999990896, 5.525000000000022560, 1.214306433183764966E-14 ) ) ;
#120738=CARTESIAN_POINT ( 'NONE',  ( 8.351459436338029008, 10.76645531385962862, -1.443375672974063439 ) ) ;
#120740=CARTESIAN_POINT ( 'NONE',  ( -5.233084104750526322, 5.207612331738130429, 0.000000000000000000 ) ) ;
#120746=ORIENTED_EDGE ( 'NONE', *, *, #167641, .T. ) ;
#120747=CARTESIAN_POINT ( 'NONE',  ( 8.988692655735958326, 12.47026328412523988, -1.082531754730543083 ) ) ;
#120751=CARTESIAN_POINT ( 'NONE',  ( 8.717529583462649612, 10.23316793787035195, 1.082531754730558626 ) ) ;
#120752=CARTESIAN_POINT ( 'NONE',  ( 7.721532178182734185, 8.967207948423393304, 1.199719254218462483 ) ) ;
#120753=CARTESIAN_POINT ( 'NONE',  ( -6.891622154448065807, 6.934647356477856128, 1.040834085586084257E-14 ) ) ;
#120757=DIRECTION ( 'NONE',  ( 5.578564026256490882E-16, 1.000000000000000000, 9.066213480720158442E-32 ) ) ;
#120759=CARTESIAN_POINT ( 'NONE',  ( 4.365362273920250225, 5.155639410070820716, 1.082531754730560403 ) ) ;
#120760=ORIENTED_EDGE ( 'NONE', *, *, #89709, .F. ) ;
#120761=CARTESIAN_POINT ( 'NONE',  ( -3.972702704004144714, 4.593573561881607148, 1.199719254218462483 ) ) ;
#120772=ORIENTED_EDGE ( 'NONE', *, *, #201935, .T. ) ;
#120775=CARTESIAN_POINT ( 'NONE',  ( 6.259060471003163428, 10.45398764947904624, -0.7998128361456291469 ) ) ;
#120781=CARTESIAN_POINT ( 'NONE',  ( 1.533805080506458030, 8.737074443703258808, 2.508413646267935171 ) ) ;
#120786=CARTESIAN_POINT ( 'NONE',  ( -0.1841574206260490065, 7.053066645632062759, 4.037422194176029322 ) ) ;
#120788=CARTESIAN_POINT ( 'NONE',  ( -5.225778143063529946, 8.184159369294361497, 1.199719254218452047 ) ) ;
#120790=CARTESIAN_POINT ( 'NONE',  ( -4.416205349749324327, 6.175325546172740765, 1.599625672291267398 ) ) ;
#120801=CARTESIAN_POINT ( 'NONE',  ( -3.144601563365788444, 5.756120026313656268, -1.199719254218452935 ) ) ;
#120804=CARTESIAN_POINT ( 'NONE',  ( 5.750629710490689384, 9.860818428881154674, -0.7998128361456291469 ) ) ;
#120805=CARTESIAN_POINT ( 'NONE',  ( 0.6823417656249899377, 4.176041667008085767, -1.181850606188754593 ) ) ;
#120811=CARTESIAN_POINT ( 'NONE',  ( 5.680503174001485078, 6.689970460165617361, -1.082531754730543083 ) ) ;
#120812=CARTESIAN_POINT ( 'NONE',  ( -7.426115451983156923, 9.686887332112256388, -1.599625672291263179 ) ) ;
#120815=CARTESIAN_POINT ( 'NONE',  ( -7.049349804101573191, 10.31165964050546258, -1.199719254218440723 ) ) ;
#120816=CARTESIAN_POINT ( 'NONE',  ( -4.062639585589296942, 7.891496616496157301, 0.7998128361456341429 ) ) ;
#120820=CARTESIAN_POINT ( 'NONE',  ( 4.900944506803885936, 4.854540586819195092, 0.6419561201193320077 ) ) ;
#120824=CARTESIAN_POINT ( 'NONE',  ( 6.100279051144945619, 9.204410428722734849, -1.199719254218440723 ) ) ;
#120840=CARTESIAN_POINT ( 'NONE',  ( -1.500000000000011324, 5.129166666666691299, -0.8660254037844313801 ) ) ;
#120841=CARTESIAN_POINT ( 'NONE',  ( 2.347533153460546806, 5.890539112345938300, 0.000000000000000000 ) ) ;
#120843=CARTESIAN_POINT ( 'NONE',  ( 5.900823170445728572, 7.907379670318584353, 1.599625672291267398 ) ) ;
#120845=CARTESIAN_POINT ( 'NONE',  ( -9.029367117021344313, 9.636609179387466639, 0.7216878364870438212 ) ) ;
#120848=CARTESIAN_POINT ( 'NONE',  ( 4.500943810056890371, 8.194925511800951412, -0.7216878364870207285 ) ) ;
#120849=CARTESIAN_POINT ( 'NONE',  ( -8.039621902779392926, 9.442275643739831636, 1.082531754730558626 ) ) ;
#120852=CARTESIAN_POINT ( 'NONE',  ( 7.938462636001388795, 9.220293482545153907, -1.199719254218441611 ) ) ;
#120858=CARTESIAN_POINT ( 'NONE',  ( 0.6823417656249899377, 2.092708333674753174, 1.181850606188767472 ) ) ;
#120864=CARTESIAN_POINT ( 'NONE',  ( 7.747594715205354809, 11.12627870345989756, -1.199719254218446718 ) ) ;
#120867=CARTESIAN_POINT ( 'NONE',  ( -8.319899820280397762, 12.85830022363583147, -0.7998128361456281477 ) ) ;
#120871=CARTESIAN_POINT ( 'NONE',  ( 0.7499999999999920064, 4.264583334016150751, 1.299038105676669330 ) ) ;
#120873=CARTESIAN_POINT ( 'NONE',  ( 9.890836756369282057, 11.49806328964105617, -1.199719254218440723 ) ) ;
#120877=CARTESIAN_POINT ( 'NONE',  ( -7.967387826325084355, 12.44703623068796361, 0.7998128361456481317 ) ) ;
#120880=CARTESIAN_POINT ( 'NONE',  ( 4.897706171852771462, 4.871974472535213430, 0.6676900015689657408 ) ) ;
#120883=CARTESIAN_POINT ( 'NONE',  ( 5.804557637360799660, 6.030435022130575362, 0.4940411958238543066 ) ) ;
#120885=CARTESIAN_POINT ( 'NONE',  ( -5.739179097286464248, 5.590130456455974617, -0.7998128361456221525 ) ) ;
#120889=CARTESIAN_POINT ( 'NONE',  ( 7.263417608619159083, 9.497073181520933716, -1.599625672291262513 ) ) ;
#120891=CARTESIAN_POINT ( 'NONE',  ( 7.298366762858032430, 7.409182732956175244, 1.040834085586084257E-14 ) ) ;
#120892=CARTESIAN_POINT ( 'NONE',  ( 4.253507506385319381, 5.985511395581417204, 1.599625672291267398 ) ) ;
#120894=CARTESIAN_POINT ( 'NONE',  ( -9.517460647113315630, 10.20605163116143821, 0.7216878364870438212 ) ) ;
#120902=CARTESIAN_POINT ( 'NONE',  ( -5.289711001425910553, 6.400709951683444920, -1.138330407662338617 ) ) ;
#120905=CARTESIAN_POINT ( 'NONE',  ( 4.677199807034550183, 8.400557508274889784, 1.040834085586084257E-14 ) ) ;
#120909=CARTESIAN_POINT ( 'NONE',  ( -9.937763408692596556, 11.65677406730528887, -1.082531754730537976 ) ) ;
#120914=CARTESIAN_POINT ( 'NONE',  ( 6.938893903907228378E-15, 10.64264068711930733, 1.214306433183764966E-14 ) ) ;
#120916=ORIENTED_EDGE ( 'NONE', *, *, #183589, .F. ) ;
#120926=CARTESIAN_POINT ( 'NONE',  ( 6.598014311344812199, 10.84943379654430906, 1.040834085586084257E-14 ) ) ;
#120930=CARTESIAN_POINT ( 'NONE',  ( -1.201851678989727383E-14, 1.493750000682814383, 1.732050807568877637 ) ) ;
#120932=CARTESIAN_POINT ( 'NONE',  ( -6.501298352952815662, 7.543601818988450169, -1.199719254218446718 ) ) ;
#120935=CARTESIAN_POINT ( 'NONE',  ( -8.513630394377489807, 12.01998699582738972, -1.199719254218446718 ) ) ;
#120938=ADVANCED_FACE ( 'NONE', ( #68514 ), #38181, .F. ) ;
#120941=CARTESIAN_POINT ( 'NONE',  ( -1.387358672534699799, 7.315968950353656020, 4.254625267138158584 ) ) ;
#120942=CARTESIAN_POINT ( 'NONE',  ( 5.991813822235618758, 9.077867661661846554, 1.199719254218462483 ) ) ;
#120945=CARTESIAN_POINT ( 'NONE',  ( -6.551614543901706611, 8.666636272683888365, 1.599625672291283607 ) ) ;
#120947=CARTESIAN_POINT ( 'NONE',  ( 9.447334110624092673, 9.916311305349925220, -0.7998128361456281477 ) ) ;
#120948=CARTESIAN_POINT ( 'NONE',  ( 1.364683531249992088, 5.634375000341417916, 1.214306433183764966E-14 ) ) ;
#120954=CARTESIAN_POINT ( 'NONE',  ( -6.710922849084449915, 10.77323439066645783, 0.000000000000000000 ) ) ;
#120958=CARTESIAN_POINT ( 'NONE',  ( -1.364683531250012516, 4.051041667008088432, -0.7879004041258300672 ) ) ;
#120965=CARTESIAN_POINT ( 'NONE',  ( 1.364683531249988535, 4.655208333674755394, -0.7879004041258300672 ) ) ;
#120969=CARTESIAN_POINT ( 'NONE',  ( 4.351804119862229037, 4.179452349368450115, -0.7216878364870188411 ) ) ;
#120977=CARTESIAN_POINT ( 'NONE',  ( 0.6823417656249899377, 0.8427083336747520637, 1.181850606188755259 ) ) ;
#120978=CARTESIAN_POINT ( 'NONE',  ( -3.687454593236990430, 4.364747115940301292, 1.082531754730560403 ) ) ;
#120979=CARTESIAN_POINT ( 'NONE',  ( 5.229694566569264680, 7.124396299129368337, 1.599625672291267398 ) ) ;
#120982=CARTESIAN_POINT ( 'NONE',  ( 3.850152436600940753, 7.435668909435635854, -0.7216878364870309426 ) ) ;
#120984=CARTESIAN_POINT ( 'NONE',  ( -4.067937748088393590, 7.725456827083305278, 0.6547958487484796253 ) ) ;
#120985=CARTESIAN_POINT ( 'NONE',  ( 2.846849069189655967, 5.304779099821139710, -1.082531754730543083 ) ) ;
#120989=CARTESIAN_POINT ( 'NONE',  ( -7.158341918335454857, 10.33485409049125003, 1.082531754730549967 ) ) ;
#120994=CARTESIAN_POINT ( 'NONE',  ( -9.643927338022246332, 10.14567007064778004, -0.7998128361456291469 ) ) ;
#120995=CARTESIAN_POINT ( 'NONE',  ( -4.555176424067209240, 8.258196894812975586, 1.040834085586084257E-14 ) ) ;
#120996=CARTESIAN_POINT ( 'NONE',  ( -1.364683531250014514, 1.551041667008084435, -0.7879004041258289570 ) ) ;
#121010=ORIENTED_EDGE ( 'NONE', *, *, #19034, .F. ) ;
#121021=CARTESIAN_POINT ( 'NONE',  ( 0.6823417656249899377, 2.905208333674754062, 1.181850606188765695 ) ) ;
#121032=CARTESIAN_POINT ( 'NONE',  ( -1.364683531250012516, 1.530208333674756505, 0.7879004041258379498 ) ) ;
#121042=CARTESIAN_POINT ( 'NONE',  ( 6.030679399980265920, 5.930214142932100252, -0.7998128361456281477 ) ) ;
#121045=ORIENTED_EDGE ( 'NONE', *, *, #131446, .F. ) ;
#121048=CARTESIAN_POINT ( 'NONE',  ( 6.934105498385400246, 10.17720795050327354, -1.199719254218441611 ) ) ;
#121052=CARTESIAN_POINT ( 'NONE',  ( 8.772289083241844310, 10.19309100432570148, -1.199719254218446718 ) ) ;
#121064=CARTESIAN_POINT ( 'NONE',  ( -8.365017589951714072, 8.861534731139549592, 1.040834085586084257E-14 ) ) ;
#121068=CARTESIAN_POINT ( 'NONE',  ( -8.296699936558862731, 11.76690146170562201, 1.199719254218453823 ) ) ;
#121073=CARTESIAN_POINT ( 'NONE',  ( -2.625475302540713152, 6.214804952939456228, -0.7998128361456281477 ) ) ;
#121074=EDGE_CURVE ( 'NONE', #152353, #23324, #89226, .T. ) ;
#121076=CARTESIAN_POINT ( 'NONE',  ( 9.154780037725547714, 11.70366268214508487, 1.599625672291279388 ) ) ;
#121078=CARTESIAN_POINT ( 'NONE',  ( 2.842405760359353106, 6.467890487061221272, -0.7998128361456291469 ) ) ;
#121084=CARTESIAN_POINT ( 'NONE',  ( 4.528060117284240071, 5.345453560662148718, 1.082531754730560403 ) ) ;
#121086=CARTESIAN_POINT ( 'NONE',  ( -3.716906668440817185, 7.488141546489591072, 0.7998128361456341429 ) ) ;
#121087=FACE_OUTER_BOUND ( 'NONE', #73794, .T. ) ;
#121089=CARTESIAN_POINT ( 'NONE',  ( -9.646789991323334590, 11.21334206375407305, 1.199719254218462483 ) ) ;
#121095=CARTESIAN_POINT ( 'NONE',  ( 8.595506201384013778, 10.09080732544527592, 1.082531754730558626 ) ) ;
#121096=CARTESIAN_POINT ( 'NONE',  ( -0.6823417656249969321, 3.780208333674754506, -1.181850606188749264 ) ) ;
#121099=CARTESIAN_POINT ( 'NONE',  ( 2.998324526916512411, 6.649795714711241423, 0.000000000000000000 ) ) ;
#121112=ORIENTED_EDGE ( 'NONE', *, *, #179509, .F. ) ;
#121114=CARTESIAN_POINT ( 'NONE',  ( -1.364683531250012516, 3.051041667008083547, -0.7879004041258289570 ) ) ;
#121116=CARTESIAN_POINT ( 'NONE',  ( 2.218730694130720771, 5.740269576461138890, 0.7998128361456462443 ) ) ;
#121118=CARTESIAN_POINT ( 'NONE',  ( -7.063434843039784639, 7.343021526408956667, 1.040834085586084257E-14 ) ) ;
#121120=CARTESIAN_POINT ( 'NONE',  ( -2.535011536075371996, 5.133042487381361596, 2.420000000000010587 ) ) ;
#121121=CARTESIAN_POINT ( 'NONE',  ( -4.406036734316882253, 8.084200590104265061, -0.7216878364870257245 ) ) ;
#121125=CARTESIAN_POINT ( 'NONE',  ( 6.145923705696426431, 6.064665832934283962, 0.7998128361456341429 ) ) ;
#121136=ADVANCED_FACE ( 'NONE', ( #191875 ), #76011, .F. ) ;
#121137=CARTESIAN_POINT ( 'NONE',  ( 4.659198344590585350, 8.587481835331020719, 0.7998128361456462443 ) ) ;
#121140=CARTESIAN_POINT ( 'NONE',  ( -5.575427483717760424, 7.527751369135936343, 1.599625672291269396 ) ) ;
#121144=CARTESIAN_POINT ( 'NONE',  ( 7.884230021546724920, 9.157022099014721306, 1.199719254218462483 ) ) ;
#121147=CARTESIAN_POINT ( 'NONE',  ( -7.874588291438845644, 8.081441182967111558, -0.7998128361456291469 ) ) ;
#121148=CARTESIAN_POINT ( 'NONE',  ( 6.439759776366769550, 8.536139043893143707, 1.443375672974076540 ) ) ;
#121149=CARTESIAN_POINT ( 'NONE',  ( 4.901917485988815493, 6.882077164048857831, 1.422854466155202502 ) ) ;
#121150=CARTESIAN_POINT ( 'NONE',  ( -5.599681137644054729, 6.491715067794862293, 1.199719254218450271 ) ) ;
#121153=CARTESIAN_POINT ( 'NONE',  ( -5.900823170445743671, 7.907379670318584353, 1.599625672291269396 ) ) ;
#121156=CARTESIAN_POINT ( 'NONE',  ( 0.6823417656249899377, 2.092708333674753174, 1.181850606188767472 ) ) ;
#121158=CARTESIAN_POINT ( 'NONE',  ( -6.263503779833496488, 6.409768619334935913, 0.7216878364870317197 ) ) ;
#121163=CARTESIAN_POINT ( 'NONE',  ( 5.575427483717746213, 7.527751369135936343, 1.599625672291267398 ) ) ;
#121165=CARTESIAN_POINT ( 'NONE',  ( -5.660981573724272131, 6.153771497223376130, 0.8018600159674215133 ) ) ;
#121166=CARTESIAN_POINT ( 'NONE',  ( -0.6823417656250003738, 1.030208333674752286, -1.181850606188749264 ) ) ;
#121169=CARTESIAN_POINT ( 'NONE',  ( -1.402160292154681736E-14, -1.115624999658584082, 1.575800808251672791 ) ) ;
#121173=CARTESIAN_POINT ( 'NONE',  ( -3.086452525405351643, 6.752611712948207057, 0.7998128361456341429 ) ) ;
#121174=CARTESIAN_POINT ( 'NONE',  ( -6.507550544435101614, 10.53596670190887963, 0.000000000000000000 ) ) ;
#121182=CARTESIAN_POINT ( 'NONE',  ( -8.039621902779392926, 9.442275643739831636, 1.082531754730558626 ) ) ;
#121187=CARTESIAN_POINT ( 'NONE',  ( -6.182154857707119255, 10.15633840072622363, 0.000000000000000000 ) ) ;
#121194=CARTESIAN_POINT ( 'NONE',  ( 4.264789376140788235, 7.497597942732838305, -1.024658161349981444 ) ) ;
#121201=CARTESIAN_POINT ( 'NONE',  ( -7.019370843573183194, 9.212351955633947043, 1.599625672291283607 ) ) ;
#121204=EDGE_CURVE ( 'NONE', #207748, #20507, #73882, .T. ) ;
#121205=CARTESIAN_POINT ( 'NONE',  ( 5.345992642490140057, 5.131412925860272090, 1.040834085586084257E-14 ) ) ;
#121209=CARTESIAN_POINT ( 'NONE',  ( 6.681470773436232413, 6.689470745297396270, -0.7998128361456281477 ) ) ;
#121213=CARTESIAN_POINT ( 'NONE',  ( -5.924549939491850381, 6.014322472269677533, 0.000000000000000000 ) ) ;
#121223=CARTESIAN_POINT ( 'NONE',  ( -1.201851678989727383E-14, 1.321875000341419248, 1.575800808251672791 ) ) ;
#121225=CARTESIAN_POINT ( 'NONE',  ( -9.664264568442742842, 10.16939683947169115, -0.7998128361456291469 ) ) ;
#121227=CARTESIAN_POINT ( 'NONE',  ( 7.151035956204054855, 10.43029348462504124, 1.199719254218460707 ) ) ;
#121229=CARTESIAN_POINT ( 'NONE',  ( -7.283754839039664475, 9.520799950344851936, -1.599625672291263179 ) ) ;
#121232=CARTESIAN_POINT ( 'NONE',  ( -0.6823417656249969321, 4.467708333674755394, -1.181850606188749264 ) ) ;
#121234=CARTESIAN_POINT ( 'NONE',  ( 9.463228032658635769, 11.10314946193233965, -1.082531754730543083 ) ) ;
#121237=CARTESIAN_POINT ( 'NONE',  ( 1.364683531249986981, -1.053124999658580752, 0.000000000000000000 ) ) ;
#121240=CARTESIAN_POINT ( 'NONE',  ( 6.439759776366758892, 10.45687747249582955, 0.7216878364870438212 ) ) ;
#121243=CARTESIAN_POINT ( 'NONE',  ( -4.744990575102892905, 8.479646737687938085, 0.7216878364870458196 ) ) ;
#121245=CARTESIAN_POINT ( 'NONE',  ( 1.364683531249990311, 3.134375000341423245, 1.214306433183764966E-14 ) ) ;
#121249=CARTESIAN_POINT ( 'NONE',  ( -6.728924311084075960, 6.744833205886536120, 1.040834085586084257E-14 ) ) ;
#121250=CARTESIAN_POINT ( 'NONE',  ( -1.201851678989727383E-14, 5.509375000341415252, -1.575800808251660134 ) ) ;
#121257=CARTESIAN_POINT ( 'NONE',  ( -1.500000000000011324, 2.670833333333352044, 0.8660254037844403729 ) ) ;
#121260=CARTESIAN_POINT ( 'NONE',  ( -0.006768871532359390167, 8.210909518262125673, -2.038649385027042626 ) ) ;
#121263=CARTESIAN_POINT ( 'NONE',  ( 7.321039761699430493, 7.643560598178549270, -0.7216878364870257245 ) ) ;
#121264=CARTESIAN_POINT ( 'NONE',  ( -1.364683531250000748, -0.1781249996585798634, 0.000000000000000000 ) ) ;
#121270=CARTESIAN_POINT ( 'NONE',  ( -1.402160292154681736E-14, 0.3375000000000208389, -1.732050807568870754 ) ) ;
#121271=CARTESIAN_POINT ( 'NONE',  ( 6.751070424600909448, 9.963667031088037973, -1.199719254218441611 ) ) ;
#121272=CARTESIAN_POINT ( 'NONE',  ( -8.533967624797991647, 12.04371376465130439, -1.199719254218446718 ) ) ;
#121274=CARTESIAN_POINT ( 'NONE',  ( 0.6823417656249882723, 0.4260416670080896528, -1.181850606188749264 ) ) ;
#121275=CARTESIAN_POINT ( 'NONE',  ( -1.500000000000013101, 1.420833333333354043, 0.8660254037844403729 ) ) ;
#121277=CARTESIAN_POINT ( 'NONE',  ( 5.983225862332436584, 5.874851682342960402, 0.7998128361456341429 ) ) ;
#121283=CARTESIAN_POINT ( 'NONE',  ( 1.364683531249988535, 5.155208333674749177, -0.7879004041258300672 ) ) ;
#121286=CARTESIAN_POINT ( 'NONE',  ( -7.374745490829552885, 10.69128794168811680, -1.199719254218446718 ) ) ;
#121287=CARTESIAN_POINT ( 'NONE',  ( -4.229780737783618072, 6.918199379847403740, 1.082531754730560403 ) ) ;
#121295=EDGE_CURVE ( 'NONE', #153422, #56362, #186446, .T. ) ;
#121296=CARTESIAN_POINT ( 'NONE',  ( 6.753933077901968396, 11.03133902419432566, 0.7998128361456462443 ) ) ;
#121300=CARTESIAN_POINT ( 'NONE',  ( 6.426201622753093368, 10.44105962661321563, 1.040834085586084257E-14 ) ) ;
#121303=CARTESIAN_POINT ( 'NONE',  ( -6.496328159242330536, 10.73079995242472862, 0.000000000000000000 ) ) ;
#121304=CARTESIAN_POINT ( 'NONE',  ( 6.179819089730593795, 6.104210447640811665, 1.040834085586084257E-14 ) ) ;
#121308=CARTESIAN_POINT ( 'NONE',  ( 2.198393463710220264, 5.716542807637226886, 0.7998128361456462443 ) ) ;
#121315=CARTESIAN_POINT ( 'NONE',  ( -4.284013352238250860, 7.941839977679187257, -0.7216878364870267237 ) ) ;
#121316=CARTESIAN_POINT ( 'NONE',  ( 10.22248463502393001, 11.02857961705718282, 0.7216878364870438212 ) ) ;
#121319=CARTESIAN_POINT ( 'NONE',  ( -7.314787569772770226, 8.492672571945082183, -1.199719254218452935 ) ) ;
#121322=DIRECTION ( 'NONE',  ( 0.000000000000000000, -0.7999999999999973799, -0.6000000000000034195 ) ) ;
#121324=CARTESIAN_POINT ( 'NONE',  ( -6.482770005628665011, 10.71498210654212002, 0.7998128361456481317 ) ) ;
#121342=CARTESIAN_POINT ( 'NONE',  ( -7.314787569772770226, 8.492672571945082183, -1.199719254218452935 ) ) ;
#121345=CARTESIAN_POINT ( 'NONE',  ( 6.480434237652135998, 6.662854153456708950, 0.7216878364870317197 ) ) ;
#121349=CARTESIAN_POINT ( 'NONE',  ( -6.410307701162927252, 6.373113827645189744, -0.7998128361456291469 ) ) ;
#121352=CARTESIAN_POINT ( 'NONE',  ( 1.000000000000003553, 6.120000000000020535, 1.214306433183764966E-14 ) ) ;
#121353=CARTESIAN_POINT ( 'NONE',  ( -6.007394966791244961, 6.077829431809393945, -0.6506939885215150543 ) ) ;
#121354=CARTESIAN_POINT ( 'NONE',  ( -5.693534442735004752, 8.729875052244421951, 1.199719254218452047 ) ) ;
#121355=CARTESIAN_POINT ( 'NONE',  ( -5.854831387906667572, 6.034345315880532468, 0.4035957558334040685 ) ) ;
#121360=CARTESIAN_POINT ( 'NONE',  ( -8.154339323615371171, 11.60081407993821045, 1.199719254218453823 ) ) ;
#121361=CARTESIAN_POINT ( 'NONE',  ( 6.076025397218672630, 10.24044673006381245, -0.7998128361456291469 ) ) ;
#121364=CARTESIAN_POINT ( 'NONE',  ( -10.08065090696061716, 11.71951313199760136, -1.199719254218441611 ) ) ;
#121371=CARTESIAN_POINT ( 'NONE',  ( 8.866669273657322492, 12.32790267170016207, -1.082531754730543083 ) ) ;
#121378=CARTESIAN_POINT ( 'NONE',  ( -5.623048529261291506, 6.177845134385851367, -0.8520226256489031869 ) ) ;
#121379=EDGE_CURVE ( 'NONE', #44633, #65489, #133989, .T. ) ;
#121381=CARTESIAN_POINT ( 'NONE',  ( -0.3532385256851401367, 6.953154881905717843, -3.904206509207633680 ) ) ;
#121393=CARTESIAN_POINT ( 'NONE',  ( -4.973143418114339021, 4.696422164088486895, 0.7998128361456341429 ) ) ;
#121396=CARTESIAN_POINT ( 'NONE',  ( -4.783329267523015460, 4.474972321731942593, -0.7998128361456221525 ) ) ;
#121401=CARTESIAN_POINT ( 'NONE',  ( -0.7500000000000006661, -0.8604166659838472508, -1.299038105676652011 ) ) ;
#121406=ORIENTED_EDGE ( 'NONE', *, *, #211660, .F. ) ;
#121407=CARTESIAN_POINT ( 'NONE',  ( 1.468321960011987670, 7.242494692102993348, -4.289992922803929076 ) ) ;
#121409=CARTESIAN_POINT ( 'NONE',  ( 2.205172540517054802, 5.724451730578533848, 1.040834085586084257E-14 ) ) ;
#121411=DIRECTION ( 'NONE',  ( 0.000000000000000000, 0.000000000000000000, 1.000000000000000000 ) ) ;
#121414=CARTESIAN_POINT ( 'NONE',  ( 4.852928918687680948, 7.749168607522574526, 1.199719254218462483 ) ) ;
#121415=CARTESIAN_POINT ( 'NONE',  ( -1.364683531250012516, 2.842708333674754506, 0.7879004041258379498 ) ) ;
#121418=CARTESIAN_POINT ( 'NONE',  ( -8.727698198895085469, 11.20540053684285553, -1.599625672291263179 ) ) ;
#121420=CARTESIAN_POINT ( 'NONE',  ( -5.056828107772872727, 5.001980335264194721, -0.7216878364870197293 ) ) ;
#121423=CARTESIAN_POINT ( 'NONE',  ( -4.557512192488103686, 8.468847991211438497, -0.7998128361456281477 ) ) ;
#121425=CARTESIAN_POINT ( 'NONE',  ( -1.500000000000015099, -1.089583332650509773, -0.8660254037844383745 ) ) ;
#121434=CARTESIAN_POINT ( 'NONE',  ( -6.195713011320807873, 6.330679389403470303, -0.7216878364870267237 ) ) ;
#121440=CARTESIAN_POINT ( 'NONE',  ( -3.375617059678305054, 5.921675088724528635, 1.082531754730560403 ) ) ;
#121442=CARTESIAN_POINT ( 'NONE',  ( 9.694243528971124846, 11.26870452434320491, 1.199719254218450271 ) ) ;
#121448=VERTEX_POINT ( 'NONE', #4863 ) ;
#121452=FACE_OUTER_BOUND ( 'NONE', #187309, .T. ) ;
#121457=CARTESIAN_POINT ( 'NONE',  ( 4.984594031318565932, 8.967110136513669616, 0.7998128361456462443 ) ) ;
#121463=CARTESIAN_POINT ( 'NONE',  ( 4.891794496432329886, 4.601515088792824670, -0.7998128361456211532 ) ) ;
#121474=CARTESIAN_POINT ( 'NONE',  ( 7.584896871841365851, 10.93646455286856956, -1.199719254218446718 ) ) ;
#121475=CARTESIAN_POINT ( 'NONE',  ( -5.925076824372040640, 6.871343368977510302, 1.199719254218450271 ) ) ;
#121478=CARTESIAN_POINT ( 'NONE',  ( 4.702146809683721784, 5.356480858934594025, 2.420000000000010587 ) ) ;
#121481=CARTESIAN_POINT ( 'NONE',  ( 1.364683531249990311, 4.863541667008084879, 0.7879004041258500513 ) ) ;
#121485=CARTESIAN_POINT ( 'NONE',  ( -1.451998047843646500, 7.315968950353777700, -4.301760722578332086 ) ) ;
#121486=CARTESIAN_POINT ( 'NONE',  ( 3.680148631105580215, 6.380924938676771241, -1.199719254218446718 ) ) ;
#121487=CARTESIAN_POINT ( 'NONE',  ( -5.935772324684618795, 5.819489221753827657, 0.000000000000000000 ) ) ;
#121493=CARTESIAN_POINT ( 'NONE',  ( 5.612712406377503349, 8.531619659873665995, -1.082531754730543083 ) ) ;
#121495=CARTESIAN_POINT ( 'NONE',  ( 7.171900071504736296, 9.390302721554109056, -1.443375672974058777 ) ) ;
#121496=CARTESIAN_POINT ( 'NONE',  ( -1.201851678989727383E-14, 3.509375000341421469, -1.575800808251660134 ) ) ;
#121498=CARTESIAN_POINT ( 'NONE',  ( 3.823036128929238942, 7.404033217152015567, 1.040834085586084257E-14 ) ) ;
#121505=CARTESIAN_POINT ( 'NONE',  ( -4.127447729399665199, 7.650344214561823009, 0.8192481249636590634 ) ) ;
#121513=CARTESIAN_POINT ( 'NONE',  ( -8.696665468161981494, 12.23352791524263239, -1.199719254218446718 ) ) ;
#121525=CARTESIAN_POINT ( 'NONE',  ( 2.223174002961016082, 5.537527403522402025, -0.7216878364870267237 ) ) ;
#121526=CARTESIAN_POINT ( 'NONE',  ( 0.6823417656249899377, 3.988541667008085767, -1.181850606188754593 ) ) ;
#121528=CARTESIAN_POINT ( 'NONE',  ( 6.317209508963599340, 9.457495962844502557, 1.199719254218462483 ) ) ;
#121530=CARTESIAN_POINT ( 'NONE',  ( -10.10098813738111545, 11.74323990082152491, -1.199719254218441611 ) ) ;
#121532=CARTESIAN_POINT ( 'NONE',  ( -5.278201874421822204, 5.052323696447222900, 0.7998128361456341429 ) ) ;
#121536=CARTESIAN_POINT ( 'NONE',  ( -0.7500000000000215383, 4.691666666666684193, 1.299038105676671107 ) ) ;
#121537=CARTESIAN_POINT ( 'NONE',  ( 5.443762371086860341, 6.309809840144842141, 1.199719254218462483 ) ) ;
#121540=CARTESIAN_POINT ( 'NONE',  ( -1.201851678989727383E-14, 4.071875000341425022, 1.575800808251672791 ) ) ;
#121543=CARTESIAN_POINT ( 'NONE',  ( 9.002250809793993724, 11.52571191622492464, -1.443375672974057666 ) ) ;
#121548=CARTESIAN_POINT ( 'NONE',  ( -1.201851678989727383E-14, 1.993750000682816381, 1.732050807568877637 ) ) ;
#121550=CARTESIAN_POINT ( 'NONE',  ( -5.259673527097670664, 8.223703984000886535, -1.199719254218446718 ) ) ;
#121551=CARTESIAN_POINT ( 'NONE',  ( 4.270455198180219902, 6.965652916976816655, -1.082531754730548412 ) ) ;
#121559=CARTESIAN_POINT ( 'NONE',  ( 7.416473721875251890, 8.611306416064660851, 1.199719254218462483 ) ) ;
#121560=CARTESIAN_POINT ( 'NONE',  ( 3.486418057008484617, 7.219238166485217434, 1.040834085586084257E-14 ) ) ;
#121561=DIRECTION ( 'NONE',  ( 1.000000000000000000, -7.387867266669436732E-31, 0.000000000000000000 ) ) ;
#121564=CARTESIAN_POINT ( 'NONE',  ( 5.168682875307768931, 7.053215992657626110, -1.599625672291256295 ) ) ;
#121565=CARTESIAN_POINT ( 'NONE',  ( 3.469446951953614189E-15, 8.900000000000019895, 1.214306433183764966E-14 ) ) ;
#121566=ORIENTED_EDGE ( 'NONE', *, *, #121295, .F. ) ;
#121571=CARTESIAN_POINT ( 'NONE',  ( 9.901532256681887745, 10.44620914241737530, 0.000000000000000000 ) ) ;
#121575=CARTESIAN_POINT ( 'NONE',  ( 3.469446951953614189E-15, 5.290451655907108197, 1.214306433183764966E-14 ) ) ;
#121576=CARTESIAN_POINT ( 'NONE',  ( 5.490683550995299811, 6.230756917952954055, 0.9772120879164881702 ) ) ;
#121584=CARTESIAN_POINT ( 'NONE',  ( 6.968527767744098433, 9.153035033833367251, 1.443375672974076540 ) ) ;
#121585=CARTESIAN_POINT ( 'NONE',  ( -2.740719608256871442, 6.349256642941639051, 0.7998128361456341429 ) ) ;
#121590=CARTESIAN_POINT ( 'NONE',  ( -5.148345644887285744, 7.029489223833707001, -1.599625672291256295 ) ) ;
#121597=CARTESIAN_POINT ( 'NONE',  ( -4.038971567461725698, 3.986455684509185193, -0.5169845646830102392 ) ) ;
#121603=CARTESIAN_POINT ( 'NONE',  ( 9.921869487102386032, 10.46993591124128997, 0.000000000000000000 ) ) ;
#121606=VERTEX_POINT ( 'NONE', #89016 ) ;
#121614=CARTESIAN_POINT ( 'NONE',  ( -9.653042183249970876, 11.32459930428888306, -1.082531754730539753 ) ) ;
#121618=CARTESIAN_POINT ( 'NONE',  ( 9.399880572976245574, 9.860948844760784482, 0.7998128361456462443 ) ) ;
#121620=CARTESIAN_POINT ( 'NONE',  ( -0.7158994178059416846, 2.800000000000024691, 1.161830092591057184 ) ) ;
#121623=CARTESIAN_POINT ( 'NONE',  ( -6.470265622219711688, 8.571729197388226140, -1.599625672291263179 ) ) ;
#121624=CARTESIAN_POINT ( 'NONE',  ( 3.822509244049070887, 6.547012320444182798, -1.199719254218452047 ) ) ;
#121627=CARTESIAN_POINT ( 'NONE',  ( 8.703444544968814256, 12.24143683818393313, -1.199719254218446718 ) ) ;
#121628=CARTESIAN_POINT ( 'NONE',  ( -2.318081078256692518, 5.648252324700675508, 1.040834085586084257E-14 ) ) ;
#121631=CARTESIAN_POINT ( 'NONE',  ( 0.6823417656249899377, 3.155208333674754062, 1.181850606188765695 ) ) ;
#121633=CARTESIAN_POINT ( 'NONE',  ( 5.341549334104176872, 9.175631956522799726, 0.7216878364870438212 ) ) ;
#121642=CARTESIAN_POINT ( 'NONE',  ( 7.361714222096048310, 10.57212177821199184, -1.082531754730537976 ) ) ;
#121647=CARTESIAN_POINT ( 'NONE',  ( -9.501566725078754772, 9.979582688880366703, -0.7998128361456291469 ) ) ;
#121656=CARTESIAN_POINT ( 'NONE',  ( 4.487912541323413329, 5.194651705420806564, 1.199719254218462483 ) ) ;
#121661=CARTESIAN_POINT ( 'NONE',  ( 4.123651276850781144, 7.962676922967908411, -0.7998128361456221525 ) ) ;
#121665=CARTESIAN_POINT ( 'NONE',  ( -1.500000000000011324, 3.202083334016150307, 0.8660254037844403729 ) ) ;
#121672=CARTESIAN_POINT ( 'NONE',  ( 0.7499999999999885647, 0.9833333333333569293, 1.299038105676657340 ) ) ;
#121673=CARTESIAN_POINT ( 'NONE',  ( 6.588372581236919601, 9.773852880496709972, -1.199719254218440723 ) ) ;
#121674=CARTESIAN_POINT ( 'NONE',  ( 4.758548728272192108, 7.535095368750792666, -1.082531754730549078 ) ) ;
#121678=CARTESIAN_POINT ( 'NONE',  ( 8.405692050792682224, 12.75046512599275772, -0.7216878364870328300 ) ) ;
#121683=CARTESIAN_POINT ( 'NONE',  ( -4.882907879216086933, 8.848476292394087395, -0.7998128361456281477 ) ) ;
#121684=CARTESIAN_POINT ( 'NONE',  ( 1.499999999999989120, 2.806250000682818158, 1.214306433183764966E-14 ) ) ;
#121685=CARTESIAN_POINT ( 'NONE',  ( -1.001543065824772872E-14, 5.634375000341415252, 1.575800808251672791 ) ) ;
#121690=CARTESIAN_POINT ( 'NONE',  ( -1.364683531250010295, 3.842708333674751398, 0.7879004041258379498 ) ) ;
#121700=CARTESIAN_POINT ( 'NONE',  ( -8.097244055859620815, 10.46987070330147063, -1.599625672291263179 ) ) ;
#121701=CARTESIAN_POINT ( 'NONE',  ( 4.632082037363250748, 8.555846143565791095, -0.7998128361456231517 ) ) ;
#121711=CARTESIAN_POINT ( 'NONE',  ( -5.859094939400033120, 9.987361195942037639, -0.7998128361456231517 ) ) ;
#121716=CARTESIAN_POINT ( 'NONE',  ( 4.376584659113025744, 4.000436945253625254, 0.7998128361456341429 ) ) ;
#121718=CARTESIAN_POINT ( 'NONE',  ( -4.120788623549732854, 6.895004929861607401, -1.199719254218452047 ) ) ;
#121719=CARTESIAN_POINT ( 'NONE',  ( -9.996439331977562404, 10.55693406359564790, 0.7998128361456462443 ) ) ;
#121722=CARTESIAN_POINT ( 'NONE',  ( -4.201979666139121328, 7.560802217138083314, -0.9697280773930611053 ) ) ;
#121723=CARTESIAN_POINT ( 'NONE',  ( -0.6823417656250003738, -0.2822916663252489355, -1.181850606188749264 ) ) ;
#121729=CARTESIAN_POINT ( 'NONE',  ( 4.957477724091233995, 8.935474444748447098, -0.7998128361456281477 ) ) ;
#121731=CARTESIAN_POINT ( 'NONE',  ( 6.471393748265543699, 5.229711127717882491, 2.500000000000011102 ) ) ;
#121748=ORIENTED_EDGE ( 'NONE', *, *, #16332, .F. ) ;
#121750=CARTESIAN_POINT ( 'NONE',  ( -9.158696461231359720, 10.64389961198009615, 1.199719254218462483 ) ) ;
#121756=CARTESIAN_POINT ( 'NONE',  ( 1.499999999999987121, 1.077083334016148308, -0.8660254037844253849 ) ) ;
#121762=CARTESIAN_POINT ( 'NONE',  ( -8.143643823302737061, 12.65266822716189843, 0.000000000000000000 ) ) ;
#121764=CARTESIAN_POINT ( 'NONE',  ( -0.6823417656250003738, 0.2177083336747515085, -1.181850606188749264 ) ) ;
#121769=CARTESIAN_POINT ( 'NONE',  ( -4.660252114795309097, 6.460046772059735432, -1.599625672291256295 ) ) ;
#121774=CARTESIAN_POINT ( 'NONE',  ( 1.364683531249988757, 0.1968750003414204697, 0.000000000000000000 ) ) ;
#121776=EDGE_CURVE ( 'NONE', #21552, #54906, #174834, .T. ) ;
#121781=CARTESIAN_POINT ( 'NONE',  ( -1.364683531250012516, 0.5302083336747518416, 0.7879004041258379498 ) ) ;
#121783=CARTESIAN_POINT ( 'NONE',  ( -8.199983978166823562, 8.461069484149769337, -0.7998128361456291469 ) ) ;
#121784=CARTESIAN_POINT ( 'NONE',  ( 7.879259827836241570, 12.34422023245099176, 1.040834085586084257E-14 ) ) ;
#121785=CARTESIAN_POINT ( 'NONE',  ( 6.017121246366603060, 5.914396297049491658, 1.040834085586084257E-14 ) ) ;
#121788=CARTESIAN_POINT ( 'NONE',  ( 1.364683531249986537, 0.9677083336747538400, -0.7879004041258239610 ) ) ;
#121794=CARTESIAN_POINT ( 'NONE',  ( 6.995644074971448134, 7.263932296995902149, -0.7216878364870257245 ) ) ;
#121797=CARTESIAN_POINT ( 'NONE',  ( -7.552055258011950656, 8.769484874890757453, 1.199719254218462483 ) ) ;
#121798=CARTESIAN_POINT ( 'NONE',  ( -3.253066792275140173, 5.882662793374543675, 1.199719254218462483 ) ) ;
#121799=CARTESIAN_POINT ( 'NONE',  ( -4.303094902415906198, 7.389312076987425648, -1.073240500945132236 ) ) ;
#121802=CARTESIAN_POINT ( 'NONE',  ( -2.415323921528888196, 5.969628341758991930, 0.7998128361456341429 ) ) ;
#121803=CARTESIAN_POINT ( 'NONE',  ( 4.812781342726855982, 7.598366752281232372, 1.082531754730558626 ) ) ;
#121804=CARTESIAN_POINT ( 'NONE',  ( -6.982085920913410071, 11.08959130780024260, 0.7216878364870458196 ) ) ;
#121806=CARTESIAN_POINT ( 'NONE',  ( -1.201851678989727383E-14, 4.087500000000022560, -1.732050807568863648 ) ) ;
#121810=CARTESIAN_POINT ( 'NONE',  ( 8.676855123066012254, 11.14608361504227574, -1.443375672974052559 ) ) ;
#121822=CARTESIAN_POINT ( 'NONE',  ( 6.900736999231407154, 10.99468423250458038, -0.7216878364870267237 ) ) ;
#121823=CARTESIAN_POINT ( 'NONE',  ( 8.586391356156291010, 8.911878091804165791, 0.7998128361456481317 ) ) ;
#121824=CARTESIAN_POINT ( 'NONE',  ( -6.368579470117215813, 8.453095353268645695, 1.599625672291283607 ) ) ;
#121827=CARTESIAN_POINT ( 'NONE',  ( -4.151992249809804747, 3.976174039945850502, -0.5918415319043066614 ) ) ;
#121828=CARTESIAN_POINT ( 'NONE',  ( -0.6823417656250246877, -0.8864583329919115684, 1.181850606188755259 ) ) ;
#121829=CARTESIAN_POINT ( 'NONE',  ( 4.202664430556254160, 5.926194473780837413, 1.443375672974062551 ) ) ;
#121830=EDGE_LOOP ( 'NONE', ( #52145, #190896, #11096, #98306 ) ) ;
#121831=CARTESIAN_POINT ( 'NONE',  ( -6.710922849084449915, 10.77323439066645783, 0.000000000000000000 ) ) ;
#121840=VERTEX_POINT ( 'NONE', #211261 ) ;
#121847=CARTESIAN_POINT ( 'NONE',  ( 7.741869408603235136, 8.990934717247309749, 1.199719254218462483 ) ) ;
#121859=CARTESIAN_POINT ( 'NONE',  ( -7.088215381846223906, 7.164006121775713609, 0.7998128361456341429 ) ) ;
#121861=CARTESIAN_POINT ( 'NONE',  ( -3.716906668440817185, 7.488141546489591072, 0.7998128361456341429 ) ) ;
#121865=CARTESIAN_POINT ( 'NONE',  ( 1.419999999999990603, 6.216000000000041048, 2.921333333333336668 ) ) ;
#121871=CARTESIAN_POINT ( 'NONE',  ( -4.548924232584923288, 5.265832011892554121, -1.199719254218446718 ) ) ;
#121874=CARTESIAN_POINT ( 'NONE',  ( 7.786460292950004636, 7.978625184730144149, 1.040834085586084257E-14 ) ) ;
#121877=CARTESIAN_POINT ( 'NONE',  ( 5.904500254309781759, 6.149185751451256898, 0.8064407133735688182 ) ) ;
#121883=CARTESIAN_POINT ( 'NONE',  ( 6.466876083594112146, 6.647036307055676829, -0.7216878364870257245 ) ) ;
#121884=CARTESIAN_POINT ( 'NONE',  ( -8.355902744723985975, 8.642974711799791265, 1.040834085586084257E-14 ) ) ;
#121887=CARTESIAN_POINT ( 'NONE',  ( -9.345647958521597687, 9.797677461230342999, 0.7998128361456462443 ) ) ;
#121888=CARTESIAN_POINT ( 'NONE',  ( -4.564291269294938225, 8.476756914152748124, 1.040834085586084257E-14 ) ) ;
#121893=CARTESIAN_POINT ( 'NONE',  ( -1.499999999999997780, 3.431250000682818602, 1.214306433183764966E-14 ) ) ;
#121897=CARTESIAN_POINT ( 'NONE',  ( 6.577677080924314801, 10.82570702772039262, 1.040834085586084257E-14 ) ) ;
#121912=CARTESIAN_POINT ( 'NONE',  ( -0.7500000000000215383, 4.191666666666690411, 1.299038105676671107 ) ) ;
#121913=CARTESIAN_POINT ( 'NONE',  ( 3.486418057008484617, 7.219238166485217434, 1.040834085586084257E-14 ) ) ;
#121914=CARTESIAN_POINT ( 'NONE',  ( 6.817052309572890323, 6.847649204123507083, 0.7998128361456341429 ) ) ;
#121916=CARTESIAN_POINT ( 'NONE',  ( -9.015808963407680565, 9.620791333504852716, 1.040834085586084257E-14 ) ) ;
#121918=CARTESIAN_POINT ( 'NONE',  ( 6.480434237652124452, 8.583592582059388576, 1.443375672974076540 ) ) ;
#121919=CARTESIAN_POINT ( 'NONE',  ( -7.483737604619046913, 11.67485160545682987, 0.000000000000000000 ) ) ;
#121922=ORIENTED_EDGE ( 'NONE', *, *, #66705, .T. ) ;
#121924=CARTESIAN_POINT ( 'NONE',  ( 8.535021395002688749, 9.916278701380017324, 1.199719254218462483 ) ) ;
#121928=CARTESIAN_POINT ( 'NONE',  ( -2.300042508418743914, 5.503185706334628335, -0.7429425145402666075 ) ) ;
#121929=CARTESIAN_POINT ( 'NONE',  ( 0.6823417656249899377, 2.592708333674753618, 1.181850606188767472 ) ) ;
#121935=CARTESIAN_POINT ( 'NONE',  ( 9.284636267260101050, 9.726497154758602548, -0.7998128361456281477 ) ) ;
#121939=CARTESIAN_POINT ( 'NONE',  ( -9.317477881089553549, 11.89347683273641820, 1.599625672291281386 ) ) ;
#121945=CARTESIAN_POINT ( 'NONE',  ( 4.390142812726693045, 4.016254791136236513, 1.214306433183764966E-14 ) ) ;
#121948=CARTESIAN_POINT ( 'NONE',  ( -9.677822722056413696, 10.18521468535430685, 1.040834085586084257E-14 ) ) ;
#121951=CARTESIAN_POINT ( 'NONE',  ( 9.368847842243145152, 10.88907622316056312, 1.199719254218453823 ) ) ;
#121953=CARTESIAN_POINT ( 'NONE',  ( 5.335014106237911946, 6.336523053015567619, 1.100733037772538170 ) ) ;
#121955=CARTESIAN_POINT ( 'NONE',  ( -4.765854690403601879, 5.518917546014321829, 1.199719254218462483 ) ) ;
#121959=CARTESIAN_POINT ( 'NONE',  ( 7.426115451983150706, 9.686887332112256388, -1.599625672291262513 ) ) ;
#121961=CARTESIAN_POINT ( 'NONE',  ( 7.786460292950004636, 7.978625184730144149, 1.040834085586084257E-14 ) ) ;
#121964=CARTESIAN_POINT ( 'NONE',  ( -7.361714222540411967, 11.53249099303175385, 0.000000000000000000 ) ) ;
#121975=CARTESIAN_POINT ( 'NONE',  ( -4.610256348478378285, 6.944848931137240555, -1.199160056556654697 ) ) ;
#121977=CARTESIAN_POINT ( 'NONE',  ( 6.399085315970131305, 8.488685506763726352, -1.443375672974057666 ) ) ;
#121999=CARTESIAN_POINT ( 'NONE',  ( 6.611572464958476836, 10.86525164242692298, 0.7998128361456462443 ) ) ;
#122003=CARTESIAN_POINT ( 'NONE',  ( -1.500000000000013101, 2.202083334016153859, 0.8660254037844403729 ) ) ;
#122004=CARTESIAN_POINT ( 'NONE',  ( -3.810004860640155311, 4.403759411290286252, 1.199719254218462483 ) ) ;
#122005=CARTESIAN_POINT ( 'NONE',  ( -7.542413527904030524, 7.693903958843159252, 1.040834085586084257E-14 ) ) ;
#122008=CARTESIAN_POINT ( 'NONE',  ( -10.08065090696061716, 11.71951313199760136, -1.199719254218441611 ) ) ;
#122012=CARTESIAN_POINT ( 'NONE',  ( 6.449928391799196525, 8.548002428564306143, -1.599625672291262513 ) ) ;
#122015=CARTESIAN_POINT ( 'NONE',  ( -7.901704598666176693, 8.113076874732334076, 0.7998128361456602331 ) ) ;
#122017=CARTESIAN_POINT ( 'NONE',  ( 1.364683531249988535, 4.905208333674756283, -0.7879004041258300672 ) ) ;
#122022=B_SPLINE_CURVE_WITH_KNOTS ( 'NONE', 3,
 ( #99502, #196989, #133098, #82165, #146141, #78968, #96321, #162375, #214259, #179688 ),
 .UNSPECIFIED., .F., .F.,
 ( 4, 3, 3, 4 ),
 ( 0.000000000000000000, 8.736270215687113379E-05, 0.0001565438449761693651, 0.0002258025094466979254 ),
 .UNSPECIFIED. ) ;
#122024=CARTESIAN_POINT ( 'NONE',  ( -8.703971430293361067, 9.256980878204810637, 0.7216878364870438212 ) ) ;
#122028=CARTESIAN_POINT ( 'NONE',  ( 1.364683531249988535, 4.717708333674756283, -0.7879004041258300672 ) ) ;
#122029=ADVANCED_FACE ( 'NONE', ( #51977, #152664, #86598 ), #184087, .T. ) ;
#122035=CARTESIAN_POINT ( 'NONE',  ( -1.201851678989727383E-14, 3.946875000341423689, -1.575800808251660134 ) ) ;
#122040=CARTESIAN_POINT ( 'NONE',  ( 3.592547517496925913, 5.214391408544949869, -1.443375672974058777 ) ) ;
#122041=CARTESIAN_POINT ( 'NONE',  ( -0.6823417656249969321, 5.280208333674756283, -1.181850606188749264 ) ) ;
#122046=CARTESIAN_POINT ( 'NONE',  ( 0.6823417656249899377, 1.342708333674752508, 1.181850606188755259 ) ) ;
#122047=CARTESIAN_POINT ( 'NONE',  ( -4.772106882330247046, 4.669805572247793357, -0.7216878364870207285 ) ) ;
#122048=CARTESIAN_POINT ( 'NONE',  ( 3.811813743736467419, 7.598866467667865443, 1.040834085586084257E-14 ) ) ;
#122054=CARTESIAN_POINT ( 'NONE',  ( 3.063779527008311021, 5.557864633942907417, 1.082531754730546636 ) ) ;
#122057=CARTESIAN_POINT ( 'NONE',  ( -6.697364695470783502, 10.75741654478384035, 0.7216878364870458196 ) ) ;
#122062=CARTESIAN_POINT ( 'NONE',  ( -7.947050595904583403, 12.42330946186405249, 0.7998128361456481317 ) ) ;
#122063=CARTESIAN_POINT ( 'NONE',  ( -4.406036734316882253, 8.084200590104265061, -0.7216878364870257245 ) ) ;
#122065=CARTESIAN_POINT ( 'NONE',  ( 1.364683531249988535, 2.426041667008088432, 0.7879004041258500513 ) ) ;
#122074=CARTESIAN_POINT ( 'NONE',  ( 10.07387183015377197, 11.71160420905630062, -1.199719254218440723 ) ) ;
#122081=EDGE_LOOP ( 'NONE', ( #29307, #145433, #2496, #192979 ) ) ;
#122087=CARTESIAN_POINT ( 'NONE',  ( -3.277320446201389181, 4.846626492033466072, 1.599625672291267398 ) ) ;
#122089=CARTESIAN_POINT ( 'NONE',  ( -3.939498435241230556, 2.812004590916141744, 0.7750000000000135669 ) ) ;
#122090=CARTESIAN_POINT ( 'NONE',  ( 0.6823417656249899377, 3.155208333674754062, 1.181850606188765695 ) ) ;
#122099=CARTESIAN_POINT ( 'NONE',  ( 0.6823417656249882723, 0.6760416670080898749, -1.181850606188749264 ) ) ;
#122105=ORIENTED_EDGE ( 'NONE', *, *, #137465, .F. ) ;
#122109=CARTESIAN_POINT ( 'NONE',  ( 4.924636110261782385, 6.768494766770632332, 1.599625672291267398 ) ) ;
#122117=CARTESIAN_POINT ( 'NONE',  ( 7.096803341749390981, 10.36702210109460154, -1.199719254218441611 ) ) ;
#122121=CARTESIAN_POINT ( 'NONE',  ( 9.094822116668764167, 9.505047312402055582, 0.7998128361456462443 ) ) ;
#122133=CARTESIAN_POINT ( 'NONE',  ( -7.619319141200077361, 9.912291636198670375, 1.443375672974090751 ) ) ;
#122137=CARTESIAN_POINT ( 'NONE',  ( -9.215791728987058562, 11.77484298861683598, -1.599625672291263179 ) ) ;
#122141=CARTESIAN_POINT ( 'NONE',  ( -3.574546055497324737, 7.322054164722185732, 0.7998128361456341429 ) ) ;
#122143=CARTESIAN_POINT ( 'NONE',  ( 8.224992744984721327, 12.74757530245756243, 1.040834085586084257E-14 ) ) ;
#122145=CARTESIAN_POINT ( 'NONE',  ( 3.845709127770629010, 7.638411082374393146, 0.7998128361456321445 ) ) ;
#122147=ORIENTED_EDGE ( 'NONE', *, *, #160202, .T. ) ;
#122151=CARTESIAN_POINT ( 'NONE',  ( 3.199361063144961825, 6.676412307070352270, -0.7216878364870267237 ) ) ;
#122153=CARTESIAN_POINT ( 'NONE',  ( -4.543954038874438162, 8.453030145328826350, 1.040834085586084257E-14 ) ) ;
#122156=CARTESIAN_POINT ( 'NONE',  ( -9.215791728987058562, 11.77484298861683598, -1.599625672291263179 ) ) ;
#122163=CARTESIAN_POINT ( 'NONE',  ( 7.104109303880752790, 11.23195192126214970, -0.7216878364870267237 ) ) ;
#122165=CARTESIAN_POINT ( 'NONE',  ( -1.201851678989727383E-14, 4.259375000341417028, -1.575800808251660134 ) ) ;
#122168=CARTESIAN_POINT ( 'NONE',  ( 5.495132332240461714, 5.305409230568988832, 0.7998128361456341429 ) ) ;
#122183=CARTESIAN_POINT ( 'NONE',  ( -1.364683531250012516, 2.551041667008089320, -0.7879004041258289570 ) ) ;
#122185=CARTESIAN_POINT ( 'NONE',  ( 10.53876547652418338, 11.18964789890005918, 0.7998128361456462443 ) ) ;
#122187=CARTESIAN_POINT ( 'NONE',  ( -4.758548728716557541, 8.495464583570553785, 1.040834085586084257E-14 ) ) ;
#122188=CARTESIAN_POINT ( 'NONE',  ( 3.958617665510264949, 5.641473247893851628, -1.443375672974051449 ) ) ;
#122190=CARTESIAN_POINT ( 'NONE',  ( -4.894130264408862452, 7.693273827576896373, -1.082531754730548412 ) ) ;
#122196=CARTESIAN_POINT ( 'NONE',  ( 3.825371897350130723, 7.614684313550482031, 0.7998128361456321445 ) ) ;
#122206=CARTESIAN_POINT ( 'NONE',  ( 6.830610463186557624, 6.863467050006115677, 1.040834085586084257E-14 ) ) ;
#122209=FACE_OUTER_BOUND ( 'NONE', #213508, .T. ) ;
#122211=CARTESIAN_POINT ( 'NONE',  ( -7.335124800193271177, 8.516399340768996851, -1.199719254218452935 ) ) ;
#122215=CARTESIAN_POINT ( 'NONE',  ( 6.428537391173986038, 10.65171072301167854, 0.7998128361456462443 ) ) ;
#122218=CARTESIAN_POINT ( 'NONE',  ( -7.400052914960538963, 7.527816577075747695, 1.040834085586084257E-14 ) ) ;
#122219=CARTESIAN_POINT ( 'NONE',  ( 5.138177029454829459, 8.938364267765221527, 0.7216878364870438212 ) ) ;
#122220=CARTESIAN_POINT ( 'NONE',  ( 4.197832665289490173, 7.575126408543901846, 0.9117821302269245587 ) ) ;
#122222=CARTESIAN_POINT ( 'NONE',  ( -5.111587607552082524, 5.922272616020886282, 1.199719254218450271 ) ) ;
#122225=CARTESIAN_POINT ( 'NONE',  ( -6.196239896645333367, 7.187700286629718605, -1.199719254218446718 ) ) ;
#122230=CARTESIAN_POINT ( 'NONE',  ( 0.6823417656249899377, 2.342708333674753618, 1.181850606188767472 ) ) ;
#122232=CARTESIAN_POINT ( 'NONE',  ( -7.049876689426121779, 7.327203680526343632, -0.7216878364870278340 ) ) ;
#122233=ORIENTED_EDGE ( 'NONE', *, *, #210306, .T. ) ;
#122238=CARTESIAN_POINT ( 'NONE',  ( 4.821896187954575197, 8.777295985922343391, 0.7998128361456462443 ) ) ;
#122241=CARTESIAN_POINT ( 'NONE',  ( -5.892944143475336460, 6.011535633345318708, 0.2346759862181871381 ) ) ;
#122242=CARTESIAN_POINT ( 'NONE',  ( 0.6823417656249899377, 1.905208333674752952, 1.181850606188755259 ) ) ;
#122247=CARTESIAN_POINT ( 'NONE',  ( -3.249150368769345043, 6.942425863539538611, 0.7998128361456341429 ) ) ;
#122248=CARTESIAN_POINT ( 'NONE',  ( -8.310784975052685652, 9.758632561392040827, -1.082531754730543083 ) ) ;
#122256=CARTESIAN_POINT ( 'NONE',  ( -8.798878505144665851, 9.367705798864669475, -0.7216878364870267237 ) ) ;
#122262=CARTESIAN_POINT ( 'NONE',  ( -8.161645285302366659, 8.624267042381978499, 1.040834085586084257E-14 ) ) ;
#122269=CARTESIAN_POINT ( 'NONE',  ( -1.500000000000011324, 5.160416667349487341, -0.8660254037844313801 ) ) ;
#122276=CARTESIAN_POINT ( 'NONE',  ( -6.449928391799210736, 8.548002428564306143, -1.599625672291263179 ) ) ;
#122279=CARTESIAN_POINT ( 'NONE',  ( 5.495132332240461714, 5.305409230568988832, 0.7998128361456341429 ) ) ;
#122283=CARTESIAN_POINT ( 'NONE',  ( 5.524057522564145728, 8.532151978711786100, 1.199719254218462483 ) ) ;
#122289=CARTESIAN_POINT ( 'NONE',  ( -5.287316719649550301, 5.270883715786984780, 0.7216878364870317197 ) ) ;
#122300=CARTESIAN_POINT ( 'NONE',  ( 1.364683531249988757, 0.3843750003414206362, 0.000000000000000000 ) ) ;
#122302=CARTESIAN_POINT ( 'NONE',  ( -7.018317073368468328, 11.33978701890523233, -0.7998128361456291469 ) ) ;
#122304=CARTESIAN_POINT ( 'NONE',  ( 6.909851844459134362, 11.21324425184434936, -0.7998128361456291469 ) ) ;
#122306=CARTESIAN_POINT ( 'NONE',  ( -7.178152263431422320, 10.46192917639026554, 1.199719254218453823 ) ) ;
#122309=CARTESIAN_POINT ( 'NONE',  ( -1.364683531250012516, 4.738541667008091096, -0.7879004041258300672 ) ) ;
#122310=EDGE_CURVE ( 'NONE', #145502, #188383, #6301, .T. ) ;
#122312=CARTESIAN_POINT ( 'NONE',  ( 8.080296364064698977, 12.37083682481011060, -0.7216878364870328300 ) ) ;
#122315=CARTESIAN_POINT ( 'NONE',  ( -1.402160292154681736E-14, -0.3656249996585805295, 1.575800808251672791 ) ) ;
#122318=CARTESIAN_POINT ( 'NONE',  ( 7.917598520256366790, 8.339545816494993602, 1.040834085586084257E-14 ) ) ;
#122320=CARTESIAN_POINT ( 'NONE',  ( 1.608462485350599769, 8.735270501766756013, 2.463594439587641904 ) ) ;
#122321=CARTESIAN_POINT ( 'NONE',  ( -4.772106882330227506, 7.550913215151819458, -1.082531754730549967 ) ) ;
#122323=CARTESIAN_POINT ( 'NONE',  ( -0.6823417656250212460, 3.801041667008085767, 1.181850606188767472 ) ) ;
#122327=CARTESIAN_POINT ( 'NONE',  ( -6.718228810771495141, 7.796687353110217877, 1.199719254218450271 ) ) ;
#122334=CARTESIAN_POINT ( 'NONE',  ( 8.178592977541601527, 10.56477777859713463, 1.599625672291281386 ) ) ;
#122343=CARTESIAN_POINT ( 'NONE',  ( 5.477130870240836558, 9.333810415348903433, -0.7216878364870267237 ) ) ;
#122344=CARTESIAN_POINT ( 'NONE',  ( 1.364683531249986537, -0.3239583329919163424, 0.7879004041258500513 ) ) ;
#122351=CARTESIAN_POINT ( 'NONE',  ( 7.670162217029129259, 9.971608557999250166, 1.599625672291281386 ) ) ;
#122352=CARTESIAN_POINT ( 'NONE',  ( -9.016335848287868160, 10.47781223021269170, 1.199719254218462483 ) ) ;
#122356=CARTESIAN_POINT ( 'NONE',  ( -1.364683531250014514, -0.2197916663252438285, 0.7879004041258379498 ) ) ;
#122357=CARTESIAN_POINT ( 'NONE',  ( -1.500000000000013101, 1.670833333333355153, 0.8660254037844403729 ) ) ;
#122359=CARTESIAN_POINT ( 'NONE',  ( 3.988069740714122791, 7.804498464141805592, 0.7998128361456321445 ) ) ;
#122366=CARTESIAN_POINT ( 'NONE',  ( -1.001543065824772872E-14, 5.071875000341421469, 1.575800808251672791 ) ) ;
#122368=CARTESIAN_POINT ( 'NONE',  ( -7.645908563102897126, 11.00764485934031889, 1.199719254218453823 ) ) ;
#122369=CARTESIAN_POINT ( 'NONE',  ( -5.341549334104202629, 7.254893527920112994, 1.443375672974064550 ) ) ;
#122378=CARTESIAN_POINT ( 'NONE',  ( 7.613066949273408213, 8.840665181362512115, -1.199719254218441611 ) ) ;
#122379=CARTESIAN_POINT ( 'NONE',  ( -6.078132937628113908, 5.985576603521232109, 1.040834085586084257E-14 ) ) ;
#122380=CARTESIAN_POINT ( 'NONE',  ( 5.327714171786221975, 6.335452698179637743, -1.103974704194911283 ) ) ;
#122382=CARTESIAN_POINT ( 'NONE',  ( 6.249945625775433555, 10.23542763013927726, -0.7216878364870267237 ) ) ;
#122385=CARTESIAN_POINT ( 'NONE',  ( -8.857554428429624593, 9.228235009456373206, 0.7998128361456462443 ) ) ;
#122386=CARTESIAN_POINT ( 'NONE',  ( 6.356075086708249167, 6.309842444114747373, -0.7998128361456281477 ) ) ;
#122389=CARTESIAN_POINT ( 'NONE',  ( 4.857899112398166075, 4.561970474086296079, 1.040834085586084257E-14 ) ) ;
#122395=CARTESIAN_POINT ( 'NONE',  ( -4.772106882330234612, 6.590544000850479200, -1.443375672974053447 ) ) ;
#122396=CARTESIAN_POINT ( 'NONE',  ( 2.683624340501134853, 5.218313266304903664, -1.199719254218446718 ) ) ;
#122399=CARTESIAN_POINT ( 'NONE',  ( -5.181187258716735577, 9.196468901811520880, 0.7998128361456481317 ) ) ;
#122404=CARTESIAN_POINT ( 'NONE',  ( -9.158696461231359720, 10.64389961198009615, 1.199719254218462483 ) ) ;
#122408=CARTESIAN_POINT ( 'NONE',  ( 4.310602774141044868, 7.116454772218158809, -1.199719254218452047 ) ) ;
#122411=ORIENTED_EDGE ( 'NONE', *, *, #157331, .F. ) ;
#122421=CARTESIAN_POINT ( 'NONE',  ( -6.826694039680798021, 7.923230120171105284, -1.199719254218446718 ) ) ;
#122425=CARTESIAN_POINT ( 'NONE',  ( 6.182154858151487353, 6.314861544039274577, -0.7216878364870257245 ) ) ;
#122430=CARTESIAN_POINT ( 'NONE',  ( -4.466521540698216164, 7.298359999868178960, -1.199719254218452047 ) ) ;
#122434=CARTESIAN_POINT ( 'NONE',  ( -6.124532705071231931, 8.168374127381657246, -1.599625672291263179 ) ) ;
#122440=CARTESIAN_POINT ( 'NONE',  ( -7.641992139597101108, 12.06740792950531649, 0.7998128361456481317 ) ) ;
#122441=CARTESIAN_POINT ( 'NONE',  ( 6.751070424600909448, 9.963667031088037973, -1.199719254218441611 ) ) ;
#122444=CARTESIAN_POINT ( 'NONE',  ( -1.499999999999997780, 4.400000000000021672, 1.214306433183764966E-14 ) ) ;
#122448=CARTESIAN_POINT ( 'NONE',  ( -1.364683531250000748, -0.9281249996585805295, 0.000000000000000000 ) ) ;
#122452=CARTESIAN_POINT ( 'NONE',  ( 7.944714827928033962, 12.21265836598400689, 0.7216878364870438212 ) ) ;
#122456=CARTESIAN_POINT ( 'NONE',  ( 1.445103857048100515, 8.688264192037886247, 2.625611233228254182 ) ) ;
#122473=CARTESIAN_POINT ( 'NONE',  ( -3.460355519985875983, 5.060167411448709629, 1.599625672291267398 ) ) ;
#122479=CARTESIAN_POINT ( 'NONE',  ( -0.7500000000000249800, -1.277083332650516656, 1.299038105676659116 ) ) ;
#122482=CARTESIAN_POINT ( 'NONE',  ( -4.311129659465605002, 4.131998812239033647, 0.7216878364870317197 ) ) ;
#122487=CARTESIAN_POINT ( 'NONE',  ( 5.680503174445848735, 5.729601246382692636, 1.040834085586084257E-14 ) ) ;
#122488=CARTESIAN_POINT ( 'NONE',  ( 4.403700966340357681, 4.032072637018845107, -0.7998128361456211532 ) ) ;
#122489=CARTESIAN_POINT ( 'NONE',  ( -5.382223794500848868, 5.381608636446845395, -0.7216878364870227269 ) ) ;
#122490=CARTESIAN_POINT ( 'NONE',  ( 1.499999999999989120, 6.280000000000042881, 2.500000000000003997 ) ) ;
#122492=CARTESIAN_POINT ( 'NONE',  ( 10.01911233037457905, 11.75168114260095109, 1.082531754730548412 ) ) ;
#122494=CARTESIAN_POINT ( 'NONE',  ( -1.402160292154681736E-14, 2.009375000341422801, -1.575800808251660134 ) ) ;
#122496=CARTESIAN_POINT ( 'NONE',  ( 4.217276354152451390, 3.814577256132954730, 1.214306433183764966E-14 ) ) ;
#122497=AXIS2_PLACEMENT_3D ( 'NONE', #162850, #146615, #114164 ) ;
#122499=CARTESIAN_POINT ( 'NONE',  ( -9.657485491635913633, 10.16148791653038330, 1.040834085586084257E-14 ) ) ;
#122500=CARTESIAN_POINT ( 'NONE',  ( -3.416291520519271874, 6.929497840673697340, 1.040834085586084257E-14 ) ) ;
#122502=CARTESIAN_POINT ( 'NONE',  ( -7.054319997812058318, 7.124461507069184130, 1.040834085586084257E-14 ) ) ;
#122504=CARTESIAN_POINT ( 'NONE',  ( -1.364683531250010295, 5.488541667008087543, -0.7879004041258300672 ) ) ;
#122507=AXIS2_PLACEMENT_3D ( 'NONE', #126098, #74066, #192058 ) ;
#122513=CARTESIAN_POINT ( 'NONE',  ( -5.707619481228832115, 6.721606151930833661, -1.082531754730543971 ) ) ;
#122516=DIRECTION ( 'NONE',  ( 7.387867266669436732E-31, -1.000000000000000000, -8.546850786086424434E-32 ) ) ;
#122518=CARTESIAN_POINT ( 'NONE',  ( -5.721177634842498527, 5.777054783512106440, 0.000000000000000000 ) ) ;
#122520=CARTESIAN_POINT ( 'NONE',  ( 9.911173986789782120, 11.52179005846497972, -1.199719254218440723 ) ) ;
#122530=CARTESIAN_POINT ( 'NONE',  ( -3.307299406729781399, 5.945934176904983381, -1.199719254218452935 ) ) ;
#122531=CARTESIAN_POINT ( 'NONE',  ( -8.448702279610222021, 13.00856975952063088, 1.040834085586084257E-14 ) ) ;
#122536=CARTESIAN_POINT ( 'NONE',  ( 4.632082037363250748, 8.555846143565791095, -0.7998128361456231517 ) ) ;
#122540=CARTESIAN_POINT ( 'NONE',  ( 2.920214025141053327, 6.445393704534057022, 0.4458799699700779495 ) ) ;
#122541=CARTESIAN_POINT ( 'NONE',  ( 4.227444969362701421, 3.826440640544909400, 1.214306433183764966E-14 ) ) ;
#122547=DIRECTION ( 'NONE',  ( 1.000000000000000000, 0.000000000000000000, 0.000000000000000000 ) ) ;
#122552=CARTESIAN_POINT ( 'NONE',  ( 8.934986926605834157, 10.38290515491702770, -1.199719254218446718 ) ) ;
#122553=CARTESIAN_POINT ( 'NONE',  ( -4.225337428953291230, 8.081310767087481750, 0.7998128361456341429 ) ) ;
#122558=CARTESIAN_POINT ( 'NONE',  ( -0.6823417656249969321, 4.217708333674755394, -1.181850606188749264 ) ) ;
#122560=CARTESIAN_POINT ( 'NONE',  ( -4.954615070790188369, 7.867802451642154082, -1.199719254218452047 ) ) ;
#122562=CARTESIAN_POINT ( 'NONE',  ( -1.436717785781610024, 7.422226822640078048, -4.237127798884826824 ) ) ;
#122563=CARTESIAN_POINT ( 'NONE',  ( 5.789495288235341874, 6.713164910151406595, 1.199719254218462483 ) ) ;
#122564=CARTESIAN_POINT ( 'NONE',  ( -5.925076824372040640, 6.871343368977510302, 1.199719254218450271 ) ) ;
#122571=CARTESIAN_POINT ( 'NONE',  ( 7.307481608085759639, 7.627742752295940676, 1.040834085586084257E-14 ) ) ;
#122573=CARTESIAN_POINT ( 'NONE',  ( 6.277061933002769045, 10.26706332190449622, 0.7216878364870438212 ) ) ;
#122574=CARTESIAN_POINT ( 'NONE',  ( 0.6823417656249882723, 2.988541667008084879, -1.181850606188754593 ) ) ;
#122576=CARTESIAN_POINT ( 'NONE',  ( 4.324687812634882000, 7.028924300507257250, 1.082531754730558626 ) ) ;
#122585=CARTESIAN_POINT ( 'NONE',  ( -4.081306271799089558, 7.708262650413779227, 0.6970576149333465032 ) ) ;
#122591=CARTESIAN_POINT ( 'NONE',  ( -10.15522075183580419, 11.80651128435196462, 1.199719254218462483 ) ) ;
#122593=CARTESIAN_POINT ( 'NONE',  ( -1.499999999999997780, 4.150000000000021672, 1.214306433183764966E-14 ) ) ;
#122596=CARTESIAN_POINT ( 'NONE',  ( -4.308793891044708779, 3.921347715840572956, 1.214306433183764966E-14 ) ) ;
#122601=CARTESIAN_POINT ( 'NONE',  ( 2.738383840280328663, 5.178236332760252303, 1.082531754730548412 ) ) ;
#122602=CARTESIAN_POINT ( 'NONE',  ( -0.6823417656250212460, 3.363541667008085323, 1.181850606188767472 ) ) ;
#122604=CARTESIAN_POINT ( 'NONE',  ( 7.995557903757111617, 10.35123685918189729, 1.599625672291281386 ) ) ;
#122605=CARTESIAN_POINT ( 'NONE',  ( -10.50487009249003378, 11.15010328419353947, 0.7998128361456462443 ) ) ;
#122612=CARTESIAN_POINT ( 'NONE',  ( -0.7500000000000215383, 3.691666666666690411, 1.299038105676671107 ) ) ;
#122613=CARTESIAN_POINT ( 'NONE',  ( 4.150767584078112193, 7.994312614733129152, 0.7998128361456321445 ) ) ;
#122616=EDGE_CURVE ( 'NONE', #120076, #69400, #132944, .T. ) ;
#122617=CARTESIAN_POINT ( 'NONE',  ( 1.499999999999999556, 7.809254910141758543, 3.635752117236003667 ) ) ;
#122618=CARTESIAN_POINT ( 'NONE',  ( 0.6823417656249917140, 4.342708333674755394, 1.181850606188765695 ) ) ;
#122619=EDGE_CURVE ( 'NONE', #173996, #137701, #145999, .T. ) ;
#122621=CARTESIAN_POINT ( 'NONE',  ( 8.676855123066012254, 11.14608361504227574, -1.443375672974052559 ) ) ;
#122626=CARTESIAN_POINT ( 'NONE',  ( -0.7500000000000006661, 1.889583334016155192, -1.299038105676652011 ) ) ;
#122628=CARTESIAN_POINT ( 'NONE',  ( -4.543954038874438162, 8.453030145328826350, 1.040834085586084257E-14 ) ) ;
#122629=CARTESIAN_POINT ( 'NONE',  ( 4.107757354816228279, 6.775838766385488654, -1.082531754730548412 ) ) ;
#122638=CARTESIAN_POINT ( 'NONE',  ( 7.308008492965924141, 8.484763649003774333, -1.199719254218451159 ) ) ;
#122639=CARTESIAN_POINT ( 'NONE',  ( 5.148345644887269756, 7.029489223833707001, -1.599625672291256295 ) ) ;
#122640=DIRECTION ( 'NONE',  ( 1.000000000000000000, -5.578564026256504688E-16, 0.000000000000000000 ) ) ;
#122642=CARTESIAN_POINT ( 'NONE',  ( 5.681030059326015014, 6.586622143090519188, -1.199719254218445830 ) ) ;
#122649=CARTESIAN_POINT ( 'NONE',  ( 8.516493047678546091, 13.08765898893368629, -0.7998128361456352531 ) ) ;
#122654=CARTESIAN_POINT ( 'NONE',  ( 5.039007818866061861, 6.552116822607409574, 1.229770346242751389 ) ) ;
#122664=CARTESIAN_POINT ( 'NONE',  ( -1.608462485350604876, 8.735270501766756013, -2.463594439587629914 ) ) ;
#122667=CARTESIAN_POINT ( 'NONE',  ( 8.120970824905713314, 8.576813505252564696, 1.040834085586084257E-14 ) ) ;
#122668=CARTESIAN_POINT ( 'NONE',  ( -3.093231602212184850, 6.760520635889515795, -0.7998128361456281477 ) ) ;
#122672=CARTESIAN_POINT ( 'NONE',  ( -5.199715606040888005, 6.025088614257851027, -1.199719254218446718 ) ) ;
#122679=ORIENTED_EDGE ( 'NONE', *, *, #70772, .T. ) ;
#122685=CARTESIAN_POINT ( 'NONE',  ( -6.961139734775127152, 5.290451655907111750, 1.299555808129863194E-14 ) ) ;
#122688=FACE_OUTER_BOUND ( 'NONE', #184404, .T. ) ;
#122695=CARTESIAN_POINT ( 'NONE',  ( -10.31739171031960822, 11.13930453823545186, 1.040834085586084257E-14 ) ) ;
#122699=CARTESIAN_POINT ( 'NONE',  ( 8.076906825439115423, 10.44614393447756129, -1.599625672291262513 ) ) ;
#122703=CARTESIAN_POINT ( 'NONE',  ( -4.876128802409253282, 8.840567369452784874, 0.7998128361456481317 ) ) ;
#122704=CARTESIAN_POINT ( 'NONE',  ( 3.659811400685081040, 6.357198169852855685, -1.199719254218446718 ) ) ;
#122709=CARTESIAN_POINT ( 'NONE',  ( -2.657034918598345730, 5.083329257464595408, -1.082531754730543971 ) ) ;
#122712=CARTESIAN_POINT ( 'NONE',  ( -1.364683531250012516, 2.092708333674750953, 0.7879004041258379498 ) ) ;
#122715=CARTESIAN_POINT ( 'NONE',  ( 6.968527767744109980, 7.232296605230681408, 0.7216878364870317197 ) ) ;
#122723=CARTESIAN_POINT ( 'NONE',  ( 8.554831740098649107, 11.96409221588171157, 1.082531754730546636 ) ) ;
#122724=EDGE_LOOP ( 'NONE', ( #143650, #151789, #12119, #142422, #192508, #181419, #181587 ) ) ;
#122727=CARTESIAN_POINT ( 'NONE',  ( -8.696665468161981494, 12.23352791524263239, -1.199719254218446718 ) ) ;
#122736=CARTESIAN_POINT ( 'NONE',  ( 3.032219910950674890, 6.689340329417765574, 0.7998128361456321445 ) ) ;
#122742=CARTESIAN_POINT ( 'NONE',  ( 4.635998460869027227, 7.496083073400806818, -1.199719254218452047 ) ) ;
#122745=( BOUNDED_SURFACE ( )  B_SPLINE_SURFACE ( 1, 2, ( 
 ( #142951, #99499, #148255, #16079, #149308, #114739, #33421, #50739, #889, #166628, #115799, #18220, #83225, #180737, #100557, #196985, #164493, #17149, #181787, #65887, #66956, #165556, #48624, #82162, #32364, #214256, #132035, #49674, #116865, #133095, #98428, #198045, #199093, #182867, #34483, #15543, #47024, #130466, #97906, #148770, #212681, #115264, #67479, #147713, #131501, #129411, #146667, #162896, #197505, #83756, #16607, #96849, #79499, #80568, #30769, #165012, #195394, #48099, #133625, #13424, #1417, #82688, #199627, #34999, #339, #51273, #66412, #132557, #196456, #114211, #149848, #117397, #145618, #183394, #211614, #179146, #14479, #213731, #65354, #100018, #33943, #198556, #161836, #166082, #64322, #180209, #63250, #31831, #113139, #163967, #81628, #49148, #50205, #116323, #181257, #32884, #98961, #182314, #17670, #20722, #88967, #69473, #203736, #106318, #6606, #123679, #153958, #41292, #22853, #3404, #205888, #189641, #36990, #187507, #87884, #136648, #171259, #5524, #57521, #135580, #139857, #201602, #53250, #4460, #72687, #71605, #168070, #155022, #70530, #39136, #121537, #21775, #119381, #202673, #104142, #138782, #54321, #105219, #73762, #137716, #55382, #185367, #152882, #169128, #204802, #90034, #56453, #103073, #85749, #86816, #120462, #122613, #186434, #38072, #19670, #151831, #7678, #188576, #170189, #40208, #172342, #23930, #156093, #78024, #75898, #142002, #29284, #161427, #173422, #13010, #157167, #124738, #190697, #93242, #159276, #45551, #193903, #176603, #107400, #111667, #42358, #174492, #145205, #92181, #62836, #158231, #59643, #10875, #94308, #110602, #192827, #108470, #177674, #26069, #208017, #44485, #76950, #128998, #79087, #143075, #160349, #28215, #11951, #144148, #211211, #9822, #210140, #61784, #125801, #209068, #191763, #127950, #60705, #43419, #126869, #95378, #194975, #25004, #91106, #27136, #109543, #8759, #74840, #140940, #206954, #175547, #58583, #180850, #134273, #33534, #97496, #132148, #214368, #114850, #146258, #15136, #197096, #99606, #163553, #65998, #166744, #32472, #16193, #14066, #31420, #47687, #82274, #182981, #115913, #196055, #178743, #179801, #130062, #49787, #80153, #147306, #18338, #112733, #100666, #181899, #84419, #46611, #165672, #150508, #17261, #83337, #81224, #213332, #34598, #2069, #30356, #68140, #96443, #63906, #113799, #98544, #164608, #199209, #133205, #149422, #162494, #50856, #64957, #131109, #212271, #48737, #148369, #198154, #1005, #67069, #116981, #203472, #71341, #3137, #72417, #135327, #86554, #137457, #186171, #155829, #106057, #37805, #38873, #55126, #121271, #187246, #23672, #52981, #170999, #22597, #168865, #103880, #119117, #88704, #169928, #152618, #21512, #154762, #104958, #6345, #138518, #120195, #202405, #87624, #153695, #70273, #151570, #5264, #36723, #185096, #204542, #101737, #56190, #122351, #188308, #7413, #39950, #73495, #172079, #35658, #89782, #200281, #69207, #51932, #118056, #20468, #184041, #167806, #19405, #85484, #201341, #102809, #4205, #136389, #54060, #123421, #109279, #189383, #206694, #205619, #141749, #25807, #43166, #208811, #77760, #176343, #27951, #94044, #95106, #207756, #174233, #111403, #91916, #124478, #160084, #58322, #11686, #75642, #143882, #157976, #74575, #110340, #59383, #191500, #60443, #139596, #90841, #125538, #209875, #175288, #140678, #9565, #26874, #92977, #159023, #126601, #61514, #127679, #193639, #190435, #45281, #177405, #42095, #29022, #108210, #8493, #173159, #161154, #156904, #12741, #57259, #41026, #107135, #24740, #114101, #180092, #81520, #147598, #53284, #37022, #121571, #123713, #189675, #103106, #41325, #137754, #70565, #72723, #54360, #107435, #205923, #187542, #185404, #39172, #38108, #136684, #173459, #170229, #55417, #156132, #120501, #4496, #57556, #104180, #5560, #169164, #20759, #87918, #25039, #91139, #119417, #40244, #21813, #203773, #202709, #186472, #152918, #23967, #153992, #71641, #105256, #157196, #188612, #138817, #140978, #86853, #171297, #22888, #89004, #155057, #204838, #6644, #56490, #122649, #74872, #106355, #172378, #90069, #7714, #73797, #139892 ),
 ( #8793, #193939, #43456, #160385, #112770, #192863, #176638, #174527, #191795, #208050, #28250, #129038, #61818, #142034, #124772, #125836, #75933, #210178, #26105, #93275, #178782, #58616, #46647, #127986, #30395, #80191, #45586, #96481, #111703, #177710, #175581, #27171, #195014, #162528, #190731, #14101, #42394, #9857, #59677, #44519, #110636, #145241, #79125, #29320, #206987, #211246, #109577, #159313, #108503, #10910, #92217, #76986, #143112, #94343, #95414, #161466, #78061, #209104, #62871, #60742, #126904, #144186, #11985, #158268, #13046, #132183, #199245, #149458, #67104, #83375, #184075, #213369, #117017, #183014, #114887, #198189, #64991, #34631, #49824, #98583, #115949, #100702, #1041, #166778, #18374, #66036, #148406, #181939, #33569, #16228, #97535, #99641, #197134, #131145, #133240, #47725, #165708, #84451, #50892, #101770, #17297, #19436, #150539, #196092, #35694, #167838, #15175, #2103, #68177, #180886, #134308, #200315, #51966, #48773, #214405, #118090, #32508, #163592, #146296, #164645, #82312, #130098, #113841, #212308, #63943, #179837, #31458, #81262, #147341, #169961, #20502, #102843, #185132, #56224, #4237, #54094, #36758, #89816, #6380, #104990, #173191, #85516, #203506, #168900, #121304, #103915, #171031, #55157, #53016, #70307, #107166, #154793, #22627, #135359, #88737, #57290, #120231, #122386, #172113, #69241, #187279, #201375, #152654, #151602, #87658, #186205, #38906, #72451, #23707, #188343, #39982, #106091, #41059, #153727, #37839, #123453, #21547, #136423, #155861, #202439, #7449, #5296, #73528, #71376, #86588, #138551, #137490, #204574, #139630, #3170, #205653, #189415, #119150, #93008, #25836, #43194, #60473, #126630, #26903, #192594, #159052, #12772, #59412, #91944, #77791, #29053, #75671, #95136, #158006, #108239, #58353, #141778, #42126, #174263, #142837, #62600, #9594, #74606, #11717, #208843, #112493, #207785, #24771, #8525, #10645, #161186, #78846, #140710, #144966, #109307, #125569, #44248, #191530, #210972, #177436, #76720, #156936, #110370, #175317, #176375, #143912, #27981, #94075, #160115, #209906, #124508, #61543, #127710, #193670, #190467, #128763, #45313, #111432, #90874, #206725, #194737, #46374, #214143, #196872, #197926, #148141, #146025, #97263, #200059, #33300, #49553, #13840, #115679, #150276, #147081, #767, #50623, #162254, #65769, #79916, #31190, #30114, #180620, #64734, #82048, #181673, #116749, #66833, #132976, #198978, #134051, #32244, #213103, #1846, #130878, #163317, #182748, #14899, #34366, #114629, #100440, #48509, #113566, #17034, #98315, #15964, #99385, #178504, #129831, #164380, #166511, #131916, #179571, #165437, #83111, #149192, #18102, #84189, #67905, #51710, #96204, #80993, #212035, #63677, #195814, #47451, #184875, #201115, #151341, #168640, #135101, #52756, #21298, #155605, #102579, #167579, #104730, #87404, #205397, #118891, #117830, #101509, #185944, #188085, #39715, #19178, #105823, #202179, #36501, #137234, #20242, #171849, #55968, #37577, #85253, #103659, #86328, #152399, #23444, #3978, #119967, #6119, #70047, #68983, #122121, #136161, #53836, #2910, #169708, #153469, #89554, #7189, #183821, #5042, #71118, #72187, #203256, #54899, #73262, #121052, #187018, #38651, #170777, #22366, #139366, #88479, #154538, #138296, #204311, #141532, #206471, #74355, #156680, #27733, #190218, #25586, #8272, #61300, #192344, #76474, #144729, #57036, #175070, #140459, #92760, #75420, #142585, #26657, #24512, #41877, #78607, #126384, #208593, #106910, #60225, #28804, #91697, #93827, #143665, #40803, #158804, #172935, #124259, #123203, #59160, #157750, #10401, #44002, #209659, #159868, #11472, #77543, #12535, #125318, #9348, #94889, #207540, #107988, #127462, #174016, #193433, #191277, #45077, #42944, #58100, #110121, #109052, #176133, #111186, #189164, #177189, #160941, #90622, #64500, #211799, #14664, #32007, #98089, #212864, #164142, #130642, #198732, #30954, #63435, #49327, #517, #47212, #66585, #129587, #79680, #29878, #113326, #13605, #145793, #114388, #34119, #195574, #46139, #197682, #180383, #83930, #179333, #210740, #194495, #196635, #132728 ) ),
 .UNSPECIFIED., .F., .F., .T. ) 
 B_SPLINE_SURFACE_WITH_KNOTS ( ( 2, 2 ),
 ( 3, 2, 2, 2, 2, 2, 2, 2, 2, 2, 2, 2, 2, 2, 2, 2, 2, 2, 2, 2, 2, 2, 2, 2, 2, 2, 2, 2, 2, 2, 2, 2, 2, 2, 2, 2, 2, 2, 2, 2, 2, 2, 2, 2, 2, 2, 2, 2, 2, 2, 2, 2, 2, 2, 2, 2, 2, 2, 2, 2, 2, 2, 2, 2, 2, 2, 2, 2, 2, 2, 2, 2, 2, 2, 2, 2, 2, 2, 2, 2, 2, 2, 2, 2, 2, 2, 2, 2, 2, 2, 2, 2, 2, 2, 2, 2, 2, 2, 2, 2, 2, 2, 2, 2, 2, 2, 2, 2, 2, 2, 2, 2, 2, 2, 2, 2, 2, 2, 2, 2, 2, 2, 2, 2, 2, 2, 2, 2, 2, 2, 2, 2, 2, 2, 2, 2, 2, 2, 2, 2, 2, 2, 2, 2, 2, 2, 2, 2, 2, 2, 2, 2, 2, 2, 2, 2, 2, 2, 2, 2, 2, 2, 2, 2, 2, 2, 2, 2, 2, 2, 2, 2, 2, 2, 2, 2, 2, 2, 2, 2, 2, 2, 2, 2, 2, 2, 2, 2, 2, 2, 2, 2, 2, 2, 2, 2, 2, 2, 2, 2, 2, 2, 2, 2, 2, 2, 2, 2, 2, 2, 2, 2, 2, 2, 2, 2, 2, 2, 2, 2, 2, 2, 2, 2, 2, 2, 2, 2, 2, 2, 2, 2, 2, 2, 2, 2, 2, 2, 2, 2, 3 ),
 ( 0.000000000000000000, 1.000000000000000000 ),
 ( 0.000000000000000000, 0.004166666666666666609, 0.008333333333333333218, 0.01250000000000000069, 0.01666666666666666644, 0.02083333333333333218, 0.02500000000000000139, 0.02916666666666666713, 0.03333333333333333287, 0.03749999999999999861, 0.04166666666666666435, 0.04583333333333333010, 0.05000000000000000278, 0.05416666666666666852, 0.05833333333333333426, 0.06250000000000000000, 0.06666666666666666574, 0.07083333333333333148, 0.07499999999999999722, 0.07916666666666666297, 0.08333333333333332871, 0.08749999999999999445, 0.09166666666666666019, 0.09583333333333333981, 0.1000000000000000056, 0.1041666666666666713, 0.1083333333333333370, 0.1125000000000000028, 0.1166666666666666685, 0.1208333333333333343, 0.1250000000000000000, 0.1291666666666666796, 0.1333333333333333315, 0.1375000000000000111, 0.1416666666666666630, 0.1458333333333333426, 0.1499999999999999944, 0.1541666666666666741, 0.1583333333333333259, 0.1625000000000000056, 0.1666666666666666574, 0.1708333333333333370, 0.1749999999999999889, 0.1791666666666666685, 0.1833333333333333204, 0.1875000000000000000, 0.1916666666666666796, 0.1958333333333333315, 0.2000000000000000111, 0.2041666666666666630, 0.2083333333333333426, 0.2124999999999999944, 0.2166666666666666741, 0.2208333333333333259, 0.2250000000000000056, 0.2291666666666666574, 0.2333333333333333370, 0.2374999999999999889, 0.2416666666666666685, 0.2458333333333333204, 0.2500000000000000000, 0.2541666666666666519, 0.2583333333333333592, 0.2625000000000000111, 0.2666666666666666630, 0.2708333333333333148, 0.2750000000000000222, 0.2791666666666666741, 0.2833333333333333259, 0.2874999999999999778, 0.2916666666666666852, 0.2958333333333333370, 0.2999999999999999889, 0.3041666666666666408, 0.3083333333333333481, 0.3125000000000000000, 0.3166666666666666519, 0.3208333333333333592, 0.3250000000000000111, 0.3291666666666666630, 0.3333333333333333148, 0.3375000000000000222, 0.3416666666666666741, 0.3458333333333333259, 0.3499999999999999778, 0.3541666666666666852, 0.3583333333333333370, 0.3624999999999999889, 0.3666666666666666408, 0.3708333333333333481, 0.3750000000000000000, 0.3791666666666666519, 0.3833333333333333592, 0.3875000000000000111, 0.3916666666666666630, 0.3958333333333333148, 0.4000000000000000222, 0.4041666666666666741, 0.4083333333333333259, 0.4124999999999999778, 0.4166666666666666852, 0.4208333333333333370, 0.4249999999999999889, 0.4291666666666666408, 0.4333333333333333481, 0.4375000000000000000, 0.4416666666666666519, 0.4458333333333333592, 0.4500000000000000111, 0.4541666666666666630, 0.4583333333333333148, 0.4625000000000000222, 0.4666666666666666741, 0.4708333333333333259, 0.4749999999999999778, 0.4791666666666666852, 0.4833333333333333370, 0.4874999999999999889, 0.4916666666666666408, 0.4958333333333333481, 0.5000000000000000000, 0.5041666666666666519, 0.5083333333333333037, 0.5124999999999999556, 0.5166666666666667185, 0.5208333333333333703, 0.5250000000000000222, 0.5291666666666666741, 0.5333333333333333259, 0.5374999999999999778, 0.5416666666666666297, 0.5458333333333332815, 0.5500000000000000444, 0.5541666666666666963, 0.5583333333333333481, 0.5625000000000000000, 0.5666666666666666519, 0.5708333333333333037, 0.5749999999999999556, 0.5791666666666667185, 0.5833333333333333703, 0.5875000000000000222, 0.5916666666666666741, 0.5958333333333333259, 0.5999999999999999778, 0.6041666666666666297, 0.6083333333333332815, 0.6125000000000000444, 0.6166666666666666963, 0.6208333333333333481, 0.6250000000000000000, 0.6291666666666666519, 0.6333333333333333037, 0.6374999999999999556, 0.6416666666666667185, 0.6458333333333333703, 0.6500000000000000222, 0.6541666666666666741, 0.6583333333333333259, 0.6624999999999999778, 0.6666666666666666297, 0.6708333333333332815, 0.6750000000000000444, 0.6791666666666666963, 0.6833333333333333481, 0.6875000000000000000, 0.6916666666666666519, 0.6958333333333333037, 0.6999999999999999556, 0.7041666666666667185, 0.7083333333333333703, 0.7125000000000000222, 0.7166666666666666741, 0.7208333333333333259, 0.7249999999999999778, 0.7291666666666666297, 0.7333333333333332815, 0.7375000000000000444, 0.7416666666666666963, 0.7458333333333333481, 0.7500000000000000000, 0.7541666666666666519, 0.7583333333333333037, 0.7624999999999999556, 0.7666666666666667185, 0.7708333333333333703, 0.7750000000000000222, 0.7791666666666666741, 0.7833333333333333259, 0.7874999999999999778, 0.7916666666666666297, 0.7958333333333332815, 0.8000000000000000444, 0.8041666666666666963, 0.8083333333333333481, 0.8125000000000000000, 0.8166666666666666519, 0.8208333333333333037, 0.8249999999999999556, 0.8291666666666667185, 0.8333333333333333703, 0.8375000000000000222, 0.8416666666666666741, 0.8458333333333333259, 0.8499999999999999778, 0.8541666666666666297, 0.8583333333333332815, 0.8625000000000000444, 0.8666666666666666963, 0.8708333333333333481, 0.8750000000000000000, 0.8791666666666666519, 0.8833333333333333037, 0.8874999999999999556, 0.8916666666666667185, 0.8958333333333333703, 0.9000000000000000222, 0.9041666666666666741, 0.9083333333333333259, 0.9124999999999999778, 0.9166666666666666297, 0.9208333333333332815, 0.9250000000000000444, 0.9291666666666666963, 0.9333333333333333481, 0.9375000000000000000, 0.9416666666666666519, 0.9458333333333333037, 0.9499999999999999556, 0.9541666666666667185, 0.9583333333333333703, 0.9625000000000000222, 0.9666666666666666741, 0.9708333333333333259, 0.9749999999999999778, 0.9791666666666666297, 0.9833333333333332815, 0.9875000000000000444, 0.9916666666666666963, 0.9958333333333333481, 1.000000000000000000 ),
 .UNSPECIFIED. ) 
 GEOMETRIC_REPRESENTATION_ITEM ( )  RATIONAL_B_SPLINE_SURFACE ( (
 ( 1.000000000000000000, 0.8660254037844387076, 1.000000000000000000, 0.8660254037844387076, 1.000000000000000000, 0.8660254037844387076, 1.000000000000000000, 0.8660254037844387076, 1.000000000000000000, 0.8660254037844387076, 1.000000000000000000, 0.8660254037844387076, 1.000000000000000000, 0.8660254037844387076, 1.000000000000000000, 0.8660254037844387076, 1.000000000000000000, 0.8660254037844387076, 1.000000000000000000, 0.8660254037844387076, 1.000000000000000000, 0.8660254037844387076, 1.000000000000000000, 0.8660254037844387076, 1.000000000000000000, 0.8660254037844387076, 1.000000000000000000, 0.8660254037844387076, 1.000000000000000000, 0.8660254037844387076, 1.000000000000000000, 0.8660254037844387076, 1.000000000000000000, 0.8660254037844387076, 1.000000000000000000, 0.8660254037844387076, 1.000000000000000000, 0.8660254037844387076, 1.000000000000000000, 0.8660254037844387076, 1.000000000000000000, 0.8660254037844387076, 1.000000000000000000, 0.8660254037844387076, 1.000000000000000000, 0.8660254037844387076, 1.000000000000000000, 0.8660254037844387076, 1.000000000000000000, 0.8660254037844387076, 1.000000000000000000, 0.8660254037844387076, 1.000000000000000000, 0.8660254037844387076, 1.000000000000000000, 0.8660254037844387076, 1.000000000000000000, 0.8660254037844387076, 1.000000000000000000, 0.8660254037844387076, 1.000000000000000000, 0.8660254037844387076, 1.000000000000000000, 0.8660254037844387076, 1.000000000000000000, 0.8660254037844387076, 1.000000000000000000, 0.8660254037844387076, 1.000000000000000000, 0.8660254037844387076, 1.000000000000000000, 0.8660254037844387076, 1.000000000000000000, 0.8660254037844387076, 1.000000000000000000, 0.8660254037844387076, 1.000000000000000000, 0.8660254037844387076, 1.000000000000000000, 0.8660254037844387076, 1.000000000000000000, 0.8660254037844387076, 1.000000000000000000, 0.8660254037844387076, 1.000000000000000000, 0.8660254037844387076, 1.000000000000000000, 0.8660254037844387076, 1.000000000000000000, 0.8660254037844387076, 1.000000000000000000, 0.8660254037844387076, 1.000000000000000000, 0.8660254037844387076, 1.000000000000000000, 0.8660254037844387076, 1.000000000000000000, 0.8660254037844387076, 1.000000000000000000, 0.8660254037844387076, 1.000000000000000000, 0.8660254037844387076, 1.000000000000000000, 0.8660254037844387076, 1.000000000000000000, 0.8660254037844387076, 1.000000000000000000, 0.8660254037844387076, 1.000000000000000000, 0.8660254037844387076, 1.000000000000000000, 0.8660254037844387076, 1.000000000000000000, 0.8660254037844387076, 1.000000000000000000, 0.8660254037844387076, 1.000000000000000000, 0.8660254037844387076, 1.000000000000000000, 0.8660254037844387076, 1.000000000000000000, 0.8660254037844387076, 1.000000000000000000, 0.8660254037844387076, 1.000000000000000000, 0.8660254037844387076, 1.000000000000000000, 0.8660254037844387076, 1.000000000000000000, 0.8660254037844387076, 1.000000000000000000, 0.8660254037844387076, 1.000000000000000000, 0.8660254037844387076, 1.000000000000000000, 0.8660254037844387076, 1.000000000000000000, 0.8660254037844387076, 1.000000000000000000, 0.8660254037844387076, 1.000000000000000000, 0.8660254037844387076, 1.000000000000000000, 0.8660254037844387076, 1.000000000000000000, 0.8660254037844387076, 1.000000000000000000, 0.8660254037844387076, 1.000000000000000000, 0.8660254037844387076, 1.000000000000000000, 0.8660254037844387076, 1.000000000000000000, 0.8660254037844387076, 1.000000000000000000, 0.8660254037844387076, 1.000000000000000000, 0.8660254037844387076, 1.000000000000000000, 0.8660254037844387076, 1.000000000000000000, 0.8660254037844387076, 1.000000000000000000, 0.8660254037844387076, 1.000000000000000000, 0.8660254037844387076, 1.000000000000000000, 0.8660254037844387076, 1.000000000000000000, 0.8660254037844387076, 1.000000000000000000, 0.8660254037844387076, 1.000000000000000000, 0.8660254037844387076, 1.000000000000000000, 0.8660254037844387076, 1.000000000000000000, 0.8660254037844387076, 1.000000000000000000, 0.8660254037844387076, 1.000000000000000000, 0.8660254037844387076, 1.000000000000000000, 0.8660254037844387076, 1.000000000000000000, 0.8660254037844387076, 1.000000000000000000, 0.8660254037844387076, 1.000000000000000000, 0.8660254037844387076, 1.000000000000000000, 0.8660254037844387076, 1.000000000000000000, 0.8660254037844387076, 1.000000000000000000, 0.8660254037844387076, 1.000000000000000000, 0.8660254037844387076, 1.000000000000000000, 0.8660254037844387076, 1.000000000000000000, 0.8660254037844387076, 1.000000000000000000, 0.8660254037844387076, 1.000000000000000000, 0.8660254037844387076, 1.000000000000000000, 0.8660254037844387076, 1.000000000000000000, 0.8660254037844387076, 1.000000000000000000, 0.8660254037844387076, 1.000000000000000000, 0.8660254037844387076, 1.000000000000000000, 0.8660254037844387076, 1.000000000000000000, 0.8660254037844387076, 1.000000000000000000, 0.8660254037844387076, 1.000000000000000000, 0.8660254037844387076, 1.000000000000000000, 0.8660254037844387076, 1.000000000000000000, 0.8660254037844387076, 1.000000000000000000, 0.8660254037844387076, 1.000000000000000000, 0.8660254037844387076, 1.000000000000000000, 0.8660254037844387076, 1.000000000000000000, 0.8660254037844387076, 1.000000000000000000, 0.8660254037844387076, 1.000000000000000000, 0.8660254037844387076, 1.000000000000000000, 0.8660254037844387076, 1.000000000000000000, 0.8660254037844387076, 1.000000000000000000, 0.8660254037844387076, 1.000000000000000000, 0.8660254037844387076, 1.000000000000000000, 0.8660254037844387076, 1.000000000000000000, 0.8660254037844387076, 1.000000000000000000, 0.8660254037844387076, 1.000000000000000000, 0.8660254037844387076, 1.000000000000000000, 0.8660254037844387076, 1.000000000000000000, 0.8660254037844387076, 1.000000000000000000, 0.8660254037844387076, 1.000000000000000000, 0.8660254037844387076, 1.000000000000000000, 0.8660254037844387076, 1.000000000000000000, 0.8660254037844387076, 1.000000000000000000, 0.8660254037844387076, 1.000000000000000000, 0.8660254037844387076, 1.000000000000000000, 0.8660254037844387076, 1.000000000000000000, 0.8660254037844387076, 1.000000000000000000, 0.8660254037844387076, 1.000000000000000000, 0.8660254037844387076, 1.000000000000000000, 0.8660254037844387076, 1.000000000000000000, 0.8660254037844387076, 1.000000000000000000, 0.8660254037844387076, 1.000000000000000000, 0.8660254037844387076, 1.000000000000000000, 0.8660254037844387076, 1.000000000000000000, 0.8660254037844387076, 1.000000000000000000, 0.8660254037844387076, 1.000000000000000000, 0.8660254037844387076, 1.000000000000000000, 0.8660254037844387076, 1.000000000000000000, 0.8660254037844387076, 1.000000000000000000, 0.8660254037844387076, 1.000000000000000000, 0.8660254037844387076, 1.000000000000000000, 0.8660254037844387076, 1.000000000000000000, 0.8660254037844387076, 1.000000000000000000, 0.8660254037844387076, 1.000000000000000000, 0.8660254037844387076, 1.000000000000000000, 0.8660254037844387076, 1.000000000000000000, 0.8660254037844387076, 1.000000000000000000, 0.8660254037844387076, 1.000000000000000000, 0.8660254037844387076, 1.000000000000000000, 0.8660254037844387076, 1.000000000000000000, 0.8660254037844387076, 1.000000000000000000, 0.8660254037844387076, 1.000000000000000000, 0.8660254037844387076, 1.000000000000000000, 0.8660254037844387076, 1.000000000000000000, 0.8660254037844387076, 1.000000000000000000, 0.8660254037844387076, 1.000000000000000000, 0.8660254037844387076, 1.000000000000000000, 0.8660254037844387076, 1.000000000000000000, 0.8660254037844387076, 1.000000000000000000, 0.8660254037844387076, 1.000000000000000000, 0.8660254037844387076, 1.000000000000000000, 0.8660254037844387076, 1.000000000000000000, 0.8660254037844387076, 1.000000000000000000, 0.8660254037844387076, 1.000000000000000000, 0.8660254037844387076, 1.000000000000000000, 0.8660254037844387076, 1.000000000000000000, 0.8660254037844387076, 1.000000000000000000, 0.8660254037844387076, 1.000000000000000000, 0.8660254037844387076, 1.000000000000000000, 0.8660254037844387076, 1.000000000000000000, 0.8660254037844387076, 1.000000000000000000, 0.8660254037844387076, 1.000000000000000000, 0.8660254037844387076, 1.000000000000000000, 0.8660254037844387076, 1.000000000000000000, 0.8660254037844387076, 1.000000000000000000, 0.8660254037844387076, 1.000000000000000000, 0.8660254037844387076, 1.000000000000000000, 0.8660254037844387076, 1.000000000000000000, 0.8660254037844387076, 1.000000000000000000, 0.8660254037844387076, 1.000000000000000000, 0.8660254037844387076, 1.000000000000000000, 0.8660254037844387076, 1.000000000000000000, 0.8660254037844387076, 1.000000000000000000, 0.8660254037844387076, 1.000000000000000000, 0.8660254037844387076, 1.000000000000000000, 0.8660254037844387076, 1.000000000000000000, 0.8660254037844387076, 1.000000000000000000, 0.8660254037844387076, 1.000000000000000000, 0.8660254037844387076, 1.000000000000000000, 0.8660254037844387076, 1.000000000000000000, 0.8660254037844387076, 1.000000000000000000, 0.8660254037844387076, 1.000000000000000000, 0.8660254037844387076, 1.000000000000000000, 0.8660254037844387076, 1.000000000000000000, 0.8660254037844387076, 1.000000000000000000, 0.8660254037844387076, 1.000000000000000000, 0.8660254037844387076, 1.000000000000000000, 0.8660254037844387076, 1.000000000000000000, 0.8660254037844387076, 1.000000000000000000, 0.8660254037844387076, 1.000000000000000000, 0.8660254037844387076, 1.000000000000000000, 0.8660254037844387076, 1.000000000000000000, 0.8660254037844387076, 1.000000000000000000, 0.8660254037844387076, 1.000000000000000000, 0.8660254037844387076, 1.000000000000000000, 0.8660254037844387076, 1.000000000000000000, 0.8660254037844387076, 1.000000000000000000, 0.8660254037844387076, 1.000000000000000000, 0.8660254037844387076, 1.000000000000000000, 0.8660254037844387076, 1.000000000000000000, 0.8660254037844387076, 1.000000000000000000, 0.8660254037844387076, 1.000000000000000000, 0.8660254037844387076, 1.000000000000000000, 0.8660254037844387076, 1.000000000000000000, 0.8660254037844387076, 1.000000000000000000, 0.8660254037844387076, 1.000000000000000000, 0.8660254037844387076, 1.000000000000000000, 0.8660254037844387076, 1.000000000000000000, 0.8660254037844387076, 1.000000000000000000, 0.8660254037844387076, 1.000000000000000000, 0.8660254037844387076, 1.000000000000000000, 0.8660254037844387076, 1.000000000000000000, 0.8660254037844387076, 1.000000000000000000, 0.8660254037844387076, 1.000000000000000000, 0.8660254037844387076, 1.000000000000000000, 0.8660254037844387076, 1.000000000000000000, 0.8660254037844387076, 1.000000000000000000, 0.8660254037844387076, 1.000000000000000000, 0.8660254037844387076, 1.000000000000000000, 0.8660254037844387076, 1.000000000000000000),
 ( 1.000000000000000000, 0.8660254037844387076, 1.000000000000000000, 0.8660254037844387076, 1.000000000000000000, 0.8660254037844387076, 1.000000000000000000, 0.8660254037844387076, 1.000000000000000000, 0.8660254037844387076, 1.000000000000000000, 0.8660254037844387076, 1.000000000000000000, 0.8660254037844387076, 1.000000000000000000, 0.8660254037844387076, 1.000000000000000000, 0.8660254037844387076, 1.000000000000000000, 0.8660254037844387076, 1.000000000000000000, 0.8660254037844387076, 1.000000000000000000, 0.8660254037844387076, 1.000000000000000000, 0.8660254037844387076, 1.000000000000000000, 0.8660254037844387076, 1.000000000000000000, 0.8660254037844387076, 1.000000000000000000, 0.8660254037844387076, 1.000000000000000000, 0.8660254037844387076, 1.000000000000000000, 0.8660254037844387076, 1.000000000000000000, 0.8660254037844387076, 1.000000000000000000, 0.8660254037844387076, 1.000000000000000000, 0.8660254037844387076, 1.000000000000000000, 0.8660254037844387076, 1.000000000000000000, 0.8660254037844387076, 1.000000000000000000, 0.8660254037844387076, 1.000000000000000000, 0.8660254037844387076, 1.000000000000000000, 0.8660254037844387076, 1.000000000000000000, 0.8660254037844387076, 1.000000000000000000, 0.8660254037844387076, 1.000000000000000000, 0.8660254037844387076, 1.000000000000000000, 0.8660254037844387076, 1.000000000000000000, 0.8660254037844387076, 1.000000000000000000, 0.8660254037844387076, 1.000000000000000000, 0.8660254037844387076, 1.000000000000000000, 0.8660254037844387076, 1.000000000000000000, 0.8660254037844387076, 1.000000000000000000, 0.8660254037844387076, 1.000000000000000000, 0.8660254037844387076, 1.000000000000000000, 0.8660254037844387076, 1.000000000000000000, 0.8660254037844387076, 1.000000000000000000, 0.8660254037844387076, 1.000000000000000000, 0.8660254037844387076, 1.000000000000000000, 0.8660254037844387076, 1.000000000000000000, 0.8660254037844387076, 1.000000000000000000, 0.8660254037844387076, 1.000000000000000000, 0.8660254037844387076, 1.000000000000000000, 0.8660254037844387076, 1.000000000000000000, 0.8660254037844387076, 1.000000000000000000, 0.8660254037844387076, 1.000000000000000000, 0.8660254037844387076, 1.000000000000000000, 0.8660254037844387076, 1.000000000000000000, 0.8660254037844387076, 1.000000000000000000, 0.8660254037844387076, 1.000000000000000000, 0.8660254037844387076, 1.000000000000000000, 0.8660254037844387076, 1.000000000000000000, 0.8660254037844387076, 1.000000000000000000, 0.8660254037844387076, 1.000000000000000000, 0.8660254037844387076, 1.000000000000000000, 0.8660254037844387076, 1.000000000000000000, 0.8660254037844387076, 1.000000000000000000, 0.8660254037844387076, 1.000000000000000000, 0.8660254037844387076, 1.000000000000000000, 0.8660254037844387076, 1.000000000000000000, 0.8660254037844387076, 1.000000000000000000, 0.8660254037844387076, 1.000000000000000000, 0.8660254037844387076, 1.000000000000000000, 0.8660254037844387076, 1.000000000000000000, 0.8660254037844387076, 1.000000000000000000, 0.8660254037844387076, 1.000000000000000000, 0.8660254037844387076, 1.000000000000000000, 0.8660254037844387076, 1.000000000000000000, 0.8660254037844387076, 1.000000000000000000, 0.8660254037844387076, 1.000000000000000000, 0.8660254037844387076, 1.000000000000000000, 0.8660254037844387076, 1.000000000000000000, 0.8660254037844387076, 1.000000000000000000, 0.8660254037844387076, 1.000000000000000000, 0.8660254037844387076, 1.000000000000000000, 0.8660254037844387076, 1.000000000000000000, 0.8660254037844387076, 1.000000000000000000, 0.8660254037844387076, 1.000000000000000000, 0.8660254037844387076, 1.000000000000000000, 0.8660254037844387076, 1.000000000000000000, 0.8660254037844387076, 1.000000000000000000, 0.8660254037844387076, 1.000000000000000000, 0.8660254037844387076, 1.000000000000000000, 0.8660254037844387076, 1.000000000000000000, 0.8660254037844387076, 1.000000000000000000, 0.8660254037844387076, 1.000000000000000000, 0.8660254037844387076, 1.000000000000000000, 0.8660254037844387076, 1.000000000000000000, 0.8660254037844387076, 1.000000000000000000, 0.8660254037844387076, 1.000000000000000000, 0.8660254037844387076, 1.000000000000000000, 0.8660254037844387076, 1.000000000000000000, 0.8660254037844387076, 1.000000000000000000, 0.8660254037844387076, 1.000000000000000000, 0.8660254037844387076, 1.000000000000000000, 0.8660254037844387076, 1.000000000000000000, 0.8660254037844387076, 1.000000000000000000, 0.8660254037844387076, 1.000000000000000000, 0.8660254037844387076, 1.000000000000000000, 0.8660254037844387076, 1.000000000000000000, 0.8660254037844387076, 1.000000000000000000, 0.8660254037844387076, 1.000000000000000000, 0.8660254037844387076, 1.000000000000000000, 0.8660254037844387076, 1.000000000000000000, 0.8660254037844387076, 1.000000000000000000, 0.8660254037844387076, 1.000000000000000000, 0.8660254037844387076, 1.000000000000000000, 0.8660254037844387076, 1.000000000000000000, 0.8660254037844387076, 1.000000000000000000, 0.8660254037844387076, 1.000000000000000000, 0.8660254037844387076, 1.000000000000000000, 0.8660254037844387076, 1.000000000000000000, 0.8660254037844387076, 1.000000000000000000, 0.8660254037844387076, 1.000000000000000000, 0.8660254037844387076, 1.000000000000000000, 0.8660254037844387076, 1.000000000000000000, 0.8660254037844387076, 1.000000000000000000, 0.8660254037844387076, 1.000000000000000000, 0.8660254037844387076, 1.000000000000000000, 0.8660254037844387076, 1.000000000000000000, 0.8660254037844387076, 1.000000000000000000, 0.8660254037844387076, 1.000000000000000000, 0.8660254037844387076, 1.000000000000000000, 0.8660254037844387076, 1.000000000000000000, 0.8660254037844387076, 1.000000000000000000, 0.8660254037844387076, 1.000000000000000000, 0.8660254037844387076, 1.000000000000000000, 0.8660254037844387076, 1.000000000000000000, 0.8660254037844387076, 1.000000000000000000, 0.8660254037844387076, 1.000000000000000000, 0.8660254037844387076, 1.000000000000000000, 0.8660254037844387076, 1.000000000000000000, 0.8660254037844387076, 1.000000000000000000, 0.8660254037844387076, 1.000000000000000000, 0.8660254037844387076, 1.000000000000000000, 0.8660254037844387076, 1.000000000000000000, 0.8660254037844387076, 1.000000000000000000, 0.8660254037844387076, 1.000000000000000000, 0.8660254037844387076, 1.000000000000000000, 0.8660254037844387076, 1.000000000000000000, 0.8660254037844387076, 1.000000000000000000, 0.8660254037844387076, 1.000000000000000000, 0.8660254037844387076, 1.000000000000000000, 0.8660254037844387076, 1.000000000000000000, 0.8660254037844387076, 1.000000000000000000, 0.8660254037844387076, 1.000000000000000000, 0.8660254037844387076, 1.000000000000000000, 0.8660254037844387076, 1.000000000000000000, 0.8660254037844387076, 1.000000000000000000, 0.8660254037844387076, 1.000000000000000000, 0.8660254037844387076, 1.000000000000000000, 0.8660254037844387076, 1.000000000000000000, 0.8660254037844387076, 1.000000000000000000, 0.8660254037844387076, 1.000000000000000000, 0.8660254037844387076, 1.000000000000000000, 0.8660254037844387076, 1.000000000000000000, 0.8660254037844387076, 1.000000000000000000, 0.8660254037844387076, 1.000000000000000000, 0.8660254037844387076, 1.000000000000000000, 0.8660254037844387076, 1.000000000000000000, 0.8660254037844387076, 1.000000000000000000, 0.8660254037844387076, 1.000000000000000000, 0.8660254037844387076, 1.000000000000000000, 0.8660254037844387076, 1.000000000000000000, 0.8660254037844387076, 1.000000000000000000, 0.8660254037844387076, 1.000000000000000000, 0.8660254037844387076, 1.000000000000000000, 0.8660254037844387076, 1.000000000000000000, 0.8660254037844387076, 1.000000000000000000, 0.8660254037844387076, 1.000000000000000000, 0.8660254037844387076, 1.000000000000000000, 0.8660254037844387076, 1.000000000000000000, 0.8660254037844387076, 1.000000000000000000, 0.8660254037844387076, 1.000000000000000000, 0.8660254037844387076, 1.000000000000000000, 0.8660254037844387076, 1.000000000000000000, 0.8660254037844387076, 1.000000000000000000, 0.8660254037844387076, 1.000000000000000000, 0.8660254037844387076, 1.000000000000000000, 0.8660254037844387076, 1.000000000000000000, 0.8660254037844387076, 1.000000000000000000, 0.8660254037844387076, 1.000000000000000000, 0.8660254037844387076, 1.000000000000000000, 0.8660254037844387076, 1.000000000000000000, 0.8660254037844387076, 1.000000000000000000, 0.8660254037844387076, 1.000000000000000000, 0.8660254037844387076, 1.000000000000000000, 0.8660254037844387076, 1.000000000000000000, 0.8660254037844387076, 1.000000000000000000, 0.8660254037844387076, 1.000000000000000000, 0.8660254037844387076, 1.000000000000000000, 0.8660254037844387076, 1.000000000000000000, 0.8660254037844387076, 1.000000000000000000, 0.8660254037844387076, 1.000000000000000000, 0.8660254037844387076, 1.000000000000000000, 0.8660254037844387076, 1.000000000000000000, 0.8660254037844387076, 1.000000000000000000, 0.8660254037844387076, 1.000000000000000000, 0.8660254037844387076, 1.000000000000000000, 0.8660254037844387076, 1.000000000000000000, 0.8660254037844387076, 1.000000000000000000, 0.8660254037844387076, 1.000000000000000000, 0.8660254037844387076, 1.000000000000000000, 0.8660254037844387076, 1.000000000000000000, 0.8660254037844387076, 1.000000000000000000, 0.8660254037844387076, 1.000000000000000000, 0.8660254037844387076, 1.000000000000000000, 0.8660254037844387076, 1.000000000000000000, 0.8660254037844387076, 1.000000000000000000, 0.8660254037844387076, 1.000000000000000000, 0.8660254037844387076, 1.000000000000000000, 0.8660254037844387076, 1.000000000000000000, 0.8660254037844387076, 1.000000000000000000, 0.8660254037844387076, 1.000000000000000000, 0.8660254037844387076, 1.000000000000000000, 0.8660254037844387076, 1.000000000000000000, 0.8660254037844387076, 1.000000000000000000, 0.8660254037844387076, 1.000000000000000000, 0.8660254037844387076, 1.000000000000000000, 0.8660254037844387076, 1.000000000000000000, 0.8660254037844387076, 1.000000000000000000, 0.8660254037844387076, 1.000000000000000000, 0.8660254037844387076, 1.000000000000000000, 0.8660254037844387076, 1.000000000000000000, 0.8660254037844387076, 1.000000000000000000, 0.8660254037844387076, 1.000000000000000000, 0.8660254037844387076, 1.000000000000000000, 0.8660254037844387076, 1.000000000000000000, 0.8660254037844387076, 1.000000000000000000, 0.8660254037844387076, 1.000000000000000000, 0.8660254037844387076, 1.000000000000000000, 0.8660254037844387076, 1.000000000000000000, 0.8660254037844387076, 1.000000000000000000, 0.8660254037844387076, 1.000000000000000000, 0.8660254037844387076, 1.000000000000000000, 0.8660254037844387076, 1.000000000000000000, 0.8660254037844387076, 1.000000000000000000, 0.8660254037844387076, 1.000000000000000000) ) ) 
 REPRESENTATION_ITEM ( '' )  SURFACE ( )  );
#122746=CARTESIAN_POINT ( 'NONE',  ( 1.499999999999989120, 2.556250000682817713, 1.214306433183764966E-14 ) ) ;
#122750=ORIENTED_EDGE ( 'NONE', *, *, #33691, .T. ) ;
#122752=CARTESIAN_POINT ( 'NONE',  ( 0.7499999999999867883, -0.1833333333333131421, -1.299038105676652899 ) ) ;
#122753=CARTESIAN_POINT ( 'NONE',  ( 8.274553823041976841, 8.548067636504127265, 1.040834085586084257E-14 ) ) ;
#122754=CARTESIAN_POINT ( 'NONE',  ( 0.6823417656249882723, 0.1760416670080894308, -1.181850606188749264 ) ) ;
#122758=CARTESIAN_POINT ( 'NONE',  ( 8.093854517678360949, 12.38665467069271386, 1.040834085586084257E-14 ) ) ;
#122765=CARTESIAN_POINT ( 'NONE',  ( -6.728924311084075960, 6.744833205886536120, 1.040834085586084257E-14 ) ) ;
#122766=CARTESIAN_POINT ( 'NONE',  ( 1.499999999999987121, 2.577083334016147198, -0.8660254037844262731 ) ) ;
#122767=CARTESIAN_POINT ( 'NONE',  ( -1.364683531250012516, 4.801041667008083991, -0.7879004041258300672 ) ) ;
#122780=CARTESIAN_POINT ( 'NONE',  ( -7.980945979938748103, 12.46285407657057220, 0.000000000000000000 ) ) ;
#122781=CARTESIAN_POINT ( 'NONE',  ( 8.118635056484817980, 8.366162408854107113, 0.7998128361456481317 ) ) ;
#122789=CARTESIAN_POINT ( 'NONE',  ( -6.561256274009600986, 9.742217188731485678, -1.199719254218440723 ) ) ;
#122795=CARTESIAN_POINT ( 'NONE',  ( 2.544126380858701797, 6.119897877643793116, 0.7998128361456462443 ) ) ;
#122798=CARTESIAN_POINT ( 'NONE',  ( -4.066556009095094737, 6.831733546331167695, 1.199719254218464037 ) ) ;
#122799=CARTESIAN_POINT ( 'NONE',  ( -7.486073373039941359, 11.88550270185529278, -0.7998128361456291469 ) ) ;
#122802=CARTESIAN_POINT ( 'NONE',  ( -3.992976280936286759, 7.825322551632388546, 0.2949607357299148802 ) ) ;
#122809=CARTESIAN_POINT ( 'NONE',  ( 6.681470773436232413, 6.689470745297396270, -0.7998128361456281477 ) ) ;
#122811=CARTESIAN_POINT ( 'NONE',  ( 4.183485216215318658, 3.563207579971337413, 2.499999999999998668 ) ) ;
#122830=CARTESIAN_POINT ( 'NONE',  ( 4.392478581147586603, 4.226905887534702977, -0.7216878364870188411 ) ) ;
#122834=CARTESIAN_POINT ( 'NONE',  ( -9.484092147959342967, 11.02352791316275216, 1.199719254218462483 ) ) ;
#122840=CARTESIAN_POINT ( 'NONE',  ( 1.499999999999989120, 2.306250000682817713, 1.214306433183764966E-14 ) ) ;
#122845=CARTESIAN_POINT ( 'NONE',  ( -8.805130697071332335, 12.36007068230351358, 1.199719254218462483 ) ) ;
#122847=CARTESIAN_POINT ( 'NONE',  ( 1.364683531249988757, 0.6343750003414208027, 0.000000000000000000 ) ) ;
#122849=EDGE_CURVE ( 'NONE', #62256, #63949, #46963, .T. ) ;
#122855=CARTESIAN_POINT ( 'NONE',  ( -3.846762897975357198, 5.510976019103107859, -1.599625672291256295 ) ) ;
#122860=CARTESIAN_POINT ( 'NONE',  ( 1.364683531249988757, -0.3031249996585799744, 0.000000000000000000 ) ) ;
#122865=CARTESIAN_POINT ( 'NONE',  ( -0.6823417656250246877, 0.5510416670080897639, 1.181850606188755259 ) ) ;
#122867=CARTESIAN_POINT ( 'NONE',  ( -6.204827856548512877, 10.39071626594860476, -0.7998128361456291469 ) ) ;
#122868=CARTESIAN_POINT ( 'NONE',  ( 9.413438726589914651, 9.876766690643398405, 0.000000000000000000 ) ) ;
#122869=CARTESIAN_POINT ( 'NONE',  ( 4.355193658487812591, 6.104145239700998538, -1.599625672291255185 ) ) ;
#122872=CARTESIAN_POINT ( 'NONE',  ( -1.402160292154681736E-14, -0.2406249996585799189, -1.575800808251665908 ) ) ;
#122878=CIRCLE ( 'NONE', #112468, 0.07999999999999986289 ) ;
#122882=CARTESIAN_POINT ( 'NONE',  ( 6.643132081016124069, 7.813037518349371879, 1.082531754730558626 ) ) ;
#122885=CARTESIAN_POINT ( 'NONE',  ( -4.416205349749324327, 6.175325546172740765, 1.599625672291267398 ) ) ;
#122886=CARTESIAN_POINT ( 'NONE',  ( 1.499999999999989120, 5.577083334016153415, -0.8660254037844323793 ) ) ;
#122888=CARTESIAN_POINT ( 'NONE',  ( -2.656508033273816238, 5.186677574539687363, -1.199719254218446718 ) ) ;
#122889=CARTESIAN_POINT ( 'NONE',  ( 4.758548728272192108, 7.535095368750792666, -1.082531754730549078 ) ) ;
#122890=CARTESIAN_POINT ( 'NONE',  ( -6.683806541412756985, 10.74159869838281622, -0.7216878364870267237 ) ) ;
#122892=CARTESIAN_POINT ( 'NONE',  ( -1.201851678989727383E-14, 3.962500000000022116, 1.732050807568877637 ) ) ;
#122896=CARTESIAN_POINT ( 'NONE',  ( 8.541273586929342798, 11.94827437051752206, -1.082531754730543083 ) ) ;
#122908=CARTESIAN_POINT ( 'NONE',  ( 8.229436053370676518, 9.663725486096376827, 1.082531754730558626 ) ) ;
#122909=CARTESIAN_POINT ( 'NONE',  ( 7.751511138711133064, 10.06651563329490529, -1.599625672291262513 ) ) ;
#122910=CARTESIAN_POINT ( 'NONE',  ( -6.338600509588822263, 7.353787668397130162, -1.199719254218446718 ) ) ;
#122915=CARTESIAN_POINT ( 'NONE',  ( 5.504247177468190699, 5.523969249908757817, 0.7216878364870317197 ) ) ;
#122917=CARTESIAN_POINT ( 'NONE',  ( -8.026063749610061748, 9.426457798375635022, -1.082531754730543971 ) ) ;
#122944=CARTESIAN_POINT ( 'NONE',  ( -4.876128802409253282, 8.840567369452784874, 0.7998128361456481317 ) ) ;
#122947=CARTESIAN_POINT ( 'NONE',  ( 4.937140493670735708, 8.911747675924535983, -0.7998128361456281477 ) ) ;
#122957=CARTESIAN_POINT ( 'NONE',  ( -3.632695093457760649, 6.325562478087638496, -1.199719254218452047 ) ) ;
#122961=CARTESIAN_POINT ( 'NONE',  ( 7.884230021546724920, 9.157022099014721306, 1.199719254218462483 ) ) ;
#122962=CARTESIAN_POINT ( 'NONE',  ( 1.364683531249990311, 3.884375000341417028, 1.214306433183764966E-14 ) ) ;
#122964=CARTESIAN_POINT ( 'NONE',  ( 6.064713176501767222, 6.047104440226040545, 0.4075101515045934097 ) ) ;
#122969=CARTESIAN_POINT ( 'NONE',  ( 7.280365300414074703, 7.596107060012304402, -0.7216878364870257245 ) ) ;
#122970=CARTESIAN_POINT ( 'NONE',  ( -8.532158741701643123, 8.848606708273724308, 0.7998128361456462443 ) ) ;
#122971=EDGE_CURVE ( 'NONE', #25151, #210539, #83398, .T. ) ;
#122974=CARTESIAN_POINT ( 'NONE',  ( -8.993135964566285168, 9.386413468282476913, -0.7998128361456291469 ) ) ;
#122975=CARTESIAN_POINT ( 'NONE',  ( -5.280010757518168063, 8.247430752824802980, -1.199719254218446718 ) ) ;
#122983=CARTESIAN_POINT ( 'NONE',  ( 7.052212457402625922, 11.37933163361175382, -0.7998128361456291469 ) ) ;
#122998=CARTESIAN_POINT ( 'NONE',  ( -0.7499999999999972244, 4.108333333333360038, -1.299038105676652011 ) ) ;
#122999=CARTESIAN_POINT ( 'NONE',  ( 5.345992642490140057, 5.131412925860272090, 1.040834085586084257E-14 ) ) ;
#123000=CARTESIAN_POINT ( 'NONE',  ( 5.632522751473472589, 8.658694745772667289, -1.199719254218440723 ) ) ;
#123003=CARTESIAN_POINT ( 'NONE',  ( -9.341204650135658483, 10.00041963468749984, 1.040834085586084257E-14 ) ) ;
#123005=CARTESIAN_POINT ( 'NONE',  ( 6.724481002698112775, 8.868313807946373473, -1.443375672974057666 ) ) ;
#123006=EDGE_CURVE ( 'NONE', #129569, #180365, #169308, .T. ) ;
#123007=CARTESIAN_POINT ( 'NONE',  ( -9.042925270190641740, 11.57316545335434199, 1.443375672974064550 ) ) ;
#123009=B_SPLINE_CURVE_WITH_KNOTS ( 'NONE', 3,
 ( #207557, #75438, #7208, #24533, #40821, #205418, #123220, #90641, #176153, #44022 ),
 .UNSPECIFIED., .F., .F.,
 ( 4, 3, 3, 4 ),
 ( 9.838398445787047234E-17, 3.125150876928134587E-05, 6.280292424941480802E-05, 9.436683654567485139E-05 ),
 .UNSPECIFIED. ) ;
#123012=CARTESIAN_POINT ( 'NONE',  ( 6.903072767652295383, 11.20533532890304684, 1.040834085586084257E-14 ) ) ;
#123018=CARTESIAN_POINT ( 'NONE',  ( -1.364683531250012516, 2.238541667008087988, -0.7879004041258289570 ) ) ;
#123024=AXIS2_PLACEMENT_3D ( 'NONE', #66870, #187054, #38686 ) ;
#123025=CARTESIAN_POINT ( 'NONE',  ( 10.26082332744404368, 10.86538205830655279, -0.7998128361456281477 ) ) ;
#123029=CARTESIAN_POINT ( 'NONE',  ( -8.642432853707342488, 12.17025653171218558, 1.199719254218462483 ) ) ;
#123035=CARTESIAN_POINT ( 'NONE',  ( 3.867100128395839942, 5.534702787927018974, -1.599625672291255185 ) ) ;
#123039=CARTESIAN_POINT ( 'NONE',  ( -10.32861409551237486, 10.94447128771960287, 1.040834085586084257E-14 ) ) ;
#123043=CARTESIAN_POINT ( 'NONE',  ( 8.341290820905593151, 10.75459192918846618, 1.599625672291281386 ) ) ;
#123045=CARTESIAN_POINT ( 'NONE',  ( 4.662511749779700843, 6.863130753939731932, 1.222702295491843616 ) ) ;
#123047=CARTESIAN_POINT ( 'NONE',  ( -5.766295404513795297, 5.621766148221195358, 0.7998128361456341429 ) ) ;
#123051=CARTESIAN_POINT ( 'NONE',  ( 8.599949509769960088, 8.927695937686774386, 1.040834085586084257E-14 ) ) ;
#123053=CARTESIAN_POINT ( 'NONE',  ( 5.940443861082012944, 10.08226827123770697, 0.7998128361456462443 ) ) ;
#123055=CARTESIAN_POINT ( 'NONE',  ( -7.700668062882059850, 11.92793714009701311, -0.7216878364870267237 ) ) ;
#123063=CARTESIAN_POINT ( 'NONE',  ( -5.297426666345223190, 6.395294968284933823, -1.134026229594787383 ) ) ;
#123064=CARTESIAN_POINT ( 'NONE',  ( 0.6823417656249899377, 1.592708333674752730, 1.181850606188755259 ) ) ;
#123066=CARTESIAN_POINT ( 'NONE',  ( 5.287316719649520991, 8.151991358691011769, -1.082531754730549078 ) ) ;
#123081=LINE ( 'NONE', #24379, #104338 ) ;
#123086=CARTESIAN_POINT ( 'NONE',  ( 7.723341061279088038, 12.16231500480096983, -0.7998128361456291469 ) ) ;
#123088=ORIENTED_EDGE ( 'NONE', *, *, #144045, .T. ) ;
#123091=CARTESIAN_POINT ( 'NONE',  ( -6.531277313481209212, 8.642909503859968368, 1.599625672291283607 ) ) ;
#123094=CARTESIAN_POINT ( 'NONE',  ( -8.839026081105473054, 12.39961529701003684, -1.199719254218446718 ) ) ;
#123098=CARTESIAN_POINT ( 'NONE',  ( -1.001543065824772872E-14, 5.243750000682815937, 1.732050807568877637 ) ) ;
#123099=CARTESIAN_POINT ( 'NONE',  ( 8.450809820019639318, 8.753699632978056755, -0.7998128361456291469 ) ) ;
#123102=CARTESIAN_POINT ( 'NONE',  ( -7.063961727919978451, 8.200042423116789436, 1.199719254218450271 ) ) ;
#123104=CARTESIAN_POINT ( 'NONE',  ( -1.364683531250012516, 4.988541667008084879, -0.7879004041258300672 ) ) ;
#123105=CARTESIAN_POINT ( 'NONE',  ( -5.966965883657915803, 5.998778352662823998, -0.3115505981291895043 ) ) ;
#123110=CARTESIAN_POINT ( 'NONE',  ( -6.873620692448438874, 10.96304854125777695, 0.000000000000000000 ) ) ;
#123114=CARTESIAN_POINT ( 'NONE',  ( -1.364683531250012516, 4.801041667008083991, -0.7879004041258300672 ) ) ;
#123120=CARTESIAN_POINT ( 'NONE',  ( -0.6823417656250212460, 3.801041667008085767, 1.181850606188767472 ) ) ;
#123121=AXIS2_PLACEMENT_3D ( 'NONE', #156684, #53025, #206474 ) ;
#123122=CARTESIAN_POINT ( 'NONE',  ( -5.284980951228653190, 5.060232619388524533, 0.000000000000000000 ) ) ;
#123123=CARTESIAN_POINT ( 'NONE',  ( 6.368579470117202490, 8.453095353268645695, 1.599625672291281386 ) ) ;
#123124=CARTESIAN_POINT ( 'NONE',  ( -6.518203450479830963, 5.167241622962448488, -2.437504649502885368 ) ) ;
#123126=CARTESIAN_POINT ( 'NONE',  ( 3.009546912109283934, 6.454962464195385330, 0.000000000000000000 ) ) ;
#123127=CARTESIAN_POINT ( 'NONE',  ( -0.6823417656249969321, 5.030208333674755394, -1.181850606188749264 ) ) ;
#123134=CARTESIAN_POINT ( 'NONE',  ( -1.402160292154681736E-14, 0.5718750003414239114, 1.575800808251672791 ) ) ;
#123135=CARTESIAN_POINT ( 'NONE',  ( -2.331639231870358930, 5.664070170583284103, -0.7216878364870267237 ) ) ;
#123136=CARTESIAN_POINT ( 'NONE',  ( 4.473300617505036492, 7.306268922809479704, -1.199719254218452047 ) ) ;
#123140=CARTESIAN_POINT ( 'NONE',  ( 3.958617665510264949, 5.641473247893851628, -1.443375672974051449 ) ) ;
#123143=CARTESIAN_POINT ( 'NONE',  ( -9.354762803749327560, 10.01623748057011376, 0.7216878364870438212 ) ) ;
#123150=CARTESIAN_POINT ( 'NONE',  ( -4.568734577680880093, 7.313645526394248364, -1.082531754730548412 ) ) ;
#123152=CARTESIAN_POINT ( 'NONE',  ( 1.364683531249988757, 1.196875000341421469, 0.000000000000000000 ) ) ;
#123160=CARTESIAN_POINT ( 'NONE',  ( 9.205623113554628034, 9.842241175342985926, 0.7216878364870458196 ) ) ;
#123166=VERTEX_POINT ( 'NONE', #50231 ) ;
#123170=LINE ( 'NONE', #142551, #88260 ) ;
#123173=CARTESIAN_POINT ( 'NONE',  ( -1.364683531250012516, 2.801041667008090652, -0.7879004041258289570 ) ) ;
#123183=CARTESIAN_POINT ( 'NONE',  ( -1.402160292154681736E-14, 0.5718750003414239114, 1.575800808251672791 ) ) ;
#123187=DIRECTION ( 'NONE',  ( 0.000000000000000000, 1.000000000000000000, -8.546850786086437571E-32 ) ) ;
#123192=CARTESIAN_POINT ( 'NONE',  ( 6.518772930072240790, 6.499656594706071822, -0.7998128361456281477 ) ) ;
#123200=CARTESIAN_POINT ( 'NONE',  ( 5.960781091502512119, 10.10599504006161986, 0.7998128361456462443 ) ) ;
#123201=CARTESIAN_POINT ( 'NONE',  ( -5.911983611117388904, 6.103112485921549535, -0.7233604532801055642 ) ) ;
#123203=CARTESIAN_POINT ( 'NONE',  ( 9.368847842243145152, 10.88907622316056312, 1.199719254218453823 ) ) ;
#123213=CARTESIAN_POINT ( 'NONE',  ( -6.548225005720456515, 10.58342024007512983, 0.000000000000000000 ) ) ;
#123218=CARTESIAN_POINT ( 'NONE',  ( -10.29471871147821282, 10.90492667301307605, -0.7998128361456291469 ) ) ;
#123220=CARTESIAN_POINT ( 'NONE',  ( -4.202365068134823467, 3.977385433202452969, -0.5578299018209158522 ) ) ;
#123224=CARTESIAN_POINT ( 'NONE',  ( 10.40996301719436090, 11.03937836301526687, 0.000000000000000000 ) ) ;
#123226=CARTESIAN_POINT ( 'NONE',  ( 3.357615597678655917, 7.068968630600412695, 0.7998128361456321445 ) ) ;
#123233=CARTESIAN_POINT ( 'NONE',  ( -5.799137018343247796, 7.788745826199009237, -1.599625672291256295 ) ) ;
#123235=CARTESIAN_POINT ( 'NONE',  ( -3.002240950422295995, 5.590032644546251817, -1.199719254218452935 ) ) ;
#123241=CARTESIAN_POINT ( 'NONE',  ( 8.188761592974039161, 10.57664116326830595, -1.443375672974063439 ) ) ;
#123243=CARTESIAN_POINT ( 'NONE',  ( 1.364683531249988535, 4.717708333674755394, -0.7879004041258300672 ) ) ;
#123245=CARTESIAN_POINT ( 'NONE',  ( 5.986088515633498197, 6.942523675449257858, -1.199719254218446718 ) ) ;
#123254=CARTESIAN_POINT ( 'NONE',  ( 1.536181705502183137, 8.701161256998862115, -2.509509933406538273 ) ) ;
#123259=CARTESIAN_POINT ( 'NONE',  ( 0.6823417656249899377, 0.6552083336747518416, 1.181850606188755259 ) ) ;
#123261=CARTESIAN_POINT ( 'NONE',  ( 4.704842999142070603, 5.447737239542574272, -1.199719254218452047 ) ) ;
#123264=CARTESIAN_POINT ( 'NONE',  ( -4.907688418466881863, 8.669460888279271416, 0.7216878364870458196 ) ) ;
#123266=CARTESIAN_POINT ( 'NONE',  ( 3.795919822146273326, 5.451659097302528068, -1.443375672974051449 ) ) ;
#123267=CARTESIAN_POINT ( 'NONE',  ( -5.816084710138169633, 8.768887347594400694, 1.082531754730548412 ) ) ;
#123268=( BOUNDED_CURVE ( )  B_SPLINE_CURVE ( 2, ( #157241, #24007, #91181 ),
 .UNSPECIFIED., .F., .T. ) 
 B_SPLINE_CURVE_WITH_KNOTS ( ( 3, 3 ),
 ( 0.000000000000000000, 0.002450381106065499439 ),
 .UNSPECIFIED. ) 
 CURVE ( )  GEOMETRIC_REPRESENTATION_ITEM ( )  RATIONAL_B_SPLINE_CURVE ( ( 1.000000000000000000, 0.9212106833777522485, 0.9350920161047693302 ) ) 
 REPRESENTATION_ITEM ( '' )  );
#123273=CARTESIAN_POINT ( 'NONE',  ( 4.741601036477289810, 6.554953847355395880, 1.599625672291267398 ) ) ;
#123283=CARTESIAN_POINT ( 'NONE',  ( 6.114890974963323345, 7.092793211334054604, 1.199719254218462483 ) ) ;
#123285=CARTESIAN_POINT ( 'NONE',  ( -6.714312387265696458, 8.856450423275211037, 1.599625672291283607 ) ) ;
#123289=CARTESIAN_POINT ( 'NONE',  ( 7.588813295347141441, 9.876701482703580837, -1.599625672291262513 ) ) ;
#123291=CARTESIAN_POINT ( 'NONE',  ( -6.144869935491728441, 8.192100896205577243, -1.599625672291263179 ) ) ;
#123292=CARTESIAN_POINT ( 'NONE',  ( 7.931156673870037643, 8.355363662377600420, -0.7216878364870267237 ) ) ;
#123293=CARTESIAN_POINT ( 'NONE',  ( 4.048816217420559305, 7.761621341895022397, 0.4883610165275272808 ) ) ;
#123294=CARTESIAN_POINT ( 'NONE',  ( -3.574546055497324737, 7.322054164722185732, 0.7998128361456341429 ) ) ;
#123301=CARTESIAN_POINT ( 'NONE',  ( 9.890836756369282057, 11.49806328964105617, -1.199719254218440723 ) ) ;
#123303=CARTESIAN_POINT ( 'NONE',  ( -0.6823417656250003738, 2.467708333674753618, -1.181850606188749264 ) ) ;
#123305=CARTESIAN_POINT ( 'NONE',  ( -7.212574532790110737, 7.517017831117667193, -0.7216878364870278340 ) ) ;
#123310=CARTESIAN_POINT ( 'NONE',  ( -5.788012183699196456, 6.074875824575221017, 0.5810633148162994699 ) ) ;
#123311=CARTESIAN_POINT ( 'NONE',  ( -1.364683531250012516, 1.342708333674755616, 0.7879004041258379498 ) ) ;
#123314=CARTESIAN_POINT ( 'NONE',  ( 2.385871846325007706, 5.727341554113725586, -0.7216878364870267237 ) ) ;
#123318=CARTESIAN_POINT ( 'NONE',  ( -5.274285450916075035, 6.112086766612214284, 1.199719254218450271 ) ) ;
#123320=CARTESIAN_POINT ( 'NONE',  ( -6.832946231163084860, 10.91559500309152675, 0.000000000000000000 ) ) ;
#123327=CARTESIAN_POINT ( 'NONE',  ( -8.649738815394339753, 9.193709494155953621, 1.040834085586084257E-14 ) ) ;
#123331=ORIENTED_EDGE ( 'NONE', *, *, #125522, .T. ) ;
#123332=CARTESIAN_POINT ( 'NONE',  ( -8.148087131688692253, 9.568818410800712826, -1.082531754730543083 ) ) ;
#123338=CARTESIAN_POINT ( 'NONE',  ( 1.499999999999990896, 5.306250000682820378, 1.214306433183764966E-14 ) ) ;
#123339=CARTESIAN_POINT ( 'NONE',  ( 4.499531974119707733, 7.248992493261455117, -1.273121237324711386 ) ) ;
#123343=ORIENTED_EDGE ( 'NONE', *, *, #170700, .F. ) ;
#123346=CARTESIAN_POINT ( 'NONE',  ( -7.528855374290365887, 7.678086112960552434, -0.7998128361456291469 ) ) ;
#123348=CARTESIAN_POINT ( 'NONE',  ( 5.820528018968444961, 5.685037531751635953, 0.7998128361456341429 ) ) ;
#123352=CARTESIAN_POINT ( 'NONE',  ( 7.253775878511261155, 8.421492265473332850, 1.199719254218462483 ) ) ;
#123353=( BOUNDED_CURVE ( )  B_SPLINE_CURVE ( 2, ( #84619, #200483, #67274, #213530, #66203, #165877, #181057 ),
 .UNSPECIFIED., .F., .T. ) 
 B_SPLINE_CURVE_WITH_KNOTS ( ( 3, 2, 2, 3 ),
 ( 0.3962798098108560874, 0.3988095238095238360, 0.4047619047619047672, 0.4072916187605991611 ),
 .UNSPECIFIED. ) 
 CURVE ( )  GEOMETRIC_REPRESENTATION_ITEM ( )  RATIONAL_B_SPLINE_CURVE ( ( 0.9345202395942615592, 0.9430618748659230777, 1.000000000000000000, 0.8660254037844387076, 1.000000000000000000, 0.9430618748653227801, 0.9345202395940813700 ) ) 
 REPRESENTATION_ITEM ( '' )  );
#123359=CARTESIAN_POINT ( 'NONE',  ( -5.097502569058210753, 7.930541516334467467, -1.082531754730549967 ) ) ;
#123368=CARTESIAN_POINT ( 'NONE',  ( 1.364683531249986537, 1.113541667008082658, 0.7879004041258500513 ) ) ;
#123370=CARTESIAN_POINT ( 'NONE',  ( -8.178592977541617515, 10.56477777859713463, 1.599625672291295375 ) ) ;
#123372=CARTESIAN_POINT ( 'NONE',  ( 7.741869408603235136, 8.990934717247309749, 1.199719254218462483 ) ) ;
#123374=CARTESIAN_POINT ( 'NONE',  ( -7.666245793523398078, 11.03137162816423356, 1.199719254218453823 ) ) ;
#123378=CARTESIAN_POINT ( 'NONE',  ( -0.6823417656250212460, 4.551041667008086655, 1.181850606188767472 ) ) ;
#123379=CARTESIAN_POINT ( 'NONE',  ( 8.432808358020015049, 11.82173160345663376, 1.082531754730546636 ) ) ;
#123382=CARTESIAN_POINT ( 'NONE',  ( 1.364683531249986537, -0.8239583329919186738, 0.7879004041258500513 ) ) ;
#123385=CARTESIAN_POINT ( 'NONE',  ( 8.609064354553323639, 10.10662517080946543, -1.082531754730543083 ) ) ;
#123388=CARTESIAN_POINT ( 'NONE',  ( -4.107757355260591936, 7.736207981205250661, 1.040834085586084257E-14 ) ) ;
#123391=CARTESIAN_POINT ( 'NONE',  ( -0.6823417656250212460, 1.801041667008083991, 1.181850606188755259 ) ) ;
#123395=CARTESIAN_POINT ( 'NONE',  ( -7.802881099864745984, 9.062115023719057305, -1.199719254218446718 ) ) ;
#123396=CARTESIAN_POINT ( 'NONE',  ( 1.364683531249988535, 4.967708333674756283, -0.7879004041258300672 ) ) ;
#123401=CARTESIAN_POINT ( 'NONE',  ( 8.609591239877852686, 10.00327685373437347, -1.199719254218445830 ) ) ;
#123404=CARTESIAN_POINT ( 'NONE',  ( -1.201851678989727383E-14, 0.9625000000000237810, 1.732050807568877637 ) ) ;
#123409=VERTEX_POINT ( 'NONE', #173612 ) ;
#123410=CARTESIAN_POINT ( 'NONE',  ( 5.816084710582486217, 9.729256562414162701, 1.040834085586084257E-14 ) ) ;
#123411=CARTESIAN_POINT ( 'NONE',  ( 8.723781775389312543, 12.26516360700784958, -1.199719254218446718 ) ) ;
#123414=CARTESIAN_POINT ( 'NONE',  ( 2.517010073631369860, 6.088262185878572375, -0.7998128361456281477 ) ) ;
#123417=ADVANCED_FACE ( 'NONE', ( #73944, #55562 ), #24108, .F. ) ;
#123421=CARTESIAN_POINT ( 'NONE',  ( 6.916630921265960019, 11.22115317478565188, 0.7998128361456462443 ) ) ;
#123422=CARTESIAN_POINT ( 'NONE',  ( -9.775592450653132204, 11.36361159963886891, -1.199719254218441611 ) ) ;
#123425=CARTESIAN_POINT ( 'NONE',  ( -1.402160292154681736E-14, -0.1781249996585796136, 1.575800808251672791 ) ) ;
#123426=CARTESIAN_POINT ( 'NONE',  ( -1.500000000000015099, 0.6291666666666863028, -0.8660254037844313801 ) ) ;
#123430=CARTESIAN_POINT ( 'NONE',  ( -4.953446695184517523, 4.881368687244443727, 0.2706067644340372502 ) ) ;
#123433=CARTESIAN_POINT ( 'NONE',  ( -1.364683531250010295, 5.488541667008087543, -0.7879004041258300672 ) ) ;
#123435=CARTESIAN_POINT ( 'NONE',  ( -7.458957065812611198, 11.85386701009007204, 0.7998128361456481317 ) ) ;
#123436=CARTESIAN_POINT ( 'NONE',  ( -6.127922243696855453, 7.211959374810172463, 1.082531754730549967 ) ) ;
#123438=CARTESIAN_POINT ( 'NONE',  ( -1.500000000000025091, 4.952083334016149863, 0.8660254037844322683 ) ) ;
#123445=CARTESIAN_POINT ( 'NONE',  ( 7.567422294721922960, 11.98040977715095323, 0.7998128361456462443 ) ) ;
#123449=CARTESIAN_POINT ( 'NONE',  ( 8.405692050348340771, 8.908988268268968724, 1.040834085586084257E-14 ) ) ;
#123452=CARTESIAN_POINT ( 'NONE',  ( -7.811469059767924605, 12.26513100303794168, -0.7998128361456281477 ) ) ;
#123453=CARTESIAN_POINT ( 'NONE',  ( 4.496500501226593727, 8.397667684739696270, 0.7998128361456462443 ) ) ;
#123455=CARTESIAN_POINT ( 'NONE',  ( 2.860407222358963608, 5.320596945185329218, 1.082531754730548412 ) ) ;
#123457=CARTESIAN_POINT ( 'NONE',  ( 2.184835310096557404, 5.700724961754617404, 1.040834085586084257E-14 ) ) ;
#123465=CARTESIAN_POINT ( 'NONE',  ( -4.121315508874255684, 7.752025827087861920, -0.7216878364870267237 ) ) ;
#123466=CARTESIAN_POINT ( 'NONE',  ( 4.518945272056516416, 4.166524327021037699, 0.7998128361456341429 ) ) ;
#123469=CARTESIAN_POINT ( 'NONE',  ( -6.205881626753225966, 8.263281202677319470, 1.599625672291283607 ) ) ;
#123475=CARTESIAN_POINT ( 'NONE',  ( -9.671043645249580933, 10.17730576241299900, 0.7998128361456462443 ) ) ;
#123479=CARTESIAN_POINT ( 'NONE',  ( 4.313465427442102929, 8.184126765324453601, 0.7998128361456462443 ) ) ;
#123482=ORIENTED_EDGE ( 'NONE', *, *, #178819, .T. ) ;
#123488=CARTESIAN_POINT ( 'NONE',  ( 0.000000000000000000, 2.800000000000024691, 1.214306433183764966E-14 ) ) ;
#123489=DIRECTION ( 'NONE',  ( 0.000000000000000000, -0.7999999999972235987, -0.6000000000037019054 ) ) ;
#123490=CARTESIAN_POINT ( 'NONE',  ( -5.682838942422375084, 9.781729199468104596, 0.000000000000000000 ) ) ;
#123493=CARTESIAN_POINT ( 'NONE',  ( 6.168596704537822717, 6.299043698156668647, 1.040834085586084257E-14 ) ) ;
#123497=CARTESIAN_POINT ( 'NONE',  ( 3.181359600701000989, 6.863336634126477875, 0.000000000000000000 ) ) ;
#123499=CARTESIAN_POINT ( 'NONE',  ( -5.331380718671772101, 7.243030143248949670, -1.599625672291256295 ) ) ;
#123502=CARTESIAN_POINT ( 'NONE',  ( 1.387358672534390935, 7.315968950353690659, -4.254625267138188782 ) ) ;
#123507=FACE_OUTER_BOUND ( 'NONE', #35845, .T. ) ;
#123508=CARTESIAN_POINT ( 'NONE',  ( -9.829825065107822724, 11.42688298316931572, 1.199719254218462483 ) ) ;
#123509=CARTESIAN_POINT ( 'NONE',  ( 8.423693512792301163, 8.722063941212843119, 0.7998128361456481317 ) ) ;
#123513=CARTESIAN_POINT ( 'NONE',  ( -5.762678113124475310, 6.090388861115007657, -0.6347866013659544393 ) ) ;
#123520=CARTESIAN_POINT ( 'NONE',  ( 10.39874063200158893, 11.23421161353111586, 0.000000000000000000 ) ) ;
#123526=CARTESIAN_POINT ( 'NONE',  ( -5.775621779818983725, 6.082434804166422460, -0.6095328524017195049 ) ) ;
#123530=( BOUNDED_SURFACE ( )  B_SPLINE_SURFACE ( 3, 2, ( 
 ( #203607, #21645, #84550 ),
 ( #101871, #87752, #166880 ),
 ( #153829, #121407, #5399 ),
 ( #55260, #105093, #138655 ) ),
 .UNSPECIFIED., .F., .F., .T. ) 
 B_SPLINE_SURFACE_WITH_KNOTS ( ( 4, 4 ),
 ( 3, 3 ),
 ( 1.570796326794896114, 2.200856270471036158 ),
 ( 0.000000000000000000, 1.000000000000000000 ),
 .UNSPECIFIED. ) 
 GEOMETRIC_REPRESENTATION_ITEM ( )  RATIONAL_B_SPLINE_SURFACE ( (
 ( 1.000000000000000000, 0.7071067811865544561, 1.000000000000000000),
 ( 1.000000000000000000, 0.7517196685950666701, 1.000000000000000000),
 ( 1.000000000000000000, 0.7917671131335243251, 1.000000000000000000),
 ( 1.000000000000000000, 0.8226529996948415135, 1.000000000000000000) ) ) 
 REPRESENTATION_ITEM ( '' )  SURFACE ( )  );
#123538=CARTESIAN_POINT ( 'NONE',  ( -3.086452525405351643, 6.752611712948207057, 0.7998128361456341429 ) ) ;
#123541=CARTESIAN_POINT ( 'NONE',  ( -4.243865776277440993, 4.909930479533815451, -1.199719254218446718 ) ) ;
#123545=CARTESIAN_POINT ( 'NONE',  ( -1.500000000000001332, -0.8187499993171781787, 0.000000000000000000 ) ) ;
#123550=CARTESIAN_POINT ( 'NONE',  ( 2.835626683552519012, 6.459981564119914310, 0.000000000000000000 ) ) ;
#123554=CARTESIAN_POINT ( 'NONE',  ( 9.028840231696797503, 12.62106513936658203, -1.199719254218446718 ) ) ;
#123560=CARTESIAN_POINT ( 'NONE',  ( 1.364683531249988535, 1.676041667008085101, 0.7879004041258500513 ) ) ;
#123561=CARTESIAN_POINT ( 'NONE',  ( -1.500000000000043299, 3.670833333333355153, 0.8660254037844216102 ) ) ;
#123564=CARTESIAN_POINT ( 'NONE',  ( -8.809047120577080392, 11.30030761213851953, 1.599625672291269396 ) ) ;
#123565=CARTESIAN_POINT ( 'NONE',  ( -4.243338890952892406, 7.894386439512932618, -0.7216878364870257245 ) ) ;
#123567=CARTESIAN_POINT ( 'NONE',  ( -4.381256195510448315, 8.263215994737505454, 1.040834085586084257E-14 ) ) ;
#123569=CARTESIAN_POINT ( 'NONE',  ( 0.7499999999999885647, -1.235416665983847473, 1.299038105676657340 ) ) ;
#123570=EDGE_CURVE ( 'NONE', #146015, #19327, #145621, .T. ) ;
#123578=CARTESIAN_POINT ( 'NONE',  ( -6.358410854684796831, 6.520493539994793863, -0.7216878364870267237 ) ) ;
#123582=CARTESIAN_POINT ( 'NONE',  ( -6.033015167956818026, 6.140865238812146742, -0.7216878364870267237 ) ) ;
#123584=CARTESIAN_POINT ( 'NONE',  ( 10.07387183015377197, 11.71160420905630062, -1.199719254218440723 ) ) ;
#123589=VERTEX_POINT ( 'NONE', #140039 ) ;
#123593=CARTESIAN_POINT ( 'NONE',  ( -4.090809663021341969, 5.795697244990093644, 1.599625672291267398 ) ) ;
#123594=CARTESIAN_POINT ( 'NONE',  ( -9.110189153378817295, 12.71597221466224603, 1.199719254218462483 ) ) ;
#123599=CARTESIAN_POINT ( 'NONE',  ( 8.785320351975350661, 9.351887953500479966, -0.7216878364870197293 ) ) ;
#123600=CARTESIAN_POINT ( 'NONE',  ( 4.957477724091233995, 8.935474444748447098, -0.7998128361456281477 ) ) ;
#123605=CARTESIAN_POINT ( 'NONE',  ( 4.704842999142070603, 5.447737239542574272, -1.199719254218452047 ) ) ;
#123606=CIRCLE ( 'NONE', #151191, 6.959052028703005099 ) ;
#123616=CARTESIAN_POINT ( 'NONE',  ( 9.772729797352075920, 10.29593960653257234, -0.7998128361456281477 ) ) ;
#123617=CARTESIAN_POINT ( 'NONE',  ( -5.551173829791513192, 8.563787670477010394, 1.199719254218452047 ) ) ;
#123623=CARTESIAN_POINT ( 'NONE',  ( 0.6823417656249899377, 5.176041667008086655, -1.181850606188754593 ) ) ;
#123625=CARTESIAN_POINT ( 'NONE',  ( -5.819474248763749635, 7.812472595022922128, -1.599625672291256295 ) ) ;
#123627=CARTESIAN_POINT ( 'NONE',  ( -1.403499169902657995, 7.376709478543001630, -4.304123474984410613 ) ) ;
#123628=CARTESIAN_POINT ( 'NONE',  ( 5.087333953625774008, 6.958308917361963886, 1.599625672291267398 ) ) ;
#123629=CARTESIAN_POINT ( 'NONE',  ( -4.388035272317281077, 8.271124917678806199, 0.7998128361456481317 ) ) ;
#123636=CARTESIAN_POINT ( 'NONE',  ( 7.483737605063422116, 7.833374748769873719, -0.7216878364870257245 ) ) ;
#123638=CARTESIAN_POINT ( 'NONE',  ( 7.931156673870037643, 8.355363662377600420, -0.7216878364870267237 ) ) ;
#123639=CARTESIAN_POINT ( 'NONE',  ( 1.364683531249988535, 3.926041667008087543, 0.7879004041258500513 ) ) ;
#123641=CARTESIAN_POINT ( 'NONE',  ( 5.626270559546821204, 6.626699076635176766, 1.082531754730560403 ) ) ;
#123646=CARTESIAN_POINT ( 'NONE',  ( 1.364683531249990311, 5.613541667008087543, 0.7879004041258500513 ) ) ;
#123651=CARTESIAN_POINT ( 'NONE',  ( -4.565105001785453531, 7.177652750280781646, 1.346018956990787885 ) ) ;
#123658=CARTESIAN_POINT ( 'NONE',  ( -4.406036734316900905, 5.203092947200234519, -1.082531754730543971 ) ) ;
#123660=CARTESIAN_POINT ( 'NONE',  ( 2.333974999846879061, 5.874721266463329705, -0.7998128361456291469 ) ) ;
#123663=CARTESIAN_POINT ( 'NONE',  ( -2.948008335967658322, 5.526761261015804116, 1.199719254218462483 ) ) ;
#123668=CARTESIAN_POINT ( 'NONE',  ( 3.985733972737593778, 6.633478153960411738, -1.082531754730548412 ) ) ;
#123669=CARTESIAN_POINT ( 'NONE',  ( -1.364683531250012516, 3.051041667008083547, -0.7879004041258289570 ) ) ;
#123671=CARTESIAN_POINT ( 'NONE',  ( 7.401861798056875053, 10.72292363345333399, -1.199719254218441611 ) ) ;
#123674=CARTESIAN_POINT ( 'NONE',  ( -4.578903193113314174, 6.365139696764064325, 1.599625672291267175 ) ) ;
#123678=CARTESIAN_POINT ( 'NONE',  ( 1.499999999999987121, 3.045833333333353377, -0.8660254037844262731 ) ) ;
#123679=CARTESIAN_POINT ( 'NONE',  ( 4.578903193113299963, 6.365139696764064325, 1.599625672291267398 ) ) ;
#123684=CARTESIAN_POINT ( 'NONE',  ( -1.201851678989727383E-14, 3.446875000341421469, -1.575800808251660134 ) ) ;
#123686=CARTESIAN_POINT ( 'NONE',  ( 9.571693261567961741, 11.22969222899322617, 1.082531754730548412 ) ) ;
#123691=CARTESIAN_POINT ( 'NONE',  ( -0.7500000000000215383, 2.222916667349486453, 1.299038105676671107 ) ) ;
#123694=CARTESIAN_POINT ( 'NONE',  ( -5.555090253297260361, 7.504024600312024340, 1.599625672291269396 ) ) ;
#123703=CARTESIAN_POINT ( 'NONE',  ( 5.671388329218120639, 5.511041227042920099, 1.040834085586084257E-14 ) ) ;
#123707=CARTESIAN_POINT ( 'NONE',  ( 6.356075086708249167, 6.309842444114747373, -0.7998128361456281477 ) ) ;
#123713=CARTESIAN_POINT ( 'NONE',  ( 9.915090410295563927, 10.46202698829998567, -0.7998128361456281477 ) ) ;
#123718=CARTESIAN_POINT ( 'NONE',  ( 5.892592298951464969, 5.976936425253049912, 0.01597356071081010298 ) ) ;
#123728=DIRECTION ( 'NONE',  ( 0.6507913734559640506, -0.7592566023653004592, 0.000000000000000000 ) ) ;
#123730=CARTESIAN_POINT ( 'NONE',  ( 7.293923454472087897, 8.572294120714675003, 1.082531754730558626 ) ) ;
#123732=CARTESIAN_POINT ( 'NONE',  ( -2.415323921528888196, 5.969628341758991930, 0.7998128361456341429 ) ) ;
#123736=CARTESIAN_POINT ( 'NONE',  ( -5.311043488251275591, 7.219303374425030562, -1.599625672291256295 ) ) ;
#123743=ORIENTED_EDGE ( 'NONE', *, *, #87019, .T. ) ;
#123744=CARTESIAN_POINT ( 'NONE',  ( 3.128205532383693921, 2.800000000000115730, 2.480558432692051340 ) ) ;
#123749=CARTESIAN_POINT ( 'NONE',  ( 9.911173986789782120, 11.52179005846497972, -1.199719254218440723 ) ) ;
#123752=CARTESIAN_POINT ( 'NONE',  ( 4.229780737783593203, 4.037091736943370535, -0.7216878364870188411 ) ) ;
#123754=CARTESIAN_POINT ( 'NONE',  ( 6.471393748265519719, 5.229711127717882491, -2.419999999999995044 ) ) ;
#123757=CARTESIAN_POINT ( 'NONE',  ( -8.622622508611375025, 12.04318144581317895, 1.082531754730560403 ) ) ;
#123761=CARTESIAN_POINT ( 'NONE',  ( 7.214910300766615769, 11.56914578420308715, -0.7998128361456291469 ) ) ;
#123766=CARTESIAN_POINT ( 'NONE',  ( -5.879432169820529630, 10.01108796476595764, -0.7998128361456221525 ) ) ;
#123767=CARTESIAN_POINT ( 'NONE',  ( 4.090809663021327758, 5.795697244990093644, 1.599625672291267398 ) ) ;
#123770=CARTESIAN_POINT ( 'NONE',  ( 8.530051201292206287, 13.10347683481629488, 0.000000000000000000 ) ) ;
#123774=CARTESIAN_POINT ( 'NONE',  ( 0.6823417656249882723, 2.488541667008084435, -1.181850606188749264 ) ) ;
#123776=CARTESIAN_POINT ( 'NONE',  ( 6.155038550924139429, 9.164333495178082600, 1.082531754730558626 ) ) ;
#123778=CARTESIAN_POINT ( 'NONE',  ( 1.499999999999990896, 4.556250000682819490, 1.214306433183764966E-14 ) ) ;
#123781=AXIS2_PLACEMENT_3D ( 'NONE', #71194, #21374, #138373 ) ;
#123785=CARTESIAN_POINT ( 'NONE',  ( 8.229436053370667636, 11.58446391469906267, 1.082531754730558626 ) ) ;
#123791=CARTESIAN_POINT ( 'NONE',  ( -9.826962411806732689, 10.35921099006301382, -0.7998128361456291469 ) ) ;
#123800=CARTESIAN_POINT ( 'NONE',  ( 5.027376032568989572, 4.759693547618927489, 0.7998128361456341429 ) ) ;
#123806=CARTESIAN_POINT ( 'NONE',  ( 6.094553744542824170, 7.069066442510145265, 1.199719254218462483 ) ) ;
#123809=CARTESIAN_POINT ( 'NONE',  ( -1.499999999999997780, 2.681250000682818158, 1.214306433183764966E-14 ) ) ;
#123815=CARTESIAN_POINT ( 'NONE',  ( -1.500000000000001332, 0.1500000000000251132, 0.000000000000000000 ) ) ;
#123816=CARTESIAN_POINT ( 'NONE',  ( 7.426115451983150706, 9.686887332112256388, -1.599625672291262513 ) ) ;
#123818=CARTESIAN_POINT ( 'NONE',  ( -1.364683531250000748, -0.4906249996585801409, 0.000000000000000000 ) ) ;
#123821=CARTESIAN_POINT ( 'NONE',  ( 9.408995418203963013, 12.00024729270324286, 1.443375672974076540 ) ) ;
#123825=CARTESIAN_POINT ( 'NONE',  ( -5.530836599371015794, 8.540060901653093950, 1.199719254218452047 ) ) ;
#123826=CARTESIAN_POINT ( 'NONE',  ( -1.402160292154681736E-14, 2.118750000682816825, -1.732050807568863648 ) ) ;
#123828=CARTESIAN_POINT ( 'NONE',  ( 1.364683531249988535, 4.426041667008082214, 0.7879004041258500513 ) ) ;
#123841=CARTESIAN_POINT ( 'NONE',  ( -8.585337585951595685, 11.03931315507545108, -1.599625672291263179 ) ) ;
#123842=CARTESIAN_POINT ( 'NONE',  ( 7.969495366734495434, 8.192166104145387706, 1.040834085586084257E-14 ) ) ;
#123848=CARTESIAN_POINT ( 'NONE',  ( 2.209183025140937673, 5.729130629306395051, 0.2365836213946782840 ) ) ;
#123850=CARTESIAN_POINT ( 'NONE',  ( -7.043624497499477499, 8.176315654292865887, 1.199719254218450271 ) ) ;
#123854=CARTESIAN_POINT ( 'NONE',  ( 8.920375002787457319, 12.49452237230570084, 1.199719254218450271 ) ) ;
#123856=CARTESIAN_POINT ( 'NONE',  ( -3.893162665418476109, 7.693773542963529444, 1.040834085586084257E-14 ) ) ;
#123857=CARTESIAN_POINT ( 'NONE',  ( -7.811469059767924605, 12.26513100303794168, -0.7998128361456281477 ) ) ;
#123861=CARTESIAN_POINT ( 'NONE',  ( -3.975508435578610555, 7.849559089036333148, -0.01386331990411299175 ) ) ;
#123868=CARTESIAN_POINT ( 'NONE',  ( 5.608269097547198712, 9.694731047113750222, -0.7998128361456281477 ) ) ;
#123870=CARTESIAN_POINT ( 'NONE',  ( 3.039951802757222765, 2.724153688964670028, 2.451370731312843443 ) ) ;
#123888=CARTESIAN_POINT ( 'NONE',  ( 3.009546912553647147, 5.494593250412460606, -1.082531754730543083 ) ) ;
#123892=CARTESIAN_POINT ( 'NONE',  ( -8.109748439268576803, 12.61312361245537517, 0.7998128361456481317 ) ) ;
#123904=CARTESIAN_POINT ( 'NONE',  ( 1.364683531249988757, 0.1343750003414204142, 0.000000000000000000 ) ) ;
#123906=ORIENTED_EDGE ( 'NONE', *, *, #80361, .T. ) ;
#123912=CARTESIAN_POINT ( 'NONE',  ( -5.576481253922474401, 5.400316305864651056, -0.7998128361456221525 ) ) ;
#123913=CARTESIAN_POINT ( 'NONE',  ( -0.4875155550656232184, 6.677512024511295330, -3.385544892646772386 ) ) ;
#123915=CARTESIAN_POINT ( 'NONE',  ( 1.499999999999985123, -0.4541666666666469010, -0.8660254037844323793 ) ) ;
#123917=CARTESIAN_POINT ( 'NONE',  ( -1.364683531250000748, -1.178124999658580752, 0.000000000000000000 ) ) ;
#123923=CARTESIAN_POINT ( 'NONE',  ( -1.364683531250014514, 0.7385416670080887647, -0.7879004041258289570 ) ) ;
#123925=CARTESIAN_POINT ( 'NONE',  ( -5.865874016206865882, 9.995270118883347266, 0.000000000000000000 ) ) ;
#123926=CARTESIAN_POINT ( 'NONE',  ( 9.589694723567584234, 10.08239868711733855, -0.7998128361456281477 ) ) ;
#123927=CARTESIAN_POINT ( 'NONE',  ( 3.330499290451325312, 7.037332938835193730, -0.7998128361456291469 ) ) ;
#123931=CARTESIAN_POINT ( 'NONE',  ( 0.6823417656249882723, -0.09479166632524876901, 1.181850606188755259 ) ) ;
#123938=CARTESIAN_POINT ( 'NONE',  ( 7.619319141200072920, 7.991553207595983643, 0.7216878364870317197 ) ) ;
#123941=CARTESIAN_POINT ( 'NONE',  ( -4.205000198532790279, 8.057583998263570635, 0.7998128361456341429 ) ) ;
#123943=CARTESIAN_POINT ( 'NONE',  ( -0.7499999999999972244, 5.389583334016151639, -1.299038105676652899 ) ) ;
#123945=CARTESIAN_POINT ( 'NONE',  ( 4.311129659021211147, 7.973475668925984472, 1.040834085586084257E-14 ) ) ;
#123946=CARTESIAN_POINT ( 'NONE',  ( -8.690413276235355866, 10.20153224610512943, 1.082531754730558626 ) ) ;
#123948=CARTESIAN_POINT ( 'NONE',  ( 0.7499999999999902300, 3.483333333333352044, 1.299038105676669330 ) ) ;
#123952=CARTESIAN_POINT ( 'NONE',  ( 9.924205255523292024, 10.68058700763975466, -0.7216878364870257245 ) ) ;
#123959=VERTEX_POINT ( 'NONE', #144329 ) ;
#123963=TOROIDAL_SURFACE ( 'NONE', #203458, 0.1600000000000000033, 0.08000000000000000167 ) ;
#123964=CARTESIAN_POINT ( 'NONE',  ( -2.535011536075347571, 5.133042487381361596, -0.9999999999999956701 ) ) ;
#123966=CARTESIAN_POINT ( 'NONE',  ( 6.765155463094740362, 10.83650577367847667, 0.7216878364870438212 ) ) ;
#123968=CARTESIAN_POINT ( 'NONE',  ( 7.065770611016287006, 11.39514947949436774, 1.040834085586084257E-14 ) ) ;
#123972=CARTESIAN_POINT ( 'NONE',  ( 4.080641048033257334, 5.783833860837341412, 1.214306433183764966E-14 ) ) ;
#123973=CARTESIAN_POINT ( 'NONE',  ( 4.284013352238246419, 6.021101549076499637, -1.443375672974051449 ) ) ;
#123974=ORIENTED_EDGE ( 'NONE', *, *, #170032, .T. ) ;
#123975=CARTESIAN_POINT ( 'NONE',  ( -7.863365906246061243, 10.19701286208565705, -1.443375672974059665 ) ) ;
#123979=CARTESIAN_POINT ( 'NONE',  ( -3.735435015764967837, 4.316761258935923884, -1.199719254218452047 ) ) ;
#123984=VERTEX_POINT ( 'NONE', #147776 ) ;
#124002=CARTESIAN_POINT ( 'NONE',  ( -4.903245109636583443, 8.872203061218007392, -0.7998128361456281477 ) ) ;
#124006=CARTESIAN_POINT ( 'NONE',  ( 4.611744806942754238, 8.532119374741881757, -0.7998128361456231517 ) ) ;
#124014=CARTESIAN_POINT ( 'NONE',  ( -3.744022975668147790, 7.519777238254810925, -0.7998128361456281477 ) ) ;
#124019=CARTESIAN_POINT ( 'NONE',  ( 7.637320603199683866, 7.804628880021436288, -0.7998128361456281477 ) ) ;
#124022=CARTESIAN_POINT ( 'NONE',  ( 5.396677706949416731, 6.496517479030419651, 1.312881173378084521 ) ) ;
#124028=CARTESIAN_POINT ( 'NONE',  ( 6.493992390821439642, 7.639041213122241381, -1.082531754730543971 ) ) ;
#124030=CARTESIAN_POINT ( 'NONE',  ( -6.482770005628665011, 10.71498210654212002, 0.7998128361456481317 ) ) ;
#124033=CARTESIAN_POINT ( 'NONE',  ( -8.320953590485107298, 10.73086516036454618, 1.599625672291269396 ) ) ;
#124034=CARTESIAN_POINT ( 'NONE',  ( -7.549192604710863286, 7.701812881784464437, -0.7998128361456291469 ) ) ;
#124041=CARTESIAN_POINT ( 'NONE',  ( 8.158255747121103241, 10.54105100977322174, 1.599625672291281386 ) ) ;
#124056=CARTESIAN_POINT ( 'NONE',  ( -1.499999999999997780, 4.900000000000022560, 1.214306433183764966E-14 ) ) ;
#124057=CARTESIAN_POINT ( 'NONE',  ( 4.660252114795294887, 6.460046772059735432, -1.599625672291256295 ) ) ;
#124058=CARTESIAN_POINT ( 'NONE',  ( 6.226218857173709154, 8.287007971501239467, 1.599625672291281386 ) ) ;
#124061=CARTESIAN_POINT ( 'NONE',  ( -8.839552966430012759, 10.37552855133225904, -1.082531754730543971 ) ) ;
#124063=CARTESIAN_POINT ( 'NONE',  ( 7.307481608085759639, 7.627742752295940676, 1.040834085586084257E-14 ) ) ;
#124064=CARTESIAN_POINT ( 'NONE',  ( -7.659993601596706725, 11.88048360193076647, -0.7216878364870267237 ) ) ;
#124067=CARTESIAN_POINT ( 'NONE',  ( 9.589694723567584234, 10.08239868711733855, -0.7998128361456281477 ) ) ;
#124071=CARTESIAN_POINT ( 'NONE',  ( -2.310360766237192109, 5.468970595003730395, -0.7883092092346147828 ) ) ;
#124073=CARTESIAN_POINT ( 'NONE',  ( -1.364683531250014514, 1.738541667008085545, -0.7879004041258289570 ) ) ;
#124078=CARTESIAN_POINT ( 'NONE',  ( -1.402160292154681736E-14, -0.6781249996585819728, 1.575800808251672791 ) ) ;
#124081=CARTESIAN_POINT ( 'NONE',  ( 8.224992744984721327, 12.74757530245756243, 1.040834085586084257E-14 ) ) ;
#124085=CARTESIAN_POINT ( 'NONE',  ( -8.482597663644387609, 13.04811437422715414, -0.7998128361456281477 ) ) ;
#124091=CARTESIAN_POINT ( 'NONE',  ( 5.054492339796319733, 4.791329239384148231, -0.7998128361456211532 ) ) ;
#124094=CARTESIAN_POINT ( 'NONE',  ( -9.992522908471816123, 11.61669713376064372, 1.199719254218462483 ) ) ;
#124097=CARTESIAN_POINT ( 'NONE',  ( 8.829384350997564468, 11.32403438096243775, 1.599625672291281386 ) ) ;
#124099=CARTESIAN_POINT ( 'NONE',  ( 4.546345379095670047, 6.970243970676179401, 1.177900817425497904 ) ) ;
#124100=CARTESIAN_POINT ( 'NONE',  ( 0.7869457366334648984, 2.800000000000024247, -1.251086691529569306 ) ) ;
#124102=CARTESIAN_POINT ( 'NONE',  ( -3.228813138348844536, 6.918699094715619502, 0.7998128361456341429 ) ) ;
#124106=CARTESIAN_POINT ( 'NONE',  ( 6.889514614038635187, 11.18951748302043114, -0.7998128361456291469 ) ) ;
#124108=CARTESIAN_POINT ( 'NONE',  ( 8.288111976655649471, 8.563885482386732306, -0.7998128361456291469 ) ) ;
#124111=CARTESIAN_POINT ( 'NONE',  ( -7.510853912290736289, 11.70648729774046792, 0.7216878364870458196 ) ) ;
#124118=CARTESIAN_POINT ( 'NONE',  ( -4.791002085003811750, 6.784460936665063890, -1.245152473204954591 ) ) ;
#124119=CARTESIAN_POINT ( 'NONE',  ( -1.402160292154681736E-14, 2.196875000341423689, -1.575800808251660134 ) ) ;
#124121=AXIS2_PLACEMENT_3D ( 'NONE', #173391, #24974, #176574 ) ;
#124122=CARTESIAN_POINT ( 'NONE',  ( 5.016153647376196290, 8.796003655340152605, 0.7216878364870438212 ) ) ;
#124140=CARTESIAN_POINT ( 'NONE',  ( 8.398386088661320414, 11.88553530582519357, -1.199719254218446718 ) ) ;
#124144=CARTESIAN_POINT ( 'NONE',  ( -3.972702704004144714, 4.593573561881607148, 1.199719254218462483 ) ) ;
#124145=CARTESIAN_POINT ( 'NONE',  ( -7.314787569772770226, 8.492672571945082183, -1.199719254218452935 ) ) ;
#124148=CARTESIAN_POINT ( 'NONE',  ( -9.972185678051314284, 11.59297036493672017, 1.199719254218462483 ) ) ;
#124152=CARTESIAN_POINT ( 'NONE',  ( 1.499999999999990896, 4.306250000682819490, 1.214306433183764966E-14 ) ) ;
#124153=CARTESIAN_POINT ( 'NONE',  ( 6.103141704446003679, 10.27208242182903142, 0.7998128361456462443 ) ) ;
#124156=CARTESIAN_POINT ( 'NONE',  ( -6.093499974338126179, 9.196501505781426999, -1.199719254218440723 ) ) ;
#124158=CARTESIAN_POINT ( 'NONE',  ( -1.364683531250012516, 4.738541667008091096, -0.7879004041258300672 ) ) ;
#124164=CARTESIAN_POINT ( 'NONE',  ( -7.700668062882065179, 10.96756792579566664, -1.082531754730543971 ) ) ;
#124168=CARTESIAN_POINT ( 'NONE',  ( -0.6823417656250212460, 2.613541667008084879, 1.181850606188767472 ) ) ;
#124174=CARTESIAN_POINT ( 'NONE',  ( 1.364683531249988535, 4.155208333674753618, -0.7879004041258239610 ) ) ;
#124176=CARTESIAN_POINT ( 'NONE',  ( -3.750802052474980108, 7.527686161196117887, 1.040834085586084257E-14 ) ) ;
#124177=CARTESIAN_POINT ( 'NONE',  ( 5.452350330990040739, 9.512825819463730070, 0.7998128361456462443 ) ) ;
#124180=CARTESIAN_POINT ( 'NONE',  ( 3.999292125906905859, 5.688926785023260102, 1.443375672974062551 ) ) ;
#124181=CARTESIAN_POINT ( 'NONE',  ( 1.364683531249988535, 3.467708333674749621, -0.7879004041258239610 ) ) ;
#124182=CARTESIAN_POINT ( 'NONE',  ( 1.403499169902377552, 7.376709478543040710, 4.304123474984470121 ) ) ;
#124186=CARTESIAN_POINT ( 'NONE',  ( -1.402160292154681736E-14, 1.446875000341420137, -1.575800808251659024 ) ) ;
#124187=CARTESIAN_POINT ( 'NONE',  ( -5.260200412422213923, 6.199617238323108737, -1.082531754730544860 ) ) ;
#124188=CARTESIAN_POINT ( 'NONE',  ( 6.471319392424407901, 6.444294134116939077, 0.7998128361456341429 ) ) ;
#124192=CARTESIAN_POINT ( 'NONE',  ( 5.016153647376217606, 4.954526798134778254, 0.7216878364870317197 ) ) ;
#124195=CARTESIAN_POINT ( 'NONE',  ( -7.836249599018719536, 12.08611559892311504, 0.7216878364870478180 ) ) ;
#124200=CARTESIAN_POINT ( 'NONE',  ( -10.14557902172788495, 10.73093036830436553, 1.040834085586084257E-14 ) ) ;
#124201=CARTESIAN_POINT ( 'NONE',  ( -6.033015167956810920, 7.101234453113482559, -1.082531754730543083 ) ) ;
#124203=CARTESIAN_POINT ( 'NONE',  ( 1.364683531249986537, 0.7177083336747527298, -0.7879004041258239610 ) ) ;
#124216=CARTESIAN_POINT ( 'NONE',  ( 7.402388682937041331, 11.57994453016116587, 1.040834085586084257E-14 ) ) ;
#124222=EDGE_CURVE ( 'NONE', #214172, #162715, #51331, .T. ) ;
#124227=CARTESIAN_POINT ( 'NONE',  ( -2.442440228756222353, 6.001264033524212671, -0.7998128361456281477 ) ) ;
#124231=CARTESIAN_POINT ( 'NONE',  ( -0.6823417656250003738, 1.280208333674752508, -1.181850606188749264 ) ) ;
#124240=VERTEX_POINT ( 'NONE', #66471 ) ;
#124245=ORIENTED_EDGE ( 'NONE', *, *, #65741, .F. ) ;
#124249=CARTESIAN_POINT ( 'NONE',  ( 4.710568305744190276, 7.583081225755162968, 1.199719254218462483 ) ) ;
#124256=CARTESIAN_POINT ( 'NONE',  ( 6.448874621594486989, 10.67543749183559143, 0.7998128361456462443 ) ) ;
#124259=CARTESIAN_POINT ( 'NONE',  ( 8.829384350997564468, 11.32403438096243775, 1.599625672291281386 ) ) ;
#124261=CARTESIAN_POINT ( 'NONE',  ( 1.541006503187393850, 8.695732182938039401, -2.510084419394968513 ) ) ;
#124264=ORIENTED_EDGE ( 'NONE', *, *, #114516, .F. ) ;
#124272=CARTESIAN_POINT ( 'NONE',  ( -6.724481002698120768, 9.828683022247721723, -1.082531754730538864 ) ) ;
#124277=CARTESIAN_POINT ( 'NONE',  ( -10.08065090696061716, 11.71951313199760136, -1.199719254218441611 ) ) ;
#124279=CARTESIAN_POINT ( 'NONE',  ( -4.649416048473335117, 6.918063047017545486, -1.244856393069911915 ) ) ;
#124283=CARTESIAN_POINT ( 'NONE',  ( 2.372313692266983853, 5.711523707712699682, 0.7216878364870438212 ) ) ;
#124292=CARTESIAN_POINT ( 'NONE',  ( -4.557512192488103686, 8.468847991211438497, -0.7998128361456281477 ) ) ;
#124294=CARTESIAN_POINT ( 'NONE',  ( -2.625475302540713152, 6.214804952939456228, -0.7998128361456281477 ) ) ;
#124300=CARTESIAN_POINT ( 'NONE',  ( 7.619319141200051604, 11.83303006480134911, 0.7216878364870438212 ) ) ;
#124302=CARTESIAN_POINT ( 'NONE',  ( -1.201851678989727383E-14, 3.884375000341423689, 1.575800808251672791 ) ) ;
#124304=CARTESIAN_POINT ( 'NONE',  ( 6.145923705696426431, 6.064665832934283962, 0.7998128361456341429 ) ) ;
#124309=EDGE_CURVE ( 'NONE', #40788, #44957, #18941, .T. ) ;
#124316=EDGE_LOOP ( 'NONE', ( #53721, #156403 ) ) ;
#124318=CARTESIAN_POINT ( 'NONE',  ( 0.6823417656249882723, 1.488541667008083547, -1.181850606188749264 ) ) ;
#124320=CARTESIAN_POINT ( 'NONE',  ( 4.715538499454675403, 4.395883092318884522, 1.214306433183764966E-14 ) ) ;
#124322=CARTESIAN_POINT ( 'NONE',  ( -5.531363484695544841, 8.436712584578003771, 1.082531754730548412 ) ) ;
#124323=CARTESIAN_POINT ( 'NONE',  ( 4.365362273920250225, 5.155639410070820716, 1.082531754730560403 ) ) ;
#124324=CARTESIAN_POINT ( 'NONE',  ( -7.036318535368094373, 7.311385834125318617, 0.7216878364870317197 ) ) ;
#124328=CARTESIAN_POINT ( 'NONE',  ( 6.257251587906815793, 7.258880593101466161, 1.199719254218462483 ) ) ;
#124339=CARTESIAN_POINT ( 'NONE',  ( 6.632963465583686435, 8.761543347979550589, -1.599625672291262513 ) ) ;
#124341=CARTESIAN_POINT ( 'NONE',  ( -6.738566041191992539, 7.820414121934134322, 1.199719254218450271 ) ) ;
#124345=CARTESIAN_POINT ( 'NONE',  ( 6.726816770674637347, 10.99970333242910669, -0.7998128361456291469 ) ) ;
#124348=CARTESIAN_POINT ( 'NONE',  ( -7.386494761346872551, 7.511998731193139989, -0.7998128361456291469 ) ) ;
#124350=CARTESIAN_POINT ( 'NONE',  ( 7.470179451005385829, 8.777926116670192513, -1.082531754730537976 ) ) ;
#124351=CARTESIAN_POINT ( 'NONE',  ( 4.383065840713377348, 7.132475524829186675, -1.069666325224464032 ) ) ;
#124352=CARTESIAN_POINT ( 'NONE',  ( -4.574986769607567894, 7.424902766929059261, 1.199719254218464037 ) ) ;
#124359=CARTESIAN_POINT ( 'NONE',  ( 9.752392566931574081, 10.27221283770866300, -0.7998128361456281477 ) ) ;
#124360=CARTESIAN_POINT ( 'NONE',  ( -5.602744053211161201, 6.190815373437144942, 0.8771416995774529157 ) ) ;
#124362=CARTESIAN_POINT ( 'NONE',  ( 0.6823417656249882723, 1.176041667008083325, -1.181850606188749264 ) ) ;
#124364=CARTESIAN_POINT ( 'NONE',  ( -6.914295153289458540, 7.169025221700239925, 0.7216878364870317197 ) ) ;
#124370=CARTESIAN_POINT ( 'NONE',  ( -5.762141863986474100, 6.090740110424618159, 0.6348889758391648153 ) ) ;
#124371=CARTESIAN_POINT ( 'NONE',  ( -1.402160292154681736E-14, 1.759375000341421469, -1.575800808251659024 ) ) ;
#124374=CARTESIAN_POINT ( 'NONE',  ( 3.226477370372305753, 4.787309570232886280, 1.443375672974062551 ) ) ;
#124379=CARTESIAN_POINT ( 'NONE',  ( -6.982085920913410071, 11.08959130780024260, 0.7216878364870458196 ) ) ;
#124386=CARTESIAN_POINT ( 'NONE',  ( -7.144783764277399030, 11.27940545839156528, 0.7216878364870458196 ) ) ;
#124389=DIRECTION ( 'NONE',  ( -5.578564026256490882E-16, -1.000000000000000000, -9.066213480720158442E-32 ) ) ;
#124392=CARTESIAN_POINT ( 'NONE',  ( -6.670248387799091461, 10.72578085250020585, 0.000000000000000000 ) ) ;
#124399=CARTESIAN_POINT ( 'NONE',  ( 1.499999999999990896, 5.056250000682820378, 1.214306433183764966E-14 ) ) ;
#124405=CARTESIAN_POINT ( 'NONE',  ( -6.693975156845199059, 8.832723654451292816, 1.599625672291283607 ) ) ;
#124406=CARTESIAN_POINT ( 'NONE',  ( -2.916975605234527702, 6.554888639415577423, 1.040834085586084257E-14 ) ) ;
#124409=CARTESIAN_POINT ( 'NONE',  ( 4.741601036477289810, 6.554953847355395880, 1.599625672291267398 ) ) ;
#124413=CARTESIAN_POINT ( 'NONE',  ( 6.662942426112080874, 9.860851032851066122, 1.199719254218460707 ) ) ;
#124421=CARTESIAN_POINT ( 'NONE',  ( -5.178851490740209229, 7.065079377328788546, 1.443375672974064550 ) ) ;
#124424=CARTESIAN_POINT ( 'NONE',  ( -6.385527162356468445, 10.39360608948380538, 1.040834085586084257E-14 ) ) ;
#124432=CARTESIAN_POINT ( 'NONE',  ( -9.176171038350775078, 9.599954387697719582, -0.7998128361456291469 ) ) ;
#124434=CARTESIAN_POINT ( 'NONE',  ( 6.448874621594486989, 10.67543749183559143, 0.7998128361456462443 ) ) ;
#124435=CARTESIAN_POINT ( 'NONE',  ( 0.7499999999999885647, -0.2666666666666442365, 1.299038105676657340 ) ) ;
#124436=CARTESIAN_POINT ( 'NONE',  ( -7.609150525767646833, 9.900428251527500834, -1.599625672291263179 ) ) ;
#124439=CARTESIAN_POINT ( 'NONE',  ( 1.364683531249990311, 4.863541667008084879, 0.7879004041258500513 ) ) ;
#124440=CARTESIAN_POINT ( 'NONE',  ( 8.758204044747998296, 11.24099069033793974, 1.443375672974076540 ) ) ;
#124444=CARTESIAN_POINT ( 'NONE',  ( -1.500000000000011324, 5.129166666666691299, -0.8660254037844313801 ) ) ;
#124446=CARTESIAN_POINT ( 'NONE',  ( 9.219181267168295335, 9.858059021225592744, 1.040834085586084257E-14 ) ) ;
#124448=CARTESIAN_POINT ( 'NONE',  ( 5.738313685646321716, 5.917571446856333850, 2.440166996132847377 ) ) ;
#124449=CARTESIAN_POINT ( 'NONE',  ( -4.433153041988574294, 8.115836282387899558, 1.040834085586084257E-14 ) ) ;
#124451=CARTESIAN_POINT ( 'NONE',  ( -1.201851678989727383E-14, 1.821875000341421691, 1.575800808251672791 ) ) ;
#124455=CARTESIAN_POINT ( 'NONE',  ( -6.181627972826976958, 9.299317504018391745, 1.199719254218452047 ) ) ;
#124456=CARTESIAN_POINT ( 'NONE',  ( 0.6823417656249917140, 5.155208333674749177, 1.181850606188765695 ) ) ;
#124462=CARTESIAN_POINT ( 'NONE',  ( 8.555358625423188812, 9.940005470203933768, 1.199719254218462483 ) ) ;
#124465=CARTESIAN_POINT ( 'NONE',  ( 0.7499999999999885647, 1.566666666666688412, -1.299038105676652899 ) ) ;
#124470=CARTESIAN_POINT ( 'NONE',  ( 6.805829924380105034, 9.923590097543378619, 1.082531754730558626 ) ) ;
#124471=EDGE_CURVE ( 'NONE', #195242, #27525, #94012, .T. ) ;
#124478=CARTESIAN_POINT ( 'NONE',  ( 9.264299036839600987, 9.702770385934682551, -0.7998128361456281477 ) ) ;
#124479=CARTESIAN_POINT ( 'NONE',  ( -10.64045162862669081, 11.30828174301964140, -0.7998128361456221525 ) ) ;
#124481=CARTESIAN_POINT ( 'NONE',  ( 7.334597915313080918, 9.580116872663850813, 1.040834085586084257E-14 ) ) ;
#124482=CARTESIAN_POINT ( 'NONE',  ( 1.364683531249986981, -1.115624999658580752, 0.000000000000000000 ) ) ;
#124483=CARTESIAN_POINT ( 'NONE',  ( 1.499999999999989120, 0.5250000000000185629, 0.000000000000000000 ) ) ;
#124486=EDGE_CURVE ( 'NONE', #54906, #182393, #86096, .T. ) ;
#124490=CARTESIAN_POINT ( 'NONE',  ( -0.6823417656249969321, 4.967708333674755394, -1.181850606188749264 ) ) ;
#124492=CARTESIAN_POINT ( 'NONE',  ( -4.744990575102892905, 8.479646737687938085, 0.7216878364870458196 ) ) ;
#124501=CARTESIAN_POINT ( 'NONE',  ( 7.401861798056875053, 10.72292363345333399, -1.199719254218441611 ) ) ;
#124507=CARTESIAN_POINT ( 'NONE',  ( -8.971744963941075568, 11.49012176272984931, 1.599625672291269396 ) ) ;
#124508=CARTESIAN_POINT ( 'NONE',  ( 5.445571254183207088, 9.504916896522420444, -0.7998128361456281477 ) ) ;
#124510=CARTESIAN_POINT ( 'NONE',  ( 3.728129053633592704, 4.412200653069714207, -1.082531754730543083 ) ) ;
#124512=CARTESIAN_POINT ( 'NONE',  ( 3.662674053986138656, 7.424870162959149589, 0.7998128361456321445 ) ) ;
#124518=CARTESIAN_POINT ( 'NONE',  ( 3.046330065665291187, 6.497876143344064381, -0.2071306710573911913 ) ) ;
#124521=CARTESIAN_POINT ( 'NONE',  ( -5.422898255786198440, 7.349800603215774331, -1.443375672974052559 ) ) ;
#124522=CARTESIAN_POINT ( 'NONE',  ( 10.05978679165993839, 10.83876546646586014, 0.7216878364870438212 ) ) ;
#124525=CARTESIAN_POINT ( 'NONE',  ( -7.263417608619167076, 9.497073181520933716, -1.599625672291263179 ) ) ;
#124530=CARTESIAN_POINT ( 'NONE',  ( -7.995557903757128493, 10.35123685918189729, 1.599625672291295375 ) ) ;
#124534=CARTESIAN_POINT ( 'NONE',  ( 7.151035956204054855, 10.43029348462504124, 1.199719254218460707 ) ) ;
#124536=CARTESIAN_POINT ( 'NONE',  ( 4.961394147597008697, 7.875711374583454827, -1.199719254218452047 ) ) ;
#124547=CARTESIAN_POINT ( 'NONE',  ( -1.123270288249902160, 2.800000000000024691, 0.7750000000000117906 ) ) ;
#124548=CARTESIAN_POINT ( 'NONE',  ( -7.965578943228732278, 9.251929174310385307, -1.199719254218446718 ) ) ;
#124551=CARTESIAN_POINT ( 'NONE',  ( 7.185458225562760148, 8.445751353653788485, -1.082531754730543083 ) ) ;
#124555=CARTESIAN_POINT ( 'NONE',  ( 4.878236342818665250, 4.585697242910212523, 1.040834085586084257E-14 ) ) ;
#124557=CARTESIAN_POINT ( 'NONE',  ( -6.084912014434944894, 5.993485526462540847, -0.7998128361456291469 ) ) ;
#124566=CARTESIAN_POINT ( 'NONE',  ( 9.264299036839600987, 9.702770385934682551, -0.7998128361456281477 ) ) ;
#124568=CARTESIAN_POINT ( 'NONE',  ( -2.331639231870358930, 5.664070170583284103, -0.7216878364870267237 ) ) ;
#124570=CARTESIAN_POINT ( 'NONE',  ( -4.981332701451811396, 6.629279788159643694, -1.242877772926734625 ) ) ;
#124573=CARTESIAN_POINT ( 'NONE',  ( 0.6823417656249864960, -1.011458332991911568, -1.181850606188749264 ) ) ;
#124575=ORIENTED_EDGE ( 'NONE', *, *, #6451, .F. ) ;
#124577=CARTESIAN_POINT ( 'NONE',  ( 8.595506201384004896, 12.01154575404795466, 1.082531754730546636 ) ) ;
#124597=CARTESIAN_POINT ( 'NONE',  ( -2.462777459176719308, 6.024990802348131780, -0.7998128361456281477 ) ) ;
#124598=CARTESIAN_POINT ( 'NONE',  ( -1.500000000000013101, 3.629166666666692187, -0.8660254037844313801 ) ) ;
#124600=CARTESIAN_POINT ( 'NONE',  ( -4.322352044658376968, 3.937165561723182883, 0.7998128361456341429 ) ) ;
#124605=( GEOMETRIC_REPRESENTATION_CONTEXT ( 3 ) GLOBAL_UNCERTAINTY_ASSIGNED_CONTEXT ( ( #33417 ) ) GLOBAL_UNIT_ASSIGNED_CONTEXT ( ( #37663, #43025, #142664 ) ) REPRESENTATION_CONTEXT ( 'NONE', 'WORKASPACE' ) );
#124606=CARTESIAN_POINT ( 'NONE',  ( -1.201851678989727383E-14, 4.071875000341425022, 1.575800808251672791 ) ) ;
#124609=CARTESIAN_POINT ( 'NONE',  ( -4.134873662487946966, 3.926366815765101936, 1.214306433183764966E-14 ) ) ;
#124615=CARTESIAN_POINT ( 'NONE',  ( 2.703961570921634028, 5.242040035128820108, -1.199719254218446718 ) ) ;
#124620=CARTESIAN_POINT ( 'NONE',  ( 1.364683531249986537, 1.176041667008082658, 0.7879004041258500513 ) ) ;
#124623=CARTESIAN_POINT ( 'NONE',  ( -9.494787648271923786, 9.971673765939062406, 1.040834085586084257E-14 ) ) ;
#124625=CARTESIAN_POINT ( 'NONE',  ( -5.436456408955534947, 6.405249234278626247, 1.082531754730546636 ) ) ;
#124629=CARTESIAN_POINT ( 'NONE',  ( -0.6823417656249969321, 5.217708333674756283, -1.181850606188749264 ) ) ;
#124638=CARTESIAN_POINT ( 'NONE',  ( -5.707619481228834779, 5.761236937629489852, -0.7216878364870197293 ) ) ;
#124643=CARTESIAN_POINT ( 'NONE',  ( -4.243338890952901288, 6.934017225211593249, -1.082531754730548412 ) ) ;
#124645=CARTESIAN_POINT ( 'NONE',  ( 10.26082332744404368, 10.86538205830655279, -0.7998128361456281477 ) ) ;
#124654=CARTESIAN_POINT ( 'NONE',  ( -4.874319919312905647, 5.645460313075203018, -1.199719254218446718 ) ) ;
#124659=CARTESIAN_POINT ( 'NONE',  ( 8.432808358020015049, 11.82173160345663376, 1.082531754730546636 ) ) ;
#124660=CARTESIAN_POINT ( 'NONE',  ( 5.575427483717746213, 7.527751369135936343, 1.599625672291267398 ) ) ;
#124663=ORIENTED_EDGE ( 'NONE', *, *, #148115, .T. ) ;
#124665=CARTESIAN_POINT ( 'NONE',  ( 5.366329872910639232, 5.155139694684188534, 1.040834085586084257E-14 ) ) ;
#124674=CARTESIAN_POINT ( 'NONE',  ( -6.749261541504576911, 6.768559974710451677, 1.040834085586084257E-14 ) ) ;
#124680=CARTESIAN_POINT ( 'NONE',  ( -0.6823417656249969321, 5.217708333674756283, -1.181850606188749264 ) ) ;
#124681=CARTESIAN_POINT ( 'NONE',  ( 9.422553571373278203, 11.05569592376608945, -1.082531754730543083 ) ) ;
#124682=CARTESIAN_POINT ( 'NONE',  ( -4.876128802409253282, 8.840567369452784874, 0.7998128361456481317 ) ) ;
#124685=CARTESIAN_POINT ( 'NONE',  ( 6.179819089730593795, 6.104210447640811665, 1.040834085586084257E-14 ) ) ;
#124686=CARTESIAN_POINT ( 'NONE',  ( -4.076197739202962467, 7.907314462378773001, 1.040834085586084257E-14 ) ) ;
#124692=CARTESIAN_POINT ( 'NONE',  ( 5.327991180490514012, 9.159814110640187579, 1.040834085586084257E-14 ) ) ;
#124694=CARTESIAN_POINT ( 'NONE',  ( 7.917598520256366790, 8.339545816494993602, 1.040834085586084257E-14 ) ) ;
#124695=CARTESIAN_POINT ( 'NONE',  ( 1.364683531249986537, 2.717708333674754062, -0.7879004041258239610 ) ) ;
#124697=CARTESIAN_POINT ( 'NONE',  ( 5.788968402910812827, 6.816513227226497662, 1.082531754730558626 ) ) ;
#124701=CARTESIAN_POINT ( 'NONE',  ( 0.6823417656249899377, 5.676041667008087543, -1.181850606188754593 ) ) ;
#124706=CARTESIAN_POINT ( 'NONE',  ( -3.999491622362644883, 7.816382810427971783, -0.3443157113667428271 ) ) ;
#124714=CARTESIAN_POINT ( 'NONE',  ( 4.469384193999260901, 8.366031992974468423, -0.7998128361456231517 ) ) ;
#124716=CARTESIAN_POINT ( 'NONE',  ( -4.582292731294565158, 4.448355729372827305, 1.214306433183764966E-14 ) ) ;
#124725=CARTESIAN_POINT ( 'NONE',  ( 3.063779527008304360, 6.518233848244248563, 0.7216878364870317197 ) ) ;
#124728=CARTESIAN_POINT ( 'NONE',  ( 1.364683531249988535, 2.176041667008087543, 0.7879004041258500513 ) ) ;
#124730=CARTESIAN_POINT ( 'NONE',  ( 7.914208982075123799, 10.25632978388623684, -1.599625672291262513 ) ) ;
#124733=CARTESIAN_POINT ( 'NONE',  ( -5.739179097286464248, 5.590130456455973729, -0.7998128361456221525 ) ) ;
#124737=CARTESIAN_POINT ( 'NONE',  ( -0.7500000000000215383, 3.191666666666689967, 1.299038105676671107 ) ) ;
#124738=CARTESIAN_POINT ( 'NONE',  ( 5.473741331615251227, 7.409117525016355010, -1.599625672291262513 ) ) ;
#124742=CARTESIAN_POINT ( 'NONE',  ( -1.364683531250012516, 3.988541667008088876, -0.7879004041258300672 ) ) ;
#124744=CARTESIAN_POINT ( 'NONE',  ( 9.571693261567965294, 10.26932301469188857, 0.7216878364870438212 ) ) ;
#124750=CARTESIAN_POINT ( 'NONE',  ( -1.500000000000013101, 1.702083334016151417, 0.8660254037844403729 ) ) ;
#124753=CARTESIAN_POINT ( 'NONE',  ( -5.880485940025243607, 7.883652901494672349, 1.599625672291269396 ) ) ;
#124754=CARTESIAN_POINT ( 'NONE',  ( -4.121315508874276112, 4.870918184183829602, -1.082531754730549967 ) ) ;
#124762=CARTESIAN_POINT ( 'NONE',  ( 6.419949431270806528, 7.448694743692793274, 1.199719254218462483 ) ) ;
#124766=CARTESIAN_POINT ( 'NONE',  ( 4.981731378017507872, 7.899438143407371271, -1.199719254218452047 ) ) ;
#124772=CARTESIAN_POINT ( 'NONE',  ( 3.891353782322113375, 4.498666486585943147, -1.199719254218446718 ) ) ;
#124777=CARTESIAN_POINT ( 'NONE',  ( 5.530423754462008290, 6.204488192500752675, 0.9375459734879583173 ) ) ;
#124786=LINE ( 'NONE', #191808, #88081 ) ;
#124787=CARTESIAN_POINT ( 'NONE',  ( -4.128963376203445890, 3.977025402421431544, 0.4311926875460708186 ) ) ;
#124788=CARTESIAN_POINT ( 'NONE',  ( 5.978782553946477840, 9.919070713005490703, 1.040834085586084257E-14 ) ) ;
#124790=CARTESIAN_POINT ( 'NONE',  ( -3.684065054611367351, 5.321161868511784299, -1.599625672291256295 ) ) ;
#124794=CARTESIAN_POINT ( 'NONE',  ( -6.124532705071231931, 8.168374127381657246, -1.599625672291263179 ) ) ;
#124808=CARTESIAN_POINT ( 'NONE',  ( 8.723781775389312543, 12.26516360700784958, -1.199719254218446718 ) ) ;
#124812=DIRECTION ( 'NONE',  ( 5.176899690512889097E-31, -0.6000000000000018652, -0.7999999999999984901 ) ) ;
#124814=CARTESIAN_POINT ( 'NONE',  ( -4.274898507010545856, 3.881803101134051470, -0.7998128361456221525 ) ) ;
#124816=CARTESIAN_POINT ( 'NONE',  ( 7.079328764629950754, 11.41096732537697633, 0.7998128361456462443 ) ) ;
#124820=CARTESIAN_POINT ( 'NONE',  ( -6.527360889975461156, 9.702672574024962415, 1.199719254218452047 ) ) ;
#124821=CARTESIAN_POINT ( 'NONE',  ( 5.229694566569264680, 7.124396299129368337, 1.599625672291267398 ) ) ;
#124824=CARTESIAN_POINT ( 'NONE',  ( -2.819732761962335577, 5.273143408055916304, -1.082531754730543971 ) ) ;
#124827=CARTESIAN_POINT ( 'NONE',  ( -0.6823417656250212460, 2.613541667008084879, 1.181850606188767472 ) ) ;
#124829=CARTESIAN_POINT ( 'NONE',  ( 6.236387472606139681, 8.298871356172400127, -1.443375672974057666 ) ) ;
#124837=CARTESIAN_POINT ( 'NONE',  ( 8.663296969007976855, 12.09063498294259809, -1.082531754730543083 ) ) ;
#124838=ORIENTED_EDGE ( 'NONE', *, *, #52342, .T. ) ;
#124842=CARTESIAN_POINT ( 'NONE',  ( -9.179033691651859783, 10.66762638080401260, 1.199719254218462483 ) ) ;
#124861=CARTESIAN_POINT ( 'NONE',  ( 1.499999999999987121, 1.285416667349485120, 0.8660254037844524744 ) ) ;
#124867=CARTESIAN_POINT ( 'NONE',  ( -1.402160292154681736E-14, 0.4625000000000214495, 1.732050807568877637 ) ) ;
#124868=CARTESIAN_POINT ( 'NONE',  ( 6.591235234537977661, 10.84152487360300299, 0.7998128361456462443 ) ) ;
#124869=CARTESIAN_POINT ( 'NONE',  ( -1.364683531250014514, -0.7614583329919104582, -0.7879004041258359514 ) ) ;
#124873=CARTESIAN_POINT ( 'NONE',  ( 8.270110514656016321, 12.59228666716665401, 0.7216878364870438212 ) ) ;
#124874=CARTESIAN_POINT ( 'NONE',  ( -6.317736394288148816, 8.393778431468064127, 1.443375672974078761 ) ) ;
#124880=CARTESIAN_POINT ( 'NONE',  ( -6.124532705071231931, 8.168374127381657246, -1.599625672291263179 ) ) ;
#124883=CARTESIAN_POINT ( 'NONE',  ( 0.7499999999999885647, 2.097916667349486453, -1.299038105676652899 ) ) ;
#124884=CARTESIAN_POINT ( 'NONE',  ( -1.201851678989727383E-14, 3.759375000341422801, -1.575800808251660134 ) ) ;
#124898=CARTESIAN_POINT ( 'NONE',  ( -7.720478407978036195, 11.09464301169468037, -1.199719254218446718 ) ) ;
#124899=CARTESIAN_POINT ( 'NONE',  ( 8.132193210098487057, 8.381980254736715708, 1.040834085586084257E-14 ) ) ;
#124906=CARTESIAN_POINT ( 'NONE',  ( -7.157815033010924921, 10.43820240756634199, 1.199719254218453823 ) ) ;
#124911=CARTESIAN_POINT ( 'NONE',  ( 4.566398809704347528, 4.221886787610169556, -0.7998128361456211532 ) ) ;
#124912=CARTESIAN_POINT ( 'NONE',  ( -4.911894908834722351, 4.738238661368090909, 0.4458799699701230246 ) ) ;
#124913=ORIENTED_EDGE ( 'NONE', *, *, #207112, .T. ) ;
#124914=CARTESIAN_POINT ( 'NONE',  ( -4.741601036477307574, 6.554953847355395880, 1.599625672291267398 ) ) ;
#124916=CARTESIAN_POINT ( 'NONE',  ( -9.169391961543940539, 9.592045464756413509, 1.040834085586084257E-14 ) ) ;
#124920=CARTESIAN_POINT ( 'NONE',  ( -5.747250929305832479, 6.247137566976777912, -1.064685594968674209 ) ) ;
#124928=CARTESIAN_POINT ( 'NONE',  ( 7.308008492965924141, 8.484763649003774333, -1.199719254218451159 ) ) ;
#124930=CARTESIAN_POINT ( 'NONE',  ( 5.335766472694954743, 4.384919054141799499, 2.499999999999998668 ) ) ;
#124948=CARTESIAN_POINT ( 'NONE',  ( 4.853455804012228647, 4.764712647543454693, 0.7216878364870317197 ) ) ;
#124952=CARTESIAN_POINT ( 'NONE',  ( -10.13202086811422475, 10.71511252242175161, -0.7998128361456291469 ) ) ;
#124953=CARTESIAN_POINT ( 'NONE',  ( -0.7500000000000215383, 4.191666666666690411, 1.299038105676671107 ) ) ;
#124955=CARTESIAN_POINT ( 'NONE',  ( 10.26082332744404368, 10.86538205830655279, -0.7998128361456281477 ) ) ;
#124959=CARTESIAN_POINT ( 'NONE',  ( -3.159872497350062481, 2.806782174840205091, 2.466584723216629360 ) ) ;
#124964=CARTESIAN_POINT ( 'NONE',  ( -1.402160292154681736E-14, 0.07187500034142156602, 1.575800808251672791 ) ) ;
#124970=CARTESIAN_POINT ( 'NONE',  ( -4.416205349749324327, 6.175325546172740765, 1.599625672291267398 ) ) ;
#124973=CARTESIAN_POINT ( 'NONE',  ( -1.402160292154681736E-14, -0.03749999999998095135, 1.732050807568877637 ) ) ;
#124975=CARTESIAN_POINT ( 'NONE',  ( -0.7499999999999972244, 5.608333333333353821, -1.299038105676652011 ) ) ;
#124981=CARTESIAN_POINT ( 'NONE',  ( 0.6823417656249882723, 0.3427083336747516196, 1.181850606188755259 ) ) ;
#124983=CARTESIAN_POINT ( 'NONE',  ( -7.725448601688521322, 7.907444878258402809, 1.040834085586084257E-14 ) ) ;
#124984=CARTESIAN_POINT ( 'NONE',  ( 8.751951852821344247, 10.16936423550178503, -1.199719254218446718 ) ) ;
#124985=CARTESIAN_POINT ( 'NONE',  ( 6.003563092752935759, 5.898578451166879510, 0.7998128361456341429 ) ) ;
#124986=CIRCLE ( 'NONE', #117996, 0.07999999999999998779 ) ;
#124990=CARTESIAN_POINT ( 'NONE',  ( 1.364683531249986537, -0.07395833299191513499, 0.7879004041258500513 ) ) ;
#124997=EDGE_CURVE ( 'NONE', #71069, #143793, #150856, .T. ) ;
#124999=CARTESIAN_POINT ( 'NONE',  ( 5.938108093105483931, 8.911247961056314892, -1.082531754730537088 ) ) ;
#125002=CARTESIAN_POINT ( 'NONE',  ( -4.042302355168801320, 7.867769847672247074, 0.7998128361456341429 ) ) ;
#125004=CARTESIAN_POINT ( 'NONE',  ( -1.499999999999997780, 5.900000000000023448, 1.214306433183764966E-14 ) ) ;
#125006=CARTESIAN_POINT ( 'NONE',  ( -2.819205876637805641, 5.376491725131008259, -1.199719254218446718 ) ) ;
#125007=CARTESIAN_POINT ( 'NONE',  ( 4.921246571636183731, 7.724909519342112674, -1.082531754730549078 ) ) ;
#125008=CARTESIAN_POINT ( 'NONE',  ( -8.134528978075012517, 12.43410820782212767, 1.040834085586084257E-14 ) ) ;
#125010=CARTESIAN_POINT ( 'NONE',  ( 1.499999999999989120, 4.254166666666687746, 0.8660254037844524744 ) ) ;
#125014=CARTESIAN_POINT ( 'NONE',  ( 3.708318708537623021, 4.285125567170706695, -1.199719254218446718 ) ) ;
#125018=CARTESIAN_POINT ( 'NONE',  ( 1.220000000000003304, 6.400000000000022560, 1.229247124133362667E-14 ) ) ;
#125024=ADVANCED_FACE ( 'NONE', ( #6050 ), #109789, .T. ) ;
#125029=CARTESIAN_POINT ( 'NONE',  ( 9.693716643646601128, 10.41168362711695750, 0.7216878364870438212 ) ) ;
#125031=CARTESIAN_POINT ( 'NONE',  ( 6.805303039055573322, 10.02693841461847057, 1.199719254218460707 ) ) ;
#125037=CARTESIAN_POINT ( 'NONE',  ( 4.202664430556247055, 6.886563688082179446, 1.082531754730558626 ) ) ;
#125038=ORIENTED_EDGE ( 'NONE', *, *, #121204, .F. ) ;
#125039=CARTESIAN_POINT ( 'NONE',  ( -6.724481002698115439, 10.78905223654906109, -0.7216878364870267237 ) ) ;
#125065=PRODUCT_DEFINITION_FORMATION_WITH_SPECIFIED_SOURCE ( 'ANY', '', #26328, .NOT_KNOWN. ) ;
#125068=CARTESIAN_POINT ( 'NONE',  ( -6.413170354464012846, 7.440785820751486312, 1.199719254218450271 ) ) ;
#125073=CARTESIAN_POINT ( 'NONE',  ( 6.474182045725470402, 7.511966127223233869, -1.199719254218446718 ) ) ;
#125075=CARTESIAN_POINT ( 'NONE',  ( -3.100010679019018500, 6.768429558830820980, 1.040834085586084257E-14 ) ) ;
#125077=CARTESIAN_POINT ( 'NONE',  ( -5.721177634842498527, 5.777054783512106440, 0.000000000000000000 ) ) ;
#125082=CARTESIAN_POINT ( 'NONE',  ( -5.091250377131585125, 5.898545847196970726, 1.199719254218450271 ) ) ;
#125085=CARTESIAN_POINT ( 'NONE',  ( 8.762647353133951711, 9.117510088278095282, 1.040834085586084257E-14 ) ) ;
#125088=CARTESIAN_POINT ( 'NONE',  ( 6.080382892099663650, 6.037283676876850969, 0.3399492115118609714 ) ) ;
#125094=CARTESIAN_POINT ( 'NONE',  ( 4.961921032477176752, 8.732732271291288484, 1.040834085586084257E-14 ) ) ;
#125095=CARTESIAN_POINT ( 'NONE',  ( -7.263417608619167076, 9.497073181520933716, -1.599625672291263179 ) ) ;
#125098=CARTESIAN_POINT ( 'NONE',  ( -8.402302512167102222, 10.82577223566020841, -1.599625672291263179 ) ) ;
#125099=CARTESIAN_POINT ( 'NONE',  ( -6.575868197828002693, 7.630599971342813426, 1.199719254218450271 ) ) ;
#125104=EDGE_CURVE ( 'NONE', #116176, #158436, #178483, .T. ) ;
#125107=CARTESIAN_POINT ( 'NONE',  ( 7.618792255875527886, 10.97600916757510170, 1.199719254218460707 ) ) ;
#125119=ORIENTED_EDGE ( 'NONE', *, *, #71283, .F. ) ;
#125120=CARTESIAN_POINT ( 'NONE',  ( -1.001543065824772872E-14, 4.712500000000017231, 1.732050807568877637 ) ) ;
#125121=CARTESIAN_POINT ( 'NONE',  ( 4.473300617505036492, 7.306268922809479704, -1.199719254218452047 ) ) ;
#125122=CARTESIAN_POINT ( 'NONE',  ( 7.793239369756836510, 7.986534107671458216, 0.7998128361456341429 ) ) ;
#125124=CARTESIAN_POINT ( 'NONE',  ( 6.534666852106798096, 7.686494751288491578, -1.082531754730543083 ) ) ;
#125125=EDGE_CURVE ( 'NONE', #65489, #160319, #36715, .T. ) ;
#125126=CARTESIAN_POINT ( 'NONE',  ( -8.961576348508641487, 11.47825837805867799, -1.443375672974058777 ) ) ;
#125129=CARTESIAN_POINT ( 'NONE',  ( 7.377608144130607393, 11.75895993479440982, -0.7998128361456291469 ) ) ;
#125131=CARTESIAN_POINT ( 'NONE',  ( 1.499999999999989120, 6.280000000000042881, -2.873333333333329520 ) ) ;
#125135=CARTESIAN_POINT ( 'NONE',  ( -0.6823417656250212460, 1.051041667008083325, 1.181850606188755259 ) ) ;
#125140=CARTESIAN_POINT ( 'NONE',  ( 0.6823417656249882723, 0.09270833367475139752, 1.181850606188755259 ) ) ;
#125143=CARTESIAN_POINT ( 'NONE',  ( 8.563946585326370098, 13.14302144952281814, 0.7998128361456462443 ) ) ;
#125147=CARTESIAN_POINT ( 'NONE',  ( -10.47775378526269918, 11.11846759242831872, -0.7998128361456221525 ) ) ;
#125152=CARTESIAN_POINT ( 'NONE',  ( 3.506755287428983792, 7.242964935309132990, 1.040834085586084257E-14 ) ) ;
#125158=CARTESIAN_POINT ( 'NONE',  ( 7.723341061279088038, 12.16231500480096983, -0.7998128361456291469 ) ) ;
#125161=CARTESIAN_POINT ( 'NONE',  ( -4.009460741339347045, 5.700790169694431420, -1.599625672291256295 ) ) ;
#125165=CARTESIAN_POINT ( 'NONE',  ( 8.426556166093362776, 9.789735934319136135, -1.199719254218446718 ) ) ;
#125167=CARTESIAN_POINT ( 'NONE',  ( 6.913768267964901071, 10.15348118167935709, -1.199719254218441611 ) ) ;
#125170=CARTESIAN_POINT ( 'NONE',  ( -9.354762803749327560, 10.01623748057011376, 0.7216878364870438212 ) ) ;
#125176=CARTESIAN_POINT ( 'NONE',  ( -5.408724846006345288, 6.482216231307839749, 1.333832282565196925 ) ) ;
#125177=CARTESIAN_POINT ( 'NONE',  ( -1.402160292154681736E-14, 1.696875000341421469, -1.575800808251659024 ) ) ;
#125179=CARTESIAN_POINT ( 'NONE',  ( 5.178851490740187913, 8.985817805931475277, 0.7216878364870438212 ) ) ;
#125181=CIRCLE ( 'NONE', #100801, 0.07999999999999972411 ) ;
#125197=CARTESIAN_POINT ( 'NONE',  ( 7.584896871841365851, 10.93646455286856956, -1.199719254218446718 ) ) ;
#125201=CARTESIAN_POINT ( 'NONE',  ( -2.774614992291035698, 6.388801257648172971, 1.040834085586084257E-14 ) ) ;
#125202=CARTESIAN_POINT ( 'NONE',  ( -7.477485413136760073, 8.682486722536401302, -1.199719254218446718 ) ) ;
#125206=CARTESIAN_POINT ( 'NONE',  ( -1.500000000000079936, 7.176846818246208848, 4.202462424328226476 ) ) ;
#125208=CARTESIAN_POINT ( 'NONE',  ( -1.500000000000011324, 4.410416667349484676, -0.8660254037844313801 ) ) ;
#125209=CARTESIAN_POINT ( 'NONE',  ( 8.776205506747620788, 9.133327934160710981, -0.7998128361456221525 ) ) ;
#125212=CARTESIAN_POINT ( 'NONE',  ( -7.283754839039664475, 9.520799950344851936, -1.599625672291263179 ) ) ;
#125214=CARTESIAN_POINT ( 'NONE',  ( -1.364683531250012516, 4.238541667008090208, -0.7879004041258300672 ) ) ;
#125223=CARTESIAN_POINT ( 'NONE',  ( -7.809133291791416909, 11.09411069285655493, 1.082531754730549967 ) ) ;
#125228=CARTESIAN_POINT ( 'NONE',  ( -1.402160292154681736E-14, 2.509375000341417028, -1.575800808251660134 ) ) ;
#125235=CARTESIAN_POINT ( 'NONE',  ( -1.364683531250012516, 3.738541667008087099, -0.7879004041258300672 ) ) ;
#125236=CARTESIAN_POINT ( 'NONE',  ( -3.438964519360665051, 7.163875705896082913, -0.7998128361456281477 ) ) ;
#125237=CARTESIAN_POINT ( 'NONE',  ( 5.961834861707224320, 7.978559976790334574, -1.599625672291262513 ) ) ;
#125240=CARTESIAN_POINT ( 'NONE',  ( 1.364683531249988535, 4.217708333674752730, -0.7879004041258239610 ) ) ;
#125245=CARTESIAN_POINT ( 'NONE',  ( -1.402160292154681736E-14, 0.07187500034142156602, 1.575800808251672791 ) ) ;
#125246=CARTESIAN_POINT ( 'NONE',  ( -3.145128448690310830, 6.613140923539910787, -0.7216878364870267237 ) ) ;
#125247=EDGE_CURVE ( 'NONE', #63949, #184190, #213115, .T. ) ;
#125251=CARTESIAN_POINT ( 'NONE',  ( 2.901081683644312736, 6.328419697652925002, 0.7216878364870338292 ) ) ;
#125254=CARTESIAN_POINT ( 'NONE',  ( -9.002250809794000830, 11.52571191622492464, -1.443375672974059665 ) ) ;
#125259=CARTESIAN_POINT ( 'NONE',  ( -10.29471871147821282, 10.90492667301307605, -0.7998128361456291469 ) ) ;
#125260=CARTESIAN_POINT ( 'NONE',  ( -5.056828107772852299, 7.883087978168217269, -1.082531754730548412 ) ) ;
#125262=CARTESIAN_POINT ( 'NONE',  ( -1.201851678989727383E-14, 0.8843750003414173610, 1.575800808251672791 ) ) ;
#125273=CARTESIAN_POINT ( 'NONE',  ( 1.499999999999987121, -0.4958333333333110882, 0.8660254037844524744 ) ) ;
#125274=CARTESIAN_POINT ( 'NONE',  ( 8.283668667825342169, 9.726996869626816533, -1.082531754730543083 ) ) ;
#125278=ORIENTED_EDGE ( 'NONE', *, *, #96134, .F. ) ;
#125282=CARTESIAN_POINT ( 'NONE',  ( 4.704842999142070603, 5.447737239542574272, -1.199719254218452047 ) ) ;
#125285=CARTESIAN_POINT ( 'NONE',  ( -3.735435015764967837, 4.316761258935923884, -1.199719254218452047 ) ) ;
#125289=CARTESIAN_POINT ( 'NONE',  ( -0.6823417656250212460, 1.113541667008083325, 1.181850606188755259 ) ) ;
#125308=CARTESIAN_POINT ( 'NONE',  ( 7.318703993278529829, 7.432909501780090800, 1.040834085586084257E-14 ) ) ;
#125315=CARTESIAN_POINT ( 'NONE',  ( 8.446893396513862839, 9.813462703143045474, -1.199719254218445830 ) ) ;
#125318=CARTESIAN_POINT ( 'NONE',  ( 8.452618703115982512, 11.94880668935564216, 1.199719254218450271 ) ) ;
#125325=CARTESIAN_POINT ( 'NONE',  ( 10.07387183015377197, 11.71160420905630062, -1.199719254218440723 ) ) ;
#125329=CARTESIAN_POINT ( 'NONE',  ( -9.680158490477310806, 10.39586578175276266, 0.7216878364870438212 ) ) ;
#125340=CARTESIAN_POINT ( 'NONE',  ( 2.833290915131624566, 6.249330467721451399, -0.7216878364870267237 ) ) ;
#125343=ORIENTED_EDGE ( 'NONE', *, *, #81050, .F. ) ;
#125348=CARTESIAN_POINT ( 'NONE',  ( -4.693093728624763372, 8.627026450037540428, 0.7998128361456481317 ) ) ;
#125350=CARTESIAN_POINT ( 'NONE',  ( -4.796887421136680985, 4.490790167614548523, 1.214306433183764966E-14 ) ) ;
#125357=CARTESIAN_POINT ( 'NONE',  ( -1.364683531250012516, 4.301041667008089320, -0.7879004041258300672 ) ) ;
#125359=CARTESIAN_POINT ( 'NONE',  ( 5.996784015946103885, 5.890669528225568996, 1.040834085586084257E-14 ) ) ;
#125360=CARTESIAN_POINT ( 'NONE',  ( 1.510809298642989296, 8.679800937805028482, 2.538927604451451270 ) ) ;
#125369=AXIS2_PLACEMENT_3D ( 'NONE', #1287, #67345, #199493 ) ;
#125370=DIRECTION ( 'NONE',  ( 0.000000000000000000, 0.8000000000000117018, -0.5999999999999843237 ) ) ;
#125373=CARTESIAN_POINT ( 'NONE',  ( 0.6823417656249899377, 1.905208333674752952, 1.181850606188755259 ) ) ;
#125375=CARTESIAN_POINT ( 'NONE',  ( 2.544126380858701797, 6.119897877643793116, 0.7998128361456462443 ) ) ;
#125377=CARTESIAN_POINT ( 'NONE',  ( -6.073689629242160493, 8.109057205581079231, -1.443375672974059665 ) ) ;
#125378=CARTESIAN_POINT ( 'NONE',  ( 4.094199201646931741, 4.839282492418613302, -1.082531754730543083 ) ) ;
#125379=CARTESIAN_POINT ( 'NONE',  ( -7.497295758232736418, 7.849192594134070333, -0.7216878364870267237 ) ) ;
#125383=CARTESIAN_POINT ( 'NONE',  ( 6.823831386379729302, 6.855558127064808716, -0.7998128361456281477 ) ) ;
#125388=CARTESIAN_POINT ( 'NONE',  ( -1.364683531250012516, 4.988541667008084879, -0.7879004041258300672 ) ) ;
#125392=CARTESIAN_POINT ( 'NONE',  ( 5.296431564432884542, 9.330920591813708143, 1.040834085586084257E-14 ) ) ;
#125396=CARTESIAN_POINT ( 'NONE',  ( -7.226659571283968297, 8.389856573708110332, 1.199719254218450271 ) ) ;
#125401=CARTESIAN_POINT ( 'NONE',  ( 8.914649696185335870, 10.35917838609310593, -1.199719254218446718 ) ) ;
#125403=CARTESIAN_POINT ( 'NONE',  ( -8.040148788103921973, 9.338927326664741457, 1.199719254218462483 ) ) ;
#125405=CARTESIAN_POINT ( 'NONE',  ( 6.738039155867407537, 10.80487008191325771, -0.7216878364870267237 ) ) ;
#125406=CARTESIAN_POINT ( 'NONE',  ( 3.999300167945916584, 7.828775037665852921, -0.06519116529766534607 ) ) ;
#125407=CARTESIAN_POINT ( 'NONE',  ( -5.005985031943793295, 6.863401842066301661, -1.599625672291256295 ) ) ;
#125412=CARTESIAN_POINT ( 'NONE',  ( 6.335737856287750880, 6.286115675290828264, -0.7998128361456281477 ) ) ;
#125414=CARTESIAN_POINT ( 'NONE',  ( 7.703003830858588863, 12.13858823597705872, -0.7998128361456291469 ) ) ;
#125415=CARTESIAN_POINT ( 'NONE',  ( -4.789689200157987159, 6.785576372466274542, 1.244997348908165602 ) ) ;
#125416=CARTESIAN_POINT ( 'NONE',  ( 4.220665892555866883, 3.818531717603609987, -0.7998128361456211532 ) ) ;
#125417=CARTESIAN_POINT ( 'NONE',  ( -1.201851678989727383E-14, 0.8218750003414171390, 1.575800808251672791 ) ) ;
#125419=CARTESIAN_POINT ( 'NONE',  ( -6.399085315970155285, 6.567947078161039620, -0.7216878364870278340 ) ) ;
#125420=ORIENTED_EDGE ( 'NONE', *, *, #46917, .F. ) ;
#125426=CARTESIAN_POINT ( 'NONE',  ( -5.505981461394960697, 6.253680794909101337, 0.9796770575781436063 ) ) ;
#125427=CARTESIAN_POINT ( 'NONE',  ( -1.402160292154681736E-14, 1.259375000341419248, -1.575800808251659024 ) ) ;
#125432=CARTESIAN_POINT ( 'NONE',  ( 4.717874267875568961, 4.606534188717351874, -0.7216878364870188411 ) ) ;
#125438=CARTESIAN_POINT ( 'NONE',  ( -7.822691444960700125, 11.10992853822074444, -1.082531754730543083 ) ) ;
#125446=CARTESIAN_POINT ( 'NONE',  ( -8.148087131688683371, 11.48955683940339867, -1.082531754730543083 ) ) ;
#125448=ORIENTED_EDGE ( 'NONE', *, *, #113684, .T. ) ;
#125450=DIRECTION ( 'NONE',  ( -0.6507913734559640506, -0.7592566023653004592, 0.000000000000000000 ) ) ;
#125452=ORIENTED_EDGE ( 'NONE', *, *, #141149, .F. ) ;
#125453=CARTESIAN_POINT ( 'NONE',  ( -7.171900071504738072, 10.35067193585544665, -1.082531754730543083 ) ) ;
#125458=CARTESIAN_POINT ( 'NONE',  ( -1.001543065824772872E-14, 4.243750000682819490, 1.732050807568877637 ) ) ;
#125465=CARTESIAN_POINT ( 'NONE',  ( -8.030507057996002729, 8.263346410617135263, 1.040834085586084257E-14 ) ) ;
#125466=CARTESIAN_POINT ( 'NONE',  ( -3.070003471035267495, 6.451017196056028524, -0.6895117023006979151 ) ) ;
#125469=CARTESIAN_POINT ( 'NONE',  ( 5.671388329218120639, 5.511041227042920099, 1.040834085586084257E-14 ) ) ;
#125476=CARTESIAN_POINT ( 'NONE',  ( 8.118635056484817980, 8.366162408854107113, 0.7998128361456481317 ) ) ;
#125483=CARTESIAN_POINT ( 'NONE',  ( -5.043269954603569083, 7.867270132804026872, 1.082531754730560403 ) ) ;
#125486=CARTESIAN_POINT ( 'NONE',  ( -4.609606157881824373, 5.330435195252891667, 1.197383514668200144 ) ) ;
#125492=CARTESIAN_POINT ( 'NONE',  ( -7.479294296233107708, 11.87759377891399204, 0.7998128361456481317 ) ) ;
#125494=CARTESIAN_POINT ( 'NONE',  ( 8.229962938695207342, 9.560377169021284871, 1.199719254218462483 ) ) ;
#125495=CARTESIAN_POINT ( 'NONE',  ( -1.500000000000001332, -0.09999999999997510880, 0.000000000000000000 ) ) ;
#125496=CARTESIAN_POINT ( 'NONE',  ( -8.877891658850122880, 9.251961778280284321, 0.7998128361456462443 ) ) ;
#125498=CARTESIAN_POINT ( 'NONE',  ( -1.364683531250010295, 5.030208333674757171, 0.7879004041258379498 ) ) ;
#125499=CARTESIAN_POINT ( 'NONE',  ( 8.595506201384004896, 12.01154575404795466, 1.082531754730546636 ) ) ;
#125503=CARTESIAN_POINT ( 'NONE',  ( 1.499999999999989120, 5.254166666666684193, 0.8660254037844524744 ) ) ;
#125506=CARTESIAN_POINT ( 'NONE',  ( 7.551528372687370094, 11.75394083486988528, -0.7216878364870267237 ) ) ;
#125509=CARTESIAN_POINT ( 'NONE',  ( -7.565086526745425033, 7.928281824065535055, 0.7216878364870317197 ) ) ;
#125511=CARTESIAN_POINT ( 'NONE',  ( 1.364683531249990311, 2.634375000341422801, 1.214306433183764966E-14 ) ) ;
#125516=CARTESIAN_POINT ( 'NONE',  ( -5.682838942422375084, 9.781729199468104596, 0.000000000000000000 ) ) ;
#125518=CARTESIAN_POINT ( 'NONE',  ( 0.6823417656249917140, 5.405208333674749177, 1.181850606188765695 ) ) ;
#125522=EDGE_CURVE ( 'NONE', #60515, #85555, #60404, .T. ) ;
#125525=CARTESIAN_POINT ( 'NONE',  ( 9.447334110624092673, 9.916311305349925220, -0.7998128361456281477 ) ) ;
#125529=CARTESIAN_POINT ( 'NONE',  ( -1.500000000000013101, 1.379166666666689745, -0.8660254037844313801 ) ) ;
#125533=CARTESIAN_POINT ( 'NONE',  ( 6.643132081016117851, 8.773406732650713025, 1.443375672974076540 ) ) ;
#125534=CARTESIAN_POINT ( 'NONE',  ( 8.615316546479974136, 12.13862083994696839, 1.199719254218450271 ) ) ;
#125538=CARTESIAN_POINT ( 'NONE',  ( 8.402302512167096893, 10.82577223566020841, -1.599625672291268286 ) ) ;
#125539=CARTESIAN_POINT ( 'NONE',  ( -9.398826802771548472, 11.98838390803207865, -1.599625672291263179 ) ) ;
#125542=ADVANCED_FACE ( 'NONE', ( #153951 ), #3398, .F. ) ;
#125543=CARTESIAN_POINT ( 'NONE',  ( 0.6823417656249917140, 5.405208333674749177, 1.181850606188765695 ) ) ;
#125550=CARTESIAN_POINT ( 'NONE',  ( -1.364683531250012516, 3.988541667008088876, -0.7879004041258300672 ) ) ;
#125552=CARTESIAN_POINT ( 'NONE',  ( -6.724481002698130538, 7.907944593645035880, -1.082531754730544860 ) ) ;
#125558=CARTESIAN_POINT ( 'NONE',  ( 2.866659414285625651, 5.431854185720147221, -1.199719254218446718 ) ) ;
#125561=CARTESIAN_POINT ( 'NONE',  ( 9.023114925094663619, 10.48572115315399245, 1.199719254218453823 ) ) ;
#125562=CARTESIAN_POINT ( 'NONE',  ( 3.697672731464857421, 7.367968498737394789, -2.499999999999995115 ) ) ;
#125568=CARTESIAN_POINT ( 'NONE',  ( -8.995998617867369873, 10.45408546138876993, 1.199719254218462483 ) ) ;
#125569=CARTESIAN_POINT ( 'NONE',  ( 6.819914962873951936, 7.915321197229798322, -1.199719254218446718 ) ) ;
#125571=CARTESIAN_POINT ( 'NONE',  ( 4.541618270453549044, 5.361271406026338227, -1.082531754730548412 ) ) ;
#125573=CARTESIAN_POINT ( 'NONE',  ( 5.020596955762157698, 4.751784624677624080, 1.040834085586084257E-14 ) ) ;
#125574=ORIENTED_EDGE ( 'NONE', *, *, #80137, .T. ) ;
#125582=CARTESIAN_POINT ( 'NONE',  ( -4.582292731738899505, 8.289832587096611860, 0.7216878364870458196 ) ) ;
#125583=CARTESIAN_POINT ( 'NONE',  ( 3.063252641683779753, 5.661212951017999373, 1.199719254218450271 ) ) ;
#125586=CARTESIAN_POINT ( 'NONE',  ( -6.021792782764022078, 10.17717534653336209, -0.7998128361456291469 ) ) ;
#125591=CARTESIAN_POINT ( 'NONE',  ( -8.188234707649510113, 11.64035869464474082, -1.199719254218446718 ) ) ;
#125594=CARTESIAN_POINT ( 'NONE',  ( 7.096803341749390981, 10.36702210109460154, -1.199719254218441611 ) ) ;
#125595=AXIS2_PLACEMENT_3D ( 'NONE', #185211, #36835, #133323 ) ;
#125596=CARTESIAN_POINT ( 'NONE',  ( 5.281064527722868718, 6.119995689553514140, 1.199719254218462483 ) ) ;
#125599=ORIENTED_EDGE ( 'NONE', *, *, #25593, .T. ) ;
#125609=CARTESIAN_POINT ( 'NONE',  ( -6.821723845970312894, 11.11042825360738284, 0.000000000000000000 ) ) ;
#125612=CARTESIAN_POINT ( 'NONE',  ( 5.151735183512854199, 8.954182114166247430, -0.7216878364870257245 ) ) ;
#125617=CARTESIAN_POINT ( 'NONE',  ( -5.382750679825375251, 6.238629533673094585, -1.199719254218446718 ) ) ;
#125627=CARTESIAN_POINT ( 'NONE',  ( -1.201851678989727383E-14, 5.587500000000021672, -1.732050807568863648 ) ) ;
#125628=CARTESIAN_POINT ( 'NONE',  ( 6.740374924288304648, 11.01552117831172062, 1.040834085586084257E-14 ) ) ;
#125630=CARTESIAN_POINT ( 'NONE',  ( -4.121315508874280553, 3.910548969882488901, -0.7216878364870207285 ) ) ;
#125631=CARTESIAN_POINT ( 'NONE',  ( -5.266540691475234404, 6.417032612176464923, -1.150853802781536039 ) ) ;
#125638=CARTESIAN_POINT ( 'NONE',  ( 3.195971524519376494, 4.751719416737803847, -1.599625672291262513 ) ) ;
#125655=CARTESIAN_POINT ( 'NONE',  ( -3.262708522383007903, 6.958243709422141876, 1.040834085586084257E-14 ) ) ;
#125656=CARTESIAN_POINT ( 'NONE',  ( 5.517805330637495231, 6.500156309574290248, -1.082531754730543083 ) ) ;
#125657=CARTESIAN_POINT ( 'NONE',  ( 0.7499999999999885647, 3.566666666666690411, -1.299038105676658228 ) ) ;
#125659=CARTESIAN_POINT ( 'NONE',  ( -3.216308754939891212, 4.775446185561722956, -1.599625672291262513 ) ) ;
#125663=CARTESIAN_POINT ( 'NONE',  ( -1.364683531249997417, 4.259375000341424133, 1.214306433183764966E-14 ) ) ;
#125666=CARTESIAN_POINT ( 'NONE',  ( -3.551873057100300990, 5.166937871415542283, 1.443375672974064550 ) ) ;
#125672=CARTESIAN_POINT ( 'NONE',  ( 3.357615597678655917, 7.068968630600412695, 0.7998128361456321445 ) ) ;
#125675=CARTESIAN_POINT ( 'NONE',  ( 3.922984035321162022, 2.804646012044671899, -0.7749999999999935829 ) ) ;
#125676=CARTESIAN_POINT ( 'NONE',  ( 10.68346185744421462, 11.56638637654751989, 0.000000000000000000 ) ) ;
#125678=EDGE_CURVE ( 'NONE', #145532, #94342, #49635, .T. ) ;
#125679=CARTESIAN_POINT ( 'NONE',  ( -0.6823417656250212460, 1.113541667008083325, 1.181850606188755259 ) ) ;
#125683=CARTESIAN_POINT ( 'NONE',  ( -8.239604668803112375, 10.63595808506888396, -1.599625672291263179 ) ) ;
#125684=CARTESIAN_POINT ( 'NONE',  ( -4.839897649954225223, 7.630002444046455778, 1.082531754730560403 ) ) ;
#125688=CARTESIAN_POINT ( 'NONE',  ( -1.001543065824772872E-14, 5.071875000341421469, 1.575800808251672791 ) ) ;
#125696=CARTESIAN_POINT ( 'NONE',  ( -6.222829318548141586, 6.362315081168691044, 0.7216878364870317197 ) ) ;
#125702=CARTESIAN_POINT ( 'NONE',  ( -4.677199806590235376, 7.440188293455128665, 1.082531754730560403 ) ) ;
#125704=CARTESIAN_POINT ( 'NONE',  ( 9.398826802771546696, 11.98838390803207865, -1.599625672291262513 ) ) ;
#125705=CARTESIAN_POINT ( 'NONE',  ( -5.000000000000000888, 0.2350621082554960051, -0.7749999999999935829 ) ) ;
#125713=CARTESIAN_POINT ( 'NONE',  ( -4.776550190716183586, 4.467063398790632966, 1.214306433183764966E-14 ) ) ;
#125714=CARTESIAN_POINT ( 'NONE',  ( -5.470505178835490590, 6.436924650462506392, 1.307677400191203709 ) ) ;
#125716=CARTESIAN_POINT ( 'NONE',  ( 0.7499999999999885647, 0.9833333333333569293, 1.299038105676657340 ) ) ;
#125719=CARTESIAN_POINT ( 'NONE',  ( 8.215877900201359552, 11.56864606933486606, -1.082531754730543083 ) ) ;
#125720=AXIS2_PLACEMENT_3D ( 'NONE', #4725, #149963, #54583 ) ;
#125721=CARTESIAN_POINT ( 'NONE',  ( 6.602984505055297326, 7.662235663108029726, 1.199719254218462483 ) ) ;
#125726=CARTESIAN_POINT ( 'NONE',  ( 5.352771719296971042, 5.139321848801576387, 0.7998128361456341429 ) ) ;
#125727=CARTESIAN_POINT ( 'NONE',  ( 0.006800380015300722461, 7.009756401597622144, -1.999988438675401881 ) ) ;
#125734=CARTESIAN_POINT ( 'NONE',  ( -7.400052914960538963, 7.527816577075747695, 1.040834085586084257E-14 ) ) ;
#125738=VECTOR ( 'NONE', #87525, 1000.000000000000000 ) ;
#125742=CARTESIAN_POINT ( 'NONE',  ( -0.6823417656249969321, 4.967708333674755394, -1.181850606188749264 ) ) ;
#125743=CARTESIAN_POINT ( 'NONE',  ( 9.219181267168295335, 9.858059021225592744, 1.040834085586084257E-14 ) ) ;
#125744=CARTESIAN_POINT ( 'NONE',  ( -4.889686956022917919, 8.856385215335397021, 1.214306433183764966E-14 ) ) ;
#125747=CARTESIAN_POINT ( 'NONE',  ( 5.705283713252285338, 5.550585841749444249, -0.7998128361456211532 ) ) ;
#125748=CARTESIAN_POINT ( 'NONE',  ( -5.225778143063529946, 8.184159369294361497, 1.199719254218452047 ) ) ;
#125754=CARTESIAN_POINT ( 'NONE',  ( 5.829642864196157070, 8.784705193995428374, 1.082531754730558626 ) ) ;
#125759=CARTESIAN_POINT ( 'NONE',  ( -0.6823417656250212460, 2.363541667008084435, 1.181850606188767472 ) ) ;
#125761=CARTESIAN_POINT ( 'NONE',  ( 6.954969613686092345, 7.216478758829655504, -0.7216878364870257245 ) ) ;
#125763=CARTESIAN_POINT ( 'NONE',  ( -3.795919822146293754, 4.491289883001181593, -1.082531754730549967 ) ) ;
#125765=CARTESIAN_POINT ( 'NONE',  ( -1.364683531250010295, 5.738541667008088432, -0.7879004041258300672 ) ) ;
#125771=CARTESIAN_POINT ( 'NONE',  ( -4.127707017443506210, 7.650024674618332021, -0.8198546088712642677 ) ) ;
#125778=CARTESIAN_POINT ( 'NONE',  ( 4.794779880727245036, 8.745660294157122649, -0.7998128361456281477 ) ) ;
#125787=ORIENTED_EDGE ( 'NONE', *, *, #77070, .T. ) ;
#125789=CARTESIAN_POINT ( 'NONE',  ( 5.355107487717867265, 5.349972945200037522, 1.040834085586084257E-14 ) ) ;
#125790=CARTESIAN_POINT ( 'NONE',  ( 0.6823417656249899377, 1.655208333674752730, 1.181850606188755259 ) ) ;
#125792=CARTESIAN_POINT ( 'NONE',  ( 8.426556166093362776, 9.789735934319136135, -1.199719254218446718 ) ) ;
#125794=CARTESIAN_POINT ( 'NONE',  ( -3.445171926680890451, 6.328521679139374356, -0.9347783054773143308 ) ) ;
#125795=CARTESIAN_POINT ( 'NONE',  ( -4.283486466913726254, 7.084819080452935403, -1.199719254218452047 ) ) ;
#125800=CARTESIAN_POINT ( 'NONE',  ( 1.499999999999989120, 3.525000000000021227, 1.214306433183764966E-14 ) ) ;
#125801=CARTESIAN_POINT ( 'NONE',  ( 5.449487677688982679, 8.445153826357429949, -1.199719254218446718 ) ) ;
#125802=CARTESIAN_POINT ( 'NONE',  ( -6.015013705957189316, 10.16926642359206134, 0.7998128361456481317 ) ) ;
#125807=CARTESIAN_POINT ( 'NONE',  ( -1.402160292154681736E-14, 1.946875000341422579, -1.575800808251660134 ) ) ;
#125809=CARTESIAN_POINT ( 'NONE',  ( 2.523789150438203510, 6.096171108819874007, 0.7998128361456462443 ) ) ;
#125814=CARTESIAN_POINT ( 'NONE',  ( -1.201851678989727383E-14, 0.7437500006828187127, 1.732050807568877637 ) ) ;
#125817=CARTESIAN_POINT ( 'NONE',  ( -7.067878151425722955, 7.140279352951794500, 0.7998128361456341429 ) ) ;
#125819=CARTESIAN_POINT ( 'NONE',  ( -2.168941388506379742, 5.474256019991960542, -0.7216878364870267237 ) ) ;
#125826=CARTESIAN_POINT ( 'NONE',  ( 4.462605117192430804, 8.358123070033169455, 1.040834085586084257E-14 ) ) ;
#125830=CARTESIAN_POINT ( 'NONE',  ( 4.873266149108180123, 7.772895376346490970, 1.199719254218462483 ) ) ;
#125835=ORIENTED_EDGE ( 'NONE', *, *, #72672, .F. ) ;
#125836=CARTESIAN_POINT ( 'NONE',  ( 3.379006598303866848, 4.965260336153046516, -1.599625672291262513 ) ) ;
#125842=CARTESIAN_POINT ( 'NONE',  ( 5.290189798603822879, 6.367883502209223501, 1.128355864069837455 ) ) ;
#125854=CARTESIAN_POINT ( 'NONE',  ( 6.453317930424781856, 10.47269531889685545, -0.7216878364870267237 ) ) ;
#125856=CARTESIAN_POINT ( 'NONE',  ( -5.603597561149804562, 5.431951997629870910, 0.7998128361456341429 ) ) ;
#125857=CARTESIAN_POINT ( 'NONE',  ( -0.2462715347619852391, 7.026474760181363521, 3.914608670279890568 ) ) ;
#125859=CARTESIAN_POINT ( 'NONE',  ( 7.527801604085637699, 9.805521176231838609, 1.599625672291281386 ) ) ;
#125861=CARTESIAN_POINT ( 'NONE',  ( -4.869349725602420520, 8.832658446511480577, 1.040834085586084257E-14 ) ) ;
#125864=CYLINDRICAL_SURFACE ( 'NONE', #44726, 1.500000000000000222 ) ;
#125874=CARTESIAN_POINT ( 'NONE',  ( 8.401248741962376698, 12.95320729893149370, 0.7998128361456462443 ) ) ;
#125875=CARTESIAN_POINT ( 'NONE',  ( -3.906720819032141190, 7.709591388846142479, -0.7998128361456281477 ) ) ;
#125878=CARTESIAN_POINT ( 'NONE',  ( 2.846849069189655967, 5.304779099821139710, -1.082531754730543083 ) ) ;
#125882=FACE_OUTER_BOUND ( 'NONE', #1732, .T. ) ;
#125883=CARTESIAN_POINT ( 'NONE',  ( -4.711622075948912247, 5.455646162483875017, -1.199719254218446718 ) ) ;
#125884=( BOUNDED_SURFACE ( )  B_SPLINE_SURFACE ( 3, 2, ( 
 ( #170666, #138188, #154429 ),
 ( #75307, #8163, #88363 ),
 ( #72077, #6007, #156568 ),
 ( #4929, #125206, #7074 ) ),
 .UNSPECIFIED., .F., .F., .T. ) 
 B_SPLINE_SURFACE_WITH_KNOTS ( ( 4, 4 ),
 ( 3, 3 ),
 ( 4.082329036714114956, 4.712388980384689674 ),
 ( 0.000000000000000000, 1.000000000000000000 ),
 .UNSPECIFIED. ) 
 GEOMETRIC_REPRESENTATION_ITEM ( )  RATIONAL_B_SPLINE_SURFACE ( (
 ( 1.000000000000000000, 0.8226529996940167289, 1.000000000000000000),
 ( 1.000000000000000000, 0.7917671131328077871, 1.000000000000000000),
 ( 1.000000000000000000, 0.7517196685946685442, 1.000000000000000000),
 ( 1.000000000000000000, 0.7071067811865475727, 1.000000000000000000) ) ) 
 REPRESENTATION_ITEM ( '' )  SURFACE ( )  );
#125887=CARTESIAN_POINT ( 'NONE',  ( 9.738834413317897898, 10.25639499182604730, 0.000000000000000000 ) ) ;
#125891=CARTESIAN_POINT ( 'NONE',  ( -7.714753101375940503, 8.959299025482085455, 1.199719254218462483 ) ) ;
#125892=CARTESIAN_POINT ( 'NONE',  ( 3.988069740714122791, 7.804498464141805592, 0.7998128361456321445 ) ) ;
#125895=CARTESIAN_POINT ( 'NONE',  ( 4.334856428067314305, 6.080418470877079429, -1.599625672291256517 ) ) ;
#125898=CARTESIAN_POINT ( 'NONE',  ( -1.364683531250000748, 2.321875000341422357, 1.214306433183764966E-14 ) ) ;
#125902=CARTESIAN_POINT ( 'NONE',  ( 7.456621297836078632, 8.762108271306003004, 1.082531754730558626 ) ) ;
#125910=CARTESIAN_POINT ( 'NONE',  ( 10.20892648096591770, 11.01276177065614981, -0.7216878364870257245 ) ) ;
#125915=CARTESIAN_POINT ( 'NONE',  ( -10.15235809853472126, 10.73883929124566983, -0.7998128361456291469 ) ) ;
#125932=CARTESIAN_POINT ( 'NONE',  ( 1.499999999999989120, 2.035416667349480679, 0.8660254037844524744 ) ) ;
#125938=CARTESIAN_POINT ( 'NONE',  ( -1.402160292154681736E-14, 0.8375000000000232259, -1.732050807568863648 ) ) ;
#125939=CARTESIAN_POINT ( 'NONE',  ( 9.077347539549325717, 10.54899253668443393, -1.199719254218446718 ) ) ;
#125940=CARTESIAN_POINT ( 'NONE',  ( -0.6823417656250246877, -0.9489583329919115684, 1.181850606188755259 ) ) ;
#125945=CARTESIAN_POINT ( 'NONE',  ( 3.602716132929354664, 5.226254793216122074, 1.599625672291267398 ) ) ;
#125946=CARTESIAN_POINT ( 'NONE',  ( -5.910991785878170646, 7.919243054989755670, -1.443375672974059665 ) ) ;
#125950=CARTESIAN_POINT ( 'NONE',  ( -5.555090253297260361, 7.504024600312024340, 1.599625672291269396 ) ) ;
#125952=CARTESIAN_POINT ( 'NONE',  ( -1.499999999999997780, 2.431250000682817713, 1.214306433183764966E-14 ) ) ;
#125964=CARTESIAN_POINT ( 'NONE',  ( -10.01677656239806247, 10.58066083241955901, 0.7998128361456462443 ) ) ;
#125965=CARTESIAN_POINT ( 'NONE',  ( 5.770966940911189447, 9.884545197705074671, -0.7998128361456291469 ) ) ;
#125972=CARTESIAN_POINT ( 'NONE',  ( -7.344766530301162000, 9.591980256816594164, 1.599625672291295375 ) ) ;
#125974=CARTESIAN_POINT ( 'NONE',  ( -2.081668171172168513E-14, 6.468705557303652931, 4.925226524755076163 ) ) ;
#125977=CARTESIAN_POINT ( 'NONE',  ( 2.517010073631369860, 6.088262185878572375, -0.7998128361456281477 ) ) ;
#125979=ORIENTED_EDGE ( 'NONE', *, *, #20075, .T. ) ;
#125980=CARTESIAN_POINT ( 'NONE',  ( -8.483651433849100698, 10.92067931095586886, 1.599625672291269396 ) ) ;
#125983=CARTESIAN_POINT ( 'NONE',  ( -4.957984823605727343, 6.829280066411827832, -1.450623857674667283 ) ) ;
#125984=ORIENTED_EDGE ( 'NONE', *, *, #17814, .T. ) ;
#125998=CARTESIAN_POINT ( 'NONE',  ( -1.500000000000013101, 0.9520833340161557468, 0.8660254037844403729 ) ) ;
#126010=CARTESIAN_POINT ( 'NONE',  ( 3.172244755917638770, 5.684407401003788607, -1.082531754730543083 ) ) ;
#126013=ORIENTED_EDGE ( 'NONE', *, *, #30361, .F. ) ;
#126015=CARTESIAN_POINT ( 'NONE',  ( -9.110189153378817295, 12.71597221466224603, 1.199719254218462483 ) ) ;
#126018=CARTESIAN_POINT ( 'NONE',  ( 10.23370702021670020, 10.83374636654133383, 0.7998128361456462443 ) ) ;
#126025=CARTESIAN_POINT ( 'NONE',  ( -1.201851678989727383E-14, 0.8218750003414171390, 1.575800808251672791 ) ) ;
#126030=CARTESIAN_POINT ( 'NONE',  ( -3.567766978690493307, 7.314145241780881435, 1.040834085586084257E-14 ) ) ;
#126033=CARTESIAN_POINT ( 'NONE',  ( 0.7499999999999867883, -0.4333333333333133641, -1.299038105676652899 ) ) ;
#126035=CARTESIAN_POINT ( 'NONE',  ( -1.500000000000011324, 5.420833333333356485, 0.8660254037844403729 ) ) ;
#126040=CARTESIAN_POINT ( 'NONE',  ( -1.364683531250014514, -0.7197916663252461600, 0.7879004041258379498 ) ) ;
#126043=CARTESIAN_POINT ( 'NONE',  ( -6.744291347794091784, 9.955758108146730123, -1.199719254218440723 ) ) ;
#126045=CARTESIAN_POINT ( 'NONE',  ( 8.809047120577066181, 11.30030761213851953, 1.599625672291281386 ) ) ;
#126053=CARTESIAN_POINT ( 'NONE',  ( -0.6823417656250246877, -0.1364583329919108468, 1.181850606188755259 ) ) ;
#126060=CARTESIAN_POINT ( 'NONE',  ( 7.470179451449751262, 7.817556902887268677, 1.040834085586084257E-14 ) ) ;
#126063=CARTESIAN_POINT ( 'NONE',  ( -4.741601036477307574, 6.554953847355395880, 1.599625672291267398 ) ) ;
#126070=CARTESIAN_POINT ( 'NONE',  ( 5.951666246274807115, 6.045958163516475636, 0.7216878364870317197 ) ) ;
#126071=CARTESIAN_POINT ( 'NONE',  ( -9.625925875578284163, 10.33259439770390564, 1.040834085586084257E-14 ) ) ;
#126076=CARTESIAN_POINT ( 'NONE',  ( 8.703971430293332645, 12.13808852110884118, -1.082531754730543083 ) ) ;
#126090=CARTESIAN_POINT ( 'NONE',  ( 8.229436053370667636, 11.58446391469906267, 1.082531754730558626 ) ) ;
#126092=CARTESIAN_POINT ( 'NONE',  ( 8.046927864910717432, 9.346836249606042202, 1.199719254218462483 ) ) ;
#126096=EDGE_CURVE ( 'NONE', #162715, #213175, #207312, .T. ) ;
#126098=CARTESIAN_POINT ( 'NONE',  ( -1.387358672534890536, 7.315968950354793776, -4.254625267136668221 ) ) ;
#126099=CARTESIAN_POINT ( 'NONE',  ( 3.362058906508953449, 6.866226457661676719, -0.7216878364870267237 ) ) ;
#126101=CARTESIAN_POINT ( 'NONE',  ( -7.809133291791416909, 11.09411069285655493, 1.082531754730549967 ) ) ;
#126129=CARTESIAN_POINT ( 'NONE',  ( -6.995644074971465010, 10.14503993989993091, 1.082531754730549967 ) ) ;
#126133=CARTESIAN_POINT ( 'NONE',  ( 5.717788096661236885, 7.693838750903348789, 1.599625672291267398 ) ) ;
#126135=CARTESIAN_POINT ( 'NONE',  ( 2.191614386903386613, 5.708633884695917260, -0.7998128361456281477 ) ) ;
#126137=CARTESIAN_POINT ( 'NONE',  ( -5.271422797614987665, 5.044414773505913274, -0.7998128361456221525 ) ) ;
#126142=CARTESIAN_POINT ( 'NONE',  ( -3.391510981712833939, 7.108513245306943062, 0.7998128361456341429 ) ) ;
#126145=CARTESIAN_POINT ( 'NONE',  ( 6.577677080924314801, 10.82570702772039262, 1.040834085586084257E-14 ) ) ;
#126148=CARTESIAN_POINT ( 'NONE',  ( 5.936406840065503232, 6.128608848081334770, 0.7476236741628620175 ) ) ;
#126149=CARTESIAN_POINT ( 'NONE',  ( 4.392478581147586603, 4.226905887534702977, -0.7216878364870188411 ) ) ;
#126156=CARTESIAN_POINT ( 'NONE',  ( 7.090551149822739596, 8.335026431957096804, 1.082531754730558626 ) ) ;
#126157=CARTESIAN_POINT ( 'NONE',  ( -8.995998617867369873, 10.45408546138876993, 1.199719254218462483 ) ) ;
#126160=CARTESIAN_POINT ( 'NONE',  ( -9.318531651294266638, 9.766041769465124034, -0.7998128361456291469 ) ) ;
#126161=CARTESIAN_POINT ( 'NONE',  ( -5.391338639728555648, 9.441645512991978961, -0.7998128361456231517 ) ) ;
#126168=CARTESIAN_POINT ( 'NONE',  ( 8.776205506747620788, 9.133327934160710981, -0.7998128361456221525 ) ) ;
#126176=CARTESIAN_POINT ( 'NONE',  ( 1.499999999999991118, 5.535416667349481123, 0.8660254037844524744 ) ) ;
#126181=CARTESIAN_POINT ( 'NONE',  ( -1.499999999999997780, 3.900000000000021672, 1.214306433183764966E-14 ) ) ;
#126182=CARTESIAN_POINT ( 'NONE',  ( 6.257251587906815793, 7.258880593101466161, 1.199719254218462483 ) ) ;
#126183=CARTESIAN_POINT ( 'NONE',  ( 5.795220594837462436, 8.848508896363995291, -1.199719254218440723 ) ) ;
#126187=CARTESIAN_POINT ( 'NONE',  ( 6.426201623197458801, 9.480690412830290015, -1.082531754730537088 ) ) ;
#126188=CARTESIAN_POINT ( 'NONE',  ( -8.798878505144648088, 12.24881344176869469, -1.082531754730543083 ) ) ;
#126192=CARTESIAN_POINT ( 'NONE',  ( 7.865701674222579598, 12.32840238656838139, -0.7998128361456352531 ) ) ;
#126195=CARTESIAN_POINT ( 'NONE',  ( -3.521367211247373508, 5.131347717920458962, -1.599625672291256295 ) ) ;
#126199=CARTESIAN_POINT ( 'NONE',  ( 0.6823417656249899377, 1.342708333674752508, 1.181850606188755259 ) ) ;
#126204=CARTESIAN_POINT ( 'NONE',  ( 1.364683531249986537, 0.1135416670080857532, 0.7879004041258500513 ) ) ;
#126206=CARTESIAN_POINT ( 'NONE',  ( 8.387690588348714726, 12.93738945304888333, 1.040834085586084257E-14 ) ) ;
#126210=CARTESIAN_POINT ( 'NONE',  ( -4.582292731294565158, 4.448355729372827305, 1.214306433183764966E-14 ) ) ;
#126211=CARTESIAN_POINT ( 'NONE',  ( 5.802526556524483681, 5.871961858807763335, 1.040834085586084257E-14 ) ) ;
#126213=CARTESIAN_POINT ( 'NONE',  ( -4.713430959045263435, 8.650753218861462202, 0.7998128361456481317 ) ) ;
#126215=AXIS2_PLACEMENT_3D ( 'NONE', #26946, #192640, #41102 ) ;
#126217=CARTESIAN_POINT ( 'NONE',  ( 3.517450787741589036, 6.191110788085444128, -1.199719254218446718 ) ) ;
#126223=CARTESIAN_POINT ( 'NONE',  ( 7.964525173024008531, 11.37936423758166526, 1.199719254218460707 ) ) ;
#126226=CARTESIAN_POINT ( 'NONE',  ( -5.687809136132860210, 6.594531066031826150, -1.199719254218446718 ) ) ;
#126230=CARTESIAN_POINT ( 'NONE',  ( 7.456094412511537151, 10.78619501698377370, 1.199719254218460707 ) ) ;
#126232=CARTESIAN_POINT ( 'NONE',  ( 8.423693512792301163, 8.722063941212843119, 0.7998128361456481317 ) ) ;
#126236=CARTESIAN_POINT ( 'NONE',  ( -9.869972641068651242, 11.57768483841065787, 1.082531754730558626 ) ) ;
#126243=CARTESIAN_POINT ( 'NONE',  ( -5.903366504444580443, 6.144480293219754863, 0.8539384941207116553 ) ) ;
#126244=CARTESIAN_POINT ( 'NONE',  ( 0.6823417656249882723, 1.176041667008083325, -1.181850606188749264 ) ) ;
#126245=EDGE_CURVE ( 'NONE', #189420, #42278, #22185, .T. ) ;
#126248=CARTESIAN_POINT ( 'NONE',  ( 7.144783764721768904, 7.437928601704619780, 1.040834085586084257E-14 ) ) ;
#126249=B_SPLINE_CURVE_WITH_KNOTS ( 'NONE', 3,
 ( #105587, #38426, #103427, #138072 ),
 .UNSPECIFIED., .F., .F.,
 ( 4, 4 ),
 ( 3.313539133636207956E-16, 0.0001949197170424516140 ),
 .UNSPECIFIED. ) ;
#126268=CARTESIAN_POINT ( 'NONE',  ( 7.235247531187115833, 11.59287255302699648, -0.7998128361456291469 ) ) ;
#126272=CARTESIAN_POINT ( 'NONE',  ( -3.002240950422295995, 5.590032644546251817, -1.199719254218452935 ) ) ;
#126273=CARTESIAN_POINT ( 'NONE',  ( -7.881367368245678406, 8.089350105908421185, 0.7998128361456602331 ) ) ;
#126278=CARTESIAN_POINT ( 'NONE',  ( 0.7499999999999902300, 4.347916667349481123, -1.299038105676658228 ) ) ;
#126279=CARTESIAN_POINT ( 'NONE',  ( 6.076025397218672630, 10.24044673006381245, -0.7998128361456291469 ) ) ;
#126282=CARTESIAN_POINT ( 'NONE',  ( -8.148614017013223076, 9.465470093725620870, -1.199719254218446718 ) ) ;
#126284=CARTESIAN_POINT ( 'NONE',  ( -1.201851678989727383E-14, 4.196875000341417028, -1.575800808251660134 ) ) ;
#126288=CARTESIAN_POINT ( 'NONE',  ( -9.327646496521992958, 9.984601788804893019, -0.7216878364870267237 ) ) ;
#126292=CARTESIAN_POINT ( 'NONE',  ( 1.364683531249988535, 3.426041667008085323, 0.7879004041258500513 ) ) ;
#126299=CARTESIAN_POINT ( 'NONE',  ( -0.6823417656250003738, 2.717708333674753618, -1.181850606188749264 ) ) ;
#126302=CARTESIAN_POINT ( 'NONE',  ( -3.588104209110990706, 7.337872010604796991, 1.040834085586084257E-14 ) ) ;
#126303=CARTESIAN_POINT ( 'NONE',  ( 5.991813822235618758, 9.077867661661846554, 1.199719254218462483 ) ) ;
#126306=CARTESIAN_POINT ( 'NONE',  ( 0.6823417656249917140, 3.905208333674754950, 1.181850606188765695 ) ) ;
#126309=CARTESIAN_POINT ( 'NONE',  ( 1.364683531249986537, -0.8447916663252468261, -0.7879004041258309554 ) ) ;
#126310=CARTESIAN_POINT ( 'NONE',  ( -4.609409038966248318, 5.440360635957812718, -1.082531754730544860 ) ) ;
#126313=CARTESIAN_POINT ( 'NONE',  ( 3.551873057100283226, 6.127307085716883428, 1.082531754730558626 ) ) ;
#126316=CARTESIAN_POINT ( 'NONE',  ( -8.351459436338023679, 12.68719374246231624, -0.7216878364870267237 ) ) ;
#126324=CARTESIAN_POINT ( 'NONE',  ( -6.358410854684793279, 7.480862754296137673, -1.082531754730543083 ) ) ;
#126326=CARTESIAN_POINT ( 'NONE',  ( -1.402160292154681736E-14, 0.3843750003414230232, 1.575800808251672791 ) ) ;
#126332=CARTESIAN_POINT ( 'NONE',  ( -0.6823417656250246877, -0.1364583329919108468, 1.181850606188755259 ) ) ;
#126339=CARTESIAN_POINT ( 'NONE',  ( -0.7500000000000249800, -0.3083333333333132531, 1.299038105676659116 ) ) ;
#126340=CARTESIAN_POINT ( 'NONE',  ( 6.765155463094740362, 10.83650577367847667, 0.7216878364870438212 ) ) ;
#126349=CARTESIAN_POINT ( 'NONE',  ( 4.462605117192430804, 8.358123070033169455, 1.040834085586084257E-14 ) ) ;
#126351=CARTESIAN_POINT ( 'NONE',  ( -4.288456660624211381, 3.897620947016656956, 1.214306433183764966E-14 ) ) ;
#126353=FACE_BOUND ( 'NONE', #26298, .T. ) ;
#126356=CARTESIAN_POINT ( 'NONE',  ( 0.6823417656249882723, 2.238541667008084435, -1.181850606188749264 ) ) ;
#126357=B_SPLINE_CURVE_WITH_KNOTS ( 'NONE', 3,
 ( #54029, #88676, #89754, #168837 ),
 .UNSPECIFIED., .F., .F.,
 ( 4, 4 ),
 ( 0.0006335992342243043293, 0.001020988003094174239 ),
 .UNSPECIFIED. ) ;
#126368=CARTESIAN_POINT ( 'NONE',  ( -0.2527754068639477270, 7.036719836771394121, -4.015626449028464329 ) ) ;
#126375=CARTESIAN_POINT ( 'NONE',  ( 5.686755365928134687, 8.721966129303114101, 1.199719254218462483 ) ) ;
#126384=CARTESIAN_POINT ( 'NONE',  ( 9.206149998879153529, 10.69926207256923689, 1.199719254218453823 ) ) ;
#126387=CARTESIAN_POINT ( 'NONE',  ( -0.007772928215657127701, 8.279395425053859725, -2.079985476292311564 ) ) ;
#126391=CARTESIAN_POINT ( 'NONE',  ( 10.57266086055835075, 11.22919251360659310, 0.000000000000000000 ) ) ;
#126397=CARTESIAN_POINT ( 'NONE',  ( -8.297226821883391779, 11.66355314463053006, 1.082531754730549967 ) ) ;
#126402=CARTESIAN_POINT ( 'NONE',  ( 4.961394147597008697, 7.875711374583454827, -1.199719254218452047 ) ) ;
#126409=CARTESIAN_POINT ( 'NONE',  ( 2.860407222358956503, 6.280966159486672140, 0.7216878364870338292 ) ) ;
#126417=CARTESIAN_POINT ( 'NONE',  ( -5.687809136132860210, 6.594531066031826150, -1.199719254218446718 ) ) ;
#126419=CARTESIAN_POINT ( 'NONE',  ( -2.788173145904702555, 6.404619103530779789, -0.7998128361456281477 ) ) ;
#126424=CARTESIAN_POINT ( 'NONE',  ( -1.084637062511556005, 2.932371192708034702, 1.105835307554803082 ) ) ;
#126428=CARTESIAN_POINT ( 'NONE',  ( 5.015626762051672571, 7.938982758113895422, 1.199719254218462483 ) ) ;
#126439=EDGE_CURVE ( 'NONE', #188860, #1110, #39284, .T. ) ;
#126442=CARTESIAN_POINT ( 'NONE',  ( 1.364683531249986537, 1.176041667008082658, 0.7879004041258500513 ) ) ;
#126444=CARTESIAN_POINT ( 'NONE',  ( 4.162516854595432747, 4.815023404238158555, 1.199719254218464037 ) ) ;
#126446=CARTESIAN_POINT ( 'NONE',  ( -6.778713617152821058, 7.971215977175476475, 1.082531754730549967 ) ) ;
#126447=EDGE_CURVE ( 'NONE', #197822, #62722, #47270, .T. ) ;
#126448=CARTESIAN_POINT ( 'NONE',  ( 4.704316114261903436, 4.590716342834741504, 1.214306433183764966E-14 ) ) ;
#126449=CARTESIAN_POINT ( 'NONE',  ( -5.694061327615147050, 9.586895948952255608, 0.000000000000000000 ) ) ;
#126453=CARTESIAN_POINT ( 'NONE',  ( 6.972971076130050072, 7.029554431773520129, 1.040834085586084257E-14 ) ) ;
#126458=CARTESIAN_POINT ( 'NONE',  ( -1.364683531250012516, 4.738541667008091096, -0.7879004041258300672 ) ) ;
#126463=CARTESIAN_POINT ( 'NONE',  ( 6.795661308947685164, 8.951357498570873261, -1.599625672291262513 ) ) ;
#126465=CARTESIAN_POINT ( 'NONE',  ( -6.551614543901706611, 8.666636272683888365, 1.599625672291283607 ) ) ;
#126470=CARTESIAN_POINT ( 'NONE',  ( 9.399880572976245574, 9.860948844760784482, 0.7998128361456462443 ) ) ;
#126473=CARTESIAN_POINT ( 'NONE',  ( -6.744291347794091784, 9.955758108146730123, -1.199719254218440723 ) ) ;
#126475=CARTESIAN_POINT ( 'NONE',  ( 7.578644679914713578, 8.904468883731073703, 1.082531754730558626 ) ) ;
#126476=CARTESIAN_POINT ( 'NONE',  ( 4.033840454514115770, 7.781623563118116316, -0.4120627063678127255 ) ) ;
#126477=CARTESIAN_POINT ( 'NONE',  ( -9.653042183249970876, 11.32459930428888306, -1.082531754730539753 ) ) ;
#126482=CARTESIAN_POINT ( 'NONE',  ( 4.822949958159288286, 6.649860922651058992, -1.599625672291256295 ) ) ;
#126484=CARTESIAN_POINT ( 'NONE',  ( 7.879259827836241570, 12.34422023245099176, 1.040834085586084257E-14 ) ) ;
#126485=CARTESIAN_POINT ( 'NONE',  ( -5.590496338642190643, 6.198678163000841401, 0.8915474099989786350 ) ) ;
#126486=( BOUNDED_CURVE ( )  B_SPLINE_CURVE ( 2, ( #120400, #39076, #105162, #196513, #6547, #171201, #22792 ),
 .UNSPECIFIED., .F., .T. ) 
 B_SPLINE_CURVE_WITH_KNOTS ( ( 3, 2, 2, 3 ),
 ( 0.2142857142857144681, 0.2202380952380953438, 0.2261904761904762196, 0.2321428571428570953 ),
 .UNSPECIFIED. ) 
 CURVE ( )  GEOMETRIC_REPRESENTATION_ITEM ( )  RATIONAL_B_SPLINE_CURVE ( ( 0.9999999999999956701, 0.8660254037844430375, 1.000000000000000000, 0.8660254037844387076, 1.000000000000000000, 0.8660254037844399289, 0.9999999999999987788 ) ) 
 REPRESENTATION_ITEM ( '' )  );
#126487=CARTESIAN_POINT ( 'NONE',  ( 2.737856954955798727, 5.281584649835344258, 1.199719254218452047 ) ) ;
#126488=CARTESIAN_POINT ( 'NONE',  ( -1.364683531250000748, 0.7593750003414210248, 0.000000000000000000 ) ) ;
#126490=CARTESIAN_POINT ( 'NONE',  ( -5.531363484695544841, 8.436712584578003771, 1.082531754730548412 ) ) ;
#126491=VERTEX_POINT ( 'NONE', #11946 ) ;
#126496=CARTESIAN_POINT ( 'NONE',  ( -4.728240158028945928, 6.838416746360681309, 1.235430216343525567 ) ) ;
#126497=CARTESIAN_POINT ( 'NONE',  ( 0.6823417656249882723, 0.4052083336747516751, 1.181850606188755259 ) ) ;
#126500=CARTESIAN_POINT ( 'NONE',  ( 2.399429999938675007, 5.743159399996332404, 0.000000000000000000 ) ) ;
#126505=CARTESIAN_POINT ( 'NONE',  ( -8.853111119599343937, 10.39134639669645566, 1.082531754730558626 ) ) ;
#126513=CARTESIAN_POINT ( 'NONE',  ( -9.788623718942277563, 10.52240854829523187, 1.040834085586084257E-14 ) ) ;
#126517=EDGE_CURVE ( 'NONE', #66184, #174777, #109190, .T. ) ;
#126521=CARTESIAN_POINT ( 'NONE',  ( -7.497295758232712437, 11.69066945133944380, -0.7216878364870267237 ) ) ;
#126525=CARTESIAN_POINT ( 'NONE',  ( 1.364683531249992088, 5.446875000341417916, 1.214306433183764966E-14 ) ) ;
#126526=CARTESIAN_POINT ( 'NONE',  ( -0.7499999999999972244, 4.389583334016150751, -1.299038105676652899 ) ) ;
#126527=CARTESIAN_POINT ( 'NONE',  ( 5.232446707518059625, 6.618332276934084213, -1.382299536160000120 ) ) ;
#126533=CARTESIAN_POINT ( 'NONE',  ( -7.344766530301162000, 9.591980256816594164, 1.599625672291295375 ) ) ;
#126534=DIRECTION ( 'NONE',  ( -5.578564026256490882E-16, -1.000000000000000000, -9.066213480720158442E-32 ) ) ;
#126537=CARTESIAN_POINT ( 'NONE',  ( 5.769158057814842699, 6.689438141327490150, 1.199719254218462483 ) ) ;
#126542=CARTESIAN_POINT ( 'NONE',  ( 6.771407655021410399, 9.987393799911945536, -1.199719254218441611 ) ) ;
#126543=CARTESIAN_POINT ( 'NONE',  ( -4.911894908834722351, 4.738238661368090909, 0.4458799699701230246 ) ) ;
#126550=CARTESIAN_POINT ( 'NONE',  ( -4.433153041988574294, 8.115836282387899558, 1.040834085586084257E-14 ) ) ;
#126560=CARTESIAN_POINT ( 'NONE',  ( -10.49131193887636826, 11.13428543831092909, 1.040834085586084257E-14 ) ) ;
#126562=CARTESIAN_POINT ( 'NONE',  ( 8.910733272679570049, 11.41894145625809820, -1.599625672291255185 ) ) ;
#126563=CARTESIAN_POINT ( 'NONE',  ( -1.402160292154681736E-14, -0.7874999999999764411, 1.732050807568877637 ) ) ;
#126564=CARTESIAN_POINT ( 'NONE',  ( -8.799405390469187793, 10.22472669609091689, -1.199719254218446718 ) ) ;
#126566=CARTESIAN_POINT ( 'NONE',  ( -1.201851678989727383E-14, 2.946875000341419248, -1.575800808251660134 ) ) ;
#126568=CARTESIAN_POINT ( 'NONE',  ( 3.195971524519376494, 4.751719416737803847, -1.599625672291262513 ) ) ;
#126571=CARTESIAN_POINT ( 'NONE',  ( -1.499999999999997780, 5.150000000000022560, 1.214306433183764966E-14 ) ) ;
#126574=CARTESIAN_POINT ( 'NONE',  ( 7.741342523278692767, 11.01502146292508044, 1.082531754730558626 ) ) ;
#126577=CARTESIAN_POINT ( 'NONE',  ( -6.561783159334137139, 8.678499657355050800, -1.443375672974059665 ) ) ;
#126579=CARTESIAN_POINT ( 'NONE',  ( -1.364683531250012516, 2.030208333674750953, 0.7879004041258379498 ) ) ;
#126583=CARTESIAN_POINT ( 'NONE',  ( -6.612626235163205024, 8.737816579155630592, -1.599625672291263179 ) ) ;
#126584=CARTESIAN_POINT ( 'NONE',  ( 1.364683531249988535, 4.217708333674752730, -0.7879004041258239610 ) ) ;
#126589=CARTESIAN_POINT ( 'NONE',  ( 7.913155211870404493, 12.38376484715752213, 0.7998128361456462443 ) ) ;
#126592=CARTESIAN_POINT ( 'NONE',  ( 1.499999999999987121, 1.795833333333355819, -0.8660254037844253849 ) ) ;
#126596=ORIENTED_EDGE ( 'NONE', *, *, #209460, .F. ) ;
#126601=CARTESIAN_POINT ( 'NONE',  ( 9.562578416340237197, 10.05076299535211781, 0.7998128361456462443 ) ) ;
#126602=CARTESIAN_POINT ( 'NONE',  ( -8.642432853707342488, 12.17025653171218558, 1.199719254218462483 ) ) ;
#126605=CARTESIAN_POINT ( 'NONE',  ( 1.364683531249984538, -1.094791666325247936, -0.7879004041258309554 ) ) ;
#126609=CARTESIAN_POINT ( 'NONE',  ( 8.446893396513862839, 9.813462703143045474, -1.199719254218445830 ) ) ;
#126612=CARTESIAN_POINT ( 'NONE',  ( -1.364683531250010295, 4.030208333674751842, 0.7879004041258379498 ) ) ;
#126614=CARTESIAN_POINT ( 'NONE',  ( -6.073689629242165822, 7.148687991279732756, -1.082531754730544860 ) ) ;
#126623=CARTESIAN_POINT ( 'NONE',  ( 8.426556166093362776, 9.789735934319136135, -1.199719254218446718 ) ) ;
#126624=CARTESIAN_POINT ( 'NONE',  ( 4.839532526265843515, 5.050905555379832990, 0.6780825091596712761 ) ) ;
#126629=CARTESIAN_POINT ( 'NONE',  ( -7.160677686311960777, 11.50587440067263678, -0.7998128361456291469 ) ) ;
#126630=CARTESIAN_POINT ( 'NONE',  ( 4.794779880727245036, 8.745660294157122649, -0.7998128361456281477 ) ) ;
#126632=CARTESIAN_POINT ( 'NONE',  ( 2.670593071767634719, 6.059516317130127838, -0.7216878364870267237 ) ) ;
#126634=CARTESIAN_POINT ( 'NONE',  ( 5.508690485854129903, 5.321227076451600091, 1.040834085586084257E-14 ) ) ;
#126642=CARTESIAN_POINT ( 'NONE',  ( -4.907688418466881863, 8.669460888279271416, 0.7216878364870458196 ) ) ;
#126643=CARTESIAN_POINT ( 'NONE',  ( 4.630273154266905777, 5.360739087188218122, 1.199719254218464037 ) ) ;
#126646=CARTESIAN_POINT ( 'NONE',  ( -5.994676475536691029, 10.14553965476814845, 0.7998128361456481317 ) ) ;
#126652=CARTESIAN_POINT ( 'NONE',  ( -7.700141177557535244, 11.07091624287075859, -1.199719254218446718 ) ) ;
#126653=CARTESIAN_POINT ( 'NONE',  ( 1.244150428498994376, 3.053773246564666977, 0.7750000000000100142 ) ) ;
#126656=CARTESIAN_POINT ( 'NONE',  ( 7.958799866421889746, 9.244020251369077457, -1.199719254218441611 ) ) ;
#126657=CARTESIAN_POINT ( 'NONE',  ( 5.178324605415663306, 8.128796908705222535, 1.199719254218462483 ) ) ;
#126658=( BOUNDED_CURVE ( )  B_SPLINE_CURVE ( 2, ( #212832, #160907, #12504, #144698, #64470 ),
 .UNSPECIFIED., .F., .T. ) 
 B_SPLINE_CURVE_WITH_KNOTS ( ( 3, 2, 3 ),
 ( 0.1232094925783373957, 0.1250000000000000000, 0.1270731450466760504 ),
 .UNSPECIFIED. ) 
 CURVE ( )  GEOMETRIC_REPRESENTATION_ITEM ( )  RATIONAL_B_SPLINE_CURVE ( ( 0.9343361104663525651, 0.9424281978788288106, 1.000000000000000000, 0.9333402950740685711, 0.9330143039465762511 ) ) 
 REPRESENTATION_ITEM ( '' )  );
#126659=CARTESIAN_POINT ( 'NONE',  ( -5.736990052180565236, 5.898621588815100125, -2.499999999999995115 ) ) ;
#126671=CARTESIAN_POINT ( 'NONE',  ( -7.212047647465563038, 10.50147379109678880, -1.199719254218446718 ) ) ;
#126675=CARTESIAN_POINT ( 'NONE',  ( 7.307481608085759639, 7.627742752295940676, 1.040834085586084257E-14 ) ) ;
#126679=LINE ( 'NONE', #44294, #79063 ) ;
#126681=CARTESIAN_POINT ( 'NONE',  ( -5.819474248763749635, 7.812472595022922128, -1.599625672291256295 ) ) ;
#126691=CARTESIAN_POINT ( 'NONE',  ( -9.130526383799315582, 12.73969898348616070, 1.199719254218462483 ) ) ;
#126692=CARTESIAN_POINT ( 'NONE',  ( 7.995557903757111617, 10.35123685918189729, 1.599625672291281386 ) ) ;
#126694=CARTESIAN_POINT ( 'NONE',  ( -3.687454593236990430, 4.364747115940301292, 1.082531754730560403 ) ) ;
#126696=CARTESIAN_POINT ( 'NONE',  ( -4.775553520644376881, 6.797630844710244702, -1.243162211532616857 ) ) ;
#126698=DIRECTION ( 'NONE',  ( -1.000000000000000000, 4.336808689942017736E-16, 8.881784197001260212E-16 ) ) ;
#126703=CARTESIAN_POINT ( 'NONE',  ( 3.009020027229115879, 5.597941567487558778, -1.199719254218446718 ) ) ;
#126723=CARTESIAN_POINT ( 'NONE',  ( -4.436542580169821726, 6.199052314996659874, 1.599625672291267398 ) ) ;
#126724=CARTESIAN_POINT ( 'NONE',  ( 6.304178240230120522, 6.457222156464352381, -0.7216878364870257245 ) ) ;
#126725=CARTESIAN_POINT ( 'NONE',  ( 0.7499999999999885647, 3.316666666666689967, -1.299038105676658228 ) ) ;
#126727=CARTESIAN_POINT ( 'NONE',  ( -4.029797971759847997, 5.724516938518342535, -1.599625672291256295 ) ) ;
#126728=CARTESIAN_POINT ( 'NONE',  ( 0.3006164276378255340, 8.220220202720884828, -1.980250916746227441 ) ) ;
#126732=CARTESIAN_POINT ( 'NONE',  ( -1.364683531250012516, 4.988541667008084879, -0.7879004041258300672 ) ) ;
#126735=CARTESIAN_POINT ( 'NONE',  ( -3.850152436600983386, 4.554561266531622188, 1.082531754730560403 ) ) ;
#126739=CARTESIAN_POINT ( 'NONE',  ( -6.471393748265563239, 5.229711127717889596, 2.419999999999998597 ) ) ;
#126740=CARTESIAN_POINT ( 'NONE',  ( 5.217190183160311356, 4.981143389975473568, -0.7998128361456211532 ) ) ;
#126741=DIRECTION ( 'NONE',  ( 1.000000000000000000, 1.045014142154703195E-15, 0.000000000000000000 ) ) ;
#126743=CARTESIAN_POINT ( 'NONE',  ( 0.04971382200798128703, 7.069534788352777710, -4.059379717803641263 ) ) ;
#126746=CARTESIAN_POINT ( 'NONE',  ( -1.201851678989727383E-14, 1.384375000341419693, 1.575800808251672791 ) ) ;
#126749=CARTESIAN_POINT ( 'NONE',  ( -7.947050595904583403, 12.42330946186405249, 0.7998128361456481317 ) ) ;
#126750=CARTESIAN_POINT ( 'NONE',  ( -6.697364695026446491, 6.915939687060050467, 1.040834085586084257E-14 ) ) ;
#126754=CARTESIAN_POINT ( 'NONE',  ( -1.201851678989727383E-14, 3.946875000341423689, -1.575800808251660134 ) ) ;
#126763=CARTESIAN_POINT ( 'NONE',  ( -5.544921637864824504, 8.452530429942200385, -1.082531754730543971 ) ) ;
#126770=CARTESIAN_POINT ( 'NONE',  ( -5.707619481228834779, 5.761236937629489852, -0.7216878364870197293 ) ) ;
#126775=LINE ( 'NONE', #112642, #203254 ) ;
#126777=CARTESIAN_POINT ( 'NONE',  ( 3.863710590214593399, 7.451486755318259547, 1.040834085586084257E-14 ) ) ;
#126779=CARTESIAN_POINT ( 'NONE',  ( 1.474093356799754062, 8.744500914157981697, -2.533844564144165812 ) ) ;
#126785=CARTESIAN_POINT ( 'NONE',  ( -3.090368948911150770, 5.692848642783215674, 1.199719254218462483 ) ) ;
#126788=CARTESIAN_POINT ( 'NONE',  ( -1.201851678989727383E-14, 1.462500000000018119, 1.732050807568877637 ) ) ;
#126791=CARTESIAN_POINT ( 'NONE',  ( 9.598809568795314107, 10.30095870645710754, -0.7216878364870257245 ) ) ;
#126792=CARTESIAN_POINT ( 'NONE',  ( 7.820355676984174664, 8.018169799436671852, -0.7998128361456281477 ) ) ;
#126795=VERTEX_POINT ( 'NONE', #110225 ) ;
#126797=CARTESIAN_POINT ( 'NONE',  ( 4.005544317833563461, 6.760553239859419250, -1.199719254218452047 ) ) ;
#126805=CARTESIAN_POINT ( 'NONE',  ( -7.250913225210214641, 7.353820272367037170, 0.7998128361456341429 ) ) ;
#126811=CARTESIAN_POINT ( 'NONE',  ( -1.201851678989727383E-14, 3.446875000341421469, -1.575800808251660134 ) ) ;
#126812=CARTESIAN_POINT ( 'NONE',  ( 7.714226216051361718, 11.94375498546120795, -0.7216878364870267237 ) ) ;
#126813=CARTESIAN_POINT ( 'NONE',  ( -7.901704598666176693, 8.113076874732334076, 0.7998128361456602331 ) ) ;
#126816=CARTESIAN_POINT ( 'NONE',  ( 4.632082037363250748, 8.555846143565791095, -0.7998128361456231517 ) ) ;
#126817=CARTESIAN_POINT ( 'NONE',  ( -6.762819695118240659, 6.784377820593065600, 0.7998128361456341429 ) ) ;
#126821=CARTESIAN_POINT ( 'NONE',  ( -1.402160292154681736E-14, 0.6187500006828180465, -1.732050807568863648 ) ) ;
#126824=CARTESIAN_POINT ( 'NONE',  ( 6.805829924380105034, 9.923590097543378619, 1.082531754730558626 ) ) ;
#126827=CARTESIAN_POINT ( 'NONE',  ( 0.6823417656249899377, 2.655208333674753618, 1.181850606188767472 ) ) ;
#126829=CARTESIAN_POINT ( 'NONE',  ( 5.246642258364164313, 8.104537820524768676, -1.082531754730549078 ) ) ;
#126832=CARTESIAN_POINT ( 'NONE',  ( -4.609409038966248318, 5.440360635957812718, -1.082531754730544860 ) ) ;
#126837=LINE ( 'NONE', #61750, #53140 ) ;
#126839=CARTESIAN_POINT ( 'NONE',  ( -4.043597078347817231, 7.757176853022865082, 0.5683662157932849457 ) ) ;
#126844=EDGE_CURVE ( 'NONE', #26788, #120076, #37401, .T. ) ;
#126847=CARTESIAN_POINT ( 'NONE',  ( 5.819474248763732760, 7.812472595022922128, -1.599625672291262513 ) ) ;
#126858=CARTESIAN_POINT ( 'NONE',  ( 4.039966587192257208, 6.696749537490852333, 1.082531754730558626 ) ) ;
#126859=VECTOR ( 'NONE', #150720, 1000.000000000000000 ) ;
#126860=CARTESIAN_POINT ( 'NONE',  ( 0.6823417656249882723, 1.488541667008083547, -1.181850606188749264 ) ) ;
#126861=CARTESIAN_POINT ( 'NONE',  ( 9.101601193475611140, 9.512956235343358102, -0.7998128361456221525 ) ) ;
#126862=DIRECTION ( 'NONE',  ( 3.347138415753903010E-16, 0.6000000000000019762, -0.7999999999999986011 ) ) ;
#126863=DIRECTION ( 'NONE',  ( -0.5996521035822321988, -0.8002608041566222630, 0.000000000000000000 ) ) ;
#126864=CARTESIAN_POINT ( 'NONE',  ( -3.893162665418476109, 7.693773542963529444, 1.040834085586084257E-14 ) ) ;
#126865=DIRECTION ( 'NONE',  ( 1.000000000000000000, 0.000000000000000000, 0.000000000000000000 ) ) ;
#126868=CARTESIAN_POINT ( 'NONE',  ( -1.201851678989727383E-14, 2.962500000000025224, 1.732050807568877637 ) ) ;
#126869=CARTESIAN_POINT ( 'NONE',  ( 6.582647274634798151, 7.638508894284114170, 1.199719254218462483 ) ) ;
#126870=CARTESIAN_POINT ( 'NONE',  ( -6.418895661066105873, 9.576129806964074120, -1.199719254218440723 ) ) ;
#126873=CARTESIAN_POINT ( 'NONE',  ( 0.7499999999999902300, 5.816666666666685082, -1.299038105676658228 ) ) ;
#126874=CARTESIAN_POINT ( 'NONE',  ( -1.201851678989727383E-14, 2.571875000341417472, 1.575800808251672791 ) ) ;
#126877=CARTESIAN_POINT ( 'NONE',  ( 4.695201269034174452, 4.372156323494968966, 1.214306433183764966E-14 ) ) ;
#126882=CARTESIAN_POINT ( 'NONE',  ( -0.7500000000000215383, 0.9729166673494854534, 1.299038105676659116 ) ) ;
#126884=CARTESIAN_POINT ( 'NONE',  ( -7.705111371268023923, 7.883718109434487253, 1.040834085586084257E-14 ) ) ;
#126885=CARTESIAN_POINT ( 'NONE',  ( -3.389175213736311587, 4.977123720824209840, 1.443375672974064550 ) ) ;
#126891=ORIENTED_EDGE ( 'NONE', *, *, #122971, .T. ) ;
#126893=CARTESIAN_POINT ( 'NONE',  ( 5.799137018343234473, 7.788745826199009237, -1.599625672291262513 ) ) ;
#126894=ADVANCED_FACE ( 'NONE', ( #8373 ), #156361, .T. ) ;
#126898=CARTESIAN_POINT ( 'NONE',  ( 5.632522751473472589, 8.658694745772667289, -1.199719254218440723 ) ) ;
#126902=CARTESIAN_POINT ( 'NONE',  ( -6.124532705071231931, 8.168374127381657246, -1.599625672291263179 ) ) ;
#126903=ORIENTED_EDGE ( 'NONE', *, *, #36635, .F. ) ;
#126904=CARTESIAN_POINT ( 'NONE',  ( 5.040934186182656873, 4.775511393501539636, 1.040834085586084257E-14 ) ) ;
#126910=CARTESIAN_POINT ( 'NONE',  ( 4.062392026992976746, 7.509557588607558287, 0.5198811075141016591 ) ) ;
#126911=EDGE_CURVE ( 'NONE', #140339, #19327, #29193, .T. ) ;
#126913=EDGE_CURVE ( 'NONE', #201094, #177962, #171858, .T. ) ;
#126921=CARTESIAN_POINT ( 'NONE',  ( 7.375272376154084597, 9.627570410311676596, -1.443375672974057666 ) ) ;
#126924=CARTESIAN_POINT ( 'NONE',  ( -5.199715606040888005, 6.025088614257851027, -1.199719254218446718 ) ) ;
#126925=CARTESIAN_POINT ( 'NONE',  ( 4.800089777832203808, 5.120415418395356077, -0.7784788408505428636 ) ) ;
#126927=CARTESIAN_POINT ( 'NONE',  ( 8.620286740190458374, 8.951422706510690830, 1.040834085586084257E-14 ) ) ;
#126929=CARTESIAN_POINT ( 'NONE',  ( -6.891622154448065807, 6.934647356477856128, 1.040834085586084257E-14 ) ) ;
#126944=CARTESIAN_POINT ( 'NONE',  ( -5.199715606040888005, 6.025088614257851027, -1.199719254218446718 ) ) ;
#126947=CARTESIAN_POINT ( 'NONE',  ( 4.582292731738905722, 5.408724944192588424, -1.082531754730548412 ) ) ;
#126951=CARTESIAN_POINT ( 'NONE',  ( -4.298098390732130625, 4.973201863064262263, 1.199719254218462483 ) ) ;
#126952=CARTESIAN_POINT ( 'NONE',  ( -3.144601563365788444, 5.756120026313656268, -1.199719254218452935 ) ) ;
#126955=CARTESIAN_POINT ( 'NONE',  ( 8.191097360950562845, 12.70803068775103739, -0.7998128361456352531 ) ) ;
#126959=CARTESIAN_POINT ( 'NONE',  ( -6.093499974338126179, 9.196501505781426999, -1.199719254218440723 ) ) ;
#126960=CARTESIAN_POINT ( 'NONE',  ( 5.769158057814842699, 6.689438141327490150, 1.199719254218462483 ) ) ;
#126964=CARTESIAN_POINT ( 'NONE',  ( 5.522248639467795428, 5.337044922334209573, -0.7998128361456231517 ) ) ;
#126967=CARTESIAN_POINT ( 'NONE',  ( 1.364683531249988535, 1.426041667008083991, 0.7879004041258500513 ) ) ;
#126968=ORIENTED_EDGE ( 'NONE', *, *, #166950, .F. ) ;
#126970=CARTESIAN_POINT ( 'NONE',  ( 6.127922243696800386, 10.09306701771420656, -0.7216878364870267237 ) ) ;
#126971=ORIENTED_EDGE ( 'NONE', *, *, #95161, .F. ) ;
#126978=CARTESIAN_POINT ( 'NONE',  ( 9.531018800282605952, 11.18223869082697597, 1.082531754730548412 ) ) ;
#126980=ORIENTED_EDGE ( 'NONE', *, *, #141538, .T. ) ;
#126984=CARTESIAN_POINT ( 'NONE',  ( -2.065088895208807340, 8.523968132013855836, 2.459875961809343092 ) ) ;
#126987=DIRECTION ( 'NONE',  ( 5.578564026256490882E-16, 1.000000000000000000, 9.066213480720158442E-32 ) ) ;
#127003=CARTESIAN_POINT ( 'NONE',  ( 0.7499999999999885647, 1.847916667349486231, -1.299038105676652899 ) ) ;
#127009=CARTESIAN_POINT ( 'NONE',  ( -1.500000000000015099, -0.8291666666666407393, 0.8660254037844403729 ) ) ;
#127010=CARTESIAN_POINT ( 'NONE',  ( 8.911787042884274257, 9.291506392986812912, 0.7998128361456462443 ) ) ;
#127011=CARTESIAN_POINT ( 'NONE',  ( -1.364683531250014514, -0.2197916663252438285, 0.7879004041258379498 ) ) ;
#127014=CARTESIAN_POINT ( 'NONE',  ( 8.581948047770334043, 12.95609712246668899, 0.000000000000000000 ) ) ;
#127015=CARTESIAN_POINT ( 'NONE',  ( -5.422898255786186006, 9.270539031818461950, -0.7216878364870207285 ) ) ;
#127019=CARTESIAN_POINT ( 'NONE',  ( -6.018930129462987999, 9.109503353427070849, 1.199719254218452047 ) ) ;
#127021=CARTESIAN_POINT ( 'NONE',  ( -1.500000000000001332, 1.431250000682816825, 0.000000000000000000 ) ) ;
#127024=ADVANCED_FACE ( 'NONE', ( #185575 ), #136855, .T. ) ;
#127029=CIRCLE ( 'NONE', #161434, 4.021913119055696484 ) ;
#127034=CARTESIAN_POINT ( 'NONE',  ( -7.641992139597101108, 12.06740792950531649, 0.7998128361456481317 ) ) ;
#127035=CARTESIAN_POINT ( 'NONE',  ( 6.096362627639171805, 10.26417349888772179, -0.7998128361456291469 ) ) ;
#127039=ORIENTED_EDGE ( 'NONE', *, *, #198453, .F. ) ;
#127042=CARTESIAN_POINT ( 'NONE',  ( -7.426115451983156923, 9.686887332112256388, -1.599625672291263179 ) ) ;
#127046=EDGE_LOOP ( 'NONE', ( #196150, #65528, #3326, #22359 ) ) ;
#127049=CARTESIAN_POINT ( 'NONE',  ( 5.203632029546647608, 4.965325544092860532, 1.040834085586084257E-14 ) ) ;
#127057=CARTESIAN_POINT ( 'NONE',  ( -4.922147708203060468, 6.858988491581952118, -1.449652397630277756 ) ) ;
#127073=( BOUNDED_CURVE ( )  B_SPLINE_CURVE ( 3, ( #53542, #71900, #153177, #119674 ),
 .UNSPECIFIED., .F., .T. ) 
 B_SPLINE_CURVE_WITH_KNOTS ( ( 4, 4 ),
 ( 1.570796326794896114, 2.200856270471019283 ),
 .UNSPECIFIED. ) 
 CURVE ( )  GEOMETRIC_REPRESENTATION_ITEM ( )  RATIONAL_B_SPLINE_CURVE ( ( 1.000000000000000000, 0.9671913951452630887, 0.9671913951452630887, 1.000000000000000000 ) ) 
 REPRESENTATION_ITEM ( '' )  );
#127075=CARTESIAN_POINT ( 'NONE',  ( -1.402160292154681736E-14, 0.3687500006828169363, -1.732050807568870754 ) ) ;
#127078=CARTESIAN_POINT ( 'NONE',  ( -1.598423149421388523, 8.713846000020799565, -2.500000000000119016 ) ) ;
#127084=DIRECTION ( 'NONE',  ( -0.1674078377062507283, 3.252606517456525293E-14, 0.9858877298529065136 ) ) ;
#127086=CARTESIAN_POINT ( 'NONE',  ( 4.121315508874254796, 5.831287398485176077, -1.443375672974051449 ) ) ;
#127090=CARTESIAN_POINT ( 'NONE',  ( -9.541187415715041809, 12.15447128979948310, -1.599625672291263179 ) ) ;
#127091=( BOUNDED_SURFACE ( )  B_SPLINE_SURFACE ( 1, 2, ( 
 ( #54967, #187084, #38717, #200120, #116813, #51774, #104797, #84255, #170844, #167642, #135167, #1909, #22434, #182814, #85323, #151406, #201183, #67968, #134111, #117892, #183884, #35496, #101574, #52821, #156747, #190283, #154606, #27796, #157814, #8337, #74422, #91760, #89618, #6185, #140522, #41940, #138361, #208658, #125378, #189230, #26722, #204379, #109120, #76538, #172999, #23513, #24580, #206535, #126448, #9412, #108053, #123266, #58165, #72254, #174077, #142649, #110184, #25649, #124323, #40869, #56035, #75483, #43008, #122188, #155671, #191342, #192411, #92823, #175135, #188154, #141594, #60289, #7253, #90687, #158868, #10464, #207601, #39786, #44066, #59220, #176195, #57099, #73329, #105892, #106974, #171917, #139431, #205466, #209724, #31014, #146906, #63497, #210801, #94953, #62424, #193497, #181493, #197742, #177254, #127526, #64560, #212925, #194555, #93894, #11536, #47271, #32061, #147955, #28866, #161001, #128589, #178331, #180445, #130704, #213968, #77606, #49380, #46198, #81870, #65588, #12595, #196695, #211860, #48335, #114445, #112316, #159933, #143730, #113385, #98148, #131736, #78668, #144794, #29939, #96024, #164197, #15784, #115498, #61368, #45139, #162076, #111251, #13665, #79737, #145853, #129652, #195637, #179394, #97088, #163141, #14724, #80815, #185743, #52563, #17905, #82926, #83991, #119764, #116558, #153262, #199866, #101308, #132786, #36301, #102378, #51509, #117634, #183625, #134908, #103452, #69848, #168447, #151147, #120848, #148999, #35233, #68789, #33122, #99201, #20046, #167389, #18979, #184679, #182551, #165251, #85062, #200915, #16844, #87198, #3773, #67708, #37377, #576, #201974, #169512, #2716, #34175, #118694, #86133, #4837, #152205, #135959, #1650, #53631, #66642, #21094, #70916, #203053, #137026, #54697, #133857, #198789, #50438, #100247, #166315, #150078, #157554, #158612, #125124, #9149, #88271, #172732, #108855, #39514, #56834, #191083, #42751, #173817, #22156, #174881, #188960, #75224, #89352, #55762, #8073, #155401, #40601, #140253, #141336, #154338, #124063, #25395, #156484, #6984, #187886, #73064, #71988, #60034, #76284, #121918, #5914, #139163, #26461, #90414, #57898, #206275, #190028, #38449, #41680, #91494, #106707, #186821, #104529, #207350, #170574, #58970, #205193, #123005, #138099, #24309, #74159, #107791, #92570, #10210, #142392, #208401, #204110, #105613, #171643, #23240, #126187, #194302, #210545, #127264, #78416, #31818, #193235, #176993, #143464, #211600, #163954, #80555, #96835, #160740, #178065, #45945, #15531, #209461, #12335, #64308, #27533, #61105, #159671, #29683, #110988, #146653, #161822, #130454, #212667, #43814, #162884, #147700, #192150, #97894, #93629, #129399, #44883, #113126, #81616, #196442, #14464, #13410, #213718, #179131, #112065, #48086, #128338, #114199, #180197, #144536, #95767, #195378, #28610, #11273, #109927, #79486, #145605, #63236, #47010, #77351, #94700, #175938, #62180, #30755, #185506, #165001, #101057, #329, #1404, #33930, #119518, #118452, #151964, #183381, #50191, #52323, #169270, #68542, #66400, #134671, #65341, #16593, #82675, #69609, #148759, #115252, #37129, #98947, #36056, #49135, #200674, #184439, #85888, #103208, #86955, #102137, #132546, #131489, #198545, #20856, #2466, #3536, #84816, #116311, #181243, #182302, #135716, #100005, #153023, #17659, #133611, #166071, #168205, #19804, #83742, #149835, #67465, #167146, #201742, #53383, #197494, #34987, #32871, #199615, #51260, #18733, #117384, #150905, #7818, #6747, #72825, #156241, #154095, #4598, #138928, #40357, #202811, #58722, #189781, #39271, #91245, #54460, #173574, #141084, #22993, #88023, #89110, #204945, #190838, #73911, #106461, #187643, #56596, #136782, #24072, #207094, #174634, #172485, #122758, #105365, #120603, #90178, #107540, #186580, #5664, #41432, #42499, #157305, #25143, #38209, #188719, #124873, #71743, #155164, #8895, #74975, #206025, #104282, #108606, #140004, #26210, #121678, #137858, #57663, #171402, #123821, #92328, #70672, #170327, #21914, #203878, #55523, #60851, #159419, #127014, #43563, #31565, #47835, #27275, #191901, #129148 ),
 ( #130198, #179941, #62979, #109683, #9962, #175686, #44625, #162631, #61926, #29431, #177815, #95522, #76039, #161572, #176740, #28354, #94449, #45695, #14206, #195124, #13159, #128085, #158369, #59786, #160488, #194042, #142142, #208156, #79236, #12095, #78163, #145354, #93382, #125945, #144293, #111810, #11019, #212412, #46762, #192973, #30502, #77094, #112873, #80301, #210286, #143221, #211355, #178888, #196192, #96583, #146398, #110740, #64055, #209211, #113946, #19547, #53124, #51002, #149567, #132285, #147446, #117122, #200421, #213470, #98689, #68285, #69348, #35802, #134417, #65093, #83484, #85625, #164746, #182041, #101880, #167946, #84558, #131250, #151712, #99747, #52068, #75, #180992, #133348, #66140, #165817, #183125, #118194, #197237, #34731, #150647, #67213, #198290, #16338, #49932, #48876, #185242, #201482, #32612, #114994, #184182, #2208, #116053, #97640, #15279, #100803, #3281, #135459, #82419, #148508, #33672, #17400, #119257, #163697, #81366, #1150, #199354, #166889, #18479, #159968, #120338, #158904, #157850, #126482, #86692, #71485, #10500, #209759, #191378, #192446, #59254, #21654, #152761, #87761, #44101, #186314, #11573, #203615, #105099, #136528, #43044, #77643, #20606, #61400, #55267, #27831, #143765, #37949, #76573, #9444, #110221, #4343, #137598, #142685, #127563, #109157, #176229, #125412, #153837, #70410, #5407, #93927, #104021, #36864, #121414, #171140, #202548, #175169, #26756, #187386, #39017, #22732, #141627, #102948, #208695, #92857, #75515, #169008, #54198, #88848, #207636, #170068, #60322, #196731, #195673, #47309, #130738, #128625, #193532, #113423, #14763, #177292, #33159, #164233, #13702, #65626, #28906, #147994, #115536, #211898, #62463, #63535, #179429, #165289, #48372, #80853, #162112, #31050, #111286, #212959, #181531, #149038, #146944, #97126, #79775, #94991, #64597, #81906, #161037, #194592, #15821, #16883, #131775, #214004, #12632, #163178, #99240, #46236, #129690, #197778, #49416, #180481, #78703, #82965, #114484, #613, #96059, #112353, #32100, #145887, #98185, #66681, #45174, #144829, #210837, #178366, #29974, #35272, #133898, #101350, #17945, #5957, #22203, #1694, #166355, #103494, #185784, #19021, #132828, #50477, #86174, #70959, #186863, #67748, #199905, #167429, #2758, #4880, #37418, #203094, #134949, #21137, #85101, #51551, #168487, #151186, #200956, #152244, #169555, #34215, #69888, #87240, #102419, #68827, #117676, #52604, #84032, #198832, #88316, #183669, #150121, #153305, #137069, #118733, #116598, #182592, #3817, #54739, #38493, #184717, #36341, #20086, #136001, #120889, #104571, #170616, #100288, #154380, #202014, #53673, #119805, #155442, #191124, #190069, #158652, #121959, #106748, #42790, #27573, #9192, #10250, #91538, #56875, #187926, #123051, #76326, #7027, #192191, #24349, #140298, #171685, #75263, #141377, #90459, #156525, #8116, #173856, #142432, #108899, #207388, #41721, #159714, #39556, #74204, #107831, #72028, #138140, #59009, #206317, #57941, #125165, #73103, #204149, #124106, #25432, #55805, #126230, #174922, #172775, #208440, #105657, #26502, #60074, #157597, #139204, #92609, #43855, #109969, #175980, #93671, #40645, #23282, #89394, #205234, #189002, #181283, #179173, #63278, #45985, #61143, #30797, #114238, #127305, #12377, #196484, #197530, #163993, #48126, #193276, #211643, #147742, #78457, #95807, #15568, #81655, #212710, #44921, #129440, #210589, #180236, #47053, #213758, #97935, #143506, #31860, #32910, #77390, #131527, #111029, #14507, #144575, #64351, #115292, #65381, #49175, #113169, #98987, #130497, #145647, #11312, #13453, #209503, #177034, #29725, #195423, #80598, #62219, #28651, #94738, #96876, #162926, #146694, #160784, #128376, #194344, #112106, #178109, #161863, #79529, #50228, #200709, #100043, #101093, #133650, #4632, #3570, #37167, #68578, #149871, #151999, #54493, #168240, #166106, #19839, #165040, #116348, #182338, #169305, #33966, #364, #70704, #198582, #135753, #148794, #85925, #69644, #185539, #136817, #186615, #201776, #17692, #16633, #83779, #51296, #20890, #134704, #36089, #184472, #102173, #82717, #53416 ) ),
 .UNSPECIFIED., .F., .F., .F. ) 
 B_SPLINE_SURFACE_WITH_KNOTS ( ( 2, 2 ),
 ( 3, 2, 2, 2, 2, 2, 2, 2, 2, 2, 2, 2, 2, 2, 2, 2, 2, 2, 2, 2, 2, 2, 2, 2, 2, 2, 2, 2, 2, 2, 2, 2, 2, 2, 2, 2, 2, 2, 2, 2, 2, 2, 2, 2, 2, 2, 2, 2, 2, 2, 2, 2, 2, 2, 2, 2, 2, 2, 2, 2, 2, 2, 2, 2, 2, 2, 2, 2, 2, 2, 2, 2, 2, 2, 2, 2, 2, 2, 2, 2, 2, 2, 2, 2, 2, 2, 2, 2, 2, 2, 2, 2, 2, 2, 2, 2, 2, 2, 2, 2, 2, 2, 2, 2, 2, 2, 2, 2, 2, 2, 2, 2, 2, 2, 2, 2, 2, 2, 2, 2, 2, 2, 2, 2, 2, 2, 2, 2, 2, 2, 2, 2, 2, 2, 2, 2, 2, 2, 2, 2, 2, 2, 2, 2, 2, 2, 2, 2, 2, 2, 2, 2, 2, 2, 2, 2, 2, 2, 2, 2, 2, 2, 2, 2, 2, 2, 2, 2, 2, 2, 2, 2, 2, 2, 2, 2, 2, 2, 2, 2, 2, 2, 2, 2, 2, 2, 2, 2, 2, 2, 2, 2, 2, 2, 2, 2, 2, 2, 2, 2, 2, 2, 2, 2, 2, 2, 2, 2, 2, 2, 2, 2, 2, 2, 2, 2, 2, 2, 2, 2, 2, 2, 2, 2, 2, 2, 2, 2, 2, 2, 2, 2, 2, 2, 2, 2, 2, 2, 2, 2, 3 ),
 ( 0.000000000000000000, 1.000000000000000000 ),
 ( 0.000000000000000000, 0.004166666666666666609, 0.008333333333333333218, 0.01250000000000000069, 0.01666666666666666644, 0.02083333333333333218, 0.02500000000000000139, 0.02916666666666666713, 0.03333333333333333287, 0.03749999999999999861, 0.04166666666666666435, 0.04583333333333333010, 0.05000000000000000278, 0.05416666666666666852, 0.05833333333333333426, 0.06250000000000000000, 0.06666666666666666574, 0.07083333333333333148, 0.07499999999999999722, 0.07916666666666666297, 0.08333333333333332871, 0.08749999999999999445, 0.09166666666666666019, 0.09583333333333333981, 0.1000000000000000056, 0.1041666666666666713, 0.1083333333333333370, 0.1125000000000000028, 0.1166666666666666685, 0.1208333333333333343, 0.1250000000000000000, 0.1291666666666666796, 0.1333333333333333315, 0.1375000000000000111, 0.1416666666666666630, 0.1458333333333333426, 0.1499999999999999944, 0.1541666666666666741, 0.1583333333333333259, 0.1625000000000000056, 0.1666666666666666574, 0.1708333333333333370, 0.1749999999999999889, 0.1791666666666666685, 0.1833333333333333204, 0.1875000000000000000, 0.1916666666666666796, 0.1958333333333333315, 0.2000000000000000111, 0.2041666666666666630, 0.2083333333333333426, 0.2124999999999999944, 0.2166666666666666741, 0.2208333333333333259, 0.2250000000000000056, 0.2291666666666666574, 0.2333333333333333370, 0.2374999999999999889, 0.2416666666666666685, 0.2458333333333333204, 0.2500000000000000000, 0.2541666666666666519, 0.2583333333333333592, 0.2625000000000000111, 0.2666666666666666630, 0.2708333333333333148, 0.2750000000000000222, 0.2791666666666666741, 0.2833333333333333259, 0.2874999999999999778, 0.2916666666666666852, 0.2958333333333333370, 0.2999999999999999889, 0.3041666666666666408, 0.3083333333333333481, 0.3125000000000000000, 0.3166666666666666519, 0.3208333333333333592, 0.3250000000000000111, 0.3291666666666666630, 0.3333333333333333148, 0.3375000000000000222, 0.3416666666666666741, 0.3458333333333333259, 0.3499999999999999778, 0.3541666666666666852, 0.3583333333333333370, 0.3624999999999999889, 0.3666666666666666408, 0.3708333333333333481, 0.3750000000000000000, 0.3791666666666666519, 0.3833333333333333592, 0.3875000000000000111, 0.3916666666666666630, 0.3958333333333333148, 0.4000000000000000222, 0.4041666666666666741, 0.4083333333333333259, 0.4124999999999999778, 0.4166666666666666852, 0.4208333333333333370, 0.4249999999999999889, 0.4291666666666666408, 0.4333333333333333481, 0.4375000000000000000, 0.4416666666666666519, 0.4458333333333333592, 0.4500000000000000111, 0.4541666666666666630, 0.4583333333333333148, 0.4625000000000000222, 0.4666666666666666741, 0.4708333333333333259, 0.4749999999999999778, 0.4791666666666666852, 0.4833333333333333370, 0.4874999999999999889, 0.4916666666666666408, 0.4958333333333333481, 0.5000000000000000000, 0.5041666666666666519, 0.5083333333333333037, 0.5124999999999999556, 0.5166666666666667185, 0.5208333333333333703, 0.5250000000000000222, 0.5291666666666666741, 0.5333333333333333259, 0.5374999999999999778, 0.5416666666666666297, 0.5458333333333332815, 0.5500000000000000444, 0.5541666666666666963, 0.5583333333333333481, 0.5625000000000000000, 0.5666666666666666519, 0.5708333333333333037, 0.5749999999999999556, 0.5791666666666667185, 0.5833333333333333703, 0.5875000000000000222, 0.5916666666666666741, 0.5958333333333333259, 0.5999999999999999778, 0.6041666666666666297, 0.6083333333333332815, 0.6125000000000000444, 0.6166666666666666963, 0.6208333333333333481, 0.6250000000000000000, 0.6291666666666666519, 0.6333333333333333037, 0.6374999999999999556, 0.6416666666666667185, 0.6458333333333333703, 0.6500000000000000222, 0.6541666666666666741, 0.6583333333333333259, 0.6624999999999999778, 0.6666666666666666297, 0.6708333333333332815, 0.6750000000000000444, 0.6791666666666666963, 0.6833333333333333481, 0.6875000000000000000, 0.6916666666666666519, 0.6958333333333333037, 0.6999999999999999556, 0.7041666666666667185, 0.7083333333333333703, 0.7125000000000000222, 0.7166666666666666741, 0.7208333333333333259, 0.7249999999999999778, 0.7291666666666666297, 0.7333333333333332815, 0.7375000000000000444, 0.7416666666666666963, 0.7458333333333333481, 0.7500000000000000000, 0.7541666666666666519, 0.7583333333333333037, 0.7624999999999999556, 0.7666666666666667185, 0.7708333333333333703, 0.7750000000000000222, 0.7791666666666666741, 0.7833333333333333259, 0.7874999999999999778, 0.7916666666666666297, 0.7958333333333332815, 0.8000000000000000444, 0.8041666666666666963, 0.8083333333333333481, 0.8125000000000000000, 0.8166666666666666519, 0.8208333333333333037, 0.8249999999999999556, 0.8291666666666667185, 0.8333333333333333703, 0.8375000000000000222, 0.8416666666666666741, 0.8458333333333333259, 0.8499999999999999778, 0.8541666666666666297, 0.8583333333333332815, 0.8625000000000000444, 0.8666666666666666963, 0.8708333333333333481, 0.8750000000000000000, 0.8791666666666666519, 0.8833333333333333037, 0.8874999999999999556, 0.8916666666666667185, 0.8958333333333333703, 0.9000000000000000222, 0.9041666666666666741, 0.9083333333333333259, 0.9124999999999999778, 0.9166666666666666297, 0.9208333333333332815, 0.9250000000000000444, 0.9291666666666666963, 0.9333333333333333481, 0.9375000000000000000, 0.9416666666666666519, 0.9458333333333333037, 0.9499999999999999556, 0.9541666666666667185, 0.9583333333333333703, 0.9625000000000000222, 0.9666666666666666741, 0.9708333333333333259, 0.9749999999999999778, 0.9791666666666666297, 0.9833333333333332815, 0.9875000000000000444, 0.9916666666666666963, 0.9958333333333333481, 1.000000000000000000 ),
 .UNSPECIFIED. ) 
 GEOMETRIC_REPRESENTATION_ITEM ( )  RATIONAL_B_SPLINE_SURFACE ( (
 ( 1.000000000000000000, 0.8660254037844387076, 1.000000000000000000, 0.8660254037844387076, 1.000000000000000000, 0.8660254037844387076, 1.000000000000000000, 0.8660254037844387076, 1.000000000000000000, 0.8660254037844387076, 1.000000000000000000, 0.8660254037844387076, 1.000000000000000000, 0.8660254037844387076, 1.000000000000000000, 0.8660254037844387076, 1.000000000000000000, 0.8660254037844387076, 1.000000000000000000, 0.8660254037844387076, 1.000000000000000000, 0.8660254037844387076, 1.000000000000000000, 0.8660254037844387076, 1.000000000000000000, 0.8660254037844387076, 1.000000000000000000, 0.8660254037844387076, 1.000000000000000000, 0.8660254037844387076, 1.000000000000000000, 0.8660254037844387076, 1.000000000000000000, 0.8660254037844387076, 1.000000000000000000, 0.8660254037844387076, 1.000000000000000000, 0.8660254037844387076, 1.000000000000000000, 0.8660254037844387076, 1.000000000000000000, 0.8660254037844387076, 1.000000000000000000, 0.8660254037844387076, 1.000000000000000000, 0.8660254037844387076, 1.000000000000000000, 0.8660254037844387076, 1.000000000000000000, 0.8660254037844387076, 1.000000000000000000, 0.8660254037844387076, 1.000000000000000000, 0.8660254037844387076, 1.000000000000000000, 0.8660254037844387076, 1.000000000000000000, 0.8660254037844387076, 1.000000000000000000, 0.8660254037844387076, 1.000000000000000000, 0.8660254037844387076, 1.000000000000000000, 0.8660254037844387076, 1.000000000000000000, 0.8660254037844387076, 1.000000000000000000, 0.8660254037844387076, 1.000000000000000000, 0.8660254037844387076, 1.000000000000000000, 0.8660254037844387076, 1.000000000000000000, 0.8660254037844387076, 1.000000000000000000, 0.8660254037844387076, 1.000000000000000000, 0.8660254037844387076, 1.000000000000000000, 0.8660254037844387076, 1.000000000000000000, 0.8660254037844387076, 1.000000000000000000, 0.8660254037844387076, 1.000000000000000000, 0.8660254037844387076, 1.000000000000000000, 0.8660254037844387076, 1.000000000000000000, 0.8660254037844387076, 1.000000000000000000, 0.8660254037844387076, 1.000000000000000000, 0.8660254037844387076, 1.000000000000000000, 0.8660254037844387076, 1.000000000000000000, 0.8660254037844387076, 1.000000000000000000, 0.8660254037844387076, 1.000000000000000000, 0.8660254037844387076, 1.000000000000000000, 0.8660254037844387076, 1.000000000000000000, 0.8660254037844387076, 1.000000000000000000, 0.8660254037844387076, 1.000000000000000000, 0.8660254037844387076, 1.000000000000000000, 0.8660254037844387076, 1.000000000000000000, 0.8660254037844387076, 1.000000000000000000, 0.8660254037844387076, 1.000000000000000000, 0.8660254037844387076, 1.000000000000000000, 0.8660254037844387076, 1.000000000000000000, 0.8660254037844387076, 1.000000000000000000, 0.8660254037844387076, 1.000000000000000000, 0.8660254037844387076, 1.000000000000000000, 0.8660254037844387076, 1.000000000000000000, 0.8660254037844387076, 1.000000000000000000, 0.8660254037844387076, 1.000000000000000000, 0.8660254037844387076, 1.000000000000000000, 0.8660254037844387076, 1.000000000000000000, 0.8660254037844387076, 1.000000000000000000, 0.8660254037844387076, 1.000000000000000000, 0.8660254037844387076, 1.000000000000000000, 0.8660254037844387076, 1.000000000000000000, 0.8660254037844387076, 1.000000000000000000, 0.8660254037844387076, 1.000000000000000000, 0.8660254037844387076, 1.000000000000000000, 0.8660254037844387076, 1.000000000000000000, 0.8660254037844387076, 1.000000000000000000, 0.8660254037844387076, 1.000000000000000000, 0.8660254037844387076, 1.000000000000000000, 0.8660254037844387076, 1.000000000000000000, 0.8660254037844387076, 1.000000000000000000, 0.8660254037844387076, 1.000000000000000000, 0.8660254037844387076, 1.000000000000000000, 0.8660254037844387076, 1.000000000000000000, 0.8660254037844387076, 1.000000000000000000, 0.8660254037844387076, 1.000000000000000000, 0.8660254037844387076, 1.000000000000000000, 0.8660254037844387076, 1.000000000000000000, 0.8660254037844387076, 1.000000000000000000, 0.8660254037844387076, 1.000000000000000000, 0.8660254037844387076, 1.000000000000000000, 0.8660254037844387076, 1.000000000000000000, 0.8660254037844387076, 1.000000000000000000, 0.8660254037844387076, 1.000000000000000000, 0.8660254037844387076, 1.000000000000000000, 0.8660254037844387076, 1.000000000000000000, 0.8660254037844387076, 1.000000000000000000, 0.8660254037844387076, 1.000000000000000000, 0.8660254037844387076, 1.000000000000000000, 0.8660254037844387076, 1.000000000000000000, 0.8660254037844387076, 1.000000000000000000, 0.8660254037844387076, 1.000000000000000000, 0.8660254037844387076, 1.000000000000000000, 0.8660254037844387076, 1.000000000000000000, 0.8660254037844387076, 1.000000000000000000, 0.8660254037844387076, 1.000000000000000000, 0.8660254037844387076, 1.000000000000000000, 0.8660254037844387076, 1.000000000000000000, 0.8660254037844387076, 1.000000000000000000, 0.8660254037844387076, 1.000000000000000000, 0.8660254037844387076, 1.000000000000000000, 0.8660254037844387076, 1.000000000000000000, 0.8660254037844387076, 1.000000000000000000, 0.8660254037844387076, 1.000000000000000000, 0.8660254037844387076, 1.000000000000000000, 0.8660254037844387076, 1.000000000000000000, 0.8660254037844387076, 1.000000000000000000, 0.8660254037844387076, 1.000000000000000000, 0.8660254037844387076, 1.000000000000000000, 0.8660254037844387076, 1.000000000000000000, 0.8660254037844387076, 1.000000000000000000, 0.8660254037844387076, 1.000000000000000000, 0.8660254037844387076, 1.000000000000000000, 0.8660254037844387076, 1.000000000000000000, 0.8660254037844387076, 1.000000000000000000, 0.8660254037844387076, 1.000000000000000000, 0.8660254037844387076, 1.000000000000000000, 0.8660254037844387076, 1.000000000000000000, 0.8660254037844387076, 1.000000000000000000, 0.8660254037844387076, 1.000000000000000000, 0.8660254037844387076, 1.000000000000000000, 0.8660254037844387076, 1.000000000000000000, 0.8660254037844387076, 1.000000000000000000, 0.8660254037844387076, 1.000000000000000000, 0.8660254037844387076, 1.000000000000000000, 0.8660254037844387076, 1.000000000000000000, 0.8660254037844387076, 1.000000000000000000, 0.8660254037844387076, 1.000000000000000000, 0.8660254037844387076, 1.000000000000000000, 0.8660254037844387076, 1.000000000000000000, 0.8660254037844387076, 1.000000000000000000, 0.8660254037844387076, 1.000000000000000000, 0.8660254037844387076, 1.000000000000000000, 0.8660254037844387076, 1.000000000000000000, 0.8660254037844387076, 1.000000000000000000, 0.8660254037844387076, 1.000000000000000000, 0.8660254037844387076, 1.000000000000000000, 0.8660254037844387076, 1.000000000000000000, 0.8660254037844387076, 1.000000000000000000, 0.8660254037844387076, 1.000000000000000000, 0.8660254037844387076, 1.000000000000000000, 0.8660254037844387076, 1.000000000000000000, 0.8660254037844387076, 1.000000000000000000, 0.8660254037844387076, 1.000000000000000000, 0.8660254037844387076, 1.000000000000000000, 0.8660254037844387076, 1.000000000000000000, 0.8660254037844387076, 1.000000000000000000, 0.8660254037844387076, 1.000000000000000000, 0.8660254037844387076, 1.000000000000000000, 0.8660254037844387076, 1.000000000000000000, 0.8660254037844387076, 1.000000000000000000, 0.8660254037844387076, 1.000000000000000000, 0.8660254037844387076, 1.000000000000000000, 0.8660254037844387076, 1.000000000000000000, 0.8660254037844387076, 1.000000000000000000, 0.8660254037844387076, 1.000000000000000000, 0.8660254037844387076, 1.000000000000000000, 0.8660254037844387076, 1.000000000000000000, 0.8660254037844387076, 1.000000000000000000, 0.8660254037844387076, 1.000000000000000000, 0.8660254037844387076, 1.000000000000000000, 0.8660254037844387076, 1.000000000000000000, 0.8660254037844387076, 1.000000000000000000, 0.8660254037844387076, 1.000000000000000000, 0.8660254037844387076, 1.000000000000000000, 0.8660254037844387076, 1.000000000000000000, 0.8660254037844387076, 1.000000000000000000, 0.8660254037844387076, 1.000000000000000000, 0.8660254037844387076, 1.000000000000000000, 0.8660254037844387076, 1.000000000000000000, 0.8660254037844387076, 1.000000000000000000, 0.8660254037844387076, 1.000000000000000000, 0.8660254037844387076, 1.000000000000000000, 0.8660254037844387076, 1.000000000000000000, 0.8660254037844387076, 1.000000000000000000, 0.8660254037844387076, 1.000000000000000000, 0.8660254037844387076, 1.000000000000000000, 0.8660254037844387076, 1.000000000000000000, 0.8660254037844387076, 1.000000000000000000, 0.8660254037844387076, 1.000000000000000000, 0.8660254037844387076, 1.000000000000000000, 0.8660254037844387076, 1.000000000000000000, 0.8660254037844387076, 1.000000000000000000, 0.8660254037844387076, 1.000000000000000000, 0.8660254037844387076, 1.000000000000000000, 0.8660254037844387076, 1.000000000000000000, 0.8660254037844387076, 1.000000000000000000, 0.8660254037844387076, 1.000000000000000000, 0.8660254037844387076, 1.000000000000000000, 0.8660254037844387076, 1.000000000000000000, 0.8660254037844387076, 1.000000000000000000, 0.8660254037844387076, 1.000000000000000000, 0.8660254037844387076, 1.000000000000000000, 0.8660254037844387076, 1.000000000000000000, 0.8660254037844387076, 1.000000000000000000, 0.8660254037844387076, 1.000000000000000000, 0.8660254037844387076, 1.000000000000000000, 0.8660254037844387076, 1.000000000000000000, 0.8660254037844387076, 1.000000000000000000, 0.8660254037844387076, 1.000000000000000000, 0.8660254037844387076, 1.000000000000000000, 0.8660254037844387076, 1.000000000000000000, 0.8660254037844387076, 1.000000000000000000, 0.8660254037844387076, 1.000000000000000000, 0.8660254037844387076, 1.000000000000000000, 0.8660254037844387076, 1.000000000000000000, 0.8660254037844387076, 1.000000000000000000, 0.8660254037844387076, 1.000000000000000000, 0.8660254037844387076, 1.000000000000000000, 0.8660254037844387076, 1.000000000000000000, 0.8660254037844387076, 1.000000000000000000, 0.8660254037844387076, 1.000000000000000000, 0.8660254037844387076, 1.000000000000000000, 0.8660254037844387076, 1.000000000000000000, 0.8660254037844387076, 1.000000000000000000, 0.8660254037844387076, 1.000000000000000000, 0.8660254037844387076, 1.000000000000000000, 0.8660254037844387076, 1.000000000000000000, 0.8660254037844387076, 1.000000000000000000, 0.8660254037844387076, 1.000000000000000000, 0.8660254037844387076, 1.000000000000000000, 0.8660254037844387076, 1.000000000000000000, 0.8660254037844387076, 1.000000000000000000, 0.8660254037844387076, 1.000000000000000000, 0.8660254037844387076, 1.000000000000000000, 0.8660254037844387076, 1.000000000000000000, 0.8660254037844387076, 1.000000000000000000, 0.8660254037844387076, 1.000000000000000000, 0.8660254037844387076, 1.000000000000000000, 0.8660254037844387076, 1.000000000000000000),
 ( 1.000000000000000000, 0.8660254037844387076, 1.000000000000000000, 0.8660254037844387076, 1.000000000000000000, 0.8660254037844387076, 1.000000000000000000, 0.8660254037844387076, 1.000000000000000000, 0.8660254037844387076, 1.000000000000000000, 0.8660254037844387076, 1.000000000000000000, 0.8660254037844387076, 1.000000000000000000, 0.8660254037844387076, 1.000000000000000000, 0.8660254037844387076, 1.000000000000000000, 0.8660254037844387076, 1.000000000000000000, 0.8660254037844387076, 1.000000000000000000, 0.8660254037844387076, 1.000000000000000000, 0.8660254037844387076, 1.000000000000000000, 0.8660254037844387076, 1.000000000000000000, 0.8660254037844387076, 1.000000000000000000, 0.8660254037844387076, 1.000000000000000000, 0.8660254037844387076, 1.000000000000000000, 0.8660254037844387076, 1.000000000000000000, 0.8660254037844387076, 1.000000000000000000, 0.8660254037844387076, 1.000000000000000000, 0.8660254037844387076, 1.000000000000000000, 0.8660254037844387076, 1.000000000000000000, 0.8660254037844387076, 1.000000000000000000, 0.8660254037844387076, 1.000000000000000000, 0.8660254037844387076, 1.000000000000000000, 0.8660254037844387076, 1.000000000000000000, 0.8660254037844387076, 1.000000000000000000, 0.8660254037844387076, 1.000000000000000000, 0.8660254037844387076, 1.000000000000000000, 0.8660254037844387076, 1.000000000000000000, 0.8660254037844387076, 1.000000000000000000, 0.8660254037844387076, 1.000000000000000000, 0.8660254037844387076, 1.000000000000000000, 0.8660254037844387076, 1.000000000000000000, 0.8660254037844387076, 1.000000000000000000, 0.8660254037844387076, 1.000000000000000000, 0.8660254037844387076, 1.000000000000000000, 0.8660254037844387076, 1.000000000000000000, 0.8660254037844387076, 1.000000000000000000, 0.8660254037844387076, 1.000000000000000000, 0.8660254037844387076, 1.000000000000000000, 0.8660254037844387076, 1.000000000000000000, 0.8660254037844387076, 1.000000000000000000, 0.8660254037844387076, 1.000000000000000000, 0.8660254037844387076, 1.000000000000000000, 0.8660254037844387076, 1.000000000000000000, 0.8660254037844387076, 1.000000000000000000, 0.8660254037844387076, 1.000000000000000000, 0.8660254037844387076, 1.000000000000000000, 0.8660254037844387076, 1.000000000000000000, 0.8660254037844387076, 1.000000000000000000, 0.8660254037844387076, 1.000000000000000000, 0.8660254037844387076, 1.000000000000000000, 0.8660254037844387076, 1.000000000000000000, 0.8660254037844387076, 1.000000000000000000, 0.8660254037844387076, 1.000000000000000000, 0.8660254037844387076, 1.000000000000000000, 0.8660254037844387076, 1.000000000000000000, 0.8660254037844387076, 1.000000000000000000, 0.8660254037844387076, 1.000000000000000000, 0.8660254037844387076, 1.000000000000000000, 0.8660254037844387076, 1.000000000000000000, 0.8660254037844387076, 1.000000000000000000, 0.8660254037844387076, 1.000000000000000000, 0.8660254037844387076, 1.000000000000000000, 0.8660254037844387076, 1.000000000000000000, 0.8660254037844387076, 1.000000000000000000, 0.8660254037844387076, 1.000000000000000000, 0.8660254037844387076, 1.000000000000000000, 0.8660254037844387076, 1.000000000000000000, 0.8660254037844387076, 1.000000000000000000, 0.8660254037844387076, 1.000000000000000000, 0.8660254037844387076, 1.000000000000000000, 0.8660254037844387076, 1.000000000000000000, 0.8660254037844387076, 1.000000000000000000, 0.8660254037844387076, 1.000000000000000000, 0.8660254037844387076, 1.000000000000000000, 0.8660254037844387076, 1.000000000000000000, 0.8660254037844387076, 1.000000000000000000, 0.8660254037844387076, 1.000000000000000000, 0.8660254037844387076, 1.000000000000000000, 0.8660254037844387076, 1.000000000000000000, 0.8660254037844387076, 1.000000000000000000, 0.8660254037844387076, 1.000000000000000000, 0.8660254037844387076, 1.000000000000000000, 0.8660254037844387076, 1.000000000000000000, 0.8660254037844387076, 1.000000000000000000, 0.8660254037844387076, 1.000000000000000000, 0.8660254037844387076, 1.000000000000000000, 0.8660254037844387076, 1.000000000000000000, 0.8660254037844387076, 1.000000000000000000, 0.8660254037844387076, 1.000000000000000000, 0.8660254037844387076, 1.000000000000000000, 0.8660254037844387076, 1.000000000000000000, 0.8660254037844387076, 1.000000000000000000, 0.8660254037844387076, 1.000000000000000000, 0.8660254037844387076, 1.000000000000000000, 0.8660254037844387076, 1.000000000000000000, 0.8660254037844387076, 1.000000000000000000, 0.8660254037844387076, 1.000000000000000000, 0.8660254037844387076, 1.000000000000000000, 0.8660254037844387076, 1.000000000000000000, 0.8660254037844387076, 1.000000000000000000, 0.8660254037844387076, 1.000000000000000000, 0.8660254037844387076, 1.000000000000000000, 0.8660254037844387076, 1.000000000000000000, 0.8660254037844387076, 1.000000000000000000, 0.8660254037844387076, 1.000000000000000000, 0.8660254037844387076, 1.000000000000000000, 0.8660254037844387076, 1.000000000000000000, 0.8660254037844387076, 1.000000000000000000, 0.8660254037844387076, 1.000000000000000000, 0.8660254037844387076, 1.000000000000000000, 0.8660254037844387076, 1.000000000000000000, 0.8660254037844387076, 1.000000000000000000, 0.8660254037844387076, 1.000000000000000000, 0.8660254037844387076, 1.000000000000000000, 0.8660254037844387076, 1.000000000000000000, 0.8660254037844387076, 1.000000000000000000, 0.8660254037844387076, 1.000000000000000000, 0.8660254037844387076, 1.000000000000000000, 0.8660254037844387076, 1.000000000000000000, 0.8660254037844387076, 1.000000000000000000, 0.8660254037844387076, 1.000000000000000000, 0.8660254037844387076, 1.000000000000000000, 0.8660254037844387076, 1.000000000000000000, 0.8660254037844387076, 1.000000000000000000, 0.8660254037844387076, 1.000000000000000000, 0.8660254037844387076, 1.000000000000000000, 0.8660254037844387076, 1.000000000000000000, 0.8660254037844387076, 1.000000000000000000, 0.8660254037844387076, 1.000000000000000000, 0.8660254037844387076, 1.000000000000000000, 0.8660254037844387076, 1.000000000000000000, 0.8660254037844387076, 1.000000000000000000, 0.8660254037844387076, 1.000000000000000000, 0.8660254037844387076, 1.000000000000000000, 0.8660254037844387076, 1.000000000000000000, 0.8660254037844387076, 1.000000000000000000, 0.8660254037844387076, 1.000000000000000000, 0.8660254037844387076, 1.000000000000000000, 0.8660254037844387076, 1.000000000000000000, 0.8660254037844387076, 1.000000000000000000, 0.8660254037844387076, 1.000000000000000000, 0.8660254037844387076, 1.000000000000000000, 0.8660254037844387076, 1.000000000000000000, 0.8660254037844387076, 1.000000000000000000, 0.8660254037844387076, 1.000000000000000000, 0.8660254037844387076, 1.000000000000000000, 0.8660254037844387076, 1.000000000000000000, 0.8660254037844387076, 1.000000000000000000, 0.8660254037844387076, 1.000000000000000000, 0.8660254037844387076, 1.000000000000000000, 0.8660254037844387076, 1.000000000000000000, 0.8660254037844387076, 1.000000000000000000, 0.8660254037844387076, 1.000000000000000000, 0.8660254037844387076, 1.000000000000000000, 0.8660254037844387076, 1.000000000000000000, 0.8660254037844387076, 1.000000000000000000, 0.8660254037844387076, 1.000000000000000000, 0.8660254037844387076, 1.000000000000000000, 0.8660254037844387076, 1.000000000000000000, 0.8660254037844387076, 1.000000000000000000, 0.8660254037844387076, 1.000000000000000000, 0.8660254037844387076, 1.000000000000000000, 0.8660254037844387076, 1.000000000000000000, 0.8660254037844387076, 1.000000000000000000, 0.8660254037844387076, 1.000000000000000000, 0.8660254037844387076, 1.000000000000000000, 0.8660254037844387076, 1.000000000000000000, 0.8660254037844387076, 1.000000000000000000, 0.8660254037844387076, 1.000000000000000000, 0.8660254037844387076, 1.000000000000000000, 0.8660254037844387076, 1.000000000000000000, 0.8660254037844387076, 1.000000000000000000, 0.8660254037844387076, 1.000000000000000000, 0.8660254037844387076, 1.000000000000000000, 0.8660254037844387076, 1.000000000000000000, 0.8660254037844387076, 1.000000000000000000, 0.8660254037844387076, 1.000000000000000000, 0.8660254037844387076, 1.000000000000000000, 0.8660254037844387076, 1.000000000000000000, 0.8660254037844387076, 1.000000000000000000, 0.8660254037844387076, 1.000000000000000000, 0.8660254037844387076, 1.000000000000000000, 0.8660254037844387076, 1.000000000000000000, 0.8660254037844387076, 1.000000000000000000, 0.8660254037844387076, 1.000000000000000000, 0.8660254037844387076, 1.000000000000000000, 0.8660254037844387076, 1.000000000000000000, 0.8660254037844387076, 1.000000000000000000, 0.8660254037844387076, 1.000000000000000000, 0.8660254037844387076, 1.000000000000000000, 0.8660254037844387076, 1.000000000000000000, 0.8660254037844387076, 1.000000000000000000, 0.8660254037844387076, 1.000000000000000000, 0.8660254037844387076, 1.000000000000000000, 0.8660254037844387076, 1.000000000000000000, 0.8660254037844387076, 1.000000000000000000, 0.8660254037844387076, 1.000000000000000000, 0.8660254037844387076, 1.000000000000000000, 0.8660254037844387076, 1.000000000000000000, 0.8660254037844387076, 1.000000000000000000, 0.8660254037844387076, 1.000000000000000000, 0.8660254037844387076, 1.000000000000000000, 0.8660254037844387076, 1.000000000000000000, 0.8660254037844387076, 1.000000000000000000, 0.8660254037844387076, 1.000000000000000000, 0.8660254037844387076, 1.000000000000000000, 0.8660254037844387076, 1.000000000000000000, 0.8660254037844387076, 1.000000000000000000, 0.8660254037844387076, 1.000000000000000000, 0.8660254037844387076, 1.000000000000000000, 0.8660254037844387076, 1.000000000000000000, 0.8660254037844387076, 1.000000000000000000, 0.8660254037844387076, 1.000000000000000000, 0.8660254037844387076, 1.000000000000000000, 0.8660254037844387076, 1.000000000000000000, 0.8660254037844387076, 1.000000000000000000, 0.8660254037844387076, 1.000000000000000000, 0.8660254037844387076, 1.000000000000000000, 0.8660254037844387076, 1.000000000000000000, 0.8660254037844387076, 1.000000000000000000, 0.8660254037844387076, 1.000000000000000000, 0.8660254037844387076, 1.000000000000000000, 0.8660254037844387076, 1.000000000000000000, 0.8660254037844387076, 1.000000000000000000, 0.8660254037844387076, 1.000000000000000000, 0.8660254037844387076, 1.000000000000000000, 0.8660254037844387076, 1.000000000000000000, 0.8660254037844387076, 1.000000000000000000, 0.8660254037844387076, 1.000000000000000000, 0.8660254037844387076, 1.000000000000000000, 0.8660254037844387076, 1.000000000000000000, 0.8660254037844387076, 1.000000000000000000, 0.8660254037844387076, 1.000000000000000000, 0.8660254037844387076, 1.000000000000000000, 0.8660254037844387076, 1.000000000000000000, 0.8660254037844387076, 1.000000000000000000, 0.8660254037844387076, 1.000000000000000000) ) ) 
 REPRESENTATION_ITEM ( '' )  SURFACE ( )  );
#127092=CARTESIAN_POINT ( 'NONE',  ( 8.723781775389312543, 12.26516360700784958, -1.199719254218446718 ) ) ;
#127094=AXIS2_PLACEMENT_3D ( 'NONE', #156993, #24827, #107223 ) ;
#127101=CARTESIAN_POINT ( 'NONE',  ( -1.364683531250014514, -1.011458332991911568, -0.7879004041258359514 ) ) ;
#127107=CARTESIAN_POINT ( 'NONE',  ( -4.741601036477307574, 6.554953847355395880, 1.599625672291267398 ) ) ;
#127110=CARTESIAN_POINT ( 'NONE',  ( -0.7500000000000006661, -0.1416666666666441254, -1.299038105676652011 ) ) ;
#127112=CARTESIAN_POINT ( 'NONE',  ( -0.7499999999999972244, 5.358333333333353821, -1.299038105676652011 ) ) ;
#127118=CARTESIAN_POINT ( 'NONE',  ( 1.364683531249992088, 5.696875000341418804, 1.214306433183764966E-14 ) ) ;
#127120=CARTESIAN_POINT ( 'NONE',  ( -7.004758919754800139, 11.32396917302262018, 0.000000000000000000 ) ) ;
#127126=CARTESIAN_POINT ( 'NONE',  ( -1.364683531250014514, 0.3427083336747508424, 0.7879004041258379498 ) ) ;
#127130=CARTESIAN_POINT ( 'NONE',  ( -2.034713692888051373, 8.461455076002923903, 2.500000000000011102 ) ) ;
#127133=CARTESIAN_POINT ( 'NONE',  ( 8.622622508611357262, 9.162073802909148412, -0.7216878364870197293 ) ) ;
#127136=CARTESIAN_POINT ( 'NONE',  ( -6.240830780992103755, 6.175390754112560110, 1.040834085586084257E-14 ) ) ;
#127138=CARTESIAN_POINT ( 'NONE',  ( -1.001543065824772872E-14, 4.743750000682822154, 1.732050807568877637 ) ) ;
#127140=CARTESIAN_POINT ( 'NONE',  ( -4.060830702492950195, 4.696389560118578999, -1.199719254218452047 ) ) ;
#127141=CARTESIAN_POINT ( 'NONE',  ( 6.439759776366769550, 8.536139043893143707, 1.443375672974076540 ) ) ;
#127142=CARTESIAN_POINT ( 'NONE',  ( -9.042925270190641740, 11.57316545335434199, 1.443375672974064550 ) ) ;
#127148=CARTESIAN_POINT ( 'NONE',  ( 10.54788032175191326, 11.40820791823982994, 0.7216878364870317197 ) ) ;
#127151=CARTESIAN_POINT ( 'NONE',  ( 2.319698010557100343, 5.424362912284642846, 0.6383152452940642485 ) ) ;
#127154=( BOUNDED_CURVE ( )  B_SPLINE_CURVE ( 2, ( #168537, #3866, #184767, #131820, #33205, #20135, #165336 ),
 .UNSPECIFIED., .F., .T. ) 
 B_SPLINE_CURVE_WITH_KNOTS ( ( 3, 2, 2, 3 ),
 ( 0.1750000000000002942, 0.1791666666666668628, 0.1833333333333334036, 0.1874999999999999722 ),
 .UNSPECIFIED. ) 
 CURVE ( )  GEOMETRIC_REPRESENTATION_ITEM ( )  RATIONAL_B_SPLINE_CURVE ( ( 0.9999999999999902300, 0.8660254037844484776, 1.000000000000000000, 0.8660254037844387076, 1.000000000000000000, 0.8660254037844395958, 0.9999999999999991118 ) ) 
 REPRESENTATION_ITEM ( '' )  );
#127155=CARTESIAN_POINT ( 'NONE',  ( -1.500000000000053513, 7.267697830503716538, -4.207111467970358731 ) ) ;
#127156=ORIENTED_EDGE ( 'NONE', *, *, #92482, .T. ) ;
#127167=CARTESIAN_POINT ( 'NONE',  ( 9.565441069641300587, 11.11843498845840905, -1.199719254218440723 ) ) ;
#127170=FACE_OUTER_BOUND ( 'NONE', #105605, .T. ) ;
#127173=CARTESIAN_POINT ( 'NONE',  ( -1.364683531250000748, 0.009375000341420303140, 0.000000000000000000 ) ) ;
#127174=CARTESIAN_POINT ( 'NONE',  ( 6.507550544879468823, 6.694489845221929691, -0.7216878364870257245 ) ) ;
#127176=CARTESIAN_POINT ( 'NONE',  ( -7.510853912290736289, 11.70648729774046792, 0.7216878364870458196 ) ) ;
#127198=CARTESIAN_POINT ( 'NONE',  ( 5.634486230560368902, 6.328851001874927107, -1.145628596103397623 ) ) ;
#127206=CARTESIAN_POINT ( 'NONE',  ( -8.365017589951714072, 8.861534731139549592, 1.040834085586084257E-14 ) ) ;
#127210=CARTESIAN_POINT ( 'NONE',  ( 5.913327553854682783, 10.05063257947248800, -0.7998128361456291469 ) ) ;
#127211=DIRECTION ( 'NONE',  ( -0.000000000000000000, -8.546850786086437571E-32, -1.000000000000000000 ) ) ;
#127212=CARTESIAN_POINT ( 'NONE',  ( 2.866659414285625651, 5.431854185720147221, -1.199719254218446718 ) ) ;
#127214=CARTESIAN_POINT ( 'NONE',  ( -4.948889764188092677, 5.732458465429559169, 1.199719254218462483 ) ) ;
#127218=CARTESIAN_POINT ( 'NONE',  ( -4.578903193113314174, 6.365139696764064325, 1.599625672291267398 ) ) ;
#127221=CARTESIAN_POINT ( 'NONE',  ( 3.897079088924235712, 6.634010472798538949, 1.199719254218462483 ) ) ;
#127222=CARTESIAN_POINT ( 'NONE',  ( 8.076906825439115423, 10.44614393447756129, -1.599625672291262513 ) ) ;
#127225=CARTESIAN_POINT ( 'NONE',  ( 4.815752433886056671, 6.955745678547994970, 1.411323681429425880 ) ) ;
#127226=CARTESIAN_POINT ( 'NONE',  ( 4.907688418466886304, 5.788353245375237321, -1.082531754730548412 ) ) ;
#127233=CARTESIAN_POINT ( 'NONE',  ( 5.761852095683461350, 9.665985178365305686, -0.7216878364870267237 ) ) ;
#127234=CARTESIAN_POINT ( 'NONE',  ( -9.833741488613570780, 10.36711991300432345, 0.7998128361456462443 ) ) ;
#127238=CARTESIAN_POINT ( 'NONE',  ( -9.809487834687324437, 11.40315621434539395, 1.199719254218462483 ) ) ;
#127239=CARTESIAN_POINT ( 'NONE',  ( -7.562750758324527922, 7.717630727667075696, 1.040834085586084257E-14 ) ) ;
#127240=CARTESIAN_POINT ( 'NONE',  ( -5.273758565591545988, 6.215435083687305351, 1.082531754730546636 ) ) ;
#127247=CARTESIAN_POINT ( 'NONE',  ( 7.377608144130607393, 11.75895993479440982, -0.7998128361456291469 ) ) ;
#127260=CARTESIAN_POINT ( 'NONE',  ( -1.500000000000011324, 2.670833333333352044, 0.8660254037844403729 ) ) ;
#127261=CARTESIAN_POINT ( 'NONE',  ( 5.449487677688982679, 8.445153826357429949, -1.199719254218446718 ) ) ;
#127264=CARTESIAN_POINT ( 'NONE',  ( 5.992340707560141588, 9.934888558888093968, 0.7216878364870438212 ) ) ;
#127265=CARTESIAN_POINT ( 'NONE',  ( -8.771762197917311710, 13.17754696430482042, 0.7216878364870317197 ) ) ;
#127269=CARTESIAN_POINT ( 'NONE',  ( 8.540746701604824409, 12.05162268759261224, -1.199719254218446718 ) ) ;
#127272=CARTESIAN_POINT ( 'NONE',  ( 1.499999999999990896, 5.056250000682820378, 1.214306433183764966E-14 ) ) ;
#127273=CARTESIAN_POINT ( 'NONE',  ( 1.364683531249988535, 1.613541667008084879, 0.7879004041258500513 ) ) ;
#127277=ADVANCED_FACE ( 'NONE', ( #169341 ), #52588, .T. ) ;
#127279=CARTESIAN_POINT ( 'NONE',  ( -1.364683531250014514, 0.2385416670080863499, -0.7879004041258359514 ) ) ;
#127281=CARTESIAN_POINT ( 'NONE',  ( 10.42352117080803708, 11.05519620889787724, -0.7998128361456281477 ) ) ;
#127284=CARTESIAN_POINT ( 'NONE',  ( -2.453662613948990323, 5.806430783008362795, -0.7216878364870257245 ) ) ;
#127287=CARTESIAN_POINT ( 'NONE',  ( -5.876569516519495551, 8.943415971659659292, 1.199719254218452047 ) ) ;
#127290=CARTESIAN_POINT ( 'NONE',  ( 2.855963913973019963, 6.483708332943829866, 0.000000000000000000 ) ) ;
#127296=ORIENTED_EDGE ( 'NONE', *, *, #5002, .T. ) ;
#127298=CARTESIAN_POINT ( 'NONE',  ( 8.563946585326370098, 13.14302144952281814, 0.7998128361456462443 ) ) ;
#127301=CARTESIAN_POINT ( 'NONE',  ( -5.473741331615264549, 7.409117525016355010, -1.599625672291256295 ) ) ;
#127305=CARTESIAN_POINT ( 'NONE',  ( 8.860417081730671995, 10.29590700256267155, 1.199719254218453823 ) ) ;
#127307=CARTESIAN_POINT ( 'NONE',  ( 6.591235234537977661, 10.84152487360300299, 0.7998128361456462443 ) ) ;
#127311=CARTESIAN_POINT ( 'NONE',  ( -3.735435015764967837, 4.316761258935923884, -1.199719254218452047 ) ) ;
#127314=CARTESIAN_POINT ( 'NONE',  ( -6.021792782764022078, 10.17717534653336209, -0.7998128361456291469 ) ) ;
#127318=CARTESIAN_POINT ( 'NONE',  ( -6.133306371789854161, 5.998871118906519584, 0.1305517085098181207 ) ) ;
#127319=CARTESIAN_POINT ( 'NONE',  ( 1.364683531249988757, 2.384375000341422357, 1.214306433183764966E-14 ) ) ;
#127322=CARTESIAN_POINT ( 'NONE',  ( 7.185458225562760148, 8.445751353653788485, -1.082531754730543083 ) ) ;
#127339=CARTESIAN_POINT ( 'NONE',  ( 9.284636267260101050, 9.726497154758602548, -0.7998128361456281477 ) ) ;
#127343=CARTESIAN_POINT ( 'NONE',  ( -4.192495815123836955, 5.914331089109674089, -1.599625672291256295 ) ) ;
#127344=CARTESIAN_POINT ( 'NONE',  ( -5.994676475536691029, 10.14553965476814845, 0.7998128361456481317 ) ) ;
#127350=CARTESIAN_POINT ( 'NONE',  ( 1.499999999999990896, 4.806250000682819490, 1.214306433183764966E-14 ) ) ;
#127351=CARTESIAN_POINT ( 'NONE',  ( 8.426556166093362776, 9.789735934319136135, -1.199719254218446718 ) ) ;
#127354=CARTESIAN_POINT ( 'NONE',  ( -6.842061076390810292, 11.13415502243129218, 0.000000000000000000 ) ) ;
#127356=CARTESIAN_POINT ( 'NONE',  ( -1.201851678989727383E-14, 3.321875000341421025, 1.575800808251672791 ) ) ;
#127361=CARTESIAN_POINT ( 'NONE',  ( -10.00555417720528872, 10.77549408293541866, 0.7216878364870438212 ) ) ;
#127365=CARTESIAN_POINT ( 'NONE',  ( -0.6823417656250003738, 2.280208333674753174, -1.181850606188749264 ) ) ;
#127372=CARTESIAN_POINT ( 'NONE',  ( -0.6823417656250003738, 2.967708333674754062, -1.181850606188749264 ) ) ;
#127374=CARTESIAN_POINT ( 'NONE',  ( -4.948889764188092677, 5.732458465429559169, 1.199719254218462483 ) ) ;
#127375=CARTESIAN_POINT ( 'NONE',  ( 7.135668919494039031, 7.219368582364847242, 1.040834085586084257E-14 ) ) ;
#127378=CARTESIAN_POINT ( 'NONE',  ( -1.001543065824772872E-14, 4.634375000341418804, 1.575800808251672791 ) ) ;
#127381=CARTESIAN_POINT ( 'NONE',  ( 1.364683531249988757, -0.6156249996585803075, 0.000000000000000000 ) ) ;
#127382=CARTESIAN_POINT ( 'NONE',  ( -3.782361668532609134, 7.356579680022602652, 1.040834085586084257E-14 ) ) ;
#127385=CARTESIAN_POINT ( 'NONE',  ( 5.341549334104200852, 5.334155099317434257, 0.7216878364870317197 ) ) ;
#127388=CARTESIAN_POINT ( 'NONE',  ( -7.446452682403657874, 9.710614100936176385, -1.599625672291263179 ) ) ;
#127389=CARTESIAN_POINT ( 'NONE',  ( -8.161645285746702783, 12.46574390010577105, 0.7216878364870478180 ) ) ;
#127397=CARTESIAN_POINT ( 'NONE',  ( -6.602457619730773608, 8.725953194484466380, 1.443375672974078761 ) ) ;
#127399=CARTESIAN_POINT ( 'NONE',  ( 0.6823417656249882723, 0.2385416670080825474, -1.181850606188749264 ) ) ;
#127400=CARTESIAN_POINT ( 'NONE',  ( 1.441119962213327499, 8.287674021641846522, 3.161270278916411325 ) ) ;
#127412=CARTESIAN_POINT ( 'NONE',  ( 0.7499999999999867883, -0.9333333333333138082, -1.299038105676652011 ) ) ;
#127413=CARTESIAN_POINT ( 'NONE',  ( 9.232739420781973294, 9.873876867108206667, -0.7216878364870257245 ) ) ;
#127419=ORIENTED_EDGE ( 'NONE', *, *, #82451, .F. ) ;
#127422=CARTESIAN_POINT ( 'NONE',  ( 4.473300617505036492, 7.306268922809479704, -1.199719254218452047 ) ) ;
#127424=CARTESIAN_POINT ( 'NONE',  ( -4.548924232584923288, 5.265832011892554121, -1.199719254218446718 ) ) ;
#127429=CARTESIAN_POINT ( 'NONE',  ( -4.880680834860089412, 4.940735376530475342, -0.5749358470996156489 ) ) ;
#127431=CARTESIAN_POINT ( 'NONE',  ( 0.6823417656249899377, 1.655208333674752730, 1.181850606188755259 ) ) ;
#127433=CARTESIAN_POINT ( 'NONE',  ( -7.862839020921525091, 11.26073039346208660, -1.199719254218446718 ) ) ;
#127447=VERTEX_POINT ( 'NONE', #85628 ) ;
#127451=CARTESIAN_POINT ( 'NONE',  ( 5.282873410819217241, 9.315102745931094219, -0.7998128361456281477 ) ) ;
#127458=CARTESIAN_POINT ( 'NONE',  ( 8.772289083241844310, 10.19309100432570148, -1.199719254218446718 ) ) ;
#127462=CARTESIAN_POINT ( 'NONE',  ( 10.09812548408005384, 10.67556790771522124, -0.7998128361456281477 ) ) ;
#127464=CARTESIAN_POINT ( 'NONE',  ( 1.550536438491937563, 8.693843051952859113, -2.505472492508726834 ) ) ;
#127467=ORIENTED_EDGE ( 'NONE', *, *, #179709, .F. ) ;
#127468=CARTESIAN_POINT ( 'NONE',  ( 10.58621901417202515, 11.24501035948919991, -0.7998128361456281477 ) ) ;
#127471=CARTESIAN_POINT ( 'NONE',  ( -0.3176981287468134685, 7.220460999378147449, 2.081427265489085521 ) ) ;
#127476=CARTESIAN_POINT ( 'NONE',  ( -7.185458225562757484, 11.32685899655781903, 0.7216878364870458196 ) ) ;
#127482=CARTESIAN_POINT ( 'NONE',  ( 4.904298879841284098, 6.744767997946721216, 1.599625672291267398 ) ) ;
#127483=CARTESIAN_POINT ( 'NONE',  ( -5.290478191143363595, 6.407017486086630242, -1.170018636208163043 ) ) ;
#127488=CARTESIAN_POINT ( 'NONE',  ( 3.836594282542920009, 4.538743420130594508, 1.082531754730560403 ) ) ;
#127496=CARTESIAN_POINT ( 'NONE',  ( -7.217017841176048165, 7.314275657660511243, 1.040834085586084257E-14 ) ) ;
#127498=CARTESIAN_POINT ( 'NONE',  ( -2.937312835655025101, 6.578615408239493867, 1.040834085586084257E-14 ) ) ;
#127507=CARTESIAN_POINT ( 'NONE',  ( 6.335737856287750880, 6.286115675290828264, -0.7998128361456281477 ) ) ;
#127509=CARTESIAN_POINT ( 'NONE',  ( 1.527330013470509673, 8.693738994866436087, 2.519751708053329153 ) ) ;
#127521=CARTESIAN_POINT ( 'NONE',  ( -1.402160292154681736E-14, 1.759375000341421469, -1.575800808251659024 ) ) ;
#127523=CARTESIAN_POINT ( 'NONE',  ( 4.864678189204997949, 4.569879397027603929, 0.7998128361456341429 ) ) ;
#127525=CARTESIAN_POINT ( 'NONE',  ( -5.422898255786186006, 9.270539031818461950, -0.7216878364870207285 ) ) ;
#127526=CARTESIAN_POINT ( 'NONE',  ( 4.446711195602238931, 6.210915699667823198, -1.443375672974051449 ) ) ;
#127527=CARTESIAN_POINT ( 'NONE',  ( -5.653386866774179786, 8.579073197003079798, 1.082531754730548412 ) ) ;
#127531=CARTESIAN_POINT ( 'NONE',  ( 6.205881626753210867, 8.263281202677319470, 1.599625672291281386 ) ) ;
#127536=CARTESIAN_POINT ( 'NONE',  ( -0.6823417656249969321, 5.467708333674756283, -1.181850606188749264 ) ) ;
#127540=CARTESIAN_POINT ( 'NONE',  ( 5.933664784275179294, 10.07435934829639912, -0.7998128361456291469 ) ) ;
#127544=CARTESIAN_POINT ( 'NONE',  ( -6.015013705957189316, 10.16926642359206134, 0.7998128361456481317 ) ) ;
#127549=CARTESIAN_POINT ( 'NONE',  ( 8.263858322729371153, 9.599921783727809910, -1.199719254218446718 ) ) ;
#127552=CARTESIAN_POINT ( 'NONE',  ( -8.389798128758148010, 8.682519326506312751, 0.7998128361456462443 ) ) ;
#127556=CARTESIAN_POINT ( 'NONE',  ( 7.415946836550722843, 8.714654733139752807, 1.082531754730558626 ) ) ;
#127557=CARTESIAN_POINT ( 'NONE',  ( 4.044190953901719787, 7.767772900817621284, 0.4663397696828552874 ) ) ;
#127558=CARTESIAN_POINT ( 'NONE',  ( -7.687109909268394325, 11.91211929421440097, 0.000000000000000000 ) ) ;
#127563=CARTESIAN_POINT ( 'NONE',  ( 5.769158057814842699, 6.689438141327490150, 1.199719254218462483 ) ) ;
#127565=CARTESIAN_POINT ( 'NONE',  ( 10.06423010004587759, 10.63602329300870153, 0.000000000000000000 ) ) ;
#127566=CARTESIAN_POINT ( 'NONE',  ( -5.660981573724272131, 6.153771497223376130, 0.8018600159674215133 ) ) ;
#127567=CARTESIAN_POINT ( 'NONE',  ( 2.333974999846879061, 5.874721266463329705, -0.7998128361456291469 ) ) ;
#127569=CARTESIAN_POINT ( 'NONE',  ( -7.890482213473404727, 8.307910125248191946, 0.7216878364870578100 ) ) ;
#127576=CARTESIAN_POINT ( 'NONE',  ( -4.245236785304952853, 7.324258608653995140, 0.8904289178662868620 ) ) ;
#127577=CARTESIAN_POINT ( 'NONE',  ( -1.364683531250014514, -0.4489583329919089039, -0.7879004041258359514 ) ) ;
#127580=CARTESIAN_POINT ( 'NONE',  ( 4.867013957625893283, 4.780530493426062399, 1.040834085586084257E-14 ) ) ;
#127581=CARTESIAN_POINT ( 'NONE',  ( -0.7499999999999972244, 3.639583334016149863, -1.299038105676652011 ) ) ;
#127584=CARTESIAN_POINT ( 'NONE',  ( -10.12757755928392456, 10.91785469536048758, 0.7216878364870438212 ) ) ;
#127587=EDGE_CURVE ( 'NONE', #77611, #155158, #163296, .T. ) ;
#127588=B_SPLINE_CURVE_WITH_KNOTS ( 'NONE', 1,
 ( #115081, #95603 ),
 .UNSPECIFIED., .F., .F.,
 ( 2, 2 ),
 ( 0.7585745852332145267, 1.000000000000000000 ),
 .UNSPECIFIED. ) ;
#127591=CARTESIAN_POINT ( 'NONE',  ( -8.798878505144649864, 11.28844422746735532, -1.443375672974058777 ) ) ;
#127597=VERTEX_POINT ( 'NONE', #150650 ) ;
#127598=CARTESIAN_POINT ( 'NONE',  ( -7.659993601596710278, 10.92011438762942355, -1.082531754730543083 ) ) ;
#127602=CARTESIAN_POINT ( 'NONE',  ( -0.6823417656250212460, 4.863541667008086655, 1.181850606188767472 ) ) ;
#127603=CARTESIAN_POINT ( 'NONE',  ( -1.500000000000011324, 4.410416667349484676, -0.8660254037844313801 ) ) ;
#127604=CARTESIAN_POINT ( 'NONE',  ( 5.763841807162588537, 6.241519824923047466, -1.009562751112670576 ) ) ;
#127608=EDGE_LOOP ( 'NONE', ( #122105, #86592, #158759, #155646 ) ) ;
#127610=CARTESIAN_POINT ( 'NONE',  ( -7.670162217029145246, 9.971608557999250166, 1.599625672291295375 ) ) ;
#127614=CARTESIAN_POINT ( 'NONE',  ( 5.823390672269506574, 6.752709524857930745, -1.199719254218446718 ) ) ;
#127619=CARTESIAN_POINT ( 'NONE',  ( 5.459129407796876166, 9.520734742405036144, 1.040834085586084257E-14 ) ) ;
#127626=CARTESIAN_POINT ( 'NONE',  ( -6.738039156311804945, 6.963393225226301553, 1.040834085586084257E-14 ) ) ;
#127629=CARTESIAN_POINT ( 'NONE',  ( -2.428612866367529932E-14, 2.800000000000024691, 0.7750000000000117906 ) ) ;
#127632=CARTESIAN_POINT ( 'NONE',  ( 4.528060117284232966, 6.305822774963486310, 1.443375672974062551 ) ) ;
#127635=CARTESIAN_POINT ( 'NONE',  ( -9.612894607289142357, 11.17379744904754801, -1.199719254218441611 ) ) ;
#127637=CARTESIAN_POINT ( 'NONE',  ( 7.086107841436786181, 11.41887624831828418, 1.040834085586084257E-14 ) ) ;
#127638=CARTESIAN_POINT ( 'NONE',  ( -1.402160292154681736E-14, -0.4124999999999747202, -1.732050807568870754 ) ) ;
#127639=CARTESIAN_POINT ( 'NONE',  ( -10.00321840878439339, 10.56484298653695397, 1.040834085586084257E-14 ) ) ;
#127643=CARTESIAN_POINT ( 'NONE',  ( 0.6823417656249899377, 3.676041667008085767, -1.181850606188754593 ) ) ;
#127644=CARTESIAN_POINT ( 'NONE',  ( 3.816783937446950770, 4.411668334231586996, 1.199719254218464037 ) ) ;
#127647=CARTESIAN_POINT ( 'NONE',  ( -1.201851678989727383E-14, 4.587500000000025224, -1.732050807568863648 ) ) ;
#127650=CARTESIAN_POINT ( 'NONE',  ( 7.063434842595398777, 11.18449838309590483, -0.7216878364870267237 ) ) ;
#127653=CARTESIAN_POINT ( 'NONE',  ( -6.236387472606153892, 8.298871356172400127, -1.443375672974059665 ) ) ;
#127654=CARTESIAN_POINT ( 'NONE',  ( -0.6823417656250212460, 1.551041667008083769, 1.181850606188755259 ) ) ;
#127658=CARTESIAN_POINT ( 'NONE',  ( -7.100719765255177229, 9.307259030929609267, -1.599625672291263179 ) ) ;
#127660=CARTESIAN_POINT ( 'NONE',  ( -1.364683531250010295, 5.301041667008085767, -0.7879004041258300672 ) ) ;
#127661=AXIS2_PLACEMENT_3D ( 'NONE', #180004, #44686, #159477 ) ;
#127666=CARTESIAN_POINT ( 'NONE',  ( 7.964525173024008531, 11.37936423758166526, 1.199719254218460707 ) ) ;
#127674=CARTESIAN_POINT ( 'NONE',  ( 9.480175724453529185, 12.08329098332774265, 1.599625672291279388 ) ) ;
#127679=CARTESIAN_POINT ( 'NONE',  ( 9.589694723567584234, 10.08239868711733855, -0.7998128361456281477 ) ) ;
#127680=CARTESIAN_POINT ( 'NONE',  ( -8.859363311525973117, 12.42334206583395328, -1.199719254218446718 ) ) ;
#127683=CARTESIAN_POINT ( 'NONE',  ( -1.364683531250014514, -1.011458332991911568, -0.7879004041258359514 ) ) ;
#127688=CARTESIAN_POINT ( 'NONE',  ( 8.945682426918439845, 9.331051007693339727, 1.040834085586084257E-14 ) ) ;
#127691=CARTESIAN_POINT ( 'NONE',  ( 1.364683531249990311, 3.384375000341416140, 1.214306433183764966E-14 ) ) ;
#127693=CARTESIAN_POINT ( 'NONE',  ( -6.887178846062128379, 7.137389529935019183, -0.7216878364870278340 ) ) ;
#127702=CARTESIAN_POINT ( 'NONE',  ( 7.079328764629950754, 11.41096732537697633, 0.7998128361456462443 ) ) ;
#127708=CARTESIAN_POINT ( 'NONE',  ( -8.188234707649510113, 11.64035869464474082, -1.199719254218446718 ) ) ;
#127710=CARTESIAN_POINT ( 'NONE',  ( 5.472687561410540802, 9.536552588287639409, 0.7998128361456462443 ) ) ;
#127712=CARTESIAN_POINT ( 'NONE',  ( 3.673896439178923057, 5.309298483840612093, 1.443375672974066548 ) ) ;
#127715=CARTESIAN_POINT ( 'NONE',  ( 5.522248639467795428, 5.337044922334209573, -0.7998128361456231517 ) ) ;
#127716=ORIENTED_EDGE ( 'NONE', *, *, #4614, .T. ) ;
#127721=CIRCLE ( 'NONE', #172164, 0.07999999999999975187 ) ;
#127723=CARTESIAN_POINT ( 'NONE',  ( -6.914295153289458540, 7.169025221700239925, 0.7216878364870317197 ) ) ;
#127724=CARTESIAN_POINT ( 'NONE',  ( 4.708759422647839976, 4.387974169377582001, -0.7998128361456211532 ) ) ;
#127728=CARTESIAN_POINT ( 'NONE',  ( -5.845536785786364931, 9.971543350059432598, 0.000000000000000000 ) ) ;
#127732=DIRECTION ( 'NONE',  ( -5.578564026256490882E-16, -1.000000000000000000, -9.066213480720158442E-32 ) ) ;
#127734=CARTESIAN_POINT ( 'NONE',  ( -7.811469059767924605, 12.26513100303794168, -0.7998128361456281477 ) ) ;
#127739=CARTESIAN_POINT ( 'NONE',  ( 8.446893396513862839, 9.813462703143045474, -1.199719254218445830 ) ) ;
#127740=CARTESIAN_POINT ( 'NONE',  ( 6.148786358997489820, 7.132337826040578754, -1.199719254218446718 ) ) ;
#127741=CARTESIAN_POINT ( 'NONE',  ( 2.703961570921634028, 5.242040035128820108, -1.199719254218446718 ) ) ;
#127752=CARTESIAN_POINT ( 'NONE',  ( -6.645467848992654858, 10.90479625713344625, 0.7998128361456481317 ) ) ;
#127757=CARTESIAN_POINT ( 'NONE',  ( 7.131225611108096274, 8.382479970123348778, 1.082531754730558626 ) ) ;
#127763=CARTESIAN_POINT ( 'NONE',  ( -7.237355071596549116, 7.338002426484427687, 1.040834085586084257E-14 ) ) ;
#127764=( BOUNDED_SURFACE ( )  B_SPLINE_SURFACE ( 3, 2, ( 
 ( #104145, #188579, #70533 ),
 ( #122617, #153961, #156096 ),
 ( #54325, #200544, #35927 ),
 ( #7681, #106321, #56456 ) ),
 .UNSPECIFIED., .F., .F., .T. ) 
 B_SPLINE_SURFACE_WITH_KNOTS ( ( 4, 4 ),
 ( 3, 3 ),
 ( 8.673617379884035472E-19, 0.002003486994853858651 ),
 ( 0.000000000000000000, 1.000000000000000000 ),
 .UNSPECIFIED. ) 
 GEOMETRIC_REPRESENTATION_ITEM ( )  RATIONAL_B_SPLINE_SURFACE ( (
 ( 1.000000000000000000, 0.7779734834199515392, 1.000000000000000000),
 ( 1.000000000000000000, 0.7856061901475751563, 1.000000000000000000),
 ( 1.000000000000000000, 0.7951961705782221168, 1.000000000000000000),
 ( 1.000000000000000000, 0.8104931255419017821, 1.000000000000000000) ) ) 
 REPRESENTATION_ITEM ( '' )  SURFACE ( )  );
#127774=CARTESIAN_POINT ( 'NONE',  ( 7.065770611016287006, 11.39514947949436774, 1.040834085586084257E-14 ) ) ;
#127776=CARTESIAN_POINT ( 'NONE',  ( -5.273758566035884776, 5.255065869904374409, 0.000000000000000000 ) ) ;
#127779=CARTESIAN_POINT ( 'NONE',  ( -5.204229338117261072, 6.461601495962581154, -1.180324454998063377 ) ) ;
#127786=CARTESIAN_POINT ( 'NONE',  ( 4.532503425670185493, 4.182342172903648070, 1.214306433183764966E-14 ) ) ;
#127792=CARTESIAN_POINT ( 'NONE',  ( 4.867540842506059562, 5.637551390133895168, -1.199719254218452047 ) ) ;
#127796=CARTESIAN_POINT ( 'NONE',  ( -1.201851678989727383E-14, 3.509375000341421469, -1.575800808251660134 ) ) ;
#127801=ADVANCED_BREP_SHAPE_REPRESENTATION ( '', ( #93359, #200407 ), #124605 ) ;
#127802=CARTESIAN_POINT ( 'NONE',  ( 4.801558957534076022, 8.753569217098425170, 0.7998128361456462443 ) ) ;
#127806=CARTESIAN_POINT ( 'NONE',  ( -4.303823697334223652, 7.108545849276850959, -1.199719254218452047 ) ) ;
#127807=EDGE_CURVE ( 'NONE', #57442, #201902, #144242, .T. ) ;
#127808=CARTESIAN_POINT ( 'NONE',  ( 4.975479186090852046, 6.827811688571220117, 1.443375672974062551 ) ) ;
#127809=CARTESIAN_POINT ( 'NONE',  ( -1.201851678989727383E-14, 3.837500000000021227, -1.732050807568863648 ) ) ;
#127811=CARTESIAN_POINT ( 'NONE',  ( -5.434120640978981065, 5.234228924097238611, -0.7998128361456221525 ) ) ;
#127812=CARTESIAN_POINT ( 'NONE',  ( 0.1447443628656777947, 7.100480071729100118, -2.114679381859644547 ) ) ;
#127813=DIRECTION ( 'NONE',  ( -5.578564026256490882E-16, -1.000000000000000000, -9.066213480720158442E-32 ) ) ;
#127814=CARTESIAN_POINT ( 'NONE',  ( -1.201851678989727383E-14, 5.196875000341422357, -1.575800808251660134 ) ) ;
#127817=CARTESIAN_POINT ( 'NONE',  ( -4.500943810056945438, 5.313817868896925312, 1.082531754730560403 ) ) ;
#127821=CARTESIAN_POINT ( 'NONE',  ( 4.028709946750490545, 3.988235255965033588, -0.8025987720412866011 ) ) ;
#127822=CARTESIAN_POINT ( 'NONE',  ( 3.842846474469570062, 6.570739089268092137, -1.199719254218452047 ) ) ;
#127826=CARTESIAN_POINT ( 'NONE',  ( 0.1021010164683408133, 6.360493866598983637, -3.113991822131907838 ) ) ;
#127830=CARTESIAN_POINT ( 'NONE',  ( 1.364683531249986537, 0.7177083336747527298, -0.7879004041258239610 ) ) ;
#127833=CARTESIAN_POINT ( 'NONE',  ( -9.755255220232635693, 11.33988483081495957, -1.199719254218441611 ) ) ;
#127834=CARTESIAN_POINT ( 'NONE',  ( -5.883875478206491927, 5.966868934103426447, 0.000000000000000000 ) ) ;
#127837=EDGE_LOOP ( 'NONE', ( #85470, #102570, #763, #175419, #110081 ) ) ;
#127838=CARTESIAN_POINT ( 'NONE',  ( -1.364683531250010295, 4.030208333674751842, 0.7879004041258379498 ) ) ;
#127846=CARTESIAN_POINT ( 'NONE',  ( -6.575341312503472757, 7.733948288417905381, 1.082531754730549967 ) ) ;
#127853=CARTESIAN_POINT ( 'NONE',  ( -5.327991180046197428, 8.199444895820425572, 1.082531754730548412 ) ) ;
#127866=CARTESIAN_POINT ( 'NONE',  ( -3.958090780185743451, 6.705190779270287393, -1.199719254218452047 ) ) ;
#127869=CARTESIAN_POINT ( 'NONE',  ( 1.499999999999985123, 0.5458333333333577064, -0.8660254037844253849 ) ) ;
#127871=CARTESIAN_POINT ( 'NONE',  ( 9.436111725431318931, 10.11114455586577776, -0.7216878364870257245 ) ) ;
#127872=CARTESIAN_POINT ( 'NONE',  ( 5.770966940911189447, 9.884545197705074671, -0.7998128361456291469 ) ) ;
#127877=CARTESIAN_POINT ( 'NONE',  ( 5.379888026524302980, 5.170957540566797128, -0.7998128361456211532 ) ) ;
#127878=CARTESIAN_POINT ( 'NONE',  ( -0.5059764118015118717, 7.965522150964809533, -1.935091031283027174 ) ) ;
#127885=CARTESIAN_POINT ( 'NONE',  ( 9.043452155515161905, 10.50944792197790889, 1.199719254218453823 ) ) ;
#127886=CARTESIAN_POINT ( 'NONE',  ( -5.819474248763749635, 7.812472595022922128, -1.599625672291256295 ) ) ;
#127887=ADVANCED_FACE ( 'NONE', ( #56336 ), #23816, .F. ) ;
#127892=CARTESIAN_POINT ( 'NONE',  ( -0.6823417656249969321, 3.217708333674754062, -1.181850606188749264 ) ) ;
#127893=CARTESIAN_POINT ( 'NONE',  ( 9.558135107509954764, 10.25350516829085379, -0.7216878364870257245 ) ) ;
#127894=CARTESIAN_POINT ( 'NONE',  ( -5.364222332501225488, 9.410009821226765325, 0.7998128361456481317 ) ) ;
#127897=CARTESIAN_POINT ( 'NONE',  ( 5.361359679200154105, 8.342337828120466980, 1.199719254218462483 ) ) ;
#127898=CARTESIAN_POINT ( 'NONE',  ( -6.358937740009323214, 7.377514437221045718, -1.199719254218446718 ) ) ;
#127902=CARTESIAN_POINT ( 'NONE',  ( -0.7500000000000249800, -0.02708333265051543481, 1.299038105676659116 ) ) ;
#127905=CARTESIAN_POINT ( 'NONE',  ( 8.446366511633696561, 8.956441806435218922, 1.040834085586084257E-14 ) ) ;
#127908=CARTESIAN_POINT ( 'NONE',  ( 1.364683531249988535, 2.176041667008087543, 0.7879004041258500513 ) ) ;
#127910=CARTESIAN_POINT ( 'NONE',  ( 4.799223189113185128, 8.542918120699967588, 1.040834085586084257E-14 ) ) ;
#127912=CARTESIAN_POINT ( 'NONE',  ( -3.307826292054310890, 5.842585859829892314, -1.082531754730549967 ) ) ;
#127921=CARTESIAN_POINT ( 'NONE',  ( -4.475961918153980257, 7.265020140467052023, -1.287590260893024086 ) ) ;
#127929=CARTESIAN_POINT ( 'NONE',  ( 7.481401836642521452, 7.622723652371411696, 1.040834085586084257E-14 ) ) ;
#127932=CARTESIAN_POINT ( 'NONE',  ( 2.984766373302843778, 6.633977868828633717, -0.7998128361456291469 ) ) ;
#127934=EDGE_CURVE ( 'NONE', #212596, #102537, #185428, .T. ) ;
#127941=CARTESIAN_POINT ( 'NONE',  ( 5.205967797967541166, 5.175976640491323444, -0.7216878364870197293 ) ) ;
#127942=CARTESIAN_POINT ( 'NONE',  ( -1.364683531250014514, 1.801041667008085767, -0.7879004041258289570 ) ) ;
#127943=CARTESIAN_POINT ( 'NONE',  ( 9.399880572976245574, 9.860948844760784482, 0.7998128361456462443 ) ) ;
#127946=CARTESIAN_POINT ( 'NONE',  ( -4.391951695823077984, 7.211361847513815704, 1.199719254218464037 ) ) ;
#127949=CARTESIAN_POINT ( 'NONE',  ( 0.7499999999999885647, 2.066666666666688634, -1.299038105676652899 ) ) ;
#127950=CARTESIAN_POINT ( 'NONE',  ( 4.964256800898067645, 8.943383367689749619, 0.7998128361456462443 ) ) ;
#127951=CARTESIAN_POINT ( 'NONE',  ( -6.204827856548512877, 10.39071626594860476, -0.7998128361456291469 ) ) ;
#127954=CARTESIAN_POINT ( 'NONE',  ( -0.6823417656250212460, 2.301041667008084435, 1.181850606188767472 ) ) ;
#127958=CARTESIAN_POINT ( 'NONE',  ( 4.220665892555866883, 3.818531717603609987, -0.7998128361456211532 ) ) ;
#127965=CARTESIAN_POINT ( 'NONE',  ( -1.500000000000001332, 1.181250000682816603, 0.000000000000000000 ) ) ;
#127967=CARTESIAN_POINT ( 'NONE',  ( -7.691553217654356622, 7.867900263551875994, -0.7998128361456291469 ) ) ;
#127968=CARTESIAN_POINT ( 'NONE',  ( -3.633221978782299910, 5.261844946711204507, -1.443375672974053447 ) ) ;
#127974=ORIENTED_EDGE ( 'NONE', *, *, #198453, .T. ) ;
#127976=CARTESIAN_POINT ( 'NONE',  ( 4.950698647284403009, 8.927565521807144577, 1.040834085586084257E-14 ) ) ;
#127979=CARTESIAN_POINT ( 'NONE',  ( 7.318703993278529829, 7.432909501780090800, 1.040834085586084257E-14 ) ) ;
#127984=CARTESIAN_POINT ( 'NONE',  ( -7.379715684540041565, 7.504089808251839244, 1.040834085586084257E-14 ) ) ;
#127986=CARTESIAN_POINT ( 'NONE',  ( 4.539282502477016479, 4.190251095844947926, 0.7998128361456341429 ) ) ;
#127990=CARTESIAN_POINT ( 'NONE',  ( 4.413087178904756769, 7.101426714207548230, 1.094556639780567053 ) ) ;
#127998=CARTESIAN_POINT ( 'NONE',  ( -3.958617665510283601, 4.681104033592509595, -1.082531754730549967 ) ) ;
#127999=CARTESIAN_POINT ( 'NONE',  ( 6.643132081016105417, 10.69414516125339887, 0.7216878364870438212 ) ) ;
#128002=CARTESIAN_POINT ( 'NONE',  ( -4.578903193113314174, 6.365139696764064325, 1.599625672291267398 ) ) ;
#128007=CARTESIAN_POINT ( 'NONE',  ( -6.368579470117215813, 8.453095353268645695, 1.599625672291283607 ) ) ;
#128021=CARTESIAN_POINT ( 'NONE',  ( -5.253948220495577637, 6.088359997788290734, 1.199719254218450271 ) ) ;
#128024=CARTESIAN_POINT ( 'NONE',  ( 4.121315508874254796, 5.831287398485176077, -1.443375672974051449 ) ) ;
#128026=FACE_OUTER_BOUND ( 'NONE', #169966, .T. ) ;
#128028=CARTESIAN_POINT ( 'NONE',  ( -4.308793891044708779, 3.921347715840572956, 1.214306433183764966E-14 ) ) ;
#128029=CARTESIAN_POINT ( 'NONE',  ( -4.925689880466507908, 4.641059703499347044, -0.7998128361456221525 ) ) ;
#128032=CARTESIAN_POINT ( 'NONE',  ( 10.22692794340986921, 10.82583744360002243, 0.000000000000000000 ) ) ;
#128035=CARTESIAN_POINT ( 'NONE',  ( -7.901704598666176693, 8.113076874732334076, 0.7998128361456602331 ) ) ;
#128036=CARTESIAN_POINT ( 'NONE',  ( 4.313465427442102929, 8.184126765324453601, 0.7998128361456462443 ) ) ;
#128038=CARTESIAN_POINT ( 'NONE',  ( 4.497554271431305040, 6.270232621468402989, -1.599625672291256517 ) ) ;
#128041=CARTESIAN_POINT ( 'NONE',  ( 1.364683531249988757, 1.946875000341415030, 0.000000000000000000 ) ) ;
#128044=CARTESIAN_POINT ( 'NONE',  ( 6.317736394288122170, 10.31451686007074997, 0.7216878364870438212 ) ) ;
#128052=CARTESIAN_POINT ( 'NONE',  ( 10.53432216769390095, 11.39239007183880581, -0.7216878364870257245 ) ) ;
#128057=CARTESIAN_POINT ( 'NONE',  ( 5.355107487717867265, 5.349972945200037522, 1.040834085586084257E-14 ) ) ;
#128059=CARTESIAN_POINT ( 'NONE',  ( -8.319899820280397762, 12.85830022363583147, -0.7998128361456281477 ) ) ;
#128068=FACE_OUTER_BOUND ( 'NONE', #207644, .T. ) ;
#128075=CARTESIAN_POINT ( 'NONE',  ( -1.500000000000013101, 1.702083334016151417, 0.8660254037844403729 ) ) ;
#128079=ORIENTED_EDGE ( 'NONE', *, *, #39947, .T. ) ;
#128081=CARTESIAN_POINT ( 'NONE',  ( -1.500000000000015099, -1.079166666666641961, 0.8660254037844403729 ) ) ;
#128082=CARTESIAN_POINT ( 'NONE',  ( 9.413438726589914651, 9.876766690643398405, 0.000000000000000000 ) ) ;
#128085=CARTESIAN_POINT ( 'NONE',  ( 3.440018289565364817, 5.036440642624797626, 1.599625672291267398 ) ) ;
#128086=CARTESIAN_POINT ( 'NONE',  ( -6.914295153289458540, 7.169025221700239925, 0.7216878364870317197 ) ) ;
#128090=CARTESIAN_POINT ( 'NONE',  ( -5.357443255694392725, 9.402100898285455699, 0.000000000000000000 ) ) ;
#128092=CARTESIAN_POINT ( 'NONE',  ( 1.499999999999989120, 0.8062500006828163812, 0.000000000000000000 ) ) ;
#128099=CARTESIAN_POINT ( 'NONE',  ( -4.744990574658554117, 4.638169879964154418, 1.214306433183764966E-14 ) ) ;
#128102=CARTESIAN_POINT ( 'NONE',  ( 4.147051400439892177, 7.400425289818373109, 0.7480841269332880739 ) ) ;
#128107=CARTESIAN_POINT ( 'NONE',  ( -2.779058300676980675, 5.225689869889666106, -1.082531754730543083 ) ) ;
#128108=CARTESIAN_POINT ( 'NONE',  ( 8.959240580532112475, 9.346868853575953651, -0.7998128361456221525 ) ) ;
#128109=LINE ( 'NONE', #176762, #91075 ) ;
#128115=CARTESIAN_POINT ( 'NONE',  ( -8.694856585065634746, 9.038420858865048757, 0.7998128361456462443 ) ) ;
#128120=CARTESIAN_POINT ( 'NONE',  ( 5.040934186182656873, 4.775511393501539636, 1.040834085586084257E-14 ) ) ;
#128123=ORIENTED_EDGE ( 'NONE', *, *, #16995, .T. ) ;
#128125=CARTESIAN_POINT ( 'NONE',  ( -8.611400122974211868, 13.19838391011195888, 1.040834085586084257E-14 ) ) ;
#128128=CARTESIAN_POINT ( 'NONE',  ( -5.594971466091354095, 6.350553869658721595, -1.210626573312810761 ) ) ;
#128136=CARTESIAN_POINT ( 'NONE',  ( 6.470265622219697477, 8.571729197388226140, -1.599625672291262513 ) ) ;
#128146=ORIENTED_EDGE ( 'NONE', *, *, #176248, .F. ) ;
#128148=CARTESIAN_POINT ( 'NONE',  ( 0.7499999999999885647, 0.5979166673494851203, -1.299038105676652899 ) ) ;
#128152=CARTESIAN_POINT ( 'NONE',  ( 2.703961570921634028, 5.242040035128820108, -1.199719254218446718 ) ) ;
#128154=CARTESIAN_POINT ( 'NONE',  ( -9.646789991323334590, 11.21334206375407305, 1.199719254218462483 ) ) ;
#128161=CARTESIAN_POINT ( 'NONE',  ( 4.202664430556247055, 6.886563688082179446, 1.082531754730558626 ) ) ;
#128164=CARTESIAN_POINT ( 'NONE',  ( 8.499999999999980460, 6.200000000000038369, 2.873333333333345951 ) ) ;
#128166=CARTESIAN_POINT ( 'NONE',  ( 10.39640486358069360, 11.02356051713265650, 0.7998128361456462443 ) ) ;
#128176=CARTESIAN_POINT ( 'NONE',  ( 1.364683531249986537, -0.8447916663252468261, -0.7879004041258309554 ) ) ;
#128181=CARTESIAN_POINT ( 'NONE',  ( -6.013204822860843457, 6.974159367214481264, -1.199719254218446718 ) ) ;
#128184=CARTESIAN_POINT ( 'NONE',  ( -1.500000000000001332, -0.5999999999999755529, 0.000000000000000000 ) ) ;
#128186=CARTESIAN_POINT ( 'NONE',  ( 1.364683531249988757, -0.5531249996585801965, 0.000000000000000000 ) ) ;
#128193=CARTESIAN_POINT ( 'NONE',  ( -0.6823417656249969321, 5.780208333674756283, -1.181850606188749264 ) ) ;
#128195=CARTESIAN_POINT ( 'NONE',  ( 6.647575389402066826, 6.649926130590872120, 1.040834085586084257E-14 ) ) ;
#128196=CARTESIAN_POINT ( 'NONE',  ( -8.701635661872465732, 9.046329781806354831, 1.040834085586084257E-14 ) ) ;
#128198=CARTESIAN_POINT ( 'NONE',  ( 8.204655514564224816, 12.72384853363364066, 1.040834085586084257E-14 ) ) ;
#128200=CARTESIAN_POINT ( 'NONE',  ( 0.000000000000000000, 6.468705557303652931, -4.925226524755051294 ) ) ;
#128204=CARTESIAN_POINT ( 'NONE',  ( 1.364683531249986981, -1.053124999658580752, 0.000000000000000000 ) ) ;
#128212=CARTESIAN_POINT ( 'NONE',  ( 7.836249599018724865, 9.205007956019091608, -1.082531754730537976 ) ) ;
#128216=CARTESIAN_POINT ( 'NONE',  ( 1.499999999999990896, 4.556250000682819490, 1.214306433183764966E-14 ) ) ;
#128218=CARTESIAN_POINT ( 'NONE',  ( -4.386226389220933441, 5.076017861301227008, -1.199719254218446718 ) ) ;
#128219=CARTESIAN_POINT ( 'NONE',  ( 7.253248993186735660, 7.564471368247083660, 0.7216878364870317197 ) ) ;
#128220=CARTESIAN_POINT ( 'NONE',  ( -8.798878505144648088, 12.24881344176869469, -1.082531754730543083 ) ) ;
#128226=CARTESIAN_POINT ( 'NONE',  ( 2.846322183865124700, 5.408127416896231665, -1.199719254218446718 ) ) ;
#128227=CARTESIAN_POINT ( 'NONE',  ( -1.499999999999997780, 4.650000000000022560, 1.214306433183764966E-14 ) ) ;
#128240=ORIENTED_EDGE ( 'NONE', *, *, #58178, .T. ) ;
#128242=CARTESIAN_POINT ( 'NONE',  ( 8.914649696185335870, 10.35917838609310593, -1.199719254218446718 ) ) ;
#128247=CARTESIAN_POINT ( 'NONE',  ( 1.364683531249986537, 0.1135416670080857532, 0.7879004041258500513 ) ) ;
#128248=CARTESIAN_POINT ( 'NONE',  ( 4.189106276942576201, 7.831115056500907556, 1.040834085586084257E-14 ) ) ;
#128251=CARTESIAN_POINT ( 'NONE',  ( -8.839552966430012759, 10.37552855133225904, -1.082531754730543971 ) ) ;
#128271=ORIENTED_EDGE ( 'NONE', *, *, #166654, .T. ) ;
#128272=CARTESIAN_POINT ( 'NONE',  ( 4.286934996870309433, 7.472684718058654418, -1.056577385247484457 ) ) ;
#128273=CARTESIAN_POINT ( 'NONE',  ( -2.103486388414573138, 5.605817886458954291, 1.040834085586084257E-14 ) ) ;
#128280=CARTESIAN_POINT ( 'NONE',  ( -8.676855123066030018, 9.225345186439589895, -0.7216878364870267237 ) ) ;
#128284=CARTESIAN_POINT ( 'NONE',  ( 6.262976894508937242, 9.394224579314053969, -1.199719254218440723 ) ) ;
#128285=CARTESIAN_POINT ( 'NONE',  ( -4.192495815123837843, 5.914331089109674977, -1.599625672291256517 ) ) ;
#128286=CARTESIAN_POINT ( 'NONE',  ( 4.701980345841006326, 4.380065246436280368, 0.7998128361456341429 ) ) ;
#128288=CARTESIAN_POINT ( 'NONE',  ( -4.680589345215810049, 6.483773540883647435, -1.599625672291256295 ) ) ;
#128292=CARTESIAN_POINT ( 'NONE',  ( -6.091691091241777656, 6.001394449403842479, 0.7998128361456341429 ) ) ;
#128295=CARTESIAN_POINT ( 'NONE',  ( 3.669453130792974971, 7.432779085900453886, 1.040834085586084257E-14 ) ) ;
#128296=CARTESIAN_POINT ( 'NONE',  ( 7.065770611016287006, 11.39514947949436774, 1.040834085586084257E-14 ) ) ;
#128297=CARTESIAN_POINT ( 'NONE',  ( -0.1004607481840987110, 6.432248552227529004, 3.209664736303321497 ) ) ;
#128299=CARTESIAN_POINT ( 'NONE',  ( 4.369547513234953939, 7.382648021784232739, 1.157447143386416188 ) ) ;
#128300=CARTESIAN_POINT ( 'NONE',  ( 4.473827502829567315, 7.202920605734387749, -1.082531754730548412 ) ) ;
#128307=CARTESIAN_POINT ( 'NONE',  ( 7.768458830506048685, 8.165549511786275971, -0.7216878364870267237 ) ) ;
#128308=CARTESIAN_POINT ( 'NONE',  ( -7.700141177557535244, 11.07091624287075859, -1.199719254218446718 ) ) ;
#128311=CARTESIAN_POINT ( 'NONE',  ( -8.134002093194872884, 11.57708731111429401, 1.199719254218453823 ) ) ;
#128312=CARTESIAN_POINT ( 'NONE',  ( -8.525379664894808585, 8.840697785332414682, -0.7998128361456291469 ) ) ;
#128313=CARTESIAN_POINT ( 'NONE',  ( -3.890826896997543471, 7.483122446565097619, 0.7216878364870037421 ) ) ;
#128320=CARTESIAN_POINT ( 'NONE',  ( 10.24048609702354717, 10.84165528948263457, -0.7998128361456281477 ) ) ;
#128325=CARTESIAN_POINT ( 'NONE',  ( 2.523789150438203510, 6.096171108819874007, 0.7998128361456462443 ) ) ;
#128328=CARTESIAN_POINT ( 'NONE',  ( 1.499999999999989120, 5.327083334016152527, -0.8660254037844323793 ) ) ;
#128332=VERTEX_POINT ( 'NONE', #18006 ) ;
#128334=CARTESIAN_POINT ( 'NONE',  ( -1.500000000000013101, 2.879166666666688634, -0.8660254037844313801 ) ) ;
#128335=CARTESIAN_POINT ( 'NONE',  ( 5.311043488251262268, 7.219303374425030562, -1.599625672291256295 ) ) ;
#128338=CARTESIAN_POINT ( 'NONE',  ( 7.998947442382716488, 9.394822106610419610, -1.082531754730543083 ) ) ;
#128339=CARTESIAN_POINT ( 'NONE',  ( -10.42585693878457853, 11.26584730477792284, -0.7216878364870267237 ) ) ;
#128342=CARTESIAN_POINT ( 'NONE',  ( 8.809047120577066181, 11.30030761213851953, 1.599625672291281386 ) ) ;
#128345=CARTESIAN_POINT ( 'NONE',  ( -2.916975605234527702, 6.554888639415577423, 1.040834085586084257E-14 ) ) ;
#128346=CARTESIAN_POINT ( 'NONE',  ( -1.364683531250000748, 1.259375000341421469, 0.000000000000000000 ) ) ;
#128351=CARTESIAN_POINT ( 'NONE',  ( -1.364683531250014514, -0.7614583329919104582, -0.7879004041258359514 ) ) ;
#128359=CARTESIAN_POINT ( 'NONE',  ( -7.877450944739929461, 9.149113176073413456, 1.199719254218462483 ) ) ;
#128363=CARTESIAN_POINT ( 'NONE',  ( 5.412729640353754590, 7.337937218544611895, 1.599625672291267398 ) ) ;
#128369=CARTESIAN_POINT ( 'NONE',  ( 10.72180055030867329, 11.40318881831530540, 0.7998128361456341429 ) ) ;
#128372=CARTESIAN_POINT ( 'NONE',  ( -3.906720819032141190, 7.709591388846142479, -0.7998128361456281477 ) ) ;
#128376=CARTESIAN_POINT ( 'NONE',  ( 10.07778825365955733, 10.65184113889131012, -0.7998128361456281477 ) ) ;
#128378=CARTESIAN_POINT ( 'NONE',  ( 7.079328764629950754, 11.41096732537697633, 0.7998128361456462443 ) ) ;
#128379=( BOUNDED_SURFACE ( )  B_SPLINE_SURFACE ( 1, 2, ( 
 ( #59609, #125765, #95344, #176568, #124701, #28178, #160314, #123646, #190660, #161394, #42321, #11918, #191727, #26032, #107364, #173385, #24968, #92144, #158198, #27101, #47657, #50823, #145170, #130030, #64930, #974, #146224, #163519, #67040, #79053, #214337, #182949, #149392, #81195, #181869, #196021, #164576, #98514, #148337, #82246, #32445, #49758, #194942, #16161, #65967, #212242, #199177, #132116, #113768, #178707, #166712, #34564, #162457, #112697, #115884, #198126, #179771, #211175, #62801, #33505, #133177, #116950, #46578, #48706, #31388, #15106, #165642, #99578, #100635, #17230, #147273, #83305, #128962, #30322, #14033, #96407, #197069, #80119, #63876, #97463, #213305, #131080, #114820, #180818, #37775, #3104, #68105, #69175, #104927, #101703, #138490, #185067, #87596, #18302, #122323, #84388, #36693, #102778, #168835, #120164, #88674, #55096, #153667, #136357, #106029, #134241, #20438, #54027, #52949, #86521, #184011, #200248, #103849, #135295, #150475, #201309, #152586, #186140, #2035, #72390, #70242, #21486, #202377, #119087, #51900, #169897, #121245, #118022, #19371, #203442, #4173, #204511, #35625, #5235, #71311, #154733, #85451, #137423, #6316, #167774, #187215, #188280, #56160, #38844, #170969, #22568, #39921, #151536, #26848, #175263, #125511, #142783, #73465, #109255, #158999, #24710, #77737, #10592, #140650, #57230, #45259, #61489, #40995, #205593, #208788, #76668, #58295, #172051, #89752, #191474, #27926, #160059, #139566, #141723, #206663, #42066, #44193, #60419, #193618, #126579, #108180, #43142, #11663, #143858, #107106, #192539, #75613, #110313, #7385, #124451, #123391, #92952, #25779, #207732, #176320, #156876, #189355, #8463, #94020, #173129, #209851, #190410, #127654, #23644, #155802, #90812, #174206, #91891, #157947, #59355, #74550, #9538, #147029, #113511, #115622, #161131, #63625, #179520, #96151, #79863, #144915, #95083, #163265, #30062, #111379, #162202, #195760, #31138, #12719, #214087, #97213, #65715, #13789, #114574, #32188, #148082, #145972, #128711, #211984, #129779, #131863, #80937, #194682, #14847, #213051, #28996, #210922, #197870, #46324, #178453, #78792, #47399, #98264, #112440, #49502, #64680, #130826, #177382, #62548, #196818, #48460, #180566, #164322, #15912, #81995, #127279, #159686, #208415, #178082, #206289, #92586, #126204, #125140, #108873, #41694, #140269, #175952, #207364, #90430, #58984, #10225, #192166, #74177, #144552, #142407, #210560, #141349, #193250, #44897, #12350, #174897, #173830, #26476, #158628, #62195, #27548, #91510, #43827, #109943, #156499, #107805, #194318, #157570, #93643, #60049, #191098, #57913, #11287, #111004, #124078, #9163, #61118, #42766, #128351, #8089, #76299, #77366, #78430, #75239, #143480, #45959, #190042, #209476, #112080, #160755, #177008, #28625, #94713, #25407, #49150, #98963, #32886, #197507, #341, #145620, #181259, #16609 ),
 ( #165014, #29699, #195396, #129413, #33945, #95781, #162899, #17672, #212683, #66414, #13426, #82690, #148772, #132559, #47026, #80570, #113141, #179148, #161838, #63252, #130468, #100020, #147715, #115267, #198559, #31834, #131503, #50207, #14481, #97909, #30772, #116325, #182316, #79502, #96851, #133627, #146669, #166084, #81630, #64324, #211616, #83758, #149850, #196458, #48101, #1419, #114213, #67482, #180211, #163969, #15545, #199629, #213733, #65356, #51275, #117399, #104294, #72836, #39283, #185518, #71755, #85904, #54472, #202823, #38221, #186594, #136798, #154108, #84832, #120616, #170342, #36071, #89123, #21927, #151978, #68558, #56608, #138940, #52339, #2482, #5677, #88036, #69622, #183396, #101073, #137871, #105378, #171417, #150921, #153037, #3552, #53395, #55536, #203891, #204960, #121690, #119532, #187657, #23005, #155177, #118467, #6761, #86968, #35001, #18747, #135732, #134685, #167160, #37142, #4611, #200688, #168219, #184453, #19819, #102153, #201754, #103224, #169283, #20869, #70685, #24026, #158326, #142098, #92281, #73862, #189734, #204898, #41386, #121631, #104238, #172439, #188675, #105318, #57616, #7771, #106416, #22950, #74931, #170284, #173524, #190792, #141041, #138880, #156195, #90128, #58679, #59740, #208111, #89064, #5619, #187600, #137813, #139956, #155122, #124827, #205981, #108561, #107497, #39227, #40308, #123774, #75993, #25098, #171356, #91199, #157259, #21872, #55477, #125898, #6704, #8851, #207048, #56551, #154052, #42454, #174589, #71701, #72781, #26164, #122712, #191857, #87978, #9919, #203832, #179898, #110694, #128041, #31521, #43518, #178843, #147402, #113903, #45645, #146355, #160441, #129102, #62934, #112827, #46714, #211309, #14161, #159374, #195074, #30454, #176694, #163654, #96540, #12047, #143175, #131207, #213428, #126967, #77046, #80256, #162587, #144247, #109641, #175644, #212367, #97595, #15236, #10973, #13111, #78117, #193996, #130157, #64009, #65051, #196149, #111762, #47789, #81323, #27230, #192925, #93338, #161526, #209168, #60806, #210239, #44581, #28307, #177768, #79188, #94403, #61876, #29384, #95478, #145303, #66100, #102901, #149523, #50956, #82377, #200377, #52025, #1109, #67170, #133305, #84513, #53076, #19500, #118151, #100760, #70368, #98647, #199310, #18438, #17359, #117080, #148468, #32570, #68239, #99704, #197195, #165776, #183079, #150602, #180948, #36820, #34691, #168960, #33631, #85576, #151665, #119211, #166842, #48834, #83443, #2162, #134373, #164704, #20564, #184135, #86647, #35759, #3237, #69302, #185195, #101833, #132242, #167902, #135415, #152715, #201436, #198250, #4297, #114948, #16292, #36, #49889, #116014, #182000, #188406, #171093, #186267, #89874, #24837, #37902, #137552, #107235, #105057, #108305, #202505, #187342, #122448, #58420, #203570, #6440, #124573, #136482, #57353, #25900, #206788, #138614, #90936, #38971, #7511 ) ),
 .UNSPECIFIED., .F., .F., .F. ) 
 B_SPLINE_SURFACE_WITH_KNOTS ( ( 2, 2 ),
 ( 3, 2, 2, 2, 2, 2, 2, 2, 2, 2, 2, 2, 2, 2, 2, 2, 2, 2, 2, 2, 2, 2, 2, 2, 2, 2, 2, 2, 2, 2, 2, 2, 2, 2, 2, 2, 2, 2, 2, 2, 2, 2, 2, 2, 2, 2, 2, 2, 2, 2, 2, 2, 2, 2, 2, 2, 2, 2, 2, 2, 2, 2, 2, 2, 2, 2, 2, 2, 2, 2, 2, 2, 2, 2, 2, 2, 2, 2, 2, 2, 2, 2, 2, 2, 2, 2, 2, 2, 2, 2, 2, 2, 2, 2, 2, 2, 2, 2, 2, 2, 2, 2, 2, 2, 2, 2, 2, 2, 2, 2, 2, 2, 2, 2, 2, 2, 2, 2, 2, 2, 2, 2, 2, 2, 2, 2, 2, 2, 2, 2, 2, 2, 2, 2, 2, 2, 2, 2, 2, 2, 2, 2, 2, 2, 2, 2, 2, 2, 2, 2, 2, 2, 2, 2, 2, 2, 2, 2, 2, 2, 2, 2, 2, 2, 2, 2, 2, 2, 3 ),
 ( 0.000000000000000000, 1.000000000000000000 ),
 ( 0.000000000000000000, 0.005952380952380952051, 0.01190476190476190410, 0.01785714285714285615, 0.02380952380952380820, 0.02976190476190476025, 0.03571428571428571230, 0.04166666666666666435, 0.04761904761904761640, 0.05357142857142856845, 0.05952380952380952051, 0.06547619047619047949, 0.07142857142857142461, 0.07738095238095238360, 0.08333333333333332871, 0.08928571428571428770, 0.09523809523809523281, 0.1011904761904761918, 0.1071428571428571369, 0.1130952380952380959, 0.1190476190476190410, 0.1250000000000000000, 0.1309523809523809590, 0.1369047619047619180, 0.1428571428571428492, 0.1488095238095238082, 0.1547619047619047672, 0.1607142857142857262, 0.1666666666666666574, 0.1726190476190476164, 0.1785714285714285754, 0.1845238095238095344, 0.1904761904761904656, 0.1964285714285714246, 0.2023809523809523836, 0.2083333333333333426, 0.2142857142857142738, 0.2202380952380952328, 0.2261904761904761918, 0.2321428571428571508, 0.2380952380952380820, 0.2440476190476190410, 0.2500000000000000000, 0.2559523809523809312, 0.2619047619047619180, 0.2678571428571428492, 0.2738095238095238360, 0.2797619047619047672, 0.2857142857142856984, 0.2916666666666666852, 0.2976190476190476164, 0.3035714285714285476, 0.3095238095238095344, 0.3154761904761904656, 0.3214285714285714524, 0.3273809523809523836, 0.3333333333333333148, 0.3392857142857143016, 0.3452380952380952328, 0.3511904761904761640, 0.3571428571428571508, 0.3630952380952380820, 0.3690476190476190688, 0.3750000000000000000, 0.3809523809523809312, 0.3869047619047619180, 0.3928571428571428492, 0.3988095238095238360, 0.4047619047619047672, 0.4107142857142856984, 0.4166666666666666852, 0.4226190476190476164, 0.4285714285714285476, 0.4345238095238095344, 0.4404761904761904656, 0.4464285714285714524, 0.4523809523809523836, 0.4583333333333333148, 0.4642857142857143016, 0.4702380952380952328, 0.4761904761904761640, 0.4821428571428571508, 0.4880952380952380820, 0.4940476190476190688, 0.5000000000000000000, 0.5059523809523809312, 0.5119047619047618625, 0.5178571428571429047, 0.5238095238095238360, 0.5297619047619047672, 0.5357142857142856984, 0.5416666666666666297, 0.5476190476190476719, 0.5535714285714286031, 0.5595238095238095344, 0.5654761904761904656, 0.5714285714285713969, 0.5773809523809523281, 0.5833333333333333703, 0.5892857142857143016, 0.5952380952380952328, 0.6011904761904761640, 0.6071428571428570953, 0.6130952380952381375, 0.6190476190476190688, 0.6250000000000000000, 0.6309523809523809312, 0.6369047619047618625, 0.6428571428571429047, 0.6488095238095238360, 0.6547619047619047672, 0.6607142857142856984, 0.6666666666666666297, 0.6726190476190476719, 0.6785714285714286031, 0.6845238095238095344, 0.6904761904761904656, 0.6964285714285713969, 0.7023809523809523281, 0.7083333333333333703, 0.7142857142857143016, 0.7202380952380952328, 0.7261904761904761640, 0.7321428571428570953, 0.7380952380952381375, 0.7440476190476190688, 0.7500000000000000000, 0.7559523809523809312, 0.7619047619047618625, 0.7678571428571429047, 0.7738095238095238360, 0.7797619047619047672, 0.7857142857142856984, 0.7916666666666666297, 0.7976190476190476719, 0.8035714285714286031, 0.8095238095238095344, 0.8154761904761904656, 0.8214285714285713969, 0.8273809523809523281, 0.8333333333333333703, 0.8392857142857143016, 0.8452380952380952328, 0.8511904761904761640, 0.8571428571428570953, 0.8630952380952381375, 0.8690476190476190688, 0.8750000000000000000, 0.8809523809523809312, 0.8869047619047618625, 0.8928571428571429047, 0.8988095238095238360, 0.9047619047619047672, 0.9107142857142856984, 0.9166666666666666297, 0.9226190476190476719, 0.9285714285714286031, 0.9345238095238095344, 0.9404761904761904656, 0.9464285714285713969, 0.9523809523809523281, 0.9583333333333333703, 0.9642857142857143016, 0.9702380952380952328, 0.9761904761904761640, 0.9821428571428570953, 0.9880952380952381375, 0.9940476190476190688, 1.000000000000000000 ),
 .UNSPECIFIED. ) 
 GEOMETRIC_REPRESENTATION_ITEM ( )  RATIONAL_B_SPLINE_SURFACE ( (
 ( 1.000000000000000000, 0.8660254037844387076, 1.000000000000000000, 0.8660254037844387076, 1.000000000000000000, 0.8660254037844387076, 1.000000000000000000, 0.8660254037844387076, 1.000000000000000000, 0.8660254037844387076, 1.000000000000000000, 0.8660254037844387076, 1.000000000000000000, 0.8660254037844387076, 1.000000000000000000, 0.8660254037844387076, 1.000000000000000000, 0.8660254037844387076, 1.000000000000000000, 0.8660254037844387076, 1.000000000000000000, 0.8660254037844387076, 1.000000000000000000, 0.8660254037844387076, 1.000000000000000000, 0.8660254037844387076, 1.000000000000000000, 0.8660254037844387076, 1.000000000000000000, 0.8660254037844387076, 1.000000000000000000, 0.8660254037844387076, 1.000000000000000000, 0.8660254037844387076, 1.000000000000000000, 0.8660254037844387076, 1.000000000000000000, 0.8660254037844387076, 1.000000000000000000, 0.8660254037844387076, 1.000000000000000000, 0.8660254037844387076, 1.000000000000000000, 0.8660254037844387076, 1.000000000000000000, 0.8660254037844387076, 1.000000000000000000, 0.8660254037844387076, 1.000000000000000000, 0.8660254037844387076, 1.000000000000000000, 0.8660254037844387076, 1.000000000000000000, 0.8660254037844387076, 1.000000000000000000, 0.8660254037844387076, 1.000000000000000000, 0.8660254037844387076, 1.000000000000000000, 0.8660254037844387076, 1.000000000000000000, 0.8660254037844387076, 1.000000000000000000, 0.8660254037844387076, 1.000000000000000000, 0.8660254037844387076, 1.000000000000000000, 0.8660254037844387076, 1.000000000000000000, 0.8660254037844387076, 1.000000000000000000, 0.8660254037844387076, 1.000000000000000000, 0.8660254037844387076, 1.000000000000000000, 0.8660254037844387076, 1.000000000000000000, 0.8660254037844387076, 1.000000000000000000, 0.8660254037844387076, 1.000000000000000000, 0.8660254037844387076, 1.000000000000000000, 0.8660254037844387076, 1.000000000000000000, 0.8660254037844387076, 1.000000000000000000, 0.8660254037844387076, 1.000000000000000000, 0.8660254037844387076, 1.000000000000000000, 0.8660254037844387076, 1.000000000000000000, 0.8660254037844387076, 1.000000000000000000, 0.8660254037844387076, 1.000000000000000000, 0.8660254037844387076, 1.000000000000000000, 0.8660254037844387076, 1.000000000000000000, 0.8660254037844387076, 1.000000000000000000, 0.8660254037844387076, 1.000000000000000000, 0.8660254037844387076, 1.000000000000000000, 0.8660254037844387076, 1.000000000000000000, 0.8660254037844387076, 1.000000000000000000, 0.8660254037844387076, 1.000000000000000000, 0.8660254037844387076, 1.000000000000000000, 0.8660254037844387076, 1.000000000000000000, 0.8660254037844387076, 1.000000000000000000, 0.8660254037844387076, 1.000000000000000000, 0.8660254037844387076, 1.000000000000000000, 0.8660254037844387076, 1.000000000000000000, 0.8660254037844387076, 1.000000000000000000, 0.8660254037844387076, 1.000000000000000000, 0.8660254037844387076, 1.000000000000000000, 0.8660254037844387076, 1.000000000000000000, 0.8660254037844387076, 1.000000000000000000, 0.8660254037844387076, 1.000000000000000000, 0.8660254037844387076, 1.000000000000000000, 0.8660254037844387076, 1.000000000000000000, 0.8660254037844387076, 1.000000000000000000, 0.8660254037844387076, 1.000000000000000000, 0.8660254037844387076, 1.000000000000000000, 0.8660254037844387076, 1.000000000000000000, 0.8660254037844387076, 1.000000000000000000, 0.8660254037844387076, 1.000000000000000000, 0.8660254037844387076, 1.000000000000000000, 0.8660254037844387076, 1.000000000000000000, 0.8660254037844387076, 1.000000000000000000, 0.8660254037844387076, 1.000000000000000000, 0.8660254037844387076, 1.000000000000000000, 0.8660254037844387076, 1.000000000000000000, 0.8660254037844387076, 1.000000000000000000, 0.8660254037844387076, 1.000000000000000000, 0.8660254037844387076, 1.000000000000000000, 0.8660254037844387076, 1.000000000000000000, 0.8660254037844387076, 1.000000000000000000, 0.8660254037844387076, 1.000000000000000000, 0.8660254037844387076, 1.000000000000000000, 0.8660254037844387076, 1.000000000000000000, 0.8660254037844387076, 1.000000000000000000, 0.8660254037844387076, 1.000000000000000000, 0.8660254037844387076, 1.000000000000000000, 0.8660254037844387076, 1.000000000000000000, 0.8660254037844387076, 1.000000000000000000, 0.8660254037844387076, 1.000000000000000000, 0.8660254037844387076, 1.000000000000000000, 0.8660254037844387076, 1.000000000000000000, 0.8660254037844387076, 1.000000000000000000, 0.8660254037844387076, 1.000000000000000000, 0.8660254037844387076, 1.000000000000000000, 0.8660254037844387076, 1.000000000000000000, 0.8660254037844387076, 1.000000000000000000, 0.8660254037844387076, 1.000000000000000000, 0.8660254037844387076, 1.000000000000000000, 0.8660254037844387076, 1.000000000000000000, 0.8660254037844387076, 1.000000000000000000, 0.8660254037844387076, 1.000000000000000000, 0.8660254037844387076, 1.000000000000000000, 0.8660254037844387076, 1.000000000000000000, 0.8660254037844387076, 1.000000000000000000, 0.8660254037844387076, 1.000000000000000000, 0.8660254037844387076, 1.000000000000000000, 0.8660254037844387076, 1.000000000000000000, 0.8660254037844387076, 1.000000000000000000, 0.8660254037844387076, 1.000000000000000000, 0.8660254037844387076, 1.000000000000000000, 0.8660254037844387076, 1.000000000000000000, 0.8660254037844387076, 1.000000000000000000, 0.8660254037844387076, 1.000000000000000000, 0.8660254037844387076, 1.000000000000000000, 0.8660254037844387076, 1.000000000000000000, 0.8660254037844387076, 1.000000000000000000, 0.8660254037844387076, 1.000000000000000000, 0.8660254037844387076, 1.000000000000000000, 0.8660254037844387076, 1.000000000000000000, 0.8660254037844387076, 1.000000000000000000, 0.8660254037844387076, 1.000000000000000000, 0.8660254037844387076, 1.000000000000000000, 0.8660254037844387076, 1.000000000000000000, 0.8660254037844387076, 1.000000000000000000, 0.8660254037844387076, 1.000000000000000000, 0.8660254037844387076, 1.000000000000000000, 0.8660254037844387076, 1.000000000000000000, 0.8660254037844387076, 1.000000000000000000, 0.8660254037844387076, 1.000000000000000000, 0.8660254037844387076, 1.000000000000000000, 0.8660254037844387076, 1.000000000000000000, 0.8660254037844387076, 1.000000000000000000, 0.8660254037844387076, 1.000000000000000000, 0.8660254037844387076, 1.000000000000000000, 0.8660254037844387076, 1.000000000000000000, 0.8660254037844387076, 1.000000000000000000, 0.8660254037844387076, 1.000000000000000000, 0.8660254037844387076, 1.000000000000000000, 0.8660254037844387076, 1.000000000000000000, 0.8660254037844387076, 1.000000000000000000, 0.8660254037844387076, 1.000000000000000000, 0.8660254037844387076, 1.000000000000000000, 0.8660254037844387076, 1.000000000000000000, 0.8660254037844387076, 1.000000000000000000, 0.8660254037844387076, 1.000000000000000000, 0.8660254037844387076, 1.000000000000000000, 0.8660254037844387076, 1.000000000000000000, 0.8660254037844387076, 1.000000000000000000, 0.8660254037844387076, 1.000000000000000000, 0.8660254037844387076, 1.000000000000000000, 0.8660254037844387076, 1.000000000000000000, 0.8660254037844387076, 1.000000000000000000, 0.8660254037844387076, 1.000000000000000000, 0.8660254037844387076, 1.000000000000000000, 0.8660254037844387076, 1.000000000000000000, 0.8660254037844387076, 1.000000000000000000, 0.8660254037844387076, 1.000000000000000000, 0.8660254037844387076, 1.000000000000000000, 0.8660254037844387076, 1.000000000000000000, 0.8660254037844387076, 1.000000000000000000, 0.8660254037844387076, 1.000000000000000000),
 ( 1.000000000000000000, 0.8660254037844387076, 1.000000000000000000, 0.8660254037844387076, 1.000000000000000000, 0.8660254037844387076, 1.000000000000000000, 0.8660254037844387076, 1.000000000000000000, 0.8660254037844387076, 1.000000000000000000, 0.8660254037844387076, 1.000000000000000000, 0.8660254037844387076, 1.000000000000000000, 0.8660254037844387076, 1.000000000000000000, 0.8660254037844387076, 1.000000000000000000, 0.8660254037844387076, 1.000000000000000000, 0.8660254037844387076, 1.000000000000000000, 0.8660254037844387076, 1.000000000000000000, 0.8660254037844387076, 1.000000000000000000, 0.8660254037844387076, 1.000000000000000000, 0.8660254037844387076, 1.000000000000000000, 0.8660254037844387076, 1.000000000000000000, 0.8660254037844387076, 1.000000000000000000, 0.8660254037844387076, 1.000000000000000000, 0.8660254037844387076, 1.000000000000000000, 0.8660254037844387076, 1.000000000000000000, 0.8660254037844387076, 1.000000000000000000, 0.8660254037844387076, 1.000000000000000000, 0.8660254037844387076, 1.000000000000000000, 0.8660254037844387076, 1.000000000000000000, 0.8660254037844387076, 1.000000000000000000, 0.8660254037844387076, 1.000000000000000000, 0.8660254037844387076, 1.000000000000000000, 0.8660254037844387076, 1.000000000000000000, 0.8660254037844387076, 1.000000000000000000, 0.8660254037844387076, 1.000000000000000000, 0.8660254037844387076, 1.000000000000000000, 0.8660254037844387076, 1.000000000000000000, 0.8660254037844387076, 1.000000000000000000, 0.8660254037844387076, 1.000000000000000000, 0.8660254037844387076, 1.000000000000000000, 0.8660254037844387076, 1.000000000000000000, 0.8660254037844387076, 1.000000000000000000, 0.8660254037844387076, 1.000000000000000000, 0.8660254037844387076, 1.000000000000000000, 0.8660254037844387076, 1.000000000000000000, 0.8660254037844387076, 1.000000000000000000, 0.8660254037844387076, 1.000000000000000000, 0.8660254037844387076, 1.000000000000000000, 0.8660254037844387076, 1.000000000000000000, 0.8660254037844387076, 1.000000000000000000, 0.8660254037844387076, 1.000000000000000000, 0.8660254037844387076, 1.000000000000000000, 0.8660254037844387076, 1.000000000000000000, 0.8660254037844387076, 1.000000000000000000, 0.8660254037844387076, 1.000000000000000000, 0.8660254037844387076, 1.000000000000000000, 0.8660254037844387076, 1.000000000000000000, 0.8660254037844387076, 1.000000000000000000, 0.8660254037844387076, 1.000000000000000000, 0.8660254037844387076, 1.000000000000000000, 0.8660254037844387076, 1.000000000000000000, 0.8660254037844387076, 1.000000000000000000, 0.8660254037844387076, 1.000000000000000000, 0.8660254037844387076, 1.000000000000000000, 0.8660254037844387076, 1.000000000000000000, 0.8660254037844387076, 1.000000000000000000, 0.8660254037844387076, 1.000000000000000000, 0.8660254037844387076, 1.000000000000000000, 0.8660254037844387076, 1.000000000000000000, 0.8660254037844387076, 1.000000000000000000, 0.8660254037844387076, 1.000000000000000000, 0.8660254037844387076, 1.000000000000000000, 0.8660254037844387076, 1.000000000000000000, 0.8660254037844387076, 1.000000000000000000, 0.8660254037844387076, 1.000000000000000000, 0.8660254037844387076, 1.000000000000000000, 0.8660254037844387076, 1.000000000000000000, 0.8660254037844387076, 1.000000000000000000, 0.8660254037844387076, 1.000000000000000000, 0.8660254037844387076, 1.000000000000000000, 0.8660254037844387076, 1.000000000000000000, 0.8660254037844387076, 1.000000000000000000, 0.8660254037844387076, 1.000000000000000000, 0.8660254037844387076, 1.000000000000000000, 0.8660254037844387076, 1.000000000000000000, 0.8660254037844387076, 1.000000000000000000, 0.8660254037844387076, 1.000000000000000000, 0.8660254037844387076, 1.000000000000000000, 0.8660254037844387076, 1.000000000000000000, 0.8660254037844387076, 1.000000000000000000, 0.8660254037844387076, 1.000000000000000000, 0.8660254037844387076, 1.000000000000000000, 0.8660254037844387076, 1.000000000000000000, 0.8660254037844387076, 1.000000000000000000, 0.8660254037844387076, 1.000000000000000000, 0.8660254037844387076, 1.000000000000000000, 0.8660254037844387076, 1.000000000000000000, 0.8660254037844387076, 1.000000000000000000, 0.8660254037844387076, 1.000000000000000000, 0.8660254037844387076, 1.000000000000000000, 0.8660254037844387076, 1.000000000000000000, 0.8660254037844387076, 1.000000000000000000, 0.8660254037844387076, 1.000000000000000000, 0.8660254037844387076, 1.000000000000000000, 0.8660254037844387076, 1.000000000000000000, 0.8660254037844387076, 1.000000000000000000, 0.8660254037844387076, 1.000000000000000000, 0.8660254037844387076, 1.000000000000000000, 0.8660254037844387076, 1.000000000000000000, 0.8660254037844387076, 1.000000000000000000, 0.8660254037844387076, 1.000000000000000000, 0.8660254037844387076, 1.000000000000000000, 0.8660254037844387076, 1.000000000000000000, 0.8660254037844387076, 1.000000000000000000, 0.8660254037844387076, 1.000000000000000000, 0.8660254037844387076, 1.000000000000000000, 0.8660254037844387076, 1.000000000000000000, 0.8660254037844387076, 1.000000000000000000, 0.8660254037844387076, 1.000000000000000000, 0.8660254037844387076, 1.000000000000000000, 0.8660254037844387076, 1.000000000000000000, 0.8660254037844387076, 1.000000000000000000, 0.8660254037844387076, 1.000000000000000000, 0.8660254037844387076, 1.000000000000000000, 0.8660254037844387076, 1.000000000000000000, 0.8660254037844387076, 1.000000000000000000, 0.8660254037844387076, 1.000000000000000000, 0.8660254037844387076, 1.000000000000000000, 0.8660254037844387076, 1.000000000000000000, 0.8660254037844387076, 1.000000000000000000, 0.8660254037844387076, 1.000000000000000000, 0.8660254037844387076, 1.000000000000000000, 0.8660254037844387076, 1.000000000000000000, 0.8660254037844387076, 1.000000000000000000, 0.8660254037844387076, 1.000000000000000000, 0.8660254037844387076, 1.000000000000000000, 0.8660254037844387076, 1.000000000000000000, 0.8660254037844387076, 1.000000000000000000, 0.8660254037844387076, 1.000000000000000000, 0.8660254037844387076, 1.000000000000000000, 0.8660254037844387076, 1.000000000000000000, 0.8660254037844387076, 1.000000000000000000, 0.8660254037844387076, 1.000000000000000000, 0.8660254037844387076, 1.000000000000000000, 0.8660254037844387076, 1.000000000000000000, 0.8660254037844387076, 1.000000000000000000, 0.8660254037844387076, 1.000000000000000000, 0.8660254037844387076, 1.000000000000000000, 0.8660254037844387076, 1.000000000000000000, 0.8660254037844387076, 1.000000000000000000, 0.8660254037844387076, 1.000000000000000000, 0.8660254037844387076, 1.000000000000000000, 0.8660254037844387076, 1.000000000000000000, 0.8660254037844387076, 1.000000000000000000, 0.8660254037844387076, 1.000000000000000000, 0.8660254037844387076, 1.000000000000000000, 0.8660254037844387076, 1.000000000000000000, 0.8660254037844387076, 1.000000000000000000, 0.8660254037844387076, 1.000000000000000000, 0.8660254037844387076, 1.000000000000000000, 0.8660254037844387076, 1.000000000000000000, 0.8660254037844387076, 1.000000000000000000, 0.8660254037844387076, 1.000000000000000000, 0.8660254037844387076, 1.000000000000000000, 0.8660254037844387076, 1.000000000000000000, 0.8660254037844387076, 1.000000000000000000, 0.8660254037844387076, 1.000000000000000000, 0.8660254037844387076, 1.000000000000000000, 0.8660254037844387076, 1.000000000000000000, 0.8660254037844387076, 1.000000000000000000, 0.8660254037844387076, 1.000000000000000000, 0.8660254037844387076, 1.000000000000000000, 0.8660254037844387076, 1.000000000000000000) ) ) 
 REPRESENTATION_ITEM ( '' )  SURFACE ( )  );
#128382=CARTESIAN_POINT ( 'NONE',  ( -8.175203439360366531, 12.48156174598837787, 1.040834085586084257E-14 ) ) ;
#128383=CARTESIAN_POINT ( 'NONE',  ( -7.206322340863467346, 8.366129804884193888, 1.199719254218450271 ) ) ;
#128388=CARTESIAN_POINT ( 'NONE',  ( -6.082092046053040768, 6.030765914320626919, 0.4329532585971782033 ) ) ;
#128389=CARTESIAN_POINT ( 'NONE',  ( -0.6823417656250246877, -0.1989583329919109023, 1.181850606188755259 ) ) ;
#128392=CARTESIAN_POINT ( 'NONE',  ( 7.809133291791403586, 8.213003049952529722, -0.7216878364870257245 ) ) ;
#128410=CARTESIAN_POINT ( 'NONE',  ( 8.723781775389312543, 12.26516360700784958, -1.199719254218446718 ) ) ;
#128412=ORIENTED_EDGE ( 'NONE', *, *, #111969, .F. ) ;
#128414=CARTESIAN_POINT ( 'NONE',  ( -5.298539104842322267, 5.076050465271134016, 0.7998128361456341429 ) ) ;
#128415=CARTESIAN_POINT ( 'NONE',  ( -7.344766530301162000, 9.591980256816594164, 1.599625672291295375 ) ) ;
#128420=CARTESIAN_POINT ( 'NONE',  ( -1.500000000000013101, 3.910416667349482012, -0.8660254037844313801 ) ) ;
#128421=CARTESIAN_POINT ( 'NONE',  ( 9.399880572976245574, 9.860948844760784482, 0.7998128361456462443 ) ) ;
#128424=CARTESIAN_POINT ( 'NONE',  ( -6.991200766141138168, 11.30815132714001159, 0.7998128361456481317 ) ) ;
#128426=CARTESIAN_POINT ( 'NONE',  ( -0.6823417656249969321, 3.967708333674754950, -1.181850606188749264 ) ) ;
#128430=CARTESIAN_POINT ( 'NONE',  ( -5.111060722227552588, 6.025620933095978238, 1.082531754730546636 ) ) ;
#128432=CARTESIAN_POINT ( 'NONE',  ( -9.680158490477310806, 10.39586578175276266, 0.7216878364870438212 ) ) ;
#128436=CARTESIAN_POINT ( 'NONE',  ( 0.6823417656249882723, 2.238541667008084435, -1.181850606188749264 ) ) ;
#128444=CARTESIAN_POINT ( 'NONE',  ( -1.364683531250012516, 3.530208333674758059, 0.7879004041258379498 ) ) ;
#128446=CARTESIAN_POINT ( 'NONE',  ( -4.466521540698216164, 7.298359999868178960, -1.199719254218452047 ) ) ;
#128449=CARTESIAN_POINT ( 'NONE',  ( -1.201851678989727383E-14, 3.759375000341422801, -1.575800808251660134 ) ) ;
#128452=CARTESIAN_POINT ( 'NONE',  ( 0.6823417656249882723, -0.1572916663252488245, 1.181850606188755259 ) ) ;
#128453=CARTESIAN_POINT ( 'NONE',  ( -5.775410249741523394, 5.840326167560965231, 0.7216878364870317197 ) ) ;
#128457=CARTESIAN_POINT ( 'NONE',  ( 5.856759171423504107, 5.935233242856626568, -0.7216878364870257245 ) ) ;
#128460=CARTESIAN_POINT ( 'NONE',  ( -8.525379664894808585, 8.840697785332414682, -0.7998128361456291469 ) ) ;
#128461=CARTESIAN_POINT ( 'NONE',  ( -10.14113571334194930, 10.93367254176152059, -0.7216878364870267237 ) ) ;
#128463=CARTESIAN_POINT ( 'NONE',  ( 1.364683531249990311, 4.634375000341417916, 1.214306433183764966E-14 ) ) ;
#128468=CARTESIAN_POINT ( 'NONE',  ( -6.873620692004104527, 7.121571683533994168, 0.7216878364870317197 ) ) ;
#128470=CARTESIAN_POINT ( 'NONE',  ( -1.364683531250014514, -0.4489583329919089039, -0.7879004041258359514 ) ) ;
#128482=CARTESIAN_POINT ( 'NONE',  ( -1.500000000000001332, -0.3499999999999753308, 0.000000000000000000 ) ) ;
#128484=CARTESIAN_POINT ( 'NONE',  ( 9.585251414737269826, 11.24551007435741568, -1.082531754730537088 ) ) ;
#128492=CARTESIAN_POINT ( 'NONE',  ( 5.289652487626049115, 9.323011668872403845, 0.7998128361456462443 ) ) ;
#128493=CARTESIAN_POINT ( 'NONE',  ( -5.251085567194491155, 5.020688004682002159, -0.7998128361456221525 ) ) ;
#128496=CARTESIAN_POINT ( 'NONE',  ( 1.499999999999822586, 7.360382131182487520, 4.205521753552998732 ) ) ;
#128497=CARTESIAN_POINT ( 'NONE',  ( -1.402160292154681736E-14, 2.259375000341416140, -1.575800808251660134 ) ) ;
#128499=CARTESIAN_POINT ( 'NONE',  ( -7.960608749518247151, 12.43912730774665576, 0.000000000000000000 ) ) ;
#128510=EDGE_CURVE ( 'NONE', #123166, #211245, #44267, .T. ) ;
#128517=CARTESIAN_POINT ( 'NONE',  ( 6.440286661691305703, 7.472421512516709718, 1.199719254218462483 ) ) ;
#128523=CARTESIAN_POINT ( 'NONE',  ( 6.747154001095143627, 11.02343010125301959, -0.7998128361456291469 ) ) ;
#128528=CARTESIAN_POINT ( 'NONE',  ( -4.302014814237876017, 3.913438792899272212, 0.7998128361456341429 ) ) ;
#128531=DIRECTION ( 'NONE',  ( -3.347138415753903010E-16, -0.6000000000000018652, 0.7999999999999984901 ) ) ;
#128533=CARTESIAN_POINT ( 'NONE',  ( -0.1447443628656817916, 7.100480071729094789, 2.114679381859663199 ) ) ;
#128539=EDGE_CURVE ( 'NONE', #135745, #63949, #152834, .T. ) ;
#128540=CARTESIAN_POINT ( 'NONE',  ( -9.164948653158003111, 9.794787638213568570, -0.7216878364870267237 ) ) ;
#128544=CARTESIAN_POINT ( 'NONE',  ( 3.825371897350130723, 7.614684313550482031, 0.7998128361456321445 ) ) ;
#128545=CARTESIAN_POINT ( 'NONE',  ( -1.001543065824772872E-14, 5.571875000341416140, 1.575800808251672791 ) ) ;
#128551=CARTESIAN_POINT ( 'NONE',  ( 4.324687812634897988, 4.147816657603229373, 0.7216878364870317197 ) ) ;
#128559=CARTESIAN_POINT ( 'NONE',  ( -5.018489415352746619, 9.006654751220198207, 0.7998128361456481317 ) ) ;
#128561=CARTESIAN_POINT ( 'NONE',  ( -3.750802052474980108, 7.527686161196117887, 1.040834085586084257E-14 ) ) ;
#128566=CARTESIAN_POINT ( 'NONE',  ( -0.003079562120915812617, 7.078201604703583172, 2.121336893758693609 ) ) ;
#128567=CARTESIAN_POINT ( 'NONE',  ( 1.364683531249988535, 3.467708333674749621, -0.7879004041258239610 ) ) ;
#128570=CARTESIAN_POINT ( 'NONE',  ( 7.070740804726770357, 8.207951346058097286, 1.199719254218462483 ) ) ;
#128572=CARTESIAN_POINT ( 'NONE',  ( 1.547033095191288954, 8.694673270357780481, 2.507079848779477871 ) ) ;
#128581=ORIENTED_EDGE ( 'NONE', *, *, #55578, .F. ) ;
#128583=CARTESIAN_POINT ( 'NONE',  ( 0.6823417656249864960, -0.5114583329919111243, -1.181850606188749264 ) ) ;
#128584=CARTESIAN_POINT ( 'NONE',  ( 3.708318708537623021, 4.285125567170706695, -1.199719254218446718 ) ) ;
#128585=CARTESIAN_POINT ( 'NONE',  ( 3.357615597678655917, 7.068968630600412695, 0.7998128361456321445 ) ) ;
#128588=CARTESIAN_POINT ( 'NONE',  ( -5.721177635286839092, 9.618531641235897212, 0.7216878364870458196 ) ) ;
#128589=CARTESIAN_POINT ( 'NONE',  ( 5.070386261830877928, 5.978167395966564435, -1.082531754730548412 ) ) ;
#128590=CARTESIAN_POINT ( 'NONE',  ( -8.473482818416682605, 8.988077497682020578, -0.7216878364870267237 ) ) ;
#128594=CARTESIAN_POINT ( 'NONE',  ( 5.636439174979242850, 7.598931675607687453, -1.599625672291262513 ) ) ;
#128599=CARTESIAN_POINT ( 'NONE',  ( 1.364683531249992088, 5.384375000341417916, 1.214306433183764966E-14 ) ) ;
#128603=CARTESIAN_POINT ( 'NONE',  ( 8.932124273304774320, 9.315233161810734686, 0.7998128361456462443 ) ) ;
#128607=CARTESIAN_POINT ( 'NONE',  ( -6.353967546298838087, 10.56471257065732416, 0.000000000000000000 ) ) ;
#128612=CARTESIAN_POINT ( 'NONE',  ( 8.239604668803105270, 10.63595808506888396, -1.599625672291268286 ) ) ;
#128615=CARTESIAN_POINT ( 'NONE',  ( -7.283754839039664475, 9.520799950344851936, -1.599625672291263179 ) ) ;
#128619=CARTESIAN_POINT ( 'NONE',  ( 5.112599315731837457, 6.496590726105775815, -1.208607640439966158 ) ) ;
#128620=CARTESIAN_POINT ( 'NONE',  ( -9.164948653157999559, 10.75515685251491504, -1.082531754730539753 ) ) ;
#128625=CARTESIAN_POINT ( 'NONE',  ( 4.638861114170084399, 8.563755066507100722, 0.7998128361456462443 ) ) ;
#128627=CARTESIAN_POINT ( 'NONE',  ( 6.484877546038077867, 6.460111979999551224, 1.040834085586084257E-14 ) ) ;
#128628=CARTESIAN_POINT ( 'NONE',  ( -4.235850332497944848, 7.335353122692886529, 0.8760575672057471230 ) ) ;
#128629=CARTESIAN_POINT ( 'NONE',  ( 4.684505768721569652, 5.424010470718658716, -1.199719254218452047 ) ) ;
#128631=CARTESIAN_POINT ( 'NONE',  ( -6.399085315970142851, 8.488685506763726352, -1.443375672974059665 ) ) ;
#128637=TOROIDAL_SURFACE ( 'NONE', #476, 3.971937515251341644, 0.08000000000000000167 ) ;
#128638=CARTESIAN_POINT ( 'NONE',  ( -4.698067037153471404, 6.865000302791745668, 1.228424997642649563 ) ) ;
#128639=CARTESIAN_POINT ( 'NONE',  ( -0.6823417656250246877, -0.1364583329919108468, 1.181850606188755259 ) ) ;
#128642=CARTESIAN_POINT ( 'NONE',  ( 5.341549334104194635, 6.294524313618772737, 1.082531754730558626 ) ) ;
#128647=CARTESIAN_POINT ( 'NONE',  ( -9.503902493055310430, 11.15060299906175167, 1.082531754730558626 ) ) ;
#128652=CARTESIAN_POINT ( 'NONE',  ( -9.503902493055310430, 11.15060299906175167, 1.082531754730558626 ) ) ;
#128659=CARTESIAN_POINT ( 'NONE',  ( -8.093854517234044366, 11.42628545587295186, 1.082531754730549967 ) ) ;
#128663=CARTESIAN_POINT ( 'NONE',  ( 1.364683531249990311, 5.196875000341417916, 1.214306433183764966E-14 ) ) ;
#128664=CARTESIAN_POINT ( 'NONE',  ( -1.500000000000011324, 4.660416667349484676, -0.8660254037844313801 ) ) ;
#128665=CARTESIAN_POINT ( 'NONE',  ( 5.089368577813358385, 6.729159871965151751, -1.415889853396500975 ) ) ;
#128670=CARTESIAN_POINT ( 'NONE',  ( -6.659026002606323047, 10.92061410301605662, 0.000000000000000000 ) ) ;
#128674=CARTESIAN_POINT ( 'NONE',  ( 5.124091990960999432, 8.065525525174782828, -1.199719254218452047 ) ) ;
#128679=CARTESIAN_POINT ( 'NONE',  ( 7.096803341749390981, 10.36702210109460154, -1.199719254218441611 ) ) ;
#128685=CARTESIAN_POINT ( 'NONE',  ( -5.395781948558855845, 9.238903340053241209, 0.7216878364870458196 ) ) ;
#128688=DIRECTION ( 'NONE',  ( 1.000000000000000000, -8.673617379884035472E-16, 0.000000000000000000 ) ) ;
#128690=CARTESIAN_POINT ( 'NONE',  ( 5.517805331081858888, 5.539787095791365523, 1.040834085586084257E-14 ) ) ;
#128694=CARTESIAN_POINT ( 'NONE',  ( -10.00321840878439339, 10.56484298653695397, 1.040834085586084257E-14 ) ) ;
#128696=CARTESIAN_POINT ( 'NONE',  ( 8.718056468787178659, 10.12981962079525289, 1.199719254218462483 ) ) ;
#128697=CARTESIAN_POINT ( 'NONE',  ( 1.499999999999985123, -0.2041666666666457353, -0.8660254037844323793 ) ) ;
#128698=CARTESIAN_POINT ( 'NONE',  ( -8.666686507633592385, 11.13422023037111330, 1.599625672291269396 ) ) ;
#128701=CARTESIAN_POINT ( 'NONE',  ( -1.364683531250012516, 3.738541667008087099, -0.7879004041258300672 ) ) ;
#128702=CARTESIAN_POINT ( 'NONE',  ( 3.009020027229115879, 5.597941567487558778, -1.199719254218446718 ) ) ;
#128707=CARTESIAN_POINT ( 'NONE',  ( 9.042925270190625753, 11.57316545335434199, 1.443375672974076540 ) ) ;
#128710=CARTESIAN_POINT ( 'NONE',  ( -5.856759171423528088, 8.816340885760650892, 1.082531754730548412 ) ) ;
#128711=CARTESIAN_POINT ( 'NONE',  ( -1.201851678989727383E-14, 0.8218750003414171390, 1.575800808251672791 ) ) ;
#128713=CARTESIAN_POINT ( 'NONE',  ( 0.4680205011783269420, 8.035366863023833517, 1.945178226287680223 ) ) ;
#128715=CARTESIAN_POINT ( 'NONE',  ( -6.808165692356648258, 11.09461040772476714, 0.7998128361456481317 ) ) ;
#128716=CARTESIAN_POINT ( 'NONE',  ( -3.429849674132948500, 5.024577257953626308, -1.443375672974051449 ) ) ;
#128717=CARTESIAN_POINT ( 'NONE',  ( 0.6823417656249917140, 3.905208333674754950, 1.181850606188765695 ) ) ;
#128723=CARTESIAN_POINT ( 'NONE',  ( 8.062294901620731480, 12.55776115186623620, 1.040834085586084257E-14 ) ) ;
#128736=CARTESIAN_POINT ( 'NONE',  ( -1.001543065824772872E-14, 5.634375000341415252, 1.575800808251672791 ) ) ;
#128740=CARTESIAN_POINT ( 'NONE',  ( 7.584896871841365851, 10.93646455286856956, -1.199719254218446718 ) ) ;
#128743=CARTESIAN_POINT ( 'NONE',  ( -1.201851678989727383E-14, 4.196875000341417028, -1.575800808251660134 ) ) ;
#128745=CARTESIAN_POINT ( 'NONE',  ( -7.049876689426106680, 9.247942109129029475, -1.443375672974059665 ) ) ;
#128752=CARTESIAN_POINT ( 'NONE',  ( 4.715538499454675403, 4.395883092318884522, 1.214306433183764966E-14 ) ) ;
#128755=CARTESIAN_POINT ( 'NONE',  ( 9.134442807305049428, 11.67993591332117376, 1.599625672291281386 ) ) ;
#128756=CARTESIAN_POINT ( 'NONE',  ( 5.690973801507735352, 5.856266416820083975, -2.499999999999995115 ) ) ;
#128761=CARTESIAN_POINT ( 'NONE',  ( -10.62011439820619429, 11.28455497419572318, -0.7998128361456221525 ) ) ;
#128763=CARTESIAN_POINT ( 'NONE',  ( 7.091078035147269532, 8.231678114882006625, 1.199719254218462483 ) ) ;
#128765=CARTESIAN_POINT ( 'NONE',  ( 3.497113557321089861, 6.167384019261527683, -1.199719254218446718 ) ) ;
#128771=FACE_OUTER_BOUND ( 'NONE', #49129, .T. ) ;
#128774=CARTESIAN_POINT ( 'NONE',  ( -6.900736999675794792, 7.153207375817628666, 1.040834085586084257E-14 ) ) ;
#128775=CARTESIAN_POINT ( 'NONE',  ( 5.345992642490140057, 5.131412925860272090, 1.040834085586084257E-14 ) ) ;
#128778=CARTESIAN_POINT ( 'NONE',  ( -6.008234629150358330, 10.16135750065076060, 0.000000000000000000 ) ) ;
#128781=CARTESIAN_POINT ( 'NONE',  ( -8.890396042259075315, 11.39521468743417998, -1.599625672291263179 ) ) ;
#128785=CARTESIAN_POINT ( 'NONE',  ( 6.774270308322468459, 11.05506579301824743, 0.7998128361456462443 ) ) ;
#128795=CARTESIAN_POINT ( 'NONE',  ( -7.344766530301162000, 9.591980256816594164, 1.599625672291295375 ) ) ;
#128799=CARTESIAN_POINT ( 'NONE',  ( 5.341549334104176872, 9.175631956522799726, 0.7216878364870438212 ) ) ;
#128802=CARTESIAN_POINT ( 'NONE',  ( 2.510230996824538430, 6.080353262937265413, 0.000000000000000000 ) ) ;
#128805=CARTESIAN_POINT ( 'NONE',  ( -5.982172092127739482, 8.002286745614243912, -1.599625672291263179 ) ) ;
#128807=CARTESIAN_POINT ( 'NONE',  ( -1.499999999999997780, 7.388542872122518368, -4.154462424328208670 ) ) ;
#128814=CARTESIAN_POINT ( 'NONE',  ( 1.364683531249988535, 4.426041667008082214, 0.7879004041258500513 ) ) ;
#128815=CARTESIAN_POINT ( 'NONE',  ( 3.999405481576134846, 7.808394548344907093, -0.08844146109573064463 ) ) ;
#128816=CARTESIAN_POINT ( 'NONE',  ( 8.925345196497941558, 9.307324238869423283, 1.040834085586084257E-14 ) ) ;
#128818=CARTESIAN_POINT ( 'NONE',  ( -2.955314298098991266, 6.391691081183366485, 0.7216878364870317197 ) ) ;
#128821=CARTESIAN_POINT ( 'NONE',  ( -3.755245360860919757, 7.324943987738961049, -0.7216878364870257245 ) ) ;
#128828=CARTESIAN_POINT ( 'NONE',  ( 2.672928840188529609, 6.270167413528593414, 0.000000000000000000 ) ) ;
#128835=CARTESIAN_POINT ( 'NONE',  ( 4.650610384687404952, 5.384465856012134566, 1.199719254218462483 ) ) ;
#128840=CARTESIAN_POINT ( 'NONE',  ( -1.364683531250010295, 4.342708333674753618, 0.7879004041258379498 ) ) ;
#128845=CARTESIAN_POINT ( 'NONE',  ( 5.229694566569264680, 7.124396299129368337, 1.599625672291267398 ) ) ;
#128849=CARTESIAN_POINT ( 'NONE',  ( -3.737243898861318137, 7.511868315313511069, 0.7998128361456341429 ) ) ;
#128850=CARTESIAN_POINT ( 'NONE',  ( 5.626270559546814098, 7.587068290936515247, 1.443375672974062551 ) ) ;
#128851=CARTESIAN_POINT ( 'NONE',  ( -0.7499999999999972244, 3.858333333333359594, -1.299038105676652011 ) ) ;
#128855=CARTESIAN_POINT ( 'NONE',  ( -3.588104209110990706, 7.337872010604796991, 1.040834085586084257E-14 ) ) ;
#128856=CARTESIAN_POINT ( 'NONE',  ( 0.08369048095983153135, 7.010987279216816859, -1.999726996211172336 ) ) ;
#128858=CARTESIAN_POINT ( 'NONE',  ( 1.364683531249988535, 4.405208333674754506, -0.7879004041258300672 ) ) ;
#128861=CARTESIAN_POINT ( 'NONE',  ( -2.806174608348664723, 6.217694776474651519, 1.040834085586084257E-14 ) ) ;
#128867=CARTESIAN_POINT ( 'NONE',  ( 3.005103603723342953, 6.657704637652544832, -0.7998128361456291469 ) ) ;
#128870=CARTESIAN_POINT ( 'NONE',  ( 0.08888683327021046354, 6.492044364012832247, -3.106763327641855810 ) ) ;
#128871=CARTESIAN_POINT ( 'NONE',  ( -1.001543065824772872E-14, 4.384375000341417916, 1.575800808251672791 ) ) ;
#128875=CARTESIAN_POINT ( 'NONE',  ( -0.6823417656250003738, 0.2802083336747515641, -1.181850606188749264 ) ) ;
#128876=CARTESIAN_POINT ( 'NONE',  ( 2.295757763869426871, 5.519548059767960702, 0.4031905389056070765 ) ) ;
#128879=CARTESIAN_POINT ( 'NONE',  ( -9.134442807305063639, 11.67993591332117376, 1.599625672291281386 ) ) ;
#128880=CARTESIAN_POINT ( 'NONE',  ( -5.192409643909507544, 9.001635651295671892, 0.7216878364870458196 ) ) ;
#128883=ORIENTED_EDGE ( 'NONE', *, *, #187231, .T. ) ;
#128884=CARTESIAN_POINT ( 'NONE',  ( -0.6823417656250212460, 3.801041667008085767, 1.181850606188767472 ) ) ;
#128892=CARTESIAN_POINT ( 'NONE',  ( -6.900736999231456004, 8.113576589600553390, 1.082531754730549967 ) ) ;
#128897=CARTESIAN_POINT ( 'NONE',  ( -5.626270559546828309, 7.587068290936515247, 1.443375672974064550 ) ) ;
#128905=CARTESIAN_POINT ( 'NONE',  ( 1.594690046439222630, 8.741643652401167586, -2.463706593913769893 ) ) ;
#128909=CARTESIAN_POINT ( 'NONE',  ( 0.1254057754173175943, 7.054063922337675763, -3.955400951015573874 ) ) ;
#128910=CARTESIAN_POINT ( 'NONE',  ( -4.717347382551060342, 7.590990148696470818, 1.199719254218464037 ) ) ;
#128911=CARTESIAN_POINT ( 'NONE',  ( -4.417564364067771088, 7.323841156470280112, 1.242459261498860323 ) ) ;
#128913=CARTESIAN_POINT ( 'NONE',  ( 1.499999999999989120, 1.275000000000019229, 0.000000000000000000 ) ) ;
#128915=CARTESIAN_POINT ( 'NONE',  ( 8.920901888111989919, 11.43080484092926241, 1.443375672974076540 ) ) ;
#128916=CARTESIAN_POINT ( 'NONE',  ( 7.467843683028853263, 7.606905806488803101, 0.7998128361456341429 ) ) ;
#128920=CARTESIAN_POINT ( 'NONE',  ( 4.547870462380197765, 7.393267075163835855, 1.199719254218462483 ) ) ;
#128923=CARTESIAN_POINT ( 'NONE',  ( -0.1332994001262414741, 7.096108761198731685, -2.115961662170576574 ) ) ;
#128924=ORIENTED_EDGE ( 'NONE', *, *, #141157, .F. ) ;
#128932=CARTESIAN_POINT ( 'NONE',  ( -2.657034918598338180, 6.043698471765932112, -0.7216878364870267237 ) ) ;
#128938=CARTESIAN_POINT ( 'NONE',  ( -0.6823417656250003738, 2.967708333674754062, -1.181850606188749264 ) ) ;
#128939=CARTESIAN_POINT ( 'NONE',  ( 8.717529583462649612, 10.23316793787035195, 1.082531754730558626 ) ) ;
#128940=ADVANCED_FACE ( 'NONE', ( #153368 ), #49, .T. ) ;
#128941=CARTESIAN_POINT ( 'NONE',  ( -6.256197817702116026, 9.386315656372753224, -1.199719254218440723 ) ) ;
#128944=CARTESIAN_POINT ( 'NONE',  ( 4.957477724091233995, 8.935474444748447098, -0.7998128361456281477 ) ) ;
#128945=CARTESIAN_POINT ( 'NONE',  ( -5.201524489137236529, 9.220195670635433771, 0.7998128361456481317 ) ) ;
#128949=CARTESIAN_POINT ( 'NONE',  ( -0.7500000000000006661, 0.3895833340161539149, -1.299038105676652011 ) ) ;
#128952=CARTESIAN_POINT ( 'NONE',  ( 7.782016984564060103, 9.141736572488651902, 1.082531754730558626 ) ) ;
#128955=CARTESIAN_POINT ( 'NONE',  ( -1.364683531250014514, 1.801041667008085767, -0.7879004041258289570 ) ) ;
#128957=CARTESIAN_POINT ( 'NONE',  ( 4.975479186090847605, 7.788180902872553268, 1.082531754730558626 ) ) ;
#128960=CARTESIAN_POINT ( 'NONE',  ( -4.446711195602255806, 5.250546485366484717, -1.082531754730544860 ) ) ;
#128962=CARTESIAN_POINT ( 'NONE',  ( -1.364683531249997417, 4.259375000341424133, 1.214306433183764966E-14 ) ) ;
#128968=CARTESIAN_POINT ( 'NONE',  ( -5.140457058134151325, 6.683247392444177315, -1.432107399977754270 ) ) ;
#128970=PRODUCT_DEFINITION ( 'UNKNOWN', '', #125065, #35183 ) ;
#128975=CARTESIAN_POINT ( 'NONE',  ( 6.979750152936881058, 7.037463354714830643, 0.7998128361456341429 ) ) ;
#128978=CARTESIAN_POINT ( 'NONE',  ( 2.510230996824538430, 6.080353262937265413, 0.000000000000000000 ) ) ;
#128987=CARTESIAN_POINT ( 'NONE',  ( 5.178851490740196795, 7.065079377328788546, 1.443375672974062551 ) ) ;
#128988=CARTESIAN_POINT ( 'NONE',  ( -1.364683531250000748, 1.571875000341421691, 0.000000000000000000 ) ) ;
#128989=CARTESIAN_POINT ( 'NONE',  ( 8.239604668803105270, 10.63595808506888396, -1.599625672291268286 ) ) ;
#128997=CARTESIAN_POINT ( 'NONE',  ( 0.7499999999999885647, 1.566666666666688412, -1.299038105676652899 ) ) ;
#128998=CARTESIAN_POINT ( 'NONE',  ( 4.774442650306744085, 8.721933525333202653, -0.7998128361456281477 ) ) ;
#128999=CARTESIAN_POINT ( 'NONE',  ( -6.855619230004478482, 11.14997286831390788, -0.7998128361456291469 ) ) ;
#129003=CARTESIAN_POINT ( 'NONE',  ( 1.364683531249988535, 2.863541667008082658, 0.7879004041258500513 ) ) ;
#129005=CARTESIAN_POINT ( 'NONE',  ( 1.499999999999989120, 3.504166666666683749, 0.8660254037844524744 ) ) ;
#129007=CARTESIAN_POINT ( 'NONE',  ( 3.602716132929354664, 5.226254793216122074, 1.599625672291267398 ) ) ;
#129013=CARTESIAN_POINT ( 'NONE',  ( 1.499999999999987121, 0.2854166673494805684, 0.8660254037844524744 ) ) ;
#129015=CARTESIAN_POINT ( 'NONE',  ( -5.533699252672048985, 9.607732894759390518, -0.7998128361456231517 ) ) ;
#129016=CARTESIAN_POINT ( 'NONE',  ( -4.284013352238265959, 5.060732334775157604, -1.082531754730544860 ) ) ;
#129025=CARTESIAN_POINT ( 'NONE',  ( 6.796715079152391148, 6.823922435299587974, 0.7998128361456341429 ) ) ;
#129026=VECTOR ( 'NONE', #150837, 1000.000000000000000 ) ;
#129030=CARTESIAN_POINT ( 'NONE',  ( 6.144869935491714230, 8.192100896205568361, -1.599625672291262513 ) ) ;
#129033=( BOUNDED_CURVE ( )  B_SPLINE_CURVE ( 2, ( #160906, #12503, #129555, #144697, #81779, #163048, #15693 ),
 .UNSPECIFIED., .F., .T. ) 
 B_SPLINE_CURVE_WITH_KNOTS ( ( 3, 2, 2, 3 ),
 ( 0.3392857142857143571, 0.3452380952380953438, 0.3511904761904763861, 0.3571428571428574283 ),
 .UNSPECIFIED. ) 
 CURVE ( )  GEOMETRIC_REPRESENTATION_ITEM ( )  RATIONAL_B_SPLINE_CURVE ( ( 0.9999999999999987788, 0.8660254037844399289, 1.000000000000000000, 0.8660254037844387076, 1.000000000000000000, 0.8660254037844324904, 1.000000000000006217 ) ) 
 REPRESENTATION_ITEM ( '' )  );
#129036=CARTESIAN_POINT ( 'NONE',  ( -6.184490626128011925, 10.36698949712469364, -0.7998128361456291469 ) ) ;
#129038=CARTESIAN_POINT ( 'NONE',  ( 4.376584659113025744, 4.000436945253625254, 0.7998128361456341429 ) ) ;
#129039=EDGE_LOOP ( 'NONE', ( #59751, #163222, #134046, #995, #148660, #145517, #41016, #184332, #17992 ) ) ;
#129044=CARTESIAN_POINT ( 'NONE',  ( 8.563946585326370098, 13.14302144952281814, 0.7998128361456462443 ) ) ;
#129045=CARTESIAN_POINT ( 'NONE',  ( 4.677432586336220055, 6.849818891840005364, 1.226792522213099979 ) ) ;
#129055=CARTESIAN_POINT ( 'NONE',  ( -2.331639231870358930, 5.664070170583284103, -0.7216878364870267237 ) ) ;
#129056=CARTESIAN_POINT ( 'NONE',  ( 7.076992996653421741, 10.23994701519558781, -1.082531754730537976 ) ) ;
#129058=CARTESIAN_POINT ( 'NONE',  ( -4.554649539187067830, 7.401175998105142817, 1.199719254218464037 ) ) ;
#129064=CARTESIAN_POINT ( 'NONE',  ( -7.854251061018346469, 8.057714414143200443, -0.7998128361456291469 ) ) ;
#129070=ORIENTED_EDGE ( 'NONE', *, *, #14168, .T. ) ;
#129079=FACE_OUTER_BOUND ( 'NONE', #198257, .T. ) ;
#129080=CARTESIAN_POINT ( 'NONE',  ( -4.554649539187067830, 7.401175998105142817, 1.199719254218464037 ) ) ;
#129083=CARTESIAN_POINT ( 'NONE',  ( 4.256897045010922476, 5.029096643009940415, -1.082531754730548412 ) ) ;
#129087=CARTESIAN_POINT ( 'NONE',  ( -3.216308754939891212, 4.775446185561722956, -1.599625672291262513 ) ) ;
#129088=CARTESIAN_POINT ( 'NONE',  ( -2.930533758848195447, 6.570706485298192234, -0.7998128361456281477 ) ) ;
#129091=CARTESIAN_POINT ( 'NONE',  ( 8.432281472695482449, 11.92507992053172572, 1.199719254218450271 ) ) ;
#129095=CARTESIAN_POINT ( 'NONE',  ( -6.503107236049161521, 10.73870887536603291, 0.7998128361456481317 ) ) ;
#129096=CARTESIAN_POINT ( 'NONE',  ( 6.647575389402066826, 6.649926130590872120, 1.040834085586084257E-14 ) ) ;
#129099=CARTESIAN_POINT ( 'NONE',  ( 3.822509244049070887, 6.547012320444182798, -1.199719254218452047 ) ) ;
#129102=CARTESIAN_POINT ( 'NONE',  ( -1.402160292154681736E-14, 1.759375000341421469, -1.575800808251659024 ) ) ;
#129105=CARTESIAN_POINT ( 'NONE',  ( 6.290620087060792009, 10.28288116830553101, -0.7216878364870267237 ) ) ;
#129118=CARTESIAN_POINT ( 'NONE',  ( -2.030969412801321816, 8.463209591663684250, 2.499999999999998668 ) ) ;
#129136=CARTESIAN_POINT ( 'NONE',  ( 0.7499999999999885647, 2.097916667349486453, -1.299038105676652899 ) ) ;
#129142=CARTESIAN_POINT ( 'NONE',  ( 1.499999999999987566, -0.9749999999999827693, 0.000000000000000000 ) ) ;
#129143=CARTESIAN_POINT ( 'NONE',  ( 7.239163954692881653, 10.53310948286200599, -1.199719254218441611 ) ) ;
#129148=CARTESIAN_POINT ( 'NONE',  ( 10.56143847536557878, 11.42402576412244386, 0.000000000000000000 ) ) ;
#129149=CARTESIAN_POINT ( 'NONE',  ( -4.907688418466881863, 8.669460888279271416, 0.7216878364870458196 ) ) ;
#129154=CARTESIAN_POINT ( 'NONE',  ( -5.831978632172702071, 9.955725504176825780, 0.7998128361456481317 ) ) ;
#129157=CARTESIAN_POINT ( 'NONE',  ( 1.499999999999987121, 1.535416667349486453, 0.8660254037844524744 ) ) ;
#129164=CARTESIAN_POINT ( 'NONE',  ( -3.511198595814942980, 5.119484333249288532, 1.443375672974064550 ) ) ;
#129165=ADVANCED_FACE ( 'NONE', ( #1492 ), #197585, .F. ) ;
#129168=CARTESIAN_POINT ( 'NONE',  ( 4.139348914150634329, 7.410017372392475821, 0.7316189255667099323 ) ) ;
#129171=CARTESIAN_POINT ( 'NONE',  ( -3.160134022698144918, 2.806877976488492354, -2.466440901443690326 ) ) ;
#129174=CARTESIAN_POINT ( 'NONE',  ( -10.64045162862669081, 11.30828174301964140, -0.7998128361456221525 ) ) ;
#129175=CARTESIAN_POINT ( 'NONE',  ( 7.609150525767641504, 9.900428251527500834, -1.599625672291262513 ) ) ;
#129178=CARTESIAN_POINT ( 'NONE',  ( 0.7499999999999920064, 5.233333333333353821, 1.299038105676669330 ) ) ;
#129179=ORIENTED_EDGE ( 'NONE', *, *, #187231, .F. ) ;
#129182=CARTESIAN_POINT ( 'NONE',  ( -7.537443334193545397, 10.88110209227943770, -1.199719254218446718 ) ) ;
#129188=CARTESIAN_POINT ( 'NONE',  ( 4.059776932288224671, 6.823824623389866950, 1.199719254218462483 ) ) ;
#129194=CARTESIAN_POINT ( 'NONE',  ( -8.784793466650835825, 12.33634391347959713, 1.199719254218462483 ) ) ;
#129198=ORIENTED_EDGE ( 'NONE', *, *, #124471, .T. ) ;
#129206=CARTESIAN_POINT ( 'NONE',  ( 8.606728586576791074, 8.935604860628076906, 0.7998128361456462443 ) ) ;
#129208=CARTESIAN_POINT ( 'NONE',  ( -4.948889764188092677, 5.732458465429559169, 1.199719254218462483 ) ) ;
#129211=CARTESIAN_POINT ( 'NONE',  ( -4.161989969715274462, 4.726297878971393196, -2.420000000000000373 ) ) ;
#129215=CARTESIAN_POINT ( 'NONE',  ( 0.7499999999999885647, 0.8479166673494853423, -1.299038105676652899 ) ) ;
#129220=CARTESIAN_POINT ( 'NONE',  ( 4.539282502477016479, 4.190251095844947926, 0.7998128361456341429 ) ) ;
#129222=CARTESIAN_POINT ( 'NONE',  ( -2.676845263694313637, 5.210404343363602919, -1.199719254218446718 ) ) ;
#129229=CARTESIAN_POINT ( 'NONE',  ( 4.365362273920244007, 6.116008624372160973, 1.443375672974062551 ) ) ;
#129235=CARTESIAN_POINT ( 'NONE',  ( 10.24726517383036928, 10.84956421242393887, 0.000000000000000000 ) ) ;
#129245=CARTESIAN_POINT ( 'NONE',  ( -1.364683531250000748, -0.9906249996585805295, 0.000000000000000000 ) ) ;
#129247=VECTOR ( 'NONE', #5158, 1000.000000000000000 ) ;
#129251=CARTESIAN_POINT ( 'NONE',  ( -5.311043488251275591, 7.219303374425030562, -1.599625672291256295 ) ) ;
#129256=CARTESIAN_POINT ( 'NONE',  ( -1.201851678989727383E-14, 4.587500000000025224, -1.732050807568863648 ) ) ;
#129263=CARTESIAN_POINT ( 'NONE',  ( 1.364683531249986537, -0.8864583329919110133, 0.7879004041258500513 ) ) ;
#129265=CARTESIAN_POINT ( 'NONE',  ( 6.205881626753210867, 8.263281202677319470, 1.599625672291281386 ) ) ;
#129266=CARTESIAN_POINT ( 'NONE',  ( -8.474009703741204547, 9.845098394908269768, -1.199719254218446718 ) ) ;
#129268=DIRECTION ( 'NONE',  ( 0.000000000000000000, -1.000000000000000000, 0.000000000000000000 ) ) ;
#129272=CARTESIAN_POINT ( 'NONE',  ( -0.6823417656250246877, -0.8864583329919115684, 1.181850606188755259 ) ) ;
#129279=CARTESIAN_POINT ( 'NONE',  ( 7.456621297836072415, 9.722477485607340597, 1.443375672974076540 ) ) ;
#129283=CARTESIAN_POINT ( 'NONE',  ( -1.201851678989727383E-14, 4.118750000682818602, -1.732050807568863648 ) ) ;
#129285=CARTESIAN_POINT ( 'NONE',  ( -2.740719608256871442, 6.349256642941639051, 0.7998128361456341429 ) ) ;
#129286=CARTESIAN_POINT ( 'NONE',  ( 4.799223189113185128, 8.542918120699967588, 1.040834085586084257E-14 ) ) ;
#129287=CARTESIAN_POINT ( 'NONE',  ( -8.581948047326017459, 11.99572790764693409, 1.082531754730558626 ) ) ;
#129293=CARTESIAN_POINT ( 'NONE',  ( 4.220665892555866883, 3.818531717603609987, -0.7998128361456211532 ) ) ;
#129294=CARTESIAN_POINT ( 'NONE',  ( 0.7499999999999920064, 4.733333333333352932, 1.299038105676669330 ) ) ;
#129295=CARTESIAN_POINT ( 'NONE',  ( 5.190073875932979419, 4.949507698210251938, 0.7998128361456341429 ) ) ;
#129305=CARTESIAN_POINT ( 'NONE',  ( 0.6823417656249899377, 3.238541667008085323, -1.181850606188754593 ) ) ;
#129309=CARTESIAN_POINT ( 'NONE',  ( 9.185812768458653466, 10.67553530374532045, 1.199719254218453823 ) ) ;
#129315=CARTESIAN_POINT ( 'NONE',  ( -0.6823417656250246877, -0.6989583329919113464, 1.181850606188755259 ) ) ;
#129316=VECTOR ( 'NONE', #75865, 1000.000000000000000 ) ;
#129317=CARTESIAN_POINT ( 'NONE',  ( 3.877268743828258479, 7.467304601200877023, 0.7216878364870298324 ) ) ;
#129318=CARTESIAN_POINT ( 'NONE',  ( -9.517460647113315630, 10.20605163116143821, 0.7216878364870438212 ) ) ;
#129323=CARTESIAN_POINT ( 'NONE',  ( -2.930533758848195447, 6.570706485298192234, -0.7998128361456281477 ) ) ;
#129331=ORIENTED_EDGE ( 'NONE', *, *, #194628, .T. ) ;
#129337=CARTESIAN_POINT ( 'NONE',  ( 5.250185332887272516, 6.604911474350376288, -1.376424501724478944 ) ) ;
#129341=CARTESIAN_POINT ( 'NONE',  ( -4.229856262585510507, 7.526865594461044751, -1.029777601131131037 ) ) ;
#129344=CARTESIAN_POINT ( 'NONE',  ( -7.483737605063437215, 10.71448239167390604, 1.082531754730549967 ) ) ;
#129348=CARTESIAN_POINT ( 'NONE',  ( 6.636879889089462026, 7.701780277814560982, -1.199719254218446718 ) ) ;
#129349=CARTESIAN_POINT ( 'NONE',  ( 4.566398809704347528, 4.221886787610169556, -0.7998128361456211532 ) ) ;
#129351=CARTESIAN_POINT ( 'NONE',  ( -3.262708522383007903, 6.958243709422141876, 1.040834085586084257E-14 ) ) ;
#129355=CARTESIAN_POINT ( 'NONE',  ( -5.066996723205291708, 6.934582148538044777, 1.599625672291267398 ) ) ;
#129358=CARTESIAN_POINT ( 'NONE',  ( 8.239604668803105270, 10.63595808506888396, -1.599625672291268286 ) ) ;
#129361=CARTESIAN_POINT ( 'NONE',  ( 4.058723290341089474, 7.748532961531467755, 0.5319316551511514835 ) ) ;
#129362=CARTESIAN_POINT ( 'NONE',  ( 5.341549334104194635, 6.294524313618772737, 1.082531754730558626 ) ) ;
#129369=CARTESIAN_POINT ( 'NONE',  ( 5.951666246274784910, 9.887435020721849099, 0.7216878364870438212 ) ) ;
#129372=CARTESIAN_POINT ( 'NONE',  ( -10.13202086811422475, 10.71511252242175161, -0.7998128361456291469 ) ) ;
#129373=CARTESIAN_POINT ( 'NONE',  ( -6.632963465583701534, 8.761543347979550589, -1.599625672291263179 ) ) ;
#129378=CARTESIAN_POINT ( 'NONE',  ( 1.495221130952435029, 8.717880658893497170, -2.557745341056325117 ) ) ;
#129381=CARTESIAN_POINT ( 'NONE',  ( 9.402743226277308963, 10.92862083786708816, -1.199719254218446718 ) ) ;
#129382=CARTESIAN_POINT ( 'NONE',  ( -1.201851678989727383E-14, 4.087500000000022560, -1.732050807568863648 ) ) ;
#129386=CARTESIAN_POINT ( 'NONE',  ( 4.681643115420508039, 4.356338477612361260, 0.7998128361456341429 ) ) ;
#129389=CARTESIAN_POINT ( 'NONE',  ( -1.500000000000011324, 5.410416667349489117, -0.8660254037844313801 ) ) ;
#129393=ORIENTED_EDGE ( 'NONE', *, *, #46380, .T. ) ;
#129395=CARTESIAN_POINT ( 'NONE',  ( 1.499999999999989120, 3.254166666666690855, 0.8660254037844524744 ) ) ;
#129396=CARTESIAN_POINT ( 'NONE',  ( 6.661133543015731462, 6.665743976473484267, -0.7998128361456281477 ) ) ;
#129399=CARTESIAN_POINT ( 'NONE',  ( 7.375272376154084597, 9.627570410311676596, -1.443375672974057666 ) ) ;
#129400=CARTESIAN_POINT ( 'NONE',  ( -8.961576348508637935, 12.43862759236002269, -1.082531754730543083 ) ) ;
#129403=CARTESIAN_POINT ( 'NONE',  ( 10.56588178375152864, 11.22128359066528169, -0.7998128361456281477 ) ) ;
#129405=CARTESIAN_POINT ( 'NONE',  ( -3.928111819657352566, 5.605883094398769195, 1.599625672291267398 ) ) ;
#129407=CARTESIAN_POINT ( 'NONE',  ( -0.6823417656250212460, 0.8010416670080899859, 1.181850606188755259 ) ) ;
#129411=CARTESIAN_POINT ( 'NONE',  ( 3.765413976293345844, 5.416068943807445635, 1.599625672291267398 ) ) ;
#129413=CARTESIAN_POINT ( 'NONE',  ( -1.201851678989727383E-14, 5.759375000341417028, -1.575800808251660801 ) ) ;
#129423=CARTESIAN_POINT ( 'NONE',  ( -7.823218330285243383, 9.085841792542966644, -1.199719254218446718 ) ) ;
#129426=CARTESIAN_POINT ( 'NONE',  ( 4.333802657862601215, 8.207853534148366492, 0.7998128361456462443 ) ) ;
#129433=CARTESIAN_POINT ( 'NONE',  ( 7.886038904643079661, 12.35212915539230139, -0.7998128361456352531 ) ) ;
#129436=CARTESIAN_POINT ( 'NONE',  ( -6.091691091241777656, 6.001394449403842479, 0.7998128361456341429 ) ) ;
#129440=CARTESIAN_POINT ( 'NONE',  ( 9.589694723567584234, 10.08239868711733855, -0.7998128361456281477 ) ) ;
#129442=CARTESIAN_POINT ( 'NONE',  ( 6.903072767652295383, 11.20533532890304684, 1.040834085586084257E-14 ) ) ;
#129443=ADVANCED_FACE ( 'NONE', ( #99042 ), #58289, .T. ) ;
#129446=CARTESIAN_POINT ( 'NONE',  ( -10.33094986393327197, 11.15512238411806578, 0.7216878364870438212 ) ) ;
#129447=CARTESIAN_POINT ( 'NONE',  ( -6.880926654135487652, 7.986501503701545879, 1.199719254218450271 ) ) ;
#129451=CARTESIAN_POINT ( 'NONE',  ( -5.829309506874599478, 6.192769411583809003, 0.9639237645304669089 ) ) ;
#129452=CARTESIAN_POINT ( 'NONE',  ( 1.364683531249986537, 0.6552083336747522857, -0.7879004041258239610 ) ) ;
#129455=CARTESIAN_POINT ( 'NONE',  ( 6.914295153289432783, 10.05013286460426691, -1.082531754730537976 ) ) ;
#129464=EDGE_CURVE ( 'NONE', #186824, #190586, #29402, .T. ) ;
#129470=EDGE_CURVE ( 'NONE', #63977, #69507, #44386, .T. ) ;
#129474=CARTESIAN_POINT ( 'NONE',  ( 10.55910270694468345, 11.21337466772398095, 0.7998128361456462443 ) ) ;
#129476=ORIENTED_EDGE ( 'NONE', *, *, #148860, .F. ) ;
#129478=CARTESIAN_POINT ( 'NONE',  ( -4.634189577772691138, 4.300976017023221409, 1.214306433183764966E-14 ) ) ;
#129479=CARTESIAN_POINT ( 'NONE',  ( -8.532158741701643123, 8.848606708273724308, 0.7998128361456462443 ) ) ;
#129485=CARTESIAN_POINT ( 'NONE',  ( 0.7499999999999902300, 3.264583334016149418, 1.299038105676669330 ) ) ;
#129486=CARTESIAN_POINT ( 'NONE',  ( 9.576136569953906275, 10.06658084123472641, 0.000000000000000000 ) ) ;
#129489=CARTESIAN_POINT ( 'NONE',  ( -8.552495972122143186, 8.872333477097637200, 0.7998128361456462443 ) ) ;
#129491=CARTESIAN_POINT ( 'NONE',  ( -1.364683531249997417, 4.009375000341424133, 1.214306433183764966E-14 ) ) ;
#129496=CARTESIAN_POINT ( 'NONE',  ( -7.673551755654729689, 11.89630144833179060, 0.7216878364870458196 ) ) ;
#129500=CARTESIAN_POINT ( 'NONE',  ( 1.364683531249988757, 1.696875000341414808, 0.000000000000000000 ) ) ;
#129507=CARTESIAN_POINT ( 'NONE',  ( -1.364683531249997417, 2.509375000341422357, 1.214306433183764966E-14 ) ) ;
#129509=CARTESIAN_POINT ( 'NONE',  ( -6.586563698140583512, 6.578745824119123675, 1.040834085586084257E-14 ) ) ;
#129510=CARTESIAN_POINT ( 'NONE',  ( 7.775764792637399836, 9.030479331953833011, -1.199719254218441611 ) ) ;
#129512=VECTOR ( 'NONE', #213017, 1000.000000000000000 ) ;
#129514=CARTESIAN_POINT ( 'NONE',  ( -0.6823417656250212460, 2.113541667008083991, 1.181850606188767472 ) ) ;
#129517=CARTESIAN_POINT ( 'NONE',  ( -0.6823417656250003738, -0.03229166632524871350, -1.181850606188749264 ) ) ;
#129518=CARTESIAN_POINT ( 'NONE',  ( -5.314433026876900001, 6.262888621853549331, 1.082531754730548412 ) ) ;
#129521=CARTESIAN_POINT ( 'NONE',  ( 4.853455804012222430, 5.725081861844796727, 1.082531754730560403 ) ) ;
#129524=CARTESIAN_POINT ( 'NONE',  ( -8.227100285394159940, 8.492705175914988303, 0.7998128361456602331 ) ) ;
#129525=CARTESIAN_POINT ( 'NONE',  ( -2.819205876637805641, 5.376491725131008259, -1.199719254218446718 ) ) ;
#129527=FACE_OUTER_BOUND ( 'NONE', #50407, .T. ) ;
#129532=CARTESIAN_POINT ( 'NONE',  ( -5.056828107772848746, 8.843457192469559303, -0.7216878364870207285 ) ) ;
#129534=CARTESIAN_POINT ( 'NONE',  ( 1.364683531249986537, -0.5322916663252452718, -0.7879004041258309554 ) ) ;
#129537=CARTESIAN_POINT ( 'NONE',  ( 6.290620087060792009, 10.28288116830553101, -0.7216878364870267237 ) ) ;
#129546=CARTESIAN_POINT ( 'NONE',  ( 8.961576348508637935, 11.47825837805867799, -1.443375672974052559 ) ) ;
#129550=ORIENTED_EDGE ( 'NONE', *, *, #114672, .T. ) ;
#129552=CARTESIAN_POINT ( 'NONE',  ( 5.880485940025228508, 7.883652901494672349, 1.599625672291267398 ) ) ;
#129553=CARTESIAN_POINT ( 'NONE',  ( -2.903417451620861289, 6.539070793532962611, 0.7998128361456341429 ) ) ;
#129555=CARTESIAN_POINT ( 'NONE',  ( 0.7499999999999902300, 3.483333333333352044, 1.299038105676669330 ) ) ;
#129557=CARTESIAN_POINT ( 'NONE',  ( 5.463572716182819811, 8.357623354646536384, 1.082531754730558626 ) ) ;
#129558=CARTESIAN_POINT ( 'NONE',  ( 0.6823417656249882723, -0.09479166632524876901, 1.181850606188755259 ) ) ;
#129559=CARTESIAN_POINT ( 'NONE',  ( -9.755255220232635693, 11.33988483081495957, -1.199719254218441611 ) ) ;
#129565=CARTESIAN_POINT ( 'NONE',  ( 1.500000000000007105, 10.64264068711930733, 1.214306433183764966E-14 ) ) ;
#129569=VERTEX_POINT ( 'NONE', #179915 ) ;
#129578=CARTESIAN_POINT ( 'NONE',  ( 6.979750152936881058, 7.037463354714830643, 0.7998128361456341429 ) ) ;
#129581=ORIENTED_EDGE ( 'NONE', *, *, #187141, .T. ) ;
#129587=CARTESIAN_POINT ( 'NONE',  ( 8.401248741962376698, 12.95320729893149370, 0.7998128361456462443 ) ) ;
#129602=CARTESIAN_POINT ( 'NONE',  ( -7.700668062882059850, 11.92793714009701311, -0.7216878364870267237 ) ) ;
#129607=CARTESIAN_POINT ( 'NONE',  ( 4.364835388595708743, 7.179726155748598515, 1.199719254218462483 ) ) ;
#129613=CARTESIAN_POINT ( 'NONE',  ( 4.243338890952890630, 5.973648010910253880, -1.443375672974051449 ) ) ;
#129616=ORIENTED_EDGE ( 'NONE', *, *, #30361, .T. ) ;
#129622=CARTESIAN_POINT ( 'NONE',  ( -7.366157530926372488, 7.488271962369228874, -0.7998128361456291469 ) ) ;
#129623=CARTESIAN_POINT ( 'NONE',  ( -4.355193658487827690, 6.104145239700998538, -1.599625672291256295 ) ) ;
#129631=CARTESIAN_POINT ( 'NONE',  ( 5.099838337034727331, 9.101561826515851550, -0.7998128361456281477 ) ) ;
#129635=( BOUNDED_CURVE ( )  B_SPLINE_CURVE ( 2, ( #109287, #91925, #175297, #123430, #189392 ),
 .UNSPECIFIED., .F., .T. ) 
 B_SPLINE_CURVE_WITH_KNOTS ( ( 3, 2, 3 ),
 ( 0.1361778335736238132, 0.1375000000000000111, 0.1392051351651958091 ),
 .UNSPECIFIED. ) 
 CURVE ( )  GEOMETRIC_REPRESENTATION_ITEM ( )  RATIONAL_B_SPLINE_CURVE ( ( 0.9419547032718706969, 0.9574871888551546029, 1.000000000000000000, 0.9451732491399851277, 0.9352202683046937359 ) ) 
 REPRESENTATION_ITEM ( '' )  );
#129641=CARTESIAN_POINT ( 'NONE',  ( 1.244123718695673952, 3.098244533904601195, -0.7749999999999926947 ) ) ;
#129644=CARTESIAN_POINT ( 'NONE',  ( -5.233084104750526322, 5.207612331738130429, 0.000000000000000000 ) ) ;
#129647=CARTESIAN_POINT ( 'NONE',  ( 1.364683531249986537, -0.2822916663252520997, -0.7879004041258309554 ) ) ;
#129649=CARTESIAN_POINT ( 'NONE',  ( 4.008406971134620633, 7.828225232965717595, 0.7998128361456321445 ) ) ;
#129651=CARTESIAN_POINT ( 'NONE',  ( -5.856759171423528088, 8.816340885760650892, 1.082531754730548412 ) ) ;
#129652=CARTESIAN_POINT ( 'NONE',  ( 6.019457014787495730, 6.125047393447951016, -0.7216878364870257245 ) ) ;
#129653=CARTESIAN_POINT ( 'NONE',  ( -8.161645285302366659, 8.624267042381978499, 1.040834085586084257E-14 ) ) ;
#129658=CARTESIAN_POINT ( 'NONE',  ( 5.601490020740366838, 9.686822124172440596, 1.040834085586084257E-14 ) ) ;
#129662=CARTESIAN_POINT ( 'NONE',  ( 1.364683531249988535, 5.405208333674750953, -0.7879004041258300672 ) ) ;
#129668=CARTESIAN_POINT ( 'NONE',  ( 6.123478934866503742, 10.29580919065294431, 0.7998128361456462443 ) ) ;
#129672=CARTESIAN_POINT ( 'NONE',  ( -6.690058733339450114, 9.892486724616283311, 1.199719254218452047 ) ) ;
#129677=CARTESIAN_POINT ( 'NONE',  ( 7.892817981449907982, 12.36003807833360391, 0.7998128361456462443 ) ) ;
#129678=DIRECTION ( 'NONE',  ( -1.000000000000000000, 0.000000000000000000, 0.000000000000000000 ) ) ;
#129680=CARTESIAN_POINT ( 'NONE',  ( -7.823218330285243383, 9.085841792542966644, -1.199719254218446718 ) ) ;
#129682=CARTESIAN_POINT ( 'NONE',  ( 0.1263921868141488214, 7.050106634747087320, 4.033475512996062662 ) ) ;
#129684=CARTESIAN_POINT ( 'NONE',  ( 5.064587263324675348, 6.532718652379178259, -1.222898410871699593 ) ) ;
#129685=CARTESIAN_POINT ( 'NONE',  ( -8.839552966430002101, 12.29626697993494666, -1.082531754730543971 ) ) ;
#129690=CARTESIAN_POINT ( 'NONE',  ( 7.298366762858032430, 7.409182732956175244, 1.040834085586084257E-14 ) ) ;
#129692=CARTESIAN_POINT ( 'NONE',  ( 5.555090253297246150, 7.504024600312024340, 1.599625672291267398 ) ) ;
#129693=CARTESIAN_POINT ( 'NONE',  ( -4.059107376188687333, 7.562469429224047524, 0.4300614504739261879 ) ) ;
#129694=CARTESIAN_POINT ( 'NONE',  ( 3.846762897975340767, 5.510976019103107859, -1.599625672291256295 ) ) ;
#129696=CARTESIAN_POINT ( 'NONE',  ( -5.558479791922849245, 9.428717490644563881, 0.7216878364870458196 ) ) ;
#129697=( BOUNDED_SURFACE ( )  B_SPLINE_SURFACE ( 1, 2, ( 
 ( #41158, #7546, #106189, #107267, #23803, #24869, #124609, #44349, #157035, #75769, #60577, #8623, #140808, #206820, #6476, #56322, #58454, #76821, #208941, #122482, #126735, #42223, #108340, #25939, #158103, #110471, #159149, #9692, #138651, #141877, #207886, #59509, #28082, #125666, #191628, #109412, #43292, #172214, #10750, #175417, #27001, #188444, #93107, #94178, #72553, #16067, #160217, #147183, #128861, #30221, #95242, #177541, #45418, #130983, #78952, #194843, #111534, #164481, #81094, #179673, #33409, #11818, #63775, #29152, #195922, #178611, #31293, #129934, #127817, #145074, #181776, #15003, #97368, #210008, #163426, #132024, #46476, #196974, #32351, #144015, #47559, #61650, #12876, #77894, #162361, #112600, #113669, #213208, #98416, #48613, #114728, #180726, #115787, #13940, #96305, #198034, #80023, #211077, #82151, #62700, #148243, #146126, #214245, #212139, #161290, #64837, #65876, #49664, #193772, #99487, #50728, #167682, #136267, #19283, #100545, #117932, #135208, #201224, #101615, #52865, #85364, #69087, #66944, #84294, #166618, #118999, #21402, #168747, #34473, #17138, #18210, #182855, #102689, #133084, #200160, #71223, #165545, #153576, #20351, #137338, #187125, #86436, #5146, #152501, #70155, #68011, #134151, #87512, #203355, #83215, #55008, #149297, #116853, #150379, #151446, #3019, #37686, #186051, #4084, #878, #103763, #1950, #51814, #121158, #183926, #199082, #35538, #184977, #36603, #202287, #53939, #120075, #169814, #125419, #188192, #139476, #190321, #24619, #208702, #158911, #90727, #91800, #41980, #174119, #108090, #76580, #105936, #9451, #75522, #7293, #156790, #171960, #141635, #8376, #205505, #74459, #207643, #25692, #59262, #191385, #173037, #142692, #60329, #140564, #206576, #204421, #58204, #89658, #23549, #157858, #154643, #124364, #43051, #109164, #126490, #175176, #38756, #26763, #88586, #104837, #170882, #122232, #92864, #10507, #73371, #22474, #6224, #72294, #138402, #56076, #39827, #155711, #57137, #123305, #189268, #40907, #107013, #28912, #63541, #145893, #46242, #77650, #161043, #128631, #179435, #94997, #211904, #98191, #178372, #214010, #47316, #129696, #27838, #195679, #164239, #12639, #14769, #64604, #176236, #162118, #93934, #45180, #44107, #194598, #78709, #96066, #113429, #130744, #80860, #146950, #212965, #148000, #112359, #144835, #15827, #210843, #177298, #196737, #111293, #48378, #29981, #114490, #62469, #127569, #31056, #13708, #79781, #97132, #192454, #143772, #163184, #180487, #32106, #193538, #81913, #65633, #110228, #159975, #11579, #209767, #61407, #166361, #198838, #184722, #136006, #182598, #202019, #50484, #619, #165295, #34221, #149044, #66687, #35279, #169560, #116605, #200962, #185790, #100294, #150127, #132834, #131781, #115542, #199911, #53678, #119810, #181537, #37423, #1700, #17951, #151192, #84038, #103499, #69894, #51557, #49422, #117683, #67754, #133905, #21142, #183675, #101356, #20092, #167434, #82971, #87245, #19026, #85106, #33165, #99246, #2763, #153311, #4886, #197784, #118738, #68832, #134954, #52609, #36346, #16889, #102424, #168493, #86179, #152249, #3822, #206321, #90463, #158658, #70964, #189009, #170622, #106753, #89399, #156530, #40651, #38498, #204155, #55810, #72033, #172780, #207393, #140303, #5963, #203099, #121964, #154385, #74208, #104576, #171690, #42795, #137074, #125170, #57946, #108904, #54744, #124111, #191129, #190074, #41726, #39561, #105663, #59013, #174927, #120894, #26507, #22208, #88321, #138145, #56880, #123055, #9197, #157602, #107836, #187931, #75269, #23288, #155447, #92616, #7031, #73108, #205239, #24354, #8121, #173861, #25437, #91543, #141383, #96881, #159719, #111034, #161869, #210594, #180240, #130501, #62224, #63284, #13458, #145652, #79534, #48130, #77396, #195428, #47058, #193281, #128382, #143512, #113175, #194349, #177040, #45991, #179179, #211648, #30802, #162931, #144581, #114242, #31864, #112112, #178115, #175985, #29730, #61148, #209508, #129446, #126236, #95812, #14512, #80604, #97940, #146699, #10257, #212715, #60078, #76331, #142437, #93677, #64355, #196488, #44926, #208444, #192196 ),
 ( #109975, #28657, #160790, #43860, #127311, #27578, #11317, #94743, #12382, #78462, #52366, #119557, #17696, #198586, #135758, #116352, #148798, #184476, #16638, #200714, #100047, #36094, #182342, #98991, #2510, #166110, #1443, #101097, #163997, #115296, #83783, #118495, #149876, #165045, #33972, #199655, #51301, #67508, #117426, #133654, #152003, #50232, #82722, #68583, #168245, #368, #19844, #66442, #32914, #197534, #132583, #181287, #183423, #35025, #201780, #167183, #18772, #3575, #84857, #150946, #134708, #15572, #147746, #102178, #85930, #69650, #213764, #53421, #185545, #37174, #81660, #65385, #131531, #49179, #23034, #20894, #171444, #88064, #120641, #91289, #5705, #105407, #206065, #170369, #54497, #41471, #154136, #55563, #86990, #153063, #137897, #8937, #173614, #103249, #90212, #71782, #187683, #38246, #186620, #202849, #73947, #21954, #203916, #104321, #107580, #24110, #122798, #190878, #169310, #6784, #121718, #138967, #39311, #188756, #72860, #70709, #89149, #124914, #172526, #40396, #4638, #106498, #75017, #155203, #140041, #189822, #136822, #204989, #56632, #156277, #7861, #57700, #123856, #25185, #157348, #141127, #207138, #58762, #112918, #145397, #63026, #108646, #174675, #178929, #27320, #30545, #60893, #64101, #11060, #78746, #113464, #99284, #143807, #179469, #66726, #168533, #203143, #199950, #53719, #103539, #659, #201003, #132869, #84080, #83005, #19067, #117721, #134993, #20131, #169599, #119852, #185830, #37461, #186905, #85145, #51597, #54785, #183711, #1736, #21182, #150168, #87285, #167471, #153354, #35318, #166399, #69935, #151232, #68873, #86217, #16925, #182638, #2801, #4924, #52648, #17990, #101397, #118777, #184762, #36389, #102467, #152288, #71001, #3862, #67793, #136047, #137114, #133943, #120932, #202059, #100332, #50520, #38537, #34260, #104614, #149081, #198873, #116643, #25474, #10289, #155487, #189048, #171729, #170662, #154424, #24388, #26541, #92649, #6002, #158691, #40685, #187971, #190107, #23327, #76363, #108938, #90500, #88359, #156564, #7070, #39598, #142470, #73142, #172816, #59044, #89435, #122005, #174959, #139248, #123091, #72073, #138183, #205279, #208478, #60114, #22249, #157633, #56918, #106788, #105701, #8159, #55848, #141418, #74243, #140336, #206355, #204193, #57982, #124145, #41760, #107872, #126273, #42832, #91581, #173898, #192230, #9231, #75303, #43893, #207425, #125202, #191165, #62254, #13490, #96915, #113208, #195461, #127344, #196522, #44960, #210628, #47090, #95847, #65419, #15609, #161903, #162966, #179213, #30838, #14545, #147780, #177074, #80642, #146734, #78496, #79565, #28690, #212752, #145684, #128415, #211682, #64386, #130531, #48165, #114277, #29762, #213796, #131568, #63318, #129479, #61184, #180274, #160824, #94776, #31898, #11350, #97975, #164034, #81697, #197569, #110007, #176020, #27612, #159753, #93712, #77431, #193314, #143548, #209542, #144613, #111068, #12416, #194382, #46025, #112145, #178148, #16673, #100080, #102213, #35060, #136859, #36129, #166142, #200750, #2543, #101131, #148831, #83817, #199691, #168279, #149910, #68618, #169345, #167219, #84891, #82758, #34006, #182376, #150978, #185579, #118526, #1477, #181324, #133686, #51336, #52399, #66476, #184510, #20930, #115333, #103283, #19879, #87026, #49213, #85962, #153098, #152038, #69686, #135790, #201814, #37209, #4673, #32952, #70746, #53458, #99026, #165082, #119596, #88099, #24143, #6818, #7895, #172559, #170402, #121750, #10039, #57735, #73983, #38280, #140077, #174711, #171479, #25221, #75050, #186654, #90245, #104357, #55595, #54531, #56670, #89185, #106533, #206101, #141165, #91324, #157382, #8976, #158438, #122834, #23069, #26286, #155237, #187718, #207173, #72897, #58797, #139002, #124952, #188795, #137927, #41503, #40431, #156311, #123892, #202883, #154172, #189859, #190914, #107616, #203948, #173647, #42579, #108682, #92400, #76113, #120676, #21990, #5739, #209286, #195205, #146479, #193053, #212498, #60933, #11097, #175766, #44707, #159499, #77173, #45775, #180024, #127090, #211434, #196271, #110814, #160565, #143295, #142217, #126015, #210368, #64139 ) ),
 .UNSPECIFIED., .F., .F., .T. ) 
 B_SPLINE_SURFACE_WITH_KNOTS ( ( 2, 2 ),
 ( 3, 2, 2, 2, 2, 2, 2, 2, 2, 2, 2, 2, 2, 2, 2, 2, 2, 2, 2, 2, 2, 2, 2, 2, 2, 2, 2, 2, 2, 2, 2, 2, 2, 2, 2, 2, 2, 2, 2, 2, 2, 2, 2, 2, 2, 2, 2, 2, 2, 2, 2, 2, 2, 2, 2, 2, 2, 2, 2, 2, 2, 2, 2, 2, 2, 2, 2, 2, 2, 2, 2, 2, 2, 2, 2, 2, 2, 2, 2, 2, 2, 2, 2, 2, 2, 2, 2, 2, 2, 2, 2, 2, 2, 2, 2, 2, 2, 2, 2, 2, 2, 2, 2, 2, 2, 2, 2, 2, 2, 2, 2, 2, 2, 2, 2, 2, 2, 2, 2, 2, 2, 2, 2, 2, 2, 2, 2, 2, 2, 2, 2, 2, 2, 2, 2, 2, 2, 2, 2, 2, 2, 2, 2, 2, 2, 2, 2, 2, 2, 2, 2, 2, 2, 2, 2, 2, 2, 2, 2, 2, 2, 2, 2, 2, 2, 2, 2, 2, 2, 2, 2, 2, 2, 2, 2, 2, 2, 2, 2, 2, 2, 2, 2, 2, 2, 2, 2, 2, 2, 2, 2, 2, 2, 2, 2, 2, 2, 2, 2, 2, 2, 2, 2, 2, 2, 2, 2, 2, 2, 2, 2, 2, 2, 2, 2, 2, 2, 2, 2, 2, 2, 2, 2, 2, 2, 2, 2, 2, 2, 2, 2, 2, 2, 2, 2, 2, 2, 2, 2, 2, 3 ),
 ( 0.000000000000000000, 1.000000000000000000 ),
 ( 0.000000000000000000, 0.004166666666666666609, 0.008333333333333333218, 0.01250000000000000069, 0.01666666666666666644, 0.02083333333333333218, 0.02500000000000000139, 0.02916666666666666713, 0.03333333333333333287, 0.03749999999999999861, 0.04166666666666666435, 0.04583333333333333010, 0.05000000000000000278, 0.05416666666666666852, 0.05833333333333333426, 0.06250000000000000000, 0.06666666666666666574, 0.07083333333333333148, 0.07499999999999999722, 0.07916666666666666297, 0.08333333333333332871, 0.08749999999999999445, 0.09166666666666666019, 0.09583333333333333981, 0.1000000000000000056, 0.1041666666666666713, 0.1083333333333333370, 0.1125000000000000028, 0.1166666666666666685, 0.1208333333333333343, 0.1250000000000000000, 0.1291666666666666796, 0.1333333333333333315, 0.1375000000000000111, 0.1416666666666666630, 0.1458333333333333426, 0.1499999999999999944, 0.1541666666666666741, 0.1583333333333333259, 0.1625000000000000056, 0.1666666666666666574, 0.1708333333333333370, 0.1749999999999999889, 0.1791666666666666685, 0.1833333333333333204, 0.1875000000000000000, 0.1916666666666666796, 0.1958333333333333315, 0.2000000000000000111, 0.2041666666666666630, 0.2083333333333333426, 0.2124999999999999944, 0.2166666666666666741, 0.2208333333333333259, 0.2250000000000000056, 0.2291666666666666574, 0.2333333333333333370, 0.2374999999999999889, 0.2416666666666666685, 0.2458333333333333204, 0.2500000000000000000, 0.2541666666666666519, 0.2583333333333333592, 0.2625000000000000111, 0.2666666666666666630, 0.2708333333333333148, 0.2750000000000000222, 0.2791666666666666741, 0.2833333333333333259, 0.2874999999999999778, 0.2916666666666666852, 0.2958333333333333370, 0.2999999999999999889, 0.3041666666666666408, 0.3083333333333333481, 0.3125000000000000000, 0.3166666666666666519, 0.3208333333333333592, 0.3250000000000000111, 0.3291666666666666630, 0.3333333333333333148, 0.3375000000000000222, 0.3416666666666666741, 0.3458333333333333259, 0.3499999999999999778, 0.3541666666666666852, 0.3583333333333333370, 0.3624999999999999889, 0.3666666666666666408, 0.3708333333333333481, 0.3750000000000000000, 0.3791666666666666519, 0.3833333333333333592, 0.3875000000000000111, 0.3916666666666666630, 0.3958333333333333148, 0.4000000000000000222, 0.4041666666666666741, 0.4083333333333333259, 0.4124999999999999778, 0.4166666666666666852, 0.4208333333333333370, 0.4249999999999999889, 0.4291666666666666408, 0.4333333333333333481, 0.4375000000000000000, 0.4416666666666666519, 0.4458333333333333592, 0.4500000000000000111, 0.4541666666666666630, 0.4583333333333333148, 0.4625000000000000222, 0.4666666666666666741, 0.4708333333333333259, 0.4749999999999999778, 0.4791666666666666852, 0.4833333333333333370, 0.4874999999999999889, 0.4916666666666666408, 0.4958333333333333481, 0.5000000000000000000, 0.5041666666666666519, 0.5083333333333333037, 0.5124999999999999556, 0.5166666666666667185, 0.5208333333333333703, 0.5250000000000000222, 0.5291666666666666741, 0.5333333333333333259, 0.5374999999999999778, 0.5416666666666666297, 0.5458333333333332815, 0.5500000000000000444, 0.5541666666666666963, 0.5583333333333333481, 0.5625000000000000000, 0.5666666666666666519, 0.5708333333333333037, 0.5749999999999999556, 0.5791666666666667185, 0.5833333333333333703, 0.5875000000000000222, 0.5916666666666666741, 0.5958333333333333259, 0.5999999999999999778, 0.6041666666666666297, 0.6083333333333332815, 0.6125000000000000444, 0.6166666666666666963, 0.6208333333333333481, 0.6250000000000000000, 0.6291666666666666519, 0.6333333333333333037, 0.6374999999999999556, 0.6416666666666667185, 0.6458333333333333703, 0.6500000000000000222, 0.6541666666666666741, 0.6583333333333333259, 0.6624999999999999778, 0.6666666666666666297, 0.6708333333333332815, 0.6750000000000000444, 0.6791666666666666963, 0.6833333333333333481, 0.6875000000000000000, 0.6916666666666666519, 0.6958333333333333037, 0.6999999999999999556, 0.7041666666666667185, 0.7083333333333333703, 0.7125000000000000222, 0.7166666666666666741, 0.7208333333333333259, 0.7249999999999999778, 0.7291666666666666297, 0.7333333333333332815, 0.7375000000000000444, 0.7416666666666666963, 0.7458333333333333481, 0.7500000000000000000, 0.7541666666666666519, 0.7583333333333333037, 0.7624999999999999556, 0.7666666666666667185, 0.7708333333333333703, 0.7750000000000000222, 0.7791666666666666741, 0.7833333333333333259, 0.7874999999999999778, 0.7916666666666666297, 0.7958333333333332815, 0.8000000000000000444, 0.8041666666666666963, 0.8083333333333333481, 0.8125000000000000000, 0.8166666666666666519, 0.8208333333333333037, 0.8249999999999999556, 0.8291666666666667185, 0.8333333333333333703, 0.8375000000000000222, 0.8416666666666666741, 0.8458333333333333259, 0.8499999999999999778, 0.8541666666666666297, 0.8583333333333332815, 0.8625000000000000444, 0.8666666666666666963, 0.8708333333333333481, 0.8750000000000000000, 0.8791666666666666519, 0.8833333333333333037, 0.8874999999999999556, 0.8916666666666667185, 0.8958333333333333703, 0.9000000000000000222, 0.9041666666666666741, 0.9083333333333333259, 0.9124999999999999778, 0.9166666666666666297, 0.9208333333333332815, 0.9250000000000000444, 0.9291666666666666963, 0.9333333333333333481, 0.9375000000000000000, 0.9416666666666666519, 0.9458333333333333037, 0.9499999999999999556, 0.9541666666666667185, 0.9583333333333333703, 0.9625000000000000222, 0.9666666666666666741, 0.9708333333333333259, 0.9749999999999999778, 0.9791666666666666297, 0.9833333333333332815, 0.9875000000000000444, 0.9916666666666666963, 0.9958333333333333481, 1.000000000000000000 ),
 .UNSPECIFIED. ) 
 GEOMETRIC_REPRESENTATION_ITEM ( )  RATIONAL_B_SPLINE_SURFACE ( (
 ( 1.000000000000000000, 0.8660254037844387076, 1.000000000000000000, 0.8660254037844387076, 1.000000000000000000, 0.8660254037844387076, 1.000000000000000000, 0.8660254037844387076, 1.000000000000000000, 0.8660254037844387076, 1.000000000000000000, 0.8660254037844387076, 1.000000000000000000, 0.8660254037844387076, 1.000000000000000000, 0.8660254037844387076, 1.000000000000000000, 0.8660254037844387076, 1.000000000000000000, 0.8660254037844387076, 1.000000000000000000, 0.8660254037844387076, 1.000000000000000000, 0.8660254037844387076, 1.000000000000000000, 0.8660254037844387076, 1.000000000000000000, 0.8660254037844387076, 1.000000000000000000, 0.8660254037844387076, 1.000000000000000000, 0.8660254037844387076, 1.000000000000000000, 0.8660254037844387076, 1.000000000000000000, 0.8660254037844387076, 1.000000000000000000, 0.8660254037844387076, 1.000000000000000000, 0.8660254037844387076, 1.000000000000000000, 0.8660254037844387076, 1.000000000000000000, 0.8660254037844387076, 1.000000000000000000, 0.8660254037844387076, 1.000000000000000000, 0.8660254037844387076, 1.000000000000000000, 0.8660254037844387076, 1.000000000000000000, 0.8660254037844387076, 1.000000000000000000, 0.8660254037844387076, 1.000000000000000000, 0.8660254037844387076, 1.000000000000000000, 0.8660254037844387076, 1.000000000000000000, 0.8660254037844387076, 1.000000000000000000, 0.8660254037844387076, 1.000000000000000000, 0.8660254037844387076, 1.000000000000000000, 0.8660254037844387076, 1.000000000000000000, 0.8660254037844387076, 1.000000000000000000, 0.8660254037844387076, 1.000000000000000000, 0.8660254037844387076, 1.000000000000000000, 0.8660254037844387076, 1.000000000000000000, 0.8660254037844387076, 1.000000000000000000, 0.8660254037844387076, 1.000000000000000000, 0.8660254037844387076, 1.000000000000000000, 0.8660254037844387076, 1.000000000000000000, 0.8660254037844387076, 1.000000000000000000, 0.8660254037844387076, 1.000000000000000000, 0.8660254037844387076, 1.000000000000000000, 0.8660254037844387076, 1.000000000000000000, 0.8660254037844387076, 1.000000000000000000, 0.8660254037844387076, 1.000000000000000000, 0.8660254037844387076, 1.000000000000000000, 0.8660254037844387076, 1.000000000000000000, 0.8660254037844387076, 1.000000000000000000, 0.8660254037844387076, 1.000000000000000000, 0.8660254037844387076, 1.000000000000000000, 0.8660254037844387076, 1.000000000000000000, 0.8660254037844387076, 1.000000000000000000, 0.8660254037844387076, 1.000000000000000000, 0.8660254037844387076, 1.000000000000000000, 0.8660254037844387076, 1.000000000000000000, 0.8660254037844387076, 1.000000000000000000, 0.8660254037844387076, 1.000000000000000000, 0.8660254037844387076, 1.000000000000000000, 0.8660254037844387076, 1.000000000000000000, 0.8660254037844387076, 1.000000000000000000, 0.8660254037844387076, 1.000000000000000000, 0.8660254037844387076, 1.000000000000000000, 0.8660254037844387076, 1.000000000000000000, 0.8660254037844387076, 1.000000000000000000, 0.8660254037844387076, 1.000000000000000000, 0.8660254037844387076, 1.000000000000000000, 0.8660254037844387076, 1.000000000000000000, 0.8660254037844387076, 1.000000000000000000, 0.8660254037844387076, 1.000000000000000000, 0.8660254037844387076, 1.000000000000000000, 0.8660254037844387076, 1.000000000000000000, 0.8660254037844387076, 1.000000000000000000, 0.8660254037844387076, 1.000000000000000000, 0.8660254037844387076, 1.000000000000000000, 0.8660254037844387076, 1.000000000000000000, 0.8660254037844387076, 1.000000000000000000, 0.8660254037844387076, 1.000000000000000000, 0.8660254037844387076, 1.000000000000000000, 0.8660254037844387076, 1.000000000000000000, 0.8660254037844387076, 1.000000000000000000, 0.8660254037844387076, 1.000000000000000000, 0.8660254037844387076, 1.000000000000000000, 0.8660254037844387076, 1.000000000000000000, 0.8660254037844387076, 1.000000000000000000, 0.8660254037844387076, 1.000000000000000000, 0.8660254037844387076, 1.000000000000000000, 0.8660254037844387076, 1.000000000000000000, 0.8660254037844387076, 1.000000000000000000, 0.8660254037844387076, 1.000000000000000000, 0.8660254037844387076, 1.000000000000000000, 0.8660254037844387076, 1.000000000000000000, 0.8660254037844387076, 1.000000000000000000, 0.8660254037844387076, 1.000000000000000000, 0.8660254037844387076, 1.000000000000000000, 0.8660254037844387076, 1.000000000000000000, 0.8660254037844387076, 1.000000000000000000, 0.8660254037844387076, 1.000000000000000000, 0.8660254037844387076, 1.000000000000000000, 0.8660254037844387076, 1.000000000000000000, 0.8660254037844387076, 1.000000000000000000, 0.8660254037844387076, 1.000000000000000000, 0.8660254037844387076, 1.000000000000000000, 0.8660254037844387076, 1.000000000000000000, 0.8660254037844387076, 1.000000000000000000, 0.8660254037844387076, 1.000000000000000000, 0.8660254037844387076, 1.000000000000000000, 0.8660254037844387076, 1.000000000000000000, 0.8660254037844387076, 1.000000000000000000, 0.8660254037844387076, 1.000000000000000000, 0.8660254037844387076, 1.000000000000000000, 0.8660254037844387076, 1.000000000000000000, 0.8660254037844387076, 1.000000000000000000, 0.8660254037844387076, 1.000000000000000000, 0.8660254037844387076, 1.000000000000000000, 0.8660254037844387076, 1.000000000000000000, 0.8660254037844387076, 1.000000000000000000, 0.8660254037844387076, 1.000000000000000000, 0.8660254037844387076, 1.000000000000000000, 0.8660254037844387076, 1.000000000000000000, 0.8660254037844387076, 1.000000000000000000, 0.8660254037844387076, 1.000000000000000000, 0.8660254037844387076, 1.000000000000000000, 0.8660254037844387076, 1.000000000000000000, 0.8660254037844387076, 1.000000000000000000, 0.8660254037844387076, 1.000000000000000000, 0.8660254037844387076, 1.000000000000000000, 0.8660254037844387076, 1.000000000000000000, 0.8660254037844387076, 1.000000000000000000, 0.8660254037844387076, 1.000000000000000000, 0.8660254037844387076, 1.000000000000000000, 0.8660254037844387076, 1.000000000000000000, 0.8660254037844387076, 1.000000000000000000, 0.8660254037844387076, 1.000000000000000000, 0.8660254037844387076, 1.000000000000000000, 0.8660254037844387076, 1.000000000000000000, 0.8660254037844387076, 1.000000000000000000, 0.8660254037844387076, 1.000000000000000000, 0.8660254037844387076, 1.000000000000000000, 0.8660254037844387076, 1.000000000000000000, 0.8660254037844387076, 1.000000000000000000, 0.8660254037844387076, 1.000000000000000000, 0.8660254037844387076, 1.000000000000000000, 0.8660254037844387076, 1.000000000000000000, 0.8660254037844387076, 1.000000000000000000, 0.8660254037844387076, 1.000000000000000000, 0.8660254037844387076, 1.000000000000000000, 0.8660254037844387076, 1.000000000000000000, 0.8660254037844387076, 1.000000000000000000, 0.8660254037844387076, 1.000000000000000000, 0.8660254037844387076, 1.000000000000000000, 0.8660254037844387076, 1.000000000000000000, 0.8660254037844387076, 1.000000000000000000, 0.8660254037844387076, 1.000000000000000000, 0.8660254037844387076, 1.000000000000000000, 0.8660254037844387076, 1.000000000000000000, 0.8660254037844387076, 1.000000000000000000, 0.8660254037844387076, 1.000000000000000000, 0.8660254037844387076, 1.000000000000000000, 0.8660254037844387076, 1.000000000000000000, 0.8660254037844387076, 1.000000000000000000, 0.8660254037844387076, 1.000000000000000000, 0.8660254037844387076, 1.000000000000000000, 0.8660254037844387076, 1.000000000000000000, 0.8660254037844387076, 1.000000000000000000, 0.8660254037844387076, 1.000000000000000000, 0.8660254037844387076, 1.000000000000000000, 0.8660254037844387076, 1.000000000000000000, 0.8660254037844387076, 1.000000000000000000, 0.8660254037844387076, 1.000000000000000000, 0.8660254037844387076, 1.000000000000000000, 0.8660254037844387076, 1.000000000000000000, 0.8660254037844387076, 1.000000000000000000, 0.8660254037844387076, 1.000000000000000000, 0.8660254037844387076, 1.000000000000000000, 0.8660254037844387076, 1.000000000000000000, 0.8660254037844387076, 1.000000000000000000, 0.8660254037844387076, 1.000000000000000000, 0.8660254037844387076, 1.000000000000000000, 0.8660254037844387076, 1.000000000000000000, 0.8660254037844387076, 1.000000000000000000, 0.8660254037844387076, 1.000000000000000000, 0.8660254037844387076, 1.000000000000000000, 0.8660254037844387076, 1.000000000000000000, 0.8660254037844387076, 1.000000000000000000, 0.8660254037844387076, 1.000000000000000000, 0.8660254037844387076, 1.000000000000000000, 0.8660254037844387076, 1.000000000000000000, 0.8660254037844387076, 1.000000000000000000, 0.8660254037844387076, 1.000000000000000000, 0.8660254037844387076, 1.000000000000000000, 0.8660254037844387076, 1.000000000000000000, 0.8660254037844387076, 1.000000000000000000, 0.8660254037844387076, 1.000000000000000000, 0.8660254037844387076, 1.000000000000000000, 0.8660254037844387076, 1.000000000000000000, 0.8660254037844387076, 1.000000000000000000, 0.8660254037844387076, 1.000000000000000000, 0.8660254037844387076, 1.000000000000000000, 0.8660254037844387076, 1.000000000000000000, 0.8660254037844387076, 1.000000000000000000, 0.8660254037844387076, 1.000000000000000000, 0.8660254037844387076, 1.000000000000000000, 0.8660254037844387076, 1.000000000000000000, 0.8660254037844387076, 1.000000000000000000, 0.8660254037844387076, 1.000000000000000000, 0.8660254037844387076, 1.000000000000000000, 0.8660254037844387076, 1.000000000000000000, 0.8660254037844387076, 1.000000000000000000, 0.8660254037844387076, 1.000000000000000000, 0.8660254037844387076, 1.000000000000000000, 0.8660254037844387076, 1.000000000000000000, 0.8660254037844387076, 1.000000000000000000, 0.8660254037844387076, 1.000000000000000000, 0.8660254037844387076, 1.000000000000000000, 0.8660254037844387076, 1.000000000000000000, 0.8660254037844387076, 1.000000000000000000, 0.8660254037844387076, 1.000000000000000000, 0.8660254037844387076, 1.000000000000000000, 0.8660254037844387076, 1.000000000000000000, 0.8660254037844387076, 1.000000000000000000, 0.8660254037844387076, 1.000000000000000000, 0.8660254037844387076, 1.000000000000000000, 0.8660254037844387076, 1.000000000000000000, 0.8660254037844387076, 1.000000000000000000, 0.8660254037844387076, 1.000000000000000000, 0.8660254037844387076, 1.000000000000000000, 0.8660254037844387076, 1.000000000000000000, 0.8660254037844387076, 1.000000000000000000, 0.8660254037844387076, 1.000000000000000000, 0.8660254037844387076, 1.000000000000000000, 0.8660254037844387076, 1.000000000000000000, 0.8660254037844387076, 1.000000000000000000, 0.8660254037844387076, 1.000000000000000000, 0.8660254037844387076, 1.000000000000000000, 0.8660254037844387076, 1.000000000000000000, 0.8660254037844387076, 1.000000000000000000, 0.8660254037844387076, 1.000000000000000000, 0.8660254037844387076, 1.000000000000000000),
 ( 1.000000000000000000, 0.8660254037844387076, 1.000000000000000000, 0.8660254037844387076, 1.000000000000000000, 0.8660254037844387076, 1.000000000000000000, 0.8660254037844387076, 1.000000000000000000, 0.8660254037844387076, 1.000000000000000000, 0.8660254037844387076, 1.000000000000000000, 0.8660254037844387076, 1.000000000000000000, 0.8660254037844387076, 1.000000000000000000, 0.8660254037844387076, 1.000000000000000000, 0.8660254037844387076, 1.000000000000000000, 0.8660254037844387076, 1.000000000000000000, 0.8660254037844387076, 1.000000000000000000, 0.8660254037844387076, 1.000000000000000000, 0.8660254037844387076, 1.000000000000000000, 0.8660254037844387076, 1.000000000000000000, 0.8660254037844387076, 1.000000000000000000, 0.8660254037844387076, 1.000000000000000000, 0.8660254037844387076, 1.000000000000000000, 0.8660254037844387076, 1.000000000000000000, 0.8660254037844387076, 1.000000000000000000, 0.8660254037844387076, 1.000000000000000000, 0.8660254037844387076, 1.000000000000000000, 0.8660254037844387076, 1.000000000000000000, 0.8660254037844387076, 1.000000000000000000, 0.8660254037844387076, 1.000000000000000000, 0.8660254037844387076, 1.000000000000000000, 0.8660254037844387076, 1.000000000000000000, 0.8660254037844387076, 1.000000000000000000, 0.8660254037844387076, 1.000000000000000000, 0.8660254037844387076, 1.000000000000000000, 0.8660254037844387076, 1.000000000000000000, 0.8660254037844387076, 1.000000000000000000, 0.8660254037844387076, 1.000000000000000000, 0.8660254037844387076, 1.000000000000000000, 0.8660254037844387076, 1.000000000000000000, 0.8660254037844387076, 1.000000000000000000, 0.8660254037844387076, 1.000000000000000000, 0.8660254037844387076, 1.000000000000000000, 0.8660254037844387076, 1.000000000000000000, 0.8660254037844387076, 1.000000000000000000, 0.8660254037844387076, 1.000000000000000000, 0.8660254037844387076, 1.000000000000000000, 0.8660254037844387076, 1.000000000000000000, 0.8660254037844387076, 1.000000000000000000, 0.8660254037844387076, 1.000000000000000000, 0.8660254037844387076, 1.000000000000000000, 0.8660254037844387076, 1.000000000000000000, 0.8660254037844387076, 1.000000000000000000, 0.8660254037844387076, 1.000000000000000000, 0.8660254037844387076, 1.000000000000000000, 0.8660254037844387076, 1.000000000000000000, 0.8660254037844387076, 1.000000000000000000, 0.8660254037844387076, 1.000000000000000000, 0.8660254037844387076, 1.000000000000000000, 0.8660254037844387076, 1.000000000000000000, 0.8660254037844387076, 1.000000000000000000, 0.8660254037844387076, 1.000000000000000000, 0.8660254037844387076, 1.000000000000000000, 0.8660254037844387076, 1.000000000000000000, 0.8660254037844387076, 1.000000000000000000, 0.8660254037844387076, 1.000000000000000000, 0.8660254037844387076, 1.000000000000000000, 0.8660254037844387076, 1.000000000000000000, 0.8660254037844387076, 1.000000000000000000, 0.8660254037844387076, 1.000000000000000000, 0.8660254037844387076, 1.000000000000000000, 0.8660254037844387076, 1.000000000000000000, 0.8660254037844387076, 1.000000000000000000, 0.8660254037844387076, 1.000000000000000000, 0.8660254037844387076, 1.000000000000000000, 0.8660254037844387076, 1.000000000000000000, 0.8660254037844387076, 1.000000000000000000, 0.8660254037844387076, 1.000000000000000000, 0.8660254037844387076, 1.000000000000000000, 0.8660254037844387076, 1.000000000000000000, 0.8660254037844387076, 1.000000000000000000, 0.8660254037844387076, 1.000000000000000000, 0.8660254037844387076, 1.000000000000000000, 0.8660254037844387076, 1.000000000000000000, 0.8660254037844387076, 1.000000000000000000, 0.8660254037844387076, 1.000000000000000000, 0.8660254037844387076, 1.000000000000000000, 0.8660254037844387076, 1.000000000000000000, 0.8660254037844387076, 1.000000000000000000, 0.8660254037844387076, 1.000000000000000000, 0.8660254037844387076, 1.000000000000000000, 0.8660254037844387076, 1.000000000000000000, 0.8660254037844387076, 1.000000000000000000, 0.8660254037844387076, 1.000000000000000000, 0.8660254037844387076, 1.000000000000000000, 0.8660254037844387076, 1.000000000000000000, 0.8660254037844387076, 1.000000000000000000, 0.8660254037844387076, 1.000000000000000000, 0.8660254037844387076, 1.000000000000000000, 0.8660254037844387076, 1.000000000000000000, 0.8660254037844387076, 1.000000000000000000, 0.8660254037844387076, 1.000000000000000000, 0.8660254037844387076, 1.000000000000000000, 0.8660254037844387076, 1.000000000000000000, 0.8660254037844387076, 1.000000000000000000, 0.8660254037844387076, 1.000000000000000000, 0.8660254037844387076, 1.000000000000000000, 0.8660254037844387076, 1.000000000000000000, 0.8660254037844387076, 1.000000000000000000, 0.8660254037844387076, 1.000000000000000000, 0.8660254037844387076, 1.000000000000000000, 0.8660254037844387076, 1.000000000000000000, 0.8660254037844387076, 1.000000000000000000, 0.8660254037844387076, 1.000000000000000000, 0.8660254037844387076, 1.000000000000000000, 0.8660254037844387076, 1.000000000000000000, 0.8660254037844387076, 1.000000000000000000, 0.8660254037844387076, 1.000000000000000000, 0.8660254037844387076, 1.000000000000000000, 0.8660254037844387076, 1.000000000000000000, 0.8660254037844387076, 1.000000000000000000, 0.8660254037844387076, 1.000000000000000000, 0.8660254037844387076, 1.000000000000000000, 0.8660254037844387076, 1.000000000000000000, 0.8660254037844387076, 1.000000000000000000, 0.8660254037844387076, 1.000000000000000000, 0.8660254037844387076, 1.000000000000000000, 0.8660254037844387076, 1.000000000000000000, 0.8660254037844387076, 1.000000000000000000, 0.8660254037844387076, 1.000000000000000000, 0.8660254037844387076, 1.000000000000000000, 0.8660254037844387076, 1.000000000000000000, 0.8660254037844387076, 1.000000000000000000, 0.8660254037844387076, 1.000000000000000000, 0.8660254037844387076, 1.000000000000000000, 0.8660254037844387076, 1.000000000000000000, 0.8660254037844387076, 1.000000000000000000, 0.8660254037844387076, 1.000000000000000000, 0.8660254037844387076, 1.000000000000000000, 0.8660254037844387076, 1.000000000000000000, 0.8660254037844387076, 1.000000000000000000, 0.8660254037844387076, 1.000000000000000000, 0.8660254037844387076, 1.000000000000000000, 0.8660254037844387076, 1.000000000000000000, 0.8660254037844387076, 1.000000000000000000, 0.8660254037844387076, 1.000000000000000000, 0.8660254037844387076, 1.000000000000000000, 0.8660254037844387076, 1.000000000000000000, 0.8660254037844387076, 1.000000000000000000, 0.8660254037844387076, 1.000000000000000000, 0.8660254037844387076, 1.000000000000000000, 0.8660254037844387076, 1.000000000000000000, 0.8660254037844387076, 1.000000000000000000, 0.8660254037844387076, 1.000000000000000000, 0.8660254037844387076, 1.000000000000000000, 0.8660254037844387076, 1.000000000000000000, 0.8660254037844387076, 1.000000000000000000, 0.8660254037844387076, 1.000000000000000000, 0.8660254037844387076, 1.000000000000000000, 0.8660254037844387076, 1.000000000000000000, 0.8660254037844387076, 1.000000000000000000, 0.8660254037844387076, 1.000000000000000000, 0.8660254037844387076, 1.000000000000000000, 0.8660254037844387076, 1.000000000000000000, 0.8660254037844387076, 1.000000000000000000, 0.8660254037844387076, 1.000000000000000000, 0.8660254037844387076, 1.000000000000000000, 0.8660254037844387076, 1.000000000000000000, 0.8660254037844387076, 1.000000000000000000, 0.8660254037844387076, 1.000000000000000000, 0.8660254037844387076, 1.000000000000000000, 0.8660254037844387076, 1.000000000000000000, 0.8660254037844387076, 1.000000000000000000, 0.8660254037844387076, 1.000000000000000000, 0.8660254037844387076, 1.000000000000000000, 0.8660254037844387076, 1.000000000000000000, 0.8660254037844387076, 1.000000000000000000, 0.8660254037844387076, 1.000000000000000000, 0.8660254037844387076, 1.000000000000000000, 0.8660254037844387076, 1.000000000000000000, 0.8660254037844387076, 1.000000000000000000, 0.8660254037844387076, 1.000000000000000000, 0.8660254037844387076, 1.000000000000000000, 0.8660254037844387076, 1.000000000000000000, 0.8660254037844387076, 1.000000000000000000, 0.8660254037844387076, 1.000000000000000000, 0.8660254037844387076, 1.000000000000000000, 0.8660254037844387076, 1.000000000000000000, 0.8660254037844387076, 1.000000000000000000, 0.8660254037844387076, 1.000000000000000000, 0.8660254037844387076, 1.000000000000000000, 0.8660254037844387076, 1.000000000000000000, 0.8660254037844387076, 1.000000000000000000, 0.8660254037844387076, 1.000000000000000000, 0.8660254037844387076, 1.000000000000000000, 0.8660254037844387076, 1.000000000000000000, 0.8660254037844387076, 1.000000000000000000, 0.8660254037844387076, 1.000000000000000000, 0.8660254037844387076, 1.000000000000000000, 0.8660254037844387076, 1.000000000000000000, 0.8660254037844387076, 1.000000000000000000, 0.8660254037844387076, 1.000000000000000000, 0.8660254037844387076, 1.000000000000000000, 0.8660254037844387076, 1.000000000000000000, 0.8660254037844387076, 1.000000000000000000, 0.8660254037844387076, 1.000000000000000000, 0.8660254037844387076, 1.000000000000000000, 0.8660254037844387076, 1.000000000000000000, 0.8660254037844387076, 1.000000000000000000, 0.8660254037844387076, 1.000000000000000000, 0.8660254037844387076, 1.000000000000000000, 0.8660254037844387076, 1.000000000000000000, 0.8660254037844387076, 1.000000000000000000, 0.8660254037844387076, 1.000000000000000000, 0.8660254037844387076, 1.000000000000000000, 0.8660254037844387076, 1.000000000000000000, 0.8660254037844387076, 1.000000000000000000, 0.8660254037844387076, 1.000000000000000000, 0.8660254037844387076, 1.000000000000000000, 0.8660254037844387076, 1.000000000000000000, 0.8660254037844387076, 1.000000000000000000, 0.8660254037844387076, 1.000000000000000000, 0.8660254037844387076, 1.000000000000000000, 0.8660254037844387076, 1.000000000000000000, 0.8660254037844387076, 1.000000000000000000, 0.8660254037844387076, 1.000000000000000000, 0.8660254037844387076, 1.000000000000000000, 0.8660254037844387076, 1.000000000000000000, 0.8660254037844387076, 1.000000000000000000, 0.8660254037844387076, 1.000000000000000000, 0.8660254037844387076, 1.000000000000000000, 0.8660254037844387076, 1.000000000000000000, 0.8660254037844387076, 1.000000000000000000, 0.8660254037844387076, 1.000000000000000000, 0.8660254037844387076, 1.000000000000000000, 0.8660254037844387076, 1.000000000000000000, 0.8660254037844387076, 1.000000000000000000, 0.8660254037844387076, 1.000000000000000000, 0.8660254037844387076, 1.000000000000000000, 0.8660254037844387076, 1.000000000000000000, 0.8660254037844387076, 1.000000000000000000, 0.8660254037844387076, 1.000000000000000000, 0.8660254037844387076, 1.000000000000000000, 0.8660254037844387076, 1.000000000000000000, 0.8660254037844387076, 1.000000000000000000) ) ) 
 REPRESENTATION_ITEM ( '' )  SURFACE ( )  );
#129702=CARTESIAN_POINT ( 'NONE',  ( -4.305726085941478765, 7.254707473775878768, 0.9719050602644065950 ) ) ;
#129703=CARTESIAN_POINT ( 'NONE',  ( 1.364683531249986537, -0.07395833299191513499, 0.7879004041258500513 ) ) ;
#129706=CARTESIAN_POINT ( 'NONE',  ( 5.368665641331531013, 5.365790791082654998, -0.7216878364870207285 ) ) ;
#129707=CARTESIAN_POINT ( 'NONE',  ( 1.499999999999990896, 3.556250000682818602, 1.214306433183764966E-14 ) ) ;
#129710=CARTESIAN_POINT ( 'NONE',  ( -9.775065565328612038, 10.50659070241261794, -0.7216878364870267237 ) ) ;
#129715=CARTESIAN_POINT ( 'NONE',  ( -9.124274191872645545, 9.747334100047323702, -0.7216878364870267237 ) ) ;
#129723=CARTESIAN_POINT ( 'NONE',  ( -9.015808962963337336, 10.58116054728778366, 1.082531754730558626 ) ) ;
#129727=CARTESIAN_POINT ( 'NONE',  ( -1.364683531250010295, 5.801041667008088432, -0.7879004041258300672 ) ) ;
#129728=CARTESIAN_POINT ( 'NONE',  ( -0.7499999999999972244, 4.889583334016150751, -1.299038105676652899 ) ) ;
#129729=CARTESIAN_POINT ( 'NONE',  ( 5.196774945655527667, 6.645529799594804388, -1.392961322168507765 ) ) ;
#129735=CARTESIAN_POINT ( 'NONE',  ( -6.482770005628665011, 10.71498210654212002, 0.7998128361456481317 ) ) ;
#129739=CARTESIAN_POINT ( 'NONE',  ( 6.647575389402066826, 6.649926130590872120, 1.040834085586084257E-14 ) ) ;
#129744=CARTESIAN_POINT ( 'NONE',  ( 9.094822116668764167, 9.505047312402055582, 0.7998128361456462443 ) ) ;
#129750=CARTESIAN_POINT ( 'NONE',  ( -6.724481002698130538, 7.907944593645035880, -1.082531754730544860 ) ) ;
#129753=CARTESIAN_POINT ( 'NONE',  ( 7.334597915313080918, 9.580116872663850813, 1.040834085586084257E-14 ) ) ;
#129760=CARTESIAN_POINT ( 'NONE',  ( -9.840520565420403543, 10.37502883594562597, 1.040834085586084257E-14 ) ) ;
#129763=CARTESIAN_POINT ( 'NONE',  ( 9.260382613333817403, 10.76253345609967660, -1.199719254218446718 ) ) ;
#129765=CARTESIAN_POINT ( 'NONE',  ( -10.16591625214838679, 10.75465713712827487, 1.040834085586084257E-14 ) ) ;
#129768=CARTESIAN_POINT ( 'NONE',  ( 1.364683531249988535, 3.155208333674756283, -0.7879004041258239610 ) ) ;
#129769=CARTESIAN_POINT ( 'NONE',  ( 2.496672843210871129, 6.064535417054653266, -0.7998128361456291469 ) ) ;
#129774=CARTESIAN_POINT ( 'NONE',  ( 10.20892648096591770, 11.01276177065614981, -0.7216878364870257245 ) ) ;
#129778=CARTESIAN_POINT ( 'NONE',  ( -5.572037945536512105, 9.444535336527177805, 0.000000000000000000 ) ) ;
#129779=CARTESIAN_POINT ( 'NONE',  ( -1.364683531250012516, 0.7802083336747528408, 0.7879004041258379498 ) ) ;
#129781=CARTESIAN_POINT ( 'NONE',  ( 0.07021666366551572447, 7.008523639393767546, 2.000250312771564065 ) ) ;
#129783=CARTESIAN_POINT ( 'NONE',  ( -6.347188469492005325, 10.55680364771601809, -0.7998128361456291469 ) ) ;
#129784=CARTESIAN_POINT ( 'NONE',  ( -2.914639836813632812, 6.344237543017112735, 0.7216878364870317197 ) ) ;
#129785=CARTESIAN_POINT ( 'NONE',  ( 1.364683531249990311, 3.946875000341417028, 1.214306433183764966E-14 ) ) ;
#129791=CARTESIAN_POINT ( 'NONE',  ( 9.073431116043567002, 11.60875560684942265, -1.599625672291262513 ) ) ;
#129798=ORIENTED_EDGE ( 'NONE', *, *, #97607, .T. ) ;
#129801=FACE_OUTER_BOUND ( 'NONE', #103764, .T. ) ;
#129804=CARTESIAN_POINT ( 'NONE',  ( -1.580000000000022276, 8.674529973577531194, 2.500000000000011102 ) ) ;
#129806=CARTESIAN_POINT ( 'NONE',  ( 0.6823417656249899377, 3.738541667008085767, -1.181850606188754593 ) ) ;
#129811=CARTESIAN_POINT ( 'NONE',  ( 9.121938423896107651, 9.536683004167278099, -0.7998128361456221525 ) ) ;
#129813=CARTESIAN_POINT ( 'NONE',  ( -1.201851678989727383E-14, 3.821875000341423689, 1.575800808251672791 ) ) ;
#129815=CARTESIAN_POINT ( 'NONE',  ( -6.507550544879489252, 9.575597488125954015, 1.082531754730548412 ) ) ;
#129821=CARTESIAN_POINT ( 'NONE',  ( 3.192055101013606233, 5.811482486902795230, -1.199719254218446718 ) ) ;
#129824=CARTESIAN_POINT ( 'NONE',  ( 8.380911511541880188, 12.92948053010758258, 0.7998128361456462443 ) ) ;
#129830=CARTESIAN_POINT ( 'NONE',  ( -9.622536337397040285, 12.24937836509514710, 1.599625672291281386 ) ) ;
#129831=CARTESIAN_POINT ( 'NONE',  ( 7.283754839039659146, 9.520799950344851936, -1.599625672291262513 ) ) ;
#129833=CARTESIAN_POINT ( 'NONE',  ( 3.348500752450937590, 5.890039396959305229, 1.082531754730558626 ) ) ;
#129844=CARTESIAN_POINT ( 'NONE',  ( -6.738039156311804945, 6.963393225226301553, 1.040834085586084257E-14 ) ) ;
#129845=CARTESIAN_POINT ( 'NONE',  ( 3.684065054611349144, 5.321161868511784299, -1.599625672291262513 ) ) ;
#129848=CARTESIAN_POINT ( 'NONE',  ( -9.494787648271923786, 9.971673765939062406, 1.040834085586084257E-14 ) ) ;
#129853=CARTESIAN_POINT ( 'NONE',  ( -8.350932551013499960, 11.83017284523606172, -1.199719254218446718 ) ) ;
#129856=CARTESIAN_POINT ( 'NONE',  ( 9.257519960032755790, 9.694861462993381807, 0.7998128361456462443 ) ) ;
#129858=CARTESIAN_POINT ( 'NONE',  ( 6.647575389402066826, 6.649926130590872120, 1.040834085586084257E-14 ) ) ;
#129859=CARTESIAN_POINT ( 'NONE',  ( -3.332168893502572171, 7.719402352560116753, -2.450693629706319321 ) ) ;
#129865=CARTESIAN_POINT ( 'NONE',  ( 3.128199800776516160, 2.800000000000115730, -2.480560084996043191 ) ) ;
#129870=CARTESIAN_POINT ( 'NONE',  ( -9.657485491635913633, 10.16148791653038330, 1.040834085586084257E-14 ) ) ;
#129871=CIRCLE ( 'NONE', #8721, 0.08000000000000020983 ) ;
#129875=CARTESIAN_POINT ( 'NONE',  ( 8.459924665247367415, 8.972259652317825740, -0.7216878364870267237 ) ) ;
#129877=CARTESIAN_POINT ( 'NONE',  ( 2.496672843210871129, 6.064535417054653266, -0.7998128361456291469 ) ) ;
#129880=CARTESIAN_POINT ( 'NONE',  ( -5.768104287610143821, 8.816873204598778102, -1.199719254218440723 ) ) ;
#129882=DIRECTION ( 'NONE',  ( 5.578564026256490882E-16, 1.000000000000000000, 9.066213480720158442E-32 ) ) ;
#129889=CARTESIAN_POINT ( 'NONE',  ( -1.364683531250010295, 4.592708333674755394, 0.7879004041258379498 ) ) ;
#129890=CARTESIAN_POINT ( 'NONE',  ( 2.030969412801347573, 8.463209591663295228, 2.499999999999998668 ) ) ;
#129891=CARTESIAN_POINT ( 'NONE',  ( 9.240045382913317340, 10.73880668727576015, -1.199719254218446718 ) ) ;
#129893=CARTESIAN_POINT ( 'NONE',  ( -3.294268138440636928, 6.787137228248626641, 1.040834085586084257E-14 ) ) ;
#129895=CARTESIAN_POINT ( 'NONE',  ( -5.883875478206491927, 5.966868934103426447, 0.000000000000000000 ) ) ;
#129903=CARTESIAN_POINT ( 'NONE',  ( 4.844340958784499662, 4.546152628203684820, 0.7998128361456341429 ) ) ;
#129912=CARTESIAN_POINT ( 'NONE',  ( 5.705283713252285338, 5.550585841749444249, -0.7998128361456211532 ) ) ;
#129917=CARTESIAN_POINT ( 'NONE',  ( -1.201851678989727383E-14, 4.509375000341417916, -1.575800808251660134 ) ) ;
#129922=CARTESIAN_POINT ( 'NONE',  ( 6.205881626753210867, 8.263281202677319470, 1.599625672291281386 ) ) ;
#129924=CARTESIAN_POINT ( 'NONE',  ( -5.922214171070950606, 5.803671375871217286, -0.7998128361456291469 ) ) ;
#129925=CARTESIAN_POINT ( 'NONE',  ( 1.499999999999989120, 2.525000000000020339, 1.214306433183764966E-14 ) ) ;
#129928=CARTESIAN_POINT ( 'NONE',  ( -3.086452525405351643, 6.752611712948207057, 0.7998128361456341429 ) ) ;
#129929=CARTESIAN_POINT ( 'NONE',  ( 0.4829820140310078780, 7.516281308464741961, -1.942130999994612139 ) ) ;
#129931=CARTESIAN_POINT ( 'NONE',  ( 1.364683531249988535, 2.905208333674754506, -0.7879004041258239610 ) ) ;
#129934=CARTESIAN_POINT ( 'NONE',  ( -4.961921032921567054, 4.891255414604337659, 0.7216878364870317197 ) ) ;
#129939=CARTESIAN_POINT ( 'NONE',  ( 4.496500501226593727, 8.397667684739696270, 0.7998128361456462443 ) ) ;
#129943=CARTESIAN_POINT ( 'NONE',  ( -1.201851678989727383E-14, 3.634375000341422357, 1.575800808251672791 ) ) ;
#129947=CARTESIAN_POINT ( 'NONE',  ( 1.364683531249986537, -0.03229166632525094088, -0.7879004041258309554 ) ) ;
#129950=CARTESIAN_POINT ( 'NONE',  ( -9.996439331977562404, 10.55693406359564790, 0.7998128361456462443 ) ) ;
#129951=CARTESIAN_POINT ( 'NONE',  ( -7.036318535368094373, 7.311385834125318617, 0.7216878364870317197 ) ) ;
#129955=EDGE_LOOP ( 'NONE', ( #213576, #66965, #96274, #82546 ) ) ;
#129956=CARTESIAN_POINT ( 'NONE',  ( 1.364683531249988535, 4.905208333674756283, -0.7879004041258300672 ) ) ;
#129964=CARTESIAN_POINT ( 'NONE',  ( -5.382223794500827552, 9.223085493652217082, -0.7216878364870207285 ) ) ;
#129972=CARTESIAN_POINT ( 'NONE',  ( -6.412643469139482910, 7.544134137826577380, 1.082531754730549967 ) ) ;
#129986=CARTESIAN_POINT ( 'NONE',  ( -4.771579997005698459, 7.654261532226910525, -1.199719254218452047 ) ) ;
#129989=CARTESIAN_POINT ( 'NONE',  ( 1.499999999999987121, 1.254166666666689300, 0.8660254037844524744 ) ) ;
#129990=CARTESIAN_POINT ( 'NONE',  ( 9.327646496521982300, 11.90534021740758064, -1.443375672974057666 ) ) ;
#129991=CARTESIAN_POINT ( 'NONE',  ( 7.579171565239241737, 8.801120566655981747, 1.199719254218462483 ) ) ;
#129993=CARTESIAN_POINT ( 'NONE',  ( 1.419999999999989049, 6.216000000000041048, -2.921333333333328675 ) ) ;
#129994=CARTESIAN_POINT ( 'NONE',  ( 4.493637847925535667, 7.329995691633395261, -1.199719254218452047 ) ) ;
#129995=CARTESIAN_POINT ( 'NONE',  ( -4.257741265285667431, 3.982435197156672491, 0.4597581080974452727 ) ) ;
#130000=CARTESIAN_POINT ( 'NONE',  ( -3.578989364327652467, 6.158942777482099729, 1.082531754730560403 ) ) ;
#130007=CARTESIAN_POINT ( 'NONE',  ( -1.364683531249997417, 3.009375000341422801, 1.214306433183764966E-14 ) ) ;
#130008=CARTESIAN_POINT ( 'NONE',  ( 10.34450801710256584, 11.17094022948226240, 0.7216878364870438212 ) ) ;
#130009=CARTESIAN_POINT ( 'NONE',  ( -5.228640796364566690, 9.251831362400652736, -0.7998128361456231517 ) ) ;
#130012=CARTESIAN_POINT ( 'NONE',  ( 5.307127064745490230, 8.279066444590018392, -1.199719254218452935 ) ) ;
#130013=CARTESIAN_POINT ( 'NONE',  ( -6.470265622219711688, 8.571729197388226140, -1.599625672291263179 ) ) ;
#130014=CARTESIAN_POINT ( 'NONE',  ( -1.524175555628288992, 8.756493634679708649, 2.487619788734857007 ) ) ;
#130017=CARTESIAN_POINT ( 'NONE',  ( -1.201851678989727383E-14, 0.7437500006828187127, 1.732050807568877637 ) ) ;
#130020=CARTESIAN_POINT ( 'NONE',  ( 6.480434237652115570, 10.50433101066207442, 0.7216878364870438212 ) ) ;
#130023=CARTESIAN_POINT ( 'NONE',  ( -1.201851678989727383E-14, 1.884375000341422135, 1.575800808251672791 ) ) ;
#130025=CARTESIAN_POINT ( 'NONE',  ( 6.765155463094759014, 7.955398130774449683, 1.082531754730558626 ) ) ;
#130028=CARTESIAN_POINT ( 'NONE',  ( -2.629918611371007575, 6.012062780000711371, 0.7216878364870317197 ) ) ;
#130030=CARTESIAN_POINT ( 'NONE',  ( -1.364683531250010295, 5.280208333674758059, 0.7879004041258379498 ) ) ;
#130034=CARTESIAN_POINT ( 'NONE',  ( -4.646091124696241081, 7.101299429195864654, -1.386232413501260474 ) ) ;
#130041=CARTESIAN_POINT ( 'NONE',  ( 5.957918438201454059, 9.038323046955323292, -1.199719254218440723 ) ) ;
#130044=CARTESIAN_POINT ( 'NONE',  ( 5.183294799126148433, 4.941598775268944976, 1.040834085586084257E-14 ) ) ;
#130052=CARTESIAN_POINT ( 'NONE',  ( 5.585596099150174965, 7.539614753807099667, -1.443375672974057666 ) ) ;
#130053=CARTESIAN_POINT ( 'NONE',  ( -0.6823417656250246877, 0.3635416670080895973, 1.181850606188755259 ) ) ;
#130056=CARTESIAN_POINT ( 'NONE',  ( 0.1021010164683408550, 6.360493866598974755, -3.113991822131910059 ) ) ;
#130061=CARTESIAN_POINT ( 'NONE',  ( -1.500000000000013101, 1.670833333333355153, 0.8660254037844403729 ) ) ;
#130062=CARTESIAN_POINT ( 'NONE',  ( 7.623762449586013901, 7.788811034138823253, 1.040834085586084257E-14 ) ) ;
#130063=CARTESIAN_POINT ( 'NONE',  ( -6.503107236049161521, 10.73870887536603291, 0.7998128361456481317 ) ) ;
#130067=CARTESIAN_POINT ( 'NONE',  ( -1.364683531250012516, 2.988541667008091096, -0.7879004041258289570 ) ) ;
#130068=CARTESIAN_POINT ( 'NONE',  ( 1.499999999999987121, 2.545833333333351156, -0.8660254037844262731 ) ) ;
#130070=CARTESIAN_POINT ( 'NONE',  ( 2.333974999846879061, 5.874721266463329705, -0.7998128361456291469 ) ) ;
#130073=DIRECTION ( 'NONE',  ( 0.7592566023653005702, -0.6507913734559639396, 0.000000000000000000 ) ) ;
#130075=CARTESIAN_POINT ( 'NONE',  ( 6.471393748265519719, 5.229711127717882491, -2.419999999999995044 ) ) ;
#130076=CARTESIAN_POINT ( 'NONE',  ( 1.499999999999987121, 1.285416667349485120, 0.8660254037844524744 ) ) ;
#130077=CARTESIAN_POINT ( 'NONE',  ( -7.314787569772770226, 8.492672571945082183, -1.199719254218452935 ) ) ;
#130078=CARTESIAN_POINT ( 'NONE',  ( -4.284013352238262407, 6.021101549076499637, -1.443375672974053447 ) ) ;
#130085=CARTESIAN_POINT ( 'NONE',  ( 5.587931867126699537, 9.671004278289832001, -0.7998128361456291469 ) ) ;
#130089=CARTESIAN_POINT ( 'NONE',  ( 7.091078035147269532, 8.231678114882006625, 1.199719254218462483 ) ) ;
#130090=CARTESIAN_POINT ( 'NONE',  ( 9.395437264145964917, 10.06369101769952934, -0.7216878364870257245 ) ) ;
#130097=CARTESIAN_POINT ( 'NONE',  ( -7.718669524881690336, 7.899535955317097624, 0.7998128361456462443 ) ) ;
#130098=CARTESIAN_POINT ( 'NONE',  ( 5.867981556616276073, 5.740399992340775803, -0.7998128361456281477 ) ) ;
#130102=CARTESIAN_POINT ( 'NONE',  ( 4.023704138721054591, 7.562441369377219225, 0.3480857562657164173 ) ) ;
#130103=CARTESIAN_POINT ( 'NONE',  ( 10.41229878561526512, 11.25002945941372623, -0.7216878364870257245 ) ) ;
#130104=ADVANCED_FACE ( 'NONE', ( #134389 ), #201451, .F. ) ;
#130114=CARTESIAN_POINT ( 'NONE',  ( -2.304522924643024773, 5.632434478818063361, 0.7216878364870317197 ) ) ;
#130115=CARTESIAN_POINT ( 'NONE',  ( 7.239690840017413365, 10.42976116578691403, -1.082531754730537976 ) ) ;
#130118=CARTESIAN_POINT ( 'NONE',  ( -6.389970470742427189, 6.349387058821269747, -0.7998128361456291469 ) ) ;
#130119=CARTESIAN_POINT ( 'NONE',  ( -5.070386261386537363, 5.017798181146802428, 1.214306433183764966E-14 ) ) ;
#130125=CARTESIAN_POINT ( 'NONE',  ( -5.208303565944065738, 9.228104593576741621, -0.7998128361456231517 ) ) ;
#130139=CARTESIAN_POINT ( 'NONE',  ( -4.706651882238427120, 8.642844295920152575, 1.040834085586084257E-14 ) ) ;
#130142=CARTESIAN_POINT ( 'NONE',  ( 3.795919822146273326, 5.451659097302528068, -1.443375672974051449 ) ) ;
#130146=CARTESIAN_POINT ( 'NONE',  ( -2.625475302540713152, 6.214804952939456228, -0.7998128361456281477 ) ) ;
#130149=CARTESIAN_POINT ( 'NONE',  ( 8.269583629331492602, 11.73526576994040482, 1.199719254218450271 ) ) ;
#130152=CARTESIAN_POINT ( 'NONE',  ( -8.259941899223614215, 10.65968485389279508, -1.599625672291263179 ) ) ;
#130153=CARTESIAN_POINT ( 'NONE',  ( 5.113396490648394632, 9.117379672398465473, 1.040834085586084257E-14 ) ) ;
#130157=CARTESIAN_POINT ( 'NONE',  ( -1.201851678989727383E-14, 1.134375000341418582, 1.575800808251672791 ) ) ;
#130160=CARTESIAN_POINT ( 'NONE',  ( 7.076992996653421741, 10.23994701519558781, -1.082531754730537976 ) ) ;
#130173=CARTESIAN_POINT ( 'NONE',  ( -1.580000000000018723, 8.674529973577529418, 2.499999999999998668 ) ) ;
#130175=CARTESIAN_POINT ( 'NONE',  ( -9.130526383799315582, 12.73969898348616070, 1.199719254218462483 ) ) ;
#130181=CARTESIAN_POINT ( 'NONE',  ( -1.387358672534890536, 7.315968950354793776, -4.254625267136668221 ) ) ;
#130187=CARTESIAN_POINT ( 'NONE',  ( -1.500000000000015099, 0.6604166673494823447, -0.8660254037844313801 ) ) ;
#130193=CARTESIAN_POINT ( 'NONE',  ( -1.500000000000015099, -0.5791666666666476226, 0.8660254037844403729 ) ) ;
#130194=CARTESIAN_POINT ( 'NONE',  ( 9.576136569953906275, 10.06658084123472641, 0.000000000000000000 ) ) ;
#130198=CARTESIAN_POINT ( 'NONE',  ( 4.207107738942202246, 3.802713871720993399, 1.214306433183764966E-14 ) ) ;
#130199=CARTESIAN_POINT ( 'NONE',  ( -7.104109303880803417, 8.350844278358124484, 1.082531754730549967 ) ) ;
#130203=CARTESIAN_POINT ( 'NONE',  ( -5.682838942422375084, 9.781729199468104596, 0.000000000000000000 ) ) ;
#130208=CARTESIAN_POINT ( 'NONE',  ( -0.7500000000000006661, 1.889583334016155192, -1.299038105676652011 ) ) ;
#130215=CARTESIAN_POINT ( 'NONE',  ( -4.270455198180246548, 4.084545274072787890, 0.7216878364870317197 ) ) ;
#130218=CARTESIAN_POINT ( 'NONE',  ( 5.039007818866061861, 6.552116822607409574, 1.229770346242751389 ) ) ;
#130223=CARTESIAN_POINT ( 'NONE',  ( -8.469039510030723861, 13.03229652834454733, 1.040834085586084257E-14 ) ) ;
#130224=CARTESIAN_POINT ( 'NONE',  ( 6.259060471003163428, 10.45398764947904624, -0.7998128361456291469 ) ) ;
#130233=CARTESIAN_POINT ( 'NONE',  ( -7.797910906154257304, 12.24931315715533486, 0.000000000000000000 ) ) ;
#130238=CARTESIAN_POINT ( 'NONE',  ( 3.897079088924235712, 6.634010472798538949, 1.199719254218462483 ) ) ;
#130243=CARTESIAN_POINT ( 'NONE',  ( -9.215791728987058562, 11.77484298861683598, -1.599625672291263179 ) ) ;
#130256=CARTESIAN_POINT ( 'NONE',  ( 7.470706336329915764, 8.674577799595093452, -1.199719254218441611 ) ) ;
#130258=CARTESIAN_POINT ( 'NONE',  ( -4.894657149733403045, 5.669187081899118574, -1.199719254218446718 ) ) ;
#130267=CARTESIAN_POINT ( 'NONE',  ( 0.7499999999999885647, 0.3479166673494848983, -1.299038105676652899 ) ) ;
#130270=CARTESIAN_POINT ( 'NONE',  ( -1.445367865411041564, 8.714818166637975594, -2.590103969856726085 ) ) ;
#130271=CARTESIAN_POINT ( 'NONE',  ( 3.999819011231439347, 4.625209253646830554, 1.199719254218464037 ) ) ;
#130273=CARTESIAN_POINT ( 'NONE',  ( -4.457933580795036654, 4.095344020549286590, -0.7998128361456221525 ) ) ;
#130280=CARTESIAN_POINT ( 'NONE',  ( 3.687454593236936251, 7.245854758844324728, -0.7216878364870267237 ) ) ;
#130285=CARTESIAN_POINT ( 'NONE',  ( 4.161989969270902812, 4.918371721313249623, 1.082531754730560403 ) ) ;
#130292=CARTESIAN_POINT ( 'NONE',  ( -5.775368881829861856, 6.228402001981104164, 1.032258425150527126 ) ) ;
#130294=CARTESIAN_POINT ( 'NONE',  ( 1.364683531249986537, -1.136458332991912235, 0.7879004041258500513 ) ) ;
#130296=( BOUNDED_SURFACE ( )  B_SPLINE_SURFACE ( 1, 2, ( 
 ( #52685, #87326, #89479, #86255, #72116, #23370, #54828, #205323, #120978, #36429, #35360, #19106, #103580, #123135, #155534, #7114, #85184, #151268, #71042, #4964, #73187, #102506, #119893, #101435, #22287, #6045, #152325, #68909, #137157, #204238, #3903, #168568, #201042, #55890, #88400, #139293, #69973, #38579, #136084, #167508, #20168, #135029, #138225, #118815, #184800, #202101, #53760, #185869, #186946, #37504, #104654, #154468, #169638, #122047, #21221, #203181, #170702, #188011, #39639, #105747, #171774, #26584, #42871, #172862, #43931, #12459, #141460, #60153, #77469, #193354, #190150, #157675, #159789, #125246, #191206, #75344, #126310, #176058, #108979, #40726, #107917, #207467, #156609, #78535, #62294, #144652, #210667, #173943, #28729, #143588, #11391, #189093, #94815, #25516, #106832, #59086, #192270, #24433, #208518, #27654, #41804, #61227, #160865, #91624, #140378, #58023, #9273, #44998, #76401, #92685, #174998, #90545, #110046, #8199, #158731, #93751, #209581, #111108, #10327, #142510, #127382, #177113, #74284, #206398, #124187, #81740, #212790, #128453, #129518, #163005, #95889, #447, #194421, #198661, #46062, #47134, #66515, #181366, #64427, #115374, #146774, #132657, #49253, #161943, #112184, #30878, #80682, #180314, #79605, #130572, #196561, #164072, #165122, #195498, #14586, #147822, #213840, #179255, #178188, #31934, #32990, #65458, #197609, #131608, #113250, #99068, #145724, #29803, #13535, #48203, #96957, #211723, #16713, #98016, #82798, #148872, #63360, #114315, #15652, #92329, #145355, #111811, #79237, #28355, #58723, #60852, #158370, #174635, #211356, #94450, #25144, #142143, #61927, #208157, #160489, #9963, #144294, #76040, #62980, #95523, #194043, #190839, #44626, #129149, #59787, #91246, #26211, #125946, #45696, #195125, #191902, #128086, #43564, #107541, #109684, #173575, #175687, #157306, #11020, #12096, #110741, #78164, #176741, #42500, #210287, #8896, #29432, #74976, #27276, #141085, #161573, #93383, #159420, #77095, #177816, #13160, #207095, #124874, #143222, #108607, #209212, #127015, #192974, #212413, #76, #97641, #113947, #18480, #182042, #178889, #81367, #1151, #147447, #33673, #31566, #83485, #163698, #84559, #34732, #133349, #130199, #198291, #68286, #15280, #30503, #179942, #213471, #199355, #134418, #65094, #67214, #131251, #2209, #197238, #150648, #48877, #46763, #149568, #112874, #166890, #114995, #96584, #180993, #49933, #162632, #66141, #99748, #47836, #51003, #14207, #32613, #64056, #196193, #98690, #117123, #148509, #164747, #16339, #80302, #116054, #146399, #82420, #132286, #183126, #100804, #165818, #17401, #143405, #48027, #178008, #46953, #195322, #176932, #59975, #193173, #44823, #62120, #110928, #127206, #28550, #29625, #163898, #126129, #160683, #27471, #192089, #114143, #14407, #211544, #80498, #43755, #144477, #146595, #12278, #209401, #94639, #112007, #210482, #15474, #208344, #159614, #128280, #30697, #61045, #78354, #194241, #212613, #45886, #95709, #161763, #13354, #79429, #81558, #109869, #11212, #145547, #96779, #63179, #129344, #180135, #175881, #113070, #179076, #162830, #64253, #93569, #77293, #31762, #130395, #196386, #97833, #181188, #19744, #16534, #32814, #198488, #164941, #199555, #201677, #50133, #184377, #135654, #167087, #103146, #18678, #148701, #147641, #131432, #1345, #20798, #53324, #119457, #197434, #49075, #183320, #51200, #185444, #270, #17596, #213660, #134611, #118388, #116255, #115195, #117322, #102077, #182243, #66340, #98889, #168145, #200615, #37064, #33869, #169206, #68485, #67407, #65285, #99946, #132486, #166011, #83680, #149770, #82616, #133548, #34924, #85825, #52262, #35996, #100997, #84757, #150844, #2406, #151903, #3478, #69545, #7757, #87960, #55459, #154034, #38149, #86894, #105300, #123757, #104221, #39209, #73846, #189720, #108544, #121614, #21853, #141024, #56533, #139940, #205967, #187582, #152960, #71681, #137795, #155104, #203814, #5600, #171336, #122695, #42439, #4535, #22931, #120540, #70609, #207033, #107483, #90112, #173508, #136724, #89046, #188657, #6688, #54400, #186517, #58662, #72764, #40287 ),
 ( #57599, #170267, #106396, #138863, #204880, #124814, #41372, #202748, #172421, #25080, #24010, #91183, #156178, #157244, #8837, #190777, #74916, #174575, #109626, #177754, #50659, #77031, #9903, #93322, #159359, #181707, #116785, #143160, #49593, #209154, #199014, #60793, #66869, #10957, #26152, #62920, #133014, #149226, #126952, #92266, #192910, #29369, #158311, #45631, #79174, #27217, #115717, #801, #44566, #191842, #175630, #110681, #99419, #128029, #78105, #94388, #75979, #95464, #142082, #176681, #111748, #129088, #33337, #28293, #160428, #12033, #144232, #210226, #43505, #161513, #13094, #61864, #208097, #193983, #145291, #59724, #125883, #211295, #195060, #165474, #17069, #83148, #137267, #184909, #71150, #52790, #22404, #153505, #166547, #138328, #19212, #135135, #86363, #150312, #201152, #102620, #70083, #54934, #117863, #69018, #120002, #185979, #101545, #154575, #152434, #21331, #37612, #118929, #88513, #5075, #18135, #204344, #85291, #36533, #4013, #1878, #168675, #20279, #136197, #121086, #183855, #202215, #103693, #169742, #167614, #6151, #53869, #87437, #203287, #187053, #38685, #35467, #104764, #84224, #170813, #56002, #151377, #67938, #72221, #182782, #34400, #100472, #134083, #200091, #51740, #2946, #106944, #159900, #126417, #93862, #42979, #73295, #75451, #172967, #189198, #11507, #109089, #39752, #156715, #76507, #8306, #175104, #24546, #158838, #90654, #77578, #110153, #208626, #205431, #59193, #143701, #74390, #105857, #40835, #140491, #60260, #209693, #206502, #142618, #58133, #122153, #124292, #188121, #190251, #171883, #10435, #23480, #27766, #41909, #89587, #108020, #125348, #155636, #141564, #26691, #123233, #192380, #7221, #174046, #139398, #57069, #25619, #44035, #9380, #91731, #157782, #207572, #191311, #92793, #176166, #146879, #164172, #65562, #62394, #29909, #128559, #63467, #145825, #78638, #212899, #48305, #195608, #127496, #194524, #79710, #28837, #99169, #148972, #16814, #82899, #46172, #115473, #15757, #129622, #81841, #211830, #94925, #165222, #61337, #193467, #45111, #112286, #181466, #147925, #47243, #213941, #113358, #33095, #32034, #111221, #177224, #178302, #13637, #179363, #160974, #30985, #97060, #163113, #131709, #210774, #162047, #64531, #130676, #95994, #12564, #14694, #114416, #196664, #180416, #98120, #80789, #197713, #144763, #49355, #170544, #67681, #182519, #54667, #200887, #167361, #52533, #185714, #169483, #22128, #104500, #199838, #38420, #4806, #186792, #135928, #166287, #168419, #51480, #133825, #88241, #201946, #132758, #35202, #21067, #101277, #53602, #117603, #37348, #183595, #546, #203025, #87165, #83961, #152176, #66611, #18949, #198761, #85033, #151121, #153235, #50410, #2687, #70887, #68760, #116529, #134880, #34149, #118667, #100219, #103422, #17876, #120815, #184650, #150050, #36271, #3745, #1622, #20016, #119736, #102348, #136998, #86104, #69820, #105582, #23210, #205162, #10183, #41649, #206245, #8039, #138067, #9121, #192123, #106678, #25365, #42721, #158583, #155370, #122974, #6955, #156454, #24279, #171616, #91465, #141308, #74129, #5883, #73036, #57870, #208375, #56804, #191056, #142366, #173789, #109901, #157526, #139134, #154311, #204080, #140224, #27504, #60007, #126160, #55733, #121887, #189999, #124033, #43789, #188933, #90385, #71957, #207320, #125098, #40572, #187857, #107763, #108829, #172701, #75196, #89323, #174855, #58941, #175913, #26433, #39484, #92543, #76257, #181217, #62152, #160714, #144509, #128311, #210517, #77324, #45919, #44854, #48059, #14437, #196414, #110960, #194274, #28584, #209434, #30727, #63208, #112038, #80527, #94672, #178040, #12308, #176967, #93604, #29656, #130429, #78389, #95742, #146624, #114172, #115227, #161793, #13384, #147674, #129372, #212641, #64283, #79460, #159649, #145576, #211574, #195351, #46983, #113099, #179105, #96810, #49106, #11246, #162859, #127238, #143437, #213691, #180166, #31792, #97866, #61078, #163927, #15502, #81589, #65313, #131462, #197463, #193207, #54431, #32843, #198517, #101026, #69576, #99978, #149802, #152993, #120573, #134639, #34955, #200644, #167117, #300, #132519 ) ),
 .UNSPECIFIED., .F., .F., .T. ) 
 B_SPLINE_SURFACE_WITH_KNOTS ( ( 2, 2 ),
 ( 3, 2, 2, 2, 2, 2, 2, 2, 2, 2, 2, 2, 2, 2, 2, 2, 2, 2, 2, 2, 2, 2, 2, 2, 2, 2, 2, 2, 2, 2, 2, 2, 2, 2, 2, 2, 2, 2, 2, 2, 2, 2, 2, 2, 2, 2, 2, 2, 2, 2, 2, 2, 2, 2, 2, 2, 2, 2, 2, 2, 2, 2, 2, 2, 2, 2, 2, 2, 2, 2, 2, 2, 2, 2, 2, 2, 2, 2, 2, 2, 2, 2, 2, 2, 2, 2, 2, 2, 2, 2, 2, 2, 2, 2, 2, 2, 2, 2, 2, 2, 2, 2, 2, 2, 2, 2, 2, 2, 2, 2, 2, 2, 2, 2, 2, 2, 2, 2, 2, 2, 2, 2, 2, 2, 2, 2, 2, 2, 2, 2, 2, 2, 2, 2, 2, 2, 2, 2, 2, 2, 2, 2, 2, 2, 2, 2, 2, 2, 2, 2, 2, 2, 2, 2, 2, 2, 2, 2, 2, 2, 2, 2, 2, 2, 2, 2, 2, 2, 2, 2, 2, 2, 2, 2, 2, 2, 2, 2, 2, 2, 2, 2, 2, 2, 2, 2, 2, 2, 2, 2, 2, 2, 2, 2, 2, 2, 2, 2, 2, 2, 2, 2, 2, 2, 2, 2, 2, 2, 2, 2, 2, 2, 2, 2, 2, 2, 2, 2, 2, 2, 2, 2, 2, 2, 2, 2, 2, 2, 2, 2, 2, 2, 2, 2, 2, 2, 2, 2, 2, 2, 3 ),
 ( 0.000000000000000000, 1.000000000000000000 ),
 ( 0.000000000000000000, 0.004166666666666666609, 0.008333333333333333218, 0.01250000000000000069, 0.01666666666666666644, 0.02083333333333333218, 0.02500000000000000139, 0.02916666666666666713, 0.03333333333333333287, 0.03749999999999999861, 0.04166666666666666435, 0.04583333333333333010, 0.05000000000000000278, 0.05416666666666666852, 0.05833333333333333426, 0.06250000000000000000, 0.06666666666666666574, 0.07083333333333333148, 0.07499999999999999722, 0.07916666666666666297, 0.08333333333333332871, 0.08749999999999999445, 0.09166666666666666019, 0.09583333333333333981, 0.1000000000000000056, 0.1041666666666666713, 0.1083333333333333370, 0.1125000000000000028, 0.1166666666666666685, 0.1208333333333333343, 0.1250000000000000000, 0.1291666666666666796, 0.1333333333333333315, 0.1375000000000000111, 0.1416666666666666630, 0.1458333333333333426, 0.1499999999999999944, 0.1541666666666666741, 0.1583333333333333259, 0.1625000000000000056, 0.1666666666666666574, 0.1708333333333333370, 0.1749999999999999889, 0.1791666666666666685, 0.1833333333333333204, 0.1875000000000000000, 0.1916666666666666796, 0.1958333333333333315, 0.2000000000000000111, 0.2041666666666666630, 0.2083333333333333426, 0.2124999999999999944, 0.2166666666666666741, 0.2208333333333333259, 0.2250000000000000056, 0.2291666666666666574, 0.2333333333333333370, 0.2374999999999999889, 0.2416666666666666685, 0.2458333333333333204, 0.2500000000000000000, 0.2541666666666666519, 0.2583333333333333592, 0.2625000000000000111, 0.2666666666666666630, 0.2708333333333333148, 0.2750000000000000222, 0.2791666666666666741, 0.2833333333333333259, 0.2874999999999999778, 0.2916666666666666852, 0.2958333333333333370, 0.2999999999999999889, 0.3041666666666666408, 0.3083333333333333481, 0.3125000000000000000, 0.3166666666666666519, 0.3208333333333333592, 0.3250000000000000111, 0.3291666666666666630, 0.3333333333333333148, 0.3375000000000000222, 0.3416666666666666741, 0.3458333333333333259, 0.3499999999999999778, 0.3541666666666666852, 0.3583333333333333370, 0.3624999999999999889, 0.3666666666666666408, 0.3708333333333333481, 0.3750000000000000000, 0.3791666666666666519, 0.3833333333333333592, 0.3875000000000000111, 0.3916666666666666630, 0.3958333333333333148, 0.4000000000000000222, 0.4041666666666666741, 0.4083333333333333259, 0.4124999999999999778, 0.4166666666666666852, 0.4208333333333333370, 0.4249999999999999889, 0.4291666666666666408, 0.4333333333333333481, 0.4375000000000000000, 0.4416666666666666519, 0.4458333333333333592, 0.4500000000000000111, 0.4541666666666666630, 0.4583333333333333148, 0.4625000000000000222, 0.4666666666666666741, 0.4708333333333333259, 0.4749999999999999778, 0.4791666666666666852, 0.4833333333333333370, 0.4874999999999999889, 0.4916666666666666408, 0.4958333333333333481, 0.5000000000000000000, 0.5041666666666666519, 0.5083333333333333037, 0.5124999999999999556, 0.5166666666666667185, 0.5208333333333333703, 0.5250000000000000222, 0.5291666666666666741, 0.5333333333333333259, 0.5374999999999999778, 0.5416666666666666297, 0.5458333333333332815, 0.5500000000000000444, 0.5541666666666666963, 0.5583333333333333481, 0.5625000000000000000, 0.5666666666666666519, 0.5708333333333333037, 0.5749999999999999556, 0.5791666666666667185, 0.5833333333333333703, 0.5875000000000000222, 0.5916666666666666741, 0.5958333333333333259, 0.5999999999999999778, 0.6041666666666666297, 0.6083333333333332815, 0.6125000000000000444, 0.6166666666666666963, 0.6208333333333333481, 0.6250000000000000000, 0.6291666666666666519, 0.6333333333333333037, 0.6374999999999999556, 0.6416666666666667185, 0.6458333333333333703, 0.6500000000000000222, 0.6541666666666666741, 0.6583333333333333259, 0.6624999999999999778, 0.6666666666666666297, 0.6708333333333332815, 0.6750000000000000444, 0.6791666666666666963, 0.6833333333333333481, 0.6875000000000000000, 0.6916666666666666519, 0.6958333333333333037, 0.6999999999999999556, 0.7041666666666667185, 0.7083333333333333703, 0.7125000000000000222, 0.7166666666666666741, 0.7208333333333333259, 0.7249999999999999778, 0.7291666666666666297, 0.7333333333333332815, 0.7375000000000000444, 0.7416666666666666963, 0.7458333333333333481, 0.7500000000000000000, 0.7541666666666666519, 0.7583333333333333037, 0.7624999999999999556, 0.7666666666666667185, 0.7708333333333333703, 0.7750000000000000222, 0.7791666666666666741, 0.7833333333333333259, 0.7874999999999999778, 0.7916666666666666297, 0.7958333333333332815, 0.8000000000000000444, 0.8041666666666666963, 0.8083333333333333481, 0.8125000000000000000, 0.8166666666666666519, 0.8208333333333333037, 0.8249999999999999556, 0.8291666666666667185, 0.8333333333333333703, 0.8375000000000000222, 0.8416666666666666741, 0.8458333333333333259, 0.8499999999999999778, 0.8541666666666666297, 0.8583333333333332815, 0.8625000000000000444, 0.8666666666666666963, 0.8708333333333333481, 0.8750000000000000000, 0.8791666666666666519, 0.8833333333333333037, 0.8874999999999999556, 0.8916666666666667185, 0.8958333333333333703, 0.9000000000000000222, 0.9041666666666666741, 0.9083333333333333259, 0.9124999999999999778, 0.9166666666666666297, 0.9208333333333332815, 0.9250000000000000444, 0.9291666666666666963, 0.9333333333333333481, 0.9375000000000000000, 0.9416666666666666519, 0.9458333333333333037, 0.9499999999999999556, 0.9541666666666667185, 0.9583333333333333703, 0.9625000000000000222, 0.9666666666666666741, 0.9708333333333333259, 0.9749999999999999778, 0.9791666666666666297, 0.9833333333333332815, 0.9875000000000000444, 0.9916666666666666963, 0.9958333333333333481, 1.000000000000000000 ),
 .UNSPECIFIED. ) 
 GEOMETRIC_REPRESENTATION_ITEM ( )  RATIONAL_B_SPLINE_SURFACE ( (
 ( 1.000000000000000000, 0.8660254037844387076, 1.000000000000000000, 0.8660254037844387076, 1.000000000000000000, 0.8660254037844387076, 1.000000000000000000, 0.8660254037844387076, 1.000000000000000000, 0.8660254037844387076, 1.000000000000000000, 0.8660254037844387076, 1.000000000000000000, 0.8660254037844387076, 1.000000000000000000, 0.8660254037844387076, 1.000000000000000000, 0.8660254037844387076, 1.000000000000000000, 0.8660254037844387076, 1.000000000000000000, 0.8660254037844387076, 1.000000000000000000, 0.8660254037844387076, 1.000000000000000000, 0.8660254037844387076, 1.000000000000000000, 0.8660254037844387076, 1.000000000000000000, 0.8660254037844387076, 1.000000000000000000, 0.8660254037844387076, 1.000000000000000000, 0.8660254037844387076, 1.000000000000000000, 0.8660254037844387076, 1.000000000000000000, 0.8660254037844387076, 1.000000000000000000, 0.8660254037844387076, 1.000000000000000000, 0.8660254037844387076, 1.000000000000000000, 0.8660254037844387076, 1.000000000000000000, 0.8660254037844387076, 1.000000000000000000, 0.8660254037844387076, 1.000000000000000000, 0.8660254037844387076, 1.000000000000000000, 0.8660254037844387076, 1.000000000000000000, 0.8660254037844387076, 1.000000000000000000, 0.8660254037844387076, 1.000000000000000000, 0.8660254037844387076, 1.000000000000000000, 0.8660254037844387076, 1.000000000000000000, 0.8660254037844387076, 1.000000000000000000, 0.8660254037844387076, 1.000000000000000000, 0.8660254037844387076, 1.000000000000000000, 0.8660254037844387076, 1.000000000000000000, 0.8660254037844387076, 1.000000000000000000, 0.8660254037844387076, 1.000000000000000000, 0.8660254037844387076, 1.000000000000000000, 0.8660254037844387076, 1.000000000000000000, 0.8660254037844387076, 1.000000000000000000, 0.8660254037844387076, 1.000000000000000000, 0.8660254037844387076, 1.000000000000000000, 0.8660254037844387076, 1.000000000000000000, 0.8660254037844387076, 1.000000000000000000, 0.8660254037844387076, 1.000000000000000000, 0.8660254037844387076, 1.000000000000000000, 0.8660254037844387076, 1.000000000000000000, 0.8660254037844387076, 1.000000000000000000, 0.8660254037844387076, 1.000000000000000000, 0.8660254037844387076, 1.000000000000000000, 0.8660254037844387076, 1.000000000000000000, 0.8660254037844387076, 1.000000000000000000, 0.8660254037844387076, 1.000000000000000000, 0.8660254037844387076, 1.000000000000000000, 0.8660254037844387076, 1.000000000000000000, 0.8660254037844387076, 1.000000000000000000, 0.8660254037844387076, 1.000000000000000000, 0.8660254037844387076, 1.000000000000000000, 0.8660254037844387076, 1.000000000000000000, 0.8660254037844387076, 1.000000000000000000, 0.8660254037844387076, 1.000000000000000000, 0.8660254037844387076, 1.000000000000000000, 0.8660254037844387076, 1.000000000000000000, 0.8660254037844387076, 1.000000000000000000, 0.8660254037844387076, 1.000000000000000000, 0.8660254037844387076, 1.000000000000000000, 0.8660254037844387076, 1.000000000000000000, 0.8660254037844387076, 1.000000000000000000, 0.8660254037844387076, 1.000000000000000000, 0.8660254037844387076, 1.000000000000000000, 0.8660254037844387076, 1.000000000000000000, 0.8660254037844387076, 1.000000000000000000, 0.8660254037844387076, 1.000000000000000000, 0.8660254037844387076, 1.000000000000000000, 0.8660254037844387076, 1.000000000000000000, 0.8660254037844387076, 1.000000000000000000, 0.8660254037844387076, 1.000000000000000000, 0.8660254037844387076, 1.000000000000000000, 0.8660254037844387076, 1.000000000000000000, 0.8660254037844387076, 1.000000000000000000, 0.8660254037844387076, 1.000000000000000000, 0.8660254037844387076, 1.000000000000000000, 0.8660254037844387076, 1.000000000000000000, 0.8660254037844387076, 1.000000000000000000, 0.8660254037844387076, 1.000000000000000000, 0.8660254037844387076, 1.000000000000000000, 0.8660254037844387076, 1.000000000000000000, 0.8660254037844387076, 1.000000000000000000, 0.8660254037844387076, 1.000000000000000000, 0.8660254037844387076, 1.000000000000000000, 0.8660254037844387076, 1.000000000000000000, 0.8660254037844387076, 1.000000000000000000, 0.8660254037844387076, 1.000000000000000000, 0.8660254037844387076, 1.000000000000000000, 0.8660254037844387076, 1.000000000000000000, 0.8660254037844387076, 1.000000000000000000, 0.8660254037844387076, 1.000000000000000000, 0.8660254037844387076, 1.000000000000000000, 0.8660254037844387076, 1.000000000000000000, 0.8660254037844387076, 1.000000000000000000, 0.8660254037844387076, 1.000000000000000000, 0.8660254037844387076, 1.000000000000000000, 0.8660254037844387076, 1.000000000000000000, 0.8660254037844387076, 1.000000000000000000, 0.8660254037844387076, 1.000000000000000000, 0.8660254037844387076, 1.000000000000000000, 0.8660254037844387076, 1.000000000000000000, 0.8660254037844387076, 1.000000000000000000, 0.8660254037844387076, 1.000000000000000000, 0.8660254037844387076, 1.000000000000000000, 0.8660254037844387076, 1.000000000000000000, 0.8660254037844387076, 1.000000000000000000, 0.8660254037844387076, 1.000000000000000000, 0.8660254037844387076, 1.000000000000000000, 0.8660254037844387076, 1.000000000000000000, 0.8660254037844387076, 1.000000000000000000, 0.8660254037844387076, 1.000000000000000000, 0.8660254037844387076, 1.000000000000000000, 0.8660254037844387076, 1.000000000000000000, 0.8660254037844387076, 1.000000000000000000, 0.8660254037844387076, 1.000000000000000000, 0.8660254037844387076, 1.000000000000000000, 0.8660254037844387076, 1.000000000000000000, 0.8660254037844387076, 1.000000000000000000, 0.8660254037844387076, 1.000000000000000000, 0.8660254037844387076, 1.000000000000000000, 0.8660254037844387076, 1.000000000000000000, 0.8660254037844387076, 1.000000000000000000, 0.8660254037844387076, 1.000000000000000000, 0.8660254037844387076, 1.000000000000000000, 0.8660254037844387076, 1.000000000000000000, 0.8660254037844387076, 1.000000000000000000, 0.8660254037844387076, 1.000000000000000000, 0.8660254037844387076, 1.000000000000000000, 0.8660254037844387076, 1.000000000000000000, 0.8660254037844387076, 1.000000000000000000, 0.8660254037844387076, 1.000000000000000000, 0.8660254037844387076, 1.000000000000000000, 0.8660254037844387076, 1.000000000000000000, 0.8660254037844387076, 1.000000000000000000, 0.8660254037844387076, 1.000000000000000000, 0.8660254037844387076, 1.000000000000000000, 0.8660254037844387076, 1.000000000000000000, 0.8660254037844387076, 1.000000000000000000, 0.8660254037844387076, 1.000000000000000000, 0.8660254037844387076, 1.000000000000000000, 0.8660254037844387076, 1.000000000000000000, 0.8660254037844387076, 1.000000000000000000, 0.8660254037844387076, 1.000000000000000000, 0.8660254037844387076, 1.000000000000000000, 0.8660254037844387076, 1.000000000000000000, 0.8660254037844387076, 1.000000000000000000, 0.8660254037844387076, 1.000000000000000000, 0.8660254037844387076, 1.000000000000000000, 0.8660254037844387076, 1.000000000000000000, 0.8660254037844387076, 1.000000000000000000, 0.8660254037844387076, 1.000000000000000000, 0.8660254037844387076, 1.000000000000000000, 0.8660254037844387076, 1.000000000000000000, 0.8660254037844387076, 1.000000000000000000, 0.8660254037844387076, 1.000000000000000000, 0.8660254037844387076, 1.000000000000000000, 0.8660254037844387076, 1.000000000000000000, 0.8660254037844387076, 1.000000000000000000, 0.8660254037844387076, 1.000000000000000000, 0.8660254037844387076, 1.000000000000000000, 0.8660254037844387076, 1.000000000000000000, 0.8660254037844387076, 1.000000000000000000, 0.8660254037844387076, 1.000000000000000000, 0.8660254037844387076, 1.000000000000000000, 0.8660254037844387076, 1.000000000000000000, 0.8660254037844387076, 1.000000000000000000, 0.8660254037844387076, 1.000000000000000000, 0.8660254037844387076, 1.000000000000000000, 0.8660254037844387076, 1.000000000000000000, 0.8660254037844387076, 1.000000000000000000, 0.8660254037844387076, 1.000000000000000000, 0.8660254037844387076, 1.000000000000000000, 0.8660254037844387076, 1.000000000000000000, 0.8660254037844387076, 1.000000000000000000, 0.8660254037844387076, 1.000000000000000000, 0.8660254037844387076, 1.000000000000000000, 0.8660254037844387076, 1.000000000000000000, 0.8660254037844387076, 1.000000000000000000, 0.8660254037844387076, 1.000000000000000000, 0.8660254037844387076, 1.000000000000000000, 0.8660254037844387076, 1.000000000000000000, 0.8660254037844387076, 1.000000000000000000, 0.8660254037844387076, 1.000000000000000000, 0.8660254037844387076, 1.000000000000000000, 0.8660254037844387076, 1.000000000000000000, 0.8660254037844387076, 1.000000000000000000, 0.8660254037844387076, 1.000000000000000000, 0.8660254037844387076, 1.000000000000000000, 0.8660254037844387076, 1.000000000000000000, 0.8660254037844387076, 1.000000000000000000, 0.8660254037844387076, 1.000000000000000000, 0.8660254037844387076, 1.000000000000000000, 0.8660254037844387076, 1.000000000000000000, 0.8660254037844387076, 1.000000000000000000, 0.8660254037844387076, 1.000000000000000000, 0.8660254037844387076, 1.000000000000000000, 0.8660254037844387076, 1.000000000000000000, 0.8660254037844387076, 1.000000000000000000, 0.8660254037844387076, 1.000000000000000000, 0.8660254037844387076, 1.000000000000000000, 0.8660254037844387076, 1.000000000000000000, 0.8660254037844387076, 1.000000000000000000, 0.8660254037844387076, 1.000000000000000000, 0.8660254037844387076, 1.000000000000000000, 0.8660254037844387076, 1.000000000000000000, 0.8660254037844387076, 1.000000000000000000, 0.8660254037844387076, 1.000000000000000000, 0.8660254037844387076, 1.000000000000000000, 0.8660254037844387076, 1.000000000000000000, 0.8660254037844387076, 1.000000000000000000, 0.8660254037844387076, 1.000000000000000000, 0.8660254037844387076, 1.000000000000000000, 0.8660254037844387076, 1.000000000000000000, 0.8660254037844387076, 1.000000000000000000, 0.8660254037844387076, 1.000000000000000000, 0.8660254037844387076, 1.000000000000000000, 0.8660254037844387076, 1.000000000000000000, 0.8660254037844387076, 1.000000000000000000, 0.8660254037844387076, 1.000000000000000000, 0.8660254037844387076, 1.000000000000000000, 0.8660254037844387076, 1.000000000000000000, 0.8660254037844387076, 1.000000000000000000, 0.8660254037844387076, 1.000000000000000000, 0.8660254037844387076, 1.000000000000000000, 0.8660254037844387076, 1.000000000000000000, 0.8660254037844387076, 1.000000000000000000, 0.8660254037844387076, 1.000000000000000000, 0.8660254037844387076, 1.000000000000000000, 0.8660254037844387076, 1.000000000000000000, 0.8660254037844387076, 1.000000000000000000, 0.8660254037844387076, 1.000000000000000000, 0.8660254037844387076, 1.000000000000000000, 0.8660254037844387076, 1.000000000000000000, 0.8660254037844387076, 1.000000000000000000, 0.8660254037844387076, 1.000000000000000000),
 ( 1.000000000000000000, 0.8660254037844387076, 1.000000000000000000, 0.8660254037844387076, 1.000000000000000000, 0.8660254037844387076, 1.000000000000000000, 0.8660254037844387076, 1.000000000000000000, 0.8660254037844387076, 1.000000000000000000, 0.8660254037844387076, 1.000000000000000000, 0.8660254037844387076, 1.000000000000000000, 0.8660254037844387076, 1.000000000000000000, 0.8660254037844387076, 1.000000000000000000, 0.8660254037844387076, 1.000000000000000000, 0.8660254037844387076, 1.000000000000000000, 0.8660254037844387076, 1.000000000000000000, 0.8660254037844387076, 1.000000000000000000, 0.8660254037844387076, 1.000000000000000000, 0.8660254037844387076, 1.000000000000000000, 0.8660254037844387076, 1.000000000000000000, 0.8660254037844387076, 1.000000000000000000, 0.8660254037844387076, 1.000000000000000000, 0.8660254037844387076, 1.000000000000000000, 0.8660254037844387076, 1.000000000000000000, 0.8660254037844387076, 1.000000000000000000, 0.8660254037844387076, 1.000000000000000000, 0.8660254037844387076, 1.000000000000000000, 0.8660254037844387076, 1.000000000000000000, 0.8660254037844387076, 1.000000000000000000, 0.8660254037844387076, 1.000000000000000000, 0.8660254037844387076, 1.000000000000000000, 0.8660254037844387076, 1.000000000000000000, 0.8660254037844387076, 1.000000000000000000, 0.8660254037844387076, 1.000000000000000000, 0.8660254037844387076, 1.000000000000000000, 0.8660254037844387076, 1.000000000000000000, 0.8660254037844387076, 1.000000000000000000, 0.8660254037844387076, 1.000000000000000000, 0.8660254037844387076, 1.000000000000000000, 0.8660254037844387076, 1.000000000000000000, 0.8660254037844387076, 1.000000000000000000, 0.8660254037844387076, 1.000000000000000000, 0.8660254037844387076, 1.000000000000000000, 0.8660254037844387076, 1.000000000000000000, 0.8660254037844387076, 1.000000000000000000, 0.8660254037844387076, 1.000000000000000000, 0.8660254037844387076, 1.000000000000000000, 0.8660254037844387076, 1.000000000000000000, 0.8660254037844387076, 1.000000000000000000, 0.8660254037844387076, 1.000000000000000000, 0.8660254037844387076, 1.000000000000000000, 0.8660254037844387076, 1.000000000000000000, 0.8660254037844387076, 1.000000000000000000, 0.8660254037844387076, 1.000000000000000000, 0.8660254037844387076, 1.000000000000000000, 0.8660254037844387076, 1.000000000000000000, 0.8660254037844387076, 1.000000000000000000, 0.8660254037844387076, 1.000000000000000000, 0.8660254037844387076, 1.000000000000000000, 0.8660254037844387076, 1.000000000000000000, 0.8660254037844387076, 1.000000000000000000, 0.8660254037844387076, 1.000000000000000000, 0.8660254037844387076, 1.000000000000000000, 0.8660254037844387076, 1.000000000000000000, 0.8660254037844387076, 1.000000000000000000, 0.8660254037844387076, 1.000000000000000000, 0.8660254037844387076, 1.000000000000000000, 0.8660254037844387076, 1.000000000000000000, 0.8660254037844387076, 1.000000000000000000, 0.8660254037844387076, 1.000000000000000000, 0.8660254037844387076, 1.000000000000000000, 0.8660254037844387076, 1.000000000000000000, 0.8660254037844387076, 1.000000000000000000, 0.8660254037844387076, 1.000000000000000000, 0.8660254037844387076, 1.000000000000000000, 0.8660254037844387076, 1.000000000000000000, 0.8660254037844387076, 1.000000000000000000, 0.8660254037844387076, 1.000000000000000000, 0.8660254037844387076, 1.000000000000000000, 0.8660254037844387076, 1.000000000000000000, 0.8660254037844387076, 1.000000000000000000, 0.8660254037844387076, 1.000000000000000000, 0.8660254037844387076, 1.000000000000000000, 0.8660254037844387076, 1.000000000000000000, 0.8660254037844387076, 1.000000000000000000, 0.8660254037844387076, 1.000000000000000000, 0.8660254037844387076, 1.000000000000000000, 0.8660254037844387076, 1.000000000000000000, 0.8660254037844387076, 1.000000000000000000, 0.8660254037844387076, 1.000000000000000000, 0.8660254037844387076, 1.000000000000000000, 0.8660254037844387076, 1.000000000000000000, 0.8660254037844387076, 1.000000000000000000, 0.8660254037844387076, 1.000000000000000000, 0.8660254037844387076, 1.000000000000000000, 0.8660254037844387076, 1.000000000000000000, 0.8660254037844387076, 1.000000000000000000, 0.8660254037844387076, 1.000000000000000000, 0.8660254037844387076, 1.000000000000000000, 0.8660254037844387076, 1.000000000000000000, 0.8660254037844387076, 1.000000000000000000, 0.8660254037844387076, 1.000000000000000000, 0.8660254037844387076, 1.000000000000000000, 0.8660254037844387076, 1.000000000000000000, 0.8660254037844387076, 1.000000000000000000, 0.8660254037844387076, 1.000000000000000000, 0.8660254037844387076, 1.000000000000000000, 0.8660254037844387076, 1.000000000000000000, 0.8660254037844387076, 1.000000000000000000, 0.8660254037844387076, 1.000000000000000000, 0.8660254037844387076, 1.000000000000000000, 0.8660254037844387076, 1.000000000000000000, 0.8660254037844387076, 1.000000000000000000, 0.8660254037844387076, 1.000000000000000000, 0.8660254037844387076, 1.000000000000000000, 0.8660254037844387076, 1.000000000000000000, 0.8660254037844387076, 1.000000000000000000, 0.8660254037844387076, 1.000000000000000000, 0.8660254037844387076, 1.000000000000000000, 0.8660254037844387076, 1.000000000000000000, 0.8660254037844387076, 1.000000000000000000, 0.8660254037844387076, 1.000000000000000000, 0.8660254037844387076, 1.000000000000000000, 0.8660254037844387076, 1.000000000000000000, 0.8660254037844387076, 1.000000000000000000, 0.8660254037844387076, 1.000000000000000000, 0.8660254037844387076, 1.000000000000000000, 0.8660254037844387076, 1.000000000000000000, 0.8660254037844387076, 1.000000000000000000, 0.8660254037844387076, 1.000000000000000000, 0.8660254037844387076, 1.000000000000000000, 0.8660254037844387076, 1.000000000000000000, 0.8660254037844387076, 1.000000000000000000, 0.8660254037844387076, 1.000000000000000000, 0.8660254037844387076, 1.000000000000000000, 0.8660254037844387076, 1.000000000000000000, 0.8660254037844387076, 1.000000000000000000, 0.8660254037844387076, 1.000000000000000000, 0.8660254037844387076, 1.000000000000000000, 0.8660254037844387076, 1.000000000000000000, 0.8660254037844387076, 1.000000000000000000, 0.8660254037844387076, 1.000000000000000000, 0.8660254037844387076, 1.000000000000000000, 0.8660254037844387076, 1.000000000000000000, 0.8660254037844387076, 1.000000000000000000, 0.8660254037844387076, 1.000000000000000000, 0.8660254037844387076, 1.000000000000000000, 0.8660254037844387076, 1.000000000000000000, 0.8660254037844387076, 1.000000000000000000, 0.8660254037844387076, 1.000000000000000000, 0.8660254037844387076, 1.000000000000000000, 0.8660254037844387076, 1.000000000000000000, 0.8660254037844387076, 1.000000000000000000, 0.8660254037844387076, 1.000000000000000000, 0.8660254037844387076, 1.000000000000000000, 0.8660254037844387076, 1.000000000000000000, 0.8660254037844387076, 1.000000000000000000, 0.8660254037844387076, 1.000000000000000000, 0.8660254037844387076, 1.000000000000000000, 0.8660254037844387076, 1.000000000000000000, 0.8660254037844387076, 1.000000000000000000, 0.8660254037844387076, 1.000000000000000000, 0.8660254037844387076, 1.000000000000000000, 0.8660254037844387076, 1.000000000000000000, 0.8660254037844387076, 1.000000000000000000, 0.8660254037844387076, 1.000000000000000000, 0.8660254037844387076, 1.000000000000000000, 0.8660254037844387076, 1.000000000000000000, 0.8660254037844387076, 1.000000000000000000, 0.8660254037844387076, 1.000000000000000000, 0.8660254037844387076, 1.000000000000000000, 0.8660254037844387076, 1.000000000000000000, 0.8660254037844387076, 1.000000000000000000, 0.8660254037844387076, 1.000000000000000000, 0.8660254037844387076, 1.000000000000000000, 0.8660254037844387076, 1.000000000000000000, 0.8660254037844387076, 1.000000000000000000, 0.8660254037844387076, 1.000000000000000000, 0.8660254037844387076, 1.000000000000000000, 0.8660254037844387076, 1.000000000000000000, 0.8660254037844387076, 1.000000000000000000, 0.8660254037844387076, 1.000000000000000000, 0.8660254037844387076, 1.000000000000000000, 0.8660254037844387076, 1.000000000000000000, 0.8660254037844387076, 1.000000000000000000, 0.8660254037844387076, 1.000000000000000000, 0.8660254037844387076, 1.000000000000000000, 0.8660254037844387076, 1.000000000000000000, 0.8660254037844387076, 1.000000000000000000, 0.8660254037844387076, 1.000000000000000000, 0.8660254037844387076, 1.000000000000000000, 0.8660254037844387076, 1.000000000000000000, 0.8660254037844387076, 1.000000000000000000, 0.8660254037844387076, 1.000000000000000000, 0.8660254037844387076, 1.000000000000000000, 0.8660254037844387076, 1.000000000000000000, 0.8660254037844387076, 1.000000000000000000, 0.8660254037844387076, 1.000000000000000000, 0.8660254037844387076, 1.000000000000000000, 0.8660254037844387076, 1.000000000000000000, 0.8660254037844387076, 1.000000000000000000, 0.8660254037844387076, 1.000000000000000000, 0.8660254037844387076, 1.000000000000000000, 0.8660254037844387076, 1.000000000000000000, 0.8660254037844387076, 1.000000000000000000, 0.8660254037844387076, 1.000000000000000000, 0.8660254037844387076, 1.000000000000000000, 0.8660254037844387076, 1.000000000000000000, 0.8660254037844387076, 1.000000000000000000, 0.8660254037844387076, 1.000000000000000000, 0.8660254037844387076, 1.000000000000000000, 0.8660254037844387076, 1.000000000000000000, 0.8660254037844387076, 1.000000000000000000, 0.8660254037844387076, 1.000000000000000000, 0.8660254037844387076, 1.000000000000000000, 0.8660254037844387076, 1.000000000000000000, 0.8660254037844387076, 1.000000000000000000, 0.8660254037844387076, 1.000000000000000000, 0.8660254037844387076, 1.000000000000000000, 0.8660254037844387076, 1.000000000000000000, 0.8660254037844387076, 1.000000000000000000, 0.8660254037844387076, 1.000000000000000000, 0.8660254037844387076, 1.000000000000000000, 0.8660254037844387076, 1.000000000000000000, 0.8660254037844387076, 1.000000000000000000, 0.8660254037844387076, 1.000000000000000000, 0.8660254037844387076, 1.000000000000000000, 0.8660254037844387076, 1.000000000000000000, 0.8660254037844387076, 1.000000000000000000, 0.8660254037844387076, 1.000000000000000000, 0.8660254037844387076, 1.000000000000000000, 0.8660254037844387076, 1.000000000000000000, 0.8660254037844387076, 1.000000000000000000, 0.8660254037844387076, 1.000000000000000000, 0.8660254037844387076, 1.000000000000000000, 0.8660254037844387076, 1.000000000000000000, 0.8660254037844387076, 1.000000000000000000, 0.8660254037844387076, 1.000000000000000000, 0.8660254037844387076, 1.000000000000000000, 0.8660254037844387076, 1.000000000000000000, 0.8660254037844387076, 1.000000000000000000, 0.8660254037844387076, 1.000000000000000000, 0.8660254037844387076, 1.000000000000000000, 0.8660254037844387076, 1.000000000000000000) ) ) 
 REPRESENTATION_ITEM ( '' )  SURFACE ( )  );
#130299=CARTESIAN_POINT ( 'NONE',  ( -5.253948220495577637, 6.088359997788290734, 1.199719254218450271 ) ) ;
#130303=CARTESIAN_POINT ( 'NONE',  ( -1.201851678989727383E-14, 4.337500000000023448, -1.732050807568863648 ) ) ;
#130311=CARTESIAN_POINT ( 'NONE',  ( -0.6823417656250246877, -1.198958332991911790, 1.181850606188755259 ) ) ;
#130313=CARTESIAN_POINT ( 'NONE',  ( 6.148786358997489820, 7.132337826040578754, -1.199719254218446718 ) ) ;
#130314=CARTESIAN_POINT ( 'NONE',  ( -7.018317073368468328, 11.33978701890523233, -0.7998128361456291469 ) ) ;
#130316=CARTESIAN_POINT ( 'NONE',  ( 9.297140650669039275, 11.86975006391249643, 1.599625672291281386 ) ) ;
#130321=CARTESIAN_POINT ( 'NONE',  ( 1.499999999999990896, 5.775000000000023448, 1.040834085586084257E-14 ) ) ;
#130325=CARTESIAN_POINT ( 'NONE',  ( 4.324687812634882000, 7.028924300507257250, 1.082531754730558626 ) ) ;
#130329=CARTESIAN_POINT ( 'NONE',  ( 6.751597309925441159, 9.860318714012938912, -1.082531754730537088 ) ) ;
#130334=CARTESIAN_POINT ( 'NONE',  ( -1.001543065824772872E-14, 4.493750000682820378, 1.732050807568877637 ) ) ;
#130336=CARTESIAN_POINT ( 'NONE',  ( -4.762992037102518950, 4.451245552908022596, -0.7998128361456221525 ) ) ;
#130337=CARTESIAN_POINT ( 'NONE',  ( 5.287316719205157334, 9.112360572473935605, 1.040834085586084257E-14 ) ) ;
#130338=CARTESIAN_POINT ( 'NONE',  ( -10.42585693878457853, 11.26584730477792284, -0.7216878364870267237 ) ) ;
#130345=CARTESIAN_POINT ( 'NONE',  ( 4.196412238629597447, 4.854568018944682706, -1.199719254218452047 ) ) ;
#130346=CARTESIAN_POINT ( 'NONE',  ( 1.499999999999990896, 3.806250000682819046, 1.214306433183764966E-14 ) ) ;
#130347=CARTESIAN_POINT ( 'NONE',  ( 2.295757763869426871, 5.519548059767960702, 0.4031905389056070765 ) ) ;
#130362=CARTESIAN_POINT ( 'NONE',  ( 8.860417081730671995, 10.29590700256267155, 1.199719254218453823 ) ) ;
#130364=CARTESIAN_POINT ( 'NONE',  ( 0.000000000000000000, 2.880000000000021210, 1.214306433183764966E-14 ) ) ;
#130366=CARTESIAN_POINT ( 'NONE',  ( 0.6823417656249882723, 0.4260416670080896528, -1.181850606188749264 ) ) ;
#130367=CARTESIAN_POINT ( 'NONE',  ( 5.843201017809841247, 5.919415396974013532, 1.040834085586084257E-14 ) ) ;
#130368=CARTESIAN_POINT ( 'NONE',  ( -8.459924665247381625, 11.85336729522185806, 1.082531754730560403 ) ) ;
#130374=CARTESIAN_POINT ( 'NONE',  ( -4.776550190716183586, 4.467063398790632966, 1.214306433183764966E-14 ) ) ;
#130387=CARTESIAN_POINT ( 'NONE',  ( 5.693912546396379781, 6.288398852508453096, -1.088204328156989087 ) ) ;
#130390=CARTESIAN_POINT ( 'NONE',  ( 5.172599298813543633, 5.993452922492633839, -1.199719254218452047 ) ) ;
#130395=CARTESIAN_POINT ( 'NONE',  ( -8.568389894156720032, 10.05917163368005163, 1.082531754730558626 ) ) ;
#130400=CARTESIAN_POINT ( 'NONE',  ( 7.623762449586013901, 7.788811034138823253, 1.040834085586084257E-14 ) ) ;
#130402=CARTESIAN_POINT ( 'NONE',  ( -4.894657149733403045, 5.669187081899118574, -1.199719254218446718 ) ) ;
#130406=CARTESIAN_POINT ( 'NONE',  ( -4.076197739202962467, 7.907314462378773001, 1.040834085586084257E-14 ) ) ;
#130409=CARTESIAN_POINT ( 'NONE',  ( -5.850506979496850057, 6.784345216623154151, -1.199719254218446718 ) ) ;
#130412=CARTESIAN_POINT ( 'NONE',  ( 8.914649696185335870, 10.35917838609310593, -1.199719254218446718 ) ) ;
#130413=DIRECTION ( 'NONE',  ( -5.578564026256490882E-16, -1.000000000000000000, -9.066213480720158442E-32 ) ) ;
#130416=CARTESIAN_POINT ( 'NONE',  ( 4.326045746746942200, 7.429495238844160632, 1.107669923005821344 ) ) ;
#130417=CARTESIAN_POINT ( 'NONE',  ( 3.850152436600926542, 7.435668909435648288, -0.7216878364870197293 ) ) ;
#130426=CARTESIAN_POINT ( 'NONE',  ( 8.256552360598020002, 8.734991963560254646, -0.7216878364870267237 ) ) ;
#130429=CARTESIAN_POINT ( 'NONE',  ( -9.484092147959342967, 11.02352791316275216, 1.199719254218462483 ) ) ;
#130430=CARTESIAN_POINT ( 'NONE',  ( -7.877450944739929461, 9.149113176073413456, 1.199719254218462483 ) ) ;
#130437=CARTESIAN_POINT ( 'NONE',  ( 9.511208455186636712, 11.05516360492796935, 1.199719254218453823 ) ) ;
#130441=CARTESIAN_POINT ( 'NONE',  ( 3.225950485047770933, 5.851027101609320269, 1.199719254218450271 ) ) ;
#130444=CARTESIAN_POINT ( 'NONE',  ( -4.199533704925234368, 7.510932310329544670, -0.9222493318717175370 ) ) ;
#130450=CARTESIAN_POINT ( 'NONE',  ( 0.7499999999999902300, 2.983333333333351600, 1.299038105676669330 ) ) ;
#130451=CARTESIAN_POINT ( 'NONE',  ( 6.474182045725470402, 7.511966127223233869, -1.199719254218446718 ) ) ;
#130453=CARTESIAN_POINT ( 'NONE',  ( 1.499999999999970912, 4.795833333333354709, -0.8660254037844417052 ) ) ;
#130454=CARTESIAN_POINT ( 'NONE',  ( 6.317736394288122170, 10.31451686007074997, 0.7216878364870438212 ) ) ;
#130455=CARTESIAN_POINT ( 'NONE',  ( 0.07118442604959854259, 7.078193277237673442, 2.121339347286374633 ) ) ;
#130458=CARTESIAN_POINT ( 'NONE',  ( 9.297140650669039275, 11.86975006391249643, 1.599625672291281386 ) ) ;
#130460=CARTESIAN_POINT ( 'NONE',  ( -4.711622075948912247, 5.455646162483875017, -1.199719254218446718 ) ) ;
#130461=CARTESIAN_POINT ( 'NONE',  ( -0.7500000000000215383, 4.722916667349482012, 1.299038105676671107 ) ) ;
#130462=CARTESIAN_POINT ( 'NONE',  ( -1.364683531250014514, -0.2614583329919080157, -0.7879004041258359514 ) ) ;
#130466=CARTESIAN_POINT ( 'NONE',  ( 4.708759422647839976, 4.387974169377582001, -0.7998128361456211532 ) ) ;
#130468=CARTESIAN_POINT ( 'NONE',  ( 0.6823417656249917140, 5.405208333674749177, 1.181850606188765695 ) ) ;
#130470=DIRECTION ( 'NONE',  ( 5.578564026256491869E-16, 1.000000000000000000, 9.066213480720160632E-32 ) ) ;
#130476=CARTESIAN_POINT ( 'NONE',  ( -6.581593504430098385, 9.765943957555402122, -1.199719254218440723 ) ) ;
#130478=( BOUNDED_CURVE ( )  B_SPLINE_CURVE ( 2, ( #154896, #6478, #123550, #21643, #137588 ),
 .UNSPECIFIED., .F., .T. ) 
 B_SPLINE_CURVE_WITH_KNOTS ( ( 3, 2, 3 ),
 ( 0.1116300932268863011, 0.1125000000000000028, 0.1135379806157290478 ),
 .UNSPECIFIED. ) 
 CURVE ( )  GEOMETRIC_REPRESENTATION_ITEM ( )  RATIONAL_B_SPLINE_CURVE ( ( 0.9557375992086956096, 0.9720291019184583714, 1.000000000000000000, 0.9666248718707491916, 0.9498782570434034511 ) ) 
 REPRESENTATION_ITEM ( '' )  );
#130480=CARTESIAN_POINT ( 'NONE',  ( 5.518332215962025167, 6.396807992499198292, -1.199719254218445830 ) ) ;
#130485=CARTESIAN_POINT ( 'NONE',  ( 0.6823417656249882723, 0.09270833367475139752, 1.181850606188755259 ) ) ;
#130490=CARTESIAN_POINT ( 'NONE',  ( 10.57266086055835075, 11.22919251360659310, 0.000000000000000000 ) ) ;
#130493=CARTESIAN_POINT ( 'NONE',  ( -5.880485940025243607, 7.883652901494672349, 1.599625672291269396 ) ) ;
#130497=CARTESIAN_POINT ( 'NONE',  ( 8.809047120577066181, 11.30030761213851953, 1.599625672291281386 ) ) ;
#130499=CARTESIAN_POINT ( 'NONE',  ( 7.456094412511537151, 10.78619501698377370, 1.199719254218460707 ) ) ;
#130501=CARTESIAN_POINT ( 'NONE',  ( -8.026063749610043985, 12.30756544127966912, -0.7216878364870267237 ) ) ;
#130502=CARTESIAN_POINT ( 'NONE',  ( -6.669721502918952716, 9.868759955792373972, 1.199719254218452047 ) ) ;
#130505=CARTESIAN_POINT ( 'NONE',  ( -4.027792083363366693, 7.778134382787397882, 0.5015608049221946807 ) ) ;
#130506=CARTESIAN_POINT ( 'NONE',  ( 0.6823417656249882723, 0.3427083336747516196, 1.181850606188755259 ) ) ;
#130510=CARTESIAN_POINT ( 'NONE',  ( 7.795575138177731844, 8.197185204069915798, 1.040834085586084257E-14 ) ) ;
#130526=CARTESIAN_POINT ( 'NONE',  ( -4.911894908834722351, 4.738238661368090021, 0.4458799699701230246 ) ) ;
#130530=CARTESIAN_POINT ( 'NONE',  ( -4.089755892816631544, 7.923132308261379819, -0.7998128361456281477 ) ) ;
#130531=CARTESIAN_POINT ( 'NONE',  ( -6.333630315878337136, 10.54098580183340772, 0.000000000000000000 ) ) ;
#130537=CARTESIAN_POINT ( 'NONE',  ( -0.7500000000000215383, 3.472916667349487785, 1.299038105676671107 ) ) ;
#130538=CARTESIAN_POINT ( 'NONE',  ( 7.228468454380276853, 11.58496363008569574, 1.040834085586084257E-14 ) ) ;
#130541=CARTESIAN_POINT ( 'NONE',  ( -7.655550293210764856, 12.08322577538792331, 0.000000000000000000 ) ) ;
#130543=CARTESIAN_POINT ( 'NONE',  ( 0.6823417656249882723, 2.926041667008084879, -1.181850606188754593 ) ) ;
#130549=CARTESIAN_POINT ( 'NONE',  ( -10.30383355670593737, 11.12348669235284504, -0.7216878364870267237 ) ) ;
#130553=CARTESIAN_POINT ( 'NONE',  ( -1.364683531250014514, 1.801041667008085767, -0.7879004041258289570 ) ) ;
#130560=CARTESIAN_POINT ( 'NONE',  ( -1.402160292154681736E-14, 2.446875000341416584, -1.575800808251660134 ) ) ;
#130562=CARTESIAN_POINT ( 'NONE',  ( -6.084912014434944894, 5.993485526462540847, -0.7998128361456291469 ) ) ;
#130563=CARTESIAN_POINT ( 'NONE',  ( 7.721532178182734185, 8.967207948423393304, 1.199719254218462483 ) ) ;
#130566=CARTESIAN_POINT ( 'NONE',  ( -1.201851678989727383E-14, 3.384375000341421469, 1.575800808251672791 ) ) ;
#130572=CARTESIAN_POINT ( 'NONE',  ( -6.073689629242176480, 6.188318776978391611, -0.7216878364870278340 ) ) ;
#130575=CARTESIAN_POINT ( 'NONE',  ( 4.148431816101584957, 6.823292304551739740, -1.082531754730548412 ) ) ;
#130578=CARTESIAN_POINT ( 'NONE',  ( -7.283754839039664475, 9.520799950344851936, -1.599625672291263179 ) ) ;
#130579=CARTESIAN_POINT ( 'NONE',  ( -4.613852347352193739, 4.277249248199312071, 1.214306433183764966E-14 ) ) ;
#130581=CARTESIAN_POINT ( 'NONE',  ( -1.364683531250010295, 5.238541667008086655, -0.7879004041258300672 ) ) ;
#130586=CARTESIAN_POINT ( 'NONE',  ( -5.816084710138169633, 8.768887347594400694, 1.082531754730548412 ) ) ;
#130588=CARTESIAN_POINT ( 'NONE',  ( -1.402160292154681736E-14, -1.115624999658584082, 1.575800808251672791 ) ) ;
#130592=CARTESIAN_POINT ( 'NONE',  ( 6.155038550924139429, 9.164333495178082600, 1.082531754730558626 ) ) ;
#130601=CARTESIAN_POINT ( 'NONE',  ( 9.544576953896278582, 10.23768732240824164, 0.000000000000000000 ) ) ;
#130608=CARTESIAN_POINT ( 'NONE',  ( 5.774883364416965037, 8.824782127540085952, -1.199719254218440723 ) ) ;
#130609=CARTESIAN_POINT ( 'NONE',  ( -3.093231602212184850, 6.760520635889515795, -0.7998128361456281477 ) ) ;
#130612=CARTESIAN_POINT ( 'NONE',  ( 6.114364089638795186, 7.196141528409145671, 1.082531754730558626 ) ) ;
#130613=CARTESIAN_POINT ( 'NONE',  ( 1.364683531249986537, 0.4677083336747514530, -0.7879004041258309554 ) ) ;
#130615=CARTESIAN_POINT ( 'NONE',  ( -7.811469059767924605, 12.26513100303794168, -0.7998128361456281477 ) ) ;
#130624=ORIENTED_EDGE ( 'NONE', *, *, #69865, .T. ) ;
#130633=CARTESIAN_POINT ( 'NONE',  ( 7.630541526392844887, 7.796719957080126662, 0.7998128361456341429 ) ) ;
#130642=CARTESIAN_POINT ( 'NONE',  ( 10.39640486358069360, 11.02356051713265650, 0.7998128361456462443 ) ) ;
#130645=CARTESIAN_POINT ( 'NONE',  ( -2.656508033273816238, 5.186677574539687363, -1.199719254218446718 ) ) ;
#130648=DIRECTION ( 'NONE',  ( -5.578564026256490882E-16, -1.000000000000000000, -9.066213480720158442E-32 ) ) ;
#130650=CARTESIAN_POINT ( 'NONE',  ( 0.006913841192817556623, 8.234242197375175820, 1.999988128101762408 ) ) ;
#130656=CARTESIAN_POINT ( 'NONE',  ( -8.012505595996376684, 12.29174759539704986, 0.000000000000000000 ) ) ;
#130661=CARTESIAN_POINT ( 'NONE',  ( 5.392392409933256303, 7.314210449720692786, 1.599625672291267398 ) ) ;
#130662=CARTESIAN_POINT ( 'NONE',  ( -0.6823417656249969321, 5.467708333674756283, -1.181850606188749264 ) ) ;
#130669=CARTESIAN_POINT ( 'NONE',  ( 5.300874872818840622, 6.247070775452521652, 1.082531754730560403 ) ) ;
#130676=CARTESIAN_POINT ( 'NONE',  ( -6.181627972826976958, 9.299317504018391745, 1.199719254218452047 ) ) ;
#130677=CARTESIAN_POINT ( 'NONE',  ( -3.761497552787613330, 6.475832013972435242, 1.199719254218464037 ) ) ;
#130678=CARTESIAN_POINT ( 'NONE',  ( -0.9999999999999965583, 6.120000000000022311, 1.226552901175238481E-14 ) ) ;
#130682=CARTESIAN_POINT ( 'NONE',  ( -1.201851678989727383E-14, 2.962500000000025224, 1.732050807568877637 ) ) ;
#130686=CARTESIAN_POINT ( 'NONE',  ( 6.810273232766058449, 6.839740281182199233, 1.040834085586084257E-14 ) ) ;
#130693=CARTESIAN_POINT ( 'NONE',  ( -1.270904146967334336, 2.959693569853255823, 0.7750000000000152323 ) ) ;
#130697=CARTESIAN_POINT ( 'NONE',  ( -1.402160292154681736E-14, 0.1343750003414218575, 1.575800808251672791 ) ) ;
#130698=CARTESIAN_POINT ( 'NONE',  ( 2.333974999846879061, 5.874721266463329705, -0.7998128361456291469 ) ) ;
#130699=CARTESIAN_POINT ( 'NONE',  ( 3.683011284406639607, 7.448596931783069586, 0.7998128361456321445 ) ) ;
#130702=CARTESIAN_POINT ( 'NONE',  ( -7.876924059859742755, 8.292092279365579799, 1.040834085586084257E-14 ) ) ;
#130704=CARTESIAN_POINT ( 'NONE',  ( 3.687454593236936251, 7.245854758844324728, -0.7216878364870267237 ) ) ;
#130705=CARTESIAN_POINT ( 'NONE',  ( -6.521108698048772467, 9.591415333490143524, -1.082531754730537976 ) ) ;
#130709=CARTESIAN_POINT ( 'NONE',  ( 7.558834334818744338, 8.777393797832065303, 1.199719254218462483 ) ) ;
#130713=CARTESIAN_POINT ( 'NONE',  ( -5.599154252763867134, 5.634694171087028636, 0.000000000000000000 ) ) ;
#130714=CARTESIAN_POINT ( 'NONE',  ( -0.6823417656249969321, 3.717708333674754506, -1.181850606188749264 ) ) ;
#130718=CARTESIAN_POINT ( 'NONE',  ( 8.471147050440139381, 8.777426401801974976, -0.7998128361456281477 ) ) ;
#130721=CARTESIAN_POINT ( 'NONE',  ( -7.771848369131641121, 10.09024240211882351, -1.599625672291263179 ) ) ;
#130727=CARTESIAN_POINT ( 'NONE',  ( 9.901532256681887745, 10.44620914241737530, 0.000000000000000000 ) ) ;
#130729=CARTESIAN_POINT ( 'NONE',  ( -8.503988664269602538, 10.94440607977979063, 1.599625672291269396 ) ) ;
#130730=DIRECTION ( 'NONE',  ( -0.6507913734559640506, -0.7592566023653004592, 0.000000000000000000 ) ) ;
#130732=CARTESIAN_POINT ( 'NONE',  ( 4.540820729390463661, 6.975461451583557348, -1.175308324676842542 ) ) ;
#130733=CARTESIAN_POINT ( 'NONE',  ( -9.408995418203979000, 12.00024729270324286, 1.443375672974076540 ) ) ;
#130738=CARTESIAN_POINT ( 'NONE',  ( 4.625302960556422427, 8.547937220624488575, 1.040834085586084257E-14 ) ) ;
#130740=CARTESIAN_POINT ( 'NONE',  ( 5.229694566569264680, 7.124396299129368337, 1.599625672291267398 ) ) ;
#130741=CARTESIAN_POINT ( 'NONE',  ( -4.264599663924041550, 7.301641052403419430, 0.9184948912712449509 ) ) ;
#130742=CARTESIAN_POINT ( 'NONE',  ( 4.708759422647839976, 4.387974169377582001, -0.7998128361456211532 ) ) ;
#130744=CARTESIAN_POINT ( 'NONE',  ( -6.724481002698126098, 8.868313807946373473, -1.443375672974059665 ) ) ;
#130750=CARTESIAN_POINT ( 'NONE',  ( -4.789689200157987159, 6.785576372466274542, 1.244997348908165602 ) ) ;
#130751=CARTESIAN_POINT ( 'NONE',  ( -0.6823417656250246877, -0.3864583329919110688, 1.181850606188755259 ) ) ;
#130754=CARTESIAN_POINT ( 'NONE',  ( 3.985733972737593778, 6.633478153960411738, -1.082531754730548412 ) ) ;
#130755=CARTESIAN_POINT ( 'NONE',  ( -1.499999999999997780, 3.681250000682819046, 1.214306433183764966E-14 ) ) ;
#130758=CARTESIAN_POINT ( 'NONE',  ( -9.639484029191951464, 10.34841224358651601, 0.7216878364870438212 ) ) ;
#130763=CARTESIAN_POINT ( 'NONE',  ( -8.961576348508637935, 12.43862759236002269, -1.082531754730543083 ) ) ;
#130770=CARTESIAN_POINT ( 'NONE',  ( -8.853111119599343937, 10.39134639669645566, 1.082531754730558626 ) ) ;
#130774=CARTESIAN_POINT ( 'NONE',  ( 1.364683531249990311, 4.676041667008083103, 0.7879004041258500513 ) ) ;
#130775=CARTESIAN_POINT ( 'NONE',  ( -1.500000000000011324, 2.952083334016149418, 0.8660254037844403729 ) ) ;
#130779=APPLICATION_CONTEXT ( 'automotive_design' ) ;
#130781=CARTESIAN_POINT ( 'NONE',  ( -7.320512876374914768, 10.62801655815766999, 1.199719254218453823 ) ) ;
#130784=CARTESIAN_POINT ( 'NONE',  ( 4.788000803920411386, 8.737751371215816576, 1.040834085586084257E-14 ) ) ;
#130790=CARTESIAN_POINT ( 'NONE',  ( 7.099665995050449041, 11.43469409420089455, 0.7998128361456462443 ) ) ;
#130793=CARTESIAN_POINT ( 'NONE',  ( 4.161989969715248705, 4.726297878971393196, -2.500000000000000444 ) ) ;
#130797=CARTESIAN_POINT ( 'NONE',  ( -5.422898255786186006, 9.270539031818461950, -0.7216878364870207285 ) ) ;
#130802=CARTESIAN_POINT ( 'NONE',  ( -0.6823417656250212460, 5.613541667008087543, 1.181850606188767472 ) ) ;
#130806=CARTESIAN_POINT ( 'NONE',  ( -7.334597915313094241, 9.580116872663850813, 1.040834085586084257E-14 ) ) ;
#130810=CARTESIAN_POINT ( 'NONE',  ( -9.480175724453545172, 12.08329098332774265, 1.599625672291281386 ) ) ;
#130812=CARTESIAN_POINT ( 'NONE',  ( 7.072549687823125097, 11.40305840243567381, -0.7998128361456291469 ) ) ;
#130814=CARTESIAN_POINT ( 'NONE',  ( -8.143643823302737061, 12.65266822716189843, 0.000000000000000000 ) ) ;
#130817=CARTESIAN_POINT ( 'NONE',  ( -0.6823417656250003738, 2.217708333674753174, -1.181850606188749264 ) ) ;
#130818=CARTESIAN_POINT ( 'NONE',  ( 2.171277156482887882, 5.684907115872006145, -0.7998128361456291469 ) ) ;
#130822=CARTESIAN_POINT ( 'NONE',  ( 3.469446951953614189E-15, 8.900000000000025224, 1.214306433183764966E-14 ) ) ;
#130823=CARTESIAN_POINT ( 'NONE',  ( 8.378575743120986630, 12.71882943370911789, 1.040834085586084257E-14 ) ) ;
#130825=CARTESIAN_POINT ( 'NONE',  ( -6.561783159334121152, 10.59923808595773664, -0.7216878364870278340 ) ) ;
#130826=CARTESIAN_POINT ( 'NONE',  ( 0.6823417656249882723, 0.4260416670080896528, -1.181850606188749264 ) ) ;
#130828=CARTESIAN_POINT ( 'NONE',  ( 0.2828007905113860132, 7.102855049428861811, 1.981079112686755517 ) ) ;
#130830=CARTESIAN_POINT ( 'NONE',  ( -8.128276786592724790, 9.441743324901704426, -1.199719254218446718 ) ) ;
#130831=CARTESIAN_POINT ( 'NONE',  ( -4.460269348771590536, 5.266364330730674226, 1.082531754730558626 ) ) ;
#130832=CARTESIAN_POINT ( 'NONE',  ( 1.364683531249988535, 3.926041667008087543, 0.7879004041258500513 ) ) ;
#130837=CIRCLE ( 'NONE', #85780, 0.08000000000000020983 ) ;
#130842=ORIENTED_EDGE ( 'NONE', *, *, #101284, .F. ) ;
#130846=DIRECTION ( 'NONE',  ( 0.000000000000000000, -0.7996470168499970610, 0.6004703560067728985 ) ) ;
#130848=CARTESIAN_POINT ( 'NONE',  ( -1.364683531250010295, 4.342708333674753618, 0.7879004041258379498 ) ) ;
#130854=CARTESIAN_POINT ( 'NONE',  ( 9.284636267260101050, 9.726497154758602548, -0.7998128361456281477 ) ) ;
#130857=CARTESIAN_POINT ( 'NONE',  ( -1.364683531249997417, 2.759375000341422801, 1.214306433183764966E-14 ) ) ;
#130858=CARTESIAN_POINT ( 'NONE',  ( -6.236387472606145010, 9.259240570473746601, -1.082531754730538864 ) ) ;
#130864=CARTESIAN_POINT ( 'NONE',  ( 5.217190183160311356, 4.981143389975473568, -0.7998128361456211532 ) ) ;
#130867=CARTESIAN_POINT ( 'NONE',  ( 9.887974103068218668, 10.43039129653476493, 0.7998128361456462443 ) ) ;
#130877=CARTESIAN_POINT ( 'NONE',  ( -3.810004860640155311, 4.403759411290286252, 1.199719254218462483 ) ) ;
#130878=CARTESIAN_POINT ( 'NONE',  ( 8.145751363712157911, 8.397798100619326078, -0.7998128361456281477 ) ) ;
#130880=CARTESIAN_POINT ( 'NONE',  ( 4.406036734316882253, 6.163462161501577441, -1.443375672974051449 ) ) ;
#130890=CARTESIAN_POINT ( 'NONE',  ( -7.429504990608782222, 8.730472579540773381, 1.082531754730549967 ) ) ;
#130891=CARTESIAN_POINT ( 'NONE',  ( 5.172599298813543633, 5.993452922492633839, -1.199719254218452047 ) ) ;
#130894=CARTESIAN_POINT ( 'NONE',  ( -8.345207244411405156, 9.694828859023472134, 1.199719254218462483 ) ) ;
#130900=CARTESIAN_POINT ( 'NONE',  ( -8.513630394377489807, 12.01998699582738972, -1.199719254218446718 ) ) ;
#130901=CARTESIAN_POINT ( 'NONE',  ( 3.701012746850603996, 7.261672604726938651, 1.040834085586084257E-14 ) ) ;
#130904=CARTESIAN_POINT ( 'NONE',  ( 7.235247531187115833, 11.59287255302699648, -0.7998128361456291469 ) ) ;
#130905=CARTESIAN_POINT ( 'NONE',  ( 6.661133543015731462, 6.665743976473484267, -0.7998128361456281477 ) ) ;
#130912=CARTESIAN_POINT ( 'NONE',  ( 3.714570900464285064, 4.396382807705524698, 1.082531754730560403 ) ) ;
#130916=CARTESIAN_POINT ( 'NONE',  ( -8.158255747121117452, 10.54105100977322174, 1.599625672291295375 ) ) ;
#130920=CARTESIAN_POINT ( 'NONE',  ( 7.944714827928050838, 9.331550723079971021, 1.082531754730558626 ) ) ;
#130922=CARTESIAN_POINT ( 'NONE',  ( 2.822068529938852155, 6.444163718237301275, -0.7998128361456291469 ) ) ;
#130924=CARTESIAN_POINT ( 'NONE',  ( 5.515469562660962666, 5.329135999392899947, 0.7998128361456341429 ) ) ;
#130926=CARTESIAN_POINT ( 'NONE',  ( -5.575427483717760424, 7.527751369135936343, 1.599625672291269396 ) ) ;
#130929=( BOUNDED_CURVE ( )  B_SPLINE_CURVE ( 1, ( #143889, #13819 ),
 .UNSPECIFIED., .F., .T. ) 
 B_SPLINE_CURVE_WITH_KNOTS ( ( 2, 2 ),
 ( 0.000000000000000000, 6.249999999999788711E-05 ),
 .UNSPECIFIED. ) 
 CURVE ( )  GEOMETRIC_REPRESENTATION_ITEM ( )  RATIONAL_B_SPLINE_CURVE ( ( 0.9345202395942815432, 0.9345202395942815432 ) ) 
 REPRESENTATION_ITEM ( '' )  );
#130930=VECTOR ( 'NONE', #96248, 1000.000000000000000 ) ;
#130937=CARTESIAN_POINT ( 'NONE',  ( 1.364683531249990311, 4.446875000341417028, 1.214306433183764966E-14 ) ) ;
#130938=CARTESIAN_POINT ( 'NONE',  ( -4.257741265285667431, 3.982435197156672491, 0.4597581080974452172 ) ) ;
#130939=CARTESIAN_POINT ( 'NONE',  ( 7.391166297744269365, 11.77477778067701664, 1.040834085586084257E-14 ) ) ;
#130941=CARTESIAN_POINT ( 'NONE',  ( -3.633221978782299910, 5.261844946711204507, -1.443375672974053447 ) ) ;
#130943=CARTESIAN_POINT ( 'NONE',  ( -3.917943204224914933, 6.554388924028945240, -1.082531754730548412 ) ) ;
#130951=ORIENTED_EDGE ( 'NONE', *, *, #167443, .T. ) ;
#130953=CARTESIAN_POINT ( 'NONE',  ( 4.955668840994886359, 5.740367388370866131, 1.199719254218462483 ) ) ;
#130961=CARTESIAN_POINT ( 'NONE',  ( 5.005985031943777308, 6.863401842066294556, -1.599625672291256295 ) ) ;
#130965=CARTESIAN_POINT ( 'NONE',  ( 1.364683531249988535, 3.676041667008087099, 0.7879004041258500513 ) ) ;
#130970=CARTESIAN_POINT ( 'NONE',  ( 5.991813822235618758, 9.077867661661846554, 1.199719254218462483 ) ) ;
#130974=CARTESIAN_POINT ( 'NONE',  ( -6.274726165026268454, 6.214935368819085149, 0.7998128361456341429 ) ) ;
#130975=CARTESIAN_POINT ( 'NONE',  ( 0.7499999999999885647, 2.816666666666689522, -1.299038105676658228 ) ) ;
#130978=CARTESIAN_POINT ( 'NONE',  ( -4.786191920824102830, 5.542644314838231168, 1.199719254218462483 ) ) ;
#130979=CARTESIAN_POINT ( 'NONE',  ( 0.006158830626129450057, 7.078243236992583398, -2.121324627965403220 ) ) ;
#130981=CARTESIAN_POINT ( 'NONE',  ( 1.364683531249990311, 3.384375000341416140, 1.214306433183764966E-14 ) ) ;
#130983=CARTESIAN_POINT ( 'NONE',  ( -4.772106882330247046, 4.669805572247793357, -0.7216878364870207285 ) ) ;
#130988=CARTESIAN_POINT ( 'NONE',  ( 3.967488985650382549, 3.999290593069634081, -0.7827604779067200980 ) ) ;
#130989=CARTESIAN_POINT ( 'NONE',  ( 4.222474775652216294, 7.013638773981186958, 1.199719254218462483 ) ) ;
#130992=CARTESIAN_POINT ( 'NONE',  ( 0.4682352675917088591, 6.596815194046603104, -3.429086925395263385 ) ) ;
#130993=CARTESIAN_POINT ( 'NONE',  ( -1.364683531250010295, 4.342708333674753618, 0.7879004041258379498 ) ) ;
#130998=CARTESIAN_POINT ( 'NONE',  ( -0.6823417656250246877, 0.3635416670080895973, 1.181850606188755259 ) ) ;
#131001=CARTESIAN_POINT ( 'NONE',  ( -9.110189153378817295, 12.71597221466224603, 1.199719254218462483 ) ) ;
#131002=CARTESIAN_POINT ( 'NONE',  ( -7.361714222096077620, 7.691014135307965738, 0.7216878364870317197 ) ) ;
#131006=CARTESIAN_POINT ( 'NONE',  ( 1.364683531249988535, 2.863541667008082658, 0.7879004041258500513 ) ) ;
#131014=CARTESIAN_POINT ( 'NONE',  ( -4.731432421044865499, 8.463828891286912182, -0.7216878364870257245 ) ) ;
#131020=CARTESIAN_POINT ( 'NONE',  ( -5.761852095683518193, 6.784877535461274256, 1.082531754730546636 ) ) ;
#131033=CARTESIAN_POINT ( 'NONE',  ( -5.362413449404877852, 6.214902764849178141, -1.199719254218446718 ) ) ;
#131035=CARTESIAN_POINT ( 'NONE',  ( 1.499999999999987566, -0.2249999999999821587, 0.000000000000000000 ) ) ;
#131037=CARTESIAN_POINT ( 'NONE',  ( 8.270110514656016321, 12.59228666716665401, 0.7216878364870438212 ) ) ;
#131038=CARTESIAN_POINT ( 'NONE',  ( 6.608709811657416999, 9.797579649320619311, -1.199719254218440723 ) ) ;
#131040=CARTESIAN_POINT ( 'NONE',  ( 3.795362611133989095, 4.068874996780127873, 0.8733349908450734889 ) ) ;
#131041=CARTESIAN_POINT ( 'NONE',  ( 6.003563092752934871, 5.898578451166879510, 0.7998128361456341429 ) ) ;
#131049=CARTESIAN_POINT ( 'NONE',  ( -3.470524135418300737, 6.032400010421219427, -1.082531754730549967 ) ) ;
#131054=CARTESIAN_POINT ( 'NONE',  ( -0.3275477585932070057, 6.485062452714529080, 3.280083270285460983 ) ) ;
#131057=CARTESIAN_POINT ( 'NONE',  ( -1.201851678989727383E-14, 3.946875000341423689, -1.575800808251660134 ) ) ;
#131058=CARTESIAN_POINT ( 'NONE',  ( 10.07334494482924292, 11.81495252613139257, -1.082531754730537088 ) ) ;
#131059=CARTESIAN_POINT ( 'NONE',  ( -5.201524489137236529, 9.220195670635433771, 0.7998128361456481317 ) ) ;
#131062=CARTESIAN_POINT ( 'NONE',  ( 4.821896187954575197, 8.777295985922343391, 0.7998128361456462443 ) ) ;
#131063=CARTESIAN_POINT ( 'NONE',  ( -6.063521013809733518, 8.097193820909906137, 1.599625672291283607 ) ) ;
#131066=CARTESIAN_POINT ( 'NONE',  ( -0.7500000000000006661, 0.1395833340161536928, -1.299038105676652011 ) ) ;
#131069=CARTESIAN_POINT ( 'NONE',  ( 7.782016984564065432, 8.181367358187307204, 0.7216878364870458196 ) ) ;
#131073=CARTESIAN_POINT ( 'NONE',  ( -1.364683531250000748, 0.5718750003414208027, 0.000000000000000000 ) ) ;
#131075=CARTESIAN_POINT ( 'NONE',  ( 7.415946836550727284, 7.754285518838408109, 0.7216878364870317197 ) ) ;
#131078=CARTESIAN_POINT ( 'NONE',  ( -5.938108093105513241, 6.030140318152288792, 0.7216878364870317197 ) ) ;
#131080=CARTESIAN_POINT ( 'NONE',  ( -1.201851678989727383E-14, 4.071875000341425022, 1.575800808251672791 ) ) ;
#131084=CARTESIAN_POINT ( 'NONE',  ( -5.796555320980813164, 6.214368590181693186, -1.006237437275556257 ) ) ;
#131091=CARTESIAN_POINT ( 'NONE',  ( 5.770966940911189447, 9.884545197705074671, -0.7998128361456291469 ) ) ;
#131094=CARTESIAN_POINT ( 'NONE',  ( 4.196412238629597447, 4.854568018944682706, -1.199719254218452047 ) ) ;
#131099=ORIENTED_EDGE ( 'NONE', *, *, #159943, .F. ) ;
#131100=CARTESIAN_POINT ( 'NONE',  ( 5.504247177468186258, 6.484338464210099851, 1.082531754730558626 ) ) ;
#131101=CARTESIAN_POINT ( 'NONE',  ( -0.6823417656250246877, 0.6135416670080897639, 1.181850606188755259 ) ) ;
#131108=CARTESIAN_POINT ( 'NONE',  ( -0.7500000000000006661, 1.358333333333357151, -1.299038105676652011 ) ) ;
#131109=CARTESIAN_POINT ( 'NONE',  ( 5.940443861082012944, 10.08226827123770697, 0.7998128361456462443 ) ) ;
#131110=CARTESIAN_POINT ( 'NONE',  ( -6.991200766141138168, 11.30815132714001159, 0.7998128361456481317 ) ) ;
#131114=CARTESIAN_POINT ( 'NONE',  ( -0.6823417656250212460, 0.8010416670080899859, 1.181850606188755259 ) ) ;
#131116=CARTESIAN_POINT ( 'NONE',  ( 1.499999999999989120, 2.025000000000019895, 1.214306433183764966E-14 ) ) ;
#131118=CARTESIAN_POINT ( 'NONE',  ( 5.196852952739813070, 4.957416621151553571, -0.7998128361456221525 ) ) ;
#131125=CARTESIAN_POINT ( 'NONE',  ( -1.402160292154681736E-14, -0.8812499993171809543, -1.732050807568870754 ) ) ;
#131127=CARTESIAN_POINT ( 'NONE',  ( -7.528855374290365887, 7.678086112960552434, -0.7998128361456291469 ) ) ;
#131128=CARTESIAN_POINT ( 'NONE',  ( -4.989037340148921196, 5.883260320670900434, 1.082531754730560403 ) ) ;
#131135=CARTESIAN_POINT ( 'NONE',  ( 7.124973419181436007, 8.271222729588529887, -1.199719254218446718 ) ) ;
#131140=CARTESIAN_POINT ( 'NONE',  ( 4.971035877704902184, 8.951292290631053916, 1.040834085586084257E-14 ) ) ;
#131141=CARTESIAN_POINT ( 'NONE',  ( 8.554831740098649107, 11.96409221588171157, 1.082531754730546636 ) ) ;
#131144=CARTESIAN_POINT ( 'NONE',  ( -8.044065211609668253, 8.279164256499745633, 0.7998128361456602331 ) ) ;
#131145=CARTESIAN_POINT ( 'NONE',  ( 4.436542580169809291, 6.199052314996659874, 1.599625672291267398 ) ) ;
#131149=CARTESIAN_POINT ( 'NONE',  ( 4.012968703617612931, 7.577496623363801476, 0.2782505873175616373 ) ) ;
#131150=CARTESIAN_POINT ( 'NONE',  ( 9.246297574839974942, 11.81043314211192019, 1.443375672974076540 ) ) ;
#131159=CARTESIAN_POINT ( 'NONE',  ( 9.910647101909615841, 10.66476916175714607, 0.000000000000000000 ) ) ;
#131162=CARTESIAN_POINT ( 'NONE',  ( -5.850506979496850057, 6.784345216623154151, -1.199719254218446718 ) ) ;
#131167=DIRECTION ( 'NONE',  ( 0.6507913734559627184, 0.7592566023653016805, 0.000000000000000000 ) ) ;
#131169=CARTESIAN_POINT ( 'NONE',  ( -6.181627972826976958, 9.299317504018391745, 1.199719254218452047 ) ) ;
#131170=CARTESIAN_POINT ( 'NONE',  ( -1.500000000000022204, 6.120000000000041851, 2.500000000000011102 ) ) ;
#131184=ADVANCED_FACE ( 'NONE', ( #175411 ), #26994, .F. ) ;
#131186=CARTESIAN_POINT ( 'NONE',  ( -6.742482464697739708, 6.760651051769146491, 0.7998128361456341429 ) ) ;
#131189=CARTESIAN_POINT ( 'NONE',  ( 4.528060117284229413, 7.266191989264828344, 1.082531754730558626 ) ) ;
#131192=DIRECTION ( 'NONE',  ( 1.000000000000000000, 0.000000000000000000, 0.000000000000000000 ) ) ;
#131194=CARTESIAN_POINT ( 'NONE',  ( -1.387358672534711346, 7.251968950353628429, 4.302625267138136422 ) ) ;
#131197=CARTESIAN_POINT ( 'NONE',  ( 8.727698198895078363, 11.20540053684285553, -1.599625672291257406 ) ) ;
#131200=CARTESIAN_POINT ( 'NONE',  ( -8.552495972122143186, 8.872333477097637200, 0.7998128361456462443 ) ) ;
#131201=CARTESIAN_POINT ( 'NONE',  ( 7.311924916471702396, 7.425000578838787391, -0.7998128361456281477 ) ) ;
#131207=CARTESIAN_POINT ( 'NONE',  ( 1.364683531249986537, 1.467708333674748289, -0.7879004041258239610 ) ) ;
#131210=CARTESIAN_POINT ( 'NONE',  ( 8.785320351975350661, 9.351887953500479966, -0.7216878364870197293 ) ) ;
#131217=CARTESIAN_POINT ( 'NONE',  ( 5.178851490740205676, 6.104710163027444736, 1.082531754730558626 ) ) ;
#131237=CARTESIAN_POINT ( 'NONE',  ( 0.7499999999999867883, 0.09791666734948467621, -1.299038105676652899 ) ) ;
#131244=CARTESIAN_POINT ( 'NONE',  ( -1.500000000000013101, -0.3291666666666463459, 0.8660254037844403729 ) ) ;
#131245=CARTESIAN_POINT ( 'NONE',  ( 8.367353357928214663, 12.91366268422496688, 1.040834085586084257E-14 ) ) ;
#131250=CARTESIAN_POINT ( 'NONE',  ( 3.147464216666835402, 6.823792019419957278, -0.7998128361456291469 ) ) ;
#131251=CARTESIAN_POINT ( 'NONE',  ( -7.727784370109414880, 8.118095974656867497, 0.7216878364870578100 ) ) ;
#131255=CARTESIAN_POINT ( 'NONE',  ( -6.826694039680798021, 7.923230120171105284, -1.199719254218446718 ) ) ;
#131256=CARTESIAN_POINT ( 'NONE',  ( -4.744990574658554117, 4.638169879964154418, 1.214306433183764966E-14 ) ) ;
#131259=CARTESIAN_POINT ( 'NONE',  ( -1.500000000000013101, 0.9520833340161557468, 0.8660254037844403729 ) ) ;
#131266=CARTESIAN_POINT ( 'NONE',  ( -3.673896439178936824, 5.309298483840612093, 1.443375672974064550 ) ) ;
#131269=CARTESIAN_POINT ( 'NONE',  ( 3.998873522394119195, 7.597518543056763995, -0.1390531931140040478 ) ) ;
#131273=CARTESIAN_POINT ( 'NONE',  ( -8.967828540435322182, 12.54988483289483980, 1.199719254218462483 ) ) ;
#131274=CARTESIAN_POINT ( 'NONE',  ( 8.606728586576791074, 8.935604860628076906, 0.7998128361456462443 ) ) ;
#131284=CARTESIAN_POINT ( 'NONE',  ( -9.481229494658258261, 9.955855920056455588, -0.7998128361456291469 ) ) ;
#131289=CARTESIAN_POINT ( 'NONE',  ( 3.680148631105580215, 6.380924938676771241, -1.199719254218446718 ) ) ;
#131293=CARTESIAN_POINT ( 'NONE',  ( -8.971744963941075568, 11.49012176272984931, 1.599625672291269396 ) ) ;
#131296=ORIENTED_EDGE ( 'NONE', *, *, #18560, .F. ) ;
#131304=CARTESIAN_POINT ( 'NONE',  ( 6.283314124929436417, 9.417951348137970413, -1.199719254218440723 ) ) ;
#131306=CARTESIAN_POINT ( 'NONE',  ( -2.761056838677368397, 6.372983411765559048, 0.7998128361456341429 ) ) ;
#131307=ORIENTED_EDGE ( 'NONE', *, *, #8949, .F. ) ;
#131314=CARTESIAN_POINT ( 'NONE',  ( -1.402160292154681736E-14, 0.8687500006828192678, -1.732050807568863648 ) ) ;
#131319=CARTESIAN_POINT ( 'NONE',  ( -4.485049888022365927, 4.126979712314507331, 0.7998128361456341429 ) ) ;
#131325=CARTESIAN_POINT ( 'NONE',  ( 3.863710590214593399, 7.451486755318259547, 1.040834085586084257E-14 ) ) ;
#131328=CARTESIAN_POINT ( 'NONE',  ( -0.6823417656250212460, 4.863541667008086655, 1.181850606188767472 ) ) ;
#131330=CARTESIAN_POINT ( 'NONE',  ( 3.158686601859607368, 6.628958768904106513, -0.7216878364870267237 ) ) ;
#131337=CARTESIAN_POINT ( 'NONE',  ( -6.113138475847556208, 6.011394290285472231, -0.2943476003282770037 ) ) ;
#131339=CARTESIAN_POINT ( 'NONE',  ( -0.6823417656250003738, -0.2822916663252489355, -1.181850606188749264 ) ) ;
#131346=CARTESIAN_POINT ( 'NONE',  ( 1.499999999999989120, 5.254166666666684193, 0.8660254037844524744 ) ) ;
#131354=CARTESIAN_POINT ( 'NONE',  ( -1.001543065824772872E-14, 5.134375000341421469, 1.575800808251672791 ) ) ;
#131356=CARTESIAN_POINT ( 'NONE',  ( 7.149227073107712549, 7.235186428247455837, -0.7998128361456281477 ) ) ;
#131357=CARTESIAN_POINT ( 'NONE',  ( -8.311311860377216476, 9.655284244316948872, -1.199719254218446718 ) ) ;
#131360=DIRECTION ( 'NONE',  ( 7.387867266669436732E-31, -1.000000000000000000, -8.546850786086424434E-32 ) ) ;
#131361=ORIENTED_EDGE ( 'NONE', *, *, #126096, .F. ) ;
#131363=CARTESIAN_POINT ( 'NONE',  ( 1.499999999999989120, 5.295833333333356485, -0.8660254037844323793 ) ) ;
#131370=CARTESIAN_POINT ( 'NONE',  ( 8.188761592974039161, 10.57664116326830595, -1.443375672974063439 ) ) ;
#131374=CARTESIAN_POINT ( 'NONE',  ( -1.499999999999997780, 5.181250000682820378, 1.214306433183764966E-14 ) ) ;
#131376=CARTESIAN_POINT ( 'NONE',  ( -3.255929445576174697, 6.950334786480840243, -0.7998128361456281477 ) ) ;
#131378=CARTESIAN_POINT ( 'NONE',  ( 6.439759776366775768, 7.575769829591800786, 1.082531754730558626 ) ) ;
#131379=CARTESIAN_POINT ( 'NONE',  ( -10.27671724903424888, 11.09185100006920877, 1.040834085586084257E-14 ) ) ;
#131386=CARTESIAN_POINT ( 'NONE',  ( 2.686486993802192913, 6.285985259411197568, 0.7998128361456362523 ) ) ;
#131388=CARTESIAN_POINT ( 'NONE',  ( 4.864678189204997949, 4.569879397027603929, 0.7998128361456341429 ) ) ;
#131401=CARTESIAN_POINT ( 'NONE',  ( 7.540305987494599016, 11.94877408538573427, -0.7998128361456291469 ) ) ;
#131403=CARTESIAN_POINT ( 'NONE',  ( -1.499999999999995559, 8.266799604815048497, 3.162088779279327966 ) ) ;
#131404=CARTESIAN_POINT ( 'NONE',  ( 1.364683531249986537, -0.6364583329919177856, 0.7879004041258500513 ) ) ;
#131405=CARTESIAN_POINT ( 'NONE',  ( 5.829642864196168617, 6.863966765392747860, 1.082531754730558626 ) ) ;
#131406=CARTESIAN_POINT ( 'NONE',  ( -9.327646496521984076, 11.90534021740758064, -1.443375672974059665 ) ) ;
#131412=CARTESIAN_POINT ( 'NONE',  ( -4.440459003675619520, 5.139289244831666714, 1.199719254218462483 ) ) ;
#131424=CARTESIAN_POINT ( 'NONE',  ( 5.854153468347242040, 6.181931306435468620, -0.8879621099797951889 ) ) ;
#131432=CARTESIAN_POINT ( 'NONE',  ( -8.351459436338037889, 10.76645531385962862, -1.443375672974059665 ) ) ;
#131436=CARTESIAN_POINT ( 'NONE',  ( 7.298366762858032430, 7.409182732956175244, 1.040834085586084257E-14 ) ) ;
#131437=CARTESIAN_POINT ( 'NONE',  ( -3.438964519360664607, 7.163875705896082913, -0.7998128361456282587 ) ) ;
#131439=CARTESIAN_POINT ( 'NONE',  ( -4.388035272317281077, 8.271124917678806199, 0.7998128361456481317 ) ) ;
#131440=CARTESIAN_POINT ( 'NONE',  ( 2.333974999846879061, 5.874721266463329705, -0.7998128361456291469 ) ) ;
#131443=CARTESIAN_POINT ( 'NONE',  ( -5.717788096661253761, 7.693838750903348789, 1.599625672291269396 ) ) ;
#131446=EDGE_CURVE ( 'NONE', #172377, #163352, #139607, .T. ) ;
#131448=CARTESIAN_POINT ( 'NONE',  ( 8.215351014876830504, 11.67199438640995801, -1.199719254218446718 ) ) ;
#131451=CARTESIAN_POINT ( 'NONE',  ( 4.188544580023894071, 7.586160867502751870, 0.8937768461303140510 ) ) ;
#131452=CARTESIAN_POINT ( 'NONE',  ( 4.311129659465574804, 7.013106455143060636, -1.082531754730548412 ) ) ;
#131454=CARTESIAN_POINT ( 'NONE',  ( 6.471393748265540147, 5.229711127717882491, 2.420000000000010587 ) ) ;
#131459=CARTESIAN_POINT ( 'NONE',  ( 6.277061933002774374, 9.306694107603160404, 1.082531754730558626 ) ) ;
#131462=CARTESIAN_POINT ( 'NONE',  ( -10.48453286206953727, 11.12637651536962125, 0.7998128361456462443 ) ) ;
#131463=CARTESIAN_POINT ( 'NONE',  ( -8.037286134802835491, 8.271255333558444889, -0.7998128361456291469 ) ) ;
#131471=CARTESIAN_POINT ( 'NONE',  ( 9.134442807305049428, 11.67993591332117376, 1.599625672291281386 ) ) ;
#131475=CARTESIAN_POINT ( 'NONE',  ( 3.334415713957098681, 5.977569868670206787, -1.199719254218446718 ) ) ;
#131478=CARTESIAN_POINT ( 'NONE',  ( 0.7499999999999902300, 3.514583334016149863, 1.299038105676669330 ) ) ;
#131484=CARTESIAN_POINT ( 'NONE',  ( 0.7499999999999902300, 2.733333333333351600, 1.299038105676669330 ) ) ;
#131485=CARTESIAN_POINT ( 'NONE',  ( 7.474622759835693131, 7.614814729430110951, -0.7998128361456281477 ) ) ;
#131489=CARTESIAN_POINT ( 'NONE',  ( 7.266807147244743526, 11.42176607185347414, -0.7216878364870267237 ) ) ;
#131493=CARTESIAN_POINT ( 'NONE',  ( 10.71502147350184231, 11.39527989537399755, 0.000000000000000000 ) ) ;
#131495=CARTESIAN_POINT ( 'NONE',  ( -3.415764635639130020, 6.072476943965863683, 1.199719254218462483 ) ) ;
#131497=CARTESIAN_POINT ( 'NONE',  ( -0.6823417656250246877, 0.05104166700808931978, 1.181850606188755259 ) ) ;
#131501=CARTESIAN_POINT ( 'NONE',  ( 3.225950485047770933, 5.851027101609320269, 1.199719254218450271 ) ) ;
#131503=CARTESIAN_POINT ( 'NONE',  ( -0.6823417656249969321, 5.280208333674756283, -1.181850606188749264 ) ) ;
#131511=CARTESIAN_POINT ( 'NONE',  ( -7.335124800193271177, 8.516399340768996851, -1.199719254218452935 ) ) ;
#131513=CARTESIAN_POINT ( 'NONE',  ( 5.843727902690005749, 6.776436293681846301, -1.199719254218445830 ) ) ;
#131516=CARTESIAN_POINT ( 'NONE',  ( 1.364683531249986537, -0.8864583329919110133, 0.7879004041258500513 ) ) ;
#131520=CARTESIAN_POINT ( 'NONE',  ( 9.049177462117294013, 12.64479190819049670, -1.199719254218446718 ) ) ;
#131523=CARTESIAN_POINT ( 'NONE',  ( -6.338600509588822263, 7.353787668397130162, -1.199719254218446718 ) ) ;
#131527=CARTESIAN_POINT ( 'NONE',  ( 9.725276259704228821, 10.24057714594344048, 0.7998128361456462443 ) ) ;
#131529=CARTESIAN_POINT ( 'NONE',  ( 9.576136569953906275, 10.06658084123472641, 0.000000000000000000 ) ) ;
#131530=CARTESIAN_POINT ( 'NONE',  ( 4.885223684246801312, 4.924875305092577982, -0.7419332605567361405 ) ) ;
#131531=CARTESIAN_POINT ( 'NONE',  ( -3.079673448598517549, 6.744702790006905424, 1.040834085586084257E-14 ) ) ;
#131533=CARTESIAN_POINT ( 'NONE',  ( -7.314787569772770226, 8.492672571945082183, -1.199719254218452935 ) ) ;
#131536=CARTESIAN_POINT ( 'NONE',  ( -5.084594181526506773, 6.727074486938107611, 1.441884573159227578 ) ) ;
#131537=CARTESIAN_POINT ( 'NONE',  ( -1.364683531250014514, 0.2385416670080863499, -0.7879004041258359514 ) ) ;
#131541=CARTESIAN_POINT ( 'NONE',  ( 6.155038550924139429, 9.164333495178082600, 1.082531754730558626 ) ) ;
#131544=CARTESIAN_POINT ( 'NONE',  ( 4.143988507271280319, 7.986403691791820414, -0.7998128361456221525 ) ) ;
#131545=ADVANCED_FACE ( 'NONE', ( #110465 ), #148119, .T. ) ;
#131563=CARTESIAN_POINT ( 'NONE',  ( 8.536830278099042602, 13.11138575775759563, -0.7998128361456352531 ) ) ;
#131567=CARTESIAN_POINT ( 'NONE',  ( -4.843287188579803448, 6.673587691474970107, -1.599625672291256295 ) ) ;
#131568=CARTESIAN_POINT ( 'NONE',  ( -8.505042434474312074, 8.816971016508505343, -0.7998128361456291469 ) ) ;
#131574=CARTESIAN_POINT ( 'NONE',  ( 1.499999999999989120, 3.535416667349488229, 0.8660254037844524744 ) ) ;
#131575=CARTESIAN_POINT ( 'NONE',  ( 9.589694723567584234, 10.08239868711733855, -0.7998128361456281477 ) ) ;
#131579=CARTESIAN_POINT ( 'NONE',  ( -8.799405390469187793, 10.22472669609091689, -1.199719254218446718 ) ) ;
#131581=CARTESIAN_POINT ( 'NONE',  ( -1.364683531250012516, 2.780208333674754506, 0.7879004041258379498 ) ) ;
#131583=CARTESIAN_POINT ( 'NONE',  ( -3.741371894207468074, 7.428709027653146890, 2.448389769268642713 ) ) ;
#131587=CARTESIAN_POINT ( 'NONE',  ( -9.219181267612684749, 10.81842823604534765, 1.082531754730558626 ) ) ;
#131592=CARTESIAN_POINT ( 'NONE',  ( -1.364683531250012516, 1.342708333674755616, 0.7879004041258379498 ) ) ;
#131597=CARTESIAN_POINT ( 'NONE',  ( -1.364683531250000748, 1.259375000341421469, 0.000000000000000000 ) ) ;
#131599=CARTESIAN_POINT ( 'NONE',  ( -5.762378981008047241, 6.681529218386182301, 1.199719254218450271 ) ) ;
#131600=CARTESIAN_POINT ( 'NONE',  ( 8.098297826064319693, 8.342435640030188893, 0.7998128361456481317 ) ) ;
#131602=CARTESIAN_POINT ( 'NONE',  ( -0.7499999999999972244, 5.358333333333353821, -1.299038105676652011 ) ) ;
#131604=CARTESIAN_POINT ( 'NONE',  ( -1.364683531250012516, 3.092708333674755838, 0.7879004041258379498 ) ) ;
#131608=CARTESIAN_POINT ( 'NONE',  ( -6.263503779833496488, 6.409768619334935913, 0.7216878364870317197 ) ) ;
#131613=CARTESIAN_POINT ( 'NONE',  ( 5.517805331081858888, 5.539787095791365523, 1.040834085586084257E-14 ) ) ;
#131616=CARTESIAN_POINT ( 'NONE',  ( -9.027031348600448979, 9.425958082989001952, 1.040834085586084257E-14 ) ) ;
#131617=CARTESIAN_POINT ( 'NONE',  ( -9.869972641068651242, 11.57768483841065787, 1.082531754730558626 ) ) ;
#131619=CARTESIAN_POINT ( 'NONE',  ( -1.001543065824772872E-14, 4.821875000341419693, 1.575800808251672791 ) ) ;
#131622=CARTESIAN_POINT ( 'NONE',  ( -1.124828079527723457, 3.298464558332917740, -0.7749999999999970246 ) ) ;
#131624=CARTESIAN_POINT ( 'NONE',  ( -7.822691444960716112, 8.228820895316715678, -0.7216878364870267237 ) ) ;
#131626=CARTESIAN_POINT ( 'NONE',  ( -1.500000000000011324, 5.879166666666686858, -0.8660254037844313801 ) ) ;
#131629=CARTESIAN_POINT ( 'NONE',  ( 8.595506201384020883, 9.130438111143927671, 0.7216878364870438212 ) ) ;
#131637=CARTESIAN_POINT ( 'NONE',  ( 9.558135107509954764, 10.25350516829085379, -0.7216878364870257245 ) ) ;
#131644=CARTESIAN_POINT ( 'NONE',  ( 6.799577732453452761, 7.891594428405881878, -1.199719254218446718 ) ) ;
#131645=CARTESIAN_POINT ( 'NONE',  ( -4.066556009095094737, 6.831733546331167695, 1.199719254218464037 ) ) ;
#131648=DIRECTION ( 'NONE',  ( -5.578564026256490882E-16, -1.000000000000000000, -9.066213480720158442E-32 ) ) ;
#131649=CARTESIAN_POINT ( 'NONE',  ( 6.439759776366780208, 6.615400615290456088, 0.7216878364870317197 ) ) ;
#131650=CARTESIAN_POINT ( 'NONE',  ( 1.364683531249988757, -0.3031249996585799744, 0.000000000000000000 ) ) ;
#131652=CARTESIAN_POINT ( 'NONE',  ( -9.969323024750229578, 10.52529837183042716, -0.7998128361456291469 ) ) ;
#131657=CARTESIAN_POINT ( 'NONE',  ( 4.175484721775176489, 3.976419294354625933, -0.06592222766770190756 ) ) ;
#131660=ORIENTED_EDGE ( 'NONE', *, *, #143969, .T. ) ;
#131665=CARTESIAN_POINT ( 'NONE',  ( 2.282078984650023123, 5.585856895725574311, 0.4608960419188404822 ) ) ;
#131669=CARTESIAN_POINT ( 'NONE',  ( 5.933664784275179294, 10.07435934829639912, -0.7998128361456291469 ) ) ;
#131670=CARTESIAN_POINT ( 'NONE',  ( 6.096362627639171805, 10.26417349888772179, -0.7998128361456291469 ) ) ;
#131672=EDGE_CURVE ( 'NONE', #171990, #193490, #2381, .T. ) ;
#131682=CARTESIAN_POINT ( 'NONE',  ( -3.521367211247373508, 5.131347717920458962, -1.599625672291256295 ) ) ;
#131691=CARTESIAN_POINT ( 'NONE',  ( -8.324343129110692630, 12.65555805069709550, 0.7216878364870338292 ) ) ;
#131694=CARTESIAN_POINT ( 'NONE',  ( 4.937140493670735708, 8.911747675924535983, -0.7998128361456281477 ) ) ;
#131695=CARTESIAN_POINT ( 'NONE',  ( 1.364683531249988535, 5.655208333674751842, -0.7879004041258300672 ) ) ;
#131701=CARTESIAN_POINT ( 'NONE',  ( 5.626270559546826533, 5.666329862333828515, 0.7216878364870317197 ) ) ;
#131702=CARTESIAN_POINT ( 'NONE',  ( -6.073162743917628781, 9.172774736957510555, -1.199719254218440723 ) ) ;
#131709=CARTESIAN_POINT ( 'NONE',  ( -7.705111371268023923, 7.883718109434487253, 1.040834085586084257E-14 ) ) ;
#131710=CARTESIAN_POINT ( 'NONE',  ( -5.057354993097396445, 5.859001232490445688, -1.199719254218446718 ) ) ;
#131718=CARTESIAN_POINT ( 'NONE',  ( 6.205881626753210867, 8.263281202677319470, 1.599625672291281386 ) ) ;
#131724=CARTESIAN_POINT ( 'NONE',  ( -1.230728480726517748, 2.980010058876359835, 0.7750000000000170086 ) ) ;
#131729=CARTESIAN_POINT ( 'NONE',  ( -1.402160292154681736E-14, 0.3843750003414230232, 1.575800808251672791 ) ) ;
#131731=CARTESIAN_POINT ( 'NONE',  ( 5.518332215962025167, 6.396807992499198292, -1.199719254218445830 ) ) ;
#131733=CARTESIAN_POINT ( 'NONE',  ( -8.026063749610063525, 8.466088584074293877, -0.7216878364870278340 ) ) ;
#131735=CARTESIAN_POINT ( 'NONE',  ( -3.740297717422789159, 7.429476292658450554, -2.448395595369508015 ) ) ;
#131736=CARTESIAN_POINT ( 'NONE',  ( 5.341549334104194635, 6.294524313618772737, 1.082531754730558626 ) ) ;
#131737=CARTESIAN_POINT ( 'NONE',  ( -6.507550544435101614, 10.53596670190887963, 0.000000000000000000 ) ) ;
#131742=CARTESIAN_POINT ( 'NONE',  ( 6.425674737872927089, 9.584038729905381970, -1.199719254218440723 ) ) ;
#131747=CARTESIAN_POINT ( 'NONE',  ( 0.6823417656249917140, 3.342708333674754506, 1.181850606188765695 ) ) ;
#131751=CARTESIAN_POINT ( 'NONE',  ( 8.118635056484817980, 8.366162408854107113, 0.7998128361456481317 ) ) ;
#131755=CARTESIAN_POINT ( 'NONE',  ( -7.283754839039664475, 9.520799950344851936, -1.599625672291263179 ) ) ;
#131761=CARTESIAN_POINT ( 'NONE',  ( 10.24048609702354717, 10.84165528948263457, -0.7998128361456281477 ) ) ;
#131764=CARTESIAN_POINT ( 'NONE',  ( -7.934546212495630968, 10.28005655271014795, -1.599625672291263179 ) ) ;
#131768=CARTESIAN_POINT ( 'NONE',  ( 5.718470792885002041, 6.083800970187063228, -0.6820517675651931455 ) ) ;
#131769=CARTESIAN_POINT ( 'NONE',  ( -9.110716038703348119, 12.61262389758715408, 1.082531754730560403 ) ) ;
#131772=CARTESIAN_POINT ( 'NONE',  ( -1.500000000000022204, 7.388542872122518368, 4.154462424328226433 ) ) ;
#131775=CARTESIAN_POINT ( 'NONE',  ( 5.113396490648394632, 9.117379672398465473, 1.040834085586084257E-14 ) ) ;
#131777=CARTESIAN_POINT ( 'NONE',  ( 5.986088515633498197, 6.942523675449257858, -1.199719254218446718 ) ) ;
#131778=CARTESIAN_POINT ( 'NONE',  ( -4.274576072154308903, 7.290118009659216192, 0.9321895248279310486 ) ) ;
#131779=CARTESIAN_POINT ( 'NONE',  ( 3.440018289565364817, 5.036440642624797626, 1.599625672291267398 ) ) ;
#131781=CARTESIAN_POINT ( 'NONE',  ( -7.456621297836087514, 9.722477485607340597, 1.443375672974090751 ) ) ;
#131787=CARTESIAN_POINT ( 'NONE',  ( -4.105200985651542567, 7.499488806860944656, 0.5979674706809139373 ) ) ;
#131788=CARTESIAN_POINT ( 'NONE',  ( 1.364683531249986537, -1.073958332991911790, 0.7879004041258500513 ) ) ;
#131791=CARTESIAN_POINT ( 'NONE',  ( -1.123270288250318494, 3.297697346350006331, -0.7749999999993560929 ) ) ;
#131792=CARTESIAN_POINT ( 'NONE',  ( 5.205967797967541166, 5.175976640491323444, -0.7216878364870197293 ) ) ;
#131796=CARTESIAN_POINT ( 'NONE',  ( -9.666600336419303829, 11.34041714965307968, 1.082531754730558626 ) ) ;
#131809=CARTESIAN_POINT ( 'NONE',  ( -9.531018800282611281, 12.14260790512831889, 1.443375672974076540 ) ) ;
#131815=CARTESIAN_POINT ( 'NONE',  ( -1.201851678989727383E-14, 2.993750000682821266, 1.732050807568877637 ) ) ;
#131818=ORIENTED_EDGE ( 'NONE', *, *, #168064, .F. ) ;
#131819=CARTESIAN_POINT ( 'NONE',  ( -9.643927338022246332, 10.14567007064778004, -0.7998128361456291469 ) ) ;
#131820=CARTESIAN_POINT ( 'NONE',  ( -4.284013352238262407, 6.021101549076499637, -1.443375672974053892 ) ) ;
#131823=CARTESIAN_POINT ( 'NONE',  ( 5.099838337034727331, 9.101561826515851550, -0.7998128361456281477 ) ) ;
#131824=ORIENTED_EDGE ( 'NONE', *, *, #77409, .T. ) ;
#131829=CARTESIAN_POINT ( 'NONE',  ( 8.769426429940780920, 9.125419011219408461, 0.7998128361456462443 ) ) ;
#131831=CARTESIAN_POINT ( 'NONE',  ( -4.826164018371312814, 5.074823732154670530, -0.9293088092043750859 ) ) ;
#131836=CARTESIAN_POINT ( 'NONE',  ( -6.073689629242160493, 8.109057205581079231, -1.443375672974059665 ) ) ;
#131839=CARTESIAN_POINT ( 'NONE',  ( -0.6823417656250212460, 4.863541667008086655, 1.181850606188767472 ) ) ;
#131843=FACE_OUTER_BOUND ( 'NONE', #138252, .T. ) ;
#131844=CARTESIAN_POINT ( 'NONE',  ( -2.941756144040963417, 6.375873234782333476, -0.7216878364870257245 ) ) ;
#131847=CARTESIAN_POINT ( 'NONE',  ( 3.728129053633592704, 4.412200653069714207, -1.082531754730543083 ) ) ;
#131848=FACE_OUTER_BOUND ( 'NONE', #87649, .T. ) ;
#131849=CARTESIAN_POINT ( 'NONE',  ( -10.17947440576205054, 10.77047498301088346, 0.7998128361456462443 ) ) ;
#131852=CARTESIAN_POINT ( 'NONE',  ( 1.364683531249986537, 1.905208333674750287, -0.7879004041258239610 ) ) ;
#131854=CARTESIAN_POINT ( 'NONE',  ( 2.835626683552519012, 6.459981564119914310, 0.000000000000000000 ) ) ;
#131860=CARTESIAN_POINT ( 'NONE',  ( 9.124274191872634887, 11.66807252865000244, -1.443375672974058777 ) ) ;
#131862=CARTESIAN_POINT ( 'NONE',  ( -6.399085315970132193, 10.40942393536641397, -0.7216878364870278340 ) ) ;
#131863=CARTESIAN_POINT ( 'NONE',  ( -1.364683531250000748, 0.7593750003414210248, 0.000000000000000000 ) ) ;
#131865=CARTESIAN_POINT ( 'NONE',  ( 0.4886806171078367234, 7.337544960129623206, 1.941936010599545792 ) ) ;
#131867=CARTESIAN_POINT ( 'NONE',  ( -8.532158741701643123, 8.848606708273724308, 0.7998128361456462443 ) ) ;
#131868=CARTESIAN_POINT ( 'NONE',  ( -5.246642258364192735, 5.223430177620739023, 0.7216878364870317197 ) ) ;
#131869=CARTESIAN_POINT ( 'NONE',  ( -0.6823417656250212460, 3.113541667008084879, 1.181850606188767472 ) ) ;
#131874=CARTESIAN_POINT ( 'NONE',  ( 8.238550898598388628, 12.76339314834017102, 0.7998128361456462443 ) ) ;
#131889=CARTESIAN_POINT ( 'NONE',  ( 1.364683531249990311, 4.676041667008083103, 0.7879004041258500513 ) ) ;
#131894=CARTESIAN_POINT ( 'NONE',  ( 10.24726517383036928, 10.84956421242393887, 0.000000000000000000 ) ) ;
#131897=CARTESIAN_POINT ( 'NONE',  ( -1.402160292154681736E-14, 2.446875000341416584, -1.575800808251660134 ) ) ;
#131900=CARTESIAN_POINT ( 'NONE',  ( -5.910991785878158211, 9.839981483592442402, -0.7216878364870278340 ) ) ;
#131906=CARTESIAN_POINT ( 'NONE',  ( 5.529027716274630855, 5.344953845275508542, 1.040834085586084257E-14 ) ) ;
#131909=CARTESIAN_POINT ( 'NONE',  ( 9.028840231696797503, 12.62106513936658203, -1.199719254218446718 ) ) ;
#131915=CARTESIAN_POINT ( 'NONE',  ( -9.646789991323334590, 11.21334206375407305, 1.199719254218462483 ) ) ;
#131916=CARTESIAN_POINT ( 'NONE',  ( 6.272618624616828953, 10.46980549536166016, 1.040834085586084257E-14 ) ) ;
#131919=CARTESIAN_POINT ( 'NONE',  ( 5.300874872818843286, 5.286701561151180506, 0.7216878364870317197 ) ) ;
#131925=VECTOR ( 'NONE', #4743, 1000.000000000000000 ) ;
#131930=CARTESIAN_POINT ( 'NONE',  ( -6.968527767744110868, 9.153035033833367251, 1.443375672974078761 ) ) ;
#131931=CARTESIAN_POINT ( 'NONE',  ( 4.690231075323689325, 7.559354456931247412, 1.199719254218462483 ) ) ;
#131934=CARTESIAN_POINT ( 'NONE',  ( -8.857554428429624593, 9.228235009456373206, 0.7998128361456462443 ) ) ;
#131939=CARTESIAN_POINT ( 'NONE',  ( -9.378489572351046633, 11.96465713920816043, -1.599625672291263179 ) ) ;
#131940=DIRECTION ( 'NONE',  ( -1.207943261119674327E-30, -2.168404344971008079E-15, -1.000000000000000000 ) ) ;
#131943=CARTESIAN_POINT ( 'NONE',  ( 9.094822116668764167, 9.505047312402055582, 0.7998128361456462443 ) ) ;
#131944=CARTESIAN_POINT ( 'NONE',  ( -2.065088895208611941, 8.523968132013475696, -2.459875961809982137 ) ) ;
#131946=ORIENTED_EDGE ( 'NONE', *, *, #84582, .F. ) ;
#131950=CARTESIAN_POINT ( 'NONE',  ( -3.104453987849326690, 4.644948957289396496, 1.040834085586084257E-14 ) ) ;
#131955=CARTESIAN_POINT ( 'NONE',  ( -9.806625181386236179, 10.33548422123910449, -0.7998128361456291469 ) ) ;
#131959=CARTESIAN_POINT ( 'NONE',  ( 7.293923454472087897, 8.572294120714675003, 1.082531754730558626 ) ) ;
#131960=CARTESIAN_POINT ( 'NONE',  ( 0.6823417656249899377, 4.988541667008086655, -1.181850606188754593 ) ) ;
#131962=CARTESIAN_POINT ( 'NONE',  ( 3.928111819657337911, 5.605883094398769195, 1.599625672291267398 ) ) ;
#131965=CARTESIAN_POINT ( 'NONE',  ( -6.470265622219711688, 8.571729197388226140, -1.599625672291263179 ) ) ;
#131971=CARTESIAN_POINT ( 'NONE',  ( 3.863710590214593399, 7.451486755318259547, 1.040834085586084257E-14 ) ) ;
#131979=CARTESIAN_POINT ( 'NONE',  ( 1.364683531249990311, 3.696875000341416584, 1.214306433183764966E-14 ) ) ;
#131980=CARTESIAN_POINT ( 'NONE',  ( 6.471393748265540147, 5.229711127717882491, 2.500000000000011102 ) ) ;
#131981=CARTESIAN_POINT ( 'NONE',  ( 8.106885785967500979, 11.54545161934907682, 1.199719254218460707 ) ) ;
#131983=CARTESIAN_POINT ( 'NONE',  ( -4.473827502829599290, 4.321812962830357208, 0.7216878364870317197 ) ) ;
#131986=CARTESIAN_POINT ( 'NONE',  ( -5.070386261386537363, 5.017798181146802428, 1.214306433183764966E-14 ) ) ;
#131993=CARTESIAN_POINT ( 'NONE',  ( 4.521807925357579805, 5.234196320127330715, -1.199719254218452047 ) ) ;
#131999=CARTESIAN_POINT ( 'NONE',  ( 1.177073619093315759, 2.949321498342245995, 0.7750000000000100142 ) ) ;
#132001=CARTESIAN_POINT ( 'NONE',  ( 4.656335691289526402, 7.519809842224722374, -1.199719254218452047 ) ) ;
#132002=DIRECTION ( 'NONE',  ( 0.000000000000000000, 0.000000000000000000, 1.000000000000000000 ) ) ;
#132006=CARTESIAN_POINT ( 'NONE',  ( -0.6823417656250212460, 4.363541667008085767, 1.181850606188767472 ) ) ;
#132011=CARTESIAN_POINT ( 'NONE',  ( 6.154511665599609493, 9.267681812253174556, 1.199719254218462483 ) ) ;
#132013=CARTESIAN_POINT ( 'NONE',  ( -4.415151579544611238, 8.302760609444034046, -0.7998128361456281477 ) ) ;
#132015=CARTESIAN_POINT ( 'NONE',  ( 1.499999999999989120, 1.775000000000019673, 0.000000000000000000 ) ) ;
#132016=CARTESIAN_POINT ( 'NONE',  ( -3.086452525405351643, 6.752611712948207057, 0.7998128361456341429 ) ) ;
#132019=CARTESIAN_POINT ( 'NONE',  ( -4.249591082879585535, 7.045274465746411252, 1.199719254218464037 ) ) ;
#132022=CARTESIAN_POINT ( 'NONE',  ( 1.364683531249988535, 3.613541667008086211, 0.7879004041258500513 ) ) ;
#132024=CARTESIAN_POINT ( 'NONE',  ( -4.121315508874269007, 5.831287398485176077, -1.443375672974053447 ) ) ;
#132027=ORIENTED_EDGE ( 'NONE', *, *, #157816, .F. ) ;
#132030=CARTESIAN_POINT ( 'NONE',  ( 5.840865249388943248, 5.708764300575555062, 0.7998128361456341429 ) ) ;
#132033=CARTESIAN_POINT ( 'NONE',  ( -1.364683531250012516, 3.051041667008083547, -0.7879004041258289570 ) ) ;
#132035=CARTESIAN_POINT ( 'NONE',  ( 4.033714395265605823, 4.664753868353354704, -1.199719254218446718 ) ) ;
#132037=CARTESIAN_POINT ( 'NONE',  ( 0.6823417656249882723, -0.5947916663252492686, 1.181850606188755259 ) ) ;
#132039=CARTESIAN_POINT ( 'NONE',  ( -2.449219305563052895, 6.009172956465517856, 1.040834085586084257E-14 ) ) ;
#132041=CARTESIAN_POINT ( 'NONE',  ( -6.412643469139482910, 7.544134137826577380, 1.082531754730549967 ) ) ;
#132044=ORIENTED_EDGE ( 'NONE', *, *, #11497, .T. ) ;
#132045=CARTESIAN_POINT ( 'NONE',  ( 0.6823417656249899377, 3.426041667008085323, -1.181850606188754593 ) ) ;
#132053=CARTESIAN_POINT ( 'NONE',  ( -5.694061327615147050, 9.586895948952255608, 0.000000000000000000 ) ) ;
#132060=CARTESIAN_POINT ( 'NONE',  ( -7.348156068482412095, 7.675196289425353591, 1.040834085586084257E-14 ) ) ;
#132064=CARTESIAN_POINT ( 'NONE',  ( 2.854315967138055132, 6.433244981884085334, -0.2941531795266367211 ) ) ;
#132072=CARTESIAN_POINT ( 'NONE',  ( -3.716906668440817185, 7.488141546489591072, 0.7998128361456341429 ) ) ;
#132074=CARTESIAN_POINT ( 'NONE',  ( -1.500000000000015099, -0.8708333333333129200, -0.8660254037844383745 ) ) ;
#132075=CARTESIAN_POINT ( 'NONE',  ( 2.846322183865124700, 5.408127416896231665, -1.199719254218446718 ) ) ;
#132078=EDGE_CURVE ( 'NONE', #60775, #158934, #22241, .T. ) ;
#132079=CARTESIAN_POINT ( 'NONE',  ( 3.968218245261731170, 4.000131783038177957, 0.6440902300205559872 ) ) ;
#132080=CARTESIAN_POINT ( 'NONE',  ( 6.193377243344257543, 6.120028293523423812, -0.7998128361456281477 ) ) ;
#132086=CARTESIAN_POINT ( 'NONE',  ( -2.643476764984671767, 6.027880625883323518, 1.040834085586084257E-14 ) ) ;
#132094=CARTESIAN_POINT ( 'NONE',  ( 1.364683531249986537, 2.655208333674754062, -0.7879004041258239610 ) ) ;
#132095=CARTESIAN_POINT ( 'NONE',  ( -6.204827856548512877, 10.39071626594860476, -0.7998128361456291469 ) ) ;
#132099=CARTESIAN_POINT ( 'NONE',  ( 5.947222937888848371, 10.09017719417900416, 1.040834085586084257E-14 ) ) ;
#132100=CARTESIAN_POINT ( 'NONE',  ( -4.889686956022917919, 8.856385215335397021, 1.214306433183764966E-14 ) ) ;
#132103=CARTESIAN_POINT ( 'NONE',  ( -1.500000000000015099, -1.297916665983847029, 0.8660254037844403729 ) ) ;
#132107=CARTESIAN_POINT ( 'NONE',  ( 7.619319141200057821, 10.87266085050000974, 1.082531754730557072 ) ) ;
#132110=CARTESIAN_POINT ( 'NONE',  ( 1.364683531249986537, 0.2177083336747502595, -0.7879004041258309554 ) ) ;
#132112=CARTESIAN_POINT ( 'NONE',  ( 5.788968402910795064, 9.697620870130524651, 0.7216878364870438212 ) ) ;
#132114=CARTESIAN_POINT ( 'NONE',  ( -4.446711195602252253, 6.210915699667823198, -1.443375672974053447 ) ) ;
#132116=CARTESIAN_POINT ( 'NONE',  ( -1.364683531250010295, 4.780208333674755394, 0.7879004041258379498 ) ) ;
#132120=CARTESIAN_POINT ( 'NONE',  ( -4.816275411463948330, 6.948951914485960835, -1.437501944199247372 ) ) ;
#132128=CARTESIAN_POINT ( 'NONE',  ( 5.621827251160867789, 9.710548892996357040, 1.040834085586084257E-14 ) ) ;
#132132=CARTESIAN_POINT ( 'NONE',  ( 2.998324526916512411, 6.649795714711241423, 0.000000000000000000 ) ) ;
#132137=ORIENTED_EDGE ( 'NONE', *, *, #99758, .T. ) ;
#132138=CARTESIAN_POINT ( 'NONE',  ( 6.317736394288147039, 6.473040002865377396, 0.7216878364870317197 ) ) ;
#132139=CARTESIAN_POINT ( 'NONE',  ( 1.364683531249986537, 1.176041667008082658, 0.7879004041258500513 ) ) ;
#132141=CARTESIAN_POINT ( 'NONE',  ( 10.70146331988817323, 11.37946204949139251, 0.7998128361456341429 ) ) ;
#132147=CARTESIAN_POINT ( 'NONE',  ( -1.201851678989727383E-14, 2.212500000000021672, 1.732050807568877637 ) ) ;
#132148=CARTESIAN_POINT ( 'NONE',  ( 6.287230548435207567, 8.358188277972981695, -1.599625672291262513 ) ) ;
#132149=CARTESIAN_POINT ( 'NONE',  ( -8.799405390469187793, 10.22472669609091689, -1.199719254218446718 ) ) ;
#132153=CARTESIAN_POINT ( 'NONE',  ( 0.6823417656249882723, 1.176041667008083325, -1.181850606188749264 ) ) ;
#132154=VERTEX_POINT ( 'NONE', #8152 ) ;
#132155=CARTESIAN_POINT ( 'NONE',  ( -1.201851678989727383E-14, 2.837500000000024780, -1.732050807568863648 ) ) ;
#132157=CARTESIAN_POINT ( 'NONE',  ( 3.822509244049070887, 6.547012320444182798, -1.199719254218452047 ) ) ;
#132164=CARTESIAN_POINT ( 'NONE',  ( 1.499999999999987566, -0.9437499993171851731, 0.000000000000000000 ) ) ;
#132165=CARTESIAN_POINT ( 'NONE',  ( -6.008234629150358330, 10.16135750065076060, 0.000000000000000000 ) ) ;
#132166=CARTESIAN_POINT ( 'NONE',  ( -5.273758566035884776, 5.255065869904374409, 0.000000000000000000 ) ) ;
#132174=CARTESIAN_POINT ( 'NONE',  ( 6.368579470117202490, 8.453095353268645695, 1.599625672291281386 ) ) ;
#132176=AXIS2_PLACEMENT_3D ( 'NONE', #51951, #36742, #187265 ) ;
#132177=CARTESIAN_POINT ( 'NONE',  ( 0.000000000000000000, 2.817530495244580102, 1.214306433183764966E-14 ) ) ;
#132178=CARTESIAN_POINT ( 'NONE',  ( 7.876924059415351564, 12.13356913605253240, -0.7216878364870267237 ) ) ;
#132182=CARTESIAN_POINT ( 'NONE',  ( -6.021792782764022078, 10.17717534653336209, -0.7998128361456291469 ) ) ;
#132183=CARTESIAN_POINT ( 'NONE',  ( 3.005103603723342953, 6.657704637652544832, -0.7998128361456291469 ) ) ;
#132187=CARTESIAN_POINT ( 'NONE',  ( 9.327646496521982300, 11.90534021740758064, -1.443375672974057666 ) ) ;
#132196=CARTESIAN_POINT ( 'NONE',  ( -3.416291520963659512, 5.969128626890772615, 1.082531754730560403 ) ) ;
#132197=CARTESIAN_POINT ( 'NONE',  ( 7.768458830950378591, 12.00702636951006497, 1.040834085586084257E-14 ) ) ;
#132200=CARTESIAN_POINT ( 'NONE',  ( -6.891622154448065807, 6.934647356477856128, 1.040834085586084257E-14 ) ) ;
#132205=CARTESIAN_POINT ( 'NONE',  ( -7.867809214632013770, 8.073532260025807261, 1.040834085586084257E-14 ) ) ;
#132218=CARTESIAN_POINT ( 'NONE',  ( -4.557512192488103686, 8.468847991211438497, -0.7998128361456281477 ) ) ;
#132221=CARTESIAN_POINT ( 'NONE',  ( 5.341549334104194635, 6.294524313618772737, 1.082531754730558626 ) ) ;
#132223=EDGE_CURVE ( 'NONE', #87474, #57507, #104606, .T. ) ;
#132227=CARTESIAN_POINT ( 'NONE',  ( -5.298539104842322267, 5.076050465271134016, 0.7998128361456341429 ) ) ;
#132231=CARTESIAN_POINT ( 'NONE',  ( 4.559605246071182449, 3.300000000000025135, -0.7749999999999944711 ) ) ;
#132235=CARTESIAN_POINT ( 'NONE',  ( -8.636707547105197946, 10.03491254549959777, -1.199719254218446718 ) ) ;
#132236=CARTESIAN_POINT ( 'NONE',  ( 6.796715079152391148, 6.823922435299587974, 0.7998128361456341429 ) ) ;
#132238=CARTESIAN_POINT ( 'NONE',  ( -7.160677686311960777, 11.50587440067263678, -0.7998128361456291469 ) ) ;
#132239=CARTESIAN_POINT ( 'NONE',  ( 5.983225862332436584, 5.874851682342960402, 0.7998128361456341429 ) ) ;
#132242=CARTESIAN_POINT ( 'NONE',  ( -1.364683531250014514, -0.4072916663252447167, 0.7879004041258379498 ) ) ;
#132245=CARTESIAN_POINT ( 'NONE',  ( 9.408995418203975447, 10.07950886410055524, 0.7216878364870438212 ) ) ;
#132251=CARTESIAN_POINT ( 'NONE',  ( 10.66990370383054731, 11.55056853066490952, 0.7216878364870317197 ) ) ;
#132271=VECTOR ( 'NONE', #185864, 1000.000000000000000 ) ;
#132272=CARTESIAN_POINT ( 'NONE',  ( -1.402160292154681736E-14, -0.006249999317184824418, 1.732050807568877637 ) ) ;
#132277=CARTESIAN_POINT ( 'NONE',  ( 0.2802162696002897246, 8.153957901067531822, -2.020850277443529741 ) ) ;
#132278=AXIS2_PLACEMENT_3D ( 'NONE', #117260, #171276, #3421 ) ;
#132280=CARTESIAN_POINT ( 'NONE',  ( 8.920375002787457319, 12.49452237230570084, 1.199719254218450271 ) ) ;
#132281=DIRECTION ( 'NONE',  ( -5.578564026256490882E-16, -1.000000000000000000, -9.066213480720158442E-32 ) ) ;
#132285=CARTESIAN_POINT ( 'NONE',  ( 5.007038802148489509, 4.735966778795008381, 0.7998128361456341429 ) ) ;
#132286=CARTESIAN_POINT ( 'NONE',  ( -6.724481002698120768, 9.828683022247721723, -1.082531754730538864 ) ) ;
#132290=CARTESIAN_POINT ( 'NONE',  ( -6.333630315878337136, 10.54098580183340772, 0.000000000000000000 ) ) ;
#132291=CARTESIAN_POINT ( 'NONE',  ( -4.595850884908229794, 4.464173575255435011, 0.7216878364870317197 ) ) ;
#132293=ORIENTED_EDGE ( 'NONE', *, *, #6240, .F. ) ;
#132294=CARTESIAN_POINT ( 'NONE',  ( -1.402160292154681736E-14, -0.3812499993171785673, -1.732050807568870754 ) ) ;
#132301=CARTESIAN_POINT ( 'NONE',  ( -4.568734577680894304, 5.392907097791561633, -1.082531754730543971 ) ) ;
#132310=CARTESIAN_POINT ( 'NONE',  ( -2.290964770585000920, 5.616616632417037458, -0.7216878364870257245 ) ) ;
#132311=( BOUNDED_CURVE ( )  B_SPLINE_CURVE ( 2, ( #29380, #92278, #161523 ),
 .UNSPECIFIED., .F., .T. ) 
 B_SPLINE_CURVE_WITH_KNOTS ( ( 3, 3 ),
 ( 0.000000000000000000, 0.002781257751169560668 ),
 .UNSPECIFIED. ) 
 CURVE ( )  GEOMETRIC_REPRESENTATION_ITEM ( )  RATIONAL_B_SPLINE_CURVE ( ( 1.000000000000000000, 0.9105717077957579120, 0.9405305184076300229 ) ) 
 REPRESENTATION_ITEM ( '' )  );
#132312=CARTESIAN_POINT ( 'NONE',  ( 6.611572464958476836, 10.86525164242692298, 0.7998128361456462443 ) ) ;
#132321=CARTESIAN_POINT ( 'NONE',  ( -9.484092147959342967, 11.02352791316275216, 1.199719254218462483 ) ) ;
#132324=ORIENTED_EDGE ( 'NONE', *, *, #102521, .T. ) ;
#132327=CARTESIAN_POINT ( 'NONE',  ( 6.342516933094585418, 6.294024598232139667, 1.040834085586084257E-14 ) ) ;
#132330=ORIENTED_EDGE ( 'NONE', *, *, #128510, .F. ) ;
#132345=CARTESIAN_POINT ( 'NONE',  ( 8.444030743212801227, 8.745790710036752458, 0.7998128361456462443 ) ) ;
#132347=CARTESIAN_POINT ( 'NONE',  ( -5.447678794592645701, 5.250046769979851646, 0.000000000000000000 ) ) ;
#132355=CARTESIAN_POINT ( 'NONE',  ( -0.6823417656249969321, 5.717708333674756283, -1.181850606188749264 ) ) ;
#132360=CARTESIAN_POINT ( 'NONE',  ( 2.205172540517054802, 5.724451730578533848, 1.040834085586084257E-14 ) ) ;
#132362=CARTESIAN_POINT ( 'NONE',  ( -2.598358995313378550, 6.183169261174235487, 0.7998128361456341429 ) ) ;
#132368=CARTESIAN_POINT ( 'NONE',  ( 5.856759171423504107, 5.935233242856626568, -0.7216878364870257245 ) ) ;
#132371=CARTESIAN_POINT ( 'NONE',  ( 1.364683531249990311, 4.696875000341417916, 1.214306433183764966E-14 ) ) ;
#132373=CARTESIAN_POINT ( 'NONE',  ( 2.684151225381301575, 6.075334163012737321, 0.000000000000000000 ) ) ;
#132383=CARTESIAN_POINT ( 'NONE',  ( -5.867374215541069304, 6.167859493020809047, 0.9100554989533160555 ) ) ;
#132386=CARTESIAN_POINT ( 'NONE',  ( 1.364683531249992088, 5.696875000341418804, 1.214306433183764966E-14 ) ) ;
#132393=CARTESIAN_POINT ( 'NONE',  ( -1.001543065824772872E-14, 4.962500000000019007, 1.732050807568877637 ) ) ;
#132401=CARTESIAN_POINT ( 'NONE',  ( 1.364683531249988535, 4.717708333674756283, -0.7879004041258300672 ) ) ;
#132403=CARTESIAN_POINT ( 'NONE',  ( 5.099838337034727331, 9.101561826515851550, -0.7998128361456281477 ) ) ;
#132404=CARTESIAN_POINT ( 'NONE',  ( -8.642432853707342488, 12.17025653171218558, 1.199719254218462483 ) ) ;
#132407=EDGE_CURVE ( 'NONE', #123409, #79803, #177218, .T. ) ;
#132411=CARTESIAN_POINT ( 'NONE',  ( -1.402160292154681736E-14, -0.9906249996585834161, -1.575800808251665908 ) ) ;
#132419=CARTESIAN_POINT ( 'NONE',  ( 6.778713617152772208, 10.85232362007950258, -0.7216878364870267237 ) ) ;
#132422=CYLINDRICAL_SURFACE ( 'NONE', #62130, 1.250000000000000000 ) ;
#132424=CARTESIAN_POINT ( 'NONE',  ( 1.499999999999987121, 3.077083334016149863, -0.8660254037844262731 ) ) ;
#132426=CARTESIAN_POINT ( 'NONE',  ( -6.064574784014443942, 5.969758757638621738, -0.7998128361456291469 ) ) ;
#132427=CARTESIAN_POINT ( 'NONE',  ( 4.867013957181530515, 5.740899707208986236, -1.082531754730548412 ) ) ;
#132435=CARTESIAN_POINT ( 'NONE',  ( 3.171717870593107058, 5.787755718078879674, -1.199719254218446718 ) ) ;
#132439=CARTESIAN_POINT ( 'NONE',  ( 2.855963913973019963, 6.483708332943829866, 0.000000000000000000 ) ) ;
#132444=ADVANCED_FACE ( 'NONE', ( #37793 ), #88690, .F. ) ;
#132447=ORIENTED_EDGE ( 'NONE', *, *, #159943, .T. ) ;
#132448=CIRCLE ( 'NONE', #42444, 0.07999999999999968248 ) ;
#132453=DIRECTION ( 'NONE',  ( 3.347138415753902517E-16, 0.6000000000000019762, 0.7999999999999986011 ) ) ;
#132454=CARTESIAN_POINT ( 'NONE',  ( 5.678179657697552507, 6.109196432984326464, -0.7486794562398890740 ) ) ;
#132456=CARTESIAN_POINT ( 'NONE',  ( 10.55232363013785246, 11.20546574478267132, 0.000000000000000000 ) ) ;
#132459=CARTESIAN_POINT ( 'NONE',  ( 5.829642864196162400, 7.824335979694092558, 1.443375672974062551 ) ) ;
#132460=CARTESIAN_POINT ( 'NONE',  ( -8.663296969452339624, 13.05100419776235299, 1.040834085586084257E-14 ) ) ;
#132466=CARTESIAN_POINT ( 'NONE',  ( -4.172158584703340445, 5.890604320285754980, -1.599625672291256295 ) ) ;
#132478=CARTESIAN_POINT ( 'NONE',  ( 6.110807642276722795, 6.018297815386236316, -0.1222484578899986352 ) ) ;
#132480=CARTESIAN_POINT ( 'NONE',  ( -4.650083499807243115, 5.295740330745369207, -1.052294140492322283 ) ) ;
#132486=CARTESIAN_POINT ( 'NONE',  ( -8.297226821883391779, 11.66355314463053006, 1.082531754730549967 ) ) ;
#132488=CARTESIAN_POINT ( 'NONE',  ( 1.203907071533380613, 2.868479746939697872, -0.7749999999999910294 ) ) ;
#132490=CARTESIAN_POINT ( 'NONE',  ( 8.776205506747620788, 9.133327934160710981, -0.7998128361456221525 ) ) ;
#132491=CARTESIAN_POINT ( 'NONE',  ( -4.924636110261798372, 6.768494766770632332, 1.599625672291267175 ) ) ;
#132493=CARTESIAN_POINT ( 'NONE',  ( 3.083589872104280705, 5.684939719841914929, 1.199719254218450271 ) ) ;
#132495=CARTESIAN_POINT ( 'NONE',  ( -4.550733115681270036, 8.460939068270139529, 0.7998128361456481317 ) ) ;
#132496=CARTESIAN_POINT ( 'NONE',  ( 2.686486993802192913, 6.285985259411197568, 0.7998128361456362523 ) ) ;
#132499=CARTESIAN_POINT ( 'NONE',  ( -4.367698041896780126, 8.247398148854895084, 0.7998128361456481317 ) ) ;
#132503=CARTESIAN_POINT ( 'NONE',  ( 8.565000355531088516, 11.01558638625153286, -1.599625672291257406 ) ) ;
#132504=CARTESIAN_POINT ( 'NONE',  ( 0.5056851195614943117, 6.800201140161028945, 3.700268186881439547 ) ) ;
#132506=CARTESIAN_POINT ( 'NONE',  ( 4.420695050690802930, 7.093836324768183488, -1.099706215833176515 ) ) ;
#132507=CARTESIAN_POINT ( 'NONE',  ( 6.493992391265805075, 6.678671999339316656, 1.040834085586084257E-14 ) ) ;
#132514=VERTEX_POINT ( 'NONE', #7402 ) ;
#132515=CARTESIAN_POINT ( 'NONE',  ( 8.066738210006686671, 9.473911335505048825, 1.082531754730558626 ) ) ;
#132519=CARTESIAN_POINT ( 'NONE',  ( -8.611400122974211868, 13.19838391011195888, 1.040834085586084257E-14 ) ) ;
#132520=CARTESIAN_POINT ( 'NONE',  ( -7.446452682403657874, 9.710614100936176385, -1.599625672291263179 ) ) ;
#132524=CARTESIAN_POINT ( 'NONE',  ( 3.988012250146443449, 7.596505358572088085, 0.1212705993496351053 ) ) ;
#132529=CARTESIAN_POINT ( 'NONE',  ( 3.460355519985863548, 5.060167411448709629, 1.599625672291267398 ) ) ;
#132533=CARTESIAN_POINT ( 'NONE',  ( 2.347533153460546806, 5.890539112345938300, 0.000000000000000000 ) ) ;
#132536=CARTESIAN_POINT ( 'NONE',  ( -0.7500000000000215383, 4.472916667349482012, 1.299038105676671107 ) ) ;
#132542=CARTESIAN_POINT ( 'NONE',  ( -1.201851678989727383E-14, 2.212500000000021672, 1.732050807568877637 ) ) ;
#132543=CARTESIAN_POINT ( 'NONE',  ( 5.750629710490689384, 9.860818428881154674, -0.7998128361456291469 ) ) ;
#132544=CARTESIAN_POINT ( 'NONE',  ( 5.639828713160493834, 5.682147708216442439, 1.040834085586084257E-14 ) ) ;
#132546=CARTESIAN_POINT ( 'NONE',  ( 7.727784370109387346, 10.99920361756089093, -1.082531754730543083 ) ) ;
#132551=CARTESIAN_POINT ( 'NONE',  ( -4.391951695823077984, 7.211361847513815704, 1.199719254218464037 ) ) ;
#132552=CARTESIAN_POINT ( 'NONE',  ( -0.7499999999999972244, 3.889583334016149863, -1.299038105676652011 ) ) ;
#132553=CARTESIAN_POINT ( 'NONE',  ( -1.364683531250014514, 0.2802083336747505649, 0.7879004041258379498 ) ) ;
#132557=CARTESIAN_POINT ( 'NONE',  ( 3.011882680530176604, 6.665613560593854459, 0.7998128361456341429 ) ) ;
#132559=CARTESIAN_POINT ( 'NONE',  ( -1.364683531250010295, 5.551041667008087543, -0.7879004041258300672 ) ) ;
#132563=CARTESIAN_POINT ( 'NONE',  ( 3.563261906135761770, 6.332667919118538435, 2.420000000000010587 ) ) ;
#132565=CARTESIAN_POINT ( 'NONE',  ( -7.660520486921249983, 8.896027641951645748, -1.199719254218446718 ) ) ;
#132566=CARTESIAN_POINT ( 'NONE',  ( 3.832150974156964818, 7.622593236491780999, 1.040834085586084257E-14 ) ) ;
#132569=CARTESIAN_POINT ( 'NONE',  ( -1.364683531250014514, -0.4697916663252449943, 0.7879004041258379498 ) ) ;
#132575=CARTESIAN_POINT ( 'NONE',  ( -5.194745412330402878, 9.212286747694129474, 0.000000000000000000 ) ) ;
#132581=CARTESIAN_POINT ( 'NONE',  ( 9.399880572976245574, 9.860948844760784482, 0.7998128361456462443 ) ) ;
#132583=CARTESIAN_POINT ( 'NONE',  ( -3.307299406729781399, 5.945934176904983381, -1.199719254218452935 ) ) ;
#132584=CARTESIAN_POINT ( 'NONE',  ( -8.518600588087975822, 8.832788862391110385, 1.040834085586084257E-14 ) ) ;
#132588=CARTESIAN_POINT ( 'NONE',  ( -4.243318646243602998, 7.513047557524930475, 1.036732258902311354 ) ) ;
#132589=CARTESIAN_POINT ( 'NONE',  ( -1.364683531250014514, 0.03020833367475737191, 0.7879004041258379498 ) ) ;
#132593=CARTESIAN_POINT ( 'NONE',  ( 8.107412671292035355, 10.48173408797264194, 1.443375672974076540 ) ) ;
#132611=CARTESIAN_POINT ( 'NONE',  ( 9.856941372335116469, 11.45851867493453291, 1.199719254218450271 ) ) ;
#132615=CARTESIAN_POINT ( 'NONE',  ( -3.276266675996675204, 6.974061555304760240, -0.7998128361456281477 ) ) ;
#132621=CARTESIAN_POINT ( 'NONE',  ( -1.500000000000013101, 2.452083334016154748, 0.8660254037844403729 ) ) ;
#132622=CARTESIAN_POINT ( 'NONE',  ( 9.725276259704228821, 10.24057714594344048, 0.7998128361456462443 ) ) ;
#132627=CARTESIAN_POINT ( 'NONE',  ( -8.208571938070008400, 11.66408546346865016, -1.199719254218446718 ) ) ;
#132629=CARTESIAN_POINT ( 'NONE',  ( -0.6823417656250003738, 1.967708333674753174, -1.181850606188749264 ) ) ;
#132630=DIRECTION ( 'NONE',  ( -5.578564026256490882E-16, -1.000000000000000000, -9.066213480720158442E-32 ) ) ;
#132635=CARTESIAN_POINT ( 'NONE',  ( -3.789667630219657912, 4.380032642466370696, 1.199719254218462483 ) ) ;
#132639=CARTESIAN_POINT ( 'NONE',  ( -1.364683531250000748, 1.071875000341421247, 0.000000000000000000 ) ) ;
#132644=CARTESIAN_POINT ( 'NONE',  ( -1.201851678989727383E-14, 1.321875000341419248, 1.575800808251672791 ) ) ;
#132648=CARTESIAN_POINT ( 'NONE',  ( -5.412729640353771465, 7.337937218544611895, 1.599625672291269396 ) ) ;
#132649=CARTESIAN_POINT ( 'NONE',  ( 1.000000000000001554, 6.468705557303653819, -4.925226524755053958 ) ) ;
#132652=CARTESIAN_POINT ( 'NONE',  ( -0.7499999999999972244, 3.608333333333359150, -1.299038105676652011 ) ) ;
#132653=CARTESIAN_POINT ( 'NONE',  ( -1.364683531250012516, 3.301041667008084879, -0.7879004041258289570 ) ) ;
#132657=CARTESIAN_POINT ( 'NONE',  ( -5.016153647376219382, 6.875265226737464985, 1.443375672974064550 ) ) ;
#132661=CARTESIAN_POINT ( 'NONE',  ( 5.585596099150174965, 7.539614753807099667, -1.443375672974057666 ) ) ;
#132664=CARTESIAN_POINT ( 'NONE',  ( -7.004758919754800139, 11.32396917302262018, 0.000000000000000000 ) ) ;
#132665=CARTESIAN_POINT ( 'NONE',  ( -3.521367211247373508, 5.131347717920458962, -1.599625672291256295 ) ) ;
#132667=CARTESIAN_POINT ( 'NONE',  ( -1.201851678989727383E-14, 5.446875000341422357, -1.575800808251660134 ) ) ;
#132672=CARTESIAN_POINT ( 'NONE',  ( -6.521108698048772467, 9.591415333490143524, -1.082531754730537976 ) ) ;
#132674=CARTESIAN_POINT ( 'NONE',  ( 0.7499999999999902300, 5.066666666666684193, -1.299038105676658228 ) ) ;
#132677=CARTESIAN_POINT ( 'NONE',  ( 7.836249599018724865, 9.205007956019091608, -1.082531754730537976 ) ) ;
#132684=ORIENTED_EDGE ( 'NONE', *, *, #89482, .T. ) ;
#132685=CARTESIAN_POINT ( 'NONE',  ( 10.01911233037458260, 10.79131192829960462, 0.7216878364870438212 ) ) ;
#132692=CARTESIAN_POINT ( 'NONE',  ( 5.503720292143644777, 8.508425209887878538, 1.199719254218462483 ) ) ;
#132693=CARTESIAN_POINT ( 'NONE',  ( -5.687809136132860210, 6.594531066031826150, -1.199719254218446718 ) ) ;
#132696=CARTESIAN_POINT ( 'NONE',  ( 1.579999999999989413, 6.280000000000042881, 2.500000000000000444 ) ) ;
#132697=( BOUNDED_CURVE ( )  B_SPLINE_CURVE ( 2, ( #168400, #100198, #99150, #1598, #82875, #67659, #524 ),
 .UNSPECIFIED., .F., .T. ) 
 B_SPLINE_CURVE_WITH_KNOTS ( ( 3, 2, 2, 3 ),
 ( 0.1249999999999998612, 0.1309523809523809035, 0.1369047619047619735, 0.1428571428571429880 ),
 .UNSPECIFIED. ) 
 CURVE ( )  GEOMETRIC_REPRESENTATION_ITEM ( )  RATIONAL_B_SPLINE_CURVE ( ( 1.000000000000003109, 0.8660254037844355990, 1.000000000000000000, 0.8660254037844387076, 1.000000000000000000, 0.8660254037844355990, 1.000000000000003109 ) ) 
 REPRESENTATION_ITEM ( '' )  );
#132698=CARTESIAN_POINT ( 'NONE',  ( 4.636525345749193505, 8.353103970108639587, 1.040834085586084257E-14 ) ) ;
#132699=CARTESIAN_POINT ( 'NONE',  ( 1.364683531249986537, 0.1760416670080860446, 0.7879004041258500513 ) ) ;
#132700=CARTESIAN_POINT ( 'NONE',  ( 2.901081683644312736, 6.328419697652925002, 0.7216878364870338292 ) ) ;
#132701=CARTESIAN_POINT ( 'NONE',  ( -7.648771216403934758, 12.07531685244661723, -0.7998128361456291469 ) ) ;
#132717=CARTESIAN_POINT ( 'NONE',  ( 6.337546739384100292, 9.481222731668410120, 1.199719254218460707 ) ) ;
#132718=CARTESIAN_POINT ( 'NONE',  ( 6.551614543901692400, 8.666636272683888365, 1.599625672291281386 ) ) ;
#132728=CARTESIAN_POINT ( 'NONE',  ( 10.73535870392234237, 11.41900666419791399, 0.000000000000000000 ) ) ;
#132730=CARTESIAN_POINT ( 'NONE',  ( -5.063080299699540987, 7.994345218703034384, 1.199719254218464037 ) ) ;
#132732=CARTESIAN_POINT ( 'NONE',  ( -4.952806187693842510, 4.672695395264567786, 0.7998128361456341429 ) ) ;
#132737=EDGE_CURVE ( 'NONE', #12149, #103805, #113747, .T. ) ;
#132742=VECTOR ( 'NONE', #39044, 1000.000000000000000 ) ;
#132743=CARTESIAN_POINT ( 'NONE',  ( -2.103486388414573138, 5.605817886458954291, 1.040834085586084257E-14 ) ) ;
#132746=CARTESIAN_POINT ( 'NONE',  ( 6.124532705071213279, 8.168374127381657246, -1.599625672291262513 ) ) ;
#132747=CARTESIAN_POINT ( 'NONE',  ( -1.364683531250010740, 5.280208333674758947, 0.7879004041258379498 ) ) ;
#132752=CARTESIAN_POINT ( 'NONE',  ( 4.650083499362867911, 6.448183387388563226, 1.443375672974062551 ) ) ;
#132753=CARTESIAN_POINT ( 'NONE',  ( -5.343885102080728977, 9.386283052402845328, 0.7998128361456481317 ) ) ;
#132758=CARTESIAN_POINT ( 'NONE',  ( -7.694415870955439551, 8.935572256658169010, 1.199719254218462483 ) ) ;
#132759=CARTESIAN_POINT ( 'NONE',  ( -4.436542580169821726, 6.199052314996659874, 1.599625672291267398 ) ) ;
#132766=CARTESIAN_POINT ( 'NONE',  ( 6.799577732453452761, 7.891594428405881878, -1.199719254218446718 ) ) ;
#132772=( BOUNDED_SURFACE ( )  B_SPLINE_SURFACE ( 3, 2, ( 
 ( #169188, #136706, #104203 ),
 ( #137776, #170249, #203794 ),
 ( #117302, #53308, #19729 ),
 ( #55440, #20780, #17577 ),
 ( #199537, #202730, #21834 ),
 ( #87942, #85808, #34905 ) ),
 .UNSPECIFIED., .F., .F., .T. ) 
 B_SPLINE_SURFACE_WITH_KNOTS ( ( 4, 2, 4 ),
 ( 3, 3 ),
 ( 0.000000000000000000, 0.002122857551078453833, 0.004245715102156907665 ),
 ( 0.000000000000000000, 1.000000000000000000 ),
 .UNSPECIFIED. ) 
 GEOMETRIC_REPRESENTATION_ITEM ( )  RATIONAL_B_SPLINE_SURFACE ( (
 ( 1.000000000000000000, 0.7806433624857550546, 1.000000000000000000),
 ( 1.000000000000000000, 0.7860453980259737294, 1.000000000000000000),
 ( 1.000000000000000000, 0.7924770197564218188, 1.000000000000000000),
 ( 1.000000000000000000, 0.8094762427233131996, 1.000000000000000000),
 ( 1.000000000000000000, 0.8200718518785200528, 1.000000000000000000),
 ( 1.000000000000000000, 0.8343063410434338190, 1.000000000000000000) ) ) 
 REPRESENTATION_ITEM ( '' )  SURFACE ( )  );
#132780=CARTESIAN_POINT ( 'NONE',  ( 0.7499999999999920064, 5.483333333333353821, 1.299038105676669330 ) ) ;
#132781=CARTESIAN_POINT ( 'NONE',  ( 4.253507506385319381, 5.985511395581417204, 1.599625672291267398 ) ) ;
#132782=CARTESIAN_POINT ( 'NONE',  ( 4.656335691289526402, 7.519809842224722374, -1.199719254218452047 ) ) ;
#132784=CARTESIAN_POINT ( 'NONE',  ( -6.399085315970132193, 10.40942393536641397, -0.7216878364870278340 ) ) ;
#132785=CARTESIAN_POINT ( 'NONE',  ( -2.065456695249157981, 8.523797939977241001, -2.459872958007379928 ) ) ;
#132786=CARTESIAN_POINT ( 'NONE',  ( 4.351804120306567825, 8.020929207092235558, 1.040834085586084257E-14 ) ) ;
#132787=CARTESIAN_POINT ( 'NONE',  ( -8.690413276235355866, 10.20153224610512943, 1.082531754730558626 ) ) ;
#132792=CARTESIAN_POINT ( 'NONE',  ( 7.721532178182734185, 8.967207948423393304, 1.199719254218462483 ) ) ;
#132794=CARTESIAN_POINT ( 'NONE',  ( -1.420000000000001039, 6.200000000000045475, -2.579999999999995630 ) ) ;
#132798=CARTESIAN_POINT ( 'NONE',  ( 1.364683531249988535, 3.863541667008087543, 0.7879004041258500513 ) ) ;
#132804=CARTESIAN_POINT ( 'NONE',  ( 6.747154001095143627, 11.02343010125301959, -0.7998128361456291469 ) ) ;
#132808=CARTESIAN_POINT ( 'NONE',  ( -8.799405390469187793, 10.22472669609091689, -1.199719254218446718 ) ) ;
#132814=CARTESIAN_POINT ( 'NONE',  ( 7.540305987494599016, 11.94877408538573427, -0.7998128361456291469 ) ) ;
#132815=CARTESIAN_POINT ( 'NONE',  ( -3.096765176264313357, 6.450054161018508481, 0.6354748981389554130 ) ) ;
#132818=CARTESIAN_POINT ( 'NONE',  ( -7.666245793523398078, 11.03137162816423356, 1.199719254218453823 ) ) ;
#132820=CARTESIAN_POINT ( 'NONE',  ( 0.1861310709357004711, 6.361154168393027497, 3.114872224523889344 ) ) ;
#132822=CARTESIAN_POINT ( 'NONE',  ( 5.343583877570073248, 6.330574952785890552, -1.095086179472234189 ) ) ;
#132823=CARTESIAN_POINT ( 'NONE',  ( -4.627410500965859264, 4.293067094081919777, 0.7998128361456341429 ) ) ;
#132828=CARTESIAN_POINT ( 'NONE',  ( 5.601490020740366838, 9.686822124172440596, 1.040834085586084257E-14 ) ) ;
#132830=CARTESIAN_POINT ( 'NONE',  ( 5.148345644887269756, 7.029489223833707001, -1.599625672291256295 ) ) ;
#132831=CARTESIAN_POINT ( 'NONE',  ( -4.022774286133019572, 7.614368594009178537, 0.1926593524083572428 ) ) ;
#132832=CARTESIAN_POINT ( 'NONE',  ( 4.202137545231717120, 6.989912005157271402, 1.199719254218462483 ) ) ;
#132834=CARTESIAN_POINT ( 'NONE',  ( -7.917598520700757980, 9.299915031314755609, 1.082531754730558626 ) ) ;
#132840=CARTESIAN_POINT ( 'NONE',  ( -4.022774286133019572, 7.614368594009178537, 0.1926593524083572428 ) ) ;
#132841=CARTESIAN_POINT ( 'NONE',  ( 1.364683531249988757, -0.8031249996585804185, 0.000000000000000000 ) ) ;
#132844=CARTESIAN_POINT ( 'NONE',  ( 3.199361063144961825, 6.676412307070352270, -0.7216878364870267237 ) ) ;
#132848=CARTESIAN_POINT ( 'NONE',  ( -8.785320351530977234, 13.19336481018743079, 1.040834085586084257E-14 ) ) ;
#132853=CARTESIAN_POINT ( 'NONE',  ( -10.29027540264791440, 11.10766884595181203, 0.7216878364870438212 ) ) ;
#132860=CARTESIAN_POINT ( 'NONE',  ( -7.795575137733361970, 12.03866206075687018, 0.7216878364870458196 ) ) ;
#132867=CARTESIAN_POINT ( 'NONE',  ( 1.499999999999987121, 2.327083334016154303, -0.8660254037844262731 ) ) ;
#132868=CARTESIAN_POINT ( 'NONE',  ( 4.786522169170392971, 5.141580351323885800, 0.8077998227834035649 ) ) ;
#132869=CARTESIAN_POINT ( 'NONE',  ( -6.403528624356093601, 6.365204904703887223, 1.040834085586084257E-14 ) ) ;
#132873=CARTESIAN_POINT ( 'NONE',  ( -7.808606406466886973, 11.19745900993164511, 1.199719254218453823 ) ) ;
#132878=CARTESIAN_POINT ( 'NONE',  ( 5.126954644262057492, 9.133197518281081173, 0.7998128361456462443 ) ) ;
#132883=CARTESIAN_POINT ( 'NONE',  ( 8.633844893804129228, 8.967240552393299424, -0.7998128361456211532 ) ) ;
#132884=CARTESIAN_POINT ( 'NONE',  ( 0.9399888277777949108, 7.435091042679344397, 4.383624543540939555 ) ) ;
#132885=DIRECTION ( 'NONE',  ( 0.7592566023652995710, -0.6507913734559652719, 0.000000000000000000 ) ) ;
#132888=CARTESIAN_POINT ( 'NONE',  ( -6.561783159334130922, 9.638868871656395498, -1.082531754730538864 ) ) ;
#132894=CARTESIAN_POINT ( 'NONE',  ( -1.364683531250010295, 5.030208333674757171, 0.7879004041258379498 ) ) ;
#132897=CARTESIAN_POINT ( 'NONE',  ( -3.267151830768959098, 4.834763107362302748, -1.443375672974058777 ) ) ;
#132899=CARTESIAN_POINT ( 'NONE',  ( 8.238550898598388628, 12.76339314834017102, 0.7998128361456462443 ) ) ;
#132900=CARTESIAN_POINT ( 'NONE',  ( 1.499999999999822586, 7.268077025657071033, 4.207854987878929975 ) ) ;
#132901=CARTESIAN_POINT ( 'NONE',  ( -8.859363311525973117, 12.42334206583395328, -1.199719254218446718 ) ) ;
#132904=CARTESIAN_POINT ( 'NONE',  ( -1.364683531250000748, 2.259375000341422357, 1.214306433183764966E-14 ) ) ;
#132906=CARTESIAN_POINT ( 'NONE',  ( 4.684505768721569652, 5.424010470718658716, -1.199719254218452047 ) ) ;
#132911=CARTESIAN_POINT ( 'NONE',  ( -3.028993686180011746, 2.741750000184231428, -2.499999999999996003 ) ) ;
#132913=CARTESIAN_POINT ( 'NONE',  ( 8.961576348508637935, 11.47825837805867799, -1.443375672974052559 ) ) ;
#132915=CARTESIAN_POINT ( 'NONE',  ( -6.887178846062116833, 9.058127958537705027, -1.443375672974059665 ) ) ;
#132917=CARTESIAN_POINT ( 'NONE',  ( 0.3421332810201426211, 7.155223633118597881, 1.971148363701352269 ) ) ;
#132919=CARTESIAN_POINT ( 'NONE',  ( -8.158255747121117452, 10.54105100977322174, 1.599625672291295375 ) ) ;
#132920=CARTESIAN_POINT ( 'NONE',  ( -4.622967192135580383, 5.456178481322002227, 1.082531754730558626 ) ) ;
#132921=CARTESIAN_POINT ( 'NONE',  ( -1.201851678989727383E-14, 3.884375000341423689, 1.575800808251672791 ) ) ;
#132926=CARTESIAN_POINT ( 'NONE',  ( 8.778014389843965759, 12.32843499053828928, 1.199719254218450271 ) ) ;
#132942=CARTESIAN_POINT ( 'NONE',  ( 1.364683531249990311, 3.946875000341417028, 1.214306433183764966E-14 ) ) ;
#132944=B_SPLINE_CURVE_WITH_KNOTS ( 'NONE', 3,
 ( #13456, #178112, #194347, #212714 ),
 .UNSPECIFIED., .F., .F.,
 ( 4, 4 ),
 ( 8.673617379883660879E-19, 0.0006776115001627299730 ),
 .UNSPECIFIED. ) ;
#132947=CARTESIAN_POINT ( 'NONE',  ( -3.189213936345670852, 2.817530495244580102, -2.450448857954567572 ) ) ;
#132950=CARTESIAN_POINT ( 'NONE',  ( 8.075853055234393452, 12.57357899774884658, 0.7998128361456462443 ) ) ;
#132951=CARTESIAN_POINT ( 'NONE',  ( -2.279673327426058105, 5.603443282065057929, -0.02210016498917465738 ) ) ;
#132954=CARTESIAN_POINT ( 'NONE',  ( -1.364683531249997417, 3.009375000341422801, 1.214306433183764966E-14 ) ) ;
#132956=CARTESIAN_POINT ( 'NONE',  ( -5.721177635286839092, 9.618531641235897212, 0.7216878364870458196 ) ) ;
#132964=CARTESIAN_POINT ( 'NONE',  ( 5.190073875932979419, 4.949507698210251938, 0.7998128361456341429 ) ) ;
#132968=CARTESIAN_POINT ( 'NONE',  ( 8.215351014876830504, 11.67199438640995801, -1.199719254218446718 ) ) ;
#132975=CARTESIAN_POINT ( 'NONE',  ( -8.272446282632566650, 12.80293776304669962, 0.7998128361456481317 ) ) ;
#132976=CARTESIAN_POINT ( 'NONE',  ( 5.960781091502512119, 10.10599504006161986, 0.7998128361456462443 ) ) ;
#132978=CARTESIAN_POINT ( 'NONE',  ( 5.626270559546826533, 5.666329862333828515, 0.7216878364870317197 ) ) ;
#132989=CARTESIAN_POINT ( 'NONE',  ( -7.863365906246074566, 8.276274433482971205, -0.7216878364870278340 ) ) ;
#132990=CARTESIAN_POINT ( 'NONE',  ( 3.649115900372475796, 7.409052317076538330, 1.040834085586084257E-14 ) ) ;
#132993=CARTESIAN_POINT ( 'NONE',  ( -8.158255747121117452, 10.54105100977322174, 1.599625672291295375 ) ) ;
#132998=CARTESIAN_POINT ( 'NONE',  ( -3.327636637150278798, 5.969660945728899826, -1.199719254218452935 ) ) ;
#133001=AXIS2_PLACEMENT_3D ( 'NONE', #69291, #135402, #201425 ) ;
#133002=EDGE_CURVE ( 'NONE', #66184, #132154, #61885, .T. ) ;
#133004=CARTESIAN_POINT ( 'NONE',  ( 9.759171643738394408, 10.28012176064996197, 0.000000000000000000 ) ) ;
#133005=CARTESIAN_POINT ( 'NONE',  ( 3.005103603723342953, 6.657704637652544832, -0.7998128361456291469 ) ) ;
#133007=ORIENTED_EDGE ( 'NONE', *, *, #172864, .T. ) ;
#133011=CARTESIAN_POINT ( 'NONE',  ( 2.250290310188348464, 5.569163095287620990, 0.7216878364870438212 ) ) ;
#133014=CARTESIAN_POINT ( 'NONE',  ( -2.591579918506545344, 6.175260338232929413, 1.040834085586084257E-14 ) ) ;
#133015=CYLINDRICAL_SURFACE ( 'NONE', #81495, 1.500000000000000222 ) ;
#133017=CARTESIAN_POINT ( 'NONE',  ( -7.309817376062285099, 11.67987070538135264, 0.000000000000000000 ) ) ;
#133021=CARTESIAN_POINT ( 'NONE',  ( 5.829642864196151741, 9.745074408296771296, 0.7216878364870438212 ) ) ;
#133022=CARTESIAN_POINT ( 'NONE',  ( -1.364683531249997417, 5.071875000341417916, 1.214306433183764966E-14 ) ) ;
#133024=CARTESIAN_POINT ( 'NONE',  ( 2.347533153460546806, 5.890539112345938300, 0.000000000000000000 ) ) ;
#133025=CARTESIAN_POINT ( 'NONE',  ( 5.908755808680682620, 6.041823544852629624, 0.5163281919262531217 ) ) ;
#133027=CARTESIAN_POINT ( 'NONE',  ( -6.877010230629689858, 9.046264573866535486, 1.599625672291283607 ) ) ;
#133037=CARTESIAN_POINT ( 'NONE',  ( -1.364683531250012516, 3.801041667008087099, -0.7879004041258300672 ) ) ;
#133038=CARTESIAN_POINT ( 'NONE',  ( 9.023114925094663619, 10.48572115315399245, 1.199719254218453823 ) ) ;
#133040=CARTESIAN_POINT ( 'NONE',  ( -4.256897045010916258, 7.910204285913967404, 0.7216878364870317197 ) ) ;
#133042=CARTESIAN_POINT ( 'NONE',  ( -4.243338890952901288, 6.934017225211593249, -1.082531754730548412 ) ) ;
#133049=CARTESIAN_POINT ( 'NONE',  ( 4.253507506385319381, 5.985511395581417204, 1.599625672291267398 ) ) ;
#133061=CARTESIAN_POINT ( 'NONE',  ( 6.328958779480917229, 6.278206752349526631, 0.7998128361456341429 ) ) ;
#133067=CARTESIAN_POINT ( 'NONE',  ( -6.423865854776591000, 6.388931673527803667, 1.040834085586084257E-14 ) ) ;
#133071=CARTESIAN_POINT ( 'NONE',  ( 6.693975156845185737, 8.832723654451292816, 1.599625672291281386 ) ) ;
#133075=CARTESIAN_POINT ( 'NONE',  ( -6.911959384868566758, 6.958374125301778790, 1.040834085586084257E-14 ) ) ;
#133076=CARTESIAN_POINT ( 'NONE',  ( 0.7499999999999902300, 2.733333333333351600, 1.299038105676669330 ) ) ;
#133077=CARTESIAN_POINT ( 'NONE',  ( -4.029797971759847997, 5.724516938518342535, -1.599625672291256295 ) ) ;
#133080=CARTESIAN_POINT ( 'NONE',  ( -3.913499895838973508, 7.717500311787445000, 1.040834085586084257E-14 ) ) ;
#133082=CARTESIAN_POINT ( 'NONE',  ( -1.364683531249997417, 3.009375000341422801, 1.214306433183764966E-14 ) ) ;
#133084=CARTESIAN_POINT ( 'NONE',  ( -3.958617665510266725, 7.562211676496538360, -0.7216878364870267237 ) ) ;
#133090=CARTESIAN_POINT ( 'NONE',  ( 3.683011284406639607, 7.448596931783069586, 0.7998128361456321445 ) ) ;
#133093=CARTESIAN_POINT ( 'NONE',  ( -1.402160292154681736E-14, 2.259375000341416140, -1.575800808251660134 ) ) ;
#133095=CARTESIAN_POINT ( 'NONE',  ( 2.496672843210871129, 6.064535417054653266, -0.7998128361456291469 ) ) ;
#133097=CARTESIAN_POINT ( 'NONE',  ( 1.364683531249986537, 0.4260416670080872659, 0.7879004041258500513 ) ) ;
#133098=CARTESIAN_POINT ( 'NONE',  ( -4.246261168552931231, 7.356898243746066157, -0.9190081729578998271 ) ) ;
#133101=CARTESIAN_POINT ( 'NONE',  ( -2.598358995313378550, 6.183169261174235487, 0.7998128361456341429 ) ) ;
#133102=CARTESIAN_POINT ( 'NONE',  ( -6.141480396866151992, 9.148515648777049591, 1.082531754730548412 ) ) ;
#133105=CARTESIAN_POINT ( 'NONE',  ( -1.364683531250012516, 3.488541667008085767, -0.7879004041258300672 ) ) ;
#133114=CARTESIAN_POINT ( 'NONE',  ( -6.033015167956800262, 9.021972881716168402, -1.082531754730537976 ) ) ;
#133119=CARTESIAN_POINT ( 'NONE',  ( -5.978782553502159480, 8.958701498185728695, 1.082531754730548412 ) ) ;
#133132=CARTESIAN_POINT ( 'NONE',  ( -7.040761844198392794, 7.108643661186573759, -0.7998128361456291469 ) ) ;
#133134=CARTESIAN_POINT ( 'NONE',  ( -1.500000000000015099, -0.3708333333333105331, -0.8660254037844383745 ) ) ;
#133135=CARTESIAN_POINT ( 'NONE',  ( 8.866669273657322492, 12.32790267170016207, -1.082531754730543083 ) ) ;
#133137=CARTESIAN_POINT ( 'NONE',  ( 4.177814833339259515, 3.976464848425037779, 0.1981503615792765127 ) ) ;
#133139=CARTESIAN_POINT ( 'NONE',  ( 4.981731378017507872, 7.899438143407371271, -1.199719254218452047 ) ) ;
#133145=CARTESIAN_POINT ( 'NONE',  ( -3.850152436600983386, 4.554561266531622188, 1.082531754730560403 ) ) ;
#133147=CARTESIAN_POINT ( 'NONE',  ( -0.1695794614869980399, 7.019966546936163176, 3.993288729248444024 ) ) ;
#133152=CARTESIAN_POINT ( 'NONE',  ( 1.364683531249988757, 1.884375000341421913, 0.000000000000000000 ) ) ;
#133153=CARTESIAN_POINT ( 'NONE',  ( 8.663296969007976855, 12.09063498294259809, -1.082531754730543083 ) ) ;
#133154=CARTESIAN_POINT ( 'NONE',  ( -8.389798128758148010, 8.682519326506312751, 0.7998128361456462443 ) ) ;
#133158=CARTESIAN_POINT ( 'NONE',  ( 5.849453209292126310, 8.911780279894442103, 1.199719254218462483 ) ) ;
#133159=CARTESIAN_POINT ( 'NONE',  ( -6.177711549321182716, 10.35908057418338402, 0.7998128361456481317 ) ) ;
#133162=CARTESIAN_POINT ( 'NONE',  ( 0.7499999999999867883, -0.6520833326505159899, -1.299038105676652899 ) ) ;
#133165=CARTESIAN_POINT ( 'NONE',  ( 8.622622508611357262, 9.162073802909148412, -0.7216878364870197293 ) ) ;
#133168=CARTESIAN_POINT ( 'NONE',  ( 1.364683531249986537, 0.9677083336747538400, -0.7879004041258239610 ) ) ;
#133171=CARTESIAN_POINT ( 'NONE',  ( 6.060131475184119765, 9.053608573481392696, -1.082531754730537976 ) ) ;
#133175=CARTESIAN_POINT ( 'NONE',  ( -4.067082894419624672, 6.728385229256075739, 1.082531754730560403 ) ) ;
#133177=CARTESIAN_POINT ( 'NONE',  ( -1.364683531249997417, 4.509375000341424133, 1.214306433183764966E-14 ) ) ;
#133187=CARTESIAN_POINT ( 'NONE',  ( 7.983053520348166288, 8.207983950027992748, -0.7998128361456281477 ) ) ;
#133196=CARTESIAN_POINT ( 'NONE',  ( 4.473827502829567315, 7.202920605734387749, -1.082531754730548412 ) ) ;
#133197=CARTESIAN_POINT ( 'NONE',  ( -0.6823417656250212460, 1.363541667008083547, 1.181850606188755259 ) ) ;
#133200=CARTESIAN_POINT ( 'NONE',  ( 9.028840231696797503, 12.62106513936658203, -1.199719254218446718 ) ) ;
#133204=CARTESIAN_POINT ( 'NONE',  ( -0.7500000000000006661, 0.8583333333333567072, -1.299038105676652011 ) ) ;
#133205=CARTESIAN_POINT ( 'NONE',  ( 7.450369105909416589, 8.650851030771185890, -1.199719254218441611 ) ) ;
#133206=CARTESIAN_POINT ( 'NONE',  ( -9.013473194986783454, 9.410140237106395134, -0.7998128361456291469 ) ) ;
#133209=CARTESIAN_POINT ( 'NONE',  ( -0.6823417656250212460, 1.551041667008083769, 1.181850606188755259 ) ) ;
#133210=CARTESIAN_POINT ( 'NONE',  ( 1.499999999999989120, 2.254166666666685970, 0.8660254037844524744 ) ) ;
#133212=CARTESIAN_POINT ( 'NONE',  ( 3.310162060030825248, 7.013606170011280838, -0.7998128361456291469 ) ) ;
#133219=CARTESIAN_POINT ( 'NONE',  ( 1.499999999999989120, -0.1937499993171845625, 0.000000000000000000 ) ) ;
#133220=CARTESIAN_POINT ( 'NONE',  ( -7.588813295347149435, 9.876701482703580837, -1.599625672291263179 ) ) ;
#133221=CARTESIAN_POINT ( 'NONE',  ( -3.456965981804629884, 6.976951378839947537, 1.040834085586084257E-14 ) ) ;
#133224=VECTOR ( 'NONE', #29509, 1000.000000000000000 ) ;
#133229=VERTEX_POINT ( 'NONE', #195278 ) ;
#133230=ADVANCED_FACE ( 'NONE', ( #111963 ), #196344, .F. ) ;
#133231=CARTESIAN_POINT ( 'NONE',  ( 6.124532705071213279, 8.168374127381657246, -1.599625672291262513 ) ) ;
#133235=CARTESIAN_POINT ( 'NONE',  ( 7.470179451005385829, 8.777926116670192513, -1.082531754730537976 ) ) ;
#133239=CARTESIAN_POINT ( 'NONE',  ( -6.157374318900681764, 10.33535380535947290, 0.7998128361456481317 ) ) ;
#133240=CARTESIAN_POINT ( 'NONE',  ( 4.976006071415387311, 5.764094157194782575, 1.199719254218462483 ) ) ;
#133243=CARTESIAN_POINT ( 'NONE',  ( 1.387358672533593129, 7.315968950352074174, -4.254625267140469624 ) ) ;
#133245=CARTESIAN_POINT ( 'NONE',  ( 4.041346116833469893, 7.538066791021210022, -0.4365389052301202333 ) ) ;
#133246=CARTESIAN_POINT ( 'NONE',  ( 7.917598520700710019, 12.18102267421877727, -0.7216878364870328300 ) ) ;
#133254=CARTESIAN_POINT ( 'NONE',  ( -1.525860493984666055, 8.693043820721571890, -2.521102513734311046 ) ) ;
#133255=CARTESIAN_POINT ( 'NONE',  ( -4.609409038966248318, 5.440360635957812718, -1.082531754730544860 ) ) ;
#133256=CARTESIAN_POINT ( 'NONE',  ( 7.456621297836061757, 11.64321591421002644, 0.7216878364870438212 ) ) ;
#133259=CARTESIAN_POINT ( 'NONE',  ( -6.175902666224832416, 7.163973517805802160, -1.199719254218446718 ) ) ;
#133260=SPHERICAL_SURFACE ( 'NONE', #207780, 0.08000000000000000167 ) ;
#133261=CARTESIAN_POINT ( 'NONE',  ( -3.129460678718345878, 6.444905630999884671, -0.7687999843507524744 ) ) ;
#133263=CARTESIAN_POINT ( 'NONE',  ( 3.922244425448867311, 2.804391244181456244, 0.7750000000000135669 ) ) ;
#133265=CARTESIAN_POINT ( 'NONE',  ( -7.049349804101573191, 10.31165964050546258, -1.199719254218440723 ) ) ;
#133281=CARTESIAN_POINT ( 'NONE',  ( -5.042743069279040036, 7.970618449879118828, 1.199719254218464037 ) ) ;
#133284=CARTESIAN_POINT ( 'NONE',  ( 3.389175213736285386, 6.897862149426897460, 0.7216878364870317197 ) ) ;
#133289=CARTESIAN_POINT ( 'NONE',  ( -3.761497552787613330, 6.475832013972435242, 1.199719254218464037 ) ) ;
#133296=CARTESIAN_POINT ( 'NONE',  ( -7.069687034522070590, 10.33538640932937724, -1.199719254218440723 ) ) ;
#133297=CARTESIAN_POINT ( 'NONE',  ( 7.284808609244363353, 7.393364887073558656, 0.7998128361456341429 ) ) ;
#133300=CARTESIAN_POINT ( 'NONE',  ( -7.133561379084627063, 11.47423870890741782, 0.7998128361456481317 ) ) ;
#133302=CARTESIAN_POINT ( 'NONE',  ( 4.147904930777053245, 6.926640621626830807, -1.199719254218452047 ) ) ;
#133305=CARTESIAN_POINT ( 'NONE',  ( 1.364683531249986537, 0.4677083336747514530, -0.7879004041258309554 ) ) ;
#133308=CARTESIAN_POINT ( 'NONE',  ( 9.246297574839983824, 9.889694713509232571, 0.7216878364870438212 ) ) ;
#133314=VERTEX_POINT ( 'NONE', #212574 ) ;
#133319=CARTESIAN_POINT ( 'NONE',  ( -0.2309780072035732823, 7.005396854623739067, -3.973862472851087624 ) ) ;
#133323=DIRECTION ( 'NONE',  ( 0.7592566023653005702, 0.6507913734559639396, 0.000000000000000000 ) ) ;
#133330=CARTESIAN_POINT ( 'NONE',  ( -2.785310492603665367, 5.336947110424484109, 1.199719254218462483 ) ) ;
#133331=CARTESIAN_POINT ( 'NONE',  ( 6.471393748265519719, 5.229711127717882491, -2.419999999999995044 ) ) ;
#133337=CARTESIAN_POINT ( 'NONE',  ( -0.7500000000000249800, -0.2770833326505156569, 1.299038105676659116 ) ) ;
#133344=CARTESIAN_POINT ( 'NONE',  ( 8.432281472695482449, 11.92507992053172572, 1.199719254218450271 ) ) ;
#133348=CARTESIAN_POINT ( 'NONE',  ( 5.332434488876471868, 5.115595079977664383, 0.7998128361456341429 ) ) ;
#133349=CARTESIAN_POINT ( 'NONE',  ( -7.565086526745425033, 7.928281824065535055, 0.7216878364870317197 ) ) ;
#133350=CARTESIAN_POINT ( 'NONE',  ( -5.788012183699196456, 6.074875824575221017, 0.5810633148162994699 ) ) ;
#133354=CARTESIAN_POINT ( 'NONE',  ( -7.694415870955439551, 8.935572256658169010, 1.199719254218462483 ) ) ;
#133355=CARTESIAN_POINT ( 'NONE',  ( -4.080641047588918546, 4.823464646017586510, -1.082531754730548412 ) ) ;
#133357=ORIENTED_EDGE ( 'NONE', *, *, #98548, .T. ) ;
#133358=CARTESIAN_POINT ( 'NONE',  ( -1.500000000000015099, -0.3395833326505143801, -0.8660254037844383745 ) ) ;
#133365=CARTESIAN_POINT ( 'NONE',  ( -3.728129053633589152, 7.293308295973741195, 0.7216878364870317197 ) ) ;
#133374=CARTESIAN_POINT ( 'NONE',  ( -2.779058300676974014, 6.186059084191009916, -0.7216878364870257245 ) ) ;
#133375=CARTESIAN_POINT ( 'NONE',  ( 7.248805684800777804, 11.60869039890961218, 1.040834085586084257E-14 ) ) ;
#133384=CARTESIAN_POINT ( 'NONE',  ( -2.415323921528888196, 5.969628341758991930, 0.7998128361456341429 ) ) ;
#133385=CARTESIAN_POINT ( 'NONE',  ( -9.267161690140662600, 10.77044237904097734, -1.199719254218441611 ) ) ;
#133389=CARTESIAN_POINT ( 'NONE',  ( 5.854423403002611437, 5.724582146458163656, 1.040834085586084257E-14 ) ) ;
#133395=CARTESIAN_POINT ( 'NONE',  ( 2.901707926954590899, 6.442594886792162967, 0.4081411060850581585 ) ) ;
#133408=CARTESIAN_POINT ( 'NONE',  ( 5.947222937888848371, 10.09017719417900416, 1.040834085586084257E-14 ) ) ;
#133410=CARTESIAN_POINT ( 'NONE',  ( -3.978428010606240850, 6.728917548094202949, -1.199719254218452047 ) ) ;
#133417=CARTESIAN_POINT ( 'NONE',  ( 1.364683531249988535, 5.655208333674751842, -0.7879004041258300672 ) ) ;
#133421=CARTESIAN_POINT ( 'NONE',  ( 5.529027716274630855, 5.344953845275508542, 1.040834085586084257E-14 ) ) ;
#133423=CARTESIAN_POINT ( 'NONE',  ( -4.460796234096120472, 5.163016013655583158, 1.199719254218462483 ) ) ;
#133429=CARTESIAN_POINT ( 'NONE',  ( 6.643132081016125845, 6.852668304048034287, 0.7216878364870317197 ) ) ;
#133432=CARTESIAN_POINT ( 'NONE',  ( 7.741342523278705201, 9.094283034322399928, 1.082531754730558626 ) ) ;
#133433=CARTESIAN_POINT ( 'NONE',  ( -1.001543065824772872E-14, 4.384375000341417916, 1.575800808251672791 ) ) ;
#133435=CARTESIAN_POINT ( 'NONE',  ( 3.999292125906905859, 5.688926785023260102, 1.443375672974062551 ) ) ;
#133439=CARTESIAN_POINT ( 'NONE',  ( 5.608800697670862867, 6.153485950588945208, -0.8468207216996347375 ) ) ;
#133442=CARTESIAN_POINT ( 'NONE',  ( -6.116367690567846793, 6.009388118678342217, 0.2715307625813894177 ) ) ;
#133446=CARTESIAN_POINT ( 'NONE',  ( 0.6823417656249899377, 4.988541667008086655, -1.181850606188754593 ) ) ;
#133462=CARTESIAN_POINT ( 'NONE',  ( -1.201851678989727383E-14, 4.337500000000023448, -1.732050807568863648 ) ) ;
#133463=CARTESIAN_POINT ( 'NONE',  ( 1.364683531249990311, 4.196875000341417028, 1.214306433183764966E-14 ) ) ;
#133465=CARTESIAN_POINT ( 'NONE',  ( 5.587931867126699537, 9.671004278289832001, -0.7998128361456291469 ) ) ;
#133467=CARTESIAN_POINT ( 'NONE',  ( -9.341731535015849630, 10.85744053139533349, 1.199719254218462483 ) ) ;
#133470=VECTOR ( 'NONE', #144197, 1000.000000000000114 ) ;
#133474=CARTESIAN_POINT ( 'NONE',  ( 1.499999999999989120, 5.045833333333354709, -0.8660254037844323793 ) ) ;
#133481=CARTESIAN_POINT ( 'NONE',  ( 9.097157885089661278, 9.715698408800516717, 1.040834085586084257E-14 ) ) ;
#133486=CARTESIAN_POINT ( 'NONE',  ( -0.7500000000000215383, 2.972916667349487341, 1.299038105676671107 ) ) ;
#133488=CARTESIAN_POINT ( 'NONE',  ( -3.958090780185743451, 6.705190779270287393, -1.199719254218452047 ) ) ;
#133489=CARTESIAN_POINT ( 'NONE',  ( 4.650083499362875017, 5.487814173087225633, 1.082531754730560403 ) ) ;
#133497=CARTESIAN_POINT ( 'NONE',  ( 3.147464216666835402, 6.823792019419957278, -0.7998128361456291469 ) ) ;
#133501=CARTESIAN_POINT ( 'NONE',  ( 5.464099601507359516, 6.333536608968757697, 1.199719254218462483 ) ) ;
#133503=ORIENTED_EDGE ( 'NONE', *, *, #157159, .T. ) ;
#133504=DIRECTION ( 'NONE',  ( 0.7592566023653005702, -0.6507913734559639396, 0.000000000000000000 ) ) ;
#133505=ORIENTED_EDGE ( 'NONE', *, *, #160202, .F. ) ;
#133507=ORIENTED_EDGE ( 'NONE', *, *, #13805, .T. ) ;
#133513=CARTESIAN_POINT ( 'NONE',  ( 4.904330715672160501, 6.657863961833647259, -1.249385787368818113 ) ) ;
#133515=CARTESIAN_POINT ( 'NONE',  ( 10.40318394038753702, 11.03146944007395724, -0.7998128361456281477 ) ) ;
#133521=CARTESIAN_POINT ( 'NONE',  ( 5.992340707560151358, 8.014150130285418783, 1.443375672974062551 ) ) ;
#133522=CARTESIAN_POINT ( 'NONE',  ( -3.789667630219657912, 4.380032642466370696, 1.199719254218462483 ) ) ;
#133527=CARTESIAN_POINT ( 'NONE',  ( -2.754277761870538299, 6.365074488824250309, 1.040834085586084257E-14 ) ) ;
#133530=FACE_OUTER_BOUND ( 'NONE', #1183, .T. ) ;
#133540=CARTESIAN_POINT ( 'NONE',  ( 5.943008360174058424, 6.124345481070006869, -0.7360307644482602107 ) ) ;
#133544=CARTESIAN_POINT ( 'NONE',  ( 3.323720213644492993, 7.029424015893889433, 1.040834085586084257E-14 ) ) ;
#133548=CARTESIAN_POINT ( 'NONE',  ( -8.839552966430007430, 11.33589776563360019, -1.443375672974059665 ) ) ;
#133552=CARTESIAN_POINT ( 'NONE',  ( 6.089583550832340819, 10.25626457594641749, 1.040834085586084257E-14 ) ) ;
#133553=CARTESIAN_POINT ( 'NONE',  ( -3.764360206088648297, 7.543504007078730922, -0.7998128361456282587 ) ) ;
#133554=CARTESIAN_POINT ( 'NONE',  ( 3.357615597678655917, 7.068968630600412695, 0.7998128361456321445 ) ) ;
#133556=CARTESIAN_POINT ( 'NONE',  ( -5.656776405399756236, 7.622658444431597680, -1.599625672291256295 ) ) ;
#133557=CARTESIAN_POINT ( 'NONE',  ( 2.683624340501134853, 5.218313266304903664, -1.199719254218446718 ) ) ;
#133560=CARTESIAN_POINT ( 'NONE',  ( -4.205000198532790279, 8.057583998263570635, 0.7998128361456341429 ) ) ;
#133564=CARTESIAN_POINT ( 'NONE',  ( 8.646349277213076334, 11.11049346154719508, 1.599625672291281386 ) ) ;
#133568=CARTESIAN_POINT ( 'NONE',  ( 4.031617349472986334, 7.784614636675013521, 0.3993128758026931457 ) ) ;
#133569=CARTESIAN_POINT ( 'NONE',  ( 4.500943810056890371, 8.194925511800951412, -0.7216878364870207285 ) ) ;
#133573=CARTESIAN_POINT ( 'NONE',  ( -1.367741837319783604, 3.300000000000193001, -0.09290545499925643991 ) ) ;
#133576=VERTEX_POINT ( 'NONE', #45844 ) ;
#133577=CARTESIAN_POINT ( 'NONE',  ( 7.388830529323379359, 11.56412668427855195, -0.7216878364870267237 ) ) ;
#133583=CARTESIAN_POINT ( 'NONE',  ( -8.688077508258798431, 9.030511935923748013, -0.7998128361456291469 ) ) ;
#133589=CARTESIAN_POINT ( 'NONE',  ( 2.280903940472752467, 5.594607745005274246, -0.6109567437776646237 ) ) ;
#133592=CARTESIAN_POINT ( 'NONE',  ( 10.53876547652418338, 11.18964789890005918, 0.7998128361456462443 ) ) ;
#133595=CARTESIAN_POINT ( 'NONE',  ( 3.486418057008484617, 7.219238166485217434, 1.040834085586084257E-14 ) ) ;
#133599=CARTESIAN_POINT ( 'NONE',  ( -1.001543065824772872E-14, 4.243750000682819490, 1.732050807568877637 ) ) ;
#133605=CARTESIAN_POINT ( 'NONE',  ( -1.500000000000013101, 2.379166666666686414, -0.8660254037844313801 ) ) ;
#133606=CARTESIAN_POINT ( 'NONE',  ( 5.774883364416965037, 8.824782127540085952, -1.199719254218440723 ) ) ;
#133607=CARTESIAN_POINT ( 'NONE',  ( 5.300874872818840622, 6.247070775452521652, 1.082531754730560403 ) ) ;
#133610=CARTESIAN_POINT ( 'NONE',  ( -1.499999999999990896, 4.879166666666689522, -0.8660254037844429265 ) ) ;
#133611=CARTESIAN_POINT ( 'NONE',  ( 7.443063144222396232, 11.62739806832741785, 1.040834085586084257E-14 ) ) ;
#133614=CIRCLE ( 'NONE', #19299, 0.07999999999999975187 ) ;
#133619=CARTESIAN_POINT ( 'NONE',  ( -5.066996723205291708, 6.934582148538044777, 1.599625672291267398 ) ) ;
#133620=CARTESIAN_POINT ( 'NONE',  ( -1.500000000000011324, 4.452083334016148086, 0.8660254037844403729 ) ) ;
#133621=CARTESIAN_POINT ( 'NONE',  ( -0.6823417656250003738, 0.2177083336747515085, -1.181850606188749264 ) ) ;
#133625=CARTESIAN_POINT ( 'NONE',  ( 4.467575310902914154, 5.170924936596891008, 1.199719254218464037 ) ) ;
#133627=CARTESIAN_POINT ( 'NONE',  ( -1.364683531250010295, 5.092708333674757171, 0.7879004041258379498 ) ) ;
#133630=CIRCLE ( 'NONE', #188927, 1.250000000000000222 ) ;
#133635=CARTESIAN_POINT ( 'NONE',  ( -7.609150525767646833, 9.900428251527500834, -1.599625672291263179 ) ) ;
#133636=CARTESIAN_POINT ( 'NONE',  ( 5.656776405399742025, 7.622658444431597680, -1.599625672291262513 ) ) ;
#133639=CARTESIAN_POINT ( 'NONE',  ( -0.6823417656250246877, -0.6989583329919113464, 1.181850606188755259 ) ) ;
#133647=CARTESIAN_POINT ( 'NONE',  ( -6.501298352952815662, 7.543601818988450169, -1.199719254218446718 ) ) ;
#133650=CARTESIAN_POINT ( 'NONE',  ( 10.21336978979620191, 10.81001959771741205, 0.7998128361456462443 ) ) ;
#133652=CARTESIAN_POINT ( 'NONE',  ( 10.24048609702354717, 10.84165528948263457, -0.7998128361456281477 ) ) ;
#133653=CARTESIAN_POINT ( 'NONE',  ( 3.146123468421266001, 6.442327133617253843, 0.5169845646841256803 ) ) ;
#133654=CARTESIAN_POINT ( 'NONE',  ( -3.684065054611367351, 5.321161868511784299, -1.599625672291256295 ) ) ;
#133655=CARTESIAN_POINT ( 'NONE',  ( -8.355902744723985975, 8.642974711799791265, 1.040834085586084257E-14 ) ) ;
#133657=CARTESIAN_POINT ( 'NONE',  ( -4.712061673757400371, 7.041017223283659199, 1.411098259540758182 ) ) ;
#133658=CARTESIAN_POINT ( 'NONE',  ( 0.6823417656249882723, -0.4072916663252490466, 1.181850606188755259 ) ) ;
#133662=CARTESIAN_POINT ( 'NONE',  ( 7.537970219518073556, 9.817384560903001045, -1.443375672974057666 ) ) ;
#133665=CARTESIAN_POINT ( 'NONE',  ( 5.331380718671758778, 7.243030143248949670, -1.599625672291256295 ) ) ;
#133685=CARTESIAN_POINT ( 'NONE',  ( -5.220052836461385404, 6.048815383081766583, -1.199719254218446718 ) ) ;
#133686=CARTESIAN_POINT ( 'NONE',  ( -7.160677686311960777, 11.50587440067263678, -0.7998128361456291469 ) ) ;
#133687=FACE_OUTER_BOUND ( 'NONE', #118418, .T. ) ;
#133692=CARTESIAN_POINT ( 'NONE',  ( -1.201851678989727383E-14, 3.118750000682814161, -1.732050807568863648 ) ) ;
#133693=CARTESIAN_POINT ( 'NONE',  ( 7.865701674222579598, 12.32840238656838139, -0.7998128361456352531 ) ) ;
#133697=CARTESIAN_POINT ( 'NONE',  ( -9.124801077197171040, 10.60435499727357289, -1.199719254218441611 ) ) ;
#133699=CARTESIAN_POINT ( 'NONE',  ( -0.6823417656250003738, 2.217708333674753174, -1.181850606188749264 ) ) ;
#133706=CARTESIAN_POINT ( 'NONE',  ( -2.764973262183167968, 5.313220341600567664, 1.199719254218462483 ) ) ;
#133710=CARTESIAN_POINT ( 'NONE',  ( -1.402160292154681736E-14, 1.259375000341419248, -1.575800808251659024 ) ) ;
#133716=CARTESIAN_POINT ( 'NONE',  ( 1.364683531249988535, 2.113541667008087099, 0.7879004041258500513 ) ) ;
#133719=CARTESIAN_POINT ( 'NONE',  ( -6.901263884555985051, 8.010228272525461435, 1.199719254218450271 ) ) ;
#133720=CARTESIAN_POINT ( 'NONE',  ( 7.564559641420864899, 10.91273778404466199, -1.199719254218446718 ) ) ;
#133721=CARTESIAN_POINT ( 'NONE',  ( -1.177110729581227089, 2.870878374463987193, 0.7750000000000083489 ) ) ;
#133723=CARTESIAN_POINT ( 'NONE',  ( -1.499999999999997780, 3.400000000000021227, 1.214306433183764966E-14 ) ) ;
#133725=CARTESIAN_POINT ( 'NONE',  ( -1.201851678989727383E-14, 2.134375000341423689, 1.575800808251672791 ) ) ;
#133728=LINE ( 'NONE', #101174, #184335 ) ;
#133729=ADVANCED_FACE ( 'NONE', ( #54361 ), #102039, .F. ) ;
#133732=CARTESIAN_POINT ( 'NONE',  ( 6.182154858151487353, 6.314861544039274577, -0.7216878364870257245 ) ) ;
#133735=CARTESIAN_POINT ( 'NONE',  ( -9.528683032306089373, 10.01121838064558744, 0.7998128361456462443 ) ) ;
#133736=CARTESIAN_POINT ( 'NONE',  ( -8.500599126088349777, 12.86119004717103209, 1.040834085586084257E-14 ) ) ;
#133742=CARTESIAN_POINT ( 'NONE',  ( -7.714226216051410567, 9.062647342557177410, 1.082531754730558626 ) ) ;
#133744=CARTESIAN_POINT ( 'NONE',  ( 0.7499999999999902300, 5.816666666666685082, -1.299038105676658228 ) ) ;
#133747=CARTESIAN_POINT ( 'NONE',  ( 8.487040972474689582, 9.964264558384387627, -1.082531754730543083 ) ) ;
#133754=ORIENTED_EDGE ( 'NONE', *, *, #104548, .T. ) ;
#133761=CARTESIAN_POINT ( 'NONE',  ( 6.100279051144945619, 9.204410428722734849, -1.199719254218440723 ) ) ;
#133762=CARTESIAN_POINT ( 'NONE',  ( -4.069418662396130593, 7.899405539437467816, -0.7998128361456281477 ) ) ;
#133766=CARTESIAN_POINT ( 'NONE',  ( 4.311129659021211147, 7.973475668925984472, 1.040834085586084257E-14 ) ) ;
#133767=CARTESIAN_POINT ( 'NONE',  ( -1.364683531250000748, 0.5718750003414208027, 0.000000000000000000 ) ) ;
#133768=CARTESIAN_POINT ( 'NONE',  ( 4.039966587192267866, 4.776011108888172707, 1.082531754730560403 ) ) ;
#133769=CARTESIAN_POINT ( 'NONE',  ( -2.286521462199063492, 5.819358805874190743, 1.040834085586084257E-14 ) ) ;
#133779=EDGE_LOOP ( 'NONE', ( #197521, #159312, #51354, #48869 ) ) ;
#133787=CARTESIAN_POINT ( 'NONE',  ( 7.121056995675668411, 9.330985799753529264, -1.599625672291262513 ) ) ;
#133788=CARTESIAN_POINT ( 'NONE',  ( 5.309989718046547402, 9.346738437696316737, 0.7998128361456462443 ) ) ;
#133798=CARTESIAN_POINT ( 'NONE',  ( -6.423865854776591000, 6.388931673527803667, 1.040834085586084257E-14 ) ) ;
#133800=CARTESIAN_POINT ( 'NONE',  ( -2.591579918506545344, 6.175260338232929413, 1.040834085586084257E-14 ) ) ;
#133808=CARTESIAN_POINT ( 'NONE',  ( -8.459924665247381625, 11.85336729522185806, 1.082531754730560403 ) ) ;
#133811=CARTESIAN_POINT ( 'NONE',  ( 6.810273232766058449, 6.839740281182199233, 1.040834085586084257E-14 ) ) ;
#133812=CARTESIAN_POINT ( 'NONE',  ( -0.6823417656249969321, 4.967708333674755394, -1.181850606188749264 ) ) ;
#133819=CARTESIAN_POINT ( 'NONE',  ( 5.477130869796502211, 5.492333557625114437, 1.040834085586084257E-14 ) ) ;
#133820=CARTESIAN_POINT ( 'NONE',  ( -8.044065211609668253, 8.279164256499745633, 0.7998128361456602331 ) ) ;
#133825=CARTESIAN_POINT ( 'NONE',  ( -8.179646747746328828, 8.437342715325849341, -0.7998128361456291469 ) ) ;
#133827=CARTESIAN_POINT ( 'NONE',  ( -6.423865854776591000, 6.388931673527803667, 1.040834085586084257E-14 ) ) ;
#133835=CARTESIAN_POINT ( 'NONE',  ( 8.288111976655649471, 8.563885482386732306, -0.7998128361456291469 ) ) ;
#133849=CARTESIAN_POINT ( 'NONE',  ( -1.201851678989727383E-14, 5.587500000000021672, -1.732050807568863648 ) ) ;
#133850=CARTESIAN_POINT ( 'NONE',  ( 3.846762897975340767, 5.510976019103107859, -1.599625672291256295 ) ) ;
#133852=CARTESIAN_POINT ( 'NONE',  ( 5.469824908109481854, 8.468880595181346393, -1.199719254218446718 ) ) ;
#133854=CARTESIAN_POINT ( 'NONE',  ( -8.188761592974058701, 8.655902734665618325, -0.7216878364870278340 ) ) ;
#133857=CARTESIAN_POINT ( 'NONE',  ( 5.002595493762530765, 8.780185809457538681, 1.040834085586084257E-14 ) ) ;
#133858=CARTESIAN_POINT ( 'NONE',  ( -7.904040366642703930, 10.24446639921506552, 1.443375672974090751 ) ) ;
#133862=ORIENTED_EDGE ( 'NONE', *, *, #127587, .F. ) ;
#133864=CARTESIAN_POINT ( 'NONE',  ( 8.288111976655649471, 8.563885482386732306, -0.7998128361456291469 ) ) ;
#133869=CARTESIAN_POINT ( 'NONE',  ( -1.364683531250012516, 3.238541667008084879, -0.7879004041258289570 ) ) ;
#133875=CARTESIAN_POINT ( 'NONE',  ( 6.923409998072794558, 11.22906209772695618, 1.040834085586084257E-14 ) ) ;
#133878=CARTESIAN_POINT ( 'NONE',  ( -7.181014916732457287, 11.52960116949655678, -0.7998128361456291469 ) ) ;
#133880=DIRECTION ( 'NONE',  ( -1.000000000000000000, 4.984021416236792516E-16, 0.000000000000000000 ) ) ;
#133883=CARTESIAN_POINT ( 'NONE',  ( 9.215791728987056786, 11.77484298861683598, -1.599625672291262513 ) ) ;
#133886=CARTESIAN_POINT ( 'NONE',  ( -8.311311860377216476, 9.655284244316948872, -1.199719254218446718 ) ) ;
#133889=CARTESIAN_POINT ( 'NONE',  ( 4.831368594223144797, 5.066186338679537826, -0.7556405859116925861 ) ) ;
#133892=CARTESIAN_POINT ( 'NONE',  ( 5.811422509517683466, 6.026224704000590293, 0.4751317933852049480 ) ) ;
#133893=CARTESIAN_POINT ( 'NONE',  ( -4.302014814237876017, 3.913438792899272212, 0.7998128361456341429 ) ) ;
#133898=CARTESIAN_POINT ( 'NONE',  ( 5.991813822235618758, 9.077867661661846554, 1.199719254218462483 ) ) ;
#133900=CARTESIAN_POINT ( 'NONE',  ( 4.950698647284403009, 8.927565521807144577, 1.040834085586084257E-14 ) ) ;
#133901=CARTESIAN_POINT ( 'NONE',  ( -4.236586233130071655, 7.334480220043515075, -0.8772045297030308664 ) ) ;
#133902=CARTESIAN_POINT ( 'NONE',  ( 4.364835388595708743, 7.179726155748598515, 1.199719254218462483 ) ) ;
#133905=CARTESIAN_POINT ( 'NONE',  ( -7.212574532790092974, 10.39812547402169862, -1.082531754730543971 ) ) ;
#133912=CARTESIAN_POINT ( 'NONE',  ( -4.047283575590383542, 7.579128156381162107, 0.3715214982176785474 ) ) ;
#133913=FACE_OUTER_BOUND ( 'NONE', #122724, .T. ) ;
#133916=CARTESIAN_POINT ( 'NONE',  ( 6.656690234629796699, 6.868486149930637552, 1.040834085586084257E-14 ) ) ;
#133918=CONICAL_SURFACE ( 'NONE', #61208, 1.000000000000000000, 0.7853981633974508325 ) ;
#133921=CARTESIAN_POINT ( 'NONE',  ( -10.29027540264791440, 11.10766884595181203, 0.7216878364870438212 ) ) ;
#133926=CARTESIAN_POINT ( 'NONE',  ( -10.27671724903424888, 11.09185100006920877, 1.040834085586084257E-14 ) ) ;
#133928=ORIENTED_EDGE ( 'NONE', *, *, #178431, .F. ) ;
#133934=CARTESIAN_POINT ( 'NONE',  ( -9.286972035236626510, 11.85788667924133399, -1.443375672974058777 ) ) ;
#133941=CARTESIAN_POINT ( 'NONE',  ( 1.499999999999989120, 3.285416667349486897, 0.8660254037844524744 ) ) ;
#133943=CARTESIAN_POINT ( 'NONE',  ( -5.961834861707238531, 7.978559976790334574, -1.599625672291263179 ) ) ;
#133946=CARTESIAN_POINT ( 'NONE',  ( -7.645908563102897126, 11.00764485934031889, 1.199719254218453823 ) ) ;
#133950=CARTESIAN_POINT ( 'NONE',  ( 5.276094334012385367, 9.307193822989793475, 1.040834085586084257E-14 ) ) ;
#133955=CARTESIAN_POINT ( 'NONE',  ( 8.910733272679570049, 11.41894145625809820, -1.599625672291255185 ) ) ;
#133957=CARTESIAN_POINT ( 'NONE',  ( -3.975497760493641675, 7.849573349659754840, -7.471960471057975262E-11 ) ) ;
#133960=CARTESIAN_POINT ( 'NONE',  ( -7.863365906246074566, 8.276274433482971205, -0.7216878364870278340 ) ) ;
#133963=CARTESIAN_POINT ( 'NONE',  ( -1.201851678989727383E-14, 5.509375000341415252, -1.575800808251660134 ) ) ;
#133968=CARTESIAN_POINT ( 'NONE',  ( -0.6823417656249969321, 5.467708333674756283, -1.181850606188749264 ) ) ;
#133971=CARTESIAN_POINT ( 'NONE',  ( -9.022061154889962964, 12.61315621642528129, -1.199719254218446718 ) ) ;
#133973=CARTESIAN_POINT ( 'NONE',  ( 8.940712233207955606, 12.51824914112961729, 1.199719254218450271 ) ) ;
#133979=CARTESIAN_POINT ( 'NONE',  ( -0.6823417656250003738, 2.717708333674753618, -1.181850606188749264 ) ) ;
#133981=CARTESIAN_POINT ( 'NONE',  ( 2.984766373302843778, 6.633977868828633717, -0.7998128361456291469 ) ) ;
#133982=ORIENTED_EDGE ( 'NONE', *, *, #181883, .F. ) ;
#133987=CARTESIAN_POINT ( 'NONE',  ( 1.499999999999990896, 3.306250000682818602, 1.214306433183764966E-14 ) ) ;
#133989=( BOUNDED_CURVE ( )  B_SPLINE_CURVE ( 3, ( #185768, #21117, #82950, #137052 ),
 .UNSPECIFIED., .F., .T. ) 
 B_SPLINE_CURVE_WITH_KNOTS ( ( 4, 4 ),
 ( 3.059570999471033392, 3.223614307708452031 ),
 .UNSPECIFIED. ) 
 CURVE ( )  GEOMETRIC_REPRESENTATION_ITEM ( )  RATIONAL_B_SPLINE_CURVE ( ( 1.000000000000000000, 0.9977587396908789152, 0.9977587396908789152, 1.000000000000000000 ) ) 
 REPRESENTATION_ITEM ( '' )  );
#133990=CARTESIAN_POINT ( 'NONE',  ( -8.351459436338048548, 8.845716885256940998, -0.7216878364870278340 ) ) ;
#133996=CARTESIAN_POINT ( 'NONE',  ( -7.621654909176601045, 12.04368116068139472, 0.7998128361456481317 ) ) ;
#133998=CARTESIAN_POINT ( 'NONE',  ( -3.890826896997578999, 7.483122446565064756, 0.7216878364870317197 ) ) ;
#133999=CARTESIAN_POINT ( 'NONE',  ( -1.364683531250012516, 2.301041667008087988, -0.7879004041258289570 ) ) ;
#134007=ORIENTED_EDGE ( 'NONE', *, *, #80476, .F. ) ;
#134017=CARTESIAN_POINT ( 'NONE',  ( 0.6823417656249899377, 4.988541667008086655, -1.181850606188754593 ) ) ;
#134024=CARTESIAN_POINT ( 'NONE',  ( 7.750457368506414646, 12.19395069656619945, 0.7998128361456462443 ) ) ;
#134027=CARTESIAN_POINT ( 'NONE',  ( -1.364683531250000748, 2.009375000341421913, 1.214306433183764966E-14 ) ) ;
#134029=ORIENTED_EDGE ( 'NONE', *, *, #183780, .T. ) ;
#134030=CARTESIAN_POINT ( 'NONE',  ( -8.351459436338048548, 8.845716885256940998, -0.7216878364870278340 ) ) ;
#134038=CARTESIAN_POINT ( 'NONE',  ( 5.678167406024951624, 5.518950149984223508, 0.7998128361456341429 ) ) ;
#134041=ORIENTED_EDGE ( 'NONE', *, *, #68597, .T. ) ;
#134046=ORIENTED_EDGE ( 'NONE', *, *, #157427, .F. ) ;
#134049=CARTESIAN_POINT ( 'NONE',  ( -4.406563619641430840, 5.099744630125142564, -1.199719254218446718 ) ) ;
#134051=CARTESIAN_POINT ( 'NONE',  ( 7.039708073993665494, 9.236078724457858158, 1.599625672291281386 ) ) ;
#134053=CARTESIAN_POINT ( 'NONE',  ( 3.673896439178911066, 7.230036912443299713, 0.7216878364870317197 ) ) ;
#134055=CARTESIAN_POINT ( 'NONE',  ( 3.469446951953614189E-15, 5.167241622962441383, 1.214306433183764966E-14 ) ) ;
#134062=CARTESIAN_POINT ( 'NONE',  ( -5.422898255786186006, 9.270539031818461950, -0.7216878364870207285 ) ) ;
#134063=CARTESIAN_POINT ( 'NONE',  ( 3.988069740714122791, 7.804498464141805592, 0.7998128361456321445 ) ) ;
#134066=CARTESIAN_POINT ( 'NONE',  ( -7.486073373039941359, 11.88550270185529278, -0.7998128361456291469 ) ) ;
#134071=CARTESIAN_POINT ( 'NONE',  ( -3.002240950422295995, 5.590032644546251817, -1.199719254218452935 ) ) ;
#134073=CARTESIAN_POINT ( 'NONE',  ( 9.908311333488716954, 10.45411806535867782, 0.7998128361456462443 ) ) ;
#134074=CARTESIAN_POINT ( 'NONE',  ( 4.111146893441827821, 5.819424013814004759, 1.599625672291267398 ) ) ;
#134080=CARTESIAN_POINT ( 'NONE',  ( 2.385871846325007706, 5.727341554113725586, -0.7216878364870267237 ) ) ;
#134083=CARTESIAN_POINT ( 'NONE',  ( -4.554649539187067830, 7.401175998105142817, 1.199719254218464037 ) ) ;
#134085=CARTESIAN_POINT ( 'NONE',  ( -7.458957065812611198, 11.85386701009007204, 0.7998128361456481317 ) ) ;
#134091=CARTESIAN_POINT ( 'NONE',  ( 6.317736394288131052, 9.354147645769410602, 1.082531754730558626 ) ) ;
#134092=CARTESIAN_POINT ( 'NONE',  ( 0.6823417656249899377, 5.488541667008087543, -1.181850606188754593 ) ) ;
#134094=CARTESIAN_POINT ( 'NONE',  ( 4.578903193113299963, 6.365139696764064325, 1.599625672291267398 ) ) ;
#134097=CARTESIAN_POINT ( 'NONE',  ( -7.552055258011950656, 8.769484874890757453, 1.199719254218462483 ) ) ;
#134107=CARTESIAN_POINT ( 'NONE',  ( 0.6823417656249899377, 3.238541667008085323, -1.181850606188754593 ) ) ;
#134108=CARTESIAN_POINT ( 'NONE',  ( 8.041957671200231417, 12.53403438304231976, 1.040834085586084257E-14 ) ) ;
#134110=CARTESIAN_POINT ( 'NONE',  ( -3.945059511896602089, 7.546393830613923548, 1.040834085586084257E-14 ) ) ;
#134111=CARTESIAN_POINT ( 'NONE',  ( 2.399429999938675007, 5.743159399996332404, 0.000000000000000000 ) ) ;
#134112=CARTESIAN_POINT ( 'NONE',  ( -6.697364695026446491, 6.915939687060050467, 1.040834085586084257E-14 ) ) ;
#134115=CARTESIAN_POINT ( 'NONE',  ( -1.420000000000079865, 7.204077025658377487, 4.238769367544453992 ) ) ;
#134120=CARTESIAN_POINT ( 'NONE',  ( 5.172599298813543633, 5.993452922492633839, -1.199719254218452047 ) ) ;
#134130=CARTESIAN_POINT ( 'NONE',  ( 5.854423403002611437, 5.724582146458163656, 1.040834085586084257E-14 ) ) ;
#134135=CARTESIAN_POINT ( 'NONE',  ( -4.401593425930945713, 8.286942763561420122, 1.040834085586084257E-14 ) ) ;
#134139=CARTESIAN_POINT ( 'NONE',  ( 6.582647274634798151, 7.638508894284114170, 1.199719254218462483 ) ) ;
#134142=CARTESIAN_POINT ( 'NONE',  ( -6.247609857798938293, 6.183299677053865295, -0.7998128361456291469 ) ) ;
#134143=CARTESIAN_POINT ( 'NONE',  ( 1.499999999999989120, 2.275000000000019895, 1.214306433183764966E-14 ) ) ;
#134144=CARTESIAN_POINT ( 'NONE',  ( -5.461236948206312114, 5.265864615862458464, 0.7998128361456341429 ) ) ;
#134147=CARTESIAN_POINT ( 'NONE',  ( -6.586563698140583512, 6.578745824119123675, 1.040834085586084257E-14 ) ) ;
#134149=CARTESIAN_POINT ( 'NONE',  ( 0.6823417656249899377, 3.092708333674754062, 1.181850606188765695 ) ) ;
#134151=CARTESIAN_POINT ( 'NONE',  ( -4.609409038966234995, 7.361099064560491456, -1.082531754730549967 ) ) ;
#134158=CARTESIAN_POINT ( 'NONE',  ( 6.006425746053997372, 6.966250444273174303, -1.199719254218445830 ) ) ;
#134160=CARTESIAN_POINT ( 'NONE',  ( -0.6823417656250212460, 3.363541667008085323, 1.181850606188767472 ) ) ;
#134163=CARTESIAN_POINT ( 'NONE',  ( -0.5160254906862650204, 7.984099418343994614, 1.935262202534214548 ) ) ;
#134166=CARTESIAN_POINT ( 'NONE',  ( -3.002240950422295995, 5.590032644546251817, -1.199719254218452935 ) ) ;
#134167=CARTESIAN_POINT ( 'NONE',  ( -7.822691444960713447, 9.189190109618056823, -1.082531754730543083 ) ) ;
#134168=VECTOR ( 'NONE', #174023, 1000.000000000000000 ) ;
#134171=CARTESIAN_POINT ( 'NONE',  ( -1.402160292154681736E-14, 2.446875000341416584, -1.575800808251660134 ) ) ;
#134178=CARTESIAN_POINT ( 'NONE',  ( -7.171900071504745178, 9.390302721554109056, -1.443375672974058777 ) ) ;
#134182=CARTESIAN_POINT ( 'NONE',  ( -5.653386866774179786, 8.579073197003079798, 1.082531754730548412 ) ) ;
#134195=CARTESIAN_POINT ( 'NONE',  ( -6.067437437315529536, 7.037430750744921859, 1.199719254218450271 ) ) ;
#134197=CARTESIAN_POINT ( 'NONE',  ( 0.7499999999999885647, -0.01666666666664401442, 1.299038105676657340 ) ) ;
#134198=CARTESIAN_POINT ( 'NONE',  ( 3.195971524519376494, 4.751719416737803847, -1.599625672291262513 ) ) ;
#134202=CARTESIAN_POINT ( 'NONE',  ( 7.142447996300871793, 7.227277505306155092, 0.7998128361456341429 ) ) ;
#134209=CARTESIAN_POINT ( 'NONE',  ( -5.775410249741523394, 5.840326167560965231, 0.7216878364870317197 ) ) ;
#134213=DIRECTION ( 'NONE',  ( 1.000000000000000000, -5.578564026256504688E-16, -0.000000000000000000 ) ) ;
#134218=CARTESIAN_POINT ( 'NONE',  ( -1.201851678989727383E-14, 1.571875000341420581, 1.575800808251672791 ) ) ;
#134219=CARTESIAN_POINT ( 'NONE',  ( 10.52076401408022299, 11.37657222595619189, 0.000000000000000000 ) ) ;
#134220=CARTESIAN_POINT ( 'NONE',  ( -6.516665389662827934, 10.75452672124865217, 0.000000000000000000 ) ) ;
#134222=CARTESIAN_POINT ( 'NONE',  ( 7.644099680006512187, 7.812537802962739697, 1.040834085586084257E-14 ) ) ;
#134223=CARTESIAN_POINT ( 'NONE',  ( -7.121056995675673740, 9.330985799753529264, -1.599625672291263179 ) ) ;
#134226=CARTESIAN_POINT ( 'NONE',  ( -1.402160292154681736E-14, -1.256249999317182953, 1.732050807568877637 ) ) ;
#134229=CARTESIAN_POINT ( 'NONE',  ( 7.117667457494414762, 11.24776976714476184, 1.040834085586084257E-14 ) ) ;
#134232=CARTESIAN_POINT ( 'NONE',  ( -1.364683531250000748, 0.3218750003414205807, 0.000000000000000000 ) ) ;
#134235=( BOUNDED_CURVE ( )  B_SPLINE_CURVE ( 2, ( #48547, #15999, #178541, #29090, #82084 ),
 .UNSPECIFIED., .F., .T. ) 
 B_SPLINE_CURVE_WITH_KNOTS ( ( 3, 2, 3 ),
 ( 0.01079486483480432586, 0.01250000000000000069, 0.01382216642637611702 ),
 .UNSPECIFIED. ) 
 CURVE ( )  GEOMETRIC_REPRESENTATION_ITEM ( )  RATIONAL_B_SPLINE_CURVE ( ( 0.9352202683046952902, 0.9451732491399892355, 1.000000000000000000, 0.9574871888551572674, 0.9419547032718726953 ) ) 
 REPRESENTATION_ITEM ( '' )  );
#134236=CARTESIAN_POINT ( 'NONE',  ( 5.788968402910802169, 8.737251655829183505, 1.082531754730558626 ) ) ;
#134239=CARTESIAN_POINT ( 'NONE',  ( -4.934804725694224459, 6.780358151441803649, -1.443375672974053447 ) ) ;
#134241=CARTESIAN_POINT ( 'NONE',  ( -1.201851678989727383E-14, 3.571875000341422357, 1.575800808251672791 ) ) ;
#134245=CARTESIAN_POINT ( 'NONE',  ( -4.391951695823077984, 7.211361847513815704, 1.199719254218464037 ) ) ;
#134246=CARTESIAN_POINT ( 'NONE',  ( 0.1021010164683408550, 6.424493866598983693, -3.065991822131907352 ) ) ;
#134253=CARTESIAN_POINT ( 'NONE',  ( 7.806797523370503811, 8.002351953554066810, 1.040834085586084257E-14 ) ) ;
#134257=CARTESIAN_POINT ( 'NONE',  ( -1.402160292154681736E-14, 2.337500000000022560, -1.732050807568863648 ) ) ;
#134263=ORIENTED_EDGE ( 'NONE', *, *, #142048, .F. ) ;
#134264=CARTESIAN_POINT ( 'NONE',  ( 5.612712406377503349, 8.531619659873665995, -1.082531754730543083 ) ) ;
#134265=CARTESIAN_POINT ( 'NONE',  ( -1.364683531250014514, 0.09270833367475767028, 0.7879004041258379498 ) ) ;
#134272=CARTESIAN_POINT ( 'NONE',  ( 0.7499999999999867883, 0.06666666666668707997, -1.299038105676652899 ) ) ;
#134273=CARTESIAN_POINT ( 'NONE',  ( 7.298366762858032430, 7.409182732956175244, 1.040834085586084257E-14 ) ) ;
#134274=CARTESIAN_POINT ( 'NONE',  ( -9.287498920561160887, 10.79416914786490089, -1.199719254218441611 ) ) ;
#134277=CARTESIAN_POINT ( 'NONE',  ( 1.364683531249986537, 1.113541667008082658, 0.7879004041258500513 ) ) ;
#134280=CARTESIAN_POINT ( 'NONE',  ( 1.499999999999989120, 2.754166666666688190, 0.8660254037844524744 ) ) ;
#134282=CARTESIAN_POINT ( 'NONE',  ( 3.472859903394816872, 7.203420320602605287, -0.7998128361456291469 ) ) ;
#134289=CARTESIAN_POINT ( 'NONE',  ( -1.402160292154681736E-14, -0.2562499993171780122, 1.732050807568877637 ) ) ;
#134290=CARTESIAN_POINT ( 'NONE',  ( -7.694415870955439551, 8.935572256658169010, 1.199719254218462483 ) ) ;
#134291=CARTESIAN_POINT ( 'NONE',  ( -4.609409038966245653, 6.400729850259146758, -1.443375672974053447 ) ) ;
#134297=ORIENTED_EDGE ( 'NONE', *, *, #180525, .F. ) ;
#134298=CARTESIAN_POINT ( 'NONE',  ( 5.126954644262057492, 9.133197518281081173, 0.7998128361456462443 ) ) ;
#134302=CARTESIAN_POINT ( 'NONE',  ( 6.277061933002777927, 8.346324893301817482, 1.443375672974076540 ) ) ;
#134306=CARTESIAN_POINT ( 'NONE',  ( -7.344766530301162000, 9.591980256816594164, 1.599625672291295375 ) ) ;
#134308=CARTESIAN_POINT ( 'NONE',  ( 5.192936529234042808, 6.017179691316550283, -1.199719254218452047 ) ) ;
#134312=CARTESIAN_POINT ( 'NONE',  ( 4.128490713069958851, 7.423566268403333446, -0.7082486411538677640 ) ) ;
#134313=CARTESIAN_POINT ( 'NONE',  ( 10.05978679165993839, 10.83876546646586014, 0.7216878364870438212 ) ) ;
#134322=CARTESIAN_POINT ( 'NONE',  ( -5.422898255786209099, 5.429062174613087599, -0.7216878364870207285 ) ) ;
#134323=CARTESIAN_POINT ( 'NONE',  ( 9.897088948295946764, 10.64895131587453569, 0.7216878364870438212 ) ) ;
#134326=CARTESIAN_POINT ( 'NONE',  ( -6.742482464697739708, 6.760651051769146491, 0.7998128361456341429 ) ) ;
#134332=CARTESIAN_POINT ( 'NONE',  ( -7.157815033010924921, 10.43820240756634199, 1.199719254218453823 ) ) ;
#134336=ORIENTED_EDGE ( 'NONE', *, *, #162394, .F. ) ;
#134338=ORIENTED_EDGE ( 'NONE', *, *, #15120, .T. ) ;
#134347=CARTESIAN_POINT ( 'NONE',  ( -5.032047568966410367, 9.022472597102808578, 1.214306433183764966E-14 ) ) ;
#134351=CARTESIAN_POINT ( 'NONE',  ( 5.504247177468186258, 6.484338464210099851, 1.082531754730558626 ) ) ;
#134356=CARTESIAN_POINT ( 'NONE',  ( -2.937312835655025101, 6.578615408239493867, 1.040834085586084257E-14 ) ) ;
#134365=CARTESIAN_POINT ( 'NONE',  ( -10.17947440576205054, 10.77047498301088346, 0.7998128361456462443 ) ) ;
#134366=CARTESIAN_POINT ( 'NONE',  ( 6.799577732453452761, 7.891594428405881878, -1.199719254218446718 ) ) ;
#134370=CARTESIAN_POINT ( 'NONE',  ( -7.947050595904583403, 12.42330946186405249, 0.7998128361456481317 ) ) ;
#134373=CARTESIAN_POINT ( 'NONE',  ( -1.364683531250014514, -0.1989583329919157317, -0.7879004041258359514 ) ) ;
#134377=CARTESIAN_POINT ( 'NONE',  ( 6.792271770766432404, 10.86814146596211472, 1.040834085586084257E-14 ) ) ;
#134383=CARTESIAN_POINT ( 'NONE',  ( -5.436165250227197987, 6.300106160968032221, -1.040272029539757170 ) ) ;
#134385=CARTESIAN_POINT ( 'NONE',  ( -3.511198596259295535, 6.271927390929313617, -2.420000000000000373 ) ) ;
#134389=FACE_OUTER_BOUND ( 'NONE', #44400, .T. ) ;
#134404=CARTESIAN_POINT ( 'NONE',  ( -1.500000000000013101, -0.04791666598384902026, 0.8660254037844403729 ) ) ;
#134408=EDGE_LOOP ( 'NONE', ( #195560, #38107, #72894, #30285 ) ) ;
#134410=CARTESIAN_POINT ( 'NONE',  ( 0.1460981902779634745, 7.101100029736093333, -2.114500818361211287 ) ) ;
#134412=CARTESIAN_POINT ( 'NONE',  ( 8.757677159423465696, 12.30470822171437284, 1.199719254218450271 ) ) ;
#134417=CARTESIAN_POINT ( 'NONE',  ( 3.551346171775753735, 6.230655402791975384, 1.199719254218462483 ) ) ;
#134418=CARTESIAN_POINT ( 'NONE',  ( -7.212574532790102744, 8.477387045419011002, -1.082531754730550855 ) ) ;
#134420=CARTESIAN_POINT ( 'NONE',  ( -5.894595317363360287, 6.010551413984606128, 0.2245382864616944640 ) ) ;
#134423=CARTESIAN_POINT ( 'NONE',  ( -6.659026002606323047, 10.92061410301605662, 0.000000000000000000 ) ) ;
#134424=CARTESIAN_POINT ( 'NONE',  ( -4.161989969270909917, 5.878740935614591656, 1.443375672974064550 ) ) ;
#134427=CARTESIAN_POINT ( 'NONE',  ( 1.499999999999987121, 0.5354166673494816786, 0.8660254037844524744 ) ) ;
#134435=CARTESIAN_POINT ( 'NONE',  ( -3.402733366905605905, 6.913679994791092298, 0.7216878364870317197 ) ) ;
#134442=CARTESIAN_POINT ( 'NONE',  ( -2.616360457312984167, 5.996244933599686355, -0.7216878364870257245 ) ) ;
#134443=CARTESIAN_POINT ( 'NONE',  ( 9.257519960032755790, 9.694861462993381807, 0.7998128361456462443 ) ) ;
#134453=CARTESIAN_POINT ( 'NONE',  ( -7.635213062790267458, 12.05949900656400686, 0.000000000000000000 ) ) ;
#134458=CARTESIAN_POINT ( 'NONE',  ( 5.789495288235341874, 6.713164910151406595, 1.199719254218462483 ) ) ;
#134477=CARTESIAN_POINT ( 'NONE',  ( 7.411503528164766763, 11.79850454950093841, 1.040834085586084257E-14 ) ) ;
#134479=CARTESIAN_POINT ( 'NONE',  ( -6.033542053281340856, 6.997886136038390603, -1.199719254218446718 ) ) ;
#134484=CARTESIAN_POINT ( 'NONE',  ( 0.6823417656249917140, 5.592708333674749177, 1.181850606188765695 ) ) ;
#134488=CARTESIAN_POINT ( 'NONE',  ( 4.325214697959421706, 5.004837554829479451, 1.199719254218462483 ) ) ;
#134490=CARTESIAN_POINT ( 'NONE',  ( -5.623934791570306402, 5.455678766453782913, 0.7998128361456341429 ) ) ;
#134497=CARTESIAN_POINT ( 'NONE',  ( 6.371969008742804697, 7.496680600697164465, -1.082531754730543083 ) ) ;
#134500=CARTESIAN_POINT ( 'NONE',  ( 7.578644679914702031, 10.82520731233375955, 1.082531754730558626 ) ) ;
#134501=CARTESIAN_POINT ( 'NONE',  ( -0.6823417656249969321, 5.030208333674755394, -1.181850606188749264 ) ) ;
#134502=CARTESIAN_POINT ( 'NONE',  ( 4.053524740361575063, 4.791828954252362216, -1.082531754730543083 ) ) ;
#134505=CARTESIAN_POINT ( 'NONE',  ( 5.417385717461801420, 6.279972267429607236, -1.041140759853006026 ) ) ;
#134508=CARTESIAN_POINT ( 'NONE',  ( -6.131331467106510225, 6.000095466447766590, 0.1540833971661673130 ) ) ;
#134511=CARTESIAN_POINT ( 'NONE',  ( 1.364683531249990311, 4.676041667008083103, 0.7879004041258500513 ) ) ;
#134525=CARTESIAN_POINT ( 'NONE',  ( -1.364683531250010295, 5.092708333674757171, 0.7879004041258379498 ) ) ;
#134527=CARTESIAN_POINT ( 'NONE',  ( 7.558834334818744338, 8.777393797832065303, 1.199719254218462483 ) ) ;
#134528=CARTESIAN_POINT ( 'NONE',  ( -7.655550293210764856, 12.08322577538792331, 0.000000000000000000 ) ) ;
#134534=CARTESIAN_POINT ( 'NONE',  ( -1.500000000000011324, 4.670833333333353821, 0.8660254037844403729 ) ) ;
#134539=ORIENTED_EDGE ( 'NONE', *, *, #1901, .T. ) ;
#134542=CARTESIAN_POINT ( 'NONE',  ( 8.758204044748005401, 10.28062147603659504, 1.082531754730549967 ) ) ;
#134547=CARTESIAN_POINT ( 'NONE',  ( 0.7499999999999885647, 2.847916667349487341, -1.299038105676658228 ) ) ;
#134550=CARTESIAN_POINT ( 'NONE',  ( -5.603597561149804562, 5.431951997629870910, 0.7998128361456341429 ) ) ;
#134551=CARTESIAN_POINT ( 'NONE',  ( 5.314433026432511475, 5.302519407033794430, 1.040834085586084257E-14 ) ) ;
#134560=CARTESIAN_POINT ( 'NONE',  ( 8.471147050440139381, 8.777426401801974976, -0.7998128361456281477 ) ) ;
#134561=CARTESIAN_POINT ( 'NONE',  ( 3.928111819657337911, 5.605883094398769195, 1.599625672291267398 ) ) ;
#134562=DIRECTION ( 'NONE',  ( -0.000000000000000000, -8.546850786086437571E-32, -1.000000000000000000 ) ) ;
#134564=SURFACE_SIDE_STYLE ('',( #104172 ) ) ;
#134565=CARTESIAN_POINT ( 'NONE',  ( 6.030679399980265920, 5.930214142932100252, -0.7998128361456281477 ) ) ;
#134567=EDGE_CURVE ( 'NONE', #94342, #119510, #163877, .T. ) ;
#134579=CARTESIAN_POINT ( 'NONE',  ( 5.343583877570073248, 6.330574952785890552, -1.095086179472234189 ) ) ;
#134581=CARTESIAN_POINT ( 'NONE',  ( 8.540746701604824409, 12.05162268759261224, -1.199719254218446718 ) ) ;
#134587=CARTESIAN_POINT ( 'NONE',  ( 5.151735183512854199, 8.954182114166247430, -0.7216878364870257245 ) ) ;
#134588=CARTESIAN_POINT ( 'NONE',  ( -8.785320351975364872, 12.23299559640450518, 1.082531754730560403 ) ) ;
#134593=CARTESIAN_POINT ( 'NONE',  ( -5.742041750587549842, 6.657802449562273850, 1.199719254218450271 ) ) ;
#134603=CARTESIAN_POINT ( 'NONE',  ( 7.910292558569346433, 11.31609285405122556, -1.199719254218446718 ) ) ;
#134604=CARTESIAN_POINT ( 'NONE',  ( 6.093061176370408560, 6.029359313278345844, 0.2718797729955486631 ) ) ;
#134611=CARTESIAN_POINT ( 'NONE',  ( -9.002250809794006159, 10.56534270192358704, -1.082531754730543971 ) ) ;
#134612=AXIS2_PLACEMENT_3D ( 'NONE', #137008, #155380, #171625 ) ;
#134617=CARTESIAN_POINT ( 'NONE',  ( 6.238723240582662477, 10.43026088065513513, -0.7998128361456291469 ) ) ;
#134619=CARTESIAN_POINT ( 'NONE',  ( -5.949330478298284319, 5.835307067636438916, 0.7998128361456341429 ) ) ;
#134621=CARTESIAN_POINT ( 'NONE',  ( -5.215082642750900277, 9.236013516518044142, 0.000000000000000000 ) ) ;
#134622=CARTESIAN_POINT ( 'NONE',  ( 4.359110081993588182, 5.044382169536003602, -1.199719254218452047 ) ) ;
#134626=CARTESIAN_POINT ( 'NONE',  ( 8.106885785967500979, 11.54545161934907682, 1.199719254218460707 ) ) ;
#134630=CARTESIAN_POINT ( 'NONE',  ( 4.118656133465138147, 7.671478758617087834, -0.7332979114653701558 ) ) ;
#134631=CARTESIAN_POINT ( 'NONE',  ( 6.331294547901813452, 6.488857848747989543, 1.040834085586084257E-14 ) ) ;
#134633=CARTESIAN_POINT ( 'NONE',  ( 0.5100945355815690307, 6.808349925817971382, 3.584950416132734130 ) ) ;
#134637=CARTESIAN_POINT ( 'NONE',  ( 8.717529583462649612, 10.23316793787035195, 1.082531754730558626 ) ) ;
#134639=CARTESIAN_POINT ( 'NONE',  ( -10.64723070543352712, 11.31619066596094392, 0.7998128361456462443 ) ) ;
#134640=CARTESIAN_POINT ( 'NONE',  ( -8.148614017013223076, 9.465470093725620870, -1.199719254218446718 ) ) ;
#134649=CARTESIAN_POINT ( 'NONE',  ( 8.218213668177886788, 12.73966637951625813, 0.7998128361456462443 ) ) ;
#134655=CARTESIAN_POINT ( 'NONE',  ( 4.578903193113299963, 6.365139696764064325, 1.599625672291267398 ) ) ;
#134658=CARTESIAN_POINT ( 'NONE',  ( -0.7499999999999972244, 4.389583334016150751, -1.299038105676652899 ) ) ;
#134664=CARTESIAN_POINT ( 'NONE',  ( 0.7499999999999902300, 2.233333333333351156, 1.299038105676669330 ) ) ;
#134665=CARTESIAN_POINT ( 'NONE',  ( 6.368579470117202490, 8.453095353268645695, 1.599625672291281386 ) ) ;
#134666=CARTESIAN_POINT ( 'NONE',  ( 4.541618270453549044, 5.361271406026338227, -1.082531754730548412 ) ) ;
#134671=CARTESIAN_POINT ( 'NONE',  ( 8.920901888112002354, 9.510066412326583674, 0.7216878364870438212 ) ) ;
#134677=CARTESIAN_POINT ( 'NONE',  ( -4.446184310277715213, 7.274633231044262516, -1.199719254218452047 ) ) ;
#134678=CARTESIAN_POINT ( 'NONE',  ( 1.499999999999989120, 3.785416667349481123, 0.8660254037844524744 ) ) ;
#134679=CARTESIAN_POINT ( 'NONE',  ( -1.364683531250014514, -0.7614583329919104582, -0.7879004041258359514 ) ) ;
#134683=CARTESIAN_POINT ( 'NONE',  ( 9.612367721964607981, 12.23751498042398289, -1.443375672974058777 ) ) ;
#134685=CARTESIAN_POINT ( 'NONE',  ( -0.6823417656250212460, 3.613541667008085767, 1.181850606188767472 ) ) ;
#134692=CARTESIAN_POINT ( 'NONE',  ( -6.530223543276495235, 10.77034456713125188, -0.7998128361456291469 ) ) ;
#134693=CARTESIAN_POINT ( 'NONE',  ( 4.957477724091233995, 8.935474444748447098, -0.7998128361456281477 ) ) ;
#134695=CARTESIAN_POINT ( 'NONE',  ( 0.6823417656249882723, -1.157291666325249713, 1.181850606188755259 ) ) ;
#134697=ORIENTED_EDGE ( 'NONE', *, *, #170700, .T. ) ;
#134701=CARTESIAN_POINT ( 'NONE',  ( -6.043183783389232566, 8.073467052085995022, 1.599625672291269396 ) ) ;
#134704=CARTESIAN_POINT ( 'NONE',  ( 8.543609354905870035, 13.11929468069890525, 0.7998128361456462443 ) ) ;
#134706=CARTESIAN_POINT ( 'NONE',  ( 8.866142388332804103, 12.43125098877526113, -1.199719254218446718 ) ) ;
#134708=CARTESIAN_POINT ( 'NONE',  ( -2.916975605234527702, 6.554888639415577423, 1.040834085586084257E-14 ) ) ;
#134709=CARTESIAN_POINT ( 'NONE',  ( -8.857554428429624593, 9.228235009456373206, 0.7998128361456462443 ) ) ;
#134711=CARTESIAN_POINT ( 'NONE',  ( -4.172014829671058855, 7.596244486910340044, 0.9145543751994407167 ) ) ;
#134712=CARTESIAN_POINT ( 'NONE',  ( 0.6823417656249864960, -0.5739583329919112353, -1.181850606188749264 ) ) ;
#134717=CARTESIAN_POINT ( 'NONE',  ( 7.131225611108079399, 11.26358761302737754, 0.7216878364870438212 ) ) ;
#134738=CARTESIAN_POINT ( 'NONE',  ( 3.307826292054301121, 4.882216645528547616, -1.443375672974057666 ) ) ;
#134740=EDGE_LOOP ( 'NONE', ( #165396, #117470, #59861, #22725 ) ) ;
#134742=CARTESIAN_POINT ( 'NONE',  ( -5.949330478298285207, 5.835307067636438028, 0.7998128361456341429 ) ) ;
#134746=CARTESIAN_POINT ( 'NONE',  ( -1.500000000000013101, 2.160416667349489561, -0.8660254037844313801 ) ) ;
#134747=CARTESIAN_POINT ( 'NONE',  ( 10.07778825365955733, 10.65184113889131012, -0.7998128361456281477 ) ) ;
#134751=CARTESIAN_POINT ( 'NONE',  ( -10.10098813738111545, 11.74323990082152491, -1.199719254218441611 ) ) ;
#134753=CARTESIAN_POINT ( 'NONE',  ( -1.402160292154681736E-14, 1.946875000341422579, -1.575800808251660134 ) ) ;
#134754=CARTESIAN_POINT ( 'NONE',  ( -1.499999999999997780, 4.181250000682819490, 1.214306433183764966E-14 ) ) ;
#134757=ORIENTED_EDGE ( 'NONE', *, *, #142755, .F. ) ;
#134761=CARTESIAN_POINT ( 'NONE',  ( -2.442440228756222353, 6.001264033524212671, -0.7998128361456281477 ) ) ;
#134765=CARTESIAN_POINT ( 'NONE',  ( -0.6823417656250003738, 0.7802083336747520637, -1.181850606188749264 ) ) ;
#134770=CARTESIAN_POINT ( 'NONE',  ( -1.364683531250014514, 1.238541667008091096, -0.7879004041258289570 ) ) ;
#134772=CARTESIAN_POINT ( 'NONE',  ( -7.576308911938196999, 7.733448573549685179, 0.7998128361456462443 ) ) ;
#134773=CARTESIAN_POINT ( 'NONE',  ( 8.158255747121103241, 10.54105100977322174, 1.599625672291281386 ) ) ;
#134774=CARTESIAN_POINT ( 'NONE',  ( -3.189213936345698830, 2.817530495244580102, 2.450448857954578230 ) ) ;
#134775=CARTESIAN_POINT ( 'NONE',  ( 6.017121246366603060, 5.914396297049491658, 1.040834085586084257E-14 ) ) ;
#134777=CARTESIAN_POINT ( 'NONE',  ( -1.201851678989727383E-14, 3.962500000000022116, 1.732050807568877637 ) ) ;
#134779=CARTESIAN_POINT ( 'NONE',  ( -1.364683531250014514, 0.8010416670080889867, -0.7879004041258289570 ) ) ;
#134787=CARTESIAN_POINT ( 'NONE',  ( 6.331294547901813452, 6.488857848747989543, 1.040834085586084257E-14 ) ) ;
#134790=CARTESIAN_POINT ( 'NONE',  ( -7.167456763118792651, 11.51378332361394818, 0.000000000000000000 ) ) ;
#134791=CARTESIAN_POINT ( 'NONE',  ( -4.603156847039612920, 5.329103395422994716, 1.199719254218462483 ) ) ;
#134794=CARTESIAN_POINT ( 'NONE',  ( 0.000000000000000000, 6.487495393664096888, -3.100011470320000573 ) ) ;
#134796=CARTESIAN_POINT ( 'NONE',  ( -6.927853306458756855, 9.105581495667113501, 1.443375672974078761 ) ) ;
#134798=CARTESIAN_POINT ( 'NONE',  ( 1.499999999999989120, 5.795833333333350268, -0.8660254037844323793 ) ) ;
#134801=CARTESIAN_POINT ( 'NONE',  ( 7.131225611108079399, 11.26358761302737754, 0.7216878364870438212 ) ) ;
#134810=CARTESIAN_POINT ( 'NONE',  ( 8.527715432871318058, 12.89282573841782664, -0.7216878364870338292 ) ) ;
#134816=CARTESIAN_POINT ( 'NONE',  ( 7.637320603199683866, 7.804628880021436288, -0.7998128361456281477 ) ) ;
#134817=CARTESIAN_POINT ( 'NONE',  ( -6.389970470742427189, 6.349387058821269747, -0.7998128361456291469 ) ) ;
#134821=CARTESIAN_POINT ( 'NONE',  ( 0.6823417656249864960, -0.7614583329919113464, -1.181850606188749264 ) ) ;
#134822=CARTESIAN_POINT ( 'NONE',  ( 3.877268743828276243, 4.586196958296845594, 1.082531754730560403 ) ) ;
#134823=CARTESIAN_POINT ( 'NONE',  ( -10.64723070543352712, 11.31619066596094392, 0.7998128361456462443 ) ) ;
#134830=( BOUNDED_SURFACE ( )  B_SPLINE_SURFACE ( 3, 2, ( 
 ( #14444, #210523, #160721 ),
 ( #79466, #145583, #12314 ),
 ( #123254, #146630, #211580 ),
 ( #171906, #129378, #112045 ),
 ( #74412, #73318, #205456 ),
 ( #80534, #78395, #189219 ) ),
 .UNSPECIFIED., .F., .F., .T. ) 
 B_SPLINE_SURFACE_WITH_KNOTS ( ( 4, 2, 4 ),
 ( 3, 3 ),
 ( 0.0001465838689801550747, 0.0002810652682710439903, 0.0004155466675619328516 ),
 ( 0.000000000000000000, 1.000000000000000000 ),
 .UNSPECIFIED. ) 
 GEOMETRIC_REPRESENTATION_ITEM ( )  RATIONAL_B_SPLINE_SURFACE ( (
 ( 1.000000000000000000, 0.8789000212895440312, 1.000000000000000000),
 ( 1.000000000000000000, 0.9073166784884890701, 1.000000000000000000),
 ( 1.000000000000000000, 0.9160359019619150889, 1.000000000000000000),
 ( 1.000000000000000000, 0.8858134948703313416, 1.000000000000000000),
 ( 1.000000000000000000, 0.8506312074210923280, 1.000000000000000000),
 ( 1.000000000000000000, 0.8104931255412307634, 1.000000000000000000) ) ) 
 REPRESENTATION_ITEM ( '' )  SURFACE ( )  );
#134841=CARTESIAN_POINT ( 'NONE',  ( 6.446011968293428041, 9.607765498729298415, -1.199719254218440723 ) ) ;
#134850=CARTESIAN_POINT ( 'NONE',  ( -2.279673327426077645, 5.603443282064907827, 0.1981503615792774842 ) ) ;
#134851=CARTESIAN_POINT ( 'NONE',  ( -0.02299836291579685638, 7.070324784597906920, 4.060433046130490276 ) ) ;
#134853=CARTESIAN_POINT ( 'NONE',  ( -5.117312914154178216, 8.057616602233474978, -1.199719254218452047 ) ) ;
#134855=CARTESIAN_POINT ( 'NONE',  ( -4.386226389220933441, 5.076017861301227008, -1.199719254218446718 ) ) ;
#134866=CARTESIAN_POINT ( 'NONE',  ( -9.707274797704657843, 11.38787068781932987, 1.082531754730558626 ) ) ;
#134869=CARTESIAN_POINT ( 'NONE',  ( 7.474622759835693131, 7.614814729430110951, -0.7998128361456281477 ) ) ;
#134870=CARTESIAN_POINT ( 'NONE',  ( 0.6823417656249917140, 5.092708333674749177, 1.181850606188765695 ) ) ;
#134876=CARTESIAN_POINT ( 'NONE',  ( 6.439759776366780208, 6.615400615290456088, 0.7216878364870317197 ) ) ;
#134877=CARTESIAN_POINT ( 'NONE',  ( -5.357443255694392725, 9.402100898285455699, 0.000000000000000000 ) ) ;
#134880=CARTESIAN_POINT ( 'NONE',  ( -8.019811557683421910, 9.315200557840817908, 1.199719254218462483 ) ) ;
#134881=CARTESIAN_POINT ( 'NONE',  ( -4.574986769607567894, 7.424902766929059261, 1.199719254218464037 ) ) ;
#134885=DIRECTION ( 'NONE',  ( 0.6507913734559596097, -0.7592566023653043450, 0.000000000000000000 ) ) ;
#134888=CARTESIAN_POINT ( 'NONE',  ( 8.437251666405968464, 8.737881787095446384, 1.040834085586084257E-14 ) ) ;
#134896=FACE_OUTER_BOUND ( 'NONE', #191016, .T. ) ;
#134902=CARTESIAN_POINT ( 'NONE',  ( -1.499999999999997780, 5.150000000000022560, 1.214306433183764966E-14 ) ) ;
#134903=CARTESIAN_POINT ( 'NONE',  ( 3.684065054611349144, 5.321161868511784299, -1.599625672291262513 ) ) ;
#134904=CARTESIAN_POINT ( 'NONE',  ( 4.808338034340912337, 8.761478140039733020, 1.040834085586084257E-14 ) ) ;
#134905=ADVANCED_FACE ( 'NONE', ( #108536 ), #193973, .F. ) ;
#134907=CARTESIAN_POINT ( 'NONE',  ( -8.039621903223732602, 8.481906429956900695, 1.040834085586084257E-14 ) ) ;
#134908=CARTESIAN_POINT ( 'NONE',  ( 6.331294547901813452, 6.488857848747989543, 1.040834085586084257E-14 ) ) ;
#134909=CARTESIAN_POINT ( 'NONE',  ( -7.578644679914719795, 9.864838098032418401, 1.443375672974090751 ) ) ;
#134913=CARTESIAN_POINT ( 'NONE',  ( 7.130698725783555680, 10.40656671580112658, 1.199719254218460707 ) ) ;
#134918=CARTESIAN_POINT ( 'NONE',  ( -1.201851678989727383E-14, 3.821875000341423689, 1.575800808251672791 ) ) ;
#134925=CARTESIAN_POINT ( 'NONE',  ( 9.260382613333817403, 10.76253345609967660, -1.199719254218446718 ) ) ;
#134930=CARTESIAN_POINT ( 'NONE',  ( -7.330154606482786050, 11.70359747420527619, 0.000000000000000000 ) ) ;
#134935=CARTESIAN_POINT ( 'NONE',  ( 3.379006598303866848, 4.965260336153046516, -1.599625672291262513 ) ) ;
#134938=CARTESIAN_POINT ( 'NONE',  ( -8.962103233833181193, 10.41454084668224489, -1.199719254218446718 ) ) ;
#134943=CARTESIAN_POINT ( 'NONE',  ( 5.890517129559706078, 5.978185313570312687, -0.07684424279984919393 ) ) ;
#134945=CARTESIAN_POINT ( 'NONE',  ( -3.440018289565379028, 5.036440642624797626, 1.599625672291267398 ) ) ;
#134949=CARTESIAN_POINT ( 'NONE',  ( 5.764187864104357573, 9.876636274763768597, 1.040834085586084257E-14 ) ) ;
#134951=CARTESIAN_POINT ( 'NONE',  ( 5.961834861707224320, 7.978559976790334574, -1.599625672291262513 ) ) ;
#134952=CARTESIAN_POINT ( 'NONE',  ( 3.974511587100456822, 7.788680618259193444, 1.040834085586084257E-14 ) ) ;
#134954=CARTESIAN_POINT ( 'NONE',  ( -8.405692050792730186, 9.869357483088723626, 1.082531754730558626 ) ) ;
#134961=CARTESIAN_POINT ( 'NONE',  ( -4.167783244592077274, 7.418453011031667543, -0.7534271236282058526 ) ) ;
#134962=CARTESIAN_POINT ( 'NONE',  ( 4.222827212797172436, 7.545785358913557950, -0.9571512059609885714 ) ) ;
#134965=CARTESIAN_POINT ( 'NONE',  ( 5.504247177468186258, 6.484338464210099851, 1.082531754730558626 ) ) ;
#134970=CARTESIAN_POINT ( 'NONE',  ( -9.232739420781982176, 12.75498451001223010, 1.082531754730558626 ) ) ;
#134975=CARTESIAN_POINT ( 'NONE',  ( -9.991996023147281747, 11.72004545083573568, 1.082531754730558626 ) ) ;
#134982=CARTESIAN_POINT ( 'NONE',  ( -9.951321562306267410, 10.71222269888655987, 1.040834085586084257E-14 ) ) ;
#134987=CARTESIAN_POINT ( 'NONE',  ( 8.294891053462476904, 8.571794405328034827, 1.040834085586084257E-14 ) ) ;
#134991=CARTESIAN_POINT ( 'NONE',  ( -1.500000000000013101, 1.702083334016151417, 0.8660254037844403729 ) ) ;
#134993=CARTESIAN_POINT ( 'NONE',  ( -4.367698041896780126, 8.247398148854895084, 0.7998128361456481317 ) ) ;
#134996=CARTESIAN_POINT ( 'NONE',  ( -9.806625181386236179, 10.33548422123910449, -0.7998128361456291469 ) ) ;
#134999=CARTESIAN_POINT ( 'NONE',  ( 7.233438648090761980, 8.397765496649418182, 1.199719254218462483 ) ) ;
#135003=CARTESIAN_POINT ( 'NONE',  ( 7.425061681778431399, 11.81432239538354345, 0.7998128361456462443 ) ) ;
#135004=CARTESIAN_POINT ( 'NONE',  ( 6.115103934187892776, 6.015625209457229339, 1.345820777640227805E-10 ) ) ;
#135009=CARTESIAN_POINT ( 'NONE',  ( -6.060131475628484310, 10.01397778830115470, 0.000000000000000000 ) ) ;
#135012=CARTESIAN_POINT ( 'NONE',  ( 1.364683531249988535, 3.717708333674750953, -0.7879004041258239610 ) ) ;
#135019=CARTESIAN_POINT ( 'NONE',  ( -3.050221372950322252, 5.542046787541873520, 1.082531754730560403 ) ) ;
#135021=CARTESIAN_POINT ( 'NONE',  ( 10.55910270694468345, 11.21337466772398095, 0.7998128361456462443 ) ) ;
#135022=CARTESIAN_POINT ( 'NONE',  ( -1.364683531249997417, 5.571875000341417916, 1.214306433183764966E-14 ) ) ;
#135023=CARTESIAN_POINT ( 'NONE',  ( -8.631737353394710155, 13.22211067893587533, 1.040834085586084257E-14 ) ) ;
#135028=CARTESIAN_POINT ( 'NONE',  ( -1.201851678989727383E-14, 1.821875000341421691, 1.575800808251672791 ) ) ;
#135029=CARTESIAN_POINT ( 'NONE',  ( -4.609409038966253647, 4.479991421656468908, -0.7216878364870207285 ) ) ;
#135030=CARTESIAN_POINT ( 'NONE',  ( 5.359550796103802028, 5.147230771742885125, -0.7998128361456231517 ) ) ;
#135031=ORIENTED_EDGE ( 'NONE', *, *, #54130, .T. ) ;
#135035=CARTESIAN_POINT ( 'NONE',  ( -3.039951802757221877, 2.724153688964683351, -2.451370731312840778 ) ) ;
#135036=CARTESIAN_POINT ( 'NONE',  ( 2.684151225825664788, 5.114964949229812596, -1.082531754730543083 ) ) ;
#135037=DIRECTION ( 'NONE',  ( 0.9754920898435691656, -0.1320207019938371973, -0.1760276026584480513 ) ) ;
#135039=CARTESIAN_POINT ( 'NONE',  ( -6.385527162356466668, 10.39360608948380182, 0.000000000000000000 ) ) ;
#135045=CARTESIAN_POINT ( 'NONE',  ( -7.472515219426274946, 11.86968485597268064, 0.000000000000000000 ) ) ;
#135046=CARTESIAN_POINT ( 'NONE',  ( -5.870317324592829067, 5.951051088220814300, -0.7216878364870197293 ) ) ;
#135047=CARTESIAN_POINT ( 'NONE',  ( 0.6823417656249882723, 2.488541667008084435, -1.181850606188749264 ) ) ;
#135055=CARTESIAN_POINT ( 'NONE',  ( 9.236128959407556849, 11.79856975744075598, -1.599625672291262513 ) ) ;
#135063=ADVANCED_FACE ( 'NONE', ( #15212 ), #156438, .F. ) ;
#135069=CARTESIAN_POINT ( 'NONE',  ( -1.364683531250012516, 3.342708333674756727, 0.7879004041258379498 ) ) ;
#135073=CARTESIAN_POINT ( 'NONE',  ( -5.786256696412555911, 6.075953140482280190, 0.5845640519336701146 ) ) ;
#135076=CARTESIAN_POINT ( 'NONE',  ( 10.26082332744404368, 10.86538205830655279, -0.7998128361456281477 ) ) ;
#135079=CARTESIAN_POINT ( 'NONE',  ( -1.201851678989727383E-14, 2.946875000341419248, -1.575800808251660134 ) ) ;
#135089=CARTESIAN_POINT ( 'NONE',  ( 3.194917754314666514, 6.879154480009089134, 0.7998128361456321445 ) ) ;
#135100=CARTESIAN_POINT ( 'NONE',  ( -2.950870989268691957, 6.594433254122103349, -0.7998128361456281477 ) ) ;
#135101=CARTESIAN_POINT ( 'NONE',  ( 8.633844893804129228, 8.967240552393299424, -0.7998128361456211532 ) ) ;
#135104=CARTESIAN_POINT ( 'NONE',  ( 3.945059511452237100, 6.586024615794168646, -1.082531754730548412 ) ) ;
#135113=CARTESIAN_POINT ( 'NONE',  ( -6.805829924380121909, 8.963220883242035697, 1.443375672974078761 ) ) ;
#135115=CARTESIAN_POINT ( 'NONE',  ( 4.416205349749311004, 6.175325546172740765, 1.599625672291267398 ) ) ;
#135118=CARTESIAN_POINT ( 'NONE',  ( -7.648771216403934758, 12.07531685244661723, -0.7998128361456291469 ) ) ;
#135123=CARTESIAN_POINT ( 'NONE',  ( -3.297657676621885692, 4.870353260857385180, 1.599625672291267398 ) ) ;
#135125=CARTESIAN_POINT ( 'NONE',  ( 10.07387183015377197, 11.71160420905630062, -1.199719254218440723 ) ) ;
#135126=CARTESIAN_POINT ( 'NONE',  ( 3.029357257649615054, 5.621668336311468117, -1.199719254218446718 ) ) ;
#135132=CARTESIAN_POINT ( 'NONE',  ( 3.050221373394638835, 6.502416002361635528, 0.000000000000000000 ) ) ;
#135135=CARTESIAN_POINT ( 'NONE',  ( -5.440899717785814715, 5.242137847038546461, 0.7998128361456341429 ) ) ;
#135138=CARTESIAN_POINT ( 'NONE',  ( -8.448702279610222021, 13.00856975952063088, 1.040834085586084257E-14 ) ) ;
#135143=CARTESIAN_POINT ( 'NONE',  ( 7.700668062882064291, 10.00719871149432549, -1.443375672974057666 ) ) ;
#135144=CARTESIAN_POINT ( 'NONE',  ( -1.201851678989727383E-14, 5.259375000341422357, -1.575800808251660134 ) ) ;
#135146=CARTESIAN_POINT ( 'NONE',  ( 5.508690485854129903, 5.321227076451600091, 1.040834085586084257E-14 ) ) ;
#135148=CARTESIAN_POINT ( 'NONE',  ( 5.867981556616276073, 5.740399992340775803, -0.7998128361456281477 ) ) ;
#135150=CARTESIAN_POINT ( 'NONE',  ( -8.050844288416501016, 8.287073179441051707, 1.040834085586084257E-14 ) ) ;
#135153=DIRECTION ( 'NONE',  ( 0.1674078377060222722, 0.000000000000000000, 0.9858877298529452604 ) ) ;
#135159=CARTESIAN_POINT ( 'NONE',  ( -1.364683531250012516, 2.592708333674753174, 0.7879004041258379498 ) ) ;
#135161=CARTESIAN_POINT ( 'NONE',  ( 3.297657676621871925, 4.870353260857385180, 1.599625672291267398 ) ) ;
#135166=CARTESIAN_POINT ( 'NONE',  ( -4.609409038966234995, 7.361099064560491456, -1.082531754730549967 ) ) ;
#135167=CARTESIAN_POINT ( 'NONE',  ( 3.714570900464285064, 4.396382807705524698, 1.082531754730560403 ) ) ;
#135169=CARTESIAN_POINT ( 'NONE',  ( -6.195713011320807873, 6.330679389403470303, -0.7216878364870267237 ) ) ;
#135174=CARTESIAN_POINT ( 'NONE',  ( 3.662674053986138656, 7.424870162959149589, 0.7998128361456321445 ) ) ;
#135180=CARTESIAN_POINT ( 'NONE',  ( 1.150196859685079342, 2.935958678954801115, 0.7750000000000065725 ) ) ;
#135184=CARTESIAN_POINT ( 'NONE',  ( 6.144869935491714230, 8.192100896205568361, -1.599625672291262513 ) ) ;
#135189=CARTESIAN_POINT ( 'NONE',  ( -6.087774667736030487, 7.061157519568837415, 1.199719254218450271 ) ) ;
#135193=CARTESIAN_POINT ( 'NONE',  ( 6.103141704446003679, 10.27208242182903142, 0.7998128361456462443 ) ) ;
#135196=CARTESIAN_POINT ( 'NONE',  ( -4.900382456335551140, 7.804531068111707270, 1.199719254218464037 ) ) ;
#135197=CARTESIAN_POINT ( 'NONE',  ( 6.277061933002777927, 8.346324893301817482, 1.443375672974076540 ) ) ;
#135198=CARTESIAN_POINT ( 'NONE',  ( 4.526804827544169463, 7.221866427374837194, 1.292974732014543271 ) ) ;
#135199=CARTESIAN_POINT ( 'NONE',  ( -4.973143418114339021, 4.696422164088486895, 0.7998128361456341429 ) ) ;
#135202=CARTESIAN_POINT ( 'NONE',  ( -4.062639585589296942, 7.891496616496157301, 0.7998128361456341429 ) ) ;
#135206=CARTESIAN_POINT ( 'NONE',  ( -0.6823417656250003738, 1.467708333674752730, -1.181850606188749264 ) ) ;
#135208=CARTESIAN_POINT ( 'NONE',  ( -5.151735183512911043, 6.073074471262228435, 1.082531754730548412 ) ) ;
#135214=CARTESIAN_POINT ( 'NONE',  ( -0.006158830626153827259, 7.078243236992583398, 2.121324627965421872 ) ) ;
#135215=CARTESIAN_POINT ( 'NONE',  ( 6.169123589417988995, 7.156064594864501416, -1.199719254218445830 ) ) ;
#135220=CARTESIAN_POINT ( 'NONE',  ( 1.364683531249988535, 3.217708333674748289, -0.7879004041258239610 ) ) ;
#135223=CARTESIAN_POINT ( 'NONE',  ( -1.364683531250014514, -0.9489583329919112353, -0.7879004041258359514 ) ) ;
#135226=CARTESIAN_POINT ( 'NONE',  ( -2.761056838677368397, 6.372983411765559048, 0.7998128361456341429 ) ) ;
#135227=CARTESIAN_POINT ( 'NONE',  ( -6.466876083594135238, 9.528143949959703818, 1.082531754730548412 ) ) ;
#135229=CARTESIAN_POINT ( 'NONE',  ( -1.364683531250012516, 2.738541667008090208, -0.7879004041258289570 ) ) ;
#135236=CARTESIAN_POINT ( 'NONE',  ( -6.521108698048772467, 9.591415333490143524, -1.082531754730537976 ) ) ;
#135240=CARTESIAN_POINT ( 'NONE',  ( -7.388830529323428209, 8.683019041374528513, 1.082531754730549967 ) ) ;
#135254=CARTESIAN_POINT ( 'NONE',  ( -7.203459687562382641, 7.298457811777897319, -0.7998128361456291469 ) ) ;
#135256=CARTESIAN_POINT ( 'NONE',  ( 1.499999999999985123, 0.04583333333335545129, -0.8660254037844323793 ) ) ;
#135257=CARTESIAN_POINT ( 'NONE',  ( 2.672928840188529609, 6.270167413528593414, 0.000000000000000000 ) ) ;
#135259=( BOUNDED_SURFACE ( )  B_SPLINE_SURFACE ( 3, 2, ( 
 ( #73586, #41115, #131980 ),
 ( #13898, #79980, #146083 ),
 ( #164436, #48569, #81054 ),
 ( #115741, #95193, #212095 ),
 ( #63731, #97326, #196931 ),
 ( #163382, #178563, #45374 ),
 ( #162313, #47513, #129890 ),
 ( #49616, #197988, #112552 ) ),
 .UNSPECIFIED., .F., .F., .T. ) 
 B_SPLINE_SURFACE_WITH_KNOTS ( ( 4, 2, 2, 4 ),
 ( 3, 3 ),
 ( 0.000000000000000000, 0.003001918495469456383, 0.004502877743204184574, 0.006003836990938912765 ),
 ( 0.000000000000000000, 1.000000000000000000 ),
 .UNSPECIFIED. ) 
 GEOMETRIC_REPRESENTATION_ITEM ( )  RATIONAL_B_SPLINE_SURFACE ( (
 ( 1.000000000000000000, 0.7835651598521251593, 1.000000000000000000),
 ( 1.000000000000000000, 0.7913519369905593903, 1.000000000000000000),
 ( 1.000000000000000000, 0.8009496234844375451, 1.000000000000000000),
 ( 1.000000000000000000, 0.8230981486283348580, 1.000000000000000000),
 ( 1.000000000000000000, 0.8318333311017230836, 1.000000000000000000),
 ( 1.000000000000000000, 0.8529518727575170489, 1.000000000000000000),
 ( 1.000000000000000000, 0.8654984584225912103, 1.000000000000000000),
 ( 1.000000000000000000, 0.8789000212895414776, 1.000000000000000000) ) ) 
 REPRESENTATION_ITEM ( '' )  SURFACE ( )  );
#135262=CARTESIAN_POINT ( 'NONE',  ( 4.821896187954575197, 8.777295985922343391, 0.7998128361456462443 ) ) ;
#135266=CARTESIAN_POINT ( 'NONE',  ( -3.768803514918943609, 7.340761834139994058, 0.7216878364870317197 ) ) ;
#135268=CARTESIAN_POINT ( 'NONE',  ( -0.2172799280667317978, 6.446489533111720682, 3.228652710814125193 ) ) ;
#135269=CARTESIAN_POINT ( 'NONE',  ( 3.215772567386471437, 6.427315425527130088, -0.8732430475888955934 ) ) ;
#135273=CARTESIAN_POINT ( 'NONE',  ( -0.6823417656250003738, 1.467708333674752730, -1.181850606188749264 ) ) ;
#135276=CARTESIAN_POINT ( 'NONE',  ( -8.199983978166823562, 8.461069484149769337, -0.7998128361456291469 ) ) ;
#135278=CARTESIAN_POINT ( 'NONE',  ( 5.445571254183207088, 9.504916896522420444, -0.7998128361456281477 ) ) ;
#135279=CARTESIAN_POINT ( 'NONE',  ( -6.714312387265696458, 8.856450423275211037, 1.599625672291283607 ) ) ;
#135282=CARTESIAN_POINT ( 'NONE',  ( -1.500000000000015099, -0.8395833326505166561, -0.8660254037844383745 ) ) ;
#135284=CARTESIAN_POINT ( 'NONE',  ( 7.293923454472069245, 11.45340176361870199, 0.7216878364870438212 ) ) ;
#135287=CARTESIAN_POINT ( 'NONE',  ( -1.402160292154681736E-14, 1.009375000341417916, -1.575800808251659024 ) ) ;
#135290=CARTESIAN_POINT ( 'NONE',  ( 7.199016378732056687, 10.38230762762066384, -1.082531754730537976 ) ) ;
#135292=CARTESIAN_POINT ( 'NONE',  ( -3.294268138440636928, 6.787137228248626641, 1.040834085586084257E-14 ) ) ;
#135295=CARTESIAN_POINT ( 'NONE',  ( 1.364683531249988535, 3.405208333674749621, -0.7879004041258239610 ) ) ;
#135299=CARTESIAN_POINT ( 'NONE',  ( -5.096975683733680818, 8.033889833409558534, -1.199719254218452047 ) ) ;
#135308=CARTESIAN_POINT ( 'NONE',  ( 6.934105498385400246, 10.17720795050327354, -1.199719254218441611 ) ) ;
#135311=CARTESIAN_POINT ( 'NONE',  ( 0.7499999999999902300, 1.983333333333357817, 1.299038105676669330 ) ) ;
#135317=CARTESIAN_POINT ( 'NONE',  ( 6.371969008742804697, 7.496680600697164465, -1.082531754730543083 ) ) ;
#135318=CARTESIAN_POINT ( 'NONE',  ( -0.6823417656250246877, -0.3864583329919110688, 1.181850606188755259 ) ) ;
#135326=CARTESIAN_POINT ( 'NONE',  ( 1.499999999999987566, 0.02500000000001806333, 0.000000000000000000 ) ) ;
#135327=CARTESIAN_POINT ( 'NONE',  ( 6.103141704446003679, 10.27208242182903142, 0.7998128361456462443 ) ) ;
#135328=CARTESIAN_POINT ( 'NONE',  ( -9.365985188942097750, 9.821404230054264772, 0.7998128361456462443 ) ) ;
#135330=CARTESIAN_POINT ( 'NONE',  ( -1.402160292154681736E-14, -0.3031249996585801965, -1.575800808251665908 ) ) ;
#135331=CARTESIAN_POINT ( 'NONE',  ( -0.7500000000000006661, 1.858333333333357595, -1.299038105676652011 ) ) ;
#135333=CARTESIAN_POINT ( 'NONE',  ( 4.497554271431305040, 6.270232621468402989, -1.599625672291256295 ) ) ;
#135336=CARTESIAN_POINT ( 'NONE',  ( 0.7499999999999920064, 4.514583334016150751, 1.299038105676669330 ) ) ;
#135340=CARTESIAN_POINT ( 'NONE',  ( 1.499999999999985123, -0.6729166659838520248, -0.8660254037844323793 ) ) ;
#135342=CARTESIAN_POINT ( 'NONE',  ( -6.659026002606323047, 10.92061410301605662, 0.000000000000000000 ) ) ;
#135343=CARTESIAN_POINT ( 'NONE',  ( -4.853455804012230423, 6.685451076146141425, 1.443375672974064550 ) ) ;
#135351=CARTESIAN_POINT ( 'NONE',  ( 8.586391356156291010, 8.911878091804165791, 0.7998128361456481317 ) ) ;
#135353=CARTESIAN_POINT ( 'NONE',  ( 6.195713011320782115, 8.251417818006149929, -1.443375672974057666 ) ) ;
#135357=CARTESIAN_POINT ( 'NONE',  ( -7.537443334193545397, 10.88110209227943770, -1.199719254218446718 ) ) ;
#135359=CARTESIAN_POINT ( 'NONE',  ( 5.250031796989762967, 7.148123067953287446, 1.599625672291267398 ) ) ;
#135363=CARTESIAN_POINT ( 'NONE',  ( 3.765413976293345844, 5.416068943807445635, 1.599625672291267398 ) ) ;
#135370=CARTESIAN_POINT ( 'NONE',  ( -5.273758566035884776, 5.255065869904374409, 0.000000000000000000 ) ) ;
#135371=CARTESIAN_POINT ( 'NONE',  ( 8.920901888111997025, 10.47043562662792304, 1.082531754730549967 ) ) ;
#135374=CARTESIAN_POINT ( 'NONE',  ( -5.747767057189642870, 8.793146435774861658, -1.199719254218440723 ) ) ;
#135377=CARTESIAN_POINT ( 'NONE',  ( 3.904598122329021148, 2.800000000000017586, 0.7750000000000135669 ) ) ;
#135379=CARTESIAN_POINT ( 'NONE',  ( -6.561256274009600986, 9.742217188731485678, -1.199719254218440723 ) ) ;
#135381=VERTEX_POINT ( 'NONE', #46688 ) ;
#135391=CARTESIAN_POINT ( 'NONE',  ( -5.506582945444718824, 9.576097202994168001, 0.7998128361456481317 ) ) ;
#135394=CARTESIAN_POINT ( 'NONE',  ( 3.375617060122621194, 6.882044303544283537, 1.040834085586084257E-14 ) ) ;
#135398=CARTESIAN_POINT ( 'NONE',  ( -4.086893239515592136, 6.855460315155083251, 1.199719254218464037 ) ) ;
#135400=CARTESIAN_POINT ( 'NONE',  ( -1.499999999999997780, 5.400000000000022560, 1.214306433183764966E-14 ) ) ;
#135402=DIRECTION ( 'NONE',  ( -5.578564026256490882E-16, -1.000000000000000000, -9.066213480720158442E-32 ) ) ;
#135406=CARTESIAN_POINT ( 'NONE',  ( -7.980945979938748103, 12.46285407657057220, 0.000000000000000000 ) ) ;
#135407=CARTESIAN_POINT ( 'NONE',  ( 5.940443861082012944, 10.08226827123770697, 0.7998128361456462443 ) ) ;
#135411=CARTESIAN_POINT ( 'NONE',  ( -8.839026081105473054, 12.39961529701003684, -1.199719254218446718 ) ) ;
#135412=AXIS2_PLACEMENT_3D ( 'NONE', #109758, #111893, #78246 ) ;
#135415=CARTESIAN_POINT ( 'NONE',  ( -1.364683531250014514, -0.4489583329919089039, -0.7879004041258359514 ) ) ;
#135419=CARTESIAN_POINT ( 'NONE',  ( 8.053180056837369705, 11.37883191874353805, -1.082531754730543083 ) ) ;
#135423=CARTESIAN_POINT ( 'NONE',  ( -5.492770192564149667, 6.262391236846517550, -0.9919644673941154789 ) ) ;
#135425=CARTESIAN_POINT ( 'NONE',  ( 0.000000000000000000, 3.300000000000025135, 1.561251128379126385E-14 ) ) ;
#135445=CARTESIAN_POINT ( 'NONE',  ( -1.364683531249997417, 5.759375000341418804, 1.214306433183764966E-14 ) ) ;
#135449=CARTESIAN_POINT ( 'NONE',  ( 10.16199982864259788, 11.81442020729326536, 1.199719254218452047 ) ) ;
#135451=CARTESIAN_POINT ( 'NONE',  ( 0.5028141819148617131, 7.728236690828134137, -1.993924427468488414 ) ) ;
#135453=CARTESIAN_POINT ( 'NONE',  ( 9.565441069641300587, 11.11843498845840905, -1.199719254218440723 ) ) ;
#135454=ADVANCED_FACE ( 'NONE', ( #136458 ), #85550, .F. ) ;
#135459=CARTESIAN_POINT ( 'NONE',  ( 5.657830175604453338, 5.495223381160312393, 0.7998128361456341429 ) ) ;
#135460=CARTESIAN_POINT ( 'NONE',  ( 1.364683531249988535, 3.217708333674748289, -0.7879004041258239610 ) ) ;
#135461=CARTESIAN_POINT ( 'NONE',  ( -5.899211624428097878, 6.007801130575932014, 0.1941222073163356709 ) ) ;
#135462=CARTESIAN_POINT ( 'NONE',  ( 9.083072846151447166, 12.68433652289702884, 1.199719254218450271 ) ) ;
#135464=CARTESIAN_POINT ( 'NONE',  ( -8.290974629956718189, 9.631557475493025322, -1.199719254218446718 ) ) ;
#135465=CARTESIAN_POINT ( 'NONE',  ( -4.026408433134269771, 6.680931691089825541, 1.082531754730560403 ) ) ;
#135467=CARTESIAN_POINT ( 'NONE',  ( -4.720210035852093533, 8.658662141802762946, -0.7998128361456281477 ) ) ;
#135469=CARTESIAN_POINT ( 'NONE',  ( -1.500000000000015099, 0.4104166673494891726, -0.8660254037844383745 ) ) ;
#135477=CARTESIAN_POINT ( 'NONE',  ( -5.219525951136862574, 5.191794485855519170, -0.7216878364870197293 ) ) ;
#135479=CARTESIAN_POINT ( 'NONE',  ( 3.994353263318512148, 7.604006752988897055, -0.01585061804776008443 ) ) ;
#135484=CARTESIAN_POINT ( 'NONE',  ( -3.104453987404957260, 6.565687385373657925, -0.7216878364870257245 ) ) ;
#135485=CARTESIAN_POINT ( 'NONE',  ( 7.723341061279088038, 12.16231500480096983, -0.7998128361456291469 ) ) ;
#135493=CARTESIAN_POINT ( 'NONE',  ( -2.266184231778562541, 5.795632037050281404, 1.040834085586084257E-14 ) ) ;
#135494=CARTESIAN_POINT ( 'NONE',  ( -9.917953063596627317, 11.52969898140628047, -1.199719254218441611 ) ) ;
#135499=CARTESIAN_POINT ( 'NONE',  ( 4.547870462380197765, 7.393267075163835855, 1.199719254218462483 ) ) ;
#135502=VERTEX_POINT ( 'NONE', #169994 ) ;
#135505=CARTESIAN_POINT ( 'NONE',  ( 4.390142812726693045, 4.016254791136236513, 1.214306433183764966E-14 ) ) ;
#135516=CARTESIAN_POINT ( 'NONE',  ( 8.097244055859613709, 10.46987070330147063, -1.599625672291262513 ) ) ;
#135519=CARTESIAN_POINT ( 'NONE',  ( -5.382750679825375251, 6.238629533673094585, -1.199719254218446718 ) ) ;
#135524=CARTESIAN_POINT ( 'NONE',  ( 1.499999999999987566, -0.9437499993171851731, 0.000000000000000000 ) ) ;
#135528=CARTESIAN_POINT ( 'NONE',  ( -2.535011536075371996, 5.133042487381361596, 2.420000000000010587 ) ) ;
#135529=CARTESIAN_POINT ( 'NONE',  ( 4.704842999142070603, 5.447737239542574272, -1.199719254218452047 ) ) ;
#135530=CARTESIAN_POINT ( 'NONE',  ( -5.434120640978981065, 5.234228924097238611, -0.7998128361456221525 ) ) ;
#135536=CARTESIAN_POINT ( 'NONE',  ( 5.097502569058200983, 6.970172302033127210, -1.443375672974051449 ) ) ;
#135539=CARTESIAN_POINT ( 'NONE',  ( 7.497295758232718654, 9.769931022736756177, -1.443375672974058777 ) ) ;
#135540=CARTESIAN_POINT ( 'NONE',  ( 0.6823417656249917140, 5.155208333674749177, 1.181850606188765695 ) ) ;
#135542=CARTESIAN_POINT ( 'NONE',  ( 3.945059511452237100, 6.586024615794168646, -1.082531754730548412 ) ) ;
#135550=CARTESIAN_POINT ( 'NONE',  ( -4.596643646408070438, 7.147595147647359148, 1.363028123281652793 ) ) ;
#135551=CARTESIAN_POINT ( 'NONE',  ( 1.500000000000003997, 3.300000000000018030, 1.214306433183764966E-14 ) ) ;
#135553=CARTESIAN_POINT ( 'NONE',  ( -1.001543065824772872E-14, 5.384375000341415252, 1.575800808251672791 ) ) ;
#135557=CARTESIAN_POINT ( 'NONE',  ( -8.859363311525973117, 12.42334206583395328, -1.199719254218446718 ) ) ;
#135567=CARTESIAN_POINT ( 'NONE',  ( 3.877268743828270470, 5.546566172598190292, 1.443375672974062551 ) ) ;
#135568=CARTESIAN_POINT ( 'NONE',  ( 0.6823417656249899377, 5.238541667008086655, -1.181850606188754593 ) ) ;
#135570=CARTESIAN_POINT ( 'NONE',  ( 7.772902139336337335, 7.962807338847539107, 0.7998128361456341429 ) ) ;
#135571=CARTESIAN_POINT ( 'NONE',  ( -9.450196763925152510, 10.98398329845622001, -1.199719254218441611 ) ) ;
#135573=CARTESIAN_POINT ( 'NONE',  ( -3.958090780185743451, 6.705190779270287393, -1.199719254218452047 ) ) ;
#135579=CARTESIAN_POINT ( 'NONE',  ( -1.201851678989727383E-14, 4.837500000000018119, -1.732050807568863648 ) ) ;
#135580=CARTESIAN_POINT ( 'NONE',  ( 5.820528018968444961, 5.685037531751635953, 0.7998128361456341429 ) ) ;
#135583=FACE_OUTER_BOUND ( 'NONE', #206511, .T. ) ;
#135586=CARTESIAN_POINT ( 'NONE',  ( 7.565086526745395723, 10.80938946696957004, -1.082531754730543083 ) ) ;
#135591=CARTESIAN_POINT ( 'NONE',  ( 0.7499999999999920064, 4.014583334016149863, 1.299038105676669330 ) ) ;
#135593=CARTESIAN_POINT ( 'NONE',  ( -4.066556009095094737, 6.831733546331167695, 1.199719254218464037 ) ) ;
#135594=CARTESIAN_POINT ( 'NONE',  ( 4.704316113817540668, 5.551085556617666228, -1.082531754730548412 ) ) ;
#135595=DIRECTION ( 'NONE',  ( -5.578564026256490882E-16, -1.000000000000000000, -9.066213480720158442E-32 ) ) ;
#135603=CARTESIAN_POINT ( 'NONE',  ( 5.947222937888848371, 10.09017719417900416, 1.040834085586084257E-14 ) ) ;
#135604=CARTESIAN_POINT ( 'NONE',  ( 6.159481859310094620, 6.080483678816896109, 1.040834085586084257E-14 ) ) ;
#135606=CARTESIAN_POINT ( 'NONE',  ( 1.419999999999989049, 6.280000000000042881, -2.499999999999995115 ) ) ;
#135608=FILL_AREA_STYLE_COLOUR ( '', #116002 ) ;
#135609=CARTESIAN_POINT ( 'NONE',  ( 5.691725559638619814, 5.534767995866836543, 1.040834085586084257E-14 ) ) ;
#135613=VERTEX_POINT ( 'NONE', #87686 ) ;
#135621=CARTESIAN_POINT ( 'NONE',  ( 4.716373530444390560, 6.815548562371487762, -1.235710759775530798 ) ) ;
#135628=CARTESIAN_POINT ( 'NONE',  ( -0.6823417656250003738, -1.032291666325242607, -1.181850606188749264 ) ) ;
#135629=CARTESIAN_POINT ( 'NONE',  ( 5.002595493762530765, 8.780185809457538681, 1.040834085586084257E-14 ) ) ;
#135630=CARTESIAN_POINT ( 'NONE',  ( -8.514157279702017078, 12.87700789305364069, -0.7216878364870267237 ) ) ;
#135636=CARTESIAN_POINT ( 'NONE',  ( -4.232116505760120440, 8.089219690028791376, -0.7998128361456281477 ) ) ;
#135646=CARTESIAN_POINT ( 'NONE',  ( 9.772729797352075920, 10.29593960653257234, -0.7998128361456281477 ) ) ;
#135647=CARTESIAN_POINT ( 'NONE',  ( 6.108345433475511399, 6.019830046288782377, 0.1574382575924727079 ) ) ;
#135648=CARTESIAN_POINT ( 'NONE',  ( -1.203907071533397932, 3.087770253743141069, -0.7749999999999918066 ) ) ;
#135654=CARTESIAN_POINT ( 'NONE',  ( -8.270110514656041190, 10.67154823856396817, 1.443375672974090751 ) ) ;
#135659=CARTESIAN_POINT ( 'NONE',  ( 7.588813295347141441, 9.876701482703580837, -1.599625672291262513 ) ) ;
#135662=CARTESIAN_POINT ( 'NONE',  ( -0.2958088229434103766, 2.800000000000024691, 1.358438285410177748 ) ) ;
#135665=CARTESIAN_POINT ( 'NONE',  ( -5.065942953000576843, 9.062017211809330064, -0.7998128361456231517 ) ) ;
#135666=CARTESIAN_POINT ( 'NONE',  ( 2.849184837166184536, 6.475799410002530898, 0.7998128361456362523 ) ) ;
#135670=CARTESIAN_POINT ( 'NONE',  ( 9.028840231696797503, 12.62106513936658203, -1.199719254218446718 ) ) ;
#135674=CARTESIAN_POINT ( 'NONE',  ( 4.014041799177766379, 7.808471211821870206, -0.2759448393452879067 ) ) ;
#135676=CARTESIAN_POINT ( 'NONE',  ( 5.002595493762530765, 8.780185809457538681, 1.040834085586084257E-14 ) ) ;
#135684=CARTESIAN_POINT ( 'NONE',  ( 9.368320956918616105, 10.03205532593431037, 0.7216878364870458196 ) ) ;
#135688=CARTESIAN_POINT ( 'NONE',  ( -8.690940161559884913, 10.09818392903003748, 1.199719254218462483 ) ) ;
#135689=DIRECTION ( 'NONE',  ( 0.000000000000000000, 8.546850786086437571E-32, 1.000000000000000000 ) ) ;
#135697=CARTESIAN_POINT ( 'NONE',  ( 3.837121167867449945, 4.435395103055503441, 1.199719254218464037 ) ) ;
#135701=CARTESIAN_POINT ( 'NONE',  ( 5.657830175604453338, 5.495223381160312393, 0.7998128361456341429 ) ) ;
#135704=CARTESIAN_POINT ( 'NONE',  ( -1.500000000000013101, 3.660416667349488673, -0.8660254037844313801 ) ) ;
#135710=CARTESIAN_POINT ( 'NONE',  ( -0.7500000000000006661, 1.858333333333357595, -1.299038105676652011 ) ) ;
#135711=CARTESIAN_POINT ( 'NONE',  ( 6.745345117998789775, 7.828323044875442172, 1.199719254218462483 ) ) ;
#135712=CARTESIAN_POINT ( 'NONE',  ( 5.300874872818843286, 5.286701561151180506, 0.7216878364870317197 ) ) ;
#135716=CARTESIAN_POINT ( 'NONE',  ( 8.812436659202669276, 10.34389285956704363, -1.082531754730543083 ) ) ;
#135719=VECTOR ( 'NONE', #76890, 1000.000000000000000 ) ;
#135724=CARTESIAN_POINT ( 'NONE',  ( -6.064574784014443942, 5.969758757638621738, -0.7998128361456291469 ) ) ;
#135725=CARTESIAN_POINT ( 'NONE',  ( 0.7499999999999902300, 3.514583334016149863, 1.299038105676669330 ) ) ;
#135727=CARTESIAN_POINT ( 'NONE',  ( -1.602468905319636405E-14, -1.053124999658583638, -1.575800808251665908 ) ) ;
#135732=CARTESIAN_POINT ( 'NONE',  ( -1.201851678989727383E-14, 3.634375000341422357, 1.575800808251672791 ) ) ;
#135740=CARTESIAN_POINT ( 'NONE',  ( -7.934546212495630968, 10.28005655271014795, -1.599625672291263179 ) ) ;
#135741=CARTESIAN_POINT ( 'NONE',  ( 6.144869935491714230, 8.192100896205568361, -1.599625672291262513 ) ) ;
#135745=VERTEX_POINT ( 'NONE', #74641 ) ;
#135747=CARTESIAN_POINT ( 'NONE',  ( -1.580000000000022276, 6.280000000000042881, 2.580000000000011173 ) ) ;
#135749=CARTESIAN_POINT ( 'NONE',  ( -8.206763054973658100, 8.468978407091068306, 0.7998128361456602331 ) ) ;
#135753=CARTESIAN_POINT ( 'NONE',  ( 8.367353357928214663, 12.91366268422496688, 1.040834085586084257E-14 ) ) ;
#135755=CARTESIAN_POINT ( 'NONE',  ( 8.703444544968814256, 12.24143683818393313, -1.199719254218446718 ) ) ;
#135758=CARTESIAN_POINT ( 'NONE',  ( -2.819205876637805641, 5.376491725131008259, -1.199719254218446718 ) ) ;
#135759=CARTESIAN_POINT ( 'NONE',  ( -7.751511138711140170, 10.06651563329490529, -1.599625672291263179 ) ) ;
#135762=CARTESIAN_POINT ( 'NONE',  ( -3.978601536817720330, 7.845232424458246534, -0.1334687937623244003 ) ) ;
#135767=CARTESIAN_POINT ( 'NONE',  ( 7.944714827928043732, 10.29191993738131927, 1.443375672974076540 ) ) ;
#135770=CARTESIAN_POINT ( 'NONE',  ( 6.830610463186557624, 6.863467050006115677, 1.040834085586084257E-14 ) ) ;
#135790=CARTESIAN_POINT ( 'NONE',  ( -8.941766003412679353, 10.39081407785832845, -1.199719254218446718 ) ) ;
#135795=CARTESIAN_POINT ( 'NONE',  ( -0.7500000000000215383, 1.722916667349486008, 1.299038105676659116 ) ) ;
#135796=CARTESIAN_POINT ( 'NONE',  ( 10.53876547652418338, 11.18964789890005918, 0.7998128361456462443 ) ) ;
#135800=CARTESIAN_POINT ( 'NONE',  ( -10.31505594189871111, 10.92865344183699428, -0.7998128361456291469 ) ) ;
#135802=CARTESIAN_POINT ( 'NONE',  ( -1.201851678989727383E-14, 2.571875000341417472, 1.575800808251672791 ) ) ;
#135809=CARTESIAN_POINT ( 'NONE',  ( -4.288456660624211381, 3.897620947016656956, 1.214306433183764966E-14 ) ) ;
#135811=CARTESIAN_POINT ( 'NONE',  ( 3.978581756310789252, 7.793429149004582612, 0.2401044915457872797 ) ) ;
#135814=CARTESIAN_POINT ( 'NONE',  ( 1.364683531249986537, 0.6760416670080884316, 0.7879004041258500513 ) ) ;
#135819=CARTESIAN_POINT ( 'NONE',  ( 0.6823417656249882723, 1.926041667008083991, -1.181850606188749264 ) ) ;
#135821=CARTESIAN_POINT ( 'NONE',  ( -5.377780486114890124, 9.425827667109372143, 0.000000000000000000 ) ) ;
#135822=CARTESIAN_POINT ( 'NONE',  ( 7.938462636001388795, 9.220293482545153907, -1.199719254218441611 ) ) ;
#135823=CARTESIAN_POINT ( 'NONE',  ( 3.009347262367756848, 6.662655572737694598, -0.5494739808164535999 ) ) ;
#135825=CARTESIAN_POINT ( 'NONE',  ( 5.518332215962025167, 6.396807992499198292, -1.199719254218445830 ) ) ;
#135827=CARTESIAN_POINT ( 'NONE',  ( -1.500000000000011324, 3.670833333333356485, 0.8660254037844403729 ) ) ;
#135829=CARTESIAN_POINT ( 'NONE',  ( 1.364683531249986537, 1.467708333674748289, -0.7879004041258239610 ) ) ;
#135835=CARTESIAN_POINT ( 'NONE',  ( 5.341549334104188418, 7.254893527920112994, 1.443375672974062551 ) ) ;
#135838=CARTESIAN_POINT ( 'NONE',  ( -8.097244055859620815, 10.46987070330147063, -1.599625672291263179 ) ) ;
#135839=CARTESIAN_POINT ( 'NONE',  ( -4.066556009095094737, 6.831733546331167695, 1.199719254218464037 ) ) ;
#135844=CARTESIAN_POINT ( 'NONE',  ( -7.388830529323428209, 8.683019041374528513, 1.082531754730549967 ) ) ;
#135846=CARTESIAN_POINT ( 'NONE',  ( -0.7500000000000215383, 5.441666666666685082, 1.299038105676671107 ) ) ;
#135850=CARTESIAN_POINT ( 'NONE',  ( 6.466876084038451822, 10.48851316477946582, 1.040834085586084257E-14 ) ) ;
#135858=CARTESIAN_POINT ( 'NONE',  ( 10.18181017373857067, 11.94149529319227909, 1.082531754730548412 ) ) ;
#135863=CARTESIAN_POINT ( 'NONE',  ( 7.578644679914702031, 10.82520731233375955, 1.082531754730558626 ) ) ;
#135865=CARTESIAN_POINT ( 'NONE',  ( 6.154511665599609493, 9.267681812253174556, 1.199719254218462483 ) ) ;
#135867=CARTESIAN_POINT ( 'NONE',  ( -4.042302355168801320, 7.867769847672247074, 0.7998128361456341429 ) ) ;
#135869=AXIS2_PLACEMENT_3D ( 'NONE', #130793, #114543, #180536 ) ;
#135871=CARTESIAN_POINT ( 'NONE',  ( -0.6823417656250246877, -1.136458332991911790, 1.181850606188755259 ) ) ;
#135872=CARTESIAN_POINT ( 'NONE',  ( 3.795919822146273326, 5.451659097302528068, -1.443375672974051449 ) ) ;
#135874=CARTESIAN_POINT ( 'NONE',  ( -4.620631424159025613, 4.285158171140619032, -0.7998128361456221525 ) ) ;
#135887=B_SPLINE_CURVE_WITH_KNOTS ( 'NONE', 3,
 ( #68090, #199161, #80103, #100620, #147257, #212224, #130014, #198110, #196005, #179755, #97448, #163504, #166695, #49740, #33489, #18286, #84372, #2021, #15088 ),
 .UNSPECIFIED., .F., .F.,
 ( 4, 3, 3, 3, 3, 3, 4 ),
 ( 0.000000000000000000, 4.552787399504409541E-05, 9.164501444053858924E-05, 0.0001336247809766599628, 0.0001748474261958555187, 0.0002334031072667163169, 0.0002737127687883810032 ),
 .UNSPECIFIED. ) ;
#135888=EDGE_LOOP ( 'NONE', ( #123974, #70919, #107507, #96639, #82573 ) ) ;
#135891=CARTESIAN_POINT ( 'NONE',  ( 7.416473721875251890, 8.611306416064660851, 1.199719254218462483 ) ) ;
#135896=CARTESIAN_POINT ( 'NONE',  ( 1.598423149420390210, 8.713846000021385763, 2.499999999999967581 ) ) ;
#135903=CARTESIAN_POINT ( 'NONE',  ( -4.252453736180621391, 8.112946458852704268, -0.7998128361456281477 ) ) ;
#135905=CARTESIAN_POINT ( 'NONE',  ( -4.790108344329849110, 4.482881244673243337, 0.7998128361456341429 ) ) ;
#135907=CARTESIAN_POINT ( 'NONE',  ( -3.416291520519271874, 6.929497840673697340, 1.040834085586084257E-14 ) ) ;
#135912=CARTESIAN_POINT ( 'NONE',  ( -3.253066792275140173, 5.882662793374543675, 1.199719254218462483 ) ) ;
#135915=CARTESIAN_POINT ( 'NONE',  ( 6.311484202361478779, 7.322151976631905868, -1.199719254218446718 ) ) ;
#135916=CARTESIAN_POINT ( 'NONE',  ( 1.364683531249990311, 5.134375000341417916, 1.214306433183764966E-14 ) ) ;
#135922=CARTESIAN_POINT ( 'NONE',  ( 4.460269348771534581, 8.147471973634706544, -0.7216878364870207285 ) ) ;
#135924=CARTESIAN_POINT ( 'NONE',  ( -6.398558430645608475, 9.552403038140164782, -1.199719254218440723 ) ) ;
#135928=CARTESIAN_POINT ( 'NONE',  ( -6.021792782764022078, 10.17717534653336209, -0.7998128361456291469 ) ) ;
#135929=CARTESIAN_POINT ( 'NONE',  ( -3.913499895838973508, 7.717500311787445000, 1.040834085586084257E-14 ) ) ;
#135933=DIRECTION ( 'NONE',  ( 1.000000000000000000, 0.000000000000000000, 0.000000000000000000 ) ) ;
#135936=CARTESIAN_POINT ( 'NONE',  ( 6.238723240582662477, 10.43026088065513513, -0.7998128361456291469 ) ) ;
#135946=CARTESIAN_POINT ( 'NONE',  ( 1.499999999999990896, 4.025000000000021672, 1.214306433183764966E-14 ) ) ;
#135953=CARTESIAN_POINT ( 'NONE',  ( -1.402160292154681736E-14, -0.7406249996585823059, -1.575800808251665908 ) ) ;
#135954=CARTESIAN_POINT ( 'NONE',  ( 3.602716132929354664, 5.226254793216122074, 1.599625672291267398 ) ) ;
#135955=CARTESIAN_POINT ( 'NONE',  ( 4.873266149108180123, 7.772895376346490970, 1.199719254218462483 ) ) ;
#135957=CARTESIAN_POINT ( 'NONE',  ( -7.049876689426106680, 9.247942109129029475, -1.443375672974059665 ) ) ;
#135959=CARTESIAN_POINT ( 'NONE',  ( 5.829642864196162400, 7.824335979694092558, 1.443375672974062551 ) ) ;
#135960=CARTESIAN_POINT ( 'NONE',  ( -8.825994812371996900, 9.399341490629888440, 0.7216878364870438212 ) ) ;
#135963=CARTESIAN_POINT ( 'NONE',  ( 8.426556166093362776, 9.789735934319136135, -1.199719254218446718 ) ) ;
#135968=CARTESIAN_POINT ( 'NONE',  ( -1.364683531250012516, 2.988541667008091096, -0.7879004041258289570 ) ) ;
#135975=CARTESIAN_POINT ( 'NONE',  ( 8.097244055859613709, 10.46987070330147063, -1.599625672291262513 ) ) ;
#135978=CARTESIAN_POINT ( 'NONE',  ( -8.666686507633592385, 11.13422023037111330, 1.599625672291269396 ) ) ;
#135984=CARTESIAN_POINT ( 'NONE',  ( 3.297657676621871925, 4.870353260857385180, 1.599625672291267398 ) ) ;
#135988=CARTESIAN_POINT ( 'NONE',  ( -8.306341666666730461, 12.84248237775322643, 1.040834085586084257E-14 ) ) ;
#135994=CARTESIAN_POINT ( 'NONE',  ( 5.702249273124194495, 6.094009171513759426, 0.7094654760324905496 ) ) ;
#135996=CARTESIAN_POINT ( 'NONE',  ( -2.927671105547157371, 5.503034492191895666, 1.199719254218462483 ) ) ;
#136001=CARTESIAN_POINT ( 'NONE',  ( 7.775764792637399836, 9.030479331953833011, -1.199719254218441611 ) ) ;
#136003=CARTESIAN_POINT ( 'NONE',  ( 6.962275575817444384, 8.081408578997208991, -1.199719254218446718 ) ) ;
#136004=CARTESIAN_POINT ( 'NONE',  ( 4.578903193113299963, 6.365139696764064325, 1.599625672291267398 ) ) ;
#136006=CARTESIAN_POINT ( 'NONE',  ( -7.700668062882078502, 9.046829497192987901, -1.082531754730543971 ) ) ;
#136014=CARTESIAN_POINT ( 'NONE',  ( -4.067982317475717480, 7.550107770606433455, 0.4684429539664070608 ) ) ;
#136017=CARTESIAN_POINT ( 'NONE',  ( 4.690757960648213931, 8.416375354157496602, 0.7216878364870438212 ) ) ;
#136021=CARTESIAN_POINT ( 'NONE',  ( -8.622622508166983835, 13.00355065959610279, 1.040834085586084257E-14 ) ) ;
#136036=CARTESIAN_POINT ( 'NONE',  ( -7.958272981097355370, 12.22847621134819285, 0.7216878364870458196 ) ) ;
#136041=CARTESIAN_POINT ( 'NONE',  ( 8.796542737168120851, 9.157054702984622097, -0.7998128361456211532 ) ) ;
#136045=CARTESIAN_POINT ( 'NONE',  ( -1.201851678989727383E-14, 1.993750000682816381, 1.732050807568877637 ) ) ;
#136047=CARTESIAN_POINT ( 'NONE',  ( -4.882907879216086933, 8.848476292394087395, -0.7998128361456281477 ) ) ;
#136050=CARTESIAN_POINT ( 'NONE',  ( -8.158255747121117452, 10.54105100977322174, 1.599625672291295375 ) ) ;
#136053=CARTESIAN_POINT ( 'NONE',  ( -1.001543065824772872E-14, 5.493750000682816825, 1.732050807568877637 ) ) ;
#136054=CARTESIAN_POINT ( 'NONE',  ( 5.764187864104357573, 9.876636274763768597, 1.040834085586084257E-14 ) ) ;
#136056=CARTESIAN_POINT ( 'NONE',  ( -6.795661308947694934, 8.951357498570873261, -1.599625672291263179 ) ) ;
#136058=CARTESIAN_POINT ( 'NONE',  ( 9.260382613333817403, 10.76253345609967660, -1.199719254218446718 ) ) ;
#136059=CARTESIAN_POINT ( 'NONE',  ( 1.364683531249990311, 5.613541667008087543, 0.7879004041258500513 ) ) ;
#136065=CARTESIAN_POINT ( 'NONE',  ( -6.548225005720456515, 10.58342024007512983, 0.000000000000000000 ) ) ;
#136068=CARTESIAN_POINT ( 'NONE',  ( -0.6823417656250212460, 4.113541667008085767, 1.181850606188767472 ) ) ;
#136073=CARTESIAN_POINT ( 'NONE',  ( 1.364683531249988535, 5.155208333674749177, -0.7879004041258300672 ) ) ;
#136074=SPHERICAL_SURFACE ( 'NONE', #44683, 0.08000000000000000167 ) ;
#136075=CARTESIAN_POINT ( 'NONE',  ( -4.582292731294565158, 4.448355729372827305, 1.214306433183764966E-14 ) ) ;
#136077=CARTESIAN_POINT ( 'NONE',  ( 7.886038904643079661, 12.35212915539230139, -0.7998128361456352531 ) ) ;
#136078=CARTESIAN_POINT ( 'NONE',  ( -1.364683531250012516, 4.801041667008083991, -0.7879004041258300672 ) ) ;
#136079=CARTESIAN_POINT ( 'NONE',  ( -1.258302072444749564, 2.865146149352002514, -0.7749999999999892530 ) ) ;
#136083=CARTESIAN_POINT ( 'NONE',  ( 1.364683531249986537, 0.4052083336747511200, -0.7879004041258309554 ) ) ;
#136084=CARTESIAN_POINT ( 'NONE',  ( -3.145128448690317935, 5.652771709238564313, -1.082531754730549967 ) ) ;
#136085=CARTESIAN_POINT ( 'NONE',  ( 5.684946482831785275, 5.526859072925533134, -0.7998128361456231517 ) ) ;
#136090=CARTESIAN_POINT ( 'NONE',  ( -5.381422217466647062, 4.322449550048936828, -2.440471613107404902 ) ) ;
#136093=DIRECTION ( 'NONE',  ( -0.1775819850076547912, 0.000000000000000000, -0.9841060098387475197 ) ) ;
#136095=CARTESIAN_POINT ( 'NONE',  ( -7.036318535812428721, 11.15286269184909784, 0.000000000000000000 ) ) ;
#136100=CARTESIAN_POINT ( 'NONE',  ( -7.147119532698295252, 11.49005655479003174, 0.000000000000000000 ) ) ;
#136101=CARTESIAN_POINT ( 'NONE',  ( -3.917943204224913156, 7.514758138330285497, -0.7216878364870257245 ) ) ;
#136102=CARTESIAN_POINT ( 'NONE',  ( -1.364683531250014514, 1.801041667008085767, -0.7879004041258289570 ) ) ;
#136128=CARTESIAN_POINT ( 'NONE',  ( 1.364683531249988757, 2.446875000341415696, 1.214306433183764966E-14 ) ) ;
#136135=CARTESIAN_POINT ( 'NONE',  ( 7.913155211870404493, 12.38376484715752213, 0.7998128361456462443 ) ) ;
#136138=CARTESIAN_POINT ( 'NONE',  ( -1.201851678989727383E-14, 0.8218750003414171390, 1.575800808251672791 ) ) ;
#136149=CARTESIAN_POINT ( 'NONE',  ( 3.981290663907289140, 7.796589541200495965, -0.7998128361456221525 ) ) ;
#136160=CARTESIAN_POINT ( 'NONE',  ( -2.611917148927046295, 6.198987107056845858, 1.040834085586084257E-14 ) ) ;
#136161=CARTESIAN_POINT ( 'NONE',  ( 9.108380270282433244, 9.520865158284665952, 1.040834085586084257E-14 ) ) ;
#136172=CARTESIAN_POINT ( 'NONE',  ( -7.158341918335454857, 10.33485409049125003, 1.082531754730549967 ) ) ;
#136174=CARTESIAN_POINT ( 'NONE',  ( 5.341022448779654930, 8.318611059296550536, 1.199719254218462483 ) ) ;
#136178=CARTESIAN_POINT ( 'NONE',  ( -8.272446282632566650, 12.80293776304669962, 0.7998128361456481317 ) ) ;
#136183=CARTESIAN_POINT ( 'NONE',  ( -2.774614992291035698, 6.388801257648172971, 1.040834085586084257E-14 ) ) ;
#136185=CARTESIAN_POINT ( 'NONE',  ( 10.55910270694468345, 11.21337466772398095, 0.7998128361456462443 ) ) ;
#136188=CARTESIAN_POINT ( 'NONE',  ( 2.706824224222692088, 6.309712028235118453, 0.7998128361456362523 ) ) ;
#136194=CARTESIAN_POINT ( 'NONE',  ( 5.192409644353875642, 5.160158794608717514, 1.040834085586084257E-14 ) ) ;
#136197=CARTESIAN_POINT ( 'NONE',  ( -4.229253852459088137, 7.021547696922494808, 1.199719254218464037 ) ) ;
#136200=CARTESIAN_POINT ( 'NONE',  ( -7.797910906154257304, 12.24931315715533486, 0.000000000000000000 ) ) ;
#136205=CARTESIAN_POINT ( 'NONE',  ( 8.758204044748010730, 9.320252261735261001, 0.7216878364870438212 ) ) ;
#136206=CARTESIAN_POINT ( 'NONE',  ( 1.364683531249988535, 4.967708333674756283, -0.7879004041258300672 ) ) ;
#136208=CARTESIAN_POINT ( 'NONE',  ( 5.684946482831785275, 5.526859072925533134, -0.7998128361456231517 ) ) ;
#136218=EDGE_LOOP ( 'NONE', ( #141420, #157298, #79383, #165965, #128079, #192585, #212572, #199700, #22373, #160002, #176017, #27799, #61371 ) ) ;
#136220=CARTESIAN_POINT ( 'NONE',  ( -0.6823417656249969321, 3.280208333674754062, -1.181850606188749264 ) ) ;
#136222=CARTESIAN_POINT ( 'NONE',  ( 8.530051201292206287, 13.10347683481629488, 0.000000000000000000 ) ) ;
#136224=CARTESIAN_POINT ( 'NONE',  ( -3.619663825168619731, 7.166765529431275539, 1.040834085586084257E-14 ) ) ;
#136226=CARTESIAN_POINT ( 'NONE',  ( -6.033015167956810920, 7.101234453113482559, -1.082531754730543083 ) ) ;
#136231=CARTESIAN_POINT ( 'NONE',  ( 4.798696304233017074, 7.685897223992134819, -1.199719254218452047 ) ) ;
#136238=EDGE_CURVE ( 'NONE', #170224, #44633, #122878, .T. ) ;
#136244=CARTESIAN_POINT ( 'NONE',  ( 4.469384193999260901, 8.366031992974468423, -0.7998128361456231517 ) ) ;
#136246=CARTESIAN_POINT ( 'NONE',  ( -3.358669367883384105, 4.941533567329135401, -1.599625672291262513 ) ) ;
#136248=CARTESIAN_POINT ( 'NONE',  ( -5.065942953000576843, 9.062017211809330064, -0.7998128361456231517 ) ) ;
#136252=CARTESIAN_POINT ( 'NONE',  ( 6.938021921891177612, 9.117444880338284818, -1.599625672291262513 ) ) ;
#136255=CARTESIAN_POINT ( 'NONE',  ( -7.562750758324527922, 7.717630727667075696, 1.040834085586084257E-14 ) ) ;
#136256=CARTESIAN_POINT ( 'NONE',  ( 7.090551149822744925, 7.374657217655760100, 0.7216878364870317197 ) ) ;
#136257=CARTESIAN_POINT ( 'NONE',  ( 4.226642156305554288, 7.541242530477547668, 0.9646342093552334740 ) ) ;
#136258=CARTESIAN_POINT ( 'NONE',  ( -4.355193658487827690, 6.104145239700998538, -1.599625672291256295 ) ) ;
#136261=CARTESIAN_POINT ( 'NONE',  ( -3.737243898861318137, 7.511868315313511069, 0.7998128361456341429 ) ) ;
#136265=CARTESIAN_POINT ( 'NONE',  ( -1.201851678989727383E-14, 2.571875000341417472, 1.575800808251672791 ) ) ;
#136267=CARTESIAN_POINT ( 'NONE',  ( -5.097502569058221411, 6.009803087731781623, -1.082531754730544860 ) ) ;
#136273=CARTESIAN_POINT ( 'NONE',  ( 6.765682348419287173, 7.852049813699357728, 1.199719254218462483 ) ) ;
#136276=CARTESIAN_POINT ( 'NONE',  ( -1.364683531250012516, 2.801041667008090652, -0.7879004041258289570 ) ) ;
#136282=CARTESIAN_POINT ( 'NONE',  ( -4.192495815123836955, 5.914331089109674089, -1.599625672291256295 ) ) ;
#136283=ADVANCED_FACE ( 'NONE', ( #59449 ), #25872, .T. ) ;
#136284=CARTESIAN_POINT ( 'NONE',  ( -7.226132685959434809, 8.493204890783200511, 1.082531754730549967 ) ) ;
#136286=CARTESIAN_POINT ( 'NONE',  ( -1.364683531250000748, 2.259375000341422357, 1.214306433183764966E-14 ) ) ;
#136293=CARTESIAN_POINT ( 'NONE',  ( -7.551528372687420720, 8.872833191965849409, 1.082531754730558626 ) ) ;
#136297=CARTESIAN_POINT ( 'NONE',  ( -6.141480396866151992, 9.148515648777049591, 1.082531754730548412 ) ) ;
#136312=CARTESIAN_POINT ( 'NONE',  ( -4.706651882238427120, 8.642844295920152575, 1.040834085586084257E-14 ) ) ;
#136315=CARTESIAN_POINT ( 'NONE',  ( 4.847203612085560387, 5.613824621309978724, -1.199719254218452047 ) ) ;
#136319=CARTESIAN_POINT ( 'NONE',  ( 6.982612806237943559, 8.105135347821125436, -1.199719254218446718 ) ) ;
#136324=CARTESIAN_POINT ( 'NONE',  ( -4.121315508874255684, 7.752025827087861920, -0.7216878364870267237 ) ) ;
#136333=CARTESIAN_POINT ( 'NONE',  ( -1.364683531250000748, 2.259375000341422357, 1.214306433183764966E-14 ) ) ;
#136335=CARTESIAN_POINT ( 'NONE',  ( -6.852756576703439961, 10.08230087520760954, 1.199719254218453823 ) ) ;
#136337=CARTESIAN_POINT ( 'NONE',  ( 5.309989718046547402, 9.346738437696316737, 0.7998128361456462443 ) ) ;
#136339=CARTESIAN_POINT ( 'NONE',  ( -7.497822643557261024, 8.706213491360317747, -1.199719254218446718 ) ) ;
#136342=CARTESIAN_POINT ( 'NONE',  ( -0.7500000000000249800, -0.7770833326505161009, 1.299038105676659116 ) ) ;
#136344=CARTESIAN_POINT ( 'NONE',  ( 8.351459436338029008, 10.76645531385962862, -1.443375672974063439 ) ) ;
#136348=CARTESIAN_POINT ( 'NONE',  ( 0.6823417656249882723, -0.2614583329919109578, -1.181850606188749264 ) ) ;
#136351=B_SPLINE_CURVE_WITH_KNOTS ( 'NONE', 3,
 ( #207584, #141577, #25632, #42990, #59204, #125360, #44048, #162059, #109103, #91744, #127509, #176178, #13648, #26704, #140505, #92806, #60273, #128572, #194536, #158850, #58148, #10447, #192393, #142631, #209705, #27778, #93876, #159913 ),
 .UNSPECIFIED., .F., .F.,
 ( 4, 3, 3, 3, 3, 3, 3, 3, 3, 4 ),
 ( 0.000000000000000000, 4.667319012710265200E-05, 7.775567177467941214E-05, 9.418433154889146845E-05, 0.0001004198801466371470, 0.0001156098471385010821, 0.0001218465752387289092, 0.0001431384767120459612, 0.0001435705847349271001, 0.0001594483893922525955 ),
 .UNSPECIFIED. ) ;
#136352=CARTESIAN_POINT ( 'NONE',  ( 8.717529583462654941, 9.272798723569005475, 0.7216878364870458196 ) ) ;
#136355=CARTESIAN_POINT ( 'NONE',  ( -4.609409038966229666, 8.321468278861834378, -0.7216878364870267237 ) ) ;
#136357=CARTESIAN_POINT ( 'NONE',  ( 1.364683531249988535, 3.613541667008086211, 0.7879004041258500513 ) ) ;
#136361=CARTESIAN_POINT ( 'NONE',  ( -5.208303565944065738, 9.228104593576741621, -0.7998128361456231517 ) ) ;
#136362=CARTESIAN_POINT ( 'NONE',  ( 0.6823417656249917140, 5.655208333674749177, 1.181850606188765695 ) ) ;
#136369=CARTESIAN_POINT ( 'NONE',  ( 9.257519960032755790, 9.694861462993381807, 0.7998128361456462443 ) ) ;
#136372=CARTESIAN_POINT ( 'NONE',  ( -1.500000000000013101, 2.879166666666688634, -0.8660254037844313801 ) ) ;
#136378=CARTESIAN_POINT ( 'NONE',  ( 7.144783764721768904, 7.437928601704619780, 1.040834085586084257E-14 ) ) ;
#136380=CARTESIAN_POINT ( 'NONE',  ( -1.402160292154681736E-14, -1.115624999658584082, 1.575800808251672791 ) ) ;
#136388=CARTESIAN_POINT ( 'NONE',  ( -1.500000000000015099, -0.1208333333333093396, -0.8660254037844383745 ) ) ;
#136389=CARTESIAN_POINT ( 'NONE',  ( 6.889514614038635187, 11.18951748302043114, -0.7998128361456291469 ) ) ;
#136390=CARTESIAN_POINT ( 'NONE',  ( -7.818248136574758256, 12.27303992597924420, 0.000000000000000000 ) ) ;
#136392=CARTESIAN_POINT ( 'NONE',  ( -0.6823417656250003738, 0.4677083336747517306, -1.181850606188749264 ) ) ;
#136393=CARTESIAN_POINT ( 'NONE',  ( 1.499999999999987121, 1.254166666666689300, 0.8660254037844524744 ) ) ;
#136395=CARTESIAN_POINT ( 'NONE',  ( 5.769158057814842699, 6.689438141327490150, 1.199719254218462483 ) ) ;
#136403=CARTESIAN_POINT ( 'NONE',  ( 1.364683531249992088, 5.384375000341417916, 1.214306433183764966E-14 ) ) ;
#136405=CARTESIAN_POINT ( 'NONE',  ( -8.290974629956718189, 9.631557475493025322, -1.199719254218446718 ) ) ;
#136406=CARTESIAN_POINT ( 'NONE',  ( -4.772106882330227506, 7.550913215151819458, -1.082531754730549967 ) ) ;
#136414=CARTESIAN_POINT ( 'NONE',  ( 7.182068686937156166, 9.402166106225269715, 1.599625672291281386 ) ) ;
#136415=CARTESIAN_POINT ( 'NONE',  ( -5.422898255786213539, 5.429062174613084935, -0.7216878364870178419 ) ) ;
#136418=CARTESIAN_POINT ( 'NONE',  ( 7.578644679914718019, 7.944099669429731669, 0.7216878364870317197 ) ) ;
#136422=CARTESIAN_POINT ( 'NONE',  ( -6.509886312855995172, 10.74661779830734254, -0.7998128361456291469 ) ) ;
#136423=CARTESIAN_POINT ( 'NONE',  ( 5.575427483717746213, 7.527751369135936343, 1.599625672291267398 ) ) ;
#136425=CARTESIAN_POINT ( 'NONE',  ( 4.189106276498237413, 3.989638198777126110, -0.7216878364870188411 ) ) ;
#136426=LINE ( 'NONE', #82317, #179030 ) ;
#136427=CARTESIAN_POINT ( 'NONE',  ( 2.523789150438203510, 6.096171108819874007, 0.7998128361456462443 ) ) ;
#136428=ORIENTED_EDGE ( 'NONE', *, *, #169120, .F. ) ;
#136435=CARTESIAN_POINT ( 'NONE',  ( -3.131570295076647525, 6.597323077657299528, 1.040834085586084257E-14 ) ) ;
#136436=CARTESIAN_POINT ( 'NONE',  ( 10.54788032175191326, 11.40820791823982994, 0.7216878364870317197 ) ) ;
#136439=CARTESIAN_POINT ( 'NONE',  ( -6.043183783389232566, 8.073467052085995022, 1.599625672291269396 ) ) ;
#136443=CARTESIAN_POINT ( 'NONE',  ( -1.201851678989727383E-14, 3.009375000341419693, -1.575800808251660134 ) ) ;
#136445=CARTESIAN_POINT ( 'NONE',  ( -8.518600588087975822, 8.832788862391110385, 1.040834085586084257E-14 ) ) ;
#136458=FACE_OUTER_BOUND ( 'NONE', #53833, .T. ) ;
#136460=CARTESIAN_POINT ( 'NONE',  ( -7.477485413136760073, 8.682486722536401302, -1.199719254218446718 ) ) ;
#136463=CARTESIAN_POINT ( 'NONE',  ( 6.819388077993785657, 7.058300300521964665, 1.040834085586084257E-14 ) ) ;
#136468=CARTESIAN_POINT ( 'NONE',  ( -4.959585264500673496, 4.680604318205876524, 1.214306433183764966E-14 ) ) ;
#136470=CARTESIAN_POINT ( 'NONE',  ( -6.138158007735671440, 5.995864564798076835, -0.1121503744203552477 ) ) ;
#136475=CARTESIAN_POINT ( 'NONE',  ( -7.343712760096452463, 11.71941532008788833, -0.7998128361456291469 ) ) ;
#136476=CARTESIAN_POINT ( 'NONE',  ( 6.805303039055573322, 10.02693841461847057, 1.199719254218460707 ) ) ;
#136482=CARTESIAN_POINT ( 'NONE',  ( 1.364683531249984538, -1.032291666325247714, -0.7879004041258309554 ) ) ;
#136487=CARTESIAN_POINT ( 'NONE',  ( 9.747949258545622442, 10.47495501116581984, 0.000000000000000000 ) ) ;
#136490=EDGE_CURVE ( 'NONE', #11835, #64117, #134235, .T. ) ;
#136495=CARTESIAN_POINT ( 'NONE',  ( -0.04822499102144637423, 6.344199970485692397, -3.092266627314186334 ) ) ;
#136507=CARTESIAN_POINT ( 'NONE',  ( -4.647747731386360215, 4.316793862905830892, 0.7998128361456341429 ) ) ;
#136512=( BOUNDED_CURVE ( )  B_SPLINE_CURVE ( 2, ( #31119, #145953, #48439, #45239, #111355 ),
 .UNSPECIFIED., .F., .T. ) 
 B_SPLINE_CURVE_WITH_KNOTS ( ( 3, 2, 3 ),
 ( 0.2585522869718673844, 0.2625000000000000111, 0.2644396091801784476 ),
 .UNSPECIFIED. ) 
 CURVE ( )  GEOMETRIC_REPRESENTATION_ITEM ( )  RATIONAL_B_SPLINE_CURVE ( ( 0.9866594824841232736, 0.8730656178594444761, 1.000000000000000000, 0.9376339943847032954, 0.9333315137402016237 ) ) 
 REPRESENTATION_ITEM ( '' )  );
#136515=CARTESIAN_POINT ( 'NONE',  ( -1.500000000000015099, -0.8395833326505166561, -0.8660254037844383745 ) ) ;
#136520=CARTESIAN_POINT ( 'NONE',  ( 8.703444544968814256, 12.24143683818393313, -1.199719254218446718 ) ) ;
#136521=ORIENTED_EDGE ( 'NONE', *, *, #41655, .T. ) ;
#136524=CARTESIAN_POINT ( 'NONE',  ( 3.623053363349855172, 5.249981562040033189, 1.599625672291267398 ) ) ;
#136528=CARTESIAN_POINT ( 'NONE',  ( 3.988069740714122791, 7.804498464141805592, 0.7998128361456321445 ) ) ;
#136529=CARTESIAN_POINT ( 'NONE',  ( -0.6823417656249969321, 3.280208333674754062, -1.181850606188749264 ) ) ;
#136530=CARTESIAN_POINT ( 'NONE',  ( -4.884136011505287200, 6.706951837855620546, 1.250136565965910274 ) ) ;
#136533=CARTESIAN_POINT ( 'NONE',  ( -6.886651960737580680, 10.12184548991413457, -1.199719254218440723 ) ) ;
#136535=CARTESIAN_POINT ( 'NONE',  ( -3.755245360860919757, 7.324943987738961049, -0.7216878364870257245 ) ) ;
#136538=CARTESIAN_POINT ( 'NONE',  ( -5.693534442735004752, 8.729875052244421951, 1.199719254218452047 ) ) ;
#136540=CARTESIAN_POINT ( 'NONE',  ( 0.7499999999999867883, -0.4020833326505157679, -1.299038105676652899 ) ) ;
#136547=CARTESIAN_POINT ( 'NONE',  ( -5.056828107772872727, 5.001980335264194721, -0.7216878364870197293 ) ) ;
#136552=CARTESIAN_POINT ( 'NONE',  ( -3.836594282542926226, 5.499112634431936542, 1.443375672974064550 ) ) ;
#136554=CARTESIAN_POINT ( 'NONE',  ( 7.086107841436786181, 11.41887624831828418, 1.040834085586084257E-14 ) ) ;
#136563=CARTESIAN_POINT ( 'NONE',  ( -4.115063316947640715, 4.759660943649018705, 1.199719254218462483 ) ) ;
#136569=CARTESIAN_POINT ( 'NONE',  ( 6.518772930072240790, 6.499656594706071822, -0.7998128361456281477 ) ) ;
#136575=CARTESIAN_POINT ( 'NONE',  ( 3.728655938958122196, 4.308852335994623139, -1.199719254218446718 ) ) ;
#136586=CARTESIAN_POINT ( 'NONE',  ( 7.934546212495622086, 10.28005655271014795, -1.599625672291262513 ) ) ;
#136588=CARTESIAN_POINT ( 'NONE',  ( -4.141125853970233806, 6.918731698685530063, -1.199719254218452047 ) ) ;
#136590=CARTESIAN_POINT ( 'NONE',  ( -5.056828107772866510, 5.962349549565537643, -1.082531754730543971 ) ) ;
#136593=CARTESIAN_POINT ( 'NONE',  ( 1.499999999999985123, -1.172916665983846363, -0.8660254037844323793 ) ) ;
#136598=CARTESIAN_POINT ( 'NONE',  ( 4.029797971759831121, 5.724516938518342535, -1.599625672291255185 ) ) ;
#136599=CARTESIAN_POINT ( 'NONE',  ( -5.382750679825375251, 6.238629533673094585, -1.199719254218446718 ) ) ;
#136605=CARTESIAN_POINT ( 'NONE',  ( 5.287316719649520991, 8.151991358691011769, -1.082531754730549078 ) ) ;
#136608=CARTESIAN_POINT ( 'NONE',  ( 7.361714222096048310, 10.57212177821199184, -1.082531754730537976 ) ) ;
#136609=CARTESIAN_POINT ( 'NONE',  ( -1.201851678989727383E-14, 3.134375000341420137, 1.575800808251672791 ) ) ;
#136611=CARTESIAN_POINT ( 'NONE',  ( 4.595850884908202261, 7.345281218159464665, -1.082531754730549078 ) ) ;
#136618=CARTESIAN_POINT ( 'NONE',  ( -5.229776604766065873, 6.614552831964506829, 1.409540066939333425 ) ) ;
#136624=CARTESIAN_POINT ( 'NONE',  ( -9.775592450653132204, 11.36361159963886891, -1.199719254218441611 ) ) ;
#136629=CARTESIAN_POINT ( 'NONE',  ( -3.002240950422295995, 5.590032644546251817, -1.199719254218452935 ) ) ;
#136634=CARTESIAN_POINT ( 'NONE',  ( 2.236732156574683827, 5.553345249405011508, 1.040834085586084257E-14 ) ) ;
#136635=EDGE_CURVE ( 'NONE', #193266, #14088, #195450, .T. ) ;
#136636=CARTESIAN_POINT ( 'NONE',  ( 0.6823417656249899377, 3.238541667008085323, -1.181850606188754593 ) ) ;
#136638=CARTESIAN_POINT ( 'NONE',  ( 6.262976894508937242, 9.394224579314053969, -1.199719254218440723 ) ) ;
#136640=CARTESIAN_POINT ( 'NONE',  ( -8.157201976916404362, 12.66848607304450702, -0.7998128361456281477 ) ) ;
#136642=CARTESIAN_POINT ( 'NONE',  ( -3.632695093457760649, 6.325562478087638496, -1.199719254218452047 ) ) ;
#136647=CARTESIAN_POINT ( 'NONE',  ( -1.499999999999997780, 4.150000000000021672, 1.214306433183764966E-14 ) ) ;
#136648=CARTESIAN_POINT ( 'NONE',  ( 3.662674053986138656, 7.424870162959149589, 0.7998128361456321445 ) ) ;
#136653=CARTESIAN_POINT ( 'NONE',  ( 1.364683531249988535, 3.863541667008087543, 0.7879004041258500513 ) ) ;
#136656=CARTESIAN_POINT ( 'NONE',  ( 8.270110514656021650, 11.63191745286530576, 1.082531754730557072 ) ) ;
#136661=CARTESIAN_POINT ( 'NONE',  ( -1.402160292154681736E-14, 1.868750000682816381, -1.732050807568863648 ) ) ;
#136663=CARTESIAN_POINT ( 'NONE',  ( -4.608882153641705059, 7.464447381635583412, -1.199719254218452047 ) ) ;
#136664=CARTESIAN_POINT ( 'NONE',  ( 3.185802909086937973, 6.660594460669327255, 0.7216878364870317197 ) ) ;
#136671=ORIENTED_EDGE ( 'NONE', *, *, #89227, .F. ) ;
#136673=CARTESIAN_POINT ( 'NONE',  ( 7.983053520348166288, 8.207983950027992748, -0.7998128361456281477 ) ) ;
#136674=CARTESIAN_POINT ( 'NONE',  ( 4.955668840994886359, 5.740367388370866131, 1.199719254218462483 ) ) ;
#136678=CARTESIAN_POINT ( 'NONE',  ( 3.506755287428983792, 7.242964935309132990, 1.040834085586084257E-14 ) ) ;
#136680=ORIENTED_EDGE ( 'NONE', *, *, #158371, .T. ) ;
#136682=AXIS2_PLACEMENT_3D ( 'NONE', #47681, #126862, #162487 ) ;
#136683=ORIENTED_EDGE ( 'NONE', *, *, #58248, .F. ) ;
#136684=CARTESIAN_POINT ( 'NONE',  ( 9.053093885623066939, 11.58502883802551153, -1.599625672291262513 ) ) ;
#136689=CARTESIAN_POINT ( 'NONE',  ( 5.880650534977156063, 5.984130091214588276, -0.1889179825720621597 ) ) ;
#136691=CARTESIAN_POINT ( 'NONE',  ( 9.728138913005292210, 11.30824913904973705, -1.199719254218440723 ) ) ;
#136697=CARTESIAN_POINT ( 'NONE',  ( 7.782016984564060103, 9.141736572488651902, 1.082531754730558626 ) ) ;
#136698=CARTESIAN_POINT ( 'NONE',  ( -3.469997250093771246, 6.135748327496311383, -1.199719254218452935 ) ) ;
#136704=CARTESIAN_POINT ( 'NONE',  ( -3.554208825076827782, 7.298327395898266623, 0.7998128361456341429 ) ) ;
#136706=CARTESIAN_POINT ( 'NONE',  ( -6.509799877575655813, 5.178456542363094606, 2.499999999999998668 ) ) ;
#136711=CARTESIAN_POINT ( 'NONE',  ( -4.911752498546917423, 4.707425932596563278, -0.3822207396134598145 ) ) ;
#136716=CARTESIAN_POINT ( 'NONE',  ( 7.411503528164766763, 11.79850454950093841, 1.040834085586084257E-14 ) ) ;
#136717=CARTESIAN_POINT ( 'NONE',  ( 6.114332400817464652, 6.016105027659348181, -0.05221600309115309591 ) ) ;
#136720=DIRECTION ( 'NONE',  ( 1.000000000000000000, 0.000000000000000000, 0.000000000000000000 ) ) ;
#136724=CARTESIAN_POINT ( 'NONE',  ( -9.978437869977950569, 11.70422760547153906, -1.082531754730539753 ) ) ;
#136728=CARTESIAN_POINT ( 'NONE',  ( 8.762647353133951711, 9.117510088278095282, 1.040834085586084257E-14 ) ) ;
#136732=CARTESIAN_POINT ( 'NONE',  ( -5.377780486114890124, 9.425827667109372143, 0.000000000000000000 ) ) ;
#136733=CARTESIAN_POINT ( 'NONE',  ( 4.630273154266905777, 5.360739087188218122, 1.199719254218464037 ) ) ;
#136737=CARTESIAN_POINT ( 'NONE',  ( 10.70146331988817323, 11.37946204949139251, 0.7998128361456341429 ) ) ;
#136740=CARTESIAN_POINT ( 'NONE',  ( 4.051511279158463985, 7.758049153162790645, -0.5006740859710266944 ) ) ;
#136742=CARTESIAN_POINT ( 'NONE',  ( 4.202664430556241726, 7.846932902383524144, 0.7216878364870298324 ) ) ;
#136749=ORIENTED_EDGE ( 'NONE', *, *, #177765, .T. ) ;
#136750=CARTESIAN_POINT ( 'NONE',  ( 6.751597309481075726, 10.82068792779586985, 1.040834085586084257E-14 ) ) ;
#136754=CARTESIAN_POINT ( 'NONE',  ( -8.877891658850122880, 9.251961778280284321, 0.7998128361456462443 ) ) ;
#136763=CARTESIAN_POINT ( 'NONE',  ( 4.566398809704347528, 4.221886787610169556, -0.7998128361456211532 ) ) ;
#136767=CARTESIAN_POINT ( 'NONE',  ( 5.820528018968444961, 5.685037531751635953, 0.7998128361456341429 ) ) ;
#136770=CARTESIAN_POINT ( 'NONE',  ( 0.7499999999999885647, 2.347916667349486453, -1.299038105676652899 ) ) ;
#136776=CARTESIAN_POINT ( 'NONE',  ( -0.7500000000000215383, 1.941666666666688634, 1.299038105676659116 ) ) ;
#136777=CARTESIAN_POINT ( 'NONE',  ( 7.935599982700328958, 8.152621489438862667, 0.7998128361456481317 ) ) ;
#136778=CARTESIAN_POINT ( 'NONE',  ( 4.324687812634882000, 7.028924300507257250, 1.082531754730558626 ) ) ;
#136782=CARTESIAN_POINT ( 'NONE',  ( 9.924205255523292024, 10.68058700763975466, -0.7216878364870257245 ) ) ;
#136788=CARTESIAN_POINT ( 'NONE',  ( -4.771579997005698459, 7.654261532226910525, -1.199719254218452047 ) ) ;
#136790=AXIS2_PLACEMENT_3D ( 'NONE', #66364, #33892, #17620 ) ;
#136791=CARTESIAN_POINT ( 'NONE',  ( -1.499999999999997780, 4.431250000682819490, 1.214306433183764966E-14 ) ) ;
#136792=CARTESIAN_POINT ( 'NONE',  ( 1.364683531249990311, 4.926041667008083991, 0.7879004041258500513 ) ) ;
#136798=CARTESIAN_POINT ( 'NONE',  ( 1.364683531249990311, 4.446875000341417028, 1.214306433183764966E-14 ) ) ;
#136805=CARTESIAN_POINT ( 'NONE',  ( -8.552495972122143186, 8.872333477097637200, 0.7998128361456462443 ) ) ;
#136806=CARTESIAN_POINT ( 'NONE',  ( 6.765682348419287173, 7.852049813699357728, 1.199719254218462483 ) ) ;
#136814=CARTESIAN_POINT ( 'NONE',  ( -8.369460898337653276, 8.658792557682392754, 0.7998128361456462443 ) ) ;
#136817=CARTESIAN_POINT ( 'NONE',  ( 10.53876547652418338, 11.18964789890005918, 0.7998128361456462443 ) ) ;
#136819=CARTESIAN_POINT ( 'NONE',  ( 8.540746701604824409, 12.05162268759261224, -1.199719254218446718 ) ) ;
#136822=CARTESIAN_POINT ( 'NONE',  ( -5.915435094264120508, 5.795762452929912101, 0.000000000000000000 ) ) ;
#136823=CARTESIAN_POINT ( 'NONE',  ( -7.537443334193545397, 10.88110209227943770, -1.199719254218446718 ) ) ;
#136827=CARTESIAN_POINT ( 'NONE',  ( -3.990270464981529486, 7.829052896380438220, 0.2716399205876223744 ) ) ;
#136828=CARTESIAN_POINT ( 'NONE',  ( -1.364683531250000748, -0.9906249996585805295, 0.000000000000000000 ) ) ;
#136834=CARTESIAN_POINT ( 'NONE',  ( 6.518772930072240790, 6.499656594706071822, -0.7998128361456281477 ) ) ;
#136847=VECTOR ( 'NONE', #148977, 1000.000000000000000 ) ;
#136855=SPHERICAL_SURFACE ( 'NONE', #16132, 0.08000000000000000167 ) ;
#136859=CARTESIAN_POINT ( 'NONE',  ( -7.374745490829552885, 10.69128794168811680, -1.199719254218446718 ) ) ;
#136864=CARTESIAN_POINT ( 'NONE',  ( 0.7499999999999885647, 1.597916667349486008, -1.299038105676652899 ) ) ;
#136865=CARTESIAN_POINT ( 'NONE',  ( 9.402743226277308963, 10.92862083786708816, -1.199719254218446718 ) ) ;
#136870=CARTESIAN_POINT ( 'NONE',  ( -9.130526383799315582, 12.73969898348616070, 1.199719254218462483 ) ) ;
#136872=CARTESIAN_POINT ( 'NONE',  ( 0.6823417656249882723, 1.426041667008083547, -1.181850606188749264 ) ) ;
#136878=CARTESIAN_POINT ( 'NONE',  ( -3.440018289565379028, 5.036440642624797626, 1.599625672291267398 ) ) ;
#136880=CARTESIAN_POINT ( 'NONE',  ( -0.4308379095628913080, 6.611440747340219914, -3.285375171801879990 ) ) ;
#136883=CARTESIAN_POINT ( 'NONE',  ( -1.364683531250012516, 0.8427083336747532849, 0.7879004041258379498 ) ) ;
#136889=CARTESIAN_POINT ( 'NONE',  ( 1.364683531249986537, -0.1364583329919154264, 0.7879004041258500513 ) ) ;
#136891=CARTESIAN_POINT ( 'NONE',  ( -5.280010757518168063, 8.247430752824802980, -1.199719254218446718 ) ) ;
#136892=CARTESIAN_POINT ( 'NONE',  ( 6.740374924288304648, 11.01552117831172062, 1.040834085586084257E-14 ) ) ;
#136894=CARTESIAN_POINT ( 'NONE',  ( 4.493637847925535667, 7.329995691633395261, -1.199719254218452047 ) ) ;
#136896=CARTESIAN_POINT ( 'NONE',  ( 1.499999999999989120, 3.275000000000020783, 1.214306433183764966E-14 ) ) ;
#136898=CARTESIAN_POINT ( 'NONE',  ( 1.364683531249988535, 1.676041667008085101, 0.7879004041258500513 ) ) ;
#136905=CARTESIAN_POINT ( 'NONE',  ( 4.500943810056890371, 8.194925511800951412, -0.7216878364870207285 ) ) ;
#136908=CARTESIAN_POINT ( 'NONE',  ( -9.040589502214116280, 9.441775928871617651, 0.7998128361456462443 ) ) ;
#136909=CARTESIAN_POINT ( 'NONE',  ( -3.632695093457760649, 6.325562478087638496, -1.199719254218452047 ) ) ;
#136911=CARTESIAN_POINT ( 'NONE',  ( 1.499999999999990674, 8.226407212580419070, 3.114167208185194990 ) ) ;
#136913=CARTESIAN_POINT ( 'NONE',  ( 8.499999999999980460, 6.216000000000041048, 2.921333333333346882 ) ) ;
#136914=CARTESIAN_POINT ( 'NONE',  ( -7.659993601596710278, 10.92011438762942355, -1.082531754730543083 ) ) ;
#136916=CARTESIAN_POINT ( 'NONE',  ( -1.499999999999997780, 5.650000000000023448, 1.214306433183764966E-14 ) ) ;
#136920=CARTESIAN_POINT ( 'NONE',  ( 8.839552966430002101, 11.33589776563360019, -1.443375672974052559 ) ) ;
#136927=CARTESIAN_POINT ( 'NONE',  ( -1.468321960012591409, 7.242494692102439124, -4.289992922803198994 ) ) ;
#136929=CARTESIAN_POINT ( 'NONE',  ( 8.365017589507326434, 12.70301158782650397, -0.7216878364870338292 ) ) ;
#136931=ADVANCED_FACE ( 'NONE', ( #121087 ), #802, .F. ) ;
#136935=CARTESIAN_POINT ( 'NONE',  ( 7.578644679914706472, 9.864838098032418401, 1.443375672974076540 ) ) ;
#136937=CARTESIAN_POINT ( 'NONE',  ( 7.070740804726770357, 8.207951346058097286, 1.199719254218462483 ) ) ;
#136938=CARTESIAN_POINT ( 'NONE',  ( -6.579784621333750749, 6.570836901177822931, 0.7998128361456341429 ) ) ;
#136942=ADVANCED_FACE ( 'NONE', ( #104765 ), #133015, .F. ) ;
#136944=CARTESIAN_POINT ( 'NONE',  ( 2.873965376416980355, 6.296784005887697155, -0.7216878364870267237 ) ) ;
#136946=CARTESIAN_POINT ( 'NONE',  ( -2.839543107058306592, 5.400218493954923815, -1.199719254218446718 ) ) ;
#136958=VERTEX_POINT ( 'NONE', #1879 ) ;
#136961=CARTESIAN_POINT ( 'NONE',  ( 8.555358625423188812, 9.940005470203933768, 1.199719254218462483 ) ) ;
#136970=CARTESIAN_POINT ( 'NONE',  ( -0.2766633939784177154, 6.383776174518168034, 3.145034899357514124 ) ) ;
#136972=CARTESIAN_POINT ( 'NONE',  ( -4.574986769607567894, 7.424902766929059261, 1.199719254218464037 ) ) ;
#136973=AXIS2_PLACEMENT_3D ( 'NONE', #155775, #139540, #26826 ) ;
#136975=CARTESIAN_POINT ( 'NONE',  ( -5.440899717785814715, 5.242137847038546461, 0.7998128361456341429 ) ) ;
#136979=CARTESIAN_POINT ( 'NONE',  ( -5.426287360647527258, 6.306760859481674864, -1.047964138152550406 ) ) ;
#136984=CARTESIAN_POINT ( 'NONE',  ( -4.223528545856940042, 4.886203710709899006, -1.199719254218446718 ) ) ;
#136987=CARTESIAN_POINT ( 'NONE',  ( 7.558834334818744338, 8.777393797832065303, 1.199719254218462483 ) ) ;
#136988=CARTESIAN_POINT ( 'NONE',  ( -1.201851678989727383E-14, 4.696875000341419693, -1.575800808251660134 ) ) ;
#136994=CARTESIAN_POINT ( 'NONE',  ( 6.168596704093459060, 7.259412911939593371, -1.082531754730543083 ) ) ;
#136995=CARTESIAN_POINT ( 'NONE',  ( -7.914208982075130905, 10.25632978388623684, -1.599625672291263179 ) ) ;
#136998=CARTESIAN_POINT ( 'NONE',  ( -6.645467848992654858, 10.90479625713344625, 0.7998128361456481317 ) ) ;
#136999=CARTESIAN_POINT ( 'NONE',  ( -4.924636110261798372, 6.768494766770632332, 1.599625672291267398 ) ) ;
#137004=EDGE_CURVE ( 'NONE', #155662, #93347, #23474, .T. ) ;
#137007=CARTESIAN_POINT ( 'NONE',  ( 5.777746017718023097, 9.892454120646377191, 0.7998128361456462443 ) ) ;
#137008=CARTESIAN_POINT ( 'NONE',  ( 3.469446951953614189E-15, 8.900000000000025224, 1.214306433183764966E-14 ) ) ;
#137019=EDGE_LOOP ( 'NONE', ( #120760, #52173, #161004, #110250 ) ) ;
#137021=CARTESIAN_POINT ( 'NONE',  ( -0.7499999999999972244, 5.858333333333353821, -1.299038105676652011 ) ) ;
#137022=CARTESIAN_POINT ( 'NONE',  ( 5.183294799126148433, 4.941598775268944976, 1.040834085586084257E-14 ) ) ;
#137023=CARTESIAN_POINT ( 'NONE',  ( 6.844168616800228477, 6.879284895888727824, -0.7998128361456281477 ) ) ;
#137025=CARTESIAN_POINT ( 'NONE',  ( -8.568389894156720032, 10.05917163368005163, 1.082531754730558626 ) ) ;
#137026=CARTESIAN_POINT ( 'NONE',  ( 5.450014563013511726, 8.341805509282339770, -1.082531754730543083 ) ) ;
#137028=CARTESIAN_POINT ( 'NONE',  ( -8.527715432871366019, 10.01171809551380143, 1.082531754730558626 ) ) ;
#137032=CARTESIAN_POINT ( 'NONE',  ( 8.423693512792301163, 8.722063941212843119, 0.7998128361456481317 ) ) ;
#137037=CARTESIAN_POINT ( 'NONE',  ( 1.364683531249988535, 2.113541667008087099, 0.7879004041258500513 ) ) ;
#137044=CARTESIAN_POINT ( 'NONE',  ( 7.397945374551106568, 11.78268670361832093, -0.7998128361456291469 ) ) ;
#137048=CARTESIAN_POINT ( 'NONE',  ( -7.994504133552415404, 12.47867192245318435, -0.7998128361456281477 ) ) ;
#137052=CARTESIAN_POINT ( 'NONE',  ( 1.387358672525637715, 7.251968950354889643, -4.302625267139783993 ) ) ;
#137054=CARTESIAN_POINT ( 'NONE',  ( 4.701980345841006326, 4.380065246436280368, 0.7998128361456341429 ) ) ;
#137058=CARTESIAN_POINT ( 'NONE',  ( -8.642432853707342488, 12.17025653171218558, 1.199719254218462483 ) ) ;
#137063=CARTESIAN_POINT ( 'NONE',  ( 5.891030527642284298, 5.977876296848656956, -0.06656325335930267373 ) ) ;
#137065=CARTESIAN_POINT ( 'NONE',  ( -5.576481253922474401, 5.400316305864651056, -0.7998128361456221525 ) ) ;
#137069=CARTESIAN_POINT ( 'NONE',  ( 6.588372581236919601, 9.773852880496709972, -1.199719254218440723 ) ) ;
#137071=CARTESIAN_POINT ( 'NONE',  ( 4.964256800898067645, 8.943383367689749619, 0.7998128361456462443 ) ) ;
#137072=CARTESIAN_POINT ( 'NONE',  ( 3.499976210622149253, 7.235056012367825140, 0.7998128361456321445 ) ) ;
#137074=CARTESIAN_POINT ( 'NONE',  ( -9.341204650135658483, 10.00041963468749984, 1.040834085586084257E-14 ) ) ;
#137082=CARTESIAN_POINT ( 'NONE',  ( -4.822091459260241741, 6.758233420496813082, -1.248138317850192580 ) ) ;
#137085=CARTESIAN_POINT ( 'NONE',  ( 5.666945020832177882, 6.674152614801420746, 1.082531754730558626 ) ) ;
#137108=CARTESIAN_POINT ( 'NONE',  ( 6.421758314367153275, 10.64380180007036891, -0.7998128361456291469 ) ) ;
#137112=CARTESIAN_POINT ( 'NONE',  ( 1.499999999999989120, 1.556250000682817047, 0.000000000000000000 ) ) ;
#137113=CARTESIAN_POINT ( 'NONE',  ( -2.785310492603665367, 5.336947110424484109, 1.199719254218462483 ) ) ;
#137114=CARTESIAN_POINT ( 'NONE',  ( -5.422371370461663176, 8.413518134592214537, -1.199719254218446718 ) ) ;
#137117=CARTESIAN_POINT ( 'NONE',  ( -10.13202086811422475, 10.71511252242175161, -0.7998128361456291469 ) ) ;
#137120=CARTESIAN_POINT ( 'NONE',  ( 5.452350330990040739, 9.512825819463730070, 0.7998128361456462443 ) ) ;
#137123=CARTESIAN_POINT ( 'NONE',  ( -6.958359152311683893, 9.141171649162195934, -1.599625672291263179 ) ) ;
#137125=CARTESIAN_POINT ( 'NONE',  ( 9.284636267260101050, 9.726497154758602548, -0.7998128361456281477 ) ) ;
#137132=CARTESIAN_POINT ( 'NONE',  ( -7.158341918335454857, 10.33485409049125003, 1.082531754730549967 ) ) ;
#137137=CARTESIAN_POINT ( 'NONE',  ( 1.364683531249988535, 4.426041667008082214, 0.7879004041258500513 ) ) ;
#137144=CARTESIAN_POINT ( 'NONE',  ( -1.201851678989727383E-14, 5.196875000341422357, -1.575800808251660134 ) ) ;
#137146=CARTESIAN_POINT ( 'NONE',  ( -4.907688418022547516, 4.827984030555475314, 1.214306433183764966E-14 ) ) ;
#137148=CARTESIAN_POINT ( 'NONE',  ( 4.677199806590210507, 4.559080650551097236, -0.7216878364870197293 ) ) ;
#137149=CARTESIAN_POINT ( 'NONE',  ( 1.364683531249988535, 5.467708333674750953, -0.7879004041258300672 ) ) ;
#137150=CARTESIAN_POINT ( 'NONE',  ( -9.992522908471816123, 11.61669713376064372, 1.199719254218462483 ) ) ;
#137155=CARTESIAN_POINT ( 'NONE',  ( 0.6823417656249899377, 1.092708333674752286, 1.181850606188755259 ) ) ;
#137157=CARTESIAN_POINT ( 'NONE',  ( -3.958617665510283601, 4.681104033592509595, -1.082531754730549967 ) ) ;
#137158=CARTESIAN_POINT ( 'NONE',  ( 5.281064527722868718, 6.119995689553514140, 1.199719254218462483 ) ) ;
#137168=CARTESIAN_POINT ( 'NONE',  ( -7.049876689426097798, 11.16868053773170821, -0.7216878364870267237 ) ) ;
#137173=CARTESIAN_POINT ( 'NONE',  ( -7.811469059767924605, 12.26513100303794168, -0.7998128361456281477 ) ) ;
#137174=CARTESIAN_POINT ( 'NONE',  ( -4.067082893975237035, 7.688754443039000464, 1.040834085586084257E-14 ) ) ;
#137175=CARTESIAN_POINT ( 'NONE',  ( -1.364683531250012516, 2.551041667008089320, -0.7879004041258289570 ) ) ;
#137176=CARTESIAN_POINT ( 'NONE',  ( 1.499999999999990896, 4.525000000000021672, 1.214306433183764966E-14 ) ) ;
#137181=( BOUNDED_CURVE ( )  B_SPLINE_CURVE ( 2, ( #189644, #10879, #109547 ),
 .UNSPECIFIED., .F., .T. ) 
 B_SPLINE_CURVE_WITH_KNOTS ( ( 3, 3 ),
 ( 0.1229783203405390019, 0.1249999999999998751 ),
 .UNSPECIFIED. ) 
 CURVE ( )  GEOMETRIC_REPRESENTATION_ITEM ( )  RATIONAL_B_SPLINE_CURVE ( ( 0.9330713687540070911, 0.9349951081471596925, 0.9999999999999960032 ) ) 
 REPRESENTATION_ITEM ( '' )  );
#137183=CARTESIAN_POINT ( 'NONE',  ( 9.049177462117294013, 12.64479190819049670, -1.199719254218446718 ) ) ;
#137193=ORIENTED_EDGE ( 'NONE', *, *, #125522, .F. ) ;
#137201=CARTESIAN_POINT ( 'NONE',  ( -1.201851678989727383E-14, 2.884375000341418804, 1.575800808251672791 ) ) ;
#137205=ADVANCED_FACE ( 'NONE', ( #115219 ), #111222, .F. ) ;
#137212=CARTESIAN_POINT ( 'NONE',  ( -1.402160292154681736E-14, 0.6968750003414164729, -1.575800808251659024 ) ) ;
#137222=ORIENTED_EDGE ( 'NONE', *, *, #166535, .T. ) ;
#137224=CARTESIAN_POINT ( 'NONE',  ( 4.680589345215795838, 6.483773540883647435, -1.599625672291256295 ) ) ;
#137230=CARTESIAN_POINT ( 'NONE',  ( 7.958799866421889746, 9.244020251369077457, -1.199719254218441611 ) ) ;
#137233=CARTESIAN_POINT ( 'NONE',  ( -3.327636637150278798, 5.969660945728899826, -1.199719254218452935 ) ) ;
#137234=CARTESIAN_POINT ( 'NONE',  ( 7.313733799568044702, 10.62010763521636214, 1.199719254218460707 ) ) ;
#137246=CARTESIAN_POINT ( 'NONE',  ( -8.215877900201387973, 8.687538426430837291, 0.7216878364870578100 ) ) ;
#137247=AXIS2_PLACEMENT_3D ( 'NONE', #92580, #26470, #139172 ) ;
#137251=CARTESIAN_POINT ( 'NONE',  ( -8.459397779922852578, 11.95671561229694824, 1.199719254218453823 ) ) ;
#137256=CARTESIAN_POINT ( 'NONE',  ( -3.755772246185468788, 4.340488027759846545, -1.199719254218452047 ) ) ;
#137258=CARTESIAN_POINT ( 'NONE',  ( 10.07100917685271035, 10.64393221595000938, 0.7998128361456462443 ) ) ;
#137259=CARTESIAN_POINT ( 'NONE',  ( 4.704842999142070603, 5.447737239542574272, -1.199719254218452047 ) ) ;
#137265=CARTESIAN_POINT ( 'NONE',  ( 3.172244755917638770, 5.684407401003788607, -1.082531754730543083 ) ) ;
#137267=CARTESIAN_POINT ( 'NONE',  ( -3.741160322367112379, 6.452105245148518797, 1.199719254218464037 ) ) ;
#137270=CARTESIAN_POINT ( 'NONE',  ( -9.996439331977562404, 10.55693406359564790, 0.7998128361456462443 ) ) ;
#137276=CARTESIAN_POINT ( 'NONE',  ( 6.968527767744088663, 11.07377346243604599, 0.7216878364870438212 ) ) ;
#137277=CARTESIAN_POINT ( 'NONE',  ( -1.364683531250010740, 4.592708333674755394, 0.7879004041258379498 ) ) ;
#137279=CARTESIAN_POINT ( 'NONE',  ( 4.009460741339333723, 5.700790169694431420, -1.599625672291256295 ) ) ;
#137291=CARTESIAN_POINT ( 'NONE',  ( 5.847644326195775122, 5.716673223516857583, -0.7998128361456282587 ) ) ;
#137294=CARTESIAN_POINT ( 'NONE',  ( -1.364683531250012516, 3.301041667008084879, -0.7879004041258289570 ) ) ;
#137296=CARTESIAN_POINT ( 'NONE',  ( 9.028840231696797503, 12.62106513936658203, -1.199719254218446718 ) ) ;
#137299=CARTESIAN_POINT ( 'NONE',  ( -5.910991785878183080, 5.998504626387068051, -0.7216878364870278340 ) ) ;
#137301=CARTESIAN_POINT ( 'NONE',  ( -4.677199806590235376, 7.440188293455128665, 1.082531754730560403 ) ) ;
#137305=CARTESIAN_POINT ( 'NONE',  ( 5.823390672269506574, 6.752709524857930745, -1.199719254218446718 ) ) ;
#137315=CARTESIAN_POINT ( 'NONE',  ( 4.632082037363250748, 8.555846143565791095, -0.7998128361456231517 ) ) ;
#137319=CARTESIAN_POINT ( 'NONE',  ( -7.061099074618889304, 7.132370430010492868, -0.7998128361456291469 ) ) ;
#137323=CARTESIAN_POINT ( 'NONE',  ( 6.076025397218672630, 10.24044673006381245, -0.7998128361456291469 ) ) ;
#137326=CARTESIAN_POINT ( 'NONE',  ( -5.215082642750900277, 9.236013516518044142, 0.000000000000000000 ) ) ;
#137327=CARTESIAN_POINT ( 'NONE',  ( 5.761852095683461350, 9.665985178365305686, -0.7216878364870267237 ) ) ;
#137328=CARTESIAN_POINT ( 'NONE',  ( 4.363209728991265024, 7.389406413240373617, 1.150570763150955633 ) ) ;
#137330=CARTESIAN_POINT ( 'NONE',  ( -3.913499895838973508, 7.717500311787445000, 1.040834085586084257E-14 ) ) ;
#137333=CARTESIAN_POINT ( 'NONE',  ( -5.065942953000576843, 9.062017211809330064, -0.7998128361456231517 ) ) ;
#137336=CARTESIAN_POINT ( 'NONE',  ( 1.364683531249988535, 2.363541667008088432, 0.7879004041258500513 ) ) ;
#137338=CARTESIAN_POINT ( 'NONE',  ( -5.938108093105513241, 6.030140318152288792, 0.7216878364870317197 ) ) ;
#137344=CARTESIAN_POINT ( 'NONE',  ( 4.984594031318565932, 8.967110136513669616, 0.7998128361456462443 ) ) ;
#137346=CARTESIAN_POINT ( 'NONE',  ( -5.672026259827416261, 6.146810915570031675, 0.7861540255039052294 ) ) ;
#137347=CARTESIAN_POINT ( 'NONE',  ( -1.201851678989727383E-14, 1.384375000341419693, 1.575800808251672791 ) ) ;
#137350=EDGE_CURVE ( 'NONE', #42278, #85030, #67731, .T. ) ;
#137351=CARTESIAN_POINT ( 'NONE',  ( -0.1638468497727919582, 7.035416012003069319, 1.994423973928958205 ) ) ;
#137355=CARTESIAN_POINT ( 'NONE',  ( -5.298539104842322267, 5.076050465271134016, 0.7998128361456341429 ) ) ;
#137356=CARTESIAN_POINT ( 'NONE',  ( -6.358410854684777291, 10.36197039720016022, -0.7216878364870267237 ) ) ;
#137364=CARTESIAN_POINT ( 'NONE',  ( -7.822691444960709006, 10.14955932391940330, -1.443375672974058777 ) ) ;
#137368=CARTESIAN_POINT ( 'NONE',  ( -6.507550544435101614, 10.53596670190887963, 0.000000000000000000 ) ) ;
#137371=VERTEX_POINT ( 'NONE', #159901 ) ;
#137382=CARTESIAN_POINT ( 'NONE',  ( -4.381256195510448315, 8.263215994737505454, 1.040834085586084257E-14 ) ) ;
#137385=CARTESIAN_POINT ( 'NONE',  ( 4.359110081993588182, 5.044382169536003602, -1.199719254218452047 ) ) ;
#137387=CARTESIAN_POINT ( 'NONE',  ( 4.888966637111398228, 4.912082840724287358, 0.6391686513922645307 ) ) ;
#137389=CARTESIAN_POINT ( 'NONE',  ( 5.307127064745490230, 8.279066444590018392, -1.199719254218452935 ) ) ;
#137393=CARTESIAN_POINT ( 'NONE',  ( -3.294268138440636928, 6.787137228248626641, 1.040834085586084257E-14 ) ) ;
#137401=CARTESIAN_POINT ( 'NONE',  ( -1.402160292154681736E-14, 0.5718750003414239114, 1.575800808251672791 ) ) ;
#137402=CARTESIAN_POINT ( 'NONE',  ( -8.962103233833181193, 10.41454084668224489, -1.199719254218446718 ) ) ;
#137404=CARTESIAN_POINT ( 'NONE',  ( 8.782984583554449998, 9.141236857102018831, 1.040834085586084257E-14 ) ) ;
#137406=CARTESIAN_POINT ( 'NONE',  ( -6.852756576703439961, 10.08230087520760954, 1.199719254218453823 ) ) ;
#137409=CARTESIAN_POINT ( 'NONE',  ( -1.001543065824772872E-14, 4.571875000341418804, 1.575800808251672791 ) ) ;
#137411=CARTESIAN_POINT ( 'NONE',  ( 8.432808358020004391, 12.78210081775797669, 0.7216878364870438212 ) ) ;
#137415=CARTESIAN_POINT ( 'NONE',  ( -1.402160292154681736E-14, -0.9906249996585834161, -1.575800808251665908 ) ) ;
#137418=CARTESIAN_POINT ( 'NONE',  ( 7.741342523278698096, 10.05465224862374285, 1.443375672974076540 ) ) ;
#137421=CARTESIAN_POINT ( 'NONE',  ( -5.205967797967562483, 8.057084283395347768, 1.082531754730548412 ) ) ;
#137423=CARTESIAN_POINT ( 'NONE',  ( 1.364683531249988535, 2.905208333674754506, -0.7879004041258239610 ) ) ;
#137427=CARTESIAN_POINT ( 'NONE',  ( -7.040761844198392794, 7.108643661186573759, -0.7998128361456291469 ) ) ;
#137429=CARTESIAN_POINT ( 'NONE',  ( 0.6823417656249899377, 5.738541667008087543, -1.181850606188754593 ) ) ;
#137435=CIRCLE ( 'NONE', #210070, 0.7500000000000011102 ) ;
#137437=CARTESIAN_POINT ( 'NONE',  ( 7.072549687823125097, 11.40305840243567381, -0.7998128361456291469 ) ) ;
#137440=CARTESIAN_POINT ( 'NONE',  ( -0.7500000000000215383, 2.191666666666689078, 1.299038105676671107 ) ) ;
#137446=CARTESIAN_POINT ( 'NONE',  ( 6.317736394288140822, 7.433409217166723870, 1.082531754730558626 ) ) ;
#137448=CARTESIAN_POINT ( 'NONE',  ( -1.402160292154681736E-14, -0.2406249996585799189, -1.575800808251665908 ) ) ;
#137450=CARTESIAN_POINT ( 'NONE',  ( 2.354312230267378236, 5.898448035287240820, -0.7998128361456281477 ) ) ;
#137456=CARTESIAN_POINT ( 'NONE',  ( 1.499999999999987121, 0.5041666666666856367, 0.8660254037844524744 ) ) ;
#137457=CARTESIAN_POINT ( 'NONE',  ( 7.182068686937156166, 9.402166106225269715, 1.599625672291281386 ) ) ;
#137458=CARTESIAN_POINT ( 'NONE',  ( -7.994504133552415404, 12.47867192245318435, -0.7998128361456281477 ) ) ;
#137461=CARTESIAN_POINT ( 'NONE',  ( -0.6823417656250246877, 0.3010416670080895418, 1.181850606188755259 ) ) ;
#137462=CARTESIAN_POINT ( 'NONE',  ( 0.7499999999999885647, 1.316666666666688190, -1.299038105676652899 ) ) ;
#137464=CARTESIAN_POINT ( 'NONE',  ( 4.822949958159288286, 6.649860922651058992, -1.599625672291256295 ) ) ;
#137465=EDGE_CURVE ( 'NONE', #86628, #148246, #157572, .T. ) ;
#137471=CARTESIAN_POINT ( 'NONE',  ( -1.364683531250010295, 5.238541667008086655, -0.7879004041258300672 ) ) ;
#137473=CARTESIAN_POINT ( 'NONE',  ( -7.635213062790267458, 12.05949900656400686, 0.000000000000000000 ) ) ;
#137474=CARTESIAN_POINT ( 'NONE',  ( -6.426201623197489887, 6.599582769926260362, 0.7216878364870317197 ) ) ;
#137482=CARTESIAN_POINT ( 'NONE',  ( 6.076025397218672630, 10.24044673006381245, -0.7998128361456291469 ) ) ;
#137484=CARTESIAN_POINT ( 'NONE',  ( 5.802526556524483681, 5.871961858807763335, 1.040834085586084257E-14 ) ) ;
#137486=CARTESIAN_POINT ( 'NONE',  ( 6.819388077549422889, 8.018669514304889390, -1.082531754730543971 ) ) ;
#137489=CARTESIAN_POINT ( 'NONE',  ( -7.965578943228732278, 9.251929174310385307, -1.199719254218446718 ) ) ;
#137490=CARTESIAN_POINT ( 'NONE',  ( 4.645640190976921602, 8.571663989448405019, 1.040834085586084257E-14 ) ) ;
#137492=CARTESIAN_POINT ( 'NONE',  ( 0.000000000000000000, 8.600000000000017408, -0.3999999999999819811 ) ) ;
#137493=CARTESIAN_POINT ( 'NONE',  ( 3.358669367883368118, 4.941533567329135401, -1.599625672291262513 ) ) ;
#137494=ORIENTED_EDGE ( 'NONE', *, *, #58928, .F. ) ;
#137499=CARTESIAN_POINT ( 'NONE',  ( -6.073689629242176480, 6.188318776978391611, -0.7216878364870278340 ) ) ;
#137500=CARTESIAN_POINT ( 'NONE',  ( 10.08690309888728187, 10.87040115823107911, -0.7216878364870257245 ) ) ;
#137503=CARTESIAN_POINT ( 'NONE',  ( -6.073162743917628781, 9.172774736957510555, -1.199719254218440723 ) ) ;
#137508=CARTESIAN_POINT ( 'NONE',  ( -7.751511138711140170, 10.06651563329490529, -1.599625672291263179 ) ) ;
#137526=CARTESIAN_POINT ( 'NONE',  ( -7.369020184227459858, 8.555943955475521889, 1.199719254218450271 ) ) ;
#137529=CARTESIAN_POINT ( 'NONE',  ( 5.883875478650832491, 6.927238148923188454, -1.082531754730543083 ) ) ;
#137533=CARTESIAN_POINT ( 'NONE',  ( -4.076197739202962467, 7.907314462378773001, 1.040834085586084257E-14 ) ) ;
#137538=CARTESIAN_POINT ( 'NONE',  ( -5.208303565944065738, 9.228104593576741621, -0.7998128361456231517 ) ) ;
#137544=CARTESIAN_POINT ( 'NONE',  ( -8.045874094706015001, 11.47427131287732927, -1.199719254218446718 ) ) ;
#137545=CARTESIAN_POINT ( 'NONE',  ( 7.935599982700328958, 8.152621489438862667, 0.7998128361456481317 ) ) ;
#137548=CARTESIAN_POINT ( 'NONE',  ( -8.676328237741483207, 12.20980114641871062, -1.199719254218446718 ) ) ;
#137552=CARTESIAN_POINT ( 'NONE',  ( 1.364683531249988757, -0.8031249996585804185, 0.000000000000000000 ) ) ;
#137556=CARTESIAN_POINT ( 'NONE',  ( 9.571693261567961741, 11.22969222899322617, 1.082531754730548412 ) ) ;
#137563=CARTESIAN_POINT ( 'NONE',  ( -5.576221682296247373, 6.207884856865704570, -0.9076712001952822462 ) ) ;
#137565=CARTESIAN_POINT ( 'NONE',  ( -0.4573399425327669965, 6.471653648908428202, -3.262204865211126403 ) ) ;
#137576=CARTESIAN_POINT ( 'NONE',  ( -3.110706179331648169, 5.716575411607132118, 1.199719254218462483 ) ) ;
#137579=CARTESIAN_POINT ( 'NONE',  ( -2.123823618835070537, 5.629544655282869847, 1.040834085586084257E-14 ) ) ;
#137584=CARTESIAN_POINT ( 'NONE',  ( -1.364683531250010295, 5.738541667008088432, -0.7879004041258300672 ) ) ;
#137588=CARTESIAN_POINT ( 'NONE',  ( 2.876381804795541619, 6.437993120328354024, 0.3511878651327338674 ) ) ;
#137589=VERTEX_POINT ( 'NONE', #61338 ) ;
#137591=CARTESIAN_POINT ( 'NONE',  ( 2.191614386903386613, 5.708633884695917260, -0.7998128361456281477 ) ) ;
#137593=LINE ( 'NONE', #122490, #59568 ) ;
#137598=CARTESIAN_POINT ( 'NONE',  ( 4.690231075323689325, 7.559354456931247412, 1.199719254218462483 ) ) ;
#137599=CARTESIAN_POINT ( 'NONE',  ( 1.364683531249988757, 2.446875000341415696, 1.214306433183764966E-14 ) ) ;
#137600=CARTESIAN_POINT ( 'NONE',  ( -4.932365459154965492, 6.668011768565191844, 1.248136097290372337 ) ) ;
#137601=CARTESIAN_POINT ( 'NONE',  ( 10.05353459973327368, 11.68787744023238417, -1.199719254218440723 ) ) ;
#137603=CARTESIAN_POINT ( 'NONE',  ( -7.635213062790267458, 12.05949900656400686, 0.000000000000000000 ) ) ;
#137604=CARTESIAN_POINT ( 'NONE',  ( -5.409340101728186134, 5.413244328212063472, 0.7216878364870317197 ) ) ;
#137607=CARTESIAN_POINT ( 'NONE',  ( -5.717788096661253761, 7.693838750903348789, 1.599625672291269396 ) ) ;
#137609=CARTESIAN_POINT ( 'NONE',  ( 0.6823417656249899377, 5.426041667008087543, -1.181850606188754593 ) ) ;
#137617=CARTESIAN_POINT ( 'NONE',  ( -4.812781342726871969, 6.637997537979888563, 1.443375672974064550 ) ) ;
#137619=EDGE_CURVE ( 'NONE', #17249, #12495, #140271, .T. ) ;
#137622=CARTESIAN_POINT ( 'NONE',  ( -3.416291520519271874, 6.929497840673697340, 1.040834085586084257E-14 ) ) ;
#137624=CARTESIAN_POINT ( 'NONE',  ( 9.260382613333817403, 10.76253345609967660, -1.199719254218446718 ) ) ;
#137630=ORIENTED_EDGE ( 'NONE', *, *, #132078, .F. ) ;
#137634=CARTESIAN_POINT ( 'NONE',  ( -8.462260433223891098, 13.02438760540324481, -0.7998128361456281477 ) ) ;
#137639=CARTESIAN_POINT ( 'NONE',  ( 7.006866460164219212, 7.069099046480051385, -0.7998128361456281477 ) ) ;
#137644=CARTESIAN_POINT ( 'NONE',  ( 2.920892028740289081, 5.495125569250587816, 1.199719254218452047 ) ) ;
#137654=CARTESIAN_POINT ( 'NONE',  ( 8.341290820905593151, 10.75459192918846618, 1.599625672291281386 ) ) ;
#137656=CARTESIAN_POINT ( 'NONE',  ( -4.900382456335551140, 7.804531068111707270, 1.199719254218464037 ) ) ;
#137661=CARTESIAN_POINT ( 'NONE',  ( 0.6823417656249899377, 4.926041667008086655, -1.181850606188754593 ) ) ;
#137666=CARTESIAN_POINT ( 'NONE',  ( 5.203632029546647608, 4.965325544092860532, 1.040834085586084257E-14 ) ) ;
#137667=CARTESIAN_POINT ( 'NONE',  ( -4.517891501851816649, 6.293959390292322986, -1.599625672291256295 ) ) ;
#137673=CARTESIAN_POINT ( 'NONE',  ( 6.182154858151487353, 6.314861544039274577, -0.7216878364870257245 ) ) ;
#137676=CARTESIAN_POINT ( 'NONE',  ( 8.405692050348340771, 8.908988268268968724, 1.040834085586084257E-14 ) ) ;
#137677=CARTESIAN_POINT ( 'NONE',  ( 1.364683531249988535, 3.967708333674751842, -0.7879004041258239610 ) ) ;
#137679=CARTESIAN_POINT ( 'NONE',  ( 3.646780131951580461, 7.198401220678078971, -0.7216878364870267237 ) ) ;
#137686=CARTESIAN_POINT ( 'NONE',  ( -5.029856876702963220, 6.770753873564038017, 1.447965164949674310 ) ) ;
#137693=CARTESIAN_POINT ( 'NONE',  ( -10.66756793585402363, 11.33991743478486391, 0.7998128361456462443 ) ) ;
#137701=VERTEX_POINT ( 'NONE', #64538 ) ;
#137703=CARTESIAN_POINT ( 'NONE',  ( 2.575685996916329046, 5.948791396470269888, 0.7216878364870438212 ) ) ;
#137704=CARTESIAN_POINT ( 'NONE',  ( -1.201851678989727383E-14, 2.884375000341418804, 1.575800808251672791 ) ) ;
#137706=CARTESIAN_POINT ( 'NONE',  ( 7.100719765255169236, 9.307259030929609267, -1.599625672291262513 ) ) ;
#137707=CARTESIAN_POINT ( 'NONE',  ( -10.49131193887636826, 11.13428543831092909, 1.040834085586084257E-14 ) ) ;
#137709=CARTESIAN_POINT ( 'NONE',  ( -3.903858165731105778, 6.641919395739846799, 1.199719254218464037 ) ) ;
#137713=ORIENTED_EDGE ( 'NONE', *, *, #57944, .F. ) ;
#137715=CARTESIAN_POINT ( 'NONE',  ( 1.499999999999989120, 4.754166666666689522, 0.8660254037844524744 ) ) ;
#137716=CARTESIAN_POINT ( 'NONE',  ( 3.988069740714122791, 7.804498464141805592, 0.7998128361456321445 ) ) ;
#137719=CARTESIAN_POINT ( 'NONE',  ( -1.201851678989727383E-14, 2.884375000341418804, 1.575800808251672791 ) ) ;
#137720=EDGE_CURVE ( 'NONE', #207748, #69931, #89945, .T. ) ;
#137721=CARTESIAN_POINT ( 'NONE',  ( 1.364683531249988535, 3.905208333674751842, -0.7879004041258239610 ) ) ;
#137724=CARTESIAN_POINT ( 'NONE',  ( 7.768458830950378591, 12.00702636951006497, 1.040834085586084257E-14 ) ) ;
#137729=CARTESIAN_POINT ( 'NONE',  ( 0.7499999999999885647, 2.347916667349486453, -1.299038105676652899 ) ) ;
#137731=CARTESIAN_POINT ( 'NONE',  ( -4.706651882238427120, 8.642844295920152575, 1.040834085586084257E-14 ) ) ;
#137732=EDGE_CURVE ( 'NONE', #55162, #146442, #102748, .T. ) ;
#137733=CARTESIAN_POINT ( 'NONE',  ( 4.487385655998878953, 6.258369236797239665, 1.443375672974062551 ) ) ;
#137742=CARTESIAN_POINT ( 'NONE',  ( 6.446011968293428041, 9.607765498729298415, -1.199719254218440723 ) ) ;
#137743=CARTESIAN_POINT ( 'NONE',  ( 4.904298879841284098, 6.744767997946721216, 1.599625672291267398 ) ) ;
#137744=PLANE ( 'NONE',  #95565 ) ;
#137746=CYLINDRICAL_SURFACE ( 'NONE', #53621, 1.000000000000000000 ) ;
#137747=CARTESIAN_POINT ( 'NONE',  ( 5.138703914779377158, 5.953908307786102583, 1.199719254218462483 ) ) ;
#137748=CARTESIAN_POINT ( 'NONE',  ( 3.673896439623286714, 4.156855427197417185, -0.9999999999999940048 ) ) ;
#137749=EDGE_LOOP ( 'NONE', ( #150693, #35954, #103921, #122679, #139295, #134336, #190793, #94344, #176626 ) ) ;
#137751=ORIENTED_EDGE ( 'NONE', *, *, #198196, .T. ) ;
#137754=CARTESIAN_POINT ( 'NONE',  ( 7.865701674222579598, 12.32840238656838139, -0.7998128361456352531 ) ) ;
#137758=CARTESIAN_POINT ( 'NONE',  ( 5.102592784488711786, 6.504070869828495027, 1.211835919174956366 ) ) ;
#137765=EDGE_CURVE ( 'NONE', #73840, #171296, #178291, .T. ) ;
#137766=CARTESIAN_POINT ( 'NONE',  ( -1.084637062511556005, 3.182371192708035146, 1.105835307554803082 ) ) ;
#137768=CARTESIAN_POINT ( 'NONE',  ( 7.836249599018724865, 9.205007956019091608, -1.082531754730537976 ) ) ;
#137769=CARTESIAN_POINT ( 'NONE',  ( -2.591579918506545344, 6.175260338232929413, 1.040834085586084257E-14 ) ) ;
#137774=CARTESIAN_POINT ( 'NONE',  ( -3.879604511804807032, 7.677955697080923514, 0.7998128361456341429 ) ) ;
#137776=CARTESIAN_POINT ( 'NONE',  ( -5.951324661304366437, 4.742844146919000359, 2.438848701836275001 ) ) ;
#137786=CARTESIAN_POINT ( 'NONE',  ( 8.561083932025322696, 12.07534945641652158, -1.199719254218446718 ) ) ;
#137795=CARTESIAN_POINT ( 'NONE',  ( -8.351459436338023679, 12.68719374246231624, -0.7216878364870267237 ) ) ;
#137797=CARTESIAN_POINT ( 'NONE',  ( 3.880185816268708177, 5.955652630921238533, -1.265242915204408458 ) ) ;
#137799=CARTESIAN_POINT ( 'NONE',  ( 7.391166297744269365, 11.77477778067701664, 1.040834085586084257E-14 ) ) ;
#137801=CARTESIAN_POINT ( 'NONE',  ( 1.145901822213557075, 2.800000000000024247, 0.9291478600312689240 ) ) ;
#137804=CARTESIAN_POINT ( 'NONE',  ( -7.074657228232555717, 7.148188275893099686, 1.040834085586084257E-14 ) ) ;
#137805=CARTESIAN_POINT ( 'NONE',  ( 4.792970997630896512, 5.550553237779539018, 1.199719254218464037 ) ) ;
#137808=CARTESIAN_POINT ( 'NONE',  ( 8.380911511541880188, 12.92948053010758258, 0.7998128361456462443 ) ) ;
#137813=CARTESIAN_POINT ( 'NONE',  ( 1.364683531249988535, 2.676041667008082214, 0.7879004041258500513 ) ) ;
#137815=CARTESIAN_POINT ( 'NONE',  ( 5.314433026876846711, 9.143996264757578984, -0.7216878364870267237 ) ) ;
#137823=CARTESIAN_POINT ( 'NONE',  ( 8.066738210006679566, 10.43428054980638997, 1.443375672974076540 ) ) ;
#137827=CARTESIAN_POINT ( 'NONE',  ( -8.715193815486133033, 9.062147627688959872, 0.7998128361456462443 ) ) ;
#137836=CARTESIAN_POINT ( 'NONE',  ( 2.842405760359353106, 6.467890487061221272, -0.7998128361456291469 ) ) ;
#137840=CARTESIAN_POINT ( 'NONE',  ( 5.341022448779654930, 8.318611059296550536, 1.199719254218462483 ) ) ;
#137843=( BOUNDED_CURVE ( )  B_SPLINE_CURVE ( 2, ( #184035, #166738, #18330, #2062, #68134, #51925, #82269 ),
 .UNSPECIFIED., .F., .T. ) 
 B_SPLINE_CURVE_WITH_KNOTS ( ( 3, 2, 2, 3 ),
 ( 0.4141369526679988811, 0.4166666666666666852, 0.4226190476190476164, 0.4227888527529243823 ),
 .UNSPECIFIED. ) 
 CURVE ( )  GEOMETRIC_REPRESENTATION_ITEM ( )  RATIONAL_B_SPLINE_CURVE ( ( 0.9345202395942611151, 0.9430618748659218564, 1.000000000000000000, 0.8660254037844387076, 1.000000000000000000, 0.9961780715265932118, 0.9925742013667540053 ) ) 
 REPRESENTATION_ITEM ( '' )  );
#137845=CARTESIAN_POINT ( 'NONE',  ( -1.201851678989727383E-14, 2.868750000682821266, -1.732050807568863648 ) ) ;
#137851=CARTESIAN_POINT ( 'NONE',  ( -0.7500000000000006661, -0.1416666666666441254, -1.299038105676652011 ) ) ;
#137852=CARTESIAN_POINT ( 'NONE',  ( 7.019370843573166319, 9.212351955633947043, 1.599625672291281386 ) ) ;
#137853=CARTESIAN_POINT ( 'NONE',  ( 5.246642258364164313, 8.104537820524768676, -1.082531754730549078 ) ) ;
#137857=EDGE_CURVE ( 'NONE', #190246, #116745, #17558, .T. ) ;
#137858=CARTESIAN_POINT ( 'NONE',  ( 8.419250204406344196, 12.76628297187536809, 1.040834085586084257E-14 ) ) ;
#137864=CARTESIAN_POINT ( 'NONE',  ( -4.381256195510448315, 8.263215994737505454, 1.040834085586084257E-14 ) ) ;
#137865=CARTESIAN_POINT ( 'NONE',  ( 1.499999999999989120, 3.285416667349486897, 0.8660254037844524744 ) ) ;
#137866=CARTESIAN_POINT ( 'NONE',  ( -1.001543065824772872E-14, 5.134375000341421469, 1.575800808251672791 ) ) ;
#137871=CARTESIAN_POINT ( 'NONE',  ( -1.364683531250012516, 4.051041667008088432, -0.7879004041258300672 ) ) ;
#137879=CARTESIAN_POINT ( 'NONE',  ( -2.937312835655025101, 6.578615408239493867, 1.040834085586084257E-14 ) ) ;
#137880=CARTESIAN_POINT ( 'NONE',  ( -8.202846631467911820, 9.528741477256060577, 1.199719254218462483 ) ) ;
#137881=CARTESIAN_POINT ( 'NONE',  ( 4.981731378017507872, 7.899438143407371271, -1.199719254218452047 ) ) ;
#137885=ORIENTED_EDGE ( 'NONE', *, *, #156347, .T. ) ;
#137890=CARTESIAN_POINT ( 'NONE',  ( -6.398558430645608475, 9.552403038140164782, -1.199719254218440723 ) ) ;
#137895=CARTESIAN_POINT ( 'NONE',  ( 3.728655938958122196, 4.308852335994623139, -1.199719254218446718 ) ) ;
#137897=CARTESIAN_POINT ( 'NONE',  ( -5.427341564172148303, 5.226320001155936090, 0.000000000000000000 ) ) ;
#137898=CARTESIAN_POINT ( 'NONE',  ( -8.320953590485107298, 10.73086516036454618, 1.599625672291269396 ) ) ;
#137901=CARTESIAN_POINT ( 'NONE',  ( -3.975490874141025088, 7.849583646728635955, 0.01022619435145193101 ) ) ;
#137902=CARTESIAN_POINT ( 'NONE',  ( -1.364683531250014514, -0.4697916663252449943, 0.7879004041258379498 ) ) ;
#137923=CARTESIAN_POINT ( 'NONE',  ( 2.684151225825664788, 5.114964949229812596, -1.082531754730543083 ) ) ;
#137927=CARTESIAN_POINT ( 'NONE',  ( -10.15913717534155047, 10.74674821418697057, 0.7998128361456462443 ) ) ;
#137928=DIRECTION ( 'NONE',  ( -0.9998757926790047268, 0.01538962834599434497, -0.003399787332182534986 ) ) ;
#137932=CARTESIAN_POINT ( 'NONE',  ( -1.402160292154681736E-14, 1.118750000682820378, -1.732050807568863648 ) ) ;
#137933=CARTESIAN_POINT ( 'NONE',  ( 8.543609354905870035, 13.11929468069890525, 0.7998128361456462443 ) ) ;
#137938=CARTESIAN_POINT ( 'NONE',  ( -7.967387826325084355, 12.44703623068796361, 0.7998128361456481317 ) ) ;
#137939=CARTESIAN_POINT ( 'NONE',  ( -5.692136587293078698, 5.855332880448203881, -2.499999999999996003 ) ) ;
#137940=CARTESIAN_POINT ( 'NONE',  ( 1.364683531249986537, 0.9052083336747533959, -0.7879004041258239610 ) ) ;
#137946=CARTESIAN_POINT ( 'NONE',  ( -3.242371291962510504, 6.934516940598226320, 1.040834085586084257E-14 ) ) ;
#137952=CARTESIAN_POINT ( 'NONE',  ( -1.402160292154681736E-14, -0.3656249996585805295, 1.575800808251672791 ) ) ;
#137957=CARTESIAN_POINT ( 'NONE',  ( 0.6823417656249882723, 0.09270833367475139752, 1.181850606188755259 ) ) ;
#137959=CARTESIAN_POINT ( 'NONE',  ( -6.911959384868566758, 6.958374125301778790, 1.040834085586084257E-14 ) ) ;
#137960=CARTESIAN_POINT ( 'NONE',  ( 7.242026607993941489, 11.60078147596829901, 0.7998128361456462443 ) ) ;
#137961=CARTESIAN_POINT ( 'NONE',  ( 3.357615597678655917, 7.068968630600413583, 0.7998128361456321445 ) ) ;
#137964=CARTESIAN_POINT ( 'NONE',  ( 1.364683531249988535, 1.926041667008086211, 0.7879004041258500513 ) ) ;
#137971=CARTESIAN_POINT ( 'NONE',  ( 5.666945020832160118, 9.555260257705446847, 0.7216878364870438212 ) ) ;
#137974=CARTESIAN_POINT ( 'NONE',  ( -7.823218330285243383, 9.085841792542966644, -1.199719254218446718 ) ) ;
#137975=CARTESIAN_POINT ( 'NONE',  ( -4.874319919312905647, 5.645460313075203018, -1.199719254218446718 ) ) ;
#137981=CARTESIAN_POINT ( 'NONE',  ( 5.517805330637495231, 6.500156309574290248, -1.082531754730543083 ) ) ;
#137982=CARTESIAN_POINT ( 'NONE',  ( -8.825994812371996900, 9.399341490629888440, 0.7216878364870438212 ) ) ;
#137984=CARTESIAN_POINT ( 'NONE',  ( 1.499999999999990896, 4.275000000000021672, 1.214306433183764966E-14 ) ) ;
#137988=CARTESIAN_POINT ( 'NONE',  ( 9.246297574839980271, 10.85006392781057905, 1.082531754730549967 ) ) ;
#137994=CIRCLE ( 'NONE', #134612, 2.750000000000000000 ) ;
#138001=CARTESIAN_POINT ( 'NONE',  ( 8.731087737076324018, 9.288616569451617622, 1.040834085586084257E-14 ) ) ;
#138002=CARTESIAN_POINT ( 'NONE',  ( 7.564559641420864899, 10.91273778404466199, -1.199719254218446718 ) ) ;
#138003=CARTESIAN_POINT ( 'NONE',  ( -6.555530967407501741, 7.606873202518897870, 1.199719254218450271 ) ) ;
#138007=CARTESIAN_POINT ( 'NONE',  ( -3.565431210269620621, 7.103494145382398095, 0.7216878364870484841 ) ) ;
#138010=CARTESIAN_POINT ( 'NONE',  ( 5.178851490740207453, 5.144340948726102702, 0.7216878364870317197 ) ) ;
#138012=CARTESIAN_POINT ( 'NONE',  ( -8.351459436338041442, 9.806086099558291025, -1.082531754730543971 ) ) ;
#138028=CARTESIAN_POINT ( 'NONE',  ( 8.308449207076147758, 8.587612251210650527, -0.7998128361456281477 ) ) ;
#138031=ORIENTED_EDGE ( 'NONE', *, *, #26674, .F. ) ;
#138040=CARTESIAN_POINT ( 'NONE',  ( -6.911959384868566758, 6.958374125301778790, 1.040834085586084257E-14 ) ) ;
#138042=CARTESIAN_POINT ( 'NONE',  ( -5.901876940650454095, 5.779944607047298177, -0.7998128361456291469 ) ) ;
#138052=CARTESIAN_POINT ( 'NONE',  ( -2.279742385392243165, 5.811449882932888222, -0.7998128361456281477 ) ) ;
#138055=CARTESIAN_POINT ( 'NONE',  ( 8.111855979677986994, 8.358253485912799263, 1.040834085586084257E-14 ) ) ;
#138058=CARTESIAN_POINT ( 'NONE',  ( 6.115167699822185554, 6.015585554489271125, 0.01814796302670486361 ) ) ;
#138063=CARTESIAN_POINT ( 'NONE',  ( 4.650083499362856365, 8.368921815991249957, 0.7216878364870438212 ) ) ;
#138064=CARTESIAN_POINT ( 'NONE',  ( -6.170932472514347289, 10.35117165124207972, 0.000000000000000000 ) ) ;
#138067=CARTESIAN_POINT ( 'NONE',  ( -7.832860060393135093, 10.16142270859057462, 1.599625672291295375 ) ) ;
#138068=CARTESIAN_POINT ( 'NONE',  ( -6.033542053281340856, 6.997886136038390603, -1.199719254218446718 ) ) ;
#138072=CARTESIAN_POINT ( 'NONE',  ( -2.398572866711294438, 5.287202466803544887, -0.8077998227820496480 ) ) ;
#138075=CARTESIAN_POINT ( 'NONE',  ( 7.800018446563675489, 7.994443030612759848, -0.7998128361456281477 ) ) ;
#138082=DIRECTION ( 'NONE',  ( 6.314299915563594049E-62, 8.546850786086437571E-32, 1.000000000000000000 ) ) ;
#138091=CARTESIAN_POINT ( 'NONE',  ( -1.001543065824772872E-14, 4.962500000000019007, 1.732050807568877637 ) ) ;
#138092=CARTESIAN_POINT ( 'NONE',  ( 3.310162060030825248, 7.013606170011280838, -0.7998128361456291469 ) ) ;
#138093=CARTESIAN_POINT ( 'NONE',  ( 6.667912619822566000, 6.673652899414787676, 1.040834085586084257E-14 ) ) ;
#138095=CARTESIAN_POINT ( 'NONE',  ( -7.049876689426097798, 11.16868053773170821, -0.7216878364870267237 ) ) ;
#138099=CARTESIAN_POINT ( 'NONE',  ( 6.263503779833467178, 9.290876262238963790, -1.082531754730537088 ) ) ;
#138100=CARTESIAN_POINT ( 'NONE',  ( -9.802181872555943087, 10.53822639417784046, 0.7216878364870438212 ) ) ;
#138104=CARTESIAN_POINT ( 'NONE',  ( 7.052212457402625922, 11.37933163361175382, -0.7998128361456291469 ) ) ;
#138109=CARTESIAN_POINT ( 'NONE',  ( -1.364683531250014514, 1.988541667008086655, -0.7879004041258289570 ) ) ;
#138115=ADVANCED_FACE ( 'NONE', ( #53607 ), #95273, .F. ) ;
#138116=CARTESIAN_POINT ( 'NONE',  ( 9.108380270282433244, 9.520865158284665952, 1.040834085586084257E-14 ) ) ;
#138120=CARTESIAN_POINT ( 'NONE',  ( -9.450196763925152510, 10.98398329845622001, -1.199719254218441611 ) ) ;
#138126=CARTESIAN_POINT ( 'NONE',  ( 4.241003122976366058, 3.842258486427521103, -0.7998128361456211532 ) ) ;
#138129=CARTESIAN_POINT ( 'NONE',  ( -9.341731535015849630, 10.85744053139533349, 1.199719254218462483 ) ) ;
#138134=CARTESIAN_POINT ( 'NONE',  ( 5.880650534977156063, 5.984130091214588276, -0.1889179825720621597 ) ) ;
#138136=CARTESIAN_POINT ( 'NONE',  ( -3.255929445576174697, 6.950334786480840243, -0.7998128361456281477 ) ) ;
#138140=CARTESIAN_POINT ( 'NONE',  ( 8.372323551638698902, 9.726464550788689323, 1.199719254218462483 ) ) ;
#138142=CARTESIAN_POINT ( 'NONE',  ( 7.311924916471702396, 7.425000578838787391, -0.7998128361456281477 ) ) ;
#138143=CARTESIAN_POINT ( 'NONE',  ( -1.499999999999997780, 8.627523663848661428, -2.579999999999990301 ) ) ;
#138145=CARTESIAN_POINT ( 'NONE',  ( -7.673551755654729689, 11.89630144833179060, 0.7216878364870458196 ) ) ;
#138154=CARTESIAN_POINT ( 'NONE',  ( -6.025499844618653178, 6.066343344509915525, -0.6079853925319089747 ) ) ;
#138155=ADVANCED_FACE ( 'NONE', ( #198766 ), #119584, .T. ) ;
#138157=CARTESIAN_POINT ( 'NONE',  ( 5.395781948558860286, 6.357795697149212444, -1.082531754730542195 ) ) ;
#138161=CARTESIAN_POINT ( 'NONE',  ( 4.650083499807233345, 5.295740330745369207, -7.499999999999997335 ) ) ;
#138177=CARTESIAN_POINT ( 'NONE',  ( 8.392660782059197189, 9.750191319612612872, 1.199719254218462483 ) ) ;
#138181=CARTESIAN_POINT ( 'NONE',  ( 1.499999999999987121, 1.077083334016148308, -0.8660254037844253849 ) ) ;
#138183=CARTESIAN_POINT ( 'NONE',  ( -5.506582945444718824, 9.576097202994168001, 0.7998128361456481317 ) ) ;
#138187=CARTESIAN_POINT ( 'NONE',  ( -8.448702279610222021, 13.00856975952063088, 1.040834085586084257E-14 ) ) ;
#138188=CARTESIAN_POINT ( 'NONE',  ( -1.435115314735526448, 7.268684689231142748, 4.324912918974801457 ) ) ;
#138191=CARTESIAN_POINT ( 'NONE',  ( -1.500000000000011324, 5.410416667349489117, -0.8660254037844313801 ) ) ;
#138192=CARTESIAN_POINT ( 'NONE',  ( 7.298366762858032430, 7.409182732956175244, 1.040834085586084257E-14 ) ) ;
#138196=CARTESIAN_POINT ( 'NONE',  ( -7.389357414647957256, 8.579670724299436557, 1.199719254218450271 ) ) ;
#138198=CARTESIAN_POINT ( 'NONE',  ( 5.751721435176966324, 6.248267645806530268, -1.064211863609406672 ) ) ;
#138203=CARTESIAN_POINT ( 'NONE',  ( -7.361714222540411967, 11.53249099303175385, 0.000000000000000000 ) ) ;
#138207=CARTESIAN_POINT ( 'NONE',  ( -1.364683531249997417, 3.821875000341416584, 1.214306433183764966E-14 ) ) ;
#138214=CARTESIAN_POINT ( 'NONE',  ( -1.364683531249997417, 4.009375000341424133, 1.214306433183764966E-14 ) ) ;
#138217=CARTESIAN_POINT ( 'NONE',  ( 3.511198595814932766, 5.119484333249288532, 1.443375672974066548 ) ) ;
#138218=CARTESIAN_POINT ( 'NONE',  ( -0.6823417656250212460, 5.363541667008087543, 1.181850606188767472 ) ) ;
#138224=CARTESIAN_POINT ( 'NONE',  ( 0.6823417656249882723, 0.9260416670080831025, -1.181850606188749264 ) ) ;
#138225=CARTESIAN_POINT ( 'NONE',  ( -4.622967192579922724, 4.495809267539077503, 1.214306433183764966E-14 ) ) ;
#138226=CARTESIAN_POINT ( 'NONE',  ( 3.960953433486789521, 7.772862772376584850, -0.7998128361456221525 ) ) ;
#138231=CARTESIAN_POINT ( 'NONE',  ( 3.389175213736292047, 5.937492935125556315, 1.082531754730558626 ) ) ;
#138234=CARTESIAN_POINT ( 'NONE',  ( -8.107412671292051343, 10.48173408797264194, 1.443375672974090751 ) ) ;
#138239=CARTESIAN_POINT ( 'NONE',  ( -7.323375529675950624, 11.69568855126397011, -0.7998128361456291469 ) ) ;
#138240=EDGE_CURVE ( 'NONE', #110521, #206877, #181471, .T. ) ;
#138241=CARTESIAN_POINT ( 'NONE',  ( -4.894130264408858899, 8.653643041878236630, -0.7216878364870207285 ) ) ;
#138243=CARTESIAN_POINT ( 'NONE',  ( -1.364683531250012516, 2.342708333674752286, 0.7879004041258379498 ) ) ;
#138250=CARTESIAN_POINT ( 'NONE',  ( 8.387690588348714726, 12.93738945304888333, 1.040834085586084257E-14 ) ) ;
#138252=EDGE_LOOP ( 'NONE', ( #111438, #71044, #202581 ) ) ;
#138261=CARTESIAN_POINT ( 'NONE',  ( 1.499999999999821032, 7.268077025657388113, -4.207854987879545483 ) ) ;
#138263=CARTESIAN_POINT ( 'NONE',  ( -2.764973262183167968, 5.313220341600567664, 1.199719254218462483 ) ) ;
#138265=CARTESIAN_POINT ( 'NONE',  ( -0.6823417656250003738, 2.530208333674753618, -1.181850606188749264 ) ) ;
#138275=CARTESIAN_POINT ( 'NONE',  ( -0.6823417656250246877, 0.5510416670080897639, 1.181850606188755259 ) ) ;
#138277=VERTEX_POINT ( 'NONE', #65568 ) ;
#138281=ORIENTED_EDGE ( 'NONE', *, *, #211661, .T. ) ;
#138285=CARTESIAN_POINT ( 'NONE',  ( 3.832150974156964818, 7.622593236491780999, 1.040834085586084257E-14 ) ) ;
#138296=CARTESIAN_POINT ( 'NONE',  ( 8.880754312151170282, 10.31963377138658089, 1.199719254218453823 ) ) ;
#138308=CARTESIAN_POINT ( 'NONE',  ( -8.703971430293361067, 9.256980878204810637, 0.7216878364870438212 ) ) ;
#138312=CARTESIAN_POINT ( 'NONE',  ( -9.321394304595349567, 10.83371376257142416, 1.199719254218462483 ) ) ;
#138316=CARTESIAN_POINT ( 'NONE',  ( -3.737243898861318137, 7.511868315313511069, 0.7998128361456341429 ) ) ;
#138318=CARTESIAN_POINT ( 'NONE',  ( 9.585778300061798873, 11.14216175728232550, -1.199719254218440723 ) ) ;
#138320=CARTESIAN_POINT ( 'NONE',  ( 4.330940004561544043, 7.140181541042074365, -1.199719254218452047 ) ) ;
#138326=CARTESIAN_POINT ( 'NONE',  ( 3.063779527008304360, 6.518233848244248563, 0.7216878364870317197 ) ) ;
#138328=CARTESIAN_POINT ( 'NONE',  ( -5.413783410558481002, 5.210502155273325720, -0.7998128361456221525 ) ) ;
#138331=CARTESIAN_POINT ( 'NONE',  ( -9.429859533504656000, 10.96025652963230534, -1.199719254218441611 ) ) ;
#138337=CARTESIAN_POINT ( 'NONE',  ( 7.863365906246055914, 10.19701286208565705, -1.443375672974057666 ) ) ;
#138338=CARTESIAN_POINT ( 'NONE',  ( -1.201851678989727383E-14, 3.509375000341421469, -1.575800808251660134 ) ) ;
#138341=CARTESIAN_POINT ( 'NONE',  ( 4.253507506385319381, 5.985511395581417204, 1.599625672291267398 ) ) ;
#138350=DIRECTION ( 'NONE',  ( 0.7592566023653004592, -0.6507913734559641616, -1.725633230170963105E-31 ) ) ;
#138356=CARTESIAN_POINT ( 'NONE',  ( -1.364683531249997417, 2.821875000341422801, 1.214306433183764966E-14 ) ) ;
#138358=CARTESIAN_POINT ( 'NONE',  ( 8.866142388332804103, 12.43125098877526113, -1.199719254218446718 ) ) ;
#138360=CARTESIAN_POINT ( 'NONE',  ( -6.249945626219832739, 6.393950773452325542, 1.040834085586084257E-14 ) ) ;
#138361=CARTESIAN_POINT ( 'NONE',  ( 4.541618270897912701, 4.400902192243413502, 1.214306433183764966E-14 ) ) ;
#138362=CARTESIAN_POINT ( 'NONE',  ( -4.704316113817535339, 8.432193199521691440, 0.7216878364870458196 ) ) ;
#138367=CARTESIAN_POINT ( 'NONE',  ( 5.996784015946103885, 5.890669528225568996, 1.040834085586084257E-14 ) ) ;
#138373=DIRECTION ( 'NONE',  ( 0.000000000000000000, 1.000000000000000000, 0.000000000000000000 ) ) ;
#138378=CARTESIAN_POINT ( 'NONE',  ( 5.575427483717746213, 7.527751369135936343, 1.599625672291267398 ) ) ;
#138379=SURFACE_STYLE_USAGE ( .BOTH. , #6201 ) ;
#138381=CARTESIAN_POINT ( 'NONE',  ( -3.440018289565379028, 5.036440642624797626, 1.599625672291267398 ) ) ;
#138383=CARTESIAN_POINT ( 'NONE',  ( -5.540478329478883524, 9.615641817700700145, 0.000000000000000000 ) ) ;
#138387=CARTESIAN_POINT ( 'NONE',  ( 8.437251666405968464, 8.737881787095446384, 1.040834085586084257E-14 ) ) ;
#138390=CARTESIAN_POINT ( 'NONE',  ( -7.172426956829277778, 8.326585190177668849, -1.199719254218452935 ) ) ;
#138391=CARTESIAN_POINT ( 'NONE',  ( 7.253248993186731219, 8.524840582548424806, 1.082531754730558626 ) ) ;
#138392=CARTESIAN_POINT ( 'NONE',  ( 4.145277420728366025, 7.638539262984231470, 0.7997124044470202975 ) ) ;
#138393=CARTESIAN_POINT ( 'NONE',  ( -5.596818484342970912, 5.424043074688562172, -0.7998128361456221525 ) ) ;
#138396=CARTESIAN_POINT ( 'NONE',  ( -6.063521013809733518, 8.097193820909906137, 1.599625672291283607 ) ) ;
#138400=CARTESIAN_POINT ( 'NONE',  ( 1.364683531249988535, 1.363541667008083769, 0.7879004041258500513 ) ) ;
#138402=CARTESIAN_POINT ( 'NONE',  ( -5.246642258808529746, 9.064907035344523578, 0.000000000000000000 ) ) ;
#138407=CARTESIAN_POINT ( 'NONE',  ( 6.063521013809720195, 8.097193820909906137, 1.599625672291281386 ) ) ;
#138409=CARTESIAN_POINT ( 'NONE',  ( -5.903030530102264528, 6.005529115149156993, -0.1628943571830038795 ) ) ;
#138410=CARTESIAN_POINT ( 'NONE',  ( -1.201851678989727383E-14, 0.8843750003414173610, 1.575800808251672791 ) ) ;
#138417=CARTESIAN_POINT ( 'NONE',  ( -3.100010679019018500, 6.768429558830820980, 1.040834085586084257E-14 ) ) ;
#138418=CARTESIAN_POINT ( 'NONE',  ( -5.870317324592805086, 9.792527945426188651, -0.7216878364870197293 ) ) ;
#138422=EDGE_CURVE ( 'NONE', #159827, #121606, #53805, .T. ) ;
#138427=CARTESIAN_POINT ( 'NONE',  ( -7.334597914868727919, 10.54048608644677465, -1.082531754730543083 ) ) ;
#138430=DIRECTION ( 'NONE',  ( 0.6507913734559640506, -0.7592566023653004592, 0.000000000000000000 ) ) ;
#138433=CARTESIAN_POINT ( 'NONE',  ( -6.331294547457448019, 10.33033470543493770, 0.7216878364870458196 ) ) ;
#138439=CARTESIAN_POINT ( 'NONE',  ( -1.499999999999997780, 5.681250000682820378, 1.214306433183764966E-14 ) ) ;
#138440=CARTESIAN_POINT ( 'NONE',  ( 4.232984923718338344, 7.533997312158466464, -0.9744250676351111640 ) ) ;
#138447=CARTESIAN_POINT ( 'NONE',  ( -6.989391883044787868, 8.113044270762433285, -1.199719254218446718 ) ) ;
#138448=CARTESIAN_POINT ( 'NONE',  ( 4.955668840994886359, 5.740367388370866131, 1.199719254218462483 ) ) ;
#138451=CARTESIAN_POINT ( 'NONE',  ( 6.494519276145969577, 7.535692896047149425, -1.199719254218446718 ) ) ;
#138458=CARTESIAN_POINT ( 'NONE',  ( -3.904385051055635270, 6.538571078664754843, 1.082531754730560403 ) ) ;
#138467=CARTESIAN_POINT ( 'NONE',  ( -0.6823417656250212460, 1.301041667008083547, 1.181850606188755259 ) ) ;
#138469=CARTESIAN_POINT ( 'NONE',  ( -7.828943636887387925, 11.22118577875556156, 1.199719254218453823 ) ) ;
#138471=CARTESIAN_POINT ( 'NONE',  ( 6.259060471003163428, 10.45398764947904624, -0.7998128361456291469 ) ) ;
#138473=CARTESIAN_POINT ( 'NONE',  ( -6.503107236049161521, 10.73870887536603291, 0.7998128361456481317 ) ) ;
#138476=CARTESIAN_POINT ( 'NONE',  ( -1.001543065824772872E-14, 5.071875000341421469, 1.575800808251672791 ) ) ;
#138478=CARTESIAN_POINT ( 'NONE',  ( 9.897088948295946764, 10.64895131587453569, 0.7216878364870438212 ) ) ;
#138481=CARTESIAN_POINT ( 'NONE',  ( -0.6823417656250246877, -1.136458332991911790, 1.181850606188755259 ) ) ;
#138484=CARTESIAN_POINT ( 'NONE',  ( 7.931156673870037643, 8.355363662377600420, -0.7216878364870267237 ) ) ;
#138487=CARTESIAN_POINT ( 'NONE',  ( -4.555176424511596878, 7.297827681030051750, 1.082531754730560403 ) ) ;
#138489=B_SPLINE_CURVE_WITH_KNOTS ( 'NONE', 3,
 ( #17342, #138595, #141827, #204618 ),
 .UNSPECIFIED., .F., .F.,
 ( 4, 4 ),
 ( 0.000000000000000000, 7.241384396098642291E-05 ),
 .UNSPECIFIED. ) ;
#138490=CARTESIAN_POINT ( 'NONE',  ( 1.364683531249990311, 3.884375000341417028, 1.214306433183764966E-14 ) ) ;
#138494=CARTESIAN_POINT ( 'NONE',  ( -4.720210035852093533, 8.658662141802762946, -0.7998128361456281477 ) ) ;
#138500=CARTESIAN_POINT ( 'NONE',  ( 8.932124273304774320, 9.315233161810734686, 0.7998128361456462443 ) ) ;
#138503=CARTESIAN_POINT ( 'NONE',  ( -0.7500000000000215383, 0.6916666666666876351, 1.299038105676659116 ) ) ;
#138509=CARTESIAN_POINT ( 'NONE',  ( 6.534666852106798096, 7.686494751288491578, -1.082531754730543083 ) ) ;
#138510=CARTESIAN_POINT ( 'NONE',  ( -1.364683531250014514, -0.9072916663252470482, 0.7879004041258379498 ) ) ;
#138512=CARTESIAN_POINT ( 'NONE',  ( 2.381428537494710618, 5.930083727052461562, 0.7998128361456462443 ) ) ;
#138518=CARTESIAN_POINT ( 'NONE',  ( 6.968000882419564945, 10.21675256520979858, 1.199719254218460707 ) ) ;
#138519=CARTESIAN_POINT ( 'NONE',  ( -10.17947440576205054, 10.77047498301088346, 0.7998128361456462443 ) ) ;
#138521=B_SPLINE_CURVE_WITH_KNOTS ( 'NONE', 3,
 ( #10925, #77000, #209121, #60759 ),
 .UNSPECIFIED., .F., .F.,
 ( 4, 4 ),
 ( 0.003703980837549441640, 0.004484133753724313387 ),
 .UNSPECIFIED. ) ;
#138522=CARTESIAN_POINT ( 'NONE',  ( 1.364683531249988757, 0.1343750003414204142, 0.000000000000000000 ) ) ;
#138523=CARTESIAN_POINT ( 'NONE',  ( -1.402160292154681736E-14, 1.337500000000025446, -1.732050807568863648 ) ) ;
#138525=CARTESIAN_POINT ( 'NONE',  ( 4.137209430464448445, 7.978494768850520558, 1.040834085586084257E-14 ) ) ;
#138531=CARTESIAN_POINT ( 'NONE',  ( -1.500000000000001332, -1.318749999317178734, 0.000000000000000000 ) ) ;
#138533=CARTESIAN_POINT ( 'NONE',  ( -7.995557903757128493, 10.35123685918189729, 1.599625672291295375 ) ) ;
#138534=CARTESIAN_POINT ( 'NONE',  ( -5.761852096127856981, 5.824508321678349532, 0.000000000000000000 ) ) ;
#138542=CARTESIAN_POINT ( 'NONE',  ( 7.938462636001388795, 9.220293482545153907, -1.199719254218441611 ) ) ;
#138547=CARTESIAN_POINT ( 'NONE',  ( 8.093854517234030155, 8.545177812968924869, -0.7216878364870267237 ) ) ;
#138550=CARTESIAN_POINT ( 'NONE',  ( -6.995117189646935962, 10.24838825697502109, 1.199719254218453823 ) ) ;
#138551=CARTESIAN_POINT ( 'NONE',  ( 4.632082037363250748, 8.555846143565791095, -0.7998128361456231517 ) ) ;
#138552=DIRECTION ( 'NONE',  ( 0.7592566023653005702, -0.6507913734559639396, 0.000000000000000000 ) ) ;
#138554=CARTESIAN_POINT ( 'NONE',  ( 4.304877467538922531, 4.981110786005563007, 1.199719254218464037 ) ) ;
#138555=VERTEX_POINT ( 'NONE', #37353 ) ;
#138558=EDGE_CURVE ( 'NONE', #19519, #106155, #203613, .T. ) ;
#138563=CARTESIAN_POINT ( 'NONE',  ( -6.249945626219832739, 6.393950773452325542, 1.040834085586084257E-14 ) ) ;
#138564=CARTESIAN_POINT ( 'NONE',  ( 4.356247428692526569, 3.976710176429713250, 0.7998128361456341429 ) ) ;
#138567=CARTESIAN_POINT ( 'NONE',  ( -7.528855374290365887, 7.678086112960552434, -0.7998128361456291469 ) ) ;
#138571=CARTESIAN_POINT ( 'NONE',  ( -9.169391961543940539, 9.592045464756413509, 1.040834085586084257E-14 ) ) ;
#138576=CARTESIAN_POINT ( 'NONE',  ( 4.462605117192430804, 8.358123070033169455, 1.040834085586084257E-14 ) ) ;
#138589=CARTESIAN_POINT ( 'NONE',  ( -7.691553217654356622, 7.867900263551875994, -0.7998128361456291469 ) ) ;
#138592=CARTESIAN_POINT ( 'NONE',  ( 6.155038550924155416, 6.283225852274053835, 0.7216878364870317197 ) ) ;
#138593=VERTEX_POINT ( 'NONE', #203031 ) ;
#138595=CARTESIAN_POINT ( 'NONE',  ( 3.046854503059200248, 2.800000000000017586, -2.499999999999995115 ) ) ;
#138597=CARTESIAN_POINT ( 'NONE',  ( -5.922214171070950606, 5.803671375871217286, -0.7998128361456291469 ) ) ;
#138601=CARTESIAN_POINT ( 'NONE',  ( -7.203459687562382641, 7.298457811777897319, -0.7998128361456291469 ) ) ;
#138602=CARTESIAN_POINT ( 'NONE',  ( -5.805552323418545768, 6.064174366559389462, -0.5408148663509839693 ) ) ;
#138607=CARTESIAN_POINT ( 'NONE',  ( -9.612894607289142357, 11.17379744904754801, -1.199719254218441611 ) ) ;
#138608=CARTESIAN_POINT ( 'NONE',  ( 6.262976894508937242, 9.394224579314053969, -1.199719254218440723 ) ) ;
#138611=CARTESIAN_POINT ( 'NONE',  ( -9.541187415715041809, 12.15447128979948310, -1.599625672291263179 ) ) ;
#138614=CARTESIAN_POINT ( 'NONE',  ( -1.402160292154681736E-14, -1.115624999658584082, 1.575800808251672791 ) ) ;
#138618=CARTESIAN_POINT ( 'NONE',  ( 8.256552361042350796, 12.57646882128404187, 1.040834085586084257E-14 ) ) ;
#138635=ORIENTED_EDGE ( 'NONE', *, *, #118861, .T. ) ;
#138640=CARTESIAN_POINT ( 'NONE',  ( -2.788173145904702555, 6.404619103530779789, -0.7998128361456281477 ) ) ;
#138643=CARTESIAN_POINT ( 'NONE',  ( -4.810445574750349174, 4.506608013497163334, 0.7998128361456341429 ) ) ;
#138645=EDGE_CURVE ( 'NONE', #4590, #13599, #126249, .T. ) ;
#138648=CARTESIAN_POINT ( 'NONE',  ( 0.6823417656249899377, 5.676041667008087543, -1.181850606188754593 ) ) ;
#138651=CARTESIAN_POINT ( 'NONE',  ( -3.958617665510283601, 4.681104033592509595, -1.082531754730549967 ) ) ;
#138655=CARTESIAN_POINT ( 'NONE',  ( 1.451998047839290207, 7.315968950356647404, -4.301760722583974683 ) ) ;
#138657=CARTESIAN_POINT ( 'NONE',  ( 10.53876547652418338, 11.18964789890005918, 0.7998128361456462443 ) ) ;
#138658=CARTESIAN_POINT ( 'NONE',  ( -3.917943204224914933, 6.554388924028945240, -1.082531754730548412 ) ) ;
#138660=LINE ( 'NONE', #203612, #92404 ) ;
#138661=CARTESIAN_POINT ( 'NONE',  ( 8.527715432871318058, 12.89282573841782664, -0.7216878364870338292 ) ) ;
#138663=CARTESIAN_POINT ( 'NONE',  ( -1.364683531250000748, 2.321875000341422357, 1.214306433183764966E-14 ) ) ;
#138666=CARTESIAN_POINT ( 'NONE',  ( -9.481229494658258261, 9.955855920056455588, -0.7998128361456291469 ) ) ;
#138668=CARTESIAN_POINT ( 'NONE',  ( -4.894130264408866893, 6.732904613275549899, -1.443375672974051449 ) ) ;
#138671=CARTESIAN_POINT ( 'NONE',  ( -4.543954038874438162, 8.453030145328826350, 1.040834085586084257E-14 ) ) ;
#138673=CARTESIAN_POINT ( 'NONE',  ( -1.500000000000015099, -0.7979166659838445863, 0.8660254037844403729 ) ) ;
#138676=EDGE_CURVE ( 'NONE', #30492, #204725, #19680, .T. ) ;
#138682=CARTESIAN_POINT ( 'NONE',  ( -5.056828107772860292, 6.922718763866881453, -1.443375672974051449 ) ) ;
#138686=CARTESIAN_POINT ( 'NONE',  ( 1.249999999999822364, 10.00000000000000178, 4.154462424328221104 ) ) ;
#138688=CARTESIAN_POINT ( 'NONE',  ( -5.382223794500852421, 5.381608636446842731, -0.7216878364870197293 ) ) ;
#138699=CARTESIAN_POINT ( 'NONE',  ( -4.253507506385335368, 5.985511395581417204, 1.599625672291267398 ) ) ;
#138700=CARTESIAN_POINT ( 'NONE',  ( -8.272446282632566650, 12.80293776304669962, 0.7998128361456481317 ) ) ;
#138703=VERTEX_POINT ( 'NONE', #188938 ) ;
#138705=CARTESIAN_POINT ( 'NONE',  ( 5.120175567455225618, 9.125288595339771547, -0.7998128361456281477 ) ) ;
#138711=CARTESIAN_POINT ( 'NONE',  ( 2.205172540517054802, 5.724451730578533848, 1.040834085586084257E-14 ) ) ;
#138721=CARTESIAN_POINT ( 'NONE',  ( 7.099665995050449041, 11.43469409420089455, 0.7998128361456462443 ) ) ;
#138722=CARTESIAN_POINT ( 'NONE',  ( -5.250031796989778066, 7.148123067953287446, 1.599625672291267398 ) ) ;
#138723=AXIS2_PLACEMENT_3D ( 'NONE', #161471, #209109, #157200 ) ;
#138728=CARTESIAN_POINT ( 'NONE',  ( -1.364683531249997417, 4.259375000341424133, 1.214306433183764966E-14 ) ) ;
#138730=CARTESIAN_POINT ( 'NONE',  ( -4.550733115681270036, 8.460939068270139529, 0.7998128361456481317 ) ) ;
#138733=CARTESIAN_POINT ( 'NONE',  ( 4.656335691289526402, 7.519809842224722374, -1.199719254218452047 ) ) ;
#138734=CARTESIAN_POINT ( 'NONE',  ( -5.271422797614987665, 5.044414773505913274, -0.7998128361456221525 ) ) ;
#138740=CARTESIAN_POINT ( 'NONE',  ( 5.992340707560151358, 8.014150130285418783, 1.443375672974062551 ) ) ;
#138742=CARTESIAN_POINT ( 'NONE',  ( 7.090551149822735155, 9.295395646258437949, 1.443375672974076540 ) ) ;
#138743=CARTESIAN_POINT ( 'NONE',  ( -0.6823417656250212460, 3.363541667008085323, 1.181850606188767472 ) ) ;
#138745=CARTESIAN_POINT ( 'NONE',  ( 4.867013957181530515, 5.740899707208986236, -1.082531754730548412 ) ) ;
#138753=CARTESIAN_POINT ( 'NONE',  ( -4.849785647588779725, 6.920107565692508622, 1.442884047295606820 ) ) ;
#138761=CARTESIAN_POINT ( 'NONE',  ( -10.49131193887636826, 11.13428543831092909, 1.040834085586084257E-14 ) ) ;
#138763=VECTOR ( 'NONE', #127813, 1000.000000000000000 ) ;
#138771=CARTESIAN_POINT ( 'NONE',  ( 3.334942599281629949, 5.874221551595115720, -1.082531754730543083 ) ) ;
#138772=CARTESIAN_POINT ( 'NONE',  ( -1.201851678989727383E-14, 3.759375000341422801, -1.575800808251660134 ) ) ;
#138774=CARTESIAN_POINT ( 'NONE',  ( 6.740374924288304648, 11.01552117831172062, 1.040834085586084257E-14 ) ) ;
#138775=CARTESIAN_POINT ( 'NONE',  ( -9.561524646135538319, 12.17819805862340310, -1.599625672291263179 ) ) ;
#138777=CARTESIAN_POINT ( 'NONE',  ( -4.475070042639309520, 5.445751865460756846, 1.284222742053057642 ) ) ;
#138781=CARTESIAN_POINT ( 'NONE',  ( -1.201851678989727383E-14, 3.337500000000019007, -1.732050807568863648 ) ) ;
#138782=CARTESIAN_POINT ( 'NONE',  ( 4.985647801523278133, 6.839675073242382553, -1.599625672291256295 ) ) ;
#138786=CARTESIAN_POINT ( 'NONE',  ( 0.6823417656249899377, 3.676041667008085767, -1.181850606188754593 ) ) ;
#138788=CARTESIAN_POINT ( 'NONE',  ( 8.595506201384008449, 11.05117653974661529, 1.443375672974076540 ) ) ;
#138793=CARTESIAN_POINT ( 'NONE',  ( 1.499999999999989120, 2.285416667349482012, 0.8660254037844524744 ) ) ;
#138795=CARTESIAN_POINT ( 'NONE',  ( -4.367698041896780126, 8.247398148854895084, 0.7998128361456481317 ) ) ;
#138796=CARTESIAN_POINT ( 'NONE',  ( 3.999292125906899198, 6.649295999324608353, 1.082531754730558626 ) ) ;
#138805=CARTESIAN_POINT ( 'NONE',  ( 6.096362627639171805, 10.26417349888772179, -0.7998128361456291469 ) ) ;
#138806=CARTESIAN_POINT ( 'NONE',  ( 5.606460214450851964, 6.499623990736163037, 1.199719254218462483 ) ) ;
#138808=PLANE ( 'NONE',  #182088 ) ;
#138811=CARTESIAN_POINT ( 'NONE',  ( 6.844168616800228477, 6.879284895888727824, -0.7998128361456281477 ) ) ;
#138816=ORIENTED_EDGE ( 'NONE', *, *, #59430, .T. ) ;
#138817=CARTESIAN_POINT ( 'NONE',  ( 8.380911511541880188, 12.92948053010758258, 0.7998128361456462443 ) ) ;
#138822=CARTESIAN_POINT ( 'NONE',  ( 5.364345920411571100, 6.316227854031381206, 1.080878399565273540 ) ) ;
#138835=CARTESIAN_POINT ( 'NONE',  ( 7.456621297836082185, 7.801739057004660971, 0.7216878364870317197 ) ) ;
#138836=CARTESIAN_POINT ( 'NONE',  ( -3.415764635639130020, 6.072476943965863683, 1.199719254218462483 ) ) ;
#138840=CARTESIAN_POINT ( 'NONE',  ( -5.590039407536138150, 5.416134151747256986, 0.000000000000000000 ) ) ;
#138847=VERTEX_POINT ( 'NONE', #117359 ) ;
#138853=CARTESIAN_POINT ( 'NONE',  ( 9.317477881089539338, 11.89347683273640932, 1.599625672291279388 ) ) ;
#138856=CARTESIAN_POINT ( 'NONE',  ( 3.714570900464285064, 4.396382807705524698, 1.082531754730560403 ) ) ;
#138863=CARTESIAN_POINT ( 'NONE',  ( -3.195971524519394702, 4.751719416737803847, -1.599625672291262513 ) ) ;
#138867=CARTESIAN_POINT ( 'NONE',  ( 9.413438726589914651, 9.876766690643398405, 0.000000000000000000 ) ) ;
#138872=CARTESIAN_POINT ( 'NONE',  ( -5.554036483092550824, 9.631459663583308739, -0.7998128361456231517 ) ) ;
#138873=CARTESIAN_POINT ( 'NONE',  ( 5.495132332240461714, 5.305409230568988832, 0.7998128361456341429 ) ) ;
#138876=CARTESIAN_POINT ( 'NONE',  ( 10.56588178375152864, 11.22128359066528169, -0.7998128361456281477 ) ) ;
#138880=CARTESIAN_POINT ( 'NONE',  ( -0.6823417656250212460, 2.863541667008084879, 1.181850606188767472 ) ) ;
#138883=CARTESIAN_POINT ( 'NONE',  ( 7.456621297836082185, 7.801739057004660971, 0.7216878364870317197 ) ) ;
#138891=CARTESIAN_POINT ( 'NONE',  ( 9.205623113554624481, 10.80261038964432707, 1.082531754730549967 ) ) ;
#138896=CARTESIAN_POINT ( 'NONE',  ( -7.330154606482786050, 11.70359747420527619, 0.000000000000000000 ) ) ;
#138906=CARTESIAN_POINT ( 'NONE',  ( 3.867100128395839942, 5.534702787927018974, -1.599625672291255185 ) ) ;
#138912=CARTESIAN_POINT ( 'NONE',  ( 4.150767584078112193, 7.994312614733129152, 0.7998128361456321445 ) ) ;
#138915=CIRCLE ( 'NONE', #45527, 0.08000000000000015432 ) ;
#138916=CARTESIAN_POINT ( 'NONE',  ( -1.201851678989727383E-14, 3.118750000682814161, -1.732050807568863648 ) ) ;
#138922=CIRCLE ( 'NONE', #11013, 0.08000000000000025147 ) ;
#138923=CARTESIAN_POINT ( 'NONE',  ( -1.402160292154681736E-14, -0.1624999999999815481, -1.732050807568870754 ) ) ;
#138924=CARTESIAN_POINT ( 'NONE',  ( 6.805303039055573322, 10.02693841461847057, 1.199719254218460707 ) ) ;
#138925=CARTESIAN_POINT ( 'NONE',  ( -0.6823417656250003738, -0.7822916663252423852, -1.181850606188749264 ) ) ;
#138928=CARTESIAN_POINT ( 'NONE',  ( 7.768458830950378591, 12.00702636951006497, 1.040834085586084257E-14 ) ) ;
#138932=CARTESIAN_POINT ( 'NONE',  ( -6.555530967407501741, 7.606873202518897870, 1.199719254218450271 ) ) ;
#138933=CARTESIAN_POINT ( 'NONE',  ( 1.499999999999987121, 2.827083334016148530, -0.8660254037844262731 ) ) ;
#138934=CARTESIAN_POINT ( 'NONE',  ( -0.6823417656249969321, 5.030208333674755394, -1.181850606188749264 ) ) ;
#138940=CARTESIAN_POINT ( 'NONE',  ( 1.364683531249988535, 4.217708333674752730, -0.7879004041258239610 ) ) ;
#138948=CARTESIAN_POINT ( 'NONE',  ( -1.249999999999997558, 10.00000000000000178, -4.154462424328202452 ) ) ;
#138949=CARTESIAN_POINT ( 'NONE',  ( -8.479735010343349089, 11.98044238112085758, 1.199719254218453823 ) ) ;
#138950=CARTESIAN_POINT ( 'NONE',  ( 6.632963465583686435, 8.761543347979550589, -1.599625672291262513 ) ) ;
#138953=ADVANCED_FACE ( 'NONE', ( #116289 ), #97872, .T. ) ;
#138958=CARTESIAN_POINT ( 'NONE',  ( -7.477485413136760073, 8.682486722536401302, -1.199719254218446718 ) ) ;
#138963=CARTESIAN_POINT ( 'NONE',  ( 2.381428537494710618, 5.930083727052461562, 0.7998128361456462443 ) ) ;
#138964=DIRECTION ( 'NONE',  ( -1.000000000000000000, 6.505213034913026604E-16, 0.000000000000000000 ) ) ;
#138967=CARTESIAN_POINT ( 'NONE',  ( -4.660252114795309097, 6.460046772059735432, -1.599625672291256295 ) ) ;
#138968=CARTESIAN_POINT ( 'NONE',  ( -8.134002093194872884, 11.57708731111429401, 1.199719254218453823 ) ) ;
#138971=CARTESIAN_POINT ( 'NONE',  ( -4.014048110574687911, 7.796590492392542870, 0.4333429611983550256 ) ) ;
#138978=CARTESIAN_POINT ( 'NONE',  ( 6.657217119509961201, 7.725507046638470321, -1.199719254218446718 ) ) ;
#138980=CARTESIAN_POINT ( 'NONE',  ( 5.951324661306437669, 4.742844146916157300, 2.438848701820569786 ) ) ;
#138998=CARTESIAN_POINT ( 'NONE',  ( 3.063779527008311021, 5.557864633942907417, 1.082531754730546636 ) ) ;
#139000=ORIENTED_EDGE ( 'NONE', *, *, #22500, .F. ) ;
#139002=CARTESIAN_POINT ( 'NONE',  ( -9.592557376868645846, 11.15007068022363157, -1.199719254218441611 ) ) ;
#139008=CARTESIAN_POINT ( 'NONE',  ( 0.7499999999999902300, 1.264583334016147642, 1.299038105676657340 ) ) ;
#139013=CARTESIAN_POINT ( 'NONE',  ( -9.612894607289142357, 11.17379744904754801, -1.199719254218441611 ) ) ;
#139015=CARTESIAN_POINT ( 'NONE',  ( 0.6823417656249882723, 0.6760416670080898749, -1.181850606188749264 ) ) ;
#139021=CARTESIAN_POINT ( 'NONE',  ( -5.590039407536138150, 5.416134151747256986, 0.000000000000000000 ) ) ;
#139023=CARTESIAN_POINT ( 'NONE',  ( 1.499999999999990896, 8.673756432004010364, -2.614717076620595826 ) ) ;
#139026=CARTESIAN_POINT ( 'NONE',  ( -1.402160292154681736E-14, 0.2593750003414224681, -1.575800808251665908 ) ) ;
#139032=CARTESIAN_POINT ( 'NONE',  ( 0.6823417656249882723, 0.4260416670080896528, -1.181850606188749264 ) ) ;
#139034=CARTESIAN_POINT ( 'NONE',  ( -6.906989191158078079, 10.14557225873805812, -1.199719254218440723 ) ) ;
#139035=CARTESIAN_POINT ( 'NONE',  ( 9.023114925094663619, 10.48572115315399245, 1.199719254218453823 ) ) ;
#139038=CARTESIAN_POINT ( 'NONE',  ( -0.6823417656250212460, 0.8635416670080899859, 1.181850606188755259 ) ) ;
#139045=CARTESIAN_POINT ( 'NONE',  ( 5.477130870240836558, 9.333810415348903433, -0.7216878364870267237 ) ) ;
#139048=CARTESIAN_POINT ( 'NONE',  ( -4.548924232584923288, 5.265832011892554121, -1.199719254218446718 ) ) ;
#139049=CARTESIAN_POINT ( 'NONE',  ( 1.499999999999822586, 7.388542872122531691, 4.154462424328221104 ) ) ;
#139052=CARTESIAN_POINT ( 'NONE',  ( 4.595850884908202261, 7.345281218159464665, -1.082531754730549078 ) ) ;
#139053=CARTESIAN_POINT ( 'NONE',  ( -9.300530188850304469, 9.952966096521256745, 1.040834085586084257E-14 ) ) ;
#139055=CARTESIAN_POINT ( 'NONE',  ( -0.7499999999999972244, 4.108333333333360038, -1.299038105676652011 ) ) ;
#139059=CARTESIAN_POINT ( 'NONE',  ( 7.944714827928033962, 12.21265836598400689, 0.7216878364870438212 ) ) ;
#139067=EDGE_LOOP ( 'NONE', ( #12879, #22652, #110766 ) ) ;
#139068=CIRCLE ( 'NONE', #45688, 0.08000000000000032085 ) ;
#139073=CARTESIAN_POINT ( 'NONE',  ( -2.432941034296860483, 5.235517099077979353, -0.8783347955927902628 ) ) ;
#139075=CARTESIAN_POINT ( 'NONE',  ( 7.524412065460039933, 10.76193592880331984, -1.082531754730537976 ) ) ;
#139076=CARTESIAN_POINT ( 'NONE',  ( 6.428537391173986038, 10.65171072301167854, 0.7998128361456462443 ) ) ;
#139077=CARTESIAN_POINT ( 'NONE',  ( -6.728924311084075960, 6.744833205886536120, 1.040834085586084257E-14 ) ) ;
#139079=CARTESIAN_POINT ( 'NONE',  ( -5.409340101728189687, 5.413244328212059031, 0.7216878364870288332 ) ) ;
#139080=CARTESIAN_POINT ( 'NONE',  ( 4.528060117284232966, 6.305822774963486310, 1.443375672974062551 ) ) ;
#139082=CARTESIAN_POINT ( 'NONE',  ( -8.676855123066030018, 9.225345186439589895, -0.7216878364870267237 ) ) ;
#139104=CARTESIAN_POINT ( 'NONE',  ( 0.5221183067616939066, 7.970647359861179559, 1.933437843119054866 ) ) ;
#139107=CARTESIAN_POINT ( 'NONE',  ( -5.038826645773246682, 9.030381520044109322, 0.7998128361456481317 ) ) ;
#139113=CARTESIAN_POINT ( 'NONE',  ( 4.390142812726693045, 4.016254791136236513, 1.214306433183764966E-14 ) ) ;
#139119=CARTESIAN_POINT ( 'NONE',  ( -4.603156847039612920, 5.329103395422994716, 1.199719254218462483 ) ) ;
#139122=CARTESIAN_POINT ( 'NONE',  ( 7.396136491454752715, 8.587579647240744407, 1.199719254218462483 ) ) ;
#139123=CARTESIAN_POINT ( 'NONE',  ( 0.6823417656249899377, 3.676041667008085767, -1.181850606188754593 ) ) ;
#139125=CARTESIAN_POINT ( 'NONE',  ( 5.497327176576959573, 6.424397595302826502, 1.252573174869066941 ) ) ;
#139130=CARTESIAN_POINT ( 'NONE',  ( 6.114364089638798738, 6.235772314107808079, 0.7216878364870317197 ) ) ;
#139131=CARTESIAN_POINT ( 'NONE',  ( -8.369460898337653276, 8.658792557682392754, 0.7998128361456462443 ) ) ;
#139134=CARTESIAN_POINT ( 'NONE',  ( -7.133561379084627063, 11.47423870890741782, 0.7998128361456481317 ) ) ;
#139135=CARTESIAN_POINT ( 'NONE',  ( -6.738566041191992539, 7.820414121934134322, 1.199719254218450271 ) ) ;
#139139=CARTESIAN_POINT ( 'NONE',  ( -1.499999999999981126, 3.410416667349486897, -0.8660254037844499209 ) ) ;
#139143=CARTESIAN_POINT ( 'NONE',  ( 7.293396569147545527, 10.59638086639245280, 1.199719254218460707 ) ) ;
#139150=CARTESIAN_POINT ( 'NONE',  ( 2.737856954955798727, 5.281584649835344258, 1.199719254218452047 ) ) ;
#139157=CARTESIAN_POINT ( 'NONE',  ( -0.7500000000000215383, 4.941666666666684193, 1.299038105676671107 ) ) ;
#139158=CARTESIAN_POINT ( 'NONE',  ( 3.974511587100456822, 7.788680618259193444, 1.040834085586084257E-14 ) ) ;
#139159=CARTESIAN_POINT ( 'NONE',  ( 6.551614543901692400, 8.666636272683888365, 1.599625672291281386 ) ) ;
#139161=CARTESIAN_POINT ( 'NONE',  ( -7.361714222540411967, 11.53249099303175385, 0.000000000000000000 ) ) ;
#139163=CARTESIAN_POINT ( 'NONE',  ( 7.456621297836082185, 7.801739057004660971, 0.7216878364870317197 ) ) ;
#139164=CARTESIAN_POINT ( 'NONE',  ( -7.985389288324685531, 12.26011190311341537, -0.7216878364870267237 ) ) ;
#139167=CARTESIAN_POINT ( 'NONE',  ( 8.762647353133951711, 9.117510088278095282, 1.040834085586084257E-14 ) ) ;
#139172=DIRECTION ( 'NONE',  ( 1.000000000000000000, 0.000000000000000000, 0.000000000000000000 ) ) ;
#139173=CARTESIAN_POINT ( 'NONE',  ( 1.364683531249988535, 1.863541667008086211, 0.7879004041258500513 ) ) ;
#139179=CARTESIAN_POINT ( 'NONE',  ( 10.58621901417202515, 11.24501035948919991, -0.7998128361456281477 ) ) ;
#139183=CARTESIAN_POINT ( 'NONE',  ( -7.967387826325084355, 12.44703623068796361, 0.7998128361456481317 ) ) ;
#139189=CARTESIAN_POINT ( 'NONE',  ( 3.999819011231439347, 4.625209253646830554, 1.199719254218464037 ) ) ;
#139192=CARTESIAN_POINT ( 'NONE',  ( -9.236128959407555072, 11.79856975744075598, -1.599625672291263179 ) ) ;
#139196=CARTESIAN_POINT ( 'NONE',  ( 7.801827329660018684, 11.18955008699033726, 1.199719254218460707 ) ) ;
#139198=CARTESIAN_POINT ( 'NONE',  ( 4.464323212750023195, 7.049731028713583925, 1.131627047429624167 ) ) ;
#139200=CARTESIAN_POINT ( 'NONE',  ( -3.741160322367112379, 6.452105245148518797, 1.199719254218464037 ) ) ;
#139204=CARTESIAN_POINT ( 'NONE',  ( 7.564559641420864899, 10.91273778404466199, -1.199719254218446718 ) ) ;
#139206=CARTESIAN_POINT ( 'NONE',  ( 7.019370843573166319, 9.212351955633947043, 1.599625672291281386 ) ) ;
#139217=CARTESIAN_POINT ( 'NONE',  ( -4.744851797206062649, 6.824086272657805985, -1.238183395270262999 ) ) ;
#139219=CARTESIAN_POINT ( 'NONE',  ( 6.480434237652132445, 7.623223367758051872, 1.082531754730558626 ) ) ;
#139223=CARTESIAN_POINT ( 'NONE',  ( -3.022498986271275001, 2.800000000000024691, 2.500000000000011102 ) ) ;
#139225=EDGE_CURVE ( 'NONE', #92745, #148246, #157723, .T. ) ;
#139237=CARTESIAN_POINT ( 'NONE',  ( -10.10046125205658463, 11.84658821789661509, -1.082531754730537976 ) ) ;
#139242=CARTESIAN_POINT ( 'NONE',  ( 8.121497709785879593, 9.433834401960398353, -1.199719254218445830 ) ) ;
#139246=CARTESIAN_POINT ( 'NONE',  ( -1.500000000000015099, 1.160416667349484898, -0.8660254037844313801 ) ) ;
#139248=CARTESIAN_POINT ( 'NONE',  ( -7.043624497499477499, 8.176315654292865887, 1.199719254218450271 ) ) ;
#139251=CARTESIAN_POINT ( 'NONE',  ( -8.611400122974211868, 13.19838391011195888, 1.040834085586084257E-14 ) ) ;
#139255=CARTESIAN_POINT ( 'NONE',  ( 1.499999999999990896, 5.306250000682820378, 1.214306433183764966E-14 ) ) ;
#139256=B_SPLINE_CURVE_WITH_KNOTS ( 'NONE', 3,
 ( #63938, #198185, #199241, #50888, #165704, #83368 ),
 .UNSPECIFIED., .F., .F.,
 ( 4, 2, 4 ),
 ( 5.135960789614000585E-18, 0.001422024648551338099, 0.002844049297102670994 ),
 .UNSPECIFIED. ) ;
#139257=CARTESIAN_POINT ( 'NONE',  ( 6.428537391173986038, 10.65171072301167854, 0.7998128361456462443 ) ) ;
#139260=AXIS2_PLACEMENT_3D ( 'NONE', #212326, #165730, #179856 ) ;
#139261=CARTESIAN_POINT ( 'NONE',  ( -7.725448601688521322, 7.907444878258402809, 1.040834085586084257E-14 ) ) ;
#139263=CARTESIAN_POINT ( 'NONE',  ( 1.364683531249988535, 5.155208333674749177, -0.7879004041258300672 ) ) ;
#139269=CARTESIAN_POINT ( 'NONE',  ( -6.860062538834774237, 10.94723069537516302, 0.7216878364870458196 ) ) ;
#139273=CARTESIAN_POINT ( 'NONE',  ( -1.364683531250012516, 4.551041667008082214, -0.7879004041258300672 ) ) ;
#139279=CARTESIAN_POINT ( 'NONE',  ( 0.6823417656249917140, 3.842708333674754506, 1.181850606188765695 ) ) ;
#139282=CARTESIAN_POINT ( 'NONE',  ( -3.262708522383007903, 6.958243709422141876, 1.040834085586084257E-14 ) ) ;
#139283=CARTESIAN_POINT ( 'NONE',  ( 6.745345117998789775, 7.828323044875442172, 1.199719254218462483 ) ) ;
#139286=CARTESIAN_POINT ( 'NONE',  ( 3.917943204224906939, 5.594019709727598766, -1.443375672974051449 ) ) ;
#139287=CARTESIAN_POINT ( 'NONE',  ( -1.364683531250010295, 5.342708333674750953, 0.7879004041258379498 ) ) ;
#139292=CARTESIAN_POINT ( 'NONE',  ( 0.6823417656249882723, 0.6760416670080898749, -1.181850606188749264 ) ) ;
#139293=CARTESIAN_POINT ( 'NONE',  ( -2.629918611371007575, 6.012062780000711371, 0.7216878364870317197 ) ) ;
#139294=CARTESIAN_POINT ( 'NONE',  ( 4.150767584078112193, 7.994312614733129152, 0.7998128361456321445 ) ) ;
#139295=ORIENTED_EDGE ( 'NONE', *, *, #52572, .F. ) ;
#139300=CARTESIAN_POINT ( 'NONE',  ( 3.660338286009610975, 6.253849852777763729, -1.082531754730543083 ) ) ;
#139303=CARTESIAN_POINT ( 'NONE',  ( -8.866669273657352690, 9.446795028796142191, 0.7216878364870438212 ) ) ;
#139308=CARTESIAN_POINT ( 'NONE',  ( -8.136864746495904299, 12.64475930422059768, -0.7998128361456281477 ) ) ;
#139309=CARTESIAN_POINT ( 'NONE',  ( -5.056828107772860292, 6.922718763866881453, -1.443375672974051449 ) ) ;
#139311=CARTESIAN_POINT ( 'NONE',  ( -1.364683531250014514, 0.3427083336747508424, 0.7879004041258379498 ) ) ;
#139321=ORIENTED_EDGE ( 'NONE', *, *, #73148, .F. ) ;
#139322=CARTESIAN_POINT ( 'NONE',  ( 9.070041577417981671, 9.684062716516882219, -0.7216878364870197293 ) ) ;
#139327=ORIENTED_EDGE ( 'NONE', *, *, #66049, .T. ) ;
#139329=ORIENTED_EDGE ( 'NONE', *, *, #38831, .T. ) ;
#139333=CARTESIAN_POINT ( 'NONE',  ( -2.117044542028253318, 5.621635732341564662, -0.7998128361456281477 ) ) ;
#139336=CARTESIAN_POINT ( 'NONE',  ( 1.364683531249988535, 3.467708333674749621, -0.7879004041258239610 ) ) ;
#139338=B_SPLINE_CURVE_WITH_KNOTS ( 'NONE', 3,
 ( #143453, #62169, #208391, #212657, #79476, #194291 ),
 .UNSPECIFIED., .F., .F.,
 ( 4, 2, 4 ),
 ( 1.685978275629812889E-15, 0.0001724549256341273700, 0.0003449098512665687514 ),
 .UNSPECIFIED. ) ;
#139346=CARTESIAN_POINT ( 'NONE',  ( -1.364683531250000748, 1.759375000341421913, 0.000000000000000000 ) ) ;
#139356=CARTESIAN_POINT ( 'NONE',  ( 6.017121246366603060, 5.914396297049491658, 1.040834085586084257E-14 ) ) ;
#139366=CARTESIAN_POINT ( 'NONE',  ( 7.262363838414439776, 11.62450824479221900, 0.7998128361456462443 ) ) ;
#139369=CARTESIAN_POINT ( 'NONE',  ( 1.546240757466833093, 8.694816975860053532, -2.507471980975701342 ) ) ;
#139377=CARTESIAN_POINT ( 'NONE',  ( -7.212574532790092974, 10.39812547402169862, -1.082531754730543971 ) ) ;
#139383=CARTESIAN_POINT ( 'NONE',  ( -9.996439331977562404, 10.55693406359564790, 0.7998128361456462443 ) ) ;
#139389=CARTESIAN_POINT ( 'NONE',  ( 9.856941372335116469, 11.45851867493453291, 1.199719254218450271 ) ) ;
#139391=CARTESIAN_POINT ( 'NONE',  ( 4.599240423533799138, 6.388866465587984322, 1.599625672291267398 ) ) ;
#139398=CARTESIAN_POINT ( 'NONE',  ( -6.905180308061733996, 6.950465202360470052, 0.7998128361456341429 ) ) ;
#139401=CARTESIAN_POINT ( 'NONE',  ( -2.449219305563052895, 6.009172956465517856, 1.040834085586084257E-14 ) ) ;
#139402=CARTESIAN_POINT ( 'NONE',  ( -1.580000000000025828, -1.099999999999976108, 2.579999999999999183 ) ) ;
#139407=CARTESIAN_POINT ( 'NONE',  ( 8.975134502566660899, 10.53370701015836275, -1.082531754730543083 ) ) ;
#139409=CARTESIAN_POINT ( 'NONE',  ( -1.001543065824772872E-14, 4.634375000341418804, 1.575800808251672791 ) ) ;
#139411=CIRCLE ( 'NONE', #4530, 3.971937515251341644 ) ;
#139412=CARTESIAN_POINT ( 'NONE',  ( 6.173040012923759257, 6.096301524699504704, -0.7998128361456281477 ) ) ;
#139424=ORIENTED_EDGE ( 'NONE', *, *, #48451, .T. ) ;
#139426=CARTESIAN_POINT ( 'NONE',  ( -1.364683531250014514, 0.8010416670080889867, -0.7879004041258289570 ) ) ;
#139428=CARTESIAN_POINT ( 'NONE',  ( 10.37606763316019531, 10.99983374830873650, 0.7998128361456462443 ) ) ;
#139430=CARTESIAN_POINT ( 'NONE',  ( -5.829642864196175722, 7.824335979694092558, 1.443375672974064550 ) ) ;
#139431=CARTESIAN_POINT ( 'NONE',  ( 4.744990575102895569, 5.598539094783909320, -1.082531754730548412 ) ) ;
#139432=CARTESIAN_POINT ( 'NONE',  ( -6.114364089638801403, 8.156510742710487705, 1.443375672974078761 ) ) ;
#139437=CARTESIAN_POINT ( 'NONE',  ( 3.988069740714122791, 7.804498464141805592, 0.7998128361456321445 ) ) ;
#139447=CARTESIAN_POINT ( 'NONE',  ( 4.971035877704902184, 8.951292290631053916, 1.040834085586084257E-14 ) ) ;
#139450=AXIS2_PLACEMENT_3D ( 'NONE', #49228, #132630, #16688 ) ;
#139452=CARTESIAN_POINT ( 'NONE',  ( -7.576308911938196999, 7.733448573549685179, 0.7998128361456462443 ) ) ;
#139456=CARTESIAN_POINT ( 'NONE',  ( 6.913768267964901071, 10.15348118167935709, -1.199719254218441611 ) ) ;
#139459=CARTESIAN_POINT ( 'NONE',  ( -5.038826645773246682, 9.030381520044109322, 0.7998128361456481317 ) ) ;
#139461=CARTESIAN_POINT ( 'NONE',  ( 5.951666246274792016, 8.927065806420504401, 1.082531754730558626 ) ) ;
#139462=CARTESIAN_POINT ( 'NONE',  ( 5.291954866116698852, 6.573566887673666592, 1.361072633976003310 ) ) ;
#139464=CARTESIAN_POINT ( 'NONE',  ( -4.629219384062206011, 7.488174150459498968, -1.199719254218452047 ) ) ;
#139468=CARTESIAN_POINT ( 'NONE',  ( -6.735703387890906946, 6.752742128827836865, -0.7998128361456291469 ) ) ;
#139472=CARTESIAN_POINT ( 'NONE',  ( 8.703444544968814256, 12.24143683818393313, -1.199719254218446718 ) ) ;
#139474=CARTESIAN_POINT ( 'NONE',  ( -0.6823417656250003738, 1.717708333674752730, -1.181850606188749264 ) ) ;
#139476=CARTESIAN_POINT ( 'NONE',  ( -6.426201623197489887, 6.599582769926260362, 0.7216878364870317197 ) ) ;
#139481=CARTESIAN_POINT ( 'NONE',  ( 5.632522751473472589, 8.658694745772667289, -1.199719254218440723 ) ) ;
#139484=CARTESIAN_POINT ( 'NONE',  ( -5.899175937014327076, 6.007822909898694164, -0.1935691424272238670 ) ) ;
#139485=CARTESIAN_POINT ( 'NONE',  ( 1.364683531249988757, 1.446875000341421469, 0.000000000000000000 ) ) ;
#139488=CARTESIAN_POINT ( 'NONE',  ( 3.497640442645619796, 6.064035702186436616, -1.082531754730543083 ) ) ;
#139491=CARTESIAN_POINT ( 'NONE',  ( -5.786632634934295361, 5.645492917045106473, 0.7998128361456341429 ) ) ;
#139493=CARTESIAN_POINT ( 'NONE',  ( -8.473482818416675499, 9.948446711983361723, -1.082531754730543083 ) ) ;
#139501=CARTESIAN_POINT ( 'NONE',  ( -8.365017589507372620, 9.821903944922480534, 1.082531754730558626 ) ) ;
#139506=CARTESIAN_POINT ( 'NONE',  ( -6.168596704093453731, 10.14052055484361325, 0.7216878364870458196 ) ) ;
#139512=CARTESIAN_POINT ( 'NONE',  ( -0.7499999999999972244, 5.139583334016151639, -1.299038105676652899 ) ) ;
#139513=CARTESIAN_POINT ( 'NONE',  ( 4.774589472192324102, 6.991777125168484375, -1.402305405395011251 ) ) ;
#139515=CARTESIAN_POINT ( 'NONE',  ( -1.436716030283634371, 7.421837552815579109, -4.237608343040895953 ) ) ;
#139520=CARTESIAN_POINT ( 'NONE',  ( -5.669280788808708671, 9.765911353585494226, 0.7998128361456481317 ) ) ;
#139523=CARTESIAN_POINT ( 'NONE',  ( 5.183294799126148433, 4.941598775268944976, 1.040834085586084257E-14 ) ) ;
#139527=CARTESIAN_POINT ( 'NONE',  ( 7.657657833620182153, 7.828355648845348291, -0.7998128361456281477 ) ) ;
#139534=CARTESIAN_POINT ( 'NONE',  ( -6.426201623197489887, 6.599582769926260362, 0.7216878364870317197 ) ) ;
#139539=CARTESIAN_POINT ( 'NONE',  ( -0.1263102688159843945, 6.363441598446243574, 3.117922131261606999 ) ) ;
#139540=DIRECTION ( 'NONE',  ( 0.000000000000000000, 8.546850786086437571E-32, 1.000000000000000000 ) ) ;
#139544=CARTESIAN_POINT ( 'NONE',  ( -0.6823417656250246877, 0.3010416670080895418, 1.181850606188755259 ) ) ;
#139545=DIRECTION ( 'NONE',  ( 0.000000000000000000, 1.000000000000000000, -8.546850786086437571E-32 ) ) ;
#139546=CARTESIAN_POINT ( 'NONE',  ( -9.013473194986783454, 9.410140237106395134, -0.7998128361456291469 ) ) ;
#139548=CARTESIAN_POINT ( 'NONE',  ( 8.555358625423188812, 9.940005470203933768, 1.199719254218462483 ) ) ;
#139550=CARTESIAN_POINT ( 'NONE',  ( -8.864333505236459132, 9.236143932397675727, 1.040834085586084257E-14 ) ) ;
#139553=CARTESIAN_POINT ( 'NONE',  ( -0.6823417656250212460, 5.051041667008086655, 1.181850606188767472 ) ) ;
#139555=CARTESIAN_POINT ( 'NONE',  ( 7.917598520700710019, 12.18102267421877727, -0.7216878364870328300 ) ) ;
#139558=CARTESIAN_POINT ( 'NONE',  ( 0.6823417656249882723, -0.3447916663252489911, 1.181850606188755259 ) ) ;
#139561=CARTESIAN_POINT ( 'NONE',  ( 7.497295758232718654, 9.769931022736756177, -1.443375672974058777 ) ) ;
#139564=CARTESIAN_POINT ( 'NONE',  ( -5.422898255786198440, 7.349800603215774331, -1.443375672974052559 ) ) ;
#139566=CARTESIAN_POINT ( 'NONE',  ( 0.6823417656249882723, 2.176041667008084435, -1.181850606188749264 ) ) ;
#139570=CARTESIAN_POINT ( 'NONE',  ( -6.669721502918952716, 9.868759955792373972, 1.199719254218452047 ) ) ;
#139571=CARTESIAN_POINT ( 'NONE',  ( -1.364683531250012516, 4.551041667008082214, -0.7879004041258300672 ) ) ;
#139577=CARTESIAN_POINT ( 'NONE',  ( 9.108380270282433244, 9.520865158284665952, 1.040834085586084257E-14 ) ) ;
#139580=CARTESIAN_POINT ( 'NONE',  ( 1.499999999999987121, 1.545833333333354487, -0.8660254037844253849 ) ) ;
#139586=CARTESIAN_POINT ( 'NONE',  ( 7.782016984564060103, 9.141736572488651902, 1.082531754730558626 ) ) ;
#139587=EDGE_CURVE ( 'NONE', #137371, #201176, #198073, .T. ) ;
#139596=CARTESIAN_POINT ( 'NONE',  ( 9.426996880203592610, 9.892584536526015881, -0.7998128361456281477 ) ) ;
#139597=CARTESIAN_POINT ( 'NONE',  ( -8.130085669689073313, 12.63685038127928806, 0.7998128361456481317 ) ) ;
#139600=DIRECTION ( 'NONE',  ( -5.578564026256491869E-16, -1.000000000000000000, -9.066213480720160632E-32 ) ) ;
#139601=CARTESIAN_POINT ( 'NONE',  ( -1.364683531250012516, 0.5302083336747518416, 0.7879004041258379498 ) ) ;
#139602=CARTESIAN_POINT ( 'NONE',  ( 1.499999999999987121, 1.754166666666691521, 0.8660254037844524744 ) ) ;
#139604=CARTESIAN_POINT ( 'NONE',  ( 6.484877546038077867, 6.460111979999551224, 1.040834085586084257E-14 ) ) ;
#139607=CIRCLE ( 'NONE', #205271, 0.08000000000000004330 ) ;
#139611=CARTESIAN_POINT ( 'NONE',  ( 1.364683531249990311, 4.863541667008084879, 0.7879004041258500513 ) ) ;
#139613=CARTESIAN_POINT ( 'NONE',  ( -9.508345801885592863, 9.987491611821676329, 0.7998128361456462443 ) ) ;
#139614=CARTESIAN_POINT ( 'NONE',  ( -6.236387472606166327, 6.378132927569716060, -0.7216878364870278340 ) ) ;
#139622=CARTESIAN_POINT ( 'NONE',  ( 6.642605195691581699, 9.837124264027149678, 1.199719254218462483 ) ) ;
#139626=CARTESIAN_POINT ( 'NONE',  ( 7.415946836550714849, 9.675023947441092176, 1.443375672974076540 ) ) ;
#139629=CARTESIAN_POINT ( 'NONE',  ( -9.494787648271923786, 9.971673765939062406, 1.040834085586084257E-14 ) ) ;
#139630=CARTESIAN_POINT ( 'NONE',  ( 5.198661835836162481, 8.152523677529138979, 1.199719254218462483 ) ) ;
#139633=FACE_OUTER_BOUND ( 'NONE', #89481, .T. ) ;
#139634=CARTESIAN_POINT ( 'NONE',  ( 2.361091307074211887, 5.906356958228550447, 0.7998128361456462443 ) ) ;
#139642=CARTESIAN_POINT ( 'NONE',  ( -4.717874267875590277, 7.487641831621378863, 1.082531754730560403 ) ) ;
#139643=CARTESIAN_POINT ( 'NONE',  ( 3.440018289565364817, 5.036440642624797626, 1.599625672291267398 ) ) ;
#139647=CARTESIAN_POINT ( 'NONE',  ( -6.344325816190970357, 9.489131654609717970, 1.199719254218452047 ) ) ;
#139652=CARTESIAN_POINT ( 'NONE',  ( -8.076906825439122528, 10.44614393447756129, -1.599625672291263179 ) ) ;
#139658=CARTESIAN_POINT ( 'NONE',  ( 5.823390672269506574, 6.752709524857930745, -1.199719254218446718 ) ) ;
#139659=CARTESIAN_POINT ( 'NONE',  ( -3.697672731464866747, 7.367968498737385019, -2.499999999999995115 ) ) ;
#139669=CARTESIAN_POINT ( 'NONE',  ( -6.018930129462987999, 9.109503353427070849, 1.199719254218452047 ) ) ;
#139672=CARTESIAN_POINT ( 'NONE',  ( 6.317736394288147039, 6.473040002865377396, 0.7216878364870317197 ) ) ;
#139675=CARTESIAN_POINT ( 'NONE',  ( 4.111146893441827821, 5.819424013814004759, 1.599625672291267398 ) ) ;
#139677=CARTESIAN_POINT ( 'NONE',  ( -3.764360206088648297, 7.543504007078730922, -0.7998128361456281477 ) ) ;
#139681=CARTESIAN_POINT ( 'NONE',  ( 0.7499999999999920064, 5.514583334016151639, 1.299038105676669330 ) ) ;
#139682=CARTESIAN_POINT ( 'NONE',  ( -5.032047568966410367, 9.022472597102808578, 1.214306433183764966E-14 ) ) ;
#139683=CARTESIAN_POINT ( 'NONE',  ( -1.201851678989727383E-14, 3.337500000000019007, -1.732050807568863648 ) ) ;
#139688=CARTESIAN_POINT ( 'NONE',  ( -10.66756793585402363, 11.33991743478486391, 0.7998128361456462443 ) ) ;
#139689=CARTESIAN_POINT ( 'NONE',  ( 6.154511665599609493, 9.267681812253174556, 1.199719254218462483 ) ) ;
#139692=CARTESIAN_POINT ( 'NONE',  ( -5.639314450680645407, 6.167449467472198243, -0.8320033040390877321 ) ) ;
#139697=EDGE_LOOP ( 'NONE', ( #171394, #60859, #136749, #184137 ) ) ;
#139699=CARTESIAN_POINT ( 'NONE',  ( 10.38518247838791986, 11.21839376764850726, 0.7216878364870438212 ) ) ;
#139718=CARTESIAN_POINT ( 'NONE',  ( -4.243865776277440993, 4.909930479533815451, -1.199719254218446718 ) ) ;
#139722=CARTESIAN_POINT ( 'NONE',  ( -4.620631424159025613, 4.285158171140619032, -0.7998128361456221525 ) ) ;
#139727=CARTESIAN_POINT ( 'NONE',  ( -1.402160292154681736E-14, -0.7562499993171803991, 1.732050807568877637 ) ) ;
#139733=ORIENTED_EDGE ( 'NONE', *, *, #177164, .T. ) ;
#139736=CARTESIAN_POINT ( 'NONE',  ( 2.693266070609028784, 6.293894182352508970, 0.000000000000000000 ) ) ;
#139740=CARTESIAN_POINT ( 'NONE',  ( 8.554831740098642001, 12.92446143018304916, 0.7216878364870438212 ) ) ;
#139742=CARTESIAN_POINT ( 'NONE',  ( 0.6823417656249882723, 0.9885416670080832136, -1.181850606188749264 ) ) ;
#139746=CARTESIAN_POINT ( 'NONE',  ( -9.820183334999905256, 10.35130206712171130, 1.040834085586084257E-14 ) ) ;
#139747=CARTESIAN_POINT ( 'NONE',  ( -4.392478580703220281, 8.068382744221649361, 1.040834085586084257E-14 ) ) ;
#139749=CARTESIAN_POINT ( 'NONE',  ( -4.855791571988752331, 8.816840600628864877, 0.7998128361456481317 ) ) ;
#139751=CARTESIAN_POINT ( 'NONE',  ( 1.499999999999987566, -1.193749999317185395, 0.000000000000000000 ) ) ;
#139760=CARTESIAN_POINT ( 'NONE',  ( -5.056828107772852299, 7.883087978168217269, -1.082531754730548412 ) ) ;
#139764=CARTESIAN_POINT ( 'NONE',  ( -5.544921637864838715, 6.531792001339513654, -1.082531754730543971 ) ) ;
#139766=CARTESIAN_POINT ( 'NONE',  ( 8.723781775389312543, 12.26516360700784958, -1.199719254218446718 ) ) ;
#139774=CARTESIAN_POINT ( 'NONE',  ( -2.903417451620861289, 6.539070793532962611, 0.7998128361456341429 ) ) ;
#139775=CARTESIAN_POINT ( 'NONE',  ( -9.001723924469462901, 12.58942944760136484, -1.199719254218446718 ) ) ;
#139780=CARTESIAN_POINT ( 'NONE',  ( 8.270110514656026979, 10.67154823856396817, 1.443375672974076540 ) ) ;
#139781=CARTESIAN_POINT ( 'NONE',  ( 5.307127064745490230, 8.279066444590018392, -1.199719254218452935 ) ) ;
#139786=CARTESIAN_POINT ( 'NONE',  ( 3.683011284406639607, 7.448596931783069586, 0.7998128361456321445 ) ) ;
#139796=CARTESIAN_POINT ( 'NONE',  ( -5.052384799386910430, 9.046199365926717917, 1.214306433183764966E-14 ) ) ;
#139803=CARTESIAN_POINT ( 'NONE',  ( 1.364683531249988535, 5.155208333674749177, -0.7879004041258300672 ) ) ;
#139805=CARTESIAN_POINT ( 'NONE',  ( -6.423865854776591000, 6.388931673527803667, 1.040834085586084257E-14 ) ) ;
#139808=CARTESIAN_POINT ( 'NONE',  ( 6.166260936116925606, 6.088392601758203071, 0.7998128361456341429 ) ) ;
#139809=CARTESIAN_POINT ( 'NONE',  ( -4.401593425930945713, 8.286942763561420122, 1.040834085586084257E-14 ) ) ;
#139815=CARTESIAN_POINT ( 'NONE',  ( 6.317736394288135493, 8.393778431468064127, 1.443375672974076540 ) ) ;
#139817=CARTESIAN_POINT ( 'NONE',  ( 7.144783764277405247, 8.398297815487545392, -1.082531754730543971 ) ) ;
#139818=CARTESIAN_POINT ( 'NONE',  ( -0.6823417656250212460, 2.863541667008084879, 1.181850606188767472 ) ) ;
#139819=CARTESIAN_POINT ( 'NONE',  ( 3.836594282542902246, 7.419851063034623273, 0.7216878364870317197 ) ) ;
#139821=DIRECTION ( 'NONE',  ( 0.7592566023652994600, -0.6507913734559651608, -0.000000000000000000 ) ) ;
#139822=CARTESIAN_POINT ( 'NONE',  ( -3.145128448690323264, 4.692402494937224056, -1.443375672974059665 ) ) ;
#139830=CARTESIAN_POINT ( 'NONE',  ( -4.645415345243833372, 7.101964347008438594, 1.385782282575825919 ) ) ;
#139837=CARTESIAN_POINT ( 'NONE',  ( -9.073431116043565225, 11.60875560684942265, -1.599625672291263179 ) ) ;
#139841=CARTESIAN_POINT ( 'NONE',  ( -2.137381772448751605, 5.645362501165475777, -0.7998128361456281477 ) ) ;
#139846=CARTESIAN_POINT ( 'NONE',  ( 3.714570900464274850, 6.317121236308204324, 1.082531754730558626 ) ) ;
#139847=CARTESIAN_POINT ( 'NONE',  ( 1.364683531249990311, 3.446875000341416584, 1.214306433183764966E-14 ) ) ;
#139849=CARTESIAN_POINT ( 'NONE',  ( 7.052212457402625922, 11.37933163361175382, -0.7998128361456291469 ) ) ;
#139850=DIRECTION ( 'NONE',  ( -0.6507913734559640506, -0.7592566023653004592, 0.000000000000000000 ) ) ;
#139852=CARTESIAN_POINT ( 'NONE',  ( -3.242371291962510504, 6.934516940598226320, 1.040834085586084257E-14 ) ) ;
#139856=CARTESIAN_POINT ( 'NONE',  ( -1.500000000000013101, 3.379166666666691299, -0.8660254037844313801 ) ) ;
#139857=CARTESIAN_POINT ( 'NONE',  ( 5.834086172582112262, 5.700855377634248100, 1.040834085586084257E-14 ) ) ;
#139861=CARTESIAN_POINT ( 'NONE',  ( -1.364683531250012516, 3.530208333674758059, 0.7879004041258379498 ) ) ;
#139864=CARTESIAN_POINT ( 'NONE',  ( 10.22248463502393001, 11.02857961705718282, 0.7216878364870438212 ) ) ;
#139869=CARTESIAN_POINT ( 'NONE',  ( -1.500000000000013101, 2.702083334016155636, 0.8660254037844403729 ) ) ;
#139871=CARTESIAN_POINT ( 'NONE',  ( -6.552668314106420588, 6.539201209412602189, -0.7998128361456291469 ) ) ;
#139880=CARTESIAN_POINT ( 'NONE',  ( 6.923409998072794558, 11.22906209772695618, 1.040834085586084257E-14 ) ) ;
#139881=CARTESIAN_POINT ( 'NONE',  ( 5.497994985541524215, 6.373081223675282736, -1.199719254218445830 ) ) ;
#139884=FACE_OUTER_BOUND ( 'NONE', #155963, .T. ) ;
#139885=CARTESIAN_POINT ( 'NONE',  ( 6.654354466208897811, 6.657835053532175529, 0.7998128361456341429 ) ) ;
#139892=CARTESIAN_POINT ( 'NONE',  ( 10.71502147350184231, 11.39527989537399755, 0.000000000000000000 ) ) ;
#139897=CARTESIAN_POINT ( 'NONE',  ( 5.849510849484250485, 6.002983934024645585, 0.3487602046992159810 ) ) ;
#139903=CARTESIAN_POINT ( 'NONE',  ( 1.499999999999985789, -1.099999999999976108, 2.579999999999999183 ) ) ;
#139908=AXIS2_PLACEMENT_3D ( 'NONE', #134055, #51715, #164384 ) ;
#139909=CARTESIAN_POINT ( 'NONE',  ( 7.348156068926750883, 8.635565504245116486, -1.082531754730537976 ) ) ;
#139911=CARTESIAN_POINT ( 'NONE',  ( -3.253066792275140173, 5.882662793374543675, 1.199719254218462483 ) ) ;
#139915=CARTESIAN_POINT ( 'NONE',  ( -6.715366157470410435, 6.729015360003925750, -0.7998128361456291469 ) ) ;
#139932=CARTESIAN_POINT ( 'NONE',  ( 10.01963921569910632, 11.64833282552586091, 1.199719254218450271 ) ) ;
#139935=CARTESIAN_POINT ( 'NONE',  ( 2.223174002961016082, 5.537527403522402025, -0.7216878364870267237 ) ) ;
#139940=CARTESIAN_POINT ( 'NONE',  ( -9.707274797704657843, 11.38787068781932987, 1.082531754730558626 ) ) ;
#139942=DIRECTION ( 'NONE',  ( 0.000000000000000000, 8.546850786086437571E-32, 1.000000000000000000 ) ) ;
#139944=CARTESIAN_POINT ( 'NONE',  ( 9.088043039861931405, 9.497138389460751284, 1.040834085586084257E-14 ) ) ;
#139948=CARTESIAN_POINT ( 'NONE',  ( -7.660520486921249983, 8.896027641951645748, -1.199719254218446718 ) ) ;
#139949=CARTESIAN_POINT ( 'NONE',  ( 4.147904930777053245, 6.926640621626830807, -1.199719254218452047 ) ) ;
#139952=CARTESIAN_POINT ( 'NONE',  ( 9.999301985278609806, 11.62460605670194447, 1.199719254218452047 ) ) ;
#139956=CARTESIAN_POINT ( 'NONE',  ( 0.6823417656249899377, 2.655208333674753618, 1.181850606188767472 ) ) ;
#139958=EDGE_LOOP ( 'NONE', ( #178218, #65309, #50184, #91391, #132330, #123343, #35812, #20393, #81373, #29199, #155674, #53903, #91264, #47942, #47523, #142198, #140598, #68293, #97010, #29552, #105146, #95018, #45488, #86947, #193013 ) ) ;
#139960=CARTESIAN_POINT ( 'NONE',  ( 6.697364695470787943, 7.876308901879812474, -1.082531754730543083 ) ) ;
#139967=ORIENTED_EDGE ( 'NONE', *, *, #8949, .T. ) ;
#139969=CARTESIAN_POINT ( 'NONE',  ( 9.544576953896278582, 10.23768732240824164, 0.000000000000000000 ) ) ;
#139974=CARTESIAN_POINT ( 'NONE',  ( -9.664264568442742842, 10.16939683947169115, -0.7998128361456291469 ) ) ;
#139983=CARTESIAN_POINT ( 'NONE',  ( 3.842846474469570062, 6.570739089268092137, -1.199719254218452047 ) ) ;
#139990=CARTESIAN_POINT ( 'NONE',  ( 5.769158057814842699, 6.689438141327490150, 1.199719254218462483 ) ) ;
#139993=CARTESIAN_POINT ( 'NONE',  ( -1.201851678989727383E-14, 3.368750000682815049, -1.732050807568863648 ) ) ;
#139999=CARTESIAN_POINT ( 'NONE',  ( -1.402160292154681736E-14, 0.3375000000000208389, -1.732050807568870754 ) ) ;
#140000=CARTESIAN_POINT ( 'NONE',  ( 6.401421083946654100, 10.62007503124645957, -0.7998128361456291469 ) ) ;
#140001=CARTESIAN_POINT ( 'NONE',  ( -1.402160292154681736E-14, -0.3031249996585801965, -1.575800808251665908 ) ) ;
#140004=CARTESIAN_POINT ( 'NONE',  ( 9.327646496521982300, 11.90534021740758064, -1.443375672974057666 ) ) ;
#140009=CARTESIAN_POINT ( 'NONE',  ( -5.961834861707238531, 7.978559976790334574, -1.599625672291263179 ) ) ;
#140010=CARTESIAN_POINT ( 'NONE',  ( -1.500000000000013101, 2.452083334016154748, 0.8660254037844403729 ) ) ;
#140011=CARTESIAN_POINT ( 'NONE',  ( -0.6823417656249969321, 5.780208333674756283, -1.181850606188749264 ) ) ;
#140024=CARTESIAN_POINT ( 'NONE',  ( -8.853638004923878313, 10.28799807962136548, 1.199719254218462483 ) ) ;
#140025=CARTESIAN_POINT ( 'NONE',  ( 5.849453209292126310, 8.911780279894442103, 1.199719254218462483 ) ) ;
#140033=CARTESIAN_POINT ( 'NONE',  ( -5.831978632172702071, 9.955725504176825780, 0.7998128361456481317 ) ) ;
#140038=CARTESIAN_POINT ( 'NONE',  ( 8.516493047678546091, 13.08765898893368629, -0.7998128361456352531 ) ) ;
#140039=CARTESIAN_POINT ( 'NONE',  ( 1.252085211431710698, 2.800000000000024691, 0.7750000000000152323 ) ) ;
#140041=CARTESIAN_POINT ( 'NONE',  ( -5.362413449404877852, 6.214902764849178141, -1.199719254218446718 ) ) ;
#140042=CARTESIAN_POINT ( 'NONE',  ( -7.700141177557535244, 11.07091624287075859, -1.199719254218446718 ) ) ;
#140045=CARTESIAN_POINT ( 'NONE',  ( -4.550628574872730425, 7.191434026324334816, -1.338276217581878980 ) ) ;
#140052=CARTESIAN_POINT ( 'NONE',  ( 5.412729640353754590, 7.337937218544611895, 1.599625672291267398 ) ) ;
#140056=CARTESIAN_POINT ( 'NONE',  ( 3.028993686180013079, 2.741750000184217217, 2.499999999999997335 ) ) ;
#140073=CARTESIAN_POINT ( 'NONE',  ( 2.575685996916329046, 5.948791396470269888, 0.7216878364870438212 ) ) ;
#140075=ORIENTED_EDGE ( 'NONE', *, *, #132078, .T. ) ;
#140077=CARTESIAN_POINT ( 'NONE',  ( -7.648771216403934758, 12.07531685244661723, -0.7998128361456291469 ) ) ;
#140083=CARTESIAN_POINT ( 'NONE',  ( -0.7500000000000215383, 0.7229166673494852313, 1.299038105676659116 ) ) ;
#140088=CARTESIAN_POINT ( 'NONE',  ( 4.350813900535696277, 4.000456626940672500, 0.2320863031703649382 ) ) ;
#140089=CARTESIAN_POINT ( 'NONE',  ( -1.364683531250014514, 0.2385416670080863499, -0.7879004041258359514 ) ) ;
#140095=CARTESIAN_POINT ( 'NONE',  ( -4.172158584703340445, 5.890604320285754980, -1.599625672291256295 ) ) ;
#140096=CARTESIAN_POINT ( 'NONE',  ( -0.2497763946155639181, 6.515865096501928910, -3.141954037565825253 ) ) ;
#140098=CARTESIAN_POINT ( 'NONE',  ( -0.7500000000000006661, 0.1083333333333560966, -1.299038105676652011 ) ) ;
#140100=CARTESIAN_POINT ( 'NONE',  ( 1.364683531249986537, -0.5322916663252452718, -0.7879004041258309554 ) ) ;
#140105=CARTESIAN_POINT ( 'NONE',  ( -1.402160292154681736E-14, 0.9468750003414176941, -1.575800808251659024 ) ) ;
#140107=CARTESIAN_POINT ( 'NONE',  ( -7.389357414647957256, 8.579670724299436557, 1.199719254218450271 ) ) ;
#140108=CARTESIAN_POINT ( 'NONE',  ( 8.432281472695482449, 11.92507992053172572, 1.199719254218450271 ) ) ;
#140109=CARTESIAN_POINT ( 'NONE',  ( 4.059776932288224671, 6.823824623389866950, 1.199719254218462483 ) ) ;
#140113=CARTESIAN_POINT ( 'NONE',  ( 1.364683531249986537, -0.5322916663252452718, -0.7879004041258309554 ) ) ;
#140123=CARTESIAN_POINT ( 'NONE',  ( 5.829642864196157070, 8.784705193995428374, 1.082531754730558626 ) ) ;
#140126=CARTESIAN_POINT ( 'NONE',  ( -4.717347382551060342, 7.590990148696470818, 1.199719254218464037 ) ) ;
#140130=CARTESIAN_POINT ( 'NONE',  ( -4.288456660624211381, 3.897620947016656956, 1.214306433183764966E-14 ) ) ;
#140131=CARTESIAN_POINT ( 'NONE',  ( 5.463572716182829581, 6.436884926043849653, 1.082531754730560403 ) ) ;
#140132=CARTESIAN_POINT ( 'NONE',  ( -6.846504384776750385, 10.93141284897413890, -0.7216878364870267237 ) ) ;
#140134=CARTESIAN_POINT ( 'NONE',  ( -1.500000000000013101, 3.629166666666692187, -0.8660254037844313801 ) ) ;
#140138=CARTESIAN_POINT ( 'NONE',  ( 7.931156674314368438, 12.19684052010138586, 1.040834085586084257E-14 ) ) ;
#140145=EDGE_LOOP ( 'NONE', ( #22005, #148785, #94407, #50920 ) ) ;
#140150=CYLINDRICAL_SURFACE ( 'NONE', #3835, 0.08000000000000012657 ) ;
#140151=ORIENTED_EDGE ( 'NONE', *, *, #181542, .T. ) ;
#140152=CARTESIAN_POINT ( 'NONE',  ( 8.581948047326003248, 9.114620264742901767, -0.7216878364870197293 ) ) ;
#140153=CARTESIAN_POINT ( 'NONE',  ( 7.456094412511537151, 10.78619501698377370, 1.199719254218460707 ) ) ;
#140158=FACE_OUTER_BOUND ( 'NONE', #86213, .T. ) ;
#140159=CARTESIAN_POINT ( 'NONE',  ( 3.538314903486612817, 7.071858454135611538, 1.040834085586084257E-14 ) ) ;
#140160=ORIENTED_EDGE ( 'NONE', *, *, #93332, .F. ) ;
#140162=CARTESIAN_POINT ( 'NONE',  ( -9.029367117021344313, 9.636609179387466639, 0.7216878364870438212 ) ) ;
#140166=CARTESIAN_POINT ( 'NONE',  ( -3.789667630219657912, 4.380032642466370696, 1.199719254218462483 ) ) ;
#140167=ADVANCED_FACE ( 'NONE', ( #60080 ), #175987, .F. ) ;
#140172=ORIENTED_EDGE ( 'NONE', *, *, #118661, .T. ) ;
#140192=CARTESIAN_POINT ( 'NONE',  ( -6.521635583373313061, 7.567328587812373719, -1.199719254218446718 ) ) ;
#140195=CARTESIAN_POINT ( 'NONE',  ( 4.852928918687680948, 7.749168607522574526, 1.199719254218462483 ) ) ;
#140196=FACE_OUTER_BOUND ( 'NONE', #116462, .T. ) ;
#140198=ADVANCED_FACE ( 'NONE', ( #9199 ), #160792, .F. ) ;
#140207=CARTESIAN_POINT ( 'NONE',  ( -4.060830702492950195, 4.696389560118578999, -1.199719254218452047 ) ) ;
#140211=CARTESIAN_POINT ( 'NONE',  ( 6.103141704446003679, 10.27208242182903142, 0.7998128361456462443 ) ) ;
#140214=CARTESIAN_POINT ( 'NONE',  ( 5.447554933476544292, 6.459834866240243834, 1.284201090641323040 ) ) ;
#140220=CARTESIAN_POINT ( 'NONE',  ( 7.605760987142057061, 7.975735361194951523, -0.7216878364870267237 ) ) ;
#140221=CARTESIAN_POINT ( 'NONE',  ( -6.659026002606323047, 10.92061410301605662, 0.000000000000000000 ) ) ;
#140224=CARTESIAN_POINT ( 'NONE',  ( -7.700141177557535244, 11.07091624287075859, -1.199719254218446718 ) ) ;
#140225=CARTESIAN_POINT ( 'NONE',  ( -5.930802130974132780, 9.006687355190106103, -1.199719254218440723 ) ) ;
#140229=CARTESIAN_POINT ( 'NONE',  ( 4.899944684240791659, 4.860301720779024670, 0.6505774570350670860 ) ) ;
#140232=CARTESIAN_POINT ( 'NONE',  ( 6.889514614038635187, 11.18951748302043114, -0.7998128361456291469 ) ) ;
#140238=CARTESIAN_POINT ( 'NONE',  ( 3.195971524519376494, 4.751719416737803847, -1.599625672291262513 ) ) ;
#140246=ORIENTED_EDGE ( 'NONE', *, *, #127807, .T. ) ;
#140247=CARTESIAN_POINT ( 'NONE',  ( -1.201851678989727383E-14, 4.587500000000025224, -1.732050807568863648 ) ) ;
#140248=CARTESIAN_POINT ( 'NONE',  ( 4.792970997630896512, 5.550553237779539018, 1.199719254218464037 ) ) ;
#140249=CARTESIAN_POINT ( 'NONE',  ( 6.144869935491714230, 8.192100896205568361, -1.599625672291262513 ) ) ;
#140251=CARTESIAN_POINT ( 'NONE',  ( -8.188761592974046266, 10.57664116326830595, -1.443375672974059665 ) ) ;
#140252=CARTESIAN_POINT ( 'NONE',  ( 4.386855106046934516, 4.010796903234440158, -0.04314253085381029862 ) ) ;
#140253=CARTESIAN_POINT ( 'NONE',  ( 6.317736394288135493, 8.393778431468064127, 1.443375672974076540 ) ) ;
#140254=CARTESIAN_POINT ( 'NONE',  ( -7.822691444960696572, 12.07029775252209092, -0.7216878364870267237 ) ) ;
#140258=CARTESIAN_POINT ( 'NONE',  ( 7.553864141108259211, 11.96459193126834464, 1.040834085586084257E-14 ) ) ;
#140264=CARTESIAN_POINT ( 'NONE',  ( -1.364683531250000748, 1.759375000341421913, 0.000000000000000000 ) ) ;
#140269=CARTESIAN_POINT ( 'NONE',  ( -1.364683531250014514, 0.03020833367475737191, 0.7879004041258379498 ) ) ;
#140271=CIRCLE ( 'NONE', #84880, 0.07999999999999998779 ) ;
#140272=CARTESIAN_POINT ( 'NONE',  ( 8.452618703115982512, 11.94880668935564216, 1.199719254218450271 ) ) ;
#140276=CARTESIAN_POINT ( 'NONE',  ( -8.967828540435322182, 12.54988483289483980, 1.199719254218462483 ) ) ;
#140282=CARTESIAN_POINT ( 'NONE',  ( 4.273844736805816780, 6.009238164405336313, 1.599625672291267398 ) ) ;
#140286=CARTESIAN_POINT ( 'NONE',  ( -2.453662613948990323, 5.806430783008362795, -0.7216878364870257245 ) ) ;
#140290=CARTESIAN_POINT ( 'NONE',  ( 8.422639742587595180, 10.84949900448412130, -1.599625672291268286 ) ) ;
#140292=CARTESIAN_POINT ( 'NONE',  ( 4.103641366189806128, 7.455328040159560743, 0.6459977421944228526 ) ) ;
#140294=CARTESIAN_POINT ( 'NONE',  ( -3.578462479003122976, 6.262291094557191684, 1.199719254218464037 ) ) ;
#140298=CARTESIAN_POINT ( 'NONE',  ( 6.564118927310645724, 10.80988918183778225, -0.7998128361456291469 ) ) ;
#140300=CARTESIAN_POINT ( 'NONE',  ( 7.884230021546724920, 9.157022099014721306, 1.199719254218462483 ) ) ;
#140303=CARTESIAN_POINT ( 'NONE',  ( -8.270110514656041190, 10.67154823856396817, 1.443375672974090751 ) ) ;
#140310=CARTESIAN_POINT ( 'NONE',  ( -5.157125652413038885, 6.495829312680758250, -1.199528311315662510 ) ) ;
#140311=CARTESIAN_POINT ( 'NONE',  ( 0.6823417656249882723, 1.926041667008083991, -1.181850606188749264 ) ) ;
#140313=CARTESIAN_POINT ( 'NONE',  ( 5.327991180490514012, 9.159814110640187579, 1.040834085586084257E-14 ) ) ;
#140327=CARTESIAN_POINT ( 'NONE',  ( -9.232739420781982176, 12.75498451001223010, 1.082531754730558626 ) ) ;
#140331=CARTESIAN_POINT ( 'NONE',  ( 9.423080456697809026, 10.95234760669099749, -1.199719254218446718 ) ) ;
#140335=CARTESIAN_POINT ( 'NONE',  ( -4.322352044658376968, 3.937165561723182883, 0.7998128361456341429 ) ) ;
#140336=CARTESIAN_POINT ( 'NONE',  ( -5.682838942422375084, 9.781729199468104596, 0.000000000000000000 ) ) ;
#140339=VERTEX_POINT ( 'NONE', #136711 ) ;
#140340=CARTESIAN_POINT ( 'NONE',  ( -9.755255220232635693, 11.33988483081495957, -1.199719254218441611 ) ) ;
#140344=CARTESIAN_POINT ( 'NONE',  ( -1.201851678989727383E-14, 5.118750000682815937, -1.732050807568863648 ) ) ;
#140345=CARTESIAN_POINT ( 'NONE',  ( 6.751070424600909448, 9.963667031088037973, -1.199719254218441611 ) ) ;
#140348=CARTESIAN_POINT ( 'NONE',  ( -6.042130013184518589, 10.20090211535728031, -0.7998128361456291469 ) ) ;
#140350=CARTESIAN_POINT ( 'NONE',  ( -0.6823417656249969321, 4.967708333674755394, -1.181850606188749264 ) ) ;
#140355=CARTESIAN_POINT ( 'NONE',  ( -9.015808963407680565, 9.620791333504852716, 1.040834085586084257E-14 ) ) ;
#140359=CARTESIAN_POINT ( 'NONE',  ( -1.364683531250012516, 3.051041667008083547, -0.7879004041258289570 ) ) ;
#140365=CARTESIAN_POINT ( 'NONE',  ( 0.6823417656249917140, 4.092708333674755394, 1.181850606188765695 ) ) ;
#140367=CARTESIAN_POINT ( 'NONE',  ( -4.680589345215810049, 6.483773540883647435, -1.599625672291256295 ) ) ;
#140368=CARTESIAN_POINT ( 'NONE',  ( 5.262536180398716290, 9.291375977107183104, -0.7998128361456291469 ) ) ;
#140372=CARTESIAN_POINT ( 'NONE',  ( 4.514501963226220660, 4.369266499959774563, -0.7216878364870197293 ) ) ;
#140373=CARTESIAN_POINT ( 'NONE',  ( -1.364683531250010295, 3.842708333674751398, 0.7879004041258379498 ) ) ;
#140377=CARTESIAN_POINT ( 'NONE',  ( -0.6823417656250003738, 0.2177083336747515085, -1.181850606188749264 ) ) ;
#140378=CARTESIAN_POINT ( 'NONE',  ( -4.989037340148921196, 5.883260320670900434, 1.082531754730560403 ) ) ;
#140379=CARTESIAN_POINT ( 'NONE',  ( 5.392392409933256303, 7.314210449720692786, 1.599625672291267398 ) ) ;
#140381=EDGE_CURVE ( 'NONE', #177962, #213399, #171322, .T. ) ;
#140384=CARTESIAN_POINT ( 'NONE',  ( 3.714570900464278846, 5.356752022006865843, 1.443375672974062551 ) ) ;
#140387=CARTESIAN_POINT ( 'NONE',  ( -6.724481002698115439, 10.78905223654906109, -0.7216878364870267237 ) ) ;
#140393=CARTESIAN_POINT ( 'NONE',  ( -9.622536337397040285, 12.24937836509514710, 1.599625672291281386 ) ) ;
#140394=CARTESIAN_POINT ( 'NONE',  ( -6.358410854684796831, 6.520493539994793863, -0.7216878364870267237 ) ) ;
#140396=CARTESIAN_POINT ( 'NONE',  ( 0.6823417656249882723, 0.9885416670080832136, -1.181850606188749264 ) ) ;
#140397=DIRECTION ( 'NONE',  ( -1.000000000000000000, 7.387867266669436732E-31, -0.000000000000000000 ) ) ;
#140405=CARTESIAN_POINT ( 'NONE',  ( 8.401248741962376698, 12.95320729893149370, 0.7998128361456462443 ) ) ;
#140409=CARTESIAN_POINT ( 'NONE',  ( 8.012505595552012139, 11.33137838057728786, -1.082531754730543083 ) ) ;
#140419=CARTESIAN_POINT ( 'NONE',  ( -2.819205876637805641, 5.376491725131008259, -1.199719254218446718 ) ) ;
#140424=B_SPLINE_CURVE_WITH_KNOTS ( 'NONE', 3,
 ( #170358, #84847, #150937, #186609, #183412 ),
 .UNSPECIFIED., .F., .F.,
 ( 4, 1, 4 ),
 ( 0.001713136426838359665, 0.001716577612580400414, 0.001720018798322440947 ),
 .UNSPECIFIED. ) ;
#140425=CARTESIAN_POINT ( 'NONE',  ( -1.201851678989727383E-14, 1.384375000341419693, 1.575800808251672791 ) ) ;
#140445=EDGE_LOOP ( 'NONE', ( #143637, #76985 ) ) ;
#140449=CARTESIAN_POINT ( 'NONE',  ( 4.469384193999260901, 8.366031992974468423, -0.7998128361456231517 ) ) ;
#140453=ORIENTED_EDGE ( 'NONE', *, *, #193237, .F. ) ;
#140459=CARTESIAN_POINT ( 'NONE',  ( 9.097684769969825780, 10.57271930550834860, -1.199719254218446718 ) ) ;
#140461=CARTESIAN_POINT ( 'NONE',  ( 1.543624195544782474, 8.695410207106890610, -2.508689898543530639 ) ) ;
#140462=CARTESIAN_POINT ( 'NONE',  ( -1.538818179733931313, 8.696032261897956417, -2.511230101280735649 ) ) ;
#140464=VERTEX_POINT ( 'NONE', #40274 ) ;
#140471=CARTESIAN_POINT ( 'NONE',  ( -6.710922849084449915, 10.77323439066645783, 0.000000000000000000 ) ) ;
#140476=CARTESIAN_POINT ( 'NONE',  ( -10.64723070543352712, 11.31619066596094392, 0.7998128361456462443 ) ) ;
#140482=CARTESIAN_POINT ( 'NONE',  ( 4.487385655998885170, 5.298000022495898520, 1.082531754730560403 ) ) ;
#140484=CARTESIAN_POINT ( 'NONE',  ( 4.680589345215795838, 6.483773540883647435, -1.599625672291256295 ) ) ;
#140486=ORIENTED_EDGE ( 'NONE', *, *, #31725, .T. ) ;
#140491=CARTESIAN_POINT ( 'NONE',  ( -6.566226467720086113, 6.555019055295208119, 1.040834085586084257E-14 ) ) ;
#140494=CARTESIAN_POINT ( 'NONE',  ( -4.295235737431041478, 3.905529869957963029, -0.7998128361456221525 ) ) ;
#140500=CARTESIAN_POINT ( 'NONE',  ( 9.137832345930652522, 10.72352116074969075, -1.082531754730543083 ) ) ;
#140501=CARTESIAN_POINT ( 'NONE',  ( 0.6823417656249917140, 3.905208333674754950, 1.181850606188765695 ) ) ;
#140503=CARTESIAN_POINT ( 'NONE',  ( 5.983225862332436584, 5.874851682342960402, 0.7998128361456341429 ) ) ;
#140505=CARTESIAN_POINT ( 'NONE',  ( 1.538818179733923541, 8.696032261897956417, 2.511230101280747196 ) ) ;
#140516=CARTESIAN_POINT ( 'NONE',  ( -1.402160292154681736E-14, 1.509375000341420359, -1.575800808251659024 ) ) ;
#140518=CARTESIAN_POINT ( 'NONE',  ( 4.542145155778077203, 5.257923088951247159, -1.199719254218452047 ) ) ;
#140520=CARTESIAN_POINT ( 'NONE',  ( -6.399085315970151733, 7.528316292462387871, -1.082531754730544860 ) ) ;
#140522=CARTESIAN_POINT ( 'NONE',  ( 4.039966587192267866, 4.776011108888172707, 1.082531754730560403 ) ) ;
#140523=CARTESIAN_POINT ( 'NONE',  ( -7.361714222096077620, 7.691014135307965738, 0.7216878364870317197 ) ) ;
#140525=CIRCLE ( 'NONE', #109483, 0.08000000000000020983 ) ;
#140528=CARTESIAN_POINT ( 'NONE',  ( 6.159481859310094620, 6.080483678816896109, 1.040834085586084257E-14 ) ) ;
#140533=FACE_OUTER_BOUND ( 'NONE', #91213, .T. ) ;
#140537=CARTESIAN_POINT ( 'NONE',  ( 5.459129407796876166, 9.520734742405036144, 1.040834085586084257E-14 ) ) ;
#140541=CARTESIAN_POINT ( 'NONE',  ( -7.901704598666176693, 8.113076874732334076, 0.7998128361456602331 ) ) ;
#140546=CARTESIAN_POINT ( 'NONE',  ( 8.938903350111612411, 9.323142084752035430, -0.7998128361456221525 ) ) ;
#140549=CARTESIAN_POINT ( 'NONE',  ( -6.226218857173722476, 8.287007971501239467, 1.599625672291283607 ) ) ;
#140551=CARTESIAN_POINT ( 'NONE',  ( 7.917598520256366790, 8.339545816494993602, 1.040834085586084257E-14 ) ) ;
#140552=CARTESIAN_POINT ( 'NONE',  ( 4.291716407524416077, 7.230775179981989709, -0.9765121647202840149 ) ) ;
#140553=CARTESIAN_POINT ( 'NONE',  ( -3.601662362724658895, 7.353689856487406473, -0.7998128361456281477 ) ) ;
#140559=CARTESIAN_POINT ( 'NONE',  ( 8.866142388332804103, 12.43125098877526113, -1.199719254218446718 ) ) ;
#140561=CARTESIAN_POINT ( 'NONE',  ( -1.364683531250000748, 1.009375000341421247, 0.000000000000000000 ) ) ;
#140564=CARTESIAN_POINT ( 'NONE',  ( -4.907688418466881863, 8.669460888279271416, 0.7216878364870458196 ) ) ;
#140570=CARTESIAN_POINT ( 'NONE',  ( -5.812277037385564782, 6.060071624232533871, -0.5253754717876522040 ) ) ;
#140571=CARTESIAN_POINT ( 'NONE',  ( -1.364683531250014514, 0.8010416670080889867, -0.7879004041258289570 ) ) ;
#140574=CARTESIAN_POINT ( 'NONE',  ( 3.714570900464285064, 4.396382807705524698, 1.082531754730560403 ) ) ;
#140579=CARTESIAN_POINT ( 'NONE',  ( -3.653032323878261600, 6.349289246911547835, -1.199719254218452047 ) ) ;
#140581=CARTESIAN_POINT ( 'NONE',  ( -7.009202228140739344, 11.12122699956546334, -0.7216878364870267237 ) ) ;
#140583=B_SPLINE_CURVE_WITH_KNOTS ( 'NONE', 3,
 ( #110273, #176282, #96110, #27884 ),
 .UNSPECIFIED., .F., .F.,
 ( 4, 4 ),
 ( 0.002059939351769825289, 0.002341702326271046831 ),
 .UNSPECIFIED. ) ;
#140588=CARTESIAN_POINT ( 'NONE',  ( -6.683806541412756985, 10.74159869838281622, -0.7216878364870267237 ) ) ;
#140589=VERTEX_POINT ( 'NONE', #186504 ) ;
#140590=AXIS2_PLACEMENT_3D ( 'NONE', #206822, #89910, #189514 ) ;
#140595=CARTESIAN_POINT ( 'NONE',  ( -7.334597914868735025, 9.580116872145431728, -1.443375672974058777 ) ) ;
#140598=ORIENTED_EDGE ( 'NONE', *, *, #22500, .T. ) ;
#140608=CARTESIAN_POINT ( 'NONE',  ( -6.398558430645608475, 9.552403038140164782, -1.199719254218440723 ) ) ;
#140611=CARTESIAN_POINT ( 'NONE',  ( 4.635998460869027227, 7.496083073400806818, -1.199719254218452047 ) ) ;
#140615=CARTESIAN_POINT ( 'NONE',  ( 6.012151052656117933, 9.101594430485762999, 1.199719254218460707 ) ) ;
#140621=CARTESIAN_POINT ( 'NONE',  ( -4.934804725694220906, 7.740727365743146571, -1.082531754730549967 ) ) ;
#140630=CARTESIAN_POINT ( 'NONE',  ( -7.883176251342026042, 11.28445716228600126, -1.199719254218446718 ) ) ;
#140632=CARTESIAN_POINT ( 'NONE',  ( 8.945682426918439845, 9.331051007693339727, 1.040834085586084257E-14 ) ) ;
#140634=CARTESIAN_POINT ( 'NONE',  ( -8.311311860377216476, 9.655284244316948872, -1.199719254218446718 ) ) ;
#140638=CARTESIAN_POINT ( 'NONE',  ( 0.6823417656249917140, 4.592708333674755394, 1.181850606188765695 ) ) ;
#140639=CARTESIAN_POINT ( 'NONE',  ( 8.758204044747994743, 12.20135990463928266, 1.082531754730546636 ) ) ;
#140642=CARTESIAN_POINT ( 'NONE',  ( -1.402160292154681736E-14, 0.009375000341421267647, -1.575800808251665908 ) ) ;
#140644=CARTESIAN_POINT ( 'NONE',  ( 9.070041577417981671, 9.684062716516882219, -0.7216878364870197293 ) ) ;
#140647=CARTESIAN_POINT ( 'NONE',  ( -4.270455198624581783, 7.926022131796578662, 1.040834085586084257E-14 ) ) ;
#140650=CARTESIAN_POINT ( 'NONE',  ( -0.6823417656250003738, 2.467708333674753618, -1.181850606188749264 ) ) ;
#140654=CARTESIAN_POINT ( 'NONE',  ( -7.152089726408780379, 8.302858421353754181, -1.199719254218446718 ) ) ;
#140655=CARTESIAN_POINT ( 'NONE',  ( -1.201851678989727383E-14, 4.509375000341417916, -1.575800808251660134 ) ) ;
#140660=CARTESIAN_POINT ( 'NONE',  ( 7.609150525767641504, 9.900428251527500834, -1.599625672291262513 ) ) ;
#140663=CARTESIAN_POINT ( 'NONE',  ( 1.499999999999989120, 1.275000000000019229, 0.000000000000000000 ) ) ;
#140666=CARTESIAN_POINT ( 'NONE',  ( -0.4967775439449015895, 7.792564024146572343, -1.990974371293803280 ) ) ;
#140669=CARTESIAN_POINT ( 'NONE',  ( 6.426201623197458801, 9.480690412830290015, -1.082531754730537088 ) ) ;
#140670=CARTESIAN_POINT ( 'NONE',  ( 8.048736748007069508, 12.54194330598362406, -0.7998128361456352531 ) ) ;
#140678=CARTESIAN_POINT ( 'NONE',  ( 7.391166297744269365, 11.77477778067701664, 1.040834085586084257E-14 ) ) ;
#140679=CARTESIAN_POINT ( 'NONE',  ( -8.482597663644387609, 13.04811437422715414, -0.7998128361456281477 ) ) ;
#140681=EDGE_CURVE ( 'NONE', #110280, #26662, #189858, .T. ) ;
#140682=CARTESIAN_POINT ( 'NONE',  ( -4.911752498546917423, 4.707425932596563278, -0.3822207396134598145 ) ) ;
#140683=CARTESIAN_POINT ( 'NONE',  ( -1.364683531250010295, 5.592708333674750953, 0.7879004041258379498 ) ) ;
#140684=CARTESIAN_POINT ( 'NONE',  ( -1.500000000000013101, 0.4208333333333572068, 0.8660254037844403729 ) ) ;
#140691=CARTESIAN_POINT ( 'NONE',  ( -0.6823417656250212460, 5.051041667008086655, 1.181850606188767472 ) ) ;
#140693=CARTESIAN_POINT ( 'NONE',  ( -6.453317930424837812, 7.591587675992828466, 1.082531754730549967 ) ) ;
#140696=EDGE_CURVE ( 'NONE', #162407, #113693, #203214, .T. ) ;
#140703=CARTESIAN_POINT ( 'NONE',  ( 6.903072767652295383, 11.20533532890304684, 1.040834085586084257E-14 ) ) ;
#140709=CARTESIAN_POINT ( 'NONE',  ( -9.104463846776669200, 10.58062822844965645, -1.199719254218441611 ) ) ;
#140710=CARTESIAN_POINT ( 'NONE',  ( 7.305145839664861640, 7.417091655897478653, 0.7998128361456341429 ) ) ;
#140712=CARTESIAN_POINT ( 'NONE',  ( 4.487385655998888723, 4.337630808194552934, 0.7216878364870317197 ) ) ;
#140713=CARTESIAN_POINT ( 'NONE',  ( -1.000000000000017097, 5.868705557303652398, 4.125226524755080781 ) ) ;
#140714=CARTESIAN_POINT ( 'NONE',  ( 5.495132332240461714, 5.305409230568988832, 0.7998128361456341429 ) ) ;
#140723=CARTESIAN_POINT ( 'NONE',  ( -4.433153041988574294, 8.115836282387899558, 1.040834085586084257E-14 ) ) ;
#140724=CARTESIAN_POINT ( 'NONE',  ( 8.581948047770334043, 12.95609712246668899, 0.000000000000000000 ) ) ;
#140727=CARTESIAN_POINT ( 'NONE',  ( -8.355902744723985975, 8.642974711799791265, 1.040834085586084257E-14 ) ) ;
#140733=CARTESIAN_POINT ( 'NONE',  ( -8.616370316684697883, 10.01118577667568132, -1.199719254218446718 ) ) ;
#140737=CARTESIAN_POINT ( 'NONE',  ( 8.284195553149872993, 9.623648552551724578, -1.199719254218445830 ) ) ;
#140738=CARTESIAN_POINT ( 'NONE',  ( 4.476163270806094552, 8.373940915915776273, 0.7998128361456462443 ) ) ;
#140749=CARTESIAN_POINT ( 'NONE',  ( -6.669721502918952716, 9.868759955792373972, 1.199719254218452047 ) ) ;
#140752=CARTESIAN_POINT ( 'NONE',  ( 6.832946231607457399, 7.074118146404578589, -0.7216878364870257245 ) ) ;
#140754=CARTESIAN_POINT ( 'NONE',  ( -1.500000000000079492, 7.438721522839117917, 4.195160983902621155 ) ) ;
#140757=CARTESIAN_POINT ( 'NONE',  ( -4.238895582566952314, 8.097128612970093897, 1.040834085586084257E-14 ) ) ;
#140765=CARTESIAN_POINT ( 'NONE',  ( -8.967828540435322182, 12.54988483289483980, 1.199719254218462483 ) ) ;
#140766=CARTESIAN_POINT ( 'NONE',  ( 7.938462636001388795, 9.220293482545153907, -1.199719254218441611 ) ) ;
#140770=CARTESIAN_POINT ( 'NONE',  ( -4.610256348478378285, 6.944848931137240555, -1.199160056556654697 ) ) ;
#140777=CARTESIAN_POINT ( 'NONE',  ( 8.432808358020015049, 11.82173160345663376, 1.082531754730546636 ) ) ;
#140792=CIRCLE ( 'NONE', #47398, 0.8300000000000008482 ) ;
#140798=CARTESIAN_POINT ( 'NONE',  ( -3.436101866059630527, 6.096203712789787232, 1.199719254218462483 ) ) ;
#140799=CARTESIAN_POINT ( 'NONE',  ( 0.7499999999999902300, 3.483333333333352044, 1.299038105676669330 ) ) ;
#140801=CARTESIAN_POINT ( 'NONE',  ( -3.867100128395853709, 5.534702787927018974, -1.599625672291256295 ) ) ;
#140805=CARTESIAN_POINT ( 'NONE',  ( -0.6823417656249969321, 5.217708333674756283, -1.181850606188749264 ) ) ;
#140808=CARTESIAN_POINT ( 'NONE',  ( -2.318081078256692518, 5.648252324700675508, 1.040834085586084257E-14 ) ) ;
#140811=ORIENTED_EDGE ( 'NONE', *, *, #165849, .T. ) ;
#140813=CARTESIAN_POINT ( 'NONE',  ( 3.029357257649615054, 5.621668336311468117, -1.199719254218446718 ) ) ;
#140815=CARTESIAN_POINT ( 'NONE',  ( 4.702146809683721784, 5.356480858934594025, 2.500000000000011102 ) ) ;
#140819=CARTESIAN_POINT ( 'NONE',  ( 0.6823417656249899377, 1.905208333674752952, 1.181850606188755259 ) ) ;
#140820=EDGE_CURVE ( 'NONE', #47677, #11835, #105047, .T. ) ;
#140823=CARTESIAN_POINT ( 'NONE',  ( -8.076906825439122528, 10.44614393447756129, -1.599625672291263179 ) ) ;
#140824=CARTESIAN_POINT ( 'NONE',  ( -5.599154252319524794, 6.595063384869953360, 1.082531754730546636 ) ) ;
#140829=CARTESIAN_POINT ( 'NONE',  ( 0.7499999999999867883, -1.152083332650516434, -1.299038105676652011 ) ) ;
#140837=CARTESIAN_POINT ( 'NONE',  ( -5.734735788456164940, 5.792872629394710593, 0.7216878364870317197 ) ) ;
#140843=CARTESIAN_POINT ( 'NONE',  ( -5.883875478206491927, 5.966868934103426447, 0.000000000000000000 ) ) ;
#140845=CARTESIAN_POINT ( 'NONE',  ( 10.09812548408005384, 10.67556790771522124, -0.7998128361456281477 ) ) ;
#140849=CARTESIAN_POINT ( 'NONE',  ( 1.512220381301902616, 8.756542408759468543, -2.494878041824251547 ) ) ;
#140853=DIRECTION ( 'NONE',  ( 0.5996521035822445223, -0.8002608041566132702, 0.000000000000000000 ) ) ;
#140854=CARTESIAN_POINT ( 'NONE',  ( -4.939248034080176097, 4.656877549381960080, 1.214306433183764966E-14 ) ) ;
#140859=CARTESIAN_POINT ( 'NONE',  ( 8.378575743565351175, 11.75846021992619406, -1.082531754730543083 ) ) ;
#140860=CARTESIAN_POINT ( 'NONE',  ( 6.844168616800228477, 6.879284895888727824, -0.7998128361456281477 ) ) ;
#140865=CARTESIAN_POINT ( 'NONE',  ( 3.734381245560244089, 6.444196322207211836, 1.199719254218462483 ) ) ;
#140876=CARTESIAN_POINT ( 'NONE',  ( -5.117312914154178216, 8.057616602233474978, -1.199719254218452047 ) ) ;
#140881=CARTESIAN_POINT ( 'NONE',  ( -1.364683531250010295, 4.030208333674751842, 0.7879004041258379498 ) ) ;
#140882=CARTESIAN_POINT ( 'NONE',  ( 9.205623113554624481, 10.80261038964432707, 1.082531754730549967 ) ) ;
#140884=CARTESIAN_POINT ( 'NONE',  ( -6.749261541504576911, 6.768559974710451677, 1.040834085586084257E-14 ) ) ;
#140887=CARTESIAN_POINT ( 'NONE',  ( 3.981290663907289140, 7.796589541200495965, -0.7998128361456221525 ) ) ;
#140888=CARTESIAN_POINT ( 'NONE',  ( -4.062639585589296942, 7.891496616496157301, 0.7998128361456341429 ) ) ;
#140892=EDGE_CURVE ( 'NONE', #132514, #63111, #160767, .T. ) ;
#140896=CARTESIAN_POINT ( 'NONE',  ( 5.775410249741494972, 8.721433810464993996, -1.082531754730537088 ) ) ;
#140898=CARTESIAN_POINT ( 'NONE',  ( 7.415946836550722843, 8.714654733139752807, 1.082531754730558626 ) ) ;
#140899=CARTESIAN_POINT ( 'NONE',  ( 0.6823417656249899377, 3.738541667008085767, -1.181850606188754593 ) ) ;
#140901=CARTESIAN_POINT ( 'NONE',  ( 4.636525345749193505, 8.353103970108639587, 1.040834085586084257E-14 ) ) ;
#140903=CARTESIAN_POINT ( 'NONE',  ( -3.226477370372317743, 4.787309570232886280, 1.443375672974064550 ) ) ;
#140910=CARTESIAN_POINT ( 'NONE',  ( -3.985474048508588663, 7.835680043367737824, -0.2278754907324483936 ) ) ;
#140917=CARTESIAN_POINT ( 'NONE',  ( 6.169123589417988995, 7.156064594864501416, -1.199719254218445830 ) ) ;
#140919=CARTESIAN_POINT ( 'NONE',  ( -2.765500147063310266, 6.170241238308400433, 1.040834085586084257E-14 ) ) ;
#140921=DIRECTION ( 'NONE',  ( -5.578564026256490882E-16, -1.000000000000000000, -9.066213480720158442E-32 ) ) ;
#140928=CARTESIAN_POINT ( 'NONE',  ( 3.660338286009610975, 6.253849852777763729, -1.082531754730543083 ) ) ;
#140929=CARTESIAN_POINT ( 'NONE',  ( -1.364683531250012516, 2.842708333674754506, 0.7879004041258379498 ) ) ;
#140931=CARTESIAN_POINT ( 'NONE',  ( 6.577677080924314801, 10.82570702772039262, 1.040834085586084257E-14 ) ) ;
#140932=CARTESIAN_POINT ( 'NONE',  ( -10.34217224912604571, 10.96028913360221502, 0.7998128361456462443 ) ) ;
#140936=( BOUNDED_SURFACE ( )  B_SPLINE_SURFACE ( 3, 2, ( 
 ( #96651, #164818, #212485 ),
 ( #94515, #181064, #130270 ),
 ( #44694, #196259, #31633 ),
 ( #47906, #114016, #97710 ),
 ( #16409, #163768, #32682 ),
 ( #148576, #127078, #110802 ) ),
 .UNSPECIFIED., .F., .F., .T. ) 
 B_SPLINE_SURFACE_WITH_KNOTS ( ( 4, 2, 4 ),
 ( 3, 3 ),
 ( 8.104322365866072748E-05, 0.0002156911409644568555, 0.0003503390582702529564 ),
 ( 0.000000000000000000, 1.000000000000000000 ),
 .UNSPECIFIED. ) 
 GEOMETRIC_REPRESENTATION_ITEM ( )  RATIONAL_B_SPLINE_SURFACE ( (
 ( 1.000000000000000000, 0.8104931255419008940, 1.000000000000000000),
 ( 1.000000000000000000, 0.8505897838743379236, 1.000000000000000000),
 ( 1.000000000000000000, 0.8859283899327281553, 1.000000000000000000),
 ( 1.000000000000000000, 0.9158911669206120099, 1.000000000000000000),
 ( 1.000000000000000000, 0.9074584363674400578, 1.000000000000000000),
 ( 1.000000000000000000, 0.8789000212885805796, 1.000000000000000000) ) ) 
 REPRESENTATION_ITEM ( '' )  SURFACE ( )  );
#140939=CARTESIAN_POINT ( 'NONE',  ( -1.201851678989727383E-14, 2.712500000000023892, 1.732050807568877637 ) ) ;
#140940=CARTESIAN_POINT ( 'NONE',  ( 5.126954644262057492, 9.133197518281081173, 0.7998128361456462443 ) ) ;
#140944=CARTESIAN_POINT ( 'NONE',  ( 0.6823417656249899377, 3.926041667008085767, -1.181850606188754593 ) ) ;
#140945=EDGE_LOOP ( 'NONE', ( #192856, #193033, #206940 ) ) ;
#140947=CARTESIAN_POINT ( 'NONE',  ( 9.327646496521982300, 11.90534021740758064, -1.443375672974057666 ) ) ;
#140954=CARTESIAN_POINT ( 'NONE',  ( -1.402160292154681736E-14, 2.368750000682818602, -1.732050807568863648 ) ) ;
#140955=AXIS2_PLACEMENT_3D ( 'NONE', #202542, #27822, #11565 ) ;
#140957=CARTESIAN_POINT ( 'NONE',  ( -6.230135280679522936, 7.227244901336242755, 1.199719254218450271 ) ) ;
#140958=CARTESIAN_POINT ( 'NONE',  ( -4.311129659465605002, 4.131998812239033647, 0.7216878364870317197 ) ) ;
#140967=CARTESIAN_POINT ( 'NONE',  ( 5.769158057814842699, 6.689438141327490150, 1.199719254218462483 ) ) ;
#140972=CARTESIAN_POINT ( 'NONE',  ( 5.656776405399742025, 7.622658444431597680, -1.599625672291262513 ) ) ;
#140978=CARTESIAN_POINT ( 'NONE',  ( 8.920375002787457319, 12.49452237230570084, 1.199719254218450271 ) ) ;
#140981=CARTESIAN_POINT ( 'NONE',  ( -4.769568550827871789, 5.176413985123565986, -0.9566739868914522216 ) ) ;
#140983=CARTESIAN_POINT ( 'NONE',  ( 5.616475580598488726, 6.148514233939430973, 0.8375902553012237739 ) ) ;
#140986=EDGE_CURVE ( 'NONE', #132154, #161726, #64487, .T. ) ;
#140990=DIRECTION ( 'NONE',  ( 1.000000000000000000, 0.000000000000000000, 0.000000000000000000 ) ) ;
#140995=CARTESIAN_POINT ( 'NONE',  ( -4.181699849152211712, 3.976283482609832109, 0.4846375484205614481 ) ) ;
#140996=CARTESIAN_POINT ( 'NONE',  ( 6.141480397310468575, 10.10888486359680982, 1.040834085586084257E-14 ) ) ;
#140998=CARTESIAN_POINT ( 'NONE',  ( -4.762992037102518950, 4.451245552908022596, -0.7998128361456221525 ) ) ;
#141002=CARTESIAN_POINT ( 'NONE',  ( -5.530836599371015794, 8.540060901653093950, 1.199719254218452047 ) ) ;
#141016=CARTESIAN_POINT ( 'NONE',  ( 4.028709946750490545, 3.988235255965033588, -0.8025987720412866011 ) ) ;
#141024=CARTESIAN_POINT ( 'NONE',  ( -10.15469386695561482, 10.94949038764413096, 1.040834085586084257E-14 ) ) ;
#141026=( BOUNDED_SURFACE ( )  B_SPLINE_SURFACE ( 3, 2, ( 
 ( #49091, #128297, #181201 ),
 ( #11230, #143423, #77310 ),
 ( #61064, #193192, #94656 ),
 ( #44840, #110946, #176953 ),
 ( #33885, #102091, #186533 ),
 ( #150860, #202763, #66358 ),
 ( #287, #132504, #1360 ),
 ( #84773, #38162, #151918 ),
 ( #164958, #201695, #54413 ),
 ( #67422, #120554, #51215 ) ),
 .UNSPECIFIED., .F., .F., .T. ) 
 B_SPLINE_SURFACE_WITH_KNOTS ( ( 4, 2, 2, 2, 4 ),
 ( 3, 3 ),
 ( 0.000000000000000000, 0.0004557608768731892805, 0.0009115217537463785611, 0.001367282630619567896, 0.001823043507492757122 ),
 ( 0.000000000000000000, 1.000000000000000000 ),
 .UNSPECIFIED. ) 
 GEOMETRIC_REPRESENTATION_ITEM ( )  RATIONAL_B_SPLINE_SURFACE ( (
 ( 1.000000000000000000, 0.5626093260850774103, 1.000000000000000000),
 ( 1.000000000000000000, 0.5538465755378986222, 1.000000000000000000),
 ( 1.000000000000000000, 0.5614387302410062119, 1.000000000000000000),
 ( 1.000000000000000000, 0.6035072769098912548, 1.000000000000000000),
 ( 1.000000000000000000, 0.6388423421880006225, 1.000000000000000000),
 ( 1.000000000000000000, 0.7131546070456026287, 1.000000000000000000),
 ( 1.000000000000000000, 0.7507011191611827616, 1.000000000000000000),
 ( 1.000000000000000000, 0.8047563548239682341, 1.000000000000000000),
 ( 1.000000000000000000, 0.8208891226306104238, 1.000000000000000000),
 ( 1.000000000000000000, 0.8267197332297674395, 1.000000000000000000) ) ) 
 REPRESENTATION_ITEM ( '' )  SURFACE ( )  );
#141029=CARTESIAN_POINT ( 'NONE',  ( 9.589694723567584234, 10.08239868711733855, -0.7998128361456281477 ) ) ;
#141032=TOROIDAL_SURFACE ( 'NONE', #12946, 0.8300000000000010703, 0.08000000000000000167 ) ;
#141034=CARTESIAN_POINT ( 'NONE',  ( -6.906989191158078079, 10.14557225873805812, -1.199719254218440723 ) ) ;
#141035=CARTESIAN_POINT ( 'NONE',  ( 3.635557746758808495, 7.393234471193928847, -0.7998128361456291469 ) ) ;
#141041=CARTESIAN_POINT ( 'NONE',  ( -1.201851678989727383E-14, 2.884375000341418804, 1.575800808251672791 ) ) ;
#141043=CARTESIAN_POINT ( 'NONE',  ( 7.131225611108100715, 7.422110755822004968, 0.7216878364870317197 ) ) ;
#141052=CARTESIAN_POINT ( 'NONE',  ( 10.03267048398825168, 10.80712977418221676, 0.000000000000000000 ) ) ;
#141057=CARTESIAN_POINT ( 'NONE',  ( -9.124801077197171040, 10.60435499727357289, -1.199719254218441611 ) ) ;
#141073=CARTESIAN_POINT ( 'NONE',  ( -1.201851678989727383E-14, 2.493750000682819046, 1.732050807568877637 ) ) ;
#141079=CARTESIAN_POINT ( 'NONE',  ( -0.7500000000000215383, 0.6916666666666876351, 1.299038105676659116 ) ) ;
#141080=CARTESIAN_POINT ( 'NONE',  ( 7.450369105909416589, 8.650851030771185890, -1.199719254218441611 ) ) ;
#141081=CARTESIAN_POINT ( 'NONE',  ( -1.364683531250014514, 0.2802083336747505649, 0.7879004041258379498 ) ) ;
#141084=CARTESIAN_POINT ( 'NONE',  ( 8.839552966430002101, 11.33589776563360019, -1.443375672974052559 ) ) ;
#141085=CARTESIAN_POINT ( 'NONE',  ( -5.260200412422196159, 9.080724881227137502, -0.7216878364870207285 ) ) ;
#141090=CARTESIAN_POINT ( 'NONE',  ( -6.878064000834399394, 6.918829510595249310, -0.7998128361456291469 ) ) ;
#141092=CARTESIAN_POINT ( 'NONE',  ( 0.7499999999999902300, 2.764583334016148974, 1.299038105676669330 ) ) ;
#141093=CARTESIAN_POINT ( 'NONE',  ( -1.201851678989727383E-14, 3.884375000341423689, 1.575800808251672791 ) ) ;
#141109=CARTESIAN_POINT ( 'NONE',  ( -9.515124878692420296, 9.995400534762978850, 1.040834085586084257E-14 ) ) ;
#141110=CARTESIAN_POINT ( 'NONE',  ( 6.283314124929436417, 9.417951348137970413, -1.199719254218440723 ) ) ;
#141114=ORIENTED_EDGE ( 'NONE', *, *, #136635, .T. ) ;
#141117=CARTESIAN_POINT ( 'NONE',  ( -7.483210719738908168, 10.81783070874899799, 1.199719254218453823 ) ) ;
#141123=CARTESIAN_POINT ( 'NONE',  ( 4.390142812726693045, 4.016254791136236513, 1.214306433183764966E-14 ) ) ;
#141127=CARTESIAN_POINT ( 'NONE',  ( -4.985647801523292344, 6.839675073242382553, -1.599625672291256295 ) ) ;
#141128=CARTESIAN_POINT ( 'NONE',  ( -9.657485491635913633, 10.16148791653038330, 1.040834085586084257E-14 ) ) ;
#141132=CARTESIAN_POINT ( 'NONE',  ( -5.732732414299474222, 6.256854150074313559, -1.080652830874342163 ) ) ;
#141140=CARTESIAN_POINT ( 'NONE',  ( 5.849453209292126310, 8.911780279894442103, 1.199719254218462483 ) ) ;
#141149=EDGE_CURVE ( 'NONE', #80197, #127597, #27528, .T. ) ;
#141157=EDGE_CURVE ( 'NONE', #93347, #84679, #161818, .T. ) ;
#141161=CARTESIAN_POINT ( 'NONE',  ( 3.226477370372302644, 5.747678784534228313, 1.082531754730546636 ) ) ;
#141165=CARTESIAN_POINT ( 'NONE',  ( -8.890396042259075315, 11.39521468743417998, -1.599625672291263179 ) ) ;
#141167=CARTESIAN_POINT ( 'NONE',  ( 8.503988664269582998, 10.94440607977979063, 1.599625672291281386 ) ) ;
#141169=CARTESIAN_POINT ( 'NONE',  ( 3.284841267552055299, 6.405332120898776793, -0.9495590844852130896 ) ) ;
#141173=DIRECTION ( 'NONE',  ( 1.000000000000000000, 0.000000000000000000, 0.000000000000000000 ) ) ;
#141175=CARTESIAN_POINT ( 'NONE',  ( -1.402160292154681736E-14, 0.6968750003414164729, -1.575800808251659024 ) ) ;
#141176=DIRECTION ( 'NONE',  ( -0.7592566023653016805, -0.6507913734559627184, 4.115938288792108699E-15 ) ) ;
#141177=EDGE_LOOP ( 'NONE', ( #111331, #37560, #168276, #150800, #3351 ) ) ;
#141182=CARTESIAN_POINT ( 'NONE',  ( -4.939248034080176097, 4.656877549381960080, 1.214306433183764966E-14 ) ) ;
#141185=CARTESIAN_POINT ( 'NONE',  ( -1.402160292154681736E-14, 0.3375000000000208389, -1.732050807568870754 ) ) ;
#141187=CARTESIAN_POINT ( 'NONE',  ( 1.364683531249984538, -1.032291666325247714, -0.7879004041258309554 ) ) ;
#141192=CARTESIAN_POINT ( 'NONE',  ( 0.6823417656249899377, 0.5927083336747518416, 1.181850606188755259 ) ) ;
#141194=CARTESIAN_POINT ( 'NONE',  ( -7.497822643557261024, 8.706213491360317747, -1.199719254218446718 ) ) ;
#141195=CARTESIAN_POINT ( 'NONE',  ( 7.391166297744269365, 11.77477778067701664, 1.040834085586084257E-14 ) ) ;
#141196=CARTESIAN_POINT ( 'NONE',  ( 3.683011284406639163, 7.448596931783069586, 0.7998128361456321445 ) ) ;
#141200=CARTESIAN_POINT ( 'NONE',  ( 1.364683531249988757, 0.1968750003414204697, 0.000000000000000000 ) ) ;
#141205=CARTESIAN_POINT ( 'NONE',  ( -1.580000000000022276, 8.674529973577531194, 2.500000000000011102 ) ) ;
#141208=CARTESIAN_POINT ( 'NONE',  ( 5.802526556968819804, 9.713438716531550554, -0.7216878364870267237 ) ) ;
#141211=CARTESIAN_POINT ( 'NONE',  ( -4.446184310277715213, 7.274633231044262516, -1.199719254218452047 ) ) ;
#141216=CARTESIAN_POINT ( 'NONE',  ( -3.735435015764967837, 4.316761258935923884, -1.199719254218452047 ) ) ;
#141218=CARTESIAN_POINT ( 'NONE',  ( -6.995644074527074707, 11.10540915368285475, 0.000000000000000000 ) ) ;
#141220=CARTESIAN_POINT ( 'NONE',  ( 1.499999999999987121, 3.795833333333356929, -0.8660254037844262731 ) ) ;
#141225=CARTESIAN_POINT ( 'NONE',  ( 8.514157279702022407, 10.95626946445095307, -1.443375672974063439 ) ) ;
#141235=CIRCLE ( 'NONE', #61550, 0.7499999999999997780 ) ;
#141238=CARTESIAN_POINT ( 'NONE',  ( 7.388830529323379359, 11.56412668427855195, -0.7216878364870267237 ) ) ;
#141240=CARTESIAN_POINT ( 'NONE',  ( 8.076906825439115423, 10.44614393447756129, -1.599625672291262513 ) ) ;
#141242=CARTESIAN_POINT ( 'NONE',  ( -3.578989363883261277, 7.119311991265024453, 1.040834085586084257E-14 ) ) ;
#141243=CARTESIAN_POINT ( 'NONE',  ( 8.550388431712704573, 13.12720360364021133, 0.000000000000000000 ) ) ;
#141245=CARTESIAN_POINT ( 'NONE',  ( 3.701012746850603996, 7.261672604726938651, 1.040834085586084257E-14 ) ) ;
#141247=CARTESIAN_POINT ( 'NONE',  ( -7.199016379176422120, 11.34267684244042584, 0.000000000000000000 ) ) ;
#141260=ORIENTED_EDGE ( 'NONE', *, *, #174519, .T. ) ;
#141272=CARTESIAN_POINT ( 'NONE',  ( -0.006800380015319074101, 7.009756401597622144, 1.999988438674507485 ) ) ;
#141275=CARTESIAN_POINT ( 'NONE',  ( -2.314109536355652530, 5.457892750589173225, -0.8025987720412944837 ) ) ;
#141277=CARTESIAN_POINT ( 'NONE',  ( -5.280010757518168063, 8.247430752824802980, -1.199719254218446718 ) ) ;
#141280=CARTESIAN_POINT ( 'NONE',  ( 1.230728480726485330, 2.855010058876359835, -0.7749999999999926947 ) ) ;
#141282=CARTESIAN_POINT ( 'NONE',  ( 4.788000803920411386, 8.737751371215816576, 1.040834085586084257E-14 ) ) ;
#141291=CARTESIAN_POINT ( 'NONE',  ( -5.576481253922474401, 5.400316305864651056, -0.7998128361456221525 ) ) ;
#141295=CARTESIAN_POINT ( 'NONE',  ( 5.940443861082012944, 10.08226827123770697, 0.7998128361456462443 ) ) ;
#141298=CARTESIAN_POINT ( 'NONE',  ( 6.112872195911107198, 6.017013290715023111, -0.08730524813132384265 ) ) ;
#141304=CARTESIAN_POINT ( 'NONE',  ( 7.253248993186735660, 7.564471368247083660, 0.7216878364870317197 ) ) ;
#141305=CARTESIAN_POINT ( 'NONE',  ( -8.830438121202295321, 9.196599317691152464, -0.7998128361456291469 ) ) ;
#141308=CARTESIAN_POINT ( 'NONE',  ( -6.970863535720637216, 11.28442455831609337, 0.7998128361456481317 ) ) ;
#141309=CARTESIAN_POINT ( 'NONE',  ( -7.061099074618889304, 7.132370430010492868, -0.7998128361456291469 ) ) ;
#141316=CARTESIAN_POINT ( 'NONE',  ( 7.065770611016287006, 11.39514947949436774, 1.040834085586084257E-14 ) ) ;
#141322=CARTESIAN_POINT ( 'NONE',  ( 2.683624340501134853, 5.218313266304903664, -1.199719254218446718 ) ) ;
#141330=CARTESIAN_POINT ( 'NONE',  ( -1.201851678989727383E-14, 4.087500000000022560, -1.732050807568863648 ) ) ;
#141331=CARTESIAN_POINT ( 'NONE',  ( 5.497994985541524215, 6.373081223675282736, -1.199719254218445830 ) ) ;
#141332=CARTESIAN_POINT ( 'NONE',  ( 7.145310649601935182, 8.294949498412453437, -1.199719254218446718 ) ) ;
#141336=CARTESIAN_POINT ( 'NONE',  ( 6.805829924380114804, 8.002851668940699881, 1.082531754730558626 ) ) ;
#141337=CARTESIAN_POINT ( 'NONE',  ( -10.10046125205659173, 10.88621900359527572, -0.7216878364870267237 ) ) ;
#141340=CARTESIAN_POINT ( 'NONE',  ( 9.413438726589914651, 9.876766690643398405, 0.000000000000000000 ) ) ;
#141344=CARTESIAN_POINT ( 'NONE',  ( -1.364683531250012516, 0.7802083336747528408, 0.7879004041258379498 ) ) ;
#141349=CARTESIAN_POINT ( 'NONE',  ( -0.6823417656250246877, -0.1989583329919109023, 1.181850606188755259 ) ) ;
#141352=CARTESIAN_POINT ( 'NONE',  ( 9.049177462117294013, 12.64479190819049670, -1.199719254218446718 ) ) ;
#141356=CARTESIAN_POINT ( 'NONE',  ( -10.15522075183580419, 11.80651128435196462, 1.199719254218462483 ) ) ;
#141363=CARTESIAN_POINT ( 'NONE',  ( 3.357615597678655917, 7.068968630600412695, 0.7998128361456321445 ) ) ;
#141369=CARTESIAN_POINT ( 'NONE',  ( 9.094822116668764167, 9.505047312402055582, 0.7998128361456462443 ) ) ;
#141373=CARTESIAN_POINT ( 'NONE',  ( -5.590039407536138150, 5.416134151747256986, 0.000000000000000000 ) ) ;
#141377=CARTESIAN_POINT ( 'NONE',  ( 7.130698725783555680, 10.40656671580112658, 1.199719254218460707 ) ) ;
#141379=CARTESIAN_POINT ( 'NONE',  ( 8.450809820019639318, 8.753699632978056755, -0.7998128361456291469 ) ) ;
#141383=CARTESIAN_POINT ( 'NONE',  ( -9.829298180227631576, 10.56986208646148384, 1.040834085586084257E-14 ) ) ;
#141391=CARTESIAN_POINT ( 'NONE',  ( -4.885033903151685841, 6.706220529795296592, -1.250124166851230845 ) ) ;
#141392=CARTESIAN_POINT ( 'NONE',  ( 1.364683531249986537, 2.155208333674751398, -0.7879004041258239610 ) ) ;
#141394=CARTESIAN_POINT ( 'NONE',  ( 6.982085921357777281, 7.248114451113292667, 1.040834085586084257E-14 ) ) ;
#141400=B_SPLINE_CURVE_WITH_KNOTS ( 'NONE', 3,
 ( #67707, #81868, #101307, #147954 ),
 .UNSPECIFIED., .F., .F.,
 ( 4, 4 ),
 ( 0.000000000000000000, 7.308104204455707247E-05 ),
 .UNSPECIFIED. ) ;
#141413=CARTESIAN_POINT ( 'NONE',  ( 7.574201371528760163, 11.98831870009225931, 1.040834085586084257E-14 ) ) ;
#141417=CARTESIAN_POINT ( 'NONE',  ( -4.783329267523015460, 4.474972321731942593, -0.7998128361456221525 ) ) ;
#141418=CARTESIAN_POINT ( 'NONE',  ( -6.181627972826976958, 9.299317504018391745, 1.199719254218452047 ) ) ;
#141420=ORIENTED_EDGE ( 'NONE', *, *, #133002, .F. ) ;
#141422=CARTESIAN_POINT ( 'NONE',  ( -8.286004436246233951, 12.81875560892930466, 1.040834085586084257E-14 ) ) ;
#141425=CARTESIAN_POINT ( 'NONE',  ( -1.201851678989727383E-14, 4.118750000682818602, -1.732050807568863648 ) ) ;
#141426=CARTESIAN_POINT ( 'NONE',  ( 7.670162217029129259, 9.971608557999250166, 1.599625672291281386 ) ) ;
#141429=CARTESIAN_POINT ( 'NONE',  ( -8.365544474831901667, 9.718555627847388578, 1.199719254218462483 ) ) ;
#141431=CARTESIAN_POINT ( 'NONE',  ( 1.364683531249990311, 4.384375000341417028, 1.214306433183764966E-14 ) ) ;
#141432=CARTESIAN_POINT ( 'NONE',  ( -1.608462485350604876, 8.735270501766756013, -2.463594439587629914 ) ) ;
#141438=CARTESIAN_POINT ( 'NONE',  ( -8.351459436338037889, 10.76645531385962862, -1.443375672974059665 ) ) ;
#141442=CARTESIAN_POINT ( 'NONE',  ( -1.201851678989727383E-14, 2.634375000341417916, 1.575800808251672791 ) ) ;
#141449=CARTESIAN_POINT ( 'NONE',  ( -1.364683531250010295, 4.280208333674753618, 0.7879004041258379498 ) ) ;
#141451=CARTESIAN_POINT ( 'NONE',  ( -3.653032323878261600, 6.349289246911547835, -1.199719254218452047 ) ) ;
#141454=CARTESIAN_POINT ( 'NONE',  ( -1.364683531249997417, 4.571875000341417028, 1.214306433183764966E-14 ) ) ;
#141459=CARTESIAN_POINT ( 'NONE',  ( -1.364683531250000748, -0.9906249996585805295, 0.000000000000000000 ) ) ;
#141460=CARTESIAN_POINT ( 'NONE',  ( -4.948362879307902418, 4.875437568721725512, 1.214306433183764966E-14 ) ) ;
#141461=CARTESIAN_POINT ( 'NONE',  ( 5.986088515633498197, 6.942523675449257858, -1.199719254218446718 ) ) ;
#141464=CARTESIAN_POINT ( 'NONE',  ( 3.009546912553647147, 5.494593250412460606, -1.082531754730543083 ) ) ;
#141467=CARTESIAN_POINT ( 'NONE',  ( -8.839552966430007430, 11.33589776563360019, -1.443375672974059665 ) ) ;
#141472=CARTESIAN_POINT ( 'NONE',  ( -10.45741655484220267, 11.09474082360439873, -0.7998128361456221525 ) ) ;
#141473=CARTESIAN_POINT ( 'NONE',  ( -4.514501963226242864, 7.250374142863800664, 1.082531754730560403 ) ) ;
#141475=CARTESIAN_POINT ( 'NONE',  ( -0.6823417656250003738, 0.7802083336747520637, -1.181850606188749264 ) ) ;
#141477=DIRECTION ( 'NONE',  ( -0.7592566023653004592, 0.6507913734559639396, 0.000000000000000000 ) ) ;
#141488=CARTESIAN_POINT ( 'NONE',  ( 0.7499999999999885647, -0.5166666666666444030, 1.299038105676657340 ) ) ;
#141489=CARTESIAN_POINT ( 'NONE',  ( 7.565086526301031178, 11.76975868075249387, 1.040834085586084257E-14 ) ) ;
#141497=CARTESIAN_POINT ( 'NONE',  ( 5.203632029546647608, 4.965325544092860532, 1.040834085586084257E-14 ) ) ;
#141500=CARTESIAN_POINT ( 'NONE',  ( -2.591579918506545344, 6.175260338232929413, 1.040834085586084257E-14 ) ) ;
#141504=CARTESIAN_POINT ( 'NONE',  ( -1.364683531250014514, 1.051041667008090208, -0.7879004041258289570 ) ) ;
#141516=CARTESIAN_POINT ( 'NONE',  ( -1.499999999999997780, 5.650000000000023448, 1.214306433183764966E-14 ) ) ;
#141523=CARTESIAN_POINT ( 'NONE',  ( 5.133733721068893807, 9.141106441222381918, 1.040834085586084257E-14 ) ) ;
#141532=CARTESIAN_POINT ( 'NONE',  ( 9.433775957010412938, 9.900493459467314850, 0.000000000000000000 ) ) ;
#141534=CARTESIAN_POINT ( 'NONE',  ( 1.499999999922324134, 8.635424801869593381, -2.574739023100856006 ) ) ;
#141538=EDGE_CURVE ( 'NONE', #199393, #133314, #133630, .T. ) ;
#141544=CARTESIAN_POINT ( 'NONE',  ( -8.514157279702027736, 10.95626946445095307, -1.443375672974059665 ) ) ;
#141555=CARTESIAN_POINT ( 'NONE',  ( 4.663641652976547647, 4.543262804668490418, 1.214306433183764966E-14 ) ) ;
#141556=EDGE_CURVE ( 'NONE', #17304, #60595, #53230, .T. ) ;
#141559=VERTEX_POINT ( 'NONE', #50656 ) ;
#141564=CARTESIAN_POINT ( 'NONE',  ( -4.720210035852093533, 8.658662141802762946, -0.7998128361456281477 ) ) ;
#141566=CARTESIAN_POINT ( 'NONE',  ( -3.460355519985875983, 5.060167411448709629, 1.599625672291267398 ) ) ;
#141573=CARTESIAN_POINT ( 'NONE',  ( 0.6823417656249917140, 3.655208333674754506, 1.181850606188765695 ) ) ;
#141575=CARTESIAN_POINT ( 'NONE',  ( 5.311043488251262268, 7.219303374425030562, -1.599625672291256295 ) ) ;
#141577=CARTESIAN_POINT ( 'NONE',  ( 1.499999999999990896, 8.640473353474858342, 2.571377442220807996 ) ) ;
#141589=CARTESIAN_POINT ( 'NONE',  ( -0.6823417656250003738, 1.530208333674752730, -1.181850606188749264 ) ) ;
#141591=CARTESIAN_POINT ( 'NONE',  ( 5.352771719296971042, 5.139321848801576387, 0.7998128361456341429 ) ) ;
#141593=CARTESIAN_POINT ( 'NONE',  ( -5.097502569058207200, 8.890910730635814829, -0.7216878364870207285 ) ) ;
#141594=CARTESIAN_POINT ( 'NONE',  ( 4.528060117284240071, 5.345453560662148718, 1.082531754730560403 ) ) ;
#141595=CARTESIAN_POINT ( 'NONE',  ( -5.544921637864820951, 9.412899644243539754, -0.7216878364870207285 ) ) ;
#141597=ORIENTED_EDGE ( 'NONE', *, *, #107203, .T. ) ;
#141599=CARTESIAN_POINT ( 'NONE',  ( 6.962275575817444384, 8.081408578997208991, -1.199719254218446718 ) ) ;
#141601=CARTESIAN_POINT ( 'NONE',  ( -3.830881975230008507, 4.022296396677373487, 0.8449283794988144969 ) ) ;
#141604=CARTESIAN_POINT ( 'NONE',  ( -1.364683531249997417, 5.009375000341425022, 1.214306433183764966E-14 ) ) ;
#141609=CARTESIAN_POINT ( 'NONE',  ( 7.657657833620182153, 7.828355648845348291, -0.7998128361456281477 ) ) ;
#141611=CARTESIAN_POINT ( 'NONE',  ( -7.888146445052511169, 8.097259028849730811, 1.040834085586084257E-14 ) ) ;
#141615=CARTESIAN_POINT ( 'NONE',  ( 8.860417081730671995, 10.29590700256267155, 1.199719254218453823 ) ) ;
#141618=CARTESIAN_POINT ( 'NONE',  ( -5.865874016206865882, 9.995270118883347266, 0.000000000000000000 ) ) ;
#141620=CARTESIAN_POINT ( 'NONE',  ( 6.277061933002769045, 10.26706332190449622, 0.7216878364870438212 ) ) ;
#141621=CARTESIAN_POINT ( 'NONE',  ( 4.007874524826865681, 7.816931064126571016, 0.2151701594551927443 ) ) ;
#141622=CARTESIAN_POINT ( 'NONE',  ( -4.076197739202962467, 7.907314462378773001, 1.040834085586084257E-14 ) ) ;
#141627=CARTESIAN_POINT ( 'NONE',  ( 4.961394147597008697, 7.875711374583454827, -1.199719254218452047 ) ) ;
#141629=CARTESIAN_POINT ( 'NONE',  ( 9.077347539549325717, 10.54899253668443393, -1.199719254218446718 ) ) ;
#141630=CARTESIAN_POINT ( 'NONE',  ( -4.980508561475621043, 6.629897003107849685, 1.243112925831350246 ) ) ;
#141633=CARTESIAN_POINT ( 'NONE',  ( -0.6823417656250003738, -0.03229166632524871350, -1.181850606188749264 ) ) ;
#141635=CARTESIAN_POINT ( 'NONE',  ( -4.758548728716557541, 8.495464583570553785, 1.040834085586084257E-14 ) ) ;
#141641=CARTESIAN_POINT ( 'NONE',  ( -5.626640144655740805, 6.175545741207232098, 0.8476793345565808435 ) ) ;
#141642=CARTESIAN_POINT ( 'NONE',  ( 0.6823417656249882723, 0.9885416670080832136, -1.181850606188749264 ) ) ;
#141645=CARTESIAN_POINT ( 'NONE',  ( 2.250290310188348464, 5.569163095287620990, 0.7216878364870438212 ) ) ;
#141649=CARTESIAN_POINT ( 'NONE',  ( -7.768458830506062007, 11.04665715469030296, 1.082531754730549967 ) ) ;
#141656=CARTESIAN_POINT ( 'NONE',  ( -7.497295758232720431, 10.73030023703809555, -1.082531754730543083 ) ) ;
#141658=ADVANCED_FACE ( 'NONE', ( #67935 ), #163356, .F. ) ;
#141663=ORIENTED_EDGE ( 'NONE', *, *, #46527, .F. ) ;
#141664=CARTESIAN_POINT ( 'NONE',  ( -7.090551149822745813, 9.295395646258437949, 1.443375672974078761 ) ) ;
#141669=CARTESIAN_POINT ( 'NONE',  ( 1.499999999999989120, 4.785416667349486453, 0.8660254037844524744 ) ) ;
#141676=ADVANCED_FACE ( 'NONE', ( #181704 ), #5738, .T. ) ;
#141677=CARTESIAN_POINT ( 'NONE',  ( -8.016948904382338981, 8.247528564734524892, -0.7998128361456291469 ) ) ;
#141680=CARTESIAN_POINT ( 'NONE',  ( 5.281064527722868718, 6.119995689553514140, 1.199719254218462483 ) ) ;
#141685=CARTESIAN_POINT ( 'NONE',  ( 6.958359152311676787, 9.141171649162195934, -1.599625672291262513 ) ) ;
#141693=CARTESIAN_POINT ( 'NONE',  ( -4.419594888374909658, 8.100018436505289188, 0.7216878364870458196 ) ) ;
#141696=CARTESIAN_POINT ( 'NONE',  ( -4.623281625960056651, 5.318713365471549714, 1.186903574614258439 ) ) ;
#141704=CARTESIAN_POINT ( 'NONE',  ( -8.877891658850122880, 9.251961778280284321, 0.7998128361456462443 ) ) ;
#141706=CARTESIAN_POINT ( 'NONE',  ( 7.476431642932036326, 10.80992178580769014, 1.199719254218460707 ) ) ;
#141707=CARTESIAN_POINT ( 'NONE',  ( 1.499999999999987566, -0.4749999999999823808, 0.000000000000000000 ) ) ;
#141708=CARTESIAN_POINT ( 'NONE',  ( -9.338868881714763148, 9.789768538289042255, -0.7998128361456291469 ) ) ;
#141711=CARTESIAN_POINT ( 'NONE',  ( 1.364683531249988535, 4.155208333674753618, -0.7879004041258239610 ) ) ;
#141712=CARTESIAN_POINT ( 'NONE',  ( 8.419250204406344196, 12.76628297187536809, 1.040834085586084257E-14 ) ) ;
#141715=CARTESIAN_POINT ( 'NONE',  ( -0.7499999999999972244, 5.608333333333353821, -1.299038105676652011 ) ) ;
#141717=FACE_OUTER_BOUND ( 'NONE', #166573, .T. ) ;
#141718=CARTESIAN_POINT ( 'NONE',  ( 7.361714222096048310, 10.57212177821199184, -1.082531754730537976 ) ) ;
#141721=CARTESIAN_POINT ( 'NONE',  ( -6.480434237652138663, 8.583592582059388576, 1.443375672974078761 ) ) ;
#141723=CARTESIAN_POINT ( 'NONE',  ( 1.364683531249986537, 2.155208333674751398, -0.7879004041258239610 ) ) ;
#141724=B_SPLINE_CURVE_WITH_KNOTS ( 'NONE', 3,
 ( #42105, #141757, #92986, #45291 ),
 .UNSPECIFIED., .F., .F.,
 ( 4, 4 ),
 ( 0.000000000000000000, 0.0002564548269640155843 ),
 .UNSPECIFIED. ) ;
#141728=CARTESIAN_POINT ( 'NONE',  ( -6.723954117373590833, 9.932031339322813679, -1.199719254218440723 ) ) ;
#141729=CARTESIAN_POINT ( 'NONE',  ( 0.6823417656249899377, 4.488541667008086655, -1.181850606188754593 ) ) ;
#141735=CARTESIAN_POINT ( 'NONE',  ( 9.694243528971124846, 11.26870452434320491, 1.199719254218450271 ) ) ;
#141738=CARTESIAN_POINT ( 'NONE',  ( -1.201851678989727383E-14, 1.712500000000019229, 1.732050807568877637 ) ) ;
#141743=CARTESIAN_POINT ( 'NONE',  ( 6.480434237652121787, 9.543961796360731498, 1.082531754730558626 ) ) ;
#141749=CARTESIAN_POINT ( 'NONE',  ( 9.088043039861931405, 9.497138389460751284, 1.040834085586084257E-14 ) ) ;
#141750=CARTESIAN_POINT ( 'NONE',  ( -10.10098813738111545, 11.74323990082152491, -1.199719254218441611 ) ) ;
#141753=CARTESIAN_POINT ( 'NONE',  ( 1.364683531249990311, 5.176041667008085767, 0.7879004041258500513 ) ) ;
#141757=CARTESIAN_POINT ( 'NONE',  ( 4.097995649369902793, 7.467253099217946222, -0.6374303210496650163 ) ) ;
#141759=CARTESIAN_POINT ( 'NONE',  ( 1.364683531249988535, 3.905208333674751842, -0.7879004041258239610 ) ) ;
#141761=CARTESIAN_POINT ( 'NONE',  ( -7.076992996653451939, 7.358839372291564374, 0.7216878364870317197 ) ) ;
#141769=ORIENTED_EDGE ( 'NONE', *, *, #20625, .F. ) ;
#141770=CARTESIAN_POINT ( 'NONE',  ( 8.320953590485093088, 10.73086516036454618, 1.599625672291281386 ) ) ;
#141771=CARTESIAN_POINT ( 'NONE',  ( 3.332168893502668539, 7.719402352560120306, -2.450693629706207854 ) ) ;
#141773=CIRCLE ( 'NONE', #197075, 0.08000000000000012657 ) ;
#141777=CARTESIAN_POINT ( 'NONE',  ( -8.646349277213090545, 11.11049346154719508, 1.599625672291269396 ) ) ;
#141778=CARTESIAN_POINT ( 'NONE',  ( 4.984594031318565932, 8.967110136513669616, 0.7998128361456462443 ) ) ;
#141779=CARTESIAN_POINT ( 'NONE',  ( 2.860407222358956503, 6.280966159486672140, 0.7216878364870338292 ) ) ;
#141781=CARTESIAN_POINT ( 'NONE',  ( 3.551346171775753735, 6.230655402791975384, 1.199719254218462483 ) ) ;
#141783=ADVANCED_FACE ( 'NONE', ( #36854 ), #113130, .F. ) ;
#141792=CARTESIAN_POINT ( 'NONE',  ( -5.612712406377534435, 5.650512016969639895, 0.7216878364870317197 ) ) ;
#141793=CARTESIAN_POINT ( 'NONE',  ( 3.602716132929354664, 5.226254793216122074, 1.599625672291267398 ) ) ;
#141796=CARTESIAN_POINT ( 'NONE',  ( -8.128276786592724790, 9.441743324901704426, -1.199719254218446718 ) ) ;
#141801=CARTESIAN_POINT ( 'NONE',  ( -7.971304249830880373, 11.38727316052296601, 1.199719254218453823 ) ) ;
#141805=CARTESIAN_POINT ( 'NONE',  ( 6.747154001095143627, 11.02343010125301959, -0.7998128361456291469 ) ) ;
#141807=CARTESIAN_POINT ( 'NONE',  ( 5.931855901178834323, 6.879252291918818152, 1.199719254218462483 ) ) ;
#141818=DIRECTION ( 'NONE',  ( -1.000000000000000000, 5.421010862427522170E-16, 0.000000000000000000 ) ) ;
#141819=CARTESIAN_POINT ( 'NONE',  ( -1.387358672534890536, 7.315968950354793776, -4.254625267136668221 ) ) ;
#141821=CARTESIAN_POINT ( 'NONE',  ( -7.670162217029145246, 9.971608557999250166, 1.599625672291295375 ) ) ;
#141824=CARTESIAN_POINT ( 'NONE',  ( 7.158341918335438869, 7.453746447587225710, -0.7216878364870257245 ) ) ;
#141827=CARTESIAN_POINT ( 'NONE',  ( 3.070819976954436203, 2.800000000000017586, -2.497101503361887076 ) ) ;
#141829=CARTESIAN_POINT ( 'NONE',  ( -4.680589345215810049, 6.483773540883647435, -1.599625672291256295 ) ) ;
#141831=CARTESIAN_POINT ( 'NONE',  ( 1.579999999999991189, 8.674529973577531194, 2.500000000000000444 ) ) ;
#141832=CARTESIAN_POINT ( 'NONE',  ( -5.840764256335890359, 6.042828518458865261, -0.4463971771759592810 ) ) ;
#141837=CARTESIAN_POINT ( 'NONE',  ( -10.15522075183580419, 11.80651128435196462, 1.199719254218462483 ) ) ;
#141838=CARTESIAN_POINT ( 'NONE',  ( 8.437251666405968464, 8.737881787095446384, 1.040834085586084257E-14 ) ) ;
#141843=CARTESIAN_POINT ( 'NONE',  ( -5.013591113304329383, 6.604120902668014992, -1.237928687022475494 ) ) ;
#141850=CARTESIAN_POINT ( 'NONE',  ( 2.510230996824538430, 6.080353262937265413, 0.000000000000000000 ) ) ;
#141866=CARTESIAN_POINT ( 'NONE',  ( -5.786632634934295361, 5.645492917045106473, 0.7998128361456341429 ) ) ;
#141867=CARTESIAN_POINT ( 'NONE',  ( 4.975479186090847605, 7.788180902872553268, 1.082531754730558626 ) ) ;
#141868=CARTESIAN_POINT ( 'NONE',  ( -1.201851678989727383E-14, 3.962500000000022116, 1.732050807568877637 ) ) ;
#141870=CARTESIAN_POINT ( 'NONE',  ( -4.946027110887008860, 4.664786472323266153, -0.7998128361456221525 ) ) ;
#141874=CARTESIAN_POINT ( 'NONE',  ( 1.364683531249988535, 4.905208333674756283, -0.7879004041258300672 ) ) ;
#141877=CARTESIAN_POINT ( 'NONE',  ( -4.446711195602264688, 4.290177271065136466, -0.7216878364870207285 ) ) ;
#141882=CARTESIAN_POINT ( 'NONE',  ( 3.181359600701000989, 6.863336634126477875, 0.000000000000000000 ) ) ;
#141886=CARTESIAN_POINT ( 'NONE',  ( 8.202319746143333035, 12.51319743723517952, -0.7216878364870328300 ) ) ;
#141888=CARTESIAN_POINT ( 'NONE',  ( 1.364683531249988757, 1.446875000341421469, 0.000000000000000000 ) ) ;
#141891=CARTESIAN_POINT ( 'NONE',  ( -9.332089804907933939, 9.781859615347734405, 1.040834085586084257E-14 ) ) ;
#141892=CARTESIAN_POINT ( 'NONE',  ( -5.544921637864833386, 7.492161215640853023, -1.443375672974051449 ) ) ;
#141896=CARTESIAN_POINT ( 'NONE',  ( 0.7499999999999885647, -0.7354166659838470288, 1.299038105676657340 ) ) ;
#141905=CARTESIAN_POINT ( 'NONE',  ( -4.067082893975237035, 7.688754443039000464, 1.040834085586084257E-14 ) ) ;
#141909=CARTESIAN_POINT ( 'NONE',  ( -4.568734577680880093, 7.313645526394248364, -1.082531754730548412 ) ) ;
#141911=CARTESIAN_POINT ( 'NONE',  ( 8.224992744984721327, 12.74757530245756243, 1.040834085586084257E-14 ) ) ;
#141915=CARTESIAN_POINT ( 'NONE',  ( 1.491528662501849123, 8.751894132169937279, -2.513572095680560281 ) ) ;
#141920=CARTESIAN_POINT ( 'NONE',  ( 6.471393748265543699, 5.229711127717882491, 2.420000000000010587 ) ) ;
#141921=CARTESIAN_POINT ( 'NONE',  ( -5.440899717785814715, 5.242137847038546461, 0.7998128361456341429 ) ) ;
#141923=CARTESIAN_POINT ( 'NONE',  ( -1.500000000000001332, 0.9000000000000187850, 0.000000000000000000 ) ) ;
#141924=ORIENTED_EDGE ( 'NONE', *, *, #142048, .T. ) ;
#141926=CARTESIAN_POINT ( 'NONE',  ( 8.080296364064698977, 12.37083682481011060, -0.7216878364870328300 ) ) ;
#141927=CARTESIAN_POINT ( 'NONE',  ( 5.524057522564145728, 8.532151978711786100, 1.199719254218462483 ) ) ;
#141932=CARTESIAN_POINT ( 'NONE',  ( 4.517891501851804215, 6.293959390292322986, -1.599625672291255185 ) ) ;
#141934=VERTEX_POINT ( 'NONE', #114203 ) ;
#141941=CARTESIAN_POINT ( 'NONE',  ( 9.582915646760733708, 10.07448976417602893, 0.7998128361456462443 ) ) ;
#141942=CARTESIAN_POINT ( 'NONE',  ( -6.250472511100020334, 7.250971670160158311, 1.199719254218450271 ) ) ;
#141947=CARTESIAN_POINT ( 'NONE',  ( 0.6823417656249899377, 4.676041667008086655, -1.181850606188754593 ) ) ;
#141948=CARTESIAN_POINT ( 'NONE',  ( 9.042925270190632858, 10.61279623905300085, 1.082531754730549967 ) ) ;
#141949=CARTESIAN_POINT ( 'NONE',  ( -5.063080299699540987, 7.994345218703034384, 1.199719254218464037 ) ) ;
#141952=CARTESIAN_POINT ( 'NONE',  ( 5.843727902690005749, 6.776436293681846301, -1.199719254218445830 ) ) ;
#141953=CARTESIAN_POINT ( 'NONE',  ( -4.574986769607567894, 7.424902766929059261, 1.199719254218464037 ) ) ;
#141959=CARTESIAN_POINT ( 'NONE',  ( 5.450014563013511726, 8.341805509282339770, -1.082531754730543083 ) ) ;
#141962=CARTESIAN_POINT ( 'NONE',  ( 1.364683531249988757, 1.446875000341421469, 0.000000000000000000 ) ) ;
#141964=CARTESIAN_POINT ( 'NONE',  ( 5.083944415000174466, 7.914723669933440675, -1.082531754730549078 ) ) ;
#141966=CARTESIAN_POINT ( 'NONE',  ( 4.586165880992498778, 5.350526861157986147, -2.420000000000000373 ) ) ;
#141967=CARTESIAN_POINT ( 'NONE',  ( -4.799223189557577207, 4.701441264013013210, 0.7216878364870317197 ) ) ;
#141974=CARTESIAN_POINT ( 'NONE',  ( -4.044288467547167976, 7.756266588949179308, -0.5710662792986564984 ) ) ;
#141981=CARTESIAN_POINT ( 'NONE',  ( 6.440286661691305703, 7.472421512516709718, 1.199719254218462483 ) ) ;
#141992=CARTESIAN_POINT ( 'NONE',  ( 3.199361063144961825, 6.676412307070352270, -0.7216878364870267237 ) ) ;
#141994=CARTESIAN_POINT ( 'NONE',  ( -1.364683531250000748, 1.821875000341421913, 0.000000000000000000 ) ) ;
#141996=CARTESIAN_POINT ( 'NONE',  ( 8.911787042884274257, 9.291506392986812912, 0.7998128361456462443 ) ) ;
#142001=CARTESIAN_POINT ( 'NONE',  ( 0.7499999999999902300, 2.733333333333351600, 1.299038105676669330 ) ) ;
#142002=CARTESIAN_POINT ( 'NONE',  ( 5.392392409933256303, 7.314210449720692786, 1.599625672291267398 ) ) ;
#142003=CARTESIAN_POINT ( 'NONE',  ( -8.064402442030170093, 8.302891025323665630, 0.7998128361456602331 ) ) ;
#142007=CARTESIAN_POINT ( 'NONE',  ( 0.6823417656249882723, 2.176041667008084435, -1.181850606188749264 ) ) ;
#142009=CARTESIAN_POINT ( 'NONE',  ( 4.518945272056516416, 4.166524327021037699, 0.7998128361456341429 ) ) ;
#142014=CARTESIAN_POINT ( 'NONE',  ( 1.499999999999987121, 0.3270833340161527492, -0.8660254037844323793 ) ) ;
#142017=CARTESIAN_POINT ( 'NONE',  ( -7.040761844198392794, 7.108643661186573759, -0.7998128361456291469 ) ) ;
#142018=FACE_OUTER_BOUND ( 'NONE', #35417, .T. ) ;
#142024=EDGE_LOOP ( 'NONE', ( #120772, #29716, #134697, #138816 ) ) ;
#142026=CARTESIAN_POINT ( 'NONE',  ( 5.717788096661236885, 7.693838750903348789, 1.599625672291267398 ) ) ;
#142030=CARTESIAN_POINT ( 'NONE',  ( 5.626797444871351139, 6.523350759560078593, 1.199719254218462483 ) ) ;
#142034=CARTESIAN_POINT ( 'NONE',  ( 4.403700966340357681, 4.032072637018845107, -0.7998128361456211532 ) ) ;
#142039=CARTESIAN_POINT ( 'NONE',  ( 5.378845419373885051, 6.306261619127770501, 1.070519943709395960 ) ) ;
#142044=DIRECTION ( 'NONE',  ( 0.3502638921866464417, -1.953969548649013438E-16, 0.9366510587354618389 ) ) ;
#142048=EDGE_CURVE ( 'NONE', #157004, #24729, #130478, .T. ) ;
#142050=FACE_OUTER_BOUND ( 'NONE', #40053, .T. ) ;
#142051=CARTESIAN_POINT ( 'NONE',  ( 7.456621297836072415, 9.722477485607340597, 1.443375672974076540 ) ) ;
#142053=CARTESIAN_POINT ( 'NONE',  ( -4.822949958159302497, 6.649860922651058992, -1.599625672291256295 ) ) ;
#142055=CARTESIAN_POINT ( 'NONE',  ( -0.1099460098627005888, 6.494484681433106310, 3.110387376256865011 ) ) ;
#142057=CARTESIAN_POINT ( 'NONE',  ( 7.690499447449630210, 9.995335326823163058, 1.599625672291281386 ) ) ;
#142059=CARTESIAN_POINT ( 'NONE',  ( -5.096975683733680818, 8.033889833409558534, -1.199719254218452047 ) ) ;
#142073=CARTESIAN_POINT ( 'NONE',  ( 8.940712233207955606, 12.51824914112961729, 1.199719254218450271 ) ) ;
#142074=CARTESIAN_POINT ( 'NONE',  ( -4.660252114795309097, 6.460046772059735432, -1.599625672291256295 ) ) ;
#142077=CARTESIAN_POINT ( 'NONE',  ( 5.043269954603547767, 4.986162489899998995, -0.7216878364870197293 ) ) ;
#142078=CARTESIAN_POINT ( 'NONE',  ( 1.499999999999990896, 4.525000000000021672, 1.214306433183764966E-14 ) ) ;
#142082=CARTESIAN_POINT ( 'NONE',  ( -3.415764635639130020, 6.072476943965863683, 1.199719254218462483 ) ) ;
#142085=CARTESIAN_POINT ( 'NONE',  ( 7.564559641420864899, 10.91273778404466199, -1.199719254218446718 ) ) ;
#142090=CARTESIAN_POINT ( 'NONE',  ( -8.037286134802835491, 8.271255333558444889, -0.7998128361456291469 ) ) ;
#142091=CARTESIAN_POINT ( 'NONE',  ( 4.904298879841284098, 6.744767997946721216, 1.599625672291267398 ) ) ;
#142094=DIRECTION ( 'NONE',  ( 0.3321398189114310173, 0.9432301631592798774, 3.697785493223492838E-32 ) ) ;
#142098=CARTESIAN_POINT ( 'NONE',  ( -0.6823417656249969321, 3.280208333674754062, -1.181850606188749264 ) ) ;
#142101=CARTESIAN_POINT ( 'NONE',  ( 5.802526556968819804, 9.713438716531550554, -0.7216878364870267237 ) ) ;
#142103=CARTESIAN_POINT ( 'NONE',  ( 1.499999999999972911, 4.577083334016149863, -0.8660254037844417052 ) ) ;
#142108=CARTESIAN_POINT ( 'NONE',  ( 10.04622863760192963, 10.82294762006482713, -0.7216878364870257245 ) ) ;
#142113=CARTESIAN_POINT ( 'NONE',  ( -7.967387826325084355, 12.44703623068796361, 0.7998128361456481317 ) ) ;
#142130=CARTESIAN_POINT ( 'NONE',  ( 1.499999999999987121, 1.577083334016150751, -0.8660254037844253849 ) ) ;
#142136=CARTESIAN_POINT ( 'NONE',  ( 1.499999999999987121, 0.004166666666691258049, 0.8660254037844524744 ) ) ;
#142137=CARTESIAN_POINT ( 'NONE',  ( 7.751511138711133064, 10.06651563329490529, -1.599625672291262513 ) ) ;
#142138=CARTESIAN_POINT ( 'NONE',  ( 0.6823417656249882723, -0.07395833299191079124, -1.181850606188749264 ) ) ;
#142142=CARTESIAN_POINT ( 'NONE',  ( 4.033714395265605823, 4.664753868353354704, -1.199719254218446718 ) ) ;
#142143=CARTESIAN_POINT ( 'NONE',  ( -4.744990575102892905, 8.479646737687938085, 0.7216878364870458196 ) ) ;
#142147=CARTESIAN_POINT ( 'NONE',  ( -5.693534442735004752, 8.729875052244421951, 1.199719254218452047 ) ) ;
#142149=CARTESIAN_POINT ( 'NONE',  ( -0.7500000000000215383, 2.972916667349487341, 1.299038105676671107 ) ) ;
#142160=CARTESIAN_POINT ( 'NONE',  ( -8.910733272679575379, 11.41894145625809820, -1.599625672291263179 ) ) ;
#142161=CARTESIAN_POINT ( 'NONE',  ( 7.253775878511261155, 8.421492265473332850, 1.199719254218462483 ) ) ;
#142167=ADVANCED_FACE ( 'NONE', ( #72555 ), #157037, .F. ) ;
#142169=CARTESIAN_POINT ( 'NONE',  ( -6.509886312855995172, 10.74661779830734254, -0.7998128361456291469 ) ) ;
#142171=CARTESIAN_POINT ( 'NONE',  ( -2.081668171172168513E-14, 5.868705557303649734, 4.125226524755077229 ) ) ;
#142175=CARTESIAN_POINT ( 'NONE',  ( 4.715538499454675403, 4.395883092318884522, 1.214306433183764966E-14 ) ) ;
#142177=ORIENTED_EDGE ( 'NONE', *, *, #183780, .F. ) ;
#142179=CARTESIAN_POINT ( 'NONE',  ( -9.155833807930273238, 9.576227618873799585, -0.7998128361456291469 ) ) ;
#142183=CARTESIAN_POINT ( 'NONE',  ( -5.030466903028923298, 6.770262730772157234, -1.447917484242104758 ) ) ;
#142187=AXIS2_PLACEMENT_3D ( 'NONE', #7908, #141176, #159511 ) ;
#142191=CARTESIAN_POINT ( 'NONE',  ( 7.630541526392844887, 7.796719957080126662, 0.7998128361456341429 ) ) ;
#142198=ORIENTED_EDGE ( 'NONE', *, *, #90702, .T. ) ;
#142210=DIRECTION ( 'NONE',  ( 1.000000000000000000, 0.000000000000000000, 0.000000000000000000 ) ) ;
#142212=CARTESIAN_POINT ( 'NONE',  ( 4.541618270897912701, 4.400902192243413502, 1.214306433183764966E-14 ) ) ;
#142217=CARTESIAN_POINT ( 'NONE',  ( -9.622536337397040285, 12.24937836509514710, 1.599625672291281386 ) ) ;
#142221=CARTESIAN_POINT ( 'NONE',  ( 8.940712233207955606, 12.51824914112961729, 1.199719254218450271 ) ) ;
#142229=CARTESIAN_POINT ( 'NONE',  ( -1.364683531250012516, 1.030208333674754062, 0.7879004041258379498 ) ) ;
#142235=CARTESIAN_POINT ( 'NONE',  ( -5.091250377131585125, 5.898545847196970726, 1.199719254218450271 ) ) ;
#142238=CARTESIAN_POINT ( 'NONE',  ( -0.7500000000000006661, -0.3916666666666443475, -1.299038105676652011 ) ) ;
#142240=CARTESIAN_POINT ( 'NONE',  ( 1.364683531249988757, -0.8031249996585804185, 0.000000000000000000 ) ) ;
#142245=CARTESIAN_POINT ( 'NONE',  ( 1.364683531249988535, 5.717708333674752730, -0.7879004041258300672 ) ) ;
#142247=CARTESIAN_POINT ( 'NONE',  ( -7.874588291438845644, 8.081441182967111558, -0.7998128361456291469 ) ) ;
#142248=CARTESIAN_POINT ( 'NONE',  ( 7.781490099239519509, 11.16582331816642260, 1.199719254218460707 ) ) ;
#142255=CARTESIAN_POINT ( 'NONE',  ( -1.364683531250014514, 0.5510416670080878765, -0.7879004041258289570 ) ) ;
#142263=CARTESIAN_POINT ( 'NONE',  ( 6.860062538834778678, 8.066123052471139587, -1.082531754730543083 ) ) ;
#142266=CARTESIAN_POINT ( 'NONE',  ( -5.752737250900127997, 5.605948302338584099, 0.000000000000000000 ) ) ;
#142270=CARTESIAN_POINT ( 'NONE',  ( -4.451154503988200339, 4.087435097607984957, 1.214306433183764966E-14 ) ) ;
#142271=CARTESIAN_POINT ( 'NONE',  ( 5.707619481228810798, 7.681975366232176583, -1.443375672974057666 ) ) ;
#142272=CARTESIAN_POINT ( 'NONE',  ( -8.310784975052669665, 12.63974020429606249, -0.7216878364870267237 ) ) ;
#142277=CARTESIAN_POINT ( 'NONE',  ( 8.920901888111986366, 12.39117405523060889, 1.082531754730546636 ) ) ;
#142283=( BOUNDED_CURVE ( )  B_SPLINE_CURVE ( 2, ( #60314, #193524, #192438, #110213, #12624 ),
 .UNSPECIFIED., .F., .T. ) 
 B_SPLINE_CURVE_WITH_KNOTS ( ( 3, 2, 3 ),
 ( 0.1347995350948868465, 0.1375000000000000111, 0.1409922313975706942 ),
 .UNSPECIFIED. ) 
 CURVE ( )  GEOMETRIC_REPRESENTATION_ITEM ( )  RATIONAL_B_SPLINE_CURVE ( ( 0.9388907138593196589, 0.9131695131383610331, 1.000000000000000000, 0.8877111300685985862, 0.9636488443798396641 ) ) 
 REPRESENTATION_ITEM ( '' )  );
#142290=ADVANCED_FACE ( 'NONE', ( #205687 ), #209790, .T. ) ;
#142294=CARTESIAN_POINT ( 'NONE',  ( 9.368320956918616105, 10.03205532593431037, 0.7216878364870458196 ) ) ;
#142297=CARTESIAN_POINT ( 'NONE',  ( 8.437251666405968464, 8.737881787095446384, 1.040834085586084257E-14 ) ) ;
#142302=CARTESIAN_POINT ( 'NONE',  ( 5.694061328059515148, 5.745419092265303007, -0.7216878364870207285 ) ) ;
#142304=CARTESIAN_POINT ( 'NONE',  ( -9.002250809794006159, 10.56534270192358704, -1.082531754730543971 ) ) ;
#142309=CARTESIAN_POINT ( 'NONE',  ( -2.656508033273816238, 5.186677574539687363, -1.199719254218446718 ) ) ;
#142333=CARTESIAN_POINT ( 'NONE',  ( -6.738566041191992539, 7.820414121934134322, 1.199719254218450271 ) ) ;
#142338=CARTESIAN_POINT ( 'NONE',  ( 7.135668919494039031, 7.219368582364847242, 1.040834085586084257E-14 ) ) ;
#142340=CARTESIAN_POINT ( 'NONE',  ( -5.135841261478327979, 4.886236314679810455, 0.7998128361456341429 ) ) ;
#142344=CARTESIAN_POINT ( 'NONE',  ( -3.764360206088648297, 7.543504007078730922, -0.7998128361456281477 ) ) ;
#142345=DIRECTION ( 'NONE',  ( -1.000000000000000000, 7.387867266669436732E-31, 0.000000000000000000 ) ) ;
#142348=CARTESIAN_POINT ( 'NONE',  ( -3.903858165731105778, 6.641919395739846799, 1.199719254218464037 ) ) ;
#142351=CARTESIAN_POINT ( 'NONE',  ( 6.889514614038635187, 11.18951748302043114, -0.7998128361456291469 ) ) ;
#142354=CARTESIAN_POINT ( 'NONE',  ( 6.017762162252820346, 6.076696597586958681, 0.5614182107811436229 ) ) ;
#142355=CARTESIAN_POINT ( 'NONE',  ( 4.880572111239557920, 4.796348339308675435, -0.7216878364870197293 ) ) ;
#142362=CARTESIAN_POINT ( 'NONE',  ( 6.060131475184119765, 9.053608573481392696, -1.082531754730537976 ) ) ;
#142363=CARTESIAN_POINT ( 'NONE',  ( -7.648771216403934758, 12.07531685244661723, -0.7998128361456291469 ) ) ;
#142366=CARTESIAN_POINT ( 'NONE',  ( -9.182950115157607840, 9.607863310639020327, 0.7998128361456462443 ) ) ;
#142367=CARTESIAN_POINT ( 'NONE',  ( -6.847031270101295419, 7.946956888995021728, -1.199719254218446718 ) ) ;
#142374=CARTESIAN_POINT ( 'NONE',  ( 6.428537391173986038, 10.65171072301167854, 0.7998128361456462443 ) ) ;
#142382=CARTESIAN_POINT ( 'NONE',  ( -1.499999999999997780, 5.431250000682820378, 1.214306433183764966E-14 ) ) ;
#142387=CARTESIAN_POINT ( 'NONE',  ( 1.499999999999990896, 4.525000000000021672, 1.214306433183764966E-14 ) ) ;
#142388=CARTESIAN_POINT ( 'NONE',  ( 4.847203612085560387, 5.613824621309978724, -1.199719254218452047 ) ) ;
#142389=CARTESIAN_POINT ( 'NONE',  ( 7.253775878511261155, 8.421492265473332850, 1.199719254218462483 ) ) ;
#142392=CARTESIAN_POINT ( 'NONE',  ( 7.293923454472087897, 8.572294120714675003, 1.082531754730558626 ) ) ;
#142393=CARTESIAN_POINT ( 'NONE',  ( -9.124274191872636663, 11.66807252865000244, -1.443375672974058777 ) ) ;
#142397=CARTESIAN_POINT ( 'NONE',  ( 8.751951852821344247, 10.16936423550178503, -1.199719254218446718 ) ) ;
#142399=CARTESIAN_POINT ( 'NONE',  ( -1.201851678989727383E-14, 5.337500000000019895, -1.732050807568863648 ) ) ;
#142400=FACE_OUTER_BOUND ( 'NONE', #29212, .T. ) ;
#142402=CARTESIAN_POINT ( 'NONE',  ( -1.402160292154681736E-14, 0.4468750003414233563, -1.575800808251665908 ) ) ;
#142407=CARTESIAN_POINT ( 'NONE',  ( 0.6823417656249882723, -0.1572916663252488245, 1.181850606188755259 ) ) ;
#142409=CARTESIAN_POINT ( 'NONE',  ( 10.01963921569910632, 11.64833282552586091, 1.199719254218450271 ) ) ;
#142413=CARTESIAN_POINT ( 'NONE',  ( -8.618179199781044630, 13.20629283305325963, 0.7998128361456341429 ) ) ;
#142418=CARTESIAN_POINT ( 'NONE',  ( 2.679707916995359263, 6.278076336469897711, -0.7998128361456291469 ) ) ;
#142422=ORIENTED_EDGE ( 'NONE', *, *, #64571, .F. ) ;
#142424=CARTESIAN_POINT ( 'NONE',  ( 8.072990401933337168, 11.50590700464255356, -1.199719254218446718 ) ) ;
#142427=CARTESIAN_POINT ( 'NONE',  ( -4.381256195510448315, 8.263215994737505454, 1.040834085586084257E-14 ) ) ;
#142432=CARTESIAN_POINT ( 'NONE',  ( 8.776205506747620788, 9.133327934160710981, -0.7998128361456221525 ) ) ;
#142434=CARTESIAN_POINT ( 'NONE',  ( 6.805303039055573322, 10.02693841461847057, 1.199719254218460707 ) ) ;
#142437=CARTESIAN_POINT ( 'NONE',  ( -10.48008955368359629, 11.32911868882677986, 1.040834085586084257E-14 ) ) ;
#142445=CARTESIAN_POINT ( 'NONE',  ( -6.133411998150831046, 5.998805638374869353, -0.1291943307598683033 ) ) ;
#142446=CARTESIAN_POINT ( 'NONE',  ( -1.201851678989727383E-14, 1.821875000341421691, 1.575800808251672791 ) ) ;
#142448=CARTESIAN_POINT ( 'NONE',  ( 6.317736394288135493, 8.393778431468064127, 1.443375672974076540 ) ) ;
#142461=CARTESIAN_POINT ( 'NONE',  ( 3.782361668088245921, 6.396210465202840645, -1.082531754730548412 ) ) ;
#142465=CARTESIAN_POINT ( 'NONE',  ( 7.964525173024008531, 11.37936423758166526, 1.199719254218460707 ) ) ;
#142467=ORIENTED_EDGE ( 'NONE', *, *, #31970, .F. ) ;
#142469=CARTESIAN_POINT ( 'NONE',  ( -3.541704441667874903, 5.155074486744371853, -1.599625672291256295 ) ) ;
#142470=CARTESIAN_POINT ( 'NONE',  ( -5.371001409308059138, 9.417918744168066070, -0.7998128361456231517 ) ) ;
#142475=CARTESIAN_POINT ( 'NONE',  ( -1.499999999999997780, 4.431250000682819490, 1.214306433183764966E-14 ) ) ;
#142476=CARTESIAN_POINT ( 'NONE',  ( 7.182068686937156166, 9.402166106225269715, 1.599625672291281386 ) ) ;
#142479=CARTESIAN_POINT ( 'NONE',  ( -7.771848369131641121, 10.09024240211882351, -1.599625672291263179 ) ) ;
#142481=CARTESIAN_POINT ( 'NONE',  ( -1.364683531250010295, 4.780208333674755394, 0.7879004041258379498 ) ) ;
#142484=CARTESIAN_POINT ( 'NONE',  ( 2.881411693390222961, 6.438990010880548454, -0.3632046419933783743 ) ) ;
#142488=VECTOR ( 'NONE', #70608, 1000.000000000000000 ) ;
#142489=CARTESIAN_POINT ( 'NONE',  ( -7.971831135155409420, 11.28392484344787405, 1.082531754730549967 ) ) ;
#142493=CARTESIAN_POINT ( 'NONE',  ( -0.6823417656250003738, 2.780208333674753618, -1.181850606188749264 ) ) ;
#142501=CARTESIAN_POINT ( 'NONE',  ( -1.201851678989727383E-14, 3.696875000341422801, -1.575800808251660134 ) ) ;
#142502=CARTESIAN_POINT ( 'NONE',  ( -3.113568832632681360, 6.784247404713427798, -0.7998128361456281477 ) ) ;
#142503=CARTESIAN_POINT ( 'NONE',  ( 7.461064606222022277, 7.598996883547496139, 1.040834085586084257E-14 ) ) ;
#142506=CARTESIAN_POINT ( 'NONE',  ( 1.364683531249990311, 4.676041667008083103, 0.7879004041258500513 ) ) ;
#142509=CARTESIAN_POINT ( 'NONE',  ( -0.6823417656250003738, -0.7822916663252423852, -1.181850606188749264 ) ) ;
#142510=CARTESIAN_POINT ( 'NONE',  ( -3.768803514918943609, 7.340761834139994058, 0.7216878364870317197 ) ) ;
#142513=CARTESIAN_POINT ( 'NONE',  ( 3.551873057100287223, 5.166937871415542283, 1.443375672974062551 ) ) ;
#142516=CARTESIAN_POINT ( 'NONE',  ( -10.15469386695561482, 10.94949038764413096, 1.040834085586084257E-14 ) ) ;
#142522=CARTESIAN_POINT ( 'NONE',  ( -7.199016378732087773, 7.501199984716642177, 0.7216878364870317197 ) ) ;
#142524=CARTESIAN_POINT ( 'NONE',  ( 0.6823417656249899377, 0.6552083336747518416, 1.181850606188755259 ) ) ;
#142532=CARTESIAN_POINT ( 'NONE',  ( 1.364683531249986537, -0.7822916663252464931, -0.7879004041258309554 ) ) ;
#142536=CARTESIAN_POINT ( 'NONE',  ( 2.860407222358963608, 5.320596945185329218, 1.082531754730548412 ) ) ;
#142541=CARTESIAN_POINT ( 'NONE',  ( 6.751597309481075726, 10.82068792779586985, 1.040834085586084257E-14 ) ) ;
#142545=ORIENTED_EDGE ( 'NONE', *, *, #125104, .F. ) ;
#142547=ORIENTED_EDGE ( 'NONE', *, *, #50310, .T. ) ;
#142551=CARTESIAN_POINT ( 'NONE',  ( -1.499999999999993339, 10.64264068711930733, 1.232676135170975238E-14 ) ) ;
#142554=CARTESIAN_POINT ( 'NONE',  ( -0.6823417656250212460, 2.113541667008083991, 1.181850606188767472 ) ) ;
#142555=DIRECTION ( 'NONE',  ( 0.9366510587354612838, 0.000000000000000000, 0.3502638921866474409 ) ) ;
#142565=ORIENTED_EDGE ( 'NONE', *, *, #85154, .T. ) ;
#142574=CARTESIAN_POINT ( 'NONE',  ( 7.006866460164219212, 7.069099046480051385, -0.7998128361456281477 ) ) ;
#142580=AXIS2_PLACEMENT_3D ( 'NONE', #134246, #86526, #168840 ) ;
#142585=CARTESIAN_POINT ( 'NONE',  ( 7.560643217915098191, 11.97250085420964716, -0.7998128361456291469 ) ) ;
#142587=CARTESIAN_POINT ( 'NONE',  ( 1.579999999999991189, 8.674529973577531194, -2.499999999999989342 ) ) ;
#142593=CARTESIAN_POINT ( 'NONE',  ( -0.3006164276377518707, 8.220220202721305824, 1.980250916746241652 ) ) ;
#142596=CARTESIAN_POINT ( 'NONE',  ( -8.188761592974040937, 11.53701037756964887, -1.082531754730543971 ) ) ;
#142602=CARTESIAN_POINT ( 'NONE',  ( 5.335297142177534369, 6.183267073083954735, -1.199719254218452047 ) ) ;
#142610=CARTESIAN_POINT ( 'NONE',  ( 3.429849674132933846, 5.024577257953626308, -1.443375672974058777 ) ) ;
#142618=CARTESIAN_POINT ( 'NONE',  ( -5.042743069279040036, 7.970618449879118828, 1.199719254218464037 ) ) ;
#142620=CARTESIAN_POINT ( 'NONE',  ( -2.286521462199063492, 5.819358805874190743, 1.040834085586084257E-14 ) ) ;
#142626=ORIENTED_EDGE ( 'NONE', *, *, #64812, .T. ) ;
#142629=CARTESIAN_POINT ( 'NONE',  ( 6.634017235788401301, 6.634108284708264414, 0.7998128361456341429 ) ) ;
#142631=CARTESIAN_POINT ( 'NONE',  ( 1.567523721964578121, 8.684745761082966808, 2.500978756717656015 ) ) ;
#142641=AXIS2_PLACEMENT_3D ( 'NONE', #5760, #89205, #208248 ) ;
#142645=CARTESIAN_POINT ( 'NONE',  ( -1.402160292154681736E-14, 1.259375000341419248, -1.575800808251659024 ) ) ;
#142646=CARTESIAN_POINT ( 'NONE',  ( 4.325214697959421706, 5.004837554829479451, 1.199719254218462483 ) ) ;
#142648=CARTESIAN_POINT ( 'NONE',  ( -6.155038550924159857, 8.203964280876741455, 1.443375672974078761 ) ) ;
#142649=CARTESIAN_POINT ( 'NONE',  ( 2.901081683644312736, 6.328419697652925002, 0.7216878364870338292 ) ) ;
#142650=CARTESIAN_POINT ( 'NONE',  ( -5.029711800545518585, 8.811821500704338561, 0.7216878364870458196 ) ) ;
#142654=CARTESIAN_POINT ( 'NONE',  ( 7.474622759835693131, 7.614814729430110951, -0.7998128361456281477 ) ) ;
#142659=CARTESIAN_POINT ( 'NONE',  ( -1.001543065824772872E-14, 4.821875000341419693, 1.575800808251672791 ) ) ;
#142663=CARTESIAN_POINT ( 'NONE',  ( 6.928380191783277908, 8.041863964290678624, 1.199719254218462483 ) ) ;
#142664=( NAMED_UNIT ( * ) SI_UNIT ( $, .STERADIAN. ) SOLID_ANGLE_UNIT ( ) );
#142666=CARTESIAN_POINT ( 'NONE',  ( -6.877010230629689858, 9.046264573866535486, 1.599625672291283607 ) ) ;
#142671=CARTESIAN_POINT ( 'NONE',  ( 8.749089199520284410, 9.101692242395490240, 0.7998128361456481317 ) ) ;
#142674=CARTESIAN_POINT ( 'NONE',  ( -6.015013705957189316, 10.16926642359206134, 0.7998128361456481317 ) ) ;
#142677=CARTESIAN_POINT ( 'NONE',  ( 6.602457619730749627, 10.64669162308715222, 0.7216878364870438212 ) ) ;
#142678=CARTESIAN_POINT ( 'NONE',  ( 4.167679133687917314, 7.375052378509237450, -0.7893339205088979460 ) ) ;
#142679=CARTESIAN_POINT ( 'NONE',  ( -8.459924665247381625, 11.85336729522185806, 1.082531754730560403 ) ) ;
#142685=CARTESIAN_POINT ( 'NONE',  ( 5.229694566569264680, 7.124396299129368337, 1.599625672291267398 ) ) ;
#142687=CARTESIAN_POINT ( 'NONE',  ( 7.540305987494599016, 11.94877408538573427, -0.7998128361456291469 ) ) ;
#142688=CARTESIAN_POINT ( 'NONE',  ( -5.266216980226317013, 6.417262052691032004, 1.151019644853501944 ) ) ;
#142690=CARTESIAN_POINT ( 'NONE',  ( -1.364683531250012516, 1.030208333674754062, 0.7879004041258379498 ) ) ;
#142692=CARTESIAN_POINT ( 'NONE',  ( -5.829642864196175722, 7.824335979694092558, 1.443375672974064550 ) ) ;
#142699=CARTESIAN_POINT ( 'NONE',  ( -5.155981903556834389, 6.496760599866445496, 1.199444197134313272 ) ) ;
#142700=CARTESIAN_POINT ( 'NONE',  ( -1.364683531250014514, 0.3010416670080866552, -0.7879004041258359514 ) ) ;
#142703=CARTESIAN_POINT ( 'NONE',  ( 2.738383840280320669, 6.138605547061593448, 0.7216878364870338292 ) ) ;
#142708=CARTESIAN_POINT ( 'NONE',  ( -7.443063143778079649, 10.66702885350765584, 1.082531754730549967 ) ) ;
#142709=AXIS2_PLACEMENT_3D ( 'NONE', #23999, #205958, #58654 ) ;
#142715=CARTESIAN_POINT ( 'NONE',  ( -9.015808962963337336, 10.58116054728778366, 1.082531754730558626 ) ) ;
#142722=CARTESIAN_POINT ( 'NONE',  ( -7.931156673870055407, 11.23647130528163096, 1.082531754730549967 ) ) ;
#142726=CARTESIAN_POINT ( 'NONE',  ( -1.201851678989727383E-14, 4.759375000341419693, -1.575800808251660134 ) ) ;
#142727=CARTESIAN_POINT ( 'NONE',  ( -0.7499999999999972244, 3.889583334016149863, -1.299038105676652011 ) ) ;
#142728=CARTESIAN_POINT ( 'NONE',  ( 4.834557559160812978, 6.939504195329335268, -1.414529171088283688 ) ) ;
#142734=CARTESIAN_POINT ( 'NONE',  ( -8.694856585065634746, 9.038420858865048757, 0.7998128361456462443 ) ) ;
#142738=CARTESIAN_POINT ( 'NONE',  ( 4.039439701867726384, 6.800097854565950506, 1.199719254218462483 ) ) ;
#142740=EDGE_CURVE ( 'NONE', #64117, #152385, #33924, .T. ) ;
#142745=CARTESIAN_POINT ( 'NONE',  ( 5.635385404774530649, 9.726366738878972740, 0.7998128361456462443 ) ) ;
#142752=CARTESIAN_POINT ( 'NONE',  ( -5.368665641331555882, 8.246898433986675769, 1.082531754730548412 ) ) ;
#142755=EDGE_CURVE ( 'NONE', #192824, #196589, #26256, .T. ) ;
#142756=CARTESIAN_POINT ( 'NONE',  ( -4.636780943466218829, 5.307142521894840037, 1.176014350056652225 ) ) ;
#142763=CARTESIAN_POINT ( 'NONE',  ( -8.666686507633592385, 11.13422023037111330, 1.599625672291269396 ) ) ;
#142765=CARTESIAN_POINT ( 'NONE',  ( 8.178592977541601527, 10.56477777859713463, 1.599625672291281386 ) ) ;
#142766=CARTESIAN_POINT ( 'NONE',  ( -1.402160292154681736E-14, -0.6624999999999758860, -1.732050807568870754 ) ) ;
#142767=CARTESIAN_POINT ( 'NONE',  ( -8.850775351622791831, 9.220326086515070685, -0.7998128361456291469 ) ) ;
#142770=CARTESIAN_POINT ( 'NONE',  ( -1.364683531249997417, 3.509375000341423245, 1.214306433183764966E-14 ) ) ;
#142771=CARTESIAN_POINT ( 'NONE',  ( 9.083599731475976213, 12.58098820582193689, 1.082531754730546636 ) ) ;
#142774=CARTESIAN_POINT ( 'NONE',  ( 1.499999999999990896, 5.025000000000022560, 1.214306433183764966E-14 ) ) ;
#142777=CARTESIAN_POINT ( 'NONE',  ( 7.904040366642689719, 10.24446639921506552, 1.443375672974076540 ) ) ;
#142780=CARTESIAN_POINT ( 'NONE',  ( -7.402388683381436074, 7.738467673474211495, 0.7216878364870317197 ) ) ;
#142782=B_SPLINE_CURVE_WITH_KNOTS ( 'NONE', 3,
 ( #185385, #40224, #107415, #203753 ),
 .UNSPECIFIED., .F., .F.,
 ( 4, 4 ),
 ( 0.000000000000000000, 0.0003389024754017963548 ),
 .UNSPECIFIED. ) ;
#142783=CARTESIAN_POINT ( 'NONE',  ( 1.364683531249988535, 2.613541667008089764, 0.7879004041258500513 ) ) ;
#142785=DIRECTION ( 'NONE',  ( 0.000000000000000000, 8.546850786086437571E-32, 1.000000000000000000 ) ) ;
#142787=CARTESIAN_POINT ( 'NONE',  ( -7.043624497499477499, 8.176315654292865887, 1.199719254218450271 ) ) ;
#142788=CARTESIAN_POINT ( 'NONE',  ( -1.201851678989727383E-14, 4.259375000341417028, -1.575800808251660134 ) ) ;
#142794=CARTESIAN_POINT ( 'NONE',  ( 8.289920859751990889, 11.75899253876431416, 1.199719254218450271 ) ) ;
#142798=CARTESIAN_POINT ( 'NONE',  ( -1.402160292154681736E-14, 0.8375000000000232259, -1.732050807568863648 ) ) ;
#142802=ORIENTED_EDGE ( 'NONE', *, *, #140986, .T. ) ;
#142808=CARTESIAN_POINT ( 'NONE',  ( -1.500511526392867001, 8.643217832945683909, 2.569261818345993653 ) ) ;
#142811=CARTESIAN_POINT ( 'NONE',  ( 0.6823417656249899377, 5.238541667008086655, -1.181850606188754593 ) ) ;
#142818=CARTESIAN_POINT ( 'NONE',  ( 1.364683531249990311, 4.384375000341417028, 1.214306433183764966E-14 ) ) ;
#142820=CARTESIAN_POINT ( 'NONE',  ( -4.907688418466881863, 8.669460888279271416, 0.7216878364870458196 ) ) ;
#142826=CARTESIAN_POINT ( 'NONE',  ( 4.390142812726693045, 4.016254791136236513, 1.214306433183764966E-14 ) ) ;
#142829=CARTESIAN_POINT ( 'NONE',  ( 9.101601193475611140, 9.512956235343358102, -0.7998128361456221525 ) ) ;
#142830=CARTESIAN_POINT ( 'NONE',  ( 3.325722479477188021, 7.699077257575913436, -2.500000000000104361 ) ) ;
#142836=CARTESIAN_POINT ( 'NONE',  ( -7.458957065812611198, 11.85386701009007204, 0.7998128361456481317 ) ) ;
#142837=CARTESIAN_POINT ( 'NONE',  ( 6.602984505055297326, 7.662235663108029726, 1.199719254218462483 ) ) ;
#142840=CARTESIAN_POINT ( 'NONE',  ( 5.118366684358879759, 5.930181538962194132, 1.199719254218462483 ) ) ;
#142849=CARTESIAN_POINT ( 'NONE',  ( -6.561783159334141580, 7.718130443053708767, -1.082531754730544860 ) ) ;
#142850=CARTESIAN_POINT ( 'NONE',  ( 2.849184837166184536, 6.475799410002530898, 0.7998128361456362523 ) ) ;
#142853=CARTESIAN_POINT ( 'NONE',  ( -6.509886312855995172, 10.74661779830734254, -0.7998128361456291469 ) ) ;
#142860=CARTESIAN_POINT ( 'NONE',  ( -7.160677686311960777, 11.50587440067263678, -0.7998128361456291469 ) ) ;
#142861=CARTESIAN_POINT ( 'NONE',  ( 1.230761180058548954, 3.060133534840178360, 0.7750000000000100142 ) ) ;
#142863=EDGE_CURVE ( 'NONE', #25107, #2091, #147521, .T. ) ;
#142865=CARTESIAN_POINT ( 'NONE',  ( 7.690499447449630210, 9.995335326823163058, 1.599625672291281386 ) ) ;
#142867=CARTESIAN_POINT ( 'NONE',  ( 5.660692828905515839, 6.562895374266609849, -1.199719254218445830 ) ) ;
#142878=CARTESIAN_POINT ( 'NONE',  ( -6.496328159242330536, 10.73079995242472862, 0.000000000000000000 ) ) ;
#142882=CARTESIAN_POINT ( 'NONE',  ( 5.504247177468168495, 9.365446107114122398, 0.7216878364870438212 ) ) ;
#142888=CARTESIAN_POINT ( 'NONE',  ( -6.358937740009323214, 7.377514437221045718, -1.199719254218446718 ) ) ;
#142889=( BOUNDED_CURVE ( )  B_SPLINE_CURVE ( 3, ( #57838, #73003, #74097, #156419 ),
 .UNSPECIFIED., .F., .T. ) 
 B_SPLINE_CURVE_WITH_KNOTS ( ( 4, 4 ),
 ( 1.570796326794897002, 2.200856270465477937 ),
 .UNSPECIFIED. ) 
 CURVE ( )  GEOMETRIC_REPRESENTATION_ITEM ( )  RATIONAL_B_SPLINE_CURVE ( ( 1.000000000000000000, 0.9671913951458355196, 0.9671913951458355196, 1.000000000000000000 ) ) 
 REPRESENTATION_ITEM ( '' )  );
#142898=CARTESIAN_POINT ( 'NONE',  ( -9.480175724453545172, 12.08329098332774265, 1.599625672291281386 ) ) ;
#142899=CARTESIAN_POINT ( 'NONE',  ( 7.076466111328892694, 10.34329533227067799, -1.199719254218441611 ) ) ;
#142901=CARTESIAN_POINT ( 'NONE',  ( -2.765500147507697459, 5.209872024525476597, 1.082531754730560403 ) ) ;
#142904=CARTESIAN_POINT ( 'NONE',  ( -5.565591498217608013, 6.214750235347503704, -0.9194985501971261188 ) ) ;
#142911=CARTESIAN_POINT ( 'NONE',  ( 4.546061579283848353, 4.198160018786257552, -0.7998128361456211532 ) ) ;
#142917=CARTESIAN_POINT ( 'NONE',  ( -5.669981010301158086, 6.148093781360158161, -0.7892279793065083426 ) ) ;
#142929=CARTESIAN_POINT ( 'NONE',  ( -3.927058049452637700, 7.733318157670055371, -0.7998128361456281477 ) ) ;
#142930=CARTESIAN_POINT ( 'NONE',  ( 6.290620086616457662, 6.441404310581745563, 1.040834085586084257E-14 ) ) ;
#142931=CARTESIAN_POINT ( 'NONE',  ( -0.7499999999999972244, 4.108333333333360038, -1.299038105676652011 ) ) ;
#142933=CARTESIAN_POINT ( 'NONE',  ( -3.924195396151603177, 6.665646164563756138, 1.199719254218464037 ) ) ;
#142934=CARTESIAN_POINT ( 'NONE',  ( 0.4491468415840123019, 7.944909564338990648, -1.993991491228294777 ) ) ;
#142938=CARTESIAN_POINT ( 'NONE',  ( -1.364683531250012516, 4.738541667008091096, -0.7879004041258300672 ) ) ;
#142947=CARTESIAN_POINT ( 'NONE',  ( 3.408985558832261731, 6.064568021024562938, 1.199719254218462483 ) ) ;
#142950=CARTESIAN_POINT ( 'NONE',  ( 4.894543267554960053, 4.887125941896303338, -0.6895117023006970269 ) ) ;
#142951=CARTESIAN_POINT ( 'NONE',  ( 4.207107738942202246, 3.802713871720993399, 1.214306433183764966E-14 ) ) ;
#142953=CARTESIAN_POINT ( 'NONE',  ( -1.364683531250012516, 0.8427083336747532849, 0.7879004041258379498 ) ) ;
#142954=DIRECTION ( 'NONE',  ( 6.314299915563594049E-62, 8.546850786086437571E-32, 1.000000000000000000 ) ) ;
#142956=CARTESIAN_POINT ( 'NONE',  ( -10.48453286206953727, 11.12637651536962125, 0.7998128361456462443 ) ) ;
#142957=CARTESIAN_POINT ( 'NONE',  ( -6.195713011320804320, 7.291048603704809672, -1.082531754730543083 ) ) ;
#142961=CARTESIAN_POINT ( 'NONE',  ( -1.364683531250010295, 4.530208333674754506, 0.7879004041258379498 ) ) ;
#142969=CARTESIAN_POINT ( 'NONE',  ( -4.867013957181525186, 8.622007350113015889, 0.7216878364870458196 ) ) ;
#142974=CARTESIAN_POINT ( 'NONE',  ( -5.572037945092175981, 5.603058478803387032, 0.7216878364870317197 ) ) ;
#142982=CARTESIAN_POINT ( 'NONE',  ( 1.467638673046481657, 8.739153922842808342, -2.544768421592523033 ) ) ;
#142983=ORIENTED_EDGE ( 'NONE', *, *, #140681, .T. ) ;
#142987=CARTESIAN_POINT ( 'NONE',  ( -3.684065054611367351, 5.321161868511784299, -1.599625672291256295 ) ) ;
#142990=CARTESIAN_POINT ( 'NONE',  ( -1.402160292154681736E-14, 0.2125000000000202283, 1.732050807568877637 ) ) ;
#142993=CARTESIAN_POINT ( 'NONE',  ( 8.595506201384008449, 11.05117653974661529, 1.443375672974076540 ) ) ;
#142995=CARTESIAN_POINT ( 'NONE',  ( 7.481401836642521452, 7.622723652371411696, 1.040834085586084257E-14 ) ) ;
#142999=DIRECTION ( 'NONE',  ( 1.000000000000000000, -5.578564026256504688E-16, 0.000000000000000000 ) ) ;
#143000=CARTESIAN_POINT ( 'NONE',  ( 5.217190183160311356, 4.981143389975473568, -0.7998128361456211532 ) ) ;
#143008=CARTESIAN_POINT ( 'NONE',  ( -6.684333426737305572, 7.757142738403693727, -1.199719254218446718 ) ) ;
#143011=ORIENTED_EDGE ( 'NONE', *, *, #99066, .T. ) ;
#143017=CARTESIAN_POINT ( 'NONE',  ( -1.201851678989727383E-14, 3.196875000341420137, -1.575800808251660134 ) ) ;
#143018=CARTESIAN_POINT ( 'NONE',  ( 9.395437264145964917, 10.06369101769952934, -0.7216878364870257245 ) ) ;
#143019=CARTESIAN_POINT ( 'NONE',  ( -5.526920175865215334, 9.599823971818089774, 0.7998128361456481317 ) ) ;
#143022=CARTESIAN_POINT ( 'NONE',  ( 4.168242161197552420, 6.950367390450747251, -1.199719254218452047 ) ) ;
#143023=CARTESIAN_POINT ( 'NONE',  ( -4.412288926243578935, 7.235088616337731260, 1.199719254218464037 ) ) ;
#143029=CARTESIAN_POINT ( 'NONE',  ( 6.534666852106798096, 7.686494751288491578, -1.082531754730543083 ) ) ;
#143034=CARTESIAN_POINT ( 'NONE',  ( 0.6823417656249899377, 1.655208333674752730, 1.181850606188755259 ) ) ;
#143036=CARTESIAN_POINT ( 'NONE',  ( 5.463572716182819811, 8.357623354646536384, 1.082531754730558626 ) ) ;
#143038=CARTESIAN_POINT ( 'NONE',  ( -4.175548123328963079, 4.934189567714277302, 1.082531754730560403 ) ) ;
#143045=CARTESIAN_POINT ( 'NONE',  ( -4.027792083363366693, 7.778134382787397882, 0.5015608049221946807 ) ) ;
#143052=CARTESIAN_POINT ( 'NONE',  ( 6.144869935491714230, 8.192100896205568361, -1.599625672291262513 ) ) ;
#143055=CARTESIAN_POINT ( 'NONE',  ( 4.369805582306193870, 3.992528022312320957, 1.214306433183764966E-14 ) ) ;
#143063=CARTESIAN_POINT ( 'NONE',  ( 4.284013352238246419, 6.021101549076499637, -1.443375672974051449 ) ) ;
#143064=CARTESIAN_POINT ( 'NONE',  ( 1.364683531249988535, 1.676041667008085101, 0.7879004041258500513 ) ) ;
#143066=CARTESIAN_POINT ( 'NONE',  ( 7.426115451983150706, 9.686887332112256388, -1.599625672291262513 ) ) ;
#143069=CARTESIAN_POINT ( 'NONE',  ( -3.716906668440817185, 7.488141546489591072, 0.7998128361456341429 ) ) ;
#143074=CARTESIAN_POINT ( 'NONE',  ( 1.499999999999987121, 2.545833333333351156, -0.8660254037844262731 ) ) ;
#143075=CARTESIAN_POINT ( 'NONE',  ( 4.801558957534076022, 8.753569217098425170, 0.7998128361456462443 ) ) ;
#143076=CARTESIAN_POINT ( 'NONE',  ( -6.191269702934848240, 10.37489842006599616, 0.000000000000000000 ) ) ;
#143080=CARTESIAN_POINT ( 'NONE',  ( 0.6823417656249899377, 3.092708333674754062, 1.181850606188765695 ) ) ;
#143082=CARTESIAN_POINT ( 'NONE',  ( 9.083599731475976213, 12.58098820582193689, 1.082531754730546636 ) ) ;
#143090=CARTESIAN_POINT ( 'NONE',  ( -1.201851678989727383E-14, 1.243750000682821044, 1.732050807568877637 ) ) ;
#143093=CARTESIAN_POINT ( 'NONE',  ( -6.880926654135487652, 7.986501503701545879, 1.199719254218450271 ) ) ;
#143094=CARTESIAN_POINT ( 'NONE',  ( -4.609409038966253647, 4.479991421656468908, -0.7216878364870207285 ) ) ;
#143100=ORIENTED_EDGE ( 'NONE', *, *, #17125, .T. ) ;
#143102=CARTESIAN_POINT ( 'NONE',  ( 5.823390672269506574, 6.752709524857930745, -1.199719254218446718 ) ) ;
#143106=CARTESIAN_POINT ( 'NONE',  ( 4.794779880727245036, 8.745660294157122649, -0.7998128361456281477 ) ) ;
#143107=CARTESIAN_POINT ( 'NONE',  ( 3.070819976953864661, 2.800000000000017586, 2.497101503370694253 ) ) ;
#143110=CARTESIAN_POINT ( 'NONE',  ( -7.040761844198392794, 7.108643661186573759, -0.7998128361456291469 ) ) ;
#143112=CARTESIAN_POINT ( 'NONE',  ( 3.354752944377597856, 6.001296637494123232, -1.199719254218446718 ) ) ;
#143118=CARTESIAN_POINT ( 'NONE',  ( -7.334597915313094241, 9.580116872663850813, 1.040834085586084257E-14 ) ) ;
#143119=CARTESIAN_POINT ( 'NONE',  ( 4.163006777067105091, 7.380761635867615134, 0.7803290320304544503 ) ) ;
#143127=CARTESIAN_POINT ( 'NONE',  ( -4.012850279964973232, 4.744375417122949301, 1.082531754730560403 ) ) ;
#143128=CARTESIAN_POINT ( 'NONE',  ( 8.107412671292042461, 9.521364873671299023, 1.082531754730558626 ) ) ;
#143130=CARTESIAN_POINT ( 'NONE',  ( -3.405069135326500351, 7.124331091189553433, 1.040834085586084257E-14 ) ) ;
#143134=CARTESIAN_POINT ( 'NONE',  ( 7.934546212495622086, 10.28005655271014795, -1.599625672291262513 ) ) ;
#143136=CARTESIAN_POINT ( 'NONE',  ( -5.259673527097670664, 8.223703984000886535, -1.199719254218446718 ) ) ;
#143151=CARTESIAN_POINT ( 'NONE',  ( 9.856941372335116469, 11.45851867493453291, 1.199719254218450271 ) ) ;
#143152=CARTESIAN_POINT ( 'NONE',  ( -5.091250377131585125, 5.898545847196970726, 1.199719254218450271 ) ) ;
#143155=CARTESIAN_POINT ( 'NONE',  ( 3.551873057100287223, 5.166937871415542283, 1.443375672974062551 ) ) ;
#143159=CARTESIAN_POINT ( 'NONE',  ( -4.243865776277440993, 4.909930479533815451, -1.199719254218446718 ) ) ;
#143160=CARTESIAN_POINT ( 'NONE',  ( -3.521367211247373508, 5.131347717920458962, -1.599625672291256295 ) ) ;
#143163=CARTESIAN_POINT ( 'NONE',  ( 8.516493047678546091, 13.08765898893368629, -0.7998128361456352531 ) ) ;
#143167=CARTESIAN_POINT ( 'NONE',  ( -6.795661308947694934, 8.951357498570873261, -1.599625672291263179 ) ) ;
#143168=CARTESIAN_POINT ( 'NONE',  ( 4.364835388595708743, 7.179726155748598515, 1.199719254218462483 ) ) ;
#143175=CARTESIAN_POINT ( 'NONE',  ( 0.6823417656249882723, 1.488541667008083547, -1.181850606188749264 ) ) ;
#143179=CARTESIAN_POINT ( 'NONE',  ( 7.456621297836072415, 9.722477485607340597, 1.443375672974076540 ) ) ;
#143187=CARTESIAN_POINT ( 'NONE',  ( 8.012505595552012139, 11.33137838057728786, -1.082531754730543083 ) ) ;
#143188=ORIENTED_EDGE ( 'NONE', *, *, #147466, .F. ) ;
#143194=CARTESIAN_POINT ( 'NONE',  ( 5.843201017809841247, 5.919415396974013532, 1.040834085586084257E-14 ) ) ;
#143198=B_SPLINE_CURVE_WITH_KNOTS ( 'NONE', 3,
 ( #84787, #66371, #50163, #98920, #33899, #52293 ),
 .UNSPECIFIED., .F., .F.,
 ( 4, 2, 4 ),
 ( 1.039251754646360662E-16, 0.002037829324722970417, 0.004075658649445835884 ),
 .UNSPECIFIED. ) ;
#143204=PLANE ( 'NONE',  #187030 ) ;
#143211=CARTESIAN_POINT ( 'NONE',  ( -1.402160292154681736E-14, 1.368750000682821710, -1.732050807568863648 ) ) ;
#143215=EDGE_LOOP ( 'NONE', ( #72978, #63502, #200571, #97167 ) ) ;
#143217=CARTESIAN_POINT ( 'NONE',  ( 1.499999999999985123, -0.4541666666666469010, -0.8660254037844323793 ) ) ;
#143218=CARTESIAN_POINT ( 'NONE',  ( 7.293396569147545527, 10.59638086639245280, 1.199719254218460707 ) ) ;
#143219=CARTESIAN_POINT ( 'NONE',  ( -1.364683531250014514, 0.2385416670080863499, -0.7879004041258359514 ) ) ;
#143221=CARTESIAN_POINT ( 'NONE',  ( 3.765413976293345844, 5.416068943807445635, 1.599625672291267398 ) ) ;
#143222=CARTESIAN_POINT ( 'NONE',  ( -5.856759171423528088, 8.816340885760650892, 1.082531754730548412 ) ) ;
#143226=CARTESIAN_POINT ( 'NONE',  ( -8.044065211609668253, 8.279164256499745633, 0.7998128361456602331 ) ) ;
#143228=CARTESIAN_POINT ( 'NONE',  ( 1.499999999999987121, 1.327083334016149641, -0.8660254037844253849 ) ) ;
#143241=CARTESIAN_POINT ( 'NONE',  ( -9.691380875670077444, 10.20103253123691189, 0.7998128361456462443 ) ) ;
#143242=CARTESIAN_POINT ( 'NONE',  ( 6.958359152311676787, 9.141171649162195934, -1.599625672291262513 ) ) ;
#143249=CARTESIAN_POINT ( 'NONE',  ( -8.518600588087975822, 8.832788862391110385, 1.040834085586084257E-14 ) ) ;
#143256=CARTESIAN_POINT ( 'NONE',  ( 3.018661757337009810, 6.673522483535157868, 0.000000000000000000 ) ) ;
#143259=ORIENTED_EDGE ( 'NONE', *, *, #150826, .F. ) ;
#143261=CARTESIAN_POINT ( 'NONE',  ( -10.63367255181986160, 11.30037282007833532, 1.040834085586084257E-14 ) ) ;
#143264=CARTESIAN_POINT ( 'NONE',  ( -5.140457058134151325, 6.683247392444177315, -1.432107399977754270 ) ) ;
#143278=EDGE_LOOP ( 'NONE', ( #110254, #140246, #110588, #155744 ) ) ;
#143280=CARTESIAN_POINT ( 'NONE',  ( -1.500000000000013101, -0.04791666598384902026, 0.8660254037844403729 ) ) ;
#143291=CARTESIAN_POINT ( 'NONE',  ( 4.419594888374914099, 5.218910793601261311, -1.082531754730548412 ) ) ;
#143295=CARTESIAN_POINT ( 'NONE',  ( -10.13488352141530768, 11.78278451552804817, 1.199719254218462483 ) ) ;
#143297=CARTESIAN_POINT ( 'NONE',  ( 8.374132434735052755, 12.92157160716627295, -0.7998128361456352531 ) ) ;
#143306=CARTESIAN_POINT ( 'NONE',  ( -1.364683531250000748, -1.240624999658580752, 0.000000000000000000 ) ) ;
#143311=CARTESIAN_POINT ( 'NONE',  ( -4.232116505760120440, 8.089219690028791376, -0.7998128361456281477 ) ) ;
#143313=CARTESIAN_POINT ( 'NONE',  ( 0.7499999999999885647, -0.01666666666664401442, 1.299038105676657340 ) ) ;
#143315=CARTESIAN_POINT ( 'NONE',  ( -1.499999999999997780, 5.400000000000022560, 1.214306433183764966E-14 ) ) ;
#143320=CARTESIAN_POINT ( 'NONE',  ( -1.364683531250010295, 5.551041667008087543, -0.7879004041258300672 ) ) ;
#143323=CARTESIAN_POINT ( 'NONE',  ( -7.226659571283968297, 8.389856573708110332, 1.199719254218450271 ) ) ;
#143327=ORIENTED_EDGE ( 'NONE', *, *, #41574, .T. ) ;
#143330=CARTESIAN_POINT ( 'NONE',  ( -1.364683531250014514, -0.1572916663252435232, 0.7879004041258379498 ) ) ;
#143337=CARTESIAN_POINT ( 'NONE',  ( 7.212574532790092974, 9.437756259720353924, -1.443375672974057666 ) ) ;
#143340=CARTESIAN_POINT ( 'NONE',  ( -4.120788623549732854, 6.895004929861607401, -1.199719254218452047 ) ) ;
#143342=CARTESIAN_POINT ( 'NONE',  ( -1.001543065824772872E-14, 4.243750000682819490, 1.732050807568877637 ) ) ;
#143344=CARTESIAN_POINT ( 'NONE',  ( -3.521367211247373508, 5.131347717920458962, -1.599625672291256295 ) ) ;
#143345=CARTESIAN_POINT ( 'NONE',  ( 5.450014562569148957, 9.302174723065263606, 1.040834085586084257E-14 ) ) ;
#143346=CARTESIAN_POINT ( 'NONE',  ( -9.937763408692600109, 10.69640485300394417, -0.7216878364870267237 ) ) ;
#143352=CARTESIAN_POINT ( 'NONE',  ( 10.38518247838791986, 11.21839376764850726, 0.7216878364870438212 ) ) ;
#143367=CARTESIAN_POINT ( 'NONE',  ( 9.738834413317897898, 10.25639499182604730, 0.000000000000000000 ) ) ;
#143372=CARTESIAN_POINT ( 'NONE',  ( -1.402160292154681736E-14, 0.07187500034142156602, 1.575800808251672791 ) ) ;
#143373=CARTESIAN_POINT ( 'NONE',  ( 6.168596704537822717, 6.299043698156668647, 1.040834085586084257E-14 ) ) ;
#143375=CARTESIAN_POINT ( 'NONE',  ( -7.700668062882059850, 11.92793714009701311, -0.7216878364870267237 ) ) ;
#143378=CIRCLE ( 'NONE', #32630, 0.08000000000000025147 ) ;
#143396=CARTESIAN_POINT ( 'NONE',  ( 4.912861335034773624, 6.872882102868723919, -1.423633489635463878 ) ) ;
#143405=CARTESIAN_POINT ( 'NONE',  ( -8.215877900201387973, 8.687538426430837291, 0.7216878364870578100 ) ) ;
#143409=CARTESIAN_POINT ( 'NONE',  ( 6.425674737872927089, 9.584038729905381970, -1.199719254218440723 ) ) ;
#143412=CARTESIAN_POINT ( 'NONE',  ( 4.376584659113025744, 4.000436945253625254, 0.7998128361456341429 ) ) ;
#143414=CARTESIAN_POINT ( 'NONE',  ( -5.298539104842322267, 5.076050465271134016, 0.7998128361456341429 ) ) ;
#143418=CARTESIAN_POINT ( 'NONE',  ( -4.765854690403601879, 5.518917546014321829, 1.199719254218462483 ) ) ;
#143422=CARTESIAN_POINT ( 'NONE',  ( 8.599949509769960088, 8.927695937686774386, 1.040834085586084257E-14 ) ) ;
#143423=CARTESIAN_POINT ( 'NONE',  ( 0.02006731904125590854, 6.417555505232583002, 3.190074006977743792 ) ) ;
#143425=CARTESIAN_POINT ( 'NONE',  ( 4.699069518069377338, 7.059409271092678573, 1.379435410134820295 ) ) ;
#143426=CARTESIAN_POINT ( 'NONE',  ( 3.389175213736285386, 6.897862149426897460, 0.7216878364870317197 ) ) ;
#143433=CARTESIAN_POINT ( 'NONE',  ( 5.599154252319471503, 9.476171027773981237, -0.7216878364870267237 ) ) ;
#143434=CARTESIAN_POINT ( 'NONE',  ( -9.806625181386236179, 10.33548422123910449, -0.7998128361456291469 ) ) ;
#143437=CARTESIAN_POINT ( 'NONE',  ( -9.297140650669053485, 11.86975006391249643, 1.599625672291281386 ) ) ;
#143438=CARTESIAN_POINT ( 'NONE',  ( -7.400052914960538963, 7.527816577075747695, 1.040834085586084257E-14 ) ) ;
#143446=CARTESIAN_POINT ( 'NONE',  ( 8.762647353133951711, 9.117510088278095282, 1.040834085586084257E-14 ) ) ;
#143453=CARTESIAN_POINT ( 'NONE',  ( -3.337985173046072340, 6.383183490859034137, 0.8077998227833966816 ) ) ;
#143459=CARTESIAN_POINT ( 'NONE',  ( -1.499999999999997780, 2.650000000000020339, 1.214306433183764966E-14 ) ) ;
#143460=CARTESIAN_POINT ( 'NONE',  ( 6.419949431270806528, 7.448694743692793274, 1.199719254218462483 ) ) ;
#143464=CARTESIAN_POINT ( 'NONE',  ( 7.958272981541723468, 8.386999354661243800, 1.040834085586084257E-14 ) ) ;
#143469=CARTESIAN_POINT ( 'NONE',  ( 9.725276259704228821, 10.24057714594344048, 0.7998128361456462443 ) ) ;
#143471=CARTESIAN_POINT ( 'NONE',  ( 3.686212053427321056, 6.121915856213854923, 1.284222742053100941 ) ) ;
#143472=CARTESIAN_POINT ( 'NONE',  ( -2.578021764892882040, 6.159442492350315490, 0.7998128361456341429 ) ) ;
#143475=CARTESIAN_POINT ( 'NONE',  ( 1.364683531249986537, 0.6552083336747522857, -0.7879004041258239610 ) ) ;
#143480=CARTESIAN_POINT ( 'NONE',  ( 1.364683531249986537, -0.8864583329919110133, 0.7879004041258500513 ) ) ;
#143482=CARTESIAN_POINT ( 'NONE',  ( 8.829384350997564468, 11.32403438096243775, 1.599625672291281386 ) ) ;
#143486=CARTESIAN_POINT ( 'NONE',  ( -2.589244150085650009, 5.964609241834465614, 0.7216878364870317197 ) ) ;
#143489=CARTESIAN_POINT ( 'NONE',  ( -5.713871673155502151, 8.753601821068331290, 1.199719254218452047 ) ) ;
#143493=CARTESIAN_POINT ( 'NONE',  ( 3.344057444064992168, 7.053150784717805877, 1.040834085586084257E-14 ) ) ;
#143497=B_SPLINE_CURVE_WITH_KNOTS ( 'NONE', 3,
 ( #104015, #1144, #36857, #35795, #70404, #182035, #18472, #102941, #87753, #69341 ),
 .UNSPECIFIED., .F., .F.,
 ( 4, 3, 3, 4 ),
 ( 0.000000000000000000, 4.502046072368973497E-05, 9.004093402560359031E-05, 0.0001800865003231039206 ),
 .UNSPECIFIED. ) ;
#143500=CARTESIAN_POINT ( 'NONE',  ( 7.750457368506414646, 12.19395069656619945, 0.7998128361456462443 ) ) ;
#143502=CARTESIAN_POINT ( 'NONE',  ( -5.229694566569281555, 7.124396299129368337, 1.599625672291267398 ) ) ;
#143506=CARTESIAN_POINT ( 'NONE',  ( 7.567422294721922960, 11.98040977715095323, 0.7998128361456462443 ) ) ;
#143508=CARTESIAN_POINT ( 'NONE',  ( 7.076466111328892694, 10.34329533227067799, -1.199719254218441611 ) ) ;
#143512=CARTESIAN_POINT ( 'NONE',  ( -8.188761592974033832, 12.49737959187099179, -0.7216878364870267237 ) ) ;
#143515=CARTESIAN_POINT ( 'NONE',  ( -5.371001409308059138, 9.417918744168066070, -0.7998128361456231517 ) ) ;
#143520=CARTESIAN_POINT ( 'NONE',  ( -6.126358594793636314, 6.003181085514223803, -0.2003443317756918585 ) ) ;
#143521=CARTESIAN_POINT ( 'NONE',  ( 1.364683531249986537, 1.905208333674750287, -0.7879004041258239610 ) ) ;
#143524=CARTESIAN_POINT ( 'NONE',  ( 7.348156068926750883, 8.635565504245116486, -1.082531754730537976 ) ) ;
#143543=CARTESIAN_POINT ( 'NONE',  ( 7.910292558569346433, 11.31609285405122556, -1.199719254218446718 ) ) ;
#143545=VERTEX_POINT ( 'NONE', #132794 ) ;
#143547=CARTESIAN_POINT ( 'NONE',  ( -3.598799709423620374, 6.286017863381107240, 1.199719254218464037 ) ) ;
#143548=CARTESIAN_POINT ( 'NONE',  ( -6.672584156219988571, 10.93643194889866521, -0.7998128361456291469 ) ) ;
#143550=ORIENTED_EDGE ( 'NONE', *, *, #26050, .F. ) ;
#143553=CARTESIAN_POINT ( 'NONE',  ( -0.7500000000000215383, 3.972916667349481123, 1.299038105676671107 ) ) ;
#143554=CARTESIAN_POINT ( 'NONE',  ( 7.426115451983150706, 9.686887332112256388, -1.599625672291262513 ) ) ;
#143557=CARTESIAN_POINT ( 'NONE',  ( -6.503107236049161521, 10.73870887536603291, 0.7998128361456481317 ) ) ;
#143559=CARTESIAN_POINT ( 'NONE',  ( -1.364683531249997417, 4.759375000341424133, 1.214306433183764966E-14 ) ) ;
#143562=( BOUNDED_CURVE ( )  B_SPLINE_CURVE ( 2, ( #197310, #94516, #78233, #96652, #144356, #47907, #213539 ),
 .UNSPECIFIED., .F., .T. ) 
 B_SPLINE_CURVE_WITH_KNOTS ( ( 3, 2, 2, 3 ),
 ( 0.1375000000000000111, 0.1416666666666667462, 0.1458333333333334814, 0.1500000000000002165 ),
 .UNSPECIFIED. ) 
 CURVE ( )  GEOMETRIC_REPRESENTATION_ITEM ( )  RATIONAL_B_SPLINE_CURVE ( ( 1.000000000000000000, 0.8660254037844387076, 1.000000000000000000, 0.8660254037844387076, 1.000000000000000000, 0.8660254037844316022, 1.000000000000007105 ) ) 
 REPRESENTATION_ITEM ( '' )  );
#143565=CARTESIAN_POINT ( 'NONE',  ( -9.991996023591624976, 10.75967623705280296, 1.040834085586084257E-14 ) ) ;
#143570=CARTESIAN_POINT ( 'NONE',  ( -0.6823417656250212460, 2.363541667008084435, 1.181850606188767472 ) ) ;
#143577=CARTESIAN_POINT ( 'NONE',  ( -1.201851678989727383E-14, 3.196875000341420137, -1.575800808251660134 ) ) ;
#143579=CARTESIAN_POINT ( 'NONE',  ( -3.086452525405351643, 6.752611712948207057, 0.7998128361456341429 ) ) ;
#143580=CARTESIAN_POINT ( 'NONE',  ( 7.122110765880372618, 7.203550736482235095, 0.7998128361456341429 ) ) ;
#143584=CARTESIAN_POINT ( 'NONE',  ( -1.201851678989727383E-14, 4.259375000341417028, -1.575800808251660134 ) ) ;
#143587=CARTESIAN_POINT ( 'NONE',  ( -0.6823417656250003738, -1.032291666325242607, -1.181850606188749264 ) ) ;
#143588=CARTESIAN_POINT ( 'NONE',  ( -5.260200412422220140, 5.239248024021764039, -0.7216878364870207285 ) ) ;
#143592=CARTESIAN_POINT ( 'NONE',  ( 5.341549334104194635, 6.294524313618772737, 1.082531754730558626 ) ) ;
#143595=CARTESIAN_POINT ( 'NONE',  ( -6.828502922777144768, 11.11833717654868892, 0.7998128361456481317 ) ) ;
#143596=CARTESIAN_POINT ( 'NONE',  ( -9.056483424248693126, 10.62861408545402675, 1.082531754730558626 ) ) ;
#143602=CARTESIAN_POINT ( 'NONE',  ( -9.541187415715041809, 12.15447128979948310, -1.599625672291263179 ) ) ;
#143603=CARTESIAN_POINT ( 'NONE',  ( -6.846504384776765484, 8.050305206070113684, -1.082531754730543083 ) ) ;
#143605=CARTESIAN_POINT ( 'NONE',  ( -0.6823417656250246877, 0.3635416670080895973, 1.181850606188755259 ) ) ;
#143606=CARTESIAN_POINT ( 'NONE',  ( 1.445103857048100515, 8.688264192037886247, 2.625611233228254182 ) ) ;
#143617=CARTESIAN_POINT ( 'NONE',  ( -0.7500000000000006661, -0.3916666666666443475, -1.299038105676652011 ) ) ;
#143618=CARTESIAN_POINT ( 'NONE',  ( 9.056483423804305488, 9.668244870634271848, 1.040834085586084257E-14 ) ) ;
#143626=AXIS2_PLACEMENT_3D ( 'NONE', #123502, #42174, #108290 ) ;
#143627=CARTESIAN_POINT ( 'NONE',  ( 5.311043488251262268, 7.219303374425030562, -1.599625672291256295 ) ) ;
#143629=CARTESIAN_POINT ( 'NONE',  ( -3.079673448598517549, 6.744702790006905424, 1.040834085586084257E-14 ) ) ;
#143632=CARTESIAN_POINT ( 'NONE',  ( 1.499999999999822586, 7.388542872122531691, 4.154462424328221104 ) ) ;
#143633=CIRCLE ( 'NONE', #63959, 0.08000000000000012657 ) ;
#143634=CARTESIAN_POINT ( 'NONE',  ( -1.364683531250000748, 1.071875000341421247, 0.000000000000000000 ) ) ;
#143635=DIRECTION ( 'NONE',  ( 5.578564026256490882E-16, 1.000000000000000000, 9.066213480720158442E-32 ) ) ;
#143636=CARTESIAN_POINT ( 'NONE',  ( -7.537443334193545397, 10.88110209227943770, -1.199719254218446718 ) ) ;
#143637=ORIENTED_EDGE ( 'NONE', *, *, #4338, .T. ) ;
#143650=ORIENTED_EDGE ( 'NONE', *, *, #181542, .F. ) ;
#143654=CARTESIAN_POINT ( 'NONE',  ( 5.632522751473472589, 8.658694745772667289, -1.199719254218440723 ) ) ;
#143662=CARTESIAN_POINT ( 'NONE',  ( 7.086107841436786181, 11.41887624831828418, 1.040834085586084257E-14 ) ) ;
#143665=CARTESIAN_POINT ( 'NONE',  ( 7.723341061279088038, 12.16231500480096983, -0.7998128361456291469 ) ) ;
#143668=CARTESIAN_POINT ( 'NONE',  ( 1.538487831126108762, 8.695753106490483830, -2.511613306591210293 ) ) ;
#143672=CARTESIAN_POINT ( 'NONE',  ( 8.886479618753304166, 12.45497775759917758, -1.199719254218446718 ) ) ;
#143680=CARTESIAN_POINT ( 'NONE',  ( -7.971831135155409420, 11.28392484344787405, 1.082531754730549967 ) ) ;
#143686=CARTESIAN_POINT ( 'NONE',  ( 6.159481859310094620, 6.080483678816896109, 1.040834085586084257E-14 ) ) ;
#143691=AXIS2_PLACEMENT_3D ( 'NONE', #117348, #116278, #210775 ) ;
#143693=CARTESIAN_POINT ( 'NONE',  ( 3.619663824724254741, 6.206396314611513532, -1.082531754730543971 ) ) ;
#143696=ORIENTED_EDGE ( 'NONE', *, *, #3649, .F. ) ;
#143701=CARTESIAN_POINT ( 'NONE',  ( -4.934277840369690971, 7.844075682818238526, -1.199719254218452047 ) ) ;
#143703=CARTESIAN_POINT ( 'NONE',  ( -2.923754682041362241, 6.562797562356882608, 0.7998128361456341429 ) ) ;
#143711=CARTESIAN_POINT ( 'NONE',  ( 6.471319392424407901, 6.444294134116939077, 0.7998128361456341429 ) ) ;
#143722=ORIENTED_EDGE ( 'NONE', *, *, #214235, .T. ) ;
#143724=CARTESIAN_POINT ( 'NONE',  ( 0.6823417656249899377, 0.9052083336747520637, 1.181850606188755259 ) ) ;
#143726=CARTESIAN_POINT ( 'NONE',  ( 2.706824224222692088, 6.309712028235118453, 0.7998128361456362523 ) ) ;
#143728=CARTESIAN_POINT ( 'NONE',  ( -7.700668062882084719, 8.086460282891644979, -0.7216878364870278340 ) ) ;
#143730=CARTESIAN_POINT ( 'NONE',  ( 3.877268743828258479, 7.467304601200877023, 0.7216878364870298324 ) ) ;
#143732=CARTESIAN_POINT ( 'NONE',  ( -7.022760381754429737, 7.295567988242705582, 1.040834085586084257E-14 ) ) ;
#143736=CARTESIAN_POINT ( 'NONE',  ( 6.287230548435207567, 8.358188277972981695, -1.599625672291262513 ) ) ;
#143741=CARTESIAN_POINT ( 'NONE',  ( -0.6823417656250212460, 5.551041667008087543, 1.181850606188767472 ) ) ;
#143745=CARTESIAN_POINT ( 'NONE',  ( 6.765682348419287173, 7.852049813699357728, 1.199719254218462483 ) ) ;
#143748=CARTESIAN_POINT ( 'NONE',  ( -6.679363233026820446, 10.94434087183997129, 0.000000000000000000 ) ) ;
#143753=CARTESIAN_POINT ( 'NONE',  ( 6.916630921265960019, 11.22115317478565188, 0.7998128361456462443 ) ) ;
#143756=CARTESIAN_POINT ( 'NONE',  ( -8.688077508258798431, 9.030511935923748013, -0.7998128361456291469 ) ) ;
#143758=CARTESIAN_POINT ( 'NONE',  ( 6.927853306458739979, 10.06595070996845642, 1.082531754730558626 ) ) ;
#143759=CARTESIAN_POINT ( 'NONE',  ( 4.260617097460324132, 7.265790484119571957, -0.9368387426427534637 ) ) ;
#143760=CARTESIAN_POINT ( 'NONE',  ( -9.002250809794000830, 11.52571191622492464, -1.443375672974059665 ) ) ;
#143765=CARTESIAN_POINT ( 'NONE',  ( 5.660692828905515839, 6.562895374266609849, -1.199719254218445830 ) ) ;
#143767=CARTESIAN_POINT ( 'NONE',  ( 9.134442807305049428, 11.67993591332117376, 1.599625672291281386 ) ) ;
#143768=CARTESIAN_POINT ( 'NONE',  ( -4.588080609115144703, 6.965600104441714180, 1.189663598451236926 ) ) ;
#143769=CARTESIAN_POINT ( 'NONE',  ( 5.034155109375821446, 4.767602470560229122, -0.7998128361456221525 ) ) ;
#143770=CARTESIAN_POINT ( 'NONE',  ( 0.6823417656249882723, 0.3427083336747516196, 1.181850606188755259 ) ) ;
#143772=CARTESIAN_POINT ( 'NONE',  ( -6.073689629242151611, 10.02979563418376685, -0.7216878364870278340 ) ) ;
#143778=CARTESIAN_POINT ( 'NONE',  ( -5.108350220830032207, 6.531958715577594887, 1.215759808322430136 ) ) ;
#143779=CARTESIAN_POINT ( 'NONE',  ( -1.364683531250000748, 0.3218750003414205807, 0.000000000000000000 ) ) ;
#143781=CARTESIAN_POINT ( 'NONE',  ( 1.499999999999989120, 3.303247596591511126, 0.1248075943439479751 ) ) ;
#143782=CARTESIAN_POINT ( 'NONE',  ( 3.389175213736292047, 5.937492935125556315, 1.082531754730558626 ) ) ;
#143786=CARTESIAN_POINT ( 'NONE',  ( -9.042925270190641740, 11.57316545335434199, 1.443375672974064550 ) ) ;
#143791=CARTESIAN_POINT ( 'NONE',  ( -8.717529583462656717, 11.19353715217169309, 1.443375672974064550 ) ) ;
#143793=VERTEX_POINT ( 'NONE', #125131 ) ;
#143799=CARTESIAN_POINT ( 'NONE',  ( -9.151390499099978371, 9.778969791812544443, 0.7216878364870438212 ) ) ;
#143803=CARTESIAN_POINT ( 'NONE',  ( 1.364683531249990311, 4.926041667008083991, 0.7879004041258500513 ) ) ;
#143804=CARTESIAN_POINT ( 'NONE',  ( -0.7500000000000215383, 4.722916667349482012, 1.299038105676671107 ) ) ;
#143805=CARTESIAN_POINT ( 'NONE',  ( 4.808669324434905690, 6.961940934708692019, -1.409791361277392241 ) ) ;
#143807=CARTESIAN_POINT ( 'NONE',  ( -5.742041750587549842, 6.657802449562273850, 1.199719254218450271 ) ) ;
#143811=CARTESIAN_POINT ( 'NONE',  ( -6.669721502918952716, 9.868759955792373972, 1.199719254218452047 ) ) ;
#143815=CARTESIAN_POINT ( 'NONE',  ( 6.173040012923759257, 6.096301524699504704, -0.7998128361456281477 ) ) ;
#143820=CARTESIAN_POINT ( 'NONE',  ( 6.337546739384100292, 9.481222731668410120, 1.199719254218460707 ) ) ;
#143827=CARTESIAN_POINT ( 'NONE',  ( -6.887178846062128379, 7.137389529935019183, -0.7216878364870278340 ) ) ;
#143831=CARTESIAN_POINT ( 'NONE',  ( -4.566062713072708057, 5.367758147946414482, 1.229400682838634573 ) ) ;
#143834=DIRECTION ( 'NONE',  ( 0.6507913734559640506, -0.7592566023653004592, 0.000000000000000000 ) ) ;
#143838=CARTESIAN_POINT ( 'NONE',  ( -8.533967624797991647, 12.04371376465130439, -1.199719254218446718 ) ) ;
#143841=CARTESIAN_POINT ( 'NONE',  ( 8.422639742587595180, 10.84949900448412130, -1.599625672291268286 ) ) ;
#143842=CARTESIAN_POINT ( 'NONE',  ( -0.7500000000000006661, -0.6416666666666446250, -1.299038105676652011 ) ) ;
#143843=CARTESIAN_POINT ( 'NONE',  ( -7.991641480251377772, 11.41099992934688956, 1.199719254218453823 ) ) ;
#143846=CARTESIAN_POINT ( 'NONE',  ( -1.364683531250012516, 3.238541667008084879, -0.7879004041258289570 ) ) ;
#143848=CARTESIAN_POINT ( 'NONE',  ( 10.39874063200158893, 11.23421161353111586, 0.000000000000000000 ) ) ;
#143851=CARTESIAN_POINT ( 'NONE',  ( -1.500000000000011324, 4.670833333333353821, 0.8660254037844403729 ) ) ;
#143854=CARTESIAN_POINT ( 'NONE',  ( 8.175203438916005538, 11.52119253116861586, -1.082531754730543083 ) ) ;
#143857=CARTESIAN_POINT ( 'NONE',  ( -5.910991785878165317, 8.879612269291090598, -1.082531754730538864 ) ) ;
#143858=CARTESIAN_POINT ( 'NONE',  ( -1.402160292154681736E-14, 1.946875000341422579, -1.575800808251660134 ) ) ;
#143862=CARTESIAN_POINT ( 'NONE',  ( -6.856673000209188906, 9.022537805042615489, 1.599625672291283607 ) ) ;
#143863=CARTESIAN_POINT ( 'NONE',  ( -0.6823417656249969321, 4.280208333674755394, -1.181850606188749264 ) ) ;
#143869=CARTESIAN_POINT ( 'NONE',  ( 7.736899214892750010, 12.17813285068358020, 1.040834085586084257E-14 ) ) ;
#143872=CARTESIAN_POINT ( 'NONE',  ( 1.499999999999987121, 0.5041666666666856367, 0.8660254037844524744 ) ) ;
#143877=CARTESIAN_POINT ( 'NONE',  ( 8.940712233207955606, 12.51824914112961729, 1.199719254218450271 ) ) ;
#143882=CARTESIAN_POINT ( 'NONE',  ( 7.228468454380276853, 11.58496363008569574, 1.040834085586084257E-14 ) ) ;
#143883=CARTESIAN_POINT ( 'NONE',  ( -1.534377212605050333, 8.695787254938599276, 2.514108538948842675 ) ) ;
#143885=CARTESIAN_POINT ( 'NONE',  ( -4.909967638851771454, 4.671257834700952571, -0.2941531795261614346 ) ) ;
#143886=CARTESIAN_POINT ( 'NONE',  ( 0.6823417656249917140, 5.155208333674749177, 1.181850606188765695 ) ) ;
#143889=CARTESIAN_POINT ( 'NONE',  ( 1.123270288254022198, 2.908552654332631437, -0.7749999999939810591 ) ) ;
#143890=CARTESIAN_POINT ( 'NONE',  ( 7.099665995050449041, 11.43469409420089455, 0.7998128361456462443 ) ) ;
#143893=CARTESIAN_POINT ( 'NONE',  ( -1.364683531249997417, 3.509375000341423245, 1.214306433183764966E-14 ) ) ;
#143895=CARTESIAN_POINT ( 'NONE',  ( -6.561783159334141580, 7.718130443053708767, -1.082531754730544860 ) ) ;
#143902=CARTESIAN_POINT ( 'NONE',  ( 4.539282502477016479, 4.190251095844947926, 0.7998128361456341429 ) ) ;
#143904=EDGE_LOOP ( 'NONE', ( #112999, #119220 ) ) ;
#143905=CARTESIAN_POINT ( 'NONE',  ( 9.725276259704228821, 10.24057714594344048, 0.7998128361456462443 ) ) ;
#143906=CARTESIAN_POINT ( 'NONE',  ( 2.456316247939560160, 8.205176026796141997, -2.499999999999995115 ) ) ;
#143911=CARTESIAN_POINT ( 'NONE',  ( -9.158696461231359720, 10.64389961198009615, 1.199719254218462483 ) ) ;
#143912=CARTESIAN_POINT ( 'NONE',  ( 7.481401836642521452, 7.622723652371411696, 1.040834085586084257E-14 ) ) ;
#143915=CARTESIAN_POINT ( 'NONE',  ( 4.847203612085560387, 5.613824621309978724, -1.199719254218452047 ) ) ;
#143923=CARTESIAN_POINT ( 'NONE',  ( -5.097502569058207200, 8.890910730635814829, -0.7216878364870207285 ) ) ;
#143925=CARTESIAN_POINT ( 'NONE',  ( 3.147464216666835402, 6.823792019419957278, -0.7998128361456291469 ) ) ;
#143928=CARTESIAN_POINT ( 'NONE',  ( -8.532158741701643123, 8.848606708273724308, 0.7998128361456462443 ) ) ;
#143934=CARTESIAN_POINT ( 'NONE',  ( -8.784793466650835825, 12.33634391347959713, 1.199719254218462483 ) ) ;
#143935=CARTESIAN_POINT ( 'NONE',  ( 1.177110729581195780, 3.085371626218851748, 0.7750000000000065725 ) ) ;
#143938=CARTESIAN_POINT ( 'NONE',  ( 6.272618624616828953, 10.46980549536166016, 1.040834085586084257E-14 ) ) ;
#143950=CARTESIAN_POINT ( 'NONE',  ( -6.509886312855995172, 10.74661779830734254, -0.7998128361456291469 ) ) ;
#143954=CARTESIAN_POINT ( 'NONE',  ( 6.317736394288135493, 8.393778431468064127, 1.443375672974076540 ) ) ;
#143957=DIRECTION ( 'NONE',  ( -9.912705607951403669E-16, -1.000000000000000000, -8.227696745425610178E-32 ) ) ;
#143960=CARTESIAN_POINT ( 'NONE',  ( -5.065942953000576843, 9.062017211809330064, -0.7998128361456231517 ) ) ;
#143969=EDGE_CURVE ( 'NONE', #197571, #21610, #63974, .T. ) ;
#143970=CARTESIAN_POINT ( 'NONE',  ( -8.696665468161981494, 12.23352791524263239, -1.199719254218446718 ) ) ;
#143971=CARTESIAN_POINT ( 'NONE',  ( 8.613507663383630941, 8.943513783569379427, -0.7998128361456221525 ) ) ;
#143973=CARTESIAN_POINT ( 'NONE',  ( -4.772106882330241717, 5.630174786549132726, -1.082531754730544860 ) ) ;
#143977=CARTESIAN_POINT ( 'NONE',  ( -4.932901803036217281, 6.667582871412107259, -1.248097486420626900 ) ) ;
#143984=CARTESIAN_POINT ( 'NONE',  ( 3.979481780810941949, 4.601482484822914998, 1.199719254218464037 ) ) ;
#143992=CARTESIAN_POINT ( 'NONE',  ( 4.273844736805816780, 6.009238164405336313, 1.599625672291267398 ) ) ;
#143996=CARTESIAN_POINT ( 'NONE',  ( -1.201851678989727383E-14, 3.634375000341422357, 1.575800808251672791 ) ) ;
#144001=CARTESIAN_POINT ( 'NONE',  ( 4.774442650306744085, 8.721933525333202653, -0.7998128361456281477 ) ) ;
#144005=CARTESIAN_POINT ( 'NONE',  ( -3.978428010606240850, 6.728917548094202949, -1.199719254218452047 ) ) ;
#144006=CARTESIAN_POINT ( 'NONE',  ( 4.636525345749193505, 8.353103970108639587, 1.040834085586084257E-14 ) ) ;
#144007=CARTESIAN_POINT ( 'NONE',  ( -1.500000000000011324, 4.170833333333359150, 0.8660254037844403729 ) ) ;
#144009=CARTESIAN_POINT ( 'NONE',  ( -3.598799709423620374, 6.286017863381107240, 1.199719254218464037 ) ) ;
#144010=CARTESIAN_POINT ( 'NONE',  ( 0.5021762176675715894, 7.740673110510241983, -1.993154341637451088 ) ) ;
#144012=CARTESIAN_POINT ( 'NONE',  ( 1.364683531249990311, 4.134375000341417028, 1.214306433183764966E-14 ) ) ;
#144015=CARTESIAN_POINT ( 'NONE',  ( -5.124618876285560454, 5.081069565195661220, 0.7216878364870317197 ) ) ;
#144019=CARTESIAN_POINT ( 'NONE',  ( 4.111146893441827821, 5.819424013814004759, 1.599625672291267398 ) ) ;
#144022=CARTESIAN_POINT ( 'NONE',  ( 0.1815159415691200706, 7.045075310427906246, -3.942267139059067560 ) ) ;
#144023=CARTESIAN_POINT ( 'NONE',  ( 4.284013352238246419, 6.021101549076499637, -1.443375672974051449 ) ) ;
#144025=CARTESIAN_POINT ( 'NONE',  ( -1.364683531250014514, 1.551041667008084435, -0.7879004041258289570 ) ) ;
#144028=CARTESIAN_POINT ( 'NONE',  ( -7.811469059767924605, 12.26513100303794168, -0.7998128361456281477 ) ) ;
#144029=CARTESIAN_POINT ( 'NONE',  ( -4.894130264408862452, 7.693273827576896373, -1.082531754730548412 ) ) ;
#144033=CARTESIAN_POINT ( 'NONE',  ( -1.364683531250010295, 4.780208333674755394, 0.7879004041258379498 ) ) ;
#144041=CARTESIAN_POINT ( 'NONE',  ( -6.358410854684789726, 8.441231968597481483, -1.443375672974058777 ) ) ;
#144045=EDGE_CURVE ( 'NONE', #141934, #66184, #127029, .T. ) ;
#144049=CARTESIAN_POINT ( 'NONE',  ( -5.870317324592821073, 6.911420302522161663, -1.082531754730543083 ) ) ;
#144063=CARTESIAN_POINT ( 'NONE',  ( -5.229694566569281555, 7.124396299129368337, 1.599625672291267398 ) ) ;
#144066=CARTESIAN_POINT ( 'NONE',  ( -0.7500000000000215383, 0.6916666666666876351, 1.299038105676659116 ) ) ;
#144068=CARTESIAN_POINT ( 'NONE',  ( 10.08690309888728187, 10.87040115823107911, -0.7216878364870257245 ) ) ;
#144069=CARTESIAN_POINT ( 'NONE',  ( 6.470265622219697477, 8.571729197388226140, -1.599625672291262513 ) ) ;
#144073=EDGE_CURVE ( 'NONE', #3126, #197889, #80351, .T. ) ;
#144074=CARTESIAN_POINT ( 'NONE',  ( 4.542145155778077203, 5.257923088951247159, -1.199719254218452047 ) ) ;
#144075=CARTESIAN_POINT ( 'NONE',  ( -0.4020909550004448385, 7.366597533580868884, -1.962779437971320595 ) ) ;
#144082=CARTESIAN_POINT ( 'NONE',  ( -5.215082642750900277, 9.236013516518044142, 0.000000000000000000 ) ) ;
#144089=CARTESIAN_POINT ( 'NONE',  ( 0.6823417656249917140, 3.592708333674754506, 1.181850606188765695 ) ) ;
#144090=CARTESIAN_POINT ( 'NONE',  ( 7.551528372687370094, 11.75394083486988528, -0.7216878364870267237 ) ) ;
#144091=CARTESIAN_POINT ( 'NONE',  ( -5.038826645773246682, 9.030381520044109322, 0.7998128361456481317 ) ) ;
#144095=CARTESIAN_POINT ( 'NONE',  ( 4.808338034340912337, 8.761478140039733020, 1.040834085586084257E-14 ) ) ;
#144096=CARTESIAN_POINT ( 'NONE',  ( -6.087774667736030487, 7.061157519568837415, 1.199719254218450271 ) ) ;
#144100=CARTESIAN_POINT ( 'NONE',  ( -1.500000000000001332, 0.1812500006828157706, 0.000000000000000000 ) ) ;
#144102=EDGE_CURVE ( 'NONE', #157452, #20719, #209613, .T. ) ;
#144104=CARTESIAN_POINT ( 'NONE',  ( 8.283668668269706714, 8.766627655843892697, 1.040834085586084257E-14 ) ) ;
#144107=CARTESIAN_POINT ( 'NONE',  ( -0.6823417656250212460, 2.113541667008083991, 1.181850606188767472 ) ) ;
#144109=CARTESIAN_POINT ( 'NONE',  ( 4.961921032477176752, 8.732732271291288484, 1.040834085586084257E-14 ) ) ;
#144111=CARTESIAN_POINT ( 'NONE',  ( -4.012850279964973232, 4.744375417122949301, 1.082531754730560403 ) ) ;
#144119=CARTESIAN_POINT ( 'NONE',  ( -4.119491766144414591, 7.660190618428146081, -0.8001636830725885607 ) ) ;
#144127=CARTESIAN_POINT ( 'NONE',  ( 5.795220594837462436, 8.848508896363995291, -1.199719254218440723 ) ) ;
#144138=CARTESIAN_POINT ( 'NONE',  ( 3.389175213736285386, 6.897862149426897460, 0.7216878364870317197 ) ) ;
#144140=CARTESIAN_POINT ( 'NONE',  ( -1.201851678989727383E-14, 2.134375000341423689, 1.575800808251672791 ) ) ;
#144141=CARTESIAN_POINT ( 'NONE',  ( 9.413438726589914651, 9.876766690643398405, 0.000000000000000000 ) ) ;
#144147=CARTESIAN_POINT ( 'NONE',  ( -1.500000000000013101, 1.920833333333356263, 0.8660254037844403729 ) ) ;
#144148=CARTESIAN_POINT ( 'NONE',  ( 6.959412922516382771, 7.013736585890911535, 0.7998128361456341429 ) ) ;
#144149=CARTESIAN_POINT ( 'NONE',  ( -5.879432169820529630, 10.01108796476595764, -0.7998128361456221525 ) ) ;
#144153=CARTESIAN_POINT ( 'NONE',  ( 1.364683531249990311, 2.884375000341422801, 1.214306433183764966E-14 ) ) ;
#144154=ORIENTED_EDGE ( 'NONE', *, *, #134567, .T. ) ;
#144157=CARTESIAN_POINT ( 'NONE',  ( 3.871016551901614200, 4.474939717762034697, -1.199719254218446718 ) ) ;
#144162=CARTESIAN_POINT ( 'NONE',  ( 0.7499999999999885647, 0.7645833340161543035, 1.299038105676657340 ) ) ;
#144164=CARTESIAN_POINT ( 'NONE',  ( -7.555971681517696936, 7.709721804725773175, 0.7998128361456462443 ) ) ;
#144166=CARTESIAN_POINT ( 'NONE',  ( -2.318081078256692518, 5.648252324700675508, 1.040834085586084257E-14 ) ) ;
#144172=ORIENTED_EDGE ( 'NONE', *, *, #211621, .F. ) ;
#144174=CARTESIAN_POINT ( 'NONE',  ( 4.611744806942754238, 8.532119374741881757, -0.7998128361456231517 ) ) ;
#144178=CARTESIAN_POINT ( 'NONE',  ( 6.982612806237943559, 8.105135347821125436, -1.199719254218446718 ) ) ;
#144185=CARTESIAN_POINT ( 'NONE',  ( -7.366157530926372488, 7.488271962369228874, -0.7998128361456291469 ) ) ;
#144186=CARTESIAN_POINT ( 'NONE',  ( 5.054492339796319733, 4.791329239384148231, -0.7998128361456211532 ) ) ;
#144192=CARTESIAN_POINT ( 'NONE',  ( 4.799922300691145338, 6.743925459469453543, 1.247687964948118733 ) ) ;
#144197=DIRECTION ( 'NONE',  ( 0.6507913734559708230, 0.7592566023652946861, 2.465190328815661618E-32 ) ) ;
#144200=CARTESIAN_POINT ( 'NONE',  ( -3.633221978782299910, 5.261844946711204507, -1.443375672974053447 ) ) ;
#144201=CARTESIAN_POINT ( 'NONE',  ( 8.771762198361678031, 9.336070107617867819, 1.040834085586084257E-14 ) ) ;
#144203=CARTESIAN_POINT ( 'NONE',  ( -4.985647801523292344, 6.839675073242382553, -1.599625672291256295 ) ) ;
#144208=CARTESIAN_POINT ( 'NONE',  ( -7.203459687562382641, 7.298457811777897319, -0.7998128361456291469 ) ) ;
#144213=ORIENTED_EDGE ( 'NONE', *, *, #60938, .T. ) ;
#144217=ORIENTED_EDGE ( 'NONE', *, *, #85154, .F. ) ;
#144224=CARTESIAN_POINT ( 'NONE',  ( -5.037017762676898158, 5.835274463666530131, -1.199719254218446718 ) ) ;
#144227=CARTESIAN_POINT ( 'NONE',  ( 3.036663219780971978, 6.486598156479028709, -0.7216878364870267237 ) ) ;
#144231=CARTESIAN_POINT ( 'NONE',  ( -1.403499169903686727, 7.376709478542852416, 4.304123474984240083 ) ) ;
#144232=CARTESIAN_POINT ( 'NONE',  ( -5.101945877444165944, 4.846691699973280976, 0.000000000000000000 ) ) ;
#144235=CARTESIAN_POINT ( 'NONE',  ( 10.05067194643221207, 10.62020544712608938, 0.7998128361456462443 ) ) ;
#144238=ADVANCED_FACE ( 'NONE', ( #102940 ), #123530, .T. ) ;
#144239=CARTESIAN_POINT ( 'NONE',  ( -7.739006755302186846, 7.923262724141010516, 0.7998128361456462443 ) ) ;
#144240=CARTESIAN_POINT ( 'NONE',  ( 4.137209430464448445, 7.978494768850520558, 1.040834085586084257E-14 ) ) ;
#144242=CIRCLE ( 'NONE', #2372, 0.08000000000000020983 ) ;
#144247=CARTESIAN_POINT ( 'NONE',  ( -1.364683531250012516, 1.342708333674755616, 0.7879004041258379498 ) ) ;
#144248=EDGE_LOOP ( 'NONE', ( #97567, #100729, #122750, #206538, #48338, #11680, #183697, #4495, #57733, #187981, #59041 ) ) ;
#144250=CARTESIAN_POINT ( 'NONE',  ( 7.375272376154084597, 9.627570410311676596, -1.443375672974057666 ) ) ;
#144255=LINE ( 'NONE', #177777, #19768 ) ;
#144258=CARTESIAN_POINT ( 'NONE',  ( 10.35806617071623315, 11.18675807536486566, 0.000000000000000000 ) ) ;
#144267=CARTESIAN_POINT ( 'NONE',  ( -9.561524646135538319, 12.17819805862340310, -1.599625672291263179 ) ) ;
#144282=CARTESIAN_POINT ( 'NONE',  ( -1.499999999999997780, 1.931250000682817269, 0.000000000000000000 ) ) ;
#144286=ORIENTED_EDGE ( 'NONE', *, *, #87710, .T. ) ;
#144288=CARTESIAN_POINT ( 'NONE',  ( -1.500000000000001332, -1.099999999999976108, 0.000000000000000000 ) ) ;
#144289=CARTESIAN_POINT ( 'NONE',  ( 6.726816770674637347, 10.99970333242910669, -0.7998128361456291469 ) ) ;
#144293=CARTESIAN_POINT ( 'NONE',  ( 4.142179624174931796, 4.791296635414242111, 1.199719254218464037 ) ) ;
#144294=CARTESIAN_POINT ( 'NONE',  ( -6.236387472606158333, 7.338502141871059870, -1.082531754730544860 ) ) ;
#144298=CARTESIAN_POINT ( 'NONE',  ( -7.691553217654356622, 7.867900263551875994, -0.7998128361456291469 ) ) ;
#144300=CARTESIAN_POINT ( 'NONE',  ( 0.7499999999999885647, 0.8479166673494853423, -1.299038105676652899 ) ) ;
#144307=CARTESIAN_POINT ( 'NONE',  ( -3.755245360860931303, 5.404205559136275205, -1.443375672974051449 ) ) ;
#144309=CARTESIAN_POINT ( 'NONE',  ( 4.943270704524102221, 6.626842455454077907, 1.245637569283185586 ) ) ;
#144314=CARTESIAN_POINT ( 'NONE',  ( -8.143643823302737061, 12.65266822716189843, 0.000000000000000000 ) ) ;
#144315=CARTESIAN_POINT ( 'NONE',  ( 6.747154001095143627, 11.02343010125301959, -0.7998128361456291469 ) ) ;
#144322=CARTESIAN_POINT ( 'NONE',  ( -6.832419346282942563, 10.05857410638369487, 1.199719254218453823 ) ) ;
#144327=CARTESIAN_POINT ( 'NONE',  ( 3.506755287428983792, 7.242964935309132990, 1.040834085586084257E-14 ) ) ;
#144329=CARTESIAN_POINT ( 'NONE',  ( -3.895595285070201808, 2.800000000000024691, 0.7750000000000135669 ) ) ;
#144332=CARTESIAN_POINT ( 'NONE',  ( -10.64723070543352712, 11.31619066596094392, 0.7998128361456462443 ) ) ;
#144335=CARTESIAN_POINT ( 'NONE',  ( -5.495703055830178485, 6.420018438214686540, -1.282350674470073448 ) ) ;
#144344=ORIENTED_EDGE ( 'NONE', *, *, #193336, .T. ) ;
#144351=CARTESIAN_POINT ( 'NONE',  ( -1.500000000000015099, 0.9104166673494835660, -0.8660254037844313801 ) ) ;
#144354=EDGE_CURVE ( 'NONE', #78710, #21552, #101051, .T. ) ;
#144355=CARTESIAN_POINT ( 'NONE',  ( -4.263518483283433191, 7.399640243518209815, 1.003058986863963220 ) ) ;
#144356=CARTESIAN_POINT ( 'NONE',  ( 4.650083499362875017, 5.487814173087225633, 1.082531754730560403 ) ) ;
#144364=CARTESIAN_POINT ( 'NONE',  ( 3.389175213736285386, 6.897862149426897460, 0.7216878364870317197 ) ) ;
#144368=CARTESIAN_POINT ( 'NONE',  ( 0.6823417656249899377, 5.738541667008087543, -1.181850606188754593 ) ) ;
#144370=CARTESIAN_POINT ( 'NONE',  ( 2.860407222358963608, 5.320596945185329218, 1.082531754730548412 ) ) ;
#144380=CARTESIAN_POINT ( 'NONE',  ( 0.6823417656249882723, -0.07395833299191079124, -1.181850606188749264 ) ) ;
#144384=CARTESIAN_POINT ( 'NONE',  ( -6.091691091241777656, 6.001394449403842479, 0.7998128361456341429 ) ) ;
#144387=CARTESIAN_POINT ( 'NONE',  ( -0.7500000000000215383, 0.4416666666666874130, 1.299038105676659116 ) ) ;
#144389=CARTESIAN_POINT ( 'NONE',  ( -1.001543065824772872E-14, 5.712500000000021672, 1.732050807568877637 ) ) ;
#144393=ORIENTED_EDGE ( 'NONE', *, *, #93332, .T. ) ;
#144396=CARTESIAN_POINT ( 'NONE',  ( -1.402160292154681736E-14, -0.9281249996585830830, 1.575800808251672791 ) ) ;
#144398=CARTESIAN_POINT ( 'NONE',  ( -7.316596452869116973, 11.68777962832266049, 0.7998128361456481317 ) ) ;
#144400=CARTESIAN_POINT ( 'NONE',  ( 8.703444544968814256, 12.24143683818393313, -1.199719254218446718 ) ) ;
#144407=CARTESIAN_POINT ( 'NONE',  ( -1.364683531250000748, 0.07187500034142035865, 0.000000000000000000 ) ) ;
#144413=CARTESIAN_POINT ( 'NONE',  ( 6.304178240674458422, 10.29869901418813782, 1.040834085586084257E-14 ) ) ;
#144417=CARTESIAN_POINT ( 'NONE',  ( -1.500000000000011324, 4.202083334016156080, 0.8660254037844403729 ) ) ;
#144419=CARTESIAN_POINT ( 'NONE',  ( -2.981903720001798597, 5.566305875722335372, -1.199719254218446718 ) ) ;
#144420=CARTESIAN_POINT ( 'NONE',  ( 6.927853306458749749, 8.145212281365775908, 1.082531754730558626 ) ) ;
#144421=CARTESIAN_POINT ( 'NONE',  ( -8.744645890690007306, 12.18554205823825498, 1.082531754730558626 ) ) ;
#144427=CARTESIAN_POINT ( 'NONE',  ( 4.356247428692526569, 3.976710176429713250, 0.7998128361456341429 ) ) ;
#144431=CARTESIAN_POINT ( 'NONE',  ( -1.490514837427310058, 7.209629588552702195, -4.246172784736847561 ) ) ;
#144443=CARTESIAN_POINT ( 'NONE',  ( 9.576136569953906275, 10.06658084123472641, 0.000000000000000000 ) ) ;
#144448=CARTESIAN_POINT ( 'NONE',  ( -1.364683531250014514, -0.01145833299191483488, -0.7879004041258359514 ) ) ;
#144449=CARTESIAN_POINT ( 'NONE',  ( 5.178851490740196795, 7.065079377328788546, 1.443375672974062551 ) ) ;
#144450=ORIENTED_EDGE ( 'NONE', *, *, #22894, .T. ) ;
#144451=CARTESIAN_POINT ( 'NONE',  ( -9.680158490477310806, 10.39586578175276266, 0.7216878364870438212 ) ) ;
#144470=CARTESIAN_POINT ( 'NONE',  ( 4.566373025097719029, 7.183545020864719355, -1.317121582780217404 ) ) ;
#144477=CARTESIAN_POINT ( 'NONE',  ( -8.541273586929371220, 9.067166727613487964, 0.7216878364870438212 ) ) ;
#144481=CARTESIAN_POINT ( 'NONE',  ( 6.287230548435207567, 8.358188277972981695, -1.599625672291262513 ) ) ;
#144485=CARTESIAN_POINT ( 'NONE',  ( -5.623934791570306402, 5.455678766453782913, 0.7998128361456341429 ) ) ;
#144489=CARTESIAN_POINT ( 'NONE',  ( -4.229253852459088137, 7.021547696922494808, 1.199719254218464037 ) ) ;
#144492=CARTESIAN_POINT ( 'NONE',  ( 3.330499290451326200, 7.037332938835193730, -0.7998128361456291469 ) ) ;
#144493=CARTESIAN_POINT ( 'NONE',  ( 7.293396569147545527, 10.59638086639245280, 1.199719254218460707 ) ) ;
#144496=CARTESIAN_POINT ( 'NONE',  ( 4.798800619506367049, 6.970516071510092893, 1.407892184351482889 ) ) ;
#144498=CARTESIAN_POINT ( 'NONE',  ( 3.375617060122621194, 6.882044303544283537, 1.040834085586084257E-14 ) ) ;
#144500=CARTESIAN_POINT ( 'NONE',  ( 3.189213936345665523, 2.817530495244580102, 2.450448857954567572 ) ) ;
#144505=CARTESIAN_POINT ( 'NONE',  ( 6.602457619730756733, 9.686322408785807525, 1.082531754730558626 ) ) ;
#144506=CARTESIAN_POINT ( 'NONE',  ( -7.296259222448620463, 11.66405285949874759, 0.7998128361456481317 ) ) ;
#144509=CARTESIAN_POINT ( 'NONE',  ( -8.646349277213090545, 11.11049346154719508, 1.599625672291269396 ) ) ;
#144510=CARTESIAN_POINT ( 'NONE',  ( -8.213542131780492639, 8.476887330032372603, 1.040834085586084257E-14 ) ) ;
#144518=CARTESIAN_POINT ( 'NONE',  ( 7.540305987494599016, 11.94877408538573427, -0.7998128361456291469 ) ) ;
#144522=CARTESIAN_POINT ( 'NONE',  ( 5.020596955762157698, 4.751784624677624080, 1.040834085586084257E-14 ) ) ;
#144532=CARTESIAN_POINT ( 'NONE',  ( -1.201851678989727383E-14, 3.462500000000019895, 1.732050807568877637 ) ) ;
#144533=CARTESIAN_POINT ( 'NONE',  ( 4.635998460869027227, 7.496083073400806818, -1.199719254218452047 ) ) ;
#144536=CARTESIAN_POINT ( 'NONE',  ( 6.616015773788773480, 10.66250946948817813, -0.7216878364870267237 ) ) ;
#144537=CARTESIAN_POINT ( 'NONE',  ( -8.636180661780651135, 13.01936850547871138, -0.7216878364870257245 ) ) ;
#144539=AXIS2_PLACEMENT_3D ( 'NONE', #72195, #157757, #92769 ) ;
#144542=CARTESIAN_POINT ( 'NONE',  ( 9.185812768458653466, 10.67553530374532045, 1.199719254218453823 ) ) ;
#144545=CARTESIAN_POINT ( 'NONE',  ( -5.101945877444165944, 4.846691699973280976, 0.000000000000000000 ) ) ;
#144546=CARTESIAN_POINT ( 'NONE',  ( -1.201851678989727383E-14, 5.618750000682818602, -1.732050807568863648 ) ) ;
#144547=CARTESIAN_POINT ( 'NONE',  ( 1.364683531249986537, 0.8635416670080893198, 0.7879004041258500513 ) ) ;
#144552=CARTESIAN_POINT ( 'NONE',  ( 1.364683531249986537, -0.1364583329919154264, 0.7879004041258500513 ) ) ;
#144559=CARTESIAN_POINT ( 'NONE',  ( -5.038826645773246682, 9.030381520044109322, 0.7998128361456481317 ) ) ;
#144562=CARTESIAN_POINT ( 'NONE',  ( 4.306686350635271054, 8.176217842383143974, -0.7998128361456221525 ) ) ;
#144568=CARTESIAN_POINT ( 'NONE',  ( 8.075853055234393452, 12.57357899774884658, 0.7998128361456462443 ) ) ;
#144571=CARTESIAN_POINT ( 'NONE',  ( -5.253948220495577637, 6.088359997788290734, 1.199719254218450271 ) ) ;
#144575=CARTESIAN_POINT ( 'NONE',  ( 9.240045382913317340, 10.73880668727576015, -1.199719254218446718 ) ) ;
#144577=CARTESIAN_POINT ( 'NONE',  ( 7.832860060393120882, 10.16142270859057462, 1.599625672291281386 ) ) ;
#144581=CARTESIAN_POINT ( 'NONE',  ( -8.785320351975364872, 12.23299559640450518, 1.082531754730560403 ) ) ;
#144583=CARTESIAN_POINT ( 'NONE',  ( -6.989391883044787868, 8.113044270762433285, -1.199719254218446718 ) ) ;
#144587=CARTESIAN_POINT ( 'NONE',  ( -6.138273485042783584, 5.995793210058552702, 0.01269068828805425264 ) ) ;
#144588=CARTESIAN_POINT ( 'NONE',  ( -1.402160292154681736E-14, -0.1781249996585796136, 1.575800808251672791 ) ) ;
#144591=CARTESIAN_POINT ( 'NONE',  ( 6.805829924380108586, 8.963220883242035697, 1.443375672974076540 ) ) ;
#144608=CARTESIAN_POINT ( 'NONE',  ( 8.075853055234393452, 12.57357899774884658, 0.7998128361456462443 ) ) ;
#144612=CARTESIAN_POINT ( 'NONE',  ( -2.449219305563052895, 6.009172956465517856, 1.040834085586084257E-14 ) ) ;
#144613=CARTESIAN_POINT ( 'NONE',  ( -7.751511138711140170, 10.06651563329490529, -1.599625672291263179 ) ) ;
#144619=CARTESIAN_POINT ( 'NONE',  ( 1.499999999999990896, 4.556250000682819490, 1.214306433183764966E-14 ) ) ;
#144620=CARTESIAN_POINT ( 'NONE',  ( 9.185812768458653466, 10.67553530374532045, 1.199719254218453823 ) ) ;
#144623=CARTESIAN_POINT ( 'NONE',  ( -8.528242318195895066, 9.908369778438709474, 1.199719254218462483 ) ) ;
#144625=CARTESIAN_POINT ( 'NONE',  ( 1.364683531249990311, 3.634375000341416584, 1.214306433183764966E-14 ) ) ;
#144630=CARTESIAN_POINT ( 'NONE',  ( -8.459924665247381625, 11.85336729522185806, 1.082531754730560403 ) ) ;
#144634=CARTESIAN_POINT ( 'NONE',  ( 1.364683531249988757, 2.196875000341415252, 1.214306433183764966E-14 ) ) ;
#144641=CARTESIAN_POINT ( 'NONE',  ( 0.6823417656249899377, 3.176041667008085323, -1.181850606188754593 ) ) ;
#144643=CARTESIAN_POINT ( 'NONE',  ( -6.410307701162927252, 6.373113827645189744, -0.7998128361456291469 ) ) ;
#144644=CARTESIAN_POINT ( 'NONE',  ( 6.076025397218672630, 10.24044673006381245, -0.7998128361456291469 ) ) ;
#144648=CARTESIAN_POINT ( 'NONE',  ( 1.364683531249990311, 4.446875000341417028, 1.214306433183764966E-14 ) ) ;
#144651=CARTESIAN_POINT ( 'NONE',  ( -1.364683531250014514, -1.011458332991911568, -0.7879004041258359514 ) ) ;
#144652=CARTESIAN_POINT ( 'NONE',  ( -3.307826292054304673, 6.802955074131234348, -0.7216878364870267237 ) ) ;
#144655=CARTESIAN_POINT ( 'NONE',  ( 5.355107487717867265, 5.349972945200037522, 1.040834085586084257E-14 ) ) ;
#144658=CARTESIAN_POINT ( 'NONE',  ( -8.538937818508475885, 8.856515631215026829, 1.040834085586084257E-14 ) ) ;
#144659=CARTESIAN_POINT ( 'NONE',  ( -7.863365906246048809, 12.11775129068834289, -0.7216878364870267237 ) ) ;
#144662=CARTESIAN_POINT ( 'NONE',  ( -1.201851678989727383E-14, 4.696875000341419693, -1.575800808251660134 ) ) ;
#144667=CARTESIAN_POINT ( 'NONE',  ( -6.277061933002790362, 8.346324893301817482, 1.443375672974078761 ) ) ;
#144669=CARTESIAN_POINT ( 'NONE',  ( -0.6823417656250003738, -0.9697916663252494907, -1.181850606188749264 ) ) ;
#144678=CARTESIAN_POINT ( 'NONE',  ( 10.73535870392234237, 11.41900666419791399, 0.000000000000000000 ) ) ;
#144682=ORIENTED_EDGE ( 'NONE', *, *, #28619, .F. ) ;
#144683=CARTESIAN_POINT ( 'NONE',  ( -1.402160292154681736E-14, -0.7874999999999764411, 1.732050807568877637 ) ) ;
#144684=CARTESIAN_POINT ( 'NONE',  ( 10.03267048398825168, 10.80712977418221676, 0.000000000000000000 ) ) ;
#144690=ORIENTED_EDGE ( 'NONE', *, *, #137857, .T. ) ;
#144692=CARTESIAN_POINT ( 'NONE',  ( 6.287230548435207567, 8.358188277972981695, -1.599625672291262513 ) ) ;
#144693=CARTESIAN_POINT ( 'NONE',  ( -4.603156847039612920, 5.329103395422994716, 1.199719254218462483 ) ) ;
#144697=CARTESIAN_POINT ( 'NONE',  ( -1.201851678989727383E-14, 3.462500000000019895, 1.732050807568877637 ) ) ;
#144698=CARTESIAN_POINT ( 'NONE',  ( 5.026856346975741019, 4.759087247760136918, -0.3692494997280463265 ) ) ;
#144699=CARTESIAN_POINT ( 'NONE',  ( -1.364683531250014514, 1.551041667008084435, -0.7879004041258289570 ) ) ;
#144700=CARTESIAN_POINT ( 'NONE',  ( 2.854315967138055132, 6.433244981884085334, -0.2941531795266367211 ) ) ;
#144701=CARTESIAN_POINT ( 'NONE',  ( -8.646349277213090545, 11.11049346154719508, 1.599625672291269396 ) ) ;
#144718=CARTESIAN_POINT ( 'NONE',  ( 4.645640190976921602, 8.571663989448405019, 1.040834085586084257E-14 ) ) ;
#144725=CARTESIAN_POINT ( 'NONE',  ( 7.151035956204054855, 10.43029348462504124, 1.199719254218460707 ) ) ;
#144729=CARTESIAN_POINT ( 'NONE',  ( 9.582915646760733708, 10.07448976417602893, 0.7998128361456462443 ) ) ;
#144731=CARTESIAN_POINT ( 'NONE',  ( 0.7499999999999902300, 3.816666666666690411, -1.299038105676658228 ) ) ;
#144737=CARTESIAN_POINT ( 'NONE',  ( -0.4933182949323664523, 7.812106778933141982, 1.990607459109340560 ) ) ;
#144743=CARTESIAN_POINT ( 'NONE',  ( -8.920901888112002354, 11.43080484092926241, 1.443375672974064550 ) ) ;
#144748=CARTESIAN_POINT ( 'NONE',  ( 6.498435699651741615, 6.475929825882159818, -0.7998128361456281477 ) ) ;
#144749=CARTESIAN_POINT ( 'NONE',  ( 0.6823417656249917140, 5.592708333674749177, 1.181850606188765695 ) ) ;
#144755=CARTESIAN_POINT ( 'NONE',  ( 3.009546912109283934, 6.454962464195385330, 0.000000000000000000 ) ) ;
#144763=CARTESIAN_POINT ( 'NONE',  ( -7.369020184227459858, 8.555943955475521889, 1.199719254218450271 ) ) ;
#144765=CARTESIAN_POINT ( 'NONE',  ( -3.737243898861318137, 7.511868315313511069, 0.7998128361456341429 ) ) ;
#144774=CARTESIAN_POINT ( 'NONE',  ( 7.610204295972345712, 7.772993188256215547, 0.7998128361456341429 ) ) ;
#144789=CARTESIAN_POINT ( 'NONE',  ( -1.402160292154681736E-14, 0.5093750003414236893, -1.575800808251659024 ) ) ;
#144791=CARTESIAN_POINT ( 'NONE',  ( 3.032219910950674890, 6.689340329417765574, 0.7998128361456321445 ) ) ;
#144793=CARTESIAN_POINT ( 'NONE',  ( -7.565086526745425033, 7.928281824065535055, 0.7216878364870317197 ) ) ;
#144794=CARTESIAN_POINT ( 'NONE',  ( 5.843201017809841247, 5.919415396974013532, 1.040834085586084257E-14 ) ) ;
#144795=CARTESIAN_POINT ( 'NONE',  ( -7.497295758232731089, 8.809561808435409702, -1.082531754730543083 ) ) ;
#144799=CARTESIAN_POINT ( 'NONE',  ( 5.341022448779654930, 8.318611059296550536, 1.199719254218462483 ) ) ;
#144805=CARTESIAN_POINT ( 'NONE',  ( -1.201851678989727383E-14, 4.696875000341419693, -1.575800808251660134 ) ) ;
#144809=CARTESIAN_POINT ( 'NONE',  ( 5.947222937888848371, 10.09017719417900416, 1.040834085586084257E-14 ) ) ;
#144812=CARTESIAN_POINT ( 'NONE',  ( -8.213542131780492639, 8.476887330032372603, 1.040834085586084257E-14 ) ) ;
#144817=CARTESIAN_POINT ( 'NONE',  ( 7.618792255875527886, 10.97600916757510170, 1.199719254218460707 ) ) ;
#144818=CARTESIAN_POINT ( 'NONE',  ( 4.076122527140082497, 7.725281555510842502, -0.6205295181239127711 ) ) ;
#144820=CARTESIAN_POINT ( 'NONE',  ( -6.690058733339450114, 9.892486724616283311, 1.199719254218452047 ) ) ;
#144824=CARTESIAN_POINT ( 'NONE',  ( 4.003607682157598546, 7.822813005323850710, -0.1595685970469905290 ) ) ;
#144825=CARTESIAN_POINT ( 'NONE',  ( -10.15469386695561482, 10.94949038764413096, 1.040834085586084257E-14 ) ) ;
#144827=CARTESIAN_POINT ( 'NONE',  ( 3.234284411020655003, 6.422206199346979894, -0.8943276771341170939 ) ) ;
#144829=CARTESIAN_POINT ( 'NONE',  ( 6.449928391799196525, 8.548002428564306143, -1.599625672291262513 ) ) ;
#144831=CARTESIAN_POINT ( 'NONE',  ( 4.801558957534076022, 8.753569217098425170, 0.7998128361456462443 ) ) ;
#144832=CARTESIAN_POINT ( 'NONE',  ( -4.160056744896282410, 7.428205994021240599, -0.7369721661574859528 ) ) ;
#144833=CARTESIAN_POINT ( 'NONE',  ( 3.388648328411762556, 6.040841252200647382, 1.199719254218462483 ) ) ;
#144835=CARTESIAN_POINT ( 'NONE',  ( -6.805829924380121909, 8.963220883242035697, 1.443375672974078761 ) ) ;
#144838=TOROIDAL_SURFACE ( 'NONE', #179283, 0.1600000000000000033, 0.08000000000000000167 ) ;
#144843=CARTESIAN_POINT ( 'NONE',  ( -5.250693970737303928, 6.428279158139240224, 1.158874695820178324 ) ) ;
#144844=CARTESIAN_POINT ( 'NONE',  ( 0.6823417656249882723, 0.4885416670080827695, -1.181850606188749264 ) ) ;
#144847=CARTESIAN_POINT ( 'NONE',  ( 4.365362273920238678, 7.076377838673507448, 1.082531754730558626 ) ) ;
#144851=CARTESIAN_POINT ( 'NONE',  ( -8.717529583462656717, 11.19353715217169309, 1.443375672974064550 ) ) ;
#144855=CARTESIAN_POINT ( 'NONE',  ( -7.470179451005382276, 11.65903375957422128, 0.7216878364870458196 ) ) ;
#144862=CARTESIAN_POINT ( 'NONE',  ( -7.144783764277399030, 11.27940545839156528, 0.7216878364870458196 ) ) ;
#144867=CARTESIAN_POINT ( 'NONE',  ( 0.7499999999999902300, 4.597916667349482012, -1.299038105676658228 ) ) ;
#144868=CARTESIAN_POINT ( 'NONE',  ( 5.531458889030211878, 6.400359360821498811, -1.228567739025695493 ) ) ;
#144873=CARTESIAN_POINT ( 'NONE',  ( -8.532158741701643123, 8.848606708273724308, 0.7998128361456462443 ) ) ;
#144878=CARTESIAN_POINT ( 'NONE',  ( 5.684946482831785275, 5.526859072925533134, -0.7998128361456231517 ) ) ;
#144883=CARTESIAN_POINT ( 'NONE',  ( 7.690499447449630210, 9.995335326823163058, 1.599625672291281386 ) ) ;
#144889=CARTESIAN_POINT ( 'NONE',  ( -5.585596099150182958, 8.499983968108443477, -1.082531754730544860 ) ) ;
#144892=CARTESIAN_POINT ( 'NONE',  ( -4.475070042639309520, 5.445751865460756846, 1.284222742053057642 ) ) ;
#144894=CARTESIAN_POINT ( 'NONE',  ( -7.334597915313094241, 9.580116872663850813, 1.040834085586084257E-14 ) ) ;
#144897=CARTESIAN_POINT ( 'NONE',  ( -7.967387826325084355, 12.44703623068796361, 0.7998128361456481317 ) ) ;
#144899=CARTESIAN_POINT ( 'NONE',  ( 7.587759525142423911, 12.00413654597487501, 0.7998128361456462443 ) ) ;
#144900=CARTESIAN_POINT ( 'NONE',  ( 1.499999999999987566, -0.9749999999999827693, 0.000000000000000000 ) ) ;
#144901=CARTESIAN_POINT ( 'NONE',  ( -7.994504133552415404, 12.47867192245318435, -0.7998128361456281477 ) ) ;
#144904=CARTESIAN_POINT ( 'NONE',  ( 1.364683531249988535, 2.863541667008082658, 0.7879004041258500513 ) ) ;
#144906=CARTESIAN_POINT ( 'NONE',  ( 8.581948047770334043, 12.95609712246668899, 0.000000000000000000 ) ) ;
#144908=CARTESIAN_POINT ( 'NONE',  ( 1.441120163477462413, 8.287694259231834337, -3.161243217722550458 ) ) ;
#144911=CARTESIAN_POINT ( 'NONE',  ( 7.714226216051361718, 11.94375498546120795, -0.7216878364870267237 ) ) ;
#144914=CARTESIAN_POINT ( 'NONE',  ( -7.226132686403777150, 7.532835677000276675, 1.040834085586084257E-14 ) ) ;
#144915=CARTESIAN_POINT ( 'NONE',  ( 0.6823417656249882723, 1.176041667008083325, -1.181850606188749264 ) ) ;
#144919=CARTESIAN_POINT ( 'NONE',  ( -7.507464373665155399, 9.781794407407920389, 1.599625672291295375 ) ) ;
#144920=CARTESIAN_POINT ( 'NONE',  ( -2.928197990427299668, 6.360055388899728435, 1.040834085586084257E-14 ) ) ;
#144921=CARTESIAN_POINT ( 'NONE',  ( 0.6823417656249899377, 2.905208333674754062, 1.181850606188765695 ) ) ;
#144927=CARTESIAN_POINT ( 'NONE',  ( 8.561083932025322696, 12.07534945641652158, -1.199719254218446718 ) ) ;
#144935=CARTESIAN_POINT ( 'NONE',  ( 8.452618703115982512, 11.94880668935564216, 1.199719254218450271 ) ) ;
#144939=DIRECTION ( 'NONE',  ( 0.7592566023653005702, 0.6507913734559639396, 0.000000000000000000 ) ) ;
#144941=CARTESIAN_POINT ( 'NONE',  ( -1.201851678989727383E-14, 5.009375000341421469, -1.575800808251660134 ) ) ;
#144945=CARTESIAN_POINT ( 'NONE',  ( 7.262363838414439776, 11.62450824479221900, 0.7998128361456462443 ) ) ;
#144948=CARTESIAN_POINT ( 'NONE',  ( 0.6823417656249917140, 3.842708333674754506, 1.181850606188765695 ) ) ;
#144950=CARTESIAN_POINT ( 'NONE',  ( -4.934804725694212912, 8.701096580044490381, -0.7216878364870207285 ) ) ;
#144956=CARTESIAN_POINT ( 'NONE',  ( 4.162516854595432747, 4.815023404238158555, 1.199719254218464037 ) ) ;
#144959=CARTESIAN_POINT ( 'NONE',  ( 8.911787042884274257, 9.291506392986812912, 0.7998128361456462443 ) ) ;
#144965=CARTESIAN_POINT ( 'NONE',  ( -10.48453286206953727, 11.12637651536962125, 0.7998128361456462443 ) ) ;
#144966=CARTESIAN_POINT ( 'NONE',  ( 7.318703993278529829, 7.432909501780090800, 1.040834085586084257E-14 ) ) ;
#144970=CARTESIAN_POINT ( 'NONE',  ( 4.792970997630896512, 5.550553237779539018, 1.199719254218464037 ) ) ;
#144971=EDGE_LOOP ( 'NONE', ( #203721, #82386, #176542, #108307, #39762, #44590, #163446, #1029, #125119, #140172, #21178 ) ) ;
#144980=CARTESIAN_POINT ( 'NONE',  ( -6.073689629242165822, 7.148687991279732756, -1.082531754730544860 ) ) ;
#144981=CARTESIAN_POINT ( 'NONE',  ( 4.792970997630896512, 5.550553237779539018, 1.199719254218464037 ) ) ;
#144984=CARTESIAN_POINT ( 'NONE',  ( -7.751511138711140170, 10.06651563329490529, -1.599625672291263179 ) ) ;
#144990=CARTESIAN_POINT ( 'NONE',  ( -8.123306592882240551, 12.62894145833798376, 0.000000000000000000 ) ) ;
#144991=CARTESIAN_POINT ( 'NONE',  ( 0.9486429539237137831, 3.100839070649073381, 1.028101543438981080 ) ) ;
#144995=CARTESIAN_POINT ( 'NONE',  ( 8.392660782059197189, 9.750191319612612872, 1.199719254218462483 ) ) ;
#144996=CARTESIAN_POINT ( 'NONE',  ( 4.801558957534076022, 8.753569217098425170, 0.7998128361456462443 ) ) ;
#145008=CARTESIAN_POINT ( 'NONE',  ( -7.100719765255177229, 9.307259030929609267, -1.599625672291263179 ) ) ;
#145012=CARTESIAN_POINT ( 'NONE',  ( 6.480434237652124452, 8.583592582059388576, 1.443375672974076540 ) ) ;
#145015=DIRECTION ( 'NONE',  ( -5.578564026256490882E-16, -1.000000000000000000, -9.066213480720158442E-32 ) ) ;
#145017=CARTESIAN_POINT ( 'NONE',  ( -5.738125327081750271, 7.717565519727259904, 1.599625672291269396 ) ) ;
#145019=CARTESIAN_POINT ( 'NONE',  ( -1.436838838544753694, 7.449283400311743186, 4.203727439823589762 ) ) ;
#145026=CARTESIAN_POINT ( 'NONE',  ( -1.201851678989727383E-14, 4.134375000341417028, 1.575800808251672791 ) ) ;
#145027=CARTESIAN_POINT ( 'NONE',  ( 3.334942598837264960, 6.834590765378040444, 1.214306433183764966E-14 ) ) ;
#145028=CARTESIAN_POINT ( 'NONE',  ( 8.776205506747620788, 9.133327934160710981, -0.7998128361456221525 ) ) ;
#145030=CARTESIAN_POINT ( 'NONE',  ( -4.785665035943912571, 4.685623418130398399, 1.214306433183764966E-14 ) ) ;
#145033=CARTESIAN_POINT ( 'NONE',  ( -3.592547517496929466, 7.135129837147637488, -0.7216878364870257245 ) ) ;
#145040=CARTESIAN_POINT ( 'NONE',  ( 2.496672843210871129, 6.064535417054653266, -0.7998128361456291469 ) ) ;
#145044=EDGE_CURVE ( 'NONE', #47756, #69090, #144255, .T. ) ;
#145049=CARTESIAN_POINT ( 'NONE',  ( 3.785751206713845018, 5.439795712631356750, 1.599625672291267398 ) ) ;
#145053=CARTESIAN_POINT ( 'NONE',  ( -1.001543065824772872E-14, 4.634375000341418804, 1.575800808251672791 ) ) ;
#145058=CARTESIAN_POINT ( 'NONE',  ( 5.931855901178834323, 6.879252291918818152, 1.199719254218462483 ) ) ;
#145062=CARTESIAN_POINT ( 'NONE',  ( -5.596818484342970912, 5.424043074688562172, -0.7998128361456221525 ) ) ;
#145065=CARTESIAN_POINT ( 'NONE',  ( 3.985733972293228344, 7.593847367743336463, 1.040834085586084257E-14 ) ) ;
#145066=CARTESIAN_POINT ( 'NONE',  ( 1.499999999999989120, 3.275000000000020783, 1.214306433183764966E-14 ) ) ;
#145068=CARTESIAN_POINT ( 'NONE',  ( -4.623494077460110319, 5.352830164246910272, 1.199719254218462483 ) ) ;
#145069=CARTESIAN_POINT ( 'NONE',  ( 0.4444767461200390124, 7.387363020590400176, -2.040826832792550505 ) ) ;
#145071=CARTESIAN_POINT ( 'NONE',  ( -1.001543065824772872E-14, 4.571875000341418804, 1.575800808251672791 ) ) ;
#145074=CARTESIAN_POINT ( 'NONE',  ( -4.039966587192274083, 5.736380323189513852, 1.443375672974064550 ) ) ;
#145080=CARTESIAN_POINT ( 'NONE',  ( 5.705283713252285338, 5.550585841749444249, -0.7998128361456211532 ) ) ;
#145084=CARTESIAN_POINT ( 'NONE',  ( -0.6823417656249969321, 3.530208333674754506, -1.181850606188749264 ) ) ;
#145087=CARTESIAN_POINT ( 'NONE',  ( -1.364683531250014514, 0.3010416670080866552, -0.7879004041258359514 ) ) ;
#145090=CARTESIAN_POINT ( 'NONE',  ( -8.513630394377489807, 12.01998699582738972, -1.199719254218446718 ) ) ;
#145091=CARTESIAN_POINT ( 'NONE',  ( -5.517805330637490790, 9.381263952478319013, 0.7216878364870458196 ) ) ;
#145094=VERTEX_POINT ( 'NONE', #100766 ) ;
#145095=CARTESIAN_POINT ( 'NONE',  ( 0.6823417656249899377, 4.426041667008086655, -1.181850606188754593 ) ) ;
#145103=CARTESIAN_POINT ( 'NONE',  ( -6.860062538390436337, 7.105753837651378468, 1.040834085586084257E-14 ) ) ;
#145107=CARTESIAN_POINT ( 'NONE',  ( -6.521108698048791119, 6.710307690586118312, -0.7216878364870267237 ) ) ;
#145120=CARTESIAN_POINT ( 'NONE',  ( -6.227272627378437342, 6.159572908229946187, -0.7998128361456291469 ) ) ;
#145123=CARTESIAN_POINT ( 'NONE',  ( 1.499999999999987121, 1.295833333333353377, -0.8660254037844253849 ) ) ;
#145125=CARTESIAN_POINT ( 'NONE',  ( 8.514157279702022407, 10.95626946445095307, -1.443375672974063439 ) ) ;
#145126=CARTESIAN_POINT ( 'NONE',  ( 6.388916700537700777, 8.476822122092563916, 1.599625672291281386 ) ) ;
#145131=CARTESIAN_POINT ( 'NONE',  ( 3.832150974156964818, 7.622593236491780999, 1.040834085586084257E-14 ) ) ;
#145133=CARTESIAN_POINT ( 'NONE',  ( -0.4396101492293769120, 7.376551424357159270, -2.043156636846727991 ) ) ;
#145140=CARTESIAN_POINT ( 'NONE',  ( -4.446711195602264688, 4.290177271065136466, -0.7216878364870207285 ) ) ;
#145143=CARTESIAN_POINT ( 'NONE',  ( 3.039951802757216548, 2.724153688964676689, -2.451370731312840778 ) ) ;
#145146=CARTESIAN_POINT ( 'NONE',  ( -0.6823417656250212460, 2.801041667008084879, 1.181850606188767472 ) ) ;
#145147=CARTESIAN_POINT ( 'NONE',  ( 8.229436053370667636, 11.58446391469906267, 1.082531754730558626 ) ) ;
#145148=CARTESIAN_POINT ( 'NONE',  ( -7.386494761346872551, 7.511998731193139989, -0.7998128361456291469 ) ) ;
#145151=CARTESIAN_POINT ( 'NONE',  ( 6.993308306550549247, 7.053281200597435685, 1.040834085586084257E-14 ) ) ;
#145152=CARTESIAN_POINT ( 'NONE',  ( -7.237355071596549116, 7.338002426484427687, 1.040834085586084257E-14 ) ) ;
#145156=CARTESIAN_POINT ( 'NONE',  ( 1.499999999999987121, 0.3270833340161527492, -0.8660254037844323793 ) ) ;
#145160=CARTESIAN_POINT ( 'NONE',  ( 7.809133291791403586, 8.213003049952529722, -0.7216878364870257245 ) ) ;
#145163=CARTESIAN_POINT ( 'NONE',  ( -1.364683531250000748, 1.821875000341421913, 0.000000000000000000 ) ) ;
#145165=CARTESIAN_POINT ( 'NONE',  ( 5.626270559546814098, 7.587068290936515247, 1.443375672974062551 ) ) ;
#145167=CARTESIAN_POINT ( 'NONE',  ( -3.314994193297896796, 6.393354490853021765, -0.7784788408506218005 ) ) ;
#145168=CARTESIAN_POINT ( 'NONE',  ( -3.470524135418300737, 6.032400010421219427, -1.082531754730549967 ) ) ;
#145170=CARTESIAN_POINT ( 'NONE',  ( -0.6823417656250212460, 5.301041667008086655, 1.181850606188767472 ) ) ;
#145175=ORIENTED_EDGE ( 'NONE', *, *, #105176, .F. ) ;
#145176=CARTESIAN_POINT ( 'NONE',  ( -4.244195945626527688, 7.512047922924973697, -1.038054094898384294 ) ) ;
#145183=CARTESIAN_POINT ( 'NONE',  ( 6.470265622219697477, 8.571729197388226140, -1.599625672291262513 ) ) ;
#145186=CARTESIAN_POINT ( 'NONE',  ( 4.467575310902914154, 5.170924936596891008, 1.199719254218464037 ) ) ;
#145195=CARTESIAN_POINT ( 'NONE',  ( 4.175548123328908900, 7.815297210618305179, -0.7216878364870197293 ) ) ;
#145196=CARTESIAN_POINT ( 'NONE',  ( -1.364683531249997417, 2.571875000341422357, 1.214306433183764966E-14 ) ) ;
#145197=CARTESIAN_POINT ( 'NONE',  ( 7.079328764629950754, 11.41096732537697633, 0.7998128361456462443 ) ) ;
#145199=CYLINDRICAL_SURFACE ( 'NONE', #136682, 0.08000000000000004330 ) ;
#145200=CARTESIAN_POINT ( 'NONE',  ( 0.5972946010069523082, 6.677937103010220810, -3.537249470680236652 ) ) ;
#145204=CARTESIAN_POINT ( 'NONE',  ( -0.7500000000000006661, 1.858333333333357595, -1.299038105676652011 ) ) ;
#145205=CARTESIAN_POINT ( 'NONE',  ( 6.148786358997489820, 7.132337826040578754, -1.199719254218446718 ) ) ;
#145206=CARTESIAN_POINT ( 'NONE',  ( -6.632963465583701534, 8.761543347979550589, -1.599625672291263179 ) ) ;
#145210=CARTESIAN_POINT ( 'NONE',  ( -0.6823417656250212460, 2.051041667008083991, 1.181850606188767472 ) ) ;
#145211=CARTESIAN_POINT ( 'NONE',  ( 1.499999999999989120, 4.004166666666685970, 0.8660254037844524744 ) ) ;
#145213=CARTESIAN_POINT ( 'NONE',  ( 4.871457266011829823, 4.577788319968905562, -0.7998128361456221525 ) ) ;
#145219=CARTESIAN_POINT ( 'NONE',  ( -1.500000000000015099, 0.1604166673494879791, -0.8660254037844383745 ) ) ;
#145221=CARTESIAN_POINT ( 'NONE',  ( -7.854251061018346469, 8.057714414143200443, -0.7998128361456291469 ) ) ;
#145222=CARTESIAN_POINT ( 'NONE',  ( -4.636525346193588248, 4.511627113421689650, 0.7216878364870317197 ) ) ;
#145230=CARTESIAN_POINT ( 'NONE',  ( 6.582647274634798151, 7.638508894284114170, 1.199719254218462483 ) ) ;
#145233=CARTESIAN_POINT ( 'NONE',  ( 7.494959990256193194, 7.638541498254023843, -0.7998128361456281477 ) ) ;
#145239=CARTESIAN_POINT ( 'NONE',  ( -7.881367368245678406, 8.089350105908421185, 0.7998128361456602331 ) ) ;
#145240=ORIENTED_EDGE ( 'NONE', *, *, #103885, .T. ) ;
#145241=CARTESIAN_POINT ( 'NONE',  ( 2.679707916995359263, 6.278076336469897711, -0.7998128361456291469 ) ) ;
#145247=CARTESIAN_POINT ( 'NONE',  ( 4.244147651705390878, 7.284590634535035747, 0.9143829328417275581 ) ) ;
#145257=CARTESIAN_POINT ( 'NONE',  ( -2.765500147507697459, 5.209872024525476597, 1.082531754730560403 ) ) ;
#145258=CARTESIAN_POINT ( 'NONE',  ( 8.948018195339340508, 9.541702104091804415, -0.7216878364870197293 ) ) ;
#145260=CARTESIAN_POINT ( 'NONE',  ( -4.334856428067329404, 6.080418470877079429, -1.599625672291256295 ) ) ;
#145264=CARTESIAN_POINT ( 'NONE',  ( -5.859094939400033120, 9.987361195942037639, -0.7998128361456231517 ) ) ;
#145274=ORIENTED_EDGE ( 'NONE', *, *, #80361, .F. ) ;
#145281=CARTESIAN_POINT ( 'NONE',  ( -5.928993247877788697, 5.811580298812519807, 0.7998128361456341429 ) ) ;
#145284=CARTESIAN_POINT ( 'NONE',  ( 2.385871846325007706, 5.727341554113725586, -0.7216878364870267237 ) ) ;
#145290=CARTESIAN_POINT ( 'NONE',  ( 0.4702634422464547770, 7.494255424139249833, 4.464191613398297953 ) ) ;
#145291=CARTESIAN_POINT ( 'NONE',  ( -3.632695093457760649, 6.325562478087638496, -1.199719254218452047 ) ) ;
#145294=CARTESIAN_POINT ( 'NONE',  ( 10.38962578677386084, 11.01565159419135043, 0.000000000000000000 ) ) ;
#145297=CARTESIAN_POINT ( 'NONE',  ( -6.530223543276495235, 10.77034456713125188, -0.7998128361456291469 ) ) ;
#145298=CARTESIAN_POINT ( 'NONE',  ( 5.473741331615251227, 7.409117525016355010, -1.599625672291262513 ) ) ;
#145303=CARTESIAN_POINT ( 'NONE',  ( 1.364683531249986537, 0.6760416670080884316, 0.7879004041258500513 ) ) ;
#145307=CARTESIAN_POINT ( 'NONE',  ( 6.616015773788773480, 10.66250946948817813, -0.7216878364870267237 ) ) ;
#145313=B_SPLINE_CURVE_WITH_KNOTS ( 'NONE', 3,
 ( #3875, #123105, #89450, #69948 ),
 .UNSPECIFIED., .F., .F.,
 ( 4, 4 ),
 ( 0.0001647631253658502772, 0.001106915643567259362 ),
 .UNSPECIFIED. ) ;
#145318=ORIENTED_EDGE ( 'NONE', *, *, #178819, .F. ) ;
#145320=FACE_OUTER_BOUND ( 'NONE', #5253, .T. ) ;
#145333=AXIS2_PLACEMENT_3D ( 'NONE', #181613, #48457, #707 ) ;
#145334=CARTESIAN_POINT ( 'NONE',  ( 2.981521246686049231, 6.451858035227898469, -0.1755584056236529911 ) ) ;
#145341=CARTESIAN_POINT ( 'NONE',  ( -1.201851678989727383E-14, 0.9937500006828198229, 1.732050807568877637 ) ) ;
#145347=DIRECTION ( 'NONE',  ( -1.000000000000000000, 5.421010862427522170E-16, 0.000000000000000000 ) ) ;
#145348=CARTESIAN_POINT ( 'NONE',  ( 8.402302512167096893, 10.82577223566020841, -1.599625672291268286 ) ) ;
#145350=CARTESIAN_POINT ( 'NONE',  ( -1.364683531250000748, -1.240624999658580752, 0.000000000000000000 ) ) ;
#145354=CARTESIAN_POINT ( 'NONE',  ( 2.523789150438203510, 6.096171108819874007, 0.7998128361456462443 ) ) ;
#145355=CARTESIAN_POINT ( 'NONE',  ( -4.595850885352567694, 8.305650432979225783, 1.040834085586084257E-14 ) ) ;
#145356=AXIS2_PLACEMENT_3D ( 'NONE', #138948, #189802, #92347 ) ;
#145360=CARTESIAN_POINT ( 'NONE',  ( -6.775324078527193983, 8.927630729746953264, -1.599625672291263179 ) ) ;
#145364=CARTESIAN_POINT ( 'NONE',  ( -0.7500000000000006661, 1.639583334016154970, -1.299038105676652011 ) ) ;
#145371=CARTESIAN_POINT ( 'NONE',  ( -2.426546306721660606, 5.774795091243142053, 0.7216878364870317197 ) ) ;
#145374=CARTESIAN_POINT ( 'NONE',  ( 4.047743032765107607, 7.529339606631276105, 0.4638284745723305624 ) ) ;
#145379=CARTESIAN_POINT ( 'NONE',  ( -10.32861409551237486, 10.94447128771960287, 1.040834085586084257E-14 ) ) ;
#145380=CARTESIAN_POINT ( 'NONE',  ( 8.392660782059197189, 9.750191319612612872, 1.199719254218462483 ) ) ;
#145384=EDGE_LOOP ( 'NONE', ( #180875, #137630, #3325, #196086 ) ) ;
#145387=CARTESIAN_POINT ( 'NONE',  ( -6.645467848992654858, 10.90479625713344625, 0.7998128361456481317 ) ) ;
#145393=CARTESIAN_POINT ( 'NONE',  ( 4.891794496432329886, 4.601515088792824670, -0.7998128361456211532 ) ) ;
#145397=CARTESIAN_POINT ( 'NONE',  ( -6.091691091241777656, 6.001394449403842479, 0.7998128361456341429 ) ) ;
#145398=CARTESIAN_POINT ( 'NONE',  ( -9.541187415715041809, 12.15447128979948310, -1.599625672291263179 ) ) ;
#145409=CARTESIAN_POINT ( 'NONE',  ( 6.226218857173709154, 8.287007971501239467, 1.599625672291281386 ) ) ;
#145418=CARTESIAN_POINT ( 'NONE',  ( -0.7500000000000006661, 0.3895833340161539149, -1.299038105676652011 ) ) ;
#145422=CARTESIAN_POINT ( 'NONE',  ( 2.530568227245037605, 6.104080031761181857, 0.000000000000000000 ) ) ;
#145424=CARTESIAN_POINT ( 'NONE',  ( -3.755772246185468788, 4.340488027759846545, -1.199719254218452047 ) ) ;
#145431=CARTESIAN_POINT ( 'NONE',  ( 5.178851490740205676, 6.104710163027444736, 1.082531754730558626 ) ) ;
#145433=ORIENTED_EDGE ( 'NONE', *, *, #74793, .F. ) ;
#145434=CARTESIAN_POINT ( 'NONE',  ( -0.6823417656250212460, 5.613541667008087543, 1.181850606188767472 ) ) ;
#145436=CARTESIAN_POINT ( 'NONE',  ( 10.18233705906309972, 11.83814697611718714, 1.199719254218450271 ) ) ;
#145440=CARTESIAN_POINT ( 'NONE',  ( 3.511198596259283544, 6.271927390929313617, 2.420000000000010587 ) ) ;
#145446=CARTESIAN_POINT ( 'NONE',  ( -0.6823417656250246877, -0.1989583329919109023, 1.181850606188755259 ) ) ;
#145451=CARTESIAN_POINT ( 'NONE',  ( -5.742041750587549842, 6.657802449562273850, 1.199719254218450271 ) ) ;
#145455=CARTESIAN_POINT ( 'NONE',  ( 0.7499999999999920064, 4.983333333333353821, 1.299038105676669330 ) ) ;
#145464=CARTESIAN_POINT ( 'NONE',  ( 0.6823417656249917140, 5.655208333674749177, 1.181850606188765695 ) ) ;
#145466=CARTESIAN_POINT ( 'NONE',  ( 4.788000803920411386, 8.737751371215816576, 1.040834085586084257E-14 ) ) ;
#145467=CARTESIAN_POINT ( 'NONE',  ( -7.343712760096452463, 11.71941532008788833, -0.7998128361456291469 ) ) ;
#145469=CARTESIAN_POINT ( 'NONE',  ( 8.218213668177886788, 12.73966637951625813, 0.7998128361456462443 ) ) ;
#145471=CARTESIAN_POINT ( 'NONE',  ( 0.000000000000000000, 5.868705557303649734, -4.125226524755057689 ) ) ;
#145473=ORIENTED_EDGE ( 'NONE', *, *, #153202, .T. ) ;
#145475=CARTESIAN_POINT ( 'NONE',  ( 1.499999999999990896, 5.525000000000022560, 1.214306433183764966E-14 ) ) ;
#145482=CARTESIAN_POINT ( 'NONE',  ( 7.348156068926750883, 8.635565504245116486, -1.082531754730537976 ) ) ;
#145487=CARTESIAN_POINT ( 'NONE',  ( 1.499999999999989120, 5.077083334016151639, -0.8660254037844323793 ) ) ;
#145489=CARTESIAN_POINT ( 'NONE',  ( -2.591579918506545344, 6.175260338232929413, 1.040834085586084257E-14 ) ) ;
#145490=CARTESIAN_POINT ( 'NONE',  ( 5.734735788456138295, 8.673980272298743799, -1.082531754730537976 ) ) ;
#145491=CARTESIAN_POINT ( 'NONE',  ( -7.632877294369372123, 11.84884791016554573, 0.7216878364870458196 ) ) ;
#145497=CARTESIAN_POINT ( 'NONE',  ( 10.07334494527360569, 10.85458331234846696, 0.000000000000000000 ) ) ;
#145499=CARTESIAN_POINT ( 'NONE',  ( 4.891794496432329886, 4.601515088792824670, -0.7998128361456211532 ) ) ;
#145502=VERTEX_POINT ( 'NONE', #153796 ) ;
#145512=CARTESIAN_POINT ( 'NONE',  ( 8.239604668803105270, 10.63595808506888396, -1.599625672291268286 ) ) ;
#145514=CARTESIAN_POINT ( 'NONE',  ( -1.499999999999995781, 8.627523663848663205, 2.580000000000011173 ) ) ;
#145515=CARTESIAN_POINT ( 'NONE',  ( 0.6823417656249882723, 0.1760416670080894308, -1.181850606188749264 ) ) ;
#145516=CARTESIAN_POINT ( 'NONE',  ( 4.351804120306567825, 8.020929207092235558, 1.040834085586084257E-14 ) ) ;
#145517=ORIENTED_EDGE ( 'NONE', *, *, #79248, .T. ) ;
#145518=CARTESIAN_POINT ( 'NONE',  ( -8.676855123066022912, 10.18571440074093282, -1.082531754730543971 ) ) ;
#145523=CARTESIAN_POINT ( 'NONE',  ( -3.795392936821753604, 6.515376628678959392, -1.199719254218452047 ) ) ;
#145532=VERTEX_POINT ( 'NONE', #122456 ) ;
#145538=CARTESIAN_POINT ( 'NONE',  ( 4.834557559160812978, 6.939504195329335268, -1.414529171088283688 ) ) ;
#145544=FACE_BOUND ( 'NONE', #75808, .T. ) ;
#145547=CARTESIAN_POINT ( 'NONE',  ( -8.866669273657352690, 9.446795028796142191, 0.7216878364870438212 ) ) ;
#145551=CARTESIAN_POINT ( 'NONE',  ( 6.205881626753210867, 8.263281202677319470, 1.599625672291281386 ) ) ;
#145554=CARTESIAN_POINT ( 'NONE',  ( -3.653032323878261600, 6.349289246911547835, -1.199719254218452047 ) ) ;
#145558=CARTESIAN_POINT ( 'NONE',  ( -5.901876940650454095, 5.779944607047298177, -0.7998128361456291469 ) ) ;
#145561=CARTESIAN_POINT ( 'NONE',  ( 6.564118927310645724, 10.80988918183778225, -0.7998128361456291469 ) ) ;
#145564=CARTESIAN_POINT ( 'NONE',  ( 4.064005108223194718, 7.741596126659699983, 0.5534810405699239766 ) ) ;
#145565=CARTESIAN_POINT ( 'NONE',  ( 4.148431816101584957, 6.823292304551739740, -1.082531754730548412 ) ) ;
#145570=ADVANCED_FACE ( 'NONE', ( #43265 ), #154766, .T. ) ;
#145573=CARTESIAN_POINT ( 'NONE',  ( 5.938108092661121162, 9.871617174839238729, 1.040834085586084257E-14 ) ) ;
#145576=CARTESIAN_POINT ( 'NONE',  ( -8.622095623286845978, 12.14652976288826913, 1.199719254218462483 ) ) ;
#145577=CARTESIAN_POINT ( 'NONE',  ( -6.877010230629689858, 9.046264573866535486, 1.599625672291283607 ) ) ;
#145583=CARTESIAN_POINT ( 'NONE',  ( 1.569538198872422630, 8.730447571941267526, -2.495330465741606218 ) ) ;
#145586=CARTESIAN_POINT ( 'NONE',  ( 9.901532256681887745, 10.44620914241737530, 0.000000000000000000 ) ) ;
#145587=CARTESIAN_POINT ( 'NONE',  ( 1.499999999999987121, 4.045833333333359150, -0.8660254037844323793 ) ) ;
#145591=CARTESIAN_POINT ( 'NONE',  ( 2.849184837166184536, 6.475799410002530898, 0.7998128361456362523 ) ) ;
#145594=CARTESIAN_POINT ( 'NONE',  ( 0.7499999999999902300, 5.097916667349482012, -1.299038105676658228 ) ) ;
#145601=CARTESIAN_POINT ( 'NONE',  ( 0.7499999999999885647, 3.566666666666690411, -1.299038105676658228 ) ) ;
#145602=CARTESIAN_POINT ( 'NONE',  ( 6.498435699651741615, 6.475929825882159818, -0.7998128361456281477 ) ) ;
#145605=CARTESIAN_POINT ( 'NONE',  ( 8.609064354997688184, 9.146255957026539818, 1.040834085586084257E-14 ) ) ;
#145609=DIRECTION ( 'NONE',  ( 1.000000000000000000, 0.000000000000000000, 0.000000000000000000 ) ) ;
#145612=CARTESIAN_POINT ( 'NONE',  ( -2.767835915484202047, 6.380892334706859792, -0.7998128361456281477 ) ) ;
#145614=CARTESIAN_POINT ( 'NONE',  ( -1.402160292154681736E-14, 0.9468750003414176941, -1.575800808251659024 ) ) ;
#145618=CARTESIAN_POINT ( 'NONE',  ( 5.183294799126148433, 4.941598775268944976, 1.040834085586084257E-14 ) ) ;
#145620=CARTESIAN_POINT ( 'NONE',  ( -0.6823417656250246877, -1.198958332991911790, 1.181850606188755259 ) ) ;
#145621=B_SPLINE_CURVE_WITH_KNOTS ( 'NONE', 3,
 ( #75014, #186618, #157345, #124912 ),
 .UNSPECIFIED., .F., .F.,
 ( 4, 4 ),
 ( 1.810030818090551184E-16, 0.0003120095058623759956 ),
 .UNSPECIFIED. ) ;
#145629=CARTESIAN_POINT ( 'NONE',  ( -6.028571859570855729, 10.18508426947466816, 0.000000000000000000 ) ) ;
#145633=CARTESIAN_POINT ( 'NONE',  ( 5.250031796989762967, 7.148123067953287446, 1.599625672291267398 ) ) ;
#145638=ORIENTED_EDGE ( 'NONE', *, *, #115408, .T. ) ;
#145640=CARTESIAN_POINT ( 'NONE',  ( 9.073431116043567002, 11.60875560684942265, -1.599625672291262513 ) ) ;
#145643=CARTESIAN_POINT ( 'NONE',  ( -6.227272627378437342, 6.159572908229946187, -0.7998128361456291469 ) ) ;
#145647=CARTESIAN_POINT ( 'NONE',  ( 9.348510611822643313, 10.86534945433664134, 1.199719254218453823 ) ) ;
#145649=CARTESIAN_POINT ( 'NONE',  ( 6.753933077901968396, 11.03133902419432566, 0.7998128361456462443 ) ) ;
#145650=CARTESIAN_POINT ( 'NONE',  ( 4.887048565581556758, 4.918228951918932168, -0.7329281915080710919 ) ) ;
#145652=CARTESIAN_POINT ( 'NONE',  ( -9.978437869977959451, 10.74385839117019614, -0.7216878364870267237 ) ) ;
#145653=CARTESIAN_POINT ( 'NONE',  ( -8.193204901359996128, 8.453160561208463264, 1.040834085586084257E-14 ) ) ;
#145657=CARTESIAN_POINT ( 'NONE',  ( -6.087928554039494067, 6.027116558704463500, 0.4103310871990673014 ) ) ;
#145658=CARTESIAN_POINT ( 'NONE',  ( -1.364683531250014514, 0.7385416670080887647, -0.7879004041258289570 ) ) ;
#145661=CARTESIAN_POINT ( 'NONE',  ( 6.805829924380105034, 9.923590097543378619, 1.082531754730558626 ) ) ;
#145675=CARTESIAN_POINT ( 'NONE',  ( 3.334942598837264960, 6.834590765378040444, 1.214306433183764966E-14 ) ) ;
#145679=CARTESIAN_POINT ( 'NONE',  ( 8.992082194361556091, 11.51384853155376220, 1.599625672291279388 ) ) ;
#145683=CARTESIAN_POINT ( 'NONE',  ( -3.110706179331648169, 5.716575411607132118, 1.199719254218462483 ) ) ;
#145684=CARTESIAN_POINT ( 'NONE',  ( -7.857113714319432063, 9.125386407249497012, 1.199719254218462483 ) ) ;
#145690=CARTESIAN_POINT ( 'NONE',  ( 0.7499999999999920064, 5.014583334016150751, 1.299038105676669330 ) ) ;
#145691=CARTESIAN_POINT ( 'NONE',  ( 8.239604668803105270, 10.63595808506888396, -1.599625672291268286 ) ) ;
#145695=CARTESIAN_POINT ( 'NONE',  ( -8.097244055859620815, 10.46987070330147063, -1.599625672291263179 ) ) ;
#145697=CARTESIAN_POINT ( 'NONE',  ( 0.6823417656249917140, 3.342708333674754506, 1.181850606188765695 ) ) ;
#145701=CARTESIAN_POINT ( 'NONE',  ( -7.836249599018719536, 12.08611559892311504, 0.7216878364870478180 ) ) ;
#145706=CARTESIAN_POINT ( 'NONE',  ( -1.402160292154681736E-14, 1.759375000341421469, -1.575800808251659024 ) ) ;
#145714=CARTESIAN_POINT ( 'NONE',  ( -1.364683531249997417, 3.509375000341423245, 1.214306433183764966E-14 ) ) ;
#145716=CARTESIAN_POINT ( 'NONE',  ( -4.062639585589296942, 7.891496616496157301, 0.7998128361456341429 ) ) ;
#145717=CARTESIAN_POINT ( 'NONE',  ( 7.786460292950004636, 7.978625184730144149, 1.040834085586084257E-14 ) ) ;
#145720=CARTESIAN_POINT ( 'NONE',  ( 0.6823417656249899377, 3.155208333674754062, 1.181850606188765695 ) ) ;
#145723=CARTESIAN_POINT ( 'NONE',  ( -1.364683531250014514, -0.7614583329919104582, -0.7879004041258359514 ) ) ;
#145724=CARTESIAN_POINT ( 'NONE',  ( -4.880572111239580124, 7.677455982212699759, 1.082531754730560403 ) ) ;
#145727=CARTESIAN_POINT ( 'NONE',  ( 4.039966587192257208, 6.696749537490852333, 1.082531754730558626 ) ) ;
#145730=CARTESIAN_POINT ( 'NONE',  ( -7.178152263431422320, 10.46192917639026554, 1.199719254218453823 ) ) ;
#145731=CARTESIAN_POINT ( 'NONE',  ( -8.514157279702017078, 12.87700789305364069, -0.7216878364870267237 ) ) ;
#145733=CARTESIAN_POINT ( 'NONE',  ( -0.6823417656249969321, 5.467708333674756283, -1.181850606188749264 ) ) ;
#145738=CARTESIAN_POINT ( 'NONE',  ( -5.029711800545518585, 8.811821500704338561, 0.7216878364870458196 ) ) ;
#145740=CARTESIAN_POINT ( 'NONE',  ( -1.364683531250014514, -0.9489583329919112353, -0.7879004041258359514 ) ) ;
#145743=CARTESIAN_POINT ( 'NONE',  ( 7.673551755654734130, 9.015193805427763607, -1.082531754730537976 ) ) ;
#145751=EDGE_LOOP ( 'NONE', ( #147853, #110473 ) ) ;
#145752=CARTESIAN_POINT ( 'NONE',  ( 0.7499999999999867883, -0.1833333333333131421, -1.299038105676652899 ) ) ;
#145754=CARTESIAN_POINT ( 'NONE',  ( 7.727784369665023689, 11.95957283134381477, 1.040834085586084257E-14 ) ) ;
#145760=CARTESIAN_POINT ( 'NONE',  ( 4.774442650306744085, 8.721933525333202653, -0.7998128361456281477 ) ) ;
#145761=CARTESIAN_POINT ( 'NONE',  ( -3.567766978690493307, 7.314145241780881435, 1.040834085586084257E-14 ) ) ;
#145764=CARTESIAN_POINT ( 'NONE',  ( -4.856601257608931022, 5.009828881649966092, -0.8247166059246564540 ) ) ;
#145765=CARTESIAN_POINT ( 'NONE',  ( 4.148431815657221300, 7.783661518334664464, 1.040834085586084257E-14 ) ) ;
#145766=CARTESIAN_POINT ( 'NONE',  ( -1.402160292154681736E-14, 0.009375000341421267647, -1.575800808251665908 ) ) ;
#145768=CARTESIAN_POINT ( 'NONE',  ( -10.29471871147821282, 10.90492667301307605, -0.7998128361456291469 ) ) ;
#145780=ORIENTED_EDGE ( 'NONE', *, *, #186980, .F. ) ;
#145785=CARTESIAN_POINT ( 'NONE',  ( 6.226218857173709154, 8.287007971501239467, 1.599625672291281386 ) ) ;
#145788=ORIENTED_EDGE ( 'NONE', *, *, #169120, .T. ) ;
#145793=CARTESIAN_POINT ( 'NONE',  ( 10.57266086055835075, 11.22919251360659310, 0.000000000000000000 ) ) ;
#145795=CARTESIAN_POINT ( 'NONE',  ( 3.022498986271242138, 2.800000000000017586, 2.500000000000000444 ) ) ;
#145799=CARTESIAN_POINT ( 'NONE',  ( -0.08369048095984887858, 7.010987279218348078, 1.999726996211184549 ) ) ;
#145804=CIRCLE ( 'NONE', #135412, 0.8300000000000008482 ) ;
#145805=CARTESIAN_POINT ( 'NONE',  ( -9.327646496521992958, 9.984601788804893019, -0.7216878364870267237 ) ) ;
#145809=CARTESIAN_POINT ( 'NONE',  ( 5.996784015946103885, 5.890669528225568996, 1.040834085586084257E-14 ) ) ;
#145817=CARTESIAN_POINT ( 'NONE',  ( 5.463572716182829581, 6.436884926043849653, 1.082531754730560403 ) ) ;
#145825=CARTESIAN_POINT ( 'NONE',  ( -5.045605722580076780, 9.038290442985410067, -0.7998128361456231517 ) ) ;
#145826=CARTESIAN_POINT ( 'NONE',  ( -3.425406365747000859, 7.148057860013469877, 1.040834085586084257E-14 ) ) ;
#145832=CARTESIAN_POINT ( 'NONE',  ( -1.364683531250005188, 3.311721076625156357, -0.3840134687763438470 ) ) ;
#145835=CARTESIAN_POINT ( 'NONE',  ( 7.311924916471702396, 7.425000578838787391, -0.7998128361456281477 ) ) ;
#145845=CARTESIAN_POINT ( 'NONE',  ( 4.975479186090857375, 5.867442474269873642, 1.082531754730560403 ) ) ;
#145848=CARTESIAN_POINT ( 'NONE',  ( -1.402160292154681736E-14, -0.6156249996585817508, 1.575800808251672791 ) ) ;
#145849=CARTESIAN_POINT ( 'NONE',  ( 6.017121246366603060, 5.914396297049491658, 1.040834085586084257E-14 ) ) ;
#145852=CARTESIAN_POINT ( 'NONE',  ( -6.344852701515500293, 9.385783337534627790, 1.082531754730548412 ) ) ;
#145853=CARTESIAN_POINT ( 'NONE',  ( 6.005898861173831094, 6.109229547565340646, 1.040834085586084257E-14 ) ) ;
#145854=CARTESIAN_POINT ( 'NONE',  ( -7.497295758232724872, 9.769931022736756177, -1.443375672974058777 ) ) ;
#145859=CARTESIAN_POINT ( 'NONE',  ( 5.276094334012385367, 9.307193822989793475, 1.040834085586084257E-14 ) ) ;
#145864=CARTESIAN_POINT ( 'NONE',  ( -1.364683531250010295, 5.030208333674757171, 0.7879004041258379498 ) ) ;
#145868=CARTESIAN_POINT ( 'NONE',  ( 6.774270308322468459, 11.05506579301824743, 0.7998128361456462443 ) ) ;
#145871=CARTESIAN_POINT ( 'NONE',  ( -6.665805079413154921, 10.92852302595736447, 0.7998128361456481317 ) ) ;
#145876=CARTESIAN_POINT ( 'NONE',  ( 10.38962578677386084, 11.01565159419135043, 0.000000000000000000 ) ) ;
#145879=CARTESIAN_POINT ( 'NONE',  ( -6.367525699912501835, 10.58053041653993098, -0.7998128361456291469 ) ) ;
#145880=CARTESIAN_POINT ( 'NONE',  ( -5.111060722671894929, 5.065251719313053513, 0.000000000000000000 ) ) ;
#145882=CARTESIAN_POINT ( 'NONE',  ( 5.000138648025401977, 6.582195279309941860, -1.237349059142704988 ) ) ;
#145883=CARTESIAN_POINT ( 'NONE',  ( -9.666600336863641729, 10.38004793587015584, 1.040834085586084257E-14 ) ) ;
#145887=CARTESIAN_POINT ( 'NONE',  ( 7.447506452608354088, 7.583179037664891098, 0.7998128361456341429 ) ) ;
#145889=CARTESIAN_POINT ( 'NONE',  ( 6.972971076130050072, 7.029554431773520129, 1.040834085586084257E-14 ) ) ;
#145890=CARTESIAN_POINT ( 'NONE',  ( -4.034408581249735448, 7.597519823075112200, 0.2926387080343200164 ) ) ;
#145891=CARTESIAN_POINT ( 'NONE',  ( 2.523789150438203510, 6.096171108819874007, 0.7998128361456462443 ) ) ;
#145893=CARTESIAN_POINT ( 'NONE',  ( -5.395781948558855845, 9.238903340053241209, 0.7216878364870458196 ) ) ;
#145900=CARTESIAN_POINT ( 'NONE',  ( -4.964471428385745178, 6.642511170548884181, 1.245120630419704888 ) ) ;
#145901=CARTESIAN_POINT ( 'NONE',  ( -1.402160292154681736E-14, 0.7593750003414168059, -1.575800808251659024 ) ) ;
#145904=CARTESIAN_POINT ( 'NONE',  ( 3.375617060122621194, 6.882044303544283537, 1.040834085586084257E-14 ) ) ;
#145908=CARTESIAN_POINT ( 'NONE',  ( -8.744645890690007306, 12.18554205823825498, 1.082531754730558626 ) ) ;
#145913=CARTESIAN_POINT ( 'NONE',  ( -8.690413276235355866, 10.20153224610512943, 1.082531754730558626 ) ) ;
#145919=ORIENTED_EDGE ( 'NONE', *, *, #27402, .F. ) ;
#145920=CARTESIAN_POINT ( 'NONE',  ( -8.690413276235355866, 10.20153224610512943, 1.082531754730558626 ) ) ;
#145924=CARTESIAN_POINT ( 'NONE',  ( 1.364683531249990311, 5.426041667008086655, 0.7879004041258500513 ) ) ;
#145925=CARTESIAN_POINT ( 'NONE',  ( 0.7499999999999920064, 4.264583334016150751, 1.299038105676669330 ) ) ;
#145926=CARTESIAN_POINT ( 'NONE',  ( 4.825890400613210396, 6.946991693042408045, -1.413043630229819048 ) ) ;
#145931=CARTESIAN_POINT ( 'NONE',  ( -8.993135964566285168, 9.386413468282476913, -0.7998128361456291469 ) ) ;
#145935=CARTESIAN_POINT ( 'NONE',  ( 5.286789834324991055, 8.255339675766103724, -1.199719254218452935 ) ) ;
#145940=CARTESIAN_POINT ( 'NONE',  ( 8.620286740190458374, 8.951422706510690830, 1.040834085586084257E-14 ) ) ;
#145946=CARTESIAN_POINT ( 'NONE',  ( -7.049876689426121779, 7.327203680526343632, -0.7216878364870278340 ) ) ;
#145953=CARTESIAN_POINT ( 'NONE',  ( -5.871133375163540613, 5.952003147219978807, -0.6782502278256223871 ) ) ;
#145956=CARTESIAN_POINT ( 'NONE',  ( -8.479735010343349089, 11.98044238112085758, 1.199719254218453823 ) ) ;
#145958=CARTESIAN_POINT ( 'NONE',  ( 7.747594715205354809, 11.12627870345989756, -1.199719254218446718 ) ) ;
#145959=CARTESIAN_POINT ( 'NONE',  ( 0.7499999999999867883, 0.06666666666668707997, -1.299038105676652899 ) ) ;
#145960=CARTESIAN_POINT ( 'NONE',  ( -9.612894607289142357, 11.17379744904754801, -1.199719254218441611 ) ) ;
#145963=CARTESIAN_POINT ( 'NONE',  ( -1.201851678989727383E-14, 3.571875000341422357, 1.575800808251672791 ) ) ;
#145964=CARTESIAN_POINT ( 'NONE',  ( 10.05978679165993483, 11.79913468076720306, 1.082531754730548412 ) ) ;
#145966=CARTESIAN_POINT ( 'NONE',  ( 1.436838838544733044, 7.449283400311756509, -4.203727439823553347 ) ) ;
#145968=CARTESIAN_POINT ( 'NONE',  ( 9.422553571373278203, 11.05569592376608945, -1.082531754730543083 ) ) ;
#145971=CARTESIAN_POINT ( 'NONE',  ( -6.887178846062123938, 8.097758744236356776, -1.082531754730544860 ) ) ;
#145972=CARTESIAN_POINT ( 'NONE',  ( 0.6823417656249899377, 0.8427083336747520637, 1.181850606188755259 ) ) ;
#145974=CARTESIAN_POINT ( 'NONE',  ( 0.5029403714634882450, 7.727853499551113003, 1.993913793680534452 ) ) ;
#145976=CARTESIAN_POINT ( 'NONE',  ( -6.496328159242330536, 10.73079995242472862, 0.000000000000000000 ) ) ;
#145977=CARTESIAN_POINT ( 'NONE',  ( -4.297571505407598025, 5.076550180139354218, 1.082531754730558626 ) ) ;
#145978=CARTESIAN_POINT ( 'NONE',  ( -1.201851678989727383E-14, 3.384375000341421469, 1.575800808251672791 ) ) ;
#145984=CARTESIAN_POINT ( 'NONE',  ( 8.452618703115982512, 11.94880668935564216, 1.199719254218450271 ) ) ;
#145995=CYLINDRICAL_SURFACE ( 'NONE', #82416, 1.250000000000000000 ) ;
#145998=CARTESIAN_POINT ( 'NONE',  ( -1.364683531250012516, 3.801041667008087099, -0.7879004041258300672 ) ) ;
#145999=B_SPLINE_CURVE_WITH_KNOTS ( 'NONE', 3,
 ( #114241, #79532, #64354, #211646, #28654, #145650, #131530, #160787, #197533, #11315 ),
 .UNSPECIFIED., .F., .F.,
 ( 4, 3, 3, 4 ),
 ( 1.849923431806924672E-17, 3.125162491452015815E-05, 6.527199249539997140E-05, 9.931020432975908203E-05 ),
 .UNSPECIFIED. ) ;
#146003=CARTESIAN_POINT ( 'NONE',  ( 8.934986926605834157, 10.38290515491702770, -1.199719254218446718 ) ) ;
#146005=CARTESIAN_POINT ( 'NONE',  ( 0.6823417656249899377, 3.676041667008085767, -1.181850606188754593 ) ) ;
#146007=CARTESIAN_POINT ( 'NONE',  ( -6.643132081016132062, 8.773406732650713025, 1.443375672974078761 ) ) ;
#146013=CARTESIAN_POINT ( 'NONE',  ( 4.403700966340357681, 4.032072637018845107, -0.7998128361456211532 ) ) ;
#146015=VERTEX_POINT ( 'NONE', #82126 ) ;
#146016=CARTESIAN_POINT ( 'NONE',  ( 10.07778825365955733, 10.65184113889131012, -0.7998128361456281477 ) ) ;
#146017=CARTESIAN_POINT ( 'NONE',  ( 1.579999999999990523, 8.674529973577531194, -2.499999999999995115 ) ) ;
#146023=CARTESIAN_POINT ( 'NONE',  ( -9.215791728987058562, 11.77484298861683598, -1.599625672291263179 ) ) ;
#146025=CARTESIAN_POINT ( 'NONE',  ( 6.714312387265682247, 8.856450423275211037, 1.599625672291281386 ) ) ;
#146028=CARTESIAN_POINT ( 'NONE',  ( 3.456965981360264895, 6.016582164020185530, -1.082531754730543971 ) ) ;
#146036=CARTESIAN_POINT ( 'NONE',  ( -6.236387472606158333, 7.338502141871059870, -1.082531754730544860 ) ) ;
#146037=CARTESIAN_POINT ( 'NONE',  ( 5.196852952739813070, 4.957416621151553571, -0.7998128361456221525 ) ) ;
#146040=CARTESIAN_POINT ( 'NONE',  ( -9.318531651294266638, 9.766041769465124034, -0.7998128361456291469 ) ) ;
#146045=CARTESIAN_POINT ( 'NONE',  ( -9.755255220232635693, 11.33988483081495957, -1.199719254218441611 ) ) ;
#146047=CARTESIAN_POINT ( 'NONE',  ( 3.687454593236886513, 7.245854758844370913, -0.7216878364869879769 ) ) ;
#146049=CARTESIAN_POINT ( 'NONE',  ( 8.072990401933337168, 11.50590700464255356, -1.199719254218446718 ) ) ;
#146050=CARTESIAN_POINT ( 'NONE',  ( -3.289951133708662212, 7.658661826346112811, -2.499999999999995115 ) ) ;
#146060=CARTESIAN_POINT ( 'NONE',  ( -7.971304249830880373, 11.38727316052296601, 1.199719254218453823 ) ) ;
#146065=CARTESIAN_POINT ( 'NONE',  ( 6.141480397310468575, 10.10888486359680982, 1.040834085586084257E-14 ) ) ;
#146068=CARTESIAN_POINT ( 'NONE',  ( 3.225950485047770933, 5.851027101609320269, 1.199719254218450271 ) ) ;
#146071=CARTESIAN_POINT ( 'NONE',  ( -4.577849422908604637, 8.492574760035358494, -0.7998128361456281477 ) ) ;
#146082=CARTESIAN_POINT ( 'NONE',  ( 0.6823417656249917140, 4.405208333674755394, 1.181850606188765695 ) ) ;
#146083=CARTESIAN_POINT ( 'NONE',  ( 5.690973801500785356, 5.856266416811339859, 2.500000000000011102 ) ) ;
#146084=CARTESIAN_POINT ( 'NONE',  ( 9.511208455186636712, 11.05516360492796935, 1.199719254218453823 ) ) ;
#146086=CARTESIAN_POINT ( 'NONE',  ( -3.145128448690310830, 6.613140923539910787, -0.7216878364870267237 ) ) ;
#146088=CARTESIAN_POINT ( 'NONE',  ( -5.870317324592829067, 5.951051088220814300, -0.7216878364870197293 ) ) ;
#146096=CARTESIAN_POINT ( 'NONE',  ( 3.684065054611349144, 5.321161868511784299, -1.599625672291262513 ) ) ;
#146104=CARTESIAN_POINT ( 'NONE',  ( 5.087333953625774008, 6.958308917361963886, 1.599625672291267398 ) ) ;
#146108=CARTESIAN_POINT ( 'NONE',  ( 1.364683531249988535, 3.717708333674750953, -0.7879004041258239610 ) ) ;
#146113=CARTESIAN_POINT ( 'NONE',  ( 5.666418135507635512, 8.698239360479199433, 1.199719254218462483 ) ) ;
#146116=CARTESIAN_POINT ( 'NONE',  ( -4.086893239515592136, 6.855460315155083251, 1.199719254218464037 ) ) ;
#146117=CARTESIAN_POINT ( 'NONE',  ( 1.499999999999989120, 2.254166666666685970, 0.8660254037844524744 ) ) ;
#146120=CARTESIAN_POINT ( 'NONE',  ( -4.973143418114339021, 4.696422164088486895, 0.7998128361456341429 ) ) ;
#146121=CARTESIAN_POINT ( 'NONE',  ( 0.5500358407890573176, 7.827628757559660144, -1.923053904898945232 ) ) ;
#146123=CARTESIAN_POINT ( 'NONE',  ( 0.6823417656249917140, 3.342708333674754506, 1.181850606188765695 ) ) ;
#146126=CARTESIAN_POINT ( 'NONE',  ( -5.422898255786209099, 5.429062174613087599, -0.7216878364870207285 ) ) ;
#146129=EDGE_LOOP ( 'NONE', ( #58234, #104273, #125787, #151720 ) ) ;
#146132=CARTESIAN_POINT ( 'NONE',  ( 3.571683402196252910, 6.254382171615883834, 1.199719254218462483 ) ) ;
#146135=CARTESIAN_POINT ( 'NONE',  ( 4.909844308960606085, 4.783825108070185905, -0.2656215318195585540 ) ) ;
#146136=CARTESIAN_POINT ( 'NONE',  ( 1.364683531249990311, 3.946875000341417028, 1.214306433183764966E-14 ) ) ;
#146138=CARTESIAN_POINT ( 'NONE',  ( 3.375617060122621194, 6.882044303544283537, 1.040834085586084257E-14 ) ) ;
#146140=CARTESIAN_POINT ( 'NONE',  ( 1.364683531249986537, 0.4677083336747514530, -0.7879004041258309554 ) ) ;
#146141=CARTESIAN_POINT ( 'NONE',  ( -4.262896864317852419, 7.367918308143647010, -0.9672248769079903052 ) ) ;
#146143=CARTESIAN_POINT ( 'NONE',  ( -8.622095623286845978, 12.14652976288826913, 1.199719254218462483 ) ) ;
#146144=CARTESIAN_POINT ( 'NONE',  ( -6.521108698048783126, 7.670676904887464786, -1.082531754730543083 ) ) ;
#146148=CARTESIAN_POINT ( 'NONE',  ( 1.364683531249988535, 4.405208333674754506, -0.7879004041258300672 ) ) ;
#146156=CARTESIAN_POINT ( 'NONE',  ( -4.717874267431199087, 8.448011045404303587, 1.040834085586084257E-14 ) ) ;
#146162=CARTESIAN_POINT ( 'NONE',  ( -6.249945625775490399, 7.354319987235250267, 1.082531754730549967 ) ) ;
#146175=CARTESIAN_POINT ( 'NONE',  ( -4.218558352146454915, 8.073401844146177453, 1.040834085586084257E-14 ) ) ;
#146178=CARTESIAN_POINT ( 'NONE',  ( -1.500000000000015099, 0.8791666666666874130, -0.8660254037844313801 ) ) ;
#146179=CARTESIAN_POINT ( 'NONE',  ( 3.440018289565364817, 5.036440642624797626, 1.599625672291267398 ) ) ;
#146180=CARTESIAN_POINT ( 'NONE',  ( 8.145751363712157911, 8.397798100619326078, -0.7998128361456281477 ) ) ;
#146184=CARTESIAN_POINT ( 'NONE',  ( 6.017121246366603060, 5.914396297049491658, 1.040834085586084257E-14 ) ) ;
#146186=CARTESIAN_POINT ( 'NONE',  ( -0.3421332810201531127, 7.155223633118590776, -1.971148363701348050 ) ) ;
#146192=CARTESIAN_POINT ( 'NONE',  ( -3.416291520963659512, 5.969128626890772615, 1.082531754730560403 ) ) ;
#146200=CARTESIAN_POINT ( 'NONE',  ( 0.6823417656249899377, 3.926041667008085767, -1.181850606188754593 ) ) ;
#146201=FACE_OUTER_BOUND ( 'NONE', #36093, .T. ) ;
#146202=CARTESIAN_POINT ( 'NONE',  ( -6.063521013809733518, 8.097193820909906137, 1.599625672291283607 ) ) ;
#146205=CARTESIAN_POINT ( 'NONE',  ( 5.133733721068893807, 9.141106441222381918, 1.040834085586084257E-14 ) ) ;
#146206=CARTESIAN_POINT ( 'NONE',  ( -5.526920175865215334, 9.599823971818089774, 0.7998128361456481317 ) ) ;
#146210=CARTESIAN_POINT ( 'NONE',  ( 1.499999999999987121, -0.2145833326505137972, 0.8660254037844524744 ) ) ;
#146212=EDGE_CURVE ( 'NONE', #207748, #57355, #25838, .T. ) ;
#146214=CARTESIAN_POINT ( 'NONE',  ( 8.270110514656037637, 8.750809809961280550, 0.7216878364870458196 ) ) ;
#146217=CARTESIAN_POINT ( 'NONE',  ( 1.364683531249988535, 2.676041667008082214, 0.7879004041258500513 ) ) ;
#146219=CARTESIAN_POINT ( 'NONE',  ( 7.307481607641395094, 8.588111966078864512, -1.082531754730537976 ) ) ;
#146221=CARTESIAN_POINT ( 'NONE',  ( -3.286906687871170352, 6.405221329422087884, -0.7651497088209441300 ) ) ;
#146222=CARTESIAN_POINT ( 'NONE',  ( -2.968872451712654126, 6.407508927065978632, 1.040834085586084257E-14 ) ) ;
#146224=CARTESIAN_POINT ( 'NONE',  ( -0.6823417656249969321, 5.217708333674756283, -1.181850606188749264 ) ) ;
#146229=CARTESIAN_POINT ( 'NONE',  ( -5.356222800695524811, 6.520424213373273936, -1.360004217313095953 ) ) ;
#146235=CARTESIAN_POINT ( 'NONE',  ( 6.063521013809720195, 8.097193820909906137, 1.599625672291281386 ) ) ;
#146238=CARTESIAN_POINT ( 'NONE',  ( 3.551346171775753735, 6.230655402791975384, 1.199719254218462483 ) ) ;
#146247=CARTESIAN_POINT ( 'NONE',  ( 4.636525346193557162, 7.392734756325715750, -1.082531754730549078 ) ) ;
#146248=CARTESIAN_POINT ( 'NONE',  ( 0.6823417656249899377, 1.405208333674752508, 1.181850606188755259 ) ) ;
#146251=CARTESIAN_POINT ( 'NONE',  ( 2.341816809502491381, 5.373577454990479119, -0.7037892630772487612 ) ) ;
#146252=VECTOR ( 'NONE', #33424, 1000.000000000000000 ) ;
#146257=CARTESIAN_POINT ( 'NONE',  ( 0.7499999999999885647, 1.316666666666688190, -1.299038105676652899 ) ) ;
#146258=CARTESIAN_POINT ( 'NONE',  ( 5.276094334012385367, 9.307193822989793475, 1.040834085586084257E-14 ) ) ;
#146259=CARTESIAN_POINT ( 'NONE',  ( -6.692921386640485082, 10.96015871772258521, -0.7998128361456291469 ) ) ;
#146264=CARTESIAN_POINT ( 'NONE',  ( -1.364683531250012516, 2.030208333674750953, 0.7879004041258379498 ) ) ;
#146266=CARTESIAN_POINT ( 'NONE',  ( -1.499999999999997780, 2.400000000000020339, 1.214306433183764966E-14 ) ) ;
#146268=CARTESIAN_POINT ( 'NONE',  ( 4.857899112398166075, 4.561970474086296079, 1.040834085586084257E-14 ) ) ;
#146275=CARTESIAN_POINT ( 'NONE',  ( -0.7500000000000006661, 0.8895833340161543035, -1.299038105676652011 ) ) ;
#146277=CARTESIAN_POINT ( 'NONE',  ( -5.845536785786364931, 9.971543350059432598, 0.000000000000000000 ) ) ;
#146278=CARTESIAN_POINT ( 'NONE',  ( -3.280709984826970516, 6.771319382366015383, 0.7216878364870317197 ) ) ;
#146285=CARTESIAN_POINT ( 'NONE',  ( 5.937581207780954884, 9.014596278131406848, -1.199719254218440723 ) ) ;
#146289=CARTESIAN_POINT ( 'NONE',  ( 6.120616281565444794, 9.228137197546649517, -1.199719254218440723 ) ) ;
#146290=CARTESIAN_POINT ( 'NONE',  ( 9.531018800282609504, 10.22186947652563305, 0.7216878364870458196 ) ) ;
#146295=CARTESIAN_POINT ( 'NONE',  ( -6.612626235163205024, 8.737816579155630592, -1.599625672291263179 ) ) ;
#146296=CARTESIAN_POINT ( 'NONE',  ( 5.301401758143367893, 6.143722458377430584, 1.199719254218462483 ) ) ;
#146299=CARTESIAN_POINT ( 'NONE',  ( 4.318426605249491068, 7.201576024430431211, 1.005918518748824875 ) ) ;
#146300=CARTESIAN_POINT ( 'NONE',  ( 8.432808358020004391, 12.78210081775797669, 0.7216878364870438212 ) ) ;
#146305=FACE_OUTER_BOUND ( 'NONE', #40682, .T. ) ;
#146307=CARTESIAN_POINT ( 'NONE',  ( -2.168941388506379742, 5.474256019991960542, -0.7216878364870267237 ) ) ;
#146308=CARTESIAN_POINT ( 'NONE',  ( 8.107412671292035355, 10.48173408797264194, 1.443375672974076540 ) ) ;
#146310=CARTESIAN_POINT ( 'NONE',  ( -3.242371291962510504, 6.934516940598226320, 1.040834085586084257E-14 ) ) ;
#146316=CARTESIAN_POINT ( 'NONE',  ( -6.531277313481209212, 8.642909503859968368, 1.599625672291283607 ) ) ;
#146329=CARTESIAN_POINT ( 'NONE',  ( 3.469446951953614189E-15, 6.120000000000021423, 1.214306433183764966E-14 ) ) ;
#146330=CARTESIAN_POINT ( 'NONE',  ( 1.440240048128890171, 7.355731858842234239, -4.317885097517412341 ) ) ;
#146331=CARTESIAN_POINT ( 'NONE',  ( -5.259673527097670664, 8.223703984000886535, -1.199719254218446718 ) ) ;
#146332=ADVANCED_FACE ( 'NONE', ( #8348 ), #38729, .F. ) ;
#146335=CARTESIAN_POINT ( 'NONE',  ( 3.714570900464278846, 5.356752022006865843, 1.443375672974062551 ) ) ;
#146340=CARTESIAN_POINT ( 'NONE',  ( -2.598358995313378550, 6.183169261174235487, 0.7998128361456341429 ) ) ;
#146344=CARTESIAN_POINT ( 'NONE',  ( 8.380911511541880188, 12.92948053010758258, 0.7998128361456462443 ) ) ;
#146348=CARTESIAN_POINT ( 'NONE',  ( -6.828502922777144768, 11.11833717654868892, 0.7998128361456481317 ) ) ;
#146349=CARTESIAN_POINT ( 'NONE',  ( 5.983225862332436584, 5.874851682342960402, 0.7998128361456341429 ) ) ;
#146355=CARTESIAN_POINT ( 'NONE',  ( -1.364683531250014514, 1.801041667008085767, -0.7879004041258289570 ) ) ;
#146358=CARTESIAN_POINT ( 'NONE',  ( 7.944714827928050838, 9.331550723079971021, 1.082531754730558626 ) ) ;
#146360=CARTESIAN_POINT ( 'NONE',  ( -4.989037340148921196, 5.883260320670900434, 1.082531754730560403 ) ) ;
#146372=CARTESIAN_POINT ( 'NONE',  ( -8.469039510030723861, 13.03229652834454733, 1.040834085586084257E-14 ) ) ;
#146386=CARTESIAN_POINT ( 'NONE',  ( -0.7500000000000006661, 1.889583334016155192, -1.299038105676652011 ) ) ;
#146392=FACE_OUTER_BOUND ( 'NONE', #164283, .T. ) ;
#146393=CARTESIAN_POINT ( 'NONE',  ( 8.535021395002688749, 9.916278701380017324, 1.199719254218462483 ) ) ;
#146398=CARTESIAN_POINT ( 'NONE',  ( 4.359110081993588182, 5.044382169536003602, -1.199719254218452047 ) ) ;
#146399=CARTESIAN_POINT ( 'NONE',  ( -6.222829318992474157, 10.20379193889247382, 0.000000000000000000 ) ) ;
#146404=AXIS2_PLACEMENT_3D ( 'NONE', #68855, #49443, #181558 ) ;
#146406=CARTESIAN_POINT ( 'NONE',  ( -7.366157530926372488, 7.488271962369228874, -0.7998128361456291469 ) ) ;
#146409=CARTESIAN_POINT ( 'NONE',  ( 1.499999999999987121, 1.077083334016148308, -0.8660254037844253849 ) ) ;
#146416=CARTESIAN_POINT ( 'NONE',  ( -8.967828540435322182, 12.54988483289483980, 1.199719254218462483 ) ) ;
#146420=CARTESIAN_POINT ( 'NONE',  ( 4.062392026992976746, 7.509557588607558287, 0.5198811075141016591 ) ) ;
#146424=CARTESIAN_POINT ( 'NONE',  ( -3.267151830768959098, 4.834763107362302748, -1.443375672974058777 ) ) ;
#146425=CARTESIAN_POINT ( 'NONE',  ( 6.825640269476072497, 10.05066518344239412, 1.199719254218460707 ) ) ;
#146433=CARTESIAN_POINT ( 'NONE',  ( -7.160677686311960777, 11.50587440067263678, -0.7998128361456291469 ) ) ;
#146439=CARTESIAN_POINT ( 'NONE',  ( 3.354752944377597856, 6.001296637494123232, -1.199719254218446718 ) ) ;
#146442=VERTEX_POINT ( 'NONE', #72265 ) ;
#146444=CARTESIAN_POINT ( 'NONE',  ( -8.513630394377489807, 12.01998699582738972, -1.199719254218446718 ) ) ;
#146447=ORIENTED_EDGE ( 'NONE', *, *, #108295, .T. ) ;
#146455=CARTESIAN_POINT ( 'NONE',  ( 6.500244582748090139, 9.671036882259738121, 1.199719254218460707 ) ) ;
#146457=CARTESIAN_POINT ( 'NONE',  ( -2.950870989268691957, 6.594433254122103349, -0.7998128361456281477 ) ) ;
#146464=CARTESIAN_POINT ( 'NONE',  ( -1.500000000000001332, -0.3187499993171846735, 0.000000000000000000 ) ) ;
#146467=CARTESIAN_POINT ( 'NONE',  ( 4.729096653068339151, 4.411700938201493116, -0.7998128361456211532 ) ) ;
#146469=CARTESIAN_POINT ( 'NONE',  ( -2.272963308585411735, 5.803540959991587478, 0.7998128361456341429 ) ) ;
#146476=CARTESIAN_POINT ( 'NONE',  ( 3.538314903486612817, 7.071858454135611538, 1.040834085586084257E-14 ) ) ;
#146478=ORIENTED_EDGE ( 'NONE', *, *, #142755, .T. ) ;
#146479=CARTESIAN_POINT ( 'NONE',  ( -9.917953063596627317, 11.52969898140628047, -1.199719254218441611 ) ) ;
#146481=CARTESIAN_POINT ( 'NONE',  ( 3.348500752450929596, 6.850408611260650815, 0.7216878364870317197 ) ) ;
#146489=CARTESIAN_POINT ( 'NONE',  ( -6.123385318682658784, 6.005027156464323390, -0.2239653954101868127 ) ) ;
#146491=CARTESIAN_POINT ( 'NONE',  ( -1.364683531250000748, 0.009375000341420303140, 0.000000000000000000 ) ) ;
#146498=CARTESIAN_POINT ( 'NONE',  ( -5.904739593951539689, 6.847616600153594746, 1.199719254218450271 ) ) ;
#146502=CARTESIAN_POINT ( 'NONE',  ( 0.7499999999999902300, 4.566666666666691299, -1.299038105676658228 ) ) ;
#146509=CARTESIAN_POINT ( 'NONE',  ( -0.7499999999999972244, 4.358333333333352932, -1.299038105676652011 ) ) ;
#146510=CARTESIAN_POINT ( 'NONE',  ( -1.402160292154681736E-14, -1.178124999658576311, 1.575800808251672791 ) ) ;
#146512=CARTESIAN_POINT ( 'NONE',  ( 5.113396490648394632, 9.117379672398465473, 1.040834085586084257E-14 ) ) ;
#146513=CARTESIAN_POINT ( 'NONE',  ( -6.828502922777144768, 11.11833717654868892, 0.7998128361456481317 ) ) ;
#146514=CARTESIAN_POINT ( 'NONE',  ( 8.028399517586572998, 12.51821653715971472, -0.7998128361456352531 ) ) ;
#146521=CARTESIAN_POINT ( 'NONE',  ( -1.001543065824772872E-14, 5.712500000000021672, 1.732050807568877637 ) ) ;
#146525=ADVANCED_FACE ( 'NONE', ( #140533 ), #72165, .F. ) ;
#146526=CARTESIAN_POINT ( 'NONE',  ( 3.836594282542955092, 7.419851063034579752, 0.7216878364870705775 ) ) ;
#146527=VERTEX_POINT ( 'NONE', #99254 ) ;
#146530=CARTESIAN_POINT ( 'NONE',  ( 6.629573927402440781, 10.67832731537079383, 1.040834085586084257E-14 ) ) ;
#146535=CARTESIAN_POINT ( 'NONE',  ( -1.500000000000011324, 4.952083334016150751, 0.8660254037844403729 ) ) ;
#146537=CARTESIAN_POINT ( 'NONE',  ( -3.093231602212184850, 6.760520635889515795, -0.7998128361456281477 ) ) ;
#146538=CARTESIAN_POINT ( 'NONE',  ( 5.124618875841165710, 8.922546421882614709, 1.040834085586084257E-14 ) ) ;
#146539=CARTESIAN_POINT ( 'NONE',  ( -9.775065565328612038, 10.50659070241261794, -0.7216878364870267237 ) ) ;
#146541=B_SPLINE_CURVE_WITH_KNOTS ( 'NONE', 3,
 ( #112545, #179621, #29104, #160167 ),
 .UNSPECIFIED., .F., .F.,
 ( 4, 4 ),
 ( 9.058118219994478620E-18, 0.0001726908832626409531 ),
 .UNSPECIFIED. ) ;
#146546=DIRECTION ( 'NONE',  ( 6.314299915563594049E-62, 8.546850786086437571E-32, 1.000000000000000000 ) ) ;
#146547=CARTESIAN_POINT ( 'NONE',  ( 3.174580523894166006, 6.855427711185178019, 0.7998128361456341429 ) ) ;
#146561=CARTESIAN_POINT ( 'NONE',  ( 8.215351014876830504, 11.67199438640995801, -1.199719254218446718 ) ) ;
#146566=CARTESIAN_POINT ( 'NONE',  ( -1.364683531250014514, -0.5114583329919092369, -0.7879004041258359514 ) ) ;
#146568=CARTESIAN_POINT ( 'NONE',  ( 5.558479791922850133, 6.547609847740540445, -1.082531754730542195 ) ) ;
#146569=CARTESIAN_POINT ( 'NONE',  ( -7.700668062882065179, 10.96756792579566664, -1.082531754730543971 ) ) ;
#146574=CARTESIAN_POINT ( 'NONE',  ( -4.627410500965859264, 4.293067094081919777, 0.7998128361456341429 ) ) ;
#146581=ORIENTED_EDGE ( 'NONE', *, *, #102005, .T. ) ;
#146588=CARTESIAN_POINT ( 'NONE',  ( 5.531458889030211878, 6.400359360821498811, -1.228567739025695493 ) ) ;
#146595=CARTESIAN_POINT ( 'NONE',  ( -8.080296364064746939, 9.489729181906076505, 1.082531754730558626 ) ) ;
#146597=CARTESIAN_POINT ( 'NONE',  ( 1.177073619093308432, 2.881928502340592058, -0.7749999999999910294 ) ) ;
#146599=CARTESIAN_POINT ( 'NONE',  ( 7.311924916471702396, 7.425000578838787391, -0.7998128361456281477 ) ) ;
#146602=CARTESIAN_POINT ( 'NONE',  ( -6.735703387890906946, 6.752742128827836865, -0.7998128361456291469 ) ) ;
#146605=CARTESIAN_POINT ( 'NONE',  ( -5.555090253297260361, 7.504024600312024340, 1.599625672291269396 ) ) ;
#146609=CARTESIAN_POINT ( 'NONE',  ( 8.055515824813896941, 12.54985222892493368, 0.7998128361456462443 ) ) ;
#146612=CARTESIAN_POINT ( 'NONE',  ( 4.526804827544169463, 7.221866427374837194, 1.292974732014543271 ) ) ;
#146613=CARTESIAN_POINT ( 'NONE',  ( 4.365362273920244007, 6.116008624372160973, 1.443375672974062551 ) ) ;
#146615=DIRECTION ( 'NONE',  ( -5.578564026256490882E-16, -1.000000000000000000, -9.066213480720158442E-32 ) ) ;
#146621=CARTESIAN_POINT ( 'NONE',  ( 7.171900071504736296, 9.390302721554109056, -1.443375672974058777 ) ) ;
#146624=CARTESIAN_POINT ( 'NONE',  ( -7.947050595904583403, 12.42330946186405249, 0.7998128361456481317 ) ) ;
#146625=CARTESIAN_POINT ( 'NONE',  ( -6.204827856548512877, 10.39071626594860476, -0.7998128361456291469 ) ) ;
#146630=CARTESIAN_POINT ( 'NONE',  ( 1.534012367094065077, 8.737164261768352702, -2.508166476568407965 ) ) ;
#146634=CARTESIAN_POINT ( 'NONE',  ( 7.889955328148847258, 11.29236608522730911, -1.199719254218446718 ) ) ;
#146639=CARTESIAN_POINT ( 'NONE',  ( 2.984766373302843778, 6.633977868828633717, -0.7998128361456291469 ) ) ;
#146642=CARTESIAN_POINT ( 'NONE',  ( -0.7499999999999972244, 4.889583334016150751, -1.299038105676652899 ) ) ;
#146646=ORIENTED_EDGE ( 'NONE', *, *, #163416, .T. ) ;
#146648=CARTESIAN_POINT ( 'NONE',  ( -0.7499999999999972244, 3.608333333333359150, -1.299038105676652011 ) ) ;
#146649=CARTESIAN_POINT ( 'NONE',  ( 6.959412922516382771, 7.013736585890911535, 0.7998128361456341429 ) ) ;
#146650=ADVANCED_FACE ( 'NONE', ( #67762, #133913 ), #81382, .T. ) ;
#146652=DIRECTION ( 'NONE',  ( 1.000000000000000000, 0.000000000000000000, 0.000000000000000000 ) ) ;
#146653=CARTESIAN_POINT ( 'NONE',  ( 6.290620087060792009, 10.28288116830553101, -0.7216878364870267237 ) ) ;
#146655=CARTESIAN_POINT ( 'NONE',  ( 0.2607081404540609326, 7.167562920730477849, 2.095805658632963642 ) ) ;
#146661=CARTESIAN_POINT ( 'NONE',  ( -4.928552533767591726, 5.708731696605642725, 1.199719254218462483 ) ) ;
#146662=CARTESIAN_POINT ( 'NONE',  ( 1.499999999999990896, 4.806250000682819490, 1.214306433183764966E-14 ) ) ;
#146663=CARTESIAN_POINT ( 'NONE',  ( -1.364683531250000748, 0.2593750003414205252, 0.000000000000000000 ) ) ;
#146667=CARTESIAN_POINT ( 'NONE',  ( 4.304877467538922531, 4.981110786005563007, 1.199719254218464037 ) ) ;
#146669=CARTESIAN_POINT ( 'NONE',  ( -1.364683531249997417, 5.071875000341417916, 1.214306433183764966E-14 ) ) ;
#146671=CARTESIAN_POINT ( 'NONE',  ( 4.425744359874354217, 7.314857078510163646, 1.252187566917076778 ) ) ;
#146678=CARTESIAN_POINT ( 'NONE',  ( -6.191269702934848240, 10.37489842006599616, 0.000000000000000000 ) ) ;
#146681=CARTESIAN_POINT ( 'NONE',  ( 4.761938266897790761, 6.578680616179308771, 1.599625672291267398 ) ) ;
#146687=CARTESIAN_POINT ( 'NONE',  ( 9.911173986789782120, 11.52179005846497972, -1.199719254218440723 ) ) ;
#146690=CARTESIAN_POINT ( 'NONE',  ( -5.742041750587549842, 6.657802449562273850, 1.199719254218450271 ) ) ;
#146694=CARTESIAN_POINT ( 'NONE',  ( 10.05067194643221207, 10.62020544712608938, 0.7998128361456462443 ) ) ;
#146696=CARTESIAN_POINT ( 'NONE',  ( 9.237182729612253951, 9.671134694169463586, 0.7998128361456462443 ) ) ;
#146699=CARTESIAN_POINT ( 'NONE',  ( -8.514157279702017078, 12.87700789305364069, -0.7216878364870267237 ) ) ;
#146700=( BOUNDED_CURVE ( )  B_SPLINE_CURVE ( 3, ( #72746, #171317, #93304, #155081 ),
 .UNSPECIFIED., .F., .T. ) 
 B_SPLINE_CURVE_WITH_KNOTS ( ( 4, 4 ),
 ( 4.082329036708564729, 4.712388980384689674 ),
 .UNSPECIFIED. ) 
 CURVE ( )  GEOMETRIC_REPRESENTATION_ITEM ( )  RATIONAL_B_SPLINE_CURVE ( ( 1.000000000000000000, 0.9671913951452629776, 0.9671913951452629776, 1.000000000000000000 ) ) 
 REPRESENTATION_ITEM ( '' )  );
#146701=CARTESIAN_POINT ( 'NONE',  ( -8.044065211609668253, 8.279164256499745633, 0.7998128361456602331 ) ) ;
#146704=CARTESIAN_POINT ( 'NONE',  ( -4.055257346293188014, 7.741894102302186553, 0.6119906029944787162 ) ) ;
#146705=CARTESIAN_POINT ( 'NONE',  ( -1.364683531250000748, 0.2593750003414205252, 0.000000000000000000 ) ) ;
#146709=CARTESIAN_POINT ( 'NONE',  ( 6.968527767744098433, 9.153035033833367251, 1.443375672974076540 ) ) ;
#146729=CARTESIAN_POINT ( 'NONE',  ( -4.963467767100621764, 4.685133904572482244, 0.2290337979854002448 ) ) ;
#146733=CARTESIAN_POINT ( 'NONE',  ( -5.461236948206312114, 5.265864615862458464, 0.7998128361456341429 ) ) ;
#146734=CARTESIAN_POINT ( 'NONE',  ( -7.263417608619167076, 9.497073181520933716, -1.599625672291263179 ) ) ;
#146740=CARTESIAN_POINT ( 'NONE',  ( -1.500000000000013101, 2.660416667349483788, -0.8660254037844313801 ) ) ;
#146741=CARTESIAN_POINT ( 'NONE',  ( 7.079328764629950754, 11.41096732537697633, 0.7998128361456462443 ) ) ;
#146743=CARTESIAN_POINT ( 'NONE',  ( -8.178592977541617515, 10.56477777859713463, 1.599625672291295375 ) ) ;
#146745=CARTESIAN_POINT ( 'NONE',  ( -0.6823417656250003738, 2.967708333674754062, -1.181850606188749264 ) ) ;
#146747=EDGE_CURVE ( 'NONE', #109653, #1642, #70433, .T. ) ;
#146751=CARTESIAN_POINT ( 'NONE',  ( -8.351459436338023679, 12.68719374246231624, -0.7216878364870267237 ) ) ;
#146755=CARTESIAN_POINT ( 'NONE',  ( 1.364683531249986537, 0.9260416670080896528, 0.7879004041258500513 ) ) ;
#146762=CARTESIAN_POINT ( 'NONE',  ( -1.364683531250012516, 2.780208333674754506, 0.7879004041258379498 ) ) ;
#146764=CARTESIAN_POINT ( 'NONE',  ( -4.564291269294938225, 8.476756914152748124, 1.040834085586084257E-14 ) ) ;
#146766=VECTOR ( 'NONE', #47578, 1000.000000000000000 ) ;
#146768=CARTESIAN_POINT ( 'NONE',  ( 1.364683531249990311, 2.696875000341415696, 1.214306433183764966E-14 ) ) ;
#146772=ADVANCED_FACE ( 'NONE', ( #173319 ), #151275, .T. ) ;
#146774=CARTESIAN_POINT ( 'NONE',  ( -5.477130870240893401, 6.452702772444876445, 1.082531754730548412 ) ) ;
#146778=CARTESIAN_POINT ( 'NONE',  ( 5.666945020832181434, 5.713783400500082266, 0.7216878364870317197 ) ) ;
#146781=CARTESIAN_POINT ( 'NONE',  ( -6.842061076390810292, 11.13415502243129218, 0.000000000000000000 ) ) ;
#146782=CARTESIAN_POINT ( 'NONE',  ( -4.464712657601869417, 4.103252943490596216, 0.7998128361456341429 ) ) ;
#146784=CARTESIAN_POINT ( 'NONE',  ( 1.364683531249988535, 5.405208333674750953, -0.7879004041258300672 ) ) ;
#146789=CARTESIAN_POINT ( 'NONE',  ( -6.846504384776774366, 7.089935991768773427, -0.7216878364870267237 ) ) ;
#146791=CARTESIAN_POINT ( 'NONE',  ( 1.364683531249986981, -1.053124999658580752, 0.000000000000000000 ) ) ;
#146794=CARTESIAN_POINT ( 'NONE',  ( 5.965224400332808763, 9.903252867122883885, -0.7216878364870267237 ) ) ;
#146809=CARTESIAN_POINT ( 'NONE',  ( 6.745345117998789775, 7.828323044875442172, 1.199719254218462483 ) ) ;
#146811=CARTESIAN_POINT ( 'NONE',  ( -4.334856428067329404, 6.080418470877079429, -1.599625672291256295 ) ) ;
#146815=CARTESIAN_POINT ( 'NONE',  ( 5.300874872818830852, 7.207439989753867238, 1.443375672974062551 ) ) ;
#146816=CARTESIAN_POINT ( 'NONE',  ( -1.364683531250000748, -0.1781249996585798634, 0.000000000000000000 ) ) ;
#146818=CARTESIAN_POINT ( 'NONE',  ( -10.30827686509187835, 10.92074451889568643, 1.040834085586084257E-14 ) ) ;
#146835=CARTESIAN_POINT ( 'NONE',  ( 6.632963465583686435, 8.761543347979550589, -1.599625672291262513 ) ) ;
#146841=CARTESIAN_POINT ( 'NONE',  ( 6.923409998072794558, 11.22906209772695618, 1.040834085586084257E-14 ) ) ;
#146847=ADVANCED_FACE ( 'NONE', ( #37969 ), #40107, .F. ) ;
#146848=CARTESIAN_POINT ( 'NONE',  ( -2.279742385392243165, 5.811449882932888222, -0.7998128361456281477 ) ) ;
#146853=CARTESIAN_POINT ( 'NONE',  ( -0.4444767461201751813, 7.387363020590631990, 2.040826832792407508 ) ) ;
#146859=CARTESIAN_POINT ( 'NONE',  ( -9.002250809793991948, 12.48608113052627289, -1.082531754730543971 ) ) ;
#146864=CARTESIAN_POINT ( 'NONE',  ( 5.311043488251262268, 7.219303374425030562, -1.599625672291256295 ) ) ;
#146870=CARTESIAN_POINT ( 'NONE',  ( 3.823036128929238942, 7.404033217152015567, 1.040834085586084257E-14 ) ) ;
#146879=CARTESIAN_POINT ( 'NONE',  ( -7.054319997812058318, 7.124461507069184130, 1.040834085586084257E-14 ) ) ;
#146880=CARTESIAN_POINT ( 'NONE',  ( -5.447678794592645701, 5.250046769979851646, 0.000000000000000000 ) ) ;
#146885=CARTESIAN_POINT ( 'NONE',  ( 0.7499999999999902300, 2.983333333333351600, 1.299038105676669330 ) ) ;
#146889=CARTESIAN_POINT ( 'NONE',  ( 6.043183783389218355, 8.073467052085995022, 1.599625672291267398 ) ) ;
#146900=CARTESIAN_POINT ( 'NONE',  ( 0.6823417656249882723, 0.4885416670080827695, -1.181850606188749264 ) ) ;
#146901=FACE_OUTER_BOUND ( 'NONE', #30544, .T. ) ;
#146902=CARTESIAN_POINT ( 'NONE',  ( 5.705283713252285338, 5.550585841749444249, -0.7998128361456211532 ) ) ;
#146905=CARTESIAN_POINT ( 'NONE',  ( -6.805829924380121909, 8.963220883242035697, 1.443375672974078761 ) ) ;
#146906=CARTESIAN_POINT ( 'NONE',  ( 3.375617060122621194, 6.882044303544283537, 1.040834085586084257E-14 ) ) ;
#146907=CARTESIAN_POINT ( 'NONE',  ( -7.171900071504745178, 9.390302721554109056, -1.443375672974058777 ) ) ;
#146912=CARTESIAN_POINT ( 'NONE',  ( 6.775324078527185989, 8.927630729746953264, -1.599625672291262513 ) ) ;
#146917=CARTESIAN_POINT ( 'NONE',  ( 1.364683531249988535, 3.655208333674750509, -0.7879004041258239610 ) ) ;
#146922=CARTESIAN_POINT ( 'NONE',  ( 6.109920781252839994, 10.27999134477033216, 1.040834085586084257E-14 ) ) ;
#146926=CARTESIAN_POINT ( 'NONE',  ( -8.850775351622791831, 9.220326086515070685, -0.7998128361456291469 ) ) ;
#146932=CARTESIAN_POINT ( 'NONE',  ( 8.028399517586572998, 12.51821653715971472, -0.7998128361456352531 ) ) ;
#146935=CARTESIAN_POINT ( 'NONE',  ( -9.176171038350775078, 9.599954387697719582, -0.7998128361456291469 ) ) ;
#146937=FACE_OUTER_BOUND ( 'NONE', #28509, .T. ) ;
#146939=CARTESIAN_POINT ( 'NONE',  ( 4.685856777024981490, 6.842343872427582241, -1.228950205364977899 ) ) ;
#146940=CARTESIAN_POINT ( 'NONE',  ( -10.33094986393327197, 11.15512238411806578, 0.7216878364870438212 ) ) ;
#146944=CARTESIAN_POINT ( 'NONE',  ( 5.503720292143644777, 8.508425209887878538, 1.199719254218462483 ) ) ;
#146946=CARTESIAN_POINT ( 'NONE',  ( 5.311043488251262268, 7.219303374425030562, -1.599625672291256295 ) ) ;
#146947=CARTESIAN_POINT ( 'NONE',  ( -4.015218494013213402, 7.625434522713817387, 0.07065147036973244699 ) ) ;
#146948=CARTESIAN_POINT ( 'NONE',  ( 4.857899112398166075, 4.561970474086296079, 1.040834085586084257E-14 ) ) ;
#146950=CARTESIAN_POINT ( 'NONE',  ( -7.700668062882084719, 8.086460282891644979, -0.7216878364870278340 ) ) ;
#146955=CARTESIAN_POINT ( 'NONE',  ( -4.145011909418054863, 7.447386798385191575, 0.7030492056920457644 ) ) ;
#146956=CARTESIAN_POINT ( 'NONE',  ( 1.364683531249988757, 0.6968750003414209138, 0.000000000000000000 ) ) ;
#146959=CARTESIAN_POINT ( 'NONE',  ( 4.772106882330221289, 6.590544000850479200, -1.443375672974051449 ) ) ;
#146962=AXIS2_PLACEMENT_3D ( 'NONE', #165464, #792, #48537 ) ;
#146964=CARTESIAN_POINT ( 'NONE',  ( -7.659993601596706725, 11.88048360193076647, -0.7216878364870267237 ) ) ;
#146969=CARTESIAN_POINT ( 'NONE',  ( -9.775065565328603157, 11.46695991671396087, -1.082531754730537976 ) ) ;
#146970=CARTESIAN_POINT ( 'NONE',  ( 6.471393748265540147, 5.229711127717882491, 2.500000000000011102 ) ) ;
#146976=CARTESIAN_POINT ( 'NONE',  ( -7.483737604619046913, 11.67485160545682987, 0.000000000000000000 ) ) ;
#146981=CARTESIAN_POINT ( 'NONE',  ( -0.6823417656250212460, 5.613541667008087543, 1.181850606188767472 ) ) ;
#146982=CARTESIAN_POINT ( 'NONE',  ( 0.7499999999999902300, 2.764583334016148974, 1.299038105676669330 ) ) ;
#146987=CARTESIAN_POINT ( 'NONE',  ( -7.426115451983156923, 9.686887332112256388, -1.599625672291263179 ) ) ;
#146991=CARTESIAN_POINT ( 'NONE',  ( 6.823831386379729302, 6.855558127064808716, -0.7998128361456281477 ) ) ;
#146997=CARTESIAN_POINT ( 'NONE',  ( 9.108380270282433244, 9.520865158284665952, 1.040834085586084257E-14 ) ) ;
#147003=CARTESIAN_POINT ( 'NONE',  ( -6.019457014787517046, 9.006155036351978893, 1.082531754730548412 ) ) ;
#147006=CARTESIAN_POINT ( 'NONE',  ( -1.201851678989727383E-14, 5.259375000341421469, -1.575800808251660134 ) ) ;
#147011=CARTESIAN_POINT ( 'NONE',  ( -8.208571938070008400, 11.66408546346865016, -1.199719254218446718 ) ) ;
#147014=CARTESIAN_POINT ( 'NONE',  ( 8.748035429315576650, 11.22912730566677553, -1.599625672291255185 ) ) ;
#147016=CARTESIAN_POINT ( 'NONE',  ( -8.317037166979361018, 11.79062823052953668, 1.199719254218453823 ) ) ;
#147019=CARTESIAN_POINT ( 'NONE',  ( -1.364683531250010295, 4.030208333674751842, 0.7879004041258379498 ) ) ;
#147020=CARTESIAN_POINT ( 'NONE',  ( 4.708759422647839976, 4.387974169377582001, -0.7998128361456211532 ) ) ;
#147024=CARTESIAN_POINT ( 'NONE',  ( 8.798878505144646311, 11.28844422746735532, -1.443375672974052559 ) ) ;
#147027=CARTESIAN_POINT ( 'NONE',  ( -8.053180056837398126, 8.497724275839514618, 0.7216878364870578100 ) ) ;
#147029=CARTESIAN_POINT ( 'NONE',  ( 0.6823417656249899377, 1.342708333674752508, 1.181850606188755259 ) ) ;
#147031=CARTESIAN_POINT ( 'NONE',  ( 0.5059764118015197543, 7.965522150964524428, 1.935091031283028506 ) ) ;
#147033=CARTESIAN_POINT ( 'NONE',  ( -6.672584156219988571, 10.93643194889866521, -0.7998128361456291469 ) ) ;
#147034=CARTESIAN_POINT ( 'NONE',  ( -3.538314903042294457, 6.111489239315849531, 1.082531754730560403 ) ) ;
#147035=CARTESIAN_POINT ( 'NONE',  ( -1.201851678989727383E-14, 3.009375000341419248, -1.575800808251660134 ) ) ;
#147053=FACE_OUTER_BOUND ( 'NONE', #210317, .T. ) ;
#147054=CARTESIAN_POINT ( 'NONE',  ( 0.6823417656249917140, 4.905208333674755394, 1.181850606188765695 ) ) ;
#147060=CARTESIAN_POINT ( 'NONE',  ( 8.772289083241844310, 10.19309100432570148, -1.199719254218446718 ) ) ;
#147063=CARTESIAN_POINT ( 'NONE',  ( 1.364683531249988535, 2.863541667008082658, 0.7879004041258500513 ) ) ;
#147065=CARTESIAN_POINT ( 'NONE',  ( -7.727784370109414880, 8.118095974656867497, 0.7216878364870578100 ) ) ;
#147071=CARTESIAN_POINT ( 'NONE',  ( 2.920892028740289081, 5.495125569250587816, 1.199719254218452047 ) ) ;
#147074=CARTESIAN_POINT ( 'NONE',  ( 8.971744963941056028, 11.49012176272984931, 1.599625672291281386 ) ) ;
#147080=CARTESIAN_POINT ( 'NONE',  ( -4.308793891044708779, 3.921347715840572956, 1.214306433183764966E-14 ) ) ;
#147081=CARTESIAN_POINT ( 'NONE',  ( 5.770966940911189447, 9.884545197705074671, -0.7998128361456291469 ) ) ;
#147083=CARTESIAN_POINT ( 'NONE',  ( 4.894130264408854458, 6.732904613275549899, -1.443375672974051449 ) ) ;
#147092=DIRECTION ( 'NONE',  ( -1.207943261119674327E-30, -2.168404344971008079E-15, -1.000000000000000000 ) ) ;
#147094=CARTESIAN_POINT ( 'NONE',  ( -5.395781948558855845, 9.238903340053241209, 0.7216878364870458196 ) ) ;
#147095=CARTESIAN_POINT ( 'NONE',  ( 5.834086172582112262, 5.700855377634248100, 1.040834085586084257E-14 ) ) ;
#147098=CARTESIAN_POINT ( 'NONE',  ( -9.169391961543940539, 9.592045464756413509, 1.040834085586084257E-14 ) ) ;
#147100=DIRECTION ( 'NONE',  ( 1.000000000000000000, 0.000000000000000000, 0.000000000000000000 ) ) ;
#147103=CARTESIAN_POINT ( 'NONE',  ( -8.459397779922852578, 11.95671561229694824, 1.199719254218453823 ) ) ;
#147104=CARTESIAN_POINT ( 'NONE',  ( -1.499999999999997780, 7.388542872122518368, -4.154462424328208670 ) ) ;
#147105=CARTESIAN_POINT ( 'NONE',  ( 4.609409038966229666, 6.400729850259146758, -1.443375672974051449 ) ) ;
#147107=CARTESIAN_POINT ( 'NONE',  ( 8.880754312151170282, 10.31963377138658089, 1.199719254218453823 ) ) ;
#147119=CARTESIAN_POINT ( 'NONE',  ( -7.133561379084627063, 11.47423870890741782, 0.7998128361456481317 ) ) ;
#147123=CARTESIAN_POINT ( 'NONE',  ( 7.782016984564060103, 9.141736572488651902, 1.082531754730558626 ) ) ;
#147125=CARTESIAN_POINT ( 'NONE',  ( 2.184835310096557404, 5.700724961754617404, 1.040834085586084257E-14 ) ) ;
#147126=CARTESIAN_POINT ( 'NONE',  ( 4.843287188579786573, 6.673587691474970107, -1.599625672291256295 ) ) ;
#147128=CARTESIAN_POINT ( 'NONE',  ( -5.038826645773246682, 9.030381520044109322, 0.7998128361456481317 ) ) ;
#147137=CARTESIAN_POINT ( 'NONE',  ( 0.6823417656249899377, 3.488541667008085323, -1.181850606188754593 ) ) ;
#147138=CARTESIAN_POINT ( 'NONE',  ( -1.499999999999993339, 10.64264068711930733, 1.232676135170975238E-14 ) ) ;
#147139=CARTESIAN_POINT ( 'NONE',  ( 8.727698198895078363, 11.20540053684285553, -1.599625672291257406 ) ) ;
#147142=CARTESIAN_POINT ( 'NONE',  ( -3.253593677599670109, 5.779314476299451719, 1.082531754730560403 ) ) ;
#147144=CARTESIAN_POINT ( 'NONE',  ( -3.240035523541616502, 6.723865844199768738, 0.7216878364870317197 ) ) ;
#147152=CARTESIAN_POINT ( 'NONE',  ( 3.174580523894166006, 6.855427711185178019, 0.7998128361456341429 ) ) ;
#147160=CARTESIAN_POINT ( 'NONE',  ( 5.464099601507359516, 6.333536608968757697, 1.199719254218462483 ) ) ;
#147165=CARTESIAN_POINT ( 'NONE',  ( 1.364683531249990311, 3.946875000341417028, 1.214306433183764966E-14 ) ) ;
#147170=CARTESIAN_POINT ( 'NONE',  ( 7.461064606222022277, 7.598996883547496139, 1.040834085586084257E-14 ) ) ;
#147172=CARTESIAN_POINT ( 'NONE',  ( -5.388475986427523345, 8.373973519885682393, 1.199719254218452047 ) ) ;
#147174=CARTESIAN_POINT ( 'NONE',  ( -1.499999999999997780, 1.900000000000019673, 0.000000000000000000 ) ) ;
#147177=CARTESIAN_POINT ( 'NONE',  ( -5.135841261478327979, 4.886236314679810455, 0.7998128361456341429 ) ) ;
#147178=CARTESIAN_POINT ( 'NONE',  ( 0.3176981287468615966, 7.220460999378246036, -2.081427265489023348 ) ) ;
#147179=CARTESIAN_POINT ( 'NONE',  ( -3.456965981804629884, 6.976951378839947537, 1.040834085586084257E-14 ) ) ;
#147180=CARTESIAN_POINT ( 'NONE',  ( 1.364683531249990311, 3.634375000341416584, 1.214306433183764966E-14 ) ) ;
#147183=CARTESIAN_POINT ( 'NONE',  ( -2.792616454734997866, 6.201876930592042925, 0.7216878364870317197 ) ) ;
#147186=VERTEX_POINT ( 'NONE', #11847 ) ;
#147189=CARTESIAN_POINT ( 'NONE',  ( 4.320244504248938355, 8.192035688265757898, 1.040834085586084257E-14 ) ) ;
#147191=CARTESIAN_POINT ( 'NONE',  ( 0.04331300497836985952, 7.063164988974223846, -3.968916547456744492 ) ) ;
#147192=CARTESIAN_POINT ( 'NONE',  ( 1.364683531249988535, 4.217708333674752730, -0.7879004041258239610 ) ) ;
#147196=CARTESIAN_POINT ( 'NONE',  ( 1.364683531249988757, -0.3031249996585799744, 0.000000000000000000 ) ) ;
#147198=CARTESIAN_POINT ( 'NONE',  ( -7.797910906154257304, 12.24931315715533486, 0.000000000000000000 ) ) ;
#147199=CARTESIAN_POINT ( 'NONE',  ( -6.738039155867462604, 7.923762439009225389, 1.082531754730549967 ) ) ;
#147204=CARTESIAN_POINT ( 'NONE',  ( 0.6823417656249917140, 4.592708333674755394, 1.181850606188765695 ) ) ;
#147212=CARTESIAN_POINT ( 'NONE',  ( -7.036318535368094373, 7.311385834125318617, 0.7216878364870317197 ) ) ;
#147219=CARTESIAN_POINT ( 'NONE',  ( -4.406036734316882253, 8.084200590104265061, -0.7216878364870257245 ) ) ;
#147221=CARTESIAN_POINT ( 'NONE',  ( -4.741649638052999549, 5.202212439478444139, 1.069586989871945670 ) ) ;
#147232=CARTESIAN_POINT ( 'NONE',  ( -3.879604511804807032, 7.677955697080923514, 0.7998128361456341429 ) ) ;
#147234=CARTESIAN_POINT ( 'NONE',  ( -1.500000000000001332, 0.1500000000000251132, 0.000000000000000000 ) ) ;
#147235=CARTESIAN_POINT ( 'NONE',  ( 8.758204044747994743, 12.20135990463928266, 1.082531754730546636 ) ) ;
#147236=CARTESIAN_POINT ( 'NONE',  ( 6.500244582748090139, 9.671036882259738121, 1.199719254218460707 ) ) ;
#147239=CARTESIAN_POINT ( 'NONE',  ( 5.854423403002611437, 5.724582146458163656, 1.040834085586084257E-14 ) ) ;
#147245=CARTESIAN_POINT ( 'NONE',  ( -2.968872451712654126, 6.407508927065978632, 1.040834085586084257E-14 ) ) ;
#147250=CARTESIAN_POINT ( 'NONE',  ( -1.364683531250012516, 3.988541667008088876, -0.7879004041258300672 ) ) ;
#147251=CARTESIAN_POINT ( 'NONE',  ( 8.365017589507326434, 12.70301158782650397, -0.7216878364870338292 ) ) ;
#147252=CARTESIAN_POINT ( 'NONE',  ( -5.713871673155502151, 8.753601821068331290, 1.199719254218452047 ) ) ;
#147255=CARTESIAN_POINT ( 'NONE',  ( 6.494519276145969577, 7.535692896047149425, -1.199719254218446718 ) ) ;
#147256=CARTESIAN_POINT ( 'NONE',  ( -6.575868197828002693, 7.630599971342813426, 1.199719254218450271 ) ) ;
#147257=CARTESIAN_POINT ( 'NONE',  ( -1.551702917632625356, 8.754377144105260911, 2.473499015030076631 ) ) ;
#147259=CARTESIAN_POINT ( 'NONE',  ( -0.7500000000000249800, -0.2770833326505156569, 1.299038105676659116 ) ) ;
#147262=CARTESIAN_POINT ( 'NONE',  ( 6.968527767744093993, 10.11340424813470662, 1.082531754730558626 ) ) ;
#147265=CARTESIAN_POINT ( 'NONE',  ( -1.364683531250014514, 0.8010416670080889867, -0.7879004041258289570 ) ) ;
#147267=CARTESIAN_POINT ( 'NONE',  ( 5.300874872818821082, 9.128178418356554857, 0.7216878364870438212 ) ) ;
#147270=CARTESIAN_POINT ( 'NONE',  ( -5.260200412422213923, 6.199617238323108737, -1.082531754730544860 ) ) ;
#147273=CARTESIAN_POINT ( 'NONE',  ( -0.6823417656250212460, 4.301041667008085767, 1.181850606188767472 ) ) ;
#147277=CARTESIAN_POINT ( 'NONE',  ( -5.562564655730993124, 6.373022183664215135, -1.235959600235781330 ) ) ;
#147281=( BOUNDED_CURVE ( )  B_SPLINE_CURVE ( 2, ( #199614, #133610, #14463, #50190, #213717, #130453, #81615 ),
 .UNSPECIFIED., .F., .T. ) 
 B_SPLINE_CURVE_WITH_KNOTS ( ( 3, 2, 2, 3 ),
 ( 0.1428571428571429880, 0.1488095238095238637, 0.1547619047619047394, 0.1607142857142856152 ),
 .UNSPECIFIED. ) 
 CURVE ( )  GEOMETRIC_REPRESENTATION_ITEM ( )  RATIONAL_B_SPLINE_CURVE ( ( 0.9999999999999968914, 0.8660254037844418162, 1.000000000000000000, 0.8660254037844387076, 1.000000000000000000, 0.8660254037844412611, 0.9999999999999974465 ) ) 
 REPRESENTATION_ITEM ( '' )  );
#147284=CARTESIAN_POINT ( 'NONE',  ( 6.421758314367153275, 10.64380180007036891, -0.7998128361456291469 ) ) ;
#147287=CARTESIAN_POINT ( 'NONE',  ( 3.161022370280501814, 6.839609865302569425, 0.000000000000000000 ) ) ;
#147296=CARTESIAN_POINT ( 'NONE',  ( 4.772106882330221289, 6.590544000850479200, -1.443375672974051449 ) ) ;
#147297=CARTESIAN_POINT ( 'NONE',  ( -1.364683531250012516, 0.8427083336747532849, 0.7879004041258379498 ) ) ;
#147305=CARTESIAN_POINT ( 'NONE',  ( -1.402160292154681736E-14, 2.337500000000022560, -1.732050807568863648 ) ) ;
#147306=CARTESIAN_POINT ( 'NONE',  ( 6.612626235163189925, 8.737816579155630592, -1.599625672291262513 ) ) ;
#147307=CARTESIAN_POINT ( 'NONE',  ( -7.853197290813634268, 10.18514947741448573, 1.599625672291295375 ) ) ;
#147311=CARTESIAN_POINT ( 'NONE',  ( -1.201851678989727383E-14, 1.821875000341421691, 1.575800808251672791 ) ) ;
#147312=VERTEX_POINT ( 'NONE', #113704 ) ;
#147313=CARTESIAN_POINT ( 'NONE',  ( -1.499999999999997780, 2.650000000000020339, 1.214306433183764966E-14 ) ) ;
#147315=CARTESIAN_POINT ( 'NONE',  ( 5.495132332240461714, 5.305409230568988832, 0.7998128361456341429 ) ) ;
#147320=DIRECTION ( 'NONE',  ( 1.000000000000000000, 0.000000000000000000, 0.000000000000000000 ) ) ;
#147322=CARTESIAN_POINT ( 'NONE',  ( -1.402160292154681736E-14, -0.5062499993171791779, 1.732050807568877637 ) ) ;
#147323=CARTESIAN_POINT ( 'NONE',  ( -6.718228810771495141, 7.796687353110217877, 1.199719254218450271 ) ) ;
#147324=CARTESIAN_POINT ( 'NONE',  ( -5.124618876285560454, 5.081069565195661220, 0.7216878364870317197 ) ) ;
#147331=CARTESIAN_POINT ( 'NONE',  ( 6.962275575817444384, 8.081408578997208991, -1.199719254218446718 ) ) ;
#147334=CARTESIAN_POINT ( 'NONE',  ( 6.657217119509961201, 7.725507046638470321, -1.199719254218446718 ) ) ;
#147335=CARTESIAN_POINT ( 'NONE',  ( 7.904040366642678173, 12.16520482781775137, 0.7216878364870438212 ) ) ;
#147340=CARTESIAN_POINT ( 'NONE',  ( -6.018930129462987999, 9.109503353427070849, 1.199719254218452047 ) ) ;
#147341=CARTESIAN_POINT ( 'NONE',  ( 4.385172619016207918, 7.203452924572514959, 1.199719254218462483 ) ) ;
#147345=CARTESIAN_POINT ( 'NONE',  ( 4.018854549923576158, 7.569224129587659888, 0.3183394790292719545 ) ) ;
#147346=CARTESIAN_POINT ( 'NONE',  ( 9.246297574839980271, 10.85006392781057905, 1.082531754730549967 ) ) ;
#147354=DIRECTION ( 'NONE',  ( 0.000000000000000000, -0.7996470168499917319, 0.6004703560067797818 ) ) ;
#147355=CARTESIAN_POINT ( 'NONE',  ( -2.629918611371007575, 6.012062780000711371, 0.7216878364870317197 ) ) ;
#147356=CARTESIAN_POINT ( 'NONE',  ( 8.676855123066012254, 11.14608361504227574, -1.443375672974052559 ) ) ;
#147359=CARTESIAN_POINT ( 'NONE',  ( -4.693093728624763372, 8.627026450037540428, 0.7998128361456481317 ) ) ;
#147360=CARTESIAN_POINT ( 'NONE',  ( -4.622967192135580383, 5.456178481322002227, 1.082531754730558626 ) ) ;
#147366=CARTESIAN_POINT ( 'NONE',  ( -5.831978632172702071, 9.955725504176825780, 0.7998128361456481317 ) ) ;
#147371=ORIENTED_EDGE ( 'NONE', *, *, #57965, .T. ) ;
#147372=CARTESIAN_POINT ( 'NONE',  ( 3.104453987849314700, 4.644948957289396496, 0.000000000000000000 ) ) ;
#147373=EDGE_LOOP ( 'NONE', ( #125343, #92216, #140486, #131307 ) ) ;
#147381=CARTESIAN_POINT ( 'NONE',  ( 4.059495096955338056, 3.983312706056738595, -0.7638817160546188534 ) ) ;
#147382=CARTESIAN_POINT ( 'NONE',  ( -7.230575994789712801, 7.330093503543126054, 0.7998128361456341429 ) ) ;
#147385=CARTESIAN_POINT ( 'NONE',  ( 5.829642864196171281, 5.903597551091405826, 0.7216878364870317197 ) ) ;
#147386=CARTESIAN_POINT ( 'NONE',  ( 2.034713692888019843, 8.461455076002923903, 2.500000000000000444 ) ) ;
#147388=CARTESIAN_POINT ( 'NONE',  ( -3.972702704004144714, 4.593573561881607148, 1.199719254218462483 ) ) ;
#147391=CARTESIAN_POINT ( 'NONE',  ( 7.892817981449907982, 12.36003807833360391, 0.7998128361456462443 ) ) ;
#147394=CARTESIAN_POINT ( 'NONE',  ( -9.189729191964438826, 9.615772233580322848, 1.040834085586084257E-14 ) ) ;
#147395=CARTESIAN_POINT ( 'NONE',  ( 5.126954644262057492, 9.133197518281081173, 0.7998128361456462443 ) ) ;
#147399=CARTESIAN_POINT ( 'NONE',  ( 4.822949958159289174, 6.649860922651057216, -1.599625672291256517 ) ) ;
#147402=CARTESIAN_POINT ( 'NONE',  ( -0.6823417656250212460, 1.863541667008083991, 1.181850606188755259 ) ) ;
#147405=CARTESIAN_POINT ( 'NONE',  ( 6.155038550924133212, 10.12470270947942730, 0.7216878364870438212 ) ) ;
#147407=CARTESIAN_POINT ( 'NONE',  ( -5.450014563013541036, 5.460697866378312781, 0.7216878364870346063 ) ) ;
#147412=CARTESIAN_POINT ( 'NONE',  ( 4.202664430556247055, 6.886563688082179446, 1.082531754730558626 ) ) ;
#147419=CARTESIAN_POINT ( 'NONE',  ( 3.985733972737593778, 6.633478153960411738, -1.082531754730548412 ) ) ;
#147434=CARTESIAN_POINT ( 'NONE',  ( -1.402160292154681736E-14, -0.1312499993171854229, -1.732050807568870754 ) ) ;
#147440=CARTESIAN_POINT ( 'NONE',  ( 8.866142388332804103, 12.43125098877526113, -1.199719254218446718 ) ) ;
#147442=CARTESIAN_POINT ( 'NONE',  ( 0.7499999999999920064, 5.264583334016151639, 1.299038105676669330 ) ) ;
#147446=CARTESIAN_POINT ( 'NONE',  ( 5.020596955762157698, 4.751784624677624080, 1.040834085586084257E-14 ) ) ;
#147447=CARTESIAN_POINT ( 'NONE',  ( -5.572037945536512105, 9.444535336527177805, 0.000000000000000000 ) ) ;
#147452=CARTESIAN_POINT ( 'NONE',  ( -8.016948904382338981, 8.247528564734524892, -0.7998128361456291469 ) ) ;
#147453=CARTESIAN_POINT ( 'NONE',  ( -2.779058300676980675, 5.225689869889666106, -1.082531754730543083 ) ) ;
#147457=CARTESIAN_POINT ( 'NONE',  ( -1.201851678989727383E-14, 1.243750000682821044, 1.732050807568877637 ) ) ;
#147465=CARTESIAN_POINT ( 'NONE',  ( -10.66756793585402363, 11.33991743478486391, 0.7998128361456462443 ) ) ;
#147466=EDGE_CURVE ( 'NONE', #160603, #172377, #33442, .T. ) ;
#147469=CARTESIAN_POINT ( 'NONE',  ( 4.029290343944737174, 7.554674111305462070, -0.3786771240106376890 ) ) ;
#147472=CARTESIAN_POINT ( 'NONE',  ( -3.094265954482842140, 2.800000000000024691, -2.490342512183689294 ) ) ;
#147474=CARTESIAN_POINT ( 'NONE',  ( -9.236128959407555072, 11.79856975744075598, -1.599625672291263179 ) ) ;
#147476=CARTESIAN_POINT ( 'NONE',  ( 8.281332899848809603, 8.555976559445431562, 0.7998128361456481317 ) ) ;
#147479=CARTESIAN_POINT ( 'NONE',  ( 3.469446951953614189E-15, 5.167241622962441383, 1.214306433183764966E-14 ) ) ;
#147483=CARTESIAN_POINT ( 'NONE',  ( -7.309817376062285099, 11.67987070538135264, 0.000000000000000000 ) ) ;
#147488=CARTESIAN_POINT ( 'NONE',  ( 5.542585869888291938, 5.360771691158120689, -0.7998128361456211532 ) ) ;
#147491=ORIENTED_EDGE ( 'NONE', *, *, #146747, .F. ) ;
#147492=CARTESIAN_POINT ( 'NONE',  ( -8.947491310014823895, 12.52615806407091803, 1.199719254218462483 ) ) ;
#147493=CYLINDRICAL_SURFACE ( 'NONE', #175895, 1.250000000000000000 ) ;
#147494=VECTOR ( 'NONE', #121561, 1000.000000000000000 ) ;
#147500=CARTESIAN_POINT ( 'NONE',  ( -4.951779652976519230, 6.537757797665403992, 2.442612065051306125 ) ) ;
#147504=CARTESIAN_POINT ( 'NONE',  ( 6.771407655021410399, 9.987393799911945536, -1.199719254218441611 ) ) ;
#147506=CARTESIAN_POINT ( 'NONE',  ( -3.086452525405351643, 6.752611712948207057, 0.7998128361456341429 ) ) ;
#147514=CARTESIAN_POINT ( 'NONE',  ( 1.499999999999987121, 0.5354166673494816786, 0.8660254037844524744 ) ) ;
#147520=CARTESIAN_POINT ( 'NONE',  ( -3.327636637150278798, 5.969660945728899826, -1.199719254218452935 ) ) ;
#147521=CIRCLE ( 'NONE', #192477, 0.08000000000000020983 ) ;
#147526=CARTESIAN_POINT ( 'NONE',  ( 4.772106882330221289, 6.590544000850479200, -1.443375672974051449 ) ) ;
#147529=CARTESIAN_POINT ( 'NONE',  ( 1.364683531249990311, 5.176041667008085767, 0.7879004041258500513 ) ) ;
#147531=CARTESIAN_POINT ( 'NONE',  ( 3.619663824724254741, 6.206396314611513532, -1.082531754730543971 ) ) ;
#147540=CARTESIAN_POINT ( 'NONE',  ( -6.118227108790639690, 6.008232112836603633, 0.2598000991895776934 ) ) ;
#147542=CARTESIAN_POINT ( 'NONE',  ( -1.364683531250014514, -0.7614583329919104582, -0.7879004041258359514 ) ) ;
#147549=CARTESIAN_POINT ( 'NONE',  ( -1.499999999999997780, 4.650000000000022560, 1.214306433183764966E-14 ) ) ;
#147557=CARTESIAN_POINT ( 'NONE',  ( -1.364683531249997417, 5.071875000341417916, 1.214306433183764966E-14 ) ) ;
#147559=CARTESIAN_POINT ( 'NONE',  ( 5.961834861707224320, 7.978559976790334574, -1.599625672291262513 ) ) ;
#147560=CARTESIAN_POINT ( 'NONE',  ( -7.771848369131641121, 10.09024240211882351, -1.599625672291263179 ) ) ;
#147566=CARTESIAN_POINT ( 'NONE',  ( -1.001543065824772872E-14, 5.462500000000020783, 1.732050807568877637 ) ) ;
#147575=CARTESIAN_POINT ( 'NONE',  ( 7.239690840017413365, 10.42976116578691403, -1.082531754730537976 ) ) ;
#147579=CARTESIAN_POINT ( 'NONE',  ( 0.7499999999999902300, 4.347916667349481123, -1.299038105676658228 ) ) ;
#147582=CARTESIAN_POINT ( 'NONE',  ( -3.741160322367112379, 6.452105245148518797, 1.199719254218464037 ) ) ;
#147583=CARTESIAN_POINT ( 'NONE',  ( 6.331294547457450683, 7.449227062530913379, -1.082531754730543083 ) ) ;
#147591=CARTESIAN_POINT ( 'NONE',  ( 4.857899112398166075, 4.561970474086296079, 1.040834085586084257E-14 ) ) ;
#147595=ORIENTED_EDGE ( 'NONE', *, *, #164073, .T. ) ;
#147598=CARTESIAN_POINT ( 'NONE',  ( 8.809047120577066181, 11.30030761213851953, 1.599625672291281386 ) ) ;
#147605=EDGE_CURVE ( 'NONE', #24517, #18401, #8048, .T. ) ;
#147608=CARTESIAN_POINT ( 'NONE',  ( 9.399880572976245574, 9.860948844760784482, 0.7998128361456462443 ) ) ;
#147613=CARTESIAN_POINT ( 'NONE',  ( -1.364683531250014514, -0.2614583329919080157, -0.7879004041258359514 ) ) ;
#147614=CARTESIAN_POINT ( 'NONE',  ( 6.019457014787495730, 6.125047393447951016, -0.7216878364870257245 ) ) ;
#147615=CARTESIAN_POINT ( 'NONE',  ( -3.735435015764967837, 4.316761258935923884, -1.199719254218452047 ) ) ;
#147621=CARTESIAN_POINT ( 'NONE',  ( -5.251085567194491155, 5.020688004682002159, -0.7998128361456221525 ) ) ;
#147634=CARTESIAN_POINT ( 'NONE',  ( 4.877963630130927264, 6.902327454639943127, -1.420620101560632342 ) ) ;
#147635=CARTESIAN_POINT ( 'NONE',  ( -2.279673327430177476, 5.603443282069742182, 1.040551764627347231E-14 ) ) ;
#147638=CARTESIAN_POINT ( 'NONE',  ( -6.007394966791244961, 6.077829431809393945, -0.6506939885215150543 ) ) ;
#147641=CARTESIAN_POINT ( 'NONE',  ( -7.863365906246054138, 11.15738207638699464, -1.082531754730543971 ) ) ;
#147646=CARTESIAN_POINT ( 'NONE',  ( 5.777746017718023097, 9.892454120646377191, 0.7998128361456462443 ) ) ;
#147647=CARTESIAN_POINT ( 'NONE',  ( -4.412288926243578935, 7.235088616337731260, 1.199719254218464037 ) ) ;
#147650=CARTESIAN_POINT ( 'NONE',  ( 2.544126380858701797, 6.119897877643793116, 0.7998128361456462443 ) ) ;
#147652=CARTESIAN_POINT ( 'NONE',  ( -5.925076824372040640, 6.871343368977510302, 1.199719254218450271 ) ) ;
#147653=CARTESIAN_POINT ( 'NONE',  ( 4.857899112398166075, 4.561970474086296079, 1.040834085586084257E-14 ) ) ;
#147656=CARTESIAN_POINT ( 'NONE',  ( -6.728924311084075960, 6.744833205886536120, 1.040834085586084257E-14 ) ) ;
#147659=CARTESIAN_POINT ( 'NONE',  ( 7.889955328148847258, 11.29236608522730911, -1.199719254218446718 ) ) ;
#147660=DIRECTION ( 'NONE',  ( -1.000000000000000000, 5.459311322609750190E-16, 0.000000000000000000 ) ) ;
#147662=CARTESIAN_POINT ( 'NONE',  ( 4.626555186793138930, 7.126393038833472637, 1.348983236782254957 ) ) ;
#147663=CARTESIAN_POINT ( 'NONE',  ( 4.284013352238246419, 6.021101549076499637, -1.443375672974051449 ) ) ;
#147670=CARTESIAN_POINT ( 'NONE',  ( 8.419250203962011625, 8.924806114151579095, -0.7216878364870267237 ) ) ;
#147674=CARTESIAN_POINT ( 'NONE',  ( -9.592557376868645846, 11.15007068022363157, -1.199719254218441611 ) ) ;
#147675=CARTESIAN_POINT ( 'NONE',  ( -6.256197817702116026, 9.386315656372753224, -1.199719254218440723 ) ) ;
#147676=CARTESIAN_POINT ( 'NONE',  ( -3.904385050611244079, 7.498940292447679568, 1.040834085586084257E-14 ) ) ;
#147683=CARTESIAN_POINT ( 'NONE',  ( 10.07778825365955733, 10.65184113889131012, -0.7998128361456281477 ) ) ;
#147687=CARTESIAN_POINT ( 'NONE',  ( 2.835626683552519012, 6.459981564119914310, 0.000000000000000000 ) ) ;
#147690=CARTESIAN_POINT ( 'NONE',  ( -1.500000000000013101, 3.910416667349482012, -0.8660254037844313801 ) ) ;
#147696=CARTESIAN_POINT ( 'NONE',  ( 0.7499999999999885647, 2.816666666666689522, -1.299038105676658228 ) ) ;
#147697=CARTESIAN_POINT ( 'NONE',  ( 4.961394147597008697, 7.875711374583454827, -1.199719254218452047 ) ) ;
#147700=CARTESIAN_POINT ( 'NONE',  ( 8.270110514656037637, 8.750809809961280550, 0.7216878364870458196 ) ) ;
#147701=CARTESIAN_POINT ( 'NONE',  ( -8.609064354553318310, 12.98773281371349775, 0.7216878364870317197 ) ) ;
#147706=CARTESIAN_POINT ( 'NONE',  ( -5.413783410558481002, 5.210502155273325720, -0.7998128361456221525 ) ) ;
#147707=CARTESIAN_POINT ( 'NONE',  ( 0.7499999999999902300, 5.597916667349482900, -1.299038105676658228 ) ) ;
#147709=CARTESIAN_POINT ( 'NONE',  ( -1.402160292154681736E-14, -0.5531249996585814177, -1.575800808251665908 ) ) ;
#147713=CARTESIAN_POINT ( 'NONE',  ( 2.686486993802192913, 6.285985259411197568, 0.7998128361456362523 ) ) ;
#147715=CARTESIAN_POINT ( 'NONE',  ( -0.6823417656250212460, 5.363541667008087543, 1.181850606188767472 ) ) ;
#147724=CARTESIAN_POINT ( 'NONE',  ( -7.901704598666176693, 8.113076874732334076, 0.7998128361456602331 ) ) ;
#147726=CARTESIAN_POINT ( 'NONE',  ( 4.008406971134620633, 7.828225232965717595, 0.7998128361456321445 ) ) ;
#147729=B_SPLINE_CURVE_WITH_KNOTS ( 'NONE', 3,
 ( #141205, #127130, #110856, #94567, #160610, #12212, #177938, #164870 ),
 .UNSPECIFIED., .F., .F.,
 ( 4, 2, 2, 4 ),
 ( 0.000000000000000000, 0.001495953190030211571, 0.002991906380060423143, 0.005983812760120844551 ),
 .UNSPECIFIED. ) ;
#147731=CARTESIAN_POINT ( 'NONE',  ( -1.364683531250014514, 0.03020833367475737191, 0.7879004041258379498 ) ) ;
#147735=CARTESIAN_POINT ( 'NONE',  ( 9.642873567817520808, 12.27310513391906532, 1.599625672291279388 ) ) ;
#147738=CARTESIAN_POINT ( 'NONE',  ( -6.449928391799210736, 8.548002428564306143, -1.599625672291263179 ) ) ;
#147742=CARTESIAN_POINT ( 'NONE',  ( 7.391166297744269365, 11.77477778067701664, 1.040834085586084257E-14 ) ) ;
#147744=CARTESIAN_POINT ( 'NONE',  ( 7.228468454380276853, 11.58496363008569574, 1.040834085586084257E-14 ) ) ;
#147746=CARTESIAN_POINT ( 'NONE',  ( -3.469997250093771246, 6.135748327496311383, -1.199719254218452935 ) ) ;
#147747=CARTESIAN_POINT ( 'NONE',  ( -5.856232286098998152, 8.919689202835742847, 1.199719254218452047 ) ) ;
#147750=CARTESIAN_POINT ( 'NONE',  ( -4.637175514440688318, 7.109613026884349374, 1.382187809737724704 ) ) ;
#147751=CARTESIAN_POINT ( 'NONE',  ( -1.364683531250000748, 0.5093750003414208027, 0.000000000000000000 ) ) ;
#147755=CARTESIAN_POINT ( 'NONE',  ( 7.510853912290742507, 8.825379654836435606, -1.082531754730537976 ) ) ;
#147758=CARTESIAN_POINT ( 'NONE',  ( 4.710568305744190276, 7.583081225755162968, 1.199719254218462483 ) ) ;
#147775=CARTESIAN_POINT ( 'NONE',  ( 8.211434591371064684, 12.73175745657494851, -0.7998128361456352531 ) ) ;
#147776=CARTESIAN_POINT ( 'NONE',  ( 1.499999999999990896, 6.280000000000042881, 2.873333333333337070 ) ) ;
#147777=ORIENTED_EDGE ( 'NONE', *, *, #10652, .T. ) ;
#147779=CARTESIAN_POINT ( 'NONE',  ( -5.922214171070950606, 5.803671375871217286, -0.7998128361456291469 ) ) ;
#147780=CARTESIAN_POINT ( 'NONE',  ( -6.170932472514347289, 10.35117165124207972, 0.000000000000000000 ) ) ;
#147786=CARTESIAN_POINT ( 'NONE',  ( 0.7499999999999902300, 3.514583334016149863, 1.299038105676669330 ) ) ;
#147787=CARTESIAN_POINT ( 'NONE',  ( 7.703003830858588863, 12.13858823597705872, -0.7998128361456291469 ) ) ;
#147791=CARTESIAN_POINT ( 'NONE',  ( -7.720478407978036195, 11.09464301169468037, -1.199719254218446718 ) ) ;
#147793=CARTESIAN_POINT ( 'NONE',  ( 1.364683531249988535, 3.655208333674750509, -0.7879004041258239610 ) ) ;
#147797=VECTOR ( 'NONE', #191969, 1000.000000000000000 ) ;
#147800=CARTESIAN_POINT ( 'NONE',  ( -10.33094986393327197, 11.15512238411806578, 0.7216878364870438212 ) ) ;
#147804=CARTESIAN_POINT ( 'NONE',  ( 0.6823417656249899377, 1.405208333674752508, 1.181850606188755259 ) ) ;
#147810=CARTESIAN_POINT ( 'NONE',  ( 1.364683531249988757, 2.384375000341422357, 1.214306433183764966E-14 ) ) ;
#147812=CARTESIAN_POINT ( 'NONE',  ( -6.098470168048611306, 6.009303372345148553, 1.040834085586084257E-14 ) ) ;
#147813=CARTESIAN_POINT ( 'NONE',  ( 8.274553823041976841, 8.548067636504127265, 1.040834085586084257E-14 ) ) ;
#147814=CARTESIAN_POINT ( 'NONE',  ( 0.000000000000000000, 8.600000000000017408, 0.4000000000000045186 ) ) ;
#147816=CARTESIAN_POINT ( 'NONE',  ( -1.500000000000011324, 5.170833333333356485, 0.8660254037844403729 ) ) ;
#147817=CARTESIAN_POINT ( 'NONE',  ( -1.201851678989727383E-14, 2.384375000341416584, 1.575800808251672791 ) ) ;
#147822=CARTESIAN_POINT ( 'NONE',  ( -4.256897045010916258, 7.910204285913967404, 0.7216878364870317197 ) ) ;
#147825=CARTESIAN_POINT ( 'NONE',  ( 5.097502569058200983, 6.970172302033127210, -1.443375672974051449 ) ) ;
#147828=CARTESIAN_POINT ( 'NONE',  ( -8.148614017013223076, 9.465470093725620870, -1.199719254218446718 ) ) ;
#147829=CARTESIAN_POINT ( 'NONE',  ( -10.46653140006992899, 11.31330084294416771, -0.7216878364870267237 ) ) ;
#147831=CARTESIAN_POINT ( 'NONE',  ( 1.364683531249990311, 5.134375000341417916, 1.214306433183764966E-14 ) ) ;
#147836=CARTESIAN_POINT ( 'NONE',  ( -6.331294547457448019, 10.33033470543493770, 0.7216878364870458196 ) ) ;
#147838=CARTESIAN_POINT ( 'NONE',  ( 0.6823417656249882723, -0.09479166632524876901, 1.181850606188755259 ) ) ;
#147841=CARTESIAN_POINT ( 'NONE',  ( 7.998947442382716488, 9.394822106610419610, -1.082531754730543083 ) ) ;
#147845=CARTESIAN_POINT ( 'NONE',  ( 3.348500752450942031, 4.929670182657964084, 1.443375672974066548 ) ) ;
#147848=VERTEX_POINT ( 'NONE', #86465 ) ;
#147849=CARTESIAN_POINT ( 'NONE',  ( 7.876924059415351564, 12.13356913605253240, -0.7216878364870267237 ) ) ;
#147853=ORIENTED_EDGE ( 'NONE', *, *, #77726, .T. ) ;
#147857=EDGE_CURVE ( 'NONE', #20507, #154752, #70884, .T. ) ;
#147858=CARTESIAN_POINT ( 'NONE',  ( 4.638861114170084399, 8.563755066507100722, 0.7998128361456462443 ) ) ;
#147859=CARTESIAN_POINT ( 'NONE',  ( -3.242371291962510504, 6.934516940598226320, 1.040834085586084257E-14 ) ) ;
#147864=CARTESIAN_POINT ( 'NONE',  ( 5.626270559546821204, 6.626699076635176766, 1.082531754730560403 ) ) ;
#147865=CARTESIAN_POINT ( 'NONE',  ( -0.6823417656250003738, 0.7802083336747520637, -1.181850606188749264 ) ) ;
#147867=CARTESIAN_POINT ( 'NONE',  ( -8.123306592882240551, 12.62894145833798376, 0.000000000000000000 ) ) ;
#147873=CARTESIAN_POINT ( 'NONE',  ( 4.177814833339410505, 3.976464848425038223, -0.02210016498919950903 ) ) ;
#147885=CARTESIAN_POINT ( 'NONE',  ( 7.467843683028853263, 7.606905806488803101, 0.7998128361456341429 ) ) ;
#147886=CARTESIAN_POINT ( 'NONE',  ( 6.632963465583686435, 8.761543347979550589, -1.599625672291262513 ) ) ;
#147897=CARTESIAN_POINT ( 'NONE',  ( -2.764973262183167968, 5.313220341600567664, 1.199719254218462483 ) ) ;
#147900=LINE ( 'NONE', #98095, #65833 ) ;
#147902=CARTESIAN_POINT ( 'NONE',  ( 1.468321960012000549, 7.242494692103044862, 4.289992922803952169 ) ) ;
#147907=CARTESIAN_POINT ( 'NONE',  ( -8.161645285746702783, 12.46574390010577105, 0.7216878364870478180 ) ) ;
#147911=CARTESIAN_POINT ( 'NONE',  ( 5.991813822235618758, 9.077867661661846554, 1.199719254218462483 ) ) ;
#147917=CARTESIAN_POINT ( 'NONE',  ( 5.802526556524483681, 5.871961858807763335, 1.040834085586084257E-14 ) ) ;
#147919=CARTESIAN_POINT ( 'NONE',  ( -7.528855374290365887, 7.678086112960552434, -0.7998128361456291469 ) ) ;
#147925=CARTESIAN_POINT ( 'NONE',  ( -6.449928391799210736, 8.548002428564306143, -1.599625672291263179 ) ) ;
#147926=CARTESIAN_POINT ( 'NONE',  ( -4.786191920824102830, 5.542644314838231168, 1.199719254218462483 ) ) ;
#147934=CARTESIAN_POINT ( 'NONE',  ( 7.447506452608354088, 7.583179037664891098, 0.7998128361456341429 ) ) ;
#147940=AXIS2_PLACEMENT_3D ( 'NONE', #83255, #214285, #68050 ) ;
#147948=CARTESIAN_POINT ( 'NONE',  ( -1.364683531250014514, -0.4072916663252447167, 0.7879004041258379498 ) ) ;
#147950=CARTESIAN_POINT ( 'NONE',  ( 3.845709127770629010, 7.638411082374393146, 0.7998128361456321445 ) ) ;
#147953=CARTESIAN_POINT ( 'NONE',  ( -6.222829318992474157, 10.20379193889247382, 0.000000000000000000 ) ) ;
#147954=CARTESIAN_POINT ( 'NONE',  ( -1.127943160727153060, 3.300000000000025135, -0.7749999999999935829 ) ) ;
#147955=CARTESIAN_POINT ( 'NONE',  ( 5.504247177468190699, 5.523969249908757817, 0.7216878364870317197 ) ) ;
#147956=CARTESIAN_POINT ( 'NONE',  ( -6.182154857707119255, 10.15633840072622363, 0.000000000000000000 ) ) ;
#147960=CARTESIAN_POINT ( 'NONE',  ( 7.637320603199683866, 7.804628880021436288, -0.7998128361456281477 ) ) ;
#147962=DIRECTION ( 'NONE',  ( -7.387867266669436732E-31, -1.000000000000000000, 8.546850786086437571E-32 ) ) ;
#147966=CARTESIAN_POINT ( 'NONE',  ( 0.6823417656249899377, 3.426041667008085323, -1.181850606188754593 ) ) ;
#147971=CARTESIAN_POINT ( 'NONE',  ( 7.039708073993665494, 9.236078724457858158, 1.599625672291281386 ) ) ;
#147975=CARTESIAN_POINT ( 'NONE',  ( -6.855619230004478482, 11.14997286831390788, -0.7998128361456291469 ) ) ;
#147981=CARTESIAN_POINT ( 'NONE',  ( 8.540746701604824409, 12.05162268759261224, -1.199719254218446718 ) ) ;
#147985=CARTESIAN_POINT ( 'NONE',  ( -6.842061076390810292, 11.13415502243129218, 0.000000000000000000 ) ) ;
#147986=CARTESIAN_POINT ( 'NONE',  ( 0.4410926847035671616, 6.460511719969816546, 3.247348959959607484 ) ) ;
#147988=CARTESIAN_POINT ( 'NONE',  ( 5.688518940989607309, 6.102662425301288884, -0.7322136710279708582 ) ) ;
#147989=CARTESIAN_POINT ( 'NONE',  ( -3.735435015764967837, 4.316761258935923884, -1.199719254218452047 ) ) ;
#147992=CARTESIAN_POINT ( 'NONE',  ( 3.264161633363777959, 6.412690354096299394, -0.9273118095389889515 ) ) ;
#147994=CARTESIAN_POINT ( 'NONE',  ( 4.774442650306744085, 8.721933525333202653, -0.7998128361456281477 ) ) ;
#147996=CARTESIAN_POINT ( 'NONE',  ( 6.145923705696426431, 6.064665832934283962, 0.7998128361456341429 ) ) ;
#147997=CARTESIAN_POINT ( 'NONE',  ( -4.117634752470962667, 7.483002602015099924, 0.6335975934644126895 ) ) ;
#147998=CARTESIAN_POINT ( 'NONE',  ( 4.521807925357579805, 5.234196320127330715, -1.199719254218452047 ) ) ;
#148000=CARTESIAN_POINT ( 'NONE',  ( -7.727784370109414880, 8.118095974656867497, 0.7216878364870578100 ) ) ;
#148006=CARTESIAN_POINT ( 'NONE',  ( -4.160056744896282410, 7.428205994021240599, -0.7369721661574859528 ) ) ;
#148007=CARTESIAN_POINT ( 'NONE',  ( -1.402160292154681736E-14, -0.6156249996585817508, 1.575800808251672791 ) ) ;
#148010=CARTESIAN_POINT ( 'NONE',  ( 4.528060117284240071, 5.345453560662148718, 1.082531754730560403 ) ) ;
#148014=CARTESIAN_POINT ( 'NONE',  ( -8.473482818416664841, 11.86918514058604757, -1.082531754730543083 ) ) ;
#148019=CARTESIAN_POINT ( 'NONE',  ( -10.58855478214856660, 11.45566145536924552, -0.7216878364870217277 ) ) ;
#148026=CARTESIAN_POINT ( 'NONE',  ( -8.134528978075012517, 12.43410820782212767, 1.040834085586084257E-14 ) ) ;
#148031=CARTESIAN_POINT ( 'NONE',  ( -0.7500000000000215383, 2.472916667349486897, 1.299038105676671107 ) ) ;
#148034=EDGE_LOOP ( 'NONE', ( #157548, #125448, #150604, #119919 ) ) ;
#148035=ADVANCED_FACE ( 'NONE', ( #187154 ), #104864, .F. ) ;
#148037=CARTESIAN_POINT ( 'NONE',  ( -7.147119532698295252, 11.49005655479003174, 0.000000000000000000 ) ) ;
#148040=CARTESIAN_POINT ( 'NONE',  ( 6.636879889089462026, 7.701780277814560982, -1.199719254218446718 ) ) ;
#148046=CARTESIAN_POINT ( 'NONE',  ( 7.086107841436786181, 11.41887624831828418, 1.040834085586084257E-14 ) ) ;
#148051=CIRCLE ( 'NONE', #203357, 0.07999999999999998779 ) ;
#148054=CARTESIAN_POINT ( 'NONE',  ( -7.551528373131759508, 7.912463978182924684, 1.040834085586084257E-14 ) ) ;
#148057=CARTESIAN_POINT ( 'NONE',  ( 1.364683531249992088, 5.696875000341418804, 1.214306433183764966E-14 ) ) ;
#148065=CARTESIAN_POINT ( 'NONE',  ( -3.375617059678305054, 5.921675088724528635, 1.082531754730560403 ) ) ;
#148067=CARTESIAN_POINT ( 'NONE',  ( 8.048736748007069508, 12.54194330598362406, -0.7998128361456352531 ) ) ;
#148069=CARTESIAN_POINT ( 'NONE',  ( -9.504429378379839477, 11.04725468198666150, 1.199719254218462483 ) ) ;
#148072=CARTESIAN_POINT ( 'NONE',  ( -0.6823417656250003738, 1.967708333674753174, -1.181850606188749264 ) ) ;
#148073=CARTESIAN_POINT ( 'NONE',  ( 3.011882680530176604, 6.665613560593854459, 0.7998128361456341429 ) ) ;
#148079=CARTESIAN_POINT ( 'NONE',  ( 7.904040366642678173, 12.16520482781775137, 0.7216878364870438212 ) ) ;
#148080=CARTESIAN_POINT ( 'NONE',  ( -2.280006499904862149, 5.600973625046616000, -0.2919740144436631102 ) ) ;
#148081=CARTESIAN_POINT ( 'NONE',  ( -6.561783159334130922, 9.638868871656395498, -1.082531754730538864 ) ) ;
#148082=CARTESIAN_POINT ( 'NONE',  ( 1.364683531249986537, 0.8635416670080893198, 0.7879004041258500513 ) ) ;
#148084=CARTESIAN_POINT ( 'NONE',  ( 0.4782691259469203371, 7.503280781840964586, 1.943353214563591003 ) ) ;
#148086=CARTESIAN_POINT ( 'NONE',  ( -8.616370316684697883, 10.01118577667568132, -1.199719254218446718 ) ) ;
#148087=CARTESIAN_POINT ( 'NONE',  ( -4.487385655998893164, 6.258369236797239665, 1.443375672974064550 ) ) ;
#148088=CARTESIAN_POINT ( 'NONE',  ( -1.201851678989727383E-14, 3.509375000341421469, -1.575800808251660134 ) ) ;
#148095=CARTESIAN_POINT ( 'NONE',  ( 9.748476143425788720, 11.33197590787365172, -1.199719254218440723 ) ) ;
#148111=CARTESIAN_POINT ( 'NONE',  ( -1.364683531250010295, 4.842708333674756283, 0.7879004041258379498 ) ) ;
#148115=EDGE_CURVE ( 'NONE', #167173, #11923, #112382, .T. ) ;
#148117=CARTESIAN_POINT ( 'NONE',  ( 10.07100917685271035, 10.64393221595000938, 0.7998128361456462443 ) ) ;
#148119=( BOUNDED_SURFACE ( )  B_SPLINE_SURFACE ( 3, 2, ( 
 ( #29147, #96300, #11813 ),
 ( #211072, #176465, #60569 ),
 ( #13935, #178606, #126728 ),
 ( #64833, #196970, #77889 ),
 ( #142934, #94172, #98412 ),
 ( #47554, #32346, #146121 ),
 ( #144010, #95236, #161285 ),
 ( #46471, #129929, #208935 ),
 ( #145069, #210002, #63770 ),
 ( #147178, #112594, #163422 ),
 ( #61644, #162355, #164476 ),
 ( #127812, #62695, #113665 ),
 ( #76815, #213204, #128856 ),
 ( #130979, #48607, #45412 ) ),
 .UNSPECIFIED., .F., .F., .T. ) 
 B_SPLINE_SURFACE_WITH_KNOTS ( ( 4, 2, 2, 2, 2, 2, 4 ),
 ( 3, 3 ),
 ( 0.001912008033049058262, 0.002390010041311322556, 0.002629011045442455029, 0.002868012049573587068, 0.003346014057835851145, 0.003585015061966983184, 0.003824016066098115656 ),
 ( 0.000000000000000000, 1.000000000000000000 ),
 .UNSPECIFIED. ) 
 GEOMETRIC_REPRESENTATION_ITEM ( )  RATIONAL_B_SPLINE_SURFACE ( (
 ( 1.000000000000000000, 0.8708456909032173954, 1.000000000000000000),
 ( 1.000000000000000000, 0.8699862225465916366, 1.000000000000000000),
 ( 1.000000000000000000, 0.8740515128125330158, 1.000000000000000000),
 ( 1.000000000000000000, 0.8627336009020147856, 1.000000000000000000),
 ( 1.000000000000000000, 0.8557431983335841430, 1.000000000000000000),
 ( 1.000000000000000000, 0.8314605231442517841, 1.000000000000000000),
 ( 1.000000000000000000, 0.8141324793653522685, 1.000000000000000000),
 ( 1.000000000000000000, 0.7486317046913882889, 1.000000000000000000),
 ( 1.000000000000000000, 0.6849789572268089044, 1.000000000000000000),
 ( 1.000000000000000000, 0.5903265755408019233, 1.000000000000000000),
 ( 1.000000000000000000, 0.5583523351997250472, 1.000000000000000000),
 ( 1.000000000000000000, 0.5090820572710972325, 1.000000000000000000),
 ( 1.000000000000000000, 0.4920791080017826169, 1.000000000000000000),
 ( 1.000000000000000000, 0.4915962107220928079, 1.000000000000000000) ) ) 
 REPRESENTATION_ITEM ( '' )  SURFACE ( )  );
#148121=CARTESIAN_POINT ( 'NONE',  ( 1.364683531249988535, 2.113541667008087099, 0.7879004041258500513 ) ) ;
#148124=CARTESIAN_POINT ( 'NONE',  ( -7.700668062882078502, 9.046829497192987901, -1.082531754730543971 ) ) ;
#148130=CARTESIAN_POINT ( 'NONE',  ( 2.842405760359353106, 6.467890487061221272, -0.7998128361456291469 ) ) ;
#148133=CARTESIAN_POINT ( 'NONE',  ( 10.05353459973327368, 11.68787744023238417, -1.199719254218440723 ) ) ;
#148134=DIRECTION ( 'NONE',  ( -5.578564026256490882E-16, -1.000000000000000000, -9.066213480720158442E-32 ) ) ;
#148140=CARTESIAN_POINT ( 'NONE',  ( -8.435144125996554720, 12.99275191363802229, 0.7998128361456341429 ) ) ;
#148141=CARTESIAN_POINT ( 'NONE',  ( 6.174848896020108668, 9.291408581077091000, 1.199719254218460707 ) ) ;
#148143=CARTESIAN_POINT ( 'NONE',  ( 5.192409643909512873, 6.120528008391641350, -1.082531754730549078 ) ) ;
#148153=CARTESIAN_POINT ( 'NONE',  ( -7.700668062882084719, 8.086460282891644979, -0.7216878364870278340 ) ) ;
#148154=CARTESIAN_POINT ( 'NONE',  ( 4.123651276850781144, 7.962676922967908411, -0.7998128361456221525 ) ) ;
#148157=CARTESIAN_POINT ( 'NONE',  ( -8.483651433849100698, 10.92067931095586886, 1.599625672291269396 ) ) ;
#148162=CARTESIAN_POINT ( 'NONE',  ( -7.797910906154257304, 12.24931315715533486, 0.000000000000000000 ) ) ;
#148163=CARTESIAN_POINT ( 'NONE',  ( 3.823036128929238942, 7.404033217152015567, 1.040834085586084257E-14 ) ) ;
#148166=CARTESIAN_POINT ( 'NONE',  ( 7.072549687823125097, 11.40305840243567381, -0.7998128361456291469 ) ) ;
#148168=CARTESIAN_POINT ( 'NONE',  ( 4.241003122976366058, 3.842258486427521103, -0.7998128361456211532 ) ) ;
#148179=CARTESIAN_POINT ( 'NONE',  ( -9.318531651294266638, 9.766041769465124034, -0.7998128361456291469 ) ) ;
#148183=CARTESIAN_POINT ( 'NONE',  ( 7.619319141200070256, 8.951922421897323900, 1.082531754730558626 ) ) ;
#148184=CARTESIAN_POINT ( 'NONE',  ( 0.6823417656249917140, 4.905208333674755394, 1.181850606188765695 ) ) ;
#148186=CARTESIAN_POINT ( 'NONE',  ( 2.333974999846879061, 5.874721266463329705, -0.7998128361456291469 ) ) ;
#148189=CARTESIAN_POINT ( 'NONE',  ( -5.703176172842872482, 9.805455968292021041, 0.000000000000000000 ) ) ;
#148200=CARTESIAN_POINT ( 'NONE',  ( -1.364683531250012516, 4.551041667008082214, -0.7879004041258300672 ) ) ;
#148201=CARTESIAN_POINT ( 'NONE',  ( -4.304117108723031215, 3.915891469798615354, -0.2758893754505397644 ) ) ;
#148202=CARTESIAN_POINT ( 'NONE',  ( 7.889955328148847258, 11.29236608522730911, -1.199719254218446718 ) ) ;
#148204=CARTESIAN_POINT ( 'NONE',  ( -2.792616454734997866, 6.201876930592042925, 0.7216878364870317197 ) ) ;
#148206=CARTESIAN_POINT ( 'NONE',  ( -3.728129053633589152, 7.293308295973741195, 0.7216878364870317197 ) ) ;
#148213=CARTESIAN_POINT ( 'NONE',  ( 5.118366684358879759, 5.930181538962194132, 1.199719254218462483 ) ) ;
#148219=EDGE_CURVE ( 'NONE', #59141, #179291, #177322, .T. ) ;
#148222=CARTESIAN_POINT ( 'NONE',  ( 3.994848817520957773, 7.812407387083109001, 1.040834085586084257E-14 ) ) ;
#148226=CARTESIAN_POINT ( 'NONE',  ( 0.6823417656249917140, 3.405208333674754506, 1.181850606188765695 ) ) ;
#148231=CARTESIAN_POINT ( 'NONE',  ( 6.612626235163189925, 8.737816579155630592, -1.599625672291262513 ) ) ;
#148234=CARTESIAN_POINT ( 'NONE',  ( -4.577849422908604637, 8.492574760035358494, -0.7998128361456281477 ) ) ;
#148235=CARTESIAN_POINT ( 'NONE',  ( 0.7499999999999885647, 1.816666666666688634, -1.299038105676652899 ) ) ;
#148238=CARTESIAN_POINT ( 'NONE',  ( -3.750802052474980108, 7.527686161196117887, 1.040834085586084257E-14 ) ) ;
#148241=CARTESIAN_POINT ( 'NONE',  ( 1.364683531249988535, 3.155208333674756283, -0.7879004041258239610 ) ) ;
#148243=CARTESIAN_POINT ( 'NONE',  ( -4.934804725694231564, 5.819988937140460727, -1.082531754730544860 ) ) ;
#148246=VERTEX_POINT ( 'NONE', #174145 ) ;
#148248=CARTESIAN_POINT ( 'NONE',  ( 5.355634372598031767, 6.206993841907870291, -1.199719254218445830 ) ) ;
#148253=CARTESIAN_POINT ( 'NONE',  ( -1.364683531250012516, 2.301041667008087988, -0.7879004041258289570 ) ) ;
#148255=CARTESIAN_POINT ( 'NONE',  ( 3.708318708537623021, 4.285125567170706695, -1.199719254218446718 ) ) ;
#148258=CARTESIAN_POINT ( 'NONE',  ( 1.364683531249986537, -0.5322916663252452718, -0.7879004041258309554 ) ) ;
#148261=CARTESIAN_POINT ( 'NONE',  ( -4.471491734408701291, 4.111161866431900513, 1.214306433183764966E-14 ) ) ;
#148263=CARTESIAN_POINT ( 'NONE',  ( -7.334597914868743018, 7.659378443542744996, -0.7216878364870267237 ) ) ;
#148267=CARTESIAN_POINT ( 'NONE',  ( -1.201851678989727383E-14, 3.196875000341420137, -1.575800808251660134 ) ) ;
#148275=CARTESIAN_POINT ( 'NONE',  ( -6.005898860729463884, 9.950706404252290582, 0.7216878364870458196 ) ) ;
#148281=CARTESIAN_POINT ( 'NONE',  ( -7.009202228140764213, 7.279750142360097875, -0.7216878364870267237 ) ) ;
#148284=CARTESIAN_POINT ( 'NONE',  ( -1.123270288250318494, 3.297697346350006331, -0.7749999999993560929 ) ) ;
#148290=ORIENTED_EDGE ( 'NONE', *, *, #186210, .F. ) ;
#148293=CARTESIAN_POINT ( 'NONE',  ( -4.446184310277715213, 7.274633231044262516, -1.199719254218452047 ) ) ;
#148295=CARTESIAN_POINT ( 'NONE',  ( -1.500000000000015099, -0.8291666666666407393, 0.8660254037844403729 ) ) ;
#148296=AXIS2_PLACEMENT_3D ( 'NONE', #129211, #96642, #11075 ) ;
#148297=CARTESIAN_POINT ( 'NONE',  ( 10.39874063200158893, 11.23421161353111586, 0.000000000000000000 ) ) ;
#148298=CARTESIAN_POINT ( 'NONE',  ( 8.471147050440139381, 8.777426401801974976, -0.7998128361456281477 ) ) ;
#148300=CARTESIAN_POINT ( 'NONE',  ( 4.177814833343409084, 3.976464848429826393, 1.040551764647542070E-14 ) ) ;
#148301=CARTESIAN_POINT ( 'NONE',  ( 4.819033534653518025, 7.709623992816043270, -1.199719254218452047 ) ) ;
#148308=CARTESIAN_POINT ( 'NONE',  ( -4.622967192579922724, 4.495809267539077503, 1.214306433183764966E-14 ) ) ;
#148310=CARTESIAN_POINT ( 'NONE',  ( 6.471393748265519719, 5.229711127717882491, -2.499999999999995115 ) ) ;
#148314=CARTESIAN_POINT ( 'NONE',  ( -1.402160292154681736E-14, 1.696875000341421469, -1.575800808251659024 ) ) ;
#148315=CARTESIAN_POINT ( 'NONE',  ( 8.554831740098649107, 11.96409221588171157, 1.082531754730546636 ) ) ;
#148316=CARTESIAN_POINT ( 'NONE',  ( -7.660520486921249983, 8.896027641951645748, -1.199719254218446718 ) ) ;
#148319=CARTESIAN_POINT ( 'NONE',  ( 6.817052309572890323, 6.847649204123507083, 0.7998128361456341429 ) ) ;
#148320=CARTESIAN_POINT ( 'NONE',  ( -5.228640796364566690, 9.251831362400652736, -0.7998128361456231517 ) ) ;
#148323=CARTESIAN_POINT ( 'NONE',  ( 1.499999999999985123, -0.6729166659838520248, -0.8660254037844323793 ) ) ;
#148326=CARTESIAN_POINT ( 'NONE',  ( 8.432808358020025707, 9.900993174853955026, 1.082531754730558626 ) ) ;
#148329=CARTESIAN_POINT ( 'NONE',  ( 0.6823417656249899377, 0.6552083336747518416, 1.181850606188755259 ) ) ;
#148331=CARTESIAN_POINT ( 'NONE',  ( 7.090551149822739596, 8.335026431957096804, 1.082531754730558626 ) ) ;
#148335=CARTESIAN_POINT ( 'NONE',  ( -3.958617665510272943, 6.601842462195195438, -1.082531754730549967 ) ) ;
#148337=CARTESIAN_POINT ( 'NONE',  ( -0.6823417656249969321, 4.967708333674755394, -1.181850606188749264 ) ) ;
#148348=CARTESIAN_POINT ( 'NONE',  ( 5.635385404774530649, 9.726366738878972740, 0.7998128361456462443 ) ) ;
#148351=CARTESIAN_POINT ( 'NONE',  ( 3.174580523894166006, 6.855427711185178019, 0.7998128361456341429 ) ) ;
#148359=CARTESIAN_POINT ( 'NONE',  ( 5.097502569058200983, 6.970172302033127210, -1.443375672974051449 ) ) ;
#148361=CARTESIAN_POINT ( 'NONE',  ( -1.364683531250000748, 0.8218750003414210248, 0.000000000000000000 ) ) ;
#148363=CARTESIAN_POINT ( 'NONE',  ( 8.353795204314554468, 12.89784483834236184, -0.7998128361456352531 ) ) ;
#148364=CARTESIAN_POINT ( 'NONE',  ( -2.482948226198874231, 5.072301959192136778, -2.499999999999995115 ) ) ;
#148368=CARTESIAN_POINT ( 'NONE',  ( -1.402160292154681736E-14, 1.337500000000025446, -1.732050807568863648 ) ) ;
#148369=CARTESIAN_POINT ( 'NONE',  ( 7.558834334818744338, 8.777393797832065303, 1.199719254218462483 ) ) ;
#148370=CARTESIAN_POINT ( 'NONE',  ( -8.259941899223614215, 10.65968485389279508, -1.599625672291263179 ) ) ;
#148373=CARTESIAN_POINT ( 'NONE',  ( 0.6823417656249882723, 1.676041667008083769, -1.181850606188749264 ) ) ;
#148374=CARTESIAN_POINT ( 'NONE',  ( -1.201851678989727383E-14, 3.087500000000026112, -1.732050807568863648 ) ) ;
#148376=CARTESIAN_POINT ( 'NONE',  ( 5.345992642490140057, 5.131412925860272090, 1.040834085586084257E-14 ) ) ;
#148384=CARTESIAN_POINT ( 'NONE',  ( -0.7500000000000006661, -0.3604166659838467512, -1.299038105676652011 ) ) ;
#148386=CARTESIAN_POINT ( 'NONE',  ( -6.507023659554960204, 9.678945805201045971, 1.199719254218452047 ) ) ;
#148387=CARTESIAN_POINT ( 'NONE',  ( -3.118012141462980669, 6.581505231774690046, 0.7216878364870317197 ) ) ;
#148394=ORIENTED_EDGE ( 'NONE', *, *, #198992, .T. ) ;
#148395=CARTESIAN_POINT ( 'NONE',  ( 5.276094334012385367, 9.307193822989793475, 1.040834085586084257E-14 ) ) ;
#148396=DIRECTION ( 'NONE',  ( -1.000000000000000000, 0.000000000000000000, 0.000000000000000000 ) ) ;
#148400=CARTESIAN_POINT ( 'NONE',  ( 5.798083248138522272, 9.916180889470295412, 0.7998128361456462443 ) ) ;
#148401=CARTESIAN_POINT ( 'NONE',  ( 8.310784975052673218, 10.71900177569337487, -1.443375672974063439 ) ) ;
#148405=CARTESIAN_POINT ( 'NONE',  ( -8.030507057996002729, 8.263346410617135263, 1.040834085586084257E-14 ) ) ;
#148406=CARTESIAN_POINT ( 'NONE',  ( 4.867540842506059562, 5.637551390133895168, -1.199719254218452047 ) ) ;
#148410=CARTESIAN_POINT ( 'NONE',  ( -2.535011536075354677, 5.133042487381361596, -7.499999999999997335 ) ) ;
#148412=CARTESIAN_POINT ( 'NONE',  ( 8.080296364064698977, 12.37083682481011060, -0.7216878364870328300 ) ) ;
#148413=ORIENTED_EDGE ( 'NONE', *, *, #71089, .T. ) ;
#148420=CARTESIAN_POINT ( 'NONE',  ( -3.904385051055635270, 6.538571078664754843, 1.082531754730560403 ) ) ;
#148421=CARTESIAN_POINT ( 'NONE',  ( 8.514157279702022407, 10.95626946445095307, -1.443375672974063439 ) ) ;
#148424=CARTESIAN_POINT ( 'NONE',  ( -5.799137018343247796, 7.788745826199009237, -1.599625672291256295 ) ) ;
#148425=CARTESIAN_POINT ( 'NONE',  ( 1.499999999999989120, 3.525000000000021227, 1.214306433183764966E-14 ) ) ;
#148430=CARTESIAN_POINT ( 'NONE',  ( -7.152089726408780379, 8.302858421353754181, -1.199719254218446718 ) ) ;
#148433=EDGE_LOOP ( 'NONE', ( #55306, #214374, #154135, #63417 ) ) ;
#148434=CARTESIAN_POINT ( 'NONE',  ( 8.500000000000000000, 6.280000000000042881, -2.873333333333334405 ) ) ;
#148443=CARTESIAN_POINT ( 'NONE',  ( -6.566226467720086113, 6.555019055295208119, 1.040834085586084257E-14 ) ) ;
#148446=CARTESIAN_POINT ( 'NONE',  ( 4.365362273920238678, 7.076377838673507448, 1.082531754730558626 ) ) ;
#148451=CARTESIAN_POINT ( 'NONE',  ( -4.273844736805832767, 6.009238164405336313, 1.599625672291267398 ) ) ;
#148459=CARTESIAN_POINT ( 'NONE',  ( -8.850775351622791831, 9.220326086515070685, -0.7998128361456291469 ) ) ;
#148460=CARTESIAN_POINT ( 'NONE',  ( 5.438792177376376991, 9.497007973581119700, 1.040834085586084257E-14 ) ) ;
#148463=CARTESIAN_POINT ( 'NONE',  ( -8.565000355531095622, 11.01558638625153286, -1.599625672291263179 ) ) ;
#148464=CARTESIAN_POINT ( 'NONE',  ( 4.039439701867726384, 6.800097854565950506, 1.199719254218462483 ) ) ;
#148466=ADVANCED_FACE ( 'NONE', ( #178394 ), #156814, .F. ) ;
#148468=CARTESIAN_POINT ( 'NONE',  ( 1.364683531249986537, 0.2177083336747502595, -0.7879004041258309554 ) ) ;
#148471=CARTESIAN_POINT ( 'NONE',  ( 9.273413882067330860, 9.921330405274451536, -0.7216878364870257245 ) ) ;
#148496=CARTESIAN_POINT ( 'NONE',  ( -1.201851678989727383E-14, 0.7437500006828187127, 1.732050807568877637 ) ) ;
#148503=CARTESIAN_POINT ( 'NONE',  ( 10.38962578677386084, 11.01565159419135043, 0.000000000000000000 ) ) ;
#148504=CARTESIAN_POINT ( 'NONE',  ( -1.499999999999997780, 5.181250000682820378, 1.214306433183764966E-14 ) ) ;
#148505=CARTESIAN_POINT ( 'NONE',  ( -0.6823417656250246877, -1.198958332991911790, 1.181850606188755259 ) ) ;
#148508=CARTESIAN_POINT ( 'NONE',  ( 5.684946482831785275, 5.526859072925533134, -0.7998128361456231517 ) ) ;
#148509=CARTESIAN_POINT ( 'NONE',  ( -8.053180056837398126, 8.497724275839514618, 0.7216878364870578100 ) ) ;
#148510=CARTESIAN_POINT ( 'NONE',  ( -5.779651213448679492, 6.079991247305356339, 0.5991391260298760679 ) ) ;
#148513=CARTESIAN_POINT ( 'NONE',  ( -7.751511138711140170, 10.06651563329490529, -1.599625672291263179 ) ) ;
#148515=CARTESIAN_POINT ( 'NONE',  ( -4.921246571636213929, 4.843801876438091902, 0.7216878364870317197 ) ) ;
#148518=CARTESIAN_POINT ( 'NONE',  ( -1.500000000000001332, 0.4312500006828159926, 0.000000000000000000 ) ) ;
#148525=CARTESIAN_POINT ( 'NONE',  ( -4.406036734316898240, 6.163462161501577441, -1.443375672974051449 ) ) ;
#148532=CARTESIAN_POINT ( 'NONE',  ( -9.775592450653132204, 11.36361159963886891, -1.199719254218441611 ) ) ;
#148533=CARTESIAN_POINT ( 'NONE',  ( 7.096803341749390981, 10.36702210109460154, -1.199719254218441611 ) ) ;
#148536=CARTESIAN_POINT ( 'NONE',  ( 1.284279953904121641, 2.800000000000024691, -0.7749999999999892530 ) ) ;
#148537=CARTESIAN_POINT ( 'NONE',  ( -1.500000000000025091, 5.170833333333355597, 0.8660254037844322683 ) ) ;
#148543=CARTESIAN_POINT ( 'NONE',  ( -9.969323024750229578, 10.52529837183042716, -0.7998128361456291469 ) ) ;
#148548=CARTESIAN_POINT ( 'NONE',  ( 4.157546660884947620, 8.002221537674429896, 1.040834085586084257E-14 ) ) ;
#148557=CARTESIAN_POINT ( 'NONE',  ( -1.217358635584794291, 3.191465920220512231, -0.7749999999999883649 ) ) ;
#148558=ORIENTED_EDGE ( 'NONE', *, *, #92359, .F. ) ;
#148567=CARTESIAN_POINT ( 'NONE',  ( -3.815730167242251003, 6.539103397502874948, -1.199719254218452047 ) ) ;
#148573=CARTESIAN_POINT ( 'NONE',  ( 1.499999999999985123, -0.9229166659838452524, -0.8660254037844323793 ) ) ;
#148576=CARTESIAN_POINT ( 'NONE',  ( -1.580000000000721716, 8.674529973576886377, -2.499999999999952038 ) ) ;
#148577=CARTESIAN_POINT ( 'NONE',  ( 2.758194185376297902, 5.305311418659259814, 1.199719254218452047 ) ) ;
#148579=CARTESIAN_POINT ( 'NONE',  ( -3.436101866059630527, 6.096203712789787232, 1.199719254218462483 ) ) ;
#148585=CARTESIAN_POINT ( 'NONE',  ( 3.375617060122621194, 6.882044303544283537, 1.040834085586084257E-14 ) ) ;
#148588=CARTESIAN_POINT ( 'NONE',  ( -1.201851678989727383E-14, 4.759375000341419693, -1.575800808251660134 ) ) ;
#148590=CARTESIAN_POINT ( 'NONE',  ( 2.697709378994964879, 6.091152008895348580, 0.7216878364870338292 ) ) ;
#148598=CARTESIAN_POINT ( 'NONE',  ( -6.123425537405413621, 6.005001634332811200, 0.2246051741978810634 ) ) ;
#148601=CARTESIAN_POINT ( 'NONE',  ( 0.6823417656249899377, 5.488541667008087543, -1.181850606188754593 ) ) ;
#148608=CARTESIAN_POINT ( 'NONE',  ( -1.001543065824772872E-14, 5.212500000000019895, 1.732050807568877637 ) ) ;
#148617=CARTESIAN_POINT ( 'NONE',  ( 1.364683531249990311, 4.696875000341417916, 1.214306433183764966E-14 ) ) ;
#148619=CARTESIAN_POINT ( 'NONE',  ( 6.823831386379729302, 6.855558127064808716, -0.7998128361456281477 ) ) ;
#148620=CARTESIAN_POINT ( 'NONE',  ( -9.826962411806732689, 10.35921099006301382, -0.7998128361456291469 ) ) ;
#148625=ORIENTED_EDGE ( 'NONE', *, *, #30821, .F. ) ;
#148628=CARTESIAN_POINT ( 'NONE',  ( -1.500000000000011324, 5.170833333333356485, 0.8660254037844403729 ) ) ;
#148633=VERTEX_POINT ( 'NONE', #24680 ) ;
#148635=CARTESIAN_POINT ( 'NONE',  ( 7.782016984564049444, 11.06247500109133064, 1.082531754730557072 ) ) ;
#148640=CARTESIAN_POINT ( 'NONE',  ( -1.500000000000013101, 3.910416667349482012, -0.8660254037844313801 ) ) ;
#148642=CARTESIAN_POINT ( 'NONE',  ( -3.405069135326500351, 7.124331091189553433, 1.040834085586084257E-14 ) ) ;
#148643=CARTESIAN_POINT ( 'NONE',  ( 4.053524740361575063, 4.791828954252362216, -1.082531754730543083 ) ) ;
#148651=CARTESIAN_POINT ( 'NONE',  ( 4.871457266011829823, 4.577788319968905562, -0.7998128361456221525 ) ) ;
#148652=CARTESIAN_POINT ( 'NONE',  ( -1.270916165646603035, 2.916024509562820111, -0.7749999999999892530 ) ) ;
#148653=CARTESIAN_POINT ( 'NONE',  ( -1.500000000000022204, 7.388542872122518368, 4.154462424328226433 ) ) ;
#148654=CARTESIAN_POINT ( 'NONE',  ( 3.704402285031850539, 5.344888637335695414, -1.599625672291262513 ) ) ;
#148658=VERTEX_POINT ( 'NONE', #149639 ) ;
#148660=ORIENTED_EDGE ( 'NONE', *, *, #55578, .T. ) ;
#148663=EDGE_CURVE ( 'NONE', #177025, #205532, #155771, .T. ) ;
#148666=CARTESIAN_POINT ( 'NONE',  ( 2.278644679984271892, 5.611497393830711111, -0.5843877675706611319 ) ) ;
#148667=CARTESIAN_POINT ( 'NONE',  ( 4.762865522572231392, 6.775349848016087861, -1.243673390893657471 ) ) ;
#148674=CARTESIAN_POINT ( 'NONE',  ( 1.364683531249984538, -1.094791666325247936, -0.7879004041258309554 ) ) ;
#148675=CARTESIAN_POINT ( 'NONE',  ( 6.534666852106798096, 7.686494751288491578, -1.082531754730543083 ) ) ;
#148676=CARTESIAN_POINT ( 'NONE',  ( -8.500599126088349777, 12.86119004717103209, 1.040834085586084257E-14 ) ) ;
#148682=CARTESIAN_POINT ( 'NONE',  ( -4.952806187693842510, 4.672695395264567786, 0.7998128361456341429 ) ) ;
#148693=CARTESIAN_POINT ( 'NONE',  ( 6.046415161660691595, 6.058605959254545148, 0.4744590674741564484 ) ) ;
#148696=CARTESIAN_POINT ( 'NONE',  ( 4.847203612085560387, 5.613824621309978724, -1.199719254218452047 ) ) ;
#148701=CARTESIAN_POINT ( 'NONE',  ( -7.375272376154077492, 11.54830883891436422, -0.7216878364870267237 ) ) ;
#148705=CARTESIAN_POINT ( 'NONE',  ( 7.100719765255169236, 9.307259030929609267, -1.599625672291262513 ) ) ;
#148706=CARTESIAN_POINT ( 'NONE',  ( -3.262708522383007903, 6.958243709422141876, 1.040834085586084257E-14 ) ) ;
#148707=CARTESIAN_POINT ( 'NONE',  ( 3.999819011231439347, 4.625209253646830554, 1.199719254218464037 ) ) ;
#148709=CARTESIAN_POINT ( 'NONE',  ( -6.586563698140583512, 6.578745824119123675, 1.040834085586084257E-14 ) ) ;
#148710=CARTESIAN_POINT ( 'NONE',  ( 4.681643115420508039, 4.356338477612361260, 0.7998128361456341429 ) ) ;
#148713=CARTESIAN_POINT ( 'NONE',  ( -6.338600509588822263, 7.353787668397130162, -1.199719254218446718 ) ) ;
#148716=CARTESIAN_POINT ( 'NONE',  ( 9.185812768458653466, 10.67553530374532045, 1.199719254218453823 ) ) ;
#148719=CARTESIAN_POINT ( 'NONE',  ( 4.597200498174307981, 6.922409349013787683, -1.201048452015600843 ) ) ;
#148720=CARTESIAN_POINT ( 'NONE',  ( 4.338245966692901412, 8.005111361209628740, -0.7216878364870197293 ) ) ;
#148727=ORIENTED_EDGE ( 'NONE', *, *, #63358, .F. ) ;
#148728=CARTESIAN_POINT ( 'NONE',  ( 6.412643469139427843, 10.42524178073059993, -0.7216878364870267237 ) ) ;
#148729=( BOUNDED_CURVE ( )  B_SPLINE_CURVE ( 2, ( #89699, #155749, #7334, #73411, #156825, #8412, #124399 ),
 .UNSPECIFIED., .F., .T. ) 
 B_SPLINE_CURVE_WITH_KNOTS ( ( 3, 2, 2, 3 ),
 ( 0.07142857142857149400, 0.07738095238095236972, 0.08333333333333324544, 0.08928571428571412116 ),
 .UNSPECIFIED. ) 
 CURVE ( )  GEOMETRIC_REPRESENTATION_ITEM ( )  RATIONAL_B_SPLINE_CURVE ( ( 0.9999999999999984457, 0.8660254037844402619, 1.000000000000000000, 0.8660254037844387076, 1.000000000000000000, 0.8660254037844424824, 0.9999999999999962252 ) ) 
 REPRESENTATION_ITEM ( '' )  );
#148733=CARTESIAN_POINT ( 'NONE',  ( -7.283754839039664475, 9.520799950344851936, -1.599625672291263179 ) ) ;
#148737=CARTESIAN_POINT ( 'NONE',  ( 3.980184376345591968, 7.587372839137763059, -0.2953998019899722882 ) ) ;
#148741=CARTESIAN_POINT ( 'NONE',  ( 7.892817981449907982, 12.36003807833360391, 0.7998128361456462443 ) ) ;
#148745=CARTESIAN_POINT ( 'NONE',  ( 3.011882680530176604, 6.665613560593854459, 0.7998128361456341429 ) ) ;
#148748=CARTESIAN_POINT ( 'NONE',  ( 1.499999999999990896, 3.806250000682819046, 1.214306433183764966E-14 ) ) ;
#148754=CARTESIAN_POINT ( 'NONE',  ( -1.201851678989727383E-14, 1.712500000000019229, 1.732050807568877637 ) ) ;
#148755=CARTESIAN_POINT ( 'NONE',  ( 7.122110765880372618, 7.203550736482235095, 0.7998128361456341429 ) ) ;
#148756=CARTESIAN_POINT ( 'NONE',  ( 4.568734577680873876, 6.353276312092901890, -1.443375672974051449 ) ) ;
#148759=CARTESIAN_POINT ( 'NONE',  ( 7.565086526745395723, 10.80938946696957004, -1.082531754730543083 ) ) ;
#148764=CARTESIAN_POINT ( 'NONE',  ( -2.740719608256871442, 6.349256642941639051, 0.7998128361456341429 ) ) ;
#148765=CARTESIAN_POINT ( 'NONE',  ( 0.7499999999999920064, 5.514583334016151639, 1.299038105676669330 ) ) ;
#148766=CARTESIAN_POINT ( 'NONE',  ( -1.402160292154681736E-14, 0.3218750003414227456, 1.575800808251672791 ) ) ;
#148770=CARTESIAN_POINT ( 'NONE',  ( 3.684065054611349144, 5.321161868511784299, -1.599625672291262513 ) ) ;
#148772=CARTESIAN_POINT ( 'NONE',  ( -1.364683531249997417, 5.571875000341417916, 1.214306433183764966E-14 ) ) ;
#148779=CARTESIAN_POINT ( 'NONE',  ( -7.888146445052511169, 8.097259028849730811, 1.040834085586084257E-14 ) ) ;
#148780=CARTESIAN_POINT ( 'NONE',  ( 3.683011284406639607, 7.448596931783069586, 0.7998128361456321445 ) ) ;
#148783=CARTESIAN_POINT ( 'NONE',  ( 0.6823417656249864960, -1.073958332991911568, -1.181850606188749264 ) ) ;
#148785=ORIENTED_EDGE ( 'NONE', *, *, #182043, .F. ) ;
#148790=CARTESIAN_POINT ( 'NONE',  ( -5.018489415352746619, 9.006654751220198207, 0.7998128361456481317 ) ) ;
#148794=CARTESIAN_POINT ( 'NONE',  ( 8.380911511541880188, 12.92948053010758258, 0.7998128361456462443 ) ) ;
#148796=CARTESIAN_POINT ( 'NONE',  ( 8.860417081730671995, 10.29590700256267155, 1.199719254218453823 ) ) ;
#148797=CARTESIAN_POINT ( 'NONE',  ( 3.344425985610775864, 6.383782420805063751, 0.9919173777418579530 ) ) ;
#148798=CARTESIAN_POINT ( 'NONE',  ( -3.898132859128961236, 4.506575409527250997, -1.199719254218452047 ) ) ;
#148800=CARTESIAN_POINT ( 'NONE',  ( -6.995117189646935962, 10.24838825697502109, 1.199719254218453823 ) ) ;
#148803=CARTESIAN_POINT ( 'NONE',  ( -5.283800884368243800, 6.573997454655339467, 1.390413726763789937 ) ) ;
#148804=CARTESIAN_POINT ( 'NONE',  ( -0.6823417656250003738, 0.7177083336747519526, -1.181850606188749264 ) ) ;
#148808=CARTESIAN_POINT ( 'NONE',  ( 6.968527767744088663, 11.07377346243604599, 0.7216878364870438212 ) ) ;
#148826=CARTESIAN_POINT ( 'NONE',  ( 8.374132434735052755, 12.92157160716627295, -0.7998128361456352531 ) ) ;
#148828=ORIENTED_EDGE ( 'NONE', *, *, #171612, .T. ) ;
#148830=CARTESIAN_POINT ( 'NONE',  ( -3.978428010606240850, 6.728917548094202949, -1.199719254218452047 ) ) ;
#148831=CARTESIAN_POINT ( 'NONE',  ( -8.507905087775398556, 9.884643009614800135, 1.199719254218462483 ) ) ;
#148837=CARTESIAN_POINT ( 'NONE',  ( 1.499999999999989120, 3.035416667349485564, 0.8660254037844524744 ) ) ;
#148838=CARTESIAN_POINT ( 'NONE',  ( 7.727257484784855635, 11.10255193463598111, -1.199719254218446718 ) ) ;
#148842=CARTESIAN_POINT ( 'NONE',  ( -7.669108446824431269, 12.09904362127053545, -0.7998128361456291469 ) ) ;
#148844=CARTESIAN_POINT ( 'NONE',  ( -1.364683531250012516, 3.530208333674758059, 0.7879004041258379498 ) ) ;
#148850=CARTESIAN_POINT ( 'NONE',  ( -4.451154503988200339, 4.087435097607984957, 1.214306433183764966E-14 ) ) ;
#148855=CARTESIAN_POINT ( 'NONE',  ( -1.364683531250012516, 1.092708333674754506, 0.7879004041258379498 ) ) ;
#148860=EDGE_CURVE ( 'NONE', #71636, #179842, #183361, .T. ) ;
#148861=CARTESIAN_POINT ( 'NONE',  ( 1.364683531249986537, 1.113541667008082658, 0.7879004041258500513 ) ) ;
#148863=CARTESIAN_POINT ( 'NONE',  ( -4.791917227426195858, 7.677988301050826969, -1.199719254218452047 ) ) ;
#148864=CARTESIAN_POINT ( 'NONE',  ( 5.750629710490689384, 9.860818428881154674, -0.7998128361456291469 ) ) ;
#148865=CARTESIAN_POINT ( 'NONE',  ( 0.000000000000000000, 6.468705557303652931, -4.925226524755051294 ) ) ;
#148867=CARTESIAN_POINT ( 'NONE',  ( -0.7500000000000215383, 4.441666666666691299, 1.299038105676671107 ) ) ;
#148868=CARTESIAN_POINT ( 'NONE',  ( -1.402160292154681736E-14, 2.509375000341417028, -1.575800808251660134 ) ) ;
#148872=CARTESIAN_POINT ( 'NONE',  ( -6.426201623197489887, 6.599582769926260362, 0.7216878364870317197 ) ) ;
#148874=ADVANCED_FACE ( 'NONE', ( #92927 ), #209827, .F. ) ;
#148877=CARTESIAN_POINT ( 'NONE',  ( 6.317736394288147039, 6.473040002865377396, 0.7216878364870317197 ) ) ;
#148880=CARTESIAN_POINT ( 'NONE',  ( -8.015895134177625891, 10.37496362800581018, 1.599625672291295375 ) ) ;
#148881=CARTESIAN_POINT ( 'NONE',  ( -8.649738815838677652, 13.03518635187974262, 0.7216878364870357165 ) ) ;
#148882=DIRECTION ( 'NONE',  ( 7.387867266669436732E-31, -1.000000000000000000, -8.546850786086424434E-32 ) ) ;
#148883=CARTESIAN_POINT ( 'NONE',  ( 1.364683531249992088, 5.634375000341417916, 1.214306433183764966E-14 ) ) ;
#148888=CARTESIAN_POINT ( 'NONE',  ( -7.687109908824056426, 8.070642436490613747, 0.7216878364870438212 ) ) ;
#148890=CARTESIAN_POINT ( 'NONE',  ( 0.6823417656249882723, -0.5947916663252492686, 1.181850606188755259 ) ) ;
#148893=CARTESIAN_POINT ( 'NONE',  ( 7.944714827928050838, 9.331550723079971021, 1.082531754730558626 ) ) ;
#148899=CARTESIAN_POINT ( 'NONE',  ( -4.257741265285667431, 3.982435197156672491, 0.4597581080974452727 ) ) ;
#148902=CARTESIAN_POINT ( 'NONE',  ( 9.042925270190625753, 11.57316545335434199, 1.443375672974076540 ) ) ;
#148909=CARTESIAN_POINT ( 'NONE',  ( 7.461064606222022277, 7.598996883547496139, 1.040834085586084257E-14 ) ) ;
#148910=CARTESIAN_POINT ( 'NONE',  ( -3.906720819032141190, 7.709591388846142479, -0.7998128361456281477 ) ) ;
#148913=CARTESIAN_POINT ( 'NONE',  ( 6.453317929980448397, 6.631218461173066459, 1.040834085586084257E-14 ) ) ;
#148915=CARTESIAN_POINT ( 'NONE',  ( -1.402160292154681736E-14, 0.6343750003414162508, 1.575800808251672791 ) ) ;
#148916=CARTESIAN_POINT ( 'NONE',  ( 3.063779527008311021, 5.557864633942907417, 1.082531754730546636 ) ) ;
#148917=CARTESIAN_POINT ( 'NONE',  ( -10.32183501870554387, 10.93656236477829502, 0.7998128361456462443 ) ) ;
#148935=CARTESIAN_POINT ( 'NONE',  ( 6.012151052656117933, 9.101594430485762999, 1.199719254218460707 ) ) ;
#148936=CARTESIAN_POINT ( 'NONE',  ( 5.770966940911189447, 9.884545197705074671, -0.7998128361456291469 ) ) ;
#148945=DIRECTION ( 'NONE',  ( 1.000000000000000000, 0.000000000000000000, 0.000000000000000000 ) ) ;
#148948=CARTESIAN_POINT ( 'NONE',  ( -6.600121851754250812, 6.594563670001734046, 0.7998128361456341429 ) ) ;
#148952=CARTESIAN_POINT ( 'NONE',  ( -1.127943160727153060, 3.300000000000025135, -0.7749999999999935829 ) ) ;
#148958=CARTESIAN_POINT ( 'NONE',  ( -9.490344339885977476, 11.13478515369756217, -1.082531754730539753 ) ) ;
#148961=CARTESIAN_POINT ( 'NONE',  ( 7.284808609244363353, 7.393364887073558656, 0.7998128361456341429 ) ) ;
#148962=CARTESIAN_POINT ( 'NONE',  ( 0.6823417656249899377, 5.426041667008087543, -1.181850606188754593 ) ) ;
#148967=CARTESIAN_POINT ( 'NONE',  ( 4.107757354816228279, 6.775838766385488654, -1.082531754730548412 ) ) ;
#148968=CARTESIAN_POINT ( 'NONE',  ( -6.449928391799210736, 8.548002428564306143, -1.599625672291263179 ) ) ;
#148972=CARTESIAN_POINT ( 'NONE',  ( -5.181187258716735577, 9.196468901811520880, 0.7998128361456481317 ) ) ;
#148973=CARTESIAN_POINT ( 'NONE',  ( -5.108724954250998707, 4.854600622914589714, -0.7998128361456221525 ) ) ;
#148974=DIRECTION ( 'NONE',  ( 0.000000000000000000, 8.546850786086437571E-32, 1.000000000000000000 ) ) ;
#148977=DIRECTION ( 'NONE',  ( 0.6507913734559640506, -0.7592566023653004592, 0.000000000000000000 ) ) ;
#148980=CARTESIAN_POINT ( 'NONE',  ( 4.788000803920411386, 8.737751371215816576, 1.040834085586084257E-14 ) ) ;
#148991=ORIENTED_EDGE ( 'NONE', *, *, #19510, .F. ) ;
#148993=CARTESIAN_POINT ( 'NONE',  ( -1.364683531250000748, 0.5718750003414208027, 0.000000000000000000 ) ) ;
#148994=CARTESIAN_POINT ( 'NONE',  ( 2.835626683552519012, 6.459981564119914310, 0.000000000000000000 ) ) ;
#148995=CARTESIAN_POINT ( 'NONE',  ( 6.193377243344257543, 6.120028293523423812, -0.7998128361456281477 ) ) ;
#148997=CARTESIAN_POINT ( 'NONE',  ( -6.670248388243482651, 9.765411638717282017, 1.082531754730548412 ) ) ;
#148999=CARTESIAN_POINT ( 'NONE',  ( 4.514501963670558560, 8.210743357683563559, 1.040834085586084257E-14 ) ) ;
#149000=CARTESIAN_POINT ( 'NONE',  ( -6.168596704093453731, 10.14052055484361325, 0.7216878364870458196 ) ) ;
#149005=CARTESIAN_POINT ( 'NONE',  ( 7.623762449586013901, 7.788811034138823253, 1.040834085586084257E-14 ) ) ;
#149010=CARTESIAN_POINT ( 'NONE',  ( 1.364683531249988535, 3.113541667008083991, 0.7879004041258500513 ) ) ;
#149015=EDGE_CURVE ( 'NONE', #123589, #138847, #27899, .T. ) ;
#149016=CARTESIAN_POINT ( 'NONE',  ( 6.611572464958476836, 10.86525164242692298, 0.7998128361456462443 ) ) ;
#149020=CARTESIAN_POINT ( 'NONE',  ( -9.013473194986783454, 9.410140237106395134, -0.7998128361456291469 ) ) ;
#149026=CARTESIAN_POINT ( 'NONE',  ( 9.348510611822643313, 10.86534945433664134, 1.199719254218453823 ) ) ;
#149028=CARTESIAN_POINT ( 'NONE',  ( -9.013473194986783454, 9.410140237106395134, -0.7998128361456291469 ) ) ;
#149031=CARTESIAN_POINT ( 'NONE',  ( 4.597200498174307981, 6.922409349013787683, -1.201048452015600843 ) ) ;
#149032=CARTESIAN_POINT ( 'NONE',  ( -4.464712657601869417, 4.103252943490596216, 0.7998128361456341429 ) ) ;
#149038=CARTESIAN_POINT ( 'NONE',  ( 4.964256800898067645, 8.943383367689749619, 0.7998128361456462443 ) ) ;
#149040=CARTESIAN_POINT ( 'NONE',  ( 5.823390672269506574, 6.752709524857930745, -1.199719254218446718 ) ) ;
#149041=CARTESIAN_POINT ( 'NONE',  ( -4.029167574269930441, 7.605081013511371779, 0.2528308249854539502 ) ) ;
#149042=CARTESIAN_POINT ( 'NONE',  ( 3.822509244049070887, 6.547012320444182798, -1.199719254218452047 ) ) ;
#149044=CARTESIAN_POINT ( 'NONE',  ( -6.371969008742801144, 10.37778824360119145, 0.7216878364870458196 ) ) ;
#149050=CARTESIAN_POINT ( 'NONE',  ( -4.373759202716216876, 7.180157790548314267, -1.044885312346154782 ) ) ;
#149051=CARTESIAN_POINT ( 'NONE',  ( -0.6823417656250003738, -0.7197916663252492686, -1.181850606188749264 ) ) ;
#149054=CARTESIAN_POINT ( 'NONE',  ( 4.365362273920244007, 6.116008624372160973, 1.443375672974062551 ) ) ;
#149058=EDGE_CURVE ( 'NONE', #171990, #57016, #72493, .T. ) ;
#149060=CARTESIAN_POINT ( 'NONE',  ( -9.070041577417988776, 12.56517035942090388, 1.082531754730558626 ) ) ;
#149066=CARTESIAN_POINT ( 'NONE',  ( -10.11401940567025548, 10.90203684947788076, 1.040834085586084257E-14 ) ) ;
#149072=EDGE_LOOP ( 'NONE', ( #170566, #177858, #204102, #133754 ) ) ;
#149073=CARTESIAN_POINT ( 'NONE',  ( -9.964879715919934711, 10.72804054476916313, 0.7216878364870438212 ) ) ;
#149079=CARTESIAN_POINT ( 'NONE',  ( 1.499999999999987121, 3.077083334016149863, -0.8660254037844262731 ) ) ;
#149081=CARTESIAN_POINT ( 'NONE',  ( -5.018489415352746619, 9.006654751220198207, 0.7998128361456481317 ) ) ;
#149084=CARTESIAN_POINT ( 'NONE',  ( -9.182950115157607840, 9.607863310639020327, 0.7998128361456462443 ) ) ;
#149087=CARTESIAN_POINT ( 'NONE',  ( 6.796715079152391148, 6.823922435299587974, 0.7998128361456341429 ) ) ;
#149088=EDGE_CURVE ( 'NONE', #25476, #63977, #181614, .T. ) ;
#149092=CARTESIAN_POINT ( 'NONE',  ( 9.121938423896107651, 9.536683004167278099, -0.7998128361456221525 ) ) ;
#149101=CARTESIAN_POINT ( 'NONE',  ( -7.266807147244793263, 8.540658428949452485, 1.082531754730549967 ) ) ;
#149107=CARTESIAN_POINT ( 'NONE',  ( -1.364683531250012516, 4.988541667008084879, -0.7879004041258300672 ) ) ;
#149111=CARTESIAN_POINT ( 'NONE',  ( -4.433153041544240835, 4.274359424664112339, 0.7216878364870317197 ) ) ;
#149113=CARTESIAN_POINT ( 'NONE',  ( 8.992082194361556091, 11.51384853155376220, 1.599625672291279388 ) ) ;
#149114=CARTESIAN_POINT ( 'NONE',  ( -9.317477881089553549, 11.89347683273641820, 1.599625672291281386 ) ) ;
#149117=CARTESIAN_POINT ( 'NONE',  ( 0.6823417656249899377, 2.342708333674753618, 1.181850606188767472 ) ) ;
#149118=CARTESIAN_POINT ( 'NONE',  ( 3.497113557321089861, 6.167384019261527683, -1.199719254218446718 ) ) ;
#149124=CARTESIAN_POINT ( 'NONE',  ( -4.183485216215313329, 3.563207579971348515, -2.499999999999995115 ) ) ;
#149126=CARTESIAN_POINT ( 'NONE',  ( 9.042925270190622200, 12.53353466765568669, 1.082531754730546636 ) ) ;
#149129=CARTESIAN_POINT ( 'NONE',  ( -8.080296364064746939, 9.489729181906076505, 1.082531754730558626 ) ) ;
#149133=CARTESIAN_POINT ( 'NONE',  ( -9.169391961543940539, 9.592045464756413509, 1.040834085586084257E-14 ) ) ;
#149134=CARTESIAN_POINT ( 'NONE',  ( -3.741687207247254676, 7.309126141856352454, 1.040834085586084257E-14 ) ) ;
#149135=CARTESIAN_POINT ( 'NONE',  ( 0.6823417656249899377, 3.488541667008085323, -1.181850606188754593 ) ) ;
#149139=( BOUNDED_CURVE ( )  B_SPLINE_CURVE ( 2, ( #33293, #180612, #1839, #17026, #200052, #181666, #149183 ),
 .UNSPECIFIED., .F., .T. ) 
 B_SPLINE_CURVE_WITH_KNOTS ( ( 3, 2, 2, 3 ),
 ( 0.4316551096257628672, 0.4345238095238095344, 0.4404761904761904656, 0.4428956208513696868 ),
 .UNSPECIFIED. ) 
 CURVE ( )  GEOMETRIC_REPRESENTATION_ITEM ( )  RATIONAL_B_SPLINE_CURVE ( ( 0.9331000818465632340, 0.9354320710352570512, 1.000000000000000000, 0.8660254037844387076, 1.000000000000000000, 0.9455441091255019082, 0.9353569697113766068 ) ) 
 REPRESENTATION_ITEM ( '' )  );
#149151=CARTESIAN_POINT ( 'NONE',  ( -2.277406616971334508, 5.600798786534425311, 1.040834085586084257E-14 ) ) ;
#149156=ADVANCED_FACE ( 'NONE', ( #192514 ), #133918, .F. ) ;
#149157=CARTESIAN_POINT ( 'NONE',  ( -1.201851678989727383E-14, 4.009375000341416140, -1.575800808251660134 ) ) ;
#149161=EDGE_CURVE ( 'NONE', #63704, #49215, #3196, .T. ) ;
#149162=CARTESIAN_POINT ( 'NONE',  ( -5.974410882859528371, 4.760127796209656204, -2.438793965253434060 ) ) ;
#149165=CARTESIAN_POINT ( 'NONE',  ( 9.921869487102386032, 10.46993591124128997, 0.000000000000000000 ) ) ;
#149168=CARTESIAN_POINT ( 'NONE',  ( 0.6823417656249882723, 2.676041667008084879, -1.181850606188749264 ) ) ;
#149170=CARTESIAN_POINT ( 'NONE',  ( -7.537970219518091319, 7.896646132300314314, -0.7216878364870278340 ) ) ;
#149172=CARTESIAN_POINT ( 'NONE',  ( 1.499999999999823475, 7.438721522839173872, 4.195160983902624707 ) ) ;
#149179=CARTESIAN_POINT ( 'NONE',  ( 4.599240423533799138, 6.388866465587984322, 1.599625672291267398 ) ) ;
#149182=CARTESIAN_POINT ( 'NONE',  ( 8.757677159423465696, 12.30470822171437284, 1.199719254218450271 ) ) ;
#149183=CARTESIAN_POINT ( 'NONE',  ( 1.217526595471194906, 2.800000000000017586, -0.8761443883974121549 ) ) ;
#149188=ORIENTED_EDGE ( 'NONE', *, *, #76938, .T. ) ;
#149190=CARTESIAN_POINT ( 'NONE',  ( -4.295235737431041478, 3.905529869957963029, -0.7998128361456221525 ) ) ;
#149191=( BOUNDED_CURVE ( )  B_SPLINE_CURVE ( 2, ( #113308, #179314, #81794, #80738, #212846, #196617, #48256 ),
 .UNSPECIFIED., .F., .T. ) 
 B_SPLINE_CURVE_WITH_KNOTS ( ( 3, 2, 2, 3 ),
 ( 0.1785714285714287142, 0.1845238095238095899, 0.1904761904761904656, 0.1964285714285713413 ),
 .UNSPECIFIED. ) 
 CURVE ( )  GEOMETRIC_REPRESENTATION_ITEM ( )  RATIONAL_B_SPLINE_CURVE ( ( 0.9999999999999968914, 0.8660254037844418162, 1.000000000000000000, 0.8660254037844387076, 1.000000000000000000, 0.8660254037844405950, 0.9999999999999981126 ) ) 
 REPRESENTATION_ITEM ( '' )  );
#149192=CARTESIAN_POINT ( 'NONE',  ( 7.904567251967224095, 9.180748867838630645, 1.199719254218462483 ) ) ;
#149194=CARTESIAN_POINT ( 'NONE',  ( 4.704316113817540668, 5.551085556617666228, -1.082531754730548412 ) ) ;
#149203=CARTESIAN_POINT ( 'NONE',  ( -5.585596099150174965, 9.460353182409786399, -0.7216878364870207285 ) ) ;
#149204=CARTESIAN_POINT ( 'NONE',  ( 5.657830175604453338, 5.495223381160312393, 0.7998128361456341429 ) ) ;
#149207=CARTESIAN_POINT ( 'NONE',  ( -9.020252271793614440, 9.418049160047695878, 0.7998128361456462443 ) ) ;
#149212=CARTESIAN_POINT ( 'NONE',  ( -3.216308754939891212, 4.775446185561722956, -1.599625672291262513 ) ) ;
#149216=CARTESIAN_POINT ( 'NONE',  ( 7.099665995050449041, 11.43469409420089455, 0.7998128361456462443 ) ) ;
#149217=CARTESIAN_POINT ( 'NONE',  ( 3.728655938958122196, 4.308852335994623139, -1.199719254218446718 ) ) ;
#149223=DIRECTION ( 'NONE',  ( 1.000000000000000000, -7.387867266669436732E-31, 0.000000000000000000 ) ) ;
#149226=CARTESIAN_POINT ( 'NONE',  ( -2.605138072120212200, 6.191078184115536232, -0.7998128361456281477 ) ) ;
#149229=CARTESIAN_POINT ( 'NONE',  ( -9.155833807930273238, 9.576227618873799585, -0.7998128361456291469 ) ) ;
#149234=CARTESIAN_POINT ( 'NONE',  ( 6.643132081016105417, 10.69414516125339887, 0.7216878364870438212 ) ) ;
#149235=CARTESIAN_POINT ( 'NONE',  ( -1.364683531250010740, 5.301041667008085767, -0.7879004041258300672 ) ) ;
#149237=CARTESIAN_POINT ( 'NONE',  ( 2.846322183865124700, 5.408127416896231665, -1.199719254218446718 ) ) ;
#149240=CARTESIAN_POINT ( 'NONE',  ( -6.201965203247477909, 9.323044272842313518, 1.199719254218452047 ) ) ;
#149254=CARTESIAN_POINT ( 'NONE',  ( -1.364683531250012516, 4.051041667008088432, -0.7879004041258300672 ) ) ;
#149255=CARTESIAN_POINT ( 'NONE',  ( 8.432281472695482449, 11.92507992053172572, 1.199719254218450271 ) ) ;
#149257=CARTESIAN_POINT ( 'NONE',  ( -6.087247782855839340, 6.204136622861004646, 0.000000000000000000 ) ) ;
#149258=CARTESIAN_POINT ( 'NONE',  ( -5.056828107772872727, 5.001980335264194721, -0.7216878364870197293 ) ) ;
#149265=CARTESIAN_POINT ( 'NONE',  ( 5.169736645512481132, 4.925780929386339935, 0.7998128361456341429 ) ) ;
#149274=CARTESIAN_POINT ( 'NONE',  ( 4.330940004561544043, 7.140181541042074365, -1.199719254218452047 ) ) ;
#149278=CARTESIAN_POINT ( 'NONE',  ( -4.577849422908604637, 8.492574760035358494, -0.7998128361456281477 ) ) ;
#149282=CARTESIAN_POINT ( 'NONE',  ( 4.937140493670735708, 8.911747675924535983, -0.7998128361456281477 ) ) ;
#149285=CARTESIAN_POINT ( 'NONE',  ( -4.740547266272593596, 8.682388910626682943, -0.7998128361456281477 ) ) ;
#149287=CARTESIAN_POINT ( 'NONE',  ( 1.499999999999987121, 2.004166666666684637, 0.8660254037844524744 ) ) ;
#149289=CARTESIAN_POINT ( 'NONE',  ( -3.113568832632681360, 6.784247404713427798, -0.7998128361456281477 ) ) ;
#149292=CARTESIAN_POINT ( 'NONE',  ( -5.922214171070950606, 5.803671375871217286, -0.7998128361456291469 ) ) ;
#149295=CARTESIAN_POINT ( 'NONE',  ( -0.6823417656250003738, 2.967708333674754062, -1.181850606188749264 ) ) ;
#149297=CARTESIAN_POINT ( 'NONE',  ( -6.100805936469506641, 6.219954468743612352, 0.7216878364870317197 ) ) ;
#149303=CARTESIAN_POINT ( 'NONE',  ( 3.655894977179307226, 7.416961240017848844, -0.7998128361456291469 ) ) ;
#149306=CARTESIAN_POINT ( 'NONE',  ( 1.364683531249986537, 2.217708333674751398, -0.7879004041258239610 ) ) ;
#149308=CARTESIAN_POINT ( 'NONE',  ( 2.683624340501134853, 5.218313266304903664, -1.199719254218446718 ) ) ;
#149310=ADVANCED_FACE ( 'NONE', ( #65691 ), #195553, .F. ) ;
#149311=CARTESIAN_POINT ( 'NONE',  ( -1.364683531250000748, -0.6781249996585803075, 0.000000000000000000 ) ) ;
#149312=CARTESIAN_POINT ( 'NONE',  ( 1.419999999999989049, 6.200000000000045475, -2.899999999999995470 ) ) ;
#149315=CARTESIAN_POINT ( 'NONE',  ( -4.457933580795036654, 4.095344020549286590, -0.7998128361456221525 ) ) ;
#149316=CARTESIAN_POINT ( 'NONE',  ( -6.900736999231456004, 8.113576589600553390, 1.082531754730549967 ) ) ;
#149319=ORIENTED_EDGE ( 'NONE', *, *, #211516, .T. ) ;
#149320=CARTESIAN_POINT ( 'NONE',  ( 1.364683531249990311, 2.634375000341422801, 1.214306433183764966E-14 ) ) ;
#149328=CARTESIAN_POINT ( 'NONE',  ( -6.358410854684783509, 9.401601182898824405, -1.082531754730537976 ) ) ;
#149334=CARTESIAN_POINT ( 'NONE',  ( -5.205967797523171292, 9.017453497178271604, 0.000000000000000000 ) ) ;
#149347=CARTESIAN_POINT ( 'NONE',  ( -5.422371370461663176, 8.413518134592214537, -1.199719254218446718 ) ) ;
#149349=CARTESIAN_POINT ( 'NONE',  ( 1.499999999999985123, -0.4541666666666469010, -0.8660254037844323793 ) ) ;
#149350=CARTESIAN_POINT ( 'NONE',  ( 4.518945272056516416, 4.166524327021037699, 0.7998128361456341429 ) ) ;
#149355=CARTESIAN_POINT ( 'NONE',  ( 4.873266149108180123, 7.772895376346490970, 1.199719254218462483 ) ) ;
#149361=CARTESIAN_POINT ( 'NONE',  ( -4.799223189557577207, 4.701441264013013210, 0.7216878364870317197 ) ) ;
#149364=FACE_OUTER_BOUND ( 'NONE', #181040, .T. ) ;
#149368=CARTESIAN_POINT ( 'NONE',  ( 1.364683531249986537, 2.155208333674751398, -0.7879004041258239610 ) ) ;
#149369=CARTESIAN_POINT ( 'NONE',  ( 8.527715432871318058, 12.89282573841782664, -0.7216878364870338292 ) ) ;
#149370=CARTESIAN_POINT ( 'NONE',  ( -6.191269702934848240, 10.37489842006599616, 0.000000000000000000 ) ) ;
#149373=CARTESIAN_POINT ( 'NONE',  ( 6.388916700537700777, 8.476822122092563916, 1.599625672291281386 ) ) ;
#149374=CARTESIAN_POINT ( 'NONE',  ( -6.418895661066105873, 9.576129806964074120, -1.199719254218440723 ) ) ;
#149377=CARTESIAN_POINT ( 'NONE',  ( 0.7499999999999885647, -0.4854166659838468623, 1.299038105676657340 ) ) ;
#149380=CARTESIAN_POINT ( 'NONE',  ( 9.259855728453651125, 9.905512559391842942, 1.040834085586084257E-14 ) ) ;
#149384=CARTESIAN_POINT ( 'NONE',  ( 1.364683531249988757, 1.196875000341421469, 0.000000000000000000 ) ) ;
#149386=CARTESIAN_POINT ( 'NONE',  ( 6.114364089638782751, 9.116879957011832403, 1.082531754730558626 ) ) ;
#149390=CARTESIAN_POINT ( 'NONE',  ( -4.365362273920257330, 6.116008624372160973, 1.443375672974064550 ) ) ;
#149392=CARTESIAN_POINT ( 'NONE',  ( 0.6823417656249917140, 5.092708333674749177, 1.181850606188765695 ) ) ;
#149403=CARTESIAN_POINT ( 'NONE',  ( 7.121056995675668411, 9.330985799753529264, -1.599625672291262513 ) ) ;
#149408=CARTESIAN_POINT ( 'NONE',  ( 3.388648328411762556, 6.040841252200647382, 1.199719254218462483 ) ) ;
#149414=CARTESIAN_POINT ( 'NONE',  ( 5.558479791922850133, 6.547609847740540445, -1.082531754730542195 ) ) ;
#149415=CARTESIAN_POINT ( 'NONE',  ( 0.6823417656249899377, 1.155208333674752286, 1.181850606188755259 ) ) ;
#149421=CARTESIAN_POINT ( 'NONE',  ( -1.500000000000013101, -0.07916666666664513852, 0.8660254037844403729 ) ) ;
#149422=CARTESIAN_POINT ( 'NONE',  ( 6.938021921891177612, 9.117444880338284818, -1.599625672291262513 ) ) ;
#149423=CARTESIAN_POINT ( 'NONE',  ( -6.679363233026820446, 10.94434087183997129, 0.000000000000000000 ) ) ;
#149427=CARTESIAN_POINT ( 'NONE',  ( -0.6823417656250003738, 1.717708333674752730, -1.181850606188749264 ) ) ;
#149428=CARTESIAN_POINT ( 'NONE',  ( 0.7499999999999902300, 2.233333333333351156, 1.299038105676669330 ) ) ;
#149430=CARTESIAN_POINT ( 'NONE',  ( 5.183294799126148433, 4.941598775268944976, 1.040834085586084257E-14 ) ) ;
#149438=CARTESIAN_POINT ( 'NONE',  ( 1.499999999999987121, -0.4645833326505149907, 0.8660254037844524744 ) ) ;
#149439=CARTESIAN_POINT ( 'NONE',  ( -8.193204901359996128, 8.453160561208463264, 1.040834085586084257E-14 ) ) ;
#149440=CARTESIAN_POINT ( 'NONE',  ( -3.904385051055635270, 6.538571078664754843, 1.082531754730560403 ) ) ;
#149448=CARTESIAN_POINT ( 'NONE',  ( 7.070740804726770357, 8.207951346058097286, 1.199719254218462483 ) ) ;
#149453=CARTESIAN_POINT ( 'NONE',  ( 7.931156673870037643, 8.355363662377600420, -0.7216878364870267237 ) ) ;
#149454=CARTESIAN_POINT ( 'NONE',  ( 1.419999999999989049, 6.280000000000035776, 2.775557561562891351E-14 ) ) ;
#149457=CARTESIAN_POINT ( 'NONE',  ( -7.182068686937172153, 9.402166106225269715, 1.599625672291283607 ) ) ;
#149458=CARTESIAN_POINT ( 'NONE',  ( 3.032219910950674890, 6.689340329417765574, 0.7998128361456321445 ) ) ;
#149464=CARTESIAN_POINT ( 'NONE',  ( 8.866669273657322492, 12.32790267170016207, -1.082531754730543083 ) ) ;
#149473=CARTESIAN_POINT ( 'NONE',  ( -1.579999999999998073, 8.674529973577531194, -2.499999999999990230 ) ) ;
#149474=CARTESIAN_POINT ( 'NONE',  ( -4.961921032921567054, 4.891255414604337659, 0.7216878364870317197 ) ) ;
#149475=CARTESIAN_POINT ( 'NONE',  ( 8.215877900201359552, 11.56864606933486606, -1.082531754730543083 ) ) ;
#149478=CARTESIAN_POINT ( 'NONE',  ( -6.067437437315529536, 7.037430750744921859, 1.199719254218450271 ) ) ;
#149479=DIRECTION ( 'NONE',  ( -1.000000000000000000, 5.578564026256490882E-16, 2.058387550816952846E-48 ) ) ;
#149484=CARTESIAN_POINT ( 'NONE',  ( -5.845536785786364931, 9.971543350059432598, 0.000000000000000000 ) ) ;
#149487=CARTESIAN_POINT ( 'NONE',  ( -0.1399574524686796051, 8.210952333604124576, 2.038660652713628618 ) ) ;
#149489=DIRECTION ( 'NONE',  ( -0.6507913734559642727, -0.7592566023653003482, -2.775557561562895049E-17 ) ) ;
#149490=ORIENTED_EDGE ( 'NONE', *, *, #44167, .F. ) ;
#149499=CARTESIAN_POINT ( 'NONE',  ( -5.530836599371015794, 8.540060901653093950, 1.199719254218452047 ) ) ;
#149502=CARTESIAN_POINT ( 'NONE',  ( 5.368665641331531013, 5.365790791082654998, -0.7216878364870207285 ) ) ;
#149507=CARTESIAN_POINT ( 'NONE',  ( -2.774614992291035698, 6.388801257648172971, 1.040834085586084257E-14 ) ) ;
#149515=CARTESIAN_POINT ( 'NONE',  ( -8.148614017013223076, 9.465470093725620870, -1.199719254218446718 ) ) ;
#149516=CARTESIAN_POINT ( 'NONE',  ( 5.341022448779654930, 8.318611059296550536, 1.199719254218462483 ) ) ;
#149519=CARTESIAN_POINT ( 'NONE',  ( -9.169391961543940539, 9.592045464756413509, 1.040834085586084257E-14 ) ) ;
#149520=CARTESIAN_POINT ( 'NONE',  ( 5.465584804120450002, 6.402597129658848196, -1.225016630617669744 ) ) ;
#149522=CARTESIAN_POINT ( 'NONE',  ( 3.332481584934672281, 7.719208080883574574, -2.450691333334232613 ) ) ;
#149523=CARTESIAN_POINT ( 'NONE',  ( -0.6823417656250246877, 0.6135416670080897639, 1.181850606188755259 ) ) ;
#149526=CARTESIAN_POINT ( 'NONE',  ( 8.920901888112002354, 9.510066412326583674, 0.7216878364870438212 ) ) ;
#149534=CARTESIAN_POINT ( 'NONE',  ( 0.08113548435146850091, 6.430127061359857343, -3.206836081813071004 ) ) ;
#149553=CARTESIAN_POINT ( 'NONE',  ( 1.499999999999987121, 0.07708333401615156955, -0.8660254037844323793 ) ) ;
#149558=CARTESIAN_POINT ( 'NONE',  ( -6.385527162356468445, 10.39360608948380538, 1.040834085586084257E-14 ) ) ;
#149561=CARTESIAN_POINT ( 'NONE',  ( 10.21336978979620191, 10.81001959771741205, 0.7998128361456462443 ) ) ;
#149567=CARTESIAN_POINT ( 'NONE',  ( 4.467575310902914154, 5.170924936596891008, 1.199719254218464037 ) ) ;
#149568=CARTESIAN_POINT ( 'NONE',  ( -5.910991785878158211, 9.839981483592442402, -0.7216878364870278340 ) ) ;
#149569=CARTESIAN_POINT ( 'NONE',  ( -5.811497925844209433, 6.060560459143458978, 0.5261113891226586459 ) ) ;
#149570=CARTESIAN_POINT ( 'NONE',  ( 8.380911511541880188, 12.92948053010758258, 0.7998128361456462443 ) ) ;
#149572=CARTESIAN_POINT ( 'NONE',  ( -6.482770005628665011, 10.71498210654212002, 0.7998128361456481317 ) ) ;
#149573=CARTESIAN_POINT ( 'NONE',  ( -3.077337680177623103, 6.534051693608437184, 0.7216878364870317197 ) ) ;
#149576=CARTESIAN_POINT ( 'NONE',  ( -1.402160292154681736E-14, 0.1187500006828157706, -1.732050807568870754 ) ) ;
#149583=CARTESIAN_POINT ( 'NONE',  ( -3.077337680177623103, 6.534051693608437184, 0.7216878364870317197 ) ) ;
#149586=CARTESIAN_POINT ( 'NONE',  ( 4.000938479675252069, 7.594566414207783112, 0.1672846332331431873 ) ) ;
#149589=EDGE_CURVE ( 'NONE', #30492, #160543, #62507, .T. ) ;
#149592=CARTESIAN_POINT ( 'NONE',  ( -3.701012746406287413, 6.301303389907177532, 1.082531754730560403 ) ) ;
#149593=CARTESIAN_POINT ( 'NONE',  ( 9.908311333488716954, 10.45411806535867782, 0.7998128361456462443 ) ) ;
#149599=CARTESIAN_POINT ( 'NONE',  ( -2.656508033273816238, 5.186677574539687363, -1.199719254218446718 ) ) ;
#149601=CARTESIAN_POINT ( 'NONE',  ( -7.296259222448620463, 11.66405285949874759, 0.7998128361456481317 ) ) ;
#149604=ORIENTED_EDGE ( 'NONE', *, *, #42311, .T. ) ;
#149607=CIRCLE ( 'NONE', #83878, 0.7500000000000011102 ) ;
#149608=CARTESIAN_POINT ( 'NONE',  ( 4.171104814498611368, 8.018039383557042044, 0.7998128361456321445 ) ) ;
#149613=CARTESIAN_POINT ( 'NONE',  ( 2.876381804795541619, 6.437993120328354024, 0.3511878651327338674 ) ) ;
#149614=DIRECTION ( 'NONE',  ( 0.7592566023653005702, 0.6507913734559639396, 0.000000000000000000 ) ) ;
#149625=CARTESIAN_POINT ( 'NONE',  ( 6.435316467980822353, 10.65961964595298817, 1.040834085586084257E-14 ) ) ;
#149627=CARTESIAN_POINT ( 'NONE',  ( -3.425406365747000859, 7.148057860013469877, 1.040834085586084257E-14 ) ) ;
#149634=CARTESIAN_POINT ( 'NONE',  ( -1.500000000000015099, -1.047916665983845919, 0.8660254037844403729 ) ) ;
#149638=CARTESIAN_POINT ( 'NONE',  ( 4.436542580169809291, 6.199052314996659874, 1.599625672291267398 ) ) ;
#149639=CARTESIAN_POINT ( 'NONE',  ( 1.217526595471194906, 2.800000000000017586, -0.8761443883974120439 ) ) ;
#149640=CARTESIAN_POINT ( 'NONE',  ( -3.972702704004144714, 4.593573561881607148, 1.199719254218462483 ) ) ;
#149646=CARTESIAN_POINT ( 'NONE',  ( 4.202664430556241726, 7.846932902383524144, 0.7216878364870298324 ) ) ;
#149650=CARTESIAN_POINT ( 'NONE',  ( 6.588899466117086767, 10.63087377720454363, 1.040834085586084257E-14 ) ) ;
#149651=CARTESIAN_POINT ( 'NONE',  ( 1.364683531249988535, 4.426041667008082214, 0.7879004041258500513 ) ) ;
#149653=CARTESIAN_POINT ( 'NONE',  ( 2.670593071767634719, 6.059516317130127838, -0.7216878364870267237 ) ) ;
#149657=CARTESIAN_POINT ( 'NONE',  ( 5.620091457764528897, 6.146229702208615642, -0.8320832460304794509 ) ) ;
#149662=CARTESIAN_POINT ( 'NONE',  ( -5.891600325674557048, 6.152103933748189313, 0.8728944348482190474 ) ) ;
#149665=CARTESIAN_POINT ( 'NONE',  ( -0.6823417656250212460, 5.613541667008087543, 1.181850606188767472 ) ) ;
#149671=CARTESIAN_POINT ( 'NONE',  ( 0.7499999999999867883, -0.9333333333333138082, -1.299038105676652011 ) ) ;
#149680=CARTESIAN_POINT ( 'NONE',  ( 0.6823417656249917140, 4.655208333674755394, 1.181850606188765695 ) ) ;
#149682=CARTESIAN_POINT ( 'NONE',  ( 4.476163270806094552, 8.373940915915776273, 0.7998128361456462443 ) ) ;
#149683=CARTESIAN_POINT ( 'NONE',  ( -9.677822722056413696, 10.18521468535430685, 1.040834085586084257E-14 ) ) ;
#149689=CARTESIAN_POINT ( 'NONE',  ( -0.6823417656250003738, -0.7197916663252492686, -1.181850606188749264 ) ) ;
#149697=CARTESIAN_POINT ( 'NONE',  ( 8.107412671292035355, 10.48173408797264194, 1.443375672974076540 ) ) ;
#149702=CARTESIAN_POINT ( 'NONE',  ( -1.499999999999997780, 3.431250000682818602, 1.214306433183764966E-14 ) ) ;
#149704=CARTESIAN_POINT ( 'NONE',  ( -5.739179097286464248, 5.590130456455974617, -0.7998128361456221525 ) ) ;
#149706=CARTESIAN_POINT ( 'NONE',  ( 4.839897649954202130, 4.748894801142428790, -0.7216878364870197293 ) ) ;
#149707=FACE_OUTER_BOUND ( 'NONE', #116280, .T. ) ;
#149714=CARTESIAN_POINT ( 'NONE',  ( 4.684505768721569652, 5.424010470718658716, -1.199719254218452047 ) ) ;
#149718=CARTESIAN_POINT ( 'NONE',  ( 3.845709127770629010, 7.638411082374393146, 0.7998128361456321445 ) ) ;
#149730=CARTESIAN_POINT ( 'NONE',  ( -1.420000000000001039, 2.244000000000016648, -2.508000000000002228 ) ) ;
#149731=CARTESIAN_POINT ( 'NONE',  ( 5.373129273518238769, 6.310201232541126970, -1.074510414011679016 ) ) ;
#149733=CARTESIAN_POINT ( 'NONE',  ( 8.380911511541880188, 12.92948053010758258, 0.7998128361456462443 ) ) ;
#149740=CARTESIAN_POINT ( 'NONE',  ( 0.6823417656249882723, -0.9072916663252494907, 1.181850606188755259 ) ) ;
#149741=CARTESIAN_POINT ( 'NONE',  ( 7.293923454472091450, 7.611924906413328529, 0.7216878364870317197 ) ) ;
#149743=CARTESIAN_POINT ( 'NONE',  ( -10.30383355670593737, 11.12348669235284504, -0.7216878364870267237 ) ) ;
#149749=CARTESIAN_POINT ( 'NONE',  ( -4.090809663021341969, 5.795697244990093644, 1.599625672291267398 ) ) ;
#149761=CARTESIAN_POINT ( 'NONE',  ( 6.058883744127357751, 6.050764970021646150, 0.4299300578466564993 ) ) ;
#149770=CARTESIAN_POINT ( 'NONE',  ( -7.863365906246048809, 12.11775129068834289, -0.7216878364870267237 ) ) ;
#149774=CARTESIAN_POINT ( 'NONE',  ( 8.450809820019639318, 8.753699632978056755, -0.7998128361456291469 ) ) ;
#149775=CARTESIAN_POINT ( 'NONE',  ( -5.935772324684618795, 5.819489221753827657, 0.000000000000000000 ) ) ;
#149776=CARTESIAN_POINT ( 'NONE',  ( 3.842846474469570062, 6.570739089268092137, -1.199719254218452047 ) ) ;
#149778=CARTESIAN_POINT ( 'NONE',  ( -4.577849422908604637, 8.492574760035358494, -0.7998128361456281477 ) ) ;
#149779=CARTESIAN_POINT ( 'NONE',  ( 4.356247428692526569, 3.976710176429713250, 0.7998128361456341429 ) ) ;
#149781=CARTESIAN_POINT ( 'NONE',  ( -5.229694566569281555, 7.124396299129368337, 1.599625672291267398 ) ) ;
#149785=CARTESIAN_POINT ( 'NONE',  ( 7.781490099239519509, 11.16582331816642260, 1.199719254218460707 ) ) ;
#149789=CARTESIAN_POINT ( 'NONE',  ( 4.022946295931974170, 7.796337852756115794, -0.3444838504574644356 ) ) ;
#149790=CARTESIAN_POINT ( 'NONE',  ( 5.178851490740196795, 7.065079377328788546, 1.443375672974062551 ) ) ;
#149795=DIRECTION ( 'NONE',  ( -5.578564026256490882E-16, -1.000000000000000000, -9.066213480720158442E-32 ) ) ;
#149798=CARTESIAN_POINT ( 'NONE',  ( 6.914295152845067349, 11.01050207838719075, 1.040834085586084257E-14 ) ) ;
#149802=CARTESIAN_POINT ( 'NONE',  ( -10.08065090696061716, 11.71951313199760136, -1.199719254218441611 ) ) ;
#149803=CARTESIAN_POINT ( 'NONE',  ( -7.666245793523398078, 11.03137162816423356, 1.199719254218453823 ) ) ;
#149812=AXIS2_PLACEMENT_3D ( 'NONE', #108631, #89135, #207122 ) ;
#149813=CARTESIAN_POINT ( 'NONE',  ( 10.37606763316019531, 10.99983374830873650, 0.7998128361456462443 ) ) ;
#149816=( BOUNDED_CURVE ( )  B_SPLINE_CURVE ( 2, ( #205620, #109280, #175289, #26875, #10617 ),
 .UNSPECIFIED., .F., .T. ) 
 B_SPLINE_CURVE_WITH_KNOTS ( ( 3, 2, 3 ),
 ( 0.1312500000637054354, 0.1333333333333333592, 0.1375000000000000666 ),
 .UNSPECIFIED. ) 
 CURVE ( )  GEOMETRIC_REPRESENTATION_ITEM ( )  RATIONAL_B_SPLINE_CURVE ( ( 0.9330127018922194093, 0.9330127039405975431, 1.000000000000000000, 0.8660254037844369313, 1.000000000000001776 ) ) 
 REPRESENTATION_ITEM ( '' )  );
#149818=CARTESIAN_POINT ( 'NONE',  ( 3.659811400685081040, 6.357198169852855685, -1.199719254218446718 ) ) ;
#149821=B_SPLINE_CURVE_WITH_KNOTS ( 'NONE', 3,
 ( #55771, #121928, #34183, #84000, #1661, #67717, #208409, #124071, #76292, #8082 ),
 .UNSPECIFIED., .F., .F.,
 ( 4, 3, 3, 4 ),
 ( 0.000000000000000000, 3.125173617800492537E-05, 5.893797102792729749E-05, 8.663451821266118878E-05 ),
 .UNSPECIFIED. ) ;
#149822=CARTESIAN_POINT ( 'NONE',  ( -0.7499999999999972244, 4.639583334016150751, -1.299038105676652899 ) ) ;
#149828=CARTESIAN_POINT ( 'NONE',  ( -0.7500000000000215383, 2.191666666666689078, 1.299038105676671107 ) ) ;
#149829=CARTESIAN_POINT ( 'NONE',  ( 5.425234023762710578, 9.481190127698507553, -0.7998128361456291469 ) ) ;
#149830=CARTESIAN_POINT ( 'NONE',  ( 4.161989969270895706, 5.878740935614591656, 1.443375672974062551 ) ) ;
#149835=CARTESIAN_POINT ( 'NONE',  ( 9.408995418203975447, 10.07950886410055524, 0.7216878364870438212 ) ) ;
#149841=CARTESIAN_POINT ( 'NONE',  ( -4.717347382551060342, 7.590990148696470818, 1.199719254218464037 ) ) ;
#149842=CARTESIAN_POINT ( 'NONE',  ( -1.201851678989727383E-14, 4.618750000682821266, -1.732050807568863648 ) ) ;
#149843=CARTESIAN_POINT ( 'NONE',  ( 0.6823417656249864960, -0.5739583329919112353, -1.181850606188749264 ) ) ;
#149845=B_SPLINE_CURVE_WITH_KNOTS ( 'NONE', 3,
 ( #122320, #71307, #169894, #91888, #58292, #40992, #124448, #21483 ),
 .UNSPECIFIED., .F., .F.,
 ( 4, 2, 2, 4 ),
 ( 0.000000000000000000, 0.001499836411158095902, 0.002999672822316190503, 0.005999345644632378405 ),
 .UNSPECIFIED. ) ;
#149848=CARTESIAN_POINT ( 'NONE',  ( 4.630273154266905777, 5.360739087188218122, 1.199719254218464037 ) ) ;
#149850=CARTESIAN_POINT ( 'NONE',  ( 1.364683531249990311, 4.946875000341417916, 1.214306433183764966E-14 ) ) ;
#149856=CARTESIAN_POINT ( 'NONE',  ( -3.741687207247254676, 7.309126141856352454, 1.040834085586084257E-14 ) ) ;
#149858=CARTESIAN_POINT ( 'NONE',  ( -8.389798128758148010, 8.682519326506312751, 0.7998128361456462443 ) ) ;
#149859=CARTESIAN_POINT ( 'NONE',  ( 6.169123589417988995, 7.156064594864501416, -1.199719254218445830 ) ) ;
#149862=CARTESIAN_POINT ( 'NONE',  ( -1.364683531250014514, -0.5114583329919092369, -0.7879004041258359514 ) ) ;
#149868=CARTESIAN_POINT ( 'NONE',  ( -7.054319997812058318, 7.124461507069184130, 1.040834085586084257E-14 ) ) ;
#149871=CARTESIAN_POINT ( 'NONE',  ( 8.703444544968814256, 12.24143683818393313, -1.199719254218446718 ) ) ;
#149873=CARTESIAN_POINT ( 'NONE',  ( 10.21336978979620191, 10.81001959771741205, 0.7998128361456462443 ) ) ;
#149876=CARTESIAN_POINT ( 'NONE',  ( -4.115063316947640715, 4.759660943649018705, 1.199719254218462483 ) ) ;
#149878=CARTESIAN_POINT ( 'NONE',  ( -8.342344591110322227, 8.627156865917170236, -0.7998128361456291469 ) ) ;
#149882=CARTESIAN_POINT ( 'NONE',  ( -4.695247098932518348, 7.056227087241170537, 1.405392365797274445 ) ) ;
#149887=CARTESIAN_POINT ( 'NONE',  ( 8.609064354997688184, 9.146255957026539818, 1.040834085586084257E-14 ) ) ;
#149909=CARTESIAN_POINT ( 'NONE',  ( -3.737243898861318137, 7.511868315313511069, 0.7998128361456341429 ) ) ;
#149910=CARTESIAN_POINT ( 'NONE',  ( -6.984421689334302741, 11.30024240419870374, 0.000000000000000000 ) ) ;
#149915=CARTESIAN_POINT ( 'NONE',  ( -0.7500000000000006661, 2.889583334016148974, -1.299038105676652011 ) ) ;
#149916=CARTESIAN_POINT ( 'NONE',  ( 9.901532256681887745, 10.44620914241737530, 0.000000000000000000 ) ) ;
#149917=CARTESIAN_POINT ( 'NONE',  ( -4.909967638851771454, 4.671257834700952571, -0.2941531795261614346 ) ) ;
#149920=CARTESIAN_POINT ( 'NONE',  ( -8.045874094706015001, 11.47427131287732927, -1.199719254218446718 ) ) ;
#149921=CARTESIAN_POINT ( 'NONE',  ( 0.6823417656249882723, 2.676041667008084879, -1.181850606188749264 ) ) ;
#149928=CARTESIAN_POINT ( 'NONE',  ( -8.663296969452339624, 13.05100419776235299, 1.040834085586084257E-14 ) ) ;
#149932=CARTESIAN_POINT ( 'NONE',  ( 1.364683531249988535, 2.176041667008087543, 0.7879004041258500513 ) ) ;
#149937=CARTESIAN_POINT ( 'NONE',  ( -1.364683531250012516, 2.280208333674751842, 0.7879004041258379498 ) ) ;
#149940=CARTESIAN_POINT ( 'NONE',  ( -5.442708600882160574, 8.437244903416123876, -1.199719254218446718 ) ) ;
#149941=CARTESIAN_POINT ( 'NONE',  ( 8.749089199520284410, 9.101692242395490240, 0.7998128361456481317 ) ) ;
#149942=CARTESIAN_POINT ( 'NONE',  ( 0.000000000000000000, 5.868705557303649734, -4.125226524755057689 ) ) ;
#149944=CARTESIAN_POINT ( 'NONE',  ( -1.500000000000011324, 3.420833333333355597, 0.8660254037844403729 ) ) ;
#149947=CARTESIAN_POINT ( 'NONE',  ( -0.6823417656250212460, 3.363541667008085323, 1.181850606188767472 ) ) ;
#149954=CARTESIAN_POINT ( 'NONE',  ( 5.504247177468179153, 7.444707678511436555, 1.443375672974062551 ) ) ;
#149957=CARTESIAN_POINT ( 'NONE',  ( -7.330154606482786050, 11.70359747420527619, 0.000000000000000000 ) ) ;
#149958=CARTESIAN_POINT ( 'NONE',  ( -2.927671105547157371, 5.503034492191895666, 1.199719254218462483 ) ) ;
#149960=CARTESIAN_POINT ( 'NONE',  ( 0.6823417656249917140, 4.092708333674755394, 1.181850606188765695 ) ) ;
#149963=DIRECTION ( 'NONE',  ( -5.578564026256490882E-16, -1.000000000000000000, -9.066213480720158442E-32 ) ) ;
#149965=CARTESIAN_POINT ( 'NONE',  ( -5.843201017365469596, 9.760892253660966134, 0.7216878364870458196 ) ) ;
#149967=CARTESIAN_POINT ( 'NONE',  ( -1.500000000000011324, 4.629166666666689522, -0.8660254037844313801 ) ) ;
#149970=CARTESIAN_POINT ( 'NONE',  ( 7.700668062882064291, 10.00719871149432549, -1.443375672974057666 ) ) ;
#149975=CARTESIAN_POINT ( 'NONE',  ( 3.023105065722954787, 5.510411095776657220, 1.082531754730546636 ) ) ;
#149983=CARTESIAN_POINT ( 'NONE',  ( 7.233438648090761980, 8.397765496649418182, 1.199719254218462483 ) ) ;
#149984=CARTESIAN_POINT ( 'NONE',  ( -6.254388934605767503, 6.191208599995166040, 0.7998128361456341429 ) ) ;
#149989=CARTESIAN_POINT ( 'NONE',  ( 4.799223189113185128, 8.542918120699967588, 1.040834085586084257E-14 ) ) ;
#149990=CARTESIAN_POINT ( 'NONE',  ( 0.6823417656249899377, 0.9052083336747520637, 1.181850606188755259 ) ) ;
#149992=CARTESIAN_POINT ( 'NONE',  ( -2.137381772448751605, 5.645362501165475777, -0.7998128361456281477 ) ) ;
#150009=CARTESIAN_POINT ( 'NONE',  ( 5.608269097547198712, 9.694731047113750222, -0.7998128361456281477 ) ) ;
#150010=CARTESIAN_POINT ( 'NONE',  ( 7.955937213120826357, 8.176348258262782664, 0.7998128361456481317 ) ) ;
#150019=CARTESIAN_POINT ( 'NONE',  ( -0.1263102688159843667, 6.363441598446241798, 3.117922131261609664 ) ) ;
#150021=CARTESIAN_POINT ( 'NONE',  ( -4.238895582566952314, 8.097128612970093897, 1.040834085586084257E-14 ) ) ;
#150024=CARTESIAN_POINT ( 'NONE',  ( -3.469997250093771246, 6.135748327496311383, -1.199719254218452935 ) ) ;
#150027=CARTESIAN_POINT ( 'NONE',  ( 6.938893903907228378E-15, 10.64264068711930733, 1.214306433183764966E-14 ) ) ;
#150034=CARTESIAN_POINT ( 'NONE',  ( -2.656508033273816238, 5.186677574539687363, -1.199719254218446718 ) ) ;
#150037=CARTESIAN_POINT ( 'NONE',  ( 7.135668919494039031, 7.219368582364847242, 1.040834085586084257E-14 ) ) ;
#150038=CARTESIAN_POINT ( 'NONE',  ( 0.6823417656249899377, 5.176041667008086655, -1.181850606188754593 ) ) ;
#150044=CARTESIAN_POINT ( 'NONE',  ( 3.985733972293228344, 7.593847367743336463, 1.040834085586084257E-14 ) ) ;
#150045=CARTESIAN_POINT ( 'NONE',  ( -6.856673000209188906, 9.022537805042615489, 1.599625672291283607 ) ) ;
#150050=CARTESIAN_POINT ( 'NONE',  ( -8.128276786592724790, 9.441743324901704426, -1.199719254218446718 ) ) ;
#150051=CARTESIAN_POINT ( 'NONE',  ( -6.573005544526917099, 6.562927978236513304, -0.7998128361456291469 ) ) ;
#150058=CARTESIAN_POINT ( 'NONE',  ( 7.721532178182734185, 8.967207948423393304, 1.199719254218462483 ) ) ;
#150070=EDGE_LOOP ( 'NONE', ( #77673, #72408, #75486, #149319 ) ) ;
#150072=CARTESIAN_POINT ( 'NONE',  ( -1.500000000000011324, 5.879166666666686858, -0.8660254037844313801 ) ) ;
#150073=CARTESIAN_POINT ( 'NONE',  ( 4.857899112398166075, 4.561970474086296079, 1.040834085586084257E-14 ) ) ;
#150074=CARTESIAN_POINT ( 'NONE',  ( 5.301401758143367893, 6.143722458377430584, 1.199719254218462483 ) ) ;
#150076=CARTESIAN_POINT ( 'NONE',  ( -6.073689629242151611, 10.02979563418376685, -0.7216878364870278340 ) ) ;
#150078=CARTESIAN_POINT ( 'NONE',  ( 6.968527767744109980, 7.232296605230681408, 0.7216878364870317197 ) ) ;
#150080=CARTESIAN_POINT ( 'NONE',  ( -8.392133896734675247, 10.81390885098904420, 1.443375672974064550 ) ) ;
#150085=CARTESIAN_POINT ( 'NONE',  ( 7.233438648090761980, 8.397765496649418182, 1.199719254218462483 ) ) ;
#150091=CARTESIAN_POINT ( 'NONE',  ( -1.364683531250012516, 3.988541667008088876, -0.7879004041258300672 ) ) ;
#150097=ADVANCED_FACE ( 'NONE', ( #10788 ), #68130, .T. ) ;
#150098=CARTESIAN_POINT ( 'NONE',  ( 7.741869408603235136, 8.990934717247309749, 1.199719254218462483 ) ) ;
#150101=CARTESIAN_POINT ( 'NONE',  ( -7.503547950159405566, 10.84155747757291266, 1.199719254218453823 ) ) ;
#150107=CARTESIAN_POINT ( 'NONE',  ( 8.594979316059474073, 12.11489407112305372, 1.199719254218450271 ) ) ;
#150110=CARTESIAN_POINT ( 'NONE',  ( -8.474009703741204547, 9.845098394908269768, -1.199719254218446718 ) ) ;
#150115=CARTESIAN_POINT ( 'NONE',  ( 5.320181785876097358, 6.346852008952179602, 1.110229221197155169 ) ) ;
#150116=CARTESIAN_POINT ( 'NONE',  ( -4.223528545856940042, 4.886203710709899006, -1.199719254218446718 ) ) ;
#150121=CARTESIAN_POINT ( 'NONE',  ( 7.613066949273408213, 8.840665181362512115, -1.199719254218441611 ) ) ;
#150123=CARTESIAN_POINT ( 'NONE',  ( 6.745345117998789775, 7.828323044875442172, 1.199719254218462483 ) ) ;
#150124=CARTESIAN_POINT ( 'NONE',  ( -4.218308198147158627, 7.356310275799033960, -0.8477421400144637964 ) ) ;
#150125=CARTESIAN_POINT ( 'NONE',  ( 4.822949958159288286, 6.649860922651058992, -1.599625672291256295 ) ) ;
#150127=CARTESIAN_POINT ( 'NONE',  ( -8.378575743565381373, 8.877352577022161739, 0.7216878364870438212 ) ) ;
#150134=CARTESIAN_POINT ( 'NONE',  ( -4.026842413655439046, 7.608452276161581374, 0.2328349793435397497 ) ) ;
#150136=CARTESIAN_POINT ( 'NONE',  ( -0.6823417656250246877, -1.136458332991911790, 1.181850606188755259 ) ) ;
#150139=CARTESIAN_POINT ( 'NONE',  ( 4.961921032921539521, 7.772363057508363759, -1.082531754730549078 ) ) ;
#150143=CARTESIAN_POINT ( 'NONE',  ( -9.286972035236626510, 11.85788667924133399, -1.443375672974058777 ) ) ;
#150150=CARTESIAN_POINT ( 'NONE',  ( -8.636180661780658241, 12.05899929117736846, -1.082531754730543083 ) ) ;
#150152=ORIENTED_EDGE ( 'NONE', *, *, #932, .F. ) ;
#150158=ORIENTED_EDGE ( 'NONE', *, *, #185760, .T. ) ;
#150159=CARTESIAN_POINT ( 'NONE',  ( -8.283668667825340393, 12.60810451253083997, 0.7216878364870458196 ) ) ;
#150166=CARTESIAN_POINT ( 'NONE',  ( 0.7499999999999902300, 3.514583334016149863, 1.299038105676669330 ) ) ;
#150168=CARTESIAN_POINT ( 'NONE',  ( -4.543954038874438162, 8.453030145328826350, 1.040834085586084257E-14 ) ) ;
#150172=CARTESIAN_POINT ( 'NONE',  ( -6.970863535720637216, 11.28442455831609337, 0.7998128361456481317 ) ) ;
#150176=CARTESIAN_POINT ( 'NONE',  ( 5.262536180398716290, 9.291375977107183104, -0.7998128361456291469 ) ) ;
#150181=CARTESIAN_POINT ( 'NONE',  ( 9.610031953988080744, 10.10612545594124967, -0.7998128361456281477 ) ) ;
#150182=CARTESIAN_POINT ( 'NONE',  ( 4.875256056531546811, 6.897355949014277954, -1.450507286032868270 ) ) ;
#150187=CARTESIAN_POINT ( 'NONE',  ( -8.188761592974058701, 8.655902734665618325, -0.7216878364870278340 ) ) ;
#150190=CARTESIAN_POINT ( 'NONE',  ( -1.364683531249997417, 5.071875000341417916, 1.214306433183764966E-14 ) ) ;
#150194=CARTESIAN_POINT ( 'NONE',  ( -0.6823417656249969321, 5.717708333674756283, -1.181850606188749264 ) ) ;
#150196=DIRECTION ( 'NONE',  ( 0.000000000000000000, 1.000000000000000000, -8.546850786086437571E-32 ) ) ;
#150197=CARTESIAN_POINT ( 'NONE',  ( -3.917943204224928699, 4.633650495426258509, -1.082531754730548412 ) ) ;
#150199=CARTESIAN_POINT ( 'NONE',  ( 8.886479618753304166, 12.45497775759917758, -1.199719254218446718 ) ) ;
#150200=CARTESIAN_POINT ( 'NONE',  ( 1.426546532658254263, 7.396047039057247474, -4.272878514717298515 ) ) ;
#150201=CARTESIAN_POINT ( 'NONE',  ( -1.180180411290526976, 2.825872823607642914, -0.7749999999999979128 ) ) ;
#150204=CARTESIAN_POINT ( 'NONE',  ( 1.364683531249988535, 1.613541667008084879, 0.7879004041258500513 ) ) ;
#150206=CARTESIAN_POINT ( 'NONE',  ( 3.876741858503734761, 6.610283703974623393, 1.199719254218462483 ) ) ;
#150207=ORIENTED_EDGE ( 'NONE', *, *, #68027, .F. ) ;
#150215=CARTESIAN_POINT ( 'NONE',  ( -7.592202833972775622, 8.920286730132099606, 1.082531754730558626 ) ) ;
#150217=CARTESIAN_POINT ( 'NONE',  ( 0.2089193878861559939, 7.199905994521539121, 1.991006660531130512 ) ) ;
#150220=CARTESIAN_POINT ( 'NONE',  ( -7.974166903131914452, 12.45494515362926435, -0.7998128361456281477 ) ) ;
#150223=CARTESIAN_POINT ( 'NONE',  ( -5.409340101728186134, 5.413244328212063472, 0.7216878364870317197 ) ) ;
#150224=CARTESIAN_POINT ( 'NONE',  ( 0.6823417656249882723, 2.738541667008084879, -1.181850606188749264 ) ) ;
#150235=EDGE_CURVE ( 'NONE', #10132, #54906, #23388, .T. ) ;
#150237=CIRCLE ( 'NONE', #70575, 0.07999999999999994615 ) ;
#150244=CARTESIAN_POINT ( 'NONE',  ( -0.6823417656250212460, 4.113541667008085767, 1.181850606188767472 ) ) ;
#150252=CARTESIAN_POINT ( 'NONE',  ( 9.610031953988080744, 10.10612545594124967, -0.7998128361456281477 ) ) ;
#150255=CARTESIAN_POINT ( 'NONE',  ( -1.364683531250012516, 2.238541667008087988, -0.7879004041258289570 ) ) ;
#150258=CARTESIAN_POINT ( 'NONE',  ( -7.212574532790102744, 8.477387045419011002, -1.082531754730550855 ) ) ;
#150266=CARTESIAN_POINT ( 'NONE',  ( 4.650610384687404952, 5.384465856012134566, 1.199719254218462483 ) ) ;
#150275=CARTESIAN_POINT ( 'NONE',  ( -2.937312835655025101, 6.578615408239493867, 1.040834085586084257E-14 ) ) ;
#150276=CARTESIAN_POINT ( 'NONE',  ( 6.283314124929436417, 9.417951348137970413, -1.199719254218440723 ) ) ;
#150278=CARTESIAN_POINT ( 'NONE',  ( 5.463572716182834910, 5.476515711742504067, 0.7216878364870317197 ) ) ;
#150285=ADVANCED_FACE ( 'NONE', ( #84337 ), #109832, .T. ) ;
#150290=CARTESIAN_POINT ( 'NONE',  ( -6.670248388243482651, 9.765411638717282017, 1.082531754730548412 ) ) ;
#150291=CARTESIAN_POINT ( 'NONE',  ( 5.660692828905515839, 6.562895374266609849, -1.199719254218445830 ) ) ;
#150294=CARTESIAN_POINT ( 'NONE',  ( -9.657485491635913633, 10.16148791653038330, 1.040834085586084257E-14 ) ) ;
#150299=CARTESIAN_POINT ( 'NONE',  ( -3.436101866059630527, 6.096203712789787232, 1.199719254218462483 ) ) ;
#150300=AXIS2_PLACEMENT_3D ( 'NONE', #65504, #143635, #210711 ) ;
#150302=CARTESIAN_POINT ( 'NONE',  ( 7.639129486296027061, 10.99973593639901814, 1.199719254218460707 ) ) ;
#150303=CARTESIAN_POINT ( 'NONE',  ( 4.864678189204997949, 4.569879397027603929, 0.7998128361456341429 ) ) ;
#150312=CARTESIAN_POINT ( 'NONE',  ( -4.416205349749324327, 6.175325546172740765, 1.599625672291267398 ) ) ;
#150315=CARTESIAN_POINT ( 'NONE',  ( -9.508345801885592863, 9.987491611821676329, 0.7998128361456462443 ) ) ;
#150320=CARTESIAN_POINT ( 'NONE',  ( 6.466876084038451822, 10.48851316477946582, 1.040834085586084257E-14 ) ) ;
#150321=CARTESIAN_POINT ( 'NONE',  ( -1.201851678989727383E-14, 5.759375000341417028, -1.575800808251661023 ) ) ;
#150323=CARTESIAN_POINT ( 'NONE',  ( 5.332434488876471868, 5.115595079977664383, 0.7998128361456341429 ) ) ;
#150326=CARTESIAN_POINT ( 'NONE',  ( -5.364222332501225488, 9.410009821226765325, 0.7998128361456481317 ) ) ;
#150336=CARTESIAN_POINT ( 'NONE',  ( -1.364683531249997417, 2.571875000341422357, 1.214306433183764966E-14 ) ) ;
#150337=CARTESIAN_POINT ( 'NONE',  ( 7.404724451357931336, 11.79059562655963056, 0.7998128361456462443 ) ) ;
#150339=CARTESIAN_POINT ( 'NONE',  ( -4.121315508874262790, 6.791656612786516334, -1.082531754730549967 ) ) ;
#150341=CARTESIAN_POINT ( 'NONE',  ( -6.087247782411500552, 7.164505836643929371, 1.082531754730549967 ) ) ;
#150348=CARTESIAN_POINT ( 'NONE',  ( 4.039439701867726384, 6.800097854565950506, 1.199719254218462483 ) ) ;
#150359=CARTESIAN_POINT ( 'NONE',  ( 3.669453130792974971, 7.432779085900453886, 1.040834085586084257E-14 ) ) ;
#150363=CARTESIAN_POINT ( 'NONE',  ( -4.954615070790188369, 7.867802451642154082, -1.199719254218452047 ) ) ;
#150367=CARTESIAN_POINT ( 'NONE',  ( 6.449928391799196525, 8.548002428564306143, -1.599625672291262513 ) ) ;
#150370=CARTESIAN_POINT ( 'NONE',  ( -6.898401231254901234, 6.942556279419168419, -0.7998128361456291469 ) ) ;
#150371=CARTESIAN_POINT ( 'NONE',  ( -1.500000000000013101, 2.420833333333359150, 0.8660254037844403729 ) ) ;
#150372=CARTESIAN_POINT ( 'NONE',  ( -5.135841261478327979, 4.886236314679810455, 0.7998128361456341429 ) ) ;
#150375=CARTESIAN_POINT ( 'NONE',  ( -5.331380718671772101, 7.243030143248949670, -1.599625672291256295 ) ) ;
#150377=CARTESIAN_POINT ( 'NONE',  ( 0.6823417656249899377, 3.926041667008085767, -1.181850606188754593 ) ) ;
#150379=CARTESIAN_POINT ( 'NONE',  ( -5.178851490740209229, 7.065079377328788546, 1.443375672974064550 ) ) ;
#150382=ORIENTED_EDGE ( 'NONE', *, *, #58928, .T. ) ;
#150385=CARTESIAN_POINT ( 'NONE',  ( 5.854423403002611437, 5.724582146458163656, 1.040834085586084257E-14 ) ) ;
#150389=CARTESIAN_POINT ( 'NONE',  ( 0.6823417656249899377, 3.155208333674754062, 1.181850606188765695 ) ) ;
#150391=FACE_OUTER_BOUND ( 'NONE', #77139, .T. ) ;
#150392=CARTESIAN_POINT ( 'NONE',  ( -0.1501718367240184870, 8.265200931437576060, 1.995665264648829096 ) ) ;
#150396=CARTESIAN_POINT ( 'NONE',  ( -3.867100128395853709, 5.534702787927018974, -1.599625672291256295 ) ) ;
#150397=CARTESIAN_POINT ( 'NONE',  ( -8.337901282280023807, 8.829899038855916871, 0.7216878364870438212 ) ) ;
#150399=CARTESIAN_POINT ( 'NONE',  ( 1.364683531249988535, 3.655208333674750509, -0.7879004041258239610 ) ) ;
#150408=CARTESIAN_POINT ( 'NONE',  ( -6.019457014343129408, 9.966524250134902729, 0.000000000000000000 ) ) ;
#150411=CARTESIAN_POINT ( 'NONE',  ( 4.720248583150478794, 5.235598830736874376, 1.011424349686943280 ) ) ;
#150414=CARTESIAN_POINT ( 'NONE',  ( -6.358410854684783509, 9.401601182898824405, -1.082531754730537976 ) ) ;
#150429=CARTESIAN_POINT ( 'NONE',  ( -5.018489415352746619, 9.006654751220198207, 0.7998128361456481317 ) ) ;
#150431=CARTESIAN_POINT ( 'NONE',  ( -0.7500000000000249800, -1.058333333333314030, 1.299038105676659116 ) ) ;
#150432=CARTESIAN_POINT ( 'NONE',  ( 2.510230996824538430, 6.080353262937265413, 0.000000000000000000 ) ) ;
#150434=( BOUNDED_CURVE ( )  B_SPLINE_CURVE ( 2, ( #27420, #212566, #213610, #176884, #64205, #179028, #130346 ),
 .UNSPECIFIED., .F., .T. ) 
 B_SPLINE_CURVE_WITH_KNOTS ( ( 3, 2, 2, 3 ),
 ( 0.2500000000000002220, 0.2559523809523810978, 0.2619047619047619735, 0.2678571428571428492 ),
 .UNSPECIFIED. ) 
 CURVE ( )  GEOMETRIC_REPRESENTATION_ITEM ( )  RATIONAL_B_SPLINE_CURVE ( ( 0.9999999999999950040, 0.8660254037844437036, 1.000000000000000000, 0.8660254037844387076, 1.000000000000000000, 0.8660254037844387076, 1.000000000000000000 ) ) 
 REPRESENTATION_ITEM ( '' )  );
#150435=CARTESIAN_POINT ( 'NONE',  ( -3.267151830768976417, 6.755501535964965498, -0.7216878364870478180 ) ) ;
#150437=EDGE_CURVE ( 'NONE', #196229, #78732, #105921, .T. ) ;
#150438=CARTESIAN_POINT ( 'NONE',  ( 6.657217119509961201, 7.725507046638470321, -1.199719254218446718 ) ) ;
#150445=CARTESIAN_POINT ( 'NONE',  ( -3.470524135418294520, 6.992769224722559684, -0.7216878364870267237 ) ) ;
#150453=CARTESIAN_POINT ( 'NONE',  ( 0.6823417656249899377, 1.592708333674752730, 1.181850606188755259 ) ) ;
#150454=CARTESIAN_POINT ( 'NONE',  ( 9.693716643646595799, 11.37205284141829686, 1.082531754730548412 ) ) ;
#150455=CARTESIAN_POINT ( 'NONE',  ( -7.527801604085656351, 9.805521176231838609, 1.599625672291295375 ) ) ;
#150458=CARTESIAN_POINT ( 'NONE',  ( 5.608269097547198712, 9.694731047113750222, -0.7998128361456281477 ) ) ;
#150459=CARTESIAN_POINT ( 'NONE',  ( -6.340409392685171674, 10.54889472477470846, 0.7998128361456481317 ) ) ;
#150462=CARTESIAN_POINT ( 'NONE',  ( 1.499999999999985123, -1.172916665983846363, -0.8660254037844323793 ) ) ;
#150464=CARTESIAN_POINT ( 'NONE',  ( 7.456621297836067086, 10.68284669990868174, 1.082531754730558626 ) ) ;
#150467=CARTESIAN_POINT ( 'NONE',  ( 1.364683531249986537, 0.4677083336747514530, -0.7879004041258309554 ) ) ;
#150470=CARTESIAN_POINT ( 'NONE',  ( 6.765155463094751909, 8.915767345075790828, 1.443375672974076540 ) ) ;
#150473=CARTESIAN_POINT ( 'NONE',  ( -5.775410249741523394, 5.840326167560965231, 0.7216878364870317197 ) ) ;
#150475=CARTESIAN_POINT ( 'NONE',  ( 1.364683531249990311, 3.384375000341416140, 1.214306433183764966E-14 ) ) ;
#150479=CARTESIAN_POINT ( 'NONE',  ( -5.362413449404877852, 6.214902764849178141, -1.199719254218446718 ) ) ;
#150480=CARTESIAN_POINT ( 'NONE',  ( -5.094707486240121597, 6.719114383638050469, -1.440239009331502062 ) ) ;
#150485=( BOUNDED_CURVE ( )  B_SPLINE_CURVE ( 2, ( #69003, #55987, #88497, #187038, #35449 ),
 .UNSPECIFIED., .F., .T. ) 
 B_SPLINE_CURVE_WITH_KNOTS ( ( 3, 2, 3 ),
 ( 0.01079486483480429637, 0.01250000000000000069, 0.01382216642637607365 ),
 .UNSPECIFIED. ) 
 CURVE ( )  GEOMETRIC_REPRESENTATION_ITEM ( )  RATIONAL_B_SPLINE_CURVE ( ( 0.9352202683046948462, 0.9451732491399882363, 1.000000000000000000, 0.9574871888551585997, 0.9419547032718735835 ) ) 
 REPRESENTATION_ITEM ( '' )  );
#150487=CARTESIAN_POINT ( 'NONE',  ( 6.283314124929436417, 9.417951348137970413, -1.199719254218440723 ) ) ;
#150491=CARTESIAN_POINT ( 'NONE',  ( 1.499999999999987121, 2.795833333333352488, -0.8660254037844262731 ) ) ;
#150497=CARTESIAN_POINT ( 'NONE',  ( 5.341549334104184865, 8.215262742221458581, 1.082531754730558626 ) ) ;
#150498=CARTESIAN_POINT ( 'NONE',  ( 1.364683531249986537, 0.4260416670080872659, 0.7879004041258500513 ) ) ;
#150500=CARTESIAN_POINT ( 'NONE',  ( 8.516493047678546091, 13.08765898893368629, -0.7998128361456352531 ) ) ;
#150502=B_SPLINE_CURVE_WITH_KNOTS ( 'NONE', 3,
 ( #58330, #59391, #111409, #44226, #30092, #177413 ),
 .UNSPECIFIED., .F., .F.,
 ( 4, 2, 4 ),
 ( 0.4261085947076337921, 0.4631192677600871610, 0.5001299408125404744 ),
 .UNSPECIFIED. ) ;
#150507=CARTESIAN_POINT ( 'NONE',  ( -0.7500000000000215383, 0.1916666666666871910, 1.299038105676659116 ) ) ;
#150508=CARTESIAN_POINT ( 'NONE',  ( 7.772902139336337335, 7.962807338847539107, 0.7998128361456341429 ) ) ;
#150509=CARTESIAN_POINT ( 'NONE',  ( -7.178152263431422320, 10.46192917639026554, 1.199719254218453823 ) ) ;
#150511=CARTESIAN_POINT ( 'NONE',  ( -1.402160292154681736E-14, 1.696875000341421469, -1.575800808251659024 ) ) ;
#150512=CARTESIAN_POINT ( 'NONE',  ( -0.7500000000000215383, 3.191666666666689967, 1.299038105676671107 ) ) ;
#150514=CARTESIAN_POINT ( 'NONE',  ( 5.508690485854129903, 5.321227076451600091, 1.040834085586084257E-14 ) ) ;
#150521=CARTESIAN_POINT ( 'NONE',  ( -0.7500000000000249800, -1.277083332650516656, 1.299038105676659116 ) ) ;
#150522=CARTESIAN_POINT ( 'NONE',  ( -8.030507057996002729, 8.263346410617135263, 1.040834085586084257E-14 ) ) ;
#150523=CARTESIAN_POINT ( 'NONE',  ( -4.663641653420935285, 5.503632019488245319, 1.082531754730560403 ) ) ;
#150528=CARTESIAN_POINT ( 'NONE',  ( 4.006649928318074316, 7.586413011018040997, -0.2369455770718699450 ) ) ;
#150531=CARTESIAN_POINT ( 'NONE',  ( 5.425234023762710578, 9.481190127698507553, -0.7998128361456291469 ) ) ;
#150534=CARTESIAN_POINT ( 'NONE',  ( 7.144783764277405247, 8.398297815487545392, -1.082531754730543971 ) ) ;
#150538=CARTESIAN_POINT ( 'NONE',  ( -8.369460898337653276, 8.658792557682392754, 0.7998128361456462443 ) ) ;
#150539=CARTESIAN_POINT ( 'NONE',  ( 3.506755287428983792, 7.242964935309132990, 1.040834085586084257E-14 ) ) ;
#150544=CARTESIAN_POINT ( 'NONE',  ( 9.910647101909615841, 10.66476916175714607, 0.000000000000000000 ) ) ;
#150545=ORIENTED_EDGE ( 'NONE', *, *, #96134, .T. ) ;
#150551=DIRECTION ( 'NONE',  ( 0.7592566023653005702, 0.6507913734559639396, 0.000000000000000000 ) ) ;
#150553=CARTESIAN_POINT ( 'NONE',  ( -1.567642296063691987, 8.684662666223690763, -2.500960217906271321 ) ) ;
#150554=CARTESIAN_POINT ( 'NONE',  ( -3.741687207691642314, 6.348756928073427730, 1.082531754730560403 ) ) ;
#150556=CARTESIAN_POINT ( 'NONE',  ( 7.944714827928033962, 12.21265836598400689, 0.7216878364870438212 ) ) ;
#150559=CARTESIAN_POINT ( 'NONE',  ( -6.728924311084075960, 6.744833205886536120, 1.040834085586084257E-14 ) ) ;
#150564=CARTESIAN_POINT ( 'NONE',  ( -8.843996274815957293, 9.212417163573759282, 1.040834085586084257E-14 ) ) ;
#150567=DIRECTION ( 'NONE',  ( -5.578564026256490882E-16, -1.000000000000000000, -9.066213480720158442E-32 ) ) ;
#150578=CARTESIAN_POINT ( 'NONE',  ( -6.501298352952815662, 7.543601818988450169, -1.199719254218446718 ) ) ;
#150581=CARTESIAN_POINT ( 'NONE',  ( 4.690757960648231695, 5.535267711253469614, 1.082531754730560403 ) ) ;
#150583=CARTESIAN_POINT ( 'NONE',  ( 4.907894938888484937, 6.474487383728033230, 2.499999999999998668 ) ) ;
#150584=CARTESIAN_POINT ( 'NONE',  ( 3.404766800216717737, 6.348112014766642552, 1.069586989871921467 ) ) ;
#150586=CARTESIAN_POINT ( 'NONE',  ( -4.029797971759847997, 5.724516938518342535, -1.599625672291256295 ) ) ;
#150593=CARTESIAN_POINT ( 'NONE',  ( -9.073431116043565225, 11.60875560684942265, -1.599625672291263179 ) ) ;
#150594=CARTESIAN_POINT ( 'NONE',  ( 4.774442650306744085, 8.721933525333202653, -0.7998128361456281477 ) ) ;
#150597=CARTESIAN_POINT ( 'NONE',  ( -10.29471871147821282, 10.90492667301307605, -0.7998128361456291469 ) ) ;
#150599=CARTESIAN_POINT ( 'NONE',  ( 4.202137545231717120, 6.989912005157271402, 1.199719254218462483 ) ) ;
#150602=CARTESIAN_POINT ( 'NONE',  ( -1.364683531250000748, 0.07187500034142035865, 0.000000000000000000 ) ) ;
#150604=ORIENTED_EDGE ( 'NONE', *, *, #196542, .F. ) ;
#150606=CARTESIAN_POINT ( 'NONE',  ( 8.188761592974039161, 10.57664116326830595, -1.443375672974063439 ) ) ;
#150615=CARTESIAN_POINT ( 'NONE',  ( -0.2542610327306510931, 7.036558673036513056, -4.015411564048622317 ) ) ;
#150627=CARTESIAN_POINT ( 'NONE',  ( -3.755772246185468788, 4.340488027759846545, -1.199719254218452047 ) ) ;
#150634=CARTESIAN_POINT ( 'NONE',  ( 1.499999999999987121, -0.2145833326505137972, 0.8660254037844524744 ) ) ;
#150642=CARTESIAN_POINT ( 'NONE',  ( 8.028399517586572998, 12.51821653715971472, -0.7998128361456352531 ) ) ;
#150643=FACE_OUTER_BOUND ( 'NONE', #53794, .T. ) ;
#150647=CARTESIAN_POINT ( 'NONE',  ( 3.323720213644492993, 7.029424015893889433, 1.040834085586084257E-14 ) ) ;
#150648=CARTESIAN_POINT ( 'NONE',  ( -6.344852701515500293, 9.385783337534627790, 1.082531754730548412 ) ) ;
#150649=CARTESIAN_POINT ( 'NONE',  ( -5.910693218230258061, 6.000975156485434781, -0.07073762994192281384 ) ) ;
#150650=CARTESIAN_POINT ( 'NONE',  ( 2.275435306267621804, 5.643409308550367598, 0.5316758947214432762 ) ) ;
#150652=CARTESIAN_POINT ( 'NONE',  ( -6.320072162264675164, 10.52516795595079557, 0.7998128361456481317 ) ) ;
#150653=CARTESIAN_POINT ( 'NONE',  ( -5.558479791478509568, 5.587240632920778438, 0.000000000000000000 ) ) ;
#150656=CARTESIAN_POINT ( 'NONE',  ( -1.500000000000015099, -0.08958333265051321437, -0.8660254037844383745 ) ) ;
#150664=CARTESIAN_POINT ( 'NONE',  ( -3.253593677155282471, 6.739683690082376444, 1.040834085586084257E-14 ) ) ;
#150668=CARTESIAN_POINT ( 'NONE',  ( 3.995705304526904200, 7.602062626508213405, -0.07732544726959944548 ) ) ;
#150673=CARTESIAN_POINT ( 'NONE',  ( -4.161989969270909917, 5.878740935614591656, 1.443375672974064550 ) ) ;
#150674=CARTESIAN_POINT ( 'NONE',  ( 7.910292558569346433, 11.31609285405122556, -1.199719254218446718 ) ) ;
#150683=CARTESIAN_POINT ( 'NONE',  ( -2.764973262183167968, 5.313220341600567664, 1.199719254218462483 ) ) ;
#150684=CARTESIAN_POINT ( 'NONE',  ( -7.960608749518247151, 12.43912730774665576, 0.000000000000000000 ) ) ;
#150689=CARTESIAN_POINT ( 'NONE',  ( 4.710568305744190276, 7.583081225755162968, 1.199719254218462483 ) ) ;
#150693=ORIENTED_EDGE ( 'NONE', *, *, #24957, .F. ) ;
#150705=CARTESIAN_POINT ( 'NONE',  ( 6.123478934866503742, 10.29580919065294431, 0.7998128361456462443 ) ) ;
#150707=CARTESIAN_POINT ( 'NONE',  ( -4.786191920824102830, 5.542644314838231168, 1.199719254218462483 ) ) ;
#150715=CARTESIAN_POINT ( 'NONE',  ( -0.7500000000000006661, -0.8604166659838472508, -1.299038105676652011 ) ) ;
#150719=CARTESIAN_POINT ( 'NONE',  ( 4.005544317833563461, 6.760553239859419250, -1.199719254218452047 ) ) ;
#150720=DIRECTION ( 'NONE',  ( 0.6507913734559640506, -0.7592566023653004592, 0.000000000000000000 ) ) ;
#150721=CARTESIAN_POINT ( 'NONE',  ( -3.425406365747000859, 7.148057860013469877, 1.040834085586084257E-14 ) ) ;
#150727=CARTESIAN_POINT ( 'NONE',  ( 6.819388077993785657, 7.058300300521964665, 1.040834085586084257E-14 ) ) ;
#150729=ORIENTED_EDGE ( 'NONE', *, *, #14091, .F. ) ;
#150730=CARTESIAN_POINT ( 'NONE',  ( 8.066738210006686671, 9.473911335505048825, 1.082531754730558626 ) ) ;
#150731=CARTESIAN_POINT ( 'NONE',  ( -0.6823417656250212460, 5.363541667008087543, 1.181850606188767472 ) ) ;
#150733=CARTESIAN_POINT ( 'NONE',  ( 4.378920427089557421, 5.171457255435017331, -1.082531754730548412 ) ) ;
#150737=CARTESIAN_POINT ( 'NONE',  ( 5.445097452434600527, 6.261244994358417415, -1.018272717561970353 ) ) ;
#150740=CARTESIAN_POINT ( 'NONE',  ( -6.024621019446552594, 6.066914679173425640, 0.6088392743194663836 ) ) ;
#150743=CARTESIAN_POINT ( 'NONE',  ( -0.6823417656249969321, 5.530208333674756283, -1.181850606188749264 ) ) ;
#150759=CARTESIAN_POINT ( 'NONE',  ( 1.364683531249990311, 5.176041667008085767, 0.7879004041258500513 ) ) ;
#150761=CARTESIAN_POINT ( 'NONE',  ( 6.693975156845185737, 8.832723654451292816, 1.599625672291281386 ) ) ;
#150762=CARTESIAN_POINT ( 'NONE',  ( -9.501566725078754772, 9.979582688880366703, -0.7998128361456291469 ) ) ;
#150767=EDGE_LOOP ( 'NONE', ( #4920, #170807, #149188, #8936, #175075, #144344, #34769, #203125, #126980 ) ) ;
#150769=CARTESIAN_POINT ( 'NONE',  ( -1.499999999999997780, 5.150000000000022560, 1.214306433183764966E-14 ) ) ;
#150776=CARTESIAN_POINT ( 'NONE',  ( 8.812436659202669276, 10.34389285956704363, -1.082531754730543083 ) ) ;
#150779=CARTESIAN_POINT ( 'NONE',  ( 1.608462485350599769, 8.735270501766756013, -2.463594439587629914 ) ) ;
#150781=CARTESIAN_POINT ( 'NONE',  ( -1.500000000000013101, 2.910416667349485120, -0.8660254037844313801 ) ) ;
#150783=CARTESIAN_POINT ( 'NONE',  ( -4.497554271431319250, 6.270232621468402989, -1.599625672291256295 ) ) ;
#150784=CARTESIAN_POINT ( 'NONE',  ( 4.324687812634887329, 6.068555086205916105, 1.443375672974062551 ) ) ;
#150792=CARTESIAN_POINT ( 'NONE',  ( 5.169736645512481132, 4.925780929386339935, 0.7998128361456341429 ) ) ;
#150796=CARTESIAN_POINT ( 'NONE',  ( 4.385172619016207918, 7.203452924572514959, 1.199719254218462483 ) ) ;
#150800=ORIENTED_EDGE ( 'NONE', *, *, #11172, .F. ) ;
#150807=CARTESIAN_POINT ( 'NONE',  ( 5.016205007133085481, 6.569753085731051989, -1.234251006731339917 ) ) ;
#150808=ADVANCED_FACE ( 'NONE', ( #1478 ), #36131, .F. ) ;
#150810=CARTESIAN_POINT ( 'NONE',  ( 8.041957671200231417, 12.53403438304231976, 1.040834085586084257E-14 ) ) ;
#150815=CARTESIAN_POINT ( 'NONE',  ( -5.000000000000024869, 0.2350621082554960051, 0.7750000000000117906 ) ) ;
#150816=CARTESIAN_POINT ( 'NONE',  ( -1.364683531250000748, -1.240624999658580752, 0.000000000000000000 ) ) ;
#150817=( BOUNDED_CURVE ( )  B_SPLINE_CURVE ( 3, ( #186057, #69092, #49669, #16072 ),
 .UNSPECIFIED., .F., .T. ) 
 B_SPLINE_CURVE_WITH_KNOTS ( ( 4, 4 ),
 ( 1.570796326794897224, 2.200856270442954621 ),
 .UNSPECIFIED. ) 
 CURVE ( )  GEOMETRIC_REPRESENTATION_ITEM ( )  RATIONAL_B_SPLINE_CURVE ( ( 1.000000000000000000, 0.9671913951481618810, 0.9671913951481618810, 1.000000000000000000 ) ) 
 REPRESENTATION_ITEM ( '' )  );
#150818=CARTESIAN_POINT ( 'NONE',  ( 6.656690234629796699, 6.868486149930637552, 1.040834085586084257E-14 ) ) ;
#150819=CARTESIAN_POINT ( 'NONE',  ( -2.252626078164912560, 5.779814191167667481, 0.7998128361456341429 ) ) ;
#150824=CARTESIAN_POINT ( 'NONE',  ( -4.497554271431319250, 6.270232621468402989, -1.599625672291256295 ) ) ;
#150826=EDGE_CURVE ( 'NONE', #116745, #73904, #9409, .T. ) ;
#150835=CARTESIAN_POINT ( 'NONE',  ( 7.913155211870404493, 12.38376484715752213, 0.7998128361456462443 ) ) ;
#150836=CARTESIAN_POINT ( 'NONE',  ( 5.624517712206933417, 6.335738387217328516, 1.153896037602806013 ) ) ;
#150837=DIRECTION ( 'NONE',  ( 1.207943261119674327E-30, 2.168404344971008079E-15, -1.000000000000000000 ) ) ;
#150839=CARTESIAN_POINT ( 'NONE',  ( 5.359550796103802028, 5.147230771742885125, -0.7998128361456231517 ) ) ;
#150844=CARTESIAN_POINT ( 'NONE',  ( -8.459924665247381625, 11.85336729522185806, 1.082531754730560403 ) ) ;
#150848=CARTESIAN_POINT ( 'NONE',  ( 8.288111976655649471, 8.563885482386732306, -0.7998128361456291469 ) ) ;
#150851=CARTESIAN_POINT ( 'NONE',  ( 3.571683402196252910, 6.254382171615883834, 1.199719254218462483 ) ) ;
#150853=CARTESIAN_POINT ( 'NONE',  ( -6.762819695118240659, 6.784377820593065600, 0.7998128361456341429 ) ) ;
#150856=CIRCLE ( 'NONE', #202612, 0.08000000000000004330 ) ;
#150859=CARTESIAN_POINT ( 'NONE',  ( 9.565441069641300587, 11.11843498845840905, -1.199719254218440723 ) ) ;
#150860=CARTESIAN_POINT ( 'NONE',  ( 0.5988494165465870767, 6.720065942961383598, 3.593421257281793402 ) ) ;
#150863=CARTESIAN_POINT ( 'NONE',  ( 4.009205846845453003, 7.815100513429686480, -0.2297154615349787654 ) ) ;
#150864=CARTESIAN_POINT ( 'NONE',  ( 6.155038550924150087, 7.243595066575396757, 1.082531754730558626 ) ) ;
#150868=CARTESIAN_POINT ( 'NONE',  ( -1.284945213870648306, 3.300000000000025135, -0.4778516606550328727 ) ) ;
#150871=CARTESIAN_POINT ( 'NONE',  ( 7.985389288324691748, 10.33937347451072775, -1.443375672974058777 ) ) ;
#150872=ADVANCED_FACE ( 'NONE', ( #133687 ), #71844, .F. ) ;
#150876=CARTESIAN_POINT ( 'NONE',  ( -7.069687034522070590, 10.33538640932937724, -1.199719254218440723 ) ) ;
#150885=CARTESIAN_POINT ( 'NONE',  ( 8.380911511541880188, 12.92948053010758258, 0.7998128361456462443 ) ) ;
#150889=CARTESIAN_POINT ( 'NONE',  ( 3.825371897350130723, 7.614684313550482031, 0.7998128361456321445 ) ) ;
#150893=CARTESIAN_POINT ( 'NONE',  ( -1.500000000000011324, 3.952083334016153415, 0.8660254037844403729 ) ) ;
#150899=CARTESIAN_POINT ( 'NONE',  ( -1.500000000000013101, 1.129166666666688634, -0.8660254037844313801 ) ) ;
#150900=CARTESIAN_POINT ( 'NONE',  ( 5.666418135507635512, 8.698239360479199433, 1.199719254218462483 ) ) ;
#150901=CARTESIAN_POINT ( 'NONE',  ( 4.894130264408854458, 6.732904613275549899, -1.443375672974051449 ) ) ;
#150905=CARTESIAN_POINT ( 'NONE',  ( 9.571693261567965294, 10.26932301469188857, 0.7216878364870438212 ) ) ;
#150911=CARTESIAN_POINT ( 'NONE',  ( -5.901876940650454095, 5.779944607047298177, -0.7998128361456291469 ) ) ;
#150913=CARTESIAN_POINT ( 'NONE',  ( -0.7500000000000215383, 3.722916667349487785, 1.299038105676671107 ) ) ;
#150914=CARTESIAN_POINT ( 'NONE',  ( -0.6823417656250246877, -0.4489583329919111243, 1.181850606188755259 ) ) ;
#150921=CARTESIAN_POINT ( 'NONE',  ( 0.6823417656249899377, 3.988541667008085767, -1.181850606188754593 ) ) ;
#150929=CARTESIAN_POINT ( 'NONE',  ( -8.148614017013223076, 9.465470093725620870, -1.199719254218446718 ) ) ;
#150930=CARTESIAN_POINT ( 'NONE',  ( 6.979750152936881058, 7.037463354714830643, 0.7998128361456341429 ) ) ;
#150932=CARTESIAN_POINT ( 'NONE',  ( -0.6823417656250003738, -1.032291666325242607, -1.181850606188749264 ) ) ;
#150937=CARTESIAN_POINT ( 'NONE',  ( -0.003385325826195171531, 8.210945192570349604, -2.038658773260200174 ) ) ;
#150939=CARTESIAN_POINT ( 'NONE',  ( -5.799137018343247796, 7.788745826199009237, -1.599625672291256295 ) ) ;
#150944=CARTESIAN_POINT ( 'NONE',  ( 9.890836756369282057, 11.49806328964105617, -1.199719254218440723 ) ) ;
#150946=CARTESIAN_POINT ( 'NONE',  ( -2.903417451620861289, 6.539070793532962611, 0.7998128361456341429 ) ) ;
#150947=CARTESIAN_POINT ( 'NONE',  ( -6.723954117373590833, 9.932031339322813679, -1.199719254218440723 ) ) ;
#150949=CARTESIAN_POINT ( 'NONE',  ( -4.474540158260005285, 7.266292661500576955, 1.287230779100386968 ) ) ;
#150950=CARTESIAN_POINT ( 'NONE',  ( -1.402160292154681736E-14, -0.8031249996585825279, -1.575800808251665908 ) ) ;
#150954=CARTESIAN_POINT ( 'NONE',  ( 7.619319141200057821, 10.87266085050000974, 1.082531754730557072 ) ) ;
#150977=CARTESIAN_POINT ( 'NONE',  ( -5.773074481320628948, 5.629675071162500544, 0.000000000000000000 ) ) ;
#150978=CARTESIAN_POINT ( 'NONE',  ( -8.670602931139386627, 10.07445716020612103, 1.199719254218462483 ) ) ;
#150984=CARTESIAN_POINT ( 'NONE',  ( -0.7500000000000215383, 2.972916667349487341, 1.299038105676671107 ) ) ;
#150985=CARTESIAN_POINT ( 'NONE',  ( 8.890396042259068210, 11.39521468743417998, -1.599625672291257406 ) ) ;
#150989=CARTESIAN_POINT ( 'NONE',  ( -8.503988664269602538, 10.94440607977979063, 1.599625672291269396 ) ) ;
#150991=CARTESIAN_POINT ( 'NONE',  ( -0.6823417656250212460, 2.051041667008083991, 1.181850606188767472 ) ) ;
#150993=CARTESIAN_POINT ( 'NONE',  ( -4.952636518945644717, 6.537114055553945313, 2.442608363190701404 ) ) ;
#150994=VERTEX_POINT ( 'NONE', #54532 ) ;
#150998=CARTESIAN_POINT ( 'NONE',  ( -2.428882075142555497, 5.985446187641602300, 1.040834085586084257E-14 ) ) ;
#151002=CARTESIAN_POINT ( 'NONE',  ( 1.364683531249986537, 0.2177083336747502595, -0.7879004041258309554 ) ) ;
#151007=CARTESIAN_POINT ( 'NONE',  ( -0.6823417656250212460, 1.801041667008083991, 1.181850606188755259 ) ) ;
#151010=CARTESIAN_POINT ( 'NONE',  ( -7.413611068574208041, 7.543634422958360730, 0.7998128361456341429 ) ) ;
#151011=CARTESIAN_POINT ( 'NONE',  ( 8.599949509769960088, 8.927695937686774386, 1.040834085586084257E-14 ) ) ;
#151012=CARTESIAN_POINT ( 'NONE',  ( -1.217358635584817383, 2.889784080462333371, 0.7750000000000083489 ) ) ;
#151014=CARTESIAN_POINT ( 'NONE',  ( 3.994848817520957773, 7.812407387083109001, 1.040834085586084257E-14 ) ) ;
#151016=CARTESIAN_POINT ( 'NONE',  ( -1.499999999999997780, 3.150000000000020783, 1.214306433183764966E-14 ) ) ;
#151019=CARTESIAN_POINT ( 'NONE',  ( 0.6823417656249899377, 0.9052083336747520637, 1.181850606188755259 ) ) ;
#151025=CARTESIAN_POINT ( 'NONE',  ( 5.992340707560160240, 7.053780915984068756, 1.082531754730558626 ) ) ;
#151028=CARTESIAN_POINT ( 'NONE',  ( -7.479294296233107708, 11.87759377891399204, 0.7998128361456481317 ) ) ;
#151029=CARTESIAN_POINT ( 'NONE',  ( -4.939248034080176097, 4.656877549381960080, 1.214306433183764966E-14 ) ) ;
#151030=DIRECTION ( 'NONE',  ( 0.000000000000000000, 0.000000000000000000, 1.000000000000000000 ) ) ;
#151035=CARTESIAN_POINT ( 'NONE',  ( -7.334597914868735025, 9.580116872145431728, -1.443375672974058777 ) ) ;
#151037=CARTESIAN_POINT ( 'NONE',  ( -0.7500000000000215383, 5.191666666666685082, 1.299038105676671107 ) ) ;
#151040=CARTESIAN_POINT ( 'NONE',  ( 8.107412671292035355, 10.48173408797264194, 1.443375672974076540 ) ) ;
#151049=CARTESIAN_POINT ( 'NONE',  ( 9.151390499099949949, 12.66007743471656788, -1.082531754730543971 ) ) ;
#151055=ORIENTED_EDGE ( 'NONE', *, *, #150235, .T. ) ;
#151059=CARTESIAN_POINT ( 'NONE',  ( 6.103141704446003679, 10.27208242182903142, 0.7998128361456462443 ) ) ;
#151060=CARTESIAN_POINT ( 'NONE',  ( -6.091691091241777656, 6.001394449403842479, 0.7998128361456341429 ) ) ;
#151064=CARTESIAN_POINT ( 'NONE',  ( -0.6823417656250003738, -0.7197916663252492686, -1.181850606188749264 ) ) ;
#151065=CARTESIAN_POINT ( 'NONE',  ( 4.229780737783593203, 4.037091736943370535, -0.7216878364870188411 ) ) ;
#151066=CARTESIAN_POINT ( 'NONE',  ( -4.322352044658376968, 3.937165561723182883, 0.7998128361456341429 ) ) ;
#151078=ORIENTED_EDGE ( 'NONE', *, *, #122616, .F. ) ;
#151082=CARTESIAN_POINT ( 'NONE',  ( 7.579171565239241737, 8.801120566655981747, 1.199719254218462483 ) ) ;
#151095=CARTESIAN_POINT ( 'NONE',  ( -4.550733115681270036, 8.460939068270139529, 0.7998128361456481317 ) ) ;
#151097=CARTESIAN_POINT ( 'NONE',  ( -4.765854690403601879, 5.518917546014321829, 1.199719254218462483 ) ) ;
#151106=CARTESIAN_POINT ( 'NONE',  ( -9.408995418203979000, 12.00024729270324286, 1.443375672974076540 ) ) ;
#151109=CARTESIAN_POINT ( 'NONE',  ( 6.368579470117202490, 8.453095353268645695, 1.599625672291281386 ) ) ;
#151110=CARTESIAN_POINT ( 'NONE',  ( 0.6823417656249917140, 4.092708333674755394, 1.181850606188765695 ) ) ;
#151116=CARTESIAN_POINT ( 'NONE',  ( 5.246642258364164313, 8.104537820524768676, -1.082531754730549078 ) ) ;
#151117=CARTESIAN_POINT ( 'NONE',  ( -5.910464900553636269, 8.982960586366182554, -1.199719254218440723 ) ) ;
#151121=CARTESIAN_POINT ( 'NONE',  ( -6.347188469492005325, 10.55680364771601809, -0.7998128361456291469 ) ) ;
#151123=CARTESIAN_POINT ( 'NONE',  ( -5.762378981008047241, 6.681529218386182301, 1.199719254218450271 ) ) ;
#151129=CARTESIAN_POINT ( 'NONE',  ( 7.124973419181436007, 8.271222729588529887, -1.199719254218446718 ) ) ;
#151140=ORIENTED_EDGE ( 'NONE', *, *, #16981, .F. ) ;
#151142=CARTESIAN_POINT ( 'NONE',  ( 1.499999999999989120, 5.295833333333356485, -0.8660254037844323793 ) ) ;
#151143=CARTESIAN_POINT ( 'NONE',  ( 4.630273154266905777, 5.360739087188218122, 1.199719254218464037 ) ) ;
#151144=CARTESIAN_POINT ( 'NONE',  ( 6.114890974963323345, 7.092793211334054604, 1.199719254218462483 ) ) ;
#151146=CARTESIAN_POINT ( 'NONE',  ( -7.212574532790092974, 10.39812547402169862, -1.082531754730543971 ) ) ;
#151147=CARTESIAN_POINT ( 'NONE',  ( 4.961921032921539521, 7.772363057508363759, -1.082531754730549078 ) ) ;
#151148=CARTESIAN_POINT ( 'NONE',  ( -8.636180661780672452, 9.177891648273343250, -0.7216878364870267237 ) ) ;
#151152=CARTESIAN_POINT ( 'NONE',  ( 7.182068686937156166, 9.402166106225269715, 1.599625672291281386 ) ) ;
#151156=DIRECTION ( 'NONE',  ( 0.000000000000000000, 8.546850786086437571E-32, 1.000000000000000000 ) ) ;
#151157=CARTESIAN_POINT ( 'NONE',  ( 0.6823417656249899377, 3.092708333674754062, 1.181850606188765695 ) ) ;
#151163=CARTESIAN_POINT ( 'NONE',  ( 9.772729797352075920, 10.29593960653257234, -0.7998128361456281477 ) ) ;
#151166=CARTESIAN_POINT ( 'NONE',  ( -9.528683032306089373, 10.01121838064558744, 0.7998128361456462443 ) ) ;
#151172=CARTESIAN_POINT ( 'NONE',  ( 10.55232363013785246, 11.20546574478267132, 0.000000000000000000 ) ) ;
#151175=CARTESIAN_POINT ( 'NONE',  ( -8.799405390469187793, 10.22472669609091689, -1.199719254218446718 ) ) ;
#151178=CARTESIAN_POINT ( 'NONE',  ( 4.858666941289190078, 5.005999693891180158, -0.7510321973731617362 ) ) ;
#151181=CARTESIAN_POINT ( 'NONE',  ( 5.712091369430416066, 6.087825614771766425, 0.6924918054137980672 ) ) ;
#151182=CARTESIAN_POINT ( 'NONE',  ( -4.274898507010545856, 3.881803101134051470, -0.7998128361456221525 ) ) ;
#151186=CARTESIAN_POINT ( 'NONE',  ( 7.935599982700328958, 8.152621489438862667, 0.7998128361456481317 ) ) ;
#151188=CARTESIAN_POINT ( 'NONE',  ( 6.986529229743720926, 7.045372277656132276, -0.7998128361456281477 ) ) ;
#151189=CARTESIAN_POINT ( 'NONE',  ( 4.955668840994886359, 5.740367388370866131, 1.199719254218462483 ) ) ;
#151191=AXIS2_PLACEMENT_3D ( 'NONE', #147479, #97669, #14233 ) ;
#151192=CARTESIAN_POINT ( 'NONE',  ( -8.527715433315703919, 9.051348881730875817, 1.040834085586084257E-14 ) ) ;
#151199=CARTESIAN_POINT ( 'NONE',  ( -4.022721148277657477, 7.614442113290216696, -0.1953124528039917873 ) ) ;
#151200=CARTESIAN_POINT ( 'NONE',  ( 4.264789376140788235, 7.497597942732838305, -1.024658161349981444 ) ) ;
#151203=CARTESIAN_POINT ( 'NONE',  ( 6.168596704537822717, 6.299043698156668647, 1.040834085586084257E-14 ) ) ;
#151205=CARTESIAN_POINT ( 'NONE',  ( 7.750457368506414646, 12.19395069656619945, 0.7998128361456462443 ) ) ;
#151208=CARTESIAN_POINT ( 'NONE',  ( -8.771762197917311710, 13.17754696430482042, 0.7216878364870317197 ) ) ;
#151214=CYLINDRICAL_SURFACE ( 'NONE', #146404, 1.250000000000000000 ) ;
#151223=CARTESIAN_POINT ( 'NONE',  ( -9.286972035236630063, 10.89751746493999107, -1.082531754730537976 ) ) ;
#151230=CARTESIAN_POINT ( 'NONE',  ( 1.499999999999987121, 3.577083334016152527, -0.8660254037844262731 ) ) ;
#151232=CARTESIAN_POINT ( 'NONE',  ( -6.742482464697739708, 6.760651051769146491, 0.7998128361456341429 ) ) ;
#151235=CARTESIAN_POINT ( 'NONE',  ( -9.321394304595349567, 10.83371376257142416, 1.199719254218462483 ) ) ;
#151236=CARTESIAN_POINT ( 'NONE',  ( 0.006768871532346317291, 8.210909518262139883, 2.038649385027042626 ) ) ;
#151238=CARTESIAN_POINT ( 'NONE',  ( 0.7499999999999902300, 4.347916667349481123, -1.299038105676658228 ) ) ;
#151239=CARTESIAN_POINT ( 'NONE',  ( 5.774883364416965037, 8.824782127540085952, -1.199719254218440723 ) ) ;
#151243=CARTESIAN_POINT ( 'NONE',  ( 10.08456733046637765, 10.65975006183261087, 0.000000000000000000 ) ) ;
#151246=CARTESIAN_POINT ( 'NONE',  ( 3.701012746850603996, 7.261672604726938651, 1.040834085586084257E-14 ) ) ;
#151250=CARTESIAN_POINT ( 'NONE',  ( -7.429504990608782222, 8.730472579540773381, 1.082531754730549967 ) ) ;
#151253=CARTESIAN_POINT ( 'NONE',  ( -0.6823417656249969321, 5.030208333674755394, -1.181850606188749264 ) ) ;
#151259=CARTESIAN_POINT ( 'NONE',  ( -2.941756144040970522, 5.415504020480993219, -1.082531754730543083 ) ) ;
#151261=CARTESIAN_POINT ( 'NONE',  ( 9.049177462117294013, 12.64479190819049670, -1.199719254218446718 ) ) ;
#151262=CARTESIAN_POINT ( 'NONE',  ( 0.6823417656249917140, 4.905208333674755394, 1.181850606188765695 ) ) ;
#151267=CARTESIAN_POINT ( 'NONE',  ( -0.6823417656250003738, 2.467708333674753618, -1.181850606188749264 ) ) ;
#151268=CARTESIAN_POINT ( 'NONE',  ( -4.284013352238274841, 4.100363120473813794, -0.7216878364870207285 ) ) ;
#151269=CARTESIAN_POINT ( 'NONE',  ( 3.551346171775753735, 6.230655402791975384, 1.199719254218462483 ) ) ;
#151275=( BOUNDED_SURFACE ( )  B_SPLINE_SURFACE ( 3, 2, ( 
 ( #73661, #58483, #104043 ),
 ( #102970, #202569, #54220 ),
 ( #8655, #106218, #91004 ),
 ( #172244, #71507, #89937 ) ),
 .UNSPECIFIED., .F., .F., .T. ) 
 B_SPLINE_SURFACE_WITH_KNOTS ( ( 4, 4 ),
 ( 3, 3 ),
 ( 3.059570999470615060, 3.223614307708551951 ),
 ( 0.000000000000000000, 1.000000000000000000 ),
 .UNSPECIFIED. ) 
 GEOMETRIC_REPRESENTATION_ITEM ( )  RATIONAL_B_SPLINE_SURFACE ( (
 ( 1.000000000000000000, 0.6179932349765480115, 1.000000000000000000),
 ( 1.000000000000000000, 0.6282795510880925249, 1.000000000000000000),
 ( 1.000000000000000000, 0.6282795510881205026, 1.000000000000000000),
 ( 1.000000000000000000, 0.6179932349766239508, 1.000000000000000000) ) ) 
 REPRESENTATION_ITEM ( '' )  SURFACE ( )  );
#151278=CARTESIAN_POINT ( 'NONE',  ( -6.995644074971465010, 10.14503993989993091, 1.082531754730549967 ) ) ;
#151284=CARTESIAN_POINT ( 'NONE',  ( -9.657485491635913633, 10.16148791653038330, 1.040834085586084257E-14 ) ) ;
#151285=CARTESIAN_POINT ( 'NONE',  ( -4.161989969270909917, 5.878740935614591656, 1.443375672974064550 ) ) ;
#151286=CARTESIAN_POINT ( 'NONE',  ( -1.402160292154681736E-14, 2.009375000341422801, -1.575800808251660134 ) ) ;
#151299=ORIENTED_EDGE ( 'NONE', *, *, #96162, .F. ) ;
#151302=DIRECTION ( 'NONE',  ( 0.7592566023653005702, 0.6507913734559639396, 0.000000000000000000 ) ) ;
#151304=CARTESIAN_POINT ( 'NONE',  ( 1.500000000000003997, 5.900000000000022560, 1.214306433183764966E-14 ) ) ;
#151309=CARTESIAN_POINT ( 'NONE',  ( 0.6823417656249917140, 3.405208333674754506, 1.181850606188765695 ) ) ;
#151316=CARTESIAN_POINT ( 'NONE',  ( 8.615316546479974136, 12.13862083994696839, 1.199719254218450271 ) ) ;
#151319=CARTESIAN_POINT ( 'NONE',  ( 1.364683531249986537, 2.405208333674752286, -0.7879004041258239610 ) ) ;
#151329=CARTESIAN_POINT ( 'NONE',  ( 3.506755287428983792, 7.242964935309132990, 1.040834085586084257E-14 ) ) ;
#151340=CARTESIAN_POINT ( 'NONE',  ( -2.435661151949389147, 5.993355110582911038, 0.7998128361456341429 ) ) ;
#151341=CARTESIAN_POINT ( 'NONE',  ( 8.606728586576791074, 8.935604860628076906, 0.7998128361456462443 ) ) ;
#151344=CARTESIAN_POINT ( 'NONE',  ( 5.951666246274807115, 6.045958163516475636, 0.7216878364870317197 ) ) ;
#151354=CARTESIAN_POINT ( 'NONE',  ( -5.721177635286839092, 9.618531641235897212, 0.7216878364870458196 ) ) ;
#151356=CARTESIAN_POINT ( 'NONE',  ( 4.955668840994886359, 5.740367388370866131, 1.199719254218462483 ) ) ;
#151360=CARTESIAN_POINT ( 'NONE',  ( -9.484092147959342967, 11.02352791316275216, 1.199719254218462483 ) ) ;
#151364=CARTESIAN_POINT ( 'NONE',  ( -8.597841969360544567, 13.18256606422934674, 0.7998128361456341429 ) ) ;
#151365=EDGE_CURVE ( 'NONE', #103797, #6371, #50069, .T. ) ;
#151367=CARTESIAN_POINT ( 'NONE',  ( 8.723781775389312543, 12.26516360700784958, -1.199719254218446718 ) ) ;
#151368=CARTESIAN_POINT ( 'NONE',  ( 4.192495815123822744, 5.914331089109666983, -1.599625672291255185 ) ) ;
#151370=ORIENTED_EDGE ( 'NONE', *, *, #104548, .F. ) ;
#151374=CARTESIAN_POINT ( 'NONE',  ( 3.009546912553647147, 5.494593250412460606, -1.082531754730543083 ) ) ;
#151377=CARTESIAN_POINT ( 'NONE',  ( -5.525111292768871252, 6.404716915440499037, -1.199719254218446718 ) ) ;
#151378=DIRECTION ( 'NONE',  ( 5.578564026256490882E-16, 1.000000000000000000, 9.066213480720158442E-32 ) ) ;
#151380=CARTESIAN_POINT ( 'NONE',  ( -8.286004436246233951, 12.81875560892930466, 1.040834085586084257E-14 ) ) ;
#151385=CARTESIAN_POINT ( 'NONE',  ( 9.110716038703335684, 9.731516254683127087, -0.7216878364870197293 ) ) ;
#151386=CARTESIAN_POINT ( 'NONE',  ( -1.364683531250010740, 5.592708333674751842, 0.7879004041258379498 ) ) ;
#151388=CARTESIAN_POINT ( 'NONE',  ( 4.090809663021327758, 5.795697244990093644, 1.599625672291267398 ) ) ;
#151390=CARTESIAN_POINT ( 'NONE',  ( 5.301401758143367893, 6.143722458377430584, 1.199719254218462483 ) ) ;
#151392=CARTESIAN_POINT ( 'NONE',  ( -6.042130013184518589, 10.20090211535728031, -0.7998128361456291469 ) ) ;
#151398=DIRECTION ( 'NONE',  ( 0.000000000000000000, 8.546850786086437571E-32, 1.000000000000000000 ) ) ;
#151402=CARTESIAN_POINT ( 'NONE',  ( 0.6823417656249899377, 2.905208333674754062, 1.181850606188765695 ) ) ;
#151403=CARTESIAN_POINT ( 'NONE',  ( 10.24048609702354717, 10.84165528948263457, -0.7998128361456281477 ) ) ;
#151405=CARTESIAN_POINT ( 'NONE',  ( -3.606105671554953318, 7.150947683548662503, 0.7216878364870317197 ) ) ;
#151406=CARTESIAN_POINT ( 'NONE',  ( 3.307826292054301121, 4.882216645528547616, -1.443375672974057666 ) ) ;
#151407=CARTESIAN_POINT ( 'NONE',  ( -5.138177029454855216, 7.017625839162543677, 1.443375672974064550 ) ) ;
#151413=CARTESIAN_POINT ( 'NONE',  ( 4.660252114795294887, 6.460046772059735432, -1.599625672291256295 ) ) ;
#151423=CARTESIAN_POINT ( 'NONE',  ( 5.361359679200154105, 8.342337828120466980, 1.199719254218462483 ) ) ;
#151427=CARTESIAN_POINT ( 'NONE',  ( -6.898401231254901234, 6.942556279419168419, -0.7998128361456291469 ) ) ;
#151431=CARTESIAN_POINT ( 'NONE',  ( 7.450369105909416589, 8.650851030771185890, -1.199719254218441611 ) ) ;
#151434=CARTESIAN_POINT ( 'NONE',  ( -4.062639585589296942, 7.891496616496157301, 0.7998128361456341429 ) ) ;
#151436=CARTESIAN_POINT ( 'NONE',  ( 6.656690234185433042, 7.828855363713562276, -1.082531754730543971 ) ) ;
#151437=CARTESIAN_POINT ( 'NONE',  ( 5.327099315257549428, 6.547468694062620997, 1.346473575380419563 ) ) ;
#151438=CARTESIAN_POINT ( 'NONE',  ( -3.924195396151603177, 6.665646164563756138, 1.199719254218464037 ) ) ;
#151441=CARTESIAN_POINT ( 'NONE',  ( -3.899941742225307539, 7.701682465904834629, 0.7998128361456341429 ) ) ;
#151444=CARTESIAN_POINT ( 'NONE',  ( -1.364683531250012516, 2.530208333674753174, 0.7879004041258379498 ) ) ;
#151446=CARTESIAN_POINT ( 'NONE',  ( -4.717874267875590277, 7.487641831621378863, 1.082531754730560403 ) ) ;
#151453=CARTESIAN_POINT ( 'NONE',  ( 3.832150974156964818, 7.622593236491780999, 1.040834085586084257E-14 ) ) ;
#151456=CARTESIAN_POINT ( 'NONE',  ( -1.364683531249997417, 2.571875000341422357, 1.214306433183764966E-14 ) ) ;
#151459=CARTESIAN_POINT ( 'NONE',  ( -1.402160292154681736E-14, -0.8656249996585829720, 1.575800808251672791 ) ) ;
#151462=CARTESIAN_POINT ( 'NONE',  ( -4.485049888022365927, 4.126979712314507331, 0.7998128361456341429 ) ) ;
#151463=CARTESIAN_POINT ( 'NONE',  ( -7.171900071504748730, 8.429933507252760805, -1.082531754730549078 ) ) ;
#151467=CARTESIAN_POINT ( 'NONE',  ( -0.6823417656250212460, 2.801041667008084879, 1.181850606188767472 ) ) ;
#151474=CARTESIAN_POINT ( 'NONE',  ( -8.012505595552038784, 8.450270737673262644, 0.7216878364870578100 ) ) ;
#151476=EDGE_CURVE ( 'NONE', #99491, #54687, #85623, .T. ) ;
#151480=CARTESIAN_POINT ( 'NONE',  ( -7.510853911846401942, 7.865010440016681592, 1.040834085586084257E-14 ) ) ;
#151493=CARTESIAN_POINT ( 'NONE',  ( -6.663996196316808174, 7.733415969579778171, -1.199719254218446718 ) ) ;
#151496=CARTESIAN_POINT ( 'NONE',  ( 3.684065054611349144, 5.321161868511784299, -1.599625672291262513 ) ) ;
#151499=CARTESIAN_POINT ( 'NONE',  ( 5.738125327081736060, 7.717565519727259904, 1.599625672291267398 ) ) ;
#151505=CARTESIAN_POINT ( 'NONE',  ( -3.307826292054304673, 6.802955074131234348, -0.7216878364870267237 ) ) ;
#151510=CARTESIAN_POINT ( 'NONE',  ( 1.499999999999989120, 6.200000000000045475, 2.580000000000000515 ) ) ;
#151511=DIRECTION ( 'NONE',  ( 0.7592566023653004592, -0.6507913734559639396, -0.000000000000000000 ) ) ;
#151515=CARTESIAN_POINT ( 'NONE',  ( 1.364683531249986537, 2.405208333674752286, -0.7879004041258239610 ) ) ;
#151516=DIRECTION ( 'NONE',  ( -5.578564026256490882E-16, -1.000000000000000000, -9.066213480720158442E-32 ) ) ;
#151517=CARTESIAN_POINT ( 'NONE',  ( -6.340409392685171674, 10.54889472477470846, 0.7998128361456481317 ) ) ;
#151519=CARTESIAN_POINT ( 'NONE',  ( 6.958359152311676787, 9.141171649162195934, -1.599625672291262513 ) ) ;
#151520=CARTESIAN_POINT ( 'NONE',  ( -7.660520486921249983, 8.896027641951645748, -1.199719254218446718 ) ) ;
#151523=CARTESIAN_POINT ( 'NONE',  ( -1.364683531249997417, 5.759375000341418804, 1.214306433183764966E-14 ) ) ;
#151525=CARTESIAN_POINT ( 'NONE',  ( 7.293923454472077239, 10.49303254931736262, 1.082531754730558626 ) ) ;
#151528=CARTESIAN_POINT ( 'NONE',  ( -0.6823417656250003738, 1.030208333674752286, -1.181850606188749264 ) ) ;
#151531=CARTESIAN_POINT ( 'NONE',  ( 8.066738210006686671, 9.473911335505048825, 1.082531754730558626 ) ) ;
#151534=CARTESIAN_POINT ( 'NONE',  ( -3.931501358282937009, 7.530575984731317618, 0.7216878364870317197 ) ) ;
#151536=CARTESIAN_POINT ( 'NONE',  ( -1.201851678989727383E-14, 2.696875000341417916, -1.575800808251660134 ) ) ;
#151540=CARTESIAN_POINT ( 'NONE',  ( -6.338600509588822263, 7.353787668397130162, -1.199719254218446718 ) ) ;
#151548=CARTESIAN_POINT ( 'NONE',  ( 7.958799866421889746, 9.244020251369077457, -1.199719254218441611 ) ) ;
#151551=CARTESIAN_POINT ( 'NONE',  ( 0.7499999999999885647, 2.066666666666688634, -1.299038105676652899 ) ) ;
#151553=EDGE_CURVE ( 'NONE', #197417, #40273, #184295, .T. ) ;
#151559=CARTESIAN_POINT ( 'NONE',  ( 6.670248388243460447, 6.884303995813253252, -0.7216878364870257245 ) ) ;
#151560=CARTESIAN_POINT ( 'NONE',  ( -1.364683531250000748, 1.321875000341421469, 0.000000000000000000 ) ) ;
#151561=EDGE_CURVE ( 'NONE', #71636, #6682, #21771, .T. ) ;
#151563=CARTESIAN_POINT ( 'NONE',  ( 3.297657676621871925, 4.870353260857385180, 1.599625672291267398 ) ) ;
#151569=CARTESIAN_POINT ( 'NONE',  ( -1.402160292154681736E-14, 0.4625000000000214495, 1.732050807568877637 ) ) ;
#151570=CARTESIAN_POINT ( 'NONE',  ( 8.101160479365381306, 9.410107633136481908, -1.199719254218446718 ) ) ;
#151571=CARTESIAN_POINT ( 'NONE',  ( -8.910733272679575379, 11.41894145625809820, -1.599625672291263179 ) ) ;
#151573=CARTESIAN_POINT ( 'NONE',  ( 0.6823417656249882723, 0.9260416670080831025, -1.181850606188749264 ) ) ;
#151574=CARTESIAN_POINT ( 'NONE',  ( 0.7499999999999885647, 1.066666666666687968, -1.299038105676652899 ) ) ;
#151577=CARTESIAN_POINT ( 'NONE',  ( 4.660252114795294887, 6.460046772059735432, -1.599625672291256295 ) ) ;
#151580=CARTESIAN_POINT ( 'NONE',  ( 1.499999999999990896, 4.556250000682819490, 1.214306433183764966E-14 ) ) ;
#151584=CARTESIAN_POINT ( 'NONE',  ( 0.7499999999999867883, -0.6520833326505159899, -1.299038105676652899 ) ) ;
#151585=CARTESIAN_POINT ( 'NONE',  ( -7.157815033010924921, 10.43820240756634199, 1.199719254218453823 ) ) ;
#151586=CARTESIAN_POINT ( 'NONE',  ( -5.748293942514189681, 5.808690475795744490, -0.7216878364870207285 ) ) ;
#151594=CARTESIAN_POINT ( 'NONE',  ( 6.479907352327590964, 9.647310113435821677, 1.199719254218462483 ) ) ;
#151597=CARTESIAN_POINT ( 'NONE',  ( 5.788968402910802169, 8.737251655829183505, 1.082531754730558626 ) ) ;
#151601=CARTESIAN_POINT ( 'NONE',  ( -9.155833807930273238, 9.576227618873799585, -0.7998128361456291469 ) ) ;
#151602=CARTESIAN_POINT ( 'NONE',  ( 4.333802657862601215, 8.207853534148366492, 0.7998128361456462443 ) ) ;
#151605=CARTESIAN_POINT ( 'NONE',  ( 3.997610708356745146, 7.599328567695712522, -0.1184163795967980992 ) ) ;
#151606=CARTESIAN_POINT ( 'NONE',  ( 2.659370686574860976, 6.254349567645977714, -0.7998128361456291469 ) ) ;
#151610=CARTESIAN_POINT ( 'NONE',  ( 3.092648394857516525, 6.449253795920727228, -0.4031905389056261724 ) ) ;
#151611=CIRCLE ( 'NONE', #75388, 0.8299999999999999600 ) ;
#151615=CARTESIAN_POINT ( 'NONE',  ( -3.145128448690310830, 6.613140923539910787, -0.7216878364870267237 ) ) ;
#151616=CARTESIAN_POINT ( 'NONE',  ( 8.107412671292022921, 12.40247251657532956, 0.7216878364870438212 ) ) ;
#151620=CARTESIAN_POINT ( 'NONE',  ( -7.067878151425722955, 7.140279352951794500, 0.7998128361456341429 ) ) ;
#151624=CARTESIAN_POINT ( 'NONE',  ( 1.123270288250309612, 2.971052654332832610, -0.7749999999993620881 ) ) ;
#151626=CARTESIAN_POINT ( 'NONE',  ( -7.344766530301162000, 9.591980256816594164, 1.599625672291295375 ) ) ;
#151641=CARTESIAN_POINT ( 'NONE',  ( -6.507023659554960204, 9.678945805201045971, 1.199719254218452047 ) ) ;
#151644=CARTESIAN_POINT ( 'NONE',  ( 4.772106882330221289, 6.590544000850479200, -1.443375672974051449 ) ) ;
#151649=CARTESIAN_POINT ( 'NONE',  ( -3.425406365747000859, 7.148057860013469877, 1.040834085586084257E-14 ) ) ;
#151653=CYLINDRICAL_SURFACE ( 'NONE', #133001, 1.500000000000000222 ) ;
#151658=CARTESIAN_POINT ( 'NONE',  ( -7.506410603460441422, 11.90922947067921278, -0.7998128361456291469 ) ) ;
#151659=CARTESIAN_POINT ( 'NONE',  ( 8.125414133291656071, 8.374071331795406081, -0.7998128361456291469 ) ) ;
#151665=CARTESIAN_POINT ( 'NONE',  ( 1.364683531249986537, -0.07395833299191513499, 0.7879004041258500513 ) ) ;
#151670=CARTESIAN_POINT ( 'NONE',  ( 8.351459436338029008, 10.76645531385962862, -1.443375672974063439 ) ) ;
#151695=( BOUNDED_CURVE ( )  B_SPLINE_CURVE ( 2, ( #62163, #93613, #63220, #129382, #45929, #145587, #109911 ),
 .UNSPECIFIED., .F., .T. ) 
 B_SPLINE_CURVE_WITH_KNOTS ( ( 3, 2, 2, 3 ),
 ( 0.2500000000000002220, 0.2559523809523810978, 0.2619047619047619735, 0.2678571428571428492 ),
 .UNSPECIFIED. ) 
 CURVE ( )  GEOMETRIC_REPRESENTATION_ITEM ( )  RATIONAL_B_SPLINE_CURVE ( ( 0.9999999999999950040, 0.8660254037844437036, 1.000000000000000000, 0.8660254037844387076, 1.000000000000000000, 0.8660254037844387076, 1.000000000000000000 ) ) 
 REPRESENTATION_ITEM ( '' )  );
#151698=CARTESIAN_POINT ( 'NONE',  ( -1.402160292154681736E-14, 0.4937500006828175469, 1.732050807568877637 ) ) ;
#151702=CARTESIAN_POINT ( 'NONE',  ( 8.367353357928214663, 12.91366268422496688, 1.040834085586084257E-14 ) ) ;
#151707=CARTESIAN_POINT ( 'NONE',  ( 9.752392566931574081, 10.27221283770866300, -0.7998128361456281477 ) ) ;
#151712=CARTESIAN_POINT ( 'NONE',  ( 3.161022370280501814, 6.839609865302569425, 0.000000000000000000 ) ) ;
#151713=CARTESIAN_POINT ( 'NONE',  ( -1.364683531250012516, 3.092708333674755838, 0.7879004041258379498 ) ) ;
#151714=CARTESIAN_POINT ( 'NONE',  ( -5.912409256564314930, 5.999956524776160371, -0.009440138123966573813 ) ) ;
#151717=CARTESIAN_POINT ( 'NONE',  ( -7.914208982075130905, 10.25632978388623684, -1.599625672291263179 ) ) ;
#151718=CARTESIAN_POINT ( 'NONE',  ( -4.324687812634898876, 6.068555086205916105, 1.443375672974064550 ) ) ;
#151720=ORIENTED_EDGE ( 'NONE', *, *, #95454, .F. ) ;
#151721=CARTESIAN_POINT ( 'NONE',  ( 0.7499999999999867883, -0.6520833326505159899, -1.299038105676652899 ) ) ;
#151728=CARTESIAN_POINT ( 'NONE',  ( -3.429849674132936066, 6.945315686556313040, -0.7216878364870257245 ) ) ;
#151731=CARTESIAN_POINT ( 'NONE',  ( 4.002655450416458649, 7.592114961386800864, 0.1875155472659401079 ) ) ;
#151736=CARTESIAN_POINT ( 'NONE',  ( -3.090895833791289071, 6.549869539491048442, 1.040834085586084257E-14 ) ) ;
#151737=CARTESIAN_POINT ( 'NONE',  ( 8.585337585951586803, 11.03931315507545108, -1.599625672291255185 ) ) ;
#151746=CARTESIAN_POINT ( 'NONE',  ( -4.112233706258869859, 7.668264228514641623, 0.7994708601795056380 ) ) ;
#151751=CARTESIAN_POINT ( 'NONE',  ( 6.491656622844908853, 6.468020902940851968, 0.7998128361456341429 ) ) ;
#151757=CARTESIAN_POINT ( 'NONE',  ( 3.379006598303866848, 4.965260336153046516, -1.599625672291262513 ) ) ;
#151765=CARTESIAN_POINT ( 'NONE',  ( -2.492951620383208944, 8.266420250602596553, 2.456391984604374024 ) ) ;
#151769=CARTESIAN_POINT ( 'NONE',  ( 7.313733799568044702, 10.62010763521636214, 1.199719254218460707 ) ) ;
#151771=CARTESIAN_POINT ( 'NONE',  ( -4.954615070790188369, 7.867802451642154082, -1.199719254218452047 ) ) ;
#151776=CARTESIAN_POINT ( 'NONE',  ( -1.500000000000001332, -0.5687499993171779566, 0.000000000000000000 ) ) ;
#151780=CARTESIAN_POINT ( 'NONE',  ( 5.054492339796319733, 4.791329239384148231, -0.7998128361456211532 ) ) ;
#151781=CARTESIAN_POINT ( 'NONE',  ( -3.100010679019018500, 6.768429558830820980, 1.040834085586084257E-14 ) ) ;
#151787=CARTESIAN_POINT ( 'NONE',  ( 6.670248388243460447, 6.884303995813253252, -0.7216878364870257245 ) ) ;
#151789=ORIENTED_EDGE ( 'NONE', *, *, #6451, .T. ) ;
#151790=CARTESIAN_POINT ( 'NONE',  ( 7.822691444960700125, 10.14955932391940330, -1.443375672974058777 ) ) ;
#151791=CARTESIAN_POINT ( 'NONE',  ( 1.364683531249990311, 4.676041667008083103, 0.7879004041258500513 ) ) ;
#151793=CARTESIAN_POINT ( 'NONE',  ( 5.816084710138150093, 5.887779704690372817, -0.7216878364870257245 ) ) ;
#151797=CARTESIAN_POINT ( 'NONE',  ( 5.315329802055971165, 6.350237698360829519, -1.113282574169037531 ) ) ;
#151800=CARTESIAN_POINT ( 'NONE',  ( -4.920796802804098924, 6.860114910817498135, 1.449587651302047364 ) ) ;
#151804=CARTESIAN_POINT ( 'NONE',  ( -1.201851678989727383E-14, 4.759375000341419693, -1.575800808251660134 ) ) ;
#151809=CARTESIAN_POINT ( 'NONE',  ( -2.290964770585000920, 5.616616632417037458, -0.7216878364870257245 ) ) ;
#151811=DIRECTION ( 'NONE',  ( 1.000000000000000000, 0.000000000000000000, 0.000000000000000000 ) ) ;
#151819=CARTESIAN_POINT ( 'NONE',  ( 2.399429999938675007, 5.743159399996332404, 0.000000000000000000 ) ) ;
#151820=CARTESIAN_POINT ( 'NONE',  ( -1.201851678989727383E-14, 4.509375000341417916, -1.575800808251660134 ) ) ;
#151822=CARTESIAN_POINT ( 'NONE',  ( 8.274553823041976841, 8.548067636504127265, 1.040834085586084257E-14 ) ) ;
#151824=CARTESIAN_POINT ( 'NONE',  ( -7.479294296233107708, 11.87759377891399204, 0.7998128361456481317 ) ) ;
#151830=CARTESIAN_POINT ( 'NONE',  ( -1.001543065824772872E-14, 4.962500000000019007, 1.732050807568877637 ) ) ;
#151831=CARTESIAN_POINT ( 'NONE',  ( 6.308621549060418054, 6.254479983525607523, 0.7998128361456341429 ) ) ;
#151836=CARTESIAN_POINT ( 'NONE',  ( 8.487040972474689582, 9.964264558384387627, -1.082531754730543083 ) ) ;
#151840=CARTESIAN_POINT ( 'NONE',  ( -1.500000000000011324, 3.952083334016153415, 0.8660254037844403729 ) ) ;
#151842=CARTESIAN_POINT ( 'NONE',  ( -6.078132937628113908, 5.985576603521232109, 1.040834085586084257E-14 ) ) ;
#151843=CARTESIAN_POINT ( 'NONE',  ( 4.826339496340538382, 4.733076955259818419, 1.040834085586084257E-14 ) ) ;
#151853=CARTESIAN_POINT ( 'NONE',  ( 6.825640269476072497, 10.05066518344239412, 1.199719254218460707 ) ) ;
#151854=CARTESIAN_POINT ( 'NONE',  ( 3.472859903394816872, 7.203420320602605287, -0.7998128361456291469 ) ) ;
#151858=CARTESIAN_POINT ( 'NONE',  ( 1.123270288250308280, 2.860197346350005887, 0.7749999999993786304 ) ) ;
#151864=EDGE_LOOP ( 'NONE', ( #136683, #194384, #184902 ) ) ;
#151871=CARTESIAN_POINT ( 'NONE',  ( 5.786614514570532997, 6.041473168147688533, -0.5398422057949890940 ) ) ;
#151878=CARTESIAN_POINT ( 'NONE',  ( 5.938108093105483931, 8.911247961056314892, -1.082531754730537088 ) ) ;
#151880=CARTESIAN_POINT ( 'NONE',  ( -9.815740026613960723, 11.51441345488021106, -1.082531754730539753 ) ) ;
#151885=CARTESIAN_POINT ( 'NONE',  ( -3.744022975668147790, 7.519777238254810925, -0.7998128361456281477 ) ) ;
#151895=CARTESIAN_POINT ( 'NONE',  ( 8.341290820905593151, 10.75459192918846618, 1.599625672291281386 ) ) ;
#151897=CARTESIAN_POINT ( 'NONE',  ( 6.055847235078346991, 6.052673195394750572, 0.4411178842869938888 ) ) ;
#151903=CARTESIAN_POINT ( 'NONE',  ( -8.012505595996376684, 12.29174759539704986, 0.000000000000000000 ) ) ;
#151908=CARTESIAN_POINT ( 'NONE',  ( 7.938462636001388795, 9.220293482545153907, -1.199719254218441611 ) ) ;
#151911=CARTESIAN_POINT ( 'NONE',  ( 3.005103603723342953, 6.657704637652544832, -0.7998128361456291469 ) ) ;
#151913=CARTESIAN_POINT ( 'NONE',  ( -5.540478329478883524, 9.615641817700700145, 0.000000000000000000 ) ) ;
#151914=CARTESIAN_POINT ( 'NONE',  ( 3.225950485047770933, 5.851027101609320269, 1.199719254218450271 ) ) ;
#151917=CARTESIAN_POINT ( 'NONE',  ( 9.215791728987056786, 11.77484298861683598, -1.599625672291262513 ) ) ;
#151918=CARTESIAN_POINT ( 'NONE',  ( 0.3542539638296999804, 6.983552608457117117, 3.850577409504350346 ) ) ;
#151921=CARTESIAN_POINT ( 'NONE',  ( 4.015052158831055706, 7.807088067957844046, 0.2846288760043579336 ) ) ;
#151923=CARTESIAN_POINT ( 'NONE',  ( 6.317736394288140822, 7.433409217166723870, 1.082531754730558626 ) ) ;
#151926=CARTESIAN_POINT ( 'NONE',  ( -1.164422670175135899, 3.300000000000025135, -0.7116747751938151678 ) ) ;
#151929=CARTESIAN_POINT ( 'NONE',  ( 8.907343734053986495, 9.494248565925552441, -0.7216878364870197293 ) ) ;
#151932=CARTESIAN_POINT ( 'NONE',  ( -7.178152263431422320, 10.46192917639026554, 1.199719254218453823 ) ) ;
#151943=CARTESIAN_POINT ( 'NONE',  ( 10.70146331988817323, 11.37946204949139251, 0.7998128361456341429 ) ) ;
#151944=VECTOR ( 'NONE', #63579, 1000.000000000000000 ) ;
#151948=CARTESIAN_POINT ( 'NONE',  ( 6.010342169559767633, 5.906487374108181143, -0.7998128361456281477 ) ) ;
#151952=CARTESIAN_POINT ( 'NONE',  ( -1.500000000000011324, 4.452083334016148086, 0.8660254037844403729 ) ) ;
#151956=ORIENTED_EDGE ( 'NONE', *, *, #192264, .T. ) ;
#151958=CARTESIAN_POINT ( 'NONE',  ( -1.402160292154681736E-14, 2.337500000000022560, -1.732050807568863648 ) ) ;
#151959=CARTESIAN_POINT ( 'NONE',  ( 5.126954644262057492, 9.133197518281081173, 0.7998128361456462443 ) ) ;
#151960=CARTESIAN_POINT ( 'NONE',  ( 5.477130869796502211, 5.492333557625114437, 1.040834085586084257E-14 ) ) ;
#151964=CARTESIAN_POINT ( 'NONE',  ( 7.402388683381404988, 10.61957531637824204, -1.082531754730537976 ) ) ;
#151971=CARTESIAN_POINT ( 'NONE',  ( -6.091691091241777656, 6.001394449403842479, 0.7998128361456341429 ) ) ;
#151972=CARTESIAN_POINT ( 'NONE',  ( -1.201851678989727383E-14, 3.868750000682817713, -1.732050807568863648 ) ) ;
#151973=CARTESIAN_POINT ( 'NONE',  ( -1.364683531250010295, 5.801041667008088432, -0.7879004041258300672 ) ) ;
#151978=CARTESIAN_POINT ( 'NONE',  ( -0.6823417656249969321, 4.280208333674755394, -1.181850606188749264 ) ) ;
#151981=CARTESIAN_POINT ( 'NONE',  ( 3.469446951953614189E-15, 5.167241622962441383, 1.214306433183764966E-14 ) ) ;
#151985=CARTESIAN_POINT ( 'NONE',  ( -6.692921386640485082, 10.96015871772258521, -0.7998128361456291469 ) ) ;
#151986=CARTESIAN_POINT ( 'NONE',  ( 6.657217119509961201, 7.725507046638470321, -1.199719254218446718 ) ) ;
#151988=CARTESIAN_POINT ( 'NONE',  ( -1.402160292154681736E-14, -0.6781249996585819728, 1.575800808251672791 ) ) ;
#151990=ORIENTED_EDGE ( 'NONE', *, *, #70772, .F. ) ;
#151995=CARTESIAN_POINT ( 'NONE',  ( -6.742482464697739708, 6.760651051769146491, 0.7998128361456341429 ) ) ;
#151999=CARTESIAN_POINT ( 'NONE',  ( 8.191097360950562845, 12.70803068775103739, -0.7998128361456352531 ) ) ;
#152001=CARTESIAN_POINT ( 'NONE',  ( 8.971744963941056028, 11.49012176272984931, 1.599625672291281386 ) ) ;
#152003=CARTESIAN_POINT ( 'NONE',  ( -4.223528545856940042, 4.886203710709899006, -1.199719254218446718 ) ) ;
#152004=CARTESIAN_POINT ( 'NONE',  ( -8.667740277838301921, 9.006785167099828016, -0.7998128361456291469 ) ) ;
#152007=CARTESIAN_POINT ( 'NONE',  ( -4.023696502211203452, 7.783621949832661535, -0.4819376843918365960 ) ) ;
#152008=CARTESIAN_POINT ( 'NONE',  ( -1.602468905319636405E-14, -1.053124999658583638, -1.575800808251665908 ) ) ;
#152013=CARTESIAN_POINT ( 'NONE',  ( 7.293923454472077239, 10.49303254931736262, 1.082531754730558626 ) ) ;
#152016=ADVANCED_FACE ( 'NONE', ( #28210 ), #141032, .T. ) ;
#152038=CARTESIAN_POINT ( 'NONE',  ( -7.862839020921525091, 11.26073039346208660, -1.199719254218446718 ) ) ;
#152043=CARTESIAN_POINT ( 'NONE',  ( -1.500000000000013101, 1.660416667349487119, -0.8660254037844313801 ) ) ;
#152044=CARTESIAN_POINT ( 'NONE',  ( 10.05067194643221207, 10.62020544712608938, 0.7998128361456462443 ) ) ;
#152049=CARTESIAN_POINT ( 'NONE',  ( -10.32861409551237486, 10.94447128771960287, 1.040834085586084257E-14 ) ) ;
#152051=CARTESIAN_POINT ( 'NONE',  ( 1.364683531249990311, 2.634375000341422801, 1.214306433183764966E-14 ) ) ;
#152053=EDGE_LOOP ( 'NONE', ( #29083, #184173, #203606 ) ) ;
#152057=CARTESIAN_POINT ( 'NONE',  ( -4.274898507010545856, 3.881803101134051470, -0.7998128361456221525 ) ) ;
#152059=CARTESIAN_POINT ( 'NONE',  ( -0.08896015503664694846, 7.049507384514476449, -3.948637857580539201 ) ) ;
#152062=CARTESIAN_POINT ( 'NONE',  ( -1.364683531250014514, -0.1989583329919157317, -0.7879004041258359514 ) ) ;
#152067=CARTESIAN_POINT ( 'NONE',  ( -0.6823417656250212460, 1.551041667008083769, 1.181850606188755259 ) ) ;
#152069=CARTESIAN_POINT ( 'NONE',  ( -5.364222332501225488, 9.410009821226765325, 0.7998128361456481317 ) ) ;
#152070=CARTESIAN_POINT ( 'NONE',  ( 8.762647353133951711, 9.117510088278095282, 1.040834085586084257E-14 ) ) ;
#152071=CARTESIAN_POINT ( 'NONE',  ( 5.352771719296971042, 5.139321848801576387, 0.7998128361456341429 ) ) ;
#152072=CARTESIAN_POINT ( 'NONE',  ( 6.114890974963323345, 7.092793211334054604, 1.199719254218462483 ) ) ;
#152074=CARTESIAN_POINT ( 'NONE',  ( 1.499999999999987121, 3.795833333333356929, -0.8660254037844262731 ) ) ;
#152076=CARTESIAN_POINT ( 'NONE',  ( -1.402160292154681736E-14, 1.509375000341420359, -1.575800808251659024 ) ) ;
#152083=CARTESIAN_POINT ( 'NONE',  ( 4.514501963670558560, 8.210743357683563559, 1.040834085586084257E-14 ) ) ;
#152086=CARTESIAN_POINT ( 'NONE',  ( -7.669108446824431269, 12.09904362127053545, -0.7998128361456291469 ) ) ;
#152087=CARTESIAN_POINT ( 'NONE',  ( -3.405069135326500351, 7.124331091189553433, 1.040834085586084257E-14 ) ) ;
#152091=CARTESIAN_POINT ( 'NONE',  ( -8.039621902779392926, 9.442275643739831636, 1.082531754730558626 ) ) ;
#152093=CARTESIAN_POINT ( 'NONE',  ( -1.500000000000011324, 5.670833333333358262, 0.8660254037844403729 ) ) ;
#152096=CARTESIAN_POINT ( 'NONE',  ( 6.778713617152772208, 10.85232362007950258, -0.7216878364870267237 ) ) ;
#152105=CARTESIAN_POINT ( 'NONE',  ( 8.378575743120986630, 12.71882943370911789, 1.040834085586084257E-14 ) ) ;
#152110=CARTESIAN_POINT ( 'NONE',  ( 7.036318535368067728, 10.19249347702934294, -1.082531754730537976 ) ) ;
#152112=CARTESIAN_POINT ( 'NONE',  ( 5.777746017718023097, 9.892454120646377191, 0.7998128361456462443 ) ) ;
#152113=CARTESIAN_POINT ( 'NONE',  ( -5.148345644887285744, 7.029489223833707001, -1.599625672291256295 ) ) ;
#152117=CARTESIAN_POINT ( 'NONE',  ( 1.364683531249986537, -1.073958332991911790, 0.7879004041258500513 ) ) ;
#152118=CARTESIAN_POINT ( 'NONE',  ( 4.717874267875568961, 4.606534188717351874, -0.7216878364870188411 ) ) ;
#152120=CARTESIAN_POINT ( 'NONE',  ( -3.810004860640155311, 4.403759411290286252, 1.199719254218462483 ) ) ;
#152121=EDGE_CURVE ( 'NONE', #46131, #152273, #185952, .T. ) ;
#152132=ADVANCED_FACE ( 'NONE', ( #113795 ), #162491, .T. ) ;
#152138=CARTESIAN_POINT ( 'NONE',  ( 8.132193210098487057, 8.381980254736715708, 1.040834085586084257E-14 ) ) ;
#152141=ORIENTED_EDGE ( 'NONE', *, *, #155670, .T. ) ;
#152149=CARTESIAN_POINT ( 'NONE',  ( -4.412288926243578935, 7.235088616337731260, 1.199719254218464037 ) ) ;
#152151=CARTESIAN_POINT ( 'NONE',  ( -3.795392936821753604, 6.515376628678959392, -1.199719254218452047 ) ) ;
#152156=CARTESIAN_POINT ( 'NONE',  ( 1.499999999999822586, 7.240846818246208905, 4.154462424328221104 ) ) ;
#152157=AXIS2_PLACEMENT_3D ( 'NONE', #113589, #131940, #21049 ) ;
#152162=CARTESIAN_POINT ( 'NONE',  ( -4.939248034080176097, 4.656877549381960080, 1.214306433183764966E-14 ) ) ;
#152165=CARTESIAN_POINT ( 'NONE',  ( 6.287230548435207567, 8.358188277972981695, -1.599625672291262513 ) ) ;
#152166=CARTESIAN_POINT ( 'NONE',  ( -1.201851678989727383E-14, 4.946875000341420581, -1.575800808251660134 ) ) ;
#152172=CARTESIAN_POINT ( 'NONE',  ( 4.799223189113185128, 8.542918120699967588, 1.040834085586084257E-14 ) ) ;
#152173=CARTESIAN_POINT ( 'NONE',  ( -7.043624497499477499, 8.176315654292865887, 1.199719254218450271 ) ) ;
#152176=CARTESIAN_POINT ( 'NONE',  ( -7.857113714319432063, 9.125386407249497012, 1.199719254218462483 ) ) ;
#152177=CARTESIAN_POINT ( 'NONE',  ( -4.225337428953291230, 8.081310767087481750, 0.7998128361456341429 ) ) ;
#152184=CARTESIAN_POINT ( 'NONE',  ( 7.558834334818744338, 8.777393797832065303, 1.199719254218462483 ) ) ;
#152200=CARTESIAN_POINT ( 'NONE',  ( -0.7500000000000215383, 5.691666666666685082, 1.299038105676671107 ) ) ;
#152201=CARTESIAN_POINT ( 'NONE',  ( 4.196412238629597447, 4.854568018944682706, -1.199719254218452047 ) ) ;
#152202=CARTESIAN_POINT ( 'NONE',  ( 7.006866460164219212, 7.069099046480051385, -0.7998128361456281477 ) ) ;
#152204=CARTESIAN_POINT ( 'NONE',  ( -8.242994207428740339, 9.679543332497402730, 1.082531754730558626 ) ) ;
#152205=CARTESIAN_POINT ( 'NONE',  ( 5.341549334104184865, 8.215262742221458581, 1.082531754730558626 ) ) ;
#152206=CARTESIAN_POINT ( 'NONE',  ( -7.822691444960709006, 10.14955932391940330, -1.443375672974058777 ) ) ;
#152209=CARTESIAN_POINT ( 'NONE',  ( 8.372323551638698902, 9.726464550788689323, 1.199719254218462483 ) ) ;
#152215=CARTESIAN_POINT ( 'NONE',  ( -1.364683531250012516, 2.780208333674754506, 0.7879004041258379498 ) ) ;
#152221=CARTESIAN_POINT ( 'NONE',  ( 7.086107841436786181, 11.41887624831828418, 1.040834085586084257E-14 ) ) ;
#152224=CARTESIAN_POINT ( 'NONE',  ( -9.338868881714763148, 9.789768538289042255, -0.7998128361456291469 ) ) ;
#152230=CARTESIAN_POINT ( 'NONE',  ( 4.715538499454675403, 4.395883092318884522, 1.214306433183764966E-14 ) ) ;
#152233=CARTESIAN_POINT ( 'NONE',  ( -8.805130697071332335, 12.36007068230351358, 1.199719254218462483 ) ) ;
#152238=CARTESIAN_POINT ( 'NONE',  ( 5.846986258851572416, 6.004518191619921730, 0.3586427151269864222 ) ) ;
#152240=CARTESIAN_POINT ( 'NONE',  ( -2.656508033273816238, 5.186677574539687363, -1.199719254218446718 ) ) ;
#152244=CARTESIAN_POINT ( 'NONE',  ( 7.962716289927667113, 8.184257181204083409, -0.7998128361456291469 ) ) ;
#152246=CARTESIAN_POINT ( 'NONE',  ( 5.276094334012385367, 9.307193822989793475, 1.040834085586084257E-14 ) ) ;
#152247=CARTESIAN_POINT ( 'NONE',  ( 3.649115900372475796, 7.409052317076538330, 1.040834085586084257E-14 ) ) ;
#152249=CARTESIAN_POINT ( 'NONE',  ( -8.026063749610056419, 10.38682701267698150, -1.443375672974059665 ) ) ;
#152256=CARTESIAN_POINT ( 'NONE',  ( -4.059747316280317264, 7.561585642977368238, -0.4325785229164439416 ) ) ;
#152259=CARTESIAN_POINT ( 'NONE',  ( 5.178851490740196795, 7.065079377328788546, 1.443375672974062551 ) ) ;
#152265=CARTESIAN_POINT ( 'NONE',  ( -8.446366511189330240, 12.79791866312216442, 0.7216878364870317197 ) ) ;
#152273=VERTEX_POINT ( 'NONE', #117275 ) ;
#152278=CARTESIAN_POINT ( 'NONE',  ( -9.829298179783291900, 11.53023130024440768, 1.082531754730558626 ) ) ;
#152283=CARTESIAN_POINT ( 'NONE',  ( 6.771407655021410399, 9.987393799911945536, -1.199719254218441611 ) ) ;
#152286=CARTESIAN_POINT ( 'NONE',  ( -0.7500000000000215383, 2.222916667349486453, 1.299038105676671107 ) ) ;
#152288=CARTESIAN_POINT ( 'NONE',  ( -5.880485940025243607, 7.883652901494672349, 1.599625672291269396 ) ) ;
#152291=CARTESIAN_POINT ( 'NONE',  ( -9.345647958521597687, 9.797677461230342999, 0.7998128361456462443 ) ) ;
#152294=CARTESIAN_POINT ( 'NONE',  ( 1.499999999999991118, 5.535416667349481123, 0.8660254037844524744 ) ) ;
#152296=CARTESIAN_POINT ( 'NONE',  ( 6.775324078527185989, 8.927630729746953264, -1.599625672291262513 ) ) ;
#152298=CARTESIAN_POINT ( 'NONE',  ( -8.064402442030170093, 8.302891025323665630, 0.7998128361456602331 ) ) ;
#152300=CARTESIAN_POINT ( 'NONE',  ( 9.759171643738394408, 10.28012176064996197, 0.000000000000000000 ) ) ;
#152301=CARTESIAN_POINT ( 'NONE',  ( -1.201851678989727383E-14, 5.696875000341416140, -1.575800808251660134 ) ) ;
#152306=CARTESIAN_POINT ( 'NONE',  ( -8.351459436338048548, 8.845716885256940998, -0.7216878364870278340 ) ) ;
#152309=CARTESIAN_POINT ( 'NONE',  ( -0.6823417656249969321, 4.530208333674755394, -1.181850606188749264 ) ) ;
#152314=CARTESIAN_POINT ( 'NONE',  ( -1.201851678989727383E-14, 5.696875000341416140, -1.575800808251660134 ) ) ;
#152316=CARTESIAN_POINT ( 'NONE',  ( -4.758548728272219641, 4.653987725846768342, 0.7216878364870317197 ) ) ;
#152318=CARTESIAN_POINT ( 'NONE',  ( 8.452618703115982512, 11.94880668935564216, 1.199719254218450271 ) ) ;
#152319=CARTESIAN_POINT ( 'NONE',  ( -1.364683531249997417, 4.821875000341417916, 1.214306433183764966E-14 ) ) ;
#152320=CARTESIAN_POINT ( 'NONE',  ( -9.642873567817536795, 12.27310513391906532, 1.599625672291281386 ) ) ;
#152324=CARTESIAN_POINT ( 'NONE',  ( -1.364683531250012516, 2.238541667008087988, -0.7879004041258289570 ) ) ;
#152325=CARTESIAN_POINT ( 'NONE',  ( -2.982430605326328532, 5.462957558647244305, -1.082531754730543971 ) ) ;
#152326=CARTESIAN_POINT ( 'NONE',  ( 4.847203612085560387, 5.613824621309978724, -1.199719254218452047 ) ) ;
#152329=CARTESIAN_POINT ( 'NONE',  ( 5.680503174445848735, 5.729601246382692636, 1.040834085586084257E-14 ) ) ;
#152330=ADVANCED_FACE ( 'NONE', ( #50088 ), #182198, .F. ) ;
#152332=CARTESIAN_POINT ( 'NONE',  ( -3.642672431166898317, 3.097590952613070492, -2.447572309174330218 ) ) ;
#152335=CARTESIAN_POINT ( 'NONE',  ( 0.000000000000000000, 2.800000000000024691, 1.214306433183764966E-14 ) ) ;
#152336=CARTESIAN_POINT ( 'NONE',  ( -9.178506806771670412, 9.810605484096178941, 1.040834085586084257E-14 ) ) ;
#152341=CARTESIAN_POINT ( 'NONE',  ( -9.318531651294266638, 9.766041769465124034, -0.7998128361456291469 ) ) ;
#152342=CARTESIAN_POINT ( 'NONE',  ( -5.219525951136856357, 6.152163700156858539, -1.082531754730543971 ) ) ;
#152343=CARTESIAN_POINT ( 'NONE',  ( -1.201851678989727383E-14, 2.759375000341417916, -1.575800808251660134 ) ) ;
#152351=CARTESIAN_POINT ( 'NONE',  ( 10.39640486358069360, 11.02356051713265650, 0.7998128361456462443 ) ) ;
#152353=VERTEX_POINT ( 'NONE', #199508 ) ;
#152362=CARTESIAN_POINT ( 'NONE',  ( 1.579999999999991189, 8.674529973577531194, -2.499999999999989342 ) ) ;
#152366=CARTESIAN_POINT ( 'NONE',  ( -0.6823417656250212460, 2.863541667008084879, 1.181850606188767472 ) ) ;
#152374=CARTESIAN_POINT ( 'NONE',  ( 9.856941372335116469, 11.45851867493453291, 1.199719254218450271 ) ) ;
#152376=CARTESIAN_POINT ( 'NONE',  ( 1.364683531249986537, 1.655208333674748955, -0.7879004041258239610 ) ) ;
#152385=VERTEX_POINT ( 'NONE', #105252 ) ;
#152387=CARTESIAN_POINT ( 'NONE',  ( 5.789495288235341874, 6.713164910151406595, 1.199719254218462483 ) ) ;
#152390=EDGE_LOOP ( 'NONE', ( #111168, #182448 ) ) ;
#152398=CARTESIAN_POINT ( 'NONE',  ( -2.449219305563052895, 6.009172956465517856, 1.040834085586084257E-14 ) ) ;
#152399=CARTESIAN_POINT ( 'NONE',  ( 7.422199028477372451, 10.74665040227725044, -1.199719254218441611 ) ) ;
#152402=CARTESIAN_POINT ( 'NONE',  ( 4.134873662043553111, 7.767843672452050541, -0.7216878364870197293 ) ) ;
#152406=ORIENTED_EDGE ( 'NONE', *, *, #24898, .F. ) ;
#152412=CARTESIAN_POINT ( 'NONE',  ( -8.527715433315703919, 9.051348881730875817, 1.040834085586084257E-14 ) ) ;
#152414=CARTESIAN_POINT ( 'NONE',  ( 5.178324605415663306, 8.128796908705222535, 1.199719254218462483 ) ) ;
#152417=CARTESIAN_POINT ( 'NONE',  ( -9.833741488613570780, 10.36711991300432345, 0.7998128361456462443 ) ) ;
#152422=CARTESIAN_POINT ( 'NONE',  ( -3.704402285031864306, 5.344888637335695414, -1.599625672291256295 ) ) ;
#152424=CARTESIAN_POINT ( 'NONE',  ( 8.075853055234393452, 12.57357899774884658, 0.7998128361456462443 ) ) ;
#152425=CARTESIAN_POINT ( 'NONE',  ( 4.054051625686104998, 4.688480637177271149, -1.199719254218446718 ) ) ;
#152431=CARTESIAN_POINT ( 'NONE',  ( 3.660338286009610975, 6.253849852777763729, -1.082531754730543083 ) ) ;
#152434=CARTESIAN_POINT ( 'NONE',  ( -5.091250377131585125, 5.898545847196970726, 1.199719254218450271 ) ) ;
#152437=CARTESIAN_POINT ( 'NONE',  ( -8.597841969360544567, 13.18256606422934674, 0.7998128361456341429 ) ) ;
#152442=CARTESIAN_POINT ( 'NONE',  ( 8.609064354997688184, 9.146255957026539818, 1.040834085586084257E-14 ) ) ;
#152443=CARTESIAN_POINT ( 'NONE',  ( -1.364683531250012516, 5.051041667008084879, -0.7879004041258300672 ) ) ;
#152445=CARTESIAN_POINT ( 'NONE',  ( 4.334856428067313416, 6.080418470877079429, -1.599625672291256295 ) ) ;
#152447=CARTESIAN_POINT ( 'NONE',  ( 4.107757354816228279, 6.775838766385488654, -1.082531754730548412 ) ) ;
#152456=ORIENTED_EDGE ( 'NONE', *, *, #75356, .F. ) ;
#152458=CARTESIAN_POINT ( 'NONE',  ( 1.364683531249988535, 2.426041667008088432, 0.7879004041258500513 ) ) ;
#152460=CARTESIAN_POINT ( 'NONE',  ( 9.728138913005292210, 11.30824913904973705, -1.199719254218440723 ) ) ;
#152461=AXIS2_PLACEMENT_3D ( 'NONE', #172427, #202754, #169213 ) ;
#152463=CARTESIAN_POINT ( 'NONE',  ( -3.443407828190963915, 6.961133532957338943, 0.7216878364870317197 ) ) ;
#152465=CARTESIAN_POINT ( 'NONE',  ( -5.599154252319524794, 6.595063384869953360, 1.082531754730546636 ) ) ;
#152470=CARTESIAN_POINT ( 'NONE',  ( 5.769158057814842699, 6.689438141327490150, 1.199719254218462483 ) ) ;
#152480=CARTESIAN_POINT ( 'NONE',  ( 4.957477724091233995, 8.935474444748447098, -0.7998128361456281477 ) ) ;
#152484=CARTESIAN_POINT ( 'NONE',  ( -5.925076824372040640, 6.871343368977510302, 1.199719254218450271 ) ) ;
#152488=CARTESIAN_POINT ( 'NONE',  ( 7.949158136313996259, 8.168439335321471262, 1.040834085586084257E-14 ) ) ;
#152490=CARTESIAN_POINT ( 'NONE',  ( -6.063521013809733518, 8.097193820909906137, 1.599625672291283607 ) ) ;
#152491=CARTESIAN_POINT ( 'NONE',  ( 6.060131475184119765, 9.053608573481392696, -1.082531754730537976 ) ) ;
#152492=CARTESIAN_POINT ( 'NONE',  ( 4.699069518069377338, 7.059409271092678573, 1.379435410134820295 ) ) ;
#152493=CARTESIAN_POINT ( 'NONE',  ( -3.273404022695637572, 5.906389562198459231, 1.199719254218462483 ) ) ;
#152496=CARTESIAN_POINT ( 'NONE',  ( -4.629219384062206011, 7.488174150459498968, -1.199719254218452047 ) ) ;
#152499=CARTESIAN_POINT ( 'NONE',  ( -0.6823417656250212460, 2.551041667008084435, 1.181850606188767472 ) ) ;
#152501=CARTESIAN_POINT ( 'NONE',  ( -4.094199201646926412, 7.720390135322642067, 0.7216878364870317197 ) ) ;
#152507=CARTESIAN_POINT ( 'NONE',  ( 6.844168616800228477, 6.879284895888727824, -0.7998128361456281477 ) ) ;
#152510=CARTESIAN_POINT ( 'NONE',  ( -1.364683531249997417, 2.821875000341422801, 1.214306433183764966E-14 ) ) ;
#152517=CARTESIAN_POINT ( 'NONE',  ( -3.948449050077848632, 5.629609863222681199, 1.599625672291267398 ) ) ;
#152518=CARTESIAN_POINT ( 'NONE',  ( -6.331294547457448019, 10.33033470543493770, 0.7216878364870458196 ) ) ;
#152520=CARTESIAN_POINT ( 'NONE',  ( 1.364683531249990311, 3.384375000341416140, 1.214306433183764966E-14 ) ) ;
#152527=CARTESIAN_POINT ( 'NONE',  ( -7.510853911846401942, 7.865010440016681592, 1.040834085586084257E-14 ) ) ;
#152529=CARTESIAN_POINT ( 'NONE',  ( 0.7499999999999902300, 3.014583334016149418, 1.299038105676669330 ) ) ;
#152531=CARTESIAN_POINT ( 'NONE',  ( -6.602457619730773608, 8.725953194484466380, 1.443375672974078761 ) ) ;
#152544=CARTESIAN_POINT ( 'NONE',  ( -6.579784621333750749, 6.570836901177822931, 0.7998128361456341429 ) ) ;
#152547=CARTESIAN_POINT ( 'NONE',  ( 3.161022370280501814, 6.839609865302569425, 0.000000000000000000 ) ) ;
#152549=CARTESIAN_POINT ( 'NONE',  ( 4.861705877774147311, 4.996687906539577284, 0.6087874222351703501 ) ) ;
#152551=CARTESIAN_POINT ( 'NONE',  ( 5.795220594837462436, 8.848508896363995291, -1.199719254218440723 ) ) ;
#152555=CARTESIAN_POINT ( 'NONE',  ( -5.748293942514189681, 5.808690475795744490, -0.7216878364870207285 ) ) ;
#152564=CARTESIAN_POINT ( 'NONE',  ( 1.364683531249988757, 1.384375000341421469, 0.000000000000000000 ) ) ;
#152566=CARTESIAN_POINT ( 'NONE',  ( -8.362681821530818738, 8.650883634741092010, -0.7998128361456291469 ) ) ;
#152568=CARTESIAN_POINT ( 'NONE',  ( 6.123478934866503742, 10.29580919065294431, 0.7998128361456462443 ) ) ;
#152570=CARTESIAN_POINT ( 'NONE',  ( -8.362681821530818738, 8.650883634741092010, -0.7998128361456291469 ) ) ;
#152573=CARTESIAN_POINT ( 'NONE',  ( -1.364683531250010295, 5.488541667008087543, -0.7879004041258300672 ) ) ;
#152575=CARTESIAN_POINT ( 'NONE',  ( 8.270110514656034084, 9.711179024262627024, 1.082531754730558626 ) ) ;
#152578=CARTESIAN_POINT ( 'NONE',  ( -1.364683531250014514, -0.9072916663252470482, 0.7879004041258379498 ) ) ;
#152581=CARTESIAN_POINT ( 'NONE',  ( 6.263503779389103521, 10.25124547602188763, 1.040834085586084257E-14 ) ) ;
#152584=CARTESIAN_POINT ( 'NONE',  ( -5.666945020832185875, 7.634521829102760115, 1.443375672974064550 ) ) ;
#152586=CARTESIAN_POINT ( 'NONE',  ( 0.6823417656249917140, 3.342708333674754506, 1.181850606188765695 ) ) ;
#152590=CARTESIAN_POINT ( 'NONE',  ( -5.422371370461663176, 8.413518134592214537, -1.199719254218446718 ) ) ;
#152591=CARTESIAN_POINT ( 'NONE',  ( 1.364683531249988535, 5.717708333674752730, -0.7879004041258300672 ) ) ;
#152598=B_SPLINE_CURVE_WITH_KNOTS ( 'NONE', 3,
 ( #60585, #61658, #11825, #146135, #77900, #142950 ),
 .UNSPECIFIED., .F., .F.,
 ( 4, 2, 4 ),
 ( 3.471140604459606978E-18, 0.0006533246752568837691, 0.001306649350513764069 ),
 .UNSPECIFIED. ) ;
#152599=CARTESIAN_POINT ( 'NONE',  ( 8.015895134177609904, 10.37496362800581018, 1.599625672291281386 ) ) ;
#152602=CARTESIAN_POINT ( 'NONE',  ( -1.201851678989727383E-14, 1.962500000000020783, 1.732050807568877637 ) ) ;
#152608=CARTESIAN_POINT ( 'NONE',  ( 4.839897650398541806, 8.590371658866210680, 1.040834085586084257E-14 ) ) ;
#152610=CARTESIAN_POINT ( 'NONE',  ( -0.6823417656250003738, -0.7197916663252492686, -1.181850606188749264 ) ) ;
#152612=CARTESIAN_POINT ( 'NONE',  ( 3.216308754939877446, 4.775446185561722956, -1.599625672291262513 ) ) ;
#152617=CARTESIAN_POINT ( 'NONE',  ( 1.499999999999989120, 0.2750000000000182854, 0.000000000000000000 ) ) ;
#152618=CARTESIAN_POINT ( 'NONE',  ( 7.426115451983150706, 9.686887332112256388, -1.599625672291262513 ) ) ;
#152619=CARTESIAN_POINT ( 'NONE',  ( -8.317037166979361018, 11.79062823052953668, 1.199719254218453823 ) ) ;
#152621=CARTESIAN_POINT ( 'NONE',  ( -1.364683531250000748, 0.009375000341420303140, 0.000000000000000000 ) ) ;
#152622=CARTESIAN_POINT ( 'NONE',  ( 0.7499999999999902300, 1.483333333333357373, 1.299038105676657340 ) ) ;
#152624=CARTESIAN_POINT ( 'NONE',  ( 5.335297142177534369, 6.183267073083954735, -1.199719254218452047 ) ) ;
#152631=CARTESIAN_POINT ( 'NONE',  ( 1.364683531249990311, 5.134375000341417916, 1.214306433183764966E-14 ) ) ;
#152633=CARTESIAN_POINT ( 'NONE',  ( -7.100719765255177229, 9.307259030929609267, -1.599625672291263179 ) ) ;
#152634=CARTESIAN_POINT ( 'NONE',  ( -5.924549939491850381, 6.014322472269677533, 0.000000000000000000 ) ) ;
#152643=CARTESIAN_POINT ( 'NONE',  ( 6.726816770674637347, 10.99970333242910669, -0.7998128361456291469 ) ) ;
#152647=CARTESIAN_POINT ( 'NONE',  ( 6.439759776366769550, 8.536139043893143707, 1.443375672974076540 ) ) ;
#152652=CARTESIAN_POINT ( 'NONE',  ( -7.212047647465563038, 10.50147379109678880, -1.199719254218446718 ) ) ;
#152654=CARTESIAN_POINT ( 'NONE',  ( 4.320244504248938355, 8.192035688265757898, 1.040834085586084257E-14 ) ) ;
#152657=CARTESIAN_POINT ( 'NONE',  ( 4.000938479675252069, 7.594566414207783112, 0.1672846332331431873 ) ) ;
#152658=CARTESIAN_POINT ( 'NONE',  ( 4.033714395265605823, 4.664753868353354704, -1.199719254218446718 ) ) ;
#152664=FACE_BOUND ( 'NONE', #135888, .T. ) ;
#152665=CARTESIAN_POINT ( 'NONE',  ( -3.795919822146289313, 5.451659097302528068, -1.443375672974053447 ) ) ;
#152666=CARTESIAN_POINT ( 'NONE',  ( 9.571693261567954636, 12.19006144329456731, 1.443375672974076540 ) ) ;
#152669=CARTESIAN_POINT ( 'NONE',  ( -5.682838942422375084, 9.781729199468104596, 0.000000000000000000 ) ) ;
#152675=CARTESIAN_POINT ( 'NONE',  ( -6.347188469492005325, 10.55680364771601809, -0.7998128361456291469 ) ) ;
#152678=CARTESIAN_POINT ( 'NONE',  ( -0.4206437366318691584, 7.996079560418738907, 1.998769755887072286 ) ) ;
#152681=VERTEX_POINT ( 'NONE', #55413 ) ;
#152691=CARTESIAN_POINT ( 'NONE',  ( -7.019370843573183194, 9.212351955633947043, 1.599625672291283607 ) ) ;
#152694=CARTESIAN_POINT ( 'NONE',  ( 4.853455804012203778, 8.606189504748821051, 0.7216878364870438212 ) ) ;
#152699=CARTESIAN_POINT ( 'NONE',  ( -4.786191920824102830, 5.542644314838231168, 1.199719254218462483 ) ) ;
#152703=CARTESIAN_POINT ( 'NONE',  ( -1.499999999999972689, 3.379166666666690411, -0.8660254037844548058 ) ) ;
#152707=CARTESIAN_POINT ( 'NONE',  ( -7.994504133552415404, 12.47867192245318435, -0.7998128361456281477 ) ) ;
#152708=CARTESIAN_POINT ( 'NONE',  ( 7.610204295972345712, 7.772993188256215547, 0.7998128361456341429 ) ) ;
#152711=CARTESIAN_POINT ( 'NONE',  ( -8.286004436246233951, 12.81875560892930466, 1.040834085586084257E-14 ) ) ;
#152715=CARTESIAN_POINT ( 'NONE',  ( -0.6823417656250003738, -0.4697916663252491021, -1.181850606188749264 ) ) ;
#152719=CARTESIAN_POINT ( 'NONE',  ( 10.24960094225127172, 11.06021530882240356, -0.7216878364870257245 ) ) ;
#152726=CARTESIAN_POINT ( 'NONE',  ( 0.1021010164683408133, 6.360493866598983637, -3.113991822131907838 ) ) ;
#152746=CARTESIAN_POINT ( 'NONE',  ( -1.364683531250010295, 5.280208333674758059, 0.7879004041258379498 ) ) ;
#152750=CARTESIAN_POINT ( 'NONE',  ( 9.728138913005292210, 11.30824913904973705, -1.199719254218440723 ) ) ;
#152752=CARTESIAN_POINT ( 'NONE',  ( 1.257539916218596732, 3.033837156058346807, -0.7749999999999874767 ) ) ;
#152753=CARTESIAN_POINT ( 'NONE',  ( 0.4956004317509306034, 7.799479031273147456, -1.990828115380115282 ) ) ;
#152754=CARTESIAN_POINT ( 'NONE',  ( 3.215772567386471437, 6.427315425527130088, -0.8732430475888955934 ) ) ;
#152755=CARTESIAN_POINT ( 'NONE',  ( 10.71502147350184231, 11.39527989537399755, 0.000000000000000000 ) ) ;
#152761=CARTESIAN_POINT ( 'NONE',  ( 5.996784015946103885, 5.890669528225568996, 1.040834085586084257E-14 ) ) ;
#152762=CARTESIAN_POINT ( 'NONE',  ( -1.364683531250012516, 2.551041667008089320, -0.7879004041258289570 ) ) ;
#152765=CARTESIAN_POINT ( 'NONE',  ( 10.71502147350184231, 11.39527989537399755, 0.000000000000000000 ) ) ;
#152767=CARTESIAN_POINT ( 'NONE',  ( -8.128276786592724790, 9.441743324901704426, -1.199719254218446718 ) ) ;
#152768=CARTESIAN_POINT ( 'NONE',  ( -4.080641047588907888, 6.744203074620265248, -1.082531754730548412 ) ) ;
#152771=CARTESIAN_POINT ( 'NONE',  ( -4.706651882238427120, 8.642844295920152575, 1.040834085586084257E-14 ) ) ;
#152773=CARTESIAN_POINT ( 'NONE',  ( -1.402160292154681736E-14, -0.006249999317184824418, 1.732050807568877637 ) ) ;
#152780=CARTESIAN_POINT ( 'NONE',  ( -3.104453987404957260, 6.565687385373657925, -0.7216878364870257245 ) ) ;
#152786=CARTESIAN_POINT ( 'NONE',  ( -3.755245360860931303, 5.404205559136275205, -1.443375672974051449 ) ) ;
#152788=CARTESIAN_POINT ( 'NONE',  ( 8.178592977541601527, 10.56477777859713463, 1.599625672291281386 ) ) ;
#152798=CARTESIAN_POINT ( 'NONE',  ( -10.13488352141530768, 11.78278451552804817, 1.199719254218462483 ) ) ;
#152803=CARTESIAN_POINT ( 'NONE',  ( 5.192936529234042808, 6.017179691316550283, -1.199719254218452047 ) ) ;
#152809=CARTESIAN_POINT ( 'NONE',  ( 3.192055101013606233, 5.811482486902795230, -1.199719254218446718 ) ) ;
#152822=CARTESIAN_POINT ( 'NONE',  ( 6.747154001095143627, 11.02343010125301959, -0.7998128361456291469 ) ) ;
#152824=CARTESIAN_POINT ( 'NONE',  ( -6.423865854776591000, 6.388931673527803667, 1.040834085586084257E-14 ) ) ;
#152829=CARTESIAN_POINT ( 'NONE',  ( 1.364683531249990311, 5.613541667008087543, 0.7879004041258500513 ) ) ;
#152834=B_SPLINE_CURVE_WITH_KNOTS ( 'NONE', 3,
 ( #100347, #102482, #87299, #115591, #132884, #116656 ),
 .UNSPECIFIED., .F., .F.,
 ( 4, 2, 4 ),
 ( 5.346776843295201289E-18, 0.001422024648551337882, 0.002844049297102670126 ),
 .UNSPECIFIED. ) ;
#152836=CARTESIAN_POINT ( 'NONE',  ( 3.571683402196252910, 6.254382171615883834, 1.199719254218462483 ) ) ;
#152837=CARTESIAN_POINT ( 'NONE',  ( -4.948889764188092677, 5.732458465429559169, 1.199719254218462483 ) ) ;
#152844=CARTESIAN_POINT ( 'NONE',  ( 4.514501963670558560, 8.210743357683563559, 1.040834085586084257E-14 ) ) ;
#152847=CARTESIAN_POINT ( 'NONE',  ( 8.392133896734668141, 9.853539636687704828, 1.082531754730558626 ) ) ;
#152848=CARTESIAN_POINT ( 'NONE',  ( 1.364683531249988535, 2.926041667008082658, 0.7879004041258500513 ) ) ;
#152850=CARTESIAN_POINT ( 'NONE',  ( 4.487385655998878953, 6.258369236797239665, 1.443375672974062551 ) ) ;
#152853=CARTESIAN_POINT ( 'NONE',  ( 5.630352418794719149, 6.139657267270441920, -0.8181431533968346326 ) ) ;
#152855=CARTESIAN_POINT ( 'NONE',  ( -5.066364649336571269, 6.741537443998309342, 1.444296757982476587 ) ) ;
#152861=CARTESIAN_POINT ( 'NONE',  ( -10.17947440576205054, 10.77047498301088346, 0.7998128361456462443 ) ) ;
#152871=CARTESIAN_POINT ( 'NONE',  ( 4.392478581147586603, 4.226905887534702977, -0.7216878364870188411 ) ) ;
#152872=CARTESIAN_POINT ( 'NONE',  ( -1.201851678989727383E-14, 3.009375000341419248, -1.575800808251660134 ) ) ;
#152874=CARTESIAN_POINT ( 'NONE',  ( 6.154511665599609493, 9.267681812253174556, 1.199719254218462483 ) ) ;
#152875=CARTESIAN_POINT ( 'NONE',  ( -10.16591625214838679, 10.75465713712827487, 1.040834085586084257E-14 ) ) ;
#152877=CARTESIAN_POINT ( 'NONE',  ( -5.037017762676898158, 5.835274463666530131, -1.199719254218446718 ) ) ;
#152881=CARTESIAN_POINT ( 'NONE',  ( -1.500000000000011324, 4.920833333333354709, 0.8660254037844403729 ) ) ;
#152882=CARTESIAN_POINT ( 'NONE',  ( 5.606460214450851964, 6.499623990736163037, 1.199719254218462483 ) ) ;
#152887=CARTESIAN_POINT ( 'NONE',  ( 7.605760987586388744, 11.81721221891873697, 1.040834085586084257E-14 ) ) ;
#152892=CARTESIAN_POINT ( 'NONE',  ( -1.201851678989727383E-14, 3.493750000682815493, 1.732050807568877637 ) ) ;
#152894=CARTESIAN_POINT ( 'NONE',  ( -5.766295404513795297, 5.621766148221195358, 0.7998128361456341429 ) ) ;
#152895=CARTESIAN_POINT ( 'NONE',  ( 3.456965981360264895, 6.016582164020185530, -1.082531754730543971 ) ) ;
#152905=CARTESIAN_POINT ( 'NONE',  ( 7.446452682403650769, 9.710614100936176385, -1.599625672291262513 ) ) ;
#152906=CARTESIAN_POINT ( 'NONE',  ( 4.822949958159288286, 6.649860922651058992, -1.599625672291256295 ) ) ;
#152907=AXIS2_PLACEMENT_3D ( 'NONE', #68110, #36698, #104932 ) ;
#152908=DIRECTION ( 'NONE',  ( -0.6507913734559640506, -0.7592566023653004592, 0.000000000000000000 ) ) ;
#152910=DIRECTION ( 'NONE',  ( 1.000000000000000000, -8.673617379884035472E-16, 0.000000000000000000 ) ) ;
#152911=CARTESIAN_POINT ( 'NONE',  ( 3.897079088924235712, 6.634010472798538949, 1.199719254218462483 ) ) ;
#152918=CARTESIAN_POINT ( 'NONE',  ( 10.38962578677386084, 11.01565159419135043, 0.000000000000000000 ) ) ;
#152923=CARTESIAN_POINT ( 'NONE',  ( 5.844719547729445353, 6.005894922780862899, -0.3676955087418033452 ) ) ;
#152931=CARTESIAN_POINT ( 'NONE',  ( 6.968527767744104651, 8.192665819532020777, 1.082531754730558626 ) ) ;
#152933=CARTESIAN_POINT ( 'NONE',  ( -2.767835915484202047, 6.380892334706859792, -0.7998128361456281477 ) ) ;
#152939=CARTESIAN_POINT ( 'NONE',  ( -4.660252114795309097, 6.460046772059735432, -1.599625672291256295 ) ) ;
#152946=ORIENTED_EDGE ( 'NONE', *, *, #79298, .F. ) ;
#152952=CARTESIAN_POINT ( 'NONE',  ( 8.666686507633574621, 11.13422023037111330, 1.599625672291281386 ) ) ;
#152953=CARTESIAN_POINT ( 'NONE',  ( 5.684994455280509840, 6.294486374732538359, 1.096603583888225764 ) ) ;
#152957=( BOUNDED_CURVE ( )  B_SPLINE_CURVE ( 2, ( #36617, #104849, #84308 ),
 .UNSPECIFIED., .F., .T. ) 
 B_SPLINE_CURVE_WITH_KNOTS ( ( 3, 3 ),
 ( 0.2750000000000000777, 0.2778239691812269263 ),
 .UNSPECIFIED. ) 
 CURVE ( )  GEOMETRIC_REPRESENTATION_ITEM ( )  RATIONAL_B_SPLINE_CURVE ( ( 0.9999999999999982236, 0.9091983686127850239, 0.9414788213740286071 ) ) 
 REPRESENTATION_ITEM ( '' )  );
#152959=CARTESIAN_POINT ( 'NONE',  ( -8.283668668269720925, 8.766627655843896250, 1.056142170575426150E-14 ) ) ;
#152960=CARTESIAN_POINT ( 'NONE',  ( -8.324343129110692630, 12.65555805069709550, 0.7216878364870338292 ) ) ;
#152965=CARTESIAN_POINT ( 'NONE',  ( 8.209625708274705502, 9.536650400197368427, 1.199719254218462483 ) ) ;
#152968=CARTESIAN_POINT ( 'NONE',  ( 3.094265954482837255, 2.800000000000017586, 2.490342512183689294 ) ) ;
#152969=CARTESIAN_POINT ( 'NONE',  ( 3.680148631105580215, 6.380924938676771241, -1.199719254218446718 ) ) ;
#152971=CARTESIAN_POINT ( 'NONE',  ( -6.898401231254901234, 6.942556279419168419, -0.7998128361456291469 ) ) ;
#152972=CARTESIAN_POINT ( 'NONE',  ( 4.741601036477289810, 6.554953847355395880, 1.599625672291267398 ) ) ;
#152980=CARTESIAN_POINT ( 'NONE',  ( 4.005937425286727027, 7.819599604358462130, 0.1919598339409686050 ) ) ;
#152982=CARTESIAN_POINT ( 'NONE',  ( 6.507550544879468823, 6.694489845221929691, -0.7216878364870257245 ) ) ;
#152984=CARTESIAN_POINT ( 'NONE',  ( 0.2305739854149619072, 7.031539004852044528, 3.921949077993606370 ) ) ;
#152989=EDGE_LOOP ( 'NONE', ( #90464, #137713, #49940, #105816 ) ) ;
#152990=CARTESIAN_POINT ( 'NONE',  ( 8.717529583462654941, 9.272798723569005475, 0.7216878364870458196 ) ) ;
#152993=CARTESIAN_POINT ( 'NONE',  ( -10.62011439820619429, 11.28455497419572318, -0.7998128361456221525 ) ) ;
#152994=CARTESIAN_POINT ( 'NONE',  ( -8.701635661872465732, 9.046329781806354831, 1.040834085586084257E-14 ) ) ;
#153002=CARTESIAN_POINT ( 'NONE',  ( 8.703444544968814256, 12.24143683818393313, -1.199719254218446718 ) ) ;
#153006=CARTESIAN_POINT ( 'NONE',  ( 3.174580523894166006, 6.855427711185178019, 0.7998128361456341429 ) ) ;
#153009=( BOUNDED_CURVE ( )  B_SPLINE_CURVE ( 2, ( #157326, #11038, #137879, #41453, #23014 ),
 .UNSPECIFIED., .F., .T. ) 
 B_SPLINE_CURVE_WITH_KNOTS ( ( 3, 2, 3 ),
 ( 0.1229971016045082050, 0.1250000000000000000, 0.1273350245274847692 ),
 .UNSPECIFIED. ) 
 CURVE ( )  GEOMETRIC_REPRESENTATION_ITEM ( )  RATIONAL_B_SPLINE_CURVE ( ( 0.9331125556462565029, 0.9355989990887658703, 1.000000000000000000, 0.9249198476264313129, 0.9339904139662591476 ) ) 
 REPRESENTATION_ITEM ( '' )  );
#153010=CARTESIAN_POINT ( 'NONE',  ( -1.500000000000011324, 2.952083334016149418, 0.8660254037844403729 ) ) ;
#153016=CARTESIAN_POINT ( 'NONE',  ( 0.7499999999999902300, 1.233333333333357151, 1.299038105676657340 ) ) ;
#153017=CARTESIAN_POINT ( 'NONE',  ( 7.070740804726770357, 8.207951346058097286, 1.199719254218462483 ) ) ;
#153019=CARTESIAN_POINT ( 'NONE',  ( 5.192409643909512873, 6.120528008391641350, -1.082531754730549078 ) ) ;
#153023=CARTESIAN_POINT ( 'NONE',  ( 7.890482213473377193, 11.18901776815221716, -1.082531754730543083 ) ) ;
#153028=AXIS2_PLACEMENT_3D ( 'NONE', #52221, #37023, #155058 ) ;
#153030=CARTESIAN_POINT ( 'NONE',  ( -4.232116505760120440, 8.089219690028791376, -0.7998128361456281477 ) ) ;
#153031=CARTESIAN_POINT ( 'NONE',  ( -1.499999999999997780, 3.681250000682819046, 1.214306433183764966E-14 ) ) ;
#153032=CARTESIAN_POINT ( 'NONE',  ( -1.201851678989727383E-14, 5.009375000341421469, -1.575800808251660134 ) ) ;
#153037=CARTESIAN_POINT ( 'NONE',  ( 1.364683531249988535, 3.967708333674751842, -0.7879004041258239610 ) ) ;
#153045=CARTESIAN_POINT ( 'NONE',  ( -7.167456763118792651, 11.51378332361394818, 0.000000000000000000 ) ) ;
#153046=CARTESIAN_POINT ( 'NONE',  ( 4.984594031318565932, 8.967110136513669616, 0.7998128361456462443 ) ) ;
#153053=CARTESIAN_POINT ( 'NONE',  ( -6.856673000209188906, 9.022537805042615489, 1.599625672291283607 ) ) ;
#153059=CARTESIAN_POINT ( 'NONE',  ( 9.240045382913317340, 10.73880668727576015, -1.199719254218446718 ) ) ;
#153063=CARTESIAN_POINT ( 'NONE',  ( -5.413783410558481002, 5.210502155273325720, -0.7998128361456221525 ) ) ;
#153064=CARTESIAN_POINT ( 'NONE',  ( -6.970863535720637216, 11.28442455831609337, 0.7998128361456481317 ) ) ;
#153067=CARTESIAN_POINT ( 'NONE',  ( -4.182100719528288657, 7.584231438125928371, -0.9338283797597360936 ) ) ;
#153074=CARTESIAN_POINT ( 'NONE',  ( 6.817052309572890323, 6.847649204123507083, 0.7998128361456341429 ) ) ;
#153081=EDGE_CURVE ( 'NONE', #162407, #104139, #185636, .T. ) ;
#153088=VERTEX_POINT ( 'NONE', #109573 ) ;
#153096=ORIENTED_EDGE ( 'NONE', *, *, #65958, .T. ) ;
#153098=CARTESIAN_POINT ( 'NONE',  ( -7.323375529675950624, 11.69568855126397011, -0.7998128361456291469 ) ) ;
#153103=CARTESIAN_POINT ( 'NONE',  ( 0.7499999999999902300, 1.514583334016148086, 1.299038105676657340 ) ) ;
#153104=CARTESIAN_POINT ( 'NONE',  ( 9.348510611822643313, 10.86534945433664134, 1.199719254218453823 ) ) ;
#153109=CARTESIAN_POINT ( 'NONE',  ( -9.775592450653132204, 11.36361159963886891, -1.199719254218441611 ) ) ;
#153110=CARTESIAN_POINT ( 'NONE',  ( -1.579999999999998073, 8.674529973577531194, -2.499999999999990230 ) ) ;
#153111=CARTESIAN_POINT ( 'NONE',  ( 0.6823417656249899377, 1.842708333674752952, 1.181850606188755259 ) ) ;
#153118=CARTESIAN_POINT ( 'NONE',  ( -4.790108344329849110, 4.482881244673243337, 0.7998128361456341429 ) ) ;
#153123=CARTESIAN_POINT ( 'NONE',  ( -1.364683531250014514, 0.09270833367475767028, 0.7879004041258379498 ) ) ;
#153128=CARTESIAN_POINT ( 'NONE',  ( 0.6823417656249882723, 0.6760416670080898749, -1.181850606188749264 ) ) ;
#153130=CARTESIAN_POINT ( 'NONE',  ( -5.605406444246153974, 8.627059054007450101, -1.199719254218440723 ) ) ;
#153131=CARTESIAN_POINT ( 'NONE',  ( 8.101160479365381306, 9.410107633136481908, -1.199719254218446718 ) ) ;
#153133=CARTESIAN_POINT ( 'NONE',  ( 5.168682875307768931, 7.053215992657626110, -1.599625672291256295 ) ) ;
#153135=CARTESIAN_POINT ( 'NONE',  ( 0.7499999999999902300, 3.483333333333352044, 1.299038105676669330 ) ) ;
#153137=CARTESIAN_POINT ( 'NONE',  ( 1.364683531249988757, 1.196875000341421469, 0.000000000000000000 ) ) ;
#153142=CARTESIAN_POINT ( 'NONE',  ( 4.853455804012212660, 7.645820290447483458, 1.082531754730558626 ) ) ;
#153145=CARTESIAN_POINT ( 'NONE',  ( -8.178592977541617515, 10.56477777859713463, 1.599625672291295375 ) ) ;
#153146=CARTESIAN_POINT ( 'NONE',  ( -4.440459003675619520, 5.139289244831666714, 1.199719254218462483 ) ) ;
#153151=CARTESIAN_POINT ( 'NONE',  ( -7.280365300414089802, 10.47721470291632784, 1.082531754730549967 ) ) ;
#153153=CARTESIAN_POINT ( 'NONE',  ( 0.7499999999999920064, 5.733333333333353821, 1.299038105676669330 ) ) ;
#153157=CARTESIAN_POINT ( 'NONE',  ( 8.758204044747998296, 11.24099069033793974, 1.443375672974076540 ) ) ;
#153163=CARTESIAN_POINT ( 'NONE',  ( -1.451998047840333594, 7.315968950356099398, -4.301760722582879559 ) ) ;
#153165=CARTESIAN_POINT ( 'NONE',  ( 9.612367721964607981, 12.23751498042398289, -1.443375672974058777 ) ) ;
#153169=CARTESIAN_POINT ( 'NONE',  ( 8.744645890689993095, 9.304434415334227992, -0.7216878364870197293 ) ) ;
#153170=CARTESIAN_POINT ( 'NONE',  ( 5.991813822235618758, 9.077867661661846554, 1.199719254218462483 ) ) ;
#153172=CARTESIAN_POINT ( 'NONE',  ( -5.473741331615264549, 7.409117525016355010, -1.599625672291256295 ) ) ;
#153177=CARTESIAN_POINT ( 'NONE',  ( 1.408750476333324952, 7.229967155398369982, 4.273289540531094666 ) ) ;
#153178=CARTESIAN_POINT ( 'NONE',  ( 2.385871846325007706, 5.727341554113725586, -0.7216878364870267237 ) ) ;
#153180=CARTESIAN_POINT ( 'NONE',  ( -2.598358995313378550, 6.183169261174235487, 0.7998128361456341429 ) ) ;
#153197=CARTESIAN_POINT ( 'NONE',  ( 6.272618624616828953, 10.46980549536166016, 1.040834085586084257E-14 ) ) ;
#153202=EDGE_CURVE ( 'NONE', #3975, #59123, #110632, .T. ) ;
#153210=CARTESIAN_POINT ( 'NONE',  ( -4.089755892816631544, 7.923132308261379819, -0.7998128361456281477 ) ) ;
#153212=CARTESIAN_POINT ( 'NONE',  ( -5.413783410558481002, 5.210502155273325720, -0.7998128361456221525 ) ) ;
#153221=CARTESIAN_POINT ( 'NONE',  ( -2.415323921528888196, 5.969628341758991930, 0.7998128361456341429 ) ) ;
#153224=CARTESIAN_POINT ( 'NONE',  ( 7.124973419181436007, 8.271222729588529887, -1.199719254218446718 ) ) ;
#153225=CARTESIAN_POINT ( 'NONE',  ( -1.364683531249997417, 4.759375000341424133, 1.214306433183764966E-14 ) ) ;
#153231=CARTESIAN_POINT ( 'NONE',  ( 4.595850884908202261, 7.345281218159464665, -1.082531754730549078 ) ) ;
#153232=CARTESIAN_POINT ( 'NONE',  ( -6.509886312855995172, 10.74661779830734254, -0.7998128361456291469 ) ) ;
#153235=CARTESIAN_POINT ( 'NONE',  ( -6.886651960737580680, 10.12184548991413457, -1.199719254218440723 ) ) ;
#153236=CARTESIAN_POINT ( 'NONE',  ( -4.550733115681270036, 8.460939068270139529, 0.7998128361456481317 ) ) ;
#153242=CARTESIAN_POINT ( 'NONE',  ( 8.125414133291656071, 8.374071331795406081, -0.7998128361456291469 ) ) ;
#153249=DIRECTION ( 'NONE',  ( 1.000000000000000000, -7.387867266669436732E-31, 0.000000000000000000 ) ) ;
#153254=ORIENTED_EDGE ( 'NONE', *, *, #137619, .T. ) ;
#153256=CARTESIAN_POINT ( 'NONE',  ( 1.364683531249986537, -0.7822916663252464931, -0.7879004041258309554 ) ) ;
#153257=CARTESIAN_POINT ( 'NONE',  ( 3.161022370280501814, 6.839609865302569425, 0.000000000000000000 ) ) ;
#153258=CARTESIAN_POINT ( 'NONE',  ( 5.819474248763732760, 7.812472595022922128, -1.599625672291262513 ) ) ;
#153260=CARTESIAN_POINT ( 'NONE',  ( -8.351459436338041442, 9.806086099558291025, -1.082531754730543971 ) ) ;
#153262=CARTESIAN_POINT ( 'NONE',  ( 5.260200412422194383, 7.159986452624450770, -1.443375672974051449 ) ) ;
#153263=CARTESIAN_POINT ( 'NONE',  ( -8.473482818416675499, 9.948446711983361723, -1.082531754730543083 ) ) ;
#153267=CARTESIAN_POINT ( 'NONE',  ( 8.158255747121103241, 10.54105100977322174, 1.599625672291281386 ) ) ;
#153272=CARTESIAN_POINT ( 'NONE',  ( 1.364683531249986537, 2.155208333674751398, -0.7879004041258239610 ) ) ;
#153279=CARTESIAN_POINT ( 'NONE',  ( 9.257519960032755790, 9.694861462993381807, 0.7998128361456462443 ) ) ;
#153283=CARTESIAN_POINT ( 'NONE',  ( -7.506410603460441422, 11.90922947067921278, -0.7998128361456291469 ) ) ;
#153289=CARTESIAN_POINT ( 'NONE',  ( 2.205172540517054802, 5.724451730578533848, 1.040834085586084257E-14 ) ) ;
#153292=CARTESIAN_POINT ( 'NONE',  ( -8.748035429315585532, 11.22912730566677553, -1.599625672291263179 ) ) ;
#153298=CARTESIAN_POINT ( 'NONE',  ( 5.568360837313221623, 6.179671487343128433, 0.8958872440008452953 ) ) ;
#153300=CARTESIAN_POINT ( 'NONE',  ( -3.418627288940168096, 7.140148937072163804, -0.7998128361456281477 ) ) ;
#153302=AXIS2_PLACEMENT_3D ( 'NONE', #52774, #54919, #118911 ) ;
#153305=CARTESIAN_POINT ( 'NONE',  ( 7.100719765255169236, 9.307259030929609267, -1.599625672291262513 ) ) ;
#153307=CARTESIAN_POINT ( 'NONE',  ( 6.154511665599609493, 9.267681812253174556, 1.199719254218462483 ) ) ;
#153309=CARTESIAN_POINT ( 'NONE',  ( 6.010342169559767633, 5.906487374108181143, -0.7998128361456281477 ) ) ;
#153311=CARTESIAN_POINT ( 'NONE',  ( -7.863365906246061243, 10.19701286208565705, -1.443375672974059665 ) ) ;
#153319=CARTESIAN_POINT ( 'NONE',  ( -4.989408424308831691, 6.622959204541034595, -1.241733208710007696 ) ) ;
#153322=CARTESIAN_POINT ( 'NONE',  ( 5.016153647376205171, 6.875265226737464985, 1.443375672974062551 ) ) ;
#153327=CARTESIAN_POINT ( 'NONE',  ( -10.15469386651127515, 11.90985960142705657, 1.082531754730558626 ) ) ;
#153342=CARTESIAN_POINT ( 'NONE',  ( -8.771762197917311710, 13.17754696430482042, 0.7216878364870317197 ) ) ;
#153348=CARTESIAN_POINT ( 'NONE',  ( 8.932124273304774320, 9.315233161810734686, 0.7998128361456462443 ) ) ;
#153352=CARTESIAN_POINT ( 'NONE',  ( 0.7499999999999902300, 1.764583334016148086, 1.299038105676657340 ) ) ;
#153354=CARTESIAN_POINT ( 'NONE',  ( -5.636439174979254396, 7.598931675607687453, -1.599625672291256295 ) ) ;
#153356=ORIENTED_EDGE ( 'NONE', *, *, #214235, .F. ) ;
#153357=CARTESIAN_POINT ( 'NONE',  ( -9.484092147959342967, 11.02352791316275216, 1.199719254218462483 ) ) ;
#153361=CARTESIAN_POINT ( 'NONE',  ( 6.154511665599609493, 9.267681812253174556, 1.199719254218462483 ) ) ;
#153363=CARTESIAN_POINT ( 'NONE',  ( -7.552055258011950656, 8.769484874890757453, 1.199719254218462483 ) ) ;
#153365=CARTESIAN_POINT ( 'NONE',  ( 8.235688245297327015, 11.69572115523387268, -1.199719254218446718 ) ) ;
#153366=CARTESIAN_POINT ( 'NONE',  ( -0.6823417656249969321, 5.717708333674756283, -1.181850606188749264 ) ) ;
#153368=FACE_OUTER_BOUND ( 'NONE', #8000, .T. ) ;
#153372=CARTESIAN_POINT ( 'NONE',  ( -7.890482213473404727, 8.307910125248191946, 0.7216878364870578100 ) ) ;
#153375=CARTESIAN_POINT ( 'NONE',  ( -1.364683531250010295, 4.842708333674756283, 0.7879004041258379498 ) ) ;
#153381=CARTESIAN_POINT ( 'NONE',  ( -0.6823417656250212460, 5.051041667008086655, 1.181850606188767472 ) ) ;
#153383=CARTESIAN_POINT ( 'NONE',  ( -3.538314903042294457, 6.111489239315849531, 1.082531754730560403 ) ) ;
#153385=CARTESIAN_POINT ( 'NONE',  ( 3.131570294632282092, 5.636953862837537521, -1.082531754730543971 ) ) ;
#153387=CARTESIAN_POINT ( 'NONE',  ( -10.66756793585402363, 11.33991743478486391, 0.7998128361456462443 ) ) ;
#153392=CARTESIAN_POINT ( 'NONE',  ( 0.6823417656249882723, 0.4260416670080896528, -1.181850606188749264 ) ) ;
#153394=CARTESIAN_POINT ( 'NONE',  ( 4.660252114795294887, 6.460046772059735432, -1.599625672291256295 ) ) ;
#153395=ORIENTED_EDGE ( 'NONE', *, *, #137004, .F. ) ;
#153403=CARTESIAN_POINT ( 'NONE',  ( -7.700668062882065179, 10.96756792579566664, -1.082531754730543971 ) ) ;
#153410=CARTESIAN_POINT ( 'NONE',  ( -7.797910906154257304, 12.24931315715533486, 0.000000000000000000 ) ) ;
#153411=CARTESIAN_POINT ( 'NONE',  ( -5.002595493318215070, 7.819816594637776674, 1.082531754730560403 ) ) ;
#153412=CARTESIAN_POINT ( 'NONE',  ( 1.364683531249986537, 2.217708333674751398, -0.7879004041258239610 ) ) ;
#153422=VERTEX_POINT ( 'NONE', #66030 ) ;
#153439=CARTESIAN_POINT ( 'NONE',  ( -1.201851678989727383E-14, 3.134375000341420137, 1.575800808251672791 ) ) ;
#153448=CARTESIAN_POINT ( 'NONE',  ( 0.6823417656249882723, 1.176041667008083325, -1.181850606188749264 ) ) ;
#153450=ORIENTED_EDGE ( 'NONE', *, *, #113143, .F. ) ;
#153458=CARTESIAN_POINT ( 'NONE',  ( 5.626797444871351139, 6.523350759560078593, 1.199719254218462483 ) ) ;
#153468=CARTESIAN_POINT ( 'NONE',  ( -2.761056838677368397, 6.372983411765559048, 0.7998128361456341429 ) ) ;
#153469=CARTESIAN_POINT ( 'NONE',  ( 7.584896871841365851, 10.93646455286856956, -1.199719254218446718 ) ) ;
#153483=CARTESIAN_POINT ( 'NONE',  ( -6.385527162356466668, 10.39360608948380182, 0.000000000000000000 ) ) ;
#153488=CARTESIAN_POINT ( 'NONE',  ( -7.947050595904583403, 12.42330946186405249, 0.7998128361456481317 ) ) ;
#153493=CARTESIAN_POINT ( 'NONE',  ( -8.611400122974211868, 13.19838391011195888, 1.040834085586084257E-14 ) ) ;
#153495=CARTESIAN_POINT ( 'NONE',  ( 9.480175724453529185, 12.08329098332774265, 1.599625672291279388 ) ) ;
#153497=CARTESIAN_POINT ( 'NONE',  ( 3.867100128395839942, 5.534702787927018974, -1.599625672291255185 ) ) ;
#153503=CARTESIAN_POINT ( 'NONE',  ( 2.548569689688999329, 5.917155704705049146, -0.7216878364870267237 ) ) ;
#153505=CARTESIAN_POINT ( 'NONE',  ( -4.334856428067329404, 6.080418470877079429, -1.599625672291256295 ) ) ;
#153508=B_SPLINE_CURVE_WITH_KNOTS ( 'NONE', 3,
 ( #193640, #76692, #142808, #107136, #173160, #94045, #24741, #208812, #60444, #44219, #110341, #45282, #176344, #160085, #143883, #11687, #29023, #73496, #96176, #95107, #78816, #66799, #15935, #12742, #129804 ),
 .UNSPECIFIED., .F., .F.,
 ( 4, 3, 3, 3, 3, 3, 3, 3, 4 ),
 ( 0.000000000000000000, 2.847723191052633419E-05, 6.630505566359037818E-05, 8.958118362427361825E-05, 9.621695898307921417E-05, 0.0001106671188294728486, 0.0001194291616091207911, 0.0001339184197518205287, 0.0001602236158699500094 ),
 .UNSPECIFIED. ) ;
#153509=CARTESIAN_POINT ( 'NONE',  ( -8.809047120577080392, 11.30030761213851953, 1.599625672291269396 ) ) ;
#153515=CARTESIAN_POINT ( 'NONE',  ( 7.619319141200057821, 10.87266085050000974, 1.082531754730557072 ) ) ;
#153516=CARTESIAN_POINT ( 'NONE',  ( 0.6823417656249899377, 3.988541667008085767, -1.181850606188754593 ) ) ;
#153518=CARTESIAN_POINT ( 'NONE',  ( 3.011882680530176604, 6.665613560593854459, 0.7998128361456341429 ) ) ;
#153531=CARTESIAN_POINT ( 'NONE',  ( -1.201851678989727383E-14, 2.384375000341416584, 1.575800808251672791 ) ) ;
#153533=CARTESIAN_POINT ( 'NONE',  ( 8.204655514564224816, 12.72384853363364066, 1.040834085586084257E-14 ) ) ;
#153535=CARTESIAN_POINT ( 'NONE',  ( -4.717874267875590277, 7.487641831621378863, 1.082531754730560403 ) ) ;
#153537=CARTESIAN_POINT ( 'NONE',  ( -5.870317324592821073, 6.911420302522161663, -1.082531754730543083 ) ) ;
#153542=CARTESIAN_POINT ( 'NONE',  ( 5.660692828905515839, 6.562895374266609849, -1.199719254218445830 ) ) ;
#153553=CARTESIAN_POINT ( 'NONE',  ( 6.006425746053997372, 6.966250444273174303, -1.199719254218445830 ) ) ;
#153555=CARTESIAN_POINT ( 'NONE',  ( -3.621833129746822255, 4.096114899008192367, -2.500000000000000444 ) ) ;
#153557=CARTESIAN_POINT ( 'NONE',  ( -6.437424008390261854, 6.404749519410410485, 0.7998128361456341429 ) ) ;
#153561=CARTESIAN_POINT ( 'NONE',  ( 6.751070424600909448, 9.963667031088037973, -1.199719254218441611 ) ) ;
#153564=CARTESIAN_POINT ( 'NONE',  ( -6.795661308947694934, 8.951357498570873261, -1.599625672291263179 ) ) ;
#153566=CARTESIAN_POINT ( 'NONE',  ( 5.788968402910802169, 8.737251655829183505, 1.082531754730558626 ) ) ;
#153567=CARTESIAN_POINT ( 'NONE',  ( 4.954777096267108050, 6.838018505022927407, 1.425084580847448379 ) ) ;
#153568=CARTESIAN_POINT ( 'NONE',  ( -4.731959306369413198, 5.479372931307791461, -1.199719254218446718 ) ) ;
#153571=CARTESIAN_POINT ( 'NONE',  ( -6.250472511100020334, 7.250971670160158311, 1.199719254218450271 ) ) ;
#153574=CARTESIAN_POINT ( 'NONE',  ( 1.364683531249986537, 1.655208333674748955, -0.7879004041258239610 ) ) ;
#153576=CARTESIAN_POINT ( 'NONE',  ( -5.910991785878183080, 5.998504626387068051, -0.7216878364870278340 ) ) ;
#153577=ORIENTED_EDGE ( 'NONE', *, *, #28211, .F. ) ;
#153583=CARTESIAN_POINT ( 'NONE',  ( 4.971035877704902184, 8.951292290631053916, 1.040834085586084257E-14 ) ) ;
#153586=CARTESIAN_POINT ( 'NONE',  ( -1.364683531250014514, 2.051041667008086655, -0.7879004041258289570 ) ) ;
#153589=CARTESIAN_POINT ( 'NONE',  ( 0.6823417656249882723, -1.094791666325249713, 1.181850606188755259 ) ) ;
#153592=CARTESIAN_POINT ( 'NONE',  ( -3.598799709423620374, 6.286017863381107240, 1.199719254218464037 ) ) ;
#153594=CARTESIAN_POINT ( 'NONE',  ( -7.334597914868735025, 9.580116872145431728, -1.443375672974058777 ) ) ;
#153603=CARTESIAN_POINT ( 'NONE',  ( -8.487040972030346353, 9.003895343564625620, 1.040834085586084257E-14 ) ) ;
#153608=CARTESIAN_POINT ( 'NONE',  ( -5.355107487273497391, 9.191449801886996340, 0.7216878364870458196 ) ) ;
#153621=EDGE_CURVE ( 'NONE', #170502, #108282, #139256, .T. ) ;
#153622=CARTESIAN_POINT ( 'NONE',  ( -6.230135280679522936, 7.227244901336242755, 1.199719254218450271 ) ) ;
#153624=CARTESIAN_POINT ( 'NONE',  ( 4.521807925357579805, 5.234196320127330715, -1.199719254218452047 ) ) ;
#153628=CARTESIAN_POINT ( 'NONE',  ( 7.305145839664861640, 7.417091655897478653, 0.7998128361456341429 ) ) ;
#153633=CARTESIAN_POINT ( 'NONE',  ( -4.934804725694231564, 5.819988937140460727, -1.082531754730544860 ) ) ;
#153637=CARTESIAN_POINT ( 'NONE',  ( 3.121116478100642411, 6.446053203092279027, -0.5571924983477014592 ) ) ;
#153643=CARTESIAN_POINT ( 'NONE',  ( 1.364683531249988757, 0.8843750003414210248, 0.000000000000000000 ) ) ;
#153645=CARTESIAN_POINT ( 'NONE',  ( -9.365985188942097750, 9.821404230054264772, 0.7998128361456462443 ) ) ;
#153648=CARTESIAN_POINT ( 'NONE',  ( 6.662942426112080874, 9.860851032851066122, 1.199719254218460707 ) ) ;
#153650=CARTESIAN_POINT ( 'NONE',  ( -8.376239975144482486, 8.666701480623698828, 1.040834085586084257E-14 ) ) ;
#153654=CARTESIAN_POINT ( 'NONE',  ( 1.364683531249988535, 4.655208333674755394, -0.7879004041258300672 ) ) ;
#153656=CARTESIAN_POINT ( 'NONE',  ( 7.592202833972727660, 11.80139437303613015, -0.7216878364870267237 ) ) ;
#153659=CARTESIAN_POINT ( 'NONE',  ( 0.6823417656249882723, -0.5947916663252492686, 1.181850606188755259 ) ) ;
#153662=CARTESIAN_POINT ( 'NONE',  ( 8.731087737076324018, 9.288616569451617622, 1.040834085586084257E-14 ) ) ;
#153665=CARTESIAN_POINT ( 'NONE',  ( -4.582292731738899505, 8.289832587096611860, 0.7216878364870458196 ) ) ;
#153667=CARTESIAN_POINT ( 'NONE',  ( 1.364683531249990311, 3.634375000341416584, 1.214306433183764966E-14 ) ) ;
#153671=CARTESIAN_POINT ( 'NONE',  ( -4.693093728624763372, 8.627026450037540428, 0.7998128361456481317 ) ) ;
#153677=CARTESIAN_POINT ( 'NONE',  ( 6.909851844459134362, 11.21324425184434936, -0.7998128361456291469 ) ) ;
#153680=CARTESIAN_POINT ( 'NONE',  ( 1.499999999999989120, 2.254166666666685970, 0.8660254037844524744 ) ) ;
#153686=CARTESIAN_POINT ( 'NONE',  ( 6.819388077993785657, 7.058300300521964665, 1.040834085586084257E-14 ) ) ;
#153687=CARTESIAN_POINT ( 'NONE',  ( 0.6823417656249882723, -0.8447916663252494907, 1.181850606188755259 ) ) ;
#153694=CARTESIAN_POINT ( 'NONE',  ( 0.7499999999999885647, 0.5666666666666875241, -1.299038105676652899 ) ) ;
#153695=CARTESIAN_POINT ( 'NONE',  ( 8.599949509769960088, 8.927695937686774386, 1.040834085586084257E-14 ) ) ;
#153696=CARTESIAN_POINT ( 'NONE',  ( -7.492852449846775897, 11.89341162479659531, 0.000000000000000000 ) ) ;
#153698=CARTESIAN_POINT ( 'NONE',  ( -0.6823417656250246877, -0.6989583329919113464, 1.181850606188755259 ) ) ;
#153699=CARTESIAN_POINT ( 'NONE',  ( -1.499999999999997780, 1.650000000000019451, 0.000000000000000000 ) ) ;
#153702=CARTESIAN_POINT ( 'NONE',  ( 3.825371897350130723, 7.614684313550482031, 0.7998128361456321445 ) ) ;
#153709=CARTESIAN_POINT ( 'NONE',  ( -0.6823417656249969321, 5.217708333674756283, -1.181850606188749264 ) ) ;
#153711=CARTESIAN_POINT ( 'NONE',  ( -7.621654909176601045, 12.04368116068139472, 0.7998128361456481317 ) ) ;
#153712=CARTESIAN_POINT ( 'NONE',  ( -3.931501358282937009, 7.530575984731317618, 0.7216878364870317197 ) ) ;
#153720=CARTESIAN_POINT ( 'NONE',  ( 7.076466111328892694, 10.34329533227067799, -1.199719254218441611 ) ) ;
#153721=CARTESIAN_POINT ( 'NONE',  ( -4.406036734316890247, 7.123831375802920363, -1.082531754730548412 ) ) ;
#153723=CARTESIAN_POINT ( 'NONE',  ( 6.683806541412754321, 8.820860269780128604, -1.443375672974058777 ) ) ;
#153726=CARTESIAN_POINT ( 'NONE',  ( -7.914208982075130905, 10.25632978388623684, -1.599625672291263179 ) ) ;
#153727=CARTESIAN_POINT ( 'NONE',  ( 4.469384193999260901, 8.366031992974468423, -0.7998128361456231517 ) ) ;
#153730=CARTESIAN_POINT ( 'NONE',  ( 3.195971524519376494, 4.751719416737803847, -1.599625672291262513 ) ) ;
#153732=ADVANCED_FACE ( 'NONE', ( #18370 ), #84447, .T. ) ;
#153738=CARTESIAN_POINT ( 'NONE',  ( -3.958617665510266725, 7.562211676496538360, -0.7216878364870267237 ) ) ;
#153739=CARTESIAN_POINT ( 'NONE',  ( 10.41229878561526512, 11.25002945941372623, -0.7216878364870257245 ) ) ;
#153742=CARTESIAN_POINT ( 'NONE',  ( -6.018930129462987999, 9.109503353427070849, 1.199719254218452047 ) ) ;
#153747=CARTESIAN_POINT ( 'NONE',  ( -6.723954117373590833, 9.932031339322813679, -1.199719254218440723 ) ) ;
#153762=CARTESIAN_POINT ( 'NONE',  ( -7.867809214632013770, 8.073532260025807261, 1.040834085586084257E-14 ) ) ;
#153766=CARTESIAN_POINT ( 'NONE',  ( 6.344852701515477200, 6.504675694630598137, -0.7216878364870257245 ) ) ;
#153771=CARTESIAN_POINT ( 'NONE',  ( -4.249591082879585535, 7.045274465746411252, 1.199719254218464037 ) ) ;
#153774=CARTESIAN_POINT ( 'NONE',  ( -5.045605722580076780, 9.038290442985410067, -0.7998128361456231517 ) ) ;
#153775=CARTESIAN_POINT ( 'NONE',  ( -5.900304042155601003, 6.007113627712965531, 0.2101855125488115983 ) ) ;
#153780=CARTESIAN_POINT ( 'NONE',  ( -8.479735010343349089, 11.98044238112085758, 1.199719254218453823 ) ) ;
#153781=CARTESIAN_POINT ( 'NONE',  ( 6.425674737872927089, 9.584038729905381970, -1.199719254218440723 ) ) ;
#153785=CARTESIAN_POINT ( 'NONE',  ( -7.811469059767924605, 12.26513100303794168, -0.7998128361456281477 ) ) ;
#153793=CARTESIAN_POINT ( 'NONE',  ( 9.734391104931955141, 10.45913716528321125, 0.7216878364870438212 ) ) ;
#153796=CARTESIAN_POINT ( 'NONE',  ( -1.579999999999998073, 8.674529973577531194, -2.499999999999990230 ) ) ;
#153815=CARTESIAN_POINT ( 'NONE',  ( -4.634189577772691138, 4.300976017023221409, 1.214306433183764966E-14 ) ) ;
#153818=CARTESIAN_POINT ( 'NONE',  ( -3.164938793786285842, 5.779846795137578930, -1.199719254218452935 ) ) ;
#153822=CARTESIAN_POINT ( 'NONE',  ( -0.7500000000000006661, -0.6104166659838470288, -1.299038105676652011 ) ) ;
#153829=CARTESIAN_POINT ( 'NONE',  ( 1.408440994508639577, 7.230285460703519185, -4.273713947604624863 ) ) ;
#153831=CARTESIAN_POINT ( 'NONE',  ( -3.145128448690340139, 6.613140923539886806, -0.7216878364870489282 ) ) ;
#153832=CARTESIAN_POINT ( 'NONE',  ( 2.920892028740289081, 5.495125569250587816, 1.199719254218452047 ) ) ;
#153834=DIRECTION ( 'NONE',  ( 0.6507913734559658270, 0.7592566023652989049, 0.000000000000000000 ) ) ;
#153837=CARTESIAN_POINT ( 'NONE',  ( 5.823390672269506574, 6.752709524857930745, -1.199719254218446718 ) ) ;
#153838=CARTESIAN_POINT ( 'NONE',  ( 0.6823417656249899377, 2.905208333674754062, 1.181850606188765695 ) ) ;
#153839=CARTESIAN_POINT ( 'NONE',  ( -4.373253022481784491, 7.180661499490419430, 1.044565980707335529 ) ) ;
#153842=CARTESIAN_POINT ( 'NONE',  ( -9.671043645249580933, 10.17730576241299900, 0.7998128361456462443 ) ) ;
#153843=CARTESIAN_POINT ( 'NONE',  ( -4.568734577680894304, 5.392907097791561633, -1.082531754730543971 ) ) ;
#153846=CARTESIAN_POINT ( 'NONE',  ( -6.067437437315529536, 7.037430750744921859, 1.199719254218450271 ) ) ;
#153848=CARTESIAN_POINT ( 'NONE',  ( -1.402160292154681736E-14, -0.7562499993171803991, 1.732050807568877637 ) ) ;
#153856=CARTESIAN_POINT ( 'NONE',  ( -4.894130264408862452, 7.693273827576896373, -1.082531754730548412 ) ) ;
#153862=CARTESIAN_POINT ( 'NONE',  ( -2.941756144040963417, 6.375873234782333476, -0.7216878364870257245 ) ) ;
#153864=CARTESIAN_POINT ( 'NONE',  ( 8.072990401933337168, 11.50590700464255356, -1.199719254218446718 ) ) ;
#153866=CARTESIAN_POINT ( 'NONE',  ( 3.660338285565247762, 7.214219066560688454, 1.040834085586084257E-14 ) ) ;
#153874=CARTESIAN_POINT ( 'NONE',  ( -4.288456660624211381, 3.897620947016656956, 1.214306433183764966E-14 ) ) ;
#153875=CARTESIAN_POINT ( 'NONE',  ( -9.972185678051314284, 11.59297036493672017, 1.199719254218462483 ) ) ;
#153880=CARTESIAN_POINT ( 'NONE',  ( 5.309989718046547402, 9.346738437696316737, 0.7998128361456462443 ) ) ;
#153885=CARTESIAN_POINT ( 'NONE',  ( 4.878236342818665250, 4.585697242910212523, 1.040834085586084257E-14 ) ) ;
#153895=CARTESIAN_POINT ( 'NONE',  ( 8.945682426918439845, 9.331051007693339727, 1.040834085586084257E-14 ) ) ;
#153896=CARTESIAN_POINT ( 'NONE',  ( -4.737684612971557740, 7.614716917520386374, 1.199719254218464037 ) ) ;
#153899=CARTESIAN_POINT ( 'NONE',  ( 1.230687378724321990, 2.810186076401617772, 0.7750000000000152323 ) ) ;
#153903=CARTESIAN_POINT ( 'NONE',  ( -0.6823417656250212460, 4.551041667008086655, 1.181850606188767472 ) ) ;
#153906=ORIENTED_EDGE ( 'NONE', *, *, #142863, .F. ) ;
#153907=CARTESIAN_POINT ( 'NONE',  ( -4.741649638052999549, 5.202212439478444139, 1.069586989871945670 ) ) ;
#153908=CARTESIAN_POINT ( 'NONE',  ( 4.379447312414087357, 5.068108938359919158, -1.199719254218452047 ) ) ;
#153909=CARTESIAN_POINT ( 'NONE',  ( -4.731959306369413198, 5.479372931307791461, -1.199719254218446718 ) ) ;
#153915=CARTESIAN_POINT ( 'NONE',  ( 5.016153647376201619, 7.835634441038803466, 1.082531754730558626 ) ) ;
#153917=CARTESIAN_POINT ( 'NONE',  ( 7.415946836550712185, 10.63539316174243865, 1.082531754730558626 ) ) ;
#153918=CARTESIAN_POINT ( 'NONE',  ( -0.6823417656249969321, 3.530208333674754506, -1.181850606188749264 ) ) ;
#153920=CARTESIAN_POINT ( 'NONE',  ( 4.812781342726858647, 6.637997537979888563, 1.443375672974062551 ) ) ;
#153922=CARTESIAN_POINT ( 'NONE',  ( -0.01485505708498172442, 7.054063922337708625, -3.955400951015620947 ) ) ;
#153929=CARTESIAN_POINT ( 'NONE',  ( -4.390790479118549250, 7.352160220884910835, 1.215098293768980930 ) ) ;
#153935=CARTESIAN_POINT ( 'NONE',  ( -9.829825065107822724, 11.42688298316931572, 1.199719254218462483 ) ) ;
#153943=ORIENTED_EDGE ( 'NONE', *, *, #126911, .T. ) ;
#153945=CARTESIAN_POINT ( 'NONE',  ( 3.714570900464285064, 4.396382807705524698, 1.082531754730560403 ) ) ;
#153946=CARTESIAN_POINT ( 'NONE',  ( -1.201851678989727383E-14, 3.634375000341422357, 1.575800808251672791 ) ) ;
#153948=CARTESIAN_POINT ( 'NONE',  ( 5.750629710490689384, 9.860818428881154674, -0.7998128361456291469 ) ) ;
#153950=CARTESIAN_POINT ( 'NONE',  ( -8.618179199781044630, 13.20629283305325963, 0.7998128361456341429 ) ) ;
#153951=FACE_OUTER_BOUND ( 'NONE', #147373, .T. ) ;
#153956=AXIS2_PLACEMENT_3D ( 'NONE', #162278, #212060, #116773 ) ;
#153957=CARTESIAN_POINT ( 'NONE',  ( -0.7499999999999972244, 3.858333333333359594, -1.299038105676652011 ) ) ;
#153958=CARTESIAN_POINT ( 'NONE',  ( 5.118366684358879759, 5.930181538962194132, 1.199719254218462483 ) ) ;
#153961=CARTESIAN_POINT ( 'NONE',  ( 1.499999999990964339, 7.854386371700860181, 3.680172642296245744 ) ) ;
#153962=CARTESIAN_POINT ( 'NONE',  ( 0.6823417656249917140, 3.342708333674754506, 1.181850606188765695 ) ) ;
#153964=CARTESIAN_POINT ( 'NONE',  ( 8.405692050792682224, 12.75046512599275772, -0.7216878364870328300 ) ) ;
#153969=CARTESIAN_POINT ( 'NONE',  ( -1.500000000000013101, 2.452083334016154748, 0.8660254037844403729 ) ) ;
#153971=CARTESIAN_POINT ( 'NONE',  ( -5.850506979496850057, 6.784345216623154151, -1.199719254218446718 ) ) ;
#153972=CARTESIAN_POINT ( 'NONE',  ( 3.497640442201256139, 7.024404915969360452, 1.040834085586084257E-14 ) ) ;
#153980=CARTESIAN_POINT ( 'NONE',  ( 6.608709811657416999, 9.797579649320619311, -1.199719254218440723 ) ) ;
#153981=CARTESIAN_POINT ( 'NONE',  ( 4.660252114795294887, 6.460046772059735432, -1.599625672291256295 ) ) ;
#153982=FACE_OUTER_BOUND ( 'NONE', #12938, .T. ) ;
#153984=CARTESIAN_POINT ( 'NONE',  ( 3.330499290451326200, 7.037332938835193730, -0.7998128361456291469 ) ) ;
#153988=ORIENTED_EDGE ( 'NONE', *, *, #174354, .T. ) ;
#153990=STYLED_ITEM ( 'NONE', ( #169156 ), #93359 ) ;
#153992=CARTESIAN_POINT ( 'NONE',  ( 9.890836756369282057, 11.49806328964105617, -1.199719254218440723 ) ) ;
#153997=CARTESIAN_POINT ( 'NONE',  ( 5.811422509517683466, 6.026224704000590293, 0.4751317933852049480 ) ) ;
#154007=CARTESIAN_POINT ( 'NONE',  ( 6.155038550924133212, 10.12470270947942730, 0.7216878364870438212 ) ) ;
#154008=CARTESIAN_POINT ( 'NONE',  ( -4.060830702492950195, 4.696389560118578999, -1.199719254218452047 ) ) ;
#154014=CARTESIAN_POINT ( 'NONE',  ( -4.042302355168801320, 7.867769847672247074, 0.7998128361456341429 ) ) ;
#154021=CARTESIAN_POINT ( 'NONE',  ( 0.7499999999999902300, 3.264583334016149418, 1.299038105676669330 ) ) ;
#154026=CARTESIAN_POINT ( 'NONE',  ( 10.08456733046637765, 10.65975006183261087, 0.000000000000000000 ) ) ;
#154028=CARTESIAN_POINT ( 'NONE',  ( 3.606105671554957759, 4.269840040644637291, -1.082531754730543083 ) ) ;
#154034=CARTESIAN_POINT ( 'NONE',  ( -9.991996023591624976, 10.75967623705280296, 1.040834085586084257E-14 ) ) ;
#154038=CARTESIAN_POINT ( 'NONE',  ( 9.237182729612253951, 9.671134694169463586, 0.7998128361456462443 ) ) ;
#154040=EDGE_CURVE ( 'NONE', #154752, #69931, #120227, .T. ) ;
#154043=CARTESIAN_POINT ( 'NONE',  ( -6.039267359883488950, 9.133230122250985517, 1.199719254218452047 ) ) ;
#154044=CARTESIAN_POINT ( 'NONE',  ( 3.174580523894166006, 6.855427711185178019, 0.7998128361456341429 ) ) ;
#154047=CARTESIAN_POINT ( 'NONE',  ( 10.38962578677386084, 11.01565159419135043, 0.000000000000000000 ) ) ;
#154048=DIRECTION ( 'NONE',  ( -0.000000000000000000, -8.546850786086437571E-32, -1.000000000000000000 ) ) ;
#154052=CARTESIAN_POINT ( 'NONE',  ( 1.364683531249986537, 2.217708333674751398, -0.7879004041258239610 ) ) ;
#154055=CARTESIAN_POINT ( 'NONE',  ( 5.829642864196157070, 8.784705193995428374, 1.082531754730558626 ) ) ;
#154064=CARTESIAN_POINT ( 'NONE',  ( 8.554831740098659765, 10.04335378727902395, 1.082531754730558626 ) ) ;
#154065=ORIENTED_EDGE ( 'NONE', *, *, #210306, .F. ) ;
#154068=CARTESIAN_POINT ( 'NONE',  ( -7.167456763118792651, 11.51378332361394818, 0.000000000000000000 ) ) ;
#154076=CARTESIAN_POINT ( 'NONE',  ( 2.544126380858701797, 6.119897877643793116, 0.7998128361456462443 ) ) ;
#154080=CARTESIAN_POINT ( 'NONE',  ( 5.172599298813543633, 5.993452922492633839, -1.199719254218452047 ) ) ;
#154083=CARTESIAN_POINT ( 'NONE',  ( -1.499999999999997780, 2.931250000682818158, 1.214306433183764966E-14 ) ) ;
#154089=CARTESIAN_POINT ( 'NONE',  ( -1.500000000000013101, 0.6708333333333583726, 0.8660254037844403729 ) ) ;
#154090=CARTESIAN_POINT ( 'NONE',  ( 6.577677080924314801, 10.82570702772039262, 1.040834085586084257E-14 ) ) ;
#154091=CARTESIAN_POINT ( 'NONE',  ( 6.629573926958101993, 6.836850457647000390, -0.7216878364870257245 ) ) ;
#154095=CARTESIAN_POINT ( 'NONE',  ( 8.215877900201359552, 11.56864606933486606, -1.082531754730543083 ) ) ;
#154100=CARTESIAN_POINT ( 'NONE',  ( -5.253948220495577637, 6.088359997788290734, 1.199719254218450271 ) ) ;
#154102=CARTESIAN_POINT ( 'NONE',  ( -1.500000000000011324, 4.410416667349484676, -0.8660254037844313801 ) ) ;
#154103=CARTESIAN_POINT ( 'NONE',  ( -1.001543065824772872E-14, 5.384375000341415252, 1.575800808251672791 ) ) ;
#154108=CARTESIAN_POINT ( 'NONE',  ( 1.364683531249988535, 4.426041667008082214, 0.7879004041258500513 ) ) ;
#154117=CARTESIAN_POINT ( 'NONE',  ( -7.503547950159405566, 10.84155747757291266, 1.199719254218453823 ) ) ;
#154118=CARTESIAN_POINT ( 'NONE',  ( 5.900823170445728572, 7.907379670318584353, 1.599625672291267398 ) ) ;
#154124=EDGE_CURVE ( 'NONE', #164674, #161364, #30688, .T. ) ;
#154125=CARTESIAN_POINT ( 'NONE',  ( 2.205172540517054802, 5.724451730578533848, 1.040834085586084257E-14 ) ) ;
#154127=CARTESIAN_POINT ( 'NONE',  ( -6.344325816190970357, 9.489131654609717970, 1.199719254218452047 ) ) ;
#154132=CARTESIAN_POINT ( 'NONE',  ( 8.204655514564224816, 12.72384853363364066, 1.040834085586084257E-14 ) ) ;
#154135=ORIENTED_EDGE ( 'NONE', *, *, #17378, .T. ) ;
#154136=CARTESIAN_POINT ( 'NONE',  ( -3.795392936821753604, 6.515376628678959392, -1.199719254218452047 ) ) ;
#154137=CARTESIAN_POINT ( 'NONE',  ( -7.797910906154257304, 12.24931315715533486, 0.000000000000000000 ) ) ;
#154141=CARTESIAN_POINT ( 'NONE',  ( -4.398207409718558836, 7.344456035913847103, -1.221965942340837552 ) ) ;
#154149=CARTESIAN_POINT ( 'NONE',  ( 6.979750152936881058, 7.037463354714830643, 0.7998128361456341429 ) ) ;
#154168=CARTESIAN_POINT ( 'NONE',  ( 3.145128448690309053, 4.692402494937224056, -1.443375672974057666 ) ) ;
#154172=CARTESIAN_POINT ( 'NONE',  ( -8.136864746495904299, 12.64475930422059768, -0.7998128361456281477 ) ) ;
#154177=CARTESIAN_POINT ( 'NONE',  ( -0.7500000000000006661, 1.639583334016154970, -1.299038105676652011 ) ) ;
#154178=CARTESIAN_POINT ( 'NONE',  ( 9.459838494033030898, 12.05956421450382088, 1.599625672291281386 ) ) ;
#154182=FACE_OUTER_BOUND ( 'NONE', #129955, .T. ) ;
#154183=CARTESIAN_POINT ( 'NONE',  ( -2.034713692888026060, 8.461455076002922127, -2.499999999999990230 ) ) ;
#154184=CARTESIAN_POINT ( 'NONE',  ( 0.6823417656249882723, 0.9260416670080831025, -1.181850606188749264 ) ) ;
#154190=CARTESIAN_POINT ( 'NONE',  ( -5.199715606040888005, 6.025088614257851027, -1.199719254218446718 ) ) ;
#154195=CARTESIAN_POINT ( 'NONE',  ( -1.402160292154681736E-14, 0.3843750003414230232, 1.575800808251672791 ) ) ;
#154201=CARTESIAN_POINT ( 'NONE',  ( -0.6823417656250003738, -0.03229166632524871350, -1.181850606188749264 ) ) ;
#154203=CARTESIAN_POINT ( 'NONE',  ( -7.562750758324527922, 7.717630727667075696, 1.040834085586084257E-14 ) ) ;
#154204=CARTESIAN_POINT ( 'NONE',  ( 6.805303039055573322, 10.02693841461847057, 1.199719254218460707 ) ) ;
#154205=CARTESIAN_POINT ( 'NONE',  ( 5.840865249388944136, 5.708764300575555950, 0.7998128361456341429 ) ) ;
#154208=CARTESIAN_POINT ( 'NONE',  ( -1.364683531250012516, 1.592708333674756727, 0.7879004041258379498 ) ) ;
#154213=CARTESIAN_POINT ( 'NONE',  ( 7.456621297836082185, 7.801739057004660971, 0.7216878364870317197 ) ) ;
#154216=CARTESIAN_POINT ( 'NONE',  ( -6.364663046611467756, 9.512858423433634414, 1.199719254218452047 ) ) ;
#154217=CARTESIAN_POINT ( 'NONE',  ( -2.740719608256871442, 6.349256642941639051, 0.7998128361456341429 ) ) ;
#154219=CARTESIAN_POINT ( 'NONE',  ( 3.809477975315520570, 7.388215371269448717, -0.7216878364869808715 ) ) ;
#154222=CARTESIAN_POINT ( 'NONE',  ( 5.300874872818830852, 7.207439989753867238, 1.443375672974062551 ) ) ;
#154223=CARTESIAN_POINT ( 'NONE',  ( -8.636180661780672452, 9.177891648273343250, -0.7216878364870267237 ) ) ;
#154225=CARTESIAN_POINT ( 'NONE',  ( -1.500000000000011324, 5.129166666666691299, -0.8660254037844313801 ) ) ;
#154229=CARTESIAN_POINT ( 'NONE',  ( 8.595506201384004896, 12.01154575404795466, 1.082531754730546636 ) ) ;
#154230=CARTESIAN_POINT ( 'NONE',  ( -5.111060722671894929, 5.065251719313053513, 0.000000000000000000 ) ) ;
#154239=CARTESIAN_POINT ( 'NONE',  ( 10.07334494482924292, 11.81495252613139257, -1.082531754730537088 ) ) ;
#154245=CARTESIAN_POINT ( 'NONE',  ( 7.497295758232718654, 9.769931022736756177, -1.443375672974058777 ) ) ;
#154247=CARTESIAN_POINT ( 'NONE',  ( 6.238723240582662477, 10.43026088065513513, -0.7998128361456291469 ) ) ;
#154248=CARTESIAN_POINT ( 'NONE',  ( -6.880926654135487652, 7.986501503701545879, 1.199719254218450271 ) ) ;
#154252=VECTOR ( 'NONE', #114418, 1000.000000000000000 ) ;
#154253=CARTESIAN_POINT ( 'NONE',  ( -1.364683531250000748, -1.178124999658580752, 0.000000000000000000 ) ) ;
#154254=CARTESIAN_POINT ( 'NONE',  ( 5.016153647376217606, 4.954526798134778254, 0.7216878364870317197 ) ) ;
#154256=CARTESIAN_POINT ( 'NONE',  ( -4.298098390732130625, 4.973201863064262263, 1.199719254218462483 ) ) ;
#154257=CARTESIAN_POINT ( 'NONE',  ( -7.049876689426103127, 10.20831132343037062, -1.082531754730537976 ) ) ;
#154260=EDGE_CURVE ( 'NONE', #212749, #190586, #107046, .T. ) ;
#154273=CARTESIAN_POINT ( 'NONE',  ( 6.747154001095143627, 11.02343010125301959, -0.7998128361456291469 ) ) ;
#154276=ORIENTED_EDGE ( 'NONE', *, *, #82451, .T. ) ;
#154284=CARTESIAN_POINT ( 'NONE',  ( -5.364222332501225488, 9.410009821226765325, 0.7998128361456481317 ) ) ;
#154286=CARTESIAN_POINT ( 'NONE',  ( -3.307299406729781399, 5.945934176904983381, -1.199719254218452935 ) ) ;
#154294=CARTESIAN_POINT ( 'NONE',  ( -4.790108344329849110, 4.482881244673243337, 0.7998128361456341429 ) ) ;
#154297=CARTESIAN_POINT ( 'NONE',  ( 6.252281394196331554, 10.44607872653774372, 1.040834085586084257E-14 ) ) ;
#154298=CARTESIAN_POINT ( 'NONE',  ( -0.6823417656250212460, 5.301041667008086655, 1.181850606188767472 ) ) ;
#154307=CARTESIAN_POINT ( 'NONE',  ( 4.311129659021211147, 7.973475668925984472, 1.040834085586084257E-14 ) ) ;
#154308=CARTESIAN_POINT ( 'NONE',  ( -6.157374318900681764, 10.33535380535947290, 0.7998128361456481317 ) ) ;
#154311=CARTESIAN_POINT ( 'NONE',  ( -7.147119532698295252, 11.49005655479003174, 0.000000000000000000 ) ) ;
#154312=CARTESIAN_POINT ( 'NONE',  ( -6.261168011412601153, 6.199117522936475666, 1.040834085586084257E-14 ) ) ;
#154319=CARTESIAN_POINT ( 'NONE',  ( 6.938021921891177612, 9.117444880338284818, -1.599625672291262513 ) ) ;
#154333=CARTESIAN_POINT ( 'NONE',  ( 0.6823417656249882723, -1.094791666325249713, 1.181850606188755259 ) ) ;
#154334=CARTESIAN_POINT ( 'NONE',  ( 4.985647801523278133, 6.839675073242382553, -1.599625672291256295 ) ) ;
#154335=CARTESIAN_POINT ( 'NONE',  ( 4.971035877704902184, 8.951292290631053916, 1.040834085586084257E-14 ) ) ;
#154337=CARTESIAN_POINT ( 'NONE',  ( -7.483737605063437215, 10.71448239167390604, 1.082531754730549967 ) ) ;
#154338=CARTESIAN_POINT ( 'NONE',  ( 7.293923454472091450, 7.611924906413328529, 0.7216878364870317197 ) ) ;
#154339=CARTESIAN_POINT ( 'NONE',  ( -8.066738210006693777, 10.43428054980638997, 1.443375672974090751 ) ) ;
#154342=CARTESIAN_POINT ( 'NONE',  ( 7.884230021546724920, 9.157022099014721306, 1.199719254218462483 ) ) ;
#154347=DIRECTION ( 'NONE',  ( 1.000000000000000000, 0.000000000000000000, 0.000000000000000000 ) ) ;
#154348=CARTESIAN_POINT ( 'NONE',  ( -1.364683531250012516, 2.738541667008090208, -0.7879004041258289570 ) ) ;
#154354=CARTESIAN_POINT ( 'NONE',  ( 7.422199028477372451, 10.74665040227725044, -1.199719254218441611 ) ) ;
#154357=CARTESIAN_POINT ( 'NONE',  ( -10.32861409551237486, 10.94447128771960287, 1.040834085586084257E-14 ) ) ;
#154363=CARTESIAN_POINT ( 'NONE',  ( 2.191614386903386613, 5.708633884695917260, -0.7998128361456281477 ) ) ;
#154369=CARTESIAN_POINT ( 'NONE',  ( -10.47775378526269918, 11.11846759242831872, -0.7998128361456221525 ) ) ;
#154374=CARTESIAN_POINT ( 'NONE',  ( 5.543269800280802073, 6.196057874731542015, 0.9238780061134096444 ) ) ;
#154376=CARTESIAN_POINT ( 'NONE',  ( -3.079673448598517549, 6.744702790006905424, 1.040834085586084257E-14 ) ) ;
#154380=CARTESIAN_POINT ( 'NONE',  ( 6.265839547809997079, 10.46189657242035587, 0.7998128361456462443 ) ) ;
#154382=CARTESIAN_POINT ( 'NONE',  ( 4.937140493670735708, 8.911747675924535983, -0.7998128361456281477 ) ) ;
#154385=CARTESIAN_POINT ( 'NONE',  ( -7.375272376154077492, 11.54830883891436422, -0.7216878364870267237 ) ) ;
#154393=CARTESIAN_POINT ( 'NONE',  ( -5.486276195386677657, 6.266678140956847720, -0.9979454321464575894 ) ) ;
#154395=CARTESIAN_POINT ( 'NONE',  ( 4.500943810056890371, 8.194925511800951412, -0.7216878364870207285 ) ) ;
#154398=AXIS2_PLACEMENT_3D ( 'NONE', #50051, #186428, #36983 ) ;
#154400=LINE ( 'NONE', #138161, #68768 ) ;
#154413=CARTESIAN_POINT ( 'NONE',  ( -9.693716643646601128, 12.33242205571964512, 1.443375672974076540 ) ) ;
#154417=( BOUNDED_CURVE ( )  B_SPLINE_CURVE ( 2, ( #128273, #196378, #77285 ),
 .UNSPECIFIED., .F., .T. ) 
 B_SPLINE_CURVE_WITH_KNOTS ( ( 3, 3 ),
 ( 0.000000000000000000, 0.002450381106065508980 ),
 .UNSPECIFIED. ) 
 CURVE ( )  GEOMETRIC_REPRESENTATION_ITEM ( )  RATIONAL_B_SPLINE_CURVE ( ( 1.000000000000000000, 0.9212106833777519155, 0.9350920161047693302 ) ) 
 REPRESENTATION_ITEM ( '' )  );
#154418=CARTESIAN_POINT ( 'NONE',  ( 8.782984583554449998, 9.141236857102018831, 1.040834085586084257E-14 ) ) ;
#154420=VERTEX_POINT ( 'NONE', #60223 ) ;
#154422=CARTESIAN_POINT ( 'NONE',  ( -1.500000000000013101, 1.202083334016148974, 0.8660254037844403729 ) ) ;
#154423=DIRECTION ( 'NONE',  ( -1.000000000000000000, 5.578564026256504688E-16, 0.000000000000000000 ) ) ;
#154424=CARTESIAN_POINT ( 'NONE',  ( -6.718228810771495141, 7.796687353110217877, 1.199719254218450271 ) ) ;
#154428=CARTESIAN_POINT ( 'NONE',  ( -9.378489572351046633, 11.96465713920816043, -1.599625672291263179 ) ) ;
#154429=CARTESIAN_POINT ( 'NONE',  ( -1.387358672531466386, 7.251968950356099342, 4.302625267141412913 ) ) ;
#154433=CARTESIAN_POINT ( 'NONE',  ( 6.479907352327590964, 9.647310113435821677, 1.199719254218462483 ) ) ;
#154435=CARTESIAN_POINT ( 'NONE',  ( -6.256197817702116026, 9.386315656372753224, -1.199719254218440723 ) ) ;
#154437=CARTESIAN_POINT ( 'NONE',  ( 1.364683531249990311, 5.363541667008086655, 0.7879004041258500513 ) ) ;
#154443=CARTESIAN_POINT ( 'NONE',  ( -6.073689629242151611, 10.02979563418376685, -0.7216878364870278340 ) ) ;
#154448=CARTESIAN_POINT ( 'NONE',  ( -0.6823417656250212460, 4.363541667008085767, 1.181850606188767472 ) ) ;
#154456=CARTESIAN_POINT ( 'NONE',  ( -1.364683531250012516, 4.738541667008091096, -0.7879004041258300672 ) ) ;
#154459=CARTESIAN_POINT ( 'NONE',  ( 3.673896439178923057, 5.309298483840612093, 1.443375672974066548 ) ) ;
#154466=CARTESIAN_POINT ( 'NONE',  ( -1.364683531250012516, 0.5302083336747518416, 0.7879004041258379498 ) ) ;
#154468=CARTESIAN_POINT ( 'NONE',  ( -3.795919822146289313, 5.451659097302528068, -1.443375672974053447 ) ) ;
#154469=CARTESIAN_POINT ( 'NONE',  ( 3.649115900372475796, 7.409052317076538330, 1.040834085586084257E-14 ) ) ;
#154475=CARTESIAN_POINT ( 'NONE',  ( 2.399429999938675007, 5.743159399996332404, 0.000000000000000000 ) ) ;
#154476=CARTESIAN_POINT ( 'NONE',  ( 9.612367721964607981, 12.23751498042398289, -1.443375672974058777 ) ) ;
#154478=CARTESIAN_POINT ( 'NONE',  ( -7.375272376154081932, 10.58793962461302485, -1.082531754730543971 ) ) ;
#154483=CARTESIAN_POINT ( 'NONE',  ( -8.971744963941075568, 11.49012176272984931, 1.599625672291269396 ) ) ;
#154484=CARTESIAN_POINT ( 'NONE',  ( -5.219525951136850139, 7.112532914458205013, -1.443375672974051449 ) ) ;
#154486=CARTESIAN_POINT ( 'NONE',  ( 1.364683531249986537, 1.467708333674748289, -0.7879004041258239610 ) ) ;
#154499=ORIENTED_EDGE ( 'NONE', *, *, #196828, .F. ) ;
#154501=ORIENTED_EDGE ( 'NONE', *, *, #77263, .T. ) ;
#154505=CARTESIAN_POINT ( 'NONE',  ( -2.415323921528888196, 5.969628341758991930, 0.7998128361456341429 ) ) ;
#154507=CARTESIAN_POINT ( 'NONE',  ( -1.201851678989727383E-14, 3.009375000341419248, -1.575800808251660134 ) ) ;
#154517=CARTESIAN_POINT ( 'NONE',  ( -1.364683531250000748, 0.7593750003414210248, 0.000000000000000000 ) ) ;
#154519=ORIENTED_EDGE ( 'NONE', *, *, #80217, .T. ) ;
#154528=CARTESIAN_POINT ( 'NONE',  ( 5.464099601507359516, 6.333536608968757697, 1.199719254218462483 ) ) ;
#154534=CARTESIAN_POINT ( 'NONE',  ( 7.527801604085637699, 9.805521176231838609, 1.599625672291281386 ) ) ;
#154538=CARTESIAN_POINT ( 'NONE',  ( 8.341290820905593151, 10.75459192918846618, 1.599625672291281386 ) ) ;
#154551=CARTESIAN_POINT ( 'NONE',  ( -8.242994207428740339, 9.679543332497402730, 1.082531754730558626 ) ) ;
#154556=CARTESIAN_POINT ( 'NONE',  ( -10.48453286206953727, 11.12637651536962125, 0.7998128361456462443 ) ) ;
#154562=CARTESIAN_POINT ( 'NONE',  ( -3.086452525405351643, 6.752611712948207057, 0.7998128361456341429 ) ) ;
#154565=CARTESIAN_POINT ( 'NONE',  ( 9.642873567817520808, 12.27310513391906532, 1.599625672291279388 ) ) ;
#154567=CARTESIAN_POINT ( 'NONE',  ( 4.539282502477016479, 4.190251095844947926, 0.7998128361456341429 ) ) ;
#154573=CARTESIAN_POINT ( 'NONE',  ( 3.470524135418292300, 5.072030796119872953, -1.443375672974057666 ) ) ;
#154575=CARTESIAN_POINT ( 'NONE',  ( -5.603597561149804562, 5.431951997629870910, 0.7998128361456341429 ) ) ;
#154578=CARTESIAN_POINT ( 'NONE',  ( -10.63367255181986160, 11.30037282007833532, 1.040834085586084257E-14 ) ) ;
#154584=CARTESIAN_POINT ( 'NONE',  ( 9.408995418203975447, 10.07950886410055524, 0.7216878364870438212 ) ) ;
#154585=CARTESIAN_POINT ( 'NONE',  ( 0.6823417656249899377, 4.488541667008086655, -1.181850606188754593 ) ) ;
#154587=CARTESIAN_POINT ( 'NONE',  ( 3.714044015139744914, 6.420469553383295391, 1.199719254218462483 ) ) ;
#154601=CARTESIAN_POINT ( 'NONE',  ( -1.201851678989727383E-14, 2.759375000341417916, -1.575800808251660134 ) ) ;
#154603=CARTESIAN_POINT ( 'NONE',  ( 9.459838494033030898, 12.05956421450382088, 1.599625672291281386 ) ) ;
#154605=CARTESIAN_POINT ( 'NONE',  ( -4.772106882330223954, 8.511282429453158827, -0.7216878364870267237 ) ) ;
#154606=CARTESIAN_POINT ( 'NONE',  ( 3.931501358282940117, 4.649468341827285300, -1.082531754730543083 ) ) ;
#154607=CARTESIAN_POINT ( 'NONE',  ( -6.222829318548141586, 6.362315081168691044, 0.7216878364870317197 ) ) ;
#154609=ORIENTED_EDGE ( 'NONE', *, *, #166617, .T. ) ;
#154611=CARTESIAN_POINT ( 'NONE',  ( 6.484877546038077867, 6.460111979999551224, 1.040834085586084257E-14 ) ) ;
#154621=CARTESIAN_POINT ( 'NONE',  ( 4.808338034340912337, 8.761478140039733020, 1.040834085586084257E-14 ) ) ;
#154623=DIRECTION ( 'NONE',  ( 1.000000000000000000, 0.000000000000000000, 0.000000000000000000 ) ) ;
#154625=CARTESIAN_POINT ( 'NONE',  ( -7.400052914960538963, 7.527816577075747695, 1.040834085586084257E-14 ) ) ;
#154629=CARTESIAN_POINT ( 'NONE',  ( 8.111855979677986994, 8.358253485912799263, 1.040834085586084257E-14 ) ) ;
#154631=CARTESIAN_POINT ( 'NONE',  ( -6.738566041191992539, 7.820414121934134322, 1.199719254218450271 ) ) ;
#154632=CARTESIAN_POINT ( 'NONE',  ( 6.277061933002774374, 9.306694107603160404, 1.082531754730558626 ) ) ;
#154633=CARTESIAN_POINT ( 'NONE',  ( 4.291011075107065587, 7.468133931351726318, 1.062205608224401576 ) ) ;
#154634=CARTESIAN_POINT ( 'NONE',  ( -5.274285450916075035, 6.112086766612214284, 1.199719254218450271 ) ) ;
#154638=CARTESIAN_POINT ( 'NONE',  ( -7.088215381846223906, 7.164006121775713609, 0.7998128361456341429 ) ) ;
#154641=CARTESIAN_POINT ( 'NONE',  ( -1.402160292154681736E-14, 1.446875000341420137, -1.575800808251659024 ) ) ;
#154643=CARTESIAN_POINT ( 'NONE',  ( -6.900736999675794792, 7.153207375817628666, 1.040834085586084257E-14 ) ) ;
#154648=CARTESIAN_POINT ( 'NONE',  ( 5.738125327081736060, 7.717565519727259904, 1.599625672291267398 ) ) ;
#154650=CARTESIAN_POINT ( 'NONE',  ( -5.906232603126833958, 6.003624899985508634, 0.1331734367991978252 ) ) ;
#154651=CARTESIAN_POINT ( 'NONE',  ( 1.364683531249986537, 0.9260416670080896528, 0.7879004041258500513 ) ) ;
#154654=CARTESIAN_POINT ( 'NONE',  ( 4.053524740805938720, 3.831459740469437936, 1.214306433183764966E-14 ) ) ;
#154657=CARTESIAN_POINT ( 'NONE',  ( -5.271422797614987665, 5.044414773505913274, -0.7998128361456221525 ) ) ;
#154658=CARTESIAN_POINT ( 'NONE',  ( -7.497295758232724872, 9.769931022736756177, -1.443375672974058777 ) ) ;
#154666=CARTESIAN_POINT ( 'NONE',  ( -7.904040366642703930, 10.24446639921506552, 1.443375672974090751 ) ) ;
#154671=CARTESIAN_POINT ( 'NONE',  ( -6.656690234185426824, 10.70996300661758660, 0.7216878364870458196 ) ) ;
#154674=VERTEX_POINT ( 'NONE', #29876 ) ;
#154677=CARTESIAN_POINT ( 'NONE',  ( -0.7500000000000215383, 5.472916667349482900, 1.299038105676671107 ) ) ;
#154686=CARTESIAN_POINT ( 'NONE',  ( -5.208303565944065738, 9.228104593576741621, -0.7998128361456231517 ) ) ;
#154689=CARTESIAN_POINT ( 'NONE',  ( 4.857899112398166075, 4.561970474086296079, 1.040834085586084257E-14 ) ) ;
#154694=CARTESIAN_POINT ( 'NONE',  ( 5.900823170445728572, 7.907379670318584353, 1.599625672291267398 ) ) ;
#154699=CARTESIAN_POINT ( 'NONE',  ( -5.910991785878183080, 5.998504626387068051, -0.7216878364870278340 ) ) ;
#154702=ADVANCED_FACE ( 'NONE', ( #65531 ), #173435, .T. ) ;
#154711=CARTESIAN_POINT ( 'NONE',  ( -1.364683531250014514, 0.4885416670080875434, -0.7879004041258289570 ) ) ;
#154713=CARTESIAN_POINT ( 'NONE',  ( -8.864333505236459132, 9.236143932397675727, 1.040834085586084257E-14 ) ) ;
#154715=CARTESIAN_POINT ( 'NONE',  ( 7.259501185113382604, 10.55683625168592243, -1.199719254218441611 ) ) ;
#154717=CARTESIAN_POINT ( 'NONE',  ( -8.259941899223614215, 10.65968485389279508, -1.599625672291263179 ) ) ;
#154720=CARTESIAN_POINT ( 'NONE',  ( -0.6823417656250212460, 4.301041667008085767, 1.181850606188767472 ) ) ;
#154722=CARTESIAN_POINT ( 'NONE',  ( 7.944714827928033962, 12.21265836598400689, 0.7216878364870438212 ) ) ;
#154725=CARTESIAN_POINT ( 'NONE',  ( -1.364683531250000748, -1.178124999658580752, 0.000000000000000000 ) ) ;
#154728=CARTESIAN_POINT ( 'NONE',  ( 6.738039155867407537, 10.80487008191325771, -0.7216878364870267237 ) ) ;
#154731=CARTESIAN_POINT ( 'NONE',  ( -4.907688418466881863, 8.669460888279271416, 0.7216878364870458196 ) ) ;
#154733=CARTESIAN_POINT ( 'NONE',  ( -1.201851678989727383E-14, 2.946875000341419248, -1.575800808251660134 ) ) ;
#154737=CARTESIAN_POINT ( 'NONE',  ( -5.045605722580076780, 9.038290442985410067, -0.7998128361456231517 ) ) ;
#154738=CARTESIAN_POINT ( 'NONE',  ( 1.364683531249992088, 5.446875000341417916, 1.214306433183764966E-14 ) ) ;
#154744=CARTESIAN_POINT ( 'NONE',  ( 7.262363838414439776, 11.62450824479221900, 0.7998128361456462443 ) ) ;
#154747=CARTESIAN_POINT ( 'NONE',  ( -0.7500000000000006661, 2.608333333333358262, -1.299038105676652011 ) ) ;
#154752=VERTEX_POINT ( 'NONE', #38383 ) ;
#154753=CARTESIAN_POINT ( 'NONE',  ( 4.677199807034550183, 8.400557508274889784, 1.040834085586084257E-14 ) ) ;
#154754=CARTESIAN_POINT ( 'NONE',  ( 1.364683531249986537, -0.07395833299191513499, 0.7879004041258500513 ) ) ;
#154761=CARTESIAN_POINT ( 'NONE',  ( -1.500000000000001332, -1.099999999999976108, 0.000000000000000000 ) ) ;
#154762=CARTESIAN_POINT ( 'NONE',  ( 6.401421083946654100, 10.62007503124645957, -0.7998128361456291469 ) ) ;
#154763=CARTESIAN_POINT ( 'NONE',  ( -10.16591625214838679, 10.75465713712827487, 1.040834085586084257E-14 ) ) ;
#154765=CARTESIAN_POINT ( 'NONE',  ( 1.364683531249986537, 0.3635416670080869328, 0.7879004041258500513 ) ) ;
#154766=TOROIDAL_SURFACE ( 'NONE', #102813, 0.8299999999999998490, 0.08000000000000000167 ) ;
#154767=CARTESIAN_POINT ( 'NONE',  ( -1.201851678989727383E-14, 1.462500000000018119, 1.732050807568877637 ) ) ;
#154769=CARTESIAN_POINT ( 'NONE',  ( 4.299907273828439180, 8.168308919441841454, 1.040834085586084257E-14 ) ) ;
#154774=CARTESIAN_POINT ( 'NONE',  ( 1.499999999999990896, 5.306250000682820378, 1.214306433183764966E-14 ) ) ;
#154776=CARTESIAN_POINT ( 'NONE',  ( -1.364683531249997417, 5.509375000341417916, 1.214306433183764966E-14 ) ) ;
#154778=CARTESIAN_POINT ( 'NONE',  ( -9.169391961543940539, 9.592045464756413509, 1.040834085586084257E-14 ) ) ;
#154779=CARTESIAN_POINT ( 'NONE',  ( -4.555176424511596878, 7.297827681030051750, 1.082531754730560403 ) ) ;
#154787=CARTESIAN_POINT ( 'NONE',  ( 8.101160479365381306, 9.410107633136481908, -1.199719254218446718 ) ) ;
#154789=CARTESIAN_POINT ( 'NONE',  ( 8.080296363620359301, 8.529359967086321603, 1.040834085586084257E-14 ) ) ;
#154792=CARTESIAN_POINT ( 'NONE',  ( -7.751511138711140170, 10.06651563329490529, -1.599625672291263179 ) ) ;
#154793=CARTESIAN_POINT ( 'NONE',  ( 4.171104814498611368, 8.018039383557042044, 0.7998128361456321445 ) ) ;
#154794=B_SPLINE_CURVE_WITH_KNOTS ( 'NONE', 3,
 ( #171592, #6934, #5864, #73014, #4786, #40549 ),
 .UNSPECIFIED., .F., .F.,
 ( 4, 2, 4 ),
 ( 0.000000000000000000, 0.0003097885599249449199, 0.0006195771198498898399 ),
 .UNSPECIFIED. ) ;
#154796=CARTESIAN_POINT ( 'NONE',  ( 4.324687812634897988, 4.147816657603229373, 0.7216878364870317197 ) ) ;
#154797=CARTESIAN_POINT ( 'NONE',  ( 3.225950485047770933, 5.851027101609320269, 1.199719254218450271 ) ) ;
#154804=CARTESIAN_POINT ( 'NONE',  ( -4.772106882330227506, 7.550913215151819458, -1.082531754730549967 ) ) ;
#154805=CARTESIAN_POINT ( 'NONE',  ( 10.24960094225127172, 11.06021530882240356, -0.7216878364870257245 ) ) ;
#154808=CARTESIAN_POINT ( 'NONE',  ( -7.881367368245678406, 8.089350105908421185, 0.7998128361456602331 ) ) ;
#154809=CARTESIAN_POINT ( 'NONE',  ( -3.070003471035267939, 6.451017196056028524, -0.6895117023006979151 ) ) ;
#154814=CARTESIAN_POINT ( 'NONE',  ( -6.333630315878337136, 10.54098580183340772, 0.000000000000000000 ) ) ;
#154819=CARTESIAN_POINT ( 'NONE',  ( 4.286349120214771879, 8.152491073559232859, -0.7998128361456221525 ) ) ;
#154832=CARTESIAN_POINT ( 'NONE',  ( -7.366157530926372488, 7.488271962369228874, -0.7998128361456291469 ) ) ;
#154835=CARTESIAN_POINT ( 'NONE',  ( 5.178851490740193242, 8.025448591630130579, 1.082531754730558626 ) ) ;
#154836=VERTEX_POINT ( 'NONE', #102313 ) ;
#154839=CARTESIAN_POINT ( 'NONE',  ( -4.924636110261798372, 6.768494766770632332, 1.599625672291267398 ) ) ;
#154843=CARTESIAN_POINT ( 'NONE',  ( -6.205881626753225966, 8.263281202677319470, 1.599625672291283607 ) ) ;
#154850=CARTESIAN_POINT ( 'NONE',  ( -7.330154606482786050, 11.70359747420527619, 0.000000000000000000 ) ) ;
#154851=CARTESIAN_POINT ( 'NONE',  ( 7.070740804726770357, 8.207951346058097286, 1.199719254218462483 ) ) ;
#154853=CARTESIAN_POINT ( 'NONE',  ( -2.494337075234348777, 5.853884321174607663, -0.7216878364870267237 ) ) ;
#154854=CARTESIAN_POINT ( 'NONE',  ( -9.982881178363895103, 10.54111621771303753, 1.040834085586084257E-14 ) ) ;
#154862=CARTESIAN_POINT ( 'NONE',  ( 9.246297574839980271, 10.85006392781057905, 1.082531754730549967 ) ) ;
#154868=CARTESIAN_POINT ( 'NONE',  ( -5.718596324681298526, 6.117678329292076889, -0.7136201712047436363 ) ) ;
#154882=CARTESIAN_POINT ( 'NONE',  ( -3.972702704004144714, 4.593573561881607148, 1.199719254218462483 ) ) ;
#154889=B_SPLINE_CURVE_WITH_KNOTS ( 'NONE', 3,
 ( #968, #182942, #199170, #94536, #92410, #158449, #76125 ),
 .UNSPECIFIED., .F., .F.,
 ( 4, 3, 4 ),
 ( 4.755129718191212618E-15, 6.253302285471699906E-05, 0.0001620662963562105846 ),
 .UNSPECIFIED. ) ;
#154892=CARTESIAN_POINT ( 'NONE',  ( 0.6823417656249899377, 5.426041667008087543, -1.181850606188754593 ) ) ;
#154896=CARTESIAN_POINT ( 'NONE',  ( 2.854315967138055132, 6.433244981884085334, -0.2941531795266367211 ) ) ;
#154899=CARTESIAN_POINT ( 'NONE',  ( 4.241003122976366058, 3.842258486427521103, -0.7998128361456211532 ) ) ;
#154901=DIRECTION ( 'NONE',  ( 0.7592566023652994600, -0.6507913734559651608, -0.000000000000000000 ) ) ;
#154903=CARTESIAN_POINT ( 'NONE',  ( 8.717529583462638954, 12.15390636647303069, 1.082531754730546636 ) ) ;
#154906=CARTESIAN_POINT ( 'NONE',  ( 0.6823417656249899377, 2.655208333674753618, 1.181850606188767472 ) ) ;
#154907=DIRECTION ( 'NONE',  ( 0.000000000000000000, -1.000000000000000000, 0.000000000000000000 ) ) ;
#154909=CARTESIAN_POINT ( 'NONE',  ( -7.309817376062285099, 11.67987070538135264, 0.000000000000000000 ) ) ;
#154910=CARTESIAN_POINT ( 'NONE',  ( -4.406036734316890247, 7.123831375802920363, -1.082531754730548412 ) ) ;
#154912=CARTESIAN_POINT ( 'NONE',  ( -4.693093728624763372, 8.627026450037540428, 0.7998128361456481317 ) ) ;
#154914=CARTESIAN_POINT ( 'NONE',  ( -0.6823417656249969321, 5.717708333674756283, -1.181850606188749264 ) ) ;
#154922=CARTESIAN_POINT ( 'NONE',  ( -5.219525951136850139, 7.112532914458205013, -1.443375672974051449 ) ) ;
#154926=CARTESIAN_POINT ( 'NONE',  ( -5.056828107772866510, 5.962349549565537643, -1.082531754730543971 ) ) ;
#154928=CARTESIAN_POINT ( 'NONE',  ( 7.899597058256738968, 12.36794700127490820, 1.040834085586084257E-14 ) ) ;
#154938=CARTESIAN_POINT ( 'NONE',  ( -3.469997250093771246, 6.135748327496311383, -1.199719254218452935 ) ) ;
#154939=CARTESIAN_POINT ( 'NONE',  ( -10.30827686509187835, 10.92074451889568643, 1.040834085586084257E-14 ) ) ;
#154942=EDGE_LOOP ( 'NONE', ( #64741, #209768, #168348 ) ) ;
#154944=CARTESIAN_POINT ( 'NONE',  ( 5.035963992472171746, 7.962709526937818083, 1.199719254218462483 ) ) ;
#154949=CARTESIAN_POINT ( 'NONE',  ( 3.216308754939877446, 4.775446185561722956, -1.599625672291262513 ) ) ;
#154958=CARTESIAN_POINT ( 'NONE',  ( 6.760712154708803823, 11.03924794713562818, 1.040834085586084257E-14 ) ) ;
#154960=CARTESIAN_POINT ( 'NONE',  ( -5.274285450916075035, 6.112086766612214284, 1.199719254218450271 ) ) ;
#154966=CARTESIAN_POINT ( 'NONE',  ( -1.364683531250012516, 4.738541667008091096, -0.7879004041258300672 ) ) ;
#154968=CARTESIAN_POINT ( 'NONE',  ( -6.600121851754250812, 6.594563670001734046, 0.7998128361456341429 ) ) ;
#154971=CARTESIAN_POINT ( 'NONE',  ( 4.385172619016207918, 7.203452924572514959, 1.199719254218462483 ) ) ;
#154972=CARTESIAN_POINT ( 'NONE',  ( -5.220052836461385404, 6.048815383081766583, -1.199719254218446718 ) ) ;
#154978=CARTESIAN_POINT ( 'NONE',  ( 7.619319141200072920, 7.991553207595983643, 0.7216878364870317197 ) ) ;
#154981=CARTESIAN_POINT ( 'NONE',  ( 6.249945625775433555, 10.23542763013927726, -0.7216878364870267237 ) ) ;
#154982=CARTESIAN_POINT ( 'NONE',  ( -1.364683531249997417, 3.071875000341423245, 1.214306433183764966E-14 ) ) ;
#154984=CARTESIAN_POINT ( 'NONE',  ( 4.433153041544209749, 7.155467067568137551, -1.082531754730548412 ) ) ;
#154992=CARTESIAN_POINT ( 'NONE',  ( -4.331906098249381110, 7.414796467324478613, 1.153063172049747065 ) ) ;
#154993=DIRECTION ( 'NONE',  ( 0.000000000000000000, 8.546850786086437571E-32, 1.000000000000000000 ) ) ;
#154999=CARTESIAN_POINT ( 'NONE',  ( -8.143643823302737061, 12.65266822716189843, 0.000000000000000000 ) ) ;
#155004=CARTESIAN_POINT ( 'NONE',  ( -2.272963308585411735, 5.803540959991587478, 0.7998128361456341429 ) ) ;
#155009=CARTESIAN_POINT ( 'NONE',  ( 4.378920427533921078, 4.211088041652093494, 1.214306433183764966E-14 ) ) ;
#155010=CARTESIAN_POINT ( 'NONE',  ( 0.6823417656249917140, 3.405208333674754506, 1.181850606188765695 ) ) ;
#155012=CARTESIAN_POINT ( 'NONE',  ( 7.344766530301147789, 9.591980256816594164, 1.599625672291281386 ) ) ;
#155015=CARTESIAN_POINT ( 'NONE',  ( -5.576481253922474401, 5.400316305864649280, -0.7998128361456221525 ) ) ;
#155021=CARTESIAN_POINT ( 'NONE',  ( 1.499999999999990896, 3.775000000000021227, 1.214306433183764966E-14 ) ) ;
#155022=CARTESIAN_POINT ( 'NONE',  ( 3.825371897350130723, 7.614684313550482031, 0.7998128361456321445 ) ) ;
#155025=CARTESIAN_POINT ( 'NONE',  ( 0.9486429539237110076, 2.913339070649072493, 1.028101543438982413 ) ) ;
#155026=CARTESIAN_POINT ( 'NONE',  ( -1.201851678989727383E-14, 3.821875000341423689, 1.575800808251672791 ) ) ;
#155028=CARTESIAN_POINT ( 'NONE',  ( 7.782016984564043227, 12.02284421539267356, 0.7216878364870438212 ) ) ;
#155033=CARTESIAN_POINT ( 'NONE',  ( -1.500000000000013101, 1.410416667349486008, -0.8660254037844313801 ) ) ;
#155035=CARTESIAN_POINT ( 'NONE',  ( -4.717347382551060342, 7.590990148696470818, 1.199719254218464037 ) ) ;
#155036=CARTESIAN_POINT ( 'NONE',  ( 3.646780131951580461, 7.198401220678078971, -0.7216878364870267237 ) ) ;
#155043=ORIENTED_EDGE ( 'NONE', *, *, #1922, .T. ) ;
#155045=CARTESIAN_POINT ( 'NONE',  ( 8.145751363712157911, 8.397798100619326078, -0.7998128361456281477 ) ) ;
#155046=CARTESIAN_POINT ( 'NONE',  ( 3.974511587100456822, 7.788680618259193444, 1.040834085586084257E-14 ) ) ;
#155047=CARTESIAN_POINT ( 'NONE',  ( -5.000000000000024869, 3.300000000000025135, 0.7750000000000238920 ) ) ;
#155050=CARTESIAN_POINT ( 'NONE',  ( 5.900823170445728572, 7.907379670318584353, 1.599625672291267398 ) ) ;
#155051=DIRECTION ( 'NONE',  ( 5.578564026256490882E-16, 1.000000000000000000, 9.066213480720158442E-32 ) ) ;
#155056=ORIENTED_EDGE ( 'NONE', *, *, #45325, .F. ) ;
#155057=CARTESIAN_POINT ( 'NONE',  ( 10.56588178375152864, 11.22128359066528169, -0.7998128361456281477 ) ) ;
#155058=DIRECTION ( 'NONE',  ( 0.000000000000000000, 8.546850786086437571E-32, 1.000000000000000000 ) ) ;
#155062=CARTESIAN_POINT ( 'NONE',  ( 5.639205186016292615, 6.133955845365204773, 0.8069632701028349731 ) ) ;
#155071=CARTESIAN_POINT ( 'NONE',  ( 3.538314903486612817, 7.071858454135611538, 1.040834085586084257E-14 ) ) ;
#155072=CARTESIAN_POINT ( 'NONE',  ( 6.426201623197458801, 9.480690412830290015, -1.082531754730537088 ) ) ;
#155073=CARTESIAN_POINT ( 'NONE',  ( -4.090809663021341969, 5.795697244990093644, 1.599625672291267398 ) ) ;
#155079=CARTESIAN_POINT ( 'NONE',  ( -4.904298879841297421, 6.744767997946721216, 1.599625672291267398 ) ) ;
#155081=CARTESIAN_POINT ( 'NONE',  ( 1.420000000000001039, 7.176846818246214177, -4.202462424328213153 ) ) ;
#155094=CARTESIAN_POINT ( 'NONE',  ( 7.262363838414439776, 11.62450824479221900, 0.7998128361456462443 ) ) ;
#155098=CIRCLE ( 'NONE', #196675, 0.08000000000000012657 ) ;
#155103=DIRECTION ( 'NONE',  ( 0.000000000000000000, -0.7766560405359869135, 0.6299249119529750640 ) ) ;
#155104=CARTESIAN_POINT ( 'NONE',  ( -8.839552966430002101, 12.29626697993494666, -1.082531754730543971 ) ) ;
#155108=CARTESIAN_POINT ( 'NONE',  ( 8.158255747121103241, 10.54105100977322174, 1.599625672291281386 ) ) ;
#155113=CARTESIAN_POINT ( 'NONE',  ( -5.038826645773246682, 9.030381520044109322, 0.7998128361456481317 ) ) ;
#155114=CARTESIAN_POINT ( 'NONE',  ( 5.522248639467795428, 5.337044922334209573, -0.7998128361456231517 ) ) ;
#155122=CARTESIAN_POINT ( 'NONE',  ( -1.201851678989727383E-14, 2.634375000341417916, 1.575800808251672791 ) ) ;
#155124=CARTESIAN_POINT ( 'NONE',  ( 6.263503779833467178, 9.290876262238963790, -1.082531754730537088 ) ) ;
#155132=CARTESIAN_POINT ( 'NONE',  ( 7.904040366642678173, 12.16520482781775137, 0.7216878364870438212 ) ) ;
#155136=CARTESIAN_POINT ( 'NONE',  ( -9.854078719034067291, 10.39084668182823634, 0.7998128361456462443 ) ) ;
#155144=CARTESIAN_POINT ( 'NONE',  ( 4.813308228051395687, 5.574280006603454574, 1.199719254218462483 ) ) ;
#155150=CARTESIAN_POINT ( 'NONE',  ( 3.988069740714122791, 7.804498464141805592, 0.7998128361456321445 ) ) ;
#155154=CARTESIAN_POINT ( 'NONE',  ( 0.7499999999999885647, 2.597916667349486897, -1.299038105676658228 ) ) ;
#155158=VERTEX_POINT ( 'NONE', #155340 ) ;
#155159=CARTESIAN_POINT ( 'NONE',  ( 1.499999999999987121, 0.2541666666666844154, 0.8660254037844524744 ) ) ;
#155160=CARTESIAN_POINT ( 'NONE',  ( 6.265839547809997079, 10.46189657242035587, 0.7998128361456462443 ) ) ;
#155161=CARTESIAN_POINT ( 'NONE',  ( 1.364683531249988757, -0.1156249996585798079, 0.000000000000000000 ) ) ;
#155164=CARTESIAN_POINT ( 'NONE',  ( 9.246297574839974942, 11.81043314211192019, 1.443375672974076540 ) ) ;
#155170=CARTESIAN_POINT ( 'NONE',  ( -7.067878151425722955, 7.140279352951794500, 0.7998128361456341429 ) ) ;
#155171=CARTESIAN_POINT ( 'NONE',  ( -1.500000000000013101, 2.410416667349482456, -0.8660254037844313801 ) ) ;
#155172=CARTESIAN_POINT ( 'NONE',  ( -1.001543065824772872E-14, 4.884375000341420581, 1.575800808251672791 ) ) ;
#155177=CARTESIAN_POINT ( 'NONE',  ( -1.201851678989727383E-14, 3.759375000341422801, -1.575800808251660134 ) ) ;
#155186=CARTESIAN_POINT ( 'NONE',  ( -6.828502922777144768, 11.11833717654868892, 0.7998128361456481317 ) ) ;
#155187=CARTESIAN_POINT ( 'NONE',  ( 5.957918438201454059, 9.038323046955323292, -1.199719254218440723 ) ) ;
#155191=ORIENTED_EDGE ( 'NONE', *, *, #101780, .T. ) ;
#155195=CARTESIAN_POINT ( 'NONE',  ( -8.044065211609668253, 8.279164256499745633, 0.7998128361456602331 ) ) ;
#155200=CARTESIAN_POINT ( 'NONE',  ( 2.920892028740289081, 5.495125569250587816, 1.199719254218452047 ) ) ;
#155201=AXIS2_PLACEMENT_3D ( 'NONE', #21446, #1198, #120122 ) ;
#155203=CARTESIAN_POINT ( 'NONE',  ( -4.822949958159302497, 6.649860922651058992, -1.599625672291256295 ) ) ;
#155204=CARTESIAN_POINT ( 'NONE',  ( -7.862839020921525091, 11.26073039346208660, -1.199719254218446718 ) ) ;
#155207=CARTESIAN_POINT ( 'NONE',  ( -4.233332884224245696, 7.524468121203685023, -1.021403520103405294 ) ) ;
#155214=CARTESIAN_POINT ( 'NONE',  ( 5.469824908109481854, 8.468880595181346393, -1.199719254218446718 ) ) ;
#155233=CARTESIAN_POINT ( 'NONE',  ( 4.039966587192267866, 4.776011108888172707, 1.082531754730560403 ) ) ;
#155237=CARTESIAN_POINT ( 'NONE',  ( -7.947050595904583403, 12.42330946186405249, 0.7998128361456481317 ) ) ;
#155242=CARTESIAN_POINT ( 'NONE',  ( 1.499999999999987121, 1.327083334016149641, -0.8660254037844253849 ) ) ;
#155246=CIRCLE ( 'NONE', #210584, 0.07999999999999952982 ) ;
#155248=CARTESIAN_POINT ( 'NONE',  ( -7.994504133552415404, 12.47867192245318435, -0.7998128361456281477 ) ) ;
#155250=CARTESIAN_POINT ( 'NONE',  ( -0.6823417656250212460, 1.301041667008083547, 1.181850606188755259 ) ) ;
#155256=CARTESIAN_POINT ( 'NONE',  ( -2.930533758848195447, 6.570706485298192234, -0.7998128361456281477 ) ) ;
#155262=CARTESIAN_POINT ( 'NONE',  ( -1.364683531250014514, 0.5510416670080878765, -0.7879004041258289570 ) ) ;
#155267=CARTESIAN_POINT ( 'NONE',  ( 1.364683531249988757, -0.3656249996585800299, 0.000000000000000000 ) ) ;
#155269=CARTESIAN_POINT ( 'NONE',  ( -8.362681821530818738, 8.650883634741092010, -0.7998128361456291469 ) ) ;
#155270=CARTESIAN_POINT ( 'NONE',  ( 7.944187942603509356, 11.35563746875774882, 1.199719254218460707 ) ) ;
#155271=CARTESIAN_POINT ( 'NONE',  ( 3.669453130792974971, 7.432779085900453886, 1.040834085586084257E-14 ) ) ;
#155275=CARTESIAN_POINT ( 'NONE',  ( -1.402160292154681736E-14, 2.009375000341422801, -1.575800808251660134 ) ) ;
#155282=CARTESIAN_POINT ( 'NONE',  ( 6.697364695470787943, 7.876308901879812474, -1.082531754730543083 ) ) ;
#155285=CARTESIAN_POINT ( 'NONE',  ( -3.765413976293358278, 5.416068943807445635, 1.599625672291267398 ) ) ;
#155286=CARTESIAN_POINT ( 'NONE',  ( 4.702146809683721784, 5.356480858934594025, 2.500000000000011102 ) ) ;
#155289=CARTESIAN_POINT ( 'NONE',  ( 5.138177029454836564, 7.977995053463880382, 1.082531754730558626 ) ) ;
#155290=CARTESIAN_POINT ( 'NONE',  ( -7.171900071504738072, 10.35067193585544665, -1.082531754730543083 ) ) ;
#155292=CARTESIAN_POINT ( 'NONE',  ( -1.500000000000011324, 3.920833333333357817, 0.8660254037844403729 ) ) ;
#155296=CARTESIAN_POINT ( 'NONE',  ( 9.598809568795314107, 10.30095870645710754, -0.7216878364870257245 ) ) ;
#155309=CARTESIAN_POINT ( 'NONE',  ( 6.738039155867407537, 10.80487008191325771, -0.7216878364870267237 ) ) ;
#155310=CARTESIAN_POINT ( 'NONE',  ( 7.079328764629950754, 11.41096732537697633, 0.7998128361456462443 ) ) ;
#155311=CARTESIAN_POINT ( 'NONE',  ( -6.067437437315529536, 7.037430750744921859, 1.199719254218450271 ) ) ;
#155315=CARTESIAN_POINT ( 'NONE',  ( 1.364683531249984538, -1.032291666325247714, -0.7879004041258309554 ) ) ;
#155316=CARTESIAN_POINT ( 'NONE',  ( 3.823036129373602154, 6.443664003369091731, -1.082531754730548412 ) ) ;
#155318=CARTESIAN_POINT ( 'NONE',  ( -6.534666852106790103, 10.56760239419251590, 0.7216878364870458196 ) ) ;
#155340=CARTESIAN_POINT ( 'NONE',  ( 4.363950690066983107, 4.004001632660354915, -0.1812806842866887536 ) ) ;
#155346=CARTESIAN_POINT ( 'NONE',  ( -6.250472511100020334, 7.250971670160158311, 1.199719254218450271 ) ) ;
#155355=CARTESIAN_POINT ( 'NONE',  ( -3.521367211247373508, 5.131347717920458962, -1.599625672291256295 ) ) ;
#155358=CARTESIAN_POINT ( 'NONE',  ( 6.089583550832340819, 10.25626457594641749, 1.040834085586084257E-14 ) ) ;
#155361=CARTESIAN_POINT ( 'NONE',  ( 6.058883744127357751, 6.050764970021646150, 0.4299300578466564993 ) ) ;
#155366=CARTESIAN_POINT ( 'NONE',  ( 5.626270559546814098, 7.587068290936515247, 1.443375672974062551 ) ) ;
#155367=CARTESIAN_POINT ( 'NONE',  ( -8.193204901359996128, 8.453160561208463264, 1.040834085586084257E-14 ) ) ;
#155370=CARTESIAN_POINT ( 'NONE',  ( -8.453672473320708036, 9.821371626084353323, -1.199719254218446718 ) ) ;
#155371=CARTESIAN_POINT ( 'NONE',  ( -7.386494761346872551, 7.511998731193139989, -0.7998128361456291469 ) ) ;
#155379=CARTESIAN_POINT ( 'NONE',  ( 8.749089199520284410, 9.101692242395490240, 0.7998128361456481317 ) ) ;
#155380=DIRECTION ( 'NONE',  ( 5.578564026256490882E-16, 1.000000000000000000, 9.066213480720158442E-32 ) ) ;
#155390=CARTESIAN_POINT ( 'NONE',  ( -0.3190191529056556341, 8.208688096292659608, -1.977123213039569727 ) ) ;
#155395=CARTESIAN_POINT ( 'NONE',  ( 1.499999999999989120, 3.754166666666685082, 0.8660254037844524744 ) ) ;
#155396=CARTESIAN_POINT ( 'NONE',  ( 3.825371897350130723, 7.614684313550482031, 0.7998128361456321445 ) ) ;
#155397=CARTESIAN_POINT ( 'NONE',  ( 5.686755365928134687, 8.721966129303114101, 1.199719254218462483 ) ) ;
#155399=CARTESIAN_POINT ( 'NONE',  ( -8.026063749610056419, 10.38682701267698150, -1.443375672974059665 ) ) ;
#155401=CARTESIAN_POINT ( 'NONE',  ( 5.341549334104176872, 9.175631956522799726, 0.7216878364870438212 ) ) ;
#155402=CARTESIAN_POINT ( 'NONE',  ( -7.971831134711019118, 12.24429405723079967, 0.000000000000000000 ) ) ;
#155405=CARTESIAN_POINT ( 'NONE',  ( 9.088043039861931405, 9.497138389460751284, 1.040834085586084257E-14 ) ) ;
#155411=CARTESIAN_POINT ( 'NONE',  ( -1.201851678989727383E-14, 2.571875000341417472, 1.575800808251672791 ) ) ;
#155417=CARTESIAN_POINT ( 'NONE',  ( 8.585337585951586803, 11.03931315507545108, -1.599625672291255185 ) ) ;
#155421=CARTESIAN_POINT ( 'NONE',  ( -10.01677656239806247, 10.58066083241955901, 0.7998128361456462443 ) ) ;
#155427=CARTESIAN_POINT ( 'NONE',  ( 10.16199982864259788, 11.81442020729326536, 1.199719254218452047 ) ) ;
#155430=CARTESIAN_POINT ( 'NONE',  ( -9.989660255170729641, 10.54902514065433827, -0.7998128361456291469 ) ) ;
#155434=CARTESIAN_POINT ( 'NONE',  ( 8.503988664269582998, 10.94440607977979063, 1.599625672291281386 ) ) ;
#155436=CARTESIAN_POINT ( 'NONE',  ( 4.722716239034094876, 6.809985054512954328, 1.237095216770202954 ) ) ;
#155437=CARTESIAN_POINT ( 'NONE',  ( -1.007075241936694399, 2.800000000000025135, -0.9723682818829901819 ) ) ;
#155438=CARTESIAN_POINT ( 'NONE',  ( -5.264643720808155791, 5.036505850564608089, 0.000000000000000000 ) ) ;
#155442=CARTESIAN_POINT ( 'NONE',  ( 8.423693512792301163, 8.722063941212843119, 0.7998128361456481317 ) ) ;
#155444=CARTESIAN_POINT ( 'NONE',  ( 7.130698725783555680, 10.40656671580112658, 1.199719254218460707 ) ) ;
#155447=CARTESIAN_POINT ( 'NONE',  ( -9.219181267612684749, 10.81842823604534765, 1.082531754730558626 ) ) ;
#155456=CARTESIAN_POINT ( 'NONE',  ( -4.553630449417391368, 6.998240405024593436, -1.173447104293420473 ) ) ;
#155457=ADVANCED_FACE ( 'NONE', ( #181969 ), #33599, .T. ) ;
#155459=CARTESIAN_POINT ( 'NONE',  ( 5.477130870240836558, 9.333810415348903433, -0.7216878364870267237 ) ) ;
#155468=FACE_OUTER_BOUND ( 'NONE', #165715, .T. ) ;
#155477=CARTESIAN_POINT ( 'NONE',  ( -10.61567108937589765, 11.48729714713446803, 0.7216878364870438212 ) ) ;
#155481=CARTESIAN_POINT ( 'NONE',  ( 9.121938423896107651, 9.536683004167278099, -0.7998128361456221525 ) ) ;
#155483=ORIENTED_EDGE ( 'NONE', *, *, #114444, .F. ) ;
#155485=CARTESIAN_POINT ( 'NONE',  ( -1.500000000000001332, 1.181250000682816603, 0.000000000000000000 ) ) ;
#155486=CARTESIAN_POINT ( 'NONE',  ( -2.123823618835070537, 5.629544655282869847, 1.040834085586084257E-14 ) ) ;
#155487=CARTESIAN_POINT ( 'NONE',  ( -6.663996196316808174, 7.733415969579778171, -1.199719254218446718 ) ) ;
#155489=ORIENTED_EDGE ( 'NONE', *, *, #209460, .T. ) ;
#155490=CARTESIAN_POINT ( 'NONE',  ( -9.809487834687324437, 11.40315621434539395, 1.199719254218462483 ) ) ;
#155494=CARTESIAN_POINT ( 'NONE',  ( 1.499999999999989120, 5.327083334016152527, -0.8660254037844323793 ) ) ;
#155495=CARTESIAN_POINT ( 'NONE',  ( 7.775764792637399836, 9.030479331953833011, -1.199719254218441611 ) ) ;
#155499=CARTESIAN_POINT ( 'NONE',  ( -6.877010230629689858, 9.046264573866535486, 1.599625672291283607 ) ) ;
#155501=CARTESIAN_POINT ( 'NONE',  ( 1.364683531249988535, 4.363541667008090208, 0.7879004041258500513 ) ) ;
#155508=CARTESIAN_POINT ( 'NONE',  ( -7.199016379176422120, 11.34267684244042584, 0.000000000000000000 ) ) ;
#155510=EDGE_CURVE ( 'NONE', #60775, #128332, #9862, .T. ) ;
#155513=CARTESIAN_POINT ( 'NONE',  ( 1.364683531249988535, 3.676041667008087099, 0.7879004041258500513 ) ) ;
#155520=CARTESIAN_POINT ( 'NONE',  ( -1.201851678989727383E-14, 4.196875000341417028, -1.575800808251660134 ) ) ;
#155521=CARTESIAN_POINT ( 'NONE',  ( -5.220052836461385404, 6.048815383081766583, -1.199719254218446718 ) ) ;
#155522=CARTESIAN_POINT ( 'NONE',  ( 6.582647274634798151, 7.638508894284114170, 1.199719254218462483 ) ) ;
#155526=CARTESIAN_POINT ( 'NONE',  ( 4.487385655998888723, 4.337630808194552934, 0.7216878364870317197 ) ) ;
#155527=CARTESIAN_POINT ( 'NONE',  ( -1.364683531250010295, 5.801041667008088432, -0.7879004041258300672 ) ) ;
#155533=CARTESIAN_POINT ( 'NONE',  ( -1.402160292154681736E-14, 0.3218750003414227456, 1.575800808251672791 ) ) ;
#155534=CARTESIAN_POINT ( 'NONE',  ( -2.819732761962335577, 5.273143408055916304, -1.082531754730543971 ) ) ;
#155536=CARTESIAN_POINT ( 'NONE',  ( 5.660692828905515839, 6.562895374266609849, -1.199719254218445830 ) ) ;
#155542=CARTESIAN_POINT ( 'NONE',  ( 2.562127843302666186, 5.932973550587659517, 0.000000000000000000 ) ) ;
#155545=CARTESIAN_POINT ( 'NONE',  ( -9.164948653158003111, 9.794787638213568570, -0.7216878364870267237 ) ) ;
#155550=CARTESIAN_POINT ( 'NONE',  ( -8.435144125996554720, 12.99275191363802229, 0.7998128361456341429 ) ) ;
#155551=CARTESIAN_POINT ( 'NONE',  ( -4.378920427089552092, 8.052564898339037214, 0.7216878364870317197 ) ) ;
#155553=CARTESIAN_POINT ( 'NONE',  ( -1.402160292154681736E-14, 0.1343750003414218575, 1.575800808251672791 ) ) ;
#155567=ORIENTED_EDGE ( 'NONE', *, *, #151365, .F. ) ;
#155575=CARTESIAN_POINT ( 'NONE',  ( -0.6823417656250003738, 3.030208333674754062, -1.181850606188749264 ) ) ;
#155584=CARTESIAN_POINT ( 'NONE',  ( -1.402160292154681736E-14, 1.696875000341421469, -1.575800808251659024 ) ) ;
#155588=CARTESIAN_POINT ( 'NONE',  ( -0.3892891889261625438, 6.983571277091629170, -3.944761702788770474 ) ) ;
#155593=CARTESIAN_POINT ( 'NONE',  ( 5.355634372598031767, 6.206993841907870291, -1.199719254218445830 ) ) ;
#155601=CARTESIAN_POINT ( 'NONE',  ( 7.202405917357655341, 9.425892875049191488, 1.599625672291281386 ) ) ;
#155605=CARTESIAN_POINT ( 'NONE',  ( 7.096803341749390981, 10.36702210109460154, -1.199719254218441611 ) ) ;
#155616=CARTESIAN_POINT ( 'NONE',  ( -6.873620692448438874, 10.96304854125777695, 0.000000000000000000 ) ) ;
#155621=CARTESIAN_POINT ( 'NONE',  ( -9.820183334999905256, 10.35130206712171130, 1.040834085586084257E-14 ) ) ;
#155627=CARTESIAN_POINT ( 'NONE',  ( 9.317477881089539338, 11.89347683273640932, 1.599625672291279388 ) ) ;
#155629=CARTESIAN_POINT ( 'NONE',  ( 3.506755287428983792, 7.242964935309132990, 1.040834085586084257E-14 ) ) ;
#155636=CARTESIAN_POINT ( 'NONE',  ( -4.706651882238427120, 8.642844295920152575, 1.040834085586084257E-14 ) ) ;
#155639=CARTESIAN_POINT ( 'NONE',  ( -10.13488352141530768, 11.78278451552804817, 1.199719254218462483 ) ) ;
#155645=CARTESIAN_POINT ( 'NONE',  ( 7.944714827928039291, 11.25228915168265864, 1.082531754730557072 ) ) ;
#155646=ORIENTED_EDGE ( 'NONE', *, *, #113441, .F. ) ;
#155647=CARTESIAN_POINT ( 'NONE',  ( -1.364683531249997417, 4.321875000341417028, 1.214306433183764966E-14 ) ) ;
#155650=CARTESIAN_POINT ( 'NONE',  ( 4.123651276850781144, 7.962676922967908411, -0.7998128361456221525 ) ) ;
#155662=VERTEX_POINT ( 'NONE', #116175 ) ;
#155664=CARTESIAN_POINT ( 'NONE',  ( -1.201851678989727383E-14, 0.8843750003414173610, 1.575800808251672791 ) ) ;
#155665=DIRECTION ( 'NONE',  ( 0.6507913734559654939, -0.7592566023652992380, 0.000000000000000000 ) ) ;
#155666=CARTESIAN_POINT ( 'NONE',  ( 9.541187415715040032, 12.15447128979948310, -1.599625672291262513 ) ) ;
#155668=CARTESIAN_POINT ( 'NONE',  ( -6.724481002698138532, 6.947575379343695623, -0.7216878364870278340 ) ) ;
#155670=EDGE_CURVE ( 'NONE', #138555, #140464, #213584, .T. ) ;
#155671=CARTESIAN_POINT ( 'NONE',  ( 3.497640442645619796, 6.064035702186436616, -1.082531754730543083 ) ) ;
#155672=CARTESIAN_POINT ( 'NONE',  ( -5.043269954159181445, 8.827639346586952485, 1.214306433183764966E-14 ) ) ;
#155674=ORIENTED_EDGE ( 'NONE', *, *, #43285, .F. ) ;
#155676=CARTESIAN_POINT ( 'NONE',  ( 6.094553744542824170, 7.069066442510145265, 1.199719254218462483 ) ) ;
#155686=CARTESIAN_POINT ( 'NONE',  ( 4.482942347612929979, 8.381849838857084123, 1.040834085586084257E-14 ) ) ;
#155689=CARTESIAN_POINT ( 'NONE',  ( -6.470265622219711688, 8.571729197388226140, -1.599625672291263179 ) ) ;
#155694=CARTESIAN_POINT ( 'NONE',  ( 7.962716289927667113, 8.184257181204083409, -0.7998128361456291469 ) ) ;
#155696=CARTESIAN_POINT ( 'NONE',  ( -5.554036483092550824, 9.631459663583308739, -0.7998128361456231517 ) ) ;
#155698=CARTESIAN_POINT ( 'NONE',  ( 5.273758565591489145, 9.096542726591325234, -0.7216878364870267237 ) ) ;
#155699=CARTESIAN_POINT ( 'NONE',  ( 4.595133766160131472, 7.156059413716462814, 1.333087067838649720 ) ) ;
#155700=CARTESIAN_POINT ( 'NONE',  ( -5.545448523189368650, 6.428443684264421698, -1.199719254218446718 ) ) ;
#155704=CARTESIAN_POINT ( 'NONE',  ( -4.876128802409253282, 8.840567369452784874, 0.7998128361456481317 ) ) ;
#155709=CARTESIAN_POINT ( 'NONE',  ( -1.364683531250012516, 2.238541667008087988, -0.7879004041258289570 ) ) ;
#155711=CARTESIAN_POINT ( 'NONE',  ( -6.236387472606153892, 8.298871356172400127, -1.443375672974059665 ) ) ;
#155715=CARTESIAN_POINT ( 'NONE',  ( 6.144869935491714230, 8.192100896205568361, -1.599625672291262513 ) ) ;
#155717=CARTESIAN_POINT ( 'NONE',  ( -5.877243123607416742, 6.020912620514094371, 0.3151507616369741416 ) ) ;
#155718=CARTESIAN_POINT ( 'NONE',  ( -1.364683531250012516, 1.592708333674756727, 0.7879004041258379498 ) ) ;
#155721=CARTESIAN_POINT ( 'NONE',  ( 3.307826292054301121, 4.882216645528547616, -1.443375672974057666 ) ) ;
#155723=AXIS2_PLACEMENT_3D ( 'NONE', #30703, #127211, #94645 ) ;
#155725=CARTESIAN_POINT ( 'NONE',  ( -5.447678794592645701, 5.250046769979851646, 0.000000000000000000 ) ) ;
#155727=CARTESIAN_POINT ( 'NONE',  ( -7.605760987142072160, 10.85684300409898384, 1.082531754730549967 ) ) ;
#155735=CARTESIAN_POINT ( 'NONE',  ( -8.500599125644013654, 9.019713189447241319, 0.7216878364870438212 ) ) ;
#155737=DIRECTION ( 'NONE',  ( 0.7592566023653005702, 0.6507913734559639396, 0.000000000000000000 ) ) ;
#155741=CARTESIAN_POINT ( 'NONE',  ( -6.846504384776755714, 9.971043634672792422, -1.082531754730537088 ) ) ;
#155744=ORIENTED_EDGE ( 'NONE', *, *, #196345, .T. ) ;
#155747=CARTESIAN_POINT ( 'NONE',  ( -1.500000000000011324, 5.660416667349481123, -0.8660254037844313801 ) ) ;
#155748=CARTESIAN_POINT ( 'NONE',  ( 4.675513026854819287, 7.080785086760167601, -1.371149936167876282 ) ) ;
#155749=CARTESIAN_POINT ( 'NONE',  ( -1.500000000000001110, 5.160416667349487341, -0.8660254037844372643 ) ) ;
#155755=CARTESIAN_POINT ( 'NONE',  ( -5.520141099058386125, 9.591915048876776595, 0.000000000000000000 ) ) ;
#155758=CARTESIAN_POINT ( 'NONE',  ( 5.007038802148489509, 4.735966778795008381, 0.7998128361456341429 ) ) ;
#155763=CARTESIAN_POINT ( 'NONE',  ( 7.806797523370503811, 8.002351953554066810, 1.040834085586084257E-14 ) ) ;
#155768=CARTESIAN_POINT ( 'NONE',  ( -6.900736999675794792, 7.153207375817628666, 1.040834085586084257E-14 ) ) ;
#155771=LINE ( 'NONE', #124424, #126859 ) ;
#155775=CARTESIAN_POINT ( 'NONE',  ( -3.023105066167347310, 5.702484939155337607, 2.420000000000010587 ) ) ;
#155778=CARTESIAN_POINT ( 'NONE',  ( -1.402160292154681736E-14, 0.6968750003414164729, -1.575800808251659024 ) ) ;
#155780=CARTESIAN_POINT ( 'NONE',  ( -7.853197290813634268, 10.18514947741448573, 1.599625672291295375 ) ) ;
#155783=CARTESIAN_POINT ( 'NONE',  ( 7.853197290813620945, 10.18514947741448573, 1.599625672291281386 ) ) ;
#155785=CARTESIAN_POINT ( 'NONE',  ( -7.503547950159405566, 10.84155747757291266, 1.199719254218453823 ) ) ;
#155787=CARTESIAN_POINT ( 'NONE',  ( -0.6823417656249969321, 4.717708333674755394, -1.181850606188749264 ) ) ;
#155790=CARTESIAN_POINT ( 'NONE',  ( 8.839552966430002101, 11.33589776563360019, -1.443375672974052559 ) ) ;
#155793=CARTESIAN_POINT ( 'NONE',  ( 0.6823417656249882723, -1.094791666325249713, 1.181850606188755259 ) ) ;
#155796=CARTESIAN_POINT ( 'NONE',  ( 8.419250203962011625, 8.924806114151579095, -0.7216878364870267237 ) ) ;
#155799=CARTESIAN_POINT ( 'NONE',  ( -5.097502569058215194, 6.970172302033127210, -1.443375672974053447 ) ) ;
#155802=CARTESIAN_POINT ( 'NONE',  ( -1.364683531250000748, 1.509375000341421691, 0.000000000000000000 ) ) ;
#155806=CARTESIAN_POINT ( 'NONE',  ( -6.230135280679522936, 7.227244901336242755, 1.199719254218450271 ) ) ;
#155812=CARTESIAN_POINT ( 'NONE',  ( 6.988338112840064120, 10.24047933403371502, 1.199719254218460707 ) ) ;
#155815=CARTESIAN_POINT ( 'NONE',  ( -1.499999999999997780, 1.900000000000019673, 0.000000000000000000 ) ) ;
#155821=CARTESIAN_POINT ( 'NONE',  ( 6.155038550924133212, 10.12470270947942730, 0.7216878364870438212 ) ) ;
#155823=CARTESIAN_POINT ( 'NONE',  ( 3.999819011231439347, 4.625209253646830554, 1.199719254218464037 ) ) ;
#155829=CARTESIAN_POINT ( 'NONE',  ( 8.260995669428309540, 8.532249790621511565, 0.7998128361456481317 ) ) ;
#155830=CARTESIAN_POINT ( 'NONE',  ( -9.938290294017125603, 11.55342575023019691, -1.199719254218441611 ) ) ;
#155832=CARTESIAN_POINT ( 'NONE',  ( 3.469446951953614189E-15, 6.120000000000021423, 1.214306433183764966E-14 ) ) ;
#155833=CARTESIAN_POINT ( 'NONE',  ( 1.364683531249986537, -0.6364583329919177856, 0.7879004041258500513 ) ) ;
#155834=CARTESIAN_POINT ( 'NONE',  ( 1.499999999999987121, 1.545833333333354487, -0.8660254037844253849 ) ) ;
#155836=CARTESIAN_POINT ( 'NONE',  ( 6.145923705696426431, 6.064665832934283962, 0.7998128361456341429 ) ) ;
#155842=CARTESIAN_POINT ( 'NONE',  ( -1.364683531249997417, 4.509375000341424133, 1.214306433183764966E-14 ) ) ;
#155843=CARTESIAN_POINT ( 'NONE',  ( -7.323375529675950624, 11.69568855126397011, -0.7998128361456291469 ) ) ;
#155844=CARTESIAN_POINT ( 'NONE',  ( -4.446711195602239819, 8.131654128270509929, -0.7216878364870267237 ) ) ;
#155852=CARTESIAN_POINT ( 'NONE',  ( 6.103141704446003679, 10.27208242182903142, 0.7998128361456462443 ) ) ;
#155853=CARTESIAN_POINT ( 'NONE',  ( -3.904385050611244079, 7.498940292447679568, 1.040834085586084257E-14 ) ) ;
#155857=CARTESIAN_POINT ( 'NONE',  ( 6.439759776366758892, 10.45687747249582955, 0.7216878364870438212 ) ) ;
#155860=CARTESIAN_POINT ( 'NONE',  ( -9.182950115157607840, 9.607863310639020327, 0.7998128361456462443 ) ) ;
#155861=CARTESIAN_POINT ( 'NONE',  ( 6.114890974963323345, 7.092793211334054604, 1.199719254218462483 ) ) ;
#155864=CARTESIAN_POINT ( 'NONE',  ( 4.356247428692526569, 3.976710176429713250, 0.7998128361456341429 ) ) ;
#155866=CIRCLE ( 'NONE', #7095, 0.07999999999999972411 ) ;
#155872=CARTESIAN_POINT ( 'NONE',  ( -3.782361668532609134, 7.356579680022602652, 1.040834085586084257E-14 ) ) ;
#155873=CARTESIAN_POINT ( 'NONE',  ( 8.432808358020004391, 12.78210081775797669, 0.7216878364870438212 ) ) ;
#155876=CARTESIAN_POINT ( 'NONE',  ( -7.542413527904030524, 7.693903958843159252, 1.040834085586084257E-14 ) ) ;
#155881=CARTESIAN_POINT ( 'NONE',  ( -9.267161690140662600, 10.77044237904097734, -1.199719254218441611 ) ) ;
#155886=CARTESIAN_POINT ( 'NONE',  ( 5.066996723205273057, 6.934582148538044777, 1.599625672291267398 ) ) ;
#155898=CARTESIAN_POINT ( 'NONE',  ( -6.880926654135487652, 7.986501503701545879, 1.199719254218450271 ) ) ;
#155901=CARTESIAN_POINT ( 'NONE',  ( 6.643132081016125845, 6.852668304048034287, 0.7216878364870317197 ) ) ;
#155907=CARTESIAN_POINT ( 'NONE',  ( -6.423865854776591000, 6.388931673527803667, 1.040834085586084257E-14 ) ) ;
#155911=CARTESIAN_POINT ( 'NONE',  ( -7.393273838153706201, 7.519907654134449615, 0.7998128361456341429 ) ) ;
#155912=CARTESIAN_POINT ( 'NONE',  ( -5.824764126078942006, 6.052491103662449135, 0.4936746899740264150 ) ) ;
#155918=CARTESIAN_POINT ( 'NONE',  ( -1.500000000000005773, 5.629166666666694852, -0.8660254037844342667 ) ) ;
#155919=CARTESIAN_POINT ( 'NONE',  ( 7.623762449586013901, 7.788811034138823253, 1.040834085586084257E-14 ) ) ;
#155922=EDGE_CURVE ( 'NONE', #25107, #191425, #143378, .T. ) ;
#155930=CARTESIAN_POINT ( 'NONE',  ( 10.07334494527360569, 10.85458331234846696, 0.000000000000000000 ) ) ;
#155950=CARTESIAN_POINT ( 'NONE',  ( -5.108724954250998707, 4.854600622914589714, -0.7998128361456221525 ) ) ;
#155953=CARTESIAN_POINT ( 'NONE',  ( -2.598358995313378550, 6.183169261174235487, 0.7998128361456341429 ) ) ;
#155957=CARTESIAN_POINT ( 'NONE',  ( -1.500000000000015099, -0.5895833326505155458, -0.8660254037844383745 ) ) ;
#155960=FACE_OUTER_BOUND ( 'NONE', #208193, .T. ) ;
#155963=EDGE_LOOP ( 'NONE', ( #169113, #132324, #124663, #158871 ) ) ;
#155966=CARTESIAN_POINT ( 'NONE',  ( 10.16199982864259788, 11.81442020729326536, 1.199719254218452047 ) ) ;
#155972=CARTESIAN_POINT ( 'NONE',  ( -1.364683531250000748, 2.071875000341422357, 1.214306433183764966E-14 ) ) ;
#155974=CARTESIAN_POINT ( 'NONE',  ( -7.147119532698295252, 11.49005655479003174, 0.000000000000000000 ) ) ;
#155975=CARTESIAN_POINT ( 'NONE',  ( -4.555176424067209240, 8.258196894812975586, 1.040834085586084257E-14 ) ) ;
#155977=CARTESIAN_POINT ( 'NONE',  ( -6.392833124043511894, 7.417059051927569868, 1.199719254218450271 ) ) ;
#155979=CARTESIAN_POINT ( 'NONE',  ( -0.7500000000000249800, -1.277083332650516656, 1.299038105676659116 ) ) ;
#155987=CARTESIAN_POINT ( 'NONE',  ( -4.555176424067209240, 8.258196894812975586, 1.040834085586084257E-14 ) ) ;
#155988=DIRECTION ( 'NONE',  ( 0.7592566023653005702, -0.6507913734559639396, 0.000000000000000000 ) ) ;
#155993=CARTESIAN_POINT ( 'NONE',  ( -4.053524740361572398, 7.672936597156388316, 0.7216878364870317197 ) ) ;
#155995=CARTESIAN_POINT ( 'NONE',  ( 9.154780037725547714, 11.70366268214508487, 1.599625672291279388 ) ) ;
#156004=CARTESIAN_POINT ( 'NONE',  ( -2.591579918506545344, 6.175260338232929413, 1.040834085586084257E-14 ) ) ;
#156005=CARTESIAN_POINT ( 'NONE',  ( -10.45741655484220267, 11.09474082360439873, -0.7998128361456221525 ) ) ;
#156009=CARTESIAN_POINT ( 'NONE',  ( 7.104109303880752790, 11.23195192126214970, -0.7216878364870267237 ) ) ;
#156010=CARTESIAN_POINT ( 'NONE',  ( 6.169123589417988995, 7.156064594864501416, -1.199719254218445830 ) ) ;
#156016=CARTESIAN_POINT ( 'NONE',  ( 3.837121167867449945, 4.435395103055503441, 1.199719254218464037 ) ) ;
#156026=CARTESIAN_POINT ( 'NONE',  ( -5.599681137644054729, 6.491715067794862293, 1.199719254218450271 ) ) ;
#156030=CARTESIAN_POINT ( 'NONE',  ( 1.364683531249990311, 4.134375000341417028, 1.214306433183764966E-14 ) ) ;
#156032=CARTESIAN_POINT ( 'NONE',  ( -5.250031796989778066, 7.148123067953287446, 1.599625672291267398 ) ) ;
#156036=CARTESIAN_POINT ( 'NONE',  ( 5.355634372598031767, 6.206993841907870291, -1.199719254218445830 ) ) ;
#156037=CARTESIAN_POINT ( 'NONE',  ( -3.913499895838973508, 7.717500311787445000, 1.040834085586084257E-14 ) ) ;
#156044=CARTESIAN_POINT ( 'NONE',  ( 6.480434237652132445, 7.623223367758051872, 1.082531754730558626 ) ) ;
#156046=CARTESIAN_POINT ( 'NONE',  ( 6.846504384776753049, 9.010674420371453053, -1.443375672974058777 ) ) ;
#156047=CARTESIAN_POINT ( 'NONE',  ( 1.364683531249990311, 3.446875000341416584, 1.214306433183764966E-14 ) ) ;
#156049=CARTESIAN_POINT ( 'NONE',  ( 5.951666246274807115, 6.045958163516475636, 0.7216878364870317197 ) ) ;
#156053=B_SPLINE_CURVE_WITH_KNOTS ( 'NONE', 3,
 ( #161025, #132815, #212950, #46226 ),
 .UNSPECIFIED., .F., .F.,
 ( 4, 4 ),
 ( 0.000000000000000000, 0.0001591186035317672907 ),
 .UNSPECIFIED. ) ;
#156060=CARTESIAN_POINT ( 'NONE',  ( -5.139172151939493283, 6.684247474441955106, 1.432371535143169394 ) ) ;
#156069=CARTESIAN_POINT ( 'NONE',  ( -9.938290294017125603, 11.55342575023019691, -1.199719254218441611 ) ) ;
#156072=CARTESIAN_POINT ( 'NONE',  ( 2.184835310096557404, 5.700724961754617404, 1.040834085586084257E-14 ) ) ;
#156080=CARTESIAN_POINT ( 'NONE',  ( 2.873965376416980355, 6.296784005887697155, -0.7216878364870267237 ) ) ;
#156081=CARTESIAN_POINT ( 'NONE',  ( 0.6823417656249899377, 3.738541667008085767, -1.181850606188754593 ) ) ;
#156083=CARTESIAN_POINT ( 'NONE',  ( 6.889514614038635187, 11.18951748302043114, -0.7998128361456291469 ) ) ;
#156084=CARTESIAN_POINT ( 'NONE',  ( -8.967828540435322182, 12.54988483289483980, 1.199719254218462483 ) ) ;
#156089=( BOUNDED_CURVE ( )  B_SPLINE_CURVE ( 2, ( #6483, #72560, #138658, #204679, #189518, #122489, #53120 ),
 .UNSPECIFIED., .F., .T. ) 
 B_SPLINE_CURVE_WITH_KNOTS ( ( 3, 2, 2, 3 ),
 ( 0.1749999999999997669, 0.1791666666666665020, 0.1833333333333332371, 0.1874999999999999722 ),
 .UNSPECIFIED. ) 
 CURVE ( )  GEOMETRIC_REPRESENTATION_ITEM ( )  RATIONAL_B_SPLINE_CURVE ( ( 1.000000000000007105, 0.8660254037844316022, 1.000000000000000000, 0.8660254037844387076, 1.000000000000000000, 0.8660254037844395958, 0.9999999999999991118 ) ) 
 REPRESENTATION_ITEM ( '' )  );
#156092=CARTESIAN_POINT ( 'NONE',  ( -1.499999999999997780, 3.650000000000021227, 1.214306433183764966E-14 ) ) ;
#156093=CARTESIAN_POINT ( 'NONE',  ( 4.299907273828439180, 8.168308919441841454, 1.040834085586084257E-14 ) ) ;
#156096=CARTESIAN_POINT ( 'NONE',  ( 1.438721403194116233, 7.870009100115498590, 3.684356824108467876 ) ) ;
#156097=CARTESIAN_POINT ( 'NONE',  ( 0.6823417656249917140, 3.592708333674754506, 1.181850606188765695 ) ) ;
#156099=CARTESIAN_POINT ( 'NONE',  ( 8.703971430293332645, 12.13808852110884118, -1.082531754730543083 ) ) ;
#156105=CARTESIAN_POINT ( 'NONE',  ( 0.7499999999999902300, 1.514583334016148086, 1.299038105676657340 ) ) ;
#156108=CARTESIAN_POINT ( 'NONE',  ( -6.067437437315529536, 7.037430750744921859, 1.199719254218450271 ) ) ;
#156109=CARTESIAN_POINT ( 'NONE',  ( 5.300874872818840622, 6.247070775452521652, 1.082531754730560403 ) ) ;
#156119=CARTESIAN_POINT ( 'NONE',  ( 7.365103760721646076, 9.615707025640515937, 1.599625672291281386 ) ) ;
#156120=CARTESIAN_POINT ( 'NONE',  ( 5.684946482831785275, 5.526859072925533134, -0.7998128361456231517 ) ) ;
#156121=FACE_OUTER_BOUND ( 'NONE', #93662, .T. ) ;
#156123=( BOUNDED_SURFACE ( )  B_SPLINE_SURFACE ( 3, 2, ( 
 ( #9588, #11711, #10638 ),
 ( #128756, #95130, #29047 ),
 ( #161179, #12765, #79909 ),
 ( #125562, #78840, #77785 ),
 ( #91939, #142830, #141771 ),
 ( #143906, #209899, #61537 ),
 ( #207779, #93001, #59406 ),
 ( #146017, #62593, #208837 ) ),
 .UNSPECIFIED., .F., .F., .T. ) 
 B_SPLINE_SURFACE_WITH_KNOTS ( ( 4, 2, 2, 4 ),
 ( 3, 3 ),
 ( 0.000000000000000000, 0.003001918495469458117, 0.004502877743204187176, 0.006003836990938916235 ),
 ( 0.000000000000000000, 1.000000000000000000 ),
 .UNSPECIFIED. ) 
 GEOMETRIC_REPRESENTATION_ITEM ( )  RATIONAL_B_SPLINE_SURFACE ( (
 ( 1.000000000000000000, 0.7835651598521251593, 1.000000000000000000),
 ( 1.000000000000000000, 0.7913519369926046432, 1.000000000000000000),
 ( 1.000000000000000000, 0.8009496234817151672, 1.000000000000000000),
 ( 1.000000000000000000, 0.8230981486296959915, 1.000000000000000000),
 ( 1.000000000000000000, 0.8318333311016131715, 1.000000000000000000),
 ( 1.000000000000000000, 0.8529518727576285153, 1.000000000000000000),
 ( 1.000000000000000000, 0.8654984584225093869, 1.000000000000000000),
 ( 1.000000000000000000, 0.8789000212895426989, 1.000000000000000000) ) ) 
 REPRESENTATION_ITEM ( '' )  SURFACE ( )  );
#156125=CARTESIAN_POINT ( 'NONE',  ( 4.143988507271280319, 7.986403691791820414, -0.7998128361456221525 ) ) ;
#156132=CARTESIAN_POINT ( 'NONE',  ( 8.055515824813896941, 12.54985222892493368, 0.7998128361456462443 ) ) ;
#156137=CARTESIAN_POINT ( 'NONE',  ( 4.943270704524102221, 6.626842455454077907, 1.245637569283185586 ) ) ;
#156149=CARTESIAN_POINT ( 'NONE',  ( 7.470179451449751262, 7.817556902887268677, 1.040834085586084257E-14 ) ) ;
#156150=CARTESIAN_POINT ( 'NONE',  ( -4.765854690403601879, 5.518917546014321829, 1.199719254218462483 ) ) ;
#156154=CARTESIAN_POINT ( 'NONE',  ( -6.552668314106420588, 6.539201209412602189, -0.7998128361456291469 ) ) ;
#156168=CARTESIAN_POINT ( 'NONE',  ( 9.748476143425788720, 11.33197590787365172, -1.199719254218440723 ) ) ;
#156173=AXIS2_PLACEMENT_3D ( 'NONE', #90764, #205541, #56113 ) ;
#156178=CARTESIAN_POINT ( 'NONE',  ( -2.266184231778562541, 5.795632037050281404, 1.040834085586084257E-14 ) ) ;
#156182=CARTESIAN_POINT ( 'NONE',  ( 8.925345196497941558, 9.307324238869423283, 1.040834085586084257E-14 ) ) ;
#156187=CARTESIAN_POINT ( 'NONE',  ( -5.201524489137236529, 9.220195670635433771, 0.7998128361456481317 ) ) ;
#156188=CARTESIAN_POINT ( 'NONE',  ( 3.486418057008484617, 7.219238166485217434, 1.040834085586084257E-14 ) ) ;
#156191=CARTESIAN_POINT ( 'NONE',  ( 9.297140650669039275, 11.86975006391249643, 1.599625672291281386 ) ) ;
#156195=CARTESIAN_POINT ( 'NONE',  ( -1.364683531250012516, 2.842708333674754506, 0.7879004041258379498 ) ) ;
#156196=ORIENTED_EDGE ( 'NONE', *, *, #56646, .F. ) ;
#156198=CARTESIAN_POINT ( 'NONE',  ( 6.982085921357777281, 7.248114451113292667, 1.040834085586084257E-14 ) ) ;
#156206=CARTESIAN_POINT ( 'NONE',  ( 7.876924059415351564, 12.13356913605253240, -0.7216878364870267237 ) ) ;
#156212=CARTESIAN_POINT ( 'NONE',  ( -8.642432853707342488, 12.17025653171218558, 1.199719254218462483 ) ) ;
#156221=CARTESIAN_POINT ( 'NONE',  ( 3.734381245560244089, 6.444196322207211836, 1.199719254218462483 ) ) ;
#156227=CARTESIAN_POINT ( 'NONE',  ( 5.124091990960999432, 8.065525525174782828, -1.199719254218452047 ) ) ;
#156230=CARTESIAN_POINT ( 'NONE',  ( 1.499999999999989120, 3.035416667349485564, 0.8660254037844524744 ) ) ;
#156236=CARTESIAN_POINT ( 'NONE',  ( 1.499999999999987121, 0.5041666666666856367, 0.8660254037844524744 ) ) ;
#156237=CARTESIAN_POINT ( 'NONE',  ( 7.613066949273408213, 8.840665181362512115, -1.199719254218441611 ) ) ;
#156238=CARTESIAN_POINT ( 'NONE',  ( -1.364683531250014514, -0.01145833299191483488, -0.7879004041258359514 ) ) ;
#156241=CARTESIAN_POINT ( 'NONE',  ( 8.676855123066012254, 11.14608361504227574, -1.443375672974052559 ) ) ;
#156246=CARTESIAN_POINT ( 'NONE',  ( -4.557512192488103686, 8.468847991211438497, -0.7998128361456281477 ) ) ;
#156247=CARTESIAN_POINT ( 'NONE',  ( 0.7499999999999902300, 2.264583334016148530, 1.299038105676669330 ) ) ;
#156248=CARTESIAN_POINT ( 'NONE',  ( -1.201851678989727383E-14, 5.759375000341417028, -1.575800808251660801 ) ) ;
#156262=CARTESIAN_POINT ( 'NONE',  ( -10.15235809853472126, 10.73883929124566983, -0.7998128361456291469 ) ) ;
#156263=CARTESIAN_POINT ( 'NONE',  ( 5.608269097547198712, 9.694731047113750222, -0.7998128361456281477 ) ) ;
#156270=CARTESIAN_POINT ( 'NONE',  ( -5.682838942422375084, 9.781729199468104596, 0.000000000000000000 ) ) ;
#156274=CARTESIAN_POINT ( 'NONE',  ( 8.353795204314554468, 12.89784483834236184, -0.7998128361456352531 ) ) ;
#156277=CARTESIAN_POINT ( 'NONE',  ( -4.904298879841297421, 6.744767997946721216, 1.599625672291267398 ) ) ;
#156278=CARTESIAN_POINT ( 'NONE',  ( -9.494787648271923786, 9.971673765939062406, 1.040834085586084257E-14 ) ) ;
#156281=CARTESIAN_POINT ( 'NONE',  ( -4.597746731904842399, 7.146551969360384504, -1.363588915232381904 ) ) ;
#156288=CARTESIAN_POINT ( 'NONE',  ( 6.505214776458575265, 6.483838748823460563, 1.040834085586084257E-14 ) ) ;
#156290=CARTESIAN_POINT ( 'NONE',  ( 4.222669843016475966, 3.519858668466393947, 2.499999999999998668 ) ) ;
#156299=EDGE_CURVE ( 'NONE', #168810, #135502, #64035, .T. ) ;
#156307=CARTESIAN_POINT ( 'NONE',  ( 3.958617665510264949, 5.641473247893851628, -1.443375672974051449 ) ) ;
#156311=CARTESIAN_POINT ( 'NONE',  ( -8.622095623286845978, 12.14652976288826913, 1.199719254218462483 ) ) ;
#156317=CARTESIAN_POINT ( 'NONE',  ( -1.500000000000013101, 0.7020833340161545255, 0.8660254037844403729 ) ) ;
#156319=CARTESIAN_POINT ( 'NONE',  ( 2.535011536075336913, 5.133042487381361596, -7.499999999999997335 ) ) ;
#156323=CARTESIAN_POINT ( 'NONE',  ( -8.859363311525973117, 12.42334206583395328, -1.199719254218446718 ) ) ;
#156325=CARTESIAN_POINT ( 'NONE',  ( 0.6823417656249882723, 0.4260416670080896528, -1.181850606188749264 ) ) ;
#156331=CARTESIAN_POINT ( 'NONE',  ( -5.427341564172148303, 5.226320001155936090, 0.000000000000000000 ) ) ;
#156334=CARTESIAN_POINT ( 'NONE',  ( 1.499999999999987121, 0.004166666666691258049, 0.8660254037844524744 ) ) ;
#156336=CARTESIAN_POINT ( 'NONE',  ( 0.6823417656249864960, -0.7614583329919113464, -1.181850606188749264 ) ) ;
#156342=CARTESIAN_POINT ( 'NONE',  ( -1.402160292154681736E-14, -0.1781249996585796136, 1.575800808251672791 ) ) ;
#156344=CARTESIAN_POINT ( 'NONE',  ( -7.202405917357668663, 9.425892875049191488, 1.599625672291295375 ) ) ;
#156345=CARTESIAN_POINT ( 'NONE',  ( 7.716561984472250835, 12.15440608185967086, 1.040834085586084257E-14 ) ) ;
#156346=CARTESIAN_POINT ( 'NONE',  ( 4.761938266897790761, 6.578680616179307883, 1.599625672291267175 ) ) ;
#156347=EDGE_CURVE ( 'NONE', #33705, #82863, #191867, .T. ) ;
#156350=CARTESIAN_POINT ( 'NONE',  ( -1.402160292154681736E-14, -0.4906249996585810846, -1.575800808251665908 ) ) ;
#156357=CARTESIAN_POINT ( 'NONE',  ( 5.165293337126522388, 8.969999960048859577, 1.040834085586084257E-14 ) ) ;
#156360=CARTESIAN_POINT ( 'NONE',  ( -5.525111292768871252, 6.404716915440499037, -1.199719254218446718 ) ) ;
#156361=( BOUNDED_SURFACE ( )  B_SPLINE_SURFACE ( 1, 2, ( 
 ( #158908, #125416, #74456, #108087, #159972, #191382, #208699, #60326, #126487, #192450, #176233, #27835, #93931, #79779, #48376, #97130, #114488, #127567, #211902, #113427, #61404, #131779, #180485, #112357, #164237, #193536, #32104, #214008, #96064, #161041, #162116, #145891, #49420, #14767, #165293, #45178, #77647, #130742, #163182, #65631, #33163, #31054, #15825, #98189, #115540, #196735, #80858, #81910, #146948, #63539, #13706, #129694, #181535, #111291, #195677, #197782, #144833, #47313, #177296, #179433, #212963, #143769, #147998, #64601, #99244, #194596, #209763, #29978, #28910, #94995, #12636, #78707, #210841, #62467, #128629, #46240, #178370, #17949, #199909, #116602, #104574, #120892, #100292, #50482, #202017, #69892, #117681, #16887, #149042, #184720, #183673, #36344, #166359, #198836, #151189, #182596, #617, #20090, #168490, #102422, #169558, #38496, #4884, #137072, #84036, #136004, #82969, #34219, #66685, #21140, #53676, #186866, #86177, #87243, #152247, #1698, #132832, #67752, #119808, #101354, #54742, #3820, #85104, #150125, #19024, #185787, #37421, #103497, #133902, #2761, #52607, #51555, #70962, #153309, #35277, #203097, #167432, #68830, #134952, #200960, #118736, #14765, #50479, #147996, #113425, #163180, #112355, #132830, #78705, #198834, #194594, #15823, #179431, #130740, #80855, #97128, #63537, #98187, #149040, #146946, #62465, #165291, #34217, #16885, #615, #31052, #196733, #81908, #128627, #96061, #131777, #48374, #114486, #180483, #32102, #46238, #164235, #129692, #47311, #115538, #66683, #100290, #64599, #99242, #212961, #195675, #116600, #65628, #82967, #214006, #211900, #197780, #182594, #49418, #13704, #181533, #12634, #178368, #29976, #144831, #162114, #33161, #210839, #79777, #145889, #151188, #4882, #134951, #119807, #154382, #133900, #137071, #51553, #17947, #199907, #52606, #2760, #118735, #68829, #67750, #37420, #84034, #103496, #70961, #168489, #39558, #150123, #54741, #120891, #138142, #184719, #69890, #117678, #36343, #152246, #86176, #102421, #203096, #38495, #200958, #186865, #167431, #136003, #20088, #166357, #3819, #202016, #19023, #53675, #72030, #85103, #185786, #1696, #169557, #104573, #21139, #87242, #5959, #170618, #22205, #153307, #88318, #204151, #55807, #121961, #187928, #183671, #35274, #101352, #205236, #109971, #56877, #107833, #173858, #42792, #25434, #90461, #158654, #74206, #59011, #93673, #73105, #76328, #123053, #171687, #139206, #206319, #156527, #57943, #8118, #7029, #191126, #23284, #108901, #10252, #91540, #193278, #89396, #208442, #60076, #77392, #124108, #9194, #189004, #190071, #157599, #75265, #41723, #142434, #192193, #140300, #126232, #106750, #141379, #207390, #105659, #125167, #174924, #172777, #26504, #11314, #24351, #92611, #43857, #175982, #40647, #27575, #159716, #143508, #209505, #61145, #127307, #155444, #79531, #197532, #160786, #62221, #78459, #96878, #12379, #47055, #82719, #180238, #145649, #195425, #144577, #165042, #111031, #16635, #210591, #48128, #211645, #162928, #113171, #129442, #95809, #130499, #181285, #179175, #94740, #49177, #66439, #115294, #32912, #63280, #14509, #114240, #128378, #194346, #163995, #80600, #146696, #212712, #64353, #45987, #196486, #161865, #30799, #147744, #98989, #31862, #97937, #148796, #132581, #366, #44923, #112108, #15570, #177036, #178111, #28653, #29727, #81657, #13455, #213760, #65383, #131529, #183420, #33968, #35023, #169307, #68580, #21950, #3573, #52362, #83781, #201778, #53418, #202846, #102175, #153059, #85927, #117423, #168242, #5702, #101095, #71779, #100045, #200711, #19841, #198584, #50230, #119555, #118491, #20892, #69646, #86988, #166108, #184474, #152001, #182340, #38243, #4634, #18770, #70706, #17694, #136819, #120639, #2507, #67505, #84854, #185541, #116350, #149873, #1441, #133652, #199652, #37169, #135755, #186617, #154132, #103247, #54495, #104317, #88060, #170367, #51298, #167181, #150944, #36091, #134706, #156274, #27314, #171441, #123854, #59824, #204985, #7858, #23031, #189818, #25184, #203914, #208191, #140038, #26244, #40392, #175722, #90210, #92363, #73943, #91285 ),
 ( #190874, #24107, #137895, #55561, #157344, #206062, #8933, #72856, #105403, #57697, #89146, #121716, #141123, #41468, #187680, #39308, #75013, #107577, #207134, #138963, #155200, #173611, #6781, #56630, #58759, #124911, #42540, #76075, #159456, #125977, #43598, #122795, #108643, #188753, #106496, #11055, #142175, #174671, #93419, #158400, #191934, #9998, #172522, #109717, #61963, #47873, #161609, #115037, #96620, #145393, #176776, #80339, #146439, #81405, #195166, #31602, #178925, #210326, #46801, #98730, #128120, #164788, #193009, #79275, #112914, #77135, #143256, #212452, #211391, #113984, #162674, #179981, #127049, #63020, #30540, #60889, #131289, #97678, #111851, #163736, #44662, #15317, #213510, #95558, #160525, #177855, #64096, #209245, #110776, #28392, #94487, #12130, #130238, #14244, #65131, #32652, #196231, #147488, #197276, #181036, #48916, #78202, #144327, #194080, #129188, #13199, #45733, #29467, #49972, #2251, #152803, #83525, #100844, #116091, #68327, #118235, #82459, #86733, #18523, #119298, #133389, #54242, #183167, #185284, #34771, #184220, #101921, #166930, #102989, #69391, #200461, #199395, #17441, #51041, #182082, #104062, #120380, #99790, #33713, #201522, #135499, #84601, #1190, #53170, #117164, #35842, #4382, #198332, #36907, #165856, #148548, #149608, #150689, #67254, #134458, #52107, #132327, #167987, #114, #19592, #169047, #85665, #16380, #66181, #20644, #70454, #202590, #151751, #3322, #136569, #186355, #37990, #89959, #40129, #206874, #42275, #154944, #124660, #171183, #73683, #23852, #170109, #156010, #106239, #22773, #122536, #75819, #88890, #6528, #188497, #172265, #203658, #72605, #140860, #204722, #7598, #139781, #207939, #187428, #56373, #108389, #71528, #39057, #55308, #205808, #137639, #57439, #59561, #91026, #123600, #189565, #121457, #141927, #21696, #125721, #105143, #173341, #41210, #107317, #24921, #157087, #138705, #8676, #92098, #74758, #5449, #174413, #191681, #25990, #158152, #58505, #190617, #9745, #43342, #87807, #153880, #79010, #145126, #62756, #128916, #142995, #194897, #160269, #144069, #212195, #163477, #197027, #161348, #195979, #45470, #77948, #15059, #162417, #47612, #12929, #94231, #96363, #213264, #112656, #110524, #178665, #109462, #60629, #208993, #113726, #126792, #111587, #177597, #46535, #127872, #64891, #192747, #95299, #31349, #176524, #193822, #44404, #211132, #30277, #175469, #179730, #29209, #63833, #11871, #147236, #61704, #129991, #13994, #80078, #146180, #97423, #81151, #131038, #27055, #210064, #28135, #93162, #159199, #10800, #76874, #134987, #82204, #22243, #104609, #152283, #48664, #180778, #4918, #3856, #70995, #200997, #16121, #185824, #148298, #32404, #54779, #203137, #137108, #204187, #73137, #39593, #171723, #52642, #170656, #114780, #214295, #139242, #55843, #88353, #7064, #120926, #121999, #186899, #36383, #98470, #102461, #154418, #136041, #89430, #38531, #119846, #68867, #5996, #72067, #187965, #169594, #138177, #153348, #184756, #21176, #164535, #168527, #118772, #20125, #53713, #87279, #86211, #69929, #105696, #37455, #23322, #155481, #202053, #103534, #125197, #26536, #189043, #44955, #176015, #25468, #77426, #40680, #159747, #127339, #9226, #74238, #91576, #126268, #12411, #205273, #78491, #106783, #56913, #43888, #10284, #193309, #160819, #158686, #143543, #93707, #28685, #110002, #142465, #27607, #76358, #191160, #75298, #11345, #208473, #209537, #60109, #42827, #141413, #207420, #94771, #24383, #108933, #111063, #57977, #59039, #90496, #174954, #92644, #123086, #61179, #192225, #177069, #107867, #172811, #157628, #156559, #8154, #140331, #206350, #124140, #190102, #41755, #173893, #47085, #145679, #113203, #29757, #17724, #34001, #13485, #178143, #115328, #197564, #30833, #144608, #62249, #97970, #96909, #164029, #79560, #112139, #64381, #95842, #128410, #147775, #81691, #15604, #82753, #166137, #132611, #50265, #211677, #49208, #210623, #161898, #194377, #148826, #181319, #100075, #213791, #399, #65414, #129474, #46020, #195456, #32947, #14540, #182372, #131563, #212747, #63313, #99021, #165078, #66470, #48160, #16669 ) ),
 .UNSPECIFIED., .F., .F., .F. ) 
 B_SPLINE_SURFACE_WITH_KNOTS ( ( 2, 2 ),
 ( 3, 2, 2, 2, 2, 2, 2, 2, 2, 2, 2, 2, 2, 2, 2, 2, 2, 2, 2, 2, 2, 2, 2, 2, 2, 2, 2, 2, 2, 2, 2, 2, 2, 2, 2, 2, 2, 2, 2, 2, 2, 2, 2, 2, 2, 2, 2, 2, 2, 2, 2, 2, 2, 2, 2, 2, 2, 2, 2, 2, 2, 2, 2, 2, 2, 2, 2, 2, 2, 2, 2, 2, 2, 2, 2, 2, 2, 2, 2, 2, 2, 2, 2, 2, 2, 2, 2, 2, 2, 2, 2, 2, 2, 2, 2, 2, 2, 2, 2, 2, 2, 2, 2, 2, 2, 2, 2, 2, 2, 2, 2, 2, 2, 2, 2, 2, 2, 2, 2, 2, 2, 2, 2, 2, 2, 2, 2, 2, 2, 2, 2, 2, 2, 2, 2, 2, 2, 2, 2, 2, 2, 2, 2, 2, 2, 2, 2, 2, 2, 2, 2, 2, 2, 2, 2, 2, 2, 2, 2, 2, 2, 2, 2, 2, 2, 2, 2, 2, 2, 2, 2, 2, 2, 2, 2, 2, 2, 2, 2, 2, 2, 2, 2, 2, 2, 2, 2, 2, 2, 2, 2, 2, 2, 2, 2, 2, 2, 2, 2, 2, 2, 2, 2, 2, 2, 2, 2, 2, 2, 2, 2, 2, 2, 2, 2, 2, 2, 2, 2, 2, 2, 2, 2, 2, 2, 2, 2, 2, 2, 2, 2, 2, 2, 2, 2, 2, 2, 2, 2, 2, 3 ),
 ( 0.000000000000000000, 1.000000000000000000 ),
 ( 0.000000000000000000, 0.004166666666666666609, 0.008333333333333333218, 0.01250000000000000069, 0.01666666666666666644, 0.02083333333333333218, 0.02500000000000000139, 0.02916666666666666713, 0.03333333333333333287, 0.03749999999999999861, 0.04166666666666666435, 0.04583333333333333010, 0.05000000000000000278, 0.05416666666666666852, 0.05833333333333333426, 0.06250000000000000000, 0.06666666666666666574, 0.07083333333333333148, 0.07499999999999999722, 0.07916666666666666297, 0.08333333333333332871, 0.08749999999999999445, 0.09166666666666666019, 0.09583333333333333981, 0.1000000000000000056, 0.1041666666666666713, 0.1083333333333333370, 0.1125000000000000028, 0.1166666666666666685, 0.1208333333333333343, 0.1250000000000000000, 0.1291666666666666796, 0.1333333333333333315, 0.1375000000000000111, 0.1416666666666666630, 0.1458333333333333426, 0.1499999999999999944, 0.1541666666666666741, 0.1583333333333333259, 0.1625000000000000056, 0.1666666666666666574, 0.1708333333333333370, 0.1749999999999999889, 0.1791666666666666685, 0.1833333333333333204, 0.1875000000000000000, 0.1916666666666666796, 0.1958333333333333315, 0.2000000000000000111, 0.2041666666666666630, 0.2083333333333333426, 0.2124999999999999944, 0.2166666666666666741, 0.2208333333333333259, 0.2250000000000000056, 0.2291666666666666574, 0.2333333333333333370, 0.2374999999999999889, 0.2416666666666666685, 0.2458333333333333204, 0.2500000000000000000, 0.2541666666666666519, 0.2583333333333333592, 0.2625000000000000111, 0.2666666666666666630, 0.2708333333333333148, 0.2750000000000000222, 0.2791666666666666741, 0.2833333333333333259, 0.2874999999999999778, 0.2916666666666666852, 0.2958333333333333370, 0.2999999999999999889, 0.3041666666666666408, 0.3083333333333333481, 0.3125000000000000000, 0.3166666666666666519, 0.3208333333333333592, 0.3250000000000000111, 0.3291666666666666630, 0.3333333333333333148, 0.3375000000000000222, 0.3416666666666666741, 0.3458333333333333259, 0.3499999999999999778, 0.3541666666666666852, 0.3583333333333333370, 0.3624999999999999889, 0.3666666666666666408, 0.3708333333333333481, 0.3750000000000000000, 0.3791666666666666519, 0.3833333333333333592, 0.3875000000000000111, 0.3916666666666666630, 0.3958333333333333148, 0.4000000000000000222, 0.4041666666666666741, 0.4083333333333333259, 0.4124999999999999778, 0.4166666666666666852, 0.4208333333333333370, 0.4249999999999999889, 0.4291666666666666408, 0.4333333333333333481, 0.4375000000000000000, 0.4416666666666666519, 0.4458333333333333592, 0.4500000000000000111, 0.4541666666666666630, 0.4583333333333333148, 0.4625000000000000222, 0.4666666666666666741, 0.4708333333333333259, 0.4749999999999999778, 0.4791666666666666852, 0.4833333333333333370, 0.4874999999999999889, 0.4916666666666666408, 0.4958333333333333481, 0.5000000000000000000, 0.5041666666666666519, 0.5083333333333333037, 0.5124999999999999556, 0.5166666666666667185, 0.5208333333333333703, 0.5250000000000000222, 0.5291666666666666741, 0.5333333333333333259, 0.5374999999999999778, 0.5416666666666666297, 0.5458333333333332815, 0.5500000000000000444, 0.5541666666666666963, 0.5583333333333333481, 0.5625000000000000000, 0.5666666666666666519, 0.5708333333333333037, 0.5749999999999999556, 0.5791666666666667185, 0.5833333333333333703, 0.5875000000000000222, 0.5916666666666666741, 0.5958333333333333259, 0.5999999999999999778, 0.6041666666666666297, 0.6083333333333332815, 0.6125000000000000444, 0.6166666666666666963, 0.6208333333333333481, 0.6250000000000000000, 0.6291666666666666519, 0.6333333333333333037, 0.6374999999999999556, 0.6416666666666667185, 0.6458333333333333703, 0.6500000000000000222, 0.6541666666666666741, 0.6583333333333333259, 0.6624999999999999778, 0.6666666666666666297, 0.6708333333333332815, 0.6750000000000000444, 0.6791666666666666963, 0.6833333333333333481, 0.6875000000000000000, 0.6916666666666666519, 0.6958333333333333037, 0.6999999999999999556, 0.7041666666666667185, 0.7083333333333333703, 0.7125000000000000222, 0.7166666666666666741, 0.7208333333333333259, 0.7249999999999999778, 0.7291666666666666297, 0.7333333333333332815, 0.7375000000000000444, 0.7416666666666666963, 0.7458333333333333481, 0.7500000000000000000, 0.7541666666666666519, 0.7583333333333333037, 0.7624999999999999556, 0.7666666666666667185, 0.7708333333333333703, 0.7750000000000000222, 0.7791666666666666741, 0.7833333333333333259, 0.7874999999999999778, 0.7916666666666666297, 0.7958333333333332815, 0.8000000000000000444, 0.8041666666666666963, 0.8083333333333333481, 0.8125000000000000000, 0.8166666666666666519, 0.8208333333333333037, 0.8249999999999999556, 0.8291666666666667185, 0.8333333333333333703, 0.8375000000000000222, 0.8416666666666666741, 0.8458333333333333259, 0.8499999999999999778, 0.8541666666666666297, 0.8583333333333332815, 0.8625000000000000444, 0.8666666666666666963, 0.8708333333333333481, 0.8750000000000000000, 0.8791666666666666519, 0.8833333333333333037, 0.8874999999999999556, 0.8916666666666667185, 0.8958333333333333703, 0.9000000000000000222, 0.9041666666666666741, 0.9083333333333333259, 0.9124999999999999778, 0.9166666666666666297, 0.9208333333333332815, 0.9250000000000000444, 0.9291666666666666963, 0.9333333333333333481, 0.9375000000000000000, 0.9416666666666666519, 0.9458333333333333037, 0.9499999999999999556, 0.9541666666666667185, 0.9583333333333333703, 0.9625000000000000222, 0.9666666666666666741, 0.9708333333333333259, 0.9749999999999999778, 0.9791666666666666297, 0.9833333333333332815, 0.9875000000000000444, 0.9916666666666666963, 0.9958333333333333481, 1.000000000000000000 ),
 .UNSPECIFIED. ) 
 GEOMETRIC_REPRESENTATION_ITEM ( )  RATIONAL_B_SPLINE_SURFACE ( (
 ( 1.000000000000000000, 0.8660254037844387076, 1.000000000000000000, 0.8660254037844387076, 1.000000000000000000, 0.8660254037844387076, 1.000000000000000000, 0.8660254037844387076, 1.000000000000000000, 0.8660254037844387076, 1.000000000000000000, 0.8660254037844387076, 1.000000000000000000, 0.8660254037844387076, 1.000000000000000000, 0.8660254037844387076, 1.000000000000000000, 0.8660254037844387076, 1.000000000000000000, 0.8660254037844387076, 1.000000000000000000, 0.8660254037844387076, 1.000000000000000000, 0.8660254037844387076, 1.000000000000000000, 0.8660254037844387076, 1.000000000000000000, 0.8660254037844387076, 1.000000000000000000, 0.8660254037844387076, 1.000000000000000000, 0.8660254037844387076, 1.000000000000000000, 0.8660254037844387076, 1.000000000000000000, 0.8660254037844387076, 1.000000000000000000, 0.8660254037844387076, 1.000000000000000000, 0.8660254037844387076, 1.000000000000000000, 0.8660254037844387076, 1.000000000000000000, 0.8660254037844387076, 1.000000000000000000, 0.8660254037844387076, 1.000000000000000000, 0.8660254037844387076, 1.000000000000000000, 0.8660254037844387076, 1.000000000000000000, 0.8660254037844387076, 1.000000000000000000, 0.8660254037844387076, 1.000000000000000000, 0.8660254037844387076, 1.000000000000000000, 0.8660254037844387076, 1.000000000000000000, 0.8660254037844387076, 1.000000000000000000, 0.8660254037844387076, 1.000000000000000000, 0.8660254037844387076, 1.000000000000000000, 0.8660254037844387076, 1.000000000000000000, 0.8660254037844387076, 1.000000000000000000, 0.8660254037844387076, 1.000000000000000000, 0.8660254037844387076, 1.000000000000000000, 0.8660254037844387076, 1.000000000000000000, 0.8660254037844387076, 1.000000000000000000, 0.8660254037844387076, 1.000000000000000000, 0.8660254037844387076, 1.000000000000000000, 0.8660254037844387076, 1.000000000000000000, 0.8660254037844387076, 1.000000000000000000, 0.8660254037844387076, 1.000000000000000000, 0.8660254037844387076, 1.000000000000000000, 0.8660254037844387076, 1.000000000000000000, 0.8660254037844387076, 1.000000000000000000, 0.8660254037844387076, 1.000000000000000000, 0.8660254037844387076, 1.000000000000000000, 0.8660254037844387076, 1.000000000000000000, 0.8660254037844387076, 1.000000000000000000, 0.8660254037844387076, 1.000000000000000000, 0.8660254037844387076, 1.000000000000000000, 0.8660254037844387076, 1.000000000000000000, 0.8660254037844387076, 1.000000000000000000, 0.8660254037844387076, 1.000000000000000000, 0.8660254037844387076, 1.000000000000000000, 0.8660254037844387076, 1.000000000000000000, 0.8660254037844387076, 1.000000000000000000, 0.8660254037844387076, 1.000000000000000000, 0.8660254037844387076, 1.000000000000000000, 0.8660254037844387076, 1.000000000000000000, 0.8660254037844387076, 1.000000000000000000, 0.8660254037844387076, 1.000000000000000000, 0.8660254037844387076, 1.000000000000000000, 0.8660254037844387076, 1.000000000000000000, 0.8660254037844387076, 1.000000000000000000, 0.8660254037844387076, 1.000000000000000000, 0.8660254037844387076, 1.000000000000000000, 0.8660254037844387076, 1.000000000000000000, 0.8660254037844387076, 1.000000000000000000, 0.8660254037844387076, 1.000000000000000000, 0.8660254037844387076, 1.000000000000000000, 0.8660254037844387076, 1.000000000000000000, 0.8660254037844387076, 1.000000000000000000, 0.8660254037844387076, 1.000000000000000000, 0.8660254037844387076, 1.000000000000000000, 0.8660254037844387076, 1.000000000000000000, 0.8660254037844387076, 1.000000000000000000, 0.8660254037844387076, 1.000000000000000000, 0.8660254037844387076, 1.000000000000000000, 0.8660254037844387076, 1.000000000000000000, 0.8660254037844387076, 1.000000000000000000, 0.8660254037844387076, 1.000000000000000000, 0.8660254037844387076, 1.000000000000000000, 0.8660254037844387076, 1.000000000000000000, 0.8660254037844387076, 1.000000000000000000, 0.8660254037844387076, 1.000000000000000000, 0.8660254037844387076, 1.000000000000000000, 0.8660254037844387076, 1.000000000000000000, 0.8660254037844387076, 1.000000000000000000, 0.8660254037844387076, 1.000000000000000000, 0.8660254037844387076, 1.000000000000000000, 0.8660254037844387076, 1.000000000000000000, 0.8660254037844387076, 1.000000000000000000, 0.8660254037844387076, 1.000000000000000000, 0.8660254037844387076, 1.000000000000000000, 0.8660254037844387076, 1.000000000000000000, 0.8660254037844387076, 1.000000000000000000, 0.8660254037844387076, 1.000000000000000000, 0.8660254037844387076, 1.000000000000000000, 0.8660254037844387076, 1.000000000000000000, 0.8660254037844387076, 1.000000000000000000, 0.8660254037844387076, 1.000000000000000000, 0.8660254037844387076, 1.000000000000000000, 0.8660254037844387076, 1.000000000000000000, 0.8660254037844387076, 1.000000000000000000, 0.8660254037844387076, 1.000000000000000000, 0.8660254037844387076, 1.000000000000000000, 0.8660254037844387076, 1.000000000000000000, 0.8660254037844387076, 1.000000000000000000, 0.8660254037844387076, 1.000000000000000000, 0.8660254037844387076, 1.000000000000000000, 0.8660254037844387076, 1.000000000000000000, 0.8660254037844387076, 1.000000000000000000, 0.8660254037844387076, 1.000000000000000000, 0.8660254037844387076, 1.000000000000000000, 0.8660254037844387076, 1.000000000000000000, 0.8660254037844387076, 1.000000000000000000, 0.8660254037844387076, 1.000000000000000000, 0.8660254037844387076, 1.000000000000000000, 0.8660254037844387076, 1.000000000000000000, 0.8660254037844387076, 1.000000000000000000, 0.8660254037844387076, 1.000000000000000000, 0.8660254037844387076, 1.000000000000000000, 0.8660254037844387076, 1.000000000000000000, 0.8660254037844387076, 1.000000000000000000, 0.8660254037844387076, 1.000000000000000000, 0.8660254037844387076, 1.000000000000000000, 0.8660254037844387076, 1.000000000000000000, 0.8660254037844387076, 1.000000000000000000, 0.8660254037844387076, 1.000000000000000000, 0.8660254037844387076, 1.000000000000000000, 0.8660254037844387076, 1.000000000000000000, 0.8660254037844387076, 1.000000000000000000, 0.8660254037844387076, 1.000000000000000000, 0.8660254037844387076, 1.000000000000000000, 0.8660254037844387076, 1.000000000000000000, 0.8660254037844387076, 1.000000000000000000, 0.8660254037844387076, 1.000000000000000000, 0.8660254037844387076, 1.000000000000000000, 0.8660254037844387076, 1.000000000000000000, 0.8660254037844387076, 1.000000000000000000, 0.8660254037844387076, 1.000000000000000000, 0.8660254037844387076, 1.000000000000000000, 0.8660254037844387076, 1.000000000000000000, 0.8660254037844387076, 1.000000000000000000, 0.8660254037844387076, 1.000000000000000000, 0.8660254037844387076, 1.000000000000000000, 0.8660254037844387076, 1.000000000000000000, 0.8660254037844387076, 1.000000000000000000, 0.8660254037844387076, 1.000000000000000000, 0.8660254037844387076, 1.000000000000000000, 0.8660254037844387076, 1.000000000000000000, 0.8660254037844387076, 1.000000000000000000, 0.8660254037844387076, 1.000000000000000000, 0.8660254037844387076, 1.000000000000000000, 0.8660254037844387076, 1.000000000000000000, 0.8660254037844387076, 1.000000000000000000, 0.8660254037844387076, 1.000000000000000000, 0.8660254037844387076, 1.000000000000000000, 0.8660254037844387076, 1.000000000000000000, 0.8660254037844387076, 1.000000000000000000, 0.8660254037844387076, 1.000000000000000000, 0.8660254037844387076, 1.000000000000000000, 0.8660254037844387076, 1.000000000000000000, 0.8660254037844387076, 1.000000000000000000, 0.8660254037844387076, 1.000000000000000000, 0.8660254037844387076, 1.000000000000000000, 0.8660254037844387076, 1.000000000000000000, 0.8660254037844387076, 1.000000000000000000, 0.8660254037844387076, 1.000000000000000000, 0.8660254037844387076, 1.000000000000000000, 0.8660254037844387076, 1.000000000000000000, 0.8660254037844387076, 1.000000000000000000, 0.8660254037844387076, 1.000000000000000000, 0.8660254037844387076, 1.000000000000000000, 0.8660254037844387076, 1.000000000000000000, 0.8660254037844387076, 1.000000000000000000, 0.8660254037844387076, 1.000000000000000000, 0.8660254037844387076, 1.000000000000000000, 0.8660254037844387076, 1.000000000000000000, 0.8660254037844387076, 1.000000000000000000, 0.8660254037844387076, 1.000000000000000000, 0.8660254037844387076, 1.000000000000000000, 0.8660254037844387076, 1.000000000000000000, 0.8660254037844387076, 1.000000000000000000, 0.8660254037844387076, 1.000000000000000000, 0.8660254037844387076, 1.000000000000000000, 0.8660254037844387076, 1.000000000000000000, 0.8660254037844387076, 1.000000000000000000, 0.8660254037844387076, 1.000000000000000000, 0.8660254037844387076, 1.000000000000000000, 0.8660254037844387076, 1.000000000000000000, 0.8660254037844387076, 1.000000000000000000, 0.8660254037844387076, 1.000000000000000000, 0.8660254037844387076, 1.000000000000000000, 0.8660254037844387076, 1.000000000000000000, 0.8660254037844387076, 1.000000000000000000, 0.8660254037844387076, 1.000000000000000000, 0.8660254037844387076, 1.000000000000000000, 0.8660254037844387076, 1.000000000000000000, 0.8660254037844387076, 1.000000000000000000, 0.8660254037844387076, 1.000000000000000000, 0.8660254037844387076, 1.000000000000000000, 0.8660254037844387076, 1.000000000000000000, 0.8660254037844387076, 1.000000000000000000, 0.8660254037844387076, 1.000000000000000000, 0.8660254037844387076, 1.000000000000000000, 0.8660254037844387076, 1.000000000000000000, 0.8660254037844387076, 1.000000000000000000, 0.8660254037844387076, 1.000000000000000000, 0.8660254037844387076, 1.000000000000000000, 0.8660254037844387076, 1.000000000000000000, 0.8660254037844387076, 1.000000000000000000, 0.8660254037844387076, 1.000000000000000000, 0.8660254037844387076, 1.000000000000000000, 0.8660254037844387076, 1.000000000000000000, 0.8660254037844387076, 1.000000000000000000, 0.8660254037844387076, 1.000000000000000000, 0.8660254037844387076, 1.000000000000000000, 0.8660254037844387076, 1.000000000000000000, 0.8660254037844387076, 1.000000000000000000, 0.8660254037844387076, 1.000000000000000000, 0.8660254037844387076, 1.000000000000000000, 0.8660254037844387076, 1.000000000000000000, 0.8660254037844387076, 1.000000000000000000, 0.8660254037844387076, 1.000000000000000000, 0.8660254037844387076, 1.000000000000000000, 0.8660254037844387076, 1.000000000000000000, 0.8660254037844387076, 1.000000000000000000, 0.8660254037844387076, 1.000000000000000000, 0.8660254037844387076, 1.000000000000000000, 0.8660254037844387076, 1.000000000000000000, 0.8660254037844387076, 1.000000000000000000, 0.8660254037844387076, 1.000000000000000000, 0.8660254037844387076, 1.000000000000000000, 0.8660254037844387076, 1.000000000000000000, 0.8660254037844387076, 1.000000000000000000, 0.8660254037844387076, 1.000000000000000000, 0.8660254037844387076, 1.000000000000000000),
 ( 1.000000000000000000, 0.8660254037844387076, 1.000000000000000000, 0.8660254037844387076, 1.000000000000000000, 0.8660254037844387076, 1.000000000000000000, 0.8660254037844387076, 1.000000000000000000, 0.8660254037844387076, 1.000000000000000000, 0.8660254037844387076, 1.000000000000000000, 0.8660254037844387076, 1.000000000000000000, 0.8660254037844387076, 1.000000000000000000, 0.8660254037844387076, 1.000000000000000000, 0.8660254037844387076, 1.000000000000000000, 0.8660254037844387076, 1.000000000000000000, 0.8660254037844387076, 1.000000000000000000, 0.8660254037844387076, 1.000000000000000000, 0.8660254037844387076, 1.000000000000000000, 0.8660254037844387076, 1.000000000000000000, 0.8660254037844387076, 1.000000000000000000, 0.8660254037844387076, 1.000000000000000000, 0.8660254037844387076, 1.000000000000000000, 0.8660254037844387076, 1.000000000000000000, 0.8660254037844387076, 1.000000000000000000, 0.8660254037844387076, 1.000000000000000000, 0.8660254037844387076, 1.000000000000000000, 0.8660254037844387076, 1.000000000000000000, 0.8660254037844387076, 1.000000000000000000, 0.8660254037844387076, 1.000000000000000000, 0.8660254037844387076, 1.000000000000000000, 0.8660254037844387076, 1.000000000000000000, 0.8660254037844387076, 1.000000000000000000, 0.8660254037844387076, 1.000000000000000000, 0.8660254037844387076, 1.000000000000000000, 0.8660254037844387076, 1.000000000000000000, 0.8660254037844387076, 1.000000000000000000, 0.8660254037844387076, 1.000000000000000000, 0.8660254037844387076, 1.000000000000000000, 0.8660254037844387076, 1.000000000000000000, 0.8660254037844387076, 1.000000000000000000, 0.8660254037844387076, 1.000000000000000000, 0.8660254037844387076, 1.000000000000000000, 0.8660254037844387076, 1.000000000000000000, 0.8660254037844387076, 1.000000000000000000, 0.8660254037844387076, 1.000000000000000000, 0.8660254037844387076, 1.000000000000000000, 0.8660254037844387076, 1.000000000000000000, 0.8660254037844387076, 1.000000000000000000, 0.8660254037844387076, 1.000000000000000000, 0.8660254037844387076, 1.000000000000000000, 0.8660254037844387076, 1.000000000000000000, 0.8660254037844387076, 1.000000000000000000, 0.8660254037844387076, 1.000000000000000000, 0.8660254037844387076, 1.000000000000000000, 0.8660254037844387076, 1.000000000000000000, 0.8660254037844387076, 1.000000000000000000, 0.8660254037844387076, 1.000000000000000000, 0.8660254037844387076, 1.000000000000000000, 0.8660254037844387076, 1.000000000000000000, 0.8660254037844387076, 1.000000000000000000, 0.8660254037844387076, 1.000000000000000000, 0.8660254037844387076, 1.000000000000000000, 0.8660254037844387076, 1.000000000000000000, 0.8660254037844387076, 1.000000000000000000, 0.8660254037844387076, 1.000000000000000000, 0.8660254037844387076, 1.000000000000000000, 0.8660254037844387076, 1.000000000000000000, 0.8660254037844387076, 1.000000000000000000, 0.8660254037844387076, 1.000000000000000000, 0.8660254037844387076, 1.000000000000000000, 0.8660254037844387076, 1.000000000000000000, 0.8660254037844387076, 1.000000000000000000, 0.8660254037844387076, 1.000000000000000000, 0.8660254037844387076, 1.000000000000000000, 0.8660254037844387076, 1.000000000000000000, 0.8660254037844387076, 1.000000000000000000, 0.8660254037844387076, 1.000000000000000000, 0.8660254037844387076, 1.000000000000000000, 0.8660254037844387076, 1.000000000000000000, 0.8660254037844387076, 1.000000000000000000, 0.8660254037844387076, 1.000000000000000000, 0.8660254037844387076, 1.000000000000000000, 0.8660254037844387076, 1.000000000000000000, 0.8660254037844387076, 1.000000000000000000, 0.8660254037844387076, 1.000000000000000000, 0.8660254037844387076, 1.000000000000000000, 0.8660254037844387076, 1.000000000000000000, 0.8660254037844387076, 1.000000000000000000, 0.8660254037844387076, 1.000000000000000000, 0.8660254037844387076, 1.000000000000000000, 0.8660254037844387076, 1.000000000000000000, 0.8660254037844387076, 1.000000000000000000, 0.8660254037844387076, 1.000000000000000000, 0.8660254037844387076, 1.000000000000000000, 0.8660254037844387076, 1.000000000000000000, 0.8660254037844387076, 1.000000000000000000, 0.8660254037844387076, 1.000000000000000000, 0.8660254037844387076, 1.000000000000000000, 0.8660254037844387076, 1.000000000000000000, 0.8660254037844387076, 1.000000000000000000, 0.8660254037844387076, 1.000000000000000000, 0.8660254037844387076, 1.000000000000000000, 0.8660254037844387076, 1.000000000000000000, 0.8660254037844387076, 1.000000000000000000, 0.8660254037844387076, 1.000000000000000000, 0.8660254037844387076, 1.000000000000000000, 0.8660254037844387076, 1.000000000000000000, 0.8660254037844387076, 1.000000000000000000, 0.8660254037844387076, 1.000000000000000000, 0.8660254037844387076, 1.000000000000000000, 0.8660254037844387076, 1.000000000000000000, 0.8660254037844387076, 1.000000000000000000, 0.8660254037844387076, 1.000000000000000000, 0.8660254037844387076, 1.000000000000000000, 0.8660254037844387076, 1.000000000000000000, 0.8660254037844387076, 1.000000000000000000, 0.8660254037844387076, 1.000000000000000000, 0.8660254037844387076, 1.000000000000000000, 0.8660254037844387076, 1.000000000000000000, 0.8660254037844387076, 1.000000000000000000, 0.8660254037844387076, 1.000000000000000000, 0.8660254037844387076, 1.000000000000000000, 0.8660254037844387076, 1.000000000000000000, 0.8660254037844387076, 1.000000000000000000, 0.8660254037844387076, 1.000000000000000000, 0.8660254037844387076, 1.000000000000000000, 0.8660254037844387076, 1.000000000000000000, 0.8660254037844387076, 1.000000000000000000, 0.8660254037844387076, 1.000000000000000000, 0.8660254037844387076, 1.000000000000000000, 0.8660254037844387076, 1.000000000000000000, 0.8660254037844387076, 1.000000000000000000, 0.8660254037844387076, 1.000000000000000000, 0.8660254037844387076, 1.000000000000000000, 0.8660254037844387076, 1.000000000000000000, 0.8660254037844387076, 1.000000000000000000, 0.8660254037844387076, 1.000000000000000000, 0.8660254037844387076, 1.000000000000000000, 0.8660254037844387076, 1.000000000000000000, 0.8660254037844387076, 1.000000000000000000, 0.8660254037844387076, 1.000000000000000000, 0.8660254037844387076, 1.000000000000000000, 0.8660254037844387076, 1.000000000000000000, 0.8660254037844387076, 1.000000000000000000, 0.8660254037844387076, 1.000000000000000000, 0.8660254037844387076, 1.000000000000000000, 0.8660254037844387076, 1.000000000000000000, 0.8660254037844387076, 1.000000000000000000, 0.8660254037844387076, 1.000000000000000000, 0.8660254037844387076, 1.000000000000000000, 0.8660254037844387076, 1.000000000000000000, 0.8660254037844387076, 1.000000000000000000, 0.8660254037844387076, 1.000000000000000000, 0.8660254037844387076, 1.000000000000000000, 0.8660254037844387076, 1.000000000000000000, 0.8660254037844387076, 1.000000000000000000, 0.8660254037844387076, 1.000000000000000000, 0.8660254037844387076, 1.000000000000000000, 0.8660254037844387076, 1.000000000000000000, 0.8660254037844387076, 1.000000000000000000, 0.8660254037844387076, 1.000000000000000000, 0.8660254037844387076, 1.000000000000000000, 0.8660254037844387076, 1.000000000000000000, 0.8660254037844387076, 1.000000000000000000, 0.8660254037844387076, 1.000000000000000000, 0.8660254037844387076, 1.000000000000000000, 0.8660254037844387076, 1.000000000000000000, 0.8660254037844387076, 1.000000000000000000, 0.8660254037844387076, 1.000000000000000000, 0.8660254037844387076, 1.000000000000000000, 0.8660254037844387076, 1.000000000000000000, 0.8660254037844387076, 1.000000000000000000, 0.8660254037844387076, 1.000000000000000000, 0.8660254037844387076, 1.000000000000000000, 0.8660254037844387076, 1.000000000000000000, 0.8660254037844387076, 1.000000000000000000, 0.8660254037844387076, 1.000000000000000000, 0.8660254037844387076, 1.000000000000000000, 0.8660254037844387076, 1.000000000000000000, 0.8660254037844387076, 1.000000000000000000, 0.8660254037844387076, 1.000000000000000000, 0.8660254037844387076, 1.000000000000000000, 0.8660254037844387076, 1.000000000000000000, 0.8660254037844387076, 1.000000000000000000, 0.8660254037844387076, 1.000000000000000000, 0.8660254037844387076, 1.000000000000000000, 0.8660254037844387076, 1.000000000000000000, 0.8660254037844387076, 1.000000000000000000, 0.8660254037844387076, 1.000000000000000000, 0.8660254037844387076, 1.000000000000000000, 0.8660254037844387076, 1.000000000000000000, 0.8660254037844387076, 1.000000000000000000, 0.8660254037844387076, 1.000000000000000000, 0.8660254037844387076, 1.000000000000000000, 0.8660254037844387076, 1.000000000000000000, 0.8660254037844387076, 1.000000000000000000, 0.8660254037844387076, 1.000000000000000000, 0.8660254037844387076, 1.000000000000000000, 0.8660254037844387076, 1.000000000000000000, 0.8660254037844387076, 1.000000000000000000, 0.8660254037844387076, 1.000000000000000000, 0.8660254037844387076, 1.000000000000000000, 0.8660254037844387076, 1.000000000000000000, 0.8660254037844387076, 1.000000000000000000, 0.8660254037844387076, 1.000000000000000000, 0.8660254037844387076, 1.000000000000000000, 0.8660254037844387076, 1.000000000000000000, 0.8660254037844387076, 1.000000000000000000, 0.8660254037844387076, 1.000000000000000000, 0.8660254037844387076, 1.000000000000000000, 0.8660254037844387076, 1.000000000000000000, 0.8660254037844387076, 1.000000000000000000, 0.8660254037844387076, 1.000000000000000000, 0.8660254037844387076, 1.000000000000000000, 0.8660254037844387076, 1.000000000000000000, 0.8660254037844387076, 1.000000000000000000, 0.8660254037844387076, 1.000000000000000000, 0.8660254037844387076, 1.000000000000000000, 0.8660254037844387076, 1.000000000000000000, 0.8660254037844387076, 1.000000000000000000, 0.8660254037844387076, 1.000000000000000000, 0.8660254037844387076, 1.000000000000000000, 0.8660254037844387076, 1.000000000000000000, 0.8660254037844387076, 1.000000000000000000, 0.8660254037844387076, 1.000000000000000000, 0.8660254037844387076, 1.000000000000000000, 0.8660254037844387076, 1.000000000000000000, 0.8660254037844387076, 1.000000000000000000, 0.8660254037844387076, 1.000000000000000000, 0.8660254037844387076, 1.000000000000000000, 0.8660254037844387076, 1.000000000000000000, 0.8660254037844387076, 1.000000000000000000, 0.8660254037844387076, 1.000000000000000000, 0.8660254037844387076, 1.000000000000000000, 0.8660254037844387076, 1.000000000000000000, 0.8660254037844387076, 1.000000000000000000, 0.8660254037844387076, 1.000000000000000000, 0.8660254037844387076, 1.000000000000000000, 0.8660254037844387076, 1.000000000000000000, 0.8660254037844387076, 1.000000000000000000, 0.8660254037844387076, 1.000000000000000000, 0.8660254037844387076, 1.000000000000000000, 0.8660254037844387076, 1.000000000000000000, 0.8660254037844387076, 1.000000000000000000) ) ) 
 REPRESENTATION_ITEM ( '' )  SURFACE ( )  );
#156365=CARTESIAN_POINT ( 'NONE',  ( 4.975479186090847605, 7.788180902872553268, 1.082531754730558626 ) ) ;
#156366=CARTESIAN_POINT ( 'NONE',  ( -8.473482818416675499, 9.948446711983361723, -1.082531754730543083 ) ) ;
#156368=CARTESIAN_POINT ( 'NONE',  ( -0.7500000000000215383, 3.691666666666690411, 1.299038105676671107 ) ) ;
#156372=CARTESIAN_POINT ( 'NONE',  ( 8.270110514656021650, 11.63191745286530576, 1.082531754730557072 ) ) ;
#156386=CARTESIAN_POINT ( 'NONE',  ( 8.066738210006679566, 10.43428054980638997, 1.443375672974076540 ) ) ;
#156387=CARTESIAN_POINT ( 'NONE',  ( 6.564118927310645724, 10.80988918183778225, -0.7998128361456291469 ) ) ;
#156389=CARTESIAN_POINT ( 'NONE',  ( 3.226477370372323072, 6.708047998835549031, 0.7216878364870540352 ) ) ;
#156392=CARTESIAN_POINT ( 'NONE',  ( 4.039966587192259873, 5.736380323189513852, 1.443375672974062551 ) ) ;
#156393=ORIENTED_EDGE ( 'NONE', *, *, #141157, .T. ) ;
#156394=CARTESIAN_POINT ( 'NONE',  ( -6.832946231607472498, 9.955225789308602913, 1.082531754730549967 ) ) ;
#156398=CARTESIAN_POINT ( 'NONE',  ( -4.288456660624211381, 3.897620947016656956, 1.214306433183764966E-14 ) ) ;
#156403=ORIENTED_EDGE ( 'NONE', *, *, #17378, .F. ) ;
#156419=CARTESIAN_POINT ( 'NONE',  ( -1.387358672527334136, 7.251968950354660493, -4.302625267139479348 ) ) ;
#156423=CARTESIAN_POINT ( 'NONE',  ( -5.900823170445743671, 7.907379670318584353, 1.599625672291269396 ) ) ;
#156426=CARTESIAN_POINT ( 'NONE',  ( 5.015626762051672571, 7.938982758113895422, 1.199719254218462483 ) ) ;
#156427=DIRECTION ( 'NONE',  ( 1.000000000000000000, 0.000000000000000000, 0.000000000000000000 ) ) ;
#156437=CARTESIAN_POINT ( 'NONE',  ( -4.009460741339347045, 5.700790169694431420, -1.599625672291256295 ) ) ;
#156438=CONICAL_SURFACE ( 'NONE', #12060, 1.000000000000000000, 0.7853981633974508325 ) ;
#156441=CARTESIAN_POINT ( 'NONE',  ( 8.288111976655649471, 8.563885482386732306, -0.7998128361456291469 ) ) ;
#156442=CARTESIAN_POINT ( 'NONE',  ( 1.364683531249988535, 3.405208333674749621, -0.7879004041258239610 ) ) ;
#156444=CARTESIAN_POINT ( 'NONE',  ( 5.480859523967800406, 6.436073219340427976, 1.263442102793509880 ) ) ;
#156450=CARTESIAN_POINT ( 'NONE',  ( 5.436456408955479880, 9.286356877182658565, -0.7216878364870267237 ) ) ;
#156451=CARTESIAN_POINT ( 'NONE',  ( -8.345207244411405156, 9.694828859023472134, 1.199719254218462483 ) ) ;
#156454=CARTESIAN_POINT ( 'NONE',  ( -9.020252271793614440, 9.418049160047695878, 0.7998128361456462443 ) ) ;
#156455=CARTESIAN_POINT ( 'NONE',  ( -7.250913225210214641, 7.353820272367037170, 0.7998128361456341429 ) ) ;
#156456=CARTESIAN_POINT ( 'NONE',  ( -1.400751299551485696, 7.315968950354793776, -4.333496285525604286 ) ) ;
#156463=CARTESIAN_POINT ( 'NONE',  ( 8.046927864910717432, 9.346836249606042202, 1.199719254218462483 ) ) ;
#156478=CARTESIAN_POINT ( 'NONE',  ( -1.500000000000013101, 4.129166666666687746, -0.8660254037844313801 ) ) ;
#156479=CARTESIAN_POINT ( 'NONE',  ( 5.335297142177534369, 6.183267073083954735, -1.199719254218452047 ) ) ;
#156480=CARTESIAN_POINT ( 'NONE',  ( 7.630541526392844887, 7.796719957080126662, 0.7998128361456341429 ) ) ;
#156482=CARTESIAN_POINT ( 'NONE',  ( -9.503902493499651882, 10.19023378527882784, 1.040834085586084257E-14 ) ) ;
#156484=CARTESIAN_POINT ( 'NONE',  ( 6.860062538834778678, 8.066123052471139587, -1.082531754730543083 ) ) ;
#156485=CARTESIAN_POINT ( 'NONE',  ( -9.639484029191951464, 10.34841224358651601, 0.7216878364870438212 ) ) ;
#156488=CARTESIAN_POINT ( 'NONE',  ( 8.320953590485093088, 10.73086516036454618, 1.599625672291281386 ) ) ;
#156494=CARTESIAN_POINT ( 'NONE',  ( 1.364683531249988535, 2.613541667008089764, 0.7879004041258500513 ) ) ;
#156499=CARTESIAN_POINT ( 'NONE',  ( -1.364683531250014514, -0.4697916663252449943, 0.7879004041258379498 ) ) ;
#156501=CARTESIAN_POINT ( 'NONE',  ( 8.401248741962376698, 12.95320729893149370, 0.7998128361456462443 ) ) ;
#156505=CARTESIAN_POINT ( 'NONE',  ( -10.31505594189871111, 10.92865344183699428, -0.7998128361456291469 ) ) ;
#156511=CARTESIAN_POINT ( 'NONE',  ( 2.842405760359353106, 6.467890487061221272, -0.7998128361456291469 ) ) ;
#156514=CARTESIAN_POINT ( 'NONE',  ( -9.829825065107822724, 11.42688298316931572, 1.199719254218462483 ) ) ;
#156517=CARTESIAN_POINT ( 'NONE',  ( 8.585337585951586803, 11.03931315507545108, -1.599625672291255185 ) ) ;
#156519=CARTESIAN_POINT ( 'NONE',  ( 4.163006777067105091, 7.380761635867615134, 0.7803290320304544503 ) ) ;
#156521=CARTESIAN_POINT ( 'NONE',  ( -5.440899717785814715, 5.242137847038546461, 0.7998128361456341429 ) ) ;
#156525=CARTESIAN_POINT ( 'NONE',  ( 8.209625708274705502, 9.536650400197368427, 1.199719254218462483 ) ) ;
#156527=CARTESIAN_POINT ( 'NONE',  ( 8.098297826064319693, 8.342435640030188893, 0.7998128361456481317 ) ) ;
#156530=CARTESIAN_POINT ( 'NONE',  ( -7.212574532790087645, 11.35849468832304154, -0.7216878364870267237 ) ) ;
#156539=CARTESIAN_POINT ( 'NONE',  ( -5.320367241134011493, 6.379272830146158313, -1.120692317505559643 ) ) ;
#156540=CARTESIAN_POINT ( 'NONE',  ( 0.6823417656249899377, 2.092708333674753174, 1.181850606188767472 ) ) ;
#156542=CARTESIAN_POINT ( 'NONE',  ( 5.910991785878156435, 7.919243054989755670, -1.443375672974057666 ) ) ;
#156559=CARTESIAN_POINT ( 'NONE',  ( 9.921869487102386032, 10.46993591124128997, 0.000000000000000000 ) ) ;
#156564=CARTESIAN_POINT ( 'NONE',  ( -5.856232286098998152, 8.919689202835742847, 1.199719254218452047 ) ) ;
#156567=CARTESIAN_POINT ( 'NONE',  ( -8.136864746495904299, 12.64475930422059768, -0.7998128361456281477 ) ) ;
#156568=CARTESIAN_POINT ( 'NONE',  ( -1.419999999067559138, 7.203691543881443948, 4.238255391841873276 ) ) ;
#156572=CARTESIAN_POINT ( 'NONE',  ( 1.499999999999990896, 5.056250000682820378, 1.214306433183764966E-14 ) ) ;
#156573=CARTESIAN_POINT ( 'NONE',  ( 7.588813295347141441, 9.876701482703580837, -1.599625672291262513 ) ) ;
#156577=CARTESIAN_POINT ( 'NONE',  ( -6.191269702934848240, 10.37489842006599616, 0.000000000000000000 ) ) ;
#156579=CARTESIAN_POINT ( 'NONE',  ( -1.001543065824772872E-14, 5.321875000341422357, 1.575800808251672791 ) ) ;
#156584=CARTESIAN_POINT ( 'NONE',  ( -7.483737605063437215, 10.71448239167390604, 1.082531754730549967 ) ) ;
#156588=CARTESIAN_POINT ( 'NONE',  ( -1.364683531250012516, 3.551041667008086211, -0.7879004041258300672 ) ) ;
#156594=CARTESIAN_POINT ( 'NONE',  ( -1.364683531249997417, 4.259375000341424133, 1.214306433183764966E-14 ) ) ;
#156597=CARTESIAN_POINT ( 'NONE',  ( -5.436983294280064882, 6.301900917203534291, 1.199719254218450271 ) ) ;
#156598=CARTESIAN_POINT ( 'NONE',  ( 6.959412922516382771, 7.013736585890911535, 0.7998128361456341429 ) ) ;
#156602=CARTESIAN_POINT ( 'NONE',  ( 4.216222583725566686, 4.981643104843690217, -1.082531754730548412 ) ) ;
#156603=CARTESIAN_POINT ( 'NONE',  ( -1.364683531250012516, 4.051041667008088432, -0.7879004041258300672 ) ) ;
#156608=CARTESIAN_POINT ( 'NONE',  ( -1.364683531250000748, 1.259375000341421469, 0.000000000000000000 ) ) ;
#156609=CARTESIAN_POINT ( 'NONE',  ( -3.741687207691642314, 6.348756928073427730, 1.082531754730560403 ) ) ;
#156610=CARTESIAN_POINT ( 'NONE',  ( 5.311043488251262268, 7.219303374425030562, -1.599625672291256295 ) ) ;
#156614=CARTESIAN_POINT ( 'NONE',  ( 4.690757960648234359, 4.574898496952131133, 0.7216878364870317197 ) ) ;
#156617=CARTESIAN_POINT ( 'NONE',  ( -9.327646496521992958, 9.984601788804893019, -0.7216878364870267237 ) ) ;
#156622=CARTESIAN_POINT ( 'NONE',  ( -9.917953063596627317, 11.52969898140628047, -1.199719254218441611 ) ) ;
#156623=CARTESIAN_POINT ( 'NONE',  ( -5.382223794500843539, 7.302347065049529462, -1.443375672974051449 ) ) ;
#156625=CARTESIAN_POINT ( 'NONE',  ( -1.364683531250014514, 0.8010416670080889867, -0.7879004041258289570 ) ) ;
#156636=CARTESIAN_POINT ( 'NONE',  ( 9.395437264145964917, 10.06369101769952934, -0.7216878364870257245 ) ) ;
#156648=CARTESIAN_POINT ( 'NONE',  ( -3.946537740505278613, 2.817530495244580102, 0.7750000000000135669 ) ) ;
#156649=CARTESIAN_POINT ( 'NONE',  ( -1.364683531250012516, 1.342708333674755616, 0.7879004041258379498 ) ) ;
#156659=CARTESIAN_POINT ( 'NONE',  ( -1.364683531250014514, 1.238541667008091096, -0.7879004041258289570 ) ) ;
#156669=CARTESIAN_POINT ( 'NONE',  ( 5.840865249388943248, 5.708764300575555062, 0.7998128361456341429 ) ) ;
#156676=CARTESIAN_POINT ( 'NONE',  ( 6.500244582748090139, 9.671036882259738121, 1.199719254218460707 ) ) ;
#156679=VECTOR ( 'NONE', #69847, 1000.000000000000000 ) ;
#156680=CARTESIAN_POINT ( 'NONE',  ( 8.422639742587595180, 10.84949900448412130, -1.599625672291268286 ) ) ;
#156682=CIRCLE ( 'NONE', #52918, 0.7499999999999997780 ) ;
#156683=CARTESIAN_POINT ( 'NONE',  ( 1.499999999999990896, 8.627523663848661428, -2.579999999999989413 ) ) ;
#156684=CARTESIAN_POINT ( 'NONE',  ( -2.428612866367529932E-14, -1.099999999999976108, 2.499999999999998668 ) ) ;
#156686=ORIENTED_EDGE ( 'NONE', *, *, #140696, .F. ) ;
#156694=CARTESIAN_POINT ( 'NONE',  ( -7.049876689426097798, 11.16868053773170821, -0.7216878364870267237 ) ) ;
#156706=CARTESIAN_POINT ( 'NONE',  ( 3.755245360860917536, 5.404205559136275205, -1.443375672974051449 ) ) ;
#156708=CARTESIAN_POINT ( 'NONE',  ( 5.366329872910639232, 5.155139694684188534, 1.040834085586084257E-14 ) ) ;
#156710=EDGE_LOOP ( 'NONE', ( #148290, #129198, #70828, #57165 ) ) ;
#156715=CARTESIAN_POINT ( 'NONE',  ( -4.771579997005698459, 7.654261532226910525, -1.199719254218452047 ) ) ;
#156716=CARTESIAN_POINT ( 'NONE',  ( -3.945059511896602089, 7.546393830613923548, 1.040834085586084257E-14 ) ) ;
#156717=CARTESIAN_POINT ( 'NONE',  ( -4.647747731386360215, 4.316793862905830892, 0.7998128361456341429 ) ) ;
#156723=CARTESIAN_POINT ( 'NONE',  ( 8.595506201384008449, 11.05117653974661529, 1.443375672974076540 ) ) ;
#156725=CARTESIAN_POINT ( 'NONE',  ( 0.6823417656249917140, 4.655208333674755394, 1.181850606188765695 ) ) ;
#156728=CARTESIAN_POINT ( 'NONE',  ( 4.904298879841284098, 6.744767997946721216, 1.599625672291267398 ) ) ;
#156729=DIRECTION ( 'NONE',  ( -0.7592566023653017915, -0.6507913734559624963, 9.298211678181604981E-17 ) ) ;
#156738=CARTESIAN_POINT ( 'NONE',  ( -3.294268138440636928, 6.787137228248626641, 1.040834085586084257E-14 ) ) ;
#156739=EDGE_CURVE ( 'NONE', #93560, #3330, #14632, .T. ) ;
#156742=CARTESIAN_POINT ( 'NONE',  ( 0.6823417656249899377, 1.405208333674752508, 1.181850606188755259 ) ) ;
#156744=CARTESIAN_POINT ( 'NONE',  ( 3.408985558832261731, 6.064568021024562938, 1.199719254218462483 ) ) ;
#156746=CARTESIAN_POINT ( 'NONE',  ( -5.422898255786193111, 8.310169817517122581, -1.082531754730544860 ) ) ;
#156747=CARTESIAN_POINT ( 'NONE',  ( 4.378920427533921078, 4.211088041652093494, 1.214306433183764966E-14 ) ) ;
#156749=CARTESIAN_POINT ( 'NONE',  ( -7.348156068482412095, 7.675196289425353591, 1.040834085586084257E-14 ) ) ;
#156750=AXIS2_PLACEMENT_3D ( 'NONE', #166579, #18166, #5105 ) ;
#156754=CARTESIAN_POINT ( 'NONE',  ( 5.931855901178834323, 6.879252291918818152, 1.199719254218462483 ) ) ;
#156765=CARTESIAN_POINT ( 'NONE',  ( 7.091078035147269532, 8.231678114882006625, 1.199719254218462483 ) ) ;
#156769=CARTESIAN_POINT ( 'NONE',  ( -7.874588291438845644, 8.081441182967111558, -0.7998128361456291469 ) ) ;
#156773=CARTESIAN_POINT ( 'NONE',  ( 7.052212457402625922, 11.37933163361175382, -0.7998128361456291469 ) ) ;
#156776=CARTESIAN_POINT ( 'NONE',  ( -6.847031270101295419, 7.946956888995021728, -1.199719254218446718 ) ) ;
#156777=CARTESIAN_POINT ( 'NONE',  ( 8.419250203962011625, 8.924806114151579095, -0.7216878364870267237 ) ) ;
#156778=CARTESIAN_POINT ( 'NONE',  ( 4.002182886544830787, 7.824783036946191039, -0.1358892651178236766 ) ) ;
#156779=CIRCLE ( 'NONE', #4578, 0.8299999999999999600 ) ;
#156780=CARTESIAN_POINT ( 'NONE',  ( -3.425406365747000859, 7.148057860013469877, 1.040834085586084257E-14 ) ) ;
#156786=CARTESIAN_POINT ( 'NONE',  ( 9.915090410295563927, 10.46202698829998567, -0.7998128361456281477 ) ) ;
#156788=CARTESIAN_POINT ( 'NONE',  ( -1.364683531250012516, 0.5302083336747518416, 0.7879004041258379498 ) ) ;
#156790=CARTESIAN_POINT ( 'NONE',  ( -5.205967797967562483, 8.057084283395347768, 1.082531754730548412 ) ) ;
#156797=CARTESIAN_POINT ( 'NONE',  ( -1.364683531250014514, 1.551041667008084435, -0.7879004041258289570 ) ) ;
#156800=CARTESIAN_POINT ( 'NONE',  ( 2.575685996916329046, 5.948791396470269888, 0.7216878364870438212 ) ) ;
#156803=CARTESIAN_POINT ( 'NONE',  ( -4.273844736805832767, 6.009238164405336313, 1.599625672291267398 ) ) ;
#156805=CARTESIAN_POINT ( 'NONE',  ( -8.039621902779392926, 9.442275643739831636, 1.082531754730558626 ) ) ;
#156812=CARTESIAN_POINT ( 'NONE',  ( -8.961576348508655698, 9.557519949455999253, -0.7216878364870267237 ) ) ;
#156814=CYLINDRICAL_SURFACE ( 'NONE', #64616, 1.500000000000000222 ) ;
#156817=CARTESIAN_POINT ( 'NONE',  ( -7.822691444960709006, 10.14955932391940330, -1.443375672974058777 ) ) ;
#156825=CARTESIAN_POINT ( 'NONE',  ( 0.7499999999999902300, 5.097916667349482012, -1.299038105676658228 ) ) ;
#156828=ORIENTED_EDGE ( 'NONE', *, *, #164628, .F. ) ;
#156831=CARTESIAN_POINT ( 'NONE',  ( -6.344325816190970357, 9.489131654609717970, 1.199719254218452047 ) ) ;
#156834=CARTESIAN_POINT ( 'NONE',  ( 4.150767584078112193, 7.994312614733129152, 0.7998128361456321445 ) ) ;
#156836=CARTESIAN_POINT ( 'NONE',  ( 4.875577028304626914, 4.957510466404852600, 0.6186772747242745840 ) ) ;
#156838=CARTESIAN_POINT ( 'NONE',  ( 6.632963465583686435, 8.761543347979550589, -1.599625672291262513 ) ) ;
#156846=CARTESIAN_POINT ( 'NONE',  ( -4.284013352238250860, 7.941839977679187257, -0.7216878364870267237 ) ) ;
#156851=CARTESIAN_POINT ( 'NONE',  ( -0.2397550221597893050, 6.511191356812029873, 3.135202776928581514 ) ) ;
#156855=CARTESIAN_POINT ( 'NONE',  ( 0.6823417656249882723, 0.4260416670080896528, -1.181850606188749264 ) ) ;
#156857=CARTESIAN_POINT ( 'NONE',  ( -8.341290820905609138, 10.75459192918846618, 1.599625672291269396 ) ) ;
#156859=CARTESIAN_POINT ( 'NONE',  ( 7.904567251967224095, 9.180748867838630645, 1.199719254218462483 ) ) ;
#156861=CARTESIAN_POINT ( 'NONE',  ( -6.855619230004478482, 11.14997286831390788, -0.7998128361456291469 ) ) ;
#156864=CARTESIAN_POINT ( 'NONE',  ( -1.364683531250010295, 5.238541667008086655, -0.7879004041258300672 ) ) ;
#156865=CARTESIAN_POINT ( 'NONE',  ( 9.164948653157988900, 11.71552606681625619, -1.443375672974057666 ) ) ;
#156868=CARTESIAN_POINT ( 'NONE',  ( -0.6823417656250003738, -0.4697916663252491021, -1.181850606188749264 ) ) ;
#156871=CARTESIAN_POINT ( 'NONE',  ( 8.446366511189332016, 9.916811020218137429, -1.082531754730543083 ) ) ;
#156874=CARTESIAN_POINT ( 'NONE',  ( -4.717874267875590277, 7.487641831621378863, 1.082531754730560403 ) ) ;
#156876=CARTESIAN_POINT ( 'NONE',  ( -1.402160292154681736E-14, 1.696875000341421469, -1.575800808251659024 ) ) ;
#156880=CARTESIAN_POINT ( 'NONE',  ( -5.994676475536691029, 10.14553965476814845, 0.7998128361456481317 ) ) ;
#156881=CARTESIAN_POINT ( 'NONE',  ( 1.364683531249990311, 5.176041667008085767, 0.7879004041258500513 ) ) ;
#156886=CARTESIAN_POINT ( 'NONE',  ( 8.121497709785879593, 9.433834401960398353, -1.199719254218445830 ) ) ;
#156889=CARTESIAN_POINT ( 'NONE',  ( -0.7500000000000006661, 0.8583333333333567072, -1.299038105676652011 ) ) ;
#156895=CARTESIAN_POINT ( 'NONE',  ( 7.185458225562760148, 8.445751353653788485, -1.082531754730543083 ) ) ;
#156897=CARTESIAN_POINT ( 'NONE',  ( 8.398386088661320414, 11.88553530582519357, -1.199719254218446718 ) ) ;
#156904=CARTESIAN_POINT ( 'NONE',  ( 9.738834413317897898, 10.25639499182604730, 0.000000000000000000 ) ) ;
#156905=CARTESIAN_POINT ( 'NONE',  ( -10.50487009249003378, 11.15010328419353947, 0.7998128361456462443 ) ) ;
#156908=CARTESIAN_POINT ( 'NONE',  ( -4.911641409265215863, 4.703012472579248815, -0.3725085341543794559 ) ) ;
#156909=CARTESIAN_POINT ( 'NONE',  ( -1.402160292154681736E-14, 0.3218750003414227456, 1.575800808251672791 ) ) ;
#156910=CARTESIAN_POINT ( 'NONE',  ( 1.499999999999985123, 0.2958333333333566517, -0.8660254037844323793 ) ) ;
#156918=CARTESIAN_POINT ( 'NONE',  ( -1.364683531249997417, 4.759375000341424133, 1.214306433183764966E-14 ) ) ;
#156920=CARTESIAN_POINT ( 'NONE',  ( -7.212574532790110737, 7.517017831117667193, -0.7216878364870278340 ) ) ;
#156929=CARTESIAN_POINT ( 'NONE',  ( 8.402302512167096893, 10.82577223566020841, -1.599625672291268286 ) ) ;
#156930=CARTESIAN_POINT ( 'NONE',  ( -4.934804725694231564, 5.819988937140460727, -1.082531754730544860 ) ) ;
#156935=CARTESIAN_POINT ( 'NONE',  ( -9.484092147959342967, 11.02352791316275216, 1.199719254218462483 ) ) ;
#156936=CARTESIAN_POINT ( 'NONE',  ( 5.849453209292126310, 8.911780279894442103, 1.199719254218462483 ) ) ;
#156938=CARTESIAN_POINT ( 'NONE',  ( 3.023105065722954787, 5.510411095776657220, 1.082531754730546636 ) ) ;
#156939=CARTESIAN_POINT ( 'NONE',  ( 4.630273154266905777, 5.360739087188218122, 1.199719254218464037 ) ) ;
#156943=CARTESIAN_POINT ( 'NONE',  ( -3.997905685561188083, 7.705784594723285252, -0.04799061902135907248 ) ) ;
#156945=CARTESIAN_POINT ( 'NONE',  ( -5.341549334104202629, 7.254893527920112994, 1.443375672974064550 ) ) ;
#156946=CARTESIAN_POINT ( 'NONE',  ( 9.897088948295943212, 11.60932053017587506, 1.082531754730548412 ) ) ;
#156949=CARTESIAN_POINT ( 'NONE',  ( -5.856232286098998152, 8.919689202835742847, 1.199719254218452047 ) ) ;
#156954=CARTESIAN_POINT ( 'NONE',  ( -9.820183334999905256, 10.35130206712171130, 1.040834085586084257E-14 ) ) ;
#156960=CARTESIAN_POINT ( 'NONE',  ( 4.449046963578762615, 8.342305224150557308, -0.7998128361456231517 ) ) ;
#156961=( BOUNDED_CURVE ( )  B_SPLINE_CURVE ( 2, ( #177969, #29583, #95671, #13317, #129305, #195282, #46914 ),
 .UNSPECIFIED., .F., .T. ) 
 B_SPLINE_CURVE_WITH_KNOTS ( ( 3, 2, 2, 3 ),
 ( 0.3605655240965703334, 0.3630952380952380820, 0.3690476190476190688, 0.3715773330462868174 ),
 .UNSPECIFIED. ) 
 CURVE ( )  GEOMETRIC_REPRESENTATION_ITEM ( )  RATIONAL_B_SPLINE_CURVE ( ( 0.9345202395942613371, 0.9430618748659225226, 1.000000000000000000, 0.8660254037844387076, 1.000000000000000000, 0.9430618748659225226, 0.9345202395942613371 ) ) 
 REPRESENTATION_ITEM ( '' )  );
#156974=CARTESIAN_POINT ( 'NONE',  ( -8.342344591110322227, 8.627156865917170236, -0.7998128361456291469 ) ) ;
#156977=CARTESIAN_POINT ( 'NONE',  ( 5.829642864196162400, 7.824335979694092558, 1.443375672974062551 ) ) ;
#156978=ORIENTED_EDGE ( 'NONE', *, *, #132737, .F. ) ;
#156979=CARTESIAN_POINT ( 'NONE',  ( -1.485661138092309042, 7.335467742082953713, 4.255596723431145811 ) ) ;
#156981=CARTESIAN_POINT ( 'NONE',  ( 3.018661757337009810, 6.673522483535157868, 0.000000000000000000 ) ) ;
#156983=CARTESIAN_POINT ( 'NONE',  ( -4.574986769607567894, 7.424902766929059261, 1.199719254218464037 ) ) ;
#156988=CARTESIAN_POINT ( 'NONE',  ( -5.832844346354424836, 6.047612191973543716, -0.4696115756501819671 ) ) ;
#156993=CARTESIAN_POINT ( 'NONE',  ( -2.113655003624821838, 5.617681270870908072, 1.040834085586084257E-14 ) ) ;
#156994=CARTESIAN_POINT ( 'NONE',  ( -10.10098813738111545, 11.74323990082152491, -1.199719254218441611 ) ) ;
#156995=CARTESIAN_POINT ( 'NONE',  ( 6.414979237560321401, 10.63589287712906462, 1.040834085586084257E-14 ) ) ;
#156997=CARTESIAN_POINT ( 'NONE',  ( -2.155383234892699562, 5.458438174109348395, 1.040834085586084257E-14 ) ) ;
#156999=CARTESIAN_POINT ( 'NONE',  ( -4.791002085003811750, 6.784460936665063890, -1.245152473204954591 ) ) ;
#157004=VERTEX_POINT ( 'NONE', #144700 ) ;
#157006=CARTESIAN_POINT ( 'NONE',  ( 7.782016984564043227, 12.02284421539267356, 0.7216878364870438212 ) ) ;
#157014=ADVANCED_FACE ( 'NONE', ( #87108 ), #180362, .T. ) ;
#157026=CARTESIAN_POINT ( 'NONE',  ( -4.460796234096120472, 5.163016013655583158, 1.199719254218462483 ) ) ;
#157027=CARTESIAN_POINT ( 'NONE',  ( 1.499999999999989120, 3.254166666666690855, 0.8660254037844524744 ) ) ;
#157032=CARTESIAN_POINT ( 'NONE',  ( -1.364683531249997417, 5.009375000341425022, 1.214306433183764966E-14 ) ) ;
#157035=CARTESIAN_POINT ( 'NONE',  ( -3.687454593236990430, 4.364747115940301292, 1.082531754730560403 ) ) ;
#157037=PLANE ( 'NONE',  #140590 ) ;
#157041=CARTESIAN_POINT ( 'NONE',  ( 3.083589872104280705, 5.684939719841914929, 1.199719254218450271 ) ) ;
#157045=CARTESIAN_POINT ( 'NONE',  ( 9.856414487010587422, 11.56186699200962487, 1.082531754730548412 ) ) ;
#157047=CARTESIAN_POINT ( 'NONE',  ( 0.6823417656249899377, 0.6552083336747518416, 1.181850606188755259 ) ) ;
#157051=CARTESIAN_POINT ( 'NONE',  ( -7.483210719738908168, 10.81783070874899799, 1.199719254218453823 ) ) ;
#157052=CARTESIAN_POINT ( 'NONE',  ( -5.924549939047510705, 6.974691686052601369, 1.082531754730549967 ) ) ;
#157055=ORIENTED_EDGE ( 'NONE', *, *, #172864, .F. ) ;
#157056=CARTESIAN_POINT ( 'NONE',  ( -1.500000000000015099, -0.8395833326505166561, -0.8660254037844383745 ) ) ;
#157065=CARTESIAN_POINT ( 'NONE',  ( -6.033015167956810920, 7.101234453113482559, -1.082531754730543083 ) ) ;
#157070=CARTESIAN_POINT ( 'NONE',  ( -4.948362878863562742, 5.835806782504650236, 1.082531754730558626 ) ) ;
#157072=CARTESIAN_POINT ( 'NONE',  ( 10.72180055030867329, 11.40318881831530540, 0.7998128361456341429 ) ) ;
#157081=CARTESIAN_POINT ( 'NONE',  ( -5.101945877444165944, 4.846691699973280976, 0.000000000000000000 ) ) ;
#157082=CARTESIAN_POINT ( 'NONE',  ( -6.138157471807708987, 5.995865026538652387, 1.148737437293850421E-12 ) ) ;
#157086=CARTESIAN_POINT ( 'NONE',  ( 9.002250809793993724, 11.52571191622492464, -1.443375672974057666 ) ) ;
#157087=CARTESIAN_POINT ( 'NONE',  ( 5.632522751473472589, 8.658694745772667289, -1.199719254218440723 ) ) ;
#157091=DIRECTION ( 'NONE',  ( -0.6507913734559658270, -0.7592566023652989049, 0.000000000000000000 ) ) ;
#157092=CARTESIAN_POINT ( 'NONE',  ( 4.355193658487811703, 6.104145239700998538, -1.599625672291255185 ) ) ;
#157101=CARTESIAN_POINT ( 'NONE',  ( -6.521635583373313061, 7.567328587812373719, -1.199719254218446718 ) ) ;
#157109=CARTESIAN_POINT ( 'NONE',  ( -1.364683531250010295, 4.530208333674754506, 0.7879004041258379498 ) ) ;
#157110=CARTESIAN_POINT ( 'NONE',  ( 9.869972640624258275, 10.61731562359089587, 0.000000000000000000 ) ) ;
#157111=CARTESIAN_POINT ( 'NONE',  ( -6.250472511100020334, 7.250971670160158311, 1.199719254218450271 ) ) ;
#157114=CARTESIAN_POINT ( 'NONE',  ( 6.017121246366603060, 5.914396297049491658, 1.040834085586084257E-14 ) ) ;
#157115=CARTESIAN_POINT ( 'NONE',  ( -5.708146366553361162, 6.618257834855742594, -1.199719254218446718 ) ) ;
#157121=CARTESIAN_POINT ( 'NONE',  ( 5.938108093105483931, 8.911247961056314892, -1.082531754730537088 ) ) ;
#157123=CARTESIAN_POINT ( 'NONE',  ( 7.090551149822739596, 8.335026431957096804, 1.082531754730558626 ) ) ;
#157124=CARTESIAN_POINT ( 'NONE',  ( -1.364683531249997417, 2.821875000341422801, 1.214306433183764966E-14 ) ) ;
#157126=CARTESIAN_POINT ( 'NONE',  ( 4.311129659021211147, 7.973475668925984472, 1.040834085586084257E-14 ) ) ;
#157129=CARTESIAN_POINT ( 'NONE',  ( -4.134873662487946966, 3.926366815765101936, 1.214306433183764966E-14 ) ) ;
#157136=CARTESIAN_POINT ( 'NONE',  ( -3.990270464981529486, 7.829052896380438220, 0.2716399205876223744 ) ) ;
#157143=CARTESIAN_POINT ( 'NONE',  ( 4.659198344590585350, 8.587481835331020719, 0.7998128361456462443 ) ) ;
#157145=CARTESIAN_POINT ( 'NONE',  ( -4.256897044566581911, 4.068727428190179296, 1.214306433183764966E-14 ) ) ;
#157155=CARTESIAN_POINT ( 'NONE',  ( 5.680503174445848735, 5.729601246382692636, 1.040834085586084257E-14 ) ) ;
#157156=CARTESIAN_POINT ( 'NONE',  ( -1.364683531249997417, 3.321875000341423245, 1.214306433183764966E-14 ) ) ;
#157158=CARTESIAN_POINT ( 'NONE',  ( 7.751511138711133064, 10.06651563329490529, -1.599625672291262513 ) ) ;
#157159=EDGE_CURVE ( 'NONE', #116525, #138593, #169901, .T. ) ;
#157160=CARTESIAN_POINT ( 'NONE',  ( -9.829825065107822724, 11.42688298316931572, 1.199719254218462483 ) ) ;
#157166=CARTESIAN_POINT ( 'NONE',  ( -1.201851678989727383E-14, 2.837500000000024780, -1.732050807568863648 ) ) ;
#157167=CARTESIAN_POINT ( 'NONE',  ( 5.986088515633498197, 6.942523675449257858, -1.199719254218446718 ) ) ;
#157170=CARTESIAN_POINT ( 'NONE',  ( -1.201851678989727383E-14, 4.446875000341417916, -1.575800808251660134 ) ) ;
#157171=CARTESIAN_POINT ( 'NONE',  ( 8.432808358020004391, 12.78210081775797669, 0.7216878364870438212 ) ) ;
#157176=CARTESIAN_POINT ( 'NONE',  ( -1.499999999999997780, 1.931250000682817269, 0.000000000000000000 ) ) ;
#157178=CARTESIAN_POINT ( 'NONE',  ( -4.381256195510448315, 8.263215994737505454, 1.040834085586084257E-14 ) ) ;
#157186=CARTESIAN_POINT ( 'NONE',  ( 5.636439174979242850, 7.598931675607687453, -1.599625672291262513 ) ) ;
#157190=CARTESIAN_POINT ( 'NONE',  ( 6.667912619822566000, 6.673652899414787676, 1.040834085586084257E-14 ) ) ;
#157193=ORIENTED_EDGE ( 'NONE', *, *, #64923, .F. ) ;
#157196=CARTESIAN_POINT ( 'NONE',  ( 8.353795204314554468, 12.89784483834236184, -0.7998128361456352531 ) ) ;
#157200=DIRECTION ( 'NONE',  ( -0.7592566023653004592, -0.6507913734559641616, 0.000000000000000000 ) ) ;
#157201=CARTESIAN_POINT ( 'NONE',  ( 5.892130686423356245, 5.977214202646935703, -0.03562020706840245132 ) ) ;
#157212=CARTESIAN_POINT ( 'NONE',  ( -4.161449568064929494, 3.976298073660712529, 0.4629614534431922834 ) ) ;
#157214=CARTESIAN_POINT ( 'NONE',  ( 6.317736394288131052, 9.354147645769410602, 1.082531754730558626 ) ) ;
#157216=CARTESIAN_POINT ( 'NONE',  ( -3.952365473583647315, 4.569846793057691592, 1.199719254218462483 ) ) ;
#157220=CARTESIAN_POINT ( 'NONE',  ( -6.742482464697739708, 6.760651051769146491, 0.7998128361456341429 ) ) ;
#157231=CARTESIAN_POINT ( 'NONE',  ( -4.650083499807250220, 5.295740330745369207, -7.499999999999997335 ) ) ;
#157241=CARTESIAN_POINT ( 'NONE',  ( 4.207107738942202246, 3.802713871720993399, 1.214306433183764966E-14 ) ) ;
#157244=CARTESIAN_POINT ( 'NONE',  ( -2.279742385392243165, 5.811449882932888222, -0.7998128361456281477 ) ) ;
#157247=CARTESIAN_POINT ( 'NONE',  ( 8.483651433849084711, 10.92067931095586886, 1.599625672291281386 ) ) ;
#157251=CARTESIAN_POINT ( 'NONE',  ( -6.877010230629689858, 9.046264573866535486, 1.599625672291283607 ) ) ;
#157252=CARTESIAN_POINT ( 'NONE',  ( 5.345992642490140057, 5.131412925860272090, 1.040834085586084257E-14 ) ) ;
#157256=CARTESIAN_POINT ( 'NONE',  ( -2.155383234892699562, 5.458438174109348395, 1.040834085586084257E-14 ) ) ;
#157259=CARTESIAN_POINT ( 'NONE',  ( -1.201851678989727383E-14, 2.384375000341416584, 1.575800808251672791 ) ) ;
#157263=CARTESIAN_POINT ( 'NONE',  ( 6.073689629242148058, 8.109057205581079231, -1.443375672974057666 ) ) ;
#157272=CARTESIAN_POINT ( 'NONE',  ( 9.856414487010592751, 10.60149777770828194, 0.7216878364870438212 ) ) ;
#157273=ADVANCED_FACE ( 'NONE', ( #85564 ), #151653, .F. ) ;
#157274=ORIENTED_EDGE ( 'NONE', *, *, #157159, .F. ) ;
#157278=CARTESIAN_POINT ( 'NONE',  ( -9.612894607289142357, 11.17379744904754801, -1.199719254218441611 ) ) ;
#157294=CARTESIAN_POINT ( 'NONE',  ( -1.500000000000011324, 3.452083334016151639, 0.8660254037844403729 ) ) ;
#157298=ORIENTED_EDGE ( 'NONE', *, *, #126517, .T. ) ;
#157300=CARTESIAN_POINT ( 'NONE',  ( 1.499999999999987121, 0.7958333333333510451, -0.8660254037844253849 ) ) ;
#157301=CARTESIAN_POINT ( 'NONE',  ( 8.209625708274705502, 9.536650400197368427, 1.199719254218462483 ) ) ;
#157302=CARTESIAN_POINT ( 'NONE',  ( -1.402160292154681736E-14, -0.6781249996585819728, 1.575800808251672791 ) ) ;
#157305=CARTESIAN_POINT ( 'NONE',  ( 9.164948653157988900, 11.71552606681625619, -1.443375672974057666 ) ) ;
#157306=CARTESIAN_POINT ( 'NONE',  ( -5.097502569058207200, 8.890910730635814829, -0.7216878364870207285 ) ) ;
#157311=CARTESIAN_POINT ( 'NONE',  ( -4.855791571988752331, 8.816840600628864877, 0.7998128361456481317 ) ) ;
#157313=CARTESIAN_POINT ( 'NONE',  ( 0.7499999999999902300, 2.014583334016148530, 1.299038105676669330 ) ) ;
#157314=CARTESIAN_POINT ( 'NONE',  ( 0.6823417656249917140, 4.405208333674755394, 1.181850606188765695 ) ) ;
#157326=CARTESIAN_POINT ( 'NONE',  ( -3.054546515950523400, 6.451825606165701110, 0.6676900015689657408 ) ) ;
#157327=CARTESIAN_POINT ( 'NONE',  ( -7.831806290188425557, 12.28885777186185990, -0.7998128361456281477 ) ) ;
#157328=CARTESIAN_POINT ( 'NONE',  ( 5.621827251160867789, 9.710548892996357040, 1.040834085586084257E-14 ) ) ;
#157329=LINE ( 'NONE', #8921, #42684 ) ;
#157331=EDGE_CURVE ( 'NONE', #160543, #84121, #179102, .T. ) ;
#157339=CARTESIAN_POINT ( 'NONE',  ( -6.989391883044787868, 8.113044270762433285, -1.199719254218446718 ) ) ;
#157344=CARTESIAN_POINT ( 'NONE',  ( 2.703961570921634028, 5.242040035128820108, -1.199719254218446718 ) ) ;
#157345=CARTESIAN_POINT ( 'NONE',  ( -4.911258385257075254, 4.778213610993594429, 0.3496101188117561875 ) ) ;
#157348=CARTESIAN_POINT ( 'NONE',  ( -4.446184310277715213, 7.274633231044262516, -1.199719254218452047 ) ) ;
#157349=CARTESIAN_POINT ( 'NONE',  ( -7.635213062790267458, 12.05949900656400686, 0.000000000000000000 ) ) ;
#157378=CARTESIAN_POINT ( 'NONE',  ( 4.704316114261903436, 4.590716342834741504, 1.214306433183764966E-14 ) ) ;
#157382=CARTESIAN_POINT ( 'NONE',  ( -9.969323024750229578, 10.52529837183042716, -0.7998128361456291469 ) ) ;
#157385=CARTESIAN_POINT ( 'NONE',  ( -1.499999999999997780, 4.150000000000021672, 1.214306433183764966E-14 ) ) ;
#157387=CARTESIAN_POINT ( 'NONE',  ( 8.748035429315576650, 11.22912730566677553, -1.599625672291255185 ) ) ;
#157393=CARTESIAN_POINT ( 'NONE',  ( -4.907894938888482272, 6.474487383728027012, -2.499999999999995559 ) ) ;
#157394=CARTESIAN_POINT ( 'NONE',  ( 0.6823417656249882723, 0.09270833367475139752, 1.181850606188755259 ) ) ;
#157397=ORIENTED_EDGE ( 'NONE', *, *, #2500, .T. ) ;
#157402=CARTESIAN_POINT ( 'NONE',  ( -4.711622075948912247, 5.455646162483875017, -1.199719254218446718 ) ) ;
#157405=CARTESIAN_POINT ( 'NONE',  ( -1.402160292154681736E-14, 0.4625000000000214495, 1.732050807568877637 ) ) ;
#157407=CARTESIAN_POINT ( 'NONE',  ( -1.402160292154681736E-14, -0.9906249996585834161, -1.575800808251665908 ) ) ;
#157413=CARTESIAN_POINT ( 'NONE',  ( 1.364683531249986537, -0.09479166632524321789, -0.7879004041258309554 ) ) ;
#157415=CARTESIAN_POINT ( 'NONE',  ( -5.703176172842872482, 9.805455968292021041, 0.000000000000000000 ) ) ;
#157416=CARTESIAN_POINT ( 'NONE',  ( 8.890396042259068210, 11.39521468743417998, -1.599625672291257406 ) ) ;
#157421=CARTESIAN_POINT ( 'NONE',  ( -0.6823417656250246877, -0.3864583329919110688, 1.181850606188755259 ) ) ;
#157427=EDGE_CURVE ( 'NONE', #62417, #200114, #112808, .T. ) ;
#157428=CARTESIAN_POINT ( 'NONE',  ( -0.7500000000000215383, 3.722916667349487785, 1.299038105676671107 ) ) ;
#157430=CARTESIAN_POINT ( 'NONE',  ( 6.100805936469477331, 9.101062111647635788, -1.082531754730537088 ) ) ;
#157433=CARTESIAN_POINT ( 'NONE',  ( -5.739179097286464248, 5.590130456455974617, -0.7998128361456221525 ) ) ;
#157435=CARTESIAN_POINT ( 'NONE',  ( 4.270455198180219902, 6.965652916976816655, -1.082531754730548412 ) ) ;
#157438=CARTESIAN_POINT ( 'NONE',  ( 4.297571505407542958, 7.957657823043374989, -0.7216878364870197293 ) ) ;
#157439=CARTESIAN_POINT ( 'NONE',  ( -7.822691444960700125, 11.10992853822074444, -1.082531754730543083 ) ) ;
#157441=CARTESIAN_POINT ( 'NONE',  ( 0.7499999999999885647, 3.566666666666690411, -1.299038105676658228 ) ) ;
#157445=CARTESIAN_POINT ( 'NONE',  ( 9.246297574839983824, 9.889694713509232571, 0.7216878364870438212 ) ) ;
#157450=( BOUNDED_CURVE ( )  B_SPLINE_CURVE ( 2, ( #10548, #189313, #124406, #206621, #125466 ),
 .UNSPECIFIED., .F., .T. ) 
 B_SPLINE_CURVE_WITH_KNOTS ( ( 3, 2, 3 ),
 ( 0.1232094925783373957, 0.1250000000000000000, 0.1270731450466760504 ),
 .UNSPECIFIED. ) 
 CURVE ( )  GEOMETRIC_REPRESENTATION_ITEM ( )  RATIONAL_B_SPLINE_CURVE ( ( 0.9343361104663525651, 0.9424281978788288106, 1.000000000000000000, 0.9333402950740685711, 0.9330143039465762511 ) ) 
 REPRESENTATION_ITEM ( '' )  );
#157452=VERTEX_POINT ( 'NONE', #120280 ) ;
#157459=CARTESIAN_POINT ( 'NONE',  ( 7.890482213029013536, 12.14938698193514277, 1.040834085586084257E-14 ) ) ;
#157461=CARTESIAN_POINT ( 'NONE',  ( 7.938462636001388795, 9.220293482545153907, -1.199719254218441611 ) ) ;
#157466=CARTESIAN_POINT ( 'NONE',  ( 3.551873057100283226, 6.127307085716883428, 1.082531754730558626 ) ) ;
#157468=CARTESIAN_POINT ( 'NONE',  ( -6.548225005720456515, 10.58342024007512983, 0.000000000000000000 ) ) ;
#157472=CARTESIAN_POINT ( 'NONE',  ( -2.981903720001798597, 5.566305875722335372, -1.199719254218446718 ) ) ;
#157481=ORIENTED_EDGE ( 'NONE', *, *, #37467, .T. ) ;
#157497=CARTESIAN_POINT ( 'NONE',  ( -7.061099074618889304, 7.132370430010492868, -0.7998128361456291469 ) ) ;
#157501=CARTESIAN_POINT ( 'NONE',  ( 6.810273232766058449, 6.839740281182199233, 1.040834085586084257E-14 ) ) ;
#157502=CYLINDRICAL_SURFACE ( 'NONE', #55521, 1.250000000000000000 ) ;
#157509=CARTESIAN_POINT ( 'NONE',  ( -5.199715606040888005, 6.025088614257851027, -1.199719254218446718 ) ) ;
#157512=CARTESIAN_POINT ( 'NONE',  ( 7.962716289927667113, 8.184257181204083409, -0.7998128361456291469 ) ) ;
#157515=CARTESIAN_POINT ( 'NONE',  ( 5.993251976321238850, 6.092249680885792884, 0.6249505139499841322 ) ) ;
#157522=CARTESIAN_POINT ( 'NONE',  ( 7.090551149822744925, 7.374657217655760100, 0.7216878364870317197 ) ) ;
#157523=CARTESIAN_POINT ( 'NONE',  ( -8.182509401047415309, 9.505014708432145909, 1.199719254218462483 ) ) ;
#157526=CARTESIAN_POINT ( 'NONE',  ( -7.645908563102897126, 11.00764485934031889, 1.199719254218453823 ) ) ;
#157527=CARTESIAN_POINT ( 'NONE',  ( -4.713430959045263435, 8.650753218861462202, 0.7998128361456481317 ) ) ;
#157535=CARTESIAN_POINT ( 'NONE',  ( 8.925345196497941558, 9.307324238869423283, 1.040834085586084257E-14 ) ) ;
#157544=CARTESIAN_POINT ( 'NONE',  ( 0.006800380015298257419, 7.009756401597622144, -1.999988438674496383 ) ) ;
#157548=ORIENTED_EDGE ( 'NONE', *, *, #106610, .F. ) ;
#157549=CARTESIAN_POINT ( 'NONE',  ( 1.499999999999989120, 4.004166666666685970, 0.8660254037844524744 ) ) ;
#157550=CARTESIAN_POINT ( 'NONE',  ( 4.202137545231717120, 6.989912005157271402, 1.199719254218462483 ) ) ;
#157551=CARTESIAN_POINT ( 'NONE',  ( 7.332262146892202459, 7.448727347662698506, -0.7998128361456281477 ) ) ;
#157554=CARTESIAN_POINT ( 'NONE',  ( 6.982085921357777281, 7.248114451113292667, 1.040834085586084257E-14 ) ) ;
#157555=CARTESIAN_POINT ( 'NONE',  ( -9.612367721964613310, 11.27714576612263997, -1.082531754730537976 ) ) ;
#157560=CARTESIAN_POINT ( 'NONE',  ( 9.887974103068218668, 10.43039129653476493, 0.7998128361456462443 ) ) ;
#157565=CARTESIAN_POINT ( 'NONE',  ( 0.6823417656249882723, 0.9260416670080831025, -1.181850606188749264 ) ) ;
#157570=CARTESIAN_POINT ( 'NONE',  ( -0.6823417656250003738, -0.5322916663252491576, -1.181850606188749264 ) ) ;
#157572=CIRCLE ( 'NONE', #143691, 0.07999999999999977962 ) ;
#157573=CARTESIAN_POINT ( 'NONE',  ( 9.908311333488716954, 10.45411806535867782, 0.7998128361456462443 ) ) ;
#157576=CARTESIAN_POINT ( 'NONE',  ( -10.00321840878439339, 10.56484298653695397, 1.040834085586084257E-14 ) ) ;
#157582=CARTESIAN_POINT ( 'NONE',  ( 5.040934186182656873, 4.775511393501539636, 1.040834085586084257E-14 ) ) ;
#157586=CARTESIAN_POINT ( 'NONE',  ( -4.080641047588918546, 4.823464646017586510, -1.082531754730548412 ) ) ;
#157589=CARTESIAN_POINT ( 'NONE',  ( 7.910292558569346433, 11.31609285405122556, -1.199719254218446718 ) ) ;
#157591=CARTESIAN_POINT ( 'NONE',  ( 5.181774431428755712, 6.445567486282277159, 1.182616053296376979 ) ) ;
#157593=CARTESIAN_POINT ( 'NONE',  ( -5.115504031057831469, 4.862509545855891346, 0.7998128361456341429 ) ) ;
#157597=CARTESIAN_POINT ( 'NONE',  ( 8.076906825439115423, 10.44614393447756129, -1.599625672291262513 ) ) ;
#157599=CARTESIAN_POINT ( 'NONE',  ( 6.238723240582662477, 10.43026088065513513, -0.7998128361456291469 ) ) ;
#157602=CARTESIAN_POINT ( 'NONE',  ( -8.676855123066019360, 11.14608361504227574, -1.443375672974059665 ) ) ;
#157608=CARTESIAN_POINT ( 'NONE',  ( -5.639314450680645407, 6.167449467472198243, -0.8320033040390877321 ) ) ;
#157609=CARTESIAN_POINT ( 'NONE',  ( 1.364683531249988535, 1.613541667008084879, 0.7879004041258500513 ) ) ;
#157611=CARTESIAN_POINT ( 'NONE',  ( 5.490689023854504747, 9.349628261231513804, 1.040834085586084257E-14 ) ) ;
#157624=CARTESIAN_POINT ( 'NONE',  ( -10.60211293576223213, 11.47147930125185589, 1.040834085586084257E-14 ) ) ;
#157628=CARTESIAN_POINT ( 'NONE',  ( 9.908311333488716954, 10.45411806535867782, 0.7998128361456462443 ) ) ;
#157632=CARTESIAN_POINT ( 'NONE',  ( -3.273404022695637572, 5.906389562198459231, 1.199719254218462483 ) ) ;
#157633=CARTESIAN_POINT ( 'NONE',  ( -7.152089726408780379, 8.302858421353754181, -1.199719254218446718 ) ) ;
#157635=ORIENTED_EDGE ( 'NONE', *, *, #76553, .T. ) ;
#157636=CARTESIAN_POINT ( 'NONE',  ( -9.592557376868645846, 11.15007068022363157, -1.199719254218441611 ) ) ;
#157640=CARTESIAN_POINT ( 'NONE',  ( -1.201851678989727383E-14, 4.618750000682821266, -1.732050807568863648 ) ) ;
#157641=CARTESIAN_POINT ( 'NONE',  ( 6.238723240582662477, 10.43026088065513513, -0.7998128361456291469 ) ) ;
#157644=CARTESIAN_POINT ( 'NONE',  ( -8.877891658850122880, 9.251961778280284321, 0.7998128361456462443 ) ) ;
#157646=CARTESIAN_POINT ( 'NONE',  ( -1.364683531250012516, 4.488541667008090208, -0.7879004041258300672 ) ) ;
#157648=CARTESIAN_POINT ( 'NONE',  ( -1.506201402929161048, 8.679372656207108960, 2.542017642366253050 ) ) ;
#157652=CARTESIAN_POINT ( 'NONE',  ( -7.375272376154077492, 11.54830883891436422, -0.7216878364870267237 ) ) ;
#157656=CARTESIAN_POINT ( 'NONE',  ( -1.364683531250012516, 3.301041667008084879, -0.7879004041258289570 ) ) ;
#157663=CARTESIAN_POINT ( 'NONE',  ( -1.201851678989727383E-14, 4.446875000341417916, -1.575800808251660134 ) ) ;
#157664=CARTESIAN_POINT ( 'NONE',  ( -5.135841261478327979, 4.886236314679810455, 0.7998128361456341429 ) ) ;
#157665=CARTESIAN_POINT ( 'NONE',  ( 5.113396490648394632, 9.117379672398465473, 1.040834085586084257E-14 ) ) ;
#157669=CARTESIAN_POINT ( 'NONE',  ( -1.201851678989727383E-14, 3.509375000341421469, -1.575800808251660134 ) ) ;
#157674=CARTESIAN_POINT ( 'NONE',  ( -0.6823417656250003738, 1.467708333674752730, -1.181850606188749264 ) ) ;
#157675=CARTESIAN_POINT ( 'NONE',  ( -3.118012141462980669, 6.581505231774690046, 0.7216878364870317197 ) ) ;
#157676=CARTESIAN_POINT ( 'NONE',  ( 4.741601036477289810, 6.554953847355395880, 1.599625672291267398 ) ) ;
#157680=CARTESIAN_POINT ( 'NONE',  ( -4.083708824282378913, 7.596498746673441715, 0.5977277219625460880 ) ) ;
#157681=CARTESIAN_POINT ( 'NONE',  ( 3.389175213736297820, 4.977123720824209840, 1.443375672974062551 ) ) ;
#157684=CARTESIAN_POINT ( 'NONE',  ( -8.785320351975364872, 12.23299559640450518, 1.082531754730560403 ) ) ;
#157689=CARTESIAN_POINT ( 'NONE',  ( -10.13488352141530768, 11.78278451552804817, 1.199719254218462483 ) ) ;
#157690=CARTESIAN_POINT ( 'NONE',  ( -6.521108698048791119, 6.710307690586118312, -0.7216878364870267237 ) ) ;
#157692=CARTESIAN_POINT ( 'NONE',  ( 1.364683531249986537, 0.4260416670080872659, 0.7879004041258500513 ) ) ;
#157705=CARTESIAN_POINT ( 'NONE',  ( 9.368320956918616105, 10.03205532593431037, 0.7216878364870458196 ) ) ;
#157713=CARTESIAN_POINT ( 'NONE',  ( 4.029797971759831121, 5.724516938518342535, -1.599625672291255185 ) ) ;
#157715=CARTESIAN_POINT ( 'NONE',  ( -4.627410500965859264, 4.293067094081919777, 0.7998128361456341429 ) ) ;
#157718=CARTESIAN_POINT ( 'NONE',  ( 4.161989969715248705, 4.726297878971393196, -2.420000000000000373 ) ) ;
#157719=CARTESIAN_POINT ( 'NONE',  ( -3.922984035321194884, 2.804646012044678560, 0.7750000000000135669 ) ) ;
#157720=CARTESIAN_POINT ( 'NONE',  ( -0.6823417656250003738, 2.280208333674753174, -1.181850606188749264 ) ) ;
#157722=ORIENTED_EDGE ( 'NONE', *, *, #177164, .F. ) ;
#157723=CIRCLE ( 'NONE', #188783, 0.08000000000000020983 ) ;
#157740=CARTESIAN_POINT ( 'NONE',  ( 5.738125327081736060, 7.717565519727259904, 1.599625672291267398 ) ) ;
#157745=CARTESIAN_POINT ( 'NONE',  ( 3.048090068225879801, 6.453403318663617050, -0.2959858980189428168 ) ) ;
#157747=CARTESIAN_POINT ( 'NONE',  ( 6.259060471003163428, 10.45398764947904624, -0.7998128361456291469 ) ) ;
#157750=CARTESIAN_POINT ( 'NONE',  ( 9.921869487102386032, 10.46993591124128997, 0.000000000000000000 ) ) ;
#157752=CARTESIAN_POINT ( 'NONE',  ( 1.566570994388963856, 8.685985410138266971, -2.500753655585654656 ) ) ;
#157757=DIRECTION ( 'NONE',  ( -5.578564026256490882E-16, -1.000000000000000000, -9.066213480720158442E-32 ) ) ;
#157760=CARTESIAN_POINT ( 'NONE',  ( -9.178506806771670412, 9.810605484096178941, 1.040834085586084257E-14 ) ) ;
#157774=CARTESIAN_POINT ( 'NONE',  ( 4.351804119862229037, 4.179452349368450115, -0.7216878364870188411 ) ) ;
#157782=CARTESIAN_POINT ( 'NONE',  ( -4.882907879216086933, 8.848476292394087395, -0.7998128361456281477 ) ) ;
#157785=CARTESIAN_POINT ( 'NONE',  ( -4.783329267523015460, 4.474972321731942593, -0.7998128361456221525 ) ) ;
#157793=CARTESIAN_POINT ( 'NONE',  ( 1.364683531249988535, 3.717708333674750953, -0.7879004041258239610 ) ) ;
#157795=CARTESIAN_POINT ( 'NONE',  ( 4.462605117192430804, 8.358123070033169455, 1.040834085586084257E-14 ) ) ;
#157808=CARTESIAN_POINT ( 'NONE',  ( -0.6823417656250003738, 1.280208333674752508, -1.181850606188749264 ) ) ;
#157810=CARTESIAN_POINT ( 'NONE',  ( 3.541704441667858472, 5.155074486744371853, -1.599625672291262513 ) ) ;
#157812=CARTESIAN_POINT ( 'NONE',  ( -5.205967797967562483, 8.057084283395347768, 1.082531754730548412 ) ) ;
#157814=CARTESIAN_POINT ( 'NONE',  ( 3.009546912553647147, 5.494593250412460606, -1.082531754730543083 ) ) ;
#157815=CARTESIAN_POINT ( 'NONE',  ( -6.683806541412776525, 7.860491055478785682, -1.082531754730543083 ) ) ;
#157816=EDGE_CURVE ( 'NONE', #102987, #45840, #207348, .T. ) ;
#157821=CARTESIAN_POINT ( 'NONE',  ( 5.289652487626049115, 9.323011668872403845, 0.7998128361456462443 ) ) ;
#157830=CARTESIAN_POINT ( 'NONE',  ( 7.145310649601935182, 8.294949498412453437, -1.199719254218446718 ) ) ;
#157831=( NAMED_UNIT ( * ) SI_UNIT ( $, .STERADIAN. ) SOLID_ANGLE_UNIT ( ) );
#157833=CARTESIAN_POINT ( 'NONE',  ( -7.413611068574208041, 7.543634422958360730, 0.7998128361456341429 ) ) ;
#157837=CARTESIAN_POINT ( 'NONE',  ( 7.914208982075123799, 10.25632978388623684, -1.599625672291262513 ) ) ;
#157840=CARTESIAN_POINT ( 'NONE',  ( -6.204827856548512877, 10.39071626594860476, -0.7998128361456291469 ) ) ;
#157842=CARTESIAN_POINT ( 'NONE',  ( 7.497295758232718654, 9.769931022736756177, -1.443375672974058777 ) ) ;
#157843=CARTESIAN_POINT ( 'NONE',  ( 4.093767505759832837, 7.703081727663242617, 0.6588811006658854552 ) ) ;
#157844=CARTESIAN_POINT ( 'NONE',  ( -5.610376637956639101, 5.439860920571172542, 0.000000000000000000 ) ) ;
#157850=CARTESIAN_POINT ( 'NONE',  ( 5.335297142177534369, 6.183267073083954735, -1.199719254218452047 ) ) ;
#157852=CARTESIAN_POINT ( 'NONE',  ( 10.40318394038753702, 11.03146944007395724, -0.7998128361456281477 ) ) ;
#157853=CARTESIAN_POINT ( 'NONE',  ( -5.693503466768185639, 6.133329901302775333, 0.7540896269448340572 ) ) ;
#157854=CARTESIAN_POINT ( 'NONE',  ( -3.930962900855138553, 2.807348321460037432, -0.7749999999999944711 ) ) ;
#157855=CARTESIAN_POINT ( 'NONE',  ( 1.364683531249986537, 0.1552083336747499542, -0.7879004041258309554 ) ) ;
#157858=CARTESIAN_POINT ( 'NONE',  ( -6.887178846062128379, 7.137389529935019183, -0.7216878364870278340 ) ) ;
#157865=CARTESIAN_POINT ( 'NONE',  ( -5.552553451737586521, 6.223206628393089801, 0.9334509375357492589 ) ) ;
#157866=CARTESIAN_POINT ( 'NONE',  ( -0.6823417656250003738, 2.030208333674753174, -1.181850606188749264 ) ) ;
#157869=CARTESIAN_POINT ( 'NONE',  ( 4.555176424511575561, 4.416720038126027426, -0.7216878364870188411 ) ) ;
#157874=CARTESIAN_POINT ( 'NONE',  ( -9.137832345486311070, 9.763151945929928743, 1.040834085586084257E-14 ) ) ;
#157881=CARTESIAN_POINT ( 'NONE',  ( -8.636180661780672452, 9.177891648273343250, -0.7216878364870267237 ) ) ;
#157889=CARTESIAN_POINT ( 'NONE',  ( -6.846504384776750385, 10.93141284897413890, -0.7216878364870267237 ) ) ;
#157894=CARTESIAN_POINT ( 'NONE',  ( -1.201851678989727383E-14, 4.868750000682822154, -1.732050807568863648 ) ) ;
#157901=CARTESIAN_POINT ( 'NONE',  ( -7.314787569772770226, 8.492672571945082183, -1.199719254218452935 ) ) ;
#157905=CARTESIAN_POINT ( 'NONE',  ( 3.960953433486789521, 7.772862772376584850, -0.7998128361456221525 ) ) ;
#157909=CARTESIAN_POINT ( 'NONE',  ( 8.294891053462476904, 8.571794405328034827, 1.040834085586084257E-14 ) ) ;
#157916=CARTESIAN_POINT ( 'NONE',  ( -6.263503779833496488, 6.409768619334935913, 0.7216878364870317197 ) ) ;
#157927=CARTESIAN_POINT ( 'NONE',  ( -7.316596452869116973, 11.68777962832266049, 0.7998128361456481317 ) ) ;
#157929=CARTESIAN_POINT ( 'NONE',  ( 7.096803341749390981, 10.36702210109460154, -1.199719254218441611 ) ) ;
#157930=CARTESIAN_POINT ( 'NONE',  ( -0.7500000000000006661, 0.1083333333333560966, -1.299038105676652011 ) ) ;
#157931=CARTESIAN_POINT ( 'NONE',  ( -7.934546212495630968, 10.28005655271014795, -1.599625672291263179 ) ) ;
#157934=CARTESIAN_POINT ( 'NONE',  ( 0.6823417656249899377, 4.926041667008086655, -1.181850606188754593 ) ) ;
#157935=CARTESIAN_POINT ( 'NONE',  ( 9.327646496521982300, 11.90534021740758064, -1.443375672974057666 ) ) ;
#157938=CARTESIAN_POINT ( 'NONE',  ( -0.7500000000000215383, 4.941666666666684193, 1.299038105676671107 ) ) ;
#157941=CARTESIAN_POINT ( 'NONE',  ( 7.253248993186713456, 11.40594822545244824, 0.7216878364870438212 ) ) ;
#157944=CARTESIAN_POINT ( 'NONE',  ( -6.724481002698130538, 7.907944593645035880, -1.082531754730544860 ) ) ;
#157947=CARTESIAN_POINT ( 'NONE',  ( 0.6823417656249882723, 1.426041667008083547, -1.181850606188749264 ) ) ;
#157951=CARTESIAN_POINT ( 'NONE',  ( -7.019370843573183194, 9.212351955633947043, 1.599625672291283607 ) ) ;
#157952=CARTESIAN_POINT ( 'NONE',  ( 1.364683531249990311, 5.426041667008086655, 0.7879004041258500513 ) ) ;
#157957=CARTESIAN_POINT ( 'NONE',  ( 9.368847842243145152, 10.88907622316056312, 1.199719254218453823 ) ) ;
#157960=CARTESIAN_POINT ( 'NONE',  ( -0.7500000000000006661, 1.858333333333357595, -1.299038105676652011 ) ) ;
#157966=CARTESIAN_POINT ( 'NONE',  ( 7.131225611108096274, 8.382479970123348778, 1.082531754730558626 ) ) ;
#157967=CARTESIAN_POINT ( 'NONE',  ( 8.910733272679570049, 11.41894145625809820, -1.599625672291255185 ) ) ;
#157976=CARTESIAN_POINT ( 'NONE',  ( 7.242026607993941489, 11.60078147596829901, 0.7998128361456462443 ) ) ;
#157977=CARTESIAN_POINT ( 'NONE',  ( -8.618179199781044630, 13.20629283305325963, 0.7998128361456341429 ) ) ;
#157981=CARTESIAN_POINT ( 'NONE',  ( -0.6823417656249969321, 5.280208333674756283, -1.181850606188749264 ) ) ;
#157987=CARTESIAN_POINT ( 'NONE',  ( 1.364683531249988535, 4.155208333674753618, -0.7879004041258239610 ) ) ;
#157989=CARTESIAN_POINT ( 'NONE',  ( -6.073689629242160493, 8.109057205581079231, -1.443375672974059665 ) ) ;
#157998=CARTESIAN_POINT ( 'NONE',  ( 8.158255747121103241, 10.54105100977322174, 1.599625672291281386 ) ) ;
#158005=CARTESIAN_POINT ( 'NONE',  ( -9.643927338022246332, 10.14567007064778004, -0.7998128361456291469 ) ) ;
#158006=CARTESIAN_POINT ( 'NONE',  ( 5.469824908109481854, 8.468880595181346393, -1.199719254218446718 ) ) ;
#158009=CARTESIAN_POINT ( 'NONE',  ( 3.310162060030825248, 7.013606170011280838, -0.7998128361456291469 ) ) ;
#158010=VERTEX_POINT ( 'NONE', #177491 ) ;
#158017=CARTESIAN_POINT ( 'NONE',  ( -5.097502569058215194, 6.970172302033127210, -1.443375672974053447 ) ) ;
#158018=CARTESIAN_POINT ( 'NONE',  ( 4.090809663021327758, 5.795697244990093644, 1.599625672291267398 ) ) ;
#158021=CARTESIAN_POINT ( 'NONE',  ( -7.049349804101573191, 10.31165964050546258, -1.199719254218440723 ) ) ;
#158025=CARTESIAN_POINT ( 'NONE',  ( -8.833300774503376473, 10.26427131079744193, 1.199719254218462483 ) ) ;
#158029=CARTESIAN_POINT ( 'NONE',  ( 6.435316467980822353, 10.65961964595298817, 1.040834085586084257E-14 ) ) ;
#158030=CARTESIAN_POINT ( 'NONE',  ( 4.527533231959700366, 7.369540306339926516, 1.199719254218462483 ) ) ;
#158042=CARTESIAN_POINT ( 'NONE',  ( -8.128276786592724790, 9.441743324901704426, -1.199719254218446718 ) ) ;
#158046=CARTESIAN_POINT ( 'NONE',  ( 7.131225611108100715, 7.422110755822004968, 0.7216878364870317197 ) ) ;
#158049=CARTESIAN_POINT ( 'NONE',  ( -1.420000000000001039, 6.280000000000042881, -2.579999999999995630 ) ) ;
#158051=CARTESIAN_POINT ( 'NONE',  ( -5.220052836461385404, 6.048815383081766583, -1.199719254218446718 ) ) ;
#158052=( BOUNDED_SURFACE ( )  B_SPLINE_SURFACE ( 1, 2, ( 
 ( #38544, #57989, #203149, #104621, #170669, #22256, #88366, #152294, #6010, #136053, #73150, #72080, #171736, #138191, #204201, #23333, #89442, #155494, #139255, #205287, #56925, #123098, #189055, #40692, #106795, #184769, #74250, #140344, #172823, #90507, #156572, #160829, #145690, #158696, #59050, #178154, #93717, #177079, #111073, #92654, #190113, #108944, #127350, #159758, #28695, #61191, #10294, #11355, #79571, #41767, #76368, #157640, #107880, #29768, #144619, #193319, #210633, #173906, #60119, #62259, #142475, #125208, #208483, #27617, #126278, #211688, #124152, #75309, #192236, #12421, #9237, #209547, #44965, #25482, #91588, #141425, #43898, #77436, #207431, #191170, #95853, #42837, #143553, #174964, #26546, #128420, #94781, #110012, #78501, #176025, #194387, #161909, #46030, #112151, #13497, #212758, #164040, #409, #17733, #67548, #16679, #181330, #63324, #131574, #147786, #64393, #130537, #100086, #179219, #199696, #18810, #196528, #30844, #117466, #115339, #14552, #129485, #82764, #83822, #84897, #167224, #48171, #101136, #133692, #35065, #198627, #80648, #148837, #114284, #180281, #150984, #50274, #195467, #97981, #149915, #15615, #116393, #31904, #51341, #34011, #47098, #49220, #182381, #81705, #213802, #146740, #65425, #113214, #197575, #32958, #99033, #165088, #96922, #162972, #66481, #132621, #166147, #1483, #183459, #24147, #39352, #40438, #122840, #53464, #106539, #103288, #105448, #37215, #188801, #134746, #3613, #89191, #172564, #119601, #168287, #85968, #185585, #72904, #104362, #54535, #70752, #200755, #90250, #169350, #187724, #19884, #171484, #6824, #69691, #20935, #135795, #4678, #87031, #152043, #154177, #203954, #136864, #68623, #102218, #5745, #153103, #202890, #2548, #52404, #118531, #201819, #56676, #23075, #120682, #155242, #186659, #184514, #139008, #36135, #38285, #170407, #21996, #88106, #71822, #137932, #55601, #121756, #205030, #44436, #96393, #45503, #210095, #32432, #114807, #180806, #77977, #213291, #113754, #161380, #47643, #29239, #64917, #130017, #140083, #156317, #61734, #111619, #62786, #126821, #177631, #79041, #46564, #31375, #94261, #95331, #162444, #179758, #163506, #112684, #128949, #7900, #12964, #145156, #160300, #11903, #196008, #57740, #81180, #73988, #144100, #192778, #131066, #211162, #110553, #206107, #178694, #97451, #176555, #48692, #127902, #197054, #15090, #28165, #80106, #193853, #30308, #194927, #14019, #146210, #212228, #63861, #147259, #52937, #199163, #19358, #83292, #168822, #69162, #186128, #84374, #85438, #149377, #960, #115869, #67026, #82232, #165628, #17216, #68092, #133162, #148323, #54012, #50808, #120151, #116935, #136342, #182935, #98498, #135282, #202362, #4160, #34551, #164562, #100622, #201296, #166697, #70230, #16147, #99564, #185054, #214322, #18288, #49742, #181854, #150462, #20426, #200236, #2023, #134226, #65954, #132103, #51886 ),
 ( #151523, #3091, #33491, #198112, #35612, #118009, #183998, #119073, #101690, #167759, #36679, #102767, #86508, #152573, #207721, #206651, #174194, #24697, #74537, #59345, #72376, #187202, #91878, #7372, #90800, #156864, #6302, #103835, #22554, #40983, #73450, #8450, #189343, #138476, #139553, #125498, #169883, #204498, #71297, #21473, #157934, #58283, #107094, #124439, #87582, #188267, #190397, #56148, #38830, #122309, #155787, #39907, #37762, #153654, #203428, #106017, #140638, #137409, #123378, #173116, #5222, #55083, #121232, #172038, #205580, #104914, #170955, #9527, #88660, #57217, #154720, #23631, #42054, #108167, #89738, #25766, #75600, #141711, #31129, #27913, #13779, #179508, #210912, #147019, #62539, #192527, #191461, #175251, #45249, #64671, #97203, #163256, #26837, #92940, #12706, #28985, #14838, #128701, #178443, #63613, #127643, #79854, #113500, #158985, #177371, #145963, #94009, #44181, #142770, #194670, #161119, #211973, #195751, #80928, #112430, #111367, #43127, #160048, #110301, #11652, #77724, #143846, #10581, #209839, #208775, #129768, #76655, #46314, #78783, #61477, #213041, #109241, #47388, #60405, #30050, #126566, #176309, #193607, #95071, #144904, #96140, #162192, #117759, #99319, #196807, #115613, #133979, #166439, #183749, #67832, #165369, #100369, #86254, #48450, #83043, #164311, #114564, #184799, #151267, #199987, #2839, #180556, #66763, #68908, #149117, #65704, #16962, #34296, #132904, #152324, #130817, #81984, #198909, #167507, #15901, #1776, #51635, #32178, #3902, #98254, #50554, #18030, #148072, #214078, #36428, #131852, #84117, #197860, #49492, #135028, #35359, #181608, #19105, #33236, #182675, #102504, #698, #85183, #118814, #150204, #116676, #101434, #201041, #52684, #168567, #20167, #157674, #124186, #190149, #119891, #185868, #105746, #122046, #58022, #7113, #56960, #156608, #6044, #106831, #206396, #37503, #55889, #24432, #186945, #137155, #21220, #73186, #39638, #90544, #74283, #41803, #205322, #138224, #69972, #38578, #203180, #120977, #104653, #170701, #53759, #22286, #87325, #172861, #103579, #139292, #171772, #88399, #4963, #169637, #123134, #23369, #154466, #189091, #71041, #72115, #54827, #153392, #136083, #204237, #188010, #89478, #155533, #40725, #91623, #202100, #8198, #140377, #107916, #173942, #25515, #12458, #59085, #96956, #125245, #11390, #44997, #191205, #108978, #129517, #10326, #111107, #174997, #42870, #95887, #128452, #26582, #112183, #179254, #61225, #63359, #60152, #46061, #211722, #28728, #30877, #94814, #76400, #9271, #207466, #77468, #75343, #195497, #47133, #92684, #158730, #177112, #127381, #113248, #160864, #210666, #161942, #159788, #178187, #145723, #142509, #209580, #29802, #126309, #208517, #192269, #78533, #193353, #13534, #79604, #141459, #144651, #143587, #43930, #110045, #176057, #27653, #93750, #62293, #194420, #115373, #114314, #51381 ) ),
 .UNSPECIFIED., .F., .F., .T. ) 
 B_SPLINE_SURFACE_WITH_KNOTS ( ( 2, 2 ),
 ( 3, 2, 2, 2, 2, 2, 2, 2, 2, 2, 2, 2, 2, 2, 2, 2, 2, 2, 2, 2, 2, 2, 2, 2, 2, 2, 2, 2, 2, 2, 2, 2, 2, 2, 2, 2, 2, 2, 2, 2, 2, 2, 2, 2, 2, 2, 2, 2, 2, 2, 2, 2, 2, 2, 2, 2, 2, 2, 2, 2, 2, 2, 2, 2, 2, 2, 2, 2, 2, 2, 2, 2, 2, 2, 2, 2, 2, 2, 2, 2, 2, 2, 2, 2, 2, 2, 2, 2, 2, 2, 2, 2, 2, 2, 2, 2, 2, 2, 2, 2, 2, 2, 2, 2, 2, 2, 2, 2, 2, 2, 2, 2, 2, 2, 2, 2, 2, 2, 2, 2, 2, 2, 2, 2, 2, 2, 2, 2, 2, 2, 2, 2, 2, 2, 2, 2, 2, 2, 2, 2, 2, 2, 2, 2, 2, 2, 2, 2, 2, 2, 2, 2, 2, 2, 2, 2, 2, 2, 2, 2, 2, 2, 2, 2, 2, 2, 2, 2, 3 ),
 ( 0.000000000000000000, 1.000000000000000000 ),
 ( 0.000000000000000000, 0.005952380952380952051, 0.01190476190476190410, 0.01785714285714285615, 0.02380952380952380820, 0.02976190476190476025, 0.03571428571428571230, 0.04166666666666666435, 0.04761904761904761640, 0.05357142857142856845, 0.05952380952380952051, 0.06547619047619047949, 0.07142857142857142461, 0.07738095238095238360, 0.08333333333333332871, 0.08928571428571428770, 0.09523809523809523281, 0.1011904761904761918, 0.1071428571428571369, 0.1130952380952380959, 0.1190476190476190410, 0.1250000000000000000, 0.1309523809523809590, 0.1369047619047619180, 0.1428571428571428492, 0.1488095238095238082, 0.1547619047619047672, 0.1607142857142857262, 0.1666666666666666574, 0.1726190476190476164, 0.1785714285714285754, 0.1845238095238095344, 0.1904761904761904656, 0.1964285714285714246, 0.2023809523809523836, 0.2083333333333333426, 0.2142857142857142738, 0.2202380952380952328, 0.2261904761904761918, 0.2321428571428571508, 0.2380952380952380820, 0.2440476190476190410, 0.2500000000000000000, 0.2559523809523809312, 0.2619047619047619180, 0.2678571428571428492, 0.2738095238095238360, 0.2797619047619047672, 0.2857142857142856984, 0.2916666666666666852, 0.2976190476190476164, 0.3035714285714285476, 0.3095238095238095344, 0.3154761904761904656, 0.3214285714285714524, 0.3273809523809523836, 0.3333333333333333148, 0.3392857142857143016, 0.3452380952380952328, 0.3511904761904761640, 0.3571428571428571508, 0.3630952380952380820, 0.3690476190476190688, 0.3750000000000000000, 0.3809523809523809312, 0.3869047619047619180, 0.3928571428571428492, 0.3988095238095238360, 0.4047619047619047672, 0.4107142857142856984, 0.4166666666666666852, 0.4226190476190476164, 0.4285714285714285476, 0.4345238095238095344, 0.4404761904761904656, 0.4464285714285714524, 0.4523809523809523836, 0.4583333333333333148, 0.4642857142857143016, 0.4702380952380952328, 0.4761904761904761640, 0.4821428571428571508, 0.4880952380952380820, 0.4940476190476190688, 0.5000000000000000000, 0.5059523809523809312, 0.5119047619047618625, 0.5178571428571429047, 0.5238095238095238360, 0.5297619047619047672, 0.5357142857142856984, 0.5416666666666666297, 0.5476190476190476719, 0.5535714285714286031, 0.5595238095238095344, 0.5654761904761904656, 0.5714285714285713969, 0.5773809523809523281, 0.5833333333333333703, 0.5892857142857143016, 0.5952380952380952328, 0.6011904761904761640, 0.6071428571428570953, 0.6130952380952381375, 0.6190476190476190688, 0.6250000000000000000, 0.6309523809523809312, 0.6369047619047618625, 0.6428571428571429047, 0.6488095238095238360, 0.6547619047619047672, 0.6607142857142856984, 0.6666666666666666297, 0.6726190476190476719, 0.6785714285714286031, 0.6845238095238095344, 0.6904761904761904656, 0.6964285714285713969, 0.7023809523809523281, 0.7083333333333333703, 0.7142857142857143016, 0.7202380952380952328, 0.7261904761904761640, 0.7321428571428570953, 0.7380952380952381375, 0.7440476190476190688, 0.7500000000000000000, 0.7559523809523809312, 0.7619047619047618625, 0.7678571428571429047, 0.7738095238095238360, 0.7797619047619047672, 0.7857142857142856984, 0.7916666666666666297, 0.7976190476190476719, 0.8035714285714286031, 0.8095238095238095344, 0.8154761904761904656, 0.8214285714285713969, 0.8273809523809523281, 0.8333333333333333703, 0.8392857142857143016, 0.8452380952380952328, 0.8511904761904761640, 0.8571428571428570953, 0.8630952380952381375, 0.8690476190476190688, 0.8750000000000000000, 0.8809523809523809312, 0.8869047619047618625, 0.8928571428571429047, 0.8988095238095238360, 0.9047619047619047672, 0.9107142857142856984, 0.9166666666666666297, 0.9226190476190476719, 0.9285714285714286031, 0.9345238095238095344, 0.9404761904761904656, 0.9464285714285713969, 0.9523809523809523281, 0.9583333333333333703, 0.9642857142857143016, 0.9702380952380952328, 0.9761904761904761640, 0.9821428571428570953, 0.9880952380952381375, 0.9940476190476190688, 1.000000000000000000 ),
 .UNSPECIFIED. ) 
 GEOMETRIC_REPRESENTATION_ITEM ( )  RATIONAL_B_SPLINE_SURFACE ( (
 ( 1.000000000000000000, 0.8660254037844387076, 1.000000000000000000, 0.8660254037844387076, 1.000000000000000000, 0.8660254037844387076, 1.000000000000000000, 0.8660254037844387076, 1.000000000000000000, 0.8660254037844387076, 1.000000000000000000, 0.8660254037844387076, 1.000000000000000000, 0.8660254037844387076, 1.000000000000000000, 0.8660254037844387076, 1.000000000000000000, 0.8660254037844387076, 1.000000000000000000, 0.8660254037844387076, 1.000000000000000000, 0.8660254037844387076, 1.000000000000000000, 0.8660254037844387076, 1.000000000000000000, 0.8660254037844387076, 1.000000000000000000, 0.8660254037844387076, 1.000000000000000000, 0.8660254037844387076, 1.000000000000000000, 0.8660254037844387076, 1.000000000000000000, 0.8660254037844387076, 1.000000000000000000, 0.8660254037844387076, 1.000000000000000000, 0.8660254037844387076, 1.000000000000000000, 0.8660254037844387076, 1.000000000000000000, 0.8660254037844387076, 1.000000000000000000, 0.8660254037844387076, 1.000000000000000000, 0.8660254037844387076, 1.000000000000000000, 0.8660254037844387076, 1.000000000000000000, 0.8660254037844387076, 1.000000000000000000, 0.8660254037844387076, 1.000000000000000000, 0.8660254037844387076, 1.000000000000000000, 0.8660254037844387076, 1.000000000000000000, 0.8660254037844387076, 1.000000000000000000, 0.8660254037844387076, 1.000000000000000000, 0.8660254037844387076, 1.000000000000000000, 0.8660254037844387076, 1.000000000000000000, 0.8660254037844387076, 1.000000000000000000, 0.8660254037844387076, 1.000000000000000000, 0.8660254037844387076, 1.000000000000000000, 0.8660254037844387076, 1.000000000000000000, 0.8660254037844387076, 1.000000000000000000, 0.8660254037844387076, 1.000000000000000000, 0.8660254037844387076, 1.000000000000000000, 0.8660254037844387076, 1.000000000000000000, 0.8660254037844387076, 1.000000000000000000, 0.8660254037844387076, 1.000000000000000000, 0.8660254037844387076, 1.000000000000000000, 0.8660254037844387076, 1.000000000000000000, 0.8660254037844387076, 1.000000000000000000, 0.8660254037844387076, 1.000000000000000000, 0.8660254037844387076, 1.000000000000000000, 0.8660254037844387076, 1.000000000000000000, 0.8660254037844387076, 1.000000000000000000, 0.8660254037844387076, 1.000000000000000000, 0.8660254037844387076, 1.000000000000000000, 0.8660254037844387076, 1.000000000000000000, 0.8660254037844387076, 1.000000000000000000, 0.8660254037844387076, 1.000000000000000000, 0.8660254037844387076, 1.000000000000000000, 0.8660254037844387076, 1.000000000000000000, 0.8660254037844387076, 1.000000000000000000, 0.8660254037844387076, 1.000000000000000000, 0.8660254037844387076, 1.000000000000000000, 0.8660254037844387076, 1.000000000000000000, 0.8660254037844387076, 1.000000000000000000, 0.8660254037844387076, 1.000000000000000000, 0.8660254037844387076, 1.000000000000000000, 0.8660254037844387076, 1.000000000000000000, 0.8660254037844387076, 1.000000000000000000, 0.8660254037844387076, 1.000000000000000000, 0.8660254037844387076, 1.000000000000000000, 0.8660254037844387076, 1.000000000000000000, 0.8660254037844387076, 1.000000000000000000, 0.8660254037844387076, 1.000000000000000000, 0.8660254037844387076, 1.000000000000000000, 0.8660254037844387076, 1.000000000000000000, 0.8660254037844387076, 1.000000000000000000, 0.8660254037844387076, 1.000000000000000000, 0.8660254037844387076, 1.000000000000000000, 0.8660254037844387076, 1.000000000000000000, 0.8660254037844387076, 1.000000000000000000, 0.8660254037844387076, 1.000000000000000000, 0.8660254037844387076, 1.000000000000000000, 0.8660254037844387076, 1.000000000000000000, 0.8660254037844387076, 1.000000000000000000, 0.8660254037844387076, 1.000000000000000000, 0.8660254037844387076, 1.000000000000000000, 0.8660254037844387076, 1.000000000000000000, 0.8660254037844387076, 1.000000000000000000, 0.8660254037844387076, 1.000000000000000000, 0.8660254037844387076, 1.000000000000000000, 0.8660254037844387076, 1.000000000000000000, 0.8660254037844387076, 1.000000000000000000, 0.8660254037844387076, 1.000000000000000000, 0.8660254037844387076, 1.000000000000000000, 0.8660254037844387076, 1.000000000000000000, 0.8660254037844387076, 1.000000000000000000, 0.8660254037844387076, 1.000000000000000000, 0.8660254037844387076, 1.000000000000000000, 0.8660254037844387076, 1.000000000000000000, 0.8660254037844387076, 1.000000000000000000, 0.8660254037844387076, 1.000000000000000000, 0.8660254037844387076, 1.000000000000000000, 0.8660254037844387076, 1.000000000000000000, 0.8660254037844387076, 1.000000000000000000, 0.8660254037844387076, 1.000000000000000000, 0.8660254037844387076, 1.000000000000000000, 0.8660254037844387076, 1.000000000000000000, 0.8660254037844387076, 1.000000000000000000, 0.8660254037844387076, 1.000000000000000000, 0.8660254037844387076, 1.000000000000000000, 0.8660254037844387076, 1.000000000000000000, 0.8660254037844387076, 1.000000000000000000, 0.8660254037844387076, 1.000000000000000000, 0.8660254037844387076, 1.000000000000000000, 0.8660254037844387076, 1.000000000000000000, 0.8660254037844387076, 1.000000000000000000, 0.8660254037844387076, 1.000000000000000000, 0.8660254037844387076, 1.000000000000000000, 0.8660254037844387076, 1.000000000000000000, 0.8660254037844387076, 1.000000000000000000, 0.8660254037844387076, 1.000000000000000000, 0.8660254037844387076, 1.000000000000000000, 0.8660254037844387076, 1.000000000000000000, 0.8660254037844387076, 1.000000000000000000, 0.8660254037844387076, 1.000000000000000000, 0.8660254037844387076, 1.000000000000000000, 0.8660254037844387076, 1.000000000000000000, 0.8660254037844387076, 1.000000000000000000, 0.8660254037844387076, 1.000000000000000000, 0.8660254037844387076, 1.000000000000000000, 0.8660254037844387076, 1.000000000000000000, 0.8660254037844387076, 1.000000000000000000, 0.8660254037844387076, 1.000000000000000000, 0.8660254037844387076, 1.000000000000000000, 0.8660254037844387076, 1.000000000000000000, 0.8660254037844387076, 1.000000000000000000, 0.8660254037844387076, 1.000000000000000000, 0.8660254037844387076, 1.000000000000000000, 0.8660254037844387076, 1.000000000000000000, 0.8660254037844387076, 1.000000000000000000, 0.8660254037844387076, 1.000000000000000000, 0.8660254037844387076, 1.000000000000000000, 0.8660254037844387076, 1.000000000000000000, 0.8660254037844387076, 1.000000000000000000, 0.8660254037844387076, 1.000000000000000000, 0.8660254037844387076, 1.000000000000000000, 0.8660254037844387076, 1.000000000000000000, 0.8660254037844387076, 1.000000000000000000, 0.8660254037844387076, 1.000000000000000000, 0.8660254037844387076, 1.000000000000000000, 0.8660254037844387076, 1.000000000000000000, 0.8660254037844387076, 1.000000000000000000, 0.8660254037844387076, 1.000000000000000000, 0.8660254037844387076, 1.000000000000000000, 0.8660254037844387076, 1.000000000000000000, 0.8660254037844387076, 1.000000000000000000, 0.8660254037844387076, 1.000000000000000000, 0.8660254037844387076, 1.000000000000000000, 0.8660254037844387076, 1.000000000000000000, 0.8660254037844387076, 1.000000000000000000, 0.8660254037844387076, 1.000000000000000000, 0.8660254037844387076, 1.000000000000000000, 0.8660254037844387076, 1.000000000000000000, 0.8660254037844387076, 1.000000000000000000, 0.8660254037844387076, 1.000000000000000000, 0.8660254037844387076, 1.000000000000000000, 0.8660254037844387076, 1.000000000000000000, 0.8660254037844387076, 1.000000000000000000, 0.8660254037844387076, 1.000000000000000000, 0.8660254037844387076, 1.000000000000000000, 0.8660254037844387076, 1.000000000000000000),
 ( 1.000000000000000000, 0.8660254037844387076, 1.000000000000000000, 0.8660254037844387076, 1.000000000000000000, 0.8660254037844387076, 1.000000000000000000, 0.8660254037844387076, 1.000000000000000000, 0.8660254037844387076, 1.000000000000000000, 0.8660254037844387076, 1.000000000000000000, 0.8660254037844387076, 1.000000000000000000, 0.8660254037844387076, 1.000000000000000000, 0.8660254037844387076, 1.000000000000000000, 0.8660254037844387076, 1.000000000000000000, 0.8660254037844387076, 1.000000000000000000, 0.8660254037844387076, 1.000000000000000000, 0.8660254037844387076, 1.000000000000000000, 0.8660254037844387076, 1.000000000000000000, 0.8660254037844387076, 1.000000000000000000, 0.8660254037844387076, 1.000000000000000000, 0.8660254037844387076, 1.000000000000000000, 0.8660254037844387076, 1.000000000000000000, 0.8660254037844387076, 1.000000000000000000, 0.8660254037844387076, 1.000000000000000000, 0.8660254037844387076, 1.000000000000000000, 0.8660254037844387076, 1.000000000000000000, 0.8660254037844387076, 1.000000000000000000, 0.8660254037844387076, 1.000000000000000000, 0.8660254037844387076, 1.000000000000000000, 0.8660254037844387076, 1.000000000000000000, 0.8660254037844387076, 1.000000000000000000, 0.8660254037844387076, 1.000000000000000000, 0.8660254037844387076, 1.000000000000000000, 0.8660254037844387076, 1.000000000000000000, 0.8660254037844387076, 1.000000000000000000, 0.8660254037844387076, 1.000000000000000000, 0.8660254037844387076, 1.000000000000000000, 0.8660254037844387076, 1.000000000000000000, 0.8660254037844387076, 1.000000000000000000, 0.8660254037844387076, 1.000000000000000000, 0.8660254037844387076, 1.000000000000000000, 0.8660254037844387076, 1.000000000000000000, 0.8660254037844387076, 1.000000000000000000, 0.8660254037844387076, 1.000000000000000000, 0.8660254037844387076, 1.000000000000000000, 0.8660254037844387076, 1.000000000000000000, 0.8660254037844387076, 1.000000000000000000, 0.8660254037844387076, 1.000000000000000000, 0.8660254037844387076, 1.000000000000000000, 0.8660254037844387076, 1.000000000000000000, 0.8660254037844387076, 1.000000000000000000, 0.8660254037844387076, 1.000000000000000000, 0.8660254037844387076, 1.000000000000000000, 0.8660254037844387076, 1.000000000000000000, 0.8660254037844387076, 1.000000000000000000, 0.8660254037844387076, 1.000000000000000000, 0.8660254037844387076, 1.000000000000000000, 0.8660254037844387076, 1.000000000000000000, 0.8660254037844387076, 1.000000000000000000, 0.8660254037844387076, 1.000000000000000000, 0.8660254037844387076, 1.000000000000000000, 0.8660254037844387076, 1.000000000000000000, 0.8660254037844387076, 1.000000000000000000, 0.8660254037844387076, 1.000000000000000000, 0.8660254037844387076, 1.000000000000000000, 0.8660254037844387076, 1.000000000000000000, 0.8660254037844387076, 1.000000000000000000, 0.8660254037844387076, 1.000000000000000000, 0.8660254037844387076, 1.000000000000000000, 0.8660254037844387076, 1.000000000000000000, 0.8660254037844387076, 1.000000000000000000, 0.8660254037844387076, 1.000000000000000000, 0.8660254037844387076, 1.000000000000000000, 0.8660254037844387076, 1.000000000000000000, 0.8660254037844387076, 1.000000000000000000, 0.8660254037844387076, 1.000000000000000000, 0.8660254037844387076, 1.000000000000000000, 0.8660254037844387076, 1.000000000000000000, 0.8660254037844387076, 1.000000000000000000, 0.8660254037844387076, 1.000000000000000000, 0.8660254037844387076, 1.000000000000000000, 0.8660254037844387076, 1.000000000000000000, 0.8660254037844387076, 1.000000000000000000, 0.8660254037844387076, 1.000000000000000000, 0.8660254037844387076, 1.000000000000000000, 0.8660254037844387076, 1.000000000000000000, 0.8660254037844387076, 1.000000000000000000, 0.8660254037844387076, 1.000000000000000000, 0.8660254037844387076, 1.000000000000000000, 0.8660254037844387076, 1.000000000000000000, 0.8660254037844387076, 1.000000000000000000, 0.8660254037844387076, 1.000000000000000000, 0.8660254037844387076, 1.000000000000000000, 0.8660254037844387076, 1.000000000000000000, 0.8660254037844387076, 1.000000000000000000, 0.8660254037844387076, 1.000000000000000000, 0.8660254037844387076, 1.000000000000000000, 0.8660254037844387076, 1.000000000000000000, 0.8660254037844387076, 1.000000000000000000, 0.8660254037844387076, 1.000000000000000000, 0.8660254037844387076, 1.000000000000000000, 0.8660254037844387076, 1.000000000000000000, 0.8660254037844387076, 1.000000000000000000, 0.8660254037844387076, 1.000000000000000000, 0.8660254037844387076, 1.000000000000000000, 0.8660254037844387076, 1.000000000000000000, 0.8660254037844387076, 1.000000000000000000, 0.8660254037844387076, 1.000000000000000000, 0.8660254037844387076, 1.000000000000000000, 0.8660254037844387076, 1.000000000000000000, 0.8660254037844387076, 1.000000000000000000, 0.8660254037844387076, 1.000000000000000000, 0.8660254037844387076, 1.000000000000000000, 0.8660254037844387076, 1.000000000000000000, 0.8660254037844387076, 1.000000000000000000, 0.8660254037844387076, 1.000000000000000000, 0.8660254037844387076, 1.000000000000000000, 0.8660254037844387076, 1.000000000000000000, 0.8660254037844387076, 1.000000000000000000, 0.8660254037844387076, 1.000000000000000000, 0.8660254037844387076, 1.000000000000000000, 0.8660254037844387076, 1.000000000000000000, 0.8660254037844387076, 1.000000000000000000, 0.8660254037844387076, 1.000000000000000000, 0.8660254037844387076, 1.000000000000000000, 0.8660254037844387076, 1.000000000000000000, 0.8660254037844387076, 1.000000000000000000, 0.8660254037844387076, 1.000000000000000000, 0.8660254037844387076, 1.000000000000000000, 0.8660254037844387076, 1.000000000000000000, 0.8660254037844387076, 1.000000000000000000, 0.8660254037844387076, 1.000000000000000000, 0.8660254037844387076, 1.000000000000000000, 0.8660254037844387076, 1.000000000000000000, 0.8660254037844387076, 1.000000000000000000, 0.8660254037844387076, 1.000000000000000000, 0.8660254037844387076, 1.000000000000000000, 0.8660254037844387076, 1.000000000000000000, 0.8660254037844387076, 1.000000000000000000, 0.8660254037844387076, 1.000000000000000000, 0.8660254037844387076, 1.000000000000000000, 0.8660254037844387076, 1.000000000000000000, 0.8660254037844387076, 1.000000000000000000, 0.8660254037844387076, 1.000000000000000000, 0.8660254037844387076, 1.000000000000000000, 0.8660254037844387076, 1.000000000000000000, 0.8660254037844387076, 1.000000000000000000, 0.8660254037844387076, 1.000000000000000000, 0.8660254037844387076, 1.000000000000000000, 0.8660254037844387076, 1.000000000000000000, 0.8660254037844387076, 1.000000000000000000, 0.8660254037844387076, 1.000000000000000000, 0.8660254037844387076, 1.000000000000000000, 0.8660254037844387076, 1.000000000000000000, 0.8660254037844387076, 1.000000000000000000, 0.8660254037844387076, 1.000000000000000000, 0.8660254037844387076, 1.000000000000000000, 0.8660254037844387076, 1.000000000000000000, 0.8660254037844387076, 1.000000000000000000, 0.8660254037844387076, 1.000000000000000000, 0.8660254037844387076, 1.000000000000000000, 0.8660254037844387076, 1.000000000000000000, 0.8660254037844387076, 1.000000000000000000, 0.8660254037844387076, 1.000000000000000000, 0.8660254037844387076, 1.000000000000000000, 0.8660254037844387076, 1.000000000000000000, 0.8660254037844387076, 1.000000000000000000, 0.8660254037844387076, 1.000000000000000000, 0.8660254037844387076, 1.000000000000000000, 0.8660254037844387076, 1.000000000000000000, 0.8660254037844387076, 1.000000000000000000, 0.8660254037844387076, 1.000000000000000000) ) ) 
 REPRESENTATION_ITEM ( '' )  SURFACE ( )  );
#158061=CARTESIAN_POINT ( 'NONE',  ( -9.398826802771548472, 11.98838390803207865, -1.599625672291263179 ) ) ;
#158062=CARTESIAN_POINT ( 'NONE',  ( 6.591235234537977661, 10.84152487360300299, 0.7998128361456462443 ) ) ;
#158064=CARTESIAN_POINT ( 'NONE',  ( -4.284013352238274841, 4.100363120473813794, -0.7216878364870207285 ) ) ;
#158066=CARTESIAN_POINT ( 'NONE',  ( -5.320367241134011493, 6.379272830146158313, -1.120692317505559643 ) ) ;
#158073=CARTESIAN_POINT ( 'NONE',  ( 3.708318708537623021, 4.285125567170706695, -1.199719254218446718 ) ) ;
#158078=CARTESIAN_POINT ( 'NONE',  ( 3.511198596259283544, 6.271927390929313617, 2.420000000000010587 ) ) ;
#158092=CARTESIAN_POINT ( 'NONE',  ( -3.100010679019018500, 6.768429558830820980, 1.040834085586084257E-14 ) ) ;
#158093=CARTESIAN_POINT ( 'NONE',  ( 5.056828107772846082, 6.922718763866881453, -1.443375672974051449 ) ) ;
#158094=CARTESIAN_POINT ( 'NONE',  ( -1.500000000000011324, 3.920833333333357817, 0.8660254037844403729 ) ) ;
#158100=CARTESIAN_POINT ( 'NONE',  ( 1.364683531249988535, 4.363541667008090208, 0.7879004041258500513 ) ) ;
#158103=CARTESIAN_POINT ( 'NONE',  ( -2.480778921620681921, 5.838066475291996404, 1.040834085586084257E-14 ) ) ;
#158108=CARTESIAN_POINT ( 'NONE',  ( 3.520313441042647540, 7.258782781191745137, 0.7998128361456321445 ) ) ;
#158110=DIRECTION ( 'NONE',  ( -5.578564026256490882E-16, -1.000000000000000000, -9.066213480720158442E-32 ) ) ;
#158111=CARTESIAN_POINT ( 'NONE',  ( 8.717529583462633624, 13.11427558077437894, 0.7216878364870438212 ) ) ;
#158113=CARTESIAN_POINT ( 'NONE',  ( -1.364683531250014514, 1.301041667008083325, -0.7879004041258289570 ) ) ;
#158116=CARTESIAN_POINT ( 'NONE',  ( -8.158255747121117452, 10.54105100977322174, 1.599625672291295375 ) ) ;
#158117=CARTESIAN_POINT ( 'NONE',  ( -5.300874872818844175, 7.207439989753867238, 1.443375672974064550 ) ) ;
#158121=ORIENTED_EDGE ( 'NONE', *, *, #41574, .F. ) ;
#158122=CARTESIAN_POINT ( 'NONE',  ( 1.499999999999985123, -1.172916665983846363, -0.8660254037844323793 ) ) ;
#158130=CARTESIAN_POINT ( 'NONE',  ( -3.755245360860919757, 7.324943987738961049, -0.7216878364870257245 ) ) ;
#158135=CARTESIAN_POINT ( 'NONE',  ( -4.975479186090865369, 6.827811688571220117, 1.443375672974064550 ) ) ;
#158137=CARTESIAN_POINT ( 'NONE',  ( 9.236128959407556849, 11.79856975744075598, -1.599625672291262513 ) ) ;
#158145=CARTESIAN_POINT ( 'NONE',  ( -3.928111819657352566, 5.605883094398769195, 1.599625672291267398 ) ) ;
#158146=CARTESIAN_POINT ( 'NONE',  ( -4.976767969047747542, 6.813382189656114640, 1.452644713377107877 ) ) ;
#158149=ORIENTED_EDGE ( 'NONE', *, *, #116619, .F. ) ;
#158151=CARTESIAN_POINT ( 'NONE',  ( 8.432808358020016826, 10.86136238915529084, 1.443375672974076540 ) ) ;
#158152=CARTESIAN_POINT ( 'NONE',  ( 7.332262146892202459, 7.448727347662698506, -0.7998128361456281477 ) ) ;
#158157=CARTESIAN_POINT ( 'NONE',  ( 5.030238685870051185, 5.827365540725222282, -1.199719254218452047 ) ) ;
#158159=CARTESIAN_POINT ( 'NONE',  ( 0.006158830626129450057, 7.078243236992583398, -2.121324627965403220 ) ) ;
#158168=CARTESIAN_POINT ( 'NONE',  ( -6.307567778855718288, 8.381915046796901692, -1.599625672291263179 ) ) ;
#158169=AXIS2_PLACEMENT_3D ( 'NONE', #184511, #137928, #4674 ) ;
#158174=CARTESIAN_POINT ( 'NONE',  ( -1.001543065824772872E-14, 4.571875000341418804, 1.575800808251672791 ) ) ;
#158175=CARTESIAN_POINT ( 'NONE',  ( 8.229436053370669413, 10.62409470039771442, 1.443375672974076540 ) ) ;
#158176=CARTESIAN_POINT ( 'NONE',  ( -6.521635583373313061, 7.567328587812373719, -1.199719254218446718 ) ) ;
#158179=CARTESIAN_POINT ( 'NONE',  ( 5.626797444871351139, 6.523350759560078593, 1.199719254218462483 ) ) ;
#158180=CARTESIAN_POINT ( 'NONE',  ( -6.250472511100020334, 7.250971670160158311, 1.199719254218450271 ) ) ;
#158186=EDGE_CURVE ( 'NONE', #160603, #170224, #146541, .T. ) ;
#158188=CARTESIAN_POINT ( 'NONE',  ( 7.131225611108100715, 7.422110755822004968, 0.7216878364870317197 ) ) ;
#158190=CARTESIAN_POINT ( 'NONE',  ( 6.385527161912102123, 9.433236874664039817, -1.082531754730537976 ) ) ;
#158191=CARTESIAN_POINT ( 'NONE',  ( -1.402160292154681736E-14, 1.509375000341420359, -1.575800808251659024 ) ) ;
#158193=CARTESIAN_POINT ( 'NONE',  ( 4.921246571636183731, 7.724909519342112674, -1.082531754730549078 ) ) ;
#158198=CARTESIAN_POINT ( 'NONE',  ( 1.364683531249992088, 5.384375000341417916, 1.214306433183764966E-14 ) ) ;
#158203=CARTESIAN_POINT ( 'NONE',  ( -3.999074104275988972, 7.816954204906529924, 0.3413819327131896175 ) ) ;
#158210=CARTESIAN_POINT ( 'NONE',  ( 6.277588818327314080, 7.282607361925381717, 1.199719254218462483 ) ) ;
#158213=CARTESIAN_POINT ( 'NONE',  ( 3.469446951953614189E-15, 5.167241622962441383, 1.214306433183764966E-14 ) ) ;
#158221=CARTESIAN_POINT ( 'NONE',  ( 5.341549334104200852, 5.334155099317434257, 0.7216878364870317197 ) ) ;
#158222=CARTESIAN_POINT ( 'NONE',  ( -1.402160292154681736E-14, 2.259375000341416140, -1.575800808251660134 ) ) ;
#158224=CARTESIAN_POINT ( 'NONE',  ( 8.372323551638698902, 9.726464550788689323, 1.199719254218462483 ) ) ;
#158226=CARTESIAN_POINT ( 'NONE',  ( 3.009610312849396951, 6.452363523749469643, -0.06592220986071165023 ) ) ;
#158230=CARTESIAN_POINT ( 'NONE',  ( 1.499999999999989120, 3.504166666666683749, 0.8660254037844524744 ) ) ;
#158231=CARTESIAN_POINT ( 'NONE',  ( 4.611744806942754238, 8.532119374741881757, -0.7998128361456231517 ) ) ;
#158232=CARTESIAN_POINT ( 'NONE',  ( -7.172426956829277778, 8.326585190177668849, -1.199719254218452935 ) ) ;
#158237=CARTESIAN_POINT ( 'NONE',  ( -0.6823417656250212460, 3.051041667008084879, 1.181850606188767472 ) ) ;
#158240=CARTESIAN_POINT ( 'NONE',  ( 9.083599731475988648, 10.66024977721925104, 1.082531754730549967 ) ) ;
#158245=CARTESIAN_POINT ( 'NONE',  ( -3.280709984826931436, 6.771319382366050021, 0.7216878364870010776 ) ) ;
#158246=CARTESIAN_POINT ( 'NONE',  ( 0.7499999999999902300, 2.014583334016148530, 1.299038105676669330 ) ) ;
#158250=CARTESIAN_POINT ( 'NONE',  ( -4.720210035852093533, 8.658662141802762946, -0.7998128361456281477 ) ) ;
#158251=CARTESIAN_POINT ( 'NONE',  ( -4.121315508874280553, 3.910548969882488901, -0.7216878364870207285 ) ) ;
#158257=ORIENTED_EDGE ( 'NONE', *, *, #125247, .F. ) ;
#158259=CARTESIAN_POINT ( 'NONE',  ( 5.449487677688982679, 8.445153826357429949, -1.199719254218446718 ) ) ;
#158263=CARTESIAN_POINT ( 'NONE',  ( 5.250031796989762967, 7.148123067953287446, 1.599625672291267398 ) ) ;
#158268=CARTESIAN_POINT ( 'NONE',  ( 4.029797971759831121, 5.724516938518342535, -1.599625672291255185 ) ) ;
#158273=CARTESIAN_POINT ( 'NONE',  ( 5.886424920137334205, 5.980649323864647648, 0.1385726864747312270 ) ) ;
#158282=CARTESIAN_POINT ( 'NONE',  ( 4.175484721775176489, 3.976419294354625933, -0.06592222766770190756 ) ) ;
#158283=CARTESIAN_POINT ( 'NONE',  ( 6.805829924380105034, 9.923590097543378619, 1.082531754730558626 ) ) ;
#158285=CARTESIAN_POINT ( 'NONE',  ( -3.958090780185743451, 6.705190779270287393, -1.199719254218452047 ) ) ;
#158288=CARTESIAN_POINT ( 'NONE',  ( 7.202405917357655341, 9.425892875049191488, 1.599625672291281386 ) ) ;
#158290=CARTESIAN_POINT ( 'NONE',  ( -4.880045225915050189, 7.780804299287790826, 1.199719254218464037 ) ) ;
#158302=CARTESIAN_POINT ( 'NONE',  ( 4.053833101416107532, 3.984115073677586327, -0.7711264060391578301 ) ) ;
#158303=CARTESIAN_POINT ( 'NONE',  ( -4.822949958159302497, 6.649860922651058992, -1.599625672291256295 ) ) ;
#158306=CARTESIAN_POINT ( 'NONE',  ( 4.853455804012228647, 4.764712647543454693, 0.7216878364870317197 ) ) ;
#158311=CARTESIAN_POINT ( 'NONE',  ( -4.776550190716183586, 4.467063398790632966, 1.214306433183764966E-14 ) ) ;
#158315=CARTESIAN_POINT ( 'NONE',  ( 9.185812768458653466, 10.67553530374532045, 1.199719254218453823 ) ) ;
#158320=CARTESIAN_POINT ( 'NONE',  ( -5.703176172842872482, 9.805455968292021041, 0.000000000000000000 ) ) ;
#158321=CARTESIAN_POINT ( 'NONE',  ( 5.660692828905515839, 6.562895374266609849, -1.199719254218445830 ) ) ;
#158323=CARTESIAN_POINT ( 'NONE',  ( 5.359550796103802917, 5.147230771742885125, -0.7998128361456231517 ) ) ;
#158326=CARTESIAN_POINT ( 'NONE',  ( -1.364683531250012516, 3.301041667008084879, -0.7879004041258289570 ) ) ;
#158329=CARTESIAN_POINT ( 'NONE',  ( 6.480434237652124452, 8.583592582059388576, 1.443375672974076540 ) ) ;
#158335=EDGE_LOOP ( 'NONE', ( #90129, #60065, #37568, #34809, #159151, #197934, #104206, #157397, #21283, #72479, #193094, #168699, #47442, #75523, #3401, #17685, #24735, #81097, #10393 ) ) ;
#158336=CARTESIAN_POINT ( 'NONE',  ( 7.551528372687370094, 11.75394083486988528, -0.7216878364870267237 ) ) ;
#158341=CARTESIAN_POINT ( 'NONE',  ( -9.450196763925152510, 10.98398329845622001, -1.199719254218441611 ) ) ;
#158358=CARTESIAN_POINT ( 'NONE',  ( -1.500000000000015099, 1.160416667349484898, -0.8660254037844313801 ) ) ;
#158362=ORIENTED_EDGE ( 'NONE', *, *, #148860, .T. ) ;
#158364=CARTESIAN_POINT ( 'NONE',  ( -1.500000000000015099, 0.1291666666666918539, -0.8660254037844383745 ) ) ;
#158365=CARTESIAN_POINT ( 'NONE',  ( 9.237182729612253951, 9.671134694169463586, 0.7998128361456462443 ) ) ;
#158366=CARTESIAN_POINT ( 'NONE',  ( 1.364683531249986537, -0.8864583329919110133, 0.7879004041258500513 ) ) ;
#158369=CARTESIAN_POINT ( 'NONE',  ( 3.979481780810941949, 4.601482484822914998, 1.199719254218464037 ) ) ;
#158370=CARTESIAN_POINT ( 'NONE',  ( -6.575341312947811545, 6.773579074634973551, 1.040834085586084257E-14 ) ) ;
#158371=EDGE_CURVE ( 'NONE', #109059, #46131, #32299, .T. ) ;
#158375=CARTESIAN_POINT ( 'NONE',  ( -4.720210035852093533, 8.658662141802762946, -0.7998128361456281477 ) ) ;
#158377=CARTESIAN_POINT ( 'NONE',  ( -0.7500000000000215383, 1.972916667349486453, 1.299038105676659116 ) ) ;
#158387=CARTESIAN_POINT ( 'NONE',  ( -8.371269781434001800, 11.85389961405997816, -1.199719254218446718 ) ) ;
#158388=CARTESIAN_POINT ( 'NONE',  ( 6.928380191783277908, 8.041863964290678624, 1.199719254218462483 ) ) ;
#158394=CARTESIAN_POINT ( 'NONE',  ( -7.507464373665155399, 9.781794407407920389, 1.599625672291295375 ) ) ;
#158396=CARTESIAN_POINT ( 'NONE',  ( 0.9999999999999833467, 6.468705557303653819, 4.925226524755080604 ) ) ;
#158400=CARTESIAN_POINT ( 'NONE',  ( 3.704402285031850539, 5.344888637335695414, -1.599625672291262513 ) ) ;
#158403=CARTESIAN_POINT ( 'NONE',  ( -8.616370316684697883, 10.01118577667568132, -1.199719254218446718 ) ) ;
#158430=EDGE_CURVE ( 'NONE', #6901, #53793, #44735, .T. ) ;
#158431=LINE ( 'NONE', #10032, #147797 ) ;
#158433=CARTESIAN_POINT ( 'NONE',  ( 3.036663219780971978, 6.486598156479028709, -0.7216878364870267237 ) ) ;
#158436=VERTEX_POINT ( 'NONE', #131971 ) ;
#158438=CARTESIAN_POINT ( 'NONE',  ( -9.996439331977562404, 10.55693406359564790, 0.7998128361456462443 ) ) ;
#158441=CARTESIAN_POINT ( 'NONE',  ( 8.536830278099042602, 13.11138575775759563, -0.7998128361456352531 ) ) ;
#158445=DIRECTION ( 'NONE',  ( -0.9840448990078773939, -0.1067521860439751419, 0.1423362480586335133 ) ) ;
#158449=CARTESIAN_POINT ( 'NONE',  ( 3.490040298073151526, 6.290063075088925260, 1.146788136912090250 ) ) ;
#158450=CARTESIAN_POINT ( 'NONE',  ( 1.364683531249986537, 0.4052083336747511200, -0.7879004041258309554 ) ) ;
#158453=AXIS2_PLACEMENT_3D ( 'NONE', #186207, #22629, #37841 ) ;
#158456=CARTESIAN_POINT ( 'NONE',  ( -3.405069135326500351, 7.124331091189553433, 1.040834085586084257E-14 ) ) ;
#158458=CARTESIAN_POINT ( 'NONE',  ( 1.499999999999987121, 0.2541666666666844154, 0.8660254037844524744 ) ) ;
#158460=CARTESIAN_POINT ( 'NONE',  ( 0.6823417656249882723, -0.8447916663252494907, 1.181850606188755259 ) ) ;
#158461=VECTOR ( 'NONE', #11981, 1000.000000000000000 ) ;
#158466=CARTESIAN_POINT ( 'NONE',  ( -0.6823417656250246877, -0.6989583329919113464, 1.181850606188755259 ) ) ;
#158468=CARTESIAN_POINT ( 'NONE',  ( -5.852315862593199469, 9.979452273000736895, 0.7998128361456481317 ) ) ;
#158469=CARTESIAN_POINT ( 'NONE',  ( 8.215351014876830504, 11.67199438640995801, -1.199719254218446718 ) ) ;
#158475=CARTESIAN_POINT ( 'NONE',  ( 0.6823417656249882723, 0.4052083336747516751, 1.181850606188755259 ) ) ;
#158485=CARTESIAN_POINT ( 'NONE',  ( 6.643132081016117851, 8.773406732650713025, 1.443375672974076540 ) ) ;
#158488=CARTESIAN_POINT ( 'NONE',  ( -6.389970470742427189, 6.349387058821269747, -0.7998128361456291469 ) ) ;
#158492=CARTESIAN_POINT ( 'NONE',  ( -3.898132859128961236, 4.506575409527250997, -1.199719254218452047 ) ) ;
#158493=CARTESIAN_POINT ( 'NONE',  ( 6.602457619730771832, 6.805214765881779648, 0.7216878364870317197 ) ) ;
#158494=CARTESIAN_POINT ( 'NONE',  ( -10.12757755928392456, 10.91785469536048758, 0.7216878364870438212 ) ) ;
#158499=CARTESIAN_POINT ( 'NONE',  ( 9.029367117021314115, 12.51771682229149008, -1.082531754730543083 ) ) ;
#158502=LINE ( 'NONE', #170469, #175106 ) ;
#158505=ORIENTED_EDGE ( 'NONE', *, *, #36355, .T. ) ;
#158514=CARTESIAN_POINT ( 'NONE',  ( 9.558135107509954764, 10.25350516829085379, -0.7216878364870257245 ) ) ;
#158516=CARTESIAN_POINT ( 'NONE',  ( 8.372323551638698902, 9.726464550788689323, 1.199719254218462483 ) ) ;
#158521=CARTESIAN_POINT ( 'NONE',  ( 4.853455804012222430, 5.725081861844796727, 1.082531754730560403 ) ) ;
#158523=CARTESIAN_POINT ( 'NONE',  ( -7.863365906246048809, 12.11775129068834289, -0.7216878364870267237 ) ) ;
#158527=CARTESIAN_POINT ( 'NONE',  ( -4.464712657601869417, 4.103252943490596216, 0.7998128361456341429 ) ) ;
#158537=ORIENTED_EDGE ( 'NONE', *, *, #60236, .T. ) ;
#158549=LINE ( 'NONE', #206211, #103213 ) ;
#158551=CARTESIAN_POINT ( 'NONE',  ( -6.762819695118240659, 6.784377820593065600, 0.7998128361456341429 ) ) ;
#158556=CARTESIAN_POINT ( 'NONE',  ( 4.950698647284403009, 8.927565521807144577, 1.040834085586084257E-14 ) ) ;
#158557=CARTESIAN_POINT ( 'NONE',  ( -4.816538118508267630, 5.092449105792602460, -0.9495590845017554127 ) ) ;
#158561=CARTESIAN_POINT ( 'NONE',  ( -4.436542580169821726, 6.199052314996659874, 1.599625672291267398 ) ) ;
#158565=CARTESIAN_POINT ( 'NONE',  ( -5.915435094264120508, 5.795762452929912101, 0.000000000000000000 ) ) ;
#158569=CARTESIAN_POINT ( 'NONE',  ( 8.426556166093362776, 9.789735934319136135, -1.199719254218446718 ) ) ;
#158570=CARTESIAN_POINT ( 'NONE',  ( -1.364683531250010740, 3.780208333674751398, 0.7879004041258379498 ) ) ;
#158572=CARTESIAN_POINT ( 'NONE',  ( 6.067817914410090552, 6.045155426100865981, -0.3955105627355664510 ) ) ;
#158573=CARTESIAN_POINT ( 'NONE',  ( 4.256897045010922476, 5.029096643009940415, -1.082531754730548412 ) ) ;
#158579=CARTESIAN_POINT ( 'NONE',  ( 6.982085920913413624, 8.208483664896217391, -1.082531754730543971 ) ) ;
#158580=CARTESIAN_POINT ( 'NONE',  ( -7.537443334193545397, 10.88110209227943770, -1.199719254218446718 ) ) ;
#158583=CARTESIAN_POINT ( 'NONE',  ( -7.914208982075130905, 10.25632978388623684, -1.599625672291263179 ) ) ;
#158584=CARTESIAN_POINT ( 'NONE',  ( -7.413611068574208041, 7.543634422958360730, 0.7998128361456341429 ) ) ;
#158592=CARTESIAN_POINT ( 'NONE',  ( 9.264299036839600987, 9.702770385934682551, -0.7998128361456281477 ) ) ;
#158604=ORIENTED_EDGE ( 'NONE', *, *, #8637, .F. ) ;
#158605=CARTESIAN_POINT ( 'NONE',  ( 1.499999999999990896, 5.025000000000022560, 1.214306433183764966E-14 ) ) ;
#158606=CARTESIAN_POINT ( 'NONE',  ( 4.904298879841284098, 6.744767997946721216, 1.599625672291267398 ) ) ;
#158607=CARTESIAN_POINT ( 'NONE',  ( 5.621827251160867789, 9.710548892996357040, 1.040834085586084257E-14 ) ) ;
#158608=VECTOR ( 'NONE', #131360, 1000.000000000000000 ) ;
#158612=CARTESIAN_POINT ( 'NONE',  ( 6.995644074971448134, 7.263932296995902149, -0.7216878364870257245 ) ) ;
#158614=CARTESIAN_POINT ( 'NONE',  ( -8.283668667825340393, 12.60810451253083997, 0.7216878364870458196 ) ) ;
#158617=CARTESIAN_POINT ( 'NONE',  ( 7.228468454380276853, 11.58496363008569574, 1.040834085586084257E-14 ) ) ;
#158620=CARTESIAN_POINT ( 'NONE',  ( -2.415323921528888196, 5.969628341758991930, 0.7998128361456341429 ) ) ;
#158623=CARTESIAN_POINT ( 'NONE',  ( -1.364683531250000748, 0.5093750003414208027, 0.000000000000000000 ) ) ;
#158628=CARTESIAN_POINT ( 'NONE',  ( 1.364683531249986537, -0.3447916663252443836, -0.7879004041258309554 ) ) ;
#158630=CARTESIAN_POINT ( 'NONE',  ( 8.289920859751990889, 11.75899253876431416, 1.199719254218450271 ) ) ;
#158634=CARTESIAN_POINT ( 'NONE',  ( -7.980945979938748103, 12.46285407657057220, 0.000000000000000000 ) ) ;
#158635=CARTESIAN_POINT ( 'NONE',  ( -1.580000000000022276, 6.280000000000042881, 2.500000000000011102 ) ) ;
#158639=CARTESIAN_POINT ( 'NONE',  ( 4.487912541323413329, 5.194651705420806564, 1.199719254218462483 ) ) ;
#158645=CARTESIAN_POINT ( 'NONE',  ( 7.639129486296027061, 10.99973593639901814, 1.199719254218460707 ) ) ;
#158648=CARTESIAN_POINT ( 'NONE',  ( -5.915435094264120508, 5.795762452929912101, 0.000000000000000000 ) ) ;
#158652=CARTESIAN_POINT ( 'NONE',  ( 7.938462636001388795, 9.220293482545153907, -1.199719254218441611 ) ) ;
#158654=CARTESIAN_POINT ( 'NONE',  ( 7.962716289927667113, 8.184257181204083409, -0.7998128361456291469 ) ) ;
#158655=( BOUNDED_CURVE ( )  B_SPLINE_CURVE ( 2, ( #168891, #188336, #122379, #8519, #71367 ),
 .UNSPECIFIED., .F., .T. ) 
 B_SPLINE_CURVE_WITH_KNOTS ( ( 3, 2, 3 ),
 ( 0.2851678736916871681, 0.2874999999999999778, 0.2884211393480570207 ),
 .UNSPECIFIED. ) 
 CURVE ( )  GEOMETRIC_REPRESENTATION_ITEM ( )  RATIONAL_B_SPLINE_CURVE ( ( 0.9339680269349972530, 0.9250130366848245966, 1.000000000000000000, 0.9703817746685905465, 0.9538591554679238804 ) ) 
 REPRESENTATION_ITEM ( '' )  );
#158658=CARTESIAN_POINT ( 'NONE',  ( -9.029367117021344313, 9.636609179387466639, 0.7216878364870438212 ) ) ;
#158665=CARTESIAN_POINT ( 'NONE',  ( -6.136274411746873270, 5.997031558969919018, 0.08344787587596068368 ) ) ;
#158666=CARTESIAN_POINT ( 'NONE',  ( -1.364683531250012516, 2.238541667008087988, -0.7879004041258289570 ) ) ;
#158669=CARTESIAN_POINT ( 'NONE',  ( 4.839897650398541806, 8.590371658866210680, 1.040834085586084257E-14 ) ) ;
#158684=EDGE_CURVE ( 'NONE', #140464, #123984, #194434, .T. ) ;
#158686=CARTESIAN_POINT ( 'NONE',  ( 8.422639742587595180, 10.84949900448412130, -1.599625672291268286 ) ) ;
#158690=CARTESIAN_POINT ( 'NONE',  ( -4.460796234096120472, 5.163016013655583158, 1.199719254218462483 ) ) ;
#158691=CARTESIAN_POINT ( 'NONE',  ( -5.208303565944065738, 9.228104593576741621, -0.7998128361456231517 ) ) ;
#158696=CARTESIAN_POINT ( 'NONE',  ( -1.001543065824772872E-14, 4.993750000682814161, 1.732050807568877637 ) ) ;
#158697=CARTESIAN_POINT ( 'NONE',  ( 8.925345196497941558, 9.307324238869423283, 1.040834085586084257E-14 ) ) ;
#158700=CARTESIAN_POINT ( 'NONE',  ( -8.202846631467911820, 9.528741477256060577, 1.199719254218462483 ) ) ;
#158702=CARTESIAN_POINT ( 'NONE',  ( 1.364683531249990311, 4.863541667008084879, 0.7879004041258500513 ) ) ;
#158709=CARTESIAN_POINT ( 'NONE',  ( -9.192064960385334160, 9.826423329978791088, 0.7216878364870438212 ) ) ;
#158713=CARTESIAN_POINT ( 'NONE',  ( -1.364683531249997417, 3.321875000341423245, 1.214306433183764966E-14 ) ) ;
#158720=CARTESIAN_POINT ( 'NONE',  ( -1.364683531249997417, 3.759375000341423689, 1.214306433183764966E-14 ) ) ;
#158721=AXIS2_PLACEMENT_3D ( 'NONE', #193170, #8005, #74096 ) ;
#158722=CARTESIAN_POINT ( 'NONE',  ( -5.447678794592645701, 5.250046769979851646, 0.000000000000000000 ) ) ;
#158723=CARTESIAN_POINT ( 'NONE',  ( 4.937140493670735708, 8.911747675924535983, -0.7998128361456281477 ) ) ;
#158726=CARTESIAN_POINT ( 'NONE',  ( -1.201851678989727383E-14, 4.009375000341416140, -1.575800808251660134 ) ) ;
#158730=CARTESIAN_POINT ( 'NONE',  ( 0.6823417656249864960, -0.5739583329919112353, -1.181850606188749264 ) ) ;
#158731=CARTESIAN_POINT ( 'NONE',  ( -5.599154252763867134, 5.634694171087028636, 0.000000000000000000 ) ) ;
#158735=CARTESIAN_POINT ( 'NONE',  ( 4.202664430556257713, 4.965825259479493603, 1.082531754730560403 ) ) ;
#158738=CARTESIAN_POINT ( 'NONE',  ( -8.012505595996376684, 12.29174759539704986, 0.000000000000000000 ) ) ;
#158743=CARTESIAN_POINT ( 'NONE',  ( -8.611400122974211868, 13.19838391011195888, 1.040834085586084257E-14 ) ) ;
#158744=CARTESIAN_POINT ( 'NONE',  ( -7.510853911846401942, 7.865010440016681592, 1.040834085586084257E-14 ) ) ;
#158746=CARTESIAN_POINT ( 'NONE',  ( -1.364683531250012516, 0.8427083336747532849, 0.7879004041258379498 ) ) ;
#158753=CARTESIAN_POINT ( 'NONE',  ( -1.364683531250014514, -0.6572916663252459379, 0.7879004041258379498 ) ) ;
#158756=CARTESIAN_POINT ( 'NONE',  ( 2.806174607904299734, 5.257325561654889512, -1.082531754730543083 ) ) ;
#158759=ORIENTED_EDGE ( 'NONE', *, *, #131446, .T. ) ;
#158760=CARTESIAN_POINT ( 'NONE',  ( 1.499999999999987566, -0.2249999999999821587, 0.000000000000000000 ) ) ;
#158761=CARTESIAN_POINT ( 'NONE',  ( 8.066738210006674237, 11.39464976410773467, 1.082531754730558626 ) ) ;
#158771=CARTESIAN_POINT ( 'NONE',  ( -3.144601563365788444, 5.756120026313656268, -1.199719254218452935 ) ) ;
#158774=CARTESIAN_POINT ( 'NONE',  ( -1.364683531250014514, 1.801041667008085767, -0.7879004041258289570 ) ) ;
#158793=CARTESIAN_POINT ( 'NONE',  ( 6.667912619822566000, 6.673652899414787676, 1.040834085586084257E-14 ) ) ;
#158801=CARTESIAN_POINT ( 'NONE',  ( 8.932124273304774320, 9.315233161810734686, 0.7998128361456462443 ) ) ;
#158804=CARTESIAN_POINT ( 'NONE',  ( 7.750457368506414646, 12.19395069656619945, 0.7998128361456462443 ) ) ;
#158818=CARTESIAN_POINT ( 'NONE',  ( -8.107412671292051343, 10.48173408797264194, 1.443375672974090751 ) ) ;
#158824=CARTESIAN_POINT ( 'NONE',  ( 5.983225862332436584, 5.874851682342960402, 0.7998128361456341429 ) ) ;
#158830=CARTESIAN_POINT ( 'NONE',  ( 3.673896439178923057, 5.309298483840612093, 1.443375672974066548 ) ) ;
#158838=CARTESIAN_POINT ( 'NONE',  ( -6.417086777969760902, 6.381022750586497594, 0.7998128361456341429 ) ) ;
#158840=CARTESIAN_POINT ( 'NONE',  ( -4.298098390732130625, 4.973201863064262263, 1.199719254218462483 ) ) ;
#158845=CARTESIAN_POINT ( 'NONE',  ( 0.1638468497727625650, 7.035416012003046227, -1.994423973928960869 ) ) ;
#158846=CARTESIAN_POINT ( 'NONE',  ( 0.6823417656249917140, 3.405208333674754506, 1.181850606188765695 ) ) ;
#158848=CARTESIAN_POINT ( 'NONE',  ( 6.094553744542824170, 7.069066442510145265, 1.199719254218462483 ) ) ;
#158850=CARTESIAN_POINT ( 'NONE',  ( 1.555203039002687859, 8.692270211428450466, 2.503634413632319866 ) ) ;
#158862=CARTESIAN_POINT ( 'NONE',  ( -1.201851678989727383E-14, 1.384375000341419693, 1.575800808251672791 ) ) ;
#158864=CARTESIAN_POINT ( 'NONE',  ( 4.539282502477016479, 4.190251095844947926, 0.7998128361456341429 ) ) ;
#158867=CARTESIAN_POINT ( 'NONE',  ( -4.433153041988574294, 8.115836282387899558, 1.040834085586084257E-14 ) ) ;
#158868=CARTESIAN_POINT ( 'NONE',  ( 4.582292731738905722, 5.408724944192588424, -1.082531754730548412 ) ) ;
#158869=CARTESIAN_POINT ( 'NONE',  ( -6.141480396866151992, 9.148515648777049591, 1.082531754730548412 ) ) ;
#158871=ORIENTED_EDGE ( 'NONE', *, *, #53693, .F. ) ;
#158873=CARTESIAN_POINT ( 'NONE',  ( 6.124532705071213279, 8.168374127381657246, -1.599625672291262513 ) ) ;
#158878=CARTESIAN_POINT ( 'NONE',  ( -1.001543065824772872E-14, 5.071875000341421469, 1.575800808251672791 ) ) ;
#158882=CARTESIAN_POINT ( 'NONE',  ( 5.445571254183207088, 9.504916896522420444, -0.7998128361456281477 ) ) ;
#158886=CARTESIAN_POINT ( 'NONE',  ( -6.847031270101295419, 7.946956888995021728, -1.199719254218446718 ) ) ;
#158891=CARTESIAN_POINT ( 'NONE',  ( 7.377608144130607393, 11.75895993479440982, -0.7998128361456291469 ) ) ;
#158895=CARTESIAN_POINT ( 'NONE',  ( -6.852756576703439961, 10.08230087520760954, 1.199719254218453823 ) ) ;
#158897=CARTESIAN_POINT ( 'NONE',  ( 7.307481607641395094, 8.588111966078864512, -1.082531754730537976 ) ) ;
#158898=CARTESIAN_POINT ( 'NONE',  ( 4.058723290341089474, 7.748532961531467755, 0.5319316551511514835 ) ) ;
#158899=CARTESIAN_POINT ( 'NONE',  ( -7.836249599018719536, 12.08611559892311504, 0.7216878364870478180 ) ) ;
#158904=CARTESIAN_POINT ( 'NONE',  ( 5.847644326195776010, 5.716673223516856694, -0.7998128361456281477 ) ) ;
#158906=CARTESIAN_POINT ( 'NONE',  ( 7.730120138085914583, 12.17022392774227768, 0.7998128361456462443 ) ) ;
#158907=CARTESIAN_POINT ( 'NONE',  ( -4.820845164874406841, 6.759277571458118139, 1.248045366310134741 ) ) ;
#158908=CARTESIAN_POINT ( 'NONE',  ( 4.207107738942202246, 3.802713871720993399, 1.214306433183764966E-14 ) ) ;
#158909=CARTESIAN_POINT ( 'NONE',  ( 0.6823417656249882723, 0.6760416670080898749, -1.181850606188749264 ) ) ;
#158911=CARTESIAN_POINT ( 'NONE',  ( -4.582292731738899505, 8.289832587096611860, 0.7216878364870458196 ) ) ;
#158917=CARTESIAN_POINT ( 'NONE',  ( -4.588080609115144703, 6.965600104441714180, 1.189663598451236926 ) ) ;
#158918=CARTESIAN_POINT ( 'NONE',  ( 1.364683531249986537, -0.03229166632525094088, -0.7879004041258309554 ) ) ;
#158921=CARTESIAN_POINT ( 'NONE',  ( 3.009546912553647147, 5.494593250412460606, -1.082531754730543083 ) ) ;
#158926=CARTESIAN_POINT ( 'NONE',  ( -9.300530188850304469, 9.952966096521256745, 1.040834085586084257E-14 ) ) ;
#158932=CARTESIAN_POINT ( 'NONE',  ( -7.985389288324685531, 12.26011190311341537, -0.7216878364870267237 ) ) ;
#158933=CARTESIAN_POINT ( 'NONE',  ( -1.284279953904152949, 3.171639714193937198, 0.7750000000000152323 ) ) ;
#158934=VERTEX_POINT ( 'NONE', #103334 ) ;
#158938=EDGE_LOOP ( 'NONE', ( #22763, #85506, #211362, #83451 ) ) ;
#158939=CARTESIAN_POINT ( 'NONE',  ( -6.954969613686107444, 10.09758640173367894, 1.082531754730549967 ) ) ;
#158944=CARTESIAN_POINT ( 'NONE',  ( -1.364683531249997417, 5.071875000341417916, 1.214306433183764966E-14 ) ) ;
#158945=CARTESIAN_POINT ( 'NONE',  ( 0.7499999999999920064, 4.014583334016149863, 1.299038105676669330 ) ) ;
#158946=CARTESIAN_POINT ( 'NONE',  ( 6.006184860439112150, 6.084034629330242971, -0.5924424362405518174 ) ) ;
#158952=CARTESIAN_POINT ( 'NONE',  ( -6.531277313481209212, 8.642909503859968368, 1.599625672291283607 ) ) ;
#158956=CARTESIAN_POINT ( 'NONE',  ( 4.123651276850781144, 7.962676922967908411, -0.7998128361456221525 ) ) ;
#158961=CARTESIAN_POINT ( 'NONE',  ( 7.741869408603235136, 8.990934717247309749, 1.199719254218462483 ) ) ;
#158966=ORIENTED_EDGE ( 'NONE', *, *, #195936, .F. ) ;
#158969=CARTESIAN_POINT ( 'NONE',  ( -4.772106882330223954, 8.511282429453158827, -0.7216878364870267237 ) ) ;
#158972=DIRECTION ( 'NONE',  ( 1.000000000000000000, -5.578564026256504688E-16, 0.000000000000000000 ) ) ;
#158977=CARTESIAN_POINT ( 'NONE',  ( -9.992522908471816123, 11.61669713376064372, 1.199719254218462483 ) ) ;
#158979=CARTESIAN_POINT ( 'NONE',  ( 8.585337585951586803, 11.03931315507545108, -1.599625672291255185 ) ) ;
#158980=CARTESIAN_POINT ( 'NONE',  ( -1.500000000000015099, -0.5791666666666476226, 0.8660254037844403729 ) ) ;
#158981=CARTESIAN_POINT ( 'NONE',  ( -7.828943636887387925, 11.22118577875556156, 1.199719254218453823 ) ) ;
#158985=CARTESIAN_POINT ( 'NONE',  ( 1.364683531249988535, 3.613541667008086211, 0.7879004041258500513 ) ) ;
#158986=CARTESIAN_POINT ( 'NONE',  ( 4.369805582306193870, 3.992528022312320957, 1.214306433183764966E-14 ) ) ;
#158989=CARTESIAN_POINT ( 'NONE',  ( 0.7499999999999902300, 5.066666666666684193, -1.299038105676658228 ) ) ;
#158992=CARTESIAN_POINT ( 'NONE',  ( 6.927853306458731986, 11.02631992426980112, 0.7216878364870438212 ) ) ;
#158996=CARTESIAN_POINT ( 'NONE',  ( -6.724481002698126098, 8.868313807946373473, -1.443375672974059665 ) ) ;
#158999=CARTESIAN_POINT ( 'NONE',  ( -0.6823417656250212460, 2.551041667008084435, 1.181850606188767472 ) ) ;
#159003=CARTESIAN_POINT ( 'NONE',  ( -7.182068686937172153, 9.402166106225269715, 1.599625672291283607 ) ) ;
#159004=CARTESIAN_POINT ( 'NONE',  ( -1.364683531250012516, 4.301041667008089320, -0.7879004041258300672 ) ) ;
#159009=CARTESIAN_POINT ( 'NONE',  ( 8.748035429315576650, 11.22912730566677553, -1.599625672291255185 ) ) ;
#159012=CARTESIAN_POINT ( 'NONE',  ( 1.499999999999987121, 1.045833333333352266, -0.8660254037844253849 ) ) ;
#159017=CARTESIAN_POINT ( 'NONE',  ( 9.585778300061798873, 11.14216175728232550, -1.199719254218440723 ) ) ;
#159023=CARTESIAN_POINT ( 'NONE',  ( 9.023114925094663619, 10.48572115315399245, 1.199719254218453823 ) ) ;
#159024=CARTESIAN_POINT ( 'NONE',  ( -8.306341666666730461, 12.84248237775322643, 1.040834085586084257E-14 ) ) ;
#159027=CARTESIAN_POINT ( 'NONE',  ( 0.6823417656249899377, 5.738541667008087543, -1.181850606188754593 ) ) ;
#159033=CARTESIAN_POINT ( 'NONE',  ( 1.364683531249988535, 4.405208333674754506, -0.7879004041258300672 ) ) ;
#159035=CARTESIAN_POINT ( 'NONE',  ( -6.778713617152821058, 7.971215977175476475, 1.082531754730549967 ) ) ;
#159041=CARTESIAN_POINT ( 'NONE',  ( 3.379006598303866848, 4.965260336153046516, -1.599625672291262513 ) ) ;
#159043=VERTEX_POINT ( 'NONE', #134794 ) ;
#159044=CARTESIAN_POINT ( 'NONE',  ( 8.860417081730671995, 10.29590700256267155, 1.199719254218453823 ) ) ;
#159051=CARTESIAN_POINT ( 'NONE',  ( -9.806625181386236179, 10.33548422123910449, -0.7998128361456291469 ) ) ;
#159052=CARTESIAN_POINT ( 'NONE',  ( 5.361359679200154105, 8.342337828120466980, 1.199719254218462483 ) ) ;
#159053=CARTESIAN_POINT ( 'NONE',  ( 4.053524740361575063, 4.791828954252362216, -1.082531754730543083 ) ) ;
#159055=CARTESIAN_POINT ( 'NONE',  ( 5.345992642490140057, 5.131412925860272090, 1.040834085586084257E-14 ) ) ;
#159063=CARTESIAN_POINT ( 'NONE',  ( -5.666945020832185875, 7.634521829102760115, 1.443375672974064550 ) ) ;
#159064=CARTESIAN_POINT ( 'NONE',  ( 4.196412238629597447, 4.854568018944682706, -1.199719254218452047 ) ) ;
#159067=CARTESIAN_POINT ( 'NONE',  ( -6.832419346282942563, 10.05857410638369487, 1.199719254218453823 ) ) ;
#159072=CARTESIAN_POINT ( 'NONE',  ( -7.147119532698295252, 11.49005655479003174, 0.000000000000000000 ) ) ;
#159076=CARTESIAN_POINT ( 'NONE',  ( 6.598014311344812199, 10.84943379654430906, 1.040834085586084257E-14 ) ) ;
#159077=CARTESIAN_POINT ( 'NONE',  ( 5.983225862332436584, 5.874851682342960402, 0.7998128361456341429 ) ) ;
#159088=CARTESIAN_POINT ( 'NONE',  ( -7.320512876374914768, 10.62801655815766999, 1.199719254218453823 ) ) ;
#159092=CARTESIAN_POINT ( 'NONE',  ( 6.155038550924144758, 8.203964280876741455, 1.443375672974076540 ) ) ;
#159095=CARTESIAN_POINT ( 'NONE',  ( -6.575868197828002693, 7.630599971342813426, 1.199719254218450271 ) ) ;
#159098=CARTESIAN_POINT ( 'NONE',  ( -1.500000000000016209, 5.452083334016153415, 0.8660254037844375974 ) ) ;
#159106=CARTESIAN_POINT ( 'NONE',  ( 7.914208982075123799, 10.25632978388623684, -1.599625672291262513 ) ) ;
#159108=EDGE_CURVE ( 'NONE', #161726, #67975, #120480, .T. ) ;
#159112=CARTESIAN_POINT ( 'NONE',  ( -4.965152591087599099, 6.642004417359813395, -1.244917454897740861 ) ) ;
#159117=ORIENTED_EDGE ( 'NONE', *, *, #84646, .T. ) ;
#159119=CARTESIAN_POINT ( 'NONE',  ( 3.225950485047770933, 5.851027101609320269, 1.199719254218450271 ) ) ;
#159137=CARTESIAN_POINT ( 'NONE',  ( -4.786191920824102830, 5.542644314838231168, 1.199719254218462483 ) ) ;
#159138=CARTESIAN_POINT ( 'NONE',  ( 4.324687812634874895, 7.989293514808604613, 0.7216878364870317197 ) ) ;
#159139=CARTESIAN_POINT ( 'NONE',  ( -1.499999999999997780, 3.400000000000021227, 1.214306433183764966E-14 ) ) ;
#159141=CARTESIAN_POINT ( 'NONE',  ( -4.761938266897808525, 6.578680616179308771, 1.599625672291267398 ) ) ;
#159142=DIRECTION ( 'NONE',  ( 0.6507913734559640506, -0.7592566023653004592, 0.000000000000000000 ) ) ;
#159146=CARTESIAN_POINT ( 'NONE',  ( 0.6823417656249917140, 4.092708333674755394, 1.181850606188765695 ) ) ;
#159149=CARTESIAN_POINT ( 'NONE',  ( -2.982430605326328532, 5.462957558647244305, -1.082531754730543971 ) ) ;
#159151=ORIENTED_EDGE ( 'NONE', *, *, #95454, .T. ) ;
#159154=CARTESIAN_POINT ( 'NONE',  ( 4.867540842506059562, 5.637551390133895168, -1.199719254218452047 ) ) ;
#159160=CARTESIAN_POINT ( 'NONE',  ( 1.364683531249988757, 1.946875000341415030, 0.000000000000000000 ) ) ;
#159161=DIRECTION ( 'NONE',  ( 1.000000000000000000, -7.387867266669436732E-31, 0.000000000000000000 ) ) ;
#159163=CARTESIAN_POINT ( 'NONE',  ( -2.676845263694313637, 5.210404343363602919, -1.199719254218446718 ) ) ;
#159164=CARTESIAN_POINT ( 'NONE',  ( -4.717874267431199087, 8.448011045404303587, 1.040834085586084257E-14 ) ) ;
#159168=CARTESIAN_POINT ( 'NONE',  ( -1.201851678989727383E-14, 4.446875000341417916, -1.575800808251660134 ) ) ;
#159176=CARTESIAN_POINT ( 'NONE',  ( -5.653386866774179786, 8.579073197003079798, 1.082531754730548412 ) ) ;
#159179=CARTESIAN_POINT ( 'NONE',  ( -4.514501963226242864, 7.250374142863800664, 1.082531754730560403 ) ) ;
#159182=CARTESIAN_POINT ( 'NONE',  ( 8.563946585326370098, 13.14302144952281814, 0.7998128361456462443 ) ) ;
#159187=CARTESIAN_POINT ( 'NONE',  ( 1.501062075862685363, 8.754928401006200289, -2.503798761944566742 ) ) ;
#159190=CARTESIAN_POINT ( 'NONE',  ( 4.119726892546750285, 7.639700203672255441, -0.7297710838231908914 ) ) ;
#159193=CARTESIAN_POINT ( 'NONE',  ( -3.405069135326500351, 7.124331091189553433, 1.040834085586084257E-14 ) ) ;
#159196=CARTESIAN_POINT ( 'NONE',  ( -1.402160292154681736E-14, 0.4625000000000214495, 1.732050807568877637 ) ) ;
#159198=CARTESIAN_POINT ( 'NONE',  ( 9.585251415181632595, 10.28514086057449184, 0.000000000000000000 ) ) ;
#159199=CARTESIAN_POINT ( 'NONE',  ( 7.202405917357655341, 9.425892875049191488, 1.599625672291281386 ) ) ;
#159204=CARTESIAN_POINT ( 'NONE',  ( 5.054492339796319733, 4.791329239384148231, -0.7998128361456211532 ) ) ;
#159206=ORIENTED_EDGE ( 'NONE', *, *, #101605, .F. ) ;
#159212=CARTESIAN_POINT ( 'NONE',  ( -5.575427483717760424, 7.527751369135936343, 1.599625672291269396 ) ) ;
#159219=CARTESIAN_POINT ( 'NONE',  ( 0.6823417656249899377, 3.092708333674754062, 1.181850606188765695 ) ) ;
#159220=CARTESIAN_POINT ( 'NONE',  ( 8.880227426826641235, 10.42298208846167284, 1.082531754730549967 ) ) ;
#159221=CARTESIAN_POINT ( 'NONE',  ( -4.900382456335551140, 7.804531068111707270, 1.199719254218464037 ) ) ;
#159223=CARTESIAN_POINT ( 'NONE',  ( 3.845709127770629010, 7.638411082374393146, 0.7998128361456321445 ) ) ;
#159224=CARTESIAN_POINT ( 'NONE',  ( -3.927058049452637700, 7.733318157670055371, -0.7998128361456281477 ) ) ;
#159230=CARTESIAN_POINT ( 'NONE',  ( 5.341549334104176872, 9.175631956522799726, 0.7216878364870438212 ) ) ;
#159233=CARTESIAN_POINT ( 'NONE',  ( -1.201851678989727383E-14, 2.634375000341417916, 1.575800808251672791 ) ) ;
#159235=CARTESIAN_POINT ( 'NONE',  ( 6.927853306458752414, 7.184843067064434763, 0.7216878364870317197 ) ) ;
#159237=CARTESIAN_POINT ( 'NONE',  ( -3.633221978782290140, 6.222214161012547429, -1.082531754730549967 ) ) ;
#159245=CARTESIAN_POINT ( 'NONE',  ( -4.055257346293188014, 7.741894102302186553, 0.6119906029944787162 ) ) ;
#159252=CARTESIAN_POINT ( 'NONE',  ( 5.982172092127724383, 8.002286745614243912, -1.599625672291262513 ) ) ;
#159255=CARTESIAN_POINT ( 'NONE',  ( 2.683624340501134853, 5.218313266304903664, -1.199719254218446718 ) ) ;
#159263=CARTESIAN_POINT ( 'NONE',  ( 3.497640442645619796, 6.064035702186436616, -1.082531754730543083 ) ) ;
#159265=CARTESIAN_POINT ( 'NONE',  ( 0.6823417656249899377, 2.655208333674753618, 1.181850606188767472 ) ) ;
#159267=CARTESIAN_POINT ( 'NONE',  ( 9.088043039861931405, 9.497138389460751284, 1.040834085586084257E-14 ) ) ;
#159270=CARTESIAN_POINT ( 'NONE',  ( -5.416646063859567484, 6.278174148379618735, 1.199719254218450271 ) ) ;
#159275=CARTESIAN_POINT ( 'NONE',  ( 1.499999999999989120, 2.525000000000020339, 1.214306433183764966E-14 ) ) ;
#159276=CARTESIAN_POINT ( 'NONE',  ( 4.462605117192430804, 8.358123070033169455, 1.040834085586084257E-14 ) ) ;
#159277=CARTESIAN_POINT ( 'NONE',  ( -7.888146445052511169, 8.097259028849730811, 1.040834085586084257E-14 ) ) ;
#159281=CARTESIAN_POINT ( 'NONE',  ( 1.364683531249988535, 3.113541667008083991, 0.7879004041258500513 ) ) ;
#159283=CARTESIAN_POINT ( 'NONE',  ( 4.304877467538922531, 4.981110786005563007, 1.199719254218464037 ) ) ;
#159289=CARTESIAN_POINT ( 'NONE',  ( 1.499999999999989120, 1.306250000682816825, 0.000000000000000000 ) ) ;
#159292=CARTESIAN_POINT ( 'NONE',  ( -7.152089726408780379, 8.302858421353754181, -1.199719254218446718 ) ) ;
#159293=CARTESIAN_POINT ( 'NONE',  ( -4.460269349215930212, 4.305995116947750390, 1.214306433183764966E-14 ) ) ;
#159301=CARTESIAN_POINT ( 'NONE',  ( 6.094553744542824170, 7.069066442510145265, 1.199719254218462483 ) ) ;
#159305=CARTESIAN_POINT ( 'NONE',  ( 6.817052309572890323, 6.847649204123507083, 0.7998128361456341429 ) ) ;
#159308=( BOUNDED_SURFACE ( )  B_SPLINE_SURFACE ( 1, 2, ( 
 ( #138439, #155747, #89697, #187162, #168783, #87545, #104873, #7332, #38791, #73409, #154677, #204457, #58241, #4122, #6262, #202325, #70191, #8410, #123338, #105975, #189302, #186091, #5185, #56111, #24655, #122269, #139512, #188226, #206611, #39866, #205539, #190355, #57176, #40942, #107048, #173074, #90762, #91836, #129728, #157894, #44139, #77683, #9486, #141669, #162153, #43087, #143804, #207680, #75559, #128664, #161078, #59300, #144867, #211937, #93967, #96098, #92899, #78743, #30014, #61437, #63572, #127603, #126526, #110260, #13740, #193569, #42017, #79813, #145925, #125458, #191420, #108126, #109200, #45212, #175212, #26794, #194632, #209801, #210874, #178402, #158945, #111327, #10540, #62499, #46274, #76614, #142727, #208736, #176269, #192487, #60363, #177330, #28944, #27871, #174153, #160008, #25726, #12668, #11609, #95028, #112390, #151230, #114525, #35317, #150166, #197824, #84078, #65667, #101395, #166397, #179466, #2799, #196770, #17988, #50518, #133941, #117719, #167469, #1734, #19065, #212999, #195712, #99282, #67791, #199948, #149079, #165330, #47347, #49456, #131815, #48413, #130775, #51595, #97163, #183709, #68871, #180520, #163218, #85143, #33199, #146982, #113461, #657, #31091, #14801, #80892, #32141, #64636, #98221, #164273, #116641, #15863, #81948, #16923, #148031, #214041, #182636, #115574, #181570, #83003, #66724, #132867, #198871, #34258, #100330, #171727, #152286, #122003, #185828, #37459, #3860, #103538, #118776, #202057, #53717, #69933, #54783, #136045, #119850, #169598, #93443, #21180, #175750, #87283, #159482, #23326, #27341, #43624, #153352, #11082, #4922, #134991, #201001, #109739, #104613, #70999, #7068, #52646, #137112, #86215, #203141, #120930, #205277, #22247, #186903, #38535, #184760, #55847, #170660, #59846, #36387, #89434, #102465, #88357, #168531, #154422, #155485, #139246, #6000, #72071, #20129, #138181, #204191, #187969, #39597, #73141, #105700, #125998, #191957, #144351, #44691, #131314, #129215, #28419, #77158, #96647, #31630, #32679, #181061, #61992, #115065, #81435, #48945, #212481, #128148, #97707, #112940, #147514, #98758, #64124, #209271, #111876, #213535, #94512, #145418, #127075, #130267, #46827, #114013, #160550, #196256, #194108, #45757, #12158, #177880, #60916, #210353, #29493, #78229, #211418, #95585, #161634, #13228, #164814, #79302, #143280, #63050, #193037, #180008, #110799, #197306, #195191, #176802, #178953, #30567, #162701, #14273, #80368, #146464, #163765, #47903, #15343, #65158, #99817, #67278, #86760, #118260, #68351, #84623, #142, #151776, #33738, #85688, #182109, #119325, #20670, #17468, #199423, #83552, #18547, #100870, #165882, #168012, #3348, #150715, #82486, #183190, #148573, #135524, #202617, #104087, #186379, #38015, #149634, #70478, #185311, #2275, #36933, #166957, #136593, #201548, #66208, #16406, #1215, #53194, #69417, #169071 ),
 ( #103016, #54267, #132355, #198358, #49998, #133417, #120403, #152829, #134484, #4407, #200486, #116121, #51067, #117190, #34796, #52132, #184244, #35871, #101946, #19616, #75840, #58525, #207959, #187452, #170136, #73706, #124680, #174435, #123623, #139803, #21721, #23874, #40151, #171204, #105165, #206894, #71553, #92122, #125742, #22797, #137661, #9766, #7620, #121481, #87832, #189587, #190638, #191703, #59585, #154966, #43362, #26011, #141947, #91048, #6551, #42298, #205831, #158174, #153903, #157109, #5473, #204746, #203682, #39080, #89980, #55330, #8698, #57463, #108412, #88912, #74782, #72629, #138728, #56397, #122558, #188519, #106264, #172286, #156030, #41233, #107340, #173362, #24944, #140881, #160290, #147250, #28155, #131057, #146200, #213282, #15080, #11893, #64908, #210085, #197045, #175492, #81170, #79030, #110543, #195998, #109484, #77967, #60648, #192767, #144089, #179747, #211152, #161370, #177620, #93186, #30297, #126811, #178684, #44426, #212214, #113743, #176544, #61724, #209012, #27079, #94251, #62776, #127892, #143017, #47632, #14010, #193843, #63851, #159219, #12952, #163497, #45492, #130007, #97441, #128938, #10819, #194916, #111609, #29229, #76893, #46554, #95321, #145146, #112674, #96382, #162434, #80096, #31365, #51878, #132094, #33481, #201288, #2014, #85430, #185045, #98489, #34542, #3083, #165619, #115860, #214313, #151515, #16138, #164552, #114798, #168813, #183990, #116926, #136333, #17207, #181845, #99554, #83283, #149368, #32422, #950, #65945, #68083, #20417, #100612, #48682, #67016, #198103, #82223, #200227, #18279, #133152, #35604, #49732, #199154, #50799, #182926, #180797, #52929, #166688, #148314, #84362, #101681, #69153, #70222, #150453, #134218, #102758, #118000, #167751, #19350, #135273, #119063, #36669, #86499, #152564, #4151, #89730, #121223, #138467, #8440, #202353, #104904, #169874, #186119, #173107, #57208, #172028, #123368, #120141, #21464, #6292, #107085, #37752, #23621, #54003, #103826, #87573, #55074, #153643, #189335, #40974, #187193, #205570, #24687, #203418, #5213, #38821, #155778, #73440, #170945, #71288, #90791, #74528, #137401, #22545, #7363, #88651, #154711, #72366, #204489, #156855, #56139, #122300, #188257, #39898, #106007, #139544, #141081, #204942, #143219, #106458, #42495, #122754, #24069, #191898, #207091, #76036, #175683, #89107, #25140, #208153, #156238, #172482, #56593, #142138, #6743, #155161, #105362, #159415, #174631, #107537, #127011, #7815, #90172, #73908, #140001, #206022, #22989, #57659, #188716, #58719, #11016, #91242, #39267, #123818, #40353, #72821, #190835, #8892, #189778, #26207, #41429, #173569, #157302, #74971, #171399, #43560, #124869, #138925, #108603, #92324, #59783, #60848, #158366, #9959, #93379, #125940, #109680, #27272, #77092, #209208, #177812, #195121, #31562, #161567, #179938, #13155, #162628, #148505, #44622, #145350 ) ),
 .UNSPECIFIED., .F., .F., .T. ) 
 B_SPLINE_SURFACE_WITH_KNOTS ( ( 2, 2 ),
 ( 3, 2, 2, 2, 2, 2, 2, 2, 2, 2, 2, 2, 2, 2, 2, 2, 2, 2, 2, 2, 2, 2, 2, 2, 2, 2, 2, 2, 2, 2, 2, 2, 2, 2, 2, 2, 2, 2, 2, 2, 2, 2, 2, 2, 2, 2, 2, 2, 2, 2, 2, 2, 2, 2, 2, 2, 2, 2, 2, 2, 2, 2, 2, 2, 2, 2, 2, 2, 2, 2, 2, 2, 2, 2, 2, 2, 2, 2, 2, 2, 2, 2, 2, 2, 2, 2, 2, 2, 2, 2, 2, 2, 2, 2, 2, 2, 2, 2, 2, 2, 2, 2, 2, 2, 2, 2, 2, 2, 2, 2, 2, 2, 2, 2, 2, 2, 2, 2, 2, 2, 2, 2, 2, 2, 2, 2, 2, 2, 2, 2, 2, 2, 2, 2, 2, 2, 2, 2, 2, 2, 2, 2, 2, 2, 2, 2, 2, 2, 2, 2, 2, 2, 2, 2, 2, 2, 2, 2, 2, 2, 2, 2, 2, 2, 2, 2, 2, 2, 3 ),
 ( 0.000000000000000000, 1.000000000000000000 ),
 ( 0.000000000000000000, 0.005952380952380952051, 0.01190476190476190410, 0.01785714285714285615, 0.02380952380952380820, 0.02976190476190476025, 0.03571428571428571230, 0.04166666666666666435, 0.04761904761904761640, 0.05357142857142856845, 0.05952380952380952051, 0.06547619047619047949, 0.07142857142857142461, 0.07738095238095238360, 0.08333333333333332871, 0.08928571428571428770, 0.09523809523809523281, 0.1011904761904761918, 0.1071428571428571369, 0.1130952380952380959, 0.1190476190476190410, 0.1250000000000000000, 0.1309523809523809590, 0.1369047619047619180, 0.1428571428571428492, 0.1488095238095238082, 0.1547619047619047672, 0.1607142857142857262, 0.1666666666666666574, 0.1726190476190476164, 0.1785714285714285754, 0.1845238095238095344, 0.1904761904761904656, 0.1964285714285714246, 0.2023809523809523836, 0.2083333333333333426, 0.2142857142857142738, 0.2202380952380952328, 0.2261904761904761918, 0.2321428571428571508, 0.2380952380952380820, 0.2440476190476190410, 0.2500000000000000000, 0.2559523809523809312, 0.2619047619047619180, 0.2678571428571428492, 0.2738095238095238360, 0.2797619047619047672, 0.2857142857142856984, 0.2916666666666666852, 0.2976190476190476164, 0.3035714285714285476, 0.3095238095238095344, 0.3154761904761904656, 0.3214285714285714524, 0.3273809523809523836, 0.3333333333333333148, 0.3392857142857143016, 0.3452380952380952328, 0.3511904761904761640, 0.3571428571428571508, 0.3630952380952380820, 0.3690476190476190688, 0.3750000000000000000, 0.3809523809523809312, 0.3869047619047619180, 0.3928571428571428492, 0.3988095238095238360, 0.4047619047619047672, 0.4107142857142856984, 0.4166666666666666852, 0.4226190476190476164, 0.4285714285714285476, 0.4345238095238095344, 0.4404761904761904656, 0.4464285714285714524, 0.4523809523809523836, 0.4583333333333333148, 0.4642857142857143016, 0.4702380952380952328, 0.4761904761904761640, 0.4821428571428571508, 0.4880952380952380820, 0.4940476190476190688, 0.5000000000000000000, 0.5059523809523809312, 0.5119047619047618625, 0.5178571428571429047, 0.5238095238095238360, 0.5297619047619047672, 0.5357142857142856984, 0.5416666666666666297, 0.5476190476190476719, 0.5535714285714286031, 0.5595238095238095344, 0.5654761904761904656, 0.5714285714285713969, 0.5773809523809523281, 0.5833333333333333703, 0.5892857142857143016, 0.5952380952380952328, 0.6011904761904761640, 0.6071428571428570953, 0.6130952380952381375, 0.6190476190476190688, 0.6250000000000000000, 0.6309523809523809312, 0.6369047619047618625, 0.6428571428571429047, 0.6488095238095238360, 0.6547619047619047672, 0.6607142857142856984, 0.6666666666666666297, 0.6726190476190476719, 0.6785714285714286031, 0.6845238095238095344, 0.6904761904761904656, 0.6964285714285713969, 0.7023809523809523281, 0.7083333333333333703, 0.7142857142857143016, 0.7202380952380952328, 0.7261904761904761640, 0.7321428571428570953, 0.7380952380952381375, 0.7440476190476190688, 0.7500000000000000000, 0.7559523809523809312, 0.7619047619047618625, 0.7678571428571429047, 0.7738095238095238360, 0.7797619047619047672, 0.7857142857142856984, 0.7916666666666666297, 0.7976190476190476719, 0.8035714285714286031, 0.8095238095238095344, 0.8154761904761904656, 0.8214285714285713969, 0.8273809523809523281, 0.8333333333333333703, 0.8392857142857143016, 0.8452380952380952328, 0.8511904761904761640, 0.8571428571428570953, 0.8630952380952381375, 0.8690476190476190688, 0.8750000000000000000, 0.8809523809523809312, 0.8869047619047618625, 0.8928571428571429047, 0.8988095238095238360, 0.9047619047619047672, 0.9107142857142856984, 0.9166666666666666297, 0.9226190476190476719, 0.9285714285714286031, 0.9345238095238095344, 0.9404761904761904656, 0.9464285714285713969, 0.9523809523809523281, 0.9583333333333333703, 0.9642857142857143016, 0.9702380952380952328, 0.9761904761904761640, 0.9821428571428570953, 0.9880952380952381375, 0.9940476190476190688, 1.000000000000000000 ),
 .UNSPECIFIED. ) 
 GEOMETRIC_REPRESENTATION_ITEM ( )  RATIONAL_B_SPLINE_SURFACE ( (
 ( 1.000000000000000000, 0.8660254037844387076, 1.000000000000000000, 0.8660254037844387076, 1.000000000000000000, 0.8660254037844387076, 1.000000000000000000, 0.8660254037844387076, 1.000000000000000000, 0.8660254037844387076, 1.000000000000000000, 0.8660254037844387076, 1.000000000000000000, 0.8660254037844387076, 1.000000000000000000, 0.8660254037844387076, 1.000000000000000000, 0.8660254037844387076, 1.000000000000000000, 0.8660254037844387076, 1.000000000000000000, 0.8660254037844387076, 1.000000000000000000, 0.8660254037844387076, 1.000000000000000000, 0.8660254037844387076, 1.000000000000000000, 0.8660254037844387076, 1.000000000000000000, 0.8660254037844387076, 1.000000000000000000, 0.8660254037844387076, 1.000000000000000000, 0.8660254037844387076, 1.000000000000000000, 0.8660254037844387076, 1.000000000000000000, 0.8660254037844387076, 1.000000000000000000, 0.8660254037844387076, 1.000000000000000000, 0.8660254037844387076, 1.000000000000000000, 0.8660254037844387076, 1.000000000000000000, 0.8660254037844387076, 1.000000000000000000, 0.8660254037844387076, 1.000000000000000000, 0.8660254037844387076, 1.000000000000000000, 0.8660254037844387076, 1.000000000000000000, 0.8660254037844387076, 1.000000000000000000, 0.8660254037844387076, 1.000000000000000000, 0.8660254037844387076, 1.000000000000000000, 0.8660254037844387076, 1.000000000000000000, 0.8660254037844387076, 1.000000000000000000, 0.8660254037844387076, 1.000000000000000000, 0.8660254037844387076, 1.000000000000000000, 0.8660254037844387076, 1.000000000000000000, 0.8660254037844387076, 1.000000000000000000, 0.8660254037844387076, 1.000000000000000000, 0.8660254037844387076, 1.000000000000000000, 0.8660254037844387076, 1.000000000000000000, 0.8660254037844387076, 1.000000000000000000, 0.8660254037844387076, 1.000000000000000000, 0.8660254037844387076, 1.000000000000000000, 0.8660254037844387076, 1.000000000000000000, 0.8660254037844387076, 1.000000000000000000, 0.8660254037844387076, 1.000000000000000000, 0.8660254037844387076, 1.000000000000000000, 0.8660254037844387076, 1.000000000000000000, 0.8660254037844387076, 1.000000000000000000, 0.8660254037844387076, 1.000000000000000000, 0.8660254037844387076, 1.000000000000000000, 0.8660254037844387076, 1.000000000000000000, 0.8660254037844387076, 1.000000000000000000, 0.8660254037844387076, 1.000000000000000000, 0.8660254037844387076, 1.000000000000000000, 0.8660254037844387076, 1.000000000000000000, 0.8660254037844387076, 1.000000000000000000, 0.8660254037844387076, 1.000000000000000000, 0.8660254037844387076, 1.000000000000000000, 0.8660254037844387076, 1.000000000000000000, 0.8660254037844387076, 1.000000000000000000, 0.8660254037844387076, 1.000000000000000000, 0.8660254037844387076, 1.000000000000000000, 0.8660254037844387076, 1.000000000000000000, 0.8660254037844387076, 1.000000000000000000, 0.8660254037844387076, 1.000000000000000000, 0.8660254037844387076, 1.000000000000000000, 0.8660254037844387076, 1.000000000000000000, 0.8660254037844387076, 1.000000000000000000, 0.8660254037844387076, 1.000000000000000000, 0.8660254037844387076, 1.000000000000000000, 0.8660254037844387076, 1.000000000000000000, 0.8660254037844387076, 1.000000000000000000, 0.8660254037844387076, 1.000000000000000000, 0.8660254037844387076, 1.000000000000000000, 0.8660254037844387076, 1.000000000000000000, 0.8660254037844387076, 1.000000000000000000, 0.8660254037844387076, 1.000000000000000000, 0.8660254037844387076, 1.000000000000000000, 0.8660254037844387076, 1.000000000000000000, 0.8660254037844387076, 1.000000000000000000, 0.8660254037844387076, 1.000000000000000000, 0.8660254037844387076, 1.000000000000000000, 0.8660254037844387076, 1.000000000000000000, 0.8660254037844387076, 1.000000000000000000, 0.8660254037844387076, 1.000000000000000000, 0.8660254037844387076, 1.000000000000000000, 0.8660254037844387076, 1.000000000000000000, 0.8660254037844387076, 1.000000000000000000, 0.8660254037844387076, 1.000000000000000000, 0.8660254037844387076, 1.000000000000000000, 0.8660254037844387076, 1.000000000000000000, 0.8660254037844387076, 1.000000000000000000, 0.8660254037844387076, 1.000000000000000000, 0.8660254037844387076, 1.000000000000000000, 0.8660254037844387076, 1.000000000000000000, 0.8660254037844387076, 1.000000000000000000, 0.8660254037844387076, 1.000000000000000000, 0.8660254037844387076, 1.000000000000000000, 0.8660254037844387076, 1.000000000000000000, 0.8660254037844387076, 1.000000000000000000, 0.8660254037844387076, 1.000000000000000000, 0.8660254037844387076, 1.000000000000000000, 0.8660254037844387076, 1.000000000000000000, 0.8660254037844387076, 1.000000000000000000, 0.8660254037844387076, 1.000000000000000000, 0.8660254037844387076, 1.000000000000000000, 0.8660254037844387076, 1.000000000000000000, 0.8660254037844387076, 1.000000000000000000, 0.8660254037844387076, 1.000000000000000000, 0.8660254037844387076, 1.000000000000000000, 0.8660254037844387076, 1.000000000000000000, 0.8660254037844387076, 1.000000000000000000, 0.8660254037844387076, 1.000000000000000000, 0.8660254037844387076, 1.000000000000000000, 0.8660254037844387076, 1.000000000000000000, 0.8660254037844387076, 1.000000000000000000, 0.8660254037844387076, 1.000000000000000000, 0.8660254037844387076, 1.000000000000000000, 0.8660254037844387076, 1.000000000000000000, 0.8660254037844387076, 1.000000000000000000, 0.8660254037844387076, 1.000000000000000000, 0.8660254037844387076, 1.000000000000000000, 0.8660254037844387076, 1.000000000000000000, 0.8660254037844387076, 1.000000000000000000, 0.8660254037844387076, 1.000000000000000000, 0.8660254037844387076, 1.000000000000000000, 0.8660254037844387076, 1.000000000000000000, 0.8660254037844387076, 1.000000000000000000, 0.8660254037844387076, 1.000000000000000000, 0.8660254037844387076, 1.000000000000000000, 0.8660254037844387076, 1.000000000000000000, 0.8660254037844387076, 1.000000000000000000, 0.8660254037844387076, 1.000000000000000000, 0.8660254037844387076, 1.000000000000000000, 0.8660254037844387076, 1.000000000000000000, 0.8660254037844387076, 1.000000000000000000, 0.8660254037844387076, 1.000000000000000000, 0.8660254037844387076, 1.000000000000000000, 0.8660254037844387076, 1.000000000000000000, 0.8660254037844387076, 1.000000000000000000, 0.8660254037844387076, 1.000000000000000000, 0.8660254037844387076, 1.000000000000000000, 0.8660254037844387076, 1.000000000000000000, 0.8660254037844387076, 1.000000000000000000, 0.8660254037844387076, 1.000000000000000000, 0.8660254037844387076, 1.000000000000000000, 0.8660254037844387076, 1.000000000000000000, 0.8660254037844387076, 1.000000000000000000, 0.8660254037844387076, 1.000000000000000000, 0.8660254037844387076, 1.000000000000000000, 0.8660254037844387076, 1.000000000000000000, 0.8660254037844387076, 1.000000000000000000, 0.8660254037844387076, 1.000000000000000000, 0.8660254037844387076, 1.000000000000000000, 0.8660254037844387076, 1.000000000000000000, 0.8660254037844387076, 1.000000000000000000, 0.8660254037844387076, 1.000000000000000000, 0.8660254037844387076, 1.000000000000000000, 0.8660254037844387076, 1.000000000000000000, 0.8660254037844387076, 1.000000000000000000, 0.8660254037844387076, 1.000000000000000000, 0.8660254037844387076, 1.000000000000000000, 0.8660254037844387076, 1.000000000000000000, 0.8660254037844387076, 1.000000000000000000, 0.8660254037844387076, 1.000000000000000000, 0.8660254037844387076, 1.000000000000000000, 0.8660254037844387076, 1.000000000000000000, 0.8660254037844387076, 1.000000000000000000, 0.8660254037844387076, 1.000000000000000000),
 ( 1.000000000000000000, 0.8660254037844387076, 1.000000000000000000, 0.8660254037844387076, 1.000000000000000000, 0.8660254037844387076, 1.000000000000000000, 0.8660254037844387076, 1.000000000000000000, 0.8660254037844387076, 1.000000000000000000, 0.8660254037844387076, 1.000000000000000000, 0.8660254037844387076, 1.000000000000000000, 0.8660254037844387076, 1.000000000000000000, 0.8660254037844387076, 1.000000000000000000, 0.8660254037844387076, 1.000000000000000000, 0.8660254037844387076, 1.000000000000000000, 0.8660254037844387076, 1.000000000000000000, 0.8660254037844387076, 1.000000000000000000, 0.8660254037844387076, 1.000000000000000000, 0.8660254037844387076, 1.000000000000000000, 0.8660254037844387076, 1.000000000000000000, 0.8660254037844387076, 1.000000000000000000, 0.8660254037844387076, 1.000000000000000000, 0.8660254037844387076, 1.000000000000000000, 0.8660254037844387076, 1.000000000000000000, 0.8660254037844387076, 1.000000000000000000, 0.8660254037844387076, 1.000000000000000000, 0.8660254037844387076, 1.000000000000000000, 0.8660254037844387076, 1.000000000000000000, 0.8660254037844387076, 1.000000000000000000, 0.8660254037844387076, 1.000000000000000000, 0.8660254037844387076, 1.000000000000000000, 0.8660254037844387076, 1.000000000000000000, 0.8660254037844387076, 1.000000000000000000, 0.8660254037844387076, 1.000000000000000000, 0.8660254037844387076, 1.000000000000000000, 0.8660254037844387076, 1.000000000000000000, 0.8660254037844387076, 1.000000000000000000, 0.8660254037844387076, 1.000000000000000000, 0.8660254037844387076, 1.000000000000000000, 0.8660254037844387076, 1.000000000000000000, 0.8660254037844387076, 1.000000000000000000, 0.8660254037844387076, 1.000000000000000000, 0.8660254037844387076, 1.000000000000000000, 0.8660254037844387076, 1.000000000000000000, 0.8660254037844387076, 1.000000000000000000, 0.8660254037844387076, 1.000000000000000000, 0.8660254037844387076, 1.000000000000000000, 0.8660254037844387076, 1.000000000000000000, 0.8660254037844387076, 1.000000000000000000, 0.8660254037844387076, 1.000000000000000000, 0.8660254037844387076, 1.000000000000000000, 0.8660254037844387076, 1.000000000000000000, 0.8660254037844387076, 1.000000000000000000, 0.8660254037844387076, 1.000000000000000000, 0.8660254037844387076, 1.000000000000000000, 0.8660254037844387076, 1.000000000000000000, 0.8660254037844387076, 1.000000000000000000, 0.8660254037844387076, 1.000000000000000000, 0.8660254037844387076, 1.000000000000000000, 0.8660254037844387076, 1.000000000000000000, 0.8660254037844387076, 1.000000000000000000, 0.8660254037844387076, 1.000000000000000000, 0.8660254037844387076, 1.000000000000000000, 0.8660254037844387076, 1.000000000000000000, 0.8660254037844387076, 1.000000000000000000, 0.8660254037844387076, 1.000000000000000000, 0.8660254037844387076, 1.000000000000000000, 0.8660254037844387076, 1.000000000000000000, 0.8660254037844387076, 1.000000000000000000, 0.8660254037844387076, 1.000000000000000000, 0.8660254037844387076, 1.000000000000000000, 0.8660254037844387076, 1.000000000000000000, 0.8660254037844387076, 1.000000000000000000, 0.8660254037844387076, 1.000000000000000000, 0.8660254037844387076, 1.000000000000000000, 0.8660254037844387076, 1.000000000000000000, 0.8660254037844387076, 1.000000000000000000, 0.8660254037844387076, 1.000000000000000000, 0.8660254037844387076, 1.000000000000000000, 0.8660254037844387076, 1.000000000000000000, 0.8660254037844387076, 1.000000000000000000, 0.8660254037844387076, 1.000000000000000000, 0.8660254037844387076, 1.000000000000000000, 0.8660254037844387076, 1.000000000000000000, 0.8660254037844387076, 1.000000000000000000, 0.8660254037844387076, 1.000000000000000000, 0.8660254037844387076, 1.000000000000000000, 0.8660254037844387076, 1.000000000000000000, 0.8660254037844387076, 1.000000000000000000, 0.8660254037844387076, 1.000000000000000000, 0.8660254037844387076, 1.000000000000000000, 0.8660254037844387076, 1.000000000000000000, 0.8660254037844387076, 1.000000000000000000, 0.8660254037844387076, 1.000000000000000000, 0.8660254037844387076, 1.000000000000000000, 0.8660254037844387076, 1.000000000000000000, 0.8660254037844387076, 1.000000000000000000, 0.8660254037844387076, 1.000000000000000000, 0.8660254037844387076, 1.000000000000000000, 0.8660254037844387076, 1.000000000000000000, 0.8660254037844387076, 1.000000000000000000, 0.8660254037844387076, 1.000000000000000000, 0.8660254037844387076, 1.000000000000000000, 0.8660254037844387076, 1.000000000000000000, 0.8660254037844387076, 1.000000000000000000, 0.8660254037844387076, 1.000000000000000000, 0.8660254037844387076, 1.000000000000000000, 0.8660254037844387076, 1.000000000000000000, 0.8660254037844387076, 1.000000000000000000, 0.8660254037844387076, 1.000000000000000000, 0.8660254037844387076, 1.000000000000000000, 0.8660254037844387076, 1.000000000000000000, 0.8660254037844387076, 1.000000000000000000, 0.8660254037844387076, 1.000000000000000000, 0.8660254037844387076, 1.000000000000000000, 0.8660254037844387076, 1.000000000000000000, 0.8660254037844387076, 1.000000000000000000, 0.8660254037844387076, 1.000000000000000000, 0.8660254037844387076, 1.000000000000000000, 0.8660254037844387076, 1.000000000000000000, 0.8660254037844387076, 1.000000000000000000, 0.8660254037844387076, 1.000000000000000000, 0.8660254037844387076, 1.000000000000000000, 0.8660254037844387076, 1.000000000000000000, 0.8660254037844387076, 1.000000000000000000, 0.8660254037844387076, 1.000000000000000000, 0.8660254037844387076, 1.000000000000000000, 0.8660254037844387076, 1.000000000000000000, 0.8660254037844387076, 1.000000000000000000, 0.8660254037844387076, 1.000000000000000000, 0.8660254037844387076, 1.000000000000000000, 0.8660254037844387076, 1.000000000000000000, 0.8660254037844387076, 1.000000000000000000, 0.8660254037844387076, 1.000000000000000000, 0.8660254037844387076, 1.000000000000000000, 0.8660254037844387076, 1.000000000000000000, 0.8660254037844387076, 1.000000000000000000, 0.8660254037844387076, 1.000000000000000000, 0.8660254037844387076, 1.000000000000000000, 0.8660254037844387076, 1.000000000000000000, 0.8660254037844387076, 1.000000000000000000, 0.8660254037844387076, 1.000000000000000000, 0.8660254037844387076, 1.000000000000000000, 0.8660254037844387076, 1.000000000000000000, 0.8660254037844387076, 1.000000000000000000, 0.8660254037844387076, 1.000000000000000000, 0.8660254037844387076, 1.000000000000000000, 0.8660254037844387076, 1.000000000000000000, 0.8660254037844387076, 1.000000000000000000, 0.8660254037844387076, 1.000000000000000000, 0.8660254037844387076, 1.000000000000000000, 0.8660254037844387076, 1.000000000000000000, 0.8660254037844387076, 1.000000000000000000, 0.8660254037844387076, 1.000000000000000000, 0.8660254037844387076, 1.000000000000000000, 0.8660254037844387076, 1.000000000000000000, 0.8660254037844387076, 1.000000000000000000, 0.8660254037844387076, 1.000000000000000000, 0.8660254037844387076, 1.000000000000000000, 0.8660254037844387076, 1.000000000000000000, 0.8660254037844387076, 1.000000000000000000, 0.8660254037844387076, 1.000000000000000000, 0.8660254037844387076, 1.000000000000000000, 0.8660254037844387076, 1.000000000000000000, 0.8660254037844387076, 1.000000000000000000, 0.8660254037844387076, 1.000000000000000000, 0.8660254037844387076, 1.000000000000000000, 0.8660254037844387076, 1.000000000000000000, 0.8660254037844387076, 1.000000000000000000, 0.8660254037844387076, 1.000000000000000000, 0.8660254037844387076, 1.000000000000000000, 0.8660254037844387076, 1.000000000000000000) ) ) 
 REPRESENTATION_ITEM ( '' )  SURFACE ( )  );
#159311=CARTESIAN_POINT ( 'NONE',  ( -6.878064000834399394, 6.918829510595249310, -0.7998128361456291469 ) ) ;
#159312=ORIENTED_EDGE ( 'NONE', *, *, #144045, .F. ) ;
#159313=CARTESIAN_POINT ( 'NONE',  ( 4.864678189204997949, 4.569879397027603929, 0.7998128361456341429 ) ) ;
#159314=ORIENTED_EDGE ( 'NONE', *, *, #21930, .F. ) ;
#159318=FACE_OUTER_BOUND ( 'NONE', #59442, .T. ) ;
#159319=CARTESIAN_POINT ( 'NONE',  ( 4.815628398899983509, 6.730757278346135131, 1.248813279183153657 ) ) ;
#159329=CARTESIAN_POINT ( 'NONE',  ( -4.092446641025072829, 3.979529022206003575, 0.4031905389056175126 ) ) ;
#159330=CARTESIAN_POINT ( 'NONE',  ( 7.280365300858406385, 11.43758391773608984, 1.040834085586084257E-14 ) ) ;
#159332=CARTESIAN_POINT ( 'NONE',  ( -4.904298879841297421, 6.744767997946721216, 1.599625672291267398 ) ) ;
#159335=CARTESIAN_POINT ( 'NONE',  ( 7.259501185113382604, 10.55683625168592243, -1.199719254218441611 ) ) ;
#159337=CARTESIAN_POINT ( 'NONE',  ( -5.555090253297260361, 7.504024600312024340, 1.599625672291269396 ) ) ;
#159351=CARTESIAN_POINT ( 'NONE',  ( -4.066556009095094737, 6.831733546331167695, 1.199719254218464037 ) ) ;
#159354=CARTESIAN_POINT ( 'NONE',  ( 3.226477370372302644, 5.747678784534228313, 1.082531754730546636 ) ) ;
#159359=CARTESIAN_POINT ( 'NONE',  ( -2.428882075142555497, 5.985446187641602300, 1.040834085586084257E-14 ) ) ;
#159362=CARTESIAN_POINT ( 'NONE',  ( 9.028840231696797503, 12.62106513936658203, -1.199719254218446718 ) ) ;
#159366=CARTESIAN_POINT ( 'NONE',  ( -6.204827856548512877, 10.39071626594860476, -0.7998128361456291469 ) ) ;
#159367=CARTESIAN_POINT ( 'NONE',  ( 3.811813743736467419, 7.598866467667865443, 1.040834085586084257E-14 ) ) ;
#159371=CARTESIAN_POINT ( 'NONE',  ( 4.174301041578287297, 5.728379888396370134, 1.537733183400904036 ) ) ;
#159374=CARTESIAN_POINT ( 'NONE',  ( -1.201851678989727383E-14, 1.634375000341421025, 1.575800808251672791 ) ) ;
#159377=CARTESIAN_POINT ( 'NONE',  ( 6.968527767744098433, 9.153035033833367251, 1.443375672974076540 ) ) ;
#159384=CARTESIAN_POINT ( 'NONE',  ( 8.378575743120986630, 12.71882943370911789, 1.040834085586084257E-14 ) ) ;
#159390=CARTESIAN_POINT ( 'NONE',  ( -7.804689982961090955, 12.25722208009664094, 0.7998128361456481317 ) ) ;
#159400=DIRECTION ( 'NONE',  ( -1.000000000000000000, 5.578564026256504688E-16, 0.000000000000000000 ) ) ;
#159407=CARTESIAN_POINT ( 'NONE',  ( -1.500000000000013101, 1.202083334016148974, 0.8660254037844403729 ) ) ;
#159413=CARTESIAN_POINT ( 'NONE',  ( 8.938903350111612411, 9.323142084752035430, -0.7998128361456221525 ) ) ;
#159415=CARTESIAN_POINT ( 'NONE',  ( 0.6823417656249882723, -0.1572916663252488245, 1.181850606188755259 ) ) ;
#159419=CARTESIAN_POINT ( 'NONE',  ( 8.568389894156670294, 12.94027927658408217, -0.7216878364870257245 ) ) ;
#159420=CARTESIAN_POINT ( 'NONE',  ( -6.724481002698130538, 7.907944593645035880, -1.082531754730544860 ) ) ;
#159424=CARTESIAN_POINT ( 'NONE',  ( -6.552668314106420588, 6.539201209412602189, -0.7998128361456291469 ) ) ;
#159425=ORIENTED_EDGE ( 'NONE', *, *, #207810, .T. ) ;
#159426=CARTESIAN_POINT ( 'NONE',  ( -1.402160292154681736E-14, 0.8687500006828192678, -1.732050807568863648 ) ) ;
#159441=CARTESIAN_POINT ( 'NONE',  ( -7.343712760096452463, 11.71941532008788833, -0.7998128361456291469 ) ) ;
#159442=CARTESIAN_POINT ( 'NONE',  ( 7.308008492965924141, 8.484763649003774333, -1.199719254218451159 ) ) ;
#159450=CARTESIAN_POINT ( 'NONE',  ( -6.970863535720637216, 11.28442455831609337, 0.7998128361456481317 ) ) ;
#159456=CARTESIAN_POINT ( 'NONE',  ( 3.029357257649615054, 5.621668336311468117, -1.199719254218446718 ) ) ;
#159461=CARTESIAN_POINT ( 'NONE',  ( -8.286004436246233951, 12.81875560892930466, 1.040834085586084257E-14 ) ) ;
#159465=CARTESIAN_POINT ( 'NONE',  ( -5.642163961945882988, 6.318168449258962482, -1.169820551124676422 ) ) ;
#159469=AXIS2_PLACEMENT_3D ( 'NONE', #152335, #1786, #196816 ) ;
#159474=CARTESIAN_POINT ( 'NONE',  ( 5.309989718046547402, 9.346738437696316737, 0.7998128361456462443 ) ) ;
#159477=DIRECTION ( 'NONE',  ( -1.000000000000000000, 4.336808689942017736E-16, 0.000000000000000000 ) ) ;
#159482=CARTESIAN_POINT ( 'NONE',  ( 0.7499999999999885647, 1.847916667349486231, -1.299038105676652899 ) ) ;
#159494=CARTESIAN_POINT ( 'NONE',  ( 5.016153647376217606, 4.954526798134778254, 0.7216878364870317197 ) ) ;
#159499=CARTESIAN_POINT ( 'NONE',  ( -8.435144125996554720, 12.99275191363802229, 0.7998128361456341429 ) ) ;
#159500=DIRECTION ( 'NONE',  ( 1.000000000000000000, 0.000000000000000000, 0.000000000000000000 ) ) ;
#159501=CARTESIAN_POINT ( 'NONE',  ( 9.911173986789782120, 11.52179005846497972, -1.199719254218440723 ) ) ;
#159504=EDGE_CURVE ( 'NONE', #170226, #54971, #12513, .T. ) ;
#159510=CARTESIAN_POINT ( 'NONE',  ( 0.6823417656249864960, -0.5739583329919112353, -1.181850606188749264 ) ) ;
#159511=DIRECTION ( 'NONE',  ( 0.6507913734559627184, -0.7592566023653016805, 0.000000000000000000 ) ) ;
#159515=CARTESIAN_POINT ( 'NONE',  ( -4.822949958159302497, 6.649860922651058992, -1.599625672291256295 ) ) ;
#159518=CARTESIAN_POINT ( 'NONE',  ( -1.402160292154681736E-14, -0.5374999999999753308, 1.732050807568877637 ) ) ;
#159520=CARTESIAN_POINT ( 'NONE',  ( -1.500000000000011324, 5.629166666666693963, -0.8660254037844313801 ) ) ;
#159525=CARTESIAN_POINT ( 'NONE',  ( 1.364683531249992088, 5.446875000341417916, 1.214306433183764966E-14 ) ) ;
#159527=CARTESIAN_POINT ( 'NONE',  ( -6.177711549321182716, 10.35908057418338402, 0.7998128361456481317 ) ) ;
#159529=CARTESIAN_POINT ( 'NONE',  ( 9.077347539549325717, 10.54899253668443393, -1.199719254218446718 ) ) ;
#159532=CARTESIAN_POINT ( 'NONE',  ( 0.000000000000000000, 9.200000000000020606, -0.3999999999999941380 ) ) ;
#159536=CARTESIAN_POINT ( 'NONE',  ( -1.364683531250014514, -0.4072916663252447167, 0.7879004041258379498 ) ) ;
#159542=CARTESIAN_POINT ( 'NONE',  ( -1.201851678989727383E-14, 3.743750000682817713, 1.732050807568877637 ) ) ;
#159544=CARTESIAN_POINT ( 'NONE',  ( 7.131225611108088280, 9.342849184424693476, 1.443375672974076540 ) ) ;
#159547=CARTESIAN_POINT ( 'NONE',  ( -6.064574784014443942, 5.969758757638621738, -0.7998128361456291469 ) ) ;
#159549=CARTESIAN_POINT ( 'NONE',  ( 0.7499999999999902300, 4.597916667349482012, -1.299038105676658228 ) ) ;
#159551=CARTESIAN_POINT ( 'NONE',  ( -2.279742385392243165, 5.811449882932888222, -0.7998128361456281477 ) ) ;
#159552=CARTESIAN_POINT ( 'NONE',  ( 6.819388077549422889, 8.018669514304889390, -1.082531754730543971 ) ) ;
#159553=CARTESIAN_POINT ( 'NONE',  ( -8.310784975052671442, 11.67937098999472667, -1.082531754730543083 ) ) ;
#159559=CARTESIAN_POINT ( 'NONE',  ( 2.361091307074211887, 5.906356958228550447, 0.7998128361456462443 ) ) ;
#159575=EDGE_CURVE ( 'NONE', #183003, #27525, #69632, .T. ) ;
#159577=CARTESIAN_POINT ( 'NONE',  ( 8.423693512792301163, 8.722063941212843119, 0.7998128361456481317 ) ) ;
#159582=CARTESIAN_POINT ( 'NONE',  ( 4.365362273920230685, 8.036747052974847705, 0.7216878364870298324 ) ) ;
#159584=CARTESIAN_POINT ( 'NONE',  ( -7.673551755654729689, 11.89630144833179060, 0.7216878364870458196 ) ) ;
#159588=CARTESIAN_POINT ( 'NONE',  ( -4.600294193738529103, 4.261431402316699035, -0.7998128361456221525 ) ) ;
#159605=CARTESIAN_POINT ( 'NONE',  ( 5.196774945655527667, 6.645529799594804388, -1.392961322168507765 ) ) ;
#159614=CARTESIAN_POINT ( 'NONE',  ( -8.188761592974051595, 9.616271948966963024, -1.082531754730543971 ) ) ;
#159619=CARTESIAN_POINT ( 'NONE',  ( 5.986088515633498197, 6.942523675449257858, -1.199719254218446718 ) ) ;
#159626=CARTESIAN_POINT ( 'NONE',  ( -4.029797971759847997, 5.724516938518342535, -1.599625672291256295 ) ) ;
#159630=CARTESIAN_POINT ( 'NONE',  ( -3.893162665418476109, 7.693773542963529444, 1.040834085586084257E-14 ) ) ;
#159633=CARTESIAN_POINT ( 'NONE',  ( 6.913768267964901071, 10.15348118167935709, -1.199719254218441611 ) ) ;
#159636=CARTESIAN_POINT ( 'NONE',  ( 5.915399107357110609, 6.142141269072955545, 0.7871259410536131096 ) ) ;
#159637=CARTESIAN_POINT ( 'NONE',  ( 4.446711195602238931, 6.210915699667823198, -1.443375672974051449 ) ) ;
#159644=CARTESIAN_POINT ( 'NONE',  ( 5.951666246274792016, 8.927065806420504401, 1.082531754730558626 ) ) ;
#159646=CARTESIAN_POINT ( 'NONE',  ( -8.483651433849100698, 10.92067931095586886, 1.599625672291269396 ) ) ;
#159649=CARTESIAN_POINT ( 'NONE',  ( -9.134442807305063639, 11.67993591332117376, 1.599625672291281386 ) ) ;
#159650=CARTESIAN_POINT ( 'NONE',  ( -4.726989112658928072, 8.666571064744069020, 1.040834085586084257E-14 ) ) ;
#159657=CARTESIAN_POINT ( 'NONE',  ( 8.320953590485093088, 10.73086516036454618, 1.599625672291281386 ) ) ;
#159667=CARTESIAN_POINT ( 'NONE',  ( 0.7499999999999902300, 3.816666666666690411, -1.299038105676658228 ) ) ;
#159668=CARTESIAN_POINT ( 'NONE',  ( 6.986529229743720926, 7.045372277656132276, -0.7998128361456281477 ) ) ;
#159671=CARTESIAN_POINT ( 'NONE',  ( 7.673551755654734130, 9.015193805427763607, -1.082531754730537976 ) ) ;
#159672=CARTESIAN_POINT ( 'NONE',  ( -9.286972035236630063, 10.89751746493999107, -1.082531754730537976 ) ) ;
#159675=CARTESIAN_POINT ( 'NONE',  ( 9.511208455186636712, 11.05516360492796935, 1.199719254218453823 ) ) ;
#159678=CARTESIAN_POINT ( 'NONE',  ( -3.090368948911150770, 5.692848642783215674, 1.199719254218462483 ) ) ;
#159681=CARTESIAN_POINT ( 'NONE',  ( -0.6823417656250003738, 1.467708333674752730, -1.181850606188749264 ) ) ;
#159686=CARTESIAN_POINT ( 'NONE',  ( -0.6823417656250003738, 0.2177083336747515085, -1.181850606188749264 ) ) ;
#159689=CARTESIAN_POINT ( 'NONE',  ( 7.750457368506414646, 12.19395069656619945, 0.7998128361456462443 ) ) ;
#159693=CARTESIAN_POINT ( 'NONE',  ( -2.426546306721660606, 5.774795091243142053, 0.7216878364870317197 ) ) ;
#159696=CARTESIAN_POINT ( 'NONE',  ( -6.749261541504576911, 6.768559974710451677, 1.040834085586084257E-14 ) ) ;
#159699=CARTESIAN_POINT ( 'NONE',  ( 5.027376032568989572, 4.759693547618927489, 0.7998128361456341429 ) ) ;
#159703=B_SPLINE_CURVE_WITH_KNOTS ( 'NONE', 3,
 ( #104094, #88920, #173369, #21729 ),
 .UNSPECIFIED., .F., .F.,
 ( 4, 4 ),
 ( 0.000000000000000000, 0.0003126726301078944139 ),
 .UNSPECIFIED. ) ;
#159704=VERTEX_POINT ( 'NONE', #168371 ) ;
#159706=CARTESIAN_POINT ( 'NONE',  ( 9.745613490124728884, 10.26430391476735338, 0.7998128361456462443 ) ) ;
#159709=CARTESIAN_POINT ( 'NONE',  ( -4.985647801523292344, 6.839675073242382553, -1.599625672291256295 ) ) ;
#159712=TOROIDAL_SURFACE ( 'NONE', #166671, 6.909076424898650259, 0.08000000000000000167 ) ;
#159714=CARTESIAN_POINT ( 'NONE',  ( 6.726816770674637347, 10.99970333242910669, -0.7998128361456291469 ) ) ;
#159716=CARTESIAN_POINT ( 'NONE',  ( 7.588813295347141441, 9.876701482703580837, -1.599625672291262513 ) ) ;
#159719=CARTESIAN_POINT ( 'NONE',  ( -9.381879110976678149, 11.00824238663667565, 1.082531754730558626 ) ) ;
#159721=DIRECTION ( 'NONE',  ( 1.000000000000000000, 0.000000000000000000, 0.000000000000000000 ) ) ;
#159726=CARTESIAN_POINT ( 'NONE',  ( -5.593616938499215152, 6.351546440420595019, 1.211061620805883532 ) ) ;
#159727=CARTESIAN_POINT ( 'NONE',  ( 1.364683531249986537, 1.155208333674754728, -0.7879004041258239610 ) ) ;
#159730=CARTESIAN_POINT ( 'NONE',  ( 5.748293942514166588, 7.729428904398431222, -1.443375672974057666 ) ) ;
#159747=CARTESIAN_POINT ( 'NONE',  ( 9.271078113646423091, 9.710679308875986848, 1.040834085586084257E-14 ) ) ;
#159749=B_SPLINE_CURVE_WITH_KNOTS ( 'NONE', 3,
 ( #106644, #8007, #74098, #21742, #153922, #85707 ),
 .UNSPECIFIED., .F., .F.,
 ( 4, 2, 4 ),
 ( 0.001511140261635257956, 0.001555921757587612041, 0.001600703253539966127 ),
 .UNSPECIFIED. ) ;
#159752=CARTESIAN_POINT ( 'NONE',  ( -3.100010679019018500, 6.768429558830820980, 1.040834085586084257E-14 ) ) ;
#159753=CARTESIAN_POINT ( 'NONE',  ( -7.670162217029145246, 9.971608557999250166, 1.599625672291295375 ) ) ;
#159758=CARTESIAN_POINT ( 'NONE',  ( 1.499999999999989120, 4.785416667349486453, 0.8660254037844524744 ) ) ;
#159759=CARTESIAN_POINT ( 'NONE',  ( 7.751511138711133064, 10.06651563329490529, -1.599625672291262513 ) ) ;
#159761=CARTESIAN_POINT ( 'NONE',  ( -7.877450944739929461, 9.149113176073413456, 1.199719254218462483 ) ) ;
#159763=CARTESIAN_POINT ( 'NONE',  ( 0.6823417656249917140, 4.092708333674755394, 1.181850606188765695 ) ) ;
#159769=CARTESIAN_POINT ( 'NONE',  ( -9.503902493499651882, 10.19023378527882784, 1.040834085586084257E-14 ) ) ;
#159773=CARTESIAN_POINT ( 'NONE',  ( -0.6823417656250212460, 2.863541667008084879, 1.181850606188767472 ) ) ;
#159780=CARTESIAN_POINT ( 'NONE',  ( 1.364683531249990311, 2.884375000341422801, 1.214306433183764966E-14 ) ) ;
#159782=CARTESIAN_POINT ( 'NONE',  ( -4.894657149733403045, 5.669187081899118574, -1.199719254218446718 ) ) ;
#159785=CARTESIAN_POINT ( 'NONE',  ( 1.364683531249988535, 3.676041667008087099, 0.7879004041258500513 ) ) ;
#159788=CARTESIAN_POINT ( 'NONE',  ( -1.364683531250014514, -0.7197916663252461600, 0.7879004041258379498 ) ) ;
#159789=CARTESIAN_POINT ( 'NONE',  ( -3.131570295076647525, 6.597323077657299528, 1.040834085586084257E-14 ) ) ;
#159792=CARTESIAN_POINT ( 'NONE',  ( 5.504247177468190699, 5.523969249908757817, 0.7216878364870317197 ) ) ;
#159795=CARTESIAN_POINT ( 'NONE',  ( -8.715193815486133033, 9.062147627688959872, 0.7998128361456462443 ) ) ;
#159796=CARTESIAN_POINT ( 'NONE',  ( -9.490344339885981029, 10.17441593939621924, -0.7216878364870267237 ) ) ;
#159802=CARTESIAN_POINT ( 'NONE',  ( -8.622095623286845978, 12.14652976288826913, 1.199719254218462483 ) ) ;
#159803=CARTESIAN_POINT ( 'NONE',  ( -6.439759776366783761, 8.536139043893143707, 1.443375672974078761 ) ) ;
#159805=CARTESIAN_POINT ( 'NONE',  ( -1.402160292154681736E-14, 0.5093750003414236893, -1.575800808251659024 ) ) ;
#159807=EDGE_CURVE ( 'NONE', #96549, #69400, #195615, .T. ) ;
#159819=CARTESIAN_POINT ( 'NONE',  ( -1.500000000000015099, -0.8708333333333129200, -0.8660254037844383745 ) ) ;
#159820=CARTESIAN_POINT ( 'NONE',  ( 8.392133896734668141, 9.853539636687704828, 1.082531754730558626 ) ) ;
#159824=EDGE_LOOP ( 'NONE', ( #19893, #201074, #147595 ) ) ;
#159827=VERTEX_POINT ( 'NONE', #52484 ) ;
#159830=CARTESIAN_POINT ( 'NONE',  ( 5.986088515633498197, 6.942523675449257858, -1.199719254218446718 ) ) ;
#159833=CARTESIAN_POINT ( 'NONE',  ( -2.767835915484202047, 6.380892334706859792, -0.7998128361456281477 ) ) ;
#159837=CARTESIAN_POINT ( 'NONE',  ( -0.6823417656250212460, 1.363541667008083547, 1.181850606188755259 ) ) ;
#159839=CARTESIAN_POINT ( 'NONE',  ( -6.997979842947967377, 11.31606025008131233, -0.7998128361456291469 ) ) ;
#159853=ORIENTED_EDGE ( 'NONE', *, *, #94104, .T. ) ;
#159857=CARTESIAN_POINT ( 'NONE',  ( 5.307127064745490230, 8.279066444590018392, -1.199719254218452935 ) ) ;
#159863=AXIS2_PLACEMENT_3D ( 'NONE', #110477, #176477, #126741 ) ;
#159865=CARTESIAN_POINT ( 'NONE',  ( 8.945682426918439845, 9.331051007693339727, 1.040834085586084257E-14 ) ) ;
#159868=CARTESIAN_POINT ( 'NONE',  ( 8.398386088661320414, 11.88553530582519357, -1.199719254218446718 ) ) ;
#159870=CARTESIAN_POINT ( 'NONE',  ( -3.009396220815599321, 6.452359640394901952, 0.6004564335717228474 ) ) ;
#159875=CARTESIAN_POINT ( 'NONE',  ( 0.007473969438118412655, 8.279395425053873936, 1.999986034896453324 ) ) ;
#159880=CARTESIAN_POINT ( 'NONE',  ( -9.002250809794006159, 10.56534270192358704, -1.082531754730543971 ) ) ;
#159885=CARTESIAN_POINT ( 'NONE',  ( 4.822949958159288286, 6.649860922651058992, -1.599625672291256295 ) ) ;
#159891=CARTESIAN_POINT ( 'NONE',  ( 4.161989969270902812, 4.918371721313249623, 1.082531754730560403 ) ) ;
#159900=CARTESIAN_POINT ( 'NONE',  ( -5.148345644887285744, 7.029489223833707001, -1.599625672291256295 ) ) ;
#159901=CARTESIAN_POINT ( 'NONE',  ( 4.074186250656476993, 7.493853916489129574, -0.5595503573846259959 ) ) ;
#159902=CARTESIAN_POINT ( 'NONE',  ( -8.611400122974211868, 13.19838391011195888, 1.040834085586084257E-14 ) ) ;
#159908=VERTEX_POINT ( 'NONE', #80218 ) ;
#159911=CARTESIAN_POINT ( 'NONE',  ( 3.825371897350130723, 7.614684313550482031, 0.7998128361456321445 ) ) ;
#159913=CARTESIAN_POINT ( 'NONE',  ( 1.579999999999991189, 8.674529973577531194, 2.500000000000000444 ) ) ;
#159920=AXIS2_PLACEMENT_3D ( 'NONE', #167503, #103575, #34293 ) ;
#159926=ORIENTED_EDGE ( 'NONE', *, *, #179458, .F. ) ;
#159928=CARTESIAN_POINT ( 'NONE',  ( 1.364683531249986537, 0.9677083336747538400, -0.7879004041258239610 ) ) ;
#159929=CARTESIAN_POINT ( 'NONE',  ( 4.369805582306193870, 3.992528022312320957, 1.214306433183764966E-14 ) ) ;
#159930=CARTESIAN_POINT ( 'NONE',  ( 3.018661757337009810, 6.673522483535157868, 0.000000000000000000 ) ) ;
#159932=CARTESIAN_POINT ( 'NONE',  ( -5.246642258808529746, 9.064907035344523578, 0.000000000000000000 ) ) ;
#159933=CARTESIAN_POINT ( 'NONE',  ( 3.863710590214593399, 7.451486755318259547, 1.040834085586084257E-14 ) ) ;
#159934=CARTESIAN_POINT ( 'NONE',  ( -5.951666246274811556, 7.966696592119163256, 1.443375672974064550 ) ) ;
#159938=CARTESIAN_POINT ( 'NONE',  ( 6.799577732453452761, 7.891594428405881878, -1.199719254218446718 ) ) ;
#159943=EDGE_CURVE ( 'NONE', #73840, #81936, #97560, .T. ) ;
#159944=CARTESIAN_POINT ( 'NONE',  ( 1.364683531249990311, 4.884375000341417916, 1.214306433183764966E-14 ) ) ;
#159949=CARTESIAN_POINT ( 'NONE',  ( 6.982612806237943559, 8.105135347821125436, -1.199719254218446718 ) ) ;
#159952=CARTESIAN_POINT ( 'NONE',  ( -7.660520486921249983, 8.896027641951645748, -1.199719254218446718 ) ) ;
#159957=CARTESIAN_POINT ( 'NONE',  ( 7.214910300766615769, 11.56914578420308715, -0.7998128361456291469 ) ) ;
#159959=CARTESIAN_POINT ( 'NONE',  ( -7.069687034522070590, 10.33538640932937724, -1.199719254218440723 ) ) ;
#159961=CARTESIAN_POINT ( 'NONE',  ( 6.588899466117086767, 10.63087377720454363, 1.040834085586084257E-14 ) ) ;
#159962=CARTESIAN_POINT ( 'NONE',  ( 4.031617349472986334, 7.784614636675013521, 0.3993128758026931457 ) ) ;
#159963=CARTESIAN_POINT ( 'NONE',  ( -9.680158490477310806, 10.39586578175276266, 0.7216878364870438212 ) ) ;
#159968=CARTESIAN_POINT ( 'NONE',  ( 5.820528018968444961, 5.685037531751635953, 0.7998128361456341429 ) ) ;
#159970=CARTESIAN_POINT ( 'NONE',  ( 9.053093885623066939, 11.58502883802551153, -1.599625672291262513 ) ) ;
#159971=CARTESIAN_POINT ( 'NONE',  ( -5.195561487237588594, 6.467898337602993486, 1.183867312878450484 ) ) ;
#159972=CARTESIAN_POINT ( 'NONE',  ( 2.683624340501134853, 5.218313266304903664, -1.199719254218446718 ) ) ;
#159973=CARTESIAN_POINT ( 'NONE',  ( -1.364683531250000748, 0.2593750003414205252, 0.000000000000000000 ) ) ;
#159975=CARTESIAN_POINT ( 'NONE',  ( -7.131225611108100715, 9.342849184424693476, 1.443375672974078761 ) ) ;
#159976=VERTEX_POINT ( 'NONE', #1068 ) ;
#159982=CARTESIAN_POINT ( 'NONE',  ( -4.295139169456660078, 7.266651303919805294, 0.9588947021764819834 ) ) ;
#159983=CARTESIAN_POINT ( 'NONE',  ( 0.6823417656249882723, -0.3447916663252489911, 1.181850606188755259 ) ) ;
#159986=CARTESIAN_POINT ( 'NONE',  ( 2.724825686666657809, 6.122787701178987518, 0.000000000000000000 ) ) ;
#159991=CARTESIAN_POINT ( 'NONE',  ( -7.822691444960709006, 10.14955932391940330, -1.443375672974058777 ) ) ;
#159996=CARTESIAN_POINT ( 'NONE',  ( -7.646435447983039424, 11.86466575604815787, 0.000000000000000000 ) ) ;
#159997=CARTESIAN_POINT ( 'NONE',  ( 0.007072395215912408162, 7.009756401597622144, -2.079987976222381629 ) ) ;
#160002=ORIENTED_EDGE ( 'NONE', *, *, #21559, .F. ) ;
#160003=CARTESIAN_POINT ( 'NONE',  ( -7.646435447983039424, 11.86466575604815787, 0.000000000000000000 ) ) ;
#160007=CARTESIAN_POINT ( 'NONE',  ( -1.364683531250010295, 5.092708333674757171, 0.7879004041258379498 ) ) ;
#160008=CARTESIAN_POINT ( 'NONE',  ( -1.500000000000011324, 3.702083334016152971, 0.8660254037844403729 ) ) ;
#160009=CARTESIAN_POINT ( 'NONE',  ( 5.922464229660435286, 6.137557782886555735, -0.7752440879994120237 ) ) ;
#160013=ORIENTED_EDGE ( 'NONE', *, *, #120127, .F. ) ;
#160016=CARTESIAN_POINT ( 'NONE',  ( -6.320072162264675164, 10.52516795595079557, 0.7998128361456481317 ) ) ;
#160020=CARTESIAN_POINT ( 'NONE',  ( 5.148345644887269756, 7.029489223833707001, -1.599625672291256295 ) ) ;
#160026=CARTESIAN_POINT ( 'NONE',  ( 6.259060471003163428, 10.45398764947904624, -0.7998128361456291469 ) ) ;
#160032=CARTESIAN_POINT ( 'NONE',  ( -5.965224400332865606, 7.022145224218852455, 1.082531754730549967 ) ) ;
#160035=CARTESIAN_POINT ( 'NONE',  ( -4.588064261291555646, 5.348899678044550576, 1.213891745583789872 ) ) ;
#160038=CARTESIAN_POINT ( 'NONE',  ( 5.016153647376212277, 5.914896012436124728, 1.082531754730558626 ) ) ;
#160041=CARTESIAN_POINT ( 'NONE',  ( -8.910733272679575379, 11.41894145625809820, -1.599625672291263179 ) ) ;
#160043=CARTESIAN_POINT ( 'NONE',  ( 7.262363838414439776, 11.62450824479221900, 0.7998128361456462443 ) ) ;
#160044=CARTESIAN_POINT ( 'NONE',  ( -0.7500000000000249800, -0.5583333333333134751, 1.299038105676659116 ) ) ;
#160045=CARTESIAN_POINT ( 'NONE',  ( -9.691380875670077444, 10.20103253123691189, 0.7998128361456462443 ) ) ;
#160048=CARTESIAN_POINT ( 'NONE',  ( -1.201851678989727383E-14, 3.321875000341421025, 1.575800808251672791 ) ) ;
#160049=CARTESIAN_POINT ( 'NONE',  ( 3.765413976293345844, 5.416068943807445635, 1.599625672291267398 ) ) ;
#160052=CARTESIAN_POINT ( 'NONE',  ( -1.001543065824772872E-14, 4.712500000000017231, 1.732050807568877637 ) ) ;
#160055=CARTESIAN_POINT ( 'NONE',  ( 9.381879110532285182, 10.04787317181692075, 0.000000000000000000 ) ) ;
#160058=CARTESIAN_POINT ( 'NONE',  ( -5.748293942514172805, 8.689798118699771479, -1.082531754730538864 ) ) ;
#160059=CARTESIAN_POINT ( 'NONE',  ( -1.402160292154681736E-14, 2.196875000341423689, -1.575800808251660134 ) ) ;
#160063=CARTESIAN_POINT ( 'NONE',  ( -7.867809214632013770, 8.073532260025807261, 1.040834085586084257E-14 ) ) ;
#160064=CARTESIAN_POINT ( 'NONE',  ( 0.6823417656249917140, 4.155208333674755394, 1.181850606188765695 ) ) ;
#160070=CARTESIAN_POINT ( 'NONE',  ( 9.582915646760733708, 10.07448976417602893, 0.7998128361456462443 ) ) ;
#160072=AXIS2_PLACEMENT_3D ( 'NONE', #100926, #31689, #2335 ) ;
#160074=CARTESIAN_POINT ( 'NONE',  ( 0.7499999999999885647, 0.5666666666666875241, -1.299038105676652899 ) ) ;
#160079=CARTESIAN_POINT ( 'NONE',  ( 10.42352117080803708, 11.05519620889787724, -0.7998128361456281477 ) ) ;
#160084=CARTESIAN_POINT ( 'NONE',  ( 8.751951852821344247, 10.16936423550178503, -1.199719254218446718 ) ) ;
#160085=CARTESIAN_POINT ( 'NONE',  ( -1.530444406200916152, 8.694995975526813581, 2.517029436271791987 ) ) ;
#160088=CARTESIAN_POINT ( 'NONE',  ( 1.364683531249990311, 5.426041667008086655, 0.7879004041258500513 ) ) ;
#160093=CARTESIAN_POINT ( 'NONE',  ( 7.771848369131631351, 10.09024240211882351, -1.599625672291262513 ) ) ;
#160096=CARTESIAN_POINT ( 'NONE',  ( -1.201851678989727383E-14, 3.571875000341422357, 1.575800808251672791 ) ) ;
#160098=CARTESIAN_POINT ( 'NONE',  ( -4.772106882330223954, 8.511282429453158827, -0.7216878364870267237 ) ) ;
#160104=CARTESIAN_POINT ( 'NONE',  ( 3.837121167867449945, 4.435395103055503441, 1.199719254218464037 ) ) ;
#160107=CARTESIAN_POINT ( 'NONE',  ( 7.228468454380276853, 11.58496363008569574, 1.040834085586084257E-14 ) ) ;
#160108=FACE_OUTER_BOUND ( 'NONE', #205811, .T. ) ;
#160110=VECTOR ( 'NONE', #79445, 1000.000000000000000 ) ;
#160114=CARTESIAN_POINT ( 'NONE',  ( -8.239604668803112375, 10.63595808506888396, -1.599625672291263179 ) ) ;
#160115=CARTESIAN_POINT ( 'NONE',  ( 6.470265622219697477, 8.571729197388226140, -1.599625672291262513 ) ) ;
#160117=CARTESIAN_POINT ( 'NONE',  ( 3.009546912109283934, 6.454962464195385330, 0.000000000000000000 ) ) ;
#160119=CARTESIAN_POINT ( 'NONE',  ( 4.660252114795294887, 6.460046772059735432, -1.599625672291256295 ) ) ;
#160128=CARTESIAN_POINT ( 'NONE',  ( -5.070386261830872598, 8.859275038870594088, 0.7216878364870458196 ) ) ;
#160129=CARTESIAN_POINT ( 'NONE',  ( 3.659811400685081040, 6.357198169852855685, -1.199719254218446718 ) ) ;
#160132=CARTESIAN_POINT ( 'NONE',  ( -8.193204901359996128, 8.453160561208463264, 1.040834085586084257E-14 ) ) ;
#160138=CARTESIAN_POINT ( 'NONE',  ( -9.321394304595349567, 10.83371376257142416, 1.199719254218462483 ) ) ;
#160142=CARTESIAN_POINT ( 'NONE',  ( 8.945682426918439845, 9.331051007693339727, 1.040834085586084257E-14 ) ) ;
#160145=CARTESIAN_POINT ( 'NONE',  ( 6.257251587906815793, 7.258880593101466161, 1.199719254218462483 ) ) ;
#160148=ORIENTED_EDGE ( 'NONE', *, *, #136490, .T. ) ;
#160157=CARTESIAN_POINT ( 'NONE',  ( -7.182068686937172153, 9.402166106225269715, 1.599625672291283607 ) ) ;
#160161=CARTESIAN_POINT ( 'NONE',  ( 6.643132081016117851, 8.773406732650713025, 1.443375672974076540 ) ) ;
#160164=CARTESIAN_POINT ( 'NONE',  ( -4.889686956022917919, 8.856385215335397021, 1.214306433183764966E-14 ) ) ;
#160167=CARTESIAN_POINT ( 'NONE',  ( -1.451998047845039830, 7.315968950354585942, -4.301760722576429607 ) ) ;
#160174=CARTESIAN_POINT ( 'NONE',  ( -0.7499999999999972244, 5.608333333333353821, -1.299038105676652011 ) ) ;
#160175=CARTESIAN_POINT ( 'NONE',  ( 9.088043039861931405, 9.497138389460751284, 1.040834085586084257E-14 ) ) ;
#160177=CARTESIAN_POINT ( 'NONE',  ( -4.961921032921567054, 4.891255414604337659, 0.7216878364870317197 ) ) ;
#160179=CARTESIAN_POINT ( 'NONE',  ( -5.725072791067139732, 6.113630025739863250, -0.7036897515925732982 ) ) ;
#160186=CARTESIAN_POINT ( 'NONE',  ( 3.063252641683779753, 5.661212951017999373, 1.199719254218450271 ) ) ;
#160193=CARTESIAN_POINT ( 'NONE',  ( 5.040934186182656873, 4.775511393501539636, 1.040834085586084257E-14 ) ) ;
#160201=CARTESIAN_POINT ( 'NONE',  ( 6.311484202361478779, 7.322151976631905868, -1.199719254218446718 ) ) ;
#160202=EDGE_CURVE ( 'NONE', #12101, #20507, #24447, .T. ) ;
#160206=CARTESIAN_POINT ( 'NONE',  ( -5.623934791570306402, 5.455678766453782913, 0.7998128361456341429 ) ) ;
#160208=CARTESIAN_POINT ( 'NONE',  ( 5.083944415000174466, 7.914723669933440675, -1.082531754730549078 ) ) ;
#160209=CARTESIAN_POINT ( 'NONE',  ( -1.201851678989727383E-14, 3.087500000000026112, -1.732050807568863648 ) ) ;
#160211=CARTESIAN_POINT ( 'NONE',  ( -3.436101866059630527, 6.096203712789787232, 1.199719254218462483 ) ) ;
#160214=CARTESIAN_POINT ( 'NONE',  ( -1.201851678989727383E-14, 4.196875000341417028, -1.575800808251660134 ) ) ;
#160217=CARTESIAN_POINT ( 'NONE',  ( -3.253593677599670109, 5.779314476299451719, 1.082531754730560403 ) ) ;
#160223=CARTESIAN_POINT ( 'NONE',  ( 5.030238685870051185, 5.827365540725222282, -1.199719254218452047 ) ) ;
#160226=CARTESIAN_POINT ( 'NONE',  ( 0.4830727172305282480, 6.835855489795042317, -3.747807319729578701 ) ) ;
#160229=CARTESIAN_POINT ( 'NONE',  ( -1.364683531250012516, 1.092708333674754506, 0.7879004041258379498 ) ) ;
#160232=CARTESIAN_POINT ( 'NONE',  ( -7.960608749518247151, 12.43912730774665576, 0.000000000000000000 ) ) ;
#160233=CARTESIAN_POINT ( 'NONE',  ( -6.033015167956810920, 7.101234453113482559, -1.082531754730543083 ) ) ;
#160237=CARTESIAN_POINT ( 'NONE',  ( 1.364683531249988535, 4.113541667008088432, 0.7879004041258500513 ) ) ;
#160245=CARTESIAN_POINT ( 'NONE',  ( -6.683806541412780078, 6.900121841177441873, -0.7216878364870267237 ) ) ;
#160250=CARTESIAN_POINT ( 'NONE',  ( -6.575341312503472757, 7.733948288417905381, 1.082531754730549967 ) ) ;
#160254=FACE_OUTER_BOUND ( 'NONE', #136218, .T. ) ;
#160257=CARTESIAN_POINT ( 'NONE',  ( 4.365362273920238678, 7.076377838673507448, 1.082531754730558626 ) ) ;
#160261=CARTESIAN_POINT ( 'NONE',  ( 4.048877618987437366, 7.739821757498127397, -0.4883357188320930353 ) ) ;
#160263=CARTESIAN_POINT ( 'NONE',  ( -3.906720819032141190, 7.709591388846142479, -0.7998128361456281477 ) ) ;
#160266=CARTESIAN_POINT ( 'NONE',  ( 1.499999999999987121, 1.045833333333352266, -0.8660254037844253849 ) ) ;
#160268=CARTESIAN_POINT ( 'NONE',  ( 9.747949258545622442, 10.47495501116581984, 0.000000000000000000 ) ) ;
#160269=CARTESIAN_POINT ( 'NONE',  ( 6.982612806237943559, 8.105135347821125436, -1.199719254218446718 ) ) ;
#160272=ORIENTED_EDGE ( 'NONE', *, *, #137765, .T. ) ;
#160274=CARTESIAN_POINT ( 'NONE',  ( 5.691725559638619814, 5.534767995866836543, 1.040834085586084257E-14 ) ) ;
#160275=B_SPLINE_CURVE_WITH_KNOTS ( 'NONE', 3,
 ( #1740, #49461, #85151, #52652, #151236 ),
 .UNSPECIFIED., .F., .F.,
 ( 4, 1, 4 ),
 ( 0.001713136426838625295, 0.001716577612580663008, 0.001720018798322700722 ),
 .UNSPECIFIED. ) ;
#160276=CARTESIAN_POINT ( 'NONE',  ( -0.5610452518370884212, 7.732119650022654334, -1.919700688223590079 ) ) ;
#160283=CARTESIAN_POINT ( 'NONE',  ( -5.900823170445743671, 7.907379670318584353, 1.599625672291269396 ) ) ;
#160290=CARTESIAN_POINT ( 'NONE',  ( -1.364683531249997417, 4.009375000341424133, 1.214306433183764966E-14 ) ) ;
#160291=CARTESIAN_POINT ( 'NONE',  ( 8.771762197917315262, 10.29643932140079166, -1.082531754730543083 ) ) ;
#160292=CARTESIAN_POINT ( 'NONE',  ( -7.389357414647957256, 8.579670724299436557, 1.199719254218450271 ) ) ;
#160295=CARTESIAN_POINT ( 'NONE',  ( 6.819914962873951936, 7.915321197229798322, -1.199719254218446718 ) ) ;
#160296=CARTESIAN_POINT ( 'NONE',  ( -4.726989112658928072, 8.666571064744069020, 1.040834085586084257E-14 ) ) ;
#160300=CARTESIAN_POINT ( 'NONE',  ( 1.499999999999989120, 0.3062500006828158816, 0.000000000000000000 ) ) ;
#160303=CARTESIAN_POINT ( 'NONE',  ( 7.212574532790092974, 9.437756259720353924, -1.443375672974057666 ) ) ;
#160307=CARTESIAN_POINT ( 'NONE',  ( 1.364683531249988757, 2.196875000341415252, 1.214306433183764966E-14 ) ) ;
#160309=CARTESIAN_POINT ( 'NONE',  ( 4.622967192135525316, 8.337286124226029216, -0.7216878364870207285 ) ) ;
#160312=CARTESIAN_POINT ( 'NONE',  ( -2.480778921620681921, 5.838066475291996404, 1.040834085586084257E-14 ) ) ;
#160314=CARTESIAN_POINT ( 'NONE',  ( 1.364683531249992088, 5.634375000341417916, 1.214306433183764966E-14 ) ) ;
#160319=VERTEX_POINT ( 'NONE', #59435 ) ;
#160320=CARTESIAN_POINT ( 'NONE',  ( -4.010472434439474654, 7.801430412234481082, -0.4134458547365611469 ) ) ;
#160327=CARTESIAN_POINT ( 'NONE',  ( 5.120175567455225618, 9.125288595339771547, -0.7998128361456281477 ) ) ;
#160338=CARTESIAN_POINT ( 'NONE',  ( 3.701012746850603996, 7.261672604726938651, 1.040834085586084257E-14 ) ) ;
#160340=CARTESIAN_POINT ( 'NONE',  ( -1.364683531250014514, 2.051041667008086655, -0.7879004041258289570 ) ) ;
#160341=CARTESIAN_POINT ( 'NONE',  ( 9.250740883225924804, 9.686952540052077509, 1.040834085586084257E-14 ) ) ;
#160348=CARTESIAN_POINT ( 'NONE',  ( 1.499999999999989120, 1.775000000000019673, 0.000000000000000000 ) ) ;
#160349=CARTESIAN_POINT ( 'NONE',  ( 5.341022448779654930, 8.318611059296550536, 1.199719254218462483 ) ) ;
#160350=CARTESIAN_POINT ( 'NONE',  ( -6.093499974338126179, 9.196501505781426999, -1.199719254218440723 ) ) ;
#160353=CARTESIAN_POINT ( 'NONE',  ( 1.364683531249988535, 2.363541667008088432, 0.7879004041258500513 ) ) ;
#160356=CARTESIAN_POINT ( 'NONE',  ( 4.207107738942202246, 3.802713871720993399, 1.214306433183764966E-14 ) ) ;
#160362=CARTESIAN_POINT ( 'NONE',  ( -1.500000000000015099, 0.4104166673494891726, -0.8660254037844383745 ) ) ;
#160364=CARTESIAN_POINT ( 'NONE',  ( -6.073162743917628781, 9.172774736957510555, -1.199719254218440723 ) ) ;
#160365=CARTESIAN_POINT ( 'NONE',  ( -3.850152436600983386, 4.554561266531622188, 1.082531754730560403 ) ) ;
#160374=CARTESIAN_POINT ( 'NONE',  ( 6.471319392424407901, 6.444294134116939077, 0.7998128361456341429 ) ) ;
#160378=CARTESIAN_POINT ( 'NONE',  ( 7.332262146892202459, 7.448727347662698506, -0.7998128361456281477 ) ) ;
#160383=CARTESIAN_POINT ( 'NONE',  ( -6.718228810771495141, 7.796687353110217877, 1.199719254218450271 ) ) ;
#160385=CARTESIAN_POINT ( 'NONE',  ( 3.216308754939877446, 4.775446185561722956, -1.599625672291262513 ) ) ;
#160390=CARTESIAN_POINT ( 'NONE',  ( 4.618273733618881494, 6.903169301580018846, 1.208453198238930382 ) ) ;
#160396=VECTOR ( 'NONE', #195701, 1000.000000000000000 ) ;
#160399=CARTESIAN_POINT ( 'NONE',  ( -3.090895834235680262, 5.589500325708124606, 1.082531754730560403 ) ) ;
#160400=CARTESIAN_POINT ( 'NONE',  ( 6.805829924380097040, 10.88395931184472154, 0.7216878364870438212 ) ) ;
#160402=CARTESIAN_POINT ( 'NONE',  ( -3.581325132304157943, 7.329963087663487364, -0.7998128361456281477 ) ) ;
#160405=CARTESIAN_POINT ( 'NONE',  ( 6.662942426112080874, 9.860851032851066122, 1.199719254218460707 ) ) ;
#160407=CARTESIAN_POINT ( 'NONE',  ( -6.338600509588822263, 7.353787668397130162, -1.199719254218446718 ) ) ;
#160418=CARTESIAN_POINT ( 'NONE',  ( 8.500000000000000000, 6.200000000000038369, -2.900000000000000799 ) ) ;
#160419=CARTESIAN_POINT ( 'NONE',  ( 9.049177462117294013, 12.64479190819049670, -1.199719254218446718 ) ) ;
#160420=CARTESIAN_POINT ( 'NONE',  ( -4.446184310277715213, 7.274633231044262516, -1.199719254218452047 ) ) ;
#160423=CARTESIAN_POINT ( 'NONE',  ( 4.867013957625893283, 4.780530493426062399, 1.040834085586084257E-14 ) ) ;
#160428=CARTESIAN_POINT ( 'NONE',  ( -4.548924232584923288, 5.265832011892554121, -1.199719254218446718 ) ) ;
#160431=CARTESIAN_POINT ( 'NONE',  ( 7.865701674222579598, 12.32840238656838139, -0.7998128361456352531 ) ) ;
#160434=CARTESIAN_POINT ( 'NONE',  ( -5.716734326456539783, 9.821273814174633188, -0.7998128361456231517 ) ) ;
#160435=CARTESIAN_POINT ( 'NONE',  ( 4.527533231959700366, 7.369540306339926516, 1.199719254218462483 ) ) ;
#160439=CARTESIAN_POINT ( 'NONE',  ( -1.284279953904135407, 3.128360285806111474, -0.7749999999999892530 ) ) ;
#160441=CARTESIAN_POINT ( 'NONE',  ( -0.6823417656250003738, 1.780208333674752952, -1.181850606188749264 ) ) ;
#160445=CARTESIAN_POINT ( 'NONE',  ( 7.958272981541723468, 8.386999354661243800, 1.040834085586084257E-14 ) ) ;
#160453=CARTESIAN_POINT ( 'NONE',  ( -5.000000000000000888, 3.300000000000025135, -0.7749999999999935829 ) ) ;
#160458=CARTESIAN_POINT ( 'NONE',  ( 3.538314903486612817, 7.071858454135611538, 1.040834085586084257E-14 ) ) ;
#160465=EDGE_CURVE ( 'NONE', #123984, #57442, #31116, .T. ) ;
#160477=CARTESIAN_POINT ( 'NONE',  ( -1.500000000000001332, 1.431250000682816825, 0.000000000000000000 ) ) ;
#160483=CARTESIAN_POINT ( 'NONE',  ( -1.500000000000015099, -0.8708333333333129200, -0.8660254037844383745 ) ) ;
#160484=CARTESIAN_POINT ( 'NONE',  ( 8.426556166093362776, 9.789735934319136135, -1.199719254218446718 ) ) ;
#160488=CARTESIAN_POINT ( 'NONE',  ( 4.532503425670185493, 4.182342172903648070, 1.214306433183764966E-14 ) ) ;
#160489=CARTESIAN_POINT ( 'NONE',  ( -5.260200412422200600, 8.120355666925794580, -1.082531754730544860 ) ) ;
#160493=CARTESIAN_POINT ( 'NONE',  ( -6.531277313481209212, 8.642909503859968368, 1.599625672291283607 ) ) ;
#160495=EDGE_CURVE ( 'NONE', #12101, #110280, #22812, .T. ) ;
#160497=CARTESIAN_POINT ( 'NONE',  ( -1.500000000000015099, 0.9104166673494835660, -0.8660254037844313801 ) ) ;
#160511=CARTESIAN_POINT ( 'NONE',  ( -8.805130697071332335, 12.36007068230351358, 1.199719254218462483 ) ) ;
#160512=CARTESIAN_POINT ( 'NONE',  ( 7.741869408603235136, 8.990934717247309749, 1.199719254218462483 ) ) ;
#160519=CARTESIAN_POINT ( 'NONE',  ( -6.482770005628665011, 10.71498210654212002, 0.7998128361456481317 ) ) ;
#160525=CARTESIAN_POINT ( 'NONE',  ( 5.366329872910639232, 5.155139694684188534, 1.040834085586084257E-14 ) ) ;
#160530=CARTESIAN_POINT ( 'NONE',  ( -9.053093885623068715, 11.58502883802551153, -1.599625672291263179 ) ) ;
#160533=CARTESIAN_POINT ( 'NONE',  ( -5.057943438340505082, 6.748278329294532085, -1.445135742742007068 ) ) ;
#160541=CARTESIAN_POINT ( 'NONE',  ( 5.795220594837462436, 8.848508896363995291, -1.199719254218440723 ) ) ;
#160543=VERTEX_POINT ( 'NONE', #180645 ) ;
#160550=CARTESIAN_POINT ( 'NONE',  ( 1.499999999999987121, 0.2854166673494805684, 0.8660254037844524744 ) ) ;
#160553=CARTESIAN_POINT ( 'NONE',  ( -4.083708824282378913, 7.596498746673441715, 0.5977277219625460880 ) ) ;
#160554=CARTESIAN_POINT ( 'NONE',  ( 2.218730694130720771, 5.740269576461138890, 0.7998128361456462443 ) ) ;
#160562=CARTESIAN_POINT ( 'NONE',  ( 4.528060117284229413, 7.266191989264828344, 1.082531754730558626 ) ) ;
#160564=ORIENTED_EDGE ( 'NONE', *, *, #144073, .T. ) ;
#160565=CARTESIAN_POINT ( 'NONE',  ( -10.64723070543352712, 11.31619066596094392, 0.7998128361456462443 ) ) ;
#160567=CARTESIAN_POINT ( 'NONE',  ( 10.01963921569910632, 11.64833282552586091, 1.199719254218450271 ) ) ;
#160576=CARTESIAN_POINT ( 'NONE',  ( 1.364683531249986537, -0.3864583329919166199, 0.7879004041258500513 ) ) ;
#160579=( BOUNDED_CURVE ( )  B_SPLINE_CURVE ( 2, ( #137484, #42121, #56216, #122380, #9589 ),
 .UNSPECIFIED., .F., .T. ) 
 B_SPLINE_CURVE_WITH_KNOTS ( ( 3, 2, 3 ),
 ( 0.2499999999999997502, 0.2541666666666666519, 0.2544499682697047849 ),
 .UNSPECIFIED. ) 
 CURVE ( )  GEOMETRIC_REPRESENTATION_ITEM ( )  RATIONAL_B_SPLINE_CURVE ( ( 1.000000000000007994, 0.8660254037844307140, 1.000000000000000000, 0.9908907477101788208, 0.9830202149929265776 ) ) 
 REPRESENTATION_ITEM ( '' )  );
#160582=CARTESIAN_POINT ( 'NONE',  ( -6.064574784014443942, 5.969758757638621738, -0.7998128361456291469 ) ) ;
#160585=CARTESIAN_POINT ( 'NONE',  ( -1.500000000000013101, 0.1708333333333560411, 0.8660254037844403729 ) ) ;
#160587=CARTESIAN_POINT ( 'NONE',  ( 0.7499999999999902300, 5.316666666666685082, -1.299038105676658228 ) ) ;
#160594=CARTESIAN_POINT ( 'NONE',  ( 0.6823417656249882723, -0.6572916663252492686, 1.181850606188755259 ) ) ;
#160597=CARTESIAN_POINT ( 'NONE',  ( -7.828943636887387925, 11.22118577875556156, 1.199719254218453823 ) ) ;
#160598=CARTESIAN_POINT ( 'NONE',  ( 1.387358672533417936, 7.315968950353815892, 4.254625267138360201 ) ) ;
#160599=CARTESIAN_POINT ( 'NONE',  ( 9.134442807305049428, 11.67993591332117376, 1.599625672291281386 ) ) ;
#160603=VERTEX_POINT ( 'NONE', #147104 ) ;
#160606=CARTESIAN_POINT ( 'NONE',  ( 0.6823417656249882723, 0.2385416670080825474, -1.181850606188749264 ) ) ;
#160610=CARTESIAN_POINT ( 'NONE',  ( -3.701970883082888353, 7.364863713882347618, 2.499999999999998668 ) ) ;
#160614=CARTESIAN_POINT ( 'NONE',  ( 8.107412671292047790, 8.560995659369956101, 0.7216878364870458196 ) ) ;
#160618=CARTESIAN_POINT ( 'NONE',  ( -1.201851678989727383E-14, 4.368750000682820378, -1.732050807568863648 ) ) ;
#160620=CARTESIAN_POINT ( 'NONE',  ( -5.088387723830502196, 4.830873854090670605, -0.7998128361456221525 ) ) ;
#160621=CARTESIAN_POINT ( 'NONE',  ( 6.765155463094759014, 7.955398130774449683, 1.082531754730558626 ) ) ;
#160622=CARTESIAN_POINT ( 'NONE',  ( -9.666600336419303829, 11.34041714965307968, 1.082531754730558626 ) ) ;
#160628=CARTESIAN_POINT ( 'NONE',  ( 9.490344339885973923, 12.09515436799890331, -1.443375672974057666 ) ) ;
#160642=VERTEX_POINT ( 'NONE', #148163 ) ;
#160644=CARTESIAN_POINT ( 'NONE',  ( 9.413438726589914651, 9.876766690643398405, 0.000000000000000000 ) ) ;
#160649=EDGE_CURVE ( 'NONE', #12172, #10803, #199000, .T. ) ;
#160651=CARTESIAN_POINT ( 'NONE',  ( -1.402160292154681736E-14, 0.4468750003414233563, -1.575800808251665908 ) ) ;
#160652=CARTESIAN_POINT ( 'NONE',  ( 4.528060117284229413, 7.266191989264828344, 1.082531754730558626 ) ) ;
#160654=CARTESIAN_POINT ( 'NONE',  ( -8.188761592974040937, 11.53701037756964887, -1.082531754730543971 ) ) ;
#160661=CARTESIAN_POINT ( 'NONE',  ( -2.819205876637805641, 5.376491725131008259, -1.199719254218446718 ) ) ;
#160665=ORIENTED_EDGE ( 'NONE', *, *, #124222, .T. ) ;
#160675=CARTESIAN_POINT ( 'NONE',  ( 4.470816497852414528, 7.277750640693428252, -1.251308411505752671 ) ) ;
#160683=CARTESIAN_POINT ( 'NONE',  ( -6.534666852106790103, 10.56760239419251590, 0.7216878364870458196 ) ) ;
#160687=CARTESIAN_POINT ( 'NONE',  ( 7.450369105909416589, 8.650851030771185890, -1.199719254218441611 ) ) ;
#160691=CARTESIAN_POINT ( 'NONE',  ( -3.588104209110990706, 7.337872010604796991, 1.040834085586084257E-14 ) ) ;
#160692=PLANE ( 'NONE',  #27692 ) ;
#160695=CARTESIAN_POINT ( 'NONE',  ( -4.120788623549732854, 6.895004929861607401, -1.199719254218452047 ) ) ;
#160698=CARTESIAN_POINT ( 'NONE',  ( 3.520313441042647540, 7.258782781191745137, 0.7998128361456321445 ) ) ;
#160699=CARTESIAN_POINT ( 'NONE',  ( 8.372323551638698902, 9.726464550788689323, 1.199719254218462483 ) ) ;
#160702=CARTESIAN_POINT ( 'NONE',  ( 4.075236096247129680, 7.726954018008360237, 0.5961105570580684798 ) ) ;
#160703=CARTESIAN_POINT ( 'NONE',  ( 5.856759171423504107, 5.935233242856626568, -0.7216878364870257245 ) ) ;
#160710=CARTESIAN_POINT ( 'NONE',  ( 5.626270559546810546, 8.547437505237857280, 1.082531754730558626 ) ) ;
#160711=CARTESIAN_POINT ( 'NONE',  ( -9.318531651294266638, 9.766041769465124034, -0.7998128361456291469 ) ) ;
#160714=CARTESIAN_POINT ( 'NONE',  ( -9.158696461231359720, 10.64389961198009615, 1.199719254218462483 ) ) ;
#160715=CARTESIAN_POINT ( 'NONE',  ( -6.906989191158078079, 10.14557225873805812, -1.199719254218440723 ) ) ;
#160721=CARTESIAN_POINT ( 'NONE',  ( 1.608462485350597770, 8.735270501766754236, -2.463594439587629914 ) ) ;
#160724=CARTESIAN_POINT ( 'NONE',  ( 9.738834413317897898, 10.25639499182604730, 0.000000000000000000 ) ) ;
#160728=CARTESIAN_POINT ( 'NONE',  ( 2.510230996824538430, 6.080353262937265413, 0.000000000000000000 ) ) ;
#160731=CARTESIAN_POINT ( 'NONE',  ( 4.161989969715272686, 4.726297878971393196, 2.500000000000011102 ) ) ;
#160737=CARTESIAN_POINT ( 'NONE',  ( 1.499999999999989120, 3.504166666666683749, 0.8660254037844524744 ) ) ;
#160738=CARTESIAN_POINT ( 'NONE',  ( 4.937140493670735708, 8.911747675924535983, -0.7998128361456281477 ) ) ;
#160740=CARTESIAN_POINT ( 'NONE',  ( 6.127922243696800386, 10.09306701771420656, -0.7216878364870267237 ) ) ;
#160741=CARTESIAN_POINT ( 'NONE',  ( -10.43941509239824228, 11.28166515066052966, 1.040834085586084257E-14 ) ) ;
#160745=CARTESIAN_POINT ( 'NONE',  ( 9.399880572976245574, 9.860948844760784482, 0.7998128361456462443 ) ) ;
#160747=CARTESIAN_POINT ( 'NONE',  ( -4.253507506385335368, 5.985511395581417204, 1.599625672291267398 ) ) ;
#160749=CARTESIAN_POINT ( 'NONE',  ( -1.500000000000011324, 4.910416667349486453, -0.8660254037844313801 ) ) ;
#160750=CARTESIAN_POINT ( 'NONE',  ( 1.364683531249986537, 0.9052083336747533959, -0.7879004041258239610 ) ) ;
#160755=CARTESIAN_POINT ( 'NONE',  ( -1.364683531250000748, -0.9906249996585805295, 0.000000000000000000 ) ) ;
#160762=CARTESIAN_POINT ( 'NONE',  ( -2.765500147063310266, 6.170241238308400433, 1.040834085586084257E-14 ) ) ;
#160765=CARTESIAN_POINT ( 'NONE',  ( -5.442708600882160574, 8.437244903416123876, -1.199719254218446718 ) ) ;
#160767=( BOUNDED_CURVE ( )  B_SPLINE_CURVE ( 2, ( #70597, #38135, #154021, #5588, #71667, #203799, #55445 ),
 .UNSPECIFIED., .F., .T. ) 
 B_SPLINE_CURVE_WITH_KNOTS ( ( 3, 2, 2, 3 ),
 ( 0.3423693953400485657, 0.3452380952380952328, 0.3511904761904761640, 0.3540591760885228867 ),
 .UNSPECIFIED. ) 
 CURVE ( )  GEOMETRIC_REPRESENTATION_ITEM ( )  RATIONAL_B_SPLINE_CURVE ( ( 0.9331000818465633451, 0.9354320710352566071, 1.000000000000000000, 0.8660254037844387076, 1.000000000000000000, 0.9354320710352559409, 0.9331000818465633451 ) ) 
 REPRESENTATION_ITEM ( '' )  );
#160770=CARTESIAN_POINT ( 'NONE',  ( 3.897079088924235712, 6.634010472798538949, 1.199719254218462483 ) ) ;
#160777=CARTESIAN_POINT ( 'NONE',  ( 9.398826802771546696, 11.98838390803207865, -1.599625672291262513 ) ) ;
#160780=CARTESIAN_POINT ( 'NONE',  ( -6.067437437315529536, 7.037430750744921859, 1.199719254218450271 ) ) ;
#160784=CARTESIAN_POINT ( 'NONE',  ( 10.06423010004587759, 10.63602329300870153, 0.000000000000000000 ) ) ;
#160786=CARTESIAN_POINT ( 'NONE',  ( 8.749089199520284410, 9.101692242395490240, 0.7998128361456481317 ) ) ;
#160787=CARTESIAN_POINT ( 'NONE',  ( 4.883397849413137592, 4.931525130979966143, -0.7509430347461319988 ) ) ;
#160790=CARTESIAN_POINT ( 'NONE',  ( -2.656508033273816238, 5.186677574539687363, -1.199719254218446718 ) ) ;
#160792=CYLINDRICAL_SURFACE ( 'NONE', #213042, 1.500000000000000222 ) ;
#160793=CARTESIAN_POINT ( 'NONE',  ( -8.206763054973658100, 8.468978407091068306, 0.7998128361456602331 ) ) ;
#160798=CARTESIAN_POINT ( 'NONE',  ( -6.103605818514504122, 6.017332118737867219, 0.3415998263276952551 ) ) ;
#160799=CARTESIAN_POINT ( 'NONE',  ( 0.6823417656249899377, 1.092708333674752286, 1.181850606188755259 ) ) ;
#160802=CARTESIAN_POINT ( 'NONE',  ( 7.836249599018724865, 9.205007956019091608, -1.082531754730537976 ) ) ;
#160819=CARTESIAN_POINT ( 'NONE',  ( 8.934986926605834157, 10.38290515491702770, -1.199719254218446718 ) ) ;
#160823=CARTESIAN_POINT ( 'NONE',  ( -4.243865776277440993, 4.909930479533815451, -1.199719254218446718 ) ) ;
#160824=CARTESIAN_POINT ( 'NONE',  ( -6.995117189646935962, 10.24838825697502109, 1.199719254218453823 ) ) ;
#160829=CARTESIAN_POINT ( 'NONE',  ( 1.499999999999989120, 5.035416667349487341, 0.8660254037844524744 ) ) ;
#160830=CARTESIAN_POINT ( 'NONE',  ( 7.456094412511537151, 10.78619501698377370, 1.199719254218460707 ) ) ;
#160834=CARTESIAN_POINT ( 'NONE',  ( -9.027031348600448979, 9.425958082989001952, 1.040834085586084257E-14 ) ) ;
#160836=CARTESIAN_POINT ( 'NONE',  ( -1.364683531250010295, 3.780208333674750953, 0.7879004041258379498 ) ) ;
#160841=CARTESIAN_POINT ( 'NONE',  ( -8.595506201384022660, 11.05117653974661529, 1.443375672974064550 ) ) ;
#160846=CARTESIAN_POINT ( 'NONE',  ( -1.201851678989727383E-14, 3.509375000341421469, -1.575800808251660134 ) ) ;
#160854=CARTESIAN_POINT ( 'NONE',  ( -1.364683531249997417, 2.759375000341422801, 1.214306433183764966E-14 ) ) ;
#160856=CARTESIAN_POINT ( 'NONE',  ( -3.899941742225307539, 7.701682465904834629, 0.7998128361456341429 ) ) ;
#160857=CARTESIAN_POINT ( 'NONE',  ( 8.125414133291656071, 8.374071331795406081, -0.7998128361456291469 ) ) ;
#160861=CARTESIAN_POINT ( 'NONE',  ( -1.364683531250012516, 3.801041667008087099, -0.7879004041258300672 ) ) ;
#160864=CARTESIAN_POINT ( 'NONE',  ( 0.6823417656249882723, -0.6572916663252492686, 1.181850606188755259 ) ) ;
#160865=CARTESIAN_POINT ( 'NONE',  ( -5.436456409399874623, 5.444880020495701523, 0.000000000000000000 ) ) ;
#160869=CARTESIAN_POINT ( 'NONE',  ( 3.389175213736285386, 6.897862149426897460, 0.7216878364870317197 ) ) ;
#160872=CARTESIAN_POINT ( 'NONE',  ( -7.015454420067433361, 10.27211502579893754, 1.199719254218453823 ) ) ;
#160873=CARTESIAN_POINT ( 'NONE',  ( -9.490344339885977476, 11.13478515369756217, -1.082531754730539753 ) ) ;
#160875=CARTESIAN_POINT ( 'NONE',  ( -1.364683531249997417, 4.759375000341424133, 1.214306433183764966E-14 ) ) ;
#160880=CARTESIAN_POINT ( 'NONE',  ( -7.497295758232736418, 7.849192594134070333, -0.7216878364870267237 ) ) ;
#160882=CARTESIAN_POINT ( 'NONE',  ( -1.364683531250014514, -0.9072916663252470482, 0.7879004041258379498 ) ) ;
#160883=CARTESIAN_POINT ( 'NONE',  ( -1.499999999999997780, 4.900000000000022560, 1.214306433183764966E-14 ) ) ;
#160895=CARTESIAN_POINT ( 'NONE',  ( 8.771762197917315262, 10.29643932140079166, -1.082531754730543083 ) ) ;
#160903=CARTESIAN_POINT ( 'NONE',  ( 6.419949431270806528, 7.448694743692793274, 1.199719254218462483 ) ) ;
#160904=CARTESIAN_POINT ( 'NONE',  ( -5.037017762676898158, 5.835274463666530131, -1.199719254218446718 ) ) ;
#160906=CARTESIAN_POINT ( 'NONE',  ( 1.499999999999989120, 3.525000000000021227, 1.214306433183764966E-14 ) ) ;
#160907=CARTESIAN_POINT ( 'NONE',  ( 5.015243055491540147, 4.745538407695236494, 0.3158334299713649318 ) ) ;
#160910=CARTESIAN_POINT ( 'NONE',  ( -1.364683531250000748, 1.571875000341421691, 0.000000000000000000 ) ) ;
#160912=CARTESIAN_POINT ( 'NONE',  ( -9.657485491635913633, 10.16148791653038330, 1.040834085586084257E-14 ) ) ;
#160915=ADVANCED_FACE ( 'NONE', ( #211554 ), #160692, .F. ) ;
#160928=CARTESIAN_POINT ( 'NONE',  ( 2.290224193653310536, 5.542776064365107835, 0.4201001246203844297 ) ) ;
#160931=CARTESIAN_POINT ( 'NONE',  ( 5.982172092127724383, 8.002286745614243912, -1.599625672291262513 ) ) ;
#160934=ORIENTED_EDGE ( 'NONE', *, *, #186980, .T. ) ;
#160938=CARTESIAN_POINT ( 'NONE',  ( 7.771848369131631351, 10.09024240211882351, -1.599625672291262513 ) ) ;
#160941=CARTESIAN_POINT ( 'NONE',  ( 9.748476143425788720, 11.33197590787365172, -1.199719254218440723 ) ) ;
#160943=CARTESIAN_POINT ( 'NONE',  ( 5.342823980928593564, 4.390142039796938178, 2.499999999999998668 ) ) ;
#160946=ORIENTED_EDGE ( 'NONE', *, *, #121379, .F. ) ;
#160947=CARTESIAN_POINT ( 'NONE',  ( 10.72180055030867329, 11.40318881831530540, 0.7998128361456341429 ) ) ;
#160954=CARTESIAN_POINT ( 'NONE',  ( -7.863365906246054138, 11.15738207638699464, -1.082531754730543971 ) ) ;
#160959=CARTESIAN_POINT ( 'NONE',  ( 4.299907273828439180, 8.168308919441841454, 1.040834085586084257E-14 ) ) ;
#160966=CARTESIAN_POINT ( 'NONE',  ( 3.172244755473273781, 6.644776614786712443, 0.000000000000000000 ) ) ;
#160974=CARTESIAN_POINT ( 'NONE',  ( -6.073162743917628781, 9.172774736957510555, -1.199719254218440723 ) ) ;
#160976=CARTESIAN_POINT ( 'NONE',  ( -4.485049888022365927, 4.126979712314507331, 0.7998128361456341429 ) ) ;
#160984=CARTESIAN_POINT ( 'NONE',  ( 4.801558957534076022, 8.753569217098425170, 0.7998128361456462443 ) ) ;
#160996=CARTESIAN_POINT ( 'NONE',  ( 1.364683531249986537, -0.03229166632525094088, -0.7879004041258309554 ) ) ;
#160998=CARTESIAN_POINT ( 'NONE',  ( 4.216749469050096621, 4.878294787768598262, -1.199719254218452047 ) ) ;
#161000=CARTESIAN_POINT ( 'NONE',  ( -5.694061328059534688, 8.626526735169329996, 1.082531754730548412 ) ) ;
#161001=CARTESIAN_POINT ( 'NONE',  ( 5.531363484695522637, 5.555604941673978558, -0.7216878364870207285 ) ) ;
#161002=CARTESIAN_POINT ( 'NONE',  ( -6.521108698048767138, 10.55178454779148289, -0.7216878364870267237 ) ) ;
#161004=ORIENTED_EDGE ( 'NONE', *, *, #153202, .F. ) ;
#161006=CARTESIAN_POINT ( 'NONE',  ( 5.829115978871627135, 8.888053511070525659, 1.199719254218462483 ) ) ;
#161011=CARTESIAN_POINT ( 'NONE',  ( -0.6823417656249969321, 4.717708333674755394, -1.181850606188749264 ) ) ;
#161015=CARTESIAN_POINT ( 'NONE',  ( 5.133733721068893807, 9.141106441222381918, 1.040834085586084257E-14 ) ) ;
#161019=CARTESIAN_POINT ( 'NONE',  ( -7.877450944739929461, 9.149113176073413456, 1.199719254218462483 ) ) ;
#161024=CARTESIAN_POINT ( 'NONE',  ( 7.242026607993941489, 11.60078147596829901, 0.7998128361456462443 ) ) ;
#161025=CARTESIAN_POINT ( 'NONE',  ( -3.054546515950523400, 6.451825606165701998, 0.6676900015689657408 ) ) ;
#161028=CARTESIAN_POINT ( 'NONE',  ( -6.418895661066105873, 9.576129806964074120, -1.199719254218440723 ) ) ;
#161030=CARTESIAN_POINT ( 'NONE',  ( 7.795575137733369075, 9.157554417852841411, -1.082531754730537976 ) ) ;
#161031=CARTESIAN_POINT ( 'NONE',  ( 3.998507505471064594, 7.829874410826325182, -0.01819030738507872169 ) ) ;
#161032=CARTESIAN_POINT ( 'NONE',  ( -9.544576954340667996, 11.19805653722800365, 1.082531754730558626 ) ) ;
#161037=CARTESIAN_POINT ( 'NONE',  ( 6.636879889089462026, 7.701780277814560982, -1.199719254218446718 ) ) ;
#161039=CARTESIAN_POINT ( 'NONE',  ( 9.240045382913317340, 10.73880668727576015, -1.199719254218446718 ) ) ;
#161040=CARTESIAN_POINT ( 'NONE',  ( -5.171837412746745244, 6.485142596490002909, 1.193510785747232905 ) ) ;
#161041=CARTESIAN_POINT ( 'NONE',  ( 2.496672843210871129, 6.064535417054653266, -0.7998128361456291469 ) ) ;
#161043=CARTESIAN_POINT ( 'NONE',  ( -5.910991785878165317, 8.879612269291090598, -1.082531754730538864 ) ) ;
#161049=CARTESIAN_POINT ( 'NONE',  ( -4.980508561475621043, 6.629897003107849685, 1.243112925831350246 ) ) ;
#161050=CARTESIAN_POINT ( 'NONE',  ( -1.402160292154681736E-14, 0.009375000341421267647, -1.575800808251665908 ) ) ;
#161053=ADVANCED_FACE ( 'NONE', ( #168156 ), #187305, .T. ) ;
#161054=CARTESIAN_POINT ( 'NONE',  ( 3.687454593236936251, 7.245854758844324728, -0.7216878364870267237 ) ) ;
#161055=CARTESIAN_POINT ( 'NONE',  ( 5.314433026432511475, 5.302519407033794430, 1.040834085586084257E-14 ) ) ;
#161060=CARTESIAN_POINT ( 'NONE',  ( -9.612367721964613310, 11.27714576612263997, -1.082531754730537976 ) ) ;
#161066=CARTESIAN_POINT ( 'NONE',  ( -8.853111119599343937, 10.39134639669645566, 1.082531754730558626 ) ) ;
#161073=CARTESIAN_POINT ( 'NONE',  ( -8.392133896734675247, 10.81390885098904420, 1.443375672974064550 ) ) ;
#161077=CARTESIAN_POINT ( 'NONE',  ( -1.201851678989727383E-14, 5.009375000341421469, -1.575800808251660134 ) ) ;
#161078=CARTESIAN_POINT ( 'NONE',  ( -0.7499999999999972244, 4.639583334016150751, -1.299038105676652899 ) ) ;
#161079=CARTESIAN_POINT ( 'NONE',  ( 5.777328231396808178, 6.232550548966264259, -0.9930585829777474061 ) ) ;
#161084=CARTESIAN_POINT ( 'NONE',  ( -6.808165692356648258, 11.09461040772476714, 0.7998128361456481317 ) ) ;
#161088=CARTESIAN_POINT ( 'NONE',  ( 5.983225862332436584, 5.874851682342960402, 0.7998128361456341429 ) ) ;
#161094=CARTESIAN_POINT ( 'NONE',  ( 8.796542737168120851, 9.157054702984622097, -0.7998128361456211532 ) ) ;
#161102=CARTESIAN_POINT ( 'NONE',  ( -6.453317930424837812, 7.591587675992828466, 1.082531754730549967 ) ) ;
#161112=CARTESIAN_POINT ( 'NONE',  ( -9.854078719034067291, 10.39084668182823634, 0.7998128361456462443 ) ) ;
#161114=CARTESIAN_POINT ( 'NONE',  ( 9.596473800374404561, 10.09030761005864285, 0.000000000000000000 ) ) ;
#161115=CARTESIAN_POINT ( 'NONE',  ( 1.499999999999987121, 0.2541666666666844154, 0.8660254037844524744 ) ) ;
#161116=CARTESIAN_POINT ( 'NONE',  ( -7.980945979938748103, 12.46285407657057220, 0.000000000000000000 ) ) ;
#161119=CARTESIAN_POINT ( 'NONE',  ( -0.6823417656249969321, 3.467708333674754506, -1.181850606188749264 ) ) ;
#161120=CARTESIAN_POINT ( 'NONE',  ( 2.347533153460546806, 5.890539112345938300, 0.000000000000000000 ) ) ;
#161124=CARTESIAN_POINT ( 'NONE',  ( 1.499999999999990896, 4.525000000000021672, 1.214306433183764966E-14 ) ) ;
#161127=CARTESIAN_POINT ( 'NONE',  ( 7.741342523278686549, 11.97539067722642869, 0.7216878364870438212 ) ) ;
#161130=CARTESIAN_POINT ( 'NONE',  ( -6.616015773788831211, 7.781401826584148473, 1.082531754730549967 ) ) ;
#161131=CARTESIAN_POINT ( 'NONE',  ( -1.364683531250012516, 1.280208333674755172, 0.7879004041258379498 ) ) ;
#161135=CARTESIAN_POINT ( 'NONE',  ( -8.206763054973658100, 8.468978407091068306, 0.7998128361456602331 ) ) ;
#161136=CARTESIAN_POINT ( 'NONE',  ( -2.751941993449643409, 6.154423392425789174, 0.7216878364870317197 ) ) ;
#161137=CARTESIAN_POINT ( 'NONE',  ( -1.364683531250012516, 3.092708333674755838, 0.7879004041258379498 ) ) ;
#161143=CARTESIAN_POINT ( 'NONE',  ( 7.723341061279088038, 12.16231500480096983, -0.7998128361456291469 ) ) ;
#161148=ORIENTED_EDGE ( 'NONE', *, *, #95435, .F. ) ;
#161149=CARTESIAN_POINT ( 'NONE',  ( 9.398826802771546696, 11.98838390803207865, -1.599625672291262513 ) ) ;
#161154=CARTESIAN_POINT ( 'NONE',  ( 9.725276259704228821, 10.24057714594344048, 0.7998128361456462443 ) ) ;
#161158=EDGE_CURVE ( 'NONE', #172377, #86628, #10407, .T. ) ;
#161159=CARTESIAN_POINT ( 'NONE',  ( -1.364683531250010295, 5.092708333674757171, 0.7879004041258379498 ) ) ;
#161164=CARTESIAN_POINT ( 'NONE',  ( 7.072549687823125097, 11.40305840243567381, -0.7998128361456291469 ) ) ;
#161167=CARTESIAN_POINT ( 'NONE',  ( -0.6823417656249969321, 3.717708333674754506, -1.181850606188749264 ) ) ;
#161169=CARTESIAN_POINT ( 'NONE',  ( -6.399085315970151733, 7.528316292462387871, -1.082531754730544860 ) ) ;
#161175=CARTESIAN_POINT ( 'NONE',  ( 2.544126380858701797, 6.119897877643793116, 0.7998128361456462443 ) ) ;
#161178=CARTESIAN_POINT ( 'NONE',  ( 7.540305987494599016, 11.94877408538573427, -0.7998128361456291469 ) ) ;
#161179=CARTESIAN_POINT ( 'NONE',  ( 4.905525160107046645, 6.476373528817812364, -2.499999999999995115 ) ) ;
#161183=( BOUNDED_SURFACE ( )  B_SPLINE_SURFACE ( 3, 2, ( 
 ( #106601, #172629, #153163 ),
 ( #4738, #136927, #22057 ),
 ( #88167, #144431, #127155 ),
 ( #190977, #49808, #44775 ) ),
 .UNSPECIFIED., .F., .F., .F. ) 
 B_SPLINE_SURFACE_WITH_KNOTS ( ( 4, 4 ),
 ( 3, 3 ),
 ( 4.082329036714114956, 4.712388980384689674 ),
 ( 0.000000000000000000, 1.000000000000000000 ),
 .UNSPECIFIED. ) 
 GEOMETRIC_REPRESENTATION_ITEM ( )  RATIONAL_B_SPLINE_SURFACE ( (
 ( 1.000000000000000000, 0.8226529996940207257, 1.000000000000000000),
 ( 1.000000000000000000, 0.7917671131328134493, 1.000000000000000000),
 ( 1.000000000000000000, 0.7517196685946749835, 1.000000000000000000),
 ( 1.000000000000000000, 0.7071067811865544561, 1.000000000000000000) ) ) 
 REPRESENTATION_ITEM ( '' )  SURFACE ( )  );
#161185=CARTESIAN_POINT ( 'NONE',  ( -3.755772246185468788, 4.340488027759846545, -1.199719254218452047 ) ) ;
#161186=CARTESIAN_POINT ( 'NONE',  ( 6.226218857173709154, 8.287007971501239467, 1.599625672291281386 ) ) ;
#161189=CARTESIAN_POINT ( 'NONE',  ( 5.281064527722868718, 6.119995689553514140, 1.199719254218462483 ) ) ;
#161196=DIRECTION ( 'NONE',  ( 0.000000000000000000, 0.7996470168499970610, 0.6004703560067728985 ) ) ;
#161198=CARTESIAN_POINT ( 'NONE',  ( -6.588899466561478846, 6.789396920517583922, 0.7216878364870317197 ) ) ;
#161200=CARTESIAN_POINT ( 'NONE',  ( 4.253507506385319381, 5.985511395581417204, 1.599625672291267398 ) ) ;
#161203=CARTESIAN_POINT ( 'NONE',  ( -7.507464373665155399, 9.781794407407920389, 1.599625672291295375 ) ) ;
#161209=CARTESIAN_POINT ( 'NONE',  ( -10.13488352141530768, 11.78278451552804817, 1.199719254218462483 ) ) ;
#161212=CARTESIAN_POINT ( 'NONE',  ( 7.422199028477372451, 10.74665040227725044, -1.199719254218441611 ) ) ;
#161213=CARTESIAN_POINT ( 'NONE',  ( 5.286789834324991055, 8.255339675766103724, -1.199719254218452935 ) ) ;
#161214=CARTESIAN_POINT ( 'NONE',  ( 2.205172540517054802, 5.724451730578533848, 1.040834085586084257E-14 ) ) ;
#161225=CARTESIAN_POINT ( 'NONE',  ( -7.832860060393135093, 10.16142270859057462, 1.599625672291295375 ) ) ;
#161229=CARTESIAN_POINT ( 'NONE',  ( 7.632877294813741109, 8.007371053478589573, 1.040834085586084257E-14 ) ) ;
#161231=DIRECTION ( 'NONE',  ( -5.578564026256490882E-16, -1.000000000000000000, -9.066213480720158442E-32 ) ) ;
#161233=CARTESIAN_POINT ( 'NONE',  ( -5.388475986427523345, 8.373973519885682393, 1.199719254218452047 ) ) ;
#161235=LINE ( 'NONE', #61595, #43251 ) ;
#161243=CARTESIAN_POINT ( 'NONE',  ( -0.6823417656250212460, 3.363541667008085323, 1.181850606188767472 ) ) ;
#161245=CARTESIAN_POINT ( 'NONE',  ( 8.158255747121103241, 10.54105100977322174, 1.599625672291281386 ) ) ;
#161248=CARTESIAN_POINT ( 'NONE',  ( -4.012850279964973232, 4.744375417122949301, 1.082531754730560403 ) ) ;
#161250=CARTESIAN_POINT ( 'NONE',  ( -3.904385050611244079, 7.498940292447679568, 1.040834085586084257E-14 ) ) ;
#161257=CARTESIAN_POINT ( 'NONE',  ( 3.277320446201373638, 4.846626492033466072, 1.599625672291267398 ) ) ;
#161265=CARTESIAN_POINT ( 'NONE',  ( 2.706824224222692088, 6.309712028235118453, 0.7998128361456362523 ) ) ;
#161266=DIRECTION ( 'NONE',  ( 1.000000000000000000, 0.000000000000000000, 0.000000000000000000 ) ) ;
#161270=CARTESIAN_POINT ( 'NONE',  ( -1.364683531249997417, 3.321875000341423245, 1.214306433183764966E-14 ) ) ;
#161275=CARTESIAN_POINT ( 'NONE',  ( 6.471319392424407901, 6.444294134116939077, 0.7998128361456341429 ) ) ;
#161279=CARTESIAN_POINT ( 'NONE',  ( -3.913499895838973508, 7.717500311787445000, 1.040834085586084257E-14 ) ) ;
#161280=CARTESIAN_POINT ( 'NONE',  ( 5.382223794500827552, 7.302347065049529462, -1.443375672974051449 ) ) ;
#161281=CARTESIAN_POINT ( 'NONE',  ( 0.7499999999999902300, 2.983333333333351600, 1.299038105676669330 ) ) ;
#161284=CARTESIAN_POINT ( 'NONE',  ( -5.271422797614987665, 5.044414773505913274, -0.7998128361456221525 ) ) ;
#161285=CARTESIAN_POINT ( 'NONE',  ( 0.5601741628961998121, 7.746630099212591603, -1.919951735362950052 ) ) ;
#161287=CARTESIAN_POINT ( 'NONE',  ( -1.201851678989727383E-14, 4.696875000341419693, -1.575800808251660134 ) ) ;
#161290=CARTESIAN_POINT ( 'NONE',  ( -4.989037340148921196, 5.883260320670900434, 1.082531754730560403 ) ) ;
#161293=ORIENTED_EDGE ( 'NONE', *, *, #22449, .F. ) ;
#161295=CARTESIAN_POINT ( 'NONE',  ( 3.847109862837356786, 4.045599327266925727, -0.8077998227820462063 ) ) ;
#161296=CARTESIAN_POINT ( 'NONE',  ( 4.599240423533799138, 6.388866465587984322, 1.599625672291267398 ) ) ;
#161300=CARTESIAN_POINT ( 'NONE',  ( -0.6823417656250212460, 3.613541667008085767, 1.181850606188767472 ) ) ;
#161305=CARTESIAN_POINT ( 'NONE',  ( 1.364683531249988757, 1.196875000341421469, 0.000000000000000000 ) ) ;
#161308=CARTESIAN_POINT ( 'NONE',  ( -9.459838494033043332, 12.05956421450382088, 1.599625672291281386 ) ) ;
#161309=CARTESIAN_POINT ( 'NONE',  ( -5.694061327615147050, 9.586895948952255608, 0.000000000000000000 ) ) ;
#161312=CARTESIAN_POINT ( 'NONE',  ( -0.6823417656250212460, 4.551041667008086655, 1.181850606188767472 ) ) ;
#161320=CARTESIAN_POINT ( 'NONE',  ( -4.894130264408858899, 8.653643041878236630, -0.7216878364870207285 ) ) ;
#161327=CARTESIAN_POINT ( 'NONE',  ( -4.568734577680875653, 8.274014740695587733, -0.7216878364870257245 ) ) ;
#161336=CARTESIAN_POINT ( 'NONE',  ( 1.551702917632593826, 8.754377144105253805, -2.473499015030054871 ) ) ;
#161337=EDGE_LOOP ( 'NONE', ( #180916, #99028, #124264, #100953 ) ) ;
#161342=CARTESIAN_POINT ( 'NONE',  ( -5.525111292768871252, 6.404716915440499037, -1.199719254218446718 ) ) ;
#161343=CARTESIAN_POINT ( 'NONE',  ( -4.620413885680726196, 7.122912077659854013, 1.384570422981110216 ) ) ;
#161345=CARTESIAN_POINT ( 'NONE',  ( -1.500000000000013101, 1.129166666666688634, -0.8660254037844313801 ) ) ;
#161347=CARTESIAN_POINT ( 'NONE',  ( 7.917598520700710019, 12.18102267421877727, -0.7216878364870328300 ) ) ;
#161348=CARTESIAN_POINT ( 'NONE',  ( 5.472687561410540802, 9.536552588287639409, 0.7998128361456462443 ) ) ;
#161353=CARTESIAN_POINT ( 'NONE',  ( 4.599240423533799138, 6.388866465587984322, 1.599625672291267398 ) ) ;
#161354=CARTESIAN_POINT ( 'NONE',  ( -0.007473969438128235526, 8.279395425053861501, -1.999986034896453768 ) ) ;
#161361=CARTESIAN_POINT ( 'NONE',  ( -4.500943810056945438, 5.313817868896925312, 1.082531754730560403 ) ) ;
#161364=VERTEX_POINT ( 'NONE', #65539 ) ;
#161370=CARTESIAN_POINT ( 'NONE',  ( -1.364683531250012516, 3.530208333674758059, 0.7879004041258379498 ) ) ;
#161371=CARTESIAN_POINT ( 'NONE',  ( 8.798878505144646311, 11.28844422746735532, -1.443375672974052559 ) ) ;
#161372=CARTESIAN_POINT ( 'NONE',  ( -7.063961727919978451, 8.200042423116789436, 1.199719254218450271 ) ) ;
#161375=CARTESIAN_POINT ( 'NONE',  ( 6.114890974963323345, 7.092793211334054604, 1.199719254218462483 ) ) ;
#161376=CARTESIAN_POINT ( 'NONE',  ( -5.551173829791513192, 8.563787670477010394, 1.199719254218452047 ) ) ;
#161380=CARTESIAN_POINT ( 'NONE',  ( 1.499999999999987121, 0.8270833340161471980, -0.8660254037844253849 ) ) ;
#161383=CARTESIAN_POINT ( 'NONE',  ( 7.944714827928056167, 8.371181508778631652, 0.7216878364870458196 ) ) ;
#161388=CARTESIAN_POINT ( 'NONE',  ( -1.364683531250000748, 2.071875000341422357, 1.214306433183764966E-14 ) ) ;
#161390=CARTESIAN_POINT ( 'NONE',  ( 5.300874872818830852, 7.207439989753867238, 1.443375672974062551 ) ) ;
#161392=CARTESIAN_POINT ( 'NONE',  ( -3.090895834235680262, 5.589500325708124606, 1.082531754730560403 ) ) ;
#161394=CARTESIAN_POINT ( 'NONE',  ( -1.001543065824772872E-14, 5.571875000341416140, 1.575800808251672791 ) ) ;
#161400=CARTESIAN_POINT ( 'NONE',  ( -3.985535776513723150, 7.835598525918981316, 0.2247789072947203870 ) ) ;
#161406=CARTESIAN_POINT ( 'NONE',  ( 7.142447996300871793, 7.227277505306155092, 0.7998128361456341429 ) ) ;
#161409=CARTESIAN_POINT ( 'NONE',  ( 3.684065054611349144, 5.321161868511784299, -1.599625672291262513 ) ) ;
#161415=ORIENTED_EDGE ( 'NONE', *, *, #62562, .T. ) ;
#161417=CARTESIAN_POINT ( 'NONE',  ( 3.551873057100283226, 6.127307085716883428, 1.082531754730558626 ) ) ;
#161419=CARTESIAN_POINT ( 'NONE',  ( 0.6823417656249882723, 2.238541667008084435, -1.181850606188749264 ) ) ;
#161420=CARTESIAN_POINT ( 'NONE',  ( 7.391166297744269365, 11.77477778067701664, 1.040834085586084257E-14 ) ) ;
#161426=CARTESIAN_POINT ( 'NONE',  ( -1.500000000000013101, 2.129166666666693519, -0.8660254037844313801 ) ) ;
#161427=CARTESIAN_POINT ( 'NONE',  ( 6.471319392424407901, 6.444294134116939077, 0.7998128361456341429 ) ) ;
#161428=CARTESIAN_POINT ( 'NONE',  ( -8.389798128758148010, 8.682519326506312751, 0.7998128361456462443 ) ) ;
#161432=EDGE_CURVE ( 'NONE', #105963, #82863, #32012, .T. ) ;
#161433=CARTESIAN_POINT ( 'NONE',  ( 1.364683531249988757, 2.134375000341422357, 1.214306433183764966E-14 ) ) ;
#161434=AXIS2_PLACEMENT_3D ( 'NONE', #67205, #177000, #199346 ) ;
#161435=CARTESIAN_POINT ( 'NONE',  ( 1.499999999999989120, 3.275000000000020783, 1.214306433183764966E-14 ) ) ;
#161437=CARTESIAN_POINT ( 'NONE',  ( 3.708318708537623021, 4.285125567170706695, -1.199719254218446718 ) ) ;
#161443=CARTESIAN_POINT ( 'NONE',  ( 0.7499999999999885647, 0.2645833340161538039, 1.299038105676657340 ) ) ;
#161445=CARTESIAN_POINT ( 'NONE',  ( -6.287230548435221777, 8.358188277972981695, -1.599625672291263179 ) ) ;
#161446=ADVANCED_FACE ( 'NONE', ( #181441 ), #50385, .F. ) ;
#161447=CARTESIAN_POINT ( 'NONE',  ( -3.795919822146289313, 5.451659097302528068, -1.443375672974053447 ) ) ;
#161455=CARTESIAN_POINT ( 'NONE',  ( 6.257251587906815793, 7.258880593101466161, 1.199719254218462483 ) ) ;
#161459=CARTESIAN_POINT ( 'NONE',  ( 5.795220594837462436, 8.848508896363995291, -1.199719254218440723 ) ) ;
#161464=CARTESIAN_POINT ( 'NONE',  ( -7.393273838153706201, 7.519907654134449615, 0.7998128361456341429 ) ) ;
#161466=CARTESIAN_POINT ( 'NONE',  ( 2.869522067586683711, 6.499526178826442013, 0.7998128361456362523 ) ) ;
#161471=CARTESIAN_POINT ( 'NONE',  ( -3.104453987849326690, 4.644948957289396496, 1.040834085586084257E-14 ) ) ;
#161472=CARTESIAN_POINT ( 'NONE',  ( 4.078835981324096416, 7.487686104445945290, 0.5747339805607706298 ) ) ;
#161474=EDGE_CURVE ( 'NONE', #12264, #67678, #147900, .T. ) ;
#161482=DIRECTION ( 'NONE',  ( -5.176899690512889973E-31, 0.6004703560067813362, 0.7996470168499908437 ) ) ;
#161484=CARTESIAN_POINT ( 'NONE',  ( 6.968527767744093993, 10.11340424813470662, 1.082531754730558626 ) ) ;
#161486=CARTESIAN_POINT ( 'NONE',  ( -4.928552533767591726, 5.708731696605642725, 1.199719254218462483 ) ) ;
#161487=CARTESIAN_POINT ( 'NONE',  ( 4.997242633387394051, 4.932463948481133897, -0.4367601086738909233 ) ) ;
#161490=CARTESIAN_POINT ( 'NONE',  ( -5.696397096036042385, 9.797547045350714967, -0.7998128361456231517 ) ) ;
#161498=VECTOR ( 'NONE', #42641, 1000.000000000000114 ) ;
#161505=CARTESIAN_POINT ( 'NONE',  ( -6.254388934605767503, 6.191208599995166040, 0.7998128361456341429 ) ) ;
#161508=CARTESIAN_POINT ( 'NONE',  ( 3.877268743828270470, 5.546566172598190292, 1.443375672974062551 ) ) ;
#161512=CARTESIAN_POINT ( 'NONE',  ( 0.4867935908802952238, 7.427453578140642776, 4.536604770850393820 ) ) ;
#161513=CARTESIAN_POINT ( 'NONE',  ( -4.090809663021341969, 5.795697244990093644, 1.599625672291267398 ) ) ;
#161516=CARTESIAN_POINT ( 'NONE',  ( 10.37606763316019531, 10.99983374830873650, 0.7998128361456462443 ) ) ;
#161519=CARTESIAN_POINT ( 'NONE',  ( -6.353967546298838087, 10.56471257065732416, 0.000000000000000000 ) ) ;
#161520=CARTESIAN_POINT ( 'NONE',  ( 5.443762371086860341, 6.309809840144842141, 1.199719254218462483 ) ) ;
#161523=CARTESIAN_POINT ( 'NONE',  ( 3.847109862837357230, 4.045599327266925727, -0.8077998227820462063 ) ) ;
#161526=CARTESIAN_POINT ( 'NONE',  ( 1.364683531249986537, 0.9260416670080896528, 0.7879004041258500513 ) ) ;
#161529=CARTESIAN_POINT ( 'NONE',  ( 7.998947442382716488, 9.394822106610419610, -1.082531754730543083 ) ) ;
#161535=CARTESIAN_POINT ( 'NONE',  ( 5.680503174445848735, 5.729601246382692636, 1.040834085586084257E-14 ) ) ;
#161543=CARTESIAN_POINT ( 'NONE',  ( -9.642873567817536795, 12.27310513391906532, 1.599625672291281386 ) ) ;
#161551=DIRECTION ( 'NONE',  ( 5.578564026256504688E-16, 1.000000000000000000, 9.066213480720158442E-32 ) ) ;
#161559=CARTESIAN_POINT ( 'NONE',  ( 1.499999999999987121, 1.035416667349484232, 0.8660254037844524744 ) ) ;
#161566=CARTESIAN_POINT ( 'NONE',  ( 7.727257484784855635, 11.10255193463598111, -1.199719254218446718 ) ) ;
#161567=CARTESIAN_POINT ( 'NONE',  ( 1.364683531249986981, -1.115624999658580752, 0.000000000000000000 ) ) ;
#161572=CARTESIAN_POINT ( 'NONE',  ( 4.383363735919856730, 4.008345868194933104, -0.7998128361456211532 ) ) ;
#161573=CARTESIAN_POINT ( 'NONE',  ( -5.748293942514172805, 8.689798118699771479, -1.082531754730538864 ) ) ;
#161577=CARTESIAN_POINT ( 'NONE',  ( -7.206322340863467346, 8.366129804884193888, 1.199719254218450271 ) ) ;
#161580=CARTESIAN_POINT ( 'NONE',  ( -0.7500000000000215383, 1.722916667349486008, 1.299038105676659116 ) ) ;
#161588=CARTESIAN_POINT ( 'NONE',  ( -2.290964770585000920, 5.616616632417037458, -0.7216878364870257245 ) ) ;
#161590=CARTESIAN_POINT ( 'NONE',  ( 4.067670533747345551, 7.502496534258641603, 0.5382987142239087364 ) ) ;
#161595=CARTESIAN_POINT ( 'NONE',  ( -8.319899820280397762, 12.85830022363583147, -0.7998128361456281477 ) ) ;
#161596=CARTESIAN_POINT ( 'NONE',  ( 7.446452682403650769, 9.710614100936176385, -1.599625672291262513 ) ) ;
#161604=CARTESIAN_POINT ( 'NONE',  ( -7.914208982075130905, 10.25632978388623684, -1.599625672291263179 ) ) ;
#161609=CARTESIAN_POINT ( 'NONE',  ( 4.325214697959421706, 5.004837554829479451, 1.199719254218462483 ) ) ;
#161614=CARTESIAN_POINT ( 'NONE',  ( -10.32183501870554387, 10.93656236477829502, 0.7998128361456462443 ) ) ;
#161617=CARTESIAN_POINT ( 'NONE',  ( -5.927203485463973465, 6.129067544638190590, -0.8144944673919730649 ) ) ;
#161625=CARTESIAN_POINT ( 'NONE',  ( 7.091078035147269532, 8.231678114882006625, 1.199719254218462483 ) ) ;
#161634=CARTESIAN_POINT ( 'NONE',  ( 1.499999999999987121, 0.03541666734948738238, 0.8660254037844524744 ) ) ;
#161638=CARTESIAN_POINT ( 'NONE',  ( 4.054051625686104998, 4.688480637177271149, -1.199719254218446718 ) ) ;
#161640=CARTESIAN_POINT ( 'NONE',  ( -3.918470089549458635, 4.530302178351167441, -1.199719254218452047 ) ) ;
#161647=CARTESIAN_POINT ( 'NONE',  ( 5.829642864196171281, 5.903597551091405826, 0.7216878364870317197 ) ) ;
#161650=CARTESIAN_POINT ( 'NONE',  ( 1.364683531249990311, 5.676041667008088432, 0.7879004041258500513 ) ) ;
#161652=CARTESIAN_POINT ( 'NONE',  ( 3.836594282542920009, 4.538743420130594508, 1.082531754730560403 ) ) ;
#161662=CARTESIAN_POINT ( 'NONE',  ( -1.364683531250014514, -0.2197916663252438285, 0.7879004041258379498 ) ) ;
#161667=CARTESIAN_POINT ( 'NONE',  ( -4.934277840369690971, 7.844075682818238526, -1.199719254218452047 ) ) ;
#161670=CARTESIAN_POINT ( 'NONE',  ( -1.500000000000001332, -1.099999999999976108, 0.000000000000000000 ) ) ;
#161672=CARTESIAN_POINT ( 'NONE',  ( 1.499999999999990896, 5.275000000000022560, 1.214306433183764966E-14 ) ) ;
#161679=CARTESIAN_POINT ( 'NONE',  ( 0.6823417656249864960, -1.073958332991911568, -1.181850606188749264 ) ) ;
#161681=CARTESIAN_POINT ( 'NONE',  ( 6.972971076130050072, 7.029554431773520129, 1.040834085586084257E-14 ) ) ;
#161682=CARTESIAN_POINT ( 'NONE',  ( -6.842061076390810292, 11.13415502243129218, 0.000000000000000000 ) ) ;
#161690=CARTESIAN_POINT ( 'NONE',  ( -1.364683531250000748, -0.6781249996585803075, 0.000000000000000000 ) ) ;
#161698=CARTESIAN_POINT ( 'NONE',  ( 8.120970824905713314, 8.576813505252564696, 1.040834085586084257E-14 ) ) ;
#161702=CARTESIAN_POINT ( 'NONE',  ( 1.499999999999991118, 5.285416667349480235, 0.8660254037844524744 ) ) ;
#161704=CARTESIAN_POINT ( 'NONE',  ( -2.916975605234527702, 6.554888639415577423, 1.040834085586084257E-14 ) ) ;
#161706=CARTESIAN_POINT ( 'NONE',  ( 5.626270559546804328, 9.507806719539201978, 0.7216878364870438212 ) ) ;
#161707=CARTESIAN_POINT ( 'NONE',  ( -8.636180661780658241, 12.05899929117736846, -1.082531754730543083 ) ) ;
#161713=CARTESIAN_POINT ( 'NONE',  ( 10.05978679165993839, 10.83876546646586014, 0.7216878364870438212 ) ) ;
#161715=CARTESIAN_POINT ( 'NONE',  ( 3.571683402196252910, 6.254382171615883834, 1.199719254218462483 ) ) ;
#161716=CARTESIAN_POINT ( 'NONE',  ( -2.482948226198895103, 5.072301959192136778, 2.500000000000011102 ) ) ;
#161726=VERTEX_POINT ( 'NONE', #148952 ) ;
#161729=CARTESIAN_POINT ( 'NONE',  ( 8.432281472695482449, 11.92507992053172572, 1.199719254218450271 ) ) ;
#161731=CARTESIAN_POINT ( 'NONE',  ( -1.445103857048104512, 8.688264192037886247, 2.625611233228265284 ) ) ;
#161733=CARTESIAN_POINT ( 'NONE',  ( 0.6823417656249864960, -0.8239583329919114574, -1.181850606188749264 ) ) ;
#161734=CARTESIAN_POINT ( 'NONE',  ( 5.856759171423504107, 5.935233242856626568, -0.7216878364870257245 ) ) ;
#161736=CARTESIAN_POINT ( 'NONE',  ( -8.351459436338037889, 10.76645531385962862, -1.443375672974059665 ) ) ;
#161741=CARTESIAN_POINT ( 'NONE',  ( -5.088387723830502196, 4.830873854090670605, -0.7998128361456221525 ) ) ;
#161749=ORIENTED_EDGE ( 'NONE', *, *, #107203, .F. ) ;
#161756=CARTESIAN_POINT ( 'NONE',  ( 4.707942587747941943, 7.051207734045064512, -1.383178547476830111 ) ) ;
#161763=CARTESIAN_POINT ( 'NONE',  ( -6.887178846062105286, 10.97886638714038554, -0.7216878364870267237 ) ) ;
#161768=CARTESIAN_POINT ( 'NONE',  ( 7.772902139336337335, 7.962807338847539107, 0.7998128361456341429 ) ) ;
#161771=CARTESIAN_POINT ( 'NONE',  ( -5.596818484342970912, 5.424043074688562172, -0.7998128361456221525 ) ) ;
#161774=CARTESIAN_POINT ( 'NONE',  ( -5.603597561149804562, 5.431951997629870910, 0.7998128361456341429 ) ) ;
#161778=CARTESIAN_POINT ( 'NONE',  ( 3.493197133815315603, 7.227147089426516402, -0.7998128361456291469 ) ) ;
#161779=CARTESIAN_POINT ( 'NONE',  ( 7.076466111328892694, 10.34329533227067799, -1.199719254218441611 ) ) ;
#161782=CARTESIAN_POINT ( 'NONE',  ( 4.602920755658417740, 7.148668813305413039, 1.337190490212318839 ) ) ;
#161783=CARTESIAN_POINT ( 'NONE',  ( 4.528060117284232966, 6.305822774963486310, 1.443375672974062551 ) ) ;
#161785=CARTESIAN_POINT ( 'NONE',  ( -1.420000000000001039, 7.140846818246206595, -4.154462424328208670 ) ) ;
#161790=CARTESIAN_POINT ( 'NONE',  ( 7.741342523278707866, 8.133913820021057006, 0.7216878364870458196 ) ) ;
#161793=CARTESIAN_POINT ( 'NONE',  ( -8.513630394377489807, 12.01998699582738972, -1.199719254218446718 ) ) ;
#161794=CARTESIAN_POINT ( 'NONE',  ( -5.716734326456539783, 9.821273814174633188, -0.7998128361456231517 ) ) ;
#161802=CARTESIAN_POINT ( 'NONE',  ( 9.348510611822643313, 10.86534945433664134, 1.199719254218453823 ) ) ;
#161806=CARTESIAN_POINT ( 'NONE',  ( 3.871016551901614200, 4.474939717762034697, -1.199719254218446718 ) ) ;
#161810=CARTESIAN_POINT ( 'NONE',  ( -1.500000000000011324, 5.160416667349487341, -0.8660254037844313801 ) ) ;
#161816=CARTESIAN_POINT ( 'NONE',  ( -0.7500000000000215383, 2.441666666666689078, 1.299038105676671107 ) ) ;
#161817=CARTESIAN_POINT ( 'NONE',  ( 6.634017235788401301, 6.634108284708264414, 0.7998128361456341429 ) ) ;
#161818=B_SPLINE_CURVE_WITH_KNOTS ( 'NONE', 3,
 ( #30939, #114374, #195561, #176119, #31993, #111174, #113312, #95948, #27719, #162003, #194482, #177175, #193419, #98074, #213897 ),
 .UNSPECIFIED., .F., .F.,
 ( 4, 1, 2, 2, 2, 2, 2, 4 ),
 ( 0.6950735642280609916, 0.6991140303181444526, 0.7011342633631861831, 0.7031544964082280247, 0.7112354285883952798, 0.7193163607685624239, 0.7273972929487294570, 0.7597210216693985885 ),
 .UNSPECIFIED. ) ;
#161822=CARTESIAN_POINT ( 'NONE',  ( 6.304178240674458422, 10.29869901418813782, 1.040834085586084257E-14 ) ) ;
#161823=CARTESIAN_POINT ( 'NONE',  ( -9.232739420781982176, 12.75498451001223010, 1.082531754730558626 ) ) ;
#161828=CARTESIAN_POINT ( 'NONE',  ( 8.218213668177886788, 12.73966637951625813, 0.7998128361456462443 ) ) ;
#161830=CARTESIAN_POINT ( 'NONE',  ( -3.144601563365788444, 5.756120026313656268, -1.199719254218452935 ) ) ;
#161831=CARTESIAN_POINT ( 'NONE',  ( 1.499999999999989120, 4.785416667349486453, 0.8660254037844524744 ) ) ;
#161832=CARTESIAN_POINT ( 'NONE',  ( 1.364683531249988757, 0.3843750003414206362, 0.000000000000000000 ) ) ;
#161836=CARTESIAN_POINT ( 'NONE',  ( 4.792970997630896512, 5.550553237779539018, 1.199719254218464037 ) ) ;
#161838=CARTESIAN_POINT ( 'NONE',  ( 1.364683531249992088, 5.446875000341417916, 1.214306433183764966E-14 ) ) ;
#161840=CARTESIAN_POINT ( 'NONE',  ( 5.708314589969347708, 6.277192745311285016, 1.110195795946368635 ) ) ;
#161847=CARTESIAN_POINT ( 'NONE',  ( -6.958359152311683893, 9.141171649162195934, -1.599625672291263179 ) ) ;
#161850=CARTESIAN_POINT ( 'NONE',  ( 5.626797444871351139, 6.523350759560078593, 1.199719254218462483 ) ) ;
#161859=CARTESIAN_POINT ( 'NONE',  ( -5.311043488251275591, 7.219303374425030562, -1.599625672291256295 ) ) ;
#161863=CARTESIAN_POINT ( 'NONE',  ( 8.028399517586572998, 12.51821653715971472, -0.7998128361456352531 ) ) ;
#161865=CARTESIAN_POINT ( 'NONE',  ( 7.727257484784855635, 11.10255193463598111, -1.199719254218446718 ) ) ;
#161869=CARTESIAN_POINT ( 'NONE',  ( -8.459924665247381625, 11.85336729522185806, 1.082531754730560403 ) ) ;
#161870=( BOUNDED_SURFACE ( )  B_SPLINE_SURFACE ( 1, 2, ( 
 ( #9031, #76165, #122888, #74040, #141216, #107671, #140130, #173699, #93510, #75105, #207226, #58850, #108738, #159551, #125006, #190963, #158492, #10091, #142270, #208281, #77225, #203997, #55646, #121802, #39401, #96721, #144419, #143344, #127140, #211484, #16475, #197372, #49014, #193112, #30636, #195261, #145489, #63120, #210421, #13297, #209338, #130336, #114085, #45825, #110869, #46895, #111946, #129285, #31699, #62063, #94577, #81503, #128218, #95654, #44761, #176874, #177948, #115133, #29562, #194180, #161704, #79370, #113010, #28486, #179019, #160620, #196325, #162770, #14348, #164881, #80438, #78293, #12221, #146537, #212556, #64195, #47969, #180076, #97774, #163834, #15413, #60987, #147582, #213600, #65226, #131376, #181128, #32749, #98831, #70544, #119394, #169140, #66278, #52200, #69485, #51136, #148642, #67343, #133488, #150783, #199491, #1285, #83622, #134550, #37002, #20735, #135593, #208, #198427, #103084, #50073, #86830, #2346, #149704, #18616, #152894, #100935, #17533, #117258, #200553, #84696, #104157, #82555, #33808, #68422, #185382, #183257, #34861, #202688, #170205, #184312, #118326, #35936, #4473, #102015, #168084, #19684, #132426, #151842, #120476, #167022, #85762, #3419, #201614, #53263, #116194, #136663, #54337, #186449, #38085, #182181, #99887, #165949, #87898, #155035, #40222, #203751, #59660, #92200, #191779, #153971, #57536, #56466, #106333, #171274, #91119, #204815, #138795, #157178, #41306, #43435, #72700, #188590, #139871, #55395, #172354, #156108, #123694, #108485, #22867, #122628, #173438, #25017, #6620, #208032, #205902, #74855, #8772, #140957, #206968, #88982, #58598, #137731, #158250, #121550, #187521, #23944, #90048, #7692, #73775, #189655, #124753, #190713, #42374, #174509, #107414, #75914, #26085, #9838, #142017, #39152, #125817, #109559, #21789, #5538, #71619, #105233, #210157, #211227, #193919, #176618, #192842, #212289, #11967, #147323, #163572, #47704, #44501, #112749, #197115, #178761, #161445, #213350, #76966, #64973, #10891, #143093, #78040, #14081, #95394, #48754, #162510, #94323, #175563, #63922, #131127, #81241, #144164, #27154, #61798, #93258, #28230, #113818, #129015, #160364, #179818, #159292, #127967, #126884, #110618, #45565, #111682, #79103, #177689, #209085, #60721, #29300, #13026, #130077, #145221, #62853, #194992, #46626, #30373, #96460, #80171, #146277, #196072, #31437, #97516, #15155, #68156, #150522, #167820, #185113, #198171, #148386, #165689, #132165, #49804, #18355, #152633, #99623, #84433, #149439, #34612, #134290, #115930, #114867, #98563, #182995, #202421, #168880, #20484, #164624, #2083, #166760, #116995, #100682, #181920, #199226, #180868, #101753, #85498, #17278, #82293, #200295, #83354, #51948, #3152, #33550, #66016, #52997, #1021, #67086, #16209, #214387, #133220, #86570, #50873, #118070, #184057, #35675, #19420, #151585, #69223, #135342, #201356, #119133, #36739, #136405, #102825, #4220, #70289, #32489, #23688, #22611, #189397, #55140, #88719, #121286, #5280, #54076, #72431, #93799, #71357, #6362, #138533, #204556, #187261, #45046, #159839, #143636, #37819, #89798, #41039, #154778, #120211, #38888, #104973, #122368, #171014, #56204, #188324, #106072, #11439, #209630, #110093, #186186, #169944, #77515, #21530, #61271, #39964, #172095, #155843, #127433, #7429, #203487, #73510, #87640, #139613, #205635, #57273, #193403, #123435, #176103, #27703, #111159, #177158, #28777, #94859, #160912, #12507, #78579, #144701, #103897, #153711, #137473, #132701, #112228, #95933, #195546, #80727, #196607, #163054, #48247, #181409, #213883, #33035, #16758, #130615, #50352, #491, #47182, #131652, #161989, #164114, #113296, #63407, #182464, #197655, #128499, #30925, #31982, #14633, #211769, #13579, #99113, #179304, #34093, #198707, #82841, #79652, #147867, #17818, #65505, #97001, #129559, #145768, #146818, #148917, #212837, #64474, #194468, #46110, #114361, #116472, #180356, #98060, #15699, #81784, #49301, #178236, #115417, #165163, #66559, #100164, #166228, #83902, #210712, #62340, #29851, #119677, #3691, #134823, #103366, #18891, #200828, #84975, #35144 ),
 ( #52479, #149992, #2629, #68701, #168365, #118607, #184595, #151066, #152120, #70829, #202972, #169428, #133769, #51423, #136946, #117544, #54613, #19961, #36213, #102292, #120761, #53545, #69768, #21011, #186739, #167304, #183538, #86045, #101220, #135874, #201893, #22072, #185663, #37293, #87110, #153180, #4754, #38361, #1563, #199777, #104439, #67625, #170488, #88184, #154256, #5829, #181054, #131306, #197297, #196249, #213527, #195185, #116112, #99810, #31624, #96638, #32671, #83546, #97698, #47893, #80359, #146457, #67272, #114005, #81425, #112932, #178945, #163757, #34789, #15336, #180000, #147506, #65150, #48938, #30559, #115057, #212472, #182102, #98750, #164807, #150707, #16400, #64116, #162692, #66202, #82478, #148567, #49992, #130258, #134, #132347, #198352, #129208, #33733, #165875, #17461, #149627, #1209, #133410, #199416, #117184, #51060, #183185, #14266, #100864, #166949, #18541, #46818, #84618, #2269, #136588, #119317, #201540, #69411, #120398, #22789, #154960, #55324, #200481, #184237, #88907, #35861, #6545, #202609, #135519, #4400, #72623, #86754, #3342, #36926, #186373, #70472, #89975, #68345, #19611, #54261, #105160, #53189, #185303, #188514, #156026, #170130, #38008, #21714, #104080, #101940, #168005, #40144, #103009, #87826, #39074, #71545, #171199, #138722, #153896, #122553, #204740, #169065, #203675, #85684, #5465, #20662, #152824, #106257, #121475, #52127, #137656, #187446, #56389, #172282, #151771, #23868, #134479, #118256, #210079, #94244, #91041, #159212, #29222, #58519, #205825, #74773, #140876, #193837, #57456, #189580, #124674, #60643, #141942, #95312, #209006, #206888, #7615, #44420, #45486, #127886, #190631, #111602, #108404, #177610, #8691, #160283, #175484, #42292, #11885, #73699, #174427, #173357, #157101, #26003, #77961, #109476, #59578, #75834, #123617, #76888, #139796, #92113, #93179, #10813, #143008, #192761, #41228, #126805, #61718, #110538, #176538, #28149, #144082, #207954, #107333, #158168, #9760, #24938, #125734, #191696, #43355, #27072, #168543, #89447, #20140, #3871, #56929, #69944, #189059, #170672, #103549, #38547, #123102, #120945, #37471, #71010, #6015, #104625, #124156, #102477, #53729, #22260, #139261, #169609, #4934, #8170, #190118, #204206, #88369, #55859, #154435, #136056, #202069, #74254, #21191, #122015, #138196, #155499, #172828, #185839, #119861, #186917, #87294, #137123, #72084, #187983, #86227, #152298, #153363, #39609, #205291, #203152, #54796, #140348, #105712, #171740, #23337, #7082, #73154, #40696, #106799, #206367, #24399, #90512, #156577, #57993, #112155, #125212, #75313, #92658, #59055, #191174, #159761, #79576, #26550, #11361, #76372, #176029, #209551, #42841, #41772, #25486, #110016, #129489, #95857, #161913, #91592, #143557, #93722, #43902, #27622, #108948, #126282, #107884, #28700, #12425, #158700, #9241, #77440, #210637, #10299, #174968, #207436, #142479, #194391, #208487, #60123, #157644, #141429, #192240, #13503, #61195, #127354, #193323, #44971, #111079, #177083, #94785, #160834, #78505, #144623, #62264, #63329, #128424, #46034, #178158, #29773, #145695, #211693, #173912, #196533, #164045, #48175, #146743, #195471, #213808, #17739, #212762, #147791, #65429, #131579, #114288, #183464, #83827, #67553, #179223, #165093, #182387, #15620, #47103, #180286, #31909, #49224, #97986, #81710, #197581, #16684, #150989, #113218, #34017, #30848, #96926, #149920, #162977, #133697, #115344, #181335, #32962, #1488, #99037, #82768, #199702, #130541, #148842, #132627, #198632, #415, #167229, #66486, #100091, #50280, #116399, #166152, #51348, #117472, #14555, #35071, #80653, #64397, #101141, #18815, #84902, #2554, #68629, #105453, #137938, #171489, #155248, #54540, #188807, #139013, #185591, #55606, #85974, #88112, #37220, #201824, #106544, #121762, #52410, #169355, #170412, #153109, #135800, #152049, #23080, #103294, #172570, #122845, #6829, #3618, #71828, #156323, #20941, #118536, #53469, #119606, #24152, #184519, #102223, #87037, #187728, #120687, #7905, #39357, #4683, #134751, #89196, #90255, #40443, #70757, #200760, #136870, #36140, #202895 ) ),
 .UNSPECIFIED., .F., .F., .T. ) 
 B_SPLINE_SURFACE_WITH_KNOTS ( ( 2, 2 ),
 ( 3, 2, 2, 2, 2, 2, 2, 2, 2, 2, 2, 2, 2, 2, 2, 2, 2, 2, 2, 2, 2, 2, 2, 2, 2, 2, 2, 2, 2, 2, 2, 2, 2, 2, 2, 2, 2, 2, 2, 2, 2, 2, 2, 2, 2, 2, 2, 2, 2, 2, 2, 2, 2, 2, 2, 2, 2, 2, 2, 2, 2, 2, 2, 2, 2, 2, 2, 2, 2, 2, 2, 2, 2, 2, 2, 2, 2, 2, 2, 2, 2, 2, 2, 2, 2, 2, 2, 2, 2, 2, 2, 2, 2, 2, 2, 2, 2, 2, 2, 2, 2, 2, 2, 2, 2, 2, 2, 2, 2, 2, 2, 2, 2, 2, 2, 2, 2, 2, 2, 2, 2, 2, 2, 2, 2, 2, 2, 2, 2, 2, 2, 2, 2, 2, 2, 2, 2, 2, 2, 2, 2, 2, 2, 2, 2, 2, 2, 2, 2, 2, 2, 2, 2, 2, 2, 2, 2, 2, 2, 2, 2, 2, 2, 2, 2, 2, 2, 2, 2, 2, 2, 2, 2, 2, 2, 2, 2, 2, 2, 2, 2, 2, 2, 2, 2, 2, 2, 2, 2, 2, 2, 2, 2, 2, 2, 2, 2, 2, 2, 2, 2, 2, 2, 2, 2, 2, 2, 2, 2, 2, 2, 2, 2, 2, 2, 2, 2, 2, 2, 2, 2, 2, 2, 2, 2, 2, 2, 2, 2, 2, 2, 2, 2, 2, 2, 2, 2, 2, 2, 2, 3 ),
 ( 0.000000000000000000, 1.000000000000000000 ),
 ( 0.000000000000000000, 0.004166666666666666609, 0.008333333333333333218, 0.01250000000000000069, 0.01666666666666666644, 0.02083333333333333218, 0.02500000000000000139, 0.02916666666666666713, 0.03333333333333333287, 0.03749999999999999861, 0.04166666666666666435, 0.04583333333333333010, 0.05000000000000000278, 0.05416666666666666852, 0.05833333333333333426, 0.06250000000000000000, 0.06666666666666666574, 0.07083333333333333148, 0.07499999999999999722, 0.07916666666666666297, 0.08333333333333332871, 0.08749999999999999445, 0.09166666666666666019, 0.09583333333333333981, 0.1000000000000000056, 0.1041666666666666713, 0.1083333333333333370, 0.1125000000000000028, 0.1166666666666666685, 0.1208333333333333343, 0.1250000000000000000, 0.1291666666666666796, 0.1333333333333333315, 0.1375000000000000111, 0.1416666666666666630, 0.1458333333333333426, 0.1499999999999999944, 0.1541666666666666741, 0.1583333333333333259, 0.1625000000000000056, 0.1666666666666666574, 0.1708333333333333370, 0.1749999999999999889, 0.1791666666666666685, 0.1833333333333333204, 0.1875000000000000000, 0.1916666666666666796, 0.1958333333333333315, 0.2000000000000000111, 0.2041666666666666630, 0.2083333333333333426, 0.2124999999999999944, 0.2166666666666666741, 0.2208333333333333259, 0.2250000000000000056, 0.2291666666666666574, 0.2333333333333333370, 0.2374999999999999889, 0.2416666666666666685, 0.2458333333333333204, 0.2500000000000000000, 0.2541666666666666519, 0.2583333333333333592, 0.2625000000000000111, 0.2666666666666666630, 0.2708333333333333148, 0.2750000000000000222, 0.2791666666666666741, 0.2833333333333333259, 0.2874999999999999778, 0.2916666666666666852, 0.2958333333333333370, 0.2999999999999999889, 0.3041666666666666408, 0.3083333333333333481, 0.3125000000000000000, 0.3166666666666666519, 0.3208333333333333592, 0.3250000000000000111, 0.3291666666666666630, 0.3333333333333333148, 0.3375000000000000222, 0.3416666666666666741, 0.3458333333333333259, 0.3499999999999999778, 0.3541666666666666852, 0.3583333333333333370, 0.3624999999999999889, 0.3666666666666666408, 0.3708333333333333481, 0.3750000000000000000, 0.3791666666666666519, 0.3833333333333333592, 0.3875000000000000111, 0.3916666666666666630, 0.3958333333333333148, 0.4000000000000000222, 0.4041666666666666741, 0.4083333333333333259, 0.4124999999999999778, 0.4166666666666666852, 0.4208333333333333370, 0.4249999999999999889, 0.4291666666666666408, 0.4333333333333333481, 0.4375000000000000000, 0.4416666666666666519, 0.4458333333333333592, 0.4500000000000000111, 0.4541666666666666630, 0.4583333333333333148, 0.4625000000000000222, 0.4666666666666666741, 0.4708333333333333259, 0.4749999999999999778, 0.4791666666666666852, 0.4833333333333333370, 0.4874999999999999889, 0.4916666666666666408, 0.4958333333333333481, 0.5000000000000000000, 0.5041666666666666519, 0.5083333333333333037, 0.5124999999999999556, 0.5166666666666667185, 0.5208333333333333703, 0.5250000000000000222, 0.5291666666666666741, 0.5333333333333333259, 0.5374999999999999778, 0.5416666666666666297, 0.5458333333333332815, 0.5500000000000000444, 0.5541666666666666963, 0.5583333333333333481, 0.5625000000000000000, 0.5666666666666666519, 0.5708333333333333037, 0.5749999999999999556, 0.5791666666666667185, 0.5833333333333333703, 0.5875000000000000222, 0.5916666666666666741, 0.5958333333333333259, 0.5999999999999999778, 0.6041666666666666297, 0.6083333333333332815, 0.6125000000000000444, 0.6166666666666666963, 0.6208333333333333481, 0.6250000000000000000, 0.6291666666666666519, 0.6333333333333333037, 0.6374999999999999556, 0.6416666666666667185, 0.6458333333333333703, 0.6500000000000000222, 0.6541666666666666741, 0.6583333333333333259, 0.6624999999999999778, 0.6666666666666666297, 0.6708333333333332815, 0.6750000000000000444, 0.6791666666666666963, 0.6833333333333333481, 0.6875000000000000000, 0.6916666666666666519, 0.6958333333333333037, 0.6999999999999999556, 0.7041666666666667185, 0.7083333333333333703, 0.7125000000000000222, 0.7166666666666666741, 0.7208333333333333259, 0.7249999999999999778, 0.7291666666666666297, 0.7333333333333332815, 0.7375000000000000444, 0.7416666666666666963, 0.7458333333333333481, 0.7500000000000000000, 0.7541666666666666519, 0.7583333333333333037, 0.7624999999999999556, 0.7666666666666667185, 0.7708333333333333703, 0.7750000000000000222, 0.7791666666666666741, 0.7833333333333333259, 0.7874999999999999778, 0.7916666666666666297, 0.7958333333333332815, 0.8000000000000000444, 0.8041666666666666963, 0.8083333333333333481, 0.8125000000000000000, 0.8166666666666666519, 0.8208333333333333037, 0.8249999999999999556, 0.8291666666666667185, 0.8333333333333333703, 0.8375000000000000222, 0.8416666666666666741, 0.8458333333333333259, 0.8499999999999999778, 0.8541666666666666297, 0.8583333333333332815, 0.8625000000000000444, 0.8666666666666666963, 0.8708333333333333481, 0.8750000000000000000, 0.8791666666666666519, 0.8833333333333333037, 0.8874999999999999556, 0.8916666666666667185, 0.8958333333333333703, 0.9000000000000000222, 0.9041666666666666741, 0.9083333333333333259, 0.9124999999999999778, 0.9166666666666666297, 0.9208333333333332815, 0.9250000000000000444, 0.9291666666666666963, 0.9333333333333333481, 0.9375000000000000000, 0.9416666666666666519, 0.9458333333333333037, 0.9499999999999999556, 0.9541666666666667185, 0.9583333333333333703, 0.9625000000000000222, 0.9666666666666666741, 0.9708333333333333259, 0.9749999999999999778, 0.9791666666666666297, 0.9833333333333332815, 0.9875000000000000444, 0.9916666666666666963, 0.9958333333333333481, 1.000000000000000000 ),
 .UNSPECIFIED. ) 
 GEOMETRIC_REPRESENTATION_ITEM ( )  RATIONAL_B_SPLINE_SURFACE ( (
 ( 1.000000000000000000, 0.8660254037844387076, 1.000000000000000000, 0.8660254037844387076, 1.000000000000000000, 0.8660254037844387076, 1.000000000000000000, 0.8660254037844387076, 1.000000000000000000, 0.8660254037844387076, 1.000000000000000000, 0.8660254037844387076, 1.000000000000000000, 0.8660254037844387076, 1.000000000000000000, 0.8660254037844387076, 1.000000000000000000, 0.8660254037844387076, 1.000000000000000000, 0.8660254037844387076, 1.000000000000000000, 0.8660254037844387076, 1.000000000000000000, 0.8660254037844387076, 1.000000000000000000, 0.8660254037844387076, 1.000000000000000000, 0.8660254037844387076, 1.000000000000000000, 0.8660254037844387076, 1.000000000000000000, 0.8660254037844387076, 1.000000000000000000, 0.8660254037844387076, 1.000000000000000000, 0.8660254037844387076, 1.000000000000000000, 0.8660254037844387076, 1.000000000000000000, 0.8660254037844387076, 1.000000000000000000, 0.8660254037844387076, 1.000000000000000000, 0.8660254037844387076, 1.000000000000000000, 0.8660254037844387076, 1.000000000000000000, 0.8660254037844387076, 1.000000000000000000, 0.8660254037844387076, 1.000000000000000000, 0.8660254037844387076, 1.000000000000000000, 0.8660254037844387076, 1.000000000000000000, 0.8660254037844387076, 1.000000000000000000, 0.8660254037844387076, 1.000000000000000000, 0.8660254037844387076, 1.000000000000000000, 0.8660254037844387076, 1.000000000000000000, 0.8660254037844387076, 1.000000000000000000, 0.8660254037844387076, 1.000000000000000000, 0.8660254037844387076, 1.000000000000000000, 0.8660254037844387076, 1.000000000000000000, 0.8660254037844387076, 1.000000000000000000, 0.8660254037844387076, 1.000000000000000000, 0.8660254037844387076, 1.000000000000000000, 0.8660254037844387076, 1.000000000000000000, 0.8660254037844387076, 1.000000000000000000, 0.8660254037844387076, 1.000000000000000000, 0.8660254037844387076, 1.000000000000000000, 0.8660254037844387076, 1.000000000000000000, 0.8660254037844387076, 1.000000000000000000, 0.8660254037844387076, 1.000000000000000000, 0.8660254037844387076, 1.000000000000000000, 0.8660254037844387076, 1.000000000000000000, 0.8660254037844387076, 1.000000000000000000, 0.8660254037844387076, 1.000000000000000000, 0.8660254037844387076, 1.000000000000000000, 0.8660254037844387076, 1.000000000000000000, 0.8660254037844387076, 1.000000000000000000, 0.8660254037844387076, 1.000000000000000000, 0.8660254037844387076, 1.000000000000000000, 0.8660254037844387076, 1.000000000000000000, 0.8660254037844387076, 1.000000000000000000, 0.8660254037844387076, 1.000000000000000000, 0.8660254037844387076, 1.000000000000000000, 0.8660254037844387076, 1.000000000000000000, 0.8660254037844387076, 1.000000000000000000, 0.8660254037844387076, 1.000000000000000000, 0.8660254037844387076, 1.000000000000000000, 0.8660254037844387076, 1.000000000000000000, 0.8660254037844387076, 1.000000000000000000, 0.8660254037844387076, 1.000000000000000000, 0.8660254037844387076, 1.000000000000000000, 0.8660254037844387076, 1.000000000000000000, 0.8660254037844387076, 1.000000000000000000, 0.8660254037844387076, 1.000000000000000000, 0.8660254037844387076, 1.000000000000000000, 0.8660254037844387076, 1.000000000000000000, 0.8660254037844387076, 1.000000000000000000, 0.8660254037844387076, 1.000000000000000000, 0.8660254037844387076, 1.000000000000000000, 0.8660254037844387076, 1.000000000000000000, 0.8660254037844387076, 1.000000000000000000, 0.8660254037844387076, 1.000000000000000000, 0.8660254037844387076, 1.000000000000000000, 0.8660254037844387076, 1.000000000000000000, 0.8660254037844387076, 1.000000000000000000, 0.8660254037844387076, 1.000000000000000000, 0.8660254037844387076, 1.000000000000000000, 0.8660254037844387076, 1.000000000000000000, 0.8660254037844387076, 1.000000000000000000, 0.8660254037844387076, 1.000000000000000000, 0.8660254037844387076, 1.000000000000000000, 0.8660254037844387076, 1.000000000000000000, 0.8660254037844387076, 1.000000000000000000, 0.8660254037844387076, 1.000000000000000000, 0.8660254037844387076, 1.000000000000000000, 0.8660254037844387076, 1.000000000000000000, 0.8660254037844387076, 1.000000000000000000, 0.8660254037844387076, 1.000000000000000000, 0.8660254037844387076, 1.000000000000000000, 0.8660254037844387076, 1.000000000000000000, 0.8660254037844387076, 1.000000000000000000, 0.8660254037844387076, 1.000000000000000000, 0.8660254037844387076, 1.000000000000000000, 0.8660254037844387076, 1.000000000000000000, 0.8660254037844387076, 1.000000000000000000, 0.8660254037844387076, 1.000000000000000000, 0.8660254037844387076, 1.000000000000000000, 0.8660254037844387076, 1.000000000000000000, 0.8660254037844387076, 1.000000000000000000, 0.8660254037844387076, 1.000000000000000000, 0.8660254037844387076, 1.000000000000000000, 0.8660254037844387076, 1.000000000000000000, 0.8660254037844387076, 1.000000000000000000, 0.8660254037844387076, 1.000000000000000000, 0.8660254037844387076, 1.000000000000000000, 0.8660254037844387076, 1.000000000000000000, 0.8660254037844387076, 1.000000000000000000, 0.8660254037844387076, 1.000000000000000000, 0.8660254037844387076, 1.000000000000000000, 0.8660254037844387076, 1.000000000000000000, 0.8660254037844387076, 1.000000000000000000, 0.8660254037844387076, 1.000000000000000000, 0.8660254037844387076, 1.000000000000000000, 0.8660254037844387076, 1.000000000000000000, 0.8660254037844387076, 1.000000000000000000, 0.8660254037844387076, 1.000000000000000000, 0.8660254037844387076, 1.000000000000000000, 0.8660254037844387076, 1.000000000000000000, 0.8660254037844387076, 1.000000000000000000, 0.8660254037844387076, 1.000000000000000000, 0.8660254037844387076, 1.000000000000000000, 0.8660254037844387076, 1.000000000000000000, 0.8660254037844387076, 1.000000000000000000, 0.8660254037844387076, 1.000000000000000000, 0.8660254037844387076, 1.000000000000000000, 0.8660254037844387076, 1.000000000000000000, 0.8660254037844387076, 1.000000000000000000, 0.8660254037844387076, 1.000000000000000000, 0.8660254037844387076, 1.000000000000000000, 0.8660254037844387076, 1.000000000000000000, 0.8660254037844387076, 1.000000000000000000, 0.8660254037844387076, 1.000000000000000000, 0.8660254037844387076, 1.000000000000000000, 0.8660254037844387076, 1.000000000000000000, 0.8660254037844387076, 1.000000000000000000, 0.8660254037844387076, 1.000000000000000000, 0.8660254037844387076, 1.000000000000000000, 0.8660254037844387076, 1.000000000000000000, 0.8660254037844387076, 1.000000000000000000, 0.8660254037844387076, 1.000000000000000000, 0.8660254037844387076, 1.000000000000000000, 0.8660254037844387076, 1.000000000000000000, 0.8660254037844387076, 1.000000000000000000, 0.8660254037844387076, 1.000000000000000000, 0.8660254037844387076, 1.000000000000000000, 0.8660254037844387076, 1.000000000000000000, 0.8660254037844387076, 1.000000000000000000, 0.8660254037844387076, 1.000000000000000000, 0.8660254037844387076, 1.000000000000000000, 0.8660254037844387076, 1.000000000000000000, 0.8660254037844387076, 1.000000000000000000, 0.8660254037844387076, 1.000000000000000000, 0.8660254037844387076, 1.000000000000000000, 0.8660254037844387076, 1.000000000000000000, 0.8660254037844387076, 1.000000000000000000, 0.8660254037844387076, 1.000000000000000000, 0.8660254037844387076, 1.000000000000000000, 0.8660254037844387076, 1.000000000000000000, 0.8660254037844387076, 1.000000000000000000, 0.8660254037844387076, 1.000000000000000000, 0.8660254037844387076, 1.000000000000000000, 0.8660254037844387076, 1.000000000000000000, 0.8660254037844387076, 1.000000000000000000, 0.8660254037844387076, 1.000000000000000000, 0.8660254037844387076, 1.000000000000000000, 0.8660254037844387076, 1.000000000000000000, 0.8660254037844387076, 1.000000000000000000, 0.8660254037844387076, 1.000000000000000000, 0.8660254037844387076, 1.000000000000000000, 0.8660254037844387076, 1.000000000000000000, 0.8660254037844387076, 1.000000000000000000, 0.8660254037844387076, 1.000000000000000000, 0.8660254037844387076, 1.000000000000000000, 0.8660254037844387076, 1.000000000000000000, 0.8660254037844387076, 1.000000000000000000, 0.8660254037844387076, 1.000000000000000000, 0.8660254037844387076, 1.000000000000000000, 0.8660254037844387076, 1.000000000000000000, 0.8660254037844387076, 1.000000000000000000, 0.8660254037844387076, 1.000000000000000000, 0.8660254037844387076, 1.000000000000000000, 0.8660254037844387076, 1.000000000000000000, 0.8660254037844387076, 1.000000000000000000, 0.8660254037844387076, 1.000000000000000000, 0.8660254037844387076, 1.000000000000000000, 0.8660254037844387076, 1.000000000000000000, 0.8660254037844387076, 1.000000000000000000, 0.8660254037844387076, 1.000000000000000000, 0.8660254037844387076, 1.000000000000000000, 0.8660254037844387076, 1.000000000000000000, 0.8660254037844387076, 1.000000000000000000, 0.8660254037844387076, 1.000000000000000000, 0.8660254037844387076, 1.000000000000000000, 0.8660254037844387076, 1.000000000000000000, 0.8660254037844387076, 1.000000000000000000, 0.8660254037844387076, 1.000000000000000000, 0.8660254037844387076, 1.000000000000000000, 0.8660254037844387076, 1.000000000000000000, 0.8660254037844387076, 1.000000000000000000, 0.8660254037844387076, 1.000000000000000000, 0.8660254037844387076, 1.000000000000000000, 0.8660254037844387076, 1.000000000000000000, 0.8660254037844387076, 1.000000000000000000, 0.8660254037844387076, 1.000000000000000000, 0.8660254037844387076, 1.000000000000000000, 0.8660254037844387076, 1.000000000000000000, 0.8660254037844387076, 1.000000000000000000, 0.8660254037844387076, 1.000000000000000000, 0.8660254037844387076, 1.000000000000000000, 0.8660254037844387076, 1.000000000000000000, 0.8660254037844387076, 1.000000000000000000, 0.8660254037844387076, 1.000000000000000000, 0.8660254037844387076, 1.000000000000000000, 0.8660254037844387076, 1.000000000000000000, 0.8660254037844387076, 1.000000000000000000, 0.8660254037844387076, 1.000000000000000000, 0.8660254037844387076, 1.000000000000000000, 0.8660254037844387076, 1.000000000000000000, 0.8660254037844387076, 1.000000000000000000, 0.8660254037844387076, 1.000000000000000000, 0.8660254037844387076, 1.000000000000000000, 0.8660254037844387076, 1.000000000000000000, 0.8660254037844387076, 1.000000000000000000, 0.8660254037844387076, 1.000000000000000000, 0.8660254037844387076, 1.000000000000000000, 0.8660254037844387076, 1.000000000000000000, 0.8660254037844387076, 1.000000000000000000, 0.8660254037844387076, 1.000000000000000000, 0.8660254037844387076, 1.000000000000000000, 0.8660254037844387076, 1.000000000000000000, 0.8660254037844387076, 1.000000000000000000, 0.8660254037844387076, 1.000000000000000000, 0.8660254037844387076, 1.000000000000000000, 0.8660254037844387076, 1.000000000000000000, 0.8660254037844387076, 1.000000000000000000),
 ( 1.000000000000000000, 0.8660254037844387076, 1.000000000000000000, 0.8660254037844387076, 1.000000000000000000, 0.8660254037844387076, 1.000000000000000000, 0.8660254037844387076, 1.000000000000000000, 0.8660254037844387076, 1.000000000000000000, 0.8660254037844387076, 1.000000000000000000, 0.8660254037844387076, 1.000000000000000000, 0.8660254037844387076, 1.000000000000000000, 0.8660254037844387076, 1.000000000000000000, 0.8660254037844387076, 1.000000000000000000, 0.8660254037844387076, 1.000000000000000000, 0.8660254037844387076, 1.000000000000000000, 0.8660254037844387076, 1.000000000000000000, 0.8660254037844387076, 1.000000000000000000, 0.8660254037844387076, 1.000000000000000000, 0.8660254037844387076, 1.000000000000000000, 0.8660254037844387076, 1.000000000000000000, 0.8660254037844387076, 1.000000000000000000, 0.8660254037844387076, 1.000000000000000000, 0.8660254037844387076, 1.000000000000000000, 0.8660254037844387076, 1.000000000000000000, 0.8660254037844387076, 1.000000000000000000, 0.8660254037844387076, 1.000000000000000000, 0.8660254037844387076, 1.000000000000000000, 0.8660254037844387076, 1.000000000000000000, 0.8660254037844387076, 1.000000000000000000, 0.8660254037844387076, 1.000000000000000000, 0.8660254037844387076, 1.000000000000000000, 0.8660254037844387076, 1.000000000000000000, 0.8660254037844387076, 1.000000000000000000, 0.8660254037844387076, 1.000000000000000000, 0.8660254037844387076, 1.000000000000000000, 0.8660254037844387076, 1.000000000000000000, 0.8660254037844387076, 1.000000000000000000, 0.8660254037844387076, 1.000000000000000000, 0.8660254037844387076, 1.000000000000000000, 0.8660254037844387076, 1.000000000000000000, 0.8660254037844387076, 1.000000000000000000, 0.8660254037844387076, 1.000000000000000000, 0.8660254037844387076, 1.000000000000000000, 0.8660254037844387076, 1.000000000000000000, 0.8660254037844387076, 1.000000000000000000, 0.8660254037844387076, 1.000000000000000000, 0.8660254037844387076, 1.000000000000000000, 0.8660254037844387076, 1.000000000000000000, 0.8660254037844387076, 1.000000000000000000, 0.8660254037844387076, 1.000000000000000000, 0.8660254037844387076, 1.000000000000000000, 0.8660254037844387076, 1.000000000000000000, 0.8660254037844387076, 1.000000000000000000, 0.8660254037844387076, 1.000000000000000000, 0.8660254037844387076, 1.000000000000000000, 0.8660254037844387076, 1.000000000000000000, 0.8660254037844387076, 1.000000000000000000, 0.8660254037844387076, 1.000000000000000000, 0.8660254037844387076, 1.000000000000000000, 0.8660254037844387076, 1.000000000000000000, 0.8660254037844387076, 1.000000000000000000, 0.8660254037844387076, 1.000000000000000000, 0.8660254037844387076, 1.000000000000000000, 0.8660254037844387076, 1.000000000000000000, 0.8660254037844387076, 1.000000000000000000, 0.8660254037844387076, 1.000000000000000000, 0.8660254037844387076, 1.000000000000000000, 0.8660254037844387076, 1.000000000000000000, 0.8660254037844387076, 1.000000000000000000, 0.8660254037844387076, 1.000000000000000000, 0.8660254037844387076, 1.000000000000000000, 0.8660254037844387076, 1.000000000000000000, 0.8660254037844387076, 1.000000000000000000, 0.8660254037844387076, 1.000000000000000000, 0.8660254037844387076, 1.000000000000000000, 0.8660254037844387076, 1.000000000000000000, 0.8660254037844387076, 1.000000000000000000, 0.8660254037844387076, 1.000000000000000000, 0.8660254037844387076, 1.000000000000000000, 0.8660254037844387076, 1.000000000000000000, 0.8660254037844387076, 1.000000000000000000, 0.8660254037844387076, 1.000000000000000000, 0.8660254037844387076, 1.000000000000000000, 0.8660254037844387076, 1.000000000000000000, 0.8660254037844387076, 1.000000000000000000, 0.8660254037844387076, 1.000000000000000000, 0.8660254037844387076, 1.000000000000000000, 0.8660254037844387076, 1.000000000000000000, 0.8660254037844387076, 1.000000000000000000, 0.8660254037844387076, 1.000000000000000000, 0.8660254037844387076, 1.000000000000000000, 0.8660254037844387076, 1.000000000000000000, 0.8660254037844387076, 1.000000000000000000, 0.8660254037844387076, 1.000000000000000000, 0.8660254037844387076, 1.000000000000000000, 0.8660254037844387076, 1.000000000000000000, 0.8660254037844387076, 1.000000000000000000, 0.8660254037844387076, 1.000000000000000000, 0.8660254037844387076, 1.000000000000000000, 0.8660254037844387076, 1.000000000000000000, 0.8660254037844387076, 1.000000000000000000, 0.8660254037844387076, 1.000000000000000000, 0.8660254037844387076, 1.000000000000000000, 0.8660254037844387076, 1.000000000000000000, 0.8660254037844387076, 1.000000000000000000, 0.8660254037844387076, 1.000000000000000000, 0.8660254037844387076, 1.000000000000000000, 0.8660254037844387076, 1.000000000000000000, 0.8660254037844387076, 1.000000000000000000, 0.8660254037844387076, 1.000000000000000000, 0.8660254037844387076, 1.000000000000000000, 0.8660254037844387076, 1.000000000000000000, 0.8660254037844387076, 1.000000000000000000, 0.8660254037844387076, 1.000000000000000000, 0.8660254037844387076, 1.000000000000000000, 0.8660254037844387076, 1.000000000000000000, 0.8660254037844387076, 1.000000000000000000, 0.8660254037844387076, 1.000000000000000000, 0.8660254037844387076, 1.000000000000000000, 0.8660254037844387076, 1.000000000000000000, 0.8660254037844387076, 1.000000000000000000, 0.8660254037844387076, 1.000000000000000000, 0.8660254037844387076, 1.000000000000000000, 0.8660254037844387076, 1.000000000000000000, 0.8660254037844387076, 1.000000000000000000, 0.8660254037844387076, 1.000000000000000000, 0.8660254037844387076, 1.000000000000000000, 0.8660254037844387076, 1.000000000000000000, 0.8660254037844387076, 1.000000000000000000, 0.8660254037844387076, 1.000000000000000000, 0.8660254037844387076, 1.000000000000000000, 0.8660254037844387076, 1.000000000000000000, 0.8660254037844387076, 1.000000000000000000, 0.8660254037844387076, 1.000000000000000000, 0.8660254037844387076, 1.000000000000000000, 0.8660254037844387076, 1.000000000000000000, 0.8660254037844387076, 1.000000000000000000, 0.8660254037844387076, 1.000000000000000000, 0.8660254037844387076, 1.000000000000000000, 0.8660254037844387076, 1.000000000000000000, 0.8660254037844387076, 1.000000000000000000, 0.8660254037844387076, 1.000000000000000000, 0.8660254037844387076, 1.000000000000000000, 0.8660254037844387076, 1.000000000000000000, 0.8660254037844387076, 1.000000000000000000, 0.8660254037844387076, 1.000000000000000000, 0.8660254037844387076, 1.000000000000000000, 0.8660254037844387076, 1.000000000000000000, 0.8660254037844387076, 1.000000000000000000, 0.8660254037844387076, 1.000000000000000000, 0.8660254037844387076, 1.000000000000000000, 0.8660254037844387076, 1.000000000000000000, 0.8660254037844387076, 1.000000000000000000, 0.8660254037844387076, 1.000000000000000000, 0.8660254037844387076, 1.000000000000000000, 0.8660254037844387076, 1.000000000000000000, 0.8660254037844387076, 1.000000000000000000, 0.8660254037844387076, 1.000000000000000000, 0.8660254037844387076, 1.000000000000000000, 0.8660254037844387076, 1.000000000000000000, 0.8660254037844387076, 1.000000000000000000, 0.8660254037844387076, 1.000000000000000000, 0.8660254037844387076, 1.000000000000000000, 0.8660254037844387076, 1.000000000000000000, 0.8660254037844387076, 1.000000000000000000, 0.8660254037844387076, 1.000000000000000000, 0.8660254037844387076, 1.000000000000000000, 0.8660254037844387076, 1.000000000000000000, 0.8660254037844387076, 1.000000000000000000, 0.8660254037844387076, 1.000000000000000000, 0.8660254037844387076, 1.000000000000000000, 0.8660254037844387076, 1.000000000000000000, 0.8660254037844387076, 1.000000000000000000, 0.8660254037844387076, 1.000000000000000000, 0.8660254037844387076, 1.000000000000000000, 0.8660254037844387076, 1.000000000000000000, 0.8660254037844387076, 1.000000000000000000, 0.8660254037844387076, 1.000000000000000000, 0.8660254037844387076, 1.000000000000000000, 0.8660254037844387076, 1.000000000000000000, 0.8660254037844387076, 1.000000000000000000, 0.8660254037844387076, 1.000000000000000000, 0.8660254037844387076, 1.000000000000000000, 0.8660254037844387076, 1.000000000000000000, 0.8660254037844387076, 1.000000000000000000, 0.8660254037844387076, 1.000000000000000000, 0.8660254037844387076, 1.000000000000000000, 0.8660254037844387076, 1.000000000000000000, 0.8660254037844387076, 1.000000000000000000, 0.8660254037844387076, 1.000000000000000000, 0.8660254037844387076, 1.000000000000000000, 0.8660254037844387076, 1.000000000000000000, 0.8660254037844387076, 1.000000000000000000, 0.8660254037844387076, 1.000000000000000000, 0.8660254037844387076, 1.000000000000000000, 0.8660254037844387076, 1.000000000000000000, 0.8660254037844387076, 1.000000000000000000, 0.8660254037844387076, 1.000000000000000000, 0.8660254037844387076, 1.000000000000000000, 0.8660254037844387076, 1.000000000000000000, 0.8660254037844387076, 1.000000000000000000, 0.8660254037844387076, 1.000000000000000000, 0.8660254037844387076, 1.000000000000000000, 0.8660254037844387076, 1.000000000000000000, 0.8660254037844387076, 1.000000000000000000, 0.8660254037844387076, 1.000000000000000000, 0.8660254037844387076, 1.000000000000000000, 0.8660254037844387076, 1.000000000000000000, 0.8660254037844387076, 1.000000000000000000, 0.8660254037844387076, 1.000000000000000000, 0.8660254037844387076, 1.000000000000000000, 0.8660254037844387076, 1.000000000000000000, 0.8660254037844387076, 1.000000000000000000, 0.8660254037844387076, 1.000000000000000000, 0.8660254037844387076, 1.000000000000000000, 0.8660254037844387076, 1.000000000000000000, 0.8660254037844387076, 1.000000000000000000, 0.8660254037844387076, 1.000000000000000000, 0.8660254037844387076, 1.000000000000000000, 0.8660254037844387076, 1.000000000000000000, 0.8660254037844387076, 1.000000000000000000, 0.8660254037844387076, 1.000000000000000000, 0.8660254037844387076, 1.000000000000000000, 0.8660254037844387076, 1.000000000000000000, 0.8660254037844387076, 1.000000000000000000, 0.8660254037844387076, 1.000000000000000000, 0.8660254037844387076, 1.000000000000000000, 0.8660254037844387076, 1.000000000000000000, 0.8660254037844387076, 1.000000000000000000, 0.8660254037844387076, 1.000000000000000000, 0.8660254037844387076, 1.000000000000000000, 0.8660254037844387076, 1.000000000000000000, 0.8660254037844387076, 1.000000000000000000, 0.8660254037844387076, 1.000000000000000000, 0.8660254037844387076, 1.000000000000000000, 0.8660254037844387076, 1.000000000000000000, 0.8660254037844387076, 1.000000000000000000, 0.8660254037844387076, 1.000000000000000000, 0.8660254037844387076, 1.000000000000000000, 0.8660254037844387076, 1.000000000000000000, 0.8660254037844387076, 1.000000000000000000, 0.8660254037844387076, 1.000000000000000000, 0.8660254037844387076, 1.000000000000000000) ) ) 
 REPRESENTATION_ITEM ( '' )  SURFACE ( )  );
#161871=CARTESIAN_POINT ( 'NONE',  ( -8.179646747746328828, 8.437342715325849341, -0.7998128361456291469 ) ) ;
#161876=CARTESIAN_POINT ( 'NONE',  ( -6.082978790695654503, 6.030206930409384825, -0.4315292173028318912 ) ) ;
#161877=CARTESIAN_POINT ( 'NONE',  ( 0.6823417656249882723, 0.9260416670080831025, -1.181850606188749264 ) ) ;
#161880=CARTESIAN_POINT ( 'NONE',  ( 6.155038550924133212, 10.12470270947942730, 0.7216878364870438212 ) ) ;
#161887=ADVANCED_FACE ( 'NONE', ( #140196 ), #69799, .F. ) ;
#161898=CARTESIAN_POINT ( 'NONE',  ( 9.398826802771546696, 11.98838390803207865, -1.599625672291262513 ) ) ;
#161902=CARTESIAN_POINT ( 'NONE',  ( -4.623494077460110319, 5.352830164246910272, 1.199719254218462483 ) ) ;
#161903=CARTESIAN_POINT ( 'NONE',  ( -8.206763054973658100, 8.468978407091068306, 0.7998128361456602331 ) ) ;
#161909=CARTESIAN_POINT ( 'NONE',  ( 1.499999999999989120, 3.785416667349481123, 0.8660254037844524744 ) ) ;
#161910=CARTESIAN_POINT ( 'NONE',  ( 7.391166297744269365, 11.77477778067701664, 1.040834085586084257E-14 ) ) ;
#161913=CARTESIAN_POINT ( 'NONE',  ( -7.527801604085656351, 9.805521176231838609, 1.599625672291295375 ) ) ;
#161915=CARTESIAN_POINT ( 'NONE',  ( 1.364683531249988535, 3.155208333674756283, -0.7879004041258239610 ) ) ;
#161920=CARTESIAN_POINT ( 'NONE',  ( -8.188761592974033832, 12.49737959187099179, -0.7216878364870267237 ) ) ;
#161925=CARTESIAN_POINT ( 'NONE',  ( -1.201851678989727383E-14, 3.259375000341420581, -1.575800808251660134 ) ) ;
#161932=CARTESIAN_POINT ( 'NONE',  ( 1.364683531249988535, 3.405208333674749621, -0.7879004041258239610 ) ) ;
#161934=CARTESIAN_POINT ( 'NONE',  ( -4.900382456335551140, 7.804531068111707270, 1.199719254218464037 ) ) ;
#161935=CARTESIAN_POINT ( 'NONE',  ( 6.089583550832340819, 10.25626457594641749, 1.040834085586084257E-14 ) ) ;
#161938=CARTESIAN_POINT ( 'NONE',  ( -1.364683531250012516, 2.842708333674754506, 0.7879004041258379498 ) ) ;
#161940=B_SPLINE_CURVE_WITH_KNOTS ( 'NONE', 3,
 ( #201055, #19117, #185881, #20180 ),
 .UNSPECIFIED., .F., .F.,
 ( 4, 4 ),
 ( 0.003649387816030439866, 0.004429296091066699421 ),
 .UNSPECIFIED. ) ;
#161942=CARTESIAN_POINT ( 'NONE',  ( -0.6823417656250246877, -0.6989583329919113464, 1.181850606188755259 ) ) ;
#161943=CARTESIAN_POINT ( 'NONE',  ( -4.094199201646926412, 7.720390135322642067, 0.7216878364870317197 ) ) ;
#161946=CARTESIAN_POINT ( 'NONE',  ( 4.039966587192250103, 7.657118751792200584, 0.7216878364870298324 ) ) ;
#161949=CARTESIAN_POINT ( 'NONE',  ( -6.367525699912501835, 10.58053041653993098, -0.7998128361456291469 ) ) ;
#161950=CARTESIAN_POINT ( 'NONE',  ( -7.998947442382709383, 12.27592974951444660, 0.7216878364870478180 ) ) ;
#161952=CARTESIAN_POINT ( 'NONE',  ( -1.001543065824772872E-14, 5.071875000341421469, 1.575800808251672791 ) ) ;
#161957=CARTESIAN_POINT ( 'NONE',  ( -7.009202228140755331, 8.240119356661432803, -1.082531754730543083 ) ) ;
#161959=CARTESIAN_POINT ( 'NONE',  ( 0.6823417656249882723, -0.3447916663252489911, 1.181850606188755259 ) ) ;
#161962=CARTESIAN_POINT ( 'NONE',  ( 8.120970824905713314, 8.576813505252564696, 1.040834085586084257E-14 ) ) ;
#161969=CIRCLE ( 'NONE', #89453, 1.000000000000000000 ) ;
#161971=ORIENTED_EDGE ( 'NONE', *, *, #9881, .F. ) ;
#161972=CARTESIAN_POINT ( 'NONE',  ( -3.895595285070177383, 2.800000000000024691, -0.7749999999999944711 ) ) ;
#161973=CARTESIAN_POINT ( 'NONE',  ( 8.202319746143333035, 12.51319743723517952, -0.7216878364870328300 ) ) ;
#161980=CARTESIAN_POINT ( 'NONE',  ( 6.148786358997489820, 7.132337826040578754, -1.199719254218446718 ) ) ;
#161981=CARTESIAN_POINT ( 'NONE',  ( -4.874319919312905647, 5.645460313075203018, -1.199719254218446718 ) ) ;
#161983=VECTOR ( 'NONE', #139821, 1000.000000000000227 ) ;
#161986=CARTESIAN_POINT ( 'NONE',  ( 6.792271770322100721, 7.026664608238323950, -0.7216878364870257245 ) ) ;
#161987=CARTESIAN_POINT ( 'NONE',  ( -1.364683531250012516, 0.8427083336747532849, 0.7879004041258379498 ) ) ;
#161989=CARTESIAN_POINT ( 'NONE',  ( -9.982881178363895103, 10.54111621771303753, 1.040834085586084257E-14 ) ) ;
#162003=CARTESIAN_POINT ( 'NONE',  ( -4.308392981759444851, 7.251705977524093072, -0.9751457471971426427 ) ) ;
#162007=CARTESIAN_POINT ( 'NONE',  ( 7.169564303528210836, 7.258913197071374945, -0.7998128361456281477 ) ) ;
#162013=CARTESIAN_POINT ( 'NONE',  ( 8.178592977541601527, 10.56477777859713463, 1.599625672291281386 ) ) ;
#162018=CARTESIAN_POINT ( 'NONE',  ( -0.7499999999999972244, 3.858333333333359594, -1.299038105676652011 ) ) ;
#162021=CARTESIAN_POINT ( 'NONE',  ( 10.73535870392234237, 11.41900666419791399, 0.000000000000000000 ) ) ;
#162023=CARTESIAN_POINT ( 'NONE',  ( -0.4942839625836717987, 7.528790859548558423, 2.012357903315129537 ) ) ;
#162028=CARTESIAN_POINT ( 'NONE',  ( -8.839552966430012759, 10.37552855133225904, -1.082531754730543971 ) ) ;
#162032=CARTESIAN_POINT ( 'NONE',  ( 6.634017235788401301, 6.634108284708264414, 0.7998128361456341429 ) ) ;
#162038=CARTESIAN_POINT ( 'NONE',  ( 5.192409643909512873, 6.120528008391641350, -1.082531754730549078 ) ) ;
#162042=ORIENTED_EDGE ( 'NONE', *, *, #103885, .F. ) ;
#162047=CARTESIAN_POINT ( 'NONE',  ( -7.206322340863467346, 8.366129804884193888, 1.199719254218450271 ) ) ;
#162048=CARTESIAN_POINT ( 'NONE',  ( -4.948889764188092677, 5.732458465429559169, 1.199719254218462483 ) ) ;
#162053=CARTESIAN_POINT ( 'NONE',  ( 0.3562281372918948974, 7.169715878026163836, -1.968597608854716574 ) ) ;
#162057=CARTESIAN_POINT ( 'NONE',  ( 4.774442650306744085, 8.721933525333202653, -0.7998128361456281477 ) ) ;
#162059=CARTESIAN_POINT ( 'NONE',  ( 1.518728846951481470, 8.688592980705456270, 2.528358009378040450 ) ) ;
#162067=CARTESIAN_POINT ( 'NONE',  ( 3.497640442201256139, 7.024404915969360452, 1.040834085586084257E-14 ) ) ;
#162071=CARTESIAN_POINT ( 'NONE',  ( 1.364683531249988757, -0.05312499965857975237, 0.000000000000000000 ) ) ;
#162072=CARTESIAN_POINT ( 'NONE',  ( 4.761938266897790761, 6.578680616179308771, 1.599625672291267398 ) ) ;
#162074=CARTESIAN_POINT ( 'NONE',  ( -6.182154858151506893, 9.195969186943299789, 1.082531754730548412 ) ) ;
#162076=CARTESIAN_POINT ( 'NONE',  ( 4.528060117284229413, 7.266191989264828344, 1.082531754730558626 ) ) ;
#162077=CARTESIAN_POINT ( 'NONE',  ( -5.870317324592805086, 9.792527945426188651, -0.7216878364870197293 ) ) ;
#162081=CARTESIAN_POINT ( 'NONE',  ( 5.286789834324991055, 8.255339675766103724, -1.199719254218452935 ) ) ;
#162087=CARTESIAN_POINT ( 'NONE',  ( 1.364683531249990311, 4.384375000341417028, 1.214306433183764966E-14 ) ) ;
#162092=CARTESIAN_POINT ( 'NONE',  ( 6.584456157731144899, 10.83361595066169514, -0.7998128361456291469 ) ) ;
#162096=CARTESIAN_POINT ( 'NONE',  ( -7.178152263431422320, 10.46192917639026554, 1.199719254218453823 ) ) ;
#162101=CARTESIAN_POINT ( 'NONE',  ( 9.836604141914616406, 11.43479190611061647, 1.199719254218452047 ) ) ;
#162105=CARTESIAN_POINT ( 'NONE',  ( -6.516665389662827934, 10.75452672124865217, 0.000000000000000000 ) ) ;
#162107=CARTESIAN_POINT ( 'NONE',  ( 5.144285979226959959, 6.473071224410549718, -1.197504025336363576 ) ) ;
#162108=CARTESIAN_POINT ( 'NONE',  ( -8.324343129110692630, 12.65555805069709550, 0.7216878364870338292 ) ) ;
#162112=CARTESIAN_POINT ( 'NONE',  ( 6.474182045725470402, 7.511966127223233869, -1.199719254218446718 ) ) ;
#162114=CARTESIAN_POINT ( 'NONE',  ( 5.341022448779654930, 8.318611059296550536, 1.199719254218462483 ) ) ;
#162115=CARTESIAN_POINT ( 'NONE',  ( -4.183520347117292815, 7.398805986154902037, 0.7851016128354749712 ) ) ;
#162116=CARTESIAN_POINT ( 'NONE',  ( 2.510230996824538430, 6.080353262937265413, 0.000000000000000000 ) ) ;
#162118=CARTESIAN_POINT ( 'NONE',  ( -7.565086526745425033, 7.928281824065535055, 0.7216878364870317197 ) ) ;
#162124=CARTESIAN_POINT ( 'NONE',  ( -4.397013243575890407, 7.155424720373004810, 1.066431095959238462 ) ) ;
#162125=EDGE_CURVE ( 'NONE', #8852, #38245, #76232, .T. ) ;
#162126=CARTESIAN_POINT ( 'NONE',  ( 0.6823417656249864960, -0.5114583329919111243, -1.181850606188749264 ) ) ;
#162129=CARTESIAN_POINT ( 'NONE',  ( 5.016153647376217606, 4.954526798134778254, 0.7216878364870317197 ) ) ;
#162133=CARTESIAN_POINT ( 'NONE',  ( -9.463228032214294316, 10.14278024711257764, 1.040834085586084257E-14 ) ) ;
#162140=CARTESIAN_POINT ( 'NONE',  ( -9.124274191872640216, 10.70770331434866485, -1.082531754730537976 ) ) ;
#162148=CARTESIAN_POINT ( 'NONE',  ( -9.625925875578284163, 10.33259439770390564, 1.040834085586084257E-14 ) ) ;
#162152=FACE_OUTER_BOUND ( 'NONE', #73796, .T. ) ;
#162153=CARTESIAN_POINT ( 'NONE',  ( 0.7499999999999920064, 4.764583334016150751, 1.299038105676669330 ) ) ;
#162154=CARTESIAN_POINT ( 'NONE',  ( 4.983022828693913553, 6.814620138096638691, -1.425645453754071257 ) ) ;
#162159=CARTESIAN_POINT ( 'NONE',  ( -7.914208982075130905, 10.25632978388623684, -1.599625672291263179 ) ) ;
#162160=CYLINDRICAL_SURFACE ( 'NONE', #6580, 1.500000000000000222 ) ;
#162163=CARTESIAN_POINT ( 'NONE',  ( 5.880485940025228508, 7.883652901494672349, 1.599625672291267398 ) ) ;
#162169=CARTESIAN_POINT ( 'NONE',  ( 7.476431642932036326, 10.80992178580769014, 1.199719254218460707 ) ) ;
#162175=CARTESIAN_POINT ( 'NONE',  ( -5.531363484695544841, 8.436712584578003771, 1.082531754730548412 ) ) ;
#162180=AXIS2_PLACEMENT_3D ( 'NONE', #49781, #84412, #67064 ) ;
#162185=CARTESIAN_POINT ( 'NONE',  ( -9.450196763925152510, 10.98398329845622001, -1.199719254218441611 ) ) ;
#162187=CARTESIAN_POINT ( 'NONE',  ( 9.097684769969825780, 10.57271930550834860, -1.199719254218446718 ) ) ;
#162188=CARTESIAN_POINT ( 'NONE',  ( -1.500000000000013101, -0.07916666666664513852, 0.8660254037844403729 ) ) ;
#162189=CARTESIAN_POINT ( 'NONE',  ( -9.989660255170729641, 10.54902514065433827, -0.7998128361456291469 ) ) ;
#162192=CARTESIAN_POINT ( 'NONE',  ( -1.201851678989727383E-14, 2.821875000341418804, 1.575800808251672791 ) ) ;
#162193=CARTESIAN_POINT ( 'NONE',  ( 3.979481780810941949, 4.601482484822914998, 1.199719254218464037 ) ) ;
#162198=CARTESIAN_POINT ( 'NONE',  ( 8.053180056393003383, 12.33920113252646367, 1.040834085586084257E-14 ) ) ;
#162201=CARTESIAN_POINT ( 'NONE',  ( -5.558479791922849245, 9.428717490644563881, 0.7216878364870458196 ) ) ;
#162202=CARTESIAN_POINT ( 'NONE',  ( -1.201851678989727383E-14, 1.071875000341418138, 1.575800808251672791 ) ) ;
#162206=CARTESIAN_POINT ( 'NONE',  ( -6.984421689334302741, 11.30024240419870374, 0.000000000000000000 ) ) ;
#162207=ADVANCED_FACE ( 'NONE', ( #27477 ), #157502, .F. ) ;
#162208=CARTESIAN_POINT ( 'NONE',  ( -4.243338890952911058, 5.013278796608906518, -1.082531754730543971 ) ) ;
#162209=CARTESIAN_POINT ( 'NONE',  ( -1.201851678989727383E-14, 3.759375000341422801, -1.575800808251660134 ) ) ;
#162215=CARTESIAN_POINT ( 'NONE',  ( 9.596473800374404561, 10.09030761005864285, 0.000000000000000000 ) ) ;
#162229=CARTESIAN_POINT ( 'NONE',  ( -1.364683531250000748, -1.240624999658580752, 0.000000000000000000 ) ) ;
#162233=CARTESIAN_POINT ( 'NONE',  ( 6.909851844459134362, 11.21324425184434936, -0.7998128361456291469 ) ) ;
#162236=CARTESIAN_POINT ( 'NONE',  ( -1.364683531249997417, 3.759375000341423689, 1.214306433183764966E-14 ) ) ;
#162238=CARTESIAN_POINT ( 'NONE',  ( -7.131225611108100715, 9.342849184424693476, 1.443375672974078761 ) ) ;
#162245=ORIENTED_EDGE ( 'NONE', *, *, #14587, .F. ) ;
#162246=CARTESIAN_POINT ( 'NONE',  ( 8.204655514564224816, 12.72384853363364066, 1.040834085586084257E-14 ) ) ;
#162252=CARTESIAN_POINT ( 'NONE',  ( -9.592557376868645846, 11.15007068022363157, -1.199719254218441611 ) ) ;
#162254=CARTESIAN_POINT ( 'NONE',  ( 6.337546739384100292, 9.481222731668410120, 1.199719254218460707 ) ) ;
#162256=CARTESIAN_POINT ( 'NONE',  ( 4.216222583725566686, 4.981643104843690217, -1.082531754730548412 ) ) ;
#162265=CARTESIAN_POINT ( 'NONE',  ( -1.499999999999997558, 7.388542872122518368, -4.154462424328208670 ) ) ;
#162267=CARTESIAN_POINT ( 'NONE',  ( -5.829642864196175722, 7.824335979694092558, 1.443375672974064550 ) ) ;
#162268=CARTESIAN_POINT ( 'NONE',  ( 2.998324526916512411, 6.649795714711241423, 0.000000000000000000 ) ) ;
#162271=CARTESIAN_POINT ( 'NONE',  ( -7.374745490829552885, 10.69128794168811680, -1.199719254218446718 ) ) ;
#162276=CARTESIAN_POINT ( 'NONE',  ( -8.299562589859897699, 12.83457345481192036, -0.7998128361456281477 ) ) ;
#162277=CARTESIAN_POINT ( 'NONE',  ( -0.9486429539267164923, 3.042910930033675854, 1.028101543437260013 ) ) ;
#162278=CARTESIAN_POINT ( 'NONE',  ( 3.469446951953614189E-15, 6.400000000000023448, 1.214306433183764966E-14 ) ) ;
#162280=CARTESIAN_POINT ( 'NONE',  ( 6.923409998072794558, 11.22906209772695618, 1.040834085586084257E-14 ) ) ;
#162292=CARTESIAN_POINT ( 'NONE',  ( -7.147119532698295252, 11.49005655479003174, 0.000000000000000000 ) ) ;
#162296=CARTESIAN_POINT ( 'NONE',  ( 5.639828713604826405, 9.523624565940227882, -0.7216878364870267237 ) ) ;
#162300=FACE_OUTER_BOUND ( 'NONE', #99631, .T. ) ;
#162303=CARTESIAN_POINT ( 'NONE',  ( -6.847031270101295419, 7.946956888995021728, -1.199719254218446718 ) ) ;
#162312=CARTESIAN_POINT ( 'NONE',  ( -1.201851678989727383E-14, 4.509375000341417916, -1.575800808251660134 ) ) ;
#162313=CARTESIAN_POINT ( 'NONE',  ( 2.065088895208962327, 8.523968132013681753, 2.459875961809493639 ) ) ;
#162314=CARTESIAN_POINT ( 'NONE',  ( 9.738834413317897898, 10.25639499182604730, 0.000000000000000000 ) ) ;
#162316=CARTESIAN_POINT ( 'NONE',  ( -4.934804725694236893, 4.859619722839116918, -0.7216878364870207285 ) ) ;
#162319=CARTESIAN_POINT ( 'NONE',  ( -4.406036734316898240, 6.163462161501577441, -1.443375672974051449 ) ) ;
#162326=CARTESIAN_POINT ( 'NONE',  ( 4.033714395265605823, 4.664753868353354704, -1.199719254218446718 ) ) ;
#162333=EDGE_CURVE ( 'NONE', #211245, #178928, #24094, .T. ) ;
#162334=CARTESIAN_POINT ( 'NONE',  ( 4.008406971134620633, 7.828225232965717595, 0.7998128361456321445 ) ) ;
#162340=CARTESIAN_POINT ( 'NONE',  ( -1.201851678989727383E-14, 3.759375000341422801, -1.575800808251660134 ) ) ;
#162345=CARTESIAN_POINT ( 'NONE',  ( 6.173040012923759257, 6.096301524699504704, -0.7998128361456281477 ) ) ;
#162348=CARTESIAN_POINT ( 'NONE',  ( -3.249150368769345043, 6.942425863539538611, 0.7998128361456341429 ) ) ;
#162351=CARTESIAN_POINT ( 'NONE',  ( 6.331294547457450683, 7.449227062530913379, -1.082531754730543083 ) ) ;
#162352=CARTESIAN_POINT ( 'NONE',  ( 1.499999999999987121, 2.045833333333356929, -0.8660254037844262731 ) ) ;
#162354=CARTESIAN_POINT ( 'NONE',  ( -4.355193658487827690, 6.104145239700998538, -1.599625672291256295 ) ) ;
#162355=CARTESIAN_POINT ( 'NONE',  ( 0.2184521437216075668, 7.205153265248421590, -1.990034439536078725 ) ) ;
#162358=CARTESIAN_POINT ( 'NONE',  ( -1.364683531249997417, 3.259375000341423245, 1.214306433183764966E-14 ) ) ;
#162361=CARTESIAN_POINT ( 'NONE',  ( -3.294268138440636928, 6.787137228248626641, 1.040834085586084257E-14 ) ) ;
#162366=CARTESIAN_POINT ( 'NONE',  ( 3.506755287428983792, 7.242964935309132990, 1.040834085586084257E-14 ) ) ;
#162370=CARTESIAN_POINT ( 'NONE',  ( 0.6823417656249899377, 3.488541667008085323, -1.181850606188754593 ) ) ;
#162374=CARTESIAN_POINT ( 'NONE',  ( -1.402160292154681736E-14, 0.2593750003414224681, -1.575800808251665908 ) ) ;
#162375=CARTESIAN_POINT ( 'NONE',  ( -4.286372615631644400, 7.381325999705229179, -1.030941853605553016 ) ) ;
#162378=CARTESIAN_POINT ( 'NONE',  ( -10.62011439820619429, 11.28455497419572318, -0.7998128361456221525 ) ) ;
#162379=CARTESIAN_POINT ( 'NONE',  ( -5.029711800545518585, 8.811821500704338561, 0.7216878364870458196 ) ) ;
#162383=CARTESIAN_POINT ( 'NONE',  ( 0.6823417656249917140, 4.842708333674755394, 1.181850606188765695 ) ) ;
#162386=ADVANCED_FACE ( 'NONE', ( #31768 ), #15479, .T. ) ;
#162392=CARTESIAN_POINT ( 'NONE',  ( -5.355107487273497391, 9.191449801886996340, 0.7216878364870458196 ) ) ;
#162394=EDGE_CURVE ( 'NONE', #123589, #23747, #58250, .T. ) ;
#162398=CARTESIAN_POINT ( 'NONE',  ( -5.707619481228822345, 7.681975366232176583, -1.443375672974051449 ) ) ;
#162407=VERTEX_POINT ( 'NONE', #152968 ) ;
#162411=CARTESIAN_POINT ( 'NONE',  ( -4.069418662396130593, 7.899405539437467816, -0.7998128361456281477 ) ) ;
#162414=CARTESIAN_POINT ( 'NONE',  ( 1.499999999999987121, 0.2541666666666844154, 0.8660254037844524744 ) ) ;
#162416=CARTESIAN_POINT ( 'NONE',  ( 10.24960094225127172, 11.06021530882240356, -0.7216878364870257245 ) ) ;
#162417=CARTESIAN_POINT ( 'NONE',  ( 7.644099680006512187, 7.812537802962739697, 1.040834085586084257E-14 ) ) ;
#162421=CARTESIAN_POINT ( 'NONE',  ( 5.843727902690005749, 6.776436293681846301, -1.199719254218445830 ) ) ;
#162422=FACE_OUTER_BOUND ( 'NONE', #84599, .T. ) ;
#162427=CARTESIAN_POINT ( 'NONE',  ( -5.097502569058225852, 5.049433873430440478, -0.7216878364870207285 ) ) ;
#162434=CARTESIAN_POINT ( 'NONE',  ( -1.364683531250012516, 2.738541667008090208, -0.7879004041258289570 ) ) ;
#162435=CARTESIAN_POINT ( 'NONE',  ( 9.856414487010587422, 11.56186699200962487, 1.082531754730548412 ) ) ;
#162436=CARTESIAN_POINT ( 'NONE',  ( -6.226218857173722476, 8.287007971501239467, 1.599625672291283607 ) ) ;
#162439=CARTESIAN_POINT ( 'NONE',  ( 5.575427483717746213, 7.527751369135936343, 1.599625672291267398 ) ) ;
#162440=CARTESIAN_POINT ( 'NONE',  ( -5.280010757518168063, 8.247430752824802980, -1.199719254218446718 ) ) ;
#162444=CARTESIAN_POINT ( 'NONE',  ( -0.7500000000000215383, 0.4729166673494850093, 1.299038105676659116 ) ) ;
#162447=CARTESIAN_POINT ( 'NONE',  ( 7.510853912290742507, 8.825379654836435606, -1.082531754730537976 ) ) ;
#162450=CARTESIAN_POINT ( 'NONE',  ( -1.201851678989727383E-14, 2.134375000341423689, 1.575800808251672791 ) ) ;
#162452=CARTESIAN_POINT ( 'NONE',  ( 5.463572716182812705, 9.317992568947877530, 0.7216878364870438212 ) ) ;
#162455=CARTESIAN_POINT ( 'NONE',  ( -2.806174608348664723, 6.217694776474651519, 1.040834085586084257E-14 ) ) ;
#162457=CARTESIAN_POINT ( 'NONE',  ( 0.6823417656249899377, 4.676041667008086655, -1.181850606188754593 ) ) ;
#162462=CARTESIAN_POINT ( 'NONE',  ( -4.712932107567791462, 7.040231785572885315, -1.411385885297003373 ) ) ;
#162466=CARTESIAN_POINT ( 'NONE',  ( -9.828980619278564011E-14, 7.054063922337708625, 3.955400951015630273 ) ) ;
#162467=( BOUNDED_CURVE ( )  B_SPLINE_CURVE ( 2, ( #48423, #67803, #114536, #32152, #98230 ),
 .UNSPECIFIED., .F., .T. ) 
 B_SPLINE_CURVE_WITH_KNOTS ( ( 3, 2, 3 ),
 ( 0.01067668659529987657, 0.01250000000000000069, 0.01407841936770215865 ),
 .UNSPECIFIED. ) 
 CURVE ( )  GEOMETRIC_REPRESENTATION_ITEM ( )  RATIONAL_B_SPLINE_CURVE ( ( 0.9340561916853915569, 0.9413733574794114212, 1.000000000000000000, 0.9492476566127876492, 0.9369473844697255860 ) ) 
 REPRESENTATION_ITEM ( '' )  );
#162470=B_SPLINE_CURVE_WITH_KNOTS ( 'NONE', 3,
 ( #33275, #149162, #66805, #35401, #184847, #132947 ),
 .UNSPECIFIED., .F., .F.,
 ( 4, 2, 4 ),
 ( 0.000000000000000000, 0.002037565947615825948, 0.004075131895231652764 ),
 .UNSPECIFIED. ) ;
#162471=CARTESIAN_POINT ( 'NONE',  ( 5.459129407796876166, 9.520734742405036144, 1.040834085586084257E-14 ) ) ;
#162474=CARTESIAN_POINT ( 'NONE',  ( 3.846762897975340767, 5.510976019103107859, -1.599625672291256295 ) ) ;
#162483=CARTESIAN_POINT ( 'NONE',  ( 6.046573322014824114, 7.117052299514516456, -1.082531754730543083 ) ) ;
#162484=CARTESIAN_POINT ( 'NONE',  ( 1.364683531249988757, 1.446875000341421469, 0.000000000000000000 ) ) ;
#162485=CARTESIAN_POINT ( 'NONE',  ( 7.242026607993941489, 11.60078147596829901, 0.7998128361456462443 ) ) ;
#162487=DIRECTION ( 'NONE',  ( 0.000000000000000000, 0.7999999999999973799, 0.6000000000000034195 ) ) ;
#162491=CYLINDRICAL_SURFACE ( 'NONE', #82216, 0.08000000000000004330 ) ;
#162493=CARTESIAN_POINT ( 'NONE',  ( -1.500000000000013101, 1.420833333333354043, 0.8660254037844403729 ) ) ;
#162494=CARTESIAN_POINT ( 'NONE',  ( 6.425674737872927089, 9.584038729905381970, -1.199719254218440723 ) ) ;
#162495=CARTESIAN_POINT ( 'NONE',  ( -7.557780564614042795, 10.90482886110335414, -1.199719254218446718 ) ) ;
#162499=CARTESIAN_POINT ( 'NONE',  ( -1.364683531249997417, 2.759375000341422801, 1.214306433183764966E-14 ) ) ;
#162501=CARTESIAN_POINT ( 'NONE',  ( 0.7499999999999920064, 4.483333333333352932, 1.299038105676669330 ) ) ;
#162503=CARTESIAN_POINT ( 'NONE',  ( 3.225950485047770933, 5.851027101609320269, 1.199719254218450271 ) ) ;
#162508=CARTESIAN_POINT ( 'NONE',  ( -1.500000000000013101, 0.9520833340161557468, 0.8660254037844403729 ) ) ;
#162510=CARTESIAN_POINT ( 'NONE',  ( -5.371001409308059138, 9.417918744168066070, -0.7998128361456231517 ) ) ;
#162511=CARTESIAN_POINT ( 'NONE',  ( -2.968872451712654126, 6.407508927065978632, 1.040834085586084257E-14 ) ) ;
#162517=CARTESIAN_POINT ( 'NONE',  ( 7.298366762858032430, 7.409182732956175244, 1.040834085586084257E-14 ) ) ;
#162521=CARTESIAN_POINT ( 'NONE',  ( 6.632963465583686435, 8.761543347979550589, -1.599625672291262513 ) ) ;
#162522=CARTESIAN_POINT ( 'NONE',  ( 9.042925270190632858, 10.61279623905300085, 1.082531754730549967 ) ) ;
#162527=CARTESIAN_POINT ( 'NONE',  ( -7.043624497499477499, 8.176315654292865887, 1.199719254218450271 ) ) ;
#162528=CARTESIAN_POINT ( 'NONE',  ( 3.623053363349855172, 5.249981562040033189, 1.599625672291267398 ) ) ;
#162529=ORIENTED_EDGE ( 'NONE', *, *, #147605, .F. ) ;
#162534=CARTESIAN_POINT ( 'NONE',  ( 4.027228449831594226, 7.557535101434955216, 0.3677212997342318990 ) ) ;
#162536=EDGE_CURVE ( 'NONE', #96352, #14053, #193894, .T. ) ;
#162545=CARTESIAN_POINT ( 'NONE',  ( -4.175548123328963079, 4.934189567714277302, 1.082531754730560403 ) ) ;
#162546=CARTESIAN_POINT ( 'NONE',  ( 8.459924665247367415, 8.972259652317825740, -0.7216878364870267237 ) ) ;
#162548=CARTESIAN_POINT ( 'NONE',  ( -3.567766978690493307, 7.314145241780881435, 1.040834085586084257E-14 ) ) ;
#162553=CARTESIAN_POINT ( 'NONE',  ( -5.682838942422375084, 9.781729199468104596, 0.000000000000000000 ) ) ;
#162567=CARTESIAN_POINT ( 'NONE',  ( -5.603597561149804562, 5.431951997629870910, 0.7998128361456341429 ) ) ;
#162570=CARTESIAN_POINT ( 'NONE',  ( 3.063779527008311021, 5.557864633942907417, 1.082531754730546636 ) ) ;
#162574=CARTESIAN_POINT ( 'NONE',  ( -3.110706179331648169, 5.716575411607132118, 1.199719254218462483 ) ) ;
#162578=CARTESIAN_POINT ( 'NONE',  ( 7.716561984472250835, 12.15440608185967086, 1.040834085586084257E-14 ) ) ;
#162581=CARTESIAN_POINT ( 'NONE',  ( -7.167456763118792651, 11.51378332361394818, 0.000000000000000000 ) ) ;
#162582=CARTESIAN_POINT ( 'NONE',  ( 5.636439174979242850, 7.598931675607687453, -1.599625672291262513 ) ) ;
#162584=CARTESIAN_POINT ( 'NONE',  ( 5.671388329218120639, 5.511041227042920099, 1.040834085586084257E-14 ) ) ;
#162587=CARTESIAN_POINT ( 'NONE',  ( -0.6823417656250212460, 1.363541667008083547, 1.181850606188755259 ) ) ;
#162590=CARTESIAN_POINT ( 'NONE',  ( 7.619319141200063150, 9.912291636198670375, 1.443375672974076540 ) ) ;
#162619=CARTESIAN_POINT ( 'NONE',  ( -1.500000000000001332, 0.9312500006828163812, 0.000000000000000000 ) ) ;
#162623=VERTEX_POINT ( 'NONE', #4033 ) ;
#162625=CARTESIAN_POINT ( 'NONE',  ( 0.7499999999999885647, -0.5166666666666444030, 1.299038105676657340 ) ) ;
#162626=CARTESIAN_POINT ( 'NONE',  ( 7.944187942603509356, 11.35563746875774882, 1.199719254218460707 ) ) ;
#162628=CARTESIAN_POINT ( 'NONE',  ( -1.402160292154681736E-14, -1.178124999658576311, 1.575800808251672791 ) ) ;
#162631=CARTESIAN_POINT ( 'NONE',  ( 2.198393463710220264, 5.716542807637226886, 0.7998128361456462443 ) ) ;
#162632=CARTESIAN_POINT ( 'NONE',  ( -7.429504990608782222, 8.730472579540773381, 1.082531754730549967 ) ) ;
#162637=CARTESIAN_POINT ( 'NONE',  ( -5.506582945444718824, 9.576097202994168001, 0.7998128361456481317 ) ) ;
#162640=CARTESIAN_POINT ( 'NONE',  ( -1.500000000000013101, 1.660416667349487119, -0.8660254037844313801 ) ) ;
#162648=CARTESIAN_POINT ( 'NONE',  ( -9.130526383799315582, 12.73969898348616070, 1.199719254218462483 ) ) ;
#162652=CARTESIAN_POINT ( 'NONE',  ( 4.324073113486339714, 7.195437805949965515, 1.011975886212188813 ) ) ;
#162657=CARTESIAN_POINT ( 'NONE',  ( -4.256897044566581911, 4.068727428190179296, 1.214306433183764966E-14 ) ) ;
#162658=( BOUNDED_SURFACE ( )  B_SPLINE_SURFACE ( 1, 2, ( 
 ( #63226, #180186, #76274, #109917, #210535, #44872, #28601, #126176, #45936, #47000, #94690, #11263, #142382, #129389, #92560, #192140, #175928, #128328, #12325, #78405, #112055, #27521, #29673, #95757, #10199, #161810, #114187, #13400, #145594, #211590, #179122, #80545, #195368, #113116, #96825, #64299, #162874, #14454, #146642, #196432, #48076, #99993, #166059, #17646, #116301, #184427, #201730, #199604, #83730, #51247, #149822, #19792, #181233, #197482, #84804, #1392, #67453, #81606, #132536, #151952, #182291, #115243, #134658, #119506, #164991, #36044, #16582, #3522, #32861, #133599, #117372, #98937, #183369, #34974, #82664, #53371, #163945, #33918, #101045, #49125, #102124, #15520, #85875, #150893, #167135, #147690, #18720, #2454, #68530, #200661, #148748, #52310, #168193, #118440, #318, #69596, #66388, #135704, #31808, #213708, #50180, #198534, #65331, #97884, #131478, #71731, #55510, #157294, #5651, #105353, #20844, #139993, #171390, #56586, #37117, #203866, #90164, #173560, #106450, #121665, #88012, #107529, #8884, #138916, #22981, #170314, #7807, #156230, #89100, #21902, #187632, #153010, #154083, #73900, #103196, #137845, #72814, #57650, #25132, #169258, #6735, #104269, #91234, #86943, #123809, #41421, #39259, #74963, #155154, #204935, #122746, #188708, #189770, #141073, #40344, #172474, #24061, #206014, #207081, #120591, #136770, #58712, #185492, #4586, #70660, #202799, #54448, #186568, #38196, #13147, #212400, #43552, #129136, #109673, #30488, #125932, #192961, #110729, #59773, #12084, #144282, #175675, #146386, #42486, #127003, #78151, #76027, #195112, #108595, #178876, #29420, #128075, #26199, #44614, #210275, #60841, #28343, #142130, #61915, #46749, #194031, #191890, #94438, #27264, #160477, #45682, #174623, #143211, #93371, #92317, #211342, #124861, #11007, #209201, #96572, #159407, #176729, #158358, #79224, #111798, #177804, #190827, #95511, #161559, #112861, #145341, #62967, #77084, #162619, #14195, #80288, #9951, #208144, #100790, #34719, #116042, #114981, #148496, #31553, #48865, #183111, #130187, #97628, #17389, #18466, #16324, #197225, #47822, #166874, #151698, #113933, #81354, #182030, #180981, #164733, #32602, #179929, #65082, #66128, #64042, #98677, #85610, #83472, #163685, #82407, #33659, #15267, #35789, #131237, #149553, #64, #117109, #118181, #132272, #99733, #134404, #198280, #49921, #50988, #147434, #84544, #213458, #165805, #150634, #67200, #1138, #133337, #200408, #101865, #199341, #2195, #68272, #52054, #184169, #167933, #19533, #196180, #7543, #73628, #186299, #3267, #155957, #153822, #205750, #5393, #71471, #36850, #6473, #4328, #139727, #70397, #57381, #123545, #136515, #121401, #22720, #172211, #41155, #107264, #21639, #189510, #56319, #173284, #204670, #24866, #90970, #203601, #86679, #37935, #87746, #54183, #187373, #119243, #69334, #122479, #105088, #23800 ),
 ( #135445, #137584, #188440, #201467, #138648, #55254, #120323, #53110, #185227, #171126, #39004, #202534, #40074, #106186, #88834, #104009, #154892, #102934, #170054, #89905, #168994, #20593, #72550, #152746, #109409, #75766, #140805, #127814, #30218, #9689, #46473, #206817, #8619, #190564, #178608, #95238, #157032, #126732, #94175, #11815, #110468, #141874, #174357, #25935, #12873, #207883, #62697, #10747, #76818, #142938, #26998, #161287, #112596, #176469, #208938, #28079, #60573, #145071, #92043, #108337, #210005, #192692, #44346, #58451, #43288, #128858, #93104, #158100, #45415, #74701, #59506, #78949, #125663, #194840, #191625, #160214, #77891, #175414, #144012, #61647, #159146, #124606, #42220, #193769, #111531, #177538, #211074, #29149, #150377, #876, #99485, #212137, #98414, #115785, #32349, #214243, #47556, #181773, #166616, #165543, #163424, #65874, #147180, #132022, #17136, #80020, #114726, #97366, #63773, #182853, #117930, #196972, #180724, #68009, #130981, #16065, #146123, #50726, #82149, #33407, #162358, #164478, #66942, #84292, #83212, #148241, #213206, #18208, #134149, #49662, #198032, #81092, #133082, #199080, #149295, #64835, #116851, #129931, #48611, #34471, #13937, #195920, #100543, #1947, #200158, #15001, #113667, #51812, #183924, #96302, #179671, #31291, #20349, #136265, #152499, #151444, #36600, #37684, #123303, #86434, #57135, #55006, #202285, #137336, #122230, #23546, #101613, #71219, #168745, #155709, #167680, #188190, #103761, #35536, #4082, #19280, #121156, #53937, #203353, #39825, #89656, #85362, #187123, #70153, #7291, #3017, #105933, #171958, #120073, #73369, #169812, #21400, #87510, #186049, #139474, #205503, #38754, #153574, #104835, #5144, #69085, #184975, #201222, #88583, #170880, #22472, #135206, #154641, #52863, #6222, #118997, #138400, #102688, #72292, #204419, #56074, #97924, #190319, #43049, #175173, #124362, #76578, #208700, #25690, #213746, #107011, #191383, #142690, #140561, #196473, #173035, #31847, #93932, #192451, #90725, #109162, #60327, #125417, #92862, #206574, #126488, #48115, #44105, #41978, #158909, #91798, #10505, #110226, #24617, #207641, #108088, #156788, #61405, #65369, #75520, #59259, #163982, #9449, #26761, #8374, #143770, #176234, #27836, #40905, #159973, #11577, #180225, #77648, #209764, #157855, #114227, #15557, #130485, #81644, #174117, #147731, #189266, #74457, #141633, #58202, #98976, #116338, #36081, #197519, #165029, #84843, #85914, #83769, #50219, #115280, #102164, #117411, #182329, #68568, #33957, #100033, #17683, #166095, #32898, #132569, #353, #149862, #1430, #67495, #101082, #16622, #37157, #118478, #18758, #151988, #133639, #183407, #181272, #103234, #66426, #19830, #82704, #199640, #86978, #131516, #51286, #168232, #20879, #35011, #167171, #184463, #150932, #3562, #148783, #49163, #2494, #169294, #134695, #198570, #200699, #52351, #69635 ) ),
 .UNSPECIFIED., .F., .F., .T. ) 
 B_SPLINE_SURFACE_WITH_KNOTS ( ( 2, 2 ),
 ( 3, 2, 2, 2, 2, 2, 2, 2, 2, 2, 2, 2, 2, 2, 2, 2, 2, 2, 2, 2, 2, 2, 2, 2, 2, 2, 2, 2, 2, 2, 2, 2, 2, 2, 2, 2, 2, 2, 2, 2, 2, 2, 2, 2, 2, 2, 2, 2, 2, 2, 2, 2, 2, 2, 2, 2, 2, 2, 2, 2, 2, 2, 2, 2, 2, 2, 2, 2, 2, 2, 2, 2, 2, 2, 2, 2, 2, 2, 2, 2, 2, 2, 2, 2, 2, 2, 2, 2, 2, 2, 2, 2, 2, 2, 2, 2, 2, 2, 2, 2, 2, 2, 2, 2, 2, 2, 2, 2, 2, 2, 2, 2, 2, 2, 2, 2, 2, 2, 2, 2, 2, 2, 2, 2, 2, 2, 2, 2, 2, 2, 2, 2, 2, 2, 2, 2, 2, 2, 2, 2, 2, 2, 2, 2, 2, 2, 2, 2, 2, 2, 2, 2, 2, 2, 2, 2, 2, 2, 2, 2, 2, 2, 2, 2, 2, 2, 2, 2, 3 ),
 ( 0.000000000000000000, 1.000000000000000000 ),
 ( 0.000000000000000000, 0.005952380952380952051, 0.01190476190476190410, 0.01785714285714285615, 0.02380952380952380820, 0.02976190476190476025, 0.03571428571428571230, 0.04166666666666666435, 0.04761904761904761640, 0.05357142857142856845, 0.05952380952380952051, 0.06547619047619047949, 0.07142857142857142461, 0.07738095238095238360, 0.08333333333333332871, 0.08928571428571428770, 0.09523809523809523281, 0.1011904761904761918, 0.1071428571428571369, 0.1130952380952380959, 0.1190476190476190410, 0.1250000000000000000, 0.1309523809523809590, 0.1369047619047619180, 0.1428571428571428492, 0.1488095238095238082, 0.1547619047619047672, 0.1607142857142857262, 0.1666666666666666574, 0.1726190476190476164, 0.1785714285714285754, 0.1845238095238095344, 0.1904761904761904656, 0.1964285714285714246, 0.2023809523809523836, 0.2083333333333333426, 0.2142857142857142738, 0.2202380952380952328, 0.2261904761904761918, 0.2321428571428571508, 0.2380952380952380820, 0.2440476190476190410, 0.2500000000000000000, 0.2559523809523809312, 0.2619047619047619180, 0.2678571428571428492, 0.2738095238095238360, 0.2797619047619047672, 0.2857142857142856984, 0.2916666666666666852, 0.2976190476190476164, 0.3035714285714285476, 0.3095238095238095344, 0.3154761904761904656, 0.3214285714285714524, 0.3273809523809523836, 0.3333333333333333148, 0.3392857142857143016, 0.3452380952380952328, 0.3511904761904761640, 0.3571428571428571508, 0.3630952380952380820, 0.3690476190476190688, 0.3750000000000000000, 0.3809523809523809312, 0.3869047619047619180, 0.3928571428571428492, 0.3988095238095238360, 0.4047619047619047672, 0.4107142857142856984, 0.4166666666666666852, 0.4226190476190476164, 0.4285714285714285476, 0.4345238095238095344, 0.4404761904761904656, 0.4464285714285714524, 0.4523809523809523836, 0.4583333333333333148, 0.4642857142857143016, 0.4702380952380952328, 0.4761904761904761640, 0.4821428571428571508, 0.4880952380952380820, 0.4940476190476190688, 0.5000000000000000000, 0.5059523809523809312, 0.5119047619047618625, 0.5178571428571429047, 0.5238095238095238360, 0.5297619047619047672, 0.5357142857142856984, 0.5416666666666666297, 0.5476190476190476719, 0.5535714285714286031, 0.5595238095238095344, 0.5654761904761904656, 0.5714285714285713969, 0.5773809523809523281, 0.5833333333333333703, 0.5892857142857143016, 0.5952380952380952328, 0.6011904761904761640, 0.6071428571428570953, 0.6130952380952381375, 0.6190476190476190688, 0.6250000000000000000, 0.6309523809523809312, 0.6369047619047618625, 0.6428571428571429047, 0.6488095238095238360, 0.6547619047619047672, 0.6607142857142856984, 0.6666666666666666297, 0.6726190476190476719, 0.6785714285714286031, 0.6845238095238095344, 0.6904761904761904656, 0.6964285714285713969, 0.7023809523809523281, 0.7083333333333333703, 0.7142857142857143016, 0.7202380952380952328, 0.7261904761904761640, 0.7321428571428570953, 0.7380952380952381375, 0.7440476190476190688, 0.7500000000000000000, 0.7559523809523809312, 0.7619047619047618625, 0.7678571428571429047, 0.7738095238095238360, 0.7797619047619047672, 0.7857142857142856984, 0.7916666666666666297, 0.7976190476190476719, 0.8035714285714286031, 0.8095238095238095344, 0.8154761904761904656, 0.8214285714285713969, 0.8273809523809523281, 0.8333333333333333703, 0.8392857142857143016, 0.8452380952380952328, 0.8511904761904761640, 0.8571428571428570953, 0.8630952380952381375, 0.8690476190476190688, 0.8750000000000000000, 0.8809523809523809312, 0.8869047619047618625, 0.8928571428571429047, 0.8988095238095238360, 0.9047619047619047672, 0.9107142857142856984, 0.9166666666666666297, 0.9226190476190476719, 0.9285714285714286031, 0.9345238095238095344, 0.9404761904761904656, 0.9464285714285713969, 0.9523809523809523281, 0.9583333333333333703, 0.9642857142857143016, 0.9702380952380952328, 0.9761904761904761640, 0.9821428571428570953, 0.9880952380952381375, 0.9940476190476190688, 1.000000000000000000 ),
 .UNSPECIFIED. ) 
 GEOMETRIC_REPRESENTATION_ITEM ( )  RATIONAL_B_SPLINE_SURFACE ( (
 ( 1.000000000000000000, 0.8660254037844387076, 1.000000000000000000, 0.8660254037844387076, 1.000000000000000000, 0.8660254037844387076, 1.000000000000000000, 0.8660254037844387076, 1.000000000000000000, 0.8660254037844387076, 1.000000000000000000, 0.8660254037844387076, 1.000000000000000000, 0.8660254037844387076, 1.000000000000000000, 0.8660254037844387076, 1.000000000000000000, 0.8660254037844387076, 1.000000000000000000, 0.8660254037844387076, 1.000000000000000000, 0.8660254037844387076, 1.000000000000000000, 0.8660254037844387076, 1.000000000000000000, 0.8660254037844387076, 1.000000000000000000, 0.8660254037844387076, 1.000000000000000000, 0.8660254037844387076, 1.000000000000000000, 0.8660254037844387076, 1.000000000000000000, 0.8660254037844387076, 1.000000000000000000, 0.8660254037844387076, 1.000000000000000000, 0.8660254037844387076, 1.000000000000000000, 0.8660254037844387076, 1.000000000000000000, 0.8660254037844387076, 1.000000000000000000, 0.8660254037844387076, 1.000000000000000000, 0.8660254037844387076, 1.000000000000000000, 0.8660254037844387076, 1.000000000000000000, 0.8660254037844387076, 1.000000000000000000, 0.8660254037844387076, 1.000000000000000000, 0.8660254037844387076, 1.000000000000000000, 0.8660254037844387076, 1.000000000000000000, 0.8660254037844387076, 1.000000000000000000, 0.8660254037844387076, 1.000000000000000000, 0.8660254037844387076, 1.000000000000000000, 0.8660254037844387076, 1.000000000000000000, 0.8660254037844387076, 1.000000000000000000, 0.8660254037844387076, 1.000000000000000000, 0.8660254037844387076, 1.000000000000000000, 0.8660254037844387076, 1.000000000000000000, 0.8660254037844387076, 1.000000000000000000, 0.8660254037844387076, 1.000000000000000000, 0.8660254037844387076, 1.000000000000000000, 0.8660254037844387076, 1.000000000000000000, 0.8660254037844387076, 1.000000000000000000, 0.8660254037844387076, 1.000000000000000000, 0.8660254037844387076, 1.000000000000000000, 0.8660254037844387076, 1.000000000000000000, 0.8660254037844387076, 1.000000000000000000, 0.8660254037844387076, 1.000000000000000000, 0.8660254037844387076, 1.000000000000000000, 0.8660254037844387076, 1.000000000000000000, 0.8660254037844387076, 1.000000000000000000, 0.8660254037844387076, 1.000000000000000000, 0.8660254037844387076, 1.000000000000000000, 0.8660254037844387076, 1.000000000000000000, 0.8660254037844387076, 1.000000000000000000, 0.8660254037844387076, 1.000000000000000000, 0.8660254037844387076, 1.000000000000000000, 0.8660254037844387076, 1.000000000000000000, 0.8660254037844387076, 1.000000000000000000, 0.8660254037844387076, 1.000000000000000000, 0.8660254037844387076, 1.000000000000000000, 0.8660254037844387076, 1.000000000000000000, 0.8660254037844387076, 1.000000000000000000, 0.8660254037844387076, 1.000000000000000000, 0.8660254037844387076, 1.000000000000000000, 0.8660254037844387076, 1.000000000000000000, 0.8660254037844387076, 1.000000000000000000, 0.8660254037844387076, 1.000000000000000000, 0.8660254037844387076, 1.000000000000000000, 0.8660254037844387076, 1.000000000000000000, 0.8660254037844387076, 1.000000000000000000, 0.8660254037844387076, 1.000000000000000000, 0.8660254037844387076, 1.000000000000000000, 0.8660254037844387076, 1.000000000000000000, 0.8660254037844387076, 1.000000000000000000, 0.8660254037844387076, 1.000000000000000000, 0.8660254037844387076, 1.000000000000000000, 0.8660254037844387076, 1.000000000000000000, 0.8660254037844387076, 1.000000000000000000, 0.8660254037844387076, 1.000000000000000000, 0.8660254037844387076, 1.000000000000000000, 0.8660254037844387076, 1.000000000000000000, 0.8660254037844387076, 1.000000000000000000, 0.8660254037844387076, 1.000000000000000000, 0.8660254037844387076, 1.000000000000000000, 0.8660254037844387076, 1.000000000000000000, 0.8660254037844387076, 1.000000000000000000, 0.8660254037844387076, 1.000000000000000000, 0.8660254037844387076, 1.000000000000000000, 0.8660254037844387076, 1.000000000000000000, 0.8660254037844387076, 1.000000000000000000, 0.8660254037844387076, 1.000000000000000000, 0.8660254037844387076, 1.000000000000000000, 0.8660254037844387076, 1.000000000000000000, 0.8660254037844387076, 1.000000000000000000, 0.8660254037844387076, 1.000000000000000000, 0.8660254037844387076, 1.000000000000000000, 0.8660254037844387076, 1.000000000000000000, 0.8660254037844387076, 1.000000000000000000, 0.8660254037844387076, 1.000000000000000000, 0.8660254037844387076, 1.000000000000000000, 0.8660254037844387076, 1.000000000000000000, 0.8660254037844387076, 1.000000000000000000, 0.8660254037844387076, 1.000000000000000000, 0.8660254037844387076, 1.000000000000000000, 0.8660254037844387076, 1.000000000000000000, 0.8660254037844387076, 1.000000000000000000, 0.8660254037844387076, 1.000000000000000000, 0.8660254037844387076, 1.000000000000000000, 0.8660254037844387076, 1.000000000000000000, 0.8660254037844387076, 1.000000000000000000, 0.8660254037844387076, 1.000000000000000000, 0.8660254037844387076, 1.000000000000000000, 0.8660254037844387076, 1.000000000000000000, 0.8660254037844387076, 1.000000000000000000, 0.8660254037844387076, 1.000000000000000000, 0.8660254037844387076, 1.000000000000000000, 0.8660254037844387076, 1.000000000000000000, 0.8660254037844387076, 1.000000000000000000, 0.8660254037844387076, 1.000000000000000000, 0.8660254037844387076, 1.000000000000000000, 0.8660254037844387076, 1.000000000000000000, 0.8660254037844387076, 1.000000000000000000, 0.8660254037844387076, 1.000000000000000000, 0.8660254037844387076, 1.000000000000000000, 0.8660254037844387076, 1.000000000000000000, 0.8660254037844387076, 1.000000000000000000, 0.8660254037844387076, 1.000000000000000000, 0.8660254037844387076, 1.000000000000000000, 0.8660254037844387076, 1.000000000000000000, 0.8660254037844387076, 1.000000000000000000, 0.8660254037844387076, 1.000000000000000000, 0.8660254037844387076, 1.000000000000000000, 0.8660254037844387076, 1.000000000000000000, 0.8660254037844387076, 1.000000000000000000, 0.8660254037844387076, 1.000000000000000000, 0.8660254037844387076, 1.000000000000000000, 0.8660254037844387076, 1.000000000000000000, 0.8660254037844387076, 1.000000000000000000, 0.8660254037844387076, 1.000000000000000000, 0.8660254037844387076, 1.000000000000000000, 0.8660254037844387076, 1.000000000000000000, 0.8660254037844387076, 1.000000000000000000, 0.8660254037844387076, 1.000000000000000000, 0.8660254037844387076, 1.000000000000000000, 0.8660254037844387076, 1.000000000000000000, 0.8660254037844387076, 1.000000000000000000, 0.8660254037844387076, 1.000000000000000000, 0.8660254037844387076, 1.000000000000000000, 0.8660254037844387076, 1.000000000000000000, 0.8660254037844387076, 1.000000000000000000, 0.8660254037844387076, 1.000000000000000000, 0.8660254037844387076, 1.000000000000000000, 0.8660254037844387076, 1.000000000000000000, 0.8660254037844387076, 1.000000000000000000, 0.8660254037844387076, 1.000000000000000000, 0.8660254037844387076, 1.000000000000000000, 0.8660254037844387076, 1.000000000000000000, 0.8660254037844387076, 1.000000000000000000, 0.8660254037844387076, 1.000000000000000000, 0.8660254037844387076, 1.000000000000000000, 0.8660254037844387076, 1.000000000000000000, 0.8660254037844387076, 1.000000000000000000, 0.8660254037844387076, 1.000000000000000000, 0.8660254037844387076, 1.000000000000000000, 0.8660254037844387076, 1.000000000000000000, 0.8660254037844387076, 1.000000000000000000, 0.8660254037844387076, 1.000000000000000000, 0.8660254037844387076, 1.000000000000000000, 0.8660254037844387076, 1.000000000000000000),
 ( 1.000000000000000000, 0.8660254037844387076, 1.000000000000000000, 0.8660254037844387076, 1.000000000000000000, 0.8660254037844387076, 1.000000000000000000, 0.8660254037844387076, 1.000000000000000000, 0.8660254037844387076, 1.000000000000000000, 0.8660254037844387076, 1.000000000000000000, 0.8660254037844387076, 1.000000000000000000, 0.8660254037844387076, 1.000000000000000000, 0.8660254037844387076, 1.000000000000000000, 0.8660254037844387076, 1.000000000000000000, 0.8660254037844387076, 1.000000000000000000, 0.8660254037844387076, 1.000000000000000000, 0.8660254037844387076, 1.000000000000000000, 0.8660254037844387076, 1.000000000000000000, 0.8660254037844387076, 1.000000000000000000, 0.8660254037844387076, 1.000000000000000000, 0.8660254037844387076, 1.000000000000000000, 0.8660254037844387076, 1.000000000000000000, 0.8660254037844387076, 1.000000000000000000, 0.8660254037844387076, 1.000000000000000000, 0.8660254037844387076, 1.000000000000000000, 0.8660254037844387076, 1.000000000000000000, 0.8660254037844387076, 1.000000000000000000, 0.8660254037844387076, 1.000000000000000000, 0.8660254037844387076, 1.000000000000000000, 0.8660254037844387076, 1.000000000000000000, 0.8660254037844387076, 1.000000000000000000, 0.8660254037844387076, 1.000000000000000000, 0.8660254037844387076, 1.000000000000000000, 0.8660254037844387076, 1.000000000000000000, 0.8660254037844387076, 1.000000000000000000, 0.8660254037844387076, 1.000000000000000000, 0.8660254037844387076, 1.000000000000000000, 0.8660254037844387076, 1.000000000000000000, 0.8660254037844387076, 1.000000000000000000, 0.8660254037844387076, 1.000000000000000000, 0.8660254037844387076, 1.000000000000000000, 0.8660254037844387076, 1.000000000000000000, 0.8660254037844387076, 1.000000000000000000, 0.8660254037844387076, 1.000000000000000000, 0.8660254037844387076, 1.000000000000000000, 0.8660254037844387076, 1.000000000000000000, 0.8660254037844387076, 1.000000000000000000, 0.8660254037844387076, 1.000000000000000000, 0.8660254037844387076, 1.000000000000000000, 0.8660254037844387076, 1.000000000000000000, 0.8660254037844387076, 1.000000000000000000, 0.8660254037844387076, 1.000000000000000000, 0.8660254037844387076, 1.000000000000000000, 0.8660254037844387076, 1.000000000000000000, 0.8660254037844387076, 1.000000000000000000, 0.8660254037844387076, 1.000000000000000000, 0.8660254037844387076, 1.000000000000000000, 0.8660254037844387076, 1.000000000000000000, 0.8660254037844387076, 1.000000000000000000, 0.8660254037844387076, 1.000000000000000000, 0.8660254037844387076, 1.000000000000000000, 0.8660254037844387076, 1.000000000000000000, 0.8660254037844387076, 1.000000000000000000, 0.8660254037844387076, 1.000000000000000000, 0.8660254037844387076, 1.000000000000000000, 0.8660254037844387076, 1.000000000000000000, 0.8660254037844387076, 1.000000000000000000, 0.8660254037844387076, 1.000000000000000000, 0.8660254037844387076, 1.000000000000000000, 0.8660254037844387076, 1.000000000000000000, 0.8660254037844387076, 1.000000000000000000, 0.8660254037844387076, 1.000000000000000000, 0.8660254037844387076, 1.000000000000000000, 0.8660254037844387076, 1.000000000000000000, 0.8660254037844387076, 1.000000000000000000, 0.8660254037844387076, 1.000000000000000000, 0.8660254037844387076, 1.000000000000000000, 0.8660254037844387076, 1.000000000000000000, 0.8660254037844387076, 1.000000000000000000, 0.8660254037844387076, 1.000000000000000000, 0.8660254037844387076, 1.000000000000000000, 0.8660254037844387076, 1.000000000000000000, 0.8660254037844387076, 1.000000000000000000, 0.8660254037844387076, 1.000000000000000000, 0.8660254037844387076, 1.000000000000000000, 0.8660254037844387076, 1.000000000000000000, 0.8660254037844387076, 1.000000000000000000, 0.8660254037844387076, 1.000000000000000000, 0.8660254037844387076, 1.000000000000000000, 0.8660254037844387076, 1.000000000000000000, 0.8660254037844387076, 1.000000000000000000, 0.8660254037844387076, 1.000000000000000000, 0.8660254037844387076, 1.000000000000000000, 0.8660254037844387076, 1.000000000000000000, 0.8660254037844387076, 1.000000000000000000, 0.8660254037844387076, 1.000000000000000000, 0.8660254037844387076, 1.000000000000000000, 0.8660254037844387076, 1.000000000000000000, 0.8660254037844387076, 1.000000000000000000, 0.8660254037844387076, 1.000000000000000000, 0.8660254037844387076, 1.000000000000000000, 0.8660254037844387076, 1.000000000000000000, 0.8660254037844387076, 1.000000000000000000, 0.8660254037844387076, 1.000000000000000000, 0.8660254037844387076, 1.000000000000000000, 0.8660254037844387076, 1.000000000000000000, 0.8660254037844387076, 1.000000000000000000, 0.8660254037844387076, 1.000000000000000000, 0.8660254037844387076, 1.000000000000000000, 0.8660254037844387076, 1.000000000000000000, 0.8660254037844387076, 1.000000000000000000, 0.8660254037844387076, 1.000000000000000000, 0.8660254037844387076, 1.000000000000000000, 0.8660254037844387076, 1.000000000000000000, 0.8660254037844387076, 1.000000000000000000, 0.8660254037844387076, 1.000000000000000000, 0.8660254037844387076, 1.000000000000000000, 0.8660254037844387076, 1.000000000000000000, 0.8660254037844387076, 1.000000000000000000, 0.8660254037844387076, 1.000000000000000000, 0.8660254037844387076, 1.000000000000000000, 0.8660254037844387076, 1.000000000000000000, 0.8660254037844387076, 1.000000000000000000, 0.8660254037844387076, 1.000000000000000000, 0.8660254037844387076, 1.000000000000000000, 0.8660254037844387076, 1.000000000000000000, 0.8660254037844387076, 1.000000000000000000, 0.8660254037844387076, 1.000000000000000000, 0.8660254037844387076, 1.000000000000000000, 0.8660254037844387076, 1.000000000000000000, 0.8660254037844387076, 1.000000000000000000, 0.8660254037844387076, 1.000000000000000000, 0.8660254037844387076, 1.000000000000000000, 0.8660254037844387076, 1.000000000000000000, 0.8660254037844387076, 1.000000000000000000, 0.8660254037844387076, 1.000000000000000000, 0.8660254037844387076, 1.000000000000000000, 0.8660254037844387076, 1.000000000000000000, 0.8660254037844387076, 1.000000000000000000, 0.8660254037844387076, 1.000000000000000000, 0.8660254037844387076, 1.000000000000000000, 0.8660254037844387076, 1.000000000000000000, 0.8660254037844387076, 1.000000000000000000, 0.8660254037844387076, 1.000000000000000000, 0.8660254037844387076, 1.000000000000000000, 0.8660254037844387076, 1.000000000000000000, 0.8660254037844387076, 1.000000000000000000, 0.8660254037844387076, 1.000000000000000000, 0.8660254037844387076, 1.000000000000000000, 0.8660254037844387076, 1.000000000000000000, 0.8660254037844387076, 1.000000000000000000, 0.8660254037844387076, 1.000000000000000000, 0.8660254037844387076, 1.000000000000000000, 0.8660254037844387076, 1.000000000000000000, 0.8660254037844387076, 1.000000000000000000, 0.8660254037844387076, 1.000000000000000000, 0.8660254037844387076, 1.000000000000000000, 0.8660254037844387076, 1.000000000000000000, 0.8660254037844387076, 1.000000000000000000, 0.8660254037844387076, 1.000000000000000000, 0.8660254037844387076, 1.000000000000000000, 0.8660254037844387076, 1.000000000000000000, 0.8660254037844387076, 1.000000000000000000, 0.8660254037844387076, 1.000000000000000000, 0.8660254037844387076, 1.000000000000000000, 0.8660254037844387076, 1.000000000000000000, 0.8660254037844387076, 1.000000000000000000, 0.8660254037844387076, 1.000000000000000000, 0.8660254037844387076, 1.000000000000000000, 0.8660254037844387076, 1.000000000000000000, 0.8660254037844387076, 1.000000000000000000, 0.8660254037844387076, 1.000000000000000000) ) ) 
 REPRESENTATION_ITEM ( '' )  SURFACE ( )  );
#162659=CARTESIAN_POINT ( 'NONE',  ( 6.909851844459134362, 11.21324425184434936, -0.7998128361456291469 ) ) ;
#162668=CARTESIAN_POINT ( 'NONE',  ( -7.811469059767924605, 12.26513100303794168, -0.7998128361456281477 ) ) ;
#162674=CARTESIAN_POINT ( 'NONE',  ( 4.650610384687404952, 5.384465856012134566, 1.199719254218462483 ) ) ;
#162679=CARTESIAN_POINT ( 'NONE',  ( 0.07419657009811017612, 6.490528840037850244, -3.104513093580470340 ) ) ;
#162690=CARTESIAN_POINT ( 'NONE',  ( 8.471147050440139381, 8.777426401801974976, -0.7998128361456281477 ) ) ;
#162692=CARTESIAN_POINT ( 'NONE',  ( -3.249150368769345043, 6.942425863539538611, 0.7998128361456341429 ) ) ;
#162694=ADVANCED_FACE ( 'NONE', ( #117883 ), #14056, .T. ) ;
#162701=CARTESIAN_POINT ( 'NONE',  ( -1.402160292154681736E-14, -0.2562499993171780122, 1.732050807568877637 ) ) ;
#162707=CARTESIAN_POINT ( 'NONE',  ( -2.462777459176719308, 6.024990802348131780, -0.7998128361456281477 ) ) ;
#162713=CARTESIAN_POINT ( 'NONE',  ( 5.016153647376212277, 5.914896012436124728, 1.082531754730558626 ) ) ;
#162715=VERTEX_POINT ( 'NONE', #54956 ) ;
#162716=CARTESIAN_POINT ( 'NONE',  ( -1.201851678989727383E-14, 5.509375000341415252, -1.575800808251660134 ) ) ;
#162718=CARTESIAN_POINT ( 'NONE',  ( 2.968872451268290913, 5.447139712246216625, -1.082531754730543971 ) ) ;
#162727=CARTESIAN_POINT ( 'NONE',  ( -6.133411998150831046, 5.998805638374869353, -0.1291943307598683033 ) ) ;
#162730=CARTESIAN_POINT ( 'NONE',  ( -1.364683531250014514, -0.2614583329919080157, -0.7879004041258359514 ) ) ;
#162734=CARTESIAN_POINT ( 'NONE',  ( -6.389970470742427189, 6.349387058821269747, -0.7998128361456291469 ) ) ;
#162738=CARTESIAN_POINT ( 'NONE',  ( 1.499999999999989120, 4.504166666666688634, 0.8660254037844524744 ) ) ;
#162743=EDGE_LOOP ( 'NONE', ( #10406, #22985, #194981, #59779, #3935, #14794, #190994, #169427, #176521 ) ) ;
#162746=CARTESIAN_POINT ( 'NONE',  ( -1.364683531250014514, -0.7614583329919104582, -0.7879004041258359514 ) ) ;
#162748=CARTESIAN_POINT ( 'NONE',  ( 4.801558957534076022, 8.753569217098425170, 0.7998128361456462443 ) ) ;
#162749=B_SPLINE_CURVE_WITH_KNOTS ( 'NONE', 3,
 ( #197770, #178358, #66672, #198824, #78695, #46229 ),
 .UNSPECIFIED., .F., .F.,
 ( 4, 2, 4 ),
 ( 0.000000000000000000, 0.002109688543090480761, 0.004219377086180961522 ),
 .UNSPECIFIED. ) ;
#162750=CARTESIAN_POINT ( 'NONE',  ( -7.720478407978036195, 11.09464301169468037, -1.199719254218446718 ) ) ;
#162752=CARTESIAN_POINT ( 'NONE',  ( 9.673906298550626559, 11.24497775551929557, 1.199719254218452047 ) ) ;
#162754=CARTESIAN_POINT ( 'NONE',  ( 1.000000000000001554, 5.868705557303652398, -4.125226524755055024 ) ) ;
#162758=CARTESIAN_POINT ( 'NONE',  ( -1.500000000000011324, 5.420833333333356485, 0.8660254037844403729 ) ) ;
#162762=VERTEX_POINT ( 'NONE', #85314 ) ;
#162764=CARTESIAN_POINT ( 'NONE',  ( 6.155038550924133212, 10.12470270947942730, 0.7216878364870438212 ) ) ;
#162768=CARTESIAN_POINT ( 'NONE',  ( -0.7500000000000215383, 5.222916667349482012, 1.299038105676671107 ) ) ;
#162770=CARTESIAN_POINT ( 'NONE',  ( -5.115504031057831469, 4.862509545855891346, 0.7998128361456341429 ) ) ;
#162771=CARTESIAN_POINT ( 'NONE',  ( 6.792271770322100721, 7.026664608238323950, -0.7216878364870257245 ) ) ;
#162772=CARTESIAN_POINT ( 'NONE',  ( -9.788623718942277563, 10.52240854829523187, 1.040834085586084257E-14 ) ) ;
#162778=CARTESIAN_POINT ( 'NONE',  ( 9.164948653157988900, 11.71552606681625619, -1.443375672974057666 ) ) ;
#162780=CARTESIAN_POINT ( 'NONE',  ( 4.487912541323413329, 5.194651705420806564, 1.199719254218462483 ) ) ;
#162795=CARTESIAN_POINT ( 'NONE',  ( 9.562578416340237197, 10.05076299535211781, 0.7998128361456462443 ) ) ;
#162799=CARTESIAN_POINT ( 'NONE',  ( -1.364683531250014514, -0.4697916663252449943, 0.7879004041258379498 ) ) ;
#162800=CARTESIAN_POINT ( 'NONE',  ( 5.341549334104194635, 6.294524313618772737, 1.082531754730558626 ) ) ;
#162801=CARTESIAN_POINT ( 'NONE',  ( -9.341204650135658483, 10.00041963468749984, 1.040834085586084257E-14 ) ) ;
#162806=CARTESIAN_POINT ( 'NONE',  ( -3.090368948911150770, 5.692848642783215674, 1.199719254218462483 ) ) ;
#162822=CARTESIAN_POINT ( 'NONE',  ( 5.456969279648811622, 6.453098228331718644, -1.278498092073777626 ) ) ;
#162830=CARTESIAN_POINT ( 'NONE',  ( -8.026063749610056419, 10.38682701267698150, -1.443375672974059665 ) ) ;
#162834=CARTESIAN_POINT ( 'NONE',  ( 5.099838337034727331, 9.101561826515851550, -0.7998128361456281477 ) ) ;
#162835=CARTESIAN_POINT ( 'NONE',  ( -3.574546055497324293, 7.322054164722185732, 0.7998128361456341429 ) ) ;
#162838=CARTESIAN_POINT ( 'NONE',  ( -4.791917227426195858, 7.677988301050826969, -1.199719254218452047 ) ) ;
#162841=CARTESIAN_POINT ( 'NONE',  ( -4.608882153641705059, 7.464447381635583412, -1.199719254218452047 ) ) ;
#162844=CARTESIAN_POINT ( 'NONE',  ( 7.130698725783555680, 10.40656671580112658, 1.199719254218460707 ) ) ;
#162845=CARTESIAN_POINT ( 'NONE',  ( 0.000000000000000000, 2.800000000000024691, 1.214306433183764966E-14 ) ) ;
#162847=CARTESIAN_POINT ( 'NONE',  ( 5.168313817042160530, 6.667327647676385638, 1.400930397336812572 ) ) ;
#162848=CARTESIAN_POINT ( 'NONE',  ( 3.985733972737593778, 6.633478153960411738, -1.082531754730548412 ) ) ;
#162850=CARTESIAN_POINT ( 'NONE',  ( 0.000000000000000000, 2.800000000000024691, 1.214306433183764966E-14 ) ) ;
#162855=CARTESIAN_POINT ( 'NONE',  ( 6.087247782411444597, 10.04561347954795281, -0.7216878364870267237 ) ) ;
#162859=CARTESIAN_POINT ( 'NONE',  ( -10.32183501870554387, 10.93656236477829502, 0.7998128361456462443 ) ) ;
#162860=CARTESIAN_POINT ( 'NONE',  ( -5.703176172842872482, 9.805455968292021041, 0.000000000000000000 ) ) ;
#162867=CARTESIAN_POINT ( 'NONE',  ( 7.879259827836241570, 12.34422023245099176, 1.040834085586084257E-14 ) ) ;
#162871=CARTESIAN_POINT ( 'NONE',  ( 2.822068529938852155, 6.444163718237301275, -0.7998128361456291469 ) ) ;
#162874=CARTESIAN_POINT ( 'NONE',  ( -1.499999999999997780, 4.931250000682820378, 1.214306433183764966E-14 ) ) ;
#162881=CARTESIAN_POINT ( 'NONE',  ( -1.201851678989727383E-14, 3.587500000000020339, -1.732050807568863648 ) ) ;
#162882=CARTESIAN_POINT ( 'NONE',  ( 4.774442650306744085, 8.721933525333202653, -0.7998128361456281477 ) ) ;
#162884=CARTESIAN_POINT ( 'NONE',  ( 7.782016984564060103, 9.141736572488651902, 1.082531754730558626 ) ) ;
#162885=CARTESIAN_POINT ( 'NONE',  ( 0.4396008313321266292, 7.377972292137268795, 2.042906170116781439 ) ) ;
#162890=CARTESIAN_POINT ( 'NONE',  ( -3.253066792275140173, 5.882662793374543675, 1.199719254218462483 ) ) ;
#162891=CARTESIAN_POINT ( 'NONE',  ( 1.499999999999989120, 5.577083334016153415, -0.8660254037844323793 ) ) ;
#162892=CARTESIAN_POINT ( 'NONE',  ( 1.364683531249986537, 0.1552083336747499542, -0.7879004041258309554 ) ) ;
#162896=CARTESIAN_POINT ( 'NONE',  ( 4.844340958784499662, 4.546152628203684820, 0.7998128361456341429 ) ) ;
#162897=ADVANCED_FACE ( 'NONE', ( #113106 ), #134830, .T. ) ;
#162899=CARTESIAN_POINT ( 'NONE',  ( 1.364683531249992088, 5.696875000341418804, 1.214306433183764966E-14 ) ) ;
#162908=CARTESIAN_POINT ( 'NONE',  ( -6.418895661066105873, 9.576129806964074120, -1.199719254218440723 ) ) ;
#162911=CARTESIAN_POINT ( 'NONE',  ( 5.691725559638619814, 5.534767995866836543, 1.040834085586084257E-14 ) ) ;
#162919=CARTESIAN_POINT ( 'NONE',  ( 9.748476143425788720, 11.33197590787365172, -1.199719254218440723 ) ) ;
#162922=CARTESIAN_POINT ( 'NONE',  ( -3.716906668440817185, 7.488141546489591072, 0.7998128361456341429 ) ) ;
#162926=CARTESIAN_POINT ( 'NONE',  ( 9.511208455186636712, 11.05516360492796935, 1.199719254218453823 ) ) ;
#162928=CARTESIAN_POINT ( 'NONE',  ( 7.401861798056875053, 10.72292363345333399, -1.199719254218441611 ) ) ;
#162931=CARTESIAN_POINT ( 'NONE',  ( -9.246297574839990929, 11.81043314211192019, 1.443375672974076540 ) ) ;
#162932=CARTESIAN_POINT ( 'NONE',  ( -6.856673000209188906, 9.022537805042615489, 1.599625672291283607 ) ) ;
#162936=CARTESIAN_POINT ( 'NONE',  ( -5.391143034427437364, 6.494952464278877180, 1.342996321926675396 ) ) ;
#162937=CARTESIAN_POINT ( 'NONE',  ( -1.402160292154681736E-14, 0.9468750003414176941, -1.575800808251659024 ) ) ;
#162941=CARTESIAN_POINT ( 'NONE',  ( 7.944714827928056167, 8.371181508778631652, 0.7216878364870458196 ) ) ;
#162944=CARTESIAN_POINT ( 'NONE',  ( 6.342516933094585418, 6.294024598232139667, 1.040834085586084257E-14 ) ) ;
#162948=CIRCLE ( 'NONE', #62568, 0.08000000000000020983 ) ;
#162961=CARTESIAN_POINT ( 'NONE',  ( -4.956281507356261606, 4.676749934870729319, -0.1948928627674308134 ) ) ;
#162965=CARTESIAN_POINT ( 'NONE',  ( -5.935772324684618795, 5.819489221753827657, 0.000000000000000000 ) ) ;
#162966=CARTESIAN_POINT ( 'NONE',  ( -7.694415870955439551, 8.935572256658169010, 1.199719254218462483 ) ) ;
#162972=CARTESIAN_POINT ( 'NONE',  ( -1.201851678989727383E-14, 2.493750000682819046, 1.732050807568877637 ) ) ;
#162973=CARTESIAN_POINT ( 'NONE',  ( 7.242026607993941489, 11.60078147596829901, 0.7998128361456462443 ) ) ;
#162977=CARTESIAN_POINT ( 'NONE',  ( -8.585337585951595685, 11.03931315507545108, -1.599625672291263179 ) ) ;
#162979=CARTESIAN_POINT ( 'NONE',  ( 1.364683531249990311, 3.884375000341417028, 1.214306433183764966E-14 ) ) ;
#162983=CARTESIAN_POINT ( 'NONE',  ( -10.15469386695561482, 10.94949038764413096, 1.040834085586084257E-14 ) ) ;
#162987=CARTESIAN_POINT ( 'NONE',  ( -1.402160292154681736E-14, 1.009375000341417916, -1.575800808251659024 ) ) ;
#162988=AXIS2_PLACEMENT_3D ( 'NONE', #34201, #99228, #129678 ) ;
#162995=CARTESIAN_POINT ( 'NONE',  ( -1.364683531250012516, 3.030208333674755394, 0.7879004041258379498 ) ) ;
#162997=CARTESIAN_POINT ( 'NONE',  ( -4.252453736180621391, 8.112946458852704268, -0.7998128361456281477 ) ) ;
#163000=CARTESIAN_POINT ( 'NONE',  ( -1.201851678989727383E-14, 3.259375000341420581, -1.575800808251660134 ) ) ;
#163004=CARTESIAN_POINT ( 'NONE',  ( -4.772106882330234612, 6.590544000850480089, -1.443375672974053892 ) ) ;
#163005=CARTESIAN_POINT ( 'NONE',  ( -4.853455804012230423, 6.685451076146141425, 1.443375672974064550 ) ) ;
#163008=CARTESIAN_POINT ( 'NONE',  ( 5.070386261830877928, 5.978167395966564435, -1.082531754730548412 ) ) ;
#163011=CARTESIAN_POINT ( 'NONE',  ( -8.877891658850122880, 9.251961778280284321, 0.7998128361456462443 ) ) ;
#163012=CARTESIAN_POINT ( 'NONE',  ( -3.684065054611367351, 5.321161868511784299, -1.599625672291256295 ) ) ;
#163014=CARTESIAN_POINT ( 'NONE',  ( 1.364683531249990311, 4.884375000341417916, 1.214306433183764966E-14 ) ) ;
#163019=CARTESIAN_POINT ( 'NONE',  ( -7.659993601596726265, 8.039006744725394782, -0.7216878364870267237 ) ) ;
#163021=CARTESIAN_POINT ( 'NONE',  ( -1.402160292154681736E-14, -0.9906249996585834161, -1.575800808251665908 ) ) ;
#163024=CARTESIAN_POINT ( 'NONE',  ( 6.887178846062110615, 9.058127958537705027, -1.443375672974057666 ) ) ;
#163037=CARTESIAN_POINT ( 'NONE',  ( 9.286972035236624734, 11.85788667924133399, -1.443375672974058777 ) ) ;
#163041=ORIENTED_EDGE ( 'NONE', *, *, #126913, .T. ) ;
#163045=CARTESIAN_POINT ( 'NONE',  ( 5.961834861707224320, 7.978559976790334574, -1.599625672291262513 ) ) ;
#163046=CARTESIAN_POINT ( 'NONE',  ( -5.278201874421821316, 5.052323696447222900, 0.7998128361456341429 ) ) ;
#163048=CARTESIAN_POINT ( 'NONE',  ( -1.500000000000051514, 3.420833333333354265, 0.8660254037844170583 ) ) ;
#163049=CARTESIAN_POINT ( 'NONE',  ( -4.877338746226314470, 4.951936442570412211, -0.6255423638818237153 ) ) ;
#163051=CARTESIAN_POINT ( 'NONE',  ( 4.297571505407542958, 7.957657823043374989, -0.7216878364870197293 ) ) ;
#163052=CARTESIAN_POINT ( 'NONE',  ( -1.364683531250014514, -0.1572916663252435232, 0.7879004041258379498 ) ) ;
#163053=CARTESIAN_POINT ( 'NONE',  ( 5.939505971022265740, 6.126191976022287378, 0.7574911370455077453 ) ) ;
#163054=CARTESIAN_POINT ( 'NONE',  ( -9.833741488613570780, 10.36711991300432345, 0.7998128361456462443 ) ) ;
#163072=CARTESIAN_POINT ( 'NONE',  ( 5.445571254183207088, 9.504916896522420444, -0.7998128361456281477 ) ) ;
#163078=CARTESIAN_POINT ( 'NONE',  ( 7.476431642932036326, 10.80992178580769014, 1.199719254218460707 ) ) ;
#163085=CARTESIAN_POINT ( 'NONE',  ( -1.201851678989727383E-14, 3.837500000000022116, -1.732050807568863648 ) ) ;
#163095=CARTESIAN_POINT ( 'NONE',  ( -8.175203439360366531, 12.48156174598837787, 1.040834085586084257E-14 ) ) ;
#163099=CARTESIAN_POINT ( 'NONE',  ( 4.137209430464448445, 7.978494768850520558, 1.040834085586084257E-14 ) ) ;
#163106=CARTESIAN_POINT ( 'NONE',  ( 4.161989969270892153, 6.839110149915929249, 1.082531754730558626 ) ) ;
#163113=CARTESIAN_POINT ( 'NONE',  ( -7.691553217654356622, 7.867900263551875994, -0.7998128361456291469 ) ) ;
#163114=CARTESIAN_POINT ( 'NONE',  ( -5.935772324684618795, 5.819489221753827657, 0.000000000000000000 ) ) ;
#163123=CARTESIAN_POINT ( 'NONE',  ( 6.986529229743720926, 7.045372277656132276, -0.7998128361456281477 ) ) ;
#163135=CARTESIAN_POINT ( 'NONE',  ( -1.364683531250000748, 0.07187500034142035865, 0.000000000000000000 ) ) ;
#163137=CARTESIAN_POINT ( 'NONE',  ( 4.976006071415387311, 5.764094157194782575, 1.199719254218462483 ) ) ;
#163140=CARTESIAN_POINT ( 'NONE',  ( -7.863365906246074566, 8.276274433482971205, -0.7216878364870278340 ) ) ;
#163141=CARTESIAN_POINT ( 'NONE',  ( 4.175548123328908900, 7.815297210618305179, -0.7216878364870197293 ) ) ;
#163142=CARTESIAN_POINT ( 'NONE',  ( -5.843201017365469596, 9.760892253660966134, 0.7216878364870458196 ) ) ;
#163146=CARTESIAN_POINT ( 'NONE',  ( 6.262976894508937242, 9.394224579314053969, -1.199719254218440723 ) ) ;
#163151=CARTESIAN_POINT ( 'NONE',  ( -3.633221978782310124, 7.182583375313863705, -0.7216878364870463747 ) ) ;
#163152=CARTESIAN_POINT ( 'NONE',  ( -0.6823417656250212460, 5.051041667008086655, 1.181850606188767472 ) ) ;
#163156=CARTESIAN_POINT ( 'NONE',  ( 7.796102023057898123, 9.054206100777749455, -1.199719254218441611 ) ) ;
#163159=CARTESIAN_POINT ( 'NONE',  ( -8.199983978166823562, 8.461069484149769337, -0.7998128361456291469 ) ) ;
#163165=CARTESIAN_POINT ( 'NONE',  ( 8.204655514564224816, 12.72384853363364066, 1.040834085586084257E-14 ) ) ;
#163168=CARTESIAN_POINT ( 'NONE',  ( -7.506410603460441422, 11.90922947067921278, -0.7998128361456291469 ) ) ;
#163170=CARTESIAN_POINT ( 'NONE',  ( -0.1263102688159843667, 6.363441598446241798, 3.117922131261609664 ) ) ;
#163172=CARTESIAN_POINT ( 'NONE',  ( 4.762865522572231392, 6.775349848016087861, -1.243673390893657471 ) ) ;
#163173=CARTESIAN_POINT ( 'NONE',  ( -10.14113571334194930, 10.93367254176152059, -0.7216878364870267237 ) ) ;
#163176=CARTESIAN_POINT ( 'NONE',  ( 3.224997775515605181, 6.424863269013458833, -0.8838344238559818766 ) ) ;
#163178=CARTESIAN_POINT ( 'NONE',  ( 6.205881626753210867, 8.263281202677319470, 1.599625672291281386 ) ) ;
#163180=CARTESIAN_POINT ( 'NONE',  ( 6.173040012923759257, 6.096301524699504704, -0.7998128361456281477 ) ) ;
#163181=CARTESIAN_POINT ( 'NONE',  ( -4.191772670604852813, 7.388608026231708870, 0.8008250379338277547 ) ) ;
#163182=CARTESIAN_POINT ( 'NONE',  ( 4.196412238629597447, 4.854568018944682706, -1.199719254218452047 ) ) ;
#163184=CARTESIAN_POINT ( 'NONE',  ( -6.561783159334130922, 9.638868871656395498, -1.082531754730538864 ) ) ;
#163191=CARTESIAN_POINT ( 'NONE',  ( -4.167566996647928512, 7.418725663478599408, 0.7529690952402002813 ) ) ;
#163192=CARTESIAN_POINT ( 'NONE',  ( 1.364683531249988757, -0.3031249996585799744, 0.000000000000000000 ) ) ;
#163195=CARTESIAN_POINT ( 'NONE',  ( 4.609409038966229666, 6.400729850259146758, -1.443375672974051449 ) ) ;
#163196=CARTESIAN_POINT ( 'NONE',  ( -1.499999999999972689, 3.660416667349487341, -0.8660254037844548058 ) ) ;
#163199=CARTESIAN_POINT ( 'NONE',  ( -7.483737604619046913, 11.67485160545682987, 0.000000000000000000 ) ) ;
#163201=ADVANCED_FACE ( 'NONE', ( #29663 ), #204220, .T. ) ;
#163205=CARTESIAN_POINT ( 'NONE',  ( -8.310784975052671442, 11.67937098999472667, -1.082531754730543083 ) ) ;
#163213=CARTESIAN_POINT ( 'NONE',  ( -6.995644074527074707, 11.10540915368285475, 0.000000000000000000 ) ) ;
#163217=CARTESIAN_POINT ( 'NONE',  ( -1.364683531249997417, 4.821875000341417916, 1.214306433183764966E-14 ) ) ;
#163218=CARTESIAN_POINT ( 'NONE',  ( 1.499999999999987121, 2.827083334016148530, -0.8660254037844262731 ) ) ;
#163219=CARTESIAN_POINT ( 'NONE',  ( 5.980536202102920917, 6.100347882654393317, -0.6550157475838751520 ) ) ;
#163222=ORIENTED_EDGE ( 'NONE', *, *, #193237, .T. ) ;
#163224=CARTESIAN_POINT ( 'NONE',  ( -6.645467848992654858, 10.90479625713344625, 0.7998128361456481317 ) ) ;
#163227=CARTESIAN_POINT ( 'NONE',  ( -1.499999999999997780, 4.431250000682819490, 1.214306433183765124E-14 ) ) ;
#163228=CARTESIAN_POINT ( 'NONE',  ( 4.852928918687680948, 7.749168607522574526, 1.199719254218462483 ) ) ;
#163233=CARTESIAN_POINT ( 'NONE',  ( 6.760712154708803823, 11.03924794713562818, 1.040834085586084257E-14 ) ) ;
#163239=CARTESIAN_POINT ( 'NONE',  ( -5.910991785878165317, 8.879612269291090598, -1.082531754730538864 ) ) ;
#163242=CARTESIAN_POINT ( 'NONE',  ( 0.6823417656249917140, 5.405208333674749177, 1.181850606188765695 ) ) ;
#163249=CARTESIAN_POINT ( 'NONE',  ( -7.818248136574758256, 12.27303992597924420, 0.000000000000000000 ) ) ;
#163251=CARTESIAN_POINT ( 'NONE',  ( 7.964525173024008531, 11.37936423758166526, 1.199719254218460707 ) ) ;
#163252=CARTESIAN_POINT ( 'NONE',  ( -1.500000000000001332, -1.099999999999976108, 0.000000000000000000 ) ) ;
#163253=CARTESIAN_POINT ( 'NONE',  ( -8.130085669689073313, 12.63685038127928806, 0.7998128361456481317 ) ) ;
#163256=CARTESIAN_POINT ( 'NONE',  ( 1.364683531249988535, 3.863541667008087543, 0.7879004041258500513 ) ) ;
#163257=CARTESIAN_POINT ( 'NONE',  ( 9.897088948295943212, 11.60932053017587506, 1.082531754730548412 ) ) ;
#163262=CARTESIAN_POINT ( 'NONE',  ( 8.663296969007976855, 12.09063498294259809, -1.082531754730543083 ) ) ;
#163264=CARTESIAN_POINT ( 'NONE',  ( -7.917598520700757980, 9.299915031314755609, 1.082531754730558626 ) ) ;
#163265=CARTESIAN_POINT ( 'NONE',  ( 1.364683531249988757, 1.134375000341421247, 0.000000000000000000 ) ) ;
#163267=CARTESIAN_POINT ( 'NONE',  ( 0.2914054381963314677, 8.170846587878843437, 1.980990740193002919 ) ) ;
#163269=CARTESIAN_POINT ( 'NONE',  ( -7.914208982075130905, 10.25632978388623684, -1.599625672291263179 ) ) ;
#163270=CARTESIAN_POINT ( 'NONE',  ( -2.779058300676974014, 6.186059084191009916, -0.7216878364870257245 ) ) ;
#163271=CARTESIAN_POINT ( 'NONE',  ( 1.364683531249988535, 3.467708333674749621, -0.7879004041258239610 ) ) ;
#163281=ORIENTED_EDGE ( 'NONE', *, *, #5825, .T. ) ;
#163289=CARTESIAN_POINT ( 'NONE',  ( -1.001543065824772872E-14, 4.634375000341418804, 1.575800808251672791 ) ) ;
#163295=CARTESIAN_POINT ( 'NONE',  ( 6.774270308322468459, 11.05506579301824743, 0.7998128361456462443 ) ) ;
#163296=( BOUNDED_CURVE ( )  B_SPLINE_CURVE ( 2, ( #200424, #183128, #52070, #5410, #34734 ),
 .UNSPECIFIED., .F., .T. ) 
 B_SPLINE_CURVE_WITH_KNOTS ( ( 3, 2, 3 ),
 ( 0.02431251797087543784, 0.02500000000000000139, 0.02553812390681036229 ),
 .UNSPECIFIED. ) 
 CURVE ( )  GEOMETRIC_REPRESENTATION_ITEM ( )  RATIONAL_B_SPLINE_CURVE ( ( 0.9630840743150614891, 0.9778947694582196259, 1.000000000000000000, 0.9826972160490738961, 0.9698637321133645184 ) ) 
 REPRESENTATION_ITEM ( '' )  );
#163298=CARTESIAN_POINT ( 'NONE',  ( 0.6823417656249882723, 2.926041667008084879, -1.181850606188754593 ) ) ;
#163300=CARTESIAN_POINT ( 'NONE',  ( -5.558479791922849245, 9.428717490644563881, 0.7216878364870458196 ) ) ;
#163306=CARTESIAN_POINT ( 'NONE',  ( 3.246287715468270108, 5.874753870433235825, 1.199719254218450271 ) ) ;
#163309=CARTESIAN_POINT ( 'NONE',  ( 8.191097360950562845, 12.70803068775103739, -0.7998128361456352531 ) ) ;
#163316=CARTESIAN_POINT ( 'NONE',  ( -2.676845263694313637, 5.210404343363602919, -1.199719254218446718 ) ) ;
#163317=CARTESIAN_POINT ( 'NONE',  ( 7.633404179693907388, 8.864391950186421454, -1.199719254218441611 ) ) ;
#163320=CARTESIAN_POINT ( 'NONE',  ( 4.975479186090857375, 5.867442474269873642, 1.082531754730560403 ) ) ;
#163332=CARTESIAN_POINT ( 'NONE',  ( -7.063434843039784639, 7.343021526408956667, 1.040834085586084257E-14 ) ) ;
#163333=CARTESIAN_POINT ( 'NONE',  ( 4.578903193113299963, 6.365139696764064325, 1.599625672291267398 ) ) ;
#163335=EDGE_CURVE ( 'NONE', #104450, #127597, #186029, .T. ) ;
#163337=CARTESIAN_POINT ( 'NONE',  ( -7.320512876374914768, 10.62801655815766999, 1.199719254218453823 ) ) ;
#163342=CARTESIAN_POINT ( 'NONE',  ( -8.947491310014823895, 12.52615806407091803, 1.199719254218462483 ) ) ;
#163343=EDGE_CURVE ( 'NONE', #171443, #5554, #50170, .T. ) ;
#163345=CARTESIAN_POINT ( 'NONE',  ( -1.499999999999997780, 8.627523663848661428, -2.579999999999990301 ) ) ;
#163347=CARTESIAN_POINT ( 'NONE',  ( 9.433775957010412938, 9.900493459467314850, 0.000000000000000000 ) ) ;
#163348=CARTESIAN_POINT ( 'NONE',  ( 5.124091990960999432, 8.065525525174782828, -1.199719254218452047 ) ) ;
#163349=DIRECTION ( 'NONE',  ( -0.6507913734559640506, -0.7592566023653004592, 0.000000000000000000 ) ) ;
#163352=VERTEX_POINT ( 'NONE', #19782 ) ;
#163356=PLANE ( 'NONE',  #119892 ) ;
#163361=CARTESIAN_POINT ( 'NONE',  ( -8.779068160048691283, 10.20099992726700933, -1.199719254218446718 ) ) ;
#163365=CARTESIAN_POINT ( 'NONE',  ( 8.297226821883377568, 8.782445501726501291, -0.7216878364870267237 ) ) ;
#163368=CARTESIAN_POINT ( 'NONE',  ( 4.369805582306193870, 3.992528022312320957, 1.214306433183764966E-14 ) ) ;
#163371=CARTESIAN_POINT ( 'NONE',  ( -4.876128802409253282, 8.840567369452784874, 0.7998128361456481317 ) ) ;
#163378=B_SPLINE_CURVE_WITH_KNOTS ( 'NONE', 3,
 ( #103342, #20991, #186712, #175559 ),
 .UNSPECIFIED., .F., .F.,
 ( 4, 4 ),
 ( 8.194944171865289060E-14, 0.0009695358052320346897 ),
 .UNSPECIFIED. ) ;
#163381=CARTESIAN_POINT ( 'NONE',  ( -1.364683531250012516, 3.551041667008086211, -0.7879004041258300672 ) ) ;
#163382=CARTESIAN_POINT ( 'NONE',  ( 2.493739017040840888, 8.265916556960780426, 2.456386464945089276 ) ) ;
#163383=CARTESIAN_POINT ( 'NONE',  ( 9.576136569953906275, 10.06658084123472641, 0.000000000000000000 ) ) ;
#163385=CARTESIAN_POINT ( 'NONE',  ( -4.609409038966248318, 5.440360635957812718, -1.082531754730544860 ) ) ;
#163388=CARTESIAN_POINT ( 'NONE',  ( -4.487385655998893164, 6.258369236797239665, 1.443375672974064550 ) ) ;
#163395=CARTESIAN_POINT ( 'NONE',  ( 3.310162060030825248, 7.013606170011280838, -0.7998128361456291469 ) ) ;
#163403=CARTESIAN_POINT ( 'NONE',  ( 4.222474775652216294, 7.013638773981186958, 1.199719254218462483 ) ) ;
#163408=CARTESIAN_POINT ( 'NONE',  ( -0.6823417656249969321, 4.280208333674755394, -1.181850606188749264 ) ) ;
#163413=CARTESIAN_POINT ( 'NONE',  ( 6.799577732453452761, 7.891594428405881878, -1.199719254218446718 ) ) ;
#163415=CARTESIAN_POINT ( 'NONE',  ( -4.141125853970233806, 6.918731698685530063, -1.199719254218452047 ) ) ;
#163416=EDGE_CURVE ( 'NONE', #148633, #166401, #155866, .T. ) ;
#163417=CARTESIAN_POINT ( 'NONE',  ( -1.500000000000013101, 1.920833333333356263, 0.8660254037844403729 ) ) ;
#163421=CARTESIAN_POINT ( 'NONE',  ( -5.623934791570306402, 5.455678766453782913, 0.7998128361456341429 ) ) ;
#163422=CARTESIAN_POINT ( 'NONE',  ( 0.3520457843950711707, 7.165311474886529197, -1.969365997876474372 ) ) ;
#163424=CARTESIAN_POINT ( 'NONE',  ( 0.6823417656249899377, 3.676041667008085767, -1.181850606188754593 ) ) ;
#163426=CARTESIAN_POINT ( 'NONE',  ( -3.633221978782290140, 6.222214161012547429, -1.082531754730549967 ) ) ;
#163429=ORIENTED_EDGE ( 'NONE', *, *, #116484, .T. ) ;
#163431=CARTESIAN_POINT ( 'NONE',  ( 6.356075086708249167, 6.309842444114747373, -0.7998128361456281477 ) ) ;
#163434=CARTESIAN_POINT ( 'NONE',  ( -0.09252986283065423034, 7.021014873008922130, -3.994686497345164344 ) ) ;
#163435=CARTESIAN_POINT ( 'NONE',  ( 0.6823417656249899377, 4.488541667008086655, -1.181850606188754593 ) ) ;
#163439=CARTESIAN_POINT ( 'NONE',  ( -1.402160292154681736E-14, -0.3656249996585805295, 1.575800808251672791 ) ) ;
#163440=DIRECTION ( 'NONE',  ( 7.387867266669436732E-31, -1.000000000000000000, -8.546850786086424434E-32 ) ) ;
#163442=CARTESIAN_POINT ( 'NONE',  ( -8.597841969360544567, 13.18256606422934674, 0.7998128361456341429 ) ) ;
#163443=CARTESIAN_POINT ( 'NONE',  ( -5.870317324592812191, 7.871789516823500144, -1.443375672974051449 ) ) ;
#163446=ORIENTED_EDGE ( 'NONE', *, *, #122616, .T. ) ;
#163447=CARTESIAN_POINT ( 'NONE',  ( -0.6823417656250212460, 4.801041667008086655, 1.181850606188767472 ) ) ;
#163455=CARTESIAN_POINT ( 'NONE',  ( -6.846504384776774366, 7.089935991768773427, -0.7216878364870267237 ) ) ;
#163461=CARTESIAN_POINT ( 'NONE',  ( -4.867013957181525186, 8.622007350113015889, 0.7216878364870458196 ) ) ;
#163473=CARTESIAN_POINT ( 'NONE',  ( -5.579343907223557331, 6.467988298970945849, 1.199719254218450271 ) ) ;
#163475=CARTESIAN_POINT ( 'NONE',  ( 1.499999999999987121, 0.5041666666666856367, 0.8660254037844524744 ) ) ;
#163476=CARTESIAN_POINT ( 'NONE',  ( 10.05978679165993483, 11.79913468076720306, 1.082531754730548412 ) ) ;
#163477=CARTESIAN_POINT ( 'NONE',  ( 5.445571254183207088, 9.504916896522420444, -0.7998128361456281477 ) ) ;
#163480=CARTESIAN_POINT ( 'NONE',  ( 3.818592820543298405, 7.606775390609172405, -0.7998128361456221525 ) ) ;
#163488=CARTESIAN_POINT ( 'NONE',  ( -4.202664430556263930, 5.926194473780837413, 1.443375672974064550 ) ) ;
#163492=CARTESIAN_POINT ( 'NONE',  ( 4.183485216215308000, 3.563207579971337857, -2.499999999999995115 ) ) ;
#163497=CARTESIAN_POINT ( 'NONE',  ( -0.6823417656250212460, 3.051041667008084879, 1.181850606188767472 ) ) ;
#163498=CARTESIAN_POINT ( 'NONE',  ( 9.042925270190622200, 12.53353466765568669, 1.082531754730546636 ) ) ;
#163499=CARTESIAN_POINT ( 'NONE',  ( -7.237355071596549116, 7.338002426484427687, 1.040834085586084257E-14 ) ) ;
#163502=CARTESIAN_POINT ( 'NONE',  ( 5.469824908109481854, 8.468880595181346393, -1.199719254218446718 ) ) ;
#163503=CARTESIAN_POINT ( 'NONE',  ( -6.551614543901706611, 8.666636272683888365, 1.599625672291283607 ) ) ;
#163504=CARTESIAN_POINT ( 'NONE',  ( -1.474093356799783594, 8.744500914157981697, 2.533844564144187572 ) ) ;
#163506=CARTESIAN_POINT ( 'NONE',  ( -1.500000000000001332, 0.4312500006828159926, 0.000000000000000000 ) ) ;
#163509=CARTESIAN_POINT ( 'NONE',  ( 7.958272981541723468, 8.386999354661243800, 1.040834085586084257E-14 ) ) ;
#163512=CARTESIAN_POINT ( 'NONE',  ( -1.364683531250014514, 1.051041667008090208, -0.7879004041258289570 ) ) ;
#163514=CARTESIAN_POINT ( 'NONE',  ( 6.195713011320782115, 8.251417818006149929, -1.443375672974057666 ) ) ;
#163517=CARTESIAN_POINT ( 'NONE',  ( -3.877268743828284681, 5.546566172598190292, 1.443375672974064550 ) ) ;
#163519=CARTESIAN_POINT ( 'NONE',  ( -1.201851678989727383E-14, 5.196875000341422357, -1.575800808251660134 ) ) ;
#163523=CARTESIAN_POINT ( 'NONE',  ( -5.495703055830178485, 6.420018438214686540, -1.282350674470073448 ) ) ;
#163531=CARTESIAN_POINT ( 'NONE',  ( 7.145310649601935182, 8.294949498412453437, -1.199719254218446718 ) ) ;
#163534=CARTESIAN_POINT ( 'NONE',  ( 2.523789150438203510, 6.096171108819874007, 0.7998128361456462443 ) ) ;
#163543=CARTESIAN_POINT ( 'NONE',  ( 4.799223189557548785, 7.582548906917042864, -1.082531754730549078 ) ) ;
#163544=CARTESIAN_POINT ( 'NONE',  ( -0.6823417656250003738, 0.5302083336747518416, -1.181850606188749264 ) ) ;
#163552=CARTESIAN_POINT ( 'NONE',  ( -1.500000000000013101, 1.629166666666691077, -0.8660254037844313801 ) ) ;
#163553=CARTESIAN_POINT ( 'NONE',  ( 6.908042961362778733, 8.018137195466769285, 1.199719254218462483 ) ) ;
#163554=CARTESIAN_POINT ( 'NONE',  ( -8.688077508258798431, 9.030511935923748013, -0.7998128361456291469 ) ) ;
#163558=CARTESIAN_POINT ( 'NONE',  ( -1.364683531250014514, 1.738541667008085545, -0.7879004041258289570 ) ) ;
#163560=CARTESIAN_POINT ( 'NONE',  ( -1.499999999999997780, 2.900000000000020783, 1.214306433183764966E-14 ) ) ;
#163563=CARTESIAN_POINT ( 'NONE',  ( 5.034155109375821446, 4.767602470560229122, -0.7998128361456221525 ) ) ;
#163571=CARTESIAN_POINT ( 'NONE',  ( -1.402160292154681736E-14, 0.3687500006828169363, -1.732050807568870754 ) ) ;
#163572=CARTESIAN_POINT ( 'NONE',  ( -6.205881626753225966, 8.263281202677319470, 1.599625672291283607 ) ) ;
#163573=CARTESIAN_POINT ( 'NONE',  ( -3.443407828190963915, 6.961133532957338943, 0.7216878364870317197 ) ) ;
#163580=CARTESIAN_POINT ( 'NONE',  ( 6.745345117998789775, 7.828323044875442172, 1.199719254218462483 ) ) ;
#163585=CARTESIAN_POINT ( 'NONE',  ( 7.793239369756836510, 7.986534107671458216, 0.7998128361456341429 ) ) ;
#163586=CARTESIAN_POINT ( 'NONE',  ( 8.880227426826641235, 10.42298208846167284, 1.082531754730549967 ) ) ;
#163591=CARTESIAN_POINT ( 'NONE',  ( -6.531277313481209212, 8.642909503859968368, 1.599625672291283607 ) ) ;
#163592=CARTESIAN_POINT ( 'NONE',  ( 4.761938266897790761, 6.578680616179308771, 1.599625672291267398 ) ) ;
#163596=CARTESIAN_POINT ( 'NONE',  ( 4.097125688280337741, 7.463757567055806064, 0.6283840521477540575 ) ) ;
#163597=CARTESIAN_POINT ( 'NONE',  ( 7.931156674314368438, 12.19684052010138586, 1.040834085586084257E-14 ) ) ;
#163598=ORIENTED_EDGE ( 'NONE', *, *, #52269, .F. ) ;
#163603=CARTESIAN_POINT ( 'NONE',  ( 5.040934186182656873, 4.775511393501539636, 1.040834085586084257E-14 ) ) ;
#163606=CARTESIAN_POINT ( 'NONE',  ( -2.928197990871687306, 5.399686175116803710, 1.082531754730560403 ) ) ;
#163607=CARTESIAN_POINT ( 'NONE',  ( 8.920901888112002354, 9.510066412326583674, 0.7216878364870438212 ) ) ;
#163609=EDGE_CURVE ( 'NONE', #141559, #107270, #156053, .T. ) ;
#163611=CARTESIAN_POINT ( 'NONE',  ( -5.042743069279040036, 7.970618449879118828, 1.199719254218464037 ) ) ;
#163617=CARTESIAN_POINT ( 'NONE',  ( -5.747767057189642870, 8.793146435774861658, -1.199719254218440723 ) ) ;
#163632=CARTESIAN_POINT ( 'NONE',  ( -7.203459687562382641, 7.298457811777897319, -0.7998128361456291469 ) ) ;
#163635=CARTESIAN_POINT ( 'NONE',  ( 5.694061328059515148, 5.745419092265303007, -0.7216878364870207285 ) ) ;
#163636=ORIENTED_EDGE ( 'NONE', *, *, #137720, .F. ) ;
#163638=CARTESIAN_POINT ( 'NONE',  ( 7.334597915313080918, 9.580116872663850813, 1.040834085586084257E-14 ) ) ;
#163644=CARTESIAN_POINT ( 'NONE',  ( 9.402743226277308963, 10.92862083786708816, -1.199719254218446718 ) ) ;
#163648=CARTESIAN_POINT ( 'NONE',  ( -9.365985188942097750, 9.821404230054264772, 0.7998128361456462443 ) ) ;
#163649=CARTESIAN_POINT ( 'NONE',  ( 6.474182045725470402, 7.511966127223233869, -1.199719254218446718 ) ) ;
#163651=CARTESIAN_POINT ( 'NONE',  ( 6.010342169559767633, 5.906487374108180255, -0.7998128361456282587 ) ) ;
#163653=CARTESIAN_POINT ( 'NONE',  ( 1.608462485350599769, 8.735270501766756013, -2.463594439587629914 ) ) ;
#163654=CARTESIAN_POINT ( 'NONE',  ( -1.364683531250014514, 1.551041667008084435, -0.7879004041258289570 ) ) ;
#163657=CARTESIAN_POINT ( 'NONE',  ( 8.432808358020029260, 8.940623960552603222, 0.7216878364870438212 ) ) ;
#163664=CARTESIAN_POINT ( 'NONE',  ( 8.703971429848968100, 13.09845773489176679, 0.000000000000000000 ) ) ;
#163672=CARTESIAN_POINT ( 'NONE',  ( -10.64045162862669081, 11.30828174301964140, -0.7998128361456221525 ) ) ;
#163685=CARTESIAN_POINT ( 'NONE',  ( -1.500000000000013101, 0.2020833340161521663, 0.8660254037844403729 ) ) ;
#163691=CARTESIAN_POINT ( 'NONE',  ( 0.000000000000000000, 2.800000000000024691, 1.214306433183764966E-14 ) ) ;
#163692=CARTESIAN_POINT ( 'NONE',  ( 9.402743226277308963, 10.92862083786708816, -1.199719254218446718 ) ) ;
#163697=CARTESIAN_POINT ( 'NONE',  ( 3.635557746758808495, 7.393234471193928847, -0.7998128361456291469 ) ) ;
#163698=CARTESIAN_POINT ( 'NONE',  ( -7.049876689426113785, 8.287572894827684777, -1.082531754730544860 ) ) ;
#163704=CARTESIAN_POINT ( 'NONE',  ( -7.369020184227459858, 8.555943955475521889, 1.199719254218450271 ) ) ;
#163707=CARTESIAN_POINT ( 'NONE',  ( -0.7500000000000215383, 1.222916667349485564, 1.299038105676659116 ) ) ;
#163714=CARTESIAN_POINT ( 'NONE',  ( -8.455481356417053007, 13.01647868246193518, 0.7998128361456341429 ) ) ;
#163717=CARTESIAN_POINT ( 'NONE',  ( 4.006694938150886287, 7.586369203660299654, 0.2279062292016853508 ) ) ;
#163722=CARTESIAN_POINT ( 'NONE',  ( -2.887523529586332405, 5.352232636950553513, 1.082531754730560403 ) ) ;
#163723=CARTESIAN_POINT ( 'NONE',  ( 9.108380270282433244, 9.520865158284665952, 1.040834085586084257E-14 ) ) ;
#163729=DIRECTION ( 'NONE',  ( 0.000000000000000000, 8.546850786086437571E-32, 1.000000000000000000 ) ) ;
#163730=CARTESIAN_POINT ( 'NONE',  ( -8.833300774503376473, 10.26427131079744193, 1.199719254218462483 ) ) ;
#163734=VERTEX_POINT ( 'NONE', #33148 ) ;
#163736=CARTESIAN_POINT ( 'NONE',  ( 3.194917754314666514, 6.879154480009089134, 0.7998128361456321445 ) ) ;
#163742=CARTESIAN_POINT ( 'NONE',  ( -10.48453286206953727, 11.12637651536962125, 0.7998128361456462443 ) ) ;
#163754=CARTESIAN_POINT ( 'NONE',  ( 7.365103760721646076, 9.615707025640515937, 1.599625672291281386 ) ) ;
#163757=CARTESIAN_POINT ( 'NONE',  ( -5.135841261478327979, 4.886236314679810455, 0.7998128361456341429 ) ) ;
#163759=ADVANCED_FACE ( 'NONE', ( #97114 ), #14751, .F. ) ;
#163761=LINE ( 'NONE', #111871, #169146 ) ;
#163765=CARTESIAN_POINT ( 'NONE',  ( -1.500000000000015099, -0.3395833326505143801, -0.8660254037844383745 ) ) ;
#163768=CARTESIAN_POINT ( 'NONE',  ( -1.569519686357809585, 8.730458328474719920, -2.495327313682848214 ) ) ;
#163769=FACE_OUTER_BOUND ( 'NONE', #134408, .T. ) ;
#163771=CARTESIAN_POINT ( 'NONE',  ( -3.460355519985875983, 5.060167411448709629, 1.599625672291267398 ) ) ;
#163777=CARTESIAN_POINT ( 'NONE',  ( 3.714570900464269076, 7.277490450609545469, 0.7216878364870298324 ) ) ;
#163780=CARTESIAN_POINT ( 'NONE',  ( 0.6823417656249917140, 5.405208333674749177, 1.181850606188765695 ) ) ;
#163782=CARTESIAN_POINT ( 'NONE',  ( 3.917943204224906939, 5.594019709727598766, -1.443375672974051449 ) ) ;
#163790=CARTESIAN_POINT ( 'NONE',  ( -5.702738293170157569, 6.277038442308466415, 1.111922112425635989 ) ) ;
#163792=EDGE_CURVE ( 'NONE', #162623, #40788, #75860, .T. ) ;
#163793=CARTESIAN_POINT ( 'NONE',  ( 0.6823417656249882723, -0.1572916663252488245, 1.181850606188755259 ) ) ;
#163802=CARTESIAN_POINT ( 'NONE',  ( 0.7499999999999902300, 4.816666666666684193, -1.299038105676658228 ) ) ;
#163810=CARTESIAN_POINT ( 'NONE',  ( -1.364683531250010295, 4.092708333674751842, 0.7879004041258379498 ) ) ;
#163812=CARTESIAN_POINT ( 'NONE',  ( 5.178324605415663306, 8.128796908705222535, 1.199719254218462483 ) ) ;
#163813=CARTESIAN_POINT ( 'NONE',  ( -8.864333505236459132, 9.236143932397675727, 1.040834085586084257E-14 ) ) ;
#163819=CARTESIAN_POINT ( 'NONE',  ( 0.7499999999999920064, 5.483333333333353821, 1.299038105676669330 ) ) ;
#163828=CARTESIAN_POINT ( 'NONE',  ( 7.782016984564060103, 9.141736572488651902, 1.082531754730558626 ) ) ;
#163832=CARTESIAN_POINT ( 'NONE',  ( 1.499999999999990896, 4.806250000682819490, 1.214306433183764966E-14 ) ) ;
#163834=CARTESIAN_POINT ( 'NONE',  ( -5.278201874421821316, 5.052323696447222900, 0.7998128361456341429 ) ) ;
#163835=CARTESIAN_POINT ( 'NONE',  ( 4.975479186090839612, 8.748550117173898855, 0.7216878364870438212 ) ) ;
#163836=CARTESIAN_POINT ( 'NONE',  ( -9.070041577417988776, 12.56517035942090388, 1.082531754730558626 ) ) ;
#163842=DIRECTION ( 'NONE',  ( 1.000000000000000000, -7.387867266669436732E-31, 0.000000000000000000 ) ) ;
#163843=CARTESIAN_POINT ( 'NONE',  ( 4.792970997630896512, 5.550553237779539018, 1.199719254218464037 ) ) ;
#163851=ORIENTED_EDGE ( 'NONE', *, *, #119054, .T. ) ;
#163859=CARTESIAN_POINT ( 'NONE',  ( 7.865701674222579598, 12.32840238656838139, -0.7998128361456352531 ) ) ;
#163865=CARTESIAN_POINT ( 'NONE',  ( -1.364683531250000748, -0.2406249996585799189, 0.000000000000000000 ) ) ;
#163867=CARTESIAN_POINT ( 'NONE',  ( 4.500943810056890371, 8.194925511800951412, -0.7216878364870207285 ) ) ;
#163869=CARTESIAN_POINT ( 'NONE',  ( -10.33094986393327197, 11.15512238411806578, 0.7216878364870438212 ) ) ;
#163874=CARTESIAN_POINT ( 'NONE',  ( -5.427341564172148303, 5.226320001155936090, 0.000000000000000000 ) ) ;
#163877=CIRCLE ( 'NONE', #142709, 0.07999999999999961309 ) ;
#163884=EDGE_LOOP ( 'NONE', ( #211863, #10797, #142547, #32538 ) ) ;
#163890=CARTESIAN_POINT ( 'NONE',  ( 5.142929413680796813, 6.687119857356774055, -1.406168165883972421 ) ) ;
#163893=CARTESIAN_POINT ( 'NONE',  ( 3.876741858503734761, 6.610283703974623393, 1.199719254218462483 ) ) ;
#163898=CARTESIAN_POINT ( 'NONE',  ( -7.456621297836087514, 9.722477485607340597, 1.443375672974090751 ) ) ;
#163902=CARTESIAN_POINT ( 'NONE',  ( 6.612626235163189925, 8.737816579155630592, -1.599625672291262513 ) ) ;
#163903=CARTESIAN_POINT ( 'NONE',  ( -4.948889764188092677, 5.732458465429559169, 1.199719254218462483 ) ) ;
#163905=CARTESIAN_POINT ( 'NONE',  ( -5.436983294280064882, 6.301900917203534291, 1.199719254218450271 ) ) ;
#163906=CARTESIAN_POINT ( 'NONE',  ( 3.171717870593107058, 5.787755718078879674, -1.199719254218446718 ) ) ;
#163909=CARTESIAN_POINT ( 'NONE',  ( -6.552668314106420588, 6.539201209412602189, -0.7998128361456291469 ) ) ;
#163912=CARTESIAN_POINT ( 'NONE',  ( 10.05067194643221207, 10.62020544712608938, 0.7998128361456462443 ) ) ;
#163915=CARTESIAN_POINT ( 'NONE',  ( 4.226642156305554288, 7.541242530477547668, 0.9646342093552334740 ) ) ;
#163916=CARTESIAN_POINT ( 'NONE',  ( 6.005898861173831094, 6.109229547565340646, 1.040834085586084257E-14 ) ) ;
#163923=CARTESIAN_POINT ( 'NONE',  ( 7.415946836550714849, 9.675023947441092176, 1.443375672974076540 ) ) ;
#163927=CARTESIAN_POINT ( 'NONE',  ( -9.378489572351046633, 11.96465713920816043, -1.599625672291263179 ) ) ;
#163928=CARTESIAN_POINT ( 'NONE',  ( -6.353967546298838087, 10.56471257065732416, 0.000000000000000000 ) ) ;
#163932=CARTESIAN_POINT ( 'NONE',  ( 1.387358672533593129, 7.315968950352074174, -4.254625267140469624 ) ) ;
#163937=CARTESIAN_POINT ( 'NONE',  ( 8.540746701604824409, 12.05162268759261224, -1.199719254218446718 ) ) ;
#163942=CARTESIAN_POINT ( 'NONE',  ( 4.844340958784499662, 4.546152628203684820, 0.7998128361456341429 ) ) ;
#163945=CARTESIAN_POINT ( 'NONE',  ( 0.7499999999999902300, 4.097916667349481123, -1.299038105676658228 ) ) ;
#163951=CARTESIAN_POINT ( 'NONE',  ( 0.7499999999999885647, 3.066666666666689522, -1.299038105676658228 ) ) ;
#163952=CARTESIAN_POINT ( 'NONE',  ( 4.286349120214771879, 8.152491073559232859, -0.7998128361456221525 ) ) ;
#163954=CARTESIAN_POINT ( 'NONE',  ( 7.510853912290742507, 8.825379654836435606, -1.082531754730537976 ) ) ;
#163958=CARTESIAN_POINT ( 'NONE',  ( 10.37606763316019531, 10.99983374830873650, 0.7998128361456462443 ) ) ;
#163960=CARTESIAN_POINT ( 'NONE',  ( -4.874319919312905647, 5.645460313075203018, -1.199719254218446718 ) ) ;
#163963=CARTESIAN_POINT ( 'NONE',  ( -1.402160292154681736E-14, 0.1968750003414221628, -1.575800808251665908 ) ) ;
#163967=CARTESIAN_POINT ( 'NONE',  ( 3.310162060030825248, 7.013606170011280838, -0.7998128361456291469 ) ) ;
#163969=CARTESIAN_POINT ( 'NONE',  ( -1.364683531250012516, 4.801041667008083991, -0.7879004041258300672 ) ) ;
#163977=CARTESIAN_POINT ( 'NONE',  ( -6.093499974338126179, 9.196501505781426999, -1.199719254218440723 ) ) ;
#163979=CARTESIAN_POINT ( 'NONE',  ( 4.320244504248938355, 8.192035688265757898, 1.040834085586084257E-14 ) ) ;
#163982=CARTESIAN_POINT ( 'NONE',  ( 0.6823417656249882723, 0.4260416670080896528, -1.181850606188749264 ) ) ;
#163986=CARTESIAN_POINT ( 'NONE',  ( 9.585778300061798873, 11.14216175728232550, -1.199719254218440723 ) ) ;
#163989=CARTESIAN_POINT ( 'NONE',  ( -5.343885102080728977, 9.386283052402845328, 0.7998128361456481317 ) ) ;
#163993=CARTESIAN_POINT ( 'NONE',  ( 8.914649696185335870, 10.35917838609310593, -1.199719254218446718 ) ) ;
#163995=CARTESIAN_POINT ( 'NONE',  ( 8.158255747121103241, 10.54105100977322174, 1.599625672291281386 ) ) ;
#163997=CARTESIAN_POINT ( 'NONE',  ( -4.060830702492950195, 4.696389560118578999, -1.199719254218452047 ) ) ;
#163998=CARTESIAN_POINT ( 'NONE',  ( -7.691553217654356622, 7.867900263551875994, -0.7998128361456291469 ) ) ;
#164001=CARTESIAN_POINT ( 'NONE',  ( -4.661943307450316709, 7.086702294391122869, 1.392663581761391267 ) ) ;
#164002=CARTESIAN_POINT ( 'NONE',  ( 1.364683531249986537, 0.1135416670080857532, 0.7879004041258500513 ) ) ;
#164006=CARTESIAN_POINT ( 'NONE',  ( 6.317736394288131052, 9.354147645769410602, 1.082531754730558626 ) ) ;
#164024=CARTESIAN_POINT ( 'NONE',  ( -3.592547517496907705, 7.135129837147655252, -0.7216878364870090712 ) ) ;
#164029=CARTESIAN_POINT ( 'NONE',  ( 10.23370702021670020, 10.83374636654133383, 0.7998128361456462443 ) ) ;
#164033=CARTESIAN_POINT ( 'NONE',  ( -4.412288926243578935, 7.235088616337731260, 1.199719254218464037 ) ) ;
#164034=CARTESIAN_POINT ( 'NONE',  ( -7.588813295347149435, 9.876701482703580837, -1.599625672291263179 ) ) ;
#164040=CARTESIAN_POINT ( 'NONE',  ( -1.499999999999997780, 3.681250000682819046, 1.214306433183764966E-14 ) ) ;
#164041=CARTESIAN_POINT ( 'NONE',  ( 9.240045382913317340, 10.73880668727576015, -1.199719254218446718 ) ) ;
#164045=CARTESIAN_POINT ( 'NONE',  ( -9.203287345578106127, 9.631590079462940324, 0.7998128361456462443 ) ) ;
#164047=CARTESIAN_POINT ( 'NONE',  ( 1.364683531249988535, 2.863541667008082658, 0.7879004041258500513 ) ) ;
#164052=CARTESIAN_POINT ( 'NONE',  ( -9.544576954340667996, 11.19805653722800365, 1.082531754730558626 ) ) ;
#164056=CARTESIAN_POINT ( 'NONE',  ( -0.6823417656250003738, 1.780208333674752952, -1.181850606188749264 ) ) ;
#164061=CARTESIAN_POINT ( 'NONE',  ( -1.364683531250012516, 2.988541667008091096, -0.7879004041258289570 ) ) ;
#164063=CARTESIAN_POINT ( 'NONE',  ( -5.738125327081750271, 7.717565519727259904, 1.599625672291269396 ) ) ;
#164064=CARTESIAN_POINT ( 'NONE',  ( 8.111855979677986994, 8.358253485912799263, 1.040834085586084257E-14 ) ) ;
#164066=AXIS2_PLACEMENT_3D ( 'NONE', #198856, #48397, #16909 ) ;
#164068=CARTESIAN_POINT ( 'NONE',  ( 0.6823417656249899377, 2.405208333674753618, 1.181850606188767472 ) ) ;
#164072=CARTESIAN_POINT ( 'NONE',  ( -6.100805936469506641, 6.219954468743612352, 0.7216878364870317197 ) ) ;
#164073=EDGE_CURVE ( 'NONE', #13599, #133314, #11405, .T. ) ;
#164076=CARTESIAN_POINT ( 'NONE',  ( 6.019457014787495730, 6.125047393447951016, -0.7216878364870257245 ) ) ;
#164079=CARTESIAN_POINT ( 'NONE',  ( -7.395082721250053837, 10.71501471051202614, -1.199719254218446718 ) ) ;
#164080=CARTESIAN_POINT ( 'NONE',  ( -2.591579918506545344, 6.175260338232929413, 1.040834085586084257E-14 ) ) ;
#164086=CARTESIAN_POINT ( 'NONE',  ( -6.683806541412762314, 9.781229484081471526, -1.082531754730537976 ) ) ;
#164088=CARTESIAN_POINT ( 'NONE',  ( -1.364683531250000748, -1.178124999658580752, 0.000000000000000000 ) ) ;
#164091=CARTESIAN_POINT ( 'NONE',  ( 8.446366511633696561, 8.956441806435218922, 1.040834085586084257E-14 ) ) ;
#164099=CARTESIAN_POINT ( 'NONE',  ( 9.422553571373278203, 11.05569592376608945, -1.082531754730543083 ) ) ;
#164106=CARTESIAN_POINT ( 'NONE',  ( 7.122110765880372618, 7.203550736482235095, 0.7998128361456341429 ) ) ;
#164107=CARTESIAN_POINT ( 'NONE',  ( -3.741160322367112379, 6.452105245148518797, 1.199719254218464037 ) ) ;
#164110=CARTESIAN_POINT ( 'NONE',  ( 1.451998047844732964, 7.315968950354620581, 4.301760722576522866 ) ) ;
#164111=CARTESIAN_POINT ( 'NONE',  ( 6.331294547457450683, 7.449227062530913379, -1.082531754730543083 ) ) ;
#164112=CARTESIAN_POINT ( 'NONE',  ( 0.6823417656249882723, 0.1552083336747514530, 1.181850606188755259 ) ) ;
#164114=CARTESIAN_POINT ( 'NONE',  ( -9.996439331977562404, 10.55693406359564790, 0.7998128361456462443 ) ) ;
#164128=ORIENTED_EDGE ( 'NONE', *, *, #14587, .T. ) ;
#164133=CARTESIAN_POINT ( 'NONE',  ( 5.459129407796876166, 9.520734742405036144, 1.040834085586084257E-14 ) ) ;
#164134=CARTESIAN_POINT ( 'NONE',  ( 7.253775878511261155, 8.421492265473332850, 1.199719254218462483 ) ) ;
#164137=ORIENTED_EDGE ( 'NONE', *, *, #162333, .F. ) ;
#164141=CARTESIAN_POINT ( 'NONE',  ( -5.113031849284871200, 4.859625333787436219, 0.6539756689589106831 ) ) ;
#164142=CARTESIAN_POINT ( 'NONE',  ( 9.856941372335116469, 11.45851867493453291, 1.199719254218450271 ) ) ;
#164148=CARTESIAN_POINT ( 'NONE',  ( 1.499999999999822586, 7.267697830503921708, 4.207111467970846341 ) ) ;
#164153=EDGE_CURVE ( 'NONE', #136958, #47756, #104429, .T. ) ;
#164154=CARTESIAN_POINT ( 'NONE',  ( -10.15469386695561482, 10.94949038764413096, 1.040834085586084257E-14 ) ) ;
#164158=CARTESIAN_POINT ( 'NONE',  ( 6.636879889089462026, 7.701780277814560982, -1.199719254218446718 ) ) ;
#164159=CARTESIAN_POINT ( 'NONE',  ( 1.364683531249992088, 5.384375000341417916, 1.214306433183764966E-14 ) ) ;
#164164=CARTESIAN_POINT ( 'NONE',  ( 5.138177029454852551, 5.096887410559856946, 0.7216878364870317197 ) ) ;
#164172=CARTESIAN_POINT ( 'NONE',  ( -7.067878151425722955, 7.140279352951794500, 0.7998128361456341429 ) ) ;
#164173=CARTESIAN_POINT ( 'NONE',  ( -3.815730167242251003, 6.539103397502874948, -1.199719254218452047 ) ) ;
#164182=CARTESIAN_POINT ( 'NONE',  ( 5.289652487626049115, 9.323011668872403845, 0.7998128361456462443 ) ) ;
#164192=CARTESIAN_POINT ( 'NONE',  ( 1.364683531249988757, -0.3031249996585799744, 0.000000000000000000 ) ) ;
#164193=CARTESIAN_POINT ( 'NONE',  ( 5.030238685870051185, 5.827365540725222282, -1.199719254218452047 ) ) ;
#164195=CARTESIAN_POINT ( 'NONE',  ( -5.585596099150174965, 9.460353182409786399, -0.7216878364870207285 ) ) ;
#164197=CARTESIAN_POINT ( 'NONE',  ( 4.934804725694211136, 6.780358151441803649, -1.443375672974051449 ) ) ;
#164198=CARTESIAN_POINT ( 'NONE',  ( -7.388830529323428209, 8.683019041374528513, 1.082531754730549967 ) ) ;
#164203=CARTESIAN_POINT ( 'NONE',  ( 8.125414133291656071, 8.374071331795406081, -0.7998128361456291469 ) ) ;
#164208=CARTESIAN_POINT ( 'NONE',  ( 1.364683531249990311, 3.634375000341416584, 1.214306433183764966E-14 ) ) ;
#164212=CARTESIAN_POINT ( 'NONE',  ( 7.121056995675668411, 9.330985799753529264, -1.599625672291262513 ) ) ;
#164216=CARTESIAN_POINT ( 'NONE',  ( -8.362681821530818738, 8.650883634741092010, -0.7998128361456291469 ) ) ;
#164222=CARTESIAN_POINT ( 'NONE',  ( 7.567422294721922960, 11.98040977715095323, 0.7998128361456462443 ) ) ;
#164224=CARTESIAN_POINT ( 'NONE',  ( -7.883176251342026042, 11.28445716228600126, -1.199719254218446718 ) ) ;
#164227=CARTESIAN_POINT ( 'NONE',  ( 4.472818454536469090, 7.041451798021368447, -1.136577435397856384 ) ) ;
#164228=CARTESIAN_POINT ( 'NONE',  ( -2.252626078164912560, 5.779814191167667481, 0.7998128361456341429 ) ) ;
#164233=CARTESIAN_POINT ( 'NONE',  ( 6.823831386379729302, 6.855558127064808716, -0.7998128361456281477 ) ) ;
#164235=CARTESIAN_POINT ( 'NONE',  ( 5.015626762051672571, 7.938982758113895422, 1.199719254218462483 ) ) ;
#164236=CARTESIAN_POINT ( 'NONE',  ( -4.067982317475717480, 7.550107770606433455, 0.4684429539664070608 ) ) ;
#164237=CARTESIAN_POINT ( 'NONE',  ( 4.532503425670185493, 4.182342172903648070, 1.214306433183764966E-14 ) ) ;
#164239=CARTESIAN_POINT ( 'NONE',  ( -6.073689629242158716, 9.069426419882418600, -1.082531754730538864 ) ) ;
#164245=CARTESIAN_POINT ( 'NONE',  ( -4.044208510193211481, 7.583498396275582643, -0.3544512193057146598 ) ) ;
#164249=CARTESIAN_POINT ( 'NONE',  ( 3.524756749872944628, 7.056040608253000279, -0.7216878364870267237 ) ) ;
#164251=ADVANCED_FACE ( 'NONE', ( #106608 ), #140150, .T. ) ;
#164254=CARTESIAN_POINT ( 'NONE',  ( -8.636180661780658241, 12.05899929117736846, -1.082531754730543083 ) ) ;
#164260=CARTESIAN_POINT ( 'NONE',  ( -8.636180661780651135, 13.01936850547871138, -0.7216878364870257245 ) ) ;
#164267=CARTESIAN_POINT ( 'NONE',  ( -9.042925270190641740, 11.57316545335434199, 1.443375672974064550 ) ) ;
#164273=CARTESIAN_POINT ( 'NONE',  ( 1.499999999999987121, 2.577083334016147198, -0.8660254037844262731 ) ) ;
#164277=CARTESIAN_POINT ( 'NONE',  ( -8.667740277838301921, 9.006785167099828016, -0.7998128361456291469 ) ) ;
#164282=CARTESIAN_POINT ( 'NONE',  ( 4.950698647284403009, 8.927565521807144577, 1.040834085586084257E-14 ) ) ;
#164283=EDGE_LOOP ( 'NONE', ( #172605, #55116, #128883, #74245, #123088, #103375 ) ) ;
#164285=LINE ( 'NONE', #15873, #211465 ) ;
#164288=CARTESIAN_POINT ( 'NONE',  ( 7.446452682403650769, 9.710614100936176385, -1.599625672291262513 ) ) ;
#164294=CARTESIAN_POINT ( 'NONE',  ( -6.182154858151506893, 9.195969186943299789, 1.082531754730548412 ) ) ;
#164297=CARTESIAN_POINT ( 'NONE',  ( -1.364683531249997417, 5.821875000341418804, 1.214306433183764966E-14 ) ) ;
#164304=CARTESIAN_POINT ( 'NONE',  ( -4.080641047588918546, 4.823464646017586510, -1.082531754730548412 ) ) ;
#164307=CARTESIAN_POINT ( 'NONE',  ( 9.103410076571945453, 12.70806329172093818, 1.199719254218450271 ) ) ;
#164309=CARTESIAN_POINT ( 'NONE',  ( -9.073431116043565225, 11.60875560684942265, -1.599625672291263179 ) ) ;
#164311=CARTESIAN_POINT ( 'NONE',  ( -1.364683531250012516, 2.530208333674753174, 0.7879004041258379498 ) ) ;
#164312=CARTESIAN_POINT ( 'NONE',  ( 5.332434488876471868, 5.115595079977664383, 0.7998128361456341429 ) ) ;
#164318=CARTESIAN_POINT ( 'NONE',  ( 9.449669878600614581, 12.04770082983265844, -1.443375672974058777 ) ) ;
#164321=CARTESIAN_POINT ( 'NONE',  ( -7.537970219518083326, 9.817384560903001045, -1.443375672974059665 ) ) ;
#164322=CARTESIAN_POINT ( 'NONE',  ( -0.6823417656250246877, 0.3010416670080895418, 1.181850606188755259 ) ) ;
#164326=CARTESIAN_POINT ( 'NONE',  ( -6.997979842947967377, 11.31606025008131233, -0.7998128361456291469 ) ) ;
#164327=CARTESIAN_POINT ( 'NONE',  ( -4.080641047588918546, 4.823464646017586510, -1.082531754730548412 ) ) ;
#164328=CARTESIAN_POINT ( 'NONE',  ( -0.6823417656249969321, 3.780208333674754506, -1.181850606188749264 ) ) ;
#164351=CARTESIAN_POINT ( 'NONE',  ( 1.364683531249988535, 4.467708333674754506, -0.7879004041258300672 ) ) ;
#164357=CARTESIAN_POINT ( 'NONE',  ( 9.420217803396747414, 9.884675613584706255, 0.7998128361456462443 ) ) ;
#164360=CARTESIAN_POINT ( 'NONE',  ( -0.6823417656250003738, 2.217708333674753174, -1.181850606188749264 ) ) ;
#164362=CARTESIAN_POINT ( 'NONE',  ( -5.734735788900501952, 9.634349487118505806, 0.000000000000000000 ) ) ;
#164369=CARTESIAN_POINT ( 'NONE',  ( 4.111146893441827821, 5.819424013814004759, 1.599625672291267398 ) ) ;
#164372=CARTESIAN_POINT ( 'NONE',  ( 10.40318394038753702, 11.03146944007395724, -0.7998128361456281477 ) ) ;
#164378=CARTESIAN_POINT ( 'NONE',  ( -8.299562589859897699, 12.83457345481192036, -0.7998128361456281477 ) ) ;
#164380=CARTESIAN_POINT ( 'NONE',  ( 6.771407655021410399, 9.987393799911945536, -1.199719254218441611 ) ) ;
#164382=CARTESIAN_POINT ( 'NONE',  ( 4.731432421044862835, 6.543090462684225450, -1.443375672974051449 ) ) ;
#164384=DIRECTION ( 'NONE',  ( 1.000000000000000000, -4.985516615831701596E-16, 0.000000000000000000 ) ) ;
#164386=ORIENTED_EDGE ( 'NONE', *, *, #206253, .F. ) ;
#164393=CARTESIAN_POINT ( 'NONE',  ( -7.565086526745425033, 7.928281824065535055, 0.7216878364870317197 ) ) ;
#164394=CARTESIAN_POINT ( 'NONE',  ( 4.150767584078112193, 7.994312614733129152, 0.7998128361456321445 ) ) ;
#164397=CARTESIAN_POINT ( 'NONE',  ( -7.323375529675950624, 11.69568855126397011, -0.7998128361456291469 ) ) ;
#164402=CARTESIAN_POINT ( 'NONE',  ( -8.462260433223891098, 13.02438760540324481, -0.7998128361456281477 ) ) ;
#164405=CARTESIAN_POINT ( 'NONE',  ( 7.964525173024008531, 11.37936423758166526, 1.199719254218460707 ) ) ;
#164406=CARTESIAN_POINT ( 'NONE',  ( -1.579999999999996074, 8.674529973577525865, -2.499999999999995115 ) ) ;
#164417=CARTESIAN_POINT ( 'NONE',  ( -8.565000355531095622, 11.01558638625153286, -1.599625672291263179 ) ) ;
#164421=CARTESIAN_POINT ( 'NONE',  ( 7.809133291791403586, 8.213003049952529722, -0.7216878364870257245 ) ) ;
#164423=CARTESIAN_POINT ( 'NONE',  ( 2.672928840188529609, 6.270167413528593414, 0.000000000000000000 ) ) ;
#164425=CARTESIAN_POINT ( 'NONE',  ( 5.138703914779377158, 5.953908307786102583, 1.199719254218462483 ) ) ;
#164427=CARTESIAN_POINT ( 'NONE',  ( -7.389357414647957256, 8.579670724299436557, 1.199719254218450271 ) ) ;
#164429=CARTESIAN_POINT ( 'NONE',  ( 4.101444922696781070, 3.685019076479660427, 2.500000000000011102 ) ) ;
#164435=CARTESIAN_POINT ( 'NONE',  ( 1.364683531249988535, 4.217708333674752730, -0.7879004041258239610 ) ) ;
#164436=CARTESIAN_POINT ( 'NONE',  ( 4.952636518945290334, 6.537114055554089198, 2.442608363190974963 ) ) ;
#164437=CARTESIAN_POINT ( 'NONE',  ( 9.752392566931574081, 10.27221283770866300, -0.7998128361456281477 ) ) ;
#164439=CARTESIAN_POINT ( 'NONE',  ( -5.097502569058225852, 5.049433873430440478, -0.7216878364870207285 ) ) ;
#164442=CARTESIAN_POINT ( 'NONE',  ( -5.083944415000202888, 5.033616027029415463, 0.7216878364870317197 ) ) ;
#164450=CARTESIAN_POINT ( 'NONE',  ( 3.499976210622149253, 7.235056012367825140, 0.7998128361456321445 ) ) ;
#164458=CARTESIAN_POINT ( 'NONE',  ( 5.691725559638619814, 5.534767995866836543, 1.040834085586084257E-14 ) ) ;
#164464=CARTESIAN_POINT ( 'NONE',  ( -0.6823417656250212460, 4.613541667008086655, 1.181850606188767472 ) ) ;
#164469=CARTESIAN_POINT ( 'NONE',  ( 7.135668919494039031, 7.219368582364847242, 1.040834085586084257E-14 ) ) ;
#164471=CARTESIAN_POINT ( 'NONE',  ( -6.749261541504576911, 6.768559974710451677, 1.040834085586084257E-14 ) ) ;
#164472=CARTESIAN_POINT ( 'NONE',  ( -1.500000000000013101, 1.670833333333355153, 0.8660254037844403729 ) ) ;
#164475=CARTESIAN_POINT ( 'NONE',  ( -4.466521540698216164, 7.298359999868178960, -1.199719254218452047 ) ) ;
#164476=CARTESIAN_POINT ( 'NONE',  ( 0.2935777296394709857, 7.111227605955068753, -1.979479841891092162 ) ) ;
#164478=CARTESIAN_POINT ( 'NONE',  ( -1.364683531250012516, 3.238541667008084879, -0.7879004041258289570 ) ) ;
#164481=CARTESIAN_POINT ( 'NONE',  ( -3.877268743828284681, 5.546566172598190292, 1.443375672974064550 ) ) ;
#164486=CARTESIAN_POINT ( 'NONE',  ( -1.445103857048105844, 8.688264192037886247, -2.625611233228243968 ) ) ;
#164487=CARTESIAN_POINT ( 'NONE',  ( 5.464099601507359516, 6.333536608968757697, 1.199719254218462483 ) ) ;
#164490=CARTESIAN_POINT ( 'NONE',  ( 0.5625979914390633052, 6.581402780318009960, -3.408537040423953446 ) ) ;
#164491=CARTESIAN_POINT ( 'NONE',  ( -0.6823417656250212460, 3.863541667008085767, 1.181850606188767472 ) ) ;
#164493=CARTESIAN_POINT ( 'NONE',  ( 2.846322183865124700, 5.408127416896231665, -1.199719254218446718 ) ) ;
#164495=CARTESIAN_POINT ( 'NONE',  ( -0.6823417656250003738, -0.2197916663252488800, -1.181850606188749264 ) ) ;
#164496=CARTESIAN_POINT ( 'NONE',  ( 8.500000000000000000, 6.216000000000041048, -2.921333333333334004 ) ) ;
#164499=CARTESIAN_POINT ( 'NONE',  ( -5.108724954250998707, 4.854600622914589714, -0.7998128361456221525 ) ) ;
#164500=CARTESIAN_POINT ( 'NONE',  ( -5.951666246274811556, 7.966696592119163256, 1.443375672974064550 ) ) ;
#164501=VECTOR ( 'NONE', #200032, 1000.000000000000000 ) ;
#164505=CARTESIAN_POINT ( 'NONE',  ( -1.364683531249997417, 2.509375000341422357, 1.214306433183764966E-14 ) ) ;
#164513=CARTESIAN_POINT ( 'NONE',  ( -6.344852701071109102, 10.34615255131755163, 0.000000000000000000 ) ) ;
#164519=CARTESIAN_POINT ( 'NONE',  ( -5.544921637864824504, 8.452530429942200385, -1.082531754730543971 ) ) ;
#164522=CARTESIAN_POINT ( 'NONE',  ( 2.843981590737003629, 6.431529745484265703, 0.1377261510360130170 ) ) ;
#164526=CARTESIAN_POINT ( 'NONE',  ( 1.448804818547306139, 8.711467014680348342, -2.592604518246271361 ) ) ;
#164530=CARTESIAN_POINT ( 'NONE',  ( -3.744022975668147790, 7.519777238254810925, -0.7998128361456281477 ) ) ;
#164533=CARTESIAN_POINT ( 'NONE',  ( 0.7499999999999885647, -0.2666666666666442365, 1.299038105676657340 ) ) ;
#164534=CARTESIAN_POINT ( 'NONE',  ( 4.220665892555866883, 3.818531717603609987, -0.7998128361456211532 ) ) ;
#164535=CARTESIAN_POINT ( 'NONE',  ( 8.446893396513862839, 9.813462703143045474, -1.199719254218445830 ) ) ;
#164537=CARTESIAN_POINT ( 'NONE',  ( 3.673896439623290266, 4.156855427197417185, 1.000000000000011324 ) ) ;
#164538=CARTESIAN_POINT ( 'NONE',  ( 5.867981556616276073, 5.740399992340775803, -0.7998128361456281477 ) ) ;
#164539=CARTESIAN_POINT ( 'NONE',  ( -2.123823618835070537, 5.629544655282869847, 1.040834085586084257E-14 ) ) ;
#164545=CARTESIAN_POINT ( 'NONE',  ( -3.090895834235680262, 5.589500325708124606, 1.082531754730560403 ) ) ;
#164548=CARTESIAN_POINT ( 'NONE',  ( 5.905025204069010769, 4.805319369725367551, -2.499999999999995115 ) ) ;
#164552=CARTESIAN_POINT ( 'NONE',  ( 1.364683531249988535, 2.363541667008088432, 0.7879004041258500513 ) ) ;
#164553=CARTESIAN_POINT ( 'NONE',  ( 9.910647101465253073, 11.62513837554007168, -1.082531754730537088 ) ) ;
#164555=CARTESIAN_POINT ( 'NONE',  ( -7.576308911938196999, 7.733448573549685179, 0.7998128361456462443 ) ) ;
#164558=CARTESIAN_POINT ( 'NONE',  ( 5.738125327081736060, 7.717565519727259904, 1.599625672291267398 ) ) ;
#164559=CARTESIAN_POINT ( 'NONE',  ( -7.562750758324527922, 7.717630727667075696, 1.040834085586084257E-14 ) ) ;
#164562=CARTESIAN_POINT ( 'NONE',  ( 1.499999999999985123, -0.9229166659838452524, -0.8660254037844323793 ) ) ;
#164565=CARTESIAN_POINT ( 'NONE',  ( 6.643132081016105417, 10.69414516125339887, 0.7216878364870438212 ) ) ;
#164568=CARTESIAN_POINT ( 'NONE',  ( -0.6823417656250003738, 1.280208333674752508, -1.181850606188749264 ) ) ;
#164570=CARTESIAN_POINT ( 'NONE',  ( 5.734735788456138295, 8.673980272298743799, -1.082531754730537976 ) ) ;
#164573=CARTESIAN_POINT ( 'NONE',  ( -3.192880356576565770, 6.433770387723418693, -0.7510166236791281369 ) ) ;
#164574=CARTESIAN_POINT ( 'NONE',  ( -5.111060722671894929, 5.065251719313053513, 0.000000000000000000 ) ) ;
#164576=CARTESIAN_POINT ( 'NONE',  ( -1.364683531249997417, 5.009375000341425022, 1.214306433183764966E-14 ) ) ;
#164580=CARTESIAN_POINT ( 'NONE',  ( -5.444063778538836829, 6.456803583937833046, -1.314021404191120901 ) ) ;
#164586=CARTESIAN_POINT ( 'NONE',  ( 6.337546739384100292, 9.481222731668410120, 1.199719254218460707 ) ) ;
#164589=CARTESIAN_POINT ( 'NONE',  ( 3.497113557321089861, 6.167384019261527683, -1.199719254218446718 ) ) ;
#164596=CARTESIAN_POINT ( 'NONE',  ( 5.016153647376205171, 6.875265226737464985, 1.443375672974062551 ) ) ;
#164597=CARTESIAN_POINT ( 'NONE',  ( 0.6823417656249882723, 0.4052083336747516751, 1.181850606188755259 ) ) ;
#164600=CARTESIAN_POINT ( 'NONE',  ( 2.703961570921634028, 5.242040035128820108, -1.199719254218446718 ) ) ;
#164601=CARTESIAN_POINT ( 'NONE',  ( 1.419999999999990603, 6.200000000000045475, 2.900000000000001688 ) ) ;
#164603=CARTESIAN_POINT ( 'NONE',  ( 1.419999999999990603, 6.264000000000040203, 2.852000000000002089 ) ) ;
#164607=CARTESIAN_POINT ( 'NONE',  ( -1.499999999999997780, 2.400000000000020339, 1.214306433183764966E-14 ) ) ;
#164608=CARTESIAN_POINT ( 'NONE',  ( 7.949158136313996259, 8.168439335321471262, 1.040834085586084257E-14 ) ) ;
#164609=CARTESIAN_POINT ( 'NONE',  ( -7.181014916732457287, 11.52960116949655678, -0.7998128361456291469 ) ) ;
#164613=CARTESIAN_POINT ( 'NONE',  ( -0.6823417656250003738, 1.467708333674752730, -1.181850606188749264 ) ) ;
#164614=CARTESIAN_POINT ( 'NONE',  ( 0.7499999999999902300, 2.733333333333351600, 1.299038105676669330 ) ) ;
#164616=CARTESIAN_POINT ( 'NONE',  ( 3.334415713957098681, 5.977569868670206787, -1.199719254218446718 ) ) ;
#164623=CARTESIAN_POINT ( 'NONE',  ( 1.499999999999987121, -0.9645833326505173222, 0.8660254037844524744 ) ) ;
#164624=CARTESIAN_POINT ( 'NONE',  ( -7.802881099864745984, 9.062115023719057305, -1.199719254218446718 ) ) ;
#164625=CARTESIAN_POINT ( 'NONE',  ( -3.294268138440636928, 6.787137228248626641, 1.040834085586084257E-14 ) ) ;
#164628=EDGE_CURVE ( 'NONE', #67975, #85030, #156961, .T. ) ;
#164631=CARTESIAN_POINT ( 'NONE',  ( 4.033414559382754838, 7.548954524214963158, -0.4004916564768338794 ) ) ;
#164634=CARTESIAN_POINT ( 'NONE',  ( 6.775324078527185989, 8.927630729746953264, -1.599625672291262513 ) ) ;
#164636=DIRECTION ( 'NONE',  ( -1.000000000000000000, 5.578564026256490882E-16, -1.264049978315544409E-61 ) ) ;
#164638=CARTESIAN_POINT ( 'NONE',  ( 6.551614543901692400, 8.666636272683888365, 1.599625672291281386 ) ) ;
#164639=CARTESIAN_POINT ( 'NONE',  ( 9.883530794237934458, 10.63313346947350269, -0.7216878364870257245 ) ) ;
#164644=CARTESIAN_POINT ( 'NONE',  ( -5.371001409308059138, 9.417918744168066070, -0.7998128361456231517 ) ) ;
#164645=CARTESIAN_POINT ( 'NONE',  ( 5.840865249388943248, 5.708764300575555062, 0.7998128361456341429 ) ) ;
#164650=CARTESIAN_POINT ( 'NONE',  ( 3.998873522394119195, 7.597518543056763995, -0.1390531931140040478 ) ) ;
#164651=CARTESIAN_POINT ( 'NONE',  ( 9.164948653157988900, 11.71552606681625619, -1.443375672974057666 ) ) ;
#164652=VERTEX_POINT ( 'NONE', #113032 ) ;
#164660=CARTESIAN_POINT ( 'NONE',  ( -3.307826292054310890, 5.842585859829892314, -1.082531754730549967 ) ) ;
#164661=CARTESIAN_POINT ( 'NONE',  ( 8.351459436338029008, 10.76645531385962862, -1.443375672974063439 ) ) ;
#164664=CARTESIAN_POINT ( 'NONE',  ( -4.706651882238427120, 8.642844295920152575, 1.040834085586084257E-14 ) ) ;
#164670=CARTESIAN_POINT ( 'NONE',  ( -6.718228810771495141, 7.796687353110217877, 1.199719254218450271 ) ) ;
#164674=VERTEX_POINT ( 'NONE', #83643 ) ;
#164685=CARTESIAN_POINT ( 'NONE',  ( -7.054319997812058318, 7.124461507069184130, 1.040834085586084257E-14 ) ) ;
#164688=CARTESIAN_POINT ( 'NONE',  ( 3.362058906508953449, 6.866226457661676719, -0.7216878364870267237 ) ) ;
#164691=CARTESIAN_POINT ( 'NONE',  ( -4.796887421136680985, 4.490790167614548523, 1.214306433183764966E-14 ) ) ;
#164697=CARTESIAN_POINT ( 'NONE',  ( -7.609150525767646833, 9.900428251527500834, -1.599625672291263179 ) ) ;
#164698=CARTESIAN_POINT ( 'NONE',  ( 5.262536180398716290, 9.291375977107183104, -0.7998128361456291469 ) ) ;
#164700=CARTESIAN_POINT ( 'NONE',  ( -8.941766003412679353, 10.39081407785832845, -1.199719254218446718 ) ) ;
#164704=CARTESIAN_POINT ( 'NONE',  ( -0.6823417656250003738, -0.2197916663252488800, -1.181850606188749264 ) ) ;
#164705=VERTEX_POINT ( 'NONE', #82578 ) ;
#164707=CARTESIAN_POINT ( 'NONE',  ( 7.131225611108079399, 11.26358761302737754, 0.7216878364870438212 ) ) ;
#164712=VERTEX_POINT ( 'NONE', #98853 ) ;
#164733=CARTESIAN_POINT ( 'NONE',  ( -0.7500000000000006661, 0.3895833340161539149, -1.299038105676652011 ) ) ;
#164737=ORIENTED_EDGE ( 'NONE', *, *, #157427, .T. ) ;
#164740=CARTESIAN_POINT ( 'NONE',  ( 8.191097360950562845, 12.70803068775103739, -0.7998128361456352531 ) ) ;
#164742=EDGE_CURVE ( 'NONE', #96990, #104450, #42530, .T. ) ;
#164746=CARTESIAN_POINT ( 'NONE',  ( 5.183294799126148433, 4.941598775268944976, 1.040834085586084257E-14 ) ) ;
#164747=CARTESIAN_POINT ( 'NONE',  ( -7.592202833972775622, 8.920286730132099606, 1.082531754730558626 ) ) ;
#164749=CARTESIAN_POINT ( 'NONE',  ( -5.796211742468360129, 6.069872997065163922, -0.5622600474686073602 ) ) ;
#164753=CARTESIAN_POINT ( 'NONE',  ( -6.170932472514347289, 10.35117165124207972, 0.000000000000000000 ) ) ;
#164754=CARTESIAN_POINT ( 'NONE',  ( -3.050221372950322252, 5.542046787541873520, 1.082531754730560403 ) ) ;
#164755=AXIS2_PLACEMENT_3D ( 'NONE', #196667, #46174, #98122 ) ;
#164758=CARTESIAN_POINT ( 'NONE',  ( -1.402160292154681736E-14, -0.2562499993171780122, 1.732050807568877637 ) ) ;
#164765=CARTESIAN_POINT ( 'NONE',  ( -8.482597663644387609, 13.04811437422715414, -0.7998128361456281477 ) ) ;
#164774=CARTESIAN_POINT ( 'NONE',  ( -8.642432853707342488, 12.17025653171218558, 1.199719254218462483 ) ) ;
#164775=CARTESIAN_POINT ( 'NONE',  ( 8.284195553149872993, 9.623648552551724578, -1.199719254218445830 ) ) ;
#164778=CARTESIAN_POINT ( 'NONE',  ( -1.001543065824772872E-14, 5.212500000000019895, 1.732050807568877637 ) ) ;
#164780=ORIENTED_EDGE ( 'NONE', *, *, #3407, .F. ) ;
#164783=CARTESIAN_POINT ( 'NONE',  ( -7.784352752540590004, 12.23349531127272094, 0.7998128361456481317 ) ) ;
#164788=CARTESIAN_POINT ( 'NONE',  ( 5.054492339796319733, 4.791329239384148231, -0.7998128361456211532 ) ) ;
#164805=CARTESIAN_POINT ( 'NONE',  ( 6.337546739384100292, 9.481222731668410120, 1.199719254218460707 ) ) ;
#164807=CARTESIAN_POINT ( 'NONE',  ( -5.298539104842322267, 5.076050465271134016, 0.7998128361456341429 ) ) ;
#164808=VECTOR ( 'NONE', #125450, 1000.000000000000000 ) ;
#164814=CARTESIAN_POINT ( 'NONE',  ( -1.402160292154681736E-14, -0.006249999317184824418, 1.732050807568877637 ) ) ;
#164816=ADVANCED_FACE ( 'NONE', ( #17557 ), #47991, .T. ) ;
#164818=CARTESIAN_POINT ( 'NONE',  ( -1.499999999999998002, 8.673756432004008587, -2.614717076620595382 ) ) ;
#164819=CARTESIAN_POINT ( 'NONE',  ( 4.552840656090682891, 4.206068941727564514, 1.214306433183764966E-14 ) ) ;
#164821=CARTESIAN_POINT ( 'NONE',  ( -4.298098390732130625, 4.973201863064262263, 1.199719254218462483 ) ) ;
#164828=CARTESIAN_POINT ( 'NONE',  ( 4.528060117284232966, 6.305822774963486310, 1.443375672974062551 ) ) ;
#164831=CARTESIAN_POINT ( 'NONE',  ( -0.6823417656249969321, 5.280208333674756283, -1.181850606188749264 ) ) ;
#164833=CARTESIAN_POINT ( 'NONE',  ( 3.185802909086945967, 5.700225246367978116, 1.082531754730546636 ) ) ;
#164841=CARTESIAN_POINT ( 'NONE',  ( -5.789194372615304118, 6.219231786955013774, 1.015549131865096211 ) ) ;
#164843=CARTESIAN_POINT ( 'NONE',  ( -0.6823417656249969321, 5.030208333674755394, -1.181850606188749264 ) ) ;
#164850=CARTESIAN_POINT ( 'NONE',  ( -0.7499999999999972244, 4.358333333333352932, -1.299038105676652011 ) ) ;
#164857=CARTESIAN_POINT ( 'NONE',  ( -1.001543065824772872E-14, 4.884375000341420581, 1.575800808251672791 ) ) ;
#164859=CARTESIAN_POINT ( 'NONE',  ( 6.796715079152391148, 6.823922435299587974, 0.7998128361456341429 ) ) ;
#164860=CARTESIAN_POINT ( 'NONE',  ( -8.690940161559884913, 10.09818392903003748, 1.199719254218462483 ) ) ;
#164866=CARTESIAN_POINT ( 'NONE',  ( -1.201851678989727383E-14, 5.337500000000020783, -1.732050807568863648 ) ) ;
#164870=CARTESIAN_POINT ( 'NONE',  ( -6.471393748265563239, 5.229711127717889596, 2.499999999999998668 ) ) ;
#164873=CARTESIAN_POINT ( 'NONE',  ( 8.270110514656026979, 10.67154823856396817, 1.443375672974076540 ) ) ;
#164878=CARTESIAN_POINT ( 'NONE',  ( -1.201851678989727383E-14, 3.243750000682814161, 1.732050807568877637 ) ) ;
#164881=CARTESIAN_POINT ( 'NONE',  ( -4.090809663021341969, 5.795697244990093644, 1.599625672291267398 ) ) ;
#164882=CARTESIAN_POINT ( 'NONE',  ( 3.321384445223597659, 6.818772919495430074, -0.7216878364870267237 ) ) ;
#164883=CARTESIAN_POINT ( 'NONE',  ( -10.61567108937589765, 11.48729714713446803, 0.7216878364870438212 ) ) ;
#164890=CARTESIAN_POINT ( 'NONE',  ( 4.546061579283848353, 4.198160018786257552, -0.7998128361456211532 ) ) ;
#164891=CARTESIAN_POINT ( 'NONE',  ( -3.904385050611244079, 7.498940292447679568, 1.040834085586084257E-14 ) ) ;
#164893=CARTESIAN_POINT ( 'NONE',  ( 3.517450787741589036, 6.191110788085444128, -1.199719254218446718 ) ) ;
#164907=CARTESIAN_POINT ( 'NONE',  ( 8.052653171512838881, 11.48218023581863001, -1.199719254218446718 ) ) ;
#164912=CARTESIAN_POINT ( 'NONE',  ( -0.6823417656250003738, 0.2177083336747515085, -1.181850606188749264 ) ) ;
#164913=CARTESIAN_POINT ( 'NONE',  ( 7.321039761699430493, 7.643560598178549270, -0.7216878364870257245 ) ) ;
#164914=CARTESIAN_POINT ( 'NONE',  ( -9.246297574839990929, 11.81043314211192019, 1.443375672974076540 ) ) ;
#164920=CARTESIAN_POINT ( 'NONE',  ( -4.711622075948912247, 5.455646162483875017, -1.199719254218446718 ) ) ;
#164934=CARTESIAN_POINT ( 'NONE',  ( 5.997902985473373860, 6.089292839903872157, -0.6134941253506603909 ) ) ;
#164935=CARTESIAN_POINT ( 'NONE',  ( 7.334597915313080918, 9.580116872663850813, 1.040834085586084257E-14 ) ) ;
#164938=CARTESIAN_POINT ( 'NONE',  ( 3.469446951953614189E-15, 5.900000000000023448, 1.214306433183764966E-14 ) ) ;
#164941=CARTESIAN_POINT ( 'NONE',  ( -8.676855123066022912, 10.18571440074093282, -1.082531754730543971 ) ) ;
#164946=CARTESIAN_POINT ( 'NONE',  ( 5.126954644262057492, 9.133197518281081173, 0.7998128361456462443 ) ) ;
#164947=CARTESIAN_POINT ( 'NONE',  ( -4.141125853970233806, 6.918731698685530063, -1.199719254218452047 ) ) ;
#164950=CARTESIAN_POINT ( 'NONE',  ( -6.274726165026268454, 6.214935368819085149, 0.7998128361456341429 ) ) ;
#164951=CARTESIAN_POINT ( 'NONE',  ( 2.846322183865124700, 5.408127416896231665, -1.199719254218446718 ) ) ;
#164954=CARTESIAN_POINT ( 'NONE',  ( -4.055860508782465068, 7.883587693554856557, 1.040834085586084257E-14 ) ) ;
#164957=CARTESIAN_POINT ( 'NONE',  ( 8.402302512167096893, 10.82577223566020841, -1.599625672291268286 ) ) ;
#164958=CARTESIAN_POINT ( 'NONE',  ( 0.2771623952736271268, 7.029701766580681799, 4.006269022107524336 ) ) ;
#164960=CARTESIAN_POINT ( 'NONE',  ( 4.540820729390463661, 6.975461451583557348, -1.175308324676842542 ) ) ;
#164961=CARTESIAN_POINT ( 'NONE',  ( 5.016153647376201619, 7.835634441038803466, 1.082531754730558626 ) ) ;
#164970=CARTESIAN_POINT ( 'NONE',  ( 7.958272981097359811, 9.347368568444167636, -1.082531754730537976 ) ) ;
#164974=CARTESIAN_POINT ( 'NONE',  ( -5.852315862593199469, 9.979452273000736895, 0.7998128361456481317 ) ) ;
#164979=DIRECTION ( 'NONE',  ( 0.9999160831030532437, -0.01240418662285098193, -0.003736697214576322184 ) ) ;
#164983=CARTESIAN_POINT ( 'NONE',  ( 8.041957671200231417, 12.53403438304231976, 1.040834085586084257E-14 ) ) ;
#164988=CARTESIAN_POINT ( 'NONE',  ( 3.388648328411762556, 6.040841252200647382, 1.199719254218462483 ) ) ;
#164991=CARTESIAN_POINT ( 'NONE',  ( 0.7499999999999902300, 4.347916667349481123, -1.299038105676658228 ) ) ;
#164997=CARTESIAN_POINT ( 'NONE',  ( -1.201851678989727383E-14, 1.962500000000020783, 1.732050807568877637 ) ) ;
#164998=CARTESIAN_POINT ( 'NONE',  ( 6.262976894508937242, 9.394224579314053969, -1.199719254218440723 ) ) ;
#165001=CARTESIAN_POINT ( 'NONE',  ( 7.782016984564054773, 10.10210578678999482, 1.443375672974076540 ) ) ;
#165006=CARTESIAN_POINT ( 'NONE',  ( -3.242371291962510504, 6.934516940598226320, 1.040834085586084257E-14 ) ) ;
#165007=CARTESIAN_POINT ( 'NONE',  ( -0.7500000000000215383, 5.222916667349482012, 1.299038105676671107 ) ) ;
#165008=CARTESIAN_POINT ( 'NONE',  ( -0.6823417656250246877, -0.9489583329919115684, 1.181850606188755259 ) ) ;
#165012=CARTESIAN_POINT ( 'NONE',  ( 2.849184837166184536, 6.475799410002530898, 0.7998128361456362523 ) ) ;
#165014=CARTESIAN_POINT ( 'NONE',  ( -1.364683531249997417, 5.821875000341418804, 1.214306433183764966E-14 ) ) ;
#165018=CARTESIAN_POINT ( 'NONE',  ( 10.72180055030867329, 11.40318881831530540, 0.7998128361456341429 ) ) ;
#165023=CARTESIAN_POINT ( 'NONE',  ( -7.226659571283968297, 8.389856573708110332, 1.199719254218450271 ) ) ;
#165025=CARTESIAN_POINT ( 'NONE',  ( 4.222474775652216294, 7.013638773981186958, 1.199719254218462483 ) ) ;
#165029=CARTESIAN_POINT ( 'NONE',  ( 0.6823417656249882723, -0.1572916663252488245, 1.181850606188755259 ) ) ;
#165033=CARTESIAN_POINT ( 'NONE',  ( 8.452618703115982512, 11.94880668935564216, 1.199719254218450271 ) ) ;
#165036=CARTESIAN_POINT ( 'NONE',  ( -4.882907879216086933, 8.848476292394087395, -0.7998128361456281477 ) ) ;
#165040=CARTESIAN_POINT ( 'NONE',  ( 9.836604141914616406, 11.43479190611061647, 1.199719254218452047 ) ) ;
#165042=CARTESIAN_POINT ( 'NONE',  ( 8.372323551638698902, 9.726464550788689323, 1.199719254218462483 ) ) ;
#165043=EDGE_CURVE ( 'NONE', #6976, #30182, #180298, .T. ) ;
#165045=CARTESIAN_POINT ( 'NONE',  ( -3.602716132929368875, 5.226254793216122074, 1.599625672291267398 ) ) ;
#165047=CARTESIAN_POINT ( 'NONE',  ( -5.859094939400033120, 9.987361195942037639, -0.7998128361456231517 ) ) ;
#165050=CARTESIAN_POINT ( 'NONE',  ( -4.797329538616279976, 6.965272035667838146, 1.434408638962878957 ) ) ;
#165051=CARTESIAN_POINT ( 'NONE',  ( 1.364683531249988757, 0.3843750003414206362, 0.000000000000000000 ) ) ;
#165055=CARTESIAN_POINT ( 'NONE',  ( 7.632877294813741109, 8.007371053478589573, 1.040834085586084257E-14 ) ) ;
#165058=CARTESIAN_POINT ( 'NONE',  ( 6.356075086708249167, 6.309842444114747373, -0.7998128361456281477 ) ) ;
#165078=CARTESIAN_POINT ( 'NONE',  ( 9.642873567817520808, 12.27310513391906532, 1.599625672291279388 ) ) ;
#165081=CARTESIAN_POINT ( 'NONE',  ( -3.438964519360665051, 7.163875705896082913, -0.7998128361456281477 ) ) ;
#165082=CARTESIAN_POINT ( 'NONE',  ( -7.472515219426274946, 11.86968485597268064, 0.000000000000000000 ) ) ;
#165088=CARTESIAN_POINT ( 'NONE',  ( 1.499999999999989120, 2.535416667349483344, 0.8660254037844524744 ) ) ;
#165089=CARTESIAN_POINT ( 'NONE',  ( 8.809047120577066181, 11.30030761213851953, 1.599625672291281386 ) ) ;
#165093=CARTESIAN_POINT ( 'NONE',  ( -7.828943636887387925, 11.22118577875556156, 1.199719254218453823 ) ) ;
#165094=CARTESIAN_POINT ( 'NONE',  ( -1.201851678989727383E-14, 3.071875000341420137, 1.575800808251672791 ) ) ;
#165096=CARTESIAN_POINT ( 'NONE',  ( -4.905525160107071514, 6.476373528817366498, 2.499999999999998668 ) ) ;
#165098=CIRCLE ( 'NONE', #199709, 0.08000000000000020983 ) ;
#165101=CARTESIAN_POINT ( 'NONE',  ( -3.765413976293358278, 5.416068943807445635, 1.599625672291267398 ) ) ;
#165105=CARTESIAN_POINT ( 'NONE',  ( -1.402160292154681736E-14, 2.009375000341422801, -1.575800808251660134 ) ) ;
#165110=CARTESIAN_POINT ( 'NONE',  ( -1.364683531250014514, 1.738541667008085545, -0.7879004041258289570 ) ) ;
#165112=CARTESIAN_POINT ( 'NONE',  ( -6.196239896645333367, 7.187700286629718605, -1.199719254218446718 ) ) ;
#165113=CARTESIAN_POINT ( 'NONE',  ( 6.317209508963599340, 9.457495962844502557, 1.199719254218462483 ) ) ;
#165114=FACE_OUTER_BOUND ( 'NONE', #46754, .T. ) ;
#165116=CARTESIAN_POINT ( 'NONE',  ( -1.500000000000011324, 4.920833333333354709, 0.8660254037844403729 ) ) ;
#165117=CARTESIAN_POINT ( 'NONE',  ( 0.6823417656249882723, 2.488541667008084435, -1.181850606188749264 ) ) ;
#165122=CARTESIAN_POINT ( 'NONE',  ( -5.639828713604883248, 6.642516923036197340, 1.082531754730548412 ) ) ;
#165125=CARTESIAN_POINT ( 'NONE',  ( 5.260200412422194383, 7.159986452624450770, -1.443375672974051449 ) ) ;
#165128=CARTESIAN_POINT ( 'NONE',  ( -9.515124878692420296, 9.995400534762978850, 1.040834085586084257E-14 ) ) ;
#165129=CARTESIAN_POINT ( 'NONE',  ( -9.571693261567968847, 12.19006144329456731, 1.443375672974076540 ) ) ;
#165131=CARTESIAN_POINT ( 'NONE',  ( 0.6823417656249917140, 5.342708333674749177, 1.181850606188765695 ) ) ;
#165136=CARTESIAN_POINT ( 'NONE',  ( -6.629573926958124197, 9.717958100551031819, 1.082531754730548412 ) ) ;
#165138=CARTESIAN_POINT ( 'NONE',  ( -1.364683531250014514, -0.4072916663252447167, 0.7879004041258379498 ) ) ;
#165141=CARTESIAN_POINT ( 'NONE',  ( 6.968527767744088663, 11.07377346243604599, 0.7216878364870438212 ) ) ;
#165147=CARTESIAN_POINT ( 'NONE',  ( 3.429849674132933846, 5.024577257953626308, -1.443375672974058777 ) ) ;
#165150=CARTESIAN_POINT ( 'NONE',  ( 7.904040366642678173, 12.16520482781775137, 0.7216878364870438212 ) ) ;
#165156=CARTESIAN_POINT ( 'NONE',  ( 5.286789834324991055, 8.255339675766103724, -1.199719254218452935 ) ) ;
#165157=CARTESIAN_POINT ( 'NONE',  ( -3.744022975668147790, 7.519777238254810925, -0.7998128361456281477 ) ) ;
#165160=CARTESIAN_POINT ( 'NONE',  ( 6.141480396866128899, 6.267408005873028820, -0.7216878364870257245 ) ) ;
#165161=CARTESIAN_POINT ( 'NONE',  ( -0.6823417656250003738, 0.2802083336747515641, -1.181850606188749264 ) ) ;
#165163=CARTESIAN_POINT ( 'NONE',  ( -9.459838494033043332, 12.05956421450382088, 1.599625672291281386 ) ) ;
#165181=CARTESIAN_POINT ( 'NONE',  ( 7.579171565239241737, 8.801120566655981747, 1.199719254218462483 ) ) ;
#165182=CARTESIAN_POINT ( 'NONE',  ( 6.982612806237943559, 8.105135347821125436, -1.199719254218446718 ) ) ;
#165193=CARTESIAN_POINT ( 'NONE',  ( -4.954615070790188369, 7.867802451642154082, -1.199719254218452047 ) ) ;
#165195=CARTESIAN_POINT ( 'NONE',  ( -4.627410500965859264, 4.293067094081919777, 0.7998128361456341429 ) ) ;
#165207=CARTESIAN_POINT ( 'NONE',  ( -9.653042183249970876, 11.32459930428888306, -1.082531754730539753 ) ) ;
#165210=CARTESIAN_POINT ( 'NONE',  ( 6.823831386379729302, 6.855558127064808716, -0.7998128361456281477 ) ) ;
#165211=CARTESIAN_POINT ( 'NONE',  ( -0.6823417656250212460, 5.551041667008087543, 1.181850606188767472 ) ) ;
#165216=CARTESIAN_POINT ( 'NONE',  ( 3.945059511452237100, 6.586024615794168646, -1.082531754730548412 ) ) ;
#165217=CARTESIAN_POINT ( 'NONE',  ( -7.555971681517696936, 7.709721804725773175, 0.7998128361456462443 ) ) ;
#165222=CARTESIAN_POINT ( 'NONE',  ( -6.368579470117215813, 8.453095353268645695, 1.599625672291283607 ) ) ;
#165223=CARTESIAN_POINT ( 'NONE',  ( -3.588104209110990706, 7.337872010604796991, 1.040834085586084257E-14 ) ) ;
#165230=CARTESIAN_POINT ( 'NONE',  ( 7.298366762858032430, 7.409182732956175244, 1.040834085586084257E-14 ) ) ;
#165238=CARTESIAN_POINT ( 'NONE',  ( -1.177073619093339962, 3.006928502340592058, 0.7750000000000152323 ) ) ;
#165242=ORIENTED_EDGE ( 'NONE', *, *, #48198, .F. ) ;
#165244=CARTESIAN_POINT ( 'NONE',  ( 1.364683531249986537, 0.2177083336747502595, -0.7879004041258309554 ) ) ;
#165245=CARTESIAN_POINT ( 'NONE',  ( 3.147464216666835402, 6.823792019419957278, -0.7998128361456291469 ) ) ;
#165246=CARTESIAN_POINT ( 'NONE',  ( 6.166260936116925606, 6.088392601758203071, 0.7998128361456341429 ) ) ;
#165249=CARTESIAN_POINT ( 'NONE',  ( -8.188761592974051595, 9.616271948966963024, -1.082531754730543971 ) ) ;
#165251=CARTESIAN_POINT ( 'NONE',  ( 5.124618876285529367, 7.962177208099690873, -1.082531754730549078 ) ) ;
#165252=CARTESIAN_POINT ( 'NONE',  ( -7.171900071504748730, 8.429933507252760805, -1.082531754730549078 ) ) ;
#165256=CARTESIAN_POINT ( 'NONE',  ( 5.913327553854682783, 10.05063257947248800, -0.7998128361456291469 ) ) ;
#165261=CARTESIAN_POINT ( 'NONE',  ( -1.201851678989727383E-14, 4.196875000341417028, -1.575800808251660134 ) ) ;
#165267=CARTESIAN_POINT ( 'NONE',  ( 8.769426429940780920, 9.125419011219408461, 0.7998128361456462443 ) ) ;
#165271=CARTESIAN_POINT ( 'NONE',  ( -7.557780564614042795, 10.90482886110335414, -1.199719254218446718 ) ) ;
#165275=CARTESIAN_POINT ( 'NONE',  ( -1.499999999999997780, 4.181250000682819490, 1.214306433183764966E-14 ) ) ;
#165277=CARTESIAN_POINT ( 'NONE',  ( 10.21336978979620191, 10.81001959771741205, 0.7998128361456462443 ) ) ;
#165278=CARTESIAN_POINT ( 'NONE',  ( 4.184706906422049677, 7.590773377626947038, -0.8858016570119742195 ) ) ;
#165280=CARTESIAN_POINT ( 'NONE',  ( -6.855619230004478482, 11.14997286831390788, -0.7998128361456291469 ) ) ;
#165281=DIRECTION ( 'NONE',  ( 0.7592566023653005702, -0.6507913734559639396, 0.000000000000000000 ) ) ;
#165283=CARTESIAN_POINT ( 'NONE',  ( 4.872649465673598357, 6.683545894502381124, -1.250567445346082218 ) ) ;
#165284=CARTESIAN_POINT ( 'NONE',  ( -3.277320446201389181, 4.846626492033466072, 1.599625672291267398 ) ) ;
#165289=CARTESIAN_POINT ( 'NONE',  ( 6.959412922516382771, 7.013736585890911535, 0.7998128361456341429 ) ) ;
#165291=CARTESIAN_POINT ( 'NONE',  ( 4.286349120214771879, 8.152491073559232859, -0.7998128361456221525 ) ) ;
#165292=CARTESIAN_POINT ( 'NONE',  ( -4.044208510193211481, 7.583498396275582643, -0.3544512193057146598 ) ) ;
#165293=CARTESIAN_POINT ( 'NONE',  ( 4.142179624174931796, 4.791296635414242111, 1.199719254218464037 ) ) ;
#165295=CARTESIAN_POINT ( 'NONE',  ( -7.293923454472094114, 9.532663335016016148, 1.443375672974090751 ) ) ;
#165301=CARTESIAN_POINT ( 'NONE',  ( -4.218308198147158627, 7.356310275799033960, -0.8477421400144637964 ) ) ;
#165302=CARTESIAN_POINT ( 'NONE',  ( -1.402160292154681736E-14, -0.7406249996585823059, -1.575800808251665908 ) ) ;
#165306=CARTESIAN_POINT ( 'NONE',  ( 3.850152436600926542, 7.435668909435648288, -0.7216878364870197293 ) ) ;
#165310=CARTESIAN_POINT ( 'NONE',  ( -7.822691444960696572, 12.07029775252209092, -0.7216878364870267237 ) ) ;
#165316=CARTESIAN_POINT ( 'NONE',  ( -9.612367721964613310, 11.27714576612263997, -1.082531754730537976 ) ) ;
#165323=CARTESIAN_POINT ( 'NONE',  ( -8.256552360598034213, 11.61609960646427986, 1.082531754730549967 ) ) ;
#165330=CARTESIAN_POINT ( 'NONE',  ( 1.499999999999989120, 3.056250000682818158, 1.214306433183764966E-14 ) ) ;
#165333=ORIENTED_EDGE ( 'NONE', *, *, #120212, .T. ) ;
#165335=CARTESIAN_POINT ( 'NONE',  ( -9.158696461231359720, 10.64389961198009615, 1.199719254218462483 ) ) ;
#165336=CARTESIAN_POINT ( 'NONE',  ( -5.273758566035884776, 5.255065869904374409, 0.000000000000000000 ) ) ;
#165338=CARTESIAN_POINT ( 'NONE',  ( 6.959412922516382771, 7.013736585890911535, 0.7998128361456341429 ) ) ;
#165343=CARTESIAN_POINT ( 'NONE',  ( 8.945682426918439845, 9.331051007693339727, 1.040834085586084257E-14 ) ) ;
#165345=CARTESIAN_POINT ( 'NONE',  ( -4.843110422882263677, 5.040344427663700166, -0.8886672019048741378 ) ) ;
#165351=CARTESIAN_POINT ( 'NONE',  ( -7.700668062882084719, 8.086460282891644979, -0.7216878364870278340 ) ) ;
#165356=CARTESIAN_POINT ( 'NONE',  ( 0.6823417656249899377, 5.676041667008087543, -1.181850606188754593 ) ) ;
#165360=TOROIDAL_SURFACE ( 'NONE', #172176, 0.8299999999999998490, 0.08000000000000000167 ) ;
#165362=CARTESIAN_POINT ( 'NONE',  ( -2.453662613948990323, 5.806430783008362795, -0.7216878364870257245 ) ) ;
#165364=CARTESIAN_POINT ( 'NONE',  ( 9.073431116043567002, 11.60875560684942265, -1.599625672291262513 ) ) ;
#165369=CARTESIAN_POINT ( 'NONE',  ( 1.364683531249990311, 2.634375000341422801, 1.214306433183764966E-14 ) ) ;
#165370=CARTESIAN_POINT ( 'NONE',  ( 4.844340958784499662, 4.546152628203684820, 0.7998128361456341429 ) ) ;
#165375=CARTESIAN_POINT ( 'NONE',  ( -6.471393748265538370, 5.229711127717889596, -2.499999999999995115 ) ) ;
#165377=CARTESIAN_POINT ( 'NONE',  ( 8.988692655735958326, 12.47026328412523988, -1.082531754730543083 ) ) ;
#165379=CARTESIAN_POINT ( 'NONE',  ( -8.541273586929371220, 9.067166727613487964, 0.7216878364870438212 ) ) ;
#165381=CARTESIAN_POINT ( 'NONE',  ( -3.890471347679111513, 5.946836461140907915, 1.325960742581899110 ) ) ;
#165383=CARTESIAN_POINT ( 'NONE',  ( -8.681298431451969222, 9.022603012982438386, 1.040834085586084257E-14 ) ) ;
#165384=CARTESIAN_POINT ( 'NONE',  ( -4.189106276498259618, 6.870745841681152655, 1.082531754730560403 ) ) ;
#165385=CARTESIAN_POINT ( 'NONE',  ( -0.6823417656250212460, 3.613541667008085767, 1.181850606188767472 ) ) ;
#165396=ORIENTED_EDGE ( 'NONE', *, *, #43069, .F. ) ;
#165406=CARTESIAN_POINT ( 'NONE',  ( -1.364683531250010295, 4.092708333674751842, 0.7879004041258379498 ) ) ;
#165414=CARTESIAN_POINT ( 'NONE',  ( 8.127223016387999266, 11.56917838817298616, 1.199719254218460707 ) ) ;
#165415=CARTESIAN_POINT ( 'NONE',  ( -2.279673327430177476, 5.603443282069742182, 1.040551764627347231E-14 ) ) ;
#165417=CARTESIAN_POINT ( 'NONE',  ( -0.6823417656250212460, 2.051041667008083991, 1.181850606188767472 ) ) ;
#165419=CARTESIAN_POINT ( 'NONE',  ( -5.572037945536512105, 9.444535336527177805, 0.000000000000000000 ) ) ;
#165425=CARTESIAN_POINT ( 'NONE',  ( 3.005103603723342953, 6.657704637652544832, -0.7998128361456291469 ) ) ;
#165428=CARTESIAN_POINT ( 'NONE',  ( 8.432281472695482449, 11.92507992053172572, 1.199719254218450271 ) ) ;
#165436=CARTESIAN_POINT ( 'NONE',  ( -2.123823618835070537, 5.629544655282869847, 1.040834085586084257E-14 ) ) ;
#165437=CARTESIAN_POINT ( 'NONE',  ( 6.825640269476072497, 10.05066518344239412, 1.199719254218460707 ) ) ;
#165439=CARTESIAN_POINT ( 'NONE',  ( 3.999292125906894313, 7.609665213625947722, 0.7216878364870317197 ) ) ;
#165449=CARTESIAN_POINT ( 'NONE',  ( -6.060131475628484310, 10.01397778830115470, 0.000000000000000000 ) ) ;
#165450=CARTESIAN_POINT ( 'NONE',  ( 5.522248639467795428, 5.337044922334209573, -0.7998128361456231517 ) ) ;
#165453=CARTESIAN_POINT ( 'NONE',  ( -9.182950115157607840, 9.607863310639020327, 0.7998128361456462443 ) ) ;
#165458=CARTESIAN_POINT ( 'NONE',  ( -3.164938793786285842, 5.779846795137578930, -1.199719254218452935 ) ) ;
#165462=CARTESIAN_POINT ( 'NONE',  ( 8.127223016387999266, 11.56917838817298616, 1.199719254218460707 ) ) ;
#165463=EDGE_CURVE ( 'NONE', #42674, #199393, #211353, .T. ) ;
#165464=CARTESIAN_POINT ( 'NONE',  ( -1.387358672533697046, 7.315968950353781253, -4.254625267138305134 ) ) ;
#165470=CARTESIAN_POINT ( 'NONE',  ( 3.226477370372305753, 4.787309570232886280, 1.443375672974062551 ) ) ;
#165474=CARTESIAN_POINT ( 'NONE',  ( -5.278201874421821316, 5.052323696447222900, 0.7998128361456341429 ) ) ;
#165476=CARTESIAN_POINT ( 'NONE',  ( -8.076906825439122528, 10.44614393447756129, -1.599625672291263179 ) ) ;
#165480=CARTESIAN_POINT ( 'NONE',  ( 7.537970219518073556, 9.817384560903001045, -1.443375672974057666 ) ) ;
#165481=CARTESIAN_POINT ( 'NONE',  ( -0.6823417656250212460, 5.613541667008087543, 1.181850606188767472 ) ) ;
#165483=CARTESIAN_POINT ( 'NONE',  ( 3.440018289565364817, 5.036440642624797626, 1.599625672291267398 ) ) ;
#165484=CARTESIAN_POINT ( 'NONE',  ( 5.712296854416149650, 6.230208010187211265, -1.006048757959861151 ) ) ;
#165486=CARTESIAN_POINT ( 'NONE',  ( -7.063961727919978451, 8.200042423116789436, 1.199719254218450271 ) ) ;
#165489=CARTESIAN_POINT ( 'NONE',  ( 1.403499169902377552, 7.376709478543040710, 4.304123474984470121 ) ) ;
#165497=EDGE_LOOP ( 'NONE', ( #93159, #1722, #176263, #9228, #112141 ) ) ;
#165499=CARTESIAN_POINT ( 'NONE',  ( 1.364683531249988535, 3.717708333674750953, -0.7879004041258239610 ) ) ;
#165500=CARTESIAN_POINT ( 'NONE',  ( 8.378048858240820351, 11.86180853700128601, -1.199719254218446718 ) ) ;
#165502=CARTESIAN_POINT ( 'NONE',  ( -4.284013352238255301, 6.981470763377843447, -1.082531754730549967 ) ) ;
#165504=CARTESIAN_POINT ( 'NONE',  ( -4.324687812634898876, 6.068555086205916105, 1.443375672974064550 ) ) ;
#165512=CARTESIAN_POINT ( 'NONE',  ( 4.009460741339333723, 5.700790169694431420, -1.599625672291256295 ) ) ;
#165522=CARTESIAN_POINT ( 'NONE',  ( 5.250031796989762967, 7.148123067953287446, 1.599625672291267398 ) ) ;
#165527=CARTESIAN_POINT ( 'NONE',  ( -5.819474248763749635, 7.812472595022922128, -1.599625672291256295 ) ) ;
#165532=CARTESIAN_POINT ( 'NONE',  ( 5.289652487626049115, 9.323011668872403845, 0.7998128361456462443 ) ) ;
#165535=CARTESIAN_POINT ( 'NONE',  ( -4.726989112658928072, 8.666571064744069020, 1.040834085586084257E-14 ) ) ;
#165536=CARTESIAN_POINT ( 'NONE',  ( -1.500000000000013101, 2.379166666666686414, -0.8660254037844313801 ) ) ;
#165537=CARTESIAN_POINT ( 'NONE',  ( -3.815730167242251003, 6.539103397502874948, -1.199719254218452047 ) ) ;
#165540=CARTESIAN_POINT ( 'NONE',  ( -5.925076824372040640, 6.871343368977510302, 1.199719254218450271 ) ) ;
#165543=CARTESIAN_POINT ( 'NONE',  ( -1.201851678989727383E-14, 3.696875000341422801, -1.575800808251660134 ) ) ;
#165545=CARTESIAN_POINT ( 'NONE',  ( -5.422898255786203769, 6.389431388914436738, -1.082531754730544860 ) ) ;
#165551=CARTESIAN_POINT ( 'NONE',  ( 4.656335691289526402, 7.519809842224722374, -1.199719254218452047 ) ) ;
#165554=CARTESIAN_POINT ( 'NONE',  ( 1.364683531249988535, 2.676041667008082214, 0.7879004041258500513 ) ) ;
#165556=CARTESIAN_POINT ( 'NONE',  ( 3.440018289565364817, 5.036440642624797626, 1.599625672291267398 ) ) ;
#165558=CARTESIAN_POINT ( 'NONE',  ( -0.6823417656250003738, 0.03020833367475134201, -1.181850606188749264 ) ) ;
#165561=CARTESIAN_POINT ( 'NONE',  ( -2.272963308585411735, 5.803540959991587478, 0.7998128361456341429 ) ) ;
#165562=CARTESIAN_POINT ( 'NONE',  ( -5.490689023410187275, 8.389259046411751797, 1.082531754730548412 ) ) ;
#165566=CARTESIAN_POINT ( 'NONE',  ( 1.364683531249986537, 2.655208333674754062, -0.7879004041258239610 ) ) ;
#165574=CARTESIAN_POINT ( 'NONE',  ( -7.226132685959434809, 8.493204890783200511, 1.082531754730549967 ) ) ;
#165575=ADVANCED_FACE ( 'NONE', ( #159318 ), #193944, .F. ) ;
#165581=CARTESIAN_POINT ( 'NONE',  ( -6.927853306458756855, 9.105581495667113501, 1.443375672974078761 ) ) ;
#165595=CARTESIAN_POINT ( 'NONE',  ( -6.338600509588822263, 7.353787668397130162, -1.199719254218446718 ) ) ;
#165597=CARTESIAN_POINT ( 'NONE',  ( 1.499999999999987121, -0.9958333333333134751, 0.8660254037844524744 ) ) ;
#165599=CARTESIAN_POINT ( 'NONE',  ( 9.951321562750607086, 11.67259191370631477, -1.082531754730537088 ) ) ;
#165601=( BOUNDED_SURFACE ( )  B_SPLINE_SURFACE ( 1, 2, ( 
 ( #100358, #87312, #150194, #152314, #165356, #102494, #184789, #71030, #183739, #19093, #35347, #66753, #33225, #686, #133968, #185858, #201031, #52673, #118804, #101425, #36415, #3891, #199975, #168558, #181597, #99309, #20157, #137144, #86244, #136073, #53746, #119880, #34285, #37490, #153381, #132894, #83033, #149107, #50544, #58010, #107905, #188001, #26571, #173931, #24419, #23357, #88386, #40713, #204226, #154456, #91612, #25504, #7101, #120965, #38568, #74273, #191193, #108967, #6034, #90532, #89466, #205311, #207456, #157663, #190138, #106818, #9261, #75332, #174987, #92676, #55878, #141449, #156594, #59075, #170690, #155520, #72103, #124174, #189080, #8188, #140365, #105731, #22277, #171761, #138214, #172848, #42860, #122035, #41792, #186936, #10318, #104643, #139279, #56948, #123120, #206384, #158720, #125235, #76392, #142501, #208507, #39626, #73173, #95877, #210656, #13522, #30867, #128444, #145714, #177103, #60142, #28718, #194410, #161932, #43921, #114305, #112173, #180303, #111097, #96945, #14576, #196550, #78524, #143577, #144641, #46052, #31925, #211712, #79595, #93741, #11380, #162995, #77459, #164061, #127372, #63348, #179243, #94805, #159780, #212780, #80671, #176048, #61215, #146762, #160854, #98004, #126299, #12445, #178177, #48193, #193343, #62284, #15640, #81727, #192258, #29792, #129507, #195488, #47122, #130560, #64415, #113239, #147810, #110036, #27641, #209569, #44988, #149937, #167247, #184538, #67572, #84919, #116417, #213829, #182408, #133716, #35091, #197599, #53488, #51368, #119625, #50299, #36160, #168310, #135819, #17760, #82788, #83848, #199722, #185609, #151007, #18835, #32979, #165110, #102239, #16702, #103312, #66505, #2577, #118556, #34037, #99055, #152067, #19908, #115361, #434, #85993, #100110, #37241, #65447, #166171, #117491, #201843, #132644, #1506, #169374, #131597, #134770, #20958, #198650, #68647, #183482, #101162, #148861, #200778, #3637, #52430, #69716, #87056, #181353, #49242, #140105, #5769, #58827, #206132, #56698, #55624, #120706, #72926, #22020, #186681, #123923, #57762, #39376, #153128, #70775, #106564, #9004, #141192, #38309, #122865, #121781, #23099, #25251, #189891, #7927, #139032, #41533, #107644, #207202, #124981, #88130, #173676, #188826, #91351, #202915, #187748, #104386, #90273, #6848, #40460, #172592, #137957, #54560, #203977, #170433, #205056, #75079, #154201, #74013, #4699, #157413, #190941, #136889, #24170, #156342, #42605, #105473, #89215, #108712, #174740, #71849, #26313, #171506, #155267, #192003, #96699, #92426, #11124, #80412, #60961, #63094, #76142, #13273, #95629, #196299, #94555, #78270, #160594, #43668, #158466, #126040, #193085, #162746, #210397, #177923, #111923, #12200, #194154, #129263, #77202, #144396, #180052, #10066, #195233, #114060, #93486, #46871, #161679, #30610, #14319, #212527, #112985, #146510, #130311, #64168, #62040 ),
 ( #45802, #178995, #128193, #29538, #209314, #142245, #127118, #79347, #145464, #208258, #47945, #211459, #59891, #143320, #109785, #175794, #27386, #110842, #159525, #176848, #44736, #28461, #183233, #199467, #65202, #197349, #2321, #48991, #135568, #98804, #34838, #150759, #66253, #131354, #184289, #134525, #147557, #32722, #68397, #185, #3394, #97751, #82530, #17511, #168058, #164857, #116168, #19660, #31674, #167001, #201592, #16449, #117234, #132401, #148617, #181106, #149680, #52176, #115109, #51109, #200531, #213579, #100913, #151820, #198403, #118302, #1261, #35914, #81480, #50045, #182154, #18592, #99863, #67319, #84670, #33784, #165926, #83598, #133463, #101989, #85735, #69463, #53240, #163810, #119369, #15386, #203724, #55372, #121526, #72676, #41281, #7667, #40197, #88957, #58572, #86806, #187496, #6595, #39126, #138772, #156081, #105209, #56443, #87874, #185357, #153946, #171246, #204790, #169116, #24993, #22842, #91096, #21766, #73752, #139847, #107390, #155010, #54311, #122602, #188565, #157156, #106308, #172331, #4450, #136636, #205876, #202661, #74830, #38062, #23919, #90025, #5515, #70520, #123669, #57511, #152872, #186423, #189632, #71595, #8748, #36979, #137704, #173412, #140929, #104132, #206943, #103062, #20713, #120449, #170178, #109531, #210132, #159265, #43407, #59632, #28205, #145196, #9811, #78015, #95368, #26057, #61774, #111656, #191752, #30348, #177668, #94299, #27126, #92171, #44475, #208008, #158222, #161419, #29277, #10865, #124728, #42346, #144140, #194967, #112722, #75886, #160340, #93232, #209059, #211203, #13002, #193895, #110591, #79078, #62828, #178734, #76939, #141994, #127942, #192817, #11943, #45542, #175536, #174481, #143064, #125790, #176594, #46603, #60695, #128988, #190687, #14057, #108461, #126860, #96433, #162484, #80145, #146248, #212264, #133197, #181890, #151560, #179793, #65990, #99598, #214359, #17252, #34586, #132139, #149415, #180840, #63898, #32466, #198146, #165664, #47680, #118047, #115905, #184033, #114842, #100660, #18327, #200271, #82267, #147297, #148361, #49778, #35648, #997, #83329, #97487, #15129, #166736, #81217, #167798, #131101, #67061, #182971, #98536, #163544, #2057, #84410, #31413, #64950, #150498, #164597, #101727, #130053, #16184, #33527, #51923, #197090, #199199, #19393, #196047, #50848, #85473, #48729, #116974, #68131, #134265, #213327, #113791, #26605, #102801, #170989, #191229, #119108, #154754, #204534, #70265, #126332, #56183, #121264, #120188, #185090, #137448, #86544, #36714, #42892, #122344, #103872, #3128, #135318, #22588, #76421, #208539, #168858, #187237, #186164, #87616, #92706, #109001, #72410, #203464, #175018, #158753, #60175, #192291, #152610, #10347, #38866, #142532, #52971, #37797, #153687, #43951, #110067, #138510, #55118, #176079, #27677, #93772, #69197, #4195, #201332, #104949, #20461, #136380, #169922, #202398, #6338 ) ),
 .UNSPECIFIED., .F., .F., .T. ) 
 B_SPLINE_SURFACE_WITH_KNOTS ( ( 2, 2 ),
 ( 3, 2, 2, 2, 2, 2, 2, 2, 2, 2, 2, 2, 2, 2, 2, 2, 2, 2, 2, 2, 2, 2, 2, 2, 2, 2, 2, 2, 2, 2, 2, 2, 2, 2, 2, 2, 2, 2, 2, 2, 2, 2, 2, 2, 2, 2, 2, 2, 2, 2, 2, 2, 2, 2, 2, 2, 2, 2, 2, 2, 2, 2, 2, 2, 2, 2, 2, 2, 2, 2, 2, 2, 2, 2, 2, 2, 2, 2, 2, 2, 2, 2, 2, 2, 2, 2, 2, 2, 2, 2, 2, 2, 2, 2, 2, 2, 2, 2, 2, 2, 2, 2, 2, 2, 2, 2, 2, 2, 2, 2, 2, 2, 2, 2, 2, 2, 2, 2, 2, 2, 2, 2, 2, 2, 2, 2, 2, 2, 2, 2, 2, 2, 2, 2, 2, 2, 2, 2, 2, 2, 2, 2, 2, 2, 2, 2, 2, 2, 2, 2, 2, 2, 2, 2, 2, 2, 2, 2, 2, 2, 2, 2, 2, 2, 2, 2, 2, 2, 3 ),
 ( 0.000000000000000000, 1.000000000000000000 ),
 ( 0.000000000000000000, 0.005952380952380952051, 0.01190476190476190410, 0.01785714285714285615, 0.02380952380952380820, 0.02976190476190476025, 0.03571428571428571230, 0.04166666666666666435, 0.04761904761904761640, 0.05357142857142856845, 0.05952380952380952051, 0.06547619047619047949, 0.07142857142857142461, 0.07738095238095238360, 0.08333333333333332871, 0.08928571428571428770, 0.09523809523809523281, 0.1011904761904761918, 0.1071428571428571369, 0.1130952380952380959, 0.1190476190476190410, 0.1250000000000000000, 0.1309523809523809590, 0.1369047619047619180, 0.1428571428571428492, 0.1488095238095238082, 0.1547619047619047672, 0.1607142857142857262, 0.1666666666666666574, 0.1726190476190476164, 0.1785714285714285754, 0.1845238095238095344, 0.1904761904761904656, 0.1964285714285714246, 0.2023809523809523836, 0.2083333333333333426, 0.2142857142857142738, 0.2202380952380952328, 0.2261904761904761918, 0.2321428571428571508, 0.2380952380952380820, 0.2440476190476190410, 0.2500000000000000000, 0.2559523809523809312, 0.2619047619047619180, 0.2678571428571428492, 0.2738095238095238360, 0.2797619047619047672, 0.2857142857142856984, 0.2916666666666666852, 0.2976190476190476164, 0.3035714285714285476, 0.3095238095238095344, 0.3154761904761904656, 0.3214285714285714524, 0.3273809523809523836, 0.3333333333333333148, 0.3392857142857143016, 0.3452380952380952328, 0.3511904761904761640, 0.3571428571428571508, 0.3630952380952380820, 0.3690476190476190688, 0.3750000000000000000, 0.3809523809523809312, 0.3869047619047619180, 0.3928571428571428492, 0.3988095238095238360, 0.4047619047619047672, 0.4107142857142856984, 0.4166666666666666852, 0.4226190476190476164, 0.4285714285714285476, 0.4345238095238095344, 0.4404761904761904656, 0.4464285714285714524, 0.4523809523809523836, 0.4583333333333333148, 0.4642857142857143016, 0.4702380952380952328, 0.4761904761904761640, 0.4821428571428571508, 0.4880952380952380820, 0.4940476190476190688, 0.5000000000000000000, 0.5059523809523809312, 0.5119047619047618625, 0.5178571428571429047, 0.5238095238095238360, 0.5297619047619047672, 0.5357142857142856984, 0.5416666666666666297, 0.5476190476190476719, 0.5535714285714286031, 0.5595238095238095344, 0.5654761904761904656, 0.5714285714285713969, 0.5773809523809523281, 0.5833333333333333703, 0.5892857142857143016, 0.5952380952380952328, 0.6011904761904761640, 0.6071428571428570953, 0.6130952380952381375, 0.6190476190476190688, 0.6250000000000000000, 0.6309523809523809312, 0.6369047619047618625, 0.6428571428571429047, 0.6488095238095238360, 0.6547619047619047672, 0.6607142857142856984, 0.6666666666666666297, 0.6726190476190476719, 0.6785714285714286031, 0.6845238095238095344, 0.6904761904761904656, 0.6964285714285713969, 0.7023809523809523281, 0.7083333333333333703, 0.7142857142857143016, 0.7202380952380952328, 0.7261904761904761640, 0.7321428571428570953, 0.7380952380952381375, 0.7440476190476190688, 0.7500000000000000000, 0.7559523809523809312, 0.7619047619047618625, 0.7678571428571429047, 0.7738095238095238360, 0.7797619047619047672, 0.7857142857142856984, 0.7916666666666666297, 0.7976190476190476719, 0.8035714285714286031, 0.8095238095238095344, 0.8154761904761904656, 0.8214285714285713969, 0.8273809523809523281, 0.8333333333333333703, 0.8392857142857143016, 0.8452380952380952328, 0.8511904761904761640, 0.8571428571428570953, 0.8630952380952381375, 0.8690476190476190688, 0.8750000000000000000, 0.8809523809523809312, 0.8869047619047618625, 0.8928571428571429047, 0.8988095238095238360, 0.9047619047619047672, 0.9107142857142856984, 0.9166666666666666297, 0.9226190476190476719, 0.9285714285714286031, 0.9345238095238095344, 0.9404761904761904656, 0.9464285714285713969, 0.9523809523809523281, 0.9583333333333333703, 0.9642857142857143016, 0.9702380952380952328, 0.9761904761904761640, 0.9821428571428570953, 0.9880952380952381375, 0.9940476190476190688, 1.000000000000000000 ),
 .UNSPECIFIED. ) 
 GEOMETRIC_REPRESENTATION_ITEM ( )  RATIONAL_B_SPLINE_SURFACE ( (
 ( 1.000000000000000000, 0.8660254037844387076, 1.000000000000000000, 0.8660254037844387076, 1.000000000000000000, 0.8660254037844387076, 1.000000000000000000, 0.8660254037844387076, 1.000000000000000000, 0.8660254037844387076, 1.000000000000000000, 0.8660254037844387076, 1.000000000000000000, 0.8660254037844387076, 1.000000000000000000, 0.8660254037844387076, 1.000000000000000000, 0.8660254037844387076, 1.000000000000000000, 0.8660254037844387076, 1.000000000000000000, 0.8660254037844387076, 1.000000000000000000, 0.8660254037844387076, 1.000000000000000000, 0.8660254037844387076, 1.000000000000000000, 0.8660254037844387076, 1.000000000000000000, 0.8660254037844387076, 1.000000000000000000, 0.8660254037844387076, 1.000000000000000000, 0.8660254037844387076, 1.000000000000000000, 0.8660254037844387076, 1.000000000000000000, 0.8660254037844387076, 1.000000000000000000, 0.8660254037844387076, 1.000000000000000000, 0.8660254037844387076, 1.000000000000000000, 0.8660254037844387076, 1.000000000000000000, 0.8660254037844387076, 1.000000000000000000, 0.8660254037844387076, 1.000000000000000000, 0.8660254037844387076, 1.000000000000000000, 0.8660254037844387076, 1.000000000000000000, 0.8660254037844387076, 1.000000000000000000, 0.8660254037844387076, 1.000000000000000000, 0.8660254037844387076, 1.000000000000000000, 0.8660254037844387076, 1.000000000000000000, 0.8660254037844387076, 1.000000000000000000, 0.8660254037844387076, 1.000000000000000000, 0.8660254037844387076, 1.000000000000000000, 0.8660254037844387076, 1.000000000000000000, 0.8660254037844387076, 1.000000000000000000, 0.8660254037844387076, 1.000000000000000000, 0.8660254037844387076, 1.000000000000000000, 0.8660254037844387076, 1.000000000000000000, 0.8660254037844387076, 1.000000000000000000, 0.8660254037844387076, 1.000000000000000000, 0.8660254037844387076, 1.000000000000000000, 0.8660254037844387076, 1.000000000000000000, 0.8660254037844387076, 1.000000000000000000, 0.8660254037844387076, 1.000000000000000000, 0.8660254037844387076, 1.000000000000000000, 0.8660254037844387076, 1.000000000000000000, 0.8660254037844387076, 1.000000000000000000, 0.8660254037844387076, 1.000000000000000000, 0.8660254037844387076, 1.000000000000000000, 0.8660254037844387076, 1.000000000000000000, 0.8660254037844387076, 1.000000000000000000, 0.8660254037844387076, 1.000000000000000000, 0.8660254037844387076, 1.000000000000000000, 0.8660254037844387076, 1.000000000000000000, 0.8660254037844387076, 1.000000000000000000, 0.8660254037844387076, 1.000000000000000000, 0.8660254037844387076, 1.000000000000000000, 0.8660254037844387076, 1.000000000000000000, 0.8660254037844387076, 1.000000000000000000, 0.8660254037844387076, 1.000000000000000000, 0.8660254037844387076, 1.000000000000000000, 0.8660254037844387076, 1.000000000000000000, 0.8660254037844387076, 1.000000000000000000, 0.8660254037844387076, 1.000000000000000000, 0.8660254037844387076, 1.000000000000000000, 0.8660254037844387076, 1.000000000000000000, 0.8660254037844387076, 1.000000000000000000, 0.8660254037844387076, 1.000000000000000000, 0.8660254037844387076, 1.000000000000000000, 0.8660254037844387076, 1.000000000000000000, 0.8660254037844387076, 1.000000000000000000, 0.8660254037844387076, 1.000000000000000000, 0.8660254037844387076, 1.000000000000000000, 0.8660254037844387076, 1.000000000000000000, 0.8660254037844387076, 1.000000000000000000, 0.8660254037844387076, 1.000000000000000000, 0.8660254037844387076, 1.000000000000000000, 0.8660254037844387076, 1.000000000000000000, 0.8660254037844387076, 1.000000000000000000, 0.8660254037844387076, 1.000000000000000000, 0.8660254037844387076, 1.000000000000000000, 0.8660254037844387076, 1.000000000000000000, 0.8660254037844387076, 1.000000000000000000, 0.8660254037844387076, 1.000000000000000000, 0.8660254037844387076, 1.000000000000000000, 0.8660254037844387076, 1.000000000000000000, 0.8660254037844387076, 1.000000000000000000, 0.8660254037844387076, 1.000000000000000000, 0.8660254037844387076, 1.000000000000000000, 0.8660254037844387076, 1.000000000000000000, 0.8660254037844387076, 1.000000000000000000, 0.8660254037844387076, 1.000000000000000000, 0.8660254037844387076, 1.000000000000000000, 0.8660254037844387076, 1.000000000000000000, 0.8660254037844387076, 1.000000000000000000, 0.8660254037844387076, 1.000000000000000000, 0.8660254037844387076, 1.000000000000000000, 0.8660254037844387076, 1.000000000000000000, 0.8660254037844387076, 1.000000000000000000, 0.8660254037844387076, 1.000000000000000000, 0.8660254037844387076, 1.000000000000000000, 0.8660254037844387076, 1.000000000000000000, 0.8660254037844387076, 1.000000000000000000, 0.8660254037844387076, 1.000000000000000000, 0.8660254037844387076, 1.000000000000000000, 0.8660254037844387076, 1.000000000000000000, 0.8660254037844387076, 1.000000000000000000, 0.8660254037844387076, 1.000000000000000000, 0.8660254037844387076, 1.000000000000000000, 0.8660254037844387076, 1.000000000000000000, 0.8660254037844387076, 1.000000000000000000, 0.8660254037844387076, 1.000000000000000000, 0.8660254037844387076, 1.000000000000000000, 0.8660254037844387076, 1.000000000000000000, 0.8660254037844387076, 1.000000000000000000, 0.8660254037844387076, 1.000000000000000000, 0.8660254037844387076, 1.000000000000000000, 0.8660254037844387076, 1.000000000000000000, 0.8660254037844387076, 1.000000000000000000, 0.8660254037844387076, 1.000000000000000000, 0.8660254037844387076, 1.000000000000000000, 0.8660254037844387076, 1.000000000000000000, 0.8660254037844387076, 1.000000000000000000, 0.8660254037844387076, 1.000000000000000000, 0.8660254037844387076, 1.000000000000000000, 0.8660254037844387076, 1.000000000000000000, 0.8660254037844387076, 1.000000000000000000, 0.8660254037844387076, 1.000000000000000000, 0.8660254037844387076, 1.000000000000000000, 0.8660254037844387076, 1.000000000000000000, 0.8660254037844387076, 1.000000000000000000, 0.8660254037844387076, 1.000000000000000000, 0.8660254037844387076, 1.000000000000000000, 0.8660254037844387076, 1.000000000000000000, 0.8660254037844387076, 1.000000000000000000, 0.8660254037844387076, 1.000000000000000000, 0.8660254037844387076, 1.000000000000000000, 0.8660254037844387076, 1.000000000000000000, 0.8660254037844387076, 1.000000000000000000, 0.8660254037844387076, 1.000000000000000000, 0.8660254037844387076, 1.000000000000000000, 0.8660254037844387076, 1.000000000000000000, 0.8660254037844387076, 1.000000000000000000, 0.8660254037844387076, 1.000000000000000000, 0.8660254037844387076, 1.000000000000000000, 0.8660254037844387076, 1.000000000000000000, 0.8660254037844387076, 1.000000000000000000, 0.8660254037844387076, 1.000000000000000000, 0.8660254037844387076, 1.000000000000000000, 0.8660254037844387076, 1.000000000000000000, 0.8660254037844387076, 1.000000000000000000, 0.8660254037844387076, 1.000000000000000000, 0.8660254037844387076, 1.000000000000000000, 0.8660254037844387076, 1.000000000000000000, 0.8660254037844387076, 1.000000000000000000, 0.8660254037844387076, 1.000000000000000000, 0.8660254037844387076, 1.000000000000000000, 0.8660254037844387076, 1.000000000000000000, 0.8660254037844387076, 1.000000000000000000, 0.8660254037844387076, 1.000000000000000000, 0.8660254037844387076, 1.000000000000000000, 0.8660254037844387076, 1.000000000000000000, 0.8660254037844387076, 1.000000000000000000, 0.8660254037844387076, 1.000000000000000000, 0.8660254037844387076, 1.000000000000000000, 0.8660254037844387076, 1.000000000000000000, 0.8660254037844387076, 1.000000000000000000, 0.8660254037844387076, 1.000000000000000000),
 ( 1.000000000000000000, 0.8660254037844387076, 1.000000000000000000, 0.8660254037844387076, 1.000000000000000000, 0.8660254037844387076, 1.000000000000000000, 0.8660254037844387076, 1.000000000000000000, 0.8660254037844387076, 1.000000000000000000, 0.8660254037844387076, 1.000000000000000000, 0.8660254037844387076, 1.000000000000000000, 0.8660254037844387076, 1.000000000000000000, 0.8660254037844387076, 1.000000000000000000, 0.8660254037844387076, 1.000000000000000000, 0.8660254037844387076, 1.000000000000000000, 0.8660254037844387076, 1.000000000000000000, 0.8660254037844387076, 1.000000000000000000, 0.8660254037844387076, 1.000000000000000000, 0.8660254037844387076, 1.000000000000000000, 0.8660254037844387076, 1.000000000000000000, 0.8660254037844387076, 1.000000000000000000, 0.8660254037844387076, 1.000000000000000000, 0.8660254037844387076, 1.000000000000000000, 0.8660254037844387076, 1.000000000000000000, 0.8660254037844387076, 1.000000000000000000, 0.8660254037844387076, 1.000000000000000000, 0.8660254037844387076, 1.000000000000000000, 0.8660254037844387076, 1.000000000000000000, 0.8660254037844387076, 1.000000000000000000, 0.8660254037844387076, 1.000000000000000000, 0.8660254037844387076, 1.000000000000000000, 0.8660254037844387076, 1.000000000000000000, 0.8660254037844387076, 1.000000000000000000, 0.8660254037844387076, 1.000000000000000000, 0.8660254037844387076, 1.000000000000000000, 0.8660254037844387076, 1.000000000000000000, 0.8660254037844387076, 1.000000000000000000, 0.8660254037844387076, 1.000000000000000000, 0.8660254037844387076, 1.000000000000000000, 0.8660254037844387076, 1.000000000000000000, 0.8660254037844387076, 1.000000000000000000, 0.8660254037844387076, 1.000000000000000000, 0.8660254037844387076, 1.000000000000000000, 0.8660254037844387076, 1.000000000000000000, 0.8660254037844387076, 1.000000000000000000, 0.8660254037844387076, 1.000000000000000000, 0.8660254037844387076, 1.000000000000000000, 0.8660254037844387076, 1.000000000000000000, 0.8660254037844387076, 1.000000000000000000, 0.8660254037844387076, 1.000000000000000000, 0.8660254037844387076, 1.000000000000000000, 0.8660254037844387076, 1.000000000000000000, 0.8660254037844387076, 1.000000000000000000, 0.8660254037844387076, 1.000000000000000000, 0.8660254037844387076, 1.000000000000000000, 0.8660254037844387076, 1.000000000000000000, 0.8660254037844387076, 1.000000000000000000, 0.8660254037844387076, 1.000000000000000000, 0.8660254037844387076, 1.000000000000000000, 0.8660254037844387076, 1.000000000000000000, 0.8660254037844387076, 1.000000000000000000, 0.8660254037844387076, 1.000000000000000000, 0.8660254037844387076, 1.000000000000000000, 0.8660254037844387076, 1.000000000000000000, 0.8660254037844387076, 1.000000000000000000, 0.8660254037844387076, 1.000000000000000000, 0.8660254037844387076, 1.000000000000000000, 0.8660254037844387076, 1.000000000000000000, 0.8660254037844387076, 1.000000000000000000, 0.8660254037844387076, 1.000000000000000000, 0.8660254037844387076, 1.000000000000000000, 0.8660254037844387076, 1.000000000000000000, 0.8660254037844387076, 1.000000000000000000, 0.8660254037844387076, 1.000000000000000000, 0.8660254037844387076, 1.000000000000000000, 0.8660254037844387076, 1.000000000000000000, 0.8660254037844387076, 1.000000000000000000, 0.8660254037844387076, 1.000000000000000000, 0.8660254037844387076, 1.000000000000000000, 0.8660254037844387076, 1.000000000000000000, 0.8660254037844387076, 1.000000000000000000, 0.8660254037844387076, 1.000000000000000000, 0.8660254037844387076, 1.000000000000000000, 0.8660254037844387076, 1.000000000000000000, 0.8660254037844387076, 1.000000000000000000, 0.8660254037844387076, 1.000000000000000000, 0.8660254037844387076, 1.000000000000000000, 0.8660254037844387076, 1.000000000000000000, 0.8660254037844387076, 1.000000000000000000, 0.8660254037844387076, 1.000000000000000000, 0.8660254037844387076, 1.000000000000000000, 0.8660254037844387076, 1.000000000000000000, 0.8660254037844387076, 1.000000000000000000, 0.8660254037844387076, 1.000000000000000000, 0.8660254037844387076, 1.000000000000000000, 0.8660254037844387076, 1.000000000000000000, 0.8660254037844387076, 1.000000000000000000, 0.8660254037844387076, 1.000000000000000000, 0.8660254037844387076, 1.000000000000000000, 0.8660254037844387076, 1.000000000000000000, 0.8660254037844387076, 1.000000000000000000, 0.8660254037844387076, 1.000000000000000000, 0.8660254037844387076, 1.000000000000000000, 0.8660254037844387076, 1.000000000000000000, 0.8660254037844387076, 1.000000000000000000, 0.8660254037844387076, 1.000000000000000000, 0.8660254037844387076, 1.000000000000000000, 0.8660254037844387076, 1.000000000000000000, 0.8660254037844387076, 1.000000000000000000, 0.8660254037844387076, 1.000000000000000000, 0.8660254037844387076, 1.000000000000000000, 0.8660254037844387076, 1.000000000000000000, 0.8660254037844387076, 1.000000000000000000, 0.8660254037844387076, 1.000000000000000000, 0.8660254037844387076, 1.000000000000000000, 0.8660254037844387076, 1.000000000000000000, 0.8660254037844387076, 1.000000000000000000, 0.8660254037844387076, 1.000000000000000000, 0.8660254037844387076, 1.000000000000000000, 0.8660254037844387076, 1.000000000000000000, 0.8660254037844387076, 1.000000000000000000, 0.8660254037844387076, 1.000000000000000000, 0.8660254037844387076, 1.000000000000000000, 0.8660254037844387076, 1.000000000000000000, 0.8660254037844387076, 1.000000000000000000, 0.8660254037844387076, 1.000000000000000000, 0.8660254037844387076, 1.000000000000000000, 0.8660254037844387076, 1.000000000000000000, 0.8660254037844387076, 1.000000000000000000, 0.8660254037844387076, 1.000000000000000000, 0.8660254037844387076, 1.000000000000000000, 0.8660254037844387076, 1.000000000000000000, 0.8660254037844387076, 1.000000000000000000, 0.8660254037844387076, 1.000000000000000000, 0.8660254037844387076, 1.000000000000000000, 0.8660254037844387076, 1.000000000000000000, 0.8660254037844387076, 1.000000000000000000, 0.8660254037844387076, 1.000000000000000000, 0.8660254037844387076, 1.000000000000000000, 0.8660254037844387076, 1.000000000000000000, 0.8660254037844387076, 1.000000000000000000, 0.8660254037844387076, 1.000000000000000000, 0.8660254037844387076, 1.000000000000000000, 0.8660254037844387076, 1.000000000000000000, 0.8660254037844387076, 1.000000000000000000, 0.8660254037844387076, 1.000000000000000000, 0.8660254037844387076, 1.000000000000000000, 0.8660254037844387076, 1.000000000000000000, 0.8660254037844387076, 1.000000000000000000, 0.8660254037844387076, 1.000000000000000000, 0.8660254037844387076, 1.000000000000000000, 0.8660254037844387076, 1.000000000000000000, 0.8660254037844387076, 1.000000000000000000, 0.8660254037844387076, 1.000000000000000000, 0.8660254037844387076, 1.000000000000000000, 0.8660254037844387076, 1.000000000000000000, 0.8660254037844387076, 1.000000000000000000, 0.8660254037844387076, 1.000000000000000000, 0.8660254037844387076, 1.000000000000000000, 0.8660254037844387076, 1.000000000000000000, 0.8660254037844387076, 1.000000000000000000, 0.8660254037844387076, 1.000000000000000000, 0.8660254037844387076, 1.000000000000000000, 0.8660254037844387076, 1.000000000000000000, 0.8660254037844387076, 1.000000000000000000, 0.8660254037844387076, 1.000000000000000000, 0.8660254037844387076, 1.000000000000000000, 0.8660254037844387076, 1.000000000000000000, 0.8660254037844387076, 1.000000000000000000, 0.8660254037844387076, 1.000000000000000000, 0.8660254037844387076, 1.000000000000000000, 0.8660254037844387076, 1.000000000000000000) ) ) 
 REPRESENTATION_ITEM ( '' )  SURFACE ( )  );
#165603=CARTESIAN_POINT ( 'NONE',  ( 6.006425746053997372, 6.966250444273174303, -1.199719254218445830 ) ) ;
#165610=CARTESIAN_POINT ( 'NONE',  ( -3.795919822146289313, 5.451659097302528068, -1.443375672974053447 ) ) ;
#165619=CARTESIAN_POINT ( 'NONE',  ( -0.6823417656250003738, 2.467708333674753618, -1.181850606188749264 ) ) ;
#165620=CARTESIAN_POINT ( 'NONE',  ( 10.19536832735223975, 10.99694392477354477, 0.000000000000000000 ) ) ;
#165621=CARTESIAN_POINT ( 'NONE',  ( -7.877450944739929461, 9.149113176073413456, 1.199719254218462483 ) ) ;
#165624=CARTESIAN_POINT ( 'NONE',  ( 8.132193210098487057, 8.381980254736715708, 1.040834085586084257E-14 ) ) ;
#165625=CARTESIAN_POINT ( 'NONE',  ( -7.386494761346872551, 7.511998731193139989, -0.7998128361456291469 ) ) ;
#165628=CARTESIAN_POINT ( 'NONE',  ( -1.500000000000015099, -0.5895833326505155458, -0.8660254037844383745 ) ) ;
#165631=CARTESIAN_POINT ( 'NONE',  ( 8.758204044748005401, 10.28062147603659504, 1.082531754730549967 ) ) ;
#165634=CARTESIAN_POINT ( 'NONE',  ( -0.6823417656250212460, 1.113541667008083325, 1.181850606188755259 ) ) ;
#165636=CARTESIAN_POINT ( 'NONE',  ( 5.924549939047454750, 9.855799328956630134, -0.7216878364870267237 ) ) ;
#165640=CARTESIAN_POINT ( 'NONE',  ( -3.904385051055635270, 6.538571078664754843, 1.082531754730560403 ) ) ;
#165642=CARTESIAN_POINT ( 'NONE',  ( 1.364683531249990311, 4.384375000341417028, 1.214306433183764966E-14 ) ) ;
#165646=CARTESIAN_POINT ( 'NONE',  ( -5.789674969154799733, 6.218922551941099108, -1.014761583188450000 ) ) ;
#165651=( BOUNDED_CURVE ( )  B_SPLINE_CURVE ( 2, ( #110481, #13952, #80035, #144023, #29162, #176480, #146138 ),
 .UNSPECIFIED., .F., .T. ) 
 B_SPLINE_CURVE_WITH_KNOTS ( ( 3, 2, 2, 3 ),
 ( 0.1750000000000002942, 0.1791666666666668351, 0.1833333333333333759, 0.1874999999999999167 ),
 .UNSPECIFIED. ) 
 CURVE ( )  GEOMETRIC_REPRESENTATION_ITEM ( )  RATIONAL_B_SPLINE_CURVE ( ( 0.9999999999999902300, 0.8660254037844484776, 1.000000000000000000, 0.8660254037844387076, 1.000000000000000000, 0.8660254037844413721, 0.9999999999999973355 ) ) 
 REPRESENTATION_ITEM ( '' )  );
#165654=CARTESIAN_POINT ( 'NONE',  ( 6.632963465583686435, 8.761543347979550589, -1.599625672291262513 ) ) ;
#165657=CARTESIAN_POINT ( 'NONE',  ( 3.765413976293345844, 5.416068943807445635, 1.599625672291267398 ) ) ;
#165663=CARTESIAN_POINT ( 'NONE',  ( 5.829642864196171281, 5.903597551091405826, 0.7216878364870317197 ) ) ;
#165664=CARTESIAN_POINT ( 'NONE',  ( -1.364683531250014514, 1.051041667008090208, -0.7879004041258289570 ) ) ;
#165667=DIRECTION ( 'NONE',  ( -0.7592566023653016805, 0.6507913734559627184, 0.000000000000000000 ) ) ;
#165671=CARTESIAN_POINT ( 'NONE',  ( 0.7499999999999885647, 0.2333333333333562076, 1.299038105676657340 ) ) ;
#165672=CARTESIAN_POINT ( 'NONE',  ( 7.233438648090761980, 8.397765496649418182, 1.199719254218462483 ) ) ;
#165673=CARTESIAN_POINT ( 'NONE',  ( -7.018317073368468328, 11.33978701890523233, -0.7998128361456291469 ) ) ;
#165677=CARTESIAN_POINT ( 'NONE',  ( 0.6823417656249899377, 1.842708333674752952, 1.181850606188755259 ) ) ;
#165679=CARTESIAN_POINT ( 'NONE',  ( 0.7499999999999885647, 2.566666666666689522, -1.299038105676658228 ) ) ;
#165681=CARTESIAN_POINT ( 'NONE',  ( 4.467575310902914154, 5.170924936596891008, 1.199719254218464037 ) ) ;
#165688=CARTESIAN_POINT ( 'NONE',  ( 1.499999999999985123, -0.9229166659838452524, -0.8660254037844323793 ) ) ;
#165689=CARTESIAN_POINT ( 'NONE',  ( -5.994676475536691029, 10.14553965476814845, 0.7998128361456481317 ) ) ;
#165690=CARTESIAN_POINT ( 'NONE',  ( -4.121315508874262790, 6.791656612786516334, -1.082531754730549967 ) ) ;
#165695=CARTESIAN_POINT ( 'NONE',  ( 3.990100951807514562, 7.610040142558228915, -0.03152230841159352204 ) ) ;
#165697=ORIENTED_EDGE ( 'NONE', *, *, #126439, .T. ) ;
#165698=CARTESIAN_POINT ( 'NONE',  ( 6.100279051144945619, 9.204410428722734849, -1.199719254218440723 ) ) ;
#165703=CARTESIAN_POINT ( 'NONE',  ( 5.436456408955479880, 9.286356877182658565, -0.7216878364870267237 ) ) ;
#165704=CARTESIAN_POINT ( 'NONE',  ( -0.9399888277780873436, 7.435091042679319528, -4.383624543540896035 ) ) ;
#165707=CARTESIAN_POINT ( 'NONE',  ( -5.845536785786364931, 9.971543350059432598, 0.000000000000000000 ) ) ;
#165708=CARTESIAN_POINT ( 'NONE',  ( 5.529027716274630855, 5.344953845275508542, 1.040834085586084257E-14 ) ) ;
#165713=CARTESIAN_POINT ( 'NONE',  ( 4.100926828275982317, 7.458749316499424964, -0.6398019981258776800 ) ) ;
#165714=CARTESIAN_POINT ( 'NONE',  ( 9.463228032658635769, 11.10314946193233965, -1.082531754730543083 ) ) ;
#165715=EDGE_LOOP ( 'NONE', ( #36568, #28396, #121922, #121748 ) ) ;
#165722=CARTESIAN_POINT ( 'NONE',  ( 2.273349394227877074, 5.683342515206170731, 0.4597581080974435519 ) ) ;
#165723=CARTESIAN_POINT ( 'NONE',  ( -1.527330013470517001, 8.693738994866430758, -2.519751708053318495 ) ) ;
#165724=CARTESIAN_POINT ( 'NONE',  ( -4.338245966692955591, 5.124003718305597310, 1.082531754730560403 ) ) ;
#165725=CARTESIAN_POINT ( 'NONE',  ( 9.246297574839983824, 9.889694713509232571, 0.7216878364870438212 ) ) ;
#165728=CARTESIAN_POINT ( 'NONE',  ( -4.394814349124112951, 8.279033840620114049, -0.7998128361456281477 ) ) ;
#165730=DIRECTION ( 'NONE',  ( -5.578564026256490882E-16, -1.000000000000000000, -9.066213480720158442E-32 ) ) ;
#165734=CARTESIAN_POINT ( 'NONE',  ( -7.691553217654356622, 7.867900263551875994, -0.7998128361456291469 ) ) ;
#165750=CARTESIAN_POINT ( 'NONE',  ( -4.882907879216086933, 8.848476292394087395, -0.7998128361456281477 ) ) ;
#165753=CARTESIAN_POINT ( 'NONE',  ( 4.148431816101584957, 6.823292304551739740, -1.082531754730548412 ) ) ;
#165757=FACE_OUTER_BOUND ( 'NONE', #170346, .T. ) ;
#165759=CARTESIAN_POINT ( 'NONE',  ( -5.122283107864663343, 4.870418468797203637, 0.000000000000000000 ) ) ;
#165767=CARTESIAN_POINT ( 'NONE',  ( -8.701635661872465732, 9.046329781806354831, 1.040834085586084257E-14 ) ) ;
#165768=CARTESIAN_POINT ( 'NONE',  ( 6.205881626753210867, 8.263281202677319470, 1.599625672291281386 ) ) ;
#165772=CARTESIAN_POINT ( 'NONE',  ( -9.332089804907933939, 9.781859615347734405, 1.040834085586084257E-14 ) ) ;
#165773=CARTESIAN_POINT ( 'NONE',  ( 5.172599298813543633, 5.993452922492633839, -1.199719254218452047 ) ) ;
#165776=CARTESIAN_POINT ( 'NONE',  ( -0.6823417656250246877, 0.1135416670080893753, 1.181850606188755259 ) ) ;
#165779=CARTESIAN_POINT ( 'NONE',  ( 8.514157279702022407, 10.95626946445095307, -1.443375672974063439 ) ) ;
#165805=CARTESIAN_POINT ( 'NONE',  ( 1.499999999999989120, -0.1937499993171845625, 0.000000000000000000 ) ) ;
#165812=CARTESIAN_POINT ( 'NONE',  ( 7.730120138085914583, 12.17022392774227768, 0.7998128361456462443 ) ) ;
#165817=CARTESIAN_POINT ( 'NONE',  ( 5.359550796103802028, 5.147230771742885125, -0.7998128361456231517 ) ) ;
#165818=CARTESIAN_POINT ( 'NONE',  ( -8.188761592974058701, 8.655902734665618325, -0.7216878364870278340 ) ) ;
#165819=CARTESIAN_POINT ( 'NONE',  ( -5.867692518273577740, 6.026634161543212187, 0.3546184694816056360 ) ) ;
#165820=CARTESIAN_POINT ( 'NONE',  ( 8.367353357928214663, 12.91366268422496688, 1.040834085586084257E-14 ) ) ;
#165822=CARTESIAN_POINT ( 'NONE',  ( -7.426115451983156923, 9.686887332112256388, -1.599625672291263179 ) ) ;
#165823=CARTESIAN_POINT ( 'NONE',  ( -2.887523529586332405, 5.352232636950553513, 1.082531754730560403 ) ) ;
#165826=CARTESIAN_POINT ( 'NONE',  ( 1.499999999999987566, -0.4437499993171847845, 0.000000000000000000 ) ) ;
#165833=CARTESIAN_POINT ( 'NONE',  ( -4.161989969270909917, 5.878740935614591656, 1.443375672974064550 ) ) ;
#165840=CARTESIAN_POINT ( 'NONE',  ( -4.080641047588914994, 5.783833860318930320, -1.443375672974051449 ) ) ;
#165841=CARTESIAN_POINT ( 'NONE',  ( 9.772729797352075920, 10.29593960653257234, -0.7998128361456281477 ) ) ;
#165849=EDGE_CURVE ( 'NONE', #126795, #190246, #197469, .T. ) ;
#165851=CARTESIAN_POINT ( 'NONE',  ( -9.820183334999905256, 10.35130206712171130, 1.040834085586084257E-14 ) ) ;
#165856=CARTESIAN_POINT ( 'NONE',  ( 4.143988507271280319, 7.986403691791820414, -0.7998128361456221525 ) ) ;
#165860=ORIENTED_EDGE ( 'NONE', *, *, #113967, .F. ) ;
#165861=CARTESIAN_POINT ( 'NONE',  ( 2.884486378366592607, 6.439576038332424979, 0.3703176727237925681 ) ) ;
#165864=CARTESIAN_POINT ( 'NONE',  ( -1.123270288250318494, 3.235197346350006331, -0.7749999999993560929 ) ) ;
#165873=CARTESIAN_POINT ( 'NONE',  ( 6.421758314367153275, 10.64380180007036891, -0.7998128361456291469 ) ) ;
#165875=CARTESIAN_POINT ( 'NONE',  ( -3.924195396151603177, 6.665646164563756138, 1.199719254218464037 ) ) ;
#165877=CARTESIAN_POINT ( 'NONE',  ( 0.9486429539266807431, 2.917910930033675854, -1.028101543437250465 ) ) ;
#165880=EDGE_CURVE ( 'NONE', #39666, #143793, #113844, .T. ) ;
#165882=CARTESIAN_POINT ( 'NONE',  ( -1.500000000000015099, -0.7979166659838445863, 0.8660254037844403729 ) ) ;
#165886=CARTESIAN_POINT ( 'NONE',  ( -5.786256696412555911, 6.075953140482280190, 0.5845640519336701146 ) ) ;
#165887=CARTESIAN_POINT ( 'NONE',  ( 3.842846474469570062, 6.570739089268092137, -1.199719254218452047 ) ) ;
#165889=CARTESIAN_POINT ( 'NONE',  ( -3.490334480514268645, 6.159475096320226939, -1.199719254218452935 ) ) ;
#165895=CARTESIAN_POINT ( 'NONE',  ( 4.961921032921539521, 7.772363057508363759, -1.082531754730549078 ) ) ;
#165898=CARTESIAN_POINT ( 'NONE',  ( 6.412643469139427843, 10.42524178073059993, -0.7216878364870267237 ) ) ;
#165899=CARTESIAN_POINT ( 'NONE',  ( -1.364683531249997417, 4.571875000341417028, 1.214306433183764966E-14 ) ) ;
#165901=CARTESIAN_POINT ( 'NONE',  ( 3.456965981360264895, 6.016582164020185530, -1.082531754730543971 ) ) ;
#165909=CARTESIAN_POINT ( 'NONE',  ( -6.016097364521681534, 6.072308155256833651, 0.6301904134648171896 ) ) ;
#165911=CARTESIAN_POINT ( 'NONE',  ( -1.364683531250012516, 5.051041667008085767, -0.7879004041258300672 ) ) ;
#165926=CARTESIAN_POINT ( 'NONE',  ( 0.6823417656249899377, 4.238541667008085767, -1.181850606188754593 ) ) ;
#165928=CARTESIAN_POINT ( 'NONE',  ( 5.612185521052973414, 8.634967976948757951, -1.199719254218440723 ) ) ;
#165929=CARTESIAN_POINT ( 'NONE',  ( -8.533967624797991647, 12.04371376465130439, -1.199719254218446718 ) ) ;
#165935=CARTESIAN_POINT ( 'NONE',  ( -1.402160292154681736E-14, -0.8656249996585829720, 1.575800808251672791 ) ) ;
#165939=PLANE ( 'NONE',  #28663 ) ;
#165942=CARTESIAN_POINT ( 'NONE',  ( 8.432808358020016826, 10.86136238915529084, 1.443375672974076540 ) ) ;
#165947=CARTESIAN_POINT ( 'NONE',  ( -1.499999999999997780, 3.681250000682819046, 1.214306433183764966E-14 ) ) ;
#165949=CARTESIAN_POINT ( 'NONE',  ( -5.742041750587549842, 6.657802449562273850, 1.199719254218450271 ) ) ;
#165950=CARTESIAN_POINT ( 'NONE',  ( 3.592547517496925913, 5.214391408544949869, -1.443375672974058777 ) ) ;
#165951=CARTESIAN_POINT ( 'NONE',  ( 5.630352418794719149, 6.139657267270441920, -0.8181431533968346326 ) ) ;
#165957=FACE_OUTER_BOUND ( 'NONE', #177739, .T. ) ;
#165958=CARTESIAN_POINT ( 'NONE',  ( 2.822068529938852155, 6.444163718237301275, -0.7998128361456291469 ) ) ;
#165959=CARTESIAN_POINT ( 'NONE',  ( -4.905110356762790502, 4.827649200395154772, -0.06592220986076716138 ) ) ;
#165961=DIRECTION ( 'NONE',  ( 0.000000000000000000, 8.546850786086437571E-32, 1.000000000000000000 ) ) ;
#165962=CARTESIAN_POINT ( 'NONE',  ( 5.355634372598031767, 6.206993841907870291, -1.199719254218445830 ) ) ;
#165965=ORIENTED_EDGE ( 'NONE', *, *, #63237, .F. ) ;
#165967=EDGE_LOOP ( 'NONE', ( #129393, #42897, #43579, #35578, #176539, #115836, #48581, #180958, #34256, #6518, #119384, #69752, #158121 ) ) ;
#165972=CARTESIAN_POINT ( 'NONE',  ( 2.277354866853175341, 5.622569341069810989, -0.5665490036073304037 ) ) ;
#165973=CARTESIAN_POINT ( 'NONE',  ( 5.688518940989607309, 6.102662425301288884, -0.7322136710279708582 ) ) ;
#165974=ORIENTED_EDGE ( 'NONE', *, *, #76499, .F. ) ;
#165982=CARTESIAN_POINT ( 'NONE',  ( 5.314433026876846711, 9.143996264757578984, -0.7216878364870267237 ) ) ;
#165983=CARTESIAN_POINT ( 'NONE',  ( -10.15469386695561482, 10.94949038764413096, 1.040834085586084257E-14 ) ) ;
#165987=EDGE_CURVE ( 'NONE', #42674, #112218, #16233, .T. ) ;
#165990=CARTESIAN_POINT ( 'NONE',  ( -4.603156847039612920, 5.329103395422994716, 1.199719254218462483 ) ) ;
#166002=CARTESIAN_POINT ( 'NONE',  ( 5.882017484636844706, 6.163768100491378910, 0.8443116549854499109 ) ) ;
#166004=VERTEX_POINT ( 'NONE', #199249 ) ;
#166011=CARTESIAN_POINT ( 'NONE',  ( -7.836249599018719536, 12.08611559892311504, 0.7216878364870478180 ) ) ;
#166015=CARTESIAN_POINT ( 'NONE',  ( 7.832860060393120882, 10.16142270859057462, 1.599625672291281386 ) ) ;
#166017=CARTESIAN_POINT ( 'NONE',  ( -3.761497552787613330, 6.475832013972435242, 1.199719254218464037 ) ) ;
#166018=CARTESIAN_POINT ( 'NONE',  ( 2.855963913973019963, 6.483708332943829866, 0.000000000000000000 ) ) ;
#166020=CARTESIAN_POINT ( 'NONE',  ( -5.949330478298285207, 5.835307067636438028, 0.7998128361456341429 ) ) ;
#166023=CARTESIAN_POINT ( 'NONE',  ( -4.771579997005698459, 7.654261532226910525, -1.199719254218452047 ) ) ;
#166026=CARTESIAN_POINT ( 'NONE',  ( 7.228468454380276853, 11.58496363008569574, 1.040834085586084257E-14 ) ) ;
#166030=CARTESIAN_POINT ( 'NONE',  ( 4.433499500630886381, 7.080826916883525612, -1.109343814354251112 ) ) ;
#166031=CARTESIAN_POINT ( 'NONE',  ( 5.829642864196162400, 7.824335979694092558, 1.443375672974062551 ) ) ;
#166039=ORIENTED_EDGE ( 'NONE', *, *, #145044, .T. ) ;
#166040=CARTESIAN_POINT ( 'NONE',  ( 7.931156673870037643, 8.355363662377600420, -0.7216878364870267237 ) ) ;
#166043=CARTESIAN_POINT ( 'NONE',  ( -6.991200766141138168, 11.30815132714001159, 0.7998128361456481317 ) ) ;
#166049=DIRECTION ( 'NONE',  ( -0.6507913734559640506, -0.7592566023653004592, 0.000000000000000000 ) ) ;
#166052=CARTESIAN_POINT ( 'NONE',  ( 10.38962578677386084, 11.01565159419135043, 0.000000000000000000 ) ) ;
#166056=CARTESIAN_POINT ( 'NONE',  ( 5.345992642490140057, 5.131412925860272090, 1.040834085586084257E-14 ) ) ;
#166059=CARTESIAN_POINT ( 'NONE',  ( 1.499999999999990896, 4.806250000682819490, 1.214306433183764966E-14 ) ) ;
#166066=CARTESIAN_POINT ( 'NONE',  ( 1.499999999999987121, 2.295833333333350268, -0.8660254037844262731 ) ) ;
#166067=CARTESIAN_POINT ( 'NONE',  ( 7.610204295972345712, 7.772993188256215547, 0.7998128361456341429 ) ) ;
#166068=CARTESIAN_POINT ( 'NONE',  ( 4.812781342726858647, 6.637997537979888563, 1.443375672974062551 ) ) ;
#166071=CARTESIAN_POINT ( 'NONE',  ( 7.456621297836061757, 11.64321591421002644, 0.7216878364870438212 ) ) ;
#166076=CARTESIAN_POINT ( 'NONE',  ( -4.042302355168801320, 7.867769847672247074, 0.7998128361456341429 ) ) ;
#166077=CARTESIAN_POINT ( 'NONE',  ( 1.499999999999990896, 3.306250000682818602, 1.214306433183764966E-14 ) ) ;
#166078=CARTESIAN_POINT ( 'NONE',  ( 0.6823417656249882723, -0.07395833299191079124, -1.181850606188749264 ) ) ;
#166082=CARTESIAN_POINT ( 'NONE',  ( 5.332434488876471868, 5.115595079977664383, 0.7998128361456341429 ) ) ;
#166084=CARTESIAN_POINT ( 'NONE',  ( -1.364683531250012516, 5.051041667008085767, -0.7879004041258300672 ) ) ;
#166091=CARTESIAN_POINT ( 'NONE',  ( -7.874588291438845644, 8.081441182967111558, -0.7998128361456291469 ) ) ;
#166092=CARTESIAN_POINT ( 'NONE',  ( 4.656335691289526402, 7.519809842224722374, -1.199719254218452047 ) ) ;
#166095=CARTESIAN_POINT ( 'NONE',  ( -1.402160292154681736E-14, -0.4281249996585808071, 1.575800808251672791 ) ) ;
#166099=ADVANCED_FACE ( 'NONE', ( #88738 ), #21548, .T. ) ;
#166100=DIRECTION ( 'NONE',  ( 0.000000000000000000, 0.000000000000000000, 1.000000000000000000 ) ) ;
#166103=CARTESIAN_POINT ( 'NONE',  ( -5.208303565944065738, 9.228104593576741621, -0.7998128361456231517 ) ) ;
#166106=CARTESIAN_POINT ( 'NONE',  ( 8.757677159423465696, 12.30470822171437284, 1.199719254218450271 ) ) ;
#166108=CARTESIAN_POINT ( 'NONE',  ( 7.892817981449907982, 12.36003807833360391, 0.7998128361456462443 ) ) ;
#166110=CARTESIAN_POINT ( 'NONE',  ( -2.442440228756222353, 6.001264033524212671, -0.7998128361456281477 ) ) ;
#166112=CARTESIAN_POINT ( 'NONE',  ( -8.681298431451969222, 9.022603012982438386, 1.040834085586084257E-14 ) ) ;
#166115=CARTESIAN_POINT ( 'NONE',  ( -4.902910567894817717, 6.875085367926331514, 1.448488056007392721 ) ) ;
#166116=CARTESIAN_POINT ( 'NONE',  ( -1.402160292154681736E-14, -0.4281249996585808071, 1.575800808251672791 ) ) ;
#166120=CARTESIAN_POINT ( 'NONE',  ( 6.643132081016105417, 10.69414516125339887, 0.7216878364870438212 ) ) ;
#166123=CARTESIAN_POINT ( 'NONE',  ( 6.003563092752934871, 5.898578451166879510, 0.7998128361456341429 ) ) ;
#166137=CARTESIAN_POINT ( 'NONE',  ( 9.317477881089539338, 11.89347683273640932, 1.599625672291279388 ) ) ;
#166141=CARTESIAN_POINT ( 'NONE',  ( -4.629219384062206011, 7.488174150459498968, -1.199719254218452047 ) ) ;
#166142=CARTESIAN_POINT ( 'NONE',  ( -8.453672473320708036, 9.821371626084353323, -1.199719254218446718 ) ) ;
#166147=CARTESIAN_POINT ( 'NONE',  ( -1.499999999999997780, 2.431250000682817713, 1.214306433183764966E-14 ) ) ;
#166148=CARTESIAN_POINT ( 'NONE',  ( 8.055515824813896941, 12.54985222892493368, 0.7998128361456462443 ) ) ;
#166152=CARTESIAN_POINT ( 'NONE',  ( -8.317037166979361018, 11.79062823052953668, 1.199719254218453823 ) ) ;
#166154=CARTESIAN_POINT ( 'NONE',  ( -1.364683531250012516, 2.488541667008088876, -0.7879004041258289570 ) ) ;
#166161=CARTESIAN_POINT ( 'NONE',  ( -8.500599126088349777, 12.86119004717103209, 1.040834085586084257E-14 ) ) ;
#166165=CARTESIAN_POINT ( 'NONE',  ( -1.201851678989727383E-14, 1.384375000341419693, 1.575800808251672791 ) ) ;
#166171=CARTESIAN_POINT ( 'NONE',  ( 1.364683531249988757, 1.384375000341421469, 0.000000000000000000 ) ) ;
#166173=CARTESIAN_POINT ( 'NONE',  ( -7.400052914960538963, 7.527816577075747695, 1.040834085586084257E-14 ) ) ;
#166174=CARTESIAN_POINT ( 'NONE',  ( 8.535021395002688749, 9.916278701380017324, 1.199719254218462483 ) ) ;
#166175=CARTESIAN_POINT ( 'NONE',  ( 4.650610384687404952, 5.384465856012134566, 1.199719254218462483 ) ) ;
#166178=CARTESIAN_POINT ( 'NONE',  ( -1.201851678989727383E-14, 3.462500000000019895, 1.732050807568877637 ) ) ;
#166180=CARTESIAN_POINT ( 'NONE',  ( -1.364683531249997417, 2.571875000341422357, 1.214306433183764966E-14 ) ) ;
#166186=CARTESIAN_POINT ( 'NONE',  ( 4.365362273920230685, 8.036747052974847705, 0.7216878364870298324 ) ) ;
#166189=CARTESIAN_POINT ( 'NONE',  ( -9.189729191964438826, 9.615772233580322848, 1.040834085586084257E-14 ) ) ;
#166190=CARTESIAN_POINT ( 'NONE',  ( -4.600294193738529103, 4.261431402316699035, -0.7998128361456221525 ) ) ;
#166191=CARTESIAN_POINT ( 'NONE',  ( 0.6823417656249899377, 4.176041667008085767, -1.181850606188754593 ) ) ;
#166195=CARTESIAN_POINT ( 'NONE',  ( -7.822691444960713447, 9.189190109618056823, -1.082531754730543083 ) ) ;
#166197=CARTESIAN_POINT ( 'NONE',  ( -1.001543065824772872E-14, 5.462500000000020783, 1.732050807568877637 ) ) ;
#166201=CARTESIAN_POINT ( 'NONE',  ( 8.920901888112002354, 9.510066412326583674, 0.7216878364870438212 ) ) ;
#166208=CARTESIAN_POINT ( 'NONE',  ( 3.836594282542920009, 4.538743420130594508, 1.082531754730560403 ) ) ;
#166218=AXIS2_PLACEMENT_3D ( 'NONE', #167633, #22424, #138350 ) ;
#166219=CARTESIAN_POINT ( 'NONE',  ( 6.531277313481192337, 8.642909503859968368, 1.599625672291281386 ) ) ;
#166220=CARTESIAN_POINT ( 'NONE',  ( -4.055860508782465068, 7.883587693554856557, 1.040834085586084257E-14 ) ) ;
#166225=CARTESIAN_POINT ( 'NONE',  ( 4.921246571636183731, 7.724909519342112674, -1.082531754730549078 ) ) ;
#166226=CARTESIAN_POINT ( 'NONE',  ( -1.364683531250000748, 0.8218750003414210248, 0.000000000000000000 ) ) ;
#166227=CARTESIAN_POINT ( 'NONE',  ( 3.145128448690309053, 4.692402494937224056, -1.443375672974057666 ) ) ;
#166228=CARTESIAN_POINT ( 'NONE',  ( -8.448702279610222021, 13.00856975952063088, 1.040834085586084257E-14 ) ) ;
#166231=ADVANCED_FACE ( 'NONE', ( #102844 ), #168901, .F. ) ;
#166241=EDGE_LOOP ( 'NONE', ( #65134, #9300, #92116 ) ) ;
#166245=CARTESIAN_POINT ( 'NONE',  ( 7.657657833620182153, 7.828355648845348291, -0.7998128361456281477 ) ) ;
#166246=CARTESIAN_POINT ( 'NONE',  ( 7.806797523370503811, 8.002351953554066810, 1.040834085586084257E-14 ) ) ;
#166254=( BOUNDED_SURFACE ( )  B_SPLINE_SURFACE ( 3, 2, ( 
 ( #103303, #19899, #85983 ),
 ( #172581, #7918, #72918 ),
 ( #169365, #104378, #87047 ),
 ( #55616, #139023, #24162 ) ),
 .UNSPECIFIED., .F., .F., .T. ) 
 B_SPLINE_SURFACE_WITH_KNOTS ( ( 4, 4 ),
 ( 3, 3 ),
 ( 0.000000000000000000, 0.002003486994853853880 ),
 ( 0.000000000000000000, 1.000000000000000000 ),
 .UNSPECIFIED. ) 
 GEOMETRIC_REPRESENTATION_ITEM ( )  RATIONAL_B_SPLINE_SURFACE ( (
 ( 1.000000000000000000, 0.7779734834199515392, 1.000000000000000000),
 ( 1.000000000000000000, 0.7856061901475724918, 1.000000000000000000),
 ( 1.000000000000000000, 0.7951961705782247813, 1.000000000000000000),
 ( 1.000000000000000000, 0.8104931255419010050, 1.000000000000000000) ) ) 
 REPRESENTATION_ITEM ( '' )  SURFACE ( )  );
#166258=CARTESIAN_POINT ( 'NONE',  ( -6.274726165026268454, 6.214935368819085149, 0.7998128361456341429 ) ) ;
#166259=CARTESIAN_POINT ( 'NONE',  ( -3.684065054611367351, 5.321161868511784299, -1.599625672291256295 ) ) ;
#166264=FACE_OUTER_BOUND ( 'NONE', #52314, .T. ) ;
#166268=CARTESIAN_POINT ( 'NONE',  ( -10.00555417720528872, 10.77549408293541866, 0.7216878364870438212 ) ) ;
#166271=CARTESIAN_POINT ( 'NONE',  ( 7.298366762858032430, 7.409182732956175244, 1.040834085586084257E-14 ) ) ;
#166272=CARTESIAN_POINT ( 'NONE',  ( 1.364683531249988535, 5.155208333674750953, -0.7879004041258300672 ) ) ;
#166281=CARTESIAN_POINT ( 'NONE',  ( 4.894130264408854458, 6.732904613275549899, -1.443375672974051449 ) ) ;
#166282=CARTESIAN_POINT ( 'NONE',  ( -8.030507057996002729, 8.263346410617135263, 1.040834085586084257E-14 ) ) ;
#166287=CARTESIAN_POINT ( 'NONE',  ( -6.561256274009600986, 9.742217188731485678, -1.199719254218440723 ) ) ;
#166288=CARTESIAN_POINT ( 'NONE',  ( -3.978428010606240850, 6.728917548094202949, -1.199719254218452047 ) ) ;
#166295=CARTESIAN_POINT ( 'NONE',  ( 6.103141704446003679, 10.27208242182903142, 0.7998128361456462443 ) ) ;
#166309=CARTESIAN_POINT ( 'NONE',  ( -1.500000000000011324, 5.170833333333356485, 0.8660254037844403729 ) ) ;
#166310=CARTESIAN_POINT ( 'NONE',  ( 4.695201269034174452, 4.372156323494968966, 1.214306433183764966E-14 ) ) ;
#166311=CARTESIAN_POINT ( 'NONE',  ( 3.669453130792974971, 7.432779085900453886, 1.040834085586084257E-14 ) ) ;
#166313=CARTESIAN_POINT ( 'NONE',  ( -6.209271165378811297, 10.18797409300986878, 0.7216878364870458196 ) ) ;
#166315=CARTESIAN_POINT ( 'NONE',  ( 6.480434237652132445, 7.623223367758051872, 1.082531754730558626 ) ) ;
#166316=CARTESIAN_POINT ( 'NONE',  ( -9.124274191872645545, 9.747334100047323702, -0.7216878364870267237 ) ) ;
#166321=CARTESIAN_POINT ( 'NONE',  ( 7.949158136313996259, 8.168439335321471262, 1.040834085586084257E-14 ) ) ;
#166325=CARTESIAN_POINT ( 'NONE',  ( -1.201851678989727383E-14, 3.196875000341420137, -1.575800808251660134 ) ) ;
#166331=CARTESIAN_POINT ( 'NONE',  ( 6.934105498385400246, 10.17720795050327354, -1.199719254218441611 ) ) ;
#166334=CARTESIAN_POINT ( 'NONE',  ( -7.934546212495630968, 10.28005655271014795, -1.599625672291263179 ) ) ;
#166340=CARTESIAN_POINT ( 'NONE',  ( 8.809047120577066181, 11.30030761213851953, 1.599625672291281386 ) ) ;
#166342=PRODUCT_CONTEXT ( 'NONE', #130779, 'mechanical' ) ;
#166343=CARTESIAN_POINT ( 'NONE',  ( -8.422639742587602285, 10.84949900448412841, -1.599625672291263179 ) ) ;
#166348=CARTESIAN_POINT ( 'NONE',  ( 5.575284262857175044, 6.175169341367511500, -0.8878447928483481633 ) ) ;
#166349=CARTESIAN_POINT ( 'NONE',  ( -9.490344339885973923, 12.09515436799890331, -1.443375672974059665 ) ) ;
#166355=CARTESIAN_POINT ( 'NONE',  ( 7.124973419181436007, 8.271222729588529887, -1.199719254218446718 ) ) ;
#166357=CARTESIAN_POINT ( 'NONE',  ( 5.937581207780954884, 9.014596278131406848, -1.199719254218440723 ) ) ;
#166358=CARTESIAN_POINT ( 'NONE',  ( -4.159863475130535448, 7.428450666093093346, 0.7365534166655554049 ) ) ;
#166359=CARTESIAN_POINT ( 'NONE',  ( 3.876741858503734761, 6.610283703974623393, 1.199719254218462483 ) ) ;
#166361=CARTESIAN_POINT ( 'NONE',  ( -6.236387472606141458, 10.21960978477508952, -0.7216878364870278340 ) ) ;
#166368=CARTESIAN_POINT ( 'NONE',  ( -4.055583655087145800, 7.567422049930973671, -0.4132208808486706464 ) ) ;
#166371=CARTESIAN_POINT ( 'NONE',  ( 4.020151095146772491, 7.782762254604477015, 0.3270025911792567297 ) ) ;
#166372=CARTESIAN_POINT ( 'NONE',  ( 6.331294547901813452, 6.488857848747989543, 1.040834085586084257E-14 ) ) ;
#166377=CARTESIAN_POINT ( 'NONE',  ( -10.60211293576223213, 11.47147930125185589, 1.040834085586084257E-14 ) ) ;
#166382=CARTESIAN_POINT ( 'NONE',  ( -10.42585693878457853, 11.26584730477792284, -0.7216878364870267237 ) ) ;
#166390=CARTESIAN_POINT ( 'NONE',  ( -7.822691444960696572, 12.07029775252209092, -0.7216878364870267237 ) ) ;
#166397=CARTESIAN_POINT ( 'NONE',  ( -1.500000000000013101, 3.410416667349487785, -0.8660254037844313801 ) ) ;
#166399=CARTESIAN_POINT ( 'NONE',  ( -6.715366157470410435, 6.729015360003925750, -0.7998128361456291469 ) ) ;
#166401=VERTEX_POINT ( 'NONE', #8526 ) ;
#166402=CARTESIAN_POINT ( 'NONE',  ( -6.984421689334302741, 11.30024240419870374, 0.000000000000000000 ) ) ;
#166405=CARTESIAN_POINT ( 'NONE',  ( 5.636439174979242850, 7.598931675607687453, -1.599625672291262513 ) ) ;
#166409=CARTESIAN_POINT ( 'NONE',  ( 7.964525173024008531, 11.37936423758166526, 1.199719254218460707 ) ) ;
#166413=DIRECTION ( 'NONE',  ( 0.6507913734559640506, -0.7592566023653004592, 0.000000000000000000 ) ) ;
#166419=CARTESIAN_POINT ( 'NONE',  ( -7.212574532790100079, 9.437756259720353924, -1.443375672974059665 ) ) ;
#166423=CARTESIAN_POINT ( 'NONE',  ( 1.364683531249990311, 5.676041667008088432, 0.7879004041258500513 ) ) ;
#166431=CARTESIAN_POINT ( 'NONE',  ( -2.440104460335327463, 5.790612937125752424, 1.040834085586084257E-14 ) ) ;
#166433=CARTESIAN_POINT ( 'NONE',  ( 9.585778300061798873, 11.14216175728232550, -1.199719254218440723 ) ) ;
#166435=CARTESIAN_POINT ( 'NONE',  ( -1.154085075685135742, 2.812889018129764107, -0.7749999999999970246 ) ) ;
#166439=CARTESIAN_POINT ( 'NONE',  ( -1.201851678989727383E-14, 2.696875000341417916, -1.575800808251660134 ) ) ;
#166441=CARTESIAN_POINT ( 'NONE',  ( 4.253507506385319381, 5.985511395581417204, 1.599625672291267398 ) ) ;
#166447=CARTESIAN_POINT ( 'NONE',  ( 2.412988153552339643, 5.758977245878946327, 0.7216878364870438212 ) ) ;
#166449=CARTESIAN_POINT ( 'NONE',  ( 8.039621902779343188, 12.32338328664385507, -0.7216878364870328300 ) ) ;
#166451=CARTESIAN_POINT ( 'NONE',  ( -6.507550544879489252, 9.575597488125954015, 1.082531754730548412 ) ) ;
#166454=CARTESIAN_POINT ( 'NONE',  ( 0.2837385194700463575, 8.150966340525164000, 2.020310785919128715 ) ) ;
#166456=CARTESIAN_POINT ( 'NONE',  ( -8.355902744723985975, 8.642974711799791265, 1.040834085586084257E-14 ) ) ;
#166457=CARTESIAN_POINT ( 'NONE',  ( -4.406036734316898240, 6.163462161501577441, -1.443375672974051449 ) ) ;
#166458=CARTESIAN_POINT ( 'NONE',  ( -1.201851678989727383E-14, 2.384375000341416584, 1.575800808251672791 ) ) ;
#166467=ORIENTED_EDGE ( 'NONE', *, *, #209086, .F. ) ;
#166477=CARTESIAN_POINT ( 'NONE',  ( 1.364683531249990311, 4.946875000341417916, 1.214306433183764966E-14 ) ) ;
#166485=CARTESIAN_POINT ( 'NONE',  ( 8.289920859751990889, 11.75899253876431416, 1.199719254218450271 ) ) ;
#166488=CARTESIAN_POINT ( 'NONE',  ( 1.364683531249988535, 1.863541667008086211, 0.7879004041258500513 ) ) ;
#166490=CARTESIAN_POINT ( 'NONE',  ( -6.019457014787517046, 9.006155036351978893, 1.082531754730548412 ) ) ;
#166498=CARTESIAN_POINT ( 'NONE',  ( 3.344057444064992168, 7.053150784717805877, 1.040834085586084257E-14 ) ) ;
#166502=CARTESIAN_POINT ( 'NONE',  ( 9.915090410295563927, 10.46202698829998567, -0.7998128361456281477 ) ) ;
#166508=ORIENTED_EDGE ( 'NONE', *, *, #4338, .F. ) ;
#166510=CARTESIAN_POINT ( 'NONE',  ( -3.948449050077848632, 5.629609863222681199, 1.599625672291267398 ) ) ;
#166511=CARTESIAN_POINT ( 'NONE',  ( 6.259060471003163428, 10.45398764947904624, -0.7998128361456291469 ) ) ;
#166513=CARTESIAN_POINT ( 'NONE',  ( 5.314433026432511475, 5.302519407033794430, 1.040834085586084257E-14 ) ) ;
#166517=ORIENTED_EDGE ( 'NONE', *, *, #1511, .T. ) ;
#166522=CARTESIAN_POINT ( 'NONE',  ( -1.499999999999995559, 8.673756432004008587, -2.614717076620594050 ) ) ;
#166523=CARTESIAN_POINT ( 'NONE',  ( -6.073689629242151611, 10.02979563418376685, -0.7216878364870278340 ) ) ;
#166524=CARTESIAN_POINT ( 'NONE',  ( 4.527533231959700366, 7.369540306339926516, 1.199719254218462483 ) ) ;
#166527=CARTESIAN_POINT ( 'NONE',  ( -7.971304249830880373, 11.38727316052296601, 1.199719254218453823 ) ) ;
#166533=CARTESIAN_POINT ( 'NONE',  ( -4.973143418114339021, 4.696422164088486895, 0.7998128361456341429 ) ) ;
#166535=EDGE_CURVE ( 'NONE', #21552, #104455, #24046, .T. ) ;
#166537=CARTESIAN_POINT ( 'NONE',  ( 8.666686507633574621, 11.13422023037111330, 1.599625672291281386 ) ) ;
#166538=CARTESIAN_POINT ( 'NONE',  ( 2.517010073631369860, 6.088262185878572375, -0.7998128361456281477 ) ) ;
#166540=VERTEX_POINT ( 'NONE', #176135 ) ;
#166547=CARTESIAN_POINT ( 'NONE',  ( -4.874319919312905647, 5.645460313075203018, -1.199719254218446718 ) ) ;
#166551=CARTESIAN_POINT ( 'NONE',  ( -9.020252271793614440, 9.418049160047695878, 0.7998128361456462443 ) ) ;
#166556=CARTESIAN_POINT ( 'NONE',  ( 7.673551755654734130, 9.015193805427763607, -1.082531754730537976 ) ) ;
#166557=CARTESIAN_POINT ( 'NONE',  ( 0.6823417656249899377, 5.738541667008087543, -1.181850606188754593 ) ) ;
#166559=CARTESIAN_POINT ( 'NONE',  ( 4.207107738942202246, 3.802713871720993399, 1.214306433183764966E-14 ) ) ;
#166561=CARTESIAN_POINT ( 'NONE',  ( 4.168242161197552420, 6.950367390450747251, -1.199719254218452047 ) ) ;
#166563=CARTESIAN_POINT ( 'NONE',  ( -8.037286134802835491, 8.271255333558444889, -0.7998128361456291469 ) ) ;
#166572=VECTOR ( 'NONE', #38117, 1000.000000000000000 ) ;
#166573=EDGE_LOOP ( 'NONE', ( #111869, #41762, #7072, #8277, #65151, #5918, #172962, #22961, #151055, #26866, #153988, #19409, #74707, #186304, #28832, #153096, #1617, #114436, #138635, #44807 ) ) ;
#166575=CARTESIAN_POINT ( 'NONE',  ( 0.6823417656249899377, 2.405208333674753618, 1.181850606188767472 ) ) ;
#166576=CARTESIAN_POINT ( 'NONE',  ( 8.540746701604824409, 12.05162268759261224, -1.199719254218446718 ) ) ;
#166578=CARTESIAN_POINT ( 'NONE',  ( -3.470524135418294520, 6.992769224722559684, -0.7216878364870267237 ) ) ;
#166579=CARTESIAN_POINT ( 'NONE',  ( -7.334597915313094241, 9.580116872663850813, 1.040834085586084257E-14 ) ) ;
#166580=CARTESIAN_POINT ( 'NONE',  ( -4.514501963226242864, 7.250374142863800664, 1.082531754730560403 ) ) ;
#166587=CARTESIAN_POINT ( 'NONE',  ( 5.034155109375821446, 4.767602470560229122, -0.7998128361456221525 ) ) ;
#166597=CARTESIAN_POINT ( 'NONE',  ( 5.542585869888291938, 5.360771691158120689, -0.7998128361456211532 ) ) ;
#166602=CARTESIAN_POINT ( 'NONE',  ( -4.900382456335551140, 7.804531068111707270, 1.199719254218464037 ) ) ;
#166606=CARTESIAN_POINT ( 'NONE',  ( 5.449487677688982679, 8.445153826357429949, -1.199719254218446718 ) ) ;
#166610=CARTESIAN_POINT ( 'NONE',  ( -5.575427483717760424, 7.527751369135936343, 1.599625672291269396 ) ) ;
#166611=CARTESIAN_POINT ( 'NONE',  ( 1.499999999999987121, 1.545833333333354487, -0.8660254037844253849 ) ) ;
#166612=CARTESIAN_POINT ( 'NONE',  ( -2.774614992291035698, 6.388801257648172971, 1.040834085586084257E-14 ) ) ;
#166615=CARTESIAN_POINT ( 'NONE',  ( -5.412729640353771465, 7.337937218544611895, 1.599625672291269396 ) ) ;
#166616=CARTESIAN_POINT ( 'NONE',  ( -0.6823417656249969321, 3.717708333674754506, -1.181850606188749264 ) ) ;
#166617=EDGE_CURVE ( 'NONE', #196589, #141559, #204714, .T. ) ;
#166618=CARTESIAN_POINT ( 'NONE',  ( -5.260200412422213923, 6.199617238323108737, -1.082531754730544860 ) ) ;
#166624=CARTESIAN_POINT ( 'NONE',  ( 6.505214776458575265, 6.483838748823460563, 1.040834085586084257E-14 ) ) ;
#166626=CARTESIAN_POINT ( 'NONE',  ( 0.6823417656249899377, 2.405208333674753618, 1.181850606188767472 ) ) ;
#166628=CARTESIAN_POINT ( 'NONE',  ( 3.277320446201373638, 4.846626492033466072, 1.599625672291267398 ) ) ;
#166630=CARTESIAN_POINT ( 'NONE',  ( -1.364683531250014514, -0.1989583329919157317, -0.7879004041258359514 ) ) ;
#166631=LINE ( 'NONE', #187139, #125738 ) ;
#166633=CARTESIAN_POINT ( 'NONE',  ( -3.755772246185468788, 4.340488027759846545, -1.199719254218452047 ) ) ;
#166635=CARTESIAN_POINT ( 'NONE',  ( -6.195713011320790109, 9.211787032307496403, -1.082531754730537976 ) ) ;
#166638=CARTESIAN_POINT ( 'NONE',  ( -0.6823417656250212460, 3.051041667008084879, 1.181850606188767472 ) ) ;
#166647=CARTESIAN_POINT ( 'NONE',  ( -6.846504384776758378, 9.010674420371453053, -1.443375672974058777 ) ) ;
#166653=CARTESIAN_POINT ( 'NONE',  ( -7.226132685959434809, 8.493204890783200511, 1.082531754730549967 ) ) ;
#166654=EDGE_CURVE ( 'NONE', #12149, #55162, #125181, .T. ) ;
#166667=CARTESIAN_POINT ( 'NONE',  ( -6.555530967407501741, 7.606873202518897870, 1.199719254218450271 ) ) ;
#166669=CARTESIAN_POINT ( 'NONE',  ( -1.402160292154681736E-14, -0.1624999999999815481, -1.732050807568870754 ) ) ;
#166670=CARTESIAN_POINT ( 'NONE',  ( 2.496672843210871129, 6.064535417054653266, -0.7998128361456291469 ) ) ;
#166671=AXIS2_PLACEMENT_3D ( 'NONE', #98251, #117754, #81980 ) ;
#166675=CARTESIAN_POINT ( 'NONE',  ( 6.114890974963323345, 7.092793211334054604, 1.199719254218462483 ) ) ;
#166681=CARTESIAN_POINT ( 'NONE',  ( -4.121315508874262790, 6.791656612786516334, -1.082531754730549967 ) ) ;
#166688=CARTESIAN_POINT ( 'NONE',  ( -0.6823417656250003738, 1.717708333674752730, -1.181850606188749264 ) ) ;
#166689=CARTESIAN_POINT ( 'NONE',  ( 8.717529583462638954, 12.15390636647303069, 1.082531754730546636 ) ) ;
#166690=CARTESIAN_POINT ( 'NONE',  ( -6.367525699912501835, 10.58053041653993098, -0.7998128361456291469 ) ) ;
#166693=CARTESIAN_POINT ( 'NONE',  ( 5.621827251160867789, 9.710548892996357040, 1.040834085586084257E-14 ) ) ;
#166694=CARTESIAN_POINT ( 'NONE',  ( -8.389798128758148010, 8.682519326506312751, 0.7998128361456462443 ) ) ;
#166695=CARTESIAN_POINT ( 'NONE',  ( -1.467638673046511189, 8.739153922842808342, 2.544768421592544794 ) ) ;
#166697=CARTESIAN_POINT ( 'NONE',  ( 0.7499999999999885647, -0.9854166659838472508, 1.299038105676657340 ) ) ;
#166699=CARTESIAN_POINT ( 'NONE',  ( 7.727784370109387346, 10.99920361756089093, -1.082531754730543083 ) ) ;
#166703=CARTESIAN_POINT ( 'NONE',  ( 0.6823417656249899377, 1.155208333674752286, 1.181850606188755259 ) ) ;
#166706=CARTESIAN_POINT ( 'NONE',  ( 6.277061933002777927, 8.346324893301817482, 1.443375672974076540 ) ) ;
#166710=CARTESIAN_POINT ( 'NONE',  ( -4.772106882330241717, 5.630174786549132726, -1.082531754730544860 ) ) ;
#166712=CARTESIAN_POINT ( 'NONE',  ( -0.6823417656249969321, 4.717708333674755394, -1.181850606188749264 ) ) ;
#166716=CARTESIAN_POINT ( 'NONE',  ( -5.525111292768871252, 6.404716915440499037, -1.199719254218446718 ) ) ;
#166717=CARTESIAN_POINT ( 'NONE',  ( -4.851289806644571989, 6.918820993438449030, -1.443092038473028582 ) ) ;
#166722=CIRCLE ( 'NONE', #201320, 0.08000000000000020983 ) ;
#166724=CARTESIAN_POINT ( 'NONE',  ( 8.145751363712157911, 8.397798100619326078, -0.7998128361456281477 ) ) ;
#166729=CARTESIAN_POINT ( 'NONE',  ( -1.500000000000013101, 2.129166666666693519, -0.8660254037844313801 ) ) ;
#166735=CARTESIAN_POINT ( 'NONE',  ( 5.721177635286841756, 6.737423998331861341, -1.082531754730543083 ) ) ;
#166736=CARTESIAN_POINT ( 'NONE',  ( 1.364683531249986537, 0.6760416670080884316, 0.7879004041258500513 ) ) ;
#166738=CARTESIAN_POINT ( 'NONE',  ( 0.9486429539237110076, 2.850839070649072049, 1.028101543438982413 ) ) ;
#166743=CARTESIAN_POINT ( 'NONE',  ( -1.402160292154681736E-14, 0.5875000000000220046, -1.732050807568863648 ) ) ;
#166744=CARTESIAN_POINT ( 'NONE',  ( 7.461064606222022277, 7.598996883547496139, 1.040834085586084257E-14 ) ) ;
#166745=CARTESIAN_POINT ( 'NONE',  ( -6.906989191158078079, 10.14557225873805812, -1.199719254218440723 ) ) ;
#166747=CARTESIAN_POINT ( 'NONE',  ( 1.364683531249988535, 1.613541667008084879, 0.7879004041258500513 ) ) ;
#166748=CARTESIAN_POINT ( 'NONE',  ( 1.499999999999987121, 3.045833333333353377, -0.8660254037844262731 ) ) ;
#166750=CARTESIAN_POINT ( 'NONE',  ( 3.551346171775753735, 6.230655402791975384, 1.199719254218462483 ) ) ;
#166758=CARTESIAN_POINT ( 'NONE',  ( 0.7499999999999885647, -1.235416665983847473, 1.299038105676657340 ) ) ;
#166760=CARTESIAN_POINT ( 'NONE',  ( -8.355902744723985975, 8.642974711799791265, 1.040834085586084257E-14 ) ) ;
#166761=CARTESIAN_POINT ( 'NONE',  ( -5.151735183512911043, 6.073074471262228435, 1.082531754730548412 ) ) ;
#166763=CARTESIAN_POINT ( 'NONE',  ( -4.101444922696786399, 3.685019076479660427, -2.500000000000000444 ) ) ;
#166768=EDGE_LOOP ( 'NONE', ( #64208, #202329, #206169, #65656 ) ) ;
#166769=CARTESIAN_POINT ( 'NONE',  ( 6.317209508963599340, 9.457495962844502557, 1.199719254218462483 ) ) ;
#166773=CARTESIAN_POINT ( 'NONE',  ( 5.788968402910795064, 9.697620870130524651, 0.7216878364870438212 ) ) ;
#166777=CARTESIAN_POINT ( 'NONE',  ( -7.100719765255177229, 9.307259030929609267, -1.599625672291263179 ) ) ;
#166778=CARTESIAN_POINT ( 'NONE',  ( 5.352771719296971042, 5.139321848801576387, 0.7998128361456341429 ) ) ;
#166784=CARTESIAN_POINT ( 'NONE',  ( 9.625925876022625616, 11.29296361252366765, -1.082531754730537088 ) ) ;
#166791=CARTESIAN_POINT ( 'NONE',  ( -1.571977147778457651, 8.681624870483057421, -2.500282472944432399 ) ) ;
#166792=CARTESIAN_POINT ( 'NONE',  ( -4.826339496784927796, 5.693446170079573321, 1.082531754730560403 ) ) ;
#166793=CARTESIAN_POINT ( 'NONE',  ( 9.300530189294644146, 10.91333531134101165, -1.082531754730543083 ) ) ;
#166796=CARTESIAN_POINT ( 'NONE',  ( -5.422371370461663176, 8.413518134592214537, -1.199719254218446718 ) ) ;
#166797=FACE_OUTER_BOUND ( 'NONE', #48743, .T. ) ;
#166804=CARTESIAN_POINT ( 'NONE',  ( -7.212047647465563038, 10.50147379109678880, -1.199719254218446718 ) ) ;
#166807=CARTESIAN_POINT ( 'NONE',  ( 5.431895982697334091, 6.433277491268158954, -1.247050338538328029 ) ) ;
#166809=DIRECTION ( 'NONE',  ( 0.000000000000000000, -1.000000000000000000, 0.000000000000000000 ) ) ;
#166818=CARTESIAN_POINT ( 'NONE',  ( -4.543954038874438162, 8.453030145328826350, 1.040834085586084257E-14 ) ) ;
#166822=CARTESIAN_POINT ( 'NONE',  ( 5.178851490740205676, 6.104710163027444736, 1.082531754730558626 ) ) ;
#166827=CARTESIAN_POINT ( 'NONE',  ( -4.192495815123836955, 5.914331089109674089, -1.599625672291256295 ) ) ;
#166834=CARTESIAN_POINT ( 'NONE',  ( -9.515124878692420296, 9.995400534762978850, 1.040834085586084257E-14 ) ) ;
#166835=CARTESIAN_POINT ( 'NONE',  ( 5.425234023762710578, 9.481190127698507553, -0.7998128361456291469 ) ) ;
#166838=CARTESIAN_POINT ( 'NONE',  ( -8.350932551013499960, 11.83017284523606172, -1.199719254218446718 ) ) ;
#166842=CARTESIAN_POINT ( 'NONE',  ( -1.402160292154681736E-14, -0.1156249996585793222, 1.575800808251672791 ) ) ;
#166845=CARTESIAN_POINT ( 'NONE',  ( 8.649738815838679429, 10.15407870897571563, -1.082531754730543083 ) ) ;
#166853=CARTESIAN_POINT ( 'NONE',  ( -0.1021852871539802865, 7.053056311352817076, -4.037408415137027085 ) ) ;
#166865=FACE_OUTER_BOUND ( 'NONE', #61286, .T. ) ;
#166873=AXIS2_PLACEMENT_3D ( 'NONE', #97672, #163729, #81399 ) ;
#166874=CARTESIAN_POINT ( 'NONE',  ( 0.7499999999999885647, 0.5145833340161540814, 1.299038105676657340 ) ) ;
#166876=EDGE_CURVE ( 'NONE', #104139, #2091, #171377, .T. ) ;
#166879=EDGE_LOOP ( 'NONE', ( #194624, #183300, #108131, #113451, #133007, #106877 ) ) ;
#166880=CARTESIAN_POINT ( 'NONE',  ( 1.499999999999819034, 7.267697830503895950, -4.207111467970846341 ) ) ;
#166881=CARTESIAN_POINT ( 'NONE',  ( -2.273105066167346422, 5.702484939155337607, 2.420000000000010587 ) ) ;
#166883=CARTESIAN_POINT ( 'NONE',  ( 4.786522169170392971, 5.141580351323886688, 0.8077998227834035649 ) ) ;
#166884=CARTESIAN_POINT ( 'NONE',  ( 9.901532256681887745, 10.44620914241737530, 0.000000000000000000 ) ) ;
#166889=CARTESIAN_POINT ( 'NONE',  ( 4.741601036477289810, 6.554953847355395880, 1.599625672291267398 ) ) ;
#166890=CARTESIAN_POINT ( 'NONE',  ( -6.887178846062116833, 9.058127958537705027, -1.443375672974059665 ) ) ;
#166891=FACE_OUTER_BOUND ( 'NONE', #181145, .T. ) ;
#166892=CARTESIAN_POINT ( 'NONE',  ( 10.70146331988817323, 11.37946204949139251, 0.7998128361456341429 ) ) ;
#166894=CARTESIAN_POINT ( 'NONE',  ( -6.669721502918952716, 9.868759955792373972, 1.199719254218452047 ) ) ;
#166895=CARTESIAN_POINT ( 'NONE',  ( -3.592547517496941900, 5.214391408544949869, -1.443375672974051449 ) ) ;
#166897=VERTEX_POINT ( 'NONE', #520 ) ;
#166898=CARTESIAN_POINT ( 'NONE',  ( 0.7499999999999885647, -0.2354166659838466402, 1.299038105676657340 ) ) ;
#166905=CARTESIAN_POINT ( 'NONE',  ( -3.090895833791289071, 6.549869539491048442, 1.040834085586084257E-14 ) ) ;
#166908=CARTESIAN_POINT ( 'NONE',  ( 4.100926828275982317, 7.458749316499424964, -0.6398019981258776800 ) ) ;
#166913=CARTESIAN_POINT ( 'NONE',  ( -4.134873662043608178, 4.886736029548026217, 1.082531754730558626 ) ) ;
#166914=CARTESIAN_POINT ( 'NONE',  ( 9.368847842243145152, 10.88907622316056312, 1.199719254218453823 ) ) ;
#166923=CARTESIAN_POINT ( 'NONE',  ( -2.117044542028253318, 5.621635732341564662, -0.7998128361456281477 ) ) ;
#166924=CARTESIAN_POINT ( 'NONE',  ( -9.996439331977562404, 10.55693406359564790, 0.7998128361456462443 ) ) ;
#166927=ORIENTED_EDGE ( 'NONE', *, *, #42815, .F. ) ;
#166930=CARTESIAN_POINT ( 'NONE',  ( 3.845709127770629010, 7.638411082374393146, 0.7998128361456321445 ) ) ;
#166934=ORIENTED_EDGE ( 'NONE', *, *, #105908, .F. ) ;
#166947=CARTESIAN_POINT ( 'NONE',  ( 8.121497709785879593, 9.433834401960398353, -1.199719254218445830 ) ) ;
#166949=CARTESIAN_POINT ( 'NONE',  ( -4.599240423533815125, 6.388866465587984322, 1.599625672291267398 ) ) ;
#166950=EDGE_CURVE ( 'NONE', #117563, #212596, #91834, .T. ) ;
#166957=CARTESIAN_POINT ( 'NONE',  ( 0.7499999999999867883, -1.152083332650516434, -1.299038105676652011 ) ) ;
#166961=CARTESIAN_POINT ( 'NONE',  ( 4.542145155778077203, 5.257923088951247159, -1.199719254218452047 ) ) ;
#166963=CARTESIAN_POINT ( 'NONE',  ( -3.924195396151603177, 6.665646164563756138, 1.199719254218464037 ) ) ;
#166969=CARTESIAN_POINT ( 'NONE',  ( 4.500943810056890371, 8.194925511800951412, -0.7216878364870207285 ) ) ;
#166972=CARTESIAN_POINT ( 'NONE',  ( 7.958272981097359811, 9.347368568444167636, -1.082531754730537976 ) ) ;
#166973=CARTESIAN_POINT ( 'NONE',  ( 1.364683531249988535, 4.176041667008081326, 0.7879004041258500513 ) ) ;
#166975=CARTESIAN_POINT ( 'NONE',  ( 5.300874872818843286, 5.286701561151180506, 0.7216878364870317197 ) ) ;
#166983=CARTESIAN_POINT ( 'NONE',  ( -5.926191280687664431, 6.129739482751896062, 0.8152664440823562675 ) ) ;
#166986=CARTESIAN_POINT ( 'NONE',  ( -0.6823417656249969321, 4.780208333674755394, -1.181850606188749264 ) ) ;
#166992=DIRECTION ( 'NONE',  ( 0.000000000000000000, 8.546850786086437571E-32, 1.000000000000000000 ) ) ;
#167001=CARTESIAN_POINT ( 'NONE',  ( -1.364683531250012516, 4.801041667008083991, -0.7879004041258300672 ) ) ;
#167003=CARTESIAN_POINT ( 'NONE',  ( 7.786460292950004636, 7.978625184730144149, 1.040834085586084257E-14 ) ) ;
#167004=CARTESIAN_POINT ( 'NONE',  ( -7.994504133552415404, 12.47867192245318435, -0.7998128361456281477 ) ) ;
#167010=CARTESIAN_POINT ( 'NONE',  ( -1.500000000000011324, 3.920833333333357817, 0.8660254037844403729 ) ) ;
#167016=CARTESIAN_POINT ( 'NONE',  ( 7.293923454472069245, 11.45340176361870199, 0.7216878364870438212 ) ) ;
#167020=CARTESIAN_POINT ( 'NONE',  ( 1.499999999999987121, 3.827083334016153415, -0.8660254037844323793 ) ) ;
#167022=CARTESIAN_POINT ( 'NONE',  ( -5.579343907223557331, 6.467988298970945849, 1.199719254218450271 ) ) ;
#167023=CARTESIAN_POINT ( 'NONE',  ( 4.487385655998885170, 5.298000022495898520, 1.082531754730560403 ) ) ;
#167024=CARTESIAN_POINT ( 'NONE',  ( -9.232739420781982176, 12.75498451001223010, 1.082531754730558626 ) ) ;
#167031=CARTESIAN_POINT ( 'NONE',  ( 4.847203612085560387, 5.613824621309978724, -1.199719254218452047 ) ) ;
#167035=CARTESIAN_POINT ( 'NONE',  ( 4.680589345215795838, 6.483773540883647435, -1.599625672291256295 ) ) ;
#167049=CARTESIAN_POINT ( 'NONE',  ( 5.645731234294472323, 6.129814942853209381, -0.7970442531908157324 ) ) ;
#167051=CARTESIAN_POINT ( 'NONE',  ( 8.530051201292206287, 13.10347683481629488, 0.000000000000000000 ) ) ;
#167056=PLANE ( 'NONE',  #11839 ) ;
#167057=CARTESIAN_POINT ( 'NONE',  ( -0.6823417656250246877, -0.9489583329919115684, 1.181850606188755259 ) ) ;
#167058=CARTESIAN_POINT ( 'NONE',  ( 5.504247177468175600, 8.405076892812779477, 1.082531754730558626 ) ) ;
#167059=CARTESIAN_POINT ( 'NONE',  ( -2.764973262183167968, 5.313220341600567664, 1.199719254218462483 ) ) ;
#167064=CARTESIAN_POINT ( 'NONE',  ( -4.283486466913726254, 7.084819080452935403, -1.199719254218452047 ) ) ;
#167076=CARTESIAN_POINT ( 'NONE',  ( 9.610031953988080744, 10.10612545594124967, -0.7998128361456281477 ) ) ;
#167077=CARTESIAN_POINT ( 'NONE',  ( 6.078105975125470017, 6.038708432876411791, -0.3507111650211444109 ) ) ;
#167082=VECTOR ( 'NONE', #1533, 1000.000000000000000 ) ;
#167086=CARTESIAN_POINT ( 'NONE',  ( -5.427790276013078952, 4.356734706464544971, 2.440341524156858455 ) ) ;
#167087=CARTESIAN_POINT ( 'NONE',  ( -7.809133291791416909, 11.09411069285655493, 1.082531754730549967 ) ) ;
#167091=CARTESIAN_POINT ( 'NONE',  ( 6.642605195691581699, 9.837124264027149678, 1.199719254218462483 ) ) ;
#167093=CARTESIAN_POINT ( 'NONE',  ( -5.461236948206311226, 5.265864615862458464, 0.7998128361456341429 ) ) ;
#167094=CARTESIAN_POINT ( 'NONE',  ( 5.027376032568989572, 4.759693547618927489, 0.7998128361456341429 ) ) ;
#167096=CARTESIAN_POINT ( 'NONE',  ( -4.924636110261798372, 6.768494766770632332, 1.599625672291267398 ) ) ;
#167097=CARTESIAN_POINT ( 'NONE',  ( 2.659370686574860976, 6.254349567645977714, -0.7998128361456291469 ) ) ;
#167101=ADVANCED_FACE ( 'NONE', ( #95964 ), #89275, .T. ) ;
#167103=CARTESIAN_POINT ( 'NONE',  ( 8.378048858240820351, 11.86180853700128601, -1.199719254218446718 ) ) ;
#167107=CARTESIAN_POINT ( 'NONE',  ( 4.088248116760357931, 7.710168519003287813, -0.6407031029972446445 ) ) ;
#167108=CARTESIAN_POINT ( 'NONE',  ( 4.961921032921539521, 7.772363057508363759, -1.082531754730549078 ) ) ;
#167114=CARTESIAN_POINT ( 'NONE',  ( 7.578644679914702031, 10.82520731233375955, 1.082531754730558626 ) ) ;
#167117=CARTESIAN_POINT ( 'NONE',  ( -9.110189153378817295, 12.71597221466224603, 1.199719254218462483 ) ) ;
#167118=CARTESIAN_POINT ( 'NONE',  ( -9.176171038350775078, 9.599954387697719582, -0.7998128361456291469 ) ) ;
#167124=CARTESIAN_POINT ( 'NONE',  ( 3.469446951953614189E-15, 5.229711127717882491, 1.214306433183764966E-14 ) ) ;
#167128=CARTESIAN_POINT ( 'NONE',  ( 3.999819011231439347, 4.625209253646830554, 1.199719254218464037 ) ) ;
#167132=CARTESIAN_POINT ( 'NONE',  ( 5.335297142177534369, 6.183267073083954735, -1.199719254218452047 ) ) ;
#167135=CARTESIAN_POINT ( 'NONE',  ( -1.499999999999997780, 3.931250000682819046, 1.214306433183764966E-14 ) ) ;
#167141=CARTESIAN_POINT ( 'NONE',  ( -0.7500000000000215383, 1.691666666666688634, 1.299038105676659116 ) ) ;
#167142=CARTESIAN_POINT ( 'NONE',  ( 5.503720292143644777, 8.508425209887878538, 1.199719254218462483 ) ) ;
#167143=CARTESIAN_POINT ( 'NONE',  ( 5.802526556524483681, 5.871961858807763335, 1.040834085586084257E-14 ) ) ;
#167146=CARTESIAN_POINT ( 'NONE',  ( 9.436111725431318931, 10.11114455586577776, -0.7216878364870257245 ) ) ;
#167152=CARTESIAN_POINT ( 'NONE',  ( -5.091250377131585125, 5.898545847196970726, 1.199719254218450271 ) ) ;
#167153=CARTESIAN_POINT ( 'NONE',  ( 1.499999999999987121, 4.077083334016147198, -0.8660254037844323793 ) ) ;
#167154=CARTESIAN_POINT ( 'NONE',  ( 0.6823417656249882723, -0.3239583329919110133, -1.181850606188749264 ) ) ;
#167158=CARTESIAN_POINT ( 'NONE',  ( 8.703971429848968100, 13.09845773489176679, 0.000000000000000000 ) ) ;
#167160=CARTESIAN_POINT ( 'NONE',  ( -1.364683531250012516, 3.592708333674750509, 0.7879004041258379498 ) ) ;
#167163=DIRECTION ( 'NONE',  ( -3.347138415753902517E-16, -0.6000000000000018652, -0.7999999999999984901 ) ) ;
#167168=CARTESIAN_POINT ( 'NONE',  ( -6.340409392685171674, 10.54889472477470846, 0.7998128361456481317 ) ) ;
#167169=CARTESIAN_POINT ( 'NONE',  ( 5.738125327081736060, 7.717565519727259904, 1.599625672291267398 ) ) ;
#167171=CARTESIAN_POINT ( 'NONE',  ( -1.364683531250000748, -0.9906249996585805295, 0.000000000000000000 ) ) ;
#167173=VERTEX_POINT ( 'NONE', #143194 ) ;
#167176=CARTESIAN_POINT ( 'NONE',  ( -4.543954038874438162, 8.453030145328826350, 1.040834085586084257E-14 ) ) ;
#167181=CARTESIAN_POINT ( 'NONE',  ( 10.40318394038753702, 11.03146944007395724, -0.7998128361456281477 ) ) ;
#167183=CARTESIAN_POINT ( 'NONE',  ( -4.952806187693842510, 4.672695395264567786, 0.7998128361456341429 ) ) ;
#167184=AXIS2_PLACEMENT_3D ( 'NONE', #68023, #182868, #87523 ) ;
#167185=CARTESIAN_POINT ( 'NONE',  ( -7.157815033010924921, 10.43820240756634199, 1.199719254218453823 ) ) ;
#167188=CARTESIAN_POINT ( 'NONE',  ( -4.351171265391168497, 7.394090626460979365, 1.174491979025530597 ) ) ;
#167189=CARTESIAN_POINT ( 'NONE',  ( -0.6823417656250003738, -1.032291666325242607, -1.181850606188749264 ) ) ;
#167193=CARTESIAN_POINT ( 'NONE',  ( 8.432808358020025707, 9.900993174853955026, 1.082531754730558626 ) ) ;
#167198=CARTESIAN_POINT ( 'NONE',  ( 0.006158830626129541130, 7.078243236992583398, -2.121324627965408993 ) ) ;
#167214=CARTESIAN_POINT ( 'NONE',  ( 4.067082894419602468, 3.847277586352047862, -0.7216878364870188411 ) ) ;
#167218=CARTESIAN_POINT ( 'NONE',  ( -3.574546055497324737, 7.322054164722185732, 0.7998128361456341429 ) ) ;
#167219=CARTESIAN_POINT ( 'NONE',  ( -8.076906825439122528, 10.44614393447756129, -1.599625672291263179 ) ) ;
#167220=CARTESIAN_POINT ( 'NONE',  ( -7.334597915313094241, 9.580116872663850813, 1.040834085586084257E-14 ) ) ;
#167224=CARTESIAN_POINT ( 'NONE',  ( -1.499999999999997780, 3.181250000682818602, 1.214306433183764966E-14 ) ) ;
#167225=CARTESIAN_POINT ( 'NONE',  ( 9.053093885623066939, 11.58502883802551153, -1.599625672291262513 ) ) ;
#167229=CARTESIAN_POINT ( 'NONE',  ( -9.826962411806732689, 10.35921099006301382, -0.7998128361456291469 ) ) ;
#167230=CARTESIAN_POINT ( 'NONE',  ( 3.469446951953614189E-15, 6.400000000000023448, 1.214306433183764966E-14 ) ) ;
#167231=CARTESIAN_POINT ( 'NONE',  ( 1.364683531249988757, 2.384375000341422357, 1.214306433183764966E-14 ) ) ;
#167237=CARTESIAN_POINT ( 'NONE',  ( -2.103486388414573138, 5.605817886458954291, 1.040834085586084257E-14 ) ) ;
#167239=ADVANCED_FACE ( 'NONE', ( #191504 ), #39953, .F. ) ;
#167242=CARTESIAN_POINT ( 'NONE',  ( -0.6823417656250246877, 0.3635416670080895973, 1.181850606188755259 ) ) ;
#167247=CARTESIAN_POINT ( 'NONE',  ( -1.364683531250000748, 2.259375000341422357, 1.214306433183764966E-14 ) ) ;
#167251=CARTESIAN_POINT ( 'NONE',  ( -6.470265622219711688, 8.571729197388226140, -1.599625672291263179 ) ) ;
#167252=CARTESIAN_POINT ( 'NONE',  ( 6.428537391173986038, 10.65171072301167854, 0.7998128361456462443 ) ) ;
#167254=CARTESIAN_POINT ( 'NONE',  ( 6.830610463186557624, 6.863467050006115677, 1.040834085586084257E-14 ) ) ;
#167256=CARTESIAN_POINT ( 'NONE',  ( -0.7499999999999972244, 4.358333333333352932, -1.299038105676652011 ) ) ;
#167260=CARTESIAN_POINT ( 'NONE',  ( -1.364683531250000748, 1.321875000341421469, 0.000000000000000000 ) ) ;
#167267=CARTESIAN_POINT ( 'NONE',  ( 4.690757960648213931, 8.416375354157496602, 0.7216878364870438212 ) ) ;
#167270=CARTESIAN_POINT ( 'NONE',  ( -7.655550293210764856, 12.08322577538792331, 0.000000000000000000 ) ) ;
#167271=CARTESIAN_POINT ( 'NONE',  ( -2.981903720001798597, 5.566305875722335372, -1.199719254218446718 ) ) ;
#167277=CARTESIAN_POINT ( 'NONE',  ( -6.005898860729463884, 9.950706404252290582, 0.7216878364870458196 ) ) ;
#167279=CARTESIAN_POINT ( 'NONE',  ( -1.500000000000011324, 4.879166666666690411, -0.8660254037844313801 ) ) ;
#167282=CARTESIAN_POINT ( 'NONE',  ( 6.954969614130424027, 11.05795561655343384, 1.040834085586084257E-14 ) ) ;
#167296=CARTESIAN_POINT ( 'NONE',  ( 8.111855979677986994, 8.358253485912799263, 1.040834085586084257E-14 ) ) ;
#167297=CARTESIAN_POINT ( 'NONE',  ( -5.416646063859567484, 6.278174148379618735, 1.199719254218450271 ) ) ;
#167301=CARTESIAN_POINT ( 'NONE',  ( 6.114364089638786304, 8.156510742710487705, 1.443375672974076540 ) ) ;
#167302=CARTESIAN_POINT ( 'NONE',  ( -1.364683531250014514, -0.4489583329919089039, -0.7879004041258359514 ) ) ;
#167303=CARTESIAN_POINT ( 'NONE',  ( 3.931501358282940117, 4.649468341827285300, -1.082531754730543083 ) ) ;
#167304=CARTESIAN_POINT ( 'NONE',  ( -2.462777459176719308, 6.024990802348131780, -0.7998128361456281477 ) ) ;
#167312=ORIENTED_EDGE ( 'NONE', *, *, #70073, .F. ) ;
#167320=CARTESIAN_POINT ( 'NONE',  ( 6.928380191783277908, 8.041863964290678624, 1.199719254218462483 ) ) ;
#167327=CARTESIAN_POINT ( 'NONE',  ( 1.569519686356874999, 8.730458328475176444, 2.495327313683093351 ) ) ;
#167333=CARTESIAN_POINT ( 'NONE',  ( -6.112028321662274166, 6.025121218227761588, 0.7998128361456341429 ) ) ;
#167335=CARTESIAN_POINT ( 'NONE',  ( -5.264643720808155791, 5.036505850564608089, 0.000000000000000000 ) ) ;
#167338=DIRECTION ( 'NONE',  ( 0.000000000000000000, 8.546850786086437571E-32, 1.000000000000000000 ) ) ;
#167340=CARTESIAN_POINT ( 'NONE',  ( 1.419999999999822737, 7.176846818246208848, 4.202462424328221147 ) ) ;
#167345=CARTESIAN_POINT ( 'NONE',  ( -2.266184231778562541, 5.795632037050281404, 1.040834085586084257E-14 ) ) ;
#167348=CARTESIAN_POINT ( 'NONE',  ( 6.799577732453452761, 7.891594428405881878, -1.199719254218446718 ) ) ;
#167349=CARTESIAN_POINT ( 'NONE',  ( -0.6823417656249969321, 4.217708333674755394, -1.181850606188749264 ) ) ;
#167356=CARTESIAN_POINT ( 'NONE',  ( 5.463572716182824252, 7.397254140345190798, 1.443375672974062551 ) ) ;
#167357=CARTESIAN_POINT ( 'NONE',  ( -7.314787569772770226, 8.492672571945082183, -1.199719254218452935 ) ) ;
#167361=CARTESIAN_POINT ( 'NONE',  ( -6.938021921891187382, 9.117444880338284818, -1.599625672291263179 ) ) ;
#167362=CARTESIAN_POINT ( 'NONE',  ( -4.089755892816631544, 7.923132308261379819, -0.7998128361456281477 ) ) ;
#167366=DIRECTION ( 'NONE',  ( -0.7592566023653044560, -0.6507913734559596097, -1.725633230170963762E-31 ) ) ;
#167369=CARTESIAN_POINT ( 'NONE',  ( 8.450809820019639318, 8.753699632978056755, -0.7998128361456291469 ) ) ;
#167382=CARTESIAN_POINT ( 'NONE',  ( 1.499999999999991118, 5.754166666666685970, 0.8660254037844524744 ) ) ;
#167383=CARTESIAN_POINT ( 'NONE',  ( 3.011882680530176604, 6.665613560593854459, 0.7998128361456341429 ) ) ;
#167384=CARTESIAN_POINT ( 'NONE',  ( 5.144429221381498607, 8.089252293998699272, -1.199719254218452047 ) ) ;
#167386=CARTESIAN_POINT ( 'NONE',  ( -6.697364695470783502, 10.75741654478384035, 0.7216878364870458196 ) ) ;
#167387=EDGE_CURVE ( 'NONE', #34146, #197417, #49039, .T. ) ;
#167389=CARTESIAN_POINT ( 'NONE',  ( 6.493992391265805075, 6.678671999339316656, 1.040834085586084257E-14 ) ) ;
#167390=CARTESIAN_POINT ( 'NONE',  ( -6.832946231163084860, 10.91559500309152675, 0.000000000000000000 ) ) ;
#167394=CARTESIAN_POINT ( 'NONE',  ( 7.935599982700328958, 8.152621489438862667, 0.7998128361456481317 ) ) ;
#167400=CARTESIAN_POINT ( 'NONE',  ( 1.364683531249990311, 3.384375000341416140, 1.214306433183764966E-14 ) ) ;
#167406=CARTESIAN_POINT ( 'NONE',  ( 9.745613490124728884, 10.26430391476735338, 0.7998128361456462443 ) ) ;
#167409=CARTESIAN_POINT ( 'NONE',  ( -9.189729191964438826, 9.615772233580322848, 1.040834085586084257E-14 ) ) ;
#167413=B_SPLINE_CURVE_WITH_KNOTS ( 'NONE', 3,
 ( #150019, #136970, #118637, #86072, #68730, #18917, #35171, #120786, #134851, #184622 ),
 .UNSPECIFIED., .F., .F.,
 ( 4, 2, 2, 2, 4 ),
 ( 0.0001270906692242517301, 0.0005866303604698383176, 0.001046170051715425041, 0.001505709742961011764, 0.001965249434206598270 ),
 .UNSPECIFIED. ) ;
#167416=CARTESIAN_POINT ( 'NONE',  ( 3.623053363349855172, 5.249981562040033189, 1.599625672291267398 ) ) ;
#167419=CARTESIAN_POINT ( 'NONE',  ( -7.853197290813634268, 10.18514947741448573, 1.599625672291295375 ) ) ;
#167424=CARTESIAN_POINT ( 'NONE',  ( 5.872608658597049391, 5.988986745869715023, 0.2392922861021197500 ) ) ;
#167425=CARTESIAN_POINT ( 'NONE',  ( -4.437596350374534815, 4.071617251725375475, -0.7998128361456221525 ) ) ;
#167429=CARTESIAN_POINT ( 'NONE',  ( 7.800018446563675489, 7.994443030612759848, -0.7998128361456281477 ) ) ;
#167431=CARTESIAN_POINT ( 'NONE',  ( 7.474622759835693131, 7.614814729430110951, -0.7998128361456281477 ) ) ;
#167432=CARTESIAN_POINT ( 'NONE',  ( 4.473300617505036492, 7.306268922809479704, -1.199719254218452047 ) ) ;
#167434=CARTESIAN_POINT ( 'NONE',  ( -8.703971430293361067, 9.256980878204810637, 0.7216878364870438212 ) ) ;
#167441=CARTESIAN_POINT ( 'NONE',  ( -4.061901113999940804, 7.558576442610514867, -0.4421990992426305112 ) ) ;
#167442=CARTESIAN_POINT ( 'NONE',  ( 4.254006295369892499, 7.509857431501010261, -1.008242097476583554 ) ) ;
#167443=EDGE_CURVE ( 'NONE', #133576, #140339, #62800, .T. ) ;
#167445=CARTESIAN_POINT ( 'NONE',  ( 5.666945020832170776, 7.634521829102760115, 1.443375672974062551 ) ) ;
#167454=CARTESIAN_POINT ( 'NONE',  ( -10.10046125205658463, 11.84658821789661509, -1.082531754730537976 ) ) ;
#167462=CARTESIAN_POINT ( 'NONE',  ( -10.43941509239824228, 11.28166515066052966, 1.040834085586084257E-14 ) ) ;
#167469=CARTESIAN_POINT ( 'NONE',  ( -1.201851678989727383E-14, 3.243750000682814161, 1.732050807568877637 ) ) ;
#167471=CARTESIAN_POINT ( 'NONE',  ( -5.096975683733680818, 8.033889833409558534, -1.199719254218452047 ) ) ;
#167475=CARTESIAN_POINT ( 'NONE',  ( -9.833741488613570780, 10.36711991300432345, 0.7998128361456462443 ) ) ;
#167479=CARTESIAN_POINT ( 'NONE',  ( 5.777746017718023097, 9.892454120646377191, 0.7998128361456462443 ) ) ;
#167484=CARTESIAN_POINT ( 'NONE',  ( 10.07100917685271035, 10.64393221595000938, 0.7998128361456462443 ) ) ;
#167485=CARTESIAN_POINT ( 'NONE',  ( 4.299316086327568343, 7.453850760076471182, -1.115744863390004671 ) ) ;
#167486=CARTESIAN_POINT ( 'NONE',  ( -4.848826244296223109, 5.027555131033083491, -0.8732430475888955934 ) ) ;
#167490=CARTESIAN_POINT ( 'NONE',  ( -6.371969008742801144, 10.37778824360119145, 0.7216878364870458196 ) ) ;
#167493=CARTESIAN_POINT ( 'NONE',  ( -1.001543065824772872E-14, 5.634375000341415252, 1.575800808251672791 ) ) ;
#167498=CARTESIAN_POINT ( 'NONE',  ( -10.64045162862669081, 11.30828174301964140, -0.7998128361456221525 ) ) ;
#167501=CARTESIAN_POINT ( 'NONE',  ( 7.913155211870404493, 12.38376484715752213, 0.7998128361456462443 ) ) ;
#167503=CARTESIAN_POINT ( 'NONE',  ( 0.000000000000000000, 2.800000000000024691, 1.214306433183764966E-14 ) ) ;
#167507=CARTESIAN_POINT ( 'NONE',  ( 1.364683531249986537, 2.155208333674751398, -0.7879004041258239610 ) ) ;
#167508=CARTESIAN_POINT ( 'NONE',  ( -3.633221978782299910, 5.261844946711204507, -1.443375672974053447 ) ) ;
#167510=CARTESIAN_POINT ( 'NONE',  ( 4.857899112398166075, 4.561970474086296079, 1.040834085586084257E-14 ) ) ;
#167515=CARTESIAN_POINT ( 'NONE',  ( 3.606105671554957759, 4.269840040644637291, -1.082531754730543083 ) ) ;
#167517=CARTESIAN_POINT ( 'NONE',  ( 1.499999999999997113, 4.035416667349482012, 0.8660254037844477004 ) ) ;
#167518=CARTESIAN_POINT ( 'NONE',  ( -7.212574532790100079, 9.437756259720353924, -1.443375672974059665 ) ) ;
#167523=CARTESIAN_POINT ( 'NONE',  ( -7.133561379084627063, 11.47423870890741782, 0.7998128361456481317 ) ) ;
#167524=CARTESIAN_POINT ( 'NONE',  ( -4.406036734316890247, 7.123831375802920363, -1.082531754730548412 ) ) ;
#167525=CARTESIAN_POINT ( 'NONE',  ( -1.364683531250000748, 2.071875000341422357, 1.214306433183764966E-14 ) ) ;
#167531=( BOUNDED_SURFACE ( )  B_SPLINE_SURFACE ( 1, 2, ( 
 ( #84095, #169612, #153366, #152301, #3874, #69947, #120948, #136059, #202072, #53732, #186919, #21194, #88371, #37474, #103552, #87297, #38549, #104627, #170674, #154437, #172830, #156579, #24401, #105714, #74256, #73156, #76374, #42843, #10301, #139263, #90514, #56931, #23339, #59057, #91594, #8172, #108950, #123104, #140350, #189061, #205293, #122017, #206369, #158702, #40698, #57995, #174970, #142481, #143559, #124158, #110018, #26552, #208489, #106801, #92660, #190120, #187985, #41774, #107886, #173914, #25488, #157646, #9243, #75315, #77442, #39611, #141431, #155501, #171742, #176031, #89449, #60125, #207438, #125214, #191176, #126284, #192242, #43904, #27624, #93724, #159763, #209553, #7084, #11363, #129491, #97988, #128426, #178160, #181337, #82770, #162979, #63331, #14557, #195473, #28702, #160836, #32964, #62266, #80655, #12427, #94787, #147793, #144625, #78507, #112157, #210639, #47105, #148844, #115346, #99039, #111081, #177085, #96928, #113220, #49225, #194393, #145697, #127356, #48177, #31911, #29775, #46036, #179225, #15622, #95859, #161915, #13505, #81712, #114290, #165094, #79578, #64399, #30850, #211695, #146745, #212764, #130543, #196535, #180288, #164047, #44973, #213811, #65431, #131581, #197583, #16686, #61197, #193325, #149921, #116401, #152051, #184521, #183466, #135802, #1490, #35073, #67555, #166154, #417, #18817, #37222, #17741, #167231, #201826, #103296, #22003, #101143, #202897, #53471, #87039, #133699, #119608, #84904, #66488, #199704, #51350, #68631, #117474, #150991, #2556, #36142, #170414, #132629, #134753, #34019, #198634, #54542, #182389, #153111, #200762, #52412, #118538, #20943, #102225, #168295, #19891, #85976, #3620, #88114, #50282, #83829, #69700, #169357, #185593, #4685, #120689, #100093, #70759, #136872, #186665, #38292, #104370, #39359, #59874, #155250, #41515, #105455, #187730, #26296, #23082, #171491, #205037, #89197, #175777, #55608, #58810, #40445, #142229, #173660, #109770, #25233, #6831, #154184, #137940, #107628, #56682, #72910, #126025, #75063, #71830, #188809, #108695, #106545, #141175, #139015, #190926, #122847, #191987, #208243, #92411, #172572, #91336, #27371, #24154, #203961, #90257, #156325, #158450, #5752, #7907, #174723, #73996, #57746, #8988, #207186, #140089, #121764, #42590, #43653, #206114, #123904, #189873, #157394, #124964, #10051, #76126, #146491, #94537, #180036, #65185, #144380, #44718, #176832, #210379, #163793, #195218, #145446, #161662, #77184, #162730, #131339, #45787, #178980, #196283, #97736, #160576, #62021, #64152, #29520, #95613, #194137, #30594, #80397, #13257, #159510, #12184, #111904, #60945, #197333, #181089, #48975, #115092, #78256, #147542, #47930, #79329, #114043, #128176, #177907, #14302, #112968, #93471, #211444, #63077, #129245, #127101, #46854, #96680, #212511, #31658, #28446, #130294, #15371, #81464, #213563, #11109, #143306 ),
 ( #110824, #193066, #209297, #198386, #170, #99847, #132386, #36964, #82514, #118287, #149665, #69445, #84654, #185341, #150743, #116152, #148601, #3378, #103045, #182139, #66237, #135553, #117219, #1244, #183217, #184273, #53223, #98788, #16435, #50028, #119354, #85717, #32707, #52160, #33769, #2305, #17496, #165911, #164843, #83583, #133446, #35897, #67305, #101974, #199452, #168042, #51094, #19644, #34822, #100897, #166986, #151804, #18576, #68381, #201577, #134511, #200515, #145053, #164464, #33390, #62681, #32331, #12856, #129917, #81078, #213192, #211056, #99468, #48595, #49644, #132006, #128840, #115767, #112579, #163408, #77874, #31276, #64819, #78931, #98399, #198016, #194821, #177520, #95220, #46457, #82134, #113652, #63757, #80003, #209988, #147165, #181756, #178591, #97351, #114713, #16050, #30199, #96288, #196957, #162340, #13923, #146108, #14983, #130965, #212119, #143996, #195903, #47539, #193751, #11799, #61630, #127796, #45397, #179656, #65856, #180708, #148226, #214228, #111514, #29132, #161270, #118195, #136529, #6490, #4344, #135460, #169009, #104022, #202549, #7558, #200422, #151713, #54199, #22733, #53125, #102949, #106199, #73644, #87762, #120339, #153838, #186315, #167947, #121415, #3282, #5408, #36865, #119258, #172226, #187387, #184183, #20607, #154906, #86693, #39018, #185243, #88849, #152762, #23815, #188456, #72565, #69349, #137599, #52069, #70411, #35803, #37950, #170069, #138663, #101881, #21655, #204685, #201483, #71486, #55268, #105100, #203616, #19548, #56335, #89920, #155972, #171141, #85626, #122494, #40088, #205766, #159160, #192705, #140819, #11827, #111546, #190578, #90985, #8635, #42235, #210020, #27013, #191638, #207897, #123560, #208953, #177555, #92057, #10759, #28093, #144025, #206833, #108349, #110483, #75781, #141888, #25950, #76832, #126746, #59520, #57395, #58466, #158113, #107279, #29164, #12889, #95255, #161305, #124620, #193783, #94189, #125679, #160229, #9704, #45430, #176482, #189524, #139742, #174371, #43302, #109422, #173299, #175427, #93119, #142953, #77904, #74716, #60588, #44361, #61663, #127830, #41170, #24880, #157047, #82164, #214258, #16081, #13954, #115801, #194857, #891, #34485, #146140, #46490, #133097, #64851, #31306, #130998, #49676, #116867, #145087, #128875, #162374, #182869, #83227, #50741, #112612, #178624, #199095, #80037, #180739, #30235, #96320, #165558, #212153, #63789, #129947, #195934, #100559, #47572, #198047, #179687, #66958, #98430, #166630, #164495, #113685, #78967, #62714, #147196, #211091, #97382, #163439, #15019, #81108, #114741, #196988, #213221, #48625, #32366, #148258, #65890, #181789, #132037, #33423, #99501, #17151, #149311, #85377, #183937, #38767, #71235, #72308, #69099, #21414, #202299, #151459, #184991, #201235, #3031, #135223, #52876, #119012, #1961, #36616, #35549, #187138, #153589, #121169, #101628, #102702, #167694 ) ),
 .UNSPECIFIED., .F., .F., .T. ) 
 B_SPLINE_SURFACE_WITH_KNOTS ( ( 2, 2 ),
 ( 3, 2, 2, 2, 2, 2, 2, 2, 2, 2, 2, 2, 2, 2, 2, 2, 2, 2, 2, 2, 2, 2, 2, 2, 2, 2, 2, 2, 2, 2, 2, 2, 2, 2, 2, 2, 2, 2, 2, 2, 2, 2, 2, 2, 2, 2, 2, 2, 2, 2, 2, 2, 2, 2, 2, 2, 2, 2, 2, 2, 2, 2, 2, 2, 2, 2, 2, 2, 2, 2, 2, 2, 2, 2, 2, 2, 2, 2, 2, 2, 2, 2, 2, 2, 2, 2, 2, 2, 2, 2, 2, 2, 2, 2, 2, 2, 2, 2, 2, 2, 2, 2, 2, 2, 2, 2, 2, 2, 2, 2, 2, 2, 2, 2, 2, 2, 2, 2, 2, 2, 2, 2, 2, 2, 2, 2, 2, 2, 2, 2, 2, 2, 2, 2, 2, 2, 2, 2, 2, 2, 2, 2, 2, 2, 2, 2, 2, 2, 2, 2, 2, 2, 2, 2, 2, 2, 2, 2, 2, 2, 2, 2, 2, 2, 2, 2, 2, 2, 3 ),
 ( 0.000000000000000000, 1.000000000000000000 ),
 ( 0.000000000000000000, 0.005952380952380952051, 0.01190476190476190410, 0.01785714285714285615, 0.02380952380952380820, 0.02976190476190476025, 0.03571428571428571230, 0.04166666666666666435, 0.04761904761904761640, 0.05357142857142856845, 0.05952380952380952051, 0.06547619047619047949, 0.07142857142857142461, 0.07738095238095238360, 0.08333333333333332871, 0.08928571428571428770, 0.09523809523809523281, 0.1011904761904761918, 0.1071428571428571369, 0.1130952380952380959, 0.1190476190476190410, 0.1250000000000000000, 0.1309523809523809590, 0.1369047619047619180, 0.1428571428571428492, 0.1488095238095238082, 0.1547619047619047672, 0.1607142857142857262, 0.1666666666666666574, 0.1726190476190476164, 0.1785714285714285754, 0.1845238095238095344, 0.1904761904761904656, 0.1964285714285714246, 0.2023809523809523836, 0.2083333333333333426, 0.2142857142857142738, 0.2202380952380952328, 0.2261904761904761918, 0.2321428571428571508, 0.2380952380952380820, 0.2440476190476190410, 0.2500000000000000000, 0.2559523809523809312, 0.2619047619047619180, 0.2678571428571428492, 0.2738095238095238360, 0.2797619047619047672, 0.2857142857142856984, 0.2916666666666666852, 0.2976190476190476164, 0.3035714285714285476, 0.3095238095238095344, 0.3154761904761904656, 0.3214285714285714524, 0.3273809523809523836, 0.3333333333333333148, 0.3392857142857143016, 0.3452380952380952328, 0.3511904761904761640, 0.3571428571428571508, 0.3630952380952380820, 0.3690476190476190688, 0.3750000000000000000, 0.3809523809523809312, 0.3869047619047619180, 0.3928571428571428492, 0.3988095238095238360, 0.4047619047619047672, 0.4107142857142856984, 0.4166666666666666852, 0.4226190476190476164, 0.4285714285714285476, 0.4345238095238095344, 0.4404761904761904656, 0.4464285714285714524, 0.4523809523809523836, 0.4583333333333333148, 0.4642857142857143016, 0.4702380952380952328, 0.4761904761904761640, 0.4821428571428571508, 0.4880952380952380820, 0.4940476190476190688, 0.5000000000000000000, 0.5059523809523809312, 0.5119047619047618625, 0.5178571428571429047, 0.5238095238095238360, 0.5297619047619047672, 0.5357142857142856984, 0.5416666666666666297, 0.5476190476190476719, 0.5535714285714286031, 0.5595238095238095344, 0.5654761904761904656, 0.5714285714285713969, 0.5773809523809523281, 0.5833333333333333703, 0.5892857142857143016, 0.5952380952380952328, 0.6011904761904761640, 0.6071428571428570953, 0.6130952380952381375, 0.6190476190476190688, 0.6250000000000000000, 0.6309523809523809312, 0.6369047619047618625, 0.6428571428571429047, 0.6488095238095238360, 0.6547619047619047672, 0.6607142857142856984, 0.6666666666666666297, 0.6726190476190476719, 0.6785714285714286031, 0.6845238095238095344, 0.6904761904761904656, 0.6964285714285713969, 0.7023809523809523281, 0.7083333333333333703, 0.7142857142857143016, 0.7202380952380952328, 0.7261904761904761640, 0.7321428571428570953, 0.7380952380952381375, 0.7440476190476190688, 0.7500000000000000000, 0.7559523809523809312, 0.7619047619047618625, 0.7678571428571429047, 0.7738095238095238360, 0.7797619047619047672, 0.7857142857142856984, 0.7916666666666666297, 0.7976190476190476719, 0.8035714285714286031, 0.8095238095238095344, 0.8154761904761904656, 0.8214285714285713969, 0.8273809523809523281, 0.8333333333333333703, 0.8392857142857143016, 0.8452380952380952328, 0.8511904761904761640, 0.8571428571428570953, 0.8630952380952381375, 0.8690476190476190688, 0.8750000000000000000, 0.8809523809523809312, 0.8869047619047618625, 0.8928571428571429047, 0.8988095238095238360, 0.9047619047619047672, 0.9107142857142856984, 0.9166666666666666297, 0.9226190476190476719, 0.9285714285714286031, 0.9345238095238095344, 0.9404761904761904656, 0.9464285714285713969, 0.9523809523809523281, 0.9583333333333333703, 0.9642857142857143016, 0.9702380952380952328, 0.9761904761904761640, 0.9821428571428570953, 0.9880952380952381375, 0.9940476190476190688, 1.000000000000000000 ),
 .UNSPECIFIED. ) 
 GEOMETRIC_REPRESENTATION_ITEM ( )  RATIONAL_B_SPLINE_SURFACE ( (
 ( 1.000000000000000000, 0.8660254037844387076, 1.000000000000000000, 0.8660254037844387076, 1.000000000000000000, 0.8660254037844387076, 1.000000000000000000, 0.8660254037844387076, 1.000000000000000000, 0.8660254037844387076, 1.000000000000000000, 0.8660254037844387076, 1.000000000000000000, 0.8660254037844387076, 1.000000000000000000, 0.8660254037844387076, 1.000000000000000000, 0.8660254037844387076, 1.000000000000000000, 0.8660254037844387076, 1.000000000000000000, 0.8660254037844387076, 1.000000000000000000, 0.8660254037844387076, 1.000000000000000000, 0.8660254037844387076, 1.000000000000000000, 0.8660254037844387076, 1.000000000000000000, 0.8660254037844387076, 1.000000000000000000, 0.8660254037844387076, 1.000000000000000000, 0.8660254037844387076, 1.000000000000000000, 0.8660254037844387076, 1.000000000000000000, 0.8660254037844387076, 1.000000000000000000, 0.8660254037844387076, 1.000000000000000000, 0.8660254037844387076, 1.000000000000000000, 0.8660254037844387076, 1.000000000000000000, 0.8660254037844387076, 1.000000000000000000, 0.8660254037844387076, 1.000000000000000000, 0.8660254037844387076, 1.000000000000000000, 0.8660254037844387076, 1.000000000000000000, 0.8660254037844387076, 1.000000000000000000, 0.8660254037844387076, 1.000000000000000000, 0.8660254037844387076, 1.000000000000000000, 0.8660254037844387076, 1.000000000000000000, 0.8660254037844387076, 1.000000000000000000, 0.8660254037844387076, 1.000000000000000000, 0.8660254037844387076, 1.000000000000000000, 0.8660254037844387076, 1.000000000000000000, 0.8660254037844387076, 1.000000000000000000, 0.8660254037844387076, 1.000000000000000000, 0.8660254037844387076, 1.000000000000000000, 0.8660254037844387076, 1.000000000000000000, 0.8660254037844387076, 1.000000000000000000, 0.8660254037844387076, 1.000000000000000000, 0.8660254037844387076, 1.000000000000000000, 0.8660254037844387076, 1.000000000000000000, 0.8660254037844387076, 1.000000000000000000, 0.8660254037844387076, 1.000000000000000000, 0.8660254037844387076, 1.000000000000000000, 0.8660254037844387076, 1.000000000000000000, 0.8660254037844387076, 1.000000000000000000, 0.8660254037844387076, 1.000000000000000000, 0.8660254037844387076, 1.000000000000000000, 0.8660254037844387076, 1.000000000000000000, 0.8660254037844387076, 1.000000000000000000, 0.8660254037844387076, 1.000000000000000000, 0.8660254037844387076, 1.000000000000000000, 0.8660254037844387076, 1.000000000000000000, 0.8660254037844387076, 1.000000000000000000, 0.8660254037844387076, 1.000000000000000000, 0.8660254037844387076, 1.000000000000000000, 0.8660254037844387076, 1.000000000000000000, 0.8660254037844387076, 1.000000000000000000, 0.8660254037844387076, 1.000000000000000000, 0.8660254037844387076, 1.000000000000000000, 0.8660254037844387076, 1.000000000000000000, 0.8660254037844387076, 1.000000000000000000, 0.8660254037844387076, 1.000000000000000000, 0.8660254037844387076, 1.000000000000000000, 0.8660254037844387076, 1.000000000000000000, 0.8660254037844387076, 1.000000000000000000, 0.8660254037844387076, 1.000000000000000000, 0.8660254037844387076, 1.000000000000000000, 0.8660254037844387076, 1.000000000000000000, 0.8660254037844387076, 1.000000000000000000, 0.8660254037844387076, 1.000000000000000000, 0.8660254037844387076, 1.000000000000000000, 0.8660254037844387076, 1.000000000000000000, 0.8660254037844387076, 1.000000000000000000, 0.8660254037844387076, 1.000000000000000000, 0.8660254037844387076, 1.000000000000000000, 0.8660254037844387076, 1.000000000000000000, 0.8660254037844387076, 1.000000000000000000, 0.8660254037844387076, 1.000000000000000000, 0.8660254037844387076, 1.000000000000000000, 0.8660254037844387076, 1.000000000000000000, 0.8660254037844387076, 1.000000000000000000, 0.8660254037844387076, 1.000000000000000000, 0.8660254037844387076, 1.000000000000000000, 0.8660254037844387076, 1.000000000000000000, 0.8660254037844387076, 1.000000000000000000, 0.8660254037844387076, 1.000000000000000000, 0.8660254037844387076, 1.000000000000000000, 0.8660254037844387076, 1.000000000000000000, 0.8660254037844387076, 1.000000000000000000, 0.8660254037844387076, 1.000000000000000000, 0.8660254037844387076, 1.000000000000000000, 0.8660254037844387076, 1.000000000000000000, 0.8660254037844387076, 1.000000000000000000, 0.8660254037844387076, 1.000000000000000000, 0.8660254037844387076, 1.000000000000000000, 0.8660254037844387076, 1.000000000000000000, 0.8660254037844387076, 1.000000000000000000, 0.8660254037844387076, 1.000000000000000000, 0.8660254037844387076, 1.000000000000000000, 0.8660254037844387076, 1.000000000000000000, 0.8660254037844387076, 1.000000000000000000, 0.8660254037844387076, 1.000000000000000000, 0.8660254037844387076, 1.000000000000000000, 0.8660254037844387076, 1.000000000000000000, 0.8660254037844387076, 1.000000000000000000, 0.8660254037844387076, 1.000000000000000000, 0.8660254037844387076, 1.000000000000000000, 0.8660254037844387076, 1.000000000000000000, 0.8660254037844387076, 1.000000000000000000, 0.8660254037844387076, 1.000000000000000000, 0.8660254037844387076, 1.000000000000000000, 0.8660254037844387076, 1.000000000000000000, 0.8660254037844387076, 1.000000000000000000, 0.8660254037844387076, 1.000000000000000000, 0.8660254037844387076, 1.000000000000000000, 0.8660254037844387076, 1.000000000000000000, 0.8660254037844387076, 1.000000000000000000, 0.8660254037844387076, 1.000000000000000000, 0.8660254037844387076, 1.000000000000000000, 0.8660254037844387076, 1.000000000000000000, 0.8660254037844387076, 1.000000000000000000, 0.8660254037844387076, 1.000000000000000000, 0.8660254037844387076, 1.000000000000000000, 0.8660254037844387076, 1.000000000000000000, 0.8660254037844387076, 1.000000000000000000, 0.8660254037844387076, 1.000000000000000000, 0.8660254037844387076, 1.000000000000000000, 0.8660254037844387076, 1.000000000000000000, 0.8660254037844387076, 1.000000000000000000, 0.8660254037844387076, 1.000000000000000000, 0.8660254037844387076, 1.000000000000000000, 0.8660254037844387076, 1.000000000000000000, 0.8660254037844387076, 1.000000000000000000, 0.8660254037844387076, 1.000000000000000000, 0.8660254037844387076, 1.000000000000000000, 0.8660254037844387076, 1.000000000000000000, 0.8660254037844387076, 1.000000000000000000, 0.8660254037844387076, 1.000000000000000000, 0.8660254037844387076, 1.000000000000000000, 0.8660254037844387076, 1.000000000000000000, 0.8660254037844387076, 1.000000000000000000, 0.8660254037844387076, 1.000000000000000000, 0.8660254037844387076, 1.000000000000000000, 0.8660254037844387076, 1.000000000000000000, 0.8660254037844387076, 1.000000000000000000, 0.8660254037844387076, 1.000000000000000000, 0.8660254037844387076, 1.000000000000000000, 0.8660254037844387076, 1.000000000000000000, 0.8660254037844387076, 1.000000000000000000, 0.8660254037844387076, 1.000000000000000000, 0.8660254037844387076, 1.000000000000000000, 0.8660254037844387076, 1.000000000000000000, 0.8660254037844387076, 1.000000000000000000, 0.8660254037844387076, 1.000000000000000000, 0.8660254037844387076, 1.000000000000000000, 0.8660254037844387076, 1.000000000000000000, 0.8660254037844387076, 1.000000000000000000, 0.8660254037844387076, 1.000000000000000000, 0.8660254037844387076, 1.000000000000000000, 0.8660254037844387076, 1.000000000000000000, 0.8660254037844387076, 1.000000000000000000, 0.8660254037844387076, 1.000000000000000000, 0.8660254037844387076, 1.000000000000000000, 0.8660254037844387076, 1.000000000000000000, 0.8660254037844387076, 1.000000000000000000, 0.8660254037844387076, 1.000000000000000000),
 ( 1.000000000000000000, 0.8660254037844387076, 1.000000000000000000, 0.8660254037844387076, 1.000000000000000000, 0.8660254037844387076, 1.000000000000000000, 0.8660254037844387076, 1.000000000000000000, 0.8660254037844387076, 1.000000000000000000, 0.8660254037844387076, 1.000000000000000000, 0.8660254037844387076, 1.000000000000000000, 0.8660254037844387076, 1.000000000000000000, 0.8660254037844387076, 1.000000000000000000, 0.8660254037844387076, 1.000000000000000000, 0.8660254037844387076, 1.000000000000000000, 0.8660254037844387076, 1.000000000000000000, 0.8660254037844387076, 1.000000000000000000, 0.8660254037844387076, 1.000000000000000000, 0.8660254037844387076, 1.000000000000000000, 0.8660254037844387076, 1.000000000000000000, 0.8660254037844387076, 1.000000000000000000, 0.8660254037844387076, 1.000000000000000000, 0.8660254037844387076, 1.000000000000000000, 0.8660254037844387076, 1.000000000000000000, 0.8660254037844387076, 1.000000000000000000, 0.8660254037844387076, 1.000000000000000000, 0.8660254037844387076, 1.000000000000000000, 0.8660254037844387076, 1.000000000000000000, 0.8660254037844387076, 1.000000000000000000, 0.8660254037844387076, 1.000000000000000000, 0.8660254037844387076, 1.000000000000000000, 0.8660254037844387076, 1.000000000000000000, 0.8660254037844387076, 1.000000000000000000, 0.8660254037844387076, 1.000000000000000000, 0.8660254037844387076, 1.000000000000000000, 0.8660254037844387076, 1.000000000000000000, 0.8660254037844387076, 1.000000000000000000, 0.8660254037844387076, 1.000000000000000000, 0.8660254037844387076, 1.000000000000000000, 0.8660254037844387076, 1.000000000000000000, 0.8660254037844387076, 1.000000000000000000, 0.8660254037844387076, 1.000000000000000000, 0.8660254037844387076, 1.000000000000000000, 0.8660254037844387076, 1.000000000000000000, 0.8660254037844387076, 1.000000000000000000, 0.8660254037844387076, 1.000000000000000000, 0.8660254037844387076, 1.000000000000000000, 0.8660254037844387076, 1.000000000000000000, 0.8660254037844387076, 1.000000000000000000, 0.8660254037844387076, 1.000000000000000000, 0.8660254037844387076, 1.000000000000000000, 0.8660254037844387076, 1.000000000000000000, 0.8660254037844387076, 1.000000000000000000, 0.8660254037844387076, 1.000000000000000000, 0.8660254037844387076, 1.000000000000000000, 0.8660254037844387076, 1.000000000000000000, 0.8660254037844387076, 1.000000000000000000, 0.8660254037844387076, 1.000000000000000000, 0.8660254037844387076, 1.000000000000000000, 0.8660254037844387076, 1.000000000000000000, 0.8660254037844387076, 1.000000000000000000, 0.8660254037844387076, 1.000000000000000000, 0.8660254037844387076, 1.000000000000000000, 0.8660254037844387076, 1.000000000000000000, 0.8660254037844387076, 1.000000000000000000, 0.8660254037844387076, 1.000000000000000000, 0.8660254037844387076, 1.000000000000000000, 0.8660254037844387076, 1.000000000000000000, 0.8660254037844387076, 1.000000000000000000, 0.8660254037844387076, 1.000000000000000000, 0.8660254037844387076, 1.000000000000000000, 0.8660254037844387076, 1.000000000000000000, 0.8660254037844387076, 1.000000000000000000, 0.8660254037844387076, 1.000000000000000000, 0.8660254037844387076, 1.000000000000000000, 0.8660254037844387076, 1.000000000000000000, 0.8660254037844387076, 1.000000000000000000, 0.8660254037844387076, 1.000000000000000000, 0.8660254037844387076, 1.000000000000000000, 0.8660254037844387076, 1.000000000000000000, 0.8660254037844387076, 1.000000000000000000, 0.8660254037844387076, 1.000000000000000000, 0.8660254037844387076, 1.000000000000000000, 0.8660254037844387076, 1.000000000000000000, 0.8660254037844387076, 1.000000000000000000, 0.8660254037844387076, 1.000000000000000000, 0.8660254037844387076, 1.000000000000000000, 0.8660254037844387076, 1.000000000000000000, 0.8660254037844387076, 1.000000000000000000, 0.8660254037844387076, 1.000000000000000000, 0.8660254037844387076, 1.000000000000000000, 0.8660254037844387076, 1.000000000000000000, 0.8660254037844387076, 1.000000000000000000, 0.8660254037844387076, 1.000000000000000000, 0.8660254037844387076, 1.000000000000000000, 0.8660254037844387076, 1.000000000000000000, 0.8660254037844387076, 1.000000000000000000, 0.8660254037844387076, 1.000000000000000000, 0.8660254037844387076, 1.000000000000000000, 0.8660254037844387076, 1.000000000000000000, 0.8660254037844387076, 1.000000000000000000, 0.8660254037844387076, 1.000000000000000000, 0.8660254037844387076, 1.000000000000000000, 0.8660254037844387076, 1.000000000000000000, 0.8660254037844387076, 1.000000000000000000, 0.8660254037844387076, 1.000000000000000000, 0.8660254037844387076, 1.000000000000000000, 0.8660254037844387076, 1.000000000000000000, 0.8660254037844387076, 1.000000000000000000, 0.8660254037844387076, 1.000000000000000000, 0.8660254037844387076, 1.000000000000000000, 0.8660254037844387076, 1.000000000000000000, 0.8660254037844387076, 1.000000000000000000, 0.8660254037844387076, 1.000000000000000000, 0.8660254037844387076, 1.000000000000000000, 0.8660254037844387076, 1.000000000000000000, 0.8660254037844387076, 1.000000000000000000, 0.8660254037844387076, 1.000000000000000000, 0.8660254037844387076, 1.000000000000000000, 0.8660254037844387076, 1.000000000000000000, 0.8660254037844387076, 1.000000000000000000, 0.8660254037844387076, 1.000000000000000000, 0.8660254037844387076, 1.000000000000000000, 0.8660254037844387076, 1.000000000000000000, 0.8660254037844387076, 1.000000000000000000, 0.8660254037844387076, 1.000000000000000000, 0.8660254037844387076, 1.000000000000000000, 0.8660254037844387076, 1.000000000000000000, 0.8660254037844387076, 1.000000000000000000, 0.8660254037844387076, 1.000000000000000000, 0.8660254037844387076, 1.000000000000000000, 0.8660254037844387076, 1.000000000000000000, 0.8660254037844387076, 1.000000000000000000, 0.8660254037844387076, 1.000000000000000000, 0.8660254037844387076, 1.000000000000000000, 0.8660254037844387076, 1.000000000000000000, 0.8660254037844387076, 1.000000000000000000, 0.8660254037844387076, 1.000000000000000000, 0.8660254037844387076, 1.000000000000000000, 0.8660254037844387076, 1.000000000000000000, 0.8660254037844387076, 1.000000000000000000, 0.8660254037844387076, 1.000000000000000000, 0.8660254037844387076, 1.000000000000000000, 0.8660254037844387076, 1.000000000000000000, 0.8660254037844387076, 1.000000000000000000, 0.8660254037844387076, 1.000000000000000000, 0.8660254037844387076, 1.000000000000000000, 0.8660254037844387076, 1.000000000000000000, 0.8660254037844387076, 1.000000000000000000, 0.8660254037844387076, 1.000000000000000000, 0.8660254037844387076, 1.000000000000000000, 0.8660254037844387076, 1.000000000000000000, 0.8660254037844387076, 1.000000000000000000, 0.8660254037844387076, 1.000000000000000000, 0.8660254037844387076, 1.000000000000000000, 0.8660254037844387076, 1.000000000000000000, 0.8660254037844387076, 1.000000000000000000, 0.8660254037844387076, 1.000000000000000000, 0.8660254037844387076, 1.000000000000000000, 0.8660254037844387076, 1.000000000000000000, 0.8660254037844387076, 1.000000000000000000, 0.8660254037844387076, 1.000000000000000000, 0.8660254037844387076, 1.000000000000000000, 0.8660254037844387076, 1.000000000000000000, 0.8660254037844387076, 1.000000000000000000, 0.8660254037844387076, 1.000000000000000000, 0.8660254037844387076, 1.000000000000000000, 0.8660254037844387076, 1.000000000000000000, 0.8660254037844387076, 1.000000000000000000, 0.8660254037844387076, 1.000000000000000000, 0.8660254037844387076, 1.000000000000000000, 0.8660254037844387076, 1.000000000000000000) ) ) 
 REPRESENTATION_ITEM ( '' )  SURFACE ( )  );
#167546=CARTESIAN_POINT ( 'NONE',  ( -1.364683531250012516, 2.342708333674752286, 0.7879004041258379498 ) ) ;
#167553=CARTESIAN_POINT ( 'NONE',  ( 8.452618703115982512, 11.94880668935564216, 1.199719254218450271 ) ) ;
#167556=CARTESIAN_POINT ( 'NONE',  ( -1.201851678989727383E-14, 2.821875000341418804, 1.575800808251672791 ) ) ;
#167567=CARTESIAN_POINT ( 'NONE',  ( 3.842846474469570062, 6.570739089268092137, -1.199719254218452047 ) ) ;
#167570=ORIENTED_EDGE ( 'NONE', *, *, #104659, .F. ) ;
#167578=CARTESIAN_POINT ( 'NONE',  ( -2.774614992291035698, 6.388801257648172971, 1.040834085586084257E-14 ) ) ;
#167579=CARTESIAN_POINT ( 'NONE',  ( 6.598014311344812199, 10.84943379654430906, 1.040834085586084257E-14 ) ) ;
#167582=CARTESIAN_POINT ( 'NONE',  ( 4.975479186090852046, 6.827811688571220117, 1.443375672974062551 ) ) ;
#167583=DIRECTION ( 'NONE',  ( 0.000000000000000000, 1.000000000000000000, 0.000000000000000000 ) ) ;
#167591=CARTESIAN_POINT ( 'NONE',  ( -7.727784370109414880, 8.118095974656867497, 0.7216878364870578100 ) ) ;
#167593=CARTESIAN_POINT ( 'NONE',  ( 4.822949958159288286, 6.649860922651058992, -1.599625672291256295 ) ) ;
#167596=CARTESIAN_POINT ( 'NONE',  ( -10.14557902172788495, 10.73093036830436553, 1.040834085586084257E-14 ) ) ;
#167601=CARTESIAN_POINT ( 'NONE',  ( -2.676845263694313637, 5.210404343363602919, -1.199719254218446718 ) ) ;
#167604=CARTESIAN_POINT ( 'NONE',  ( 9.582915646760733708, 10.07448976417602893, 0.7998128361456462443 ) ) ;
#167605=CARTESIAN_POINT ( 'NONE',  ( 4.325214697959421706, 5.004837554829479451, 1.199719254218462483 ) ) ;
#167611=CARTESIAN_POINT ( 'NONE',  ( 3.189213936345663747, 2.817530495244580102, -2.450448857954562243 ) ) ;
#167614=CARTESIAN_POINT ( 'NONE',  ( -5.362413449404877852, 6.214902764849178141, -1.199719254218446718 ) ) ;
#167617=CARTESIAN_POINT ( 'NONE',  ( -9.592557376868645846, 11.15007068022363157, -1.199719254218441611 ) ) ;
#167622=CARTESIAN_POINT ( 'NONE',  ( 6.805829924380108586, 8.963220883242035697, 1.443375672974076540 ) ) ;
#167625=CARTESIAN_POINT ( 'NONE',  ( 2.984766373302843778, 6.633977868828633717, -0.7998128361456291469 ) ) ;
#167627=CARTESIAN_POINT ( 'NONE',  ( -6.388916700537716764, 8.476822122092563916, 1.599625672291283607 ) ) ;
#167633=CARTESIAN_POINT ( 'NONE',  ( 3.104453987849314700, 4.644948957289396496, 0.000000000000000000 ) ) ;
#167637=CARTESIAN_POINT ( 'NONE',  ( 1.364683531249990311, 2.696875000341415696, 1.214306433183764966E-14 ) ) ;
#167638=CARTESIAN_POINT ( 'NONE',  ( 2.367870383881045981, 5.914265881169853856, 0.000000000000000000 ) ) ;
#167640=CARTESIAN_POINT ( 'NONE',  ( -5.450014563013544588, 5.460697866378308341, 0.7216878364870317197 ) ) ;
#167641=EDGE_CURVE ( 'NONE', #159908, #40273, #180441, .T. ) ;
#167642=CARTESIAN_POINT ( 'NONE',  ( 3.226477370372305753, 4.787309570232886280, 1.443375672974062551 ) ) ;
#167643=CARTESIAN_POINT ( 'NONE',  ( -4.867013957181525186, 8.622007350113015889, 0.7216878364870458196 ) ) ;
#167644=DIRECTION ( 'NONE',  ( -1.000000000000000000, 7.109522442527888164E-16, 0.000000000000000000 ) ) ;
#167649=CARTESIAN_POINT ( 'NONE',  ( 4.416205349749311004, 6.175325546172740765, 1.599625672291267398 ) ) ;
#167659=CARTESIAN_POINT ( 'NONE',  ( 6.657217119509961201, 7.725507046638470321, -1.199719254218446718 ) ) ;
#167663=CARTESIAN_POINT ( 'NONE',  ( -4.740547266272593596, 8.682388910626682943, -0.7998128361456281477 ) ) ;
#167667=CARTESIAN_POINT ( 'NONE',  ( 6.636879889089462026, 7.701780277814560982, -1.199719254218446718 ) ) ;
#167670=CARTESIAN_POINT ( 'NONE',  ( -4.629219384062206011, 7.488174150459498968, -1.199719254218452047 ) ) ;
#167671=CARTESIAN_POINT ( 'NONE',  ( 6.927853306458749749, 8.145212281365775908, 1.082531754730558626 ) ) ;
#167672=CARTESIAN_POINT ( 'NONE',  ( 4.981510052282690282, 6.816019998287410786, 1.424969591591069396 ) ) ;
#167673=CARTESIAN_POINT ( 'NONE',  ( -3.785751206713858785, 5.439795712631356750, 1.599625672291267398 ) ) ;
#167676=CARTESIAN_POINT ( 'NONE',  ( -6.573005544526917099, 6.562927978236513304, -0.7998128361456291469 ) ) ;
#167680=CARTESIAN_POINT ( 'NONE',  ( -0.6823417656250003738, 2.217708333674753174, -1.181850606188749264 ) ) ;
#167682=CARTESIAN_POINT ( 'NONE',  ( -4.609409038966245653, 6.400729850259146758, -1.443375672974053447 ) ) ;
#167687=CARTESIAN_POINT ( 'NONE',  ( 4.924636110261782385, 6.768494766770632332, 1.599625672291267398 ) ) ;
#167691=CARTESIAN_POINT ( 'NONE',  ( -1.364683531250012516, 2.842708333674754506, 0.7879004041258379498 ) ) ;
#167694=CARTESIAN_POINT ( 'NONE',  ( -1.364683531250000748, -1.178124999658580752, 0.000000000000000000 ) ) ;
#167698=CARTESIAN_POINT ( 'NONE',  ( -3.273404022695637572, 5.906389562198459231, 1.199719254218462483 ) ) ;
#167699=CARTESIAN_POINT ( 'NONE',  ( -7.836249598574384301, 8.244638741199329601, 1.040834085586084257E-14 ) ) ;
#167701=CARTESIAN_POINT ( 'NONE',  ( 0.6823417656249882723, 2.926041667008084879, -1.181850606188754593 ) ) ;
#167709=CARTESIAN_POINT ( 'NONE',  ( -7.714226216051410567, 9.062647342557177410, 1.082531754730558626 ) ) ;
#167715=CARTESIAN_POINT ( 'NONE',  ( -7.687109908824056426, 8.070642436490613747, 0.7216878364870438212 ) ) ;
#167721=CARTESIAN_POINT ( 'NONE',  ( -0.1263102688159843667, 6.363441598446241798, 3.117922131261609664 ) ) ;
#167729=CARTESIAN_POINT ( 'NONE',  ( -4.693093728624763372, 8.627026450037540428, 0.7998128361456481317 ) ) ;
#167731=CARTESIAN_POINT ( 'NONE',  ( -1.500000000000001332, -0.09999999999997510880, 0.000000000000000000 ) ) ;
#167732=CARTESIAN_POINT ( 'NONE',  ( 5.020596955762157698, 4.751784624677624080, 1.040834085586084257E-14 ) ) ;
#167737=CARTESIAN_POINT ( 'NONE',  ( 5.686755365928134687, 8.721966129303114101, 1.199719254218462483 ) ) ;
#167739=VECTOR ( 'NONE', #202139, 1000.000000000000000 ) ;
#167743=CARTESIAN_POINT ( 'NONE',  ( -5.151735183512911043, 6.073074471262228435, 1.082531754730548412 ) ) ;
#167746=CARTESIAN_POINT ( 'NONE',  ( -0.5707955116133547335, 6.595905893872795467, 3.427874525163681074 ) ) ;
#167751=CARTESIAN_POINT ( 'NONE',  ( -1.364683531250000748, 1.509375000341421691, 0.000000000000000000 ) ) ;
#167752=CARTESIAN_POINT ( 'NONE',  ( -8.701635661872465732, 9.046329781806354831, 1.040834085586084257E-14 ) ) ;
#167755=CARTESIAN_POINT ( 'NONE',  ( 7.955937213120826357, 8.176348258262782664, 0.7998128361456481317 ) ) ;
#167756=CARTESIAN_POINT ( 'NONE',  ( -8.213542131780492639, 8.476887330032372603, 1.040834085586084257E-14 ) ) ;
#167759=CARTESIAN_POINT ( 'NONE',  ( -1.001543065824772872E-14, 5.571875000341416140, 1.575800808251672791 ) ) ;
#167763=CARTESIAN_POINT ( 'NONE',  ( 6.778713617152772208, 10.85232362007950258, -0.7216878364870267237 ) ) ;
#167766=CARTESIAN_POINT ( 'NONE',  ( -1.364683531250000748, 0.07187500034142035865, 0.000000000000000000 ) ) ;
#167769=CARTESIAN_POINT ( 'NONE',  ( 8.229436053370683624, 8.703356271795033905, 0.7216878364870458196 ) ) ;
#167771=CARTESIAN_POINT ( 'NONE',  ( -3.782361668532609134, 7.356579680022602652, 1.040834085586084257E-14 ) ) ;
#167774=CARTESIAN_POINT ( 'NONE',  ( 1.364683531249988535, 2.863541667008082658, 0.7879004041258500513 ) ) ;
#167779=CARTESIAN_POINT ( 'NONE',  ( -7.067878151425722955, 7.140279352951794500, 0.7998128361456341429 ) ) ;
#167780=CARTESIAN_POINT ( 'NONE',  ( -1.364683531249997417, 5.821875000341418804, 1.214306433183764966E-14 ) ) ;
#167787=CARTESIAN_POINT ( 'NONE',  ( 8.457588896826466751, 8.761608555919362828, 1.040834085586084257E-14 ) ) ;
#167791=CARTESIAN_POINT ( 'NONE',  ( 0.7499999999999902300, 2.733333333333351600, 1.299038105676669330 ) ) ;
#167797=CARTESIAN_POINT ( 'NONE',  ( 5.341549334104176872, 9.175631956522799726, 0.7216878364870438212 ) ) ;
#167798=CARTESIAN_POINT ( 'NONE',  ( -1.402160292154681736E-14, 0.6343750003414162508, 1.575800808251672791 ) ) ;
#167800=CARTESIAN_POINT ( 'NONE',  ( 10.71502147350184231, 11.39527989537399755, 0.000000000000000000 ) ) ;
#167805=CARTESIAN_POINT ( 'NONE',  ( -1.500000000000013101, 0.9208333333333594828, 0.8660254037844403729 ) ) ;
#167806=CARTESIAN_POINT ( 'NONE',  ( 8.911787042884274257, 9.291506392986812912, 0.7998128361456462443 ) ) ;
#167807=CARTESIAN_POINT ( 'NONE',  ( -9.179033691651859783, 10.66762638080401260, 1.199719254218462483 ) ) ;
#167809=CARTESIAN_POINT ( 'NONE',  ( -0.6823417656250212460, 1.051041667008083325, 1.181850606188755259 ) ) ;
#167810=CARTESIAN_POINT ( 'NONE',  ( 1.499999999999987121, 1.004166666666687968, 0.8660254037844524744 ) ) ;
#167812=CARTESIAN_POINT ( 'NONE',  ( 5.684946482831785275, 5.526859072925533134, -0.7998128361456231517 ) ) ;
#167819=CARTESIAN_POINT ( 'NONE',  ( -1.402160292154681736E-14, -0.6312499993171797330, -1.732050807568870754 ) ) ;
#167820=CARTESIAN_POINT ( 'NONE',  ( -8.044065211609668253, 8.279164256499745633, 0.7998128361456602331 ) ) ;
#167821=CARTESIAN_POINT ( 'NONE',  ( -5.422898255786198440, 7.349800603215774331, -1.443375672974052559 ) ) ;
#167823=DIRECTION ( 'NONE',  ( -5.578564026256490882E-16, -1.000000000000000000, -9.066213480720158442E-32 ) ) ;
#167829=CARTESIAN_POINT ( 'NONE',  ( 8.423693512792301163, 8.722063941212843119, 0.7998128361456481317 ) ) ;
#167831=FACE_OUTER_BOUND ( 'NONE', #192182, .T. ) ;
#167832=CARTESIAN_POINT ( 'NONE',  ( 6.846504384776753049, 9.010674420371453053, -1.443375672974058777 ) ) ;
#167837=CARTESIAN_POINT ( 'NONE',  ( -8.290974629956718189, 9.631557475493025322, -1.199719254218446718 ) ) ;
#167838=CARTESIAN_POINT ( 'NONE',  ( 4.599240423533799138, 6.388866465587984322, 1.599625672291267398 ) ) ;
#167843=CARTESIAN_POINT ( 'NONE',  ( 4.518945272056516416, 4.166524327021037699, 0.7998128361456341429 ) ) ;
#167850=CARTESIAN_POINT ( 'NONE',  ( -1.499999999999997780, 8.640473353474856566, -2.571377442220798670 ) ) ;
#167851=CARTESIAN_POINT ( 'NONE',  ( -4.284013352238262407, 6.021101549076499637, -1.443375672974053447 ) ) ;
#167853=CARTESIAN_POINT ( 'NONE',  ( 7.782016984564049444, 11.06247500109133064, 1.082531754730557072 ) ) ;
#167857=CARTESIAN_POINT ( 'NONE',  ( -7.040761844198392794, 7.108643661186573759, -0.7998128361456291469 ) ) ;
#167861=CARTESIAN_POINT ( 'NONE',  ( -0.9486429539237204445, 3.038339070649072493, -1.028101543438967980 ) ) ;
#167863=CARTESIAN_POINT ( 'NONE',  ( -8.857554428429624593, 9.228235009456373206, 0.7998128361456462443 ) ) ;
#167867=ORIENTED_EDGE ( 'NONE', *, *, #72583, .T. ) ;
#167876=CARTESIAN_POINT ( 'NONE',  ( -6.938021921891187382, 9.117444880338284818, -1.599625672291263179 ) ) ;
#167879=CARTESIAN_POINT ( 'NONE',  ( 3.714570900464269076, 7.277490450609545469, 0.7216878364870298324 ) ) ;
#167884=CARTESIAN_POINT ( 'NONE',  ( -4.623494077460110319, 5.352830164246910272, 1.199719254218462483 ) ) ;
#167893=CARTESIAN_POINT ( 'NONE',  ( -8.503988664269602538, 10.94440607977979063, 1.599625672291269396 ) ) ;
#167894=CARTESIAN_POINT ( 'NONE',  ( 6.287230548435207567, 8.358188277972981695, -1.599625672291262513 ) ) ;
#167898=CARTESIAN_POINT ( 'NONE',  ( -8.611400122974211868, 13.19838391011195888, 1.040834085586084257E-14 ) ) ;
#167902=CARTESIAN_POINT ( 'NONE',  ( -1.364683531250000748, -0.4281249996585800854, 0.000000000000000000 ) ) ;
#167906=CARTESIAN_POINT ( 'NONE',  ( 7.456621297836067086, 10.68284669990868174, 1.082531754730558626 ) ) ;
#167910=LINE ( 'NONE', #101842, #192875 ) ;
#167933=CARTESIAN_POINT ( 'NONE',  ( 1.499999999999987566, -0.4437499993171847845, 0.000000000000000000 ) ) ;
#167937=ORIENTED_EDGE ( 'NONE', *, *, #117124, .T. ) ;
#167939=CARTESIAN_POINT ( 'NONE',  ( 0.1399574524686736654, 8.210952333604119247, -2.038660652713630395 ) ) ;
#167941=CARTESIAN_POINT ( 'NONE',  ( 9.887974103068218668, 10.43039129653476493, 0.7998128361456462443 ) ) ;
#167946=CARTESIAN_POINT ( 'NONE',  ( 4.172158584703322681, 5.890604320285754980, -1.599625672291256295 ) ) ;
#167947=CARTESIAN_POINT ( 'NONE',  ( -0.6823417656250212460, 2.863541667008084879, 1.181850606188767472 ) ) ;
#167950=CARTESIAN_POINT ( 'NONE',  ( -6.808165692356648258, 11.09461040772476714, 0.7998128361456481317 ) ) ;
#167951=CARTESIAN_POINT ( 'NONE',  ( -4.622967192135580383, 5.456178481322002227, 1.082531754730558626 ) ) ;
#167955=CARTESIAN_POINT ( 'NONE',  ( -1.500000000000001332, -0.5687499993171779566, 0.000000000000000000 ) ) ;
#167962=CARTESIAN_POINT ( 'NONE',  ( -5.544921637864841379, 5.571422787038166291, -0.7216878364870197293 ) ) ;
#167964=CARTESIAN_POINT ( 'NONE',  ( 4.023704138721054591, 7.562441369377219225, 0.3480857562657164173 ) ) ;
#167966=EDGE_CURVE ( 'NONE', #33385, #137589, #15861, .T. ) ;
#167970=CARTESIAN_POINT ( 'NONE',  ( -4.921246571636213929, 4.843801876438091902, 0.7216878364870317197 ) ) ;
#167971=CARTESIAN_POINT ( 'NONE',  ( 8.666686507633574621, 11.13422023037111330, 1.599625672291281386 ) ) ;
#167978=EDGE_LOOP ( 'NONE', ( #180522, #125452, #181401, #150152 ) ) ;
#167981=CARTESIAN_POINT ( 'NONE',  ( -2.981903720001798597, 5.566305875722335372, -1.199719254218446718 ) ) ;
#167982=PLANE ( 'NONE',  #13138 ) ;
#167987=CARTESIAN_POINT ( 'NONE',  ( 6.356075086708249167, 6.309842444114747373, -0.7998128361456281477 ) ) ;
#167993=CARTESIAN_POINT ( 'NONE',  ( 3.623053363349855172, 5.249981562040033189, 1.599625672291267398 ) ) ;
#167995=ORIENTED_EDGE ( 'NONE', *, *, #69670, .T. ) ;
#167999=CARTESIAN_POINT ( 'NONE',  ( -5.738512597764678702, 5.917411899002910758, 2.440166504834945904 ) ) ;
#168003=CARTESIAN_POINT ( 'NONE',  ( 8.446893396513862839, 9.813462703143045474, -1.199719254218445830 ) ) ;
#168005=CARTESIAN_POINT ( 'NONE',  ( -4.629219384062206011, 7.488174150459498968, -1.199719254218452047 ) ) ;
#168012=CARTESIAN_POINT ( 'NONE',  ( -1.500000000000001332, -0.8187499993171781787, 0.000000000000000000 ) ) ;
#168015=EDGE_CURVE ( 'NONE', #78732, #77955, #93918, .T. ) ;
#168016=CARTESIAN_POINT ( 'NONE',  ( 4.982944139801846362, 4.915782372631361419, 0.3243353321068405126 ) ) ;
#168017=CARTESIAN_POINT ( 'NONE',  ( 5.190073875932979419, 4.949507698210251938, 0.7998128361456341429 ) ) ;
#168018=CARTESIAN_POINT ( 'NONE',  ( -4.680589345215810049, 6.483773540883647435, -1.599625672291256295 ) ) ;
#168024=CARTESIAN_POINT ( 'NONE',  ( 6.317736394288140822, 7.433409217166723870, 1.082531754730558626 ) ) ;
#168027=CARTESIAN_POINT ( 'NONE',  ( 8.581948047326003248, 9.114620264742901767, -0.7216878364870197293 ) ) ;
#168028=CARTESIAN_POINT ( 'NONE',  ( -1.364683531250012516, 4.051041667008088432, -0.7879004041258300672 ) ) ;
#168030=CARTESIAN_POINT ( 'NONE',  ( 4.243338890952890630, 5.973648010910253880, -1.443375672974051449 ) ) ;
#168039=CARTESIAN_POINT ( 'NONE',  ( -4.474540158260005285, 7.266292661500576955, 1.287230779100386968 ) ) ;
#168042=CARTESIAN_POINT ( 'NONE',  ( -1.001543065824772872E-14, 4.884375000341420581, 1.575800808251672791 ) ) ;
#168047=CARTESIAN_POINT ( 'NONE',  ( -10.32861409551237486, 10.94447128771960287, 1.040834085586084257E-14 ) ) ;
#168057=CARTESIAN_POINT ( 'NONE',  ( 3.877268743828276243, 4.586196958296845594, 1.082531754730560403 ) ) ;
#168058=CARTESIAN_POINT ( 'NONE',  ( 0.6823417656249917140, 4.905208333674755394, 1.181850606188765695 ) ) ;
#168060=CARTESIAN_POINT ( 'NONE',  ( 7.474622759835693131, 7.614814729430110951, -0.7998128361456281477 ) ) ;
#168061=CARTESIAN_POINT ( 'NONE',  ( -8.143643823302737061, 12.65266822716189843, 0.000000000000000000 ) ) ;
#168064=EDGE_CURVE ( 'NONE', #133229, #115335, #55503, .T. ) ;
#168069=CARTESIAN_POINT ( 'NONE',  ( -1.201851678989727383E-14, 3.962500000000022116, 1.732050807568877637 ) ) ;
#168070=CARTESIAN_POINT ( 'NONE',  ( 3.811813743736467419, 7.598866467667865443, 1.040834085586084257E-14 ) ) ;
#168073=CARTESIAN_POINT ( 'NONE',  ( -1.500000000000011324, 5.879166666666686858, -0.8660254037844312691 ) ) ;
#168074=ORIENTED_EDGE ( 'NONE', *, *, #167387, .T. ) ;
#168077=CARTESIAN_POINT ( 'NONE',  ( 6.805829924380097040, 10.88395931184472154, 0.7216878364870438212 ) ) ;
#168082=CARTESIAN_POINT ( 'NONE',  ( 1.499999999999989120, 2.785416667349484676, 0.8660254037844524744 ) ) ;
#168084=CARTESIAN_POINT ( 'NONE',  ( -4.985647801523292344, 6.839675073242382553, -1.599625672291256295 ) ) ;
#168085=CARTESIAN_POINT ( 'NONE',  ( 3.294268137996273715, 5.826768013428865522, -1.082531754730543971 ) ) ;
#168086=CARTESIAN_POINT ( 'NONE',  ( -9.991996023147281747, 11.72004545083573568, 1.082531754730558626 ) ) ;
#168095=CARTESIAN_POINT ( 'NONE',  ( 7.796102023057898123, 9.054206100777749455, -1.199719254218441611 ) ) ;
#168096=CARTESIAN_POINT ( 'NONE',  ( 3.334415713957098681, 5.977569868670206787, -1.199719254218446718 ) ) ;
#168099=( NAMED_UNIT ( * ) SI_UNIT ( $, .STERADIAN. ) SOLID_ANGLE_UNIT ( ) );
#168100=CARTESIAN_POINT ( 'NONE',  ( 5.366329872910639232, 5.155139694684188534, 1.040834085586084257E-14 ) ) ;
#168112=CARTESIAN_POINT ( 'NONE',  ( 5.144285979226959959, 6.473071224410549718, -1.197504025336363576 ) ) ;
#168114=CARTESIAN_POINT ( 'NONE',  ( 10.16199982864259788, 11.81442020729326536, 1.199719254218452047 ) ) ;
#168119=CARTESIAN_POINT ( 'NONE',  ( 6.860062538834778678, 8.066123052471139587, -1.082531754730543083 ) ) ;
#168120=CARTESIAN_POINT ( 'NONE',  ( -4.451154503988200339, 4.087435097607984957, 1.214306433183764966E-14 ) ) ;
#168125=CARTESIAN_POINT ( 'NONE',  ( -6.227272627378437342, 6.159572908229946187, -0.7998128361456291469 ) ) ;
#168135=CARTESIAN_POINT ( 'NONE',  ( 7.587759525142423911, 12.00413654597487501, 0.7998128361456462443 ) ) ;
#168136=CARTESIAN_POINT ( 'NONE',  ( 6.017762162252820346, 6.076696597586958681, 0.5614182107811436229 ) ) ;
#168138=ORIENTED_EDGE ( 'NONE', *, *, #92189, .F. ) ;
#168141=( BOUNDED_CURVE ( )  B_SPLINE_CURVE ( 1, ( #43544, #28334 ),
 .UNSPECIFIED., .F., .T. ) 
 B_SPLINE_CURVE_WITH_KNOTS ( ( 2, 2 ),
 ( 0.000000000000000000, 1.644734566718861202E-05 ),
 .UNSPECIFIED. ) 
 CURVE ( )  GEOMETRIC_REPRESENTATION_ITEM ( )  RATIONAL_B_SPLINE_CURVE ( ( 0.9345202395942817652, 0.9345202395942817652 ) ) 
 REPRESENTATION_ITEM ( '' )  );
#168145=CARTESIAN_POINT ( 'NONE',  ( -7.700668062882059850, 11.92793714009701311, -0.7216878364870267237 ) ) ;
#168149=CARTESIAN_POINT ( 'NONE',  ( 6.968000882419564945, 10.21675256520979858, 1.199719254218460707 ) ) ;
#168151=CARTESIAN_POINT ( 'NONE',  ( 0.1664695996868958416, 2.800000000000018030, 1.413346573192864497 ) ) ;
#168153=CARTESIAN_POINT ( 'NONE',  ( 4.029797971759831121, 5.724516938518342535, -1.599625672291255185 ) ) ;
#168155=CARTESIAN_POINT ( 'NONE',  ( -6.063521013809733518, 8.097193820909906137, 1.599625672291283607 ) ) ;
#168156=FACE_OUTER_BOUND ( 'NONE', #95703, .T. ) ;
#168160=CARTESIAN_POINT ( 'NONE',  ( 7.404724451357931336, 11.79059562655963056, 0.7998128361456462443 ) ) ;
#168164=CARTESIAN_POINT ( 'NONE',  ( 4.078932850288060408, 7.722175824222965446, -0.6089670364913578604 ) ) ;
#168166=CARTESIAN_POINT ( 'NONE',  ( 5.422898255786183341, 7.349800603215774331, -1.443375672974051449 ) ) ;
#168173=CARTESIAN_POINT ( 'NONE',  ( 8.446366511189332016, 9.916811020218137429, -1.082531754730543083 ) ) ;
#168174=ADVANCED_FACE ( 'NONE', ( #110655 ), #27191, .F. ) ;
#168177=CARTESIAN_POINT ( 'NONE',  ( -6.516665389662827934, 10.75452672124865217, 0.000000000000000000 ) ) ;
#168179=DIRECTION ( 'NONE',  ( 0.000000000000000000, -1.000000000000000000, 0.000000000000000000 ) ) ;
#168186=CARTESIAN_POINT ( 'NONE',  ( 8.204655514564224816, 12.72384853363364066, 1.040834085586084257E-14 ) ) ;
#168190=CARTESIAN_POINT ( 'NONE',  ( 3.662674053986138656, 7.424870162959149589, 0.7998128361456321445 ) ) ;
#168193=CARTESIAN_POINT ( 'NONE',  ( 0.7499999999999902300, 3.764583334016149863, 1.299038105676669330 ) ) ;
#168199=CARTESIAN_POINT ( 'NONE',  ( 1.499999999999987121, 2.004166666666684637, 0.8660254037844524744 ) ) ;
#168200=CARTESIAN_POINT ( 'NONE',  ( 6.693975156845185737, 8.832723654451292816, 1.599625672291281386 ) ) ;
#168201=CARTESIAN_POINT ( 'NONE',  ( 4.704316113817540668, 5.551085556617666228, -1.082531754730548412 ) ) ;
#168205=CARTESIAN_POINT ( 'NONE',  ( 7.944714827928039291, 11.25228915168265864, 1.082531754730557072 ) ) ;
#168211=CARTESIAN_POINT ( 'NONE',  ( -4.205000198532790279, 8.057583998263570635, 0.7998128361456341429 ) ) ;
#168212=CARTESIAN_POINT ( 'NONE',  ( 0.7499999999999902300, 4.347916667349481123, -1.299038105676658228 ) ) ;
#168213=CARTESIAN_POINT ( 'NONE',  ( -0.6823417656250003738, -1.032291666325242607, -1.181850606188749264 ) ) ;
#168217=CARTESIAN_POINT ( 'NONE',  ( 8.663296969007976855, 12.09063498294259809, -1.082531754730543083 ) ) ;
#168219=CARTESIAN_POINT ( 'NONE',  ( -1.201851678989727383E-14, 3.509375000341421469, -1.575800808251660134 ) ) ;
#168227=DIRECTION ( 'NONE',  ( 0.6507913734559712671, 0.7592566023652943530, 0.000000000000000000 ) ) ;
#168229=CARTESIAN_POINT ( 'NONE',  ( -8.311311860377216476, 9.655284244316948872, -1.199719254218446718 ) ) ;
#168230=CARTESIAN_POINT ( 'NONE',  ( 4.482942347612929979, 8.381849838857084123, 1.040834085586084257E-14 ) ) ;
#168232=CARTESIAN_POINT ( 'NONE',  ( -1.402160292154681736E-14, -0.9281249996585830830, 1.575800808251672791 ) ) ;
#168237=CARTESIAN_POINT ( 'NONE',  ( -4.855791571988752331, 8.816840600628864877, 0.7998128361456481317 ) ) ;
#168240=CARTESIAN_POINT ( 'NONE',  ( 8.218213668177886788, 12.73966637951625813, 0.7998128361456462443 ) ) ;
#168242=CARTESIAN_POINT ( 'NONE',  ( 7.703003830858588863, 12.13858823597705872, -0.7998128361456291469 ) ) ;
#168245=CARTESIAN_POINT ( 'NONE',  ( -4.277761160311629673, 4.949475094240346706, 1.199719254218462483 ) ) ;
#168246=CARTESIAN_POINT ( 'NONE',  ( -9.020252271793614440, 9.418049160047695878, 0.7998128361456462443 ) ) ;
#168249=CARTESIAN_POINT ( 'NONE',  ( -4.503925953283787642, 7.237052973511334919, 1.308369160636771333 ) ) ;
#168250=CARTESIAN_POINT ( 'NONE',  ( -0.6823417656250246877, -1.198958332991911790, 1.181850606188755259 ) ) ;
#168254=CARTESIAN_POINT ( 'NONE',  ( 9.110716038703335684, 9.731516254683127087, -0.7216878364870197293 ) ) ;
#168257=CARTESIAN_POINT ( 'NONE',  ( 5.307127064745490230, 8.279066444590018392, -1.199719254218452935 ) ) ;
#168276=ORIENTED_EDGE ( 'NONE', *, *, #109130, .F. ) ;
#168279=CARTESIAN_POINT ( 'NONE',  ( -6.970863535720637216, 11.28442455831609337, 0.7998128361456481317 ) ) ;
#168287=CARTESIAN_POINT ( 'NONE',  ( 1.499999999999989120, 2.056250000682817269, 1.214306433183764966E-14 ) ) ;
#168288=CARTESIAN_POINT ( 'NONE',  ( 9.890836756369282057, 11.49806328964105617, -1.199719254218440723 ) ) ;
#168291=VERTEX_POINT ( 'NONE', #148425 ) ;
#168295=CARTESIAN_POINT ( 'NONE',  ( -0.6823417656250003738, 1.717708333674752730, -1.181850606188749264 ) ) ;
#168296=CARTESIAN_POINT ( 'NONE',  ( 0.7499999999999920064, 5.483333333333353821, 1.299038105676669330 ) ) ;
#168301=CARTESIAN_POINT ( 'NONE',  ( -4.115063316947640715, 4.759660943649018705, 1.199719254218462483 ) ) ;
#168305=CARTESIAN_POINT ( 'NONE',  ( -0.6823417656250003738, 0.03020833367475134201, -1.181850606188749264 ) ) ;
#168310=CARTESIAN_POINT ( 'NONE',  ( -1.402160292154681736E-14, 1.946875000341422579, -1.575800808251660134 ) ) ;
#168313=CARTESIAN_POINT ( 'NONE',  ( -7.549192604710863286, 7.701812881784464437, -0.7998128361456291469 ) ) ;
#168314=CARTESIAN_POINT ( 'NONE',  ( 8.613507663383630941, 8.943513783569379427, -0.7998128361456221525 ) ) ;
#168317=CARTESIAN_POINT ( 'NONE',  ( 4.873266149108180123, 7.772895376346490970, 1.199719254218462483 ) ) ;
#168319=CARTESIAN_POINT ( 'NONE',  ( -1.201851678989727383E-14, 4.337500000000023448, -1.732050807568863648 ) ) ;
#168322=CARTESIAN_POINT ( 'NONE',  ( -1.201851678989727383E-14, 1.634375000341421025, 1.575800808251672791 ) ) ;
#168328=CARTESIAN_POINT ( 'NONE',  ( 6.819388077993785657, 7.058300300521964665, 1.040834085586084257E-14 ) ) ;
#168331=CARTESIAN_POINT ( 'NONE',  ( -8.799405390469187793, 10.22472669609091689, -1.199719254218446718 ) ) ;
#168332=CARTESIAN_POINT ( 'NONE',  ( -3.079673448598517549, 6.744702790006905424, 1.040834085586084257E-14 ) ) ;
#168333=CARTESIAN_POINT ( 'NONE',  ( -0.6823417656250212460, 3.113541667008084879, 1.181850606188767472 ) ) ;
#168337=CARTESIAN_POINT ( 'NONE',  ( -6.507550544435101614, 10.53596670190887963, 0.000000000000000000 ) ) ;
#168339=CARTESIAN_POINT ( 'NONE',  ( -1.500000000000011324, 4.920833333333354709, 0.8660254037844403729 ) ) ;
#168342=CARTESIAN_POINT ( 'NONE',  ( 9.083599731475992201, 9.699880562917908122, 0.7216878364870438212 ) ) ;
#168348=ORIENTED_EDGE ( 'NONE', *, *, #136238, .F. ) ;
#168352=CARTESIAN_POINT ( 'NONE',  ( 9.449669878600614581, 12.04770082983265844, -1.443375672974058777 ) ) ;
#168356=VECTOR ( 'NONE', #109192, 1000.000000000000000 ) ;
#168357=CARTESIAN_POINT ( 'NONE',  ( 7.962716289927667113, 8.184257181204083409, -0.7998128361456291469 ) ) ;
#168358=CARTESIAN_POINT ( 'NONE',  ( -4.446184310277715213, 7.274633231044262516, -1.199719254218452047 ) ) ;
#168361=CARTESIAN_POINT ( 'NONE',  ( 6.602457619730767391, 7.765583980183128787, 1.082531754730558626 ) ) ;
#168362=CARTESIAN_POINT ( 'NONE',  ( -1.364683531250014514, -0.4072916663252447167, 0.7879004041258379498 ) ) ;
#168363=CARTESIAN_POINT ( 'NONE',  ( 3.714570900464278846, 5.356752022006865843, 1.443375672974062551 ) ) ;
#168365=CARTESIAN_POINT ( 'NONE',  ( -3.755772246185468788, 4.340488027759846545, -1.199719254218452047 ) ) ;
#168371=CARTESIAN_POINT ( 'NONE',  ( -1.499999999999997780, 3.931250000682819046, 1.214306433183764966E-14 ) ) ;
#168380=CARTESIAN_POINT ( 'NONE',  ( 6.938893903907228378E-15, 10.64264068711930733, 1.214306433183764966E-14 ) ) ;
#168381=CARTESIAN_POINT ( 'NONE',  ( 5.933664784275179294, 10.07435934829639912, -0.7998128361456291469 ) ) ;
#168384=ORIENTED_EDGE ( 'NONE', *, *, #31325, .T. ) ;
#168393=CARTESIAN_POINT ( 'NONE',  ( -5.922214171070950606, 5.803671375871217286, -0.7998128361456291469 ) ) ;
#168395=CARTESIAN_POINT ( 'NONE',  ( -3.242371291962510504, 6.934516940598226320, 1.040834085586084257E-14 ) ) ;
#168400=CARTESIAN_POINT ( 'NONE',  ( 1.499999999999990896, 4.806250000682819490, 1.214306433183764966E-14 ) ) ;
#168401=ADVANCED_FACE ( 'NONE', ( #166797 ), #133260, .T. ) ;
#168405=CARTESIAN_POINT ( 'NONE',  ( -4.386226389220933441, 5.076017861301227008, -1.199719254218446718 ) ) ;
#168408=CARTESIAN_POINT ( 'NONE',  ( 5.880485940025228508, 7.883652901494672349, 1.599625672291267398 ) ) ;
#168409=CARTESIAN_POINT ( 'NONE',  ( -1.201851678989727383E-14, 5.196875000341421469, -1.575800808251660134 ) ) ;
#168415=CARTESIAN_POINT ( 'NONE',  ( 6.114364089638795186, 7.196141528409145671, 1.082531754730558626 ) ) ;
#168416=CARTESIAN_POINT ( 'NONE',  ( -5.194745412330402878, 9.212286747694129474, 0.000000000000000000 ) ) ;
#168419=CARTESIAN_POINT ( 'NONE',  ( -7.100719765255177229, 9.307259030929609267, -1.599625672291263179 ) ) ;
#168421=CARTESIAN_POINT ( 'NONE',  ( -5.870844209917351009, 6.808071985447069707, -1.199719254218446718 ) ) ;
#168428=CARTESIAN_POINT ( 'NONE',  ( 5.913327553854682783, 10.05063257947248800, -0.7998128361456291469 ) ) ;
#168441=CARTESIAN_POINT ( 'NONE',  ( 1.499999999999989120, 5.504166666666685970, 0.8660254037844524744 ) ) ;
#168442=CARTESIAN_POINT ( 'NONE',  ( 4.871457266011829823, 4.577788319968905562, -0.7998128361456221525 ) ) ;
#168443=CARTESIAN_POINT ( 'NONE',  ( 4.794779880727245036, 8.745660294157122649, -0.7998128361456281477 ) ) ;
#168445=CARTESIAN_POINT ( 'NONE',  ( -8.690413276679693766, 9.241163032322203819, 1.040834085586084257E-14 ) ) ;
#168447=CARTESIAN_POINT ( 'NONE',  ( 5.422898255786183341, 7.349800603215774331, -1.443375672974051449 ) ) ;
#168448=CARTESIAN_POINT ( 'NONE',  ( -7.334597914868722590, 11.50085530074811935, -0.7216878364870267237 ) ) ;
#168451=CARTESIAN_POINT ( 'NONE',  ( 7.670162217029129259, 9.971608557999250166, 1.599625672291281386 ) ) ;
#168457=CARTESIAN_POINT ( 'NONE',  ( 1.364683531249990311, 4.134375000341417028, 1.214306433183764966E-14 ) ) ;
#168462=CARTESIAN_POINT ( 'NONE',  ( 7.801827329660018684, 11.18955008699033726, 1.199719254218460707 ) ) ;
#168466=CARTESIAN_POINT ( 'NONE',  ( -9.179033691651859783, 10.66762638080401260, 1.199719254218462483 ) ) ;
#168472=CARTESIAN_POINT ( 'NONE',  ( 3.029357257649615054, 5.621668336311468117, -1.199719254218446718 ) ) ;
#168475=CARTESIAN_POINT ( 'NONE',  ( -9.504429378379839477, 11.04725468198666150, 1.199719254218462483 ) ) ;
#168481=CARTESIAN_POINT ( 'NONE',  ( 5.863316726098953602, 5.994608360591326068, -0.2888550730815123702 ) ) ;
#168483=CARTESIAN_POINT ( 'NONE',  ( -3.144601563365788444, 5.756120026313656268, -1.199719254218452935 ) ) ;
#168487=CARTESIAN_POINT ( 'NONE',  ( 7.396136491454752715, 8.587579647240744407, 1.199719254218462483 ) ) ;
#168489=CARTESIAN_POINT ( 'NONE',  ( 5.666418135507635512, 8.698239360479199433, 1.199719254218462483 ) ) ;
#168490=CARTESIAN_POINT ( 'NONE',  ( 5.009901455449552010, 5.803638771901306725, -1.199719254218452047 ) ) ;
#168492=CIRCLE ( 'NONE', #33658, 0.08000000000000025147 ) ;
#168493=CARTESIAN_POINT ( 'NONE',  ( -7.049876689426097798, 11.16868053773170821, -0.7216878364870267237 ) ) ;
#168500=CARTESIAN_POINT ( 'NONE',  ( -4.245996903372413200, 7.323364108789364835, -0.8915694317389293300 ) ) ;
#168503=CARTESIAN_POINT ( 'NONE',  ( 4.175548123328908900, 7.815297210618305179, -0.7216878364870197293 ) ) ;
#168523=CARTESIAN_POINT ( 'NONE',  ( -8.717529583462656717, 11.19353715217169309, 1.443375672974064550 ) ) ;
#168527=CARTESIAN_POINT ( 'NONE',  ( 7.934546212495622086, 10.28005655271014795, -1.599625672291262513 ) ) ;
#168531=CARTESIAN_POINT ( 'NONE',  ( -0.7500000000000215383, 1.222916667349485564, 1.299038105676659116 ) ) ;
#168533=CARTESIAN_POINT ( 'NONE',  ( -4.205000198532790279, 8.057583998263570635, 0.7998128361456341429 ) ) ;
#168536=CARTESIAN_POINT ( 'NONE',  ( -7.296259222448620463, 11.66405285949874759, 0.7998128361456481317 ) ) ;
#168537=CARTESIAN_POINT ( 'NONE',  ( -3.294268138440636928, 6.787137228248626641, 1.040834085586084257E-14 ) ) ;
#168539=ADVANCED_FACE ( 'NONE', ( #117039 ), #190462, .T. ) ;
#168541=CARTESIAN_POINT ( 'NONE',  ( 7.800018446563675489, 7.994443030612759848, -0.7998128361456281477 ) ) ;
#168543=CARTESIAN_POINT ( 'NONE',  ( -5.876569516519495551, 8.943415971659659292, 1.199719254218452047 ) ) ;
#168545=CARTESIAN_POINT ( 'NONE',  ( 9.908311333488716954, 10.45411806535867782, 0.7998128361456462443 ) ) ;
#168546=DIRECTION ( 'NONE',  ( -0.9366510587354612838, 1.084202172485500963E-14, -0.3502638921866474409 ) ) ;
#168551=CARTESIAN_POINT ( 'NONE',  ( -6.832946231607472498, 9.955225789308602913, 1.082531754730549967 ) ) ;
#168554=CARTESIAN_POINT ( 'NONE',  ( 0.6823417656249917140, 4.655208333674755394, 1.181850606188765695 ) ) ;
#168558=CARTESIAN_POINT ( 'NONE',  ( -1.364683531250010295, 5.280208333674758059, 0.7879004041258379498 ) ) ;
#168560=CARTESIAN_POINT ( 'NONE',  ( -2.589244150085650009, 5.964609241834465614, 0.7216878364870317197 ) ) ;
#168562=CARTESIAN_POINT ( 'NONE',  ( 4.175548122884573665, 3.973820352894515295, 1.214306433183764966E-14 ) ) ;
#168563=CARTESIAN_POINT ( 'NONE',  ( -1.001543065824772872E-14, 5.384375000341415252, 1.575800808251672791 ) ) ;
#168567=CARTESIAN_POINT ( 'NONE',  ( -1.364683531250000748, 1.509375000341421691, 0.000000000000000000 ) ) ;
#168568=CARTESIAN_POINT ( 'NONE',  ( -4.473827502829599290, 4.321812962830357208, 0.7216878364870317197 ) ) ;
#168569=CARTESIAN_POINT ( 'NONE',  ( 2.998324526916512411, 6.649795714711241423, 0.000000000000000000 ) ) ;
#168574=FACE_OUTER_BOUND ( 'NONE', #192639, .T. ) ;
#168577=CARTESIAN_POINT ( 'NONE',  ( -7.212574532790092974, 10.39812547402169862, -1.082531754730543971 ) ) ;
#168583=CARTESIAN_POINT ( 'NONE',  ( -9.267161690140662600, 10.77044237904097734, -1.199719254218441611 ) ) ;
#168584=CARTESIAN_POINT ( 'NONE',  ( -4.324687812634898876, 6.068555086205916105, 1.443375672974064550 ) ) ;
#168585=CARTESIAN_POINT ( 'NONE',  ( 0.6823417656249899377, 1.905208333674752952, 1.181850606188755259 ) ) ;
#168592=CARTESIAN_POINT ( 'NONE',  ( 9.103410076571945453, 12.70806329172093818, 1.199719254218450271 ) ) ;
#168607=CARTESIAN_POINT ( 'NONE',  ( -1.201851678989727383E-14, 3.509375000341421469, -1.575800808251660134 ) ) ;
#168611=CARTESIAN_POINT ( 'NONE',  ( -7.334597915313094241, 9.580116872663850813, 1.040834085586084257E-14 ) ) ;
#168614=CARTESIAN_POINT ( 'NONE',  ( 7.723341061279088038, 12.16231500480096983, -0.7998128361456291469 ) ) ;
#168617=CARTESIAN_POINT ( 'NONE',  ( -1.364683531250014514, 0.9885416670080898749, -0.7879004041258289570 ) ) ;
#168619=ORIENTED_EDGE ( 'NONE', *, *, #42815, .T. ) ;
#168627=CARTESIAN_POINT ( 'NONE',  ( 3.032219910950674890, 6.689340329417765574, 0.7998128361456321445 ) ) ;
#168639=CARTESIAN_POINT ( 'NONE',  ( -3.704402285031864306, 5.344888637335695414, -1.599625672291256295 ) ) ;
#168640=CARTESIAN_POINT ( 'NONE',  ( 8.620286740190458374, 8.951422706510690830, 1.040834085586084257E-14 ) ) ;
#168643=CARTESIAN_POINT ( 'NONE',  ( 5.965224399888476192, 6.061776009399090448, 1.040834085586084257E-14 ) ) ;
#168651=DIRECTION ( 'NONE',  ( -0.6507913734559640506, -0.7592566023653004592, 0.000000000000000000 ) ) ;
#168652=CARTESIAN_POINT ( 'NONE',  ( -6.399085315970142851, 8.488685506763726352, -1.443375672974059665 ) ) ;
#168654=CARTESIAN_POINT ( 'NONE',  ( 6.647575389402066826, 6.649926130590872120, 1.040834085586084257E-14 ) ) ;
#168657=CARTESIAN_POINT ( 'NONE',  ( -7.811469059767924605, 12.26513100303794168, -0.7998128361456281477 ) ) ;
#168662=CARTESIAN_POINT ( 'NONE',  ( -4.634189577772691138, 4.300976017023221409, 1.214306433183764966E-14 ) ) ;
#168665=CARTESIAN_POINT ( 'NONE',  ( 10.57266086055835075, 11.22919251360659310, 0.000000000000000000 ) ) ;
#168666=CARTESIAN_POINT ( 'NONE',  ( 4.379447312414087357, 5.068108938359919158, -1.199719254218452047 ) ) ;
#168672=CARTESIAN_POINT ( 'NONE',  ( 2.738383840280320669, 6.138605547061593448, 0.7216878364870338292 ) ) ;
#168675=CARTESIAN_POINT ( 'NONE',  ( -5.253948220495577637, 6.088359997788290734, 1.199719254218450271 ) ) ;
#168676=CARTESIAN_POINT ( 'NONE',  ( 0.000000000000000000, 2.817530495244580102, 1.214306433183764966E-14 ) ) ;
#168679=CARTESIAN_POINT ( 'NONE',  ( -8.513630394377489807, 12.01998699582738972, -1.199719254218446718 ) ) ;
#168684=CARTESIAN_POINT ( 'NONE',  ( 8.161645285746708112, 9.584636257201740506, -1.082531754730543083 ) ) ;
#168687=CARTESIAN_POINT ( 'NONE',  ( 3.486418057008484617, 7.219238166485217434, 1.040834085586084257E-14 ) ) ;
#168698=EDGE_CURVE ( 'NONE', #55454, #193812, #82288, .T. ) ;
#168699=ORIENTED_EDGE ( 'NONE', *, *, #36264, .T. ) ;
#168701=CARTESIAN_POINT ( 'NONE',  ( -1.201851678989727383E-14, 3.134375000341420137, 1.575800808251672791 ) ) ;
#168703=CARTESIAN_POINT ( 'NONE',  ( 10.56588178375152864, 11.22128359066528169, -0.7998128361456281477 ) ) ;
#168705=CARTESIAN_POINT ( 'NONE',  ( -3.768803514918943609, 7.340761834139994058, 0.7216878364870317197 ) ) ;
#168707=CARTESIAN_POINT ( 'NONE',  ( -4.541618270453545492, 8.242379048930368768, 0.7216878364870458196 ) ) ;
#168713=CARTESIAN_POINT ( 'NONE',  ( 5.311043488251262268, 7.219303374425030562, -1.599625672291256295 ) ) ;
#168720=CARTESIAN_POINT ( 'NONE',  ( 1.257518954445002723, 2.989770990628810132, 0.7750000000000100142 ) ) ;
#168725=CARTESIAN_POINT ( 'NONE',  ( 6.654354466208897811, 6.657835053532175529, 0.7998128361456341429 ) ) ;
#168727=CARTESIAN_POINT ( 'NONE',  ( -2.428882075142555497, 5.985446187641602300, 1.040834085586084257E-14 ) ) ;
#168729=CARTESIAN_POINT ( 'NONE',  ( -6.575868197828002693, 7.630599971342813426, 1.199719254218450271 ) ) ;
#168734=CARTESIAN_POINT ( 'NONE',  ( 6.262976894508937242, 9.394224579314053969, -1.199719254218440723 ) ) ;
#168736=CARTESIAN_POINT ( 'NONE',  ( -7.074657228232555717, 7.148188275893099686, 1.040834085586084257E-14 ) ) ;
#168737=CARTESIAN_POINT ( 'NONE',  ( 7.266807146800403849, 7.580289214129690478, 1.040834085586084257E-14 ) ) ;
#168738=CARTESIAN_POINT ( 'NONE',  ( 4.748509658595381211, 7.014904321862622361, 1.395353610025750646 ) ) ;
#168739=CARTESIAN_POINT ( 'NONE',  ( -3.623053363349869382, 5.249981562040033189, 1.599625672291267398 ) ) ;
#168742=CARTESIAN_POINT ( 'NONE',  ( -4.900382456335551140, 7.804531068111707270, 1.199719254218464037 ) ) ;
#168745=CARTESIAN_POINT ( 'NONE',  ( -1.364683531250000748, 2.259375000341422357, 1.214306433183764966E-14 ) ) ;
#168747=CARTESIAN_POINT ( 'NONE',  ( -5.775410249741523394, 5.840326167560965231, 0.7216878364870317197 ) ) ;
#168754=CARTESIAN_POINT ( 'NONE',  ( 5.900823170445728572, 7.907379670318584353, 1.599625672291267398 ) ) ;
#168757=CARTESIAN_POINT ( 'NONE',  ( 0.6823417656249899377, 2.905208333674754062, 1.181850606188765695 ) ) ;
#168762=CARTESIAN_POINT ( 'NONE',  ( -3.490334480514268645, 6.159475096320226939, -1.199719254218452935 ) ) ;
#168763=CARTESIAN_POINT ( 'NONE',  ( -7.253248993186740989, 9.485209796849769504, 1.443375672974090751 ) ) ;
#168766=CARTESIAN_POINT ( 'NONE',  ( 0.6823417656249899377, 3.676041667008085767, -1.181850606188754593 ) ) ;
#168773=CARTESIAN_POINT ( 'NONE',  ( -7.497295758232736418, 7.849192594134070333, -0.7216878364870267237 ) ) ;
#168778=CARTESIAN_POINT ( 'NONE',  ( -5.517805330637490790, 9.381263952478319013, 0.7216878364870458196 ) ) ;
#168783=CARTESIAN_POINT ( 'NONE',  ( 0.7499999999999902300, 5.597916667349482900, -1.299038105676658228 ) ) ;
#168788=ORIENTED_EDGE ( 'NONE', *, *, #55029, .T. ) ;
#168791=CARTESIAN_POINT ( 'NONE',  ( -4.880045225915050189, 7.780804299287790826, 1.199719254218464037 ) ) ;
#168794=CARTESIAN_POINT ( 'NONE',  ( 2.686486993802192913, 6.285985259411197568, 0.7998128361456362523 ) ) ;
#168796=CARTESIAN_POINT ( 'NONE',  ( -1.499999999999997780, 7.240846818246208905, -4.154462424328208670 ) ) ;
#168798=CARTESIAN_POINT ( 'NONE',  ( 6.830610463186557624, 6.863467050006115677, 1.040834085586084257E-14 ) ) ;
#168803=CARTESIAN_POINT ( 'NONE',  ( -5.761852096127856981, 5.824508321678349532, 0.000000000000000000 ) ) ;
#168809=CARTESIAN_POINT ( 'NONE',  ( 3.092648394857516525, 6.449253795920727228, -0.4031905389056261724 ) ) ;
#168810=VERTEX_POINT ( 'NONE', #192351 ) ;
#168813=CARTESIAN_POINT ( 'NONE',  ( -1.201851678989727383E-14, 2.321875000341416584, 1.575800808251672791 ) ) ;
#168815=CARTESIAN_POINT ( 'NONE',  ( -7.690499447449645309, 9.995335326823163058, 1.599625672291295375 ) ) ;
#168817=CARTESIAN_POINT ( 'NONE',  ( 5.798083248138522272, 9.916180889470295412, 0.7998128361456462443 ) ) ;
#168819=CARTESIAN_POINT ( 'NONE',  ( -7.985916173649233230, 9.275655943134292869, -1.199719254218446718 ) ) ;
#168822=CARTESIAN_POINT ( 'NONE',  ( -1.402160292154681736E-14, -0.3812499993171785673, -1.732050807568870754 ) ) ;
#168824=CARTESIAN_POINT ( 'NONE',  ( 8.595506201384013778, 10.09080732544527592, 1.082531754730558626 ) ) ;
#168826=CARTESIAN_POINT ( 'NONE',  ( -0.6823417656250003738, -0.7197916663252492686, -1.181850606188749264 ) ) ;
#168828=CARTESIAN_POINT ( 'NONE',  ( 3.146123468421266001, 6.442327133617253843, 0.5169845646841256803 ) ) ;
#168829=CARTESIAN_POINT ( 'NONE',  ( 8.581948047326003248, 9.114620264742901767, -0.7216878364870197293 ) ) ;
#168832=CARTESIAN_POINT ( 'NONE',  ( -4.392478581147607031, 7.108013530438723748, 1.082531754730560403 ) ) ;
#168835=CARTESIAN_POINT ( 'NONE',  ( -0.6823417656249969321, 3.717708333674754506, -1.181850606188749264 ) ) ;
#168837=CARTESIAN_POINT ( 'NONE',  ( 3.019342412789784547, 6.452475500722323787, 0.1501914610189964416 ) ) ;
#168839=CARTESIAN_POINT ( 'NONE',  ( -6.175902666224832416, 7.163973517805802160, -1.199719254218446718 ) ) ;
#168840=DIRECTION ( 'NONE',  ( -0.1430349330369308225, 0.000000000000000000, -0.9897176405071906879 ) ) ;
#168847=CARTESIAN_POINT ( 'NONE',  ( 6.795661308947685164, 8.951357498570873261, -1.599625672291262513 ) ) ;
#168850=CARTESIAN_POINT ( 'NONE',  ( -1.500000000000011324, 2.920833333333352932, 0.8660254037844403729 ) ) ;
#168854=CARTESIAN_POINT ( 'NONE',  ( -1.500000000000005773, 5.410416667349489117, -0.8660254037844342667 ) ) ;
#168857=CARTESIAN_POINT ( 'NONE',  ( 6.832946231607457399, 7.074118146404578589, -0.7216878364870257245 ) ) ;
#168858=CARTESIAN_POINT ( 'NONE',  ( -0.6823417656250003738, -0.4697916663252491021, -1.181850606188749264 ) ) ;
#168862=DIRECTION ( 'NONE',  ( 7.387867266669436732E-31, -1.000000000000000000, -8.546850786086424434E-32 ) ) ;
#168864=CARTESIAN_POINT ( 'NONE',  ( -0.7500000000000006661, 0.6083333333333564852, -1.299038105676652011 ) ) ;
#168865=CARTESIAN_POINT ( 'NONE',  ( 7.884230021546724920, 9.157022099014721306, 1.199719254218462483 ) ) ;
#168866=CARTESIAN_POINT ( 'NONE',  ( -9.691380875670077444, 10.20103253123691189, 0.7998128361456462443 ) ) ;
#168868=CARTESIAN_POINT ( 'NONE',  ( -1.402160292154681736E-14, -0.4281249996585808071, 1.575800808251672791 ) ) ;
#168869=CARTESIAN_POINT ( 'NONE',  ( -0.7500000000000006661, 0.8583333333333567072, -1.299038105676652011 ) ) ;
#168871=CARTESIAN_POINT ( 'NONE',  ( 6.498435699651741615, 6.475929825882159818, -0.7998128361456281477 ) ) ;
#168878=CARTESIAN_POINT ( 'NONE',  ( -1.364683531249997417, 5.009375000341425022, 1.214306433183764966E-14 ) ) ;
#168880=CARTESIAN_POINT ( 'NONE',  ( -6.723954117373590833, 9.932031339322813679, -1.199719254218440723 ) ) ;
#168881=CARTESIAN_POINT ( 'NONE',  ( -5.585596099150193616, 6.579245539505756746, -1.082531754730544860 ) ) ;
#168890=CARTESIAN_POINT ( 'NONE',  ( 8.762647353133951711, 9.117510088278095282, 1.040834085586084257E-14 ) ) ;
#168891=CARTESIAN_POINT ( 'NONE',  ( -5.886439722289627419, 6.118937485343680649, -0.7679415244158313003 ) ) ;
#168893=DIRECTION ( 'NONE',  ( 5.578564026256490882E-16, 1.000000000000000000, 9.066213480720158442E-32 ) ) ;
#168894=CARTESIAN_POINT ( 'NONE',  ( 7.768458830506048685, 8.165549511786275971, -0.7216878364870267237 ) ) ;
#168898=CARTESIAN_POINT ( 'NONE',  ( -7.320512876374914768, 10.62801655815766999, 1.199719254218453823 ) ) ;
#168900=CARTESIAN_POINT ( 'NONE',  ( 6.166260936116925606, 6.088392601758203071, 0.7998128361456341429 ) ) ;
#168901=CYLINDRICAL_SURFACE ( 'NONE', #73120, 1.250000000000000000 ) ;
#168903=CARTESIAN_POINT ( 'NONE',  ( 9.571693261567954636, 12.19006144329456731, 1.443375672974076540 ) ) ;
#168904=ORIENTED_EDGE ( 'NONE', *, *, #932, .T. ) ;
#168910=CARTESIAN_POINT ( 'NONE',  ( -1.576106191276491542, 8.678179183658462748, -2.499999999999308109 ) ) ;
#168911=CARTESIAN_POINT ( 'NONE',  ( -3.307826292054304673, 6.802955074131234348, -0.7216878364870267237 ) ) ;
#168912=CARTESIAN_POINT ( 'NONE',  ( 10.07334494527360569, 10.85458331234846696, 0.000000000000000000 ) ) ;
#168915=CARTESIAN_POINT ( 'NONE',  ( -5.669280788808708671, 9.765911353585494226, 0.7998128361456481317 ) ) ;
#168919=CARTESIAN_POINT ( 'NONE',  ( 3.895595285070167169, 2.800000000000017586, 0.7750000000000135669 ) ) ;
#168921=CARTESIAN_POINT ( 'NONE',  ( -6.832419346282942563, 10.05857410638369487, 1.199719254218453823 ) ) ;
#168938=CARTESIAN_POINT ( 'NONE',  ( -5.371001409308059138, 9.417918744168066070, -0.7998128361456231517 ) ) ;
#168941=CARTESIAN_POINT ( 'NONE',  ( 4.175548123328908900, 7.815297210618305179, -0.7216878364870197293 ) ) ;
#168942=ORIENTED_EDGE ( 'NONE', *, *, #54130, .F. ) ;
#168946=CARTESIAN_POINT ( 'NONE',  ( -4.599240423533815125, 6.388866465587984322, 1.599625672291267398 ) ) ;
#168953=CARTESIAN_POINT ( 'NONE',  ( -8.992082194361570302, 11.51384853155376220, 1.599625672291269396 ) ) ;
#168954=CARTESIAN_POINT ( 'NONE',  ( 6.612626235163189925, 8.737816579155630592, -1.599625672291262513 ) ) ;
#168957=CARTESIAN_POINT ( 'NONE',  ( -10.32183501870554387, 10.93656236477829502, 0.7998128361456462443 ) ) ;
#168960=CARTESIAN_POINT ( 'NONE',  ( 0.6823417656249882723, -0.01145833299191073573, -1.181850606188749264 ) ) ;
#168964=CARTESIAN_POINT ( 'NONE',  ( 7.605760987586388744, 11.81721221891873697, 1.040834085586084257E-14 ) ) ;
#168970=ORIENTED_EDGE ( 'NONE', *, *, #211914, .T. ) ;
#168974=CARTESIAN_POINT ( 'NONE',  ( -0.4702976403610291678, 6.650664745223592966, -3.344716071613587971 ) ) ;
#168994=CARTESIAN_POINT ( 'NONE',  ( 0.6823417656249917140, 5.342708333674749177, 1.181850606188765695 ) ) ;
#169000=CARTESIAN_POINT ( 'NONE',  ( 4.176167785551761824, 3.974543292672902961, -0.03298406423014330069 ) ) ;
#169001=DIRECTION ( 'NONE',  ( -0.000000000000000000, -8.546850786086437571E-32, -1.000000000000000000 ) ) ;
#169002=CARTESIAN_POINT ( 'NONE',  ( 2.517010073631369860, 6.088262185878572375, -0.7998128361456281477 ) ) ;
#169004=DIRECTION ( 'NONE',  ( 0.000000000000000000, 1.000000000000000000, -8.546850786086437571E-32 ) ) ;
#169008=CARTESIAN_POINT ( 'NONE',  ( 5.555090253297246150, 7.504024600312024340, 1.599625672291267398 ) ) ;
#169009=CARTESIAN_POINT ( 'NONE',  ( 1.364683531249990311, 3.196875000341416140, 1.214306433183764966E-14 ) ) ;
#169010=CARTESIAN_POINT ( 'NONE',  ( -5.906331710381417466, 6.003565991635761989, -0.1321356564752910190 ) ) ;
#169012=CARTESIAN_POINT ( 'NONE',  ( -7.374745490829552885, 10.69128794168811680, -1.199719254218446718 ) ) ;
#169013=CARTESIAN_POINT ( 'NONE',  ( -3.565431210269599749, 7.103494145382415859, 0.7216878364870317197 ) ) ;
#169016=CARTESIAN_POINT ( 'NONE',  ( -6.663996196316808174, 7.733415969579778171, -1.199719254218446718 ) ) ;
#169018=CARTESIAN_POINT ( 'NONE',  ( 1.499999999999987121, -0.4645833326505149907, 0.8660254037844524744 ) ) ;
#169025=CARTESIAN_POINT ( 'NONE',  ( -3.755245360860925086, 6.364574773437617239, -1.082531754730548412 ) ) ;
#169031=CARTESIAN_POINT ( 'NONE',  ( -4.731432421044883263, 5.582721248382882528, -1.082531754730543971 ) ) ;
#169033=CARTESIAN_POINT ( 'NONE',  ( 9.043452155515161905, 10.50944792197790889, 1.199719254218453823 ) ) ;
#169042=CARTESIAN_POINT ( 'NONE',  ( -9.378489572351046633, 11.96465713920816043, -1.599625672291263179 ) ) ;
#169047=CARTESIAN_POINT ( 'NONE',  ( 4.819033534653518025, 7.709623992816043270, -1.199719254218452047 ) ) ;
#169051=ORIENTED_EDGE ( 'NONE', *, *, #120432, .T. ) ;
#169053=CARTESIAN_POINT ( 'NONE',  ( 3.460355519985863548, 5.060167411448709629, 1.599625672291267398 ) ) ;
#169063=CARTESIAN_POINT ( 'NONE',  ( 8.782984583554449998, 9.141236857102018831, 1.040834085586084257E-14 ) ) ;
#169065=CARTESIAN_POINT ( 'NONE',  ( -4.252453736180621391, 8.112946458852704268, -0.7998128361456281477 ) ) ;
#169069=AXIS2_PLACEMENT_3D ( 'NONE', #90935, #57352, #126698 ) ;
#169071=CARTESIAN_POINT ( 'NONE',  ( -1.500000000000001332, -1.318749999317178734, 0.000000000000000000 ) ) ;
#169075=CARTESIAN_POINT ( 'NONE',  ( 4.989037339704528229, 4.922891105851139315, 1.040834085586084257E-14 ) ) ;
#169076=CARTESIAN_POINT ( 'NONE',  ( 2.855963913973019963, 6.483708332943829866, 0.000000000000000000 ) ) ;
#169077=CARTESIAN_POINT ( 'NONE',  ( -3.750802052474980108, 7.527686161196117887, 1.040834085586084257E-14 ) ) ;
#169083=CARTESIAN_POINT ( 'NONE',  ( 6.493992391265805075, 6.678671999339316656, 1.040834085586084257E-14 ) ) ;
#169086=CARTESIAN_POINT ( 'NONE',  ( 7.578644679914706472, 9.864838098032418401, 1.443375672974076540 ) ) ;
#169087=CARTESIAN_POINT ( 'NONE',  ( -1.364683531250010295, 5.092708333674757171, 0.7879004041258379498 ) ) ;
#169089=CARTESIAN_POINT ( 'NONE',  ( 5.327991180046175224, 5.318337252916401248, -0.7216878364870207285 ) ) ;
#169096=CARTESIAN_POINT ( 'NONE',  ( -4.277165953568806245, 7.474871692096041187, 1.085114461911325101 ) ) ;
#169104=CARTESIAN_POINT ( 'NONE',  ( -7.831806290188425557, 12.28885777186185990, -0.7998128361456281477 ) ) ;
#169113=ORIENTED_EDGE ( 'NONE', *, *, #92074, .F. ) ;
#169115=CARTESIAN_POINT ( 'NONE',  ( 3.063779527008311021, 5.557864633942907417, 1.082531754730546636 ) ) ;
#169116=CARTESIAN_POINT ( 'NONE',  ( -1.364683531249997417, 3.571875000341423245, 1.214306433183764966E-14 ) ) ;
#169118=CARTESIAN_POINT ( 'NONE',  ( 7.447506452608354088, 7.583179037664891098, 0.7998128361456341429 ) ) ;
#169120=EDGE_CURVE ( 'NONE', #138703, #170885, #202002, .T. ) ;
#169121=CARTESIAN_POINT ( 'NONE',  ( -8.748035429315585532, 11.22912730566677553, -1.599625672291263179 ) ) ;
#169127=CARTESIAN_POINT ( 'NONE',  ( -1.001543065824772872E-14, 4.212500000000023448, 1.732050807568877637 ) ) ;
#169128=CARTESIAN_POINT ( 'NONE',  ( 6.145923705696426431, 6.064665832934283962, 0.7998128361456341429 ) ) ;
#169131=CARTESIAN_POINT ( 'NONE',  ( -0.9999999999999965583, 6.180000000000019256, 1.226552901175238481E-14 ) ) ;
#169133=CARTESIAN_POINT ( 'NONE',  ( 7.863365906246055914, 10.19701286208565705, -1.443375672974057666 ) ) ;
#169138=CARTESIAN_POINT ( 'NONE',  ( -0.7500000000000215383, 3.222916667349487341, 1.299038105676671107 ) ) ;
#169140=CARTESIAN_POINT ( 'NONE',  ( -5.440899717785814715, 5.242137847038546461, 0.7998128361456341429 ) ) ;
#169142=CARTESIAN_POINT ( 'NONE',  ( 3.917943204224906939, 5.594019709727598766, -1.443375672974051449 ) ) ;
#169143=CARTESIAN_POINT ( 'NONE',  ( 3.469446951953614189E-15, 3.300000000000018030, 1.214306433183764966E-14 ) ) ;
#169146=VECTOR ( 'NONE', #208209, 1000.000000000000000 ) ;
#169152=CARTESIAN_POINT ( 'NONE',  ( 6.877010230629674759, 9.046264573866535486, 1.599625672291281386 ) ) ;
#169153=CARTESIAN_POINT ( 'NONE',  ( 5.443762371086860341, 6.309809840144842141, 1.199719254218462483 ) ) ;
#169156=PRESENTATION_STYLE_ASSIGNMENT (( #54352 ) ) ;
#169157=CARTESIAN_POINT ( 'NONE',  ( 5.379888026524302980, 5.170957540566797128, -0.7998128361456211532 ) ) ;
#169164=CARTESIAN_POINT ( 'NONE',  ( 10.24048609702354717, 10.84165528948263457, -0.7998128361456281477 ) ) ;
#169170=CARTESIAN_POINT ( 'NONE',  ( 5.656792095876843618, 6.122768675584825182, -0.7810860850652520115 ) ) ;
#169172=CARTESIAN_POINT ( 'NONE',  ( 9.459838494033030898, 12.05956421450382088, 1.599625672291281386 ) ) ;
#169178=CARTESIAN_POINT ( 'NONE',  ( 5.477130870240836558, 9.333810415348903433, -0.7216878364870267237 ) ) ;
#169179=CARTESIAN_POINT ( 'NONE',  ( -3.440018289565379028, 5.036440642624797626, 1.599625672291267398 ) ) ;
#169185=CARTESIAN_POINT ( 'NONE',  ( -5.253948220495577637, 6.088359997788290734, 1.199719254218450271 ) ) ;
#169188=CARTESIAN_POINT ( 'NONE',  ( -6.518203450479854943, 5.167241622962447600, 2.437504649502888920 ) ) ;
#169197=CARTESIAN_POINT ( 'NONE',  ( 7.736899214892750010, 12.17813285068358020, 1.040834085586084257E-14 ) ) ;
#169198=CARTESIAN_POINT ( 'NONE',  ( 5.834672162164848075, 6.194663582219344988, 0.9174233710642684114 ) ) ;
#169200=ORIENTED_EDGE ( 'NONE', *, *, #161158, .T. ) ;
#169205=CARTESIAN_POINT ( 'NONE',  ( 1.284279953904121641, 3.077889714876734573, -0.7749999999999892530 ) ) ;
#169206=CARTESIAN_POINT ( 'NONE',  ( -9.653042183249972652, 10.36423008998754192, -0.7216878364870267237 ) ) ;
#169211=CARTESIAN_POINT ( 'NONE',  ( 6.252281394196331554, 10.44607872653774372, 1.040834085586084257E-14 ) ) ;
#169213=DIRECTION ( 'NONE',  ( 0.6507913734559658270, -0.7592566023652989049, 0.000000000000000000 ) ) ;
#169214=CARTESIAN_POINT ( 'NONE',  ( 2.842405760359353106, 6.467890487061221272, -0.7998128361456291469 ) ) ;
#169216=CARTESIAN_POINT ( 'NONE',  ( -6.575868197828002693, 7.630599971342813426, 1.199719254218450271 ) ) ;
#169217=CARTESIAN_POINT ( 'NONE',  ( 3.662674053986138656, 7.424870162959149589, 0.7998128361456321445 ) ) ;
#169220=CARTESIAN_POINT ( 'NONE',  ( 9.083072846151447166, 12.68433652289702884, 1.199719254218450271 ) ) ;
#169224=CARTESIAN_POINT ( 'NONE',  ( 4.037917249208685000, 7.776151245443112536, -0.4343759663945709892 ) ) ;
#169226=CARTESIAN_POINT ( 'NONE',  ( 5.883875478650832491, 6.927238148923188454, -1.082531754730543083 ) ) ;
#169235=CARTESIAN_POINT ( 'NONE',  ( 9.395437264145964917, 10.06369101769952934, -0.7216878364870257245 ) ) ;
#169236=ADVANCED_FACE ( 'NONE', ( #196642 ), #81819, .F. ) ;
#169240=CARTESIAN_POINT ( 'NONE',  ( -9.203287345578106127, 9.631590079462940324, 0.7998128361456462443 ) ) ;
#169241=DIRECTION ( 'NONE',  ( 1.000000000000000000, 0.000000000000000000, 0.000000000000000000 ) ) ;
#169249=CARTESIAN_POINT ( 'NONE',  ( 4.376584659113025744, 4.000436945253625254, 0.7998128361456341429 ) ) ;
#169255=CARTESIAN_POINT ( 'NONE',  ( 3.323720213644492993, 7.029424015893889433, 1.040834085586084257E-14 ) ) ;
#169258=CARTESIAN_POINT ( 'NONE',  ( 1.499999999999989120, 2.785416667349484676, 0.8660254037844524744 ) ) ;
#169262=VERTEX_POINT ( 'NONE', #135907 ) ;
#169264=CARTESIAN_POINT ( 'NONE',  ( 0.7499999999999885647, 1.316666666666688190, -1.299038105676652899 ) ) ;
#169265=CARTESIAN_POINT ( 'NONE',  ( 7.772902139336337335, 7.962807338847539107, 0.7998128361456341429 ) ) ;
#169266=CARTESIAN_POINT ( 'NONE',  ( 3.999292125906899198, 6.649295999324608353, 1.082531754730558626 ) ) ;
#169270=CARTESIAN_POINT ( 'NONE',  ( 7.456621297836067086, 10.68284669990868174, 1.082531754730558626 ) ) ;
#169276=CARTESIAN_POINT ( 'NONE',  ( -3.581325132304157943, 7.329963087663487364, -0.7998128361456281477 ) ) ;
#169277=CARTESIAN_POINT ( 'NONE',  ( -1.500000000000013101, 3.660416667349488673, -0.8660254037844313801 ) ) ;
#169278=CARTESIAN_POINT ( 'NONE',  ( -1.364683531250014514, -1.011458332991911568, -0.7879004041258359514 ) ) ;
#169283=CARTESIAN_POINT ( 'NONE',  ( -1.201851678989727383E-14, 3.384375000341421469, 1.575800808251672791 ) ) ;
#169286=DIRECTION ( 'NONE',  ( -1.000000000000000000, 7.387867266669436732E-31, 0.000000000000000000 ) ) ;
#169291=CARTESIAN_POINT ( 'NONE',  ( -8.474009703741204547, 9.845098394908269768, -1.199719254218446718 ) ) ;
#169292=CARTESIAN_POINT ( 'NONE',  ( 6.844168616800228477, 6.879284895888727824, -0.7998128361456281477 ) ) ;
#169294=CARTESIAN_POINT ( 'NONE',  ( 1.364683531249986537, -1.136458332991912235, 0.7879004041258500513 ) ) ;
#169302=CARTESIAN_POINT ( 'NONE',  ( -6.723954117373590833, 9.932031339322813679, -1.199719254218440723 ) ) ;
#169305=CARTESIAN_POINT ( 'NONE',  ( 10.40318394038753702, 11.03146944007395724, -0.7998128361456281477 ) ) ;
#169307=CARTESIAN_POINT ( 'NONE',  ( 8.052653171512838881, 11.48218023581863001, -1.199719254218446718 ) ) ;
#169308=LINE ( 'NONE', #185542, #19394 ) ;
#169310=CARTESIAN_POINT ( 'NONE',  ( -3.567766978690493307, 7.314145241780881435, 1.040834085586084257E-14 ) ) ;
#169311=CARTESIAN_POINT ( 'NONE',  ( -7.995557903757128493, 10.35123685918189729, 1.599625672291295375 ) ) ;
#169314=CARTESIAN_POINT ( 'NONE',  ( -3.978769281187482854, 7.845005453061479450, 0.1301786893823601021 ) ) ;
#169319=CARTESIAN_POINT ( 'NONE',  ( 6.629573927402440781, 10.67832731537079383, 1.040834085586084257E-14 ) ) ;
#169322=CARTESIAN_POINT ( 'NONE',  ( 6.006425746053997372, 6.966250444273174303, -1.199719254218445830 ) ) ;
#169323=VECTOR ( 'NONE', #182802, 1000.000000000000114 ) ;
#169341=FACE_OUTER_BOUND ( 'NONE', #71676, .T. ) ;
#169345=CARTESIAN_POINT ( 'NONE',  ( -7.537443334193545397, 10.88110209227943770, -1.199719254218446718 ) ) ;
#169350=CARTESIAN_POINT ( 'NONE',  ( -1.402160292154681736E-14, 1.868750000682816381, -1.732050807568863648 ) ) ;
#169351=CARTESIAN_POINT ( 'NONE',  ( 8.757677159423465696, 12.30470822171437284, 1.199719254218450271 ) ) ;
#169355=CARTESIAN_POINT ( 'NONE',  ( -8.696665468161981494, 12.23352791524263239, -1.199719254218446718 ) ) ;
#169357=CARTESIAN_POINT ( 'NONE',  ( -0.6823417656250212460, 1.551041667008083769, 1.181850606188755259 ) ) ;
#169363=CARTESIAN_POINT ( 'NONE',  ( -4.762992037102518950, 4.451245552908022596, -0.7998128361456221525 ) ) ;
#169365=CARTESIAN_POINT ( 'NONE',  ( 1.441115678600851213, 8.287243072884326267, -3.161846531485696499 ) ) ;
#169368=CARTESIAN_POINT ( 'NONE',  ( -1.364683531250000748, 0.3218750003414205807, 0.000000000000000000 ) ) ;
#169374=CARTESIAN_POINT ( 'NONE',  ( -1.364683531250012516, 1.280208333674755172, 0.7879004041258379498 ) ) ;
#169376=CARTESIAN_POINT ( 'NONE',  ( -4.876128802409253282, 8.840567369452784874, 0.7998128361456481317 ) ) ;
#169377=CARTESIAN_POINT ( 'NONE',  ( 6.401421083946654100, 10.62007503124645957, -0.7998128361456291469 ) ) ;
#169378=CARTESIAN_POINT ( 'NONE',  ( 5.605114358992041801, 6.317488171369740613, -1.123711807521186490 ) ) ;
#169379=CARTESIAN_POINT ( 'NONE',  ( 6.491656622844908853, 6.468020902940851968, 0.7998128361456341429 ) ) ;
#169381=CARTESIAN_POINT ( 'NONE',  ( 1.499999999999987121, 4.045833333333359150, -0.8660254037844323793 ) ) ;
#169383=CARTESIAN_POINT ( 'NONE',  ( 0.6823417656249899377, 1.905208333674752952, 1.181850606188755259 ) ) ;
#169390=CARTESIAN_POINT ( 'NONE',  ( 5.721177635286841756, 6.737423998331861341, -1.082531754730543083 ) ) ;
#169393=CARTESIAN_POINT ( 'NONE',  ( -7.883176251342026042, 11.28445716228600126, -1.199719254218446718 ) ) ;
#169394=CARTESIAN_POINT ( 'NONE',  ( -3.093231602212184850, 6.760520635889515795, -0.7998128361456281477 ) ) ;
#169398=CARTESIAN_POINT ( 'NONE',  ( -8.310784975052685652, 9.758632561392040827, -1.082531754730543083 ) ) ;
#169400=CARTESIAN_POINT ( 'NONE',  ( -1.201851678989727383E-14, 4.587500000000025224, -1.732050807568863648 ) ) ;
#169404=CARTESIAN_POINT ( 'NONE',  ( 9.083599731475988648, 10.66024977721925104, 1.082531754730549967 ) ) ;
#169406=AXIS2_PLACEMENT_3D ( 'NONE', #60412, #92946, #23638 ) ;
#169412=CARTESIAN_POINT ( 'NONE',  ( -4.650083499807250220, 5.295740330745369207, -7.499999999999997335 ) ) ;
#169419=CARTESIAN_POINT ( 'NONE',  ( 7.741342523278692767, 11.01502146292508044, 1.082531754730558626 ) ) ;
#169421=CARTESIAN_POINT ( 'NONE',  ( 6.479907352327590964, 9.647310113435821677, 1.199719254218462483 ) ) ;
#169422=CARTESIAN_POINT ( 'NONE',  ( -6.227272627378437342, 6.159572908229946187, -0.7998128361456291469 ) ) ;
#169425=CARTESIAN_POINT ( 'NONE',  ( -1.364683531250000748, -0.4281249996585800854, 0.000000000000000000 ) ) ;
#169426=CARTESIAN_POINT ( 'NONE',  ( 2.223174002961016082, 5.537527403522402025, -0.7216878364870267237 ) ) ;
#169427=ORIENTED_EDGE ( 'NONE', *, *, #81943, .T. ) ;
#169428=CARTESIAN_POINT ( 'NONE',  ( -2.272963308585411735, 5.803540959991587478, 0.7998128361456341429 ) ) ;
#169441=ORIENTED_EDGE ( 'NONE', *, *, #19647, .F. ) ;
#169444=CARTESIAN_POINT ( 'NONE',  ( 8.284195553149872993, 9.623648552551724578, -1.199719254218445830 ) ) ;
#169455=CARTESIAN_POINT ( 'NONE',  ( -5.545448523189368650, 6.428443684264421698, -1.199719254218446718 ) ) ;
#169457=CARTESIAN_POINT ( 'NONE',  ( -4.172158584703340445, 5.890604320285754980, -1.599625672291256295 ) ) ;
#169464=CARTESIAN_POINT ( 'NONE',  ( 5.181758602633672162, 4.945385036406048762, -2.500000000000000444 ) ) ;
#169468=CARTESIAN_POINT ( 'NONE',  ( -3.846762897975357198, 5.510976019103107859, -1.599625672291256295 ) ) ;
#169471=CARTESIAN_POINT ( 'NONE',  ( 7.100719765255169236, 9.307259030929609267, -1.599625672291262513 ) ) ;
#169472=CARTESIAN_POINT ( 'NONE',  ( -0.6823417656249969321, 5.217708333674756283, -1.181850606188749264 ) ) ;
#169479=CARTESIAN_POINT ( 'NONE',  ( 5.788968402910812827, 6.816513227226497662, 1.082531754730558626 ) ) ;
#169480=CARTESIAN_POINT ( 'NONE',  ( -7.718669524881690336, 7.899535955317097624, 0.7998128361456462443 ) ) ;
#169483=CARTESIAN_POINT ( 'NONE',  ( -8.030507057996002729, 8.263346410617135263, 1.040834085586084257E-14 ) ) ;
#169484=CARTESIAN_POINT ( 'NONE',  ( -6.196239896645333367, 7.187700286629718605, -1.199719254218446718 ) ) ;
#169489=CARTESIAN_POINT ( 'NONE',  ( 1.499999999999990896, 3.306250000682818602, 1.214306433183764966E-14 ) ) ;
#169492=CARTESIAN_POINT ( 'NONE',  ( 7.233438648090761980, 8.397765496649418182, 1.199719254218462483 ) ) ;
#169506=CARTESIAN_POINT ( 'NONE',  ( 0.6823417656249864960, -0.7614583329919113464, -1.181850606188749264 ) ) ;
#169507=CARTESIAN_POINT ( 'NONE',  ( 5.169736645512481132, 4.925780929386339935, 0.7998128361456341429 ) ) ;
#169508=CARTESIAN_POINT ( 'NONE',  ( 6.830610463186557624, 6.863467050006115677, 1.040834085586084257E-14 ) ) ;
#169510=CARTESIAN_POINT ( 'NONE',  ( -6.561783159334130922, 9.638868871656395498, -1.082531754730538864 ) ) ;
#169512=CARTESIAN_POINT ( 'NONE',  ( 6.209271165378815738, 7.306866450105836464, -1.082531754730543083 ) ) ;
#169513=CARTESIAN_POINT ( 'NONE',  ( -9.137832345486311070, 9.763151945929928743, 1.040834085586084257E-14 ) ) ;
#169518=CARTESIAN_POINT ( 'NONE',  ( 9.250740883225924804, 9.686952540052077509, 1.040834085586084257E-14 ) ) ;
#169524=CARTESIAN_POINT ( 'NONE',  ( 1.364683531249986537, 2.405208333674752286, -0.7879004041258239610 ) ) ;
#169530=CARTESIAN_POINT ( 'NONE',  ( 7.934546212495622086, 10.28005655271014795, -1.599625672291262513 ) ) ;
#169533=CARTESIAN_POINT ( 'NONE',  ( -8.748035429315585532, 11.22912730566677553, -1.599625672291263179 ) ) ;
#169539=CARTESIAN_POINT ( 'NONE',  ( 4.216749469050096621, 4.878294787768598262, -1.199719254218452047 ) ) ;
#169544=CARTESIAN_POINT ( 'NONE',  ( -8.143643823302737061, 12.65266822716189843, 0.000000000000000000 ) ) ;
#169549=CARTESIAN_POINT ( 'NONE',  ( 5.830449476509543594, 6.014588727829297987, 0.4175459632603968352 ) ) ;
#169551=CARTESIAN_POINT ( 'NONE',  ( -4.497554271431319250, 6.270232621468402989, -1.599625672291256295 ) ) ;
#169555=CARTESIAN_POINT ( 'NONE',  ( 7.450369105909416589, 8.650851030771185890, -1.199719254218441611 ) ) ;
#169557=CARTESIAN_POINT ( 'NONE',  ( 7.637320603199683866, 7.804628880021436288, -0.7998128361456281477 ) ) ;
#169558=CARTESIAN_POINT ( 'NONE',  ( 3.985207087413062066, 6.736826471035503694, -1.199719254218452047 ) ) ;
#169560=CARTESIAN_POINT ( 'NONE',  ( -6.887178846062109727, 10.01849717283904262, -1.082531754730537976 ) ) ;
#169568=CARTESIAN_POINT ( 'NONE',  ( -5.762678113124475310, 6.090388861115007657, -0.6347866013659544393 ) ) ;
#169570=CARTESIAN_POINT ( 'NONE',  ( 4.026131012922935959, 7.773685636243294006, 0.3673651676878584849 ) ) ;
#169571=CARTESIAN_POINT ( 'NONE',  ( 4.663641653420880218, 8.384739662392275861, -0.7216878364870207285 ) ) ;
#169575=CARTESIAN_POINT ( 'NONE',  ( -9.124274191872631334, 12.62844174295135069, -1.082531754730543083 ) ) ;
#169594=CARTESIAN_POINT ( 'NONE',  ( 7.853197290813620945, 10.18514947741448573, 1.599625672291281386 ) ) ;
#169598=CARTESIAN_POINT ( 'NONE',  ( -1.500000000000013101, 1.952083334016152527, 0.8660254037844403729 ) ) ;
#169599=CARTESIAN_POINT ( 'NONE',  ( -4.394814349124112951, 8.279033840620114049, -0.7998128361456281477 ) ) ;
#169603=CARTESIAN_POINT ( 'NONE',  ( -9.657485491635913633, 10.16148791653038330, 1.040834085586084257E-14 ) ) ;
#169606=DIRECTION ( 'NONE',  ( -0.1674078377062480916, 2.168404344971017388E-14, 0.9858877298529068467 ) ) ;
#169607=CARTESIAN_POINT ( 'NONE',  ( 7.311924916471702396, 7.425000578838787391, -0.7998128361456281477 ) ) ;
#169609=CARTESIAN_POINT ( 'NONE',  ( -7.739006755302186846, 7.923262724141010516, 0.7998128361456462443 ) ) ;
#169611=CARTESIAN_POINT ( 'NONE',  ( 10.09812548408005384, 10.67556790771522124, -0.7998128361456281477 ) ) ;
#169612=CARTESIAN_POINT ( 'NONE',  ( -1.364683531250010295, 5.738541667008088432, -0.7879004041258300672 ) ) ;
#169617=CARTESIAN_POINT ( 'NONE',  ( -8.026063749610063525, 8.466088584074293877, -0.7216878364870278340 ) ) ;
#169620=CARTESIAN_POINT ( 'NONE',  ( 1.364683531249990311, 4.196875000341417028, 1.214306433183764966E-14 ) ) ;
#169629=CARTESIAN_POINT ( 'NONE',  ( -4.080641047588914994, 5.783833860318930320, -1.443375672974051449 ) ) ;
#169631=CARTESIAN_POINT ( 'NONE',  ( 4.989037339704528229, 4.922891105851139315, 1.040834085586084257E-14 ) ) ;
#169633=CARTESIAN_POINT ( 'NONE',  ( -8.482597663644387609, 13.04811437422715414, -0.7998128361456281477 ) ) ;
#169637=CARTESIAN_POINT ( 'NONE',  ( 0.6823417656249899377, 0.5927083336747518416, 1.181850606188755259 ) ) ;
#169638=CARTESIAN_POINT ( 'NONE',  ( -4.284013352238265959, 5.060732334775157604, -1.082531754730544860 ) ) ;
#169639=CARTESIAN_POINT ( 'NONE',  ( 6.335737856287750880, 6.286115675290828264, -0.7998128361456281477 ) ) ;
#169642=CARTESIAN_POINT ( 'NONE',  ( 5.694061328059478733, 5.745419092265336758, -0.7216878364870484841 ) ) ;
#169644=CARTESIAN_POINT ( 'NONE',  ( 2.738383840280328663, 5.178236332760252303, 1.082531754730548412 ) ) ;
#169647=CARTESIAN_POINT ( 'NONE',  ( -7.524412065904404479, 11.72230514362308185, 0.000000000000000000 ) ) ;
#169652=CARTESIAN_POINT ( 'NONE',  ( -9.820183334999905256, 10.35130206712171130, 1.040834085586084257E-14 ) ) ;
#169653=CARTESIAN_POINT ( 'NONE',  ( -4.948362878863562742, 5.835806782504650236, 1.082531754730558626 ) ) ;
#169654=CARTESIAN_POINT ( 'NONE',  ( -1.402160292154681736E-14, 1.759375000341421469, -1.575800808251659024 ) ) ;
#169661=CARTESIAN_POINT ( 'NONE',  ( 10.01963921569910632, 11.64833282552586091, 1.199719254218450271 ) ) ;
#169667=ORIENTED_EDGE ( 'NONE', *, *, #69490, .F. ) ;
#169669=EDGE_LOOP ( 'NONE', ( #181631, #61969, #18821 ) ) ;
#169675=LINE ( 'NONE', #35396, #7232 ) ;
#169676=CARTESIAN_POINT ( 'NONE',  ( 1.364683531249990311, 3.446875000341416584, 1.214306433183764966E-14 ) ) ;
#169686=CARTESIAN_POINT ( 'NONE',  ( 0.6823417656249882723, 1.426041667008083547, -1.181850606188749264 ) ) ;
#169697=CARTESIAN_POINT ( 'NONE',  ( 5.005985031943777308, 6.863401842066294556, -1.599625672291256295 ) ) ;
#169700=ORIENTED_EDGE ( 'NONE', *, *, #175957, .F. ) ;
#169703=CARTESIAN_POINT ( 'NONE',  ( 6.771407655021410399, 9.987393799911945536, -1.199719254218441611 ) ) ;
#169707=CARTESIAN_POINT ( 'NONE',  ( -3.273404022695637572, 5.906389562198459231, 1.199719254218462483 ) ) ;
#169708=CARTESIAN_POINT ( 'NONE',  ( 8.097244055859613709, 10.46987070330147063, -1.599625672291262513 ) ) ;
#169720=CARTESIAN_POINT ( 'NONE',  ( -6.887178846062109727, 10.01849717283904262, -1.082531754730537976 ) ) ;
#169725=CARTESIAN_POINT ( 'NONE',  ( -9.429859533504656000, 10.96025652963230534, -1.199719254218441611 ) ) ;
#169730=CARTESIAN_POINT ( 'NONE',  ( -4.243865776277440993, 4.909930479533815451, -1.199719254218446718 ) ) ;
#169732=CARTESIAN_POINT ( 'NONE',  ( 10.01963921569910632, 11.64833282552586091, 1.199719254218450271 ) ) ;
#169733=CARTESIAN_POINT ( 'NONE',  ( 5.027376032568989572, 4.759693547618927489, 0.7998128361456341429 ) ) ;
#169735=ORIENTED_EDGE ( 'NONE', *, *, #40172, .T. ) ;
#169739=CARTESIAN_POINT ( 'NONE',  ( 4.555176424511575561, 4.416720038126027426, -0.7216878364870188411 ) ) ;
#169742=CARTESIAN_POINT ( 'NONE',  ( -4.822949958159302497, 6.649860922651058992, -1.599625672291256295 ) ) ;
#169745=CARTESIAN_POINT ( 'NONE',  ( -9.982881178363895103, 10.54111621771303753, 1.040834085586084257E-14 ) ) ;
#169751=CARTESIAN_POINT ( 'NONE',  ( 8.948018195339340508, 9.541702104091804415, -0.7216878364870197293 ) ) ;
#169752=CARTESIAN_POINT ( 'NONE',  ( 1.364683531249990311, 4.926041667008084879, 0.7879004041258499402 ) ) ;
#169755=CARTESIAN_POINT ( 'NONE',  ( 3.174580523894166006, 6.855427711185178019, 0.7998128361456341429 ) ) ;
#169767=CARTESIAN_POINT ( 'NONE',  ( 1.364683531249988535, 2.967708333674755394, -0.7879004041258239610 ) ) ;
#169769=CARTESIAN_POINT ( 'NONE',  ( 2.381428537494710618, 5.930083727052461562, 0.7998128361456462443 ) ) ;
#169771=CARTESIAN_POINT ( 'NONE',  ( -4.107757355260591936, 7.736207981205250661, 1.040834085586084257E-14 ) ) ;
#169773=CARTESIAN_POINT ( 'NONE',  ( -5.165293336682207581, 8.009630745229104676, 1.082531754730548412 ) ) ;
#169777=ORIENTED_EDGE ( 'NONE', *, *, #38831, .F. ) ;
#169779=CARTESIAN_POINT ( 'NONE',  ( 4.822949958159288286, 6.649860922651058992, -1.599625672291256295 ) ) ;
#169789=CARTESIAN_POINT ( 'NONE',  ( 5.843727902690005749, 6.776436293681846301, -1.199719254218445830 ) ) ;
#169792=CARTESIAN_POINT ( 'NONE',  ( 4.161989969715248705, 4.726297878971393196, -2.420000000000000373 ) ) ;
#169794=CARTESIAN_POINT ( 'NONE',  ( -5.551173829791513192, 8.563787670477010394, 1.199719254218452047 ) ) ;
#169798=CARTESIAN_POINT ( 'NONE',  ( 8.274553823041976841, 8.548067636504127265, 1.040834085586084257E-14 ) ) ;
#169801=CARTESIAN_POINT ( 'NONE',  ( -5.391338639728555648, 9.441645512991978961, -0.7998128361456231517 ) ) ;
#169802=CARTESIAN_POINT ( 'NONE',  ( 6.521108698048765362, 8.631046119188804155, -1.443375672974058777 ) ) ;
#169803=CARTESIAN_POINT ( 'NONE',  ( 5.529887635128906354, 6.401445659467410287, 1.229860404580757072 ) ) ;
#169804=CARTESIAN_POINT ( 'NONE',  ( -3.653032323878261600, 6.349289246911547835, -1.199719254218452047 ) ) ;
#169807=CARTESIAN_POINT ( 'NONE',  ( -5.280010757518168063, 8.247430752824802980, -1.199719254218446718 ) ) ;
#169812=CARTESIAN_POINT ( 'NONE',  ( -0.6823417656250212460, 1.801041667008083991, 1.181850606188755259 ) ) ;
#169814=CARTESIAN_POINT ( 'NONE',  ( -5.910991785878175975, 6.958873840688411860, -1.082531754730544860 ) ) ;
#169818=ORIENTED_EDGE ( 'NONE', *, *, #46527, .T. ) ;
#169821=CARTESIAN_POINT ( 'NONE',  ( 5.307127064745490230, 8.279066444590018392, -1.199719254218452935 ) ) ;
#169825=CARTESIAN_POINT ( 'NONE',  ( -1.364683531250012516, 2.342708333674752286, 0.7879004041258379498 ) ) ;
#169828=CARTESIAN_POINT ( 'NONE',  ( 0.007473969438204840048, 8.279395425053873936, 1.999986034896453324 ) ) ;
#169831=CARTESIAN_POINT ( 'NONE',  ( -4.894657149733403045, 5.669187081899118574, -1.199719254218446718 ) ) ;
#169832=CARTESIAN_POINT ( 'NONE',  ( -6.683806541412768532, 8.820860269780128604, -1.443375672974058777 ) ) ;
#169840=CARTESIAN_POINT ( 'NONE',  ( -8.066738210006693777, 10.43428054980638997, 1.443375672974090751 ) ) ;
#169844=CARTESIAN_POINT ( 'NONE',  ( -5.870317324592805086, 9.792527945426188651, -0.7216878364870197293 ) ) ;
#169854=VERTEX_POINT ( 'NONE', #182714 ) ;
#169857=CARTESIAN_POINT ( 'NONE',  ( -5.555090253297260361, 7.504024600312024340, 1.599625672291269396 ) ) ;
#169859=CARTESIAN_POINT ( 'NONE',  ( 3.765413976293345844, 5.416068943807445635, 1.599625672291267398 ) ) ;
#169863=CARTESIAN_POINT ( 'NONE',  ( 4.808338034340912337, 8.761478140039733020, 1.040834085586084257E-14 ) ) ;
#169866=CARTESIAN_POINT ( 'NONE',  ( -5.314433026876900001, 6.262888621853549331, 1.082531754730548412 ) ) ;
#169874=CARTESIAN_POINT ( 'NONE',  ( -0.6823417656250003738, 1.217708333674752286, -1.181850606188749264 ) ) ;
#169876=CARTESIAN_POINT ( 'NONE',  ( -8.050844288416501016, 8.287073179441051707, 1.040834085586084257E-14 ) ) ;
#169878=CARTESIAN_POINT ( 'NONE',  ( 5.933664784275179294, 10.07435934829639912, -0.7998128361456291469 ) ) ;
#169880=CARTESIAN_POINT ( 'NONE',  ( -8.037286134802835491, 8.271255333558444889, -0.7998128361456291469 ) ) ;
#169883=CARTESIAN_POINT ( 'NONE',  ( -1.364683531249997417, 5.009375000341425022, 1.214306433183764966E-14 ) ) ;
#169886=CARTESIAN_POINT ( 'NONE',  ( 7.402388683381404988, 10.61957531637824204, -1.082531754730537976 ) ) ;
#169889=CARTESIAN_POINT ( 'NONE',  ( -1.364683531250000748, -0.9281249996585805295, 0.000000000000000000 ) ) ;
#169891=LINE ( 'NONE', #6310, #44970 ) ;
#169892=CARTESIAN_POINT ( 'NONE',  ( 6.575341312503417690, 10.61505593132193326, -0.7216878364870267237 ) ) ;
#169894=CARTESIAN_POINT ( 'NONE',  ( 2.493766133720156652, 8.265889183060442846, 2.456386456769295901 ) ) ;
#169895=CARTESIAN_POINT ( 'NONE',  ( -5.260200412422208593, 7.159986452624450770, -1.443375672974053447 ) ) ;
#169897=CARTESIAN_POINT ( 'NONE',  ( 1.364683531249988535, 3.155208333674756283, -0.7879004041258239610 ) ) ;
#169901=B_SPLINE_CURVE_WITH_KNOTS ( 'NONE', 3,
 ( #132231, #100749, #49878, #2152 ),
 .UNSPECIFIED., .F., .F.,
 ( 4, 4 ),
 ( 0.002966363312150372029, 0.003746507044012918359 ),
 .UNSPECIFIED. ) ;
#169902=CARTESIAN_POINT ( 'NONE',  ( -6.368579470117215813, 8.453095353268645695, 1.599625672291283607 ) ) ;
#169910=CARTESIAN_POINT ( 'NONE',  ( 7.259501185113382604, 10.55683625168592243, -1.199719254218441611 ) ) ;
#169913=CARTESIAN_POINT ( 'NONE',  ( 1.499999999999987121, 2.004166666666684637, 0.8660254037844524744 ) ) ;
#169919=ORIENTED_EDGE ( 'NONE', *, *, #205893, .T. ) ;
#169920=CARTESIAN_POINT ( 'NONE',  ( 5.165293337126522388, 8.969999960048859577, 1.040834085586084257E-14 ) ) ;
#169922=CARTESIAN_POINT ( 'NONE',  ( -0.6823417656250246877, -1.136458332991911790, 1.181850606188755259 ) ) ;
#169927=CARTESIAN_POINT ( 'NONE',  ( 1.499999999999989120, 1.025000000000019007, 0.000000000000000000 ) ) ;
#169928=CARTESIAN_POINT ( 'NONE',  ( 7.938462636001388795, 9.220293482545153907, -1.199719254218441611 ) ) ;
#169929=CARTESIAN_POINT ( 'NONE',  ( -9.504429378379839477, 11.04725468198666150, 1.199719254218462483 ) ) ;
#169932=CARTESIAN_POINT ( 'NONE',  ( 0.6823417656249882723, -0.6572916663252492686, 1.181850606188755259 ) ) ;
#169933=CARTESIAN_POINT ( 'NONE',  ( -1.201851678989727383E-14, 0.9625000000000237810, 1.732050807568877637 ) ) ;
#169935=CARTESIAN_POINT ( 'NONE',  ( 4.202137545231717120, 6.989912005157271402, 1.199719254218462483 ) ) ;
#169942=CARTESIAN_POINT ( 'NONE',  ( -1.201851678989727383E-14, 4.946875000341420581, -1.575800808251660134 ) ) ;
#169944=CARTESIAN_POINT ( 'NONE',  ( -9.345647958521597687, 9.797677461230342999, 0.7998128361456462443 ) ) ;
#169945=CARTESIAN_POINT ( 'NONE',  ( -6.263503779833496488, 6.409768619334935913, 0.7216878364870317197 ) ) ;
#169952=CARTESIAN_POINT ( 'NONE',  ( 6.913768267964901071, 10.15348118167935709, -1.199719254218441611 ) ) ;
#169956=CARTESIAN_POINT ( 'NONE',  ( 6.439759776366765998, 9.496508258194486629, 1.082531754730558626 ) ) ;
#169959=CARTESIAN_POINT ( 'NONE',  ( -8.681298431451969222, 9.022603012982438386, 1.040834085586084257E-14 ) ) ;
#169961=CARTESIAN_POINT ( 'NONE',  ( 4.924636110261782385, 6.768494766770632332, 1.599625672291267398 ) ) ;
#169964=PLANE ( 'NONE',  #158453 ) ;
#169965=CARTESIAN_POINT ( 'NONE',  ( 10.05978679165993483, 11.79913468076720306, 1.082531754730548412 ) ) ;
#169966=EDGE_LOOP ( 'NONE', ( #14362, #186080, #112, #134029 ) ) ;
#169970=CARTESIAN_POINT ( 'NONE',  ( 2.273450361290503263, 5.679387915302107182, 0.4672911629945233347 ) ) ;
#169972=CARTESIAN_POINT ( 'NONE',  ( -5.938108093105513241, 6.030140318152288792, 0.7216878364870317197 ) ) ;
#169973=CARTESIAN_POINT ( 'NONE',  ( 4.220665892555866883, 3.818531717603609987, -0.7998128361456211532 ) ) ;
#169976=CARTESIAN_POINT ( 'NONE',  ( -5.208303565944065738, 9.228104593576741621, -0.7998128361456231517 ) ) ;
#169981=CARTESIAN_POINT ( 'NONE',  ( -7.694415870955439551, 8.935572256658169010, 1.199719254218462483 ) ) ;
#169984=CARTESIAN_POINT ( 'NONE',  ( 5.605114358992040913, 6.317488171369740613, -1.123711807521186490 ) ) ;
#169987=VERTEX_POINT ( 'NONE', #38618 ) ;
#169994=CARTESIAN_POINT ( 'NONE',  ( 5.858512798400357546, 6.179092012920288646, 0.8810539604525641222 ) ) ;
#169995=CARTESIAN_POINT ( 'NONE',  ( -6.368579470117215813, 8.453095353268645695, 1.599625672291283607 ) ) ;
#169999=CARTESIAN_POINT ( 'NONE',  ( 5.124618876285529367, 7.962177208099690873, -1.082531754730549078 ) ) ;
#170004=CARTESIAN_POINT ( 'NONE',  ( -4.412288926243578935, 7.235088616337731260, 1.199719254218464037 ) ) ;
#170008=CARTESIAN_POINT ( 'NONE',  ( -5.636439174979254396, 7.598931675607687453, -1.599625672291256295 ) ) ;
#170014=CARTESIAN_POINT ( 'NONE',  ( -8.317037166979361018, 11.79062823052953668, 1.199719254218453823 ) ) ;
#170015=CARTESIAN_POINT ( 'NONE',  ( 7.233438648090761980, 8.397765496649418182, 1.199719254218462483 ) ) ;
#170018=CARTESIAN_POINT ( 'NONE',  ( -8.299562589859897699, 12.83457345481192036, -0.7998128361456281477 ) ) ;
#170024=ORIENTED_EDGE ( 'NONE', *, *, #7830, .T. ) ;
#170026=CARTESIAN_POINT ( 'NONE',  ( 8.758204044747998296, 11.24099069033793974, 1.443375672974076540 ) ) ;
#170032=EDGE_CURVE ( 'NONE', #16921, #159827, #169675, .T. ) ;
#170034=CARTESIAN_POINT ( 'NONE',  ( -0.1609840471590594513, 6.431820245570142980, -3.209093660759736899 ) ) ;
#170045=CARTESIAN_POINT ( 'NONE',  ( -4.946027110887008860, 4.664786472323266153, -0.7998128361456221525 ) ) ;
#170053=( BOUNDED_CURVE ( )  B_SPLINE_CURVE ( 2, ( #208829, #75656, #91931, #89801, #107151, #123438, #205638 ),
 .UNSPECIFIED., .F., .T. ) 
 B_SPLINE_CURVE_WITH_KNOTS ( ( 3, 2, 2, 3 ),
 ( 0.08928571428571412116, 0.09523809523809514954, 0.1011904761904762057, 0.1071428571428572341 ),
 .UNSPECIFIED. ) 
 CURVE ( )  GEOMETRIC_REPRESENTATION_ITEM ( )  RATIONAL_B_SPLINE_CURVE ( ( 1.000000000000003775, 0.8660254037844349329, 1.000000000000000000, 0.8660254037844387076, 1.000000000000000000, 0.8660254037844364872, 1.000000000000002220 ) ) 
 REPRESENTATION_ITEM ( '' )  );
#170054=CARTESIAN_POINT ( 'NONE',  ( 1.364683531249992088, 5.384375000341417916, 1.214306433183764966E-14 ) ) ;
#170059=ORIENTED_EDGE ( 'NONE', *, *, #151561, .F. ) ;
#170061=CARTESIAN_POINT ( 'NONE',  ( 0.3171178118501411514, 7.220087385434813321, -2.081545611384603145 ) ) ;
#170062=CARTESIAN_POINT ( 'NONE',  ( 3.704402285031850539, 5.344888637335695414, -1.599625672291262513 ) ) ;
#170064=CARTESIAN_POINT ( 'NONE',  ( 4.702146809683701356, 5.356480858934594025, -2.420000000000000373 ) ) ;
#170068=CARTESIAN_POINT ( 'NONE',  ( 6.661133543015731462, 6.665743976473484267, -0.7998128361456281477 ) ) ;
#170069=CARTESIAN_POINT ( 'NONE',  ( -1.364683531250012516, 2.342708333674752286, 0.7879004041258379498 ) ) ;
#170071=CARTESIAN_POINT ( 'NONE',  ( -4.446147712686649989, 7.104319146577407373, 1.107073289137233241 ) ) ;
#170074=CARTESIAN_POINT ( 'NONE',  ( -7.472515219426274946, 11.86968485597268064, 0.000000000000000000 ) ) ;
#170075=CARTESIAN_POINT ( 'NONE',  ( -3.701012746406287413, 6.301303389907177532, 1.082531754730560403 ) ) ;
#170077=CARTESIAN_POINT ( 'NONE',  ( -4.394814349124112951, 8.279033840620114049, -0.7998128361456281477 ) ) ;
#170079=CARTESIAN_POINT ( 'NONE',  ( -0.7500000000000006661, -0.8604166659838472508, -1.299038105676652011 ) ) ;
#170087=CARTESIAN_POINT ( 'NONE',  ( -4.324687812634898876, 6.068555086205916105, 1.443375672974064550 ) ) ;
#170088=CARTESIAN_POINT ( 'NONE',  ( 6.385527162356455122, 10.39360608948380538, 1.056142170575426150E-14 ) ) ;
#170092=CARTESIAN_POINT ( 'NONE',  ( -3.863710589770277259, 6.491117540498504646, 1.082531754730560403 ) ) ;
#170094=CARTESIAN_POINT ( 'NONE',  ( 7.639129486296027061, 10.99973593639901814, 1.199719254218460707 ) ) ;
#170103=CARTESIAN_POINT ( 'NONE',  ( -3.195971524519394702, 4.751719416737803847, -1.599625672291262513 ) ) ;
#170104=CARTESIAN_POINT ( 'NONE',  ( -4.173017639316489280, 7.592962374094866185, 0.9320401348096055694 ) ) ;
#170109=CARTESIAN_POINT ( 'NONE',  ( 6.681470773436232413, 6.689470745297396270, -0.7998128361456281477 ) ) ;
#170114=CARTESIAN_POINT ( 'NONE',  ( 2.381428537494710618, 5.930083727052461562, 0.7998128361456462443 ) ) ;
#170122=DIRECTION ( 'NONE',  ( 0.000000000000000000, 8.546850786086437571E-32, 1.000000000000000000 ) ) ;
#170127=CARTESIAN_POINT ( 'NONE',  ( 9.094822116668764167, 9.505047312402055582, 0.7998128361456462443 ) ) ;
#170130=CARTESIAN_POINT ( 'NONE',  ( -5.087333953625788219, 6.958308917361963886, 1.599625672291267398 ) ) ;
#170136=CARTESIAN_POINT ( 'NONE',  ( -1.364683531249997417, 5.259375000341425022, 1.214306433183764966E-14 ) ) ;
#170141=CARTESIAN_POINT ( 'NONE',  ( 4.273844736805816780, 6.009238164405336313, 1.599625672291267398 ) ) ;
#170142=CARTESIAN_POINT ( 'NONE',  ( -3.761497552787613330, 6.475832013972435242, 1.199719254218464037 ) ) ;
#170149=CARTESIAN_POINT ( 'NONE',  ( 4.853455804012203778, 8.606189504748821051, 0.7216878364870438212 ) ) ;
#170151=CARTESIAN_POINT ( 'NONE',  ( 8.568389893712330618, 9.098802418860289620, 1.040834085586084257E-14 ) ) ;
#170152=CARTESIAN_POINT ( 'NONE',  ( -0.6823417656250212460, 3.613541667008085767, 1.181850606188767472 ) ) ;
#170154=CARTESIAN_POINT ( 'NONE',  ( 5.463572716182829581, 6.436884926043849653, 1.082531754730560403 ) ) ;
#170160=CARTESIAN_POINT ( 'NONE',  ( -4.300870446666812619, 7.448604017583265957, 1.116033750828262949 ) ) ;
#170167=CARTESIAN_POINT ( 'NONE',  ( -8.469039510030723861, 13.03229652834454733, 1.040834085586084257E-14 ) ) ;
#170175=ORIENTED_EDGE ( 'NONE', *, *, #167966, .T. ) ;
#170177=CARTESIAN_POINT ( 'NONE',  ( 2.385871846325007706, 5.727341554113725586, -0.7216878364870267237 ) ) ;
#170178=CARTESIAN_POINT ( 'NONE',  ( 1.364683531249986537, 2.717708333674754062, -0.7879004041258239610 ) ) ;
#170180=CARTESIAN_POINT ( 'NONE',  ( 8.111855979677986994, 8.358253485912799263, 1.040834085586084257E-14 ) ) ;
#170181=CARTESIAN_POINT ( 'NONE',  ( -10.00321840878439339, 10.56484298653695397, 1.040834085586084257E-14 ) ) ;
#170183=CARTESIAN_POINT ( 'NONE',  ( -3.405069135326500351, 7.124331091189553433, 1.040834085586084257E-14 ) ) ;
#170188=CARTESIAN_POINT ( 'NONE',  ( -0.7499999999999972244, 4.608333333333352932, -1.299038105676652011 ) ) ;
#170189=CARTESIAN_POINT ( 'NONE',  ( 5.823390672269506574, 6.752709524857930745, -1.199719254218446718 ) ) ;
#170193=CARTESIAN_POINT ( 'NONE',  ( 4.161989969715272686, 4.726297878971393196, 2.420000000000010587 ) ) ;
#170194=CARTESIAN_POINT ( 'NONE',  ( -0.6823417656250212460, 4.051041667008085767, 1.181850606188767472 ) ) ;
#170198=CARTESIAN_POINT ( 'NONE',  ( 10.24960094225127172, 11.06021530882240356, -0.7216878364870257245 ) ) ;
#170203=CARTESIAN_POINT ( 'NONE',  ( 1.499999999999989120, 1.556250000682817047, 0.000000000000000000 ) ) ;
#170205=CARTESIAN_POINT ( 'NONE',  ( -4.904298879841297421, 6.744767997946721216, 1.599625672291267398 ) ) ;
#170206=CARTESIAN_POINT ( 'NONE',  ( 4.894130264408854458, 6.732904613275549899, -1.443375672974051449 ) ) ;
#170215=CARTESIAN_POINT ( 'NONE',  ( 5.770966940911189447, 9.884545197705074671, -0.7998128361456291469 ) ) ;
#170216=CARTESIAN_POINT ( 'NONE',  ( 3.635557746758808495, 7.393234471193928847, -0.7998128361456291469 ) ) ;
#170220=( LENGTH_UNIT ( ) NAMED_UNIT ( * ) SI_UNIT ( .MILLI., .METRE. ) );
#170221=CARTESIAN_POINT ( 'NONE',  ( 5.867981556616276073, 5.740399992340775803, -0.7998128361456281477 ) ) ;
#170223=B_SPLINE_CURVE_WITH_KNOTS ( 'NONE', 3,
 ( #140088, #188808, #187729, #8987 ),
 .UNSPECIFIED., .F., .F.,
 ( 4, 4 ),
 ( 0.000000000000000000, 0.0004136821696107355730 ),
 .UNSPECIFIED. ) ;
#170224=VERTEX_POINT ( 'NONE', #74324 ) ;
#170226=VERTEX_POINT ( 'NONE', #170746 ) ;
#170229=CARTESIAN_POINT ( 'NONE',  ( 8.028399517586572998, 12.51821653715971472, -0.7998128361456352531 ) ) ;
#170234=CARTESIAN_POINT ( 'NONE',  ( 5.504159067553832330, 6.221818635116664886, 0.9641881782859774708 ) ) ;
#170239=CARTESIAN_POINT ( 'NONE',  ( -1.500000000000011324, 5.660416667349481123, -0.8660254037844312691 ) ) ;
#170240=CARTESIAN_POINT ( 'NONE',  ( 0.6823417656249882723, -1.157291666325249713, 1.181850606188755259 ) ) ;
#170241=CARTESIAN_POINT ( 'NONE',  ( 5.816084710582486217, 9.729256562414162701, 1.040834085586084257E-14 ) ) ;
#170242=CARTESIAN_POINT ( 'NONE',  ( -3.144601563365788444, 5.756120026313656268, -1.199719254218452935 ) ) ;
#170247=CARTESIAN_POINT ( 'NONE',  ( -4.120788623549732854, 6.895004929861607401, -1.199719254218452047 ) ) ;
#170249=CARTESIAN_POINT ( 'NONE',  ( -5.946383829923330921, 4.757679660048923509, 2.499999999998779199 ) ) ;
#170254=CARTESIAN_POINT ( 'NONE',  ( -3.673896439623302257, 4.156855427197417185, -0.9999999999999991118 ) ) ;
#170259=CARTESIAN_POINT ( 'NONE',  ( 9.260382613333817403, 10.76253345609967660, -1.199719254218446718 ) ) ;
#170261=CARTESIAN_POINT ( 'NONE',  ( 4.053524740805938720, 3.831459740469437936, 1.214306433183764966E-14 ) ) ;
#170267=CARTESIAN_POINT ( 'NONE',  ( -2.117044542028253318, 5.621635732341564662, -0.7998128361456281477 ) ) ;
#170272=CARTESIAN_POINT ( 'NONE',  ( 8.274553823041976841, 8.548067636504127265, 1.040834085586084257E-14 ) ) ;
#170276=CARTESIAN_POINT ( 'NONE',  ( -5.930802130974132780, 9.006687355190106103, -1.199719254218440723 ) ) ;
#170277=CARTESIAN_POINT ( 'NONE',  ( 2.984766373302843778, 6.633977868828633717, -0.7998128361456291469 ) ) ;
#170280=CARTESIAN_POINT ( 'NONE',  ( 9.378489572351044856, 11.96465713920816043, -1.599625672291262513 ) ) ;
#170281=CARTESIAN_POINT ( 'NONE',  ( -4.284013352238274841, 4.100363120473813794, -0.7216878364870207285 ) ) ;
#170284=CARTESIAN_POINT ( 'NONE',  ( 1.364683531249990311, 2.946875000341416140, 1.214306433183764966E-14 ) ) ;
#170286=CARTESIAN_POINT ( 'NONE',  ( 6.995644074971448134, 7.263932296995902149, -0.7216878364870257245 ) ) ;
#170290=CARTESIAN_POINT ( 'NONE',  ( 3.172244755473273781, 6.644776614786712443, 0.000000000000000000 ) ) ;
#170294=CARTESIAN_POINT ( 'NONE',  ( 7.687109908824030668, 10.95175007939464606, -1.082531754730543083 ) ) ;
#170298=CARTESIAN_POINT ( 'NONE',  ( -7.609150525767646833, 9.900428251527500834, -1.599625672291263179 ) ) ;
#170306=CARTESIAN_POINT ( 'NONE',  ( 8.191097360950562845, 12.70803068775103739, -0.7998128361456352531 ) ) ;
#170307=CIRCLE ( 'NONE', #118583, 0.08000000000000004330 ) ;
#170311=CARTESIAN_POINT ( 'NONE',  ( 3.499976210622149253, 7.235056012367825140, 0.7998128361456321445 ) ) ;
#170314=CARTESIAN_POINT ( 'NONE',  ( 1.499999999999987121, 3.077083334016149863, -0.8660254037844262731 ) ) ;
#170320=CARTESIAN_POINT ( 'NONE',  ( 0.7499999999999885647, -0.01666666666664401442, 1.299038105676657340 ) ) ;
#170321=CARTESIAN_POINT ( 'NONE',  ( 7.962716289927667113, 8.184257181204083409, -0.7998128361456291469 ) ) ;
#170322=CARTESIAN_POINT ( 'NONE',  ( 5.219525951136835928, 7.112532914458205013, -1.443375672974051449 ) ) ;
#170327=CARTESIAN_POINT ( 'NONE',  ( 10.39874063200158893, 11.23421161353111586, 0.000000000000000000 ) ) ;
#170328=EDGE_CURVE ( 'NONE', #123959, #193266, #181328, .T. ) ;
#170335=CARTESIAN_POINT ( 'NONE',  ( -4.660252114795309097, 6.460046772059735432, -1.599625672291256295 ) ) ;
#170336=CARTESIAN_POINT ( 'NONE',  ( 1.499999999999989120, 3.535416667349488229, 0.8660254037844524744 ) ) ;
#170337=CARTESIAN_POINT ( 'NONE',  ( -1.364683531249997417, 4.821875000341417916, 1.214306433183764966E-14 ) ) ;
#170342=CARTESIAN_POINT ( 'NONE',  ( -0.6823417656250212460, 4.363541667008085767, 1.181850606188767472 ) ) ;
#170345=PLANE ( 'NONE',  #36269 ) ;
#170346=EDGE_LOOP ( 'NONE', ( #76981, #122233, #68684, #186752 ) ) ;
#170351=CARTESIAN_POINT ( 'NONE',  ( -8.715193815486133033, 9.062147627688959872, 0.7998128361456462443 ) ) ;
#170352=CARTESIAN_POINT ( 'NONE',  ( 6.307567778855705853, 8.381915046796901692, -1.599625672291262513 ) ) ;
#170358=CARTESIAN_POINT ( 'NONE',  ( -7.815970093360414158E-14, 8.210952333604092601, -2.038660652713623733 ) ) ;
#170360=CARTESIAN_POINT ( 'NONE',  ( -6.235860587281615075, 9.362588887548838557, -1.199719254218440723 ) ) ;
#170367=CARTESIAN_POINT ( 'NONE',  ( 10.37606763316019531, 10.99983374830873650, 0.7998128361456462443 ) ) ;
#170369=CARTESIAN_POINT ( 'NONE',  ( -3.228813138348844536, 6.918699094715619502, 0.7998128361456341429 ) ) ;
#170370=CARTESIAN_POINT ( 'NONE',  ( -7.263417608619167076, 9.497073181520933716, -1.599625672291263179 ) ) ;
#170373=CARTESIAN_POINT ( 'NONE',  ( -4.475961918153980257, 7.265020140467052023, -1.287590260893024086 ) ) ;
#170374=CARTESIAN_POINT ( 'NONE',  ( 1.364683531249986537, -0.3447916663252443836, -0.7879004041258309554 ) ) ;
#170402=CARTESIAN_POINT ( 'NONE',  ( -9.671043645249580933, 10.17730576241299900, 0.7998128361456462443 ) ) ;
#170407=CARTESIAN_POINT ( 'NONE',  ( -1.500000000000013101, 1.202083334016148974, 0.8660254037844403729 ) ) ;
#170408=CARTESIAN_POINT ( 'NONE',  ( 8.516493047678546091, 13.08765898893368629, -0.7998128361456352531 ) ) ;
#170412=CARTESIAN_POINT ( 'NONE',  ( -9.236128959407555072, 11.79856975744075598, -1.599625672291263179 ) ) ;
#170414=CARTESIAN_POINT ( 'NONE',  ( -1.364683531250014514, 1.988541667008086655, -0.7879004041258289570 ) ) ;
#170415=CARTESIAN_POINT ( 'NONE',  ( -1.499999999999997780, 5.400000000000022560, 1.214306433183764966E-14 ) ) ;
#170416=EDGE_CURVE ( 'NONE', #108753, #179933, #93796, .T. ) ;
#170423=CARTESIAN_POINT ( 'NONE',  ( -2.916975605234527702, 6.554888639415577423, 1.040834085586084257E-14 ) ) ;
#170425=FACE_OUTER_BOUND ( 'NONE', #30626, .T. ) ;
#170428=CARTESIAN_POINT ( 'NONE',  ( -1.402160292154681736E-14, -0.1156249996585793222, 1.575800808251672791 ) ) ;
#170433=CARTESIAN_POINT ( 'NONE',  ( -1.364683531250014514, 0.03020833367475737191, 0.7879004041258379498 ) ) ;
#170435=CARTESIAN_POINT ( 'NONE',  ( -7.386494761346872551, 7.511998731193139989, -0.7998128361456291469 ) ) ;
#170436=CARTESIAN_POINT ( 'NONE',  ( 9.074484886248265880, 9.481320543578137361, 0.7998128361456462443 ) ) ;
#170437=CARTESIAN_POINT ( 'NONE',  ( 3.655894977179307226, 7.416961240017848844, -0.7998128361456291469 ) ) ;
#170438=CARTESIAN_POINT ( 'NONE',  ( 4.632082037363250748, 8.555846143565791095, -0.7998128361456231517 ) ) ;
#170439=CARTESIAN_POINT ( 'NONE',  ( 1.499999999999989120, 4.254166666666687746, 0.8660254037844524744 ) ) ;
#170441=CARTESIAN_POINT ( 'NONE',  ( 0.6823417656249882723, 0.9885416670080832136, -1.181850606188749264 ) ) ;
#170450=CARTESIAN_POINT ( 'NONE',  ( 5.327991180490514012, 9.159814110640187579, 1.040834085586084257E-14 ) ) ;
#170453=CARTESIAN_POINT ( 'NONE',  ( -7.497822643557261024, 8.706213491360317747, -1.199719254218446718 ) ) ;
#170454=CARTESIAN_POINT ( 'NONE',  ( -3.242371291962510504, 6.934516940598226320, 1.040834085586084257E-14 ) ) ;
#170455=CARTESIAN_POINT ( 'NONE',  ( -1.123270288250343141, 3.096052654332833054, 0.7749999999993751887 ) ) ;
#170459=CARTESIAN_POINT ( 'NONE',  ( -7.768458830506062007, 11.04665715469030296, 1.082531754730549967 ) ) ;
#170461=CARTESIAN_POINT ( 'NONE',  ( 0.7499999999999920064, 5.233333333333353821, 1.299038105676669330 ) ) ;
#170465=CARTESIAN_POINT ( 'NONE',  ( 8.080296364064698977, 12.37083682481011060, -0.7216878364870328300 ) ) ;
#170469=CARTESIAN_POINT ( 'NONE',  ( 1.500000000000007105, 10.64264068711930733, 1.214306433183764966E-14 ) ) ;
#170477=CARTESIAN_POINT ( 'NONE',  ( 9.219181267168295335, 9.858059021225592744, 1.040834085586084257E-14 ) ) ;
#170478=CARTESIAN_POINT ( 'NONE',  ( 7.775764792637399836, 9.030479331953833011, -1.199719254218441611 ) ) ;
#170480=CARTESIAN_POINT ( 'NONE',  ( -7.217017841176048165, 7.314275657660511243, 1.040834085586084257E-14 ) ) ;
#170485=CARTESIAN_POINT ( 'NONE',  ( 1.364683531249988757, -0.8031249996585804185, 0.000000000000000000 ) ) ;
#170486=CARTESIAN_POINT ( 'NONE',  ( 3.714570900464274850, 6.317121236308204324, 1.082531754730558626 ) ) ;
#170488=CARTESIAN_POINT ( 'NONE',  ( -4.796887421136680985, 4.490790167614548523, 1.214306433183764966E-14 ) ) ;
#170489=CARTESIAN_POINT ( 'NONE',  ( -8.080296364064746939, 9.489729181906076505, 1.082531754730558626 ) ) ;
#170502=VERTEX_POINT ( 'NONE', #11436 ) ;
#170505=DIRECTION ( 'NONE',  ( -5.578564026256490882E-16, -1.000000000000000000, -9.066213480720158442E-32 ) ) ;
#170506=CARTESIAN_POINT ( 'NONE',  ( 7.096803341749390981, 10.36702210109460154, -1.199719254218441611 ) ) ;
#170518=CARTESIAN_POINT ( 'NONE',  ( -5.228640796364566690, 9.251831362400652736, -0.7998128361456231517 ) ) ;
#170520=CARTESIAN_POINT ( 'NONE',  ( -4.115063316947640715, 4.759660943649018705, 1.199719254218462483 ) ) ;
#170529=CARTESIAN_POINT ( 'NONE',  ( -4.090809663021341969, 5.795697244990093644, 1.599625672291267398 ) ) ;
#170532=CARTESIAN_POINT ( 'NONE',  ( 6.805303039055573322, 10.02693841461847057, 1.199719254218460707 ) ) ;
#170533=CARTESIAN_POINT ( 'NONE',  ( 1.364683531249988535, 4.113541667008088432, 0.7879004041258499402 ) ) ;
#170539=CARTESIAN_POINT ( 'NONE',  ( 5.870317324592803310, 7.871789516823500144, -1.443375672974057666 ) ) ;
#170540=CARTESIAN_POINT ( 'NONE',  ( -6.184490626128011925, 10.36698949712469364, -0.7998128361456291469 ) ) ;
#170544=CARTESIAN_POINT ( 'NONE',  ( -6.344325816190970357, 9.489131654609717970, 1.199719254218452047 ) ) ;
#170545=CARTESIAN_POINT ( 'NONE',  ( -4.954615070790188369, 7.867802451642154082, -1.199719254218452047 ) ) ;
#170553=CARTESIAN_POINT ( 'NONE',  ( 5.601490020740366838, 9.686822124172440596, 1.040834085586084257E-14 ) ) ;
#170566=ORIENTED_EDGE ( 'NONE', *, *, #57726, .T. ) ;
#170568=CARTESIAN_POINT ( 'NONE',  ( -1.500000000000011324, 5.670833333333358262, 0.8660254037844403729 ) ) ;
#170569=CARTESIAN_POINT ( 'NONE',  ( 3.649115900372475796, 7.409052317076538330, 1.040834085586084257E-14 ) ) ;
#170570=CARTESIAN_POINT ( 'NONE',  ( 6.993308306550549247, 7.053281200597435685, 1.040834085586084257E-14 ) ) ;
#170571=EDGE_CURVE ( 'NONE', #138555, #184190, #41709, .T. ) ;
#170573=CARTESIAN_POINT ( 'NONE',  ( -8.270110514656041190, 10.67154823856396817, 1.443375672974090751 ) ) ;
#170574=CARTESIAN_POINT ( 'NONE',  ( 7.632877294813741109, 8.007371053478589573, 1.040834085586084257E-14 ) ) ;
#170576=CARTESIAN_POINT ( 'NONE',  ( -6.982085920913410071, 11.08959130780024260, 0.7216878364870458196 ) ) ;
#170579=CARTESIAN_POINT ( 'NONE',  ( 7.914208982075123799, 10.25632978388623684, -1.599625672291262513 ) ) ;
#170584=CARTESIAN_POINT ( 'NONE',  ( -0.6823417656250212460, 2.301041667008084435, 1.181850606188767472 ) ) ;
#170590=CARTESIAN_POINT ( 'NONE',  ( 9.596473800374404561, 10.09030761005864285, 0.000000000000000000 ) ) ;
#170594=CARTESIAN_POINT ( 'NONE',  ( -8.317037166979361018, 11.79062823052953668, 1.199719254218453823 ) ) ;
#170600=CARTESIAN_POINT ( 'NONE',  ( 2.354312230267378236, 5.898448035287240820, -0.7998128361456281477 ) ) ;
#170604=CARTESIAN_POINT ( 'NONE',  ( -9.073431116043565225, 11.60875560684942265, -1.599625672291263179 ) ) ;
#170610=CARTESIAN_POINT ( 'NONE',  ( 5.891550962509589873, 5.977563058329811163, 0.05700887847147687038 ) ) ;
#170611=CARTESIAN_POINT ( 'NONE',  ( 1.177110729581195114, 3.245878374463980975, -0.7749999999999840350 ) ) ;
#170612=CARTESIAN_POINT ( 'NONE',  ( -2.903417451620861289, 6.539070793532962611, 0.7998128361456341429 ) ) ;
#170616=CARTESIAN_POINT ( 'NONE',  ( 6.238723240582662477, 10.43026088065513513, -0.7998128361456291469 ) ) ;
#170618=CARTESIAN_POINT ( 'NONE',  ( 5.601490020740366838, 9.686822124172440596, 1.040834085586084257E-14 ) ) ;
#170622=CARTESIAN_POINT ( 'NONE',  ( -7.646435448427427062, 10.90429654226522693, 1.082531754730549967 ) ) ;
#170630=CARTESIAN_POINT ( 'NONE',  ( -5.402149754905330781, 6.322992007072439691, -1.066970298751448443 ) ) ;
#170632=CARTESIAN_POINT ( 'NONE',  ( 5.992340707560163793, 6.093411701682730275, 0.7216878364870317197 ) ) ;
#170637=CARTESIAN_POINT ( 'NONE',  ( -8.961576348508637935, 12.43862759236002269, -1.082531754730543083 ) ) ;
#170654=EDGE_CURVE ( 'NONE', #106155, #173996, #126658, .T. ) ;
#170656=CARTESIAN_POINT ( 'NONE',  ( 8.606728586576791074, 8.935604860628076906, 0.7998128361456462443 ) ) ;
#170660=CARTESIAN_POINT ( 'NONE',  ( 0.7499999999999885647, 1.347916667349485786, -1.299038105676652899 ) ) ;
#170662=CARTESIAN_POINT ( 'NONE',  ( -7.230575994789712801, 7.330093503543126054, 0.7998128361456341429 ) ) ;
#170665=CARTESIAN_POINT ( 'NONE',  ( -8.784793466650835825, 12.33634391347959713, 1.199719254218462483 ) ) ;
#170666=CARTESIAN_POINT ( 'NONE',  ( -1.451998047840359130, 7.315968950356099398, 4.301760722582896435 ) ) ;
#170669=CARTESIAN_POINT ( 'NONE',  ( 0.7499999999999902300, 5.597916667349482900, -1.299038105676658228 ) ) ;
#170670=CARTESIAN_POINT ( 'NONE',  ( 6.100279051144945619, 9.204410428722734849, -1.199719254218440723 ) ) ;
#170672=CARTESIAN_POINT ( 'NONE',  ( -7.549192604710863286, 7.701812881784464437, -0.7998128361456291469 ) ) ;
#170674=CARTESIAN_POINT ( 'NONE',  ( 1.364683531249992088, 5.384375000341417916, 1.214306433183764966E-14 ) ) ;
#170680=CARTESIAN_POINT ( 'NONE',  ( -7.754900677336769022, 9.110100880723427608, 1.082531754730558626 ) ) ;
#170684=CARTESIAN_POINT ( 'NONE',  ( -1.001543065824772872E-14, 4.384375000341417916, 1.575800808251672791 ) ) ;
#170690=CARTESIAN_POINT ( 'NONE',  ( -0.6823417656249969321, 4.217708333674755394, -1.181850606188749264 ) ) ;
#170691=DIRECTION ( 'NONE',  ( -1.000000000000000000, 4.984021416236792516E-16, 0.000000000000000000 ) ) ;
#170693=CARTESIAN_POINT ( 'NONE',  ( 2.507895228403643539, 5.869702166538802501, -0.7216878364870267237 ) ) ;
#170700=EDGE_CURVE ( 'NONE', #7066, #123166, #196665, .T. ) ;
#170701=CARTESIAN_POINT ( 'NONE',  ( -0.6823417656250212460, 0.8010416670080899859, 1.181850606188755259 ) ) ;
#170702=CARTESIAN_POINT ( 'NONE',  ( -4.338245966692955591, 5.124003718305597310, 1.082531754730560403 ) ) ;
#170703=CARTESIAN_POINT ( 'NONE',  ( 5.066996723205273057, 6.934582148538044777, 1.599625672291267398 ) ) ;
#170709=CARTESIAN_POINT ( 'NONE',  ( 2.385871846325007706, 5.727341554113725586, -0.7216878364870267237 ) ) ;
#170710=CARTESIAN_POINT ( 'NONE',  ( 9.151390499099949949, 12.66007743471656788, -1.082531754730543971 ) ) ;
#170712=CARTESIAN_POINT ( 'NONE',  ( -6.710922849084449915, 10.77323439066645783, 0.000000000000000000 ) ) ;
#170718=CARTESIAN_POINT ( 'NONE',  ( -9.158696461231359720, 10.64389961198009615, 1.199719254218462483 ) ) ;
#170719=CARTESIAN_POINT ( 'NONE',  ( -4.867013957181525186, 8.622007350113015889, 0.7216878364870458196 ) ) ;
#170720=CARTESIAN_POINT ( 'NONE',  ( 1.364683531249986537, 1.967708333674750731, -0.7879004041258239610 ) ) ;
#170730=EDGE_LOOP ( 'NONE', ( #166934, #178844, #128123, #64486, #21952 ) ) ;
#170741=CARTESIAN_POINT ( 'NONE',  ( 2.460826785407678408, 8.202405370174465915, -2.499999999999995559 ) ) ;
#170744=CARTESIAN_POINT ( 'NONE',  ( -4.613852347352193739, 4.277249248199312071, 1.214306433183764966E-14 ) ) ;
#170746=CARTESIAN_POINT ( 'NONE',  ( 1.499999999999990896, 4.056250000682819490, 1.214306433183764966E-14 ) ) ;
#170747=CARTESIAN_POINT ( 'NONE',  ( -0.6823417656249969321, 3.530208333674754506, -1.181850606188749264 ) ) ;
#170756=CARTESIAN_POINT ( 'NONE',  ( -1.201851678989727383E-14, 1.571875000341420581, 1.575800808251672791 ) ) ;
#170758=ORIENTED_EDGE ( 'NONE', *, *, #208798, .T. ) ;
#170767=CARTESIAN_POINT ( 'NONE',  ( 6.179819089730593795, 6.104210447640811665, 1.040834085586084257E-14 ) ) ;
#170774=CARTESIAN_POINT ( 'NONE',  ( 6.096362627639171805, 10.26417349888772179, -0.7998128361456291469 ) ) ;
#170777=CARTESIAN_POINT ( 'NONE',  ( 7.235247531187115833, 11.59287255302699648, -0.7998128361456291469 ) ) ;
#170790=CARTESIAN_POINT ( 'NONE',  ( -8.514157279702036618, 9.035531035848267223, -0.7216878364870278340 ) ) ;
#170794=VECTOR ( 'NONE', #167163, 1000.000000000000114 ) ;
#170795=CARTESIAN_POINT ( 'NONE',  ( -8.136864746495904299, 12.64475930422059768, -0.7998128361456281477 ) ) ;
#170801=CARTESIAN_POINT ( 'NONE',  ( -3.924195396151603177, 6.665646164563756138, 1.199719254218464037 ) ) ;
#170803=CARTESIAN_POINT ( 'NONE',  ( 3.728129053633592704, 4.412200653069714207, -1.082531754730543083 ) ) ;
#170805=CARTESIAN_POINT ( 'NONE',  ( 2.869522067586683711, 6.499526178826442013, 0.7998128361456362523 ) ) ;
#170807=ORIENTED_EDGE ( 'NONE', *, *, #183332, .T. ) ;
#170811=CARTESIAN_POINT ( 'NONE',  ( 4.202664430556254160, 5.926194473780837413, 1.443375672974062551 ) ) ;
#170813=CARTESIAN_POINT ( 'NONE',  ( -4.446184310277715213, 7.274633231044262516, -1.199719254218452047 ) ) ;
#170816=CARTESIAN_POINT ( 'NONE',  ( -10.47097470845587175, 11.11055866948701443, 1.040834085586084257E-14 ) ) ;
#170822=CARTESIAN_POINT ( 'NONE',  ( 7.429504990608736037, 11.61158022244479682, -0.7216878364870267237 ) ) ;
#170823=CARTESIAN_POINT ( 'NONE',  ( 1.364683531249990311, 4.196875000341417028, 1.214306433183764966E-14 ) ) ;
#170825=CARTESIAN_POINT ( 'NONE',  ( 3.659811400685081040, 6.357198169852855685, -1.199719254218446718 ) ) ;
#170838=CARTESIAN_POINT ( 'NONE',  ( 1.364683531249988757, 2.196875000341415252, 1.214306433183764966E-14 ) ) ;
#170840=CARTESIAN_POINT ( 'NONE',  ( 9.890836756369282057, 11.49806328964105617, -1.199719254218440723 ) ) ;
#170843=CARTESIAN_POINT ( 'NONE',  ( -6.127922243696855453, 7.211959374810172463, 1.082531754730549967 ) ) ;
#170844=CARTESIAN_POINT ( 'NONE',  ( 2.738383840280328663, 5.178236332760252303, 1.082531754730548412 ) ) ;
#170845=CARTESIAN_POINT ( 'NONE',  ( -5.219525951136845698, 8.072902128759544382, -1.082531754730543971 ) ) ;
#170849=CARTESIAN_POINT ( 'NONE',  ( 5.983225862332436584, 5.874851682342960402, 0.7998128361456341429 ) ) ;
#170859=CARTESIAN_POINT ( 'NONE',  ( 4.821896187954575197, 8.777295985922343391, 0.7998128361456462443 ) ) ;
#170862=CARTESIAN_POINT ( 'NONE',  ( -4.302014814237876017, 3.913438792899272212, 0.7998128361456341429 ) ) ;
#170865=CARTESIAN_POINT ( 'NONE',  ( -5.391338639728555648, 9.441645512991978961, -0.7998128361456231517 ) ) ;
#170869=CARTESIAN_POINT ( 'NONE',  ( 7.938462636001388795, 9.220293482545153907, -1.199719254218441611 ) ) ;
#170871=CARTESIAN_POINT ( 'NONE',  ( -5.442708600882160574, 8.437244903416123876, -1.199719254218446718 ) ) ;
#170872=CARTESIAN_POINT ( 'NONE',  ( 7.605760987142057061, 7.975735361194951523, -0.7216878364870267237 ) ) ;
#170873=CARTESIAN_POINT ( 'NONE',  ( 4.344452866495080556, 7.409550296852231099, 1.129427019999120985 ) ) ;
#170874=CARTESIAN_POINT ( 'NONE',  ( -5.168682875307782254, 7.053215992657626110, -1.599625672291256295 ) ) ;
#170877=CARTESIAN_POINT ( 'NONE',  ( -7.237355071596549116, 7.338002426484427687, 1.040834085586084257E-14 ) ) ;
#170880=CARTESIAN_POINT ( 'NONE',  ( -1.364683531250000748, 1.509375000341421691, 0.000000000000000000 ) ) ;
#170882=CARTESIAN_POINT ( 'NONE',  ( -6.561783159334141580, 7.718130443053708767, -1.082531754730544860 ) ) ;
#170885=VERTEX_POINT ( 'NONE', #67620 ) ;
#170887=CARTESIAN_POINT ( 'NONE',  ( 5.361359679200154105, 8.342337828120466980, 1.199719254218462483 ) ) ;
#170890=CARTESIAN_POINT ( 'NONE',  ( -5.897748123441601820, 6.008673066555767051, -0.2037434952626964724 ) ) ;
#170891=CARTESIAN_POINT ( 'NONE',  ( -1.364683531250014514, 1.301041667008083325, -0.7879004041258289570 ) ) ;
#170894=CARTESIAN_POINT ( 'NONE',  ( -0.3562281372919119393, 7.169715878026186928, 1.968597608854712133 ) ) ;
#170897=CARTESIAN_POINT ( 'NONE',  ( -3.574546055497324737, 7.322054164722185732, 0.7998128361456341429 ) ) ;
#170898=CARTESIAN_POINT ( 'NONE',  ( -6.846504384776758378, 9.010674420371453053, -1.443375672974058777 ) ) ;
#170906=CARTESIAN_POINT ( 'NONE',  ( -7.605760987142072160, 10.85684300409898384, 1.082531754730549967 ) ) ;
#170908=CARTESIAN_POINT ( 'NONE',  ( -1.284279953904152949, 2.952889714876734573, 0.7750000000000152323 ) ) ;
#170911=CARTESIAN_POINT ( 'NONE',  ( -7.117667457050096402, 10.28740055232499984, 1.082531754730549967 ) ) ;
#170916=CARTESIAN_POINT ( 'NONE',  ( 4.435735274902380176, 7.313263296268260660, -1.222879399185505367 ) ) ;
#170923=CARTESIAN_POINT ( 'NONE',  ( -5.831978632172702071, 9.955725504176825780, 0.7998128361456481317 ) ) ;
#170926=CARTESIAN_POINT ( 'NONE',  ( 3.323720213644492993, 7.029424015893889433, 1.040834085586084257E-14 ) ) ;
#170930=CARTESIAN_POINT ( 'NONE',  ( 4.632082037363250748, 8.555846143565791095, -0.7998128361456231517 ) ) ;
#170934=CARTESIAN_POINT ( 'NONE',  ( -4.772106882330234612, 6.590544000850479200, -1.443375672974053447 ) ) ;
#170939=CARTESIAN_POINT ( 'NONE',  ( -0.3549189177861599154, 6.558674322353176933, 3.205845166494230902 ) ) ;
#170941=EDGE_LOOP ( 'NONE', ( #52632, #18983, #202061, #68582 ) ) ;
#170945=CARTESIAN_POINT ( 'NONE',  ( 1.364683531249986537, 0.6552083336747522857, -0.7879004041258239610 ) ) ;
#170947=CARTESIAN_POINT ( 'NONE',  ( -9.040589502214116280, 9.441775928871617651, 0.7998128361456462443 ) ) ;
#170950=CARTESIAN_POINT ( 'NONE',  ( 6.760712154708803823, 11.03924794713562818, 1.040834085586084257E-14 ) ) ;
#170952=CARTESIAN_POINT ( 'NONE',  ( -8.050844288416501016, 8.287073179441051707, 1.040834085586084257E-14 ) ) ;
#170955=CARTESIAN_POINT ( 'NONE',  ( 1.364683531249990311, 4.384375000341417028, 1.214306433183764966E-14 ) ) ;
#170957=CARTESIAN_POINT ( 'NONE',  ( 10.08690309888728187, 10.87040115823107911, -0.7216878364870257245 ) ) ;
#170960=CARTESIAN_POINT ( 'NONE',  ( 1.364683531249986537, -0.7822916663252464931, -0.7879004041258309554 ) ) ;
#170963=CARTESIAN_POINT ( 'NONE',  ( 8.066738210006692000, 8.513542121203711233, 0.7216878364870458196 ) ) ;
#170965=CARTESIAN_POINT ( 'NONE',  ( -5.395781948114519722, 5.397426482329451325, 0.000000000000000000 ) ) ;
#170966=CARTESIAN_POINT ( 'NONE',  ( -5.748293942514186128, 6.769059690097084747, -1.082531754730544860 ) ) ;
#170969=CARTESIAN_POINT ( 'NONE',  ( -1.364683531249997417, 2.759375000341422801, 1.214306433183764966E-14 ) ) ;
#170973=CARTESIAN_POINT ( 'NONE',  ( -7.054319997812058318, 7.124461507069184130, 1.040834085586084257E-14 ) ) ;
#170979=CARTESIAN_POINT ( 'NONE',  ( 8.718056468787178659, 10.12981962079525289, 1.199719254218462483 ) ) ;
#170982=CARTESIAN_POINT ( 'NONE',  ( 0.7499999999999885647, 2.566666666666689522, -1.299038105676658228 ) ) ;
#170988=CARTESIAN_POINT ( 'NONE',  ( 6.399085315970131305, 8.488685506763726352, -1.443375672974057666 ) ) ;
#170989=CARTESIAN_POINT ( 'NONE',  ( 0.6823417656249882723, -0.01145833299191073573, -1.181850606188749264 ) ) ;
#170991=CARTESIAN_POINT ( 'NONE',  ( 2.367870383881045981, 5.914265881169853856, 0.000000000000000000 ) ) ;
#170998=CARTESIAN_POINT ( 'NONE',  ( 1.499999999999987121, -0.9958333333333134751, 0.8660254037844524744 ) ) ;
#170999=CARTESIAN_POINT ( 'NONE',  ( 6.805303039055573322, 10.02693841461847057, 1.199719254218460707 ) ) ;
#171000=CARTESIAN_POINT ( 'NONE',  ( -9.073431116043565225, 11.60875560684942265, -1.599625672291263179 ) ) ;
#171002=CARTESIAN_POINT ( 'NONE',  ( 1.364683531249986537, -0.3447916663252443836, -0.7879004041258309554 ) ) ;
#171003=CARTESIAN_POINT ( 'NONE',  ( -1.500000000000001332, 1.150000000000019007, 0.000000000000000000 ) ) ;
#171006=CARTESIAN_POINT ( 'NONE',  ( 6.308621549060418054, 6.254479983525607523, 0.7998128361456341429 ) ) ;
#171008=CARTESIAN_POINT ( 'NONE',  ( -4.650083499807267984, 5.295740330745369207, 2.420000000000010587 ) ) ;
#171012=CARTESIAN_POINT ( 'NONE',  ( -1.364683531250012516, 4.738541667008091096, -0.7879004041258300672 ) ) ;
#171014=CARTESIAN_POINT ( 'NONE',  ( -7.133561379084627063, 11.47423870890741782, 0.7998128361456481317 ) ) ;
#171015=CARTESIAN_POINT ( 'NONE',  ( -3.768803514918943609, 7.340761834139994058, 0.7216878364870317197 ) ) ;
#171023=CARTESIAN_POINT ( 'NONE',  ( 8.260995669428309540, 8.532249790621511565, 0.7998128361456481317 ) ) ;
#171027=CARTESIAN_POINT ( 'NONE',  ( 6.710922848640084482, 9.812865175846695820, -1.082531754730537976 ) ) ;
#171030=CARTESIAN_POINT ( 'NONE',  ( -6.333630315878337136, 10.54098580183340772, 0.000000000000000000 ) ) ;
#171031=CARTESIAN_POINT ( 'NONE',  ( 5.681030059326015014, 6.586622143090519188, -1.199719254218445830 ) ) ;
#171033=CARTESIAN_POINT ( 'NONE',  ( -1.000000000000017097, 9.200000000000018829, 0.4000000000000144551 ) ) ;
#171034=CARTESIAN_POINT ( 'NONE',  ( 3.602716132929354664, 5.226254793216122074, 1.599625672291267398 ) ) ;
#171040=CARTESIAN_POINT ( 'NONE',  ( -5.477130870240893401, 6.452702772444876445, 1.082531754730548412 ) ) ;
#171041=CARTESIAN_POINT ( 'NONE',  ( 8.866669273657322492, 12.32790267170016207, -1.082531754730543083 ) ) ;
#171044=CARTESIAN_POINT ( 'NONE',  ( -6.368579470117215813, 8.453095353268645695, 1.599625672291283607 ) ) ;
#171049=CARTESIAN_POINT ( 'NONE',  ( -5.994676475536691029, 10.14553965476814845, 0.7998128361456481317 ) ) ;
#171054=CARTESIAN_POINT ( 'NONE',  ( 6.173040012923759257, 6.096301524699504704, -0.7998128361456281477 ) ) ;
#171055=ORIENTED_EDGE ( 'NONE', *, *, #150437, .F. ) ;
#171066=CARTESIAN_POINT ( 'NONE',  ( -5.357443255694392725, 9.402100898285455699, 0.000000000000000000 ) ) ;
#171069=CARTESIAN_POINT ( 'NONE',  ( 5.178851490740196795, 7.065079377328788546, 1.443375672974062551 ) ) ;
#171074=CARTESIAN_POINT ( 'NONE',  ( -5.087333953625788219, 6.958308917361963886, 1.599625672291267398 ) ) ;
#171078=CARTESIAN_POINT ( 'NONE',  ( -7.040761844198392794, 7.108643661186573759, -0.7998128361456291469 ) ) ;
#171084=CARTESIAN_POINT ( 'NONE',  ( -7.991641480251377772, 11.41099992934688956, 1.199719254218453823 ) ) ;
#171085=CARTESIAN_POINT ( 'NONE',  ( 8.274553823041976841, 8.548067636504127265, 1.040834085586084257E-14 ) ) ;
#171090=CARTESIAN_POINT ( 'NONE',  ( -8.272446282632566650, 12.80293776304669962, 0.7998128361456481317 ) ) ;
#171093=CARTESIAN_POINT ( 'NONE',  ( -1.364683531250014514, -0.6989583329919100141, -0.7879004041258359514 ) ) ;
#171099=CARTESIAN_POINT ( 'NONE',  ( 9.002250809793993724, 11.52571191622492464, -1.443375672974057666 ) ) ;
#171119=CARTESIAN_POINT ( 'NONE',  ( -4.457933580795036654, 4.095344020549286590, -0.7998128361456221525 ) ) ;
#171122=CARTESIAN_POINT ( 'NONE',  ( -4.471491734408701291, 4.111161866431900513, 1.214306433183764966E-14 ) ) ;
#171126=CARTESIAN_POINT ( 'NONE',  ( -1.001543065824772872E-14, 5.571875000341416140, 1.575800808251672791 ) ) ;
#171135=CARTESIAN_POINT ( 'NONE',  ( 3.297657676621871925, 4.870353260857385180, 1.599625672291267398 ) ) ;
#171138=CARTESIAN_POINT ( 'NONE',  ( 3.939498435241196805, 2.812004590916141300, -0.7749999999999935829 ) ) ;
#171140=CARTESIAN_POINT ( 'NONE',  ( 5.392392409933256303, 7.314210449720692786, 1.599625672291267398 ) ) ;
#171141=CARTESIAN_POINT ( 'NONE',  ( -1.364683531250014514, 2.051041667008086655, -0.7879004041258289570 ) ) ;
#171144=CARTESIAN_POINT ( 'NONE',  ( -9.182950115157607840, 9.607863310639020327, 0.7998128361456462443 ) ) ;
#171145=CARTESIAN_POINT ( 'NONE',  ( -3.741687207247254676, 7.309126141856352454, 1.040834085586084257E-14 ) ) ;
#171148=CARTESIAN_POINT ( 'NONE',  ( -5.799137018343247796, 7.788745826199009237, -1.599625672291256295 ) ) ;
#171150=CARTESIAN_POINT ( 'NONE',  ( 0.6823417656249917140, 5.342708333674749177, 1.181850606188765695 ) ) ;
#171159=CARTESIAN_POINT ( 'NONE',  ( -5.761852095683518193, 6.784877535461274256, 1.082531754730546636 ) ) ;
#171165=CARTESIAN_POINT ( 'NONE',  ( -5.111060722227552588, 6.025620933095978238, 1.082531754730546636 ) ) ;
#171167=CARTESIAN_POINT ( 'NONE',  ( 10.08456733046637765, 10.65975006183261087, 0.000000000000000000 ) ) ;
#171177=CARTESIAN_POINT ( 'NONE',  ( -3.632695093457760649, 6.325562478087638496, -1.199719254218452047 ) ) ;
#171178=CARTESIAN_POINT ( 'NONE',  ( -10.32183501870554387, 10.93656236477829502, 0.7998128361456462443 ) ) ;
#171183=CARTESIAN_POINT ( 'NONE',  ( 6.114890974963323345, 7.092793211334054604, 1.199719254218462483 ) ) ;
#171187=FACE_OUTER_BOUND ( 'NONE', #196760, .T. ) ;
#171188=CARTESIAN_POINT ( 'NONE',  ( 3.704402285031850539, 5.344888637335695414, -1.599625672291262513 ) ) ;
#171198=CARTESIAN_POINT ( 'NONE',  ( 6.611572464958476836, 10.86525164242692298, 0.7998128361456462443 ) ) ;
#171199=CARTESIAN_POINT ( 'NONE',  ( -5.762378981008047241, 6.681529218386182301, 1.199719254218450271 ) ) ;
#171201=CARTESIAN_POINT ( 'NONE',  ( 1.499999999999978906, 4.077083334016147198, -0.8660254037844369313 ) ) ;
#171204=CARTESIAN_POINT ( 'NONE',  ( -1.001543065824772872E-14, 5.071875000341421469, 1.575800808251672791 ) ) ;
#171206=CARTESIAN_POINT ( 'NONE',  ( -4.238895582566952314, 8.097128612970093897, 1.040834085586084257E-14 ) ) ;
#171209=CARTESIAN_POINT ( 'NONE',  ( 4.320244504248938355, 8.192035688265757898, 1.040834085586084257E-14 ) ) ;
#171210=CARTESIAN_POINT ( 'NONE',  ( -4.786191920824102830, 5.542644314838231168, 1.199719254218462483 ) ) ;
#171216=CARTESIAN_POINT ( 'NONE',  ( 6.968527767744104651, 8.192665819532020777, 1.082531754730558626 ) ) ;
#171218=CARTESIAN_POINT ( 'NONE',  ( 6.710922848640084482, 9.812865175846695820, -1.082531754730537976 ) ) ;
#171219=CARTESIAN_POINT ( 'NONE',  ( -1.364683531250012516, 3.301041667008084879, -0.7879004041258289570 ) ) ;
#171220=CARTESIAN_POINT ( 'NONE',  ( -1.500000000000022204, 8.627523663848661428, 2.580000000000011173 ) ) ;
#171221=CARTESIAN_POINT ( 'NONE',  ( 4.975479186090857375, 5.867442474269873642, 1.082531754730560403 ) ) ;
#171229=CARTESIAN_POINT ( 'NONE',  ( -4.103288207896339301, 7.680416417065718093, 0.7589585138018557497 ) ) ;
#171235=CARTESIAN_POINT ( 'NONE',  ( -9.561524646135538319, 12.17819805862340310, -1.599625672291263179 ) ) ;
#171240=CARTESIAN_POINT ( 'NONE',  ( -3.810004860640155311, 4.403759411290286252, 1.199719254218462483 ) ) ;
#171245=CARTESIAN_POINT ( 'NONE',  ( 3.009546912553647147, 5.494593250412460606, -1.082531754730543083 ) ) ;
#171246=CARTESIAN_POINT ( 'NONE',  ( -0.6823417656250212460, 3.613541667008085767, 1.181850606188767472 ) ) ;
#171248=CARTESIAN_POINT ( 'NONE',  ( 6.425674737872927089, 9.584038729905381970, -1.199719254218440723 ) ) ;
#171250=CARTESIAN_POINT ( 'NONE',  ( -8.859363311525973117, 12.42334206583395328, -1.199719254218446718 ) ) ;
#171252=CARTESIAN_POINT ( 'NONE',  ( -5.590039407536138150, 5.416134151747256986, 0.000000000000000000 ) ) ;
#171258=CARTESIAN_POINT ( 'NONE',  ( 0.7499999999999920064, 4.483333333333352932, 1.299038105676669330 ) ) ;
#171259=CARTESIAN_POINT ( 'NONE',  ( 4.202137545231717120, 6.989912005157271402, 1.199719254218462483 ) ) ;
#171263=CARTESIAN_POINT ( 'NONE',  ( -1.001543065824772872E-14, 4.321875000341417916, 1.575800808251672791 ) ) ;
#171266=CARTESIAN_POINT ( 'NONE',  ( 9.463228032658635769, 11.10314946193233965, -1.082531754730543083 ) ) ;
#171271=( BOUNDED_CURVE ( )  B_SPLINE_CURVE ( 2, ( #188391, #206771, #139681, #109359, #190518, #159098, #41109 ),
 .UNSPECIFIED., .F., .T. ) 
 B_SPLINE_CURVE_WITH_KNOTS ( ( 3, 2, 2, 3 ),
 ( 0.01785714285714263064, 0.02380952380952366942, 0.02976190476190470821, 0.03571428571428574700 ),
 .UNSPECIFIED. ) 
 CURVE ( )  GEOMETRIC_REPRESENTATION_ITEM ( )  RATIONAL_B_SPLINE_CURVE ( ( 1.000000000000005107, 0.8660254037844337116, 1.000000000000000000, 0.8660254037844387076, 1.000000000000000000, 0.8660254037844379305, 1.000000000000000666 ) ) 
 REPRESENTATION_ITEM ( '' )  );
#171272=CARTESIAN_POINT ( 'NONE',  ( -1.402160292154681736E-14, 1.618750000682814827, -1.732050807568863648 ) ) ;
#171274=CARTESIAN_POINT ( 'NONE',  ( -5.904739593951539689, 6.847616600153594746, 1.199719254218450271 ) ) ;
#171275=CARTESIAN_POINT ( 'NONE',  ( 4.568734577680873876, 6.353276312092901890, -1.443375672974051449 ) ) ;
#171276=DIRECTION ( 'NONE',  ( -0.5265943820692667865, 0.4485553919953594315, -0.7221470882617865295 ) ) ;
#171282=ORIENTED_EDGE ( 'NONE', *, *, #154124, .T. ) ;
#171284=CARTESIAN_POINT ( 'NONE',  ( 8.457588896826466751, 8.761608555919362828, 1.040834085586084257E-14 ) ) ;
#171285=CARTESIAN_POINT ( 'NONE',  ( 5.281064527722868718, 6.119995689553514140, 1.199719254218462483 ) ) ;
#171290=CARTESIAN_POINT ( 'NONE',  ( 4.821896187954575197, 8.777295985922343391, 0.7998128361456462443 ) ) ;
#171291=CARTESIAN_POINT ( 'NONE',  ( -4.874313559192080092, 4.961021341527962036, 0.5169845646830675268 ) ) ;
#171296=VERTEX_POINT ( 'NONE', #132696 ) ;
#171297=CARTESIAN_POINT ( 'NONE',  ( 9.999301985278609806, 11.62460605670194447, 1.199719254218452047 ) ) ;
#171302=CARTESIAN_POINT ( 'NONE',  ( 5.804557637360799660, 6.030435022130575362, 0.4940411958238543066 ) ) ;
#171309=CARTESIAN_POINT ( 'NONE',  ( 6.100805936469477331, 9.101062111647635788, -1.082531754730537088 ) ) ;
#171310=CARTESIAN_POINT ( 'NONE',  ( -4.009460741339347045, 5.700790169694431420, -1.599625672291256295 ) ) ;
#171315=CARTESIAN_POINT ( 'NONE',  ( -3.958090780185743451, 6.705190779270287393, -1.199719254218452047 ) ) ;
#171317=CARTESIAN_POINT ( 'NONE',  ( 1.408750476333323176, 7.229967155398369982, -4.273289540531086672 ) ) ;
#171322=LINE ( 'NONE', #157231, #33237 ) ;
#171328=CARTESIAN_POINT ( 'NONE',  ( 9.582915646760733708, 10.07448976417602893, 0.7998128361456462443 ) ) ;
#171336=CARTESIAN_POINT ( 'NONE',  ( -10.30383355670593737, 11.12348669235284504, -0.7216878364870267237 ) ) ;
#171337=( BOUNDED_SURFACE ( )  B_SPLINE_SURFACE ( 3, 2, ( 
 ( #46485, #163434, #81103 ),
 ( #126743, #176479, #147191 ),
 ( #213216, #211086, #144022 ),
 ( #95250, #30229, #195929 ),
 ( #13949, #160226, #64846 ),
 ( #29159, #80032, #111542 ),
 ( #164490, #130992, #47567 ),
 ( #113678, #212148, #62709 ),
 ( #192702, #210016, #28090 ),
 ( #127826, #78961, #128870 ) ),
 .UNSPECIFIED., .F., .F., .T. ) 
 B_SPLINE_SURFACE_WITH_KNOTS ( ( 4, 2, 2, 2, 4 ),
 ( 3, 3 ),
 ( 0.001823084239704076889, 0.002278855299642388362, 0.002734626359580699835, 0.003190397419519010874, 0.003646168479457322347 ),
 ( 0.000000000000000000, 1.000000000000000000 ),
 .UNSPECIFIED. ) 
 GEOMETRIC_REPRESENTATION_ITEM ( )  RATIONAL_B_SPLINE_SURFACE ( (
 ( 1.000000000000000000, 0.8275596917163435817, 1.000000000000000000),
 ( 1.000000000000000000, 0.8320789365404243076, 1.000000000000000000),
 ( 1.000000000000000000, 0.8266768160090710582, 1.000000000000000000),
 ( 1.000000000000000000, 0.7938580293400921972, 1.000000000000000000),
 ( 1.000000000000000000, 0.7658694575135178706, 1.000000000000000000),
 ( 1.000000000000000000, 0.6964599583665085358, 1.000000000000000000),
 ( 1.000000000000000000, 0.6553951921932222868, 1.000000000000000000),
 ( 1.000000000000000000, 0.5911026409457650344, 1.000000000000000000),
 ( 1.000000000000000000, 0.5677445233671155611, 1.000000000000000000),
 ( 1.000000000000000000, 0.5613739026647618369, 1.000000000000000000) ) ) 
 REPRESENTATION_ITEM ( '' )  SURFACE ( )  );
#171341=CARTESIAN_POINT ( 'NONE',  ( 7.995557903757111617, 10.35123685918189729, 1.599625672291281386 ) ) ;
#171346=CARTESIAN_POINT ( 'NONE',  ( -5.280010757518168063, 8.247430752824802980, -1.199719254218446718 ) ) ;
#171347=CARTESIAN_POINT ( 'NONE',  ( 3.497113557321089861, 6.167384019261527683, -1.199719254218446718 ) ) ;
#171352=CARTESIAN_POINT ( 'NONE',  ( 8.920375002787457319, 12.49452237230570084, 1.199719254218450271 ) ) ;
#171356=CARTESIAN_POINT ( 'NONE',  ( 1.364683531249988535, 2.426041667008088432, 0.7879004041258500513 ) ) ;
#171358=CARTESIAN_POINT ( 'NONE',  ( 7.321039761699430493, 7.643560598178549270, -0.7216878364870257245 ) ) ;
#171366=CARTESIAN_POINT ( 'NONE',  ( 8.310784975052673218, 10.71900177569337487, -1.443375672974063439 ) ) ;
#171371=CARTESIAN_POINT ( 'NONE',  ( -7.506410603460441422, 11.90922947067921278, -0.7998128361456291469 ) ) ;
#171377=B_SPLINE_CURVE_WITH_KNOTS ( 'NONE', 3,
 ( #145795, #82871, #97031, #160943, #78609, #194497 ),
 .UNSPECIFIED., .F., .F.,
 ( 4, 2, 4 ),
 ( 0.000000000000000000, 0.002110194456903486098, 0.004220388913806971329 ),
 .UNSPECIFIED. ) ;
#171381=CARTESIAN_POINT ( 'NONE',  ( 3.517450787741589036, 6.191110788085444128, -1.199719254218446718 ) ) ;
#171387=CARTESIAN_POINT ( 'NONE',  ( 5.392392409933256303, 7.314210449720692786, 1.599625672291267398 ) ) ;
#171390=CARTESIAN_POINT ( 'NONE',  ( 0.7499999999999885647, 3.347916667349487341, -1.299038105676658228 ) ) ;
#171394=ORIENTED_EDGE ( 'NONE', *, *, #138645, .T. ) ;
#171396=CARTESIAN_POINT ( 'NONE',  ( 0.7499999999999885647, 0.5666666666666875241, -1.299038105676652899 ) ) ;
#171397=CARTESIAN_POINT ( 'NONE',  ( 6.479907352327590964, 9.647310113435821677, 1.199719254218462483 ) ) ;
#171399=CARTESIAN_POINT ( 'NONE',  ( -1.364683531250014514, -0.7197916663252461600, 0.7879004041258379498 ) ) ;
#171402=CARTESIAN_POINT ( 'NONE',  ( 8.920901888111986366, 12.39117405523060889, 1.082531754730546636 ) ) ;
#171408=CARTESIAN_POINT ( 'NONE',  ( -6.501298352952815662, 7.543601818988450169, -1.199719254218446718 ) ) ;
#171409=VECTOR ( 'NONE', #127732, 1000.000000000000000 ) ;
#171410=CARTESIAN_POINT ( 'NONE',  ( -1.201851678989727383E-14, 2.993750000682821266, 1.732050807568877637 ) ) ;
#171412=CARTESIAN_POINT ( 'NONE',  ( 0.6823417656249864960, -1.073958332991911568, -1.181850606188749264 ) ) ;
#171417=CARTESIAN_POINT ( 'NONE',  ( -1.201851678989727383E-14, 4.009375000341416140, -1.575800808251660134 ) ) ;
#171427=CARTESIAN_POINT ( 'NONE',  ( -7.985916173649233230, 9.275655943134292869, -1.199719254218446718 ) ) ;
#171428=CARTESIAN_POINT ( 'NONE',  ( 5.035963992472171746, 7.962709526937818083, 1.199719254218462483 ) ) ;
#171436=CARTESIAN_POINT ( 'NONE',  ( -5.669280788808708671, 9.765911353585494226, 0.7998128361456481317 ) ) ;
#171441=CARTESIAN_POINT ( 'NONE',  ( 8.380911511541880188, 12.92948053010758258, 0.7998128361456462443 ) ) ;
#171443=VERTEX_POINT ( 'NONE', #91404 ) ;
#171444=CARTESIAN_POINT ( 'NONE',  ( -4.711622075948912247, 5.455646162483875017, -1.199719254218446718 ) ) ;
#171445=CARTESIAN_POINT ( 'NONE',  ( -9.345647958521597687, 9.797677461230342999, 0.7998128361456462443 ) ) ;
#171449=CARTESIAN_POINT ( 'NONE',  ( -4.432925279414208219, 7.308574008990986748, -1.253226476263115341 ) ) ;
#171456=CARTESIAN_POINT ( 'NONE',  ( 6.440286661691305703, 7.472421512516709718, 1.199719254218462483 ) ) ;
#171479=CARTESIAN_POINT ( 'NONE',  ( -8.727698198895085469, 11.20540053684285553, -1.599625672291263179 ) ) ;
#171480=DIRECTION ( 'NONE',  ( -0.000000000000000000, -8.546850786086437571E-32, -1.000000000000000000 ) ) ;
#171484=CARTESIAN_POINT ( 'NONE',  ( 1.499999999999989120, 1.806250000682817269, 0.000000000000000000 ) ) ;
#171489=CARTESIAN_POINT ( 'NONE',  ( -7.980945979938748103, 12.46285407657057220, 0.000000000000000000 ) ) ;
#171491=CARTESIAN_POINT ( 'NONE',  ( 0.6823417656249882723, 1.176041667008083325, -1.181850606188749264 ) ) ;
#171497=CARTESIAN_POINT ( 'NONE',  ( -4.765854690403601879, 5.518917546014321829, 1.199719254218462483 ) ) ;
#171501=CARTESIAN_POINT ( 'NONE',  ( 0.6823417656249882723, -0.01145833299191073573, -1.181850606188749264 ) ) ;
#171506=CARTESIAN_POINT ( 'NONE',  ( 1.364683531249986537, -0.3447916663252443836, -0.7879004041258309554 ) ) ;
#171508=CARTESIAN_POINT ( 'NONE',  ( -6.714312387265696458, 8.856450423275211037, 1.599625672291283607 ) ) ;
#171509=CARTESIAN_POINT ( 'NONE',  ( 10.06423010004587759, 10.63602329300870153, 0.000000000000000000 ) ) ;
#171510=CARTESIAN_POINT ( 'NONE',  ( 3.818592820543299293, 7.606775390609172405, -0.7998128361456221525 ) ) ;
#171513=CARTESIAN_POINT ( 'NONE',  ( -1.364683531250014514, 1.801041667008085767, -0.7879004041258289570 ) ) ;
#171520=CARTESIAN_POINT ( 'NONE',  ( 7.293923454472091450, 7.611924906413328529, 0.7216878364870317197 ) ) ;
#171523=CARTESIAN_POINT ( 'NONE',  ( -5.115504031057831469, 4.862509545855891346, 0.7998128361456341429 ) ) ;
#171524=CARTESIAN_POINT ( 'NONE',  ( -4.227109282828894088, 7.477533499778591164, -0.9684700126486052163 ) ) ;
#171527=CARTESIAN_POINT ( 'NONE',  ( -1.499999999999997780, 4.431250000682819490, 1.214306433183764966E-14 ) ) ;
#171528=CARTESIAN_POINT ( 'NONE',  ( 3.972175818679561043, 7.578029521860726092, -0.7216878364870197293 ) ) ;
#171529=CARTESIAN_POINT ( 'NONE',  ( -7.334597914868722590, 11.50085530074811935, -0.7216878364870267237 ) ) ;
#171531=CARTESIAN_POINT ( 'NONE',  ( 1.499999999999989120, 4.504166666666688634, 0.8660254037844524744 ) ) ;
#171535=CARTESIAN_POINT ( 'NONE',  ( 7.890482213473377193, 11.18901776815221716, -1.082531754730543083 ) ) ;
#171546=CARTESIAN_POINT ( 'NONE',  ( 8.066738210006686671, 9.473911335505048825, 1.082531754730558626 ) ) ;
#171549=CARTESIAN_POINT ( 'NONE',  ( 8.426556166093362776, 9.789735934319136135, -1.199719254218446718 ) ) ;
#171550=CARTESIAN_POINT ( 'NONE',  ( -7.203459687562382641, 7.298457811777897319, -0.7998128361456291469 ) ) ;
#171554=CARTESIAN_POINT ( 'NONE',  ( -0.6823417656250003738, -0.4697916663252491021, -1.181850606188749264 ) ) ;
#171555=CARTESIAN_POINT ( 'NONE',  ( 4.690757960648231695, 5.535267711253469614, 1.082531754730560403 ) ) ;
#171557=CARTESIAN_POINT ( 'NONE',  ( -7.375272376154093479, 9.627570410311676596, -1.443375672974059665 ) ) ;
#171573=CARTESIAN_POINT ( 'NONE',  ( 6.598014311344812199, 10.84943379654430906, 1.040834085586084257E-14 ) ) ;
#171579=EDGE_CURVE ( 'NONE', #57507, #195170, #1932, .T. ) ;
#171586=CARTESIAN_POINT ( 'NONE',  ( -6.358937740009323214, 7.377514437221045718, -1.199719254218446718 ) ) ;
#171587=VECTOR ( 'NONE', #101196, 1000.000000000000000 ) ;
#171589=CARTESIAN_POINT ( 'NONE',  ( -3.418627288940168096, 7.140148937072163804, -0.7998128361456281477 ) ) ;
#171592=CARTESIAN_POINT ( 'NONE',  ( -4.741649638052999549, 5.202212439478444139, 1.069586989871945670 ) ) ;
#171599=CARTESIAN_POINT ( 'NONE',  ( -3.602716132929368875, 5.226254793216122074, 1.599625672291267398 ) ) ;
#171602=CARTESIAN_POINT ( 'NONE',  ( 6.856673000209174695, 9.022537805042615489, 1.599625672291281386 ) ) ;
#171605=CARTESIAN_POINT ( 'NONE',  ( 6.114657076318319007, 6.015903114251479167, -0.04046911893108330605 ) ) ;
#171611=CARTESIAN_POINT ( 'NONE',  ( 4.297571505407542958, 7.957657823043374989, -0.7216878364870197293 ) ) ;
#171612=EDGE_CURVE ( 'NONE', #11745, #21505, #22068, .T. ) ;
#171613=CARTESIAN_POINT ( 'NONE',  ( -8.206763054973658100, 8.468978407091068306, 0.7998128361456602331 ) ) ;
#171616=CARTESIAN_POINT ( 'NONE',  ( -7.995557903757128493, 10.35123685918189729, 1.599625672291295375 ) ) ;
#171617=CARTESIAN_POINT ( 'NONE',  ( -6.226218857173722476, 8.287007971501239467, 1.599625672291283607 ) ) ;
#171621=CARTESIAN_POINT ( 'NONE',  ( -1.201851678989727383E-14, 3.368750000682815049, -1.732050807568863648 ) ) ;
#171624=CARTESIAN_POINT ( 'NONE',  ( 7.588813295347141441, 9.876701482703580837, -1.599625672291262513 ) ) ;
#171625=DIRECTION ( 'NONE',  ( -1.000000000000000000, 6.308085367188389255E-16, 0.000000000000000000 ) ) ;
#171638=CARTESIAN_POINT ( 'NONE',  ( 1.499999999999990896, 3.775000000000021227, 1.214306433183764966E-14 ) ) ;
#171639=CARTESIAN_POINT ( 'NONE',  ( 5.359550796103802028, 5.147230771742885125, -0.7998128361456231517 ) ) ;
#171640=CARTESIAN_POINT ( 'NONE',  ( 6.331821432781979730, 7.345878745455822312, -1.199719254218445830 ) ) ;
#171642=CARTESIAN_POINT ( 'NONE',  ( -9.178506806771670412, 9.810605484096178941, 1.040834085586084257E-14 ) ) ;
#171643=CARTESIAN_POINT ( 'NONE',  ( 7.348156068926750883, 8.635565504245116486, -1.082531754730537976 ) ) ;
#171644=CARTESIAN_POINT ( 'NONE',  ( -8.798878505144649864, 11.28844422746735532, -1.443375672974058777 ) ) ;
#171648=CARTESIAN_POINT ( 'NONE',  ( 6.564118927310645724, 10.80988918183778225, -0.7998128361456291469 ) ) ;
#171653=CARTESIAN_POINT ( 'NONE',  ( -0.6823417656250003738, 2.217708333674753174, -1.181850606188749264 ) ) ;
#171660=CARTESIAN_POINT ( 'NONE',  ( 8.422639742587595180, 10.84949900448412130, -1.599625672291268286 ) ) ;
#171664=CARTESIAN_POINT ( 'NONE',  ( -8.292783513053063160, 12.82666453187061073, 0.7998128361456481317 ) ) ;
#171669=CARTESIAN_POINT ( 'NONE',  ( 3.837121167867449945, 4.435395103055503441, 1.199719254218464037 ) ) ;
#171674=CARTESIAN_POINT ( 'NONE',  ( -9.124801077197171040, 10.60435499727357289, -1.199719254218441611 ) ) ;
#171677=CARTESIAN_POINT ( 'NONE',  ( 9.908311333488716954, 10.45411806535867782, 0.7998128361456462443 ) ) ;
#171679=CARTESIAN_POINT ( 'NONE',  ( 5.244386534325491844, 6.400378350754194479, 1.153371672928265479 ) ) ;
#171681=CARTESIAN_POINT ( 'NONE',  ( -3.928111819657352566, 5.605883094398769195, 1.599625672291267398 ) ) ;
#171685=CARTESIAN_POINT ( 'NONE',  ( 6.577677080924314801, 10.82570702772039262, 1.040834085586084257E-14 ) ) ;
#171687=CARTESIAN_POINT ( 'NONE',  ( 6.479907352327590964, 9.647310113435821677, 1.199719254218462483 ) ) ;
#171690=CARTESIAN_POINT ( 'NONE',  ( -8.839552966430012759, 10.37552855133225904, -1.082531754730543971 ) ) ;
#171698=CARTESIAN_POINT ( 'NONE',  ( -6.041716223103725802, 6.056113169402001617, -0.5645603026655892087 ) ) ;
#171700=CARTESIAN_POINT ( 'NONE',  ( 4.989037340148863464, 8.764367963574922982, -0.7216878364870257245 ) ) ;
#171702=CARTESIAN_POINT ( 'NONE',  ( 8.829384350997564468, 11.32403438096243775, 1.599625672291281386 ) ) ;
#171704=AXIS2_PLACEMENT_3D ( 'NONE', #160598, #97756, #31678 ) ;
#171723=CARTESIAN_POINT ( 'NONE',  ( 7.527801604085637699, 9.805521176231838609, 1.599625672291281386 ) ) ;
#171727=CARTESIAN_POINT ( 'NONE',  ( -1.201851678989727383E-14, 2.243750000682818158, 1.732050807568877637 ) ) ;
#171728=CARTESIAN_POINT ( 'NONE',  ( -3.755772246185468788, 4.340488027759846545, -1.199719254218452047 ) ) ;
#171729=CARTESIAN_POINT ( 'NONE',  ( -7.217017841176048165, 7.314275657660511243, 1.040834085586084257E-14 ) ) ;
#171731=ORIENTED_EDGE ( 'NONE', *, *, #19236, .F. ) ;
#171732=CARTESIAN_POINT ( 'NONE',  ( -8.597841969360544567, 13.18256606422934674, 0.7998128361456341429 ) ) ;
#171736=CARTESIAN_POINT ( 'NONE',  ( -1.499999999999997780, 5.431250000682820378, 1.214306433183764966E-14 ) ) ;
#171737=CARTESIAN_POINT ( 'NONE',  ( 8.125414133291656071, 8.374071331795406081, -0.7998128361456291469 ) ) ;
#171740=CARTESIAN_POINT ( 'NONE',  ( -7.121056995675673740, 9.330985799753529264, -1.599625672291263179 ) ) ;
#171742=CARTESIAN_POINT ( 'NONE',  ( 0.6823417656249917140, 4.342708333674755394, 1.181850606188765695 ) ) ;
#171749=CARTESIAN_POINT ( 'NONE',  ( -7.524412065904404479, 11.72230514362308185, 0.000000000000000000 ) ) ;
#171754=CARTESIAN_POINT ( 'NONE',  ( -0.6823417656250212460, 3.863541667008085767, 1.181850606188767472 ) ) ;
#171761=CARTESIAN_POINT ( 'NONE',  ( -1.364683531250010295, 4.030208333674751842, 0.7879004041258379498 ) ) ;
#171763=CARTESIAN_POINT ( 'NONE',  ( 6.531277313481192337, 8.642909503859968368, 1.599625672291281386 ) ) ;
#171766=CARTESIAN_POINT ( 'NONE',  ( 2.860407222358956503, 6.280966159486672140, 0.7216878364870338292 ) ) ;
#171767=CARTESIAN_POINT ( 'NONE',  ( 1.364683531249990311, 5.176041667008085767, 0.7879004041258500513 ) ) ;
#171770=CARTESIAN_POINT ( 'NONE',  ( -1.284279953904128524, 10.64264068711930733, -0.7749999999999892530 ) ) ;
#171772=CARTESIAN_POINT ( 'NONE',  ( 1.364683531249986537, 0.6552083336747522857, -0.7879004041258239610 ) ) ;
#171774=CARTESIAN_POINT ( 'NONE',  ( -2.968872451712654126, 6.407508927065978632, 1.040834085586084257E-14 ) ) ;
#171775=CARTESIAN_POINT ( 'NONE',  ( 3.662674053986138656, 7.424870162959149589, 0.7998128361456321445 ) ) ;
#171781=CARTESIAN_POINT ( 'NONE',  ( 4.256897045010922476, 5.029096643009940415, -1.082531754730548412 ) ) ;
#171784=CARTESIAN_POINT ( 'NONE',  ( -8.676855123066022912, 10.18571440074093282, -1.082531754730543971 ) ) ;
#171786=CARTESIAN_POINT ( 'NONE',  ( -5.273758566035884776, 5.255065869904374409, 0.000000000000000000 ) ) ;
#171789=CARTESIAN_POINT ( 'NONE',  ( -8.513630394377489807, 12.01998699582738972, -1.199719254218446718 ) ) ;
#171790=CARTESIAN_POINT ( 'NONE',  ( -4.704316113817535339, 8.432193199521691440, 0.7216878364870458196 ) ) ;
#171792=CARTESIAN_POINT ( 'NONE',  ( 1.364683531249986537, 0.1760416670080860446, 0.7879004041258500513 ) ) ;
#171800=CARTESIAN_POINT ( 'NONE',  ( 8.374132434735052755, 12.92157160716627295, -0.7998128361456352531 ) ) ;
#171813=EDGE_CURVE ( 'NONE', #11835, #61877, #114117, .T. ) ;
#171815=CARTESIAN_POINT ( 'NONE',  ( -3.765413976293358278, 5.416068943807445635, 1.599625672291267398 ) ) ;
#171818=CARTESIAN_POINT ( 'NONE',  ( 0.6823417656249899377, 2.405208333674753618, 1.181850606188767472 ) ) ;
#171827=CARTESIAN_POINT ( 'NONE',  ( -1.364683531250012516, 0.5302083336747518416, 0.7879004041258379498 ) ) ;
#171838=CARTESIAN_POINT ( 'NONE',  ( 5.331380718671758778, 7.243030143248949670, -1.599625672291256295 ) ) ;
#171846=CARTESIAN_POINT ( 'NONE',  ( 5.933664784275179294, 10.07435934829639912, -0.7998128361456291469 ) ) ;
#171849=CARTESIAN_POINT ( 'NONE',  ( 8.392660782059197189, 9.750191319612612872, 1.199719254218462483 ) ) ;
#171858=CIRCLE ( 'NONE', #5770, 0.08000000000000041800 ) ;
#171860=CARTESIAN_POINT ( 'NONE',  ( -8.866669273657352690, 9.446795028796142191, 0.7216878364870438212 ) ) ;
#171866=CARTESIAN_POINT ( 'NONE',  ( -10.45741655484220267, 11.09474082360439873, -0.7998128361456221525 ) ) ;
#171871=CARTESIAN_POINT ( 'NONE',  ( -5.382750679825375251, 6.238629533673094585, -1.199719254218446718 ) ) ;
#171873=CARTESIAN_POINT ( 'NONE',  ( 8.778014389843965759, 12.32843499053828928, 1.199719254218450271 ) ) ;
#171876=CARTESIAN_POINT ( 'NONE',  ( 5.867981556616276073, 5.740399992340775803, -0.7998128361456281477 ) ) ;
#171883=CARTESIAN_POINT ( 'NONE',  ( -6.175902666224832416, 7.163973517805802160, -1.199719254218446718 ) ) ;
#171886=CARTESIAN_POINT ( 'NONE',  ( -9.917953063596627317, 11.52969898140628047, -1.199719254218441611 ) ) ;
#171892=CARTESIAN_POINT ( 'NONE',  ( 9.273413882067330860, 9.921330405274451536, -0.7216878364870257245 ) ) ;
#171893=VERTEX_POINT ( 'NONE', #187164 ) ;
#171894=CARTESIAN_POINT ( 'NONE',  ( 0.6823417656249899377, 4.738541667008086655, -1.181850606188754593 ) ) ;
#171896=CARTESIAN_POINT ( 'NONE',  ( 3.985207087413062066, 6.736826471035503694, -1.199719254218452047 ) ) ;
#171897=CARTESIAN_POINT ( 'NONE',  ( 0.000000000000000000, 3.300000000000025135, 1.561251128379126385E-14 ) ) ;
#171903=AXIS2_PLACEMENT_3D ( 'NONE', #114877, #100692, #148396 ) ;
#171906=CARTESIAN_POINT ( 'NONE',  ( 1.506201402929115973, 8.679372656207114289, -2.542017642366260155 ) ) ;
#171911=CARTESIAN_POINT ( 'NONE',  ( 0.6823417656249882723, 1.738541667008083991, -1.181850606188749264 ) ) ;
#171913=CARTESIAN_POINT ( 'NONE',  ( 9.999301985278609806, 11.62460605670194447, 1.199719254218452047 ) ) ;
#171916=CARTESIAN_POINT ( 'NONE',  ( -4.609409038966229666, 8.321468278861834378, -0.7216878364870267237 ) ) ;
#171917=CARTESIAN_POINT ( 'NONE',  ( 5.205967797967541166, 5.175976640491323444, -0.7216878364870197293 ) ) ;
#171918=CARTESIAN_POINT ( 'NONE',  ( -6.738039155867462604, 7.923762439009225389, 1.082531754730549967 ) ) ;
#171922=CARTESIAN_POINT ( 'NONE',  ( 5.015626762051672571, 7.938982758113895422, 1.199719254218462483 ) ) ;
#171928=ADVANCED_FACE ( 'NONE', ( #38793 ), #171999, .T. ) ;
#171935=CARTESIAN_POINT ( 'NONE',  ( 5.982172092127724383, 8.002286745614243912, -1.599625672291262513 ) ) ;
#171938=CARTESIAN_POINT ( 'NONE',  ( -5.876569516519495551, 8.943415971659659292, 1.199719254218452047 ) ) ;
#171942=CARTESIAN_POINT ( 'NONE',  ( 8.423693512792301163, 8.722063941212843119, 0.7998128361456481317 ) ) ;
#171946=CARTESIAN_POINT ( 'NONE',  ( -5.713871673155502151, 8.753601821068331290, 1.199719254218452047 ) ) ;
#171947=CARTESIAN_POINT ( 'NONE',  ( 5.124618875841165710, 8.922546421882614709, 1.040834085586084257E-14 ) ) ;
#171948=CARTESIAN_POINT ( 'NONE',  ( 5.447554933476544292, 6.459834866240243834, 1.284201090641323040 ) ) ;
#171949=CARTESIAN_POINT ( 'NONE',  ( -5.922214171070950606, 5.803671375871217286, -0.7998128361456291469 ) ) ;
#171952=CARTESIAN_POINT ( 'NONE',  ( -7.061099074618889304, 7.132370430010492868, -0.7998128361456291469 ) ) ;
#171957=CARTESIAN_POINT ( 'NONE',  ( -3.922244425448907279, 2.804391244181470011, -0.7749999999999944711 ) ) ;
#171958=CARTESIAN_POINT ( 'NONE',  ( 1.364683531249988535, 1.863541667008086211, 0.7879004041258500513 ) ) ;
#171960=CARTESIAN_POINT ( 'NONE',  ( -4.744990575102892905, 8.479646737687938085, 0.7216878364870458196 ) ) ;
#171965=CARTESIAN_POINT ( 'NONE',  ( 6.277588818327314080, 7.282607361925381717, 1.199719254218462483 ) ) ;
#171968=CARTESIAN_POINT ( 'NONE',  ( 1.364683531249986537, 1.717708333674749399, -0.7879004041258239610 ) ) ;
#171971=CARTESIAN_POINT ( 'NONE',  ( 3.551873057100287223, 5.166937871415542283, 1.443375672974062551 ) ) ;
#171974=CARTESIAN_POINT ( 'NONE',  ( -5.220052836461385404, 6.048815383081766583, -1.199719254218446718 ) ) ;
#171975=EDGE_CURVE ( 'NONE', #186977, #182051, #148729, .T. ) ;
#171977=CARTESIAN_POINT ( 'NONE',  ( -6.670248387799091461, 10.72578085250020585, 0.000000000000000000 ) ) ;
#171985=CARTESIAN_POINT ( 'NONE',  ( -7.334597914868735025, 9.580116872145431728, -1.443375672974058777 ) ) ;
#171990=VERTEX_POINT ( 'NONE', #74498 ) ;
#171991=CARTESIAN_POINT ( 'NONE',  ( -8.337901282280023807, 8.829899038855916871, 0.7216878364870438212 ) ) ;
#171999=SPHERICAL_SURFACE ( 'NONE', #156173, 0.08000000000000000167 ) ;
#172006=CARTESIAN_POINT ( 'NONE',  ( -5.357443255694392725, 9.402100898285455699, 0.000000000000000000 ) ) ;
#172008=CARTESIAN_POINT ( 'NONE',  ( 4.304877467538922531, 4.981110786005563007, 1.199719254218464037 ) ) ;
#172012=CARTESIAN_POINT ( 'NONE',  ( 6.714312387265682247, 8.856450423275211037, 1.599625672291281386 ) ) ;
#172018=CARTESIAN_POINT ( 'NONE',  ( -6.399085315970151733, 7.528316292462387871, -1.082531754730544860 ) ) ;
#172026=AXIS2_PLACEMENT_3D ( 'NONE', #168611, #3949, #99360 ) ;
#172028=CARTESIAN_POINT ( 'NONE',  ( 1.364683531249988757, 1.134375000341421247, 0.000000000000000000 ) ) ;
#172031=CARTESIAN_POINT ( 'NONE',  ( -7.934546212495630968, 10.28005655271014795, -1.599625672291263179 ) ) ;
#172033=CARTESIAN_POINT ( 'NONE',  ( 8.284195553149872993, 9.623648552551724578, -1.199719254218445830 ) ) ;
#172035=CARTESIAN_POINT ( 'NONE',  ( -9.027031348600448979, 9.425958082989001952, 1.040834085586084257E-14 ) ) ;
#172038=CARTESIAN_POINT ( 'NONE',  ( -1.201851678989727383E-14, 4.446875000341417916, -1.575800808251660134 ) ) ;
#172040=CARTESIAN_POINT ( 'NONE',  ( 8.270110514656021650, 11.63191745286530576, 1.082531754730557072 ) ) ;
#172043=CARTESIAN_POINT ( 'NONE',  ( 1.364683531249988757, -0.5531249996585801965, 0.000000000000000000 ) ) ;
#172046=CARTESIAN_POINT ( 'NONE',  ( 7.334597914868727919, 9.580116872145431728, -1.443375672974058777 ) ) ;
#172049=CARTESIAN_POINT ( 'NONE',  ( -4.772106882330223954, 8.511282429453158827, -0.7216878364870267237 ) ) ;
#172051=CARTESIAN_POINT ( 'NONE',  ( -1.364683531250012516, 2.280208333674751842, 0.7879004041258379498 ) ) ;
#172055=CARTESIAN_POINT ( 'NONE',  ( -5.259673527097670664, 8.223703984000886535, -1.199719254218446718 ) ) ;
#172062=CARTESIAN_POINT ( 'NONE',  ( 6.936968151686458306, 11.24487994360957188, 0.7998128361456462443 ) ) ;
#172065=CARTESIAN_POINT ( 'NONE',  ( -1.402160292154681736E-14, 1.337500000000025446, -1.732050807568863648 ) ) ;
#172070=ORIENTED_EDGE ( 'NONE', *, *, #122310, .F. ) ;
#172071=CARTESIAN_POINT ( 'NONE',  ( 7.971831135155394321, 8.402817200543854170, -0.7216878364870267237 ) ) ;
#172073=EDGE_CURVE ( 'NONE', #199311, #210868, #59363, .T. ) ;
#172079=CARTESIAN_POINT ( 'NONE',  ( 8.263858322729371153, 9.599921783727809910, -1.199719254218446718 ) ) ;
#172080=CARTESIAN_POINT ( 'NONE',  ( -7.316596452869116973, 11.68777962832266049, 0.7998128361456481317 ) ) ;
#172083=CARTESIAN_POINT ( 'NONE',  ( -0.6823417656250246877, -0.4489583329919111243, 1.181850606188755259 ) ) ;
#172085=CARTESIAN_POINT ( 'NONE',  ( 1.499999999999987121, 1.045833333333352266, -0.8660254037844253849 ) ) ;
#172087=CARTESIAN_POINT ( 'NONE',  ( 4.852928918687680948, 7.749168607522574526, 1.199719254218462483 ) ) ;
#172094=CARTESIAN_POINT ( 'NONE',  ( 0.6823417656249899377, 5.676041667008087543, -1.181850606188754593 ) ) ;
#172095=CARTESIAN_POINT ( 'NONE',  ( -7.309817376062285099, 11.67987070538135264, 0.000000000000000000 ) ) ;
#172096=CARTESIAN_POINT ( 'NONE',  ( -4.690757960648240577, 6.495636925554817864, 1.443375672974064550 ) ) ;
#172105=CARTESIAN_POINT ( 'NONE',  ( 7.721532178182734185, 8.967207948423393304, 1.199719254218462483 ) ) ;
#172109=CARTESIAN_POINT ( 'NONE',  ( 8.256552360598020002, 8.734991963560254646, -0.7216878364870267237 ) ) ;
#172110=CARTESIAN_POINT ( 'NONE',  ( -1.284279953904125193, 10.64264068711930733, 0.7750000000000117906 ) ) ;
#172112=CARTESIAN_POINT ( 'NONE',  ( -9.332089804907933939, 9.781859615347734405, 1.040834085586084257E-14 ) ) ;
#172113=CARTESIAN_POINT ( 'NONE',  ( 5.843727902690005749, 6.776436293681846301, -1.199719254218445830 ) ) ;
#172115=CARTESIAN_POINT ( 'NONE',  ( 10.73535870392234237, 11.41900666419791399, 0.000000000000000000 ) ) ;
#172116=CARTESIAN_POINT ( 'NONE',  ( -1.000000000000014433, 6.468705557303653819, 4.925226524755080604 ) ) ;
#172117=CARTESIAN_POINT ( 'NONE',  ( 4.546061579283848353, 4.198160018786257552, -0.7998128361456211532 ) ) ;
#172120=CARTESIAN_POINT ( 'NONE',  ( -4.048498009130195641, 7.637439037563395594, 0.4772038154421194278 ) ) ;
#172123=CARTESIAN_POINT ( 'NONE',  ( -4.121315508874262790, 6.791656612786516334, -1.082531754730549967 ) ) ;
#172124=CARTESIAN_POINT ( 'NONE',  ( 2.361091307074211887, 5.906356958228550447, 0.7998128361456462443 ) ) ;
#172127=CARTESIAN_POINT ( 'NONE',  ( -7.718669524881690336, 7.899535955317097624, 0.7998128361456462443 ) ) ;
#172132=CARTESIAN_POINT ( 'NONE',  ( -7.648771216403934758, 12.07531685244661723, -0.7998128361456291469 ) ) ;
#172138=CARTESIAN_POINT ( 'NONE',  ( 5.820528018968444961, 5.685037531751635953, 0.7998128361456341429 ) ) ;
#172140=CARTESIAN_POINT ( 'NONE',  ( -6.511106444359256784, 5.279176164187211917, -2.499999999999995115 ) ) ;
#172151=CARTESIAN_POINT ( 'NONE',  ( -5.747767057189642870, 8.793146435774861658, -1.199719254218440723 ) ) ;
#172154=CARTESIAN_POINT ( 'NONE',  ( 5.097502569058200983, 6.970172302033127210, -1.443375672974051449 ) ) ;
#172155=EDGE_LOOP ( 'NONE', ( #49006, #42294, #209640, #186358 ) ) ;
#172159=CARTESIAN_POINT ( 'NONE',  ( -6.274726165026268454, 6.214935368819085149, 0.7998128361456341429 ) ) ;
#172163=CARTESIAN_POINT ( 'NONE',  ( -5.747767057189642870, 8.793146435774861658, -1.199719254218440723 ) ) ;
#172164=AXIS2_PLACEMENT_3D ( 'NONE', #90400, #27518, #108842 ) ;
#172170=CARTESIAN_POINT ( 'NONE',  ( -10.49131193887636826, 11.13428543831092909, 1.040834085586084257E-14 ) ) ;
#172171=CARTESIAN_POINT ( 'NONE',  ( 5.587931867126699537, 9.671004278289832001, -0.7998128361456291469 ) ) ;
#172173=CARTESIAN_POINT ( 'NONE',  ( -4.460269349215930212, 4.305995116947750390, 1.214306433183764966E-14 ) ) ;
#172175=AXIS2_PLACEMENT_3D ( 'NONE', #117801, #70016, #2881 ) ;
#172176=AXIS2_PLACEMENT_3D ( 'NONE', #61349, #45123, #111233 ) ;
#172183=CARTESIAN_POINT ( 'NONE',  ( 7.768458830950378591, 12.00702636951006497, 1.040834085586084257E-14 ) ) ;
#172204=CARTESIAN_POINT ( 'NONE',  ( -4.959585264500673496, 4.680604318205876524, 1.214306433183764966E-14 ) ) ;
#172206=CARTESIAN_POINT ( 'NONE',  ( -4.298098390732130625, 4.973201863064262263, 1.199719254218462483 ) ) ;
#172211=CARTESIAN_POINT ( 'NONE',  ( 0.7499999999999867883, -0.9020833326505162120, -1.299038105676652011 ) ) ;
#172214=CARTESIAN_POINT ( 'NONE',  ( -2.657034918598338180, 6.043698471765932112, -0.7216878364870267237 ) ) ;
#172219=CARTESIAN_POINT ( 'NONE',  ( 2.367870383881045981, 5.914265881169853856, 0.000000000000000000 ) ) ;
#172222=CARTESIAN_POINT ( 'NONE',  ( 3.904855289079228076, 2.800000000000017586, -0.7749999999999935829 ) ) ;
#172223=CARTESIAN_POINT ( 'NONE',  ( 8.378575743120986630, 12.71882943370911789, 1.040834085586084257E-14 ) ) ;
#172226=CARTESIAN_POINT ( 'NONE',  ( 0.6823417656249882723, 2.738541667008084879, -1.181850606188749264 ) ) ;
#172229=CARTESIAN_POINT ( 'NONE',  ( -8.188234707649510113, 11.64035869464474082, -1.199719254218446718 ) ) ;
#172231=CARTESIAN_POINT ( 'NONE',  ( -4.229780737339226881, 7.878568593630327577, 1.040834085586084257E-14 ) ) ;
#172233=CARTESIAN_POINT ( 'NONE',  ( -5.368138756007025947, 8.350246751061767725, 1.199719254218452047 ) ) ;
#172235=CARTESIAN_POINT ( 'NONE',  ( -1.602468905319636405E-14, -1.131249999317182064, -1.732050807568870754 ) ) ;
#172243=CARTESIAN_POINT ( 'NONE',  ( -5.463572716182839351, 7.397254140345190798, 1.443375672974064550 ) ) ;
#172244=CARTESIAN_POINT ( 'NONE',  ( -1.387358672527289727, 7.251968950354596544, -4.302625267139392307 ) ) ;
#172248=CARTESIAN_POINT ( 'NONE',  ( -4.080641047588902559, 7.704572288921609058, -0.7216878364870257245 ) ) ;
#172250=CARTESIAN_POINT ( 'NONE',  ( 8.452618703115982512, 11.94880668935564216, 1.199719254218450271 ) ) ;
#172255=EDGE_LOOP ( 'NONE', ( #213905, #172893, #87881, #151078 ) ) ;
#172258=CARTESIAN_POINT ( 'NONE',  ( -5.115504031057831469, 4.862509545855891346, 0.7998128361456341429 ) ) ;
#172265=CARTESIAN_POINT ( 'NONE',  ( 6.277588818327314080, 7.282607361925381717, 1.199719254218462483 ) ) ;
#172270=CARTESIAN_POINT ( 'NONE',  ( 3.999819011231439347, 4.625209253646830554, 1.199719254218464037 ) ) ;
#172280=CARTESIAN_POINT ( 'NONE',  ( 7.151035956204054855, 10.43029348462504124, 1.199719254218460707 ) ) ;
#172282=CARTESIAN_POINT ( 'NONE',  ( -4.415151579544611238, 8.302760609444034046, -0.7998128361456281477 ) ) ;
#172286=CARTESIAN_POINT ( 'NONE',  ( 1.364683531249988535, 4.155208333674753618, -0.7879004041258239610 ) ) ;
#172288=CARTESIAN_POINT ( 'NONE',  ( -5.117312914154178216, 8.057616602233474978, -1.199719254218452047 ) ) ;
#172291=CARTESIAN_POINT ( 'NONE',  ( 4.143988507271280319, 7.986403691791820414, -0.7998128361456221525 ) ) ;
#172292=CARTESIAN_POINT ( 'NONE',  ( -5.870844209917351009, 6.808071985447069707, -1.199719254218446718 ) ) ;
#172298=CARTESIAN_POINT ( 'NONE',  ( 6.480434237652124452, 8.583592582059388576, 1.443375672974076540 ) ) ;
#172300=CARTESIAN_POINT ( 'NONE',  ( 6.087247782411444597, 10.04561347954795281, -0.7216878364870267237 ) ) ;
#172301=CARTESIAN_POINT ( 'NONE',  ( 0.6823417656249899377, 3.155208333674754062, 1.181850606188765695 ) ) ;
#172303=CARTESIAN_POINT ( 'NONE',  ( 3.809477975315569864, 7.388215371269402532, -0.7216878364870197293 ) ) ;
#172311=CARTESIAN_POINT ( 'NONE',  ( -5.443514322282436702, 6.457176790571845792, 1.314492736914568027 ) ) ;
#172312=CARTESIAN_POINT ( 'NONE',  ( -4.101444922696786399, 3.685019076479660427, -2.420000000000000373 ) ) ;
#172319=CARTESIAN_POINT ( 'NONE',  ( -7.980945979938748103, 12.46285407657057220, 0.000000000000000000 ) ) ;
#172321=CARTESIAN_POINT ( 'NONE',  ( 4.383363735919856730, 4.008345868194933104, -0.7998128361456211532 ) ) ;
#172324=CARTESIAN_POINT ( 'NONE',  ( -2.839543107058306592, 5.400218493954923815, -1.199719254218446718 ) ) ;
#172329=CARTESIAN_POINT ( 'NONE',  ( 3.226477370372305753, 4.787309570232886280, 1.443375672974062551 ) ) ;
#172330=ADVANCED_FACE ( 'NONE', ( #47349 ), #180426, .T. ) ;
#172331=CARTESIAN_POINT ( 'NONE',  ( -0.6823417656249969321, 3.280208333674754062, -1.181850606188749264 ) ) ;
#172333=CARTESIAN_POINT ( 'NONE',  ( 8.076906825439115423, 10.44614393447756129, -1.599625672291262513 ) ) ;
#172336=CARTESIAN_POINT ( 'NONE',  ( -3.079673448598517549, 6.744702790006905424, 1.040834085586084257E-14 ) ) ;
#172341=CARTESIAN_POINT ( 'NONE',  ( -1.201851678989727383E-14, 3.212500000000018119, 1.732050807568877637 ) ) ;
#172342=CARTESIAN_POINT ( 'NONE',  ( 4.798696304233017074, 7.685897223992134819, -1.199719254218452047 ) ) ;
#172345=CARTESIAN_POINT ( 'NONE',  ( -0.6823417656249969321, 4.217708333674755394, -1.181850606188749264 ) ) ;
#172347=CARTESIAN_POINT ( 'NONE',  ( 9.137832345930652522, 10.72352116074969075, -1.082531754730543083 ) ) ;
#172352=CARTESIAN_POINT ( 'NONE',  ( -1.201851678989727383E-14, 1.493750000682814383, 1.732050807568877637 ) ) ;
#172354=CARTESIAN_POINT ( 'NONE',  ( -6.579784621333750749, 6.570836901177822931, 0.7998128361456341429 ) ) ;
#172356=CARTESIAN_POINT ( 'NONE',  ( 3.836594282542902246, 7.419851063034623273, 0.7216878364870317197 ) ) ;
#172365=CARTESIAN_POINT ( 'NONE',  ( 6.500244582748090139, 9.671036882259738121, 1.199719254218460707 ) ) ;
#172366=CARTESIAN_POINT ( 'NONE',  ( 4.497554271431305040, 6.270232621468402989, -1.599625672291256295 ) ) ;
#172367=CARTESIAN_POINT ( 'NONE',  ( 2.482948226198858688, 5.072301959192136778, -2.499999999999995115 ) ) ;
#172370=CARTESIAN_POINT ( 'NONE',  ( 6.277588818327314080, 7.282607361925381717, 1.199719254218462483 ) ) ;
#172377=VERTEX_POINT ( 'NONE', #76616 ) ;
#172378=CARTESIAN_POINT ( 'NONE',  ( 9.083072846151447166, 12.68433652289702884, 1.199719254218450271 ) ) ;
#172381=CARTESIAN_POINT ( 'NONE',  ( -1.499999999999997780, 6.280000000000042881, -2.579999999999995630 ) ) ;
#172383=CARTESIAN_POINT ( 'NONE',  ( 5.134314571617769829, 6.480444997182255307, 1.201143065674977528 ) ) ;
#172395=CARTESIAN_POINT ( 'NONE',  ( 6.724481002698112775, 8.868313807946373473, -1.443375672974057666 ) ) ;
#172396=CARTESIAN_POINT ( 'NONE',  ( -5.264643720808155791, 5.036505850564608089, 0.000000000000000000 ) ) ;
#172400=CARTESIAN_POINT ( 'NONE',  ( -5.585069213825653023, 8.603332285183535433, -1.199719254218440723 ) ) ;
#172420=CARTESIAN_POINT ( 'NONE',  ( 1.419999999999820739, 7.388542872122566330, -4.154462424328212222 ) ) ;
#172421=CARTESIAN_POINT ( 'NONE',  ( -3.789667630219657912, 4.380032642466370696, 1.199719254218462483 ) ) ;
#172425=CARTESIAN_POINT ( 'NONE',  ( 6.889514614038635187, 11.18951748302043114, -0.7998128361456291469 ) ) ;
#172427=CARTESIAN_POINT ( 'NONE',  ( -4.638229190868998764, 5.411267389347211854, -2.420000000000000373 ) ) ;
#172430=CARTESIAN_POINT ( 'NONE',  ( -6.684333426737305572, 7.757142738403693727, -1.199719254218446718 ) ) ;
#172431=CARTESIAN_POINT ( 'NONE',  ( 5.172599298813543633, 5.993452922492633839, -1.199719254218452047 ) ) ;
#172434=CARTESIAN_POINT ( 'NONE',  ( 10.24048609702354717, 10.84165528948263457, -0.7998128361456281477 ) ) ;
#172439=CARTESIAN_POINT ( 'NONE',  ( -0.6823417656250212460, 3.113541667008084879, 1.181850606188767472 ) ) ;
#172441=CARTESIAN_POINT ( 'NONE',  ( 7.185458225562760148, 8.445751353653788485, -1.082531754730543083 ) ) ;
#172443=CARTESIAN_POINT ( 'NONE',  ( 0.7499999999999902300, 4.597916667349482012, -1.299038105676658228 ) ) ;
#172449=CARTESIAN_POINT ( 'NONE',  ( 8.717529583462646059, 11.19353715217169309, 1.443375672974076540 ) ) ;
#172454=CARTESIAN_POINT ( 'NONE',  ( -7.831806290188425557, 12.28885777186185990, -0.7998128361456281477 ) ) ;
#172459=EDGE_CURVE ( 'NONE', #18401, #179696, #192994, .T. ) ;
#172463=CARTESIAN_POINT ( 'NONE',  ( 5.217190183160311356, 4.981143389975473568, -0.7998128361456211532 ) ) ;
#172470=CARTESIAN_POINT ( 'NONE',  ( 6.484877546038077867, 6.460111979999551224, 1.040834085586084257E-14 ) ) ;
#172474=CARTESIAN_POINT ( 'NONE',  ( -1.500000000000013101, 2.452083334016154748, 0.8660254037844403729 ) ) ;
#172480=CARTESIAN_POINT ( 'NONE',  ( -0.7500000000000215383, 0.1916666666666871910, 1.299038105676659116 ) ) ;
#172481=CARTESIAN_POINT ( 'NONE',  ( 5.926885707468349196, 10.06645042535509660, 1.040834085586084257E-14 ) ) ;
#172482=CARTESIAN_POINT ( 'NONE',  ( -0.6823417656250003738, -0.03229166632524871350, -1.181850606188749264 ) ) ;
#172485=CARTESIAN_POINT ( 'NONE',  ( 8.080296364064698977, 12.37083682481011060, -0.7216878364870328300 ) ) ;
#172488=AXIS2_PLACEMENT_3D ( 'NONE', #20204, #119928, #151302 ) ;
#172491=CARTESIAN_POINT ( 'NONE',  ( -5.799137018343247796, 7.788745826199009237, -1.599625672291256295 ) ) ;
#172493=CARTESIAN_POINT ( 'NONE',  ( 0.7499999999999885647, 2.847916667349487341, -1.299038105676658228 ) ) ;
#172494=CARTESIAN_POINT ( 'NONE',  ( 1.364683531249992088, 5.446875000341417916, 1.214306433183764966E-14 ) ) ;
#172509=CARTESIAN_POINT ( 'NONE',  ( -7.655550293210764856, 12.08322577538792331, 0.000000000000000000 ) ) ;
#172510=CARTESIAN_POINT ( 'NONE',  ( 6.012151052656117933, 9.101594430485762999, 1.199719254218460707 ) ) ;
#172517=CARTESIAN_POINT ( 'NONE',  ( -5.506582945444718824, 9.576097202994168001, 0.7998128361456481317 ) ) ;
#172522=CARTESIAN_POINT ( 'NONE',  ( 2.693266070609028784, 6.293894182352508970, 0.000000000000000000 ) ) ;
#172526=CARTESIAN_POINT ( 'NONE',  ( -4.229253852459088137, 7.021547696922494808, 1.199719254218464037 ) ) ;
#172527=CARTESIAN_POINT ( 'NONE',  ( -8.296699936558862731, 11.76690146170562201, 1.199719254218453823 ) ) ;
#172530=CARTESIAN_POINT ( 'NONE',  ( -3.980123661693549142, 7.843117270353603843, 0.1539385989055529202 ) ) ;
#172537=CARTESIAN_POINT ( 'NONE',  ( 6.667912619822566000, 6.673652899414787676, 1.040834085586084257E-14 ) ) ;
#172539=CARTESIAN_POINT ( 'NONE',  ( 6.518203450479836292, 5.167241622962440495, 2.437504649502901799 ) ) ;
#172555=CARTESIAN_POINT ( 'NONE',  ( 3.199361063144961825, 6.676412307070352270, -0.7216878364870267237 ) ) ;
#172559=CARTESIAN_POINT ( 'NONE',  ( -9.657485491635913633, 10.16148791653038330, 1.040834085586084257E-14 ) ) ;
#172564=CARTESIAN_POINT ( 'NONE',  ( 0.7499999999999885647, 2.097916667349486453, -1.299038105676652899 ) ) ;
#172570=CARTESIAN_POINT ( 'NONE',  ( -9.317477881089553549, 11.89347683273641820, 1.599625672291281386 ) ) ;
#172572=CARTESIAN_POINT ( 'NONE',  ( -0.6823417656250246877, 0.5510416670080897639, 1.181850606188755259 ) ) ;
#172575=ORIENTED_EDGE ( 'NONE', *, *, #25641, .T. ) ;
#172579=CARTESIAN_POINT ( 'NONE',  ( -5.413783410558481002, 5.210502155273325720, -0.7998128361456221525 ) ) ;
#172581=CARTESIAN_POINT ( 'NONE',  ( 1.438721403194443083, 7.870009100115442635, -3.684356824108416362 ) ) ;
#172586=CARTESIAN_POINT ( 'NONE',  ( 0.6823417656249864960, -0.5114583329919111243, -1.181850606188749264 ) ) ;
#172592=CARTESIAN_POINT ( 'NONE',  ( 1.364683531249986537, 0.1135416670080857532, 0.7879004041258500513 ) ) ;
#172594=CARTESIAN_POINT ( 'NONE',  ( -8.552495972122143186, 8.872333477097637200, 0.7998128361456462443 ) ) ;
#172595=CARTESIAN_POINT ( 'NONE',  ( 9.752392566931574081, 10.27221283770866300, -0.7998128361456281477 ) ) ;
#172596=CARTESIAN_POINT ( 'NONE',  ( 4.517891501851804215, 6.293959390292322986, -1.599625672291255185 ) ) ;
#172599=CARTESIAN_POINT ( 'NONE',  ( -1.402160292154681736E-14, 0.3843750003414230232, 1.575800808251672791 ) ) ;
#172605=ORIENTED_EDGE ( 'NONE', *, *, #212483, .T. ) ;
#172608=CARTESIAN_POINT ( 'NONE',  ( 5.639828713604826405, 9.523624565940227882, -0.7216878364870267237 ) ) ;
#172611=CARTESIAN_POINT ( 'NONE',  ( -2.767835915484202047, 6.380892334706859792, -0.7998128361456281477 ) ) ;
#172613=CARTESIAN_POINT ( 'NONE',  ( -0.7499999999999972244, 5.639583334016151639, -1.299038105676652899 ) ) ;
#172616=CARTESIAN_POINT ( 'NONE',  ( 6.466876083594112146, 6.647036307055676829, -0.7216878364870257245 ) ) ;
#172617=CARTESIAN_POINT ( 'NONE',  ( -7.659993601596713830, 9.959745173328078849, -1.443375672974058777 ) ) ;
#172619=CARTESIAN_POINT ( 'NONE',  ( 0.7499999999999902300, 3.733333333333352488, 1.299038105676669330 ) ) ;
#172623=CARTESIAN_POINT ( 'NONE',  ( 9.436111725431318931, 10.11114455586577776, -0.7216878364870257245 ) ) ;
#172629=CARTESIAN_POINT ( 'NONE',  ( -1.435115314735500691, 7.268684689231141860, -4.324912918974784581 ) ) ;
#172632=CARTESIAN_POINT ( 'NONE',  ( -3.946537740501743219, 2.817530495241825417, -0.7749999999999944711 ) ) ;
#172637=CARTESIAN_POINT ( 'NONE',  ( 7.958272981097359811, 9.347368568444167636, -1.082531754730537976 ) ) ;
#172638=CARTESIAN_POINT ( 'NONE',  ( 8.599949509769960088, 8.927695937686774386, 1.040834085586084257E-14 ) ) ;
#172639=CARTESIAN_POINT ( 'NONE',  ( -6.742482464697739708, 6.760651051769146491, 0.7998128361456341429 ) ) ;
#172645=CARTESIAN_POINT ( 'NONE',  ( 4.880572111239557920, 4.796348339308675435, -0.7216878364870197293 ) ) ;
#172647=CARTESIAN_POINT ( 'NONE',  ( -9.002250809794013264, 9.604973487622245898, -0.7216878364870267237 ) ) ;
#172649=ADVANCED_FACE ( 'NONE', ( #74242, #189047 ), #4923, .T. ) ;
#172670=CARTESIAN_POINT ( 'NONE',  ( 0.5654481856764899117, 7.808910395760752188, 1.918425245283303715 ) ) ;
#172674=CARTESIAN_POINT ( 'NONE',  ( -6.847031270101295419, 7.946956888995021728, -1.199719254218446718 ) ) ;
#172677=CARTESIAN_POINT ( 'NONE',  ( 4.961394147597008697, 7.875711374583454827, -1.199719254218452047 ) ) ;
#172681=CARTESIAN_POINT ( 'NONE',  ( 2.354312230267378236, 5.898448035287240820, -0.7998128361456281477 ) ) ;
#172686=CARTESIAN_POINT ( 'NONE',  ( -4.627410500965859264, 4.293067094081919777, 0.7998128361456341429 ) ) ;
#172689=CARTESIAN_POINT ( 'NONE',  ( 6.076025397218672630, 10.24044673006381245, -0.7998128361456291469 ) ) ;
#172690=CARTESIAN_POINT ( 'NONE',  ( 0.6823417656249917140, 3.842708333674754506, 1.181850606188765695 ) ) ;
#172692=CARTESIAN_POINT ( 'NONE',  ( 6.025359521845701671, 6.071890788804434891, 0.5399204162177869692 ) ) ;
#172697=CARTESIAN_POINT ( 'NONE',  ( 6.927853306458749749, 8.145212281365775908, 1.082531754730558626 ) ) ;
#172698=CARTESIAN_POINT ( 'NONE',  ( -7.100719765255177229, 9.307259030929609267, -1.599625672291263179 ) ) ;
#172701=CARTESIAN_POINT ( 'NONE',  ( -8.995998617867369873, 10.45408546138876993, 1.199719254218462483 ) ) ;
#172702=CARTESIAN_POINT ( 'NONE',  ( -7.088215381846223906, 7.164006121775713609, 0.7998128361456341429 ) ) ;
#172707=ADVANCED_FACE ( 'NONE', ( #6001 ), #6357, .T. ) ;
#172711=CARTESIAN_POINT ( 'NONE',  ( 6.753933077901968396, 11.03133902419432566, 0.7998128361456462443 ) ) ;
#172724=EDGE_LOOP ( 'NONE', ( #146478, #209139 ) ) ;
#172725=CARTESIAN_POINT ( 'NONE',  ( -1.499999999999997780, 4.150000000000021672, 1.214306433183764966E-14 ) ) ;
#172726=CARTESIAN_POINT ( 'NONE',  ( 3.499976210622149253, 7.235056012367825140, 0.7998128361456321445 ) ) ;
#172727=CARTESIAN_POINT ( 'NONE',  ( 5.472687561410540802, 9.536552588287639409, 0.7998128361456462443 ) ) ;
#172729=CARTESIAN_POINT ( 'NONE',  ( -8.432808358020034589, 10.86136238915529084, 1.443375672974064550 ) ) ;
#172732=CARTESIAN_POINT ( 'NONE',  ( 5.151735183512854199, 8.954182114166247430, -0.7216878364870257245 ) ) ;
#172734=CARTESIAN_POINT ( 'NONE',  ( -8.961576348508652146, 10.51788916375733685, -1.082531754730543083 ) ) ;
#172737=CARTESIAN_POINT ( 'NONE',  ( 7.344766530301147789, 9.591980256816594164, 1.599625672291281386 ) ) ;
#172743=CARTESIAN_POINT ( 'NONE',  ( -1.364683531250012516, 1.780208333674757615, 0.7879004041258379498 ) ) ;
#172750=CARTESIAN_POINT ( 'NONE',  ( 8.374132434735052755, 12.92157160716627295, -0.7998128361456352531 ) ) ;
#172754=CARTESIAN_POINT ( 'NONE',  ( -9.480175724453545172, 12.08329098332774265, 1.599625672291281386 ) ) ;
#172760=CARTESIAN_POINT ( 'NONE',  ( 3.948449050077836642, 5.629609863222681199, 1.599625672291267398 ) ) ;
#172764=CARTESIAN_POINT ( 'NONE',  ( -8.666686507633592385, 11.13422023037111330, 1.599625672291269396 ) ) ;
#172768=CARTESIAN_POINT ( 'NONE',  ( 7.397945374551106568, 11.78268670361832093, -0.7998128361456291469 ) ) ;
#172769=CARTESIAN_POINT ( 'NONE',  ( 5.102592784488711786, 6.504070869828495027, 1.211835919174956366 ) ) ;
#172770=CARTESIAN_POINT ( 'NONE',  ( 1.217526595471194906, 2.800000000000017586, -0.8761443883974120439 ) ) ;
#172771=CARTESIAN_POINT ( 'NONE',  ( -3.093231602212184850, 6.760520635889515795, -0.7998128361456281477 ) ) ;
#172775=CARTESIAN_POINT ( 'NONE',  ( 8.535021395002688749, 9.916278701380017324, 1.199719254218462483 ) ) ;
#172777=CARTESIAN_POINT ( 'NONE',  ( 6.414979237560321401, 10.63589287712906462, 1.040834085586084257E-14 ) ) ;
#172780=CARTESIAN_POINT ( 'NONE',  ( -9.192064960385334160, 9.826423329978791088, 0.7216878364870438212 ) ) ;
#172789=CARTESIAN_POINT ( 'NONE',  ( -4.837732268475038566, 6.745175811576873848, -1.249133900884531467 ) ) ;
#172790=CARTESIAN_POINT ( 'NONE',  ( -1.201851678989727383E-14, 1.321875000341419248, 1.575800808251672791 ) ) ;
#172792=CARTESIAN_POINT ( 'NONE',  ( 5.504247177468168495, 9.365446107114122398, 0.7216878364870438212 ) ) ;
#172811=CARTESIAN_POINT ( 'NONE',  ( 9.368847842243145152, 10.88907622316056312, 1.199719254218453823 ) ) ;
#172815=CARTESIAN_POINT ( 'NONE',  ( -2.839543107058306592, 5.400218493954923815, -1.199719254218446718 ) ) ;
#172816=CARTESIAN_POINT ( 'NONE',  ( -6.449928391799210736, 8.548002428564306143, -1.599625672291263179 ) ) ;
#172819=CARTESIAN_POINT ( 'NONE',  ( -8.123306592882240551, 12.62894145833798376, 0.000000000000000000 ) ) ;
#172823=CARTESIAN_POINT ( 'NONE',  ( 0.7499999999999902300, 5.097916667349482012, -1.299038105676658228 ) ) ;
#172824=CARTESIAN_POINT ( 'NONE',  ( 7.130698725783555680, 10.40656671580112658, 1.199719254218460707 ) ) ;
#172828=CARTESIAN_POINT ( 'NONE',  ( -6.364663046611467756, 9.512858423433634414, 1.199719254218452047 ) ) ;
#172830=CARTESIAN_POINT ( 'NONE',  ( 0.6823417656249917140, 5.342708333674749177, 1.181850606188765695 ) ) ;
#172831=CARTESIAN_POINT ( 'NONE',  ( -1.608462485350631077, 8.735270501766754236, 2.463594439587651230 ) ) ;
#172832=CARTESIAN_POINT ( 'NONE',  ( 2.877399083922144385, 6.438195321532787396, -0.3536239397737388490 ) ) ;
#172836=CARTESIAN_POINT ( 'NONE',  ( -6.887178846062105286, 10.97886638714038554, -0.7216878364870267237 ) ) ;
#172841=CARTESIAN_POINT ( 'NONE',  ( -1.364683531250012516, 3.592708333674750509, 0.7879004041258379498 ) ) ;
#172848=CARTESIAN_POINT ( 'NONE',  ( -1.364683531250012516, 3.988541667008088876, -0.7879004041258300672 ) ) ;
#172849=CARTESIAN_POINT ( 'NONE',  ( -5.922214171070950606, 5.803671375871217286, -0.7998128361456291469 ) ) ;
#172850=CARTESIAN_POINT ( 'NONE',  ( 6.972971076130050072, 7.029554431773520129, 1.040834085586084257E-14 ) ) ;
#172853=B_SPLINE_CURVE_WITH_KNOTS ( 'NONE', 3,
 ( #132064, #84333, #164522, #198075 ),
 .UNSPECIFIED., .F., .F.,
 ( 4, 4 ),
 ( 3.900039219166819614E-15, 0.0006467211803968906259 ),
 .UNSPECIFIED. ) ;
#172854=CARTESIAN_POINT ( 'NONE',  ( 3.511198595814926993, 6.079853547550633230, 1.082531754730558626 ) ) ;
#172855=CARTESIAN_POINT ( 'NONE',  ( 1.364683531249992088, 5.696875000341418804, 1.214306433183764966E-14 ) ) ;
#172861=CARTESIAN_POINT ( 'NONE',  ( -0.6823417656250003738, 0.7177083336747519526, -1.181850606188749264 ) ) ;
#172862=CARTESIAN_POINT ( 'NONE',  ( -3.958617665510279160, 5.641473247893851628, -1.443375672974053447 ) ) ;
#172863=CARTESIAN_POINT ( 'NONE',  ( 4.798696304233017074, 7.685897223992134819, -1.199719254218452047 ) ) ;
#172864=EDGE_CURVE ( 'NONE', #148633, #190246, #26172, .T. ) ;
#172868=CARTESIAN_POINT ( 'NONE',  ( 3.633221978782282147, 5.261844946711204507, -1.443375672974057666 ) ) ;
#172871=CARTESIAN_POINT ( 'NONE',  ( -7.863365906246054138, 11.15738207638699464, -1.082531754730543971 ) ) ;
#172876=CARTESIAN_POINT ( 'NONE',  ( -9.134442807305063639, 11.67993591332117376, 1.599625672291281386 ) ) ;
#172877=CARTESIAN_POINT ( 'NONE',  ( -6.249945625775490399, 7.354319987235250267, 1.082531754730549967 ) ) ;
#172879=CARTESIAN_POINT ( 'NONE',  ( -1.364683531250014514, 1.051041667008090208, -0.7879004041258289570 ) ) ;
#172888=CARTESIAN_POINT ( 'NONE',  ( 8.907343734053986495, 9.494248565925552441, -0.7216878364870197293 ) ) ;
#172893=ORIENTED_EDGE ( 'NONE', *, *, #200959, .T. ) ;
#172899=CARTESIAN_POINT ( 'NONE',  ( -4.464712657601869417, 4.103252943490596216, 0.7998128361456341429 ) ) ;
#172900=DIRECTION ( 'NONE',  ( 1.000000000000000000, 0.000000000000000000, 0.000000000000000000 ) ) ;
#172903=CARTESIAN_POINT ( 'NONE',  ( -1.201851678989727383E-14, 2.134375000341423689, 1.575800808251672791 ) ) ;
#172913=CARTESIAN_POINT ( 'NONE',  ( -0.6823417656250003738, 0.9677083336747521747, -1.181850606188749264 ) ) ;
#172923=CARTESIAN_POINT ( 'NONE',  ( 6.491656622844908853, 6.468020902940851968, 0.7998128361456341429 ) ) ;
#172931=CARTESIAN_POINT ( 'NONE',  ( 8.281332899848809603, 8.555976559445431562, 0.7998128361456481317 ) ) ;
#172935=CARTESIAN_POINT ( 'NONE',  ( 8.289920859751990889, 11.75899253876431416, 1.199719254218450271 ) ) ;
#172937=CARTESIAN_POINT ( 'NONE',  ( -3.035736007439495232, 6.452393136558649545, 0.6403810252995913999 ) ) ;
#172938=CARTESIAN_POINT ( 'NONE',  ( -1.545144449789736862, 8.695096949162934408, -2.507961912884401734 ) ) ;
#172946=CARTESIAN_POINT ( 'NONE',  ( -7.022760382198764084, 11.13704484596649635, 0.7216878364870458196 ) ) ;
#172958=CARTESIAN_POINT ( 'NONE',  ( 2.860407222358963608, 5.320596945185329218, 1.082531754730548412 ) ) ;
#172960=CARTESIAN_POINT ( 'NONE',  ( 4.843287188579786573, 6.673587691474970107, -1.599625672291256295 ) ) ;
#172962=ORIENTED_EDGE ( 'NONE', *, *, #11637, .T. ) ;
#172967=CARTESIAN_POINT ( 'NONE',  ( -5.229694566569281555, 7.124396299129368337, 1.599625672291267398 ) ) ;
#172969=CARTESIAN_POINT ( 'NONE',  ( -3.810004860640155311, 4.403759411290286252, 1.199719254218462483 ) ) ;
#172975=CARTESIAN_POINT ( 'NONE',  ( 7.782016984564049444, 11.06247500109133064, 1.082531754730557072 ) ) ;
#172977=CARTESIAN_POINT ( 'NONE',  ( -1.364683531249997417, 4.071875000341417028, 1.214306433183764966E-14 ) ) ;
#172980=CARTESIAN_POINT ( 'NONE',  ( 4.286349120214771879, 8.152491073559232859, -0.7998128361456221525 ) ) ;
#172981=CARTESIAN_POINT ( 'NONE',  ( -7.034482758620708154, 5.227586206896615018, 1.300454001123785972E-14 ) ) ;
#172993=CARTESIAN_POINT ( 'NONE',  ( -1.364683531250000748, 0.8218750003414210248, 0.000000000000000000 ) ) ;
#172995=CARTESIAN_POINT ( 'NONE',  ( 4.813308228051395687, 5.574280006603454574, 1.199719254218462483 ) ) ;
#172997=CARTESIAN_POINT ( 'NONE',  ( -6.751597309925468693, 6.979211071108916364, 0.7216878364870317197 ) ) ;
#172998=VECTOR ( 'NONE', #112895, 1000.000000000000000 ) ;
#172999=CARTESIAN_POINT ( 'NONE',  ( 3.226477370372302644, 5.747678784534228313, 1.082531754730546636 ) ) ;
#173000=CARTESIAN_POINT ( 'NONE',  ( -6.358410854684789726, 8.441231968597481483, -1.443375672974058777 ) ) ;
#173004=CARTESIAN_POINT ( 'NONE',  ( 5.847644326195776010, 5.716673223516856694, -0.7998128361456281477 ) ) ;
#173014=CARTESIAN_POINT ( 'NONE',  ( 7.955937213120826357, 8.176348258262782664, 0.7998128361456481317 ) ) ;
#173017=CARTESIAN_POINT ( 'NONE',  ( -5.768104287610143821, 8.816873204598778102, -1.199719254218440723 ) ) ;
#173021=CARTESIAN_POINT ( 'NONE',  ( 7.995557903757111617, 10.35123685918189729, 1.599625672291281386 ) ) ;
#173024=CARTESIAN_POINT ( 'NONE',  ( -7.009729113465285266, 8.136771039586342624, -1.199719254218446718 ) ) ;
#173025=CARTESIAN_POINT ( 'NONE',  ( 5.938108092661121162, 9.871617174839238729, 1.040834085586084257E-14 ) ) ;
#173026=CARTESIAN_POINT ( 'NONE',  ( 4.012431654125413694, 7.810675627703163038, 0.2615036927465386740 ) ) ;
#173027=CARTESIAN_POINT ( 'NONE',  ( -5.250031796989778066, 7.148123067953287446, 1.599625672291267398 ) ) ;
#173033=CARTESIAN_POINT ( 'NONE',  ( 8.565000355531088516, 11.01558638625153286, -1.599625672291257406 ) ) ;
#173034=CARTESIAN_POINT ( 'NONE',  ( -3.895595285070177383, 2.800000000000024691, -0.7749999999999944711 ) ) ;
#173035=CARTESIAN_POINT ( 'NONE',  ( -0.6823417656250003738, 0.9677083336747521747, -1.181850606188749264 ) ) ;
#173037=CARTESIAN_POINT ( 'NONE',  ( -6.290620087060847965, 7.401773525401500464, 1.082531754730549967 ) ) ;
#173043=CARTESIAN_POINT ( 'NONE',  ( -5.703936002245207249, 6.126809468943200443, 0.7377312291968595170 ) ) ;
#173044=CARTESIAN_POINT ( 'NONE',  ( 1.364683531249988757, 1.196875000341421469, 0.000000000000000000 ) ) ;
#173048=CARTESIAN_POINT ( 'NONE',  ( 2.548569689688999329, 5.917155704705049146, -0.7216878364870267237 ) ) ;
#173053=CARTESIAN_POINT ( 'NONE',  ( -4.141125853970233806, 6.918731698685530063, -1.199719254218452047 ) ) ;
#173055=CARTESIAN_POINT ( 'NONE',  ( -8.649738815394339753, 9.193709494155953621, 1.040834085586084257E-14 ) ) ;
#173062=CARTESIAN_POINT ( 'NONE',  ( -6.995644074527074707, 11.10540915368285475, 0.000000000000000000 ) ) ;
#173068=CARTESIAN_POINT ( 'NONE',  ( -7.280365300414089802, 10.47721470291632784, 1.082531754730549967 ) ) ;
#173074=CARTESIAN_POINT ( 'NONE',  ( -1.500000000000011324, 4.952083334016150751, 0.8660254037844403729 ) ) ;
#173082=CARTESIAN_POINT ( 'NONE',  ( -7.366157530926372488, 7.488271962369228874, -0.7998128361456291469 ) ) ;
#173086=CARTESIAN_POINT ( 'NONE',  ( 3.635557746758808495, 7.393234471193928847, -0.7998128361456291469 ) ) ;
#173088=CARTESIAN_POINT ( 'NONE',  ( 4.871399016515830738, 4.969688109501518625, 0.6151586745235249065 ) ) ;
#173090=CARTESIAN_POINT ( 'NONE',  ( 6.446011968293428041, 9.607765498729298415, -1.199719254218440723 ) ) ;
#173096=CARTESIAN_POINT ( 'NONE',  ( -5.097502569058215194, 6.970172302033127210, -1.443375672974053447 ) ) ;
#173107=CARTESIAN_POINT ( 'NONE',  ( 0.6823417656249882723, 1.176041667008083325, -1.181850606188749264 ) ) ;
#173109=CARTESIAN_POINT ( 'NONE',  ( -8.799405390469187793, 10.22472669609091689, -1.199719254218446718 ) ) ;
#173111=CARTESIAN_POINT ( 'NONE',  ( 8.121497709785879593, 9.433834401960398353, -1.199719254218445830 ) ) ;
#173113=CARTESIAN_POINT ( 'NONE',  ( -6.842061076390810292, 11.13415502243129218, 0.000000000000000000 ) ) ;
#173116=CARTESIAN_POINT ( 'NONE',  ( -1.364683531250010295, 4.530208333674754506, 0.7879004041258379498 ) ) ;
#173117=CARTESIAN_POINT ( 'NONE',  ( 8.053180056837369705, 11.37883191874353805, -1.082531754730543083 ) ) ;
#173121=CARTESIAN_POINT ( 'NONE',  ( -1.364683531250014514, -0.1572916663252435232, 0.7879004041258379498 ) ) ;
#173124=CARTESIAN_POINT ( 'NONE',  ( 8.473482818416664841, 10.90881592628469932, -1.443375672974063439 ) ) ;
#173127=CARTESIAN_POINT ( 'NONE',  ( -6.588899466561478846, 6.789396920517583922, 0.7216878364870317197 ) ) ;
#173129=CARTESIAN_POINT ( 'NONE',  ( 1.364683531249988535, 1.613541667008084879, 0.7879004041258500513 ) ) ;
#173133=CARTESIAN_POINT ( 'NONE',  ( -6.157374318900681764, 10.33535380535947290, 0.7998128361456481317 ) ) ;
#173134=CARTESIAN_POINT ( 'NONE',  ( -1.001543065824772872E-14, 5.384375000341415252, 1.575800808251672791 ) ) ;
#173140=CARTESIAN_POINT ( 'NONE',  ( 8.769426429940780920, 9.125419011219408461, 0.7998128361456462443 ) ) ;
#173143=CARTESIAN_POINT ( 'NONE',  ( 0.7499999999999902300, 1.483333333333357373, 1.299038105676657340 ) ) ;
#173149=CARTESIAN_POINT ( 'NONE',  ( 5.978782553946477840, 9.919070713005490703, 1.040834085586084257E-14 ) ) ;
#173150=CARTESIAN_POINT ( 'NONE',  ( 9.694243528971124846, 11.26870452434320491, 1.199719254218450271 ) ) ;
#173152=CARTESIAN_POINT ( 'NONE',  ( 3.623053363349855172, 5.249981562040033189, 1.599625672291267398 ) ) ;
#173153=EDGE_LOOP ( 'NONE', ( #165697, #78498 ) ) ;
#173159=CARTESIAN_POINT ( 'NONE',  ( 9.185812768458653466, 10.67553530374532045, 1.199719254218453823 ) ) ;
#173160=CARTESIAN_POINT ( 'NONE',  ( -1.503277409322750779, 8.660639097433820766, 2.556074651073470427 ) ) ;
#173165=CARTESIAN_POINT ( 'NONE',  ( -1.364683531250000748, -0.2406249996585799189, 0.000000000000000000 ) ) ;
#173166=CARTESIAN_POINT ( 'NONE',  ( -1.402160292154681736E-14, 0.3375000000000208389, -1.732050807568870754 ) ) ;
#173173=CARTESIAN_POINT ( 'NONE',  ( -0.6823417656250212460, 4.801041667008086655, 1.181850606188767472 ) ) ;
#173174=CARTESIAN_POINT ( 'NONE',  ( -5.694061328059534688, 8.626526735169329996, 1.082531754730548412 ) ) ;
#173183=CARTESIAN_POINT ( 'NONE',  ( 9.738834413317897898, 10.25639499182604730, 0.000000000000000000 ) ) ;
#173184=CARTESIAN_POINT ( 'NONE',  ( -4.446711195602252253, 6.210915699667824974, -1.443375672974053892 ) ) ;
#173187=CARTESIAN_POINT ( 'NONE',  ( 6.277061933002769045, 10.26706332190449622, 0.7216878364870438212 ) ) ;
#173190=CARTESIAN_POINT ( 'NONE',  ( -8.809047120577080392, 11.30030761213851953, 1.599625672291269396 ) ) ;
#173191=CARTESIAN_POINT ( 'NONE',  ( 4.547870462380197765, 7.393267075163835855, 1.199719254218462483 ) ) ;
#173193=CARTESIAN_POINT ( 'NONE',  ( 0.9999999999999833467, 5.868705557303652398, 4.125226524755083446 ) ) ;
#173194=CARTESIAN_POINT ( 'NONE',  ( 4.684505768721569652, 5.424010470718658716, -1.199719254218452047 ) ) ;
#173203=CARTESIAN_POINT ( 'NONE',  ( -5.585596099150199834, 5.618876325204420930, -0.7216878364870207285 ) ) ;
#173204=CARTESIAN_POINT ( 'NONE',  ( 3.195971524519376494, 4.751719416737803847, -1.599625672291262513 ) ) ;
#173207=CARTESIAN_POINT ( 'NONE',  ( -5.032047568966410367, 9.022472597102808578, 1.214306433183764966E-14 ) ) ;
#173212=CARTESIAN_POINT ( 'NONE',  ( -8.320953590485107298, 10.73086516036454618, 1.599625672291269396 ) ) ;
#173217=CARTESIAN_POINT ( 'NONE',  ( 4.137209430464448445, 7.978494768850520558, 1.040834085586084257E-14 ) ) ;
#173228=CARTESIAN_POINT ( 'NONE',  ( -6.333630315878337136, 10.54098580183340772, 0.000000000000000000 ) ) ;
#173231=CARTESIAN_POINT ( 'NONE',  ( 5.341549334104184865, 8.215262742221458581, 1.082531754730558626 ) ) ;
#173233=FACE_OUTER_BOUND ( 'NONE', #187321, .T. ) ;
#173235=CARTESIAN_POINT ( 'NONE',  ( 4.650610384687404952, 5.384465856012134566, 1.199719254218462483 ) ) ;
#173237=CARTESIAN_POINT ( 'NONE',  ( -4.737684612971557740, 7.614716917520386374, 1.199719254218464037 ) ) ;
#173249=CARTESIAN_POINT ( 'NONE',  ( 7.182068686937156166, 9.402166106225269715, 1.599625672291281386 ) ) ;
#173253=CARTESIAN_POINT ( 'NONE',  ( -4.744851797206062649, 6.824086272657805985, -1.238183395270262999 ) ) ;
#173260=CARTESIAN_POINT ( 'NONE',  ( 8.676855123066012254, 11.14608361504227574, -1.443375672974052559 ) ) ;
#173266=CARTESIAN_POINT ( 'NONE',  ( -5.796211742350026341, 6.069872996917573538, -0.5622600474562855499 ) ) ;
#173278=CARTESIAN_POINT ( 'NONE',  ( -4.810445574750349174, 4.506608013497163334, 0.7998128361456341429 ) ) ;
#173280=CARTESIAN_POINT ( 'NONE',  ( -2.788173145904702555, 6.404619103530779789, -0.7998128361456281477 ) ) ;
#173284=CARTESIAN_POINT ( 'NONE',  ( -0.7500000000000249800, -1.027083332650516212, 1.299038105676659116 ) ) ;
#173292=CARTESIAN_POINT ( 'NONE',  ( 3.460355519985863548, 5.060167411448709629, 1.599625672291267398 ) ) ;
#173295=DIRECTION ( 'NONE',  ( 7.387867266669436732E-31, -1.000000000000000000, -8.546850786086424434E-32 ) ) ;
#173296=CARTESIAN_POINT ( 'NONE',  ( 9.531018800282598846, 12.14260790512831889, 1.443375672974076540 ) ) ;
#173299=CARTESIAN_POINT ( 'NONE',  ( 0.6823417656249899377, 0.9052083336747520637, 1.181850606188755259 ) ) ;
#173303=CARTESIAN_POINT ( 'NONE',  ( -9.104463846776669200, 10.58062822844965645, -1.199719254218441611 ) ) ;
#173305=CARTESIAN_POINT ( 'NONE',  ( -5.056828107772860292, 6.922718763866881453, -1.443375672974051449 ) ) ;
#173307=CARTESIAN_POINT ( 'NONE',  ( -5.032047568966410367, 9.022472597102808578, 1.214306433183764966E-14 ) ) ;
#173309=CARTESIAN_POINT ( 'NONE',  ( -1.001543065824772872E-14, 5.321875000341422357, 1.575800808251672791 ) ) ;
#173317=CARTESIAN_POINT ( 'NONE',  ( -4.216222583725562245, 7.862750747747711877, 0.7216878364870317197 ) ) ;
#173319=FACE_OUTER_BOUND ( 'NONE', #30910, .T. ) ;
#173324=CARTESIAN_POINT ( 'NONE',  ( -4.080641047588907888, 6.744203074620265248, -1.082531754730548412 ) ) ;
#173326=CARTESIAN_POINT ( 'NONE',  ( 7.886038904643079661, 12.35212915539230139, -0.7998128361456352531 ) ) ;
#173334=CARTESIAN_POINT ( 'NONE',  ( 3.212919216758630014, 6.692230152952963529, 0.000000000000000000 ) ) ;
#173335=CARTESIAN_POINT ( 'NONE',  ( -4.765854690403601879, 5.518917546014321829, 1.199719254218462483 ) ) ;
#173340=CARTESIAN_POINT ( 'NONE',  ( 7.700668062882064291, 10.00719871149432549, -1.443375672974057666 ) ) ;
#173341=CARTESIAN_POINT ( 'NONE',  ( 7.156006149914539982, 7.243095351188763686, 1.040834085586084257E-14 ) ) ;
#173346=CARTESIAN_POINT ( 'NONE',  ( 3.655894977179307226, 7.416961240017848844, -0.7998128361456291469 ) ) ;
#173356=CARTESIAN_POINT ( 'NONE',  ( 8.585337585951586803, 11.03931315507545108, -1.599625672291255185 ) ) ;
#173357=CARTESIAN_POINT ( 'NONE',  ( -5.982172092127739482, 8.002286745614243912, -1.599625672291263179 ) ) ;
#173362=CARTESIAN_POINT ( 'NONE',  ( -1.201851678989727383E-14, 4.071875000341425022, 1.575800808251672791 ) ) ;
#173363=CARTESIAN_POINT ( 'NONE',  ( 7.687109908824030668, 10.95175007939464606, -1.082531754730543083 ) ) ;
#173364=CARTESIAN_POINT ( 'NONE',  ( -4.564291269294938225, 8.476756914152748124, 1.040834085586084257E-14 ) ) ;
#173367=CARTESIAN_POINT ( 'NONE',  ( 3.655894977179307226, 7.416961240017848844, -0.7998128361456291469 ) ) ;
#173368=CARTESIAN_POINT ( 'NONE',  ( -6.261168011412601153, 6.199117522936475666, 1.040834085586084257E-14 ) ) ;
#173369=CARTESIAN_POINT ( 'NONE',  ( 3.001021497710600006, 6.452383585894986062, 0.2530183522923339923 ) ) ;
#173374=CARTESIAN_POINT ( 'NONE',  ( 6.100805936469477331, 9.101062111647635788, -1.082531754730537088 ) ) ;
#173377=CARTESIAN_POINT ( 'NONE',  ( 5.924549939047454750, 9.855799328956630134, -0.7216878364870267237 ) ) ;
#173378=CARTESIAN_POINT ( 'NONE',  ( -0.6823417656250212460, 3.863541667008085767, 1.181850606188767472 ) ) ;
#173380=CARTESIAN_POINT ( 'NONE',  ( 5.477130869796502211, 5.492333557625114437, 1.040834085586084257E-14 ) ) ;
#173385=CARTESIAN_POINT ( 'NONE',  ( -1.201851678989727383E-14, 5.446875000341422357, -1.575800808251660134 ) ) ;
#173390=CARTESIAN_POINT ( 'NONE',  ( -4.597746731904842399, 7.146551969360384504, -1.363588915232381904 ) ) ;
#173391=CARTESIAN_POINT ( 'NONE',  ( 3.023105066167310895, 5.702484939155337607, 2.420000000000000373 ) ) ;
#173397=AXIS2_PLACEMENT_3D ( 'NONE', #72611, #189569, #5453 ) ;
#173400=CARTESIAN_POINT ( 'NONE',  ( -4.406036734316906234, 4.242723732898890709, -0.7216878364870207285 ) ) ;
#173406=CARTESIAN_POINT ( 'NONE',  ( -4.322352044658376968, 3.937165561723182883, 0.7998128361456341429 ) ) ;
#173411=CARTESIAN_POINT ( 'NONE',  ( 5.178851490740205676, 6.104710163027444736, 1.082531754730558626 ) ) ;
#173412=CARTESIAN_POINT ( 'NONE',  ( -0.6823417656250212460, 2.863541667008084879, 1.181850606188767472 ) ) ;
#173414=CARTESIAN_POINT ( 'NONE',  ( 6.751070424600909448, 9.963667031088037973, -1.199719254218441611 ) ) ;
#173416=CARTESIAN_POINT ( 'NONE',  ( 1.458833446111210685, 8.740432391875497586, 2.548463833528534561 ) ) ;
#173417=CARTESIAN_POINT ( 'NONE',  ( -4.334856428067329404, 6.080418470877079429, -1.599625672291256517 ) ) ;
#173418=CARTESIAN_POINT ( 'NONE',  ( 3.023105066167310895, 5.702484939155337607, 2.420000000000000373 ) ) ;
#173421=CARTESIAN_POINT ( 'NONE',  ( -0.7500000000000215383, 2.941666666666689522, 1.299038105676671107 ) ) ;
#173422=CARTESIAN_POINT ( 'NONE',  ( 6.484877546038077867, 6.460111979999551224, 1.040834085586084257E-14 ) ) ;
#173427=CARTESIAN_POINT ( 'NONE',  ( -1.364683531250012516, 4.238541667008090208, -0.7879004041258300672 ) ) ;
#173430=CARTESIAN_POINT ( 'NONE',  ( 8.378575743565351175, 11.75846021992619406, -1.082531754730543083 ) ) ;
#173435=( BOUNDED_SURFACE ( )  B_SPLINE_SURFACE ( 3, 2, ( 
 ( #210738, #46136, #202994 ),
 ( #201914, #1586, #104465 ),
 ( #53567, #37313, #186759 ),
 ( #2652, #120781, #103388 ),
 ( #118633, #167327, #185684 ),
 ( #68726, #135896, #84997 ) ),
 .UNSPECIFIED., .F., .F., .T. ) 
 B_SPLINE_SURFACE_WITH_KNOTS ( ( 4, 2, 4 ),
 ( 3, 3 ),
 ( 8.104322365865941288E-05, 0.0002156911409636899451, 0.0003503390582687204908 ),
 ( 0.000000000000000000, 1.000000000000000000 ),
 .UNSPECIFIED. ) 
 GEOMETRIC_REPRESENTATION_ITEM ( )  RATIONAL_B_SPLINE_SURFACE ( (
 ( 1.000000000000000000, 0.8104931255418998948, 1.000000000000000000),
 ( 1.000000000000000000, 0.8505897838741076633, 1.000000000000000000),
 ( 1.000000000000000000, 0.8859283899323100453, 1.000000000000000000),
 ( 1.000000000000000000, 0.9158911669205149764, 1.000000000000000000),
 ( 1.000000000000000000, 0.9074584363678738219, 1.000000000000000000),
 ( 1.000000000000000000, 0.8789000212895043962, 1.000000000000000000) ) ) 
 REPRESENTATION_ITEM ( '' )  SURFACE ( )  );
#173436=CARTESIAN_POINT ( 'NONE',  ( 0.7499999999999885647, 2.097916667349486453, -1.299038105676652899 ) ) ;
#173438=CARTESIAN_POINT ( 'NONE',  ( -4.557512192488103686, 8.468847991211438497, -0.7998128361456281477 ) ) ;
#173448=CARTESIAN_POINT ( 'NONE',  ( 4.416205349749311004, 6.175325546172740765, 1.599625672291267398 ) ) ;
#173452=CARTESIAN_POINT ( 'NONE',  ( 4.157546660884947620, 8.002221537674429896, 1.040834085586084257E-14 ) ) ;
#173454=VERTEX_POINT ( 'NONE', #27278 ) ;
#173458=ORIENTED_EDGE ( 'NONE', *, *, #201653, .F. ) ;
#173459=CARTESIAN_POINT ( 'NONE',  ( 8.540746701604824409, 12.05162268759261224, -1.199719254218446718 ) ) ;
#173464=CARTESIAN_POINT ( 'NONE',  ( 5.869075745953527878, 5.991122463535357490, 0.2593076673842714119 ) ) ;
#173478=CARTESIAN_POINT ( 'NONE',  ( -4.200340102501783690, 3.977070660044089934, 0.5078479924994099282 ) ) ;
#173479=CARTESIAN_POINT ( 'NONE',  ( 8.134528978519385944, 8.592631351135175066, -0.7216878364870267237 ) ) ;
#173481=CARTESIAN_POINT ( 'NONE',  ( -3.928111819657352566, 5.605883094398769195, 1.599625672291267398 ) ) ;
#173485=CARTESIAN_POINT ( 'NONE',  ( -6.501298352952815662, 7.543601818988450169, -1.199719254218446718 ) ) ;
#173488=CARTESIAN_POINT ( 'NONE',  ( 6.938893903907228378E-15, 10.64264068711930733, 1.214306433183764966E-14 ) ) ;
#173502=CARTESIAN_POINT ( 'NONE',  ( 3.768803514918948938, 4.459654191235965293, -1.082531754730543083 ) ) ;
#173508=CARTESIAN_POINT ( 'NONE',  ( -9.490344339885973923, 12.09515436799890331, -1.443375672974059665 ) ) ;
#173511=CARTESIAN_POINT ( 'NONE',  ( 7.404724451357931336, 11.79059562655963056, 0.7998128361456462443 ) ) ;
#173516=CARTESIAN_POINT ( 'NONE',  ( -6.958359152311683893, 9.141171649162195934, -1.599625672291263179 ) ) ;
#173517=CARTESIAN_POINT ( 'NONE',  ( 5.196852952739813070, 4.957416621151553571, -0.7998128361456221525 ) ) ;
#173519=B_SPLINE_CURVE_WITH_KNOTS ( 'NONE', 3,
 ( #87829, #71550, #4402, #197560, #185306, #153899, #203678 ),
 .UNSPECIFIED., .F., .F.,
 ( 4, 3, 4 ),
 ( 0.000000000000000000, 7.109170824590711302E-05, 0.0001421874139631278545 ),
 .UNSPECIFIED. ) ;
#173520=CARTESIAN_POINT ( 'NONE',  ( 10.16199982864259788, 11.81442020729326536, 1.199719254218452047 ) ) ;
#173524=CARTESIAN_POINT ( 'NONE',  ( 1.364683531249988535, 2.926041667008082658, 0.7879004041258500513 ) ) ;
#173527=CARTESIAN_POINT ( 'NONE',  ( 6.561783159334121152, 8.678499657355050800, -1.443375672974057666 ) ) ;
#173535=CARTESIAN_POINT ( 'NONE',  ( 8.880227426826634129, 11.38335130276301754, 1.443375672974076540 ) ) ;
#173540=CARTESIAN_POINT ( 'NONE',  ( -8.748035429315585532, 11.22912730566677553, -1.599625672291263179 ) ) ;
#173541=CARTESIAN_POINT ( 'NONE',  ( 3.449892483197225523, 6.324475487839650967, -1.000715626366242450 ) ) ;
#173556=CARTESIAN_POINT ( 'NONE',  ( 6.796715079152391148, 6.823922435299587974, 0.7998128361456341429 ) ) ;
#173560=CARTESIAN_POINT ( 'NONE',  ( -1.201851678989727383E-14, 3.243750000682814161, 1.732050807568877637 ) ) ;
#173567=CARTESIAN_POINT ( 'NONE',  ( 1.499999999999989120, 0.7750000000000187850, 0.000000000000000000 ) ) ;
#173568=CARTESIAN_POINT ( 'NONE',  ( 5.940443861082012944, 10.08226827123770697, 0.7998128361456462443 ) ) ;
#173569=CARTESIAN_POINT ( 'NONE',  ( 0.6823417656249882723, -0.6572916663252492686, 1.181850606188755259 ) ) ;
#173572=ADVANCED_FACE ( 'NONE', ( #166891 ), #98707, .T. ) ;
#173574=CARTESIAN_POINT ( 'NONE',  ( 9.300530189294644146, 10.91333531134101165, -1.082531754730543083 ) ) ;
#173575=CARTESIAN_POINT ( 'NONE',  ( -5.070386261830872598, 8.859275038870594088, 0.7216878364870458196 ) ) ;
#173580=CARTESIAN_POINT ( 'NONE',  ( -4.706651882238427120, 8.642844295920152575, 1.040834085586084257E-14 ) ) ;
#173582=CARTESIAN_POINT ( 'NONE',  ( -0.7500000000000006661, 2.889583334016148974, -1.299038105676652011 ) ) ;
#173583=CARTESIAN_POINT ( 'NONE',  ( 1.364683531249990311, 4.446875000341417028, 1.214306433183764966E-14 ) ) ;
#173592=ORIENTED_EDGE ( 'NONE', *, *, #41976, .T. ) ;
#173597=CARTESIAN_POINT ( 'NONE',  ( -8.829384350997580455, 11.32403438096243775, 1.599625672291269396 ) ) ;
#173598=CARTESIAN_POINT ( 'NONE',  ( 6.174848896020108668, 9.291408581077091000, 1.199719254218460707 ) ) ;
#173606=CARTESIAN_POINT ( 'NONE',  ( -6.021792782764022078, 10.17717534653336209, -0.7998128361456291469 ) ) ;
#173611=CARTESIAN_POINT ( 'NONE',  ( 3.460355519985863548, 5.060167411448709629, 1.599625672291267398 ) ) ;
#173612=CARTESIAN_POINT ( 'NONE',  ( -1.499999999999997780, 5.431250000682820378, 1.214306433183764966E-14 ) ) ;
#173613=ORIENTED_EDGE ( 'NONE', *, *, #115527, .F. ) ;
#173614=CARTESIAN_POINT ( 'NONE',  ( -4.928552533767591726, 5.708731696605642725, 1.199719254218462483 ) ) ;
#173615=CARTESIAN_POINT ( 'NONE',  ( -9.429859533504656000, 10.96025652963230534, -1.199719254218441611 ) ) ;
#173618=CARTESIAN_POINT ( 'NONE',  ( -3.999074104275988972, 7.816954204906529924, 0.3413819327131896175 ) ) ;
#173625=CARTESIAN_POINT ( 'NONE',  ( 7.318703993278529829, 7.432909501780090800, 1.040834085586084257E-14 ) ) ;
#173627=CARTESIAN_POINT ( 'NONE',  ( 1.123270288254022198, 3.158552654332631882, -0.7749999999939810591 ) ) ;
#173643=CARTESIAN_POINT ( 'NONE',  ( 4.717874267875568961, 4.606534188717351874, -0.7216878364870188411 ) ) ;
#173647=CARTESIAN_POINT ( 'NONE',  ( -10.30827686509187835, 10.92074451889568643, 1.040834085586084257E-14 ) ) ;
#173648=CARTESIAN_POINT ( 'NONE',  ( -1.001543065824772872E-14, 4.212500000000023448, 1.732050807568877637 ) ) ;
#173650=CARTESIAN_POINT ( 'NONE',  ( 8.934986926605834157, 10.38290515491702770, -1.199719254218446718 ) ) ;
#173660=CARTESIAN_POINT ( 'NONE',  ( -1.364683531250000748, 1.009375000341421247, 0.000000000000000000 ) ) ;
#173662=ORIENTED_EDGE ( 'NONE', *, *, #83952, .T. ) ;
#173666=CARTESIAN_POINT ( 'NONE',  ( -5.251085567194491155, 5.020688004682002159, -0.7998128361456221525 ) ) ;
#173669=CARTESIAN_POINT ( 'NONE',  ( 0.7499999999999867883, 0.3166666666666873020, -1.299038105676652899 ) ) ;
#173671=CARTESIAN_POINT ( 'NONE',  ( 1.499999999999990896, 5.775000000000023448, 1.040834085586084257E-14 ) ) ;
#173676=CARTESIAN_POINT ( 'NONE',  ( -0.6823417656250246877, 0.3010416670080895418, 1.181850606188755259 ) ) ;
#173678=CARTESIAN_POINT ( 'NONE',  ( -7.739006755302186846, 7.923262724141010516, 0.7998128361456462443 ) ) ;
#173679=CARTESIAN_POINT ( 'NONE',  ( 9.240045382913317340, 10.73880668727576015, -1.199719254218446718 ) ) ;
#173680=CARTESIAN_POINT ( 'NONE',  ( 6.029140723994201423, 5.928419020948356710, -0.7090443702179377583 ) ) ;
#173684=CARTESIAN_POINT ( 'NONE',  ( 1.364683531249986537, -0.03229166632525094088, -0.7879004041258309554 ) ) ;
#173692=CARTESIAN_POINT ( 'NONE',  ( 7.131225611108100715, 7.422110755822004968, 0.7216878364870317197 ) ) ;
#173695=CARTESIAN_POINT ( 'NONE',  ( -5.066996723205291708, 6.934582148538044777, 1.599625672291267398 ) ) ;
#173699=CARTESIAN_POINT ( 'NONE',  ( -4.302014814237876017, 3.913438792899272212, 0.7998128361456341429 ) ) ;
#173701=CARTESIAN_POINT ( 'NONE',  ( 5.626270559546821204, 6.626699076635176766, 1.082531754730560403 ) ) ;
#173702=CARTESIAN_POINT ( 'NONE',  ( -6.832946231163084860, 10.91559500309152675, 0.000000000000000000 ) ) ;
#173704=CARTESIAN_POINT ( 'NONE',  ( -1.201851678989727383E-14, 3.462500000000019895, 1.732050807568877637 ) ) ;
#173708=CARTESIAN_POINT ( 'NONE',  ( 8.975134502566660899, 10.53370701015836275, -1.082531754730543083 ) ) ;
#173709=CARTESIAN_POINT ( 'NONE',  ( 2.275391796764376640, 5.643962577969389827, -0.5307291018262025872 ) ) ;
#173719=CARTESIAN_POINT ( 'NONE',  ( -3.557915510932114334, 4.150901429420823519, 2.420000000000010587 ) ) ;
#173722=CARTESIAN_POINT ( 'NONE',  ( 8.749089199520284410, 9.101692242395490240, 0.7998128361456481317 ) ) ;
#173727=CARTESIAN_POINT ( 'NONE',  ( 5.531363484695522637, 5.555604941673978558, -0.7216878364870207285 ) ) ;
#173729=CARTESIAN_POINT ( 'NONE',  ( -7.483737605063437215, 10.71448239167390604, 1.082531754730549967 ) ) ;
#173742=ORIENTED_EDGE ( 'NONE', *, *, #180914, .T. ) ;
#173744=EDGE_LOOP ( 'NONE', ( #39171, #42132, #7174, #48506, #107715, #142545, #61186, #13112, #151299, #192330, #82569, #143696, #50285, #111702, #12049, #162529 ) ) ;
#173758=CARTESIAN_POINT ( 'NONE',  ( -6.901263884555985051, 8.010228272525461435, 1.199719254218450271 ) ) ;
#173762=CARTESIAN_POINT ( 'NONE',  ( 4.638861114170084399, 8.563755066507100722, 0.7998128361456462443 ) ) ;
#173772=CARTESIAN_POINT ( 'NONE',  ( -5.427341564172148303, 5.226320001155936090, 0.000000000000000000 ) ) ;
#173776=CARTESIAN_POINT ( 'NONE',  ( 5.764187864104357573, 9.876636274763768597, 1.040834085586084257E-14 ) ) ;
#173777=CARTESIAN_POINT ( 'NONE',  ( -1.123270288250339366, 3.283552654332833054, 0.7749999999993804067 ) ) ;
#173779=CARTESIAN_POINT ( 'NONE',  ( 5.344703475446304530, 6.534489784648752853, 1.338571508491542383 ) ) ;
#173785=CARTESIAN_POINT ( 'NONE',  ( 6.927853306458752414, 7.184843067064434763, 0.7216878364870317197 ) ) ;
#173786=CARTESIAN_POINT ( 'NONE',  ( -7.507464373665155399, 9.781794407407920389, 1.599625672291295375 ) ) ;
#173789=CARTESIAN_POINT ( 'NONE',  ( -8.670602931139386627, 10.07445716020612103, 1.199719254218462483 ) ) ;
#173790=CARTESIAN_POINT ( 'NONE',  ( -5.065942953000576843, 9.062017211809330064, -0.7998128361456231517 ) ) ;
#173797=CARTESIAN_POINT ( 'NONE',  ( 7.214910300766615769, 11.56914578420308715, -0.7998128361456291469 ) ) ;
#173810=CARTESIAN_POINT ( 'NONE',  ( 1.499999999999987121, 4.295833333333352044, -0.8660254037844323793 ) ) ;
#173811=CARTESIAN_POINT ( 'NONE',  ( 3.811813743736467419, 7.598866467667865443, 1.040834085586084257E-14 ) ) ;
#173812=CARTESIAN_POINT ( 'NONE',  ( 6.819914962873951936, 7.915321197229798322, -1.199719254218446718 ) ) ;
#173814=CARTESIAN_POINT ( 'NONE',  ( -9.354762803749327560, 10.01623748057011376, 0.7216878364870438212 ) ) ;
#173816=EDGE_CURVE ( 'NONE', #197822, #30182, #197879, .T. ) ;
#173817=CARTESIAN_POINT ( 'NONE',  ( 7.131225611108100715, 7.422110755822004968, 0.7216878364870317197 ) ) ;
#173818=CARTESIAN_POINT ( 'NONE',  ( -8.093854517234044366, 11.42628545587295186, 1.082531754730549967 ) ) ;
#173821=CARTESIAN_POINT ( 'NONE',  ( 8.215351014876830504, 11.67199438640995801, -1.199719254218446718 ) ) ;
#173825=CARTESIAN_POINT ( 'NONE',  ( -1.364683531250014514, 1.488541667008084435, -0.7879004041258289570 ) ) ;
#173830=CARTESIAN_POINT ( 'NONE',  ( -1.402160292154681736E-14, -0.3031249996585801965, -1.575800808251665908 ) ) ;
#173832=CARTESIAN_POINT ( 'NONE',  ( 9.911173986789782120, 11.52179005846497972, -1.199719254218440723 ) ) ;
#173835=CARTESIAN_POINT ( 'NONE',  ( -9.612894607289142357, 11.17379744904754801, -1.199719254218441611 ) ) ;
#173837=CARTESIAN_POINT ( 'NONE',  ( 4.911989969715248705, 4.726297878971393196, -2.420000000000000373 ) ) ;
#173841=CARTESIAN_POINT ( 'NONE',  ( 5.542585869888291938, 5.360771691158120689, -0.7998128361456211532 ) ) ;
#173845=CARTESIAN_POINT ( 'NONE',  ( -10.64045162862669081, 11.30828174301964140, -0.7998128361456221525 ) ) ;
#173848=CARTESIAN_POINT ( 'NONE',  ( 8.235688245297327015, 11.69572115523387268, -1.199719254218446718 ) ) ;
#173850=CARTESIAN_POINT ( 'NONE',  ( 5.150161082644886257, 6.468739049537000518, 1.195298158575591074 ) ) ;
#173851=CARTESIAN_POINT ( 'NONE',  ( -0.2116396714000057522, 2.800000000000025135, -1.427100650709098417 ) ) ;
#173852=CARTESIAN_POINT ( 'NONE',  ( -3.958090780185743451, 6.705190779270287393, -1.199719254218452047 ) ) ;
#173856=CARTESIAN_POINT ( 'NONE',  ( 8.762647353133951711, 9.117510088278095282, 1.040834085586084257E-14 ) ) ;
#173858=CARTESIAN_POINT ( 'NONE',  ( 6.856673000209174695, 9.022537805042615489, 1.599625672291281386 ) ) ;
#173859=( BOUNDED_CURVE ( )  B_SPLINE_CURVE ( 1, ( #87077, #189910 ),
 .UNSPECIFIED., .F., .T. ) 
 B_SPLINE_CURVE_WITH_KNOTS ( ( 2, 2 ),
 ( 0.000000000000000000, 6.249999999999832079E-05 ),
 .UNSPECIFIED. ) 
 CURVE ( )  GEOMETRIC_REPRESENTATION_ITEM ( )  RATIONAL_B_SPLINE_CURVE ( ( 0.9345202395942817652, 0.9345202395942817652 ) ) 
 REPRESENTATION_ITEM ( '' )  );
#173861=CARTESIAN_POINT ( 'NONE',  ( -8.839552966430007430, 11.33589776563360019, -1.443375672974059665 ) ) ;
#173870=CARTESIAN_POINT ( 'NONE',  ( -5.609265928939476176, 6.186647267178685183, -0.8691123025580966832 ) ) ;
#173871=CARTESIAN_POINT ( 'NONE',  ( -1.364683531250012516, 2.280208333674751842, 0.7879004041258379498 ) ) ;
#173874=CARTESIAN_POINT ( 'NONE',  ( 5.612712406377503349, 8.531619659873665995, -1.082531754730543083 ) ) ;
#173883=ORIENTED_EDGE ( 'NONE', *, *, #151553, .F. ) ;
#173893=CARTESIAN_POINT ( 'NONE',  ( 7.913155211870404493, 12.38376484715752213, 0.7998128361456462443 ) ) ;
#173897=CARTESIAN_POINT ( 'NONE',  ( -4.135400547368138113, 4.783387712472935149, 1.199719254218462483 ) ) ;
#173898=CARTESIAN_POINT ( 'NONE',  ( -6.344325816190970357, 9.489131654609717970, 1.199719254218452047 ) ) ;
#173902=CARTESIAN_POINT ( 'NONE',  ( -10.45741655484220267, 11.09474082360439873, -0.7998128361456221525 ) ) ;
#173906=CARTESIAN_POINT ( 'NONE',  ( -1.001543065824772872E-14, 4.493750000682820378, 1.732050807568877637 ) ) ;
#173907=CARTESIAN_POINT ( 'NONE',  ( 8.046927864910717432, 9.346836249606042202, 1.199719254218462483 ) ) ;
#173912=CARTESIAN_POINT ( 'NONE',  ( -9.176171038350775078, 9.599954387697719582, -0.7998128361456291469 ) ) ;
#173914=CARTESIAN_POINT ( 'NONE',  ( -1.364683531250010295, 4.530208333674754506, 0.7879004041258379498 ) ) ;
#173916=CARTESIAN_POINT ( 'NONE',  ( -1.566565198595248676, 8.754658464388056061, 2.463935442259440833 ) ) ;
#173921=CARTESIAN_POINT ( 'NONE',  ( -8.676855123066022912, 10.18571440074093282, -1.082531754730543971 ) ) ;
#173925=CARTESIAN_POINT ( 'NONE',  ( -1.364683531249997417, 2.821875000341422801, 1.214306433183764966E-14 ) ) ;
#173931=CARTESIAN_POINT ( 'NONE',  ( 1.364683531249990311, 4.863541667008084879, 0.7879004041258500513 ) ) ;
#173933=CARTESIAN_POINT ( 'NONE',  ( -3.425406365747000859, 7.148057860013469877, 1.040834085586084257E-14 ) ) ;
#173934=CARTESIAN_POINT ( 'NONE',  ( 5.829115978871627135, 8.888053511070525659, 1.199719254218462483 ) ) ;
#173937=CARTESIAN_POINT ( 'NONE',  ( 0.6823417656249917140, 3.405208333674754506, 1.181850606188765695 ) ) ;
#173942=CARTESIAN_POINT ( 'NONE',  ( 0.6823417656249882723, 0.1760416670080894308, -1.181850606188749264 ) ) ;
#173943=CARTESIAN_POINT ( 'NONE',  ( -4.284013352238262407, 6.021101549076499637, -1.443375672974053447 ) ) ;
#173944=CARTESIAN_POINT ( 'NONE',  ( 6.498435699651741615, 6.475929825882159818, -0.7998128361456281477 ) ) ;
#173948=CARTESIAN_POINT ( 'NONE',  ( 3.795919822146273326, 5.451659097302528068, -1.443375672974051449 ) ) ;
#173950=CARTESIAN_POINT ( 'NONE',  ( -9.164948653157990677, 11.71552606681625619, -1.443375672974059665 ) ) ;
#173955=CARTESIAN_POINT ( 'NONE',  ( -10.64723070543352712, 11.31619066596094392, 0.7998128361456462443 ) ) ;
#173957=CARTESIAN_POINT ( 'NONE',  ( -6.060131475184148186, 6.172500930577367484, 0.7216878364870317197 ) ) ;
#173959=CARTESIAN_POINT ( 'NONE',  ( -1.364683531250014514, 0.5510416670080878765, -0.7879004041258289570 ) ) ;
#173970=CARTESIAN_POINT ( 'NONE',  ( 7.741342523278692767, 11.01502146292508044, 1.082531754730558626 ) ) ;
#173978=CARTESIAN_POINT ( 'NONE',  ( 3.246287715468270108, 5.874753870433235825, 1.199719254218450271 ) ) ;
#173981=CARTESIAN_POINT ( 'NONE',  ( -4.115063316947640715, 4.759660943649018705, 1.199719254218462483 ) ) ;
#173985=CARTESIAN_POINT ( 'NONE',  ( 0.6823417656249882723, 1.238541667008083547, -1.181850606188749264 ) ) ;
#173996=VERTEX_POINT ( 'NONE', #89758 ) ;
#174005=CARTESIAN_POINT ( 'NONE',  ( 4.143988507271280319, 7.986403691791820414, -0.7998128361456221525 ) ) ;
#174012=CARTESIAN_POINT ( 'NONE',  ( 8.633844893804129228, 8.967240552393299424, -0.7998128361456211532 ) ) ;
#174016=CARTESIAN_POINT ( 'NONE',  ( 9.585778300061798873, 11.14216175728232550, -1.199719254218440723 ) ) ;
#174018=AXIS2_PLACEMENT_3D ( 'NONE', #184553, #14585, #181365 ) ;
#174019=CARTESIAN_POINT ( 'NONE',  ( -3.031102536865480701, 6.452456358313791718, 0.6335066767141804833 ) ) ;
#174023=DIRECTION ( 'NONE',  ( -0.3321398189114301847, 0.9432301631592802105, 8.628166150854816622E-32 ) ) ;
#174027=CARTESIAN_POINT ( 'NONE',  ( -6.561783159334121152, 10.59923808595773664, -0.7216878364870278340 ) ) ;
#174038=CARTESIAN_POINT ( 'NONE',  ( 3.348500752450937590, 5.890039396959305229, 1.082531754730558626 ) ) ;
#174046=CARTESIAN_POINT ( 'NONE',  ( -6.891622154448065807, 6.934647356477856128, 1.040834085586084257E-14 ) ) ;
#174048=CARTESIAN_POINT ( 'NONE',  ( -2.761056838677368397, 6.372983411765559048, 0.7998128361456341429 ) ) ;
#174049=DIRECTION ( 'NONE',  ( 1.000000000000000000, 0.000000000000000000, 0.000000000000000000 ) ) ;
#174055=CARTESIAN_POINT ( 'NONE',  ( 0.6823417656249899377, 4.238541667008085767, -1.181850606188754593 ) ) ;
#174058=CARTESIAN_POINT ( 'NONE',  ( 5.066996723205273057, 6.934582148538044777, 1.599625672291267398 ) ) ;
#174070=EDGE_LOOP ( 'NONE', ( #61305, #164737, #24385 ) ) ;
#174072=CARTESIAN_POINT ( 'NONE',  ( 1.364683531249986537, 0.9260416670080896528, 0.7879004041258500513 ) ) ;
#174074=CARTESIAN_POINT ( 'NONE',  ( 4.552840656090682891, 4.206068941727564514, 1.214306433183764966E-14 ) ) ;
#174076=CARTESIAN_POINT ( 'NONE',  ( -6.575341312947811545, 6.773579074634973551, 1.040834085586084257E-14 ) ) ;
#174077=CARTESIAN_POINT ( 'NONE',  ( 2.887523530030648988, 6.312601851770308414, 0.000000000000000000 ) ) ;
#174079=CARTESIAN_POINT ( 'NONE',  ( -5.978782553502159480, 8.958701498185728695, 1.082531754730548412 ) ) ;
#174083=CARTESIAN_POINT ( 'NONE',  ( 6.745345117998789775, 7.828323044875442172, 1.199719254218462483 ) ) ;
#174085=CARTESIAN_POINT ( 'NONE',  ( -3.994719869312852278, 3.988629890494022057, 0.6383152452940714650 ) ) ;
#174092=EDGE_CURVE ( 'NONE', #188860, #145094, #21448, .T. ) ;
#174093=CARTESIAN_POINT ( 'NONE',  ( 7.481401836642521452, 7.622723652371411696, 1.040834085586084257E-14 ) ) ;
#174096=CARTESIAN_POINT ( 'NONE',  ( -6.418895661066105873, 9.576129806964074120, -1.199719254218440723 ) ) ;
#174100=CARTESIAN_POINT ( 'NONE',  ( 7.079328764629950754, 11.41096732537697633, 0.7998128361456462443 ) ) ;
#174104=CARTESIAN_POINT ( 'NONE',  ( -8.525379664894808585, 8.840697785332414682, -0.7998128361456291469 ) ) ;
#174106=CARTESIAN_POINT ( 'NONE',  ( 7.958272981097359811, 9.347368568444167636, -1.082531754730537976 ) ) ;
#174107=CARTESIAN_POINT ( 'NONE',  ( 4.026147685736890303, 7.792003671190927960, 0.3652107146706294882 ) ) ;
#174108=CARTESIAN_POINT ( 'NONE',  ( -3.927058049452637700, 7.733318157670055371, -0.7998128361456281477 ) ) ;
#174114=CARTESIAN_POINT ( 'NONE',  ( 8.028399517586572998, 12.51821653715971472, -0.7998128361456352531 ) ) ;
#174115=CARTESIAN_POINT ( 'NONE',  ( -5.357213605067637552, 6.353687308821166724, 1.098221101205157035 ) ) ;
#174116=CARTESIAN_POINT ( 'NONE',  ( -3.946537740501743219, 2.817530495241825417, -0.7749999999999944711 ) ) ;
#174117=CARTESIAN_POINT ( 'NONE',  ( -0.6823417656250246877, 0.05104166700808931978, 1.181850606188755259 ) ) ;
#174119=CARTESIAN_POINT ( 'NONE',  ( -5.585596099150191840, 7.539614753807099667, -1.443375672974052559 ) ) ;
#174126=CARTESIAN_POINT ( 'NONE',  ( -5.724176140219916498, 6.114206214821067853, 0.7043541215260868960 ) ) ;
#174127=CARTESIAN_POINT ( 'NONE',  ( -0.6823417656250003738, 1.280208333674752508, -1.181850606188749264 ) ) ;
#174130=CARTESIAN_POINT ( 'NONE',  ( 2.562127843302666186, 5.932973550587659517, 0.000000000000000000 ) ) ;
#174134=CARTESIAN_POINT ( 'NONE',  ( -7.334597914868727919, 10.54048608644677465, -1.082531754730543083 ) ) ;
#174137=ADVANCED_FACE ( 'NONE', ( #20444 ), #198666, .F. ) ;
#174141=CARTESIAN_POINT ( 'NONE',  ( -8.473482818416682605, 8.988077497682020578, -0.7216878364870267237 ) ) ;
#174142=ORIENTED_EDGE ( 'NONE', *, *, #189986, .T. ) ;
#174145=CARTESIAN_POINT ( 'NONE',  ( -1.420000000000001039, 6.216000000000048153, -2.921333333333328675 ) ) ;
#174148=CARTESIAN_POINT ( 'NONE',  ( -8.202319746143382773, 9.632089794331152532, 1.082531754730558626 ) ) ;
#174153=CARTESIAN_POINT ( 'NONE',  ( -0.7500000000000215383, 3.722916667349487785, 1.299038105676671107 ) ) ;
#174154=CARTESIAN_POINT ( 'NONE',  ( 4.581598608702507569, 7.168929433314090716, -1.325851593340146461 ) ) ;
#174162=CARTESIAN_POINT ( 'NONE',  ( -7.867809214632013770, 8.073532260025807261, 1.040834085586084257E-14 ) ) ;
#174165=CARTESIAN_POINT ( 'NONE',  ( 5.335297142177534369, 6.183267073083954735, -1.199719254218452047 ) ) ;
#174167=CARTESIAN_POINT ( 'NONE',  ( 4.879351199879441658, 4.945478990385278273, 0.6233296712930589401 ) ) ;
#174169=CARTESIAN_POINT ( 'NONE',  ( 7.416473721875251890, 8.611306416064660851, 1.199719254218462483 ) ) ;
#174170=CARTESIAN_POINT ( 'NONE',  ( -4.911522990386917975, 4.699272633198016358, 0.3641131004739307508 ) ) ;
#174177=CARTESIAN_POINT ( 'NONE',  ( -4.880572111239580124, 7.677455982212699759, 1.082531754730560403 ) ) ;
#174180=CARTESIAN_POINT ( 'NONE',  ( -3.022498986271247023, 2.800000000000024691, -2.500000000000000444 ) ) ;
#174185=AXIS2_PLACEMENT_3D ( 'NONE', #46261, #209788, #177318 ) ;
#174187=CARTESIAN_POINT ( 'NONE',  ( -6.842061076390810292, 11.13415502243129218, 0.000000000000000000 ) ) ;
#174189=CARTESIAN_POINT ( 'NONE',  ( 7.609150525767641504, 9.900428251527500834, -1.599625672291262513 ) ) ;
#174190=CARTESIAN_POINT ( 'NONE',  ( 0.7499999999999885647, 0.2333333333333562076, 1.299038105676657340 ) ) ;
#174191=CARTESIAN_POINT ( 'NONE',  ( -7.527801604085656351, 9.805521176231838609, 1.599625672291295375 ) ) ;
#174194=CARTESIAN_POINT ( 'NONE',  ( 0.6823417656249899377, 5.426041667008087543, -1.181850606188754593 ) ) ;
#174195=CARTESIAN_POINT ( 'NONE',  ( 9.246297574839980271, 10.85006392781057905, 1.082531754730549967 ) ) ;
#174198=CARTESIAN_POINT ( 'NONE',  ( -1.201851678989727383E-14, 4.837500000000018119, -1.732050807568863648 ) ) ;
#174201=CARTESIAN_POINT ( 'NONE',  ( 8.392133896734662812, 10.81390885098904420, 1.443375672974076540 ) ) ;
#174204=CARTESIAN_POINT ( 'NONE',  ( -7.063434843039784639, 7.343021526408956667, 1.040834085586084257E-14 ) ) ;
#174206=CARTESIAN_POINT ( 'NONE',  ( -0.6823417656250003738, 1.467708333674752730, -1.181850606188749264 ) ) ;
#174210=CARTESIAN_POINT ( 'NONE',  ( -8.044065211609668253, 8.279164256499745633, 0.7998128361456602331 ) ) ;
#174212=CARTESIAN_POINT ( 'NONE',  ( 1.364683531249990311, 4.676041667008083103, 0.7879004041258500513 ) ) ;
#174217=CARTESIAN_POINT ( 'NONE',  ( 9.433775957010412938, 9.900493459467314850, 0.000000000000000000 ) ) ;
#174220=CARTESIAN_POINT ( 'NONE',  ( -1.201851678989727383E-14, 1.212500000000025002, 1.732050807568877637 ) ) ;
#174225=CARTESIAN_POINT ( 'NONE',  ( 7.293923454472087897, 8.572294120714675003, 1.082531754730558626 ) ) ;
#174233=CARTESIAN_POINT ( 'NONE',  ( 8.697719238366680372, 10.10609285197134533, 1.199719254218462483 ) ) ;
#174234=CARTESIAN_POINT ( 'NONE',  ( -10.31505594189871111, 10.92865344183699428, -0.7998128361456291469 ) ) ;
#174238=CARTESIAN_POINT ( 'NONE',  ( -0.6823417656250212460, 5.613541667008087543, 1.181850606188767472 ) ) ;
#174245=CARTESIAN_POINT ( 'NONE',  ( -1.201851678989727383E-14, 4.071875000341425022, 1.575800808251672791 ) ) ;
#174247=CARTESIAN_POINT ( 'NONE',  ( -5.910991785878170646, 7.919243054989755670, -1.443375672974059665 ) ) ;
#174255=ORIENTED_EDGE ( 'NONE', *, *, #114444, .T. ) ;
#174256=CARTESIAN_POINT ( 'NONE',  ( 8.239604668803105270, 10.63595808506888396, -1.599625672291268286 ) ) ;
#174257=DIRECTION ( 'NONE',  ( 0.8079921913670625733, 0.000000000000000000, -0.5891931930104522541 ) ) ;
#174258=CARTESIAN_POINT ( 'NONE',  ( 2.855963913973019963, 6.483708332943829866, 0.000000000000000000 ) ) ;
#174262=CARTESIAN_POINT ( 'NONE',  ( -9.508345801885592863, 9.987491611821676329, 0.7998128361456462443 ) ) ;
#174263=CARTESIAN_POINT ( 'NONE',  ( 6.063521013809720195, 8.097193820909906137, 1.599625672291281386 ) ) ;
#174266=CARTESIAN_POINT ( 'NONE',  ( 5.834086172582112262, 5.700855377634248100, 1.040834085586084257E-14 ) ) ;
#174273=CARTESIAN_POINT ( 'NONE',  ( -6.263503779833496488, 6.409768619334935913, 0.7216878364870317197 ) ) ;
#174274=CARTESIAN_POINT ( 'NONE',  ( 4.871457266011829823, 4.577788319968905562, -0.7998128361456221525 ) ) ;
#174277=CARTESIAN_POINT ( 'NONE',  ( -6.886651960737580680, 10.12184548991413457, -1.199719254218440723 ) ) ;
#174282=CARTESIAN_POINT ( 'NONE',  ( -8.565000355531095622, 11.01558638625153286, -1.599625672291263179 ) ) ;
#174286=CARTESIAN_POINT ( 'NONE',  ( 8.308449207076147758, 8.587612251210650527, -0.7998128361456281477 ) ) ;
#174287=CARTESIAN_POINT ( 'NONE',  ( 5.497994985541524215, 6.373081223675282736, -1.199719254218445830 ) ) ;
#174299=CARTESIAN_POINT ( 'NONE',  ( -7.802881099864745984, 9.062115023719057305, -1.199719254218446718 ) ) ;
#174302=CARTESIAN_POINT ( 'NONE',  ( 6.480434237652132445, 7.623223367758051872, 1.082531754730558626 ) ) ;
#174307=CARTESIAN_POINT ( 'NONE',  ( -4.401593425930945713, 8.286942763561420122, 1.040834085586084257E-14 ) ) ;
#174312=CARTESIAN_POINT ( 'NONE',  ( -5.796211742350026341, 6.069872996917573538, -0.5622600474562855499 ) ) ;
#174317=CARTESIAN_POINT ( 'NONE',  ( -8.805130697071332335, 12.36007068230351358, 1.199719254218462483 ) ) ;
#174318=CARTESIAN_POINT ( 'NONE',  ( 8.239604668803105270, 10.63595808506888396, -1.599625672291268286 ) ) ;
#174322=CARTESIAN_POINT ( 'NONE',  ( -4.989408424308831691, 6.622959204541034595, -1.241733208710007696 ) ) ;
#174329=CARTESIAN_POINT ( 'NONE',  ( 9.327646496521982300, 11.90534021740758064, -1.443375672974057666 ) ) ;
#174335=CARTESIAN_POINT ( 'NONE',  ( -5.631423255934748795, 6.172511151708975241, -0.8413464574193817436 ) ) ;
#174336=ADVANCED_FACE ( 'NONE', ( #131848 ), #159712, .T. ) ;
#174348=CARTESIAN_POINT ( 'NONE',  ( -2.449219305563052895, 6.009172956465517856, 1.040834085586084257E-14 ) ) ;
#174349=CARTESIAN_POINT ( 'NONE',  ( 3.999292125906894313, 7.609665213625947722, 0.7216878364870317197 ) ) ;
#174350=CARTESIAN_POINT ( 'NONE',  ( -0.7500000000000215383, 3.191666666666689967, 1.299038105676671107 ) ) ;
#174352=CARTESIAN_POINT ( 'NONE',  ( -3.379006598303881059, 4.965260336153046516, -1.599625672291256295 ) ) ;
#174354=EDGE_CURVE ( 'NONE', #182393, #170502, #46687, .T. ) ;
#174357=CARTESIAN_POINT ( 'NONE',  ( 1.364683531249990311, 4.884375000341417916, 1.214306433183764966E-14 ) ) ;
#174365=CARTESIAN_POINT ( 'NONE',  ( 5.379888026524302980, 5.170957540566797128, -0.7998128361456211532 ) ) ;
#174371=CARTESIAN_POINT ( 'NONE',  ( 1.364683531249986537, 0.9677083336747538400, -0.7879004041258239610 ) ) ;
#174374=CARTESIAN_POINT ( 'NONE',  ( -9.321394304595349567, 10.83371376257142416, 1.199719254218462483 ) ) ;
#174375=CARTESIAN_POINT ( 'NONE',  ( -4.677199806590235376, 7.440188293455128665, 1.082531754730560403 ) ) ;
#174379=CARTESIAN_POINT ( 'NONE',  ( 0.6823417656249917140, 5.092708333674749177, 1.181850606188765695 ) ) ;
#174389=CARTESIAN_POINT ( 'NONE',  ( -5.219525951136856357, 6.152163700156858539, -1.082531754730543971 ) ) ;
#174394=CARTESIAN_POINT ( 'NONE',  ( -4.189106276498259618, 6.870745841681152655, 1.082531754730560403 ) ) ;
#174396=CARTESIAN_POINT ( 'NONE',  ( 10.18233705906309972, 11.83814697611718714, 1.199719254218450271 ) ) ;
#174399=CARTESIAN_POINT ( 'NONE',  ( 4.853455804012215324, 6.685451076146141425, 1.443375672974062551 ) ) ;
#174400=DIRECTION ( 'NONE',  ( -5.578564026256490882E-16, -1.000000000000000000, -9.066213480720158442E-32 ) ) ;
#174406=CARTESIAN_POINT ( 'NONE',  ( -2.740719608256871442, 6.349256642941639051, 0.7998128361456341429 ) ) ;
#174412=CARTESIAN_POINT ( 'NONE',  ( 8.676855123066012254, 11.14608361504227574, -1.443375672974052559 ) ) ;
#174413=CARTESIAN_POINT ( 'NONE',  ( 6.765682348419287173, 7.852049813699357728, 1.199719254218462483 ) ) ;
#174418=CARTESIAN_POINT ( 'NONE',  ( 5.529027716274630855, 5.344953845275508542, 1.040834085586084257E-14 ) ) ;
#174419=CARTESIAN_POINT ( 'NONE',  ( -0.09868764650532374505, 7.157731444430473822, -1.998865700660849010 ) ) ;
#174427=CARTESIAN_POINT ( 'NONE',  ( -5.442708600882160574, 8.437244903416123876, -1.199719254218446718 ) ) ;
#174432=( BOUNDED_CURVE ( )  B_SPLINE_CURVE ( 3, ( #184834, #138261, #36464, #204274 ),
 .UNSPECIFIED., .F., .T. ) 
 B_SPLINE_CURVE_WITH_KNOTS ( ( 4, 4 ),
 ( 1.570796326794895892, 2.200856270443528828 ),
 .UNSPECIFIED. ) 
 CURVE ( )  GEOMETRIC_REPRESENTATION_ITEM ( )  RATIONAL_B_SPLINE_CURVE ( ( 1.000000000000000000, 0.9671913951481023730, 0.9671913951481023730, 1.000000000000000000 ) ) 
 REPRESENTATION_ITEM ( '' )  );
#174435=CARTESIAN_POINT ( 'NONE',  ( -1.201851678989727383E-14, 5.196875000341422357, -1.575800808251660134 ) ) ;
#174436=CARTESIAN_POINT ( 'NONE',  ( 7.415946836550703303, 11.59576237604377091, 0.7216878364870438212 ) ) ;
#174437=CARTESIAN_POINT ( 'NONE',  ( -5.925076824372040640, 6.871343368977510302, 1.199719254218450271 ) ) ;
#174439=CARTESIAN_POINT ( 'NONE',  ( -1.440240048130672079, 7.355731858843376436, -4.317885097515330450 ) ) ;
#174440=CARTESIAN_POINT ( 'NONE',  ( 5.518332215962025167, 6.396807992499198292, -1.199719254218445830 ) ) ;
#174441=CARTESIAN_POINT ( 'NONE',  ( -5.656776405399756236, 7.622658444431597680, -1.599625672291256295 ) ) ;
#174447=CARTESIAN_POINT ( 'NONE',  ( 7.158341918335438869, 7.453746447587225710, -0.7216878364870257245 ) ) ;
#174449=CARTESIAN_POINT ( 'NONE',  ( 7.578644679914713578, 8.904468883731073703, 1.082531754730558626 ) ) ;
#174450=CARTESIAN_POINT ( 'NONE',  ( -1.201851678989727383E-14, 2.384375000341416584, 1.575800808251672791 ) ) ;
#174452=CARTESIAN_POINT ( 'NONE',  ( 6.616015773344440021, 6.821032611764393572, 1.040834085586084257E-14 ) ) ;
#174461=CARTESIAN_POINT ( 'NONE',  ( -3.975569122714607495, 7.849474212055944200, 0.02231197147695325456 ) ) ;
#174468=CARTESIAN_POINT ( 'NONE',  ( 6.681470773436232413, 6.689470745297396270, -0.7998128361456281477 ) ) ;
#174480=CARTESIAN_POINT ( 'NONE',  ( 3.226477370372293763, 6.708047998835573900, 0.7216878364870317197 ) ) ;
#174481=CARTESIAN_POINT ( 'NONE',  ( 1.364683531249988757, 1.696875000341414808, 0.000000000000000000 ) ) ;
#174483=CARTESIAN_POINT ( 'NONE',  ( 7.938462636001388795, 9.220293482545153907, -1.199719254218441611 ) ) ;
#174484=CARTESIAN_POINT ( 'NONE',  ( -10.32861409551237486, 10.94447128771960287, 1.040834085586084257E-14 ) ) ;
#174486=CARTESIAN_POINT ( 'NONE',  ( -4.904298879841297421, 6.744767997946720328, 1.599625672291267175 ) ) ;
#174491=CARTESIAN_POINT ( 'NONE',  ( -1.499999999999997780, 2.650000000000020339, 1.214306433183764966E-14 ) ) ;
#174492=CARTESIAN_POINT ( 'NONE',  ( 6.661133543015731462, 6.665743976473484267, -0.7998128361456281477 ) ) ;
#174493=CARTESIAN_POINT ( 'NONE',  ( -5.716734326456539783, 9.821273814174633188, -0.7998128361456231517 ) ) ;
#174497=CARTESIAN_POINT ( 'NONE',  ( -1.364683531250012516, 2.738541667008090208, -0.7879004041258289570 ) ) ;
#174499=CARTESIAN_POINT ( 'NONE',  ( 9.897088948295943212, 11.60932053017587506, 1.082531754730548412 ) ) ;
#174506=CARTESIAN_POINT ( 'NONE',  ( -1.500000000000013101, 1.660416667349487119, -0.8660254037844313801 ) ) ;
#174509=CARTESIAN_POINT ( 'NONE',  ( -4.869349725602420520, 8.832658446511480577, 1.040834085586084257E-14 ) ) ;
#174510=CARTESIAN_POINT ( 'NONE',  ( -4.134873662487946966, 3.926366815765101936, 1.214306433183764966E-14 ) ) ;
#174518=CARTESIAN_POINT ( 'NONE',  ( 6.972971076130050072, 7.029554431773520129, 1.040834085586084257E-14 ) ) ;
#174519=EDGE_CURVE ( 'NONE', #184190, #140464, #7634, .T. ) ;
#174522=CARTESIAN_POINT ( 'NONE',  ( 5.198661835836162481, 8.152523677529138979, 1.199719254218462483 ) ) ;
#174527=CARTESIAN_POINT ( 'NONE',  ( 2.218730694130720771, 5.740269576461138890, 0.7998128361456462443 ) ) ;
#174531=CARTESIAN_POINT ( 'NONE',  ( 5.681948419994366617, 6.106813310819505070, 0.7427411415691799190 ) ) ;
#174532=ORIENTED_EDGE ( 'NONE', *, *, #90702, .F. ) ;
#174540=CARTESIAN_POINT ( 'NONE',  ( -3.945059511896602089, 7.546393830613923548, 1.040834085586084257E-14 ) ) ;
#174544=CARTESIAN_POINT ( 'NONE',  ( -5.886439722289627419, 6.118937485343679761, -0.7679415244158314113 ) ) ;
#174546=CARTESIAN_POINT ( 'NONE',  ( 6.317736394288122170, 10.31451686007074997, 0.7216878364870438212 ) ) ;
#174548=CARTESIAN_POINT ( 'NONE',  ( -4.416205349749324327, 6.175325546172740765, 1.599625672291267398 ) ) ;
#174552=CARTESIAN_POINT ( 'NONE',  ( -4.706651882238427120, 8.642844295920152575, 1.040834085586084257E-14 ) ) ;
#174558=AXIS2_PLACEMENT_3D ( 'NONE', #33949, #130470, #97911 ) ;
#174567=CARTESIAN_POINT ( 'NONE',  ( 8.550388431712704573, 13.12720360364021133, 0.000000000000000000 ) ) ;
#174570=CARTESIAN_POINT ( 'NONE',  ( 4.039966587192267866, 4.776011108888172707, 1.082531754730560403 ) ) ;
#174575=CARTESIAN_POINT ( 'NONE',  ( -4.437596350374534815, 4.071617251725375475, -0.7998128361456221525 ) ) ;
#174579=CARTESIAN_POINT ( 'NONE',  ( 8.426556166093362776, 9.789735934319136135, -1.199719254218446718 ) ) ;
#174583=CARTESIAN_POINT ( 'NONE',  ( -6.632963465583701534, 8.761543347979550589, -1.599625672291263179 ) ) ;
#174584=CARTESIAN_POINT ( 'NONE',  ( 5.931855901178834323, 6.879252291918818152, 1.199719254218462483 ) ) ;
#174589=CARTESIAN_POINT ( 'NONE',  ( 1.364683531249988535, 2.176041667008087543, 0.7879004041258500513 ) ) ;
#174592=CARTESIAN_POINT ( 'NONE',  ( 5.490689023854504747, 9.349628261231513804, 1.040834085586084257E-14 ) ) ;
#174600=CARTESIAN_POINT ( 'NONE',  ( 9.693716643646601128, 10.41168362711695750, 0.7216878364870438212 ) ) ;
#174606=CARTESIAN_POINT ( 'NONE',  ( -8.371269781434001800, 11.85389961405997816, -1.199719254218446718 ) ) ;
#174623=CARTESIAN_POINT ( 'NONE',  ( -0.7500000000000006661, 1.389583334016154748, -1.299038105676652011 ) ) ;
#174629=CARTESIAN_POINT ( 'NONE',  ( -1.500000000000013101, 0.4208333333333572068, 0.8660254037844403729 ) ) ;
#174630=CARTESIAN_POINT ( 'NONE',  ( 7.588813295347141441, 9.876701482703580837, -1.599625672291262513 ) ) ;
#174631=CARTESIAN_POINT ( 'NONE',  ( -1.402160292154681736E-14, -0.1781249996585796136, 1.575800808251672791 ) ) ;
#174634=CARTESIAN_POINT ( 'NONE',  ( 8.541273586929342798, 11.94827437051752206, -1.082531754730543083 ) ) ;
#174635=CARTESIAN_POINT ( 'NONE',  ( -6.588899466561478846, 6.789396920517583922, 0.7216878364870317197 ) ) ;
#174639=CARTESIAN_POINT ( 'NONE',  ( -4.543954038874438162, 8.453030145328826350, 1.040834085586084257E-14 ) ) ;
#174641=CARTESIAN_POINT ( 'NONE',  ( -1.201851678989727383E-14, 2.868750000682821266, -1.732050807568863648 ) ) ;
#174642=CARTESIAN_POINT ( 'NONE',  ( 1.364683531249988535, 4.717708333674756283, -0.7879004041258300672 ) ) ;
#174656=CARTESIAN_POINT ( 'NONE',  ( -9.664264568442742842, 10.16939683947169115, -0.7998128361456291469 ) ) ;
#174657=CARTESIAN_POINT ( 'NONE',  ( 7.983053520348166288, 8.207983950027992748, -0.7998128361456281477 ) ) ;
#174665=CARTESIAN_POINT ( 'NONE',  ( -8.453672473320708036, 9.821371626084353323, -1.199719254218446718 ) ) ;
#174671=CARTESIAN_POINT ( 'NONE',  ( 4.729096653068339151, 4.411700938201493116, -0.7998128361456211532 ) ) ;
#174675=CARTESIAN_POINT ( 'NONE',  ( -4.554649539187067830, 7.401175998105142817, 1.199719254218464037 ) ) ;
#174676=CARTESIAN_POINT ( 'NONE',  ( -7.323375529675950624, 11.69568855126397011, -0.7998128361456291469 ) ) ;
#174679=CARTESIAN_POINT ( 'NONE',  ( -5.356222800695524811, 6.520424213373273936, -1.360004217313095953 ) ) ;
#174703=CARTESIAN_POINT ( 'NONE',  ( -3.023105066167323329, 5.702484939155337607, -2.420000000000000373 ) ) ;
#174705=CARTESIAN_POINT ( 'NONE',  ( 2.846849069189655967, 5.304779099821139710, -1.082531754730543083 ) ) ;
#174711=CARTESIAN_POINT ( 'NONE',  ( -8.188234707649510113, 11.64035869464474082, -1.199719254218446718 ) ) ;
#174714=CARTESIAN_POINT ( 'NONE',  ( 2.521453382017309952, 5.885520012421409319, 0.000000000000000000 ) ) ;
#174718=CARTESIAN_POINT ( 'NONE',  ( 5.464131616080136311, 6.363286244674468684, 1.171972476768274429 ) ) ;
#174723=CARTESIAN_POINT ( 'NONE',  ( 0.6823417656249882723, 0.3427083336747516196, 1.181850606188755259 ) ) ;
#174727=B_SPLINE_CURVE_WITH_KNOTS ( 'NONE', 3,
 ( #152362, #3939, #170741, #23404, #103618, #202137, #70007, #56996 ),
 .UNSPECIFIED., .F., .F.,
 ( 4, 2, 2, 4 ),
 ( 0.000000000000000000, 0.001495953190030211788, 0.002991906380060423577, 0.005983812760120847153 ),
 .UNSPECIFIED. ) ;
#174730=CARTESIAN_POINT ( 'NONE',  ( -3.418627288940168096, 7.140148937072163804, -0.7998128361456281477 ) ) ;
#174733=CARTESIAN_POINT ( 'NONE',  ( 1.499999999999985123, -0.2041666666666457353, -0.8660254037844323793 ) ) ;
#174735=CARTESIAN_POINT ( 'NONE',  ( 0.7499999999999902300, 5.566666666666685082, -1.299038105676658228 ) ) ;
#174740=CARTESIAN_POINT ( 'NONE',  ( -0.6823417656250003738, -0.2822916663252489355, -1.181850606188749264 ) ) ;
#174742=CARTESIAN_POINT ( 'NONE',  ( -6.418895661066105873, 9.576129806964074120, -1.199719254218440723 ) ) ;
#174743=CARTESIAN_POINT ( 'NONE',  ( 8.106885785967500979, 11.54545161934907682, 1.199719254218460707 ) ) ;
#174749=CARTESIAN_POINT ( 'NONE',  ( -1.364683531250000748, 0.5718750003414208027, 0.000000000000000000 ) ) ;
#174755=AXIS2_PLACEMENT_3D ( 'NONE', #71411, #200350, #18410 ) ;
#174758=CARTESIAN_POINT ( 'NONE',  ( 7.185458225562760148, 8.445751353653788485, -1.082531754730543083 ) ) ;
#174759=ADVANCED_FACE ( 'NONE', ( #203176 ), #87991, .F. ) ;
#174762=CARTESIAN_POINT ( 'NONE',  ( -5.311043488251275591, 7.219303374425030562, -1.599625672291256295 ) ) ;
#174767=CARTESIAN_POINT ( 'NONE',  ( -9.449669878600625239, 10.12696240122997082, -0.7216878364870267237 ) ) ;
#174772=CARTESIAN_POINT ( 'NONE',  ( 10.05978679165993483, 11.79913468076720306, 1.082531754730548412 ) ) ;
#174777=VERTEX_POINT ( 'NONE', #161972 ) ;
#174783=ORIENTED_EDGE ( 'NONE', *, *, #18312, .T. ) ;
#174785=CARTESIAN_POINT ( 'NONE',  ( 9.097157884645296733, 10.67606762258344055, -1.082531754730543083 ) ) ;
#174787=CARTESIAN_POINT ( 'NONE',  ( 7.130698725783555680, 10.40656671580112658, 1.199719254218460707 ) ) ;
#174792=CARTESIAN_POINT ( 'NONE',  ( 3.469446951953614189E-15, 6.400000000000023448, 1.214306433183764966E-14 ) ) ;
#174793=CARTESIAN_POINT ( 'NONE',  ( 5.178851490740205676, 6.104710163027444736, 1.082531754730558626 ) ) ;
#174795=CARTESIAN_POINT ( 'NONE',  ( -6.399085315970132193, 10.40942393536641397, -0.7216878364870278340 ) ) ;
#174799=CARTESIAN_POINT ( 'NONE',  ( -3.277320446201389181, 4.846626492033466072, 1.599625672291267398 ) ) ;
#174808=ORIENTED_EDGE ( 'NONE', *, *, #99577, .T. ) ;
#174825=CARTESIAN_POINT ( 'NONE',  ( -6.735703387890906946, 6.752742128827836865, -0.7998128361456291469 ) ) ;
#174828=CARTESIAN_POINT ( 'NONE',  ( 6.582647274634798151, 7.638508894284114170, 1.199719254218462483 ) ) ;
#174830=CARTESIAN_POINT ( 'NONE',  ( 4.241003122976366058, 3.842258486427521103, -0.7998128361456211532 ) ) ;
#174834=CIRCLE ( 'NONE', #102140, 0.08000000000000050127 ) ;
#174836=CARTESIAN_POINT ( 'NONE',  ( -5.766295404513795297, 5.621766148221195358, 0.7998128361456341429 ) ) ;
#174840=CARTESIAN_POINT ( 'NONE',  ( 6.428537391173986038, 10.65171072301167854, 0.7998128361456462443 ) ) ;
#174841=CARTESIAN_POINT ( 'NONE',  ( -0.6823417656249969321, 3.467708333674754506, -1.181850606188749264 ) ) ;
#174843=CARTESIAN_POINT ( 'NONE',  ( 5.882017484636844706, 6.163768100491378910, 0.8443116549854499109 ) ) ;
#174844=CARTESIAN_POINT ( 'NONE',  ( 3.226477370372302644, 5.747678784534228313, 1.082531754730546636 ) ) ;
#174850=CARTESIAN_POINT ( 'NONE',  ( 5.409340101728155936, 8.294351971116089572, -1.082531754730543971 ) ) ;
#174851=CARTESIAN_POINT ( 'NONE',  ( -6.645467848992654858, 10.90479625713344625, 0.7998128361456481317 ) ) ;
#174855=CARTESIAN_POINT ( 'NONE',  ( -7.458957065812611198, 11.85386701009007204, 0.7998128361456481317 ) ) ;
#174856=CARTESIAN_POINT ( 'NONE',  ( -7.223796917982883592, 7.322184580601816428, -0.7998128361456291469 ) ) ;
#174863=CARTESIAN_POINT ( 'NONE',  ( 6.903072767652295383, 11.20533532890304684, 1.040834085586084257E-14 ) ) ;
#174871=CARTESIAN_POINT ( 'NONE',  ( -0.1639926229446835304, 8.277376109547587291, -1.999401122995872138 ) ) ;
#174876=CARTESIAN_POINT ( 'NONE',  ( 0.7499999999999902300, 4.316666666666691299, -1.299038105676658228 ) ) ;
#174877=CARTESIAN_POINT ( 'NONE',  ( 3.472859903394816872, 7.203420320602605287, -0.7998128361456291469 ) ) ;
#174878=CARTESIAN_POINT ( 'NONE',  ( 6.632963465583686435, 8.761543347979550589, -1.599625672291262513 ) ) ;
#174881=CARTESIAN_POINT ( 'NONE',  ( 7.158341918335438869, 7.453746447587225710, -0.7216878364870257245 ) ) ;
#174882=CARTESIAN_POINT ( 'NONE',  ( -9.612367721964622191, 10.31677655182129527, -0.7216878364870267237 ) ) ;
#174886=CARTESIAN_POINT ( 'NONE',  ( 8.914649696185335870, 10.35917838609310593, -1.199719254218446718 ) ) ;
#174889=CARTESIAN_POINT ( 'NONE',  ( -2.764973262183167968, 5.313220341600567664, 1.199719254218462483 ) ) ;
#174891=CARTESIAN_POINT ( 'NONE',  ( 0.6823417656249882723, 1.426041667008083547, -1.181850606188749264 ) ) ;
#174895=EDGE_CURVE ( 'NONE', #79803, #186977, #45380, .T. ) ;
#174897=CARTESIAN_POINT ( 'NONE',  ( -0.6823417656250003738, -0.2822916663252489355, -1.181850606188749264 ) ) ;
#174899=CARTESIAN_POINT ( 'NONE',  ( 9.154780037725547714, 11.70366268214508487, 1.599625672291279388 ) ) ;
#174903=CARTESIAN_POINT ( 'NONE',  ( -9.022061154889962964, 12.61315621642528129, -1.199719254218446718 ) ) ;
#174909=CARTESIAN_POINT ( 'NONE',  ( 3.354752944377597856, 6.001296637494123232, -1.199719254218446718 ) ) ;
#174915=CARTESIAN_POINT ( 'NONE',  ( 9.284636267260101050, 9.726497154758602548, -0.7998128361456281477 ) ) ;
#174918=CARTESIAN_POINT ( 'NONE',  ( -5.525111292768871252, 6.404716915440499037, -1.199719254218446718 ) ) ;
#174922=CARTESIAN_POINT ( 'NONE',  ( 7.995557903757111617, 10.35123685918189729, 1.599625672291281386 ) ) ;
#174924=CARTESIAN_POINT ( 'NONE',  ( 6.401421083946654100, 10.62007503124645957, -0.7998128361456291469 ) ) ;
#174927=CARTESIAN_POINT ( 'NONE',  ( -9.503902493499651882, 10.19023378527882784, 1.040834085586084257E-14 ) ) ;
#174934=CARTESIAN_POINT ( 'NONE',  ( -6.104320841615721527, 6.016881168963393200, -0.3405398961462170471 ) ) ;
#174935=CARTESIAN_POINT ( 'NONE',  ( 1.364683531249988535, 1.863541667008086211, 0.7879004041258500513 ) ) ;
#174937=CARTESIAN_POINT ( 'NONE',  ( 6.805829924380118356, 7.042482454639357847, 0.7216878364870317197 ) ) ;
#174942=ADVANCED_FACE ( 'NONE', ( #150643 ), #42385, .T. ) ;
#174954=CARTESIAN_POINT ( 'NONE',  ( 8.748035429315576650, 11.22912730566677553, -1.599625672291255185 ) ) ;
#174958=CARTESIAN_POINT ( 'NONE',  ( -2.761056838677368397, 6.372983411765559048, 0.7998128361456341429 ) ) ;
#174959=CARTESIAN_POINT ( 'NONE',  ( -7.555971681517696936, 7.709721804725773175, 0.7998128361456462443 ) ) ;
#174964=CARTESIAN_POINT ( 'NONE',  ( -1.500000000000011324, 3.952083334016153415, 0.8660254037844403729 ) ) ;
#174965=CARTESIAN_POINT ( 'NONE',  ( 8.372323551638698902, 9.726464550788689323, 1.199719254218462483 ) ) ;
#174968=CARTESIAN_POINT ( 'NONE',  ( -6.692921386640485082, 10.96015871772258521, -0.7998128361456291469 ) ) ;
#174970=CARTESIAN_POINT ( 'NONE',  ( -0.6823417656250212460, 4.801041667008086655, 1.181850606188767472 ) ) ;
#174973=CARTESIAN_POINT ( 'NONE',  ( 2.865460964793633991, 6.435730012307613990, -0.3240538301300336377 ) ) ;
#174976=CARTESIAN_POINT ( 'NONE',  ( -9.178506806771670412, 9.810605484096178941, 1.040834085586084257E-14 ) ) ;
#174980=CARTESIAN_POINT ( 'NONE',  ( -0.6823417656250212460, 3.363541667008085323, 1.181850606188767472 ) ) ;
#174987=CARTESIAN_POINT ( 'NONE',  ( 0.6823417656249917140, 4.342708333674755394, 1.181850606188765695 ) ) ;
#174988=CARTESIAN_POINT ( 'NONE',  ( -5.298539104842322267, 5.076050465271134016, 0.7998128361456341429 ) ) ;
#174989=CARTESIAN_POINT ( 'NONE',  ( 6.043183783389218355, 8.073467052085995022, 1.599625672291267398 ) ) ;
#174993=CARTESIAN_POINT ( 'NONE',  ( 1.364683531249988535, 4.176041667008081326, 0.7879004041258500513 ) ) ;
#174997=CARTESIAN_POINT ( 'NONE',  ( 1.364683531249986537, -0.09479166632524321789, -0.7879004041258309554 ) ) ;
#174998=CARTESIAN_POINT ( 'NONE',  ( -4.121315508874262790, 6.791656612786516334, -1.082531754730549967 ) ) ;
#175002=CARTESIAN_POINT ( 'NONE',  ( 2.738383840280320669, 6.138605547061593448, 0.7216878364870338292 ) ) ;
#175005=CARTESIAN_POINT ( 'NONE',  ( -7.700668062882059850, 11.92793714009701311, -0.7216878364870267237 ) ) ;
#175010=CARTESIAN_POINT ( 'NONE',  ( -4.392478580703220281, 8.068382744221649361, 1.040834085586084257E-14 ) ) ;
#175012=CARTESIAN_POINT ( 'NONE',  ( -1.364683531250000748, 0.5718750003414208027, 0.000000000000000000 ) ) ;
#175018=CARTESIAN_POINT ( 'NONE',  ( -0.6823417656250246877, -0.6364583329919113464, 1.181850606188755259 ) ) ;
#175027=CARTESIAN_POINT ( 'NONE',  ( 7.253248993186713456, 11.40594822545244824, 0.7216878364870438212 ) ) ;
#175031=ORIENTED_EDGE ( 'NONE', *, *, #128539, .F. ) ;
#175037=CARTESIAN_POINT ( 'NONE',  ( -3.952365473583647315, 4.569846793057691592, 1.199719254218462483 ) ) ;
#175039=CARTESIAN_POINT ( 'NONE',  ( 1.217323170181689784, 3.219494316908636300, 0.7750000000000135669 ) ) ;
#175041=CARTESIAN_POINT ( 'NONE',  ( 1.364683531249988757, 1.946875000341415030, 0.000000000000000000 ) ) ;
#175054=CARTESIAN_POINT ( 'NONE',  ( 0.1021010164683408550, 6.360493866598974755, -3.113991822131910059 ) ) ;
#175061=CARTESIAN_POINT ( 'NONE',  ( 4.632082037363250748, 8.555846143565791095, -0.7998128361456231517 ) ) ;
#175070=CARTESIAN_POINT ( 'NONE',  ( 9.610031953988080744, 10.10612545594124967, -0.7998128361456281477 ) ) ;
#175075=ORIENTED_EDGE ( 'NONE', *, *, #93285, .T. ) ;
#175076=ORIENTED_EDGE ( 'NONE', *, *, #49744, .T. ) ;
#175078=CARTESIAN_POINT ( 'NONE',  ( -3.701012746406287413, 6.301303389907177532, 1.082531754730560403 ) ) ;
#175079=CARTESIAN_POINT ( 'NONE',  ( -4.702146809683723561, 5.356480858934594025, -2.500000000000000444 ) ) ;
#175083=CARTESIAN_POINT ( 'NONE',  ( -9.517460647113315630, 10.20605163116143821, 0.7216878364870438212 ) ) ;
#175089=CARTESIAN_POINT ( 'NONE',  ( 6.145923705696426431, 6.064665832934283962, 0.7998128361456341429 ) ) ;
#175090=CARTESIAN_POINT ( 'NONE',  ( -1.499999999999997780, 3.431250000682818602, 1.214306433183764966E-14 ) ) ;
#175096=CARTESIAN_POINT ( 'NONE',  ( 3.185802909086945967, 5.700225246367978116, 1.082531754730546636 ) ) ;
#175099=ORIENTED_EDGE ( 'NONE', *, *, #102005, .F. ) ;
#175104=CARTESIAN_POINT ( 'NONE',  ( -6.389970470742427189, 6.349387058821269747, -0.7998128361456291469 ) ) ;
#175106=VECTOR ( 'NONE', #189924, 1000.000000000000000 ) ;
#175107=CARTESIAN_POINT ( 'NONE',  ( -2.611917148927046295, 6.198987107056845858, 1.040834085586084257E-14 ) ) ;
#175115=CARTESIAN_POINT ( 'NONE',  ( 4.635998460869027227, 7.496083073400806818, -1.199719254218452047 ) ) ;
#175129=CARTESIAN_POINT ( 'NONE',  ( -1.364683531250012516, 1.842708333674749843, 0.7879004041258379498 ) ) ;
#175131=CARTESIAN_POINT ( 'NONE',  ( 3.354752944377597856, 6.001296637494123232, -1.199719254218446718 ) ) ;
#175133=CARTESIAN_POINT ( 'NONE',  ( -6.236387472606158333, 7.338502141871059870, -1.082531754730544860 ) ) ;
#175135=CARTESIAN_POINT ( 'NONE',  ( 3.551873057100283226, 6.127307085716883428, 1.082531754730558626 ) ) ;
#175136=CARTESIAN_POINT ( 'NONE',  ( -7.063434842595444962, 8.303390740191881392, 1.082531754730549967 ) ) ;
#175141=CARTESIAN_POINT ( 'NONE',  ( 5.937581207780954884, 9.014596278131406848, -1.199719254218440723 ) ) ;
#175143=CARTESIAN_POINT ( 'NONE',  ( -3.070003471035267939, 6.451017196056028524, -0.6895117023006979151 ) ) ;
#175146=CARTESIAN_POINT ( 'NONE',  ( 0.6823417656249899377, 5.426041667008087543, -1.181850606188754593 ) ) ;
#175150=CARTESIAN_POINT ( 'NONE',  ( 7.305145839664861640, 7.417091655897478653, 0.7998128361456341429 ) ) ;
#175153=CARTESIAN_POINT ( 'NONE',  ( -7.039708073993679704, 9.236078724457858158, 1.599625672291283607 ) ) ;
#175158=CARTESIAN_POINT ( 'NONE',  ( 7.239163954692881653, 10.53310948286200599, -1.199719254218441611 ) ) ;
#175160=CARTESIAN_POINT ( 'NONE',  ( -6.353967546298838087, 10.56471257065732416, 0.000000000000000000 ) ) ;
#175163=CARTESIAN_POINT ( 'NONE',  ( 5.924549939047454750, 9.855799328956630134, -0.7216878364870267237 ) ) ;
#175164=CARTESIAN_POINT ( 'NONE',  ( 4.075930520424391190, 7.726065465775651120, -0.5982635945973235891 ) ) ;
#175165=CARTESIAN_POINT ( 'NONE',  ( -4.089755892816631544, 7.923132308261379819, -0.7998128361456281477 ) ) ;
#175169=CARTESIAN_POINT ( 'NONE',  ( 6.471319392424407901, 6.444294134116939077, 0.7998128361456341429 ) ) ;
#175171=CARTESIAN_POINT ( 'NONE',  ( 8.646349277213076334, 11.11049346154719508, 1.599625672291281386 ) ) ;
#175172=CARTESIAN_POINT ( 'NONE',  ( -4.638859928512265363, 6.918491158249495676, 1.209939204767721987 ) ) ;
#175173=CARTESIAN_POINT ( 'NONE',  ( -1.402160292154681736E-14, 1.196875000341419026, -1.575800808251659024 ) ) ;
#175176=CARTESIAN_POINT ( 'NONE',  ( -5.070386261830872598, 8.859275038870594088, 0.7216878364870458196 ) ) ;
#175183=CARTESIAN_POINT ( 'NONE',  ( -5.266216980226317013, 6.417262052691032004, 1.151019644853501944 ) ) ;
#175184=CARTESIAN_POINT ( 'NONE',  ( 0.6823417656249899377, 1.655208333674752730, 1.181850606188755259 ) ) ;
#175187=CARTESIAN_POINT ( 'NONE',  ( 2.236732156574683827, 5.553345249405011508, 1.040834085586084257E-14 ) ) ;
#175191=CARTESIAN_POINT ( 'NONE',  ( -9.286972035236635392, 9.937148250638648150, -0.7216878364870267237 ) ) ;
#175199=CARTESIAN_POINT ( 'NONE',  ( -8.419250203962027612, 11.80591375705560608, 1.082531754730549967 ) ) ;
#175207=CARTESIAN_POINT ( 'NONE',  ( -7.876924059415400414, 9.252461493148505411, 1.082531754730558626 ) ) ;
#175212=CARTESIAN_POINT ( 'NONE',  ( -0.7499999999999972244, 4.139583334016149863, -1.299038105676652899 ) ) ;
#175219=CARTESIAN_POINT ( 'NONE',  ( -6.008234629150358330, 10.16135750065076060, 0.000000000000000000 ) ) ;
#175223=CARTESIAN_POINT ( 'NONE',  ( 4.310602774141044868, 7.116454772218158809, -1.199719254218452047 ) ) ;
#175228=CARTESIAN_POINT ( 'NONE',  ( 5.933664784275179294, 10.07435934829639912, -0.7998128361456291469 ) ) ;
#175235=CARTESIAN_POINT ( 'NONE',  ( -4.772106882330227506, 7.550913215151819458, -1.082531754730549967 ) ) ;
#175238=CARTESIAN_POINT ( 'NONE',  ( 4.853455804012222430, 5.725081861844796727, 1.082531754730560403 ) ) ;
#175241=DIRECTION ( 'NONE',  ( 0.000000000000000000, 8.546850786086437571E-32, 1.000000000000000000 ) ) ;
#175244=CARTESIAN_POINT ( 'NONE',  ( -8.859363311525973117, 12.42334206583395328, -1.199719254218446718 ) ) ;
#175246=CARTESIAN_POINT ( 'NONE',  ( 6.611572464958476836, 10.86525164242692298, 0.7998128361456462443 ) ) ;
#175247=CARTESIAN_POINT ( 'NONE',  ( 1.499999999999985123, -0.4541666666666469010, -0.8660254037844323793 ) ) ;
#175248=CARTESIAN_POINT ( 'NONE',  ( -6.665805079413154921, 10.92852302595736447, 0.7998128361456481317 ) ) ;
#175251=CARTESIAN_POINT ( 'NONE',  ( -1.201851678989727383E-14, 3.946875000341423689, -1.575800808251660134 ) ) ;
#175252=CARTESIAN_POINT ( 'NONE',  ( 8.595506201384008449, 11.05117653974661529, 1.443375672974076540 ) ) ;
#175255=CARTESIAN_POINT ( 'NONE',  ( 0.7499999999999920064, 5.483333333333353821, 1.299038105676669330 ) ) ;
#175258=CARTESIAN_POINT ( 'NONE',  ( 7.076992996209058973, 11.20031622897851165, 1.040834085586084257E-14 ) ) ;
#175261=CARTESIAN_POINT ( 'NONE',  ( -7.104109303880803417, 8.350844278358124484, 1.082531754730549967 ) ) ;
#175263=CARTESIAN_POINT ( 'NONE',  ( 1.364683531249986537, 2.655208333674754062, -0.7879004041258239610 ) ) ;
#175267=CARTESIAN_POINT ( 'NONE',  ( -7.531718027591449705, 8.745758106066849891, 1.199719254218462483 ) ) ;
#175268=CARTESIAN_POINT ( 'NONE',  ( -1.364683531249997417, 4.321875000341417028, 1.214306433183764966E-14 ) ) ;
#175273=CARTESIAN_POINT ( 'NONE',  ( 7.397945374551106568, 11.78268670361832093, -0.7998128361456291469 ) ) ;
#175276=CARTESIAN_POINT ( 'NONE',  ( -0.7500000000000215383, 1.441666666666688190, 1.299038105676659116 ) ) ;
#175280=CARTESIAN_POINT ( 'NONE',  ( 7.510853912290742507, 8.825379654836435606, -1.082531754730537976 ) ) ;
#175282=CARTESIAN_POINT ( 'NONE',  ( 9.531545685607134999, 11.07889037375188401, 1.199719254218450271 ) ) ;
#175288=CARTESIAN_POINT ( 'NONE',  ( 7.377608144130607393, 11.75895993479440982, -0.7998128361456291469 ) ) ;
#175289=CARTESIAN_POINT ( 'NONE',  ( -4.568734577680894304, 5.392907097791561633, -1.082531754730543971 ) ) ;
#175291=CARTESIAN_POINT ( 'NONE',  ( -4.910702663797468226, 4.682374061739900561, -0.3233530799688824064 ) ) ;
#175292=CARTESIAN_POINT ( 'NONE',  ( -1.364683531249997417, 5.321875000341417916, 1.214306433183764966E-14 ) ) ;
#175297=CARTESIAN_POINT ( 'NONE',  ( -4.948362879307902418, 4.875437568721725512, 1.214306433183764966E-14 ) ) ;
#175299=CARTESIAN_POINT ( 'NONE',  ( 0.6823417656249899377, 4.426041667008086655, -1.181850606188754593 ) ) ;
#175301=CARTESIAN_POINT ( 'NONE',  ( -6.290620087060847965, 7.401773525401500464, 1.082531754730549967 ) ) ;
#175306=CARTESIAN_POINT ( 'NONE',  ( 2.218730694130720771, 5.740269576461138890, 0.7998128361456462443 ) ) ;
#175309=CARTESIAN_POINT ( 'NONE',  ( 9.589694723567584234, 10.08239868711733855, -0.7998128361456281477 ) ) ;
#175316=CARTESIAN_POINT ( 'NONE',  ( -8.727698198895085469, 11.20540053684285553, -1.599625672291263179 ) ) ;
#175317=CARTESIAN_POINT ( 'NONE',  ( 6.928380191783277908, 8.041863964290678624, 1.199719254218462483 ) ) ;
#175319=CARTESIAN_POINT ( 'NONE',  ( 3.172244755473273781, 6.644776614786712443, 0.000000000000000000 ) ) ;
#175322=CARTESIAN_POINT ( 'NONE',  ( 5.009901455449552010, 5.803638771901306725, -1.199719254218452047 ) ) ;
#175323=ORIENTED_EDGE ( 'NONE', *, *, #15931, .T. ) ;
#175330=CARTESIAN_POINT ( 'NONE',  ( -5.422898255786193111, 8.310169817517122581, -1.082531754730544860 ) ) ;
#175331=CARTESIAN_POINT ( 'NONE',  ( 5.020596955762157698, 4.751784624677624080, 1.040834085586084257E-14 ) ) ;
#175335=CARTESIAN_POINT ( 'NONE',  ( -8.681298431451969222, 9.022603012982438386, 1.040834085586084257E-14 ) ) ;
#175341=CARTESIAN_POINT ( 'NONE',  ( -8.239604668803112375, 10.63595808506888396, -1.599625672291263179 ) ) ;
#175346=CARTESIAN_POINT ( 'NONE',  ( 6.825640269476072497, 10.05066518344239412, 1.199719254218460707 ) ) ;
#175347=CARTESIAN_POINT ( 'NONE',  ( 6.145923705696426431, 6.064665832934283962, 0.7998128361456341429 ) ) ;
#175350=ORIENTED_EDGE ( 'NONE', *, *, #123006, .F. ) ;
#175357=CARTESIAN_POINT ( 'NONE',  ( -4.586165880992525423, 5.350526861157986147, -7.499999999999997335 ) ) ;
#175359=CARTESIAN_POINT ( 'NONE',  ( -6.482770005628665011, 10.71498210654212002, 0.7998128361456481317 ) ) ;
#175362=CARTESIAN_POINT ( 'NONE',  ( 5.504247177468175600, 8.405076892812779477, 1.082531754730558626 ) ) ;
#175367=CARTESIAN_POINT ( 'NONE',  ( -6.749261541504576911, 6.768559974710451677, 1.040834085586084257E-14 ) ) ;
#175369=CARTESIAN_POINT ( 'NONE',  ( -6.518203450479854943, 5.167241622962448488, 2.437504649502892473 ) ) ;
#175374=CARTESIAN_POINT ( 'NONE',  ( -10.50487009249003378, 11.15010328419353947, 0.7998128361456462443 ) ) ;
#175375=CARTESIAN_POINT ( 'NONE',  ( 7.832860060393120882, 10.16142270859057462, 1.599625672291281386 ) ) ;
#175377=CARTESIAN_POINT ( 'NONE',  ( -3.226477370372317743, 4.787309570232886280, 1.443375672974064550 ) ) ;
#175379=CARTESIAN_POINT ( 'NONE',  ( -5.552734181323573992, 6.223089306236814444, -0.9332588772281782408 ) ) ;
#175386=CARTESIAN_POINT ( 'NONE',  ( 4.207107738942202246, 3.802713871720993399, 1.214306433183764966E-14 ) ) ;
#175405=CARTESIAN_POINT ( 'NONE',  ( -4.517891501851816649, 6.293959390292322986, -1.599625672291256295 ) ) ;
#175407=CARTESIAN_POINT ( 'NONE',  ( 6.127922243252466039, 6.251590159990418449, 1.040834085586084257E-14 ) ) ;
#175408=CARTESIAN_POINT ( 'NONE',  ( 0.7499999999999902300, 3.983333333333352488, 1.299038105676669330 ) ) ;
#175411=FACE_OUTER_BOUND ( 'NONE', #159824, .T. ) ;
#175414=CARTESIAN_POINT ( 'NONE',  ( 1.364683531249988535, 4.155208333674753618, -0.7879004041258239610 ) ) ;
#175417=CARTESIAN_POINT ( 'NONE',  ( -3.633221978782299910, 5.261844946711204507, -1.443375672974053447 ) ) ;
#175419=ORIENTED_EDGE ( 'NONE', *, *, #166876, .F. ) ;
#175420=CARTESIAN_POINT ( 'NONE',  ( 1.500000000000001554, 7.809273069926260469, -3.635729725621137831 ) ) ;
#175422=CARTESIAN_POINT ( 'NONE',  ( 4.704842999142070603, 5.447737239542574272, -1.199719254218452047 ) ) ;
#175423=DIRECTION ( 'NONE',  ( 0.7592566023652995710, 0.6507913734559652719, 0.000000000000000000 ) ) ;
#175427=CARTESIAN_POINT ( 'NONE',  ( -1.201851678989727383E-14, 0.8843750003414173610, 1.575800808251672791 ) ) ;
#175430=CARTESIAN_POINT ( 'NONE',  ( -9.297140650669053485, 11.86975006391249643, 1.599625672291281386 ) ) ;
#175431=CARTESIAN_POINT ( 'NONE',  ( -5.626270559546828309, 7.587068290936515247, 1.443375672974064550 ) ) ;
#175432=AXIS2_PLACEMENT_3D ( 'NONE', #7134, #140397, #88420 ) ;
#175436=CARTESIAN_POINT ( 'NONE',  ( -1.001543065824772872E-14, 4.571875000341418804, 1.575800808251672791 ) ) ;
#175444=CARTESIAN_POINT ( 'NONE',  ( -5.029711800545518585, 8.811821500704338561, 0.7216878364870458196 ) ) ;
#175450=CARTESIAN_POINT ( 'NONE',  ( -4.568734577680887199, 6.353276312092901890, -1.443375672974051449 ) ) ;
#175452=CARTESIAN_POINT ( 'NONE',  ( 8.238550898598388628, 12.76339314834017102, 0.7998128361456462443 ) ) ;
#175453=DIRECTION ( 'NONE',  ( -1.000000000000000000, 7.387867266669436732E-31, 0.000000000000000000 ) ) ;
#175460=LINE ( 'NONE', #97417, #106331 ) ;
#175462=CARTESIAN_POINT ( 'NONE',  ( -3.144601563365788444, 5.756120026313656268, -1.199719254218452935 ) ) ;
#175465=CARTESIAN_POINT ( 'NONE',  ( -1.201851678989727383E-14, 0.9625000000000237810, 1.732050807568877637 ) ) ;
#175468=CARTESIAN_POINT ( 'NONE',  ( 9.571693261567965294, 10.26932301469188857, 0.7216878364870438212 ) ) ;
#175469=CARTESIAN_POINT ( 'NONE',  ( 6.958359152311676787, 9.141171649162195934, -1.599625672291262513 ) ) ;
#175473=CARTESIAN_POINT ( 'NONE',  ( 1.419999999999990603, 6.280000000000042881, 2.873333333333337070 ) ) ;
#175474=CARTESIAN_POINT ( 'NONE',  ( 3.032219910950674890, 6.689340329417765574, 0.7998128361456321445 ) ) ;
#175476=CARTESIAN_POINT ( 'NONE',  ( -0.1495493664682910895, 8.232402834744856790, -1.999498275785964507 ) ) ;
#175477=ORIENTED_EDGE ( 'NONE', *, *, #160465, .F. ) ;
#175483=CARTESIAN_POINT ( 'NONE',  ( 9.759171643738394408, 10.28012176064996197, 0.000000000000000000 ) ) ;
#175484=CARTESIAN_POINT ( 'NONE',  ( -5.388475986427523345, 8.373973519885682393, 1.199719254218452047 ) ) ;
#175492=CARTESIAN_POINT ( 'NONE',  ( -1.364683531250010295, 3.780208333674750953, 0.7879004041258379498 ) ) ;
#175493=CARTESIAN_POINT ( 'NONE',  ( 9.368320956918614328, 10.99242454023565507, 1.082531754730549967 ) ) ;
#175494=CARTESIAN_POINT ( 'NONE',  ( -6.358937740009323214, 7.377514437221045718, -1.199719254218446718 ) ) ;
#175496=CARTESIAN_POINT ( 'NONE',  ( 6.505214776458575265, 6.483838748823460563, 1.040834085586084257E-14 ) ) ;
#175497=CARTESIAN_POINT ( 'NONE',  ( -3.899941742225307539, 7.701682465904834629, 0.7998128361456341429 ) ) ;
#175502=CARTESIAN_POINT ( 'NONE',  ( 5.490689023854504747, 9.349628261231513804, 1.040834085586084257E-14 ) ) ;
#175505=CARTESIAN_POINT ( 'NONE',  ( -0.6823417656250003738, 2.280208333674753174, -1.181850606188749264 ) ) ;
#175507=CARTESIAN_POINT ( 'NONE',  ( 6.493992390821439642, 7.639041213122241381, -1.082531754730543971 ) ) ;
#175509=CARTESIAN_POINT ( 'NONE',  ( -2.819732761962332024, 6.233512622357263666, -0.7216878364870267237 ) ) ;
#175516=EDGE_CURVE ( 'NONE', #199311, #11347, #5403, .T. ) ;
#175517=CARTESIAN_POINT ( 'NONE',  ( -4.301340604499551468, 7.447936736316801642, -1.117465989868490883 ) ) ;
#175524=CARTESIAN_POINT ( 'NONE',  ( 5.309989718046547402, 9.346738437696316737, 0.7998128361456462443 ) ) ;
#175529=EDGE_CURVE ( 'NONE', #169262, #57507, #156089, .T. ) ;
#175535=CARTESIAN_POINT ( 'NONE',  ( 3.036663219780971978, 6.486598156479028709, -0.7216878364870267237 ) ) ;
#175536=CARTESIAN_POINT ( 'NONE',  ( 1.364683531249986537, 1.717708333674749399, -0.7879004041258239610 ) ) ;
#175538=CARTESIAN_POINT ( 'NONE',  ( 7.293396569147545527, 10.59638086639245280, 1.199719254218460707 ) ) ;
#175541=CARTESIAN_POINT ( 'NONE',  ( 3.010962844182406783, 6.456614384947361174, 0.07536873999088607168 ) ) ;
#175546=CARTESIAN_POINT ( 'NONE',  ( -1.402160292154681736E-14, 2.587500000000023892, -1.732050807568863648 ) ) ;
#175547=CARTESIAN_POINT ( 'NONE',  ( 6.205881626753210867, 8.263281202677319470, 1.599625672291281386 ) ) ;
#175548=CARTESIAN_POINT ( 'NONE',  ( -6.690058733339450114, 9.892486724616283311, 1.199719254218452047 ) ) ;
#175552=CARTESIAN_POINT ( 'NONE',  ( -1.364683531250012516, 2.780208333674754506, 0.7879004041258379498 ) ) ;
#175555=CARTESIAN_POINT ( 'NONE',  ( 2.683624340501134853, 5.218313266304903664, -1.199719254218446718 ) ) ;
#175559=CARTESIAN_POINT ( 'NONE',  ( -5.956409969451652131, 6.075908546082715134, -0.6293437877468227581 ) ) ;
#175560=CARTESIAN_POINT ( 'NONE',  ( 1.499999999999989120, 0.05625000068281565957, 0.000000000000000000 ) ) ;
#175563=CARTESIAN_POINT ( 'NONE',  ( -6.449928391799210736, 8.548002428564306143, -1.599625672291263179 ) ) ;
#175564=CARTESIAN_POINT ( 'NONE',  ( -2.928197990871687306, 5.399686175116803710, 1.082531754730560403 ) ) ;
#175572=CARTESIAN_POINT ( 'NONE',  ( 6.335737856287750880, 6.286115675290828264, -0.7998128361456281477 ) ) ;
#175576=CARTESIAN_POINT ( 'NONE',  ( 5.738125327081736060, 7.717565519727259904, 1.599625672291267398 ) ) ;
#175577=CARTESIAN_POINT ( 'NONE',  ( 3.094265954482837255, 2.800000000000017586, 2.490342512183689294 ) ) ;
#175578=ORIENTED_EDGE ( 'NONE', *, *, #92189, .T. ) ;
#175581=CARTESIAN_POINT ( 'NONE',  ( 2.530568227245037605, 6.104080031761181857, 0.000000000000000000 ) ) ;
#175587=CARTESIAN_POINT ( 'NONE',  ( 4.009017875521604601, 7.583074288825860876, 0.2480677224083651655 ) ) ;
#175597=CARTESIAN_POINT ( 'NONE',  ( 3.212919216758630014, 6.692230152952963529, 0.000000000000000000 ) ) ;
#175598=CARTESIAN_POINT ( 'NONE',  ( 8.785320351975350661, 9.351887953500479966, -0.7216878364870197293 ) ) ;
#175601=CARTESIAN_POINT ( 'NONE',  ( -3.554208825076827782, 7.298327395898266623, 0.7998128361456341429 ) ) ;
#175604=CARTESIAN_POINT ( 'NONE',  ( 7.313733799568044702, 10.62010763521636214, 1.199719254218460707 ) ) ;
#175606=CARTESIAN_POINT ( 'NONE',  ( -4.367698041896780126, 8.247398148854895084, 0.7998128361456481317 ) ) ;
#175612=EDGE_LOOP ( 'NONE', ( #80026, #1474, #90502, #184524 ) ) ;
#175622=CARTESIAN_POINT ( 'NONE',  ( -3.730464822054482710, 7.503959392372201442, 1.040834085586084257E-14 ) ) ;
#175625=CARTESIAN_POINT ( 'NONE',  ( 2.901081683644319842, 5.368050483351580304, 1.082531754730548412 ) ) ;
#175627=FACE_BOUND ( 'NONE', #140445, .T. ) ;
#175629=CARTESIAN_POINT ( 'NONE',  ( 3.945059511452237100, 6.586024615794168646, -1.082531754730548412 ) ) ;
#175630=CARTESIAN_POINT ( 'NONE',  ( -3.307299406729781399, 5.945934176904983381, -1.199719254218452935 ) ) ;
#175634=CARTESIAN_POINT ( 'NONE',  ( 9.378489572351044856, 11.96465713920816043, -1.599625672291262513 ) ) ;
#175639=CARTESIAN_POINT ( 'NONE',  ( -6.177711549321182716, 10.35908057418338402, 0.7998128361456481317 ) ) ;
#175640=CARTESIAN_POINT ( 'NONE',  ( 4.150767584078112193, 7.994312614733129152, 0.7998128361456321445 ) ) ;
#175642=CARTESIAN_POINT ( 'NONE',  ( 3.174580523894165562, 6.855427711185177131, 0.7998128361456341429 ) ) ;
#175644=CARTESIAN_POINT ( 'NONE',  ( -1.364683531250014514, 1.301041667008083325, -0.7879004041258289570 ) ) ;
#175647=CARTESIAN_POINT ( 'NONE',  ( 6.588899466561449536, 9.670504563421618016, -1.082531754730537088 ) ) ;
#175654=CARTESIAN_POINT ( 'NONE',  ( 8.392133896734655707, 11.77427806529038357, 1.082531754730546636 ) ) ;
#175659=CARTESIAN_POINT ( 'NONE',  ( -9.073431116043565225, 11.60875560684942265, -1.599625672291263179 ) ) ;
#175675=CARTESIAN_POINT ( 'NONE',  ( -1.500000000000013101, 1.910416667349488451, -0.8660254037844313801 ) ) ;
#175681=CARTESIAN_POINT ( 'NONE',  ( -1.402160292154681736E-14, -0.7874999999999764411, 1.732050807568877637 ) ) ;
#175682=CARTESIAN_POINT ( 'NONE',  ( 7.540305987494599016, 11.94877408538573427, -0.7998128361456291469 ) ) ;
#175683=CARTESIAN_POINT ( 'NONE',  ( -1.402160292154681736E-14, 0.07187500034142156602, 1.575800808251672791 ) ) ;
#175686=CARTESIAN_POINT ( 'NONE',  ( 2.171277156482887882, 5.684907115872006145, -0.7998128361456291469 ) ) ;
#175687=CARTESIAN_POINT ( 'NONE',  ( -5.083944415444539899, 8.875092884753202682, 0.000000000000000000 ) ) ;
#175691=CARTESIAN_POINT ( 'NONE',  ( -7.040761844198392794, 7.108643661186573759, -0.7998128361456291469 ) ) ;
#175694=CARTESIAN_POINT ( 'NONE',  ( -0.7500000000000006661, 2.639583334016156080, -1.299038105676652011 ) ) ;
#175707=CARTESIAN_POINT ( 'NONE',  ( -9.528683032306089373, 10.01121838064558744, 0.7998128361456462443 ) ) ;
#175708=CARTESIAN_POINT ( 'NONE',  ( 6.714312387265682247, 8.856450423275211037, 1.599625672291281386 ) ) ;
#175715=CARTESIAN_POINT ( 'NONE',  ( -6.886651960737580680, 10.12184548991413457, -1.199719254218440723 ) ) ;
#175722=CARTESIAN_POINT ( 'NONE',  ( 9.083072846151447166, 12.68433652289702884, 1.199719254218450271 ) ) ;
#175726=CARTESIAN_POINT ( 'NONE',  ( -10.13202086811422475, 10.71511252242175161, -0.7998128361456291469 ) ) ;
#175730=CARTESIAN_POINT ( 'NONE',  ( -5.435328143874127882, 6.463069452080541843, -1.319038057358821403 ) ) ;
#175739=CARTESIAN_POINT ( 'NONE',  ( 6.714312387265682247, 8.856450423275211037, 1.599625672291281386 ) ) ;
#175743=CARTESIAN_POINT ( 'NONE',  ( -2.535011536075375105, 5.133042487381368701, 1.000000000000011324 ) ) ;
#175750=CARTESIAN_POINT ( 'NONE',  ( -0.7500000000000006661, 1.889583334016155192, -1.299038105676652011 ) ) ;
#175762=CARTESIAN_POINT ( 'NONE',  ( 3.551873057100283226, 6.127307085716883428, 1.082531754730558626 ) ) ;
#175766=CARTESIAN_POINT ( 'NONE',  ( -9.459838494033043332, 12.05956421450382088, 1.599625672291281386 ) ) ;
#175768=CARTESIAN_POINT ( 'NONE',  ( 8.238550898598388628, 12.76339314834017102, 0.7998128361456462443 ) ) ;
#175777=CARTESIAN_POINT ( 'NONE',  ( 1.364683531249986537, 1.113541667008082658, 0.7879004041258500513 ) ) ;
#175784=CARTESIAN_POINT ( 'NONE',  ( -5.579343907223557331, 6.467988298970945849, 1.199719254218450271 ) ) ;
#175786=CARTESIAN_POINT ( 'NONE',  ( 0.7499999999999885647, 0.4833333333333564297, 1.299038105676657340 ) ) ;
#175788=CARTESIAN_POINT ( 'NONE',  ( -1.364683531250014514, -0.6572916663252459379, 0.7879004041258379498 ) ) ;
#175794=CARTESIAN_POINT ( 'NONE',  ( -1.201851678989727383E-14, 5.509375000341415252, -1.575800808251660134 ) ) ;
#175796=CARTESIAN_POINT ( 'NONE',  ( -7.714753101375940503, 8.959299025482085455, 1.199719254218462483 ) ) ;
#175797=DIRECTION ( 'NONE',  ( -1.000000000000000000, 5.578564026256490882E-16, -1.264049978315544409E-61 ) ) ;
#175798=CARTESIAN_POINT ( 'NONE',  ( 9.399880572976245574, 9.860948844760784482, 0.7998128361456462443 ) ) ;
#175804=CARTESIAN_POINT ( 'NONE',  ( 1.364683531249988757, 0.4468750003414206917, 0.000000000000000000 ) ) ;
#175809=EDGE_CURVE ( 'NONE', #159827, #185972, #4277, .T. ) ;
#175812=CARTESIAN_POINT ( 'NONE',  ( 5.965224400332808763, 9.903252867122883885, -0.7216878364870267237 ) ) ;
#175815=CARTESIAN_POINT ( 'NONE',  ( -3.893162665418476109, 7.693773542963529444, 1.040834085586084257E-14 ) ) ;
#175817=CARTESIAN_POINT ( 'NONE',  ( -0.7500000000000215383, 4.972916667349482012, 1.299038105676671107 ) ) ;
#175820=CARTESIAN_POINT ( 'NONE',  ( 4.161989969270883272, 7.799479364217271282, 0.7216878364870317197 ) ) ;
#175821=CARTESIAN_POINT ( 'NONE',  ( -8.148087131688683371, 11.48955683940339867, -1.082531754730543083 ) ) ;
#175827=CARTESIAN_POINT ( 'NONE',  ( 2.347533153460546806, 5.890539112345938300, 0.000000000000000000 ) ) ;
#175844=CARTESIAN_POINT ( 'NONE',  ( 7.239163954692881653, 10.53310948286200599, -1.199719254218441611 ) ) ;
#175849=CARTESIAN_POINT ( 'NONE',  ( 6.182154858151487353, 6.314861544039274577, -0.7216878364870257245 ) ) ;
#175853=CARTESIAN_POINT ( 'NONE',  ( -9.056483424248693126, 10.62861408545402675, 1.082531754730558626 ) ) ;
#175857=CARTESIAN_POINT ( 'NONE',  ( -3.952365473583647315, 4.569846793057691592, 1.199719254218462483 ) ) ;
#175881=CARTESIAN_POINT ( 'NONE',  ( -7.036318535812428721, 11.15286269184909784, 0.000000000000000000 ) ) ;
#175886=CARTESIAN_POINT ( 'NONE',  ( 7.149227073107712549, 7.235186428247455837, -0.7998128361456281477 ) ) ;
#175888=CARTESIAN_POINT ( 'NONE',  ( 2.758194185376297902, 5.305311418659259814, 1.199719254218452047 ) ) ;
#175890=CARTESIAN_POINT ( 'NONE',  ( -4.111146893441842920, 5.819424013814012753, 1.599625672291267398 ) ) ;
#175894=CARTESIAN_POINT ( 'NONE',  ( -5.362413449404877852, 6.214902764849178141, -1.199719254218446718 ) ) ;
#175895=AXIS2_PLACEMENT_3D ( 'NONE', #49978, #181042, #149614 ) ;
#175898=CARTESIAN_POINT ( 'NONE',  ( 7.914208982075123799, 10.25632978388623684, -1.599625672291262513 ) ) ;
#175899=CARTESIAN_POINT ( 'NONE',  ( 1.364683531249988535, 3.863541667008087543, 0.7879004041258499402 ) ) ;
#175901=CARTESIAN_POINT ( 'NONE',  ( 6.101957686160805139, 6.023808750328159434, -0.2146407016825630509 ) ) ;
#175902=CARTESIAN_POINT ( 'NONE',  ( 4.039966587192267866, 4.776011108888172707, 1.082531754730560403 ) ) ;
#175909=CARTESIAN_POINT ( 'NONE',  ( 7.144783764277405247, 8.398297815487545392, -1.082531754730543971 ) ) ;
#175910=CARTESIAN_POINT ( 'NONE',  ( -9.104463846776669200, 10.58062822844965645, -1.199719254218441611 ) ) ;
#175913=CARTESIAN_POINT ( 'NONE',  ( -7.486073373039941359, 11.88550270185529278, -0.7998128361456291469 ) ) ;
#175914=CARTESIAN_POINT ( 'NONE',  ( -5.442708600882160574, 8.437244903416123876, -1.199719254218446718 ) ) ;
#175921=CARTESIAN_POINT ( 'NONE',  ( 6.916630921265960019, 11.22115317478565188, 0.7998128361456462443 ) ) ;
#175928=CARTESIAN_POINT ( 'NONE',  ( 0.7499999999999902300, 5.347916667349482012, -1.299038105676658228 ) ) ;
#175933=CARTESIAN_POINT ( 'NONE',  ( -0.7499999999999972244, 3.858333333333359594, -1.299038105676652011 ) ) ;
#175934=CARTESIAN_POINT ( 'NONE',  ( 6.094553744542824170, 7.069066442510145265, 1.199719254218462483 ) ) ;
#175938=CARTESIAN_POINT ( 'NONE',  ( 6.778713617152772208, 10.85232362007950258, -0.7216878364870267237 ) ) ;
#175939=CARTESIAN_POINT ( 'NONE',  ( -7.809133291347029271, 12.05447990663947877, 0.000000000000000000 ) ) ;
#175942=CARTESIAN_POINT ( 'NONE',  ( 7.716561984472250835, 12.15440608185967086, 1.040834085586084257E-14 ) ) ;
#175944=CARTESIAN_POINT ( 'NONE',  ( 1.499999999999990896, 5.275000000000022560, 1.214306433183764966E-14 ) ) ;
#175945=CARTESIAN_POINT ( 'NONE',  ( -4.115063316947640715, 4.759660943649018705, 1.199719254218462483 ) ) ;
#175947=CARTESIAN_POINT ( 'NONE',  ( -1.402160292154681736E-14, 1.196875000341419026, -1.575800808251659024 ) ) ;
#175952=CARTESIAN_POINT ( 'NONE',  ( -1.364683531250000748, 0.009375000341420303140, 0.000000000000000000 ) ) ;
#175954=CARTESIAN_POINT ( 'NONE',  ( 8.910733272679570049, 11.41894145625809820, -1.599625672291255185 ) ) ;
#175957=EDGE_CURVE ( 'NONE', #177712, #20719, #67472, .T. ) ;
#175959=CARTESIAN_POINT ( 'NONE',  ( -3.755245360860939297, 4.443836344834937613, -1.082531754730548412 ) ) ;
#175960=CARTESIAN_POINT ( 'NONE',  ( 4.702146809683701356, 5.356480858934594025, -2.500000000000000444 ) ) ;
#175962=CARTESIAN_POINT ( 'NONE',  ( -6.898401231254901234, 6.942556279419168419, -0.7998128361456291469 ) ) ;
#175966=CARTESIAN_POINT ( 'NONE',  ( 4.029797971759831121, 5.724516938518342535, -1.599625672291255185 ) ) ;
#175972=CARTESIAN_POINT ( 'NONE',  ( 9.772729797352075920, 10.29593960653257234, -0.7998128361456281477 ) ) ;
#175976=CARTESIAN_POINT ( 'NONE',  ( -6.078132937628113908, 5.985576603521232109, 1.040834085586084257E-14 ) ) ;
#175980=CARTESIAN_POINT ( 'NONE',  ( 7.618792255875527886, 10.97600916757510170, 1.199719254218460707 ) ) ;
#175982=CARTESIAN_POINT ( 'NONE',  ( 8.599949509769960088, 8.927695937686774386, 1.040834085586084257E-14 ) ) ;
#175985=CARTESIAN_POINT ( 'NONE',  ( -9.327646496521984076, 11.90534021740758064, -1.443375672974059665 ) ) ;
#175987=CYLINDRICAL_SURFACE ( 'NONE', #22697, 0.7500000000000011102 ) ;
#175992=CARTESIAN_POINT ( 'NONE',  ( -5.747036748294815922, 6.247280920146251582, 1.064921034751656226 ) ) ;
#175993=CARTESIAN_POINT ( 'NONE',  ( 0.6823417656249882723, 1.676041667008083769, -1.181850606188749264 ) ) ;
#175997=CARTESIAN_POINT ( 'NONE',  ( 6.073689629242148058, 8.109057205581079231, -1.443375672974057666 ) ) ;
#176015=CARTESIAN_POINT ( 'NONE',  ( 7.639129486296027061, 10.99973593639901814, 1.199719254218460707 ) ) ;
#176017=ORIENTED_EDGE ( 'NONE', *, *, #17814, .F. ) ;
#176019=CARTESIAN_POINT ( 'NONE',  ( -4.569261463005423352, 5.289558780716470565, -1.199719254218446718 ) ) ;
#176020=CARTESIAN_POINT ( 'NONE',  ( -8.694856585065634746, 9.038420858865048757, 0.7998128361456462443 ) ) ;
#176025=CARTESIAN_POINT ( 'NONE',  ( 1.499999999999987121, 3.827083334016153415, -0.8660254037844323793 ) ) ;
#176026=CARTESIAN_POINT ( 'NONE',  ( 7.721532178182734185, 8.967207948423393304, 1.199719254218462483 ) ) ;
#176029=CARTESIAN_POINT ( 'NONE',  ( -6.367525699912501835, 10.58053041653993098, -0.7998128361456291469 ) ) ;
#176031=CARTESIAN_POINT ( 'NONE',  ( -1.001543065824772872E-14, 4.321875000341417916, 1.575800808251672791 ) ) ;
#176037=CARTESIAN_POINT ( 'NONE',  ( -9.002250809794006159, 10.56534270192358704, -1.082531754730543971 ) ) ;
#176041=CARTESIAN_POINT ( 'NONE',  ( 1.364683531249986537, 2.217708333674751398, -0.7879004041258239610 ) ) ;
#176048=CARTESIAN_POINT ( 'NONE',  ( -1.201851678989727383E-14, 2.821875000341418804, 1.575800808251672791 ) ) ;
#176050=CARTESIAN_POINT ( 'NONE',  ( -5.786632634934295361, 5.645492917045106473, 0.7998128361456341429 ) ) ;
#176051=CARTESIAN_POINT ( 'NONE',  ( 6.612626235163189925, 8.737816579155630592, -1.599625672291262513 ) ) ;
#176054=CARTESIAN_POINT ( 'NONE',  ( 1.364683531249988535, 3.717708333674750953, -0.7879004041258239610 ) ) ;
#176057=CARTESIAN_POINT ( 'NONE',  ( 1.364683531249984538, -1.094791666325247936, -0.7879004041258309554 ) ) ;
#176058=CARTESIAN_POINT ( 'NONE',  ( -5.097502569058225852, 5.049433873430440478, -0.7216878364870207285 ) ) ;
#176062=CARTESIAN_POINT ( 'NONE',  ( 4.704316114261903436, 4.590716342834741504, 1.214306433183764966E-14 ) ) ;
#176065=CARTESIAN_POINT ( 'NONE',  ( -8.134528978519403708, 11.47373899403920205, 1.082531754730549967 ) ) ;
#176071=CARTESIAN_POINT ( 'NONE',  ( -5.978782553502159480, 8.958701498185728695, 1.082531754730548412 ) ) ;
#176073=CARTESIAN_POINT ( 'NONE',  ( 0.6823417656249899377, 1.155208333674752286, 1.181850606188755259 ) ) ;
#176079=CARTESIAN_POINT ( 'NONE',  ( -1.364683531250014514, -0.9489583329919112353, -0.7879004041258359514 ) ) ;
#176082=CARTESIAN_POINT ( 'NONE',  ( 4.189106276498237413, 3.989638198777126110, -0.7216878364870188411 ) ) ;
#176086=CARTESIAN_POINT ( 'NONE',  ( 1.499999999999985123, -0.4541666666666469010, -0.8660254037844323793 ) ) ;
#176087=CARTESIAN_POINT ( 'NONE',  ( 8.731087737076324018, 9.288616569451617622, 1.040834085586084257E-14 ) ) ;
#176091=ORIENTED_EDGE ( 'NONE', *, *, #184288, .F. ) ;
#176095=CARTESIAN_POINT ( 'NONE',  ( 4.690231075323689325, 7.559354456931247412, 1.199719254218462483 ) ) ;
#176097=CARTESIAN_POINT ( 'NONE',  ( -3.846762897975357198, 5.510976019103107859, -1.599625672291256295 ) ) ;
#176101=CARTESIAN_POINT ( 'NONE',  ( -1.364683531250012516, 1.592708333674756727, 0.7879004041258379498 ) ) ;
#176103=CARTESIAN_POINT ( 'NONE',  ( -7.472515219426274946, 11.86968485597268064, 0.000000000000000000 ) ) ;
#176119=CARTESIAN_POINT ( 'NONE',  ( -4.247512733928926920, 7.321623457166534621, -0.8935899926269799121 ) ) ;
#176122=CARTESIAN_POINT ( 'NONE',  ( 6.169123589417988995, 7.156064594864501416, -1.199719254218445830 ) ) ;
#176130=CARTESIAN_POINT ( 'NONE',  ( 8.796542737168120851, 9.157054702984622097, -0.7998128361456211532 ) ) ;
#176133=CARTESIAN_POINT ( 'NONE',  ( 9.694243528971124846, 11.26870452434320491, 1.199719254218450271 ) ) ;
#176135=CARTESIAN_POINT ( 'NONE',  ( -1.123270288249902160, 2.800000000000024691, 0.7750000000000117906 ) ) ;
#176139=CARTESIAN_POINT ( 'NONE',  ( 9.561524646135536543, 12.17819805862340310, -1.599625672291262513 ) ) ;
#176141=AXIS2_PLACEMENT_3D ( 'NONE', #100492, #82101, #183873 ) ;
#176146=CARTESIAN_POINT ( 'NONE',  ( -8.839552966430007430, 11.33589776563360019, -1.443375672974059665 ) ) ;
#176151=CARTESIAN_POINT ( 'NONE',  ( -4.904003162269379601, 4.835767286957110223, -0.1818790228878807702 ) ) ;
#176152=CARTESIAN_POINT ( 'NONE',  ( 5.066996723205273057, 6.934582148538044777, 1.599625672291267398 ) ) ;
#176153=CARTESIAN_POINT ( 'NONE',  ( -4.213209511989692402, 3.978029986984279898, -0.5398075284353744951 ) ) ;
#176158=CARTESIAN_POINT ( 'NONE',  ( 4.500943809612556024, 4.353448654077163305, 1.214306433183764966E-14 ) ) ;
#176166=CARTESIAN_POINT ( 'NONE',  ( -7.040761844198392794, 7.108643661186573759, -0.7998128361456291469 ) ) ;
#176168=CARTESIAN_POINT ( 'NONE',  ( -4.959585264500673496, 4.680604318205876524, 1.214306433183764966E-14 ) ) ;
#176173=CARTESIAN_POINT ( 'NONE',  ( 0.5631007116328431428, 7.823254984196703177, -1.919102855466201518 ) ) ;
#176174=CARTESIAN_POINT ( 'NONE',  ( -1.201851678989727383E-14, 3.384375000341421025, 1.575800808251672791 ) ) ;
#176176=CARTESIAN_POINT ( 'NONE',  ( 3.974511587100456822, 7.788680618259193444, 1.040834085586084257E-14 ) ) ;
#176178=CARTESIAN_POINT ( 'NONE',  ( 1.528885273045258231, 8.694317336386671258, 2.518424357262873059 ) ) ;
#176190=CARTESIAN_POINT ( 'NONE',  ( -1.402160292154681736E-14, 1.009375000341417916, -1.575800808251659024 ) ) ;
#176192=CARTESIAN_POINT ( 'NONE',  ( 5.054492339796319733, 4.791329239384148231, -0.7998128361456211532 ) ) ;
#176194=CARTESIAN_POINT ( 'NONE',  ( -5.558479791922849245, 9.428717490644563881, 0.7216878364870458196 ) ) ;
#176195=CARTESIAN_POINT ( 'NONE',  ( 3.714570900464274850, 6.317121236308204324, 1.082531754730558626 ) ) ;
#176196=CARTESIAN_POINT ( 'NONE',  ( -5.707619481228814351, 9.602713794834864203, -0.7216878364870207285 ) ) ;
#176200=CARTESIAN_POINT ( 'NONE',  ( 4.801558957534076022, 8.753569217098425170, 0.7998128361456462443 ) ) ;
#176205=CARTESIAN_POINT ( 'NONE',  ( 0.6823417656249917140, 5.342708333674749177, 1.181850606188765695 ) ) ;
#176209=CARTESIAN_POINT ( 'NONE',  ( 7.470706336329915764, 8.674577799595093452, -1.199719254218441611 ) ) ;
#176212=CARTESIAN_POINT ( 'NONE',  ( -7.395082721250053837, 10.71501471051202614, -1.199719254218446718 ) ) ;
#176217=CARTESIAN_POINT ( 'NONE',  ( 7.670162217029129259, 9.971608557999250166, 1.599625672291281386 ) ) ;
#176219=CARTESIAN_POINT ( 'NONE',  ( -7.446452682403657874, 9.710614100936176385, -1.599625672291263179 ) ) ;
#176221=CARTESIAN_POINT ( 'NONE',  ( 6.710922848640084482, 9.812865175846695820, -1.082531754730537976 ) ) ;
#176222=CARTESIAN_POINT ( 'NONE',  ( 4.026354976812863917, 7.791716866330316904, -0.3671166487079768892 ) ) ;
#176223=CARTESIAN_POINT ( 'NONE',  ( -8.297226821883391779, 11.66355314463053006, 1.082531754730549967 ) ) ;
#176229=CARTESIAN_POINT ( 'NONE',  ( 6.322179702674084467, 6.270297829408224111, 1.040834085586084257E-14 ) ) ;
#176231=CARTESIAN_POINT ( 'NONE',  ( 10.05067194643221207, 10.62020544712608938, 0.7998128361456462443 ) ) ;
#176232=CARTESIAN_POINT ( 'NONE',  ( -5.512743837300482674, 6.249232958799082027, 0.9732600881407500459 ) ) ;
#176233=CARTESIAN_POINT ( 'NONE',  ( 3.816783937446950770, 4.411668334231586996, 1.199719254218464037 ) ) ;
#176234=CARTESIAN_POINT ( 'NONE',  ( -1.402160292154681736E-14, 0.3218750003414227456, 1.575800808251672791 ) ) ;
#176236=CARTESIAN_POINT ( 'NONE',  ( -7.551528373131759508, 7.912463978182924684, 1.040834085586084257E-14 ) ) ;
#176242=CARTESIAN_POINT ( 'NONE',  ( -4.511607644515479798, 7.038970647229928268, 1.150300019105324978 ) ) ;
#176243=CARTESIAN_POINT ( 'NONE',  ( -0.6823417656250003738, -0.2197916663252488800, -1.181850606188749264 ) ) ;
#176246=CARTESIAN_POINT ( 'NONE',  ( 2.873965376416980355, 6.296784005887697155, -0.7216878364870267237 ) ) ;
#176248=EDGE_CURVE ( 'NONE', #147848, #4590, #154417, .T. ) ;
#176250=AXIS2_PLACEMENT_3D ( 'NONE', #205343, #56980, #141477 ) ;
#176252=CARTESIAN_POINT ( 'NONE',  ( -7.307481607641392429, 11.46921960898288972, 0.7216878364870458196 ) ) ;
#176257=CARTESIAN_POINT ( 'NONE',  ( -9.300530188850304469, 9.952966096521256745, 1.040834085586084257E-14 ) ) ;
#176263=ORIENTED_EDGE ( 'NONE', *, *, #109624, .T. ) ;
#176264=CARTESIAN_POINT ( 'NONE',  ( -8.961576348508655698, 9.557519949455999253, -0.7216878364870267237 ) ) ;
#176268=CARTESIAN_POINT ( 'NONE',  ( 0.6823417656249899377, 5.488541667008087543, -1.181850606188754593 ) ) ;
#176269=CARTESIAN_POINT ( 'NONE',  ( 0.7499999999999902300, 3.847916667349481123, -1.299038105676658228 ) ) ;
#176270=CARTESIAN_POINT ( 'NONE',  ( 5.877843389052785028, 6.166481636157870483, -0.8510708418205383818 ) ) ;
#176276=CARTESIAN_POINT ( 'NONE',  ( -8.830438121202295321, 9.196599317691152464, -0.7998128361456291469 ) ) ;
#176277=CARTESIAN_POINT ( 'NONE',  ( -4.161989969715295778, 4.726297878971393196, 2.420000000000010587 ) ) ;
#176280=CARTESIAN_POINT ( 'NONE',  ( 6.308621549060418054, 6.254479983525607523, 0.7998128361456341429 ) ) ;
#176282=CARTESIAN_POINT ( 'NONE',  ( 3.790776250277827941, 4.071658342522865404, -0.8783347955927873763 ) ) ;
#176285=CARTESIAN_POINT ( 'NONE',  ( 5.947222937888848371, 10.09017719417900416, 1.040834085586084257E-14 ) ) ;
#176292=CARTESIAN_POINT ( 'NONE',  ( -4.609409038966229666, 8.321468278861834378, -0.7216878364870267237 ) ) ;
#176295=DIRECTION ( 'NONE',  ( 0.7592566023653005702, -0.6507913734559639396, 0.000000000000000000 ) ) ;
#176302=CARTESIAN_POINT ( 'NONE',  ( -8.805130697071332335, 12.36007068230351358, 1.199719254218462483 ) ) ;
#176304=CARTESIAN_POINT ( 'NONE',  ( 9.423080456697809026, 10.95234760669099749, -1.199719254218446718 ) ) ;
#176305=CARTESIAN_POINT ( 'NONE',  ( -1.500000000000001332, 0.1500000000000251132, 0.000000000000000000 ) ) ;
#176306=CARTESIAN_POINT ( 'NONE',  ( -6.516665389662827934, 10.75452672124865217, 0.000000000000000000 ) ) ;
#176309=CARTESIAN_POINT ( 'NONE',  ( 0.6823417656249882723, 2.926041667008084879, -1.181850606188754593 ) ) ;
#176310=CARTESIAN_POINT ( 'NONE',  ( 2.184835310096557404, 5.700724961754617404, 1.040834085586084257E-14 ) ) ;
#176313=CARTESIAN_POINT ( 'NONE',  ( -1.499999999999997780, 4.900000000000022560, 1.214306433183764966E-14 ) ) ;
#176316=CARTESIAN_POINT ( 'NONE',  ( 8.554831740098654436, 11.00372300158037042, 1.443375672974076540 ) ) ;
#176319=CARTESIAN_POINT ( 'NONE',  ( -6.561783159334141580, 7.718130443053708767, -1.082531754730544860 ) ) ;
#176320=CARTESIAN_POINT ( 'NONE',  ( -0.6823417656250003738, 1.717708333674752730, -1.181850606188749264 ) ) ;
#176324=CARTESIAN_POINT ( 'NONE',  ( -7.691553217654356622, 7.867900263551875994, -0.7998128361456291469 ) ) ;
#176325=CARTESIAN_POINT ( 'NONE',  ( -0.6823417656250212460, 5.113541667008086655, 1.181850606188767472 ) ) ;
#176330=CARTESIAN_POINT ( 'NONE',  ( 8.503988664269582998, 10.94440607977979063, 1.599625672291281386 ) ) ;
#176333=CARTESIAN_POINT ( 'NONE',  ( 0.7499999999999885647, 1.816666666666688634, -1.299038105676652899 ) ) ;
#176338=CARTESIAN_POINT ( 'NONE',  ( 8.211434591371064684, 12.73175745657494851, -0.7998128361456352531 ) ) ;
#176343=CARTESIAN_POINT ( 'NONE',  ( 7.052212457402625922, 11.37933163361175382, -0.7998128361456291469 ) ) ;
#176344=CARTESIAN_POINT ( 'NONE',  ( -1.527007413433568939, 8.693555224946434734, 2.520068491016817624 ) ) ;
#176348=CARTESIAN_POINT ( 'NONE',  ( -0.6823417656250003738, -1.032291666325242607, -1.181850606188749264 ) ) ;
#176352=CARTESIAN_POINT ( 'NONE',  ( 7.397945374551106568, 11.78268670361832093, -0.7998128361456291469 ) ) ;
#176354=CARTESIAN_POINT ( 'NONE',  ( 1.364683531249990311, 3.884375000341417028, 1.214306433183764966E-14 ) ) ;
#176356=CARTESIAN_POINT ( 'NONE',  ( -7.063434843039784639, 7.343021526408956667, 1.040834085586084257E-14 ) ) ;
#176366=CARTESIAN_POINT ( 'NONE',  ( 8.565000355531088516, 11.01558638625153286, -1.599625672291257406 ) ) ;
#176374=CARTESIAN_POINT ( 'NONE',  ( -9.969323024750229578, 10.52529837183042716, -0.7998128361456291469 ) ) ;
#176375=CARTESIAN_POINT ( 'NONE',  ( 7.467843683028853263, 7.606905806488803101, 0.7998128361456341429 ) ) ;
#176377=CARTESIAN_POINT ( 'NONE',  ( 3.185802909086945967, 5.700225246367978116, 1.082531754730546636 ) ) ;
#176379=CARTESIAN_POINT ( 'NONE',  ( 4.202137545231717120, 6.989912005157271402, 1.199719254218462483 ) ) ;
#176384=CARTESIAN_POINT ( 'NONE',  ( 3.055305189271266375, 6.508347120884369730, 0.2706067644346449308 ) ) ;
#176387=CARTESIAN_POINT ( 'NONE',  ( -4.595850885352567694, 8.305650432979225783, 1.040834085586084257E-14 ) ) ;
#176388=CARTESIAN_POINT ( 'NONE',  ( 4.359110081993588182, 5.044382169536003602, -1.199719254218452047 ) ) ;
#176391=CARTESIAN_POINT ( 'NONE',  ( -7.212047647465563038, 10.50147379109678880, -1.199719254218446718 ) ) ;
#176397=CARTESIAN_POINT ( 'NONE',  ( -9.643927338022246332, 10.14567007064778004, -0.7998128361456291469 ) ) ;
#176401=CARTESIAN_POINT ( 'NONE',  ( 8.932124273304774320, 9.315233161810734686, 0.7998128361456462443 ) ) ;
#176410=DIRECTION ( 'NONE',  ( 0.6507913734559651608, -0.7592566023652994600, 0.000000000000000000 ) ) ;
#176412=CARTESIAN_POINT ( 'NONE',  ( -8.532158741701643123, 8.848606708273724308, 0.7998128361456462443 ) ) ;
#176416=CARTESIAN_POINT ( 'NONE',  ( 5.992340707560151358, 8.014150130285418783, 1.443375672974062551 ) ) ;
#176417=ORIENTED_EDGE ( 'NONE', *, *, #180914, .F. ) ;
#176421=CARTESIAN_POINT ( 'NONE',  ( -5.117312914154178216, 8.057616602233474978, -1.199719254218452047 ) ) ;
#176424=CARTESIAN_POINT ( 'NONE',  ( -1.499999999999997780, 8.627523663848661428, -2.579999999999990301 ) ) ;
#176431=CARTESIAN_POINT ( 'NONE',  ( -8.631737353394710155, 13.22211067893587533, 1.040834085586084257E-14 ) ) ;
#176432=CARTESIAN_POINT ( 'NONE',  ( 6.401421083946654100, 10.62007503124645957, -0.7998128361456291469 ) ) ;
#176434=CARTESIAN_POINT ( 'NONE',  ( -3.633221978782290140, 6.222214161012547429, -1.082531754730549967 ) ) ;
#176435=CARTESIAN_POINT ( 'NONE',  ( -5.219871119622601086, 6.450327202623305389, -1.173442693870077935 ) ) ;
#176442=CARTESIAN_POINT ( 'NONE',  ( 3.871016551901614200, 4.474939717762034697, -1.199719254218446718 ) ) ;
#176449=CARTESIAN_POINT ( 'NONE',  ( 3.357615597678655917, 7.068968630600412695, 0.7998128361456321445 ) ) ;
#176460=CARTESIAN_POINT ( 'NONE',  ( -5.949330478298285207, 5.835307067636438028, 0.7998128361456341429 ) ) ;
#176461=CARTESIAN_POINT ( 'NONE',  ( 5.951666246274803562, 7.006327377817825663, 1.082531754730558626 ) ) ;
#176462=CARTESIAN_POINT ( 'NONE',  ( -1.500000000000011324, 3.170833333333354265, 0.8660254037844403729 ) ) ;
#176464=CARTESIAN_POINT ( 'NONE',  ( -3.490334480514268645, 6.159475096320226939, -1.199719254218452935 ) ) ;
#176465=CARTESIAN_POINT ( 'NONE',  ( 0.1368715580175494662, 8.236096389522833405, -2.000481929432700756 ) ) ;
#176467=DIRECTION ( 'NONE',  ( -5.578564026256490882E-16, -1.000000000000000000, -9.066213480720158442E-32 ) ) ;
#176469=CARTESIAN_POINT ( 'NONE',  ( 1.364683531249988535, 4.655208333674755394, -0.7879004041258300672 ) ) ;
#176476=CARTESIAN_POINT ( 'NONE',  ( 3.897079088924235712, 6.634010472798538949, 1.199719254218462483 ) ) ;
#176477=DIRECTION ( 'NONE',  ( -0.000000000000000000, -8.546850786086437571E-32, -1.000000000000000000 ) ) ;
#176479=CARTESIAN_POINT ( 'NONE',  ( 0.04420220085362167040, 7.036439304898326697, -4.015252406538079022 ) ) ;
#176480=CARTESIAN_POINT ( 'NONE',  ( 3.362058906508964107, 6.866226457661666061, -0.7216878364870351614 ) ) ;
#176482=CARTESIAN_POINT ( 'NONE',  ( -0.6823417656250003738, 1.030208333674752286, -1.181850606188749264 ) ) ;
#176486=CARTESIAN_POINT ( 'NONE',  ( -8.676328237741483207, 12.20980114641871062, -1.199719254218446718 ) ) ;
#176487=CARTESIAN_POINT ( 'NONE',  ( -6.710922848640111127, 6.931757532942661726, 0.7216878364870317197 ) ) ;
#176491=CARTESIAN_POINT ( 'NONE',  ( 1.364683531249990311, 3.884375000341417028, 1.214306433183764966E-14 ) ) ;
#176499=CARTESIAN_POINT ( 'NONE',  ( -5.788968402910818156, 7.776882441527838807, 1.443375672974064550 ) ) ;
#176504=CARTESIAN_POINT ( 'NONE',  ( -6.534666851662457532, 6.726125536468730459, 1.040834085586084257E-14 ) ) ;
#176513=ORIENTED_EDGE ( 'NONE', *, *, #174092, .F. ) ;
#176515=CARTESIAN_POINT ( 'NONE',  ( 4.097261965275050599, 7.670716846599076710, -0.6648547660955180794 ) ) ;
#176517=CARTESIAN_POINT ( 'NONE',  ( -5.199715606040888005, 6.025088614257851027, -1.199719254218446718 ) ) ;
#176520=CARTESIAN_POINT ( 'NONE',  ( 1.499999999999987121, 1.004166666666687968, 0.8660254037844524744 ) ) ;
#176521=ORIENTED_EDGE ( 'NONE', *, *, #162536, .F. ) ;
#176523=CARTESIAN_POINT ( 'NONE',  ( 7.754900677336718395, 11.99120852362745460, -0.7216878364870267237 ) ) ;
#176524=CARTESIAN_POINT ( 'NONE',  ( 7.416473721875251890, 8.611306416064660851, 1.199719254218462483 ) ) ;
#176529=CARTESIAN_POINT ( 'NONE',  ( 5.138703914779377158, 5.953908307786102583, 1.199719254218462483 ) ) ;
#176530=CARTESIAN_POINT ( 'NONE',  ( -0.2828007905114904852, 7.102855049428780099, -1.981079112686744192 ) ) ;
#176531=ORIENTED_EDGE ( 'NONE', *, *, #180626, .T. ) ;
#176538=CARTESIAN_POINT ( 'NONE',  ( -5.713871673155502151, 8.753601821068331290, 1.199719254218452047 ) ) ;
#176539=ORIENTED_EDGE ( 'NONE', *, *, #147605, .T. ) ;
#176540=CARTESIAN_POINT ( 'NONE',  ( 8.283668668269706714, 8.766627655843896250, 1.040834085586084257E-14 ) ) ;
#176542=ORIENTED_EDGE ( 'NONE', *, *, #95866, .T. ) ;
#176544=CARTESIAN_POINT ( 'NONE',  ( 0.6823417656249917140, 3.342708333674754506, 1.181850606188765695 ) ) ;
#176545=CARTESIAN_POINT ( 'NONE',  ( 8.310784975052673218, 10.71900177569337487, -1.443375672974063439 ) ) ;
#176546=ADVANCED_FACE ( 'NONE', ( #194235 ), #80490, .F. ) ;
#176547=CARTESIAN_POINT ( 'NONE',  ( -7.413611068574208041, 7.543634422958360730, 0.7998128361456341429 ) ) ;
#176550=CARTESIAN_POINT ( 'NONE',  ( 4.482942347612929979, 8.381849838857084123, 1.040834085586084257E-14 ) ) ;
#176551=CARTESIAN_POINT ( 'NONE',  ( -4.550733115681270036, 8.460939068270139529, 0.7998128361456481317 ) ) ;
#176555=CARTESIAN_POINT ( 'NONE',  ( 0.7499999999999885647, 0.01458333401615358182, 1.299038105676657340 ) ) ;
#176558=CARTESIAN_POINT ( 'NONE',  ( 8.297226821883377568, 8.782445501726501291, -0.7216878364870267237 ) ) ;
#176562=CARTESIAN_POINT ( 'NONE',  ( 1.364683531249988757, 2.446875000341415696, 1.214306433183764966E-14 ) ) ;
#176564=CARTESIAN_POINT ( 'NONE',  ( 5.111060722227499298, 8.906728576000002562, -0.7216878364870267237 ) ) ;
#176566=CARTESIAN_POINT ( 'NONE',  ( -4.311129659465605002, 4.131998812239033647, 0.7216878364870317197 ) ) ;
#176568=CARTESIAN_POINT ( 'NONE',  ( -1.201851678989727383E-14, 5.696875000341416140, -1.575800808251660134 ) ) ;
#176573=CARTESIAN_POINT ( 'NONE',  ( -3.978601536817720330, 7.845232424458246534, -0.1334687937623244003 ) ) ;
#176574=DIRECTION ( 'NONE',  ( 1.000000000000000000, 0.000000000000000000, 0.000000000000000000 ) ) ;
#176581=CARTESIAN_POINT ( 'NONE',  ( 4.821896187954575197, 8.777295985922343391, 0.7998128361456462443 ) ) ;
#176592=CARTESIAN_POINT ( 'NONE',  ( 5.531363484695522637, 5.555604941673978558, -0.7216878364870207285 ) ) ;
#176594=CARTESIAN_POINT ( 'NONE',  ( -1.201851678989727383E-14, 1.634375000341421025, 1.575800808251672791 ) ) ;
#176595=CARTESIAN_POINT ( 'NONE',  ( 6.805303039055573322, 10.02693841461847057, 1.199719254218460707 ) ) ;
#176597=CARTESIAN_POINT ( 'NONE',  ( 0.04851965725442013155, 7.069405242467053263, -4.059206989956010148 ) ) ;
#176598=CARTESIAN_POINT ( 'NONE',  ( -5.362413449404877852, 6.214902764849178141, -1.199719254218446718 ) ) ;
#176599=B_SPLINE_CURVE_WITH_KNOTS ( 'NONE', 3,
 ( #208535, #58041, #127400, #143606 ),
 .UNSPECIFIED., .F., .F.,
 ( 4, 4 ),
 ( 0.000000000000000000, 0.002006560693247956984 ),
 .UNSPECIFIED. ) ;
#176602=CARTESIAN_POINT ( 'NONE',  ( 1.499999999999989120, 3.254166666666690855, 0.8660254037844524744 ) ) ;
#176603=CARTESIAN_POINT ( 'NONE',  ( 5.555090253297246150, 7.504024600312024340, 1.599625672291267398 ) ) ;
#176604=CARTESIAN_POINT ( 'NONE',  ( -7.226659571283968297, 8.389856573708110332, 1.199719254218450271 ) ) ;
#176608=CARTESIAN_POINT ( 'NONE',  ( 1.364683531249988535, 2.613541667008089764, 0.7879004041258500513 ) ) ;
#176610=CARTESIAN_POINT ( 'NONE',  ( 4.546061579283848353, 4.198160018786257552, -0.7998128361456211532 ) ) ;
#176613=CARTESIAN_POINT ( 'NONE',  ( 7.334597915313080918, 9.580116872663850813, 1.040834085586084257E-14 ) ) ;
#176616=CARTESIAN_POINT ( 'NONE',  ( 0.7499999999999902300, 1.014583334016154526, 1.299038105676657340 ) ) ;
#176618=CARTESIAN_POINT ( 'NONE',  ( -6.663996196316808174, 7.733415969579778171, -1.199719254218446718 ) ) ;
#176619=CARTESIAN_POINT ( 'NONE',  ( -2.819732761962332024, 6.233512622357263666, -0.7216878364870267237 ) ) ;
#176626=ORIENTED_EDGE ( 'NONE', *, *, #153081, .T. ) ;
#176628=CARTESIAN_POINT ( 'NONE',  ( 6.148786358997489820, 7.132337826040578754, -1.199719254218446718 ) ) ;
#176629=DIRECTION ( 'NONE',  ( 0.000000000000000000, -1.000000000000000000, 0.000000000000000000 ) ) ;
#176632=CARTESIAN_POINT ( 'NONE',  ( 5.296431564432884542, 9.330920591813708143, 1.040834085586084257E-14 ) ) ;
#176634=CARTESIAN_POINT ( 'NONE',  ( -1.499999999999997780, 6.280000000000035776, -3.469446951953614189E-15 ) ) ;
#176636=CARTESIAN_POINT ( 'NONE',  ( -4.557512192488103686, 8.468847991211438497, -0.7998128361456281477 ) ) ;
#176638=CARTESIAN_POINT ( 'NONE',  ( 2.205172540517054802, 5.724451730578533848, 1.040834085586084257E-14 ) ) ;
#176644=CARTESIAN_POINT ( 'NONE',  ( 4.014365637759117256, 7.575528411784208771, 0.2883143100938356240 ) ) ;
#176652=CARTESIAN_POINT ( 'NONE',  ( -2.155383234892699562, 5.458438174109348395, 1.040834085586084257E-14 ) ) ;
#176653=CARTESIAN_POINT ( 'NONE',  ( 7.782016984564054773, 10.10210578678999482, 1.443375672974076540 ) ) ;
#176655=CARTESIAN_POINT ( 'NONE',  ( -6.064574784014443942, 5.969758757638621738, -0.7998128361456291469 ) ) ;
#176658=CARTESIAN_POINT ( 'NONE',  ( 8.633844893804129228, 8.967240552393299424, -0.7998128361456211532 ) ) ;
#176660=CARTESIAN_POINT ( 'NONE',  ( -6.175902666224832416, 7.163973517805802160, -1.199719254218446718 ) ) ;
#176672=CARTESIAN_POINT ( 'NONE',  ( 10.42352117080803708, 11.05519620889787724, -0.7998128361456281477 ) ) ;
#176673=CARTESIAN_POINT ( 'NONE',  ( -5.416646063859567484, 6.278174148379618735, 1.199719254218450271 ) ) ;
#176676=CARTESIAN_POINT ( 'NONE',  ( 4.094199201646931741, 4.839282492418613302, -1.082531754730543083 ) ) ;
#176680=CARTESIAN_POINT ( 'NONE',  ( -4.783329267523015460, 4.474972321731942593, -0.7998128361456221525 ) ) ;
#176681=CARTESIAN_POINT ( 'NONE',  ( -2.903417451620861289, 6.539070793532962611, 0.7998128361456341429 ) ) ;
#176684=CARTESIAN_POINT ( 'NONE',  ( 8.204655514564224816, 12.72384853363364066, 1.040834085586084257E-14 ) ) ;
#176687=CARTESIAN_POINT ( 'NONE',  ( -6.744291347794091784, 9.955758108146730123, -1.199719254218440723 ) ) ;
#176688=CARTESIAN_POINT ( 'NONE',  ( 4.310602774141044868, 7.116454772218158809, -1.199719254218452047 ) ) ;
#176694=CARTESIAN_POINT ( 'NONE',  ( -1.364683531250000748, 1.571875000341421691, 0.000000000000000000 ) ) ;
#176697=CARTESIAN_POINT ( 'NONE',  ( 7.049876689426101350, 9.247942109129029475, -1.443375672974057666 ) ) ;
#176705=CARTESIAN_POINT ( 'NONE',  ( 9.368320956918608999, 11.95279375453699622, 1.443375672974076540 ) ) ;
#176706=ORIENTED_EDGE ( 'NONE', *, *, #141556, .T. ) ;
#176712=CARTESIAN_POINT ( 'NONE',  ( -8.859363311525973117, 12.42334206583395328, -1.199719254218446718 ) ) ;
#176722=CARTESIAN_POINT ( 'NONE',  ( 3.009610312849396951, 6.452363523749469643, -0.06592220986071165023 ) ) ;
#176729=CARTESIAN_POINT ( 'NONE',  ( -1.500000000000001332, 1.181250000682816603, 0.000000000000000000 ) ) ;
#176733=ORIENTED_EDGE ( 'NONE', *, *, #138676, .F. ) ;
#176735=CARTESIAN_POINT ( 'NONE',  ( -0.7500000000000249800, -0.8083333333333136972, 1.299038105676659116 ) ) ;
#176736=CARTESIAN_POINT ( 'NONE',  ( 7.618792255875527886, 10.97600916757510170, 1.199719254218460707 ) ) ;
#176740=CARTESIAN_POINT ( 'NONE',  ( 3.871016551901614200, 4.474939717762034697, -1.199719254218446718 ) ) ;
#176741=CARTESIAN_POINT ( 'NONE',  ( -7.063434843039784639, 7.343021526408956667, 1.040834085586084257E-14 ) ) ;
#176745=CARTESIAN_POINT ( 'NONE',  ( -6.449928391799210736, 8.548002428564306143, -1.599625672291263179 ) ) ;
#176747=CARTESIAN_POINT ( 'NONE',  ( 1.499999999999987121, 1.035416667349484232, 0.8660254037844524744 ) ) ;
#176760=CARTESIAN_POINT ( 'NONE',  ( -9.016335848287868160, 10.47781223021269170, 1.199719254218462483 ) ) ;
#176761=CARTESIAN_POINT ( 'NONE',  ( 6.774270308322468459, 11.05506579301824743, 0.7998128361456462443 ) ) ;
#176762=CARTESIAN_POINT ( 'NONE',  ( 1.284279953904126748, 10.64264068711930733, 0.7750000000000013545 ) ) ;
#176769=CARTESIAN_POINT ( 'NONE',  ( -8.993135964566285168, 9.386413468282476913, -0.7998128361456291469 ) ) ;
#176773=VERTEX_POINT ( 'NONE', #119451 ) ;
#176776=CARTESIAN_POINT ( 'NONE',  ( 4.379447312414087357, 5.068108938359919158, -1.199719254218452047 ) ) ;
#176781=CARTESIAN_POINT ( 'NONE',  ( -9.134442807305063639, 11.67993591332117376, 1.599625672291281386 ) ) ;
#176783=AXIS2_PLACEMENT_3D ( 'NONE', #175473, #109466, #59565 ) ;
#176785=CARTESIAN_POINT ( 'NONE',  ( -5.409091473909686698, 6.481950958801420803, -1.333638828535830045 ) ) ;
#176794=CARTESIAN_POINT ( 'NONE',  ( 6.982612806237943559, 8.105135347821125436, -1.199719254218446718 ) ) ;
#176797=CARTESIAN_POINT ( 'NONE',  ( 5.583321308294927121, 6.218571175896433267, -0.9806921612870276306 ) ) ;
#176802=CARTESIAN_POINT ( 'NONE',  ( 1.499999999999989120, -0.1937499993171845625, 0.000000000000000000 ) ) ;
#176816=CARTESIAN_POINT ( 'NONE',  ( 4.473827502829567315, 7.202920605734387749, -1.082531754730548412 ) ) ;
#176819=CARTESIAN_POINT ( 'NONE',  ( -4.893288865221945727, 4.903436309528101056, 0.4027703449977599881 ) ) ;
#176821=CARTESIAN_POINT ( 'NONE',  ( 8.563946585326370098, 13.14302144952281814, 0.7998128361456462443 ) ) ;
#176832=CARTESIAN_POINT ( 'NONE',  ( 1.364683531249988757, -0.1156249996585798079, 0.000000000000000000 ) ) ;
#176837=CARTESIAN_POINT ( 'NONE',  ( -3.893162665418476109, 7.693773542963529444, 1.040834085586084257E-14 ) ) ;
#176840=CARTESIAN_POINT ( 'NONE',  ( 0.7499999999999885647, -0.7666666666666446250, 1.299038105676657340 ) ) ;
#176842=CARTESIAN_POINT ( 'NONE',  ( 0.6823417656249864960, -1.011458332991911568, -1.181850606188749264 ) ) ;
#176848=CARTESIAN_POINT ( 'NONE',  ( 1.364683531249990311, 5.426041667008086655, 0.7879004041258500513 ) ) ;
#176850=CARTESIAN_POINT ( 'NONE',  ( -9.352427035328430449, 9.805586384171650849, 1.040834085586084257E-14 ) ) ;
#176858=CARTESIAN_POINT ( 'NONE',  ( 1.364683531249986537, 0.1760416670080860446, 0.7879004041258500513 ) ) ;
#176867=CARTESIAN_POINT ( 'NONE',  ( 6.290620087060792009, 10.28288116830553101, -0.7216878364870267237 ) ) ;
#176870=CARTESIAN_POINT ( 'NONE',  ( -4.904298879841297421, 6.744767997946721216, 1.599625672291267398 ) ) ;
#176872=CARTESIAN_POINT ( 'NONE',  ( -1.201851678989727383E-14, 5.118750000682815937, -1.732050807568863648 ) ) ;
#176874=CARTESIAN_POINT ( 'NONE',  ( -4.952806187693842510, 4.672695395264567786, 0.7998128361456341429 ) ) ;
#176875=CARTESIAN_POINT ( 'NONE',  ( 6.114364089638786304, 8.156510742710487705, 1.443375672974076540 ) ) ;
#176876=CARTESIAN_POINT ( 'NONE',  ( -10.11401940567025548, 10.90203684947788076, 1.040834085586084257E-14 ) ) ;
#176882=CARTESIAN_POINT ( 'NONE',  ( 2.333974999846879061, 5.874721266463329705, -0.7998128361456291469 ) ) ;
#176884=CARTESIAN_POINT ( 'NONE',  ( -1.201851678989727383E-14, 3.868750000682817713, -1.732050807568863648 ) ) ;
#176899=CARTESIAN_POINT ( 'NONE',  ( 7.214910300766615769, 11.56914578420308715, -0.7998128361456291469 ) ) ;
#176903=CARTESIAN_POINT ( 'NONE',  ( -0.6823417656250246877, -0.4489583329919111243, 1.181850606188755259 ) ) ;
#176904=CARTESIAN_POINT ( 'NONE',  ( 5.504247177468186258, 6.484338464210099851, 1.082531754730558626 ) ) ;
#176906=CARTESIAN_POINT ( 'NONE',  ( -9.327646496521989405, 10.94497100310623594, -1.082531754730539753 ) ) ;
#176911=FACE_OUTER_BOUND ( 'NONE', #46633, .T. ) ;
#176925=CARTESIAN_POINT ( 'NONE',  ( 5.777328231396808178, 6.232550548966264259, -0.9930585829777474061 ) ) ;
#176932=CARTESIAN_POINT ( 'NONE',  ( -6.385527162356466668, 10.39360608948380182, 0.000000000000000000 ) ) ;
#176937=CARTESIAN_POINT ( 'NONE',  ( 5.937581207780954884, 9.014596278131406848, -1.199719254218440723 ) ) ;
#176940=EDGE_CURVE ( 'NONE', #177712, #32739, #2730, .T. ) ;
#176943=CARTESIAN_POINT ( 'NONE',  ( -3.761497552787613330, 6.475832013972435242, 1.199719254218464037 ) ) ;
#176947=CARTESIAN_POINT ( 'NONE',  ( -4.066556009095094737, 6.831733546331167695, 1.199719254218464037 ) ) ;
#176951=CARTESIAN_POINT ( 'NONE',  ( 5.542585869888291938, 5.360771691158120689, -0.7998128361456211532 ) ) ;
#176952=CARTESIAN_POINT ( 'NONE',  ( 6.753933077901968396, 11.03133902419432566, 0.7998128361456462443 ) ) ;
#176953=CARTESIAN_POINT ( 'NONE',  ( 0.3819399096430804441, 6.573892064833275484, 3.228863705805710804 ) ) ;
#176955=CARTESIAN_POINT ( 'NONE',  ( 5.008269389056229315, 6.794162766424465261, 1.424127363233711252 ) ) ;
#176956=CARTESIAN_POINT ( 'NONE',  ( 4.202664430556247055, 6.886563688082179446, 1.082531754730558626 ) ) ;
#176958=CARTESIAN_POINT ( 'NONE',  ( 4.991989969715248776, 4.726297878971393196, -2.420000000000000373 ) ) ;
#176963=CARTESIAN_POINT ( 'NONE',  ( 6.277061933002777927, 8.346324893301817482, 1.443375672974076540 ) ) ;
#176964=CARTESIAN_POINT ( 'NONE',  ( -9.643927338022246332, 10.14567007064778004, -0.7998128361456291469 ) ) ;
#176967=CARTESIAN_POINT ( 'NONE',  ( -9.969323024750229578, 10.52529837183042716, -0.7998128361456291469 ) ) ;
#176968=CARTESIAN_POINT ( 'NONE',  ( -6.191269702934848240, 10.37489842006599616, 0.000000000000000000 ) ) ;
#176976=CARTESIAN_POINT ( 'NONE',  ( 8.378048858240820351, 11.86180853700128601, -1.199719254218446718 ) ) ;
#176980=CARTESIAN_POINT ( 'NONE',  ( 4.383363735919856730, 4.008345868194933104, -0.7998128361456211532 ) ) ;
#176983=DIRECTION ( 'NONE',  ( -0.000000000000000000, -8.546850786086437571E-32, -1.000000000000000000 ) ) ;
#176987=ORIENTED_EDGE ( 'NONE', *, *, #172459, .T. ) ;
#176989=CARTESIAN_POINT ( 'NONE',  ( -1.499999999999997780, 3.150000000000020783, 1.214306433183764966E-14 ) ) ;
#176990=CARTESIAN_POINT ( 'NONE',  ( 4.788000803920411386, 8.737751371215816576, 1.040834085586084257E-14 ) ) ;
#176993=CARTESIAN_POINT ( 'NONE',  ( 7.944714827928056167, 8.371181508778631652, 0.7216878364870458196 ) ) ;
#176994=CARTESIAN_POINT ( 'NONE',  ( 0.4897149945007785443, 7.513091487862237017, 2.015070445391641041 ) ) ;
#176998=CARTESIAN_POINT ( 'NONE',  ( 9.565441069641300587, 11.11843498845840905, -1.199719254218440723 ) ) ;
#177000=DIRECTION ( 'NONE',  ( 5.578564026256490882E-16, 1.000000000000000000, 9.066213480720158442E-32 ) ) ;
#177001=CARTESIAN_POINT ( 'NONE',  ( -3.846762897975357198, 5.510976019103107859, -1.599625672291256295 ) ) ;
#177002=CARTESIAN_POINT ( 'NONE',  ( -0.7500000000000215383, 5.472916667349482900, 1.299038105676671107 ) ) ;
#177003=CARTESIAN_POINT ( 'NONE',  ( -1.364683531250000748, 0.7593750003414210248, 0.000000000000000000 ) ) ;
#177008=CARTESIAN_POINT ( 'NONE',  ( -1.364683531250014514, -1.011458332991911568, -0.7879004041258359514 ) ) ;
#177010=EDGE_CURVE ( 'NONE', #150994, #213399, #41547, .T. ) ;
#177011=CARTESIAN_POINT ( 'NONE',  ( 7.913155211870404493, 12.38376484715752213, 0.7998128361456462443 ) ) ;
#177015=CARTESIAN_POINT ( 'NONE',  ( -4.419594887930571758, 4.258541578781506409, 1.214306433183764966E-14 ) ) ;
#177018=CARTESIAN_POINT ( 'NONE',  ( -7.009729113465285266, 8.136771039586342624, -1.199719254218446718 ) ) ;
#177021=CARTESIAN_POINT ( 'NONE',  ( 4.867540842506059562, 5.637551390133895168, -1.199719254218452047 ) ) ;
#177025=VERTEX_POINT ( 'NONE', #147635 ) ;
#177027=CARTESIAN_POINT ( 'NONE',  ( 8.374132434735052755, 12.92157160716627295, -0.7998128361456352531 ) ) ;
#177030=CARTESIAN_POINT ( 'NONE',  ( -4.218558352146454915, 8.073401844146177453, 1.040834085586084257E-14 ) ) ;
#177034=CARTESIAN_POINT ( 'NONE',  ( 9.402743226277308963, 10.92862083786708816, -1.199719254218446718 ) ) ;
#177036=CARTESIAN_POINT ( 'NONE',  ( 7.889955328148847258, 11.29236608522730911, -1.199719254218446718 ) ) ;
#177037=ADVANCED_FACE ( 'NONE', ( #19739 ), #198480, .F. ) ;
#177040=CARTESIAN_POINT ( 'NONE',  ( -9.653042183249970876, 11.32459930428888306, -1.082531754730539753 ) ) ;
#177044=CARTESIAN_POINT ( 'NONE',  ( -6.507023659554960204, 9.678945805201045971, 1.199719254218452047 ) ) ;
#177048=CARTESIAN_POINT ( 'NONE',  ( -5.891600325674557048, 6.152103933748189313, 0.8728944348482190474 ) ) ;
#177049=CARTESIAN_POINT ( 'NONE',  ( -1.364683531250012516, 1.780208333674757615, 0.7879004041258379498 ) ) ;
#177052=CARTESIAN_POINT ( 'NONE',  ( 6.466876084038451822, 10.48851316477946582, 1.040834085586084257E-14 ) ) ;
#177069=CARTESIAN_POINT ( 'NONE',  ( 8.289920859751990889, 11.75899253876431416, 1.199719254218450271 ) ) ;
#177073=CARTESIAN_POINT ( 'NONE',  ( -4.959585264500673496, 4.680604318205876524, 1.214306433183764966E-14 ) ) ;
#177074=CARTESIAN_POINT ( 'NONE',  ( -6.184490626128011925, 10.36698949712469364, -0.7998128361456291469 ) ) ;
#177079=CARTESIAN_POINT ( 'NONE',  ( -1.500000000000011324, 4.910416667349486453, -0.8660254037844313801 ) ) ;
#177080=CARTESIAN_POINT ( 'NONE',  ( 8.762647353133951711, 9.117510088278095282, 1.040834085586084257E-14 ) ) ;
#177083=CARTESIAN_POINT ( 'NONE',  ( -8.474009703741204547, 9.845098394908269768, -1.199719254218446718 ) ) ;
#177085=CARTESIAN_POINT ( 'NONE',  ( -1.201851678989727383E-14, 3.446875000341421469, -1.575800808251660134 ) ) ;
#177092=CARTESIAN_POINT ( 'NONE',  ( -8.676855123066019360, 11.14608361504227574, -1.443375672974059665 ) ) ;
#177096=CARTESIAN_POINT ( 'NONE',  ( -0.6823417656249969321, 3.280208333674754062, -1.181850606188749264 ) ) ;
#177103=CARTESIAN_POINT ( 'NONE',  ( -1.364683531250012516, 3.488541667008085767, -0.7879004041258300672 ) ) ;
#177105=CARTESIAN_POINT ( 'NONE',  ( -4.574986769607567894, 7.424902766929059261, 1.199719254218464037 ) ) ;
#177106=CARTESIAN_POINT ( 'NONE',  ( 6.938021921891177612, 9.117444880338284818, -1.599625672291262513 ) ) ;
#177109=CARTESIAN_POINT ( 'NONE',  ( 1.364683531249988535, 3.967708333674751842, -0.7879004041258239610 ) ) ;
#177112=CARTESIAN_POINT ( 'NONE',  ( 1.364683531249986537, -0.5947916663252456049, -0.7879004041258309554 ) ) ;
#177113=CARTESIAN_POINT ( 'NONE',  ( -3.795919822146277767, 7.372397525905215687, -0.7216878364870267237 ) ) ;
#177116=CARTESIAN_POINT ( 'NONE',  ( 3.551873057100274789, 7.087676300018221021, 0.7216878364870298324 ) ) ;
#177119=CARTESIAN_POINT ( 'NONE',  ( -6.852756576703439961, 10.08230087520760954, 1.199719254218453823 ) ) ;
#177120=CARTESIAN_POINT ( 'NONE',  ( -9.503902493499651882, 10.19023378527882784, 1.040834085586084257E-14 ) ) ;
#177127=CARTESIAN_POINT ( 'NONE',  ( -5.870317324592811303, 8.832158731124840401, -1.082531754730537976 ) ) ;
#177129=CARTESIAN_POINT ( 'NONE',  ( -0.6823417656250246877, -0.8864583329919115684, 1.181850606188755259 ) ) ;
#177143=CARTESIAN_POINT ( 'NONE',  ( 7.741342523278698096, 10.05465224862374285, 1.443375672974076540 ) ) ;
#177151=CARTESIAN_POINT ( 'NONE',  ( 5.666418135507635512, 8.698239360479199433, 1.199719254218462483 ) ) ;
#177152=AXIS2_PLACEMENT_3D ( 'NONE', #121478, #81686, #103012 ) ;
#177153=CARTESIAN_POINT ( 'NONE',  ( -3.958090780185743451, 6.705190779270287393, -1.199719254218452047 ) ) ;
#177156=CARTESIAN_POINT ( 'NONE',  ( -1.402160292154681736E-14, 2.009375000341422801, -1.575800808251660134 ) ) ;
#177158=CARTESIAN_POINT ( 'NONE',  ( -8.565000355531095622, 11.01558638625153286, -1.599625672291263179 ) ) ;
#177164=EDGE_CURVE ( 'NONE', #143545, #92745, #182236, .T. ) ;
#177175=CARTESIAN_POINT ( 'NONE',  ( -4.343881772442427014, 7.212430371758029146, -1.015018499812924135 ) ) ;
#177179=CARTESIAN_POINT ( 'NONE',  ( 5.849453209292126310, 8.911780279894442103, 1.199719254218462483 ) ) ;
#177189=CARTESIAN_POINT ( 'NONE',  ( 10.26082332744404368, 10.86538205830655279, -0.7998128361456281477 ) ) ;
#177191=CARTESIAN_POINT ( 'NONE',  ( -3.952365473583647315, 4.569846793057691592, 1.199719254218462483 ) ) ;
#177197=CARTESIAN_POINT ( 'NONE',  ( 4.002706559696581401, 7.742679268553477101, 0.2606817014456235815 ) ) ;
#177204=CARTESIAN_POINT ( 'NONE',  ( -9.815740026613967828, 10.55404424057886636, -0.7216878364870267237 ) ) ;
#177209=CARTESIAN_POINT ( 'NONE',  ( 5.606460214450851964, 6.499623990736163037, 1.199719254218462483 ) ) ;
#177215=CARTESIAN_POINT ( 'NONE',  ( 3.511198595814932766, 5.119484333249288532, 1.443375672974066548 ) ) ;
#177218=( BOUNDED_CURVE ( )  B_SPLINE_CURVE ( 2, ( #23662, #168854, #22584, #57247, #41014, #20457, #202394 ),
 .UNSPECIFIED., .F., .T. ) 
 B_SPLINE_CURVE_WITH_KNOTS ( ( 3, 2, 2, 3 ),
 ( 0.03571428571428574700, 0.04166666666666662272, 0.04761904761904750538, 0.05357142857142838110 ),
 .UNSPECIFIED. ) 
 CURVE ( )  GEOMETRIC_REPRESENTATION_ITEM ( )  RATIONAL_B_SPLINE_CURVE ( ( 0.9999999999999992228, 0.8660254037844394848, 1.000000000000000000, 0.8660254037844387076, 1.000000000000000000, 0.8660254037844429265, 0.9999999999999957812 ) ) 
 REPRESENTATION_ITEM ( '' )  );
#177224=CARTESIAN_POINT ( 'NONE',  ( -6.018930129462987999, 9.109503353427070849, 1.199719254218452047 ) ) ;
#177226=CARTESIAN_POINT ( 'NONE',  ( -2.137381772448751605, 5.645362501165475777, -0.7998128361456281477 ) ) ;
#177231=CARTESIAN_POINT ( 'NONE',  ( 0.2939347205469426960, 8.204283511488981162, -1.979604457746027446 ) ) ;
#177234=CARTESIAN_POINT ( 'NONE',  ( 4.638861114170084399, 8.563755066507100722, 0.7998128361456462443 ) ) ;
#177245=VECTOR ( 'NONE', #92417, 1000.000000000000114 ) ;
#177249=CARTESIAN_POINT ( 'NONE',  ( -1.364683531250014514, -0.1989583329919157317, -0.7879004041258359514 ) ) ;
#177251=CARTESIAN_POINT ( 'NONE',  ( 4.878236342818665250, 4.585697242910212523, 1.040834085586084257E-14 ) ) ;
#177253=CARTESIAN_POINT ( 'NONE',  ( -7.388830529767770550, 7.722649827591604677, 1.040834085586084257E-14 ) ) ;
#177254=CARTESIAN_POINT ( 'NONE',  ( 4.907688418466886304, 5.788353245375237321, -1.082531754730548412 ) ) ;
#177255=CARTESIAN_POINT ( 'NONE',  ( -8.337901282280023807, 8.829899038855916871, 0.7216878364870438212 ) ) ;
#177259=CARTESIAN_POINT ( 'NONE',  ( 7.298366762858032430, 7.409182732956175244, 1.040834085586084257E-14 ) ) ;
#177264=CARTESIAN_POINT ( 'NONE',  ( 1.364683531249988535, 4.405208333674754506, -0.7879004041258300672 ) ) ;
#177269=CARTESIAN_POINT ( 'NONE',  ( 5.795220594837462436, 8.848508896363995291, -1.199719254218440723 ) ) ;
#177273=CARTESIAN_POINT ( 'NONE',  ( -7.527801604085656351, 9.805521176231838609, 1.599625672291295375 ) ) ;
#177278=CARTESIAN_POINT ( 'NONE',  ( 7.228468454380276853, 11.58496363008569574, 1.040834085586084257E-14 ) ) ;
#177281=CARTESIAN_POINT ( 'NONE',  ( -6.527360889975461156, 9.702672574024962415, 1.199719254218452047 ) ) ;
#177284=CARTESIAN_POINT ( 'NONE',  ( 6.114364089638775646, 10.07724917131317355, 0.7216878364870438212 ) ) ;
#177285=CARTESIAN_POINT ( 'NONE',  ( 4.088248116760357931, 7.710168519003287813, -0.6407031029972446445 ) ) ;
#177286=CARTESIAN_POINT ( 'NONE',  ( -7.849807752632384172, 12.10193344480572897, 0.000000000000000000 ) ) ;
#177292=CARTESIAN_POINT ( 'NONE',  ( 6.796715079152391148, 6.823922435299587974, 0.7998128361456341429 ) ) ;
#177294=CARTESIAN_POINT ( 'NONE',  ( 10.22692794340986921, 10.82583744360002243, 0.000000000000000000 ) ) ;
#177295=CARTESIAN_POINT ( 'NONE',  ( -4.609732581575539889, 6.945374051331699938, 1.198810113796699328 ) ) ;
#177296=CARTESIAN_POINT ( 'NONE',  ( 4.467575310902914154, 5.170924936596891008, 1.199719254218464037 ) ) ;
#177298=CARTESIAN_POINT ( 'NONE',  ( -5.897433632264490910, 9.824163637709826702, 0.000000000000000000 ) ) ;
#177299=VERTEX_POINT ( 'NONE', #89040 ) ;
#177304=CARTESIAN_POINT ( 'NONE',  ( -4.446147712686649989, 7.104319146577407373, 1.107073289137233241 ) ) ;
#177305=CARTESIAN_POINT ( 'NONE',  ( -1.402160292154681736E-14, 0.5093750003414236893, -1.575800808251659024 ) ) ;
#177307=CARTESIAN_POINT ( 'NONE',  ( 4.446711195602238931, 6.210915699667823198, -1.443375672974051449 ) ) ;
#177312=CARTESIAN_POINT ( 'NONE',  ( -8.798878505144649864, 11.28844422746735532, -1.443375672974058777 ) ) ;
#177317=CARTESIAN_POINT ( 'NONE',  ( -7.497295758232712437, 11.69066945133944380, -0.7216878364870267237 ) ) ;
#177318=DIRECTION ( 'NONE',  ( -1.000000000000000000, 5.459311322609750190E-16, 0.000000000000000000 ) ) ;
#177322=LINE ( 'NONE', #61428, #168356 ) ;
#177325=CARTESIAN_POINT ( 'NONE',  ( -7.822691444960700125, 11.10992853822074444, -1.082531754730543083 ) ) ;
#177329=CARTESIAN_POINT ( 'NONE',  ( 0.6823417656249917140, 5.405208333674749177, 1.181850606188765695 ) ) ;
#177330=CARTESIAN_POINT ( 'NONE',  ( 1.499999999999989120, 3.785416667349481123, 0.8660254037844524744 ) ) ;
#177331=CARTESIAN_POINT ( 'NONE',  ( 6.050032868414796816, 6.056328681155354055, -0.4621489055621590403 ) ) ;
#177336=ADVANCED_FACE ( 'NONE', ( #122688 ), #96230, .T. ) ;
#177337=CARTESIAN_POINT ( 'NONE',  ( -8.857554428429624593, 9.228235009456373206, 0.7998128361456462443 ) ) ;
#177341=CARTESIAN_POINT ( 'NONE',  ( 5.172599298813543633, 5.993452922492633839, -1.199719254218452047 ) ) ;
#177347=CARTESIAN_POINT ( 'NONE',  ( 9.257519960032755790, 9.694861462993381807, 0.7998128361456462443 ) ) ;
#177354=CARTESIAN_POINT ( 'NONE',  ( -7.063434843039784639, 7.343021526408956667, 1.040834085586084257E-14 ) ) ;
#177357=CARTESIAN_POINT ( 'NONE',  ( 5.355107487717867265, 5.349972945200037522, 1.040834085586084257E-14 ) ) ;
#177361=EDGE_CURVE ( 'NONE', #179291, #213175, #65795, .T. ) ;
#177364=CARTESIAN_POINT ( 'NONE',  ( -8.130085669689073313, 12.63685038127928806, 0.7998128361456481317 ) ) ;
#177366=CARTESIAN_POINT ( 'NONE',  ( 8.503988664269582998, 10.94440607977979063, 1.599625672291281386 ) ) ;
#177367=CARTESIAN_POINT ( 'NONE',  ( 0.7499999999999867883, -0.6833333333333135862, -1.299038105676652899 ) ) ;
#177368=CARTESIAN_POINT ( 'NONE',  ( -8.503988664269602538, 10.94440607977979063, 1.599625672291269396 ) ) ;
#177371=CARTESIAN_POINT ( 'NONE',  ( 0.6823417656249917140, 3.592708333674754506, 1.181850606188765695 ) ) ;
#177372=CARTESIAN_POINT ( 'NONE',  ( 4.142179624174931796, 4.791296635414242111, 1.199719254218464037 ) ) ;
#177375=CARTESIAN_POINT ( 'NONE',  ( -0.7499999999999972244, 4.608333333333352932, -1.299038105676652011 ) ) ;
#177378=CARTESIAN_POINT ( 'NONE',  ( 6.914295152845067349, 11.01050207838719075, 1.040834085586084257E-14 ) ) ;
#177381=CARTESIAN_POINT ( 'NONE',  ( -6.399085315970151733, 7.528316292462387871, -1.082531754730544860 ) ) ;
#177382=CARTESIAN_POINT ( 'NONE',  ( 1.364683531249986537, 0.4052083336747511200, -0.7879004041258309554 ) ) ;
#177386=CARTESIAN_POINT ( 'NONE',  ( -7.477485413136760073, 8.682486722536401302, -1.199719254218446718 ) ) ;
#177387=CARTESIAN_POINT ( 'NONE',  ( -3.673896439178936824, 5.309298483840612093, 1.443375672974064550 ) ) ;
#177388=CARTESIAN_POINT ( 'NONE',  ( 1.364683531249990311, 4.926041667008083991, 0.7879004041258500513 ) ) ;
#177394=CARTESIAN_POINT ( 'NONE',  ( 7.899597058256738968, 12.36794700127490820, 1.040834085586084257E-14 ) ) ;
#177401=CARTESIAN_POINT ( 'NONE',  ( 10.07387183015377197, 11.71160420905630062, -1.199719254218440723 ) ) ;
#177405=CARTESIAN_POINT ( 'NONE',  ( 7.540305987494599016, 11.94877408538573427, -0.7998128361456291469 ) ) ;
#177406=CARTESIAN_POINT ( 'NONE',  ( -8.469039510030723861, 13.03229652834454733, 1.040834085586084257E-14 ) ) ;
#177410=CARTESIAN_POINT ( 'NONE',  ( -1.402160292154681736E-14, -1.178124999658576311, 1.575800808251672791 ) ) ;
#177413=CARTESIAN_POINT ( 'NONE',  ( -4.067937748088393590, 7.725456827083305278, 0.6547958487484796253 ) ) ;
#177414=CARTESIAN_POINT ( 'NONE',  ( 6.598014311344812199, 10.84943379654430906, 1.040834085586084257E-14 ) ) ;
#177417=CARTESIAN_POINT ( 'NONE',  ( -1.201851678989727383E-14, 3.321875000341421025, 1.575800808251672791 ) ) ;
#177419=CARTESIAN_POINT ( 'NONE',  ( -6.751597309925468693, 6.979211071108916364, 0.7216878364870317197 ) ) ;
#177425=CARTESIAN_POINT ( 'NONE',  ( 4.566398809704347528, 4.221886787610169556, -0.7998128361456211532 ) ) ;
#177428=CARTESIAN_POINT ( 'NONE',  ( 8.483651433849084711, 10.92067931095586886, 1.599625672291281386 ) ) ;
#177435=CARTESIAN_POINT ( 'NONE',  ( -9.053093885623068715, 11.58502883802551153, -1.599625672291263179 ) ) ;
#177436=CARTESIAN_POINT ( 'NONE',  ( 5.296431564432884542, 9.330920591813708143, 1.040834085586084257E-14 ) ) ;
#177438=CARTESIAN_POINT ( 'NONE',  ( 4.989037339704528229, 4.922891105851139315, 1.040834085586084257E-14 ) ) ;
#177440=CARTESIAN_POINT ( 'NONE',  ( 3.635557746758808495, 7.393234471193928847, -0.7998128361456291469 ) ) ;
#177448=VECTOR ( 'NONE', #45910, 1000.000000000000114 ) ;
#177450=CARTESIAN_POINT ( 'NONE',  ( -5.260200412422196159, 9.080724881227137502, -0.7216878364870207285 ) ) ;
#177451=CARTESIAN_POINT ( 'NONE',  ( 5.007038802148489509, 4.735966778795008381, 0.7998128361456341429 ) ) ;
#177454=CARTESIAN_POINT ( 'NONE',  ( -6.561256274009600986, 9.742217188731485678, -1.199719254218440723 ) ) ;
#177460=CARTESIAN_POINT ( 'NONE',  ( -9.972185678051314284, 11.59297036493672017, 1.199719254218462483 ) ) ;
#177463=CARTESIAN_POINT ( 'NONE',  ( 8.444030743212801227, 8.745790710036752458, 0.7998128361456462443 ) ) ;
#177466=CARTESIAN_POINT ( 'NONE',  ( 6.823831386379729302, 6.855558127064808716, -0.7998128361456281477 ) ) ;
#177467=CARTESIAN_POINT ( 'NONE',  ( -2.030969412800708085, 8.463209591662408826, -2.499999999999995115 ) ) ;
#177477=CARTESIAN_POINT ( 'NONE',  ( -6.659026002606323047, 10.92061410301605662, 0.000000000000000000 ) ) ;
#177481=CARTESIAN_POINT ( 'NONE',  ( 6.236387472606139681, 8.298871356172400127, -1.443375672974057666 ) ) ;
#177484=LINE ( 'NONE', #63720, #51406 ) ;
#177486=CARTESIAN_POINT ( 'NONE',  ( -4.564291269294938225, 8.476756914152748124, 1.040834085586084257E-14 ) ) ;
#177491=CARTESIAN_POINT ( 'NONE',  ( 3.563261906135761770, 6.332667919118538435, 2.500000000000011102 ) ) ;
#177497=CARTESIAN_POINT ( 'NONE',  ( 4.001749955438753226, 7.811071542261023737, 0.1299566359906061952 ) ) ;
#177498=CARTESIAN_POINT ( 'NONE',  ( 8.046927864910717432, 9.346836249606042202, 1.199719254218462483 ) ) ;
#177500=CARTESIAN_POINT ( 'NONE',  ( -3.090895834235680262, 5.589500325708124606, 1.082531754730560403 ) ) ;
#177502=CARTESIAN_POINT ( 'NONE',  ( -5.430810130430261395, 6.303639405459422917, -1.045180951442852946 ) ) ;
#177509=CARTESIAN_POINT ( 'NONE',  ( 3.440018289565364817, 5.036440642624797626, 1.599625672291267398 ) ) ;
#177515=CARTESIAN_POINT ( 'NONE',  ( 3.704402285031850539, 5.344888637335695414, -1.599625672291262513 ) ) ;
#177520=CARTESIAN_POINT ( 'NONE',  ( -0.6823417656250212460, 4.113541667008085767, 1.181850606188767472 ) ) ;
#177525=CARTESIAN_POINT ( 'NONE',  ( 4.788000803920411386, 8.737751371215816576, 1.040834085586084257E-14 ) ) ;
#177529=CARTESIAN_POINT ( 'NONE',  ( -4.599240423533815125, 6.388866465587984322, 1.599625672291267398 ) ) ;
#177530=CARTESIAN_POINT ( 'NONE',  ( 4.487385655998867406, 8.179107665399927285, 0.7216878364870438212 ) ) ;
#177531=CARTESIAN_POINT ( 'NONE',  ( 1.499999999999987121, 3.295833333333354709, -0.8660254037844262731 ) ) ;
#177534=CARTESIAN_POINT ( 'NONE',  ( -4.731959306369413198, 5.479372931307791461, -1.199719254218446718 ) ) ;
#177535=DIRECTION ( 'NONE',  ( 0.000000000000000000, -0.7999999999999973799, -0.6000000000000034195 ) ) ;
#177538=CARTESIAN_POINT ( 'NONE',  ( -1.364683531250012516, 3.988541667008088876, -0.7879004041258300672 ) ) ;
#177541=CARTESIAN_POINT ( 'NONE',  ( -3.795919822146289313, 5.451659097302528068, -1.443375672974053447 ) ) ;
#177544=EDGE_LOOP ( 'NONE', ( #97748, #127156, #181395, #42537 ) ) ;
#177548=CARTESIAN_POINT ( 'NONE',  ( 5.138703914779377158, 5.953908307786102583, 1.199719254218462483 ) ) ;
#177555=CARTESIAN_POINT ( 'NONE',  ( -1.201851678989727383E-14, 1.634375000341421025, 1.575800808251672791 ) ) ;
#177557=CARTESIAN_POINT ( 'NONE',  ( -9.809487834687324437, 11.40315621434539395, 1.199719254218462483 ) ) ;
#177558=CARTESIAN_POINT ( 'NONE',  ( -5.327991180046197428, 8.199444895820425572, 1.082531754730548412 ) ) ;
#177562=CARTESIAN_POINT ( 'NONE',  ( 1.364683531249988535, 4.655208333674755394, -0.7879004041258300672 ) ) ;
#177570=CARTESIAN_POINT ( 'NONE',  ( -7.334597914868743018, 7.659378443542744996, -0.7216878364870267237 ) ) ;
#177571=CARTESIAN_POINT ( 'NONE',  ( 2.275391796764376640, 5.643962577969389827, -0.5307291018262025872 ) ) ;
#177576=CARTESIAN_POINT ( 'NONE',  ( -6.683806541412780078, 6.900121841177441873, -0.7216878364870267237 ) ) ;
#177584=CARTESIAN_POINT ( 'NONE',  ( 1.580223361175657981, 8.746992034114501990, -2.465615386491380789 ) ) ;
#177590=CARTESIAN_POINT ( 'NONE',  ( -4.578903193113314174, 6.365139696764064325, 1.599625672291267398 ) ) ;
#177594=CARTESIAN_POINT ( 'NONE',  ( -1.402160292154681736E-14, 1.087500000000024336, -1.732050807568863648 ) ) ;
#177596=CARTESIAN_POINT ( 'NONE',  ( 9.463228032658635769, 11.10314946193233965, -1.082531754730543083 ) ) ;
#177597=CARTESIAN_POINT ( 'NONE',  ( 6.795661308947685164, 8.951357498570873261, -1.599625672291262513 ) ) ;
#177602=CARTESIAN_POINT ( 'NONE',  ( 3.408985558832261731, 6.064568021024562938, 1.199719254218462483 ) ) ;
#177610=CARTESIAN_POINT ( 'NONE',  ( -6.925517538482230506, 6.974191971184389160, 0.7998128361456341429 ) ) ;
#177614=CARTESIAN_POINT ( 'NONE',  ( 5.951324661305081420, 4.742844146917974513, -2.438848701830601318 ) ) ;
#177620=CARTESIAN_POINT ( 'NONE',  ( -1.364683531249997417, 3.509375000341423245, 1.214306433183764966E-14 ) ) ;
#177621=CARTESIAN_POINT ( 'NONE',  ( 7.226132685959389512, 11.37431253368722750, -0.7216878364870267237 ) ) ;
#177622=CARTESIAN_POINT ( 'NONE',  ( -7.888146445052511169, 8.097259028849730811, 1.040834085586084257E-14 ) ) ;
#177626=CARTESIAN_POINT ( 'NONE',  ( 6.830610463186557624, 6.863467050006115677, 1.040834085586084257E-14 ) ) ;
#177627=CARTESIAN_POINT ( 'NONE',  ( -7.074657228232555717, 7.148188275893099686, 1.040834085586084257E-14 ) ) ;
#177631=CARTESIAN_POINT ( 'NONE',  ( 0.7499999999999885647, 0.5979166673494851203, -1.299038105676652899 ) ) ;
#177634=CARTESIAN_POINT ( 'NONE',  ( 6.643132081016111634, 9.733775946952057723, 1.082531754730558626 ) ) ;
#177635=AXIS2_PLACEMENT_3D ( 'NONE', #89772, #107123, #204529 ) ;
#177638=CARTESIAN_POINT ( 'NONE',  ( -1.364683531250014514, 2.051041667008086655, -0.7879004041258289570 ) ) ;
#177640=CARTESIAN_POINT ( 'NONE',  ( 5.788968402910805722, 7.776882441527838807, 1.443375672974062551 ) ) ;
#177642=CARTESIAN_POINT ( 'NONE',  ( -3.307826292054316664, 4.882216645528547616, -1.443375672974059665 ) ) ;
#177646=CARTESIAN_POINT ( 'NONE',  ( 8.283668668269706714, 8.766627655843896250, 1.040834085586084257E-14 ) ) ;
#177649=CARTESIAN_POINT ( 'NONE',  ( -4.103765016252827635, 7.679818082383993882, -0.7602138238151506799 ) ) ;
#177656=CARTESIAN_POINT ( 'NONE',  ( 5.632522751473472589, 8.658694745772667289, -1.199719254218440723 ) ) ;
#177659=CARTESIAN_POINT ( 'NONE',  ( 3.928111819657337911, 5.605883094398769195, 1.599625672291267398 ) ) ;
#177667=CARTESIAN_POINT ( 'NONE',  ( 4.365362273920244007, 6.116008624372160973, 1.443375672974062551 ) ) ;
#177668=CARTESIAN_POINT ( 'NONE',  ( -1.201851678989727383E-14, 2.384375000341416584, 1.575800808251672791 ) ) ;
#177669=CARTESIAN_POINT ( 'NONE',  ( 7.889955328148847258, 11.29236608522730911, -1.199719254218446718 ) ) ;
#177673=CARTESIAN_POINT ( 'NONE',  ( 1.499999999999987121, 1.754166666666691521, 0.8660254037844524744 ) ) ;
#177674=CARTESIAN_POINT ( 'NONE',  ( 6.810273232766058449, 6.839740281182199233, 1.040834085586084257E-14 ) ) ;
#177675=CARTESIAN_POINT ( 'NONE',  ( -7.725448601688521322, 7.907444878258402809, 1.040834085586084257E-14 ) ) ;
#177678=CARTESIAN_POINT ( 'NONE',  ( -1.402160292154681736E-14, 2.196875000341423689, -1.575800808251660134 ) ) ;
#177679=CARTESIAN_POINT ( 'NONE',  ( -1.201851678989727383E-14, 3.337500000000019007, -1.732050807568863648 ) ) ;
#177681=CARTESIAN_POINT ( 'NONE',  ( 4.383363735919856730, 4.008345868194933104, -0.7998128361456211532 ) ) ;
#177687=CARTESIAN_POINT ( 'NONE',  ( -1.500000000000013101, 0.7020833340161545255, 0.8660254037844403729 ) ) ;
#177689=CARTESIAN_POINT ( 'NONE',  ( -5.669280788808708671, 9.765911353585494226, 0.7998128361456481317 ) ) ;
#177690=CARTESIAN_POINT ( 'NONE',  ( -3.714570900464290393, 5.356752022006865843, 1.443375672974064550 ) ) ;
#177698=CARTESIAN_POINT ( 'NONE',  ( 4.964256800898067645, 8.943383367689749619, 0.7998128361456462443 ) ) ;
#177702=CARTESIAN_POINT ( 'NONE',  ( 6.307567778855705853, 8.381915046796901692, -1.599625672291262513 ) ) ;
#177708=CARTESIAN_POINT ( 'NONE',  ( -5.208303565944065738, 9.228104593576741621, -0.7998128361456231517 ) ) ;
#177709=ORIENTED_EDGE ( 'NONE', *, *, #124222, .F. ) ;
#177710=CARTESIAN_POINT ( 'NONE',  ( 2.517010073631369860, 6.088262185878572375, -0.7998128361456281477 ) ) ;
#177712=VERTEX_POINT ( 'NONE', #160439 ) ;
#177717=CARTESIAN_POINT ( 'NONE',  ( 4.532311885504772597, 6.983620743164907552, 1.170841521963662091 ) ) ;
#177725=CARTESIAN_POINT ( 'NONE',  ( -4.636525346193588248, 4.511627113421689650, 0.7216878364870317197 ) ) ;
#177726=CARTESIAN_POINT ( 'NONE',  ( 6.954969614130424027, 11.05795561655343384, 1.040834085586084257E-14 ) ) ;
#177728=CARTESIAN_POINT ( 'NONE',  ( -6.091691091241777656, 6.001394449403842479, 0.7998128361456341429 ) ) ;
#177732=CARTESIAN_POINT ( 'NONE',  ( -8.044065211609668253, 8.279164256499745633, 0.7998128361456602331 ) ) ;
#177739=EDGE_LOOP ( 'NONE', ( #170059, #158362, #26381, #31101, #142467, #95515, #4006, #210253, #197388, #51921 ) ) ;
#177746=CARTESIAN_POINT ( 'NONE',  ( -5.362413449404877852, 6.214902764849178141, -1.199719254218446718 ) ) ;
#177749=CARTESIAN_POINT ( 'NONE',  ( 2.399429999938675007, 5.743159399996332404, 0.000000000000000000 ) ) ;
#177753=CARTESIAN_POINT ( 'NONE',  ( -4.471491734408701291, 4.111161866431900513, 1.214306433183764966E-14 ) ) ;
#177754=CARTESIAN_POINT ( 'NONE',  ( -4.464712657601869417, 4.103252943490596216, 0.7998128361456341429 ) ) ;
#177757=CARTESIAN_POINT ( 'NONE',  ( 10.24048609702354717, 10.84165528948263457, -0.7998128361456281477 ) ) ;
#177760=CARTESIAN_POINT ( 'NONE',  ( -8.199983978166823562, 8.461069484149769337, -0.7998128361456291469 ) ) ;
#177761=CARTESIAN_POINT ( 'NONE',  ( 6.484877546038077867, 6.460111979999551224, 1.040834085586084257E-14 ) ) ;
#177764=CARTESIAN_POINT ( 'NONE',  ( 3.161022370280501814, 6.839609865302569425, 0.000000000000000000 ) ) ;
#177765=EDGE_CURVE ( 'NONE', #199393, #147848, #75990, .T. ) ;
#177768=CARTESIAN_POINT ( 'NONE',  ( -1.364683531250014514, 0.8010416670080889867, -0.7879004041258289570 ) ) ;
#177769=TOROIDAL_SURFACE ( 'NONE', #87933, 0.8300000000000010703, 0.08000000000000000167 ) ;
#177772=CARTESIAN_POINT ( 'NONE',  ( 6.480434237652115570, 10.50433101066207442, 0.7216878364870438212 ) ) ;
#177777=CARTESIAN_POINT ( 'NONE',  ( -1.432341765624997709, 5.860937500170720682, 1.214306433183764966E-14 ) ) ;
#177780=CARTESIAN_POINT ( 'NONE',  ( 9.612367721964607981, 12.23751498042398289, -1.443375672974058777 ) ) ;
#177786=CARTESIAN_POINT ( 'NONE',  ( -2.456316247939693387, 8.205176026796133115, 2.499999999999998668 ) ) ;
#177804=CARTESIAN_POINT ( 'NONE',  ( 0.7499999999999885647, 1.097916667349485564, -1.299038105676652899 ) ) ;
#177810=CARTESIAN_POINT ( 'NONE',  ( -0.7500000000000249800, -0.3083333333333132531, 1.299038105676659116 ) ) ;
#177811=CARTESIAN_POINT ( 'NONE',  ( 6.903072767652295383, 11.20533532890304684, 1.040834085586084257E-14 ) ) ;
#177812=CARTESIAN_POINT ( 'NONE',  ( -1.602468905319636405E-14, -1.053124999658583638, -1.575800808251665908 ) ) ;
#177815=CARTESIAN_POINT ( 'NONE',  ( 3.816783937446950770, 4.411668334231586996, 1.199719254218464037 ) ) ;
#177816=CARTESIAN_POINT ( 'NONE',  ( -7.226132686403777150, 7.532835677000276675, 1.040834085586084257E-14 ) ) ;
#177820=CARTESIAN_POINT ( 'NONE',  ( -5.910464900553636269, 8.982960586366182554, -1.199719254218440723 ) ) ;
#177823=CARTESIAN_POINT ( 'NONE',  ( 0.7499999999999885647, 1.597916667349486008, -1.299038105676652899 ) ) ;
#177830=CARTESIAN_POINT ( 'NONE',  ( -3.104453987404963478, 5.605318171072321221, -1.082531754730549078 ) ) ;
#177835=CARTESIAN_POINT ( 'NONE',  ( 4.097125688280337741, 7.463757567055806064, 0.6283840521477540575 ) ) ;
#177840=CARTESIAN_POINT ( 'NONE',  ( -4.433153041544240835, 4.274359424664112339, 0.7216878364870317197 ) ) ;
#177842=CARTESIAN_POINT ( 'NONE',  ( 6.435316467980822353, 10.65961964595298817, 1.040834085586084257E-14 ) ) ;
#177848=EDGE_CURVE ( 'NONE', #60775, #179068, #132311, .T. ) ;
#177850=CARTESIAN_POINT ( 'NONE',  ( -7.832860060393135093, 10.16142270859057462, 1.599625672291295375 ) ) ;
#177855=CARTESIAN_POINT ( 'NONE',  ( 5.379888026524302980, 5.170957540566797128, -0.7998128361456211532 ) ) ;
#177858=ORIENTED_EDGE ( 'NONE', *, *, #207366, .F. ) ;
#177860=ORIENTED_EDGE ( 'NONE', *, *, #165043, .F. ) ;
#177861=CARTESIAN_POINT ( 'NONE',  ( -7.960608749518247151, 12.43912730774665576, 0.000000000000000000 ) ) ;
#177864=CARTESIAN_POINT ( 'NONE',  ( -5.470032677541931676, 6.438256155886466381, -1.298486150373518999 ) ) ;
#177880=CARTESIAN_POINT ( 'NONE',  ( -1.500000000000001332, 0.1812500006828157706, 0.000000000000000000 ) ) ;
#177884=CARTESIAN_POINT ( 'NONE',  ( 3.728655938958122196, 4.308852335994623139, -1.199719254218446718 ) ) ;
#177886=CARTESIAN_POINT ( 'NONE',  ( -3.273404022695637572, 5.906389562198459231, 1.199719254218462483 ) ) ;
#177893=CARTESIAN_POINT ( 'NONE',  ( 4.934804725694211136, 6.780358151441803649, -1.443375672974051449 ) ) ;
#177896=CARTESIAN_POINT ( 'NONE',  ( -1.364683531250010295, 5.801041667008088432, -0.7879004041258300672 ) ) ;
#177898=CARTESIAN_POINT ( 'NONE',  ( 10.73535870392234237, 11.41900666419791399, 0.000000000000000000 ) ) ;
#177907=CARTESIAN_POINT ( 'NONE',  ( 1.364683531249988757, -0.8656249996585805295, 0.000000000000000000 ) ) ;
#177911=CARTESIAN_POINT ( 'NONE',  ( -4.904298879841297421, 6.744767997946721216, 1.599625672291267398 ) ) ;
#177914=CARTESIAN_POINT ( 'NONE',  ( 1.499999999999987121, -0.4958333333333110882, 0.8660254037844524744 ) ) ;
#177916=CARTESIAN_POINT ( 'NONE',  ( -1.001543065824772872E-14, 4.212500000000023448, 1.732050807568877637 ) ) ;
#177923=CARTESIAN_POINT ( 'NONE',  ( -1.402160292154681736E-14, -0.8031249996585825279, -1.575800808251665908 ) ) ;
#177925=CARTESIAN_POINT ( 'NONE',  ( 5.015626762051672571, 7.938982758113895422, 1.199719254218462483 ) ) ;
#177927=CARTESIAN_POINT ( 'NONE',  ( -8.259941899223614215, 10.65968485389279508, -1.599625672291263179 ) ) ;
#177934=CARTESIAN_POINT ( 'NONE',  ( -1.500000000000011324, 5.879166666666686858, -0.8660254037844313801 ) ) ;
#177938=CARTESIAN_POINT ( 'NONE',  ( -5.692136587293105343, 5.855332880448205657, 2.499999999999999112 ) ) ;
#177940=VERTEX_POINT ( 'NONE', #191854 ) ;
#177942=CARTESIAN_POINT ( 'NONE',  ( 7.510853912290742507, 8.825379654836435606, -1.082531754730537976 ) ) ;
#177946=CARTESIAN_POINT ( 'NONE',  ( 1.499999999999989120, 4.577083334016148974, -0.8660254037844323793 ) ) ;
#177948=CARTESIAN_POINT ( 'NONE',  ( -4.440459003675619520, 5.139289244831666714, 1.199719254218462483 ) ) ;
#177949=CARTESIAN_POINT ( 'NONE',  ( 6.521108698048765362, 8.631046119188804155, -1.443375672974058777 ) ) ;
#177950=CARTESIAN_POINT ( 'NONE',  ( -9.503902493055310430, 11.15060299906175167, 1.082531754730558626 ) ) ;
#177955=FACE_BOUND ( 'NONE', #165497, .T. ) ;
#177956=CARTESIAN_POINT ( 'NONE',  ( 3.871016551901614200, 4.474939717762034697, -1.199719254218446718 ) ) ;
#177957=CARTESIAN_POINT ( 'NONE',  ( -1.500000000000031530, 4.670833333333352932, 0.8660254037844287156 ) ) ;
#177958=CARTESIAN_POINT ( 'NONE',  ( 3.005103603723342953, 6.657704637652544832, -0.7998128361456291469 ) ) ;
#177959=CARTESIAN_POINT ( 'NONE',  ( 1.419999999999989049, 6.280000000000042881, -2.873333333333328632 ) ) ;
#177962=VERTEX_POINT ( 'NONE', #74927 ) ;
#177969=CARTESIAN_POINT ( 'NONE',  ( -1.123270288250318494, 3.297697346350006331, -0.7749999999993562039 ) ) ;
#177974=CARTESIAN_POINT ( 'NONE',  ( 9.901532256681887745, 10.44620914241737530, 0.000000000000000000 ) ) ;
#177976=CARTESIAN_POINT ( 'NONE',  ( -1.499999999973776532, 7.854386371694295654, 3.680172642290445939 ) ) ;
#177978=CARTESIAN_POINT ( 'NONE',  ( -1.402160292154681736E-14, -0.8031249996585825279, -1.575800808251665908 ) ) ;
#177979=CARTESIAN_POINT ( 'NONE',  ( 3.863710590214593399, 7.451486755318259547, 1.040834085586084257E-14 ) ) ;
#177981=CARTESIAN_POINT ( 'NONE',  ( -9.192064960385334160, 9.826423329978791088, 0.7216878364870438212 ) ) ;
#177985=EDGE_CURVE ( 'NONE', #3126, #211239, #205630, .T. ) ;
#177988=CARTESIAN_POINT ( 'NONE',  ( -4.302014814237876017, 3.913438792899272212, 0.7998128361456341429 ) ) ;
#177993=ORIENTED_EDGE ( 'NONE', *, *, #115408, .F. ) ;
#178000=ORIENTED_EDGE ( 'NONE', *, *, #60399, .T. ) ;
#178001=CARTESIAN_POINT ( 'NONE',  ( 4.333225684176827741, 7.421547172477886534, -1.117180756173659084 ) ) ;
#178008=CARTESIAN_POINT ( 'NONE',  ( -7.293923454472094114, 9.532663335016016148, 1.443375672974090751 ) ) ;
#178011=CARTESIAN_POINT ( 'NONE',  ( 7.447506452608354088, 7.583179037664891098, 0.7998128361456341429 ) ) ;
#178015=CARTESIAN_POINT ( 'NONE',  ( -3.598799709423620374, 6.286017863381107240, 1.199719254218464037 ) ) ;
#178018=CLOSED_SHELL ( 'NONE', ( #173572, #146650, #10350, #138953, #60966, #127024, #184142, #108424, #214066, #31651, #150285, #62911, #2815, #101437, #79513, #70615, #150097, #185809, #135063, #188529, #14148, #165575, #68192, #18073, #174942, #88503, #162207, #109335, #96090, #199788, #112721, #112220, #132444, #148035, #130104, #204395, #140167, #177037, #8547, #152330, #133230, #136931, #93576, #10529, #10163, #166231, #146847, #19187, #90413, #183942, #123417, #157273, #29030, #36655, #113000, #200931, #18648, #148466, #35524, #125542, #129165, #26724, #32927, #8930, #168174, #53530, #121136, #135454, #137205, #136942, #161446, #22394, #174137, #5977, #149310, #18054, #146525, #96533, #43845, #185265, #196966, #52291, #60659, #178947, #29993, #26131, #32415, #161887, #140198, #160915, #186401, #133729, #46262, #26060, #194972, #105458, #211551, #284, #210040, #199820, #187943, #105120, #120938, #136283, #141783, #182121, #131184, #96023, #205607, #150808, #46010, #21265, #25227, #84626, #169236, #35989, #125024, #176546, #166099, #98501, #194799, #142290, #98552, #94644, #122029, #134905, #26513, #12454, #38129, #209792, #86006, #74977, #59965, #141658, #53763, #142167, #172649, #105343, #47228, #112572, #38043, #92463, #111267, #50809, #167101, #45192, #49901, #63112, #32070, #75296, #95113, #69803, #172707, #19967, #45896, #32761, #5813, #41084, #9958, #167239, #148874, #44213, #3359, #181290, #127277, #126894, #177336, #8692, #141676, #161053, #127887, #187695, #204668, #6871, #26171, #3901, #157014, #64763, #191981, #207203, #112458, #538, #5639, #208311, #93188, #206435, #174759, #104445, #69102, #149156, #181348, #163201, #174336, #168539, #36421, #13279, #180955, #129443, #48043, #128940, #194460, #68001, #138115, #91946, #109383, #32846, #46304, #27352, #99069, #53929, #154702, #95335, #48017, #69427, #42255, #172330, #34317, #194172, #630, #89741, #261, #193210, #138155, #50160, #163759, #77517, #155457, #210987, #27534, #7197, #153732, #146332, #99767, #51150, #150872, #162897, #51257, #184157, #162386, #34190, #42657, #21656, #70423, #25753, #45710, #39591, #162694, #152016, #109523, #118610, #61736, #164251, #145570, #78323, #20889, #131545, #201267, #146772, #49872, #88174, #201546, #152132, #70832, #67001, #23060, #164816, #202861, #168401, #144238, #92730, #171928, #185799, #90747, #189175, #66657 ) ) ;
#178019=CARTESIAN_POINT ( 'NONE',  ( -4.334856428067329404, 6.080418470877079429, -1.599625672291256295 ) ) ;
#178022=CARTESIAN_POINT ( 'NONE',  ( 3.194917754314666514, 6.879154480009089134, 0.7998128361456321445 ) ) ;
#178023=CARTESIAN_POINT ( 'NONE',  ( 9.237182729612253951, 9.671134694169463586, 0.7998128361456462443 ) ) ;
#178024=CARTESIAN_POINT ( 'NONE',  ( 1.499999999999989120, 3.535416667349488229, 0.8660254037844522523 ) ) ;
#178027=CARTESIAN_POINT ( 'NONE',  ( 4.161918892217930654, 7.618187422415517496, 0.8381857273355892701 ) ) ;
#178028=CARTESIAN_POINT ( 'NONE',  ( 5.178851490740205676, 6.104710163027444736, 1.082531754730558626 ) ) ;
#178036=CARTESIAN_POINT ( 'NONE',  ( 7.090551149822728938, 10.25576486055978442, 1.082531754730558626 ) ) ;
#178037=CARTESIAN_POINT ( 'NONE',  ( -7.458957065812611198, 11.85386701009007204, 0.7998128361456481317 ) ) ;
#178040=CARTESIAN_POINT ( 'NONE',  ( -8.890396042259075315, 11.39521468743417998, -1.599625672291263179 ) ) ;
#178041=CARTESIAN_POINT ( 'NONE',  ( -7.714753101375940503, 8.959299025482085455, 1.199719254218462483 ) ) ;
#178049=CARTESIAN_POINT ( 'NONE',  ( 9.562578416340237197, 10.05076299535211781, 0.7998128361456462443 ) ) ;
#178052=CARTESIAN_POINT ( 'NONE',  ( 3.602716132929354664, 5.226254793216122074, 1.599625672291267398 ) ) ;
#178061=CARTESIAN_POINT ( 'NONE',  ( -1.500000000000013101, 3.379166666666691299, -0.8660254037844313801 ) ) ;
#178062=CARTESIAN_POINT ( 'NONE',  ( 6.335737856287750880, 6.286115675290828264, -0.7998128361456281477 ) ) ;
#178065=CARTESIAN_POINT ( 'NONE',  ( 6.141480397310468575, 10.10888486359680982, 1.040834085586084257E-14 ) ) ;
#178066=CARTESIAN_POINT ( 'NONE',  ( -8.622622508166983835, 13.00355065959610279, 1.040834085586084257E-14 ) ) ;
#178070=CARTESIAN_POINT ( 'NONE',  ( 9.576136569953906275, 10.06658084123472641, 0.000000000000000000 ) ) ;
#178073=CARTESIAN_POINT ( 'NONE',  ( -4.223528545856940042, 4.886203710709899006, -1.199719254218446718 ) ) ;
#178075=CARTESIAN_POINT ( 'NONE',  ( -1.500000000000011324, 5.160416667349487341, -0.8660254037844313801 ) ) ;
#178076=CARTESIAN_POINT ( 'NONE',  ( 1.364683531249988757, 1.634375000341421691, 0.000000000000000000 ) ) ;
#178082=CARTESIAN_POINT ( 'NONE',  ( 0.6823417656249882723, 0.1760416670080894308, -1.181850606188749264 ) ) ;
#178091=CARTESIAN_POINT ( 'NONE',  ( -6.039267359883488950, 9.133230122250985517, 1.199719254218452047 ) ) ;
#178093=CONICAL_SURFACE ( 'NONE', #174558, 1.219999999999999751, 0.7853981633974463916 ) ;
#178095=CARTESIAN_POINT ( 'NONE',  ( 6.491656622844908853, 6.468020902940851968, 0.7998128361456341429 ) ) ;
#178099=ORIENTED_EDGE ( 'NONE', *, *, #18312, .F. ) ;
#178105=CARTESIAN_POINT ( 'NONE',  ( -5.901876940650454095, 5.779944607047298177, -0.7998128361456291469 ) ) ;
#178109=CARTESIAN_POINT ( 'NONE',  ( 8.540746701604824409, 12.05162268759261224, -1.199719254218446718 ) ) ;
#178111=CARTESIAN_POINT ( 'NONE',  ( 7.377608144130607393, 11.75895993479440982, -0.7998128361456291469 ) ) ;
#178112=CARTESIAN_POINT ( 'NONE',  ( 4.143606928732548766, 3.973957532277850646, -0.5173101462927472971 ) ) ;
#178115=CARTESIAN_POINT ( 'NONE',  ( -8.839552966430002101, 12.29626697993494666, -1.082531754730543971 ) ) ;
#178116=CARTESIAN_POINT ( 'NONE',  ( -6.073162743917628781, 9.172774736957510555, -1.199719254218440723 ) ) ;
#178120=CARTESIAN_POINT ( 'NONE',  ( -5.679923764332232672, 6.292470487948599533, 1.134535232271353999 ) ) ;
#178121=CARTESIAN_POINT ( 'NONE',  ( -1.402160292154681736E-14, 0.1968750003414221628, -1.575800808251665908 ) ) ;
#178124=CARTESIAN_POINT ( 'NONE',  ( 7.971831135155394321, 8.402817200543854170, -0.7216878364870267237 ) ) ;
#178143=CARTESIAN_POINT ( 'NONE',  ( 9.073431116043567002, 11.60875560684942265, -1.599625672291262513 ) ) ;
#178147=CARTESIAN_POINT ( 'NONE',  ( -4.406563619641430840, 5.099744630125142564, -1.199719254218446718 ) ) ;
#178148=CARTESIAN_POINT ( 'NONE',  ( -7.832860060393135093, 10.16142270859057462, 1.599625672291295375 ) ) ;
#178150=ORIENTED_EDGE ( 'NONE', *, *, #116730, .T. ) ;
#178154=CARTESIAN_POINT ( 'NONE',  ( -1.500000000000011324, 4.952083334016150751, 0.8660254037844403729 ) ) ;
#178155=CARTESIAN_POINT ( 'NONE',  ( 7.052212457402625922, 11.37933163361175382, -0.7998128361456291469 ) ) ;
#178158=CARTESIAN_POINT ( 'NONE',  ( -7.018317073368468328, 11.33978701890523233, -0.7998128361456291469 ) ) ;
#178160=CARTESIAN_POINT ( 'NONE',  ( -1.201851678989727383E-14, 3.946875000341423689, -1.575800808251660134 ) ) ;
#178165=CARTESIAN_POINT ( 'NONE',  ( -9.653042183249970876, 11.32459930428888306, -1.082531754730539753 ) ) ;
#178169=CARTESIAN_POINT ( 'NONE',  ( -0.6823417656250212460, 3.113541667008084879, 1.181850606188767472 ) ) ;
#178177=CARTESIAN_POINT ( 'NONE',  ( 0.6823417656249882723, 2.676041667008084879, -1.181850606188749264 ) ) ;
#178180=CARTESIAN_POINT ( 'NONE',  ( -4.412288926243578935, 7.235088616337731260, 1.199719254218464037 ) ) ;
#178181=CARTESIAN_POINT ( 'NONE',  ( 5.940443861082012944, 10.08226827123770697, 0.7998128361456462443 ) ) ;
#178184=CARTESIAN_POINT ( 'NONE',  ( -0.6823417656249969321, 4.280208333674755394, -1.181850606188749264 ) ) ;
#178187=CARTESIAN_POINT ( 'NONE',  ( -1.364683531250000748, -0.7406249996585803075, 0.000000000000000000 ) ) ;
#178188=CARTESIAN_POINT ( 'NONE',  ( -4.772106882330227506, 7.550913215151819458, -1.082531754730549967 ) ) ;
#178191=CARTESIAN_POINT ( 'NONE',  ( 4.934804725694211136, 6.780358151441803649, -1.443375672974051449 ) ) ;
#178194=CARTESIAN_POINT ( 'NONE',  ( -7.609150525767646833, 9.900428251527500834, -1.599625672291263179 ) ) ;
#178196=CARTESIAN_POINT ( 'NONE',  ( -8.514157279702020631, 11.91663867875229776, -1.082531754730543971 ) ) ;
#178198=CARTESIAN_POINT ( 'NONE',  ( 0.6823417656249899377, 5.176041667008086655, -1.181850606188754593 ) ) ;
#178203=CARTESIAN_POINT ( 'NONE',  ( -5.355107487273497391, 9.191449801886996340, 0.7216878364870458196 ) ) ;
#178205=CARTESIAN_POINT ( 'NONE',  ( -1.402160292154681736E-14, -0.6156249996585817508, 1.575800808251672791 ) ) ;
#178215=CARTESIAN_POINT ( 'NONE',  ( 3.267151830768944443, 4.834763107362302748, -1.443375672974058777 ) ) ;
#178218=ORIENTED_EDGE ( 'NONE', *, *, #76938, .F. ) ;
#178219=CARTESIAN_POINT ( 'NONE',  ( 1.499999999999987566, -0.4749999999999823808, 0.000000000000000000 ) ) ;
#178220=CARTESIAN_POINT ( 'NONE',  ( 9.205623113554615600, 11.76297960394566466, 1.443375672974076540 ) ) ;
#178228=CARTESIAN_POINT ( 'NONE',  ( 4.788000803920411386, 8.737751371215816576, 1.040834085586084257E-14 ) ) ;
#178229=CARTESIAN_POINT ( 'NONE',  ( -4.009460741339347045, 5.700790169694431420, -1.599625672291256295 ) ) ;
#178232=( BOUNDED_CURVE ( )  B_SPLINE_CURVE ( 2, ( #35971, #5572, #70578, #71652, #4507, #137766, #39183 ),
 .UNSPECIFIED., .F., .T. ) 
 B_SPLINE_CURVE_WITH_KNOTS ( ( 3, 2, 2, 3 ),
 ( 0.3780836810543342641, 0.3809523809523809312, 0.3869047619047619180, 0.3897734618028085851 ),
 .UNSPECIFIED. ) 
 CURVE ( )  GEOMETRIC_REPRESENTATION_ITEM ( )  RATIONAL_B_SPLINE_CURVE ( ( 0.9331000818465633451, 0.9354320710352566071, 1.000000000000000000, 0.8660254037844387076, 1.000000000000000000, 0.9354320710352564960, 0.9331000818465632340 ) ) 
 REPRESENTATION_ITEM ( '' )  );
#178234=CARTESIAN_POINT ( 'NONE',  ( -1.364683531250014514, 0.3427083336747508424, 0.7879004041258379498 ) ) ;
#178236=CARTESIAN_POINT ( 'NONE',  ( -10.48453286206953727, 11.12637651536962125, 0.7998128361456462443 ) ) ;
#178239=EDGE_CURVE ( 'NONE', #164712, #17249, #70146, .T. ) ;
#178252=CARTESIAN_POINT ( 'NONE',  ( 2.275435306267621804, 5.643409308550367598, 0.5316758947214432762 ) ) ;
#178256=CARTESIAN_POINT ( 'NONE',  ( 7.142447996300871793, 7.227277505306155092, 0.7998128361456341429 ) ) ;
#178259=VERTEX_POINT ( 'NONE', #156738 ) ;
#178262=CARTESIAN_POINT ( 'NONE',  ( 6.936968151686458306, 11.24487994360957188, 0.7998128361456462443 ) ) ;
#178269=AXIS2_PLACEMENT_3D ( 'NONE', #31707, #146546, #163842 ) ;
#178275=CARTESIAN_POINT ( 'NONE',  ( -0.4942023283147200519, 7.349555083878085426, 1.940391385854319806 ) ) ;
#178281=CARTESIAN_POINT ( 'NONE',  ( -8.351459436338037889, 10.76645531385962862, -1.443375672974059665 ) ) ;
#178285=CARTESIAN_POINT ( 'NONE',  ( 4.462605117192430804, 8.358123070033169455, 1.040834085586084257E-14 ) ) ;
#178291=CIRCLE ( 'NONE', #202514, 0.1599999999999999756 ) ;
#178294=CARTESIAN_POINT ( 'NONE',  ( 3.511198595814921219, 7.040222761851976152, 0.7216878364870317197 ) ) ;
#178302=CARTESIAN_POINT ( 'NONE',  ( -5.506582945444718824, 9.576097202994168001, 0.7998128361456481317 ) ) ;
#178303=CARTESIAN_POINT ( 'NONE',  ( -5.122283107864663343, 4.870418468797203637, 0.000000000000000000 ) ) ;
#178311=CARTESIAN_POINT ( 'NONE',  ( 7.122110765880372618, 7.203550736482235095, 0.7998128361456341429 ) ) ;
#178326=CARTESIAN_POINT ( 'NONE',  ( 1.364683531249986537, -0.5739583329919174526, 0.7879004041258500513 ) ) ;
#178327=CARTESIAN_POINT ( 'NONE',  ( 4.356247428692526569, 3.976710176429713250, 0.7998128361456341429 ) ) ;
#178328=CARTESIAN_POINT ( 'NONE',  ( 5.691725559638619814, 5.534767995866836543, 1.040834085586084257E-14 ) ) ;
#178330=CARTESIAN_POINT ( 'NONE',  ( -7.212574532790110737, 7.517017831117667193, -0.7216878364870278340 ) ) ;
#178331=CARTESIAN_POINT ( 'NONE',  ( 4.609409038966229666, 6.400729850259146758, -1.443375672974051449 ) ) ;
#178332=CARTESIAN_POINT ( 'NONE',  ( -7.009202228140751778, 9.200488570962775725, -1.443375672974058777 ) ) ;
#178336=CARTESIAN_POINT ( 'NONE',  ( 5.503720292143644777, 8.508425209887878538, 1.199719254218462483 ) ) ;
#178340=DIRECTION ( 'NONE',  ( 1.000000000000000000, -5.578564026256503701E-16, -1.479114197289397135E-31 ) ) ;
#178341=CARTESIAN_POINT ( 'NONE',  ( 1.364683531249988535, 4.905208333674756283, -0.7879004041258300672 ) ) ;
#178345=CARTESIAN_POINT ( 'NONE',  ( 6.771407655021410399, 9.987393799911945536, -1.199719254218441611 ) ) ;
#178349=CARTESIAN_POINT ( 'NONE',  ( -8.202846631467911820, 9.528741477256060577, 1.199719254218462483 ) ) ;
#178354=CARTESIAN_POINT ( 'NONE',  ( 8.890396042259068210, 11.39521468743417998, -1.599625672291257406 ) ) ;
#178357=CARTESIAN_POINT ( 'NONE',  ( -6.340409392685171674, 10.54889472477470846, 0.7998128361456481317 ) ) ;
#178358=CARTESIAN_POINT ( 'NONE',  ( 5.908535366262987587, 4.807949608181238510, -2.499999999999995115 ) ) ;
#178360=CARTESIAN_POINT ( 'NONE',  ( 5.237746300327911442, 6.405127287353401755, -1.156737470277836355 ) ) ;
#178362=CARTESIAN_POINT ( 'NONE',  ( -9.083599731475995753, 11.62061899152058686, 1.443375672974064550 ) ) ;
#178364=CARTESIAN_POINT ( 'NONE',  ( 3.271032962906592179, 6.410358100530189951, -0.9347865144461321441 ) ) ;
#178366=CARTESIAN_POINT ( 'NONE',  ( 5.425234023762710578, 9.481190127698507553, -0.7998128361456291469 ) ) ;
#178368=CARTESIAN_POINT ( 'NONE',  ( 4.774442650306744085, 8.721933525333202653, -0.7998128361456281477 ) ) ;
#178369=CARTESIAN_POINT ( 'NONE',  ( -4.059747316280317264, 7.561585642977368238, -0.4325785229164439416 ) ) ;
#178370=CARTESIAN_POINT ( 'NONE',  ( 3.659811400685081040, 6.357198169852855685, -1.199719254218446718 ) ) ;
#178372=CARTESIAN_POINT ( 'NONE',  ( -6.941411460516810017, 8.161030127766803588, 1.082531754730549967 ) ) ;
#178377=CARTESIAN_POINT ( 'NONE',  ( -4.932365459154965492, 6.668011768565191844, 1.248136097290372337 ) ) ;
#178378=CARTESIAN_POINT ( 'NONE',  ( 1.364683531249986537, 0.1760416670080860446, 0.7879004041258500513 ) ) ;
#178381=CARTESIAN_POINT ( 'NONE',  ( 3.714570900464274850, 6.317121236308204324, 1.082531754730558626 ) ) ;
#178384=CARTESIAN_POINT ( 'NONE',  ( -8.134528978075012517, 12.43410820782212767, 1.040834085586084257E-14 ) ) ;
#178390=CARTESIAN_POINT ( 'NONE',  ( -8.392133896734675247, 10.81390885098904420, 1.443375672974064550 ) ) ;
#178391=LINE ( 'NONE', #211926, #160396 ) ;
#178394=FACE_OUTER_BOUND ( 'NONE', #49459, .T. ) ;
#178397=CARTESIAN_POINT ( 'NONE',  ( -7.632877294369372123, 11.84884791016554573, 0.7216878364870458196 ) ) ;
#178401=CARTESIAN_POINT ( 'NONE',  ( -0.6823417656249969321, 5.030208333674755394, -1.181850606188749264 ) ) ;
#178402=CARTESIAN_POINT ( 'NONE',  ( 1.499999999999989120, 4.035416667349482012, 0.8660254037844524744 ) ) ;
#178403=CARTESIAN_POINT ( 'NONE',  ( 5.490304984925487908, 6.429369728800919503, -1.257259817782523381 ) ) ;
#178408=CARTESIAN_POINT ( 'NONE',  ( -6.835281999583978418, 11.12624609948998966, -0.7998128361456291469 ) ) ;
#178411=CARTESIAN_POINT ( 'NONE',  ( -0.007473969438217894709, 8.279395425053857949, -1.999986034896452880 ) ) ;
#178412=CARTESIAN_POINT ( 'NONE',  ( 5.503720292143644777, 8.508425209887878538, 1.199719254218462483 ) ) ;
#178418=CARTESIAN_POINT ( 'NONE',  ( 8.782984583554449998, 9.141236857102018831, 1.040834085586084257E-14 ) ) ;
#178425=CARTESIAN_POINT ( 'NONE',  ( -6.561783159334141580, 7.718130443053708767, -1.082531754730544860 ) ) ;
#178429=CARTESIAN_POINT ( 'NONE',  ( 5.341549334104193747, 5.334155099317440474, 0.7216878364870371598 ) ) ;
#178431=EDGE_CURVE ( 'NONE', #146527, #54417, #118420, .T. ) ;
#178437=CARTESIAN_POINT ( 'NONE',  ( -9.317477881089553549, 11.89347683273641820, 1.599625672291281386 ) ) ;
#178439=CARTESIAN_POINT ( 'NONE',  ( 8.609591239877852686, 10.00327685373437347, -1.199719254218445830 ) ) ;
#178440=CARTESIAN_POINT ( 'NONE',  ( -1.402160292154681736E-14, -1.037499999999977662, 1.732050807568877637 ) ) ;
#178441=CARTESIAN_POINT ( 'NONE',  ( -7.804689982961090955, 12.25722208009664094, 0.7998128361456481317 ) ) ;
#178443=CARTESIAN_POINT ( 'NONE',  ( -0.6823417656249969321, 3.717708333674754506, -1.181850606188749264 ) ) ;
#178444=CARTESIAN_POINT ( 'NONE',  ( 9.490344339885973923, 12.09515436799890331, -1.443375672974057666 ) ) ;
#178449=CARTESIAN_POINT ( 'NONE',  ( 9.856414487010587422, 11.56186699200962487, 1.082531754730548412 ) ) ;
#178452=CARTESIAN_POINT ( 'NONE',  ( -7.537970219518091319, 7.896646132300314314, -0.7216878364870278340 ) ) ;
#178453=CARTESIAN_POINT ( 'NONE',  ( -1.402160292154681736E-14, 0.5718750003414239114, 1.575800808251672791 ) ) ;
#178455=CARTESIAN_POINT ( 'NONE',  ( -3.807618569100454486, 6.017853128494015991, 1.294452948159442229 ) ) ;
#178457=CARTESIAN_POINT ( 'NONE',  ( -6.970863535720637216, 11.28442455831609337, 0.7998128361456481317 ) ) ;
#178458=CARTESIAN_POINT ( 'NONE',  ( -3.836594282542926226, 5.499112634431936542, 1.443375672974064550 ) ) ;
#178459=CARTESIAN_POINT ( 'NONE',  ( -1.201851678989727383E-14, 4.009375000341416140, -1.575800808251660134 ) ) ;
#178464=CARTESIAN_POINT ( 'NONE',  ( 8.072990401933337168, 11.50590700464255356, -1.199719254218446718 ) ) ;
#178469=VERTEX_POINT ( 'NONE', #129644 ) ;
#178477=CARTESIAN_POINT ( 'NONE',  ( 0.6823417656249882723, -0.9072916663252494907, 1.181850606188755259 ) ) ;
#178482=CARTESIAN_POINT ( 'NONE',  ( 8.880754312151170282, 10.31963377138658089, 1.199719254218453823 ) ) ;
#178483=( BOUNDED_CURVE ( )  B_SPLINE_CURVE ( 2, ( #152329, #169642, #119898, #21225, #37508, #120982, #103584 ),
 .UNSPECIFIED., .F., .T. ) 
 B_SPLINE_CURVE_WITH_KNOTS ( ( 3, 2, 2, 3 ),
 ( 0.2500000000000002776, 0.2541666666666668184, 0.2583333333333333592, 0.2624999999999999001 ),
 .UNSPECIFIED. ) 
 CURVE ( )  GEOMETRIC_REPRESENTATION_ITEM ( )  RATIONAL_B_SPLINE_CURVE ( ( 0.9999999999999911182, 0.8660254037844475894, 1.000000000000000000, 0.8660254037844387076, 1.000000000000000000, 0.8660254037844422603, 0.9999999999999964473 ) ) 
 REPRESENTATION_ITEM ( '' )  );
#178485=CARTESIAN_POINT ( 'NONE',  ( -1.201851678989727383E-14, 3.196875000341420137, -1.575800808251660134 ) ) ;
#178487=CARTESIAN_POINT ( 'NONE',  ( -5.897433632264490910, 9.824163637709826702, 0.000000000000000000 ) ) ;
#178489=CARTESIAN_POINT ( 'NONE',  ( 1.403499169902376664, 7.376709478543046039, 4.304123474984473674 ) ) ;
#178495=ORIENTED_EDGE ( 'NONE', *, *, #36635, .T. ) ;
#178496=CARTESIAN_POINT ( 'NONE',  ( 9.053093885623066939, 11.58502883802551153, -1.599625672291262513 ) ) ;
#178503=CARTESIAN_POINT ( 'NONE',  ( -8.286004436246233951, 12.81875560892930466, 1.040834085586084257E-14 ) ) ;
#178504=CARTESIAN_POINT ( 'NONE',  ( 7.796102023057898123, 9.054206100777749455, -1.199719254218441611 ) ) ;
#178516=CARTESIAN_POINT ( 'NONE',  ( -5.043269954603569083, 7.867270132804026872, 1.082531754730560403 ) ) ;
#178518=CARTESIAN_POINT ( 'NONE',  ( 4.847203612085560387, 5.613824621309978724, -1.199719254218452047 ) ) ;
#178521=CARTESIAN_POINT ( 'NONE',  ( -6.938021921891187382, 9.117444880338284818, -1.599625672291263179 ) ) ;
#178526=CARTESIAN_POINT ( 'NONE',  ( -8.272446282632566650, 12.80293776304669962, 0.7998128361456481317 ) ) ;
#178531=CARTESIAN_POINT ( 'NONE',  ( 8.782984583554449998, 9.141236857102018831, 1.040834085586084257E-14 ) ) ;
#178534=ORIENTED_EDGE ( 'NONE', *, *, #151553, .T. ) ;
#178541=CARTESIAN_POINT ( 'NONE',  ( -4.134873662487946966, 3.926366815765101936, 1.214306433183764966E-14 ) ) ;
#178543=CARTESIAN_POINT ( 'NONE',  ( -8.025536864285518490, 11.45054454405341282, -1.199719254218446718 ) ) ;
#178547=CARTESIAN_POINT ( 'NONE',  ( 6.968527767744109980, 7.232296605230681408, 0.7216878364870317197 ) ) ;
#178549=CARTESIAN_POINT ( 'NONE',  ( 3.602716132929354664, 5.226254793216122074, 1.599625672291267398 ) ) ;
#178552=CARTESIAN_POINT ( 'NONE',  ( -5.228640796364566690, 9.251831362400652736, -0.7998128361456231517 ) ) ;
#178562=CARTESIAN_POINT ( 'NONE',  ( -0.6823417656250212460, 3.613541667008085767, 1.181850606188767472 ) ) ;
#178563=CARTESIAN_POINT ( 'NONE',  ( 2.487170525094572149, 8.243531156567085461, 2.499999999999998224 ) ) ;
#178565=CARTESIAN_POINT ( 'NONE',  ( 8.911787042884274257, 9.291506392986812912, 0.7998128361456462443 ) ) ;
#178568=CARTESIAN_POINT ( 'NONE',  ( -4.948362879307902418, 4.875437568721725512, 1.214306433183764966E-14 ) ) ;
#178570=EDGE_CURVE ( 'NONE', #146442, #55162, #118658, .T. ) ;
#178571=CARTESIAN_POINT ( 'NONE',  ( -3.416291520519271874, 6.929497840673697340, 1.040834085586084257E-14 ) ) ;
#178578=CARTESIAN_POINT ( 'NONE',  ( 3.334415713957098681, 5.977569868670206787, -1.199719254218446718 ) ) ;
#178585=AXIS2_PLACEMENT_3D ( 'NONE', #79490, #20597, #145609 ) ;
#178586=CARTESIAN_POINT ( 'NONE',  ( 3.354752944377597856, 6.001296637494123232, -1.199719254218446718 ) ) ;
#178591=CARTESIAN_POINT ( 'NONE',  ( 0.6823417656249917140, 3.905208333674754950, 1.181850606188765695 ) ) ;
#178596=CARTESIAN_POINT ( 'NONE',  ( 6.823831386379729302, 6.855558127064808716, -0.7998128361456281477 ) ) ;
#178600=CARTESIAN_POINT ( 'NONE',  ( -5.935772324684618795, 5.819489221753827657, 0.000000000000000000 ) ) ;
#178602=CARTESIAN_POINT ( 'NONE',  ( 4.961921032477176752, 8.732732271291288484, 1.040834085586084257E-14 ) ) ;
#178603=CARTESIAN_POINT ( 'NONE',  ( 1.499999999999987121, 2.545833333333351156, -0.8660254037844262731 ) ) ;
#178605=CARTESIAN_POINT ( 'NONE',  ( -4.680589345215810049, 6.483773540883647435, -1.599625672291256295 ) ) ;
#178606=CARTESIAN_POINT ( 'NONE',  ( 0.2791710057859035921, 8.178600120974712340, -1.982899171337044297 ) ) ;
#178608=CARTESIAN_POINT ( 'NONE',  ( -0.6823417656250212460, 5.051041667008086655, 1.181850606188767472 ) ) ;
#178611=CARTESIAN_POINT ( 'NONE',  ( -4.934804725694236893, 4.859619722839116918, -0.7216878364870207285 ) ) ;
#178617=CARTESIAN_POINT ( 'NONE',  ( 5.027376032568989572, 4.759693547618927489, 0.7998128361456341429 ) ) ;
#178620=CARTESIAN_POINT ( 'NONE',  ( 1.364683531249988535, 3.676041667008087099, 0.7879004041258500513 ) ) ;
#178624=CARTESIAN_POINT ( 'NONE',  ( 0.6823417656249882723, 0.1552083336747514530, 1.181850606188755259 ) ) ;
#178625=DIRECTION ( 'NONE',  ( -3.347138415753903010E-16, -0.6000000000000018652, 0.7999999999999984901 ) ) ;
#178627=CARTESIAN_POINT ( 'NONE',  ( -9.541187415715041809, 12.15447128979948310, -1.599625672291263179 ) ) ;
#178628=CARTESIAN_POINT ( 'NONE',  ( -6.860062538390436337, 7.105753837651378468, 1.040834085586084257E-14 ) ) ;
#178632=CARTESIAN_POINT ( 'NONE',  ( -0.6823417656250212460, 4.301041667008085767, 1.181850606188767472 ) ) ;
#178640=CARTESIAN_POINT ( 'NONE',  ( -5.951666246274811556, 7.966696592119163256, 1.443375672974064550 ) ) ;
#178646=CARTESIAN_POINT ( 'NONE',  ( -4.392478580703220281, 8.068382744221649361, 1.040834085586084257E-14 ) ) ;
#178659=CARTESIAN_POINT ( 'NONE',  ( -4.822949958159302497, 6.649860922651058992, -1.599625672291256295 ) ) ;
#178662=CARTESIAN_POINT ( 'NONE',  ( -1.402160292154681736E-14, 0.8375000000000232259, -1.732050807568863648 ) ) ;
#178664=CARTESIAN_POINT ( 'NONE',  ( 8.595506201383999567, 12.97191496834930113, 0.7216878364870438212 ) ) ;
#178665=CARTESIAN_POINT ( 'NONE',  ( 6.174848896020108668, 9.291408581077091000, 1.199719254218460707 ) ) ;
#178669=CARTESIAN_POINT ( 'NONE',  ( 6.667912619822566000, 6.673652899414787676, 1.040834085586084257E-14 ) ) ;
#178670=CARTESIAN_POINT ( 'NONE',  ( -0.4782691259469663003, 7.503280781841559666, -1.943353214563636300 ) ) ;
#178675=CARTESIAN_POINT ( 'NONE',  ( -3.131570295076647525, 6.597323077657299528, 1.040834085586084257E-14 ) ) ;
#178684=CARTESIAN_POINT ( 'NONE',  ( 0.6823417656249899377, 3.426041667008085323, -1.181850606188754593 ) ) ;
#178685=CARTESIAN_POINT ( 'NONE',  ( 8.880227426826630577, 12.34372051706435869, 1.082531754730546636 ) ) ;
#178686=CARTESIAN_POINT ( 'NONE',  ( -6.877010230629689858, 9.046264573866535486, 1.599625672291283607 ) ) ;
#178689=CARTESIAN_POINT ( 'NONE',  ( 7.142447996300871793, 7.227277505306155092, 0.7998128361456341429 ) ) ;
#178690=CARTESIAN_POINT ( 'NONE',  ( -7.009729113465285266, 8.136771039586342624, -1.199719254218446718 ) ) ;
#178694=CARTESIAN_POINT ( 'NONE',  ( 1.499999999999989120, 0.05625000068281565957, 0.000000000000000000 ) ) ;
#178697=CARTESIAN_POINT ( 'NONE',  ( 6.155038550924133212, 10.12470270947942730, 0.7216878364870438212 ) ) ;
#178701=CARTESIAN_POINT ( 'NONE',  ( -0.6823417656250003738, 1.780208333674752952, -1.181850606188749264 ) ) ;
#178703=CARTESIAN_POINT ( 'NONE',  ( 5.599154252319471503, 9.476171027773981237, -0.7216878364870267237 ) ) ;
#178705=CARTESIAN_POINT ( 'NONE',  ( -3.714570900464290393, 5.356752022006865843, 1.443375672974064550 ) ) ;
#178707=CARTESIAN_POINT ( 'NONE',  ( -1.364683531250012516, 4.738541667008091096, -0.7879004041258300672 ) ) ;
#178713=CARTESIAN_POINT ( 'NONE',  ( -4.904330467487477918, 6.873893772473251396, -1.448588590679427801 ) ) ;
#178720=CARTESIAN_POINT ( 'NONE',  ( 4.957477724091233995, 8.935474444748447098, -0.7998128361456281477 ) ) ;
#178723=CARTESIAN_POINT ( 'NONE',  ( 4.518945272056516416, 4.166524327021037699, 0.7998128361456341429 ) ) ;
#178732=CARTESIAN_POINT ( 'NONE',  ( 6.507550544879468823, 6.694489845221929691, -0.7216878364870257245 ) ) ;
#178734=CARTESIAN_POINT ( 'NONE',  ( -0.6823417656250212460, 1.863541667008083991, 1.181850606188755259 ) ) ;
#178735=CARTESIAN_POINT ( 'NONE',  ( 8.483651433849084711, 10.92067931095586886, 1.599625672291281386 ) ) ;
#178737=CARTESIAN_POINT ( 'NONE',  ( 0.2537734656027313962, 6.376933751358200730, -3.135911668477547654 ) ) ;
#178742=CARTESIAN_POINT ( 'NONE',  ( 1.499999999999987121, 1.504166666666690411, 0.8660254037844524744 ) ) ;
#178743=CARTESIAN_POINT ( 'NONE',  ( 7.070740804726770357, 8.207951346058097286, 1.199719254218462483 ) ) ;
#178744=CARTESIAN_POINT ( 'NONE',  ( -8.474009703741204547, 9.845098394908269768, -1.199719254218446718 ) ) ;
#178748=CARTESIAN_POINT ( 'NONE',  ( 1.364683531249986537, 2.405208333674752286, -0.7879004041258239610 ) ) ;
#178750=CARTESIAN_POINT ( 'NONE',  ( -1.001543065824772872E-14, 4.462500000000024336, 1.732050807568877637 ) ) ;
#178752=CARTESIAN_POINT ( 'NONE',  ( 10.56143847536557878, 11.42402576412244386, 0.000000000000000000 ) ) ;
#178759=CARTESIAN_POINT ( 'NONE',  ( 0.7499999999999867883, 0.09791666734948467621, -1.299038105676652899 ) ) ;
#178761=CARTESIAN_POINT ( 'NONE',  ( -5.747767057189642870, 8.793146435774861658, -1.199719254218440723 ) ) ;
#178762=CARTESIAN_POINT ( 'NONE',  ( -2.629918611371007575, 6.012062780000711371, 0.7216878364870317197 ) ) ;
#178770=CARTESIAN_POINT ( 'NONE',  ( 6.205881626753210867, 8.263281202677319470, 1.599625672291281386 ) ) ;
#178772=DIRECTION ( 'NONE',  ( -5.578564026256490882E-16, -1.000000000000000000, -9.066213480720158442E-32 ) ) ;
#178774=CARTESIAN_POINT ( 'NONE',  ( 5.472687561410540802, 9.536552588287639409, 0.7998128361456462443 ) ) ;
#178775=CARTESIAN_POINT ( 'NONE',  ( 9.869972640624258275, 10.61731562359089587, 0.000000000000000000 ) ) ;
#178776=ORIENTED_EDGE ( 'NONE', *, *, #177765, .F. ) ;
#178777=DIRECTION ( 'NONE',  ( 0.000000000000000000, 1.000000000000000000, 2.168404344971034112E-15 ) ) ;
#178780=CARTESIAN_POINT ( 'NONE',  ( -6.008234629150358330, 10.16135750065076060, 0.000000000000000000 ) ) ;
#178782=CARTESIAN_POINT ( 'NONE',  ( 2.920892028740289081, 5.495125569250587816, 1.199719254218452047 ) ) ;
#178787=CARTESIAN_POINT ( 'NONE',  ( 4.464323212750023195, 7.049731028713583925, 1.131627047429624167 ) ) ;
#178796=CARTESIAN_POINT ( 'NONE',  ( 7.700668062882064291, 10.00719871149432549, -1.443375672974057666 ) ) ;
#178798=CARTESIAN_POINT ( 'NONE',  ( -5.148345644887285744, 7.029489223833707001, -1.599625672291256295 ) ) ;
#178800=EDGE_CURVE ( 'NONE', #110911, #109059, #156779, .T. ) ;
#178803=CARTESIAN_POINT ( 'NONE',  ( -7.528855374290365887, 7.678086112960552434, -0.7998128361456291469 ) ) ;
#178819=EDGE_CURVE ( 'NONE', #6713, #25036, #139338, .T. ) ;
#178821=CARTESIAN_POINT ( 'NONE',  ( -4.218558352146454915, 8.073401844146177453, 1.040834085586084257E-14 ) ) ;
#178824=CARTESIAN_POINT ( 'NONE',  ( 2.575685996916329046, 5.948791396470269888, 0.7216878364870438212 ) ) ;
#178829=CARTESIAN_POINT ( 'NONE',  ( -3.460355519985875983, 5.060167411448709629, 1.599625672291267398 ) ) ;
#178831=CARTESIAN_POINT ( 'NONE',  ( 8.353795204314554468, 12.89784483834236184, -0.7998128361456352531 ) ) ;
#178834=CARTESIAN_POINT ( 'NONE',  ( -8.877891658850122880, 9.251961778280284321, 0.7998128361456462443 ) ) ;
#178836=CARTESIAN_POINT ( 'NONE',  ( 3.825371897350130723, 7.614684313550482031, 0.7998128361456321445 ) ) ;
#178840=CARTESIAN_POINT ( 'NONE',  ( 5.335297142177534369, 6.183267073083954735, -1.199719254218452047 ) ) ;
#178843=CARTESIAN_POINT ( 'NONE',  ( -1.201851678989727383E-14, 1.884375000341422135, 1.575800808251672791 ) ) ;
#178844=ORIENTED_EDGE ( 'NONE', *, *, #13805, .F. ) ;
#178846=CARTESIAN_POINT ( 'NONE',  ( 6.805829924380105034, 9.923590097543378619, 1.082531754730558626 ) ) ;
#178854=CARTESIAN_POINT ( 'NONE',  ( 10.01911233037457905, 11.75168114260095109, 1.082531754730548412 ) ) ;
#178856=CARTESIAN_POINT ( 'NONE',  ( 4.716110169385688167, 5.239146042535265835, -0.9347783054772640376 ) ) ;
#178862=CARTESIAN_POINT ( 'NONE',  ( -10.31505594189871111, 10.92865344183699428, -0.7998128361456291469 ) ) ;
#178869=CARTESIAN_POINT ( 'NONE',  ( 5.133733721068893807, 9.141106441222381918, 1.040834085586084257E-14 ) ) ;
#178876=CARTESIAN_POINT ( 'NONE',  ( -1.201851678989727383E-14, 1.743750000682815493, 1.732050807568877637 ) ) ;
#178882=CARTESIAN_POINT ( 'NONE',  ( 1.499999999999985123, -0.9541666666666493990, -0.8660254037844323793 ) ) ;
#178883=CARTESIAN_POINT ( 'NONE',  ( 9.023114925094663619, 10.48572115315399245, 1.199719254218453823 ) ) ;
#178888=CARTESIAN_POINT ( 'NONE',  ( 4.844340958784499662, 4.546152628203684820, 0.7998128361456341429 ) ) ;
#178889=CARTESIAN_POINT ( 'NONE',  ( -6.480434237652138663, 8.583592582059388576, 1.443375672974078761 ) ) ;
#178893=CARTESIAN_POINT ( 'NONE',  ( -5.845536785786364931, 9.971543350059432598, 0.000000000000000000 ) ) ;
#178896=CARTESIAN_POINT ( 'NONE',  ( -1.500000000000001332, 1.181250000682816603, 0.000000000000000000 ) ) ;
#178903=CARTESIAN_POINT ( 'NONE',  ( -2.440104460335327463, 5.790612937125752424, 1.040834085586084257E-14 ) ) ;
#178905=CARTESIAN_POINT ( 'NONE',  ( 5.086710258240730198, 6.515995995190169587, 1.216687342998038934 ) ) ;
#178910=CARTESIAN_POINT ( 'NONE',  ( -9.130526383799315582, 12.73969898348616070, 1.199719254218462483 ) ) ;
#178911=CARTESIAN_POINT ( 'NONE',  ( 7.853197290813620945, 10.18514947741448573, 1.599625672291281386 ) ) ;
#178919=CARTESIAN_POINT ( 'NONE',  ( -6.333630315878337136, 10.54098580183340772, 0.000000000000000000 ) ) ;
#178922=ORIENTED_EDGE ( 'NONE', *, *, #155922, .F. ) ;
#178925=CARTESIAN_POINT ( 'NONE',  ( 3.408985558832261731, 6.064568021024562938, 1.199719254218462483 ) ) ;
#178928=VERTEX_POINT ( 'NONE', #130444 ) ;
#178929=CARTESIAN_POINT ( 'NONE',  ( -4.042302355168801320, 7.867769847672247074, 0.7998128361456341429 ) ) ;
#178930=( BOUNDED_CURVE ( )  B_SPLINE_CURVE ( 2, ( #107669, #91375, #203995, #189911, #157435, #154219, #192028 ),
 .UNSPECIFIED., .F., .T. ) 
 B_SPLINE_CURVE_WITH_KNOTS ( ( 3, 2, 2, 3 ),
 ( 0.2250000000000001998, 0.2291666666666669072, 0.2333333333333336701, 0.2375000000000003775 ),
 .UNSPECIFIED. ) 
 CURVE ( )  GEOMETRIC_REPRESENTATION_ITEM ( )  RATIONAL_B_SPLINE_CURVE ( ( 0.9999999999999937828, 0.8660254037844449249, 1.000000000000000000, 0.8660254037844387076, 1.000000000000000000, 0.8660254037844261621, 1.000000000000012434 ) ) 
 REPRESENTATION_ITEM ( '' )  );
#178934=CARTESIAN_POINT ( 'NONE',  ( -1.203941962966161627, 3.197768152887754844, -0.7749999999999883649 ) ) ;
#178943=CARTESIAN_POINT ( 'NONE',  ( 7.796102023057898123, 9.054206100777749455, -1.199719254218441611 ) ) ;
#178945=CARTESIAN_POINT ( 'NONE',  ( -5.122283107864663343, 4.870418468797203637, 0.000000000000000000 ) ) ;
#178946=ORIENTED_EDGE ( 'NONE', *, *, #163335, .F. ) ;
#178947=ADVANCED_FACE ( 'NONE', ( #43804 ), #162658, .F. ) ;
#178953=CARTESIAN_POINT ( 'NONE',  ( 1.499999999999987121, -0.2145833326505137972, 0.8660254037844524744 ) ) ;
#178956=FACE_OUTER_BOUND ( 'NONE', #85753, .T. ) ;
#178958=CARTESIAN_POINT ( 'NONE',  ( -3.164938793786285842, 5.779846795137578930, -1.199719254218452935 ) ) ;
#178964=CARTESIAN_POINT ( 'NONE',  ( 4.690757960648231695, 5.535267711253469614, 1.082531754730560403 ) ) ;
#178967=CARTESIAN_POINT ( 'NONE',  ( -1.201851678989727383E-14, 5.759375000341417028, -1.575800808251660801 ) ) ;
#178969=CARTESIAN_POINT ( 'NONE',  ( 3.890826896997583884, 4.602014803661035103, -1.082531754730543083 ) ) ;
#178971=AXIS2_PLACEMENT_3D ( 'NONE', #212953, #130730, #165281 ) ;
#178980=CARTESIAN_POINT ( 'NONE',  ( 0.6823417656249882723, -0.3239583329919110133, -1.181850606188749264 ) ) ;
#178984=CARTESIAN_POINT ( 'NONE',  ( -5.850506979496850057, 6.784345216623154151, -1.199719254218446718 ) ) ;
#178988=CARTESIAN_POINT ( 'NONE',  ( -1.499999999999997780, 5.150000000000022560, 1.214306433183764966E-14 ) ) ;
#178995=CARTESIAN_POINT ( 'NONE',  ( -1.364683531250010295, 5.801041667008088432, -0.7879004041258300672 ) ) ;
#178997=CARTESIAN_POINT ( 'NONE',  ( 5.276094334012385367, 9.307193822989793475, 1.040834085586084257E-14 ) ) ;
#178998=CARTESIAN_POINT ( 'NONE',  ( -7.340850106795412167, 10.65174332698158643, 1.199719254218453823 ) ) ;
#179001=CARTESIAN_POINT ( 'NONE',  ( -1.000000000000017097, 8.600000000000013856, 0.4000000000000026867 ) ) ;
#179006=CARTESIAN_POINT ( 'NONE',  ( 0.7499999999999902300, 5.816666666666685082, -1.299038105676658228 ) ) ;
#179013=CARTESIAN_POINT ( 'NONE',  ( 6.141480397310468575, 10.10888486359680982, 1.040834085586084257E-14 ) ) ;
#179017=CARTESIAN_POINT ( 'NONE',  ( 1.499999999999990896, 4.056250000682819490, 1.214306433183764966E-14 ) ) ;
#179019=CARTESIAN_POINT ( 'NONE',  ( -4.548924232584923288, 5.265832011892554121, -1.199719254218446718 ) ) ;
#179020=CARTESIAN_POINT ( 'NONE',  ( 7.266807146800403849, 7.580289214129690478, 1.040834085586084257E-14 ) ) ;
#179021=CARTESIAN_POINT ( 'NONE',  ( -8.473482818416670170, 10.90881592628469932, -1.443375672974058777 ) ) ;
#179027=CARTESIAN_POINT ( 'NONE',  ( 2.171277156482887882, 5.684907115872006145, -0.7998128361456291469 ) ) ;
#179028=CARTESIAN_POINT ( 'NONE',  ( 1.499999999999987121, 3.827083334016153415, -0.8660254037844323793 ) ) ;
#179030=VECTOR ( 'NONE', #67109, 1000.000000000000114 ) ;
#179043=CARTESIAN_POINT ( 'NONE',  ( 9.250740883225924804, 9.686952540052077509, 1.040834085586084257E-14 ) ) ;
#179047=CARTESIAN_POINT ( 'NONE',  ( -1.402160292154681736E-14, -0.3031249996585801965, -1.575800808251665908 ) ) ;
#179048=CARTESIAN_POINT ( 'NONE',  ( 5.883875478650832491, 6.927238148923188454, -1.082531754730543083 ) ) ;
#179049=CARTESIAN_POINT ( 'NONE',  ( -9.327646496521992958, 9.984601788804893019, -0.7216878364870267237 ) ) ;
#179054=CARTESIAN_POINT ( 'NONE',  ( -2.916975605234527702, 6.554888639415577423, 1.040834085586084257E-14 ) ) ;
#179068=VERTEX_POINT ( 'NONE', #72846 ) ;
#179069=CARTESIAN_POINT ( 'NONE',  ( 4.808669324434905690, 6.961940934708692019, -1.409791361277392241 ) ) ;
#179076=CARTESIAN_POINT ( 'NONE',  ( -7.537970219518075332, 10.77775377520434574, -1.082531754730543971 ) ) ;
#179080=CARTESIAN_POINT ( 'NONE',  ( 7.070740804726770357, 8.207951346058097286, 1.199719254218462483 ) ) ;
#179081=CARTESIAN_POINT ( 'NONE',  ( -5.298539104842322267, 5.076050465271134016, 0.7998128361456341429 ) ) ;
#179083=CARTESIAN_POINT ( 'NONE',  ( -4.900382456335551140, 7.804531068111707270, 1.199719254218464037 ) ) ;
#179086=CARTESIAN_POINT ( 'NONE',  ( -6.417086777969760902, 6.381022750586497594, 0.7998128361456341429 ) ) ;
#179088=EDGE_CURVE ( 'NONE', #184190, #32206, #208689, .T. ) ;
#179090=CARTESIAN_POINT ( 'NONE',  ( 6.903072767652295383, 11.20533532890304684, 1.040834085586084257E-14 ) ) ;
#179093=CARTESIAN_POINT ( 'NONE',  ( 5.079507498475252625, 6.736975590279616455, 1.417308049988776020 ) ) ;
#179094=CARTESIAN_POINT ( 'NONE',  ( 3.524756749872944628, 7.056040608253000279, -0.7216878364870267237 ) ) ;
#179101=CARTESIAN_POINT ( 'NONE',  ( 6.439759776366765998, 9.496508258194486629, 1.082531754730558626 ) ) ;
#179102=( BOUNDED_CURVE ( )  B_SPLINE_CURVE ( 2, ( #86636, #152703, #70356, #139683, #203556, #21597, #75718 ),
 .UNSPECIFIED., .F., .T. ) 
 B_SPLINE_CURVE_WITH_KNOTS ( ( 3, 2, 2, 3 ),
 ( 0.3571428571428574283, 0.3630952380952382486, 0.3690476190476191243, 0.3719163189456657359 ),
 .UNSPECIFIED. ) 
 CURVE ( )  GEOMETRIC_REPRESENTATION_ITEM ( )  RATIONAL_B_SPLINE_CURVE ( ( 0.9999999999999937828, 0.8660254037844449249, 1.000000000000000000, 0.8660254037844387076, 1.000000000000000000, 0.9354320710352564960, 0.9331000818465632340 ) ) 
 REPRESENTATION_ITEM ( '' )  );
#179105=CARTESIAN_POINT ( 'NONE',  ( -9.215791728987058562, 11.77484298861683598, -1.599625672291263179 ) ) ;
#179106=CARTESIAN_POINT ( 'NONE',  ( -7.121056995675673740, 9.330985799753529264, -1.599625672291263179 ) ) ;
#179114=CARTESIAN_POINT ( 'NONE',  ( 8.809047120577066181, 11.30030761213851953, 1.599625672291281386 ) ) ;
#179118=CARTESIAN_POINT ( 'NONE',  ( 2.686486993802192913, 6.285985259411197568, 0.7998128361456362523 ) ) ;
#179122=CARTESIAN_POINT ( 'NONE',  ( 1.499999999999990896, 5.056250000682820378, 1.214306433183764966E-14 ) ) ;
#179128=CARTESIAN_POINT ( 'NONE',  ( -1.500000000000013101, 3.129166666666689967, -0.8660254037844313801 ) ) ;
#179129=CARTESIAN_POINT ( 'NONE',  ( 5.178324605415663306, 8.128796908705222535, 1.199719254218462483 ) ) ;
#179131=CARTESIAN_POINT ( 'NONE',  ( 8.432808358020029260, 8.940623960552603222, 0.7216878364870438212 ) ) ;
#179132=CARTESIAN_POINT ( 'NONE',  ( -9.368320956918621434, 11.95279375453699622, 1.443375672974076540 ) ) ;
#179137=CARTESIAN_POINT ( 'NONE',  ( 8.055515824813896941, 12.54985222892493368, 0.7998128361456462443 ) ) ;
#179140=CARTESIAN_POINT ( 'NONE',  ( -3.741160322367112379, 6.452105245148518797, 1.199719254218464037 ) ) ;
#179141=CARTESIAN_POINT ( 'NONE',  ( -1.500000000000011324, 4.952083334016150751, 0.8660254037844403729 ) ) ;
#179142=CARTESIAN_POINT ( 'NONE',  ( -1.402160292154681736E-14, 0.07187500034142156602, 1.575800808251672791 ) ) ;
#179146=CARTESIAN_POINT ( 'NONE',  ( 4.172158584703322681, 5.890604320285754980, -1.599625672291256295 ) ) ;
#179148=CARTESIAN_POINT ( 'NONE',  ( 1.364683531249988535, 5.467708333674750953, -0.7879004041258300672 ) ) ;
#179150=CARTESIAN_POINT ( 'NONE',  ( 4.011676250333519711, 7.811283078717995210, 0.2953092252874019441 ) ) ;
#179157=CARTESIAN_POINT ( 'NONE',  ( -7.739006755302186846, 7.923262724141010516, 0.7998128361456462443 ) ) ;
#179160=CARTESIAN_POINT ( 'NONE',  ( 5.331380718671758778, 7.243030143248949670, -1.599625672291256295 ) ) ;
#179166=CARTESIAN_POINT ( 'NONE',  ( 8.224992744984721327, 12.74757530245756243, 1.040834085586084257E-14 ) ) ;
#179169=CARTESIAN_POINT ( 'NONE',  ( -4.391951695823077984, 7.211361847513815704, 1.199719254218464037 ) ) ;
#179173=CARTESIAN_POINT ( 'NONE',  ( 7.727257484784855635, 11.10255193463598111, -1.199719254218446718 ) ) ;
#179175=CARTESIAN_POINT ( 'NONE',  ( 8.535021395002688749, 9.916278701380017324, 1.199719254218462483 ) ) ;
#179179=CARTESIAN_POINT ( 'NONE',  ( -10.15469386695561482, 10.94949038764413096, 1.040834085586084257E-14 ) ) ;
#179180=CARTESIAN_POINT ( 'NONE',  ( -5.682838942422375084, 9.781729199468104596, 0.000000000000000000 ) ) ;
#179184=CARTESIAN_POINT ( 'NONE',  ( -5.443514322282436702, 6.457176790571845792, 1.314492736914568027 ) ) ;
#179185=CARTESIAN_POINT ( 'NONE',  ( -1.402160292154681736E-14, 0.4468750003414233563, -1.575800808251665908 ) ) ;
#179189=CARTESIAN_POINT ( 'NONE',  ( 7.456621297836072415, 9.722477485607340597, 1.443375672974076540 ) ) ;
#179192=AXIS2_PLACEMENT_3D ( 'NONE', #18632, #33825, #133504 ) ;
#179212=CARTESIAN_POINT ( 'NONE',  ( -5.087333953625788219, 6.958308917361963886, 1.599625672291267398 ) ) ;
#179213=CARTESIAN_POINT ( 'NONE',  ( -7.182068686937172153, 9.402166106225269715, 1.599625672291283607 ) ) ;
#179219=CARTESIAN_POINT ( 'NONE',  ( -1.499999999999997780, 3.431250000682818602, 1.214306433183764966E-14 ) ) ;
#179220=CARTESIAN_POINT ( 'NONE',  ( 8.589254009457354400, 9.979550084910457031, -1.199719254218446718 ) ) ;
#179223=CARTESIAN_POINT ( 'NONE',  ( -8.341290820905609138, 10.75459192918846618, 1.599625672291269396 ) ) ;
#179225=CARTESIAN_POINT ( 'NONE',  ( -0.6823417656249969321, 3.217708333674754062, -1.181850606188749264 ) ) ;
#179230=CARTESIAN_POINT ( 'NONE',  ( -7.849807752632384172, 12.10193344480572897, 0.000000000000000000 ) ) ;
#179236=CARTESIAN_POINT ( 'NONE',  ( -0.6823417656250003738, 1.280208333674752508, -1.181850606188749264 ) ) ;
#179243=CARTESIAN_POINT ( 'NONE',  ( 0.6823417656249882723, 2.926041667008084879, -1.181850606188754593 ) ) ;
#179245=CARTESIAN_POINT ( 'NONE',  ( -6.087774667736030487, 7.061157519568837415, 1.199719254218450271 ) ) ;
#179246=CARTESIAN_POINT ( 'NONE',  ( 6.265839547809997079, 10.46189657242035587, 0.7998128361456462443 ) ) ;
#179250=CARTESIAN_POINT ( 'NONE',  ( -0.6823417656250212460, 3.113541667008084879, 1.181850606188767472 ) ) ;
#179254=CARTESIAN_POINT ( 'NONE',  ( -1.364683531250014514, -0.2197916663252438285, 0.7879004041258379498 ) ) ;
#179255=CARTESIAN_POINT ( 'NONE',  ( -4.284013352238250860, 7.941839977679187257, -0.7216878364870267237 ) ) ;
#179259=CARTESIAN_POINT ( 'NONE',  ( 3.538314903486612817, 7.071858454135611538, 1.040834085586084257E-14 ) ) ;
#179262=CARTESIAN_POINT ( 'NONE',  ( -6.340409392685171674, 10.54889472477470846, 0.7998128361456481317 ) ) ;
#179263=CARTESIAN_POINT ( 'NONE',  ( -3.602716132929368875, 5.226254793216122074, 1.599625672291267398 ) ) ;
#179265=CARTESIAN_POINT ( 'NONE',  ( -1.201851678989727383E-14, 4.946875000341420581, -1.575800808251660134 ) ) ;
#179270=CARTESIAN_POINT ( 'NONE',  ( -5.382223794500827552, 9.223085493652217082, -0.7216878364870207285 ) ) ;
#179272=CARTESIAN_POINT ( 'NONE',  ( 1.364683531249988757, -0.3031249996585799744, 0.000000000000000000 ) ) ;
#179276=CARTESIAN_POINT ( 'NONE',  ( 5.666945020832160118, 9.555260257705446847, 0.7216878364870438212 ) ) ;
#179283=AXIS2_PLACEMENT_3D ( 'NONE', #158049, #73573, #8569 ) ;
#179287=CARTESIAN_POINT ( 'NONE',  ( 9.747949258101261449, 11.43532422494874368, -1.082531754730537088 ) ) ;
#179291=VERTEX_POINT ( 'NONE', #186604 ) ;
#179293=CARTESIAN_POINT ( 'NONE',  ( 6.582647274634798151, 7.638508894284114170, 1.199719254218462483 ) ) ;
#179295=CARTESIAN_POINT ( 'NONE',  ( -5.091250377131585125, 5.898545847196970726, 1.199719254218450271 ) ) ;
#179301=CARTESIAN_POINT ( 'NONE',  ( 4.650083499362864359, 7.408552601689905259, 1.082531754730558626 ) ) ;
#179302=CARTESIAN_POINT ( 'NONE',  ( 1.364683531249986537, -0.03229166632525094088, -0.7879004041258309554 ) ) ;
#179304=CARTESIAN_POINT ( 'NONE',  ( -10.15913717534155047, 10.74674821418697057, 0.7998128361456462443 ) ) ;
#179314=CARTESIAN_POINT ( 'NONE',  ( -1.499999999999990896, 4.629166666666689522, -0.8660254037844429265 ) ) ;
#179318=CARTESIAN_POINT ( 'NONE',  ( -5.000000000000000888, 3.300000000000025135, -0.7749999999999935829 ) ) ;
#179322=CARTESIAN_POINT ( 'NONE',  ( 6.830610463186557624, 6.863467050006115677, 1.040834085586084257E-14 ) ) ;
#179329=CARTESIAN_POINT ( 'NONE',  ( 7.690499447449630210, 9.995335326823163058, 1.599625672291281386 ) ) ;
#179333=CARTESIAN_POINT ( 'NONE',  ( 9.103410076571945453, 12.70806329172093818, 1.199719254218450271 ) ) ;
#179335=CARTESIAN_POINT ( 'NONE',  ( -2.252626078164912560, 5.779814191167667481, 0.7998128361456341429 ) ) ;
#179338=CARTESIAN_POINT ( 'NONE',  ( 8.387690588348714726, 12.93738945304888333, 1.040834085586084257E-14 ) ) ;
#179340=CARTESIAN_POINT ( 'NONE',  ( -0.4599077567408665357, 8.047644787141420508, 1.947158400785508947 ) ) ;
#179345=CARTESIAN_POINT ( 'NONE',  ( -10.30383355670593737, 11.12348669235284504, -0.7216878364870267237 ) ) ;
#179349=CARTESIAN_POINT ( 'NONE',  ( 4.852928918687680948, 7.749168607522574526, 1.199719254218462483 ) ) ;
#179350=CARTESIAN_POINT ( 'NONE',  ( -1.201851678989727383E-14, 5.696875000341416140, -1.575800808251660134 ) ) ;
#179355=CARTESIAN_POINT ( 'NONE',  ( 4.812781342726866640, 5.677628323678546529, 1.082531754730560403 ) ) ;
#179358=ORIENTED_EDGE ( 'NONE', *, *, #72583, .F. ) ;
#179363=CARTESIAN_POINT ( 'NONE',  ( -5.533699252672048985, 9.607732894759390518, -0.7998128361456231517 ) ) ;
#179364=CARTESIAN_POINT ( 'NONE',  ( -4.249591082879585535, 7.045274465746411252, 1.199719254218464037 ) ) ;
#179374=CARTESIAN_POINT ( 'NONE',  ( 5.126954644262057492, 9.133197518281081173, 0.7998128361456462443 ) ) ;
#179388=CARTESIAN_POINT ( 'NONE',  ( -1.364683531250014514, 0.5510416670080878765, -0.7879004041258289570 ) ) ;
#179390=CARTESIAN_POINT ( 'NONE',  ( 3.818592820543298405, 7.606775390609172405, -0.7998128361456221525 ) ) ;
#179392=CARTESIAN_POINT ( 'NONE',  ( -5.233084105194862445, 9.049089189461916760, 0.7216878364870458196 ) ) ;
#179394=CARTESIAN_POINT ( 'NONE',  ( 5.097502569058200983, 6.970172302033127210, -1.443375672974051449 ) ) ;
#179395=CARTESIAN_POINT ( 'NONE',  ( -8.487040972030346353, 9.003895343564625620, 1.040834085586084257E-14 ) ) ;
#179399=CARTESIAN_POINT ( 'NONE',  ( 8.098297826064319693, 8.342435640030188893, 0.7998128361456481317 ) ) ;
#179404=CARTESIAN_POINT ( 'NONE',  ( 0.6823417656249899377, 5.176041667008086655, -1.181850606188754593 ) ) ;
#179408=CARTESIAN_POINT ( 'NONE',  ( 7.633404179693907388, 8.864391950186421454, -1.199719254218441611 ) ) ;
#179412=CARTESIAN_POINT ( 'NONE',  ( -8.311311860377216476, 9.655284244316948872, -1.199719254218446718 ) ) ;
#179417=CARTESIAN_POINT ( 'NONE',  ( 8.055515824813896941, 12.54985222892493368, 0.7998128361456462443 ) ) ;
#179420=CARTESIAN_POINT ( 'NONE',  ( -8.850775351622791831, 9.220326086515070685, -0.7998128361456291469 ) ) ;
#179424=CARTESIAN_POINT ( 'NONE',  ( 5.622931663646434153, 6.144404617744410046, -0.8283694935172694063 ) ) ;
#179425=CARTESIAN_POINT ( 'NONE',  ( -9.246297574839990929, 11.81043314211192019, 1.443375672974076540 ) ) ;
#179429=CARTESIAN_POINT ( 'NONE',  ( 6.419949431270806528, 7.448694743692793274, 1.199719254218462483 ) ) ;
#179431=CARTESIAN_POINT ( 'NONE',  ( 4.690231075323689325, 7.559354456931247412, 1.199719254218462483 ) ) ;
#179432=CARTESIAN_POINT ( 'NONE',  ( -4.217650912117239415, 7.357101779856191293, 0.8466403022913439047 ) ) ;
#179433=CARTESIAN_POINT ( 'NONE',  ( 5.007038802148489509, 4.735966778795008381, 0.7998128361456341429 ) ) ;
#179435=CARTESIAN_POINT ( 'NONE',  ( -6.887178846062123938, 8.097758744236356776, -1.082531754730544860 ) ) ;
#179441=CARTESIAN_POINT ( 'NONE',  ( -5.386593377506219582, 6.333579893170925068, 1.078181536478119762 ) ) ;
#179442=CARTESIAN_POINT ( 'NONE',  ( -1.402160292154681736E-14, -0.1156249996585793222, 1.575800808251672791 ) ) ;
#179445=CARTESIAN_POINT ( 'NONE',  ( 4.148431816101584957, 6.823292304551739740, -1.082531754730548412 ) ) ;
#179448=CARTESIAN_POINT ( 'NONE',  ( -8.297226821439000588, 12.62392235841345389, 1.040834085586084257E-14 ) ) ;
#179449=AXIS2_PLACEMENT_3D ( 'NONE', #52693, #135037, #136093 ) ;
#179454=CARTESIAN_POINT ( 'NONE',  ( -9.775065565328612038, 10.50659070241261794, -0.7216878364870267237 ) ) ;
#179458=EDGE_CURVE ( 'NONE', #201902, #188755, #157329, .T. ) ;
#179461=CARTESIAN_POINT ( 'NONE',  ( -7.904040366642703930, 10.24446639921506552, 1.443375672974090751 ) ) ;
#179465=CARTESIAN_POINT ( 'NONE',  ( 0.6823417656249899377, 5.738541667008087543, -1.181850606188754593 ) ) ;
#179466=CARTESIAN_POINT ( 'NONE',  ( -0.7499999999999972244, 3.389583334016149863, -1.299038105676652011 ) ) ;
#179467=CARTESIAN_POINT ( 'NONE',  ( 5.854153468347242040, 6.181931306435468620, -0.8879621099797951889 ) ) ;
#179469=CARTESIAN_POINT ( 'NONE',  ( -5.229694566569281555, 7.124396299129368337, 1.599625672291267398 ) ) ;
#179473=CARTESIAN_POINT ( 'NONE',  ( -8.290974629956718189, 9.631557475493025322, -1.199719254218446718 ) ) ;
#179477=CARTESIAN_POINT ( 'NONE',  ( 4.462605117192430804, 8.358123070033169455, 1.040834085586084257E-14 ) ) ;
#179484=CARTESIAN_POINT ( 'NONE',  ( 7.609150525767641504, 9.900428251527500834, -1.599625672291262513 ) ) ;
#179487=CYLINDRICAL_SURFACE ( 'NONE', #14784, 0.08000000000000041800 ) ;
#179490=CARTESIAN_POINT ( 'NONE',  ( -6.399085315970142851, 8.488685506763726352, -1.443375672974059665 ) ) ;
#179493=CARTESIAN_POINT ( 'NONE',  ( 1.364683531249988535, 5.217708333674750065, -0.7879004041258300672 ) ) ;
#179500=CARTESIAN_POINT ( 'NONE',  ( -9.775592450653132204, 11.36361159963886891, -1.199719254218441611 ) ) ;
#179503=CARTESIAN_POINT ( 'NONE',  ( 7.910292558569346433, 11.31609285405122556, -1.199719254218446718 ) ) ;
#179504=CARTESIAN_POINT ( 'NONE',  ( 1.436715752608449748, 7.421775496532144523, -4.237684949271973700 ) ) ;
#179505=CARTESIAN_POINT ( 'NONE',  ( -7.479294296233107708, 11.87759377891399204, 0.7998128361456481317 ) ) ;
#179508=CARTESIAN_POINT ( 'NONE',  ( -1.201851678989727383E-14, 4.071875000341425022, 1.575800808251672791 ) ) ;
#179509=EDGE_CURVE ( 'NONE', #184190, #62256, #35685, .T. ) ;
#179510=CARTESIAN_POINT ( 'NONE',  ( 4.532503425670185493, 4.182342172903648070, 1.214306433183764966E-14 ) ) ;
#179515=CARTESIAN_POINT ( 'NONE',  ( 8.066738210006668908, 12.35501897840907581, 0.7216878364870438212 ) ) ;
#179519=CARTESIAN_POINT ( 'NONE',  ( -6.209271165378811297, 10.18797409300986878, 0.7216878364870458196 ) ) ;
#179520=CARTESIAN_POINT ( 'NONE',  ( -1.364683531250014514, 1.238541667008091096, -0.7879004041258289570 ) ) ;
#179523=CARTESIAN_POINT ( 'NONE',  ( -7.426115451983156923, 9.686887332112256388, -1.599625672291263179 ) ) ;
#179524=CARTESIAN_POINT ( 'NONE',  ( -3.090895833791289071, 6.549869539491048442, 1.040834085586084257E-14 ) ) ;
#179525=CARTESIAN_POINT ( 'NONE',  ( -1.364683531249997417, 3.821875000341416584, 1.214306433183764966E-14 ) ) ;
#179542=CARTESIAN_POINT ( 'NONE',  ( -0.6823417656250212460, 4.613541667008086655, 1.181850606188767472 ) ) ;
#179547=CARTESIAN_POINT ( 'NONE',  ( 9.271078113646423091, 9.710679308875986848, 1.040834085586084257E-14 ) ) ;
#179550=CARTESIAN_POINT ( 'NONE',  ( -1.364683531250012516, 2.488541667008088876, -0.7879004041258289570 ) ) ;
#179552=CARTESIAN_POINT ( 'NONE',  ( -7.565086526745425033, 7.928281824065535055, 0.7216878364870317197 ) ) ;
#179554=CARTESIAN_POINT ( 'NONE',  ( 1.499999999999823475, 7.361490936993391188, 4.203511340218978987 ) ) ;
#179558=CARTESIAN_POINT ( 'NONE',  ( 2.354312230267378236, 5.898448035287240820, -0.7998128361456281477 ) ) ;
#179561=CARTESIAN_POINT ( 'NONE',  ( 8.055515824813896941, 12.54985222892493368, 0.7998128361456462443 ) ) ;
#179568=CARTESIAN_POINT ( 'NONE',  ( -10.15913717534155047, 10.74674821418697057, 0.7998128361456462443 ) ) ;
#179571=CARTESIAN_POINT ( 'NONE',  ( 6.286176778230493589, 10.48562334124426698, 0.7998128361456462443 ) ) ;
#179582=CARTESIAN_POINT ( 'NONE',  ( -5.585596099150191840, 7.539614753807099667, -1.443375672974052559 ) ) ;
#179583=CARTESIAN_POINT ( 'NONE',  ( 5.606460214450851964, 6.499623990736163037, 1.199719254218462483 ) ) ;
#179586=CARTESIAN_POINT ( 'NONE',  ( -8.995998617867369873, 10.45408546138876993, 1.199719254218462483 ) ) ;
#179588=FACE_OUTER_BOUND ( 'NONE', #141177, .T. ) ;
#179591=CARTESIAN_POINT ( 'NONE',  ( -8.109748439268576803, 12.61312361245537517, 0.7998128361456481317 ) ) ;
#179595=CARTESIAN_POINT ( 'NONE',  ( 9.921869487102386032, 10.46993591124128997, 0.000000000000000000 ) ) ;
#179607=CARTESIAN_POINT ( 'NONE',  ( -8.670602931139386627, 10.07445716020612103, 1.199719254218462483 ) ) ;
#179611=CARTESIAN_POINT ( 'NONE',  ( 7.212574532790092974, 9.437756259720353924, -1.443375672974057666 ) ) ;
#179614=CARTESIAN_POINT ( 'NONE',  ( 3.708318708537623021, 4.285125567170706695, -1.199719254218446718 ) ) ;
#179616=CARTESIAN_POINT ( 'NONE',  ( 3.493197133815315603, 7.227147089426516402, -0.7998128361456291469 ) ) ;
#179618=CARTESIAN_POINT ( 'NONE',  ( -7.413611068574208041, 7.543634422958360730, 0.7998128361456341429 ) ) ;
#179621=CARTESIAN_POINT ( 'NONE',  ( -1.500000000000058398, 7.360382131182438670, -4.205521753552950770 ) ) ;
#179628=CARTESIAN_POINT ( 'NONE',  ( -1.364683531250010295, 4.092708333674751842, 0.7879004041258379498 ) ) ;
#179629=LINE ( 'NONE', #147138, #5502 ) ;
#179630=CARTESIAN_POINT ( 'NONE',  ( 9.413438726589914651, 9.876766690643398405, 0.000000000000000000 ) ) ;
#179632=CARTESIAN_POINT ( 'NONE',  ( -4.622967192579922724, 4.495809267539077503, 1.214306433183764966E-14 ) ) ;
#179636=CARTESIAN_POINT ( 'NONE',  ( -5.897433631820158340, 5.982686779986042147, 0.7216878364870317197 ) ) ;
#179643=CARTESIAN_POINT ( 'NONE',  ( 9.490344339885973923, 12.09515436799890331, -1.443375672974057666 ) ) ;
#179651=CARTESIAN_POINT ( 'NONE',  ( 4.157546660884947620, 8.002221537674429896, 1.040834085586084257E-14 ) ) ;
#179656=CARTESIAN_POINT ( 'NONE',  ( 1.364683531249988535, 3.467708333674749621, -0.7879004041258239610 ) ) ;
#179661=CARTESIAN_POINT ( 'NONE',  ( 5.113396490648394632, 9.117379672398465473, 1.040834085586084257E-14 ) ) ;
#179663=CARTESIAN_POINT ( 'NONE',  ( -5.005985031943793295, 6.863401842066301661, -1.599625672291256295 ) ) ;
#179665=CARTESIAN_POINT ( 'NONE',  ( 1.499999999999989120, 2.025000000000019895, 1.214306433183764966E-14 ) ) ;
#179668=CARTESIAN_POINT ( 'NONE',  ( -4.948889764188092677, 5.732458465429559169, 1.199719254218462483 ) ) ;
#179671=CARTESIAN_POINT ( 'NONE',  ( 1.364683531249990311, 2.634375000341422801, 1.214306433183764966E-14 ) ) ;
#179673=CARTESIAN_POINT ( 'NONE',  ( -2.955314298098991266, 6.391691081183366485, 0.7216878364870317197 ) ) ;
#179678=CARTESIAN_POINT ( 'NONE',  ( 6.017121246366603060, 5.914396297049491658, 1.040834085586084257E-14 ) ) ;
#179683=CARTESIAN_POINT ( 'NONE',  ( -1.364683531250012516, 3.801041667008087099, -0.7879004041258300672 ) ) ;
#179687=CARTESIAN_POINT ( 'NONE',  ( -0.6823417656250246877, -0.1364583329919108468, 1.181850606188755259 ) ) ;
#179688=CARTESIAN_POINT ( 'NONE',  ( -4.303094902415906198, 7.389312076987425648, -1.073240500945132236 ) ) ;
#179691=CARTESIAN_POINT ( 'NONE',  ( -2.137381772448751605, 5.645362501165475777, -0.7998128361456281477 ) ) ;
#179692=CARTESIAN_POINT ( 'NONE',  ( -6.277061933002790362, 8.346324893301817482, 1.443375672974078761 ) ) ;
#179696=VERTEX_POINT ( 'NONE', #212440 ) ;
#179697=CARTESIAN_POINT ( 'NONE',  ( -1.364683531249997417, 4.259375000341424133, 1.214306433183764966E-14 ) ) ;
#179706=CARTESIAN_POINT ( 'NONE',  ( -6.249945625775490399, 7.354319987235250267, 1.082531754730549967 ) ) ;
#179709=EDGE_CURVE ( 'NONE', #55695, #132514, #128109, .T. ) ;
#179712=CARTESIAN_POINT ( 'NONE',  ( -6.846504384776774366, 7.089935991768773427, -0.7216878364870267237 ) ) ;
#179720=CARTESIAN_POINT ( 'NONE',  ( -9.828980619278564011E-14, 7.054063922337708625, 3.955400951015630273 ) ) ;
#179725=CARTESIAN_POINT ( 'NONE',  ( -4.497554271431319250, 6.270232621468402989, -1.599625672291256295 ) ) ;
#179728=CARTESIAN_POINT ( 'NONE',  ( -1.402160292154681736E-14, 0.5875000000000220046, -1.732050807568863648 ) ) ;
#179729=CARTESIAN_POINT ( 'NONE',  ( 9.490344339885973923, 12.09515436799890331, -1.443375672974057666 ) ) ;
#179730=CARTESIAN_POINT ( 'NONE',  ( 6.446011968293428041, 9.607765498729298415, -1.199719254218440723 ) ) ;
#179734=CARTESIAN_POINT ( 'NONE',  ( 3.845709127770629010, 7.638411082374393146, 0.7998128361456321445 ) ) ;
#179735=COLOUR_RGB ( '', 0.72549020, 0.75294118, 0.79215686) ;
#179741=CARTESIAN_POINT ( 'NONE',  ( -2.982430605326321427, 6.423326772948587227, -0.7216878364870267237 ) ) ;
#179743=CARTESIAN_POINT ( 'NONE',  ( 4.226925616482860804, 3.500738074553328527, -2.444828727306142202 ) ) ;
#179747=CARTESIAN_POINT ( 'NONE',  ( -1.201851678989727383E-14, 3.571875000341422357, 1.575800808251672791 ) ) ;
#179748=CARTESIAN_POINT ( 'NONE',  ( 10.35806617071623315, 11.18675807536486566, 0.000000000000000000 ) ) ;
#179749=CARTESIAN_POINT ( 'NONE',  ( -5.865874016206865882, 9.995270118883347266, 0.000000000000000000 ) ) ;
#179753=CARTESIAN_POINT ( 'NONE',  ( 6.518772930072240790, 6.499656594706071822, -0.7998128361456281477 ) ) ;
#179754=CARTESIAN_POINT ( 'NONE',  ( -6.632963465583701534, 8.761543347979550589, -1.599625672291263179 ) ) ;
#179755=CARTESIAN_POINT ( 'NONE',  ( -1.491528662501878655, 8.751894132169937279, 2.513572095680582041 ) ) ;
#179758=CARTESIAN_POINT ( 'NONE',  ( -1.500000000000013101, 0.4520833340161533598, 0.8660254037844403729 ) ) ;
#179762=CARTESIAN_POINT ( 'NONE',  ( 6.751597309925441159, 9.860318714012938912, -1.082531754730537088 ) ) ;
#179765=CARTESIAN_POINT ( 'NONE',  ( -0.6823417656250246877, 0.1135416670080893753, 1.181850606188755259 ) ) ;
#179767=CARTESIAN_POINT ( 'NONE',  ( 7.592202833528386208, 7.959917515312338487, 1.040834085586084257E-14 ) ) ;
#179769=CARTESIAN_POINT ( 'NONE',  ( -3.253593677599670109, 5.779314476299451719, 1.082531754730560403 ) ) ;
#179771=CARTESIAN_POINT ( 'NONE',  ( 0.6823417656249917140, 4.592708333674755394, 1.181850606188765695 ) ) ;
#179773=CARTESIAN_POINT ( 'NONE',  ( 1.500000000000007105, 10.64264068711930733, 1.214306433183764966E-14 ) ) ;
#179775=CARTESIAN_POINT ( 'NONE',  ( -5.057943438340505082, 6.748278329294532085, -1.445135742742007068 ) ) ;
#179781=CARTESIAN_POINT ( 'NONE',  ( 7.630541526392844887, 7.796719957080126662, 0.7998128361456341429 ) ) ;
#179784=CARTESIAN_POINT ( 'NONE',  ( 5.020596955762157698, 4.751784624677624080, 1.040834085586084257E-14 ) ) ;
#179792=CARTESIAN_POINT ( 'NONE',  ( 5.260200412422194383, 7.159986452624450770, -1.443375672974051449 ) ) ;
#179793=CARTESIAN_POINT ( 'NONE',  ( -1.364683531250014514, 1.301041667008083325, -0.7879004041258289570 ) ) ;
#179800=CARTESIAN_POINT ( 'NONE',  ( -1.500000000000001332, 1.400000000000019229, 0.000000000000000000 ) ) ;
#179801=CARTESIAN_POINT ( 'NONE',  ( 7.610204295972345712, 7.772993188256215547, 0.7998128361456341429 ) ) ;
#179802=CARTESIAN_POINT ( 'NONE',  ( -8.715193815486133033, 9.062147627688959872, 0.7998128361456462443 ) ) ;
#179806=CARTESIAN_POINT ( 'NONE',  ( 1.364683531249988757, 1.634375000341421691, 0.000000000000000000 ) ) ;
#179808=CARTESIAN_POINT ( 'NONE',  ( -1.500000000000013101, 2.879166666666688634, -0.8660254037844313801 ) ) ;
#179810=CARTESIAN_POINT ( 'NONE',  ( 3.171717870593107058, 5.787755718078879674, -1.199719254218446718 ) ) ;
#179817=CARTESIAN_POINT ( 'NONE',  ( 0.7499999999999885647, 1.097916667349485564, -1.299038105676652899 ) ) ;
#179818=CARTESIAN_POINT ( 'NONE',  ( -6.612626235163205024, 8.737816579155630592, -1.599625672291263179 ) ) ;
#179819=CARTESIAN_POINT ( 'NONE',  ( -4.039966587192274083, 5.736380323189513852, 1.443375672974064550 ) ) ;
#179826=CARTESIAN_POINT ( 'NONE',  ( 5.615048174354031474, 9.702639970055050966, 0.7998128361456462443 ) ) ;
#179830=CARTESIAN_POINT ( 'NONE',  ( 5.445571254183207088, 9.504916896522420444, -0.7998128361456281477 ) ) ;
#179831=CARTESIAN_POINT ( 'NONE',  ( 9.205623113554624481, 10.80261038964432707, 1.082531754730549967 ) ) ;
#179836=CARTESIAN_POINT ( 'NONE',  ( -6.181627972826976958, 9.299317504018391745, 1.199719254218452047 ) ) ;
#179837=CARTESIAN_POINT ( 'NONE',  ( 3.818592820543298405, 7.606775390609172405, -0.7998128361456221525 ) ) ;
#179840=CARTESIAN_POINT ( 'NONE',  ( 4.324073113486339714, 7.195437805949965515, 1.011975886212188813 ) ) ;
#179841=CARTESIAN_POINT ( 'NONE',  ( 8.378575743565351175, 11.75846021992619406, -1.082531754730543083 ) ) ;
#179842=VERTEX_POINT ( 'NONE', #27299 ) ;
#179848=CARTESIAN_POINT ( 'NONE',  ( -1.499999999999997780, 3.681250000682819046, 1.214306433183764966E-14 ) ) ;
#179851=CARTESIAN_POINT ( 'NONE',  ( -2.318081078256692518, 5.648252324700675508, 1.040834085586084257E-14 ) ) ;
#179852=CARTESIAN_POINT ( 'NONE',  ( 8.161645285746708112, 9.584636257201740506, -1.082531754730543083 ) ) ;
#179855=CARTESIAN_POINT ( 'NONE',  ( -6.403528624356093601, 6.365204904703887223, 1.040834085586084257E-14 ) ) ;
#179856=DIRECTION ( 'NONE',  ( 1.000000000000000000, 0.000000000000000000, 0.000000000000000000 ) ) ;
#179860=CARTESIAN_POINT ( 'NONE',  ( -6.449928391799210736, 8.548002428564306143, -1.599625672291263179 ) ) ;
#179865=VERTEX_POINT ( 'NONE', #64082 ) ;
#179876=CARTESIAN_POINT ( 'NONE',  ( -6.905180308061733996, 6.950465202360470052, 0.7998128361456341429 ) ) ;
#179879=CARTESIAN_POINT ( 'NONE',  ( 5.355107487717867265, 5.349972945200037522, 1.040834085586084257E-14 ) ) ;
#179880=ORIENTED_EDGE ( 'NONE', *, *, #158684, .T. ) ;
#179881=CARTESIAN_POINT ( 'NONE',  ( 3.701970883082871921, 7.364863713882360052, 2.499999999999999556 ) ) ;
#179882=CYLINDRICAL_SURFACE ( 'NONE', #51246, 1.250000000000000000 ) ;
#179884=CARTESIAN_POINT ( 'NONE',  ( -3.541704441667874903, 5.155074486744371853, -1.599625672291256295 ) ) ;
#179886=LINE ( 'NONE', #31510, #181446 ) ;
#179887=CARTESIAN_POINT ( 'NONE',  ( 9.565441069641300587, 11.11843498845840905, -1.199719254218440723 ) ) ;
#179891=CARTESIAN_POINT ( 'NONE',  ( -7.018317073368468328, 11.33978701890523233, -0.7998128361456291469 ) ) ;
#179892=CARTESIAN_POINT ( 'NONE',  ( 6.810273232766058449, 6.839740281182199233, 1.040834085586084257E-14 ) ) ;
#179898=CARTESIAN_POINT ( 'NONE',  ( 0.6823417656249882723, 1.988541667008083991, -1.181850606188749264 ) ) ;
#179901=CARTESIAN_POINT ( 'NONE',  ( 7.673551755654734130, 9.015193805427763607, -1.082531754730537976 ) ) ;
#179903=CARTESIAN_POINT ( 'NONE',  ( -4.528060117284247177, 6.305822774963486310, 1.443375672974064550 ) ) ;
#179908=CARTESIAN_POINT ( 'NONE',  ( 8.541273586484978253, 12.90864358430044589, 0.000000000000000000 ) ) ;
#179915=CARTESIAN_POINT ( 'NONE',  ( -4.559605246071217088, 3.300000000000025135, 0.7750000000000135669 ) ) ;
#179917=CARTESIAN_POINT ( 'NONE',  ( -10.10098813738111545, 11.74323990082152491, -1.199719254218441611 ) ) ;
#179929=CARTESIAN_POINT ( 'NONE',  ( 0.7499999999999885647, 0.3479166673494848983, -1.299038105676652899 ) ) ;
#179933=VERTEX_POINT ( 'NONE', #142078 ) ;
#179935=CARTESIAN_POINT ( 'NONE',  ( 1.499999999999987566, -0.7249999999999825473, 0.000000000000000000 ) ) ;
#179936=CARTESIAN_POINT ( 'NONE',  ( 6.889514614038635187, 11.18951748302043114, -0.7998128361456291469 ) ) ;
#179938=CARTESIAN_POINT ( 'NONE',  ( 1.364683531249986537, -1.136458332991912235, 0.7879004041258500513 ) ) ;
#179941=CARTESIAN_POINT ( 'NONE',  ( 4.220665892555866883, 3.818531717603609987, -0.7998128361456211532 ) ) ;
#179942=CARTESIAN_POINT ( 'NONE',  ( -5.748293942514169252, 9.650167333001109071, -0.7216878364870207285 ) ) ;
#179947=CARTESIAN_POINT ( 'NONE',  ( -6.989391883044787868, 8.113044270762433285, -1.199719254218446718 ) ) ;
#179950=CARTESIAN_POINT ( 'NONE',  ( -1.500000000000001332, 0.6812500006828161592, 0.000000000000000000 ) ) ;
#179958=CARTESIAN_POINT ( 'NONE',  ( -4.256897044566581911, 4.068727428190179296, 1.214306433183764966E-14 ) ) ;
#179961=CARTESIAN_POINT ( 'NONE',  ( 4.799922300691145338, 6.743925459469453543, 1.247687964948118733 ) ) ;
#179967=CARTESIAN_POINT ( 'NONE',  ( -8.631737353394710155, 13.22211067893587533, 1.040834085586084257E-14 ) ) ;
#179968=CARTESIAN_POINT ( 'NONE',  ( 9.094822116668764167, 9.505047312402055582, 0.7998128361456462443 ) ) ;
#179976=CARTESIAN_POINT ( 'NONE',  ( -7.974166903131914452, 12.45494515362926435, -0.7998128361456281477 ) ) ;
#179981=CARTESIAN_POINT ( 'NONE',  ( 5.190073875932979419, 4.949507698210251938, 0.7998128361456341429 ) ) ;
#179986=CARTESIAN_POINT ( 'NONE',  ( -9.297140650669053485, 11.86975006391249643, 1.599625672291281386 ) ) ;
#179998=CARTESIAN_POINT ( 'NONE',  ( 7.579171565239241737, 8.801120566655981747, 1.199719254218462483 ) ) ;
#180000=CARTESIAN_POINT ( 'NONE',  ( -3.598799709423620374, 6.286017863381107240, 1.199719254218464037 ) ) ;
#180004=CARTESIAN_POINT ( 'NONE',  ( 3.469446951953614189E-15, 6.400000000000023448, 1.214306433183764966E-14 ) ) ;
#180008=CARTESIAN_POINT ( 'NONE',  ( -0.7500000000000006661, -0.1104166659838465292, -1.299038105676652011 ) ) ;
#180013=CARTESIAN_POINT ( 'NONE',  ( 3.192055101013606233, 5.811482486902795230, -1.199719254218446718 ) ) ;
#180015=CARTESIAN_POINT ( 'NONE',  ( -2.774614992291035698, 6.388801257648172971, 1.040834085586084257E-14 ) ) ;
#180021=CARTESIAN_POINT ( 'NONE',  ( 3.877268743828266029, 6.506935386899531437, 1.082531754730558626 ) ) ;
#180023=ORIENTED_EDGE ( 'NONE', *, *, #100231, .T. ) ;
#180024=CARTESIAN_POINT ( 'NONE',  ( -9.001723924469462901, 12.58942944760136484, -1.199719254218446718 ) ) ;
#180026=CARTESIAN_POINT ( 'NONE',  ( 3.009546912109283934, 6.454962464195385330, 0.000000000000000000 ) ) ;
#180034=CARTESIAN_POINT ( 'NONE',  ( -5.460715490240072079, 6.444878312648672392, 1.304320558087665782 ) ) ;
#180036=CARTESIAN_POINT ( 'NONE',  ( -0.6823417656250003738, -0.03229166632524871350, -1.181850606188749264 ) ) ;
#180044=CARTESIAN_POINT ( 'NONE',  ( 1.499999999999990896, 5.025000000000022560, 1.214306433183764966E-14 ) ) ;
#180052=CARTESIAN_POINT ( 'NONE',  ( -0.6823417656250246877, -0.9489583329919115684, 1.181850606188755259 ) ) ;
#180054=CARTESIAN_POINT ( 'NONE',  ( 7.298366762858032430, 7.409182732956175244, 1.040834085586084257E-14 ) ) ;
#180055=CARTESIAN_POINT ( 'NONE',  ( -8.688077508258798431, 9.030511935923748013, -0.7998128361456291469 ) ) ;
#180060=ORIENTED_EDGE ( 'NONE', *, *, #55029, .F. ) ;
#180062=CARTESIAN_POINT ( 'NONE',  ( -0.6823417656250246877, -0.6364583329919113464, 1.181850606188755259 ) ) ;
#180069=CARTESIAN_POINT ( 'NONE',  ( 7.619319141200063150, 9.912291636198670375, 1.443375672974076540 ) ) ;
#180074=CARTESIAN_POINT ( 'NONE',  ( 1.499999999999989120, 4.827083334016149863, -0.8660254037844323793 ) ) ;
#180076=CARTESIAN_POINT ( 'NONE',  ( -5.251085567194491155, 5.020688004682002159, -0.7998128361456221525 ) ) ;
#180077=CARTESIAN_POINT ( 'NONE',  ( 5.572037945092146671, 8.484166121707415797, -1.082531754730543971 ) ) ;
#180085=CARTESIAN_POINT ( 'NONE',  ( 4.521807925357579805, 5.234196320127330715, -1.199719254218452047 ) ) ;
#180092=CARTESIAN_POINT ( 'NONE',  ( 7.730120138085914583, 12.17022392774227768, 0.7998128361456462443 ) ) ;
#180101=CARTESIAN_POINT ( 'NONE',  ( 9.348510611822643313, 10.86534945433664134, 1.199719254218453823 ) ) ;
#180107=CARTESIAN_POINT ( 'NONE',  ( -0.6823417656250003738, -0.03229166632524871350, -1.181850606188749264 ) ) ;
#180108=CARTESIAN_POINT ( 'NONE',  ( 5.992340707560160240, 7.053780915984068756, 1.082531754730558626 ) ) ;
#180109=CARTESIAN_POINT ( 'NONE',  ( -8.351459436338030784, 11.72682452816096976, -1.082531754730543971 ) ) ;
#180114=CARTESIAN_POINT ( 'NONE',  ( -2.578021764892882040, 6.159442492350315490, 0.7998128361456341429 ) ) ;
#180127=CARTESIAN_POINT ( 'NONE',  ( 5.490304984925487908, 6.429369728800919503, -1.257259817782523381 ) ) ;
#180129=ORIENTED_EDGE ( 'NONE', *, *, #126913, .F. ) ;
#180135=CARTESIAN_POINT ( 'NONE',  ( -7.022760382198764084, 11.13704484596649635, 0.7216878364870458196 ) ) ;
#180139=CARTESIAN_POINT ( 'NONE',  ( 7.786460292950004636, 7.978625184730144149, 1.040834085586084257E-14 ) ) ;
#180140=CARTESIAN_POINT ( 'NONE',  ( -3.924195396151603177, 6.665646164563756138, 1.199719254218464037 ) ) ;
#180144=CARTESIAN_POINT ( 'NONE',  ( -5.599681137644054729, 6.491715067794862293, 1.199719254218450271 ) ) ;
#180145=CARTESIAN_POINT ( 'NONE',  ( 3.816783937446950770, 4.411668334231586996, 1.199719254218464037 ) ) ;
#180148=CARTESIAN_POINT ( 'NONE',  ( -4.934277840369690971, 7.844075682818238526, -1.199719254218452047 ) ) ;
#180151=CARTESIAN_POINT ( 'NONE',  ( 9.348510611822643313, 10.86534945433664134, 1.199719254218453823 ) ) ;
#180154=CARTESIAN_POINT ( 'NONE',  ( 4.388746605030885206, 7.362284722717403085, 1.177686187499202619 ) ) ;
#180155=CARTESIAN_POINT ( 'NONE',  ( 5.504247177468186258, 6.484338464210099851, 1.082531754730558626 ) ) ;
#180157=DIRECTION ( 'NONE',  ( -7.387867266669436732E-31, -1.000000000000000000, 8.546850786086437571E-32 ) ) ;
#180162=CARTESIAN_POINT ( 'NONE',  ( 6.439759776366758892, 10.45687747249582955, 0.7216878364870438212 ) ) ;
#180166=CARTESIAN_POINT ( 'NONE',  ( -8.272446282632566650, 12.80293776304669962, 0.7998128361456481317 ) ) ;
#180167=CARTESIAN_POINT ( 'NONE',  ( -8.064402442030170093, 8.302891025323665630, 0.7998128361456602331 ) ) ;
#180175=CARTESIAN_POINT ( 'NONE',  ( 7.404724451357931336, 11.79059562655963056, 0.7998128361456462443 ) ) ;
#180182=CARTESIAN_POINT ( 'NONE',  ( 4.518945272056516416, 4.166524327021037699, 0.7998128361456341429 ) ) ;
#180186=CARTESIAN_POINT ( 'NONE',  ( -1.500000000000011324, 5.660416667349481123, -0.8660254037844313801 ) ) ;
#180193=CARTESIAN_POINT ( 'NONE',  ( 1.499999999999987121, 3.295833333333354709, -0.8660254037844262731 ) ) ;
#180194=CARTESIAN_POINT ( 'NONE',  ( 5.392392409933256303, 7.314210449720692786, 1.599625672291267398 ) ) ;
#180197=CARTESIAN_POINT ( 'NONE',  ( 7.076992996653421741, 10.23994701519558781, -1.082531754730537976 ) ) ;
#180198=CARTESIAN_POINT ( 'NONE',  ( -9.991996023147281747, 11.72004545083573568, 1.082531754730558626 ) ) ;
#180201=CARTESIAN_POINT ( 'NONE',  ( 8.041957671200231417, 12.53403438304231976, 1.040834085586084257E-14 ) ) ;
#180203=CARTESIAN_POINT ( 'NONE',  ( -2.605138072120212200, 6.191078184115536232, -0.7998128361456281477 ) ) ;
#180204=CARTESIAN_POINT ( 'NONE',  ( -0.7499999999999972244, 4.639583334016150751, -1.299038105676652899 ) ) ;
#180205=CARTESIAN_POINT ( 'NONE',  ( -1.364683531250014514, -0.7197916663252461600, 0.7879004041258379498 ) ) ;
#180209=CARTESIAN_POINT ( 'NONE',  ( 5.359550796103802028, 5.147230771742885125, -0.7998128361456231517 ) ) ;
#180211=CARTESIAN_POINT ( 'NONE',  ( -1.364683531249997417, 4.821875000341417916, 1.214306433183764966E-14 ) ) ;
#180213=CARTESIAN_POINT ( 'NONE',  ( 10.18233705906309972, 11.83814697611718714, 1.199719254218450271 ) ) ;
#180220=CARTESIAN_POINT ( 'NONE',  ( -7.711890448074853133, 7.891627032375787998, -0.7998128361456291469 ) ) ;
#180222=CARTESIAN_POINT ( 'NONE',  ( 6.193377243344257543, 6.120028293523423812, -0.7998128361456281477 ) ) ;
#180225=CARTESIAN_POINT ( 'NONE',  ( -0.6823417656250003738, 0.2177083336747515085, -1.181850606188749264 ) ) ;
#180229=CARTESIAN_POINT ( 'NONE',  ( 8.401248741962376698, 12.95320729893149370, 0.7998128361456462443 ) ) ;
#180232=CARTESIAN_POINT ( 'NONE',  ( -7.230575994789712801, 7.330093503543126054, 0.7998128361456341429 ) ) ;
#180236=CARTESIAN_POINT ( 'NONE',  ( 8.565000355531088516, 11.01558638625153286, -1.599625672291257406 ) ) ;
#180238=CARTESIAN_POINT ( 'NONE',  ( 6.740374924288304648, 11.01552117831172062, 1.040834085586084257E-14 ) ) ;
#180240=CARTESIAN_POINT ( 'NONE',  ( -8.012505595996376684, 12.29174759539704986, 0.000000000000000000 ) ) ;
#180241=CARTESIAN_POINT ( 'NONE',  ( -7.542413527904030524, 7.693903958843159252, 1.040834085586084257E-14 ) ) ;
#180244=CARTESIAN_POINT ( 'NONE',  ( -4.022959435666734862, 7.784601250164370434, 0.4788606935734913694 ) ) ;
#180245=CARTESIAN_POINT ( 'NONE',  ( 0.6823417656249882723, 0.1760416670080894308, -1.181850606188749264 ) ) ;
#180249=CARTESIAN_POINT ( 'NONE',  ( 6.887178846062110615, 9.058127958537705027, -1.443375672974057666 ) ) ;
#180252=CARTESIAN_POINT ( 'NONE',  ( 4.924636110261782385, 6.768494766770632332, 1.599625672291267398 ) ) ;
#180273=CARTESIAN_POINT ( 'NONE',  ( -4.086893239515592136, 6.855460315155083251, 1.199719254218464037 ) ) ;
#180274=CARTESIAN_POINT ( 'NONE',  ( -7.507464373665155399, 9.781794407407920389, 1.599625672291295375 ) ) ;
#180280=EDGE_CURVE ( 'NONE', #2091, #119510, #30770, .T. ) ;
#180281=CARTESIAN_POINT ( 'NONE',  ( -1.201851678989727383E-14, 2.993750000682821266, 1.732050807568877637 ) ) ;
#180282=CARTESIAN_POINT ( 'NONE',  ( 7.540305987494599016, 11.94877408538573427, -0.7998128361456291469 ) ) ;
#180286=CARTESIAN_POINT ( 'NONE',  ( -7.883176251342026042, 11.28445716228600126, -1.199719254218446718 ) ) ;
#180288=CARTESIAN_POINT ( 'NONE',  ( 1.364683531249990311, 2.884375000341422801, 1.214306433183764966E-14 ) ) ;
#180291=CARTESIAN_POINT ( 'NONE',  ( 1.499999999999990896, 4.275000000000021672, 1.214306433183764966E-14 ) ) ;
#180293=CARTESIAN_POINT ( 'NONE',  ( -9.002250809794000830, 11.52571191622492464, -1.443375672974059665 ) ) ;
#180297=CARTESIAN_POINT ( 'NONE',  ( -0.6823417656250003738, 1.530208333674752730, -1.181850606188749264 ) ) ;
#180298=CIRCLE ( 'NONE', #104228, 6.961139734775127152 ) ;
#180303=CARTESIAN_POINT ( 'NONE',  ( -1.201851678989727383E-14, 3.321875000341421025, 1.575800808251672791 ) ) ;
#180305=CARTESIAN_POINT ( 'NONE',  ( -4.388035272317281077, 8.271124917678806199, 0.7998128361456481317 ) ) ;
#180306=CARTESIAN_POINT ( 'NONE',  ( 6.262976894508937242, 9.394224579314053969, -1.199719254218440723 ) ) ;
#180310=CARTESIAN_POINT ( 'NONE',  ( 0.6823417656249882723, 2.988541667008084879, -1.181850606188754593 ) ) ;
#180313=CARTESIAN_POINT ( 'NONE',  ( -4.284013352238255301, 6.981470763377843447, -1.082531754730549967 ) ) ;
#180314=CARTESIAN_POINT ( 'NONE',  ( -5.097502569058215194, 6.970172302033127210, -1.443375672974053447 ) ) ;
#180317=CARTESIAN_POINT ( 'NONE',  ( 5.992340707560163793, 6.093411701682730275, 0.7216878364870317197 ) ) ;
#180320=CARTESIAN_POINT ( 'NONE',  ( -6.855619230004478482, 11.14997286831390788, -0.7998128361456291469 ) ) ;
#180321=CARTESIAN_POINT ( 'NONE',  ( -2.428882075142555497, 5.985446187641602300, 1.040834085586084257E-14 ) ) ;
#180326=CARTESIAN_POINT ( 'NONE',  ( -7.836249598574384301, 8.244638741199329601, 1.040834085586084257E-14 ) ) ;
#180328=CARTESIAN_POINT ( 'NONE',  ( -1.402160292154681736E-14, -0.2406249996585799189, -1.575800808251665908 ) ) ;
#180331=CARTESIAN_POINT ( 'NONE',  ( 8.649738815838679429, 10.15407870897571563, -1.082531754730543083 ) ) ;
#180342=CARTESIAN_POINT ( 'NONE',  ( 8.798878505144646311, 11.28844422746735532, -1.443375672974052559 ) ) ;
#180348=CARTESIAN_POINT ( 'NONE',  ( 4.950698647284403009, 8.927565521807144577, 1.040834085586084257E-14 ) ) ;
#180349=CARTESIAN_POINT ( 'NONE',  ( -5.413783410558481002, 5.210502155273325720, -0.7998128361456221525 ) ) ;
#180353=CARTESIAN_POINT ( 'NONE',  ( 6.765155463094761679, 6.995028916473103209, 0.7216878364870317197 ) ) ;
#180354=CARTESIAN_POINT ( 'NONE',  ( 1.364683531249988757, 0.9468750003414211358, 0.000000000000000000 ) ) ;
#180356=CARTESIAN_POINT ( 'NONE',  ( -8.839026081105473054, 12.39961529701003684, -1.199719254218446718 ) ) ;
#180362=( BOUNDED_SURFACE ( )  B_SPLINE_SURFACE ( 1, 2, ( 
 ( #201891, #50351, #100163, #166227, #19958, #169426, #184593, #38359, #18890, #84974, #35143, #103364, #16757, #151065, #101219, #17817, #2628, #153178, #83901, #116471, #3689, #68700, #134822, #490, #51422, #70827, #167303, #34092, #53543, #82840, #67624, #21009, #148916, #182463, #133768, #198706, #200827, #199776, #52478, #36211, #117543, #186737, #66558, #102290, #183537, #168363, #4752, #86043, #119675, #152118, #69766, #135872, #185661, #136944, #37291, #132700, #202970, #54611, #120759, #42659, #104437, #172645, #188873, #105521, #90323, #92480, #39428, #55673, #157466, #156392, #7978, #154254, #205107, #10118, #40513, #187799, #207254, #192059, #23151, #108768, #170486, #121829, #171555, #138010, #74067, #89266, #206183, #123973, #155316, #126099, #22070, #106616, #204025, #6900, #158521, #107701, #189940, #72977, #71901, #88182, #24221, #41589, #140159, #57810, #56749, #139080, #25304, #122915, #76193, #173727, #91406, #9060, #5827, #75136, #141245, #58882, #125037, #190993, #174793, #26369, #59943, #142302, #208313, #30667, #93538, #212586, #177979, #129317, #109837, #62090, #162800, #31732, #130367, #161734, #28518, #96750, #15444, #211515, #95680, #94609, #160652, #110898, #176904, #47998, #61016, #147614, #146568, #97805, #12250, #194212, #128248, #79399, #78327, #144449, #210452, #45857, #143373, #175849, #77259, #111979, #29594, #13325, #145516, #159582, #44792, #63152, #131405, #195292, #46924, #113042, #179048, #14377, #196357, #163867, #27440, #80467, #64225, #114115, #180108, #209372, #11180, #127174, #81533, #213632, #65258, #43722, #193143, #198461, #199527, #70581, #33840, #51171, #150818, #117294, #183291, #69522, #185418, #49046, #18649, #19720, #82588, #132459, #50105, #52235, #201649, #2380, #197405, #34896, #100969, #67380, #135629, #115166, #167058, #133521, #116225, #84729, #37036, #182217, #148675, #35973, #68458, #134587, #32784, #83652, #103120, #200587, #66315, #85799, #181161, #99921, #53299, #98861, #243, #165982, #16506, #118362, #17568, #184351, #102052, #149741, #4509, #164913, #168119, #1319, #151878, #169178, #3453, #119431, #20770, #86866, #152931, #138835, #156149, #72738, #40260, #22903, #171309, #57572, #39184, #42412, #7731, #104193, #105272, #38121, #5574, #41343, #106372, #172395, #90086, #73816, #170241, #92232, #157214, #187555, #123730, #186489, #91158, #56505, #139909, #202722, #155072, #107452, #124788, #8810, #23983, #121584, #189692, #108517, #205940, #188629, #89019, #6661, #203786, #55432, #140996, #154007, #26121, #25056, #190748, #204851, #122667, #173479, #74888, #207004, #58635, #21825, #71654, #174546, #158283, #9873, #136697, #54375, #87934, #120512, #137768, #126921, #62887, #125854, #30412, #210197, #161484, #142051, #94358, #195030, #63960, #162546, #193953, #60761, #129056, #47741, #29338, #127999, #192879, #44534, #143128, #209124, #80207, #93294, #179852, #178796, #130115, #110652, #12002, #160400, #111718, #176653, #28266, #78076, #144201, #175598, #208066, #109593, #61833, #45601, #177726, #95431, #191811, #77002, #13062, #163607, #79141, #145258, #211263, #46664, #112785, #14116, #196105, #59691, #96496, #146308, #27188, #10926, #212322, #113857, #31475, #97550, #75949, #43475, #159330, #99656, #167853, #15189, #83391, #165725, #16243, #1058, #3183, #164661, #180901, #68190, #67123, #133256, #65007, #115966, #135371, #17313, #98600, #118104, #102856, #148421, #19451, #81280, #32524, #82329, #48787, #199262, #93774, #117035, #34646, #66053, #36770, #147356, #149475, #114904, #132197, #69254, #18387, #100716, #198204, #197150, #213383, #50907, #166793, #183030, #84464, #181955, #49839, #150556, #33583, #201389, #2116, #134323, #131159, #85527, #200329, #184089, #51979, #35708, #101785, #151616, #53027, #119160, #185146, #124522, #168912, #137500, #205665, #58368, #187291, #203517, #54106, #42138, #190479, #70319, #20515, #121316, #206737, #154805, #71388, #6391, #171041, #202452, #90887, #155873, #72464, #55171, #156946, #8537, #86600, #153739, #4250, #5307, #21561, #74619, #140724, #37850, #73541, #152666, #120241, #136436, #107178 ),
 ( #103928, #169973, #23718, #173204, #122396, #186219, #22640, #88748, #38918, #24784, #87667, #138564, #105002, #204585, #56236, #188354, #39994, #106102, #7462, #172124, #89825, #139643, #57303, #123466, #189429, #41071, #210985, #195828, #26914, #112506, #108253, #59425, #125583, #141793, #94090, #43208, #209920, #127724, #159064, #129845, #25849, #110383, #207797, #191543, #96217, #111446, #193683, #109324, #75683, #174274, #176388, #45327, #44260, #11728, #208854, #142850, #29065, #10660, #13855, #177451, #175331, #76732, #9606, #93023, #12786, #77804, #162268, #91958, #60485, #158018, #126643, #192608, #79931, #146037, #27993, #78860, #160129, #143925, #61558, #46389, #95148, #161200, #144981, #62613, #128775, #194752, #178518, #30128, #212051, #63691, #17045, #14913, #99397, #135115, #151356, #35444, #181686, #165450, #83124, #98328, #117843, #15977, #82062, #34378, #47466, #163333, #49569, #149204, #18115, #50637, #130891, #48523, #183835, #85270, #132990, #114643, #213119, #33316, #67918, #101523, #147095, #66846, #51721, #167593, #779, #182760, #2925, #198990, #19192, #115693, #197941, #81007, #116763, #180636, #68998, #32260, #100451, #64749, #113581, #134063, #166524, #84202, #179583, #196885, #65781, #31205, #150291, #97279, #1858, #148154, #200072, #164394, #131931, #214155, #90359, #36513, #20258, #189973, #91440, #52769, #59979, #206217, #92517, #106650, #140195, #118905, #24254, #10153, #102599, #8012, #159619, #201131, #172677, #26405, #93574, #74103, #156426, #86342, #77297, #11216, #168654, #184889, #57843, #27476, #41623, #124006, #107737, #173762, #152414, #126133, #191030, #25339, #157501, #192093, #3993, #9096, #75172, #202193, #141282, #43760, #136174, #70062, #42697, #207290, #58916, #53849, #125073, #109873, #108803, #122947, #158556, #188904, #40546, #208348, #174828, #76227, #142338, #175886, #129348, #78360, #30702, #162834, #194246, #164946, #61050, #145551, #28554, #12282, #131436, #146599, #14412, #144481, #110932, #16538, #211548, #80502, #79433, #46957, #29629, #178011, #64257, #45890, #49079, #212617, #176937, #112011, #44827, #210487, #48033, #113074, #179080, #96783, #130400, #94643, #98893, #163902, #95714, #196390, #193178, #97837, #63183, #114147, #209405, #161768, #180139, #197439, #15478, #31767, #128284, #81562, #115199, #147646, #195326, #13359, #213664, #62124, #65289, #181192, #160687, #32819, #143409, #127210, #51204, #18682, #101002, #118393, #117326, #67411, #1349, #199560, #182248, #148705, #116259, #183324, #133552, #34928, #167091, #198492, #83685, #84761, #170272, #150848, #2412, #36000, #68489, #134617, #169211, #70613, #274, #184381, #119461, #33873, #17601, #149774, #151908, #86898, #102081, #82620, #200619, #52266, #168149, #20802, #19749, #85829, #3482, #69549, #50136, #135659, #201682, #66346, #53328, #185449, #37069, #103150, #152965, #4539, #136728, #132490, #202752, #54405, #99951, #120544, #186523, #38153, #104225, #166015, #109629, #90116, #156182, #106401, #174579, #21857, #7760, #172425, #22935, #73849, #9906, #171341, #187587, #74918, #139944, #205970, #71686, #122699, #142085, #24014, #105304, #124816, #87964, #155108, #26155, #154038, #39213, #89051, #55463, #57602, #6693, #123761, #41376, #72768, #43508, #5604, #189722, #121618, #138867, #75982, #25084, #107486, #204885, #203818, #137799, #173511, #91186, #157247, #8840, #188662, #56537, #141029, #40291, #208100, #207036, #58666, #190780, #42443, #108547, #92269, #158315, #59728, #125887, #191845, #209158, #131197, #196139, #12037, #162578, #10960, #130149, #95468, #46702, #27220, #193986, #80246, #163644, #47779, #79178, #160431, #14152, #147391, #129091, #13098, #78108, #144235, #28296, #94392, #179887, #192914, #65041, #63998, #15225, #210229, #111751, #45634, #211299, #61867, #128032, #177757, #29373, #60796, #93326, #126955, #176684, #30445, #31511, #195063, #48822, #161516, #145294, #62923, #113893, #175634, #112818, #178831, #96529, #146344, #81315, #110686, #44570, #212357, #97586, #213418, #77035, #197185, #159362, #143163, #198240, #3223, #202492, #33622, #119198, #114938, #66089 ) ),
 .UNSPECIFIED., .F., .F., .F. ) 
 B_SPLINE_SURFACE_WITH_KNOTS ( ( 2, 2 ),
 ( 3, 2, 2, 2, 2, 2, 2, 2, 2, 2, 2, 2, 2, 2, 2, 2, 2, 2, 2, 2, 2, 2, 2, 2, 2, 2, 2, 2, 2, 2, 2, 2, 2, 2, 2, 2, 2, 2, 2, 2, 2, 2, 2, 2, 2, 2, 2, 2, 2, 2, 2, 2, 2, 2, 2, 2, 2, 2, 2, 2, 2, 2, 2, 2, 2, 2, 2, 2, 2, 2, 2, 2, 2, 2, 2, 2, 2, 2, 2, 2, 2, 2, 2, 2, 2, 2, 2, 2, 2, 2, 2, 2, 2, 2, 2, 2, 2, 2, 2, 2, 2, 2, 2, 2, 2, 2, 2, 2, 2, 2, 2, 2, 2, 2, 2, 2, 2, 2, 2, 2, 2, 2, 2, 2, 2, 2, 2, 2, 2, 2, 2, 2, 2, 2, 2, 2, 2, 2, 2, 2, 2, 2, 2, 2, 2, 2, 2, 2, 2, 2, 2, 2, 2, 2, 2, 2, 2, 2, 2, 2, 2, 2, 2, 2, 2, 2, 2, 2, 2, 2, 2, 2, 2, 2, 2, 2, 2, 2, 2, 2, 2, 2, 2, 2, 2, 2, 2, 2, 2, 2, 2, 2, 2, 2, 2, 2, 2, 2, 2, 2, 2, 2, 2, 2, 2, 2, 2, 2, 2, 2, 2, 2, 2, 2, 2, 2, 2, 2, 2, 2, 2, 2, 2, 2, 2, 2, 2, 2, 2, 2, 2, 2, 2, 2, 2, 2, 2, 2, 2, 2, 3 ),
 ( 0.000000000000000000, 1.000000000000000000 ),
 ( 0.000000000000000000, 0.004166666666666666609, 0.008333333333333333218, 0.01250000000000000069, 0.01666666666666666644, 0.02083333333333333218, 0.02500000000000000139, 0.02916666666666666713, 0.03333333333333333287, 0.03749999999999999861, 0.04166666666666666435, 0.04583333333333333010, 0.05000000000000000278, 0.05416666666666666852, 0.05833333333333333426, 0.06250000000000000000, 0.06666666666666666574, 0.07083333333333333148, 0.07499999999999999722, 0.07916666666666666297, 0.08333333333333332871, 0.08749999999999999445, 0.09166666666666666019, 0.09583333333333333981, 0.1000000000000000056, 0.1041666666666666713, 0.1083333333333333370, 0.1125000000000000028, 0.1166666666666666685, 0.1208333333333333343, 0.1250000000000000000, 0.1291666666666666796, 0.1333333333333333315, 0.1375000000000000111, 0.1416666666666666630, 0.1458333333333333426, 0.1499999999999999944, 0.1541666666666666741, 0.1583333333333333259, 0.1625000000000000056, 0.1666666666666666574, 0.1708333333333333370, 0.1749999999999999889, 0.1791666666666666685, 0.1833333333333333204, 0.1875000000000000000, 0.1916666666666666796, 0.1958333333333333315, 0.2000000000000000111, 0.2041666666666666630, 0.2083333333333333426, 0.2124999999999999944, 0.2166666666666666741, 0.2208333333333333259, 0.2250000000000000056, 0.2291666666666666574, 0.2333333333333333370, 0.2374999999999999889, 0.2416666666666666685, 0.2458333333333333204, 0.2500000000000000000, 0.2541666666666666519, 0.2583333333333333592, 0.2625000000000000111, 0.2666666666666666630, 0.2708333333333333148, 0.2750000000000000222, 0.2791666666666666741, 0.2833333333333333259, 0.2874999999999999778, 0.2916666666666666852, 0.2958333333333333370, 0.2999999999999999889, 0.3041666666666666408, 0.3083333333333333481, 0.3125000000000000000, 0.3166666666666666519, 0.3208333333333333592, 0.3250000000000000111, 0.3291666666666666630, 0.3333333333333333148, 0.3375000000000000222, 0.3416666666666666741, 0.3458333333333333259, 0.3499999999999999778, 0.3541666666666666852, 0.3583333333333333370, 0.3624999999999999889, 0.3666666666666666408, 0.3708333333333333481, 0.3750000000000000000, 0.3791666666666666519, 0.3833333333333333592, 0.3875000000000000111, 0.3916666666666666630, 0.3958333333333333148, 0.4000000000000000222, 0.4041666666666666741, 0.4083333333333333259, 0.4124999999999999778, 0.4166666666666666852, 0.4208333333333333370, 0.4249999999999999889, 0.4291666666666666408, 0.4333333333333333481, 0.4375000000000000000, 0.4416666666666666519, 0.4458333333333333592, 0.4500000000000000111, 0.4541666666666666630, 0.4583333333333333148, 0.4625000000000000222, 0.4666666666666666741, 0.4708333333333333259, 0.4749999999999999778, 0.4791666666666666852, 0.4833333333333333370, 0.4874999999999999889, 0.4916666666666666408, 0.4958333333333333481, 0.5000000000000000000, 0.5041666666666666519, 0.5083333333333333037, 0.5124999999999999556, 0.5166666666666667185, 0.5208333333333333703, 0.5250000000000000222, 0.5291666666666666741, 0.5333333333333333259, 0.5374999999999999778, 0.5416666666666666297, 0.5458333333333332815, 0.5500000000000000444, 0.5541666666666666963, 0.5583333333333333481, 0.5625000000000000000, 0.5666666666666666519, 0.5708333333333333037, 0.5749999999999999556, 0.5791666666666667185, 0.5833333333333333703, 0.5875000000000000222, 0.5916666666666666741, 0.5958333333333333259, 0.5999999999999999778, 0.6041666666666666297, 0.6083333333333332815, 0.6125000000000000444, 0.6166666666666666963, 0.6208333333333333481, 0.6250000000000000000, 0.6291666666666666519, 0.6333333333333333037, 0.6374999999999999556, 0.6416666666666667185, 0.6458333333333333703, 0.6500000000000000222, 0.6541666666666666741, 0.6583333333333333259, 0.6624999999999999778, 0.6666666666666666297, 0.6708333333333332815, 0.6750000000000000444, 0.6791666666666666963, 0.6833333333333333481, 0.6875000000000000000, 0.6916666666666666519, 0.6958333333333333037, 0.6999999999999999556, 0.7041666666666667185, 0.7083333333333333703, 0.7125000000000000222, 0.7166666666666666741, 0.7208333333333333259, 0.7249999999999999778, 0.7291666666666666297, 0.7333333333333332815, 0.7375000000000000444, 0.7416666666666666963, 0.7458333333333333481, 0.7500000000000000000, 0.7541666666666666519, 0.7583333333333333037, 0.7624999999999999556, 0.7666666666666667185, 0.7708333333333333703, 0.7750000000000000222, 0.7791666666666666741, 0.7833333333333333259, 0.7874999999999999778, 0.7916666666666666297, 0.7958333333333332815, 0.8000000000000000444, 0.8041666666666666963, 0.8083333333333333481, 0.8125000000000000000, 0.8166666666666666519, 0.8208333333333333037, 0.8249999999999999556, 0.8291666666666667185, 0.8333333333333333703, 0.8375000000000000222, 0.8416666666666666741, 0.8458333333333333259, 0.8499999999999999778, 0.8541666666666666297, 0.8583333333333332815, 0.8625000000000000444, 0.8666666666666666963, 0.8708333333333333481, 0.8750000000000000000, 0.8791666666666666519, 0.8833333333333333037, 0.8874999999999999556, 0.8916666666666667185, 0.8958333333333333703, 0.9000000000000000222, 0.9041666666666666741, 0.9083333333333333259, 0.9124999999999999778, 0.9166666666666666297, 0.9208333333333332815, 0.9250000000000000444, 0.9291666666666666963, 0.9333333333333333481, 0.9375000000000000000, 0.9416666666666666519, 0.9458333333333333037, 0.9499999999999999556, 0.9541666666666667185, 0.9583333333333333703, 0.9625000000000000222, 0.9666666666666666741, 0.9708333333333333259, 0.9749999999999999778, 0.9791666666666666297, 0.9833333333333332815, 0.9875000000000000444, 0.9916666666666666963, 0.9958333333333333481, 1.000000000000000000 ),
 .UNSPECIFIED. ) 
 GEOMETRIC_REPRESENTATION_ITEM ( )  RATIONAL_B_SPLINE_SURFACE ( (
 ( 1.000000000000000000, 0.8660254037844387076, 1.000000000000000000, 0.8660254037844387076, 1.000000000000000000, 0.8660254037844387076, 1.000000000000000000, 0.8660254037844387076, 1.000000000000000000, 0.8660254037844387076, 1.000000000000000000, 0.8660254037844387076, 1.000000000000000000, 0.8660254037844387076, 1.000000000000000000, 0.8660254037844387076, 1.000000000000000000, 0.8660254037844387076, 1.000000000000000000, 0.8660254037844387076, 1.000000000000000000, 0.8660254037844387076, 1.000000000000000000, 0.8660254037844387076, 1.000000000000000000, 0.8660254037844387076, 1.000000000000000000, 0.8660254037844387076, 1.000000000000000000, 0.8660254037844387076, 1.000000000000000000, 0.8660254037844387076, 1.000000000000000000, 0.8660254037844387076, 1.000000000000000000, 0.8660254037844387076, 1.000000000000000000, 0.8660254037844387076, 1.000000000000000000, 0.8660254037844387076, 1.000000000000000000, 0.8660254037844387076, 1.000000000000000000, 0.8660254037844387076, 1.000000000000000000, 0.8660254037844387076, 1.000000000000000000, 0.8660254037844387076, 1.000000000000000000, 0.8660254037844387076, 1.000000000000000000, 0.8660254037844387076, 1.000000000000000000, 0.8660254037844387076, 1.000000000000000000, 0.8660254037844387076, 1.000000000000000000, 0.8660254037844387076, 1.000000000000000000, 0.8660254037844387076, 1.000000000000000000, 0.8660254037844387076, 1.000000000000000000, 0.8660254037844387076, 1.000000000000000000, 0.8660254037844387076, 1.000000000000000000, 0.8660254037844387076, 1.000000000000000000, 0.8660254037844387076, 1.000000000000000000, 0.8660254037844387076, 1.000000000000000000, 0.8660254037844387076, 1.000000000000000000, 0.8660254037844387076, 1.000000000000000000, 0.8660254037844387076, 1.000000000000000000, 0.8660254037844387076, 1.000000000000000000, 0.8660254037844387076, 1.000000000000000000, 0.8660254037844387076, 1.000000000000000000, 0.8660254037844387076, 1.000000000000000000, 0.8660254037844387076, 1.000000000000000000, 0.8660254037844387076, 1.000000000000000000, 0.8660254037844387076, 1.000000000000000000, 0.8660254037844387076, 1.000000000000000000, 0.8660254037844387076, 1.000000000000000000, 0.8660254037844387076, 1.000000000000000000, 0.8660254037844387076, 1.000000000000000000, 0.8660254037844387076, 1.000000000000000000, 0.8660254037844387076, 1.000000000000000000, 0.8660254037844387076, 1.000000000000000000, 0.8660254037844387076, 1.000000000000000000, 0.8660254037844387076, 1.000000000000000000, 0.8660254037844387076, 1.000000000000000000, 0.8660254037844387076, 1.000000000000000000, 0.8660254037844387076, 1.000000000000000000, 0.8660254037844387076, 1.000000000000000000, 0.8660254037844387076, 1.000000000000000000, 0.8660254037844387076, 1.000000000000000000, 0.8660254037844387076, 1.000000000000000000, 0.8660254037844387076, 1.000000000000000000, 0.8660254037844387076, 1.000000000000000000, 0.8660254037844387076, 1.000000000000000000, 0.8660254037844387076, 1.000000000000000000, 0.8660254037844387076, 1.000000000000000000, 0.8660254037844387076, 1.000000000000000000, 0.8660254037844387076, 1.000000000000000000, 0.8660254037844387076, 1.000000000000000000, 0.8660254037844387076, 1.000000000000000000, 0.8660254037844387076, 1.000000000000000000, 0.8660254037844387076, 1.000000000000000000, 0.8660254037844387076, 1.000000000000000000, 0.8660254037844387076, 1.000000000000000000, 0.8660254037844387076, 1.000000000000000000, 0.8660254037844387076, 1.000000000000000000, 0.8660254037844387076, 1.000000000000000000, 0.8660254037844387076, 1.000000000000000000, 0.8660254037844387076, 1.000000000000000000, 0.8660254037844387076, 1.000000000000000000, 0.8660254037844387076, 1.000000000000000000, 0.8660254037844387076, 1.000000000000000000, 0.8660254037844387076, 1.000000000000000000, 0.8660254037844387076, 1.000000000000000000, 0.8660254037844387076, 1.000000000000000000, 0.8660254037844387076, 1.000000000000000000, 0.8660254037844387076, 1.000000000000000000, 0.8660254037844387076, 1.000000000000000000, 0.8660254037844387076, 1.000000000000000000, 0.8660254037844387076, 1.000000000000000000, 0.8660254037844387076, 1.000000000000000000, 0.8660254037844387076, 1.000000000000000000, 0.8660254037844387076, 1.000000000000000000, 0.8660254037844387076, 1.000000000000000000, 0.8660254037844387076, 1.000000000000000000, 0.8660254037844387076, 1.000000000000000000, 0.8660254037844387076, 1.000000000000000000, 0.8660254037844387076, 1.000000000000000000, 0.8660254037844387076, 1.000000000000000000, 0.8660254037844387076, 1.000000000000000000, 0.8660254037844387076, 1.000000000000000000, 0.8660254037844387076, 1.000000000000000000, 0.8660254037844387076, 1.000000000000000000, 0.8660254037844387076, 1.000000000000000000, 0.8660254037844387076, 1.000000000000000000, 0.8660254037844387076, 1.000000000000000000, 0.8660254037844387076, 1.000000000000000000, 0.8660254037844387076, 1.000000000000000000, 0.8660254037844387076, 1.000000000000000000, 0.8660254037844387076, 1.000000000000000000, 0.8660254037844387076, 1.000000000000000000, 0.8660254037844387076, 1.000000000000000000, 0.8660254037844387076, 1.000000000000000000, 0.8660254037844387076, 1.000000000000000000, 0.8660254037844387076, 1.000000000000000000, 0.8660254037844387076, 1.000000000000000000, 0.8660254037844387076, 1.000000000000000000, 0.8660254037844387076, 1.000000000000000000, 0.8660254037844387076, 1.000000000000000000, 0.8660254037844387076, 1.000000000000000000, 0.8660254037844387076, 1.000000000000000000, 0.8660254037844387076, 1.000000000000000000, 0.8660254037844387076, 1.000000000000000000, 0.8660254037844387076, 1.000000000000000000, 0.8660254037844387076, 1.000000000000000000, 0.8660254037844387076, 1.000000000000000000, 0.8660254037844387076, 1.000000000000000000, 0.8660254037844387076, 1.000000000000000000, 0.8660254037844387076, 1.000000000000000000, 0.8660254037844387076, 1.000000000000000000, 0.8660254037844387076, 1.000000000000000000, 0.8660254037844387076, 1.000000000000000000, 0.8660254037844387076, 1.000000000000000000, 0.8660254037844387076, 1.000000000000000000, 0.8660254037844387076, 1.000000000000000000, 0.8660254037844387076, 1.000000000000000000, 0.8660254037844387076, 1.000000000000000000, 0.8660254037844387076, 1.000000000000000000, 0.8660254037844387076, 1.000000000000000000, 0.8660254037844387076, 1.000000000000000000, 0.8660254037844387076, 1.000000000000000000, 0.8660254037844387076, 1.000000000000000000, 0.8660254037844387076, 1.000000000000000000, 0.8660254037844387076, 1.000000000000000000, 0.8660254037844387076, 1.000000000000000000, 0.8660254037844387076, 1.000000000000000000, 0.8660254037844387076, 1.000000000000000000, 0.8660254037844387076, 1.000000000000000000, 0.8660254037844387076, 1.000000000000000000, 0.8660254037844387076, 1.000000000000000000, 0.8660254037844387076, 1.000000000000000000, 0.8660254037844387076, 1.000000000000000000, 0.8660254037844387076, 1.000000000000000000, 0.8660254037844387076, 1.000000000000000000, 0.8660254037844387076, 1.000000000000000000, 0.8660254037844387076, 1.000000000000000000, 0.8660254037844387076, 1.000000000000000000, 0.8660254037844387076, 1.000000000000000000, 0.8660254037844387076, 1.000000000000000000, 0.8660254037844387076, 1.000000000000000000, 0.8660254037844387076, 1.000000000000000000, 0.8660254037844387076, 1.000000000000000000, 0.8660254037844387076, 1.000000000000000000, 0.8660254037844387076, 1.000000000000000000, 0.8660254037844387076, 1.000000000000000000, 0.8660254037844387076, 1.000000000000000000, 0.8660254037844387076, 1.000000000000000000, 0.8660254037844387076, 1.000000000000000000, 0.8660254037844387076, 1.000000000000000000, 0.8660254037844387076, 1.000000000000000000, 0.8660254037844387076, 1.000000000000000000, 0.8660254037844387076, 1.000000000000000000, 0.8660254037844387076, 1.000000000000000000, 0.8660254037844387076, 1.000000000000000000, 0.8660254037844387076, 1.000000000000000000, 0.8660254037844387076, 1.000000000000000000, 0.8660254037844387076, 1.000000000000000000, 0.8660254037844387076, 1.000000000000000000, 0.8660254037844387076, 1.000000000000000000, 0.8660254037844387076, 1.000000000000000000, 0.8660254037844387076, 1.000000000000000000, 0.8660254037844387076, 1.000000000000000000, 0.8660254037844387076, 1.000000000000000000, 0.8660254037844387076, 1.000000000000000000, 0.8660254037844387076, 1.000000000000000000, 0.8660254037844387076, 1.000000000000000000, 0.8660254037844387076, 1.000000000000000000, 0.8660254037844387076, 1.000000000000000000, 0.8660254037844387076, 1.000000000000000000, 0.8660254037844387076, 1.000000000000000000, 0.8660254037844387076, 1.000000000000000000, 0.8660254037844387076, 1.000000000000000000, 0.8660254037844387076, 1.000000000000000000, 0.8660254037844387076, 1.000000000000000000, 0.8660254037844387076, 1.000000000000000000, 0.8660254037844387076, 1.000000000000000000, 0.8660254037844387076, 1.000000000000000000, 0.8660254037844387076, 1.000000000000000000, 0.8660254037844387076, 1.000000000000000000, 0.8660254037844387076, 1.000000000000000000, 0.8660254037844387076, 1.000000000000000000, 0.8660254037844387076, 1.000000000000000000, 0.8660254037844387076, 1.000000000000000000, 0.8660254037844387076, 1.000000000000000000, 0.8660254037844387076, 1.000000000000000000, 0.8660254037844387076, 1.000000000000000000, 0.8660254037844387076, 1.000000000000000000, 0.8660254037844387076, 1.000000000000000000, 0.8660254037844387076, 1.000000000000000000, 0.8660254037844387076, 1.000000000000000000, 0.8660254037844387076, 1.000000000000000000, 0.8660254037844387076, 1.000000000000000000, 0.8660254037844387076, 1.000000000000000000, 0.8660254037844387076, 1.000000000000000000, 0.8660254037844387076, 1.000000000000000000, 0.8660254037844387076, 1.000000000000000000, 0.8660254037844387076, 1.000000000000000000, 0.8660254037844387076, 1.000000000000000000, 0.8660254037844387076, 1.000000000000000000, 0.8660254037844387076, 1.000000000000000000, 0.8660254037844387076, 1.000000000000000000, 0.8660254037844387076, 1.000000000000000000, 0.8660254037844387076, 1.000000000000000000, 0.8660254037844387076, 1.000000000000000000, 0.8660254037844387076, 1.000000000000000000, 0.8660254037844387076, 1.000000000000000000, 0.8660254037844387076, 1.000000000000000000, 0.8660254037844387076, 1.000000000000000000, 0.8660254037844387076, 1.000000000000000000, 0.8660254037844387076, 1.000000000000000000, 0.8660254037844387076, 1.000000000000000000, 0.8660254037844387076, 1.000000000000000000, 0.8660254037844387076, 1.000000000000000000, 0.8660254037844387076, 1.000000000000000000, 0.8660254037844387076, 1.000000000000000000, 0.8660254037844387076, 1.000000000000000000, 0.8660254037844387076, 1.000000000000000000, 0.8660254037844387076, 1.000000000000000000, 0.8660254037844387076, 1.000000000000000000),
 ( 1.000000000000000000, 0.8660254037844387076, 1.000000000000000000, 0.8660254037844387076, 1.000000000000000000, 0.8660254037844387076, 1.000000000000000000, 0.8660254037844387076, 1.000000000000000000, 0.8660254037844387076, 1.000000000000000000, 0.8660254037844387076, 1.000000000000000000, 0.8660254037844387076, 1.000000000000000000, 0.8660254037844387076, 1.000000000000000000, 0.8660254037844387076, 1.000000000000000000, 0.8660254037844387076, 1.000000000000000000, 0.8660254037844387076, 1.000000000000000000, 0.8660254037844387076, 1.000000000000000000, 0.8660254037844387076, 1.000000000000000000, 0.8660254037844387076, 1.000000000000000000, 0.8660254037844387076, 1.000000000000000000, 0.8660254037844387076, 1.000000000000000000, 0.8660254037844387076, 1.000000000000000000, 0.8660254037844387076, 1.000000000000000000, 0.8660254037844387076, 1.000000000000000000, 0.8660254037844387076, 1.000000000000000000, 0.8660254037844387076, 1.000000000000000000, 0.8660254037844387076, 1.000000000000000000, 0.8660254037844387076, 1.000000000000000000, 0.8660254037844387076, 1.000000000000000000, 0.8660254037844387076, 1.000000000000000000, 0.8660254037844387076, 1.000000000000000000, 0.8660254037844387076, 1.000000000000000000, 0.8660254037844387076, 1.000000000000000000, 0.8660254037844387076, 1.000000000000000000, 0.8660254037844387076, 1.000000000000000000, 0.8660254037844387076, 1.000000000000000000, 0.8660254037844387076, 1.000000000000000000, 0.8660254037844387076, 1.000000000000000000, 0.8660254037844387076, 1.000000000000000000, 0.8660254037844387076, 1.000000000000000000, 0.8660254037844387076, 1.000000000000000000, 0.8660254037844387076, 1.000000000000000000, 0.8660254037844387076, 1.000000000000000000, 0.8660254037844387076, 1.000000000000000000, 0.8660254037844387076, 1.000000000000000000, 0.8660254037844387076, 1.000000000000000000, 0.8660254037844387076, 1.000000000000000000, 0.8660254037844387076, 1.000000000000000000, 0.8660254037844387076, 1.000000000000000000, 0.8660254037844387076, 1.000000000000000000, 0.8660254037844387076, 1.000000000000000000, 0.8660254037844387076, 1.000000000000000000, 0.8660254037844387076, 1.000000000000000000, 0.8660254037844387076, 1.000000000000000000, 0.8660254037844387076, 1.000000000000000000, 0.8660254037844387076, 1.000000000000000000, 0.8660254037844387076, 1.000000000000000000, 0.8660254037844387076, 1.000000000000000000, 0.8660254037844387076, 1.000000000000000000, 0.8660254037844387076, 1.000000000000000000, 0.8660254037844387076, 1.000000000000000000, 0.8660254037844387076, 1.000000000000000000, 0.8660254037844387076, 1.000000000000000000, 0.8660254037844387076, 1.000000000000000000, 0.8660254037844387076, 1.000000000000000000, 0.8660254037844387076, 1.000000000000000000, 0.8660254037844387076, 1.000000000000000000, 0.8660254037844387076, 1.000000000000000000, 0.8660254037844387076, 1.000000000000000000, 0.8660254037844387076, 1.000000000000000000, 0.8660254037844387076, 1.000000000000000000, 0.8660254037844387076, 1.000000000000000000, 0.8660254037844387076, 1.000000000000000000, 0.8660254037844387076, 1.000000000000000000, 0.8660254037844387076, 1.000000000000000000, 0.8660254037844387076, 1.000000000000000000, 0.8660254037844387076, 1.000000000000000000, 0.8660254037844387076, 1.000000000000000000, 0.8660254037844387076, 1.000000000000000000, 0.8660254037844387076, 1.000000000000000000, 0.8660254037844387076, 1.000000000000000000, 0.8660254037844387076, 1.000000000000000000, 0.8660254037844387076, 1.000000000000000000, 0.8660254037844387076, 1.000000000000000000, 0.8660254037844387076, 1.000000000000000000, 0.8660254037844387076, 1.000000000000000000, 0.8660254037844387076, 1.000000000000000000, 0.8660254037844387076, 1.000000000000000000, 0.8660254037844387076, 1.000000000000000000, 0.8660254037844387076, 1.000000000000000000, 0.8660254037844387076, 1.000000000000000000, 0.8660254037844387076, 1.000000000000000000, 0.8660254037844387076, 1.000000000000000000, 0.8660254037844387076, 1.000000000000000000, 0.8660254037844387076, 1.000000000000000000, 0.8660254037844387076, 1.000000000000000000, 0.8660254037844387076, 1.000000000000000000, 0.8660254037844387076, 1.000000000000000000, 0.8660254037844387076, 1.000000000000000000, 0.8660254037844387076, 1.000000000000000000, 0.8660254037844387076, 1.000000000000000000, 0.8660254037844387076, 1.000000000000000000, 0.8660254037844387076, 1.000000000000000000, 0.8660254037844387076, 1.000000000000000000, 0.8660254037844387076, 1.000000000000000000, 0.8660254037844387076, 1.000000000000000000, 0.8660254037844387076, 1.000000000000000000, 0.8660254037844387076, 1.000000000000000000, 0.8660254037844387076, 1.000000000000000000, 0.8660254037844387076, 1.000000000000000000, 0.8660254037844387076, 1.000000000000000000, 0.8660254037844387076, 1.000000000000000000, 0.8660254037844387076, 1.000000000000000000, 0.8660254037844387076, 1.000000000000000000, 0.8660254037844387076, 1.000000000000000000, 0.8660254037844387076, 1.000000000000000000, 0.8660254037844387076, 1.000000000000000000, 0.8660254037844387076, 1.000000000000000000, 0.8660254037844387076, 1.000000000000000000, 0.8660254037844387076, 1.000000000000000000, 0.8660254037844387076, 1.000000000000000000, 0.8660254037844387076, 1.000000000000000000, 0.8660254037844387076, 1.000000000000000000, 0.8660254037844387076, 1.000000000000000000, 0.8660254037844387076, 1.000000000000000000, 0.8660254037844387076, 1.000000000000000000, 0.8660254037844387076, 1.000000000000000000, 0.8660254037844387076, 1.000000000000000000, 0.8660254037844387076, 1.000000000000000000, 0.8660254037844387076, 1.000000000000000000, 0.8660254037844387076, 1.000000000000000000, 0.8660254037844387076, 1.000000000000000000, 0.8660254037844387076, 1.000000000000000000, 0.8660254037844387076, 1.000000000000000000, 0.8660254037844387076, 1.000000000000000000, 0.8660254037844387076, 1.000000000000000000, 0.8660254037844387076, 1.000000000000000000, 0.8660254037844387076, 1.000000000000000000, 0.8660254037844387076, 1.000000000000000000, 0.8660254037844387076, 1.000000000000000000, 0.8660254037844387076, 1.000000000000000000, 0.8660254037844387076, 1.000000000000000000, 0.8660254037844387076, 1.000000000000000000, 0.8660254037844387076, 1.000000000000000000, 0.8660254037844387076, 1.000000000000000000, 0.8660254037844387076, 1.000000000000000000, 0.8660254037844387076, 1.000000000000000000, 0.8660254037844387076, 1.000000000000000000, 0.8660254037844387076, 1.000000000000000000, 0.8660254037844387076, 1.000000000000000000, 0.8660254037844387076, 1.000000000000000000, 0.8660254037844387076, 1.000000000000000000, 0.8660254037844387076, 1.000000000000000000, 0.8660254037844387076, 1.000000000000000000, 0.8660254037844387076, 1.000000000000000000, 0.8660254037844387076, 1.000000000000000000, 0.8660254037844387076, 1.000000000000000000, 0.8660254037844387076, 1.000000000000000000, 0.8660254037844387076, 1.000000000000000000, 0.8660254037844387076, 1.000000000000000000, 0.8660254037844387076, 1.000000000000000000, 0.8660254037844387076, 1.000000000000000000, 0.8660254037844387076, 1.000000000000000000, 0.8660254037844387076, 1.000000000000000000, 0.8660254037844387076, 1.000000000000000000, 0.8660254037844387076, 1.000000000000000000, 0.8660254037844387076, 1.000000000000000000, 0.8660254037844387076, 1.000000000000000000, 0.8660254037844387076, 1.000000000000000000, 0.8660254037844387076, 1.000000000000000000, 0.8660254037844387076, 1.000000000000000000, 0.8660254037844387076, 1.000000000000000000, 0.8660254037844387076, 1.000000000000000000, 0.8660254037844387076, 1.000000000000000000, 0.8660254037844387076, 1.000000000000000000, 0.8660254037844387076, 1.000000000000000000, 0.8660254037844387076, 1.000000000000000000, 0.8660254037844387076, 1.000000000000000000, 0.8660254037844387076, 1.000000000000000000, 0.8660254037844387076, 1.000000000000000000, 0.8660254037844387076, 1.000000000000000000, 0.8660254037844387076, 1.000000000000000000, 0.8660254037844387076, 1.000000000000000000, 0.8660254037844387076, 1.000000000000000000, 0.8660254037844387076, 1.000000000000000000, 0.8660254037844387076, 1.000000000000000000, 0.8660254037844387076, 1.000000000000000000, 0.8660254037844387076, 1.000000000000000000, 0.8660254037844387076, 1.000000000000000000, 0.8660254037844387076, 1.000000000000000000, 0.8660254037844387076, 1.000000000000000000, 0.8660254037844387076, 1.000000000000000000, 0.8660254037844387076, 1.000000000000000000, 0.8660254037844387076, 1.000000000000000000, 0.8660254037844387076, 1.000000000000000000, 0.8660254037844387076, 1.000000000000000000, 0.8660254037844387076, 1.000000000000000000, 0.8660254037844387076, 1.000000000000000000, 0.8660254037844387076, 1.000000000000000000, 0.8660254037844387076, 1.000000000000000000, 0.8660254037844387076, 1.000000000000000000, 0.8660254037844387076, 1.000000000000000000, 0.8660254037844387076, 1.000000000000000000, 0.8660254037844387076, 1.000000000000000000, 0.8660254037844387076, 1.000000000000000000, 0.8660254037844387076, 1.000000000000000000, 0.8660254037844387076, 1.000000000000000000, 0.8660254037844387076, 1.000000000000000000, 0.8660254037844387076, 1.000000000000000000, 0.8660254037844387076, 1.000000000000000000, 0.8660254037844387076, 1.000000000000000000, 0.8660254037844387076, 1.000000000000000000, 0.8660254037844387076, 1.000000000000000000, 0.8660254037844387076, 1.000000000000000000, 0.8660254037844387076, 1.000000000000000000, 0.8660254037844387076, 1.000000000000000000, 0.8660254037844387076, 1.000000000000000000, 0.8660254037844387076, 1.000000000000000000, 0.8660254037844387076, 1.000000000000000000, 0.8660254037844387076, 1.000000000000000000, 0.8660254037844387076, 1.000000000000000000, 0.8660254037844387076, 1.000000000000000000, 0.8660254037844387076, 1.000000000000000000, 0.8660254037844387076, 1.000000000000000000, 0.8660254037844387076, 1.000000000000000000, 0.8660254037844387076, 1.000000000000000000, 0.8660254037844387076, 1.000000000000000000, 0.8660254037844387076, 1.000000000000000000, 0.8660254037844387076, 1.000000000000000000, 0.8660254037844387076, 1.000000000000000000, 0.8660254037844387076, 1.000000000000000000, 0.8660254037844387076, 1.000000000000000000, 0.8660254037844387076, 1.000000000000000000, 0.8660254037844387076, 1.000000000000000000, 0.8660254037844387076, 1.000000000000000000, 0.8660254037844387076, 1.000000000000000000, 0.8660254037844387076, 1.000000000000000000, 0.8660254037844387076, 1.000000000000000000, 0.8660254037844387076, 1.000000000000000000, 0.8660254037844387076, 1.000000000000000000, 0.8660254037844387076, 1.000000000000000000, 0.8660254037844387076, 1.000000000000000000, 0.8660254037844387076, 1.000000000000000000, 0.8660254037844387076, 1.000000000000000000, 0.8660254037844387076, 1.000000000000000000) ) ) 
 REPRESENTATION_ITEM ( '' )  SURFACE ( )  );
#180365=VERTEX_POINT ( 'NONE', #63991 ) ;
#180373=CARTESIAN_POINT ( 'NONE',  ( 7.969495366734495434, 8.192166104145387706, 1.040834085586084257E-14 ) ) ;
#180374=CARTESIAN_POINT ( 'NONE',  ( 7.630541526392844887, 7.796719957080126662, 0.7998128361456341429 ) ) ;
#180382=CARTESIAN_POINT ( 'NONE',  ( -5.101945877444165944, 4.846691699973280976, 0.000000000000000000 ) ) ;
#180383=CARTESIAN_POINT ( 'NONE',  ( 8.550388431712704573, 13.12720360364021133, 0.000000000000000000 ) ) ;
#180385=CARTESIAN_POINT ( 'NONE',  ( -2.415323921528888196, 5.969628341758991930, 0.7998128361456341429 ) ) ;
#180396=AXIS2_PLACEMENT_3D ( 'NONE', #189861, #171480, #159500 ) ;
#180397=CARTESIAN_POINT ( 'NONE',  ( -10.14113571334194930, 10.93367254176152059, -0.7216878364870267237 ) ) ;
#180402=CARTESIAN_POINT ( 'NONE',  ( 5.452350330990040739, 9.512825819463730070, 0.7998128361456462443 ) ) ;
#180409=CARTESIAN_POINT ( 'NONE',  ( 5.151735183068521629, 5.112705256442466428, 1.040834085586084257E-14 ) ) ;
#180416=CARTESIAN_POINT ( 'NONE',  ( -7.314787569772770226, 8.492672571945082183, -1.199719254218452935 ) ) ;
#180417=CARTESIAN_POINT ( 'NONE',  ( -3.113568832632681360, 6.784247404713427798, -0.7998128361456281477 ) ) ;
#180426=TOROIDAL_SURFACE ( 'NONE', #14357, 3.971937515251341644, 0.08000000000000000167 ) ;
#180427=CARTESIAN_POINT ( 'NONE',  ( 6.124532705071213279, 8.168374127381657246, -1.599625672291262513 ) ) ;
#180436=VERTEX_POINT ( 'NONE', #180930 ) ;
#180438=CARTESIAN_POINT ( 'NONE',  ( -0.6823417656250246877, -0.1364583329919108468, 1.181850606188755259 ) ) ;
#180439=CARTESIAN_POINT ( 'NONE',  ( 2.683624340501134853, 5.218313266304903664, -1.199719254218446718 ) ) ;
#180440=CARTESIAN_POINT ( 'NONE',  ( 4.222474775652216294, 7.013638773981186958, 1.199719254218462483 ) ) ;
#180441=CIRCLE ( 'NONE', #35085, 1.220000000000001750 ) ;
#180443=CARTESIAN_POINT ( 'NONE',  ( -7.375272376154096143, 8.667201196010339004, -1.082531754730544860 ) ) ;
#180445=CARTESIAN_POINT ( 'NONE',  ( 4.148431816101584957, 6.823292304551739740, -1.082531754730548412 ) ) ;
#180446=CARTESIAN_POINT ( 'NONE',  ( -6.846504384776758378, 9.010674420371453053, -1.443375672974058777 ) ) ;
#180448=ORIENTED_EDGE ( 'NONE', *, *, #42311, .F. ) ;
#180450=CARTESIAN_POINT ( 'NONE',  ( 7.613066949273408213, 8.840665181362512115, -1.199719254218441611 ) ) ;
#180456=CARTESIAN_POINT ( 'NONE',  ( 1.364683531249988535, 4.155208333674753618, -0.7879004041258239610 ) ) ;
#180460=CARTESIAN_POINT ( 'NONE',  ( 6.435316467980822353, 10.65961964595298817, 1.040834085586084257E-14 ) ) ;
#180464=CARTESIAN_POINT ( 'NONE',  ( -6.828502922777144768, 11.11833717654868892, 0.7998128361456481317 ) ) ;
#180471=CARTESIAN_POINT ( 'NONE',  ( 8.646349277213076334, 11.11049346154719508, 1.599625672291281386 ) ) ;
#180472=CARTESIAN_POINT ( 'NONE',  ( 4.014051167739200565, 7.807899849707989226, -0.3196577630155780225 ) ) ;
#180473=CARTESIAN_POINT ( 'NONE',  ( -9.515124878692420296, 9.995400534762978850, 1.040834085586084257E-14 ) ) ;
#180476=CARTESIAN_POINT ( 'NONE',  ( 5.365762136054953224, 6.315268812753259020, -1.079746804988683806 ) ) ;
#180477=CARTESIAN_POINT ( 'NONE',  ( -9.327646496521984076, 11.90534021740758064, -1.443375672974059665 ) ) ;
#180481=CARTESIAN_POINT ( 'NONE',  ( 6.287230548435207567, 8.358188277972981695, -1.599625672291262513 ) ) ;
#180483=CARTESIAN_POINT ( 'NONE',  ( 4.449046963578762615, 8.342305224150557308, -0.7998128361456231517 ) ) ;
#180484=CARTESIAN_POINT ( 'NONE',  ( -4.124159483505494883, 7.474427186445510962, 0.6511861734826256409 ) ) ;
#180485=CARTESIAN_POINT ( 'NONE',  ( 3.979481780810941949, 4.601482484822914998, 1.199719254218464037 ) ) ;
#180487=CARTESIAN_POINT ( 'NONE',  ( -7.049876689426106680, 9.247942109129029475, -1.443375672974059665 ) ) ;
#180495=CARTESIAN_POINT ( 'NONE',  ( -4.014213326890253342, 7.626914324717730231, 0.01912188359321290165 ) ) ;
#180496=CARTESIAN_POINT ( 'NONE',  ( -0.6823417656250246877, -0.6364583329919113464, 1.181850606188755259 ) ) ;
#180499=CARTESIAN_POINT ( 'NONE',  ( 3.823036129373602154, 6.443664003369091731, -1.082531754730548412 ) ) ;
#180503=CARTESIAN_POINT ( 'NONE',  ( -8.256552360598034213, 11.61609960646427986, 1.082531754730549967 ) ) ;
#180515=CARTESIAN_POINT ( 'NONE',  ( -7.334597914868722590, 11.50085530074811935, -0.7216878364870267237 ) ) ;
#180520=CARTESIAN_POINT ( 'NONE',  ( 0.7499999999999885647, 2.847916667349487341, -1.299038105676658228 ) ) ;
#180522=ORIENTED_EDGE ( 'NONE', *, *, #163335, .T. ) ;
#180523=CARTESIAN_POINT ( 'NONE',  ( -8.193204901359996128, 8.453160561208463264, 1.040834085586084257E-14 ) ) ;
#180525=EDGE_CURVE ( 'NONE', #77955, #126795, #5012, .T. ) ;
#180527=CARTESIAN_POINT ( 'NONE',  ( 6.148786358997489820, 7.132337826040578754, -1.199719254218446718 ) ) ;
#180533=CARTESIAN_POINT ( 'NONE',  ( 8.932124273304774320, 9.315233161810734686, 0.7998128361456462443 ) ) ;
#180536=DIRECTION ( 'NONE',  ( 1.000000000000000000, 0.000000000000000000, 0.000000000000000000 ) ) ;
#180539=CARTESIAN_POINT ( 'NONE',  ( -7.226132686403777150, 7.532835677000276675, 1.040834085586084257E-14 ) ) ;
#180542=CARTESIAN_POINT ( 'NONE',  ( 0.7499999999999885647, 3.097916667349487341, -1.299038105676658228 ) ) ;
#180546=CYLINDRICAL_SURFACE ( 'NONE', #209608, 1.250000000000000000 ) ;
#180550=CARTESIAN_POINT ( 'NONE',  ( -2.779058300676980675, 5.225689869889666106, -1.082531754730543083 ) ) ;
#180552=CARTESIAN_POINT ( 'NONE',  ( 8.289920859751990889, 11.75899253876431416, 1.199719254218450271 ) ) ;
#180554=CARTESIAN_POINT ( 'NONE',  ( -9.179033691651859783, 10.66762638080401260, 1.199719254218462483 ) ) ;
#180556=CARTESIAN_POINT ( 'NONE',  ( 1.364683531249986537, 2.405208333674752286, -0.7879004041258239610 ) ) ;
#180557=CARTESIAN_POINT ( 'NONE',  ( 2.822068529938852155, 6.444163718237301275, -0.7998128361456291469 ) ) ;
#180563=CARTESIAN_POINT ( 'NONE',  ( 8.392133896734655707, 11.77427806529038357, 1.082531754730546636 ) ) ;
#180565=CARTESIAN_POINT ( 'NONE',  ( -8.188761592974058701, 8.655902734665618325, -0.7216878364870278340 ) ) ;
#180566=CARTESIAN_POINT ( 'NONE',  ( -1.402160292154681736E-14, 0.3218750003414227456, 1.575800808251672791 ) ) ;
#180568=CARTESIAN_POINT ( 'NONE',  ( 0.3138284133839603918, 8.211984188053584433, 1.978018658440966915 ) ) ;
#180570=CARTESIAN_POINT ( 'NONE',  ( -9.020252271793614440, 9.418049160047695878, 0.7998128361456462443 ) ) ;
#180571=CARTESIAN_POINT ( 'NONE',  ( -4.433153041544240835, 4.274359424664112339, 0.7216878364870317197 ) ) ;
#180572=CARTESIAN_POINT ( 'NONE',  ( -1.201851678989727383E-14, 3.634375000341422357, 1.575800808251672791 ) ) ;
#180577=B_SPLINE_CURVE_WITH_KNOTS ( 'NONE', 3,
 ( #117473, #1489, #67554, #66487 ),
 .UNSPECIFIED., .F., .F.,
 ( 4, 4 ),
 ( 0.000000000000000000, 0.0005756945739314307765 ),
 .UNSPECIFIED. ) ;
#180592=CARTESIAN_POINT ( 'NONE',  ( -1.201851678989727383E-14, 4.259375000341417028, -1.575800808251660134 ) ) ;
#180597=CARTESIAN_POINT ( 'NONE',  ( 9.257519960032755790, 9.694861462993381807, 0.7998128361456462443 ) ) ;
#180600=CARTESIAN_POINT ( 'NONE',  ( -1.364683531250012516, 2.280208333674751842, 0.7879004041258379498 ) ) ;
#180602=CARTESIAN_POINT ( 'NONE',  ( -6.670248388243482651, 9.765411638717282017, 1.082531754730548412 ) ) ;
#180608=CARTESIAN_POINT ( 'NONE',  ( 5.379888026524302980, 5.170957540566797128, -0.7998128361456211532 ) ) ;
#180611=CARTESIAN_POINT ( 'NONE',  ( 8.890396042259068210, 11.39521468743417998, -1.599625672291257406 ) ) ;
#180612=CARTESIAN_POINT ( 'NONE',  ( -1.084637062511542016, 2.867628807292011750, -1.105835307554790647 ) ) ;
#180618=CARTESIAN_POINT ( 'NONE',  ( -2.286521462199063492, 5.819358805874190743, 1.040834085586084257E-14 ) ) ;
#180620=CARTESIAN_POINT ( 'NONE',  ( 7.983053520348166288, 8.207983950027992748, -0.7998128361456281477 ) ) ;
#180621=VECTOR ( 'NONE', #135595, 1000.000000000000000 ) ;
#180623=CARTESIAN_POINT ( 'NONE',  ( 5.653386866774156694, 5.697965554099049257, -0.7216878364870207285 ) ) ;
#180626=EDGE_CURVE ( 'NONE', #6713, #59141, #72792, .T. ) ;
#180635=CARTESIAN_POINT ( 'NONE',  ( -8.026063749610063525, 8.466088584074293877, -0.7216878364870278340 ) ) ;
#180636=CARTESIAN_POINT ( 'NONE',  ( 6.010342169559767633, 5.906487374108181143, -0.7998128361456281477 ) ) ;
#180639=CARTESIAN_POINT ( 'NONE',  ( -7.133561379084627063, 11.47423870890741782, 0.7998128361456481317 ) ) ;
#180644=CARTESIAN_POINT ( 'NONE',  ( -8.448702279610222021, 13.00856975952063088, 1.040834085586084257E-14 ) ) ;
#180645=CARTESIAN_POINT ( 'NONE',  ( -1.499999999999997780, 3.400000000000021227, 1.214306433183764966E-14 ) ) ;
#180649=CARTESIAN_POINT ( 'NONE',  ( 8.422639742587595180, 10.84949900448412130, -1.599625672291268286 ) ) ;
#180661=CARTESIAN_POINT ( 'NONE',  ( -7.862839020921525091, 11.26073039346208660, -1.199719254218446718 ) ) ;
#180665=CARTESIAN_POINT ( 'NONE',  ( 6.155038550924133212, 10.12470270947942730, 0.7216878364870438212 ) ) ;
#180667=CARTESIAN_POINT ( 'NONE',  ( -4.229780737783618072, 6.918199379847403740, 1.082531754730560403 ) ) ;
#180668=CARTESIAN_POINT ( 'NONE',  ( 5.542585869888291938, 5.360771691158120689, -0.7998128361456211532 ) ) ;
#180670=CARTESIAN_POINT ( 'NONE',  ( -7.576308911938196999, 7.733448573549685179, 0.7998128361456462443 ) ) ;
#180680=CARTESIAN_POINT ( 'NONE',  ( -1.201851678989727383E-14, 3.759375000341422801, -1.575800808251660134 ) ) ;
#180681=CARTESIAN_POINT ( 'NONE',  ( 7.781490099239519509, 11.16582331816642260, 1.199719254218460707 ) ) ;
#180683=CARTESIAN_POINT ( 'NONE',  ( -4.284013352238265959, 5.060732334775157604, -1.082531754730544860 ) ) ;
#180685=CARTESIAN_POINT ( 'NONE',  ( -5.382223794500852421, 5.381608636446842731, -0.7216878364870197293 ) ) ;
#180693=CARTESIAN_POINT ( 'NONE',  ( 4.467575310902914154, 5.170924936596891008, 1.199719254218464037 ) ) ;
#180703=CARTESIAN_POINT ( 'NONE',  ( 6.166260936116925606, 6.088392601758203071, 0.7998128361456341429 ) ) ;
#180708=CARTESIAN_POINT ( 'NONE',  ( 1.364683531249988535, 3.426041667008085323, 0.7879004041258500513 ) ) ;
#180713=CARTESIAN_POINT ( 'NONE',  ( 7.623762449586013901, 7.788811034138823253, 1.040834085586084257E-14 ) ) ;
#180715=CARTESIAN_POINT ( 'NONE',  ( -6.762819695118240659, 6.784377820593065600, 0.7998128361456341429 ) ) ;
#180716=CARTESIAN_POINT ( 'NONE',  ( 0.7499999999999885647, 2.316666666666689078, -1.299038105676652899 ) ) ;
#180721=CARTESIAN_POINT ( 'NONE',  ( -3.574546055497324737, 7.322054164722185732, 0.7998128361456341429 ) ) ;
#180724=CARTESIAN_POINT ( 'NONE',  ( 0.6823417656249899377, 3.426041667008085323, -1.181850606188754593 ) ) ;
#180726=CARTESIAN_POINT ( 'NONE',  ( -5.287316719649550301, 5.270883715786984780, 0.7216878364870317197 ) ) ;
#180732=CARTESIAN_POINT ( 'NONE',  ( 5.412729640353754590, 7.337937218544611895, 1.599625672291267398 ) ) ;
#180735=CARTESIAN_POINT ( 'NONE',  ( -1.364683531250012516, 4.551041667008082214, -0.7879004041258300672 ) ) ;
#180737=CARTESIAN_POINT ( 'NONE',  ( 4.383363735919856730, 4.008345868194933104, -0.7998128361456211532 ) ) ;
#180739=CARTESIAN_POINT ( 'NONE',  ( -1.364683531250014514, 0.09270833367475767028, 0.7879004041258379498 ) ) ;
#180742=B_SPLINE_CURVE_WITH_KNOTS ( 'NONE', 3,
 ( #90982, #172222, #191635, #125675, #43299, #171138, #109419 ),
 .UNSPECIFIED., .F., .F.,
 ( 4, 3, 4 ),
 ( 0.000000000000000000, 2.778001202718379905E-05, 5.460790091229219688E-05 ),
 .UNSPECIFIED. ) ;
#180743=CARTESIAN_POINT ( 'NONE',  ( -3.918470089549458635, 4.530302178351167441, -1.199719254218452047 ) ) ;
#180744=CARTESIAN_POINT ( 'NONE',  ( -6.521108698048779573, 8.631046119188804155, -1.443375672974058777 ) ) ;
#180748=CARTESIAN_POINT ( 'NONE',  ( -1.201851678989727383E-14, 2.946875000341419248, -1.575800808251660134 ) ) ;
#180756=CARTESIAN_POINT ( 'NONE',  ( -7.090551149822745813, 9.295395646258437949, 1.443375672974078761 ) ) ;
#180762=CARTESIAN_POINT ( 'NONE',  ( -6.521108698048783126, 7.670676904887464786, -1.082531754730543083 ) ) ;
#180774=CARTESIAN_POINT ( 'NONE',  ( -4.042302355168801320, 7.867769847672247074, 0.7998128361456341429 ) ) ;
#180776=CARTESIAN_POINT ( 'NONE',  ( -0.7500000000000006661, -0.6416666666666446250, -1.299038105676652011 ) ) ;
#180777=CARTESIAN_POINT ( 'NONE',  ( 9.083599731475976213, 12.58098820582193689, 1.082531754730546636 ) ) ;
#180778=CARTESIAN_POINT ( 'NONE',  ( 6.272618624616828953, 10.46980549536166016, 1.040834085586084257E-14 ) ) ;
#180780=( BOUNDED_SURFACE ( )  B_SPLINE_SURFACE ( 1, 2, ( 
 ( #42665, #41596, #142309, #78334, #123979, #77266, #156398, #177988, #140166, #174799, #26375, #92488, #43728, #62097, #160661, #209378, #109843, #29601, #107707, #158527, #175857, #108774, #25310, #194219, #206189, #91412, #157472, #9067, #27446, #159588, #61022, #146574, #81539, #17575, #162806, #180114, #83659, #95687, #16513, #199534, #80475, #181168, #130374, #14383, #30673, #213640, #116233, #195300, #133527, #114122, #183297, #65266, #82596, #212593, #1326, #148682, #131412, #64231, #63158, #15451, #179054, #129323, #66322, #250, #196364, #161741, #13332, #49053, #165990, #149749, #46930, #197412, #48004, #31738, #182224, #132466, #164920, #147621, #198468, #50113, #67387, #51177, #96756, #33847, #115173, #99928, #145523, #97811, #113048, #32793, #163874, #98868, #117300, #79406, #211522, #19726, #68465, #103127, #171315, #150824, #104200, #34903, #138840, #100975, #53306, #119438, #185425, #136704, #105278, #71660, #170247, #152939, #122672, #2387, #37043, #70589, #169185, #202728, #5580, #20777, #120518, #151885, #167064, #3459, #86873, #54380, #18656, #89026, #4516, #155079, #85805, #137774, #203792, #22910, #186496, #118369, #38127, #21832, #6666, #87940, #72742, #55438, #204856, #154014, #200593, #56511, #102060, #121590, #187562, #168125, #39189, #84736, #134593, #52241, #184357, #69529, #35979, #135636, #201657, #123736, #92240, #209131, #73821, #12010, #207010, #61840, #158290, #175606, #41350, #94365, #27195, #9880, #91164, #156154, #108523, #57577, #7735, #159337, #93301, #74894, #188634, #106376, #142059, #44543, #176660, #139915, #75956, #157220, #58641, #60769, #10933, #43483, #174552, #77009, #143136, #28273, #160407, #189697, #126929, #208073, #192886, #23988, #8818, #205946, #125861, #42418, #59699, #191818, #173485, #90090, #25062, #107459, #26128, #110659, #141002, #109601, #40265, #78084, #172400, #124794, #190755, #144208, #210204, #198213, #164670, #197159, #31484, #1067, #29345, #130125, #163617, #63969, #81289, #98609, #196113, #213392, #30418, #128007, #96503, #47750, #15198, #111724, #181965, #179860, #33593, #178803, #16253, #82338, #49848, #146316, #211271, #212330, #113865, #99665, #65016, #115975, #148430, #165734, #97559, #79148, #17321, #195037, #131169, #32534, #162553, #161490, #66062, #17640, #95440, #129064, #132205, #14124, #83402, #193961, #80216, #147366, #149484, #145264, #13069, #48796, #112791, #45608, #114913, #177732, #180911, #62895, #46671, #171049, #71397, #18396, #135379, #117043, #105009, #36779, #69263, #201398, #169981, #102864, #22647, #54116, #3192, #20525, #153747, #86608, #55179, #85536, #185155, #70328, #21568, #151626, #168921, #202461, #154814, #152675, #101794, #38926, #68200, #183039, #136445, #199273, #187299, #4258, #203525, #121324, #5315, #88757, #133265, #120250, #186227, #67132, #35718, #53035, #50916, #37859, #134332, #103938, #34655, #84473, #166804, #137508, #100725, #200337, #150564, #167863, #87675, #2125, #51988, #118113, #184098, #119170, #19461, #74628, #106111, #72472, #40002, #107187, #10668, #124530, #91967, #25857, #8546, #108261, #191551, #139652, #140733, #94099, #138571, #109332, #28002, #7470, #43215, #75691, #159072, #142860, #126652, #175341, #60493, #44271, #208863, #190488, #158025, #173212, #9614, #23727, #6399, #206745, #90894, #73549, #76739, #205673, #58375, #57310, #26922, #204593, #141801, #93031, #192618, #41079, #42146, #174282, #110392, #176397, #56245, #123475, #122404, #188362, #59434, #207805, #189437, #172132, #125591, #89833, #155881, #24791, #156954, #46397, #160138, #77813, #113588, #15985, #148162, #127734, #129853, #128781, #30137, #32269, #213127, #14921, #79940, #64758, #147103, #214164, #65789, #29074, #130900, #63698, #98336, #209929, #194760, #45336, #97286, #13862, #195836, #179591, #144990, #61568, #210995, #193692, #146045, #82070, #111456, #81015, #11738, #49577, #143934, #178526, #96225, #162276, #47476, #131939, #196893, #48531, #31213, #33324, #177460, #212058, #163342, #114651, #180644, #164402, #197950, #115702, #62620, #95158, #112513, #181694, #161209, #12795, #78869, #151364, #153493 ),
 ( #103681, #50645, #167601, #149212, #137256, #69006, #101532, #19200, #202201, #135123, #203275, #86351, #35453, #52777, #185967, #118915, #87426, #117850, #2934, #102608, #53857, #183842, #201139, #20267, #187041, #184896, #134071, #71138, #100458, #787, #168662, #17053, #5063, #36521, #21319, #54922, #37599, #121073, #165458, #152422, #169730, #99405, #66854, #4001, #67926, #85278, #83133, #70070, #136183, #119990, #132998, #198999, #116772, #182769, #34386, #166533, #18123, #84211, #150299, #200080, #1865, #51728, #109878, #159626, #61055, #23467, #88500, #92522, #72209, #175890, #178015, #154562, #110937, #38673, #145554, #104752, #59984, #126137, #192099, #143414, #112014, #78365, #176943, #11220, #129351, #6139, #43765, #77302, #27481, #209408, #12284, #93581, #127214, #158561, #170801, #10159, #193182, #44831, #22390, #95718, #28558, #161771, #76235, #144485, #210492, #29632, #94647, #122141, #160691, #62127, #13363, #128288, #79437, #194250, #211553, #45893, #204331, #63186, #105844, #138316, #55990, #142344, #188109, #39739, #171871, #208353, #196394, #166020, #163905, #167096, #46961, #31770, #181195, #117331, #48037, #65292, #183329, #195330, #116262, #84767, #180144, #66351, #15481, #114151, #130406, #98897, #1354, #80505, #18685, #213668, #68494, #164950, #182253, #97840, #101007, #33877, #16543, #81566, #162838, #115202, #64261, #14416, #17606, #99955, #147652, #113079, #179083, #131439, #197443, #49084, #82624, #51209, #83690, #50140, #148709, #30705, #96788, #32822, #279, #132495, #198495, #149778, #67415, #133556, #199565, #146602, #34935, #150853, #2417, #212620, #188666, #186527, #40296, #185454, #171346, #89056, #56541, #152971, #3486, #4545, #202756, #106407, #71691, #122703, #22940, #204890, #104230, #85835, #24018, #201688, #137804, #39217, #169216, #168155, #72773, #155113, #36005, #135665, #105308, #103155, #172430, #200624, #37076, #120549, #90120, #53333, #70618, #156187, #134621, #55467, #7764, #119466, #5608, #20807, #86904, #69555, #38157, #6697, #19754, #52273, #136732, #118400, #170276, #121623, #54409, #184386, #187592, #21861, #87969, #102086, #154043, #203823, #151913, #138872, #126959, #174583, #73853, #205974, #27225, #144239, #61870, #41380, #43512, #42448, #158320, #160434, #192919, #143167, #208105, #44575, #60801, #128035, #193989, #157251, #110689, #191850, #12040, #123766, #108552, #173516, #10966, #142090, #109633, #93330, #58671, #189727, #124820, #107490, #59733, #210233, #25090, #209162, #139948, #177760, #57606, #91190, #125891, #8844, #111755, #175639, #75986, #159366, #176687, #77040, #29376, #28300, #9911, #94396, #78111, #45638, #95471, #92273, #161519, #74922, #141034, #207041, #190785, #26159, #100752, #131200, #47783, #199302, #14155, #129095, #16283, #145297, #133296, #164697, #149515, #1101, #165767, #67160, #79182, #98638, #32561, #50947, #196142, #97589, #117072, #82370, #80249, #148459, #13103, #178834, #112821, #17351, #211302, #146348, #183070, #113897, #198243, #62927, #28, #66092, #34683, #15228, #213421, #81318, #30449, #195066, #46706, #179891, #83433, #197188, #132235, #49881, #147394, #114941, #116006, #212360, #65044, #96534, #162581, #181992, #64001, #130152, #33625, #99697, #31514, #163648, #48826, #180941, #6434, #204630, #154850, #136475, #37894, #53069, #103972, #184128, #166834, #20556, #36812, #167893, #171084, #85568, #4289, #151658, #137544, #18430, #21602, #38964, #203562, #201429, #70361, #86640, #121360, #122440, #56281, #3228, #68232, #35751, #200369, #202496, #69295, #187335, #54148, #22680, #170014, #55214, #40034, #188398, #88792, #52017, #119202, #72509, #120285, #87708, #186260, #168953, #153780, #105049, #135406, #152707, #84504, #150593, #138607, #2155, #19493, #134365, #5350, #118143, #101825, #185188, #102894, #71432, #143970, #94135, #75723, #191586, #206777, #43247, #123508, #106146, #174317, #190525, #107224, #110427, #24828, #158061, #90928, #76776, #172170, #175374, #192653, #142898, #140765, #9647, #25891, #60531, #61603, #209963, #156994, #7502, #189473, #139688, #141837, #8581, #126691, #207843, #176431 ) ),
 .UNSPECIFIED., .F., .F., .F. ) 
 B_SPLINE_SURFACE_WITH_KNOTS ( ( 2, 2 ),
 ( 3, 2, 2, 2, 2, 2, 2, 2, 2, 2, 2, 2, 2, 2, 2, 2, 2, 2, 2, 2, 2, 2, 2, 2, 2, 2, 2, 2, 2, 2, 2, 2, 2, 2, 2, 2, 2, 2, 2, 2, 2, 2, 2, 2, 2, 2, 2, 2, 2, 2, 2, 2, 2, 2, 2, 2, 2, 2, 2, 2, 2, 2, 2, 2, 2, 2, 2, 2, 2, 2, 2, 2, 2, 2, 2, 2, 2, 2, 2, 2, 2, 2, 2, 2, 2, 2, 2, 2, 2, 2, 2, 2, 2, 2, 2, 2, 2, 2, 2, 2, 2, 2, 2, 2, 2, 2, 2, 2, 2, 2, 2, 2, 2, 2, 2, 2, 2, 2, 2, 2, 2, 2, 2, 2, 2, 2, 2, 2, 2, 2, 2, 2, 2, 2, 2, 2, 2, 2, 2, 2, 2, 2, 2, 2, 2, 2, 2, 2, 2, 2, 2, 2, 2, 2, 2, 2, 2, 2, 2, 2, 2, 2, 2, 2, 2, 2, 2, 2, 2, 2, 2, 2, 2, 2, 2, 2, 2, 2, 2, 2, 2, 2, 2, 2, 2, 2, 2, 2, 2, 2, 2, 2, 2, 2, 2, 2, 2, 2, 2, 2, 2, 2, 2, 2, 2, 2, 2, 2, 2, 2, 2, 2, 2, 2, 2, 2, 2, 2, 2, 2, 2, 2, 2, 2, 2, 2, 2, 2, 2, 2, 2, 2, 2, 2, 2, 2, 2, 2, 2, 2, 3 ),
 ( 0.000000000000000000, 1.000000000000000000 ),
 ( 0.000000000000000000, 0.004166666666666666609, 0.008333333333333333218, 0.01250000000000000069, 0.01666666666666666644, 0.02083333333333333218, 0.02500000000000000139, 0.02916666666666666713, 0.03333333333333333287, 0.03749999999999999861, 0.04166666666666666435, 0.04583333333333333010, 0.05000000000000000278, 0.05416666666666666852, 0.05833333333333333426, 0.06250000000000000000, 0.06666666666666666574, 0.07083333333333333148, 0.07499999999999999722, 0.07916666666666666297, 0.08333333333333332871, 0.08749999999999999445, 0.09166666666666666019, 0.09583333333333333981, 0.1000000000000000056, 0.1041666666666666713, 0.1083333333333333370, 0.1125000000000000028, 0.1166666666666666685, 0.1208333333333333343, 0.1250000000000000000, 0.1291666666666666796, 0.1333333333333333315, 0.1375000000000000111, 0.1416666666666666630, 0.1458333333333333426, 0.1499999999999999944, 0.1541666666666666741, 0.1583333333333333259, 0.1625000000000000056, 0.1666666666666666574, 0.1708333333333333370, 0.1749999999999999889, 0.1791666666666666685, 0.1833333333333333204, 0.1875000000000000000, 0.1916666666666666796, 0.1958333333333333315, 0.2000000000000000111, 0.2041666666666666630, 0.2083333333333333426, 0.2124999999999999944, 0.2166666666666666741, 0.2208333333333333259, 0.2250000000000000056, 0.2291666666666666574, 0.2333333333333333370, 0.2374999999999999889, 0.2416666666666666685, 0.2458333333333333204, 0.2500000000000000000, 0.2541666666666666519, 0.2583333333333333592, 0.2625000000000000111, 0.2666666666666666630, 0.2708333333333333148, 0.2750000000000000222, 0.2791666666666666741, 0.2833333333333333259, 0.2874999999999999778, 0.2916666666666666852, 0.2958333333333333370, 0.2999999999999999889, 0.3041666666666666408, 0.3083333333333333481, 0.3125000000000000000, 0.3166666666666666519, 0.3208333333333333592, 0.3250000000000000111, 0.3291666666666666630, 0.3333333333333333148, 0.3375000000000000222, 0.3416666666666666741, 0.3458333333333333259, 0.3499999999999999778, 0.3541666666666666852, 0.3583333333333333370, 0.3624999999999999889, 0.3666666666666666408, 0.3708333333333333481, 0.3750000000000000000, 0.3791666666666666519, 0.3833333333333333592, 0.3875000000000000111, 0.3916666666666666630, 0.3958333333333333148, 0.4000000000000000222, 0.4041666666666666741, 0.4083333333333333259, 0.4124999999999999778, 0.4166666666666666852, 0.4208333333333333370, 0.4249999999999999889, 0.4291666666666666408, 0.4333333333333333481, 0.4375000000000000000, 0.4416666666666666519, 0.4458333333333333592, 0.4500000000000000111, 0.4541666666666666630, 0.4583333333333333148, 0.4625000000000000222, 0.4666666666666666741, 0.4708333333333333259, 0.4749999999999999778, 0.4791666666666666852, 0.4833333333333333370, 0.4874999999999999889, 0.4916666666666666408, 0.4958333333333333481, 0.5000000000000000000, 0.5041666666666666519, 0.5083333333333333037, 0.5124999999999999556, 0.5166666666666667185, 0.5208333333333333703, 0.5250000000000000222, 0.5291666666666666741, 0.5333333333333333259, 0.5374999999999999778, 0.5416666666666666297, 0.5458333333333332815, 0.5500000000000000444, 0.5541666666666666963, 0.5583333333333333481, 0.5625000000000000000, 0.5666666666666666519, 0.5708333333333333037, 0.5749999999999999556, 0.5791666666666667185, 0.5833333333333333703, 0.5875000000000000222, 0.5916666666666666741, 0.5958333333333333259, 0.5999999999999999778, 0.6041666666666666297, 0.6083333333333332815, 0.6125000000000000444, 0.6166666666666666963, 0.6208333333333333481, 0.6250000000000000000, 0.6291666666666666519, 0.6333333333333333037, 0.6374999999999999556, 0.6416666666666667185, 0.6458333333333333703, 0.6500000000000000222, 0.6541666666666666741, 0.6583333333333333259, 0.6624999999999999778, 0.6666666666666666297, 0.6708333333333332815, 0.6750000000000000444, 0.6791666666666666963, 0.6833333333333333481, 0.6875000000000000000, 0.6916666666666666519, 0.6958333333333333037, 0.6999999999999999556, 0.7041666666666667185, 0.7083333333333333703, 0.7125000000000000222, 0.7166666666666666741, 0.7208333333333333259, 0.7249999999999999778, 0.7291666666666666297, 0.7333333333333332815, 0.7375000000000000444, 0.7416666666666666963, 0.7458333333333333481, 0.7500000000000000000, 0.7541666666666666519, 0.7583333333333333037, 0.7624999999999999556, 0.7666666666666667185, 0.7708333333333333703, 0.7750000000000000222, 0.7791666666666666741, 0.7833333333333333259, 0.7874999999999999778, 0.7916666666666666297, 0.7958333333333332815, 0.8000000000000000444, 0.8041666666666666963, 0.8083333333333333481, 0.8125000000000000000, 0.8166666666666666519, 0.8208333333333333037, 0.8249999999999999556, 0.8291666666666667185, 0.8333333333333333703, 0.8375000000000000222, 0.8416666666666666741, 0.8458333333333333259, 0.8499999999999999778, 0.8541666666666666297, 0.8583333333333332815, 0.8625000000000000444, 0.8666666666666666963, 0.8708333333333333481, 0.8750000000000000000, 0.8791666666666666519, 0.8833333333333333037, 0.8874999999999999556, 0.8916666666666667185, 0.8958333333333333703, 0.9000000000000000222, 0.9041666666666666741, 0.9083333333333333259, 0.9124999999999999778, 0.9166666666666666297, 0.9208333333333332815, 0.9250000000000000444, 0.9291666666666666963, 0.9333333333333333481, 0.9375000000000000000, 0.9416666666666666519, 0.9458333333333333037, 0.9499999999999999556, 0.9541666666666667185, 0.9583333333333333703, 0.9625000000000000222, 0.9666666666666666741, 0.9708333333333333259, 0.9749999999999999778, 0.9791666666666666297, 0.9833333333333332815, 0.9875000000000000444, 0.9916666666666666963, 0.9958333333333333481, 1.000000000000000000 ),
 .UNSPECIFIED. ) 
 GEOMETRIC_REPRESENTATION_ITEM ( )  RATIONAL_B_SPLINE_SURFACE ( (
 ( 1.000000000000000000, 0.8660254037844387076, 1.000000000000000000, 0.8660254037844387076, 1.000000000000000000, 0.8660254037844387076, 1.000000000000000000, 0.8660254037844387076, 1.000000000000000000, 0.8660254037844387076, 1.000000000000000000, 0.8660254037844387076, 1.000000000000000000, 0.8660254037844387076, 1.000000000000000000, 0.8660254037844387076, 1.000000000000000000, 0.8660254037844387076, 1.000000000000000000, 0.8660254037844387076, 1.000000000000000000, 0.8660254037844387076, 1.000000000000000000, 0.8660254037844387076, 1.000000000000000000, 0.8660254037844387076, 1.000000000000000000, 0.8660254037844387076, 1.000000000000000000, 0.8660254037844387076, 1.000000000000000000, 0.8660254037844387076, 1.000000000000000000, 0.8660254037844387076, 1.000000000000000000, 0.8660254037844387076, 1.000000000000000000, 0.8660254037844387076, 1.000000000000000000, 0.8660254037844387076, 1.000000000000000000, 0.8660254037844387076, 1.000000000000000000, 0.8660254037844387076, 1.000000000000000000, 0.8660254037844387076, 1.000000000000000000, 0.8660254037844387076, 1.000000000000000000, 0.8660254037844387076, 1.000000000000000000, 0.8660254037844387076, 1.000000000000000000, 0.8660254037844387076, 1.000000000000000000, 0.8660254037844387076, 1.000000000000000000, 0.8660254037844387076, 1.000000000000000000, 0.8660254037844387076, 1.000000000000000000, 0.8660254037844387076, 1.000000000000000000, 0.8660254037844387076, 1.000000000000000000, 0.8660254037844387076, 1.000000000000000000, 0.8660254037844387076, 1.000000000000000000, 0.8660254037844387076, 1.000000000000000000, 0.8660254037844387076, 1.000000000000000000, 0.8660254037844387076, 1.000000000000000000, 0.8660254037844387076, 1.000000000000000000, 0.8660254037844387076, 1.000000000000000000, 0.8660254037844387076, 1.000000000000000000, 0.8660254037844387076, 1.000000000000000000, 0.8660254037844387076, 1.000000000000000000, 0.8660254037844387076, 1.000000000000000000, 0.8660254037844387076, 1.000000000000000000, 0.8660254037844387076, 1.000000000000000000, 0.8660254037844387076, 1.000000000000000000, 0.8660254037844387076, 1.000000000000000000, 0.8660254037844387076, 1.000000000000000000, 0.8660254037844387076, 1.000000000000000000, 0.8660254037844387076, 1.000000000000000000, 0.8660254037844387076, 1.000000000000000000, 0.8660254037844387076, 1.000000000000000000, 0.8660254037844387076, 1.000000000000000000, 0.8660254037844387076, 1.000000000000000000, 0.8660254037844387076, 1.000000000000000000, 0.8660254037844387076, 1.000000000000000000, 0.8660254037844387076, 1.000000000000000000, 0.8660254037844387076, 1.000000000000000000, 0.8660254037844387076, 1.000000000000000000, 0.8660254037844387076, 1.000000000000000000, 0.8660254037844387076, 1.000000000000000000, 0.8660254037844387076, 1.000000000000000000, 0.8660254037844387076, 1.000000000000000000, 0.8660254037844387076, 1.000000000000000000, 0.8660254037844387076, 1.000000000000000000, 0.8660254037844387076, 1.000000000000000000, 0.8660254037844387076, 1.000000000000000000, 0.8660254037844387076, 1.000000000000000000, 0.8660254037844387076, 1.000000000000000000, 0.8660254037844387076, 1.000000000000000000, 0.8660254037844387076, 1.000000000000000000, 0.8660254037844387076, 1.000000000000000000, 0.8660254037844387076, 1.000000000000000000, 0.8660254037844387076, 1.000000000000000000, 0.8660254037844387076, 1.000000000000000000, 0.8660254037844387076, 1.000000000000000000, 0.8660254037844387076, 1.000000000000000000, 0.8660254037844387076, 1.000000000000000000, 0.8660254037844387076, 1.000000000000000000, 0.8660254037844387076, 1.000000000000000000, 0.8660254037844387076, 1.000000000000000000, 0.8660254037844387076, 1.000000000000000000, 0.8660254037844387076, 1.000000000000000000, 0.8660254037844387076, 1.000000000000000000, 0.8660254037844387076, 1.000000000000000000, 0.8660254037844387076, 1.000000000000000000, 0.8660254037844387076, 1.000000000000000000, 0.8660254037844387076, 1.000000000000000000, 0.8660254037844387076, 1.000000000000000000, 0.8660254037844387076, 1.000000000000000000, 0.8660254037844387076, 1.000000000000000000, 0.8660254037844387076, 1.000000000000000000, 0.8660254037844387076, 1.000000000000000000, 0.8660254037844387076, 1.000000000000000000, 0.8660254037844387076, 1.000000000000000000, 0.8660254037844387076, 1.000000000000000000, 0.8660254037844387076, 1.000000000000000000, 0.8660254037844387076, 1.000000000000000000, 0.8660254037844387076, 1.000000000000000000, 0.8660254037844387076, 1.000000000000000000, 0.8660254037844387076, 1.000000000000000000, 0.8660254037844387076, 1.000000000000000000, 0.8660254037844387076, 1.000000000000000000, 0.8660254037844387076, 1.000000000000000000, 0.8660254037844387076, 1.000000000000000000, 0.8660254037844387076, 1.000000000000000000, 0.8660254037844387076, 1.000000000000000000, 0.8660254037844387076, 1.000000000000000000, 0.8660254037844387076, 1.000000000000000000, 0.8660254037844387076, 1.000000000000000000, 0.8660254037844387076, 1.000000000000000000, 0.8660254037844387076, 1.000000000000000000, 0.8660254037844387076, 1.000000000000000000, 0.8660254037844387076, 1.000000000000000000, 0.8660254037844387076, 1.000000000000000000, 0.8660254037844387076, 1.000000000000000000, 0.8660254037844387076, 1.000000000000000000, 0.8660254037844387076, 1.000000000000000000, 0.8660254037844387076, 1.000000000000000000, 0.8660254037844387076, 1.000000000000000000, 0.8660254037844387076, 1.000000000000000000, 0.8660254037844387076, 1.000000000000000000, 0.8660254037844387076, 1.000000000000000000, 0.8660254037844387076, 1.000000000000000000, 0.8660254037844387076, 1.000000000000000000, 0.8660254037844387076, 1.000000000000000000, 0.8660254037844387076, 1.000000000000000000, 0.8660254037844387076, 1.000000000000000000, 0.8660254037844387076, 1.000000000000000000, 0.8660254037844387076, 1.000000000000000000, 0.8660254037844387076, 1.000000000000000000, 0.8660254037844387076, 1.000000000000000000, 0.8660254037844387076, 1.000000000000000000, 0.8660254037844387076, 1.000000000000000000, 0.8660254037844387076, 1.000000000000000000, 0.8660254037844387076, 1.000000000000000000, 0.8660254037844387076, 1.000000000000000000, 0.8660254037844387076, 1.000000000000000000, 0.8660254037844387076, 1.000000000000000000, 0.8660254037844387076, 1.000000000000000000, 0.8660254037844387076, 1.000000000000000000, 0.8660254037844387076, 1.000000000000000000, 0.8660254037844387076, 1.000000000000000000, 0.8660254037844387076, 1.000000000000000000, 0.8660254037844387076, 1.000000000000000000, 0.8660254037844387076, 1.000000000000000000, 0.8660254037844387076, 1.000000000000000000, 0.8660254037844387076, 1.000000000000000000, 0.8660254037844387076, 1.000000000000000000, 0.8660254037844387076, 1.000000000000000000, 0.8660254037844387076, 1.000000000000000000, 0.8660254037844387076, 1.000000000000000000, 0.8660254037844387076, 1.000000000000000000, 0.8660254037844387076, 1.000000000000000000, 0.8660254037844387076, 1.000000000000000000, 0.8660254037844387076, 1.000000000000000000, 0.8660254037844387076, 1.000000000000000000, 0.8660254037844387076, 1.000000000000000000, 0.8660254037844387076, 1.000000000000000000, 0.8660254037844387076, 1.000000000000000000, 0.8660254037844387076, 1.000000000000000000, 0.8660254037844387076, 1.000000000000000000, 0.8660254037844387076, 1.000000000000000000, 0.8660254037844387076, 1.000000000000000000, 0.8660254037844387076, 1.000000000000000000, 0.8660254037844387076, 1.000000000000000000, 0.8660254037844387076, 1.000000000000000000, 0.8660254037844387076, 1.000000000000000000, 0.8660254037844387076, 1.000000000000000000, 0.8660254037844387076, 1.000000000000000000, 0.8660254037844387076, 1.000000000000000000, 0.8660254037844387076, 1.000000000000000000, 0.8660254037844387076, 1.000000000000000000, 0.8660254037844387076, 1.000000000000000000, 0.8660254037844387076, 1.000000000000000000, 0.8660254037844387076, 1.000000000000000000, 0.8660254037844387076, 1.000000000000000000, 0.8660254037844387076, 1.000000000000000000, 0.8660254037844387076, 1.000000000000000000, 0.8660254037844387076, 1.000000000000000000, 0.8660254037844387076, 1.000000000000000000, 0.8660254037844387076, 1.000000000000000000, 0.8660254037844387076, 1.000000000000000000, 0.8660254037844387076, 1.000000000000000000, 0.8660254037844387076, 1.000000000000000000, 0.8660254037844387076, 1.000000000000000000, 0.8660254037844387076, 1.000000000000000000, 0.8660254037844387076, 1.000000000000000000, 0.8660254037844387076, 1.000000000000000000, 0.8660254037844387076, 1.000000000000000000, 0.8660254037844387076, 1.000000000000000000, 0.8660254037844387076, 1.000000000000000000, 0.8660254037844387076, 1.000000000000000000, 0.8660254037844387076, 1.000000000000000000, 0.8660254037844387076, 1.000000000000000000, 0.8660254037844387076, 1.000000000000000000, 0.8660254037844387076, 1.000000000000000000, 0.8660254037844387076, 1.000000000000000000, 0.8660254037844387076, 1.000000000000000000, 0.8660254037844387076, 1.000000000000000000, 0.8660254037844387076, 1.000000000000000000, 0.8660254037844387076, 1.000000000000000000, 0.8660254037844387076, 1.000000000000000000, 0.8660254037844387076, 1.000000000000000000, 0.8660254037844387076, 1.000000000000000000, 0.8660254037844387076, 1.000000000000000000, 0.8660254037844387076, 1.000000000000000000, 0.8660254037844387076, 1.000000000000000000, 0.8660254037844387076, 1.000000000000000000, 0.8660254037844387076, 1.000000000000000000, 0.8660254037844387076, 1.000000000000000000, 0.8660254037844387076, 1.000000000000000000, 0.8660254037844387076, 1.000000000000000000, 0.8660254037844387076, 1.000000000000000000, 0.8660254037844387076, 1.000000000000000000, 0.8660254037844387076, 1.000000000000000000, 0.8660254037844387076, 1.000000000000000000, 0.8660254037844387076, 1.000000000000000000, 0.8660254037844387076, 1.000000000000000000, 0.8660254037844387076, 1.000000000000000000, 0.8660254037844387076, 1.000000000000000000, 0.8660254037844387076, 1.000000000000000000, 0.8660254037844387076, 1.000000000000000000, 0.8660254037844387076, 1.000000000000000000, 0.8660254037844387076, 1.000000000000000000, 0.8660254037844387076, 1.000000000000000000, 0.8660254037844387076, 1.000000000000000000, 0.8660254037844387076, 1.000000000000000000, 0.8660254037844387076, 1.000000000000000000, 0.8660254037844387076, 1.000000000000000000, 0.8660254037844387076, 1.000000000000000000, 0.8660254037844387076, 1.000000000000000000, 0.8660254037844387076, 1.000000000000000000, 0.8660254037844387076, 1.000000000000000000, 0.8660254037844387076, 1.000000000000000000, 0.8660254037844387076, 1.000000000000000000, 0.8660254037844387076, 1.000000000000000000, 0.8660254037844387076, 1.000000000000000000, 0.8660254037844387076, 1.000000000000000000, 0.8660254037844387076, 1.000000000000000000),
 ( 1.000000000000000000, 0.8660254037844387076, 1.000000000000000000, 0.8660254037844387076, 1.000000000000000000, 0.8660254037844387076, 1.000000000000000000, 0.8660254037844387076, 1.000000000000000000, 0.8660254037844387076, 1.000000000000000000, 0.8660254037844387076, 1.000000000000000000, 0.8660254037844387076, 1.000000000000000000, 0.8660254037844387076, 1.000000000000000000, 0.8660254037844387076, 1.000000000000000000, 0.8660254037844387076, 1.000000000000000000, 0.8660254037844387076, 1.000000000000000000, 0.8660254037844387076, 1.000000000000000000, 0.8660254037844387076, 1.000000000000000000, 0.8660254037844387076, 1.000000000000000000, 0.8660254037844387076, 1.000000000000000000, 0.8660254037844387076, 1.000000000000000000, 0.8660254037844387076, 1.000000000000000000, 0.8660254037844387076, 1.000000000000000000, 0.8660254037844387076, 1.000000000000000000, 0.8660254037844387076, 1.000000000000000000, 0.8660254037844387076, 1.000000000000000000, 0.8660254037844387076, 1.000000000000000000, 0.8660254037844387076, 1.000000000000000000, 0.8660254037844387076, 1.000000000000000000, 0.8660254037844387076, 1.000000000000000000, 0.8660254037844387076, 1.000000000000000000, 0.8660254037844387076, 1.000000000000000000, 0.8660254037844387076, 1.000000000000000000, 0.8660254037844387076, 1.000000000000000000, 0.8660254037844387076, 1.000000000000000000, 0.8660254037844387076, 1.000000000000000000, 0.8660254037844387076, 1.000000000000000000, 0.8660254037844387076, 1.000000000000000000, 0.8660254037844387076, 1.000000000000000000, 0.8660254037844387076, 1.000000000000000000, 0.8660254037844387076, 1.000000000000000000, 0.8660254037844387076, 1.000000000000000000, 0.8660254037844387076, 1.000000000000000000, 0.8660254037844387076, 1.000000000000000000, 0.8660254037844387076, 1.000000000000000000, 0.8660254037844387076, 1.000000000000000000, 0.8660254037844387076, 1.000000000000000000, 0.8660254037844387076, 1.000000000000000000, 0.8660254037844387076, 1.000000000000000000, 0.8660254037844387076, 1.000000000000000000, 0.8660254037844387076, 1.000000000000000000, 0.8660254037844387076, 1.000000000000000000, 0.8660254037844387076, 1.000000000000000000, 0.8660254037844387076, 1.000000000000000000, 0.8660254037844387076, 1.000000000000000000, 0.8660254037844387076, 1.000000000000000000, 0.8660254037844387076, 1.000000000000000000, 0.8660254037844387076, 1.000000000000000000, 0.8660254037844387076, 1.000000000000000000, 0.8660254037844387076, 1.000000000000000000, 0.8660254037844387076, 1.000000000000000000, 0.8660254037844387076, 1.000000000000000000, 0.8660254037844387076, 1.000000000000000000, 0.8660254037844387076, 1.000000000000000000, 0.8660254037844387076, 1.000000000000000000, 0.8660254037844387076, 1.000000000000000000, 0.8660254037844387076, 1.000000000000000000, 0.8660254037844387076, 1.000000000000000000, 0.8660254037844387076, 1.000000000000000000, 0.8660254037844387076, 1.000000000000000000, 0.8660254037844387076, 1.000000000000000000, 0.8660254037844387076, 1.000000000000000000, 0.8660254037844387076, 1.000000000000000000, 0.8660254037844387076, 1.000000000000000000, 0.8660254037844387076, 1.000000000000000000, 0.8660254037844387076, 1.000000000000000000, 0.8660254037844387076, 1.000000000000000000, 0.8660254037844387076, 1.000000000000000000, 0.8660254037844387076, 1.000000000000000000, 0.8660254037844387076, 1.000000000000000000, 0.8660254037844387076, 1.000000000000000000, 0.8660254037844387076, 1.000000000000000000, 0.8660254037844387076, 1.000000000000000000, 0.8660254037844387076, 1.000000000000000000, 0.8660254037844387076, 1.000000000000000000, 0.8660254037844387076, 1.000000000000000000, 0.8660254037844387076, 1.000000000000000000, 0.8660254037844387076, 1.000000000000000000, 0.8660254037844387076, 1.000000000000000000, 0.8660254037844387076, 1.000000000000000000, 0.8660254037844387076, 1.000000000000000000, 0.8660254037844387076, 1.000000000000000000, 0.8660254037844387076, 1.000000000000000000, 0.8660254037844387076, 1.000000000000000000, 0.8660254037844387076, 1.000000000000000000, 0.8660254037844387076, 1.000000000000000000, 0.8660254037844387076, 1.000000000000000000, 0.8660254037844387076, 1.000000000000000000, 0.8660254037844387076, 1.000000000000000000, 0.8660254037844387076, 1.000000000000000000, 0.8660254037844387076, 1.000000000000000000, 0.8660254037844387076, 1.000000000000000000, 0.8660254037844387076, 1.000000000000000000, 0.8660254037844387076, 1.000000000000000000, 0.8660254037844387076, 1.000000000000000000, 0.8660254037844387076, 1.000000000000000000, 0.8660254037844387076, 1.000000000000000000, 0.8660254037844387076, 1.000000000000000000, 0.8660254037844387076, 1.000000000000000000, 0.8660254037844387076, 1.000000000000000000, 0.8660254037844387076, 1.000000000000000000, 0.8660254037844387076, 1.000000000000000000, 0.8660254037844387076, 1.000000000000000000, 0.8660254037844387076, 1.000000000000000000, 0.8660254037844387076, 1.000000000000000000, 0.8660254037844387076, 1.000000000000000000, 0.8660254037844387076, 1.000000000000000000, 0.8660254037844387076, 1.000000000000000000, 0.8660254037844387076, 1.000000000000000000, 0.8660254037844387076, 1.000000000000000000, 0.8660254037844387076, 1.000000000000000000, 0.8660254037844387076, 1.000000000000000000, 0.8660254037844387076, 1.000000000000000000, 0.8660254037844387076, 1.000000000000000000, 0.8660254037844387076, 1.000000000000000000, 0.8660254037844387076, 1.000000000000000000, 0.8660254037844387076, 1.000000000000000000, 0.8660254037844387076, 1.000000000000000000, 0.8660254037844387076, 1.000000000000000000, 0.8660254037844387076, 1.000000000000000000, 0.8660254037844387076, 1.000000000000000000, 0.8660254037844387076, 1.000000000000000000, 0.8660254037844387076, 1.000000000000000000, 0.8660254037844387076, 1.000000000000000000, 0.8660254037844387076, 1.000000000000000000, 0.8660254037844387076, 1.000000000000000000, 0.8660254037844387076, 1.000000000000000000, 0.8660254037844387076, 1.000000000000000000, 0.8660254037844387076, 1.000000000000000000, 0.8660254037844387076, 1.000000000000000000, 0.8660254037844387076, 1.000000000000000000, 0.8660254037844387076, 1.000000000000000000, 0.8660254037844387076, 1.000000000000000000, 0.8660254037844387076, 1.000000000000000000, 0.8660254037844387076, 1.000000000000000000, 0.8660254037844387076, 1.000000000000000000, 0.8660254037844387076, 1.000000000000000000, 0.8660254037844387076, 1.000000000000000000, 0.8660254037844387076, 1.000000000000000000, 0.8660254037844387076, 1.000000000000000000, 0.8660254037844387076, 1.000000000000000000, 0.8660254037844387076, 1.000000000000000000, 0.8660254037844387076, 1.000000000000000000, 0.8660254037844387076, 1.000000000000000000, 0.8660254037844387076, 1.000000000000000000, 0.8660254037844387076, 1.000000000000000000, 0.8660254037844387076, 1.000000000000000000, 0.8660254037844387076, 1.000000000000000000, 0.8660254037844387076, 1.000000000000000000, 0.8660254037844387076, 1.000000000000000000, 0.8660254037844387076, 1.000000000000000000, 0.8660254037844387076, 1.000000000000000000, 0.8660254037844387076, 1.000000000000000000, 0.8660254037844387076, 1.000000000000000000, 0.8660254037844387076, 1.000000000000000000, 0.8660254037844387076, 1.000000000000000000, 0.8660254037844387076, 1.000000000000000000, 0.8660254037844387076, 1.000000000000000000, 0.8660254037844387076, 1.000000000000000000, 0.8660254037844387076, 1.000000000000000000, 0.8660254037844387076, 1.000000000000000000, 0.8660254037844387076, 1.000000000000000000, 0.8660254037844387076, 1.000000000000000000, 0.8660254037844387076, 1.000000000000000000, 0.8660254037844387076, 1.000000000000000000, 0.8660254037844387076, 1.000000000000000000, 0.8660254037844387076, 1.000000000000000000, 0.8660254037844387076, 1.000000000000000000, 0.8660254037844387076, 1.000000000000000000, 0.8660254037844387076, 1.000000000000000000, 0.8660254037844387076, 1.000000000000000000, 0.8660254037844387076, 1.000000000000000000, 0.8660254037844387076, 1.000000000000000000, 0.8660254037844387076, 1.000000000000000000, 0.8660254037844387076, 1.000000000000000000, 0.8660254037844387076, 1.000000000000000000, 0.8660254037844387076, 1.000000000000000000, 0.8660254037844387076, 1.000000000000000000, 0.8660254037844387076, 1.000000000000000000, 0.8660254037844387076, 1.000000000000000000, 0.8660254037844387076, 1.000000000000000000, 0.8660254037844387076, 1.000000000000000000, 0.8660254037844387076, 1.000000000000000000, 0.8660254037844387076, 1.000000000000000000, 0.8660254037844387076, 1.000000000000000000, 0.8660254037844387076, 1.000000000000000000, 0.8660254037844387076, 1.000000000000000000, 0.8660254037844387076, 1.000000000000000000, 0.8660254037844387076, 1.000000000000000000, 0.8660254037844387076, 1.000000000000000000, 0.8660254037844387076, 1.000000000000000000, 0.8660254037844387076, 1.000000000000000000, 0.8660254037844387076, 1.000000000000000000, 0.8660254037844387076, 1.000000000000000000, 0.8660254037844387076, 1.000000000000000000, 0.8660254037844387076, 1.000000000000000000, 0.8660254037844387076, 1.000000000000000000, 0.8660254037844387076, 1.000000000000000000, 0.8660254037844387076, 1.000000000000000000, 0.8660254037844387076, 1.000000000000000000, 0.8660254037844387076, 1.000000000000000000, 0.8660254037844387076, 1.000000000000000000, 0.8660254037844387076, 1.000000000000000000, 0.8660254037844387076, 1.000000000000000000, 0.8660254037844387076, 1.000000000000000000, 0.8660254037844387076, 1.000000000000000000, 0.8660254037844387076, 1.000000000000000000, 0.8660254037844387076, 1.000000000000000000, 0.8660254037844387076, 1.000000000000000000, 0.8660254037844387076, 1.000000000000000000, 0.8660254037844387076, 1.000000000000000000, 0.8660254037844387076, 1.000000000000000000, 0.8660254037844387076, 1.000000000000000000, 0.8660254037844387076, 1.000000000000000000, 0.8660254037844387076, 1.000000000000000000, 0.8660254037844387076, 1.000000000000000000, 0.8660254037844387076, 1.000000000000000000, 0.8660254037844387076, 1.000000000000000000, 0.8660254037844387076, 1.000000000000000000, 0.8660254037844387076, 1.000000000000000000, 0.8660254037844387076, 1.000000000000000000, 0.8660254037844387076, 1.000000000000000000, 0.8660254037844387076, 1.000000000000000000, 0.8660254037844387076, 1.000000000000000000, 0.8660254037844387076, 1.000000000000000000, 0.8660254037844387076, 1.000000000000000000, 0.8660254037844387076, 1.000000000000000000, 0.8660254037844387076, 1.000000000000000000, 0.8660254037844387076, 1.000000000000000000, 0.8660254037844387076, 1.000000000000000000, 0.8660254037844387076, 1.000000000000000000, 0.8660254037844387076, 1.000000000000000000, 0.8660254037844387076, 1.000000000000000000, 0.8660254037844387076, 1.000000000000000000, 0.8660254037844387076, 1.000000000000000000) ) ) 
 REPRESENTATION_ITEM ( '' )  SURFACE ( )  );
#180781=CARTESIAN_POINT ( 'NONE',  ( -4.731432421044883263, 5.582721248382882528, -1.082531754730543971 ) ) ;
#180782=CARTESIAN_POINT ( 'NONE',  ( 6.356075086708249167, 6.309842444114747373, -0.7998128361456281477 ) ) ;
#180790=CARTESIAN_POINT ( 'NONE',  ( -3.741687207691642314, 6.348756928073427730, 1.082531754730560403 ) ) ;
#180797=CARTESIAN_POINT ( 'NONE',  ( -1.364683531250000748, 1.759375000341421913, 0.000000000000000000 ) ) ;
#180799=CARTESIAN_POINT ( 'NONE',  ( -5.065942953000576843, 9.062017211809330064, -0.7998128361456231517 ) ) ;
#180802=CARTESIAN_POINT ( 'NONE',  ( 5.686755365928134687, 8.721966129303114101, 1.199719254218462483 ) ) ;
#180803=CARTESIAN_POINT ( 'NONE',  ( -7.549192604710863286, 7.701812881784464437, -0.7998128361456291469 ) ) ;
#180806=CARTESIAN_POINT ( 'NONE',  ( -1.500000000000015099, 0.9104166673494835660, -0.8660254037844313801 ) ) ;
#180809=CARTESIAN_POINT ( 'NONE',  ( 7.619319141200063150, 9.912291636198670375, 1.443375672974076540 ) ) ;
#180812=CARTESIAN_POINT ( 'NONE',  ( -1.402160292154681736E-14, 1.259375000341419248, -1.575800808251659024 ) ) ;
#180813=CARTESIAN_POINT ( 'NONE',  ( 7.104109303436412226, 7.390475063538369582, 1.040834085586084257E-14 ) ) ;
#180816=CARTESIAN_POINT ( 'NONE',  ( -5.761852096127856981, 5.824508321678349532, 0.000000000000000000 ) ) ;
#180818=CARTESIAN_POINT ( 'NONE',  ( -1.364683531250010295, 4.030208333674751842, 0.7879004041258379498 ) ) ;
#180830=CARTESIAN_POINT ( 'NONE',  ( 5.947222937888848371, 10.09017719417900416, 1.040834085586084257E-14 ) ) ;
#180833=CARTESIAN_POINT ( 'NONE',  ( 4.844340958784499662, 4.546152628203684820, 0.7998128361456341429 ) ) ;
#180839=CARTESIAN_POINT ( 'NONE',  ( 3.863710590214593399, 7.451486755318259547, 1.040834085586084257E-14 ) ) ;
#180840=CARTESIAN_POINT ( 'NONE',  ( -1.201851678989727383E-14, 1.134375000341418582, 1.575800808251672791 ) ) ;
#180844=VERTEX_POINT ( 'NONE', #202484 ) ;
#180849=CARTESIAN_POINT ( 'NONE',  ( -1.201851678989727383E-14, 1.212500000000025002, 1.732050807568877637 ) ) ;
#180850=CARTESIAN_POINT ( 'NONE',  ( 7.284808609244363353, 7.393364887073558656, 0.7998128361456341429 ) ) ;
#180851=CARTESIAN_POINT ( 'NONE',  ( -9.203287345578106127, 9.631590079462940324, 0.7998128361456462443 ) ) ;
#180855=CARTESIAN_POINT ( 'NONE',  ( -1.364683531250012516, 1.530208333674756505, 0.7879004041258379498 ) ) ;
#180857=CARTESIAN_POINT ( 'NONE',  ( -1.499999999999997780, 1.900000000000019673, 0.000000000000000000 ) ) ;
#180859=CARTESIAN_POINT ( 'NONE',  ( 2.998324526916512411, 6.649795714711241423, 0.000000000000000000 ) ) ;
#180867=CARTESIAN_POINT ( 'NONE',  ( 0.7499999999999867883, -0.1520833326505155458, -1.299038105676652899 ) ) ;
#180868=CARTESIAN_POINT ( 'NONE',  ( -6.320072162264675164, 10.52516795595079557, 0.7998128361456481317 ) ) ;
#180869=CARTESIAN_POINT ( 'NONE',  ( -4.948362879307902418, 4.875437568721725512, 1.214306433183764966E-14 ) ) ;
#180875=ORIENTED_EDGE ( 'NONE', *, *, #88421, .F. ) ;
#180876=EDGE_CURVE ( 'NONE', #69090, #195242, #78891, .T. ) ;
#180877=CARTESIAN_POINT ( 'NONE',  ( 6.693975156845185737, 8.832723654451292816, 1.599625672291281386 ) ) ;
#180879=CYLINDRICAL_SURFACE ( 'NONE', #171903, 0.07999999999999998779 ) ;
#180881=CARTESIAN_POINT ( 'NONE',  ( 5.686755365928134687, 8.721966129303114101, 1.199719254218462483 ) ) ;
#180882=CARTESIAN_POINT ( 'NONE',  ( 10.03267048398825168, 10.80712977418221676, 0.000000000000000000 ) ) ;
#180885=CARTESIAN_POINT ( 'NONE',  ( -6.507023659554960204, 9.678945805201045971, 1.199719254218452047 ) ) ;
#180886=CARTESIAN_POINT ( 'NONE',  ( 5.705283713252285338, 5.550585841749444249, -0.7998128361456211532 ) ) ;
#180892=CARTESIAN_POINT ( 'NONE',  ( 10.22248463502393001, 11.02857961705718282, 0.7216878364870438212 ) ) ;
#180900=CARTESIAN_POINT ( 'NONE',  ( -5.124618876285560454, 5.081069565195661220, 0.7216878364870317197 ) ) ;
#180901=CARTESIAN_POINT ( 'NONE',  ( 7.890482213473377193, 11.18901776815221716, -1.082531754730543083 ) ) ;
#180904=B_SPLINE_CURVE_WITH_KNOTS ( 'NONE', 3,
 ( #83052, #148080, #19114, #114572 ),
 .UNSPECIFIED., .F., .F.,
 ( 4, 4 ),
 ( 1.043091274928057275E-17, 0.0006764026532485904134 ),
 .UNSPECIFIED. ) ;
#180905=CARTESIAN_POINT ( 'NONE',  ( -4.717347382551060342, 7.590990148696470818, 1.199719254218464037 ) ) ;
#180907=FACE_OUTER_BOUND ( 'NONE', #87835, .T. ) ;
#180909=CARTESIAN_POINT ( 'NONE',  ( 3.621833129746810265, 4.096114899008192367, 2.420000000000023022 ) ) ;
#180911=CARTESIAN_POINT ( 'NONE',  ( -7.531718027591449705, 8.745758106066849891, 1.199719254218462483 ) ) ;
#180914=EDGE_CURVE ( 'NONE', #162715, #150994, #53459, .T. ) ;
#180916=ORIENTED_EDGE ( 'NONE', *, *, #72672, .T. ) ;
#180918=EDGE_LOOP ( 'NONE', ( #11603, #9306, #107959, #125038 ) ) ;
#180926=CARTESIAN_POINT ( 'NONE',  ( -5.961834861707238531, 7.978559976790334574, -1.599625672291263179 ) ) ;
#180929=CARTESIAN_POINT ( 'NONE',  ( 5.843201017809841247, 5.919415396974013532, 1.040834085586084257E-14 ) ) ;
#180930=CARTESIAN_POINT ( 'NONE',  ( -2.273105066167321997, 5.702484939155337607, -2.420000000000000373 ) ) ;
#180933=CARTESIAN_POINT ( 'NONE',  ( -4.634189577772691138, 4.300976017023221409, 1.214306433183764966E-14 ) ) ;
#180941=CARTESIAN_POINT ( 'NONE',  ( -8.341290820905609138, 10.75459192918846618, 1.599625672291269396 ) ) ;
#180942=CARTESIAN_POINT ( 'NONE',  ( 5.961834861707224320, 7.978559976790334574, -1.599625672291262513 ) ) ;
#180945=CARTESIAN_POINT ( 'NONE',  ( 3.825371897350130279, 7.614684313550482031, 0.7998128361456321445 ) ) ;
#180948=CARTESIAN_POINT ( 'NONE',  ( -1.364683531250014514, 0.05104166700808546175, -0.7879004041258359514 ) ) ;
#180949=ORIENTED_EDGE ( 'NONE', *, *, #86749, .T. ) ;
#180951=CARTESIAN_POINT ( 'NONE',  ( 7.863365906246055914, 10.19701286208565705, -1.443375672974057666 ) ) ;
#180955=ADVANCED_FACE ( 'NONE', ( #173233 ), #213844, .T. ) ;
#180958=ORIENTED_EDGE ( 'NONE', *, *, #138558, .T. ) ;
#180981=CARTESIAN_POINT ( 'NONE',  ( -1.500000000000015099, 0.4104166673494891726, -0.8660254037844383745 ) ) ;
#180988=CARTESIAN_POINT ( 'NONE',  ( 8.218213668177886788, 12.73966637951625813, 0.7998128361456462443 ) ) ;
#180992=CARTESIAN_POINT ( 'NONE',  ( 4.792970997630896512, 5.550553237779539018, 1.199719254218464037 ) ) ;
#180993=CARTESIAN_POINT ( 'NONE',  ( -7.876924059859742755, 8.292092279365579799, 1.040834085586084257E-14 ) ) ;
#180998=CARTESIAN_POINT ( 'NONE',  ( -8.030507057996002729, 8.263346410617135263, 1.040834085586084257E-14 ) ) ;
#180999=CARTESIAN_POINT ( 'NONE',  ( -2.290964770585000920, 5.616616632417037458, -0.7216878364870257245 ) ) ;
#181002=CARTESIAN_POINT ( 'NONE',  ( -1.500000000000013101, 1.202083334016148974, 0.8660254037844403729 ) ) ;
#181009=CARTESIAN_POINT ( 'NONE',  ( -2.751941993449643409, 6.154423392425789174, 0.7216878364870317197 ) ) ;
#181012=CARTESIAN_POINT ( 'NONE',  ( 4.041346116833469893, 7.538066791021210022, -0.4365389052301202333 ) ) ;
#181018=CARTESIAN_POINT ( 'NONE',  ( -10.65400978224035811, 11.32409958890225710, 1.040834085586084257E-14 ) ) ;
#181019=CARTESIAN_POINT ( 'NONE',  ( 7.283754839039659146, 9.520799950344851936, -1.599625672291262513 ) ) ;
#181024=CARTESIAN_POINT ( 'NONE',  ( 1.499999999999990896, 5.275000000000022560, 1.214306433183764966E-14 ) ) ;
#181030=CARTESIAN_POINT ( 'NONE',  ( -8.134002093194872884, 11.57708731111429401, 1.199719254218453823 ) ) ;
#181036=CARTESIAN_POINT ( 'NONE',  ( 4.517891501851804215, 6.293959390292322986, -1.599625672291255185 ) ) ;
#181040=EDGE_LOOP ( 'NONE', ( #30224, #166508, #148413, #4567, #171055 ) ) ;
#181041=CARTESIAN_POINT ( 'NONE',  ( -5.342823980928611327, 4.390142039796957718, 2.499999999999999112 ) ) ;
#181042=DIRECTION ( 'NONE',  ( 0.6507913734559640506, -0.7592566023653004592, 0.000000000000000000 ) ) ;
#181052=CARTESIAN_POINT ( 'NONE',  ( 8.145751363712157911, 8.397798100619326078, -0.7998128361456281477 ) ) ;
#181054=CARTESIAN_POINT ( 'NONE',  ( -3.273404022695637572, 5.906389562198459231, 1.199719254218462483 ) ) ;
#181057=CARTESIAN_POINT ( 'NONE',  ( 1.123270288254022198, 2.908552654332631437, -0.7749999999939810591 ) ) ;
#181061=CARTESIAN_POINT ( 'NONE',  ( -0.7500000000000215383, 0.7229166673494852313, 1.299038105676659116 ) ) ;
#181064=CARTESIAN_POINT ( 'NONE',  ( -1.492681600543587006, 8.694743381153374528, -2.590460435319442922 ) ) ;
#181065=CARTESIAN_POINT ( 'NONE',  ( 3.379006598303866848, 4.965260336153046516, -1.599625672291262513 ) ) ;
#181067=CARTESIAN_POINT ( 'NONE',  ( -3.002240950422295995, 5.590032644546251817, -1.199719254218452935 ) ) ;
#181073=CARTESIAN_POINT ( 'NONE',  ( 5.341549334104194635, 6.294524313618772737, 1.082531754730558626 ) ) ;
#181075=ORIENTED_EDGE ( 'NONE', *, *, #162333, .T. ) ;
#181076=CARTESIAN_POINT ( 'NONE',  ( -0.6823417656250212460, 4.613541667008086655, 1.181850606188767472 ) ) ;
#181077=CARTESIAN_POINT ( 'NONE',  ( -2.279984679289828176, 5.601133616484927025, -0.06592222766762731445 ) ) ;
#181078=CARTESIAN_POINT ( 'NONE',  ( 4.487385655998888723, 4.337630808194552934, 0.7216878364870317197 ) ) ;
#181086=CARTESIAN_POINT ( 'NONE',  ( -6.082978790695654503, 6.030206930409384825, -0.4315292173028318912 ) ) ;
#181089=CARTESIAN_POINT ( 'NONE',  ( -1.402160292154681736E-14, -0.6781249996585819728, 1.575800808251672791 ) ) ;
#181096=CARTESIAN_POINT ( 'NONE',  ( -1.402160292154681736E-14, -1.037499999999977662, 1.732050807568877637 ) ) ;
#181098=CARTESIAN_POINT ( 'NONE',  ( -1.500000000000011324, 4.420833333333352044, 0.8660254037844403729 ) ) ;
#181104=ORIENTED_EDGE ( 'NONE', *, *, #58523, .T. ) ;
#181106=CARTESIAN_POINT ( 'NONE',  ( 1.364683531249990311, 4.676041667008083103, 0.7879004041258500513 ) ) ;
#181108=CARTESIAN_POINT ( 'NONE',  ( 6.582647274634798151, 7.638508894284114170, 1.199719254218462483 ) ) ;
#181110=CARTESIAN_POINT ( 'NONE',  ( -8.097244055859620815, 10.46987070330147063, -1.599625672291263179 ) ) ;
#181115=CARTESIAN_POINT ( 'NONE',  ( 1.499999999999989120, 5.504166666666685970, 0.8660254037844524744 ) ) ;
#181119=CARTESIAN_POINT ( 'NONE',  ( 4.771998164587357927, 6.814557936359840085, -1.288453177375107783 ) ) ;
#181122=CARTESIAN_POINT ( 'NONE',  ( 7.619319141200051604, 11.83303006480134911, 0.7216878364870438212 ) ) ;
#181126=CARTESIAN_POINT ( 'NONE',  ( -1.500000000000013101, 3.660416667349488673, -0.8660254037844313801 ) ) ;
#181128=CARTESIAN_POINT ( 'NONE',  ( -3.795392936821753604, 6.515376628678959392, -1.199719254218452047 ) ) ;
#181129=CARTESIAN_POINT ( 'NONE',  ( 4.080641047588898118, 5.783833860318930320, -1.443375672974051449 ) ) ;
#181130=CARTESIAN_POINT ( 'NONE',  ( -8.622622508166983835, 13.00355065959610279, 1.040834085586084257E-14 ) ) ;
#181137=FACE_BOUND ( 'NONE', #88964, .T. ) ;
#181138=CARTESIAN_POINT ( 'NONE',  ( 3.846762897975340767, 5.510976019103107859, -1.599625672291256295 ) ) ;
#181141=CARTESIAN_POINT ( 'NONE',  ( 5.054492339796319733, 4.791329239384148231, -0.7998128361456211532 ) ) ;
#181145=EDGE_LOOP ( 'NONE', ( #150382, #54251, #37864, #45132, #203213, #171282, #55333, #124245, #21355, #183310, #128924, #125574, #123743 ) ) ;
#181155=CARTESIAN_POINT ( 'NONE',  ( 9.402743226277308963, 10.92862083786708816, -1.199719254218446718 ) ) ;
#181159=CARTESIAN_POINT ( 'NONE',  ( 0.6823417656249882723, -0.1572916663252488245, 1.181850606188755259 ) ) ;
#181161=CARTESIAN_POINT ( 'NONE',  ( 7.144783764721768904, 7.437928601704619780, 1.040834085586084257E-14 ) ) ;
#181162=CARTESIAN_POINT ( 'NONE',  ( -4.302014814237876017, 3.913438792899272212, 0.7998128361456341429 ) ) ;
#181168=CARTESIAN_POINT ( 'NONE',  ( -4.762992037102518950, 4.451245552908022596, -0.7998128361456221525 ) ) ;
#181181=CARTESIAN_POINT ( 'NONE',  ( 5.889294496748854968, 6.159041356224602026, -0.8323295365256941913 ) ) ;
#181185=PLANE ( 'NONE',  #192861 ) ;
#181188=CARTESIAN_POINT ( 'NONE',  ( -7.185458225562757484, 11.32685899655781903, 0.7216878364870458196 ) ) ;
#181192=CARTESIAN_POINT ( 'NONE',  ( 7.962716289927667113, 8.184257181204083409, -0.7998128361456291469 ) ) ;
#181193=CARTESIAN_POINT ( 'NONE',  ( -4.843287188579803448, 6.673587691474970107, -1.599625672291256517 ) ) ;
#181195=CARTESIAN_POINT ( 'NONE',  ( -3.913499895838973508, 7.717500311787445000, 1.040834085586084257E-14 ) ) ;
#181197=CARTESIAN_POINT ( 'NONE',  ( -4.693093728624763372, 8.627026450037540428, 0.7998128361456481317 ) ) ;
#181200=CARTESIAN_POINT ( 'NONE',  ( 9.562578416340237197, 10.05076299535211781, 0.7998128361456462443 ) ) ;
#181201=CARTESIAN_POINT ( 'NONE',  ( -0.1099460098626957039, 6.494484681433106310, 3.110387376256865011 ) ) ;
#181203=CARTESIAN_POINT ( 'NONE',  ( 4.469394083494863779, 7.278994484577430590, 1.251062204184281379 ) ) ;
#181204=CARTESIAN_POINT ( 'NONE',  ( 4.690757960648221037, 7.456006139856155457, 1.082531754730558626 ) ) ;
#181206=CARTESIAN_POINT ( 'NONE',  ( 3.673896439178926610, 7.230036912443287278, 0.7216878364870428220 ) ) ;
#181213=CARTESIAN_POINT ( 'NONE',  ( 7.470179451005385829, 8.777926116670192513, -1.082531754730537976 ) ) ;
#181217=CARTESIAN_POINT ( 'NONE',  ( -9.657485491635913633, 10.16148791653038330, 1.040834085586084257E-14 ) ) ;
#181218=CARTESIAN_POINT ( 'NONE',  ( -8.362681821530818738, 8.650883634741092010, -0.7998128361456291469 ) ) ;
#181226=CARTESIAN_POINT ( 'NONE',  ( 9.565441069641300587, 11.11843498845840905, -1.199719254218440723 ) ) ;
#181230=CARTESIAN_POINT ( 'NONE',  ( 4.369805582306193870, 3.992528022312320957, 1.214306433183764966E-14 ) ) ;
#181233=CARTESIAN_POINT ( 'NONE',  ( 0.7499999999999902300, 4.597916667349482012, -1.299038105676658228 ) ) ;
#181239=CARTESIAN_POINT ( 'NONE',  ( -1.201851678989727383E-14, 3.212500000000018119, 1.732050807568877637 ) ) ;
#181240=CARTESIAN_POINT ( 'NONE',  ( 6.287230548435207567, 8.358188277972981695, -1.599625672291262513 ) ) ;
#181243=CARTESIAN_POINT ( 'NONE',  ( 9.259855728453651125, 9.905512559391842942, 1.040834085586084257E-14 ) ) ;
#181249=CARTESIAN_POINT ( 'NONE',  ( 8.516493047678546091, 13.08765898893368629, -0.7998128361456352531 ) ) ;
#181251=CARTESIAN_POINT ( 'NONE',  ( -4.497554271431319250, 6.270232621468402989, -1.599625672291256295 ) ) ;
#181253=CARTESIAN_POINT ( 'NONE',  ( -0.6823417656250003738, -0.7822916663252423852, -1.181850606188749264 ) ) ;
#181257=CARTESIAN_POINT ( 'NONE',  ( 4.955668840994886359, 5.740367388370866131, 1.199719254218462483 ) ) ;
#181259=CARTESIAN_POINT ( 'NONE',  ( -1.364683531250014514, -1.219791666325248602, 0.7879004041258379498 ) ) ;
#181262=CARTESIAN_POINT ( 'NONE',  ( 4.823331260782475205, 6.941738851361666462, 1.443736280540828032 ) ) ;
#181267=CARTESIAN_POINT ( 'NONE',  ( -7.283754839039664475, 9.520799950344851936, -1.599625672291263179 ) ) ;
#181269=CARTESIAN_POINT ( 'NONE',  ( 6.030679399980265920, 5.930214142932100252, -0.7998128361456281477 ) ) ;
#181272=CARTESIAN_POINT ( 'NONE',  ( -1.364683531250000748, -0.7406249996585803075, 0.000000000000000000 ) ) ;
#181276=CARTESIAN_POINT ( 'NONE',  ( 10.07100917685271035, 10.64393221595000938, 0.7998128361456462443 ) ) ;
#181279=CARTESIAN_POINT ( 'NONE',  ( -4.557512192488103686, 8.468847991211438497, -0.7998128361456281477 ) ) ;
#181283=CARTESIAN_POINT ( 'NONE',  ( 8.239604668803105270, 10.63595808506888396, -1.599625672291268286 ) ) ;
#181285=CARTESIAN_POINT ( 'NONE',  ( 7.995557903757111617, 10.35123685918189729, 1.599625672291281386 ) ) ;
#181287=CARTESIAN_POINT ( 'NONE',  ( -3.846762897975357198, 5.510976019103107859, -1.599625672291256295 ) ) ;
#181288=CARTESIAN_POINT ( 'NONE',  ( -5.845536785786364931, 9.971543350059432598, 0.000000000000000000 ) ) ;
#181290=ADVANCED_FACE ( 'NONE', ( #162300 ), #58891, .T. ) ;
#181292=CARTESIAN_POINT ( 'NONE',  ( -4.956836104118029773, 6.830226236571708576, 1.450618959550575182 ) ) ;
#181293=CARTESIAN_POINT ( 'NONE',  ( -1.364683531250000748, 1.009375000341421247, 0.000000000000000000 ) ) ;
#181297=CARTESIAN_POINT ( 'NONE',  ( 6.426201623197458801, 9.480690412830290015, -1.082531754730537088 ) ) ;
#181300=CARTESIAN_POINT ( 'NONE',  ( 3.994848817520957773, 7.812407387083109001, 1.040834085586084257E-14 ) ) ;
#181319=CARTESIAN_POINT ( 'NONE',  ( 8.387690588348714726, 12.93738945304888333, 1.040834085586084257E-14 ) ) ;
#181323=CARTESIAN_POINT ( 'NONE',  ( -4.894657149733403045, 5.669187081899118574, -1.199719254218446718 ) ) ;
#181324=CARTESIAN_POINT ( 'NONE',  ( -7.147119532698295252, 11.49005655479003174, 0.000000000000000000 ) ) ;
#181328=B_SPLINE_CURVE_WITH_KNOTS ( 'NONE', 3,
 ( #26626, #205365, #56999, #157719, #22331, #122089, #156648 ),
 .UNSPECIFIED., .F., .F.,
 ( 4, 3, 4 ),
 ( 0.000000000000000000, 2.778001202718471385E-05, 5.460790091229278642E-05 ),
 .UNSPECIFIED. ) ;
#181330=CARTESIAN_POINT ( 'NONE',  ( 1.499999999999987121, 3.577083334016152527, -0.8660254037844262731 ) ) ;
#181331=CARTESIAN_POINT ( 'NONE',  ( 8.076906825439115423, 10.44614393447756129, -1.599625672291262513 ) ) ;
#181335=CARTESIAN_POINT ( 'NONE',  ( -9.677822722056413696, 10.18521468535430685, 1.040834085586084257E-14 ) ) ;
#181337=CARTESIAN_POINT ( 'NONE',  ( 0.6823417656249899377, 3.926041667008085767, -1.181850606188754593 ) ) ;
#181339=CARTESIAN_POINT ( 'NONE',  ( -3.289951133708679087, 7.658661826346113699, 2.499999999999998668 ) ) ;
#181343=CARTESIAN_POINT ( 'NONE',  ( -8.948018195339354719, 12.42280974699582607, 1.082531754730560403 ) ) ;
#181347=CARTESIAN_POINT ( 'NONE',  ( 0.6823417656249899377, 1.905208333674752952, 1.181850606188755259 ) ) ;
#181348=ADVANCED_FACE ( 'NONE', ( #195399 ), #178093, .F. ) ;
#181353=CARTESIAN_POINT ( 'NONE',  ( -1.364683531250014514, 0.9885416670080898749, -0.7879004041258289570 ) ) ;
#181355=CARTESIAN_POINT ( 'NONE',  ( -4.713430959045263435, 8.650753218861462202, 0.7998128361456481317 ) ) ;
#181356=CARTESIAN_POINT ( 'NONE',  ( 7.962716289927667113, 8.184257181204083409, -0.7998128361456291469 ) ) ;
#181357=CARTESIAN_POINT ( 'NONE',  ( -1.270916165646622353, 2.915225491120026824, 0.7750000000000152323 ) ) ;
#181361=CARTESIAN_POINT ( 'NONE',  ( -0.7500000000000215383, 5.191666666666685082, 1.299038105676671107 ) ) ;
#181362=CARTESIAN_POINT ( 'NONE',  ( -1.364683531249997417, 2.821875000341422801, 1.214306433183764966E-14 ) ) ;
#181365=DIRECTION ( 'NONE',  ( 0.7592566023653004592, -0.6507913734559641616, -1.725633230170963105E-31 ) ) ;
#181366=CARTESIAN_POINT ( 'NONE',  ( -5.910991785878183080, 5.998504626387068051, -0.7216878364870278340 ) ) ;
#181371=CARTESIAN_POINT ( 'NONE',  ( 3.877268743828258479, 7.467304601200877023, 0.7216878364870298324 ) ) ;
#181374=CARTESIAN_POINT ( 'NONE',  ( -7.018317073368468328, 11.33978701890523233, -0.7998128361456291469 ) ) ;
#181375=CARTESIAN_POINT ( 'NONE',  ( -4.790108344329849110, 4.482881244673243337, 0.7998128361456341429 ) ) ;
#181377=CARTESIAN_POINT ( 'NONE',  ( -0.6823417656249969321, 4.717708333674755394, -1.181850606188749264 ) ) ;
#181382=CARTESIAN_POINT ( 'NONE',  ( -6.358410854684783509, 9.401601182898824405, -1.082531754730537976 ) ) ;
#181384=CARTESIAN_POINT ( 'NONE',  ( -1.364683531250000748, -0.1781249996585798634, 0.000000000000000000 ) ) ;
#181387=CARTESIAN_POINT ( 'NONE',  ( 8.107412671292042461, 9.521364873671299023, 1.082531754730558626 ) ) ;
#181395=ORIENTED_EDGE ( 'NONE', *, *, #12700, .T. ) ;
#181396=CARTESIAN_POINT ( 'NONE',  ( 9.707274797260268429, 10.42750147299956964, 0.000000000000000000 ) ) ;
#181401=ORIENTED_EDGE ( 'NONE', *, *, #30090, .F. ) ;
#181402=CARTESIAN_POINT ( 'NONE',  ( 6.908042961362778733, 8.018137195466769285, 1.199719254218462483 ) ) ;
#181403=CARTESIAN_POINT ( 'NONE',  ( -6.552668314106420588, 6.539201209412602189, -0.7998128361456291469 ) ) ;
#181406=CARTESIAN_POINT ( 'NONE',  ( 5.843201017365476702, 6.879784610756938257, -1.082531754730543083 ) ) ;
#181407=CARTESIAN_POINT ( 'NONE',  ( 1.364683531249986537, -0.2822916663252520997, -0.7879004041258309554 ) ) ;
#181409=CARTESIAN_POINT ( 'NONE',  ( -8.809047120577080392, 11.30030761213851953, 1.599625672291269396 ) ) ;
#181419=ORIENTED_EDGE ( 'NONE', *, *, #124309, .F. ) ;
#181424=CARTESIAN_POINT ( 'NONE',  ( 6.958359152311676787, 9.141171649162195934, -1.599625672291262513 ) ) ;
#181425=CARTESIAN_POINT ( 'NONE',  ( 6.714312387265682247, 8.856450423275211037, 1.599625672291281386 ) ) ;
#181433=( BOUNDED_CURVE ( )  B_SPLINE_CURVE ( 2, ( #41583, #156389, #204022, #27437, #7975, #93535, #74063 ),
 .UNSPECIFIED., .F., .T. ) 
 B_SPLINE_CURVE_WITH_KNOTS ( ( 3, 2, 2, 3 ),
 ( 0.1625000000000002276, 0.1666666666666669072, 0.1708333333333336146, 0.1750000000000002942 ),
 .UNSPECIFIED. ) 
 CURVE ( )  GEOMETRIC_REPRESENTATION_ITEM ( )  RATIONAL_B_SPLINE_CURVE ( ( 0.9999999999999928946, 0.8660254037844458130, 1.000000000000000000, 0.8660254037844387076, 1.000000000000000000, 0.8660254037844289376, 1.000000000000009770 ) ) 
 REPRESENTATION_ITEM ( '' )  );
#181437=CARTESIAN_POINT ( 'NONE',  ( -6.437424008390261854, 6.404749519410410485, 0.7998128361456341429 ) ) ;
#181441=FACE_OUTER_BOUND ( 'NONE', #76365, .T. ) ;
#181446=VECTOR ( 'NONE', #111750, 1000.000000000000000 ) ;
#181448=CARTESIAN_POINT ( 'NONE',  ( -9.978437869977959451, 10.74385839117019614, -0.7216878364870267237 ) ) ;
#181452=CARTESIAN_POINT ( 'NONE',  ( 6.043183783389218355, 8.073467052085995022, 1.599625672291267398 ) ) ;
#181459=CARTESIAN_POINT ( 'NONE',  ( 3.782361668088245921, 6.396210465202840645, -1.082531754730548412 ) ) ;
#181460=CARTESIAN_POINT ( 'NONE',  ( -5.520141099058386125, 9.591915048876776595, 0.000000000000000000 ) ) ;
#181466=CARTESIAN_POINT ( 'NONE',  ( -5.910464900553636269, 8.982960586366182554, -1.199719254218440723 ) ) ;
#181467=CARTESIAN_POINT ( 'NONE',  ( -4.599240423533815125, 6.388866465587984322, 1.599625672291267398 ) ) ;
#181471=LINE ( 'NONE', #33101, #136847 ) ;
#181474=CARTESIAN_POINT ( 'NONE',  ( 5.341022448779654930, 8.318611059296550536, 1.199719254218462483 ) ) ;
#181487=CARTESIAN_POINT ( 'NONE',  ( 1.364683531249988757, 0.1968750003414204697, 0.000000000000000000 ) ) ;
#181489=CARTESIAN_POINT ( 'NONE',  ( 6.179819089730593795, 6.104210447640811665, 1.040834085586084257E-14 ) ) ;
#181491=CARTESIAN_POINT ( 'NONE',  ( -8.080296364064746939, 9.489729181906076505, 1.082531754730558626 ) ) ;
#181493=CARTESIAN_POINT ( 'NONE',  ( 5.355107487717867265, 5.349972945200037522, 1.040834085586084257E-14 ) ) ;
#181494=CARTESIAN_POINT ( 'NONE',  ( -7.849807752188049825, 8.260456587081938196, 0.7216878364870578100 ) ) ;
#181497=EDGE_LOOP ( 'NONE', ( #66819, #159117, #33799 ) ) ;
#181499=CARTESIAN_POINT ( 'NONE',  ( 7.772902139336337335, 7.962807338847539107, 0.7998128361456341429 ) ) ;
#181503=CARTESIAN_POINT ( 'NONE',  ( 0.6823417656249917140, 3.842708333674754506, 1.181850606188765695 ) ) ;
#181508=CARTESIAN_POINT ( 'NONE',  ( 8.284195553149872993, 9.623648552551724578, -1.199719254218445830 ) ) ;
#181512=CARTESIAN_POINT ( 'NONE',  ( -7.720478407978036195, 11.09464301169468037, -1.199719254218446718 ) ) ;
#181518=CARTESIAN_POINT ( 'NONE',  ( 7.879259827836241570, 12.34422023245099176, 1.040834085586084257E-14 ) ) ;
#181521=CARTESIAN_POINT ( 'NONE',  ( -8.528242318195895066, 9.908369778438709474, 1.199719254218462483 ) ) ;
#181523=CARTESIAN_POINT ( 'NONE',  ( -5.097502569058280031, 5.049433873430397846, -0.7216878364869820928 ) ) ;
#181525=CARTESIAN_POINT ( 'NONE',  ( 5.512200117181983217, 6.216449928263548586, -0.9568283335872149742 ) ) ;
#181526=CARTESIAN_POINT ( 'NONE',  ( -8.663296969452339624, 13.05100419776235299, 1.040834085586084257E-14 ) ) ;
#181531=CARTESIAN_POINT ( 'NONE',  ( 4.950698647284403009, 8.927565521807144577, 1.040834085586084257E-14 ) ) ;
#181533=CARTESIAN_POINT ( 'NONE',  ( 5.799137018343234473, 7.788745826199009237, -1.599625672291262513 ) ) ;
#181534=CARTESIAN_POINT ( 'NONE',  ( -4.167566996647928512, 7.418725663478599408, 0.7529690952402002813 ) ) ;
#181535=CARTESIAN_POINT ( 'NONE',  ( 3.334415713957098681, 5.977569868670206787, -1.199719254218446718 ) ) ;
#181537=CARTESIAN_POINT ( 'NONE',  ( -7.049876689426103127, 10.20831132343037062, -1.082531754730537976 ) ) ;
#181542=EDGE_CURVE ( 'NONE', #135502, #162623, #14974, .T. ) ;
#181544=CARTESIAN_POINT ( 'NONE',  ( -4.047760499819613500, 7.578451897646762525, -0.3740945913360635977 ) ) ;
#181545=CARTESIAN_POINT ( 'NONE',  ( -1.364683531250014514, -1.157291666325248158, 0.7879004041258379498 ) ) ;
#181547=DIRECTION ( 'NONE',  ( 0.000000000000000000, -1.000000000000000000, 2.168404344971004924E-15 ) ) ;
#181548=CARTESIAN_POINT ( 'NONE',  ( 5.531363484695522637, 5.555604941673978558, -0.7216878364870207285 ) ) ;
#181553=CARTESIAN_POINT ( 'NONE',  ( -8.880227426826648340, 11.38335130276301754, 1.443375672974064550 ) ) ;
#181558=DIRECTION ( 'NONE',  ( 0.7592566023653005702, 0.6507913734559639396, 0.000000000000000000 ) ) ;
#181564=CARTESIAN_POINT ( 'NONE',  ( -8.798878505144649864, 11.28844422746735532, -1.443375672974058777 ) ) ;
#181570=CARTESIAN_POINT ( 'NONE',  ( -0.7500000000000006661, 2.389583334016155636, -1.299038105676652011 ) ) ;
#181574=CARTESIAN_POINT ( 'NONE',  ( -7.486073373039941359, 11.88550270185529278, -0.7998128361456291469 ) ) ;
#181578=CARTESIAN_POINT ( 'NONE',  ( 5.113396490648394632, 9.117379672398465473, 1.040834085586084257E-14 ) ) ;
#181583=CARTESIAN_POINT ( 'NONE',  ( 6.909851844459134362, 11.21324425184434936, -0.7998128361456291469 ) ) ;
#181586=FACE_OUTER_BOUND ( 'NONE', #106860, .T. ) ;
#181587=ORIENTED_EDGE ( 'NONE', *, *, #163792, .F. ) ;
#181590=CARTESIAN_POINT ( 'NONE',  ( -7.537970219518091319, 7.896646132300314314, -0.7216878364870278340 ) ) ;
#181594=EDGE_CURVE ( 'NONE', #182051, #24037, #48103, .T. ) ;
#181597=CARTESIAN_POINT ( 'NONE',  ( -1.364683531249997417, 5.259375000341425022, 1.214306433183764966E-14 ) ) ;
#181598=AXIS2_PLACEMENT_3D ( 'NONE', #183353, #96010, #83714 ) ;
#181601=CARTESIAN_POINT ( 'NONE',  ( -3.917943204224921150, 5.594019709727598766, -1.443375672974051449 ) ) ;
#181603=CARTESIAN_POINT ( 'NONE',  ( 8.211434591371064684, 12.73175745657494851, -0.7998128361456352531 ) ) ;
#181605=CARTESIAN_POINT ( 'NONE',  ( -1.232288786374426959, 2.852001308287894332, -0.7749999999999979128 ) ) ;
#181608=CARTESIAN_POINT ( 'NONE',  ( -1.364683531250012516, 1.780208333674757615, 0.7879004041258379498 ) ) ;
#181609=CARTESIAN_POINT ( 'NONE',  ( 3.846762897975340767, 5.510976019103107859, -1.599625672291256295 ) ) ;
#181613=CARTESIAN_POINT ( 'NONE',  ( 3.557915510932077918, 4.150901429420823519, -2.419999999999995044 ) ) ;
#181614=( BOUNDED_CURVE ( )  B_SPLINE_CURVE ( 2, ( #43113, #109228, #77710, #111352, #175238, #178429, #177357 ),
 .UNSPECIFIED., .F., .T. ) 
 B_SPLINE_CURVE_WITH_KNOTS ( ( 3, 2, 2, 3 ),
 ( 0.1874999999999999167, 0.1916666666666665964, 0.1958333333333332760, 0.1999999999999999556 ),
 .UNSPECIFIED. ) 
 CURVE ( )  GEOMETRIC_REPRESENTATION_ITEM ( )  RATIONAL_B_SPLINE_CURVE ( ( 1.000000000000002665, 0.8660254037844360431, 1.000000000000000000, 0.8660254037844387076, 1.000000000000000000, 0.8660254037844404840, 0.9999999999999982236 ) ) 
 REPRESENTATION_ITEM ( '' )  );
#181615=CARTESIAN_POINT ( 'NONE',  ( 9.707274797260268429, 10.42750147299956964, 0.000000000000000000 ) ) ;
#181617=CARTESIAN_POINT ( 'NONE',  ( -8.026063749610061748, 9.426457798375635022, -1.082531754730543971 ) ) ;
#181619=CARTESIAN_POINT ( 'NONE',  ( -4.475070042639309520, 5.445751865460756846, 1.284222742053057642 ) ) ;
#181621=CARTESIAN_POINT ( 'NONE',  ( -7.374745490829552885, 10.69128794168811680, -1.199719254218446718 ) ) ;
#181622=CARTESIAN_POINT ( 'NONE',  ( -5.233084104750526322, 5.207612331738130429, 0.000000000000000000 ) ) ;
#181623=CARTESIAN_POINT ( 'NONE',  ( 1.364683531249990311, 3.696875000341416584, 1.214306433183764966E-14 ) ) ;
#181631=ORIENTED_EDGE ( 'NONE', *, *, #139225, .F. ) ;
#181644=CARTESIAN_POINT ( 'NONE',  ( 0.6823417656249899377, 4.738541667008086655, -1.181850606188754593 ) ) ;
#181646=AXIS2_PLACEMENT_3D ( 'NONE', #168676, #151378, #85292 ) ;
#181651=CARTESIAN_POINT ( 'NONE',  ( 9.935427640716063991, 10.48575375712389679, -0.7998128361456281477 ) ) ;
#181654=CARTESIAN_POINT ( 'NONE',  ( -1.201851678989727383E-14, 2.696875000341417916, -1.575800808251660134 ) ) ;
#181656=CARTESIAN_POINT ( 'NONE',  ( -7.212574532790100079, 9.437756259720353924, -1.443375672974059665 ) ) ;
#181662=CARTESIAN_POINT ( 'NONE',  ( 4.029797971759831121, 5.724516938518342535, -1.599625672291255185 ) ) ;
#181665=CARTESIAN_POINT ( 'NONE',  ( 10.22692794340986921, 10.82583744360002243, 0.000000000000000000 ) ) ;
#181666=CARTESIAN_POINT ( 'NONE',  ( 1.029210992452657125, 2.808910805765225227, -1.137835564023402135 ) ) ;
#181672=CARTESIAN_POINT ( 'NONE',  ( -8.597841969360544567, 13.18256606422934674, 0.7998128361456341429 ) ) ;
#181673=CARTESIAN_POINT ( 'NONE',  ( 6.446011968293428041, 9.607765498729298415, -1.199719254218440723 ) ) ;
#181675=CARTESIAN_POINT ( 'NONE',  ( 5.816084710138150093, 5.887779704690372817, -0.7216878364870257245 ) ) ;
#181683=CARTESIAN_POINT ( 'NONE',  ( -1.499999999999996003, 8.266799604812621993, -3.162088779278208417 ) ) ;
#181685=CARTESIAN_POINT ( 'NONE',  ( -6.887178846062123938, 8.097758744236356776, -1.082531754730544860 ) ) ;
#181686=CARTESIAN_POINT ( 'NONE',  ( 5.508690485854129903, 5.321227076451600091, 1.040834085586084257E-14 ) ) ;
#181689=CARTESIAN_POINT ( 'NONE',  ( -8.565000355531095622, 11.01558638625153286, -1.599625672291263179 ) ) ;
#181694=CARTESIAN_POINT ( 'NONE',  ( -10.64723070543352712, 11.31619066596094392, 0.7998128361456462443 ) ) ;
#181697=CARTESIAN_POINT ( 'NONE',  ( 9.284636267260101050, 9.726497154758602548, -0.7998128361456281477 ) ) ;
#181698=CARTESIAN_POINT ( 'NONE',  ( 4.376584659113025744, 4.000436945253625254, 0.7998128361456341429 ) ) ;
#181704=FACE_OUTER_BOUND ( 'NONE', #50580, .T. ) ;
#181707=CARTESIAN_POINT ( 'NONE',  ( -2.442440228756222353, 6.001264033524212671, -0.7998128361456281477 ) ) ;
#181710=CARTESIAN_POINT ( 'NONE',  ( -9.169391961543940539, 9.592045464756413509, 1.040834085586084257E-14 ) ) ;
#181715=CARTESIAN_POINT ( 'NONE',  ( 8.134528978519385944, 8.592631351135175066, -0.7216878364870267237 ) ) ;
#181718=CARTESIAN_POINT ( 'NONE',  ( 5.034155109375821446, 4.767602470560229122, -0.7998128361456221525 ) ) ;
#181721=CARTESIAN_POINT ( 'NONE',  ( -7.562750758324527922, 7.717630727667075696, 1.040834085586084257E-14 ) ) ;
#181730=CARTESIAN_POINT ( 'NONE',  ( -1.201851678989727383E-14, 3.634375000341422357, 1.575800808251672791 ) ) ;
#181731=CARTESIAN_POINT ( 'NONE',  ( 9.887974103068218668, 10.43039129653476493, 0.7998128361456462443 ) ) ;
#181733=CARTESIAN_POINT ( 'NONE',  ( -4.270455198624581783, 7.926022131796578662, 1.040834085586084257E-14 ) ) ;
#181735=CARTESIAN_POINT ( 'NONE',  ( -4.731432421044877934, 6.543090462684225450, -1.443375672974051449 ) ) ;
#181744=CARTESIAN_POINT ( 'NONE',  ( 4.202137545231717120, 6.989912005157271402, 1.199719254218462483 ) ) ;
#181752=CARTESIAN_POINT ( 'NONE',  ( 5.301401758143367893, 6.143722458377430584, 1.199719254218462483 ) ) ;
#181756=CARTESIAN_POINT ( 'NONE',  ( 1.364683531249988535, 3.926041667008087543, 0.7879004041258500513 ) ) ;
#181762=CARTESIAN_POINT ( 'NONE',  ( 5.262536180398716290, 9.291375977107183104, -0.7998128361456291469 ) ) ;
#181764=CARTESIAN_POINT ( 'NONE',  ( -4.903245109636583443, 8.872203061218007392, -0.7998128361456281477 ) ) ;
#181765=CARTESIAN_POINT ( 'NONE',  ( 5.409340101728155936, 8.294351971116089572, -1.082531754730543971 ) ) ;
#181766=CARTESIAN_POINT ( 'NONE',  ( 0.7499999999999902300, 2.233333333333351156, 1.299038105676669330 ) ) ;
#181767=CARTESIAN_POINT ( 'NONE',  ( -2.937312835655025101, 6.578615408239493867, 1.040834085586084257E-14 ) ) ;
#181770=CARTESIAN_POINT ( 'NONE',  ( -5.599681137644054729, 6.491715067794862293, 1.199719254218450271 ) ) ;
#181773=CARTESIAN_POINT ( 'NONE',  ( -1.364683531250012516, 3.738541667008087099, -0.7879004041258300672 ) ) ;
#181776=CARTESIAN_POINT ( 'NONE',  ( -3.578989364327652467, 6.158942777482099729, 1.082531754730560403 ) ) ;
#181781=CARTESIAN_POINT ( 'NONE',  ( -1.438722679664437232, 7.870294296420953906, -3.684004759497620185 ) ) ;
#181782=CARTESIAN_POINT ( 'NONE',  ( 5.087333953625774008, 6.958308917361963886, 1.599625672291267398 ) ) ;
#181785=CARTESIAN_POINT ( 'NONE',  ( 1.364683531249990311, 2.696875000341415696, 1.214306433183764966E-14 ) ) ;
#181787=CARTESIAN_POINT ( 'NONE',  ( 2.347533153460546806, 5.890539112345938300, 0.000000000000000000 ) ) ;
#181789=CARTESIAN_POINT ( 'NONE',  ( 1.364683531249986537, -0.5739583329919174526, 0.7879004041258500513 ) ) ;
#181793=CARTESIAN_POINT ( 'NONE',  ( -2.625475302540713152, 6.214804952939456228, -0.7998128361456281477 ) ) ;
#181794=CARTESIAN_POINT ( 'NONE',  ( -7.009202228140755331, 8.240119356661432803, -1.082531754730543083 ) ) ;
#181799=CARTESIAN_POINT ( 'NONE',  ( -1.364683531250012516, 3.280208333674756727, 0.7879004041258379498 ) ) ;
#181807=CARTESIAN_POINT ( 'NONE',  ( -5.978782553502159480, 8.958701498185728695, 1.082531754730548412 ) ) ;
#181813=CARTESIAN_POINT ( 'NONE',  ( -5.707619481228814351, 9.602713794834864203, -0.7216878364870207285 ) ) ;
#181821=CARTESIAN_POINT ( 'NONE',  ( 0.01837953348866276301, 7.054063922337711290, 3.955400951015632938 ) ) ;
#181825=CARTESIAN_POINT ( 'NONE',  ( -5.392392409933270514, 7.314210449720692786, 1.599625672291269396 ) ) ;
#181827=CARTESIAN_POINT ( 'NONE',  ( -1.402160292154681736E-14, 0.08750000000001964540, -1.732050807568870754 ) ) ;
#181828=CARTESIAN_POINT ( 'NONE',  ( 3.816783937446950770, 4.411668334231586996, 1.199719254218464037 ) ) ;
#181830=CARTESIAN_POINT ( 'NONE',  ( -4.243338890952904841, 5.973648010910253880, -1.443375672974051449 ) ) ;
#181831=CARTESIAN_POINT ( 'NONE',  ( 6.179819089730593795, 6.104210447640811665, 1.040834085586084257E-14 ) ) ;
#181837=CARTESIAN_POINT ( 'NONE',  ( -2.819732761962332024, 6.233512622357263666, -0.7216878364870267237 ) ) ;
#181845=CARTESIAN_POINT ( 'NONE',  ( -0.6823417656250003738, 2.217708333674753174, -1.181850606188749264 ) ) ;
#181846=CARTESIAN_POINT ( 'NONE',  ( 9.531018800282605952, 11.18223869082697597, 1.082531754730548412 ) ) ;
#181847=CARTESIAN_POINT ( 'NONE',  ( -8.037286134802835491, 8.271255333558444889, -0.7998128361456291469 ) ) ;
#181850=CARTESIAN_POINT ( 'NONE',  ( 7.983053520348166288, 8.207983950027992748, -0.7998128361456281477 ) ) ;
#181851=CARTESIAN_POINT ( 'NONE',  ( -7.413611068574208041, 7.543634422958360730, 0.7998128361456341429 ) ) ;
#181854=CARTESIAN_POINT ( 'NONE',  ( 0.7499999999999867883, -1.152083332650516434, -1.299038105676652011 ) ) ;
#181858=CARTESIAN_POINT ( 'NONE',  ( 9.110716038703335684, 9.731516254683127087, -0.7216878364870197293 ) ) ;
#181861=CARTESIAN_POINT ( 'NONE',  ( -1.364683531250012516, 0.5927083336747520637, 0.7879004041258379498 ) ) ;
#181863=CARTESIAN_POINT ( 'NONE',  ( 6.846504384776753049, 9.010674420371453053, -1.443375672974058777 ) ) ;
#181867=CARTESIAN_POINT ( 'NONE',  ( -5.260200412422220140, 5.239248024021764039, -0.7216878364870207285 ) ) ;
#181869=CARTESIAN_POINT ( 'NONE',  ( -0.6823417656250212460, 5.051041667008086655, 1.181850606188767472 ) ) ;
#181873=CARTESIAN_POINT ( 'NONE',  ( -4.695925055628692668, 7.055611427533158064, -1.405632220554285272 ) ) ;
#181879=CARTESIAN_POINT ( 'NONE',  ( 6.096362627639171805, 10.26417349888772179, -0.7998128361456291469 ) ) ;
#181882=CARTESIAN_POINT ( 'NONE',  ( 2.686486993802192913, 6.285985259411197568, 0.7998128361456362523 ) ) ;
#181883=EDGE_CURVE ( 'NONE', #169854, #7144, #184549, .T. ) ;
#181889=CARTESIAN_POINT ( 'NONE',  ( 4.961921032921539521, 7.772363057508363759, -1.082531754730549078 ) ) ;
#181890=CARTESIAN_POINT ( 'NONE',  ( -1.364683531250012516, 1.342708333674755616, 0.7879004041258379498 ) ) ;
#181898=CARTESIAN_POINT ( 'NONE',  ( -0.7500000000000006661, 2.108333333333357817, -1.299038105676652011 ) ) ;
#181899=CARTESIAN_POINT ( 'NONE',  ( 5.615048174354031474, 9.702639970055050966, 0.7998128361456462443 ) ) ;
#181900=CARTESIAN_POINT ( 'NONE',  ( -9.040589502214116280, 9.441775928871617651, 0.7998128361456462443 ) ) ;
#181905=CARTESIAN_POINT ( 'NONE',  ( 0.6823417656249899377, 1.592708333674752730, 1.181850606188755259 ) ) ;
#181908=CARTESIAN_POINT ( 'NONE',  ( 1.499999999999989120, 3.004166666666689522, 0.8660254037844524744 ) ) ;
#181910=CARTESIAN_POINT ( 'NONE',  ( 2.849184837166184536, 6.475799410002530898, 0.7998128361456362523 ) ) ;
#181917=CARTESIAN_POINT ( 'NONE',  ( 1.499999999999987121, -0.2145833326505137972, 0.8660254037844524744 ) ) ;
#181920=CARTESIAN_POINT ( 'NONE',  ( -7.344766530301162000, 9.591980256816594164, 1.599625672291295375 ) ) ;
#181921=CARTESIAN_POINT ( 'NONE',  ( -4.772106882330247046, 4.669805572247793357, -0.7216878364870207285 ) ) ;
#181929=CARTESIAN_POINT ( 'NONE',  ( 7.623762449586013901, 7.788811034138823253, 1.040834085586084257E-14 ) ) ;
#181933=CARTESIAN_POINT ( 'NONE',  ( 6.521108698048765362, 8.631046119188804155, -1.443375672974058777 ) ) ;
#181938=CARTESIAN_POINT ( 'NONE',  ( -5.696397096036042385, 9.797547045350714967, -0.7998128361456231517 ) ) ;
#181939=CARTESIAN_POINT ( 'NONE',  ( 4.355193658487811703, 6.104145239700998538, -1.599625672291255185 ) ) ;
#181944=CARTESIAN_POINT ( 'NONE',  ( 4.037125735401803084, 7.543859425723234757, -0.4173421496808590869 ) ) ;
#181945=CARTESIAN_POINT ( 'NONE',  ( 8.568389894156670294, 12.94027927658408217, -0.7216878364870257245 ) ) ;
#181951=CIRCLE ( 'NONE', #199258, 0.07999999999999994615 ) ;
#181954=CARTESIAN_POINT ( 'NONE',  ( -2.982430605326321427, 6.423326772948587227, -0.7216878364870267237 ) ) ;
#181955=CARTESIAN_POINT ( 'NONE',  ( 7.917598520700710019, 12.18102267421877727, -0.7216878364870328300 ) ) ;
#181958=CARTESIAN_POINT ( 'NONE',  ( -4.934277840369690971, 7.844075682818238526, -1.199719254218452047 ) ) ;
#181959=DIRECTION ( 'NONE',  ( 5.578564026256490882E-16, 1.000000000000000000, 9.066213480720158442E-32 ) ) ;
#181965=CARTESIAN_POINT ( 'NONE',  ( -5.910464900553636269, 8.982960586366182554, -1.199719254218440723 ) ) ;
#181967=DIRECTION ( 'NONE',  ( -1.000000000000000000, 5.782411586589355667E-16, 0.000000000000000000 ) ) ;
#181969=FACE_OUTER_BOUND ( 'NONE', #89689, .T. ) ;
#181978=CARTESIAN_POINT ( 'NONE',  ( 1.436838838544550523, 7.449283400311791148, -4.203727439823577328 ) ) ;
#181979=CARTESIAN_POINT ( 'NONE',  ( -6.715366157470410435, 6.729015360003925750, -0.7998128361456291469 ) ) ;
#181982=CARTESIAN_POINT ( 'NONE',  ( 4.528060117284232966, 6.305822774963486310, 1.443375672974062551 ) ) ;
#181986=CARTESIAN_POINT ( 'NONE',  ( -3.815730167242251003, 6.539103397502874948, -1.199719254218452047 ) ) ;
#181992=CARTESIAN_POINT ( 'NONE',  ( -7.181014916732457287, 11.52960116949655678, -0.7998128361456291469 ) ) ;
#181993=CARTESIAN_POINT ( 'NONE',  ( 4.801558957534076022, 8.753569217098425170, 0.7998128361456462443 ) ) ;
#181996=CARTESIAN_POINT ( 'NONE',  ( -8.833300774503376473, 10.26427131079744193, 1.199719254218462483 ) ) ;
#181999=CARTESIAN_POINT ( 'NONE',  ( 6.520158902582592120, 5.290451655907108197, -2.438235897557449849 ) ) ;
#182000=CARTESIAN_POINT ( 'NONE',  ( -1.364683531250014514, -0.6572916663252459379, 0.7879004041258379498 ) ) ;
#182003=CARTESIAN_POINT ( 'NONE',  ( 9.436111725431318931, 10.11114455586577776, -0.7216878364870257245 ) ) ;
#182027=( BOUNDED_CURVE ( )  B_SPLINE_CURVE ( 2, ( #82324, #198201, #163603, #14113, #15185 ),
 .UNSPECIFIED., .F., .T. ) 
 B_SPLINE_CURVE_WITH_KNOTS ( ( 3, 2, 3 ),
 ( 0.1229971016045081911, 0.1250000000000000000, 0.1273350245274847969 ),
 .UNSPECIFIED. ) 
 CURVE ( )  GEOMETRIC_REPRESENTATION_ITEM ( )  RATIONAL_B_SPLINE_CURVE ( ( 0.9331125556462563919, 0.9355989990887654262, 1.000000000000000000, 0.9249198476264304247, 0.9339904139662593696 ) ) 
 REPRESENTATION_ITEM ( '' )  );
#182030=CARTESIAN_POINT ( 'NONE',  ( -1.500000000000001332, 0.4312500006828159926, 0.000000000000000000 ) ) ;
#182035=CARTESIAN_POINT ( 'NONE',  ( -1.217323170181725756, 3.236755683774203085, 0.7750000000000100142 ) ) ;
#182036=DIRECTION ( 'NONE',  ( 1.000000000000000000, 0.000000000000000000, 0.000000000000000000 ) ) ;
#182037=CARTESIAN_POINT ( 'NONE',  ( 7.879259827836241570, 12.34422023245099176, 1.040834085586084257E-14 ) ) ;
#182041=CARTESIAN_POINT ( 'NONE',  ( 5.196852952739813070, 4.957416621151553571, -0.7998128361456221525 ) ) ;
#182042=CARTESIAN_POINT ( 'NONE',  ( -6.941411460516810017, 8.161030127766803588, 1.082531754730549967 ) ) ;
#182043=EDGE_CURVE ( 'NONE', #91680, #162762, #52343, .T. ) ;
#182045=CARTESIAN_POINT ( 'NONE',  ( 10.55232363013785246, 11.20546574478267132, 0.000000000000000000 ) ) ;
#182048=CARTESIAN_POINT ( 'NONE',  ( -8.505042434474312074, 8.816971016508505343, -0.7998128361456291469 ) ) ;
#182049=CARTESIAN_POINT ( 'NONE',  ( -2.928197990427299668, 6.360055388899728435, 1.040834085586084257E-14 ) ) ;
#182051=VERTEX_POINT ( 'NONE', #18750 ) ;
#182052=CARTESIAN_POINT ( 'NONE',  ( 1.499999999999989120, 0.3062500006828158816, 0.000000000000000000 ) ) ;
#182059=CARTESIAN_POINT ( 'NONE',  ( -3.565431210269599749, 7.103494145382415859, 0.7216878364870317197 ) ) ;
#182066=CARTESIAN_POINT ( 'NONE',  ( -2.426546306721660606, 5.774795091243142053, 0.7216878364870317197 ) ) ;
#182067=CARTESIAN_POINT ( 'NONE',  ( 8.772289083241844310, 10.19309100432570148, -1.199719254218446718 ) ) ;
#182076=CARTESIAN_POINT ( 'NONE',  ( -7.971304249830880373, 11.38727316052296601, 1.199719254218453823 ) ) ;
#182079=EDGE_CURVE ( 'NONE', #197822, #43527, #8142, .T. ) ;
#182082=CARTESIAN_POINT ( 'NONE',  ( 5.518332215962025167, 6.396807992499198292, -1.199719254218445830 ) ) ;
#182086=CARTESIAN_POINT ( 'NONE',  ( 2.880374247444865254, 6.438789554985836716, 0.3607768799173494689 ) ) ;
#182088=AXIS2_PLACEMENT_3D ( 'NONE', #204827, #106345, #122640 ) ;
#182091=CARTESIAN_POINT ( 'NONE',  ( -1.284279953904132077, 3.159610286488902187, -0.7749999999999935829 ) ) ;
#182100=CARTESIAN_POINT ( 'NONE',  ( 6.988338112840064120, 10.24047933403371502, 1.199719254218460707 ) ) ;
#182102=CARTESIAN_POINT ( 'NONE',  ( -5.271422797614987665, 5.044414773505913274, -0.7998128361456221525 ) ) ;
#182109=CARTESIAN_POINT ( 'NONE',  ( -1.402160292154681736E-14, -0.6312499993171797330, -1.732050807568870754 ) ) ;
#182115=CARTESIAN_POINT ( 'NONE',  ( -2.937312835655025101, 6.578615408239493867, 1.040834085586084257E-14 ) ) ;
#182121=ADVANCED_FACE ( 'NONE', ( #21931 ), #170345, .T. ) ;
#182123=CARTESIAN_POINT ( 'NONE',  ( 4.351804120306567825, 8.020929207092235558, 1.040834085586084257E-14 ) ) ;
#182126=CARTESIAN_POINT ( 'NONE',  ( 8.229436053370676518, 9.663725486096376827, 1.082531754730558626 ) ) ;
#182127=CARTESIAN_POINT ( 'NONE',  ( 1.364683531249988535, 5.217708333674750065, -0.7879004041258300672 ) ) ;
#182129=CARTESIAN_POINT ( 'NONE',  ( 3.023105065722948126, 6.470780310077995701, 0.7216878364870338292 ) ) ;
#182133=CARTESIAN_POINT ( 'NONE',  ( 2.000000000000003553, 8.900000000000018119, 2.449293598294762621E-16 ) ) ;
#182136=CARTESIAN_POINT ( 'NONE',  ( -6.131443063645894753, 6.000026256920684808, -0.1528826387674747100 ) ) ;
#182139=CARTESIAN_POINT ( 'NONE',  ( 1.364683531249990311, 5.426041667008086655, 0.7879004041258500513 ) ) ;
#182145=CARTESIAN_POINT ( 'NONE',  ( -1.402160292154681736E-14, -0.9124999999999769962, -1.732050807568870754 ) ) ;
#182154=CARTESIAN_POINT ( 'NONE',  ( -0.6823417656250212460, 4.363541667008085767, 1.181850606188767472 ) ) ;
#182156=CARTESIAN_POINT ( 'NONE',  ( 5.666418135507635512, 8.698239360479199433, 1.199719254218462483 ) ) ;
#182157=CARTESIAN_POINT ( 'NONE',  ( -8.045874094706015001, 11.47427131287732927, -1.199719254218446718 ) ) ;
#182161=ORIENTED_EDGE ( 'NONE', *, *, #20526, .F. ) ;
#182163=CARTESIAN_POINT ( 'NONE',  ( -1.499999999999997780, 5.900000000000023448, 1.214306433183764966E-14 ) ) ;
#182172=CARTESIAN_POINT ( 'NONE',  ( 7.117667457494414762, 11.24776976714476184, 1.040834085586084257E-14 ) ) ;
#182177=CARTESIAN_POINT ( 'NONE',  ( 1.499999999999989120, 3.535416667349488229, 0.8660254037844524744 ) ) ;
#182181=CARTESIAN_POINT ( 'NONE',  ( -6.240830780992103755, 6.175390754112560110, 1.040834085586084257E-14 ) ) ;
#182182=CARTESIAN_POINT ( 'NONE',  ( 3.131570294632282092, 5.636953862837537521, -1.082531754730543971 ) ) ;
#182190=CARTESIAN_POINT ( 'NONE',  ( 5.007038802148489509, 4.735966778795008381, 0.7998128361456341429 ) ) ;
#182193=CARTESIAN_POINT ( 'NONE',  ( -1.500000000000022427, 8.226407212580419070, 3.114167208185206981 ) ) ;
#182194=CARTESIAN_POINT ( 'NONE',  ( 4.843287188579786573, 6.673587691474970107, -1.599625672291256295 ) ) ;
#182198=CYLINDRICAL_SURFACE ( 'NONE', #179192, 1.250000000000000000 ) ;
#182207=CARTESIAN_POINT ( 'NONE',  ( 5.849792259110643933, 6.002811869646802911, -0.3480847251615213356 ) ) ;
#182212=CARTESIAN_POINT ( 'NONE',  ( 8.920375002787457319, 12.49452237230570084, 1.199719254218450271 ) ) ;
#182217=CARTESIAN_POINT ( 'NONE',  ( 6.995644074971448134, 7.263932296995902149, -0.7216878364870257245 ) ) ;
#182218=CARTESIAN_POINT ( 'NONE',  ( -10.16825202056928390, 10.96530823352674133, 0.7216878364870438212 ) ) ;
#182224=CARTESIAN_POINT ( 'NONE',  ( -3.632695093457760649, 6.325562478087638496, -1.199719254218452047 ) ) ;
#182235=CARTESIAN_POINT ( 'NONE',  ( 6.112956004491900686, 6.016961049888108981, 0.08799760576284378077 ) ) ;
#182236=LINE ( 'NONE', #33860, #129026 ) ;
#182239=CARTESIAN_POINT ( 'NONE',  ( 4.792970997630896512, 5.550553237779539018, 1.199719254218464037 ) ) ;
#182242=LINE ( 'NONE', #152959, #142488 ) ;
#182243=CARTESIAN_POINT ( 'NONE',  ( -8.134528978519403708, 11.47373899403920205, 1.082531754730549967 ) ) ;
#182244=AXIS2_PLACEMENT_3D ( 'NONE', #213360, #1032, #50883 ) ;
#182248=CARTESIAN_POINT ( 'NONE',  ( 7.613066949273408213, 8.840665181362512115, -1.199719254218441611 ) ) ;
#182249=CARTESIAN_POINT ( 'NONE',  ( -3.588104209110990706, 7.337872010604796991, 1.040834085586084257E-14 ) ) ;
#182251=CARTESIAN_POINT ( 'NONE',  ( 2.381428537494710618, 5.930083727052461562, 0.7998128361456462443 ) ) ;
#182253=CARTESIAN_POINT ( 'NONE',  ( -5.762378981008047241, 6.681529218386182301, 1.199719254218450271 ) ) ;
#182254=CARTESIAN_POINT ( 'NONE',  ( 4.532503425670185493, 4.182342172903648070, 1.214306433183764966E-14 ) ) ;
#182256=CARTESIAN_POINT ( 'NONE',  ( -5.368138756007025947, 8.350246751061767725, 1.199719254218452047 ) ) ;
#182259=CARTESIAN_POINT ( 'NONE',  ( 9.413438726589914651, 9.876766690643398405, 0.000000000000000000 ) ) ;
#182262=CARTESIAN_POINT ( 'NONE',  ( 4.359152798643180837, 7.157646611464889119, -1.047953017514296370 ) ) ;
#182263=CARTESIAN_POINT ( 'NONE',  ( 5.666945020832170776, 7.634521829102760115, 1.443375672974062551 ) ) ;
#182265=CARTESIAN_POINT ( 'NONE',  ( 0.2458932500721333070, 6.514853439382787492, 3.140456330564937559 ) ) ;
#182272=CARTESIAN_POINT ( 'NONE',  ( 7.904040366642699489, 8.323727970612377902, 0.7216878364870458196 ) ) ;
#182276=CARTESIAN_POINT ( 'NONE',  ( -6.855619230004478482, 11.14997286831390788, -0.7998128361456291469 ) ) ;
#182284=CARTESIAN_POINT ( 'NONE',  ( 3.891353782322113375, 4.498666486585943147, -1.199719254218446718 ) ) ;
#182288=CARTESIAN_POINT ( 'NONE',  ( 3.985207087413062066, 6.736826471035503694, -1.199719254218452047 ) ) ;
#182291=CARTESIAN_POINT ( 'NONE',  ( -1.499999999999997780, 4.431250000682819490, 1.214306433183764966E-14 ) ) ;
#182297=CARTESIAN_POINT ( 'NONE',  ( -1.402160292154681736E-14, 1.337500000000025446, -1.732050807568863648 ) ) ;
#182298=CARTESIAN_POINT ( 'NONE',  ( 7.287671262545424966, 8.461036880179857889, -1.199719254218451159 ) ) ;
#182299=CARTESIAN_POINT ( 'NONE',  ( 4.975479186090857375, 5.867442474269873642, 1.082531754730560403 ) ) ;
#182302=CARTESIAN_POINT ( 'NONE',  ( 9.273413882067330860, 9.921330405274451536, -0.7216878364870257245 ) ) ;
#182308=CARTESIAN_POINT ( 'NONE',  ( -4.822949958159302497, 6.649860922651058992, -1.599625672291256295 ) ) ;
#182309=CARTESIAN_POINT ( 'NONE',  ( -0.7499999999999972244, 3.389583334016149863, -1.299038105676652011 ) ) ;
#182310=CARTESIAN_POINT ( 'NONE',  ( -1.364683531250014514, -0.9697916663252473812, 0.7879004041258379498 ) ) ;
#182314=CARTESIAN_POINT ( 'NONE',  ( 5.522248639467795428, 5.337044922334209573, -0.7998128361456231517 ) ) ;
#182316=CARTESIAN_POINT ( 'NONE',  ( 0.6823417656249917140, 5.155208333674749177, 1.181850606188765695 ) ) ;
#182324=CARTESIAN_POINT ( 'NONE',  ( -7.172426956829277778, 8.326585190177668849, -1.199719254218452935 ) ) ;
#182325=CARTESIAN_POINT ( 'NONE',  ( 6.342516933094585418, 6.294024598232139667, 1.040834085586084257E-14 ) ) ;
#182329=CARTESIAN_POINT ( 'NONE',  ( 0.6823417656249882723, -0.3239583329919110133, -1.181850606188749264 ) ) ;
#182335=CARTESIAN_POINT ( 'NONE',  ( -7.203459687562382641, 7.298457811777897319, -0.7998128361456291469 ) ) ;
#182338=CARTESIAN_POINT ( 'NONE',  ( 10.38962578677386084, 11.01565159419135043, 0.000000000000000000 ) ) ;
#182340=CARTESIAN_POINT ( 'NONE',  ( 9.511208455186636712, 11.05516360492796935, 1.199719254218453823 ) ) ;
#182342=CARTESIAN_POINT ( 'NONE',  ( -2.927671105547157371, 5.503034492191895666, 1.199719254218462483 ) ) ;
#182343=CARTESIAN_POINT ( 'NONE',  ( -6.835281999583978418, 11.12624609948998966, -0.7998128361456291469 ) ) ;
#182347=CARTESIAN_POINT ( 'NONE',  ( -4.211465482254622472, 7.549728682704877514, 0.9859626088348661943 ) ) ;
#182348=CARTESIAN_POINT ( 'NONE',  ( 1.364683531249988757, -0.1156249996585798079, 0.000000000000000000 ) ) ;
#182352=CARTESIAN_POINT ( 'NONE',  ( 9.273413882067330860, 9.921330405274451536, -0.7216878364870257245 ) ) ;
#182355=CARTESIAN_POINT ( 'NONE',  ( 6.193377243344257543, 6.120028293523423812, -0.7998128361456281477 ) ) ;
#182370=EDGE_CURVE ( 'NONE', #184579, #178469, #8913, .T. ) ;
#182372=CARTESIAN_POINT ( 'NONE',  ( 9.049177462117294013, 12.64479190819049670, -1.199719254218446718 ) ) ;
#182375=CARTESIAN_POINT ( 'NONE',  ( -5.382750679825375251, 6.238629533673094585, -1.199719254218446718 ) ) ;
#182376=CARTESIAN_POINT ( 'NONE',  ( -9.182950115157607840, 9.607863310639020327, 0.7998128361456462443 ) ) ;
#182381=CARTESIAN_POINT ( 'NONE',  ( -0.7500000000000215383, 2.722916667349486897, 1.299038105676671107 ) ) ;
#182382=CARTESIAN_POINT ( 'NONE',  ( 10.16199982864259788, 11.81442020729326536, 1.199719254218452047 ) ) ;
#182385=ORIENTED_EDGE ( 'NONE', *, *, #85850, .T. ) ;
#182387=CARTESIAN_POINT ( 'NONE',  ( -7.316596452869116973, 11.68777962832266049, 0.7998128361456481317 ) ) ;
#182389=CARTESIAN_POINT ( 'NONE',  ( 1.364683531249988535, 1.863541667008086211, 0.7879004041258500513 ) ) ;
#182393=VERTEX_POINT ( 'NONE', #64073 ) ;
#182398=CARTESIAN_POINT ( 'NONE',  ( -10.03267048443264109, 11.76749898900197877, 1.082531754730558626 ) ) ;
#182402=CARTESIAN_POINT ( 'NONE',  ( 1.364683531249986537, 0.9677083336747538400, -0.7879004041258239610 ) ) ;
#182408=CARTESIAN_POINT ( 'NONE',  ( 1.364683531249988757, 2.134375000341422357, 1.214306433183764966E-14 ) ) ;
#182410=CARTESIAN_POINT ( 'NONE',  ( -6.551614543901706611, 8.666636272683888365, 1.599625672291283607 ) ) ;
#182411=CARTESIAN_POINT ( 'NONE',  ( 7.995557903757111617, 10.35123685918189729, 1.599625672291281386 ) ) ;
#182414=CARTESIAN_POINT ( 'NONE',  ( -1.499999999999997780, 3.650000000000021227, 1.214306433183764966E-14 ) ) ;
#182415=CARTESIAN_POINT ( 'NONE',  ( 0.6823417656249899377, 2.155208333674753174, 1.181850606188767472 ) ) ;
#182419=CARTESIAN_POINT ( 'NONE',  ( -5.260200412422213923, 6.199617238323108737, -1.082531754730544860 ) ) ;
#182424=CARTESIAN_POINT ( 'NONE',  ( 6.805829924380118356, 7.042482454639357847, 0.7216878364870317197 ) ) ;
#182427=CARTESIAN_POINT ( 'NONE',  ( -9.179033691651859783, 10.66762638080401260, 1.199719254218462483 ) ) ;
#182428=CARTESIAN_POINT ( 'NONE',  ( -10.31739171031960822, 11.13930453823545186, 1.040834085586084257E-14 ) ) ;
#182429=CARTESIAN_POINT ( 'NONE',  ( -1.499999999999997780, 6.280000000000042881, -2.873333333333329520 ) ) ;
#182430=CARTESIAN_POINT ( 'NONE',  ( -1.364683531250010295, 5.738541667008088432, -0.7879004041258300672 ) ) ;
#182435=CARTESIAN_POINT ( 'NONE',  ( -7.253248993186740989, 9.485209796849769504, 1.443375672974090751 ) ) ;
#182437=CARTESIAN_POINT ( 'NONE',  ( 1.499999999999990896, 4.775000000000022560, 1.214306433183764966E-14 ) ) ;
#182440=CARTESIAN_POINT ( 'NONE',  ( 7.944714827928043732, 10.29191993738131927, 1.443375672974076540 ) ) ;
#182446=CARTESIAN_POINT ( 'NONE',  ( 2.535011535630975477, 5.901337858304024131, 0.7216878364870438212 ) ) ;
#182448=ORIENTED_EDGE ( 'NONE', *, *, #66344, .T. ) ;
#182449=CARTESIAN_POINT ( 'NONE',  ( 8.880227426826634129, 11.38335130276301754, 1.443375672974076540 ) ) ;
#182456=CARTESIAN_POINT ( 'NONE',  ( 6.642605195691581699, 9.837124264027149678, 1.199719254218462483 ) ) ;
#182457=CARTESIAN_POINT ( 'NONE',  ( -5.850506979496850057, 6.784345216623154151, -1.199719254218446718 ) ) ;
#182461=CARTESIAN_POINT ( 'NONE',  ( 6.127922243252466039, 6.251590159990418449, 1.040834085586084257E-14 ) ) ;
#182462=CARTESIAN_POINT ( 'NONE',  ( 1.364683531249988757, 0.1968750003414204697, 0.000000000000000000 ) ) ;
#182463=CARTESIAN_POINT ( 'NONE',  ( 3.551873057100287223, 5.166937871415542283, 1.443375672974062551 ) ) ;
#182464=CARTESIAN_POINT ( 'NONE',  ( -8.459397779922852578, 11.95671561229694824, 1.199719254218453823 ) ) ;
#182480=CARTESIAN_POINT ( 'NONE',  ( 7.494959990256193194, 7.638541498254023843, -0.7998128361456281477 ) ) ;
#182481=CARTESIAN_POINT ( 'NONE',  ( 6.307567778855705853, 8.381915046796901692, -1.599625672291262513 ) ) ;
#182492=CARTESIAN_POINT ( 'NONE',  ( -4.466521540698216164, 7.298359999868178960, -1.199719254218452047 ) ) ;
#182494=CARTESIAN_POINT ( 'NONE',  ( -3.253066792275140173, 5.882662793374543675, 1.199719254218462483 ) ) ;
#182502=CARTESIAN_POINT ( 'NONE',  ( -8.500599126088349777, 12.86119004717103209, 1.040834085586084257E-14 ) ) ;
#182506=CARTESIAN_POINT ( 'NONE',  ( 5.178324605415663306, 8.128796908705222535, 1.199719254218462483 ) ) ;
#182507=CARTESIAN_POINT ( 'NONE',  ( -1.364683531250012516, 4.488541667008091096, -0.7879004041258300672 ) ) ;
#182513=CARTESIAN_POINT ( 'NONE',  ( 3.809477975315569864, 7.388215371269402532, -0.7216878364870197293 ) ) ;
#182514=CARTESIAN_POINT ( 'NONE',  ( -6.938021921891187382, 9.117444880338284818, -1.599625672291263179 ) ) ;
#182519=CARTESIAN_POINT ( 'NONE',  ( -5.845536785786364931, 9.971543350059432598, 0.000000000000000000 ) ) ;
#182520=CARTESIAN_POINT ( 'NONE',  ( -5.773074481320628948, 5.629675071162500544, 0.000000000000000000 ) ) ;
#182524=DIRECTION ( 'NONE',  ( -1.000000000000000000, 5.578564026256490882E-16, 2.058387550816952846E-48 ) ) ;
#182528=CARTESIAN_POINT ( 'NONE',  ( 6.612626235163189925, 8.737816579155630592, -1.599625672291262513 ) ) ;
#182537=CARTESIAN_POINT ( 'NONE',  ( -1.284279953904152949, 2.952889714876734573, 0.7750000000000152323 ) ) ;
#182543=CARTESIAN_POINT ( 'NONE',  ( 1.499999999999990896, 5.775000000000023448, 1.040834085586084257E-14 ) ) ;
#182544=CARTESIAN_POINT ( 'NONE',  ( 4.142179624174931796, 4.791296635414242111, 1.199719254218464037 ) ) ;
#182545=CARTESIAN_POINT ( 'NONE',  ( 4.143988507271280319, 7.986403691791820414, -0.7998128361456221525 ) ) ;
#182549=CARTESIAN_POINT ( 'NONE',  ( -7.863365906246068349, 9.236643647784308797, -1.082531754730543971 ) ) ;
#182551=CARTESIAN_POINT ( 'NONE',  ( 5.585596099150174965, 7.539614753807099667, -1.443375672974057666 ) ) ;
#182552=CARTESIAN_POINT ( 'NONE',  ( -9.286972035236635392, 9.937148250638648150, -0.7216878364870267237 ) ) ;
#182556=CARTESIAN_POINT ( 'NONE',  ( 6.154511665599609493, 9.267681812253174556, 1.199719254218462483 ) ) ;
#182561=CARTESIAN_POINT ( 'NONE',  ( -1.364683531250012516, 3.738541667008087099, -0.7879004041258300672 ) ) ;
#182567=CARTESIAN_POINT ( 'NONE',  ( 8.121497709785879593, 9.433834401960398353, -1.199719254218445830 ) ) ;
#182572=CARTESIAN_POINT ( 'NONE',  ( -7.666245793523398078, 11.03137162816423356, 1.199719254218453823 ) ) ;
#182578=CARTESIAN_POINT ( 'NONE',  ( 10.05067194643221207, 10.62020544712608938, 0.7998128361456462443 ) ) ;
#182581=CARTESIAN_POINT ( 'NONE',  ( -7.343712760096452463, 11.71941532008788833, -0.7998128361456291469 ) ) ;
#182583=CYLINDRICAL_SURFACE ( 'NONE', #178971, 1.250000000000000000 ) ;
#182586=CARTESIAN_POINT ( 'NONE',  ( 5.206864636422387171, 6.427350532134703087, -1.171562478298654231 ) ) ;
#182587=CARTESIAN_POINT ( 'NONE',  ( -2.764973262183167968, 5.313220341600567664, 1.199719254218462483 ) ) ;
#182592=CARTESIAN_POINT ( 'NONE',  ( 6.103141704446003679, 10.27208242182903142, 0.7998128361456462443 ) ) ;
#182594=CARTESIAN_POINT ( 'NONE',  ( 6.810273232766058449, 6.839740281182199233, 1.040834085586084257E-14 ) ) ;
#182595=CARTESIAN_POINT ( 'NONE',  ( -4.088362842241233253, 7.522098425605555860, -0.5455919966513862462 ) ) ;
#182596=CARTESIAN_POINT ( 'NONE',  ( 5.495132332240461714, 5.305409230568988832, 0.7998128361456341429 ) ) ;
#182598=CARTESIAN_POINT ( 'NONE',  ( -8.188761592974058701, 8.655902734665618325, -0.7216878364870278340 ) ) ;
#182606=CARTESIAN_POINT ( 'NONE',  ( -4.209440762792112878, 7.367024337791516331, -0.8326445619948764643 ) ) ;
#182607=CARTESIAN_POINT ( 'NONE',  ( -1.364683531250000748, -0.9281249996585805295, 0.000000000000000000 ) ) ;
#182611=CARTESIAN_POINT ( 'NONE',  ( 6.480434237652135998, 6.662854153456708950, 0.7216878364870317197 ) ) ;
#182617=( BOUNDED_CURVE ( )  B_SPLINE_CURVE ( 2, ( #1219, #168016, #169075 ),
 .UNSPECIFIED., .F., .T. ) 
 B_SPLINE_CURVE_WITH_KNOTS ( ( 3, 3 ),
 ( 0.1229783203405389463, 0.1249999999999998751 ),
 .UNSPECIFIED. ) 
 CURVE ( )  GEOMETRIC_REPRESENTATION_ITEM ( )  RATIONAL_B_SPLINE_CURVE ( ( 0.9330713687540070911, 0.9349951081471579162, 0.9999999999999960032 ) ) 
 REPRESENTATION_ITEM ( '' )  );
#182621=CARTESIAN_POINT ( 'NONE',  ( -9.286972035236626510, 11.85788667924133399, -1.443375672974058777 ) ) ;
#182628=CARTESIAN_POINT ( 'NONE',  ( -8.446366511189330240, 12.79791866312216442, 0.7216878364870317197 ) ) ;
#182636=CARTESIAN_POINT ( 'NONE',  ( -1.499999999999997780, 2.431250000682817713, 1.214306433183764966E-14 ) ) ;
#182638=CARTESIAN_POINT ( 'NONE',  ( -4.693093728624763372, 8.627026450037540428, 0.7998128361456481317 ) ) ;
#182640=ORIENTED_EDGE ( 'NONE', *, *, #117124, .F. ) ;
#182642=CARTESIAN_POINT ( 'NONE',  ( -8.565000355531095622, 11.01558638625153286, -1.599625672291263179 ) ) ;
#182646=CARTESIAN_POINT ( 'NONE',  ( 6.582647274634798151, 7.638508894284114170, 1.199719254218462483 ) ) ;
#182651=CARTESIAN_POINT ( 'NONE',  ( 9.582915646760733708, 10.07448976417602893, 0.7998128361456462443 ) ) ;
#182655=AXIS2_PLACEMENT_3D ( 'NONE', #123754, #107479, #74913 ) ;
#182658=CARTESIAN_POINT ( 'NONE',  ( -8.365017589951714072, 8.861534731139549592, 1.040834085586084257E-14 ) ) ;
#182661=CARTESIAN_POINT ( 'NONE',  ( 0.6823417656249917140, 5.155208333674749177, 1.181850606188765695 ) ) ;
#182667=CARTESIAN_POINT ( 'NONE',  ( -3.212919216314315207, 5.731860938133201522, 1.082531754730560403 ) ) ;
#182669=CARTESIAN_POINT ( 'NONE',  ( 8.075853055234393452, 12.57357899774884658, 0.7998128361456462443 ) ) ;
#182671=CARTESIAN_POINT ( 'NONE',  ( -8.306341666666730461, 12.84248237775322643, 1.040834085586084257E-14 ) ) ;
#182675=CARTESIAN_POINT ( 'NONE',  ( -0.6823417656250003738, 1.717708333674752730, -1.181850606188749264 ) ) ;
#182677=CARTESIAN_POINT ( 'NONE',  ( 4.467575310902914154, 5.170924936596891008, 1.199719254218464037 ) ) ;
#182682=CARTESIAN_POINT ( 'NONE',  ( -5.378281411895262210, 4.339595938922584217, -2.499999999999995559 ) ) ;
#182683=DIRECTION ( 'NONE',  ( -0.7592566023652994600, 0.6507913734559651608, 0.000000000000000000 ) ) ;
#182684=CARTESIAN_POINT ( 'NONE',  ( 9.910647101465253073, 11.62513837554007168, -1.082531754730537088 ) ) ;
#182686=CARTESIAN_POINT ( 'NONE',  ( -7.375272376154096143, 8.667201196010339004, -1.082531754730544860 ) ) ;
#182689=CARTESIAN_POINT ( 'NONE',  ( 0.4396101492294202662, 7.376551424357187692, 2.043156636846811036 ) ) ;
#182691=CARTESIAN_POINT ( 'NONE',  ( -6.886651960737580680, 10.12184548991413457, -1.199719254218440723 ) ) ;
#182692=CARTESIAN_POINT ( 'NONE',  ( -3.267151830768946663, 6.755501535964989479, -0.7216878364870257245 ) ) ;
#182693=CARTESIAN_POINT ( 'NONE',  ( 1.364683531249988535, 3.176041667008084435, 0.7879004041258500513 ) ) ;
#182702=ORIENTED_EDGE ( 'NONE', *, *, #57965, .F. ) ;
#182706=ORIENTED_EDGE ( 'NONE', *, *, #208798, .F. ) ;
#182714=CARTESIAN_POINT ( 'NONE',  ( 1.419999999999989049, 6.120000000000041851, -2.499999999999995115 ) ) ;
#182715=CARTESIAN_POINT ( 'NONE',  ( -1.364683531250010295, 3.842708333674751398, 0.7879004041258379498 ) ) ;
#182719=CYLINDRICAL_SURFACE ( 'NONE', #172175, 1.250000000000000000 ) ;
#182722=CARTESIAN_POINT ( 'NONE',  ( 9.236128959407556849, 11.79856975744075598, -1.599625672291262513 ) ) ;
#182725=CARTESIAN_POINT ( 'NONE',  ( -1.364683531250012516, 2.738541667008090208, -0.7879004041258289570 ) ) ;
#182727=CARTESIAN_POINT ( 'NONE',  ( -6.941411460516810017, 8.161030127766803588, 1.082531754730549967 ) ) ;
#182735=CARTESIAN_POINT ( 'NONE',  ( 2.869522067586683711, 6.499526178826442013, 0.7998128361456362523 ) ) ;
#182739=CARTESIAN_POINT ( 'NONE',  ( 10.06423010004587759, 10.63602329300870153, 0.000000000000000000 ) ) ;
#182747=CARTESIAN_POINT ( 'NONE',  ( -4.298098390732130625, 4.973201863064262263, 1.199719254218462483 ) ) ;
#182748=CARTESIAN_POINT ( 'NONE',  ( 7.121056995675668411, 9.330985799753529264, -1.599625672291262513 ) ) ;
#182750=CARTESIAN_POINT ( 'NONE',  ( 4.324687812634887329, 6.068555086205916105, 1.443375672974062551 ) ) ;
#182752=DIRECTION ( 'NONE',  ( 0.9782075119096779181, 0.1245777785628398998, -0.1661037047504532738 ) ) ;
#182754=VECTOR ( 'NONE', #154993, 1000.000000000000000 ) ;
#182759=CARTESIAN_POINT ( 'NONE',  ( -5.748293942514169252, 9.650167333001109071, -0.7216878364870207285 ) ) ;
#182760=CARTESIAN_POINT ( 'NONE',  ( 3.798255590122797898, 7.583048621785260401, -0.7998128361456221525 ) ) ;
#182764=CARTESIAN_POINT ( 'NONE',  ( -9.345647958521597687, 9.797677461230342999, 0.7998128361456462443 ) ) ;
#182769=CARTESIAN_POINT ( 'NONE',  ( -4.946027110887008860, 4.664786472323266153, -0.7998128361456221525 ) ) ;
#182772=CARTESIAN_POINT ( 'NONE',  ( 7.736899214892750010, 12.17813285068358020, 1.040834085586084257E-14 ) ) ;
#182773=CARTESIAN_POINT ( 'NONE',  ( 2.866659414285625651, 5.431854185720147221, -1.199719254218446718 ) ) ;
#182775=ORIENTED_EDGE ( 'NONE', *, *, #178800, .T. ) ;
#182779=CARTESIAN_POINT ( 'NONE',  ( 4.229780737783593203, 4.037091736943370535, -0.7216878364870188411 ) ) ;
#182782=CARTESIAN_POINT ( 'NONE',  ( -6.091691091241777656, 6.001394449403842479, 0.7998128361456341429 ) ) ;
#182783=DIRECTION ( 'NONE',  ( 1.000000000000000000, 0.000000000000000000, 0.000000000000000000 ) ) ;
#182785=CARTESIAN_POINT ( 'NONE',  ( -7.537443334193545397, 10.88110209227943770, -1.199719254218446718 ) ) ;
#182790=CARTESIAN_POINT ( 'NONE',  ( 6.643132081016111634, 9.733775946952057723, 1.082531754730558626 ) ) ;
#182791=CARTESIAN_POINT ( 'NONE',  ( 0.6823417656249917140, 5.405208333674749177, 1.181850606188765695 ) ) ;
#182793=CARTESIAN_POINT ( 'NONE',  ( 4.359110081993588182, 5.044382169536003602, -1.199719254218452047 ) ) ;
#182795=CARTESIAN_POINT ( 'NONE',  ( 5.529027716274630855, 5.344953845275508542, 1.040834085586084257E-14 ) ) ;
#182797=CARTESIAN_POINT ( 'NONE',  ( -5.554036483092550824, 9.631459663583308739, -0.7998128361456231517 ) ) ;
#182799=CARTESIAN_POINT ( 'NONE',  ( -1.403499169903600574, 7.376709478543776122, 4.304123474983186703 ) ) ;
#182802=DIRECTION ( 'NONE',  ( -0.7592566023653004592, 0.6507913734559639396, 0.000000000000000000 ) ) ;
#182809=CARTESIAN_POINT ( 'NONE',  ( -1.364683531250012516, 3.342708333674756727, 0.7879004041258379498 ) ) ;
#182810=CARTESIAN_POINT ( 'NONE',  ( 7.214910300766615769, 11.56914578420308715, -0.7998128361456291469 ) ) ;
#182813=CARTESIAN_POINT ( 'NONE',  ( -5.585596099150199834, 5.618876325204420930, -0.7216878364870207285 ) ) ;
#182814=CARTESIAN_POINT ( 'NONE',  ( 4.229780737783593203, 4.037091736943370535, -0.7216878364870188411 ) ) ;
#182815=CARTESIAN_POINT ( 'NONE',  ( -5.409340101728186134, 5.413244328212063472, 0.7216878364870317197 ) ) ;
#182823=CARTESIAN_POINT ( 'NONE',  ( 3.388648328411762556, 6.040841252200647382, 1.199719254218462483 ) ) ;
#182829=CARTESIAN_POINT ( 'NONE',  ( 1.270904146967307025, 2.996556430829583118, 0.7750000000000065725 ) ) ;
#182833=CARTESIAN_POINT ( 'NONE',  ( 6.193377243344257543, 6.120028293523423812, -0.7998128361456281477 ) ) ;
#182838=CARTESIAN_POINT ( 'NONE',  ( -6.410307701162927252, 6.373113827645189744, -0.7998128361456291469 ) ) ;
#182842=CARTESIAN_POINT ( 'NONE',  ( 7.800018446563675489, 7.994443030612759848, -0.7998128361456281477 ) ) ;
#182845=CARTESIAN_POINT ( 'NONE',  ( -4.089755892816631544, 7.923132308261379819, -0.7998128361456281477 ) ) ;
#182846=CARTESIAN_POINT ( 'NONE',  ( 0.7499999999999885647, 2.566666666666689522, -1.299038105676658228 ) ) ;
#182847=CARTESIAN_POINT ( 'NONE',  ( -2.598358995313378550, 6.183169261174235487, 0.7998128361456341429 ) ) ;
#182850=CARTESIAN_POINT ( 'NONE',  ( -6.437424008390261854, 6.404749519410410485, 0.7998128361456341429 ) ) ;
#182853=CARTESIAN_POINT ( 'NONE',  ( -1.364683531250012516, 3.488541667008085767, -0.7879004041258300672 ) ) ;
#182854=CARTESIAN_POINT ( 'NONE',  ( -2.277406616971334508, 5.600798786534425311, 1.040834085586084257E-14 ) ) ;
#182855=CARTESIAN_POINT ( 'NONE',  ( -3.931501358282937009, 7.530575984731317618, 0.7216878364870317197 ) ) ;
#182861=CARTESIAN_POINT ( 'NONE',  ( 5.952193131599331721, 6.902979060742733708, 1.199719254218462483 ) ) ;
#182862=CARTESIAN_POINT ( 'NONE',  ( -0.7499999999999972244, 3.108333333333358706, -1.299038105676652011 ) ) ;
#182865=CARTESIAN_POINT ( 'NONE',  ( 0.6823417656249899377, 3.238541667008085323, -1.181850606188754593 ) ) ;
#182867=CARTESIAN_POINT ( 'NONE',  ( 3.602716132929354664, 5.226254793216122074, 1.599625672291267398 ) ) ;
#182868=DIRECTION ( 'NONE',  ( 0.000000000000000000, 1.000000000000000000, -8.546850786086437571E-32 ) ) ;
#182869=CARTESIAN_POINT ( 'NONE',  ( 0.6823417656249882723, 0.2385416670080825474, -1.181850606188749264 ) ) ;
#182872=CARTESIAN_POINT ( 'NONE',  ( -4.810445574750349174, 4.506608013497163334, 0.7998128361456341429 ) ) ;
#182873=CARTESIAN_POINT ( 'NONE',  ( -7.985389288324703294, 9.379004260209384825, -1.082531754730543083 ) ) ;
#182876=CARTESIAN_POINT ( 'NONE',  ( -0.6823417656250212460, 2.551041667008084435, 1.181850606188767472 ) ) ;
#182884=CARTESIAN_POINT ( 'NONE',  ( -6.195713011320790109, 9.211787032307496403, -1.082531754730537976 ) ) ;
#182890=CARTESIAN_POINT ( 'NONE',  ( -7.524412065460066579, 7.880828285899290186, 0.7216878364870317197 ) ) ;
#182900=ORIENTED_EDGE ( 'NONE', *, *, #37073, .T. ) ;
#182903=CARTESIAN_POINT ( 'NONE',  ( -5.473741331615264549, 7.409117525016355010, -1.599625672291256295 ) ) ;
#182905=CARTESIAN_POINT ( 'NONE',  ( 1.499999999999987121, -0.4958333333333110882, 0.8660254037844524744 ) ) ;
#182907=CARTESIAN_POINT ( 'NONE',  ( 4.532503425670185493, 4.182342172903648070, 1.214306433183764966E-14 ) ) ;
#182911=CARTESIAN_POINT ( 'NONE',  ( 5.035963992472171746, 7.962709526937818083, 1.199719254218462483 ) ) ;
#182919=CARTESIAN_POINT ( 'NONE',  ( -4.934804725694236893, 4.859619722839116918, -0.7216878364870207285 ) ) ;
#182921=CARTESIAN_POINT ( 'NONE',  ( -4.290995968093258561, 3.987448345753906498, 0.1285802912755794336 ) ) ;
#182922=CARTESIAN_POINT ( 'NONE',  ( -0.4746061814645892718, 6.848527939983842572, 3.764703919983649616 ) ) ;
#182923=CARTESIAN_POINT ( 'NONE',  ( 3.145207314826885092, 6.442628614629879458, -0.6582494395028383183 ) ) ;
#182926=CARTESIAN_POINT ( 'NONE',  ( -1.364683531250012516, 1.780208333674757615, 0.7879004041258379498 ) ) ;
#182927=CARTESIAN_POINT ( 'NONE',  ( 8.554831740098642001, 12.92446143018304916, 0.7216878364870438212 ) ) ;
#182928=CARTESIAN_POINT ( 'NONE',  ( -8.538937818508475885, 8.856515631215026829, 1.040834085586084257E-14 ) ) ;
#182931=CARTESIAN_POINT ( 'NONE',  ( 7.467843683028853263, 7.606905806488803101, 0.7998128361456341429 ) ) ;
#182932=CARTESIAN_POINT ( 'NONE',  ( -6.204827856548512877, 10.39071626594860476, -0.7998128361456291469 ) ) ;
#182935=CARTESIAN_POINT ( 'NONE',  ( -1.500000000000015099, -0.7979166659838445863, 0.8660254037844403729 ) ) ;
#182937=CARTESIAN_POINT ( 'NONE',  ( 9.083599731475992201, 9.699880562917908122, 0.7216878364870438212 ) ) ;
#182940=CARTESIAN_POINT ( 'NONE',  ( -1.364683531250000748, 1.071875000341421247, 0.000000000000000000 ) ) ;
#182942=CARTESIAN_POINT ( 'NONE',  ( 3.418706159394787836, 6.339871777953998588, 1.082712511304601000 ) ) ;
#182943=CARTESIAN_POINT ( 'NONE',  ( 6.602457619730767391, 7.765583980183128787, 1.082531754730558626 ) ) ;
#182946=CARTESIAN_POINT ( 'NONE',  ( -4.229780737783618072, 6.918199379847403740, 1.082531754730560403 ) ) ;
#182949=CARTESIAN_POINT ( 'NONE',  ( 1.364683531249990311, 5.113541667008084879, 0.7879004041258500513 ) ) ;
#182953=CARTESIAN_POINT ( 'NONE',  ( -4.381256195510448315, 8.263215994737505454, 1.040834085586084257E-14 ) ) ;
#182954=CARTESIAN_POINT ( 'NONE',  ( -5.642163961945882988, 6.318168449258962482, -1.169820551124676422 ) ) ;
#182960=CARTESIAN_POINT ( 'NONE',  ( 8.294891053462476904, 8.571794405328034827, 1.040834085586084257E-14 ) ) ;
#182964=CARTESIAN_POINT ( 'NONE',  ( -1.500000000000013101, 2.379166666666686414, -0.8660254037844313801 ) ) ;
#182969=ORIENTED_EDGE ( 'NONE', *, *, #177848, .T. ) ;
#182970=CARTESIAN_POINT ( 'NONE',  ( 5.016153647376201619, 7.835634441038803466, 1.082531754730558626 ) ) ;
#182971=CARTESIAN_POINT ( 'NONE',  ( -1.364683531250000748, 0.5718750003414208027, 0.000000000000000000 ) ) ;
#182973=CARTESIAN_POINT ( 'NONE',  ( 2.205172540517054802, 5.724451730578533848, 1.040834085586084257E-14 ) ) ;
#182977=CARTESIAN_POINT ( 'NONE',  ( -1.250000000000021982, 10.00000000000000178, 4.154462424328226433 ) ) ;
#182980=CARTESIAN_POINT ( 'NONE',  ( -1.500000000000001332, 1.150000000000019007, 0.000000000000000000 ) ) ;
#182981=CARTESIAN_POINT ( 'NONE',  ( 5.452350330990040739, 9.512825819463730070, 0.7998128361456462443 ) ) ;
#182982=CARTESIAN_POINT ( 'NONE',  ( -7.153898609505128015, 11.49796547773133604, 0.7998128361456481317 ) ) ;
#182984=CARTESIAN_POINT ( 'NONE',  ( 0.6823417656249899377, 0.8427083336747520637, 1.181850606188755259 ) ) ;
#182985=CARTESIAN_POINT ( 'NONE',  ( -0.7500000000000006661, 2.608333333333358262, -1.299038105676652011 ) ) ;
#182987=CARTESIAN_POINT ( 'NONE',  ( 3.147464216666835402, 6.823792019419957278, -0.7998128361456291469 ) ) ;
#182994=CARTESIAN_POINT ( 'NONE',  ( -1.500000000000015099, -0.8395833326505166561, -0.8660254037844383745 ) ) ;
#182995=CARTESIAN_POINT ( 'NONE',  ( -6.170932472514347289, 10.35117165124207972, 0.000000000000000000 ) ) ;
#182996=CARTESIAN_POINT ( 'NONE',  ( -4.961921032921567054, 4.891255414604337659, 0.7216878364870317197 ) ) ;
#182998=CYLINDRICAL_SURFACE ( 'NONE', #132176, 0.2500000000000002220 ) ;
#183003=VERTEX_POINT ( 'NONE', #36961 ) ;
#183004=CARTESIAN_POINT ( 'NONE',  ( 5.774883364416965037, 8.824782127540085952, -1.199719254218440723 ) ) ;
#183009=CARTESIAN_POINT ( 'NONE',  ( 6.982085920913413624, 8.208483664896217391, -1.082531754730543971 ) ) ;
#183013=CARTESIAN_POINT ( 'NONE',  ( -5.343885102080728977, 9.386283052402845328, 0.7998128361456481317 ) ) ;
#183014=CARTESIAN_POINT ( 'NONE',  ( 5.217190183160311356, 4.981143389975473568, -0.7998128361456211532 ) ) ;
#183020=CARTESIAN_POINT ( 'NONE',  ( 8.405692050792682224, 12.75046512599275772, -0.7216878364870328300 ) ) ;
#183028=CARTESIAN_POINT ( 'NONE',  ( -1.518728846951488354, 8.688592980705449165, -2.528358009378028903 ) ) ;
#183029=CARTESIAN_POINT ( 'NONE',  ( -2.819732761962332024, 6.233512622357263666, -0.7216878364870267237 ) ) ;
#183030=CARTESIAN_POINT ( 'NONE',  ( 8.839552966430002101, 11.33589776563360019, -1.443375672974052559 ) ) ;
#183033=CARTESIAN_POINT ( 'NONE',  ( -5.717788096661253761, 7.693838750903348789, 1.599625672291269396 ) ) ;
#183037=CYLINDRICAL_SURFACE ( 'NONE', #1607, 0.08000000000000004330 ) ;
#183039=CARTESIAN_POINT ( 'NONE',  ( -8.505042434474312074, 8.816971016508505343, -0.7998128361456291469 ) ) ;
#183042=CARTESIAN_POINT ( 'NONE',  ( 5.462746646817801199, 6.412201880991806213, -1.228565393760511215 ) ) ;
#183054=CARTESIAN_POINT ( 'NONE',  ( -6.552668314106420588, 6.539201209412602189, -0.7998128361456291469 ) ) ;
#183057=CARTESIAN_POINT ( 'NONE',  ( 5.395781948558860286, 6.357795697149212444, -1.082531754730542195 ) ) ;
#183058=AXIS2_PLACEMENT_3D ( 'NONE', #33213, #46291, #99297 ) ;
#183062=CARTESIAN_POINT ( 'NONE',  ( -2.923754682041362241, 6.562797562356882608, 0.7998128361456341429 ) ) ;
#183070=CARTESIAN_POINT ( 'NONE',  ( -6.842061076390810292, 11.13415502243129218, 0.000000000000000000 ) ) ;
#183071=CARTESIAN_POINT ( 'NONE',  ( 6.745345117998789775, 7.828323044875442172, 1.199719254218462483 ) ) ;
#183075=CARTESIAN_POINT ( 'NONE',  ( -10.45741655484220267, 11.09474082360439873, -0.7998128361456221525 ) ) ;
#183079=CARTESIAN_POINT ( 'NONE',  ( -1.364683531250014514, 0.09270833367475767028, 0.7879004041258379498 ) ) ;
#183082=CARTESIAN_POINT ( 'NONE',  ( 9.097157885089661278, 9.715698408800516717, 1.040834085586084257E-14 ) ) ;
#183090=CARTESIAN_POINT ( 'NONE',  ( -0.4866249300619188145, 6.869159268903599624, -3.677787980130352352 ) ) ;
#183101=B_SPLINE_CURVE_WITH_KNOTS ( 'NONE', 3,
 ( #147472, #94467, #129171, #78186 ),
 .UNSPECIFIED., .F., .F.,
 ( 4, 4 ),
 ( 1.908185967165630741E-16, 0.0001045641765545072172 ),
 .UNSPECIFIED. ) ;
#183103=CARTESIAN_POINT ( 'NONE',  ( -2.286521462199063492, 5.819358805874190743, 1.040834085586084257E-14 ) ) ;
#183111=CARTESIAN_POINT ( 'NONE',  ( -1.500000000000001332, 0.6812500006828161592, 0.000000000000000000 ) ) ;
#183119=CARTESIAN_POINT ( 'NONE',  ( 9.348510611822643313, 10.86534945433664134, 1.199719254218453823 ) ) ;
#183125=CARTESIAN_POINT ( 'NONE',  ( 4.847203612085560387, 5.613824621309978724, -1.199719254218452047 ) ) ;
#183126=CARTESIAN_POINT ( 'NONE',  ( -7.212574532790100079, 9.437756259720353924, -1.443375672974059665 ) ) ;
#183128=CARTESIAN_POINT ( 'NONE',  ( 4.367824458345868521, 3.990216711025275753, 0.1168690382639416964 ) ) ;
#183130=CARTESIAN_POINT ( 'NONE',  ( -8.193204901359996128, 8.453160561208463264, 1.040834085586084257E-14 ) ) ;
#183131=CARTESIAN_POINT ( 'NONE',  ( -3.104453987404957260, 6.565687385373657925, -0.7216878364870257245 ) ) ;
#183134=CARTESIAN_POINT ( 'NONE',  ( 1.499999999999987121, 0.3270833340161527492, -0.8660254037844323793 ) ) ;
#183142=CARTESIAN_POINT ( 'NONE',  ( -4.650083499362882122, 6.448183387388563226, 1.443375672974064550 ) ) ;
#183146=CARTESIAN_POINT ( 'NONE',  ( 4.016016189339381981, 7.573203028563332495, -0.3002613606930375489 ) ) ;
#183151=CARTESIAN_POINT ( 'NONE',  ( -2.765500147063310266, 6.170241238308400433, 1.040834085586084257E-14 ) ) ;
#183152=CARTESIAN_POINT ( 'NONE',  ( 7.411503528164766763, 11.79850454950093841, 1.040834085586084257E-14 ) ) ;
#183162=CARTESIAN_POINT ( 'NONE',  ( -9.345647958521597687, 9.797677461230342999, 0.7998128361456462443 ) ) ;
#183167=CARTESIAN_POINT ( 'NONE',  ( 5.355634372598031767, 6.206993841907870291, -1.199719254218445830 ) ) ;
#183168=AXIS2_PLACEMENT_3D ( 'NONE', #130822, #213047, #98260 ) ;
#183183=CARTESIAN_POINT ( 'NONE',  ( 7.283754839039659146, 9.520799950344851936, -1.599625672291262513 ) ) ;
#183185=CARTESIAN_POINT ( 'NONE',  ( -5.610376637956639101, 5.439860920571172542, 0.000000000000000000 ) ) ;
#183190=CARTESIAN_POINT ( 'NONE',  ( 0.7499999999999867883, -0.9020833326505162120, -1.299038105676652011 ) ) ;
#183193=CARTESIAN_POINT ( 'NONE',  ( 3.785751206713845018, 5.439795712631356750, 1.599625672291267398 ) ) ;
#183195=CARTESIAN_POINT ( 'NONE',  ( -3.598799709423620374, 6.286017863381107240, 1.199719254218464037 ) ) ;
#183201=CARTESIAN_POINT ( 'NONE',  ( 5.748293942514166588, 7.729428904398431222, -1.443375672974057666 ) ) ;
#183203=ORIENTED_EDGE ( 'NONE', *, *, #204199, .F. ) ;
#183204=CARTESIAN_POINT ( 'NONE',  ( 8.717529583462654941, 9.272798723569005475, 0.7216878364870458196 ) ) ;
#183205=CARTESIAN_POINT ( 'NONE',  ( 0.6823417656249899377, 4.238541667008085767, -1.181850606188754593 ) ) ;
#183207=CARTESIAN_POINT ( 'NONE',  ( 3.185802909086937973, 6.660594460669327255, 0.7216878364870317197 ) ) ;
#183215=CARTESIAN_POINT ( 'NONE',  ( -6.025499844618653178, 6.066343344509915525, -0.6079853925319089747 ) ) ;
#183217=CARTESIAN_POINT ( 'NONE',  ( -1.364683531249997417, 5.321875000341417916, 1.214306433183764966E-14 ) ) ;
#183223=CARTESIAN_POINT ( 'NONE',  ( -1.500000000000015099, -1.079166666666641961, 0.8660254037844403729 ) ) ;
#183233=CARTESIAN_POINT ( 'NONE',  ( -0.6823417656250212460, 5.363541667008087543, 1.181850606188767472 ) ) ;
#183234=EDGE_CURVE ( 'NONE', #88615, #102537, #194945, .T. ) ;
#183236=CARTESIAN_POINT ( 'NONE',  ( 7.233438648090761980, 8.397765496649418182, 1.199719254218462483 ) ) ;
#183237=CARTESIAN_POINT ( 'NONE',  ( -7.506410603460441422, 11.90922947067921278, -0.7998128361456291469 ) ) ;
#183243=CARTESIAN_POINT ( 'NONE',  ( 1.499999999999989120, 4.004166666666685970, 0.8660254037844524744 ) ) ;
#183247=CARTESIAN_POINT ( 'NONE',  ( 5.788968402910781741, 5.856144012925177833, 0.7216878364870568108 ) ) ;
#183250=CARTESIAN_POINT ( 'NONE',  ( 7.456621297836067086, 10.68284669990868174, 1.082531754730558626 ) ) ;
#183253=FACE_OUTER_BOUND ( 'NONE', #204602, .T. ) ;
#183255=CARTESIAN_POINT ( 'NONE',  ( 1.499999999999987121, 3.577083334016152527, -0.8660254037844262731 ) ) ;
#183257=CARTESIAN_POINT ( 'NONE',  ( -5.915435094264120508, 5.795762452929912101, 0.000000000000000000 ) ) ;
#183258=CARTESIAN_POINT ( 'NONE',  ( 3.348500752450929596, 6.850408611260650815, 0.7216878364870317197 ) ) ;
#183259=CARTESIAN_POINT ( 'NONE',  ( -10.15469386651127515, 11.90985960142705657, 1.082531754730558626 ) ) ;
#183266=CARTESIAN_POINT ( 'NONE',  ( 5.332434488876471868, 5.115595079977664383, 0.7998128361456341429 ) ) ;
#183270=CARTESIAN_POINT ( 'NONE',  ( 3.344057444064992168, 7.053150784717805877, 1.040834085586084257E-14 ) ) ;
#183281=CARTESIAN_POINT ( 'NONE',  ( 5.538030394937467626, 6.199453712711876285, -0.9301498999644899346 ) ) ;
#183285=CARTESIAN_POINT ( 'NONE',  ( 10.53876547652418338, 11.18964789890005918, 0.7998128361456462443 ) ) ;
#183291=CARTESIAN_POINT ( 'NONE',  ( 6.209271165378815738, 7.306866450105836464, -1.082531754730543083 ) ) ;
#183292=CARTESIAN_POINT ( 'NONE',  ( -3.277320446201389181, 4.846626492033466072, 1.599625672291267398 ) ) ;
#183297=CARTESIAN_POINT ( 'NONE',  ( -3.307299406729781399, 5.945934176904983381, -1.199719254218452935 ) ) ;
#183300=ORIENTED_EDGE ( 'NONE', *, *, #150437, .T. ) ;
#183307=CARTESIAN_POINT ( 'NONE',  ( 9.585778300061798873, 11.14216175728232550, -1.199719254218440723 ) ) ;
#183308=CARTESIAN_POINT ( 'NONE',  ( 5.639836874842681702, 6.325236607244836051, 1.140081021588116084 ) ) ;
#183310=ORIENTED_EDGE ( 'NONE', *, *, #30821, .T. ) ;
#183313=CARTESIAN_POINT ( 'NONE',  ( 5.009901455449552010, 5.803638771901306725, -1.199719254218452047 ) ) ;
#183314=AXIS2_PLACEMENT_3D ( 'NONE', #69980, #53768, #3910 ) ;
#183319=CARTESIAN_POINT ( 'NONE',  ( -5.974412749747273210, 4.760129193867236097, 2.438793960827106311 ) ) ;
#183320=CARTESIAN_POINT ( 'NONE',  ( -7.971831135155409420, 11.28392484344787405, 1.082531754730549967 ) ) ;
#183324=CARTESIAN_POINT ( 'NONE',  ( 6.076025397218672630, 10.24044673006381245, -0.7998128361456291469 ) ) ;
#183325=CARTESIAN_POINT ( 'NONE',  ( -5.786632634934295361, 5.645492917045106473, 0.7998128361456341429 ) ) ;
#183327=CARTESIAN_POINT ( 'NONE',  ( 2.869522067586683711, 6.499526178826442013, 0.7998128361456362523 ) ) ;
#183329=CARTESIAN_POINT ( 'NONE',  ( -5.545448523189368650, 6.428443684264421698, -1.199719254218446718 ) ) ;
#183330=CARTESIAN_POINT ( 'NONE',  ( 4.695201269034174452, 4.372156323494968966, 1.214306433183764966E-14 ) ) ;
#183332=EDGE_CURVE ( 'NONE', #179865, #102987, #126837, .T. ) ;
#183335=CARTESIAN_POINT ( 'NONE',  ( 7.703003830858588863, 12.13858823597705872, -0.7998128361456291469 ) ) ;
#183336=CARTESIAN_POINT ( 'NONE',  ( -1.499999999999981126, 3.629166666666691743, -0.8660254037844499209 ) ) ;
#183339=CARTESIAN_POINT ( 'NONE',  ( 4.003607682157598546, 7.822813005323850710, -0.1595685970469905290 ) ) ;
#183340=CARTESIAN_POINT ( 'NONE',  ( 4.365362273920230685, 8.036747052974847705, 0.7216878364870298324 ) ) ;
#183344=CARTESIAN_POINT ( 'NONE',  ( -1.123270288249905713, 3.300000000000025135, 0.7750000000000117906 ) ) ;
#183345=DIRECTION ( 'NONE',  ( 1.000000000000000000, 0.000000000000000000, 0.000000000000000000 ) ) ;
#183347=CARTESIAN_POINT ( 'NONE',  ( 8.771762197917315262, 10.29643932140079166, -1.082531754730543083 ) ) ;
#183348=EDGE_CURVE ( 'NONE', #179696, #33385, #111635, .T. ) ;
#183352=CARTESIAN_POINT ( 'NONE',  ( -8.202846631467911820, 9.528741477256060577, 1.199719254218462483 ) ) ;
#183353=CARTESIAN_POINT ( 'NONE',  ( 6.471393748265519719, 5.229711127717882491, -2.419999999999995044 ) ) ;
#183361=B_SPLINE_CURVE_WITH_KNOTS ( 'NONE', 3,
 ( #174180, #30037, #93994, #208764, #12693, #96123 ),
 .UNSPECIFIED., .F., .F.,
 ( 4, 2, 4 ),
 ( 0.000000000000000000, 0.002110194456903486965, 0.004220388913806973931 ),
 .UNSPECIFIED. ) ;
#183362=CARTESIAN_POINT ( 'NONE',  ( 3.216308754939877446, 4.775446185561722956, -1.599625672291262513 ) ) ;
#183366=CARTESIAN_POINT ( 'NONE',  ( 4.847203612085560387, 5.613824621309978724, -1.199719254218452047 ) ) ;
#183369=CARTESIAN_POINT ( 'NONE',  ( -1.499999999999997780, 4.181250000682819490, 1.214306433183764966E-14 ) ) ;
#183375=CARTESIAN_POINT ( 'NONE',  ( -0.7500000000000215383, 1.191666666666688190, 1.299038105676659116 ) ) ;
#183376=CARTESIAN_POINT ( 'NONE',  ( 5.289652487626049115, 9.323011668872403845, 0.7998128361456462443 ) ) ;
#183377=CARTESIAN_POINT ( 'NONE',  ( 5.788968402910816380, 5.856144012925152076, 0.7216878364870317197 ) ) ;
#183381=CARTESIAN_POINT ( 'NONE',  ( 6.941411460516762943, 11.04213777067082702, -0.7216878364870267237 ) ) ;
#183387=CARTESIAN_POINT ( 'NONE',  ( -4.120788623549732854, 6.895004929861607401, -1.199719254218452047 ) ) ;
#183388=CARTESIAN_POINT ( 'NONE',  ( -1.499999999999997780, 4.181250000682819490, 1.214306433183764966E-14 ) ) ;
#183390=CARTESIAN_POINT ( 'NONE',  ( 1.364683531249986537, -0.3447916663252443836, -0.7879004041258309554 ) ) ;
#183394=CARTESIAN_POINT ( 'NONE',  ( 5.196852952739813070, 4.957416621151553571, -0.7998128361456221525 ) ) ;
#183396=CARTESIAN_POINT ( 'NONE',  ( -1.364683531250010295, 4.092708333674751842, 0.7879004041258379498 ) ) ;
#183402=CARTESIAN_POINT ( 'NONE',  ( -5.219525951136856357, 6.152163700156858539, -1.082531754730543971 ) ) ;
#183404=CARTESIAN_POINT ( 'NONE',  ( -8.015895134177625891, 10.37496362800581018, 1.599625672291295375 ) ) ;
#183405=CARTESIAN_POINT ( 'NONE',  ( 6.667912619822566000, 6.673652899414787676, 1.040834085586084257E-14 ) ) ;
#183407=CARTESIAN_POINT ( 'NONE',  ( -1.364683531250014514, -0.7197916663252461600, 0.7879004041258379498 ) ) ;
#183411=B_SPLINE_CURVE_WITH_KNOTS ( 'NONE', 3,
 ( #101933, #167999, #147500, #66196, #85677, #151765, #3334, #119310 ),
 .UNSPECIFIED., .F., .F.,
 ( 4, 2, 2, 4 ),
 ( 0.000000000000000000, 0.003005455498261385902, 0.004508183247392079721, 0.006010910996522773539 ),
 .UNSPECIFIED. ) ;
#183412=CARTESIAN_POINT ( 'NONE',  ( -0.006768871532359390167, 8.210909518262125673, -2.038649385027042626 ) ) ;
#183415=CARTESIAN_POINT ( 'NONE',  ( -7.067878151425722955, 7.140279352951794500, 0.7998128361456341429 ) ) ;
#183420=CARTESIAN_POINT ( 'NONE',  ( 9.589694723567584234, 10.08239868711733855, -0.7998128361456281477 ) ) ;
#183423=CARTESIAN_POINT ( 'NONE',  ( -4.386226389220933441, 5.076017861301227008, -1.199719254218446718 ) ) ;
#183425=CARTESIAN_POINT ( 'NONE',  ( -8.019811557683421910, 9.315200557840817908, 1.199719254218462483 ) ) ;
#183427=CARTESIAN_POINT ( 'NONE',  ( -4.390790479118549250, 7.352160220884910835, 1.215098293768980930 ) ) ;
#183428=CARTESIAN_POINT ( 'NONE',  ( -1.364683531250000748, -0.7406249996585803075, 0.000000000000000000 ) ) ;
#183432=CARTESIAN_POINT ( 'NONE',  ( 8.432808358020029260, 8.940623960552603222, 0.7216878364870438212 ) ) ;
#183454=CARTESIAN_POINT ( 'NONE',  ( -3.924195396151603177, 6.665646164563756138, 1.199719254218464037 ) ) ;
#183459=CARTESIAN_POINT ( 'NONE',  ( -0.7500000000000006661, 2.389583334016155636, -1.299038105676652011 ) ) ;
#183460=CARTESIAN_POINT ( 'NONE',  ( 9.297140650669039275, 11.86975006391249643, 1.599625672291281386 ) ) ;
#183464=CARTESIAN_POINT ( 'NONE',  ( -9.352427035328430449, 9.805586384171650849, 1.040834085586084257E-14 ) ) ;
#183466=CARTESIAN_POINT ( 'NONE',  ( 0.6823417656249899377, 2.592708333674753618, 1.181850606188767472 ) ) ;
#183473=CARTESIAN_POINT ( 'NONE',  ( -2.927671105547157371, 5.503034492191895666, 1.199719254218462483 ) ) ;
#183477=CARTESIAN_POINT ( 'NONE',  ( 0.6823417656249899377, 1.655208333674752730, 1.181850606188755259 ) ) ;
#183482=CARTESIAN_POINT ( 'NONE',  ( 1.364683531249986537, 1.155208333674754728, -0.7879004041258239610 ) ) ;
#183484=CARTESIAN_POINT ( 'NONE',  ( -6.925517538482230506, 6.974191971184389160, 0.7998128361456341429 ) ) ;
#183485=CARTESIAN_POINT ( 'NONE',  ( 8.263858322729371153, 9.599921783727809910, -1.199719254218446718 ) ) ;
#183486=DIRECTION ( 'NONE',  ( -5.176899690512889973E-31, 0.6004703560067666812, -0.7996470168500017239 ) ) ;
#183487=CARTESIAN_POINT ( 'NONE',  ( 5.494078562035752178, 7.432844293840273231, -1.599625672291262513 ) ) ;
#183489=CARTESIAN_POINT ( 'NONE',  ( 1.499999999999989120, 3.525000000000021227, 1.214306433183764966E-14 ) ) ;
#183491=CARTESIAN_POINT ( 'NONE',  ( -1.364683531250000748, 1.071875000341421247, 0.000000000000000000 ) ) ;
#183498=CARTESIAN_POINT ( 'NONE',  ( 6.643132081016125845, 6.852668304048034287, 0.7216878364870317197 ) ) ;
#183502=CARTESIAN_POINT ( 'NONE',  ( -8.585337585951595685, 11.03931315507545108, -1.599625672291263179 ) ) ;
#183503=CARTESIAN_POINT ( 'NONE',  ( -4.451154503988200339, 4.087435097607984957, 1.214306433183764966E-14 ) ) ;
#183508=CARTESIAN_POINT ( 'NONE',  ( -6.344852701071109102, 10.34615255131755163, 0.000000000000000000 ) ) ;
#183510=CARTESIAN_POINT ( 'NONE',  ( -1.001543065824772872E-14, 4.962500000000019007, 1.732050807568877637 ) ) ;
#183513=CARTESIAN_POINT ( 'NONE',  ( 7.131225611108085616, 10.30321839872603462, 1.082531754730558626 ) ) ;
#183519=CARTESIAN_POINT ( 'NONE',  ( 4.487385655998888723, 4.337630808194552934, 0.7216878364870317197 ) ) ;
#183522=CARTESIAN_POINT ( 'NONE',  ( 10.01911233037457905, 11.75168114260095109, 1.082531754730548412 ) ) ;
#183530=CARTESIAN_POINT ( 'NONE',  ( 7.100719765255169236, 9.307259030929609267, -1.599625672291262513 ) ) ;
#183531=CARTESIAN_POINT ( 'NONE',  ( -4.367698041896780126, 8.247398148854895084, 0.7998128361456481317 ) ) ;
#183535=CARTESIAN_POINT ( 'NONE',  ( 6.277061933002785032, 7.385955679000473673, 1.082531754730558626 ) ) ;
#183537=CARTESIAN_POINT ( 'NONE',  ( 3.226477370372302644, 5.747678784534228313, 1.082531754730546636 ) ) ;
#183538=CARTESIAN_POINT ( 'NONE',  ( -3.002240950422295995, 5.590032644546251817, -1.199719254218452935 ) ) ;
#183553=CARTESIAN_POINT ( 'NONE',  ( 2.535011536075336913, 5.133042487381361596, -2.419999999999995044 ) ) ;
#183554=CARTESIAN_POINT ( 'NONE',  ( 6.174848896020108668, 9.291408581077091000, 1.199719254218460707 ) ) ;
#183555=CARTESIAN_POINT ( 'NONE',  ( 7.481401836642521452, 7.622723652371411696, 1.040834085586084257E-14 ) ) ;
#183567=CARTESIAN_POINT ( 'NONE',  ( -6.586563698140583512, 6.578745824119123675, 1.040834085586084257E-14 ) ) ;
#183569=CARTESIAN_POINT ( 'NONE',  ( -5.088387723830502196, 4.830873854090670605, -0.7998128361456221525 ) ) ;
#183578=CARTESIAN_POINT ( 'NONE',  ( -7.998947442382709383, 12.27592974951444660, 0.7216878364870478180 ) ) ;
#183581=CARTESIAN_POINT ( 'NONE',  ( 5.503720292143644777, 8.508425209887878538, 1.199719254218462483 ) ) ;
#183582=CARTESIAN_POINT ( 'NONE',  ( 0.6823417656249899377, 4.676041667008086655, -1.181850606188754593 ) ) ;
#183588=CARTESIAN_POINT ( 'NONE',  ( 5.382223794500827552, 7.302347065049529462, -1.443375672974051449 ) ) ;
#183589=EDGE_CURVE ( 'NONE', #126491, #212596, #18304, .T. ) ;
#183590=CARTESIAN_POINT ( 'NONE',  ( -6.287230548435221777, 8.358188277972981695, -1.599625672291263179 ) ) ;
#183595=CARTESIAN_POINT ( 'NONE',  ( -7.263417608619167076, 9.497073181520933716, -1.599625672291263179 ) ) ;
#183596=CARTESIAN_POINT ( 'NONE',  ( -6.762819695118240659, 6.784377820593065600, 0.7998128361456341429 ) ) ;
#183603=CARTESIAN_POINT ( 'NONE',  ( 7.884230021546724920, 9.157022099014721306, 1.199719254218462483 ) ) ;
#183613=CARTESIAN_POINT ( 'NONE',  ( -1.432341765624997709, 5.860937500170720682, 1.214306433183764966E-14 ) ) ;
#183619=CARTESIAN_POINT ( 'NONE',  ( -1.364683531250014514, -0.9489583329919112353, -0.7879004041258359514 ) ) ;
#183620=CARTESIAN_POINT ( 'NONE',  ( 4.467575310902914154, 5.170924936596891008, 1.199719254218464037 ) ) ;
#183621=CARTESIAN_POINT ( 'NONE',  ( 4.710568305744190276, 7.583081225755162968, 1.199719254218462483 ) ) ;
#183623=CARTESIAN_POINT ( 'NONE',  ( -8.514157279702036618, 9.035531035848267223, -0.7216878364870278340 ) ) ;
#183625=CARTESIAN_POINT ( 'NONE',  ( 6.317736394288147039, 6.473040002865377396, 0.7216878364870317197 ) ) ;
#183626=CARTESIAN_POINT ( 'NONE',  ( -9.151390499099978371, 9.778969791812544443, 0.7216878364870438212 ) ) ;
#183631=CARTESIAN_POINT ( 'NONE',  ( 6.751070424600909448, 9.963667031088037973, -1.199719254218441611 ) ) ;
#183637=CARTESIAN_POINT ( 'NONE',  ( -1.201851678989727383E-14, 3.071875000341420137, 1.575800808251672791 ) ) ;
#183644=CARTESIAN_POINT ( 'NONE',  ( 8.934986926605834157, 10.38290515491702770, -1.199719254218446718 ) ) ;
#183648=CARTESIAN_POINT ( 'NONE',  ( -7.883176251342026042, 11.28445716228600126, -1.199719254218446718 ) ) ;
#183653=CARTESIAN_POINT ( 'NONE',  ( 8.920375002787457319, 12.49452237230570084, 1.199719254218450271 ) ) ;
#183656=CARTESIAN_POINT ( 'NONE',  ( -8.015895134177625891, 10.37496362800581018, 1.599625672291295375 ) ) ;
#183662=CARTESIAN_POINT ( 'NONE',  ( 5.892675752748299800, 5.976886221469982274, -0.004604801460011270775 ) ) ;
#183663=CARTESIAN_POINT ( 'NONE',  ( -3.684065054611367351, 5.321161868511784299, -1.599625672291256295 ) ) ;
#183669=CARTESIAN_POINT ( 'NONE',  ( 8.125414133291656071, 8.374071331795406081, -0.7998128361456291469 ) ) ;
#183671=CARTESIAN_POINT ( 'NONE',  ( 7.287671262545424966, 8.461036880179857889, -1.199719254218451159 ) ) ;
#183672=CARTESIAN_POINT ( 'NONE',  ( -4.328009424535094851, 7.229878788426305825, -0.9977569098220413490 ) ) ;
#183673=CARTESIAN_POINT ( 'NONE',  ( 3.323720213644492993, 7.029424015893889433, 1.040834085586084257E-14 ) ) ;
#183675=CARTESIAN_POINT ( 'NONE',  ( -8.188761592974051595, 9.616271948966963024, -1.082531754730543971 ) ) ;
#183682=CARTESIAN_POINT ( 'NONE',  ( -4.356251871828045630, 7.199010410547511007, -1.027643995846918790 ) ) ;
#183686=CARTESIAN_POINT ( 'NONE',  ( 4.012850279964918165, 7.625483060026979842, -0.7216878364870197293 ) ) ;
#183690=CARTESIAN_POINT ( 'NONE',  ( -9.991996023147281747, 11.72004545083573568, 1.082531754730558626 ) ) ;
#183695=CARTESIAN_POINT ( 'NONE',  ( -9.205623113554631587, 11.76297960394566466, 1.443375672974076540 ) ) ;
#183697=ORIENTED_EDGE ( 'NONE', *, *, #57726, .F. ) ;
#183702=CARTESIAN_POINT ( 'NONE',  ( -9.205623113554631587, 11.76297960394566466, 1.443375672974076540 ) ) ;
#183709=CARTESIAN_POINT ( 'NONE',  ( -0.7500000000000006661, 2.889583334016148974, -1.299038105676652011 ) ) ;
#183711=CARTESIAN_POINT ( 'NONE',  ( -5.555090253297260361, 7.504024600312024340, 1.599625672291269396 ) ) ;
#183714=CARTESIAN_POINT ( 'NONE',  ( -9.267161690140662600, 10.77044237904097734, -1.199719254218441611 ) ) ;
#183717=CARTESIAN_POINT ( 'NONE',  ( 1.499999999999990896, 4.306250000682819490, 1.214306433183764966E-14 ) ) ;
#183718=CARTESIAN_POINT ( 'NONE',  ( 5.750629710490689384, 9.860818428881154674, -0.7998128361456291469 ) ) ;
#183723=CARTESIAN_POINT ( 'NONE',  ( 7.913155211870404493, 12.38376484715752213, 0.7998128361456462443 ) ) ;
#183726=DIRECTION ( 'NONE',  ( 0.6507913734559658270, 0.7592566023652989049, 0.000000000000000000 ) ) ;
#183732=CARTESIAN_POINT ( 'NONE',  ( -7.700668062882078502, 9.046829497192987901, -1.082531754730543971 ) ) ;
#183735=CARTESIAN_POINT ( 'NONE',  ( 0.6823417656249899377, 5.738541667008087543, -1.181850606188754593 ) ) ;
#183739=CARTESIAN_POINT ( 'NONE',  ( 0.6823417656249917140, 5.592708333674749177, 1.181850606188765695 ) ) ;
#183741=CARTESIAN_POINT ( 'NONE',  ( -3.755245360860931303, 5.404205559136275205, -1.443375672974051449 ) ) ;
#183743=CARTESIAN_POINT ( 'NONE',  ( 10.07387183015377197, 11.71160420905630062, -1.199719254218440723 ) ) ;
#183745=CARTESIAN_POINT ( 'NONE',  ( -10.34217224912604571, 10.96028913360221502, 0.7998128361456462443 ) ) ;
#183749=CARTESIAN_POINT ( 'NONE',  ( 0.6823417656249882723, 2.676041667008084879, -1.181850606188749264 ) ) ;
#183751=CARTESIAN_POINT ( 'NONE',  ( 4.359110081993588182, 5.044382169536003602, -1.199719254218452047 ) ) ;
#183758=CYLINDRICAL_SURFACE ( 'NONE', #211743, 1.500000000000000222 ) ;
#183759=CARTESIAN_POINT ( 'NONE',  ( 10.07334494482924292, 11.81495252613139257, -1.082531754730537088 ) ) ;
#183760=CARTESIAN_POINT ( 'NONE',  ( 1.499999999999990896, 4.056250000682819490, 1.214306433183764966E-14 ) ) ;
#183761=CARTESIAN_POINT ( 'NONE',  ( -6.344852701515500293, 9.385783337534627790, 1.082531754730548412 ) ) ;
#183766=CARTESIAN_POINT ( 'NONE',  ( -9.671043645249580933, 10.17730576241299900, 0.7998128361456462443 ) ) ;
#183767=CARTESIAN_POINT ( 'NONE',  ( -3.701012746406287413, 6.301303389907177532, 1.082531754730560403 ) ) ;
#183768=CARTESIAN_POINT ( 'NONE',  ( -1.364683531250012516, 2.092708333674750953, 0.7879004041258379498 ) ) ;
#183779=ORIENTED_EDGE ( 'NONE', *, *, #94104, .F. ) ;
#183780=EDGE_CURVE ( 'NONE', #25151, #185939, #126357, .T. ) ;
#183786=FACE_OUTER_BOUND ( 'NONE', #143278, .T. ) ;
#183789=CARTESIAN_POINT ( 'NONE',  ( -1.201851678989727383E-14, 4.759375000341419693, -1.575800808251660134 ) ) ;
#183796=CARTESIAN_POINT ( 'NONE',  ( 9.582915646760733708, 10.07448976417602893, 0.7998128361456462443 ) ) ;
#183798=CARTESIAN_POINT ( 'NONE',  ( -1.402160292154681736E-14, 2.196875000341423689, -1.575800808251660134 ) ) ;
#183801=CARTESIAN_POINT ( 'NONE',  ( -8.703971430293361067, 9.256980878204810637, 0.7216878364870438212 ) ) ;
#183809=CARTESIAN_POINT ( 'NONE',  ( 3.517450787741589036, 6.191110788085444128, -1.199719254218446718 ) ) ;
#183820=CARTESIAN_POINT ( 'NONE',  ( -5.108724954250998707, 4.854600622914589714, -0.7998128361456221525 ) ) ;
#183821=CARTESIAN_POINT ( 'NONE',  ( 7.099665995050449041, 11.43469409420089455, 0.7998128361456462443 ) ) ;
#183823=CARTESIAN_POINT ( 'NONE',  ( 3.972175818679561043, 7.578029521860726092, -0.7216878364870197293 ) ) ;
#183824=CARTESIAN_POINT ( 'NONE',  ( 4.905139262582266291, 4.827437033166341429, 0.6004564335717228474 ) ) ;
#183833=CARTESIAN_POINT ( 'NONE',  ( -5.910991785878165317, 8.879612269291090598, -1.082531754730538864 ) ) ;
#183835=CARTESIAN_POINT ( 'NONE',  ( 4.147904930777053245, 6.926640621626830807, -1.199719254218452047 ) ) ;
#183838=CARTESIAN_POINT ( 'NONE',  ( -7.995557903757128493, 10.35123685918189729, 1.599625672291295375 ) ) ;
#183842=CARTESIAN_POINT ( 'NONE',  ( -3.460355519985875983, 5.060167411448709629, 1.599625672291267398 ) ) ;
#183844=CARTESIAN_POINT ( 'NONE',  ( 7.425061681778431399, 11.81432239538354345, 0.7998128361456462443 ) ) ;
#183846=CARTESIAN_POINT ( 'NONE',  ( 4.566398809704347528, 4.221886787610169556, -0.7998128361456211532 ) ) ;
#183852=CARTESIAN_POINT ( 'NONE',  ( 2.901081683644319842, 5.368050483351580304, 1.082531754730548412 ) ) ;
#183855=CARTESIAN_POINT ( 'NONE',  ( -3.730464822054482710, 7.503959392372201442, 1.040834085586084257E-14 ) ) ;
#183857=CARTESIAN_POINT ( 'NONE',  ( -10.14557902172788495, 10.73093036830436553, 1.040834085586084257E-14 ) ) ;
#183862=CARTESIAN_POINT ( 'NONE',  ( 6.304178240674458422, 10.29869901418813782, 1.040834085586084257E-14 ) ) ;
#183864=CARTESIAN_POINT ( 'NONE',  ( 3.310162060030825248, 7.013606170011280838, -0.7998128361456291469 ) ) ;
#183866=CARTESIAN_POINT ( 'NONE',  ( 4.436542580169809291, 6.199052314996659874, 1.599625672291267398 ) ) ;
#183868=CARTESIAN_POINT ( 'NONE',  ( -6.527360889975461156, 9.702672574024962415, 1.199719254218452047 ) ) ;
#183873=DIRECTION ( 'NONE',  ( -1.000000000000000000, 8.673617379884035472E-16, 0.000000000000000000 ) ) ;
#183880=CARTESIAN_POINT ( 'NONE',  ( 1.364683531249990311, 2.946875000341416140, 1.214306433183764966E-14 ) ) ;
#183881=CARTESIAN_POINT ( 'NONE',  ( 2.191614386903386613, 5.708633884695917260, -0.7998128361456281477 ) ) ;
#183883=CARTESIAN_POINT ( 'NONE',  ( -4.067082894419624672, 6.728385229256075739, 1.082531754730560403 ) ) ;
#183884=CARTESIAN_POINT ( 'NONE',  ( 2.901081683644319842, 5.368050483351580304, 1.082531754730548412 ) ) ;
#183885=CARTESIAN_POINT ( 'NONE',  ( -5.327991180046197428, 8.199444895820425572, 1.082531754730548412 ) ) ;
#183886=( BOUNDED_SURFACE ( )  B_SPLINE_SURFACE ( 3, 2, ( 
 ( #97036, #130650, #159875 ),
 ( #44010, #209667, #94897 ),
 ( #98097, #47217, #142593 ),
 ( #110130, #29885, #179340 ),
 ( #11480, #210748, #61309 ),
 ( #144737, #30962, #48282 ),
 ( #78613, #95969, #114395 ),
 ( #162023, #14670, #10410 ),
 ( #146853, #76482, #178275 ),
 ( #127471, #193441, #62371 ),
 ( #208602, #45085, #32014 ),
 ( #128533, #212873, #13613 ),
 ( #79687, #111194, #145799 ),
 ( #211805, #28813, #60233 ) ),
 .UNSPECIFIED., .F., .F., .T. ) 
 B_SPLINE_SURFACE_WITH_KNOTS ( ( 4, 2, 2, 2, 2, 2, 4 ),
 ( 3, 3 ),
 ( 0.001912008033049055660, 0.002390010041311319087, 0.002629011045442450692, 0.002868012049573582731, 0.003346014057835845941, 0.003585015061966977980, 0.003824016066098109585 ),
 ( 0.000000000000000000, 1.000000000000000000 ),
 .UNSPECIFIED. ) 
 GEOMETRIC_REPRESENTATION_ITEM ( )  RATIONAL_B_SPLINE_SURFACE ( (
 ( 1.000000000000000000, 0.8708456909032173954, 1.000000000000000000),
 ( 1.000000000000000000, 0.8699862225466781229, 1.000000000000000000),
 ( 1.000000000000000000, 0.8740515128124174415, 1.000000000000000000),
 ( 1.000000000000000000, 0.8627336009020736274, 1.000000000000000000),
 ( 1.000000000000000000, 0.8557431983334260472, 1.000000000000000000),
 ( 1.000000000000000000, 0.8314605231444136546, 1.000000000000000000),
 ( 1.000000000000000000, 0.8141324793652144898, 1.000000000000000000),
 ( 1.000000000000000000, 0.7486317046916625140, 1.000000000000000000),
 ( 1.000000000000000000, 0.6849789572270683635, 1.000000000000000000),
 ( 1.000000000000000000, 0.5903265755406649218, 1.000000000000000000),
 ( 1.000000000000000000, 0.5583523351999168938, 1.000000000000000000),
 ( 1.000000000000000000, 0.5090820572709163772, 1.000000000000000000),
 ( 1.000000000000000000, 0.4920791080019514263, 1.000000000000000000),
 ( 1.000000000000000000, 0.4915962107220576138, 1.000000000000000000) ) ) 
 REPRESENTATION_ITEM ( '' )  SURFACE ( )  );
#183892=CARTESIAN_POINT ( 'NONE',  ( 2.822068529938852155, 6.444163718237301275, -0.7998128361456291469 ) ) ;
#183902=CARTESIAN_POINT ( 'NONE',  ( 3.818592820543298405, 7.606775390609172405, -0.7998128361456221525 ) ) ;
#183907=CARTESIAN_POINT ( 'NONE',  ( -5.738125327081750271, 7.717565519727259904, 1.599625672291269396 ) ) ;
#183911=CARTESIAN_POINT ( 'NONE',  ( 7.284808609244363353, 7.393364887073558656, 0.7998128361456341429 ) ) ;
#183915=CARTESIAN_POINT ( 'NONE',  ( -6.261168011412601153, 6.199117522936475666, 1.040834085586084257E-14 ) ) ;
#183916=CARTESIAN_POINT ( 'NONE',  ( 5.626270559546804328, 9.507806719539201978, 0.7216878364870438212 ) ) ;
#183917=CARTESIAN_POINT ( 'NONE',  ( 5.344703475446304530, 6.534489784648752853, 1.338571508491542383 ) ) ;
#183918=CARTESIAN_POINT ( 'NONE',  ( -4.783329267523015460, 4.474972321731942593, -0.7998128361456221525 ) ) ;
#183921=CARTESIAN_POINT ( 'NONE',  ( -4.252453736180621391, 8.112946458852704268, -0.7998128361456281477 ) ) ;
#183924=CARTESIAN_POINT ( 'NONE',  ( 0.6823417656249882723, 2.676041667008084879, -1.181850606188749264 ) ) ;
#183926=CARTESIAN_POINT ( 'NONE',  ( -5.802526556968872207, 6.832331073627524454, 1.082531754730548412 ) ) ;
#183929=ORIENTED_EDGE ( 'NONE', *, *, #2092, .T. ) ;
#183932=CARTESIAN_POINT ( 'NONE',  ( 5.789495288235341874, 6.713164910151406595, 1.199719254218462483 ) ) ;
#183934=CARTESIAN_POINT ( 'NONE',  ( -1.364683531249997417, 3.321875000341423245, 1.214306433183764966E-14 ) ) ;
#183937=CARTESIAN_POINT ( 'NONE',  ( -0.6823417656250003738, -0.7197916663252492686, -1.181850606188749264 ) ) ;
#183940=CARTESIAN_POINT ( 'NONE',  ( -3.972702704004144714, 4.593573561881607148, 1.199719254218462483 ) ) ;
#183942=ADVANCED_FACE ( 'NONE', ( #9540 ), #26850, .F. ) ;
#183943=CARTESIAN_POINT ( 'NONE',  ( -8.012505595552038784, 8.450270737673262644, 0.7216878364870578100 ) ) ;
#183945=CARTESIAN_POINT ( 'NONE',  ( -1.364683531249997417, 3.259375000341423245, 1.214306433183764966E-14 ) ) ;
#183952=CARTESIAN_POINT ( 'NONE',  ( -6.182154857707119255, 10.15633840072622363, 0.000000000000000000 ) ) ;
#183957=CARTESIAN_POINT ( 'NONE',  ( -6.195713011320790109, 9.211787032307496403, -1.082531754730537976 ) ) ;
#183970=CARTESIAN_POINT ( 'NONE',  ( -6.403528624356093601, 6.365204904703887223, 1.040834085586084257E-14 ) ) ;
#183972=CARTESIAN_POINT ( 'NONE',  ( -1.402160292154681736E-14, -0.7874999999999764411, 1.732050807568877637 ) ) ;
#183973=CARTESIAN_POINT ( 'NONE',  ( 3.011882680530176604, 6.665613560593854459, 0.7998128361456341429 ) ) ;
#183976=CARTESIAN_POINT ( 'NONE',  ( -5.233084104750526322, 5.207612331738130429, 0.000000000000000000 ) ) ;
#183978=CARTESIAN_POINT ( 'NONE',  ( 5.632522751473472589, 8.658694745772667289, -1.199719254218440723 ) ) ;
#183984=CARTESIAN_POINT ( 'NONE',  ( -5.260200412422220140, 5.239248024021764039, -0.7216878364870207285 ) ) ;
#183990=CARTESIAN_POINT ( 'NONE',  ( -0.6823417656250212460, 2.301041667008084435, 1.181850606188767472 ) ) ;
#183992=CARTESIAN_POINT ( 'NONE',  ( -7.609150525767646833, 9.900428251527500834, -1.599625672291263179 ) ) ;
#183994=CARTESIAN_POINT ( 'NONE',  ( 6.982612806237943559, 8.105135347821125436, -1.199719254218446718 ) ) ;
#183995=CARTESIAN_POINT ( 'NONE',  ( -5.879432169820529630, 10.01108796476595764, -0.7998128361456221525 ) ) ;
#183998=CARTESIAN_POINT ( 'NONE',  ( 1.364683531249992088, 5.634375000341417916, 1.214306433183764966E-14 ) ) ;
#184000=CARTESIAN_POINT ( 'NONE',  ( 7.944714827928043732, 10.29191993738131927, 1.443375672974076540 ) ) ;
#184003=CARTESIAN_POINT ( 'NONE',  ( -1.402160292154681736E-14, 0.1343750003414218575, 1.575800808251672791 ) ) ;
#184005=CARTESIAN_POINT ( 'NONE',  ( -3.511198596259319960, 6.271927390929313617, 1.082471891955974153 ) ) ;
#184006=CARTESIAN_POINT ( 'NONE',  ( 7.578644679914706472, 9.864838098032418401, 1.443375672974076540 ) ) ;
#184009=CARTESIAN_POINT ( 'NONE',  ( -3.945059511896602089, 7.546393830613923548, 1.040834085586084257E-14 ) ) ;
#184011=CARTESIAN_POINT ( 'NONE',  ( -0.6823417656249969321, 3.467708333674754506, -1.181850606188749264 ) ) ;
#184014=CARTESIAN_POINT ( 'NONE',  ( -4.855791571988752331, 8.816840600628864877, 0.7998128361456481317 ) ) ;
#184020=CARTESIAN_POINT ( 'NONE',  ( 6.771407655021410399, 9.987393799911945536, -1.199719254218441611 ) ) ;
#184025=CARTESIAN_POINT ( 'NONE',  ( -1.500000000000013101, 2.170833333333357373, 0.8660254037844403729 ) ) ;
#184030=ORIENTED_EDGE ( 'NONE', *, *, #138240, .T. ) ;
#184031=CARTESIAN_POINT ( 'NONE',  ( 6.995644074971448134, 7.263932296995902149, -0.7216878364870257245 ) ) ;
#184033=CARTESIAN_POINT ( 'NONE',  ( 1.364683531249986537, 0.9677083336747538400, -0.7879004041258239610 ) ) ;
#184035=CARTESIAN_POINT ( 'NONE',  ( 1.123270288250308280, 2.860197346350005887, 0.7749999999993786304 ) ) ;
#184040=CARTESIAN_POINT ( 'NONE',  ( 1.499999999999989120, 0.7750000000000187850, 0.000000000000000000 ) ) ;
#184041=CARTESIAN_POINT ( 'NONE',  ( 8.372323551638698902, 9.726464550788689323, 1.199719254218462483 ) ) ;
#184042=CARTESIAN_POINT ( 'NONE',  ( -10.01677656239806247, 10.58066083241955901, 0.7998128361456462443 ) ) ;
#184044=CARTESIAN_POINT ( 'NONE',  ( -1.364683531250014514, 1.238541667008091096, -0.7879004041258289570 ) ) ;
#184045=CARTESIAN_POINT ( 'NONE',  ( 1.499999999999989120, 3.025000000000020783, 1.214306433183764966E-14 ) ) ;
#184047=CARTESIAN_POINT ( 'NONE',  ( 2.835626683552519012, 6.459981564119914310, 0.000000000000000000 ) ) ;
#184055=CARTESIAN_POINT ( 'NONE',  ( -0.7500000000000249800, -0.5270833326505158789, 1.299038105676659116 ) ) ;
#184057=CARTESIAN_POINT ( 'NONE',  ( -8.694856585065634746, 9.038420858865048757, 0.7998128361456462443 ) ) ;
#184058=CARTESIAN_POINT ( 'NONE',  ( -5.748293942514186128, 6.769059690097084747, -1.082531754730544860 ) ) ;
#184066=CARTESIAN_POINT ( 'NONE',  ( 6.805303039055573322, 10.02693841461847057, 1.199719254218460707 ) ) ;
#184070=CARTESIAN_POINT ( 'NONE',  ( 7.605760987142057061, 7.975735361194951523, -0.7216878364870267237 ) ) ;
#184074=CARTESIAN_POINT ( 'NONE',  ( -8.667740277838301921, 9.006785167099828016, -0.7998128361456291469 ) ) ;
#184075=CARTESIAN_POINT ( 'NONE',  ( 4.650610384687404952, 5.384465856012134566, 1.199719254218462483 ) ) ;
#184080=CARTESIAN_POINT ( 'NONE',  ( 4.063008298707909027, 7.508743736771079647, -0.5217633019904341918 ) ) ;
#184081=CARTESIAN_POINT ( 'NONE',  ( 9.734391104931951588, 11.41950637958454706, 1.082531754730548412 ) ) ;
#184087=PLANE ( 'NONE',  #123121 ) ;
#184088=CARTESIAN_POINT ( 'NONE',  ( -3.470524135418294520, 6.992769224722559684, -0.7216878364870267237 ) ) ;
#184089=CARTESIAN_POINT ( 'NONE',  ( 9.002250809793993724, 11.52571191622492464, -1.443375672974057666 ) ) ;
#184092=CARTESIAN_POINT ( 'NONE',  ( -5.392392409933270514, 7.314210449720692786, 1.599625672291269396 ) ) ;
#184098=CARTESIAN_POINT ( 'NONE',  ( -6.821723845970312894, 11.11042825360738284, 0.000000000000000000 ) ) ;
#184101=CARTESIAN_POINT ( 'NONE',  ( -0.4417779905600746071, 7.383047307301207951, 2.041823008714554355 ) ) ;
#184112=CARTESIAN_POINT ( 'NONE',  ( -4.381256195510448315, 8.263215994737505454, 1.040834085586084257E-14 ) ) ;
#184115=CARTESIAN_POINT ( 'NONE',  ( 3.538314903486612817, 7.071858454135611538, 1.040834085586084257E-14 ) ) ;
#184118=CARTESIAN_POINT ( 'NONE',  ( -3.337985173046072340, 6.383183490859034137, 0.8077998227833966816 ) ) ;
#184121=CARTESIAN_POINT ( 'NONE',  ( -3.978428010606240850, 6.728917548094202949, -1.199719254218452047 ) ) ;
#184128=CARTESIAN_POINT ( 'NONE',  ( -9.501566725078754772, 9.979582688880366703, -0.7998128361456291469 ) ) ;
#184129=CARTESIAN_POINT ( 'NONE',  ( 7.474622759835693131, 7.614814729430110951, -0.7998128361456281477 ) ) ;
#184132=CARTESIAN_POINT ( 'NONE',  ( -9.972185678051314284, 11.59297036493672017, 1.199719254218462483 ) ) ;
#184135=CARTESIAN_POINT ( 'NONE',  ( 0.6823417656249882723, -0.2614583329919109578, -1.181850606188749264 ) ) ;
#184137=ORIENTED_EDGE ( 'NONE', *, *, #176248, .T. ) ;
#184139=CARTESIAN_POINT ( 'NONE',  ( 8.026063749610047537, 10.38682701267698150, -1.443375672974057666 ) ) ;
#184142=ADVANCED_FACE ( 'NONE', ( #8465 ), #13334, .T. ) ;
#184157=ADVANCED_FACE ( 'NONE', ( #18044 ), #177769, .T. ) ;
#184169=CARTESIAN_POINT ( 'NONE',  ( 1.499999999999985123, -0.4229166659838508036, -0.8660254037844323793 ) ) ;
#184173=ORIENTED_EDGE ( 'NONE', *, *, #162394, .T. ) ;
#184175=CARTESIAN_POINT ( 'NONE',  ( 0.4206437366318451221, 7.996079560418730026, -1.998769755887081834 ) ) ;
#184178=CARTESIAN_POINT ( 'NONE',  ( 8.106885785967500979, 11.54545161934907682, 1.199719254218460707 ) ) ;
#184182=CARTESIAN_POINT ( 'NONE',  ( 3.985207087413062066, 6.736826471035503694, -1.199719254218452047 ) ) ;
#184183=CARTESIAN_POINT ( 'NONE',  ( 1.364683531249990311, 2.696875000341415696, 1.214306433183764966E-14 ) ) ;
#184184=CARTESIAN_POINT ( 'NONE',  ( -5.889415777131212337, 6.013640170854067435, 0.2549476635474844932 ) ) ;
#184186=CARTESIAN_POINT ( 'NONE',  ( -7.965578943228732278, 9.251929174310385307, -1.199719254218446718 ) ) ;
#184188=CARTESIAN_POINT ( 'NONE',  ( -3.592547517496935683, 6.174760622846296343, -1.082531754730548412 ) ) ;
#184190=VERTEX_POINT ( 'NONE', #84131 ) ;
#184191=CARTESIAN_POINT ( 'NONE',  ( -0.7500000000000249800, -0.2770833326505156569, 1.299038105676659116 ) ) ;
#184198=CARTESIAN_POINT ( 'NONE',  ( -5.246642258364192735, 5.223430177620739023, 0.7216878364870317197 ) ) ;
#184200=CARTESIAN_POINT ( 'NONE',  ( 4.003835517601626925, 7.590433450137844318, -0.2001945245787856709 ) ) ;
#184204=CARTESIAN_POINT ( 'NONE',  ( -2.914639836813632812, 6.344237543017112735, 0.7216878364870317197 ) ) ;
#184205=CARTESIAN_POINT ( 'NONE',  ( 7.574201371528760163, 11.98831870009225931, 1.040834085586084257E-14 ) ) ;
#184215=CARTESIAN_POINT ( 'NONE',  ( -9.318531651294266638, 9.766041769465124034, -0.7998128361456291469 ) ) ;
#184220=CARTESIAN_POINT ( 'NONE',  ( 3.818592820543298405, 7.606775390609172405, -0.7998128361456221525 ) ) ;
#184225=CARTESIAN_POINT ( 'NONE',  ( 2.544126380858701797, 6.119897877643793116, 0.7998128361456462443 ) ) ;
#184227=ORIENTED_EDGE ( 'NONE', *, *, #122849, .T. ) ;
#184235=CARTESIAN_POINT ( 'NONE',  ( 7.425061681778431399, 11.81432239538354345, 0.7998128361456462443 ) ) ;
#184237=CARTESIAN_POINT ( 'NONE',  ( -3.737243898861318137, 7.511868315313511069, 0.7998128361456341429 ) ) ;
#184244=CARTESIAN_POINT ( 'NONE',  ( 0.6823417656249899377, 5.426041667008087543, -1.181850606188754593 ) ) ;
#184248=CARTESIAN_POINT ( 'NONE',  ( 3.506755287428983792, 7.242964935309132990, 1.040834085586084257E-14 ) ) ;
#184249=CARTESIAN_POINT ( 'NONE',  ( -4.623494077460110319, 5.352830164246910272, 1.199719254218462483 ) ) ;
#184255=CARTESIAN_POINT ( 'NONE',  ( 5.992340707560160240, 7.053780915984068756, 1.082531754730558626 ) ) ;
#184259=CARTESIAN_POINT ( 'NONE',  ( 8.242994206984347372, 8.719174117677642499, 1.040834085586084257E-14 ) ) ;
#184260=CARTESIAN_POINT ( 'NONE',  ( -1.201851678989727383E-14, 4.134375000341417028, 1.575800808251672791 ) ) ;
#184262=CARTESIAN_POINT ( 'NONE',  ( 3.673896439178923057, 5.309298483840612093, 1.443375672974066548 ) ) ;
#184264=CARTESIAN_POINT ( 'NONE',  ( 1.499999999999990896, 4.806250000682819490, 1.214306433183764966E-14 ) ) ;
#184270=CARTESIAN_POINT ( 'NONE',  ( -5.710256234166866562, 6.271970132040741497, 1.104226958479601173 ) ) ;
#184273=CARTESIAN_POINT ( 'NONE',  ( -1.364683531250010295, 5.301041667008085767, -0.7879004041258300672 ) ) ;
#184277=CARTESIAN_POINT ( 'NONE',  ( -8.631737353394710155, 13.22211067893587533, 1.040834085586084257E-14 ) ) ;
#184287=CARTESIAN_POINT ( 'NONE',  ( 2.846849069189655967, 5.304779099821139710, -1.082531754730543083 ) ) ;
#184288=EDGE_CURVE ( 'NONE', #57016, #25036, #24948, .T. ) ;
#184289=CARTESIAN_POINT ( 'NONE',  ( -0.6823417656250212460, 5.113541667008086655, 1.181850606188767472 ) ) ;
#184291=CARTESIAN_POINT ( 'NONE',  ( 5.452350330990040739, 9.512825819463730070, 0.7998128361456462443 ) ) ;
#184292=CARTESIAN_POINT ( 'NONE',  ( -7.980945979938748103, 12.46285407657057220, 0.000000000000000000 ) ) ;
#184295=LINE ( 'NONE', #39132, #23301 ) ;
#184298=CARTESIAN_POINT ( 'NONE',  ( -0.7499999999999972244, 4.358333333333352932, -1.299038105676652011 ) ) ;
#184305=CARTESIAN_POINT ( 'NONE',  ( 7.402388683381404988, 10.61957531637824204, -1.082531754730537976 ) ) ;
#184310=CARTESIAN_POINT ( 'NONE',  ( 0.7499999999999902300, 3.764583334016149863, 1.299038105676669330 ) ) ;
#184312=CARTESIAN_POINT ( 'NONE',  ( -4.391951695823077984, 7.211361847513815704, 1.199719254218464037 ) ) ;
#184313=CARTESIAN_POINT ( 'NONE',  ( 4.663641652976547647, 4.543262804668490418, 1.214306433183764966E-14 ) ) ;
#184314=CARTESIAN_POINT ( 'NONE',  ( -9.937763408692596556, 11.65677406730528887, -1.082531754730537976 ) ) ;
#184322=CARTESIAN_POINT ( 'NONE',  ( 8.633844893804129228, 8.967240552393299424, -0.7998128361456211532 ) ) ;
#184323=CARTESIAN_POINT ( 'NONE',  ( 4.033714395265605823, 4.664753868353354704, -1.199719254218446718 ) ) ;
#184324=CARTESIAN_POINT ( 'NONE',  ( -1.177110729581199999, 2.960371626218858410, -0.7749999999999944711 ) ) ;
#184327=CARTESIAN_POINT ( 'NONE',  ( 3.981290663907289140, 7.796589541200495965, -0.7998128361456221525 ) ) ;
#184332=ORIENTED_EDGE ( 'NONE', *, *, #118861, .F. ) ;
#184335=VECTOR ( 'NONE', #18848, 1000.000000000000000 ) ;
#184341=CARTESIAN_POINT ( 'NONE',  ( 2.275391796764376640, 5.643962577969389827, -0.5307291018262025872 ) ) ;
#184342=CARTESIAN_POINT ( 'NONE',  ( 5.328689024754546644, 6.340921230984883472, -1.104828203510083373 ) ) ;
#184344=CARTESIAN_POINT ( 'NONE',  ( 8.055515824813896941, 12.54985222892493368, 0.7998128361456462443 ) ) ;
#184351=CARTESIAN_POINT ( 'NONE',  ( 6.317736394288135493, 8.393778431468064127, 1.443375672974076540 ) ) ;
#184352=CARTESIAN_POINT ( 'NONE',  ( -9.083599731475995753, 11.62061899152058686, 1.443375672974064550 ) ) ;
#184357=CARTESIAN_POINT ( 'NONE',  ( -4.717347382551060342, 7.590990148696470818, 1.199719254218464037 ) ) ;
#184367=CARTESIAN_POINT ( 'NONE',  ( 7.248805684800777804, 11.60869039890961218, 1.040834085586084257E-14 ) ) ;
#184368=CARTESIAN_POINT ( 'NONE',  ( 6.114657076318319007, 6.015903114251479167, -0.04046911893108330605 ) ) ;
#184371=CARTESIAN_POINT ( 'NONE',  ( 6.308621549060418054, 6.254479983525607523, 0.7998128361456341429 ) ) ;
#184377=CARTESIAN_POINT ( 'NONE',  ( -8.731087737520713432, 10.24898578427137963, 1.082531754730558626 ) ) ;
#184381=CARTESIAN_POINT ( 'NONE',  ( 7.344766530301147789, 9.591980256816594164, 1.599625672291281386 ) ) ;
#184384=CARTESIAN_POINT ( 'NONE',  ( 5.040934186182656873, 4.775511393501539636, 1.040834085586084257E-14 ) ) ;
#184386=CARTESIAN_POINT ( 'NONE',  ( -7.549192604710863286, 7.701812881784464437, -0.7998128361456291469 ) ) ;
#184387=CARTESIAN_POINT ( 'NONE',  ( 3.195971524519376494, 4.751719416737803847, -1.599625672291262513 ) ) ;
#184391=CARTESIAN_POINT ( 'NONE',  ( 9.752392566931574081, 10.27221283770866300, -0.7998128361456281477 ) ) ;
#184392=CARTESIAN_POINT ( 'NONE',  ( 1.499999999999995115, 3.545833333333354709, -0.8660254037844217212 ) ) ;
#184395=CARTESIAN_POINT ( 'NONE',  ( 4.007874524826865681, 7.816931064126571016, 0.2151701594551927443 ) ) ;
#184397=CARTESIAN_POINT ( 'NONE',  ( 6.643132081016125845, 6.852668304048034287, 0.7216878364870317197 ) ) ;
#184404=EDGE_LOOP ( 'NONE', ( #28311, #136428 ) ) ;
#184405=CARTESIAN_POINT ( 'NONE',  ( 7.226132685959389512, 11.37431253368722750, -0.7216878364870267237 ) ) ;
#184409=CARTESIAN_POINT ( 'NONE',  ( -8.528242318195895066, 9.908369778438709474, 1.199719254218462483 ) ) ;
#184415=EDGE_CURVE ( 'NONE', #190459, #85365, #161940, .T. ) ;
#184419=AXIS2_PLACEMENT_3D ( 'NONE', #209232, #110763, #192996 ) ;
#184420=CARTESIAN_POINT ( 'NONE',  ( 9.028840231696797503, 12.62106513936658203, -1.199719254218446718 ) ) ;
#184424=CARTESIAN_POINT ( 'NONE',  ( 5.983225862332436584, 5.874851682342960402, 0.7998128361456341429 ) ) ;
#184427=CARTESIAN_POINT ( 'NONE',  ( -1.001543065824772872E-14, 4.743750000682822154, 1.732050807568877637 ) ) ;
#184433=CARTESIAN_POINT ( 'NONE',  ( -1.499999999999997780, 1.650000000000019451, 0.000000000000000000 ) ) ;
#184434=CARTESIAN_POINT ( 'NONE',  ( 6.043183783389218355, 8.073467052085995022, 1.599625672291267398 ) ) ;
#184435=CARTESIAN_POINT ( 'NONE',  ( 3.497640442201256139, 7.024404915969360452, 1.040834085586084257E-14 ) ) ;
#184439=CARTESIAN_POINT ( 'NONE',  ( 9.083599731475992201, 9.699880562917908122, 0.7216878364870438212 ) ) ;
#184445=CARTESIAN_POINT ( 'NONE',  ( -6.240830780992103755, 6.175390754112560110, 1.040834085586084257E-14 ) ) ;
#184446=CARTESIAN_POINT ( 'NONE',  ( -0.7500000000000215383, 4.222916667349481123, 1.299038105676671107 ) ) ;
#184447=CARTESIAN_POINT ( 'NONE',  ( 1.364683531249990311, 5.426041667008086655, 0.7879004041258500513 ) ) ;
#184451=CARTESIAN_POINT ( 'NONE',  ( 10.53432216769390095, 11.39239007183880581, -0.7216878364870257245 ) ) ;
#184453=CARTESIAN_POINT ( 'NONE',  ( 0.6823417656249899377, 3.488541667008085323, -1.181850606188754593 ) ) ;
#184460=CARTESIAN_POINT ( 'NONE',  ( -6.665805079413154921, 10.92852302595736447, 0.7998128361456481317 ) ) ;
#184461=CARTESIAN_POINT ( 'NONE',  ( 6.602984505055297326, 7.662235663108029726, 1.199719254218462483 ) ) ;
#184463=CARTESIAN_POINT ( 'NONE',  ( -1.364683531250014514, -1.011458332991911568, -0.7879004041258359514 ) ) ;
#184469=CARTESIAN_POINT ( 'NONE',  ( -7.366157530926372488, 7.488271962369228874, -0.7998128361456291469 ) ) ;
#184472=CARTESIAN_POINT ( 'NONE',  ( 9.622536337397022521, 12.24937836509514710, 1.599625672291281386 ) ) ;
#184474=CARTESIAN_POINT ( 'NONE',  ( 8.432281472695482449, 11.92507992053172572, 1.199719254218450271 ) ) ;
#184475=DIRECTION ( 'NONE',  ( 1.000000000000000000, -7.387867266669436732E-31, 0.000000000000000000 ) ) ;
#184476=CARTESIAN_POINT ( 'NONE',  ( -4.437596350374534815, 4.071617251725375475, -0.7998128361456221525 ) ) ;
#184477=CARTESIAN_POINT ( 'NONE',  ( -8.453672473320708036, 9.821371626084353323, -1.199719254218446718 ) ) ;
#184480=CARTESIAN_POINT ( 'NONE',  ( -4.074449998555902397, 7.717048951691181102, 0.6760625908293280695 ) ) ;
#184481=CARTESIAN_POINT ( 'NONE',  ( 0.6823417656249864960, -0.8239583329919114574, -1.181850606188749264 ) ) ;
#184485=CARTESIAN_POINT ( 'NONE',  ( 7.117667457494414762, 11.24776976714476184, 1.040834085586084257E-14 ) ) ;
#184488=CARTESIAN_POINT ( 'NONE',  ( 5.900823170445728572, 7.907379670318584353, 1.599625672291267398 ) ) ;
#184506=CARTESIAN_POINT ( 'NONE',  ( 2.223174002961016082, 5.537527403522402025, -0.7216878364870267237 ) ) ;
#184510=CARTESIAN_POINT ( 'NONE',  ( -9.318531651294266638, 9.766041769465124034, -0.7998128361456291469 ) ) ;
#184511=CARTESIAN_POINT ( 'NONE',  ( -0.007072395215936694290, 7.009756401597622144, 2.079987976222394952 ) ) ;
#184514=CARTESIAN_POINT ( 'NONE',  ( 1.499999999999987121, 1.285416667349485120, 0.8660254037844524744 ) ) ;
#184515=CARTESIAN_POINT ( 'NONE',  ( 9.728138913005292210, 11.30824913904973705, -1.199719254218440723 ) ) ;
#184519=CARTESIAN_POINT ( 'NONE',  ( -9.992522908471816123, 11.61669713376064372, 1.199719254218462483 ) ) ;
#184521=CARTESIAN_POINT ( 'NONE',  ( 1.364683531249988535, 2.613541667008089764, 0.7879004041258500513 ) ) ;
#184524=ORIENTED_EDGE ( 'NONE', *, *, #208497, .F. ) ;
#184528=CARTESIAN_POINT ( 'NONE',  ( -4.060830702492950195, 4.696389560118578999, -1.199719254218452047 ) ) ;
#184532=CARTESIAN_POINT ( 'NONE',  ( 0.6823417656249882723, 0.1552083336747514530, 1.181850606188755259 ) ) ;
#184538=CARTESIAN_POINT ( 'NONE',  ( -1.364683531250012516, 2.238541667008087988, -0.7879004041258289570 ) ) ;
#184542=CARTESIAN_POINT ( 'NONE',  ( -5.876569516519495551, 8.943415971659659292, 1.199719254218452047 ) ) ;
#184543=CARTESIAN_POINT ( 'NONE',  ( 7.884230021546724920, 9.157022099014721306, 1.199719254218462483 ) ) ;
#184544=CARTESIAN_POINT ( 'NONE',  ( 3.734381245560244089, 6.444196322207211836, 1.199719254218462483 ) ) ;
#184545=CARTESIAN_POINT ( 'NONE',  ( 4.306686350635271054, 8.176217842383143974, -0.7998128361456221525 ) ) ;
#184547=CARTESIAN_POINT ( 'NONE',  ( -1.500000000000011324, 4.379166666666688634, -0.8660254037844313801 ) ) ;
#184549=CIRCLE ( 'NONE', #77415, 0.08000000000000020983 ) ;
#184550=CARTESIAN_POINT ( 'NONE',  ( -0.6823417656250212460, 1.113541667008083325, 1.181850606188755259 ) ) ;
#184553=CARTESIAN_POINT ( 'NONE',  ( 3.104453987849314700, 4.644948957289396496, 0.000000000000000000 ) ) ;
#184557=CARTESIAN_POINT ( 'NONE',  ( 5.450014563013511726, 8.341805509282339770, -1.082531754730543083 ) ) ;
#184560=CARTESIAN_POINT ( 'NONE',  ( -9.854078719034067291, 10.39084668182823634, 0.7998128361456462443 ) ) ;
#184561=CARTESIAN_POINT ( 'NONE',  ( -5.427341564172148303, 5.226320001155936090, 0.000000000000000000 ) ) ;
#184566=CARTESIAN_POINT ( 'NONE',  ( -8.473482818416682605, 8.988077497682020578, -0.7216878364870267237 ) ) ;
#184568=CARTESIAN_POINT ( 'NONE',  ( 1.499999999999989120, 5.045833333333354709, -0.8660254037844323793 ) ) ;
#184571=CARTESIAN_POINT ( 'NONE',  ( 8.785320351975350661, 9.351887953500479966, -0.7216878364870197293 ) ) ;
#184579=VERTEX_POINT ( 'NONE', #171786 ) ;
#184580=CARTESIAN_POINT ( 'NONE',  ( 9.910647101465253073, 11.62513837554007168, -1.082531754730537088 ) ) ;
#184586=CARTESIAN_POINT ( 'NONE',  ( 5.764187864104357573, 9.876636274763768597, 1.040834085586084257E-14 ) ) ;
#184587=CARTESIAN_POINT ( 'NONE',  ( -5.362413449404877852, 6.214902764849178141, -1.199719254218446718 ) ) ;
#184589=CARTESIAN_POINT ( 'NONE',  ( -0.7499999999999972244, 5.108333333333353821, -1.299038105676652011 ) ) ;
#184592=CARTESIAN_POINT ( 'NONE',  ( 0.6823417656249882723, -0.8447916663252494907, 1.181850606188755259 ) ) ;
#184593=CARTESIAN_POINT ( 'NONE',  ( 2.236732156574683827, 5.553345249405011508, 1.040834085586084257E-14 ) ) ;
#184595=CARTESIAN_POINT ( 'NONE',  ( -4.308793891044708779, 3.921347715840572956, 1.214306433183764966E-14 ) ) ;
#184605=CARTESIAN_POINT ( 'NONE',  ( 1.123270288250308280, 2.860197346350005887, 0.7749999999993786304 ) ) ;
#184608=ORIENTED_EDGE ( 'NONE', *, *, #86821, .F. ) ;
#184611=CARTESIAN_POINT ( 'NONE',  ( 6.470265622219697477, 8.571729197388226140, -1.599625672291262513 ) ) ;
#184622=CARTESIAN_POINT ( 'NONE',  ( 0.1263921868141488214, 7.050106634747087320, 4.033475512996062662 ) ) ;
#184624=CARTESIAN_POINT ( 'NONE',  ( -5.436983294280064882, 6.301900917203534291, 1.199719254218450271 ) ) ;
#184626=CARTESIAN_POINT ( 'NONE',  ( -3.228813138348844536, 6.918699094715619502, 0.7998128361456341429 ) ) ;
#184636=CARTESIAN_POINT ( 'NONE',  ( -3.440018289565379028, 5.036440642624797626, 1.599625672291267398 ) ) ;
#184639=CARTESIAN_POINT ( 'NONE',  ( 4.964256800898067645, 8.943383367689749619, 0.7998128361456462443 ) ) ;
#184640=CARTESIAN_POINT ( 'NONE',  ( 0.6823417656249917140, 4.842708333674755394, 1.181850606188765695 ) ) ;
#184646=CARTESIAN_POINT ( 'NONE',  ( 5.517805330637495231, 6.500156309574290248, -1.082531754730543083 ) ) ;
#184647=CARTESIAN_POINT ( 'NONE',  ( -7.206322340863467346, 8.366129804884193888, 1.199719254218450271 ) ) ;
#184650=CARTESIAN_POINT ( 'NONE',  ( -7.588813295347149435, 9.876701482703580837, -1.599625672291263179 ) ) ;
#184651=CARTESIAN_POINT ( 'NONE',  ( -6.274726165026268454, 6.214935368819085149, 0.7998128361456341429 ) ) ;
#184659=CARTESIAN_POINT ( 'NONE',  ( 5.615048174354031474, 9.702639970055050966, 0.7998128361456462443 ) ) ;
#184673=CARTESIAN_POINT ( 'NONE',  ( -1.402160292154681736E-14, -0.8656249996585829720, 1.575800808251672791 ) ) ;
#184674=CARTESIAN_POINT ( 'NONE',  ( 2.900554798319789906, 5.471398800426671372, 1.199719254218452047 ) ) ;
#184675=CARTESIAN_POINT ( 'NONE',  ( 6.356075086708249167, 6.309842444114747373, -0.7998128361456281477 ) ) ;
#184677=CARTESIAN_POINT ( 'NONE',  ( -7.700668062882072284, 10.00719871149432549, -1.443375672974059665 ) ) ;
#184679=CARTESIAN_POINT ( 'NONE',  ( 6.046573322014824114, 7.117052299514516456, -1.082531754730543083 ) ) ;
#184680=CARTESIAN_POINT ( 'NONE',  ( -7.470179451005382276, 11.65903375957422128, 0.7216878364870458196 ) ) ;
#184685=CARTESIAN_POINT ( 'NONE',  ( 6.591235234537977661, 10.84152487360300299, 0.7998128361456462443 ) ) ;
#184688=AXIS2_PLACEMENT_3D ( 'NONE', #174792, #110896, #26368 ) ;
#184690=CARTESIAN_POINT ( 'NONE',  ( -0.6823417656249969321, 4.217708333674755394, -1.181850606188749264 ) ) ;
#184696=CARTESIAN_POINT ( 'NONE',  ( 8.748035429315576650, 11.22912730566677553, -1.599625672291255185 ) ) ;
#184699=CARTESIAN_POINT ( 'NONE',  ( -8.422639742587602285, 10.84949900448412841, -1.599625672291263179 ) ) ;
#184704=CARTESIAN_POINT ( 'NONE',  ( 8.530051201292206287, 13.10347683481629488, 0.000000000000000000 ) ) ;
#184707=CARTESIAN_POINT ( 'NONE',  ( -9.664264568442742842, 10.16939683947169115, -0.7998128361456291469 ) ) ;
#184711=CARTESIAN_POINT ( 'NONE',  ( 5.731063993565963521, 6.075950606329157289, 0.6577720730673256577 ) ) ;
#184713=CARTESIAN_POINT ( 'NONE',  ( -8.649738815838677652, 13.03518635187974262, 0.7216878364870357165 ) ) ;
#184717=CARTESIAN_POINT ( 'NONE',  ( 8.260995669428309540, 8.532249790621511565, 0.7998128361456481317 ) ) ;
#184719=CARTESIAN_POINT ( 'NONE',  ( 6.799577732453452761, 7.891594428405881878, -1.199719254218446718 ) ) ;
#184720=CARTESIAN_POINT ( 'NONE',  ( 3.310162060030825248, 7.013606170011280838, -0.7998128361456291469 ) ) ;
#184722=CARTESIAN_POINT ( 'NONE',  ( -7.212574532790100079, 9.437756259720353924, -1.443375672974059665 ) ) ;
#184729=CARTESIAN_POINT ( 'NONE',  ( -4.014638704412293535, 7.626288086010478473, 0.05010440672792437766 ) ) ;
#184732=CARTESIAN_POINT ( 'NONE',  ( 4.690757960648221037, 7.456006139856155457, 1.082531754730558626 ) ) ;
#184737=CARTESIAN_POINT ( 'NONE',  ( -9.693716643646601128, 12.33242205571964512, 1.443375672974076540 ) ) ;
#184740=AXIS2_PLACEMENT_3D ( 'NONE', #105155, #170122, #122547 ) ;
#184743=CARTESIAN_POINT ( 'NONE',  ( -10.45297324601190425, 11.29748299654313470, 0.7216878364870438212 ) ) ;
#184751=CARTESIAN_POINT ( 'NONE',  ( -8.297226821439000588, 12.62392235841345389, 1.040834085586084257E-14 ) ) ;
#184756=CARTESIAN_POINT ( 'NONE',  ( 8.945682426918439845, 9.331051007693339727, 1.040834085586084257E-14 ) ) ;
#184760=CARTESIAN_POINT ( 'NONE',  ( -0.7500000000000006661, 1.389583334016154748, -1.299038105676652011 ) ) ;
#184762=CARTESIAN_POINT ( 'NONE',  ( -6.891622154448065807, 6.934647356477856128, 1.040834085586084257E-14 ) ) ;
#184766=CARTESIAN_POINT ( 'NONE',  ( -7.621654909176601045, 12.04368116068139472, 0.7998128361456481317 ) ) ;
#184767=CARTESIAN_POINT ( 'NONE',  ( -3.795919822146283540, 6.412028311603867436, -1.082531754730549967 ) ) ;
#184769=CARTESIAN_POINT ( 'NONE',  ( -1.500000000000011324, 5.160416667349487341, -0.8660254037844313801 ) ) ;
#184770=CARTESIAN_POINT ( 'NONE',  ( 5.615048174354031474, 9.702639970055050966, 0.7998128361456462443 ) ) ;
#184775=CARTESIAN_POINT ( 'NONE',  ( 8.880754312151170282, 10.31963377138658089, 1.199719254218453823 ) ) ;
#184776=CARTESIAN_POINT ( 'NONE',  ( 6.095638044316721960, 6.027669342855261014, -0.2934597938374111092 ) ) ;
#184782=CARTESIAN_POINT ( 'NONE',  ( -6.385527162356466668, 10.39360608948380182, 0.000000000000000000 ) ) ;
#184785=CARTESIAN_POINT ( 'NONE',  ( -0.6823417656250212460, 3.613541667008085767, 1.181850606188767472 ) ) ;
#184789=CARTESIAN_POINT ( 'NONE',  ( 1.364683531249992088, 5.634375000341417916, 1.214306433183764966E-14 ) ) ;
#184792=CARTESIAN_POINT ( 'NONE',  ( -4.731432421044888592, 4.622352034081546712, -0.7216878364870207285 ) ) ;
#184794=CARTESIAN_POINT ( 'NONE',  ( 10.58621901417202515, 11.24501035948919991, -0.7998128361456281477 ) ) ;
#184795=CARTESIAN_POINT ( 'NONE',  ( -1.001543065824772872E-14, 5.134375000341421469, 1.575800808251672791 ) ) ;
#184799=CARTESIAN_POINT ( 'NONE',  ( -1.364683531250012516, 2.488541667008088876, -0.7879004041258289570 ) ) ;
#184800=CARTESIAN_POINT ( 'NONE',  ( -4.175548123328963079, 4.934189567714277302, 1.082531754730560403 ) ) ;
#184801=CARTESIAN_POINT ( 'NONE',  ( 3.388648328411762556, 6.040841252200647382, 1.199719254218462483 ) ) ;
#184802=ORIENTED_EDGE ( 'NONE', *, *, #149589, .F. ) ;
#184807=CARTESIAN_POINT ( 'NONE',  ( -1.420000000000021911, 6.280000000000042881, 2.500000000000011102 ) ) ;
#184811=CARTESIAN_POINT ( 'NONE',  ( -6.873620692448438874, 10.96304854125777695, 0.000000000000000000 ) ) ;
#184816=CARTESIAN_POINT ( 'NONE',  ( -8.134002093194872884, 11.57708731111429401, 1.199719254218453823 ) ) ;
#184817=CARTESIAN_POINT ( 'NONE',  ( -3.578989363883261277, 7.119311991265024453, 1.040834085586084257E-14 ) ) ;
#184818=CARTESIAN_POINT ( 'NONE',  ( -1.402160292154681736E-14, 2.509375000341417028, -1.575800808251660134 ) ) ;
#184834=CARTESIAN_POINT ( 'NONE',  ( 1.499999999999821032, 7.240846818246208905, -4.154462424328212222 ) ) ;
#184841=CARTESIAN_POINT ( 'NONE',  ( 0.6823417656249882723, 2.738541667008084879, -1.181850606188749264 ) ) ;
#184847=CARTESIAN_POINT ( 'NONE',  ( -3.763755302173069861, 3.180306474485406820, -2.446972558850334600 ) ) ;
#184850=CARTESIAN_POINT ( 'NONE',  ( 8.224992744984721327, 12.74757530245756243, 1.040834085586084257E-14 ) ) ;
#184853=CARTESIAN_POINT ( 'NONE',  ( 1.364683531249986537, 1.405208333674755838, -0.7879004041258239610 ) ) ;
#184863=CARTESIAN_POINT ( 'NONE',  ( 4.487912541323413329, 5.194651705420806564, 1.199719254218462483 ) ) ;
#184868=CARTESIAN_POINT ( 'NONE',  ( 4.354158978451688533, 5.549389920478685845, 1.308530732453070833 ) ) ;
#184874=CARTESIAN_POINT ( 'NONE',  ( -4.647747731386360215, 4.316793862905830892, 0.7998128361456341429 ) ) ;
#184875=CARTESIAN_POINT ( 'NONE',  ( 7.527801604085637699, 9.805521176231838609, 1.599625672291281386 ) ) ;
#184879=CARTESIAN_POINT ( 'NONE',  ( 3.348500752450929596, 6.850408611260650815, 0.7216878364870317197 ) ) ;
#184887=CARTESIAN_POINT ( 'NONE',  ( -7.049876689426113785, 8.287572894827684777, -1.082531754730544860 ) ) ;
#184889=CARTESIAN_POINT ( 'NONE',  ( 6.661133543015731462, 6.665743976473484267, -0.7998128361456281477 ) ) ;
#184892=CARTESIAN_POINT ( 'NONE',  ( -9.646789991323334590, 11.21334206375407305, 1.199719254218462483 ) ) ;
#184896=CARTESIAN_POINT ( 'NONE',  ( -2.462777459176719308, 6.024990802348131780, -0.7998128361456281477 ) ) ;
#184899=CARTESIAN_POINT ( 'NONE',  ( 8.992082194361556091, 11.51384853155376220, 1.599625672291279388 ) ) ;
#184900=CARTESIAN_POINT ( 'NONE',  ( 5.190073875932979419, 4.949507698210251938, 0.7998128361456341429 ) ) ;
#184902=ORIENTED_EDGE ( 'NONE', *, *, #54063, .T. ) ;
#184906=CARTESIAN_POINT ( 'NONE',  ( 5.043269954603547767, 4.986162489899998995, -0.7216878364870197293 ) ) ;
#184909=CARTESIAN_POINT ( 'NONE',  ( -3.228813138348844536, 6.918699094715619502, 0.7998128361456341429 ) ) ;
#184912=CARTESIAN_POINT ( 'NONE',  ( -9.972185678051314284, 11.59297036493672017, 1.199719254218462483 ) ) ;
#184917=CARTESIAN_POINT ( 'NONE',  ( 9.097157885089661278, 9.715698408800516717, 1.040834085586084257E-14 ) ) ;
#184920=CARTESIAN_POINT ( 'NONE',  ( 4.202137545231717120, 6.989912005157271402, 1.199719254218462483 ) ) ;
#184933=CARTESIAN_POINT ( 'NONE',  ( -0.6823417656250003738, 2.530208333674753618, -1.181850606188749264 ) ) ;
#184935=CARTESIAN_POINT ( 'NONE',  ( 4.390142812726693045, 4.016254791136236513, 1.214306433183764966E-14 ) ) ;
#184937=CARTESIAN_POINT ( 'NONE',  ( -3.958617665510272943, 6.601842462195195438, -1.082531754730549967 ) ) ;
#184938=CARTESIAN_POINT ( 'NONE',  ( -6.371969008298464132, 6.536311385877402458, 1.040834085586084257E-14 ) ) ;
#184943=CARTESIAN_POINT ( 'NONE',  ( 3.974511587100456822, 7.788680618259193444, 1.040834085586084257E-14 ) ) ;
#184953=CARTESIAN_POINT ( 'NONE',  ( 6.491656622844908853, 6.468020902940851968, 0.7998128361456341429 ) ) ;
#184958=CARTESIAN_POINT ( 'NONE',  ( -5.442708600882160574, 8.437244903416123876, -1.199719254218446718 ) ) ;
#184962=CARTESIAN_POINT ( 'NONE',  ( 6.252281394196331554, 10.44607872653774372, 1.040834085586084257E-14 ) ) ;
#184965=CARTESIAN_POINT ( 'NONE',  ( -4.076197739202962467, 7.907314462378773001, 1.040834085586084257E-14 ) ) ;
#184966=CARTESIAN_POINT ( 'NONE',  ( 5.734735788456138295, 8.673980272298743799, -1.082531754730537976 ) ) ;
#184967=CARTESIAN_POINT ( 'NONE',  ( 4.369547513234953939, 7.382648021784232739, 1.157447143386416188 ) ) ;
#184969=CARTESIAN_POINT ( 'NONE',  ( -3.948449050077848632, 5.629609863222681199, 1.599625672291267398 ) ) ;
#184972=CARTESIAN_POINT ( 'NONE',  ( -5.575427483717760424, 7.527751369135936343, 1.599625672291269396 ) ) ;
#184975=CARTESIAN_POINT ( 'NONE',  ( -1.201851678989727383E-14, 1.571875000341420581, 1.575800808251672791 ) ) ;
#184977=CARTESIAN_POINT ( 'NONE',  ( -4.419594888374909658, 8.100018436505289188, 0.7216878364870458196 ) ) ;
#184984=CARTESIAN_POINT ( 'NONE',  ( 5.133733721068893807, 9.141106441222381918, 1.040834085586084257E-14 ) ) ;
#184987=CARTESIAN_POINT ( 'NONE',  ( -1.364683531249997417, 3.071875000341423245, 1.214306433183764966E-14 ) ) ;
#184991=CARTESIAN_POINT ( 'NONE',  ( -0.6823417656250246877, -0.8864583329919115684, 1.181850606188755259 ) ) ;
#184996=CARTESIAN_POINT ( 'NONE',  ( -2.923754682041362241, 6.562797562356882608, 0.7998128361456341429 ) ) ;
#184997=CARTESIAN_POINT ( 'NONE',  ( -8.175203438916030407, 8.640084888264587093, 0.7216878364870578100 ) ) ;
#184999=CARTESIAN_POINT ( 'NONE',  ( -0.6823417656249969321, 3.717708333674754506, -1.181850606188749264 ) ) ;
#185007=CARTESIAN_POINT ( 'NONE',  ( -7.985389288324710400, 8.418635045908049008, -0.7216878364870267237 ) ) ;
#185010=CARTESIAN_POINT ( 'NONE',  ( -6.195713011320795438, 8.251417818006149929, -1.443375672974058777 ) ) ;
#185016=CARTESIAN_POINT ( 'NONE',  ( 0.7499999999999902300, 4.847916667349482012, -1.299038105676658228 ) ) ;
#185025=CARTESIAN_POINT ( 'NONE',  ( -6.124532705071231931, 8.168374127381657246, -1.599625672291263179 ) ) ;
#185027=CARTESIAN_POINT ( 'NONE',  ( 1.499999999999987566, -0.7249999999999825473, 0.000000000000000000 ) ) ;
#185028=CARTESIAN_POINT ( 'NONE',  ( 2.822068529938852155, 6.444163718237301275, -0.7998128361456291469 ) ) ;
#185032=CARTESIAN_POINT ( 'NONE',  ( 7.481401836642521452, 7.622723652371411696, 1.040834085586084257E-14 ) ) ;
#185037=CARTESIAN_POINT ( 'NONE',  ( -5.477130870240893401, 6.452702772444876445, 1.082531754730548412 ) ) ;
#185045=CARTESIAN_POINT ( 'NONE',  ( -0.6823417656250212460, 2.551041667008084435, 1.181850606188767472 ) ) ;
#185047=CARTESIAN_POINT ( 'NONE',  ( -7.985916173649233230, 9.275655943134292869, -1.199719254218446718 ) ) ;
#185049=CARTESIAN_POINT ( 'NONE',  ( 7.633404179693907388, 8.864391950186421454, -1.199719254218441611 ) ) ;
#185051=CARTESIAN_POINT ( 'NONE',  ( -7.202405917357668663, 9.425892875049191488, 1.599625672291295375 ) ) ;
#185054=CARTESIAN_POINT ( 'NONE',  ( -1.500000000000001332, -1.068749999317178290, 0.000000000000000000 ) ) ;
#185056=CARTESIAN_POINT ( 'NONE',  ( 8.487040972474689582, 9.964264558384387627, -1.082531754730543083 ) ) ;
#185057=EDGE_CURVE ( 'NONE', #24037, #10073, #111874, .T. ) ;
#185059=CARTESIAN_POINT ( 'NONE',  ( -1.364683531250000748, -0.6781249996585803075, 0.000000000000000000 ) ) ;
#185062=CARTESIAN_POINT ( 'NONE',  ( 7.741342523278705201, 9.094283034322399928, 1.082531754730558626 ) ) ;
#185065=CARTESIAN_POINT ( 'NONE',  ( -5.436456409399874623, 5.444880020495701523, 0.000000000000000000 ) ) ;
#185067=CARTESIAN_POINT ( 'NONE',  ( 1.364683531249988535, 3.863541667008087543, 0.7879004041258500513 ) ) ;
#185071=CARTESIAN_POINT ( 'NONE',  ( -7.230575994789712801, 7.330093503543126054, 0.7998128361456341429 ) ) ;
#185080=CARTESIAN_POINT ( 'NONE',  ( 7.470706336329915764, 8.674577799595093452, -1.199719254218441611 ) ) ;
#185083=CARTESIAN_POINT ( 'NONE',  ( 1.499999999999987121, 2.295833333333350268, -0.8660254037844262731 ) ) ;
#185089=CARTESIAN_POINT ( 'NONE',  ( 6.656690234629796699, 6.868486149930637552, 1.040834085586084257E-14 ) ) ;
#185090=CARTESIAN_POINT ( 'NONE',  ( -0.6823417656250003738, -0.2197916663252488800, -1.181850606188749264 ) ) ;
#185095=CARTESIAN_POINT ( 'NONE',  ( 0.7499999999999885647, 0.7333333333333567072, 1.299038105676657340 ) ) ;
#185096=CARTESIAN_POINT ( 'NONE',  ( 6.564118927310645724, 10.80988918183778225, -0.7998128361456291469 ) ) ;
#185097=CARTESIAN_POINT ( 'NONE',  ( -8.503988664269602538, 10.94440607977979063, 1.599625672291269396 ) ) ;
#185100=CARTESIAN_POINT ( 'NONE',  ( -1.364683531250000748, -0.4906249996585801409, 0.000000000000000000 ) ) ;
#185101=CARTESIAN_POINT ( 'NONE',  ( -1.402160292154681736E-14, 0.5875000000000220046, -1.732050807568863648 ) ) ;
#185103=CARTESIAN_POINT ( 'NONE',  ( 3.649115900372475796, 7.409052317076538330, 1.040834085586084257E-14 ) ) ;
#185111=CARTESIAN_POINT ( 'NONE',  ( -1.500000000000001332, -0.3187499993171846735, 0.000000000000000000 ) ) ;
#185113=CARTESIAN_POINT ( 'NONE',  ( -7.531718027591449705, 8.745758106066849891, 1.199719254218462483 ) ) ;
#185114=CARTESIAN_POINT ( 'NONE',  ( -4.609409038966234995, 7.361099064560491456, -1.082531754730549967 ) ) ;
#185116=DIRECTION ( 'NONE',  ( 0.7592566023653004592, 0.6507913734559639396, 0.000000000000000000 ) ) ;
#185117=AXIS2_PLACEMENT_3D ( 'NONE', #103053, #120440, #203715 ) ;
#185123=CARTESIAN_POINT ( 'NONE',  ( 7.100719765255169236, 9.307259030929609267, -1.599625672291262513 ) ) ;
#185127=CARTESIAN_POINT ( 'NONE',  ( 6.358410854684775515, 8.441231968597481483, -1.443375672974058777 ) ) ;
#185131=CARTESIAN_POINT ( 'NONE',  ( -8.019811557683421910, 9.315200557840817908, 1.199719254218462483 ) ) ;
#185132=CARTESIAN_POINT ( 'NONE',  ( 6.017121246366603060, 5.914396297049491658, 1.040834085586084257E-14 ) ) ;
#185134=CARTESIAN_POINT ( 'NONE',  ( 4.029290343944737174, 7.554674111305462070, -0.3786771240106376890 ) ) ;
#185135=CARTESIAN_POINT ( 'NONE',  ( 3.684065054611349144, 5.321161868511784299, -1.599625672291262513 ) ) ;
#185143=( BOUNDED_CURVE ( )  B_SPLINE_CURVE ( 2, ( #209436, #63210, #127240, #212643, #64285, #128313, #147676 ),
 .UNSPECIFIED., .F., .T. ) 
 B_SPLINE_CURVE_WITH_KNOTS ( ( 3, 2, 2, 3 ),
 ( 0.2375000000000001832, 0.2416666666666668906, 0.2458333333333335702, 0.2500000000000002776 ),
 .UNSPECIFIED. ) 
 CURVE ( )  GEOMETRIC_REPRESENTATION_ITEM ( )  RATIONAL_B_SPLINE_CURVE ( ( 0.9999999999999937828, 0.8660254037844449249, 1.000000000000000000, 0.8660254037844387076, 1.000000000000000000, 0.8660254037844298258, 1.000000000000008882 ) ) 
 REPRESENTATION_ITEM ( '' )  );
#185144=CARTESIAN_POINT ( 'NONE',  ( -4.934804725694231564, 5.819988937140460727, -1.082531754730544860 ) ) ;
#185146=CARTESIAN_POINT ( 'NONE',  ( 9.571693261567961741, 11.22969222899322617, 1.082531754730548412 ) ) ;
#185149=CARTESIAN_POINT ( 'NONE',  ( -6.612626235163205024, 8.737816579155630592, -1.599625672291263179 ) ) ;
#185153=CARTESIAN_POINT ( 'NONE',  ( 0.6823417656249882723, 2.988541667008084879, -1.181850606188754593 ) ) ;
#185155=CARTESIAN_POINT ( 'NONE',  ( -8.355902744723985975, 8.642974711799791265, 1.040834085586084257E-14 ) ) ;
#185171=CARTESIAN_POINT ( 'NONE',  ( -7.528855374290365887, 7.678086112960552434, -0.7998128361456291469 ) ) ;
#185174=CARTESIAN_POINT ( 'NONE',  ( 4.839897650398541806, 8.590371658866210680, 1.040834085586084257E-14 ) ) ;
#185180=CARTESIAN_POINT ( 'NONE',  ( -3.327636637150278798, 5.969660945728899826, -1.199719254218452935 ) ) ;
#185188=CARTESIAN_POINT ( 'NONE',  ( -8.130085669689073313, 12.63685038127928806, 0.7998128361456481317 ) ) ;
#185189=CARTESIAN_POINT ( 'NONE',  ( 6.531277313481192337, 8.642909503859968368, 1.599625672291281386 ) ) ;
#185192=CARTESIAN_POINT ( 'NONE',  ( -9.134442807305063639, 11.67993591332117376, 1.599625672291281386 ) ) ;
#185195=CARTESIAN_POINT ( 'NONE',  ( -1.402160292154681736E-14, -0.3656249996585805295, 1.575800808251672791 ) ) ;
#185199=CARTESIAN_POINT ( 'NONE',  ( 8.324343129110697959, 9.774450407793066731, -1.082531754730543083 ) ) ;
#185207=DIRECTION ( 'NONE',  ( -7.387867266669436732E-31, 1.000000000000000000, 8.546850786086424434E-32 ) ) ;
#185211=CARTESIAN_POINT ( 'NONE',  ( -7.334597915313094241, 9.580116872663850813, 1.040834085586084257E-14 ) ) ;
#185226=( BOUNDED_CURVE ( )  B_SPLINE_CURVE ( 2, ( #118405, #183336, #101013, #99963, #19759, #184392, #36012 ),
 .UNSPECIFIED., .F., .T. ) 
 B_SPLINE_CURVE_WITH_KNOTS ( ( 3, 2, 2, 3 ),
 ( 0.3214285714285716744, 0.3273809523809525501, 0.3333333333333334259, 0.3392857142857143571 ),
 .UNSPECIFIED. ) 
 CURVE ( )  GEOMETRIC_REPRESENTATION_ITEM ( )  RATIONAL_B_SPLINE_CURVE ( ( 0.9999999999999950040, 0.8660254037844437036, 1.000000000000000000, 0.8660254037844387076, 1.000000000000000000, 0.8660254037844374864, 1.000000000000001332 ) ) 
 REPRESENTATION_ITEM ( '' )  );
#185227=CARTESIAN_POINT ( 'NONE',  ( 0.6823417656249917140, 5.592708333674749177, 1.181850606188765695 ) ) ;
#185233=CARTESIAN_POINT ( 'NONE',  ( 1.177110729581195114, 2.995878374463980531, -0.7749999999999840350 ) ) ;
#185236=CARTESIAN_POINT ( 'NONE',  ( 8.703444544968814256, 12.24143683818393313, -1.199719254218446718 ) ) ;
#185238=CARTESIAN_POINT ( 'NONE',  ( -1.387358672536802340, 7.315968950354509559, 4.254625267136455058 ) ) ;
#185242=CARTESIAN_POINT ( 'NONE',  ( 5.508690485854129903, 5.321227076451600091, 1.040834085586084257E-14 ) ) ;
#185243=CARTESIAN_POINT ( 'NONE',  ( -1.364683531250012516, 2.592708333674753174, 0.7879004041258379498 ) ) ;
#185247=CARTESIAN_POINT ( 'NONE',  ( -8.179646747746328828, 8.437342715325849341, -0.7998128361456291469 ) ) ;
#185248=CARTESIAN_POINT ( 'NONE',  ( -3.863710589770277259, 6.491117540498504646, 1.082531754730560403 ) ) ;
#185251=CARTESIAN_POINT ( 'NONE',  ( -5.880485940025243607, 7.883652901494672349, 1.599625672291269396 ) ) ;
#185252=ORIENTED_EDGE ( 'NONE', *, *, #7040, .F. ) ;
#185253=CARTESIAN_POINT ( 'NONE',  ( -1.500000000000001332, 0.1812500006828157706, 0.000000000000000000 ) ) ;
#185260=CARTESIAN_POINT ( 'NONE',  ( -3.375617059678305054, 5.921675088724528635, 1.082531754730560403 ) ) ;
#185265=ADVANCED_FACE ( 'NONE', ( #129527 ), #104855, .F. ) ;
#185268=CARTESIAN_POINT ( 'NONE',  ( -3.240035523541616502, 6.723865844199768738, 0.7216878364870317197 ) ) ;
#185270=CARTESIAN_POINT ( 'NONE',  ( 7.235247531187115833, 11.59287255302699648, -0.7998128361456291469 ) ) ;
#185280=DIRECTION ( 'NONE',  ( 0.000000000000000000, -2.168404344971008079E-15, -1.000000000000000000 ) ) ;
#185284=CARTESIAN_POINT ( 'NONE',  ( 4.843287188579786573, 6.673587691474970107, -1.599625672291256295 ) ) ;
#185290=CARTESIAN_POINT ( 'NONE',  ( 2.758194185376297902, 5.305311418659259814, 1.199719254218452047 ) ) ;
#185301=CARTESIAN_POINT ( 'NONE',  ( 9.257519960032755790, 9.694861462993381807, 0.7998128361456462443 ) ) ;
#185303=CARTESIAN_POINT ( 'NONE',  ( -6.098470168048611306, 6.009303372345148553, 1.040834085586084257E-14 ) ) ;
#185306=CARTESIAN_POINT ( 'NONE',  ( 1.209255964962522301, 2.820301984786699023, 0.7750000000000117906 ) ) ;
#185308=ORIENTED_EDGE ( 'NONE', *, *, #43285, .T. ) ;
#185311=CARTESIAN_POINT ( 'NONE',  ( -1.500000000000015099, -1.089583332650509773, -0.8660254037844383745 ) ) ;
#185316=CARTESIAN_POINT ( 'NONE',  ( 1.252085211431714251, 3.300000000000025135, 0.7750000000000100142 ) ) ;
#185317=CARTESIAN_POINT ( 'NONE',  ( 4.864678189204997949, 4.569879397027603929, 0.7998128361456341429 ) ) ;
#185318=CARTESIAN_POINT ( 'NONE',  ( -3.653032323878261600, 6.349289246911547835, -1.199719254218452047 ) ) ;
#185324=CARTESIAN_POINT ( 'NONE',  ( 6.331294547901813452, 6.488857848747989543, 1.040834085586084257E-14 ) ) ;
#185325=EDGE_CURVE ( 'NONE', #188755, #32206, #127073, .T. ) ;
#185328=CARTESIAN_POINT ( 'NONE',  ( 8.744645890689993095, 9.304434415334227992, -0.7216878364870197293 ) ) ;
#185329=CARTESIAN_POINT ( 'NONE',  ( 1.364683531249990311, 4.926041667008083991, 0.7879004041258500513 ) ) ;
#185331=CARTESIAN_POINT ( 'NONE',  ( 4.161989969270883272, 7.799479364217271282, 0.7216878364870317197 ) ) ;
#185338=CARTESIAN_POINT ( 'NONE',  ( -5.084594181526506773, 6.727074486938107611, 1.441884573159227578 ) ) ;
#185341=CARTESIAN_POINT ( 'NONE',  ( -1.364683531250010295, 5.551041667008087543, -0.7879004041258300672 ) ) ;
#185346=CARTESIAN_POINT ( 'NONE',  ( -10.15235809853472126, 10.73883929124566983, -0.7998128361456291469 ) ) ;
#185351=DIRECTION ( 'NONE',  ( 0.9055141421511284650, 0.4243160830846573472, 0.000000000000000000 ) ) ;
#185356=CARTESIAN_POINT ( 'NONE',  ( 4.216222584169931231, 4.021273891060765493, 1.214306433183764966E-14 ) ) ;
#185357=CARTESIAN_POINT ( 'NONE',  ( 0.6823417656249917140, 3.655208333674754506, 1.181850606188765695 ) ) ;
#185359=CARTESIAN_POINT ( 'NONE',  ( 5.937581207780954884, 9.014596278131406848, -1.199719254218440723 ) ) ;
#185360=CARTESIAN_POINT ( 'NONE',  ( -7.967387826325084355, 12.44703623068796361, 0.7998128361456481317 ) ) ;
#185362=CARTESIAN_POINT ( 'NONE',  ( -3.093231602212184850, 6.760520635889516683, -0.7998128361456282587 ) ) ;
#185366=CARTESIAN_POINT ( 'NONE',  ( -0.7500000000000215383, 4.941666666666684193, 1.299038105676671107 ) ) ;
#185367=CARTESIAN_POINT ( 'NONE',  ( 5.066996723205273057, 6.934582148538044777, 1.599625672291267398 ) ) ;
#185370=DIRECTION ( 'NONE',  ( 0.000000000000000000, 8.546850786086437571E-32, 1.000000000000000000 ) ) ;
#185374=CARTESIAN_POINT ( 'NONE',  ( 7.429504990608736037, 11.61158022244479682, -0.7216878364870267237 ) ) ;
#185380=CARTESIAN_POINT ( 'NONE',  ( -0.7500000000000215383, 2.722916667349486897, 1.299038105676671107 ) ) ;
#185382=CARTESIAN_POINT ( 'NONE',  ( -5.901876940650454095, 5.779944607047298177, -0.7998128361456291469 ) ) ;
#185384=CARTESIAN_POINT ( 'NONE',  ( 5.002595493318194642, 4.938708951733754127, -0.7216878364870197293 ) ) ;
#185385=CARTESIAN_POINT ( 'NONE',  ( -4.911752498546917423, 4.707425932596563278, -0.3822207396134598145 ) ) ;
#185393=CARTESIAN_POINT ( 'NONE',  ( 5.784525094524856748, 9.900363043587685041, 1.040834085586084257E-14 ) ) ;
#185394=CARTESIAN_POINT ( 'NONE',  ( 4.137209430464448445, 7.978494768850520558, 1.040834085586084257E-14 ) ) ;
#185398=CARTESIAN_POINT ( 'NONE',  ( 3.842846474469570062, 6.570739089268092137, -1.199719254218452047 ) ) ;
#185401=VERTEX_POINT ( 'NONE', #204024 ) ;
#185403=ORIENTED_EDGE ( 'NONE', *, *, #138676, .T. ) ;
#185404=CARTESIAN_POINT ( 'NONE',  ( 10.06423010004587759, 10.63602329300870153, 0.000000000000000000 ) ) ;
#185408=DIRECTION ( 'NONE',  ( 5.578564026256490882E-16, 1.000000000000000000, 9.066213480720158442E-32 ) ) ;
#185409=CARTESIAN_POINT ( 'NONE',  ( 5.512200117181983217, 6.216449928263548586, -0.9568283335872149742 ) ) ;
#185416=CARTESIAN_POINT ( 'NONE',  ( -1.201851678989727383E-14, 5.618750000682818602, -1.732050807568863648 ) ) ;
#185418=CARTESIAN_POINT ( 'NONE',  ( 5.287316719649520991, 8.151991358691011769, -1.082531754730549078 ) ) ;
#185419=CARTESIAN_POINT ( 'NONE',  ( -9.490344339885973923, 12.09515436799890331, -1.443375672974059665 ) ) ;
#185425=CARTESIAN_POINT ( 'NONE',  ( -4.066556009095094737, 6.831733546331167695, 1.199719254218464037 ) ) ;
#185428=( BOUNDED_CURVE ( )  B_SPLINE_CURVE ( 2, ( #188458, #40089, #59521, #106200, #57397, #123561, #42236 ),
 .UNSPECIFIED., .F., .T. ) 
 B_SPLINE_CURVE_WITH_KNOTS ( ( 3, 2, 2, 3 ),
 ( 0.3035714285714285476, 0.3095238095238095899, 0.3154761904761906322, 0.3214285714285716744 ),
 .UNSPECIFIED. ) 
 CURVE ( )  GEOMETRIC_REPRESENTATION_ITEM ( )  RATIONAL_B_SPLINE_CURVE ( ( 1.000000000000000000, 0.8660254037844387076, 1.000000000000000000, 0.8660254037844387076, 1.000000000000000000, 0.8660254037844337116, 1.000000000000005107 ) ) 
 REPRESENTATION_ITEM ( '' )  );
#185436=CARTESIAN_POINT ( 'NONE',  ( 7.425061681778431399, 11.81432239538354345, 0.7998128361456462443 ) ) ;
#185437=CARTESIAN_POINT ( 'NONE',  ( 6.039686174407700392, 6.062845369715991417, 0.4964408002013191989 ) ) ;
#185444=CARTESIAN_POINT ( 'NONE',  ( -7.524412065904404479, 11.72230514362308185, 0.000000000000000000 ) ) ;
#185449=CARTESIAN_POINT ( 'NONE',  ( 6.591235234537977661, 10.84152487360300299, 0.7998128361456462443 ) ) ;
#185451=CARTESIAN_POINT ( 'NONE',  ( 1.252085211431710698, 2.800000000000024691, 0.7750000000000152323 ) ) ;
#185452=CARTESIAN_POINT ( 'NONE',  ( 5.054492339796319733, 4.791329239384148231, -0.7998128361456211532 ) ) ;
#185454=CARTESIAN_POINT ( 'NONE',  ( -4.740547266272593596, 8.682388910626682943, -0.7998128361456281477 ) ) ;
#185455=CARTESIAN_POINT ( 'NONE',  ( 3.985207087413062066, 6.736826471035503694, -1.199719254218452047 ) ) ;
#185464=CARTESIAN_POINT ( 'NONE',  ( 4.383065840713377348, 7.132475524829186675, -1.069666325224464032 ) ) ;
#185466=CARTESIAN_POINT ( 'NONE',  ( 5.178851490740193242, 8.025448591630130579, 1.082531754730558626 ) ) ;
#185473=CARTESIAN_POINT ( 'NONE',  ( 8.581948047326003248, 9.114620264742901767, -0.7216878364870197293 ) ) ;
#185476=CARTESIAN_POINT ( 'NONE',  ( -7.934546212495630968, 10.28005655271014795, -1.599625672291263179 ) ) ;
#185484=CARTESIAN_POINT ( 'NONE',  ( 4.403700966340357681, 4.032072637018845107, -0.7998128361456211532 ) ) ;
#185488=CARTESIAN_POINT ( 'NONE',  ( 4.904298879841284098, 6.744767997946721216, 1.599625672291267398 ) ) ;
#185491=CIRCLE ( 'NONE', #109515, 0.08000000000000004330 ) ;
#185492=CARTESIAN_POINT ( 'NONE',  ( 1.499999999999989120, 2.306250000682817713, 1.214306433183764966E-14 ) ) ;
#185498=CARTESIAN_POINT ( 'NONE',  ( 0.7499999999999885647, 1.566666666666688412, -1.299038105676652899 ) ) ;
#185499=CARTESIAN_POINT ( 'NONE',  ( 7.233438648090761980, 8.397765496649418182, 1.199719254218462483 ) ) ;
#185500=CARTESIAN_POINT ( 'NONE',  ( 3.511198595814921219, 7.040222761851976152, 0.7216878364870317197 ) ) ;
#185506=CARTESIAN_POINT ( 'NONE',  ( 7.293923454472077239, 10.49303254931736262, 1.082531754730558626 ) ) ;
#185511=CARTESIAN_POINT ( 'NONE',  ( -5.579343907223557331, 6.467988298970945849, 1.199719254218450271 ) ) ;
#185512=CARTESIAN_POINT ( 'NONE',  ( 1.499999999999989120, 4.327083334016148086, -0.8660254037844323793 ) ) ;
#185513=CARTESIAN_POINT ( 'NONE',  ( -1.364683531249997417, 5.071875000341417916, 1.214306433183764966E-14 ) ) ;
#185518=CARTESIAN_POINT ( 'NONE',  ( -1.364683531250010295, 4.592708333674755394, 0.7879004041258379498 ) ) ;
#185526=CARTESIAN_POINT ( 'NONE',  ( -8.864333505236459132, 9.236143932397675727, 1.040834085586084257E-14 ) ) ;
#185527=CARTESIAN_POINT ( 'NONE',  ( 6.817052309572890323, 6.847649204123507083, 0.7998128361456341429 ) ) ;
#185536=CARTESIAN_POINT ( 'NONE',  ( -6.184490626128011925, 10.36698949712469364, -0.7998128361456291469 ) ) ;
#185539=CARTESIAN_POINT ( 'NONE',  ( 9.999301985278609806, 11.62460605670194447, 1.199719254218452047 ) ) ;
#185541=CARTESIAN_POINT ( 'NONE',  ( 9.134442807305049428, 11.67993591332117376, 1.599625672291281386 ) ) ;
#185542=CARTESIAN_POINT ( 'NONE',  ( -5.000000000000024869, 3.300000000000025135, 0.7750000000000238920 ) ) ;
#185545=CARTESIAN_POINT ( 'NONE',  ( -4.603156847039612920, 5.329103395422994716, 1.199719254218462483 ) ) ;
#185546=CARTESIAN_POINT ( 'NONE',  ( -8.694856585065634746, 9.038420858865048757, 0.7998128361456462443 ) ) ;
#185549=CARTESIAN_POINT ( 'NONE',  ( -4.038790540952651220, 7.763523381248250033, -0.5490930765432913141 ) ) ;
#185550=CARTESIAN_POINT ( 'NONE',  ( -1.364683531250014514, -0.9697916663252473812, 0.7879004041258379498 ) ) ;
#185554=CARTESIAN_POINT ( 'NONE',  ( 8.771762198361678031, 9.336070107617867819, 1.040834085586084257E-14 ) ) ;
#185557=CARTESIAN_POINT ( 'NONE',  ( 6.654354466208897811, 6.657835053532175529, 0.7998128361456341429 ) ) ;
#185575=FACE_OUTER_BOUND ( 'NONE', #140945, .T. ) ;
#185579=CARTESIAN_POINT ( 'NONE',  ( -8.158255747121117452, 10.54105100977322174, 1.599625672291295375 ) ) ;
#185585=CARTESIAN_POINT ( 'NONE',  ( 0.7499999999999902300, 2.014583334016148530, 1.299038105676669330 ) ) ;
#185586=CARTESIAN_POINT ( 'NONE',  ( 9.511208455186636712, 11.05516360492796935, 1.199719254218453823 ) ) ;
#185587=CARTESIAN_POINT ( 'NONE',  ( -4.908660468810629673, 4.653493786480884964, -0.07887673679583749597 ) ) ;
#185591=CARTESIAN_POINT ( 'NONE',  ( -10.15235809853472126, 10.73883929124566983, -0.7998128361456291469 ) ) ;
#185593=CARTESIAN_POINT ( 'NONE',  ( -1.364683531250012516, 1.530208333674756505, 0.7879004041258379498 ) ) ;
#185599=CARTESIAN_POINT ( 'NONE',  ( -3.684065054611367351, 5.321161868511784299, -1.599625672291256295 ) ) ;
#185604=CARTESIAN_POINT ( 'NONE',  ( -0.6823417656250246877, -0.3864583329919110688, 1.181850606188755259 ) ) ;
#185609=CARTESIAN_POINT ( 'NONE',  ( -1.201851678989727383E-14, 1.821875000341421691, 1.575800808251672791 ) ) ;
#185612=CARTESIAN_POINT ( 'NONE',  ( -6.738566041191992539, 7.820414121934134322, 1.199719254218450271 ) ) ;
#185613=CARTESIAN_POINT ( 'NONE',  ( 7.751511138711133064, 10.06651563329490529, -1.599625672291262513 ) ) ;
#185614=CARTESIAN_POINT ( 'NONE',  ( 4.656335691289526402, 7.519809842224722374, -1.199719254218452047 ) ) ;
#185616=CARTESIAN_POINT ( 'NONE',  ( -0.7499999999999972244, 4.108333333333360038, -1.299038105676652011 ) ) ;
#185617=CIRCLE ( 'NONE', #137247, 0.8300000000000008482 ) ;
#185619=CARTESIAN_POINT ( 'NONE',  ( -0.6823417656250212460, 1.363541667008083547, 1.181850606188755259 ) ) ;
#185624=CARTESIAN_POINT ( 'NONE',  ( 5.829642864196168617, 6.863966765392747860, 1.082531754730558626 ) ) ;
#185627=CARTESIAN_POINT ( 'NONE',  ( -8.690940161559884913, 10.09818392903003748, 1.199719254218462483 ) ) ;
#185628=CARTESIAN_POINT ( 'NONE',  ( -3.795392936821753604, 6.515376628678959392, -1.199719254218452047 ) ) ;
#185633=CARTESIAN_POINT ( 'NONE',  ( -6.656690234185426824, 10.70996300661758660, 0.7216878364870458196 ) ) ;
#185635=CARTESIAN_POINT ( 'NONE',  ( -1.499999999999997780, 5.150000000000022560, 1.214306433183764966E-14 ) ) ;
#185636=B_SPLINE_CURVE_WITH_KNOTS ( 'NONE', 3,
 ( #175577, #143107, #94339, #107430 ),
 .UNSPECIFIED., .F., .F.,
 ( 4, 4 ),
 ( 2.652056914724157932E-16, 7.241384396125386848E-05 ),
 .UNSPECIFIED. ) ;
#185639=CARTESIAN_POINT ( 'NONE',  ( 8.758204044748005401, 10.28062147603659504, 1.082531754730549967 ) ) ;
#185648=CARTESIAN_POINT ( 'NONE',  ( 10.34450801710256584, 11.17094022948226240, 0.7216878364870438212 ) ) ;
#185653=CARTESIAN_POINT ( 'NONE',  ( 7.985389288324691748, 10.33937347451072775, -1.443375672974058777 ) ) ;
#185654=CARTESIAN_POINT ( 'NONE',  ( 5.425234023762710578, 9.481190127698507553, -0.7998128361456291469 ) ) ;
#185655=CARTESIAN_POINT ( 'NONE',  ( -5.742041750587549842, 6.657802449562273850, 1.199719254218450271 ) ) ;
#185661=CARTESIAN_POINT ( 'NONE',  ( 3.334942599281629949, 5.874221551595115720, -1.082531754730543083 ) ) ;
#185663=CARTESIAN_POINT ( 'NONE',  ( -4.135400547368138113, 4.783387712472935149, 1.199719254218462483 ) ) ;
#185679=CARTESIAN_POINT ( 'NONE',  ( 8.796542737168120851, 9.157054702984622097, -0.7998128361456211532 ) ) ;
#185684=CARTESIAN_POINT ( 'NONE',  ( 1.566597853258334894, 8.754643479813763562, 2.463935000416110022 ) ) ;
#185690=CARTESIAN_POINT ( 'NONE',  ( -4.388035272317281077, 8.271124917678806199, 0.7998128361456481317 ) ) ;
#185692=CARTESIAN_POINT ( 'NONE',  ( -3.144601563365788444, 5.756120026313656268, -1.199719254218452935 ) ) ;
#185695=CARTESIAN_POINT ( 'NONE',  ( 1.490514837427020067, 7.209629588552884272, 4.246172784737224148 ) ) ;
#185700=CARTESIAN_POINT ( 'NONE',  ( -4.464712657601869417, 4.103252943490596216, 0.7998128361456341429 ) ) ;
#185703=CARTESIAN_POINT ( 'NONE',  ( 6.588372581236919601, 9.773852880496709972, -1.199719254218440723 ) ) ;
#185704=CARTESIAN_POINT ( 'NONE',  ( -0.6823417656249969321, 4.467708333674755394, -1.181850606188749264 ) ) ;
#185710=CARTESIAN_POINT ( 'NONE',  ( 5.300874872818828187, 8.167809204055208383, 1.082531754730558626 ) ) ;
#185711=CARTESIAN_POINT ( 'NONE',  ( -7.705111371268023923, 7.883718109434487253, 1.040834085586084257E-14 ) ) ;
#185714=CARTESIAN_POINT ( 'NONE',  ( -8.016948904382338981, 8.247528564734524892, -0.7998128361456291469 ) ) ;
#185716=CARTESIAN_POINT ( 'NONE',  ( -5.545448523189368650, 6.428443684264421698, -1.199719254218446718 ) ) ;
#185723=CARTESIAN_POINT ( 'NONE',  ( 7.426115451983150706, 9.686887332112256388, -1.599625672291262513 ) ) ;
#185737=CARTESIAN_POINT ( 'NONE',  ( 1.364683531249986537, -1.073958332991911790, 0.7879004041258500513 ) ) ;
#185738=CARTESIAN_POINT ( 'NONE',  ( 4.090809663021327758, 5.795697244990093644, 1.599625672291267398 ) ) ;
#185739=CARTESIAN_POINT ( 'NONE',  ( 5.843727902690005749, 6.776436293681846301, -1.199719254218445830 ) ) ;
#185741=CARTESIAN_POINT ( 'NONE',  ( -6.873620692448438874, 10.96304854125777695, 0.000000000000000000 ) ) ;
#185743=CARTESIAN_POINT ( 'NONE',  ( 4.690757960648221037, 7.456006139856155457, 1.082531754730558626 ) ) ;
#185744=CARTESIAN_POINT ( 'NONE',  ( -8.649738815394339753, 9.193709494155953621, 1.040834085586084257E-14 ) ) ;
#185748=CARTESIAN_POINT ( 'NONE',  ( 6.414979237560321401, 10.63589287712906462, 1.040834085586084257E-14 ) ) ;
#185754=CARTESIAN_POINT ( 'NONE',  ( -1.364683531249997417, 2.759375000341422801, 1.214306433183764966E-14 ) ) ;
#185760=EDGE_CURVE ( 'NONE', #9480, #212749, #205415, .T. ) ;
#185761=CARTESIAN_POINT ( 'NONE',  ( 9.271078113646423091, 9.710679308875986848, 1.040834085586084257E-14 ) ) ;
#185764=CARTESIAN_POINT ( 'NONE',  ( -8.097244055859620815, 10.46987070330147063, -1.599625672291263179 ) ) ;
#185768=CARTESIAN_POINT ( 'NONE',  ( -1.387358672527334136, 7.251968950354660493, -4.302625267139479348 ) ) ;
#185770=CARTESIAN_POINT ( 'NONE',  ( 4.729096653068339151, 4.411700938201493116, -0.7998128361456211532 ) ) ;
#185774=CARTESIAN_POINT ( 'NONE',  ( -10.31505594189871111, 10.92865344183699428, -0.7998128361456291469 ) ) ;
#185778=CARTESIAN_POINT ( 'NONE',  ( 5.838973523318124137, 6.009393772954500612, 0.3882124113597507087 ) ) ;
#185780=CARTESIAN_POINT ( 'NONE',  ( -2.117044542028253318, 5.621635732341564662, -0.7998128361456281477 ) ) ;
#185784=CARTESIAN_POINT ( 'NONE',  ( 6.100279051144945619, 9.204410428722734849, -1.199719254218440723 ) ) ;
#185786=CARTESIAN_POINT ( 'NONE',  ( 7.610204295972345712, 7.772993188256215547, 0.7998128361456341429 ) ) ;
#185787=CARTESIAN_POINT ( 'NONE',  ( 3.798255590122797898, 7.583048621785260401, -0.7998128361456221525 ) ) ;
#185790=CARTESIAN_POINT ( 'NONE',  ( -8.351459436338048548, 8.845716885256940998, -0.7216878364870278340 ) ) ;
#185798=CARTESIAN_POINT ( 'NONE',  ( -5.357982633755392854, 6.353232995037386033, -1.097174801447881487 ) ) ;
#185799=ADVANCED_FACE ( 'NONE', ( #40512 ), #107700, .T. ) ;
#185801=FACE_OUTER_BOUND ( 'NONE', #137019, .T. ) ;
#185802=CARTESIAN_POINT ( 'NONE',  ( 4.853455804012212660, 7.645820290447483458, 1.082531754730558626 ) ) ;
#185809=ADVANCED_FACE ( 'NONE', ( #140158 ), #29025, .F. ) ;
#185820=CARTESIAN_POINT ( 'NONE',  ( -8.473482818416664841, 11.86918514058604757, -1.082531754730543083 ) ) ;
#185824=CARTESIAN_POINT ( 'NONE',  ( 8.457588896826466751, 8.761608555919362828, 1.040834085586084257E-14 ) ) ;
#185828=CARTESIAN_POINT ( 'NONE',  ( -1.499999999999997780, 2.181250000682817713, 1.214306433183764966E-14 ) ) ;
#185829=CARTESIAN_POINT ( 'NONE',  ( -2.137381772448751605, 5.645362501165475777, -0.7998128361456281477 ) ) ;
#185830=CARTESIAN_POINT ( 'NONE',  ( -5.473741331615264549, 7.409117525016355010, -1.599625672291256295 ) ) ;
#185833=CARTESIAN_POINT ( 'NONE',  ( -8.779068160048691283, 10.20099992726700933, -1.199719254218446718 ) ) ;
#185837=CARTESIAN_POINT ( 'NONE',  ( 7.474622759835693131, 7.614814729430110951, -0.7998128361456281477 ) ) ;
#185839=CARTESIAN_POINT ( 'NONE',  ( -5.852315862593199469, 9.979452273000736895, 0.7998128361456481317 ) ) ;
#185841=CARTESIAN_POINT ( 'NONE',  ( 9.433775957010412938, 9.900493459467314850, 0.000000000000000000 ) ) ;
#185843=( BOUNDED_SURFACE ( )  B_SPLINE_SURFACE ( 1, 2, ( 
 ( #176652, #146307, #30411, #113856, #97549, #81278, #63958, #65006, #192878, #27187, #145257, #130114, #179851, #129055, #211262, #93293, #95430, #45600, #28265, #110651, #212321, #77001, #163606, #44533, #15188, #31474, #94357, #196104, #127998, #62886, #195029, #47740, #143127, #209122, #160399, #147355, #46663, #193952, #112784, #144200, #60760, #96495, #111717, #177725, #162545, #14115, #69253, #119159, #66052, #183029, #164660, #152665, #84463, #117034, #34645, #101784, #165724, #17312, #132196, #83390, #98598, #181954, #33582, #198203, #100715, #115964, #99655, #149474, #70318, #1057, #4249, #67122, #136435, #151615, #202450, #20514, #133255, #114903, #199261, #180900, #32523, #86599, #150554, #16242, #118103, #168911, #82328, #167851, #49838, #19450, #135370, #2115, #166792, #18386, #148420, #35707, #50906, #184088, #68189, #3182, #185144, #134322, #200328, #51978, #85526, #201388, #53026, #36769, #102855, #111133, #172123, #6390, #120240, #173203, #25848, #141792, #9605, #75682, #187290, #56235, #155872, #24783, #38917, #122395, #54105, #186218, #107177, #22638, #41070, #88747, #23717, #37849, #103927, #153738, #205664, #188353, #89824, #73540, #105001, #169972, #171040, #87666, #39992, #190478, #21560, #123465, #5305, #158017, #71387, #137499, #91956, #57302, #189428, #203516, #139642, #90886, #55170, #121315, #154804, #106101, #7461, #72463, #138563, #174273, #204584, #156945, #8536, #74617, #140723, #206736, #58367, #124521, #108252, #42137, #47465, #44259, #30127, #191542, #178516, #125582, #176387, #77803, #61557, #179582, #144980, #113580, #13854, #161198, #76731, #159063, #97278, #60484, #210984, #112505, #27992, #26913, #146036, #96216, #129844, #43207, #193682, #162267, #110382, #126642, #10659, #79930, #175330, #109322, #59424, #31204, #128774, #127723, #81006, #94089, #192607, #160128, #11727, #143923, #93022, #209919, #142849, #12785, #163332, #45326, #207796, #212050, #14912, #208853, #111445, #177450, #63690, #29064, #95147, #78859, #62612, #194751, #46388, #195826, #115692, #147094, #778, #134062, #183833, #168652, #181685, #82061, #201129, #116762, #200071, #32259, #118903, #52767, #33314, #149203, #85267, #68996, #184887, #35442, #36511, #164393, #213117, #50635, #101521, #151354, #100450, #182759, #64748, #66845, #17044, #148153, #214154, #167591, #48522, #135113, #15975, #102596, #2923, #65780, #117841, #99396, #198989, #132989, #19190, #20256, #130890, #131930, #196884, #34377, #165449, #166523, #197940, #114642, #18114, #180635, #98327, #49568, #83123, #84201, #150290, #1857, #67916, #51720, #124272, #55980, #88491, #6131, #73274, #137246, #203267, #103672, #54913, #70060, #153483, #5054, #169720, #72200, #87417, #71129, #121064, #41889, #187031, #190230, #38664, #108000, #123213, #174027, #206483, #104743, #86340, #170790, #152412, #3991, #58113, #122133, #136172, #89567, #140471, #202191, #139377, #21310, #205409, #40814, #188098, #138308, #154551, #53847, #7201, #22381, #155616, #37590, #189176, #90634, #204323, #39729, #105834, #171860, #23455, #57049, #106922, #172946, #24525, #156694, #8284, #119980, #74369, #185958, #113339, #195588, #47222, #158818, #27746, #127476, #210754, #10414, #93842, #25598, #91711, #128540, #157760, #26669, #62376, #94903, #194506, #9359, #92774, #46154, #160954, #178281, #162028, #145805, #112267, #63449, #42958, #75432, #143680, #29890, #95975, #193447, #209672, #141544, #159880, #110134, #76486, #175083, #13619, #207550, #79692, #109067, #211812, #129602, #142596, #59170, #60238, #77557, #11485, #125329, #191292, #208606, #126397, #192357, #61315, #44014, #45091, #176146, #111200, #177204, #28818, #12544, #78618, #144743, #133808, #183578, #130656, #33079, #14675, #2671, #148958, #181448, #99154, #166268, #15740, #81825, #196647, #147907, #163095, #32018, #98103, #48287, #165207, #180397, #164154, #213923, #134866, #65546, #68744, #131691, #200873, #1604, #52518, #85017, #197697, #179345, #49339, #30967, #97042, #151106, #530, #80772, #182502, #18931, #146859, #17860, #114399, #83943, #199821, #66597, #16797, #82881, #212881, #100202, #115458 ),
 ( #132743, #198745, #150034, #50393, #67664, #116513, #34133, #64512, #51463, #117587, #35185, #101261, #167345, #138052, #103407, #73021, #118650, #20001, #87150, #185700, #69806, #184636, #56789, #153221, #36253, #186777, #105566, #155355, #140207, #4791, #53586, #172686, #88225, #171599, #3731, #90369, #24264, #70869, #120801, #23191, #136984, #89306, #203011, #154294, #74112, #102333, #135912, #55717, #38404, #22114, #204065, #169468, #168405, #21053, #152162, #104486, #40555, #86086, #187842, #201930, #8021, #119721, #37332, #156437, #121871, #39468, #54651, #6940, #139119, #170529, #206227, #5869, #71941, #205146, #122957, #188917, #106659, #58923, #25348, #107747, #143418, #209413, #192103, #93586, #41633, #112018, #109882, #178019, #108813, #94651, #173772, #28563, #189981, #26414, #142348, #126142, #29637, #61059, #95722, #78369, #11225, #141291, #9104, #161774, #125082, #127218, #176947, #92526, #91448, #210496, #160695, #194254, #157509, #43769, #12288, #174836, #191039, #75180, #144489, #207300, #42705, #124014, #13367, #193186, #175894, #145558, #158565, #10165, #76239, #208357, #59988, #27486, #159630, #77306, #44835, #79441, #110941, #57854, #62132, #128292, #45899, #129355, #48040, #17608, #164954, #80508, #162841, #103966, #64265, #282, #116265, #31774, #30708, #149781, #33881, #133560, #46964, #197446, #166023, #114155, #130409, #14419, #99958, #179086, #113081, #63190, #120279, #132499, #65296, #87701, #180148, #196397, #97845, #163909, #15485, #195333, #81572, #146605, #16546, #186253, #49087, #211556, #83693, #170008, #96792, #212624, #147656, #1356, #213672, #131443, #115206, #181197, #32825, #98901, #67418, #82627, #148713, #66354, #198498, #202491, #21596, #50143, #182256, #54143, #37888, #188392, #203555, #73580, #7496, #171078, #88786, #40028, #105041, #106140, #22674, #72502, #139682, #153774, #55208, #122434, #6428, #138601, #56275, #38958, #71426, #154843, #121354, #204624, #205704, #137538, #172163, #5344, #187329, #23756, #89861, #155911, #129447, #97942, #147747, #96883, #47059, #143515, #211649, #13459, #144583, #78464, #180241, #44929, #65386, #12385, #197535, #81661, #210597, #114244, #178116, #195429, #63286, #163998, #98992, #32915, #128383, #15573, #113176, #29731, #179180, #194351, #213765, #30803, #131533, #49180, #209511, #112113, #79535, #162932, #115298, #80606, #181288, #165047, #14513, #62226, #94746, #16639, #45993, #146701, #48131, #95813, #177044, #61152, #31865, #127314, #193284, #212716, #111037, #161871, #145653, #160793, #28660, #64356, #130502, #196489, #202850, #3576, #150947, #170370, #51302, #149878, #133655, #117427, #199656, #66443, #35026, #33973, #36095, #54498, #68584, #82723, #103250, #38247, #132584, #369, #183425, #37175, #148800, #198587, #101099, #83784, #85932, #69651, #100048, #152004, #166112, #185546, #86991, #1444, #167185, #67509, #84858, #18773, #17697, #135759, #2511, #201781, #200716, #134709, #50233, #53422, #120642, #116354, #104322, #182343, #52367, #118496, #184477, #119558, #102179, #168246, #19845, #169311, #20895, #153064, #4640, #70711, #136823, #186621, #158403, #142179, #124916, #108648, #41472, #23035, #7862, #190879, #26248, #189823, #140042, #21956, #90214, #106499, #89150, #171445, #58763, #137898, #10003, #105408, #76079, #174676, #155204, #207139, #56634, #73949, #156278, #42544, #191938, #125980, #6785, #92367, #206066, #122799, #208195, #71783, #75018, #72862, #141128, #59828, #43602, #25187, #138968, #91291, #157349, #39313, #8938, #187684, #109720, #88065, #204990, #188757, #40398, #24111, #172527, #57701, #154137, #123857, #5706, #107582, #173615, #203917, #55565, #121719, #48922, #131293, #197282, #94492, #177861, #63027, #146444, #160530, #29473, #175726, #27321, #64102, #93423, #176781, #212456, #30546, #113991, #97683, #81411, #130243, #47877, #195171, #28397, #161614, #196235, #179986, #129194, #79280, #159461, #95563, #45737, #12135, #110780, #31608, #77140, #163742, #44668, #15321, #147492, #78207, #213514, #210331, #13205, #145398, #65136, #11061, #143261, #144332, #209251, #211397, #61970, #46805, #128125 ) ),
 .UNSPECIFIED., .F., .F., .T. ) 
 B_SPLINE_SURFACE_WITH_KNOTS ( ( 2, 2 ),
 ( 3, 2, 2, 2, 2, 2, 2, 2, 2, 2, 2, 2, 2, 2, 2, 2, 2, 2, 2, 2, 2, 2, 2, 2, 2, 2, 2, 2, 2, 2, 2, 2, 2, 2, 2, 2, 2, 2, 2, 2, 2, 2, 2, 2, 2, 2, 2, 2, 2, 2, 2, 2, 2, 2, 2, 2, 2, 2, 2, 2, 2, 2, 2, 2, 2, 2, 2, 2, 2, 2, 2, 2, 2, 2, 2, 2, 2, 2, 2, 2, 2, 2, 2, 2, 2, 2, 2, 2, 2, 2, 2, 2, 2, 2, 2, 2, 2, 2, 2, 2, 2, 2, 2, 2, 2, 2, 2, 2, 2, 2, 2, 2, 2, 2, 2, 2, 2, 2, 2, 2, 2, 2, 2, 2, 2, 2, 2, 2, 2, 2, 2, 2, 2, 2, 2, 2, 2, 2, 2, 2, 2, 2, 2, 2, 2, 2, 2, 2, 2, 2, 2, 2, 2, 2, 2, 2, 2, 2, 2, 2, 2, 2, 2, 2, 2, 2, 2, 2, 2, 2, 2, 2, 2, 2, 2, 2, 2, 2, 2, 2, 2, 2, 2, 2, 2, 2, 2, 2, 2, 2, 2, 2, 2, 2, 2, 2, 2, 2, 2, 2, 2, 2, 2, 2, 2, 2, 2, 2, 2, 2, 2, 2, 2, 2, 2, 2, 2, 2, 2, 2, 2, 2, 2, 2, 2, 2, 2, 2, 2, 2, 2, 2, 2, 2, 2, 2, 2, 2, 2, 2, 3 ),
 ( 0.000000000000000000, 1.000000000000000000 ),
 ( 0.000000000000000000, 0.004166666666666666609, 0.008333333333333333218, 0.01250000000000000069, 0.01666666666666666644, 0.02083333333333333218, 0.02500000000000000139, 0.02916666666666666713, 0.03333333333333333287, 0.03749999999999999861, 0.04166666666666666435, 0.04583333333333333010, 0.05000000000000000278, 0.05416666666666666852, 0.05833333333333333426, 0.06250000000000000000, 0.06666666666666666574, 0.07083333333333333148, 0.07499999999999999722, 0.07916666666666666297, 0.08333333333333332871, 0.08749999999999999445, 0.09166666666666666019, 0.09583333333333333981, 0.1000000000000000056, 0.1041666666666666713, 0.1083333333333333370, 0.1125000000000000028, 0.1166666666666666685, 0.1208333333333333343, 0.1250000000000000000, 0.1291666666666666796, 0.1333333333333333315, 0.1375000000000000111, 0.1416666666666666630, 0.1458333333333333426, 0.1499999999999999944, 0.1541666666666666741, 0.1583333333333333259, 0.1625000000000000056, 0.1666666666666666574, 0.1708333333333333370, 0.1749999999999999889, 0.1791666666666666685, 0.1833333333333333204, 0.1875000000000000000, 0.1916666666666666796, 0.1958333333333333315, 0.2000000000000000111, 0.2041666666666666630, 0.2083333333333333426, 0.2124999999999999944, 0.2166666666666666741, 0.2208333333333333259, 0.2250000000000000056, 0.2291666666666666574, 0.2333333333333333370, 0.2374999999999999889, 0.2416666666666666685, 0.2458333333333333204, 0.2500000000000000000, 0.2541666666666666519, 0.2583333333333333592, 0.2625000000000000111, 0.2666666666666666630, 0.2708333333333333148, 0.2750000000000000222, 0.2791666666666666741, 0.2833333333333333259, 0.2874999999999999778, 0.2916666666666666852, 0.2958333333333333370, 0.2999999999999999889, 0.3041666666666666408, 0.3083333333333333481, 0.3125000000000000000, 0.3166666666666666519, 0.3208333333333333592, 0.3250000000000000111, 0.3291666666666666630, 0.3333333333333333148, 0.3375000000000000222, 0.3416666666666666741, 0.3458333333333333259, 0.3499999999999999778, 0.3541666666666666852, 0.3583333333333333370, 0.3624999999999999889, 0.3666666666666666408, 0.3708333333333333481, 0.3750000000000000000, 0.3791666666666666519, 0.3833333333333333592, 0.3875000000000000111, 0.3916666666666666630, 0.3958333333333333148, 0.4000000000000000222, 0.4041666666666666741, 0.4083333333333333259, 0.4124999999999999778, 0.4166666666666666852, 0.4208333333333333370, 0.4249999999999999889, 0.4291666666666666408, 0.4333333333333333481, 0.4375000000000000000, 0.4416666666666666519, 0.4458333333333333592, 0.4500000000000000111, 0.4541666666666666630, 0.4583333333333333148, 0.4625000000000000222, 0.4666666666666666741, 0.4708333333333333259, 0.4749999999999999778, 0.4791666666666666852, 0.4833333333333333370, 0.4874999999999999889, 0.4916666666666666408, 0.4958333333333333481, 0.5000000000000000000, 0.5041666666666666519, 0.5083333333333333037, 0.5124999999999999556, 0.5166666666666667185, 0.5208333333333333703, 0.5250000000000000222, 0.5291666666666666741, 0.5333333333333333259, 0.5374999999999999778, 0.5416666666666666297, 0.5458333333333332815, 0.5500000000000000444, 0.5541666666666666963, 0.5583333333333333481, 0.5625000000000000000, 0.5666666666666666519, 0.5708333333333333037, 0.5749999999999999556, 0.5791666666666667185, 0.5833333333333333703, 0.5875000000000000222, 0.5916666666666666741, 0.5958333333333333259, 0.5999999999999999778, 0.6041666666666666297, 0.6083333333333332815, 0.6125000000000000444, 0.6166666666666666963, 0.6208333333333333481, 0.6250000000000000000, 0.6291666666666666519, 0.6333333333333333037, 0.6374999999999999556, 0.6416666666666667185, 0.6458333333333333703, 0.6500000000000000222, 0.6541666666666666741, 0.6583333333333333259, 0.6624999999999999778, 0.6666666666666666297, 0.6708333333333332815, 0.6750000000000000444, 0.6791666666666666963, 0.6833333333333333481, 0.6875000000000000000, 0.6916666666666666519, 0.6958333333333333037, 0.6999999999999999556, 0.7041666666666667185, 0.7083333333333333703, 0.7125000000000000222, 0.7166666666666666741, 0.7208333333333333259, 0.7249999999999999778, 0.7291666666666666297, 0.7333333333333332815, 0.7375000000000000444, 0.7416666666666666963, 0.7458333333333333481, 0.7500000000000000000, 0.7541666666666666519, 0.7583333333333333037, 0.7624999999999999556, 0.7666666666666667185, 0.7708333333333333703, 0.7750000000000000222, 0.7791666666666666741, 0.7833333333333333259, 0.7874999999999999778, 0.7916666666666666297, 0.7958333333333332815, 0.8000000000000000444, 0.8041666666666666963, 0.8083333333333333481, 0.8125000000000000000, 0.8166666666666666519, 0.8208333333333333037, 0.8249999999999999556, 0.8291666666666667185, 0.8333333333333333703, 0.8375000000000000222, 0.8416666666666666741, 0.8458333333333333259, 0.8499999999999999778, 0.8541666666666666297, 0.8583333333333332815, 0.8625000000000000444, 0.8666666666666666963, 0.8708333333333333481, 0.8750000000000000000, 0.8791666666666666519, 0.8833333333333333037, 0.8874999999999999556, 0.8916666666666667185, 0.8958333333333333703, 0.9000000000000000222, 0.9041666666666666741, 0.9083333333333333259, 0.9124999999999999778, 0.9166666666666666297, 0.9208333333333332815, 0.9250000000000000444, 0.9291666666666666963, 0.9333333333333333481, 0.9375000000000000000, 0.9416666666666666519, 0.9458333333333333037, 0.9499999999999999556, 0.9541666666666667185, 0.9583333333333333703, 0.9625000000000000222, 0.9666666666666666741, 0.9708333333333333259, 0.9749999999999999778, 0.9791666666666666297, 0.9833333333333332815, 0.9875000000000000444, 0.9916666666666666963, 0.9958333333333333481, 1.000000000000000000 ),
 .UNSPECIFIED. ) 
 GEOMETRIC_REPRESENTATION_ITEM ( )  RATIONAL_B_SPLINE_SURFACE ( (
 ( 1.000000000000000000, 0.8660254037844387076, 1.000000000000000000, 0.8660254037844387076, 1.000000000000000000, 0.8660254037844387076, 1.000000000000000000, 0.8660254037844387076, 1.000000000000000000, 0.8660254037844387076, 1.000000000000000000, 0.8660254037844387076, 1.000000000000000000, 0.8660254037844387076, 1.000000000000000000, 0.8660254037844387076, 1.000000000000000000, 0.8660254037844387076, 1.000000000000000000, 0.8660254037844387076, 1.000000000000000000, 0.8660254037844387076, 1.000000000000000000, 0.8660254037844387076, 1.000000000000000000, 0.8660254037844387076, 1.000000000000000000, 0.8660254037844387076, 1.000000000000000000, 0.8660254037844387076, 1.000000000000000000, 0.8660254037844387076, 1.000000000000000000, 0.8660254037844387076, 1.000000000000000000, 0.8660254037844387076, 1.000000000000000000, 0.8660254037844387076, 1.000000000000000000, 0.8660254037844387076, 1.000000000000000000, 0.8660254037844387076, 1.000000000000000000, 0.8660254037844387076, 1.000000000000000000, 0.8660254037844387076, 1.000000000000000000, 0.8660254037844387076, 1.000000000000000000, 0.8660254037844387076, 1.000000000000000000, 0.8660254037844387076, 1.000000000000000000, 0.8660254037844387076, 1.000000000000000000, 0.8660254037844387076, 1.000000000000000000, 0.8660254037844387076, 1.000000000000000000, 0.8660254037844387076, 1.000000000000000000, 0.8660254037844387076, 1.000000000000000000, 0.8660254037844387076, 1.000000000000000000, 0.8660254037844387076, 1.000000000000000000, 0.8660254037844387076, 1.000000000000000000, 0.8660254037844387076, 1.000000000000000000, 0.8660254037844387076, 1.000000000000000000, 0.8660254037844387076, 1.000000000000000000, 0.8660254037844387076, 1.000000000000000000, 0.8660254037844387076, 1.000000000000000000, 0.8660254037844387076, 1.000000000000000000, 0.8660254037844387076, 1.000000000000000000, 0.8660254037844387076, 1.000000000000000000, 0.8660254037844387076, 1.000000000000000000, 0.8660254037844387076, 1.000000000000000000, 0.8660254037844387076, 1.000000000000000000, 0.8660254037844387076, 1.000000000000000000, 0.8660254037844387076, 1.000000000000000000, 0.8660254037844387076, 1.000000000000000000, 0.8660254037844387076, 1.000000000000000000, 0.8660254037844387076, 1.000000000000000000, 0.8660254037844387076, 1.000000000000000000, 0.8660254037844387076, 1.000000000000000000, 0.8660254037844387076, 1.000000000000000000, 0.8660254037844387076, 1.000000000000000000, 0.8660254037844387076, 1.000000000000000000, 0.8660254037844387076, 1.000000000000000000, 0.8660254037844387076, 1.000000000000000000, 0.8660254037844387076, 1.000000000000000000, 0.8660254037844387076, 1.000000000000000000, 0.8660254037844387076, 1.000000000000000000, 0.8660254037844387076, 1.000000000000000000, 0.8660254037844387076, 1.000000000000000000, 0.8660254037844387076, 1.000000000000000000, 0.8660254037844387076, 1.000000000000000000, 0.8660254037844387076, 1.000000000000000000, 0.8660254037844387076, 1.000000000000000000, 0.8660254037844387076, 1.000000000000000000, 0.8660254037844387076, 1.000000000000000000, 0.8660254037844387076, 1.000000000000000000, 0.8660254037844387076, 1.000000000000000000, 0.8660254037844387076, 1.000000000000000000, 0.8660254037844387076, 1.000000000000000000, 0.8660254037844387076, 1.000000000000000000, 0.8660254037844387076, 1.000000000000000000, 0.8660254037844387076, 1.000000000000000000, 0.8660254037844387076, 1.000000000000000000, 0.8660254037844387076, 1.000000000000000000, 0.8660254037844387076, 1.000000000000000000, 0.8660254037844387076, 1.000000000000000000, 0.8660254037844387076, 1.000000000000000000, 0.8660254037844387076, 1.000000000000000000, 0.8660254037844387076, 1.000000000000000000, 0.8660254037844387076, 1.000000000000000000, 0.8660254037844387076, 1.000000000000000000, 0.8660254037844387076, 1.000000000000000000, 0.8660254037844387076, 1.000000000000000000, 0.8660254037844387076, 1.000000000000000000, 0.8660254037844387076, 1.000000000000000000, 0.8660254037844387076, 1.000000000000000000, 0.8660254037844387076, 1.000000000000000000, 0.8660254037844387076, 1.000000000000000000, 0.8660254037844387076, 1.000000000000000000, 0.8660254037844387076, 1.000000000000000000, 0.8660254037844387076, 1.000000000000000000, 0.8660254037844387076, 1.000000000000000000, 0.8660254037844387076, 1.000000000000000000, 0.8660254037844387076, 1.000000000000000000, 0.8660254037844387076, 1.000000000000000000, 0.8660254037844387076, 1.000000000000000000, 0.8660254037844387076, 1.000000000000000000, 0.8660254037844387076, 1.000000000000000000, 0.8660254037844387076, 1.000000000000000000, 0.8660254037844387076, 1.000000000000000000, 0.8660254037844387076, 1.000000000000000000, 0.8660254037844387076, 1.000000000000000000, 0.8660254037844387076, 1.000000000000000000, 0.8660254037844387076, 1.000000000000000000, 0.8660254037844387076, 1.000000000000000000, 0.8660254037844387076, 1.000000000000000000, 0.8660254037844387076, 1.000000000000000000, 0.8660254037844387076, 1.000000000000000000, 0.8660254037844387076, 1.000000000000000000, 0.8660254037844387076, 1.000000000000000000, 0.8660254037844387076, 1.000000000000000000, 0.8660254037844387076, 1.000000000000000000, 0.8660254037844387076, 1.000000000000000000, 0.8660254037844387076, 1.000000000000000000, 0.8660254037844387076, 1.000000000000000000, 0.8660254037844387076, 1.000000000000000000, 0.8660254037844387076, 1.000000000000000000, 0.8660254037844387076, 1.000000000000000000, 0.8660254037844387076, 1.000000000000000000, 0.8660254037844387076, 1.000000000000000000, 0.8660254037844387076, 1.000000000000000000, 0.8660254037844387076, 1.000000000000000000, 0.8660254037844387076, 1.000000000000000000, 0.8660254037844387076, 1.000000000000000000, 0.8660254037844387076, 1.000000000000000000, 0.8660254037844387076, 1.000000000000000000, 0.8660254037844387076, 1.000000000000000000, 0.8660254037844387076, 1.000000000000000000, 0.8660254037844387076, 1.000000000000000000, 0.8660254037844387076, 1.000000000000000000, 0.8660254037844387076, 1.000000000000000000, 0.8660254037844387076, 1.000000000000000000, 0.8660254037844387076, 1.000000000000000000, 0.8660254037844387076, 1.000000000000000000, 0.8660254037844387076, 1.000000000000000000, 0.8660254037844387076, 1.000000000000000000, 0.8660254037844387076, 1.000000000000000000, 0.8660254037844387076, 1.000000000000000000, 0.8660254037844387076, 1.000000000000000000, 0.8660254037844387076, 1.000000000000000000, 0.8660254037844387076, 1.000000000000000000, 0.8660254037844387076, 1.000000000000000000, 0.8660254037844387076, 1.000000000000000000, 0.8660254037844387076, 1.000000000000000000, 0.8660254037844387076, 1.000000000000000000, 0.8660254037844387076, 1.000000000000000000, 0.8660254037844387076, 1.000000000000000000, 0.8660254037844387076, 1.000000000000000000, 0.8660254037844387076, 1.000000000000000000, 0.8660254037844387076, 1.000000000000000000, 0.8660254037844387076, 1.000000000000000000, 0.8660254037844387076, 1.000000000000000000, 0.8660254037844387076, 1.000000000000000000, 0.8660254037844387076, 1.000000000000000000, 0.8660254037844387076, 1.000000000000000000, 0.8660254037844387076, 1.000000000000000000, 0.8660254037844387076, 1.000000000000000000, 0.8660254037844387076, 1.000000000000000000, 0.8660254037844387076, 1.000000000000000000, 0.8660254037844387076, 1.000000000000000000, 0.8660254037844387076, 1.000000000000000000, 0.8660254037844387076, 1.000000000000000000, 0.8660254037844387076, 1.000000000000000000, 0.8660254037844387076, 1.000000000000000000, 0.8660254037844387076, 1.000000000000000000, 0.8660254037844387076, 1.000000000000000000, 0.8660254037844387076, 1.000000000000000000, 0.8660254037844387076, 1.000000000000000000, 0.8660254037844387076, 1.000000000000000000, 0.8660254037844387076, 1.000000000000000000, 0.8660254037844387076, 1.000000000000000000, 0.8660254037844387076, 1.000000000000000000, 0.8660254037844387076, 1.000000000000000000, 0.8660254037844387076, 1.000000000000000000, 0.8660254037844387076, 1.000000000000000000, 0.8660254037844387076, 1.000000000000000000, 0.8660254037844387076, 1.000000000000000000, 0.8660254037844387076, 1.000000000000000000, 0.8660254037844387076, 1.000000000000000000, 0.8660254037844387076, 1.000000000000000000, 0.8660254037844387076, 1.000000000000000000, 0.8660254037844387076, 1.000000000000000000, 0.8660254037844387076, 1.000000000000000000, 0.8660254037844387076, 1.000000000000000000, 0.8660254037844387076, 1.000000000000000000, 0.8660254037844387076, 1.000000000000000000, 0.8660254037844387076, 1.000000000000000000, 0.8660254037844387076, 1.000000000000000000, 0.8660254037844387076, 1.000000000000000000, 0.8660254037844387076, 1.000000000000000000, 0.8660254037844387076, 1.000000000000000000, 0.8660254037844387076, 1.000000000000000000, 0.8660254037844387076, 1.000000000000000000, 0.8660254037844387076, 1.000000000000000000, 0.8660254037844387076, 1.000000000000000000, 0.8660254037844387076, 1.000000000000000000, 0.8660254037844387076, 1.000000000000000000, 0.8660254037844387076, 1.000000000000000000, 0.8660254037844387076, 1.000000000000000000, 0.8660254037844387076, 1.000000000000000000, 0.8660254037844387076, 1.000000000000000000, 0.8660254037844387076, 1.000000000000000000, 0.8660254037844387076, 1.000000000000000000, 0.8660254037844387076, 1.000000000000000000, 0.8660254037844387076, 1.000000000000000000, 0.8660254037844387076, 1.000000000000000000, 0.8660254037844387076, 1.000000000000000000, 0.8660254037844387076, 1.000000000000000000, 0.8660254037844387076, 1.000000000000000000, 0.8660254037844387076, 1.000000000000000000, 0.8660254037844387076, 1.000000000000000000, 0.8660254037844387076, 1.000000000000000000, 0.8660254037844387076, 1.000000000000000000, 0.8660254037844387076, 1.000000000000000000, 0.8660254037844387076, 1.000000000000000000, 0.8660254037844387076, 1.000000000000000000, 0.8660254037844387076, 1.000000000000000000, 0.8660254037844387076, 1.000000000000000000, 0.8660254037844387076, 1.000000000000000000, 0.8660254037844387076, 1.000000000000000000, 0.8660254037844387076, 1.000000000000000000, 0.8660254037844387076, 1.000000000000000000, 0.8660254037844387076, 1.000000000000000000, 0.8660254037844387076, 1.000000000000000000, 0.8660254037844387076, 1.000000000000000000, 0.8660254037844387076, 1.000000000000000000, 0.8660254037844387076, 1.000000000000000000, 0.8660254037844387076, 1.000000000000000000, 0.8660254037844387076, 1.000000000000000000, 0.8660254037844387076, 1.000000000000000000, 0.8660254037844387076, 1.000000000000000000, 0.8660254037844387076, 1.000000000000000000, 0.8660254037844387076, 1.000000000000000000, 0.8660254037844387076, 1.000000000000000000, 0.8660254037844387076, 1.000000000000000000, 0.8660254037844387076, 1.000000000000000000, 0.8660254037844387076, 1.000000000000000000),
 ( 1.000000000000000000, 0.8660254037844387076, 1.000000000000000000, 0.8660254037844387076, 1.000000000000000000, 0.8660254037844387076, 1.000000000000000000, 0.8660254037844387076, 1.000000000000000000, 0.8660254037844387076, 1.000000000000000000, 0.8660254037844387076, 1.000000000000000000, 0.8660254037844387076, 1.000000000000000000, 0.8660254037844387076, 1.000000000000000000, 0.8660254037844387076, 1.000000000000000000, 0.8660254037844387076, 1.000000000000000000, 0.8660254037844387076, 1.000000000000000000, 0.8660254037844387076, 1.000000000000000000, 0.8660254037844387076, 1.000000000000000000, 0.8660254037844387076, 1.000000000000000000, 0.8660254037844387076, 1.000000000000000000, 0.8660254037844387076, 1.000000000000000000, 0.8660254037844387076, 1.000000000000000000, 0.8660254037844387076, 1.000000000000000000, 0.8660254037844387076, 1.000000000000000000, 0.8660254037844387076, 1.000000000000000000, 0.8660254037844387076, 1.000000000000000000, 0.8660254037844387076, 1.000000000000000000, 0.8660254037844387076, 1.000000000000000000, 0.8660254037844387076, 1.000000000000000000, 0.8660254037844387076, 1.000000000000000000, 0.8660254037844387076, 1.000000000000000000, 0.8660254037844387076, 1.000000000000000000, 0.8660254037844387076, 1.000000000000000000, 0.8660254037844387076, 1.000000000000000000, 0.8660254037844387076, 1.000000000000000000, 0.8660254037844387076, 1.000000000000000000, 0.8660254037844387076, 1.000000000000000000, 0.8660254037844387076, 1.000000000000000000, 0.8660254037844387076, 1.000000000000000000, 0.8660254037844387076, 1.000000000000000000, 0.8660254037844387076, 1.000000000000000000, 0.8660254037844387076, 1.000000000000000000, 0.8660254037844387076, 1.000000000000000000, 0.8660254037844387076, 1.000000000000000000, 0.8660254037844387076, 1.000000000000000000, 0.8660254037844387076, 1.000000000000000000, 0.8660254037844387076, 1.000000000000000000, 0.8660254037844387076, 1.000000000000000000, 0.8660254037844387076, 1.000000000000000000, 0.8660254037844387076, 1.000000000000000000, 0.8660254037844387076, 1.000000000000000000, 0.8660254037844387076, 1.000000000000000000, 0.8660254037844387076, 1.000000000000000000, 0.8660254037844387076, 1.000000000000000000, 0.8660254037844387076, 1.000000000000000000, 0.8660254037844387076, 1.000000000000000000, 0.8660254037844387076, 1.000000000000000000, 0.8660254037844387076, 1.000000000000000000, 0.8660254037844387076, 1.000000000000000000, 0.8660254037844387076, 1.000000000000000000, 0.8660254037844387076, 1.000000000000000000, 0.8660254037844387076, 1.000000000000000000, 0.8660254037844387076, 1.000000000000000000, 0.8660254037844387076, 1.000000000000000000, 0.8660254037844387076, 1.000000000000000000, 0.8660254037844387076, 1.000000000000000000, 0.8660254037844387076, 1.000000000000000000, 0.8660254037844387076, 1.000000000000000000, 0.8660254037844387076, 1.000000000000000000, 0.8660254037844387076, 1.000000000000000000, 0.8660254037844387076, 1.000000000000000000, 0.8660254037844387076, 1.000000000000000000, 0.8660254037844387076, 1.000000000000000000, 0.8660254037844387076, 1.000000000000000000, 0.8660254037844387076, 1.000000000000000000, 0.8660254037844387076, 1.000000000000000000, 0.8660254037844387076, 1.000000000000000000, 0.8660254037844387076, 1.000000000000000000, 0.8660254037844387076, 1.000000000000000000, 0.8660254037844387076, 1.000000000000000000, 0.8660254037844387076, 1.000000000000000000, 0.8660254037844387076, 1.000000000000000000, 0.8660254037844387076, 1.000000000000000000, 0.8660254037844387076, 1.000000000000000000, 0.8660254037844387076, 1.000000000000000000, 0.8660254037844387076, 1.000000000000000000, 0.8660254037844387076, 1.000000000000000000, 0.8660254037844387076, 1.000000000000000000, 0.8660254037844387076, 1.000000000000000000, 0.8660254037844387076, 1.000000000000000000, 0.8660254037844387076, 1.000000000000000000, 0.8660254037844387076, 1.000000000000000000, 0.8660254037844387076, 1.000000000000000000, 0.8660254037844387076, 1.000000000000000000, 0.8660254037844387076, 1.000000000000000000, 0.8660254037844387076, 1.000000000000000000, 0.8660254037844387076, 1.000000000000000000, 0.8660254037844387076, 1.000000000000000000, 0.8660254037844387076, 1.000000000000000000, 0.8660254037844387076, 1.000000000000000000, 0.8660254037844387076, 1.000000000000000000, 0.8660254037844387076, 1.000000000000000000, 0.8660254037844387076, 1.000000000000000000, 0.8660254037844387076, 1.000000000000000000, 0.8660254037844387076, 1.000000000000000000, 0.8660254037844387076, 1.000000000000000000, 0.8660254037844387076, 1.000000000000000000, 0.8660254037844387076, 1.000000000000000000, 0.8660254037844387076, 1.000000000000000000, 0.8660254037844387076, 1.000000000000000000, 0.8660254037844387076, 1.000000000000000000, 0.8660254037844387076, 1.000000000000000000, 0.8660254037844387076, 1.000000000000000000, 0.8660254037844387076, 1.000000000000000000, 0.8660254037844387076, 1.000000000000000000, 0.8660254037844387076, 1.000000000000000000, 0.8660254037844387076, 1.000000000000000000, 0.8660254037844387076, 1.000000000000000000, 0.8660254037844387076, 1.000000000000000000, 0.8660254037844387076, 1.000000000000000000, 0.8660254037844387076, 1.000000000000000000, 0.8660254037844387076, 1.000000000000000000, 0.8660254037844387076, 1.000000000000000000, 0.8660254037844387076, 1.000000000000000000, 0.8660254037844387076, 1.000000000000000000, 0.8660254037844387076, 1.000000000000000000, 0.8660254037844387076, 1.000000000000000000, 0.8660254037844387076, 1.000000000000000000, 0.8660254037844387076, 1.000000000000000000, 0.8660254037844387076, 1.000000000000000000, 0.8660254037844387076, 1.000000000000000000, 0.8660254037844387076, 1.000000000000000000, 0.8660254037844387076, 1.000000000000000000, 0.8660254037844387076, 1.000000000000000000, 0.8660254037844387076, 1.000000000000000000, 0.8660254037844387076, 1.000000000000000000, 0.8660254037844387076, 1.000000000000000000, 0.8660254037844387076, 1.000000000000000000, 0.8660254037844387076, 1.000000000000000000, 0.8660254037844387076, 1.000000000000000000, 0.8660254037844387076, 1.000000000000000000, 0.8660254037844387076, 1.000000000000000000, 0.8660254037844387076, 1.000000000000000000, 0.8660254037844387076, 1.000000000000000000, 0.8660254037844387076, 1.000000000000000000, 0.8660254037844387076, 1.000000000000000000, 0.8660254037844387076, 1.000000000000000000, 0.8660254037844387076, 1.000000000000000000, 0.8660254037844387076, 1.000000000000000000, 0.8660254037844387076, 1.000000000000000000, 0.8660254037844387076, 1.000000000000000000, 0.8660254037844387076, 1.000000000000000000, 0.8660254037844387076, 1.000000000000000000, 0.8660254037844387076, 1.000000000000000000, 0.8660254037844387076, 1.000000000000000000, 0.8660254037844387076, 1.000000000000000000, 0.8660254037844387076, 1.000000000000000000, 0.8660254037844387076, 1.000000000000000000, 0.8660254037844387076, 1.000000000000000000, 0.8660254037844387076, 1.000000000000000000, 0.8660254037844387076, 1.000000000000000000, 0.8660254037844387076, 1.000000000000000000, 0.8660254037844387076, 1.000000000000000000, 0.8660254037844387076, 1.000000000000000000, 0.8660254037844387076, 1.000000000000000000, 0.8660254037844387076, 1.000000000000000000, 0.8660254037844387076, 1.000000000000000000, 0.8660254037844387076, 1.000000000000000000, 0.8660254037844387076, 1.000000000000000000, 0.8660254037844387076, 1.000000000000000000, 0.8660254037844387076, 1.000000000000000000, 0.8660254037844387076, 1.000000000000000000, 0.8660254037844387076, 1.000000000000000000, 0.8660254037844387076, 1.000000000000000000, 0.8660254037844387076, 1.000000000000000000, 0.8660254037844387076, 1.000000000000000000, 0.8660254037844387076, 1.000000000000000000, 0.8660254037844387076, 1.000000000000000000, 0.8660254037844387076, 1.000000000000000000, 0.8660254037844387076, 1.000000000000000000, 0.8660254037844387076, 1.000000000000000000, 0.8660254037844387076, 1.000000000000000000, 0.8660254037844387076, 1.000000000000000000, 0.8660254037844387076, 1.000000000000000000, 0.8660254037844387076, 1.000000000000000000, 0.8660254037844387076, 1.000000000000000000, 0.8660254037844387076, 1.000000000000000000, 0.8660254037844387076, 1.000000000000000000, 0.8660254037844387076, 1.000000000000000000, 0.8660254037844387076, 1.000000000000000000, 0.8660254037844387076, 1.000000000000000000, 0.8660254037844387076, 1.000000000000000000, 0.8660254037844387076, 1.000000000000000000, 0.8660254037844387076, 1.000000000000000000, 0.8660254037844387076, 1.000000000000000000, 0.8660254037844387076, 1.000000000000000000, 0.8660254037844387076, 1.000000000000000000, 0.8660254037844387076, 1.000000000000000000, 0.8660254037844387076, 1.000000000000000000, 0.8660254037844387076, 1.000000000000000000, 0.8660254037844387076, 1.000000000000000000, 0.8660254037844387076, 1.000000000000000000, 0.8660254037844387076, 1.000000000000000000, 0.8660254037844387076, 1.000000000000000000, 0.8660254037844387076, 1.000000000000000000, 0.8660254037844387076, 1.000000000000000000, 0.8660254037844387076, 1.000000000000000000, 0.8660254037844387076, 1.000000000000000000, 0.8660254037844387076, 1.000000000000000000, 0.8660254037844387076, 1.000000000000000000, 0.8660254037844387076, 1.000000000000000000, 0.8660254037844387076, 1.000000000000000000, 0.8660254037844387076, 1.000000000000000000, 0.8660254037844387076, 1.000000000000000000, 0.8660254037844387076, 1.000000000000000000, 0.8660254037844387076, 1.000000000000000000, 0.8660254037844387076, 1.000000000000000000, 0.8660254037844387076, 1.000000000000000000, 0.8660254037844387076, 1.000000000000000000, 0.8660254037844387076, 1.000000000000000000, 0.8660254037844387076, 1.000000000000000000, 0.8660254037844387076, 1.000000000000000000, 0.8660254037844387076, 1.000000000000000000, 0.8660254037844387076, 1.000000000000000000, 0.8660254037844387076, 1.000000000000000000, 0.8660254037844387076, 1.000000000000000000, 0.8660254037844387076, 1.000000000000000000, 0.8660254037844387076, 1.000000000000000000, 0.8660254037844387076, 1.000000000000000000, 0.8660254037844387076, 1.000000000000000000, 0.8660254037844387076, 1.000000000000000000, 0.8660254037844387076, 1.000000000000000000, 0.8660254037844387076, 1.000000000000000000, 0.8660254037844387076, 1.000000000000000000, 0.8660254037844387076, 1.000000000000000000, 0.8660254037844387076, 1.000000000000000000, 0.8660254037844387076, 1.000000000000000000, 0.8660254037844387076, 1.000000000000000000, 0.8660254037844387076, 1.000000000000000000, 0.8660254037844387076, 1.000000000000000000, 0.8660254037844387076, 1.000000000000000000, 0.8660254037844387076, 1.000000000000000000, 0.8660254037844387076, 1.000000000000000000, 0.8660254037844387076, 1.000000000000000000, 0.8660254037844387076, 1.000000000000000000) ) ) 
 REPRESENTATION_ITEM ( '' )  SURFACE ( )  );
#185849=CARTESIAN_POINT ( 'NONE',  ( -6.222829318992474157, 10.20379193889247382, 0.000000000000000000 ) ) ;
#185852=CARTESIAN_POINT ( 'NONE',  ( 1.364683531249990311, 4.696875000341417916, 1.214306433183764966E-14 ) ) ;
#185858=CARTESIAN_POINT ( 'NONE',  ( -1.201851678989727383E-14, 5.446875000341422357, -1.575800808251660134 ) ) ;
#185860=CARTESIAN_POINT ( 'NONE',  ( -3.104453987404957260, 6.565687385373657925, -0.7216878364870257245 ) ) ;
#185862=CARTESIAN_POINT ( 'NONE',  ( 2.345197385039651472, 5.679888015947478941, -0.7216878364870267237 ) ) ;
#185863=CARTESIAN_POINT ( 'NONE',  ( -1.201851678989727383E-14, 5.009375000341421469, -1.575800808251660134 ) ) ;
#185864=DIRECTION ( 'NONE',  ( 0.7592566023653010143, -0.6507913734559633845, -5.900213523162838665E-32 ) ) ;
#185868=CARTESIAN_POINT ( 'NONE',  ( 1.364683531249988757, 1.384375000341421469, 0.000000000000000000 ) ) ;
#185869=CARTESIAN_POINT ( 'NONE',  ( -2.792616454734997866, 6.201876930592042925, 0.7216878364870317197 ) ) ;
#185870=CARTESIAN_POINT ( 'NONE',  ( 6.010342169559767633, 5.906487374108181143, -0.7998128361456281477 ) ) ;
#185878=CARTESIAN_POINT ( 'NONE',  ( -8.432808358020034589, 10.86136238915529084, 1.443375672974064550 ) ) ;
#185881=CARTESIAN_POINT ( 'NONE',  ( 4.355419904288084787, 3.138961374172543284, 0.7750000000000117906 ) ) ;
#185884=CARTESIAN_POINT ( 'NONE',  ( -9.332089804907933939, 9.781859615347734405, 1.040834085586084257E-14 ) ) ;
#185886=CARTESIAN_POINT ( 'NONE',  ( -4.351804119862249465, 7.060559992272473551, 1.082531754730560403 ) ) ;
#185887=CARTESIAN_POINT ( 'NONE',  ( 1.364683531249988535, 1.676041667008085101, 0.7879004041258500513 ) ) ;
#185909=CARTESIAN_POINT ( 'NONE',  ( -1.201851678989727383E-14, 3.384375000341421469, 1.575800808251672791 ) ) ;
#185917=CARTESIAN_POINT ( 'NONE',  ( 10.42352117080803708, 11.05519620889787724, -0.7998128361456281477 ) ) ;
#185919=CARTESIAN_POINT ( 'NONE',  ( -1.364683531250012516, 1.280208333674755172, 0.7879004041258379498 ) ) ;
#185929=CARTESIAN_POINT ( 'NONE',  ( 4.320244504248938355, 8.192035688265757898, 1.040834085586084257E-14 ) ) ;
#185932=ORIENTED_EDGE ( 'NONE', *, *, #19034, .T. ) ;
#185937=CARTESIAN_POINT ( 'NONE',  ( 7.796102023057898123, 9.054206100777749455, -1.199719254218441611 ) ) ;
#185939=VERTEX_POINT ( 'NONE', #66313 ) ;
#185943=CARTESIAN_POINT ( 'NONE',  ( -3.972702704004144714, 4.593573561881607148, 1.199719254218462483 ) ) ;
#185944=CARTESIAN_POINT ( 'NONE',  ( 8.796542737168120851, 9.157054702984622097, -0.7998128361456211532 ) ) ;
#185952=CIRCLE ( 'NONE', #26868, 0.08000000000000012657 ) ;
#185958=CARTESIAN_POINT ( 'NONE',  ( -9.002250809794013264, 9.604973487622245898, -0.7216878364870267237 ) ) ;
#185962=CARTESIAN_POINT ( 'NONE',  ( -9.378489572351046633, 11.96465713920816043, -1.599625672291263179 ) ) ;
#185967=CARTESIAN_POINT ( 'NONE',  ( -2.839543107058306592, 5.400218493954923815, -1.199719254218446718 ) ) ;
#185969=CARTESIAN_POINT ( 'NONE',  ( 10.08456733046637765, 10.65975006183261087, 0.000000000000000000 ) ) ;
#185970=CARTESIAN_POINT ( 'NONE',  ( 3.083589872104280705, 5.684939719841914929, 1.199719254218450271 ) ) ;
#185972=VERTEX_POINT ( 'NONE', #197403 ) ;
#185976=CARTESIAN_POINT ( 'NONE',  ( 3.795919822146273326, 5.451659097302528068, -1.443375672974051449 ) ) ;
#185979=CARTESIAN_POINT ( 'NONE',  ( -5.576481253922474401, 5.400316305864651056, -0.7998128361456221525 ) ) ;
#185981=CARTESIAN_POINT ( 'NONE',  ( -8.136864746495904299, 12.64475930422059768, -0.7998128361456281477 ) ) ;
#185986=CARTESIAN_POINT ( 'NONE',  ( 9.259855728453651125, 9.905512559391842942, 1.040834085586084257E-14 ) ) ;
#185987=CARTESIAN_POINT ( 'NONE',  ( -1.364683531249997417, 5.571875000341417916, 1.214306433183764966E-14 ) ) ;
#185989=CARTESIAN_POINT ( 'NONE',  ( 4.822949958159288286, 6.649860922651058992, -1.599625672291256295 ) ) ;
#186003=CARTESIAN_POINT ( 'NONE',  ( -1.364683531250000748, 2.321875000341422357, 1.214306433183764966E-14 ) ) ;
#186005=CARTESIAN_POINT ( 'NONE',  ( 3.891353782322113375, 4.498666486585943147, -1.199719254218446718 ) ) ;
#186007=CARTESIAN_POINT ( 'NONE',  ( -4.772106882330234612, 6.590544000850479200, -1.443375672974053447 ) ) ;
#186009=CARTESIAN_POINT ( 'NONE',  ( -4.975479186090865369, 6.827811688571220117, 1.443375672974064550 ) ) ;
#186014=CARTESIAN_POINT ( 'NONE',  ( 5.392392409933256303, 7.314210449720692786, 1.599625672291267398 ) ) ;
#186025=CARTESIAN_POINT ( 'NONE',  ( 4.496500501226593727, 8.397667684739696270, 0.7998128361456462443 ) ) ;
#186028=CARTESIAN_POINT ( 'NONE',  ( -2.819205876637805641, 5.376491725131008259, -1.199719254218446718 ) ) ;
#186029=( BOUNDED_CURVE ( )  B_SPLINE_CURVE ( 2, ( #133589, #82654, #31798, #15509, #99982 ),
 .UNSPECIFIED., .F., .T. ) 
 B_SPLINE_CURVE_WITH_KNOTS ( ( 3, 2, 3 ),
 ( 0.01067668659529985575, 0.01250000000000000069, 0.01407841936770214651 ),
 .UNSPECIFIED. ) 
 CURVE ( )  GEOMETRIC_REPRESENTATION_ITEM ( )  RATIONAL_B_SPLINE_CURVE ( ( 0.9340561916853913349, 0.9413733574794107550, 1.000000000000000000, 0.9492476566127880933, 0.9369473844697258080 ) ) 
 REPRESENTATION_ITEM ( '' )  );
#186031=CARTESIAN_POINT ( 'NONE',  ( -6.250472511100020334, 7.250971670160158311, 1.199719254218450271 ) ) ;
#186035=CARTESIAN_POINT ( 'NONE',  ( 7.100719765255169236, 9.307259030929609267, -1.599625672291262513 ) ) ;
#186038=CARTESIAN_POINT ( 'NONE',  ( -5.716734326456539783, 9.821273814174633188, -0.7998128361456231517 ) ) ;
#186040=CARTESIAN_POINT ( 'NONE',  ( 5.897433631820129918, 8.863794422890064695, -1.082531754730537976 ) ) ;
#186041=CARTESIAN_POINT ( 'NONE',  ( 4.133273095458231516, 7.653358944556723387, 0.7702195724684970379 ) ) ;
#186042=CARTESIAN_POINT ( 'NONE',  ( -5.447678794592645701, 5.250046769979851646, 0.000000000000000000 ) ) ;
#186046=CARTESIAN_POINT ( 'NONE',  ( -5.768104287610143821, 8.816873204598778102, -1.199719254218440723 ) ) ;
#186049=CARTESIAN_POINT ( 'NONE',  ( -1.364683531250014514, 1.738541667008085545, -0.7879004041258289570 ) ) ;
#186051=CARTESIAN_POINT ( 'NONE',  ( -4.284013352238250860, 7.941839977679187257, -0.7216878364870267237 ) ) ;
#186057=CARTESIAN_POINT ( 'NONE',  ( -1.500000000000022204, 7.240846818246208905, 4.154462424328226433 ) ) ;
#186058=CARTESIAN_POINT ( 'NONE',  ( 5.686755365928134687, 8.721966129303114101, 1.199719254218462483 ) ) ;
#186061=CARTESIAN_POINT ( 'NONE',  ( 0.6823417656249882723, 2.738541667008084879, -1.181850606188749264 ) ) ;
#186067=CARTESIAN_POINT ( 'NONE',  ( -4.517891501851816649, 6.293959390292322986, -1.599625672291256295 ) ) ;
#186068=CARTESIAN_POINT ( 'NONE',  ( -6.846504384776755714, 9.971043634672792422, -1.082531754730537088 ) ) ;
#186079=CARTESIAN_POINT ( 'NONE',  ( -6.982085920913410071, 11.08959130780024260, 0.7216878364870458196 ) ) ;
#186080=ORIENTED_EDGE ( 'NONE', *, *, #100779, .T. ) ;
#186085=CARTESIAN_POINT ( 'NONE',  ( -6.304178240230145391, 9.338329799368375816, 1.082531754730548412 ) ) ;
#186091=CARTESIAN_POINT ( 'NONE',  ( -1.001543065824772872E-14, 5.243750000682815937, 1.732050807568877637 ) ) ;
#186099=CARTESIAN_POINT ( 'NONE',  ( -6.715366157470410435, 6.729015360003925750, -0.7998128361456291469 ) ) ;
#186102=CARTESIAN_POINT ( 'NONE',  ( 3.388648328411762556, 6.040841252200647382, 1.199719254218462483 ) ) ;
#186104=CARTESIAN_POINT ( 'NONE',  ( 4.856179778084614540, 5.010200168423447842, 0.6077543439236311462 ) ) ;
#186106=CARTESIAN_POINT ( 'NONE',  ( 5.957918438201454059, 9.038323046955323292, -1.199719254218440723 ) ) ;
#186107=CARTESIAN_POINT ( 'NONE',  ( 1.420000000000001039, 7.176846818246214177, -4.202462424328213153 ) ) ;
#186110=CARTESIAN_POINT ( 'NONE',  ( -3.931501358282937009, 7.530575984731317618, 0.7216878364870317197 ) ) ;
#186114=CARTESIAN_POINT ( 'NONE',  ( -4.255895783434943347, 3.981256129034934421, -0.3686001492455212025 ) ) ;
#186119=CARTESIAN_POINT ( 'NONE',  ( -1.402160292154681736E-14, 1.196875000341419026, -1.575800808251659024 ) ) ;
#186121=CARTESIAN_POINT ( 'NONE',  ( -6.418895661066105873, 9.576129806964074120, -1.199719254218440723 ) ) ;
#186123=CARTESIAN_POINT ( 'NONE',  ( 6.283314124929436417, 9.417951348137970413, -1.199719254218440723 ) ) ;
#186125=CARTESIAN_POINT ( 'NONE',  ( -7.725448601688521322, 7.907444878258402809, 1.040834085586084257E-14 ) ) ;
#186128=CARTESIAN_POINT ( 'NONE',  ( 1.499999999999985123, -0.4229166659838508036, -0.8660254037844323793 ) ) ;
#186130=CARTESIAN_POINT ( 'NONE',  ( 7.239690840017413365, 10.42976116578691403, -1.082531754730537976 ) ) ;
#186133=CARTESIAN_POINT ( 'NONE',  ( 0.6823417656249864960, -0.7614583329919113464, -1.181850606188749264 ) ) ;
#186135=CARTESIAN_POINT ( 'NONE',  ( 6.100805936025112786, 10.06143132543056673, 1.040834085586084257E-14 ) ) ;
#186138=CARTESIAN_POINT ( 'NONE',  ( -6.399085315970155285, 6.567947078161039620, -0.7216878364870278340 ) ) ;
#186140=CARTESIAN_POINT ( 'NONE',  ( -1.201851678989727383E-14, 3.321875000341421025, 1.575800808251672791 ) ) ;
#186144=CARTESIAN_POINT ( 'NONE',  ( -6.826694039680798021, 7.923230120171105284, -1.199719254218446718 ) ) ;
#186151=VECTOR ( 'NONE', #2645, 1000.000000000000000 ) ;
#186153=CARTESIAN_POINT ( 'NONE',  ( 7.248805684800777804, 11.60869039890961218, 1.040834085586084257E-14 ) ) ;
#186156=CARTESIAN_POINT ( 'NONE',  ( 1.499999999999987121, 2.545833333333351156, -0.8660254037844262731 ) ) ;
#186163=CARTESIAN_POINT ( 'NONE',  ( 6.155038550924150087, 7.243595066575396757, 1.082531754730558626 ) ) ;
#186164=CARTESIAN_POINT ( 'NONE',  ( 0.6823417656249864960, -0.5114583329919111243, -1.181850606188749264 ) ) ;
#186167=CYLINDRICAL_SURFACE ( 'NONE', #208211, 0.2500000000000578981 ) ;
#186170=CARTESIAN_POINT ( 'NONE',  ( -1.402160292154681736E-14, -0.1624999999999815481, -1.732050807568870754 ) ) ;
#186171=CARTESIAN_POINT ( 'NONE',  ( 7.721532178182734185, 8.967207948423393304, 1.199719254218462483 ) ) ;
#186172=CARTESIAN_POINT ( 'NONE',  ( -8.853638004923878313, 10.28799807962136548, 1.199719254218462483 ) ) ;
#186174=CARTESIAN_POINT ( 'NONE',  ( -1.402160292154681736E-14, -0.5531249996585814177, -1.575800808251665908 ) ) ;
#186175=CARTESIAN_POINT ( 'NONE',  ( -1.402160292154681736E-14, 1.587500000000018785, -1.732050807568863648 ) ) ;
#186177=CARTESIAN_POINT ( 'NONE',  ( 5.229694566569264680, 7.124396299129368337, 1.599625672291267398 ) ) ;
#186184=CARTESIAN_POINT ( 'NONE',  ( 0.6823417656249899377, 5.426041667008087543, -1.181850606188754593 ) ) ;
#186186=CARTESIAN_POINT ( 'NONE',  ( -9.332089804907933939, 9.781859615347734405, 1.040834085586084257E-14 ) ) ;
#186187=CARTESIAN_POINT ( 'NONE',  ( -6.073689629242176480, 6.188318776978391611, -0.7216878364870278340 ) ) ;
#186195=CARTESIAN_POINT ( 'NONE',  ( 7.426115451983150706, 9.686887332112256388, -1.599625672291262513 ) ) ;
#186197=CARTESIAN_POINT ( 'NONE',  ( 2.920214025141053327, 6.445393704534057910, 0.4458799699700779495 ) ) ;
#186199=CARTESIAN_POINT ( 'NONE',  ( 5.775410249297131315, 9.681803024247919609, 1.040834085586084257E-14 ) ) ;
#186203=CARTESIAN_POINT ( 'NONE',  ( -7.857113714319432063, 9.125386407249497012, 1.199719254218462483 ) ) ;
#186205=CARTESIAN_POINT ( 'NONE',  ( 5.412729640353754590, 7.337937218544611895, 1.599625672291267398 ) ) ;
#186206=CARTESIAN_POINT ( 'NONE',  ( 2.345197385039651472, 5.679888015947478941, -0.7216878364870267237 ) ) ;
#186207=CARTESIAN_POINT ( 'NONE',  ( 4.586165880992507660, 5.350526861157986147, -7.499999999999997335 ) ) ;
#186208=CARTESIAN_POINT ( 'NONE',  ( 2.835626683552519012, 6.459981564119914310, 0.000000000000000000 ) ) ;
#186210=EDGE_CURVE ( 'NONE', #195242, #171893, #1056, .T. ) ;
#186211=EDGE_CURVE ( 'NONE', #55695, #152681, #178232, .T. ) ;
#186217=CARTESIAN_POINT ( 'NONE',  ( -1.543281805264341777, 8.695372333414642441, -2.508924166024196989 ) ) ;
#186218=CARTESIAN_POINT ( 'NONE',  ( -5.748293942514189681, 5.808690475795744490, -0.7216878364870207285 ) ) ;
#186219=CARTESIAN_POINT ( 'NONE',  ( 2.171277156482887882, 5.684907115872006145, -0.7998128361456291469 ) ) ;
#186222=CARTESIAN_POINT ( 'NONE',  ( -6.693975156845199059, 8.832723654451292816, 1.599625672291283607 ) ) ;
#186227=CARTESIAN_POINT ( 'NONE',  ( -8.128276786592724790, 9.441743324901704426, -1.199719254218446718 ) ) ;
#186242=CARTESIAN_POINT ( 'NONE',  ( -5.520141099058386125, 9.591915048876776595, 0.000000000000000000 ) ) ;
#186245=CARTESIAN_POINT ( 'NONE',  ( 6.805829924380118356, 7.042482454639357847, 0.7216878364870317197 ) ) ;
#186249=CARTESIAN_POINT ( 'NONE',  ( -3.273404022695637572, 5.906389562198459231, 1.199719254218462483 ) ) ;
#186253=CARTESIAN_POINT ( 'NONE',  ( -4.530395885260773525, 8.437212299446219532, 0.7998128361456481317 ) ) ;
#186260=CARTESIAN_POINT ( 'NONE',  ( -9.504429378379839477, 11.04725468198666150, 1.199719254218462483 ) ) ;
#186261=CARTESIAN_POINT ( 'NONE',  ( 6.479907352327590964, 9.647310113435821677, 1.199719254218462483 ) ) ;
#186264=CARTESIAN_POINT ( 'NONE',  ( -9.429859533504656000, 10.96025652963230534, -1.199719254218441611 ) ) ;
#186267=CARTESIAN_POINT ( 'NONE',  ( -0.6823417656250003738, -0.7197916663252492686, -1.181850606188749264 ) ) ;
#186271=CARTESIAN_POINT ( 'NONE',  ( 8.378575743565351175, 11.75846021992619406, -1.082531754730543083 ) ) ;
#186276=CARTESIAN_POINT ( 'NONE',  ( -5.465417954149238255, 6.280545163089921168, -1.016043258478748434 ) ) ;
#186279=CARTESIAN_POINT ( 'NONE',  ( -0.3695500129099597020, 6.511094381872901238, -3.314792509164075529 ) ) ;
#186290=CARTESIAN_POINT ( 'NONE',  ( -4.192495815123836955, 5.914331089109674089, -1.599625672291256295 ) ) ;
#186299=CARTESIAN_POINT ( 'NONE',  ( -1.500000000000015099, -0.5479166659838513587, 0.8660254037844403729 ) ) ;
#186303=CARTESIAN_POINT ( 'NONE',  ( 9.134442807305049428, 11.67993591332117376, 1.599625672291281386 ) ) ;
#186304=ORIENTED_EDGE ( 'NONE', *, *, #116619, .T. ) ;
#186305=CARTESIAN_POINT ( 'NONE',  ( 1.150222622689962781, 2.983395032273045366, -0.7749999999993620881 ) ) ;
#186308=CARTESIAN_POINT ( 'NONE',  ( 9.999301985278609806, 11.62460605670194447, 1.199719254218452047 ) ) ;
#186314=CARTESIAN_POINT ( 'NONE',  ( 4.985647801523278133, 6.839675073242382553, -1.599625672291256295 ) ) ;
#186315=CARTESIAN_POINT ( 'NONE',  ( -1.201851678989727383E-14, 2.884375000341418804, 1.575800808251672791 ) ) ;
#186316=CARTESIAN_POINT ( 'NONE',  ( -4.653572958549120564, 6.905085616583060748, 1.214936962016188726 ) ) ;
#186319=CARTESIAN_POINT ( 'NONE',  ( -6.157374318900681764, 10.33535380535947290, 0.7998128361456481317 ) ) ;
#186320=CARTESIAN_POINT ( 'NONE',  ( -4.731432421044877934, 6.543090462684225450, -1.443375672974051449 ) ) ;
#186323=CARTESIAN_POINT ( 'NONE',  ( -7.067878151425722955, 7.140279352951794500, 0.7998128361456341429 ) ) ;
#186325=CARTESIAN_POINT ( 'NONE',  ( 0.7499999999999885647, 0.2645833340161538039, 1.299038105676657340 ) ) ;
#186334=CARTESIAN_POINT ( 'NONE',  ( -4.948362878863562742, 5.835806782504650236, 1.082531754730558626 ) ) ;
#186338=CARTESIAN_POINT ( 'NONE',  ( -3.077337680177623103, 6.534051693608437184, 0.7216878364870317197 ) ) ;
#186340=CARTESIAN_POINT ( 'NONE',  ( 7.425061681778431399, 11.81432239538354345, 0.7998128361456462443 ) ) ;
#186349=CARTESIAN_POINT ( 'NONE',  ( -3.789667630219657912, 4.380032642466370696, 1.199719254218462483 ) ) ;
#186350=CARTESIAN_POINT ( 'NONE',  ( -10.48453286206953727, 11.12637651536962125, 0.7998128361456462443 ) ) ;
#186355=CARTESIAN_POINT ( 'NONE',  ( 6.006425746053997372, 6.966250444273174303, -1.199719254218445830 ) ) ;
#186358=ORIENTED_EDGE ( 'NONE', *, *, #192214, .T. ) ;
#186361=CARTESIAN_POINT ( 'NONE',  ( 4.054051625686104998, 4.688480637177271149, -1.199719254218446718 ) ) ;
#186363=ORIENTED_EDGE ( 'NONE', *, *, #26050, .T. ) ;
#186371=CARTESIAN_POINT ( 'NONE',  ( 9.108380270282433244, 9.520865158284665952, 1.040834085586084257E-14 ) ) ;
#186373=CARTESIAN_POINT ( 'NONE',  ( -4.412288926243578935, 7.235088616337731260, 1.199719254218464037 ) ) ;
#186379=CARTESIAN_POINT ( 'NONE',  ( -1.402160292154681736E-14, -1.006249999317181620, 1.732050807568877637 ) ) ;
#186382=ORIENTED_EDGE ( 'NONE', *, *, #180626, .F. ) ;
#186384=CARTESIAN_POINT ( 'NONE',  ( 4.650610384687404952, 5.384465856012134566, 1.199719254218462483 ) ) ;
#186385=CARTESIAN_POINT ( 'NONE',  ( -3.574546055497324737, 7.322054164722185732, 0.7998128361456341429 ) ) ;
#186391=CARTESIAN_POINT ( 'NONE',  ( 6.344852701515477200, 6.504675694630598137, -0.7216878364870257245 ) ) ;
#186394=CARTESIAN_POINT ( 'NONE',  ( 6.765155463094740362, 10.83650577367847667, 0.7216878364870438212 ) ) ;
#186395=CARTESIAN_POINT ( 'NONE',  ( -1.201851678989727383E-14, 3.884375000341423689, 1.575800808251672791 ) ) ;
#186397=CARTESIAN_POINT ( 'NONE',  ( 5.802526556524483681, 5.871961858807763335, 1.040834085586084257E-14 ) ) ;
#186401=ADVANCED_FACE ( 'NONE', ( #100967 ), #167056, .F. ) ;
#186405=CARTESIAN_POINT ( 'NONE',  ( -4.974982779204009553, 6.815313220028144769, 1.450550931683711298 ) ) ;
#186406=CARTESIAN_POINT ( 'NONE',  ( 4.989037339704528229, 4.922891105851139315, 1.040834085586084257E-14 ) ) ;
#186412=CARTESIAN_POINT ( 'NONE',  ( -8.306341666666730461, 12.84248237775322643, 1.040834085586084257E-14 ) ) ;
#186414=CARTESIAN_POINT ( 'NONE',  ( -1.420000000000021911, 6.200000000000045475, 2.873333333333347728 ) ) ;
#186417=CARTESIAN_POINT ( 'NONE',  ( -4.634189577772691138, 4.300976017023221409, 1.214306433183764966E-14 ) ) ;
#186423=CARTESIAN_POINT ( 'NONE',  ( 0.6823417656249882723, 2.988541667008084879, -1.181850606188754593 ) ) ;
#186425=CARTESIAN_POINT ( 'NONE',  ( 7.637320603199683866, 7.804628880021436288, -0.7998128361456281477 ) ) ;
#186427=CARTESIAN_POINT ( 'NONE',  ( -8.422639742587602285, 10.84949900448412841, -1.599625672291263179 ) ) ;
#186428=DIRECTION ( 'NONE',  ( -5.578564026256490882E-16, -1.000000000000000000, -9.066213480720158442E-32 ) ) ;
#186429=CARTESIAN_POINT ( 'NONE',  ( -5.440899717785814715, 5.242137847038546461, 0.7998128361456341429 ) ) ;
#186433=CARTESIAN_POINT ( 'NONE',  ( -1.499999999999997780, 3.900000000000021672, 1.214306433183764966E-14 ) ) ;
#186434=CARTESIAN_POINT ( 'NONE',  ( 4.690231075323689325, 7.559354456931247412, 1.199719254218462483 ) ) ;
#186438=CARTESIAN_POINT ( 'NONE',  ( 0.6823417656249899377, 3.426041667008085323, -1.181850606188754593 ) ) ;
#186441=CARTESIAN_POINT ( 'NONE',  ( 9.897088948295946764, 10.64895131587453569, 0.7216878364870438212 ) ) ;
#186446=( BOUNDED_CURVE ( )  B_SPLINE_CURVE ( 2, ( #1677, #3799, #120871, #20068, #84014, #86157, #165275 ),
 .UNSPECIFIED., .F., .T. ) 
 B_SPLINE_CURVE_WITH_KNOTS ( ( 3, 2, 2, 3 ),
 ( 0.1964285714285713413, 0.2023809523809523836, 0.2083333333333334536, 0.2142857142857144681 ),
 .UNSPECIFIED. ) 
 CURVE ( )  GEOMETRIC_REPRESENTATION_ITEM ( )  RATIONAL_B_SPLINE_CURVE ( ( 1.000000000000001776, 0.8660254037844368202, 1.000000000000000000, 0.8660254037844387076, 1.000000000000000000, 0.8660254037844343777, 1.000000000000004441 ) ) 
 REPRESENTATION_ITEM ( '' )  );
#186447=CARTESIAN_POINT ( 'NONE',  ( -1.500000000000013101, 2.660416667349483788, -0.8660254037844313801 ) ) ;
#186449=CARTESIAN_POINT ( 'NONE',  ( -5.687809136132860210, 6.594531066031826150, -1.199719254218446718 ) ) ;
#186450=CARTESIAN_POINT ( 'NONE',  ( 5.802526556524483681, 5.871961858807763335, 1.040834085586084257E-14 ) ) ;
#186451=LINE ( 'NONE', #57537, #180621 ) ;
#186459=CARTESIAN_POINT ( 'NONE',  ( 7.741869408603235136, 8.990934717247309749, 1.199719254218462483 ) ) ;
#186460=CARTESIAN_POINT ( 'NONE',  ( 3.825371897350130723, 7.614684313550482031, 0.7998128361456321445 ) ) ;
#186465=CARTESIAN_POINT ( 'NONE',  ( 4.222474775652216294, 7.013638773981186958, 1.199719254218462483 ) ) ;
#186466=CARTESIAN_POINT ( 'NONE',  ( 3.189213936345663747, 2.817530495244580102, -2.450448857954562243 ) ) ;
#186472=CARTESIAN_POINT ( 'NONE',  ( 10.37606763316019531, 10.99983374830873650, 0.7998128361456462443 ) ) ;
#186476=AXIS2_PLACEMENT_3D ( 'NONE', #210169, #178772, #79115 ) ;
#186478=CARTESIAN_POINT ( 'NONE',  ( 5.886971415934090679, 5.980320297827544707, -0.1280069804882408846 ) ) ;
#186489=CARTESIAN_POINT ( 'NONE',  ( 7.782016984564065432, 8.181367358187307204, 0.7216878364870458196 ) ) ;
#186491=CARTESIAN_POINT ( 'NONE',  ( -4.952806187693842510, 4.672695395264567786, 0.7998128361456341429 ) ) ;
#186496=CARTESIAN_POINT ( 'NONE',  ( -4.446184310277715213, 7.274633231044262516, -1.199719254218452047 ) ) ;
#186498=EDGE_CURVE ( 'NONE', #58494, #169262, #124786, .T. ) ;
#186504=CARTESIAN_POINT ( 'NONE',  ( -4.911285141672522059, 4.693790260148114513, 0.3511878651327460243 ) ) ;
#186509=CARTESIAN_POINT ( 'NONE',  ( 9.420217803396747414, 9.884675613584706255, 0.7998128361456462443 ) ) ;
#186510=CARTESIAN_POINT ( 'NONE',  ( 5.593492625449885125, 6.357122791843209164, 1.180528715873955692 ) ) ;
#186517=CARTESIAN_POINT ( 'NONE',  ( -9.571693261567968847, 12.19006144329456731, 1.443375672974076540 ) ) ;
#186523=CARTESIAN_POINT ( 'NONE',  ( 6.740374924288304648, 11.01552117831172062, 1.040834085586084257E-14 ) ) ;
#186527=CARTESIAN_POINT ( 'NONE',  ( -4.713430959045263435, 8.650753218861462202, 0.7998128361456481317 ) ) ;
#186528=CARTESIAN_POINT ( 'NONE',  ( 3.011882680530176604, 6.665613560593854459, 0.7998128361456341429 ) ) ;
#186530=B_SPLINE_CURVE_WITH_KNOTS ( 'NONE', 3,
 ( #38815, #186114, #21460, #182921, #85424, #67010 ),
 .UNSPECIFIED., .F., .F.,
 ( 4, 2, 4 ),
 ( 1.734723475976807865E-18, 0.0004981609494469188592, 0.0009963218988938357668 ),
 .UNSPECIFIED. ) ;
#186532=CARTESIAN_POINT ( 'NONE',  ( 8.516493047678546091, 13.08765898893368629, -0.7998128361456352531 ) ) ;
#186533=CARTESIAN_POINT ( 'NONE',  ( 0.4609910511476702499, 6.639638261665985475, 3.327981402927758570 ) ) ;
#186536=CARTESIAN_POINT ( 'NONE',  ( 4.019508774049570299, 7.801013956325979493, 0.3192432753683968061 ) ) ;
#186538=CARTESIAN_POINT ( 'NONE',  ( 5.165293337126522388, 8.969999960048859577, 1.040834085586084257E-14 ) ) ;
#186546=CARTESIAN_POINT ( 'NONE',  ( 7.822691444960700125, 10.14955932391940330, -1.443375672974058777 ) ) ;
#186551=CARTESIAN_POINT ( 'NONE',  ( -7.503547950159405566, 10.84155747757291266, 1.199719254218453823 ) ) ;
#186560=CARTESIAN_POINT ( 'NONE',  ( 10.05353459973327368, 11.68787744023238417, -1.199719254218440723 ) ) ;
#186565=CARTESIAN_POINT ( 'NONE',  ( 4.741601036477289810, 6.554953847355395880, 1.599625672291267398 ) ) ;
#186568=CARTESIAN_POINT ( 'NONE',  ( -1.500000000000013101, 2.202083334016153859, 0.8660254037844403729 ) ) ;
#186574=CARTESIAN_POINT ( 'NONE',  ( -0.7500000000000006661, 1.358333333333357151, -1.299038105676652011 ) ) ;
#186575=CARTESIAN_POINT ( 'NONE',  ( 5.913327553854682783, 10.05063257947248800, -0.7998128361456291469 ) ) ;
#186576=CARTESIAN_POINT ( 'NONE',  ( 3.809477975315569864, 7.388215371269402532, -0.7216878364870197293 ) ) ;
#186580=CARTESIAN_POINT ( 'NONE',  ( 10.05978679165993839, 10.83876546646586014, 0.7216878364870438212 ) ) ;
#186581=AXIS2_PLACEMENT_3D ( 'NONE', #74851, #206963, #108479 ) ;
#186586=CARTESIAN_POINT ( 'NONE',  ( -6.417086777969760902, 6.381022750586497594, 0.7998128361456341429 ) ) ;
#186587=CARTESIAN_POINT ( 'NONE',  ( 0.7499999999999920064, 4.014583334016149863, 1.299038105676669330 ) ) ;
#186588=CARTESIAN_POINT ( 'NONE',  ( -0.6823417656250212460, 4.863541667008086655, 1.181850606188767472 ) ) ;
#186592=EDGE_CURVE ( 'NONE', #116549, #56116, #38019, .T. ) ;
#186594=CARTESIAN_POINT ( 'NONE',  ( 1.364683531249988535, 4.467708333674754506, -0.7879004041258300672 ) ) ;
#186601=CARTESIAN_POINT ( 'NONE',  ( -7.069687034522070590, 10.33538640932937724, -1.199719254218440723 ) ) ;
#186602=CARTESIAN_POINT ( 'NONE',  ( 7.332262146892202459, 7.448727347662698506, -0.7998128361456281477 ) ) ;
#186604=CARTESIAN_POINT ( 'NONE',  ( -3.090895833791289071, 6.549869539491048442, 1.040834085586084257E-14 ) ) ;
#186609=CARTESIAN_POINT ( 'NONE',  ( -0.005641171162459664157, 8.210923785194999880, -2.038653139403752590 ) ) ;
#186612=CARTESIAN_POINT ( 'NONE',  ( -5.533699252672048985, 9.607732894759390518, -0.7998128361456231517 ) ) ;
#186615=CARTESIAN_POINT ( 'NONE',  ( 10.55232363013785246, 11.20546574478267132, 0.000000000000000000 ) ) ;
#186617=CARTESIAN_POINT ( 'NONE',  ( 8.191097360950562845, 12.70803068775103739, -0.7998128361456352531 ) ) ;
#186618=CARTESIAN_POINT ( 'NONE',  ( -4.906445432736048495, 4.819153361833998339, 0.2530815521472702390 ) ) ;
#186620=CARTESIAN_POINT ( 'NONE',  ( -3.958090780185743451, 6.705190779270287393, -1.199719254218452047 ) ) ;
#186621=CARTESIAN_POINT ( 'NONE',  ( -8.076906825439122528, 10.44614393447756129, -1.599625672291263179 ) ) ;
#186624=CARTESIAN_POINT ( 'NONE',  ( -4.338732707277040745, 7.407397761066524922, -1.160996969951762159 ) ) ;
#186625=CARTESIAN_POINT ( 'NONE',  ( -1.402160292154681736E-14, -0.5531249996585814177, -1.575800808251665908 ) ) ;
#186631=CARTESIAN_POINT ( 'NONE',  ( 5.738125327081736060, 7.717565519727259904, 1.599625672291267398 ) ) ;
#186654=CARTESIAN_POINT ( 'NONE',  ( -9.820183334999905256, 10.35130206712171130, 1.040834085586084257E-14 ) ) ;
#186659=CARTESIAN_POINT ( 'NONE',  ( 1.499999999999989120, 1.306250000682816825, 0.000000000000000000 ) ) ;
#186660=CARTESIAN_POINT ( 'NONE',  ( 9.541187415715040032, 12.15447128979948310, -1.599625672291262513 ) ) ;
#186665=CARTESIAN_POINT ( 'NONE',  ( 1.364683531249986537, 1.405208333674755838, -0.7879004041258239610 ) ) ;
#186671=CARTESIAN_POINT ( 'NONE',  ( -3.602716132929368875, 5.226254793216122074, 1.599625672291267398 ) ) ;
#186676=CARTESIAN_POINT ( 'NONE',  ( -1.402160292154681736E-14, 0.009375000341421267647, -1.575800808251665908 ) ) ;
#186681=CARTESIAN_POINT ( 'NONE',  ( -1.364683531250000748, 0.7593750003414210248, 0.000000000000000000 ) ) ;
#186683=CARTESIAN_POINT ( 'NONE',  ( -5.201524489137236529, 9.220195670635433771, 0.7998128361456481317 ) ) ;
#186684=CARTESIAN_POINT ( 'NONE',  ( 6.916630921265960019, 11.22115317478565188, 0.7998128361456462443 ) ) ;
#186685=CARTESIAN_POINT ( 'NONE',  ( 3.344057444064992168, 7.053150784717805877, 1.040834085586084257E-14 ) ) ;
#186686=CARTESIAN_POINT ( 'NONE',  ( 5.952193131599331721, 6.902979060742733708, 1.199719254218462483 ) ) ;
#186688=CARTESIAN_POINT ( 'NONE',  ( -1.500000000000013101, 3.629166666666692187, -0.8660254037844313801 ) ) ;
#186690=CARTESIAN_POINT ( 'NONE',  ( 0.6823417656249899377, 1.405208333674752508, 1.181850606188755259 ) ) ;
#186696=CARTESIAN_POINT ( 'NONE',  ( 5.504247177468175600, 8.405076892812779477, 1.082531754730558626 ) ) ;
#186699=CARTESIAN_POINT ( 'NONE',  ( -5.689618019229208734, 9.789638122409414223, 0.7998128361456481317 ) ) ;
#186700=CARTESIAN_POINT ( 'NONE',  ( -3.469997250093771246, 6.135748327496311383, -1.199719254218452935 ) ) ;
#186705=CARTESIAN_POINT ( 'NONE',  ( -8.961576348508655698, 9.557519949455999253, -0.7216878364870267237 ) ) ;
#186707=CARTESIAN_POINT ( 'NONE',  ( -1.499999999999997780, 5.400000000000022560, 1.214306433183764966E-14 ) ) ;
#186711=CARTESIAN_POINT ( 'NONE',  ( 9.408995418203971894, 11.03987807840189816, 1.082531754730549967 ) ) ;
#186712=CARTESIAN_POINT ( 'NONE',  ( -6.082945924897037671, 5.998665437213099416, -0.3423739784766628991 ) ) ;
#186714=CARTESIAN_POINT ( 'NONE',  ( -3.863710589770277259, 6.491117540498504646, 1.082531754730560403 ) ) ;
#186721=CARTESIAN_POINT ( 'NONE',  ( 9.205623113554612047, 12.72334881824701469, 1.082531754730546636 ) ) ;
#186728=CARTESIAN_POINT ( 'NONE',  ( 7.361714222096048310, 10.57212177821199184, -1.082531754730537976 ) ) ;
#186730=CARTESIAN_POINT ( 'NONE',  ( 8.274553823041976841, 8.548067636504127265, 1.040834085586084257E-14 ) ) ;
#186731=CARTESIAN_POINT ( 'NONE',  ( -6.043183783389232566, 8.073467052085995022, 1.599625672291269396 ) ) ;
#186733=CARTESIAN_POINT ( 'NONE',  ( -1.201851678989727383E-14, 5.087500000000019007, -1.732050807568863648 ) ) ;
#186735=CARTESIAN_POINT ( 'NONE',  ( 7.104109303436412226, 7.390475063538369582, 1.040834085586084257E-14 ) ) ;
#186736=CARTESIAN_POINT ( 'NONE',  ( -1.364683531250014514, -0.6989583329919100141, -0.7879004041258359514 ) ) ;
#186737=CARTESIAN_POINT ( 'NONE',  ( 2.711267533052988732, 6.106969855296372707, -0.7216878364870267237 ) ) ;
#186738=EDGE_LOOP ( 'NONE', ( #144682, #88619, #210304, #53972 ) ) ;
#186739=CARTESIAN_POINT ( 'NONE',  ( -2.449219305563052895, 6.009172956465517856, 1.040834085586084257E-14 ) ) ;
#186748=ORIENTED_EDGE ( 'NONE', *, *, #155670, .F. ) ;
#186752=ORIENTED_EDGE ( 'NONE', *, *, #31970, .T. ) ;
#186755=CARTESIAN_POINT ( 'NONE',  ( 7.796102023057898123, 9.054206100777749455, -1.199719254218441611 ) ) ;
#186759=CARTESIAN_POINT ( 'NONE',  ( 1.458525620005609147, 8.740196138359117128, 2.548959422810368913 ) ) ;
#186765=CARTESIAN_POINT ( 'NONE',  ( -5.215082642750900277, 9.236013516518044142, 0.000000000000000000 ) ) ;
#186767=CARTESIAN_POINT ( 'NONE',  ( -4.090809663021341969, 5.795697244990093644, 1.599625672291267398 ) ) ;
#186777=CARTESIAN_POINT ( 'NONE',  ( -2.442440228756222353, 6.001264033524212671, -0.7998128361456281477 ) ) ;
#186781=CARTESIAN_POINT ( 'NONE',  ( 6.317209508963599340, 9.457495962844502557, 1.199719254218462483 ) ) ;
#186782=CARTESIAN_POINT ( 'NONE',  ( -0.6823417656249969321, 4.717708333674755394, -1.181850606188749264 ) ) ;
#186788=CARTESIAN_POINT ( 'NONE',  ( 6.277061933002785032, 7.385955679000473673, 1.082531754730558626 ) ) ;
#186789=CARTESIAN_POINT ( 'NONE',  ( -8.453672473320708036, 9.821371626084353323, -1.199719254218446718 ) ) ;
#186792=CARTESIAN_POINT ( 'NONE',  ( -6.008234629150358330, 10.16135750065076060, 0.000000000000000000 ) ) ;
#186793=CARTESIAN_POINT ( 'NONE',  ( -5.168682875307782254, 7.053215992657626110, -1.599625672291256295 ) ) ;
#186797=CARTESIAN_POINT ( 'NONE',  ( 4.905139262582266291, 4.827437033166341429, 0.6004564335717228474 ) ) ;
#186800=CARTESIAN_POINT ( 'NONE',  ( 6.775324078527185989, 8.927630729746953264, -1.599625672291262513 ) ) ;
#186815=CARTESIAN_POINT ( 'NONE',  ( -0.7499999999999972244, 5.108333333333353821, -1.299038105676652011 ) ) ;
#186816=CARTESIAN_POINT ( 'NONE',  ( 3.960953433486789521, 7.772862772376584850, -0.7998128361456221525 ) ) ;
#186817=CARTESIAN_POINT ( 'NONE',  ( 5.035963992472171746, 7.962709526937818083, 1.199719254218462483 ) ) ;
#186819=CARTESIAN_POINT ( 'NONE',  ( -7.537970219518066450, 11.73812298950569044, -0.7216878364870267237 ) ) ;
#186821=CARTESIAN_POINT ( 'NONE',  ( 6.643132081016117851, 8.773406732650713025, 1.443375672974076540 ) ) ;
#186822=CARTESIAN_POINT ( 'NONE',  ( -8.663296969008007054, 9.209527340038563992, 0.7216878364870438212 ) ) ;
#186824=VERTEX_POINT ( 'NONE', #175597 ) ;
#186826=CARTESIAN_POINT ( 'NONE',  ( 8.911787042884274257, 9.291506392986812912, 0.7998128361456462443 ) ) ;
#186831=CARTESIAN_POINT ( 'NONE',  ( -0.6823417656250212460, 2.051041667008083991, 1.181850606188767472 ) ) ;
#186837=CARTESIAN_POINT ( 'NONE',  ( 9.097684769969825780, 10.57271930550834860, -1.199719254218446718 ) ) ;
#186841=CARTESIAN_POINT ( 'NONE',  ( -10.50487009249003378, 11.15010328419353947, 0.7998128361456462443 ) ) ;
#186847=CARTESIAN_POINT ( 'NONE',  ( 9.622536337397022521, 12.24937836509514710, 1.599625672291281386 ) ) ;
#186851=CARTESIAN_POINT ( 'NONE',  ( -8.479735010343349089, 11.98044238112085758, 1.199719254218453823 ) ) ;
#186857=CARTESIAN_POINT ( 'NONE',  ( 5.407503677813131127, 6.286683671216334091, 1.048937882774292785 ) ) ;
#186859=CARTESIAN_POINT ( 'NONE',  ( -3.242371291962510504, 6.934516940598226320, 1.040834085586084257E-14 ) ) ;
#186863=CARTESIAN_POINT ( 'NONE',  ( 7.233438648090761980, 8.397765496649418182, 1.199719254218462483 ) ) ;
#186865=CARTESIAN_POINT ( 'NONE',  ( 7.461064606222022277, 7.598996883547496139, 1.040834085586084257E-14 ) ) ;
#186866=CARTESIAN_POINT ( 'NONE',  ( 4.660252114795294887, 6.460046772059735432, -1.599625672291256295 ) ) ;
#186875=CARTESIAN_POINT ( 'NONE',  ( -4.932901803036217281, 6.667582871412107259, -1.248097486420626900 ) ) ;
#186877=CARTESIAN_POINT ( 'NONE',  ( 6.344852701515477200, 6.504675694630598137, -0.7216878364870257245 ) ) ;
#186881=CARTESIAN_POINT ( 'NONE',  ( -10.45297324601190425, 11.29748299654313470, 0.7216878364870438212 ) ) ;
#186899=CARTESIAN_POINT ( 'NONE',  ( 7.151035956204054855, 10.43029348462504124, 1.199719254218460707 ) ) ;
#186903=CARTESIAN_POINT ( 'NONE',  ( -1.500000000000001332, 1.431250000682816825, 0.000000000000000000 ) ) ;
#186904=CARTESIAN_POINT ( 'NONE',  ( -3.216308754939891212, 4.775446185561722956, -1.599625672291262513 ) ) ;
#186905=CARTESIAN_POINT ( 'NONE',  ( -6.552668314106420588, 6.539201209412602189, -0.7998128361456291469 ) ) ;
#186908=CARTESIAN_POINT ( 'NONE',  ( -8.676328237741483207, 12.20980114641871062, -1.199719254218446718 ) ) ;
#186913=CARTESIAN_POINT ( 'NONE',  ( 7.284808609244363353, 7.393364887073558656, 0.7998128361456341429 ) ) ;
#186914=B_SPLINE_CURVE_WITH_KNOTS ( 'NONE', 3,
 ( #198437, #37013, #184324, #2356, #83633, #16485, #68432, #66290, #148652, #50083 ),
 .UNSPECIFIED., .F., .F.,
 ( 4, 3, 3, 4 ),
 ( 0.000000000000000000, 8.893179197954873439E-05, 0.0001334007970840211997, 0.0001778705873659022839 ),
 .UNSPECIFIED. ) ;
#186917=CARTESIAN_POINT ( 'NONE',  ( -5.879432169820529630, 10.01108796476595764, -0.7998128361456221525 ) ) ;
#186919=CARTESIAN_POINT ( 'NONE',  ( -0.6823417656250212460, 5.551041667008087543, 1.181850606188767472 ) ) ;
#186925=CARTESIAN_POINT ( 'NONE',  ( -8.378575743565381373, 8.877352577022161739, 0.7216878364870438212 ) ) ;
#186929=CARTESIAN_POINT ( 'NONE',  ( -0.6823417656249969321, 4.030208333674754506, -1.181850606188749264 ) ) ;
#186936=CARTESIAN_POINT ( 'NONE',  ( 1.364683531249988535, 3.905208333674751842, -0.7879004041258239610 ) ) ;
#186939=CARTESIAN_POINT ( 'NONE',  ( 4.500943809612556024, 4.353448654077163305, 1.214306433183764966E-14 ) ) ;
#186940=CARTESIAN_POINT ( 'NONE',  ( 1.364683531249990311, 5.426041667008086655, 0.7879004041258500513 ) ) ;
#186945=CARTESIAN_POINT ( 'NONE',  ( 1.364683531249986537, 1.113541667008082658, 0.7879004041258500513 ) ) ;
#186946=CARTESIAN_POINT ( 'NONE',  ( -2.806174608348664723, 6.217694776474651519, 1.040834085586084257E-14 ) ) ;
#186947=CARTESIAN_POINT ( 'NONE',  ( 4.147904930777053245, 6.926640621626830807, -1.199719254218452047 ) ) ;
#186956=CARTESIAN_POINT ( 'NONE',  ( -8.242994207428740339, 9.679543332497402730, 1.082531754730558626 ) ) ;
#186961=CARTESIAN_POINT ( 'NONE',  ( -9.429859533504656000, 10.96025652963230534, -1.199719254218441611 ) ) ;
#186962=CARTESIAN_POINT ( 'NONE',  ( -5.327991180046197428, 8.199444895820425572, 1.082531754730548412 ) ) ;
#186963=CARTESIAN_POINT ( 'NONE',  ( -0.6823417656250003738, 1.530208333674752730, -1.181850606188749264 ) ) ;
#186964=CARTESIAN_POINT ( 'NONE',  ( -3.511198596259319960, 6.271927390929313617, 2.420000000000010587 ) ) ;
#186977=VERTEX_POINT ( 'NONE', #208064 ) ;
#186980=EDGE_CURVE ( 'NONE', #129569, #193266, #138521, .T. ) ;
#186988=CARTESIAN_POINT ( 'NONE',  ( 0.6823417656249917140, 3.655208333674754506, 1.181850606188765695 ) ) ;
#186999=CARTESIAN_POINT ( 'NONE',  ( -1.201851678989727383E-14, 1.321875000341419248, 1.575800808251672791 ) ) ;
#187009=CARTESIAN_POINT ( 'NONE',  ( 5.518332215962025167, 6.396807992499198292, -1.199719254218445830 ) ) ;
#187018=CARTESIAN_POINT ( 'NONE',  ( 8.259941899223605333, 10.65968485389279508, -1.599625672291268286 ) ) ;
#187030=AXIS2_PLACEMENT_3D ( 'NONE', #47815, #161551, #159400 ) ;
#187031=CARTESIAN_POINT ( 'NONE',  ( -7.917598520700757980, 9.299915031314755609, 1.082531754730558626 ) ) ;
#187036=CARTESIAN_POINT ( 'NONE',  ( -7.797910906154257304, 12.24931315715533486, 0.000000000000000000 ) ) ;
#187038=CARTESIAN_POINT ( 'NONE',  ( 2.240623464304030588, 5.557885108422582654, 0.2071306710573883048 ) ) ;
#187041=CARTESIAN_POINT ( 'NONE',  ( -2.449219305563052895, 6.009172956465517856, 1.040834085586084257E-14 ) ) ;
#187043=CARTESIAN_POINT ( 'NONE',  ( 8.387690588348714726, 12.93738945304888333, 1.040834085586084257E-14 ) ) ;
#187045=CARTESIAN_POINT ( 'NONE',  ( 4.701980345841006326, 4.380065246436280368, 0.7998128361456341429 ) ) ;
#187051=CARTESIAN_POINT ( 'NONE',  ( 3.226477370372293763, 6.708047998835573900, 0.7216878364870317197 ) ) ;
#187053=CARTESIAN_POINT ( 'NONE',  ( -4.904298879841297421, 6.744767997946721216, 1.599625672291267398 ) ) ;
#187054=DIRECTION ( 'NONE',  ( -0.6507913734559640506, -0.7592566023653004592, 0.000000000000000000 ) ) ;
#187056=CARTESIAN_POINT ( 'NONE',  ( -9.297140650669053485, 11.86975006391249643, 1.599625672291281386 ) ) ;
#187062=CARTESIAN_POINT ( 'NONE',  ( 7.402388683381404988, 10.61957531637824204, -1.082531754730537976 ) ) ;
#187063=CARTESIAN_POINT ( 'NONE',  ( 1.364683531249988535, 3.967708333674752286, -0.7879004041258239610 ) ) ;
#187066=CARTESIAN_POINT ( 'NONE',  ( 5.118366684358879759, 5.930181538962194132, 1.199719254218462483 ) ) ;
#187079=CARTESIAN_POINT ( 'NONE',  ( -0.6823417656250003738, 3.030208333674754062, -1.181850606188749264 ) ) ;
#187081=CARTESIAN_POINT ( 'NONE',  ( 2.354312230267378236, 5.898448035287240820, -0.7998128361456281477 ) ) ;
#187083=CARTESIAN_POINT ( 'NONE',  ( -5.910991785878175975, 6.958873840688411860, -1.082531754730544860 ) ) ;
#187084=CARTESIAN_POINT ( 'NONE',  ( 4.067082894419602468, 3.847277586352047862, -0.7216878364870188411 ) ) ;
#187085=CARTESIAN_POINT ( 'NONE',  ( -4.568734577680880093, 7.313645526394248364, -1.082531754730548412 ) ) ;
#187089=CARTESIAN_POINT ( 'NONE',  ( 4.985647801523278133, 6.839675073242382553, -1.599625672291256295 ) ) ;
#187099=CARTESIAN_POINT ( 'NONE',  ( 5.198661835836162481, 8.152523677529138979, 1.199719254218462483 ) ) ;
#187101=CARTESIAN_POINT ( 'NONE',  ( -3.195971524519394702, 4.751719416737803847, -1.599625672291262513 ) ) ;
#187103=CARTESIAN_POINT ( 'NONE',  ( -5.280010757518168063, 8.247430752824802980, -1.199719254218446718 ) ) ;
#187107=CARTESIAN_POINT ( 'NONE',  ( 8.260995669428309540, 8.532249790621511565, 0.7998128361456481317 ) ) ;
#187110=CARTESIAN_POINT ( 'NONE',  ( -7.223796917982883592, 7.322184580601816428, -0.7998128361456291469 ) ) ;
#187111=EDGE_CURVE ( 'NONE', #195163, #108282, #108865, .T. ) ;
#187112=CARTESIAN_POINT ( 'NONE',  ( 5.788968402910795064, 9.697620870130524651, 0.7216878364870438212 ) ) ;
#187113=CARTESIAN_POINT ( 'NONE',  ( 5.132834705836428313, 6.694876404991986441, 1.408819685294822932 ) ) ;
#187114=CARTESIAN_POINT ( 'NONE',  ( -4.141125853970233806, 6.918731698685530063, -1.199719254218452047 ) ) ;
#187118=CARTESIAN_POINT ( 'NONE',  ( -7.413611068574208041, 7.543634422958360730, 0.7998128361456341429 ) ) ;
#187123=CARTESIAN_POINT ( 'NONE',  ( -0.6823417656250003738, 1.967708333674753174, -1.181850606188749264 ) ) ;
#187125=CARTESIAN_POINT ( 'NONE',  ( -5.477130870240893401, 6.452702772444876445, 1.082531754730548412 ) ) ;
#187127=AXIS2_PLACEMENT_3D ( 'NONE', #29213, #12934, #79014 ) ;
#187132=CARTESIAN_POINT ( 'NONE',  ( 4.632082037363250748, 8.555846143565791095, -0.7998128361456231517 ) ) ;
#187134=CARTESIAN_POINT ( 'NONE',  ( -5.733986265252455361, 6.108121862465037744, 0.6873297539724126937 ) ) ;
#187135=CARTESIAN_POINT ( 'NONE',  ( 1.364683531249988535, 1.676041667008085101, 0.7879004041258500513 ) ) ;
#187138=CARTESIAN_POINT ( 'NONE',  ( 1.364683531249986537, -1.073958332991911790, 0.7879004041258500513 ) ) ;
#187139=CARTESIAN_POINT ( 'NONE',  ( 1.499999999999989120, 6.200000000000045475, -2.579999999999995630 ) ) ;
#187141=EDGE_CURVE ( 'NONE', #123984, #201902, #212539, .T. ) ;
#187142=CARTESIAN_POINT ( 'NONE',  ( -4.786191920824102830, 5.542644314838231168, 1.199719254218462483 ) ) ;
#187143=CARTESIAN_POINT ( 'NONE',  ( -6.521108698048767138, 10.55178454779148289, -0.7216878364870267237 ) ) ;
#187151=CARTESIAN_POINT ( 'NONE',  ( -8.663296969008007054, 9.209527340038563992, 0.7216878364870438212 ) ) ;
#187154=FACE_OUTER_BOUND ( 'NONE', #102128, .T. ) ;
#187156=CARTESIAN_POINT ( 'NONE',  ( -8.487040972030346353, 9.003895343564625620, 1.040834085586084257E-14 ) ) ;
#187162=CARTESIAN_POINT ( 'NONE',  ( -1.201851678989727383E-14, 5.618750000682818602, -1.732050807568863648 ) ) ;
#187163=CARTESIAN_POINT ( 'NONE',  ( 4.203240766677102336, 7.568734712931471265, -0.9219714408205395006 ) ) ;
#187164=CARTESIAN_POINT ( 'NONE',  ( 1.499999999999990896, 5.556250000682820378, 1.214306433183764966E-14 ) ) ;
#187170=B_SPLINE_CURVE_WITH_KNOTS ( 'NONE', 3,
 ( #100748, #136470, #5342, #55207, #119197, #121353 ),
 .UNSPECIFIED., .F., .F.,
 ( 4, 2, 4 ),
 ( 0.9260018899588919883, 0.9630662328098654745, 1.000130575660838961 ),
 .UNSPECIFIED. ) ;
#187171=CARTESIAN_POINT ( 'NONE',  ( -5.371001409308059138, 9.417918744168066070, -0.7998128361456231517 ) ) ;
#187174=CARTESIAN_POINT ( 'NONE',  ( 3.822509244049070887, 6.547012320444182798, -1.199719254218452047 ) ) ;
#187178=CARTESIAN_POINT ( 'NONE',  ( 5.144429221381498607, 8.089252293998699272, -1.199719254218452047 ) ) ;
#187182=CARTESIAN_POINT ( 'NONE',  ( -4.772106882330241717, 5.630174786549132726, -1.082531754730544860 ) ) ;
#187193=CARTESIAN_POINT ( 'NONE',  ( -1.201851678989727383E-14, 0.8218750003414171390, 1.575800808251672791 ) ) ;
#187195=CARTESIAN_POINT ( 'NONE',  ( -8.528242318195895066, 9.908369778438709474, 1.199719254218462483 ) ) ;
#187197=CARTESIAN_POINT ( 'NONE',  ( 6.771407655021410399, 9.987393799911945536, -1.199719254218441611 ) ) ;
#187199=CARTESIAN_POINT ( 'NONE',  ( -8.525379664894808585, 8.840697785332414682, -0.7998128361456291469 ) ) ;
#187202=CARTESIAN_POINT ( 'NONE',  ( -1.001543065824772872E-14, 5.321875000341422357, 1.575800808251672791 ) ) ;
#187204=CARTESIAN_POINT ( 'NONE',  ( 9.625925876022625616, 11.29296361252366765, -1.082531754730537088 ) ) ;
#187207=CARTESIAN_POINT ( 'NONE',  ( -1.364683531250014514, -1.157291666325248158, 0.7879004041258379498 ) ) ;
#187210=CARTESIAN_POINT ( 'NONE',  ( 8.093854517234030155, 8.545177812968924869, -0.7216878364870267237 ) ) ;
#187213=CARTESIAN_POINT ( 'NONE',  ( -6.751597309925468693, 6.979211071108916364, 0.7216878364870317197 ) ) ;
#187215=CARTESIAN_POINT ( 'NONE',  ( 0.6823417656249899377, 2.842708333674753618, 1.181850606188765695 ) ) ;
#187219=CARTESIAN_POINT ( 'NONE',  ( -4.869349725602420520, 8.832658446511480577, 1.040834085586084257E-14 ) ) ;
#187220=CARTESIAN_POINT ( 'NONE',  ( -0.6823417656249969321, 5.530208333674756283, -1.181850606188749264 ) ) ;
#187226=CARTESIAN_POINT ( 'NONE',  ( 8.392660782059197189, 9.750191319612612872, 1.199719254218462483 ) ) ;
#187229=CARTESIAN_POINT ( 'NONE',  ( 1.499999999999987121, 3.045833333333353377, -0.8660254037844262731 ) ) ;
#187231=EDGE_CURVE ( 'NONE', #43527, #13744, #18789, .T. ) ;
#187233=CARTESIAN_POINT ( 'NONE',  ( -0.2863318758520757568, 8.150007921796362353, -2.019927845748578310 ) ) ;
#187236=CARTESIAN_POINT ( 'NONE',  ( 6.643132081016125845, 6.852668304048034287, 0.7216878364870317197 ) ) ;
#187237=CARTESIAN_POINT ( 'NONE',  ( -1.402160292154681736E-14, -0.4906249996585810846, -1.575800808251665908 ) ) ;
#187240=CARTESIAN_POINT ( 'NONE',  ( 3.541704441667858472, 5.155074486744371853, -1.599625672291262513 ) ) ;
#187245=CARTESIAN_POINT ( 'NONE',  ( 1.499999999999985123, -0.2041666666666457353, -0.8660254037844323793 ) ) ;
#187246=CARTESIAN_POINT ( 'NONE',  ( 6.238723240582662477, 10.43026088065513513, -0.7998128361456291469 ) ) ;
#187247=CARTESIAN_POINT ( 'NONE',  ( -9.840520565420403543, 10.37502883594562597, 1.040834085586084257E-14 ) ) ;
#187249=CARTESIAN_POINT ( 'NONE',  ( -0.6823417656250246877, 0.05104166700808931978, 1.181850606188755259 ) ) ;
#187250=CARTESIAN_POINT ( 'NONE',  ( -1.402160292154681736E-14, 0.8375000000000232259, -1.732050807568863648 ) ) ;
#187253=CARTESIAN_POINT ( 'NONE',  ( 5.606460214450851964, 6.499623990736163037, 1.199719254218462483 ) ) ;
#187259=CARTESIAN_POINT ( 'NONE',  ( 1.364683531249990311, 5.113541667008084879, 0.7879004041258500513 ) ) ;
#187261=CARTESIAN_POINT ( 'NONE',  ( -6.970863535720637216, 11.28442455831609337, 0.7998128361456481317 ) ) ;
#187263=CARTESIAN_POINT ( 'NONE',  ( -4.392478581147607031, 7.108013530438723748, 1.082531754730560403 ) ) ;
#187265=DIRECTION ( 'NONE',  ( 0.000000000000000000, 0.000000000000000000, -1.000000000000000000 ) ) ;
#187271=CARTESIAN_POINT ( 'NONE',  ( 7.239163954692881653, 10.53310948286200599, -1.199719254218441611 ) ) ;
#187274=CARTESIAN_POINT ( 'NONE',  ( 7.253248993186724114, 9.485209796849769504, 1.443375672974076540 ) ) ;
#187277=CARTESIAN_POINT ( 'NONE',  ( -7.374745490829552885, 10.69128794168811680, -1.199719254218446718 ) ) ;
#187279=CARTESIAN_POINT ( 'NONE',  ( 4.819033534653518025, 7.709623992816043270, -1.199719254218452047 ) ) ;
#187283=CARTESIAN_POINT ( 'NONE',  ( 3.277320446201373638, 4.846626492033466072, 1.599625672291267398 ) ) ;
#187290=CARTESIAN_POINT ( 'NONE',  ( -4.229780737783618072, 6.918199379847403740, 1.082531754730560403 ) ) ;
#187291=CARTESIAN_POINT ( 'NONE',  ( 8.703971430293332645, 12.13808852110884118, -1.082531754730543083 ) ) ;
#187295=CARTESIAN_POINT ( 'NONE',  ( -5.533699252672048985, 9.607732894759390518, -0.7998128361456231517 ) ) ;
#187299=CARTESIAN_POINT ( 'NONE',  ( -8.019811557683421910, 9.315200557840817908, 1.199719254218462483 ) ) ;
#187305=( BOUNDED_SURFACE ( )  B_SPLINE_SURFACE ( 1, 2, ( 
 ( #115203, #32823, #34936, #184387, #133557, #53334, #99956, #83691, #50141, #118401, #180145, #149779, #116263, #98898, #67416, #19755, #164951, #131440, #18686, #199566, #51210, #15482, #66352, #85836, #182254, #49085, #68495, #31771, #16544, #36006, #97841, #197444, #82625, #213669, #117332, #148710, #183330, #101008, #280, #201689, #163906, #167097, #65293, #132496, #151914, #84768, #2418, #198496, #147653, #81567, #134622, #200625, #52274, #102087, #69556, #135666, #24019, #107491, #205975, #22941, #104231, #106408, #91191, #72774, #171347, #170277, #21862, #186528, #38158, #123767, #136733, #8845, #7765, #173517, #73854, #25091, #122704, #41381, #87970, #154044, #5609, #71692, #137805, #207042, #157252, #204891, #203824, #55468, #121624, #20808, #120550, #187593, #119467, #39218, #105309, #138873, #89057, #155114, #57607, #74923, #185455, #6698, #156188, #4546, #54410, #56542, #188667, #189728, #40297, #37077, #172431, #90121, #139949, #141035, #103156, #169217, #86905, #152972, #70619, #202757, #208106, #9912, #111756, #44576, #176688, #108553, #159367, #178836, #143168, #142091, #161520, #146349, #191851, #62928, #58672, #75987, #59734, #92274, #110690, #125892, #160435, #78112, #109634, #80250, #190786, #60802, #158321, #43513, #46707, #61871, #144240, #175640, #26160, #124821, #126960, #210234, #209163, #28301, #10967, #93331, #193990, #27226, #30450, #128036, #77041, #192920, #174584, #94397, #177761, #12041, #45639, #145298, #42449, #29377, #14156, #79183, #95472, #13104, #211303, #195067, #129096, #112822, #96535, #162582, #1102, #35752, #197189, #47784, #48827, #65045, #52018, #132236, #179892, #100753, #64002, #31515, #19494, #150594, #85569, #181993, #149516, #67161, #97590, #113898, #84505, #81319, #163649, #180942, #33626, #15229, #49882, #212361, #101826, #200370, #198244, #116007, #99698, #114942, #68233, #32562, #98639, #199303, #130153, #147395, #29, #165768, #183071, #133297, #213422, #131201, #134366, #167894, #83434, #164698, #16284, #17352, #18431, #118144, #82371, #50948, #2156, #184129, #117073, #34684, #196143, #166835, #148460, #66093, #87709, #185189, #154851, #152708, #155919, #4290, #6435, #168954, #57345, #172171, #72510, #204631, #139689, #119203, #170015, #73587, #56282, #205711, #71433, #120286, #138608, #3229, #21603, #88793, #37895, #201430, #36813, #137545, #38965, #69296, #105050, #106147, #153781, #203563, #5351, #135407, #186261, #23763, #53070, #55215, #107225, #151659, #103973, #188399, #41116, #121361, #187336, #102895, #24829, #173249, #20557, #86641, #171085, #189474, #22681, #54149, #122441, #40035, #70362, #89868, #136476, #7503, #202498, #123509, #141838, #77848, #140766, #45375, #10709, #176432, #156995, #109367, #209964, #78906, #177498, #208900, #75724, #143971, #62658, #44306, #142899, #207844, #59469, #158062, #9648, #95194, #108297, #194798, #193730, #145028, #111490, #211032, #94136, #12832, #125628, #191587, #43248, #175375, #26958, #178565, #128816, #28042, #93065, #159106, #76777, #206778, #92002, #60532, #90929, #126692, #192654, #110428, #160175, #11775, #29111, #46435, #8582, #61604, #127774, #190526, #25892, #161245, #112553, #74662, #58412, #124566, #42182, #174318, #114689, #182810, #30173, #98374, #180681, #31251, #16023, #18163, #179630, #195875, #83171, #82109, #148202, #79981, #130939, #150337, #32307, #113626, #133038, #117888, #163383, #34427, #96262, #47514, #97327, #63732, #214202, #14957, #131981, #49617, #81055, #51768, #162314, #164437, #129891, #147139, #84251, #33362, #115742, #213165, #212096, #13899, #65832, #181731, #197989, #99444, #196932, #64795, #165500, #48570, #1905, #17093, #149255, #828, #146084, #66898, #199037, #50685, #116810, #100500, #166576, #67964, #134108, #200117, #4040, #104794, #86392, #89615, #203314, #151403, #152460, #85320, #52818, #88541, #153533, #2976, #56032, #205463, #70109, #139428, #204375, #20307, #170840, #19240, #138358, #103718, #54964, #35493, #202243, #154603, #171913, #122185, #87465, #168703, #22431, #155666, #137296, #21359, #136222, #53894, #36559, #102647, #188151, #201180, #73326 ),
 ( #72250, #101571, #69044, #57096, #39782, #183881, #5102, #121116, #38714, #135161, #118956, #105888, #184935, #120029, #186005, #71178, #37640, #187081, #167638, #169769, #23510, #6182, #7249, #158864, #174074, #193494, #91757, #157810, #110181, #210798, #24576, #125375, #10461, #93890, #126444, #206530, #124320, #45136, #160998, #208655, #190279, #74419, #43004, #143726, #111246, #8334, #142646, #127523, #177251, #76534, #44062, #12590, #175131, #28863, #191338, #59217, #156744, #192407, #41936, #94950, #108049, #176192, #140518, #78663, #209719, #27792, #159930, #144791, #90683, #109117, #26718, #58162, #11533, #25646, #123261, #9408, #77603, #75479, #189226, #61364, #40866, #106971, #172995, #141591, #207597, #92820, #60285, #198785, #196691, #31010, #49376, #128585, #80812, #213964, #163137, #112313, #96019, #48330, #164193, #194551, #15779, #16840, #212922, #114440, #64556, #46195, #97085, #82922, #178328, #146902, #17900, #62421, #14721, #99195, #166311, #130699, #180440, #162072, #150074, #83986, #29936, #13662, #32057, #100243, #98144, #179390, #81865, #147950, #79734, #50434, #115494, #65584, #145849, #33118, #131731, #211857, #47267, #63493, #113382, #129649, #116553, #197736, #195634, #165246, #181489, #148995, #570, #66637, #132782, #182545, #34171, #70913, #183621, #117630, #88267, #85058, #51504, #184675, #185739, #35228, #53628, #89348, #105609, #204106, #135955, #119760, #37372, #52559, #71983, #36297, #102373, #203050, #1646, #101304, #3769, #103448, #186817, #4833, #151144, #2711, #138093, #39510, #87193, #68785, #167384, #201970, #22152, #55758, #18974, #21090, #5910, #121914, #169508, #137023, #171640, #153258, #187883, #168443, #134904, #200911, #54691, #120843, #67704, #38445, #170570, #152202, #104525, #69844, #133852, #20042, #154335, #118691, #86129, #23237, #199861, #74155, #26458, #109924, #57895, #140249, #123000, #30481, #178869, #205189, #155397, #124058, #6979, #91490, #206270, #157551, #173812, #188957, #126183, #108852, #9147, #56830, #92567, #191080, #73060, #190024, #40597, #41676, #8069, #43811, #75221, #106702, #76281, #172727, #24305, #139159, #90410, #156480, #107787, #25391, #141332, #174878, #42747, #207346, #158607, #10206, #192147, #58967, #142389, #125122, #208398, #60032, #122638, #54348, #38096, #170215, #185393, #204824, #103093, #169152, #121559, #7701, #35947, #136673, #21800, #105244, #137742, #3429, #135603, #56476, #172365, #5547, #201624, #85772, #120487, #155045, #188601, #19694, #153980, #138805, #40232, #87908, #55405, #23955, #186459, #106343, #202698, #70554, #168095, #203762, #53273, #90059, #119404, #187530, #151853, #156119, #6631, #39161, #171284, #134560, #102026, #152905, #200563, #22876, #52210, #104167, #20745, #88992, #118337, #4483, #71629, #184322, #72710, #69496, #37011, #86840, #177414, #111410, #212013, #193648, #196851, #96182, #44227, #45290, #192572, #160093, #195791, #46354, #110349, #163295, #98295, #29032, #32222, #97241, #127688, #63656, #126609, #31168, #210952, #162233, #139880, #95115, #47429, #64711, #14876, #194714, #61522, #129811, #48488, #30093, #128740, #161164, #12750, #143890, #209884, #80968, #94052, #180597, #179547, #130854, #147060, #114606, #79893, #213080, #78824, #144945, #62578, #112473, #178482, #164357, #73784, #13820, #146003, #113544, #208822, #176352, #77770, #60452, #27959, #11696, #18077, #183796, #84164, #150252, #102551, #3952, #82025, #51683, #52730, #115656, #165414, #17010, #85227, #20216, #35405, #103631, #1820, #67878, #100415, #168614, #15941, #134024, #166485, #83086, #200031, #70019, #149165, #181651, #68955, #117804, #101483, #65748, #116722, #136135, #167553, #99363, #118864, #148117, #742, #86304, #214120, #33278, #66808, #49532, #19154, #132950, #151316, #2884, #198955, #37551, #131894, #135076, #50597, #182722, #202151, #201089, #184850, #34341, #197902, #36478, #152374, #53812, #119941, #185917, #109060, #95967, #143672, #212870, #179338, #210746, #110127, #11478, #27739, #26663, #126391, #127468, #125325, #176139, #193439, #78612, #45083, #111192, #211804, #113331, #191285, #160947, #162021 ) ),
 .UNSPECIFIED., .F., .F., .T. ) 
 B_SPLINE_SURFACE_WITH_KNOTS ( ( 2, 2 ),
 ( 3, 2, 2, 2, 2, 2, 2, 2, 2, 2, 2, 2, 2, 2, 2, 2, 2, 2, 2, 2, 2, 2, 2, 2, 2, 2, 2, 2, 2, 2, 2, 2, 2, 2, 2, 2, 2, 2, 2, 2, 2, 2, 2, 2, 2, 2, 2, 2, 2, 2, 2, 2, 2, 2, 2, 2, 2, 2, 2, 2, 2, 2, 2, 2, 2, 2, 2, 2, 2, 2, 2, 2, 2, 2, 2, 2, 2, 2, 2, 2, 2, 2, 2, 2, 2, 2, 2, 2, 2, 2, 2, 2, 2, 2, 2, 2, 2, 2, 2, 2, 2, 2, 2, 2, 2, 2, 2, 2, 2, 2, 2, 2, 2, 2, 2, 2, 2, 2, 2, 2, 2, 2, 2, 2, 2, 2, 2, 2, 2, 2, 2, 2, 2, 2, 2, 2, 2, 2, 2, 2, 2, 2, 2, 2, 2, 2, 2, 2, 2, 2, 2, 2, 2, 2, 2, 2, 2, 2, 2, 2, 2, 2, 2, 2, 2, 2, 2, 2, 2, 2, 2, 2, 2, 2, 2, 2, 2, 2, 2, 2, 2, 2, 2, 2, 2, 2, 2, 2, 2, 2, 2, 2, 2, 2, 2, 2, 2, 2, 2, 2, 2, 2, 2, 2, 2, 2, 2, 2, 2, 2, 2, 2, 2, 2, 2, 2, 2, 2, 2, 2, 2, 2, 2, 2, 2, 2, 2, 2, 2, 2, 2, 2, 2, 2, 2, 2, 2, 2, 2, 2, 3 ),
 ( 0.000000000000000000, 1.000000000000000000 ),
 ( 0.000000000000000000, 0.004166666666666666609, 0.008333333333333333218, 0.01250000000000000069, 0.01666666666666666644, 0.02083333333333333218, 0.02500000000000000139, 0.02916666666666666713, 0.03333333333333333287, 0.03749999999999999861, 0.04166666666666666435, 0.04583333333333333010, 0.05000000000000000278, 0.05416666666666666852, 0.05833333333333333426, 0.06250000000000000000, 0.06666666666666666574, 0.07083333333333333148, 0.07499999999999999722, 0.07916666666666666297, 0.08333333333333332871, 0.08749999999999999445, 0.09166666666666666019, 0.09583333333333333981, 0.1000000000000000056, 0.1041666666666666713, 0.1083333333333333370, 0.1125000000000000028, 0.1166666666666666685, 0.1208333333333333343, 0.1250000000000000000, 0.1291666666666666796, 0.1333333333333333315, 0.1375000000000000111, 0.1416666666666666630, 0.1458333333333333426, 0.1499999999999999944, 0.1541666666666666741, 0.1583333333333333259, 0.1625000000000000056, 0.1666666666666666574, 0.1708333333333333370, 0.1749999999999999889, 0.1791666666666666685, 0.1833333333333333204, 0.1875000000000000000, 0.1916666666666666796, 0.1958333333333333315, 0.2000000000000000111, 0.2041666666666666630, 0.2083333333333333426, 0.2124999999999999944, 0.2166666666666666741, 0.2208333333333333259, 0.2250000000000000056, 0.2291666666666666574, 0.2333333333333333370, 0.2374999999999999889, 0.2416666666666666685, 0.2458333333333333204, 0.2500000000000000000, 0.2541666666666666519, 0.2583333333333333592, 0.2625000000000000111, 0.2666666666666666630, 0.2708333333333333148, 0.2750000000000000222, 0.2791666666666666741, 0.2833333333333333259, 0.2874999999999999778, 0.2916666666666666852, 0.2958333333333333370, 0.2999999999999999889, 0.3041666666666666408, 0.3083333333333333481, 0.3125000000000000000, 0.3166666666666666519, 0.3208333333333333592, 0.3250000000000000111, 0.3291666666666666630, 0.3333333333333333148, 0.3375000000000000222, 0.3416666666666666741, 0.3458333333333333259, 0.3499999999999999778, 0.3541666666666666852, 0.3583333333333333370, 0.3624999999999999889, 0.3666666666666666408, 0.3708333333333333481, 0.3750000000000000000, 0.3791666666666666519, 0.3833333333333333592, 0.3875000000000000111, 0.3916666666666666630, 0.3958333333333333148, 0.4000000000000000222, 0.4041666666666666741, 0.4083333333333333259, 0.4124999999999999778, 0.4166666666666666852, 0.4208333333333333370, 0.4249999999999999889, 0.4291666666666666408, 0.4333333333333333481, 0.4375000000000000000, 0.4416666666666666519, 0.4458333333333333592, 0.4500000000000000111, 0.4541666666666666630, 0.4583333333333333148, 0.4625000000000000222, 0.4666666666666666741, 0.4708333333333333259, 0.4749999999999999778, 0.4791666666666666852, 0.4833333333333333370, 0.4874999999999999889, 0.4916666666666666408, 0.4958333333333333481, 0.5000000000000000000, 0.5041666666666666519, 0.5083333333333333037, 0.5124999999999999556, 0.5166666666666667185, 0.5208333333333333703, 0.5250000000000000222, 0.5291666666666666741, 0.5333333333333333259, 0.5374999999999999778, 0.5416666666666666297, 0.5458333333333332815, 0.5500000000000000444, 0.5541666666666666963, 0.5583333333333333481, 0.5625000000000000000, 0.5666666666666666519, 0.5708333333333333037, 0.5749999999999999556, 0.5791666666666667185, 0.5833333333333333703, 0.5875000000000000222, 0.5916666666666666741, 0.5958333333333333259, 0.5999999999999999778, 0.6041666666666666297, 0.6083333333333332815, 0.6125000000000000444, 0.6166666666666666963, 0.6208333333333333481, 0.6250000000000000000, 0.6291666666666666519, 0.6333333333333333037, 0.6374999999999999556, 0.6416666666666667185, 0.6458333333333333703, 0.6500000000000000222, 0.6541666666666666741, 0.6583333333333333259, 0.6624999999999999778, 0.6666666666666666297, 0.6708333333333332815, 0.6750000000000000444, 0.6791666666666666963, 0.6833333333333333481, 0.6875000000000000000, 0.6916666666666666519, 0.6958333333333333037, 0.6999999999999999556, 0.7041666666666667185, 0.7083333333333333703, 0.7125000000000000222, 0.7166666666666666741, 0.7208333333333333259, 0.7249999999999999778, 0.7291666666666666297, 0.7333333333333332815, 0.7375000000000000444, 0.7416666666666666963, 0.7458333333333333481, 0.7500000000000000000, 0.7541666666666666519, 0.7583333333333333037, 0.7624999999999999556, 0.7666666666666667185, 0.7708333333333333703, 0.7750000000000000222, 0.7791666666666666741, 0.7833333333333333259, 0.7874999999999999778, 0.7916666666666666297, 0.7958333333333332815, 0.8000000000000000444, 0.8041666666666666963, 0.8083333333333333481, 0.8125000000000000000, 0.8166666666666666519, 0.8208333333333333037, 0.8249999999999999556, 0.8291666666666667185, 0.8333333333333333703, 0.8375000000000000222, 0.8416666666666666741, 0.8458333333333333259, 0.8499999999999999778, 0.8541666666666666297, 0.8583333333333332815, 0.8625000000000000444, 0.8666666666666666963, 0.8708333333333333481, 0.8750000000000000000, 0.8791666666666666519, 0.8833333333333333037, 0.8874999999999999556, 0.8916666666666667185, 0.8958333333333333703, 0.9000000000000000222, 0.9041666666666666741, 0.9083333333333333259, 0.9124999999999999778, 0.9166666666666666297, 0.9208333333333332815, 0.9250000000000000444, 0.9291666666666666963, 0.9333333333333333481, 0.9375000000000000000, 0.9416666666666666519, 0.9458333333333333037, 0.9499999999999999556, 0.9541666666666667185, 0.9583333333333333703, 0.9625000000000000222, 0.9666666666666666741, 0.9708333333333333259, 0.9749999999999999778, 0.9791666666666666297, 0.9833333333333332815, 0.9875000000000000444, 0.9916666666666666963, 0.9958333333333333481, 1.000000000000000000 ),
 .UNSPECIFIED. ) 
 GEOMETRIC_REPRESENTATION_ITEM ( )  RATIONAL_B_SPLINE_SURFACE ( (
 ( 1.000000000000000000, 0.8660254037844387076, 1.000000000000000000, 0.8660254037844387076, 1.000000000000000000, 0.8660254037844387076, 1.000000000000000000, 0.8660254037844387076, 1.000000000000000000, 0.8660254037844387076, 1.000000000000000000, 0.8660254037844387076, 1.000000000000000000, 0.8660254037844387076, 1.000000000000000000, 0.8660254037844387076, 1.000000000000000000, 0.8660254037844387076, 1.000000000000000000, 0.8660254037844387076, 1.000000000000000000, 0.8660254037844387076, 1.000000000000000000, 0.8660254037844387076, 1.000000000000000000, 0.8660254037844387076, 1.000000000000000000, 0.8660254037844387076, 1.000000000000000000, 0.8660254037844387076, 1.000000000000000000, 0.8660254037844387076, 1.000000000000000000, 0.8660254037844387076, 1.000000000000000000, 0.8660254037844387076, 1.000000000000000000, 0.8660254037844387076, 1.000000000000000000, 0.8660254037844387076, 1.000000000000000000, 0.8660254037844387076, 1.000000000000000000, 0.8660254037844387076, 1.000000000000000000, 0.8660254037844387076, 1.000000000000000000, 0.8660254037844387076, 1.000000000000000000, 0.8660254037844387076, 1.000000000000000000, 0.8660254037844387076, 1.000000000000000000, 0.8660254037844387076, 1.000000000000000000, 0.8660254037844387076, 1.000000000000000000, 0.8660254037844387076, 1.000000000000000000, 0.8660254037844387076, 1.000000000000000000, 0.8660254037844387076, 1.000000000000000000, 0.8660254037844387076, 1.000000000000000000, 0.8660254037844387076, 1.000000000000000000, 0.8660254037844387076, 1.000000000000000000, 0.8660254037844387076, 1.000000000000000000, 0.8660254037844387076, 1.000000000000000000, 0.8660254037844387076, 1.000000000000000000, 0.8660254037844387076, 1.000000000000000000, 0.8660254037844387076, 1.000000000000000000, 0.8660254037844387076, 1.000000000000000000, 0.8660254037844387076, 1.000000000000000000, 0.8660254037844387076, 1.000000000000000000, 0.8660254037844387076, 1.000000000000000000, 0.8660254037844387076, 1.000000000000000000, 0.8660254037844387076, 1.000000000000000000, 0.8660254037844387076, 1.000000000000000000, 0.8660254037844387076, 1.000000000000000000, 0.8660254037844387076, 1.000000000000000000, 0.8660254037844387076, 1.000000000000000000, 0.8660254037844387076, 1.000000000000000000, 0.8660254037844387076, 1.000000000000000000, 0.8660254037844387076, 1.000000000000000000, 0.8660254037844387076, 1.000000000000000000, 0.8660254037844387076, 1.000000000000000000, 0.8660254037844387076, 1.000000000000000000, 0.8660254037844387076, 1.000000000000000000, 0.8660254037844387076, 1.000000000000000000, 0.8660254037844387076, 1.000000000000000000, 0.8660254037844387076, 1.000000000000000000, 0.8660254037844387076, 1.000000000000000000, 0.8660254037844387076, 1.000000000000000000, 0.8660254037844387076, 1.000000000000000000, 0.8660254037844387076, 1.000000000000000000, 0.8660254037844387076, 1.000000000000000000, 0.8660254037844387076, 1.000000000000000000, 0.8660254037844387076, 1.000000000000000000, 0.8660254037844387076, 1.000000000000000000, 0.8660254037844387076, 1.000000000000000000, 0.8660254037844387076, 1.000000000000000000, 0.8660254037844387076, 1.000000000000000000, 0.8660254037844387076, 1.000000000000000000, 0.8660254037844387076, 1.000000000000000000, 0.8660254037844387076, 1.000000000000000000, 0.8660254037844387076, 1.000000000000000000, 0.8660254037844387076, 1.000000000000000000, 0.8660254037844387076, 1.000000000000000000, 0.8660254037844387076, 1.000000000000000000, 0.8660254037844387076, 1.000000000000000000, 0.8660254037844387076, 1.000000000000000000, 0.8660254037844387076, 1.000000000000000000, 0.8660254037844387076, 1.000000000000000000, 0.8660254037844387076, 1.000000000000000000, 0.8660254037844387076, 1.000000000000000000, 0.8660254037844387076, 1.000000000000000000, 0.8660254037844387076, 1.000000000000000000, 0.8660254037844387076, 1.000000000000000000, 0.8660254037844387076, 1.000000000000000000, 0.8660254037844387076, 1.000000000000000000, 0.8660254037844387076, 1.000000000000000000, 0.8660254037844387076, 1.000000000000000000, 0.8660254037844387076, 1.000000000000000000, 0.8660254037844387076, 1.000000000000000000, 0.8660254037844387076, 1.000000000000000000, 0.8660254037844387076, 1.000000000000000000, 0.8660254037844387076, 1.000000000000000000, 0.8660254037844387076, 1.000000000000000000, 0.8660254037844387076, 1.000000000000000000, 0.8660254037844387076, 1.000000000000000000, 0.8660254037844387076, 1.000000000000000000, 0.8660254037844387076, 1.000000000000000000, 0.8660254037844387076, 1.000000000000000000, 0.8660254037844387076, 1.000000000000000000, 0.8660254037844387076, 1.000000000000000000, 0.8660254037844387076, 1.000000000000000000, 0.8660254037844387076, 1.000000000000000000, 0.8660254037844387076, 1.000000000000000000, 0.8660254037844387076, 1.000000000000000000, 0.8660254037844387076, 1.000000000000000000, 0.8660254037844387076, 1.000000000000000000, 0.8660254037844387076, 1.000000000000000000, 0.8660254037844387076, 1.000000000000000000, 0.8660254037844387076, 1.000000000000000000, 0.8660254037844387076, 1.000000000000000000, 0.8660254037844387076, 1.000000000000000000, 0.8660254037844387076, 1.000000000000000000, 0.8660254037844387076, 1.000000000000000000, 0.8660254037844387076, 1.000000000000000000, 0.8660254037844387076, 1.000000000000000000, 0.8660254037844387076, 1.000000000000000000, 0.8660254037844387076, 1.000000000000000000, 0.8660254037844387076, 1.000000000000000000, 0.8660254037844387076, 1.000000000000000000, 0.8660254037844387076, 1.000000000000000000, 0.8660254037844387076, 1.000000000000000000, 0.8660254037844387076, 1.000000000000000000, 0.8660254037844387076, 1.000000000000000000, 0.8660254037844387076, 1.000000000000000000, 0.8660254037844387076, 1.000000000000000000, 0.8660254037844387076, 1.000000000000000000, 0.8660254037844387076, 1.000000000000000000, 0.8660254037844387076, 1.000000000000000000, 0.8660254037844387076, 1.000000000000000000, 0.8660254037844387076, 1.000000000000000000, 0.8660254037844387076, 1.000000000000000000, 0.8660254037844387076, 1.000000000000000000, 0.8660254037844387076, 1.000000000000000000, 0.8660254037844387076, 1.000000000000000000, 0.8660254037844387076, 1.000000000000000000, 0.8660254037844387076, 1.000000000000000000, 0.8660254037844387076, 1.000000000000000000, 0.8660254037844387076, 1.000000000000000000, 0.8660254037844387076, 1.000000000000000000, 0.8660254037844387076, 1.000000000000000000, 0.8660254037844387076, 1.000000000000000000, 0.8660254037844387076, 1.000000000000000000, 0.8660254037844387076, 1.000000000000000000, 0.8660254037844387076, 1.000000000000000000, 0.8660254037844387076, 1.000000000000000000, 0.8660254037844387076, 1.000000000000000000, 0.8660254037844387076, 1.000000000000000000, 0.8660254037844387076, 1.000000000000000000, 0.8660254037844387076, 1.000000000000000000, 0.8660254037844387076, 1.000000000000000000, 0.8660254037844387076, 1.000000000000000000, 0.8660254037844387076, 1.000000000000000000, 0.8660254037844387076, 1.000000000000000000, 0.8660254037844387076, 1.000000000000000000, 0.8660254037844387076, 1.000000000000000000, 0.8660254037844387076, 1.000000000000000000, 0.8660254037844387076, 1.000000000000000000, 0.8660254037844387076, 1.000000000000000000, 0.8660254037844387076, 1.000000000000000000, 0.8660254037844387076, 1.000000000000000000, 0.8660254037844387076, 1.000000000000000000, 0.8660254037844387076, 1.000000000000000000, 0.8660254037844387076, 1.000000000000000000, 0.8660254037844387076, 1.000000000000000000, 0.8660254037844387076, 1.000000000000000000, 0.8660254037844387076, 1.000000000000000000, 0.8660254037844387076, 1.000000000000000000, 0.8660254037844387076, 1.000000000000000000, 0.8660254037844387076, 1.000000000000000000, 0.8660254037844387076, 1.000000000000000000, 0.8660254037844387076, 1.000000000000000000, 0.8660254037844387076, 1.000000000000000000, 0.8660254037844387076, 1.000000000000000000, 0.8660254037844387076, 1.000000000000000000, 0.8660254037844387076, 1.000000000000000000, 0.8660254037844387076, 1.000000000000000000, 0.8660254037844387076, 1.000000000000000000, 0.8660254037844387076, 1.000000000000000000, 0.8660254037844387076, 1.000000000000000000, 0.8660254037844387076, 1.000000000000000000, 0.8660254037844387076, 1.000000000000000000, 0.8660254037844387076, 1.000000000000000000, 0.8660254037844387076, 1.000000000000000000, 0.8660254037844387076, 1.000000000000000000, 0.8660254037844387076, 1.000000000000000000, 0.8660254037844387076, 1.000000000000000000, 0.8660254037844387076, 1.000000000000000000, 0.8660254037844387076, 1.000000000000000000, 0.8660254037844387076, 1.000000000000000000, 0.8660254037844387076, 1.000000000000000000, 0.8660254037844387076, 1.000000000000000000, 0.8660254037844387076, 1.000000000000000000, 0.8660254037844387076, 1.000000000000000000, 0.8660254037844387076, 1.000000000000000000, 0.8660254037844387076, 1.000000000000000000, 0.8660254037844387076, 1.000000000000000000, 0.8660254037844387076, 1.000000000000000000, 0.8660254037844387076, 1.000000000000000000, 0.8660254037844387076, 1.000000000000000000, 0.8660254037844387076, 1.000000000000000000, 0.8660254037844387076, 1.000000000000000000, 0.8660254037844387076, 1.000000000000000000, 0.8660254037844387076, 1.000000000000000000, 0.8660254037844387076, 1.000000000000000000, 0.8660254037844387076, 1.000000000000000000, 0.8660254037844387076, 1.000000000000000000, 0.8660254037844387076, 1.000000000000000000, 0.8660254037844387076, 1.000000000000000000, 0.8660254037844387076, 1.000000000000000000, 0.8660254037844387076, 1.000000000000000000, 0.8660254037844387076, 1.000000000000000000, 0.8660254037844387076, 1.000000000000000000, 0.8660254037844387076, 1.000000000000000000, 0.8660254037844387076, 1.000000000000000000, 0.8660254037844387076, 1.000000000000000000, 0.8660254037844387076, 1.000000000000000000, 0.8660254037844387076, 1.000000000000000000, 0.8660254037844387076, 1.000000000000000000, 0.8660254037844387076, 1.000000000000000000, 0.8660254037844387076, 1.000000000000000000, 0.8660254037844387076, 1.000000000000000000, 0.8660254037844387076, 1.000000000000000000, 0.8660254037844387076, 1.000000000000000000, 0.8660254037844387076, 1.000000000000000000, 0.8660254037844387076, 1.000000000000000000, 0.8660254037844387076, 1.000000000000000000, 0.8660254037844387076, 1.000000000000000000, 0.8660254037844387076, 1.000000000000000000, 0.8660254037844387076, 1.000000000000000000, 0.8660254037844387076, 1.000000000000000000, 0.8660254037844387076, 1.000000000000000000, 0.8660254037844387076, 1.000000000000000000, 0.8660254037844387076, 1.000000000000000000, 0.8660254037844387076, 1.000000000000000000, 0.8660254037844387076, 1.000000000000000000, 0.8660254037844387076, 1.000000000000000000, 0.8660254037844387076, 1.000000000000000000),
 ( 1.000000000000000000, 0.8660254037844387076, 1.000000000000000000, 0.8660254037844387076, 1.000000000000000000, 0.8660254037844387076, 1.000000000000000000, 0.8660254037844387076, 1.000000000000000000, 0.8660254037844387076, 1.000000000000000000, 0.8660254037844387076, 1.000000000000000000, 0.8660254037844387076, 1.000000000000000000, 0.8660254037844387076, 1.000000000000000000, 0.8660254037844387076, 1.000000000000000000, 0.8660254037844387076, 1.000000000000000000, 0.8660254037844387076, 1.000000000000000000, 0.8660254037844387076, 1.000000000000000000, 0.8660254037844387076, 1.000000000000000000, 0.8660254037844387076, 1.000000000000000000, 0.8660254037844387076, 1.000000000000000000, 0.8660254037844387076, 1.000000000000000000, 0.8660254037844387076, 1.000000000000000000, 0.8660254037844387076, 1.000000000000000000, 0.8660254037844387076, 1.000000000000000000, 0.8660254037844387076, 1.000000000000000000, 0.8660254037844387076, 1.000000000000000000, 0.8660254037844387076, 1.000000000000000000, 0.8660254037844387076, 1.000000000000000000, 0.8660254037844387076, 1.000000000000000000, 0.8660254037844387076, 1.000000000000000000, 0.8660254037844387076, 1.000000000000000000, 0.8660254037844387076, 1.000000000000000000, 0.8660254037844387076, 1.000000000000000000, 0.8660254037844387076, 1.000000000000000000, 0.8660254037844387076, 1.000000000000000000, 0.8660254037844387076, 1.000000000000000000, 0.8660254037844387076, 1.000000000000000000, 0.8660254037844387076, 1.000000000000000000, 0.8660254037844387076, 1.000000000000000000, 0.8660254037844387076, 1.000000000000000000, 0.8660254037844387076, 1.000000000000000000, 0.8660254037844387076, 1.000000000000000000, 0.8660254037844387076, 1.000000000000000000, 0.8660254037844387076, 1.000000000000000000, 0.8660254037844387076, 1.000000000000000000, 0.8660254037844387076, 1.000000000000000000, 0.8660254037844387076, 1.000000000000000000, 0.8660254037844387076, 1.000000000000000000, 0.8660254037844387076, 1.000000000000000000, 0.8660254037844387076, 1.000000000000000000, 0.8660254037844387076, 1.000000000000000000, 0.8660254037844387076, 1.000000000000000000, 0.8660254037844387076, 1.000000000000000000, 0.8660254037844387076, 1.000000000000000000, 0.8660254037844387076, 1.000000000000000000, 0.8660254037844387076, 1.000000000000000000, 0.8660254037844387076, 1.000000000000000000, 0.8660254037844387076, 1.000000000000000000, 0.8660254037844387076, 1.000000000000000000, 0.8660254037844387076, 1.000000000000000000, 0.8660254037844387076, 1.000000000000000000, 0.8660254037844387076, 1.000000000000000000, 0.8660254037844387076, 1.000000000000000000, 0.8660254037844387076, 1.000000000000000000, 0.8660254037844387076, 1.000000000000000000, 0.8660254037844387076, 1.000000000000000000, 0.8660254037844387076, 1.000000000000000000, 0.8660254037844387076, 1.000000000000000000, 0.8660254037844387076, 1.000000000000000000, 0.8660254037844387076, 1.000000000000000000, 0.8660254037844387076, 1.000000000000000000, 0.8660254037844387076, 1.000000000000000000, 0.8660254037844387076, 1.000000000000000000, 0.8660254037844387076, 1.000000000000000000, 0.8660254037844387076, 1.000000000000000000, 0.8660254037844387076, 1.000000000000000000, 0.8660254037844387076, 1.000000000000000000, 0.8660254037844387076, 1.000000000000000000, 0.8660254037844387076, 1.000000000000000000, 0.8660254037844387076, 1.000000000000000000, 0.8660254037844387076, 1.000000000000000000, 0.8660254037844387076, 1.000000000000000000, 0.8660254037844387076, 1.000000000000000000, 0.8660254037844387076, 1.000000000000000000, 0.8660254037844387076, 1.000000000000000000, 0.8660254037844387076, 1.000000000000000000, 0.8660254037844387076, 1.000000000000000000, 0.8660254037844387076, 1.000000000000000000, 0.8660254037844387076, 1.000000000000000000, 0.8660254037844387076, 1.000000000000000000, 0.8660254037844387076, 1.000000000000000000, 0.8660254037844387076, 1.000000000000000000, 0.8660254037844387076, 1.000000000000000000, 0.8660254037844387076, 1.000000000000000000, 0.8660254037844387076, 1.000000000000000000, 0.8660254037844387076, 1.000000000000000000, 0.8660254037844387076, 1.000000000000000000, 0.8660254037844387076, 1.000000000000000000, 0.8660254037844387076, 1.000000000000000000, 0.8660254037844387076, 1.000000000000000000, 0.8660254037844387076, 1.000000000000000000, 0.8660254037844387076, 1.000000000000000000, 0.8660254037844387076, 1.000000000000000000, 0.8660254037844387076, 1.000000000000000000, 0.8660254037844387076, 1.000000000000000000, 0.8660254037844387076, 1.000000000000000000, 0.8660254037844387076, 1.000000000000000000, 0.8660254037844387076, 1.000000000000000000, 0.8660254037844387076, 1.000000000000000000, 0.8660254037844387076, 1.000000000000000000, 0.8660254037844387076, 1.000000000000000000, 0.8660254037844387076, 1.000000000000000000, 0.8660254037844387076, 1.000000000000000000, 0.8660254037844387076, 1.000000000000000000, 0.8660254037844387076, 1.000000000000000000, 0.8660254037844387076, 1.000000000000000000, 0.8660254037844387076, 1.000000000000000000, 0.8660254037844387076, 1.000000000000000000, 0.8660254037844387076, 1.000000000000000000, 0.8660254037844387076, 1.000000000000000000, 0.8660254037844387076, 1.000000000000000000, 0.8660254037844387076, 1.000000000000000000, 0.8660254037844387076, 1.000000000000000000, 0.8660254037844387076, 1.000000000000000000, 0.8660254037844387076, 1.000000000000000000, 0.8660254037844387076, 1.000000000000000000, 0.8660254037844387076, 1.000000000000000000, 0.8660254037844387076, 1.000000000000000000, 0.8660254037844387076, 1.000000000000000000, 0.8660254037844387076, 1.000000000000000000, 0.8660254037844387076, 1.000000000000000000, 0.8660254037844387076, 1.000000000000000000, 0.8660254037844387076, 1.000000000000000000, 0.8660254037844387076, 1.000000000000000000, 0.8660254037844387076, 1.000000000000000000, 0.8660254037844387076, 1.000000000000000000, 0.8660254037844387076, 1.000000000000000000, 0.8660254037844387076, 1.000000000000000000, 0.8660254037844387076, 1.000000000000000000, 0.8660254037844387076, 1.000000000000000000, 0.8660254037844387076, 1.000000000000000000, 0.8660254037844387076, 1.000000000000000000, 0.8660254037844387076, 1.000000000000000000, 0.8660254037844387076, 1.000000000000000000, 0.8660254037844387076, 1.000000000000000000, 0.8660254037844387076, 1.000000000000000000, 0.8660254037844387076, 1.000000000000000000, 0.8660254037844387076, 1.000000000000000000, 0.8660254037844387076, 1.000000000000000000, 0.8660254037844387076, 1.000000000000000000, 0.8660254037844387076, 1.000000000000000000, 0.8660254037844387076, 1.000000000000000000, 0.8660254037844387076, 1.000000000000000000, 0.8660254037844387076, 1.000000000000000000, 0.8660254037844387076, 1.000000000000000000, 0.8660254037844387076, 1.000000000000000000, 0.8660254037844387076, 1.000000000000000000, 0.8660254037844387076, 1.000000000000000000, 0.8660254037844387076, 1.000000000000000000, 0.8660254037844387076, 1.000000000000000000, 0.8660254037844387076, 1.000000000000000000, 0.8660254037844387076, 1.000000000000000000, 0.8660254037844387076, 1.000000000000000000, 0.8660254037844387076, 1.000000000000000000, 0.8660254037844387076, 1.000000000000000000, 0.8660254037844387076, 1.000000000000000000, 0.8660254037844387076, 1.000000000000000000, 0.8660254037844387076, 1.000000000000000000, 0.8660254037844387076, 1.000000000000000000, 0.8660254037844387076, 1.000000000000000000, 0.8660254037844387076, 1.000000000000000000, 0.8660254037844387076, 1.000000000000000000, 0.8660254037844387076, 1.000000000000000000, 0.8660254037844387076, 1.000000000000000000, 0.8660254037844387076, 1.000000000000000000, 0.8660254037844387076, 1.000000000000000000, 0.8660254037844387076, 1.000000000000000000, 0.8660254037844387076, 1.000000000000000000, 0.8660254037844387076, 1.000000000000000000, 0.8660254037844387076, 1.000000000000000000, 0.8660254037844387076, 1.000000000000000000, 0.8660254037844387076, 1.000000000000000000, 0.8660254037844387076, 1.000000000000000000, 0.8660254037844387076, 1.000000000000000000, 0.8660254037844387076, 1.000000000000000000, 0.8660254037844387076, 1.000000000000000000, 0.8660254037844387076, 1.000000000000000000, 0.8660254037844387076, 1.000000000000000000, 0.8660254037844387076, 1.000000000000000000, 0.8660254037844387076, 1.000000000000000000, 0.8660254037844387076, 1.000000000000000000, 0.8660254037844387076, 1.000000000000000000, 0.8660254037844387076, 1.000000000000000000, 0.8660254037844387076, 1.000000000000000000, 0.8660254037844387076, 1.000000000000000000, 0.8660254037844387076, 1.000000000000000000, 0.8660254037844387076, 1.000000000000000000, 0.8660254037844387076, 1.000000000000000000, 0.8660254037844387076, 1.000000000000000000, 0.8660254037844387076, 1.000000000000000000, 0.8660254037844387076, 1.000000000000000000, 0.8660254037844387076, 1.000000000000000000, 0.8660254037844387076, 1.000000000000000000, 0.8660254037844387076, 1.000000000000000000, 0.8660254037844387076, 1.000000000000000000, 0.8660254037844387076, 1.000000000000000000, 0.8660254037844387076, 1.000000000000000000, 0.8660254037844387076, 1.000000000000000000, 0.8660254037844387076, 1.000000000000000000, 0.8660254037844387076, 1.000000000000000000, 0.8660254037844387076, 1.000000000000000000, 0.8660254037844387076, 1.000000000000000000, 0.8660254037844387076, 1.000000000000000000, 0.8660254037844387076, 1.000000000000000000, 0.8660254037844387076, 1.000000000000000000, 0.8660254037844387076, 1.000000000000000000, 0.8660254037844387076, 1.000000000000000000, 0.8660254037844387076, 1.000000000000000000, 0.8660254037844387076, 1.000000000000000000, 0.8660254037844387076, 1.000000000000000000, 0.8660254037844387076, 1.000000000000000000, 0.8660254037844387076, 1.000000000000000000, 0.8660254037844387076, 1.000000000000000000, 0.8660254037844387076, 1.000000000000000000, 0.8660254037844387076, 1.000000000000000000, 0.8660254037844387076, 1.000000000000000000, 0.8660254037844387076, 1.000000000000000000, 0.8660254037844387076, 1.000000000000000000, 0.8660254037844387076, 1.000000000000000000, 0.8660254037844387076, 1.000000000000000000, 0.8660254037844387076, 1.000000000000000000, 0.8660254037844387076, 1.000000000000000000, 0.8660254037844387076, 1.000000000000000000, 0.8660254037844387076, 1.000000000000000000, 0.8660254037844387076, 1.000000000000000000, 0.8660254037844387076, 1.000000000000000000, 0.8660254037844387076, 1.000000000000000000, 0.8660254037844387076, 1.000000000000000000, 0.8660254037844387076, 1.000000000000000000, 0.8660254037844387076, 1.000000000000000000, 0.8660254037844387076, 1.000000000000000000, 0.8660254037844387076, 1.000000000000000000, 0.8660254037844387076, 1.000000000000000000, 0.8660254037844387076, 1.000000000000000000, 0.8660254037844387076, 1.000000000000000000) ) ) 
 REPRESENTATION_ITEM ( '' )  SURFACE ( )  );
#187309=EDGE_LOOP ( 'NONE', ( #57748, #25066, #134338, #163281 ) ) ;
#187317=CARTESIAN_POINT ( 'NONE',  ( -5.208303565944065738, 9.228104593576741621, -0.7998128361456231517 ) ) ;
#187320=CARTESIAN_POINT ( 'NONE',  ( 4.500943810056890371, 8.194925511800951412, -0.7216878364870207285 ) ) ;
#187321=EDGE_LOOP ( 'NONE', ( #191925, #52735, #5906, #116487 ) ) ;
#187322=CARTESIAN_POINT ( 'NONE',  ( -0.01856135223283512589, 6.487495393664096888, 3.100011470320014340 ) ) ;
#187325=CARTESIAN_POINT ( 'NONE',  ( -6.437424008390261854, 6.404749519410410485, 0.7998128361456341429 ) ) ;
#187329=CARTESIAN_POINT ( 'NONE',  ( -6.826694039680798021, 7.923230120171105284, -1.199719254218446718 ) ) ;
#187330=CARTESIAN_POINT ( 'NONE',  ( -5.862481816454102379, 6.029744924107142801, -0.3769115147483664274 ) ) ;
#187335=CARTESIAN_POINT ( 'NONE',  ( -9.854078719034067291, 10.39084668182823634, 0.7998128361456462443 ) ) ;
#187336=CARTESIAN_POINT ( 'NONE',  ( 6.089583550832340819, 10.25626457594641749, 1.040834085586084257E-14 ) ) ;
#187339=CARTESIAN_POINT ( 'NONE',  ( -7.974166903131914452, 12.45494515362926435, -0.7998128361456281477 ) ) ;
#187342=CARTESIAN_POINT ( 'NONE',  ( -1.364683531250014514, -0.9072916663252470482, 0.7879004041258379498 ) ) ;
#187346=CARTESIAN_POINT ( 'NONE',  ( 8.405692050792682224, 12.75046512599275772, -0.7216878364870328300 ) ) ;
#187352=CARTESIAN_POINT ( 'NONE',  ( -5.711861010086065171, 6.121870493066576380, -0.7247779672692231667 ) ) ;
#187366=CARTESIAN_POINT ( 'NONE',  ( -3.164938793786285842, 5.779846795137578930, -1.199719254218452935 ) ) ;
#187369=CARTESIAN_POINT ( 'NONE',  ( -2.449219305563052895, 6.009172956465517856, 1.040834085586084257E-14 ) ) ;
#187373=CARTESIAN_POINT ( 'NONE',  ( 1.499999999999987121, -1.214583332650518432, 0.8660254037844524744 ) ) ;
#187381=CARTESIAN_POINT ( 'NONE',  ( 10.56588178375152864, 11.22128359066528169, -0.7998128361456281477 ) ) ;
#187386=CARTESIAN_POINT ( 'NONE',  ( 6.498435699651741615, 6.475929825882159818, -0.7998128361456281477 ) ) ;
#187387=CARTESIAN_POINT ( 'NONE',  ( 1.364683531249986537, 2.717708333674754062, -0.7879004041258239610 ) ) ;
#187390=CARTESIAN_POINT ( 'NONE',  ( -8.565000355531095622, 11.01558638625153286, -1.599625672291263179 ) ) ;
#187391=CARTESIAN_POINT ( 'NONE',  ( -4.080641047588914994, 5.783833860318930320, -1.443375672974051449 ) ) ;
#187393=CARTESIAN_POINT ( 'NONE',  ( -4.869349725602420520, 8.832658446511480577, 1.040834085586084257E-14 ) ) ;
#187395=CARTESIAN_POINT ( 'NONE',  ( -0.6823417656250212460, 5.301041667008086655, 1.181850606188767472 ) ) ;
#187403=CARTESIAN_POINT ( 'NONE',  ( -5.300874872818844175, 7.207439989753867238, 1.443375672974064550 ) ) ;
#187409=CARTESIAN_POINT ( 'NONE',  ( -5.233084104750526322, 5.207612331738130429, 0.000000000000000000 ) ) ;
#187411=CARTESIAN_POINT ( 'NONE',  ( 8.615316546479974136, 12.13862083994696839, 1.199719254218450271 ) ) ;
#187417=VERTEX_POINT ( 'NONE', #212526 ) ;
#187422=FACE_OUTER_BOUND ( 'NONE', #91949, .T. ) ;
#187428=CARTESIAN_POINT ( 'NONE',  ( 4.808338034340912337, 8.761478140039733020, 1.040834085586084257E-14 ) ) ;
#187431=EDGE_LOOP ( 'NONE', ( #144217, #53097, #14862 ) ) ;
#187433=CARTESIAN_POINT ( 'NONE',  ( 4.379447312414087357, 5.068108938359919158, -1.199719254218452047 ) ) ;
#187436=ORIENTED_EDGE ( 'NONE', *, *, #92993, .T. ) ;
#187440=VECTOR ( 'NONE', #53837, 1000.000000000000227 ) ;
#187445=CARTESIAN_POINT ( 'NONE',  ( 9.433775957010412938, 9.900493459467314850, 0.000000000000000000 ) ) ;
#187446=CARTESIAN_POINT ( 'NONE',  ( -4.388035272317281077, 8.271124917678806199, 0.7998128361456481317 ) ) ;
#187452=CARTESIAN_POINT ( 'NONE',  ( -1.364683531250010295, 5.280208333674758059, 0.7879004041258379498 ) ) ;
#187454=CARTESIAN_POINT ( 'NONE',  ( -6.573005544526917099, 6.562927978236513304, -0.7998128361456291469 ) ) ;
#187458=CARTESIAN_POINT ( 'NONE',  ( 6.030679399980265920, 5.930214142932100252, -0.7998128361456281477 ) ) ;
#187459=CARTESIAN_POINT ( 'NONE',  ( -5.949330478298285207, 5.835307067636438028, 0.7998128361456341429 ) ) ;
#187465=CARTESIAN_POINT ( 'NONE',  ( 5.477130870240836558, 9.333810415348903433, -0.7216878364870267237 ) ) ;
#187467=CARTESIAN_POINT ( 'NONE',  ( 7.253248993186731219, 8.524840582548424806, 1.082531754730558626 ) ) ;
#187468=CARTESIAN_POINT ( 'NONE',  ( -1.364683531249997417, 3.821875000341416584, 1.214306433183764966E-14 ) ) ;
#187470=CARTESIAN_POINT ( 'NONE',  ( 5.517805330637495231, 6.500156309574290248, -1.082531754730543083 ) ) ;
#187478=CARTESIAN_POINT ( 'NONE',  ( -5.283800884368243800, 6.573997454655339467, 1.390413726763789937 ) ) ;
#187485=CARTESIAN_POINT ( 'NONE',  ( -7.994504133552415404, 12.47867192245318435, -0.7998128361456281477 ) ) ;
#187495=CARTESIAN_POINT ( 'NONE',  ( 2.738383840280320669, 6.138605547061593448, 0.7216878364870338292 ) ) ;
#187496=CARTESIAN_POINT ( 'NONE',  ( -1.364683531249997417, 3.821875000341416584, 1.214306433183764966E-14 ) ) ;
#187498=CARTESIAN_POINT ( 'NONE',  ( 7.182068686937156166, 9.402166106225269715, 1.599625672291281386 ) ) ;
#187499=CARTESIAN_POINT ( 'NONE',  ( -9.992522908471816123, 11.61669713376064372, 1.199719254218462483 ) ) ;
#187500=CARTESIAN_POINT ( 'NONE',  ( -3.314994193297896796, 6.393354490853021765, -0.7784788408506218005 ) ) ;
#187502=VECTOR ( 'NONE', #63846, 1000.000000000000114 ) ;
#187504=ORIENTED_EDGE ( 'NONE', *, *, #95474, .T. ) ;
#187506=CARTESIAN_POINT ( 'NONE',  ( 1.499999999999990896, 4.525000000000021672, 1.214306433183764966E-14 ) ) ;
#187507=CARTESIAN_POINT ( 'NONE',  ( 3.635557746758808495, 7.393234471193928847, -0.7998128361456291469 ) ) ;
#187510=CARTESIAN_POINT ( 'NONE',  ( -1.201851678989727383E-14, 3.946875000341423689, -1.575800808251660134 ) ) ;
#187514=CARTESIAN_POINT ( 'NONE',  ( 9.734391104931955141, 10.45913716528321125, 0.7216878364870438212 ) ) ;
#187519=CARTESIAN_POINT ( 'NONE',  ( -1.500000000000013101, 1.910416667349488451, -0.8660254037844313801 ) ) ;
#187521=CARTESIAN_POINT ( 'NONE',  ( -5.799137018343247796, 7.788745826199009237, -1.599625672291256295 ) ) ;
#187522=CARTESIAN_POINT ( 'NONE',  ( 4.650083499362867911, 6.448183387388563226, 1.443375672974062551 ) ) ;
#187530=CARTESIAN_POINT ( 'NONE',  ( 6.286176778230493589, 10.48562334124426698, 0.7998128361456462443 ) ) ;
#187531=CARTESIAN_POINT ( 'NONE',  ( 5.009901455449552010, 5.803638771901306725, -1.199719254218452047 ) ) ;
#187534=EDGE_CURVE ( 'NONE', #111607, #103797, #74476, .T. ) ;
#187535=CARTESIAN_POINT ( 'NONE',  ( 7.334597915313080918, 9.580116872663850813, 1.040834085586084257E-14 ) ) ;
#187536=CARTESIAN_POINT ( 'NONE',  ( 4.808338034340912337, 8.761478140039733020, 1.040834085586084257E-14 ) ) ;
#187537=DIRECTION ( 'NONE',  ( -1.000000000000000000, 8.673617379884035472E-16, 0.000000000000000000 ) ) ;
#187542=CARTESIAN_POINT ( 'NONE',  ( 10.05067194643221207, 10.62020544712608938, 0.7998128361456462443 ) ) ;
#187547=CARTESIAN_POINT ( 'NONE',  ( 5.463439706979909438, 6.248932391672394893, 1.002290858133829010 ) ) ;
#187553=CARTESIAN_POINT ( 'NONE',  ( -0.7499999999999972244, 5.639583334016151639, -1.299038105676652899 ) ) ;
#187554=CARTESIAN_POINT ( 'NONE',  ( 6.471393748265540147, 5.229711127717882491, 2.420000000000010587 ) ) ;
#187555=CARTESIAN_POINT ( 'NONE',  ( 6.805829924380108586, 8.963220883242035697, 1.443375672974076540 ) ) ;
#187557=CARTESIAN_POINT ( 'NONE',  ( -4.925689880466507908, 4.641059703499347044, -0.7998128361456221525 ) ) ;
#187562=CARTESIAN_POINT ( 'NONE',  ( -5.687809136132860210, 6.594531066031826150, -1.199719254218446718 ) ) ;
#187575=CARTESIAN_POINT ( 'NONE',  ( 8.075853055234393452, 12.57357899774884658, 0.7998128361456462443 ) ) ;
#187581=CARTESIAN_POINT ( 'NONE',  ( 5.314433026432511475, 5.302519407033794430, 1.040834085586084257E-14 ) ) ;
#187582=CARTESIAN_POINT ( 'NONE',  ( -8.785320351975364872, 12.23299559640450518, 1.082531754730560403 ) ) ;
#187583=CIRCLE ( 'NONE', #56170, 0.8300000000000008482 ) ;
#187587=CARTESIAN_POINT ( 'NONE',  ( 8.535021395002688749, 9.916278701380017324, 1.199719254218462483 ) ) ;
#187592=CARTESIAN_POINT ( 'NONE',  ( -7.562750758324527922, 7.717630727667075696, 1.040834085586084257E-14 ) ) ;
#187593=CARTESIAN_POINT ( 'NONE',  ( 3.337278367258157630, 7.045241861776501580, 0.7998128361456341429 ) ) ;
#187596=CARTESIAN_POINT ( 'NONE',  ( 10.22692794340986921, 10.82583744360002243, 0.000000000000000000 ) ) ;
#187600=CARTESIAN_POINT ( 'NONE',  ( 1.364683531249990311, 2.696875000341415696, 1.214306433183764966E-14 ) ) ;
#187602=CARTESIAN_POINT ( 'NONE',  ( 7.307481608085759639, 7.627742752295940676, 1.040834085586084257E-14 ) ) ;
#187604=CARTESIAN_POINT ( 'NONE',  ( -1.201851678989727383E-14, 4.618750000682821266, -1.732050807568863648 ) ) ;
#187610=CARTESIAN_POINT ( 'NONE',  ( 8.609064354553323639, 10.10662517080946543, -1.082531754730543083 ) ) ;
#187614=CARTESIAN_POINT ( 'NONE',  ( -8.154339323615371171, 11.60081407993821045, 1.199719254218453823 ) ) ;
#187623=CARTESIAN_POINT ( 'NONE',  ( 2.869522067586683711, 6.499526178826442013, 0.7998128361456362523 ) ) ;
#187624=VECTOR ( 'NONE', #101231, 1000.000000000000000 ) ;
#187629=CARTESIAN_POINT ( 'NONE',  ( 5.823390672269506574, 6.752709524857930745, -1.199719254218446718 ) ) ;
#187632=CARTESIAN_POINT ( 'NONE',  ( -0.7500000000000215383, 2.972916667349487341, 1.299038105676671107 ) ) ;
#187638=CARTESIAN_POINT ( 'NONE',  ( -0.7500000000000249800, -0.05833333333331303105, 1.299038105676659116 ) ) ;
#187639=CARTESIAN_POINT ( 'NONE',  ( 6.089583550832340819, 10.25626457594641749, 1.040834085586084257E-14 ) ) ;
#187643=CARTESIAN_POINT ( 'NONE',  ( 9.897088948295946764, 10.64895131587453569, 0.7216878364870438212 ) ) ;
#187650=CARTESIAN_POINT ( 'NONE',  ( -5.422371370461663176, 8.413518134592214537, -1.199719254218446718 ) ) ;
#187651=CARTESIAN_POINT ( 'NONE',  ( -1.500000000000013101, 2.910416667349485120, -0.8660254037844313801 ) ) ;
#187652=CARTESIAN_POINT ( 'NONE',  ( -1.364683531250010295, 5.092708333674757171, 0.7879004041258379498 ) ) ;
#187657=CARTESIAN_POINT ( 'NONE',  ( -1.364683531250012516, 3.801041667008087099, -0.7879004041258300672 ) ) ;
#187664=CARTESIAN_POINT ( 'NONE',  ( -8.636707547105197946, 10.03491254549959777, -1.199719254218446718 ) ) ;
#187665=CARTESIAN_POINT ( 'NONE',  ( 4.794779880727245036, 8.745660294157122649, -0.7998128361456281477 ) ) ;
#187673=CARTESIAN_POINT ( 'NONE',  ( -7.718669524881690336, 7.899535955317097624, 0.7998128361456462443 ) ) ;
#187680=CARTESIAN_POINT ( 'NONE',  ( 3.891353782322113375, 4.498666486585943147, -1.199719254218446718 ) ) ;
#187683=CARTESIAN_POINT ( 'NONE',  ( -3.405069135326500351, 7.124331091189553433, 1.040834085586084257E-14 ) ) ;
#187684=CARTESIAN_POINT ( 'NONE',  ( -8.727698198895085469, 11.20540053684285553, -1.599625672291263179 ) ) ;
#187687=CARTESIAN_POINT ( 'NONE',  ( -4.695925055628692668, 7.055611427533158064, -1.405632220554285272 ) ) ;
#187688=CARTESIAN_POINT ( 'NONE',  ( 1.364683531249986537, -0.6364583329919177856, 0.7879004041258500513 ) ) ;
#187694=CARTESIAN_POINT ( 'NONE',  ( 4.971035877704902184, 8.951292290631053916, 1.040834085586084257E-14 ) ) ;
#187695=ADVANCED_FACE ( 'NONE', ( #52175 ), #190845, .T. ) ;
#187718=CARTESIAN_POINT ( 'NONE',  ( -7.960608749518247151, 12.43912730774665576, 0.000000000000000000 ) ) ;
#187724=CARTESIAN_POINT ( 'NONE',  ( 0.7499999999999885647, 1.847916667349486231, -1.299038105676652899 ) ) ;
#187728=CARTESIAN_POINT ( 'NONE',  ( -8.455481356417053007, 13.01647868246193518, 0.7998128361456341429 ) ) ;
#187729=CARTESIAN_POINT ( 'NONE',  ( 4.337593226613512876, 3.996631841756838277, -0.04457646079592735011 ) ) ;
#187730=CARTESIAN_POINT ( 'NONE',  ( -1.364683531250014514, 1.238541667008091096, -0.7879004041258289570 ) ) ;
#187738=CARTESIAN_POINT ( 'NONE',  ( -5.739179097286464248, 5.590130456455974617, -0.7998128361456221525 ) ) ;
#187743=CARTESIAN_POINT ( 'NONE',  ( -1.364683531250000748, 0.07187500034142035865, 0.000000000000000000 ) ) ;
#187748=CARTESIAN_POINT ( 'NONE',  ( -0.6823417656250003738, 0.2177083336747515085, -1.181850606188749264 ) ) ;
#187750=CARTESIAN_POINT ( 'NONE',  ( -6.527360889975461156, 9.702672574024962415, 1.199719254218452047 ) ) ;
#187751=CARTESIAN_POINT ( 'NONE',  ( 8.971744963941056028, 11.49012176272984931, 1.599625672291281386 ) ) ;
#187755=CARTESIAN_POINT ( 'NONE',  ( 1.364683531249988757, 0.9468750003414211358, 0.000000000000000000 ) ) ;
#187762=CARTESIAN_POINT ( 'NONE',  ( 5.151735183512854199, 8.954182114166247430, -0.7216878364870257245 ) ) ;
#187765=CARTESIAN_POINT ( 'NONE',  ( -8.199983978166823562, 8.461069484149769337, -0.7998128361456291469 ) ) ;
#187766=CARTESIAN_POINT ( 'NONE',  ( -5.413783410558481002, 5.210502155273325720, -0.7998128361456221525 ) ) ;
#187769=CARTESIAN_POINT ( 'NONE',  ( -1.123270288250315163, 3.047697346350006331, -0.7749999999993613109 ) ) ;
#187770=CARTESIAN_POINT ( 'NONE',  ( 5.788968402910812827, 6.816513227226497662, 1.082531754730558626 ) ) ;
#187771=CARTESIAN_POINT ( 'NONE',  ( -7.985389288324697965, 10.33937347451072775, -1.443375672974058777 ) ) ;
#187773=CARTESIAN_POINT ( 'NONE',  ( -0.7500000000000215383, 4.441666666666691299, 1.299038105676671107 ) ) ;
#187778=CARTESIAN_POINT ( 'NONE',  ( 7.592202833972727660, 11.80139437303613015, -0.7216878364870267237 ) ) ;
#187791=CARTESIAN_POINT ( 'NONE',  ( 8.392133896734668141, 9.853539636687704828, 1.082531754730558626 ) ) ;
#187792=CARTESIAN_POINT ( 'NONE',  ( 8.209625708274705502, 9.536650400197368427, 1.199719254218462483 ) ) ;
#187794=CARTESIAN_POINT ( 'NONE',  ( -5.368138756007025947, 8.350246751061767725, 1.199719254218452047 ) ) ;
#187799=CARTESIAN_POINT ( 'NONE',  ( 4.121315508874254796, 5.831287398485176077, -1.443375672974051449 ) ) ;
#187802=CARTESIAN_POINT ( 'NONE',  ( -6.371969008742801144, 10.37778824360119145, 0.7216878364870458196 ) ) ;
#187818=CARTESIAN_POINT ( 'NONE',  ( 6.584456157731144899, 10.83361595066169514, -0.7998128361456291469 ) ) ;
#187828=CARTESIAN_POINT ( 'NONE',  ( -2.298420387838187473, 5.509269730139584986, -0.7346435760097105305 ) ) ;
#187830=CARTESIAN_POINT ( 'NONE',  ( -6.063521013809733518, 8.097193820909906137, 1.599625672291283607 ) ) ;
#187832=CARTESIAN_POINT ( 'NONE',  ( -4.205000198532790279, 8.057583998263570635, 0.7998128361456341429 ) ) ;
#187842=CARTESIAN_POINT ( 'NONE',  ( -3.415764635639130020, 6.072476943965863683, 1.199719254218462483 ) ) ;
#187845=CARTESIAN_POINT ( 'NONE',  ( 7.610204295972345712, 7.772993188256215547, 0.7998128361456341429 ) ) ;
#187848=CARTESIAN_POINT ( 'NONE',  ( 5.870433092755101612, 6.171306251675328092, 0.8628692295504901688 ) ) ;
#187853=CARTESIAN_POINT ( 'NONE',  ( 4.758548728272192108, 7.535095368750792666, -1.082531754730549078 ) ) ;
#187854=CARTESIAN_POINT ( 'NONE',  ( -6.320072162264675164, 10.52516795595079557, 0.7998128361456481317 ) ) ;
#187857=CARTESIAN_POINT ( 'NONE',  ( -9.481229494658258261, 9.955855920056455588, -0.7998128361456291469 ) ) ;
#187858=CARTESIAN_POINT ( 'NONE',  ( -6.749261541504576911, 6.768559974710451677, 1.040834085586084257E-14 ) ) ;
#187862=CARTESIAN_POINT ( 'NONE',  ( 4.902486209380604087, 4.845403771096273182, 0.6282069583892326836 ) ) ;
#187865=CARTESIAN_POINT ( 'NONE',  ( 8.209625708274705502, 9.536650400197368427, 1.199719254218462483 ) ) ;
#187881=CARTESIAN_POINT ( 'NONE',  ( -1.500000000000011324, 4.670833333333353821, 0.8660254037844403729 ) ) ;
#187882=CARTESIAN_POINT ( 'NONE',  ( 4.039439701867726384, 6.800097854565950506, 1.199719254218462483 ) ) ;
#187883=CARTESIAN_POINT ( 'NONE',  ( 5.307127064745490230, 8.279066444590018392, -1.199719254218452935 ) ) ;
#187885=CARTESIAN_POINT ( 'NONE',  ( -8.676855123066022912, 10.18571440074093282, -1.082531754730543971 ) ) ;
#187886=CARTESIAN_POINT ( 'NONE',  ( 5.938108093105483931, 8.911247961056314892, -1.082531754730537088 ) ) ;
#187887=CARTESIAN_POINT ( 'NONE',  ( -9.449669878600625239, 10.12696240122997082, -0.7216878364870267237 ) ) ;
#187891=CARTESIAN_POINT ( 'NONE',  ( 7.079328764629950754, 11.41096732537697633, 0.7998128361456462443 ) ) ;
#187896=CARTESIAN_POINT ( 'NONE',  ( -1.364683531250000748, 2.259375000341422357, 1.214306433183764966E-14 ) ) ;
#187902=CARTESIAN_POINT ( 'NONE',  ( 8.015895134177609904, 10.37496362800581018, 1.599625672291281386 ) ) ;
#187905=CARTESIAN_POINT ( 'NONE',  ( -8.805130697071332335, 12.36007068230351358, 1.199719254218462483 ) ) ;
#187911=CARTESIAN_POINT ( 'NONE',  ( 10.53876547652418338, 11.18964789890005918, 0.7998128361456462443 ) ) ;
#187914=CARTESIAN_POINT ( 'NONE',  ( -9.612894607289142357, 11.17379744904754801, -1.199719254218441611 ) ) ;
#187917=CARTESIAN_POINT ( 'NONE',  ( 9.610031953988080744, 10.10612545594124967, -0.7998128361456281477 ) ) ;
#187919=CARTESIAN_POINT ( 'NONE',  ( 5.290189798603822879, 6.367883502209223501, 1.128355864069837455 ) ) ;
#187920=CARTESIAN_POINT ( 'NONE',  ( 1.150222622689962781, 3.233395032273045810, -0.7749999999993620881 ) ) ;
#187921=CARTESIAN_POINT ( 'NONE',  ( -5.091250377131585125, 5.898545847196970726, 1.199719254218450271 ) ) ;
#187926=CARTESIAN_POINT ( 'NONE',  ( 8.586391356156291010, 8.911878091804165791, 0.7998128361456481317 ) ) ;
#187928=CARTESIAN_POINT ( 'NONE',  ( 7.800018446563675489, 7.994443030612759848, -0.7998128361456281477 ) ) ;
#187931=CARTESIAN_POINT ( 'NONE',  ( -9.653042183249972652, 10.36423008998754192, -0.7216878364870267237 ) ) ;
#187939=CARTESIAN_POINT ( 'NONE',  ( -4.869203491162207520, 6.719169366249152731, -1.250126817991310757 ) ) ;
#187941=CARTESIAN_POINT ( 'NONE',  ( 6.819388077993785657, 7.058300300521964665, 1.040834085586084257E-14 ) ) ;
#187943=ADVANCED_FACE ( 'NONE', ( #7472 ), #73551, .F. ) ;
#187953=CARTESIAN_POINT ( 'NONE',  ( 2.889785579457926801, 6.440540434672812786, -0.3822207396134719715 ) ) ;
#187955=ORIENTED_EDGE ( 'NONE', *, *, #16995, .F. ) ;
#187965=CARTESIAN_POINT ( 'NONE',  ( 7.313733799568044702, 10.62010763521636214, 1.199719254218460707 ) ) ;
#187967=ORIENTED_EDGE ( 'NONE', *, *, #190385, .F. ) ;
#187969=CARTESIAN_POINT ( 'NONE',  ( 1.499999999999987121, 1.035416667349484232, 0.8660254037844524744 ) ) ;
#187971=CARTESIAN_POINT ( 'NONE',  ( -6.287230548435221777, 8.358188277972981695, -1.599625672291263179 ) ) ;
#187974=CARTESIAN_POINT ( 'NONE',  ( -9.982881178363895103, 10.54111621771303753, 1.040834085586084257E-14 ) ) ;
#187979=CARTESIAN_POINT ( 'NONE',  ( 5.601490020740366838, 9.686822124172440596, 1.040834085586084257E-14 ) ) ;
#187981=ORIENTED_EDGE ( 'NONE', *, *, #165987, .T. ) ;
#187983=CARTESIAN_POINT ( 'NONE',  ( -8.037286134802835491, 8.271255333558444889, -0.7998128361456291469 ) ) ;
#187985=CARTESIAN_POINT ( 'NONE',  ( 0.6823417656249917140, 4.592708333674755394, 1.181850606188765695 ) ) ;
#187991=CARTESIAN_POINT ( 'NONE',  ( -7.863365906246061243, 10.19701286208565705, -1.443375672974059665 ) ) ;
#187995=CARTESIAN_POINT ( 'NONE',  ( 0.6823417656249899377, 3.738541667008085767, -1.181850606188754593 ) ) ;
#188001=CARTESIAN_POINT ( 'NONE',  ( 1.364683531249988535, 4.905208333674756283, -0.7879004041258300672 ) ) ;
#188004=CARTESIAN_POINT ( 'NONE',  ( 2.670593071767634719, 6.059516317130127838, -0.7216878364870267237 ) ) ;
#188005=CARTESIAN_POINT ( 'NONE',  ( 0.6823417656249899377, 5.238541667008086655, -1.181850606188754593 ) ) ;
#188006=DIRECTION ( 'NONE',  ( -0.000000000000000000, -8.546850786086437571E-32, -1.000000000000000000 ) ) ;
#188010=CARTESIAN_POINT ( 'NONE',  ( 1.364683531249986537, 0.3635416670080869328, 0.7879004041258500513 ) ) ;
#188011=CARTESIAN_POINT ( 'NONE',  ( -3.877268743828284681, 5.546566172598190292, 1.443375672974064550 ) ) ;
#188012=CARTESIAN_POINT ( 'NONE',  ( 3.988069740714122791, 7.804498464141805592, 0.7998128361456321445 ) ) ;
#188018=CARTESIAN_POINT ( 'NONE',  ( 4.039966587192267866, 4.776011108888172707, 1.082531754730560403 ) ) ;
#188021=CARTESIAN_POINT ( 'NONE',  ( -8.514157279702033065, 9.995900250149611921, -1.082531754730543971 ) ) ;
#188026=CARTESIAN_POINT ( 'NONE',  ( -7.960608749518247151, 12.43912730774665576, 0.000000000000000000 ) ) ;
#188027=CARTESIAN_POINT ( 'NONE',  ( -6.385527161912131433, 6.552129231760014605, 0.7216878364870317197 ) ) ;
#188029=CARTESIAN_POINT ( 'NONE',  ( 1.364683531249988757, 2.446875000341415696, 1.214306433183764966E-14 ) ) ;
#188042=ORIENTED_EDGE ( 'NONE', *, *, #158186, .T. ) ;
#188049=CARTESIAN_POINT ( 'NONE',  ( -4.776550190716183586, 4.467063398790632966, 1.214306433183764966E-14 ) ) ;
#188050=CARTESIAN_POINT ( 'NONE',  ( 1.419999999999990603, 6.280000000000042881, 2.580000000000000515 ) ) ;
#188052=CARTESIAN_POINT ( 'NONE',  ( -0.6823417656250212460, 2.613541667008084879, 1.181850606188767472 ) ) ;
#188063=CARTESIAN_POINT ( 'NONE',  ( -1.364683531250000748, 1.509375000341421691, 0.000000000000000000 ) ) ;
#188074=CARTESIAN_POINT ( 'NONE',  ( 5.301401758143367893, 6.143722458377430584, 1.199719254218462483 ) ) ;
#188082=CARTESIAN_POINT ( 'NONE',  ( 8.121497709785879593, 9.433834401960398353, -1.199719254218445830 ) ) ;
#188085=CARTESIAN_POINT ( 'NONE',  ( 8.284195553149872993, 9.623648552551724578, -1.199719254218445830 ) ) ;
#188098=CARTESIAN_POINT ( 'NONE',  ( -8.690413276679693766, 9.241163032322203819, 1.040834085586084257E-14 ) ) ;
#188104=CARTESIAN_POINT ( 'NONE',  ( -8.188234707649510113, 11.64035869464474082, -1.199719254218446718 ) ) ;
#188109=CARTESIAN_POINT ( 'NONE',  ( -4.303823697334223652, 7.108545849276850959, -1.199719254218452047 ) ) ;
#188111=CARTESIAN_POINT ( 'NONE',  ( 10.39640486358069360, 11.02356051713265650, 0.7998128361456462443 ) ) ;
#188113=CARTESIAN_POINT ( 'NONE',  ( 4.385172619016207918, 7.203452924572514959, 1.199719254218462483 ) ) ;
#188115=ORIENTED_EDGE ( 'NONE', *, *, #178239, .T. ) ;
#188119=CARTESIAN_POINT ( 'NONE',  ( 2.901081683644312736, 6.328419697652925002, 0.7216878364870338292 ) ) ;
#188121=CARTESIAN_POINT ( 'NONE',  ( -5.096975683733680818, 8.033889833409558534, -1.199719254218452047 ) ) ;
#188124=CARTESIAN_POINT ( 'NONE',  ( -8.272446282632566650, 12.80293776304669962, 0.7998128361456481317 ) ) ;
#188130=CARTESIAN_POINT ( 'NONE',  ( 8.920901888112002354, 9.510066412326583674, 0.7216878364870438212 ) ) ;
#188132=CARTESIAN_POINT ( 'NONE',  ( -0.6823417656250212460, 3.863541667008085767, 1.181850606188767472 ) ) ;
#188134=CARTESIAN_POINT ( 'NONE',  ( 5.169736645512481132, 4.925780929386339935, 0.7998128361456341429 ) ) ;
#188149=CARTESIAN_POINT ( 'NONE',  ( -0.6823417656250003738, 2.030208333674753174, -1.181850606188749264 ) ) ;
#188151=CARTESIAN_POINT ( 'NONE',  ( 10.16199982864259788, 11.81442020729326536, 1.199719254218452047 ) ) ;
#188153=CARTESIAN_POINT ( 'NONE',  ( -5.341549334104202629, 7.254893527920112994, 1.443375672974064550 ) ) ;
#188154=CARTESIAN_POINT ( 'NONE',  ( 4.039966587192259873, 5.736380323189513852, 1.443375672974062551 ) ) ;
#188155=CARTESIAN_POINT ( 'NONE',  ( -5.382223794500843539, 7.302347065049529462, -1.443375672974051449 ) ) ;
#188158=CARTESIAN_POINT ( 'NONE',  ( 4.286349120214771879, 8.152491073559232859, -0.7998128361456221525 ) ) ;
#188168=CARTESIAN_POINT ( 'NONE',  ( 4.819033534653518025, 7.709623992816043270, -1.199719254218452047 ) ) ;
#188173=CARTESIAN_POINT ( 'NONE',  ( -6.364663046611467756, 9.512858423433634414, 1.199719254218452047 ) ) ;
#188177=CARTESIAN_POINT ( 'NONE',  ( 8.046927864910717432, 9.346836249606042202, 1.199719254218462483 ) ) ;
#188179=CARTESIAN_POINT ( 'NONE',  ( -6.307567778855718288, 8.381915046796901692, -1.599625672291263179 ) ) ;
#188180=CARTESIAN_POINT ( 'NONE',  ( 7.741342523278707866, 8.133913820021057006, 0.7216878364870458196 ) ) ;
#188181=CARTESIAN_POINT ( 'NONE',  ( 4.715454802112915011, 7.044561259014620269, 1.385117731104364536 ) ) ;
#188182=CARTESIAN_POINT ( 'NONE',  ( -5.220052836461385404, 6.048815383081766583, -1.199719254218446718 ) ) ;
#188185=CARTESIAN_POINT ( 'NONE',  ( -5.117312914154178216, 8.057616602233474978, -1.199719254218452047 ) ) ;
#188190=CARTESIAN_POINT ( 'NONE',  ( -1.402160292154681736E-14, 2.196875000341423689, -1.575800808251660134 ) ) ;
#188192=CARTESIAN_POINT ( 'NONE',  ( -6.412643469583822586, 6.583764924043652655, 1.040834085586084257E-14 ) ) ;
#188197=CARTESIAN_POINT ( 'NONE',  ( 6.440286661691305703, 7.472421512516709718, 1.199719254218462483 ) ) ;
#188199=CARTESIAN_POINT ( 'NONE',  ( -5.887541547804238995, 6.014758725225416214, 0.2650624260464862214 ) ) ;
#188200=CARTESIAN_POINT ( 'NONE',  ( 1.364683531249988757, 1.696875000341414808, 0.000000000000000000 ) ) ;
#188206=CARTESIAN_POINT ( 'NONE',  ( -3.276266675996675204, 6.974061555304760240, -0.7998128361456281477 ) ) ;
#188207=CARTESIAN_POINT ( 'NONE',  ( -8.825994812371996900, 9.399341490629888440, 0.7216878364870438212 ) ) ;
#188215=CARTESIAN_POINT ( 'NONE',  ( -7.443063143778079649, 10.66702885350765584, 1.082531754730549967 ) ) ;
#188220=CARTESIAN_POINT ( 'NONE',  ( -8.175203438916030407, 8.640084888264587093, 0.7216878364870578100 ) ) ;
#188226=CARTESIAN_POINT ( 'NONE',  ( -1.201851678989727383E-14, 5.118750000682815937, -1.732050807568863648 ) ) ;
#188227=CARTESIAN_POINT ( 'NONE',  ( 4.492266506575326446, 7.256230230409263626, -1.267781117195718288 ) ) ;
#188234=CARTESIAN_POINT ( 'NONE',  ( -7.555971681517696936, 7.709721804725773175, 0.7998128361456462443 ) ) ;
#188237=CARTESIAN_POINT ( 'NONE',  ( 5.508690485854129903, 5.321227076451600091, 1.040834085586084257E-14 ) ) ;
#188241=CARTESIAN_POINT ( 'NONE',  ( 5.198661835836162481, 8.152523677529138979, 1.199719254218462483 ) ) ;
#188246=CARTESIAN_POINT ( 'NONE',  ( -5.436456409399874623, 5.444880020495701523, 0.000000000000000000 ) ) ;
#188257=CARTESIAN_POINT ( 'NONE',  ( 1.364683531249986537, 0.3635416670080869328, 0.7879004041258500513 ) ) ;
#188259=CARTESIAN_POINT ( 'NONE',  ( -9.691380875670077444, 10.20103253123691189, 0.7998128361456462443 ) ) ;
#188262=CARTESIAN_POINT ( 'NONE',  ( 8.457588896826466751, 8.761608555919362828, 1.040834085586084257E-14 ) ) ;
#188264=CARTESIAN_POINT ( 'NONE',  ( -8.688077508258798431, 9.030511935923748013, -0.7998128361456291469 ) ) ;
#188267=CARTESIAN_POINT ( 'NONE',  ( -1.001543065824772872E-14, 4.821875000341419693, 1.575800808251672791 ) ) ;
#188269=CARTESIAN_POINT ( 'NONE',  ( 9.571693261567961741, 11.22969222899322617, 1.082531754730548412 ) ) ;
#188272=CARTESIAN_POINT ( 'NONE',  ( 0.6823417656249882723, -0.01145833299191073573, -1.181850606188749264 ) ) ;
#188275=CARTESIAN_POINT ( 'NONE',  ( 6.277061933002769045, 10.26706332190449622, 0.7216878364870438212 ) ) ;
#188278=CARTESIAN_POINT ( 'NONE',  ( -6.073689629242176480, 6.188318776978391611, -0.7216878364870278340 ) ) ;
#188280=CARTESIAN_POINT ( 'NONE',  ( -1.201851678989727383E-14, 2.821875000341418804, 1.575800808251672791 ) ) ;
#188284=CARTESIAN_POINT ( 'NONE',  ( -5.181187258716735577, 9.196468901811520880, 0.7998128361456481317 ) ) ;
#188291=CARTESIAN_POINT ( 'NONE',  ( 9.271078113646423091, 9.710679308875986848, 1.040834085586084257E-14 ) ) ;
#188294=CARTESIAN_POINT ( 'NONE',  ( -1.500000000000001332, 0.6500000000000255573, 0.000000000000000000 ) ) ;
#188300=CARTESIAN_POINT ( 'NONE',  ( 5.992340707560147806, 8.974519344586754599, 1.082531754730558626 ) ) ;
#188302=ORIENTED_EDGE ( 'NONE', *, *, #136490, .F. ) ;
#188308=CARTESIAN_POINT ( 'NONE',  ( 8.209625708274705502, 9.536650400197368427, 1.199719254218462483 ) ) ;
#188309=CARTESIAN_POINT ( 'NONE',  ( -9.677822722056413696, 10.18521468535430685, 1.040834085586084257E-14 ) ) ;
#188311=DIRECTION ( 'NONE',  ( -1.000000000000000000, 8.673617379884035472E-16, 0.000000000000000000 ) ) ;
#188312=CARTESIAN_POINT ( 'NONE',  ( 1.364683531249986537, -0.3864583329919166199, 0.7879004041258500513 ) ) ;
#188313=CARTESIAN_POINT ( 'NONE',  ( -0.7500000000000215383, 1.191666666666688190, 1.299038105676659116 ) ) ;
#188316=CARTESIAN_POINT ( 'NONE',  ( 4.286349120214771879, 8.152491073559232859, -0.7998128361456221525 ) ) ;
#188322=CARTESIAN_POINT ( 'NONE',  ( 0.6823417656249917140, 4.592708333674755394, 1.181850606188765695 ) ) ;
#188324=CARTESIAN_POINT ( 'NONE',  ( -7.160677686311960777, 11.50587440067263678, -0.7998128361456291469 ) ) ;
#188325=CARTESIAN_POINT ( 'NONE',  ( -3.958617665510266725, 7.562211676496538360, -0.7216878364870267237 ) ) ;
#188334=ORIENTED_EDGE ( 'NONE', *, *, #1599, .T. ) ;
#188335=CARTESIAN_POINT ( 'NONE',  ( 8.776205506747620788, 9.133327934160710981, -0.7998128361456221525 ) ) ;
#188336=CARTESIAN_POINT ( 'NONE',  ( -6.071028223004627300, 5.977287769793835359, -0.4191162096944526239 ) ) ;
#188339=CARTESIAN_POINT ( 'NONE',  ( 6.765155463094746580, 9.876136559377135526, 1.082531754730558626 ) ) ;
#188342=CARTESIAN_POINT ( 'NONE',  ( -6.997979842947967377, 11.31606025008131233, -0.7998128361456291469 ) ) ;
#188343=CARTESIAN_POINT ( 'NONE',  ( 6.518772930072240790, 6.499656594706071822, -0.7998128361456281477 ) ) ;
#188346=CARTESIAN_POINT ( 'NONE',  ( 4.871457266011829823, 4.577788319968905562, -0.7998128361456221525 ) ) ;
#188349=CARTESIAN_POINT ( 'NONE',  ( -4.100072327556957497, 7.608104560092542101, -0.6936436459203108029 ) ) ;
#188353=CARTESIAN_POINT ( 'NONE',  ( -4.934804725694224459, 6.780358151441803649, -1.443375672974053447 ) ) ;
#188354=CARTESIAN_POINT ( 'NONE',  ( 3.358669367883368118, 4.941533567329135401, -1.599625672291262513 ) ) ;
#188357=CARTESIAN_POINT ( 'NONE',  ( -5.194745412330402878, 9.212286747694129474, 0.000000000000000000 ) ) ;
#188362=CARTESIAN_POINT ( 'NONE',  ( -8.646349277213090545, 11.11049346154719508, 1.599625672291269396 ) ) ;
#188366=CARTESIAN_POINT ( 'NONE',  ( 5.834086172582112262, 5.700855377634248100, 1.040834085586084257E-14 ) ) ;
#188367=CARTESIAN_POINT ( 'NONE',  ( -4.952636518945700672, 6.537114055553894687, -2.442608363190702292 ) ) ;
#188379=CARTESIAN_POINT ( 'NONE',  ( -5.693534442735004752, 8.729875052244421951, 1.199719254218452047 ) ) ;
#188382=CARTESIAN_POINT ( 'NONE',  ( 4.351804120306567825, 8.020929207092235558, 1.040834085586084257E-14 ) ) ;
#188383=VERTEX_POINT ( 'NONE', #163345 ) ;
#188387=CARTESIAN_POINT ( 'NONE',  ( -5.545448523189368650, 6.428443684264421698, -1.199719254218446718 ) ) ;
#188388=( BOUNDED_SURFACE ( )  B_SPLINE_SURFACE ( 1, 2, ( 
 ( #36582, #5126, #71201, #187101, #38735, #104817, #70134, #170862, #202266, #208408, #174889, #60042, #120054, #22453, #186028, #136246, #108863, #72272, #88565, #92578, #37665, #138381, #204399, #158620, #168727, #10217, #76291, #126195, #192158, #43820, #109936, #61111, #175945, #27541, #159678, #143472, #31825, #180203, #161830, #44890, #178073, #29691, #47018, #95774, #112072, #13418, #162890, #148764, #110996, #145612, #12343, #177001, #32878, #213725, #196450, #65348, #28617, #129405, #131495, #211608, #128345, #79493, #96842, #195386, #333, #193243, #144545, #113133, #15538, #45952, #63244, #98955, #66406, #97901, #48093, #114205, #130460, #194311, #81622, #94706, #115258, #160747, #179140, #78423, #165006, #30763, #14473, #80562, #163960, #147706, #210552, #82681, #146661, #16600, #197499, #62188, #49142, #212674, #64315, #181251, #199621, #104287, #53388, #50198, #167152, #86961, #18739, #119524, #117391, #169276, #183387, #170335, #120609, #4603, #1411, #69615, #154100, #34993, #116317, #51267, #101065, #102144, #84823, #182308, #88028, #150911, #5669, #2473, #21919, #68550, #132551, #20862, #198550, #38214, #134677, #33937, #200680, #135724, #100011, #151971, #185511, #133619, #70678, #166076, #52329, #83749, #67471, #118459, #202816, #19810, #184445, #36063, #17664, #201747, #149841, #168211, #3544, #153030, #136788, #85896, #37134, #103216, #54465, #186586, #89115, #8901, #58729, #206032, #137864, #204953, #90183, #39276, #109688, #159424, #27282, #93388, #56601, #125950, #26216, #73916, #174639, #156246, #191906, #42506, #55528, #71748, #122765, #24078, #189787, #105371, #7824, #57667, #173580, #158375, #6753, #172491, #74982, #141090, #188724, #43569, #41437, #91251, #203884, #157311, #72829, #121683, #187650, #140009, #171408, #175691, #22998, #155170, #138932, #107546, #123825, #59793, #40362, #25150, #106465, #124880, #108612, #207101, #190844, #92333, #9968, #76045, #142147, #208161, #14211, #195129, #31570, #15285, #131255, #146406, #79242, #98695, #194048, #78169, #61932, #45700, #128090, #209216, #177820, #176745, #179947, #212418, #113951, #28359, #111818, #160493, #127019, #162637, #46767, #29436, #64060, #12100, #95527, #144298, #94455, #11024, #161577, #47840, #210291, #13164, #130203, #97645, #32617, #145360, #211360, #65098, #112879, #196197, #163704, #62985, #77101, #129154, #178893, #30507, #96588, #80306, #81371, #147452, #180998, #143226, #213475, #44631, #60857, #197242, #48881, #114999, #192978, #110747, #100808, #185247, #183130, #99752, #133354, #68290, #166894, #186319, #164753, #116058, #18486, #201486, #17405, #67218, #70417, #37954, #52072, #84562, #118199, #150652, #132290, #49937, #136533, #165822, #184186, #182048, #198296, #36870, #33678, #83489, #1156, #149572, #2214, #4348, #199360, #53131, #152767, #202553, #16343, #120343, #82424, #51007, #54204, #119261, #134423, #102953, #34736, #148513, #135464, #80, #66145, #117128, #200426, #35808, #101885, #167950, #19553, #85630, #169012, #151717, #3287, #69354, #20610, #86698, #75784, #7561, #157051, #107282, #24883, #41174, #39022, #140823, #5412, #25953, #59523, #171144, #71491, #158116, #89923, #56338, #155974, #74719, #58469, #125683, #207900, #88853, #141891, #108352, #191641, #90988, #55271, #57399, #154909, #22736, #104026, #8639, #21660, #138666, #124623, #204688, #206836, #6493, #190581, #72568, #170074, #92059, #42239, #187390, #173303, #87766, #122499, #153842, #188460, #40091, #73647, #106203, #137603, #203620, #172229, #121418, #23818, #105105, #139746, #205770, #174374, #123564, #9708, #189527, #147198, #144028, #194860, #109425, #62717, #96323, #44364, #129950, #15022, #94192, #208958, #126749, #160232, #113689, #145090, #95258, #111548, #27016, #112615, #81113, #210023, #128879, #146143, #47574, #110487, #11831, #176486, #45433, #127833, #60591, #46493, #30239, #177557, #175430, #28096, #61665, #10762, #77908, #211094, #192708, #76836, #195938, #193785, #142956, #29168, #161308, #12891, #97385, #78970, #80039, #31308, #178627, #213224, #162378, #13956, #43305, #93124, #212157, #131001, #163442, #64854 ),
 ( #63793, #179691, #159163, #200176, #166633, #3035, #201238, #102705, #117947, #50744, #70171, #165561, #49679, #33427, #17155, #99504, #180743, #149315, #148261, #151462, #183940, #85380, #214261, #83230, #132039, #98435, #134166, #18227, #894, #35552, #198050, #66961, #115806, #65894, #196993, #133101, #19298, #181793, #199098, #101632, #69104, #4101, #116871, #182872, #36619, #84310, #167698, #135226, #34488, #48628, #100562, #150396, #1964, #68028, #51829, #52879, #119015, #152517, #114744, #184996, #16084, #32369, #168762, #20368, #86452, #164499, #82167, #22489, #57153, #104852, #153592, #121173, #138417, #88600, #140579, #136282, #21418, #154657, #205519, #137355, #187142, #156803, #206590, #122247, #6241, #188206, #72312, #103780, #169831, #8390, #155725, #204437, #202303, #203370, #56090, #87527, #74472, #53954, #120092, #186067, #38770, #37704, #5164, #23565, #71238, #89675, #55024, #170897, #7309, #39844, #173053, #105950, #171974, #189281, #73385, #139491, #123318, #40920, #107027, #24633, #90740, #52506, #34121, #87139, #18919, #168393, #118639, #36241, #184624, #50380, #152149, #16787, #37319, #70858, #182492, #82870, #169455, #101250, #67652, #167333, #86074, #69794, #136972, #4780, #100192, #153210, #119707, #203000, #102319, #66587, #68732, #166258, #17847, #115446, #19989, #33066, #150021, #135903, #1591, #3718, #83932, #201921, #133798, #181437, #103394, #53574, #198734, #185690, #99144, #199807, #165193, #51452, #117572, #85003, #183567, #148948, #519, #35173, #132730, #151095, #116502, #2658, #134853, #21041, #200859, #174825, #105552, #158551, #155346, #206213, #120788, #74100, #107732, #55704, #141277, #26401, #171586, #5858, #138040, #23180, #125068, #156423, #106646, #122944, #38390, #124002, #92513, #6929, #140192, #157497, #58913, #121859, #89295, #187830, #56778, #139107, #71929, #57840, #73007, #104471, #10148, #205135, #76223, #188900, #142333, #39456, #54639, #91436, #186765, #170518, #40543, #22100, #172674, #189970, #88213, #41619, #173758, #24251, #207286, #154284, #90354, #204053, #8009, #25335, #191026, #9091, #75168, #42693, #108798, #13011, #79088, #78025, #45552, #110603, #160350, #145206, #158232, #55641, #177675, #93243, #176604, #28216, #92182, #186699, #105490, #174493, #191764, #26070, #39395, #9823, #159277, #211212, #38328, #75899, #154216, #104404, #29285, #144149, #126870, #210141, #170453, #59644, #61785, #142003, #121797, #208018, #27137, #125802, #120726, #22038, #71865, #43420, #11952, #187765, #109544, #95379, #88149, #10876, #175548, #76951, #143076, #127951, #5788, #111668, #137974, #209069, #203993, #161428, #60706, #192828, #44486, #94309, #193904, #18339, #166745, #47688, #100667, #67070, #34599, #198155, #14067, #16194, #113800, #130063, #84420, #49788, #194976, #97497, #17262, #163554, #115914, #179802, #99607, #31421, #150509, #50857, #149423, #146259, #214369, #62837, #15137, #46612, #196056, #81225, #32473, #147307, #48738, #33535, #83338, #128999, #112734, #213333, #178744, #133206, #30357, #181900, #80154, #82275, #64958, #131110, #96444, #165673, #162495, #197097, #1006, #114851, #199210, #180851, #116982, #98545, #212272, #182982, #63907, #164609, #65999, #148370, #132149, #200282, #69208, #135328, #186172, #36724, #51933, #172080, #52982, #23673, #119118, #39951, #201342, #89783, #38874, #106058, #122352, #185097, #2070, #102810, #153696, #68141, #21513, #55127, #3138, #88705, #188309, #168866, #167807, #85485, #20469, #72418, #103881, #54061, #70274, #118057, #134274, #86555, #187247, #19406, #104959, #6346, #152619, #4206, #136390, #202406, #120196, #151571, #5265, #203473, #37806, #184042, #169929, #87625, #35659, #101738, #71342, #137458, #121272, #171000, #56191, #22598, #154763, #138519, #204543, #209876, #126602, #139597, #111404, #206695, #108211, #59384, #123422, #174234, #75643, #43167, #27952, #90842, #42096, #92978, #159024, #74576, #127680, #125539, #155830, #9566, #25808, #156905, #8494, #192564, #57260, #77761, #177406, #140679, #189384, #61515, #141750, #124479, #7414, #58323, #190436, #207757, #91917, #157977, #191501 ) ),
 .UNSPECIFIED., .F., .F., .F. ) 
 B_SPLINE_SURFACE_WITH_KNOTS ( ( 2, 2 ),
 ( 3, 2, 2, 2, 2, 2, 2, 2, 2, 2, 2, 2, 2, 2, 2, 2, 2, 2, 2, 2, 2, 2, 2, 2, 2, 2, 2, 2, 2, 2, 2, 2, 2, 2, 2, 2, 2, 2, 2, 2, 2, 2, 2, 2, 2, 2, 2, 2, 2, 2, 2, 2, 2, 2, 2, 2, 2, 2, 2, 2, 2, 2, 2, 2, 2, 2, 2, 2, 2, 2, 2, 2, 2, 2, 2, 2, 2, 2, 2, 2, 2, 2, 2, 2, 2, 2, 2, 2, 2, 2, 2, 2, 2, 2, 2, 2, 2, 2, 2, 2, 2, 2, 2, 2, 2, 2, 2, 2, 2, 2, 2, 2, 2, 2, 2, 2, 2, 2, 2, 2, 2, 2, 2, 2, 2, 2, 2, 2, 2, 2, 2, 2, 2, 2, 2, 2, 2, 2, 2, 2, 2, 2, 2, 2, 2, 2, 2, 2, 2, 2, 2, 2, 2, 2, 2, 2, 2, 2, 2, 2, 2, 2, 2, 2, 2, 2, 2, 2, 2, 2, 2, 2, 2, 2, 2, 2, 2, 2, 2, 2, 2, 2, 2, 2, 2, 2, 2, 2, 2, 2, 2, 2, 2, 2, 2, 2, 2, 2, 2, 2, 2, 2, 2, 2, 2, 2, 2, 2, 2, 2, 2, 2, 2, 2, 2, 2, 2, 2, 2, 2, 2, 2, 2, 2, 2, 2, 2, 2, 2, 2, 2, 2, 2, 2, 2, 2, 2, 2, 2, 2, 3 ),
 ( 0.000000000000000000, 1.000000000000000000 ),
 ( 0.000000000000000000, 0.004166666666666666609, 0.008333333333333333218, 0.01250000000000000069, 0.01666666666666666644, 0.02083333333333333218, 0.02500000000000000139, 0.02916666666666666713, 0.03333333333333333287, 0.03749999999999999861, 0.04166666666666666435, 0.04583333333333333010, 0.05000000000000000278, 0.05416666666666666852, 0.05833333333333333426, 0.06250000000000000000, 0.06666666666666666574, 0.07083333333333333148, 0.07499999999999999722, 0.07916666666666666297, 0.08333333333333332871, 0.08749999999999999445, 0.09166666666666666019, 0.09583333333333333981, 0.1000000000000000056, 0.1041666666666666713, 0.1083333333333333370, 0.1125000000000000028, 0.1166666666666666685, 0.1208333333333333343, 0.1250000000000000000, 0.1291666666666666796, 0.1333333333333333315, 0.1375000000000000111, 0.1416666666666666630, 0.1458333333333333426, 0.1499999999999999944, 0.1541666666666666741, 0.1583333333333333259, 0.1625000000000000056, 0.1666666666666666574, 0.1708333333333333370, 0.1749999999999999889, 0.1791666666666666685, 0.1833333333333333204, 0.1875000000000000000, 0.1916666666666666796, 0.1958333333333333315, 0.2000000000000000111, 0.2041666666666666630, 0.2083333333333333426, 0.2124999999999999944, 0.2166666666666666741, 0.2208333333333333259, 0.2250000000000000056, 0.2291666666666666574, 0.2333333333333333370, 0.2374999999999999889, 0.2416666666666666685, 0.2458333333333333204, 0.2500000000000000000, 0.2541666666666666519, 0.2583333333333333592, 0.2625000000000000111, 0.2666666666666666630, 0.2708333333333333148, 0.2750000000000000222, 0.2791666666666666741, 0.2833333333333333259, 0.2874999999999999778, 0.2916666666666666852, 0.2958333333333333370, 0.2999999999999999889, 0.3041666666666666408, 0.3083333333333333481, 0.3125000000000000000, 0.3166666666666666519, 0.3208333333333333592, 0.3250000000000000111, 0.3291666666666666630, 0.3333333333333333148, 0.3375000000000000222, 0.3416666666666666741, 0.3458333333333333259, 0.3499999999999999778, 0.3541666666666666852, 0.3583333333333333370, 0.3624999999999999889, 0.3666666666666666408, 0.3708333333333333481, 0.3750000000000000000, 0.3791666666666666519, 0.3833333333333333592, 0.3875000000000000111, 0.3916666666666666630, 0.3958333333333333148, 0.4000000000000000222, 0.4041666666666666741, 0.4083333333333333259, 0.4124999999999999778, 0.4166666666666666852, 0.4208333333333333370, 0.4249999999999999889, 0.4291666666666666408, 0.4333333333333333481, 0.4375000000000000000, 0.4416666666666666519, 0.4458333333333333592, 0.4500000000000000111, 0.4541666666666666630, 0.4583333333333333148, 0.4625000000000000222, 0.4666666666666666741, 0.4708333333333333259, 0.4749999999999999778, 0.4791666666666666852, 0.4833333333333333370, 0.4874999999999999889, 0.4916666666666666408, 0.4958333333333333481, 0.5000000000000000000, 0.5041666666666666519, 0.5083333333333333037, 0.5124999999999999556, 0.5166666666666667185, 0.5208333333333333703, 0.5250000000000000222, 0.5291666666666666741, 0.5333333333333333259, 0.5374999999999999778, 0.5416666666666666297, 0.5458333333333332815, 0.5500000000000000444, 0.5541666666666666963, 0.5583333333333333481, 0.5625000000000000000, 0.5666666666666666519, 0.5708333333333333037, 0.5749999999999999556, 0.5791666666666667185, 0.5833333333333333703, 0.5875000000000000222, 0.5916666666666666741, 0.5958333333333333259, 0.5999999999999999778, 0.6041666666666666297, 0.6083333333333332815, 0.6125000000000000444, 0.6166666666666666963, 0.6208333333333333481, 0.6250000000000000000, 0.6291666666666666519, 0.6333333333333333037, 0.6374999999999999556, 0.6416666666666667185, 0.6458333333333333703, 0.6500000000000000222, 0.6541666666666666741, 0.6583333333333333259, 0.6624999999999999778, 0.6666666666666666297, 0.6708333333333332815, 0.6750000000000000444, 0.6791666666666666963, 0.6833333333333333481, 0.6875000000000000000, 0.6916666666666666519, 0.6958333333333333037, 0.6999999999999999556, 0.7041666666666667185, 0.7083333333333333703, 0.7125000000000000222, 0.7166666666666666741, 0.7208333333333333259, 0.7249999999999999778, 0.7291666666666666297, 0.7333333333333332815, 0.7375000000000000444, 0.7416666666666666963, 0.7458333333333333481, 0.7500000000000000000, 0.7541666666666666519, 0.7583333333333333037, 0.7624999999999999556, 0.7666666666666667185, 0.7708333333333333703, 0.7750000000000000222, 0.7791666666666666741, 0.7833333333333333259, 0.7874999999999999778, 0.7916666666666666297, 0.7958333333333332815, 0.8000000000000000444, 0.8041666666666666963, 0.8083333333333333481, 0.8125000000000000000, 0.8166666666666666519, 0.8208333333333333037, 0.8249999999999999556, 0.8291666666666667185, 0.8333333333333333703, 0.8375000000000000222, 0.8416666666666666741, 0.8458333333333333259, 0.8499999999999999778, 0.8541666666666666297, 0.8583333333333332815, 0.8625000000000000444, 0.8666666666666666963, 0.8708333333333333481, 0.8750000000000000000, 0.8791666666666666519, 0.8833333333333333037, 0.8874999999999999556, 0.8916666666666667185, 0.8958333333333333703, 0.9000000000000000222, 0.9041666666666666741, 0.9083333333333333259, 0.9124999999999999778, 0.9166666666666666297, 0.9208333333333332815, 0.9250000000000000444, 0.9291666666666666963, 0.9333333333333333481, 0.9375000000000000000, 0.9416666666666666519, 0.9458333333333333037, 0.9499999999999999556, 0.9541666666666667185, 0.9583333333333333703, 0.9625000000000000222, 0.9666666666666666741, 0.9708333333333333259, 0.9749999999999999778, 0.9791666666666666297, 0.9833333333333332815, 0.9875000000000000444, 0.9916666666666666963, 0.9958333333333333481, 1.000000000000000000 ),
 .UNSPECIFIED. ) 
 GEOMETRIC_REPRESENTATION_ITEM ( )  RATIONAL_B_SPLINE_SURFACE ( (
 ( 1.000000000000000000, 0.8660254037844387076, 1.000000000000000000, 0.8660254037844387076, 1.000000000000000000, 0.8660254037844387076, 1.000000000000000000, 0.8660254037844387076, 1.000000000000000000, 0.8660254037844387076, 1.000000000000000000, 0.8660254037844387076, 1.000000000000000000, 0.8660254037844387076, 1.000000000000000000, 0.8660254037844387076, 1.000000000000000000, 0.8660254037844387076, 1.000000000000000000, 0.8660254037844387076, 1.000000000000000000, 0.8660254037844387076, 1.000000000000000000, 0.8660254037844387076, 1.000000000000000000, 0.8660254037844387076, 1.000000000000000000, 0.8660254037844387076, 1.000000000000000000, 0.8660254037844387076, 1.000000000000000000, 0.8660254037844387076, 1.000000000000000000, 0.8660254037844387076, 1.000000000000000000, 0.8660254037844387076, 1.000000000000000000, 0.8660254037844387076, 1.000000000000000000, 0.8660254037844387076, 1.000000000000000000, 0.8660254037844387076, 1.000000000000000000, 0.8660254037844387076, 1.000000000000000000, 0.8660254037844387076, 1.000000000000000000, 0.8660254037844387076, 1.000000000000000000, 0.8660254037844387076, 1.000000000000000000, 0.8660254037844387076, 1.000000000000000000, 0.8660254037844387076, 1.000000000000000000, 0.8660254037844387076, 1.000000000000000000, 0.8660254037844387076, 1.000000000000000000, 0.8660254037844387076, 1.000000000000000000, 0.8660254037844387076, 1.000000000000000000, 0.8660254037844387076, 1.000000000000000000, 0.8660254037844387076, 1.000000000000000000, 0.8660254037844387076, 1.000000000000000000, 0.8660254037844387076, 1.000000000000000000, 0.8660254037844387076, 1.000000000000000000, 0.8660254037844387076, 1.000000000000000000, 0.8660254037844387076, 1.000000000000000000, 0.8660254037844387076, 1.000000000000000000, 0.8660254037844387076, 1.000000000000000000, 0.8660254037844387076, 1.000000000000000000, 0.8660254037844387076, 1.000000000000000000, 0.8660254037844387076, 1.000000000000000000, 0.8660254037844387076, 1.000000000000000000, 0.8660254037844387076, 1.000000000000000000, 0.8660254037844387076, 1.000000000000000000, 0.8660254037844387076, 1.000000000000000000, 0.8660254037844387076, 1.000000000000000000, 0.8660254037844387076, 1.000000000000000000, 0.8660254037844387076, 1.000000000000000000, 0.8660254037844387076, 1.000000000000000000, 0.8660254037844387076, 1.000000000000000000, 0.8660254037844387076, 1.000000000000000000, 0.8660254037844387076, 1.000000000000000000, 0.8660254037844387076, 1.000000000000000000, 0.8660254037844387076, 1.000000000000000000, 0.8660254037844387076, 1.000000000000000000, 0.8660254037844387076, 1.000000000000000000, 0.8660254037844387076, 1.000000000000000000, 0.8660254037844387076, 1.000000000000000000, 0.8660254037844387076, 1.000000000000000000, 0.8660254037844387076, 1.000000000000000000, 0.8660254037844387076, 1.000000000000000000, 0.8660254037844387076, 1.000000000000000000, 0.8660254037844387076, 1.000000000000000000, 0.8660254037844387076, 1.000000000000000000, 0.8660254037844387076, 1.000000000000000000, 0.8660254037844387076, 1.000000000000000000, 0.8660254037844387076, 1.000000000000000000, 0.8660254037844387076, 1.000000000000000000, 0.8660254037844387076, 1.000000000000000000, 0.8660254037844387076, 1.000000000000000000, 0.8660254037844387076, 1.000000000000000000, 0.8660254037844387076, 1.000000000000000000, 0.8660254037844387076, 1.000000000000000000, 0.8660254037844387076, 1.000000000000000000, 0.8660254037844387076, 1.000000000000000000, 0.8660254037844387076, 1.000000000000000000, 0.8660254037844387076, 1.000000000000000000, 0.8660254037844387076, 1.000000000000000000, 0.8660254037844387076, 1.000000000000000000, 0.8660254037844387076, 1.000000000000000000, 0.8660254037844387076, 1.000000000000000000, 0.8660254037844387076, 1.000000000000000000, 0.8660254037844387076, 1.000000000000000000, 0.8660254037844387076, 1.000000000000000000, 0.8660254037844387076, 1.000000000000000000, 0.8660254037844387076, 1.000000000000000000, 0.8660254037844387076, 1.000000000000000000, 0.8660254037844387076, 1.000000000000000000, 0.8660254037844387076, 1.000000000000000000, 0.8660254037844387076, 1.000000000000000000, 0.8660254037844387076, 1.000000000000000000, 0.8660254037844387076, 1.000000000000000000, 0.8660254037844387076, 1.000000000000000000, 0.8660254037844387076, 1.000000000000000000, 0.8660254037844387076, 1.000000000000000000, 0.8660254037844387076, 1.000000000000000000, 0.8660254037844387076, 1.000000000000000000, 0.8660254037844387076, 1.000000000000000000, 0.8660254037844387076, 1.000000000000000000, 0.8660254037844387076, 1.000000000000000000, 0.8660254037844387076, 1.000000000000000000, 0.8660254037844387076, 1.000000000000000000, 0.8660254037844387076, 1.000000000000000000, 0.8660254037844387076, 1.000000000000000000, 0.8660254037844387076, 1.000000000000000000, 0.8660254037844387076, 1.000000000000000000, 0.8660254037844387076, 1.000000000000000000, 0.8660254037844387076, 1.000000000000000000, 0.8660254037844387076, 1.000000000000000000, 0.8660254037844387076, 1.000000000000000000, 0.8660254037844387076, 1.000000000000000000, 0.8660254037844387076, 1.000000000000000000, 0.8660254037844387076, 1.000000000000000000, 0.8660254037844387076, 1.000000000000000000, 0.8660254037844387076, 1.000000000000000000, 0.8660254037844387076, 1.000000000000000000, 0.8660254037844387076, 1.000000000000000000, 0.8660254037844387076, 1.000000000000000000, 0.8660254037844387076, 1.000000000000000000, 0.8660254037844387076, 1.000000000000000000, 0.8660254037844387076, 1.000000000000000000, 0.8660254037844387076, 1.000000000000000000, 0.8660254037844387076, 1.000000000000000000, 0.8660254037844387076, 1.000000000000000000, 0.8660254037844387076, 1.000000000000000000, 0.8660254037844387076, 1.000000000000000000, 0.8660254037844387076, 1.000000000000000000, 0.8660254037844387076, 1.000000000000000000, 0.8660254037844387076, 1.000000000000000000, 0.8660254037844387076, 1.000000000000000000, 0.8660254037844387076, 1.000000000000000000, 0.8660254037844387076, 1.000000000000000000, 0.8660254037844387076, 1.000000000000000000, 0.8660254037844387076, 1.000000000000000000, 0.8660254037844387076, 1.000000000000000000, 0.8660254037844387076, 1.000000000000000000, 0.8660254037844387076, 1.000000000000000000, 0.8660254037844387076, 1.000000000000000000, 0.8660254037844387076, 1.000000000000000000, 0.8660254037844387076, 1.000000000000000000, 0.8660254037844387076, 1.000000000000000000, 0.8660254037844387076, 1.000000000000000000, 0.8660254037844387076, 1.000000000000000000, 0.8660254037844387076, 1.000000000000000000, 0.8660254037844387076, 1.000000000000000000, 0.8660254037844387076, 1.000000000000000000, 0.8660254037844387076, 1.000000000000000000, 0.8660254037844387076, 1.000000000000000000, 0.8660254037844387076, 1.000000000000000000, 0.8660254037844387076, 1.000000000000000000, 0.8660254037844387076, 1.000000000000000000, 0.8660254037844387076, 1.000000000000000000, 0.8660254037844387076, 1.000000000000000000, 0.8660254037844387076, 1.000000000000000000, 0.8660254037844387076, 1.000000000000000000, 0.8660254037844387076, 1.000000000000000000, 0.8660254037844387076, 1.000000000000000000, 0.8660254037844387076, 1.000000000000000000, 0.8660254037844387076, 1.000000000000000000, 0.8660254037844387076, 1.000000000000000000, 0.8660254037844387076, 1.000000000000000000, 0.8660254037844387076, 1.000000000000000000, 0.8660254037844387076, 1.000000000000000000, 0.8660254037844387076, 1.000000000000000000, 0.8660254037844387076, 1.000000000000000000, 0.8660254037844387076, 1.000000000000000000, 0.8660254037844387076, 1.000000000000000000, 0.8660254037844387076, 1.000000000000000000, 0.8660254037844387076, 1.000000000000000000, 0.8660254037844387076, 1.000000000000000000, 0.8660254037844387076, 1.000000000000000000, 0.8660254037844387076, 1.000000000000000000, 0.8660254037844387076, 1.000000000000000000, 0.8660254037844387076, 1.000000000000000000, 0.8660254037844387076, 1.000000000000000000, 0.8660254037844387076, 1.000000000000000000, 0.8660254037844387076, 1.000000000000000000, 0.8660254037844387076, 1.000000000000000000, 0.8660254037844387076, 1.000000000000000000, 0.8660254037844387076, 1.000000000000000000, 0.8660254037844387076, 1.000000000000000000, 0.8660254037844387076, 1.000000000000000000, 0.8660254037844387076, 1.000000000000000000, 0.8660254037844387076, 1.000000000000000000, 0.8660254037844387076, 1.000000000000000000, 0.8660254037844387076, 1.000000000000000000, 0.8660254037844387076, 1.000000000000000000, 0.8660254037844387076, 1.000000000000000000, 0.8660254037844387076, 1.000000000000000000, 0.8660254037844387076, 1.000000000000000000, 0.8660254037844387076, 1.000000000000000000, 0.8660254037844387076, 1.000000000000000000, 0.8660254037844387076, 1.000000000000000000, 0.8660254037844387076, 1.000000000000000000, 0.8660254037844387076, 1.000000000000000000, 0.8660254037844387076, 1.000000000000000000, 0.8660254037844387076, 1.000000000000000000, 0.8660254037844387076, 1.000000000000000000, 0.8660254037844387076, 1.000000000000000000, 0.8660254037844387076, 1.000000000000000000, 0.8660254037844387076, 1.000000000000000000, 0.8660254037844387076, 1.000000000000000000, 0.8660254037844387076, 1.000000000000000000, 0.8660254037844387076, 1.000000000000000000, 0.8660254037844387076, 1.000000000000000000, 0.8660254037844387076, 1.000000000000000000, 0.8660254037844387076, 1.000000000000000000, 0.8660254037844387076, 1.000000000000000000, 0.8660254037844387076, 1.000000000000000000, 0.8660254037844387076, 1.000000000000000000, 0.8660254037844387076, 1.000000000000000000, 0.8660254037844387076, 1.000000000000000000, 0.8660254037844387076, 1.000000000000000000, 0.8660254037844387076, 1.000000000000000000, 0.8660254037844387076, 1.000000000000000000, 0.8660254037844387076, 1.000000000000000000, 0.8660254037844387076, 1.000000000000000000, 0.8660254037844387076, 1.000000000000000000, 0.8660254037844387076, 1.000000000000000000, 0.8660254037844387076, 1.000000000000000000, 0.8660254037844387076, 1.000000000000000000, 0.8660254037844387076, 1.000000000000000000, 0.8660254037844387076, 1.000000000000000000, 0.8660254037844387076, 1.000000000000000000, 0.8660254037844387076, 1.000000000000000000, 0.8660254037844387076, 1.000000000000000000, 0.8660254037844387076, 1.000000000000000000, 0.8660254037844387076, 1.000000000000000000, 0.8660254037844387076, 1.000000000000000000, 0.8660254037844387076, 1.000000000000000000, 0.8660254037844387076, 1.000000000000000000, 0.8660254037844387076, 1.000000000000000000, 0.8660254037844387076, 1.000000000000000000, 0.8660254037844387076, 1.000000000000000000, 0.8660254037844387076, 1.000000000000000000, 0.8660254037844387076, 1.000000000000000000, 0.8660254037844387076, 1.000000000000000000, 0.8660254037844387076, 1.000000000000000000),
 ( 1.000000000000000000, 0.8660254037844387076, 1.000000000000000000, 0.8660254037844387076, 1.000000000000000000, 0.8660254037844387076, 1.000000000000000000, 0.8660254037844387076, 1.000000000000000000, 0.8660254037844387076, 1.000000000000000000, 0.8660254037844387076, 1.000000000000000000, 0.8660254037844387076, 1.000000000000000000, 0.8660254037844387076, 1.000000000000000000, 0.8660254037844387076, 1.000000000000000000, 0.8660254037844387076, 1.000000000000000000, 0.8660254037844387076, 1.000000000000000000, 0.8660254037844387076, 1.000000000000000000, 0.8660254037844387076, 1.000000000000000000, 0.8660254037844387076, 1.000000000000000000, 0.8660254037844387076, 1.000000000000000000, 0.8660254037844387076, 1.000000000000000000, 0.8660254037844387076, 1.000000000000000000, 0.8660254037844387076, 1.000000000000000000, 0.8660254037844387076, 1.000000000000000000, 0.8660254037844387076, 1.000000000000000000, 0.8660254037844387076, 1.000000000000000000, 0.8660254037844387076, 1.000000000000000000, 0.8660254037844387076, 1.000000000000000000, 0.8660254037844387076, 1.000000000000000000, 0.8660254037844387076, 1.000000000000000000, 0.8660254037844387076, 1.000000000000000000, 0.8660254037844387076, 1.000000000000000000, 0.8660254037844387076, 1.000000000000000000, 0.8660254037844387076, 1.000000000000000000, 0.8660254037844387076, 1.000000000000000000, 0.8660254037844387076, 1.000000000000000000, 0.8660254037844387076, 1.000000000000000000, 0.8660254037844387076, 1.000000000000000000, 0.8660254037844387076, 1.000000000000000000, 0.8660254037844387076, 1.000000000000000000, 0.8660254037844387076, 1.000000000000000000, 0.8660254037844387076, 1.000000000000000000, 0.8660254037844387076, 1.000000000000000000, 0.8660254037844387076, 1.000000000000000000, 0.8660254037844387076, 1.000000000000000000, 0.8660254037844387076, 1.000000000000000000, 0.8660254037844387076, 1.000000000000000000, 0.8660254037844387076, 1.000000000000000000, 0.8660254037844387076, 1.000000000000000000, 0.8660254037844387076, 1.000000000000000000, 0.8660254037844387076, 1.000000000000000000, 0.8660254037844387076, 1.000000000000000000, 0.8660254037844387076, 1.000000000000000000, 0.8660254037844387076, 1.000000000000000000, 0.8660254037844387076, 1.000000000000000000, 0.8660254037844387076, 1.000000000000000000, 0.8660254037844387076, 1.000000000000000000, 0.8660254037844387076, 1.000000000000000000, 0.8660254037844387076, 1.000000000000000000, 0.8660254037844387076, 1.000000000000000000, 0.8660254037844387076, 1.000000000000000000, 0.8660254037844387076, 1.000000000000000000, 0.8660254037844387076, 1.000000000000000000, 0.8660254037844387076, 1.000000000000000000, 0.8660254037844387076, 1.000000000000000000, 0.8660254037844387076, 1.000000000000000000, 0.8660254037844387076, 1.000000000000000000, 0.8660254037844387076, 1.000000000000000000, 0.8660254037844387076, 1.000000000000000000, 0.8660254037844387076, 1.000000000000000000, 0.8660254037844387076, 1.000000000000000000, 0.8660254037844387076, 1.000000000000000000, 0.8660254037844387076, 1.000000000000000000, 0.8660254037844387076, 1.000000000000000000, 0.8660254037844387076, 1.000000000000000000, 0.8660254037844387076, 1.000000000000000000, 0.8660254037844387076, 1.000000000000000000, 0.8660254037844387076, 1.000000000000000000, 0.8660254037844387076, 1.000000000000000000, 0.8660254037844387076, 1.000000000000000000, 0.8660254037844387076, 1.000000000000000000, 0.8660254037844387076, 1.000000000000000000, 0.8660254037844387076, 1.000000000000000000, 0.8660254037844387076, 1.000000000000000000, 0.8660254037844387076, 1.000000000000000000, 0.8660254037844387076, 1.000000000000000000, 0.8660254037844387076, 1.000000000000000000, 0.8660254037844387076, 1.000000000000000000, 0.8660254037844387076, 1.000000000000000000, 0.8660254037844387076, 1.000000000000000000, 0.8660254037844387076, 1.000000000000000000, 0.8660254037844387076, 1.000000000000000000, 0.8660254037844387076, 1.000000000000000000, 0.8660254037844387076, 1.000000000000000000, 0.8660254037844387076, 1.000000000000000000, 0.8660254037844387076, 1.000000000000000000, 0.8660254037844387076, 1.000000000000000000, 0.8660254037844387076, 1.000000000000000000, 0.8660254037844387076, 1.000000000000000000, 0.8660254037844387076, 1.000000000000000000, 0.8660254037844387076, 1.000000000000000000, 0.8660254037844387076, 1.000000000000000000, 0.8660254037844387076, 1.000000000000000000, 0.8660254037844387076, 1.000000000000000000, 0.8660254037844387076, 1.000000000000000000, 0.8660254037844387076, 1.000000000000000000, 0.8660254037844387076, 1.000000000000000000, 0.8660254037844387076, 1.000000000000000000, 0.8660254037844387076, 1.000000000000000000, 0.8660254037844387076, 1.000000000000000000, 0.8660254037844387076, 1.000000000000000000, 0.8660254037844387076, 1.000000000000000000, 0.8660254037844387076, 1.000000000000000000, 0.8660254037844387076, 1.000000000000000000, 0.8660254037844387076, 1.000000000000000000, 0.8660254037844387076, 1.000000000000000000, 0.8660254037844387076, 1.000000000000000000, 0.8660254037844387076, 1.000000000000000000, 0.8660254037844387076, 1.000000000000000000, 0.8660254037844387076, 1.000000000000000000, 0.8660254037844387076, 1.000000000000000000, 0.8660254037844387076, 1.000000000000000000, 0.8660254037844387076, 1.000000000000000000, 0.8660254037844387076, 1.000000000000000000, 0.8660254037844387076, 1.000000000000000000, 0.8660254037844387076, 1.000000000000000000, 0.8660254037844387076, 1.000000000000000000, 0.8660254037844387076, 1.000000000000000000, 0.8660254037844387076, 1.000000000000000000, 0.8660254037844387076, 1.000000000000000000, 0.8660254037844387076, 1.000000000000000000, 0.8660254037844387076, 1.000000000000000000, 0.8660254037844387076, 1.000000000000000000, 0.8660254037844387076, 1.000000000000000000, 0.8660254037844387076, 1.000000000000000000, 0.8660254037844387076, 1.000000000000000000, 0.8660254037844387076, 1.000000000000000000, 0.8660254037844387076, 1.000000000000000000, 0.8660254037844387076, 1.000000000000000000, 0.8660254037844387076, 1.000000000000000000, 0.8660254037844387076, 1.000000000000000000, 0.8660254037844387076, 1.000000000000000000, 0.8660254037844387076, 1.000000000000000000, 0.8660254037844387076, 1.000000000000000000, 0.8660254037844387076, 1.000000000000000000, 0.8660254037844387076, 1.000000000000000000, 0.8660254037844387076, 1.000000000000000000, 0.8660254037844387076, 1.000000000000000000, 0.8660254037844387076, 1.000000000000000000, 0.8660254037844387076, 1.000000000000000000, 0.8660254037844387076, 1.000000000000000000, 0.8660254037844387076, 1.000000000000000000, 0.8660254037844387076, 1.000000000000000000, 0.8660254037844387076, 1.000000000000000000, 0.8660254037844387076, 1.000000000000000000, 0.8660254037844387076, 1.000000000000000000, 0.8660254037844387076, 1.000000000000000000, 0.8660254037844387076, 1.000000000000000000, 0.8660254037844387076, 1.000000000000000000, 0.8660254037844387076, 1.000000000000000000, 0.8660254037844387076, 1.000000000000000000, 0.8660254037844387076, 1.000000000000000000, 0.8660254037844387076, 1.000000000000000000, 0.8660254037844387076, 1.000000000000000000, 0.8660254037844387076, 1.000000000000000000, 0.8660254037844387076, 1.000000000000000000, 0.8660254037844387076, 1.000000000000000000, 0.8660254037844387076, 1.000000000000000000, 0.8660254037844387076, 1.000000000000000000, 0.8660254037844387076, 1.000000000000000000, 0.8660254037844387076, 1.000000000000000000, 0.8660254037844387076, 1.000000000000000000, 0.8660254037844387076, 1.000000000000000000, 0.8660254037844387076, 1.000000000000000000, 0.8660254037844387076, 1.000000000000000000, 0.8660254037844387076, 1.000000000000000000, 0.8660254037844387076, 1.000000000000000000, 0.8660254037844387076, 1.000000000000000000, 0.8660254037844387076, 1.000000000000000000, 0.8660254037844387076, 1.000000000000000000, 0.8660254037844387076, 1.000000000000000000, 0.8660254037844387076, 1.000000000000000000, 0.8660254037844387076, 1.000000000000000000, 0.8660254037844387076, 1.000000000000000000, 0.8660254037844387076, 1.000000000000000000, 0.8660254037844387076, 1.000000000000000000, 0.8660254037844387076, 1.000000000000000000, 0.8660254037844387076, 1.000000000000000000, 0.8660254037844387076, 1.000000000000000000, 0.8660254037844387076, 1.000000000000000000, 0.8660254037844387076, 1.000000000000000000, 0.8660254037844387076, 1.000000000000000000, 0.8660254037844387076, 1.000000000000000000, 0.8660254037844387076, 1.000000000000000000, 0.8660254037844387076, 1.000000000000000000, 0.8660254037844387076, 1.000000000000000000, 0.8660254037844387076, 1.000000000000000000, 0.8660254037844387076, 1.000000000000000000, 0.8660254037844387076, 1.000000000000000000, 0.8660254037844387076, 1.000000000000000000, 0.8660254037844387076, 1.000000000000000000, 0.8660254037844387076, 1.000000000000000000, 0.8660254037844387076, 1.000000000000000000, 0.8660254037844387076, 1.000000000000000000, 0.8660254037844387076, 1.000000000000000000, 0.8660254037844387076, 1.000000000000000000, 0.8660254037844387076, 1.000000000000000000, 0.8660254037844387076, 1.000000000000000000, 0.8660254037844387076, 1.000000000000000000, 0.8660254037844387076, 1.000000000000000000, 0.8660254037844387076, 1.000000000000000000, 0.8660254037844387076, 1.000000000000000000, 0.8660254037844387076, 1.000000000000000000, 0.8660254037844387076, 1.000000000000000000, 0.8660254037844387076, 1.000000000000000000, 0.8660254037844387076, 1.000000000000000000, 0.8660254037844387076, 1.000000000000000000, 0.8660254037844387076, 1.000000000000000000, 0.8660254037844387076, 1.000000000000000000, 0.8660254037844387076, 1.000000000000000000, 0.8660254037844387076, 1.000000000000000000, 0.8660254037844387076, 1.000000000000000000, 0.8660254037844387076, 1.000000000000000000, 0.8660254037844387076, 1.000000000000000000, 0.8660254037844387076, 1.000000000000000000, 0.8660254037844387076, 1.000000000000000000, 0.8660254037844387076, 1.000000000000000000, 0.8660254037844387076, 1.000000000000000000, 0.8660254037844387076, 1.000000000000000000, 0.8660254037844387076, 1.000000000000000000, 0.8660254037844387076, 1.000000000000000000, 0.8660254037844387076, 1.000000000000000000, 0.8660254037844387076, 1.000000000000000000, 0.8660254037844387076, 1.000000000000000000, 0.8660254037844387076, 1.000000000000000000, 0.8660254037844387076, 1.000000000000000000, 0.8660254037844387076, 1.000000000000000000, 0.8660254037844387076, 1.000000000000000000, 0.8660254037844387076, 1.000000000000000000, 0.8660254037844387076, 1.000000000000000000, 0.8660254037844387076, 1.000000000000000000, 0.8660254037844387076, 1.000000000000000000, 0.8660254037844387076, 1.000000000000000000, 0.8660254037844387076, 1.000000000000000000, 0.8660254037844387076, 1.000000000000000000) ) ) 
 REPRESENTATION_ITEM ( '' )  SURFACE ( )  );
#188391=CARTESIAN_POINT ( 'NONE',  ( 1.499999999999990896, 5.556250000682820378, 1.214306433183764966E-14 ) ) ;
#188392=CARTESIAN_POINT ( 'NONE',  ( -4.882907879216086933, 8.848476292394087395, -0.7998128361456281477 ) ) ;
#188398=CARTESIAN_POINT ( 'NONE',  ( -7.831806290188425557, 12.28885777186185990, -0.7998128361456281477 ) ) ;
#188399=CARTESIAN_POINT ( 'NONE',  ( 7.100719765255169236, 9.307259030929609267, -1.599625672291262513 ) ) ;
#188401=CARTESIAN_POINT ( 'NONE',  ( -2.318081078256692518, 5.648252324700675508, 1.040834085586084257E-14 ) ) ;
#188402=TOROIDAL_SURFACE ( 'NONE', #1602, 0.8300000000000010703, 0.08000000000000000167 ) ;
#188406=CARTESIAN_POINT ( 'NONE',  ( -1.364683531250000748, -0.6781249996585803075, 0.000000000000000000 ) ) ;
#188411=CARTESIAN_POINT ( 'NONE',  ( 9.408995418203963013, 12.00024729270324286, 1.443375672974076540 ) ) ;
#188433=CARTESIAN_POINT ( 'NONE',  ( -3.785751206713858785, 5.439795712631356750, 1.599625672291267398 ) ) ;
#188436=CARTESIAN_POINT ( 'NONE',  ( -3.297657676621885692, 4.870353260857385180, 1.599625672291267398 ) ) ;
#188440=CARTESIAN_POINT ( 'NONE',  ( -0.6823417656249969321, 5.717708333674756283, -1.181850606188749264 ) ) ;
#188444=CARTESIAN_POINT ( 'NONE',  ( -4.609409038966253647, 4.479991421656468908, -0.7216878364870207285 ) ) ;
#188450=CARTESIAN_POINT ( 'NONE',  ( 4.539282502477016479, 4.190251095844947926, 0.7998128361456341429 ) ) ;
#188452=LINE ( 'NONE', #140815, #100998 ) ;
#188454=CARTESIAN_POINT ( 'NONE',  ( 10.52076401408022299, 11.37657222595619189, 0.000000000000000000 ) ) ;
#188456=CARTESIAN_POINT ( 'NONE',  ( -1.402160292154681736E-14, 2.509375000341417028, -1.575800808251660134 ) ) ;
#188458=CARTESIAN_POINT ( 'NONE',  ( 1.499999999999990896, 3.775000000000021227, 1.214306433183764966E-14 ) ) ;
#188460=CARTESIAN_POINT ( 'NONE',  ( -9.158696461231359720, 10.64389961198009615, 1.199719254218462483 ) ) ;
#188461=CARTESIAN_POINT ( 'NONE',  ( -5.544921637864841379, 5.571422787038166291, -0.7216878364870197293 ) ) ;
#188463=CARTESIAN_POINT ( 'NONE',  ( -6.891622154448065807, 6.934647356477856128, 1.040834085586084257E-14 ) ) ;
#188464=EDGE_LOOP ( 'NONE', ( #195303, #44144, #98848, #24762 ) ) ;
#188465=CARTESIAN_POINT ( 'NONE',  ( 1.499999999999987121, -1.214583332650518432, 0.8660254037844524744 ) ) ;
#188474=CARTESIAN_POINT ( 'NONE',  ( -4.392478580703220281, 8.068382744221649361, 1.040834085586084257E-14 ) ) ;
#188476=EDGE_CURVE ( 'NONE', #2895, #109653, #109321, .T. ) ;
#188481=CARTESIAN_POINT ( 'NONE',  ( -3.917943204224913156, 7.514758138330285497, -0.7216878364870257245 ) ) ;
#188483=CARTESIAN_POINT ( 'NONE',  ( 8.886479618753304166, 12.45497775759917758, -1.199719254218446718 ) ) ;
#188491=CARTESIAN_POINT ( 'NONE',  ( -4.440459003675619520, 5.139289244831666714, 1.199719254218462483 ) ) ;
#188492=CARTESIAN_POINT ( 'NONE',  ( -8.622095623286845978, 12.14652976288826913, 1.199719254218462483 ) ) ;
#188497=CARTESIAN_POINT ( 'NONE',  ( 5.738125327081736060, 7.717565519727259904, 1.599625672291267398 ) ) ;
#188501=DIRECTION ( 'NONE',  ( 0.000000000000000000, 1.000000000000000000, -8.546850786086437571E-32 ) ) ;
#188502=CARTESIAN_POINT ( 'NONE',  ( 4.403700966340357681, 4.032072637018845107, -0.7998128361456211532 ) ) ;
#188504=ORIENTED_EDGE ( 'NONE', *, *, #95474, .F. ) ;
#188509=CARTESIAN_POINT ( 'NONE',  ( -3.197497122698730099, 6.431928158754200986, 0.6077543439236172684 ) ) ;
#188513=CARTESIAN_POINT ( 'NONE',  ( 8.769426429940780920, 9.125419011219408461, 0.7998128361456462443 ) ) ;
#188514=CARTESIAN_POINT ( 'NONE',  ( -6.112028321662274166, 6.025121218227761588, 0.7998128361456341429 ) ) ;
#188516=LINE ( 'NONE', #40147, #11077 ) ;
#188519=CARTESIAN_POINT ( 'NONE',  ( -1.201851678989727383E-14, 4.196875000341417028, -1.575800808251660134 ) ) ;
#188522=CARTESIAN_POINT ( 'NONE',  ( -5.494078562035765501, 7.432844293840273231, -1.599625672291256295 ) ) ;
#188525=CARTESIAN_POINT ( 'NONE',  ( 4.157546660884947620, 8.002221537674429896, 1.040834085586084257E-14 ) ) ;
#188526=CARTESIAN_POINT ( 'NONE',  ( -4.415151579544611238, 8.302760609444034046, -0.7998128361456281477 ) ) ;
#188529=ADVANCED_FACE ( 'NONE', ( #17055 ), #195838, .F. ) ;
#188533=CARTESIAN_POINT ( 'NONE',  ( 6.263503779833467178, 9.290876262238963790, -1.082531754730537088 ) ) ;
#188535=CARTESIAN_POINT ( 'NONE',  ( 6.765155463094746580, 9.876136559377135526, 1.082531754730558626 ) ) ;
#188536=CARTESIAN_POINT ( 'NONE',  ( 0.6823417656249899377, 2.905208333674754062, 1.181850606188765695 ) ) ;
#188538=CARTESIAN_POINT ( 'NONE',  ( 5.463572716182834910, 5.476515711742504067, 0.7216878364870317197 ) ) ;
#188547=CARTESIAN_POINT ( 'NONE',  ( -4.074449998555902397, 7.717048951691181102, 0.6760625908293280695 ) ) ;
#188553=B_SPLINE_CURVE_WITH_KNOTS ( 'NONE', 3,
 ( #70316, #51976, #71386, #35705, #100713, #54103, #38916, #84461, #169970, #165722 ),
 .UNSPECIFIED., .F., .F.,
 ( 4, 3, 3, 4 ),
 ( 3.588344277745669791E-16, 3.125155930788468421E-05, 5.676974391825271470E-05, 8.229510585278265896E-05 ),
 .UNSPECIFIED. ) ;
#188554=CARTESIAN_POINT ( 'NONE',  ( -10.50487009249003378, 11.15010328419353947, 0.7998128361456462443 ) ) ;
#188556=CARTESIAN_POINT ( 'NONE',  ( 5.756345505848640798, 6.148709499980903992, 0.8262799378709930753 ) ) ;
#188559=CARTESIAN_POINT ( 'NONE',  ( -3.918470089549458635, 4.530302178351167441, -1.199719254218452047 ) ) ;
#188564=CARTESIAN_POINT ( 'NONE',  ( 2.684151225825664788, 5.114964949229812596, -1.082531754730543083 ) ) ;
#188565=CARTESIAN_POINT ( 'NONE',  ( -1.364683531250012516, 3.342708333674756727, 0.7879004041258379498 ) ) ;
#188567=CARTESIAN_POINT ( 'NONE',  ( 8.209625708274705502, 9.536650400197368427, 1.199719254218462483 ) ) ;
#188571=CARTESIAN_POINT ( 'NONE',  ( -4.011515005667116718, 5.867910776320241162, 1.537733183400939119 ) ) ;
#188575=CARTESIAN_POINT ( 'NONE',  ( -1.201851678989727383E-14, 3.587500000000020339, -1.732050807568863648 ) ) ;
#188576=CARTESIAN_POINT ( 'NONE',  ( 6.335737856287750880, 6.286115675290828264, -0.7998128361456281477 ) ) ;
#188579=CARTESIAN_POINT ( 'NONE',  ( 1.499999999999999112, 7.438721522839136568, 4.195160983902605167 ) ) ;
#188580=CARTESIAN_POINT ( 'NONE',  ( -1.364683531249997417, 4.259375000341424133, 1.214306433183764966E-14 ) ) ;
#188582=CARTESIAN_POINT ( 'NONE',  ( 9.761507412159302177, 10.49077285704843199, -0.7216878364870257245 ) ) ;
#188588=CARTESIAN_POINT ( 'NONE',  ( 1.499999999999989120, 2.535416667349483344, 0.8660254037844524744 ) ) ;
#188590=CARTESIAN_POINT ( 'NONE',  ( -6.013204822860843457, 6.974159367214481264, -1.199719254218446718 ) ) ;
#188591=CARTESIAN_POINT ( 'NONE',  ( 3.660338285565247762, 7.214219066560688454, 1.040834085586084257E-14 ) ) ;
#188599=ORIENTED_EDGE ( 'NONE', *, *, #75356, .T. ) ;
#188601=CARTESIAN_POINT ( 'NONE',  ( 7.633404179693907388, 8.864391950186421454, -1.199719254218441611 ) ) ;
#188602=CARTESIAN_POINT ( 'NONE',  ( 5.983225862332436584, 5.874851682342960402, 0.7998128361456341429 ) ) ;
#188605=CARTESIAN_POINT ( 'NONE',  ( 4.333802657862601215, 8.207853534148366492, 0.7998128361456462443 ) ) ;
#188612=CARTESIAN_POINT ( 'NONE',  ( 8.367353357928214663, 12.91366268422496688, 1.040834085586084257E-14 ) ) ;
#188617=CARTESIAN_POINT ( 'NONE',  ( 5.881923755780003482, 5.983360633994940336, 0.1790317558759656202 ) ) ;
#188629=CARTESIAN_POINT ( 'NONE',  ( 7.971831135155394321, 8.402817200543854170, -0.7216878364870267237 ) ) ;
#188630=CARTESIAN_POINT ( 'NONE',  ( -3.632695093457760649, 6.325562478087638496, -1.199719254218452047 ) ) ;
#188634=CARTESIAN_POINT ( 'NONE',  ( -4.543954038874438162, 8.453030145328826350, 1.040834085586084257E-14 ) ) ;
#188648=CARTESIAN_POINT ( 'NONE',  ( 10.26082332744404368, 10.86538205830655279, -0.7998128361456281477 ) ) ;
#188651=CARTESIAN_POINT ( 'NONE',  ( 4.202664430556261266, 4.005456045178151570, 0.7216878364870317197 ) ) ;
#188657=CARTESIAN_POINT ( 'NONE',  ( -10.48008955368359629, 11.32911868882677986, 1.040834085586084257E-14 ) ) ;
#188662=CARTESIAN_POINT ( 'NONE',  ( 9.562578416340237197, 10.05076299535211781, 0.7998128361456462443 ) ) ;
#188666=CARTESIAN_POINT ( 'NONE',  ( -5.225778143063529946, 8.184159369294361497, 1.199719254218452047 ) ) ;
#188667=CARTESIAN_POINT ( 'NONE',  ( 5.118366684358879759, 5.930181538962194132, 1.199719254218462483 ) ) ;
#188671=CARTESIAN_POINT ( 'NONE',  ( 9.622536337397022521, 12.24937836509514710, 1.599625672291281386 ) ) ;
#188672=CARTESIAN_POINT ( 'NONE',  ( -4.121315508874280553, 3.910548969882488901, -0.7216878364870207285 ) ) ;
#188675=CARTESIAN_POINT ( 'NONE',  ( -1.364683531250012516, 3.092708333674755838, 0.7879004041258379498 ) ) ;
#188677=CARTESIAN_POINT ( 'NONE',  ( 5.327991180490514012, 9.159814110640187579, 1.040834085586084257E-14 ) ) ;
#188685=CARTESIAN_POINT ( 'NONE',  ( 8.636180661780656465, 11.09863007687603087, -1.443375672974052559 ) ) ;
#188690=CARTESIAN_POINT ( 'NONE',  ( -7.994504133552415404, 12.47867192245318435, -0.7998128361456281477 ) ) ;
#188699=CARTESIAN_POINT ( 'NONE',  ( 2.693266070609028784, 6.293894182352508970, 0.000000000000000000 ) ) ;
#188705=CARTESIAN_POINT ( 'NONE',  ( 3.974511587100456822, 7.788680618259193444, 1.040834085586084257E-14 ) ) ;
#188708=CARTESIAN_POINT ( 'NONE',  ( 1.499999999999989120, 2.535416667349483344, 0.8660254037844524744 ) ) ;
#188714=CARTESIAN_POINT ( 'NONE',  ( 1.499999999999985123, -0.2041666666666457353, -0.8660254037844323793 ) ) ;
#188715=CARTESIAN_POINT ( 'NONE',  ( 7.949158136313996259, 8.168439335321471262, 1.040834085586084257E-14 ) ) ;
#188716=CARTESIAN_POINT ( 'NONE',  ( 1.364683531249986537, -0.3864583329919166199, 0.7879004041258500513 ) ) ;
#188719=CARTESIAN_POINT ( 'NONE',  ( 8.256552361042350796, 12.57646882128404187, 1.040834085586084257E-14 ) ) ;
#188724=CARTESIAN_POINT ( 'NONE',  ( -6.891622154448065807, 6.934647356477856128, 1.040834085586084257E-14 ) ) ;
#188726=CARTESIAN_POINT ( 'NONE',  ( -1.500000000000013101, 2.202083334016153859, 0.8660254037844403729 ) ) ;
#188727=CARTESIAN_POINT ( 'NONE',  ( 1.364683531249988535, 5.717708333674752730, -0.7879004041258300672 ) ) ;
#188740=CARTESIAN_POINT ( 'NONE',  ( -8.533967624797991647, 12.04371376465130439, -1.199719254218446718 ) ) ;
#188741=CARTESIAN_POINT ( 'NONE',  ( 6.120616281565444794, 9.228137197546649517, -1.199719254218440723 ) ) ;
#188748=CARTESIAN_POINT ( 'NONE',  ( -7.640183256500752584, 8.872300873127729304, -1.199719254218446718 ) ) ;
#188753=CARTESIAN_POINT ( 'NONE',  ( 3.623053363349855172, 5.249981562040033189, 1.599625672291267398 ) ) ;
#188755=VERTEX_POINT ( 'NONE', #81287 ) ;
#188756=CARTESIAN_POINT ( 'NONE',  ( -5.739179097286464248, 5.590130456455974617, -0.7998128361456221525 ) ) ;
#188757=CARTESIAN_POINT ( 'NONE',  ( -9.833741488613570780, 10.36711991300432345, 0.7998128361456462443 ) ) ;
#188761=CARTESIAN_POINT ( 'NONE',  ( -4.028535363944735437, 7.777154369360758324, -0.5044922354892691363 ) ) ;
#188768=CARTESIAN_POINT ( 'NONE',  ( 6.844168616800228477, 6.879284895888727824, -0.7998128361456281477 ) ) ;
#188770=CARTESIAN_POINT ( 'NONE',  ( 4.226925616482873238, 3.500738074553327639, 2.444828727306146199 ) ) ;
#188783=AXIS2_PLACEMENT_3D ( 'NONE', #114177, #213696, #52299 ) ;
#188791=CARTESIAN_POINT ( 'NONE',  ( 3.714570900464278846, 5.356752022006865843, 1.443375672974062551 ) ) ;
#188795=CARTESIAN_POINT ( 'NONE',  ( -10.14557902172788495, 10.73093036830436553, 1.040834085586084257E-14 ) ) ;
#188801=CARTESIAN_POINT ( 'NONE',  ( -1.499999999999997780, 2.181250000682817713, 1.214306433183764966E-14 ) ) ;
#188807=CARTESIAN_POINT ( 'NONE',  ( -9.073431116043565225, 11.60875560684942265, -1.599625672291263179 ) ) ;
#188808=CARTESIAN_POINT ( 'NONE',  ( 4.332146500830024394, 3.995600397316412700, 0.09403405272452491914 ) ) ;
#188809=CARTESIAN_POINT ( 'NONE',  ( -1.364683531250000748, 0.7593750003414210248, 0.000000000000000000 ) ) ;
#188816=CARTESIAN_POINT ( 'NONE',  ( -3.469997250093771246, 6.135748327496311383, -1.199719254218452935 ) ) ;
#188821=CARTESIAN_POINT ( 'NONE',  ( 0.6823417656249882723, -0.3447916663252489911, 1.181850606188755259 ) ) ;
#188826=CARTESIAN_POINT ( 'NONE',  ( -1.364683531250014514, 0.2802083336747505649, 0.7879004041258379498 ) ) ;
#188828=CARTESIAN_POINT ( 'NONE',  ( -6.852756576703439961, 10.08230087520760954, 1.199719254218453823 ) ) ;
#188829=CARTESIAN_POINT ( 'NONE',  ( 8.914649696185335870, 10.35917838609310593, -1.199719254218446718 ) ) ;
#188830=CARTESIAN_POINT ( 'NONE',  ( 3.897079088924235712, 6.634010472798538949, 1.199719254218462483 ) ) ;
#188833=CARTESIAN_POINT ( 'NONE',  ( 0.6823417656249882723, -0.3447916663252489911, 1.181850606188755259 ) ) ;
#188840=CARTESIAN_POINT ( 'NONE',  ( 6.155038550924139429, 9.164333495178082600, 1.082531754730558626 ) ) ;
#188843=CARTESIAN_POINT ( 'NONE',  ( -3.958090780185743451, 6.705190779270287393, -1.199719254218452047 ) ) ;
#188845=CARTESIAN_POINT ( 'NONE',  ( 1.499999999999991118, 5.535416667349481123, 0.8660254037844524744 ) ) ;
#188848=CARTESIAN_POINT ( 'NONE',  ( 6.290620086616457662, 6.441404310581745563, 1.040834085586084257E-14 ) ) ;
#188849=CARTESIAN_POINT ( 'NONE',  ( -7.334597914868727919, 10.54048608644677465, -1.082531754730543083 ) ) ;
#188851=CARTESIAN_POINT ( 'NONE',  ( -0.7499999999999972244, 3.858333333333359594, -1.299038105676652011 ) ) ;
#188855=CARTESIAN_POINT ( 'NONE',  ( 9.083599731475983319, 11.62061899152058686, 1.443375672974076540 ) ) ;
#188860=VERTEX_POINT ( 'NONE', #65014 ) ;
#188866=CARTESIAN_POINT ( 'NONE',  ( 8.283668667825342169, 9.726996869626816533, -1.082531754730543083 ) ) ;
#188867=CARTESIAN_POINT ( 'NONE',  ( 7.293396569147545527, 10.59638086639245280, 1.199719254218460707 ) ) ;
#188868=CARTESIAN_POINT ( 'NONE',  ( -6.392833124043511894, 7.417059051927569868, 1.199719254218450271 ) ) ;
#188873=CARTESIAN_POINT ( 'NONE',  ( 4.419594888374914099, 5.218910793601261311, -1.082531754730548412 ) ) ;
#188875=CARTESIAN_POINT ( 'NONE',  ( -6.385527162356466668, 10.39360608948380182, 0.000000000000000000 ) ) ;
#188900=CARTESIAN_POINT ( 'NONE',  ( -7.250913225210214641, 7.353820272367037170, 0.7998128361456341429 ) ) ;
#188904=CARTESIAN_POINT ( 'NONE',  ( 4.964256800898067645, 8.943383367689749619, 0.7998128361456462443 ) ) ;
#188907=EDGE_CURVE ( 'NONE', #93282, #109059, #143633, .T. ) ;
#188917=CARTESIAN_POINT ( 'NONE',  ( -4.172158584703340445, 5.890604320285754980, -1.599625672291256295 ) ) ;
#188920=CARTESIAN_POINT ( 'NONE',  ( 8.437251666405968464, 8.737881787095446384, 1.040834085586084257E-14 ) ) ;
#188921=CARTESIAN_POINT ( 'NONE',  ( -0.6823417656250212460, 3.551041667008085323, 1.181850606188767472 ) ) ;
#188923=CARTESIAN_POINT ( 'NONE',  ( 5.769745475479523655, 6.237591007168648005, 1.002400605009654111 ) ) ;
#188927=AXIS2_PLACEMENT_3D ( 'NONE', #131950, #33334, #63708 ) ;
#188929=CARTESIAN_POINT ( 'NONE',  ( 6.941411460072420603, 7.200660912947041581, 1.040834085586084257E-14 ) ) ;
#188930=CARTESIAN_POINT ( 'NONE',  ( -7.157815033010924921, 10.43820240756634199, 1.199719254218453823 ) ) ;
#188933=CARTESIAN_POINT ( 'NONE',  ( -7.296259222448620463, 11.66405285949874759, 0.7998128361456481317 ) ) ;
#188934=CARTESIAN_POINT ( 'NONE',  ( -6.521635583373313061, 7.567328587812373719, -1.199719254218446718 ) ) ;
#188938=CARTESIAN_POINT ( 'NONE',  ( 4.132297641190314508, 7.622816840561035256, -0.7610026044957002300 ) ) ;
#188941=CARTESIAN_POINT ( 'NONE',  ( 8.101160479365381306, 9.410107633136481908, -1.199719254218446718 ) ) ;
#188951=CARTESIAN_POINT ( 'NONE',  ( -0.4909899725977228124, 7.342450396234926124, -1.941297109531795906 ) ) ;
#188954=ORIENTED_EDGE ( 'NONE', *, *, #36264, .F. ) ;
#188955=CARTESIAN_POINT ( 'NONE',  ( 1.499999999999987121, 4.045833333333359150, -0.8660254037844323793 ) ) ;
#188956=CARTESIAN_POINT ( 'NONE',  ( 5.657830175604453338, 5.495223381160312393, 0.7998128361456341429 ) ) ;
#188957=CARTESIAN_POINT ( 'NONE',  ( 6.307567778855705853, 8.381915046796901692, -1.599625672291262513 ) ) ;
#188959=CARTESIAN_POINT ( 'NONE',  ( -7.809133291791416909, 11.09411069285655493, 1.082531754730549967 ) ) ;
#188960=CARTESIAN_POINT ( 'NONE',  ( 6.697364695470787943, 7.876308901879812474, -1.082531754730543083 ) ) ;
#188961=CARTESIAN_POINT ( 'NONE',  ( -8.554831740098665094, 11.00372300158037042, 1.443375672974064550 ) ) ;
#188964=CARTESIAN_POINT ( 'NONE',  ( 8.101160479365381306, 9.410107633136481908, -1.199719254218446718 ) ) ;
#188969=CARTESIAN_POINT ( 'NONE',  ( 0.6823417656249899377, 2.842708333674753618, 1.181850606188765695 ) ) ;
#188976=CARTESIAN_POINT ( 'NONE',  ( 8.723781775389312543, 12.26516360700784958, -1.199719254218446718 ) ) ;
#188980=CARTESIAN_POINT ( 'NONE',  ( -8.143643823302737061, 12.65266822716189843, 0.000000000000000000 ) ) ;
#188986=CARTESIAN_POINT ( 'NONE',  ( 3.408985558832261731, 6.064568021024562938, 1.199719254218462483 ) ) ;
#188991=CARTESIAN_POINT ( 'NONE',  ( -8.533967624797991647, 12.04371376465130439, -1.199719254218446718 ) ) ;
#188994=CARTESIAN_POINT ( 'NONE',  ( 9.257519960032755790, 9.694861462993381807, 0.7998128361456462443 ) ) ;
#188996=CARTESIAN_POINT ( 'NONE',  ( 4.413087178904756769, 7.101426714207548230, 1.094556639780567053 ) ) ;
#188998=CARTESIAN_POINT ( 'NONE',  ( -4.952806187693842510, 4.672695395264567786, 0.7998128361456341429 ) ) ;
#189002=CARTESIAN_POINT ( 'NONE',  ( 8.751951852821344247, 10.16936423550178503, -1.199719254218446718 ) ) ;
#189004=CARTESIAN_POINT ( 'NONE',  ( 7.263417608619159083, 9.497073181520933716, -1.599625672291262513 ) ) ;
#189009=CARTESIAN_POINT ( 'NONE',  ( -8.107412671292051343, 10.48173408797264194, 1.443375672974090751 ) ) ;
#189017=CARTESIAN_POINT ( 'NONE',  ( -4.654334680973787108, 6.904393480334801048, -1.215188995478516221 ) ) ;
#189018=CARTESIAN_POINT ( 'NONE',  ( -1.364683531250000748, 1.759375000341421913, 0.000000000000000000 ) ) ;
#189020=CARTESIAN_POINT ( 'NONE',  ( 6.534666852106798096, 7.686494751288491578, -1.082531754730543083 ) ) ;
#189038=CARTESIAN_POINT ( 'NONE',  ( -8.636180661780651135, 13.01936850547871138, -0.7216878364870257245 ) ) ;
#189041=CARTESIAN_POINT ( 'NONE',  ( 4.130316239874070483, 3.817086806095215668, 1.214306433183764966E-14 ) ) ;
#189043=CARTESIAN_POINT ( 'NONE',  ( 7.086107841436786181, 11.41887624831828418, 1.040834085586084257E-14 ) ) ;
#189047=FACE_OUTER_BOUND ( 'NONE', #38134, .T. ) ;
#189048=CARTESIAN_POINT ( 'NONE',  ( -7.203459687562382641, 7.298457811777897319, -0.7998128361456291469 ) ) ;
#189051=CARTESIAN_POINT ( 'NONE',  ( -2.123823618835070537, 5.629544655282869847, 1.040834085586084257E-14 ) ) ;
#189055=CARTESIAN_POINT ( 'NONE',  ( -0.7500000000000215383, 5.222916667349482012, 1.299038105676671107 ) ) ;
#189056=CARTESIAN_POINT ( 'NONE',  ( 6.889514614038635187, 11.18951748302043114, -0.7998128361456291469 ) ) ;
#189059=CARTESIAN_POINT ( 'NONE',  ( -7.009729113465285266, 8.136771039586342624, -1.199719254218446718 ) ) ;
#189061=CARTESIAN_POINT ( 'NONE',  ( -1.201851678989727383E-14, 4.946875000341420581, -1.575800808251660134 ) ) ;
#189064=CIRCLE ( 'NONE', #5807, 0.07999999999999983513 ) ;
#189065=( BOUNDED_CURVE ( )  B_SPLINE_CURVE ( 2, ( #7234, #90667, #201164, #86379, #152447, #193479, #76520 ),
 .UNSPECIFIED., .F., .T. ) 
 B_SPLINE_CURVE_WITH_KNOTS ( ( 3, 2, 2, 3 ),
 ( 0.1999999999999999556, 0.2041666666666666630, 0.2083333333333333981, 0.2125000000000001055 ),
 .UNSPECIFIED. ) 
 CURVE ( )  GEOMETRIC_REPRESENTATION_ITEM ( )  RATIONAL_B_SPLINE_CURVE ( ( 1.000000000000001776, 0.8660254037844369313, 1.000000000000000000, 0.8660254037844387076, 1.000000000000000000, 0.8660254037844351549, 1.000000000000003553 ) ) 
 REPRESENTATION_ITEM ( '' )  );
#189068=CARTESIAN_POINT ( 'NONE',  ( -7.375272376154081932, 10.58793962461302485, -1.082531754730543971 ) ) ;
#189072=EDGE_CURVE ( 'NONE', #191425, #113693, #27236, .T. ) ;
#189073=CARTESIAN_POINT ( 'NONE',  ( 1.364683531249988535, 4.467708333674754506, -0.7879004041258300672 ) ) ;
#189080=CARTESIAN_POINT ( 'NONE',  ( 1.364683531249990311, 4.134375000341417028, 1.214306433183764966E-14 ) ) ;
#189081=CARTESIAN_POINT ( 'NONE',  ( -5.623934791570306402, 5.455678766453782913, 0.7998128361456341429 ) ) ;
#189082=CARTESIAN_POINT ( 'NONE',  ( 7.149227073107712549, 7.235186428247455837, -0.7998128361456281477 ) ) ;
#189085=CARTESIAN_POINT ( 'NONE',  ( 3.023105065722948126, 6.470780310077995701, 0.7216878364870338292 ) ) ;
#189086=CARTESIAN_POINT ( 'NONE',  ( 0.6823417656249899377, 4.988541667008086655, -1.181850606188754593 ) ) ;
#189091=CARTESIAN_POINT ( 'NONE',  ( -1.364683531250000748, 0.5093750003414208027, 0.000000000000000000 ) ) ;
#189093=CARTESIAN_POINT ( 'NONE',  ( -5.287316719649550301, 5.270883715786984780, 0.7216878364870317197 ) ) ;
#189094=CARTESIAN_POINT ( 'NONE',  ( 4.690231075323689325, 7.559354456931247412, 1.199719254218462483 ) ) ;
#189098=CARTESIAN_POINT ( 'NONE',  ( 3.877268743828276243, 4.586196958296845594, 1.082531754730560403 ) ) ;
#189101=CARTESIAN_POINT ( 'NONE',  ( -7.483737605063437215, 10.71448239167390604, 1.082531754730549967 ) ) ;
#189106=CARTESIAN_POINT ( 'NONE',  ( -10.13202086811422475, 10.71511252242175161, -0.7998128361456291469 ) ) ;
#189107=CARTESIAN_POINT ( 'NONE',  ( -5.870317324592821073, 6.911420302522161663, -1.082531754730543083 ) ) ;
#189109=CARTESIAN_POINT ( 'NONE',  ( -0.6823417656250003738, 1.280208333674752508, -1.181850606188749264 ) ) ;
#189117=EDGE_CURVE ( 'NONE', #190459, #138847, #197945, .T. ) ;
#189120=CARTESIAN_POINT ( 'NONE',  ( 7.687109908824030668, 10.95175007939464606, -1.082531754730543083 ) ) ;
#189130=DIRECTION ( 'NONE',  ( -5.578564026256490882E-16, -1.000000000000000000, -9.066213480720158442E-32 ) ) ;
#189133=CARTESIAN_POINT ( 'NONE',  ( -1.364683531250012516, 3.301041667008084879, -0.7879004041258289570 ) ) ;
#189143=CARTESIAN_POINT ( 'NONE',  ( -1.364683531250014514, 0.4885416670080875434, -0.7879004041258289570 ) ) ;
#189148=DIRECTION ( 'NONE',  ( 1.000000000000000000, 0.000000000000000000, 0.000000000000000000 ) ) ;
#189153=CARTESIAN_POINT ( 'NONE',  ( 4.157546660884947620, 8.002221537674429896, 1.040834085586084257E-14 ) ) ;
#189161=CARTESIAN_POINT ( 'NONE',  ( 7.283754839039659146, 9.520799950344851936, -1.599625672291262513 ) ) ;
#189162=CARTESIAN_POINT ( 'NONE',  ( 3.833604091385769408, 6.010284403505129269, -1.249999994511383772 ) ) ;
#189164=CARTESIAN_POINT ( 'NONE',  ( 10.24726517383036928, 10.84956421242393887, 0.000000000000000000 ) ) ;
#189175=ADVANCED_FACE ( 'NONE', ( #70326 ), #183037, .T. ) ;
#189176=CARTESIAN_POINT ( 'NONE',  ( -7.375272376154081932, 10.58793962461302485, -1.082531754730543971 ) ) ;
#189182=CARTESIAN_POINT ( 'NONE',  ( -9.969323024750229578, 10.52529837183042716, -0.7998128361456291469 ) ) ;
#189188=CARTESIAN_POINT ( 'NONE',  ( 8.048736748007069508, 12.54194330598362406, -0.7998128361456352531 ) ) ;
#189189=EDGE_CURVE ( 'NONE', #32739, #157452, #58014, .T. ) ;
#189191=CARTESIAN_POINT ( 'NONE',  ( 5.192936529234042808, 6.017179691316550283, -1.199719254218452047 ) ) ;
#189193=EDGE_LOOP ( 'NONE', ( #1843, #173458, #35862, #27876 ) ) ;
#189198=CARTESIAN_POINT ( 'NONE',  ( -4.717347382551060342, 7.590990148696470818, 1.199719254218464037 ) ) ;
#189200=CARTESIAN_POINT ( 'NONE',  ( -3.379006598303881059, 4.965260336153046516, -1.599625672291256295 ) ) ;
#189206=CARTESIAN_POINT ( 'NONE',  ( 7.117667457494414762, 11.24776976714476184, 1.040834085586084257E-14 ) ) ;
#189207=CARTESIAN_POINT ( 'NONE',  ( -1.364683531250012516, 4.551041667008083103, -0.7879004041258300672 ) ) ;
#189209=CARTESIAN_POINT ( 'NONE',  ( 6.484877546038077867, 6.460111979999551224, 1.040834085586084257E-14 ) ) ;
#189219=CARTESIAN_POINT ( 'NONE',  ( 1.445103857046235563, 8.688264192038509748, -2.625611233228769770 ) ) ;
#189224=CARTESIAN_POINT ( 'NONE',  ( 1.364683531249986537, 1.467708333674748289, -0.7879004041258239610 ) ) ;
#189225=CARTESIAN_POINT ( 'NONE',  ( -2.216394925932018367, 5.529618480321886409, 1.040834085586084257E-14 ) ) ;
#189226=CARTESIAN_POINT ( 'NONE',  ( 3.181359600701000989, 6.863336634126477875, 0.000000000000000000 ) ) ;
#189229=CARTESIAN_POINT ( 'NONE',  ( -4.921246572080546500, 8.685278734161874681, 1.214306433183764966E-14 ) ) ;
#189230=CARTESIAN_POINT ( 'NONE',  ( 3.633221978782282147, 5.261844946711204507, -1.443375672974057666 ) ) ;
#189231=CARTESIAN_POINT ( 'NONE',  ( -6.358410854684793279, 7.480862754296137673, -1.082531754730543083 ) ) ;
#189235=CARTESIAN_POINT ( 'NONE',  ( 4.527533231959700366, 7.369540306339926516, 1.199719254218462483 ) ) ;
#189246=CARTESIAN_POINT ( 'NONE',  ( 5.960781091502512119, 10.10599504006161986, 0.7998128361456462443 ) ) ;
#189248=CARTESIAN_POINT ( 'NONE',  ( -5.689618019229208734, 9.789638122409414223, 0.7998128361456481317 ) ) ;
#189252=CARTESIAN_POINT ( 'NONE',  ( 8.101160479365381306, 9.410107633136481908, -1.199719254218446718 ) ) ;
#189255=CARTESIAN_POINT ( 'NONE',  ( -5.364222332501225488, 9.410009821226765325, 0.7998128361456481317 ) ) ;
#189256=CARTESIAN_POINT ( 'NONE',  ( 6.263503779389103521, 10.25124547602188763, 1.040834085586084257E-14 ) ) ;
#189257=CARTESIAN_POINT ( 'NONE',  ( 4.021084497595363239, 7.798870403269500429, 0.3307836955792880507 ) ) ;
#189258=CARTESIAN_POINT ( 'NONE',  ( -5.436983294280064882, 6.301900917203534291, 1.199719254218450271 ) ) ;
#189264=CARTESIAN_POINT ( 'NONE',  ( 9.901532256681887745, 10.44620914241737530, 0.000000000000000000 ) ) ;
#189265=CARTESIAN_POINT ( 'NONE',  ( -3.904598122329041576, 2.800000000000024691, -0.7749999999999944711 ) ) ;
#189266=CARTESIAN_POINT ( 'NONE',  ( -1.364683531250000748, 0.009375000341420303140, 0.000000000000000000 ) ) ;
#189268=CARTESIAN_POINT ( 'NONE',  ( -7.226132686403777150, 7.532835677000276675, 1.040834085586084257E-14 ) ) ;
#189274=CARTESIAN_POINT ( 'NONE',  ( -5.779651213448679492, 6.079991247305356339, 0.5991391260298760679 ) ) ;
#189275=CARTESIAN_POINT ( 'NONE',  ( -1.364683531250000748, 2.071875000341422357, 1.214306433183764966E-14 ) ) ;
#189278=CARTESIAN_POINT ( 'NONE',  ( 3.389175213736297820, 4.977123720824209840, 1.443375672974062551 ) ) ;
#189281=CARTESIAN_POINT ( 'NONE',  ( -5.759516327706961647, 5.613857225279885732, -0.7998128361456221525 ) ) ;
#189283=CARTESIAN_POINT ( 'NONE',  ( -8.202319746143382773, 9.632089794331152532, 1.082531754730558626 ) ) ;
#189290=CARTESIAN_POINT ( 'NONE',  ( -8.202319746143382773, 9.632089794331152532, 1.082531754730558626 ) ) ;
#189296=CARTESIAN_POINT ( 'NONE',  ( -7.741342523278709642, 10.05465224862374285, 1.443375672974090751 ) ) ;
#189302=CARTESIAN_POINT ( 'NONE',  ( 0.7499999999999920064, 5.264583334016151639, 1.299038105676669330 ) ) ;
#189303=CARTESIAN_POINT ( 'NONE',  ( 4.333225684176827741, 7.421547172477886534, -1.117180756173659084 ) ) ;
#189312=CARTESIAN_POINT ( 'NONE',  ( -5.682838942422375084, 9.781729199468104596, 0.000000000000000000 ) ) ;
#189313=CARTESIAN_POINT ( 'NONE',  ( -2.911621704963911927, 6.548642422433190724, 0.3158334299713649318 ) ) ;
#189315=CARTESIAN_POINT ( 'NONE',  ( 4.798696304233017074, 7.685897223992134819, -1.199719254218452047 ) ) ;
#189317=CARTESIAN_POINT ( 'NONE',  ( -3.129460678718345878, 6.444905630999884671, -0.7687999843507524744 ) ) ;
#189319=CARTESIAN_POINT ( 'NONE',  ( 7.308008492965924141, 8.484763649003774333, -1.199719254218451159 ) ) ;
#189324=CARTESIAN_POINT ( 'NONE',  ( -4.717874267875590277, 7.487641831621378863, 1.082531754730560403 ) ) ;
#189335=CARTESIAN_POINT ( 'NONE',  ( 1.364683531249986537, 0.8635416670080893198, 0.7879004041258500513 ) ) ;
#189337=CARTESIAN_POINT ( 'NONE',  ( -7.167456763118792651, 11.51378332361394818, 0.000000000000000000 ) ) ;
#189339=CARTESIAN_POINT ( 'NONE',  ( 7.283754839039659146, 9.520799950344851936, -1.599625672291262513 ) ) ;
#189341=CARTESIAN_POINT ( 'NONE',  ( -9.013473194986783454, 9.410140237106395134, -0.7998128361456291469 ) ) ;
#189343=CARTESIAN_POINT ( 'NONE',  ( 0.6823417656249917140, 5.092708333674749177, 1.181850606188765695 ) ) ;
#189344=CARTESIAN_POINT ( 'NONE',  ( 9.910647101909615841, 10.66476916175714607, 0.000000000000000000 ) ) ;
#189347=CARTESIAN_POINT ( 'NONE',  ( -0.6823417656250246877, -0.1364583329919108468, 1.181850606188755259 ) ) ;
#189350=CARTESIAN_POINT ( 'NONE',  ( 7.239690839573049708, 11.39013037956983965, 1.040834085586084257E-14 ) ) ;
#189353=CARTESIAN_POINT ( 'NONE',  ( -5.585596099150191840, 7.539614753807099667, -1.443375672974052559 ) ) ;
#189355=CARTESIAN_POINT ( 'NONE',  ( 0.6823417656249882723, 1.676041667008083769, -1.181850606188749264 ) ) ;
#189359=CARTESIAN_POINT ( 'NONE',  ( -6.184490626128011925, 10.36698949712469364, -0.7998128361456291469 ) ) ;
#189360=CARTESIAN_POINT ( 'NONE',  ( -1.201851678989727383E-14, 5.259375000341421469, -1.575800808251660134 ) ) ;
#189365=CARTESIAN_POINT ( 'NONE',  ( 8.097244055859613709, 10.46987070330147063, -1.599625672291262513 ) ) ;
#189368=CARTESIAN_POINT ( 'NONE',  ( -1.402160292154681736E-14, 1.587500000000018785, -1.732050807568863648 ) ) ;
#189374=CARTESIAN_POINT ( 'NONE',  ( 6.127922243696800386, 10.09306701771420656, -0.7216878364870267237 ) ) ;
#189376=CARTESIAN_POINT ( 'NONE',  ( 10.55910270694468345, 11.21337466772398095, 0.7998128361456462443 ) ) ;
#189378=CARTESIAN_POINT ( 'NONE',  ( 2.920892028740289081, 5.495125569250587816, 1.199719254218452047 ) ) ;
#189383=CARTESIAN_POINT ( 'NONE',  ( 7.995557903757111617, 10.35123685918189729, 1.599625672291281386 ) ) ;
#189384=CARTESIAN_POINT ( 'NONE',  ( -9.022061154889962964, 12.61315621642528129, -1.199719254218446718 ) ) ;
#189387=CARTESIAN_POINT ( 'NONE',  ( 0.6823417656249882723, 0.1760416670080894308, -1.181850606188749264 ) ) ;
#189388=CARTESIAN_POINT ( 'NONE',  ( 0.7499999999999885647, 1.816666666666688634, -1.299038105676652899 ) ) ;
#189392=CARTESIAN_POINT ( 'NONE',  ( -4.874313559192080092, 4.961021341527962036, 0.5169845646830675268 ) ) ;
#189395=CARTESIAN_POINT ( 'NONE',  ( -1.500000000000015099, -1.297916665983847029, 0.8660254037844403729 ) ) ;
#189397=CARTESIAN_POINT ( 'NONE',  ( -6.808165692356648258, 11.09461040772476714, 0.7998128361456481317 ) ) ;
#189398=CARTESIAN_POINT ( 'NONE',  ( -5.368665641331555882, 8.246898433986675769, 1.082531754730548412 ) ) ;
#189407=CARTESIAN_POINT ( 'NONE',  ( 8.052653171512838881, 11.48218023581863001, -1.199719254218446718 ) ) ;
#189411=CARTESIAN_POINT ( 'NONE',  ( 7.090551149822735155, 9.295395646258437949, 1.443375672974076540 ) ) ;
#189414=CARTESIAN_POINT ( 'NONE',  ( -8.350932551013499960, 11.83017284523606172, -1.199719254218446718 ) ) ;
#189415=CARTESIAN_POINT ( 'NONE',  ( 6.817052309572890323, 6.847649204123507083, 0.7998128361456341429 ) ) ;
#189417=CARTESIAN_POINT ( 'NONE',  ( 2.535011535630975477, 5.901337858304024131, 0.7216878364870438212 ) ) ;
#189419=CARTESIAN_POINT ( 'NONE',  ( 4.681643115420508039, 4.356338477612361260, 0.7998128361456341429 ) ) ;
#189420=VERTEX_POINT ( 'NONE', #26920 ) ;
#189428=CARTESIAN_POINT ( 'NONE',  ( -5.639828713604883248, 6.642516923036197340, 1.082531754730548412 ) ) ;
#189429=CARTESIAN_POINT ( 'NONE',  ( 4.532503425670185493, 4.182342172903648070, 1.214306433183764966E-14 ) ) ;
#189432=CARTESIAN_POINT ( 'NONE',  ( -6.449928391799210736, 8.548002428564306143, -1.599625672291263179 ) ) ;
#189437=CARTESIAN_POINT ( 'NONE',  ( -7.635213062790267458, 12.05949900656400686, 0.000000000000000000 ) ) ;
#189442=CARTESIAN_POINT ( 'NONE',  ( 6.484877546038077867, 6.460111979999551224, 1.040834085586084257E-14 ) ) ;
#189454=CARTESIAN_POINT ( 'NONE',  ( -5.831978632172702071, 9.955725504176825780, 0.7998128361456481317 ) ) ;
#189457=CARTESIAN_POINT ( 'NONE',  ( 4.663641653420880218, 8.384739662392275861, -0.7216878364870207285 ) ) ;
#189459=CARTESIAN_POINT ( 'NONE',  ( -1.499999999999997780, 5.790625000341422357, 1.214306433183764966E-14 ) ) ;
#189461=CARTESIAN_POINT ( 'NONE',  ( 3.194917754314666514, 6.879154480009089134, 0.7998128361456321445 ) ) ;
#189463=CARTESIAN_POINT ( 'NONE',  ( -4.415151579544611238, 8.302760609444034046, -0.7998128361456281477 ) ) ;
#189472=CARTESIAN_POINT ( 'NONE',  ( 1.500000000000007105, 10.64264068711930733, 1.214306433183764966E-14 ) ) ;
#189473=CARTESIAN_POINT ( 'NONE',  ( -10.65400978224035811, 11.32409958890225710, 1.040834085586084257E-14 ) ) ;
#189474=CARTESIAN_POINT ( 'NONE',  ( 8.288111976655649471, 8.563885482386732306, -0.7998128361456291469 ) ) ;
#189476=FACE_OUTER_BOUND ( 'NONE', #101084, .T. ) ;
#189477=CARTESIAN_POINT ( 'NONE',  ( -4.434757016570429755, 7.116138787269118637, -1.097766128466563851 ) ) ;
#189484=CARTESIAN_POINT ( 'NONE',  ( 9.897088948295943212, 11.60932053017587506, 1.082531754730548412 ) ) ;
#189488=B_SPLINE_CURVE_WITH_KNOTS ( 'NONE', 3,
 ( #160553, #12161, #78232, #144355, #210356, #84627, #104091, #198361, #35874, #17471, #202621, #165886 ),
 .UNSPECIFIED., .F., .F.,
 ( 4, 2, 2, 2, 2, 4 ),
 ( 0.001597310297180445406, 0.001963012261066415971, 0.002328714224952386971, 0.003060118152724327668, 0.003791522080496267932, 0.004522926008268208196 ),
 .UNSPECIFIED. ) ;
#189491=CARTESIAN_POINT ( 'NONE',  ( -3.337985173046072340, 6.383183490859034137, 0.8077998227833966816 ) ) ;
#189503=CARTESIAN_POINT ( 'NONE',  ( -2.950870989268691957, 6.594433254122103349, -0.7998128361456281477 ) ) ;
#189505=CARTESIAN_POINT ( 'NONE',  ( -3.273404022695637572, 5.906389562198459231, 1.199719254218462483 ) ) ;
#189510=CARTESIAN_POINT ( 'NONE',  ( 0.7499999999999885647, -0.9854166659838472508, 1.299038105676657340 ) ) ;
#189514=DIRECTION ( 'NONE',  ( 0.7592566023653004592, 0.6507913734559639396, 0.000000000000000000 ) ) ;
#189515=ORIENTED_EDGE ( 'NONE', *, *, #213374, .T. ) ;
#189517=CARTESIAN_POINT ( 'NONE',  ( 3.216308754939877446, 4.775446185561722956, -1.599625672291262513 ) ) ;
#189518=CARTESIAN_POINT ( 'NONE',  ( -4.894130264408873110, 5.772535398974209642, -1.082531754730543971 ) ) ;
#189521=CARTESIAN_POINT ( 'NONE',  ( 10.20892648096591770, 11.01276177065614981, -0.7216878364870257245 ) ) ;
#189524=CARTESIAN_POINT ( 'NONE',  ( -1.402160292154681736E-14, 1.009375000341417916, -1.575800808251659024 ) ) ;
#189527=CARTESIAN_POINT ( 'NONE',  ( -7.784352752540590004, 12.23349531127272094, 0.7998128361456481317 ) ) ;
#189528=CARTESIAN_POINT ( 'NONE',  ( -6.358410854684796831, 6.520493539994793863, -0.7216878364870267237 ) ) ;
#189530=CARTESIAN_POINT ( 'NONE',  ( -6.501298352952815662, 7.543601818988450169, -1.199719254218446718 ) ) ;
#189532=CARTESIAN_POINT ( 'NONE',  ( -1.201851678989727383E-14, 5.446875000341422357, -1.575800808251660134 ) ) ;
#189540=CARTESIAN_POINT ( 'NONE',  ( -4.731432421044877934, 6.543090462684225450, -1.443375672974051449 ) ) ;
#189545=CARTESIAN_POINT ( 'NONE',  ( -4.812781342726871969, 6.637997537979888563, 1.443375672974064550 ) ) ;
#189547=CARTESIAN_POINT ( 'NONE',  ( 9.073431116043567002, 11.60875560684942265, -1.599625672291262513 ) ) ;
#189557=DIRECTION ( 'NONE',  ( -0.8002608041566144914, -0.5996521035822427459, -8.676445024215948894E-15 ) ) ;
#189558=CARTESIAN_POINT ( 'NONE',  ( -3.066115294984855133, 6.728884944124295053, 0.7998128361456341429 ) ) ;
#189564=CARTESIAN_POINT ( 'NONE',  ( 7.402388683381404988, 10.61957531637824204, -1.082531754730537976 ) ) ;
#189565=CARTESIAN_POINT ( 'NONE',  ( 4.971035877704902184, 8.951292290631053916, 1.040834085586084257E-14 ) ) ;
#189569=DIRECTION ( 'NONE',  ( -5.578564026256490882E-16, -1.000000000000000000, -9.066213480720158442E-32 ) ) ;
#189570=CARTESIAN_POINT ( 'NONE',  ( 3.344057444064992168, 7.053150784717805877, 1.040834085586084257E-14 ) ) ;
#189580=CARTESIAN_POINT ( 'NONE',  ( -6.735703387890906946, 6.752742128827836865, -0.7998128361456291469 ) ) ;
#189587=CARTESIAN_POINT ( 'NONE',  ( -1.001543065824772872E-14, 4.821875000341419693, 1.575800808251672791 ) ) ;
#189589=CARTESIAN_POINT ( 'NONE',  ( -6.898401231254901234, 6.942556279419168419, -0.7998128361456291469 ) ) ;
#189591=CARTESIAN_POINT ( 'NONE',  ( -1.474199074347627425, 7.377996015708403910, -4.279257749350879436 ) ) ;
#189592=CARTESIAN_POINT ( 'NONE',  ( 5.412729640353754590, 7.337937218544611895, 1.599625672291267398 ) ) ;
#189593=CARTESIAN_POINT ( 'NONE',  ( -6.196239896645333367, 7.187700286629718605, -1.199719254218446718 ) ) ;
#189599=CARTESIAN_POINT ( 'NONE',  ( 5.314433026876846711, 9.143996264757578984, -0.7216878364870267237 ) ) ;
#189601=CARTESIAN_POINT ( 'NONE',  ( 7.470179451005385829, 8.777926116670192513, -1.082531754730537976 ) ) ;
#189602=CARTESIAN_POINT ( 'NONE',  ( -1.364683531250012516, 2.842708333674754506, 0.7879004041258379498 ) ) ;
#189604=CARTESIAN_POINT ( 'NONE',  ( 6.141480396866128899, 6.267408005873028820, -0.7216878364870257245 ) ) ;
#189606=CARTESIAN_POINT ( 'NONE',  ( -2.155383234892699562, 5.458438174109348395, 1.040834085586084257E-14 ) ) ;
#189613=CARTESIAN_POINT ( 'NONE',  ( -4.277728075731661583, 7.474117497184462167, -1.086723757153153835 ) ) ;
#189621=CARTESIAN_POINT ( 'NONE',  ( -3.212919216314315207, 5.731860938133201522, 1.082531754730560403 ) ) ;
#189623=CARTESIAN_POINT ( 'NONE',  ( 5.858512798400357546, 6.179092012920288646, 0.8810539604525641222 ) ) ;
#189626=CARTESIAN_POINT ( 'NONE',  ( -2.286521462199063492, 5.819358805874190743, 1.040834085586084257E-14 ) ) ;
#189631=CARTESIAN_POINT ( 'NONE',  ( 5.504247177468190699, 5.523969249908757817, 0.7216878364870317197 ) ) ;
#189632=CARTESIAN_POINT ( 'NONE',  ( 1.364683531249988535, 2.967708333674755394, -0.7879004041258239610 ) ) ;
#189634=CARTESIAN_POINT ( 'NONE',  ( 6.903072767652295383, 11.20533532890304684, 1.040834085586084257E-14 ) ) ;
#189636=CARTESIAN_POINT ( 'NONE',  ( -4.066556009095094737, 6.831733546331167695, 1.199719254218464037 ) ) ;
#189640=CARTESIAN_POINT ( 'NONE',  ( 1.499999999999989120, 3.025000000000020783, 1.214306433183764966E-14 ) ) ;
#189641=CARTESIAN_POINT ( 'NONE',  ( 4.660252114795294887, 6.460046772059735432, -1.599625672291256295 ) ) ;
#189644=CARTESIAN_POINT ( 'NONE',  ( -3.197497122698730099, 6.431928158754201874, 0.6077543439236172684 ) ) ;
#189645=CARTESIAN_POINT ( 'NONE',  ( -0.6823417656250212460, 4.551041667008086655, 1.181850606188767472 ) ) ;
#189648=CARTESIAN_POINT ( 'NONE',  ( 8.758204044747994743, 12.20135990463928266, 1.082531754730546636 ) ) ;
#189653=CARTESIAN_POINT ( 'NONE',  ( -0.7500000000000006661, 2.639583334016156080, -1.299038105676652011 ) ) ;
#189655=CARTESIAN_POINT ( 'NONE',  ( -6.392833124043511894, 7.417059051927569868, 1.199719254218450271 ) ) ;
#189664=CARTESIAN_POINT ( 'NONE',  ( 4.473300617505036492, 7.306268922809479704, -1.199719254218452047 ) ) ;
#189665=CARTESIAN_POINT ( 'NONE',  ( 8.500000000000000000, 6.200000000000038369, -2.900000000000000799 ) ) ;
#189668=CARTESIAN_POINT ( 'NONE',  ( 6.006425746053997372, 6.966250444273174303, -1.199719254218445830 ) ) ;
#189674=ORIENTED_EDGE ( 'NONE', *, *, #116730, .F. ) ;
#189675=CARTESIAN_POINT ( 'NONE',  ( 9.402743226277308963, 10.92862083786708816, -1.199719254218446718 ) ) ;
#189680=CARTESIAN_POINT ( 'NONE',  ( 5.890592889100787488, 5.978139607520936316, 0.07745371066007235294 ) ) ;
#189692=CARTESIAN_POINT ( 'NONE',  ( 7.456621297836078632, 8.762108271306003004, 1.082531754730558626 ) ) ;
#189694=CARTESIAN_POINT ( 'NONE',  ( -3.846762897975357198, 5.510976019103107859, -1.599625672291256295 ) ) ;
#189697=CARTESIAN_POINT ( 'NONE',  ( -6.878064000834399394, 6.918829510595249310, -0.7998128361456291469 ) ) ;
#189705=CARTESIAN_POINT ( 'NONE',  ( 3.189213936345665523, 2.817530495244580102, 2.450448857954567572 ) ) ;
#189710=CARTESIAN_POINT ( 'NONE',  ( 8.886479618753304166, 12.45497775759917758, -1.199719254218446718 ) ) ;
#189720=CARTESIAN_POINT ( 'NONE',  ( -8.676855123066012254, 12.10645282934361866, -1.082531754730543971 ) ) ;
#189722=CARTESIAN_POINT ( 'NONE',  ( 8.860417081730671995, 10.29590700256267155, 1.199719254218453823 ) ) ;
#189727=CARTESIAN_POINT ( 'NONE',  ( -7.039708073993679704, 9.236078724457858158, 1.599625672291283607 ) ) ;
#189728=CARTESIAN_POINT ( 'NONE',  ( 5.657830175604453338, 5.495223381160312393, 0.7998128361456341429 ) ) ;
#189730=CARTESIAN_POINT ( 'NONE',  ( -3.090895833791289071, 6.549869539491048442, 1.040834085586084257E-14 ) ) ;
#189734=CARTESIAN_POINT ( 'NONE',  ( 1.364683531249988535, 3.217708333674748289, -0.7879004041258239610 ) ) ;
#189736=CARTESIAN_POINT ( 'NONE',  ( 7.131225611108096274, 8.382479970123348778, 1.082531754730558626 ) ) ;
#189744=CARTESIAN_POINT ( 'NONE',  ( 9.097157884645296733, 10.67606762258344055, -1.082531754730543083 ) ) ;
#189749=CARTESIAN_POINT ( 'NONE',  ( -7.316596452869116973, 11.68777962832266049, 0.7998128361456481317 ) ) ;
#189758=CARTESIAN_POINT ( 'NONE',  ( 3.571683402196252910, 6.254382171615883834, 1.199719254218462483 ) ) ;
#189766=CARTESIAN_POINT ( 'NONE',  ( 6.335737856287750880, 6.286115675290828264, -0.7998128361456281477 ) ) ;
#189770=CARTESIAN_POINT ( 'NONE',  ( 0.7499999999999902300, 2.514583334016148974, 1.299038105676669330 ) ) ;
#189774=VERTEX_POINT ( 'NONE', #108259 ) ;
#189776=CARTESIAN_POINT ( 'NONE',  ( 1.499999999999987121, 1.004166666666687968, 0.8660254037844524744 ) ) ;
#189777=CARTESIAN_POINT ( 'NONE',  ( 8.098297826064319693, 8.342435640030188893, 0.7998128361456481317 ) ) ;
#189778=CARTESIAN_POINT ( 'NONE',  ( 1.364683531249986537, -0.5947916663252456049, -0.7879004041258309554 ) ) ;
#189781=CARTESIAN_POINT ( 'NONE',  ( 9.246297574839980271, 10.85006392781057905, 1.082531754730549967 ) ) ;
#189787=CARTESIAN_POINT ( 'NONE',  ( -6.230135280679522936, 7.227244901336242755, 1.199719254218450271 ) ) ;
#189789=CARTESIAN_POINT ( 'NONE',  ( 0.7499999999999902300, 3.014583334016149418, 1.299038105676669330 ) ) ;
#189790=CARTESIAN_POINT ( 'NONE',  ( -1.201851678989727383E-14, 4.509375000341417916, -1.575800808251660134 ) ) ;
#189802=DIRECTION ( 'NONE',  ( 7.387867266669436732E-31, -1.000000000000000000, -8.546850786086424434E-32 ) ) ;
#189803=CARTESIAN_POINT ( 'NONE',  ( -9.341731535015849630, 10.85744053139533349, 1.199719254218462483 ) ) ;
#189804=CARTESIAN_POINT ( 'NONE',  ( 7.494959990256193194, 7.638541498254023843, -0.7998128361456281477 ) ) ;
#189807=ORIENTED_EDGE ( 'NONE', *, *, #2092, .F. ) ;
#189813=CARTESIAN_POINT ( 'NONE',  ( -6.507023659554960204, 9.678945805201045971, 1.199719254218452047 ) ) ;
#189815=CARTESIAN_POINT ( 'NONE',  ( -2.081668171172168513E-14, 5.868705557303649734, 4.125226524755077229 ) ) ;
#189818=CARTESIAN_POINT ( 'NONE',  ( 10.56588178375152864, 11.22128359066528169, -0.7998128361456281477 ) ) ;
#189822=CARTESIAN_POINT ( 'NONE',  ( -5.901876940650454095, 5.779944607047298177, -0.7998128361456291469 ) ) ;
#189823=CARTESIAN_POINT ( 'NONE',  ( -7.160677686311960777, 11.50587440067263678, -0.7998128361456291469 ) ) ;
#189826=CARTESIAN_POINT ( 'NONE',  ( -3.976511113072466408, 7.848157239995420476, -0.08586869108932922157 ) ) ;
#189833=CARTESIAN_POINT ( 'NONE',  ( 6.928380191783277908, 8.041863964290678624, 1.199719254218462483 ) ) ;
#189835=AXIS2_PLACEMENT_3D ( 'NONE', #204227, #89470, #170691 ) ;
#189854=CARTESIAN_POINT ( 'NONE',  ( 2.562127843302666186, 5.932973550587659517, 0.000000000000000000 ) ) ;
#189858=( BOUNDED_CURVE ( )  B_SPLINE_CURVE ( 1, ( #73831, #6674 ),
 .UNSPECIFIED., .F., .T. ) 
 B_SPLINE_CURVE_WITH_KNOTS ( ( 2, 2 ),
 ( 0.000000000000000000, 6.249999999999832079E-05 ),
 .UNSPECIFIED. ) 
 CURVE ( )  GEOMETRIC_REPRESENTATION_ITEM ( )  RATIONAL_B_SPLINE_CURVE ( ( 0.9345202395942817652, 0.9345202395942817652 ) ) 
 REPRESENTATION_ITEM ( '' )  );
#189859=CARTESIAN_POINT ( 'NONE',  ( -8.676328237741483207, 12.20980114641871062, -1.199719254218446718 ) ) ;
#189861=CARTESIAN_POINT ( 'NONE',  ( 1.419999999999990603, 6.280000000000042881, 2.580000000000000515 ) ) ;
#189862=CARTESIAN_POINT ( 'NONE',  ( 8.829384350997564468, 11.32403438096243775, 1.599625672291281386 ) ) ;
#189864=B_SPLINE_CURVE_WITH_KNOTS ( 'NONE', 3,
 ( #196161, #178856, #47802, #15249 ),
 .UNSPECIFIED., .F., .F.,
 ( 4, 4 ),
 ( 6.505213034913028530E-19, 0.0003197243294388478550 ),
 .UNSPECIFIED. ) ;
#189867=LINE ( 'NONE', #156319, #77251 ) ;
#189873=CARTESIAN_POINT ( 'NONE',  ( 1.364683531249986537, 0.1135416670080857532, 0.7879004041258500513 ) ) ;
#189879=CARTESIAN_POINT ( 'NONE',  ( -5.603597561149804562, 5.431951997629870910, 0.7998128361456341429 ) ) ;
#189883=CARTESIAN_POINT ( 'NONE',  ( 0.7499999999999867883, -0.6833333333333135862, -1.299038105676652899 ) ) ;
#189885=CARTESIAN_POINT ( 'NONE',  ( -1.402160292154681736E-14, -0.7406249996585823059, -1.575800808251665908 ) ) ;
#189891=CARTESIAN_POINT ( 'NONE',  ( -0.6823417656250003738, 0.4677083336747517306, -1.181850606188749264 ) ) ;
#189893=CARTESIAN_POINT ( 'NONE',  ( -6.690058733339450114, 9.892486724616283311, 1.199719254218452047 ) ) ;
#189894=CARTESIAN_POINT ( 'NONE',  ( 8.239604668803105270, 10.63595808506888396, -1.599625672291268286 ) ) ;
#189895=CARTESIAN_POINT ( 'NONE',  ( 5.529027716274630855, 5.344953845275508542, 1.040834085586084257E-14 ) ) ;
#189899=CARTESIAN_POINT ( 'NONE',  ( -1.364683531250000748, 0.3218750003414205807, 0.000000000000000000 ) ) ;
#189906=CARTESIAN_POINT ( 'NONE',  ( 5.490689023854504747, 9.349628261231513804, 1.040834085586084257E-14 ) ) ;
#189909=CARTESIAN_POINT ( 'NONE',  ( -4.391951695823077984, 7.211361847513815704, 1.199719254218464037 ) ) ;
#189910=CARTESIAN_POINT ( 'NONE',  ( -1.123270288250315163, 2.985197346350006331, -0.7749999999993613109 ) ) ;
#189911=CARTESIAN_POINT ( 'NONE',  ( 4.731432421044862835, 6.543090462684225450, -1.443375672974051449 ) ) ;
#189914=CARTESIAN_POINT ( 'NONE',  ( 5.843201017365476702, 6.879784610756938257, -1.082531754730543083 ) ) ;
#189915=CARTESIAN_POINT ( 'NONE',  ( -7.470179451005382276, 11.65903375957422128, 0.7216878364870458196 ) ) ;
#189917=CARTESIAN_POINT ( 'NONE',  ( -0.7499999999999972244, 4.358333333333352932, -1.299038105676652011 ) ) ;
#189921=CARTESIAN_POINT ( 'NONE',  ( 9.273413882067330860, 9.921330405274451536, -0.7216878364870257245 ) ) ;
#189924=DIRECTION ( 'NONE',  ( -5.578564026256490882E-16, -1.000000000000000000, -9.066213480720158442E-32 ) ) ;
#189934=CARTESIAN_POINT ( 'NONE',  ( 8.568389893712330618, 9.098802418860289620, 1.040834085586084257E-14 ) ) ;
#189936=CARTESIAN_POINT ( 'NONE',  ( 7.832860060393120882, 10.16142270859057462, 1.599625672291281386 ) ) ;
#189940=CARTESIAN_POINT ( 'NONE',  ( 5.355107487717867265, 5.349972945200037522, 1.040834085586084257E-14 ) ) ;
#189942=CARTESIAN_POINT ( 'NONE',  ( -7.646435448427427062, 10.90429654226522693, 1.082531754730549967 ) ) ;
#189970=CARTESIAN_POINT ( 'NONE',  ( -7.386494761346872551, 7.511998731193139989, -0.7998128361456291469 ) ) ;
#189972=CARTESIAN_POINT ( 'NONE',  ( -6.471393748265538370, 5.229711127717889596, -2.419999999999995044 ) ) ;
#189973=CARTESIAN_POINT ( 'NONE',  ( 6.335737856287750880, 6.286115675290828264, -0.7998128361456281477 ) ) ;
#189981=CARTESIAN_POINT ( 'NONE',  ( -4.928552533767591726, 5.708731696605642725, 1.199719254218462483 ) ) ;
#189984=CARTESIAN_POINT ( 'NONE',  ( 5.587931867126699537, 9.671004278289832001, -0.7998128361456291469 ) ) ;
#189986=EDGE_CURVE ( 'NONE', #186977, #86388, #94097, .T. ) ;
#189988=CARTESIAN_POINT ( 'NONE',  ( 6.078105975125470017, 6.038708432876411791, -0.3507111650211444109 ) ) ;
#189995=CARTESIAN_POINT ( 'NONE',  ( 5.124618875841165710, 8.922546421882614709, 1.040834085586084257E-14 ) ) ;
#189996=CARTESIAN_POINT ( 'NONE',  ( -7.670162217029145246, 9.971608557999250166, 1.599625672291295375 ) ) ;
#189999=CARTESIAN_POINT ( 'NONE',  ( -8.833300774503376473, 10.26427131079744193, 1.199719254218462483 ) ) ;
#190000=CARTESIAN_POINT ( 'NONE',  ( -6.093499974338126179, 9.196501505781426999, -1.199719254218440723 ) ) ;
#190008=CARTESIAN_POINT ( 'NONE',  ( 9.237182729612253951, 9.671134694169463586, 0.7998128361456462443 ) ) ;
#190022=CARTESIAN_POINT ( 'NONE',  ( 1.499999999999990896, 4.775000000000022560, 1.214306433183764966E-14 ) ) ;
#190023=CARTESIAN_POINT ( 'NONE',  ( 4.741601036477289810, 6.554953847355395880, 1.599625672291267398 ) ) ;
#190024=CARTESIAN_POINT ( 'NONE',  ( 7.467843683028853263, 7.606905806488803101, 0.7998128361456341429 ) ) ;
#190026=CARTESIAN_POINT ( 'NONE',  ( -9.517460647113315630, 10.20605163116143821, 0.7216878364870438212 ) ) ;
#190028=CARTESIAN_POINT ( 'NONE',  ( 6.100805936469477331, 9.101062111647635788, -1.082531754730537088 ) ) ;
#190029=CARTESIAN_POINT ( 'NONE',  ( -8.419250203962027612, 11.80591375705560608, 1.082531754730549967 ) ) ;
#190032=CARTESIAN_POINT ( 'NONE',  ( 9.264299036839600987, 9.702770385934682551, -0.7998128361456281477 ) ) ;
#190037=CARTESIAN_POINT ( 'NONE',  ( -0.6823417656250003738, 1.717708333674752730, -1.181850606188749264 ) ) ;
#190042=CARTESIAN_POINT ( 'NONE',  ( -1.402160292154681736E-14, -0.9281249996585830830, 1.575800808251672791 ) ) ;
#190044=CARTESIAN_POINT ( 'NONE',  ( 9.748476143425788720, 11.33197590787365172, -1.199719254218440723 ) ) ;
#190048=CARTESIAN_POINT ( 'NONE',  ( -10.10098813738111545, 11.74323990082152491, -1.199719254218441611 ) ) ;
#190054=CARTESIAN_POINT ( 'NONE',  ( 3.194917754314666514, 6.879154480009089134, 0.7998128361456321445 ) ) ;
#190058=CARTESIAN_POINT ( 'NONE',  ( -2.941756144040970522, 5.415504020480993219, -1.082531754730543083 ) ) ;
#190061=CARTESIAN_POINT ( 'NONE',  ( 9.420217803396747414, 9.884675613584706255, 0.7998128361456462443 ) ) ;
#190063=CARTESIAN_POINT ( 'NONE',  ( 4.871297188390688149, 6.684807392805372395, 1.249964738027457889 ) ) ;
#190065=CARTESIAN_POINT ( 'NONE',  ( -3.903858165731105778, 6.641919395739846799, 1.199719254218464037 ) ) ;
#190069=CARTESIAN_POINT ( 'NONE',  ( 8.450809820019639318, 8.753699632978056755, -0.7998128361456291469 ) ) ;
#190071=CARTESIAN_POINT ( 'NONE',  ( 6.751070424600909448, 9.963667031088037973, -1.199719254218441611 ) ) ;
#190074=CARTESIAN_POINT ( 'NONE',  ( -7.537970219518066450, 11.73812298950569044, -0.7216878364870267237 ) ) ;
#190081=CARTESIAN_POINT ( 'NONE',  ( -5.312752313518235958, 6.384578190230367767, -1.125208257168613502 ) ) ;
#190082=CARTESIAN_POINT ( 'NONE',  ( 1.364683531249988757, 1.884375000341421913, 0.000000000000000000 ) ) ;
#190084=CARTESIAN_POINT ( 'NONE',  ( 5.314433026876846711, 9.143996264757578984, -0.7216878364870267237 ) ) ;
#190102=CARTESIAN_POINT ( 'NONE',  ( 7.886038904643079661, 12.35212915539230139, -0.7998128361456352531 ) ) ;
#190106=CARTESIAN_POINT ( 'NONE',  ( 3.469446951953614189E-15, 6.400000000000023448, 1.214306433183764966E-14 ) ) ;
#190107=CARTESIAN_POINT ( 'NONE',  ( -6.826694039680798021, 7.923230120171105284, -1.199719254218446718 ) ) ;
#190110=CARTESIAN_POINT ( 'NONE',  ( -10.62011439820619429, 11.28455497419572318, -0.7998128361456221525 ) ) ;
#190113=CARTESIAN_POINT ( 'NONE',  ( 0.7499999999999902300, 4.847916667349482012, -1.299038105676658228 ) ) ;
#190114=CARTESIAN_POINT ( 'NONE',  ( 6.805303039055573322, 10.02693841461847057, 1.199719254218460707 ) ) ;
#190118=CARTESIAN_POINT ( 'NONE',  ( -6.201965203247477909, 9.323044272842313518, 1.199719254218452047 ) ) ;
#190120=CARTESIAN_POINT ( 'NONE',  ( 1.364683531249990311, 4.613541667008083103, 0.7879004041258500513 ) ) ;
#190122=CARTESIAN_POINT ( 'NONE',  ( -1.569538198872308055, 8.730447571940807450, 2.495330465740724701 ) ) ;
#190126=CARTESIAN_POINT ( 'NONE',  ( -8.405692050792730186, 9.869357483088723626, 1.082531754730558626 ) ) ;
#190130=CARTESIAN_POINT ( 'NONE',  ( -0.6823417656250003738, 2.530208333674753618, -1.181850606188749264 ) ) ;
#190138=CARTESIAN_POINT ( 'NONE',  ( 0.6823417656249899377, 4.426041667008086655, -1.181850606188754593 ) ) ;
#190139=CARTESIAN_POINT ( 'NONE',  ( -4.924636110261798372, 6.768494766770632332, 1.599625672291267398 ) ) ;
#190140=CARTESIAN_POINT ( 'NONE',  ( 7.124973419181436007, 8.271222729588529887, -1.199719254218446718 ) ) ;
#190143=CARTESIAN_POINT ( 'NONE',  ( 4.975479186090860928, 4.907073259968533385, 0.7216878364870317197 ) ) ;
#190144=CARTESIAN_POINT ( 'NONE',  ( 1.364683531249990311, 3.446875000341416584, 1.214306433183764966E-14 ) ) ;
#190149=CARTESIAN_POINT ( 'NONE',  ( 0.6823417656249882723, 1.426041667008083547, -1.181850606188749264 ) ) ;
#190150=CARTESIAN_POINT ( 'NONE',  ( -3.578989364327652467, 6.158942777482099729, 1.082531754730560403 ) ) ;
#190151=CARTESIAN_POINT ( 'NONE',  ( 6.484877546038077867, 6.460111979999551224, 1.040834085586084257E-14 ) ) ;
#190155=CARTESIAN_POINT ( 'NONE',  ( 3.226477370372293763, 6.708047998835573900, 0.7216878364870317197 ) ) ;
#190158=CARTESIAN_POINT ( 'NONE',  ( -8.459924665247381625, 11.85336729522185806, 1.082531754730560403 ) ) ;
#190164=CARTESIAN_POINT ( 'NONE',  ( -9.053093885623068715, 11.58502883802551153, -1.599625672291263179 ) ) ;
#190165=CARTESIAN_POINT ( 'NONE',  ( -6.697364695026446491, 6.915939687060050467, 1.040834085586084257E-14 ) ) ;
#190167=CARTESIAN_POINT ( 'NONE',  ( 1.364683531249986537, 0.6760416670080884316, 0.7879004041258500513 ) ) ;
#190178=CARTESIAN_POINT ( 'NONE',  ( 7.904040366642684390, 11.20483561351640844, 1.082531754730558626 ) ) ;
#190186=CARTESIAN_POINT ( 'NONE',  ( -2.981903720001798597, 5.566305875722335372, -1.199719254218446718 ) ) ;
#190188=FACE_OUTER_BOUND ( 'NONE', #73267, .T. ) ;
#190190=CARTESIAN_POINT ( 'NONE',  ( -1.402160292154681736E-14, 1.259375000341419248, -1.575800808251659024 ) ) ;
#190207=CARTESIAN_POINT ( 'NONE',  ( 4.385172619016207918, 7.203452924572514959, 1.199719254218462483 ) ) ;
#190210=ORIENTED_EDGE ( 'NONE', *, *, #24898, .T. ) ;
#190214=CARTESIAN_POINT ( 'NONE',  ( 6.988338112840064120, 10.24047933403371502, 1.199719254218460707 ) ) ;
#190218=CARTESIAN_POINT ( 'NONE',  ( 7.397945374551106568, 11.78268670361832093, -0.7998128361456291469 ) ) ;
#190220=CARTESIAN_POINT ( 'NONE',  ( 1.501703635994434238, 8.650726486491324252, -2.563578082221926735 ) ) ;
#190230=CARTESIAN_POINT ( 'NONE',  ( -7.456621297836087514, 9.722477485607340597, 1.443375672974090751 ) ) ;
#190235=CARTESIAN_POINT ( 'NONE',  ( -10.63367255181986160, 11.30037282007833532, 1.040834085586084257E-14 ) ) ;
#190237=CARTESIAN_POINT ( 'NONE',  ( -4.510196435976065565, 7.040407170307378060, -1.149263043085164915 ) ) ;
#190243=CARTESIAN_POINT ( 'NONE',  ( 3.592547517496925913, 5.214391408544949869, -1.443375672974058777 ) ) ;
#190246=VERTEX_POINT ( 'NONE', #83705 ) ;
#190251=CARTESIAN_POINT ( 'NONE',  ( -5.636439174979254396, 7.598931675607687453, -1.599625672291256295 ) ) ;
#190253=CARTESIAN_POINT ( 'NONE',  ( -3.704402285031864306, 5.344888637335695414, -1.599625672291256295 ) ) ;
#190259=CARTESIAN_POINT ( 'NONE',  ( 8.514157279702022407, 10.95626946445095307, -1.443375672974063439 ) ) ;
#190261=CARTESIAN_POINT ( 'NONE',  ( 0.6823417656249917140, 4.405208333674755394, 1.181850606188765695 ) ) ;
#190263=CARTESIAN_POINT ( 'NONE',  ( 4.527533231959700366, 7.369540306339926516, 1.199719254218462483 ) ) ;
#190277=CARTESIAN_POINT ( 'NONE',  ( 1.364683531249986537, 1.717708333674749399, -0.7879004041258239610 ) ) ;
#190279=CARTESIAN_POINT ( 'NONE',  ( 3.192055101013606233, 5.811482486902795230, -1.199719254218446718 ) ) ;
#190281=CARTESIAN_POINT ( 'NONE',  ( -6.561783159334145132, 6.757761228752363181, -0.7216878364870278340 ) ) ;
#190283=CARTESIAN_POINT ( 'NONE',  ( 4.392478581147586603, 4.226905887534702977, -0.7216878364870188411 ) ) ;
#190284=CARTESIAN_POINT ( 'NONE',  ( -6.860062538390436337, 7.105753837651378468, 1.040834085586084257E-14 ) ) ;
#190288=CARTESIAN_POINT ( 'NONE',  ( 5.961834861707224320, 7.978559976790334574, -1.599625672291262513 ) ) ;
#190296=CARTESIAN_POINT ( 'NONE',  ( 7.253775878511261155, 8.421492265473332850, 1.199719254218462483 ) ) ;
#190299=CARTESIAN_POINT ( 'NONE',  ( -5.713871673155502151, 8.753601821068331290, 1.199719254218452047 ) ) ;
#190303=CARTESIAN_POINT ( 'NONE',  ( 8.535021395002688749, 9.916278701380017324, 1.199719254218462483 ) ) ;
#190305=CARTESIAN_POINT ( 'NONE',  ( -5.526920175865215334, 9.599823971818089774, 0.7998128361456481317 ) ) ;
#190306=FACE_OUTER_BOUND ( 'NONE', #175612, .T. ) ;
#190307=CARTESIAN_POINT ( 'NONE',  ( 5.951666246274784910, 9.887435020721849099, 0.7216878364870438212 ) ) ;
#190308=CARTESIAN_POINT ( 'NONE',  ( 4.414360472080629094, 7.100309700288360837, -1.094782333960819809 ) ) ;
#190309=CARTESIAN_POINT ( 'NONE',  ( -4.225337428953291230, 8.081310767087481750, 0.7998128361456341429 ) ) ;
#190316=CARTESIAN_POINT ( 'NONE',  ( 8.215351014876830504, 11.67199438640995801, -1.199719254218446718 ) ) ;
#190317=CARTESIAN_POINT ( 'NONE',  ( -5.526177461252244960, 6.240421959547291841, 0.9601993850730760061 ) ) ;
#190319=CARTESIAN_POINT ( 'NONE',  ( -1.364683531250014514, 1.238541667008091096, -0.7879004041258289570 ) ) ;
#190321=CARTESIAN_POINT ( 'NONE',  ( -5.965224400332865606, 7.022145224218852455, 1.082531754730549967 ) ) ;
#190328=CARTESIAN_POINT ( 'NONE',  ( -5.602744053211161201, 6.190815373437144942, 0.8771416995774529157 ) ) ;
#190329=CARTESIAN_POINT ( 'NONE',  ( 0.6823417656249882723, 1.988541667008083991, -1.181850606188749264 ) ) ;
#190332=CARTESIAN_POINT ( 'NONE',  ( 2.846849069189655967, 5.304779099821139710, -1.082531754730543083 ) ) ;
#190337=CARTESIAN_POINT ( 'NONE',  ( -7.144783764277399030, 11.27940545839156528, 0.7216878364870458196 ) ) ;
#190344=CARTESIAN_POINT ( 'NONE',  ( -7.009202228140744673, 10.16085778526412042, -1.082531754730537088 ) ) ;
#190349=ORIENTED_EDGE ( 'NONE', *, *, #139587, .F. ) ;
#190350=CARTESIAN_POINT ( 'NONE',  ( -6.683806541412756985, 10.74159869838281622, -0.7216878364870267237 ) ) ;
#190355=CARTESIAN_POINT ( 'NONE',  ( 1.499999999999989120, 5.035416667349487341, 0.8660254037844524744 ) ) ;
#190356=CARTESIAN_POINT ( 'NONE',  ( 4.193801852926431373, 7.579907728022624802, -0.9040490846396221913 ) ) ;
#190363=CARTESIAN_POINT ( 'NONE',  ( -6.880926654135487652, 7.986501503701545879, 1.199719254218450271 ) ) ;
#190366=CARTESIAN_POINT ( 'NONE',  ( 3.825371897350130723, 7.614684313550482031, 0.7998128361456321445 ) ) ;
#190371=CARTESIAN_POINT ( 'NONE',  ( 7.202405917357655341, 9.425892875049191488, 1.599625672291281386 ) ) ;
#190379=CARTESIAN_POINT ( 'NONE',  ( -6.073689629242165822, 7.148687991279732756, -1.082531754730544860 ) ) ;
#190382=EDGE_CURVE ( 'NONE', #102987, #177962, #15695, .T. ) ;
#190385=EDGE_CURVE ( 'NONE', #180365, #116455, #68246, .T. ) ;
#190390=CARTESIAN_POINT ( 'NONE',  ( -9.528683032306089373, 10.01121838064558744, 0.7998128361456462443 ) ) ;
#190392=CARTESIAN_POINT ( 'NONE',  ( 6.774270308322468459, 11.05506579301824743, 0.7998128361456462443 ) ) ;
#190393=CARTESIAN_POINT ( 'NONE',  ( 0.7499999999999885647, -0.01666666666664401442, 1.299038105676657340 ) ) ;
#190394=CARTESIAN_POINT ( 'NONE',  ( -8.202846631467911820, 9.528741477256060577, 1.199719254218462483 ) ) ;
#190397=CARTESIAN_POINT ( 'NONE',  ( -0.6823417656250212460, 4.801041667008086655, 1.181850606188767472 ) ) ;
#190398=CARTESIAN_POINT ( 'NONE',  ( 9.571693261567965294, 10.26932301469188857, 0.7216878364870438212 ) ) ;
#190401=CARTESIAN_POINT ( 'NONE',  ( -1.499999999999997780, 5.400000000000022560, 1.214306433183764966E-14 ) ) ;
#190405=CARTESIAN_POINT ( 'NONE',  ( 7.402388682937041331, 11.57994453016116587, 1.040834085586084257E-14 ) ) ;
#190408=CARTESIAN_POINT ( 'NONE',  ( -5.748293942514180799, 7.729428904398431222, -1.443375672974052559 ) ) ;
#190410=CARTESIAN_POINT ( 'NONE',  ( -1.201851678989727383E-14, 1.571875000341420581, 1.575800808251672791 ) ) ;
#190414=CARTESIAN_POINT ( 'NONE',  ( -6.344325816190970357, 9.489131654609717970, 1.199719254218452047 ) ) ;
#190415=CARTESIAN_POINT ( 'NONE',  ( -1.001543065824772872E-14, 4.884375000341420581, 1.575800808251672791 ) ) ;
#190421=CARTESIAN_POINT ( 'NONE',  ( 7.313733799568044702, 10.62010763521636214, 1.199719254218460707 ) ) ;
#190424=CARTESIAN_POINT ( 'NONE',  ( 1.499999999999987121, 1.504166666666690411, 0.8660254037844524744 ) ) ;
#190429=CARTESIAN_POINT ( 'NONE',  ( 8.297226821883377568, 8.782445501726501291, -0.7216878364870267237 ) ) ;
#190435=CARTESIAN_POINT ( 'NONE',  ( 8.565000355531088516, 11.01558638625153286, -1.599625672291257406 ) ) ;
#190436=CARTESIAN_POINT ( 'NONE',  ( -10.15522075183580419, 11.80651128435196462, 1.199719254218462483 ) ) ;
#190440=CARTESIAN_POINT ( 'NONE',  ( -1.364683531250014514, -0.9697916663252473812, 0.7879004041258379498 ) ) ;
#190441=CARTESIAN_POINT ( 'NONE',  ( 0.7499999999999885647, 0.4833333333333564297, 1.299038105676657340 ) ) ;
#190449=CARTESIAN_POINT ( 'NONE',  ( 0.6823417656249899377, 4.926041667008086655, -1.181850606188754593 ) ) ;
#190451=CARTESIAN_POINT ( 'NONE',  ( -4.758548728716557541, 8.495464583570553785, 1.040834085586084257E-14 ) ) ;
#190459=VERTEX_POINT ( 'NONE', #15496 ) ;
#190460=CARTESIAN_POINT ( 'NONE',  ( 9.088043039861931405, 9.497138389460751284, 1.040834085586084257E-14 ) ) ;
#190462=TOROIDAL_SURFACE ( 'NONE', #93563, 3.971937515251341644, 0.08000000000000000167 ) ;
#190466=CARTESIAN_POINT ( 'NONE',  ( -8.320953590485107298, 10.73086516036454618, 1.599625672291269396 ) ) ;
#190467=CARTESIAN_POINT ( 'NONE',  ( 6.551614543901692400, 8.666636272683888365, 1.599625672291281386 ) ) ;
#190469=CARTESIAN_POINT ( 'NONE',  ( 0.000000000000000000, 9.200000000000020606, 0.4000000000000166755 ) ) ;
#190470=CARTESIAN_POINT ( 'NONE',  ( 5.820528018968444961, 5.685037531751635953, 0.7998128361456341429 ) ) ;
#190475=CARTESIAN_POINT ( 'NONE',  ( -3.999533323540116037, 7.701302116590127866, 0.08613759814882990251 ) ) ;
#190478=CARTESIAN_POINT ( 'NONE',  ( -4.094199201646926412, 7.720390135322642067, 0.7216878364870317197 ) ) ;
#190479=CARTESIAN_POINT ( 'NONE',  ( 8.758204044747994743, 12.20135990463928266, 1.082531754730546636 ) ) ;
#190482=CARTESIAN_POINT ( 'NONE',  ( -6.333630315878337136, 10.54098580183340772, 0.000000000000000000 ) ) ;
#190488=CARTESIAN_POINT ( 'NONE',  ( -9.345647958521597687, 9.797677461230342999, 0.7998128361456462443 ) ) ;
#190491=LINE ( 'NONE', #205676, #96688 ) ;
#190492=CARTESIAN_POINT ( 'NONE',  ( 8.471147050440139381, 8.777426401801974976, -0.7998128361456281477 ) ) ;
#190493=CARTESIAN_POINT ( 'NONE',  ( 4.364835388595708743, 7.179726155748598515, 1.199719254218462483 ) ) ;
#190503=DIRECTION ( 'NONE',  ( -0.5038915848335266956, -0.5182601445871922730, 0.6910135261095975423 ) ) ;
#190506=CARTESIAN_POINT ( 'NONE',  ( -7.507464373665155399, 9.781794407407920389, 1.599625672291295375 ) ) ;
#190509=CARTESIAN_POINT ( 'NONE',  ( 5.910991785878156435, 7.919243054989755670, -1.443375672974057666 ) ) ;
#190511=CARTESIAN_POINT ( 'NONE',  ( -1.500000000000079936, 7.361486028693807526, 4.203520246199945021 ) ) ;
#190512=CARTESIAN_POINT ( 'NONE',  ( 5.431895982697334091, 6.433277491268158954, -1.247050338538328029 ) ) ;
#190513=CARTESIAN_POINT ( 'NONE',  ( 3.330499290451326200, 7.037332938835193730, -0.7998128361456291469 ) ) ;
#190515=CARTESIAN_POINT ( 'NONE',  ( -4.062639585589296942, 7.891496616496157301, 0.7998128361456341429 ) ) ;
#190518=CARTESIAN_POINT ( 'NONE',  ( -0.7500000000000215383, 5.472916667349482900, 1.299038105676671107 ) ) ;
#190525=CARTESIAN_POINT ( 'NONE',  ( -8.292783513053063160, 12.82666453187061073, 0.7998128361456481317 ) ) ;
#190526=CARTESIAN_POINT ( 'NONE',  ( 7.079328764629950754, 11.41096732537697633, 0.7998128361456462443 ) ) ;
#190528=CARTESIAN_POINT ( 'NONE',  ( -2.819732761962335577, 5.273143408055916304, -1.082531754730543971 ) ) ;
#190529=DIRECTION ( 'NONE',  ( 7.387867266669436732E-31, -1.000000000000000000, -8.546850786086424434E-32 ) ) ;
#190531=CARTESIAN_POINT ( 'NONE',  ( -4.397708481796120950, 7.154691356138512148, -1.067048916732843411 ) ) ;
#190538=CARTESIAN_POINT ( 'NONE',  ( 9.924205255523292024, 10.68058700763975466, -0.7216878364870257245 ) ) ;
#190555=CARTESIAN_POINT ( 'NONE',  ( -2.435661151949389147, 5.993355110582911038, 0.7998128361456341429 ) ) ;
#190557=CARTESIAN_POINT ( 'NONE',  ( 6.005898860729467437, 7.069598761348265370, -1.082531754730543083 ) ) ;
#190558=CARTESIAN_POINT ( 'NONE',  ( -1.201851678989727383E-14, 3.587500000000020339, -1.732050807568863648 ) ) ;
#190560=CARTESIAN_POINT ( 'NONE',  ( -4.295235737431041478, 3.905529869957963029, -0.7998128361456221525 ) ) ;
#190564=CARTESIAN_POINT ( 'NONE',  ( -1.001543065824772872E-14, 5.071875000341421469, 1.575800808251672791 ) ) ;
#190573=CARTESIAN_POINT ( 'NONE',  ( 3.018661757337009810, 6.673522483535157868, 0.000000000000000000 ) ) ;
#190576=CARTESIAN_POINT ( 'NONE',  ( 9.585251414737269826, 11.24551007435741568, -1.082531754730537088 ) ) ;
#190578=CARTESIAN_POINT ( 'NONE',  ( -1.364683531250012516, 1.842708333674749843, 0.7879004041258379498 ) ) ;
#190581=CARTESIAN_POINT ( 'NONE',  ( -7.971304249830880373, 11.38727316052296601, 1.199719254218453823 ) ) ;
#190583=CARTESIAN_POINT ( 'NONE',  ( -6.046573321570485327, 6.156683084694754449, 0.000000000000000000 ) ) ;
#190586=VERTEX_POINT ( 'NONE', #170290 ) ;
#190587=CARTESIAN_POINT ( 'NONE',  ( -0.7500000000000249800, -0.7770833326505161009, 1.299038105676659116 ) ) ;
#190595=CARTESIAN_POINT ( 'NONE',  ( -5.273758565591545988, 6.215435083687305351, 1.082531754730546636 ) ) ;
#190600=CARTESIAN_POINT ( 'NONE',  ( -5.395781948114519722, 5.397426482329451325, 0.000000000000000000 ) ) ;
#190602=CARTESIAN_POINT ( 'NONE',  ( 8.536830278099042602, 13.11138575775759563, -0.7998128361456352531 ) ) ;
#190610=CARTESIAN_POINT ( 'NONE',  ( -5.427341564172148303, 5.226320001155936090, 0.000000000000000000 ) ) ;
#190616=CARTESIAN_POINT ( 'NONE',  ( 8.093854517678360949, 12.38665467069271386, 1.040834085586084257E-14 ) ) ;
#190617=CARTESIAN_POINT ( 'NONE',  ( 6.307567778855705853, 8.381915046796901692, -1.599625672291262513 ) ) ;
#190620=ORIENTED_EDGE ( 'NONE', *, *, #85341, .F. ) ;
#190622=CARTESIAN_POINT ( 'NONE',  ( 4.867540842506059562, 5.637551390133895168, -1.199719254218452047 ) ) ;
#190631=CARTESIAN_POINT ( 'NONE',  ( -6.358937740009323214, 7.377514437221045718, -1.199719254218446718 ) ) ;
#190638=CARTESIAN_POINT ( 'NONE',  ( -0.6823417656250212460, 4.801041667008086655, 1.181850606188767472 ) ) ;
#190639=CARTESIAN_POINT ( 'NONE',  ( 7.388830529323379359, 11.56412668427855195, -0.7216878364870267237 ) ) ;
#190640=CARTESIAN_POINT ( 'NONE',  ( -4.903245109636583443, 8.872203061218007392, -0.7998128361456281477 ) ) ;
#190643=CARTESIAN_POINT ( 'NONE',  ( 4.843287188579786573, 6.673587691474970107, -1.599625672291256295 ) ) ;
#190644=CARTESIAN_POINT ( 'NONE',  ( -6.573005544526917099, 6.562927978236513304, -0.7998128361456291469 ) ) ;
#190650=CARTESIAN_POINT ( 'NONE',  ( 6.968527767744109980, 7.232296605230681408, 0.7216878364870317197 ) ) ;
#190652=CARTESIAN_POINT ( 'NONE',  ( 7.009202228140744673, 9.200488570962775725, -1.443375672974058777 ) ) ;
#190653=CARTESIAN_POINT ( 'NONE',  ( 0.6823417656249882723, 2.738541667008084879, -1.181850606188749264 ) ) ;
#190655=CARTESIAN_POINT ( 'NONE',  ( 4.812781342726855982, 7.598366752281232372, 1.082531754730558626 ) ) ;
#190660=CARTESIAN_POINT ( 'NONE',  ( 0.6823417656249917140, 5.592708333674749177, 1.181850606188765695 ) ) ;
#190665=CARTESIAN_POINT ( 'NONE',  ( -4.002915605954192380, 7.811702849818844108, -0.3674259761444337302 ) ) ;
#190671=AXIS2_PLACEMENT_3D ( 'NONE', #203662, #87812, #157091 ) ;
#190673=CARTESIAN_POINT ( 'NONE',  ( 4.143988507271280319, 7.986403691791820414, -0.7998128361456221525 ) ) ;
#190675=CARTESIAN_POINT ( 'NONE',  ( -4.744990574658554117, 4.638169879964154418, 1.214306433183764966E-14 ) ) ;
#190684=ORIENTED_EDGE ( 'NONE', *, *, #115527, .T. ) ;
#190686=CARTESIAN_POINT ( 'NONE',  ( 5.016153647376217606, 4.954526798134778254, 0.7216878364870317197 ) ) ;
#190687=CARTESIAN_POINT ( 'NONE',  ( -1.364683531250014514, 1.551041667008084435, -0.7879004041258289570 ) ) ;
#190689=CARTESIAN_POINT ( 'NONE',  ( 8.589254009457354400, 9.979550084910457031, -1.199719254218446718 ) ) ;
#190692=CARTESIAN_POINT ( 'NONE',  ( -5.253948220495577637, 6.088359997788290734, 1.199719254218450271 ) ) ;
#190696=CARTESIAN_POINT ( 'NONE',  ( 1.499999999999989120, 3.004166666666689522, 0.8660254037844524744 ) ) ;
#190697=CARTESIAN_POINT ( 'NONE',  ( 4.961394147597008697, 7.875711374583454827, -1.199719254218452047 ) ) ;
#190701=CARTESIAN_POINT ( 'NONE',  ( -1.201851678989727383E-14, 3.321875000341421025, 1.575800808251672791 ) ) ;
#190703=CARTESIAN_POINT ( 'NONE',  ( 9.585251415181632595, 10.28514086057449184, 0.000000000000000000 ) ) ;
#190710=CARTESIAN_POINT ( 'NONE',  ( -1.499999999999997780, 2.681250000682818158, 1.214306433183764966E-14 ) ) ;
#190713=CARTESIAN_POINT ( 'NONE',  ( -5.368138756007025947, 8.350246751061767725, 1.199719254218452047 ) ) ;
#190714=CARTESIAN_POINT ( 'NONE',  ( -2.806174608348664723, 6.217694776474651519, 1.040834085586084257E-14 ) ) ;
#190721=CARTESIAN_POINT ( 'NONE',  ( 5.311043488251262268, 7.219303374425030562, -1.599625672291256295 ) ) ;
#190722=FACE_BOUND ( 'NONE', #124316, .T. ) ;
#190725=CARTESIAN_POINT ( 'NONE',  ( 5.144429221381498607, 8.089252293998699272, -1.199719254218452047 ) ) ;
#190731=CARTESIAN_POINT ( 'NONE',  ( 4.162516854595432747, 4.815023404238158555, 1.199719254218464037 ) ) ;
#190736=CARTESIAN_POINT ( 'NONE',  ( 5.335014106237911946, 6.336523053015567619, 1.100733037772538170 ) ) ;
#190747=CARTESIAN_POINT ( 'NONE',  ( -5.914749137557818059, 6.074338953224275528, -0.6118981238392419142 ) ) ;
#190748=CARTESIAN_POINT ( 'NONE',  ( 7.619319141200070256, 8.951922421897323900, 1.082531754730558626 ) ) ;
#190750=CARTESIAN_POINT ( 'NONE',  ( -4.120788623549732854, 6.895004929861607401, -1.199719254218452047 ) ) ;
#190752=EDGE_CURVE ( 'NONE', #119510, #171296, #120565, .T. ) ;
#190755=CARTESIAN_POINT ( 'NONE',  ( -6.663996196316808174, 7.733415969579778171, -1.199719254218446718 ) ) ;
#190769=CARTESIAN_POINT ( 'NONE',  ( 8.211434591371064684, 12.73175745657494851, -0.7998128361456352531 ) ) ;
#190772=AXIS2_PLACEMENT_3D ( 'NONE', #40944, #206613, #58243 ) ;
#190777=CARTESIAN_POINT ( 'NONE',  ( -3.358669367883384105, 4.941533567329135401, -1.599625672291262513 ) ) ;
#190780=CARTESIAN_POINT ( 'NONE',  ( 7.553864141108259211, 11.96459193126834464, 1.040834085586084257E-14 ) ) ;
#190785=CARTESIAN_POINT ( 'NONE',  ( -7.985916173649233230, 9.275655943134292869, -1.199719254218446718 ) ) ;
#190786=CARTESIAN_POINT ( 'NONE',  ( 6.159481859310094620, 6.080483678816896109, 1.040834085586084257E-14 ) ) ;
#190790=CARTESIAN_POINT ( 'NONE',  ( -3.307826292054316664, 4.882216645528547616, -1.443375672974059665 ) ) ;
#190792=CARTESIAN_POINT ( 'NONE',  ( 0.6823417656249899377, 2.905208333674754062, 1.181850606188765695 ) ) ;
#190793=ORIENTED_EDGE ( 'NONE', *, *, #149015, .T. ) ;
#190796=CARTESIAN_POINT ( 'NONE',  ( 7.144783764721768904, 7.437928601704619780, 1.040834085586084257E-14 ) ) ;
#190798=CARTESIAN_POINT ( 'NONE',  ( -1.499999999999997780, 4.681250000682819490, 1.214306433183765124E-14 ) ) ;
#190803=CARTESIAN_POINT ( 'NONE',  ( 8.175203438916005538, 11.52119253116861586, -1.082531754730543083 ) ) ;
#190808=CARTESIAN_POINT ( 'NONE',  ( -9.840520565420403543, 10.37502883594562597, 1.040834085586084257E-14 ) ) ;
#190809=DIRECTION ( 'NONE',  ( 1.000000000000000000, 0.000000000000000000, 0.000000000000000000 ) ) ;
#190827=CARTESIAN_POINT ( 'NONE',  ( 1.499999999999987121, 1.077083334016148308, -0.8660254037844253849 ) ) ;
#190833=CARTESIAN_POINT ( 'NONE',  ( -1.201851678989727383E-14, 0.9625000000000237810, 1.732050807568877637 ) ) ;
#190834=CARTESIAN_POINT ( 'NONE',  ( 6.252281394196331554, 10.44607872653774372, 1.040834085586084257E-14 ) ) ;
#190835=CARTESIAN_POINT ( 'NONE',  ( -1.402160292154681736E-14, -0.5531249996585814177, -1.575800808251665908 ) ) ;
#190838=CARTESIAN_POINT ( 'NONE',  ( 8.432808358020015049, 11.82173160345663376, 1.082531754730546636 ) ) ;
#190839=CARTESIAN_POINT ( 'NONE',  ( -5.829642864196175722, 7.824335979694092558, 1.443375672974064550 ) ) ;
#190844=CARTESIAN_POINT ( 'NONE',  ( -7.217017841176048165, 7.314275657660511243, 1.040834085586084257E-14 ) ) ;
#190845=( BOUNDED_SURFACE ( )  B_SPLINE_SURFACE ( 1, 2, ( 
 ( #71594, #118301, #4449, #105208, #188564, #121525, #136634, #103061, #122601, #172329, #153945, #38060, #185356, #54310, #70519, #23918, #184287, #170177, #151819, #40195, #85734, #35913, #168057, #5513, #155009, #152871, #119368, #101988, #171245, #21765, #36978, #137703, #169115, #20711, #86805, #120448, #19659, #201591, #87873, #73751, #203723, #7666, #55371, #187495, #39125, #72674, #106307, #3392, #22841, #88955, #90023, #69462, #138771, #156080, #200529, #56442, #6594, #135567, #208006, #9810, #78014, #95367, #93231, #59631, #159263, #175535, #75885, #124725, #161417, #206942, #76937, #190686, #42345, #26056, #108460, #41279, #140928, #141992, #13001, #174480, #139846, #10864, #92169, #27125, #11942, #127941, #205875, #143063, #58571, #45541, #57509, #144138, #61773, #177667, #210131, #158221, #125789, #191751, #43406, #193893, #123668, #209058, #109529, #60694, #126858, #192816, #44474, #189631, #110590, #176592, #91095, #28204, #94298, #111655, #160338, #8747, #29275, #107388, #173411, #24992, #157155, #74828, #80144, #147296, #64948, #14055, #180839, #98535, #15128, #100657, #81216, #165663, #32465, #30347, #83327, #62827, #133196, #198145, #82266, #194966, #213326, #164596, #131100, #197089, #96432, #16182, #149414, #148359, #146247, #145195, #50846, #48727, #214358, #128987, #97486, #212263, #46602, #17250, #166735, #179792, #163543, #116973, #113790, #114841, #112720, #33525, #65988, #132138, #211201, #49777, #115904, #67060, #181889, #99597, #196045, #996, #182970, #199198, #34585, #63897, #79077, #178732, #162483, #130052, #47679, #31412, #154753, #118045, #84409, #200270, #186163, #187236, #185089, #151559, #2056, #203463, #4194, #69196, #152608, #103871, #150497, #36713, #137446, #6337, #153686, #168857, #135317, #72409, #204532, #37796, #70264, #3127, #20460, #102799, #56182, #68129, #202397, #184031, #138509, #35647, #134264, #51922, #169920, #38865, #86543, #201331, #101726, #55117, #136378, #52969, #21506, #119107, #54049, #120186, #87615, #167797, #19392, #5254, #106048, #71331, #39940, #121263, #104948, #170988, #22587, #122343, #85471, #88693, #188300, #18326, #23665, #113271, #96976, #212810, #30899, #74570, #25800, #91909, #42086, #179276, #130592, #125533, #157966, #191492, #207749, #108201, #156895, #196581, #24730, #90833, #123410, #75635, #58315, #80704, #174225, #41017, #63382, #48223, #8483, #163024, #140669, #146794, #173149, #9558, #141743, #107126, #59376, #43160, #109272, #172071, #175280, #47155, #26867, #189374, #14607, #155821, #64447, #79624, #92971, #73486, #161962, #13552, #145743, #211744, #206683, #129537, #89775, #195518, #124470, #7405, #139586, #205613, #57250, #190429, #132677, #115394, #81759, #200807, #135850, #466, #198683, #86023, #148893, #34067, #164091, #68678, #147841, #201872, #52458, #114336, #83879, #51400, #183513, #67601, #181387, #131629, #197628, #15672, #82817, #149970, #213859, #152096, #33010, #199755, #50328, #49273, #84951, #99089, #117520, #184571, #66536, #116446, #101194, #65479, #167282, #165141, #16732, #182440, #100138, #166201, #2609, #36191, #133747, #17791, #1539, #35122, #18867, #134801, #102267, #151040, #118584, #168342, #19937, #3667, #180331, #69744, #31954, #98038, #55654, #204005, #87087, #40491, #185639, #157445, #9039, #189921, #57792, #120738, #171535, #72957, #7956, #91385, #75113, #71878, #41566, #106596, #107679, #172623, #173708, #141225, #39409, #187778, #37271, #53520, #119654, #23128, #169404, #25284, #24199, #155296, #74048, #121810, #105503, #103341, #20990, #202947, #156372, #153157, #137988, #4732, #70807, #22050, #90302, #136920, #89245, #6879, #140138, #139059, #206164, #54591, #186711, #5801, #38340, #123952, #104416, #205087, #122896, #170465, #88161, #56728, #154229, #188855, #13305, #161713, #145497, #59921, #42638, #162778, #126076, #207234, #192037, #96729, #190971, #58858, #76172, #95662, #80446, #43700, #211492, #109817, #113018, #208288, #60995, #193121, #142277, #94586, #12229, #143352, #14356, #209347, #79378, #160628, #158499, #63129, #108746, #46904, #111954, #210429, #174772, #127148, #78302 ),
 ( #26347, #129293, #125014, #93517, #77234, #179027, #27419, #44769, #92460, #195269, #110877, #144427, #10098, #11156, #177956, #30645, #128226, #176882, #175827, #159559, #28494, #62071, #194188, #45833, #29570, #164890, #184323, #64204, #116203, #97783, #68431, #31708, #212565, #114094, #99897, #100944, #98840, #65236, #130345, #117268, #132435, #197382, #83631, #131386, #49023, #32758, #115142, #47978, #147591, #148651, #19695, #181138, #168096, #165958, #16484, #33818, #18626, #134561, #196334, #182190, #82565, #52211, #180085, #84705, #200564, #35948, #2355, #217, #66288, #198436, #50082, #150792, #102027, #17542, #149714, #1294, #67352, #133497, #199500, #146547, #213609, #51144, #163843, #183266, #34870, #118338, #167031, #15422, #81512, #202699, #201625, #86841, #87909, #173448, #136674, #107423, #105245, #38097, #187531, #172366, #73785, #151854, #121560, #4484, #205911, #3430, #23956, #7702, #123703, #156120, #54349, #153981, #5548, #170216, #90060, #41316, #39162, #71630, #171285, #22877, #21801, #70555, #85773, #152906, #120488, #37012, #203763, #186460, #57546, #137743, #169153, #188602, #69497, #104168, #139881, #55406, #189664, #88993, #155046, #6632, #20746, #72711, #138806, #204825, #135604, #56477, #53274, #122639, #103094, #119405, #185394, #40233, #106344, #28239, #140967, #27163, #44510, #175572, #143102, #190721, #110627, #95403, #94332, #26094, #91127, #211235, #93268, #160374, #8781, #43444, #92208, #206977, #111691, #46635, #125826, #109568, #62860, #59667, #159301, #74864, #193928, #10900, #176628, #157186, #76975, #144174, #13035, #11976, #209095, #142026, #161455, #129025, #192851, #60730, #9848, #126893, #78050, #195001, #58608, #210166, #42384, #79112, #124762, #108494, #174518, #61807, #45575, #191788, #158259, #75923, #127976, #177698, #208040, #29309, #145230, #112758, #25027, #213359, #199235, #133231, #117005, #31445, #14089, #134298, #97524, #178770, #163580, #68166, #162517, #30382, #212298, #200305, #183004, #51957, #148395, #115940, #33560, #132174, #15163, #196080, #47712, #80180, #147331, #214396, #146285, #150531, #81251, #49814, #197124, #113827, #149448, #64980, #181929, #34622, #131135, #48763, #165698, #130085, #17287, #179826, #114875, #180877, #32498, #98572, #67095, #100691, #198180, #164634, #66025, #16218, #82302, #50882, #166769, #63930, #99632, #18364, #84442, #83363, #96468, #2093, #1030, #106082, #120221, #54085, #151594, #104983, #35684, #7439, #73520, #39975, #122378, #185123, #21540, #137482, #72441, #155852, #139622, #136414, #172105, #171023, #23698, #22620, #89808, #205645, #103906, #37828, #101762, #118079, #184066, #87650, #19428, #167829, #88729, #5288, #138542, #186195, #169952, #85508, #3161, #53006, #6372, #69233, #202430, #135351, #201365, #86579, #154787, #119141, #153720, #71366, #204567, #203496, #56214, #36748, #102834, #70298, #168890, #188335, #20493, #55149, #187271, #152643, #4228, #121296, #38897, #78838, #209898, #144959, #26896, #208836, #126623, #10637, #124501, #74599, #140703, #107158, #25828, #93000, #24763, #29046, #190460, #142829, #75663, #206717, #27973, #42119, #60466, #127702, #91938, #157998, #44241, #8518, #110362, #58345, #108231, #174256, #9587, #191522, #160107, #193662, #76713, #141770, #159044, #207778, #43187, #77784, #45305, #156929, #192586, #61536, #111424, #59405, #57283, #177428, #125561, #95129, #109300, #175309, #90865, #176366, #189407, #161178, #12764, #123445, #41049, #94067, #11710, #143905, #173183, #34358, #100431, #14890, #132968, #49545, #198971, #197917, #50615, #18093, #196863, #130867, #194728, #166502, #84181, #180611, #112487, #116740, #115671, #98307, #165428, #147074, #48501, #46367, #182739, #146016, #99376, #178496, #80985, #210965, #62592, #179561, #33292, #128755, #213095, #64725, #181665, #32236, #17025, #30106, #96196, #163309, #162246, #83102, #149182, #114620, #65762, #13833, #759, #164372, #66825, #31182, #79908, #212027, #63670, #129824, #195806, #47443, #113558, #97255, #15956, #82039, #148133, #214134, #131909, #105817, #2901, #68974, #101501, #53828, #36494, #55961, #20234 ) ),
 .UNSPECIFIED., .F., .F., .T. ) 
 B_SPLINE_SURFACE_WITH_KNOTS ( ( 2, 2 ),
 ( 3, 2, 2, 2, 2, 2, 2, 2, 2, 2, 2, 2, 2, 2, 2, 2, 2, 2, 2, 2, 2, 2, 2, 2, 2, 2, 2, 2, 2, 2, 2, 2, 2, 2, 2, 2, 2, 2, 2, 2, 2, 2, 2, 2, 2, 2, 2, 2, 2, 2, 2, 2, 2, 2, 2, 2, 2, 2, 2, 2, 2, 2, 2, 2, 2, 2, 2, 2, 2, 2, 2, 2, 2, 2, 2, 2, 2, 2, 2, 2, 2, 2, 2, 2, 2, 2, 2, 2, 2, 2, 2, 2, 2, 2, 2, 2, 2, 2, 2, 2, 2, 2, 2, 2, 2, 2, 2, 2, 2, 2, 2, 2, 2, 2, 2, 2, 2, 2, 2, 2, 2, 2, 2, 2, 2, 2, 2, 2, 2, 2, 2, 2, 2, 2, 2, 2, 2, 2, 2, 2, 2, 2, 2, 2, 2, 2, 2, 2, 2, 2, 2, 2, 2, 2, 2, 2, 2, 2, 2, 2, 2, 2, 2, 2, 2, 2, 2, 2, 2, 2, 2, 2, 2, 2, 2, 2, 2, 2, 2, 2, 2, 2, 2, 2, 2, 2, 2, 2, 2, 2, 2, 2, 2, 2, 2, 2, 2, 2, 2, 2, 2, 2, 2, 2, 2, 2, 2, 2, 2, 2, 2, 2, 2, 2, 2, 2, 2, 2, 2, 2, 2, 2, 2, 2, 2, 2, 2, 2, 2, 2, 2, 2, 2, 2, 2, 2, 2, 2, 2, 2, 3 ),
 ( 0.000000000000000000, 1.000000000000000000 ),
 ( 0.000000000000000000, 0.004166666666666666609, 0.008333333333333333218, 0.01250000000000000069, 0.01666666666666666644, 0.02083333333333333218, 0.02500000000000000139, 0.02916666666666666713, 0.03333333333333333287, 0.03749999999999999861, 0.04166666666666666435, 0.04583333333333333010, 0.05000000000000000278, 0.05416666666666666852, 0.05833333333333333426, 0.06250000000000000000, 0.06666666666666666574, 0.07083333333333333148, 0.07499999999999999722, 0.07916666666666666297, 0.08333333333333332871, 0.08749999999999999445, 0.09166666666666666019, 0.09583333333333333981, 0.1000000000000000056, 0.1041666666666666713, 0.1083333333333333370, 0.1125000000000000028, 0.1166666666666666685, 0.1208333333333333343, 0.1250000000000000000, 0.1291666666666666796, 0.1333333333333333315, 0.1375000000000000111, 0.1416666666666666630, 0.1458333333333333426, 0.1499999999999999944, 0.1541666666666666741, 0.1583333333333333259, 0.1625000000000000056, 0.1666666666666666574, 0.1708333333333333370, 0.1749999999999999889, 0.1791666666666666685, 0.1833333333333333204, 0.1875000000000000000, 0.1916666666666666796, 0.1958333333333333315, 0.2000000000000000111, 0.2041666666666666630, 0.2083333333333333426, 0.2124999999999999944, 0.2166666666666666741, 0.2208333333333333259, 0.2250000000000000056, 0.2291666666666666574, 0.2333333333333333370, 0.2374999999999999889, 0.2416666666666666685, 0.2458333333333333204, 0.2500000000000000000, 0.2541666666666666519, 0.2583333333333333592, 0.2625000000000000111, 0.2666666666666666630, 0.2708333333333333148, 0.2750000000000000222, 0.2791666666666666741, 0.2833333333333333259, 0.2874999999999999778, 0.2916666666666666852, 0.2958333333333333370, 0.2999999999999999889, 0.3041666666666666408, 0.3083333333333333481, 0.3125000000000000000, 0.3166666666666666519, 0.3208333333333333592, 0.3250000000000000111, 0.3291666666666666630, 0.3333333333333333148, 0.3375000000000000222, 0.3416666666666666741, 0.3458333333333333259, 0.3499999999999999778, 0.3541666666666666852, 0.3583333333333333370, 0.3624999999999999889, 0.3666666666666666408, 0.3708333333333333481, 0.3750000000000000000, 0.3791666666666666519, 0.3833333333333333592, 0.3875000000000000111, 0.3916666666666666630, 0.3958333333333333148, 0.4000000000000000222, 0.4041666666666666741, 0.4083333333333333259, 0.4124999999999999778, 0.4166666666666666852, 0.4208333333333333370, 0.4249999999999999889, 0.4291666666666666408, 0.4333333333333333481, 0.4375000000000000000, 0.4416666666666666519, 0.4458333333333333592, 0.4500000000000000111, 0.4541666666666666630, 0.4583333333333333148, 0.4625000000000000222, 0.4666666666666666741, 0.4708333333333333259, 0.4749999999999999778, 0.4791666666666666852, 0.4833333333333333370, 0.4874999999999999889, 0.4916666666666666408, 0.4958333333333333481, 0.5000000000000000000, 0.5041666666666666519, 0.5083333333333333037, 0.5124999999999999556, 0.5166666666666667185, 0.5208333333333333703, 0.5250000000000000222, 0.5291666666666666741, 0.5333333333333333259, 0.5374999999999999778, 0.5416666666666666297, 0.5458333333333332815, 0.5500000000000000444, 0.5541666666666666963, 0.5583333333333333481, 0.5625000000000000000, 0.5666666666666666519, 0.5708333333333333037, 0.5749999999999999556, 0.5791666666666667185, 0.5833333333333333703, 0.5875000000000000222, 0.5916666666666666741, 0.5958333333333333259, 0.5999999999999999778, 0.6041666666666666297, 0.6083333333333332815, 0.6125000000000000444, 0.6166666666666666963, 0.6208333333333333481, 0.6250000000000000000, 0.6291666666666666519, 0.6333333333333333037, 0.6374999999999999556, 0.6416666666666667185, 0.6458333333333333703, 0.6500000000000000222, 0.6541666666666666741, 0.6583333333333333259, 0.6624999999999999778, 0.6666666666666666297, 0.6708333333333332815, 0.6750000000000000444, 0.6791666666666666963, 0.6833333333333333481, 0.6875000000000000000, 0.6916666666666666519, 0.6958333333333333037, 0.6999999999999999556, 0.7041666666666667185, 0.7083333333333333703, 0.7125000000000000222, 0.7166666666666666741, 0.7208333333333333259, 0.7249999999999999778, 0.7291666666666666297, 0.7333333333333332815, 0.7375000000000000444, 0.7416666666666666963, 0.7458333333333333481, 0.7500000000000000000, 0.7541666666666666519, 0.7583333333333333037, 0.7624999999999999556, 0.7666666666666667185, 0.7708333333333333703, 0.7750000000000000222, 0.7791666666666666741, 0.7833333333333333259, 0.7874999999999999778, 0.7916666666666666297, 0.7958333333333332815, 0.8000000000000000444, 0.8041666666666666963, 0.8083333333333333481, 0.8125000000000000000, 0.8166666666666666519, 0.8208333333333333037, 0.8249999999999999556, 0.8291666666666667185, 0.8333333333333333703, 0.8375000000000000222, 0.8416666666666666741, 0.8458333333333333259, 0.8499999999999999778, 0.8541666666666666297, 0.8583333333333332815, 0.8625000000000000444, 0.8666666666666666963, 0.8708333333333333481, 0.8750000000000000000, 0.8791666666666666519, 0.8833333333333333037, 0.8874999999999999556, 0.8916666666666667185, 0.8958333333333333703, 0.9000000000000000222, 0.9041666666666666741, 0.9083333333333333259, 0.9124999999999999778, 0.9166666666666666297, 0.9208333333333332815, 0.9250000000000000444, 0.9291666666666666963, 0.9333333333333333481, 0.9375000000000000000, 0.9416666666666666519, 0.9458333333333333037, 0.9499999999999999556, 0.9541666666666667185, 0.9583333333333333703, 0.9625000000000000222, 0.9666666666666666741, 0.9708333333333333259, 0.9749999999999999778, 0.9791666666666666297, 0.9833333333333332815, 0.9875000000000000444, 0.9916666666666666963, 0.9958333333333333481, 1.000000000000000000 ),
 .UNSPECIFIED. ) 
 GEOMETRIC_REPRESENTATION_ITEM ( )  RATIONAL_B_SPLINE_SURFACE ( (
 ( 1.000000000000000000, 0.8660254037844387076, 1.000000000000000000, 0.8660254037844387076, 1.000000000000000000, 0.8660254037844387076, 1.000000000000000000, 0.8660254037844387076, 1.000000000000000000, 0.8660254037844387076, 1.000000000000000000, 0.8660254037844387076, 1.000000000000000000, 0.8660254037844387076, 1.000000000000000000, 0.8660254037844387076, 1.000000000000000000, 0.8660254037844387076, 1.000000000000000000, 0.8660254037844387076, 1.000000000000000000, 0.8660254037844387076, 1.000000000000000000, 0.8660254037844387076, 1.000000000000000000, 0.8660254037844387076, 1.000000000000000000, 0.8660254037844387076, 1.000000000000000000, 0.8660254037844387076, 1.000000000000000000, 0.8660254037844387076, 1.000000000000000000, 0.8660254037844387076, 1.000000000000000000, 0.8660254037844387076, 1.000000000000000000, 0.8660254037844387076, 1.000000000000000000, 0.8660254037844387076, 1.000000000000000000, 0.8660254037844387076, 1.000000000000000000, 0.8660254037844387076, 1.000000000000000000, 0.8660254037844387076, 1.000000000000000000, 0.8660254037844387076, 1.000000000000000000, 0.8660254037844387076, 1.000000000000000000, 0.8660254037844387076, 1.000000000000000000, 0.8660254037844387076, 1.000000000000000000, 0.8660254037844387076, 1.000000000000000000, 0.8660254037844387076, 1.000000000000000000, 0.8660254037844387076, 1.000000000000000000, 0.8660254037844387076, 1.000000000000000000, 0.8660254037844387076, 1.000000000000000000, 0.8660254037844387076, 1.000000000000000000, 0.8660254037844387076, 1.000000000000000000, 0.8660254037844387076, 1.000000000000000000, 0.8660254037844387076, 1.000000000000000000, 0.8660254037844387076, 1.000000000000000000, 0.8660254037844387076, 1.000000000000000000, 0.8660254037844387076, 1.000000000000000000, 0.8660254037844387076, 1.000000000000000000, 0.8660254037844387076, 1.000000000000000000, 0.8660254037844387076, 1.000000000000000000, 0.8660254037844387076, 1.000000000000000000, 0.8660254037844387076, 1.000000000000000000, 0.8660254037844387076, 1.000000000000000000, 0.8660254037844387076, 1.000000000000000000, 0.8660254037844387076, 1.000000000000000000, 0.8660254037844387076, 1.000000000000000000, 0.8660254037844387076, 1.000000000000000000, 0.8660254037844387076, 1.000000000000000000, 0.8660254037844387076, 1.000000000000000000, 0.8660254037844387076, 1.000000000000000000, 0.8660254037844387076, 1.000000000000000000, 0.8660254037844387076, 1.000000000000000000, 0.8660254037844387076, 1.000000000000000000, 0.8660254037844387076, 1.000000000000000000, 0.8660254037844387076, 1.000000000000000000, 0.8660254037844387076, 1.000000000000000000, 0.8660254037844387076, 1.000000000000000000, 0.8660254037844387076, 1.000000000000000000, 0.8660254037844387076, 1.000000000000000000, 0.8660254037844387076, 1.000000000000000000, 0.8660254037844387076, 1.000000000000000000, 0.8660254037844387076, 1.000000000000000000, 0.8660254037844387076, 1.000000000000000000, 0.8660254037844387076, 1.000000000000000000, 0.8660254037844387076, 1.000000000000000000, 0.8660254037844387076, 1.000000000000000000, 0.8660254037844387076, 1.000000000000000000, 0.8660254037844387076, 1.000000000000000000, 0.8660254037844387076, 1.000000000000000000, 0.8660254037844387076, 1.000000000000000000, 0.8660254037844387076, 1.000000000000000000, 0.8660254037844387076, 1.000000000000000000, 0.8660254037844387076, 1.000000000000000000, 0.8660254037844387076, 1.000000000000000000, 0.8660254037844387076, 1.000000000000000000, 0.8660254037844387076, 1.000000000000000000, 0.8660254037844387076, 1.000000000000000000, 0.8660254037844387076, 1.000000000000000000, 0.8660254037844387076, 1.000000000000000000, 0.8660254037844387076, 1.000000000000000000, 0.8660254037844387076, 1.000000000000000000, 0.8660254037844387076, 1.000000000000000000, 0.8660254037844387076, 1.000000000000000000, 0.8660254037844387076, 1.000000000000000000, 0.8660254037844387076, 1.000000000000000000, 0.8660254037844387076, 1.000000000000000000, 0.8660254037844387076, 1.000000000000000000, 0.8660254037844387076, 1.000000000000000000, 0.8660254037844387076, 1.000000000000000000, 0.8660254037844387076, 1.000000000000000000, 0.8660254037844387076, 1.000000000000000000, 0.8660254037844387076, 1.000000000000000000, 0.8660254037844387076, 1.000000000000000000, 0.8660254037844387076, 1.000000000000000000, 0.8660254037844387076, 1.000000000000000000, 0.8660254037844387076, 1.000000000000000000, 0.8660254037844387076, 1.000000000000000000, 0.8660254037844387076, 1.000000000000000000, 0.8660254037844387076, 1.000000000000000000, 0.8660254037844387076, 1.000000000000000000, 0.8660254037844387076, 1.000000000000000000, 0.8660254037844387076, 1.000000000000000000, 0.8660254037844387076, 1.000000000000000000, 0.8660254037844387076, 1.000000000000000000, 0.8660254037844387076, 1.000000000000000000, 0.8660254037844387076, 1.000000000000000000, 0.8660254037844387076, 1.000000000000000000, 0.8660254037844387076, 1.000000000000000000, 0.8660254037844387076, 1.000000000000000000, 0.8660254037844387076, 1.000000000000000000, 0.8660254037844387076, 1.000000000000000000, 0.8660254037844387076, 1.000000000000000000, 0.8660254037844387076, 1.000000000000000000, 0.8660254037844387076, 1.000000000000000000, 0.8660254037844387076, 1.000000000000000000, 0.8660254037844387076, 1.000000000000000000, 0.8660254037844387076, 1.000000000000000000, 0.8660254037844387076, 1.000000000000000000, 0.8660254037844387076, 1.000000000000000000, 0.8660254037844387076, 1.000000000000000000, 0.8660254037844387076, 1.000000000000000000, 0.8660254037844387076, 1.000000000000000000, 0.8660254037844387076, 1.000000000000000000, 0.8660254037844387076, 1.000000000000000000, 0.8660254037844387076, 1.000000000000000000, 0.8660254037844387076, 1.000000000000000000, 0.8660254037844387076, 1.000000000000000000, 0.8660254037844387076, 1.000000000000000000, 0.8660254037844387076, 1.000000000000000000, 0.8660254037844387076, 1.000000000000000000, 0.8660254037844387076, 1.000000000000000000, 0.8660254037844387076, 1.000000000000000000, 0.8660254037844387076, 1.000000000000000000, 0.8660254037844387076, 1.000000000000000000, 0.8660254037844387076, 1.000000000000000000, 0.8660254037844387076, 1.000000000000000000, 0.8660254037844387076, 1.000000000000000000, 0.8660254037844387076, 1.000000000000000000, 0.8660254037844387076, 1.000000000000000000, 0.8660254037844387076, 1.000000000000000000, 0.8660254037844387076, 1.000000000000000000, 0.8660254037844387076, 1.000000000000000000, 0.8660254037844387076, 1.000000000000000000, 0.8660254037844387076, 1.000000000000000000, 0.8660254037844387076, 1.000000000000000000, 0.8660254037844387076, 1.000000000000000000, 0.8660254037844387076, 1.000000000000000000, 0.8660254037844387076, 1.000000000000000000, 0.8660254037844387076, 1.000000000000000000, 0.8660254037844387076, 1.000000000000000000, 0.8660254037844387076, 1.000000000000000000, 0.8660254037844387076, 1.000000000000000000, 0.8660254037844387076, 1.000000000000000000, 0.8660254037844387076, 1.000000000000000000, 0.8660254037844387076, 1.000000000000000000, 0.8660254037844387076, 1.000000000000000000, 0.8660254037844387076, 1.000000000000000000, 0.8660254037844387076, 1.000000000000000000, 0.8660254037844387076, 1.000000000000000000, 0.8660254037844387076, 1.000000000000000000, 0.8660254037844387076, 1.000000000000000000, 0.8660254037844387076, 1.000000000000000000, 0.8660254037844387076, 1.000000000000000000, 0.8660254037844387076, 1.000000000000000000, 0.8660254037844387076, 1.000000000000000000, 0.8660254037844387076, 1.000000000000000000, 0.8660254037844387076, 1.000000000000000000, 0.8660254037844387076, 1.000000000000000000, 0.8660254037844387076, 1.000000000000000000, 0.8660254037844387076, 1.000000000000000000, 0.8660254037844387076, 1.000000000000000000, 0.8660254037844387076, 1.000000000000000000, 0.8660254037844387076, 1.000000000000000000, 0.8660254037844387076, 1.000000000000000000, 0.8660254037844387076, 1.000000000000000000, 0.8660254037844387076, 1.000000000000000000, 0.8660254037844387076, 1.000000000000000000, 0.8660254037844387076, 1.000000000000000000, 0.8660254037844387076, 1.000000000000000000, 0.8660254037844387076, 1.000000000000000000, 0.8660254037844387076, 1.000000000000000000, 0.8660254037844387076, 1.000000000000000000, 0.8660254037844387076, 1.000000000000000000, 0.8660254037844387076, 1.000000000000000000, 0.8660254037844387076, 1.000000000000000000, 0.8660254037844387076, 1.000000000000000000, 0.8660254037844387076, 1.000000000000000000, 0.8660254037844387076, 1.000000000000000000, 0.8660254037844387076, 1.000000000000000000, 0.8660254037844387076, 1.000000000000000000, 0.8660254037844387076, 1.000000000000000000, 0.8660254037844387076, 1.000000000000000000, 0.8660254037844387076, 1.000000000000000000, 0.8660254037844387076, 1.000000000000000000, 0.8660254037844387076, 1.000000000000000000, 0.8660254037844387076, 1.000000000000000000, 0.8660254037844387076, 1.000000000000000000, 0.8660254037844387076, 1.000000000000000000, 0.8660254037844387076, 1.000000000000000000, 0.8660254037844387076, 1.000000000000000000, 0.8660254037844387076, 1.000000000000000000, 0.8660254037844387076, 1.000000000000000000, 0.8660254037844387076, 1.000000000000000000, 0.8660254037844387076, 1.000000000000000000, 0.8660254037844387076, 1.000000000000000000, 0.8660254037844387076, 1.000000000000000000, 0.8660254037844387076, 1.000000000000000000, 0.8660254037844387076, 1.000000000000000000, 0.8660254037844387076, 1.000000000000000000, 0.8660254037844387076, 1.000000000000000000, 0.8660254037844387076, 1.000000000000000000, 0.8660254037844387076, 1.000000000000000000, 0.8660254037844387076, 1.000000000000000000, 0.8660254037844387076, 1.000000000000000000, 0.8660254037844387076, 1.000000000000000000, 0.8660254037844387076, 1.000000000000000000, 0.8660254037844387076, 1.000000000000000000, 0.8660254037844387076, 1.000000000000000000, 0.8660254037844387076, 1.000000000000000000, 0.8660254037844387076, 1.000000000000000000, 0.8660254037844387076, 1.000000000000000000, 0.8660254037844387076, 1.000000000000000000, 0.8660254037844387076, 1.000000000000000000, 0.8660254037844387076, 1.000000000000000000, 0.8660254037844387076, 1.000000000000000000, 0.8660254037844387076, 1.000000000000000000, 0.8660254037844387076, 1.000000000000000000, 0.8660254037844387076, 1.000000000000000000, 0.8660254037844387076, 1.000000000000000000, 0.8660254037844387076, 1.000000000000000000, 0.8660254037844387076, 1.000000000000000000, 0.8660254037844387076, 1.000000000000000000, 0.8660254037844387076, 1.000000000000000000, 0.8660254037844387076, 1.000000000000000000, 0.8660254037844387076, 1.000000000000000000, 0.8660254037844387076, 1.000000000000000000, 0.8660254037844387076, 1.000000000000000000, 0.8660254037844387076, 1.000000000000000000),
 ( 1.000000000000000000, 0.8660254037844387076, 1.000000000000000000, 0.8660254037844387076, 1.000000000000000000, 0.8660254037844387076, 1.000000000000000000, 0.8660254037844387076, 1.000000000000000000, 0.8660254037844387076, 1.000000000000000000, 0.8660254037844387076, 1.000000000000000000, 0.8660254037844387076, 1.000000000000000000, 0.8660254037844387076, 1.000000000000000000, 0.8660254037844387076, 1.000000000000000000, 0.8660254037844387076, 1.000000000000000000, 0.8660254037844387076, 1.000000000000000000, 0.8660254037844387076, 1.000000000000000000, 0.8660254037844387076, 1.000000000000000000, 0.8660254037844387076, 1.000000000000000000, 0.8660254037844387076, 1.000000000000000000, 0.8660254037844387076, 1.000000000000000000, 0.8660254037844387076, 1.000000000000000000, 0.8660254037844387076, 1.000000000000000000, 0.8660254037844387076, 1.000000000000000000, 0.8660254037844387076, 1.000000000000000000, 0.8660254037844387076, 1.000000000000000000, 0.8660254037844387076, 1.000000000000000000, 0.8660254037844387076, 1.000000000000000000, 0.8660254037844387076, 1.000000000000000000, 0.8660254037844387076, 1.000000000000000000, 0.8660254037844387076, 1.000000000000000000, 0.8660254037844387076, 1.000000000000000000, 0.8660254037844387076, 1.000000000000000000, 0.8660254037844387076, 1.000000000000000000, 0.8660254037844387076, 1.000000000000000000, 0.8660254037844387076, 1.000000000000000000, 0.8660254037844387076, 1.000000000000000000, 0.8660254037844387076, 1.000000000000000000, 0.8660254037844387076, 1.000000000000000000, 0.8660254037844387076, 1.000000000000000000, 0.8660254037844387076, 1.000000000000000000, 0.8660254037844387076, 1.000000000000000000, 0.8660254037844387076, 1.000000000000000000, 0.8660254037844387076, 1.000000000000000000, 0.8660254037844387076, 1.000000000000000000, 0.8660254037844387076, 1.000000000000000000, 0.8660254037844387076, 1.000000000000000000, 0.8660254037844387076, 1.000000000000000000, 0.8660254037844387076, 1.000000000000000000, 0.8660254037844387076, 1.000000000000000000, 0.8660254037844387076, 1.000000000000000000, 0.8660254037844387076, 1.000000000000000000, 0.8660254037844387076, 1.000000000000000000, 0.8660254037844387076, 1.000000000000000000, 0.8660254037844387076, 1.000000000000000000, 0.8660254037844387076, 1.000000000000000000, 0.8660254037844387076, 1.000000000000000000, 0.8660254037844387076, 1.000000000000000000, 0.8660254037844387076, 1.000000000000000000, 0.8660254037844387076, 1.000000000000000000, 0.8660254037844387076, 1.000000000000000000, 0.8660254037844387076, 1.000000000000000000, 0.8660254037844387076, 1.000000000000000000, 0.8660254037844387076, 1.000000000000000000, 0.8660254037844387076, 1.000000000000000000, 0.8660254037844387076, 1.000000000000000000, 0.8660254037844387076, 1.000000000000000000, 0.8660254037844387076, 1.000000000000000000, 0.8660254037844387076, 1.000000000000000000, 0.8660254037844387076, 1.000000000000000000, 0.8660254037844387076, 1.000000000000000000, 0.8660254037844387076, 1.000000000000000000, 0.8660254037844387076, 1.000000000000000000, 0.8660254037844387076, 1.000000000000000000, 0.8660254037844387076, 1.000000000000000000, 0.8660254037844387076, 1.000000000000000000, 0.8660254037844387076, 1.000000000000000000, 0.8660254037844387076, 1.000000000000000000, 0.8660254037844387076, 1.000000000000000000, 0.8660254037844387076, 1.000000000000000000, 0.8660254037844387076, 1.000000000000000000, 0.8660254037844387076, 1.000000000000000000, 0.8660254037844387076, 1.000000000000000000, 0.8660254037844387076, 1.000000000000000000, 0.8660254037844387076, 1.000000000000000000, 0.8660254037844387076, 1.000000000000000000, 0.8660254037844387076, 1.000000000000000000, 0.8660254037844387076, 1.000000000000000000, 0.8660254037844387076, 1.000000000000000000, 0.8660254037844387076, 1.000000000000000000, 0.8660254037844387076, 1.000000000000000000, 0.8660254037844387076, 1.000000000000000000, 0.8660254037844387076, 1.000000000000000000, 0.8660254037844387076, 1.000000000000000000, 0.8660254037844387076, 1.000000000000000000, 0.8660254037844387076, 1.000000000000000000, 0.8660254037844387076, 1.000000000000000000, 0.8660254037844387076, 1.000000000000000000, 0.8660254037844387076, 1.000000000000000000, 0.8660254037844387076, 1.000000000000000000, 0.8660254037844387076, 1.000000000000000000, 0.8660254037844387076, 1.000000000000000000, 0.8660254037844387076, 1.000000000000000000, 0.8660254037844387076, 1.000000000000000000, 0.8660254037844387076, 1.000000000000000000, 0.8660254037844387076, 1.000000000000000000, 0.8660254037844387076, 1.000000000000000000, 0.8660254037844387076, 1.000000000000000000, 0.8660254037844387076, 1.000000000000000000, 0.8660254037844387076, 1.000000000000000000, 0.8660254037844387076, 1.000000000000000000, 0.8660254037844387076, 1.000000000000000000, 0.8660254037844387076, 1.000000000000000000, 0.8660254037844387076, 1.000000000000000000, 0.8660254037844387076, 1.000000000000000000, 0.8660254037844387076, 1.000000000000000000, 0.8660254037844387076, 1.000000000000000000, 0.8660254037844387076, 1.000000000000000000, 0.8660254037844387076, 1.000000000000000000, 0.8660254037844387076, 1.000000000000000000, 0.8660254037844387076, 1.000000000000000000, 0.8660254037844387076, 1.000000000000000000, 0.8660254037844387076, 1.000000000000000000, 0.8660254037844387076, 1.000000000000000000, 0.8660254037844387076, 1.000000000000000000, 0.8660254037844387076, 1.000000000000000000, 0.8660254037844387076, 1.000000000000000000, 0.8660254037844387076, 1.000000000000000000, 0.8660254037844387076, 1.000000000000000000, 0.8660254037844387076, 1.000000000000000000, 0.8660254037844387076, 1.000000000000000000, 0.8660254037844387076, 1.000000000000000000, 0.8660254037844387076, 1.000000000000000000, 0.8660254037844387076, 1.000000000000000000, 0.8660254037844387076, 1.000000000000000000, 0.8660254037844387076, 1.000000000000000000, 0.8660254037844387076, 1.000000000000000000, 0.8660254037844387076, 1.000000000000000000, 0.8660254037844387076, 1.000000000000000000, 0.8660254037844387076, 1.000000000000000000, 0.8660254037844387076, 1.000000000000000000, 0.8660254037844387076, 1.000000000000000000, 0.8660254037844387076, 1.000000000000000000, 0.8660254037844387076, 1.000000000000000000, 0.8660254037844387076, 1.000000000000000000, 0.8660254037844387076, 1.000000000000000000, 0.8660254037844387076, 1.000000000000000000, 0.8660254037844387076, 1.000000000000000000, 0.8660254037844387076, 1.000000000000000000, 0.8660254037844387076, 1.000000000000000000, 0.8660254037844387076, 1.000000000000000000, 0.8660254037844387076, 1.000000000000000000, 0.8660254037844387076, 1.000000000000000000, 0.8660254037844387076, 1.000000000000000000, 0.8660254037844387076, 1.000000000000000000, 0.8660254037844387076, 1.000000000000000000, 0.8660254037844387076, 1.000000000000000000, 0.8660254037844387076, 1.000000000000000000, 0.8660254037844387076, 1.000000000000000000, 0.8660254037844387076, 1.000000000000000000, 0.8660254037844387076, 1.000000000000000000, 0.8660254037844387076, 1.000000000000000000, 0.8660254037844387076, 1.000000000000000000, 0.8660254037844387076, 1.000000000000000000, 0.8660254037844387076, 1.000000000000000000, 0.8660254037844387076, 1.000000000000000000, 0.8660254037844387076, 1.000000000000000000, 0.8660254037844387076, 1.000000000000000000, 0.8660254037844387076, 1.000000000000000000, 0.8660254037844387076, 1.000000000000000000, 0.8660254037844387076, 1.000000000000000000, 0.8660254037844387076, 1.000000000000000000, 0.8660254037844387076, 1.000000000000000000, 0.8660254037844387076, 1.000000000000000000, 0.8660254037844387076, 1.000000000000000000, 0.8660254037844387076, 1.000000000000000000, 0.8660254037844387076, 1.000000000000000000, 0.8660254037844387076, 1.000000000000000000, 0.8660254037844387076, 1.000000000000000000, 0.8660254037844387076, 1.000000000000000000, 0.8660254037844387076, 1.000000000000000000, 0.8660254037844387076, 1.000000000000000000, 0.8660254037844387076, 1.000000000000000000, 0.8660254037844387076, 1.000000000000000000, 0.8660254037844387076, 1.000000000000000000, 0.8660254037844387076, 1.000000000000000000, 0.8660254037844387076, 1.000000000000000000, 0.8660254037844387076, 1.000000000000000000, 0.8660254037844387076, 1.000000000000000000, 0.8660254037844387076, 1.000000000000000000, 0.8660254037844387076, 1.000000000000000000, 0.8660254037844387076, 1.000000000000000000, 0.8660254037844387076, 1.000000000000000000, 0.8660254037844387076, 1.000000000000000000, 0.8660254037844387076, 1.000000000000000000, 0.8660254037844387076, 1.000000000000000000, 0.8660254037844387076, 1.000000000000000000, 0.8660254037844387076, 1.000000000000000000, 0.8660254037844387076, 1.000000000000000000, 0.8660254037844387076, 1.000000000000000000, 0.8660254037844387076, 1.000000000000000000, 0.8660254037844387076, 1.000000000000000000, 0.8660254037844387076, 1.000000000000000000, 0.8660254037844387076, 1.000000000000000000, 0.8660254037844387076, 1.000000000000000000, 0.8660254037844387076, 1.000000000000000000, 0.8660254037844387076, 1.000000000000000000, 0.8660254037844387076, 1.000000000000000000, 0.8660254037844387076, 1.000000000000000000, 0.8660254037844387076, 1.000000000000000000, 0.8660254037844387076, 1.000000000000000000, 0.8660254037844387076, 1.000000000000000000, 0.8660254037844387076, 1.000000000000000000, 0.8660254037844387076, 1.000000000000000000, 0.8660254037844387076, 1.000000000000000000, 0.8660254037844387076, 1.000000000000000000, 0.8660254037844387076, 1.000000000000000000, 0.8660254037844387076, 1.000000000000000000, 0.8660254037844387076, 1.000000000000000000, 0.8660254037844387076, 1.000000000000000000, 0.8660254037844387076, 1.000000000000000000, 0.8660254037844387076, 1.000000000000000000, 0.8660254037844387076, 1.000000000000000000, 0.8660254037844387076, 1.000000000000000000, 0.8660254037844387076, 1.000000000000000000, 0.8660254037844387076, 1.000000000000000000, 0.8660254037844387076, 1.000000000000000000, 0.8660254037844387076, 1.000000000000000000, 0.8660254037844387076, 1.000000000000000000, 0.8660254037844387076, 1.000000000000000000, 0.8660254037844387076, 1.000000000000000000, 0.8660254037844387076, 1.000000000000000000, 0.8660254037844387076, 1.000000000000000000, 0.8660254037844387076, 1.000000000000000000, 0.8660254037844387076, 1.000000000000000000, 0.8660254037844387076, 1.000000000000000000, 0.8660254037844387076, 1.000000000000000000, 0.8660254037844387076, 1.000000000000000000, 0.8660254037844387076, 1.000000000000000000, 0.8660254037844387076, 1.000000000000000000, 0.8660254037844387076, 1.000000000000000000, 0.8660254037844387076, 1.000000000000000000, 0.8660254037844387076, 1.000000000000000000, 0.8660254037844387076, 1.000000000000000000, 0.8660254037844387076, 1.000000000000000000) ) ) 
 REPRESENTATION_ITEM ( '' )  SURFACE ( )  );
#190847=CARTESIAN_POINT ( 'NONE',  ( 1.499999999999989120, 2.785416667349484676, 0.8660254037844524744 ) ) ;
#190848=CARTESIAN_POINT ( 'NONE',  ( 1.364683531249988535, 3.717708333674750953, -0.7879004041258239610 ) ) ;
#190861=CARTESIAN_POINT ( 'NONE',  ( -9.501566725078754772, 9.979582688880366703, -0.7998128361456291469 ) ) ;
#190862=CARTESIAN_POINT ( 'NONE',  ( 6.551614543901692400, 8.666636272683888365, 1.599625672291281386 ) ) ;
#190866=ORIENTED_EDGE ( 'NONE', *, *, #164153, .F. ) ;
#190869=CARTESIAN_POINT ( 'NONE',  ( -7.965578943228732278, 9.251929174310385307, -1.199719254218446718 ) ) ;
#190874=CARTESIAN_POINT ( 'NONE',  ( 4.227444969362701421, 3.826440640544909400, 1.214306433183764966E-14 ) ) ;
#190878=CARTESIAN_POINT ( 'NONE',  ( -3.554208825076827782, 7.298327395898266623, 0.7998128361456341429 ) ) ;
#190879=CARTESIAN_POINT ( 'NONE',  ( -7.133561379084627063, 11.47423870890741782, 0.7998128361456481317 ) ) ;
#190889=CARTESIAN_POINT ( 'NONE',  ( 6.388916700537700777, 8.476822122092563916, 1.599625672291281386 ) ) ;
#190892=LINE ( 'NONE', #108660, #16822 ) ;
#190896=ORIENTED_EDGE ( 'NONE', *, *, #88030, .T. ) ;
#190910=CARTESIAN_POINT ( 'NONE',  ( 3.389175213736297820, 4.977123720824209840, 1.443375672974062551 ) ) ;
#190912=ORIENTED_EDGE ( 'NONE', *, *, #168015, .T. ) ;
#190914=CARTESIAN_POINT ( 'NONE',  ( -9.215791728987058562, 11.77484298861683598, -1.599625672291263179 ) ) ;
#190917=CARTESIAN_POINT ( 'NONE',  ( 8.778014389843965759, 12.32843499053828928, 1.199719254218450271 ) ) ;
#190921=CARTESIAN_POINT ( 'NONE',  ( 4.112618025573818947, 7.490225759230090041, 0.7307243446277329468 ) ) ;
#190925=CARTESIAN_POINT ( 'NONE',  ( -6.471393748265538370, 5.229711127717889596, -2.499999999999995115 ) ) ;
#190926=CARTESIAN_POINT ( 'NONE',  ( 1.364683531249986537, 0.6552083336747522857, -0.7879004041258239610 ) ) ;
#190932=CARTESIAN_POINT ( 'NONE',  ( -4.952806187693842510, 4.672695395264567786, 0.7998128361456341429 ) ) ;
#190934=CARTESIAN_POINT ( 'NONE',  ( 0.7499999999999867883, 0.06666666666668707997, -1.299038105676652899 ) ) ;
#190936=CARTESIAN_POINT ( 'NONE',  ( 1.499999999999989120, 5.545833333333350268, -0.8660254037844323793 ) ) ;
#190941=CARTESIAN_POINT ( 'NONE',  ( 1.364683531249988757, -0.1156249996585798079, 0.000000000000000000 ) ) ;
#190943=CARTESIAN_POINT ( 'NONE',  ( -7.901704598666176693, 8.113076874732334076, 0.7998128361456602331 ) ) ;
#190944=CARTESIAN_POINT ( 'NONE',  ( 7.377608144130607393, 11.75895993479440982, -0.7998128361456291469 ) ) ;
#190949=CARTESIAN_POINT ( 'NONE',  ( 1.364683531249986537, 0.7177083336747527298, -0.7879004041258239610 ) ) ;
#190956=CARTESIAN_POINT ( 'NONE',  ( 6.317736394288131052, 9.354147645769410602, 1.082531754730558626 ) ) ;
#190959=CARTESIAN_POINT ( 'NONE',  ( -4.660252114795309097, 6.460046772059735432, -1.599625672291256295 ) ) ;
#190961=CARTESIAN_POINT ( 'NONE',  ( 0.7499999999999902300, 5.597916667349482900, -1.299038105676658228 ) ) ;
#190963=CARTESIAN_POINT ( 'NONE',  ( -3.358669367883384105, 4.941533567329135401, -1.599625672291262513 ) ) ;
#190964=CARTESIAN_POINT ( 'NONE',  ( 6.453317929980448397, 6.631218461173066459, 1.040834085586084257E-14 ) ) ;
#190965=CARTESIAN_POINT ( 'NONE',  ( -9.449669878600623463, 11.08733161553131197, -1.082531754730537976 ) ) ;
#190967=CARTESIAN_POINT ( 'NONE',  ( 1.499999999999989120, 3.525000000000021227, 1.214306433183764966E-14 ) ) ;
#190971=CARTESIAN_POINT ( 'NONE',  ( 8.758204044747994743, 12.20135990463928266, 1.082531754730546636 ) ) ;
#190977=CARTESIAN_POINT ( 'NONE',  ( -1.420000000000055440, 7.176846818246208848, -4.202462424328208712 ) ) ;
#190986=CARTESIAN_POINT ( 'NONE',  ( 9.422553571373278203, 11.05569592376608945, -1.082531754730543083 ) ) ;
#190988=CARTESIAN_POINT ( 'NONE',  ( 6.414979237560321401, 10.63589287712906462, 1.040834085586084257E-14 ) ) ;
#190993=CARTESIAN_POINT ( 'NONE',  ( 4.690757960648224589, 6.495636925554817864, 1.443375672974062551 ) ) ;
#190994=ORIENTED_EDGE ( 'NONE', *, *, #92149, .T. ) ;
#190995=CARTESIAN_POINT ( 'NONE',  ( -7.782016984564068096, 10.10210578678999482, 1.443375672974090751 ) ) ;
#191016=EDGE_LOOP ( 'NONE', ( #166039, #204835, #149604, #40872 ) ) ;
#191026=CARTESIAN_POINT ( 'NONE',  ( -7.009729113465285266, 8.136771039586342624, -1.199719254218446718 ) ) ;
#191030=CARTESIAN_POINT ( 'NONE',  ( 6.257251587906815793, 7.258880593101466161, 1.199719254218462483 ) ) ;
#191031=CARTESIAN_POINT ( 'NONE',  ( -5.284980951228653190, 5.060232619388524533, 0.000000000000000000 ) ) ;
#191039=CARTESIAN_POINT ( 'NONE',  ( -5.253948220495577637, 6.088359997788290734, 1.199719254218450271 ) ) ;
#191043=CARTESIAN_POINT ( 'NONE',  ( 8.776205506747620788, 9.133327934160710981, -0.7998128361456221525 ) ) ;
#191046=CARTESIAN_POINT ( 'NONE',  ( 6.075519867480115188, 6.040327746143013599, 0.3625371965378897388 ) ) ;
#191052=CARTESIAN_POINT ( 'NONE',  ( 5.572037945092146671, 8.484166121707415797, -1.082531754730543971 ) ) ;
#191053=CARTESIAN_POINT ( 'NONE',  ( -7.344766530301162000, 9.591980256816594164, 1.599625672291295375 ) ) ;
#191056=CARTESIAN_POINT ( 'NONE',  ( -9.169391961543940539, 9.592045464756413509, 1.040834085586084257E-14 ) ) ;
#191057=CARTESIAN_POINT ( 'NONE',  ( -6.063521013809733518, 8.097193820909906137, 1.599625672291283607 ) ) ;
#191065=CARTESIAN_POINT ( 'NONE',  ( 6.726816770674637347, 10.99970333242910669, -0.7998128361456291469 ) ) ;
#191078=CARTESIAN_POINT ( 'NONE',  ( -1.500000000000011324, 4.920833333333354709, 0.8660254037844403729 ) ) ;
#191079=CARTESIAN_POINT ( 'NONE',  ( 5.009901455449552010, 5.803638771901306725, -1.199719254218452047 ) ) ;
#191080=CARTESIAN_POINT ( 'NONE',  ( 6.388916700537700777, 8.476822122092563916, 1.599625672291281386 ) ) ;
#191083=CARTESIAN_POINT ( 'NONE',  ( 6.155038550924144758, 8.203964280876741455, 1.443375672974076540 ) ) ;
#191084=CARTESIAN_POINT ( 'NONE',  ( -9.666600336419303829, 11.34041714965307968, 1.082531754730558626 ) ) ;
#191087=CARTESIAN_POINT ( 'NONE',  ( 8.483651433849084711, 10.92067931095586886, 1.599625672291281386 ) ) ;
#191092=CARTESIAN_POINT ( 'NONE',  ( -1.364683531250012516, 1.030208333674754062, 0.7879004041258379498 ) ) ;
#191098=CARTESIAN_POINT ( 'NONE',  ( 1.364683531249986537, -0.5947916663252456049, -0.7879004041258309554 ) ) ;
#191100=CARTESIAN_POINT ( 'NONE',  ( 8.062294901620731480, 12.55776115186623620, 1.040834085586084257E-14 ) ) ;
#191104=CARTESIAN_POINT ( 'NONE',  ( -7.818248136574758256, 12.27303992597924420, 0.000000000000000000 ) ) ;
#191111=CARTESIAN_POINT ( 'NONE',  ( 4.864678189204997949, 4.569879397027603929, 0.7998128361456341429 ) ) ;
#191117=CARTESIAN_POINT ( 'NONE',  ( 9.423080456697809026, 10.95234760669099749, -1.199719254218446718 ) ) ;
#191119=CARTESIAN_POINT ( 'NONE',  ( 0.4774187120914303861, 2.800000000000023803, -1.397118404531580316 ) ) ;
#191120=CARTESIAN_POINT ( 'NONE',  ( -5.904739593951539689, 6.847616600153594746, 1.199719254218450271 ) ) ;
#191124=CARTESIAN_POINT ( 'NONE',  ( 8.437251666405968464, 8.737881787095446384, 1.040834085586084257E-14 ) ) ;
#191126=CARTESIAN_POINT ( 'NONE',  ( 7.100719765255169236, 9.307259030929609267, -1.599625672291262513 ) ) ;
#191129=CARTESIAN_POINT ( 'NONE',  ( -7.524412065904404479, 11.72230514362308185, 0.000000000000000000 ) ) ;
#191138=CARTESIAN_POINT ( 'NONE',  ( -5.710256234166866562, 6.271970132040741497, 1.104226958479601173 ) ) ;
#191139=CARTESIAN_POINT ( 'NONE',  ( -1.364683531250014514, 1.488541667008084435, -0.7879004041258289570 ) ) ;
#191141=CARTESIAN_POINT ( 'NONE',  ( 5.666945020832167224, 8.594891043404107478, 1.082531754730558626 ) ) ;
#191145=CARTESIAN_POINT ( 'NONE',  ( -3.094265954482870118, 2.800000000000024691, 2.490342512183699508 ) ) ;
#191160=CARTESIAN_POINT ( 'NONE',  ( 9.582915646760733708, 10.07448976417602893, 0.7998128361456462443 ) ) ;
#191164=CARTESIAN_POINT ( 'NONE',  ( -2.788173145904702555, 6.404619103530779789, -0.7998128361456281477 ) ) ;
#191165=CARTESIAN_POINT ( 'NONE',  ( -8.016948904382338981, 8.247528564734524892, -0.7998128361456291469 ) ) ;
#191170=CARTESIAN_POINT ( 'NONE',  ( 1.499999999999989120, 4.035416667349482012, 0.8660254037844524744 ) ) ;
#191171=CARTESIAN_POINT ( 'NONE',  ( 6.726816770674637347, 10.99970333242910669, -0.7998128361456291469 ) ) ;
#191174=CARTESIAN_POINT ( 'NONE',  ( -8.389798128758148010, 8.682519326506312751, 0.7998128361456462443 ) ) ;
#191176=CARTESIAN_POINT ( 'NONE',  ( -0.6823417656249969321, 4.217708333674755394, -1.181850606188749264 ) ) ;
#191177=CARTESIAN_POINT ( 'NONE',  ( -1.458253848507225392, 8.740113170334302239, 2.549233421402196331 ) ) ;
#191181=CARTESIAN_POINT ( 'NONE',  ( -8.839552966430012759, 10.37552855133225904, -1.082531754730543971 ) ) ;
#191186=CARTESIAN_POINT ( 'NONE',  ( 1.364683531249990311, 3.446875000341416584, 1.214306433183764966E-14 ) ) ;
#191193=CARTESIAN_POINT ( 'NONE',  ( 0.6823417656249917140, 4.592708333674755394, 1.181850606188765695 ) ) ;
#191195=CARTESIAN_POINT ( 'NONE',  ( -4.599240423533815125, 6.388866465587984322, 1.599625672291267398 ) ) ;
#191196=CARTESIAN_POINT ( 'NONE',  ( 6.636879889089462026, 7.701780277814560982, -1.199719254218446718 ) ) ;
#191200=CARTESIAN_POINT ( 'NONE',  ( 0.6823417656249899377, 4.238541667008085767, -1.181850606188754593 ) ) ;
#191205=CARTESIAN_POINT ( 'NONE',  ( -1.364683531250000748, 0.009375000341420303140, 0.000000000000000000 ) ) ;
#191206=CARTESIAN_POINT ( 'NONE',  ( -3.633221978782290140, 6.222214161012547429, -1.082531754730549967 ) ) ;
#191209=VECTOR ( 'NONE', #65067, 1000.000000000000000 ) ;
#191212=CARTESIAN_POINT ( 'NONE',  ( 4.365362273920252889, 4.195270195769483124, 0.7216878364870317197 ) ) ;
#191215=CARTESIAN_POINT ( 'NONE',  ( -8.676855123066012254, 12.10645282934361866, -1.082531754730543971 ) ) ;
#191219=CARTESIAN_POINT ( 'NONE',  ( -9.972185678051314284, 11.59297036493672017, 1.199719254218462483 ) ) ;
#191220=CARTESIAN_POINT ( 'NONE',  ( -5.788968402910818156, 7.776882441527838807, 1.443375672974064550 ) ) ;
#191222=CARTESIAN_POINT ( 'NONE',  ( -1.201851678989727383E-14, 1.134375000341418582, 1.575800808251672791 ) ) ;
#191229=CARTESIAN_POINT ( 'NONE',  ( 1.364683531249986537, -0.03229166632525094088, -0.7879004041258309554 ) ) ;
#191235=CARTESIAN_POINT ( 'NONE',  ( -0.7500000000000006661, -0.8916666666666448471, -1.299038105676652011 ) ) ;
#191236=CARTESIAN_POINT ( 'NONE',  ( 6.900736999231407154, 10.99468423250458038, -0.7216878364870267237 ) ) ;
#191245=CARTESIAN_POINT ( 'NONE',  ( -2.279742385392243165, 5.811449882932888222, -0.7998128361456281477 ) ) ;
#191248=CARTESIAN_POINT ( 'NONE',  ( -1.201851678989727383E-14, 1.884375000341422135, 1.575800808251672791 ) ) ;
#191258=ORIENTED_EDGE ( 'NONE', *, *, #48534, .T. ) ;
#191266=CARTESIAN_POINT ( 'NONE',  ( 5.309989718046547402, 9.346738437696316737, 0.7998128361456462443 ) ) ;
#191274=CARTESIAN_POINT ( 'NONE',  ( 6.774270308322468459, 11.05506579301824743, 0.7998128361456462443 ) ) ;
#191277=CARTESIAN_POINT ( 'NONE',  ( 8.561083932025322696, 12.07534945641652158, -1.199719254218446718 ) ) ;
#191285=CARTESIAN_POINT ( 'NONE',  ( 10.18233705906309972, 11.83814697611718714, 1.199719254218450271 ) ) ;
#191292=CARTESIAN_POINT ( 'NONE',  ( -9.219181267612684749, 10.81842823604534765, 1.082531754730558626 ) ) ;
#191303=CARTESIAN_POINT ( 'NONE',  ( 3.836594282542914236, 5.499112634431936542, 1.443375672974062551 ) ) ;
#191311=CARTESIAN_POINT ( 'NONE',  ( -5.961834861707238531, 7.978559976790334574, -1.599625672291263179 ) ) ;
#191313=CARTESIAN_POINT ( 'NONE',  ( -3.867100128395853709, 5.534702787927018974, -1.599625672291256295 ) ) ;
#191320=CARTESIAN_POINT ( 'NONE',  ( 1.364683531249990311, 3.946875000341417028, 1.214306433183764966E-14 ) ) ;
#191323=CARTESIAN_POINT ( 'NONE',  ( 5.392392409933256303, 7.314210449720692786, 1.599625672291267398 ) ) ;
#191329=B_SPLINE_CURVE_WITH_KNOTS ( 'NONE', 3,
 ( #165864, #198341, #55052, #178934, #148557, #64105, #66191, #197286, #49981, #182091 ),
 .UNSPECIFIED., .F., .F.,
 ( 4, 3, 3, 4 ),
 ( 0.000000000000000000, 8.893179197954992701E-05, 0.0001334007970840233410, 0.0001778705873658995192 ),
 .UNSPECIFIED. ) ;
#191336=CARTESIAN_POINT ( 'NONE',  ( 1.364683531249986537, 1.217708333674754950, -0.7879004041258239610 ) ) ;
#191338=CARTESIAN_POINT ( 'NONE',  ( 2.855963913973019963, 6.483708332943829866, 0.000000000000000000 ) ) ;
#191340=CARTESIAN_POINT ( 'NONE',  ( -4.880572111239580124, 7.677455982212699759, 1.082531754730560403 ) ) ;
#191342=CARTESIAN_POINT ( 'NONE',  ( 3.036663219780971978, 6.486598156479028709, -0.7216878364870267237 ) ) ;
#191343=VECTOR ( 'NONE', #178625, 1000.000000000000114 ) ;
#191344=CARTESIAN_POINT ( 'NONE',  ( -7.510853911846401942, 7.865010440016681592, 1.040834085586084257E-14 ) ) ;
#191349=CARTESIAN_POINT ( 'NONE',  ( 7.284808609244363353, 7.393364887073558656, 0.7998128361456341429 ) ) ;
#191354=CARTESIAN_POINT ( 'NONE',  ( -0.6823417656249969321, 5.217708333674756283, -1.181850606188749264 ) ) ;
#191358=CARTESIAN_POINT ( 'NONE',  ( 6.174848896020108668, 9.291408581077091000, 1.199719254218460707 ) ) ;
#191361=CARTESIAN_POINT ( 'NONE',  ( -6.388916700537716764, 8.476822122092563916, 1.599625672291283607 ) ) ;
#191366=CARTESIAN_POINT ( 'NONE',  ( 8.402302512167096893, 10.82577223566020841, -1.599625672291268286 ) ) ;
#191368=CARTESIAN_POINT ( 'NONE',  ( -5.852315862593199469, 9.979452273000736895, 0.7998128361456481317 ) ) ;
#191371=CARTESIAN_POINT ( 'NONE',  ( 6.385527161912102123, 9.433236874664039817, -1.082531754730537976 ) ) ;
#191372=CARTESIAN_POINT ( 'NONE',  ( 4.016789712308713511, 7.804715019974644008, -0.2988979438510626085 ) ) ;
#191374=CARTESIAN_POINT ( 'NONE',  ( -5.759516327706961647, 5.613857225279885732, -0.7998128361456221525 ) ) ;
#191378=CARTESIAN_POINT ( 'NONE',  ( 4.364835388595708743, 7.179726155748598515, 1.199719254218462483 ) ) ;
#191380=CARTESIAN_POINT ( 'NONE',  ( 7.567422294721922960, 11.98040977715095323, 0.7998128361456462443 ) ) ;
#191381=CARTESIAN_POINT ( 'NONE',  ( -5.532833371615617502, 6.236068886146576951, 0.9535701153140889730 ) ) ;
#191382=CARTESIAN_POINT ( 'NONE',  ( 2.171277156482887882, 5.684907115872006145, -0.7998128361456291469 ) ) ;
#191383=CARTESIAN_POINT ( 'NONE',  ( -0.6823417656250212460, 1.051041667008083325, 1.181850606188755259 ) ) ;
#191385=CARTESIAN_POINT ( 'NONE',  ( -6.751597309925468693, 6.979211071108916364, 0.7216878364870317197 ) ) ;
#191392=CARTESIAN_POINT ( 'NONE',  ( -5.485560113408387117, 6.267152048184752466, 0.9985905309092910631 ) ) ;
#191393=CARTESIAN_POINT ( 'NONE',  ( 0.6823417656249882723, 1.738541667008083991, -1.181850606188749264 ) ) ;
#191396=CARTESIAN_POINT ( 'NONE',  ( 4.256897045010922476, 5.029096643009940415, -1.082531754730548412 ) ) ;
#191400=CARTESIAN_POINT ( 'NONE',  ( -7.171900071504738072, 10.35067193585544665, -1.082531754730543083 ) ) ;
#191407=CARTESIAN_POINT ( 'NONE',  ( -7.822691444960696572, 12.07029775252209092, -0.7216878364870267237 ) ) ;
#191415=CARTESIAN_POINT ( 'NONE',  ( -6.521108698048767138, 10.55178454779148289, -0.7216878364870267237 ) ) ;
#191420=CARTESIAN_POINT ( 'NONE',  ( -0.7500000000000215383, 4.222916667349481123, 1.299038105676671107 ) ) ;
#191421=CARTESIAN_POINT ( 'NONE',  ( 4.286934996870309433, 7.472684718058654418, -1.056577385247484457 ) ) ;
#191425=VERTEX_POINT ( 'NONE', #59216 ) ;
#191427=CARTESIAN_POINT ( 'NONE',  ( -7.531718027591449705, 8.745758106066849891, 1.199719254218462483 ) ) ;
#191431=CARTESIAN_POINT ( 'NONE',  ( 5.066996723205273057, 6.934582148538044777, 1.599625672291267398 ) ) ;
#191436=CARTESIAN_POINT ( 'NONE',  ( 7.793239369756836510, 7.986534107671458216, 0.7998128361456341429 ) ) ;
#191445=CARTESIAN_POINT ( 'NONE',  ( -5.422898255786198440, 7.349800603215774331, -1.443375672974052559 ) ) ;
#191454=CARTESIAN_POINT ( 'NONE',  ( -7.506410603460441422, 11.90922947067921278, -0.7998128361456291469 ) ) ;
#191457=CARTESIAN_POINT ( 'NONE',  ( 8.444030743212801227, 8.745790710036752458, 0.7998128361456462443 ) ) ;
#191458=CARTESIAN_POINT ( 'NONE',  ( -1.402160292154681736E-14, -0.1624999999999815481, -1.732050807568870754 ) ) ;
#191459=CARTESIAN_POINT ( 'NONE',  ( -7.232384877886063990, 10.52520055992070525, -1.199719254218446718 ) ) ;
#191461=CARTESIAN_POINT ( 'NONE',  ( -0.6823417656249969321, 3.967708333674754950, -1.181850606188749264 ) ) ;
#191462=EDGE_CURVE ( 'NONE', #205532, #199393, #73325, .T. ) ;
#191463=CARTESIAN_POINT ( 'NONE',  ( 8.256552361042350796, 12.57646882128404187, 1.040834085586084257E-14 ) ) ;
#191466=CARTESIAN_POINT ( 'NONE',  ( 1.499999999999989120, 5.545833333333350268, -0.8660254037844323793 ) ) ;
#191469=CARTESIAN_POINT ( 'NONE',  ( 9.368320956918616105, 10.03205532593431037, 0.7216878364870458196 ) ) ;
#191472=CARTESIAN_POINT ( 'NONE',  ( -5.734735788900501952, 9.634349487118505806, 0.000000000000000000 ) ) ;
#191474=CARTESIAN_POINT ( 'NONE',  ( -1.364683531250012516, 2.238541667008087988, -0.7879004041258289570 ) ) ;
#191478=CARTESIAN_POINT ( 'NONE',  ( -6.235860587281615075, 9.362588887548838557, -1.199719254218440723 ) ) ;
#191479=CARTESIAN_POINT ( 'NONE',  ( -1.001543065824772872E-14, 4.634375000341418804, 1.575800808251672791 ) ) ;
#191484=CARTESIAN_POINT ( 'NONE',  ( 9.745613490124728884, 10.26430391476735338, 0.7998128361456462443 ) ) ;
#191487=CARTESIAN_POINT ( 'NONE',  ( -1.500000000000013101, 1.629166666666691077, -0.8660254037844313801 ) ) ;
#191492=CARTESIAN_POINT ( 'NONE',  ( 7.619319141200072920, 7.991553207595983643, 0.7216878364870317197 ) ) ;
#191493=CARTESIAN_POINT ( 'NONE',  ( 10.39640486358069360, 11.02356051713265650, 0.7998128361456462443 ) ) ;
#191500=CARTESIAN_POINT ( 'NONE',  ( 9.399880572976245574, 9.860948844760784482, 0.7998128361456462443 ) ) ;
#191501=CARTESIAN_POINT ( 'NONE',  ( -8.631737353394710155, 13.22211067893587533, 1.040834085586084257E-14 ) ) ;
#191504=FACE_OUTER_BOUND ( 'NONE', #89148, .T. ) ;
#191505=CARTESIAN_POINT ( 'NONE',  ( -0.6823417656250212460, 5.363541667008087543, 1.181850606188767472 ) ) ;
#191511=CARTESIAN_POINT ( 'NONE',  ( -1.364683531250012516, 3.488541667008085767, -0.7879004041258300672 ) ) ;
#191513=CARTESIAN_POINT ( 'NONE',  ( -5.666945020832185875, 7.634521829102760115, 1.443375672974064550 ) ) ;
#191519=CARTESIAN_POINT ( 'NONE',  ( 3.704402285031850539, 5.344888637335695414, -1.599625672291262513 ) ) ;
#191522=CARTESIAN_POINT ( 'NONE',  ( 7.214910300766615769, 11.56914578420308715, -0.7998128361456291469 ) ) ;
#191529=CARTESIAN_POINT ( 'NONE',  ( -7.971304249830880373, 11.38727316052296601, 1.199719254218453823 ) ) ;
#191530=CARTESIAN_POINT ( 'NONE',  ( 5.795220594837462436, 8.848508896363995291, -1.199719254218440723 ) ) ;
#191532=CARTESIAN_POINT ( 'NONE',  ( 4.080641047588898118, 5.783833860318930320, -1.443375672974051449 ) ) ;
#191534=CARTESIAN_POINT ( 'NONE',  ( 2.998324526916512411, 6.649795714711241423, 0.000000000000000000 ) ) ;
#191542=CARTESIAN_POINT ( 'NONE',  ( -5.504247177468192476, 7.444707678511436555, 1.443375672974064550 ) ) ;
#191543=CARTESIAN_POINT ( 'NONE',  ( 2.686486993802192913, 6.285985259411197568, 0.7998128361456362523 ) ) ;
#191546=CARTESIAN_POINT ( 'NONE',  ( -7.965578943228732278, 9.251929174310385307, -1.199719254218446718 ) ) ;
#191551=CARTESIAN_POINT ( 'NONE',  ( -7.537443334193545397, 10.88110209227943770, -1.199719254218446718 ) ) ;
#191555=CARTESIAN_POINT ( 'NONE',  ( 6.584456157731144899, 10.83361595066169514, -0.7998128361456291469 ) ) ;
#191556=CARTESIAN_POINT ( 'NONE',  ( 4.690231075323689325, 7.559354456931247412, 1.199719254218462483 ) ) ;
#191568=CARTESIAN_POINT ( 'NONE',  ( -7.374745490829552885, 10.69128794168811680, -1.199719254218446718 ) ) ;
#191571=CARTESIAN_POINT ( 'NONE',  ( 5.002595493762530765, 8.780185809457538681, 1.040834085586084257E-14 ) ) ;
#191576=CARTESIAN_POINT ( 'NONE',  ( -5.274285450916075035, 6.112086766612214284, 1.199719254218450271 ) ) ;
#191586=CARTESIAN_POINT ( 'NONE',  ( -10.31505594189871111, 10.92865344183699428, -0.7998128361456291469 ) ) ;
#191587=CARTESIAN_POINT ( 'NONE',  ( 6.753933077901968396, 11.03133902419432566, 0.7998128361456462443 ) ) ;
#191592=CARTESIAN_POINT ( 'NONE',  ( -4.409912583257236562, 7.141888050452717351, -1.077592642408040424 ) ) ;
#191599=CARTESIAN_POINT ( 'NONE',  ( 9.951321562750607086, 11.67259191370631477, -1.082531754730537088 ) ) ;
#191617=CARTESIAN_POINT ( 'NONE',  ( -4.948889764188092677, 5.732458465429559169, 1.199719254218462483 ) ) ;
#191618=CARTESIAN_POINT ( 'NONE',  ( 5.138177029454841893, 7.017625839162543677, 1.443375672974062551 ) ) ;
#191619=CARTESIAN_POINT ( 'NONE',  ( 1.499999999999989120, 3.525000000000021227, 1.214306433183764966E-14 ) ) ;
#191621=CARTESIAN_POINT ( 'NONE',  ( -2.286521462199063492, 5.819358805874190743, 1.040834085586084257E-14 ) ) ;
#191625=CARTESIAN_POINT ( 'NONE',  ( -0.6823417656249969321, 4.217708333674755394, -1.181850606188749264 ) ) ;
#191628=CARTESIAN_POINT ( 'NONE',  ( -3.090895834235680262, 5.589500325708124606, 1.082531754730560403 ) ) ;
#191633=CARTESIAN_POINT ( 'NONE',  ( 4.379447312414087357, 5.068108938359919158, -1.199719254218452047 ) ) ;
#191635=CARTESIAN_POINT ( 'NONE',  ( 3.914243274428867103, 2.801588762746437311, -0.7749999999999935829 ) ) ;
#191636=CARTESIAN_POINT ( 'NONE',  ( 10.18181017373857067, 11.94149529319227909, 1.082531754730548412 ) ) ;
#191638=CARTESIAN_POINT ( 'NONE',  ( 1.364683531249986537, 1.717708333674749399, -0.7879004041258239610 ) ) ;
#191641=CARTESIAN_POINT ( 'NONE',  ( -8.833300774503376473, 10.26427131079744193, 1.199719254218462483 ) ) ;
#191642=CARTESIAN_POINT ( 'NONE',  ( -5.870317324592821073, 6.911420302522161663, -1.082531754730543083 ) ) ;
#191646=CARTESIAN_POINT ( 'NONE',  ( 0.6823417656249899377, 4.176041667008085767, -1.181850606188754593 ) ) ;
#191655=CARTESIAN_POINT ( 'NONE',  ( -4.243338890952901288, 6.934017225211593249, -1.082531754730548412 ) ) ;
#191661=CARTESIAN_POINT ( 'NONE',  ( -4.216222583725562245, 7.862750747747711877, 0.7216878364870317197 ) ) ;
#191667=CARTESIAN_POINT ( 'NONE',  ( 3.469446951953614189E-15, 5.229711127717882491, 1.214306433183764966E-14 ) ) ;
#191674=CARTESIAN_POINT ( 'NONE',  ( -4.928552533767591726, 5.708731696605642725, 1.199719254218462483 ) ) ;
#191677=CARTESIAN_POINT ( 'NONE',  ( -1.201851678989727383E-14, 0.7125000000000225597, 1.732050807568877637 ) ) ;
#191680=CARTESIAN_POINT ( 'NONE',  ( 8.107412671292031803, 11.44210330227398487, 1.082531754730557072 ) ) ;
#191681=CARTESIAN_POINT ( 'NONE',  ( 7.305145839664861640, 7.417091655897478653, 0.7998128361456341429 ) ) ;
#191687=CARTESIAN_POINT ( 'NONE',  ( 4.273844736805816780, 6.009238164405336313, 1.599625672291267398 ) ) ;
#191688=CARTESIAN_POINT ( 'NONE',  ( -0.2089193878862168341, 7.199905994521426322, -1.991006660531114747 ) ) ;
#191695=CARTESIAN_POINT ( 'NONE',  ( 7.574201371528760163, 11.98831870009225931, 1.040834085586084257E-14 ) ) ;
#191696=CARTESIAN_POINT ( 'NONE',  ( -7.413611068574208041, 7.543634422958360730, 0.7998128361456341429 ) ) ;
#191703=CARTESIAN_POINT ( 'NONE',  ( -1.364683531250010295, 4.780208333674755394, 0.7879004041258379498 ) ) ;
#191704=CARTESIAN_POINT ( 'NONE',  ( 9.693716643646601128, 10.41168362711695750, 0.7216878364870438212 ) ) ;
#191705=CARTESIAN_POINT ( 'NONE',  ( -7.088215381846223906, 7.164006121775713609, 0.7998128361456341429 ) ) ;
#191709=CARTESIAN_POINT ( 'NONE',  ( 5.952193131599331721, 6.902979060742733708, 1.199719254218462483 ) ) ;
#191710=CARTESIAN_POINT ( 'NONE',  ( -4.713430959045263435, 8.650753218861462202, 0.7998128361456481317 ) ) ;
#191717=CARTESIAN_POINT ( 'NONE',  ( 5.016153647376196290, 8.796003655340152605, 0.7216878364870438212 ) ) ;
#191721=CARTESIAN_POINT ( 'NONE',  ( -1.402160292154681736E-14, 2.009375000341422801, -1.575800808251660134 ) ) ;
#191723=CARTESIAN_POINT ( 'NONE',  ( 5.382223794500827552, 7.302347065049529462, -1.443375672974051449 ) ) ;
#191725=CARTESIAN_POINT ( 'NONE',  ( -3.389175213736311587, 4.977123720824209840, 1.443375672974064550 ) ) ;
#191727=CARTESIAN_POINT ( 'NONE',  ( -1.364683531249997417, 5.509375000341417916, 1.214306433183764966E-14 ) ) ;
#191732=CARTESIAN_POINT ( 'NONE',  ( -4.182100719528288657, 7.584231438125928371, -0.9338283797597360936 ) ) ;
#191740=CARTESIAN_POINT ( 'NONE',  ( 4.808338034340912337, 8.761478140039733020, 1.040834085586084257E-14 ) ) ;
#191743=CARTESIAN_POINT ( 'NONE',  ( -1.500000000000022204, 7.240846818246208905, 4.154462424328226433 ) ) ;
#191751=CARTESIAN_POINT ( 'NONE',  ( 5.368665641331531013, 5.365790791082654998, -0.7216878364870207285 ) ) ;
#191752=CARTESIAN_POINT ( 'NONE',  ( 1.364683531249988535, 2.426041667008088432, 0.7879004041258500513 ) ) ;
#191754=CARTESIAN_POINT ( 'NONE',  ( 8.586391356156291010, 8.911878091804165791, 0.7998128361456481317 ) ) ;
#191755=CARTESIAN_POINT ( 'NONE',  ( -9.130526383799315582, 12.73969898348616070, 1.199719254218462483 ) ) ;
#191756=CARTESIAN_POINT ( 'NONE',  ( -3.378415862307731832, 6.366559134822412425, -0.8608806284970575984 ) ) ;
#191757=CARTESIAN_POINT ( 'NONE',  ( -5.928993247877787809, 5.811580298812519807, 0.7998128361456341429 ) ) ;
#191760=ORIENTED_EDGE ( 'NONE', *, *, #147466, .T. ) ;
#191762=CARTESIAN_POINT ( 'NONE',  ( -0.7500000000000215383, 2.691666666666689522, 1.299038105676671107 ) ) ;
#191763=CARTESIAN_POINT ( 'NONE',  ( 4.950698647284403009, 8.927565521807144577, 1.040834085586084257E-14 ) ) ;
#191764=CARTESIAN_POINT ( 'NONE',  ( -6.256197817702116026, 9.386315656372753224, -1.199719254218440723 ) ) ;
#191769=CARTESIAN_POINT ( 'NONE',  ( 0.6823417656249882723, 1.926041667008083991, -1.181850606188749264 ) ) ;
#191771=CARTESIAN_POINT ( 'NONE',  ( 3.358669367883368118, 4.941533567329135401, -1.599625672291262513 ) ) ;
#191776=CARTESIAN_POINT ( 'NONE',  ( 0.7499999999999885647, 1.347916667349485786, -1.299038105676652899 ) ) ;
#191779=CARTESIAN_POINT ( 'NONE',  ( -5.311043488251275591, 7.219303374425030562, -1.599625672291256295 ) ) ;
#191780=CARTESIAN_POINT ( 'NONE',  ( -3.633221978782304351, 4.301475732409860697, -1.082531754730549967 ) ) ;
#191788=CARTESIAN_POINT ( 'NONE',  ( 5.961834861707224320, 7.978559976790334574, -1.599625672291262513 ) ) ;
#191791=CARTESIAN_POINT ( 'NONE',  ( 5.952193131599331721, 6.902979060742733708, 1.199719254218462483 ) ) ;
#191795=CARTESIAN_POINT ( 'NONE',  ( 2.758194185376297902, 5.305311418659259814, 1.199719254218452047 ) ) ;
#191799=CARTESIAN_POINT ( 'NONE',  ( 5.275030131637754138, 6.378586025900190748, 1.136986337720545581 ) ) ;
#191808=CARTESIAN_POINT ( 'NONE',  ( -6.385527162356468445, 10.39360608948380538, 1.040834085586084257E-14 ) ) ;
#191809=DIRECTION ( 'NONE',  ( 0.000000000000000000, 1.000000000000000000, -8.546850786086437571E-32 ) ) ;
#191811=CARTESIAN_POINT ( 'NONE',  ( 7.456621297836067086, 10.68284669990868174, 1.082531754730558626 ) ) ;
#191813=CARTESIAN_POINT ( 'NONE',  ( -5.739179097286464248, 5.590130456455974617, -0.7998128361456221525 ) ) ;
#191816=CARTESIAN_POINT ( 'NONE',  ( 8.392660782059197189, 9.750191319612612872, 1.199719254218462483 ) ) ;
#191818=CARTESIAN_POINT ( 'NONE',  ( -5.961834861707238531, 7.978559976790334574, -1.599625672291263179 ) ) ;
#191833=CARTESIAN_POINT ( 'NONE',  ( 8.563946585326370098, 13.14302144952281814, 0.7998128361456462443 ) ) ;
#191834=CARTESIAN_POINT ( 'NONE',  ( -5.525111292768871252, 6.404716915440499037, -1.199719254218446718 ) ) ;
#191837=CARTESIAN_POINT ( 'NONE',  ( 4.392478581147586603, 4.226905887534702977, -0.7216878364870188411 ) ) ;
#191842=CARTESIAN_POINT ( 'NONE',  ( -2.767835915484202047, 6.380892334706859792, -0.7998128361456281477 ) ) ;
#191845=CARTESIAN_POINT ( 'NONE',  ( 9.752392566931574081, 10.27221283770866300, -0.7998128361456281477 ) ) ;
#191850=CARTESIAN_POINT ( 'NONE',  ( -5.852315862593199469, 9.979452273000736895, 0.7998128361456481317 ) ) ;
#191851=CARTESIAN_POINT ( 'NONE',  ( 5.996784015946103885, 5.890669528225568996, 1.040834085586084257E-14 ) ) ;
#191854=CARTESIAN_POINT ( 'NONE',  ( -1.999999999999996669, 6.400000000000024336, 1.214306433183764966E-14 ) ) ;
#191857=CARTESIAN_POINT ( 'NONE',  ( -1.364683531250000748, 2.071875000341422357, 1.214306433183764966E-14 ) ) ;
#191860=CARTESIAN_POINT ( 'NONE',  ( 6.480434237652121787, 9.543961796360731498, 1.082531754730558626 ) ) ;
#191862=DIRECTION ( 'NONE',  ( 0.7592566023653044560, -0.6507913734559596097, -1.725633230170963762E-31 ) ) ;
#191867=CIRCLE ( 'NONE', #150300, 2.000000000000000000 ) ;
#191868=CARTESIAN_POINT ( 'NONE',  ( 9.720832950873944611, 10.44331931888218001, -0.7216878364870257245 ) ) ;
#191874=CARTESIAN_POINT ( 'NONE',  ( -8.503988664269602538, 10.94440607977979063, 1.599625672291269396 ) ) ;
#191875=FACE_OUTER_BOUND ( 'NONE', #18060, .T. ) ;
#191883=CARTESIAN_POINT ( 'NONE',  ( 2.934188532424650830, 6.448561212153446576, -0.2786481428285088047 ) ) ;
#191890=CARTESIAN_POINT ( 'NONE',  ( -1.201851678989727383E-14, 1.493750000682814383, 1.732050807568877637 ) ) ;
#191896=CARTESIAN_POINT ( 'NONE',  ( -0.7500000000000006661, 0.1083333333333560966, -1.299038105676652011 ) ) ;
#191897=CARTESIAN_POINT ( 'NONE',  ( 8.565000355531088516, 11.01558638625153286, -1.599625672291257406 ) ) ;
#191898=CARTESIAN_POINT ( 'NONE',  ( 1.364683531249988757, 0.1343750003414204142, 0.000000000000000000 ) ) ;
#191901=CARTESIAN_POINT ( 'NONE',  ( 10.54788032175191326, 11.40820791823982994, 0.7216878364870317197 ) ) ;
#191902=CARTESIAN_POINT ( 'NONE',  ( -6.900736999675794792, 7.153207375817628666, 1.040834085586084257E-14 ) ) ;
#191906=CARTESIAN_POINT ( 'NONE',  ( -5.096975683733680818, 8.033889833409558534, -1.199719254218452047 ) ) ;
#191908=CARTESIAN_POINT ( 'NONE',  ( 0.7499999999999902300, 3.264583334016149418, 1.299038105676669330 ) ) ;
#191914=DIRECTION ( 'NONE',  ( 0.7592566023652994600, 0.6507913734559651608, 0.000000000000000000 ) ) ;
#191920=CARTESIAN_POINT ( 'NONE',  ( -8.422639742587602285, 10.84949900448412841, -1.599625672291263179 ) ) ;
#191921=CARTESIAN_POINT ( 'NONE',  ( 6.337546739384100292, 9.481222731668410120, 1.199719254218460707 ) ) ;
#191925=ORIENTED_EDGE ( 'NONE', *, *, #198311, .F. ) ;
#191929=CARTESIAN_POINT ( 'NONE',  ( -7.857113714319432063, 9.125386407249497012, 1.199719254218462483 ) ) ;
#191934=CARTESIAN_POINT ( 'NONE',  ( 3.192055101013606233, 5.811482486902795230, -1.199719254218446718 ) ) ;
#191937=ORIENTED_EDGE ( 'NONE', *, *, #127587, .T. ) ;
#191938=CARTESIAN_POINT ( 'NONE',  ( -8.995998617867369873, 10.45408546138876993, 1.199719254218462483 ) ) ;
#191941=CARTESIAN_POINT ( 'NONE',  ( -5.122186659821378996, 6.697499048860120041, -1.435703471572645551 ) ) ;
#191948=CARTESIAN_POINT ( 'NONE',  ( 7.467843683028853263, 7.606905806488803101, 0.7998128361456341429 ) ) ;
#191957=CARTESIAN_POINT ( 'NONE',  ( -1.500000000000001332, 0.9312500006828163812, 0.000000000000000000 ) ) ;
#191969=DIRECTION ( 'NONE',  ( -5.578564026256490882E-16, -1.000000000000000000, -9.066213480720158442E-32 ) ) ;
#191971=CARTESIAN_POINT ( 'NONE',  ( 2.711267533052988732, 6.106969855296372707, -0.7216878364870267237 ) ) ;
#191978=CARTESIAN_POINT ( 'NONE',  ( 8.075853055234393452, 12.57357899774884658, 0.7998128361456462443 ) ) ;
#191981=ADVANCED_FACE ( 'NONE', ( #146901 ), #207302, .T. ) ;
#191985=FACE_OUTER_BOUND ( 'NONE', #17462, .T. ) ;
#191987=CARTESIAN_POINT ( 'NONE',  ( 1.364683531249986537, 0.6135416670080880985, 0.7879004041258500513 ) ) ;
#191991=VECTOR ( 'NONE', #139850, 1000.000000000000000 ) ;
#191993=CARTESIAN_POINT ( 'NONE',  ( -3.581325132304157943, 7.329963087663487364, -0.7998128361456281477 ) ) ;
#191996=CARTESIAN_POINT ( 'NONE',  ( -1.500000000000015099, -0.3708333333333105331, -0.8660254037844383745 ) ) ;
#191998=CARTESIAN_POINT ( 'NONE',  ( -1.001543065824772872E-14, 5.462500000000020783, 1.732050807568877637 ) ) ;
#192003=CARTESIAN_POINT ( 'NONE',  ( 1.364683531249986537, -0.3864583329919166199, 0.7879004041258500513 ) ) ;
#192005=CARTESIAN_POINT ( 'NONE',  ( -8.376239975144482486, 8.666701480623698828, 1.040834085586084257E-14 ) ) ;
#192006=CARTESIAN_POINT ( 'NONE',  ( 1.419999999999989049, 6.280000000000042881, -2.873333333333329520 ) ) ;
#192007=CARTESIAN_POINT ( 'NONE',  ( 9.348510611822643313, 10.86534945433664134, 1.199719254218453823 ) ) ;
#192013=ORIENTED_EDGE ( 'NONE', *, *, #172073, .F. ) ;
#192015=CARTESIAN_POINT ( 'NONE',  ( -1.364683531250000748, -0.1781249996585798634, 0.000000000000000000 ) ) ;
#192021=CARTESIAN_POINT ( 'NONE',  ( 1.499999999999990896, 3.806250000682819046, 1.214306433183764966E-14 ) ) ;
#192023=CARTESIAN_POINT ( 'NONE',  ( 6.426201623197458801, 9.480690412830290015, -1.082531754730537088 ) ) ;
#192026=CARTESIAN_POINT ( 'NONE',  ( -3.744022975668147790, 7.519777238254810925, -0.7998128361456281477 ) ) ;
#192028=CARTESIAN_POINT ( 'NONE',  ( 3.823036128929238942, 7.404033217152015567, 1.040834085586084257E-14 ) ) ;
#192031=CARTESIAN_POINT ( 'NONE',  ( 6.114364089638798738, 6.235772314107808079, 0.7216878364870317197 ) ) ;
#192032=CARTESIAN_POINT ( 'NONE',  ( -9.639484029191951464, 10.34841224358651601, 0.7216878364870438212 ) ) ;
#192037=CARTESIAN_POINT ( 'NONE',  ( 8.256552361042350796, 12.57646882128404187, 1.040834085586084257E-14 ) ) ;
#192038=CARTESIAN_POINT ( 'NONE',  ( -0.7500000000000215383, 4.691666666666684193, 1.299038105676671107 ) ) ;
#192051=CARTESIAN_POINT ( 'NONE',  ( 9.707274797260268429, 10.42750147299956964, 0.000000000000000000 ) ) ;
#192053=CARTESIAN_POINT ( 'NONE',  ( 6.591235234537977661, 10.84152487360300299, 0.7998128361456462443 ) ) ;
#192054=AXIS2_PLACEMENT_3D ( 'NONE', #69154, #151516, #22546 ) ;
#192058=DIRECTION ( 'NONE',  ( 1.000000000000000000, 0.000000000000000000, 0.000000000000000000 ) ) ;
#192059=CARTESIAN_POINT ( 'NONE',  ( 3.199361063144961825, 6.676412307070352270, -0.7216878364870267237 ) ) ;
#192061=CARTESIAN_POINT ( 'NONE',  ( -8.012505595996376684, 12.29174759539704986, 0.000000000000000000 ) ) ;
#192089=CARTESIAN_POINT ( 'NONE',  ( -6.561783159334121152, 10.59923808595773664, -0.7216878364870278340 ) ) ;
#192093=CARTESIAN_POINT ( 'NONE',  ( 6.823831386379729302, 6.855558127064808716, -0.7998128361456281477 ) ) ;
#192097=CARTESIAN_POINT ( 'NONE',  ( 2.205172540517054802, 5.724451730578533848, 1.040834085586084257E-14 ) ) ;
#192099=CARTESIAN_POINT ( 'NONE',  ( -5.284980951228653190, 5.060232619388524533, 0.000000000000000000 ) ) ;
#192103=CARTESIAN_POINT ( 'NONE',  ( -3.741160322367112379, 6.452105245148518797, 1.199719254218464037 ) ) ;
#192108=CARTESIAN_POINT ( 'NONE',  ( 8.586391356156291010, 8.911878091804165791, 0.7998128361456481317 ) ) ;
#192109=CARTESIAN_POINT ( 'NONE',  ( 1.364683531249988535, 3.905208333674751842, -0.7879004041258239610 ) ) ;
#192111=CARTESIAN_POINT ( 'NONE',  ( 5.670051627282618689, 6.304626411287498122, 1.111461560052000586 ) ) ;
#192112=CARTESIAN_POINT ( 'NONE',  ( 3.714570900464278846, 5.356752022006865843, 1.443375672974062551 ) ) ;
#192119=CARTESIAN_POINT ( 'NONE',  ( 4.975479186090839612, 8.748550117173898855, 0.7216878364870438212 ) ) ;
#192120=CARTESIAN_POINT ( 'NONE',  ( -8.025536864285518490, 11.45054454405341282, -1.199719254218446718 ) ) ;
#192123=CARTESIAN_POINT ( 'NONE',  ( -6.808165692356648258, 11.09461040772476714, 0.7998128361456481317 ) ) ;
#192125=CARTESIAN_POINT ( 'NONE',  ( -7.576308911938196999, 7.733448573549685179, 0.7998128361456462443 ) ) ;
#192132=CARTESIAN_POINT ( 'NONE',  ( 8.535021395002688749, 9.916278701380017324, 1.199719254218462483 ) ) ;
#192140=CARTESIAN_POINT ( 'NONE',  ( -1.201851678989727383E-14, 5.368750000682816825, -1.732050807568863648 ) ) ;
#192145=CARTESIAN_POINT ( 'NONE',  ( -1.500000000000013101, 3.879166666666685970, -0.8660254037844313801 ) ) ;
#192146=CARTESIAN_POINT ( 'NONE',  ( 5.148345644887269756, 7.029489223833707001, -1.599625672291256295 ) ) ;
#192147=CARTESIAN_POINT ( 'NONE',  ( 6.174848896020108668, 9.291408581077091000, 1.199719254218460707 ) ) ;
#192150=CARTESIAN_POINT ( 'NONE',  ( 8.283668668269706714, 8.766627655843892697, 1.040834085586084257E-14 ) ) ;
#192151=CARTESIAN_POINT ( 'NONE',  ( -8.636180661780660017, 11.09863007687603087, -1.443375672974058777 ) ) ;
#192155=CARTESIAN_POINT ( 'NONE',  ( 7.879259827836241570, 12.34422023245099176, 1.040834085586084257E-14 ) ) ;
#192158=CARTESIAN_POINT ( 'NONE',  ( -4.060830702492950195, 4.696389560118578999, -1.199719254218452047 ) ) ;
#192161=CARTESIAN_POINT ( 'NONE',  ( 0.6823417656249882723, 0.4260416670080896528, -1.181850606188749264 ) ) ;
#192166=CARTESIAN_POINT ( 'NONE',  ( 1.364683531249986537, -0.09479166632524321789, -0.7879004041258309554 ) ) ;
#192168=CARTESIAN_POINT ( 'NONE',  ( 9.480175724453529185, 12.08329098332774265, 1.599625672291279388 ) ) ;
#192172=CARTESIAN_POINT ( 'NONE',  ( -3.917943204224928699, 4.633650495426258509, -1.082531754730548412 ) ) ;
#192175=CARTESIAN_POINT ( 'NONE',  ( -5.551173829791513192, 8.563787670477010394, 1.199719254218452047 ) ) ;
#192178=CARTESIAN_POINT ( 'NONE',  ( 4.704842999142070603, 5.447737239542574272, -1.199719254218452047 ) ) ;
#192182=EDGE_LOOP ( 'NONE', ( #152141, #179880, #27839, #139424, #134041 ) ) ;
#192184=CARTESIAN_POINT ( 'NONE',  ( 9.447334110624092673, 9.916311305349925220, -0.7998128361456281477 ) ) ;
#192187=CARTESIAN_POINT ( 'NONE',  ( -6.552668314106420588, 6.539201209412602189, -0.7998128361456291469 ) ) ;
#192191=CARTESIAN_POINT ( 'NONE',  ( 7.588813295347141441, 9.876701482703580837, -1.599625672291262513 ) ) ;
#192193=CARTESIAN_POINT ( 'NONE',  ( 7.344766530301147789, 9.591980256816594164, 1.599625672291281386 ) ) ;
#192196=CARTESIAN_POINT ( 'NONE',  ( -8.663296969452339624, 13.05100419776235299, 1.040834085586084257E-14 ) ) ;
#192204=CARTESIAN_POINT ( 'NONE',  ( -6.063230027062802563, 6.042581475280591086, 0.5001817740485012820 ) ) ;
#192205=CARTESIAN_POINT ( 'NONE',  ( 0.6823417656249899377, 1.842708333674752952, 1.181850606188755259 ) ) ;
#192208=CARTESIAN_POINT ( 'NONE',  ( 7.483737605063422116, 7.833374748769873719, -0.7216878364870257245 ) ) ;
#192214=EDGE_CURVE ( 'NONE', #97926, #146015, #102285, .T. ) ;
#192225=CARTESIAN_POINT ( 'NONE',  ( 7.750457368506414646, 12.19395069656619945, 0.7998128361456462443 ) ) ;
#192229=CARTESIAN_POINT ( 'NONE',  ( -2.937312835655025101, 6.578615408239493867, 1.040834085586084257E-14 ) ) ;
#192230=CARTESIAN_POINT ( 'NONE',  ( -5.831978632172702071, 9.955725504176825780, 0.7998128361456481317 ) ) ;
#192235=EDGE_CURVE ( 'NONE', #34591, #96990, #13773, .T. ) ;
#192236=CARTESIAN_POINT ( 'NONE',  ( 0.7499999999999920064, 4.264583334016150751, 1.299038105676669330 ) ) ;
#192237=CARTESIAN_POINT ( 'NONE',  ( 6.591235234537977661, 10.84152487360300299, 0.7998128361456462443 ) ) ;
#192240=CARTESIAN_POINT ( 'NONE',  ( -7.853197290813634268, 10.18514947741448573, 1.599625672291295375 ) ) ;
#192242=CARTESIAN_POINT ( 'NONE',  ( 0.6823417656249899377, 4.176041667008085767, -1.181850606188754593 ) ) ;
#192247=CARTESIAN_POINT ( 'NONE',  ( -7.782016984564068096, 10.10210578678999482, 1.443375672974090751 ) ) ;
#192251=CARTESIAN_POINT ( 'NONE',  ( 1.364683531249986537, 2.717708333674754062, -0.7879004041258239610 ) ) ;
#192258=CARTESIAN_POINT ( 'NONE',  ( -0.6823417656250212460, 2.551041667008084435, 1.181850606188767472 ) ) ;
#192261=CARTESIAN_POINT ( 'NONE',  ( -4.141125853970233806, 6.918731698685530063, -1.199719254218452047 ) ) ;
#192262=CARTESIAN_POINT ( 'NONE',  ( 7.070740804726770357, 8.207951346058097286, 1.199719254218462483 ) ) ;
#192264=EDGE_CURVE ( 'NONE', #85555, #12149, #140424, .T. ) ;
#192266=CARTESIAN_POINT ( 'NONE',  ( 0.6823417656249899377, 3.988541667008085767, -1.181850606188754593 ) ) ;
#192269=CARTESIAN_POINT ( 'NONE',  ( 1.364683531249986537, -0.8864583329919110133, 0.7879004041258500513 ) ) ;
#192270=CARTESIAN_POINT ( 'NONE',  ( -3.456965981804629884, 6.976951378839947537, 1.040834085586084257E-14 ) ) ;
#192273=CARTESIAN_POINT ( 'NONE',  ( 2.887523530030648988, 6.312601851770308414, 0.000000000000000000 ) ) ;
#192276=CARTESIAN_POINT ( 'NONE',  ( -8.839552966430002101, 12.29626697993494666, -1.082531754730543971 ) ) ;
#192283=CARTESIAN_POINT ( 'NONE',  ( -6.412643469139482910, 7.544134137826577380, 1.082531754730549967 ) ) ;
#192285=CARTESIAN_POINT ( 'NONE',  ( -1.364683531250000748, 0.3218750003414205807, 0.000000000000000000 ) ) ;
#192291=CARTESIAN_POINT ( 'NONE',  ( -1.364683531250014514, -0.6989583329919100141, -0.7879004041258359514 ) ) ;
#192299=CARTESIAN_POINT ( 'NONE',  ( -1.402160292154681736E-14, -0.6624999999999758860, -1.732050807568870754 ) ) ;
#192300=CARTESIAN_POINT ( 'NONE',  ( 7.076992996209058973, 11.20031622897851165, 1.040834085586084257E-14 ) ) ;
#192308=CARTESIAN_POINT ( 'NONE',  ( 4.476163270806094552, 8.373940915915776273, 0.7998128361456462443 ) ) ;
#192311=CARTESIAN_POINT ( 'NONE',  ( -2.428882075142555497, 5.985446187641602300, 1.040834085586084257E-14 ) ) ;
#192314=CARTESIAN_POINT ( 'NONE',  ( -0.6823417656250003738, 1.780208333674752952, -1.181850606188749264 ) ) ;
#192330=ORIENTED_EDGE ( 'NONE', *, *, #129470, .F. ) ;
#192334=CARTESIAN_POINT ( 'NONE',  ( 6.765682348419287173, 7.852049813699357728, 1.199719254218462483 ) ) ;
#192337=ORIENTED_EDGE ( 'NONE', *, *, #38322, .T. ) ;
#192341=CARTESIAN_POINT ( 'NONE',  ( 8.284195553149872993, 9.623648552551724578, -1.199719254218445830 ) ) ;
#192344=CARTESIAN_POINT ( 'NONE',  ( 8.503988664269582998, 10.94440607977979063, 1.599625672291281386 ) ) ;
#192351=CARTESIAN_POINT ( 'NONE',  ( 6.115103934187892776, 6.015625209457229339, 1.345820777640227805E-10 ) ) ;
#192357=CARTESIAN_POINT ( 'NONE',  ( -7.836249599018719536, 12.08611559892311504, 0.7216878364870478180 ) ) ;
#192362=CARTESIAN_POINT ( 'NONE',  ( 4.985647801523278133, 6.839675073242382553, -1.599625672291256295 ) ) ;
#192371=CARTESIAN_POINT ( 'NONE',  ( 3.348500752450942031, 4.929670182657964084, 1.443375672974066548 ) ) ;
#192375=ORIENTED_EDGE ( 'NONE', *, *, #179088, .T. ) ;
#192380=CARTESIAN_POINT ( 'NONE',  ( -6.338600509588822263, 7.353787668397130162, -1.199719254218446718 ) ) ;
#192383=CARTESIAN_POINT ( 'NONE',  ( -4.322352044658376968, 3.937165561723182883, 0.7998128361456341429 ) ) ;
#192388=CARTESIAN_POINT ( 'NONE',  ( 0.1501718367240000573, 8.265200931437560072, -1.995665264648831316 ) ) ;
#192391=CARTESIAN_POINT ( 'NONE',  ( 6.647575389402066826, 6.649926130590872120, 1.040834085586084257E-14 ) ) ;
#192393=CARTESIAN_POINT ( 'NONE',  ( 1.567404983201064139, 8.684828555514158666, 2.500997594616644726 ) ) ;
#192402=EDGE_CURVE ( 'NONE', #3975, #11745, #112731, .T. ) ;
#192405=CARTESIAN_POINT ( 'NONE',  ( -1.364683531250000748, 1.071875000341421247, 0.000000000000000000 ) ) ;
#192407=CARTESIAN_POINT ( 'NONE',  ( 3.948449050077836642, 5.629609863222681199, 1.599625672291267398 ) ) ;
#192409=CARTESIAN_POINT ( 'NONE',  ( -5.572037945536512105, 9.444535336527177805, 0.000000000000000000 ) ) ;
#192411=CARTESIAN_POINT ( 'NONE',  ( 3.050221373394638835, 6.502416002361635528, 0.000000000000000000 ) ) ;
#192412=CARTESIAN_POINT ( 'NONE',  ( -6.521108698048779573, 8.631046119188804155, -1.443375672974058777 ) ) ;
#192416=CARTESIAN_POINT ( 'NONE',  ( 4.625302960556422427, 8.547937220624488575, 1.040834085586084257E-14 ) ) ;
#192422=CARTESIAN_POINT ( 'NONE',  ( 0.6823417656249917140, 4.592708333674755394, 1.181850606188765695 ) ) ;
#192426=CARTESIAN_POINT ( 'NONE',  ( 5.784525094524856748, 9.900363043587685041, 1.040834085586084257E-14 ) ) ;
#192428=CARTESIAN_POINT ( 'NONE',  ( -6.307567778855718288, 8.381915046796901692, -1.599625672291263179 ) ) ;
#192433=CARTESIAN_POINT ( 'NONE',  ( 9.074484886248265880, 9.481320543578137361, 0.7998128361456462443 ) ) ;
#192436=CARTESIAN_POINT ( 'NONE',  ( -6.028571859570855729, 10.18508426947466816, 0.000000000000000000 ) ) ;
#192438=CARTESIAN_POINT ( 'NONE',  ( 2.998324526916512411, 6.649795714711241423, 0.000000000000000000 ) ) ;
#192439=CARTESIAN_POINT ( 'NONE',  ( 8.093854517234030155, 8.545177812968924869, -0.7216878364870267237 ) ) ;
#192440=CARTESIAN_POINT ( 'NONE',  ( 4.221210552267129046, 7.311159377000789661, -0.8807526815687096722 ) ) ;
#192441=CARTESIAN_POINT ( 'NONE',  ( -8.188761592974033832, 12.49737959187099179, -0.7216878364870267237 ) ) ;
#192446=CARTESIAN_POINT ( 'NONE',  ( 4.904298879841284098, 6.744767997946721216, 1.599625672291267398 ) ) ;
#192448=CARTESIAN_POINT ( 'NONE',  ( 9.402743226277308963, 10.92862083786708816, -1.199719254218446718 ) ) ;
#192449=CARTESIAN_POINT ( 'NONE',  ( -5.108350220830032207, 6.531958715577594887, 1.215759808322430136 ) ) ;
#192450=CARTESIAN_POINT ( 'NONE',  ( 3.277320446201373638, 4.846626492033466072, 1.599625672291267398 ) ) ;
#192451=CARTESIAN_POINT ( 'NONE',  ( 1.364683531249986537, 0.9052083336747533959, -0.7879004041258239610 ) ) ;
#192453=AXIS2_PLACEMENT_3D ( 'NONE', #44511, #110628, #176629 ) ;
#192454=CARTESIAN_POINT ( 'NONE',  ( -6.060131475628484310, 10.01397778830115470, 0.000000000000000000 ) ) ;
#192459=CARTESIAN_POINT ( 'NONE',  ( -4.552667031389123764, 6.999162803142576550, 1.172958579310765970 ) ) ;
#192460=CARTESIAN_POINT ( 'NONE',  ( -1.364683531250014514, 0.3427083336747508424, 0.7879004041258379498 ) ) ;
#192464=CARTESIAN_POINT ( 'NONE',  ( 3.633221978782282147, 5.261844946711204507, -1.443375672974057666 ) ) ;
#192469=CARTESIAN_POINT ( 'NONE',  ( -6.683806541412756985, 10.74159869838281622, -0.7216878364870267237 ) ) ;
#192475=CARTESIAN_POINT ( 'NONE',  ( -9.937763408692600109, 10.69640485300394417, -0.7216878364870267237 ) ) ;
#192477=AXIS2_PLACEMENT_3D ( 'NONE', #11545, #147962, #212932 ) ;
#192482=CARTESIAN_POINT ( 'NONE',  ( -7.985389288324692636, 11.29974268881207067, -1.082531754730543083 ) ) ;
#192486=CARTESIAN_POINT ( 'NONE',  ( -1.201851678989727383E-14, 5.759375000341417028, -1.575800808251660801 ) ) ;
#192487=CARTESIAN_POINT ( 'NONE',  ( 1.499999999999987121, 3.827083334016153415, -0.8660254037844323793 ) ) ;
#192488=CARTESIAN_POINT ( 'NONE',  ( 4.860569815253008130, 6.917139861862701800, -1.418536646215622365 ) ) ;
#192494=CARTESIAN_POINT ( 'NONE',  ( -7.588813295347149435, 9.876701482703580837, -1.599625672291263179 ) ) ;
#192499=CARTESIAN_POINT ( 'NONE',  ( 5.660692828905515839, 6.562895374266609849, -1.199719254218445830 ) ) ;
#192504=CARTESIAN_POINT ( 'NONE',  ( 6.272618624616828953, 10.46980549536166016, 1.040834085586084257E-14 ) ) ;
#192507=CARTESIAN_POINT ( 'NONE',  ( 3.621833129746810265, 4.096114899008192367, 2.500000000000023093 ) ) ;
#192508=ORIENTED_EDGE ( 'NONE', *, *, #87121, .T. ) ;
#192511=CARTESIAN_POINT ( 'NONE',  ( -4.934804725694212912, 8.701096580044490381, -0.7216878364870207285 ) ) ;
#192514=FACE_OUTER_BOUND ( 'NONE', #97530, .T. ) ;
#192517=CARTESIAN_POINT ( 'NONE',  ( 4.030162213014739869, 7.767662802593035209, -0.3896624696924297360 ) ) ;
#192520=CARTESIAN_POINT ( 'NONE',  ( -10.34217224912604571, 10.96028913360221502, 0.7998128361456462443 ) ) ;
#192522=CARTESIAN_POINT ( 'NONE',  ( 9.921869487102386032, 10.46993591124128997, 0.000000000000000000 ) ) ;
#192523=CARTESIAN_POINT ( 'NONE',  ( -0.7500000000000249800, -0.8083333333333136972, 1.299038105676659116 ) ) ;
#192524=CARTESIAN_POINT ( 'NONE',  ( -8.015895134177625891, 10.37496362800581018, 1.599625672291295375 ) ) ;
#192527=CARTESIAN_POINT ( 'NONE',  ( -1.364683531250012516, 3.988541667008088876, -0.7879004041258300672 ) ) ;
#192528=CARTESIAN_POINT ( 'NONE',  ( 2.361091307074211887, 5.906356958228550447, 0.7998128361456462443 ) ) ;
#192531=CARTESIAN_POINT ( 'NONE',  ( -0.7499999999999972244, 5.108333333333353821, -1.299038105676652011 ) ) ;
#192534=CARTESIAN_POINT ( 'NONE',  ( 8.880227426826641235, 10.42298208846167284, 1.082531754730549967 ) ) ;
#192537=CARTESIAN_POINT ( 'NONE',  ( -6.900736999675794792, 7.153207375817628666, 1.040834085586084257E-14 ) ) ;
#192539=CARTESIAN_POINT ( 'NONE',  ( 1.364683531249986537, 1.905208333674750287, -0.7879004041258239610 ) ) ;
#192540=B_SPLINE_CURVE_WITH_KNOTS ( 'NONE', 3,
 ( #107735, #25337, #9094, #75170, #141280, #207288, #132488, #146597, #67409, #196388 ),
 .UNSPECIFIED., .F., .F.,
 ( 4, 3, 3, 4 ),
 ( 0.000000000000000000, 4.502046072369090049E-05, 9.004093402560593489E-05, 0.0001800865003196811486 ),
 .UNSPECIFIED. ) ;
#192544=CARTESIAN_POINT ( 'NONE',  ( -5.520141099058386125, 9.591915048876776595, 0.000000000000000000 ) ) ;
#192545=CARTESIAN_POINT ( 'NONE',  ( 1.364683531249990311, 4.446875000341417028, 1.214306433183764966E-14 ) ) ;
#192550=CARTESIAN_POINT ( 'NONE',  ( 7.411503528164766763, 11.79850454950093841, 1.040834085586084257E-14 ) ) ;
#192553=CARTESIAN_POINT ( 'NONE',  ( 1.499999999999989120, 0.7750000000000187850, 0.000000000000000000 ) ) ;
#192556=VERTEX_POINT ( 'NONE', #69639 ) ;
#192558=CARTESIAN_POINT ( 'NONE',  ( 7.899597058256738968, 12.36794700127490820, 1.040834085586084257E-14 ) ) ;
#192564=CARTESIAN_POINT ( 'NONE',  ( -9.480175724453545172, 12.08329098332774265, 1.599625672291281386 ) ) ;
#192568=CARTESIAN_POINT ( 'NONE',  ( -1.364683531250010295, 5.801041667008088432, -0.7879004041258300672 ) ) ;
#192572=CARTESIAN_POINT ( 'NONE',  ( 8.284195553149872993, 9.623648552551724578, -1.199719254218445830 ) ) ;
#192575=CARTESIAN_POINT ( 'NONE',  ( 0.6823417656249899377, 3.926041667008085767, -1.181850606188754593 ) ) ;
#192577=CARTESIAN_POINT ( 'NONE',  ( -5.422898255786186006, 9.270539031818461950, -0.7216878364870207285 ) ) ;
#192585=ORIENTED_EDGE ( 'NONE', *, *, #98066, .F. ) ;
#192586=CARTESIAN_POINT ( 'NONE',  ( 7.889955328148847258, 11.29236608522730911, -1.199719254218446718 ) ) ;
#192593=CARTESIAN_POINT ( 'NONE',  ( -7.635213062790267458, 12.05949900656400686, 0.000000000000000000 ) ) ;
#192594=CARTESIAN_POINT ( 'NONE',  ( 4.821896187954575197, 8.777295985922343391, 0.7998128361456462443 ) ) ;
#192596=CARTESIAN_POINT ( 'NONE',  ( 2.697709378994964879, 6.091152008895348580, 0.7216878364870338292 ) ) ;
#192599=CARTESIAN_POINT ( 'NONE',  ( 5.196852952739813070, 4.957416621151553571, -0.7998128361456221525 ) ) ;
#192605=CARTESIAN_POINT ( 'NONE',  ( 1.419999999999990603, 8.627523663848661428, 2.580000000000000515 ) ) ;
#192607=CARTESIAN_POINT ( 'NONE',  ( -5.531363484695544841, 8.436712584578003771, 1.082531754730548412 ) ) ;
#192608=CARTESIAN_POINT ( 'NONE',  ( 5.169736645512481132, 4.925780929386339935, 0.7998128361456341429 ) ) ;
#192611=CARTESIAN_POINT ( 'NONE',  ( -8.342344591110322227, 8.627156865917170236, -0.7998128361456291469 ) ) ;
#192618=CARTESIAN_POINT ( 'NONE',  ( -7.472515219426274946, 11.86968485597268064, 0.000000000000000000 ) ) ;
#192621=EDGE_CURVE ( 'NONE', #96990, #34591, #12451, .T. ) ;
#192623=CARTESIAN_POINT ( 'NONE',  ( 8.796542737168120851, 9.157054702984622097, -0.7998128361456211532 ) ) ;
#192634=CARTESIAN_POINT ( 'NONE',  ( -8.694856585065634746, 9.038420858865048757, 0.7998128361456462443 ) ) ;
#192638=CARTESIAN_POINT ( 'NONE',  ( 7.483737605063422116, 7.833374748769873719, -0.7216878364870257245 ) ) ;
#192639=EDGE_LOOP ( 'NONE', ( #191937, #80639 ) ) ;
#192640=DIRECTION ( 'NONE',  ( -0.6507913734559652719, 0.7592566023652995710, -0.000000000000000000 ) ) ;
#192643=CARTESIAN_POINT ( 'NONE',  ( -6.925517538482230506, 6.974191971184389160, 0.7998128361456341429 ) ) ;
#192653=CARTESIAN_POINT ( 'NONE',  ( -9.992522908471816123, 11.61669713376064372, 1.199719254218462483 ) ) ;
#192654=CARTESIAN_POINT ( 'NONE',  ( 8.535021395002688749, 9.916278701380017324, 1.199719254218462483 ) ) ;
#192657=CARTESIAN_POINT ( 'NONE',  ( -4.837732268475038566, 6.745175811576873848, -1.249133900884531467 ) ) ;
#192664=CARTESIAN_POINT ( 'NONE',  ( 9.571693261567954636, 12.19006144329456731, 1.443375672974076540 ) ) ;
#192684=CARTESIAN_POINT ( 'NONE',  ( -5.087333953625788219, 6.958308917361963886, 1.599625672291267398 ) ) ;
#192685=CARTESIAN_POINT ( 'NONE',  ( 5.843201017365476702, 6.879784610756938257, -1.082531754730543083 ) ) ;
#192686=CARTESIAN_POINT ( 'NONE',  ( -0.7499999999999972244, 3.358333333333359150, -1.299038105676652011 ) ) ;
#192688=CARTESIAN_POINT ( 'NONE',  ( -4.460796234096120472, 5.163016013655583158, 1.199719254218462483 ) ) ;
#192692=CARTESIAN_POINT ( 'NONE',  ( -1.364683531250012516, 4.488541667008090208, -0.7879004041258300672 ) ) ;
#192700=CARTESIAN_POINT ( 'NONE',  ( 3.867100128395839942, 5.534702787927018974, -1.599625672291255185 ) ) ;
#192702=CARTESIAN_POINT ( 'NONE',  ( 0.2524733864175063847, 6.376792883867242523, -3.135723845156253020 ) ) ;
#192705=CARTESIAN_POINT ( 'NONE',  ( 1.364683531249988535, 1.926041667008086211, 0.7879004041258500513 ) ) ;
#192708=CARTESIAN_POINT ( 'NONE',  ( -9.378489572351046633, 11.96465713920816043, -1.599625672291263179 ) ) ;
#192709=CARTESIAN_POINT ( 'NONE',  ( -6.033015167956818026, 6.140865238812146742, -0.7216878364870267237 ) ) ;
#192714=CARTESIAN_POINT ( 'NONE',  ( 0.6823417656249899377, 3.926041667008085767, -1.181850606188754593 ) ) ;
#192723=CARTESIAN_POINT ( 'NONE',  ( -5.490689023410187275, 8.389259046411751797, 1.082531754730548412 ) ) ;
#192728=CARTESIAN_POINT ( 'NONE',  ( -5.382223794500835545, 8.262716279350872384, -1.082531754730543971 ) ) ;
#192733=DIRECTION ( 'NONE',  ( 0.000000000000000000, 8.546850786086437571E-32, 1.000000000000000000 ) ) ;
#192739=CARTESIAN_POINT ( 'NONE',  ( 4.030162213014739869, 7.767662802593035209, -0.3896624696924297360 ) ) ;
#192741=CARTESIAN_POINT ( 'NONE',  ( -3.578462479003122976, 6.262291094557191684, 1.199719254218464037 ) ) ;
#192744=CARTESIAN_POINT ( 'NONE',  ( 0.7499999999999902300, 1.483333333333357373, 1.299038105676657340 ) ) ;
#192746=CARTESIAN_POINT ( 'NONE',  ( 9.164948653157988900, 11.71552606681625619, -1.443375672974057666 ) ) ;
#192747=CARTESIAN_POINT ( 'NONE',  ( 5.798083248138522272, 9.916180889470295412, 0.7998128361456462443 ) ) ;
#192752=CARTESIAN_POINT ( 'NONE',  ( 5.515469562660962666, 5.329135999392899947, 0.7998128361456341429 ) ) ;
#192754=CARTESIAN_POINT ( 'NONE',  ( -0.5015801190230781970, 7.801378974689814783, -1.936921611551790212 ) ) ;
#192755=EDGE_LOOP ( 'NONE', ( #191760, #169200, #58901, #76046, #3022 ) ) ;
#192761=CARTESIAN_POINT ( 'NONE',  ( -7.223796917982883592, 7.322184580601816428, -0.7998128361456291469 ) ) ;
#192767=CARTESIAN_POINT ( 'NONE',  ( 1.364683531249988535, 3.613541667008086211, 0.7879004041258500513 ) ) ;
#192768=CARTESIAN_POINT ( 'NONE',  ( 7.890482213029013536, 12.14938698193514277, 1.040834085586084257E-14 ) ) ;
#192769=CARTESIAN_POINT ( 'NONE',  ( -6.093499974338126179, 9.196501505781426999, -1.199719254218440723 ) ) ;
#192772=CARTESIAN_POINT ( 'NONE',  ( 6.681470773436232413, 6.689470745297396270, -0.7998128361456281477 ) ) ;
#192773=CARTESIAN_POINT ( 'NONE',  ( -5.738125327081750271, 7.717565519727259904, 1.599625672291269396 ) ) ;
#192778=CARTESIAN_POINT ( 'NONE',  ( -1.500000000000015099, 0.1604166673494879791, -0.8660254037844383745 ) ) ;
#192781=CARTESIAN_POINT ( 'NONE',  ( 6.914295153289432783, 10.05013286460426691, -1.082531754730537976 ) ) ;
#192784=CARTESIAN_POINT ( 'NONE',  ( -1.402160292154681736E-14, 2.509375000341417028, -1.575800808251660134 ) ) ;
#192786=CARTESIAN_POINT ( 'NONE',  ( 6.304178240230120522, 6.457222156464352381, -0.7216878364870257245 ) ) ;
#192789=CARTESIAN_POINT ( 'NONE',  ( -5.097502569058225852, 5.049433873430440478, -0.7216878364870207285 ) ) ;
#192796=CARTESIAN_POINT ( 'NONE',  ( -4.014602626671047503, 7.795841479962435372, -0.4363419845254731255 ) ) ;
#192804=CARTESIAN_POINT ( 'NONE',  ( 6.765682348419287173, 7.852049813699357728, 1.199719254218462483 ) ) ;
#192807=CARTESIAN_POINT ( 'NONE',  ( 3.871016551901614200, 4.474939717762034697, -1.199719254218446718 ) ) ;
#192814=EDGE_LOOP ( 'NONE', ( #3957, #93935, #139327, #29388 ) ) ;
#192816=CARTESIAN_POINT ( 'NONE',  ( 4.528060117284232966, 6.305822774963486310, 1.443375672974062551 ) ) ;
#192817=CARTESIAN_POINT ( 'NONE',  ( -0.6823417656250003738, 1.780208333674752952, -1.181850606188749264 ) ) ;
#192818=CARTESIAN_POINT ( 'NONE',  ( 6.968000882419564945, 10.21675256520979858, 1.199719254218460707 ) ) ;
#192824=VERTEX_POINT ( 'NONE', #89139 ) ;
#192826=CARTESIAN_POINT ( 'NONE',  ( 0.7499999999999902300, 3.733333333333352488, 1.299038105676669330 ) ) ;
#192827=CARTESIAN_POINT ( 'NONE',  ( 6.257251587906815793, 7.258880593101466161, 1.199719254218462483 ) ) ;
#192828=CARTESIAN_POINT ( 'NONE',  ( -7.365103760721662951, 9.615707025640515937, 1.599625672291295375 ) ) ;
#192832=CARTESIAN_POINT ( 'NONE',  ( -0.6823417656250003738, 2.467708333674753618, -1.181850606188749264 ) ) ;
#192834=CARTESIAN_POINT ( 'NONE',  ( 9.490344339885973923, 12.09515436799890331, -1.443375672974057666 ) ) ;
#192840=CARTESIAN_POINT ( 'NONE',  ( -1.402160292154681736E-14, 0.6187500006828180465, -1.732050807568863648 ) ) ;
#192842=CARTESIAN_POINT ( 'NONE',  ( -7.203459687562382641, 7.298457811777897319, -0.7998128361456291469 ) ) ;
#192843=CARTESIAN_POINT ( 'NONE',  ( -2.982430605326328532, 5.462957558647244305, -1.082531754730543971 ) ) ;
#192851=CARTESIAN_POINT ( 'NONE',  ( 6.810273232766058449, 6.839740281182199233, 1.040834085586084257E-14 ) ) ;
#192855=CARTESIAN_POINT ( 'NONE',  ( 5.982172092127724383, 8.002286745614243912, -1.599625672291262513 ) ) ;
#192856=ORIENTED_EDGE ( 'NONE', *, *, #179088, .F. ) ;
#192860=CARTESIAN_POINT ( 'NONE',  ( -6.826694039680798021, 7.923230120171105284, -1.199719254218446718 ) ) ;
#192861=AXIS2_PLACEMENT_3D ( 'NONE', #164938, #79426, #62117 ) ;
#192863=CARTESIAN_POINT ( 'NONE',  ( 2.191614386903386613, 5.708633884695917260, -0.7998128361456281477 ) ) ;
#192869=CARTESIAN_POINT ( 'NONE',  ( 4.871297188390688149, 6.684807392805372395, 1.249964738027457889 ) ) ;
#192875=VECTOR ( 'NONE', #84522, 1000.000000000000000 ) ;
#192878=CARTESIAN_POINT ( 'NONE',  ( -3.687454593236990430, 4.364747115940301292, 1.082531754730560403 ) ) ;
#192879=CARTESIAN_POINT ( 'NONE',  ( 7.131225611108085616, 10.30321839872603462, 1.082531754730558626 ) ) ;
#192881=CARTESIAN_POINT ( 'NONE',  ( -4.874319919312905647, 5.645460313075203018, -1.199719254218446718 ) ) ;
#192882=CARTESIAN_POINT ( 'NONE',  ( -0.2313892381897282580, 6.510114678062200788, 3.133603478753892446 ) ) ;
#192884=CARTESIAN_POINT ( 'NONE',  ( 6.988338112840064120, 10.24047933403371502, 1.199719254218460707 ) ) ;
#192886=CARTESIAN_POINT ( 'NONE',  ( -6.392833124043511894, 7.417059051927569868, 1.199719254218450271 ) ) ;
#192900=CARTESIAN_POINT ( 'NONE',  ( 9.694243528971124846, 11.26870452434320491, 1.199719254218450271 ) ) ;
#192901=CARTESIAN_POINT ( 'NONE',  ( -4.741601036477307574, 6.554953847355395880, 1.599625672291267398 ) ) ;
#192904=CARTESIAN_POINT ( 'NONE',  ( 2.873965376416980355, 6.296784005887697155, -0.7216878364870267237 ) ) ;
#192909=CARTESIAN_POINT ( 'NONE',  ( -0.4867935908897400021, 7.427453578138980994, 4.536604770853145396 ) ) ;
#192910=CARTESIAN_POINT ( 'NONE',  ( -4.223528545856940042, 4.886203710709899006, -1.199719254218446718 ) ) ;
#192914=CARTESIAN_POINT ( 'NONE',  ( 9.053093885623066939, 11.58502883802551153, -1.599625672291262513 ) ) ;
#192919=CARTESIAN_POINT ( 'NONE',  ( -6.256197817702116026, 9.386315656372753224, -1.199719254218440723 ) ) ;
#192920=CARTESIAN_POINT ( 'NONE',  ( 5.392392409933256303, 7.314210449720692786, 1.599625672291267398 ) ) ;
#192922=CARTESIAN_POINT ( 'NONE',  ( 5.009901455449552010, 5.803638771901306725, -1.199719254218452047 ) ) ;
#192925=CARTESIAN_POINT ( 'NONE',  ( 1.364683531249986537, 0.9677083336747538400, -0.7879004041258239610 ) ) ;
#192928=CARTESIAN_POINT ( 'NONE',  ( 6.968527767744093993, 10.11340424813470662, 1.082531754730558626 ) ) ;
#192937=CARTESIAN_POINT ( 'NONE',  ( 8.215877899756996783, 12.52901528311778989, 1.040834085586084257E-14 ) ) ;
#192945=CARTESIAN_POINT ( 'NONE',  ( -10.49131193887636826, 11.13428543831092909, 1.040834085586084257E-14 ) ) ;
#192961=CARTESIAN_POINT ( 'NONE',  ( 0.7499999999999902300, 2.014583334016148530, 1.299038105676669330 ) ) ;
#192967=CARTESIAN_POINT ( 'NONE',  ( 0.7499999999999885647, -0.7666666666666446250, 1.299038105676657340 ) ) ;
#192968=CARTESIAN_POINT ( 'NONE',  ( 7.401861798056875053, 10.72292363345333399, -1.199719254218441611 ) ) ;
#192973=CARTESIAN_POINT ( 'NONE',  ( 3.684065054611349144, 5.321161868511784299, -1.599625672291262513 ) ) ;
#192974=CARTESIAN_POINT ( 'NONE',  ( -5.910991785878165317, 8.879612269291090598, -1.082531754730538864 ) ) ;
#192978=CARTESIAN_POINT ( 'NONE',  ( -6.561256274009600986, 9.742217188731485678, -1.199719254218440723 ) ) ;
#192979=ORIENTED_EDGE ( 'NONE', *, *, #127934, .T. ) ;
#192980=CARTESIAN_POINT ( 'NONE',  ( 1.499999999999989120, 1.056250000682816603, 0.000000000000000000 ) ) ;
#192993=CARTESIAN_POINT ( 'NONE',  ( -7.994504133552415404, 12.47867192245318435, -0.7998128361456281477 ) ) ;
#192994=( BOUNDED_CURVE ( )  B_SPLINE_CURVE ( 2, ( #132868, #52647, #33200 ),
 .UNSPECIFIED., .F., .T. ) 
 B_SPLINE_CURVE_WITH_KNOTS ( ( 3, 3 ),
 ( 0.1472187422488249464, 0.1500000000000002165 ),
 .UNSPECIFIED. ) 
 CURVE ( )  GEOMETRIC_REPRESENTATION_ITEM ( )  RATIONAL_B_SPLINE_CURVE ( ( 0.9405305184077485947, 0.9105717077955789440, 1.000000000000007105 ) ) 
 REPRESENTATION_ITEM ( '' )  );
#192995=CARTESIAN_POINT ( 'NONE',  ( 6.109920781252839994, 10.27999134477033216, 1.040834085586084257E-14 ) ) ;
#192996=DIRECTION ( 'NONE',  ( 1.000000000000000000, 0.000000000000000000, 0.000000000000000000 ) ) ;
#193002=CARTESIAN_POINT ( 'NONE',  ( -7.588813295347149435, 9.876701482703580837, -1.599625672291263179 ) ) ;
#193009=CARTESIAN_POINT ( 'NONE',  ( 4.542145155778077203, 5.257923088951247159, -1.199719254218452047 ) ) ;
#193013=ORIENTED_EDGE ( 'NONE', *, *, #140820, .F. ) ;
#193014=CARTESIAN_POINT ( 'NONE',  ( 0.000000000000000000, 6.487495393664096888, -3.100011470320000573 ) ) ;
#193019=CARTESIAN_POINT ( 'NONE',  ( -4.747088307715054967, 7.009658186011790804, -1.421664413759090806 ) ) ;
#193033=ORIENTED_EDGE ( 'NONE', *, *, #179509, .T. ) ;
#193037=CARTESIAN_POINT ( 'NONE',  ( -1.500000000000015099, -0.08958333265051321437, -0.8660254037844383745 ) ) ;
#193049=CARTESIAN_POINT ( 'NONE',  ( 3.660338286009610975, 6.253849852777763729, -1.082531754730543083 ) ) ;
#193053=CARTESIAN_POINT ( 'NONE',  ( -10.45741655484220267, 11.09474082360439873, -0.7998128361456221525 ) ) ;
#193055=CARTESIAN_POINT ( 'NONE',  ( 8.062294901620731480, 12.55776115186623620, 1.040834085586084257E-14 ) ) ;
#193066=CARTESIAN_POINT ( 'NONE',  ( -1.364683531250010295, 5.801041667008088432, -0.7879004041258300672 ) ) ;
#193072=CARTESIAN_POINT ( 'NONE',  ( -6.227272627378437342, 6.159572908229946187, -0.7998128361456291469 ) ) ;
#193075=CARTESIAN_POINT ( 'NONE',  ( -0.7500000000000006661, -0.6416666666666446250, -1.299038105676652011 ) ) ;
#193077=CARTESIAN_POINT ( 'NONE',  ( -0.6823417656250003738, -0.7197916663252492686, -1.181850606188749264 ) ) ;
#193085=CARTESIAN_POINT ( 'NONE',  ( -1.364683531250000748, -0.7406249996585803075, 0.000000000000000000 ) ) ;
#193088=CARTESIAN_POINT ( 'NONE',  ( -8.178592977541617515, 10.56477777859713463, 1.599625672291295375 ) ) ;
#193090=CARTESIAN_POINT ( 'NONE',  ( 8.041957671200231417, 12.53403438304231976, 1.040834085586084257E-14 ) ) ;
#193094=ORIENTED_EDGE ( 'NONE', *, *, #53693, .T. ) ;
#193096=CARTESIAN_POINT ( 'NONE',  ( -0.6823417656250003738, -0.4697916663252491021, -1.181850606188749264 ) ) ;
#193104=CARTESIAN_POINT ( 'NONE',  ( 6.887178846062110615, 9.058127958537705027, -1.443375672974057666 ) ) ;
#193108=CARTESIAN_POINT ( 'NONE',  ( -6.091691091241777656, 6.001394449403842479, 0.7998128361456341429 ) ) ;
#193110=CARTESIAN_POINT ( 'NONE',  ( 0.7499999999999920064, 4.514583334016150751, 1.299038105676669330 ) ) ;
#193112=CARTESIAN_POINT ( 'NONE',  ( -3.602716132929368875, 5.226254793216122074, 1.599625672291267398 ) ) ;
#193113=CARTESIAN_POINT ( 'NONE',  ( 7.415946836550727284, 7.754285518838408109, 0.7216878364870317197 ) ) ;
#193114=CARTESIAN_POINT ( 'NONE',  ( -9.612367721964613310, 11.27714576612263997, -1.082531754730537976 ) ) ;
#193121=CARTESIAN_POINT ( 'NONE',  ( 8.432808358020004391, 12.78210081775797669, 0.7216878364870438212 ) ) ;
#193136=ORIENTED_EDGE ( 'NONE', *, *, #74793, .T. ) ;
#193138=CARTESIAN_POINT ( 'NONE',  ( 9.053093885623066939, 11.58502883802551153, -1.599625672291262513 ) ) ;
#193140=CARTESIAN_POINT ( 'NONE',  ( -1.436838838544753916, 7.449283400311742298, 4.203727439823590650 ) ) ;
#193142=CARTESIAN_POINT ( 'NONE',  ( -0.6823417656250246877, -0.1989583329919109023, 1.181850606188755259 ) ) ;
#193143=CARTESIAN_POINT ( 'NONE',  ( 4.677199807034550183, 8.400557508274889784, 1.040834085586084257E-14 ) ) ;
#193144=ORIENTED_EDGE ( 'NONE', *, *, #197058, .F. ) ;
#193145=CARTESIAN_POINT ( 'NONE',  ( -9.503902493499651882, 10.19023378527882784, 1.040834085586084257E-14 ) ) ;
#193165=CARTESIAN_POINT ( 'NONE',  ( 4.521492410791133842, 7.227233577430748568, -1.288726771885986055 ) ) ;
#193170=CARTESIAN_POINT ( 'NONE',  ( -1.420000000000021911, 6.280000000000042881, 2.873333333333347728 ) ) ;
#193173=CARTESIAN_POINT ( 'NONE',  ( -6.887178846062109727, 10.01849717283904262, -1.082531754730537976 ) ) ;
#193178=CARTESIAN_POINT ( 'NONE',  ( 5.601490020740366838, 9.686822124172440596, 1.040834085586084257E-14 ) ) ;
#193180=FACE_OUTER_BOUND ( 'NONE', #158335, .T. ) ;
#193182=CARTESIAN_POINT ( 'NONE',  ( -3.425406365747000859, 7.148057860013469877, 1.040834085586084257E-14 ) ) ;
#193186=CARTESIAN_POINT ( 'NONE',  ( -4.822949958159302497, 6.649860922651058992, -1.599625672291256295 ) ) ;
#193190=CARTESIAN_POINT ( 'NONE',  ( 4.867540842506059562, 5.637551390133895168, -1.199719254218452047 ) ) ;
#193191=CARTESIAN_POINT ( 'NONE',  ( 7.995557903757111617, 10.35123685918189729, 1.599625672291281386 ) ) ;
#193192=CARTESIAN_POINT ( 'NONE',  ( 0.1417672014102085154, 6.428417890535995660, 3.204557187381015915 ) ) ;
#193194=CARTESIAN_POINT ( 'NONE',  ( 4.279786810092509164, 7.480689796721937235, 1.046525044888670486 ) ) ;
#193195=CARTESIAN_POINT ( 'NONE',  ( 4.690757960648224589, 6.495636925554817864, 1.443375672974062551 ) ) ;
#193203=CARTESIAN_POINT ( 'NONE',  ( 5.775410249297131315, 9.681803024247919609, 1.040834085586084257E-14 ) ) ;
#193204=CARTESIAN_POINT ( 'NONE',  ( -9.321394304595349567, 10.83371376257142416, 1.199719254218462483 ) ) ;
#193207=CARTESIAN_POINT ( 'NONE',  ( -9.459838494033043332, 12.05956421450382088, 1.599625672291281386 ) ) ;
#193208=CARTESIAN_POINT ( 'NONE',  ( -5.038826645773246682, 9.030381520044109322, 0.7998128361456481317 ) ) ;
#193210=ADVANCED_FACE ( 'NONE', ( #178956 ), #140936, .T. ) ;
#193217=CARTESIAN_POINT ( 'NONE',  ( 9.752392566931574081, 10.27221283770866300, -0.7998128361456281477 ) ) ;
#193222=CARTESIAN_POINT ( 'NONE',  ( 4.207107738942202246, 3.802713871720993399, 1.214306433183764966E-14 ) ) ;
#193231=CARTESIAN_POINT ( 'NONE',  ( -1.500000000000013101, 2.629166666666687746, -0.8660254037844313801 ) ) ;
#193232=CARTESIAN_POINT ( 'NONE',  ( 5.341022448779654930, 8.318611059296550536, 1.199719254218462483 ) ) ;
#193235=CARTESIAN_POINT ( 'NONE',  ( 7.456621297836078632, 8.762108271306003004, 1.082531754730558626 ) ) ;
#193237=EDGE_CURVE ( 'NONE', #48080, #200114, #189488, .T. ) ;
#193240=CARTESIAN_POINT ( 'NONE',  ( 7.391166297744269365, 11.77477778067701664, 1.040834085586084257E-14 ) ) ;
#193243=CARTESIAN_POINT ( 'NONE',  ( -5.088387723830502196, 4.830873854090670605, -0.7998128361456221525 ) ) ;
#193244=CARTESIAN_POINT ( 'NONE',  ( 1.499999999999989120, 5.035416667349487341, 0.8660254037844524744 ) ) ;
#193245=CARTESIAN_POINT ( 'NONE',  ( 1.364683531249988757, 0.6343750003414208027, 0.000000000000000000 ) ) ;
#193250=CARTESIAN_POINT ( 'NONE',  ( -1.364683531250014514, -0.2197916663252438285, 0.7879004041258379498 ) ) ;
#193252=CARTESIAN_POINT ( 'NONE',  ( 8.211434591371064684, 12.73175745657494851, -0.7998128361456352531 ) ) ;
#193255=CARTESIAN_POINT ( 'NONE',  ( -4.134873662043608178, 4.886736029548026217, 1.082531754730558626 ) ) ;
#193258=CARTESIAN_POINT ( 'NONE',  ( -5.364222332501225488, 9.410009821226765325, 0.7998128361456481317 ) ) ;
#193261=CARTESIAN_POINT ( 'NONE',  ( 2.706824224222692088, 6.309712028235118453, 0.7998128361456362523 ) ) ;
#193266=VERTEX_POINT ( 'NONE', #3352 ) ;
#193268=CARTESIAN_POINT ( 'NONE',  ( 7.899597058256738968, 12.36794700127490820, 1.040834085586084257E-14 ) ) ;
#193272=CARTESIAN_POINT ( 'NONE',  ( -6.566226467720086113, 6.555019055295208119, 1.040834085586084257E-14 ) ) ;
#193276=CARTESIAN_POINT ( 'NONE',  ( 7.889955328148847258, 11.29236608522730911, -1.199719254218446718 ) ) ;
#193278=CARTESIAN_POINT ( 'NONE',  ( 6.642605195691581699, 9.837124264027149678, 1.199719254218462483 ) ) ;
#193281=CARTESIAN_POINT ( 'NONE',  ( -8.161645285746702783, 12.46574390010577105, 0.7216878364870478180 ) ) ;
#193284=CARTESIAN_POINT ( 'NONE',  ( -6.561256274009600986, 9.742217188731485678, -1.199719254218440723 ) ) ;
#193288=CARTESIAN_POINT ( 'NONE',  ( -6.110283559904478246, 6.013173453705326743, 0.3066926896367061506 ) ) ;
#193289=CARTESIAN_POINT ( 'NONE',  ( 1.364683531249988757, 1.134375000341421247, 0.000000000000000000 ) ) ;
#193293=CARTESIAN_POINT ( 'NONE',  ( 8.120970824905713314, 8.576813505252564696, 1.040834085586084257E-14 ) ) ;
#193309=CARTESIAN_POINT ( 'NONE',  ( 9.447334110624092673, 9.916311305349925220, -0.7998128361456281477 ) ) ;
#193313=CARTESIAN_POINT ( 'NONE',  ( -5.108724954250998707, 4.854600622914589714, -0.7998128361456221525 ) ) ;
#193314=CARTESIAN_POINT ( 'NONE',  ( -6.659026002606323047, 10.92061410301605662, 0.000000000000000000 ) ) ;
#193319=CARTESIAN_POINT ( 'NONE',  ( 1.499999999999989120, 4.535416667349484676, 0.8660254037844524744 ) ) ;
#193320=CARTESIAN_POINT ( 'NONE',  ( 7.914208982075123799, 10.25632978388623684, -1.599625672291262513 ) ) ;
#193323=CARTESIAN_POINT ( 'NONE',  ( -6.855619230004478482, 11.14997286831390788, -0.7998128361456291469 ) ) ;
#193325=CARTESIAN_POINT ( 'NONE',  ( -1.201851678989727383E-14, 2.696875000341417916, -1.575800808251660134 ) ) ;
#193329=CARTESIAN_POINT ( 'NONE',  ( -5.572037945092171540, 5.603058478803390585, 0.7216878364870346063 ) ) ;
#193331=CARTESIAN_POINT ( 'NONE',  ( -8.351459436338030784, 11.72682452816096976, -1.082531754730543971 ) ) ;
#193335=CARTESIAN_POINT ( 'NONE',  ( 0.6823417656249882723, 2.988541667008084879, -1.181850606188754593 ) ) ;
#193336=EDGE_CURVE ( 'NONE', #121606, #112218, #117194, .T. ) ;
#193343=CARTESIAN_POINT ( 'NONE',  ( 1.364683531249990311, 2.634375000341422801, 1.214306433183764966E-14 ) ) ;
#193345=VECTOR ( 'NONE', #6970, 1000.000000000000227 ) ;
#193346=CARTESIAN_POINT ( 'NONE',  ( -4.303823697334223652, 7.108545849276850959, -1.199719254218452047 ) ) ;
#193347=CARTESIAN_POINT ( 'NONE',  ( 5.503720292143644777, 8.508425209887878538, 1.199719254218462483 ) ) ;
#193350=CARTESIAN_POINT ( 'NONE',  ( -1.364683531250012516, 4.551041667008082214, -0.7879004041258300672 ) ) ;
#193353=CARTESIAN_POINT ( 'NONE',  ( -1.402160292154681736E-14, -0.9281249996585830830, 1.575800808251672791 ) ) ;
#193354=CARTESIAN_POINT ( 'NONE',  ( -4.039966587192274083, 5.736380323189513852, 1.443375672974064550 ) ) ;
#193358=CARTESIAN_POINT ( 'NONE',  ( 3.687454593236936251, 7.245854758844324728, -0.7216878364870267237 ) ) ;
#193361=CARTESIAN_POINT ( 'NONE',  ( -7.121056995675673740, 9.330985799753529264, -1.599625672291263179 ) ) ;
#193362=CARTESIAN_POINT ( 'NONE',  ( -8.188761592974033832, 12.49737959187099179, -0.7216878364870267237 ) ) ;
#193369=CARTESIAN_POINT ( 'NONE',  ( -6.141480396866151992, 9.148515648777049591, 1.082531754730548412 ) ) ;
#193371=CARTESIAN_POINT ( 'NONE',  ( -0.6823417656250003738, -0.7197916663252492686, -1.181850606188749264 ) ) ;
#193384=CARTESIAN_POINT ( 'NONE',  ( -1.402160292154681736E-14, -1.037499999999977662, 1.732050807568877637 ) ) ;
#193385=CARTESIAN_POINT ( 'NONE',  ( 7.063434842595398777, 11.18449838309590483, -0.7216878364870267237 ) ) ;
#193394=CARTESIAN_POINT ( 'NONE',  ( 4.527533231959700366, 7.369540306339926516, 1.199719254218462483 ) ) ;
#193396=CARTESIAN_POINT ( 'NONE',  ( -3.795392936821753604, 6.515376628678959392, -1.199719254218452047 ) ) ;
#193399=CARTESIAN_POINT ( 'NONE',  ( -4.848826244296223109, 5.027555131033083491, -0.8732430475888955934 ) ) ;
#193401=CARTESIAN_POINT ( 'NONE',  ( 1.364683531249988535, 2.176041667008087543, 0.7879004041258500513 ) ) ;
#193403=CARTESIAN_POINT ( 'NONE',  ( -7.971304249830880373, 11.38727316052296601, 1.199719254218453823 ) ) ;
#193419=CARTESIAN_POINT ( 'NONE',  ( -4.403059289062232651, 7.148295125103961034, -1.075145975261635911 ) ) ;
#193422=CARTESIAN_POINT ( 'NONE',  ( 4.794779880727245036, 8.745660294157122649, -0.7998128361456281477 ) ) ;
#193427=CARTESIAN_POINT ( 'NONE',  ( 3.092648394857516525, 6.449253795920727228, -0.4031905389056261724 ) ) ;
#193429=CARTESIAN_POINT ( 'NONE',  ( 8.259941899223605333, 10.65968485389279508, -1.599625672291268286 ) ) ;
#193431=( BOUNDED_CURVE ( )  B_SPLINE_CURVE ( 2, ( #181024, #116080, #129178, #164778, #104, #148537, #117154 ),
 .UNSPECIFIED., .F., .T. ) 
 B_SPLINE_CURVE_WITH_KNOTS ( ( 3, 2, 2, 3 ),
 ( 0.08928571428571412116, 0.09523809523809514954, 0.1011904761904762057, 0.1071428571428572341 ),
 .UNSPECIFIED. ) 
 CURVE ( )  GEOMETRIC_REPRESENTATION_ITEM ( )  RATIONAL_B_SPLINE_CURVE ( ( 1.000000000000003775, 0.8660254037844349329, 1.000000000000000000, 0.8660254037844387076, 1.000000000000000000, 0.8660254037844364872, 1.000000000000002220 ) ) 
 REPRESENTATION_ITEM ( '' )  );
#193433=CARTESIAN_POINT ( 'NONE',  ( 9.073431116043567002, 11.60875560684942265, -1.599625672291262513 ) ) ;
#193435=CARTESIAN_POINT ( 'NONE',  ( -4.464712657601869417, 4.103252943490596216, 0.7998128361456341429 ) ) ;
#193439=CARTESIAN_POINT ( 'NONE',  ( 9.049177462117294013, 12.64479190819049670, -1.199719254218446718 ) ) ;
#193440=CARTESIAN_POINT ( 'NONE',  ( 4.132297641190314508, 7.622816840561035256, -0.7610026044957002300 ) ) ;
#193441=CARTESIAN_POINT ( 'NONE',  ( -0.2734184563536292134, 7.240553437303447026, 1.983365796752670773 ) ) ;
#193447=CARTESIAN_POINT ( 'NONE',  ( -7.537970219518066450, 11.73812298950569044, -0.7216878364870267237 ) ) ;
#193452=CARTESIAN_POINT ( 'NONE',  ( -9.622536337397040285, 12.24937836509514710, 1.599625672291281386 ) ) ;
#193453=CARTESIAN_POINT ( 'NONE',  ( 5.148345644887269756, 7.029489223833707001, -1.599625672291256295 ) ) ;
#193454=CARTESIAN_POINT ( 'NONE',  ( -1.001543065824772872E-14, 5.321875000341422357, 1.575800808251672791 ) ) ;
#193459=CARTESIAN_POINT ( 'NONE',  ( 3.890826896997583884, 4.602014803661035103, -1.082531754730543083 ) ) ;
#193467=CARTESIAN_POINT ( 'NONE',  ( -5.343885102080728977, 9.386283052402845328, 0.7998128361456481317 ) ) ;
#193469=CARTESIAN_POINT ( 'NONE',  ( -2.950870989268691957, 6.594433254122103349, -0.7998128361456281477 ) ) ;
#193473=B_SPLINE_CURVE_WITH_KNOTS ( 'NONE', 3,
 ( #121799, #53511, #86014, #201865, #120728, #7946, #105492, #171524, #6867, #5790 ),
 .UNSPECIFIED., .F., .F.,
 ( 4, 3, 3, 4 ),
 ( 1.311158639597268106E-16, 6.251569610500030906E-05, 0.0001250312426172235419, 0.0002200345428698334245 ),
 .UNSPECIFIED. ) ;
#193477=CARTESIAN_POINT ( 'NONE',  ( 4.611744806942754238, 8.532119374741881757, -0.7998128361456231517 ) ) ;
#193479=CARTESIAN_POINT ( 'NONE',  ( 3.646780131951566251, 7.198401220678091406, -0.7216878364870155105 ) ) ;
#193490=VERTEX_POINT ( 'NONE', #153907 ) ;
#193492=CARTESIAN_POINT ( 'NONE',  ( -0.6823417656250246877, 0.1135416670080893753, 1.181850606188755259 ) ) ;
#193493=CARTESIAN_POINT ( 'NONE',  ( 3.358669367883368118, 4.941533567329135401, -1.599625672291262513 ) ) ;
#193494=CARTESIAN_POINT ( 'NONE',  ( 4.566398809704347528, 4.221886787610169556, -0.7998128361456211532 ) ) ;
#193496=CARTESIAN_POINT ( 'NONE',  ( -5.910991785878165317, 8.879612269291090598, -1.082531754730538864 ) ) ;
#193497=CARTESIAN_POINT ( 'NONE',  ( 5.341549334104200852, 5.334155099317434257, 0.7216878364870317197 ) ) ;
#193498=CARTESIAN_POINT ( 'NONE',  ( -6.344852701071109102, 10.34615255131755163, 0.000000000000000000 ) ) ;
#193503=CARTESIAN_POINT ( 'NONE',  ( 6.148786358997489820, 7.132337826040578754, -1.199719254218446718 ) ) ;
#193508=CARTESIAN_POINT ( 'NONE',  ( 1.364683531249990311, 5.363541667008086655, 0.7879004041258500513 ) ) ;
#193512=CARTESIAN_POINT ( 'NONE',  ( 5.635385404774530649, 9.726366738878972740, 0.7998128361456462443 ) ) ;
#193515=CARTESIAN_POINT ( 'NONE',  ( -7.232384877886063990, 10.52520055992070525, -1.199719254218446718 ) ) ;
#193520=CARTESIAN_POINT ( 'NONE',  ( 7.751511138711133064, 10.06651563329490529, -1.599625672291262513 ) ) ;
#193523=CARTESIAN_POINT ( 'NONE',  ( -7.527801604085656351, 9.805521176231838609, 1.599625672291295375 ) ) ;
#193524=CARTESIAN_POINT ( 'NONE',  ( 2.989990986282343055, 6.640073250638046432, -0.4916062289654400397 ) ) ;
#193525=CARTESIAN_POINT ( 'NONE',  ( 7.199016378732056687, 10.38230762762066384, -1.082531754730537976 ) ) ;
#193526=CARTESIAN_POINT ( 'NONE',  ( 4.014041799177766379, 7.808471211821870206, -0.2759448393452879067 ) ) ;
#193527=CARTESIAN_POINT ( 'NONE',  ( -9.653042183249972652, 10.36423008998754192, -0.7216878364870267237 ) ) ;
#193532=CARTESIAN_POINT ( 'NONE',  ( 5.178324605415663306, 8.128796908705222535, 1.199719254218462483 ) ) ;
#193534=CARTESIAN_POINT ( 'NONE',  ( 8.041957671200231417, 12.53403438304231976, 1.040834085586084257E-14 ) ) ;
#193535=CARTESIAN_POINT ( 'NONE',  ( -5.296940370067747317, 6.395615756200102808, 1.134431874056667233 ) ) ;
#193536=CARTESIAN_POINT ( 'NONE',  ( 4.546061579283848353, 4.198160018786257552, -0.7998128361456211532 ) ) ;
#193538=CARTESIAN_POINT ( 'NONE',  ( -8.026063749610063525, 8.466088584074293877, -0.7216878364870278340 ) ) ;
#193544=CARTESIAN_POINT ( 'NONE',  ( -5.203466197636060997, 6.462176032175228180, 1.180525766716962410 ) ) ;
#193545=CARTESIAN_POINT ( 'NONE',  ( 1.364683531249986537, -0.3239583329919163424, 0.7879004041258500513 ) ) ;
#193548=CARTESIAN_POINT ( 'NONE',  ( 3.172244755917638770, 5.684407401003788607, -1.082531754730543083 ) ) ;
#193553=CARTESIAN_POINT ( 'NONE',  ( -7.958272981097355370, 12.22847621134819285, 0.7216878364870458196 ) ) ;
#193558=CARTESIAN_POINT ( 'NONE',  ( -7.958272981097355370, 12.22847621134819285, 0.7216878364870458196 ) ) ;
#193564=CARTESIAN_POINT ( 'NONE',  ( -8.636180661780668899, 10.13826086257468795, -1.082531754730543083 ) ) ;
#193569=CARTESIAN_POINT ( 'NONE',  ( 1.499999999999989120, 4.327083334016148086, -0.8660254037844323793 ) ) ;
#193570=CARTESIAN_POINT ( 'NONE',  ( 5.506841003474272966, 6.417672382999444203, -1.246111810019270738 ) ) ;
#193575=CARTESIAN_POINT ( 'NONE',  ( -7.100719765255177229, 9.307259030929609267, -1.599625672291263179 ) ) ;
#193576=LINE ( 'NONE', #28951, #151944 ) ;
#193579=CARTESIAN_POINT ( 'NONE',  ( 5.311043488251262268, 7.219303374425030562, -1.599625672291256295 ) ) ;
#193583=CARTESIAN_POINT ( 'NONE',  ( 8.132193210098487057, 8.381980254736715708, 1.040834085586084257E-14 ) ) ;
#193587=ORIENTED_EDGE ( 'NONE', *, *, #121379, .T. ) ;
#193590=CARTESIAN_POINT ( 'NONE',  ( -6.480434237652138663, 8.583592582059388576, 1.443375672974078761 ) ) ;
#193593=CARTESIAN_POINT ( 'NONE',  ( -4.650083499807267984, 5.295740330745369207, 1.164732466530402855 ) ) ;
#193594=VECTOR ( 'NONE', #197160, 1000.000000000000000 ) ;
#193595=EDGE_CURVE ( 'NONE', #100909, #33385, #182617, .T. ) ;
#193600=CARTESIAN_POINT ( 'NONE',  ( -8.317037166979361018, 11.79062823052953668, 1.199719254218453823 ) ) ;
#193602=CARTESIAN_POINT ( 'NONE',  ( 9.433775957010412938, 9.900493459467314850, 0.000000000000000000 ) ) ;
#193603=CARTESIAN_POINT ( 'NONE',  ( -1.402160292154681736E-14, -0.9124999999999769962, -1.732050807568870754 ) ) ;
#193604=CARTESIAN_POINT ( 'NONE',  ( -8.422639742587602285, 10.84949900448412841, -1.599625672291263179 ) ) ;
#193607=CARTESIAN_POINT ( 'NONE',  ( 1.364683531249988535, 2.905208333674754506, -0.7879004041258239610 ) ) ;
#193608=CARTESIAN_POINT ( 'NONE',  ( 9.951321562750607086, 11.67259191370631477, -1.082531754730537088 ) ) ;
#193611=CARTESIAN_POINT ( 'NONE',  ( 0.7499999999999920064, 4.733333333333352932, 1.299038105676669330 ) ) ;
#193614=CARTESIAN_POINT ( 'NONE',  ( 7.578644679914702031, 10.82520731233375955, 1.082531754730558626 ) ) ;
#193617=CARTESIAN_POINT ( 'NONE',  ( -6.399085315970142851, 8.488685506763726352, -1.443375672974059665 ) ) ;
#193618=CARTESIAN_POINT ( 'NONE',  ( -0.6823417656250212460, 2.051041667008083991, 1.181850606188767472 ) ) ;
#193622=CARTESIAN_POINT ( 'NONE',  ( -7.369020184227459858, 8.555943955475521889, 1.199719254218450271 ) ) ;
#193623=CARTESIAN_POINT ( 'NONE',  ( -0.6823417656249969321, 5.030208333674755394, -1.181850606188749264 ) ) ;
#193628=CARTESIAN_POINT ( 'NONE',  ( 9.043452155515161905, 10.50944792197790889, 1.199719254218453823 ) ) ;
#193633=ORIENTED_EDGE ( 'NONE', *, *, #120712, .F. ) ;
#193634=CARTESIAN_POINT ( 'NONE',  ( 10.01963921569910632, 11.64833282552586091, 1.199719254218450271 ) ) ;
#193639=CARTESIAN_POINT ( 'NONE',  ( 9.077347539549325717, 10.54899253668443393, -1.199719254218446718 ) ) ;
#193640=CARTESIAN_POINT ( 'NONE',  ( -1.500000000000022204, 8.627523663848661428, 2.580000000000011173 ) ) ;
#193643=DIRECTION ( 'NONE',  ( -1.000000000000000000, 7.109522442527888164E-16, 0.000000000000000000 ) ) ;
#193644=CARTESIAN_POINT ( 'NONE',  ( -0.6823417656250212460, 5.113541667008086655, 1.181850606188767472 ) ) ;
#193648=CARTESIAN_POINT ( 'NONE',  ( 7.690499447449630210, 9.995335326823163058, 1.599625672291281386 ) ) ;
#193651=CARTESIAN_POINT ( 'NONE',  ( 1.364683531249988535, 3.363541667008084879, 0.7879004041258500513 ) ) ;
#193653=CARTESIAN_POINT ( 'NONE',  ( -6.616015773788831211, 7.781401826584148473, 1.082531754730549967 ) ) ;
#193662=CARTESIAN_POINT ( 'NONE',  ( 7.242026607993941489, 11.60078147596829901, 0.7998128361456462443 ) ) ;
#193663=CARTESIAN_POINT ( 'NONE',  ( 1.387358672532239989, 7.315968950352816691, -4.254625267139963363 ) ) ;
#193665=VECTOR ( 'NONE', #53470, 1000.000000000000114 ) ;
#193669=CARTESIAN_POINT ( 'NONE',  ( -9.833741488613570780, 10.36711991300432345, 0.7998128361456462443 ) ) ;
#193670=CARTESIAN_POINT ( 'NONE',  ( 6.012151052656117933, 9.101594430485762999, 1.199719254218460707 ) ) ;
#193672=CARTESIAN_POINT ( 'NONE',  ( 3.023105065722948126, 6.470780310077995701, 0.7216878364870338292 ) ) ;
#193674=CARTESIAN_POINT ( 'NONE',  ( 4.009460741339333723, 5.700790169694431420, -1.599625672291256295 ) ) ;
#193682=CARTESIAN_POINT ( 'NONE',  ( -6.290620087060847965, 7.401773525401500464, 1.082531754730549967 ) ) ;
#193683=CARTESIAN_POINT ( 'NONE',  ( 4.304877467538922531, 4.981110786005563007, 1.199719254218464037 ) ) ;
#193686=CARTESIAN_POINT ( 'NONE',  ( -6.672584156219988571, 10.93643194889866521, -0.7998128361456291469 ) ) ;
#193692=CARTESIAN_POINT ( 'NONE',  ( -9.215791728987058562, 11.77484298861683598, -1.599625672291263179 ) ) ;
#193696=CARTESIAN_POINT ( 'NONE',  ( 7.934546212495622086, 10.28005655271014795, -1.599625672291262513 ) ) ;
#193697=CARTESIAN_POINT ( 'NONE',  ( 4.638861114170084399, 8.563755066507100722, 0.7998128361456462443 ) ) ;
#193698=CARTESIAN_POINT ( 'NONE',  ( 2.218730694130720771, 5.740269576461138890, 0.7998128361456462443 ) ) ;
#193709=CARTESIAN_POINT ( 'NONE',  ( -6.808165692356648258, 11.09461040772476714, 0.7998128361456481317 ) ) ;
#193714=CARTESIAN_POINT ( 'NONE',  ( 6.643132081016124069, 7.813037518349371879, 1.082531754730558626 ) ) ;
#193719=CARTESIAN_POINT ( 'NONE',  ( -7.250913225210214641, 7.353820272367037170, 0.7998128361456341429 ) ) ;
#193730=CARTESIAN_POINT ( 'NONE',  ( 8.762647353133951711, 9.117510088278095282, 1.040834085586084257E-14 ) ) ;
#193732=CARTESIAN_POINT ( 'NONE',  ( -2.982430605326321427, 6.423326772948587227, -0.7216878364870267237 ) ) ;
#193734=CARTESIAN_POINT ( 'NONE',  ( -4.447391987980185313, 7.103198448885253313, -1.107391122544647333 ) ) ;
#193741=CARTESIAN_POINT ( 'NONE',  ( 3.602716132929354664, 5.226254793216122074, 1.599625672291267398 ) ) ;
#193746=CARTESIAN_POINT ( 'NONE',  ( 3.897079088924235712, 6.634010472798538949, 1.199719254218462483 ) ) ;
#193751=CARTESIAN_POINT ( 'NONE',  ( -1.364683531249997417, 3.571875000341423245, 1.214306433183764966E-14 ) ) ;
#193756=CARTESIAN_POINT ( 'NONE',  ( 6.159481859310094620, 6.080483678816896109, 1.040834085586084257E-14 ) ) ;
#193760=CARTESIAN_POINT ( 'NONE',  ( -3.761497552787613330, 6.475832013972435242, 1.199719254218464037 ) ) ;
#193762=CARTESIAN_POINT ( 'NONE',  ( 4.595850884908202261, 7.345281218159464665, -1.082531754730549078 ) ) ;
#193763=CARTESIAN_POINT ( 'NONE',  ( 1.499999999999989120, 3.025000000000020783, 1.214306433183764966E-14 ) ) ;
#193765=CARTESIAN_POINT ( 'NONE',  ( -5.122283107864663343, 4.870418468797203637, 0.000000000000000000 ) ) ;
#193767=DIRECTION ( 'NONE',  ( -0.6507913734559559460, 0.7592566023653074536, 0.000000000000000000 ) ) ;
#193769=CARTESIAN_POINT ( 'NONE',  ( -1.364683531250010295, 4.030208333674751842, 0.7879004041258379498 ) ) ;
#193772=CARTESIAN_POINT ( 'NONE',  ( -3.619663825168619731, 7.166765529431275539, 1.040834085586084257E-14 ) ) ;
#193777=CARTESIAN_POINT ( 'NONE',  ( 4.976006071415387311, 5.764094157194782575, 1.199719254218462483 ) ) ;
#193783=CARTESIAN_POINT ( 'NONE',  ( 0.6823417656249899377, 1.155208333674752286, 1.181850606188755259 ) ) ;
#193785=CARTESIAN_POINT ( 'NONE',  ( -10.47097470845587175, 11.11055866948701443, 1.040834085586084257E-14 ) ) ;
#193786=CARTESIAN_POINT ( 'NONE',  ( -4.216222583725562245, 7.862750747747711877, 0.7216878364870317197 ) ) ;
#193790=CARTESIAN_POINT ( 'NONE',  ( -1.364683531250012516, 4.738541667008091096, -0.7879004041258300672 ) ) ;
#193798=CARTESIAN_POINT ( 'NONE',  ( -4.880572110795192486, 8.637825195995631589, 1.214306433183764966E-14 ) ) ;
#193803=CARTESIAN_POINT ( 'NONE',  ( -5.951666246274811556, 7.966696592119163256, 1.443375672974064550 ) ) ;
#193811=CARTESIAN_POINT ( 'NONE',  ( 1.608462485350599769, 8.735270501766756013, -2.463594439587629914 ) ) ;
#193812=VERTEX_POINT ( 'NONE', #201552 ) ;
#193816=CARTESIAN_POINT ( 'NONE',  ( -3.567766978690493307, 7.314145241780881435, 1.040834085586084257E-14 ) ) ;
#193819=CARTESIAN_POINT ( 'NONE',  ( -1.500000000000013101, 0.4208333333333572068, 0.8660254037844403729 ) ) ;
#193821=CARTESIAN_POINT ( 'NONE',  ( 9.408995418203975447, 10.07950886410055524, 0.7216878364870438212 ) ) ;
#193822=CARTESIAN_POINT ( 'NONE',  ( 7.955937213120826357, 8.176348258262782664, 0.7998128361456481317 ) ) ;
#193827=CARTESIAN_POINT ( 'NONE',  ( 3.330499290451326200, 7.037332938835193730, -0.7998128361456291469 ) ) ;
#193828=CARTESIAN_POINT ( 'NONE',  ( -0.2837385194698915925, 8.150966340525300780, -2.020310785919212648 ) ) ;
#193834=EDGE_CURVE ( 'NONE', #71497, #132514, #88606, .T. ) ;
#193836=CARTESIAN_POINT ( 'NONE',  ( 8.072990401933337168, 11.50590700464255356, -1.199719254218446718 ) ) ;
#193837=CARTESIAN_POINT ( 'NONE',  ( -5.656776405399756236, 7.622658444431597680, -1.599625672291256295 ) ) ;
#193839=ORIENTED_EDGE ( 'NONE', *, *, #192621, .F. ) ;
#193843=CARTESIAN_POINT ( 'NONE',  ( 1.364683531249990311, 3.134375000341423245, 1.214306433183764966E-14 ) ) ;
#193844=CARTESIAN_POINT ( 'NONE',  ( 8.175203438916005538, 11.52119253116861586, -1.082531754730543083 ) ) ;
#193845=CARTESIAN_POINT ( 'NONE',  ( -5.930802130974132780, 9.006687355190106103, -1.199719254218440723 ) ) ;
#193848=CARTESIAN_POINT ( 'NONE',  ( 5.198661835836162481, 8.152523677529138979, 1.199719254218462483 ) ) ;
#193849=CARTESIAN_POINT ( 'NONE',  ( -5.900823170445743671, 7.907379670318584353, 1.599625672291269396 ) ) ;
#193853=CARTESIAN_POINT ( 'NONE',  ( -1.402160292154681736E-14, -0.1312499993171854229, -1.732050807568870754 ) ) ;
#193857=CARTESIAN_POINT ( 'NONE',  ( 7.537970219518073556, 9.817384560903001045, -1.443375672974057666 ) ) ;
#193860=CARTESIAN_POINT ( 'NONE',  ( -1.364683531250012516, 2.092708333674750953, 0.7879004041258379498 ) ) ;
#193862=CARTESIAN_POINT ( 'NONE',  ( 5.843201017365476702, 6.879784610756938257, -1.082531754730543083 ) ) ;
#193865=CARTESIAN_POINT ( 'NONE',  ( -3.145128448690317935, 5.652771709238564313, -1.082531754730549967 ) ) ;
#193873=CARTESIAN_POINT ( 'NONE',  ( -4.550628574872730425, 7.191434026324334816, -1.338276217581878980 ) ) ;
#193876=AXIS2_PLACEMENT_3D ( 'NONE', #32013, #49333, #27740 ) ;
#193881=CARTESIAN_POINT ( 'NONE',  ( 7.494959990256193194, 7.638541498254023843, -0.7998128361456281477 ) ) ;
#193884=CARTESIAN_POINT ( 'NONE',  ( 2.672928840188529609, 6.270167413528593414, 0.000000000000000000 ) ) ;
#193893=CARTESIAN_POINT ( 'NONE',  ( 4.446711195602238931, 6.210915699667823198, -1.443375672974051449 ) ) ;
#193894=CIRCLE ( 'NONE', #166218, 1.250000000000000222 ) ;
#193895=CARTESIAN_POINT ( 'NONE',  ( 1.364683531249988757, 1.946875000341415030, 0.000000000000000000 ) ) ;
#193896=CARTESIAN_POINT ( 'NONE',  ( 9.426996880203592610, 9.892584536526015881, -0.7998128361456281477 ) ) ;
#193900=DIRECTION ( 'NONE',  ( 0.000000000000000000, 8.546850786086437571E-32, 1.000000000000000000 ) ) ;
#193902=CARTESIAN_POINT ( 'NONE',  ( -1.500000000000013101, 2.379166666666686414, -0.8660254037844313801 ) ) ;
#193903=CARTESIAN_POINT ( 'NONE',  ( 5.015626762051672571, 7.938982758113895422, 1.199719254218462483 ) ) ;
#193904=CARTESIAN_POINT ( 'NONE',  ( -6.353967546298838087, 10.56471257065732416, 0.000000000000000000 ) ) ;
#193909=CARTESIAN_POINT ( 'NONE',  ( 1.364683531249988535, 3.155208333674756283, -0.7879004041258239610 ) ) ;
#193912=CARTESIAN_POINT ( 'NONE',  ( 10.41229878561526512, 11.25002945941372623, -0.7216878364870257245 ) ) ;
#193917=CARTESIAN_POINT ( 'NONE',  ( -1.201851678989727383E-14, 0.9937500006828198229, 1.732050807568877637 ) ) ;
#193919=CARTESIAN_POINT ( 'NONE',  ( -6.124532705071231931, 8.168374127381657246, -1.599625672291263179 ) ) ;
#193920=CARTESIAN_POINT ( 'NONE',  ( -4.297571505851936813, 4.116180966356429494, 1.214306433183764966E-14 ) ) ;
#193928=CARTESIAN_POINT ( 'NONE',  ( 6.647575389402066826, 6.649926130590872120, 1.040834085586084257E-14 ) ) ;
#193932=CARTESIAN_POINT ( 'NONE',  ( 6.979750152936881058, 7.037463354714830643, 0.7998128361456341429 ) ) ;
#193937=CARTESIAN_POINT ( 'NONE',  ( -6.905180308061733996, 6.950465202360470052, 0.7998128361456341429 ) ) ;
#193939=CARTESIAN_POINT ( 'NONE',  ( 4.241003122976366058, 3.842258486427521103, -0.7998128361456211532 ) ) ;
#193944=CYLINDRICAL_SURFACE ( 'NONE', #429, 1.250000000000000000 ) ;
#193945=CARTESIAN_POINT ( 'NONE',  ( 4.388421827844267042, 7.126904390760538277, 1.074283327121795528 ) ) ;
#193952=CARTESIAN_POINT ( 'NONE',  ( -2.657034918598338180, 6.043698471765932112, -0.7216878364870267237 ) ) ;
#193953=CARTESIAN_POINT ( 'NONE',  ( 7.998947442382716488, 9.394822106610419610, -1.082531754730543083 ) ) ;
#193956=CARTESIAN_POINT ( 'NONE',  ( -4.066556009095094737, 6.831733546331167695, 1.199719254218464037 ) ) ;
#193961=CARTESIAN_POINT ( 'NONE',  ( -6.856673000209188906, 9.022537805042615489, 1.599625672291283607 ) ) ;
#193973=PLANE ( 'NONE',  #101063 ) ;
#193974=CARTESIAN_POINT ( 'NONE',  ( 1.426745631513068657, 7.396214564680185788, -4.272608017058045604 ) ) ;
#193975=CARTESIAN_POINT ( 'NONE',  ( -4.055860508782465068, 7.883587693554856557, 1.040834085586084257E-14 ) ) ;
#193978=CARTESIAN_POINT ( 'NONE',  ( 2.562127843302666186, 5.932973550587659517, 0.000000000000000000 ) ) ;
#193982=CARTESIAN_POINT ( 'NONE',  ( -2.137381772448751605, 5.645362501165475777, -0.7998128361456281477 ) ) ;
#193983=CARTESIAN_POINT ( 'NONE',  ( -3.093231602212184850, 6.760520635889515795, -0.7998128361456281477 ) ) ;
#193986=CARTESIAN_POINT ( 'NONE',  ( 9.901532256681887745, 10.44620914241737530, 0.000000000000000000 ) ) ;
#193989=CARTESIAN_POINT ( 'NONE',  ( -7.389357414647957256, 8.579670724299436557, 1.199719254218450271 ) ) ;
#193990=CARTESIAN_POINT ( 'NONE',  ( 4.798696304233017074, 7.685897223992134819, -1.199719254218452047 ) ) ;
#193993=CARTESIAN_POINT ( 'NONE',  ( 3.985207087413062066, 6.736826471035503694, -1.199719254218452047 ) ) ;
#193995=SPHERICAL_SURFACE ( 'NONE', #68546, 0.08000000000000000167 ) ;
#193996=CARTESIAN_POINT ( 'NONE',  ( 0.6823417656249899377, 1.155208333674752286, 1.181850606188755259 ) ) ;
#193999=CARTESIAN_POINT ( 'NONE',  ( 8.297226821883377568, 8.782445501726501291, -0.7216878364870267237 ) ) ;
#194007=CARTESIAN_POINT ( 'NONE',  ( 9.151390499099949949, 12.66007743471656788, -1.082531754730543971 ) ) ;
#194015=CARTESIAN_POINT ( 'NONE',  ( -9.938290294017125603, 11.55342575023019691, -1.199719254218441611 ) ) ;
#194031=CARTESIAN_POINT ( 'NONE',  ( 0.7499999999999902300, 1.514583334016148086, 1.299038105676657340 ) ) ;
#194035=EDGE_LOOP ( 'NONE', ( #88880, #129331, #115041, #173883 ) ) ;
#194037=CARTESIAN_POINT ( 'NONE',  ( 1.499999999999987121, -0.4958333333333110882, 0.8660254037844524744 ) ) ;
#194038=CARTESIAN_POINT ( 'NONE',  ( 9.088043039861931405, 9.497138389460751284, 1.040834085586084257E-14 ) ) ;
#194042=CARTESIAN_POINT ( 'NONE',  ( 4.546061579283848353, 4.198160018786257552, -0.7998128361456211532 ) ) ;
#194043=CARTESIAN_POINT ( 'NONE',  ( -6.290620087060847965, 7.401773525401500464, 1.082531754730549967 ) ) ;
#194048=CARTESIAN_POINT ( 'NONE',  ( -6.880926654135487652, 7.986501503701545879, 1.199719254218450271 ) ) ;
#194050=CARTESIAN_POINT ( 'NONE',  ( 0.7499999999999885647, 0.7645833340161543035, 1.299038105676657340 ) ) ;
#194057=CARTESIAN_POINT ( 'NONE',  ( -4.758548728272219641, 4.653987725846768342, 0.7216878364870317197 ) ) ;
#194060=CARTESIAN_POINT ( 'NONE',  ( 4.352817808933668431, 7.164511876539561896, 1.041257065902738477 ) ) ;
#194065=CARTESIAN_POINT ( 'NONE',  ( -3.429849674132948500, 5.024577257953626308, -1.443375672974051449 ) ) ;
#194066=CARTESIAN_POINT ( 'NONE',  ( 6.771407655021410399, 9.987393799911945536, -1.199719254218441611 ) ) ;
#194073=CARTESIAN_POINT ( 'NONE',  ( -8.857554428429624593, 9.228235009456373206, 0.7998128361456462443 ) ) ;
#194080=CARTESIAN_POINT ( 'NONE',  ( 3.520313441042647540, 7.258782781191745137, 0.7998128361456321445 ) ) ;
#194088=CARTESIAN_POINT ( 'NONE',  ( 0.04469154961657068048, 6.488258805693589260, -3.101144068366980200 ) ) ;
#194091=CARTESIAN_POINT ( 'NONE',  ( -5.657660137730037953, 6.307591819868396676, -1.155748867827746995 ) ) ;
#194100=CARTESIAN_POINT ( 'NONE',  ( 5.459129407796876166, 9.520734742405036144, 1.040834085586084257E-14 ) ) ;
#194108=CARTESIAN_POINT ( 'NONE',  ( -1.402160292154681736E-14, 0.2437500006828163535, 1.732050807568877637 ) ) ;
#194112=CARTESIAN_POINT ( 'NONE',  ( 2.866659414285625651, 5.431854185720147221, -1.199719254218446718 ) ) ;
#194114=CARTESIAN_POINT ( 'NONE',  ( -9.429859533504656000, 10.96025652963230534, -1.199719254218441611 ) ) ;
#194122=CARTESIAN_POINT ( 'NONE',  ( 4.039966587192250103, 7.657118751792200584, 0.7216878364870298324 ) ) ;
#194125=FACE_OUTER_BOUND ( 'NONE', #91726, .T. ) ;
#194127=CARTESIAN_POINT ( 'NONE',  ( 3.348500752450942031, 4.929670182657964084, 1.443375672974066548 ) ) ;
#194137=CARTESIAN_POINT ( 'NONE',  ( -1.364683531250000748, -0.4906249996585801409, 0.000000000000000000 ) ) ;
#194142=CARTESIAN_POINT ( 'NONE',  ( -6.552668314106420588, 6.539201209412602189, -0.7998128361456291469 ) ) ;
#194145=CARTESIAN_POINT ( 'NONE',  ( -1.402160292154681736E-14, -0.7874999999999764411, 1.732050807568877637 ) ) ;
#194147=CARTESIAN_POINT ( 'NONE',  ( 0.6823417656249882723, -0.5947916663252492686, 1.181850606188755259 ) ) ;
#194154=CARTESIAN_POINT ( 'NONE',  ( 1.364683531249988757, -0.8656249996585805295, 0.000000000000000000 ) ) ;
#194156=CARTESIAN_POINT ( 'NONE',  ( 6.419949431270806528, 7.448694743692793274, 1.199719254218462483 ) ) ;
#194157=CARTESIAN_POINT ( 'NONE',  ( -8.528242318195895066, 9.908369778438709474, 1.199719254218462483 ) ) ;
#194165=CARTESIAN_POINT ( 'NONE',  ( 1.364683531249988757, -0.8031249996585804185, 0.000000000000000000 ) ) ;
#194172=ADVANCED_FACE ( 'NONE', ( #40155 ), #6754, .T. ) ;
#194174=CARTESIAN_POINT ( 'NONE',  ( 7.971831135155394321, 8.402817200543854170, -0.7216878364870267237 ) ) ;
#194178=CARTESIAN_POINT ( 'NONE',  ( -0.7499999999999972244, 4.139583334016149863, -1.299038105676652899 ) ) ;
#194180=CARTESIAN_POINT ( 'NONE',  ( -2.903417451620861289, 6.539070793532962611, 0.7998128361456341429 ) ) ;
#194181=CARTESIAN_POINT ( 'NONE',  ( 6.195713011320782115, 8.251417818006149929, -1.443375672974057666 ) ) ;
#194182=CARTESIAN_POINT ( 'NONE',  ( -8.880227426826648340, 11.38335130276301754, 1.443375672974064550 ) ) ;
#194188=CARTESIAN_POINT ( 'NONE',  ( 3.979481780810941949, 4.601482484822914998, 1.199719254218464037 ) ) ;
#194191=CARTESIAN_POINT ( 'NONE',  ( 3.408985558832261731, 6.064568021024562938, 1.199719254218462483 ) ) ;
#194206=CARTESIAN_POINT ( 'NONE',  ( 7.703003830858588863, 12.13858823597705872, -0.7998128361456291469 ) ) ;
#194211=CARTESIAN_POINT ( 'NONE',  ( -1.364683531250014514, -0.7197916663252461600, 0.7879004041258379498 ) ) ;
#194212=CARTESIAN_POINT ( 'NONE',  ( 4.175548123328908900, 7.815297210618305179, -0.7216878364870197293 ) ) ;
#194214=CARTESIAN_POINT ( 'NONE',  ( -9.842856333841300653, 10.58567993234409421, 0.7216878364870438212 ) ) ;
#194219=CARTESIAN_POINT ( 'NONE',  ( -2.415323921528888196, 5.969628341758991930, 0.7998128361456341429 ) ) ;
#194234=CARTESIAN_POINT ( 'NONE',  ( 5.440174215215161979, 6.465126095745926449, -1.288585324421805511 ) ) ;
#194235=FACE_OUTER_BOUND ( 'NONE', #198573, .T. ) ;
#194241=CARTESIAN_POINT ( 'NONE',  ( -7.782016984564068096, 10.10210578678999482, 1.443375672974090751 ) ) ;
#194246=CARTESIAN_POINT ( 'NONE',  ( 5.113396490648394632, 9.117379672398465473, 1.040834085586084257E-14 ) ) ;
#194248=CARTESIAN_POINT ( 'NONE',  ( 4.715538499454675403, 4.395883092318884522, 1.214306433183764966E-14 ) ) ;
#194250=CARTESIAN_POINT ( 'NONE',  ( -5.759516327706961647, 5.613857225279885732, -0.7998128361456221525 ) ) ;
#194254=CARTESIAN_POINT ( 'NONE',  ( -4.660252114795309097, 6.460046772059735432, -1.599625672291256295 ) ) ;
#194257=CARTESIAN_POINT ( 'NONE',  ( 3.683011284406639607, 7.448596931783069586, 0.7998128361456321445 ) ) ;
#194258=CARTESIAN_POINT ( 'NONE',  ( 8.209625708274705502, 9.536650400197368427, 1.199719254218462483 ) ) ;
#194261=CARTESIAN_POINT ( 'NONE',  ( 4.748509658595381211, 7.014904321862622361, 1.395353610025750646 ) ) ;
#194262=CARTESIAN_POINT ( 'NONE',  ( 4.012850279964918165, 7.625483060026979842, -0.7216878364870197293 ) ) ;
#194269=CARTESIAN_POINT ( 'NONE',  ( 8.229436053370683624, 8.703356271795033905, 0.7216878364870458196 ) ) ;
#194270=CARTESIAN_POINT ( 'NONE',  ( -9.481229494658258261, 9.955855920056455588, -0.7998128361456291469 ) ) ;
#194274=CARTESIAN_POINT ( 'NONE',  ( -9.833741488613570780, 10.36711991300432345, 0.7998128361456462443 ) ) ;
#194275=CARTESIAN_POINT ( 'NONE',  ( -8.538937818508475885, 8.856515631215026829, 1.040834085586084257E-14 ) ) ;
#194284=CARTESIAN_POINT ( 'NONE',  ( 8.106885785967500979, 11.54545161934907682, 1.199719254218460707 ) ) ;
#194288=CARTESIAN_POINT ( 'NONE',  ( 3.063252641683779753, 5.661212951017999373, 1.199719254218450271 ) ) ;
#194291=CARTESIAN_POINT ( 'NONE',  ( -3.511198596259319960, 6.271927390929313617, 1.082471891955974153 ) ) ;
#194297=CARTESIAN_POINT ( 'NONE',  ( 0.7499999999999902300, 3.733333333333352488, 1.299038105676669330 ) ) ;
#194298=CARTESIAN_POINT ( 'NONE',  ( 4.462605117192430804, 8.358123070033169455, 1.040834085586084257E-14 ) ) ;
#194302=CARTESIAN_POINT ( 'NONE',  ( 5.965224400332808763, 9.903252867122883885, -0.7216878364870267237 ) ) ;
#194304=CARTESIAN_POINT ( 'NONE',  ( -10.29027540264791440, 11.10766884595181203, 0.7216878364870438212 ) ) ;
#194308=CARTESIAN_POINT ( 'NONE',  ( 9.348510611822643313, 10.86534945433664134, 1.199719254218453823 ) ) ;
#194310=CARTESIAN_POINT ( 'NONE',  ( 3.625126395730617901, 6.174274991382457500, 1.251677269935605130 ) ) ;
#194311=CARTESIAN_POINT ( 'NONE',  ( -5.251085567194491155, 5.020688004682002159, -0.7998128361456221525 ) ) ;
#194312=CARTESIAN_POINT ( 'NONE',  ( 1.499999999999989120, 4.827083334016149863, -0.8660254037844323793 ) ) ;
#194313=CARTESIAN_POINT ( 'NONE',  ( -1.364683531250012516, 1.280208333674755172, 0.7879004041258379498 ) ) ;
#194318=CARTESIAN_POINT ( 'NONE',  ( -1.364683531250014514, -0.5114583329919092369, -0.7879004041258359514 ) ) ;
#194320=CARTESIAN_POINT ( 'NONE',  ( 5.858512798400357546, 6.179092012920288646, 0.8810539604525641222 ) ) ;
#194327=CARTESIAN_POINT ( 'NONE',  ( -7.365103760721662951, 9.615707025640515937, 1.599625672291295375 ) ) ;
#194330=CARTESIAN_POINT ( 'NONE',  ( 4.599240423533799138, 6.388866465587984322, 1.599625672291267398 ) ) ;
#194336=CARTESIAN_POINT ( 'NONE',  ( 10.73535870392234237, 11.41900666419791399, 0.000000000000000000 ) ) ;
#194339=CARTESIAN_POINT ( 'NONE',  ( -4.069418662396130593, 7.899405539437467816, -0.7998128361456281477 ) ) ;
#194344=CARTESIAN_POINT ( 'NONE',  ( 9.565441069641300587, 11.11843498845840905, -1.199719254218440723 ) ) ;
#194346=CARTESIAN_POINT ( 'NONE',  ( 7.618792255875527886, 10.97600916757510170, 1.199719254218460707 ) ) ;
#194347=CARTESIAN_POINT ( 'NONE',  ( 4.175323295466546014, 3.976416389340326596, -0.2919458039207459832 ) ) ;
#194349=CARTESIAN_POINT ( 'NONE',  ( -9.164948653157990677, 11.71552606681625619, -1.443375672974059665 ) ) ;
#194351=CARTESIAN_POINT ( 'NONE',  ( -5.696397096036042385, 9.797547045350714967, -0.7998128361456231517 ) ) ;
#194355=CARTESIAN_POINT ( 'NONE',  ( -5.775368881829861856, 6.228402001981104164, 1.032258425150527126 ) ) ;
#194356=CARTESIAN_POINT ( 'NONE',  ( -1.402160292154681736E-14, 0.6968750003414164729, -1.575800808251659024 ) ) ;
#194359=CARTESIAN_POINT ( 'NONE',  ( 7.646435448427411963, 8.023188899361205273, -0.7216878364870257245 ) ) ;
#194377=CARTESIAN_POINT ( 'NONE',  ( 8.886479618753304166, 12.45497775759917758, -1.199719254218446718 ) ) ;
#194381=CARTESIAN_POINT ( 'NONE',  ( -4.786191920824102830, 5.542644314838231168, 1.199719254218462483 ) ) ;
#194382=CARTESIAN_POINT ( 'NONE',  ( -8.843996274815957293, 9.212417163573759282, 1.040834085586084257E-14 ) ) ;
#194384=ORIENTED_EDGE ( 'NONE', *, *, #37073, .F. ) ;
#194387=CARTESIAN_POINT ( 'NONE',  ( 1.499999999999990896, 3.806250000682819046, 1.214306433183764966E-14 ) ) ;
#194388=CARTESIAN_POINT ( 'NONE',  ( 9.237182729612253951, 9.671134694169463586, 0.7998128361456462443 ) ) ;
#194391=CARTESIAN_POINT ( 'NONE',  ( -8.311311860377216476, 9.655284244316948872, -1.199719254218446718 ) ) ;
#194393=CARTESIAN_POINT ( 'NONE',  ( 1.364683531249988535, 3.363541667008084879, 0.7879004041258500513 ) ) ;
#194396=CARTESIAN_POINT ( 'NONE',  ( -3.070819976953871766, 2.800000000000024691, -2.497101503370694253 ) ) ;
#194399=CARTESIAN_POINT ( 'NONE',  ( -8.134528978519403708, 11.47373899403920205, 1.082531754730549967 ) ) ;
#194403=CARTESIAN_POINT ( 'NONE',  ( -1.364683531250012516, 3.342708333674756727, 0.7879004041258379498 ) ) ;
#194410=CARTESIAN_POINT ( 'NONE',  ( 0.6823417656249899377, 3.426041667008085323, -1.181850606188754593 ) ) ;
#194412=CARTESIAN_POINT ( 'NONE',  ( -5.925076824372040640, 6.871343368977510302, 1.199719254218450271 ) ) ;
#194413=CARTESIAN_POINT ( 'NONE',  ( 6.693975156845185737, 8.832723654451292816, 1.599625672291281386 ) ) ;
#194416=CARTESIAN_POINT ( 'NONE',  ( -1.364683531250012516, 3.551041667008086211, -0.7879004041258300672 ) ) ;
#194420=CARTESIAN_POINT ( 'NONE',  ( -1.402160292154681736E-14, -1.178124999658576311, 1.575800808251672791 ) ) ;
#194421=CARTESIAN_POINT ( 'NONE',  ( -3.945059511896602089, 7.546393830613923548, 1.040834085586084257E-14 ) ) ;
#194425=CARTESIAN_POINT ( 'NONE',  ( 3.850152436600926542, 7.435668909435648288, -0.7216878364870197293 ) ) ;
#194428=CARTESIAN_POINT ( 'NONE',  ( -8.202846631467911820, 9.528741477256060577, 1.199719254218462483 ) ) ;
#194429=CARTESIAN_POINT ( 'NONE',  ( -8.026063749610043985, 12.30756544127966912, -0.7216878364870267237 ) ) ;
#194431=CARTESIAN_POINT ( 'NONE',  ( 1.364683531249990311, 4.613541667008083103, 0.7879004041258500513 ) ) ;
#194434=LINE ( 'NONE', #46075, #58623 ) ;
#194436=CARTESIAN_POINT ( 'NONE',  ( -6.738039155867462604, 7.923762439009225389, 1.082531754730549967 ) ) ;
#194438=CARTESIAN_POINT ( 'NONE',  ( -1.364683531250000748, 0.07187500034142035865, 0.000000000000000000 ) ) ;
#194450=CARTESIAN_POINT ( 'NONE',  ( 0.7499999999999885647, -0.7666666666666446250, 1.299038105676657340 ) ) ;
#194458=CARTESIAN_POINT ( 'NONE',  ( 6.449928391799196525, 8.548002428564306143, -1.599625672291262513 ) ) ;
#194460=ADVANCED_FACE ( 'NONE', ( #41912 ), #23484, .F. ) ;
#194461=CARTESIAN_POINT ( 'NONE',  ( -5.440899717785814715, 5.242137847038546461, 0.7998128361456341429 ) ) ;
#194466=CARTESIAN_POINT ( 'NONE',  ( -1.364683531250012516, 2.301041667008087988, -0.7879004041258289570 ) ) ;
#194468=CARTESIAN_POINT ( 'NONE',  ( -8.784793466650835825, 12.33634391347959713, 1.199719254218462483 ) ) ;
#194481=ORIENTED_EDGE ( 'NONE', *, *, #29804, .F. ) ;
#194482=CARTESIAN_POINT ( 'NONE',  ( -4.332027941937599103, 7.225435059248122016, -1.002253350946308075 ) ) ;
#194485=CARTESIAN_POINT ( 'NONE',  ( 5.035963992472171746, 7.962709526937818083, 1.199719254218462483 ) ) ;
#194492=CARTESIAN_POINT ( 'NONE',  ( 8.392660782059197189, 9.750191319612612872, 1.199719254218462483 ) ) ;
#194495=CARTESIAN_POINT ( 'NONE',  ( 10.18233705906309972, 11.83814697611718714, 1.199719254218450271 ) ) ;
#194497=CARTESIAN_POINT ( 'NONE',  ( 6.471393748265540147, 5.229711127717882491, 2.500000000000011102 ) ) ;
#194502=FACE_OUTER_BOUND ( 'NONE', #53254, .T. ) ;
#194506=CARTESIAN_POINT ( 'NONE',  ( -7.809133291791416909, 11.09411069285655493, 1.082531754730549967 ) ) ;
#194510=CARTESIAN_POINT ( 'NONE',  ( 5.660692828905515839, 6.562895374266609849, -1.199719254218445830 ) ) ;
#194516=CARTESIAN_POINT ( 'NONE',  ( 4.812781342726870193, 4.717259109377208048, 0.7216878364870317197 ) ) ;
#194524=CARTESIAN_POINT ( 'NONE',  ( -7.230575994789712801, 7.330093503543126054, 0.7998128361456341429 ) ) ;
#194526=CARTESIAN_POINT ( 'NONE',  ( -4.303823697334223652, 7.108545849276850959, -1.199719254218452047 ) ) ;
#194532=CARTESIAN_POINT ( 'NONE',  ( 1.364683531249990311, 3.446875000341416584, 1.214306433183764966E-14 ) ) ;
#194534=CARTESIAN_POINT ( 'NONE',  ( 7.135668919494039031, 7.219368582364847242, 1.040834085586084257E-14 ) ) ;
#194536=CARTESIAN_POINT ( 'NONE',  ( 1.548913609767778699, 8.694120146927671655, 2.506286796689261465 ) ) ;
#194549=CARTESIAN_POINT ( 'NONE',  ( 1.364683531249986537, -0.5322916663252452718, -0.7879004041258309554 ) ) ;
#194551=CARTESIAN_POINT ( 'NONE',  ( 4.517891501851804215, 6.293959390292322986, -1.599625672291255185 ) ) ;
#194554=CARTESIAN_POINT ( 'NONE',  ( -5.748293942514169252, 9.650167333001109071, -0.7216878364870207285 ) ) ;
#194555=CARTESIAN_POINT ( 'NONE',  ( 3.538314903486612817, 7.071858454135611538, 1.040834085586084257E-14 ) ) ;
#194556=CARTESIAN_POINT ( 'NONE',  ( -6.005898860729463884, 9.950706404252290582, 0.7216878364870458196 ) ) ;
#194560=CARTESIAN_POINT ( 'NONE',  ( 4.937140493670735708, 8.911747675924535983, -0.7998128361456281477 ) ) ;
#194564=CARTESIAN_POINT ( 'NONE',  ( -1.420000000000021911, 6.280000000000042881, 2.873333333333347728 ) ) ;
#194565=CARTESIAN_POINT ( 'NONE',  ( -0.6823417656250212460, 4.801041667008086655, 1.181850606188767472 ) ) ;
#194569=CARTESIAN_POINT ( 'NONE',  ( 6.825640269476072497, 10.05066518344239412, 1.199719254218460707 ) ) ;
#194574=CARTESIAN_POINT ( 'NONE',  ( -8.701635661872465732, 9.046329781806354831, 1.040834085586084257E-14 ) ) ;
#194579=CARTESIAN_POINT ( 'NONE',  ( 7.564559641420864899, 10.91273778404466199, -1.199719254218446718 ) ) ;
#194582=CARTESIAN_POINT ( 'NONE',  ( -6.042130013184518589, 10.20090211535728031, -0.7998128361456291469 ) ) ;
#194585=CARTESIAN_POINT ( 'NONE',  ( 5.191320393234815533, 6.438618948542633724, -1.178512179637403623 ) ) ;
#194586=CARTESIAN_POINT ( 'NONE',  ( -9.842856333841300653, 10.58567993234409421, 0.7216878364870438212 ) ) ;
#194590=CARTESIAN_POINT ( 'NONE',  ( 3.277927966699532014, 6.407906593915337901, -0.9422035321714219425 ) ) ;
#194592=CARTESIAN_POINT ( 'NONE',  ( 6.124532705071213279, 8.168374127381657246, -1.599625672291262513 ) ) ;
#194594=CARTESIAN_POINT ( 'NONE',  ( 4.137209430464448445, 7.978494768850520558, 1.040834085586084257E-14 ) ) ;
#194595=CARTESIAN_POINT ( 'NONE',  ( -4.016961781477323079, 7.622873323794868483, 0.1115696107641880874 ) ) ;
#194596=CARTESIAN_POINT ( 'NONE',  ( 2.984766373302843778, 6.633977868828633717, -0.7998128361456291469 ) ) ;
#194598=CARTESIAN_POINT ( 'NONE',  ( -5.721177635286839092, 9.618531641235897212, 0.7216878364870458196 ) ) ;
#194603=CARTESIAN_POINT ( 'NONE',  ( -5.312135015290653683, 6.384990658495349081, 1.125702006352300000 ) ) ;
#194604=CARTESIAN_POINT ( 'NONE',  ( 1.364683531249988757, 0.1968750003414204697, 0.000000000000000000 ) ) ;
#194607=CARTESIAN_POINT ( 'NONE',  ( 4.121315508874254796, 5.831287398485176077, -1.443375672974051449 ) ) ;
#194612=CARTESIAN_POINT ( 'NONE',  ( -7.985389288324692636, 11.29974268881207067, -1.082531754730543083 ) ) ;
#194618=CARTESIAN_POINT ( 'NONE',  ( -7.768458830506062007, 11.04665715469030296, 1.082531754730549967 ) ) ;
#194624=ORIENTED_EDGE ( 'NONE', *, *, #113967, .T. ) ;
#194625=CARTESIAN_POINT ( 'NONE',  ( -8.798878505144665851, 9.367705798864669475, -0.7216878364870267237 ) ) ;
#194628=EDGE_CURVE ( 'NONE', #34146, #159908, #13639, .T. ) ;
#194631=CARTESIAN_POINT ( 'NONE',  ( -1.001543065824772872E-14, 5.134375000341421469, 1.575800808251672791 ) ) ;
#194632=CARTESIAN_POINT ( 'NONE',  ( 0.7499999999999902300, 4.097916667349481123, -1.299038105676658228 ) ) ;
#194633=CARTESIAN_POINT ( 'NONE',  ( 5.816641468517390834, 6.206546802344954372, -0.9418049055998338748 ) ) ;
#194638=CARTESIAN_POINT ( 'NONE',  ( -8.369460898337653276, 8.658792557682392754, 0.7998128361456462443 ) ) ;
#194639=FACE_OUTER_BOUND ( 'NONE', #50267, .T. ) ;
#194641=CARTESIAN_POINT ( 'NONE',  ( 4.638861114170084399, 8.563755066507100722, 0.7998128361456462443 ) ) ;
#194648=CARTESIAN_POINT ( 'NONE',  ( 6.584456157731144899, 10.83361595066169514, -0.7998128361456291469 ) ) ;
#194654=CARTESIAN_POINT ( 'NONE',  ( -7.375272376154101472, 7.706831981708990753, -0.7216878364870278340 ) ) ;
#194662=CARTESIAN_POINT ( 'NONE',  ( -10.31505594189871111, 10.92865344183699428, -0.7998128361456291469 ) ) ;
#194664=CARTESIAN_POINT ( 'NONE',  ( 9.610031953988080744, 10.10612545594124967, -0.7998128361456281477 ) ) ;
#194665=CARTESIAN_POINT ( 'NONE',  ( 0.7499999999999885647, -0.7666666666666446250, 1.299038105676657340 ) ) ;
#194666=CARTESIAN_POINT ( 'NONE',  ( -7.883176251342026042, 11.28445716228600126, -1.199719254218446718 ) ) ;
#194670=CARTESIAN_POINT ( 'NONE',  ( -1.364683531250012516, 3.488541667008085767, -0.7879004041258300672 ) ) ;
#194671=CARTESIAN_POINT ( 'NONE',  ( 4.383363735919856730, 4.008345868194933104, -0.7998128361456211532 ) ) ;
#194673=CARTESIAN_POINT ( 'NONE',  ( 1.438722645073102990, 7.870286565763570330, -3.684014302713757516 ) ) ;
#194676=CARTESIAN_POINT ( 'NONE',  ( 10.01911233037458260, 10.79131192829960462, 0.7216878364870438212 ) ) ;
#194680=CARTESIAN_POINT ( 'NONE',  ( -5.585596099150174965, 9.460353182409786399, -0.7216878364870207285 ) ) ;
#194682=CARTESIAN_POINT ( 'NONE',  ( -0.6823417656250003738, 0.7177083336747519526, -1.181850606188749264 ) ) ;
#194684=CARTESIAN_POINT ( 'NONE',  ( 0.5015801190230135820, 7.801378974689940904, 1.936921611551724931 ) ) ;
#194686=CARTESIAN_POINT ( 'NONE',  ( -7.670162217029145246, 9.971608557999250166, 1.599625672291295375 ) ) ;
#194688=CARTESIAN_POINT ( 'NONE',  ( -2.941756144040963417, 6.375873234782333476, -0.7216878364870257245 ) ) ;
#194689=CARTESIAN_POINT ( 'NONE',  ( 1.364683531249988535, 3.426041667008085323, 0.7879004041258500513 ) ) ;
#194693=( BOUNDED_CURVE ( )  B_SPLINE_CURVE ( 2, ( #182854, #86435, #51813 ),
 .UNSPECIFIED., .F., .T. ) 
 B_SPLINE_CURVE_WITH_KNOTS ( ( 3, 3 ),
 ( 0.000000000000000000, 0.0002183499308596753715 ),
 .UNSPECIFIED. ) 
 CURVE ( )  GEOMETRIC_REPRESENTATION_ITEM ( )  RATIONAL_B_SPLINE_CURVE ( ( 1.000000000000000000, 0.9929791974830509682, 0.9866942310032964514 ) ) 
 REPRESENTATION_ITEM ( '' )  );
#194695=CARTESIAN_POINT ( 'NONE',  ( 8.075853055234393452, 12.57357899774884658, 0.7998128361456462443 ) ) ;
#194710=CARTESIAN_POINT ( 'NONE',  ( -1.364683531250000748, -0.9906249996585805295, 0.000000000000000000 ) ) ;
#194714=CARTESIAN_POINT ( 'NONE',  ( 9.094822116668764167, 9.505047312402055582, 0.7998128361456462443 ) ) ;
#194717=CARTESIAN_POINT ( 'NONE',  ( -1.364683531249997417, 3.259375000341423245, 1.214306433183764966E-14 ) ) ;
#194719=CARTESIAN_POINT ( 'NONE',  ( -6.561783159334137139, 8.678499657355050800, -1.443375672974059665 ) ) ;
#194725=CARTESIAN_POINT ( 'NONE',  ( 2.367870383881045981, 5.914265881169853856, 0.000000000000000000 ) ) ;
#194728=CARTESIAN_POINT ( 'NONE',  ( 9.901532256681887745, 10.44620914241737530, 0.000000000000000000 ) ) ;
#194735=CARTESIAN_POINT ( 'NONE',  ( -9.459838494033043332, 12.05956421450382088, 1.599625672291281386 ) ) ;
#194737=CARTESIAN_POINT ( 'NONE',  ( 6.632963465583686435, 8.761543347979550589, -1.599625672291262513 ) ) ;
#194739=CARTESIAN_POINT ( 'NONE',  ( 4.161989969270902812, 4.918371721313249623, 1.082531754730560403 ) ) ;
#194741=CARTESIAN_POINT ( 'NONE',  ( 4.741601036477289810, 6.554953847355395880, 1.599625672291267398 ) ) ;
#194751=CARTESIAN_POINT ( 'NONE',  ( -7.239690840017442675, 7.548653522882887934, 0.7216878364870317197 ) ) ;
#194752=CARTESIAN_POINT ( 'NONE',  ( 5.359550796103802028, 5.147230771742885125, -0.7998128361456231517 ) ) ;
#194755=CARTESIAN_POINT ( 'NONE',  ( -7.100719765255177229, 9.307259030929609267, -1.599625672291263179 ) ) ;
#194760=CARTESIAN_POINT ( 'NONE',  ( -10.14557902172788495, 10.73093036830436553, 1.040834085586084257E-14 ) ) ;
#194764=CARTESIAN_POINT ( 'NONE',  ( 7.853197290813620945, 10.18514947741448573, 1.599625672291281386 ) ) ;
#194766=FACE_OUTER_BOUND ( 'NONE', #166241, .T. ) ;
#194777=CARTESIAN_POINT ( 'NONE',  ( -7.694415870955439551, 8.935572256658169010, 1.199719254218462483 ) ) ;
#194781=CARTESIAN_POINT ( 'NONE',  ( 6.860062538834778678, 8.066123052471139587, -1.082531754730543083 ) ) ;
#194784=CARTESIAN_POINT ( 'NONE',  ( 3.063252641683779753, 5.661212951017999373, 1.199719254218450271 ) ) ;
#194787=CARTESIAN_POINT ( 'NONE',  ( -7.061099074618889304, 7.132370430010492868, -0.7998128361456291469 ) ) ;
#194796=CARTESIAN_POINT ( 'NONE',  ( 1.364683531249988535, 3.676041667008087099, 0.7879004041258500513 ) ) ;
#194797=CARTESIAN_POINT ( 'NONE',  ( 4.004068906699964181, 7.801233831630747240, -0.1746446656625457727 ) ) ;
#194798=CARTESIAN_POINT ( 'NONE',  ( 8.749089199520284410, 9.101692242395490240, 0.7998128361456481317 ) ) ;
#194799=ADVANCED_FACE ( 'NONE', ( #64534 ), #54058, .T. ) ;
#194801=CARTESIAN_POINT ( 'NONE',  ( -3.470524135418300737, 6.032400010421219427, -1.082531754730549967 ) ) ;
#194803=CARTESIAN_POINT ( 'NONE',  ( -5.219525951136856357, 6.152163700156858539, -1.082531754730543971 ) ) ;
#194808=ORIENTED_EDGE ( 'NONE', *, *, #15140, .F. ) ;
#194810=CARTESIAN_POINT ( 'NONE',  ( 2.686486993802192913, 6.285985259411197568, 0.7998128361456362523 ) ) ;
#194817=CARTESIAN_POINT ( 'NONE',  ( 3.623053363349855172, 5.249981562040033189, 1.599625672291267398 ) ) ;
#194821=CARTESIAN_POINT ( 'NONE',  ( -1.201851678989727383E-14, 4.134375000341417028, 1.575800808251672791 ) ) ;
#194827=CARTESIAN_POINT ( 'NONE',  ( 6.647575389402066826, 6.649926130590872120, 1.040834085586084257E-14 ) ) ;
#194830=B_SPLINE_CURVE_WITH_KNOTS ( 'NONE', 3,
 ( #176424, #28031, #111482, #128807 ),
 .UNSPECIFIED., .F., .F.,
 ( 4, 4 ),
 ( 0.000000000000000000, 0.002003498272494342886 ),
 .UNSPECIFIED. ) ;
#194832=CARTESIAN_POINT ( 'NONE',  ( -4.273844736805832767, 6.009238164405336313, 1.599625672291267398 ) ) ;
#194833=CARTESIAN_POINT ( 'NONE',  ( 6.114364089638795186, 7.196141528409145671, 1.082531754730558626 ) ) ;
#194834=CARTESIAN_POINT ( 'NONE',  ( -1.499999999999997780, 2.900000000000020783, 1.214306433183764966E-14 ) ) ;
#194836=CARTESIAN_POINT ( 'NONE',  ( -3.601662362724658895, 7.353689856487406473, -0.7998128361456281477 ) ) ;
#194840=CARTESIAN_POINT ( 'NONE',  ( -1.364683531250012516, 4.238541667008090208, -0.7879004041258300672 ) ) ;
#194843=CARTESIAN_POINT ( 'NONE',  ( -4.799223189557577207, 4.701441264013013210, 0.7216878364870317197 ) ) ;
#194850=CARTESIAN_POINT ( 'NONE',  ( 4.355193658487811703, 6.104145239700998538, -1.599625672291255185 ) ) ;
#194853=FACE_OUTER_BOUND ( 'NONE', #56440, .T. ) ;
#194854=CARTESIAN_POINT ( 'NONE',  ( 0.6823417656249917140, 4.155208333674755394, 1.181850606188765695 ) ) ;
#194857=CARTESIAN_POINT ( 'NONE',  ( -0.6823417656250003738, 0.5302083336747518416, -1.181850606188749264 ) ) ;
#194860=CARTESIAN_POINT ( 'NONE',  ( -8.350932551013499960, 11.83017284523606172, -1.199719254218446718 ) ) ;
#194861=CARTESIAN_POINT ( 'NONE',  ( -6.195713011320795438, 8.251417818006149929, -1.443375672974058777 ) ) ;
#194865=CARTESIAN_POINT ( 'NONE',  ( 0.6823417656249899377, 4.676041667008086655, -1.181850606188754593 ) ) ;
#194873=CARTESIAN_POINT ( 'NONE',  ( -6.195713011320804320, 7.291048603704809672, -1.082531754730543083 ) ) ;
#194878=CARTESIAN_POINT ( 'NONE',  ( -6.371969008298464132, 6.536311385877402458, 1.040834085586084257E-14 ) ) ;
#194886=CARTESIAN_POINT ( 'NONE',  ( 1.537272393291603700, 8.756440202903029046, -2.479668406359592403 ) ) ;
#194890=CARTESIAN_POINT ( 'NONE',  ( 0.4304858038777367724, 6.930341212760413150, -3.770372082616246789 ) ) ;
#194891=CARTESIAN_POINT ( 'NONE',  ( -3.554208825076827782, 7.298327395898266623, 0.7998128361456341429 ) ) ;
#194894=CARTESIAN_POINT ( 'NONE',  ( -1.500000000000013101, 1.170833333333352710, 0.8660254037844403729 ) ) ;
#194896=CARTESIAN_POINT ( 'NONE',  ( 7.456621297836061757, 11.64321591421002644, 0.7216878364870438212 ) ) ;
#194897=CARTESIAN_POINT ( 'NONE',  ( 7.494959990256193194, 7.638541498254023843, -0.7998128361456281477 ) ) ;
#194901=CARTESIAN_POINT ( 'NONE',  ( 5.168682875307768931, 7.053215992657626110, -1.599625672291256295 ) ) ;
#194902=CARTESIAN_POINT ( 'NONE',  ( -0.4957404558456298682, 7.798922855753633421, -1.990826765680301591 ) ) ;
#194909=CARTESIAN_POINT ( 'NONE',  ( -4.338245966692955591, 5.124003718305597310, 1.082531754730560403 ) ) ;
#194911=CARTESIAN_POINT ( 'NONE',  ( -1.219999999999996199, 6.400000000000024336, 1.214306433183764966E-14 ) ) ;
#194916=CARTESIAN_POINT ( 'NONE',  ( 0.6823417656249882723, 2.926041667008084879, -1.181850606188754593 ) ) ;
#194917=CARTESIAN_POINT ( 'NONE',  ( 9.368320956918616105, 10.03205532593431037, 0.7216878364870458196 ) ) ;
#194918=CARTESIAN_POINT ( 'NONE',  ( -6.795661308947694934, 8.951357498570873261, -1.599625672291263179 ) ) ;
#194922=CARTESIAN_POINT ( 'NONE',  ( 6.602984505055297326, 7.662235663108029726, 1.199719254218462483 ) ) ;
#194923=CARTESIAN_POINT ( 'NONE',  ( -5.215082642750900277, 9.236013516518044142, 0.000000000000000000 ) ) ;
#194927=CARTESIAN_POINT ( 'NONE',  ( 1.499999999999985123, -0.1729166659838496101, -0.8660254037844323793 ) ) ;
#194930=CARTESIAN_POINT ( 'NONE',  ( 7.293923454472087897, 8.572294120714675003, 1.082531754730558626 ) ) ;
#194934=CARTESIAN_POINT ( 'NONE',  ( -0.6823417656250212460, 2.613541667008084879, 1.181850606188767472 ) ) ;
#194936=CARTESIAN_POINT ( 'NONE',  ( 6.765155463094761679, 6.995028916473103209, 0.7216878364870317197 ) ) ;
#194938=CARTESIAN_POINT ( 'NONE',  ( -3.160184708874208770, 6.440504254417610319, -0.7564881602227467861 ) ) ;
#194939=CARTESIAN_POINT ( 'NONE',  ( -4.934804725694236893, 4.859619722839116918, -0.7216878364870207285 ) ) ;
#194942=CARTESIAN_POINT ( 'NONE',  ( 1.364683531249990311, 4.884375000341417916, 1.214306433183764966E-14 ) ) ;
#194945=LINE ( 'NONE', #45519, #91678 ) ;
#194948=CARTESIAN_POINT ( 'NONE',  ( -5.067137445304809695, 6.740953878067043270, -1.444057985504534125 ) ) ;
#194954=CARTESIAN_POINT ( 'NONE',  ( 7.091078035147269532, 8.231678114882006625, 1.199719254218462483 ) ) ;
#194957=CARTESIAN_POINT ( 'NONE',  ( 5.007038802148489509, 4.735966778795008381, 0.7998128361456341429 ) ) ;
#194966=CARTESIAN_POINT ( 'NONE',  ( 4.039966587192250103, 7.657118751792200584, 0.7216878364870298324 ) ) ;
#194967=CARTESIAN_POINT ( 'NONE',  ( -0.6823417656250212460, 2.113541667008083991, 1.181850606188767472 ) ) ;
#194968=CARTESIAN_POINT ( 'NONE',  ( 8.320953590485093088, 10.73086516036454618, 1.599625672291281386 ) ) ;
#194970=CARTESIAN_POINT ( 'NONE',  ( -5.752737250900127997, 5.605948302338584099, 0.000000000000000000 ) ) ;
#194971=DIRECTION ( 'NONE',  ( -0.6507913734559627184, -0.7592566023653016805, 0.000000000000000000 ) ) ;
#194972=ADVANCED_FACE ( 'NONE', ( #34151 ), #37350, .F. ) ;
#194974=CARTESIAN_POINT ( 'NONE',  ( 1.499999999999987121, 1.545833333333354487, -0.8660254037844253849 ) ) ;
#194975=CARTESIAN_POINT ( 'NONE',  ( 7.135668919494039031, 7.219368582364847242, 1.040834085586084257E-14 ) ) ;
#194976=CARTESIAN_POINT ( 'NONE',  ( -7.069687034522070590, 10.33538640932937724, -1.199719254218440723 ) ) ;
#194980=CARTESIAN_POINT ( 'NONE',  ( -0.6823417656250003738, 2.717708333674753618, -1.181850606188749264 ) ) ;
#194981=ORIENTED_EDGE ( 'NONE', *, *, #118661, .F. ) ;
#194982=CARTESIAN_POINT ( 'NONE',  ( -1.201851678989727383E-14, 3.212500000000018119, 1.732050807568877637 ) ) ;
#194984=CARTESIAN_POINT ( 'NONE',  ( 4.196412238629597447, 4.854568018944682706, -1.199719254218452047 ) ) ;
#194990=CARTESIAN_POINT ( 'NONE',  ( -1.402160292154681736E-14, 0.2437500006828163535, 1.732050807568877637 ) ) ;
#194992=CARTESIAN_POINT ( 'NONE',  ( -7.881367368245678406, 8.089350105908421185, 0.7998128361456602331 ) ) ;
#194993=CARTESIAN_POINT ( 'NONE',  ( -3.687454593236990430, 4.364747115940301292, 1.082531754730560403 ) ) ;
#195001=CARTESIAN_POINT ( 'NONE',  ( 4.774442650306744085, 8.721933525333202653, -0.7998128361456281477 ) ) ;
#195003=FACE_OUTER_BOUND ( 'NONE', #72614, .T. ) ;
#195005=CARTESIAN_POINT ( 'NONE',  ( 5.120175567455225618, 9.125288595339771547, -0.7998128361456281477 ) ) ;
#195012=CARTESIAN_POINT ( 'NONE',  ( -7.152089726408780379, 8.302858421353754181, -1.199719254218446718 ) ) ;
#195014=CARTESIAN_POINT ( 'NONE',  ( 3.083589872104280705, 5.684939719841914929, 1.199719254218450271 ) ) ;
#195015=CIRCLE ( 'NONE', #142187, 0.08000000000000012657 ) ;
#195021=CARTESIAN_POINT ( 'NONE',  ( 4.147051400439892177, 7.400425289818373109, 0.7480841269332880739 ) ) ;
#195022=ORIENTED_EDGE ( 'NONE', *, *, #96265, .T. ) ;
#195029=CARTESIAN_POINT ( 'NONE',  ( -4.460269349215930212, 4.305995116947750390, 1.214306433183764966E-14 ) ) ;
#195030=CARTESIAN_POINT ( 'NONE',  ( 8.432808358020029260, 8.940623960552603222, 0.7216878364870438212 ) ) ;
#195032=CARTESIAN_POINT ( 'NONE',  ( -3.879604511804807032, 7.677955697080923514, 0.7998128361456341429 ) ) ;
#195037=CARTESIAN_POINT ( 'NONE',  ( -6.693975156845199059, 8.832723654451292816, 1.599625672291283607 ) ) ;
#195050=CARTESIAN_POINT ( 'NONE',  ( 1.436717746206296997, 7.422220963914728742, -4.237135035835245311 ) ) ;
#195051=CARTESIAN_POINT ( 'NONE',  ( -3.744022975668147790, 7.519777238254810925, -0.7998128361456281477 ) ) ;
#195054=CARTESIAN_POINT ( 'NONE',  ( 3.470524135418292300, 5.072030796119872953, -1.443375672974057666 ) ) ;
#195059=CARTESIAN_POINT ( 'NONE',  ( 1.387358672525591308, 7.251968950354787502, 4.302625267139676524 ) ) ;
#195060=CARTESIAN_POINT ( 'NONE',  ( -5.264643720808155791, 5.036505850564608089, 0.000000000000000000 ) ) ;
#195063=CARTESIAN_POINT ( 'NONE',  ( 9.297140650669039275, 11.86975006391249643, 1.599625672291281386 ) ) ;
#195066=CARTESIAN_POINT ( 'NONE',  ( -6.991200766141138168, 11.30815132714001159, 0.7998128361456481317 ) ) ;
#195067=CARTESIAN_POINT ( 'NONE',  ( 6.634017235788401301, 6.634108284708264414, 0.7998128361456341429 ) ) ;
#195071=CARTESIAN_POINT ( 'NONE',  ( 3.310162060030825248, 7.013606170011281726, -0.7998128361456291469 ) ) ;
#195074=CARTESIAN_POINT ( 'NONE',  ( -0.6823417656250212460, 1.613541667008083769, 1.181850606188755259 ) ) ;
#195075=( BOUNDED_SURFACE ( )  B_SPLINE_SURFACE ( 1, 2, ( 
 ( #16315, #198272, #83465, #36843, #150627, #68264, #118174, #116035, #99726, #1131, #133330, #50980, #183103, #34713, #24858, #202527, #107258, #171119, #38996, #104002, #154882, #122473, #56312, #190555, #174348, #124597, #106178, #7535, #22713, #73619, #153815, #136507, #204662, #6465, #137576, #88827, #42211, #203594, #187366, #5386, #139718, #25926, #90960, #173278, #72542, #188433, #40068, #92034, #71463, #138640, #74694, #37928, #55246, #170045, #172204, #121393, #157026, #23792, #140798, #8611, #206809, #189503, #89899, #54176, #120316, #155950, #58442, #205742, #108328, #57375, #105081, #123538, #158092, #41148, #9680, #186290, #21631, #87739, #63765, #195911, #159137, #194832, #193760, #162348, #125655, #110459, #46466, #31283, #12866, #13931, #95229, #60564, #191617, #126723, #80011, #10739, #47547, #28072, #144005, #175405, #78940, #145062, #94166, #160206, #11808, #177529, #146116, #112589, #211066, #45407, #163415, #43279, #77883, #111523, #75756, #141866, #62690, #209997, #61639, #128849, #76809, #207876, #127806, #29142, #59498, #129924, #178600, #176460, #212127, #109400, #30209, #113659, #161279, #142929, #96296, #179663, #97358, #26989, #93096, #44337, #208929, #192684, #34463, #151434, #184965, #182845, #167670, #117921, #52853, #134142, #183915, #130974, #16057, #200149, #201213, #19271, #51803, #196964, #866, #3006, #82141, #99476, #85353, #69076, #1940, #64828, #135196, #17128, #35526, #132013, #98406, #50719, #198023, #83204, #100535, #101602, #48602, #166610, #68000, #199072, #49651, #148234, #115774, #114720, #102678, #118987, #164471, #180715, #32338, #18198, #84283, #33397, #165535, #149285, #116844, #36591, #14991, #150370, #133075, #81085, #214236, #66932, #147172, #213199, #65863, #181764, #170871, #22462, #105920, #103750, #168736, #88574, #204408, #152490, #8362, #139459, #203342, #40894, #4073, #123291, #90714, #187110, #37674, #38743, #154631, #140549, #171946, #56060, #137326, #6211, #86425, #188179, #156776, #124348, #122218, #106999, #57125, #206562, #73356, #189255, #70143, #169801, #205491, #58189, #173024, #24604, #136255, #72281, #74445, #21390, #104825, #190305, #41963, #155696, #202275, #20337, #138390, #53926, #71210, #87499, #39814, #54995, #23535, #89644, #120063, #186038, #7279, #153564, #5134, #121147, #109148, #76564, #207627, #195665, #211887, #191368, #141618, #78694, #161028, #208684, #108074, #25676, #61392, #210827, #77634, #62452, #177281, #142674, #192436, #194582, #12622, #13693, #91783, #63527, #60313, #96051, #79762, #43036, #144820, #11564, #46228, #157840, #126473, #128615, #129680, #45164, #112345, #127552, #92849, #9436, #158895, #178357, #175160, #145879, #44091, #176219, #110211, #174104, #26748, #10491, #125403, #193523, #75506, #29964, #162105, #27821, #159959, #93919, #59245, #143756, #209751, #111277, #28897, #94981, #80845, #99230, #32089, #1682, #82955, #51539, #133886, #179420, #84019, #68816, #113414, #167419, #14753, #50467, #147985, #165280, #115526, #131764, #150110, #149028, #85091, #34203, #181521, #183656, #49406, #67736, #35261, #65615, #16874, #116586, #98176, #146935, #101337, #33150, #604, #66669, #132818, #212952, #196721, #19010, #48361, #47299, #151175, #64589, #198821, #114473, #197769, #15812, #2746, #100277, #199893, #182581, #164224, #166343, #134938, #17934, #180473, #117664, #31041, #130729, #81897, #97116, #213994, #163168, #56864, #87229, #171674, #184707, #121948, #204138, #7016, #172764, #8104, #105646, #86162, #52593, #20073, #153292, #205223, #104560, #72016, #5946, #138129, #118720, #55792, #23270, #203082, #74193, #36329, #89382, #102408, #155430, #21123, #103481, #168475, #4869, #186851, #120877, #40633, #24338, #188991, #170604, #187914, #70947, #39545, #3804, #200944, #54727, #137058, #202003, #169544, #106736, #73092, #139192, #22191, #185774, #123039, #90447, #156514, #53661, #152233, #69878, #135988, #119794, #37407, #38483, #88305, #154369, #29447, #113961, #124094, #64071, #146416, #163714, #115012, #164765, #47850, #25421, #206306, #173845, #95538, #147465, #46777, #14221, #162648, #80316, #57930 ),
 ( #212429, #161588, #13175, #79253, #30517, #213487, #179958, #130215, #112891, #16356, #41710, #145371, #178903, #140286, #190058, #196209, #211370, #62995, #31581, #78179, #107820, #129164, #96598, #91527, #197253, #97655, #177830, #15296, #157586, #81381, #65110, #195141, #9181, #131266, #48892, #181009, #32629, #98706, #111828, #144307, #210301, #61941, #128099, #194057, #45709, #20623, #185260, #120357, #201499, #36884, #198308, #83501, #53145, #54219, #86711, #119275, #49948, #68302, #4362, #149583, #166905, #152780, #70431, #69368, #132301, #136547, #84576, #102967, #199372, #165833, #118211, #51018, #150664, #35821, #169025, #116069, #19568, #135477, #2226, #184198, #82435, #170087, #85643, #134435, #200437, #151728, #17417, #148525, #52084, #101897, #66156, #202567, #186334, #117139, #37968, #182059, #104041, #91, #100820, #1167, #18498, #167962, #33690, #3300, #99766, #183142, #67231, #133365, #34747, #158130, #191655, #189540, #174389, #124638, #59536, #140837, #190595, #137617, #22749, #206850, #207915, #25967, #58482, #203633, #7575, #9721, #88867, #106217, #92072, #75797, #8653, #71506, #141905, #23831, #42252, #138682, #105119, #57413, #204701, #89936, #41188, #108365, #55285, #173317, #74732, #205784, #56351, #154922, #122513, #121434, #109438, #125696, #171159, #187403, #43320, #21674, #188474, #87782, #153856, #107295, #5427, #123578, #39035, #91002, #40105, #172243, #6506, #72581, #155987, #73660, #139760, #24896, #157065, #81127, #44377, #80053, #78984, #47588, #10776, #210038, #146156, #131014, #112630, #113702, #194873, #160245, #76850, #11845, #179706, #176499, #31323, #142969, #193798, #161320, #95272, #15035, #213237, #163455, #145103, #46508, #61678, #178640, #192723, #175444, #29183, #27029, #126763, #60604, #97399, #77922, #94205, #147212, #127846, #212172, #159176, #96336, #30252, #195952, #64869, #197006, #63806, #110500, #93137, #208972, #45447, #48641, #211107, #162392, #13969, #129964, #28110, #144041, #111562, #177570, #12904, #62731, #128892, #65907, #181807, #115820, #201249, #82181, #133114, #100574, #34500, #168773, #152527, #102716, #84322, #200186, #906, #51839, #132053, #114759, #182884, #199111, #33440, #66975, #20378, #99517, #165574, #198063, #117957, #4112, #69114, #85390, #149328, #166647, #18238, #70181, #49692, #50756, #52890, #16097, #17169, #148275, #150408, #83243, #135236, #1975, #119025, #185007, #32383, #151474, #136293, #180756, #86463, #214274, #183952, #116885, #68038, #134178, #35562, #3045, #101643, #202314, #167709, #19311, #36631, #98449, #164513, #42006, #72321, #171985, #57164, #104862, #21427, #108114, #39855, #89686, #7320, #73398, #87536, #203381, #190344, #55034, #53963, #174141, #153603, #155735, #121182, #204446, #22499, #25715, #107036, #140588, #23577, #38780, #40932, #157881, #123327, #187151, #189290, #88611, #206600, #37713, #8399, #91824, #138427, #137364, #56100, #122256, #9474, #205529, #139501, #154666, #188215, #186079, #173062, #75547, #141656, #24642, #58228, #156812, #120101, #90752, #74484, #169840, #170906, #124386, #103789, #5175, #71248, #6252, #105961, #129715, #60350, #77671, #145913, #211925, #194618, #43074, #63559, #209787, #96086, #110248, #76602, #28932, #176257, #61425, #161066, #178390, #109187, #144855, #46260, #177317, #27858, #208724, #93955, #92887, #80879, #97151, #142715, #26782, #30001, #112378, #159996, #207668, #125446, #12657, #162140, #95016, #13728, #62488, #11597, #143791, #79801, #195700, #113449, #191407, #163205, #127591, #47334, #179454, #126513, #31077, #111314, #14788, #175199, #193558, #59287, #158932, #210862, #10528, #78730, #192475, #44128, #45201, #128652, #82991, #36370, #51579, #643, #32128, #150150, #1720, #165316, #16911, #149066, #34244, #2784, #183695, #67777, #50505, #20113, #48400, #66708, #182621, #146969, #212985, #133926, #132853, #198858, #84061, #81933, #64624, #116627, #100316, #130763, #200983, #117704, #166382, #52630, #184743, #134975, #17974, #199932, #33186, #35302, #164260, #196759, #101379, #167454, #148019, #99268, #118758, #214029, #197810, #15848, #19049, #102447 ) ),
 .UNSPECIFIED., .F., .F., .F. ) 
 B_SPLINE_SURFACE_WITH_KNOTS ( ( 2, 2 ),
 ( 3, 2, 2, 2, 2, 2, 2, 2, 2, 2, 2, 2, 2, 2, 2, 2, 2, 2, 2, 2, 2, 2, 2, 2, 2, 2, 2, 2, 2, 2, 2, 2, 2, 2, 2, 2, 2, 2, 2, 2, 2, 2, 2, 2, 2, 2, 2, 2, 2, 2, 2, 2, 2, 2, 2, 2, 2, 2, 2, 2, 2, 2, 2, 2, 2, 2, 2, 2, 2, 2, 2, 2, 2, 2, 2, 2, 2, 2, 2, 2, 2, 2, 2, 2, 2, 2, 2, 2, 2, 2, 2, 2, 2, 2, 2, 2, 2, 2, 2, 2, 2, 2, 2, 2, 2, 2, 2, 2, 2, 2, 2, 2, 2, 2, 2, 2, 2, 2, 2, 2, 2, 2, 2, 2, 2, 2, 2, 2, 2, 2, 2, 2, 2, 2, 2, 2, 2, 2, 2, 2, 2, 2, 2, 2, 2, 2, 2, 2, 2, 2, 2, 2, 2, 2, 2, 2, 2, 2, 2, 2, 2, 2, 2, 2, 2, 2, 2, 2, 2, 2, 2, 2, 2, 2, 2, 2, 2, 2, 2, 2, 2, 2, 2, 2, 2, 2, 2, 2, 2, 2, 2, 2, 2, 2, 2, 2, 2, 2, 2, 2, 2, 2, 2, 2, 2, 2, 2, 2, 2, 2, 2, 2, 2, 2, 2, 2, 2, 2, 2, 2, 2, 2, 2, 2, 2, 2, 2, 2, 2, 2, 2, 2, 2, 2, 2, 2, 2, 2, 2, 2, 3 ),
 ( 0.000000000000000000, 1.000000000000000000 ),
 ( 0.000000000000000000, 0.004166666666666666609, 0.008333333333333333218, 0.01250000000000000069, 0.01666666666666666644, 0.02083333333333333218, 0.02500000000000000139, 0.02916666666666666713, 0.03333333333333333287, 0.03749999999999999861, 0.04166666666666666435, 0.04583333333333333010, 0.05000000000000000278, 0.05416666666666666852, 0.05833333333333333426, 0.06250000000000000000, 0.06666666666666666574, 0.07083333333333333148, 0.07499999999999999722, 0.07916666666666666297, 0.08333333333333332871, 0.08749999999999999445, 0.09166666666666666019, 0.09583333333333333981, 0.1000000000000000056, 0.1041666666666666713, 0.1083333333333333370, 0.1125000000000000028, 0.1166666666666666685, 0.1208333333333333343, 0.1250000000000000000, 0.1291666666666666796, 0.1333333333333333315, 0.1375000000000000111, 0.1416666666666666630, 0.1458333333333333426, 0.1499999999999999944, 0.1541666666666666741, 0.1583333333333333259, 0.1625000000000000056, 0.1666666666666666574, 0.1708333333333333370, 0.1749999999999999889, 0.1791666666666666685, 0.1833333333333333204, 0.1875000000000000000, 0.1916666666666666796, 0.1958333333333333315, 0.2000000000000000111, 0.2041666666666666630, 0.2083333333333333426, 0.2124999999999999944, 0.2166666666666666741, 0.2208333333333333259, 0.2250000000000000056, 0.2291666666666666574, 0.2333333333333333370, 0.2374999999999999889, 0.2416666666666666685, 0.2458333333333333204, 0.2500000000000000000, 0.2541666666666666519, 0.2583333333333333592, 0.2625000000000000111, 0.2666666666666666630, 0.2708333333333333148, 0.2750000000000000222, 0.2791666666666666741, 0.2833333333333333259, 0.2874999999999999778, 0.2916666666666666852, 0.2958333333333333370, 0.2999999999999999889, 0.3041666666666666408, 0.3083333333333333481, 0.3125000000000000000, 0.3166666666666666519, 0.3208333333333333592, 0.3250000000000000111, 0.3291666666666666630, 0.3333333333333333148, 0.3375000000000000222, 0.3416666666666666741, 0.3458333333333333259, 0.3499999999999999778, 0.3541666666666666852, 0.3583333333333333370, 0.3624999999999999889, 0.3666666666666666408, 0.3708333333333333481, 0.3750000000000000000, 0.3791666666666666519, 0.3833333333333333592, 0.3875000000000000111, 0.3916666666666666630, 0.3958333333333333148, 0.4000000000000000222, 0.4041666666666666741, 0.4083333333333333259, 0.4124999999999999778, 0.4166666666666666852, 0.4208333333333333370, 0.4249999999999999889, 0.4291666666666666408, 0.4333333333333333481, 0.4375000000000000000, 0.4416666666666666519, 0.4458333333333333592, 0.4500000000000000111, 0.4541666666666666630, 0.4583333333333333148, 0.4625000000000000222, 0.4666666666666666741, 0.4708333333333333259, 0.4749999999999999778, 0.4791666666666666852, 0.4833333333333333370, 0.4874999999999999889, 0.4916666666666666408, 0.4958333333333333481, 0.5000000000000000000, 0.5041666666666666519, 0.5083333333333333037, 0.5124999999999999556, 0.5166666666666667185, 0.5208333333333333703, 0.5250000000000000222, 0.5291666666666666741, 0.5333333333333333259, 0.5374999999999999778, 0.5416666666666666297, 0.5458333333333332815, 0.5500000000000000444, 0.5541666666666666963, 0.5583333333333333481, 0.5625000000000000000, 0.5666666666666666519, 0.5708333333333333037, 0.5749999999999999556, 0.5791666666666667185, 0.5833333333333333703, 0.5875000000000000222, 0.5916666666666666741, 0.5958333333333333259, 0.5999999999999999778, 0.6041666666666666297, 0.6083333333333332815, 0.6125000000000000444, 0.6166666666666666963, 0.6208333333333333481, 0.6250000000000000000, 0.6291666666666666519, 0.6333333333333333037, 0.6374999999999999556, 0.6416666666666667185, 0.6458333333333333703, 0.6500000000000000222, 0.6541666666666666741, 0.6583333333333333259, 0.6624999999999999778, 0.6666666666666666297, 0.6708333333333332815, 0.6750000000000000444, 0.6791666666666666963, 0.6833333333333333481, 0.6875000000000000000, 0.6916666666666666519, 0.6958333333333333037, 0.6999999999999999556, 0.7041666666666667185, 0.7083333333333333703, 0.7125000000000000222, 0.7166666666666666741, 0.7208333333333333259, 0.7249999999999999778, 0.7291666666666666297, 0.7333333333333332815, 0.7375000000000000444, 0.7416666666666666963, 0.7458333333333333481, 0.7500000000000000000, 0.7541666666666666519, 0.7583333333333333037, 0.7624999999999999556, 0.7666666666666667185, 0.7708333333333333703, 0.7750000000000000222, 0.7791666666666666741, 0.7833333333333333259, 0.7874999999999999778, 0.7916666666666666297, 0.7958333333333332815, 0.8000000000000000444, 0.8041666666666666963, 0.8083333333333333481, 0.8125000000000000000, 0.8166666666666666519, 0.8208333333333333037, 0.8249999999999999556, 0.8291666666666667185, 0.8333333333333333703, 0.8375000000000000222, 0.8416666666666666741, 0.8458333333333333259, 0.8499999999999999778, 0.8541666666666666297, 0.8583333333333332815, 0.8625000000000000444, 0.8666666666666666963, 0.8708333333333333481, 0.8750000000000000000, 0.8791666666666666519, 0.8833333333333333037, 0.8874999999999999556, 0.8916666666666667185, 0.8958333333333333703, 0.9000000000000000222, 0.9041666666666666741, 0.9083333333333333259, 0.9124999999999999778, 0.9166666666666666297, 0.9208333333333332815, 0.9250000000000000444, 0.9291666666666666963, 0.9333333333333333481, 0.9375000000000000000, 0.9416666666666666519, 0.9458333333333333037, 0.9499999999999999556, 0.9541666666666667185, 0.9583333333333333703, 0.9625000000000000222, 0.9666666666666666741, 0.9708333333333333259, 0.9749999999999999778, 0.9791666666666666297, 0.9833333333333332815, 0.9875000000000000444, 0.9916666666666666963, 0.9958333333333333481, 1.000000000000000000 ),
 .UNSPECIFIED. ) 
 GEOMETRIC_REPRESENTATION_ITEM ( )  RATIONAL_B_SPLINE_SURFACE ( (
 ( 1.000000000000000000, 0.8660254037844387076, 1.000000000000000000, 0.8660254037844387076, 1.000000000000000000, 0.8660254037844387076, 1.000000000000000000, 0.8660254037844387076, 1.000000000000000000, 0.8660254037844387076, 1.000000000000000000, 0.8660254037844387076, 1.000000000000000000, 0.8660254037844387076, 1.000000000000000000, 0.8660254037844387076, 1.000000000000000000, 0.8660254037844387076, 1.000000000000000000, 0.8660254037844387076, 1.000000000000000000, 0.8660254037844387076, 1.000000000000000000, 0.8660254037844387076, 1.000000000000000000, 0.8660254037844387076, 1.000000000000000000, 0.8660254037844387076, 1.000000000000000000, 0.8660254037844387076, 1.000000000000000000, 0.8660254037844387076, 1.000000000000000000, 0.8660254037844387076, 1.000000000000000000, 0.8660254037844387076, 1.000000000000000000, 0.8660254037844387076, 1.000000000000000000, 0.8660254037844387076, 1.000000000000000000, 0.8660254037844387076, 1.000000000000000000, 0.8660254037844387076, 1.000000000000000000, 0.8660254037844387076, 1.000000000000000000, 0.8660254037844387076, 1.000000000000000000, 0.8660254037844387076, 1.000000000000000000, 0.8660254037844387076, 1.000000000000000000, 0.8660254037844387076, 1.000000000000000000, 0.8660254037844387076, 1.000000000000000000, 0.8660254037844387076, 1.000000000000000000, 0.8660254037844387076, 1.000000000000000000, 0.8660254037844387076, 1.000000000000000000, 0.8660254037844387076, 1.000000000000000000, 0.8660254037844387076, 1.000000000000000000, 0.8660254037844387076, 1.000000000000000000, 0.8660254037844387076, 1.000000000000000000, 0.8660254037844387076, 1.000000000000000000, 0.8660254037844387076, 1.000000000000000000, 0.8660254037844387076, 1.000000000000000000, 0.8660254037844387076, 1.000000000000000000, 0.8660254037844387076, 1.000000000000000000, 0.8660254037844387076, 1.000000000000000000, 0.8660254037844387076, 1.000000000000000000, 0.8660254037844387076, 1.000000000000000000, 0.8660254037844387076, 1.000000000000000000, 0.8660254037844387076, 1.000000000000000000, 0.8660254037844387076, 1.000000000000000000, 0.8660254037844387076, 1.000000000000000000, 0.8660254037844387076, 1.000000000000000000, 0.8660254037844387076, 1.000000000000000000, 0.8660254037844387076, 1.000000000000000000, 0.8660254037844387076, 1.000000000000000000, 0.8660254037844387076, 1.000000000000000000, 0.8660254037844387076, 1.000000000000000000, 0.8660254037844387076, 1.000000000000000000, 0.8660254037844387076, 1.000000000000000000, 0.8660254037844387076, 1.000000000000000000, 0.8660254037844387076, 1.000000000000000000, 0.8660254037844387076, 1.000000000000000000, 0.8660254037844387076, 1.000000000000000000, 0.8660254037844387076, 1.000000000000000000, 0.8660254037844387076, 1.000000000000000000, 0.8660254037844387076, 1.000000000000000000, 0.8660254037844387076, 1.000000000000000000, 0.8660254037844387076, 1.000000000000000000, 0.8660254037844387076, 1.000000000000000000, 0.8660254037844387076, 1.000000000000000000, 0.8660254037844387076, 1.000000000000000000, 0.8660254037844387076, 1.000000000000000000, 0.8660254037844387076, 1.000000000000000000, 0.8660254037844387076, 1.000000000000000000, 0.8660254037844387076, 1.000000000000000000, 0.8660254037844387076, 1.000000000000000000, 0.8660254037844387076, 1.000000000000000000, 0.8660254037844387076, 1.000000000000000000, 0.8660254037844387076, 1.000000000000000000, 0.8660254037844387076, 1.000000000000000000, 0.8660254037844387076, 1.000000000000000000, 0.8660254037844387076, 1.000000000000000000, 0.8660254037844387076, 1.000000000000000000, 0.8660254037844387076, 1.000000000000000000, 0.8660254037844387076, 1.000000000000000000, 0.8660254037844387076, 1.000000000000000000, 0.8660254037844387076, 1.000000000000000000, 0.8660254037844387076, 1.000000000000000000, 0.8660254037844387076, 1.000000000000000000, 0.8660254037844387076, 1.000000000000000000, 0.8660254037844387076, 1.000000000000000000, 0.8660254037844387076, 1.000000000000000000, 0.8660254037844387076, 1.000000000000000000, 0.8660254037844387076, 1.000000000000000000, 0.8660254037844387076, 1.000000000000000000, 0.8660254037844387076, 1.000000000000000000, 0.8660254037844387076, 1.000000000000000000, 0.8660254037844387076, 1.000000000000000000, 0.8660254037844387076, 1.000000000000000000, 0.8660254037844387076, 1.000000000000000000, 0.8660254037844387076, 1.000000000000000000, 0.8660254037844387076, 1.000000000000000000, 0.8660254037844387076, 1.000000000000000000, 0.8660254037844387076, 1.000000000000000000, 0.8660254037844387076, 1.000000000000000000, 0.8660254037844387076, 1.000000000000000000, 0.8660254037844387076, 1.000000000000000000, 0.8660254037844387076, 1.000000000000000000, 0.8660254037844387076, 1.000000000000000000, 0.8660254037844387076, 1.000000000000000000, 0.8660254037844387076, 1.000000000000000000, 0.8660254037844387076, 1.000000000000000000, 0.8660254037844387076, 1.000000000000000000, 0.8660254037844387076, 1.000000000000000000, 0.8660254037844387076, 1.000000000000000000, 0.8660254037844387076, 1.000000000000000000, 0.8660254037844387076, 1.000000000000000000, 0.8660254037844387076, 1.000000000000000000, 0.8660254037844387076, 1.000000000000000000, 0.8660254037844387076, 1.000000000000000000, 0.8660254037844387076, 1.000000000000000000, 0.8660254037844387076, 1.000000000000000000, 0.8660254037844387076, 1.000000000000000000, 0.8660254037844387076, 1.000000000000000000, 0.8660254037844387076, 1.000000000000000000, 0.8660254037844387076, 1.000000000000000000, 0.8660254037844387076, 1.000000000000000000, 0.8660254037844387076, 1.000000000000000000, 0.8660254037844387076, 1.000000000000000000, 0.8660254037844387076, 1.000000000000000000, 0.8660254037844387076, 1.000000000000000000, 0.8660254037844387076, 1.000000000000000000, 0.8660254037844387076, 1.000000000000000000, 0.8660254037844387076, 1.000000000000000000, 0.8660254037844387076, 1.000000000000000000, 0.8660254037844387076, 1.000000000000000000, 0.8660254037844387076, 1.000000000000000000, 0.8660254037844387076, 1.000000000000000000, 0.8660254037844387076, 1.000000000000000000, 0.8660254037844387076, 1.000000000000000000, 0.8660254037844387076, 1.000000000000000000, 0.8660254037844387076, 1.000000000000000000, 0.8660254037844387076, 1.000000000000000000, 0.8660254037844387076, 1.000000000000000000, 0.8660254037844387076, 1.000000000000000000, 0.8660254037844387076, 1.000000000000000000, 0.8660254037844387076, 1.000000000000000000, 0.8660254037844387076, 1.000000000000000000, 0.8660254037844387076, 1.000000000000000000, 0.8660254037844387076, 1.000000000000000000, 0.8660254037844387076, 1.000000000000000000, 0.8660254037844387076, 1.000000000000000000, 0.8660254037844387076, 1.000000000000000000, 0.8660254037844387076, 1.000000000000000000, 0.8660254037844387076, 1.000000000000000000, 0.8660254037844387076, 1.000000000000000000, 0.8660254037844387076, 1.000000000000000000, 0.8660254037844387076, 1.000000000000000000, 0.8660254037844387076, 1.000000000000000000, 0.8660254037844387076, 1.000000000000000000, 0.8660254037844387076, 1.000000000000000000, 0.8660254037844387076, 1.000000000000000000, 0.8660254037844387076, 1.000000000000000000, 0.8660254037844387076, 1.000000000000000000, 0.8660254037844387076, 1.000000000000000000, 0.8660254037844387076, 1.000000000000000000, 0.8660254037844387076, 1.000000000000000000, 0.8660254037844387076, 1.000000000000000000, 0.8660254037844387076, 1.000000000000000000, 0.8660254037844387076, 1.000000000000000000, 0.8660254037844387076, 1.000000000000000000, 0.8660254037844387076, 1.000000000000000000, 0.8660254037844387076, 1.000000000000000000, 0.8660254037844387076, 1.000000000000000000, 0.8660254037844387076, 1.000000000000000000, 0.8660254037844387076, 1.000000000000000000, 0.8660254037844387076, 1.000000000000000000, 0.8660254037844387076, 1.000000000000000000, 0.8660254037844387076, 1.000000000000000000, 0.8660254037844387076, 1.000000000000000000, 0.8660254037844387076, 1.000000000000000000, 0.8660254037844387076, 1.000000000000000000, 0.8660254037844387076, 1.000000000000000000, 0.8660254037844387076, 1.000000000000000000, 0.8660254037844387076, 1.000000000000000000, 0.8660254037844387076, 1.000000000000000000, 0.8660254037844387076, 1.000000000000000000, 0.8660254037844387076, 1.000000000000000000, 0.8660254037844387076, 1.000000000000000000, 0.8660254037844387076, 1.000000000000000000, 0.8660254037844387076, 1.000000000000000000, 0.8660254037844387076, 1.000000000000000000, 0.8660254037844387076, 1.000000000000000000, 0.8660254037844387076, 1.000000000000000000, 0.8660254037844387076, 1.000000000000000000, 0.8660254037844387076, 1.000000000000000000, 0.8660254037844387076, 1.000000000000000000, 0.8660254037844387076, 1.000000000000000000, 0.8660254037844387076, 1.000000000000000000, 0.8660254037844387076, 1.000000000000000000, 0.8660254037844387076, 1.000000000000000000, 0.8660254037844387076, 1.000000000000000000, 0.8660254037844387076, 1.000000000000000000, 0.8660254037844387076, 1.000000000000000000, 0.8660254037844387076, 1.000000000000000000, 0.8660254037844387076, 1.000000000000000000, 0.8660254037844387076, 1.000000000000000000, 0.8660254037844387076, 1.000000000000000000, 0.8660254037844387076, 1.000000000000000000, 0.8660254037844387076, 1.000000000000000000, 0.8660254037844387076, 1.000000000000000000, 0.8660254037844387076, 1.000000000000000000, 0.8660254037844387076, 1.000000000000000000, 0.8660254037844387076, 1.000000000000000000, 0.8660254037844387076, 1.000000000000000000, 0.8660254037844387076, 1.000000000000000000, 0.8660254037844387076, 1.000000000000000000, 0.8660254037844387076, 1.000000000000000000, 0.8660254037844387076, 1.000000000000000000, 0.8660254037844387076, 1.000000000000000000, 0.8660254037844387076, 1.000000000000000000, 0.8660254037844387076, 1.000000000000000000, 0.8660254037844387076, 1.000000000000000000, 0.8660254037844387076, 1.000000000000000000, 0.8660254037844387076, 1.000000000000000000, 0.8660254037844387076, 1.000000000000000000, 0.8660254037844387076, 1.000000000000000000, 0.8660254037844387076, 1.000000000000000000, 0.8660254037844387076, 1.000000000000000000, 0.8660254037844387076, 1.000000000000000000, 0.8660254037844387076, 1.000000000000000000, 0.8660254037844387076, 1.000000000000000000, 0.8660254037844387076, 1.000000000000000000, 0.8660254037844387076, 1.000000000000000000, 0.8660254037844387076, 1.000000000000000000, 0.8660254037844387076, 1.000000000000000000, 0.8660254037844387076, 1.000000000000000000, 0.8660254037844387076, 1.000000000000000000, 0.8660254037844387076, 1.000000000000000000, 0.8660254037844387076, 1.000000000000000000, 0.8660254037844387076, 1.000000000000000000, 0.8660254037844387076, 1.000000000000000000, 0.8660254037844387076, 1.000000000000000000, 0.8660254037844387076, 1.000000000000000000),
 ( 1.000000000000000000, 0.8660254037844387076, 1.000000000000000000, 0.8660254037844387076, 1.000000000000000000, 0.8660254037844387076, 1.000000000000000000, 0.8660254037844387076, 1.000000000000000000, 0.8660254037844387076, 1.000000000000000000, 0.8660254037844387076, 1.000000000000000000, 0.8660254037844387076, 1.000000000000000000, 0.8660254037844387076, 1.000000000000000000, 0.8660254037844387076, 1.000000000000000000, 0.8660254037844387076, 1.000000000000000000, 0.8660254037844387076, 1.000000000000000000, 0.8660254037844387076, 1.000000000000000000, 0.8660254037844387076, 1.000000000000000000, 0.8660254037844387076, 1.000000000000000000, 0.8660254037844387076, 1.000000000000000000, 0.8660254037844387076, 1.000000000000000000, 0.8660254037844387076, 1.000000000000000000, 0.8660254037844387076, 1.000000000000000000, 0.8660254037844387076, 1.000000000000000000, 0.8660254037844387076, 1.000000000000000000, 0.8660254037844387076, 1.000000000000000000, 0.8660254037844387076, 1.000000000000000000, 0.8660254037844387076, 1.000000000000000000, 0.8660254037844387076, 1.000000000000000000, 0.8660254037844387076, 1.000000000000000000, 0.8660254037844387076, 1.000000000000000000, 0.8660254037844387076, 1.000000000000000000, 0.8660254037844387076, 1.000000000000000000, 0.8660254037844387076, 1.000000000000000000, 0.8660254037844387076, 1.000000000000000000, 0.8660254037844387076, 1.000000000000000000, 0.8660254037844387076, 1.000000000000000000, 0.8660254037844387076, 1.000000000000000000, 0.8660254037844387076, 1.000000000000000000, 0.8660254037844387076, 1.000000000000000000, 0.8660254037844387076, 1.000000000000000000, 0.8660254037844387076, 1.000000000000000000, 0.8660254037844387076, 1.000000000000000000, 0.8660254037844387076, 1.000000000000000000, 0.8660254037844387076, 1.000000000000000000, 0.8660254037844387076, 1.000000000000000000, 0.8660254037844387076, 1.000000000000000000, 0.8660254037844387076, 1.000000000000000000, 0.8660254037844387076, 1.000000000000000000, 0.8660254037844387076, 1.000000000000000000, 0.8660254037844387076, 1.000000000000000000, 0.8660254037844387076, 1.000000000000000000, 0.8660254037844387076, 1.000000000000000000, 0.8660254037844387076, 1.000000000000000000, 0.8660254037844387076, 1.000000000000000000, 0.8660254037844387076, 1.000000000000000000, 0.8660254037844387076, 1.000000000000000000, 0.8660254037844387076, 1.000000000000000000, 0.8660254037844387076, 1.000000000000000000, 0.8660254037844387076, 1.000000000000000000, 0.8660254037844387076, 1.000000000000000000, 0.8660254037844387076, 1.000000000000000000, 0.8660254037844387076, 1.000000000000000000, 0.8660254037844387076, 1.000000000000000000, 0.8660254037844387076, 1.000000000000000000, 0.8660254037844387076, 1.000000000000000000, 0.8660254037844387076, 1.000000000000000000, 0.8660254037844387076, 1.000000000000000000, 0.8660254037844387076, 1.000000000000000000, 0.8660254037844387076, 1.000000000000000000, 0.8660254037844387076, 1.000000000000000000, 0.8660254037844387076, 1.000000000000000000, 0.8660254037844387076, 1.000000000000000000, 0.8660254037844387076, 1.000000000000000000, 0.8660254037844387076, 1.000000000000000000, 0.8660254037844387076, 1.000000000000000000, 0.8660254037844387076, 1.000000000000000000, 0.8660254037844387076, 1.000000000000000000, 0.8660254037844387076, 1.000000000000000000, 0.8660254037844387076, 1.000000000000000000, 0.8660254037844387076, 1.000000000000000000, 0.8660254037844387076, 1.000000000000000000, 0.8660254037844387076, 1.000000000000000000, 0.8660254037844387076, 1.000000000000000000, 0.8660254037844387076, 1.000000000000000000, 0.8660254037844387076, 1.000000000000000000, 0.8660254037844387076, 1.000000000000000000, 0.8660254037844387076, 1.000000000000000000, 0.8660254037844387076, 1.000000000000000000, 0.8660254037844387076, 1.000000000000000000, 0.8660254037844387076, 1.000000000000000000, 0.8660254037844387076, 1.000000000000000000, 0.8660254037844387076, 1.000000000000000000, 0.8660254037844387076, 1.000000000000000000, 0.8660254037844387076, 1.000000000000000000, 0.8660254037844387076, 1.000000000000000000, 0.8660254037844387076, 1.000000000000000000, 0.8660254037844387076, 1.000000000000000000, 0.8660254037844387076, 1.000000000000000000, 0.8660254037844387076, 1.000000000000000000, 0.8660254037844387076, 1.000000000000000000, 0.8660254037844387076, 1.000000000000000000, 0.8660254037844387076, 1.000000000000000000, 0.8660254037844387076, 1.000000000000000000, 0.8660254037844387076, 1.000000000000000000, 0.8660254037844387076, 1.000000000000000000, 0.8660254037844387076, 1.000000000000000000, 0.8660254037844387076, 1.000000000000000000, 0.8660254037844387076, 1.000000000000000000, 0.8660254037844387076, 1.000000000000000000, 0.8660254037844387076, 1.000000000000000000, 0.8660254037844387076, 1.000000000000000000, 0.8660254037844387076, 1.000000000000000000, 0.8660254037844387076, 1.000000000000000000, 0.8660254037844387076, 1.000000000000000000, 0.8660254037844387076, 1.000000000000000000, 0.8660254037844387076, 1.000000000000000000, 0.8660254037844387076, 1.000000000000000000, 0.8660254037844387076, 1.000000000000000000, 0.8660254037844387076, 1.000000000000000000, 0.8660254037844387076, 1.000000000000000000, 0.8660254037844387076, 1.000000000000000000, 0.8660254037844387076, 1.000000000000000000, 0.8660254037844387076, 1.000000000000000000, 0.8660254037844387076, 1.000000000000000000, 0.8660254037844387076, 1.000000000000000000, 0.8660254037844387076, 1.000000000000000000, 0.8660254037844387076, 1.000000000000000000, 0.8660254037844387076, 1.000000000000000000, 0.8660254037844387076, 1.000000000000000000, 0.8660254037844387076, 1.000000000000000000, 0.8660254037844387076, 1.000000000000000000, 0.8660254037844387076, 1.000000000000000000, 0.8660254037844387076, 1.000000000000000000, 0.8660254037844387076, 1.000000000000000000, 0.8660254037844387076, 1.000000000000000000, 0.8660254037844387076, 1.000000000000000000, 0.8660254037844387076, 1.000000000000000000, 0.8660254037844387076, 1.000000000000000000, 0.8660254037844387076, 1.000000000000000000, 0.8660254037844387076, 1.000000000000000000, 0.8660254037844387076, 1.000000000000000000, 0.8660254037844387076, 1.000000000000000000, 0.8660254037844387076, 1.000000000000000000, 0.8660254037844387076, 1.000000000000000000, 0.8660254037844387076, 1.000000000000000000, 0.8660254037844387076, 1.000000000000000000, 0.8660254037844387076, 1.000000000000000000, 0.8660254037844387076, 1.000000000000000000, 0.8660254037844387076, 1.000000000000000000, 0.8660254037844387076, 1.000000000000000000, 0.8660254037844387076, 1.000000000000000000, 0.8660254037844387076, 1.000000000000000000, 0.8660254037844387076, 1.000000000000000000, 0.8660254037844387076, 1.000000000000000000, 0.8660254037844387076, 1.000000000000000000, 0.8660254037844387076, 1.000000000000000000, 0.8660254037844387076, 1.000000000000000000, 0.8660254037844387076, 1.000000000000000000, 0.8660254037844387076, 1.000000000000000000, 0.8660254037844387076, 1.000000000000000000, 0.8660254037844387076, 1.000000000000000000, 0.8660254037844387076, 1.000000000000000000, 0.8660254037844387076, 1.000000000000000000, 0.8660254037844387076, 1.000000000000000000, 0.8660254037844387076, 1.000000000000000000, 0.8660254037844387076, 1.000000000000000000, 0.8660254037844387076, 1.000000000000000000, 0.8660254037844387076, 1.000000000000000000, 0.8660254037844387076, 1.000000000000000000, 0.8660254037844387076, 1.000000000000000000, 0.8660254037844387076, 1.000000000000000000, 0.8660254037844387076, 1.000000000000000000, 0.8660254037844387076, 1.000000000000000000, 0.8660254037844387076, 1.000000000000000000, 0.8660254037844387076, 1.000000000000000000, 0.8660254037844387076, 1.000000000000000000, 0.8660254037844387076, 1.000000000000000000, 0.8660254037844387076, 1.000000000000000000, 0.8660254037844387076, 1.000000000000000000, 0.8660254037844387076, 1.000000000000000000, 0.8660254037844387076, 1.000000000000000000, 0.8660254037844387076, 1.000000000000000000, 0.8660254037844387076, 1.000000000000000000, 0.8660254037844387076, 1.000000000000000000, 0.8660254037844387076, 1.000000000000000000, 0.8660254037844387076, 1.000000000000000000, 0.8660254037844387076, 1.000000000000000000, 0.8660254037844387076, 1.000000000000000000, 0.8660254037844387076, 1.000000000000000000, 0.8660254037844387076, 1.000000000000000000, 0.8660254037844387076, 1.000000000000000000, 0.8660254037844387076, 1.000000000000000000, 0.8660254037844387076, 1.000000000000000000, 0.8660254037844387076, 1.000000000000000000, 0.8660254037844387076, 1.000000000000000000, 0.8660254037844387076, 1.000000000000000000, 0.8660254037844387076, 1.000000000000000000, 0.8660254037844387076, 1.000000000000000000, 0.8660254037844387076, 1.000000000000000000, 0.8660254037844387076, 1.000000000000000000, 0.8660254037844387076, 1.000000000000000000, 0.8660254037844387076, 1.000000000000000000, 0.8660254037844387076, 1.000000000000000000, 0.8660254037844387076, 1.000000000000000000, 0.8660254037844387076, 1.000000000000000000, 0.8660254037844387076, 1.000000000000000000, 0.8660254037844387076, 1.000000000000000000, 0.8660254037844387076, 1.000000000000000000, 0.8660254037844387076, 1.000000000000000000, 0.8660254037844387076, 1.000000000000000000, 0.8660254037844387076, 1.000000000000000000, 0.8660254037844387076, 1.000000000000000000, 0.8660254037844387076, 1.000000000000000000, 0.8660254037844387076, 1.000000000000000000, 0.8660254037844387076, 1.000000000000000000, 0.8660254037844387076, 1.000000000000000000, 0.8660254037844387076, 1.000000000000000000, 0.8660254037844387076, 1.000000000000000000, 0.8660254037844387076, 1.000000000000000000, 0.8660254037844387076, 1.000000000000000000, 0.8660254037844387076, 1.000000000000000000, 0.8660254037844387076, 1.000000000000000000, 0.8660254037844387076, 1.000000000000000000, 0.8660254037844387076, 1.000000000000000000, 0.8660254037844387076, 1.000000000000000000, 0.8660254037844387076, 1.000000000000000000, 0.8660254037844387076, 1.000000000000000000, 0.8660254037844387076, 1.000000000000000000, 0.8660254037844387076, 1.000000000000000000, 0.8660254037844387076, 1.000000000000000000, 0.8660254037844387076, 1.000000000000000000, 0.8660254037844387076, 1.000000000000000000, 0.8660254037844387076, 1.000000000000000000, 0.8660254037844387076, 1.000000000000000000, 0.8660254037844387076, 1.000000000000000000, 0.8660254037844387076, 1.000000000000000000, 0.8660254037844387076, 1.000000000000000000, 0.8660254037844387076, 1.000000000000000000, 0.8660254037844387076, 1.000000000000000000, 0.8660254037844387076, 1.000000000000000000, 0.8660254037844387076, 1.000000000000000000, 0.8660254037844387076, 1.000000000000000000, 0.8660254037844387076, 1.000000000000000000, 0.8660254037844387076, 1.000000000000000000) ) ) 
 REPRESENTATION_ITEM ( '' )  SURFACE ( )  );
#195076=AXIS2_PLACEMENT_3D ( 'NONE', #44195, #142785, #110315 ) ;
#195079=CARTESIAN_POINT ( 'NONE',  ( 8.107412671292047790, 8.560995659369956101, 0.7216878364870458196 ) ) ;
#195095=CARTESIAN_POINT ( 'NONE',  ( -1.598423149420378220, 8.713846000021357341, 2.499999999999998668 ) ) ;
#195112=CARTESIAN_POINT ( 'NONE',  ( 1.499999999999989120, 1.785416667349487563, 0.8660254037844524744 ) ) ;
#195118=CARTESIAN_POINT ( 'NONE',  ( 8.483651433849084711, 10.92067931095586886, 1.599625672291281386 ) ) ;
#195121=CARTESIAN_POINT ( 'NONE',  ( 0.6823417656249864960, -1.073958332991911568, -1.181850606188749264 ) ) ;
#195124=CARTESIAN_POINT ( 'NONE',  ( 2.361091307074211887, 5.906356958228550447, 0.7998128361456462443 ) ) ;
#195125=CARTESIAN_POINT ( 'NONE',  ( -6.887178846062128379, 7.137389529935019183, -0.7216878364870278340 ) ) ;
#195129=CARTESIAN_POINT ( 'NONE',  ( -5.208303565944065738, 9.228104593576741621, -0.7998128361456231517 ) ) ;
#195133=CARTESIAN_POINT ( 'NONE',  ( -1.402160292154681736E-14, 1.118750000682820378, -1.732050807568863648 ) ) ;
#195141=CARTESIAN_POINT ( 'NONE',  ( -4.595850884908229794, 4.464173575255435011, 0.7216878364870317197 ) ) ;
#195146=CARTESIAN_POINT ( 'NONE',  ( 4.815628398899983509, 6.730757278346135131, 1.248813279183153657 ) ) ;
#195147=CARTESIAN_POINT ( 'NONE',  ( 4.114536431845257525, 3.902640046681976393, 1.214306433183764966E-14 ) ) ;
#195151=CARTESIAN_POINT ( 'NONE',  ( -8.455481356417053007, 13.01647868246193518, 0.7998128361456341429 ) ) ;
#195152=CARTESIAN_POINT ( 'NONE',  ( 8.457588896826466751, 8.761608555919362828, 1.040834085586084257E-14 ) ) ;
#195159=CARTESIAN_POINT ( 'NONE',  ( -6.471393748265563239, 5.229711127717889596, 2.499999999999998668 ) ) ;
#195160=CARTESIAN_POINT ( 'NONE',  ( -7.049349804101573191, 10.31165964050546258, -1.199719254218440723 ) ) ;
#195163=VERTEX_POINT ( 'NONE', #156456 ) ;
#195166=CARTESIAN_POINT ( 'NONE',  ( 2.855963913973019963, 6.483708332943829866, 0.000000000000000000 ) ) ;
#195170=VERTEX_POINT ( 'NONE', #75199 ) ;
#195171=CARTESIAN_POINT ( 'NONE',  ( -10.29471871147821282, 10.90492667301307605, -0.7998128361456291469 ) ) ;
#195174=CARTESIAN_POINT ( 'NONE',  ( -4.868901516392104334, 6.903810023003053686, -1.445308410833840318 ) ) ;
#195183=CARTESIAN_POINT ( 'NONE',  ( 7.096803341749390981, 10.36702210109460154, -1.199719254218441611 ) ) ;
#195185=CARTESIAN_POINT ( 'NONE',  ( -3.867100128395853709, 5.534702787927018974, -1.599625672291256295 ) ) ;
#195191=CARTESIAN_POINT ( 'NONE',  ( 1.499999999999985123, -0.1729166659838496101, -0.8660254037844323793 ) ) ;
#195194=CARTESIAN_POINT ( 'NONE',  ( 2.191614386903386613, 5.708633884695917260, -0.7998128361456281477 ) ) ;
#195196=CARTESIAN_POINT ( 'NONE',  ( -4.471491734408701291, 4.111161866431900513, 1.214306433183764966E-14 ) ) ;
#195202=CARTESIAN_POINT ( 'NONE',  ( 3.551873057100274789, 7.087676300018221021, 0.7216878364870298324 ) ) ;
#195204=EDGE_LOOP ( 'NONE', ( #113834, #210241, #100497, #102032, #127974, #115428, #119402, #57551, #52711, #158537, #3239, #192337, #142177, #126891, #190210, #188599, #92816, #167570, #151140, #103070, #108634, #204039, #80602, #168904, #90097 ) ) ;
#195205=CARTESIAN_POINT ( 'NONE',  ( -9.378489572351046633, 11.96465713920816043, -1.599625672291263179 ) ) ;
#195207=CARTESIAN_POINT ( 'NONE',  ( 10.40996301719436090, 11.03937836301526687, 0.000000000000000000 ) ) ;
#195218=CARTESIAN_POINT ( 'NONE',  ( -1.402160292154681736E-14, -0.1781249996585796136, 1.575800808251672791 ) ) ;
#195222=CARTESIAN_POINT ( 'NONE',  ( -4.229253852459088137, 7.021547696922494808, 1.199719254218464037 ) ) ;
#195226=CARTESIAN_POINT ( 'NONE',  ( 1.499999999999990896, 4.525000000000021672, 1.214306433183764966E-14 ) ) ;
#195233=CARTESIAN_POINT ( 'NONE',  ( -1.364683531250000748, -0.9906249996585805295, 0.000000000000000000 ) ) ;
#195235=CARTESIAN_POINT ( 'NONE',  ( 5.262536180398716290, 9.291375977107183104, -0.7998128361456291469 ) ) ;
#195237=CARTESIAN_POINT ( 'NONE',  ( -9.189729191964438826, 9.615772233580322848, 1.040834085586084257E-14 ) ) ;
#195242=VERTEX_POINT ( 'NONE', #71959 ) ;
#195245=CARTESIAN_POINT ( 'NONE',  ( -1.364683531250014514, -0.9489583329919112353, -0.7879004041258359514 ) ) ;
#195253=CARTESIAN_POINT ( 'NONE',  ( 8.459924665247367415, 8.972259652317825740, -0.7216878364870267237 ) ) ;
#195258=CARTESIAN_POINT ( 'NONE',  ( 0.7499999999999902300, 4.097916667349481123, -1.299038105676658228 ) ) ;
#195261=CARTESIAN_POINT ( 'NONE',  ( -2.578021764892882040, 6.159442492350315490, 0.7998128361456341429 ) ) ;
#195262=CARTESIAN_POINT ( 'NONE',  ( 6.982085920913413624, 8.208483664896217391, -1.082531754730543971 ) ) ;
#195263=CARTESIAN_POINT ( 'NONE',  ( -9.775065565328603157, 11.46695991671396087, -1.082531754730537976 ) ) ;
#195269=CARTESIAN_POINT ( 'NONE',  ( 3.277320446201373638, 4.846626492033466072, 1.599625672291267398 ) ) ;
#195272=EDGE_LOOP ( 'NONE', ( #204565, #75127, #69775, #77677 ) ) ;
#195278=CARTESIAN_POINT ( 'NONE',  ( -2.193105066167346795, 5.702484939155337607, 2.500000000000011102 ) ) ;
#195282=CARTESIAN_POINT ( 'NONE',  ( 0.9486429539237075659, 3.230410930033764227, -1.028101543438967758 ) ) ;
#195287=CARTESIAN_POINT ( 'NONE',  ( 7.377608144130607393, 11.75895993479440982, -0.7998128361456291469 ) ) ;
#195291=CARTESIAN_POINT ( 'NONE',  ( -1.402160292154681736E-14, -0.6781249996585819728, 1.575800808251672791 ) ) ;
#195292=CARTESIAN_POINT ( 'NONE',  ( 6.317736394288147039, 6.473040002865377396, 0.7216878364870317197 ) ) ;
#195294=CARTESIAN_POINT ( 'NONE',  ( -7.998947442382709383, 12.27592974951444660, 0.7216878364870478180 ) ) ;
#195300=CARTESIAN_POINT ( 'NONE',  ( -2.740719608256871442, 6.349256642941639051, 0.7998128361456341429 ) ) ;
#195303=ORIENTED_EDGE ( 'NONE', *, *, #15281, .T. ) ;
#195305=ORIENTED_EDGE ( 'NONE', *, *, #149058, .F. ) ;
#195314=CARTESIAN_POINT ( 'NONE',  ( 4.357662274398333757, 7.395159486995275699, -1.145423081618229144 ) ) ;
#195319=CARTESIAN_POINT ( 'NONE',  ( -4.038416155542518204, 7.756558617010888668, -0.6477684560860890173 ) ) ;
#195322=CARTESIAN_POINT ( 'NONE',  ( -6.371969008742801144, 10.37778824360119145, 0.7216878364870458196 ) ) ;
#195326=CARTESIAN_POINT ( 'NONE',  ( 6.317209508963599340, 9.457495962844502557, 1.199719254218462483 ) ) ;
#195327=CARTESIAN_POINT ( 'NONE',  ( -3.653032323878261600, 6.349289246911547835, -1.199719254218452047 ) ) ;
#195330=CARTESIAN_POINT ( 'NONE',  ( -6.084912014434944894, 5.993485526462540847, -0.7998128361456291469 ) ) ;
#195333=CARTESIAN_POINT ( 'NONE',  ( -6.579784621333750749, 6.570836901177822931, 0.7998128361456341429 ) ) ;
#195336=CARTESIAN_POINT ( 'NONE',  ( 7.727257484784855635, 11.10255193463598111, -1.199719254218446718 ) ) ;
#195337=LINE ( 'NONE', #12294, #160110 ) ;
#195339=CARTESIAN_POINT ( 'NONE',  ( 4.048816217420559305, 7.761621341895022397, 0.4883610165275272808 ) ) ;
#195340=CARTESIAN_POINT ( 'NONE',  ( 5.355107487717867265, 5.349972945200037522, 1.040834085586084257E-14 ) ) ;
#195342=DIRECTION ( 'NONE',  ( 1.000000000000000000, 0.000000000000000000, 0.000000000000000000 ) ) ;
#195347=CARTESIAN_POINT ( 'NONE',  ( 6.765155463094751909, 8.915767345075790828, 1.443375672974076540 ) ) ;
#195351=CARTESIAN_POINT ( 'NONE',  ( -8.123306592882240551, 12.62894145833798376, 0.000000000000000000 ) ) ;
#195352=CARTESIAN_POINT ( 'NONE',  ( -6.527360889975461156, 9.702672574024962415, 1.199719254218452047 ) ) ;
#195360=CARTESIAN_POINT ( 'NONE',  ( 9.413438726589914651, 9.876766690643398405, 0.000000000000000000 ) ) ;
#195365=CARTESIAN_POINT ( 'NONE',  ( 3.765413976293345844, 5.416068943807445635, 1.599625672291267398 ) ) ;
#195368=CARTESIAN_POINT ( 'NONE',  ( 0.7499999999999920064, 5.014583334016150751, 1.299038105676669330 ) ) ;
#195374=CARTESIAN_POINT ( 'NONE',  ( -0.7500000000000215383, 3.191666666666689967, 1.299038105676671107 ) ) ;
#195375=CARTESIAN_POINT ( 'NONE',  ( 6.823831386379729302, 6.855558127064808716, -0.7998128361456281477 ) ) ;
#195378=CARTESIAN_POINT ( 'NONE',  ( 6.643132081016105417, 10.69414516125339887, 0.7216878364870438212 ) ) ;
#195379=CARTESIAN_POINT ( 'NONE',  ( -9.829298179783291900, 11.53023130024440768, 1.082531754730558626 ) ) ;
#195383=CARTESIAN_POINT ( 'NONE',  ( 9.541187415715040032, 12.15447128979948310, -1.599625672291262513 ) ) ;
#195386=CARTESIAN_POINT ( 'NONE',  ( -4.009460741339347045, 5.700790169694431420, -1.599625672291256295 ) ) ;
#195388=CARTESIAN_POINT ( 'NONE',  ( -1.201851678989727383E-14, 4.868750000682822154, -1.732050807568863648 ) ) ;
#195390=CARTESIAN_POINT ( 'NONE',  ( -1.402160292154681736E-14, 0.5718750003414239114, 1.575800808251672791 ) ) ;
#195394=CARTESIAN_POINT ( 'NONE',  ( 3.388648328411762556, 6.040841252200647382, 1.199719254218462483 ) ) ;
#195396=CARTESIAN_POINT ( 'NONE',  ( -0.6823417656249969321, 5.780208333674756283, -1.181850606188749264 ) ) ;
#195399=FACE_OUTER_BOUND ( 'NONE', #71418, .T. ) ;
#195406=CARTESIAN_POINT ( 'NONE',  ( -5.852315862593199469, 9.979452273000736895, 0.7998128361456481317 ) ) ;
#195410=CARTESIAN_POINT ( 'NONE',  ( 6.505214776458575265, 6.483838748823460563, 1.040834085586084257E-14 ) ) ;
#195416=CARTESIAN_POINT ( 'NONE',  ( 8.398386088661320414, 11.88553530582519357, -1.199719254218446718 ) ) ;
#195419=CARTESIAN_POINT ( 'NONE',  ( -6.389970470742427189, 6.349387058821269747, -0.7998128361456291469 ) ) ;
#195423=CARTESIAN_POINT ( 'NONE',  ( 8.378048858240820351, 11.86180853700128601, -1.199719254218446718 ) ) ;
#195425=CARTESIAN_POINT ( 'NONE',  ( 7.293396569147545527, 10.59638086639245280, 1.199719254218460707 ) ) ;
#195428=CARTESIAN_POINT ( 'NONE',  ( -9.083599731475995753, 11.62061899152058686, 1.443375672974064550 ) ) ;
#195429=CARTESIAN_POINT ( 'NONE',  ( -6.612626235163205024, 8.737816579155630592, -1.599625672291263179 ) ) ;
#195434=CARTESIAN_POINT ( 'NONE',  ( -5.544970132138452357, 6.385306161890050625, 1.248999107086716798 ) ) ;
#195435=CARTESIAN_POINT ( 'NONE',  ( 0.6823417656249899377, 0.5927083336747518416, 1.181850606188755259 ) ) ;
#195438=CARTESIAN_POINT ( 'NONE',  ( 7.619319141200070256, 8.951922421897323900, 1.082531754730558626 ) ) ;
#195450=CIRCLE ( 'NONE', #181646, 4.021913119055696484 ) ;
#195456=CARTESIAN_POINT ( 'NONE',  ( 10.58621901417202515, 11.24501035948919991, -0.7998128361456281477 ) ) ;
#195460=CARTESIAN_POINT ( 'NONE',  ( -4.620631424159025613, 4.285158171140619032, -0.7998128361456221525 ) ) ;
#195461=CARTESIAN_POINT ( 'NONE',  ( -6.507023659554960204, 9.678945805201045971, 1.199719254218452047 ) ) ;
#195467=CARTESIAN_POINT ( 'NONE',  ( -1.499999999999997780, 2.931250000682818158, 1.214306433183764966E-14 ) ) ;
#195468=CARTESIAN_POINT ( 'NONE',  ( 6.903072767652295383, 11.20533532890304684, 1.040834085586084257E-14 ) ) ;
#195471=CARTESIAN_POINT ( 'NONE',  ( -7.666245793523398078, 11.03137162816423356, 1.199719254218453823 ) ) ;
#195473=CARTESIAN_POINT ( 'NONE',  ( -1.201851678989727383E-14, 3.821875000341423689, 1.575800808251672791 ) ) ;
#195477=CARTESIAN_POINT ( 'NONE',  ( -8.161645285746702783, 12.46574390010577105, 0.7216878364870478180 ) ) ;
#195481=CARTESIAN_POINT ( 'NONE',  ( 1.364683531249988757, 1.446875000341421469, 0.000000000000000000 ) ) ;
#195488=CARTESIAN_POINT ( 'NONE',  ( -1.364683531250012516, 2.488541667008088876, -0.7879004041258289570 ) ) ;
#195490=CARTESIAN_POINT ( 'NONE',  ( -4.737684612971557740, 7.614716917520386374, 1.199719254218464037 ) ) ;
#195491=CARTESIAN_POINT ( 'NONE',  ( 7.263417608619159083, 9.497073181520933716, -1.599625672291262513 ) ) ;
#195494=CARTESIAN_POINT ( 'NONE',  ( -1.364683531250012516, 2.592708333674753174, 0.7879004041258379498 ) ) ;
#195497=CARTESIAN_POINT ( 'NONE',  ( -1.364683531250014514, -0.5114583329919092369, -0.7879004041258359514 ) ) ;
#195498=CARTESIAN_POINT ( 'NONE',  ( -5.178851490740209229, 7.065079377328788546, 1.443375672974064550 ) ) ;
#195501=CARTESIAN_POINT ( 'NONE',  ( 4.311129659465574804, 7.013106455143060636, -1.082531754730548412 ) ) ;
#195504=CARTESIAN_POINT ( 'NONE',  ( -7.232384877886063990, 10.52520055992070525, -1.199719254218446718 ) ) ;
#195505=CARTESIAN_POINT ( 'NONE',  ( -2.415323921528888196, 5.969628341758991930, 0.7998128361456341429 ) ) ;
#195507=CARTESIAN_POINT ( 'NONE',  ( -1.364683531249997417, 5.009375000341425022, 1.214306433183764966E-14 ) ) ;
#195513=CARTESIAN_POINT ( 'NONE',  ( -7.361714222096077620, 7.691014135307965738, 0.7216878364870317197 ) ) ;
#195515=CARTESIAN_POINT ( 'NONE',  ( -1.364683531250000748, -0.4281249996585800854, 0.000000000000000000 ) ) ;
#195518=CARTESIAN_POINT ( 'NONE',  ( 6.317736394288122170, 10.31451686007074997, 0.7216878364870438212 ) ) ;
#195528=CARTESIAN_POINT ( 'NONE',  ( 10.20892648096591770, 11.01276177065614981, -0.7216878364870257245 ) ) ;
#195535=EDGE_CURVE ( 'NONE', #3330, #97860, #185143, .T. ) ;
#195537=CARTESIAN_POINT ( 'NONE',  ( 6.959412922516382771, 7.013736585890911535, 0.7998128361456341429 ) ) ;
#195538=CARTESIAN_POINT ( 'NONE',  ( -4.925689880466507908, 4.641059703499347044, -0.7998128361456221525 ) ) ;
#195543=CARTESIAN_POINT ( 'NONE',  ( 5.951666246274797345, 7.966696592119163256, 1.443375672974062551 ) ) ;
#195544=CARTESIAN_POINT ( 'NONE',  ( 0.6823417656249899377, 0.6552083336747518416, 1.181850606188755259 ) ) ;
#195546=CARTESIAN_POINT ( 'NONE',  ( -9.267161690140662600, 10.77044237904097734, -1.199719254218441611 ) ) ;
#195551=CARTESIAN_POINT ( 'NONE',  ( -0.7500000000000215383, 5.691666666666685082, 1.299038105676671107 ) ) ;
#195553=( BOUNDED_SURFACE ( )  B_SPLINE_SURFACE ( 1, 2, ( 
 ( #164297, #117743, #35342, #113486, #183735, #33222, #148057, #166423, #101421, #167493, #130802, #100354, #47374, #14824, #2822, #133963, #195738, #16948, #198894, #50540, #163242, #80916, #67816, #196794, #31115, #15886, #116663, #147006, #99306, #179493, #85169, #19089, #182661, #34281, #18014, #84103, #150190, #213024, #151253, #1759, #32165, #48435, #114551, #98242, #81970, #214063, #131839, #153375, #39620, #123114, #7094, #38561, #119873, #122028, #185852, #3886, #168554, #71023, #37484, #202082, #53741, #139273, #152309, #24412, #23350, #189073, #103561, #137137, #4946, #170684, #154448, #104637, #118799, #105725, #20153, #201027, #86238, #21204, #169620, #87306, #203165, #36411, #136068, #54810, #8182, #120958, #186929, #88380, #22271, #6028, #73167, #40707, #52669, #72097, #171754, #69956, #138207, #204219, #55872, #205303, #187995, #135012, #89460, #155513, #56942, #106811, #184785, #172841, #90526, #156588, #102490, #160846, #112166, #26562, #191186, #126292, #94797, #28711, #174980, #194403, #158713, #157656, #177096, #161925, #207448, #78517, #74266, #25498, #91606, #107899, #178169, #209562, #46045, #140359, #61207, #108960, #193335, #76384, #206377, #29785, #41785, #77452, #159773, #9254, #173925, #95869, #142493, #93733, #10310, #192251, #58004, #75325, #44981, #141442, #124168, #11372, #59067, #42853, #190130, #125228, #111089, #43913, #92669, #208500, #110027, #210649, #143570, #62275, #60135, #27633, #127365, #12438, #128436, #176041, #144634, #149932, #66500, #1501, #99050, #212773, #115356, #32974, #31920, #165105, #114299, #63341, #47114, #213823, #181347, #79587, #83843, #15635, #116412, #130553, #164056, #145706, #48188, #34032, #129500, #97998, #183477, #13515, #196545, #50293, #117486, #81722, #180297, #113231, #101156, #35084, #195481, #67567, #147804, #166165, #65441, #131592, #197593, #49237, #179236, #133710, #428, #16697, #82782, #199716, #51363, #211705, #30860, #148855, #132639, #198645, #96937, #162987, #14568, #182402, #80664, #146755, #64409, #17753, #100105, #136883, #104381, #22015, #134765, #68642, #39371, #36155, #2570, #135814, #202910, #200773, #4694, #40455, #56693, #155262, #87050, #70769, #54554, #3632, #23093, #201837, #53482, #154195, #167242, #52424, #169368, #120701, #118550, #139026, #203972, #151002, #121774, #18830, #184532, #84914, #102234, #153123, #187743, #89208, #168305, #186676, #171501, #6843, #38303, #88125, #205050, #170428, #19902, #85987, #20953, #152062, #5763, #71843, #119620, #72921, #122860, #69710, #188821, #137952, #185604, #55619, #37235, #103307, #105468, #11119, #172586, #140100, #128186, #44729, #194147, #76137, #43663, #175788, #74007, #7922, #193077, #189885, #156336, #75074, #142240, #206127, #158460, #106557, #210389, #94549, #26307, #10061, #208252, #157407, #176842, #141187, #207197, #93481, #24165, #57757, #108706, #59886, #123917 ),
 ( #41527, #209308, #90268, #25246, #110837, #107639, #173671, #91346, #8999, #144389, #27380, #12194, #58822, #159520, #124975, #77195, #174735, #190936, #78265, #42600, #109779, #191998, #92421, #126035, #143315, #60955, #127112, #28455, #160587, #62031, #161672, #131346, #13265, #148608, #31666, #79338, #178988, #95621, #211452, #197341, #47937, #114051, #180044, #97743, #145455, #132393, #115101, #112976, #213571, #29530, #48983, #64161, #163802, #111916, #14310, #65192, #16442, #32714, #196291, #46863, #147549, #30602, #63086, #129256, #146502, #96691, #195226, #162738, #98796, #80405, #66245, #181098, #212519, #198395, #164850, #130303, #82521, #15378, #177, #81472, #50036, #177916, #45795, #144007, #12868, #111525, #142931, #9682, #11810, #75759, #108330, #58444, #175408, #141868, #92037, #158094, #29144, #42213, #128851, #127809, #78941, #207877, #26991, #43281, #60566, #44340, #208931, #8613, #209999, #124598, #90961, #190558, #125657, #59500, #191619, #109402, #140799, #25929, #93098, #112591, #159139, #10741, #192686, #76811, #126725, #177531, #145066, #157027, #110462, #61641, #174350, #176462, #28075, #94168, #95233, #160209, #24859, #77885, #193763, #45409, #161281, #74695, #211069, #62692, #194834, #46468, #206810, #1941, #130975, #81086, #16059, #199074, #133076, #64829, #84285, #48603, #47550, #66934, #51805, #97360, #182846, #178603, #129925, #195913, #212130, #68003, #99478, #150371, #30211, #165536, #213200, #83205, #180716, #96297, #134143, #146117, #181766, #49654, #113660, #63766, #200151, #32342, #198024, #114721, #82143, #162352, #179665, #149287, #31284, #13932, #115777, #163417, #147174, #80014, #14993, #868, #148235, #214237, #132015, #33399, #196965, #50720, #98408, #164472, #34465, #65865, #17129, #116845, #100536, #166611, #18199, #59557, #192744, #126788, #109459, #45467, #212193, #95296, #63831, #31347, #29206, #145123, #128913, #129989, #43339, #94228, #195977, #194894, #47610, #161345, #60626, #177594, #12926, #160266, #79006, #176520, #125716, #175465, #61700, #211129, #141923, #146178, #77945, #178662, #44399, #11868, #207935, #110520, #96359, #191677, #144066, #97421, #75815, #28132, #112653, #179728, #210061, #127869, #27050, #163475, #93158, #159196, #113724, #193819, #13991, #111584, #62753, #46532, #30274, #10796, #76870, #162414, #80075, #142990, #208990, #69134, #147234, #3064, #66996, #181827, #200206, #135256, #201270, #98468, #134197, #81149, #48662, #36652, #167731, #102738, #199133, #166669, #84343, #197025, #131035, #101663, #164533, #64889, #198085, #50778, #114778, #133134, #15057, #119043, #52910, #149349, #116906, #182905, #65927, #85410, #49712, #115841, #1996, #213262, #180776, #17188, #34522, #32402, #185027, #51859, #16119, #183972, #82202, #148295, #214293, #132074, #929, #33460, #117981, #83263, #99536, #165597, #100594, #18260, #150431, #68061, #35584 ) ),
 .UNSPECIFIED., .F., .F., .T. ) 
 B_SPLINE_SURFACE_WITH_KNOTS ( ( 2, 2 ),
 ( 3, 2, 2, 2, 2, 2, 2, 2, 2, 2, 2, 2, 2, 2, 2, 2, 2, 2, 2, 2, 2, 2, 2, 2, 2, 2, 2, 2, 2, 2, 2, 2, 2, 2, 2, 2, 2, 2, 2, 2, 2, 2, 2, 2, 2, 2, 2, 2, 2, 2, 2, 2, 2, 2, 2, 2, 2, 2, 2, 2, 2, 2, 2, 2, 2, 2, 2, 2, 2, 2, 2, 2, 2, 2, 2, 2, 2, 2, 2, 2, 2, 2, 2, 2, 2, 2, 2, 2, 2, 2, 2, 2, 2, 2, 2, 2, 2, 2, 2, 2, 2, 2, 2, 2, 2, 2, 2, 2, 2, 2, 2, 2, 2, 2, 2, 2, 2, 2, 2, 2, 2, 2, 2, 2, 2, 2, 2, 2, 2, 2, 2, 2, 2, 2, 2, 2, 2, 2, 2, 2, 2, 2, 2, 2, 2, 2, 2, 2, 2, 2, 2, 2, 2, 2, 2, 2, 2, 2, 2, 2, 2, 2, 2, 2, 2, 2, 2, 2, 3 ),
 ( 0.000000000000000000, 1.000000000000000000 ),
 ( 0.000000000000000000, 0.005952380952380952051, 0.01190476190476190410, 0.01785714285714285615, 0.02380952380952380820, 0.02976190476190476025, 0.03571428571428571230, 0.04166666666666666435, 0.04761904761904761640, 0.05357142857142856845, 0.05952380952380952051, 0.06547619047619047949, 0.07142857142857142461, 0.07738095238095238360, 0.08333333333333332871, 0.08928571428571428770, 0.09523809523809523281, 0.1011904761904761918, 0.1071428571428571369, 0.1130952380952380959, 0.1190476190476190410, 0.1250000000000000000, 0.1309523809523809590, 0.1369047619047619180, 0.1428571428571428492, 0.1488095238095238082, 0.1547619047619047672, 0.1607142857142857262, 0.1666666666666666574, 0.1726190476190476164, 0.1785714285714285754, 0.1845238095238095344, 0.1904761904761904656, 0.1964285714285714246, 0.2023809523809523836, 0.2083333333333333426, 0.2142857142857142738, 0.2202380952380952328, 0.2261904761904761918, 0.2321428571428571508, 0.2380952380952380820, 0.2440476190476190410, 0.2500000000000000000, 0.2559523809523809312, 0.2619047619047619180, 0.2678571428571428492, 0.2738095238095238360, 0.2797619047619047672, 0.2857142857142856984, 0.2916666666666666852, 0.2976190476190476164, 0.3035714285714285476, 0.3095238095238095344, 0.3154761904761904656, 0.3214285714285714524, 0.3273809523809523836, 0.3333333333333333148, 0.3392857142857143016, 0.3452380952380952328, 0.3511904761904761640, 0.3571428571428571508, 0.3630952380952380820, 0.3690476190476190688, 0.3750000000000000000, 0.3809523809523809312, 0.3869047619047619180, 0.3928571428571428492, 0.3988095238095238360, 0.4047619047619047672, 0.4107142857142856984, 0.4166666666666666852, 0.4226190476190476164, 0.4285714285714285476, 0.4345238095238095344, 0.4404761904761904656, 0.4464285714285714524, 0.4523809523809523836, 0.4583333333333333148, 0.4642857142857143016, 0.4702380952380952328, 0.4761904761904761640, 0.4821428571428571508, 0.4880952380952380820, 0.4940476190476190688, 0.5000000000000000000, 0.5059523809523809312, 0.5119047619047618625, 0.5178571428571429047, 0.5238095238095238360, 0.5297619047619047672, 0.5357142857142856984, 0.5416666666666666297, 0.5476190476190476719, 0.5535714285714286031, 0.5595238095238095344, 0.5654761904761904656, 0.5714285714285713969, 0.5773809523809523281, 0.5833333333333333703, 0.5892857142857143016, 0.5952380952380952328, 0.6011904761904761640, 0.6071428571428570953, 0.6130952380952381375, 0.6190476190476190688, 0.6250000000000000000, 0.6309523809523809312, 0.6369047619047618625, 0.6428571428571429047, 0.6488095238095238360, 0.6547619047619047672, 0.6607142857142856984, 0.6666666666666666297, 0.6726190476190476719, 0.6785714285714286031, 0.6845238095238095344, 0.6904761904761904656, 0.6964285714285713969, 0.7023809523809523281, 0.7083333333333333703, 0.7142857142857143016, 0.7202380952380952328, 0.7261904761904761640, 0.7321428571428570953, 0.7380952380952381375, 0.7440476190476190688, 0.7500000000000000000, 0.7559523809523809312, 0.7619047619047618625, 0.7678571428571429047, 0.7738095238095238360, 0.7797619047619047672, 0.7857142857142856984, 0.7916666666666666297, 0.7976190476190476719, 0.8035714285714286031, 0.8095238095238095344, 0.8154761904761904656, 0.8214285714285713969, 0.8273809523809523281, 0.8333333333333333703, 0.8392857142857143016, 0.8452380952380952328, 0.8511904761904761640, 0.8571428571428570953, 0.8630952380952381375, 0.8690476190476190688, 0.8750000000000000000, 0.8809523809523809312, 0.8869047619047618625, 0.8928571428571429047, 0.8988095238095238360, 0.9047619047619047672, 0.9107142857142856984, 0.9166666666666666297, 0.9226190476190476719, 0.9285714285714286031, 0.9345238095238095344, 0.9404761904761904656, 0.9464285714285713969, 0.9523809523809523281, 0.9583333333333333703, 0.9642857142857143016, 0.9702380952380952328, 0.9761904761904761640, 0.9821428571428570953, 0.9880952380952381375, 0.9940476190476190688, 1.000000000000000000 ),
 .UNSPECIFIED. ) 
 GEOMETRIC_REPRESENTATION_ITEM ( )  RATIONAL_B_SPLINE_SURFACE ( (
 ( 1.000000000000000000, 0.8660254037844387076, 1.000000000000000000, 0.8660254037844387076, 1.000000000000000000, 0.8660254037844387076, 1.000000000000000000, 0.8660254037844387076, 1.000000000000000000, 0.8660254037844387076, 1.000000000000000000, 0.8660254037844387076, 1.000000000000000000, 0.8660254037844387076, 1.000000000000000000, 0.8660254037844387076, 1.000000000000000000, 0.8660254037844387076, 1.000000000000000000, 0.8660254037844387076, 1.000000000000000000, 0.8660254037844387076, 1.000000000000000000, 0.8660254037844387076, 1.000000000000000000, 0.8660254037844387076, 1.000000000000000000, 0.8660254037844387076, 1.000000000000000000, 0.8660254037844387076, 1.000000000000000000, 0.8660254037844387076, 1.000000000000000000, 0.8660254037844387076, 1.000000000000000000, 0.8660254037844387076, 1.000000000000000000, 0.8660254037844387076, 1.000000000000000000, 0.8660254037844387076, 1.000000000000000000, 0.8660254037844387076, 1.000000000000000000, 0.8660254037844387076, 1.000000000000000000, 0.8660254037844387076, 1.000000000000000000, 0.8660254037844387076, 1.000000000000000000, 0.8660254037844387076, 1.000000000000000000, 0.8660254037844387076, 1.000000000000000000, 0.8660254037844387076, 1.000000000000000000, 0.8660254037844387076, 1.000000000000000000, 0.8660254037844387076, 1.000000000000000000, 0.8660254037844387076, 1.000000000000000000, 0.8660254037844387076, 1.000000000000000000, 0.8660254037844387076, 1.000000000000000000, 0.8660254037844387076, 1.000000000000000000, 0.8660254037844387076, 1.000000000000000000, 0.8660254037844387076, 1.000000000000000000, 0.8660254037844387076, 1.000000000000000000, 0.8660254037844387076, 1.000000000000000000, 0.8660254037844387076, 1.000000000000000000, 0.8660254037844387076, 1.000000000000000000, 0.8660254037844387076, 1.000000000000000000, 0.8660254037844387076, 1.000000000000000000, 0.8660254037844387076, 1.000000000000000000, 0.8660254037844387076, 1.000000000000000000, 0.8660254037844387076, 1.000000000000000000, 0.8660254037844387076, 1.000000000000000000, 0.8660254037844387076, 1.000000000000000000, 0.8660254037844387076, 1.000000000000000000, 0.8660254037844387076, 1.000000000000000000, 0.8660254037844387076, 1.000000000000000000, 0.8660254037844387076, 1.000000000000000000, 0.8660254037844387076, 1.000000000000000000, 0.8660254037844387076, 1.000000000000000000, 0.8660254037844387076, 1.000000000000000000, 0.8660254037844387076, 1.000000000000000000, 0.8660254037844387076, 1.000000000000000000, 0.8660254037844387076, 1.000000000000000000, 0.8660254037844387076, 1.000000000000000000, 0.8660254037844387076, 1.000000000000000000, 0.8660254037844387076, 1.000000000000000000, 0.8660254037844387076, 1.000000000000000000, 0.8660254037844387076, 1.000000000000000000, 0.8660254037844387076, 1.000000000000000000, 0.8660254037844387076, 1.000000000000000000, 0.8660254037844387076, 1.000000000000000000, 0.8660254037844387076, 1.000000000000000000, 0.8660254037844387076, 1.000000000000000000, 0.8660254037844387076, 1.000000000000000000, 0.8660254037844387076, 1.000000000000000000, 0.8660254037844387076, 1.000000000000000000, 0.8660254037844387076, 1.000000000000000000, 0.8660254037844387076, 1.000000000000000000, 0.8660254037844387076, 1.000000000000000000, 0.8660254037844387076, 1.000000000000000000, 0.8660254037844387076, 1.000000000000000000, 0.8660254037844387076, 1.000000000000000000, 0.8660254037844387076, 1.000000000000000000, 0.8660254037844387076, 1.000000000000000000, 0.8660254037844387076, 1.000000000000000000, 0.8660254037844387076, 1.000000000000000000, 0.8660254037844387076, 1.000000000000000000, 0.8660254037844387076, 1.000000000000000000, 0.8660254037844387076, 1.000000000000000000, 0.8660254037844387076, 1.000000000000000000, 0.8660254037844387076, 1.000000000000000000, 0.8660254037844387076, 1.000000000000000000, 0.8660254037844387076, 1.000000000000000000, 0.8660254037844387076, 1.000000000000000000, 0.8660254037844387076, 1.000000000000000000, 0.8660254037844387076, 1.000000000000000000, 0.8660254037844387076, 1.000000000000000000, 0.8660254037844387076, 1.000000000000000000, 0.8660254037844387076, 1.000000000000000000, 0.8660254037844387076, 1.000000000000000000, 0.8660254037844387076, 1.000000000000000000, 0.8660254037844387076, 1.000000000000000000, 0.8660254037844387076, 1.000000000000000000, 0.8660254037844387076, 1.000000000000000000, 0.8660254037844387076, 1.000000000000000000, 0.8660254037844387076, 1.000000000000000000, 0.8660254037844387076, 1.000000000000000000, 0.8660254037844387076, 1.000000000000000000, 0.8660254037844387076, 1.000000000000000000, 0.8660254037844387076, 1.000000000000000000, 0.8660254037844387076, 1.000000000000000000, 0.8660254037844387076, 1.000000000000000000, 0.8660254037844387076, 1.000000000000000000, 0.8660254037844387076, 1.000000000000000000, 0.8660254037844387076, 1.000000000000000000, 0.8660254037844387076, 1.000000000000000000, 0.8660254037844387076, 1.000000000000000000, 0.8660254037844387076, 1.000000000000000000, 0.8660254037844387076, 1.000000000000000000, 0.8660254037844387076, 1.000000000000000000, 0.8660254037844387076, 1.000000000000000000, 0.8660254037844387076, 1.000000000000000000, 0.8660254037844387076, 1.000000000000000000, 0.8660254037844387076, 1.000000000000000000, 0.8660254037844387076, 1.000000000000000000, 0.8660254037844387076, 1.000000000000000000, 0.8660254037844387076, 1.000000000000000000, 0.8660254037844387076, 1.000000000000000000, 0.8660254037844387076, 1.000000000000000000, 0.8660254037844387076, 1.000000000000000000, 0.8660254037844387076, 1.000000000000000000, 0.8660254037844387076, 1.000000000000000000, 0.8660254037844387076, 1.000000000000000000, 0.8660254037844387076, 1.000000000000000000, 0.8660254037844387076, 1.000000000000000000, 0.8660254037844387076, 1.000000000000000000, 0.8660254037844387076, 1.000000000000000000, 0.8660254037844387076, 1.000000000000000000, 0.8660254037844387076, 1.000000000000000000, 0.8660254037844387076, 1.000000000000000000, 0.8660254037844387076, 1.000000000000000000, 0.8660254037844387076, 1.000000000000000000, 0.8660254037844387076, 1.000000000000000000, 0.8660254037844387076, 1.000000000000000000, 0.8660254037844387076, 1.000000000000000000, 0.8660254037844387076, 1.000000000000000000, 0.8660254037844387076, 1.000000000000000000, 0.8660254037844387076, 1.000000000000000000, 0.8660254037844387076, 1.000000000000000000, 0.8660254037844387076, 1.000000000000000000, 0.8660254037844387076, 1.000000000000000000, 0.8660254037844387076, 1.000000000000000000, 0.8660254037844387076, 1.000000000000000000, 0.8660254037844387076, 1.000000000000000000, 0.8660254037844387076, 1.000000000000000000, 0.8660254037844387076, 1.000000000000000000, 0.8660254037844387076, 1.000000000000000000, 0.8660254037844387076, 1.000000000000000000, 0.8660254037844387076, 1.000000000000000000, 0.8660254037844387076, 1.000000000000000000, 0.8660254037844387076, 1.000000000000000000, 0.8660254037844387076, 1.000000000000000000, 0.8660254037844387076, 1.000000000000000000, 0.8660254037844387076, 1.000000000000000000, 0.8660254037844387076, 1.000000000000000000, 0.8660254037844387076, 1.000000000000000000, 0.8660254037844387076, 1.000000000000000000, 0.8660254037844387076, 1.000000000000000000, 0.8660254037844387076, 1.000000000000000000, 0.8660254037844387076, 1.000000000000000000, 0.8660254037844387076, 1.000000000000000000, 0.8660254037844387076, 1.000000000000000000, 0.8660254037844387076, 1.000000000000000000, 0.8660254037844387076, 1.000000000000000000, 0.8660254037844387076, 1.000000000000000000),
 ( 1.000000000000000000, 0.8660254037844387076, 1.000000000000000000, 0.8660254037844387076, 1.000000000000000000, 0.8660254037844387076, 1.000000000000000000, 0.8660254037844387076, 1.000000000000000000, 0.8660254037844387076, 1.000000000000000000, 0.8660254037844387076, 1.000000000000000000, 0.8660254037844387076, 1.000000000000000000, 0.8660254037844387076, 1.000000000000000000, 0.8660254037844387076, 1.000000000000000000, 0.8660254037844387076, 1.000000000000000000, 0.8660254037844387076, 1.000000000000000000, 0.8660254037844387076, 1.000000000000000000, 0.8660254037844387076, 1.000000000000000000, 0.8660254037844387076, 1.000000000000000000, 0.8660254037844387076, 1.000000000000000000, 0.8660254037844387076, 1.000000000000000000, 0.8660254037844387076, 1.000000000000000000, 0.8660254037844387076, 1.000000000000000000, 0.8660254037844387076, 1.000000000000000000, 0.8660254037844387076, 1.000000000000000000, 0.8660254037844387076, 1.000000000000000000, 0.8660254037844387076, 1.000000000000000000, 0.8660254037844387076, 1.000000000000000000, 0.8660254037844387076, 1.000000000000000000, 0.8660254037844387076, 1.000000000000000000, 0.8660254037844387076, 1.000000000000000000, 0.8660254037844387076, 1.000000000000000000, 0.8660254037844387076, 1.000000000000000000, 0.8660254037844387076, 1.000000000000000000, 0.8660254037844387076, 1.000000000000000000, 0.8660254037844387076, 1.000000000000000000, 0.8660254037844387076, 1.000000000000000000, 0.8660254037844387076, 1.000000000000000000, 0.8660254037844387076, 1.000000000000000000, 0.8660254037844387076, 1.000000000000000000, 0.8660254037844387076, 1.000000000000000000, 0.8660254037844387076, 1.000000000000000000, 0.8660254037844387076, 1.000000000000000000, 0.8660254037844387076, 1.000000000000000000, 0.8660254037844387076, 1.000000000000000000, 0.8660254037844387076, 1.000000000000000000, 0.8660254037844387076, 1.000000000000000000, 0.8660254037844387076, 1.000000000000000000, 0.8660254037844387076, 1.000000000000000000, 0.8660254037844387076, 1.000000000000000000, 0.8660254037844387076, 1.000000000000000000, 0.8660254037844387076, 1.000000000000000000, 0.8660254037844387076, 1.000000000000000000, 0.8660254037844387076, 1.000000000000000000, 0.8660254037844387076, 1.000000000000000000, 0.8660254037844387076, 1.000000000000000000, 0.8660254037844387076, 1.000000000000000000, 0.8660254037844387076, 1.000000000000000000, 0.8660254037844387076, 1.000000000000000000, 0.8660254037844387076, 1.000000000000000000, 0.8660254037844387076, 1.000000000000000000, 0.8660254037844387076, 1.000000000000000000, 0.8660254037844387076, 1.000000000000000000, 0.8660254037844387076, 1.000000000000000000, 0.8660254037844387076, 1.000000000000000000, 0.8660254037844387076, 1.000000000000000000, 0.8660254037844387076, 1.000000000000000000, 0.8660254037844387076, 1.000000000000000000, 0.8660254037844387076, 1.000000000000000000, 0.8660254037844387076, 1.000000000000000000, 0.8660254037844387076, 1.000000000000000000, 0.8660254037844387076, 1.000000000000000000, 0.8660254037844387076, 1.000000000000000000, 0.8660254037844387076, 1.000000000000000000, 0.8660254037844387076, 1.000000000000000000, 0.8660254037844387076, 1.000000000000000000, 0.8660254037844387076, 1.000000000000000000, 0.8660254037844387076, 1.000000000000000000, 0.8660254037844387076, 1.000000000000000000, 0.8660254037844387076, 1.000000000000000000, 0.8660254037844387076, 1.000000000000000000, 0.8660254037844387076, 1.000000000000000000, 0.8660254037844387076, 1.000000000000000000, 0.8660254037844387076, 1.000000000000000000, 0.8660254037844387076, 1.000000000000000000, 0.8660254037844387076, 1.000000000000000000, 0.8660254037844387076, 1.000000000000000000, 0.8660254037844387076, 1.000000000000000000, 0.8660254037844387076, 1.000000000000000000, 0.8660254037844387076, 1.000000000000000000, 0.8660254037844387076, 1.000000000000000000, 0.8660254037844387076, 1.000000000000000000, 0.8660254037844387076, 1.000000000000000000, 0.8660254037844387076, 1.000000000000000000, 0.8660254037844387076, 1.000000000000000000, 0.8660254037844387076, 1.000000000000000000, 0.8660254037844387076, 1.000000000000000000, 0.8660254037844387076, 1.000000000000000000, 0.8660254037844387076, 1.000000000000000000, 0.8660254037844387076, 1.000000000000000000, 0.8660254037844387076, 1.000000000000000000, 0.8660254037844387076, 1.000000000000000000, 0.8660254037844387076, 1.000000000000000000, 0.8660254037844387076, 1.000000000000000000, 0.8660254037844387076, 1.000000000000000000, 0.8660254037844387076, 1.000000000000000000, 0.8660254037844387076, 1.000000000000000000, 0.8660254037844387076, 1.000000000000000000, 0.8660254037844387076, 1.000000000000000000, 0.8660254037844387076, 1.000000000000000000, 0.8660254037844387076, 1.000000000000000000, 0.8660254037844387076, 1.000000000000000000, 0.8660254037844387076, 1.000000000000000000, 0.8660254037844387076, 1.000000000000000000, 0.8660254037844387076, 1.000000000000000000, 0.8660254037844387076, 1.000000000000000000, 0.8660254037844387076, 1.000000000000000000, 0.8660254037844387076, 1.000000000000000000, 0.8660254037844387076, 1.000000000000000000, 0.8660254037844387076, 1.000000000000000000, 0.8660254037844387076, 1.000000000000000000, 0.8660254037844387076, 1.000000000000000000, 0.8660254037844387076, 1.000000000000000000, 0.8660254037844387076, 1.000000000000000000, 0.8660254037844387076, 1.000000000000000000, 0.8660254037844387076, 1.000000000000000000, 0.8660254037844387076, 1.000000000000000000, 0.8660254037844387076, 1.000000000000000000, 0.8660254037844387076, 1.000000000000000000, 0.8660254037844387076, 1.000000000000000000, 0.8660254037844387076, 1.000000000000000000, 0.8660254037844387076, 1.000000000000000000, 0.8660254037844387076, 1.000000000000000000, 0.8660254037844387076, 1.000000000000000000, 0.8660254037844387076, 1.000000000000000000, 0.8660254037844387076, 1.000000000000000000, 0.8660254037844387076, 1.000000000000000000, 0.8660254037844387076, 1.000000000000000000, 0.8660254037844387076, 1.000000000000000000, 0.8660254037844387076, 1.000000000000000000, 0.8660254037844387076, 1.000000000000000000, 0.8660254037844387076, 1.000000000000000000, 0.8660254037844387076, 1.000000000000000000, 0.8660254037844387076, 1.000000000000000000, 0.8660254037844387076, 1.000000000000000000, 0.8660254037844387076, 1.000000000000000000, 0.8660254037844387076, 1.000000000000000000, 0.8660254037844387076, 1.000000000000000000, 0.8660254037844387076, 1.000000000000000000, 0.8660254037844387076, 1.000000000000000000, 0.8660254037844387076, 1.000000000000000000, 0.8660254037844387076, 1.000000000000000000, 0.8660254037844387076, 1.000000000000000000, 0.8660254037844387076, 1.000000000000000000, 0.8660254037844387076, 1.000000000000000000, 0.8660254037844387076, 1.000000000000000000, 0.8660254037844387076, 1.000000000000000000, 0.8660254037844387076, 1.000000000000000000, 0.8660254037844387076, 1.000000000000000000, 0.8660254037844387076, 1.000000000000000000, 0.8660254037844387076, 1.000000000000000000, 0.8660254037844387076, 1.000000000000000000, 0.8660254037844387076, 1.000000000000000000, 0.8660254037844387076, 1.000000000000000000, 0.8660254037844387076, 1.000000000000000000, 0.8660254037844387076, 1.000000000000000000, 0.8660254037844387076, 1.000000000000000000, 0.8660254037844387076, 1.000000000000000000, 0.8660254037844387076, 1.000000000000000000, 0.8660254037844387076, 1.000000000000000000, 0.8660254037844387076, 1.000000000000000000, 0.8660254037844387076, 1.000000000000000000, 0.8660254037844387076, 1.000000000000000000) ) ) 
 REPRESENTATION_ITEM ( '' )  SURFACE ( )  );
#195560=ORIENTED_EDGE ( 'NONE', *, *, #188476, .T. ) ;
#195561=CARTESIAN_POINT ( 'NONE',  ( -4.240783329467897822, 7.329537114711067503, -0.8835190343243297662 ) ) ;
#195565=CARTESIAN_POINT ( 'NONE',  ( 5.524057522564145728, 8.532151978711786100, 1.199719254218462483 ) ) ;
#195574=CARTESIAN_POINT ( 'NONE',  ( 9.561524646135536543, 12.17819805862340310, -1.599625672291262513 ) ) ;
#195577=CARTESIAN_POINT ( 'NONE',  ( -1.499999999999997780, 3.900000000000021672, 1.214306433183764966E-14 ) ) ;
#195587=CIRCLE ( 'NONE', #102195, 0.07999999999999997391 ) ;
#195588=CARTESIAN_POINT ( 'NONE',  ( -9.029367117021344313, 9.636609179387466639, 0.7216878364870438212 ) ) ;
#195592=CARTESIAN_POINT ( 'NONE',  ( 5.636439174979242850, 7.598931675607687453, -1.599625672291262513 ) ) ;
#195597=AXIS2_PLACEMENT_3D ( 'NONE', #117608, #167366, #134885 ) ;
#195599=CARTESIAN_POINT ( 'NONE',  ( 5.327991180046175224, 5.318337252916401248, -0.7216878364870207285 ) ) ;
#195608=CARTESIAN_POINT ( 'NONE',  ( -7.203459687562382641, 7.298457811777897319, -0.7998128361456291469 ) ) ;
#195609=CARTESIAN_POINT ( 'NONE',  ( -4.141125853970233806, 6.918731698685530063, -1.199719254218452047 ) ) ;
#195613=CARTESIAN_POINT ( 'NONE',  ( 1.284279953904125193, 3.003360285806104368, 0.7750000000000065725 ) ) ;
#195615=B_SPLINE_CURVE_WITH_KNOTS ( 'NONE', 3,
 ( #81790, #147873, #200833, #131657 ),
 .UNSPECIFIED., .F., .F.,
 ( 4, 4 ),
 ( 0.001170373960510463426, 0.001235641208627095413 ),
 .UNSPECIFIED. ) ;
#195618=CARTESIAN_POINT ( 'NONE',  ( 6.796715079152391148, 6.823922435299587974, 0.7998128361456341429 ) ) ;
#195627=CARTESIAN_POINT ( 'NONE',  ( 1.230728480726485330, 3.105010058876359835, -0.7749999999999926947 ) ) ;
#195630=ORIENTED_EDGE ( 'NONE', *, *, #99196, .F. ) ;
#195632=CARTESIAN_POINT ( 'NONE',  ( -1.364683531250000748, -0.6781249996585803075, 0.000000000000000000 ) ) ;
#195634=CARTESIAN_POINT ( 'NONE',  ( 5.626797444871351139, 6.523350759560078593, 1.199719254218462483 ) ) ;
#195636=CARTESIAN_POINT ( 'NONE',  ( -5.910991785878158211, 9.839981483592442402, -0.7216878364870278340 ) ) ;
#195637=CARTESIAN_POINT ( 'NONE',  ( 5.558479791922850133, 6.547609847740540445, -1.082531754730542195 ) ) ;
#195638=CARTESIAN_POINT ( 'NONE',  ( -8.148087131688699358, 8.608449196499371681, -0.7216878364870267237 ) ) ;
#195642=CARTESIAN_POINT ( 'NONE',  ( 7.070740804726770357, 8.207951346058097286, 1.199719254218462483 ) ) ;
#195649=CARTESIAN_POINT ( 'NONE',  ( -1.001543065824772872E-14, 5.321875000341422357, 1.575800808251672791 ) ) ;
#195654=CARTESIAN_POINT ( 'NONE',  ( 8.132193210098487057, 8.381980254736715708, 1.040834085586084257E-14 ) ) ;
#195657=CARTESIAN_POINT ( 'NONE',  ( -8.864333505236459132, 9.236143932397675727, 1.040834085586084257E-14 ) ) ;
#195662=CARTESIAN_POINT ( 'NONE',  ( 10.40318394038753702, 11.03146944007395724, -0.7998128361456281477 ) ) ;
#195665=CARTESIAN_POINT ( 'NONE',  ( -6.877010230629689858, 9.046264573866535486, 1.599625672291283607 ) ) ;
#195666=CARTESIAN_POINT ( 'NONE',  ( 0.02393948931068496516, 6.343121002295580624, 3.090828003060728246 ) ) ;
#195668=CARTESIAN_POINT ( 'NONE',  ( 5.656792095876843618, 6.122768675584825182, -0.7810860850652520115 ) ) ;
#195669=CARTESIAN_POINT ( 'NONE',  ( -7.863365906246048809, 12.11775129068834289, -0.7216878364870267237 ) ) ;
#195673=CARTESIAN_POINT ( 'NONE',  ( 5.124091990960999432, 8.065525525174782828, -1.199719254218452047 ) ) ;
#195675=CARTESIAN_POINT ( 'NONE',  ( 4.611744806942754238, 8.532119374741881757, -0.7998128361456231517 ) ) ;
#195676=CARTESIAN_POINT ( 'NONE',  ( -4.037710856648669022, 7.592775851288043221, -0.3149755216912339395 ) ) ;
#195677=CARTESIAN_POINT ( 'NONE',  ( 2.835626683552519012, 6.459981564119914310, 0.000000000000000000 ) ) ;
#195679=CARTESIAN_POINT ( 'NONE',  ( -5.585596099150174965, 9.460353182409786399, -0.7216878364870207285 ) ) ;
#195684=CARTESIAN_POINT ( 'NONE',  ( -4.884136011505287200, 6.706951837855620546, 1.250136565965910274 ) ) ;
#195685=CARTESIAN_POINT ( 'NONE',  ( -1.364683531250000748, 0.5718750003414208027, 0.000000000000000000 ) ) ;
#195688=CARTESIAN_POINT ( 'NONE',  ( 3.538314903486612817, 7.071858454135611538, 1.040834085586084257E-14 ) ) ;
#195691=AXIS2_PLACEMENT_3D ( 'NONE', #31863, #97939, #81659 ) ;
#195693=CARTESIAN_POINT ( 'NONE',  ( -9.802181872555943087, 10.53822639417784046, 0.7216878364870438212 ) ) ;
#195700=CARTESIAN_POINT ( 'NONE',  ( -7.795575137733361970, 12.03866206075687018, 0.7216878364870458196 ) ) ;
#195701=DIRECTION ( 'NONE',  ( -1.207943261119674327E-30, -2.168404344971008079E-15, 1.000000000000000000 ) ) ;
#195707=CARTESIAN_POINT ( 'NONE',  ( -7.659993601596706725, 11.88048360193076647, -0.7216878364870267237 ) ) ;
#195711=CARTESIAN_POINT ( 'NONE',  ( 0.6823417656249917140, 4.905208333674755394, 1.181850606188765695 ) ) ;
#195712=CARTESIAN_POINT ( 'NONE',  ( -1.500000000000013101, 3.160416667349486008, -0.8660254037844313801 ) ) ;
#195713=CARTESIAN_POINT ( 'NONE',  ( 5.539635733611046220, 6.394625955944754914, -1.222580188273769908 ) ) ;
#195718=CARTESIAN_POINT ( 'NONE',  ( -6.723954117373590833, 9.932031339322813679, -1.199719254218440723 ) ) ;
#195722=CARTESIAN_POINT ( 'NONE',  ( 5.015626762051672571, 7.938982758113895422, 1.199719254218462483 ) ) ;
#195727=CARTESIAN_POINT ( 'NONE',  ( 7.151035956204054855, 10.43029348462504124, 1.199719254218460707 ) ) ;
#195735=CARTESIAN_POINT ( 'NONE',  ( -5.070386261830872598, 8.859275038870594088, 0.7216878364870458196 ) ) ;
#195738=CARTESIAN_POINT ( 'NONE',  ( 0.6823417656249899377, 5.488541667008087543, -1.181850606188754593 ) ) ;
#195744=CARTESIAN_POINT ( 'NONE',  ( -8.157201976916404362, 12.66848607304450702, -0.7998128361456281477 ) ) ;
#195746=CARTESIAN_POINT ( 'NONE',  ( 7.099665995050449041, 11.43469409420089455, 0.7998128361456462443 ) ) ;
#195748=CARTESIAN_POINT ( 'NONE',  ( -8.962103233833181193, 10.41454084668224489, -1.199719254218446718 ) ) ;
#195751=CARTESIAN_POINT ( 'NONE',  ( 0.6823417656249899377, 3.426041667008085323, -1.181850606188754593 ) ) ;
#195752=CARTESIAN_POINT ( 'NONE',  ( 2.510230996824538430, 6.080353262937265413, 0.000000000000000000 ) ) ;
#195756=CARTESIAN_POINT ( 'NONE',  ( 9.205623113554615600, 11.76297960394566466, 1.443375672974076540 ) ) ;
#195759=CARTESIAN_POINT ( 'NONE',  ( -5.721177635286839092, 9.618531641235897212, 0.7216878364870458196 ) ) ;
#195760=CARTESIAN_POINT ( 'NONE',  ( -0.6823417656250212460, 1.051041667008083325, 1.181850606188755259 ) ) ;
#195762=CARTESIAN_POINT ( 'NONE',  ( 0.4957404558455620891, 7.798922855753830596, 1.990826765680269395 ) ) ;
#195764=CARTESIAN_POINT ( 'NONE',  ( -7.212047647465563038, 10.50147379109678880, -1.199719254218446718 ) ) ;
#195765=CARTESIAN_POINT ( 'NONE',  ( -3.999292125906916073, 5.688926785023260102, 1.443375672974064550 ) ) ;
#195766=CARTESIAN_POINT ( 'NONE',  ( 1.364683531249988535, 2.967708333674755394, -0.7879004041258239610 ) ) ;
#195771=CARTESIAN_POINT ( 'NONE',  ( 9.154780037725547714, 11.70366268214508487, 1.599625672291279388 ) ) ;
#195783=CARTESIAN_POINT ( 'NONE',  ( -7.334597915313094241, 9.580116872663850813, 1.040834085586084257E-14 ) ) ;
#195785=CARTESIAN_POINT ( 'NONE',  ( 1.364683531249988535, 3.717708333674750953, -0.7879004041258239610 ) ) ;
#195791=CARTESIAN_POINT ( 'NONE',  ( 7.259501185113382604, 10.55683625168592243, -1.199719254218441611 ) ) ;
#195794=CARTESIAN_POINT ( 'NONE',  ( -0.6823417656249969321, 4.467708333674755394, -1.181850606188749264 ) ) ;
#195797=CARTESIAN_POINT ( 'NONE',  ( -6.060131475628484310, 10.01397778830115470, 0.000000000000000000 ) ) ;
#195803=CARTESIAN_POINT ( 'NONE',  ( 2.205172540517054802, 5.724451730578533848, 1.040834085586084257E-14 ) ) ;
#195806=CARTESIAN_POINT ( 'NONE',  ( 8.920375002787457319, 12.49452237230570084, 1.199719254218450271 ) ) ;
#195813=CARTESIAN_POINT ( 'NONE',  ( -9.110189153378817295, 12.71597221466224603, 1.199719254218462483 ) ) ;
#195814=CARTESIAN_POINT ( 'NONE',  ( 6.448874621594486989, 10.67543749183559143, 0.7998128361456462443 ) ) ;
#195826=CARTESIAN_POINT ( 'NONE',  ( -6.317736394288148816, 8.393778431468064127, 1.443375672974078761 ) ) ;
#195828=CARTESIAN_POINT ( 'NONE',  ( 3.521367211247359741, 5.131347717920458962, -1.599625672291262513 ) ) ;
#195831=CARTESIAN_POINT ( 'NONE',  ( -8.779068160048691283, 10.20099992726700933, -1.199719254218446718 ) ) ;
#195836=CARTESIAN_POINT ( 'NONE',  ( -8.622095623286845978, 12.14652976288826913, 1.199719254218462483 ) ) ;
#195838=CYLINDRICAL_SURFACE ( 'NONE', #153956, 1.000000000000000000 ) ;
#195840=CARTESIAN_POINT ( 'NONE',  ( 7.574201371528760163, 11.98831870009225931, 1.040834085586084257E-14 ) ) ;
#195841=EDGE_CURVE ( 'NONE', #71069, #108467, #140525, .T. ) ;
#195854=CARTESIAN_POINT ( 'NONE',  ( -8.239604668803112375, 10.63595808506888396, -1.599625672291263179 ) ) ;
#195858=CARTESIAN_POINT ( 'NONE',  ( 7.944714827928056167, 8.371181508778631652, 0.7216878364870458196 ) ) ;
#195860=CARTESIAN_POINT ( 'NONE',  ( 2.523789150438203510, 6.096171108819874007, 0.7998128361456462443 ) ) ;
#195861=CYLINDRICAL_SURFACE ( 'NONE', #210483, 0.7499999999999997780 ) ;
#195863=CARTESIAN_POINT ( 'NONE',  ( -6.898401231254901234, 6.942556279419168419, -0.7998128361456291469 ) ) ;
#195873=CARTESIAN_POINT ( 'NONE',  ( 1.364683531249990311, 4.196875000341417028, 1.214306433183764966E-14 ) ) ;
#195875=CARTESIAN_POINT ( 'NONE',  ( 9.426996880203592610, 9.892584536526015881, -0.7998128361456281477 ) ) ;
#195878=CARTESIAN_POINT ( 'NONE',  ( -3.118012141462980669, 6.581505231774690046, 0.7216878364870317197 ) ) ;
#195880=CARTESIAN_POINT ( 'NONE',  ( -5.382223794500845315, 6.341977850748185652, -1.082531754730543971 ) ) ;
#195887=CARTESIAN_POINT ( 'NONE',  ( 9.029367117021314115, 12.51771682229149008, -1.082531754730543083 ) ) ;
#195897=CARTESIAN_POINT ( 'NONE',  ( 5.030238685870051185, 5.827365540725222282, -1.199719254218452047 ) ) ;
#195898=ORIENTED_EDGE ( 'NONE', *, *, #99066, .F. ) ;
#195903=CARTESIAN_POINT ( 'NONE',  ( -0.6823417656250212460, 3.613541667008085767, 1.181850606188767472 ) ) ;
#195908=CARTESIAN_POINT ( 'NONE',  ( 7.149227073107712549, 7.235186428247455837, -0.7998128361456281477 ) ) ;
#195911=CARTESIAN_POINT ( 'NONE',  ( -5.298539104842322267, 5.076050465271134016, 0.7998128361456341429 ) ) ;
#195912=CARTESIAN_POINT ( 'NONE',  ( 5.300874872818828187, 8.167809204055208383, 1.082531754730558626 ) ) ;
#195913=CARTESIAN_POINT ( 'NONE',  ( 1.499999999999989120, 2.504166666666687302, 0.8660254037844524744 ) ) ;
#195916=CARTESIAN_POINT ( 'NONE',  ( -3.113568832632681360, 6.784247404713427798, -0.7998128361456281477 ) ) ;
#195920=CARTESIAN_POINT ( 'NONE',  ( -1.201851678989727383E-14, 2.821875000341418804, 1.575800808251672791 ) ) ;
#195922=CARTESIAN_POINT ( 'NONE',  ( -4.446711195602255806, 5.250546485366484717, -1.082531754730544860 ) ) ;
#195927=CARTESIAN_POINT ( 'NONE',  ( 4.761938266897790761, 6.578680616179308771, 1.599625672291267398 ) ) ;
#195929=CARTESIAN_POINT ( 'NONE',  ( 0.3976372456648717968, 6.957695340450004373, -3.811578153443453854 ) ) ;
#195930=CARTESIAN_POINT ( 'NONE',  ( 1.364683531249990311, 4.676041667008083103, 0.7879004041258500513 ) ) ;
#195934=CARTESIAN_POINT ( 'NONE',  ( 1.364683531249988757, -0.05312499965857975237, 0.000000000000000000 ) ) ;
#195936=EDGE_CURVE ( 'NONE', #185401, #110521, #214208, .T. ) ;
#195938=CARTESIAN_POINT ( 'NONE',  ( -10.45741655484220267, 11.09474082360439873, -0.7998128361456221525 ) ) ;
#195940=CARTESIAN_POINT ( 'NONE',  ( -6.575341312503472757, 7.733948288417905381, 1.082531754730549967 ) ) ;
#195944=CARTESIAN_POINT ( 'NONE',  ( -1.364683531250012516, 4.238541667008090208, -0.7879004041258300672 ) ) ;
#195952=CARTESIAN_POINT ( 'NONE',  ( -5.219525951136837705, 9.033271343060892633, -0.7216878364870207285 ) ) ;
#195955=CARTESIAN_POINT ( 'NONE',  ( -1.499999999999997780, 10.00000000000000178, -4.154462424328202452 ) ) ;
#195959=CARTESIAN_POINT ( 'NONE',  ( -5.029711800545518585, 8.811821500704338561, 0.7216878364870458196 ) ) ;
#195974=CARTESIAN_POINT ( 'NONE',  ( -5.311043488251275591, 7.219303374425030562, -1.599625672291256295 ) ) ;
#195977=CARTESIAN_POINT ( 'NONE',  ( -0.7500000000000215383, 1.191666666666688190, 1.299038105676659116 ) ) ;
#195978=CARTESIAN_POINT ( 'NONE',  ( 8.432808358020004391, 12.78210081775797669, 0.7216878364870438212 ) ) ;
#195979=CARTESIAN_POINT ( 'NONE',  ( 6.012151052656117933, 9.101594430485762999, 1.199719254218460707 ) ) ;
#195981=( BOUNDED_CURVE ( )  B_SPLINE_CURVE ( 2, ( #151610, #124518, #60481, #176384, #91954 ),
 .UNSPECIFIED., .F., .T. ) 
 B_SPLINE_CURVE_WITH_KNOTS ( ( 3, 2, 3 ),
 ( 0.1361778335736238410, 0.1375000000000000111, 0.1392051351651994728 ),
 .UNSPECIFIED. ) 
 CURVE ( )  GEOMETRIC_REPRESENTATION_ITEM ( )  RATIONAL_B_SPLINE_CURVE ( ( 0.9419547032718713631, 0.9574871888551554910, 1.000000000000000000, 0.9451732491398672220, 0.9352202683046508813 ) ) 
 REPRESENTATION_ITEM ( '' )  );
#195983=CARTESIAN_POINT ( 'NONE',  ( 3.994848817520957773, 7.812407387083109001, 1.040834085586084257E-14 ) ) ;
#195985=ORIENTED_EDGE ( 'NONE', *, *, #43825, .T. ) ;
#195990=CARTESIAN_POINT ( 'NONE',  ( -3.633221978782290140, 6.222214161012547429, -1.082531754730549967 ) ) ;
#195998=CARTESIAN_POINT ( 'NONE',  ( -1.201851678989727383E-14, 3.696875000341422801, -1.575800808251660134 ) ) ;
#195999=CARTESIAN_POINT ( 'NONE',  ( 9.585251414737269826, 11.24551007435741568, -1.082531754730537088 ) ) ;
#196000=CARTESIAN_POINT ( 'NONE',  ( -6.039267359883488950, 9.133230122250985517, 1.199719254218452047 ) ) ;
#196003=CARTESIAN_POINT ( 'NONE',  ( 5.144429221381498607, 8.089252293998699272, -1.199719254218452047 ) ) ;
#196004=CARTESIAN_POINT ( 'NONE',  ( -5.540478329478883524, 9.615641817700700145, 0.000000000000000000 ) ) ;
#196005=CARTESIAN_POINT ( 'NONE',  ( -1.501062075862715339, 8.754928401006202066, 2.503798761944588058 ) ) ;
#196008=CARTESIAN_POINT ( 'NONE',  ( 0.7499999999999885647, 0.2645833340161538039, 1.299038105676657340 ) ) ;
#196011=CARTESIAN_POINT ( 'NONE',  ( 7.131225611108085616, 10.30321839872603462, 1.082531754730558626 ) ) ;
#196014=CARTESIAN_POINT ( 'NONE',  ( -1.364683531250012516, 1.592708333674756727, 0.7879004041258379498 ) ) ;
#196016=CARTESIAN_POINT ( 'NONE',  ( 7.443063143778065438, 7.785921210603627962, -0.7216878364870257245 ) ) ;
#196019=CARTESIAN_POINT ( 'NONE',  ( -4.284013352238274841, 4.100363120473813794, -0.7216878364870207285 ) ) ;
#196021=CARTESIAN_POINT ( 'NONE',  ( -1.364683531250010295, 5.030208333674757171, 0.7879004041258379498 ) ) ;
#196025=CARTESIAN_POINT ( 'NONE',  ( -4.868901516392104334, 6.903810023003053686, -1.445308410833840318 ) ) ;
#196034=CARTESIAN_POINT ( 'NONE',  ( 5.472687561410540802, 9.536552588287639409, 0.7998128361456462443 ) ) ;
#196037=CARTESIAN_POINT ( 'NONE',  ( 2.347533153460546806, 5.890539112345938300, 0.000000000000000000 ) ) ;
#196045=CARTESIAN_POINT ( 'NONE',  ( 4.514501963670558560, 8.210743357683563559, 1.040834085586084257E-14 ) ) ;
#196047=CARTESIAN_POINT ( 'NONE',  ( 1.364683531249986537, 0.2177083336747502595, -0.7879004041258309554 ) ) ;
#196050=CARTESIAN_POINT ( 'NONE',  ( 0.3903331394470910820, 6.430882235217429077, -3.207842980289837165 ) ) ;
#196054=CARTESIAN_POINT ( 'NONE',  ( 0.7499999999999902300, 1.483333333333357373, 1.299038105676657340 ) ) ;
#196055=CARTESIAN_POINT ( 'NONE',  ( 6.531277313481192337, 8.642909503859968368, 1.599625672291281386 ) ) ;
#196056=CARTESIAN_POINT ( 'NONE',  ( -8.864333505236459132, 9.236143932397675727, 1.040834085586084257E-14 ) ) ;
#196060=CARTESIAN_POINT ( 'NONE',  ( 0.6823417656249899377, 0.5927083336747518416, 1.181850606188755259 ) ) ;
#196063=CARTESIAN_POINT ( 'NONE',  ( -1.201851678989727383E-14, 2.212500000000021672, 1.732050807568877637 ) ) ;
#196065=CARTESIAN_POINT ( 'NONE',  ( 9.571693261567954636, 12.19006144329456731, 1.443375672974076540 ) ) ;
#196071=CARTESIAN_POINT ( 'NONE',  ( 1.499999999999989120, 0.8062500006828163812, 0.000000000000000000 ) ) ;
#196072=CARTESIAN_POINT ( 'NONE',  ( -5.859094939400033120, 9.987361195942037639, -0.7998128361456231517 ) ) ;
#196073=CARTESIAN_POINT ( 'NONE',  ( -4.121315508874269007, 5.831287398485176077, -1.443375672974053447 ) ) ;
#196080=CARTESIAN_POINT ( 'NONE',  ( 7.447506452608354088, 7.583179037664891098, 0.7998128361456341429 ) ) ;
#196084=CARTESIAN_POINT ( 'NONE',  ( 7.467843683028853263, 7.606905806488803101, 0.7998128361456341429 ) ) ;
#196085=CARTESIAN_POINT ( 'NONE',  ( 8.066738210006674237, 11.39464976410773467, 1.082531754730558626 ) ) ;
#196086=ORIENTED_EDGE ( 'NONE', *, *, #200959, .F. ) ;
#196091=CARTESIAN_POINT ( 'NONE',  ( -6.775324078527193983, 8.927630729746953264, -1.599625672291263179 ) ) ;
#196092=CARTESIAN_POINT ( 'NONE',  ( 3.520313441042647540, 7.258782781191745137, 0.7998128361456321445 ) ) ;
#196096=CARTESIAN_POINT ( 'NONE',  ( 4.839368334287259543, 6.711050605271530856, 1.249743143419468350 ) ) ;
#196097=CARTESIAN_POINT ( 'NONE',  ( 8.676855123066012254, 11.14608361504227574, -1.443375672974052559 ) ) ;
#196104=CARTESIAN_POINT ( 'NONE',  ( -3.470524135418306511, 5.072030796119872953, -1.443375672974053447 ) ) ;
#196105=CARTESIAN_POINT ( 'NONE',  ( 7.117667457494414762, 11.24776976714476184, 1.040834085586084257E-14 ) ) ;
#196108=CARTESIAN_POINT ( 'NONE',  ( -5.904739593951539689, 6.847616600153594746, 1.199719254218450271 ) ) ;
#196113=CARTESIAN_POINT ( 'NONE',  ( -7.379715684540041565, 7.504089808251839244, 1.040834085586084257E-14 ) ) ;
#196128=CARTESIAN_POINT ( 'NONE',  ( -5.904739593951539689, 6.847616600153594746, 1.199719254218450271 ) ) ;
#196131=CARTESIAN_POINT ( 'NONE',  ( 3.334942599281629949, 5.874221551595115720, -1.082531754730543083 ) ) ;
#196134=DIRECTION ( 'NONE',  ( 0.7592566023653005702, -0.6507913734559639396, 0.000000000000000000 ) ) ;
#196136=CARTESIAN_POINT ( 'NONE',  ( -3.164938793786285842, 5.779846795137578930, -1.199719254218452935 ) ) ;
#196139=CARTESIAN_POINT ( 'NONE',  ( 8.215351014876830504, 11.67199438640995801, -1.199719254218446718 ) ) ;
#196142=CARTESIAN_POINT ( 'NONE',  ( -6.679363233026820446, 10.94434087183997129, 0.000000000000000000 ) ) ;
#196143=CARTESIAN_POINT ( 'NONE',  ( 5.937581207780954884, 9.014596278131406848, -1.199719254218440723 ) ) ;
#196149=CARTESIAN_POINT ( 'NONE',  ( -1.364683531250000748, 1.071875000341421247, 0.000000000000000000 ) ) ;
#196150=ORIENTED_EDGE ( 'NONE', *, *, #150235, .F. ) ;
#196152=CARTESIAN_POINT ( 'NONE',  ( 8.609064354997688184, 9.146255957026539818, 1.040834085586084257E-14 ) ) ;
#196161=CARTESIAN_POINT ( 'NONE',  ( 4.650083499807233345, 5.295740330745369207, -1.000000000000000888 ) ) ;
#196180=CARTESIAN_POINT ( 'NONE',  ( 0.7499999999999885647, -0.4854166659838468623, 1.299038105676657340 ) ) ;
#196184=ORIENTED_EDGE ( 'NONE', *, *, #119838, .F. ) ;
#196187=CARTESIAN_POINT ( 'NONE',  ( 7.065770611016287006, 11.39514947949436774, 1.040834085586084257E-14 ) ) ;
#196192=CARTESIAN_POINT ( 'NONE',  ( 4.857899112398166075, 4.561970474086296079, 1.040834085586084257E-14 ) ) ;
#196193=CARTESIAN_POINT ( 'NONE',  ( -7.537970219518089543, 8.857015346601659900, -1.082531754730543971 ) ) ;
#196197=CARTESIAN_POINT ( 'NONE',  ( -7.881367368245678406, 8.089350105908421185, 0.7998128361456602331 ) ) ;
#196201=CARTESIAN_POINT ( 'NONE',  ( 1.499999999999989120, 1.306250000682816825, 0.000000000000000000 ) ) ;
#196209=CARTESIAN_POINT ( 'NONE',  ( -3.429849674132948500, 5.024577257953626308, -1.443375672974051449 ) ) ;
#196212=CARTESIAN_POINT ( 'NONE',  ( 4.632932323280743780, 6.889805956345480986, 1.213532624337316124 ) ) ;
#196217=CARTESIAN_POINT ( 'NONE',  ( -10.66756793585402363, 11.33991743478486391, 0.7998128361456462443 ) ) ;
#196218=CARTESIAN_POINT ( 'NONE',  ( 7.476431642932036326, 10.80992178580769014, 1.199719254218460707 ) ) ;
#196222=CARTESIAN_POINT ( 'NONE',  ( -3.023105066167347310, 5.702484939155337607, 2.420000000000010587 ) ) ;
#196223=ORIENTED_EDGE ( 'NONE', *, *, #71920, .F. ) ;
#196226=CARTESIAN_POINT ( 'NONE',  ( -8.890396042259075315, 11.39521468743417998, -1.599625672291263179 ) ) ;
#196229=VERTEX_POINT ( 'NONE', #212934 ) ;
#196231=CARTESIAN_POINT ( 'NONE',  ( 5.529027716274630855, 5.344953845275508542, 1.040834085586084257E-14 ) ) ;
#196235=CARTESIAN_POINT ( 'NONE',  ( -9.809487834687324437, 11.40315621434539395, 1.199719254218462483 ) ) ;
#196247=CARTESIAN_POINT ( 'NONE',  ( 5.960781091502512119, 10.10599504006161986, 0.7998128361456462443 ) ) ;
#196249=CARTESIAN_POINT ( 'NONE',  ( -2.788173145904702555, 6.404619103530779789, -0.7998128361456281477 ) ) ;
#196252=CARTESIAN_POINT ( 'NONE',  ( 5.431895982697334091, 6.433277491268158954, -1.247050338538328029 ) ) ;
#196256=CARTESIAN_POINT ( 'NONE',  ( 0.7499999999999885647, 0.2645833340161538039, 1.299038105676657340 ) ) ;
#196259=CARTESIAN_POINT ( 'NONE',  ( -1.495402192688975340, 8.717956978849768390, -2.557532308801403698 ) ) ;
#196260=CARTESIAN_POINT ( 'NONE',  ( 3.541704441667858472, 5.155074486744371853, -1.599625672291262513 ) ) ;
#196262=CARTESIAN_POINT ( 'NONE',  ( -2.611917148927046295, 6.198987107056845858, 1.040834085586084257E-14 ) ) ;
#196268=CARTESIAN_POINT ( 'NONE',  ( 3.701012746850603996, 7.261672604726938651, 1.040834085586084257E-14 ) ) ;
#196271=CARTESIAN_POINT ( 'NONE',  ( -10.62011439820619429, 11.28455497419572318, -0.7998128361456221525 ) ) ;
#196273=CARTESIAN_POINT ( 'NONE',  ( 3.755245360860917536, 5.404205559136275205, -1.443375672974051449 ) ) ;
#196281=CARTESIAN_POINT ( 'NONE',  ( -5.968994907891031154, 6.102274133640173126, 0.7348006213908353512 ) ) ;
#196283=CARTESIAN_POINT ( 'NONE',  ( 1.364683531249986537, -0.3447916663252443836, -0.7879004041258309554 ) ) ;
#196287=CARTESIAN_POINT ( 'NONE',  ( -4.554649539187067830, 7.401175998105142817, 1.199719254218464037 ) ) ;
#196291=CARTESIAN_POINT ( 'NONE',  ( -0.7500000000000215383, 4.691666666666684193, 1.299038105676671107 ) ) ;
#196299=CARTESIAN_POINT ( 'NONE',  ( 1.364683531249986537, -0.5947916663252456049, -0.7879004041258309554 ) ) ;
#196301=CARTESIAN_POINT ( 'NONE',  ( 4.638861114170084399, 8.563755066507100722, 0.7998128361456462443 ) ) ;
#196302=CARTESIAN_POINT ( 'NONE',  ( -9.338868881714763148, 9.789768538289042255, -0.7998128361456291469 ) ) ;
#196304=CARTESIAN_POINT ( 'NONE',  ( 9.836604141914616406, 11.43479190611061647, 1.199719254218452047 ) ) ;
#196309=ORIENTED_EDGE ( 'NONE', *, *, #49744, .F. ) ;
#196311=CARTESIAN_POINT ( 'NONE',  ( 1.499999999999991118, 5.754166666666685970, 0.8660254037844524744 ) ) ;
#196318=CARTESIAN_POINT ( 'NONE',  ( 8.432808358020029260, 8.940623960552603222, 0.7216878364870438212 ) ) ;
#196323=CARTESIAN_POINT ( 'NONE',  ( 0.7499999999999902300, 4.847916667349482012, -1.299038105676658228 ) ) ;
#196325=CARTESIAN_POINT ( 'NONE',  ( -5.101945877444165944, 4.846691699973280976, 0.000000000000000000 ) ) ;
#196326=CARTESIAN_POINT ( 'NONE',  ( 5.436456408955479880, 9.286356877182658565, -0.7216878364870267237 ) ) ;
#196327=CARTESIAN_POINT ( 'NONE',  ( -10.58855478214856660, 11.45566145536924552, -0.7216878364870217277 ) ) ;
#196334=CARTESIAN_POINT ( 'NONE',  ( 4.467575310902914154, 5.170924936596891008, 1.199719254218464037 ) ) ;
#196342=ORIENTED_EDGE ( 'NONE', *, *, #98928, .T. ) ;
#196344=CYLINDRICAL_SURFACE ( 'NONE', #59639, 1.250000000000000000 ) ;
#196345=EDGE_CURVE ( 'NONE', #162762, #6079, #71339, .T. ) ;
#196351=CARTESIAN_POINT ( 'NONE',  ( 8.106885785967500979, 11.54545161934907682, 1.199719254218460707 ) ) ;
#196356=CARTESIAN_POINT ( 'NONE',  ( 1.364683531249988757, 0.3843750003414206362, 0.000000000000000000 ) ) ;
#196357=CARTESIAN_POINT ( 'NONE',  ( 4.961921032921539521, 7.772363057508363759, -1.082531754730549078 ) ) ;
#196358=CARTESIAN_POINT ( 'NONE',  ( -9.002250809794000830, 11.52571191622492464, -1.443375672974059665 ) ) ;
#196364=CARTESIAN_POINT ( 'NONE',  ( -4.548924232584923288, 5.265832011892554121, -1.199719254218446718 ) ) ;
#196377=CARTESIAN_POINT ( 'NONE',  ( 4.408913874118179699, 7.341020650511065782, -1.198271334459002802 ) ) ;
#196378=CARTESIAN_POINT ( 'NONE',  ( -2.110982172923218325, 5.614562968385698127, -0.4421859227901755451 ) ) ;
#196381=CARTESIAN_POINT ( 'NONE',  ( 4.660252114795294887, 6.460046772059735432, -1.599625672291256295 ) ) ;
#196386=CARTESIAN_POINT ( 'NONE',  ( -8.107412671292051343, 10.48173408797264194, 1.443375672974090751 ) ) ;
#196388=CARTESIAN_POINT ( 'NONE',  ( 1.123270288254022198, 2.908552654332631437, -0.7749999999939810591 ) ) ;
#196390=CARTESIAN_POINT ( 'NONE',  ( 5.587931867126699537, 9.671004278289832001, -0.7998128361456291469 ) ) ;
#196391=CARTESIAN_POINT ( 'NONE',  ( -5.274285450916075035, 6.112086766612214284, 1.199719254218450271 ) ) ;
#196392=CARTESIAN_POINT ( 'NONE',  ( 4.552840656090682891, 4.206068941727564514, 1.214306433183764966E-14 ) ) ;
#196394=CARTESIAN_POINT ( 'NONE',  ( -5.935772324684618795, 5.819489221753827657, 0.000000000000000000 ) ) ;
#196397=CARTESIAN_POINT ( 'NONE',  ( -5.473741331615264549, 7.409117525016355010, -1.599625672291256295 ) ) ;
#196400=CARTESIAN_POINT ( 'NONE',  ( 9.589694723567584234, 10.08239868711733855, -0.7998128361456281477 ) ) ;
#196401=CARTESIAN_POINT ( 'NONE',  ( -1.201851678989727383E-14, 3.493750000682815493, 1.732050807568877637 ) ) ;
#196403=CARTESIAN_POINT ( 'NONE',  ( 4.765179230921094522, 7.000095391635957398, 1.399907146243694722 ) ) ;
#196404=CARTESIAN_POINT ( 'NONE',  ( 4.039966587192257208, 6.696749537490852333, 1.082531754730558626 ) ) ;
#196411=CARTESIAN_POINT ( 'NONE',  ( 7.253248993186724114, 9.485209796849769504, 1.443375672974076540 ) ) ;
#196414=CARTESIAN_POINT ( 'NONE',  ( -9.806625181386236179, 10.33548422123910449, -0.7998128361456291469 ) ) ;
#196416=CARTESIAN_POINT ( 'NONE',  ( -6.852756576703439961, 10.08230087520760954, 1.199719254218453823 ) ) ;
#196424=CARTESIAN_POINT ( 'NONE',  ( 8.483651433849084711, 10.92067931095586886, 1.599625672291281386 ) ) ;
#196428=CARTESIAN_POINT ( 'NONE',  ( 4.630273154266905777, 5.360739087188218122, 1.199719254218464037 ) ) ;
#196432=CARTESIAN_POINT ( 'NONE',  ( -1.201851678989727383E-14, 4.868750000682822154, -1.732050807568863648 ) ) ;
#196438=CARTESIAN_POINT ( 'NONE',  ( -1.201851678989727383E-14, 3.712500000000020339, 1.732050807568877637 ) ) ;
#196439=CARTESIAN_POINT ( 'NONE',  ( 4.625302960556422427, 8.547937220624488575, 1.040834085586084257E-14 ) ) ;
#196442=CARTESIAN_POINT ( 'NONE',  ( 6.480434237652115570, 10.50433101066207442, 0.7216878364870438212 ) ) ;
#196443=CARTESIAN_POINT ( 'NONE',  ( -8.473482818416657736, 12.82955435488738516, -0.7216878364870267237 ) ) ;
#196450=CARTESIAN_POINT ( 'NONE',  ( -4.939248034080176097, 4.656877549381960080, 1.214306433183764966E-14 ) ) ;
#196451=CARTESIAN_POINT ( 'NONE',  ( -1.500000000000011324, 4.702083334016148974, 0.8660254037844403729 ) ) ;
#196452=CARTESIAN_POINT ( 'NONE',  ( 1.364683531249988757, -0.1156249996585798079, 0.000000000000000000 ) ) ;
#196456=CARTESIAN_POINT ( 'NONE',  ( 3.551346171775753735, 6.230655402791975384, 1.199719254218462483 ) ) ;
#196458=CARTESIAN_POINT ( 'NONE',  ( 1.364683531249990311, 4.926041667008083991, 0.7879004041258500513 ) ) ;
#196467=CARTESIAN_POINT ( 'NONE',  ( -7.063961727919978451, 8.200042423116789436, 1.199719254218450271 ) ) ;
#196470=CARTESIAN_POINT ( 'NONE',  ( 5.301401758143367893, 6.143722458377430584, 1.199719254218462483 ) ) ;
#196473=CARTESIAN_POINT ( 'NONE',  ( -1.364683531250014514, 0.9885416670080898749, -0.7879004041258289570 ) ) ;
#196477=CARTESIAN_POINT ( 'NONE',  ( 10.58621901417202515, 11.24501035948919991, -0.7998128361456281477 ) ) ;
#196480=CARTESIAN_POINT ( 'NONE',  ( -7.040761844198392794, 7.108643661186573759, -0.7998128361456291469 ) ) ;
#196484=CARTESIAN_POINT ( 'NONE',  ( 9.413438726589914651, 9.876766690643398405, 0.000000000000000000 ) ) ;
#196486=CARTESIAN_POINT ( 'NONE',  ( 8.239604668803105270, 10.63595808506888396, -1.599625672291268286 ) ) ;
#196488=CARTESIAN_POINT ( 'NONE',  ( -9.571693261567968847, 12.19006144329456731, 1.443375672974076540 ) ) ;
#196489=CARTESIAN_POINT ( 'NONE',  ( -6.157374318900681764, 10.33535380535947290, 0.7998128361456481317 ) ) ;
#196492=CARTESIAN_POINT ( 'NONE',  ( -4.338283617754775889, 7.407916770541659091, 1.160293660280581785 ) ) ;
#196493=CARTESIAN_POINT ( 'NONE',  ( -1.364683531250000748, 0.7593750003414210248, 0.000000000000000000 ) ) ;
#196497=CARTESIAN_POINT ( 'NONE',  ( 7.958272981541723468, 8.386999354661243800, 1.040834085586084257E-14 ) ) ;
#196500=CARTESIAN_POINT ( 'NONE',  ( 3.818592820543298405, 7.606775390609172405, -0.7998128361456221525 ) ) ;
#196513=CARTESIAN_POINT ( 'NONE',  ( -1.201851678989727383E-14, 4.118750000682818602, -1.732050807568863648 ) ) ;
#196517=DIRECTION ( 'NONE',  ( 0.6507913734559658270, -0.7592566023652989049, 0.000000000000000000 ) ) ;
#196521=CARTESIAN_POINT ( 'NONE',  ( -4.924636110261798372, 6.768494766770632332, 1.599625672291267398 ) ) ;
#196522=CARTESIAN_POINT ( 'NONE',  ( -6.008234629150358330, 10.16135750065076060, 0.000000000000000000 ) ) ;
#196528=CARTESIAN_POINT ( 'NONE',  ( -1.201851678989727383E-14, 3.368750000682815049, -1.732050807568863648 ) ) ;
#196529=CARTESIAN_POINT ( 'NONE',  ( 7.781490099239519509, 11.16582331816642260, 1.199719254218460707 ) ) ;
#196533=CARTESIAN_POINT ( 'NONE',  ( -9.189729191964438826, 9.615772233580322848, 1.040834085586084257E-14 ) ) ;
#196535=CARTESIAN_POINT ( 'NONE',  ( 1.364683531249988535, 2.905208333674754506, -0.7879004041258239610 ) ) ;
#196540=CARTESIAN_POINT ( 'NONE',  ( -10.31739171031960822, 11.13930453823545186, 1.040834085586084257E-14 ) ) ;
#196542=EDGE_CURVE ( 'NONE', #97523, #147312, #213118, .T. ) ;
#196545=CARTESIAN_POINT ( 'NONE',  ( -0.6823417656250212460, 1.613541667008083769, 1.181850606188755259 ) ) ;
#196550=CARTESIAN_POINT ( 'NONE',  ( -1.364683531250012516, 3.238541667008084879, -0.7879004041258289570 ) ) ;
#196552=CARTESIAN_POINT ( 'NONE',  ( -5.117312914154178216, 8.057616602233474978, -1.199719254218452047 ) ) ;
#196554=( BOUNDED_SURFACE ( )  B_SPLINE_SURFACE ( 3, 2, ( 
 ( #152726, #149534, #101845 ),
 ( #136495, #2176, #203582 ),
 ( #84526, #170034, #54166 ),
 ( #137565, #186279, #119223 ),
 ( #21620, #35771, #168974 ),
 ( #55234, #4307, #120304 ),
 ( #37916, #71452, #183090 ),
 ( #103990, #121381, #3247 ),
 ( #150615, #133319, #38984 ),
 ( #166853, #87728, #19512 ) ),
 .UNSPECIFIED., .F., .F., .T. ) 
 B_SPLINE_SURFACE_WITH_KNOTS ( ( 4, 2, 2, 2, 4 ),
 ( 3, 3 ),
 ( 0.000000000000000000, 0.0004557710599321653476, 0.0009115421198643306952, 0.001367313179796496043, 0.001823084239728661390 ),
 ( 0.000000000000000000, 1.000000000000000000 ),
 .UNSPECIFIED. ) 
 GEOMETRIC_REPRESENTATION_ITEM ( )  RATIONAL_B_SPLINE_SURFACE ( (
 ( 1.000000000000000000, 0.5613739026647618369, 1.000000000000000000),
 ( 1.000000000000000000, 0.5542214518087537067, 1.000000000000000000),
 ( 1.000000000000000000, 0.5635694824811526837, 1.000000000000000000),
 ( 1.000000000000000000, 0.6084377562511148474, 1.000000000000000000),
 ( 1.000000000000000000, 0.6447860777916630814, 1.000000000000000000),
 ( 1.000000000000000000, 0.7192854197611785461, 1.000000000000000000),
 ( 1.000000000000000000, 0.7560301986938927632, 1.000000000000000000),
 ( 1.000000000000000000, 0.8079200278152608439, 1.000000000000000000),
 ( 1.000000000000000000, 0.8228378482302226571, 1.000000000000000000),
 ( 1.000000000000000000, 0.8275596917170975342, 1.000000000000000000) ) ) 
 REPRESENTATION_ITEM ( '' )  SURFACE ( )  );
#196556=CARTESIAN_POINT ( 'NONE',  ( -0.6823417656250003738, 3.030208333674754062, -1.181850606188749264 ) ) ;
#196560=CARTESIAN_POINT ( 'NONE',  ( -0.8775925178581088781, 2.800000000000024691, 1.062197627458028260 ) ) ;
#196561=CARTESIAN_POINT ( 'NONE',  ( -6.087247782855839340, 6.204136622861004646, 0.000000000000000000 ) ) ;
#196565=CARTESIAN_POINT ( 'NONE',  ( 4.528060117284232966, 6.305822774963486310, 1.443375672974062551 ) ) ;
#196568=CARTESIAN_POINT ( 'NONE',  ( -6.516665389662827934, 10.75452672124865217, 0.000000000000000000 ) ) ;
#196569=CARTESIAN_POINT ( 'NONE',  ( -4.115063316947640715, 4.759660943649018705, 1.199719254218462483 ) ) ;
#196576=CARTESIAN_POINT ( 'NONE',  ( -5.544921637864824504, 8.452530429942200385, -1.082531754730543971 ) ) ;
#196578=CARTESIAN_POINT ( 'NONE',  ( -1.364683531250014514, 0.09270833367475767028, 0.7879004041258379498 ) ) ;
#196581=CARTESIAN_POINT ( 'NONE',  ( 6.724481002698112775, 8.868313807946373473, -1.443375672974057666 ) ) ;
#196589=VERTEX_POINT ( 'NONE', #71997 ) ;
#196590=CARTESIAN_POINT ( 'NONE',  ( 9.205623113554624481, 10.80261038964432707, 1.082531754730549967 ) ) ;
#196596=CARTESIAN_POINT ( 'NONE',  ( 6.636879889089462026, 7.701780277814560982, -1.199719254218446718 ) ) ;
#196597=CARTESIAN_POINT ( 'NONE',  ( -4.440459003675619520, 5.139289244831666714, 1.199719254218462483 ) ) ;
#196603=CARTESIAN_POINT ( 'NONE',  ( 4.473827502385202770, 8.163289819517311585, 1.040834085586084257E-14 ) ) ;
#196605=CARTESIAN_POINT ( 'NONE',  ( 0.6823417656249882723, 0.7385416670080829915, -1.181850606188749264 ) ) ;
#196607=CARTESIAN_POINT ( 'NONE',  ( -9.820183334999905256, 10.35130206712171130, 1.040834085586084257E-14 ) ) ;
#196609=EDGE_CURVE ( 'NONE', #4315, #4590, #149821, .T. ) ;
#196617=CARTESIAN_POINT ( 'NONE',  ( 1.499999999999974909, 4.545833333333353821, -0.8660254037844394848 ) ) ;
#196625=CARTESIAN_POINT ( 'NONE',  ( 7.820355676984174664, 8.018169799436671852, -0.7998128361456281477 ) ) ;
#196628=ORIENTED_EDGE ( 'NONE', *, *, #31081, .T. ) ;
#196634=CARTESIAN_POINT ( 'NONE',  ( -5.093612336809997920, 4.836969235900084207, -0.4916062289654357098 ) ) ;
#196635=CARTESIAN_POINT ( 'NONE',  ( 10.72180055030867329, 11.40318881831530540, 0.7998128361456341429 ) ) ;
#196642=FACE_OUTER_BOUND ( 'NONE', #137749, .T. ) ;
#196647=CARTESIAN_POINT ( 'NONE',  ( -8.622622508611375025, 12.04318144581317895, 1.082531754730560403 ) ) ;
#196651=CARTESIAN_POINT ( 'NONE',  ( 6.173040012923759257, 6.096301524699504704, -0.7998128361456281477 ) ) ;
#196657=CARTESIAN_POINT ( 'NONE',  ( 5.314433026432511475, 5.302519407033794430, 1.040834085586084257E-14 ) ) ;
#196664=CARTESIAN_POINT ( 'NONE',  ( -6.775324078527193983, 8.927630729746953264, -1.599625672291263179 ) ) ;
#196665=B_SPLINE_CURVE_WITH_KNOTS ( 'NONE', 3,
 ( #209627, #80723, #61268, #127429, #163049, #210709, #112225, #79648, #145764, #193399 ),
 .UNSPECIFIED., .F., .F.,
 ( 4, 3, 3, 4 ),
 ( 0.000000000000000000, 0.0001748246942969784896, 0.0003306242286995172888, 0.0004873602920373641223 ),
 .UNSPECIFIED. ) ;
#196666=CARTESIAN_POINT ( 'NONE',  ( -3.100010679019018500, 6.768429558830820980, 1.040834085586084257E-14 ) ) ;
#196667=CARTESIAN_POINT ( 'NONE',  ( 0.000000000000000000, 2.800000000000024691, 1.214306433183764966E-14 ) ) ;
#196675=AXIS2_PLACEMENT_3D ( 'NONE', #86252, #20165, #35357 ) ;
#196676=CARTESIAN_POINT ( 'NONE',  ( 4.950698647284403009, 8.927565521807144577, 1.040834085586084257E-14 ) ) ;
#196689=CARTESIAN_POINT ( 'NONE',  ( -1.364683531250014514, 0.09270833367475767028, 0.7879004041258379498 ) ) ;
#196690=CARTESIAN_POINT ( 'NONE',  ( 4.220665892555866883, 3.818531717603609987, -0.7998128361456211532 ) ) ;
#196691=CARTESIAN_POINT ( 'NONE',  ( 3.842846474469570062, 6.570739089268092137, -1.199719254218452047 ) ) ;
#196693=CARTESIAN_POINT ( 'NONE',  ( -6.968527767744110868, 9.153035033833367251, 1.443375672974078761 ) ) ;
#196695=CARTESIAN_POINT ( 'NONE',  ( 5.694061328059515148, 5.745419092265303007, -0.7216878364870207285 ) ) ;
#196696=CARTESIAN_POINT ( 'NONE',  ( -6.927853306458756855, 9.105581495667113501, 1.443375672974078761 ) ) ;
#196700=CARTESIAN_POINT ( 'NONE',  ( 8.111855979677986994, 8.358253485912799263, 1.040834085586084257E-14 ) ) ;
#196705=CARTESIAN_POINT ( 'NONE',  ( 0.6823417656249917140, 4.342708333674755394, 1.181850606188765695 ) ) ;
#196709=CARTESIAN_POINT ( 'NONE',  ( 7.690499447449630210, 9.995335326823163058, 1.599625672291281386 ) ) ;
#196712=CARTESIAN_POINT ( 'NONE',  ( -8.365544474831901667, 9.718555627847388578, 1.199719254218462483 ) ) ;
#196718=CARTESIAN_POINT ( 'NONE',  ( 8.971744963941056028, 11.49012176272984931, 1.599625672291281386 ) ) ;
#196719=CARTESIAN_POINT ( 'NONE',  ( 3.998552203707626873, 7.829812396822075193, -0.1602144209190259072 ) ) ;
#196721=CARTESIAN_POINT ( 'NONE',  ( -7.167456763118792651, 11.51378332361394818, 0.000000000000000000 ) ) ;
#196723=CARTESIAN_POINT ( 'NONE',  ( 0.5717273634750134059, 6.816772624464344510, 3.722363499285739952 ) ) ;
#196725=CARTESIAN_POINT ( 'NONE',  ( 4.670798236633449285, 6.855725761985807409, -1.225018586207384352 ) ) ;
#196726=CARTESIAN_POINT ( 'NONE',  ( -8.948018195339354719, 12.42280974699582607, 1.082531754730560403 ) ) ;
#196731=CARTESIAN_POINT ( 'NONE',  ( 5.636439174979242850, 7.598931675607687453, -1.599625672291262513 ) ) ;
#196733=CARTESIAN_POINT ( 'NONE',  ( 5.931855901178834323, 6.879252291918818152, 1.199719254218462483 ) ) ;
#196734=CARTESIAN_POINT ( 'NONE',  ( -4.245236785304952853, 7.324258608653995140, 0.8904289178662868620 ) ) ;
#196735=CARTESIAN_POINT ( 'NONE',  ( 3.765413976293345844, 5.416068943807445635, 1.599625672291267398 ) ) ;
#196737=CARTESIAN_POINT ( 'NONE',  ( -5.910991785878158211, 9.839981483592442402, -0.7216878364870278340 ) ) ;
#196744=CARTESIAN_POINT ( 'NONE',  ( -5.429614816329291216, 6.304498938506903016, 1.045551501023216368 ) ) ;
#196745=CARTESIAN_POINT ( 'NONE',  ( -1.402160292154681736E-14, 0.1343750003414218575, 1.575800808251672791 ) ) ;
#196748=CARTESIAN_POINT ( 'NONE',  ( 4.690757960648224589, 6.495636925554817864, 1.443375672974062551 ) ) ;
#196753=CARTESIAN_POINT ( 'NONE',  ( -9.612367721964622191, 10.31677655182129527, -0.7216878364870267237 ) ) ;
#196759=CARTESIAN_POINT ( 'NONE',  ( -9.124274191872631334, 12.62844174295135069, -1.082531754730543083 ) ) ;
#196760=EDGE_LOOP ( 'NONE', ( #169735, #101311, #50899, #108759 ) ) ;
#196765=CARTESIAN_POINT ( 'NONE',  ( -9.639484029191951464, 10.34841224358651601, 0.7216878364870438212 ) ) ;
#196769=CARTESIAN_POINT ( 'NONE',  ( 0.6823417656249917140, 4.655208333674755394, 1.181850606188765695 ) ) ;
#196770=CARTESIAN_POINT ( 'NONE',  ( 0.7499999999999885647, 3.347916667349487341, -1.299038105676658228 ) ) ;
#196774=CARTESIAN_POINT ( 'NONE',  ( -7.157815033010924921, 10.43820240756634199, 1.199719254218453823 ) ) ;
#196778=CARTESIAN_POINT ( 'NONE',  ( 6.419949431270806528, 7.448694743692793274, 1.199719254218462483 ) ) ;
#196785=CARTESIAN_POINT ( 'NONE',  ( 6.747154001095143627, 11.02343010125301959, -0.7998128361456291469 ) ) ;
#196788=CARTESIAN_POINT ( 'NONE',  ( -2.081668171172168513E-14, 6.120000000000041851, 2.580000000000011173 ) ) ;
#196791=CARTESIAN_POINT ( 'NONE',  ( -6.073689629242158716, 9.069426419882418600, -1.082531754730538864 ) ) ;
#196794=CARTESIAN_POINT ( 'NONE',  ( -1.364683531250010295, 5.342708333674750953, 0.7879004041258379498 ) ) ;
#196800=CARTESIAN_POINT ( 'NONE',  ( -7.641992139597101108, 12.06740792950531649, 0.7998128361456481317 ) ) ;
#196802=CARTESIAN_POINT ( 'NONE',  ( 8.259941899223605333, 10.65968485389279508, -1.599625672291268286 ) ) ;
#196803=CARTESIAN_POINT ( 'NONE',  ( 1.451998047844732964, 7.315968950354620581, 4.301760722576522866 ) ) ;
#196804=CARTESIAN_POINT ( 'NONE',  ( -7.506410603460441422, 11.90922947067921278, -0.7998128361456291469 ) ) ;
#196805=FACE_OUTER_BOUND ( 'NONE', #98941, .T. ) ;
#196807=CARTESIAN_POINT ( 'NONE',  ( -1.364683531249997417, 2.759375000341422801, 1.214306433183764966E-14 ) ) ;
#196808=CARTESIAN_POINT ( 'NONE',  ( 2.686486993802192913, 6.285985259411197568, 0.7998128361456362523 ) ) ;
#196815=CARTESIAN_POINT ( 'NONE',  ( 8.717529583462638954, 12.15390636647303069, 1.082531754730546636 ) ) ;
#196816=DIRECTION ( 'NONE',  ( -1.000000000000000000, 5.459311322609750190E-16, -5.329070518200750605E-15 ) ) ;
#196817=CARTESIAN_POINT ( 'NONE',  ( -8.039621903223732602, 8.481906429956900695, 1.040834085586084257E-14 ) ) ;
#196818=CARTESIAN_POINT ( 'NONE',  ( 1.364683531249986537, 0.3635416670080869328, 0.7879004041258500513 ) ) ;
#196820=CARTESIAN_POINT ( 'NONE',  ( 0.4909524369918957798, 7.516007857509691803, 2.014442075801145648 ) ) ;
#196822=CARTESIAN_POINT ( 'NONE',  ( -8.345207244411405156, 9.694828859023472134, 1.199719254218462483 ) ) ;
#196823=CARTESIAN_POINT ( 'NONE',  ( -4.568734577680894304, 5.392907097791561633, -1.082531754730543971 ) ) ;
#196824=CARTESIAN_POINT ( 'NONE',  ( -1.364683531250012516, 3.551041667008086211, -0.7879004041258300672 ) ) ;
#196828=EDGE_CURVE ( 'NONE', #10803, #98551, #185617, .T. ) ;
#196845=CARTESIAN_POINT ( 'NONE',  ( -1.364683531249997417, 4.321875000341417028, 1.214306433183764966E-14 ) ) ;
#196851=CARTESIAN_POINT ( 'NONE',  ( 8.229962938695207342, 9.560377169021284871, 1.199719254218462483 ) ) ;
#196853=CARTESIAN_POINT ( 'NONE',  ( -1.364683531250012516, 2.530208333674753174, 0.7879004041258379498 ) ) ;
#196854=CARTESIAN_POINT ( 'NONE',  ( -7.429504990608782222, 8.730472579540773381, 1.082531754730549967 ) ) ;
#196860=CARTESIAN_POINT ( 'NONE',  ( 4.813308228051395687, 5.574280006603454574, 1.199719254218462483 ) ) ;
#196863=CARTESIAN_POINT ( 'NONE',  ( 9.348510611822643313, 10.86534945433664134, 1.199719254218453823 ) ) ;
#196870=CARTESIAN_POINT ( 'NONE',  ( -8.676328237741483207, 12.20980114641871062, -1.199719254218446718 ) ) ;
#196872=CARTESIAN_POINT ( 'NONE',  ( 5.621827251160867789, 9.710548892996357040, 1.040834085586084257E-14 ) ) ;
#196874=CARTESIAN_POINT ( 'NONE',  ( 3.484082288587588838, 7.008587070086755411, -0.7216878364870267237 ) ) ;
#196875=CARTESIAN_POINT ( 'NONE',  ( 6.909076424898653812, 5.229711127717879826, 1.214306433183764966E-14 ) ) ;
#196883=CARTESIAN_POINT ( 'NONE',  ( -1.436838838544729491, 7.449283400311742298, -4.203727439823573775 ) ) ;
#196884=CARTESIAN_POINT ( 'NONE',  ( -6.507550544879489252, 9.575597488125954015, 1.082531754730548412 ) ) ;
#196885=CARTESIAN_POINT ( 'NONE',  ( 6.145923705696426431, 6.064665832934283962, 0.7998128361456341429 ) ) ;
#196888=CARTESIAN_POINT ( 'NONE',  ( -6.808165692356648258, 11.09461040772476714, 0.7998128361456481317 ) ) ;
#196893=CARTESIAN_POINT ( 'NONE',  ( -9.917953063596627317, 11.52969898140628047, -1.199719254218441611 ) ) ;
#196897=CARTESIAN_POINT ( 'NONE',  ( 7.248805684800777804, 11.60869039890961218, 1.040834085586084257E-14 ) ) ;
#196909=CARTESIAN_POINT ( 'NONE',  ( -9.345647958521597687, 9.797677461230342999, 0.7998128361456462443 ) ) ;
#196913=CARTESIAN_POINT ( 'NONE',  ( 7.348156068926750883, 8.635565504245116486, -1.082531754730537976 ) ) ;
#196915=CARTESIAN_POINT ( 'NONE',  ( 3.388648328411762556, 6.040841252200647382, 1.199719254218462483 ) ) ;
#196916=DIRECTION ( 'NONE',  ( -1.000000000000000000, 8.673617379884035472E-16, 0.000000000000000000 ) ) ;
#196917=CARTESIAN_POINT ( 'NONE',  ( 4.059776932288224671, 6.823824623389866950, 1.199719254218462483 ) ) ;
#196919=CARTESIAN_POINT ( 'NONE',  ( -6.735703387890906946, 6.752742128827836865, -0.7998128361456291469 ) ) ;
#196930=CARTESIAN_POINT ( 'NONE',  ( -0.6823417656250212460, 4.363541667008085767, 1.181850606188767472 ) ) ;
#196931=CARTESIAN_POINT ( 'NONE',  ( 3.289951133708768793, 7.658661826345697143, 2.499999999999998668 ) ) ;
#196932=CARTESIAN_POINT ( 'NONE',  ( 9.402743226277308963, 10.92862083786708816, -1.199719254218446718 ) ) ;
#196934=CARTESIAN_POINT ( 'NONE',  ( -3.877268743828284681, 5.546566172598190292, 1.443375672974064550 ) ) ;
#196936=CARTESIAN_POINT ( 'NONE',  ( -4.650083499362882122, 6.448183387388563226, 1.443375672974064550 ) ) ;
#196943=CARTESIAN_POINT ( 'NONE',  ( 3.497113557321089861, 6.167384019261527683, -1.199719254218446718 ) ) ;
#196951=CARTESIAN_POINT ( 'NONE',  ( 5.518332215962025167, 6.396807992499198292, -1.199719254218445830 ) ) ;
#196957=CARTESIAN_POINT ( 'NONE',  ( -0.6823417656249969321, 3.780208333674754506, -1.181850606188749264 ) ) ;
#196962=CARTESIAN_POINT ( 'NONE',  ( 6.531277313481192337, 8.642909503859968368, 1.599625672291281386 ) ) ;
#196964=CARTESIAN_POINT ( 'NONE',  ( -4.252453736180621391, 8.112946458852704268, -0.7998128361456281477 ) ) ;
#196965=CARTESIAN_POINT ( 'NONE',  ( 0.7499999999999902300, 1.733333333333357595, 1.299038105676657340 ) ) ;
#196966=ADVANCED_FACE ( 'NONE', ( #110997 ), #95374, .F. ) ;
#196969=CARTESIAN_POINT ( 'NONE',  ( -3.276266675996675204, 6.974061555304760240, -0.7998128361456281477 ) ) ;
#196970=CARTESIAN_POINT ( 'NONE',  ( 0.4229270055062719358, 8.019365653748165457, -1.955756443285229240 ) ) ;
#196972=CARTESIAN_POINT ( 'NONE',  ( -1.201851678989727383E-14, 3.446875000341421469, -1.575800808251660134 ) ) ;
#196974=CARTESIAN_POINT ( 'NONE',  ( -5.097502569058225852, 5.049433873430440478, -0.7216878364870207285 ) ) ;
#196979=CARTESIAN_POINT ( 'NONE',  ( 4.981731378017507872, 7.899438143407371271, -1.199719254218452047 ) ) ;
#196983=CARTESIAN_POINT ( 'NONE',  ( -1.201851678989727383E-14, 4.259375000341417028, -1.575800808251660134 ) ) ;
#196985=CARTESIAN_POINT ( 'NONE',  ( 3.358669367883368118, 4.941533567329135401, -1.599625672291262513 ) ) ;
#196988=CARTESIAN_POINT ( 'NONE',  ( -1.364683531250014514, -0.4489583329919089039, -0.7879004041258359514 ) ) ;
#196989=CARTESIAN_POINT ( 'NONE',  ( -4.237421715137035250, 7.350374185294469953, -0.8920271880306808177 ) ) ;
#196993=CARTESIAN_POINT ( 'NONE',  ( -3.110706179331648169, 5.716575411607132118, 1.199719254218462483 ) ) ;
#196994=CARTESIAN_POINT ( 'NONE',  ( -5.978782553502159480, 8.958701498185728695, 1.082531754730548412 ) ) ;
#196997=EDGE_LOOP ( 'NONE', ( #202632, #199990, #92752, #159926 ) ) ;
#196998=CARTESIAN_POINT ( 'NONE',  ( -1.201851678989727383E-14, 3.571875000341422357, 1.575800808251672791 ) ) ;
#197006=CARTESIAN_POINT ( 'NONE',  ( -6.195713011320795438, 8.251417818006149929, -1.443375672974058777 ) ) ;
#197012=CARTESIAN_POINT ( 'NONE',  ( -6.195713011320804320, 7.291048603704809672, -1.082531754730543083 ) ) ;
#197023=CARTESIAN_POINT ( 'NONE',  ( -6.064574784014443942, 5.969758757638621738, -0.7998128361456291469 ) ) ;
#197025=CARTESIAN_POINT ( 'NONE',  ( 1.499999999999985123, -0.2041666666666457353, -0.8660254037844323793 ) ) ;
#197026=CARTESIAN_POINT ( 'NONE',  ( 9.788623719386617239, 11.48277776311499387, -1.082531754730537088 ) ) ;
#197027=CARTESIAN_POINT ( 'NONE',  ( 5.459129407796876166, 9.520734742405036144, 1.040834085586084257E-14 ) ) ;
#197030=CARTESIAN_POINT ( 'NONE',  ( 5.250031796989762967, 7.148123067953287446, 1.599625672291267398 ) ) ;
#197038=CARTESIAN_POINT ( 'NONE',  ( -4.663641653420935285, 5.503632019488245319, 1.082531754730560403 ) ) ;
#197041=DIRECTION ( 'NONE',  ( -0.7592566023652994600, -0.6507913734559651608, -0.000000000000000000 ) ) ;
#197045=CARTESIAN_POINT ( 'NONE',  ( -0.6823417656250212460, 3.801041667008085767, 1.181850606188767472 ) ) ;
#197046=CARTESIAN_POINT ( 'NONE',  ( 8.717529583462633624, 13.11427558077437894, 0.7216878364870438212 ) ) ;
#197047=CARTESIAN_POINT ( 'NONE',  ( -6.847031270101295419, 7.946956888995021728, -1.199719254218446718 ) ) ;
#197050=CARTESIAN_POINT ( 'NONE',  ( 6.654354466208897811, 6.657835053532175529, 0.7998128361456341429 ) ) ;
#197051=CARTESIAN_POINT ( 'NONE',  ( -5.052384799386910430, 9.046199365926717917, 1.214306433183764966E-14 ) ) ;
#197054=CARTESIAN_POINT ( 'NONE',  ( -1.500000000000013101, -0.04791666598384902026, 0.8660254037844403729 ) ) ;
#197057=CARTESIAN_POINT ( 'NONE',  ( 5.978782553946477840, 9.919070713005490703, 1.040834085586084257E-14 ) ) ;
#197058=EDGE_CURVE ( 'NONE', #127597, #34591, #188553, .T. ) ;
#197061=CARTESIAN_POINT ( 'NONE',  ( 0.6823417656249882723, 0.9885416670080832136, -1.181850606188749264 ) ) ;
#197063=CARTESIAN_POINT ( 'NONE',  ( 5.450014562569148957, 9.302174723065263606, 1.040834085586084257E-14 ) ) ;
#197066=CARTESIAN_POINT ( 'NONE',  ( -5.097502569058221411, 6.009803087731781623, -1.082531754730544860 ) ) ;
#197069=CARTESIAN_POINT ( 'NONE',  ( 0.6823417656249899377, 4.176041667008085767, -1.181850606188754593 ) ) ;
#197073=CARTESIAN_POINT ( 'NONE',  ( -5.830469385422084372, 6.191968629596825480, -0.9632026293319171373 ) ) ;
#197075=AXIS2_PLACEMENT_3D ( 'NONE', #95077, #12712, #33243 ) ;
#197080=CARTESIAN_POINT ( 'NONE',  ( 6.714312387265682247, 8.856450423275211037, 1.599625672291281386 ) ) ;
#197083=CARTESIAN_POINT ( 'NONE',  ( 3.602716132929354664, 5.226254793216122074, 1.599625672291267398 ) ) ;
#197089=CARTESIAN_POINT ( 'NONE',  ( 5.992340707560163793, 6.093411701682730275, 0.7216878364870317197 ) ) ;
#197090=CARTESIAN_POINT ( 'NONE',  ( -0.6823417656250003738, 0.2802083336747515641, -1.181850606188749264 ) ) ;
#197092=CARTESIAN_POINT ( 'NONE',  ( 2.535011536075338689, 5.133042487381368701, -0.9999999999999956701 ) ) ;
#197095=CARTESIAN_POINT ( 'NONE',  ( 1.499999999999987121, 2.295833333333350268, -0.8660254037844262731 ) ) ;
#197096=CARTESIAN_POINT ( 'NONE',  ( 5.829115978871627135, 8.888053511070525659, 1.199719254218462483 ) ) ;
#197097=CARTESIAN_POINT ( 'NONE',  ( -8.097244055859620815, 10.46987070330147063, -1.599625672291263179 ) ) ;
#197102=CARTESIAN_POINT ( 'NONE',  ( 0.6823417656249882723, 1.426041667008083547, -1.181850606188749264 ) ) ;
#197104=CARTESIAN_POINT ( 'NONE',  ( 0.7499999999999902300, 1.983333333333357817, 1.299038105676669330 ) ) ;
#197106=CARTESIAN_POINT ( 'NONE',  ( 3.011882680530176604, 6.665613560593854459, 0.7998128361456341429 ) ) ;
#197112=DIRECTION ( 'NONE',  ( 0.000000000000000000, 1.000000000000000000, -8.546850786086437571E-32 ) ) ;
#197114=CARTESIAN_POINT ( 'NONE',  ( -1.402160292154681736E-14, -1.006249999317181620, 1.732050807568877637 ) ) ;
#197115=CARTESIAN_POINT ( 'NONE',  ( -5.208303565944065738, 9.228104593576741621, -0.7998128361456231517 ) ) ;
#197116=EDGE_CURVE ( 'NONE', #63111, #152681, #202448, .T. ) ;
#197117=CARTESIAN_POINT ( 'NONE',  ( -3.416291520963659512, 5.969128626890772615, 1.082531754730560403 ) ) ;
#197124=CARTESIAN_POINT ( 'NONE',  ( 5.991813822235618758, 9.077867661661846554, 1.199719254218462483 ) ) ;
#197128=CARTESIAN_POINT ( 'NONE',  ( 5.524057522564145728, 8.532151978711786100, 1.199719254218462483 ) ) ;
#197129=CARTESIAN_POINT ( 'NONE',  ( 9.042925270190625753, 11.57316545335434199, 1.443375672974076540 ) ) ;
#197133=CARTESIAN_POINT ( 'NONE',  ( -7.528855374290365887, 7.678086112960552434, -0.7998128361456291469 ) ) ;
#197134=CARTESIAN_POINT ( 'NONE',  ( 3.897079088924235712, 6.634010472798538949, 1.199719254218462483 ) ) ;
#197138=CARTESIAN_POINT ( 'NONE',  ( 4.285325189395043033, 7.238007417033815116, 0.9681492361576886641 ) ) ;
#197139=CARTESIAN_POINT ( 'NONE',  ( 9.761507412159302177, 10.49077285704843199, -0.7216878364870257245 ) ) ;
#197150=CARTESIAN_POINT ( 'NONE',  ( 9.734391104931955141, 10.45913716528321125, 0.7216878364870438212 ) ) ;
#197153=CARTESIAN_POINT ( 'NONE',  ( -4.218558352146454915, 8.073401844146177453, 1.040834085586084257E-14 ) ) ;
#197159=CARTESIAN_POINT ( 'NONE',  ( -6.205881626753225966, 8.263281202677319470, 1.599625672291283607 ) ) ;
#197160=DIRECTION ( 'NONE',  ( -1.000000000000000000, 5.578564026256504688E-16, 0.000000000000000000 ) ) ;
#197175=CARTESIAN_POINT ( 'NONE',  ( -4.693093728624763372, 8.627026450037540428, 0.7998128361456481317 ) ) ;
#197178=CARTESIAN_POINT ( 'NONE',  ( 3.850152436600926542, 7.435668909435648288, -0.7216878364870197293 ) ) ;
#197182=CARTESIAN_POINT ( 'NONE',  ( -2.286521462199063492, 5.819358805874190743, 1.040834085586084257E-14 ) ) ;
#197185=CARTESIAN_POINT ( 'NONE',  ( 9.541187415715040032, 12.15447128979948310, -1.599625672291262513 ) ) ;
#197188=CARTESIAN_POINT ( 'NONE',  ( -8.097244055859620815, 10.46987070330147063, -1.599625672291263179 ) ) ;
#197189=CARTESIAN_POINT ( 'NONE',  ( 4.625302960556422427, 8.547937220624488575, 1.040834085586084257E-14 ) ) ;
#197192=CARTESIAN_POINT ( 'NONE',  ( 5.834086172582112262, 5.700855377634248100, 1.040834085586084257E-14 ) ) ;
#197195=CARTESIAN_POINT ( 'NONE',  ( -1.402160292154681736E-14, 0.1343750003414218575, 1.575800808251672791 ) ) ;
#197198=CARTESIAN_POINT ( 'NONE',  ( 7.266807147244743526, 11.42176607185347414, -0.7216878364870267237 ) ) ;
#197225=CARTESIAN_POINT ( 'NONE',  ( 1.499999999999989120, 0.5562500006828161592, 0.000000000000000000 ) ) ;
#197232=CARTESIAN_POINT ( 'NONE',  ( 8.380911511541880188, 12.92948053010758258, 0.7998128361456462443 ) ) ;
#197237=CARTESIAN_POINT ( 'NONE',  ( 3.822509244049070887, 6.547012320444182798, -1.199719254218452047 ) ) ;
#197238=CARTESIAN_POINT ( 'NONE',  ( -6.805829924380121909, 8.963220883242035697, 1.443375672974078761 ) ) ;
#197239=CARTESIAN_POINT ( 'NONE',  ( -5.833005281931015418, 6.047509994665502653, 0.4702358434125544773 ) ) ;
#197242=CARTESIAN_POINT ( 'NONE',  ( -5.994676475536691029, 10.14553965476814845, 0.7998128361456481317 ) ) ;
#197243=CARTESIAN_POINT ( 'NONE',  ( -4.894130264408878439, 4.812166184672871161, -0.7216878364870197293 ) ) ;
#197245=ORIENTED_EDGE ( 'NONE', *, *, #170654, .T. ) ;
#197246=CARTESIAN_POINT ( 'NONE',  ( 1.499999999999987121, 1.577083334016150751, -0.8660254037844253849 ) ) ;
#197253=CARTESIAN_POINT ( 'NONE',  ( -2.602802303699316866, 5.980427087717073320, 1.040834085586084257E-14 ) ) ;
#197256=CARTESIAN_POINT ( 'NONE',  ( 4.065672160753666553, 7.505179260319745360, -0.5311146244057519672 ) ) ;
#197261=CARTESIAN_POINT ( 'NONE',  ( -2.277406616971334508, 5.600798786534425311, 1.040834085586084257E-14 ) ) ;
#197262=CARTESIAN_POINT ( 'NONE',  ( 8.769426429940780920, 9.125419011219408461, 0.7998128361456462443 ) ) ;
#197271=CARTESIAN_POINT ( 'NONE',  ( -7.472515219426274946, 11.86968485597268064, 0.000000000000000000 ) ) ;
#197276=CARTESIAN_POINT ( 'NONE',  ( 5.030238685870051185, 5.827365540725222282, -1.199719254218452047 ) ) ;
#197282=CARTESIAN_POINT ( 'NONE',  ( -8.459397779922852578, 11.95671561229694824, 1.199719254218453823 ) ) ;
#197286=CARTESIAN_POINT ( 'NONE',  ( -1.257539916218606724, 3.172412844624492134, -0.7749999999999918066 ) ) ;
#197295=CARTESIAN_POINT ( 'NONE',  ( 7.955937213120826357, 8.176348258262782664, 0.7998128361456481317 ) ) ;
#197297=CARTESIAN_POINT ( 'NONE',  ( -2.774614992291035698, 6.388801257648172971, 1.040834085586084257E-14 ) ) ;
#197306=CARTESIAN_POINT ( 'NONE',  ( 0.7499999999999867883, -0.1520833326505155458, -1.299038105676652899 ) ) ;
#197310=CARTESIAN_POINT ( 'NONE',  ( 3.172244755473273781, 6.644776614786712443, 0.000000000000000000 ) ) ;
#197312=CARTESIAN_POINT ( 'NONE',  ( -4.634189577772691138, 4.300976017023221409, 1.214306433183764966E-14 ) ) ;
#197318=CARTESIAN_POINT ( 'NONE',  ( 4.365362273920238678, 7.076377838673507448, 1.082531754730558626 ) ) ;
#197322=CARTESIAN_POINT ( 'NONE',  ( -0.6823417656250212460, 4.363541667008085767, 1.181850606188767472 ) ) ;
#197324=CARTESIAN_POINT ( 'NONE',  ( 5.151735183068521629, 5.112705256442466428, 1.040834085586084257E-14 ) ) ;
#197326=CARTESIAN_POINT ( 'NONE',  ( 2.873292495919350653, 6.437382019922593734, -0.3438188498175620555 ) ) ;
#197331=CARTESIAN_POINT ( 'NONE',  ( -6.070455375431035527, 6.038045056918933895, -0.4763334965118305453 ) ) ;
#197333=CARTESIAN_POINT ( 'NONE',  ( 0.6823417656249882723, -0.6572916663252492686, 1.181850606188755259 ) ) ;
#197341=CARTESIAN_POINT ( 'NONE',  ( -1.201851678989727383E-14, 5.087500000000019007, -1.732050807568863648 ) ) ;
#197349=CARTESIAN_POINT ( 'NONE',  ( -1.364683531250010295, 5.301041667008085767, -0.7879004041258300672 ) ) ;
#197351=CARTESIAN_POINT ( 'NONE',  ( 5.341022448779654930, 8.318611059296550536, 1.199719254218462483 ) ) ;
#197352=CARTESIAN_POINT ( 'NONE',  ( -7.853197290813634268, 10.18514947741448573, 1.599625672291295375 ) ) ;
#197358=CARTESIAN_POINT ( 'NONE',  ( 1.499999999999990896, 5.275000000000022560, 1.214306433183764966E-14 ) ) ;
#197367=CARTESIAN_POINT ( 'NONE',  ( 8.785320351975350661, 9.351887953500479966, -0.7216878364870197293 ) ) ;
#197370=CARTESIAN_POINT ( 'NONE',  ( -1.201851678989727383E-14, 3.993750000682817713, 1.732050807568877637 ) ) ;
#197372=CARTESIAN_POINT ( 'NONE',  ( -4.627410500965859264, 4.293067094081919777, 0.7998128361456341429 ) ) ;
#197374=CARTESIAN_POINT ( 'NONE',  ( 7.090551149822744925, 7.374657217655760100, 0.7216878364870317197 ) ) ;
#197382=CARTESIAN_POINT ( 'NONE',  ( 2.659370686574860976, 6.254349567645977714, -0.7998128361456291469 ) ) ;
#197384=CARTESIAN_POINT ( 'NONE',  ( 4.878236342818665250, 4.585697242910212523, 1.040834085586084257E-14 ) ) ;
#197388=ORIENTED_EDGE ( 'NONE', *, *, #205767, .T. ) ;
#197398=CARTESIAN_POINT ( 'NONE',  ( 7.228468454380276853, 11.58496363008569574, 1.040834085586084257E-14 ) ) ;
#197400=CARTESIAN_POINT ( 'NONE',  ( -1.438721403180282410, 7.870009100117679068, 3.684356824110524453 ) ) ;
#197403=CARTESIAN_POINT ( 'NONE',  ( -4.702146809683744877, 5.356480858934594025, 2.500000000000011102 ) ) ;
#197404=CARTESIAN_POINT ( 'NONE',  ( -0.6823417656250003738, -0.5322916663252491576, -1.181850606188749264 ) ) ;
#197405=CARTESIAN_POINT ( 'NONE',  ( 6.371969008742804697, 7.496680600697164465, -1.082531754730543083 ) ) ;
#197406=CARTESIAN_POINT ( 'NONE',  ( -4.274898507010545856, 3.881803101134051470, -0.7998128361456221525 ) ) ;
#197412=CARTESIAN_POINT ( 'NONE',  ( -3.066115294984855133, 6.728884944124295053, 0.7998128361456341429 ) ) ;
#197417=VERTEX_POINT ( 'NONE', #121352 ) ;
#197424=CARTESIAN_POINT ( 'NONE',  ( 5.389300372041062381, 6.501875383066589187, -1.316743393031569509 ) ) ;
#197428=CARTESIAN_POINT ( 'NONE',  ( 4.253507506385319381, 5.985511395581417204, 1.599625672291267398 ) ) ;
#197434=CARTESIAN_POINT ( 'NONE',  ( -8.893785580884703279, 10.43879993486270585, 1.082531754730558626 ) ) ;
#197439=CARTESIAN_POINT ( 'NONE',  ( 7.800018446563675489, 7.994443030612759848, -0.7998128361456281477 ) ) ;
#197440=CARTESIAN_POINT ( 'NONE',  ( -5.773074481320628948, 5.629675071162500544, 0.000000000000000000 ) ) ;
#197443=CARTESIAN_POINT ( 'NONE',  ( -4.401593425930945713, 8.286942763561420122, 1.040834085586084257E-14 ) ) ;
#197444=CARTESIAN_POINT ( 'NONE',  ( 2.523789150438203510, 6.096171108819874007, 0.7998128361456462443 ) ) ;
#197446=CARTESIAN_POINT ( 'NONE',  ( -4.232116505760120440, 8.089219690028791376, -0.7998128361456281477 ) ) ;
#197449=CARTESIAN_POINT ( 'NONE',  ( 9.399880572976245574, 9.860948844760784482, 0.7998128361456462443 ) ) ;
#197452=CARTESIAN_POINT ( 'NONE',  ( 5.221388208558932931, 6.626734370510860117, 1.385765457383714816 ) ) ;
#197453=CARTESIAN_POINT ( 'NONE',  ( 4.636525346193557162, 7.392734756325715750, -1.082531754730549078 ) ) ;
#197455=CARTESIAN_POINT ( 'NONE',  ( 4.650083499362867911, 6.448183387388563226, 1.443375672974062551 ) ) ;
#197460=CARTESIAN_POINT ( 'NONE',  ( 6.710922848640084482, 9.812865175846695820, -1.082531754730537976 ) ) ;
#197463=CARTESIAN_POINT ( 'NONE',  ( -9.972185678051314284, 11.59297036493672017, 1.199719254218462483 ) ) ;
#197464=CARTESIAN_POINT ( 'NONE',  ( -7.725448601688521322, 7.907444878258402809, 1.040834085586084257E-14 ) ) ;
#197469=B_SPLINE_CURVE_WITH_KNOTS ( 'NONE', 1,
 ( #214409, #63946 ),
 .UNSPECIFIED., .F., .F.,
 ( 2, 2 ),
 ( 0.2265555213262071821, 0.4428258268412663679 ),
 .UNSPECIFIED. ) ;
#197473=CARTESIAN_POINT ( 'NONE',  ( 9.576136569953906275, 10.06658084123472641, 0.000000000000000000 ) ) ;
#197476=CARTESIAN_POINT ( 'NONE',  ( 8.920901888111986366, 12.39117405523060889, 1.082531754730546636 ) ) ;
#197478=CARTESIAN_POINT ( 'NONE',  ( 4.304877467538922531, 4.981110786005563007, 1.199719254218464037 ) ) ;
#197482=CARTESIAN_POINT ( 'NONE',  ( 1.499999999999989120, 4.577083334016148974, -0.8660254037844323793 ) ) ;
#197489=CARTESIAN_POINT ( 'NONE',  ( -0.7500000000000006661, 2.858333333333358706, -1.299038105676652011 ) ) ;
#197490=CARTESIAN_POINT ( 'NONE',  ( 6.154511665599609493, 9.267681812253174556, 1.199719254218462483 ) ) ;
#197494=CARTESIAN_POINT ( 'NONE',  ( 8.053180056837369705, 11.37883191874353805, -1.082531754730543083 ) ) ;
#197499=CARTESIAN_POINT ( 'NONE',  ( -3.903858165731105778, 6.641919395739846799, 1.199719254218464037 ) ) ;
#197501=CARTESIAN_POINT ( 'NONE',  ( -1.402160292154681736E-14, -0.9281249996585830830, 1.575800808251672791 ) ) ;
#197505=CARTESIAN_POINT ( 'NONE',  ( 4.857899112398166075, 4.561970474086296079, 1.040834085586084257E-14 ) ) ;
#197507=CARTESIAN_POINT ( 'NONE',  ( 0.6823417656249882723, -1.157291666325249713, 1.181850606188755259 ) ) ;
#197514=CARTESIAN_POINT ( 'NONE',  ( -5.865874016206865882, 9.995270118883347266, 0.000000000000000000 ) ) ;
#197516=CARTESIAN_POINT ( 'NONE',  ( 4.873266149108180123, 7.772895376346490970, 1.199719254218462483 ) ) ;
#197519=CARTESIAN_POINT ( 'NONE',  ( 1.364683531249986537, -0.1364583329919154264, 0.7879004041258500513 ) ) ;
#197521=ORIENTED_EDGE ( 'NONE', *, *, #126517, .F. ) ;
#197523=CARTESIAN_POINT ( 'NONE',  ( 8.723781775389312543, 12.26516360700784958, -1.199719254218446718 ) ) ;
#197526=CARTESIAN_POINT ( 'NONE',  ( -5.205440912643032547, 8.160432600470439723, 1.199719254218452047 ) ) ;
#197530=CARTESIAN_POINT ( 'NONE',  ( 9.426996880203592610, 9.892584536526015881, -0.7998128361456281477 ) ) ;
#197532=CARTESIAN_POINT ( 'NONE',  ( 8.209625708274705502, 9.536650400197368427, 1.199719254218462483 ) ) ;
#197533=CARTESIAN_POINT ( 'NONE',  ( 4.881461487140826172, 4.938218254980607291, -0.7598994375367192911 ) ) ;
#197534=CARTESIAN_POINT ( 'NONE',  ( -2.767835915484202047, 6.380892334706859792, -0.7998128361456281477 ) ) ;
#197535=CARTESIAN_POINT ( 'NONE',  ( -6.018930129462987999, 9.109503353427070849, 1.199719254218452047 ) ) ;
#197538=CARTESIAN_POINT ( 'NONE',  ( -4.849785647588779725, 6.920107565692508622, 1.442884047295606820 ) ) ;
#197539=CARTESIAN_POINT ( 'NONE',  ( -1.364683531250000748, 0.009375000341420303140, 0.000000000000000000 ) ) ;
#197543=CARTESIAN_POINT ( 'NONE',  ( 8.270110514656037637, 8.750809809961280550, 0.7216878364870458196 ) ) ;
#197546=CARTESIAN_POINT ( 'NONE',  ( 5.789495288235341874, 6.713164910151406595, 1.199719254218462483 ) ) ;
#197560=CARTESIAN_POINT ( 'NONE',  ( 1.187787545756531227, 2.830338437039773947, 0.7750000000000117906 ) ) ;
#197564=CARTESIAN_POINT ( 'NONE',  ( 8.048736748007069508, 12.54194330598362406, -0.7998128361456352531 ) ) ;
#197568=CARTESIAN_POINT ( 'NONE',  ( -5.596818484342970912, 5.424043074688562172, -0.7998128361456221525 ) ) ;
#197569=CARTESIAN_POINT ( 'NONE',  ( -8.667740277838301921, 9.006785167099828016, -0.7998128361456291469 ) ) ;
#197571=VERTEX_POINT ( 'NONE', #135400 ) ;
#197575=CARTESIAN_POINT ( 'NONE',  ( 0.7499999999999885647, 2.597916667349486897, -1.299038105676658228 ) ) ;
#197576=CARTESIAN_POINT ( 'NONE',  ( 7.730120138085914583, 12.17022392774227768, 0.7998128361456462443 ) ) ;
#197581=CARTESIAN_POINT ( 'NONE',  ( -9.528683032306089373, 10.01121838064558744, 0.7998128361456462443 ) ) ;
#197583=CARTESIAN_POINT ( 'NONE',  ( -1.364683531249997417, 2.759375000341422801, 1.214306433183764966E-14 ) ) ;
#197585=CYLINDRICAL_SURFACE ( 'NONE', #139450, 1.500000000000000222 ) ;
#197589=CARTESIAN_POINT ( 'NONE',  ( -9.327646496521989405, 10.94497100310623594, -1.082531754730539753 ) ) ;
#197593=CARTESIAN_POINT ( 'NONE',  ( -1.364683531250000748, 1.321875000341421469, 0.000000000000000000 ) ) ;
#197599=CARTESIAN_POINT ( 'NONE',  ( -1.201851678989727383E-14, 2.071875000341422801, 1.575800808251672791 ) ) ;
#197601=CARTESIAN_POINT ( 'NONE',  ( -6.600121851754250812, 6.594563670001734046, 0.7998128361456341429 ) ) ;
#197602=CARTESIAN_POINT ( 'NONE',  ( 3.018661757337009810, 6.673522483535157868, 0.000000000000000000 ) ) ;
#197604=CARTESIAN_POINT ( 'NONE',  ( -1.201851678989727383E-14, 5.337500000000020783, -1.732050807568863648 ) ) ;
#197605=CARTESIAN_POINT ( 'NONE',  ( 0.6823417656249882723, 2.738541667008084879, -1.181850606188749264 ) ) ;
#197609=CARTESIAN_POINT ( 'NONE',  ( -6.249945626219832739, 6.393950773452325542, 1.040834085586084257E-14 ) ) ;
#197612=CARTESIAN_POINT ( 'NONE',  ( 5.205967797967541166, 5.175976640491323444, -0.7216878364870197293 ) ) ;
#197615=CARTESIAN_POINT ( 'NONE',  ( -6.177711549321182716, 10.35908057418338402, 0.7998128361456481317 ) ) ;
#197616=CARTESIAN_POINT ( 'NONE',  ( -4.762992037102518950, 4.451245552908022596, -0.7998128361456221525 ) ) ;
#197618=CARTESIAN_POINT ( 'NONE',  ( -1.364683531250010295, 4.780208333674755394, 0.7879004041258379498 ) ) ;
#197623=CARTESIAN_POINT ( 'NONE',  ( -7.659993601596720936, 8.999375959026737704, -1.082531754730543083 ) ) ;
#197625=CARTESIAN_POINT ( 'NONE',  ( -1.364683531250014514, 0.05104166700808546175, -0.7879004041258359514 ) ) ;
#197628=CARTESIAN_POINT ( 'NONE',  ( 8.609064354997688184, 9.146255957026539818, 1.040834085586084257E-14 ) ) ;
#197634=CARTESIAN_POINT ( 'NONE',  ( 3.890826896997583884, 4.602014803661035103, -1.082531754730543083 ) ) ;
#197640=CARTESIAN_POINT ( 'NONE',  ( 8.554831740098649107, 11.96409221588171157, 1.082531754730546636 ) ) ;
#197646=CARTESIAN_POINT ( 'NONE',  ( 6.257251587906815793, 7.258880593101466161, 1.199719254218462483 ) ) ;
#197647=CARTESIAN_POINT ( 'NONE',  ( -6.064574784014443942, 5.969758757638621738, -0.7998128361456291469 ) ) ;
#197652=CARTESIAN_POINT ( 'NONE',  ( 5.626270559546814098, 7.587068290936515247, 1.443375672974062551 ) ) ;
#197653=CARTESIAN_POINT ( 'NONE',  ( 0.6823417656249882723, -0.2614583329919109578, -1.181850606188749264 ) ) ;
#197655=CARTESIAN_POINT ( 'NONE',  ( -7.947050595904583403, 12.42330946186405249, 0.7998128361456481317 ) ) ;
#197668=CARTESIAN_POINT ( 'NONE',  ( 2.278002604729090219, 5.615589014598373119, 0.4951895290833923657 ) ) ;
#197672=CARTESIAN_POINT ( 'NONE',  ( 7.955937213120826357, 8.176348258262782664, 0.7998128361456481317 ) ) ;
#197673=CARTESIAN_POINT ( 'NONE',  ( 6.500244582748090139, 9.671036882259738121, 1.199719254218460707 ) ) ;
#197682=CARTESIAN_POINT ( 'NONE',  ( 8.536830278099042602, 13.11138575775759563, -0.7998128361456352531 ) ) ;
#197684=CARTESIAN_POINT ( 'NONE',  ( -4.060830702492950195, 4.696389560118578999, -1.199719254218452047 ) ) ;
#197697=CARTESIAN_POINT ( 'NONE',  ( -9.815740026613960723, 11.51441345488021106, -1.082531754730539753 ) ) ;
#197700=CARTESIAN_POINT ( 'NONE',  ( 6.908042961362778733, 8.018137195466769285, 1.199719254218462483 ) ) ;
#197706=CARTESIAN_POINT ( 'NONE',  ( 5.816084710138150093, 5.887779704690372817, -0.7216878364870257245 ) ) ;
#197707=CARTESIAN_POINT ( 'NONE',  ( -6.018930129462987999, 9.109503353427070849, 1.199719254218452047 ) ) ;
#197713=CARTESIAN_POINT ( 'NONE',  ( -7.881367368245678406, 8.089350105908421185, 0.7998128361456602331 ) ) ;
#197714=CARTESIAN_POINT ( 'NONE',  ( -5.610376637956639101, 5.439860920571172542, 0.000000000000000000 ) ) ;
#197722=CARTESIAN_POINT ( 'NONE',  ( 5.452350330990040739, 9.512825819463730070, 0.7998128361456462443 ) ) ;
#197734=CARTESIAN_POINT ( 'NONE',  ( 1.364683531249986537, 0.1760416670080860446, 0.7879004041258500513 ) ) ;
#197736=CARTESIAN_POINT ( 'NONE',  ( 5.087333953625774008, 6.958308917361963886, 1.599625672291267398 ) ) ;
#197739=CARTESIAN_POINT ( 'NONE',  ( -6.534666852106790103, 10.56760239419251590, 0.7216878364870458196 ) ) ;
#197742=CARTESIAN_POINT ( 'NONE',  ( 5.368665641331531013, 5.365790791082654998, -0.7216878364870207285 ) ) ;
#197743=CARTESIAN_POINT ( 'NONE',  ( -6.629573926958124197, 9.717958100551031819, 1.082531754730548412 ) ) ;
#197747=CARTESIAN_POINT ( 'NONE',  ( 6.100279051144945619, 9.204410428722734849, -1.199719254218440723 ) ) ;
#197752=CARTESIAN_POINT ( 'NONE',  ( -1.364683531250012516, 3.280208333674756727, 0.7879004041258379498 ) ) ;
#197757=CARTESIAN_POINT ( 'NONE',  ( 8.796542737168120851, 9.157054702984622097, -0.7998128361456211532 ) ) ;
#197760=CARTESIAN_POINT ( 'NONE',  ( -9.027031348600448979, 9.425958082989001952, 1.040834085586084257E-14 ) ) ;
#197766=CARTESIAN_POINT ( 'NONE',  ( 7.716561984472250835, 12.15440608185967086, 1.040834085586084257E-14 ) ) ;
#197769=CARTESIAN_POINT ( 'NONE',  ( -8.853638004923878313, 10.28799807962136548, 1.199719254218462483 ) ) ;
#197770=CARTESIAN_POINT ( 'NONE',  ( 6.471393748265519719, 5.229711127717882491, -2.499999999999995115 ) ) ;
#197772=CARTESIAN_POINT ( 'NONE',  ( 5.328689024754546644, 6.340921230984883472, -1.104828203510083373 ) ) ;
#197773=CARTESIAN_POINT ( 'NONE',  ( -10.46653140006992899, 11.31330084294416771, -0.7216878364870267237 ) ) ;
#197778=CARTESIAN_POINT ( 'NONE',  ( 7.311924916471702396, 7.425000578838787391, -0.7998128361456281477 ) ) ;
#197780=CARTESIAN_POINT ( 'NONE',  ( 6.796715079152391148, 6.823922435299587974, 0.7998128361456341429 ) ) ;
#197781=CARTESIAN_POINT ( 'NONE',  ( -4.021031317475609157, 7.616913651768732585, 0.1724795716798576684 ) ) ;
#197782=CARTESIAN_POINT ( 'NONE',  ( 2.849184837166184536, 6.475799410002530898, 0.7998128361456362523 ) ) ;
#197784=CARTESIAN_POINT ( 'NONE',  ( -8.839552966430023417, 9.415159337030921449, -0.7216878364870267237 ) ) ;
#197792=CARTESIAN_POINT ( 'NONE',  ( -4.183908731771626144, 7.398323783528643283, -0.7858605482065593728 ) ) ;
#197794=CARTESIAN_POINT ( 'NONE',  ( 1.364683531249986537, -0.5739583329919174526, 0.7879004041258500513 ) ) ;
#197796=CARTESIAN_POINT ( 'NONE',  ( 4.009043883868839586, 7.799745125292699477, 0.2347419505407536966 ) ) ;
#197797=CARTESIAN_POINT ( 'NONE',  ( 4.582292731738905722, 5.408724944192588424, -1.082531754730548412 ) ) ;
#197799=CARTESIAN_POINT ( 'NONE',  ( 7.736899214892750010, 12.17813285068358020, 1.040834085586084257E-14 ) ) ;
#197802=CARTESIAN_POINT ( 'NONE',  ( -9.286972035236630063, 10.89751746493999107, -1.082531754730537976 ) ) ;
#197810=CARTESIAN_POINT ( 'NONE',  ( -9.693716643646601128, 12.33242205571964512, 1.443375672974076540 ) ) ;
#197818=CARTESIAN_POINT ( 'NONE',  ( -9.070041577417988776, 12.56517035942090388, 1.082531754730558626 ) ) ;
#197822=VERTEX_POINT ( 'NONE', #175369 ) ;
#197824=CARTESIAN_POINT ( 'NONE',  ( -1.201851678989727383E-14, 3.493750000682815493, 1.732050807568877637 ) ) ;
#197828=CARTESIAN_POINT ( 'NONE',  ( -8.616370316684697883, 10.01118577667568132, -1.199719254218446718 ) ) ;
#197832=CARTESIAN_POINT ( 'NONE',  ( 5.392392409933256303, 7.314210449720692786, 1.599625672291267398 ) ) ;
#197838=CARTESIAN_POINT ( 'NONE',  ( 8.959240580532112475, 9.346868853575953651, -0.7998128361456221525 ) ) ;
#197843=CARTESIAN_POINT ( 'NONE',  ( -5.748293942514169252, 9.650167333001109071, -0.7216878364870207285 ) ) ;
#197845=B_SPLINE_CURVE_WITH_KNOTS ( 'NONE', 3,
 ( #165415, #132951, #65749, #111411 ),
 .UNSPECIFIED., .F., .F.,
 ( 4, 4 ),
 ( 0.001170373960510464294, 0.001235641208627022772 ),
 .UNSPECIFIED. ) ;
#197854=CARTESIAN_POINT ( 'NONE',  ( -3.429849674132942727, 5.984946472254969230, -1.082531754730549078 ) ) ;
#197856=CARTESIAN_POINT ( 'NONE',  ( 2.372313692266983853, 5.711523707712699682, 0.7216878364870438212 ) ) ;
#197857=CARTESIAN_POINT ( 'NONE',  ( -8.910733272679575379, 11.41894145625809820, -1.599625672291263179 ) ) ;
#197860=CARTESIAN_POINT ( 'NONE',  ( 1.364683531249988535, 1.863541667008086211, 0.7879004041258500513 ) ) ;
#197861=CARTESIAN_POINT ( 'NONE',  ( 3.928111819657337911, 5.605883094398769195, 1.599625672291267398 ) ) ;
#197867=CARTESIAN_POINT ( 'NONE',  ( 8.365017589507326434, 12.70301158782650397, -0.7216878364870338292 ) ) ;
#197869=CARTESIAN_POINT ( 'NONE',  ( -8.215877900201387973, 8.687538426430837291, 0.7216878364870578100 ) ) ;
#197870=CARTESIAN_POINT ( 'NONE',  ( 1.364683531249986537, 0.6135416670080880985, 0.7879004041258500513 ) ) ;
#197874=CARTESIAN_POINT ( 'NONE',  ( -8.694856585065634746, 9.038420858865048757, 0.7998128361456462443 ) ) ;
#197876=CARTESIAN_POINT ( 'NONE',  ( -3.416291520519271874, 6.929497840673697340, 1.040834085586084257E-14 ) ) ;
#197877=CARTESIAN_POINT ( 'NONE',  ( -1.364683531249997417, 3.071875000341423245, 1.214306433183764966E-14 ) ) ;
#197879=CIRCLE ( 'NONE', #152907, 0.08000000000000025147 ) ;
#197889=VERTEX_POINT ( 'NONE', #113614 ) ;
#197897=CARTESIAN_POINT ( 'NONE',  ( -0.6823417656249969321, 4.530208333674755394, -1.181850606188749264 ) ) ;
#197902=CARTESIAN_POINT ( 'NONE',  ( 8.778014389843965759, 12.32843499053828928, 1.199719254218450271 ) ) ;
#197905=CARTESIAN_POINT ( 'NONE',  ( -1.402160292154681736E-14, 1.946875000341422579, -1.575800808251660134 ) ) ;
#197907=CARTESIAN_POINT ( 'NONE',  ( -6.968527767744110868, 9.153035033833367251, 1.443375672974078761 ) ) ;
#197914=CARTESIAN_POINT ( 'NONE',  ( 4.005544317833563461, 6.760553239859419250, -1.199719254218452047 ) ) ;
#197917=CARTESIAN_POINT ( 'NONE',  ( 7.730120138085914583, 12.17022392774227768, 0.7998128361456462443 ) ) ;
#197924=CARTESIAN_POINT ( 'NONE',  ( -10.32183501870554387, 10.93656236477829502, 0.7998128361456462443 ) ) ;
#197926=CARTESIAN_POINT ( 'NONE',  ( 5.635385404774530649, 9.726366738878972740, 0.7998128361456462443 ) ) ;
#197929=CARTESIAN_POINT ( 'NONE',  ( 3.646780131951580461, 7.198401220678078971, -0.7216878364870267237 ) ) ;
#197934=ORIENTED_EDGE ( 'NONE', *, *, #49638, .T. ) ;
#197939=CARTESIAN_POINT ( 'NONE',  ( -1.441115678601552652, 8.287243072884001194, -3.161846531485744460 ) ) ;
#197940=CARTESIAN_POINT ( 'NONE',  ( -6.561783159334130922, 9.638868871656395498, -1.082531754730538864 ) ) ;
#197941=CARTESIAN_POINT ( 'NONE',  ( 5.443762371086860341, 6.309809840144842141, 1.199719254218462483 ) ) ;
#197944=CARTESIAN_POINT ( 'NONE',  ( -6.997979842947967377, 11.31606025008131233, -0.7998128361456291469 ) ) ;
#197945=B_SPLINE_CURVE_WITH_KNOTS ( 'NONE', 3,
 ( #55177, #118111, #69261, #133263, #37857, #135377, #168919 ),
 .UNSPECIFIED., .F., .F.,
 ( 4, 3, 4 ),
 ( 6.124194260411441496E-16, 2.761892602837239034E-05, 5.460426739246099117E-05 ),
 .UNSPECIFIED. ) ;
#197950=CARTESIAN_POINT ( 'NONE',  ( -9.001723924469462901, 12.58942944760136484, -1.199719254218446718 ) ) ;
#197952=CARTESIAN_POINT ( 'NONE',  ( 5.517805331081858888, 5.539787095791365523, 1.040834085586084257E-14 ) ) ;
#197954=CARTESIAN_POINT ( 'NONE',  ( 9.447334110624092673, 9.916311305349925220, -0.7998128361456281477 ) ) ;
#197955=CARTESIAN_POINT ( 'NONE',  ( 4.227444969362701421, 3.826440640544909400, 1.214306433183764966E-14 ) ) ;
#197961=CARTESIAN_POINT ( 'NONE',  ( 2.236732156574683827, 5.553345249405011508, 1.040834085586084257E-14 ) ) ;
#197965=CARTESIAN_POINT ( 'NONE',  ( -7.645908563102897126, 11.00764485934031889, 1.199719254218453823 ) ) ;
#197969=CARTESIAN_POINT ( 'NONE',  ( 7.456621297836078632, 8.762108271306003004, 1.082531754730558626 ) ) ;
#197974=CARTESIAN_POINT ( 'NONE',  ( 5.020596955762157698, 4.751784624677624080, 1.040834085586084257E-14 ) ) ;
#197977=CARTESIAN_POINT ( 'NONE',  ( -6.714312387265696458, 8.856450423275211037, 1.599625672291283607 ) ) ;
#197987=CARTESIAN_POINT ( 'NONE',  ( -0.6823417656249969321, 4.030208333674754506, -1.181850606188749264 ) ) ;
#197988=CARTESIAN_POINT ( 'NONE',  ( 1.598423149420358458, 8.713846000021369775, 2.499999999999998668 ) ) ;
#197989=CARTESIAN_POINT ( 'NONE',  ( 9.901532256681887745, 10.44620914241737530, 0.000000000000000000 ) ) ;
#197991=CARTESIAN_POINT ( 'NONE',  ( -2.657034918598338180, 6.043698471765932112, -0.7216878364870267237 ) ) ;
#197994=CARTESIAN_POINT ( 'NONE',  ( -4.189106276498259618, 6.870745841681152655, 1.082531754730560403 ) ) ;
#198002=CARTESIAN_POINT ( 'NONE',  ( 5.020596955762157698, 4.751784624677624080, 1.040834085586084257E-14 ) ) ;
#198011=CARTESIAN_POINT ( 'NONE',  ( 6.179819089730593795, 6.104210447640811665, 1.040834085586084257E-14 ) ) ;
#198012=CARTESIAN_POINT ( 'NONE',  ( -4.936726087586472467, 4.653935278472638437, -0.1487728517622861069 ) ) ;
#198016=CARTESIAN_POINT ( 'NONE',  ( 0.6823417656249917140, 4.155208333674755394, 1.181850606188765695 ) ) ;
#198021=CARTESIAN_POINT ( 'NONE',  ( 6.474182045725470402, 7.511966127223233869, -1.199719254218446718 ) ) ;
#198023=CARTESIAN_POINT ( 'NONE',  ( -6.033542053281340856, 6.997886136038390603, -1.199719254218446718 ) ) ;
#198024=CARTESIAN_POINT ( 'NONE',  ( -0.7500000000000006661, 2.108333333333357817, -1.299038105676652011 ) ) ;
#198026=CARTESIAN_POINT ( 'NONE',  ( -3.262708522383007903, 6.958243709422141876, 1.040834085586084257E-14 ) ) ;
#198029=CARTESIAN_POINT ( 'NONE',  ( -4.303823697334223652, 7.108545849276850959, -1.199719254218452047 ) ) ;
#198032=CARTESIAN_POINT ( 'NONE',  ( -0.6823417656250212460, 3.051041667008084879, 1.181850606188767472 ) ) ;
#198034=CARTESIAN_POINT ( 'NONE',  ( -3.443407828190963915, 6.961133532957338943, 0.7216878364870317197 ) ) ;
#198040=CARTESIAN_POINT ( 'NONE',  ( 3.981290663907289140, 7.796589541200495965, -0.7998128361456221525 ) ) ;
#198043=CARTESIAN_POINT ( 'NONE',  ( -0.6823417656250212460, 3.113541667008084879, 1.181850606188767472 ) ) ;
#198045=CARTESIAN_POINT ( 'NONE',  ( 2.523789150438203510, 6.096171108819874007, 0.7998128361456462443 ) ) ;
#198047=CARTESIAN_POINT ( 'NONE',  ( -1.402160292154681736E-14, -0.1156249996585793222, 1.575800808251672791 ) ) ;
#198050=CARTESIAN_POINT ( 'NONE',  ( -4.634189577772691138, 4.300976017023221409, 1.214306433183764966E-14 ) ) ;
#198051=CARTESIAN_POINT ( 'NONE',  ( -5.205967797523171292, 9.017453497178271604, 0.000000000000000000 ) ) ;
#198054=CARTESIAN_POINT ( 'NONE',  ( -1.201851678989727383E-14, 3.321875000341421025, 1.575800808251672791 ) ) ;
#198063=CARTESIAN_POINT ( 'NONE',  ( -6.765155463094763455, 8.915767345075790828, 1.443375672974078761 ) ) ;
#198070=CARTESIAN_POINT ( 'NONE',  ( -7.185458225118419584, 7.485382138834033583, 1.040834085586084257E-14 ) ) ;
#198073=( BOUNDED_CURVE ( )  B_SPLINE_CURVE ( 2, ( #16570, #148737, #66376, #132524, #17632 ),
 .UNSPECIFIED., .F., .T. ) 
 B_SPLINE_CURVE_WITH_KNOTS ( ( 3, 2, 3 ),
 ( 0.2606479433802291745, 0.2625000000000000111, 0.2632879865674999098 ),
 .UNSPECIFIED. ) 
 CURVE ( )  GEOMETRIC_REPRESENTATION_ITEM ( )  RATIONAL_B_SPLINE_CURVE ( ( 0.9338382430890757036, 0.9404491509274826022, 1.000000000000000000, 0.9746631562710195151, 0.9589095569522538831 ) ) 
 REPRESENTATION_ITEM ( '' )  );
#198075=CARTESIAN_POINT ( 'NONE',  ( 2.876381804795541619, 6.437993120328354024, 0.3511878651327338674 ) ) ;
#198079=CARTESIAN_POINT ( 'NONE',  ( 0.1100172516615156165, 7.047065462482140497, 3.945011421259203566 ) ) ;
#198083=CARTESIAN_POINT ( 'NONE',  ( -4.741601036477307574, 6.554953847355395880, 1.599625672291267398 ) ) ;
#198085=CARTESIAN_POINT ( 'NONE',  ( -0.7500000000000249800, -0.3083333333333132531, 1.299038105676659116 ) ) ;
#198086=CARTESIAN_POINT ( 'NONE',  ( 2.333974999846879061, 5.874721266463329705, -0.7998128361456291469 ) ) ;
#198089=CARTESIAN_POINT ( 'NONE',  ( 4.320244504248938355, 8.192035688265757898, 1.040834085586084257E-14 ) ) ;
#198090=VECTOR ( 'NONE', #79200, 1000.000000000000000 ) ;
#198096=CARTESIAN_POINT ( 'NONE',  ( -4.609409038966253647, 4.479991421656468908, -0.7216878364870207285 ) ) ;
#198098=CARTESIAN_POINT ( 'NONE',  ( 4.350813900535696277, 4.000456626940672500, 0.2320863031703649382 ) ) ;
#198103=CARTESIAN_POINT ( 'NONE',  ( -0.6823417656250003738, 1.967708333674753174, -1.181850606188749264 ) ) ;
#198104=CARTESIAN_POINT ( 'NONE',  ( 8.703971429848968100, 13.09845773489176679, 0.000000000000000000 ) ) ;
#198105=CARTESIAN_POINT ( 'NONE',  ( -7.552055258011950656, 8.769484874890757453, 1.199719254218462483 ) ) ;
#198108=CARTESIAN_POINT ( 'NONE',  ( 7.806797523370503811, 8.002351953554066810, 1.040834085586084257E-14 ) ) ;
#198109=CARTESIAN_POINT ( 'NONE',  ( -5.876569516519495551, 8.943415971659659292, 1.199719254218452047 ) ) ;
#198110=CARTESIAN_POINT ( 'NONE',  ( -1.512220381301933259, 8.756542408759468543, 2.494878041824271975 ) ) ;
#198112=CARTESIAN_POINT ( 'NONE',  ( -1.201851678989727383E-14, 5.696875000341416140, -1.575800808251660134 ) ) ;
#198115=CARTESIAN_POINT ( 'NONE',  ( 8.609064354997688184, 9.146255957026539818, 1.040834085586084257E-14 ) ) ;
#198118=CARTESIAN_POINT ( 'NONE',  ( 1.364683531249988757, 0.1968750003414204697, 0.000000000000000000 ) ) ;
#198120=CARTESIAN_POINT ( 'NONE',  ( 7.768458830506048685, 8.165549511786275971, -0.7216878364870267237 ) ) ;
#198124=CARTESIAN_POINT ( 'NONE',  ( -5.124618876285560454, 5.081069565195661220, 0.7216878364870317197 ) ) ;
#198126=CARTESIAN_POINT ( 'NONE',  ( 1.364683531249990311, 4.613541667008083103, 0.7879004041258500513 ) ) ;
#198130=CARTESIAN_POINT ( 'NONE',  ( -5.249217764984337009, 6.599847349967512322, -1.403262209131036053 ) ) ;
#198137=CARTESIAN_POINT ( 'NONE',  ( 5.960781091502512119, 10.10599504006161986, 0.7998128361456462443 ) ) ;
#198144=ORIENTED_EDGE ( 'NONE', *, *, #146212, .F. ) ;
#198145=CARTESIAN_POINT ( 'NONE',  ( 4.012850279964918165, 7.625483060026979842, -0.7216878364870197293 ) ) ;
#198146=CARTESIAN_POINT ( 'NONE',  ( -1.364683531250000748, 1.071875000341421247, 0.000000000000000000 ) ) ;
#198148=CARTESIAN_POINT ( 'NONE',  ( 9.083072846151447166, 12.68433652289702884, 1.199719254218450271 ) ) ;
#198153=CARTESIAN_POINT ( 'NONE',  ( -1.201851678989727383E-14, 1.962500000000020783, 1.732050807568877637 ) ) ;
#198154=CARTESIAN_POINT ( 'NONE',  ( 8.098297826064319693, 8.342435640030188893, 0.7998128361456481317 ) ) ;
#198155=CARTESIAN_POINT ( 'NONE',  ( -8.552495972122143186, 8.872333477097637200, 0.7998128361456462443 ) ) ;
#198159=CARTESIAN_POINT ( 'NONE',  ( 1.364683531249986537, 1.405208333674755838, -0.7879004041258239610 ) ) ;
#198160=CARTESIAN_POINT ( 'NONE',  ( 0.7499999999999885647, 2.816666666666689522, -1.299038105676658228 ) ) ;
#198162=CARTESIAN_POINT ( 'NONE',  ( 3.323720213644492993, 7.029424015893889433, 1.040834085586084257E-14 ) ) ;
#198170=CARTESIAN_POINT ( 'NONE',  ( -0.7500000000000249800, -0.02708333265051543481, 1.299038105676659116 ) ) ;
#198171=CARTESIAN_POINT ( 'NONE',  ( -7.019370843573183194, 9.212351955633947043, 1.599625672291283607 ) ) ;
#198172=CARTESIAN_POINT ( 'NONE',  ( -3.619663825168619731, 7.166765529431275539, 1.040834085586084257E-14 ) ) ;
#198179=ORIENTED_EDGE ( 'NONE', *, *, #8087, .F. ) ;
#198180=CARTESIAN_POINT ( 'NONE',  ( 7.287671262545424966, 8.461036880179857889, -1.199719254218451159 ) ) ;
#198184=CARTESIAN_POINT ( 'NONE',  ( 8.392133896734655707, 11.77427806529038357, 1.082531754730546636 ) ) ;
#198185=CARTESIAN_POINT ( 'NONE',  ( 0.9398415344190423903, 7.435109595052201037, -4.383649807226275286 ) ) ;
#198188=CARTESIAN_POINT ( 'NONE',  ( -6.693975156845199059, 8.832723654451292816, 1.599625672291283607 ) ) ;
#198189=CARTESIAN_POINT ( 'NONE',  ( 4.192495815123822744, 5.914331089109666983, -1.599625672291255185 ) ) ;
#198194=CARTESIAN_POINT ( 'NONE',  ( 9.734391104931955141, 10.45913716528321125, 0.7216878364870438212 ) ) ;
#198195=ORIENTED_EDGE ( 'NONE', *, *, #180280, .F. ) ;
#198196=EDGE_CURVE ( 'NONE', #93714, #135745, #72299, .T. ) ;
#198201=CARTESIAN_POINT ( 'NONE',  ( 5.034901488060123498, 4.768473245691916773, 0.3558765841190755230 ) ) ;
#198203=CARTESIAN_POINT ( 'NONE',  ( -3.958617665510279160, 5.641473247893851628, -1.443375672974053447 ) ) ;
#198204=CARTESIAN_POINT ( 'NONE',  ( 9.246297574839980271, 10.85006392781057905, 1.082531754730549967 ) ) ;
#198207=CARTESIAN_POINT ( 'NONE',  ( -6.417086777969760902, 6.381022750586497594, 0.7998128361456341429 ) ) ;
#198208=DIRECTION ( 'NONE',  ( 1.000000000000000000, 0.000000000000000000, 0.000000000000000000 ) ) ;
#198211=DIRECTION ( 'NONE',  ( 0.7592566023653016805, -0.6507913734559627184, 4.115938288792103177E-15 ) ) ;
#198213=CARTESIAN_POINT ( 'NONE',  ( -7.230575994789712801, 7.330093503543126054, 0.7998128361456341429 ) ) ;
#198228=CARTESIAN_POINT ( 'NONE',  ( -5.850506979496850057, 6.784345216623154151, -1.199719254218446718 ) ) ;
#198231=CARTESIAN_POINT ( 'NONE',  ( 5.517805331081858888, 5.539787095791365523, 1.040834085586084257E-14 ) ) ;
#198233=CARTESIAN_POINT ( 'NONE',  ( 2.460826785407684181, 8.202405370174474797, 2.499999999999999112 ) ) ;
#198236=CARTESIAN_POINT ( 'NONE',  ( -2.950870989268691957, 6.594433254122103349, -0.7998128361456281477 ) ) ;
#198240=CARTESIAN_POINT ( 'NONE',  ( 8.530051201292206287, 13.10347683481629488, 0.000000000000000000 ) ) ;
#198243=CARTESIAN_POINT ( 'NONE',  ( -7.395082721250053837, 10.71501471051202614, -1.199719254218446718 ) ) ;
#198244=CARTESIAN_POINT ( 'NONE',  ( 6.582647274634798151, 7.638508894284114170, 1.199719254218462483 ) ) ;
#198246=CARTESIAN_POINT ( 'NONE',  ( -7.483210719738908168, 10.81783070874899799, 1.199719254218453823 ) ) ;
#198247=CARTESIAN_POINT ( 'NONE',  ( 5.431895982697334091, 6.433277491268158954, -1.247050338538328029 ) ) ;
#198249=DIRECTION ( 'NONE',  ( 1.000000000000000000, 0.000000000000000000, 0.000000000000000000 ) ) ;
#198250=CARTESIAN_POINT ( 'NONE',  ( 0.6823417656249864960, -0.5114583329919111243, -1.181850606188749264 ) ) ;
#198251=ORIENTED_EDGE ( 'NONE', *, *, #62562, .F. ) ;
#198253=CARTESIAN_POINT ( 'NONE',  ( 7.456621297836061757, 11.64321591421002644, 0.7216878364870438212 ) ) ;
#198257=EDGE_LOOP ( 'NONE', ( #25865, #28859, #102024, #196309 ) ) ;
#198272=CARTESIAN_POINT ( 'NONE',  ( -2.137381772448751605, 5.645362501165475777, -0.7998128361456281477 ) ) ;
#198280=CARTESIAN_POINT ( 'NONE',  ( -1.500000000000001332, -0.06874999931718445145, 0.000000000000000000 ) ) ;
#198286=CARTESIAN_POINT ( 'NONE',  ( 9.297140650669039275, 11.86975006391249643, 1.599625672291281386 ) ) ;
#198290=CARTESIAN_POINT ( 'NONE',  ( 3.876741858503734761, 6.610283703974623393, 1.199719254218462483 ) ) ;
#198291=CARTESIAN_POINT ( 'NONE',  ( -6.643132081016132062, 8.773406732650713025, 1.443375672974078761 ) ) ;
#198292=CARTESIAN_POINT ( 'NONE',  ( -5.733986265252455361, 6.108121862465037744, 0.6873297539724126937 ) ) ;
#198296=CARTESIAN_POINT ( 'NONE',  ( -8.518600588087975822, 8.832788862391110385, 1.040834085586084257E-14 ) ) ;
#198297=CARTESIAN_POINT ( 'NONE',  ( -4.406036734316906234, 4.242723732898890709, -0.7216878364870207285 ) ) ;
#198300=CARTESIAN_POINT ( 'NONE',  ( 1.499999999999987566, -0.6937499993171849511, 0.000000000000000000 ) ) ;
#198308=CARTESIAN_POINT ( 'NONE',  ( -3.429849674132942727, 5.984946472254969230, -1.082531754730549078 ) ) ;
#198311=EDGE_CURVE ( 'NONE', #17249, #127447, #111138, .T. ) ;
#198312=CARTESIAN_POINT ( 'NONE',  ( 3.996677956334552029, 7.600660605679141035, 0.1064861495668877750 ) ) ;
#198317=CARTESIAN_POINT ( 'NONE',  ( -3.755245360860939297, 4.443836344834937613, -1.082531754730548412 ) ) ;
#198318=CARTESIAN_POINT ( 'NONE',  ( 7.771848369131631351, 10.09024240211882351, -1.599625672291262513 ) ) ;
#198324=EDGE_LOOP ( 'NONE', ( #64461, #9340, #98812, #155191, #106051, #159853, #40309, #119952, #133503 ) ) ;
#198327=CARTESIAN_POINT ( 'NONE',  ( -7.621654909176601045, 12.04368116068139472, 0.7998128361456481317 ) ) ;
#198332=CARTESIAN_POINT ( 'NONE',  ( 5.168682875307768931, 7.053215992657626110, -1.599625672291256295 ) ) ;
#198338=CARTESIAN_POINT ( 'NONE',  ( 2.907691925098776942, 6.443576416979776234, 0.4208059576237854205 ) ) ;
#198341=CARTESIAN_POINT ( 'NONE',  ( -1.150222622689971441, 3.222854968409793575, -0.7749999999993560929 ) ) ;
#198350=CARTESIAN_POINT ( 'NONE',  ( 7.958799866421889746, 9.244020251369077457, -1.199719254218441611 ) ) ;
#198352=CARTESIAN_POINT ( 'NONE',  ( -5.461236948206312114, 5.265864615862458464, 0.7998128361456341429 ) ) ;
#198358=CARTESIAN_POINT ( 'NONE',  ( -1.201851678989727383E-14, 5.696875000341416140, -1.575800808251660134 ) ) ;
#198361=CARTESIAN_POINT ( 'NONE',  ( -5.088463259863680754, 6.638951673345857785, 1.365981757201965907 ) ) ;
#198362=CARTESIAN_POINT ( 'NONE',  ( 3.837121167867449945, 4.435395103055503441, 1.199719254218464037 ) ) ;
#198364=CARTESIAN_POINT ( 'NONE',  ( -3.704402285031864306, 5.344888637335695414, -1.599625672291256295 ) ) ;
#198370=CARTESIAN_POINT ( 'NONE',  ( 5.395781948558860286, 6.357795697149212444, -1.082531754730542195 ) ) ;
#198373=CARTESIAN_POINT ( 'NONE',  ( -1.001543065824772872E-14, 4.634375000341418804, 1.575800808251672791 ) ) ;
#198375=CARTESIAN_POINT ( 'NONE',  ( 4.989037339704528229, 4.922891105851139315, 1.040834085586084257E-14 ) ) ;
#198383=CARTESIAN_POINT ( 'NONE',  ( -5.854914268151548917, 6.175991412503675448, 0.9282606102084377531 ) ) ;
#198386=CARTESIAN_POINT ( 'NONE',  ( -1.201851678989727383E-14, 5.759375000341417028, -1.575800808251660801 ) ) ;
#198395=CARTESIAN_POINT ( 'NONE',  ( -1.500000000000011324, 4.379166666666688634, -0.8660254037844313801 ) ) ;
#198403=CARTESIAN_POINT ( 'NONE',  ( 0.6823417656249899377, 4.488541667008086655, -1.181850606188754593 ) ) ;
#198405=CARTESIAN_POINT ( 'NONE',  ( 5.286789834324991055, 8.255339675766103724, -1.199719254218452935 ) ) ;
#198406=CARTESIAN_POINT ( 'NONE',  ( -7.883176251342026042, 11.28445716228600126, -1.199719254218446718 ) ) ;
#198409=CIRCLE ( 'NONE', #174185, 3.971937515251341644 ) ;
#198413=CARTESIAN_POINT ( 'NONE',  ( -1.201851678989727383E-14, 5.837500000000023448, -1.732050807568863648 ) ) ;
#198417=CARTESIAN_POINT ( 'NONE',  ( 5.300874872818840622, 6.247070775452521652, 1.082531754730560403 ) ) ;
#198420=CARTESIAN_POINT ( 'NONE',  ( 6.968527767744088663, 11.07377346243604599, 0.7216878364870438212 ) ) ;
#198425=CARTESIAN_POINT ( 'NONE',  ( 1.499999999999990896, 3.556250000682818602, 1.214306433183764966E-14 ) ) ;
#198427=CARTESIAN_POINT ( 'NONE',  ( -3.567766978690493307, 7.314145241780881435, 1.040834085586084257E-14 ) ) ;
#198428=CARTESIAN_POINT ( 'NONE',  ( 3.511198595814926993, 6.079853547550633230, 1.082531754730558626 ) ) ;
#198436=CARTESIAN_POINT ( 'NONE',  ( 4.090809663021327758, 5.795697244990093644, 1.599625672291267398 ) ) ;
#198437=CARTESIAN_POINT ( 'NONE',  ( -1.123270288250315163, 2.985197346350006331, -0.7749999999993613109 ) ) ;
#198440=CARTESIAN_POINT ( 'NONE',  ( 3.032219910950674890, 6.689340329417765574, 0.7998128361456321445 ) ) ;
#198451=CARTESIAN_POINT ( 'NONE',  ( 2.276812203907196075, 5.628006997859904104, -0.5575630420769552842 ) ) ;
#198452=CARTESIAN_POINT ( 'NONE',  ( 4.952123820727618586, 6.619828698506379006, -1.244621138126526194 ) ) ;
#198453=EDGE_CURVE ( 'NONE', #23324, #18526, #90357, .T. ) ;
#198455=CARTESIAN_POINT ( 'NONE',  ( 9.890836756369282057, 11.49806328964105617, -1.199719254218440723 ) ) ;
#198457=CIRCLE ( 'NONE', #11684, 0.07999999999999984901 ) ;
#198461=CARTESIAN_POINT ( 'NONE',  ( 4.690757960648213931, 8.416375354157496602, 0.7216878364870438212 ) ) ;
#198462=CARTESIAN_POINT ( 'NONE',  ( -8.161645285746702783, 12.46574390010577105, 0.7216878364870478180 ) ) ;
#198468=CARTESIAN_POINT ( 'NONE',  ( -5.264643720808155791, 5.036505850564608089, 0.000000000000000000 ) ) ;
#198479=CARTESIAN_POINT ( 'NONE',  ( 6.113440106766272031, 6.016660024919275429, -0.07562458862005703997 ) ) ;
#198480=CYLINDRICAL_SURFACE ( 'NONE', #204982, 1.250000000000000000 ) ;
#198485=( BOUNDED_CURVE ( )  B_SPLINE_CURVE ( 2, ( #130755, #163196, #127581, #95008, #63551, #14779, #129707 ),
 .UNSPECIFIED., .F., .T. ) 
 B_SPLINE_CURVE_WITH_KNOTS ( ( 3, 2, 2, 3 ),
 ( 0.2857142857142859760, 0.2916666666666668517, 0.2976190476190477274, 0.3035714285714285476 ),
 .UNSPECIFIED. ) 
 CURVE ( )  GEOMETRIC_REPRESENTATION_ITEM ( )  RATIONAL_B_SPLINE_CURVE ( ( 0.9999999999999937828, 0.8660254037844449249, 1.000000000000000000, 0.8660254037844387076, 1.000000000000000000, 0.8660254037844387076, 1.000000000000000000 ) ) 
 REPRESENTATION_ITEM ( '' )  );
#198488=CARTESIAN_POINT ( 'NONE',  ( -8.188761592974046266, 10.57664116326830595, -1.443375672974059665 ) ) ;
#198492=CARTESIAN_POINT ( 'NONE',  ( 7.182068686937156166, 9.402166106225269715, 1.599625672291281386 ) ) ;
#198493=CARTESIAN_POINT ( 'NONE',  ( -4.273844736805831879, 6.009238164405336313, 1.599625672291267175 ) ) ;
#198495=CARTESIAN_POINT ( 'NONE',  ( -4.564291269294938225, 8.476756914152748124, 1.040834085586084257E-14 ) ) ;
#198496=CARTESIAN_POINT ( 'NONE',  ( 4.844340958784499662, 4.546152628203684820, 0.7998128361456341429 ) ) ;
#198498=CARTESIAN_POINT ( 'NONE',  ( -6.891622154448065807, 6.934647356477856128, 1.040834085586084257E-14 ) ) ;
#198501=CARTESIAN_POINT ( 'NONE',  ( 8.727698198895078363, 11.20540053684285553, -1.599625672291257406 ) ) ;
#198504=CARTESIAN_POINT ( 'NONE',  ( 4.439983357641082762, 7.074277023141499754, -1.114066652139956926 ) ) ;
#198505=B_SPLINE_CURVE_WITH_KNOTS ( 'NONE', 3,
 ( #7022, #187920, #170611, #39551, #82159, #200950, #21131, #89388, #68822, #22198 ),
 .UNSPECIFIED., .F., .F.,
 ( 4, 3, 3, 4 ),
 ( 0.000000000000000000, 8.893179197954836847E-05, 0.0001334007970840206305, 0.0001778705873658964021 ),
 .UNSPECIFIED. ) ;
#198506=CARTESIAN_POINT ( 'NONE',  ( 4.677199807034550183, 8.400557508274889784, 1.040834085586084257E-14 ) ) ;
#198513=CARTESIAN_POINT ( 'NONE',  ( 8.554831740098663317, 9.082984572977682802, 0.7216878364870458196 ) ) ;
#198517=CARTESIAN_POINT ( 'NONE',  ( -8.448702279610222021, 13.00856975952063088, 1.040834085586084257E-14 ) ) ;
#198518=CARTESIAN_POINT ( 'NONE',  ( -7.660520486921249983, 8.896027641951645748, -1.199719254218446718 ) ) ;
#198522=DIRECTION ( 'NONE',  ( 0.000000000000000000, 1.000000000000000000, -8.546850786086437571E-32 ) ) ;
#198526=CARTESIAN_POINT ( 'NONE',  ( 4.552840656090682891, 4.206068941727564514, 1.214306433183764966E-14 ) ) ;
#198530=CARTESIAN_POINT ( 'NONE',  ( 3.876741858503734761, 6.610283703974623393, 1.199719254218462483 ) ) ;
#198534=CARTESIAN_POINT ( 'NONE',  ( 1.499999999999987121, 3.577083334016152527, -0.8660254037844262731 ) ) ;
#198540=CARTESIAN_POINT ( 'NONE',  ( -1.402160292154681736E-14, 1.837500000000019895, -1.732050807568863648 ) ) ;
#198541=CARTESIAN_POINT ( 'NONE',  ( 4.950698647284403009, 8.927565521807144577, 1.040834085586084257E-14 ) ) ;
#198542=CARTESIAN_POINT ( 'NONE',  ( 3.673896439178918172, 6.269667698141953238, 1.082531754730558626 ) ) ;
#198545=CARTESIAN_POINT ( 'NONE',  ( 7.280365300858406385, 11.43758391773608984, 1.040834085586084257E-14 ) ) ;
#198550=CARTESIAN_POINT ( 'NONE',  ( -3.893162665418476109, 7.693773542963529444, 1.040834085586084257E-14 ) ) ;
#198551=CARTESIAN_POINT ( 'NONE',  ( -1.500000000000011324, 4.202083334016156080, 0.8660254037844403729 ) ) ;
#198552=CARTESIAN_POINT ( 'NONE',  ( 0.6823417656249882723, 0.09270833367475139752, 1.181850606188755259 ) ) ;
#198556=CARTESIAN_POINT ( 'NONE',  ( 4.253507506385319381, 5.985511395581417204, 1.599625672291267398 ) ) ;
#198559=CARTESIAN_POINT ( 'NONE',  ( -1.364683531249997417, 5.321875000341417916, 1.214306433183764966E-14 ) ) ;
#198566=CARTESIAN_POINT ( 'NONE',  ( -8.362681821530818738, 8.650883634741092010, -0.7998128361456291469 ) ) ;
#198567=CARTESIAN_POINT ( 'NONE',  ( 6.017121246366603060, 5.914396297049491658, 1.040834085586084257E-14 ) ) ;
#198570=CARTESIAN_POINT ( 'NONE',  ( -1.402160292154681736E-14, -1.178124999658576311, 1.575800808251672791 ) ) ;
#198573=EDGE_LOOP ( 'NONE', ( #46841, #41883, #76882, #115028, #73792 ) ) ;
#198578=CARTESIAN_POINT ( 'NONE',  ( -7.217017841176048165, 7.314275657660511243, 1.040834085586084257E-14 ) ) ;
#198582=CARTESIAN_POINT ( 'NONE',  ( 8.353795204314554468, 12.89784483834236184, -0.7998128361456352531 ) ) ;
#198584=CARTESIAN_POINT ( 'NONE',  ( 9.901532256681887745, 10.44620914241737530, 0.000000000000000000 ) ) ;
#198586=CARTESIAN_POINT ( 'NONE',  ( -2.279742385392243165, 5.811449882932888222, -0.7998128361456281477 ) ) ;
#198587=CARTESIAN_POINT ( 'NONE',  ( -6.482770005628665011, 10.71498210654212002, 0.7998128361456481317 ) ) ;
#198590=CARTESIAN_POINT ( 'NONE',  ( -5.328671718129330159, 6.540706332611327944, 1.372188321006672540 ) ) ;
#198591=CARTESIAN_POINT ( 'NONE',  ( -1.402160292154681736E-14, -0.05312499965857903073, -1.575800808251665908 ) ) ;
#198595=CARTESIAN_POINT ( 'NONE',  ( 8.758204044748005401, 10.28062147603659504, 1.082531754730549967 ) ) ;
#198598=CARTESIAN_POINT ( 'NONE',  ( 4.547870462380197765, 7.393267075163835855, 1.199719254218462483 ) ) ;
#198613=ORIENTED_EDGE ( 'NONE', *, *, #163343, .T. ) ;
#198618=CARTESIAN_POINT ( 'NONE',  ( -4.702146809683723561, 5.356480858934594025, -2.420000000000000373 ) ) ;
#198622=CARTESIAN_POINT ( 'NONE',  ( -4.680589345215810049, 6.483773540883647435, -1.599625672291256295 ) ) ;
#198627=CARTESIAN_POINT ( 'NONE',  ( 1.499999999999987121, 3.077083334016149863, -0.8660254037844262731 ) ) ;
#198628=CARTESIAN_POINT ( 'NONE',  ( 8.052653171512838881, 11.48218023581863001, -1.199719254218446718 ) ) ;
#198629=CARTESIAN_POINT ( 'NONE',  ( -4.911285141672522059, 4.693790260148114513, 0.3511878651327460243 ) ) ;
#198632=CARTESIAN_POINT ( 'NONE',  ( -8.748035429315585532, 11.22912730566677553, -1.599625672291263179 ) ) ;
#198634=CARTESIAN_POINT ( 'NONE',  ( 1.364683531249986537, 1.905208333674750287, -0.7879004041258239610 ) ) ;
#198641=CARTESIAN_POINT ( 'NONE',  ( -10.48008955368359629, 11.32911868882677986, 1.040834085586084257E-14 ) ) ;
#198645=CARTESIAN_POINT ( 'NONE',  ( -1.364683531250014514, 1.051041667008090208, -0.7879004041258289570 ) ) ;
#198650=CARTESIAN_POINT ( 'NONE',  ( -1.402160292154681736E-14, 1.196875000341419026, -1.575800808251659024 ) ) ;
#198652=CARTESIAN_POINT ( 'NONE',  ( -6.762819695118240659, 6.784377820593065600, 0.7998128361456341429 ) ) ;
#198653=CARTESIAN_POINT ( 'NONE',  ( 8.372323551638698902, 9.726464550788689323, 1.199719254218462483 ) ) ;
#198654=CARTESIAN_POINT ( 'NONE',  ( 0.9999999999999833467, 8.600000000000013856, 0.4000000000000014655 ) ) ;
#198656=CARTESIAN_POINT ( 'NONE',  ( -0.7500000000000215383, 4.191666666666690411, 1.299038105676671107 ) ) ;
#198657=CARTESIAN_POINT ( 'NONE',  ( 1.364683531249988535, 3.217708333674748289, -0.7879004041258239610 ) ) ;
#198661=CARTESIAN_POINT ( 'NONE',  ( -3.958617665510266725, 7.562211676496538360, -0.7216878364870267237 ) ) ;
#198665=CARTESIAN_POINT ( 'NONE',  ( 4.663641653420880218, 8.384739662392275861, -0.7216878364870207285 ) ) ;
#198666=( BOUNDED_SURFACE ( )  B_SPLINE_SURFACE ( 1, 2, ( 
 ( #167780, #54032, #3109, #21491, #137429, #152591, #200253, #51905, #136362, #203447, #19376, #85456, #202382, #37780, #187220, #121250, #103854, #88679, #154738, #157952, #125518, #173134, #26853, #77742, #10597, #127660, #92957, #189360, #58300, #209856, #9544, #156881, #124456, #109260, #176325, #75619, #59361, #57236, #193623, #8468, #110318, #123396, #25785, #177388, #7390, #190415, #44198, #111385, #91896, #42072, #107111, #95089, #29002, #41000, #73470, #174212, #45265, #191479, #24715, #90818, #74554, #139571, #60424, #140655, #141729, #205598, #192545, #76673, #206669, #108186, #207737, #43147, #175268, #159004, #143863, #142788, #208794, #126584, #27932, #94025, #160064, #11668, #61494, #98270, #15918, #114581, #13795, #178459, #30068, #210928, #129785, #130832, #128717, #132921, #79869, #32194, #179525, #198926, #164328, #162209, #112446, #80943, #181623, #16978, #46331, #180572, #165385, #83059, #97219, #196824, #82001, #148088, #149135, #163271, #14853, #194689, #214093, #145978, #716, #211990, #66781, #50572, #63631, #64687, #65721, #115628, #116694, #182693, #31145, #34311, #131869, #161137, #197877, #12725, #78798, #147035, #96158, #195766, #213057, #47405, #144921, #48466, #113517, #49508, #33252, #99336, #62554, #152343, #150224, #6065, #35378, #203199, #1794, #118832, #55908, #100387, #68926, #137175, #204257, #184818, #135047, #200005, #188029, #122065, #67851, #166458, #52701, #138243, #3921, #133999, #51654, #101453, #18049, #153412, #117777, #36448, #84136, #71059, #103597, #183768, #167525, #19123, #85202, #151286, #2857, #170720, #201060, #102523, #168585, #20185, #86272, #38595, #69990, #136102, #37521, #169654, #53778, #202118, #119911, #185887, #21239, #87345, #4982, #54846, #72135, #120996, #186963, #104672, #22307, #154486, #88419, #9290, #110061, #8215, #74300, #26599, #205340, #92700, #189109, #56978, #10340, #42886, #123152, #40742, #176073, #191222, #108995, #207482, #106848, #172879, #24451, #89499, #140396, #75363, #7133, #11409, #90564, #125262, #58039, #158746, #93766, #156625, #141475, #27671, #206415, #124203, #76414, #190167, #142524, #41821, #107934, #208533, #175012, #173959, #25532, #159805, #77486, #60169, #91640, #157692, #59102, #126326, #143605, #139311, #192285, #43945, #209598, #61242, #127399, #39659, #105767, #171792, #23387, #155553, #73205, #196578, #194438, #197625, #46079, #115390, #49269, #112199, #96973, #212807, #147838, #16729, #82813, #211740, #181384, #31950, #33007, #180328, #99086, #463, #179272, #62311, #161959, #63378, #29822, #165138, #195515, #128470, #95906, #80700, #213855, #129534, #30896, #28746, #148890, #178205, #81756, #94830, #47151, #66532, #193371, #13549, #15669, #45016, #113268, #79621, #78552, #111126, #177129, #160882, #12477, #145740, #144669, #163021, #210682, #14603, #146791, #64444, #98034, #130588, #48220, #114333, #164088 ),
 ( #65476, #131626, #35119, #34064, #133744, #134798, #83875, #52455, #153153, #202943, #17788, #152093, #136916, #54587, #68675, #102264, #69741, #201869, #120734, #200804, #118580, #166197, #135846, #199752, #186707, #51397, #38335, #104412, #117517, #36188, #3664, #87083, #170461, #22046, #151037, #88157, #185635, #154225, #119651, #5797, #132674, #184568, #1536, #101190, #2606, #183510, #198680, #168339, #67598, #167279, #19934, #4728, #86020, #53517, #182437, #50325, #18864, #20986, #100135, #37268, #116443, #149967, #84948, #169400, #103338, #70803, #40487, #171531, #162501, #178750, #187773, #71874, #24195, #112739, #189917, #39405, #23124, #72953, #137984, #125010, #105499, #7952, #204001, #42633, #75109, #30363, #139055, #121806, #96450, #205082, #56724, #145211, #55650, #122892, #89241, #155292, #6875, #13016, #188851, #41562, #9035, #141220, #25279, #106591, #172619, #90298, #156368, #74044, #107675, #140134, #46618, #206160, #157441, #57788, #190967, #129005, #123948, #173704, #211217, #91381, #207230, #58854, #108742, #177679, #29291, #95383, #161435, #79093, #62844, #194982, #150512, #51936, #99613, #15145, #82281, #148374, #98553, #166748, #184045, #181908, #214375, #33540, #66005, #2073, #163560, #179808, #67075, #132155, #198160, #63912, #114857, #134280, #164614, #97504, #116985, #101742, #147313, #18343, #182985, #14071, #165679, #130068, #49794, #81231, #115919, #17267, #64963, #35663, #146266, #16199, #83343, #31427, #84423, #212278, #68146, #133210, #149428, #196063, #1010, #199215, #50863, #34602, #213340, #100670, #200285, #118060, #131116, #80160, #197104, #47693, #113807, #48744, #180857, #32478, #135331, #39955, #189388, #54065, #37809, #139602, #202409, #87628, #3143, #122357, #153699, #38878, #19410, #186175, #72421, #155834, #106062, #71345, #152622, #154767, #205625, #121275, #5268, #4209, #204546, #138523, #137462, #70277, #56194, #136393, #102814, #120200, #188313, #7418, #171003, #89788, #103884, #86560, #151574, #172085, #41030, #167810, #6350, #169933, #21517, #203477, #55130, #69212, #168869, #187250, #85488, #104962, #201345, #22601, #88708, #23677, #73500, #57264, #52985, #123426, #119121, #185101, #36727, #20472, #124483, #24745, #190441, #8498, #74581, #140684, #107140, #206700, #58327, #173166, #90846, #156910, #27908, #161115, #174190, #58279, #10577, #96136, #176305, #25762, #157930, #59341, #145959, #111362, #91874, #208771, #190393, #28981, #61473, #162188, #125495, #108163, #13775, #191458, #43123, #128697, #42051, #109237, #124435, #9523, #79850, #210908, #75595, #94005, #209836, #127638, #11648, #175247, #141707, #207718, #26833, #92936, #160044, #158980, #30046, #76651, #143842, #142766, #177367, #112426, #60401, #77720, #194665, #126563, #192523, #45245, #44177, #95067, #110297, #193603, #12702, #78779, #144900, #62535, #46310, #178440, #83039, #213038, #163252 ) ),
 .UNSPECIFIED., .F., .F., .T. ) 
 B_SPLINE_SURFACE_WITH_KNOTS ( ( 2, 2 ),
 ( 3, 2, 2, 2, 2, 2, 2, 2, 2, 2, 2, 2, 2, 2, 2, 2, 2, 2, 2, 2, 2, 2, 2, 2, 2, 2, 2, 2, 2, 2, 2, 2, 2, 2, 2, 2, 2, 2, 2, 2, 2, 2, 2, 2, 2, 2, 2, 2, 2, 2, 2, 2, 2, 2, 2, 2, 2, 2, 2, 2, 2, 2, 2, 2, 2, 2, 2, 2, 2, 2, 2, 2, 2, 2, 2, 2, 2, 2, 2, 2, 2, 2, 2, 2, 2, 2, 2, 2, 2, 2, 2, 2, 2, 2, 2, 2, 2, 2, 2, 2, 2, 2, 2, 2, 2, 2, 2, 2, 2, 2, 2, 2, 2, 2, 2, 2, 2, 2, 2, 2, 2, 2, 2, 2, 2, 2, 2, 2, 2, 2, 2, 2, 2, 2, 2, 2, 2, 2, 2, 2, 2, 2, 2, 2, 2, 2, 2, 2, 2, 2, 2, 2, 2, 2, 2, 2, 2, 2, 2, 2, 2, 2, 2, 2, 2, 2, 2, 2, 3 ),
 ( 0.000000000000000000, 1.000000000000000000 ),
 ( 0.000000000000000000, 0.005952380952380952051, 0.01190476190476190410, 0.01785714285714285615, 0.02380952380952380820, 0.02976190476190476025, 0.03571428571428571230, 0.04166666666666666435, 0.04761904761904761640, 0.05357142857142856845, 0.05952380952380952051, 0.06547619047619047949, 0.07142857142857142461, 0.07738095238095238360, 0.08333333333333332871, 0.08928571428571428770, 0.09523809523809523281, 0.1011904761904761918, 0.1071428571428571369, 0.1130952380952380959, 0.1190476190476190410, 0.1250000000000000000, 0.1309523809523809590, 0.1369047619047619180, 0.1428571428571428492, 0.1488095238095238082, 0.1547619047619047672, 0.1607142857142857262, 0.1666666666666666574, 0.1726190476190476164, 0.1785714285714285754, 0.1845238095238095344, 0.1904761904761904656, 0.1964285714285714246, 0.2023809523809523836, 0.2083333333333333426, 0.2142857142857142738, 0.2202380952380952328, 0.2261904761904761918, 0.2321428571428571508, 0.2380952380952380820, 0.2440476190476190410, 0.2500000000000000000, 0.2559523809523809312, 0.2619047619047619180, 0.2678571428571428492, 0.2738095238095238360, 0.2797619047619047672, 0.2857142857142856984, 0.2916666666666666852, 0.2976190476190476164, 0.3035714285714285476, 0.3095238095238095344, 0.3154761904761904656, 0.3214285714285714524, 0.3273809523809523836, 0.3333333333333333148, 0.3392857142857143016, 0.3452380952380952328, 0.3511904761904761640, 0.3571428571428571508, 0.3630952380952380820, 0.3690476190476190688, 0.3750000000000000000, 0.3809523809523809312, 0.3869047619047619180, 0.3928571428571428492, 0.3988095238095238360, 0.4047619047619047672, 0.4107142857142856984, 0.4166666666666666852, 0.4226190476190476164, 0.4285714285714285476, 0.4345238095238095344, 0.4404761904761904656, 0.4464285714285714524, 0.4523809523809523836, 0.4583333333333333148, 0.4642857142857143016, 0.4702380952380952328, 0.4761904761904761640, 0.4821428571428571508, 0.4880952380952380820, 0.4940476190476190688, 0.5000000000000000000, 0.5059523809523809312, 0.5119047619047618625, 0.5178571428571429047, 0.5238095238095238360, 0.5297619047619047672, 0.5357142857142856984, 0.5416666666666666297, 0.5476190476190476719, 0.5535714285714286031, 0.5595238095238095344, 0.5654761904761904656, 0.5714285714285713969, 0.5773809523809523281, 0.5833333333333333703, 0.5892857142857143016, 0.5952380952380952328, 0.6011904761904761640, 0.6071428571428570953, 0.6130952380952381375, 0.6190476190476190688, 0.6250000000000000000, 0.6309523809523809312, 0.6369047619047618625, 0.6428571428571429047, 0.6488095238095238360, 0.6547619047619047672, 0.6607142857142856984, 0.6666666666666666297, 0.6726190476190476719, 0.6785714285714286031, 0.6845238095238095344, 0.6904761904761904656, 0.6964285714285713969, 0.7023809523809523281, 0.7083333333333333703, 0.7142857142857143016, 0.7202380952380952328, 0.7261904761904761640, 0.7321428571428570953, 0.7380952380952381375, 0.7440476190476190688, 0.7500000000000000000, 0.7559523809523809312, 0.7619047619047618625, 0.7678571428571429047, 0.7738095238095238360, 0.7797619047619047672, 0.7857142857142856984, 0.7916666666666666297, 0.7976190476190476719, 0.8035714285714286031, 0.8095238095238095344, 0.8154761904761904656, 0.8214285714285713969, 0.8273809523809523281, 0.8333333333333333703, 0.8392857142857143016, 0.8452380952380952328, 0.8511904761904761640, 0.8571428571428570953, 0.8630952380952381375, 0.8690476190476190688, 0.8750000000000000000, 0.8809523809523809312, 0.8869047619047618625, 0.8928571428571429047, 0.8988095238095238360, 0.9047619047619047672, 0.9107142857142856984, 0.9166666666666666297, 0.9226190476190476719, 0.9285714285714286031, 0.9345238095238095344, 0.9404761904761904656, 0.9464285714285713969, 0.9523809523809523281, 0.9583333333333333703, 0.9642857142857143016, 0.9702380952380952328, 0.9761904761904761640, 0.9821428571428570953, 0.9880952380952381375, 0.9940476190476190688, 1.000000000000000000 ),
 .UNSPECIFIED. ) 
 GEOMETRIC_REPRESENTATION_ITEM ( )  RATIONAL_B_SPLINE_SURFACE ( (
 ( 1.000000000000000000, 0.8660254037844387076, 1.000000000000000000, 0.8660254037844387076, 1.000000000000000000, 0.8660254037844387076, 1.000000000000000000, 0.8660254037844387076, 1.000000000000000000, 0.8660254037844387076, 1.000000000000000000, 0.8660254037844387076, 1.000000000000000000, 0.8660254037844387076, 1.000000000000000000, 0.8660254037844387076, 1.000000000000000000, 0.8660254037844387076, 1.000000000000000000, 0.8660254037844387076, 1.000000000000000000, 0.8660254037844387076, 1.000000000000000000, 0.8660254037844387076, 1.000000000000000000, 0.8660254037844387076, 1.000000000000000000, 0.8660254037844387076, 1.000000000000000000, 0.8660254037844387076, 1.000000000000000000, 0.8660254037844387076, 1.000000000000000000, 0.8660254037844387076, 1.000000000000000000, 0.8660254037844387076, 1.000000000000000000, 0.8660254037844387076, 1.000000000000000000, 0.8660254037844387076, 1.000000000000000000, 0.8660254037844387076, 1.000000000000000000, 0.8660254037844387076, 1.000000000000000000, 0.8660254037844387076, 1.000000000000000000, 0.8660254037844387076, 1.000000000000000000, 0.8660254037844387076, 1.000000000000000000, 0.8660254037844387076, 1.000000000000000000, 0.8660254037844387076, 1.000000000000000000, 0.8660254037844387076, 1.000000000000000000, 0.8660254037844387076, 1.000000000000000000, 0.8660254037844387076, 1.000000000000000000, 0.8660254037844387076, 1.000000000000000000, 0.8660254037844387076, 1.000000000000000000, 0.8660254037844387076, 1.000000000000000000, 0.8660254037844387076, 1.000000000000000000, 0.8660254037844387076, 1.000000000000000000, 0.8660254037844387076, 1.000000000000000000, 0.8660254037844387076, 1.000000000000000000, 0.8660254037844387076, 1.000000000000000000, 0.8660254037844387076, 1.000000000000000000, 0.8660254037844387076, 1.000000000000000000, 0.8660254037844387076, 1.000000000000000000, 0.8660254037844387076, 1.000000000000000000, 0.8660254037844387076, 1.000000000000000000, 0.8660254037844387076, 1.000000000000000000, 0.8660254037844387076, 1.000000000000000000, 0.8660254037844387076, 1.000000000000000000, 0.8660254037844387076, 1.000000000000000000, 0.8660254037844387076, 1.000000000000000000, 0.8660254037844387076, 1.000000000000000000, 0.8660254037844387076, 1.000000000000000000, 0.8660254037844387076, 1.000000000000000000, 0.8660254037844387076, 1.000000000000000000, 0.8660254037844387076, 1.000000000000000000, 0.8660254037844387076, 1.000000000000000000, 0.8660254037844387076, 1.000000000000000000, 0.8660254037844387076, 1.000000000000000000, 0.8660254037844387076, 1.000000000000000000, 0.8660254037844387076, 1.000000000000000000, 0.8660254037844387076, 1.000000000000000000, 0.8660254037844387076, 1.000000000000000000, 0.8660254037844387076, 1.000000000000000000, 0.8660254037844387076, 1.000000000000000000, 0.8660254037844387076, 1.000000000000000000, 0.8660254037844387076, 1.000000000000000000, 0.8660254037844387076, 1.000000000000000000, 0.8660254037844387076, 1.000000000000000000, 0.8660254037844387076, 1.000000000000000000, 0.8660254037844387076, 1.000000000000000000, 0.8660254037844387076, 1.000000000000000000, 0.8660254037844387076, 1.000000000000000000, 0.8660254037844387076, 1.000000000000000000, 0.8660254037844387076, 1.000000000000000000, 0.8660254037844387076, 1.000000000000000000, 0.8660254037844387076, 1.000000000000000000, 0.8660254037844387076, 1.000000000000000000, 0.8660254037844387076, 1.000000000000000000, 0.8660254037844387076, 1.000000000000000000, 0.8660254037844387076, 1.000000000000000000, 0.8660254037844387076, 1.000000000000000000, 0.8660254037844387076, 1.000000000000000000, 0.8660254037844387076, 1.000000000000000000, 0.8660254037844387076, 1.000000000000000000, 0.8660254037844387076, 1.000000000000000000, 0.8660254037844387076, 1.000000000000000000, 0.8660254037844387076, 1.000000000000000000, 0.8660254037844387076, 1.000000000000000000, 0.8660254037844387076, 1.000000000000000000, 0.8660254037844387076, 1.000000000000000000, 0.8660254037844387076, 1.000000000000000000, 0.8660254037844387076, 1.000000000000000000, 0.8660254037844387076, 1.000000000000000000, 0.8660254037844387076, 1.000000000000000000, 0.8660254037844387076, 1.000000000000000000, 0.8660254037844387076, 1.000000000000000000, 0.8660254037844387076, 1.000000000000000000, 0.8660254037844387076, 1.000000000000000000, 0.8660254037844387076, 1.000000000000000000, 0.8660254037844387076, 1.000000000000000000, 0.8660254037844387076, 1.000000000000000000, 0.8660254037844387076, 1.000000000000000000, 0.8660254037844387076, 1.000000000000000000, 0.8660254037844387076, 1.000000000000000000, 0.8660254037844387076, 1.000000000000000000, 0.8660254037844387076, 1.000000000000000000, 0.8660254037844387076, 1.000000000000000000, 0.8660254037844387076, 1.000000000000000000, 0.8660254037844387076, 1.000000000000000000, 0.8660254037844387076, 1.000000000000000000, 0.8660254037844387076, 1.000000000000000000, 0.8660254037844387076, 1.000000000000000000, 0.8660254037844387076, 1.000000000000000000, 0.8660254037844387076, 1.000000000000000000, 0.8660254037844387076, 1.000000000000000000, 0.8660254037844387076, 1.000000000000000000, 0.8660254037844387076, 1.000000000000000000, 0.8660254037844387076, 1.000000000000000000, 0.8660254037844387076, 1.000000000000000000, 0.8660254037844387076, 1.000000000000000000, 0.8660254037844387076, 1.000000000000000000, 0.8660254037844387076, 1.000000000000000000, 0.8660254037844387076, 1.000000000000000000, 0.8660254037844387076, 1.000000000000000000, 0.8660254037844387076, 1.000000000000000000, 0.8660254037844387076, 1.000000000000000000, 0.8660254037844387076, 1.000000000000000000, 0.8660254037844387076, 1.000000000000000000, 0.8660254037844387076, 1.000000000000000000, 0.8660254037844387076, 1.000000000000000000, 0.8660254037844387076, 1.000000000000000000, 0.8660254037844387076, 1.000000000000000000, 0.8660254037844387076, 1.000000000000000000, 0.8660254037844387076, 1.000000000000000000, 0.8660254037844387076, 1.000000000000000000, 0.8660254037844387076, 1.000000000000000000, 0.8660254037844387076, 1.000000000000000000, 0.8660254037844387076, 1.000000000000000000, 0.8660254037844387076, 1.000000000000000000, 0.8660254037844387076, 1.000000000000000000, 0.8660254037844387076, 1.000000000000000000, 0.8660254037844387076, 1.000000000000000000, 0.8660254037844387076, 1.000000000000000000, 0.8660254037844387076, 1.000000000000000000, 0.8660254037844387076, 1.000000000000000000, 0.8660254037844387076, 1.000000000000000000, 0.8660254037844387076, 1.000000000000000000, 0.8660254037844387076, 1.000000000000000000, 0.8660254037844387076, 1.000000000000000000, 0.8660254037844387076, 1.000000000000000000, 0.8660254037844387076, 1.000000000000000000, 0.8660254037844387076, 1.000000000000000000, 0.8660254037844387076, 1.000000000000000000, 0.8660254037844387076, 1.000000000000000000, 0.8660254037844387076, 1.000000000000000000, 0.8660254037844387076, 1.000000000000000000, 0.8660254037844387076, 1.000000000000000000, 0.8660254037844387076, 1.000000000000000000, 0.8660254037844387076, 1.000000000000000000, 0.8660254037844387076, 1.000000000000000000, 0.8660254037844387076, 1.000000000000000000, 0.8660254037844387076, 1.000000000000000000, 0.8660254037844387076, 1.000000000000000000, 0.8660254037844387076, 1.000000000000000000, 0.8660254037844387076, 1.000000000000000000, 0.8660254037844387076, 1.000000000000000000, 0.8660254037844387076, 1.000000000000000000, 0.8660254037844387076, 1.000000000000000000, 0.8660254037844387076, 1.000000000000000000, 0.8660254037844387076, 1.000000000000000000),
 ( 1.000000000000000000, 0.8660254037844387076, 1.000000000000000000, 0.8660254037844387076, 1.000000000000000000, 0.8660254037844387076, 1.000000000000000000, 0.8660254037844387076, 1.000000000000000000, 0.8660254037844387076, 1.000000000000000000, 0.8660254037844387076, 1.000000000000000000, 0.8660254037844387076, 1.000000000000000000, 0.8660254037844387076, 1.000000000000000000, 0.8660254037844387076, 1.000000000000000000, 0.8660254037844387076, 1.000000000000000000, 0.8660254037844387076, 1.000000000000000000, 0.8660254037844387076, 1.000000000000000000, 0.8660254037844387076, 1.000000000000000000, 0.8660254037844387076, 1.000000000000000000, 0.8660254037844387076, 1.000000000000000000, 0.8660254037844387076, 1.000000000000000000, 0.8660254037844387076, 1.000000000000000000, 0.8660254037844387076, 1.000000000000000000, 0.8660254037844387076, 1.000000000000000000, 0.8660254037844387076, 1.000000000000000000, 0.8660254037844387076, 1.000000000000000000, 0.8660254037844387076, 1.000000000000000000, 0.8660254037844387076, 1.000000000000000000, 0.8660254037844387076, 1.000000000000000000, 0.8660254037844387076, 1.000000000000000000, 0.8660254037844387076, 1.000000000000000000, 0.8660254037844387076, 1.000000000000000000, 0.8660254037844387076, 1.000000000000000000, 0.8660254037844387076, 1.000000000000000000, 0.8660254037844387076, 1.000000000000000000, 0.8660254037844387076, 1.000000000000000000, 0.8660254037844387076, 1.000000000000000000, 0.8660254037844387076, 1.000000000000000000, 0.8660254037844387076, 1.000000000000000000, 0.8660254037844387076, 1.000000000000000000, 0.8660254037844387076, 1.000000000000000000, 0.8660254037844387076, 1.000000000000000000, 0.8660254037844387076, 1.000000000000000000, 0.8660254037844387076, 1.000000000000000000, 0.8660254037844387076, 1.000000000000000000, 0.8660254037844387076, 1.000000000000000000, 0.8660254037844387076, 1.000000000000000000, 0.8660254037844387076, 1.000000000000000000, 0.8660254037844387076, 1.000000000000000000, 0.8660254037844387076, 1.000000000000000000, 0.8660254037844387076, 1.000000000000000000, 0.8660254037844387076, 1.000000000000000000, 0.8660254037844387076, 1.000000000000000000, 0.8660254037844387076, 1.000000000000000000, 0.8660254037844387076, 1.000000000000000000, 0.8660254037844387076, 1.000000000000000000, 0.8660254037844387076, 1.000000000000000000, 0.8660254037844387076, 1.000000000000000000, 0.8660254037844387076, 1.000000000000000000, 0.8660254037844387076, 1.000000000000000000, 0.8660254037844387076, 1.000000000000000000, 0.8660254037844387076, 1.000000000000000000, 0.8660254037844387076, 1.000000000000000000, 0.8660254037844387076, 1.000000000000000000, 0.8660254037844387076, 1.000000000000000000, 0.8660254037844387076, 1.000000000000000000, 0.8660254037844387076, 1.000000000000000000, 0.8660254037844387076, 1.000000000000000000, 0.8660254037844387076, 1.000000000000000000, 0.8660254037844387076, 1.000000000000000000, 0.8660254037844387076, 1.000000000000000000, 0.8660254037844387076, 1.000000000000000000, 0.8660254037844387076, 1.000000000000000000, 0.8660254037844387076, 1.000000000000000000, 0.8660254037844387076, 1.000000000000000000, 0.8660254037844387076, 1.000000000000000000, 0.8660254037844387076, 1.000000000000000000, 0.8660254037844387076, 1.000000000000000000, 0.8660254037844387076, 1.000000000000000000, 0.8660254037844387076, 1.000000000000000000, 0.8660254037844387076, 1.000000000000000000, 0.8660254037844387076, 1.000000000000000000, 0.8660254037844387076, 1.000000000000000000, 0.8660254037844387076, 1.000000000000000000, 0.8660254037844387076, 1.000000000000000000, 0.8660254037844387076, 1.000000000000000000, 0.8660254037844387076, 1.000000000000000000, 0.8660254037844387076, 1.000000000000000000, 0.8660254037844387076, 1.000000000000000000, 0.8660254037844387076, 1.000000000000000000, 0.8660254037844387076, 1.000000000000000000, 0.8660254037844387076, 1.000000000000000000, 0.8660254037844387076, 1.000000000000000000, 0.8660254037844387076, 1.000000000000000000, 0.8660254037844387076, 1.000000000000000000, 0.8660254037844387076, 1.000000000000000000, 0.8660254037844387076, 1.000000000000000000, 0.8660254037844387076, 1.000000000000000000, 0.8660254037844387076, 1.000000000000000000, 0.8660254037844387076, 1.000000000000000000, 0.8660254037844387076, 1.000000000000000000, 0.8660254037844387076, 1.000000000000000000, 0.8660254037844387076, 1.000000000000000000, 0.8660254037844387076, 1.000000000000000000, 0.8660254037844387076, 1.000000000000000000, 0.8660254037844387076, 1.000000000000000000, 0.8660254037844387076, 1.000000000000000000, 0.8660254037844387076, 1.000000000000000000, 0.8660254037844387076, 1.000000000000000000, 0.8660254037844387076, 1.000000000000000000, 0.8660254037844387076, 1.000000000000000000, 0.8660254037844387076, 1.000000000000000000, 0.8660254037844387076, 1.000000000000000000, 0.8660254037844387076, 1.000000000000000000, 0.8660254037844387076, 1.000000000000000000, 0.8660254037844387076, 1.000000000000000000, 0.8660254037844387076, 1.000000000000000000, 0.8660254037844387076, 1.000000000000000000, 0.8660254037844387076, 1.000000000000000000, 0.8660254037844387076, 1.000000000000000000, 0.8660254037844387076, 1.000000000000000000, 0.8660254037844387076, 1.000000000000000000, 0.8660254037844387076, 1.000000000000000000, 0.8660254037844387076, 1.000000000000000000, 0.8660254037844387076, 1.000000000000000000, 0.8660254037844387076, 1.000000000000000000, 0.8660254037844387076, 1.000000000000000000, 0.8660254037844387076, 1.000000000000000000, 0.8660254037844387076, 1.000000000000000000, 0.8660254037844387076, 1.000000000000000000, 0.8660254037844387076, 1.000000000000000000, 0.8660254037844387076, 1.000000000000000000, 0.8660254037844387076, 1.000000000000000000, 0.8660254037844387076, 1.000000000000000000, 0.8660254037844387076, 1.000000000000000000, 0.8660254037844387076, 1.000000000000000000, 0.8660254037844387076, 1.000000000000000000, 0.8660254037844387076, 1.000000000000000000, 0.8660254037844387076, 1.000000000000000000, 0.8660254037844387076, 1.000000000000000000, 0.8660254037844387076, 1.000000000000000000, 0.8660254037844387076, 1.000000000000000000, 0.8660254037844387076, 1.000000000000000000, 0.8660254037844387076, 1.000000000000000000, 0.8660254037844387076, 1.000000000000000000, 0.8660254037844387076, 1.000000000000000000, 0.8660254037844387076, 1.000000000000000000, 0.8660254037844387076, 1.000000000000000000, 0.8660254037844387076, 1.000000000000000000, 0.8660254037844387076, 1.000000000000000000, 0.8660254037844387076, 1.000000000000000000, 0.8660254037844387076, 1.000000000000000000, 0.8660254037844387076, 1.000000000000000000, 0.8660254037844387076, 1.000000000000000000, 0.8660254037844387076, 1.000000000000000000, 0.8660254037844387076, 1.000000000000000000, 0.8660254037844387076, 1.000000000000000000, 0.8660254037844387076, 1.000000000000000000, 0.8660254037844387076, 1.000000000000000000, 0.8660254037844387076, 1.000000000000000000, 0.8660254037844387076, 1.000000000000000000, 0.8660254037844387076, 1.000000000000000000, 0.8660254037844387076, 1.000000000000000000, 0.8660254037844387076, 1.000000000000000000, 0.8660254037844387076, 1.000000000000000000, 0.8660254037844387076, 1.000000000000000000, 0.8660254037844387076, 1.000000000000000000, 0.8660254037844387076, 1.000000000000000000, 0.8660254037844387076, 1.000000000000000000, 0.8660254037844387076, 1.000000000000000000, 0.8660254037844387076, 1.000000000000000000, 0.8660254037844387076, 1.000000000000000000, 0.8660254037844387076, 1.000000000000000000) ) ) 
 REPRESENTATION_ITEM ( '' )  SURFACE ( )  );
#198669=CARTESIAN_POINT ( 'NONE',  ( -7.153898609505128015, 11.49796547773133604, 0.7998128361456481317 ) ) ;
#198670=CARTESIAN_POINT ( 'NONE',  ( -2.103486388414573138, 5.605817886458954291, 1.040834085586084257E-14 ) ) ;
#198673=CARTESIAN_POINT ( 'NONE',  ( 0.6823417656249917140, 5.092708333674749177, 1.181850606188765695 ) ) ;
#198678=CARTESIAN_POINT ( 'NONE',  ( -7.551528372687420720, 8.872833191965849409, 1.082531754730558626 ) ) ;
#198680=CARTESIAN_POINT ( 'NONE',  ( -0.7500000000000215383, 4.941666666666684193, 1.299038105676671107 ) ) ;
#198683=CARTESIAN_POINT ( 'NONE',  ( 6.968527767744093993, 10.11340424813470662, 1.082531754730558626 ) ) ;
#198689=CARTESIAN_POINT ( 'NONE',  ( 4.351804119862229037, 4.179452349368450115, -0.7216878364870188411 ) ) ;
#198692=CARTESIAN_POINT ( 'NONE',  ( 9.531018800282609504, 10.22186947652563305, 0.7216878364870458196 ) ) ;
#198699=CARTESIAN_POINT ( 'NONE',  ( 6.693975156845185737, 8.832723654451292816, 1.599625672291281386 ) ) ;
#198700=CARTESIAN_POINT ( 'NONE',  ( -4.717347382551060342, 7.590990148696470818, 1.199719254218464037 ) ) ;
#198704=CARTESIAN_POINT ( 'NONE',  ( 4.650083499362856365, 8.368921815991249957, 0.7216878364870438212 ) ) ;
#198705=CARTESIAN_POINT ( 'NONE',  ( -1.402160292154681736E-14, 0.1343750003414218575, 1.575800808251672791 ) ) ;
#198706=CARTESIAN_POINT ( 'NONE',  ( 4.528060117284244512, 4.385084346360807572, 0.7216878364870317197 ) ) ;
#198707=CARTESIAN_POINT ( 'NONE',  ( -9.134442807305063639, 11.67993591332117376, 1.599625672291281386 ) ) ;
#198722=CARTESIAN_POINT ( 'NONE',  ( 6.500244582748090139, 9.671036882259738121, 1.199719254218460707 ) ) ;
#198723=CARTESIAN_POINT ( 'NONE',  ( 7.494959990256193194, 7.638541498254023843, -0.7998128361456281477 ) ) ;
#198726=EDGE_LOOP ( 'NONE', ( #54960, #181075, #201828, #162245, #195305, #112991, #34424 ) ) ;
#198732=CARTESIAN_POINT ( 'NONE',  ( 10.40996301719436090, 11.03937836301526687, 0.000000000000000000 ) ) ;
#198734=CARTESIAN_POINT ( 'NONE',  ( -4.900382456335551140, 7.804531068111707270, 1.199719254218464037 ) ) ;
#198735=CARTESIAN_POINT ( 'NONE',  ( -4.925689880466507908, 4.641059703499347044, -0.7998128361456221525 ) ) ;
#198745=CARTESIAN_POINT ( 'NONE',  ( -2.117044542028253318, 5.621635732341564662, -0.7998128361456281477 ) ) ;
#198749=CARTESIAN_POINT ( 'NONE',  ( 6.205881626753210867, 8.263281202677319470, 1.599625672291281386 ) ) ;
#198750=CARTESIAN_POINT ( 'NONE',  ( 0.6823417656249917140, 4.342708333674755394, 1.181850606188765695 ) ) ;
#198755=CARTESIAN_POINT ( 'NONE',  ( 5.138177029454847222, 6.057256624861201644, 1.082531754730560403 ) ) ;
#198756=CARTESIAN_POINT ( 'NONE',  ( -8.016948904382338981, 8.247528564734524892, -0.7998128361456291469 ) ) ;
#198761=CARTESIAN_POINT ( 'NONE',  ( -6.320072162264675164, 10.52516795595079557, 0.7998128361456481317 ) ) ;
#198762=CARTESIAN_POINT ( 'NONE',  ( -3.574546055497324737, 7.322054164722185732, 0.7998128361456341429 ) ) ;
#198766=FACE_OUTER_BOUND ( 'NONE', #205536, .T. ) ;
#198769=CARTESIAN_POINT ( 'NONE',  ( 4.937140493670735708, 8.911747675924535983, -0.7998128361456281477 ) ) ;
#198777=DIRECTION ( 'NONE',  ( 0.000000000000000000, 8.546850786086437571E-32, 1.000000000000000000 ) ) ;
#198783=CARTESIAN_POINT ( 'NONE',  ( -1.499999999999997780, 5.650000000000023448, 1.214306433183764966E-14 ) ) ;
#198784=CARTESIAN_POINT ( 'NONE',  ( 2.672928840188529609, 6.270167413528593414, 0.000000000000000000 ) ) ;
#198785=CARTESIAN_POINT ( 'NONE',  ( 4.355193658487811703, 6.104145239700998538, -1.599625672291255185 ) ) ;
#198787=CARTESIAN_POINT ( 'NONE',  ( -8.053180056837398126, 8.497724275839514618, 0.7216878364870578100 ) ) ;
#198789=CARTESIAN_POINT ( 'NONE',  ( 5.016153647376196290, 8.796003655340152605, 0.7216878364870438212 ) ) ;
#198790=CARTESIAN_POINT ( 'NONE',  ( -7.768458830506062007, 11.04665715469030296, 1.082531754730549967 ) ) ;
#198795=CARTESIAN_POINT ( 'NONE',  ( 7.610204295972345712, 7.772993188256215547, 0.7998128361456341429 ) ) ;
#198801=CARTESIAN_POINT ( 'NONE',  ( 0.6823417656249899377, 3.176041667008085323, -1.181850606188754593 ) ) ;
#198808=CARTESIAN_POINT ( 'NONE',  ( 7.579171565239241737, 8.801120566655981747, 1.199719254218462483 ) ) ;
#198812=CARTESIAN_POINT ( 'NONE',  ( -8.853638004923878313, 10.28799807962136548, 1.199719254218462483 ) ) ;
#198818=CARTESIAN_POINT ( 'NONE',  ( 9.576136569953906275, 10.06658084123472641, 0.000000000000000000 ) ) ;
#198821=CARTESIAN_POINT ( 'NONE',  ( -9.352427035328430449, 9.805586384171650849, 1.040834085586084257E-14 ) ) ;
#198824=CARTESIAN_POINT ( 'NONE',  ( 4.197870329852982252, 3.573279226090494198, -2.499999999999994671 ) ) ;
#198826=CARTESIAN_POINT ( 'NONE',  ( 5.762717851902044330, 6.056246448182416309, -0.5943541797442238872 ) ) ;
#198827=CARTESIAN_POINT ( 'NONE',  ( -2.981903720001798597, 5.566305875722335372, -1.199719254218446718 ) ) ;
#198832=CARTESIAN_POINT ( 'NONE',  ( 8.098297826064319693, 8.342435640030188893, 0.7998128361456481317 ) ) ;
#198834=CARTESIAN_POINT ( 'NONE',  ( 4.123651276850781144, 7.962676922967908411, -0.7998128361456221525 ) ) ;
#198835=CARTESIAN_POINT ( 'NONE',  ( -4.208837953572873047, 7.367755930811632936, 0.8315943877991900379 ) ) ;
#198836=CARTESIAN_POINT ( 'NONE',  ( 4.416205349749311004, 6.175325546172740765, 1.599625672291267398 ) ) ;
#198838=CARTESIAN_POINT ( 'NONE',  ( -6.724481002698120768, 9.828683022247721723, -1.082531754730538864 ) ) ;
#198844=CARTESIAN_POINT ( 'NONE',  ( -4.124159483505494883, 7.474427186445510962, 0.6511861734826256409 ) ) ;
#198848=CARTESIAN_POINT ( 'NONE',  ( 5.178851490740207453, 5.144340948726102702, 0.7216878364870317197 ) ) ;
#198856=CARTESIAN_POINT ( 'NONE',  ( 4.161989969715248705, 4.726297878971393196, -2.420000000000000373 ) ) ;
#198858=CARTESIAN_POINT ( 'NONE',  ( -9.829298179783291900, 11.53023130024440768, 1.082531754730558626 ) ) ;
#198859=CARTESIAN_POINT ( 'NONE',  ( 1.284279953904119864, 2.827889714876734129, -0.7749999999999910294 ) ) ;
#198864=CARTESIAN_POINT ( 'NONE',  ( -10.29027540264791440, 11.10766884595181203, 0.7216878364870438212 ) ) ;
#198871=CARTESIAN_POINT ( 'NONE',  ( 1.499999999999989120, 2.306250000682817713, 1.214306433183764966E-14 ) ) ;
#198873=CARTESIAN_POINT ( 'NONE',  ( -5.032047568966410367, 9.022472597102808578, 1.214306433183764966E-14 ) ) ;
#198876=CARTESIAN_POINT ( 'NONE',  ( -7.971304249830880373, 11.38727316052296601, 1.199719254218453823 ) ) ;
#198879=CARTESIAN_POINT ( 'NONE',  ( 6.498435699651741615, 6.475929825882159818, -0.7998128361456281477 ) ) ;
#198882=DIRECTION ( 'NONE',  ( 0.7592566023653016805, -0.6507913734559627184, 0.000000000000000000 ) ) ;
#198885=CARTESIAN_POINT ( 'NONE',  ( 8.178592977541601527, 10.56477777859713463, 1.599625672291281386 ) ) ;
#198891=CARTESIAN_POINT ( 'NONE',  ( -7.375272376154093479, 9.627570410311676596, -1.443375672974059665 ) ) ;
#198894=CARTESIAN_POINT ( 'NONE',  ( 1.364683531249992088, 5.446875000341417916, 1.214306433183764966E-14 ) ) ;
#198897=FACE_OUTER_BOUND ( 'NONE', #62900, .T. ) ;
#198901=CARTESIAN_POINT ( 'NONE',  ( -3.673896439178936824, 5.309298483840612093, 1.443375672974064550 ) ) ;
#198904=CARTESIAN_POINT ( 'NONE',  ( 9.856941372335116469, 11.45851867493453291, 1.199719254218450271 ) ) ;
#198905=CARTESIAN_POINT ( 'NONE',  ( 1.499999999999822586, 7.240846818246208905, 4.154462424328221104 ) ) ;
#198906=CARTESIAN_POINT ( 'NONE',  ( -10.49131193887636826, 11.13428543831092909, 1.040834085586084257E-14 ) ) ;
#198909=CARTESIAN_POINT ( 'NONE',  ( 0.6823417656249882723, 2.176041667008084435, -1.181850606188749264 ) ) ;
#198911=CARTESIAN_POINT ( 'NONE',  ( 4.334856428067313416, 6.080418470877079429, -1.599625672291256295 ) ) ;
#198918=CARTESIAN_POINT ( 'NONE',  ( 9.693716643646595799, 11.37205284141829686, 1.082531754730548412 ) ) ;
#198920=CARTESIAN_POINT ( 'NONE',  ( -6.399085315970137522, 9.449054721065074602, -1.082531754730538864 ) ) ;
#198922=CARTESIAN_POINT ( 'NONE',  ( 0.5610452518370867558, 7.732119650022924340, 1.919700688223595408 ) ) ;
#198924=CARTESIAN_POINT ( 'NONE',  ( -6.333630315878337136, 10.54098580183340772, 0.000000000000000000 ) ) ;
#198925=CARTESIAN_POINT ( 'NONE',  ( -5.721177634842498527, 5.777054783512106440, 0.000000000000000000 ) ) ;
#198926=CARTESIAN_POINT ( 'NONE',  ( -1.364683531250012516, 3.801041667008087099, -0.7879004041258300672 ) ) ;
#198931=CARTESIAN_POINT ( 'NONE',  ( 9.317477881089539338, 11.89347683273640932, 1.599625672291279388 ) ) ;
#198944=CARTESIAN_POINT ( 'NONE',  ( 8.499999999999980460, 6.280000000000042881, 2.873333333333345951 ) ) ;
#198947=CARTESIAN_POINT ( 'NONE',  ( 1.364683531249988535, 3.926041667008087543, 0.7879004041258500513 ) ) ;
#198955=CARTESIAN_POINT ( 'NONE',  ( 9.694243528971124846, 11.26870452434320491, 1.199719254218450271 ) ) ;
#198957=CARTESIAN_POINT ( 'NONE',  ( -1.201851678989727383E-14, 3.071875000341420137, 1.575800808251672791 ) ) ;
#198959=CARTESIAN_POINT ( 'NONE',  ( -8.039621903223732602, 8.481906429956900695, 1.040834085586084257E-14 ) ) ;
#198967=CARTESIAN_POINT ( 'NONE',  ( 3.181359600701000989, 6.863336634126477875, 0.000000000000000000 ) ) ;
#198971=CARTESIAN_POINT ( 'NONE',  ( 7.716561984472250835, 12.15440608185967086, 1.040834085586084257E-14 ) ) ;
#198977=CARTESIAN_POINT ( 'NONE',  ( -3.216308754939891212, 4.775446185561722956, -1.599625672291262513 ) ) ;
#198978=CARTESIAN_POINT ( 'NONE',  ( 6.500244582748090139, 9.671036882259738121, 1.199719254218460707 ) ) ;
#198980=CARTESIAN_POINT ( 'NONE',  ( 4.650083499362875017, 5.487814173087225633, 1.082531754730560403 ) ) ;
#198981=EDGE_CURVE ( 'NONE', #179933, #111607, #14962, .T. ) ;
#198989=CARTESIAN_POINT ( 'NONE',  ( -7.375272376154096143, 8.667201196010339004, -1.082531754730544860 ) ) ;
#198990=CARTESIAN_POINT ( 'NONE',  ( 3.825371897350130723, 7.614684313550482031, 0.7998128361456321445 ) ) ;
#198992=EDGE_CURVE ( 'NONE', #40394, #143545, #37033, .T. ) ;
#198994=CARTESIAN_POINT ( 'NONE',  ( -8.507905087775398556, 9.884643009614800135, 1.199719254218462483 ) ) ;
#198999=CARTESIAN_POINT ( 'NONE',  ( -3.867100128395853709, 5.534702787927018974, -1.599625672291256295 ) ) ;
#199000=LINE ( 'NONE', #169464, #86450 ) ;
#199004=CARTESIAN_POINT ( 'NONE',  ( 9.260382613333817403, 10.76253345609967660, -1.199719254218446718 ) ) ;
#199005=CARTESIAN_POINT ( 'NONE',  ( 3.785751206713845018, 5.439795712631356750, 1.599625672291267398 ) ) ;
#199014=CARTESIAN_POINT ( 'NONE',  ( -4.613852347352193739, 4.277249248199312071, 1.214306433183764966E-14 ) ) ;
#199016=CARTESIAN_POINT ( 'NONE',  ( -8.188234707649510113, 11.64035869464474082, -1.199719254218446718 ) ) ;
#199020=CARTESIAN_POINT ( 'NONE',  ( 5.978782553946477840, 9.919070713005490703, 1.040834085586084257E-14 ) ) ;
#199021=CARTESIAN_POINT ( 'NONE',  ( -1.364683531250010740, 4.842708333674756283, 0.7879004041258379498 ) ) ;
#199023=CARTESIAN_POINT ( 'NONE',  ( 4.546061579283848353, 4.198160018786257552, -0.7998128361456211532 ) ) ;
#199026=CARTESIAN_POINT ( 'NONE',  ( -5.852315862593199469, 9.979452273000736895, 0.7998128361456481317 ) ) ;
#199036=CARTESIAN_POINT ( 'NONE',  ( -0.6823417656250212460, 3.863541667008085767, 1.181850606188767472 ) ) ;
#199037=CARTESIAN_POINT ( 'NONE',  ( 10.06423010004587759, 10.63602329300870153, 0.000000000000000000 ) ) ;
#199039=CARTESIAN_POINT ( 'NONE',  ( -3.633221978782283923, 7.182583375313884133, -0.7216878364870267237 ) ) ;
#199042=CARTESIAN_POINT ( 'NONE',  ( -3.890826896997578999, 7.483122446565064756, 0.7216878364870317197 ) ) ;
#199051=CARTESIAN_POINT ( 'NONE',  ( 3.337278367258157630, 7.045241861776501580, 0.7998128361456341429 ) ) ;
#199061=CARTESIAN_POINT ( 'NONE',  ( 6.342516933094585418, 6.294024598232139667, 1.040834085586084257E-14 ) ) ;
#199065=CARTESIAN_POINT ( 'NONE',  ( -4.564291269294938225, 8.476756914152748124, 1.040834085586084257E-14 ) ) ;
#199069=CARTESIAN_POINT ( 'NONE',  ( 7.772902139336337335, 7.962807338847539107, 0.7998128361456341429 ) ) ;
#199072=CARTESIAN_POINT ( 'NONE',  ( -4.550733115681270036, 8.460939068270139529, 0.7998128361456481317 ) ) ;
#199074=CARTESIAN_POINT ( 'NONE',  ( 1.499999999999989120, 2.754166666666688190, 0.8660254037844524744 ) ) ;
#199075=CARTESIAN_POINT ( 'NONE',  ( -3.867100128395853709, 5.534702787927018974, -1.599625672291256295 ) ) ;
#199078=CARTESIAN_POINT ( 'NONE',  ( -5.935772324684618795, 5.819489221753827657, 0.000000000000000000 ) ) ;
#199080=CARTESIAN_POINT ( 'NONE',  ( -1.364683531250012516, 2.988541667008091096, -0.7879004041258289570 ) ) ;
#199082=CARTESIAN_POINT ( 'NONE',  ( -5.341549334104202629, 7.254893527920112994, 1.443375672974064550 ) ) ;
#199087=CARTESIAN_POINT ( 'NONE',  ( -1.441119962213332828, 8.287674021641837641, -3.161270278916411769 ) ) ;
#199088=CARTESIAN_POINT ( 'NONE',  ( 5.843727902690005749, 6.776436293681846301, -1.199719254218445830 ) ) ;
#199091=CARTESIAN_POINT ( 'NONE',  ( -1.364683531250012516, 3.301041667008084879, -0.7879004041258289570 ) ) ;
#199093=CARTESIAN_POINT ( 'NONE',  ( 3.063252641683779753, 5.661212951017999373, 1.199719254218450271 ) ) ;
#199095=CARTESIAN_POINT ( 'NONE',  ( -1.402160292154681736E-14, 0.1343750003414218575, 1.575800808251672791 ) ) ;
#199098=CARTESIAN_POINT ( 'NONE',  ( -3.164938793786285842, 5.779846795137578930, -1.199719254218452935 ) ) ;
#199099=CARTESIAN_POINT ( 'NONE',  ( -5.680503174001480637, 9.571078103069643461, 0.7216878364870458196 ) ) ;
#199100=VECTOR ( 'NONE', #147092, 1000.000000000000000 ) ;
#199103=CARTESIAN_POINT ( 'NONE',  ( 0.6823417656249899377, 2.842708333674753618, 1.181850606188765695 ) ) ;
#199111=CARTESIAN_POINT ( 'NONE',  ( -6.683806541412768532, 8.820860269780128604, -1.443375672974058777 ) ) ;
#199118=CARTESIAN_POINT ( 'NONE',  ( -6.114364089638801403, 8.156510742710487705, 1.443375672974078761 ) ) ;
#199131=CARTESIAN_POINT ( 'NONE',  ( -6.392833124043511894, 7.417059051927569868, 1.199719254218450271 ) ) ;
#199133=CARTESIAN_POINT ( 'NONE',  ( -0.7500000000000006661, -0.1416666666666441254, -1.299038105676652011 ) ) ;
#199134=CARTESIAN_POINT ( 'NONE',  ( 3.277320446201373638, 4.846626492033466072, 1.599625672291267398 ) ) ;
#199138=CARTESIAN_POINT ( 'NONE',  ( 4.469384193999260901, 8.366031992974468423, -0.7998128361456231517 ) ) ;
#199145=CARTESIAN_POINT ( 'NONE',  ( -4.473827502829599290, 4.321812962830357208, 0.7216878364870317197 ) ) ;
#199149=CARTESIAN_POINT ( 'NONE',  ( -0.1605634594619409494, 7.049300555817002767, 3.948520363690844359 ) ) ;
#199150=B_SPLINE_CURVE_WITH_KNOTS ( 'NONE', 3,
 ( #130347, #127151, #12231, #209350 ),
 .UNSPECIFIED., .F., .F.,
 ( 4, 4 ),
 ( 0.001582017824277144819, 0.002341702326271049434 ),
 .UNSPECIFIED. ) ;
#199154=CARTESIAN_POINT ( 'NONE',  ( -1.201851678989727383E-14, 1.821875000341421691, 1.575800808251672791 ) ) ;
#199155=CARTESIAN_POINT ( 'NONE',  ( 8.215877899756996783, 12.52901528311778989, 1.040834085586084257E-14 ) ) ;
#199156=CARTESIAN_POINT ( 'NONE',  ( -6.906989191158078079, 10.14557225873805812, -1.199719254218440723 ) ) ;
#199159=CARTESIAN_POINT ( 'NONE',  ( 7.657657833620182153, 7.828355648845348291, -0.7998128361456281477 ) ) ;
#199160=CARTESIAN_POINT ( 'NONE',  ( -7.226659571283968297, 8.389856573708110332, 1.199719254218450271 ) ) ;
#199161=CARTESIAN_POINT ( 'NONE',  ( -1.594690046439253273, 8.741643652401169362, 2.463706593913791210 ) ) ;
#199163=CARTESIAN_POINT ( 'NONE',  ( -1.500000000000001332, -0.3187499993171846735, 0.000000000000000000 ) ) ;
#199165=CARTESIAN_POINT ( 'NONE',  ( 6.941411460516762943, 11.04213777067082702, -0.7216878364870267237 ) ) ;
#199168=CARTESIAN_POINT ( 'NONE',  ( -1.402160292154681736E-14, 0.6343750003414162508, 1.575800808251672791 ) ) ;
#199170=CARTESIAN_POINT ( 'NONE',  ( 3.432607057648175530, 6.331044601171339714, 1.095529308728976137 ) ) ;
#199171=CARTESIAN_POINT ( 'NONE',  ( 7.090551149822744925, 7.374657217655760100, 0.7216878364870317197 ) ) ;
#199175=CARTESIAN_POINT ( 'NONE',  ( -3.606105671554953318, 7.150947683548662503, 0.7216878364870317197 ) ) ;
#199177=CARTESIAN_POINT ( 'NONE',  ( -0.6823417656250212460, 4.801041667008086655, 1.181850606188767472 ) ) ;
#199181=CARTESIAN_POINT ( 'NONE',  ( -5.012244793233714191, 6.784968962630095746, -1.449178643049347848 ) ) ;
#199187=CARTESIAN_POINT ( 'NONE',  ( 7.039708073993665494, 9.236078724457858158, 1.599625672291281386 ) ) ;
#199191=CARTESIAN_POINT ( 'NONE',  ( -1.201851678989727383E-14, 2.837500000000024780, -1.732050807568863648 ) ) ;
#199197=ORIENTED_EDGE ( 'NONE', *, *, #31081, .F. ) ;
#199198=CARTESIAN_POINT ( 'NONE',  ( 5.504247177468179153, 7.444707678511436555, 1.443375672974062551 ) ) ;
#199199=CARTESIAN_POINT ( 'NONE',  ( -1.402160292154681736E-14, 0.2593750003414224681, -1.575800808251665908 ) ) ;
#199203=CARTESIAN_POINT ( 'NONE',  ( 8.380911511541880188, 12.92948053010758258, 0.7998128361456462443 ) ) ;
#199208=CARTESIAN_POINT ( 'NONE',  ( -1.500000000000013101, 1.129166666666688634, -0.8660254037844313801 ) ) ;
#199209=CARTESIAN_POINT ( 'NONE',  ( 7.962716289927667113, 8.184257181204083409, -0.7998128361456291469 ) ) ;
#199210=CARTESIAN_POINT ( 'NONE',  ( -9.189729191964438826, 9.615772233580322848, 1.040834085586084257E-14 ) ) ;
#199213=CARTESIAN_POINT ( 'NONE',  ( 1.364683531249986537, 0.9052083336747533959, -0.7879004041258239610 ) ) ;
#199215=CARTESIAN_POINT ( 'NONE',  ( -1.500000000000013101, 2.170833333333357373, 0.8660254037844403729 ) ) ;
#199218=CARTESIAN_POINT ( 'NONE',  ( 2.984766373302843778, 6.633977868828633717, -0.7998128361456291469 ) ) ;
#199225=CARTESIAN_POINT ( 'NONE',  ( -0.7500000000000249800, -0.7770833326505161009, 1.299038105676659116 ) ) ;
#199226=CARTESIAN_POINT ( 'NONE',  ( -6.832419346282942563, 10.05857410638369487, 1.199719254218453823 ) ) ;
#199227=CARTESIAN_POINT ( 'NONE',  ( -5.422898255786209099, 5.429062174613087599, -0.7216878364870207285 ) ) ;
#199235=CARTESIAN_POINT ( 'NONE',  ( 6.636879889089462026, 7.701780277814560982, -1.199719254218446718 ) ) ;
#199239=CARTESIAN_POINT ( 'NONE',  ( 7.969495366734495434, 8.192166104145387706, 1.040834085586084257E-14 ) ) ;
#199240=CARTESIAN_POINT ( 'NONE',  ( 7.009202228140744673, 9.200488570962775725, -1.443375672974058777 ) ) ;
#199241=CARTESIAN_POINT ( 'NONE',  ( 0.4652293495370784515, 7.465077128757543257, -4.424517295598819011 ) ) ;
#199244=CARTESIAN_POINT ( 'NONE',  ( -8.206763054973658100, 8.468978407091068306, 0.7998128361456602331 ) ) ;
#199245=CARTESIAN_POINT ( 'NONE',  ( 3.018661757337009810, 6.673522483535157868, 0.000000000000000000 ) ) ;
#199248=DIRECTION ( 'NONE',  ( -7.387867266669436732E-31, -1.000000000000000000, 8.546850786086437571E-32 ) ) ;
#199249=CARTESIAN_POINT ( 'NONE',  ( 1.123270288250311610, 3.172697346350006331, 0.7749999999993734123 ) ) ;
#199251=CARTESIAN_POINT ( 'NONE',  ( 8.432808358020015049, 11.82173160345663376, 1.082531754730546636 ) ) ;
#199258=AXIS2_PLACEMENT_3D ( 'NONE', #72487, #108277, #208879 ) ;
#199261=CARTESIAN_POINT ( 'NONE',  ( -5.111060722671894929, 5.065251719313053513, 0.000000000000000000 ) ) ;
#199262=CARTESIAN_POINT ( 'NONE',  ( 8.595506201384008449, 11.05117653974661529, 1.443375672974076540 ) ) ;
#199266=CARTESIAN_POINT ( 'NONE',  ( -5.368138756007025947, 8.350246751061767725, 1.199719254218452047 ) ) ;
#199268=CARTESIAN_POINT ( 'NONE',  ( -3.123065541208358997, 6.445821767598281404, -0.7606279415795504928 ) ) ;
#199273=CARTESIAN_POINT ( 'NONE',  ( -8.532158741701643123, 8.848606708273724308, 0.7998128361456462443 ) ) ;
#199277=CARTESIAN_POINT ( 'NONE',  ( -0.4956004317509503099, 7.799479031273152785, 1.990828115380108176 ) ) ;
#199288=CARTESIAN_POINT ( 'NONE',  ( -5.717788096661253761, 7.693838750903348789, 1.599625672291269396 ) ) ;
#199291=CARTESIAN_POINT ( 'NONE',  ( 3.687454593236936251, 7.245854758844324728, -0.7216878364870267237 ) ) ;
#199295=CARTESIAN_POINT ( 'NONE',  ( -4.948889764188092677, 5.732458465429559169, 1.199719254218462483 ) ) ;
#199302=CARTESIAN_POINT ( 'NONE',  ( -7.527801604085656351, 9.805521176231838609, 1.599625672291295375 ) ) ;
#199303=CARTESIAN_POINT ( 'NONE',  ( 5.099838337034727331, 9.101561826515851550, -0.7998128361456281477 ) ) ;
#199306=CARTESIAN_POINT ( 'NONE',  ( -7.486073373039941359, 11.88550270185529278, -0.7998128361456291469 ) ) ;
#199307=CARTESIAN_POINT ( 'NONE',  ( 5.497994985541524215, 6.373081223675282736, -1.199719254218445830 ) ) ;
#199310=CARTESIAN_POINT ( 'NONE',  ( -1.364683531250014514, 0.3010416670080866552, -0.7879004041258359514 ) ) ;
#199311=VERTEX_POINT ( 'NONE', #186964 ) ;
#199313=CARTESIAN_POINT ( 'NONE',  ( 9.422553571817644524, 10.09532670998316384, 0.000000000000000000 ) ) ;
#199341=CARTESIAN_POINT ( 'NONE',  ( -1.500000000000015099, -0.3395833326505143801, -0.8660254037844383745 ) ) ;
#199346=DIRECTION ( 'NONE',  ( 1.000000000000000000, -5.391474854832587087E-16, 0.000000000000000000 ) ) ;
#199347=LINE ( 'NONE', #149558, #201976 ) ;
#199349=CARTESIAN_POINT ( 'NONE',  ( 9.511208455186636712, 11.05516360492796935, 1.199719254218453823 ) ) ;
#199354=CARTESIAN_POINT ( 'NONE',  ( 4.202137545231717120, 6.989912005157271402, 1.199719254218462483 ) ) ;
#199355=CARTESIAN_POINT ( 'NONE',  ( -6.724481002698126098, 8.868313807946373473, -1.443375672974059665 ) ) ;
#199357=CARTESIAN_POINT ( 'NONE',  ( 9.999301985278609806, 11.62460605670194447, 1.199719254218452047 ) ) ;
#199360=CARTESIAN_POINT ( 'NONE',  ( -7.049349804101573191, 10.31165964050546258, -1.199719254218440723 ) ) ;
#199361=CARTESIAN_POINT ( 'NONE',  ( -4.243338890952916387, 4.052909582307567149, -0.7216878364870207285 ) ) ;
#199365=CARTESIAN_POINT ( 'NONE',  ( -1.402160292154681736E-14, 0.3687500006828169363, -1.732050807568870754 ) ) ;
#199372=CARTESIAN_POINT ( 'NONE',  ( -4.622967192135580383, 5.456178481322002227, 1.082531754730558626 ) ) ;
#199375=CARTESIAN_POINT ( 'NONE',  ( 4.143432174609324115, 7.404820066527033617, -0.7413545030366501809 ) ) ;
#199379=CARTESIAN_POINT ( 'NONE',  ( -3.104453987404963478, 5.605318171072321221, -1.082531754730549078 ) ) ;
#199380=CARTESIAN_POINT ( 'NONE',  ( 9.921869487102386032, 10.46993591124128997, 0.000000000000000000 ) ) ;
#199389=CARTESIAN_POINT ( 'NONE',  ( -2.442440228756222353, 6.001264033524212671, -0.7998128361456281477 ) ) ;
#199390=CARTESIAN_POINT ( 'NONE',  ( -7.862839020921525091, 11.26073039346208660, -1.199719254218446718 ) ) ;
#199393=VERTEX_POINT ( 'NONE', #98825 ) ;
#199395=CARTESIAN_POINT ( 'NONE',  ( 6.003563092752934871, 5.898578451166879510, 0.7998128361456341429 ) ) ;
#199399=CARTESIAN_POINT ( 'NONE',  ( -4.197870329853007121, 3.573279226090508409, 2.499999999999998224 ) ) ;
#199413=CARTESIAN_POINT ( 'NONE',  ( 8.294891053462476904, 8.571794405328034827, 1.040834085586084257E-14 ) ) ;
#199416=CARTESIAN_POINT ( 'NONE',  ( -4.517891501851816649, 6.293959390292322986, -1.599625672291256295 ) ) ;
#199423=CARTESIAN_POINT ( 'NONE',  ( 1.499999999999987121, -0.7145833326505161009, 0.8660254037844524744 ) ) ;
#199427=CARTESIAN_POINT ( 'NONE',  ( 5.542585869888291938, 5.360771691158120689, -0.7998128361456211532 ) ) ;
#199429=CARTESIAN_POINT ( 'NONE',  ( -4.569261463005423352, 5.289558780716470565, -1.199719254218446718 ) ) ;
#199436=CARTESIAN_POINT ( 'NONE',  ( 4.799223189557548785, 7.582548906917042864, -1.082531754730549078 ) ) ;
#199439=CARTESIAN_POINT ( 'NONE',  ( 7.741342523278698096, 10.05465224862374285, 1.443375672974076540 ) ) ;
#199440=CARTESIAN_POINT ( 'NONE',  ( -0.6823417656249969321, 4.530208333674755394, -1.181850606188749264 ) ) ;
#199442=CARTESIAN_POINT ( 'NONE',  ( 2.995988758495615745, 6.439144618312774959, -0.7216878364870267237 ) ) ;
#199446=CARTESIAN_POINT ( 'NONE',  ( 5.568382567296971786, 6.179660279684793700, -0.8958173718428998900 ) ) ;
#199449=CARTESIAN_POINT ( 'NONE',  ( -6.098685391867989303, 6.020399689055939696, 0.3646554611961040360 ) ) ;
#199452=CARTESIAN_POINT ( 'NONE',  ( 0.6823417656249917140, 4.905208333674755394, 1.181850606188765695 ) ) ;
#199458=CARTESIAN_POINT ( 'NONE',  ( 0.7499999999999885647, -1.016666666666644847, 1.299038105676657340 ) ) ;
#199464=ORIENTED_EDGE ( 'NONE', *, *, #36958, .T. ) ;
#199467=CARTESIAN_POINT ( 'NONE',  ( -1.364683531250010295, 5.342708333674750953, 0.7879004041258379498 ) ) ;
#199469=CARTESIAN_POINT ( 'NONE',  ( 7.800018446563675489, 7.994443030612759848, -0.7998128361456281477 ) ) ;
#199470=CARTESIAN_POINT ( 'NONE',  ( -7.641992139597101108, 12.06740792950531649, 0.7998128361456481317 ) ) ;
#199476=CARTESIAN_POINT ( 'NONE',  ( -0.7499999999999972244, 4.108333333333360038, -1.299038105676652011 ) ) ;
#199483=CARTESIAN_POINT ( 'NONE',  ( 7.104109303880752790, 11.23195192126214970, -0.7216878364870267237 ) ) ;
#199486=DIRECTION ( 'NONE',  ( -0.6507913734559640506, -0.7592566023653004592, 0.000000000000000000 ) ) ;
#199488=CARTESIAN_POINT ( 'NONE',  ( 1.499999999999990896, 3.806250000682819046, 1.214306433183764966E-14 ) ) ;
#199491=CARTESIAN_POINT ( 'NONE',  ( -5.037017762676898158, 5.835274463666530131, -1.199719254218446718 ) ) ;
#199492=CARTESIAN_POINT ( 'NONE',  ( 5.138177029454852551, 5.096887410559856946, 0.7216878364870317197 ) ) ;
#199493=DIRECTION ( 'NONE',  ( 0.000000000000000000, -1.000000000000000000, 0.000000000000000000 ) ) ;
#199500=CARTESIAN_POINT ( 'NONE',  ( 3.161022370280501814, 6.839609865302569425, 0.000000000000000000 ) ) ;
#199505=CARTESIAN_POINT ( 'NONE',  ( 3.818592820543298405, 7.606775390609172405, -0.7998128361456221525 ) ) ;
#199508=CARTESIAN_POINT ( 'NONE',  ( 3.511198596259284876, 6.271927390929313617, -1.052294140492317842 ) ) ;
#199517=CARTESIAN_POINT ( 'NONE',  ( 5.874728247277303694, 5.987702652136856152, -0.2291304890473921385 ) ) ;
#199518=ORIENTED_EDGE ( 'NONE', *, *, #163609, .F. ) ;
#199521=CARTESIAN_POINT ( 'NONE',  ( 8.866142388332804103, 12.43125098877526113, -1.199719254218446718 ) ) ;
#199527=CARTESIAN_POINT ( 'NONE',  ( 5.178851490740193242, 8.025448591630130579, 1.082531754730558626 ) ) ;
#199529=CARTESIAN_POINT ( 'NONE',  ( -9.544576954340667996, 11.19805653722800365, 1.082531754730558626 ) ) ;
#199534=CARTESIAN_POINT ( 'NONE',  ( -3.684065054611367351, 5.321161868511784299, -1.599625672291256295 ) ) ;
#199537=CARTESIAN_POINT ( 'NONE',  ( -3.642672431166784186, 3.097590952613293869, 2.447572309174936844 ) ) ;
#199539=ORIENTED_EDGE ( 'NONE', *, *, #174092, .T. ) ;
#199546=CARTESIAN_POINT ( 'NONE',  ( 10.09812548408005384, 10.67556790771522124, -0.7998128361456281477 ) ) ;
#199547=CARTESIAN_POINT ( 'NONE',  ( 5.728356146706021335, 6.265246534282280066, 1.050634566151719129 ) ) ;
#199555=CARTESIAN_POINT ( 'NONE',  ( -9.164948653158003111, 9.794787638213568570, -0.7216878364870267237 ) ) ;
#199560=CARTESIAN_POINT ( 'NONE',  ( 8.125414133291656071, 8.374071331795406081, -0.7998128361456291469 ) ) ;
#199561=CARTESIAN_POINT ( 'NONE',  ( -3.899941742225307983, 7.701682465904834629, 0.7998128361456341429 ) ) ;
#199563=CARTESIAN_POINT ( 'NONE',  ( 4.192495815123822744, 5.914331089109666983, -1.599625672291255185 ) ) ;
#199565=CARTESIAN_POINT ( 'NONE',  ( -6.196239896645333367, 7.187700286629718605, -1.199719254218446718 ) ) ;
#199566=CARTESIAN_POINT ( 'NONE',  ( 2.361091307074211887, 5.906356958228550447, 0.7998128361456462443 ) ) ;
#199570=CARTESIAN_POINT ( 'NONE',  ( 10.07778825365955733, 10.65184113889131012, -0.7998128361456281477 ) ) ;
#199574=CARTESIAN_POINT ( 'NONE',  ( 4.002182886544830787, 7.824783036946191039, -0.1358892651178236766 ) ) ;
#199575=CARTESIAN_POINT ( 'NONE',  ( 4.189106276942576201, 7.831115056500907556, 1.040834085586084257E-14 ) ) ;
#199577=CARTESIAN_POINT ( 'NONE',  ( 0.1100172516615156165, 7.047065462482140497, 3.945011421259203566 ) ) ;
#199583=CARTESIAN_POINT ( 'NONE',  ( 7.076992996209058973, 11.20031622897851165, 1.040834085586084257E-14 ) ) ;
#199587=CARTESIAN_POINT ( 'NONE',  ( -8.040148788103921973, 9.338927326664741457, 1.199719254218462483 ) ) ;
#199596=CARTESIAN_POINT ( 'NONE',  ( 10.56588178375152864, 11.22128359066528169, -0.7998128361456281477 ) ) ;
#199600=CARTESIAN_POINT ( 'NONE',  ( 5.671388329218120639, 5.511041227042920099, 1.040834085586084257E-14 ) ) ;
#199604=CARTESIAN_POINT ( 'NONE',  ( -1.500000000000011324, 4.702083334016148974, 0.8660254037844403729 ) ) ;
#199610=CARTESIAN_POINT ( 'NONE',  ( -1.500000000000001332, 1.400000000000019229, 0.000000000000000000 ) ) ;
#199611=CARTESIAN_POINT ( 'NONE',  ( 5.276094334012385367, 9.307193822989793475, 1.040834085586084257E-14 ) ) ;
#199612=CARTESIAN_POINT ( 'NONE',  ( 3.782361668088245921, 6.396210465202840645, -1.082531754730548412 ) ) ;
#199614=CARTESIAN_POINT ( 'NONE',  ( -1.499999999999997780, 4.900000000000022560, 1.214306433183765124E-14 ) ) ;
#199615=CARTESIAN_POINT ( 'NONE',  ( 7.619319141200051604, 11.83303006480134911, 0.7216878364870438212 ) ) ;
#199621=CARTESIAN_POINT ( 'NONE',  ( -5.037017762676898158, 5.835274463666530131, -1.199719254218446718 ) ) ;
#199622=CARTESIAN_POINT ( 'NONE',  ( -0.7499999999999972244, 4.389583334016150751, -1.299038105676652899 ) ) ;
#199623=CARTESIAN_POINT ( 'NONE',  ( -1.364683531250014514, -0.01145833299191483488, -0.7879004041258359514 ) ) ;
#199627=CARTESIAN_POINT ( 'NONE',  ( 4.521807925357579805, 5.234196320127330715, -1.199719254218452047 ) ) ;
#199629=CARTESIAN_POINT ( 'NONE',  ( -1.201851678989727383E-14, 4.759375000341419693, -1.575800808251660134 ) ) ;
#199637=CARTESIAN_POINT ( 'NONE',  ( -8.365544474831901667, 9.718555627847388578, 1.199719254218462483 ) ) ;
#199638=CARTESIAN_POINT ( 'NONE',  ( 4.496500501226593727, 8.397667684739696270, 0.7998128361456462443 ) ) ;
#199640=CARTESIAN_POINT ( 'NONE',  ( 1.364683531249986537, -0.8447916663252468261, -0.7879004041258309554 ) ) ;
#199646=CARTESIAN_POINT ( 'NONE',  ( -6.891622154448065807, 6.934647356477856128, 1.040834085586084257E-14 ) ) ;
#199652=CARTESIAN_POINT ( 'NONE',  ( 9.728138913005292210, 11.30824913904973705, -1.199719254218440723 ) ) ;
#199655=CARTESIAN_POINT ( 'NONE',  ( -2.578021764892882040, 6.159442492350315490, 0.7998128361456341429 ) ) ;
#199656=CARTESIAN_POINT ( 'NONE',  ( -7.857113714319432063, 9.125386407249497012, 1.199719254218462483 ) ) ;
#199658=CARTESIAN_POINT ( 'NONE',  ( -4.432018112209435756, 7.309502936831247411, 1.252451368452773384 ) ) ;
#199659=CARTESIAN_POINT ( 'NONE',  ( -0.6823417656250003738, -0.7822916663252423852, -1.181850606188749264 ) ) ;
#199663=CARTESIAN_POINT ( 'NONE',  ( 8.107412671292042461, 9.521364873671299023, 1.082531754730558626 ) ) ;
#199666=CARTESIAN_POINT ( 'NONE',  ( 4.819033534653518025, 7.709623992816043270, -1.199719254218452047 ) ) ;
#199690=CARTESIAN_POINT ( 'NONE',  ( -3.913499895838973508, 7.717500311787445000, 1.040834085586084257E-14 ) ) ;
#199691=CARTESIAN_POINT ( 'NONE',  ( -7.483210719738908168, 10.81783070874899799, 1.199719254218453823 ) ) ;
#199696=CARTESIAN_POINT ( 'NONE',  ( -1.500000000000013101, 3.410416667349487785, -0.8660254037844313801 ) ) ;
#199697=CARTESIAN_POINT ( 'NONE',  ( 9.134442807305049428, 11.67993591332117376, 1.599625672291281386 ) ) ;
#199700=ORIENTED_EDGE ( 'NONE', *, *, #176940, .F. ) ;
#199702=CARTESIAN_POINT ( 'NONE',  ( -7.641992139597101108, 12.06740792950531649, 0.7998128361456481317 ) ) ;
#199704=CARTESIAN_POINT ( 'NONE',  ( 1.364683531249988757, 2.134375000341422357, 1.214306433183764966E-14 ) ) ;
#199706=CARTESIAN_POINT ( 'NONE',  ( -6.471393748265563239, 5.229711127717889596, 2.499999999999998668 ) ) ;
#199709=AXIS2_PLACEMENT_3D ( 'NONE', #43635, #109750, #27353 ) ;
#199710=CARTESIAN_POINT ( 'NONE',  ( 3.022498986271242138, 2.800000000000017586, 2.500000000000000444 ) ) ;
#199712=CARTESIAN_POINT ( 'NONE',  ( -3.898132859128961236, 4.506575409527250997, -1.199719254218452047 ) ) ;
#199716=CARTESIAN_POINT ( 'NONE',  ( 1.364683531249986537, 1.176041667008082658, 0.7879004041258500513 ) ) ;
#199722=CARTESIAN_POINT ( 'NONE',  ( 0.6823417656249899377, 1.842708333674752952, 1.181850606188755259 ) ) ;
#199724=CARTESIAN_POINT ( 'NONE',  ( -6.521635583373313061, 7.567328587812373719, -1.199719254218446718 ) ) ;
#199725=CARTESIAN_POINT ( 'NONE',  ( 7.052212457402625922, 11.37933163361175382, -0.7998128361456291469 ) ) ;
#199726=CARTESIAN_POINT ( 'NONE',  ( 3.181359600701000989, 6.863336634126477875, 0.000000000000000000 ) ) ;
#199727=CARTESIAN_POINT ( 'NONE',  ( 3.981290663907289140, 7.796589541200495965, -0.7998128361456221525 ) ) ;
#199729=CARTESIAN_POINT ( 'NONE',  ( -1.500000000000013101, 3.879166666666685970, -0.8660254037844313801 ) ) ;
#199731=CARTESIAN_POINT ( 'NONE',  ( -1.364683531250012516, 2.092708333674750953, 0.7879004041258379498 ) ) ;
#199739=CARTESIAN_POINT ( 'NONE',  ( 5.883875478650832491, 6.927238148923188454, -1.082531754730543083 ) ) ;
#199742=CARTESIAN_POINT ( 'NONE',  ( -8.503988664269602538, 10.94440607977979063, 1.599625672291269396 ) ) ;
#199743=CARTESIAN_POINT ( 'NONE',  ( -4.288456660624211381, 3.897620947016656956, 1.214306433183764966E-14 ) ) ;
#199750=CARTESIAN_POINT ( 'NONE',  ( -6.358410854684777291, 10.36197039720016022, -0.7216878364870267237 ) ) ;
#199752=CARTESIAN_POINT ( 'NONE',  ( -1.500000000000011324, 5.420833333333356485, 0.8660254037844403729 ) ) ;
#199755=CARTESIAN_POINT ( 'NONE',  ( 6.805829924380097040, 10.88395931184472154, 0.7216878364870438212 ) ) ;
#199759=( BOUNDED_CURVE ( )  B_SPLINE_CURVE ( 2, ( #53191, #164024, #31889, #70474, #136590, #119320, #20666 ),
 .UNSPECIFIED., .F., .T. ) 
 B_SPLINE_CURVE_WITH_KNOTS ( ( 3, 2, 2, 3 ),
 ( 0.1999999999999998446, 0.2041666666666665519, 0.2083333333333333148, 0.2125000000000000222 ),
 .UNSPECIFIED. ) 
 CURVE ( )  GEOMETRIC_REPRESENTATION_ITEM ( )  RATIONAL_B_SPLINE_CURVE ( ( 1.000000000000005329, 0.8660254037844333785, 1.000000000000000000, 0.8660254037844387076, 1.000000000000000000, 0.8660254037844378194, 1.000000000000000888 ) ) 
 REPRESENTATION_ITEM ( '' )  );
#199761=CARTESIAN_POINT ( 'NONE',  ( -4.222251700817149178, 3.978710388688374788, 0.5243367479217392324 ) ) ;
#199769=CARTESIAN_POINT ( 'NONE',  ( 7.623762449586013901, 7.788811034138823253, 1.040834085586084257E-14 ) ) ;
#199770=CARTESIAN_POINT ( 'NONE',  ( -4.229253852459088137, 7.021547696922494808, 1.199719254218464037 ) ) ;
#199772=DIRECTION ( 'NONE',  ( -0.000000000000000000, -8.546850786086437571E-32, -1.000000000000000000 ) ) ;
#199774=CARTESIAN_POINT ( 'NONE',  ( 5.083944415000174466, 7.914723669933440675, -1.082531754730549078 ) ) ;
#199775=CARTESIAN_POINT ( 'NONE',  ( 1.364683531249986981, -1.053124999658580752, 0.000000000000000000 ) ) ;
#199776=CARTESIAN_POINT ( 'NONE',  ( 4.555176424511575561, 4.416720038126027426, -0.7216878364870188411 ) ) ;
#199777=CARTESIAN_POINT ( 'NONE',  ( -3.704402285031864306, 5.344888637335695414, -1.599625672291256295 ) ) ;
#199788=ADVANCED_FACE ( 'NONE', ( #200028 ), #53809, .F. ) ;
#199795=CARTESIAN_POINT ( 'NONE',  ( 6.608709811657416999, 9.797579649320619311, -1.199719254218440723 ) ) ;
#199796=CARTESIAN_POINT ( 'NONE',  ( 7.308008492965924141, 8.484763649003774333, -1.199719254218451159 ) ) ;
#199807=CARTESIAN_POINT ( 'NONE',  ( -4.415151579544611238, 8.302760609444034046, -0.7998128361456281477 ) ) ;
#199810=CARTESIAN_POINT ( 'NONE',  ( -3.765413976293358278, 5.416068943807445635, 1.599625672291267398 ) ) ;
#199820=ADVANCED_FACE ( 'NONE', ( #202147 ), #182719, .F. ) ;
#199821=CARTESIAN_POINT ( 'NONE',  ( -10.48008955368359629, 11.32911868882677986, 1.040834085586084257E-14 ) ) ;
#199825=CARTESIAN_POINT ( 'NONE',  ( 6.474182045725470402, 7.511966127223233869, -1.199719254218446718 ) ) ;
#199826=CARTESIAN_POINT ( 'NONE',  ( -1.001543065824772872E-14, 4.571875000341418804, 1.575800808251672791 ) ) ;
#199832=CARTESIAN_POINT ( 'NONE',  ( 4.975479186090857375, 5.867442474269873642, 1.082531754730560403 ) ) ;
#199833=CARTESIAN_POINT ( 'NONE',  ( -6.561256274009600986, 9.742217188731485678, -1.199719254218440723 ) ) ;
#199838=CARTESIAN_POINT ( 'NONE',  ( -7.019370843573183194, 9.212351955633947043, 1.599625672291283607 ) ) ;
#199839=CARTESIAN_POINT ( 'NONE',  ( -4.401593425930945713, 8.286942763561420122, 1.040834085586084257E-14 ) ) ;
#199843=CARTESIAN_POINT ( 'NONE',  ( -1.420000000000021911, 6.280000000000042881, 2.580000000000011173 ) ) ;
#199846=CARTESIAN_POINT ( 'NONE',  ( 6.751070424600909448, 9.963667031088037973, -1.199719254218441611 ) ) ;
#199859=CARTESIAN_POINT ( 'NONE',  ( -0.6823417656250003738, -0.9697916663252494907, -1.181850606188749264 ) ) ;
#199860=CARTESIAN_POINT ( 'NONE',  ( 3.334415713957098681, 5.977569868670206787, -1.199719254218446718 ) ) ;
#199861=CARTESIAN_POINT ( 'NONE',  ( 6.602984505055297326, 7.662235663108029726, 1.199719254218462483 ) ) ;
#199864=CARTESIAN_POINT ( 'NONE',  ( -6.548225005720456515, 10.58342024007512983, 0.000000000000000000 ) ) ;
#199866=CARTESIAN_POINT ( 'NONE',  ( 4.799223189557548785, 7.582548906917042864, -1.082531754730549078 ) ) ;
#199867=CARTESIAN_POINT ( 'NONE',  ( -7.659993601596713830, 9.959745173328078849, -1.443375672974058777 ) ) ;
#199871=CARTESIAN_POINT ( 'NONE',  ( 6.238723240582662477, 10.43026088065513513, -0.7998128361456291469 ) ) ;
#199876=CARTESIAN_POINT ( 'NONE',  ( -1.364683531249997417, 4.009375000341424133, 1.214306433183764966E-14 ) ) ;
#199882=CARTESIAN_POINT ( 'NONE',  ( 8.555358625423188812, 9.940005470203933768, 1.199719254218462483 ) ) ;
#199885=CARTESIAN_POINT ( 'NONE',  ( -8.259941899223614215, 10.65968485389279508, -1.599625672291263179 ) ) ;
#199890=CARTESIAN_POINT ( 'NONE',  ( 9.077347539549325717, 10.54899253668443393, -1.199719254218446718 ) ) ;
#199893=CARTESIAN_POINT ( 'NONE',  ( -7.330154606482786050, 11.70359747420527619, 0.000000000000000000 ) ) ;
#199898=CARTESIAN_POINT ( 'NONE',  ( 5.827790676886797527, 6.016211147664318304, -0.4261259532085531765 ) ) ;
#199900=CARTESIAN_POINT ( 'NONE',  ( -9.002250809793991948, 12.48608113052627289, -1.082531754730543971 ) ) ;
#199905=CARTESIAN_POINT ( 'NONE',  ( 7.786460292950004636, 7.978625184730144149, 1.040834085586084257E-14 ) ) ;
#199907=CARTESIAN_POINT ( 'NONE',  ( 6.582647274634798151, 7.638508894284114170, 1.199719254218462483 ) ) ;
#199908=CARTESIAN_POINT ( 'NONE',  ( -4.245996903372413200, 7.323364108789364835, -0.8915694317389293300 ) ) ;
#199909=CARTESIAN_POINT ( 'NONE',  ( 3.161022370280501814, 6.839609865302569425, 0.000000000000000000 ) ) ;
#199911=CARTESIAN_POINT ( 'NONE',  ( -6.534666852106790103, 10.56760239419251590, 0.7216878364870458196 ) ) ;
#199918=CARTESIAN_POINT ( 'NONE',  ( -4.021031317475609157, 7.616913651768732585, 0.1724795716798576684 ) ) ;
#199919=CARTESIAN_POINT ( 'NONE',  ( 1.364683531249984538, -1.032291666325247714, -0.7879004041258309554 ) ) ;
#199923=CARTESIAN_POINT ( 'NONE',  ( 6.155038550924155416, 6.283225852274053835, 0.7216878364870317197 ) ) ;
#199925=EDGE_CURVE ( 'NONE', #13744, #141934, #162470, .T. ) ;
#199928=CARTESIAN_POINT ( 'NONE',  ( -10.43941509239824228, 11.28166515066052966, 1.040834085586084257E-14 ) ) ;
#199932=CARTESIAN_POINT ( 'NONE',  ( -9.070041577417988776, 12.56517035942090388, 1.082531754730558626 ) ) ;
#199939=CARTESIAN_POINT ( 'NONE',  ( -8.907343734053998929, 12.37535620882957588, 1.082531754730558626 ) ) ;
#199946=ORIENTED_EDGE ( 'NONE', *, *, #38172, .T. ) ;
#199948=CARTESIAN_POINT ( 'NONE',  ( 0.7499999999999885647, 3.097916667349487341, -1.299038105676658228 ) ) ;
#199950=CARTESIAN_POINT ( 'NONE',  ( -4.232116505760120440, 8.089219690028791376, -0.7998128361456281477 ) ) ;
#199952=ORIENTED_EDGE ( 'NONE', *, *, #97607, .F. ) ;
#199954=CARTESIAN_POINT ( 'NONE',  ( -7.995557903757128493, 10.35123685918189729, 1.599625672291295375 ) ) ;
#199958=CARTESIAN_POINT ( 'NONE',  ( 7.447506452608354088, 7.583179037664891098, 0.7998128361456341429 ) ) ;
#199962=CARTESIAN_POINT ( 'NONE',  ( 9.921869487102386032, 10.46993591124128997, 0.000000000000000000 ) ) ;
#199968=CARTESIAN_POINT ( 'NONE',  ( -8.039621903223732602, 8.481906429956900695, 1.040834085586084257E-14 ) ) ;
#199975=CARTESIAN_POINT ( 'NONE',  ( -0.6823417656250212460, 5.301041667008086655, 1.181850606188767472 ) ) ;
#199979=CARTESIAN_POINT ( 'NONE',  ( -9.130526383799315582, 12.73969898348616070, 1.199719254218462483 ) ) ;
#199981=CARTESIAN_POINT ( 'NONE',  ( 10.01963921569910632, 11.64833282552586091, 1.199719254218450271 ) ) ;
#199987=CARTESIAN_POINT ( 'NONE',  ( -1.402160292154681736E-14, 2.446875000341416584, -1.575800808251660134 ) ) ;
#199989=CARTESIAN_POINT ( 'NONE',  ( 3.985207087413062066, 6.736826471035503694, -1.199719254218452047 ) ) ;
#199990=ORIENTED_EDGE ( 'NONE', *, *, #158684, .F. ) ;
#199994=DIRECTION ( 'NONE',  ( 1.000000000000000000, 0.000000000000000000, 0.000000000000000000 ) ) ;
#199997=CARTESIAN_POINT ( 'NONE',  ( -7.754900677336769022, 9.110100880723427608, 1.082531754730558626 ) ) ;
#200002=CARTESIAN_POINT ( 'NONE',  ( -7.486073373039941359, 11.88550270185529278, -0.7998128361456291469 ) ) ;
#200004=CARTESIAN_POINT ( 'NONE',  ( -4.812781342726871969, 6.637997537979888563, 1.443375672974064550 ) ) ;
#200005=CARTESIAN_POINT ( 'NONE',  ( 1.364683531249986537, 2.467708333674753174, -0.7879004041258239610 ) ) ;
#200021=CYLINDRICAL_SURFACE ( 'NONE', #102036, 0.08000000000000020983 ) ;
#200024=CARTESIAN_POINT ( 'NONE',  ( -1.001543065824772872E-14, 4.884375000341420581, 1.575800808251672791 ) ) ;
#200028=FACE_OUTER_BOUND ( 'NONE', #104599, .T. ) ;
#200031=CARTESIAN_POINT ( 'NONE',  ( 9.368847842243145152, 10.88907622316056312, 1.199719254218453823 ) ) ;
#200032=DIRECTION ( 'NONE',  ( -1.000000000000000000, 5.578564026256504688E-16, 0.000000000000000000 ) ) ;
#200034=CARTESIAN_POINT ( 'NONE',  ( 1.364683531249988757, 2.134375000341422357, 1.214306433183764966E-14 ) ) ;
#200037=CARTESIAN_POINT ( 'NONE',  ( -6.995644074971465010, 10.14503993989993091, 1.082531754730549967 ) ) ;
#200046=CARTESIAN_POINT ( 'NONE',  ( 4.891794496432329886, 4.601515088792824670, -0.7998128361456211532 ) ) ;
#200052=CARTESIAN_POINT ( 'NONE',  ( 0.7499999999999885647, 2.816666666666689522, -1.299038105676658228 ) ) ;
#200058=CARTESIAN_POINT ( 'NONE',  ( -4.460796234096120472, 5.163016013655583158, 1.199719254218462483 ) ) ;
#200059=CARTESIAN_POINT ( 'NONE',  ( 7.793239369756836510, 7.986534107671458216, 0.7998128361456341429 ) ) ;
#200061=CARTESIAN_POINT ( 'NONE',  ( 4.270455198180219902, 6.965652916976816655, -1.082531754730548412 ) ) ;
#200071=CARTESIAN_POINT ( 'NONE',  ( -6.941411460516810017, 8.161030127766803588, 1.082531754730549967 ) ) ;
#200072=CARTESIAN_POINT ( 'NONE',  ( 4.137209430464448445, 7.978494768850520558, 1.040834085586084257E-14 ) ) ;
#200075=CARTESIAN_POINT ( 'NONE',  ( -9.671043645249580933, 10.17730576241299900, 0.7998128361456462443 ) ) ;
#200080=CARTESIAN_POINT ( 'NONE',  ( -2.923754682041362241, 6.562797562356882608, 0.7998128361456341429 ) ) ;
#200082=CARTESIAN_POINT ( 'NONE',  ( 7.584896871841365851, 10.93646455286856956, -1.199719254218446718 ) ) ;
#200088=CARTESIAN_POINT ( 'NONE',  ( 2.399429999938675007, 5.743159399996332404, 0.000000000000000000 ) ) ;
#200091=CARTESIAN_POINT ( 'NONE',  ( -4.042302355168801320, 7.867769847672247074, 0.7998128361456341429 ) ) ;
#200094=CARTESIAN_POINT ( 'NONE',  ( -8.109748439268576803, 12.61312361245537517, 0.7998128361456481317 ) ) ;
#200099=CARTESIAN_POINT ( 'NONE',  ( 8.107412671292042461, 9.521364873671299023, 1.082531754730558626 ) ) ;
#200102=CARTESIAN_POINT ( 'NONE',  ( 5.657830175604453338, 5.495223381160312393, 0.7998128361456341429 ) ) ;
#200105=CARTESIAN_POINT ( 'NONE',  ( -7.039708073993679704, 9.236078724457858158, 1.599625672291283607 ) ) ;
#200107=CARTESIAN_POINT ( 'NONE',  ( -1.387358672534977355, 7.315968950353621381, -4.254625267138091971 ) ) ;
#200114=VERTEX_POINT ( 'NONE', #135073 ) ;
#200116=CARTESIAN_POINT ( 'NONE',  ( 1.364683531249988535, 2.926041667008082658, 0.7879004041258500513 ) ) ;
#200117=CARTESIAN_POINT ( 'NONE',  ( 8.055515824813896941, 12.54985222892493368, 0.7998128361456462443 ) ) ;
#200119=CARTESIAN_POINT ( 'NONE',  ( -4.392478581147607031, 7.108013530438723748, 1.082531754730560403 ) ) ;
#200120=CARTESIAN_POINT ( 'NONE',  ( 3.145128448690309053, 4.692402494937224056, -1.443375672974057666 ) ) ;
#200121=CARTESIAN_POINT ( 'NONE',  ( -6.710922848640111127, 6.931757532942661726, 0.7216878364870317197 ) ) ;
#200124=CARTESIAN_POINT ( 'NONE',  ( -1.420000000000021911, 7.176846818246207960, 4.202462424328227364 ) ) ;
#200129=CARTESIAN_POINT ( 'NONE',  ( 4.847203612085560387, 5.613824621309978724, -1.199719254218452047 ) ) ;
#200139=CARTESIAN_POINT ( 'NONE',  ( 4.168242161197552420, 6.950367390450747251, -1.199719254218452047 ) ) ;
#200142=CARTESIAN_POINT ( 'NONE',  ( -6.600121851754250812, 6.594563670001734046, 0.7998128361456341429 ) ) ;
#200146=CARTESIAN_POINT ( 'NONE',  ( 4.964256800898067645, 8.943383367689749619, 0.7998128361456462443 ) ) ;
#200149=CARTESIAN_POINT ( 'NONE',  ( -5.250031796989778066, 7.148123067953287446, 1.599625672291267398 ) ) ;
#200150=CARTESIAN_POINT ( 'NONE',  ( 4.799223189113185128, 8.542918120699967588, 1.040834085586084257E-14 ) ) ;
#200151=CARTESIAN_POINT ( 'NONE',  ( -1.499999999999997780, 2.150000000000019895, 1.214306433183764966E-14 ) ) ;
#200152=CARTESIAN_POINT ( 'NONE',  ( -4.298098390732130625, 4.973201863064262263, 1.199719254218462483 ) ) ;
#200155=CARTESIAN_POINT ( 'NONE',  ( -5.005985031943793295, 6.863401842066301661, -1.599625672291256295 ) ) ;
#200158=CARTESIAN_POINT ( 'NONE',  ( -1.364683531249997417, 2.759375000341422801, 1.214306433183764966E-14 ) ) ;
#200160=CARTESIAN_POINT ( 'NONE',  ( -4.446711195602245148, 7.171284913969171448, -1.082531754730549967 ) ) ;
#200163=ORIENTED_EDGE ( 'NONE', *, *, #171579, .T. ) ;
#200166=CARTESIAN_POINT ( 'NONE',  ( 3.669453130792974971, 7.432779085900453886, 1.040834085586084257E-14 ) ) ;
#200169=CARTESIAN_POINT ( 'NONE',  ( 1.364683531249988535, 2.926041667008082658, 0.7879004041258500513 ) ) ;
#200172=CARTESIAN_POINT ( 'NONE',  ( -0.2981862293453914625, 7.114787932596419395, 1.978802099905853984 ) ) ;
#200176=CARTESIAN_POINT ( 'NONE',  ( -3.216308754939891212, 4.775446185561722956, -1.599625672291262513 ) ) ;
#200177=CARTESIAN_POINT ( 'NONE',  ( -8.324343128666356506, 8.814081192973304724, 1.040834085586084257E-14 ) ) ;
#200179=CARTESIAN_POINT ( 'NONE',  ( 0.6823417656249917140, 3.592708333674754506, 1.181850606188765695 ) ) ;
#200186=CARTESIAN_POINT ( 'NONE',  ( -6.602457619730773608, 8.725953194484466380, 1.443375672974078761 ) ) ;
#200191=CARTESIAN_POINT ( 'NONE',  ( -5.382223794500827552, 9.223085493652217082, -0.7216878364870207285 ) ) ;
#200196=CARTESIAN_POINT ( 'NONE',  ( 1.499999999999968914, 4.827083334016150751, -0.8660254037844440367 ) ) ;
#200204=CARTESIAN_POINT ( 'NONE',  ( -6.891622154448065807, 6.934647356477856128, 1.040834085586084257E-14 ) ) ;
#200206=CARTESIAN_POINT ( 'NONE',  ( 0.7499999999999867883, 0.06666666666668707997, -1.299038105676652899 ) ) ;
#200208=CARTESIAN_POINT ( 'NONE',  ( 2.900554798319789906, 5.471398800426671372, 1.199719254218452047 ) ) ;
#200210=CARTESIAN_POINT ( 'NONE',  ( 1.252085211431714251, 3.300000000000025135, 0.7750000000000100142 ) ) ;
#200212=CARTESIAN_POINT ( 'NONE',  ( 4.984594031318565932, 8.967110136513669616, 0.7998128361456462443 ) ) ;
#200219=CARTESIAN_POINT ( 'NONE',  ( -4.853455804012230423, 6.685451076146141425, 1.443375672974064550 ) ) ;
#200227=CARTESIAN_POINT ( 'NONE',  ( 0.6823417656249882723, 1.926041667008083991, -1.181850606188749264 ) ) ;
#200228=CARTESIAN_POINT ( 'NONE',  ( 10.18181017373857600, 10.98112607889092907, 0.7216878364870438212 ) ) ;
#200230=CARTESIAN_POINT ( 'NONE',  ( -6.028571859570855729, 10.18508426947466816, 0.000000000000000000 ) ) ;
#200232=CARTESIAN_POINT ( 'NONE',  ( 7.793239369756836510, 7.986534107671458216, 0.7998128361456341429 ) ) ;
#200233=CARTESIAN_POINT ( 'NONE',  ( -5.865874016206865882, 9.995270118883347266, 0.000000000000000000 ) ) ;
#200236=CARTESIAN_POINT ( 'NONE',  ( 1.499999999999987121, -1.214583332650518432, 0.8660254037844524744 ) ) ;
#200238=CARTESIAN_POINT ( 'NONE',  ( 8.514157279702022407, 10.95626946445095307, -1.443375672974063439 ) ) ;
#200241=CARTESIAN_POINT ( 'NONE',  ( -0.6823417656250003738, 0.2802083336747515641, -1.181850606188749264 ) ) ;
#200244=CARTESIAN_POINT ( 'NONE',  ( 7.415946836550722843, 8.714654733139752807, 1.082531754730558626 ) ) ;
#200246=CARTESIAN_POINT ( 'NONE',  ( -5.016153647376219382, 6.875265226737464985, 1.443375672974064550 ) ) ;
#200248=CARTESIAN_POINT ( 'NONE',  ( -1.201851678989727383E-14, 3.446875000341421469, -1.575800808251660134 ) ) ;
#200252=CARTESIAN_POINT ( 'NONE',  ( -6.880926654135487652, 7.986501503701545879, 1.199719254218450271 ) ) ;
#200253=CARTESIAN_POINT ( 'NONE',  ( 1.364683531249992088, 5.696875000341418804, 1.214306433183764966E-14 ) ) ;
#200260=CARTESIAN_POINT ( 'NONE',  ( 6.500244582748090139, 9.671036882259738121, 1.199719254218460707 ) ) ;
#200264=CARTESIAN_POINT ( 'NONE',  ( 0.7499999999999885647, 2.816666666666689522, -1.299038105676658228 ) ) ;
#200270=CARTESIAN_POINT ( 'NONE',  ( 5.666945020832170776, 7.634521829102760115, 1.443375672974062551 ) ) ;
#200271=CARTESIAN_POINT ( 'NONE',  ( -1.201851678989727383E-14, 0.8843750003414173610, 1.575800808251672791 ) ) ;
#200273=CARTESIAN_POINT ( 'NONE',  ( 9.890836756369282057, 11.49806328964105617, -1.199719254218440723 ) ) ;
#200280=CARTESIAN_POINT ( 'NONE',  ( 1.499999999999985123, 0.04583333333335545129, -0.8660254037844323793 ) ) ;
#200281=CARTESIAN_POINT ( 'NONE',  ( 6.726816770674637347, 10.99970333242910669, -0.7998128361456291469 ) ) ;
#200282=CARTESIAN_POINT ( 'NONE',  ( -9.338868881714763148, 9.789768538289042255, -0.7998128361456291469 ) ) ;
#200284=CARTESIAN_POINT ( 'NONE',  ( -1.402160292154681736E-14, 0.9468750003414176941, -1.575800808251659024 ) ) ;
#200285=CARTESIAN_POINT ( 'NONE',  ( 0.7499999999999885647, 2.066666666666688634, -1.299038105676652899 ) ) ;
#200287=CARTESIAN_POINT ( 'NONE',  ( 3.497113557321089861, 6.167384019261527683, -1.199719254218446718 ) ) ;
#200294=CARTESIAN_POINT ( 'NONE',  ( 1.499999999999985123, -0.4229166659838508036, -0.8660254037844323793 ) ) ;
#200295=CARTESIAN_POINT ( 'NONE',  ( -7.965578943228732278, 9.251929174310385307, -1.199719254218446718 ) ) ;
#200296=CARTESIAN_POINT ( 'NONE',  ( -4.338245966692955591, 5.124003718305597310, 1.082531754730560403 ) ) ;
#200305=CARTESIAN_POINT ( 'NONE',  ( 6.287230548435207567, 8.358188277972981695, -1.599625672291262513 ) ) ;
#200310=CARTESIAN_POINT ( 'NONE',  ( 7.741342523278707866, 8.133913820021057006, 0.7216878364870458196 ) ) ;
#200314=CARTESIAN_POINT ( 'NONE',  ( -6.645467848992654858, 10.90479625713344625, 0.7998128361456481317 ) ) ;
#200315=CARTESIAN_POINT ( 'NONE',  ( 4.680589345215795838, 6.483773540883647435, -1.599625672291256295 ) ) ;
#200320=CARTESIAN_POINT ( 'NONE',  ( 8.215877900201359552, 11.56864606933486606, -1.082531754730543083 ) ) ;
#200326=CARTESIAN_POINT ( 'NONE',  ( -1.504932104232262091, 8.664796307965627165, -2.552344783041797793 ) ) ;
#200328=CARTESIAN_POINT ( 'NONE',  ( -5.436456409399874623, 5.444880020495701523, 0.000000000000000000 ) ) ;
#200329=CARTESIAN_POINT ( 'NONE',  ( 9.463228032658635769, 11.10314946193233965, -1.082531754730543083 ) ) ;
#200332=CARTESIAN_POINT ( 'NONE',  ( -5.961834861707238531, 7.978559976790334574, -1.599625672291263179 ) ) ;
#200335=CARTESIAN_POINT ( 'NONE',  ( 3.763755302173072081, 3.180306474485404600, 2.446972558850332824 ) ) ;
#200337=CARTESIAN_POINT ( 'NONE',  ( -8.830438121202295321, 9.196599317691152464, -0.7998128361456291469 ) ) ;
#200340=CARTESIAN_POINT ( 'NONE',  ( 5.523117969621105239, 6.371578878345163233, -1.187916293638406895 ) ) ;
#200350=DIRECTION ( 'NONE',  ( -5.578564026256490882E-16, -1.000000000000000000, -9.066213480720158442E-32 ) ) ;
#200351=CARTESIAN_POINT ( 'NONE',  ( -6.175902666224832416, 7.163973517805802160, -1.199719254218446718 ) ) ;
#200354=CARTESIAN_POINT ( 'NONE',  ( 4.853455804012222430, 5.725081861844796727, 1.082531754730560403 ) ) ;
#200356=CIRCLE ( 'NONE', #68927, 0.08000000000000025147 ) ;
#200361=CARTESIAN_POINT ( 'NONE',  ( -3.100010679019018500, 6.768429558830820980, 1.040834085586084257E-14 ) ) ;
#200369=CARTESIAN_POINT ( 'NONE',  ( -9.287498920561160887, 10.79416914786490089, -1.199719254218441611 ) ) ;
#200370=CARTESIAN_POINT ( 'NONE',  ( 6.043183783389218355, 8.073467052085995022, 1.599625672291267398 ) ) ;
#200374=CARTESIAN_POINT ( 'NONE',  ( -9.917953063596627317, 11.52969898140628047, -1.199719254218441611 ) ) ;
#200377=CARTESIAN_POINT ( 'NONE',  ( -1.364683531250014514, 0.5510416670080878765, -0.7879004041258289570 ) ) ;
#200381=CARTESIAN_POINT ( 'NONE',  ( 7.782016984564054773, 10.10210578678999482, 1.443375672974076540 ) ) ;
#200407=AXIS2_PLACEMENT_3D ( 'NONE', #95216, #132002, #161266 ) ;
#200408=CARTESIAN_POINT ( 'NONE',  ( -1.500000000000013101, -0.2979166659838501929, 0.8660254037844403729 ) ) ;
#200413=CARTESIAN_POINT ( 'NONE',  ( 1.244150428498992600, 3.027476754118171964, -0.7749999999999874767 ) ) ;
#200414=CARTESIAN_POINT ( 'NONE',  ( 0.4417779905600578982, 7.383047307301190187, -2.041823008714561460 ) ) ;
#200416=CARTESIAN_POINT ( 'NONE',  ( 10.05067194643221207, 10.62020544712608938, 0.7998128361456462443 ) ) ;
#200421=CARTESIAN_POINT ( 'NONE',  ( 4.521807925357579805, 5.234196320127330715, -1.199719254218452047 ) ) ;
#200422=CARTESIAN_POINT ( 'NONE',  ( -0.6823417656250212460, 3.113541667008084879, 1.181850606188767472 ) ) ;
#200424=CARTESIAN_POINT ( 'NONE',  ( 4.350813900535696277, 4.000456626940672500, 0.2320863031703649382 ) ) ;
#200426=CARTESIAN_POINT ( 'NONE',  ( -8.345207244411405156, 9.694828859023472134, 1.199719254218462483 ) ) ;
#200427=CARTESIAN_POINT ( 'NONE',  ( -3.917943204224914933, 6.554388924028945240, -1.082531754730548412 ) ) ;
#200430=CARTESIAN_POINT ( 'NONE',  ( -1.500000000000013101, 0.2020833340161521663, 0.8660254037844403729 ) ) ;
#200437=CARTESIAN_POINT ( 'NONE',  ( -3.416291520519271874, 6.929497840673697340, 1.040834085586084257E-14 ) ) ;
#200445=CARTESIAN_POINT ( 'NONE',  ( -4.243338890952911058, 5.013278796608906518, -1.082531754730543971 ) ) ;
#200446=CARTESIAN_POINT ( 'NONE',  ( 7.801827329660018684, 11.18955008699033726, 1.199719254218460707 ) ) ;
#200456=CARTESIAN_POINT ( 'NONE',  ( -8.402302512167102222, 10.82577223566020841, -1.599625672291263179 ) ) ;
#200461=CARTESIAN_POINT ( 'NONE',  ( 5.464099601507359516, 6.333536608968757697, 1.199719254218462483 ) ) ;
#200462=CIRCLE ( 'NONE', #89810, 1.219999999999999751 ) ;
#200470=ORIENTED_EDGE ( 'NONE', *, *, #113945, .T. ) ;
#200479=CARTESIAN_POINT ( 'NONE',  ( 9.420217803396747414, 9.884675613584706255, 0.7998128361456462443 ) ) ;
#200481=CARTESIAN_POINT ( 'NONE',  ( -4.249591082879585535, 7.045274465746411252, 1.199719254218464037 ) ) ;
#200483=CARTESIAN_POINT ( 'NONE',  ( -0.9486429539237204445, 2.975839070649075158, -1.028101543438967980 ) ) ;
#200486=CARTESIAN_POINT ( 'NONE',  ( -0.6823417656250212460, 5.551041667008087543, 1.181850606188767472 ) ) ;
#200491=CARTESIAN_POINT ( 'NONE',  ( 3.005103603723342953, 6.657704637652544832, -0.7998128361456291469 ) ) ;
#200493=CARTESIAN_POINT ( 'NONE',  ( -4.086893239515592136, 6.855460315155083251, 1.199719254218464037 ) ) ;
#200500=CARTESIAN_POINT ( 'NONE',  ( 4.528060117284222308, 8.226561203566173930, 0.7216878364870438212 ) ) ;
#200503=CARTESIAN_POINT ( 'NONE',  ( 7.090551149822728938, 10.25576486055978442, 1.082531754730558626 ) ) ;
#200504=CARTESIAN_POINT ( 'NONE',  ( 0.6823417656249899377, 4.738541667008086655, -1.181850606188754593 ) ) ;
#200506=CARTESIAN_POINT ( 'NONE',  ( 4.839897649954202130, 4.748894801142428790, -0.7216878364870197293 ) ) ;
#200509=CARTESIAN_POINT ( 'NONE',  ( 2.750000000000003109, 8.900000000000023448, 1.214306433183764966E-14 ) ) ;
#200512=CARTESIAN_POINT ( 'NONE',  ( -5.903366504444580443, 6.144480293219754863, 0.8539384941207116553 ) ) ;
#200515=CARTESIAN_POINT ( 'NONE',  ( 0.6823417656249917140, 4.655208333674755394, 1.181850606188765695 ) ) ;
#200529=CARTESIAN_POINT ( 'NONE',  ( 2.887523530030648988, 6.312601851770308414, 0.000000000000000000 ) ) ;
#200531=CARTESIAN_POINT ( 'NONE',  ( -1.364683531249997417, 4.571875000341417028, 1.214306433183764966E-14 ) ) ;
#200533=CARTESIAN_POINT ( 'NONE',  ( 8.098297826064319693, 8.342435640030188893, 0.7998128361456481317 ) ) ;
#200534=CARTESIAN_POINT ( 'NONE',  ( -8.208571938070008400, 11.66408546346865016, -1.199719254218446718 ) ) ;
#200540=CARTESIAN_POINT ( 'NONE',  ( 1.499999999999989120, 4.254166666666687746, 0.8660254037844524744 ) ) ;
#200544=CARTESIAN_POINT ( 'NONE',  ( 1.499999999999990896, 8.266799604814890401, 3.162088779278453998 ) ) ;
#200547=CARTESIAN_POINT ( 'NONE',  ( 9.408995418203975447, 10.07950886410055524, 0.7216878364870438212 ) ) ;
#200551=CARTESIAN_POINT ( 'NONE',  ( -1.500000000000013101, 3.160416667349486008, -0.8660254037844313801 ) ) ;
#200553=CARTESIAN_POINT ( 'NONE',  ( -3.716906668440817185, 7.488141546489591072, 0.7998128361456341429 ) ) ;
#200554=CARTESIAN_POINT ( 'NONE',  ( 3.484082288587588838, 7.008587070086755411, -0.7216878364870267237 ) ) ;
#200555=CYLINDRICAL_SURFACE ( 'NONE', #125369, 0.08000000000000020983 ) ;
#200558=EDGE_CURVE ( 'NONE', #160319, #78710, #17798, .T. ) ;
#200563=CARTESIAN_POINT ( 'NONE',  ( 6.934105498385400246, 10.17720795050327354, -1.199719254218441611 ) ) ;
#200564=CARTESIAN_POINT ( 'NONE',  ( 3.497113557321089861, 6.167384019261527683, -1.199719254218446718 ) ) ;
#200567=CARTESIAN_POINT ( 'NONE',  ( 5.518332215962025167, 6.396807992499198292, -1.199719254218445830 ) ) ;
#200571=ORIENTED_EDGE ( 'NONE', *, *, #175529, .F. ) ;
#200579=CARTESIAN_POINT ( 'NONE',  ( 5.112599315731837457, 6.496590726105775815, -1.208607640439966158 ) ) ;
#200581=CARTESIAN_POINT ( 'NONE',  ( 9.378489572351044856, 11.96465713920816043, -1.599625672291262513 ) ) ;
#200586=CARTESIAN_POINT ( 'NONE',  ( -1.602468905319636405E-14, -1.053124999658583638, -1.575800808251665908 ) ) ;
#200587=CARTESIAN_POINT ( 'NONE',  ( 6.155038550924144758, 8.203964280876741455, 1.443375672974076540 ) ) ;
#200588=CARTESIAN_POINT ( 'NONE',  ( -2.266184231778562541, 5.795632037050281404, 1.040834085586084257E-14 ) ) ;
#200593=CARTESIAN_POINT ( 'NONE',  ( -4.055860508782465068, 7.883587693554856557, 1.040834085586084257E-14 ) ) ;
#200605=CARTESIAN_POINT ( 'NONE',  ( 9.368847842243145152, 10.88907622316056312, 1.199719254218453823 ) ) ;
#200606=CARTESIAN_POINT ( 'NONE',  ( 5.946581215072361815, 6.122072269273588496, 0.7275674859277461159 ) ) ;
#200607=CARTESIAN_POINT ( 'NONE',  ( -1.177073619093324419, 3.074321498342245995, -0.7749999999999918066 ) ) ;
#200609=CARTESIAN_POINT ( 'NONE',  ( 5.345992642490140057, 5.131412925860272090, 1.040834085586084257E-14 ) ) ;
#200614=CARTESIAN_POINT ( 'NONE',  ( -6.518203450479854943, 5.167241622962448488, 2.437504649502892473 ) ) ;
#200615=CARTESIAN_POINT ( 'NONE',  ( -8.188761592974040937, 11.53701037756964887, -1.082531754730543971 ) ) ;
#200619=CARTESIAN_POINT ( 'NONE',  ( 6.414979237560321401, 10.63589287712906462, 1.040834085586084257E-14 ) ) ;
#200621=CARTESIAN_POINT ( 'NONE',  ( -4.303823697334223652, 7.108545849276850959, -1.199719254218452047 ) ) ;
#200622=CARTESIAN_POINT ( 'NONE',  ( 3.032219910950674890, 6.689340329417765574, 0.7998128361456321445 ) ) ;
#200624=CARTESIAN_POINT ( 'NONE',  ( -7.223796917982883592, 7.322184580601816428, -0.7998128361456291469 ) ) ;
#200625=CARTESIAN_POINT ( 'NONE',  ( 3.846762897975340767, 5.510976019103107859, -1.599625672291256295 ) ) ;
#200630=CARTESIAN_POINT ( 'NONE',  ( 9.053093885623066939, 11.58502883802551153, -1.599625672291262513 ) ) ;
#200634=CARTESIAN_POINT ( 'NONE',  ( 4.159596813995052322, 7.384974941181836172, -0.7733407813514819873 ) ) ;
#200635=CARTESIAN_POINT ( 'NONE',  ( 6.371969008742804697, 7.496680600697164465, -1.082531754730543083 ) ) ;
#200637=CARTESIAN_POINT ( 'NONE',  ( 0.4841293774267214634, 6.672680601848989035, 3.378195143392549671 ) ) ;
#200642=CARTESIAN_POINT ( 'NONE',  ( 7.402388682937041331, 11.57994453016116587, 1.040834085586084257E-14 ) ) ;
#200644=CARTESIAN_POINT ( 'NONE',  ( -9.622536337397040285, 12.24937836509514710, 1.599625672291281386 ) ) ;
#200645=CARTESIAN_POINT ( 'NONE',  ( -8.015895134177625891, 10.37496362800581018, 1.599625672291295375 ) ) ;
#200654=CARTESIAN_POINT ( 'NONE',  ( 9.297140650669039275, 11.86975006391249643, 1.599625672291281386 ) ) ;
#200658=CARTESIAN_POINT ( 'NONE',  ( 4.172158584703322681, 5.890604320285754980, -1.599625672291256295 ) ) ;
#200661=CARTESIAN_POINT ( 'NONE',  ( 1.499999999999987121, 3.827083334016153415, -0.8660254037844323793 ) ) ;
#200667=CARTESIAN_POINT ( 'NONE',  ( -1.499999999999997780, 2.150000000000019895, 1.214306433183764966E-14 ) ) ;
#200668=CARTESIAN_POINT ( 'NONE',  ( 7.447506452608354088, 7.583179037664891098, 0.7998128361456341429 ) ) ;
#200669=CARTESIAN_POINT ( 'NONE',  ( 3.185802909086937973, 6.660594460669327255, 0.7216878364870317197 ) ) ;
#200674=CARTESIAN_POINT ( 'NONE',  ( 8.595506201384013778, 10.09080732544527592, 1.082531754730558626 ) ) ;
#200680=CARTESIAN_POINT ( 'NONE',  ( -5.525111292768871252, 6.404716915440499037, -1.199719254218446718 ) ) ;
#200681=CARTESIAN_POINT ( 'NONE',  ( 0.7499999999999902300, 3.597916667349487785, -1.299038105676658228 ) ) ;
#200682=CARTESIAN_POINT ( 'NONE',  ( 1.364683531249988757, -0.3656249996585800299, 0.000000000000000000 ) ) ;
#200686=CARTESIAN_POINT ( 'NONE',  ( 8.392133896734652154, 12.73464727959172293, 0.7216878364870438212 ) ) ;
#200688=CARTESIAN_POINT ( 'NONE',  ( -0.6823417656249969321, 3.530208333674754506, -1.181850606188749264 ) ) ;
#200696=CARTESIAN_POINT ( 'NONE',  ( -7.690499447449645309, 9.995335326823163058, 1.599625672291295375 ) ) ;
#200697=CARTESIAN_POINT ( 'NONE',  ( 5.469824908109481854, 8.468880595181346393, -1.199719254218446718 ) ) ;
#200699=CARTESIAN_POINT ( 'NONE',  ( -0.6823417656250246877, -1.198958332991911790, 1.181850606188755259 ) ) ;
#200704=CARTESIAN_POINT ( 'NONE',  ( -4.903732577545095062, 4.837283930932079201, 0.1501914610188368193 ) ) ;
#200706=CARTESIAN_POINT ( 'NONE',  ( -6.124532705071231931, 8.168374127381657246, -1.599625672291263179 ) ) ;
#200709=CARTESIAN_POINT ( 'NONE',  ( 8.594979316059474073, 12.11489407112305372, 1.199719254218450271 ) ) ;
#200711=CARTESIAN_POINT ( 'NONE',  ( 9.348510611822643313, 10.86534945433664134, 1.199719254218453823 ) ) ;
#200714=CARTESIAN_POINT ( 'NONE',  ( -4.464712657601869417, 4.103252943490596216, 0.7998128361456341429 ) ) ;
#200716=CARTESIAN_POINT ( 'NONE',  ( -8.843996274815957293, 9.212417163573759282, 1.040834085586084257E-14 ) ) ;
#200718=CARTESIAN_POINT ( 'NONE',  ( -4.153558989372251986, 7.618438364782146976, 0.8772435784342603737 ) ) ;
#200719=CARTESIAN_POINT ( 'NONE',  ( 1.364683531249986537, -0.5947916663252456049, -0.7879004041258309554 ) ) ;
#200723=CARTESIAN_POINT ( 'NONE',  ( 6.805829924380097040, 10.88395931184472154, 0.7216878364870438212 ) ) ;
#200726=CARTESIAN_POINT ( 'NONE',  ( 4.333802657862601215, 8.207853534148366492, 0.7998128361456462443 ) ) ;
#200745=DIRECTION ( 'NONE',  ( 0.000000000000000000, 1.000000000000000000, -8.546850786086437571E-32 ) ) ;
#200749=CARTESIAN_POINT ( 'NONE',  ( -5.762378981008047241, 6.681529218386182301, 1.199719254218450271 ) ) ;
#200750=CARTESIAN_POINT ( 'NONE',  ( -8.993135964566285168, 9.386413468282476913, -0.7998128361456291469 ) ) ;
#200755=CARTESIAN_POINT ( 'NONE',  ( -1.500000000000013101, 1.910416667349488451, -0.8660254037844313801 ) ) ;
#200756=CARTESIAN_POINT ( 'NONE',  ( 8.028399517586572998, 12.51821653715971472, -0.7998128361456352531 ) ) ;
#200760=CARTESIAN_POINT ( 'NONE',  ( -9.642873567817536795, 12.27310513391906532, 1.599625672291281386 ) ) ;
#200762=CARTESIAN_POINT ( 'NONE',  ( -1.201851678989727383E-14, 1.821875000341421691, 1.575800808251672791 ) ) ;
#200764=CARTESIAN_POINT ( 'NONE',  ( -3.733524485140432336, 7.410126666105575133, 2.499999999999998668 ) ) ;
#200769=CARTESIAN_POINT ( 'NONE',  ( -9.002250809793991948, 12.48608113052627289, -1.082531754730543971 ) ) ;
#200773=CARTESIAN_POINT ( 'NONE',  ( -1.402160292154681736E-14, 0.6343750003414162508, 1.575800808251672791 ) ) ;
#200778=CARTESIAN_POINT ( 'NONE',  ( 0.6823417656249899377, 1.092708333674752286, 1.181850606188755259 ) ) ;
#200780=CARTESIAN_POINT ( 'NONE',  ( -7.223796917982883592, 7.322184580601816428, -0.7998128361456291469 ) ) ;
#200781=CARTESIAN_POINT ( 'NONE',  ( 9.237182729612253951, 9.671134694169463586, 0.7998128361456462443 ) ) ;
#200782=CARTESIAN_POINT ( 'NONE',  ( 5.190073875932979419, 4.949507698210251938, 0.7998128361456341429 ) ) ;
#200783=CARTESIAN_POINT ( 'NONE',  ( 5.626797444871351139, 6.523350759560078593, 1.199719254218462483 ) ) ;
#200785=CARTESIAN_POINT ( 'NONE',  ( -1.201851678989727383E-14, 3.712500000000020339, 1.732050807568877637 ) ) ;
#200788=CARTESIAN_POINT ( 'NONE',  ( -0.6823417656250003738, 0.7802083336747520637, -1.181850606188749264 ) ) ;
#200794=CARTESIAN_POINT ( 'NONE',  ( 5.829642864196162400, 7.824335979694092558, 1.443375672974062551 ) ) ;
#200797=CARTESIAN_POINT ( 'NONE',  ( -7.557780564614042795, 10.90482886110335414, -1.199719254218446718 ) ) ;
#200798=CARTESIAN_POINT ( 'NONE',  ( -3.307299406729781399, 5.945934176904983381, -1.199719254218452935 ) ) ;
#200802=CARTESIAN_POINT ( 'NONE',  ( -6.493992390821436977, 10.52014885602626393, 0.7216878364870458196 ) ) ;
#200804=CARTESIAN_POINT ( 'NONE',  ( 1.499999999999989120, 5.504166666666685970, 0.8660254037844524744 ) ) ;
#200807=CARTESIAN_POINT ( 'NONE',  ( 6.453317930424781856, 10.47269531889685545, -0.7216878364870267237 ) ) ;
#200813=CARTESIAN_POINT ( 'NONE',  ( -4.230676207738683026, 3.979449701155983288, 0.5095693755076350362 ) ) ;
#200821=CARTESIAN_POINT ( 'NONE',  ( 5.601490020740366838, 9.686822124172440596, 1.040834085586084257E-14 ) ) ;
#200822=CARTESIAN_POINT ( 'NONE',  ( -4.394814349124112951, 8.279033840620114049, -0.7998128361456281477 ) ) ;
#200826=CARTESIAN_POINT ( 'NONE',  ( 1.364683531249986537, -0.7822916663252464931, -0.7879004041258309554 ) ) ;
#200827=CARTESIAN_POINT ( 'NONE',  ( 4.541618270897912701, 4.400902192243413502, 1.214306433183764966E-14 ) ) ;
#200828=CARTESIAN_POINT ( 'NONE',  ( -9.110189153378817295, 12.71597221466224603, 1.199719254218462483 ) ) ;
#200833=CARTESIAN_POINT ( 'NONE',  ( 4.177028312937637544, 3.976447072691611684, -0.04407265314626420544 ) ) ;
#200840=ORIENTED_EDGE ( 'NONE', *, *, #108295, .F. ) ;
#200843=FACE_OUTER_BOUND ( 'NONE', #163884, .T. ) ;
#200844=CARTESIAN_POINT ( 'NONE',  ( 8.118635056484817980, 8.366162408854107113, 0.7998128361456481317 ) ) ;
#200856=CARTESIAN_POINT ( 'NONE',  ( -2.335117776279159951, 5.399932185023237352, 0.6440902300205594289 ) ) ;
#200859=CARTESIAN_POINT ( 'NONE',  ( -6.196239896645333367, 7.187700286629718605, -1.199719254218446718 ) ) ;
#200861=CARTESIAN_POINT ( 'NONE',  ( -3.741160322367112379, 6.452105245148518797, 1.199719254218464037 ) ) ;
#200865=DIRECTION ( 'NONE',  ( 5.578564026256490882E-16, 1.000000000000000000, 9.066213480720158442E-32 ) ) ;
#200873=CARTESIAN_POINT ( 'NONE',  ( -8.337901282724359930, 12.67137589657970409, 1.040834085586084257E-14 ) ) ;
#200876=CARTESIAN_POINT ( 'NONE',  ( 5.113396490648394632, 9.117379672398465473, 1.040834085586084257E-14 ) ) ;
#200877=CARTESIAN_POINT ( 'NONE',  ( -1.364683531250010740, 5.238541667008085767, -0.7879004041258300672 ) ) ;
#200883=CARTESIAN_POINT ( 'NONE',  ( 4.487385655998867406, 8.179107665399927285, 0.7216878364870438212 ) ) ;
#200884=CARTESIAN_POINT ( 'NONE',  ( -6.880926654135487652, 7.986501503701545879, 1.199719254218450271 ) ) ;
#200887=CARTESIAN_POINT ( 'NONE',  ( -6.398558430645608475, 9.552403038140164782, -1.199719254218440723 ) ) ;
#200888=CARTESIAN_POINT ( 'NONE',  ( -4.076197739202962467, 7.907314462378773001, 1.040834085586084257E-14 ) ) ;
#200895=CARTESIAN_POINT ( 'NONE',  ( 7.396136491454752715, 8.587579647240744407, 1.199719254218462483 ) ) ;
#200902=CARTESIAN_POINT ( 'NONE',  ( 1.499999999999989120, 4.004166666666685970, 0.8660254037844522523 ) ) ;
#200908=CARTESIAN_POINT ( 'NONE',  ( 0.6823417656249864960, -1.011458332991911568, -1.181850606188749264 ) ) ;
#200909=CARTESIAN_POINT ( 'NONE',  ( 3.979481780810941949, 4.601482484822914998, 1.199719254218464037 ) ) ;
#200911=CARTESIAN_POINT ( 'NONE',  ( 4.821896187954575197, 8.777295985922343391, 0.7998128361456462443 ) ) ;
#200913=CARTESIAN_POINT ( 'NONE',  ( -6.371969008742801144, 10.37778824360119145, 0.7216878364870458196 ) ) ;
#200915=CARTESIAN_POINT ( 'NONE',  ( 4.677199807034550183, 8.400557508274889784, 1.040834085586084257E-14 ) ) ;
#200916=CARTESIAN_POINT ( 'NONE',  ( -8.148087131688692253, 10.52918762510205042, -1.443375672974058777 ) ) ;
#200920=CARTESIAN_POINT ( 'NONE',  ( 7.076466111328892694, 10.34329533227067799, -1.199719254218441611 ) ) ;
#200925=CARTESIAN_POINT ( 'NONE',  ( -0.6823417656250212460, 3.801041667008085767, 1.181850606188767472 ) ) ;
#200931=ADVANCED_FACE ( 'NONE', ( #207547 ), #6127, .F. ) ;
#200932=CARTESIAN_POINT ( 'NONE',  ( 7.476431642932036326, 10.80992178580769014, 1.199719254218460707 ) ) ;
#200935=CARTESIAN_POINT ( 'NONE',  ( -9.176171038350775078, 9.599954387697719582, -0.7998128361456291469 ) ) ;
#200941=CARTESIAN_POINT ( 'NONE',  ( 2.367870383881045981, 5.914265881169853856, 0.000000000000000000 ) ) ;
#200944=CARTESIAN_POINT ( 'NONE',  ( -9.667127221743832877, 11.23706883257798772, 1.199719254218462483 ) ) ;
#200949=CARTESIAN_POINT ( 'NONE',  ( 5.891837173953166307, 5.977390820968681240, -0.04595957878574669087 ) ) ;
#200950=CARTESIAN_POINT ( 'NONE',  ( 1.230761180058546289, 3.271116465842660581, -0.7749999999999874767 ) ) ;
#200951=CARTESIAN_POINT ( 'NONE',  ( -4.613852347352193739, 4.277249248199312071, 1.214306433183764966E-14 ) ) ;
#200956=CARTESIAN_POINT ( 'NONE',  ( 7.949158136313996259, 8.168439335321471262, 1.040834085586084257E-14 ) ) ;
#200958=CARTESIAN_POINT ( 'NONE',  ( 7.447506452608354088, 7.583179037664891098, 0.7998128361456341429 ) ) ;
#200959=EDGE_CURVE ( 'NONE', #26788, #95577, #26665, .T. ) ;
#200960=CARTESIAN_POINT ( 'NONE',  ( 3.988069740714122791, 7.804498464141805592, 0.7998128361456321445 ) ) ;
#200962=CARTESIAN_POINT ( 'NONE',  ( -7.863365906246068349, 9.236643647784308797, -1.082531754730543971 ) ) ;
#200969=CARTESIAN_POINT ( 'NONE',  ( -4.026828402897194792, 7.608452879803509816, -0.2354461595876176927 ) ) ;
#200973=CARTESIAN_POINT ( 'NONE',  ( 4.202664430556241726, 7.846932902383524144, 0.7216878364870298324 ) ) ;
#200978=CARTESIAN_POINT ( 'NONE',  ( -8.907343734053998929, 12.37535620882957588, 1.082531754730558626 ) ) ;
#200983=CARTESIAN_POINT ( 'NONE',  ( -9.449669878600616357, 12.04770082983265844, -1.443375672974058777 ) ) ;
#200992=CARTESIAN_POINT ( 'NONE',  ( -8.636180661780658241, 12.05899929117736846, -1.082531754730543083 ) ) ;
#200997=CARTESIAN_POINT ( 'NONE',  ( 7.904567251967224095, 9.180748867838630645, 1.199719254218462483 ) ) ;
#201001=CARTESIAN_POINT ( 'NONE',  ( -1.499999999999997780, 1.681250000682817047, 0.000000000000000000 ) ) ;
#201003=CARTESIAN_POINT ( 'NONE',  ( -6.389970470742427189, 6.349387058821269747, -0.7998128361456291469 ) ) ;
#201006=CARTESIAN_POINT ( 'NONE',  ( -9.820183334999905256, 10.35130206712171130, 1.040834085586084257E-14 ) ) ;
#201010=CARTESIAN_POINT ( 'NONE',  ( 6.745345117998789775, 7.828323044875442172, 1.199719254218462483 ) ) ;
#201014=CARTESIAN_POINT ( 'NONE',  ( 8.666686507633574621, 11.13422023037111330, 1.599625672291281386 ) ) ;
#201015=CARTESIAN_POINT ( 'NONE',  ( 4.469950146539259705, 7.269956441268025316, -1.287814263469128750 ) ) ;
#201023=CARTESIAN_POINT ( 'NONE',  ( -7.375272376154096143, 8.667201196010339004, -1.082531754730544860 ) ) ;
#201027=CARTESIAN_POINT ( 'NONE',  ( -1.201851678989727383E-14, 4.259375000341417028, -1.575800808251660134 ) ) ;
#201031=CARTESIAN_POINT ( 'NONE',  ( 0.6823417656249899377, 5.426041667008087543, -1.181850606188754593 ) ) ;
#201033=CARTESIAN_POINT ( 'NONE',  ( -4.256897044566581911, 4.068727428190179296, 1.214306433183764966E-14 ) ) ;
#201035=CARTESIAN_POINT ( 'NONE',  ( 9.317477881089539338, 11.89347683273640932, 1.599625672291279388 ) ) ;
#201036=CARTESIAN_POINT ( 'NONE',  ( 1.364683531249988535, 4.967708333674756283, -0.7879004041258300672 ) ) ;
#201037=CARTESIAN_POINT ( 'NONE',  ( -9.022061154889962964, 12.61315621642528129, -1.199719254218446718 ) ) ;
#201041=CARTESIAN_POINT ( 'NONE',  ( -0.6823417656250212460, 1.551041667008083769, 1.181850606188755259 ) ) ;
#201042=CARTESIAN_POINT ( 'NONE',  ( -4.012850279964973232, 4.744375417122949301, 1.082531754730560403 ) ) ;
#201043=CARTESIAN_POINT ( 'NONE',  ( 5.522248639467795428, 5.337044922334209573, -0.7998128361456231517 ) ) ;
#201048=CARTESIAN_POINT ( 'NONE',  ( -5.905025204060999400, 4.805319369736078094, -2.499999999999995115 ) ) ;
#201049=CARTESIAN_POINT ( 'NONE',  ( 2.236732156574683827, 5.553345249405011508, 1.040834085586084257E-14 ) ) ;
#201052=CARTESIAN_POINT ( 'NONE',  ( -7.537970219518089543, 8.857015346601659900, -1.082531754730543971 ) ) ;
#201055=CARTESIAN_POINT ( 'NONE',  ( 3.946537740505224878, 2.817530495244566335, 0.7750000000000135669 ) ) ;
#201058=CARTESIAN_POINT ( 'NONE',  ( -8.565000355531095622, 11.01558638625153286, -1.599625672291263179 ) ) ;
#201059=CARTESIAN_POINT ( 'NONE',  ( -3.240035523541616502, 6.723865844199768738, 0.7216878364870317197 ) ) ;
#201060=CARTESIAN_POINT ( 'NONE',  ( 1.364683531249988757, 1.946875000341415030, 0.000000000000000000 ) ) ;
#201074=ORIENTED_EDGE ( 'NONE', *, *, #213533, .T. ) ;
#201077=CARTESIAN_POINT ( 'NONE',  ( -1.284279953904132077, 2.909610286488902187, -0.7749999999999935829 ) ) ;
#201082=CARTESIAN_POINT ( 'NONE',  ( 1.364683531249988535, 2.676041667008082214, 0.7879004041258500513 ) ) ;
#201089=CARTESIAN_POINT ( 'NONE',  ( 8.211434591371064684, 12.73175745657494851, -0.7998128361456352531 ) ) ;
#201092=CARTESIAN_POINT ( 'NONE',  ( -1.364683531250014514, 1.738541667008085545, -0.7879004041258289570 ) ) ;
#201094=VERTEX_POINT ( 'NONE', #175079 ) ;
#201098=B_SPLINE_CURVE_WITH_KNOTS ( 'NONE', 3,
 ( #176722, #145334, #191883, #211335 ),
 .UNSPECIFIED., .F., .F.,
 ( 4, 4 ),
 ( 0.000000000000000000, 0.0003384805362160000402 ),
 .UNSPECIFIED. ) ;
#201103=CARTESIAN_POINT ( 'NONE',  ( 4.517891501851804215, 6.293959390292322986, -1.599625672291255185 ) ) ;
#201114=CARTESIAN_POINT ( 'NONE',  ( -4.029797971759847997, 5.724516938518342535, -1.599625672291256295 ) ) ;
#201115=CARTESIAN_POINT ( 'NONE',  ( 8.067265095331215718, 9.370563018429956870, 1.199719254218462483 ) ) ;
#201118=CARTESIAN_POINT ( 'NONE',  ( 3.334942598837264960, 6.834590765378040444, 1.214306433183764966E-14 ) ) ;
#201120=CARTESIAN_POINT ( 'NONE',  ( -1.387358672534977355, 7.315968950353621381, -4.254625267138091971 ) ) ;
#201129=CARTESIAN_POINT ( 'NONE',  ( -7.388830529767770550, 7.722649827591604677, 1.040834085586084257E-14 ) ) ;
#201131=CARTESIAN_POINT ( 'NONE',  ( 5.473741331615251227, 7.409117525016355010, -1.599625672291262513 ) ) ;
#201134=CARTESIAN_POINT ( 'NONE',  ( -9.158696461231359720, 10.64389961198009615, 1.199719254218462483 ) ) ;
#201139=CARTESIAN_POINT ( 'NONE',  ( -2.948008335967658322, 5.526761261015804116, 1.199719254218462483 ) ) ;
#201141=CARTESIAN_POINT ( 'NONE',  ( 10.24726517383036928, 10.84956421242393887, 0.000000000000000000 ) ) ;
#201143=CARTESIAN_POINT ( 'NONE',  ( 3.999819011231439347, 4.625209253646830554, 1.199719254218464037 ) ) ;
#201149=CARTESIAN_POINT ( 'NONE',  ( 3.931501358282940117, 4.649468341827285300, -1.082531754730543083 ) ) ;
#201152=CARTESIAN_POINT ( 'NONE',  ( -3.903858165731105778, 6.641919395739846799, 1.199719254218464037 ) ) ;
#201154=CARTESIAN_POINT ( 'NONE',  ( -9.541187415715041809, 12.15447128979948310, -1.599625672291263179 ) ) ;
#201159=CARTESIAN_POINT ( 'NONE',  ( 8.785320351975350661, 9.351887953500479966, -0.7216878364870197293 ) ) ;
#201160=CARTESIAN_POINT ( 'NONE',  ( 1.364683531249988535, 5.217708333674750065, -0.7879004041258300672 ) ) ;
#201162=CARTESIAN_POINT ( 'NONE',  ( 3.649115900372475796, 7.409052317076538330, 1.040834085586084257E-14 ) ) ;
#201164=CARTESIAN_POINT ( 'NONE',  ( 5.029711800545521250, 5.930713857800314237, -1.082531754730549078 ) ) ;
#201166=CARTESIAN_POINT ( 'NONE',  ( -6.256197817702116026, 9.386315656372753224, -1.199719254218440723 ) ) ;
#201176=VERTEX_POINT ( 'NONE', #74364 ) ;
#201178=CARTESIAN_POINT ( 'NONE',  ( -1.402160292154681736E-14, 2.509375000341417028, -1.575800808251660134 ) ) ;
#201180=CARTESIAN_POINT ( 'NONE',  ( 10.70146331988817323, 11.37946204949139251, 0.7998128361456341429 ) ) ;
#201182=CARTESIAN_POINT ( 'NONE',  ( -4.609409038966245653, 6.400729850259146758, -1.443375672974053447 ) ) ;
#201183=CARTESIAN_POINT ( 'NONE',  ( 2.846849069189655967, 5.304779099821139710, -1.082531754730543083 ) ) ;
#201184=CARTESIAN_POINT ( 'NONE',  ( -6.358410854684796831, 6.520493539994793863, -0.7216878364870267237 ) ) ;
#201189=CARTESIAN_POINT ( 'NONE',  ( 2.998324526916512411, 6.649795714711241423, 0.000000000000000000 ) ) ;
#201200=CARTESIAN_POINT ( 'NONE',  ( 6.505214776458575265, 6.483838748823460563, 1.040834085586084257E-14 ) ) ;
#201205=CARTESIAN_POINT ( 'NONE',  ( -4.889686956022917919, 8.856385215335397021, 1.214306433183764966E-14 ) ) ;
#201210=CARTESIAN_POINT ( 'NONE',  ( 6.238723240582662477, 10.43026088065513513, -0.7998128361456291469 ) ) ;
#201213=CARTESIAN_POINT ( 'NONE',  ( -4.737684612971557740, 7.614716917520386374, 1.199719254218464037 ) ) ;
#201214=CARTESIAN_POINT ( 'NONE',  ( 7.104109303436412226, 7.390475063538369582, 1.040834085586084257E-14 ) ) ;
#201215=CARTESIAN_POINT ( 'NONE',  ( 5.396677706949416731, 6.496517479030419651, 1.312881173378084521 ) ) ;
#201216=CARTESIAN_POINT ( 'NONE',  ( -2.611917148927046295, 6.198987107056845858, 1.040834085586084257E-14 ) ) ;
#201219=CARTESIAN_POINT ( 'NONE',  ( -6.247609857798938293, 6.183299677053865295, -0.7998128361456291469 ) ) ;
#201222=CARTESIAN_POINT ( 'NONE',  ( -0.6823417656250212460, 1.551041667008083769, 1.181850606188755259 ) ) ;
#201224=CARTESIAN_POINT ( 'NONE',  ( -4.690757960648240577, 6.495636925554817864, 1.443375672974064550 ) ) ;
#201230=CARTESIAN_POINT ( 'NONE',  ( 6.979750152936881058, 7.037463354714830643, 0.7998128361456341429 ) ) ;
#201232=CARTESIAN_POINT ( 'NONE',  ( 1.364683531249986537, 2.467708333674753174, -0.7879004041258239610 ) ) ;
#201235=CARTESIAN_POINT ( 'NONE',  ( -1.364683531250014514, -0.9072916663252470482, 0.7879004041258379498 ) ) ;
#201238=CARTESIAN_POINT ( 'NONE',  ( -4.308793891044708779, 3.921347715840572956, 1.214306433183764966E-14 ) ) ;
#201240=CARTESIAN_POINT ( 'NONE',  ( -8.148087131688699358, 8.608449196499371681, -0.7216878364870267237 ) ) ;
#201242=CARTESIAN_POINT ( 'NONE',  ( 0.6823417656249899377, 3.176041667008085323, -1.181850606188754593 ) ) ;
#201249=CARTESIAN_POINT ( 'NONE',  ( -5.531363484251157203, 9.397081798360927607, 0.000000000000000000 ) ) ;
#201254=CARTESIAN_POINT ( 'NONE',  ( -5.531363484251157203, 9.397081798360927607, 0.000000000000000000 ) ) ;
#201259=CARTESIAN_POINT ( 'NONE',  ( -0.7499999999999972244, 4.889583334016150751, -1.299038105676652899 ) ) ;
#201264=EDGE_LOOP ( 'NONE', ( #189807, #143100, #46936, #164780 ) ) ;
#201267=ADVANCED_FACE ( 'NONE', ( #194502 ), #183886, .T. ) ;
#201268=CARTESIAN_POINT ( 'NONE',  ( -7.217017841176048165, 7.314275657660511243, 1.040834085586084257E-14 ) ) ;
#201270=CARTESIAN_POINT ( 'NONE',  ( 1.499999999999987566, 0.02500000000001806333, 0.000000000000000000 ) ) ;
#201271=CARTESIAN_POINT ( 'NONE',  ( 2.659370686574860976, 6.254349567645977714, -0.7998128361456291469 ) ) ;
#201275=CARTESIAN_POINT ( 'NONE',  ( 5.309989718046547402, 9.346738437696316737, 0.7998128361456462443 ) ) ;
#201276=B_SPLINE_CURVE_WITH_KNOTS ( 'NONE', 3,
 ( #190925, #137939, #157393, #23081, #39358, #206113, #154183, #153110 ),
 .UNSPECIFIED., .F., .F.,
 ( 4, 2, 2, 4 ),
 ( 0.000000000000000000, 0.002997375907120270865, 0.004496063860680406081, 0.005994751814240539996 ),
 .UNSPECIFIED. ) ;
#201280=CARTESIAN_POINT ( 'NONE',  ( -4.609409038966245653, 6.400729850259146758, -1.443375672974053447 ) ) ;
#201288=CARTESIAN_POINT ( 'NONE',  ( 1.364683531249988535, 2.613541667008089764, 0.7879004041258500513 ) ) ;
#201290=CARTESIAN_POINT ( 'NONE',  ( -8.552495972122143186, 8.872333477097637200, 0.7998128361456462443 ) ) ;
#201292=CARTESIAN_POINT ( 'NONE',  ( 7.579171565239241737, 8.801120566655981747, 1.199719254218462483 ) ) ;
#201293=CARTESIAN_POINT ( 'NONE',  ( -7.365103760721662951, 9.615707025640515937, 1.599625672291295375 ) ) ;
#201296=CARTESIAN_POINT ( 'NONE',  ( 1.499999999999987121, -0.9645833326505173222, 0.8660254037844524744 ) ) ;
#201298=CARTESIAN_POINT ( 'NONE',  ( 9.273413882067330860, 9.921330405274451536, -0.7216878364870257245 ) ) ;
#201301=CARTESIAN_POINT ( 'NONE',  ( -1.364683531250012516, 1.092708333674754506, 0.7879004041258379498 ) ) ;
#201304=CARTESIAN_POINT ( 'NONE',  ( 7.795575137733369075, 9.157554417852841411, -1.082531754730537976 ) ) ;
#201307=CARTESIAN_POINT ( 'NONE',  ( -3.470524135418294520, 6.992769224722559684, -0.7216878364870267237 ) ) ;
#201309=CARTESIAN_POINT ( 'NONE',  ( 1.364683531249988535, 3.363541667008084879, 0.7879004041258500513 ) ) ;
#201313=CARTESIAN_POINT ( 'NONE',  ( -5.717788096661253761, 7.693838750903348789, 1.599625672291269396 ) ) ;
#201320=AXIS2_PLACEMENT_3D ( 'NONE', #107275, #90981, #121411 ) ;
#201321=CARTESIAN_POINT ( 'NONE',  ( 7.741869408603235136, 8.990934717247309749, 1.199719254218462483 ) ) ;
#201323=CIRCLE ( 'NONE', #52616, 1.000000000000000000 ) ;
#201325=CARTESIAN_POINT ( 'NONE',  ( -0.7500000000000215383, 1.941666666666688634, 1.299038105676659116 ) ) ;
#201331=CARTESIAN_POINT ( 'NONE',  ( 6.155038550924144758, 8.203964280876741455, 1.443375672974076540 ) ) ;
#201332=CARTESIAN_POINT ( 'NONE',  ( 1.364683531249986981, -1.053124999658580752, 0.000000000000000000 ) ) ;
#201340=CARTESIAN_POINT ( 'NONE',  ( -1.402160292154681736E-14, -0.03749999999998095135, 1.732050807568877637 ) ) ;
#201341=CARTESIAN_POINT ( 'NONE',  ( 8.426556166093362776, 9.789735934319136135, -1.199719254218446718 ) ) ;
#201342=CARTESIAN_POINT ( 'NONE',  ( -8.962103233833181193, 10.41454084668224489, -1.199719254218446718 ) ) ;
#201344=CARTESIAN_POINT ( 'NONE',  ( 1.364683531249986537, -0.09479166632524321789, -0.7879004041258309554 ) ) ;
#201345=CARTESIAN_POINT ( 'NONE',  ( 1.499999999999989120, 0.7750000000000187850, 0.000000000000000000 ) ) ;
#201347=CARTESIAN_POINT ( 'NONE',  ( 4.334856428067313416, 6.080418470877079429, -1.599625672291256295 ) ) ;
#201354=CARTESIAN_POINT ( 'NONE',  ( -0.7500000000000249800, -0.2770833326505156569, 1.299038105676659116 ) ) ;
#201356=CARTESIAN_POINT ( 'NONE',  ( -6.672584156219988571, 10.93643194889866521, -0.7998128361456291469 ) ) ;
#201357=CARTESIAN_POINT ( 'NONE',  ( -4.094199201646926412, 7.720390135322642067, 0.7216878364870317197 ) ) ;
#201365=CARTESIAN_POINT ( 'NONE',  ( 8.599949509769960088, 8.927695937686774386, 1.040834085586084257E-14 ) ) ;
#201370=CARTESIAN_POINT ( 'NONE',  ( 6.765155463094759014, 7.955398130774449683, 1.082531754730558626 ) ) ;
#201374=CARTESIAN_POINT ( 'NONE',  ( -6.347188469492005325, 10.55680364771601809, -0.7998128361456291469 ) ) ;
#201375=CARTESIAN_POINT ( 'NONE',  ( 4.306686350635271054, 8.176217842383143974, -0.7998128361456221525 ) ) ;
#201378=CARTESIAN_POINT ( 'NONE',  ( 3.388648328411762556, 6.040841252200647382, 1.199719254218462483 ) ) ;
#201388=CARTESIAN_POINT ( 'NONE',  ( -4.528060117284246289, 6.305822774963486310, 1.443375672974064550 ) ) ;
#201389=CARTESIAN_POINT ( 'NONE',  ( 8.920901888111989919, 11.43080484092926241, 1.443375672974076540 ) ) ;
#201392=CARTESIAN_POINT ( 'NONE',  ( -5.343885102080728977, 9.386283052402845328, 0.7998128361456481317 ) ) ;
#201396=CARTESIAN_POINT ( 'NONE',  ( -1.123270288250315163, 3.047697346350006331, -0.7749999999993613109 ) ) ;
#201398=CARTESIAN_POINT ( 'NONE',  ( -8.206763054973658100, 8.468978407091068306, 0.7998128361456602331 ) ) ;
#201401=CARTESIAN_POINT ( 'NONE',  ( 5.578458550106256020, 6.334871154397518467, -1.146459521134872483 ) ) ;
#201413=CARTESIAN_POINT ( 'NONE',  ( -5.343885102080728977, 9.386283052402845328, 0.7998128361456481317 ) ) ;
#201416=CARTESIAN_POINT ( 'NONE',  ( 3.823036129373602154, 6.443664003369091731, -1.082531754730548412 ) ) ;
#201421=CARTESIAN_POINT ( 'NONE',  ( -4.973143418114339021, 4.696422164088486895, 0.7998128361456341429 ) ) ;
#201425=DIRECTION ( 'NONE',  ( 1.000000000000000000, 0.000000000000000000, 0.000000000000000000 ) ) ;
#201429=CARTESIAN_POINT ( 'NONE',  ( -9.691380875670077444, 10.20103253123691189, 0.7998128361456462443 ) ) ;
#201430=CARTESIAN_POINT ( 'NONE',  ( 6.856673000209174695, 9.022537805042615489, 1.599625672291281386 ) ) ;
#201433=CARTESIAN_POINT ( 'NONE',  ( -10.30827686509187835, 10.92074451889568643, 1.040834085586084257E-14 ) ) ;
#201436=CARTESIAN_POINT ( 'NONE',  ( -1.402160292154681736E-14, -0.4906249996585810846, -1.575800808251665908 ) ) ;
#201440=CARTESIAN_POINT ( 'NONE',  ( 7.890482213473377193, 11.18901776815221716, -1.082531754730543083 ) ) ;
#201445=CARTESIAN_POINT ( 'NONE',  ( -5.503043298372868541, 6.255613091374303991, -0.9824725695728808716 ) ) ;
#201451=CYLINDRICAL_SURFACE ( 'NONE', #125595, 1.250000000000000000 ) ;
#201467=CARTESIAN_POINT ( 'NONE',  ( -1.201851678989727383E-14, 5.696875000341416140, -1.575800808251660134 ) ) ;
#201471=CARTESIAN_POINT ( 'NONE',  ( 8.594979316059474073, 12.11489407112305372, 1.199719254218450271 ) ) ;
#201477=CARTESIAN_POINT ( 'NONE',  ( 10.40318394038753702, 11.03146944007395724, -0.7998128361456281477 ) ) ;
#201482=CARTESIAN_POINT ( 'NONE',  ( 5.522248639467795428, 5.337044922334209573, -0.7998128361456231517 ) ) ;
#201483=CARTESIAN_POINT ( 'NONE',  ( 0.6823417656249882723, 2.238541667008084435, -1.181850606188749264 ) ) ;
#201486=CARTESIAN_POINT ( 'NONE',  ( -7.263417608619167076, 9.497073181520933716, -1.599625672291263179 ) ) ;
#201487=CARTESIAN_POINT ( 'NONE',  ( -5.083944415000202888, 5.033616027029415463, 0.7216878364870317197 ) ) ;
#201489=CARTESIAN_POINT ( 'NONE',  ( -6.338600509588822263, 7.353787668397130162, -1.199719254218446718 ) ) ;
#201491=CARTESIAN_POINT ( 'NONE',  ( 0.7499999999999885647, 0.5979166673494851203, -1.299038105676652899 ) ) ;
#201499=CARTESIAN_POINT ( 'NONE',  ( -2.928197990427299668, 6.360055388899728435, 1.040834085586084257E-14 ) ) ;
#201506=CARTESIAN_POINT ( 'NONE',  ( -5.083944415000202888, 5.033616027029415463, 0.7216878364870317197 ) ) ;
#201507=CARTESIAN_POINT ( 'NONE',  ( 7.072549687823125097, 11.40305840243567381, -0.7998128361456291469 ) ) ;
#201513=ORIENTED_EDGE ( 'NONE', *, *, #161432, .F. ) ;
#201516=CARTESIAN_POINT ( 'NONE',  ( -1.284279953904156280, 3.202889714876734573, 0.7750000000000117906 ) ) ;
#201522=CARTESIAN_POINT ( 'NONE',  ( 4.008406971134620633, 7.828225232965717595, 0.7998128361456321445 ) ) ;
#201526=EDGE_LOOP ( 'NONE', ( #193839, #19063 ) ) ;
#201528=CARTESIAN_POINT ( 'NONE',  ( 4.216749469050096621, 4.878294787768598262, -1.199719254218452047 ) ) ;
#201538=CARTESIAN_POINT ( 'NONE',  ( 8.796542737168120851, 9.157054702984622097, -0.7998128361456211532 ) ) ;
#201540=CARTESIAN_POINT ( 'NONE',  ( -5.220052836461385404, 6.048815383081766583, -1.199719254218446718 ) ) ;
#201546=ADVANCED_FACE ( 'NONE', ( #166264 ), #110598, .T. ) ;
#201548=CARTESIAN_POINT ( 'NONE',  ( 1.499999999999987566, -1.193749999317185395, 0.000000000000000000 ) ) ;
#201552=CARTESIAN_POINT ( 'NONE',  ( -3.253593677155282471, 6.739683690082376444, 1.040834085586084257E-14 ) ) ;
#201553=CARTESIAN_POINT ( 'NONE',  ( 4.192495815123822744, 5.914331089109666983, -1.599625672291255185 ) ) ;
#201554=CARTESIAN_POINT ( 'NONE',  ( -5.461236948206312114, 5.265864615862458464, 0.7998128361456341429 ) ) ;
#201560=CARTESIAN_POINT ( 'NONE',  ( 6.155038550924155416, 6.283225852274053835, 0.7216878364870317197 ) ) ;
#201563=ORIENTED_EDGE ( 'NONE', *, *, #80091, .T. ) ;
#201564=CARTESIAN_POINT ( 'NONE',  ( 8.554831740098663317, 9.082984572977682802, 0.7216878364870458196 ) ) ;
#201565=CARTESIAN_POINT ( 'NONE',  ( -1.364683531250012516, 5.051041667008085767, -0.7879004041258300672 ) ) ;
#201567=CARTESIAN_POINT ( 'NONE',  ( 3.999292125906899198, 6.649295999324608353, 1.082531754730558626 ) ) ;
#201575=CARTESIAN_POINT ( 'NONE',  ( -4.377387467589398007, 7.366231944554199274, 1.201952607213795821 ) ) ;
#201577=CARTESIAN_POINT ( 'NONE',  ( 1.364683531249990311, 4.696875000341417916, 1.214306433183764966E-14 ) ) ;
#201581=CARTESIAN_POINT ( 'NONE',  ( -10.31505594189871111, 10.92865344183699428, -0.7998128361456291469 ) ) ;
#201591=CARTESIAN_POINT ( 'NONE',  ( 4.555176424511575561, 4.416720038126027426, -0.7216878364870188411 ) ) ;
#201592=CARTESIAN_POINT ( 'NONE',  ( -0.6823417656249969321, 4.780208333674755394, -1.181850606188749264 ) ) ;
#201594=CARTESIAN_POINT ( 'NONE',  ( 6.089583550832340819, 10.25626457594641749, 1.040834085586084257E-14 ) ) ;
#201595=CARTESIAN_POINT ( 'NONE',  ( -9.504429378379839477, 11.04725468198666150, 1.199719254218462483 ) ) ;
#201597=CARTESIAN_POINT ( 'NONE',  ( -3.581325132304157943, 7.329963087663487364, -0.7998128361456282587 ) ) ;
#201601=CARTESIAN_POINT ( 'NONE',  ( -1.499999999999997780, 4.400000000000021672, 1.214306433183764966E-14 ) ) ;
#201602=CARTESIAN_POINT ( 'NONE',  ( 5.847644326195776010, 5.716673223516856694, -0.7998128361456281477 ) ) ;
#201605=DIRECTION ( 'NONE',  ( -7.387867266669436732E-31, 1.000000000000000000, -8.546850786086437571E-32 ) ) ;
#201607=CARTESIAN_POINT ( 'NONE',  ( 7.619319141200057821, 10.87266085050000974, 1.082531754730557072 ) ) ;
#201612=CARTESIAN_POINT ( 'NONE',  ( 1.499999999999989120, 4.035416667349482012, 0.8660254037844524744 ) ) ;
#201614=CARTESIAN_POINT ( 'NONE',  ( -4.042302355168801320, 7.867769847672247074, 0.7998128361456341429 ) ) ;
#201615=CARTESIAN_POINT ( 'NONE',  ( 4.677199806590210507, 4.559080650551097236, -0.7216878364870197293 ) ) ;
#201616=CARTESIAN_POINT ( 'NONE',  ( 3.469446951953614189E-15, 6.180000000000019256, 1.214306433183764966E-14 ) ) ;
#201624=CARTESIAN_POINT ( 'NONE',  ( 7.579171565239241737, 8.801120566655981747, 1.199719254218462483 ) ) ;
#201625=CARTESIAN_POINT ( 'NONE',  ( 3.323720213644492993, 7.029424015893889433, 1.040834085586084257E-14 ) ) ;
#201629=CARTESIAN_POINT ( 'NONE',  ( 5.192936529234042808, 6.017179691316550283, -1.199719254218452047 ) ) ;
#201641=CARTESIAN_POINT ( 'NONE',  ( 4.825424889954152086, 6.722588627200480893, -1.249340337910074705 ) ) ;
#201644=CARTESIAN_POINT ( 'NONE',  ( 10.38962578677386084, 11.01565159419135043, 0.000000000000000000 ) ) ;
#201648=CARTESIAN_POINT ( 'NONE',  ( 1.364683531249986981, -1.115624999658580752, 0.000000000000000000 ) ) ;
#201649=CARTESIAN_POINT ( 'NONE',  ( 6.819388077993785657, 7.058300300521964665, 1.040834085586084257E-14 ) ) ;
#201650=CARTESIAN_POINT ( 'NONE',  ( -8.487040972474682476, 12.84537220128841817, 0.7216878364870338292 ) ) ;
#201653=EDGE_CURVE ( 'NONE', #110797, #93128, #132697, .T. ) ;
#201657=CARTESIAN_POINT ( 'NONE',  ( -4.771579997005698459, 7.654261532226910525, -1.199719254218452047 ) ) ;
#201669=CARTESIAN_POINT ( 'NONE',  ( 8.398386088661320414, 11.88553530582519357, -1.199719254218446718 ) ) ;
#201670=CARTESIAN_POINT ( 'NONE',  ( 5.975483201341563522, 6.103571115010600678, 0.6665044388154163224 ) ) ;
#201677=CARTESIAN_POINT ( 'NONE',  ( -9.178506806771670412, 9.810605484096178941, 1.040834085586084257E-14 ) ) ;
#201682=CARTESIAN_POINT ( 'NONE',  ( 7.076466111328892694, 10.34329533227067799, -1.199719254218441611 ) ) ;
#201686=CARTESIAN_POINT ( 'NONE',  ( 4.729096653068339151, 4.411700938201493116, -0.7998128361456211532 ) ) ;
#201688=CARTESIAN_POINT ( 'NONE',  ( -7.061099074618889304, 7.132370430010492868, -0.7998128361456291469 ) ) ;
#201689=CARTESIAN_POINT ( 'NONE',  ( 3.684065054611349144, 5.321161868511784299, -1.599625672291262513 ) ) ;
#201695=CARTESIAN_POINT ( 'NONE',  ( 0.2517284219400194867, 6.998906413027644824, 3.965208550724196090 ) ) ;
#201699=CARTESIAN_POINT ( 'NONE',  ( 4.184706906298553797, 7.590773377710720915, -0.8858016571234141878 ) ) ;
#201701=CARTESIAN_POINT ( 'NONE',  ( 5.016153647376196290, 8.796003655340152605, 0.7216878364870438212 ) ) ;
#201709=CARTESIAN_POINT ( 'NONE',  ( 6.927853306458731986, 11.02631992426980112, 0.7216878364870438212 ) ) ;
#201710=AXIS2_PLACEMENT_3D ( 'NONE', #105085, #159142, #10744 ) ;
#201713=CARTESIAN_POINT ( 'NONE',  ( -8.178592977541617515, 10.56477777859713463, 1.599625672291295375 ) ) ;
#201723=CARTESIAN_POINT ( 'NONE',  ( 3.297657676621871925, 4.870353260857385180, 1.599625672291267398 ) ) ;
#201727=CARTESIAN_POINT ( 'NONE',  ( 4.147904930777053245, 6.926640621626830807, -1.199719254218452047 ) ) ;
#201730=CARTESIAN_POINT ( 'NONE',  ( -0.7500000000000215383, 4.722916667349482012, 1.299038105676671107 ) ) ;
#201736=CARTESIAN_POINT ( 'NONE',  ( 1.499999999999987121, 1.754166666666691521, 0.8660254037844524744 ) ) ;
#201737=CARTESIAN_POINT ( 'NONE',  ( 6.908042961362778733, 8.018137195466769285, 1.199719254218462483 ) ) ;
#201738=CARTESIAN_POINT ( 'NONE',  ( 3.660338285565247762, 7.214219066560688454, 1.040834085586084257E-14 ) ) ;
#201742=CARTESIAN_POINT ( 'NONE',  ( 8.975134502566660899, 10.53370701015836275, -1.082531754730543083 ) ) ;
#201747=CARTESIAN_POINT ( 'NONE',  ( -5.229694566569281555, 7.124396299129368337, 1.599625672291267398 ) ) ;
#201748=CARTESIAN_POINT ( 'NONE',  ( -1.201851678989727383E-14, 3.493750000682815493, 1.732050807568877637 ) ) ;
#201749=CARTESIAN_POINT ( 'NONE',  ( -1.364683531250010295, 5.342708333674750953, 0.7879004041258379498 ) ) ;
#201754=CARTESIAN_POINT ( 'NONE',  ( 1.364683531249988535, 3.426041667008085323, 0.7879004041258500513 ) ) ;
#201762=CARTESIAN_POINT ( 'NONE',  ( -9.040589502214116280, 9.441775928871617651, 0.7998128361456462443 ) ) ;
#201763=CARTESIAN_POINT ( 'NONE',  ( 6.440286661691305703, 7.472421512516709718, 1.199719254218462483 ) ) ;
#201768=ORIENTED_EDGE ( 'NONE', *, *, #177985, .F. ) ;
#201773=CARTESIAN_POINT ( 'NONE',  ( -6.157374318900681764, 10.33535380535947290, 0.7998128361456481317 ) ) ;
#201776=CARTESIAN_POINT ( 'NONE',  ( 10.56588178375152864, 11.22128359066528169, -0.7998128361456281477 ) ) ;
#201778=CARTESIAN_POINT ( 'NONE',  ( 9.185812768458653466, 10.67553530374532045, 1.199719254218453823 ) ) ;
#201780=CARTESIAN_POINT ( 'NONE',  ( -4.939248034080176097, 4.656877549381960080, 1.214306433183764966E-14 ) ) ;
#201781=CARTESIAN_POINT ( 'NONE',  ( -8.830438121202295321, 9.196599317691152464, -0.7998128361456291469 ) ) ;
#201785=CARTESIAN_POINT ( 'NONE',  ( -3.975603406396657213, 7.849426279905078019, -0.02588959144292704573 ) ) ;
#201786=CARTESIAN_POINT ( 'NONE',  ( 1.364683531249986537, -0.8447916663252468261, -0.7879004041258309554 ) ) ;
#201790=CARTESIAN_POINT ( 'NONE',  ( 8.595506201384013778, 10.09080732544527592, 1.082531754730558626 ) ) ;
#201812=ORIENTED_EDGE ( 'NONE', *, *, #9881, .T. ) ;
#201814=CARTESIAN_POINT ( 'NONE',  ( -9.481229494658258261, 9.955855920056455588, -0.7998128361456291469 ) ) ;
#201819=CARTESIAN_POINT ( 'NONE',  ( -1.500000000000013101, 1.410416667349486008, -0.8660254037844313801 ) ) ;
#201820=CARTESIAN_POINT ( 'NONE',  ( 8.353795204314554468, 12.89784483834236184, -0.7998128361456352531 ) ) ;
#201824=CARTESIAN_POINT ( 'NONE',  ( -8.642432853707342488, 12.17025653171218558, 1.199719254218462483 ) ) ;
#201825=CARTESIAN_POINT ( 'NONE',  ( -7.034482758620708154, 5.227586206896615018, 1.300454001123785972E-14 ) ) ;
#201826=CARTESIAN_POINT ( 'NONE',  ( 1.364683531249988535, 2.363541667008088432, 0.7879004041258500513 ) ) ;
#201828=ORIENTED_EDGE ( 'NONE', *, *, #87019, .F. ) ;
#201832=CARTESIAN_POINT ( 'NONE',  ( -2.605138072120212200, 6.191078184115536232, -0.7998128361456281477 ) ) ;
#201837=CARTESIAN_POINT ( 'NONE',  ( 1.364683531249986537, 0.4260416670080872659, 0.7879004041258500513 ) ) ;
#201843=CARTESIAN_POINT ( 'NONE',  ( 0.6823417656249899377, 1.342708333674752508, 1.181850606188755259 ) ) ;
#201846=CARTESIAN_POINT ( 'NONE',  ( -6.632963465583701534, 8.761543347979550589, -1.599625672291263179 ) ) ;
#201847=CARTESIAN_POINT ( 'NONE',  ( 8.437251666405968464, 8.737881787095446384, 1.040834085586084257E-14 ) ) ;
#201848=CARTESIAN_POINT ( 'NONE',  ( 5.379888026524302980, 5.170957540566795352, -0.7998128361456211532 ) ) ;
#201849=CARTESIAN_POINT ( 'NONE',  ( 5.681030059326015014, 6.586622143090519188, -1.199719254218445830 ) ) ;
#201851=CARTESIAN_POINT ( 'NONE',  ( 1.499999999999989120, 3.754166666666685082, 0.8660254037844524744 ) ) ;
#201854=CARTESIAN_POINT ( 'NONE',  ( -1.364683531250012516, 1.842708333674749843, 0.7879004041258379498 ) ) ;
#201860=CARTESIAN_POINT ( 'NONE',  ( 5.341549334104184865, 8.215262742221458581, 1.082531754730558626 ) ) ;
#201863=CARTESIAN_POINT ( 'NONE',  ( -9.365985188942097750, 9.821404230054264772, 0.7998128361456462443 ) ) ;
#201864=CARTESIAN_POINT ( 'NONE',  ( -3.554208825076827782, 7.298327395898266623, 0.7998128361456341429 ) ) ;
#201865=CARTESIAN_POINT ( 'NONE',  ( -4.271669656942582272, 7.425251299075903866, -1.032879151585558875 ) ) ;
#201867=CARTESIAN_POINT ( 'NONE',  ( -6.033015167956794933, 9.982342096017511324, -0.7216878364870267237 ) ) ;
#201869=CARTESIAN_POINT ( 'NONE',  ( 1.499999999999989120, 5.545833333333350268, -0.8660254037844323793 ) ) ;
#201872=CARTESIAN_POINT ( 'NONE',  ( 7.537970219518073556, 9.817384560903001045, -1.443375672974057666 ) ) ;
#201879=CARTESIAN_POINT ( 'NONE',  ( 9.531018800282598846, 12.14260790512831889, 1.443375672974076540 ) ) ;
#201885=CARTESIAN_POINT ( 'NONE',  ( 6.262976894508937242, 9.394224579314053969, -1.199719254218440723 ) ) ;
#201886=CARTESIAN_POINT ( 'NONE',  ( -4.608882153641705059, 7.464447381635583412, -1.199719254218452047 ) ) ;
#201888=CARTESIAN_POINT ( 'NONE',  ( -7.334597915313094241, 9.580116872663850813, 1.040834085586084257E-14 ) ) ;
#201890=CARTESIAN_POINT ( 'NONE',  ( -1.364683531250014514, -1.157291666325248158, 0.7879004041258379498 ) ) ;
#201891=CARTESIAN_POINT ( 'NONE',  ( 4.053524740805938720, 3.831459740469437936, 1.214306433183764966E-14 ) ) ;
#201892=ORIENTED_EDGE ( 'NONE', *, *, #126245, .T. ) ;
#201893=CARTESIAN_POINT ( 'NONE',  ( -4.634189577772691138, 4.300976017023221409, 1.214306433183764966E-14 ) ) ;
#201902=VERTEX_POINT ( 'NONE', #121865 ) ;
#201909=CARTESIAN_POINT ( 'NONE',  ( 6.936968151686458306, 11.24487994360957188, 0.7998128361456462443 ) ) ;
#201912=VERTEX_POINT ( 'NONE', #136979 ) ;
#201914=CARTESIAN_POINT ( 'NONE',  ( 1.499999999999990452, 8.654128368560188633, 2.562285273914694184 ) ) ;
#201921=CARTESIAN_POINT ( 'NONE',  ( -6.410307701162927252, 6.373113827645189744, -0.7998128361456291469 ) ) ;
#201923=CARTESIAN_POINT ( 'NONE',  ( -2.916975605234527702, 6.554888639415577423, 1.040834085586084257E-14 ) ) ;
#201930=CARTESIAN_POINT ( 'NONE',  ( -2.903417451620861289, 6.539070793532962611, 0.7998128361456341429 ) ) ;
#201933=CARTESIAN_POINT ( 'NONE',  ( 5.126954644262057492, 9.133197518281081173, 0.7998128361456462443 ) ) ;
#201934=CARTESIAN_POINT ( 'NONE',  ( -0.6823417656250212460, 4.801041667008086655, 1.181850606188767472 ) ) ;
#201935=EDGE_CURVE ( 'NONE', #193490, #17518, #154794, .T. ) ;
#201942=CARTESIAN_POINT ( 'NONE',  ( 6.778713616708431644, 7.010846762355714468, 1.040834085586084257E-14 ) ) ;
#201943=CARTESIAN_POINT ( 'NONE',  ( -7.393273838153706201, 7.519907654134449615, 0.7998128361456341429 ) ) ;
#201946=CARTESIAN_POINT ( 'NONE',  ( -8.206763054973658100, 8.468978407091068306, 0.7998128361456602331 ) ) ;
#201947=CARTESIAN_POINT ( 'NONE',  ( -5.087333953625788219, 6.958308917361963886, 1.599625672291267398 ) ) ;
#201954=CARTESIAN_POINT ( 'NONE',  ( 5.764187864104357573, 9.876636274763768597, 1.040834085586084257E-14 ) ) ;
#201968=CARTESIAN_POINT ( 'NONE',  ( 0.7499999999999902300, 5.316666666666685082, -1.299038105676658228 ) ) ;
#201969=CARTESIAN_POINT ( 'NONE',  ( 4.304877467538922531, 4.981110786005563007, 1.199719254218464037 ) ) ;
#201970=CARTESIAN_POINT ( 'NONE',  ( 4.632082037363250748, 8.555846143565791095, -0.7998128361456231517 ) ) ;
#201972=CARTESIAN_POINT ( 'NONE',  ( -7.537970219518089543, 8.857015346601659900, -1.082531754730543971 ) ) ;
#201974=CARTESIAN_POINT ( 'NONE',  ( 6.670248388243460447, 6.884303995813253252, -0.7216878364870257245 ) ) ;
#201975=CARTESIAN_POINT ( 'NONE',  ( -8.988692655735990300, 9.589155641221221771, 0.7216878364870438212 ) ) ;
#201976=VECTOR ( 'NONE', #50994, 1000.000000000000000 ) ;
#201979=CARTESIAN_POINT ( 'NONE',  ( 7.065770611016287006, 11.39514947949436774, 1.040834085586084257E-14 ) ) ;
#201984=CARTESIAN_POINT ( 'NONE',  ( -0.6823417656250212460, 2.801041667008084879, 1.181850606188767472 ) ) ;
#201990=CARTESIAN_POINT ( 'NONE',  ( 7.584896871841365851, 10.93646455286856956, -1.199719254218446718 ) ) ;
#201993=CARTESIAN_POINT ( 'NONE',  ( -8.154339323615371171, 11.60081407993821045, 1.199719254218453823 ) ) ;
#201998=CARTESIAN_POINT ( 'NONE',  ( 2.381428537494710618, 5.930083727052461562, 0.7998128361456462443 ) ) ;
#202002=B_SPLINE_CURVE_WITH_KNOTS ( 'NONE', 3,
 ( #193440, #45084, #93835, #29884, #177197, #210747 ),
 .UNSPECIFIED., .F., .F.,
 ( 4, 2, 4 ),
 ( 3.785604876262024909E-17, 0.0006272018345858698966, 0.001254403669171702063 ),
 .UNSPECIFIED. ) ;
#202003=CARTESIAN_POINT ( 'NONE',  ( -8.130085669689073313, 12.63685038127928806, 0.7998128361456481317 ) ) ;
#202008=CARTESIAN_POINT ( 'NONE',  ( 5.671489233189207724, 6.113434141373025099, 0.7590443732325997672 ) ) ;
#202010=CARTESIAN_POINT ( 'NONE',  ( -2.415323921528888196, 5.969628341758991930, 0.7998128361456341429 ) ) ;
#202014=CARTESIAN_POINT ( 'NONE',  ( 6.805303039055573322, 10.02693841461847057, 1.199719254218460707 ) ) ;
#202016=CARTESIAN_POINT ( 'NONE',  ( 5.438792177376376991, 9.497007973581119700, 1.040834085586084257E-14 ) ) ;
#202017=CARTESIAN_POINT ( 'NONE',  ( 5.345992642490140057, 5.131412925860272090, 1.040834085586084257E-14 ) ) ;
#202019=CARTESIAN_POINT ( 'NONE',  ( -8.202319746587722449, 8.671720580548228696, 1.040834085586084257E-14 ) ) ;
#202027=CARTESIAN_POINT ( 'NONE',  ( -4.043761313400059620, 7.584134902449670257, 0.3518898875958225703 ) ) ;
#202030=CARTESIAN_POINT ( 'NONE',  ( 6.182154858151487353, 6.314861544039274577, -0.7216878364870257245 ) ) ;
#202040=CYLINDRICAL_SURFACE ( 'NONE', #87619, 1.500000000000000222 ) ;
#202049=CARTESIAN_POINT ( 'NONE',  ( -8.961576348508637935, 12.43862759236002269, -1.082531754730543083 ) ) ;
#202053=CARTESIAN_POINT ( 'NONE',  ( 8.609591239877852686, 10.00327685373437347, -1.199719254218445830 ) ) ;
#202057=CARTESIAN_POINT ( 'NONE',  ( 1.499999999999987121, 2.077083334016153415, -0.8660254037844262731 ) ) ;
#202059=CARTESIAN_POINT ( 'NONE',  ( -7.040761844198392794, 7.108643661186573759, -0.7998128361456291469 ) ) ;
#202061=ORIENTED_EDGE ( 'NONE', *, *, #170654, .F. ) ;
#202062=CARTESIAN_POINT ( 'NONE',  ( -7.862839020921525091, 11.26073039346208660, -1.199719254218446718 ) ) ;
#202066=CARTESIAN_POINT ( 'NONE',  ( 6.962275575817444384, 8.081408578997208991, -1.199719254218446718 ) ) ;
#202069=CARTESIAN_POINT ( 'NONE',  ( -7.335124800193271177, 8.516399340768996851, -1.199719254218452935 ) ) ;
#202071=CARTESIAN_POINT ( 'NONE',  ( 7.723341061279088038, 12.16231500480096983, -0.7998128361456291469 ) ) ;
#202072=CARTESIAN_POINT ( 'NONE',  ( 0.6823417656249917140, 5.592708333674749177, 1.181850606188765695 ) ) ;
#202074=CARTESIAN_POINT ( 'NONE',  ( -4.840079859301741116, 5.046757083302627400, -0.8962971793361621531 ) ) ;
#202078=CARTESIAN_POINT ( 'NONE',  ( -6.561783159334121152, 10.59923808595773664, -0.7216878364870278340 ) ) ;
#202081=EDGE_CURVE ( 'NONE', #116082, #174777, #167910, .T. ) ;
#202082=CARTESIAN_POINT ( 'NONE',  ( -1.364683531250010295, 4.592708333674755394, 0.7879004041258379498 ) ) ;
#202091=CARTESIAN_POINT ( 'NONE',  ( -4.595850884908229794, 4.464173575255435011, 0.7216878364870317197 ) ) ;
#202094=CARTESIAN_POINT ( 'NONE',  ( 3.267151830768944443, 4.834763107362302748, -1.443375672974058777 ) ) ;
#202095=CARTESIAN_POINT ( 'NONE',  ( -1.201851678989727383E-14, 5.259375000341421469, -1.575800808251660134 ) ) ;
#202100=CARTESIAN_POINT ( 'NONE',  ( -1.364683531250000748, 0.2593750003414205252, 0.000000000000000000 ) ) ;
#202101=CARTESIAN_POINT ( 'NONE',  ( -3.714570900464290393, 5.356752022006865843, 1.443375672974064550 ) ) ;
#202102=CARTESIAN_POINT ( 'NONE',  ( 5.172599298813543633, 5.993452922492633839, -1.199719254218452047 ) ) ;
#202111=CARTESIAN_POINT ( 'NONE',  ( -6.860062538834774237, 10.94723069537516302, 0.7216878364870458196 ) ) ;
#202116=CARTESIAN_POINT ( 'NONE',  ( -8.239604668803112375, 10.63595808506888396, -1.599625672291263179 ) ) ;
#202117=CARTESIAN_POINT ( 'NONE',  ( -4.785665035499573783, 5.645992631913323123, 1.082531754730558626 ) ) ;
#202118=CARTESIAN_POINT ( 'NONE',  ( 1.364683531249986537, 1.717708333674749399, -0.7879004041258239610 ) ) ;
#202137=CARTESIAN_POINT ( 'NONE',  ( 4.907894938888475167, 6.474487383728034118, -2.499999999999995115 ) ) ;
#202139=DIRECTION ( 'NONE',  ( -0.6507913734559640506, -0.7592566023653004592, 0.000000000000000000 ) ) ;
#202143=CARTESIAN_POINT ( 'NONE',  ( 1.364683531249988535, 3.217708333674748289, -0.7879004041258239610 ) ) ;
#202147=FACE_OUTER_BOUND ( 'NONE', #204823, .T. ) ;
#202151=CARTESIAN_POINT ( 'NONE',  ( 8.723781775389312543, 12.26516360700784958, -1.199719254218446718 ) ) ;
#202154=CARTESIAN_POINT ( 'NONE',  ( -0.6823417656250212460, 1.301041667008083547, 1.181850606188755259 ) ) ;
#202166=CARTESIAN_POINT ( 'NONE',  ( 3.655894977179307226, 7.416961240017848844, -0.7998128361456291469 ) ) ;
#202171=CARTESIAN_POINT ( 'NONE',  ( 3.766852362949911992, 6.052795590908778500, 1.321332388365988875 ) ) ;
#202178=CARTESIAN_POINT ( 'NONE',  ( -3.002240950422295995, 5.590032644546251817, -1.199719254218452935 ) ) ;
#202179=CARTESIAN_POINT ( 'NONE',  ( 6.760712154708803823, 11.03924794713562818, 1.040834085586084257E-14 ) ) ;
#202185=CARTESIAN_POINT ( 'NONE',  ( 1.451998047843343409, 7.315968950353815892, -4.301760722578415574 ) ) ;
#202189=( BOUNDED_SURFACE ( )  B_SPLINE_SURFACE ( 1, 2, ( 
 ( #193222, #61092, #73051, #140238, #141322, #91480, #42736, #26448, #139150, #92557, #62166, #112052, #181230, #176980, #161806, #97881, #66385, #115240, #132533, #29670, #28598, #13397, #45933, #180182, #32858, #46996, #211587, #113113, #96822, #94686, #160728, #128325, #194288, #178052, #212654, #129386, #78402, #49122, #65328, #95754, #12321, #210532, #79473, #179118, #130441, #195365, #197478, #163942, #15517, #30741, #114184, #98933, #131475, #162871, #147687, #145591, #164988, #213704, #16578, #63223, #144522, #314, #14451, #80542, #82661, #146639, #64295, #148745, #48073, #81602, #196428, #31805, #44868, #110974, #4583, #200658, #149818, #102121, #21899, #153006, #53368, #70657, #104265, #17642, #166056, #38193, #183366, #68526, #99990, #71728, #169255, #116297, #198530, #83727, #3519, #50177, #33914, #1389, #88009, #5647, #182288, #67450, #133595, #170311, #85871, #134655, #69591, #135701, #199600, #120587, #154080, #51243, #201727, #202795, #54445, #168190, #117369, #186565, #19789, #136767, #34970, #101042, #167132, #18717, #119503, #84801, #52307, #150889, #2451, #185488, #118437, #184424, #36041, #151948, #37114, #103192, #20841, #86940, #188705, #155150, #204932, #62686, #55507, #40341, #193756, #162345, #211061, #13928, #122742, #121661, #106447, #138912, #61635, #128845, #139990, #90161, #206011, #189766, #187629, #39256, #6732, #72811, #56583, #94162, #7804, #171387, #145058, #161275, #172470, #105350, #89097, #24058, #57646, #11804, #73897, #78936, #45403, #111519, #123806, #209993, #194827, #12862, #41418, #29137, #156227, #46462, #95225, #112584, #107525, #22978, #96293, #173556, #25129, #178596, #160201, #77879, #30206, #144001, #177525, #127802, #137840, #203862, #34460, #100531, #82139, #31281, #198021, #117918, #166606, #149282, #18195, #200146, #113657, #47545, #134139, #64825, #164469, #195908, #167667, #50715, #212124, #80008, #179661, #99473, #146113, #129922, #97356, #183911, #101599, #63762, #163413, #14989, #51800, #181762, #16055, #165532, #17124, #81083, #1937, #35522, #147170, #83200, #84280, #150367, #49649, #213197, #67997, #115772, #130970, #196962, #48600, #114718, #180713, #863, #32336, #148231, #98404, #214233, #66929, #65861, #132011, #133071, #33395, #199069, #116841, #182842, #38741, #120060, #168734, #71207, #86422, #5132, #4070, #23533, #70140, #36588, #152488, #155694, #151431, #136252, #72278, #40892, #89641, #106996, #202272, #3004, #53923, #20335, #154629, #7276, #21387, #186035, #87496, #137323, #69073, #135193, #102675, #37671, #103747, #187107, #169798, #52848, #73353, #39811, #153561, #201210, #184962, #203339, #54992, #104823, #121144, #171942, #138387, #204405, #170869, #88571, #139456, #105917, #22459, #122215, #6209, #205488, #188177, #57122, #56058, #118983, #189252, #123289, #19268, #85350, #109145, #58187, #28894, #176217, #77631, #142671, #110208, #75504, #127549, #193520, #175158, #124345, #76561, #210824, #45161, #27819, #111275, #78692, #206559, #140546, #12619, #157837, #43033, #74443, #46225, #143753, #90711, #173021, #190303, #192433, #24602, #8359, #41960, #62449, #194579, #156773, #108072, #174100, #144817, #60311, #26744, #44088, #93916, #25673, #94978, #128612, #91780, #159957, #177278, #161024, #208682, #9434, #141615, #126470, #207625, #59243, #125401, #191366, #92847, #158891, #10488, #209748, #61390, #11561, #48359, #47296, #198818, #601, #199890, #31039, #116583, #132814, #114470, #164222, #14750, #180471, #15809, #211884, #49404, #80842, #67733, #100274, #63525, #13690, #197766, #50464, #32086, #166340, #149026, #98174, #130727, #29962, #212949, #178354, #115523, #64586, #181518, #129677, #66667, #196718, #81895, #182578, #17931, #34200, #82952, #84016, #147981, #146932, #113411, #179417, #150107, #97113, #213991, #165277, #65611, #131761, #1679, #133883, #33147, #112342, #163165, #99227, #96048, #16871, #162101, #79760, #145876, #195662, #120873, #54724, #37403, #53657, #69875, #89378, #183653, #21119, #2743, #187911, #151172, #117661, #19007, #4865, #5942, #3801, #184704, #35258, #22187, #186847, #155427, #39541, #55788 ),
 ( #52590, #138126, #88302, #87225, #105642, #154363, #153289, #118717, #204135, #135984, #171669, #68813, #121945, #7013, #23266, #134935, #101334, #170600, #200941, #201998, #72013, #73088, #139189, #103477, #86159, #36326, #102404, #51536, #168472, #119789, #104556, #20070, #70943, #167416, #85088, #137054, #152230, #185770, #169539, #203079, #38479, #142418, #56861, #193261, #57926, #60061, #208427, #191111, #207376, #9175, #28638, #123035, #174909, #156511, #127290, #90443, #188986, #172760, #158639, #159699, #157582, #124091, #40630, #175966, #126217, #94725, #44908, #209489, #8100, #10236, #43839, #106733, #26487, #107816, #192178, #24335, #75250, #27560, #109955, #190054, #111016, #140282, #206302, #77377, #93656, #92597, #177021, #11298, #76311, #41706, #143493, #141363, #160770, #74190, #61130, #12363, #78442, #173841, #25418, #205219, #91524, #58996, #125152, #42778, #108886, #194330, #115277, #49160, #162911, #80583, #79515, #16619, #32895, #17680, #63264, #148780, #165025, #146681, #196470, #47039, #212697, #48112, #29712, #81641, #113155, #100030, #132566, #95793, #45972, #15554, #82701, #64338, #198567, #181269, #130480, #14493, #62206, #30784, #210572, #147726, #96863, #213743, #161850, #98973, #114224, #180222, #350, #50216, #166092, #211629, #13438, #66423, #31844, #145633, #116335, #65366, #182325, #97921, #131513, #179160, #33954, #144562, #163979, #129426, #197516, #128363, #112093, #178095, #195410, #203901, #117409, #51284, #137881, #68566, #168230, #199638, #171428, #54481, #1427, #83766, #183405, #103232, #149859, #133636, #101080, #121701, #105389, #67491, #35009, #167169, #55547, #185527, #19827, #169292, #20877, #18756, #5688, #187665, #84841, #86976, #88047, #154118, #201763, #150930, #71765, #119542, #104303, #2491, #200697, #134693, #52349, #153046, #118476, #85912, #184461, #36079, #4621, #102162, #151986, #135741, #3560, #69633, #53404, #39295, #37153, #70693, #136806, #202832, #120626, #186602, #38229, #170352, #21937, #44648, #7844, #6769, #140025, #24095, #158388, #11040, #25170, #189804, #91271, #75001, #155187, #72845, #40380, #106483, #172510, #190862, #107563, #56617, #27298, #43586, #90199, #138950, #188741, #156263, #157328, #108630, #173598, #175708, #142161, #76062, #8920, #92349, #159442, #109703, #141110, #125965, #57686, #93405, #191921, #77119, #73932, #204971, #123842, #174657, #89133, #143242, #206051, #9984, #26232, #207121, #58746, #41455, #60876, #122781, #124899, #42525, #209231, #208178, #59810, #127035, #192995, #110762, #23016, #95545, #160512, #147476, #31590, #100, #98716, #181019, #194066, #130224, #15303, #12115, #146425, #79263, #97665, #28377, #195152, #213496, #81391, #161596, #82443, #111838, #177842, #48902, #65118, #212439, #16365, #131274, #64081, #29455, #115022, #129175, #148533, #45719, #32639, #132312, #66166, #13185, #78189, #197262, #61949, #46786, #164775, #198318, #96606, #144315, #49958, #176761, #112900, #178911, #145380, #94471, #210313, #128108, #211378, #63004, #30526, #162659, #14229, #80324, #196218, #47859, #113971, #179968, #163723, #71512, #104048, #67241, #17427, #201507, #136554, #35828, #170094, #152788, #118219, #134443, #33699, #2235, #182067, #53155, #68312, #185270, #133375, #4368, #200446, #19577, #202575, #21680, #54227, #86719, #120365, #101906, #150674, #117149, #183152, #186340, #34755, #52092, #169033, #84587, #69377, #70438, #87790, #151737, #153864, #51027, #184205, #99776, #1177, #167971, #37975, #5433, #85650, #165841, #137624, #20630, #3307, #135485, #100829, #203641, #116077, #83510, #166914, #149593, #199380, #119284, #36893, #18508, #102975, #173326, #154928, #206857, #172250, #10783, #43327, #6513, #171167, #140845, #75803, #189547, #109445, #92080, #57422, #73667, #187411, #155995, #121442, #58489, #7582, #124645, #72589, #158137, #139766, #24904, #141911, #175452, #207923, #25974, #59544, #41195, #89944, #56357, #122520, #125704, #188483, #205792, #108373, #23837, #8661, #9728, #27036, #91010, #93145, #204707, #123584, #39042, #107302, #190602, #105127, #159182, #40113, #42260, #174396, #157072, #74740 ) ),
 .UNSPECIFIED., .F., .F., .T. ) 
 B_SPLINE_SURFACE_WITH_KNOTS ( ( 2, 2 ),
 ( 3, 2, 2, 2, 2, 2, 2, 2, 2, 2, 2, 2, 2, 2, 2, 2, 2, 2, 2, 2, 2, 2, 2, 2, 2, 2, 2, 2, 2, 2, 2, 2, 2, 2, 2, 2, 2, 2, 2, 2, 2, 2, 2, 2, 2, 2, 2, 2, 2, 2, 2, 2, 2, 2, 2, 2, 2, 2, 2, 2, 2, 2, 2, 2, 2, 2, 2, 2, 2, 2, 2, 2, 2, 2, 2, 2, 2, 2, 2, 2, 2, 2, 2, 2, 2, 2, 2, 2, 2, 2, 2, 2, 2, 2, 2, 2, 2, 2, 2, 2, 2, 2, 2, 2, 2, 2, 2, 2, 2, 2, 2, 2, 2, 2, 2, 2, 2, 2, 2, 2, 2, 2, 2, 2, 2, 2, 2, 2, 2, 2, 2, 2, 2, 2, 2, 2, 2, 2, 2, 2, 2, 2, 2, 2, 2, 2, 2, 2, 2, 2, 2, 2, 2, 2, 2, 2, 2, 2, 2, 2, 2, 2, 2, 2, 2, 2, 2, 2, 2, 2, 2, 2, 2, 2, 2, 2, 2, 2, 2, 2, 2, 2, 2, 2, 2, 2, 2, 2, 2, 2, 2, 2, 2, 2, 2, 2, 2, 2, 2, 2, 2, 2, 2, 2, 2, 2, 2, 2, 2, 2, 2, 2, 2, 2, 2, 2, 2, 2, 2, 2, 2, 2, 2, 2, 2, 2, 2, 2, 2, 2, 2, 2, 2, 2, 2, 2, 2, 2, 2, 2, 3 ),
 ( 0.000000000000000000, 1.000000000000000000 ),
 ( 0.000000000000000000, 0.004166666666666666609, 0.008333333333333333218, 0.01250000000000000069, 0.01666666666666666644, 0.02083333333333333218, 0.02500000000000000139, 0.02916666666666666713, 0.03333333333333333287, 0.03749999999999999861, 0.04166666666666666435, 0.04583333333333333010, 0.05000000000000000278, 0.05416666666666666852, 0.05833333333333333426, 0.06250000000000000000, 0.06666666666666666574, 0.07083333333333333148, 0.07499999999999999722, 0.07916666666666666297, 0.08333333333333332871, 0.08749999999999999445, 0.09166666666666666019, 0.09583333333333333981, 0.1000000000000000056, 0.1041666666666666713, 0.1083333333333333370, 0.1125000000000000028, 0.1166666666666666685, 0.1208333333333333343, 0.1250000000000000000, 0.1291666666666666796, 0.1333333333333333315, 0.1375000000000000111, 0.1416666666666666630, 0.1458333333333333426, 0.1499999999999999944, 0.1541666666666666741, 0.1583333333333333259, 0.1625000000000000056, 0.1666666666666666574, 0.1708333333333333370, 0.1749999999999999889, 0.1791666666666666685, 0.1833333333333333204, 0.1875000000000000000, 0.1916666666666666796, 0.1958333333333333315, 0.2000000000000000111, 0.2041666666666666630, 0.2083333333333333426, 0.2124999999999999944, 0.2166666666666666741, 0.2208333333333333259, 0.2250000000000000056, 0.2291666666666666574, 0.2333333333333333370, 0.2374999999999999889, 0.2416666666666666685, 0.2458333333333333204, 0.2500000000000000000, 0.2541666666666666519, 0.2583333333333333592, 0.2625000000000000111, 0.2666666666666666630, 0.2708333333333333148, 0.2750000000000000222, 0.2791666666666666741, 0.2833333333333333259, 0.2874999999999999778, 0.2916666666666666852, 0.2958333333333333370, 0.2999999999999999889, 0.3041666666666666408, 0.3083333333333333481, 0.3125000000000000000, 0.3166666666666666519, 0.3208333333333333592, 0.3250000000000000111, 0.3291666666666666630, 0.3333333333333333148, 0.3375000000000000222, 0.3416666666666666741, 0.3458333333333333259, 0.3499999999999999778, 0.3541666666666666852, 0.3583333333333333370, 0.3624999999999999889, 0.3666666666666666408, 0.3708333333333333481, 0.3750000000000000000, 0.3791666666666666519, 0.3833333333333333592, 0.3875000000000000111, 0.3916666666666666630, 0.3958333333333333148, 0.4000000000000000222, 0.4041666666666666741, 0.4083333333333333259, 0.4124999999999999778, 0.4166666666666666852, 0.4208333333333333370, 0.4249999999999999889, 0.4291666666666666408, 0.4333333333333333481, 0.4375000000000000000, 0.4416666666666666519, 0.4458333333333333592, 0.4500000000000000111, 0.4541666666666666630, 0.4583333333333333148, 0.4625000000000000222, 0.4666666666666666741, 0.4708333333333333259, 0.4749999999999999778, 0.4791666666666666852, 0.4833333333333333370, 0.4874999999999999889, 0.4916666666666666408, 0.4958333333333333481, 0.5000000000000000000, 0.5041666666666666519, 0.5083333333333333037, 0.5124999999999999556, 0.5166666666666667185, 0.5208333333333333703, 0.5250000000000000222, 0.5291666666666666741, 0.5333333333333333259, 0.5374999999999999778, 0.5416666666666666297, 0.5458333333333332815, 0.5500000000000000444, 0.5541666666666666963, 0.5583333333333333481, 0.5625000000000000000, 0.5666666666666666519, 0.5708333333333333037, 0.5749999999999999556, 0.5791666666666667185, 0.5833333333333333703, 0.5875000000000000222, 0.5916666666666666741, 0.5958333333333333259, 0.5999999999999999778, 0.6041666666666666297, 0.6083333333333332815, 0.6125000000000000444, 0.6166666666666666963, 0.6208333333333333481, 0.6250000000000000000, 0.6291666666666666519, 0.6333333333333333037, 0.6374999999999999556, 0.6416666666666667185, 0.6458333333333333703, 0.6500000000000000222, 0.6541666666666666741, 0.6583333333333333259, 0.6624999999999999778, 0.6666666666666666297, 0.6708333333333332815, 0.6750000000000000444, 0.6791666666666666963, 0.6833333333333333481, 0.6875000000000000000, 0.6916666666666666519, 0.6958333333333333037, 0.6999999999999999556, 0.7041666666666667185, 0.7083333333333333703, 0.7125000000000000222, 0.7166666666666666741, 0.7208333333333333259, 0.7249999999999999778, 0.7291666666666666297, 0.7333333333333332815, 0.7375000000000000444, 0.7416666666666666963, 0.7458333333333333481, 0.7500000000000000000, 0.7541666666666666519, 0.7583333333333333037, 0.7624999999999999556, 0.7666666666666667185, 0.7708333333333333703, 0.7750000000000000222, 0.7791666666666666741, 0.7833333333333333259, 0.7874999999999999778, 0.7916666666666666297, 0.7958333333333332815, 0.8000000000000000444, 0.8041666666666666963, 0.8083333333333333481, 0.8125000000000000000, 0.8166666666666666519, 0.8208333333333333037, 0.8249999999999999556, 0.8291666666666667185, 0.8333333333333333703, 0.8375000000000000222, 0.8416666666666666741, 0.8458333333333333259, 0.8499999999999999778, 0.8541666666666666297, 0.8583333333333332815, 0.8625000000000000444, 0.8666666666666666963, 0.8708333333333333481, 0.8750000000000000000, 0.8791666666666666519, 0.8833333333333333037, 0.8874999999999999556, 0.8916666666666667185, 0.8958333333333333703, 0.9000000000000000222, 0.9041666666666666741, 0.9083333333333333259, 0.9124999999999999778, 0.9166666666666666297, 0.9208333333333332815, 0.9250000000000000444, 0.9291666666666666963, 0.9333333333333333481, 0.9375000000000000000, 0.9416666666666666519, 0.9458333333333333037, 0.9499999999999999556, 0.9541666666666667185, 0.9583333333333333703, 0.9625000000000000222, 0.9666666666666666741, 0.9708333333333333259, 0.9749999999999999778, 0.9791666666666666297, 0.9833333333333332815, 0.9875000000000000444, 0.9916666666666666963, 0.9958333333333333481, 1.000000000000000000 ),
 .UNSPECIFIED. ) 
 GEOMETRIC_REPRESENTATION_ITEM ( )  RATIONAL_B_SPLINE_SURFACE ( (
 ( 1.000000000000000000, 0.8660254037844387076, 1.000000000000000000, 0.8660254037844387076, 1.000000000000000000, 0.8660254037844387076, 1.000000000000000000, 0.8660254037844387076, 1.000000000000000000, 0.8660254037844387076, 1.000000000000000000, 0.8660254037844387076, 1.000000000000000000, 0.8660254037844387076, 1.000000000000000000, 0.8660254037844387076, 1.000000000000000000, 0.8660254037844387076, 1.000000000000000000, 0.8660254037844387076, 1.000000000000000000, 0.8660254037844387076, 1.000000000000000000, 0.8660254037844387076, 1.000000000000000000, 0.8660254037844387076, 1.000000000000000000, 0.8660254037844387076, 1.000000000000000000, 0.8660254037844387076, 1.000000000000000000, 0.8660254037844387076, 1.000000000000000000, 0.8660254037844387076, 1.000000000000000000, 0.8660254037844387076, 1.000000000000000000, 0.8660254037844387076, 1.000000000000000000, 0.8660254037844387076, 1.000000000000000000, 0.8660254037844387076, 1.000000000000000000, 0.8660254037844387076, 1.000000000000000000, 0.8660254037844387076, 1.000000000000000000, 0.8660254037844387076, 1.000000000000000000, 0.8660254037844387076, 1.000000000000000000, 0.8660254037844387076, 1.000000000000000000, 0.8660254037844387076, 1.000000000000000000, 0.8660254037844387076, 1.000000000000000000, 0.8660254037844387076, 1.000000000000000000, 0.8660254037844387076, 1.000000000000000000, 0.8660254037844387076, 1.000000000000000000, 0.8660254037844387076, 1.000000000000000000, 0.8660254037844387076, 1.000000000000000000, 0.8660254037844387076, 1.000000000000000000, 0.8660254037844387076, 1.000000000000000000, 0.8660254037844387076, 1.000000000000000000, 0.8660254037844387076, 1.000000000000000000, 0.8660254037844387076, 1.000000000000000000, 0.8660254037844387076, 1.000000000000000000, 0.8660254037844387076, 1.000000000000000000, 0.8660254037844387076, 1.000000000000000000, 0.8660254037844387076, 1.000000000000000000, 0.8660254037844387076, 1.000000000000000000, 0.8660254037844387076, 1.000000000000000000, 0.8660254037844387076, 1.000000000000000000, 0.8660254037844387076, 1.000000000000000000, 0.8660254037844387076, 1.000000000000000000, 0.8660254037844387076, 1.000000000000000000, 0.8660254037844387076, 1.000000000000000000, 0.8660254037844387076, 1.000000000000000000, 0.8660254037844387076, 1.000000000000000000, 0.8660254037844387076, 1.000000000000000000, 0.8660254037844387076, 1.000000000000000000, 0.8660254037844387076, 1.000000000000000000, 0.8660254037844387076, 1.000000000000000000, 0.8660254037844387076, 1.000000000000000000, 0.8660254037844387076, 1.000000000000000000, 0.8660254037844387076, 1.000000000000000000, 0.8660254037844387076, 1.000000000000000000, 0.8660254037844387076, 1.000000000000000000, 0.8660254037844387076, 1.000000000000000000, 0.8660254037844387076, 1.000000000000000000, 0.8660254037844387076, 1.000000000000000000, 0.8660254037844387076, 1.000000000000000000, 0.8660254037844387076, 1.000000000000000000, 0.8660254037844387076, 1.000000000000000000, 0.8660254037844387076, 1.000000000000000000, 0.8660254037844387076, 1.000000000000000000, 0.8660254037844387076, 1.000000000000000000, 0.8660254037844387076, 1.000000000000000000, 0.8660254037844387076, 1.000000000000000000, 0.8660254037844387076, 1.000000000000000000, 0.8660254037844387076, 1.000000000000000000, 0.8660254037844387076, 1.000000000000000000, 0.8660254037844387076, 1.000000000000000000, 0.8660254037844387076, 1.000000000000000000, 0.8660254037844387076, 1.000000000000000000, 0.8660254037844387076, 1.000000000000000000, 0.8660254037844387076, 1.000000000000000000, 0.8660254037844387076, 1.000000000000000000, 0.8660254037844387076, 1.000000000000000000, 0.8660254037844387076, 1.000000000000000000, 0.8660254037844387076, 1.000000000000000000, 0.8660254037844387076, 1.000000000000000000, 0.8660254037844387076, 1.000000000000000000, 0.8660254037844387076, 1.000000000000000000, 0.8660254037844387076, 1.000000000000000000, 0.8660254037844387076, 1.000000000000000000, 0.8660254037844387076, 1.000000000000000000, 0.8660254037844387076, 1.000000000000000000, 0.8660254037844387076, 1.000000000000000000, 0.8660254037844387076, 1.000000000000000000, 0.8660254037844387076, 1.000000000000000000, 0.8660254037844387076, 1.000000000000000000, 0.8660254037844387076, 1.000000000000000000, 0.8660254037844387076, 1.000000000000000000, 0.8660254037844387076, 1.000000000000000000, 0.8660254037844387076, 1.000000000000000000, 0.8660254037844387076, 1.000000000000000000, 0.8660254037844387076, 1.000000000000000000, 0.8660254037844387076, 1.000000000000000000, 0.8660254037844387076, 1.000000000000000000, 0.8660254037844387076, 1.000000000000000000, 0.8660254037844387076, 1.000000000000000000, 0.8660254037844387076, 1.000000000000000000, 0.8660254037844387076, 1.000000000000000000, 0.8660254037844387076, 1.000000000000000000, 0.8660254037844387076, 1.000000000000000000, 0.8660254037844387076, 1.000000000000000000, 0.8660254037844387076, 1.000000000000000000, 0.8660254037844387076, 1.000000000000000000, 0.8660254037844387076, 1.000000000000000000, 0.8660254037844387076, 1.000000000000000000, 0.8660254037844387076, 1.000000000000000000, 0.8660254037844387076, 1.000000000000000000, 0.8660254037844387076, 1.000000000000000000, 0.8660254037844387076, 1.000000000000000000, 0.8660254037844387076, 1.000000000000000000, 0.8660254037844387076, 1.000000000000000000, 0.8660254037844387076, 1.000000000000000000, 0.8660254037844387076, 1.000000000000000000, 0.8660254037844387076, 1.000000000000000000, 0.8660254037844387076, 1.000000000000000000, 0.8660254037844387076, 1.000000000000000000, 0.8660254037844387076, 1.000000000000000000, 0.8660254037844387076, 1.000000000000000000, 0.8660254037844387076, 1.000000000000000000, 0.8660254037844387076, 1.000000000000000000, 0.8660254037844387076, 1.000000000000000000, 0.8660254037844387076, 1.000000000000000000, 0.8660254037844387076, 1.000000000000000000, 0.8660254037844387076, 1.000000000000000000, 0.8660254037844387076, 1.000000000000000000, 0.8660254037844387076, 1.000000000000000000, 0.8660254037844387076, 1.000000000000000000, 0.8660254037844387076, 1.000000000000000000, 0.8660254037844387076, 1.000000000000000000, 0.8660254037844387076, 1.000000000000000000, 0.8660254037844387076, 1.000000000000000000, 0.8660254037844387076, 1.000000000000000000, 0.8660254037844387076, 1.000000000000000000, 0.8660254037844387076, 1.000000000000000000, 0.8660254037844387076, 1.000000000000000000, 0.8660254037844387076, 1.000000000000000000, 0.8660254037844387076, 1.000000000000000000, 0.8660254037844387076, 1.000000000000000000, 0.8660254037844387076, 1.000000000000000000, 0.8660254037844387076, 1.000000000000000000, 0.8660254037844387076, 1.000000000000000000, 0.8660254037844387076, 1.000000000000000000, 0.8660254037844387076, 1.000000000000000000, 0.8660254037844387076, 1.000000000000000000, 0.8660254037844387076, 1.000000000000000000, 0.8660254037844387076, 1.000000000000000000, 0.8660254037844387076, 1.000000000000000000, 0.8660254037844387076, 1.000000000000000000, 0.8660254037844387076, 1.000000000000000000, 0.8660254037844387076, 1.000000000000000000, 0.8660254037844387076, 1.000000000000000000, 0.8660254037844387076, 1.000000000000000000, 0.8660254037844387076, 1.000000000000000000, 0.8660254037844387076, 1.000000000000000000, 0.8660254037844387076, 1.000000000000000000, 0.8660254037844387076, 1.000000000000000000, 0.8660254037844387076, 1.000000000000000000, 0.8660254037844387076, 1.000000000000000000, 0.8660254037844387076, 1.000000000000000000, 0.8660254037844387076, 1.000000000000000000, 0.8660254037844387076, 1.000000000000000000, 0.8660254037844387076, 1.000000000000000000, 0.8660254037844387076, 1.000000000000000000, 0.8660254037844387076, 1.000000000000000000, 0.8660254037844387076, 1.000000000000000000, 0.8660254037844387076, 1.000000000000000000, 0.8660254037844387076, 1.000000000000000000, 0.8660254037844387076, 1.000000000000000000, 0.8660254037844387076, 1.000000000000000000, 0.8660254037844387076, 1.000000000000000000, 0.8660254037844387076, 1.000000000000000000, 0.8660254037844387076, 1.000000000000000000, 0.8660254037844387076, 1.000000000000000000, 0.8660254037844387076, 1.000000000000000000, 0.8660254037844387076, 1.000000000000000000, 0.8660254037844387076, 1.000000000000000000, 0.8660254037844387076, 1.000000000000000000, 0.8660254037844387076, 1.000000000000000000, 0.8660254037844387076, 1.000000000000000000, 0.8660254037844387076, 1.000000000000000000, 0.8660254037844387076, 1.000000000000000000, 0.8660254037844387076, 1.000000000000000000, 0.8660254037844387076, 1.000000000000000000, 0.8660254037844387076, 1.000000000000000000, 0.8660254037844387076, 1.000000000000000000, 0.8660254037844387076, 1.000000000000000000, 0.8660254037844387076, 1.000000000000000000, 0.8660254037844387076, 1.000000000000000000, 0.8660254037844387076, 1.000000000000000000, 0.8660254037844387076, 1.000000000000000000, 0.8660254037844387076, 1.000000000000000000, 0.8660254037844387076, 1.000000000000000000, 0.8660254037844387076, 1.000000000000000000, 0.8660254037844387076, 1.000000000000000000, 0.8660254037844387076, 1.000000000000000000, 0.8660254037844387076, 1.000000000000000000, 0.8660254037844387076, 1.000000000000000000, 0.8660254037844387076, 1.000000000000000000, 0.8660254037844387076, 1.000000000000000000, 0.8660254037844387076, 1.000000000000000000, 0.8660254037844387076, 1.000000000000000000, 0.8660254037844387076, 1.000000000000000000, 0.8660254037844387076, 1.000000000000000000, 0.8660254037844387076, 1.000000000000000000, 0.8660254037844387076, 1.000000000000000000, 0.8660254037844387076, 1.000000000000000000, 0.8660254037844387076, 1.000000000000000000, 0.8660254037844387076, 1.000000000000000000, 0.8660254037844387076, 1.000000000000000000, 0.8660254037844387076, 1.000000000000000000, 0.8660254037844387076, 1.000000000000000000, 0.8660254037844387076, 1.000000000000000000, 0.8660254037844387076, 1.000000000000000000, 0.8660254037844387076, 1.000000000000000000, 0.8660254037844387076, 1.000000000000000000, 0.8660254037844387076, 1.000000000000000000, 0.8660254037844387076, 1.000000000000000000, 0.8660254037844387076, 1.000000000000000000, 0.8660254037844387076, 1.000000000000000000, 0.8660254037844387076, 1.000000000000000000, 0.8660254037844387076, 1.000000000000000000, 0.8660254037844387076, 1.000000000000000000, 0.8660254037844387076, 1.000000000000000000, 0.8660254037844387076, 1.000000000000000000, 0.8660254037844387076, 1.000000000000000000, 0.8660254037844387076, 1.000000000000000000, 0.8660254037844387076, 1.000000000000000000, 0.8660254037844387076, 1.000000000000000000, 0.8660254037844387076, 1.000000000000000000, 0.8660254037844387076, 1.000000000000000000, 0.8660254037844387076, 1.000000000000000000, 0.8660254037844387076, 1.000000000000000000),
 ( 1.000000000000000000, 0.8660254037844387076, 1.000000000000000000, 0.8660254037844387076, 1.000000000000000000, 0.8660254037844387076, 1.000000000000000000, 0.8660254037844387076, 1.000000000000000000, 0.8660254037844387076, 1.000000000000000000, 0.8660254037844387076, 1.000000000000000000, 0.8660254037844387076, 1.000000000000000000, 0.8660254037844387076, 1.000000000000000000, 0.8660254037844387076, 1.000000000000000000, 0.8660254037844387076, 1.000000000000000000, 0.8660254037844387076, 1.000000000000000000, 0.8660254037844387076, 1.000000000000000000, 0.8660254037844387076, 1.000000000000000000, 0.8660254037844387076, 1.000000000000000000, 0.8660254037844387076, 1.000000000000000000, 0.8660254037844387076, 1.000000000000000000, 0.8660254037844387076, 1.000000000000000000, 0.8660254037844387076, 1.000000000000000000, 0.8660254037844387076, 1.000000000000000000, 0.8660254037844387076, 1.000000000000000000, 0.8660254037844387076, 1.000000000000000000, 0.8660254037844387076, 1.000000000000000000, 0.8660254037844387076, 1.000000000000000000, 0.8660254037844387076, 1.000000000000000000, 0.8660254037844387076, 1.000000000000000000, 0.8660254037844387076, 1.000000000000000000, 0.8660254037844387076, 1.000000000000000000, 0.8660254037844387076, 1.000000000000000000, 0.8660254037844387076, 1.000000000000000000, 0.8660254037844387076, 1.000000000000000000, 0.8660254037844387076, 1.000000000000000000, 0.8660254037844387076, 1.000000000000000000, 0.8660254037844387076, 1.000000000000000000, 0.8660254037844387076, 1.000000000000000000, 0.8660254037844387076, 1.000000000000000000, 0.8660254037844387076, 1.000000000000000000, 0.8660254037844387076, 1.000000000000000000, 0.8660254037844387076, 1.000000000000000000, 0.8660254037844387076, 1.000000000000000000, 0.8660254037844387076, 1.000000000000000000, 0.8660254037844387076, 1.000000000000000000, 0.8660254037844387076, 1.000000000000000000, 0.8660254037844387076, 1.000000000000000000, 0.8660254037844387076, 1.000000000000000000, 0.8660254037844387076, 1.000000000000000000, 0.8660254037844387076, 1.000000000000000000, 0.8660254037844387076, 1.000000000000000000, 0.8660254037844387076, 1.000000000000000000, 0.8660254037844387076, 1.000000000000000000, 0.8660254037844387076, 1.000000000000000000, 0.8660254037844387076, 1.000000000000000000, 0.8660254037844387076, 1.000000000000000000, 0.8660254037844387076, 1.000000000000000000, 0.8660254037844387076, 1.000000000000000000, 0.8660254037844387076, 1.000000000000000000, 0.8660254037844387076, 1.000000000000000000, 0.8660254037844387076, 1.000000000000000000, 0.8660254037844387076, 1.000000000000000000, 0.8660254037844387076, 1.000000000000000000, 0.8660254037844387076, 1.000000000000000000, 0.8660254037844387076, 1.000000000000000000, 0.8660254037844387076, 1.000000000000000000, 0.8660254037844387076, 1.000000000000000000, 0.8660254037844387076, 1.000000000000000000, 0.8660254037844387076, 1.000000000000000000, 0.8660254037844387076, 1.000000000000000000, 0.8660254037844387076, 1.000000000000000000, 0.8660254037844387076, 1.000000000000000000, 0.8660254037844387076, 1.000000000000000000, 0.8660254037844387076, 1.000000000000000000, 0.8660254037844387076, 1.000000000000000000, 0.8660254037844387076, 1.000000000000000000, 0.8660254037844387076, 1.000000000000000000, 0.8660254037844387076, 1.000000000000000000, 0.8660254037844387076, 1.000000000000000000, 0.8660254037844387076, 1.000000000000000000, 0.8660254037844387076, 1.000000000000000000, 0.8660254037844387076, 1.000000000000000000, 0.8660254037844387076, 1.000000000000000000, 0.8660254037844387076, 1.000000000000000000, 0.8660254037844387076, 1.000000000000000000, 0.8660254037844387076, 1.000000000000000000, 0.8660254037844387076, 1.000000000000000000, 0.8660254037844387076, 1.000000000000000000, 0.8660254037844387076, 1.000000000000000000, 0.8660254037844387076, 1.000000000000000000, 0.8660254037844387076, 1.000000000000000000, 0.8660254037844387076, 1.000000000000000000, 0.8660254037844387076, 1.000000000000000000, 0.8660254037844387076, 1.000000000000000000, 0.8660254037844387076, 1.000000000000000000, 0.8660254037844387076, 1.000000000000000000, 0.8660254037844387076, 1.000000000000000000, 0.8660254037844387076, 1.000000000000000000, 0.8660254037844387076, 1.000000000000000000, 0.8660254037844387076, 1.000000000000000000, 0.8660254037844387076, 1.000000000000000000, 0.8660254037844387076, 1.000000000000000000, 0.8660254037844387076, 1.000000000000000000, 0.8660254037844387076, 1.000000000000000000, 0.8660254037844387076, 1.000000000000000000, 0.8660254037844387076, 1.000000000000000000, 0.8660254037844387076, 1.000000000000000000, 0.8660254037844387076, 1.000000000000000000, 0.8660254037844387076, 1.000000000000000000, 0.8660254037844387076, 1.000000000000000000, 0.8660254037844387076, 1.000000000000000000, 0.8660254037844387076, 1.000000000000000000, 0.8660254037844387076, 1.000000000000000000, 0.8660254037844387076, 1.000000000000000000, 0.8660254037844387076, 1.000000000000000000, 0.8660254037844387076, 1.000000000000000000, 0.8660254037844387076, 1.000000000000000000, 0.8660254037844387076, 1.000000000000000000, 0.8660254037844387076, 1.000000000000000000, 0.8660254037844387076, 1.000000000000000000, 0.8660254037844387076, 1.000000000000000000, 0.8660254037844387076, 1.000000000000000000, 0.8660254037844387076, 1.000000000000000000, 0.8660254037844387076, 1.000000000000000000, 0.8660254037844387076, 1.000000000000000000, 0.8660254037844387076, 1.000000000000000000, 0.8660254037844387076, 1.000000000000000000, 0.8660254037844387076, 1.000000000000000000, 0.8660254037844387076, 1.000000000000000000, 0.8660254037844387076, 1.000000000000000000, 0.8660254037844387076, 1.000000000000000000, 0.8660254037844387076, 1.000000000000000000, 0.8660254037844387076, 1.000000000000000000, 0.8660254037844387076, 1.000000000000000000, 0.8660254037844387076, 1.000000000000000000, 0.8660254037844387076, 1.000000000000000000, 0.8660254037844387076, 1.000000000000000000, 0.8660254037844387076, 1.000000000000000000, 0.8660254037844387076, 1.000000000000000000, 0.8660254037844387076, 1.000000000000000000, 0.8660254037844387076, 1.000000000000000000, 0.8660254037844387076, 1.000000000000000000, 0.8660254037844387076, 1.000000000000000000, 0.8660254037844387076, 1.000000000000000000, 0.8660254037844387076, 1.000000000000000000, 0.8660254037844387076, 1.000000000000000000, 0.8660254037844387076, 1.000000000000000000, 0.8660254037844387076, 1.000000000000000000, 0.8660254037844387076, 1.000000000000000000, 0.8660254037844387076, 1.000000000000000000, 0.8660254037844387076, 1.000000000000000000, 0.8660254037844387076, 1.000000000000000000, 0.8660254037844387076, 1.000000000000000000, 0.8660254037844387076, 1.000000000000000000, 0.8660254037844387076, 1.000000000000000000, 0.8660254037844387076, 1.000000000000000000, 0.8660254037844387076, 1.000000000000000000, 0.8660254037844387076, 1.000000000000000000, 0.8660254037844387076, 1.000000000000000000, 0.8660254037844387076, 1.000000000000000000, 0.8660254037844387076, 1.000000000000000000, 0.8660254037844387076, 1.000000000000000000, 0.8660254037844387076, 1.000000000000000000, 0.8660254037844387076, 1.000000000000000000, 0.8660254037844387076, 1.000000000000000000, 0.8660254037844387076, 1.000000000000000000, 0.8660254037844387076, 1.000000000000000000, 0.8660254037844387076, 1.000000000000000000, 0.8660254037844387076, 1.000000000000000000, 0.8660254037844387076, 1.000000000000000000, 0.8660254037844387076, 1.000000000000000000, 0.8660254037844387076, 1.000000000000000000, 0.8660254037844387076, 1.000000000000000000, 0.8660254037844387076, 1.000000000000000000, 0.8660254037844387076, 1.000000000000000000, 0.8660254037844387076, 1.000000000000000000, 0.8660254037844387076, 1.000000000000000000, 0.8660254037844387076, 1.000000000000000000, 0.8660254037844387076, 1.000000000000000000, 0.8660254037844387076, 1.000000000000000000, 0.8660254037844387076, 1.000000000000000000, 0.8660254037844387076, 1.000000000000000000, 0.8660254037844387076, 1.000000000000000000, 0.8660254037844387076, 1.000000000000000000, 0.8660254037844387076, 1.000000000000000000, 0.8660254037844387076, 1.000000000000000000, 0.8660254037844387076, 1.000000000000000000, 0.8660254037844387076, 1.000000000000000000, 0.8660254037844387076, 1.000000000000000000, 0.8660254037844387076, 1.000000000000000000, 0.8660254037844387076, 1.000000000000000000, 0.8660254037844387076, 1.000000000000000000, 0.8660254037844387076, 1.000000000000000000, 0.8660254037844387076, 1.000000000000000000, 0.8660254037844387076, 1.000000000000000000, 0.8660254037844387076, 1.000000000000000000, 0.8660254037844387076, 1.000000000000000000, 0.8660254037844387076, 1.000000000000000000, 0.8660254037844387076, 1.000000000000000000, 0.8660254037844387076, 1.000000000000000000, 0.8660254037844387076, 1.000000000000000000, 0.8660254037844387076, 1.000000000000000000, 0.8660254037844387076, 1.000000000000000000, 0.8660254037844387076, 1.000000000000000000, 0.8660254037844387076, 1.000000000000000000, 0.8660254037844387076, 1.000000000000000000, 0.8660254037844387076, 1.000000000000000000, 0.8660254037844387076, 1.000000000000000000, 0.8660254037844387076, 1.000000000000000000, 0.8660254037844387076, 1.000000000000000000, 0.8660254037844387076, 1.000000000000000000, 0.8660254037844387076, 1.000000000000000000, 0.8660254037844387076, 1.000000000000000000, 0.8660254037844387076, 1.000000000000000000, 0.8660254037844387076, 1.000000000000000000, 0.8660254037844387076, 1.000000000000000000, 0.8660254037844387076, 1.000000000000000000, 0.8660254037844387076, 1.000000000000000000, 0.8660254037844387076, 1.000000000000000000, 0.8660254037844387076, 1.000000000000000000, 0.8660254037844387076, 1.000000000000000000, 0.8660254037844387076, 1.000000000000000000, 0.8660254037844387076, 1.000000000000000000, 0.8660254037844387076, 1.000000000000000000, 0.8660254037844387076, 1.000000000000000000, 0.8660254037844387076, 1.000000000000000000, 0.8660254037844387076, 1.000000000000000000, 0.8660254037844387076, 1.000000000000000000, 0.8660254037844387076, 1.000000000000000000, 0.8660254037844387076, 1.000000000000000000, 0.8660254037844387076, 1.000000000000000000, 0.8660254037844387076, 1.000000000000000000, 0.8660254037844387076, 1.000000000000000000, 0.8660254037844387076, 1.000000000000000000, 0.8660254037844387076, 1.000000000000000000, 0.8660254037844387076, 1.000000000000000000, 0.8660254037844387076, 1.000000000000000000, 0.8660254037844387076, 1.000000000000000000, 0.8660254037844387076, 1.000000000000000000, 0.8660254037844387076, 1.000000000000000000, 0.8660254037844387076, 1.000000000000000000, 0.8660254037844387076, 1.000000000000000000, 0.8660254037844387076, 1.000000000000000000, 0.8660254037844387076, 1.000000000000000000) ) ) 
 REPRESENTATION_ITEM ( '' )  SURFACE ( )  );
#202191=CARTESIAN_POINT ( 'NONE',  ( -6.724481002698115439, 10.78905223654906109, -0.7216878364870267237 ) ) ;
#202193=CARTESIAN_POINT ( 'NONE',  ( 4.774442650306744085, 8.721933525333202653, -0.7998128361456281477 ) ) ;
#202196=CARTESIAN_POINT ( 'NONE',  ( -8.286004436246233951, 12.81875560892930466, 1.040834085586084257E-14 ) ) ;
#202201=CARTESIAN_POINT ( 'NONE',  ( -3.810004860640155311, 4.403759411290286252, 1.199719254218462483 ) ) ;
#202205=CARTESIAN_POINT ( 'NONE',  ( 8.910733272679570049, 11.41894145625809820, -1.599625672291255185 ) ) ;
#202206=CARTESIAN_POINT ( 'NONE',  ( 2.855963913973019963, 6.483708332943829866, 0.000000000000000000 ) ) ;
#202212=CARTESIAN_POINT ( 'NONE',  ( 4.690757960648234359, 4.574898496952131133, 0.7216878364870317197 ) ) ;
#202215=CARTESIAN_POINT ( 'NONE',  ( -3.744022975668147790, 7.519777238254810925, -0.7998128361456281477 ) ) ;
#202218=CARTESIAN_POINT ( 'NONE',  ( -7.960608749518247151, 12.43912730774665576, 0.000000000000000000 ) ) ;
#202223=CARTESIAN_POINT ( 'NONE',  ( 8.758204044748005401, 10.28062147603659504, 1.082531754730549967 ) ) ;
#202224=CARTESIAN_POINT ( 'NONE',  ( 1.364683531249990311, 4.946875000341417916, 1.214306433183764966E-14 ) ) ;
#202227=CARTESIAN_POINT ( 'NONE',  ( 4.660252114795294887, 6.460046772059735432, -1.599625672291256295 ) ) ;
#202233=DIRECTION ( 'NONE',  ( 0.9782075119096779181, 0.1245777785628398998, -0.1661037047504532738 ) ) ;
#202240=CARTESIAN_POINT ( 'NONE',  ( 1.364683531249990311, 3.196875000341416140, 1.214306433183764966E-14 ) ) ;
#202243=CARTESIAN_POINT ( 'NONE',  ( 8.920375002787457319, 12.49452237230570084, 1.199719254218450271 ) ) ;
#202245=CARTESIAN_POINT ( 'NONE',  ( -5.775410249741523394, 5.840326167560965231, 0.7216878364870317197 ) ) ;
#202248=CARTESIAN_POINT ( 'NONE',  ( -6.521108698048791119, 6.710307690586118312, -0.7216878364870267237 ) ) ;
#202249=CARTESIAN_POINT ( 'NONE',  ( 3.469446951953614189E-15, 5.900000000000023448, 1.214306433183764966E-14 ) ) ;
#202254=CARTESIAN_POINT ( 'NONE',  ( 4.299907273828439180, 8.168308919441841454, 1.040834085586084257E-14 ) ) ;
#202264=CARTESIAN_POINT ( 'NONE',  ( 5.632522751473472589, 8.658694745772667289, -1.199719254218440723 ) ) ;
#202266=CARTESIAN_POINT ( 'NONE',  ( -3.789667630219657912, 4.380032642466370696, 1.199719254218462483 ) ) ;
#202268=CARTESIAN_POINT ( 'NONE',  ( -6.911959384868566758, 6.958374125301778790, 1.040834085586084257E-14 ) ) ;
#202272=CARTESIAN_POINT ( 'NONE',  ( 6.479907352327590964, 9.647310113435821677, 1.199719254218462483 ) ) ;
#202275=CARTESIAN_POINT ( 'NONE',  ( -6.093499974338126179, 9.196501505781426999, -1.199719254218440723 ) ) ;
#202276=CARTESIAN_POINT ( 'NONE',  ( 7.592202833528386208, 7.959917515312338487, 1.040834085586084257E-14 ) ) ;
#202277=CARTESIAN_POINT ( 'NONE',  ( 4.188544580023894071, 7.586160867502751870, 0.8937768461303140510 ) ) ;
#202278=CARTESIAN_POINT ( 'NONE',  ( -2.950870989268691957, 6.594433254122103349, -0.7998128361456281477 ) ) ;
#202281=CARTESIAN_POINT ( 'NONE',  ( -4.737684612971557740, 7.614716917520386374, 1.199719254218464037 ) ) ;
#202285=CARTESIAN_POINT ( 'NONE',  ( 1.364683531249988757, 2.384375000341422357, 1.214306433183764966E-14 ) ) ;
#202287=CARTESIAN_POINT ( 'NONE',  ( -4.446711195602239819, 8.131654128270509929, -0.7216878364870267237 ) ) ;
#202292=CARTESIAN_POINT ( 'NONE',  ( -1.436838838544729491, 7.449283400311743186, -4.203727439823575551 ) ) ;
#202293=CARTESIAN_POINT ( 'NONE',  ( 7.305145839664861640, 7.417091655897478653, 0.7998128361456341429 ) ) ;
#202296=CARTESIAN_POINT ( 'NONE',  ( -1.364683531250012516, 2.551041667008089320, -0.7879004041258289570 ) ) ;
#202299=CARTESIAN_POINT ( 'NONE',  ( 0.6823417656249882723, -0.8447916663252494907, 1.181850606188755259 ) ) ;
#202300=CARTESIAN_POINT ( 'NONE',  ( 3.092648394857516525, 6.449253795920727228, -0.4031905389056261724 ) ) ;
#202303=CARTESIAN_POINT ( 'NONE',  ( -4.948889764188092677, 5.732458465429559169, 1.199719254218462483 ) ) ;
#202304=CARTESIAN_POINT ( 'NONE',  ( -7.876924059415400414, 9.252461493148505411, 1.082531754730558626 ) ) ;
#202306=CARTESIAN_POINT ( 'NONE',  ( -0.6823417656250212460, 2.301041667008084435, 1.181850606188767472 ) ) ;
#202314=CARTESIAN_POINT ( 'NONE',  ( -8.175203438916030407, 8.640084888264587093, 0.7216878364870578100 ) ) ;
#202319=CARTESIAN_POINT ( 'NONE',  ( -7.659993601596726265, 8.039006744725394782, -0.7216878364870267237 ) ) ;
#202325=CARTESIAN_POINT ( 'NONE',  ( -1.201851678989727383E-14, 5.368750000682816825, -1.732050807568863648 ) ) ;
#202329=ORIENTED_EDGE ( 'NONE', *, *, #171612, .F. ) ;
#202333=CARTESIAN_POINT ( 'NONE',  ( -6.175902666224832416, 7.163973517805802160, -1.199719254218446718 ) ) ;
#202334=CARTESIAN_POINT ( 'NONE',  ( 2.998324526916512411, 6.649795714711241423, 0.000000000000000000 ) ) ;
#202337=CARTESIAN_POINT ( 'NONE',  ( 4.794779880727245036, 8.745660294157122649, -0.7998128361456281477 ) ) ;
#202342=CARTESIAN_POINT ( 'NONE',  ( -5.260200412422213923, 6.199617238323108737, -1.082531754730544860 ) ) ;
#202349=VERTEX_POINT ( 'NONE', #158078 ) ;
#202353=CARTESIAN_POINT ( 'NONE',  ( -1.364683531250000748, 1.259375000341421469, 0.000000000000000000 ) ) ;
#202355=CARTESIAN_POINT ( 'NONE',  ( -7.232384877886063990, 10.52520055992070525, -1.199719254218446718 ) ) ;
#202357=CARTESIAN_POINT ( 'NONE',  ( 7.416473721875251890, 8.611306416064660851, 1.199719254218462483 ) ) ;
#202359=CARTESIAN_POINT ( 'NONE',  ( -6.015013705957189316, 10.16926642359206134, 0.7998128361456481317 ) ) ;
#202362=CARTESIAN_POINT ( 'NONE',  ( -0.7500000000000006661, -0.8604166659838472508, -1.299038105676652011 ) ) ;
#202365=CARTESIAN_POINT ( 'NONE',  ( 8.107412671292035355, 10.48173408797264194, 1.443375672974076540 ) ) ;
#202366=EDGE_CURVE ( 'NONE', #68875, #110911, #151611, .T. ) ;
#202369=CARTESIAN_POINT ( 'NONE',  ( -1.364683531250000748, -0.4281249996585800854, 0.000000000000000000 ) ) ;
#202372=CARTESIAN_POINT ( 'NONE',  ( 8.080296363620359301, 8.529359967086321603, 1.040834085586084257E-14 ) ) ;
#202375=CARTESIAN_POINT ( 'NONE',  ( -6.724481002698138532, 6.947575379343695623, -0.7216878364870278340 ) ) ;
#202377=CARTESIAN_POINT ( 'NONE',  ( -0.6823417656249969321, 3.217708333674754062, -1.181850606188749264 ) ) ;
#202381=CARTESIAN_POINT ( 'NONE',  ( -5.747767057189642870, 8.793146435774861658, -1.199719254218440723 ) ) ;
#202382=CARTESIAN_POINT ( 'NONE',  ( -1.364683531249997417, 5.571875000341417916, 1.214306433183764966E-14 ) ) ;
#202388=CARTESIAN_POINT ( 'NONE',  ( 8.259941899223605333, 10.65968485389279508, -1.599625672291268286 ) ) ;
#202391=CARTESIAN_POINT ( 'NONE',  ( -1.499999999999997780, 2.650000000000020339, 1.214306433183764966E-14 ) ) ;
#202394=CARTESIAN_POINT ( 'NONE',  ( 1.499999999999990896, 5.306250000682820378, 1.214306433183764966E-14 ) ) ;
#202397=CARTESIAN_POINT ( 'NONE',  ( 6.982085921357777281, 7.248114451113292667, 1.040834085586084257E-14 ) ) ;
#202398=CARTESIAN_POINT ( 'NONE',  ( -1.364683531250014514, -1.157291666325248158, 0.7879004041258379498 ) ) ;
#202404=CARTESIAN_POINT ( 'NONE',  ( -1.500000000000013101, 0.4208333333333572068, 0.8660254037844403729 ) ) ;
#202405=CARTESIAN_POINT ( 'NONE',  ( 8.046927864910717432, 9.346836249606042202, 1.199719254218462483 ) ) ;
#202406=CARTESIAN_POINT ( 'NONE',  ( -7.831806290188425557, 12.28885777186185990, -0.7998128361456281477 ) ) ;
#202408=CARTESIAN_POINT ( 'NONE',  ( 0.6823417656249882723, -0.07395833299191079124, -1.181850606188749264 ) ) ;
#202409=CARTESIAN_POINT ( 'NONE',  ( 0.7499999999999902300, 1.733333333333357595, 1.299038105676657340 ) ) ;
#202411=CARTESIAN_POINT ( 'NONE',  ( 4.961394147597008697, 7.875711374583454827, -1.199719254218452047 ) ) ;
#202415=CARTESIAN_POINT ( 'NONE',  ( -0.7500000000000006661, 2.889583334016148974, -1.299038105676652011 ) ) ;
#202419=CARTESIAN_POINT ( 'NONE',  ( 1.364683531249990311, 5.613541667008087543, 0.7879004041258500513 ) ) ;
#202421=CARTESIAN_POINT ( 'NONE',  ( -6.184490626128011925, 10.36698949712469364, -0.7998128361456291469 ) ) ;
#202422=CARTESIAN_POINT ( 'NONE',  ( -5.260200412422208593, 7.159986452624450770, -1.443375672974053447 ) ) ;
#202424=CYLINDRICAL_SURFACE ( 'NONE', #42328, 1.500000000000000222 ) ;
#202430=CARTESIAN_POINT ( 'NONE',  ( 8.046927864910717432, 9.346836249606042202, 1.199719254218462483 ) ) ;
#202434=CARTESIAN_POINT ( 'NONE',  ( 6.927853306458749749, 8.145212281365775908, 1.082531754730558626 ) ) ;
#202438=CARTESIAN_POINT ( 'NONE',  ( -8.182509401047415309, 9.505014708432145909, 1.199719254218462483 ) ) ;
#202439=CARTESIAN_POINT ( 'NONE',  ( 6.654354466208897811, 6.657835053532175529, 0.7998128361456341429 ) ) ;
#202441=CARTESIAN_POINT ( 'NONE',  ( 0.9999999999999833467, 6.468705557303653819, 4.925226524755080604 ) ) ;
#202442=CARTESIAN_POINT ( 'NONE',  ( 4.142179624174931796, 4.791296635414242111, 1.199719254218464037 ) ) ;
#202448=LINE ( 'NONE', #37847, #109637 ) ;
#202449=CARTESIAN_POINT ( 'NONE',  ( -1.567523721964583450, 8.684745761082966808, -2.500978756717645357 ) ) ;
#202450=CARTESIAN_POINT ( 'NONE',  ( -3.633221978782290140, 6.222214161012547429, -1.082531754730549967 ) ) ;
#202451=VECTOR ( 'NONE', #202773, 1000.000000000000000 ) ;
#202452=CARTESIAN_POINT ( 'NONE',  ( 8.405692050792682224, 12.75046512599275772, -0.7216878364870328300 ) ) ;
#202455=CARTESIAN_POINT ( 'NONE',  ( -7.206322340863467346, 8.366129804884193888, 1.199719254218450271 ) ) ;
#202461=CARTESIAN_POINT ( 'NONE',  ( -6.320072162264675164, 10.52516795595079557, 0.7998128361456481317 ) ) ;
#202464=CARTESIAN_POINT ( 'NONE',  ( 5.477955196520937875, 6.401917805796054850, -1.218707208129303110 ) ) ;
#202466=ORIENTED_EDGE ( 'NONE', *, *, #62099, .F. ) ;
#202479=CARTESIAN_POINT ( 'NONE',  ( -6.344325816190970357, 9.489131654609717970, 1.199719254218452047 ) ) ;
#202482=CARTESIAN_POINT ( 'NONE',  ( 5.287316719649520991, 8.151991358691011769, -1.082531754730549078 ) ) ;
#202483=ORIENTED_EDGE ( 'NONE', *, *, #43620, .F. ) ;
#202484=CARTESIAN_POINT ( 'NONE',  ( 3.334942598837264960, 6.834590765378040444, 1.214306433183764966E-14 ) ) ;
#202487=CARTESIAN_POINT ( 'NONE',  ( -3.086452525405351643, 6.752611712948207057, 0.7998128361456341429 ) ) ;
#202491=CARTESIAN_POINT ( 'NONE',  ( -6.905180308061733996, 6.950465202360470052, 0.7998128361456341429 ) ) ;
#202492=CARTESIAN_POINT ( 'NONE',  ( 9.083072846151447166, 12.68433652289702884, 1.199719254218450271 ) ) ;
#202496=CARTESIAN_POINT ( 'NONE',  ( -9.826962411806732689, 10.35921099006301382, -0.7998128361456291469 ) ) ;
#202498=CARTESIAN_POINT ( 'NONE',  ( 7.884230021546724920, 9.157022099014721306, 1.199719254218462483 ) ) ;
#202501=CARTESIAN_POINT ( 'NONE',  ( -9.592557376868645846, 11.15007068022363157, -1.199719254218441611 ) ) ;
#202505=CARTESIAN_POINT ( 'NONE',  ( -0.6823417656250246877, -0.8864583329919115684, 1.181850606188755259 ) ) ;
#202509=CARTESIAN_POINT ( 'NONE',  ( 9.300530189294644146, 10.91333531134101165, -1.082531754730543083 ) ) ;
#202514=AXIS2_PLACEMENT_3D ( 'NONE', #10442, #27773, #111228 ) ;
#202527=CARTESIAN_POINT ( 'NONE',  ( -3.379006598303881059, 4.965260336153046516, -1.599625672291256295 ) ) ;
#202534=CARTESIAN_POINT ( 'NONE',  ( -1.364683531250010295, 5.530208333674751842, 0.7879004041258379498 ) ) ;
#202538=CARTESIAN_POINT ( 'NONE',  ( 10.40318394038753702, 11.03146944007395724, -0.7998128361456281477 ) ) ;
#202542=CARTESIAN_POINT ( 'NONE',  ( 6.938893903907228378E-15, 10.64264068711930733, 1.214306433183764966E-14 ) ) ;
#202543=CARTESIAN_POINT ( 'NONE',  ( 8.530051201292206287, 13.10347683481629488, 0.000000000000000000 ) ) ;
#202548=CARTESIAN_POINT ( 'NONE',  ( 5.931855901178834323, 6.879252291918818152, 1.199719254218462483 ) ) ;
#202549=CARTESIAN_POINT ( 'NONE',  ( 0.6823417656249899377, 3.155208333674754062, 1.181850606188765695 ) ) ;
#202550=CARTESIAN_POINT ( 'NONE',  ( -5.703936002245207249, 6.126809468943200443, 0.7377312291968595170 ) ) ;
#202553=CARTESIAN_POINT ( 'NONE',  ( -8.667740277838301921, 9.006785167099828016, -0.7998128361456291469 ) ) ;
#202554=CARTESIAN_POINT ( 'NONE',  ( -3.240035523541616502, 6.723865844199768738, 0.7216878364870317197 ) ) ;
#202557=CARTESIAN_POINT ( 'NONE',  ( -6.417086777969760902, 6.381022750586497594, 0.7998128361456341429 ) ) ;
#202559=CARTESIAN_POINT ( 'NONE',  ( -1.402160292154681736E-14, -0.5062499993171791779, 1.732050807568877637 ) ) ;
#202567=CARTESIAN_POINT ( 'NONE',  ( -5.409340101728186134, 5.413244328212063472, 0.7216878364870317197 ) ) ;
#202569=CARTESIAN_POINT ( 'NONE',  ( 0.4867935908847584314, 7.427453578140085888, -4.536604770854444801 ) ) ;
#202573=CARTESIAN_POINT ( 'NONE',  ( -3.999292125906916073, 5.688926785023260102, 1.443375672974064550 ) ) ;
#202575=CARTESIAN_POINT ( 'NONE',  ( 8.880754312151170282, 10.31963377138658089, 1.199719254218453823 ) ) ;
#202581=ORIENTED_EDGE ( 'NONE', *, *, #116347, .F. ) ;
#202584=CARTESIAN_POINT ( 'NONE',  ( -3.602716132929368875, 5.226254793216122074, 1.599625672291267398 ) ) ;
#202585=CARTESIAN_POINT ( 'NONE',  ( -8.123306592882240551, 12.62894145833798376, 0.000000000000000000 ) ) ;
#202590=CARTESIAN_POINT ( 'NONE',  ( 5.952193131599331721, 6.902979060742733708, 1.199719254218462483 ) ) ;
#202595=CARTESIAN_POINT ( 'NONE',  ( 6.961139734775133370, 5.290451655907104644, 1.214306433183764966E-14 ) ) ;
#202596=CARTESIAN_POINT ( 'NONE',  ( 3.891353782322113375, 4.498666486585943147, -1.199719254218446718 ) ) ;
#202606=CARTESIAN_POINT ( 'NONE',  ( 6.909851844459134362, 11.21324425184434936, -0.7998128361456291469 ) ) ;
#202609=CARTESIAN_POINT ( 'NONE',  ( -4.843287188579803448, 6.673587691474970107, -1.599625672291256295 ) ) ;
#202612=AXIS2_PLACEMENT_3D ( 'NONE', #192006, #20172, #104658 ) ;
#202617=CARTESIAN_POINT ( 'NONE',  ( 1.499999999999987121, -0.9645833326505173222, 0.8660254037844524744 ) ) ;
#202621=CARTESIAN_POINT ( 'NONE',  ( -5.710235717126113109, 6.137237704801142613, 0.8101758662225978513 ) ) ;
#202622=CARTESIAN_POINT ( 'NONE',  ( 3.032219910950674890, 6.689340329417765574, 0.7998128361456321445 ) ) ;
#202623=CARTESIAN_POINT ( 'NONE',  ( -5.274285450916075035, 6.112086766612214284, 1.199719254218450271 ) ) ;
#202629=CARTESIAN_POINT ( 'NONE',  ( 4.839897650398541806, 8.590371658866210680, 1.040834085586084257E-14 ) ) ;
#202632=ORIENTED_EDGE ( 'NONE', *, *, #187141, .F. ) ;
#202633=CARTESIAN_POINT ( 'NONE',  ( 8.907343734053986495, 9.494248565925552441, -0.7216878364870197293 ) ) ;
#202634=CARTESIAN_POINT ( 'NONE',  ( 0.6823417656249899377, 3.238541667008085323, -1.181850606188754593 ) ) ;
#202636=CARTESIAN_POINT ( 'NONE',  ( 3.660338285565247762, 7.214219066560688454, 1.040834085586084257E-14 ) ) ;
#202640=CARTESIAN_POINT ( 'NONE',  ( 5.459907696476232530, 6.251290254602066554, -1.005486610859710472 ) ) ;
#202643=B_SPLINE_CURVE_WITH_KNOTS ( 'NONE', 3,
 ( #177497, #29110, #12831, #62657, #128815, #194797, #46434, #59334, #39894, #192517 ),
 .UNSPECIFIED., .F., .F.,
 ( 4, 2, 2, 2, 4 ),
 ( 0.000000000000000000, 0.2499999999999999445, 0.4999999999999998890, 0.7499999999999997780, 1.000000000000000000 ),
 .UNSPECIFIED. ) ;
#202644=CARTESIAN_POINT ( 'NONE',  ( -4.432018112209435756, 7.309502936831247411, 1.252451368452773384 ) ) ;
#202651=CARTESIAN_POINT ( 'NONE',  ( -7.804689982961090955, 12.25722208009664094, 0.7998128361456481317 ) ) ;
#202656=CARTESIAN_POINT ( 'NONE',  ( -3.541704441667874903, 5.155074486744371853, -1.599625672291256295 ) ) ;
#202661=CARTESIAN_POINT ( 'NONE',  ( 1.364683531249990311, 3.196875000341416140, 1.214306433183764966E-14 ) ) ;
#202663=CARTESIAN_POINT ( 'NONE',  ( 5.913327553854682783, 10.05063257947248800, -0.7998128361456291469 ) ) ;
#202664=CARTESIAN_POINT ( 'NONE',  ( -8.696665468161981494, 12.23352791524263239, -1.199719254218446718 ) ) ;
#202666=CARTESIAN_POINT ( 'NONE',  ( -4.711622075948912247, 5.455646162483875017, -1.199719254218446718 ) ) ;
#202670=B_SPLINE_CURVE_WITH_KNOTS ( 'NONE', 3,
 ( #35847, #100849, #181041, #199399, #33718, #51046 ),
 .UNSPECIFIED., .F., .F.,
 ( 4, 2, 4 ),
 ( 0.000000000000000000, 0.002109688543090479894, 0.004219377086180959788 ),
 .UNSPECIFIED. ) ;
#202672=CARTESIAN_POINT ( 'NONE',  ( -1.001543065824772872E-14, 4.462500000000024336, 1.732050807568877637 ) ) ;
#202673=CARTESIAN_POINT ( 'NONE',  ( 6.010342169559767633, 5.906487374108181143, -0.7998128361456281477 ) ) ;
#202677=CARTESIAN_POINT ( 'NONE',  ( -0.6823417656249969321, 3.467708333674754506, -1.181850606188749264 ) ) ;
#202681=CARTESIAN_POINT ( 'NONE',  ( 8.866669273657322492, 12.32790267170016207, -1.082531754730543083 ) ) ;
#202686=CARTESIAN_POINT ( 'NONE',  ( -1.402160292154681736E-14, 2.118750000682816825, -1.732050807568863648 ) ) ;
#202688=CARTESIAN_POINT ( 'NONE',  ( -5.416646063859567484, 6.278174148379618735, 1.199719254218450271 ) ) ;
#202689=CARTESIAN_POINT ( 'NONE',  ( 4.161989969270895706, 5.878740935614591656, 1.443375672974062551 ) ) ;
#202698=CARTESIAN_POINT ( 'NONE',  ( 8.294891053462476904, 8.571794405328034827, 1.040834085586084257E-14 ) ) ;
#202699=CARTESIAN_POINT ( 'NONE',  ( 3.310162060030825248, 7.013606170011280838, -0.7998128361456291469 ) ) ;
#202702=CARTESIAN_POINT ( 'NONE',  ( -3.673896439623305810, 4.156855427197417185, -7.499999999999991118 ) ) ;
#202703=CARTESIAN_POINT ( 'NONE',  ( 3.520313441042647540, 7.258782781191745137, 0.7998128361456321445 ) ) ;
#202709=CARTESIAN_POINT ( 'NONE',  ( 9.836604141914616406, 11.43479190611061647, 1.199719254218452047 ) ) ;
#202714=CARTESIAN_POINT ( 'NONE',  ( 5.888650760256147088, 5.979308965038350188, -0.1076000636002025918 ) ) ;
#202716=CARTESIAN_POINT ( 'NONE',  ( 9.541187415715040032, 12.15447128979948310, -1.599625672291262513 ) ) ;
#202718=DIRECTION ( 'NONE',  ( 5.578564026256490882E-16, 1.000000000000000000, 9.066213480720158442E-32 ) ) ;
#202719=CARTESIAN_POINT ( 'NONE',  ( -5.314433026876900001, 6.262888621853549331, 1.082531754730548412 ) ) ;
#202722=CARTESIAN_POINT ( 'NONE',  ( 6.887178846062110615, 9.058127958537705027, -1.443375672974057666 ) ) ;
#202723=CARTESIAN_POINT ( 'NONE',  ( -2.981903720001798597, 5.566305875722335372, -1.199719254218446718 ) ) ;
#202728=CARTESIAN_POINT ( 'NONE',  ( -4.741601036477307574, 6.554953847355395880, 1.599625672291267398 ) ) ;
#202730=CARTESIAN_POINT ( 'NONE',  ( -3.642287698956932829, 3.120124397464415278, 2.500000000000464961 ) ) ;
#202742=CARTESIAN_POINT ( 'NONE',  ( 9.433775957010412938, 9.900493459467314850, 0.000000000000000000 ) ) ;
#202743=CARTESIAN_POINT ( 'NONE',  ( 5.714115171586898079, 6.274818061858235652, 1.066218439657661721 ) ) ;
#202748=CARTESIAN_POINT ( 'NONE',  ( -4.302014814237876017, 3.913438792899272212, 0.7998128361456341429 ) ) ;
#202752=CARTESIAN_POINT ( 'NONE',  ( 8.263858322729371153, 9.599921783727809910, -1.199719254218446718 ) ) ;
#202754=DIRECTION ( 'NONE',  ( -0.7592566023652995710, -0.6507913734559652719, 0.000000000000000000 ) ) ;
#202756=CARTESIAN_POINT ( 'NONE',  ( -6.413170354464012846, 7.440785820751486312, 1.199719254218450271 ) ) ;
#202757=CARTESIAN_POINT ( 'NONE',  ( 5.820528018968444961, 5.685037531751635953, 0.7998128361456341429 ) ) ;
#202763=CARTESIAN_POINT ( 'NONE',  ( 0.5155926040970099100, 6.713058329651131473, 3.584077772868219380 ) ) ;
#202766=CARTESIAN_POINT ( 'NONE',  ( 4.313480937648101587, 7.206793636360196764, -1.001376897629567830 ) ) ;
#202769=CARTESIAN_POINT ( 'NONE',  ( 4.799223189557548785, 7.582548906917042864, -1.082531754730549078 ) ) ;
#202773=DIRECTION ( 'NONE',  ( -5.578564026256490882E-16, -1.000000000000000000, -9.066213480720158442E-32 ) ) ;
#202776=ORIENTED_EDGE ( 'NONE', *, *, #206253, .T. ) ;
#202777=CARTESIAN_POINT ( 'NONE',  ( 9.219181267168295335, 9.858059021225592744, 1.040834085586084257E-14 ) ) ;
#202782=CARTESIAN_POINT ( 'NONE',  ( -7.395082721250053837, 10.71501471051202614, -1.199719254218446718 ) ) ;
#202791=CARTESIAN_POINT ( 'NONE',  ( 9.836604141914616406, 11.43479190611061647, 1.199719254218452047 ) ) ;
#202795=CARTESIAN_POINT ( 'NONE',  ( 3.635557746758808495, 7.393234471193928847, -0.7998128361456291469 ) ) ;
#202799=CARTESIAN_POINT ( 'NONE',  ( -1.201851678989727383E-14, 2.243750000682818158, 1.732050807568877637 ) ) ;
#202805=CARTESIAN_POINT ( 'NONE',  ( -1.500000000000013101, 1.170833333333352710, 0.8660254037844403729 ) ) ;
#202806=CARTESIAN_POINT ( 'NONE',  ( 7.558834334818744338, 8.777393797832065303, 1.199719254218462483 ) ) ;
#202807=CARTESIAN_POINT ( 'NONE',  ( 4.243338890952890630, 5.973648010910253880, -1.443375672974051449 ) ) ;
#202811=CARTESIAN_POINT ( 'NONE',  ( 8.270110514656021650, 11.63191745286530576, 1.082531754730557072 ) ) ;
#202816=CARTESIAN_POINT ( 'NONE',  ( -5.687809136132860210, 6.594531066031826150, -1.199719254218446718 ) ) ;
#202817=CARTESIAN_POINT ( 'NONE',  ( -1.201851678989727383E-14, 4.368750000682820378, -1.732050807568863648 ) ) ;
#202818=CARTESIAN_POINT ( 'NONE',  ( 0.6823417656249917140, 4.905208333674755394, 1.181850606188765695 ) ) ;
#202823=CARTESIAN_POINT ( 'NONE',  ( -1.201851678989727383E-14, 4.509375000341417916, -1.575800808251660134 ) ) ;
#202829=CARTESIAN_POINT ( 'NONE',  ( -4.243338890952901288, 6.934017225211593249, -1.082531754730548412 ) ) ;
#202831=CARTESIAN_POINT ( 'NONE',  ( -6.516665389662827934, 10.75452672124865217, 0.000000000000000000 ) ) ;
#202832=CARTESIAN_POINT ( 'NONE',  ( 7.305145839664861640, 7.417091655897478653, 0.7998128361456341429 ) ) ;
#202834=DIRECTION ( 'NONE',  ( 3.347138415753902517E-16, 0.6000000000000018652, 0.7999999999999984901 ) ) ;
#202841=CARTESIAN_POINT ( 'NONE',  ( -7.555971681517696936, 7.709721804725773175, 0.7998128361456462443 ) ) ;
#202846=CARTESIAN_POINT ( 'NONE',  ( 9.738834413317897898, 10.25639499182604730, 0.000000000000000000 ) ) ;
#202848=VERTEX_POINT ( 'NONE', #13110 ) ;
#202849=CARTESIAN_POINT ( 'NONE',  ( -4.497554271431319250, 6.270232621468402989, -1.599625672291256295 ) ) ;
#202850=CARTESIAN_POINT ( 'NONE',  ( -6.170932472514347289, 10.35117165124207972, 0.000000000000000000 ) ) ;
#202853=CARTESIAN_POINT ( 'NONE',  ( -3.990254785474510513, 7.829054500403880290, -0.2746884413801879976 ) ) ;
#202860=CARTESIAN_POINT ( 'NONE',  ( 5.035963992472171746, 7.962709526937818083, 1.199719254218462483 ) ) ;
#202861=ADVANCED_FACE ( 'NONE', ( #77045 ), #193995, .T. ) ;
#202880=CARTESIAN_POINT ( 'NONE',  ( 4.184706906422049677, 7.590773377626947038, -0.8858016570119742195 ) ) ;
#202881=ORIENTED_EDGE ( 'NONE', *, *, #175529, .T. ) ;
#202883=CARTESIAN_POINT ( 'NONE',  ( -8.123306592882240551, 12.62894145833798376, 0.000000000000000000 ) ) ;
#202889=B_SPLINE_CURVE_WITH_KNOTS ( 'NONE', 3,
 ( #161295, #80028, #130988, #127821 ),
 .UNSPECIFIED., .F., .F.,
 ( 4, 4 ),
 ( 4.470280076681866734E-19, 0.0001925329755551839501 ),
 .UNSPECIFIED. ) ;
#202890=CARTESIAN_POINT ( 'NONE',  ( -1.201851678989727383E-14, 1.493750000682814383, 1.732050807568877637 ) ) ;
#202891=CARTESIAN_POINT ( 'NONE',  ( 7.879259827836241570, 12.34422023245099176, 1.040834085586084257E-14 ) ) ;
#202895=CARTESIAN_POINT ( 'NONE',  ( -8.631737353394710155, 13.22211067893587533, 1.040834085586084257E-14 ) ) ;
#202897=CARTESIAN_POINT ( 'NONE',  ( -1.364683531250012516, 2.280208333674751842, 0.7879004041258379498 ) ) ;
#202904=CARTESIAN_POINT ( 'NONE',  ( -8.649738815838677652, 13.03518635187974262, 0.7216878364870357165 ) ) ;
#202910=CARTESIAN_POINT ( 'NONE',  ( 0.6823417656249899377, 0.6552083336747518416, 1.181850606188755259 ) ) ;
#202915=CARTESIAN_POINT ( 'NONE',  ( -1.364683531250014514, 0.2385416670080863499, -0.7879004041258359514 ) ) ;
#202918=CARTESIAN_POINT ( 'NONE',  ( -5.065942953000576843, 9.062017211809330064, -0.7998128361456231517 ) ) ;
#202919=CARTESIAN_POINT ( 'NONE',  ( 8.911787042884274257, 9.291506392986812912, 0.7998128361456462443 ) ) ;
#202921=CARTESIAN_POINT ( 'NONE',  ( 6.654354466208897811, 6.657835053532175529, 0.7998128361456341429 ) ) ;
#202923=CARTESIAN_POINT ( 'NONE',  ( 0.7499999999999902300, 3.233333333333352044, 1.299038105676669330 ) ) ;
#202925=EDGE_CURVE ( 'NONE', #31219, #10132, #113024, .T. ) ;
#202927=CARTESIAN_POINT ( 'NONE',  ( -1.364683531250012516, 1.092708333674754506, 0.7879004041258379498 ) ) ;
#202932=CARTESIAN_POINT ( 'NONE',  ( 4.989037340148863464, 8.764367963574922982, -0.7216878364870257245 ) ) ;
#202935=CARTESIAN_POINT ( 'NONE',  ( -8.636707547105197946, 10.03491254549959777, -1.199719254218446718 ) ) ;
#202936=CARTESIAN_POINT ( 'NONE',  ( -2.754277761870538299, 6.365074488824250309, 1.040834085586084257E-14 ) ) ;
#202940=DIRECTION ( 'NONE',  ( -7.387867266669436732E-31, 1.000000000000000000, 8.546850786086424434E-32 ) ) ;
#202941=CARTESIAN_POINT ( 'NONE',  ( -9.137832345486311070, 9.763151945929928743, 1.040834085586084257E-14 ) ) ;
#202943=CARTESIAN_POINT ( 'NONE',  ( -1.001543065824772872E-14, 5.712500000000021672, 1.732050807568877637 ) ) ;
#202947=CARTESIAN_POINT ( 'NONE',  ( 7.782016984564043227, 12.02284421539267356, 0.7216878364870438212 ) ) ;
#202949=CARTESIAN_POINT ( 'NONE',  ( -4.785665035499573783, 5.645992631913323123, 1.082531754730558626 ) ) ;
#202963=CARTESIAN_POINT ( 'NONE',  ( 8.717529583462654941, 9.272798723569005475, 0.7216878364870458196 ) ) ;
#202964=CARTESIAN_POINT ( 'NONE',  ( 7.613066949273408213, 8.840665181362512115, -1.199719254218441611 ) ) ;
#202965=CARTESIAN_POINT ( 'NONE',  ( -5.259673527097670664, 8.223703984000886535, -1.199719254218446718 ) ) ;
#202968=CARTESIAN_POINT ( 'NONE',  ( -4.103031383223492590, 3.978538327596326862, -0.5488639320762221940 ) ) ;
#202969=CARTESIAN_POINT ( 'NONE',  ( 1.364683531249986537, -0.8239583329919186738, 0.7879004041258500513 ) ) ;
#202970=CARTESIAN_POINT ( 'NONE',  ( 3.389175213736292047, 5.937492935125556315, 1.082531754730558626 ) ) ;
#202972=CARTESIAN_POINT ( 'NONE',  ( -2.785310492603665367, 5.336947110424484109, 1.199719254218462483 ) ) ;
#202984=B_SPLINE_CURVE_WITH_KNOTS ( 'NONE', 3,
 ( #30562, #176797, #31626, #196252 ),
 .UNSPECIFIED., .F., .F.,
 ( 4, 4 ),
 ( 0.000000000000000000, 0.0005592965258961650823 ),
 .UNSPECIFIED. ) ;
#202988=CARTESIAN_POINT ( 'NONE',  ( 6.909851844459134362, 11.21324425184434936, -0.7998128361456291469 ) ) ;
#202994=CARTESIAN_POINT ( 'NONE',  ( 1.445103857048099405, 8.688264192037884470, 2.625611233228254626 ) ) ;
#203000=CARTESIAN_POINT ( 'NONE',  ( -5.168682875307782254, 7.053215992657626110, -1.599625672291256295 ) ) ;
#203002=CARTESIAN_POINT ( 'NONE',  ( -4.928552533767591726, 5.708731696605642725, 1.199719254218462483 ) ) ;
#203011=CARTESIAN_POINT ( 'NONE',  ( -4.776550190716183586, 4.467063398790632966, 1.214306433183764966E-14 ) ) ;
#203014=CARTESIAN_POINT ( 'NONE',  ( 8.274553823041976841, 8.548067636504127265, 1.040834085586084257E-14 ) ) ;
#203015=CARTESIAN_POINT ( 'NONE',  ( -1.364683531250012516, 4.238541667008089320, -0.7879004041258300672 ) ) ;
#203021=CARTESIAN_POINT ( 'NONE',  ( 4.785665035499516051, 8.527100274817353665, -0.7216878364870207285 ) ) ;
#203022=CARTESIAN_POINT ( 'NONE',  ( -6.347188469492005325, 10.55680364771601809, -0.7998128361456291469 ) ) ;
#203025=CARTESIAN_POINT ( 'NONE',  ( -8.342344591110322227, 8.627156865917170236, -0.7998128361456291469 ) ) ;
#203027=CARTESIAN_POINT ( 'NONE',  ( -5.599681137644054729, 6.491715067794862293, 1.199719254218450271 ) ) ;
#203031=CARTESIAN_POINT ( 'NONE',  ( 3.946537740505243974, 2.817530495244580102, -0.7749999999999935829 ) ) ;
#203034=CARTESIAN_POINT ( 'NONE',  ( 7.100719765255169236, 9.307259030929609267, -1.599625672291262513 ) ) ;
#203048=CARTESIAN_POINT ( 'NONE',  ( -1.001543065824772872E-14, 5.462500000000020783, 1.732050807568877637 ) ) ;
#203049=CARTESIAN_POINT ( 'NONE',  ( 3.174580523894166006, 6.855427711185178019, 0.7998128361456341429 ) ) ;
#203050=CARTESIAN_POINT ( 'NONE',  ( 5.494078562035752178, 7.432844293840273231, -1.599625672291262513 ) ) ;
#203052=CARTESIAN_POINT ( 'NONE',  ( -7.375272376154077492, 11.54830883891436422, -0.7216878364870267237 ) ) ;
#203053=CARTESIAN_POINT ( 'NONE',  ( 5.910991785878156435, 7.919243054989755670, -1.443375672974057666 ) ) ;
#203054=CARTESIAN_POINT ( 'NONE',  ( -7.280365300414089802, 10.47721470291632784, 1.082531754730549967 ) ) ;
#203059=CARTESIAN_POINT ( 'NONE',  ( 8.450809820019639318, 8.753699632978056755, -0.7998128361456291469 ) ) ;
#203064=CARTESIAN_POINT ( 'NONE',  ( -1.201851678989727383E-14, 2.321875000341416584, 1.575800808251672791 ) ) ;
#203070=CARTESIAN_POINT ( 'NONE',  ( 7.964525173024008531, 11.37936423758166526, 1.199719254218460707 ) ) ;
#203074=CARTESIAN_POINT ( 'NONE',  ( -9.341731535015849630, 10.85744053139533349, 1.199719254218462483 ) ) ;
#203079=CARTESIAN_POINT ( 'NONE',  ( 3.704402285031850539, 5.344888637335695414, -1.599625672291262513 ) ) ;
#203082=CARTESIAN_POINT ( 'NONE',  ( -7.818248136574758256, 12.27303992597924420, 0.000000000000000000 ) ) ;
#203088=CARTESIAN_POINT ( 'NONE',  ( 5.421662447778366811, 6.277071961296246450, 1.037714289653376198 ) ) ;
#203090=CARTESIAN_POINT ( 'NONE',  ( -4.660252114795309097, 6.460046772059735432, -1.599625672291256295 ) ) ;
#203094=CARTESIAN_POINT ( 'NONE',  ( 5.750629710490689384, 9.860818428881154674, -0.7998128361456291469 ) ) ;
#203096=CARTESIAN_POINT ( 'NONE',  ( 6.368579470117202490, 8.453095353268645695, 1.599625672291281386 ) ) ;
#203097=CARTESIAN_POINT ( 'NONE',  ( 4.985647801523278133, 6.839675073242382553, -1.599625672291256295 ) ) ;
#203099=CARTESIAN_POINT ( 'NONE',  ( -7.348156068926747331, 11.51667314714914347, 0.7216878364870458196 ) ) ;
#203107=CARTESIAN_POINT ( 'NONE',  ( -5.343048727742272241, 6.363526295613923800, -1.106837213068444292 ) ) ;
#203110=FACE_OUTER_BOUND ( 'NONE', #166879, .T. ) ;
#203111=CARTESIAN_POINT ( 'NONE',  ( 5.992340707560160240, 7.053780915984068756, 1.082531754730558626 ) ) ;
#203113=CARTESIAN_POINT ( 'NONE',  ( 9.368847842243145152, 10.88907622316056312, 1.199719254218453823 ) ) ;
#203118=CARTESIAN_POINT ( 'NONE',  ( -10.42585693878457853, 11.26584730477792284, -0.7216878364870267237 ) ) ;
#203125=ORIENTED_EDGE ( 'NONE', *, *, #165463, .T. ) ;
#203137=CARTESIAN_POINT ( 'NONE',  ( 6.934105498385400246, 10.17720795050327354, -1.199719254218441611 ) ) ;
#203141=CARTESIAN_POINT ( 'NONE',  ( 0.7499999999999902300, 1.514583334016148086, 1.299038105676657340 ) ) ;
#203142=CARTESIAN_POINT ( 'NONE',  ( -3.379006598303881059, 4.965260336153046516, -1.599625672291256295 ) ) ;
#203143=CARTESIAN_POINT ( 'NONE',  ( -4.218558352146454915, 8.073401844146177453, 1.040834085586084257E-14 ) ) ;
#203146=CARTESIAN_POINT ( 'NONE',  ( -8.622095623286845978, 12.14652976288826913, 1.199719254218462483 ) ) ;
#203149=CARTESIAN_POINT ( 'NONE',  ( -0.7499999999999972244, 5.639583334016151639, -1.299038105676652899 ) ) ;
#203150=CARTESIAN_POINT ( 'NONE',  ( 5.587931867126699537, 9.671004278289832001, -0.7998128361456291469 ) ) ;
#203152=CARTESIAN_POINT ( 'NONE',  ( -6.015013705957189316, 10.16926642359206134, 0.7998128361456481317 ) ) ;
#203154=CARTESIAN_POINT ( 'NONE',  ( 7.248805684800777804, 11.60869039890961218, 1.040834085586084257E-14 ) ) ;
#203155=CARTESIAN_POINT ( 'NONE',  ( 6.039269195634717313, 6.063090950291412540, -0.5025354473536098876 ) ) ;
#203161=CARTESIAN_POINT ( 'NONE',  ( -6.236387472606141458, 10.21960978477508952, -0.7216878364870278340 ) ) ;
#203165=CARTESIAN_POINT ( 'NONE',  ( 0.6823417656249917140, 4.155208333674755394, 1.181850606188765695 ) ) ;
#203175=CARTESIAN_POINT ( 'NONE',  ( 3.999292125906911188, 4.728557570721922509, 1.082531754730560403 ) ) ;
#203176=FACE_OUTER_BOUND ( 'NONE', #110913, .T. ) ;
#203177=CARTESIAN_POINT ( 'NONE',  ( -9.561524646135538319, 12.17819805862340310, -1.599625672291263179 ) ) ;
#203180=CARTESIAN_POINT ( 'NONE',  ( 1.364683531249986537, 0.8635416670080893198, 0.7879004041258500513 ) ) ;
#203181=CARTESIAN_POINT ( 'NONE',  ( -4.799223189557577207, 4.701441264013013210, 0.7216878364870317197 ) ) ;
#203183=CARTESIAN_POINT ( 'NONE',  ( 5.335297142177534369, 6.183267073083954735, -1.199719254218452047 ) ) ;
#203189=CARTESIAN_POINT ( 'NONE',  ( 6.938893903907228378E-15, 10.64264068711930733, 1.214306433183764966E-14 ) ) ;
#203192=CARTESIAN_POINT ( 'NONE',  ( -8.839552966430012759, 10.37552855133225904, -1.082531754730543971 ) ) ;
#203197=CARTESIAN_POINT ( 'NONE',  ( -7.458957065812611198, 11.85386701009007204, 0.7998128361456481317 ) ) ;
#203198=CARTESIAN_POINT ( 'NONE',  ( -4.080641047588902559, 7.704572288921609058, -0.7216878364870257245 ) ) ;
#203199=CARTESIAN_POINT ( 'NONE',  ( 1.364683531249988535, 2.676041667008082214, 0.7879004041258500513 ) ) ;
#203200=CARTESIAN_POINT ( 'NONE',  ( -0.7500000000000215383, 4.441666666666691299, 1.299038105676671107 ) ) ;
#203213=ORIENTED_EDGE ( 'NONE', *, *, #73284, .F. ) ;
#203214=B_SPLINE_CURVE_WITH_KNOTS ( 'NONE', 3,
 ( #57587, #123744, #105286, #189705 ),
 .UNSPECIFIED., .F., .F.,
 ( 4, 4 ),
 ( 1.890032774489904948E-16, 0.0001045641765545081658 ),
 .UNSPECIFIED. ) ;
#203220=DIRECTION ( 'NONE',  ( -0.7592566023653004592, 0.6507913734559639396, 0.000000000000000000 ) ) ;
#203224=CARTESIAN_POINT ( 'NONE',  ( -1.364683531250012516, 2.842708333674754506, 0.7879004041258379498 ) ) ;
#203234=CARTESIAN_POINT ( 'NONE',  ( -0.6823417656250212460, 1.551041667008083769, 1.181850606188755259 ) ) ;
#203236=ORIENTED_EDGE ( 'NONE', *, *, #42629, .T. ) ;
#203244=CARTESIAN_POINT ( 'NONE',  ( 3.669453130792974971, 7.432779085900453886, 1.040834085586084257E-14 ) ) ;
#203249=CARTESIAN_POINT ( 'NONE',  ( 3.686212053427321056, 6.121915856213854923, 1.284222742053100941 ) ) ;
#203251=CARTESIAN_POINT ( 'NONE',  ( 6.286176778230493589, 10.48562334124426698, 0.7998128361456462443 ) ) ;
#203254=VECTOR ( 'NONE', #192733, 1000.000000000000000 ) ;
#203255=CARTESIAN_POINT ( 'NONE',  ( -4.946027110887008860, 4.664786472323266153, -0.7998128361456221525 ) ) ;
#203256=CARTESIAN_POINT ( 'NONE',  ( 9.257519960032755790, 9.694861462993381807, 0.7998128361456462443 ) ) ;
#203267=CARTESIAN_POINT ( 'NONE',  ( -7.754900677336769022, 9.110100880723427608, 1.082531754730558626 ) ) ;
#203271=CARTESIAN_POINT ( 'NONE',  ( -7.621654909176601045, 12.04368116068139472, 0.7998128361456481317 ) ) ;
#203275=CARTESIAN_POINT ( 'NONE',  ( -2.785310492603665367, 5.336947110424484109, 1.199719254218462483 ) ) ;
#203278=CARTESIAN_POINT ( 'NONE',  ( 9.398826802771546696, 11.98838390803207865, -1.599625672291262513 ) ) ;
#203279=CARTESIAN_POINT ( 'NONE',  ( 2.693266070609028784, 6.293894182352508970, 0.000000000000000000 ) ) ;
#203285=CARTESIAN_POINT ( 'NONE',  ( 4.704316114261903436, 4.590716342834741504, 1.214306433183764966E-14 ) ) ;
#203287=CARTESIAN_POINT ( 'NONE',  ( -5.416646063859567484, 6.278174148379618735, 1.199719254218450271 ) ) ;
#203290=CARTESIAN_POINT ( 'NONE',  ( -10.29471871147821282, 10.90492667301307605, -0.7998128361456291469 ) ) ;
#203296=CARTESIAN_POINT ( 'NONE',  ( 7.727784370109387346, 10.99920361756089093, -1.082531754730543083 ) ) ;
#203297=CARTESIAN_POINT ( 'NONE',  ( 1.364683531249988535, 4.217708333674753618, -0.7879004041258239610 ) ) ;
#203299=CARTESIAN_POINT ( 'NONE',  ( 3.323720213644492993, 7.029424015893889433, 1.040834085586084257E-14 ) ) ;
#203312=CARTESIAN_POINT ( 'NONE',  ( 1.364683531249986537, 2.217708333674751398, -0.7879004041258239610 ) ) ;
#203314=CARTESIAN_POINT ( 'NONE',  ( 10.22692794340986921, 10.82583744360002243, 0.000000000000000000 ) ) ;
#203316=CARTESIAN_POINT ( 'NONE',  ( -5.422898255786198440, 7.349800603215774331, -1.443375672974052559 ) ) ;
#203318=CARTESIAN_POINT ( 'NONE',  ( -4.731432421044873493, 7.503459676985569260, -1.082531754730548412 ) ) ;
#203322=CARTESIAN_POINT ( 'NONE',  ( 5.281064527722868718, 6.119995689553514140, 1.199719254218462483 ) ) ;
#203330=CARTESIAN_POINT ( 'NONE',  ( 4.320244504248938355, 8.192035688265757898, 1.040834085586084257E-14 ) ) ;
#203335=CARTESIAN_POINT ( 'NONE',  ( -5.331380718671772101, 7.243030143248949670, -1.599625672291256295 ) ) ;
#203339=CARTESIAN_POINT ( 'NONE',  ( 6.265839547809997079, 10.46189657242035587, 0.7998128361456462443 ) ) ;
#203342=CARTESIAN_POINT ( 'NONE',  ( -5.052384799386910430, 9.046199365926717917, 1.214306433183764966E-14 ) ) ;
#203344=CARTESIAN_POINT ( 'NONE',  ( 5.775410249297131315, 9.681803024247919609, 1.040834085586084257E-14 ) ) ;
#203345=CARTESIAN_POINT ( 'NONE',  ( 4.849937260509308956, 6.926242028416789154, 1.417063245053858722 ) ) ;
#203346=CARTESIAN_POINT ( 'NONE',  ( -4.517891501851816649, 6.293959390292322986, -1.599625672291256295 ) ) ;
#203349=CARTESIAN_POINT ( 'NONE',  ( -5.215082642750900277, 9.236013516518044142, 0.000000000000000000 ) ) ;
#203353=CARTESIAN_POINT ( 'NONE',  ( -0.6823417656250212460, 2.051041667008083991, 1.181850606188767472 ) ) ;
#203355=CARTESIAN_POINT ( 'NONE',  ( -5.585596099150193616, 6.579245539505756746, -1.082531754730544860 ) ) ;
#203357=AXIS2_PLACEMENT_3D ( 'NONE', #46695, #79171, #131192 ) ;
#203362=CARTESIAN_POINT ( 'NONE',  ( 5.656776405399742025, 7.622658444431597680, -1.599625672291262513 ) ) ;
#203364=CARTESIAN_POINT ( 'NONE',  ( -5.811497925844209433, 6.060560459143458978, 0.5261113891226586459 ) ) ;
#203365=CARTESIAN_POINT ( 'NONE',  ( -0.6823417656250212460, 1.863541667008083991, 1.181850606188755259 ) ) ;
#203368=CARTESIAN_POINT ( 'NONE',  ( -0.006800380015319074101, 7.009756401597622144, 1.999988438674507485 ) ) ;
#203370=CARTESIAN_POINT ( 'NONE',  ( -4.436542580169821726, 6.199052314996659874, 1.599625672291267398 ) ) ;
#203371=CARTESIAN_POINT ( 'NONE',  ( -6.954969613686107444, 10.09758640173367894, 1.082531754730549967 ) ) ;
#203381=CARTESIAN_POINT ( 'NONE',  ( -6.521108698048767138, 10.55178454779148289, -0.7216878364870267237 ) ) ;
#203385=CARTESIAN_POINT ( 'NONE',  ( -7.497295758232724872, 9.769931022736756177, -1.443375672974058777 ) ) ;
#203398=CARTESIAN_POINT ( 'NONE',  ( -7.206322340863467346, 8.366129804884193888, 1.199719254218450271 ) ) ;
#203400=CARTESIAN_POINT ( 'NONE',  ( 3.334415713957098681, 5.977569868670206787, -1.199719254218446718 ) ) ;
#203403=CARTESIAN_POINT ( 'NONE',  ( 4.893868406069843857, 4.891356491275733909, 0.6526265993265610854 ) ) ;
#203405=CARTESIAN_POINT ( 'NONE',  ( 7.169564303528210836, 7.258913197071374945, -0.7998128361456281477 ) ) ;
#203410=CARTESIAN_POINT ( 'NONE',  ( -4.067082894419624672, 6.728385229256075739, 1.082531754730560403 ) ) ;
#203415=CARTESIAN_POINT ( 'NONE',  ( -0.1099460098626957039, 6.494484681433106310, 3.110387376256865011 ) ) ;
#203418=CARTESIAN_POINT ( 'NONE',  ( -1.364683531250000748, 0.7593750003414210248, 0.000000000000000000 ) ) ;
#203419=CARTESIAN_POINT ( 'NONE',  ( 2.294141167727915320, 5.518260410454753462, -0.5312303208429024481 ) ) ;
#203420=CARTESIAN_POINT ( 'NONE',  ( -7.492852449846775897, 11.89341162479659531, 0.000000000000000000 ) ) ;
#203423=CARTESIAN_POINT ( 'NONE',  ( 7.446452682403650769, 9.710614100936176385, -1.599625672291262513 ) ) ;
#203425=CARTESIAN_POINT ( 'NONE',  ( -7.039708073993679704, 9.236078724457858158, 1.599625672291283607 ) ) ;
#203428=CARTESIAN_POINT ( 'NONE',  ( 1.364683531249990311, 4.634375000341417916, 1.214306433183764966E-14 ) ) ;
#203431=CARTESIAN_POINT ( 'NONE',  ( 10.07334494527360569, 10.85458331234846696, 0.000000000000000000 ) ) ;
#203434=CARTESIAN_POINT ( 'NONE',  ( 0.6823417656249864960, -1.011458332991911568, -1.181850606188749264 ) ) ;
#203437=CARTESIAN_POINT ( 'NONE',  ( 6.114364089638775646, 10.07724917131317355, 0.7216878364870438212 ) ) ;
#203440=CARTESIAN_POINT ( 'NONE',  ( -6.236387472606166327, 6.378132927569716060, -0.7216878364870278340 ) ) ;
#203442=CARTESIAN_POINT ( 'NONE',  ( -1.201851678989727383E-14, 3.071875000341420137, 1.575800808251672791 ) ) ;
#203446=CARTESIAN_POINT ( 'NONE',  ( -6.501298352952815662, 7.543601818988450169, -1.199719254218446718 ) ) ;
#203447=CARTESIAN_POINT ( 'NONE',  ( -1.001543065824772872E-14, 5.634375000341415252, 1.575800808251672791 ) ) ;
#203453=CARTESIAN_POINT ( 'NONE',  ( 8.620286740190458374, 8.951422706510690830, 1.040834085586084257E-14 ) ) ;
#203456=CARTESIAN_POINT ( 'NONE',  ( -1.499999999999997780, 2.900000000000020783, 1.214306433183764966E-14 ) ) ;
#203458=AXIS2_PLACEMENT_3D ( 'NONE', #188050, #8240, #172900 ) ;
#203463=CARTESIAN_POINT ( 'NONE',  ( 5.748293942514166588, 7.729428904398431222, -1.443375672974057666 ) ) ;
#203464=CARTESIAN_POINT ( 'NONE',  ( -1.402160292154681736E-14, -0.6156249996585817508, 1.575800808251672791 ) ) ;
#203471=CARTESIAN_POINT ( 'NONE',  ( -1.500000000000001332, 0.4000000000000253353, 0.000000000000000000 ) ) ;
#203472=CARTESIAN_POINT ( 'NONE',  ( 7.100719765255169236, 9.307259030929609267, -1.599625672291262513 ) ) ;
#203473=CARTESIAN_POINT ( 'NONE',  ( -9.989660255170729641, 10.54902514065433827, -0.7998128361456291469 ) ) ;
#203475=B_SPLINE_CURVE_WITH_KNOTS ( 'NONE', 3,
 ( #84113, #136079, #181605, #100365, #150201, #166435, #1772 ),
 .UNSPECIFIED., .F., .F.,
 ( 4, 3, 4 ),
 ( 3.104682540412456132E-18, 8.743668306901165302E-05, 0.0001748766834010605654 ),
 .UNSPECIFIED. ) ;
#203476=CARTESIAN_POINT ( 'NONE',  ( -1.402160292154681736E-14, 0.4468750003414233563, -1.575800808251665908 ) ) ;
#203477=CARTESIAN_POINT ( 'NONE',  ( -1.500000000000013101, 0.9208333333333594828, 0.8660254037844403729 ) ) ;
#203479=CARTESIAN_POINT ( 'NONE',  ( 4.364835388595708743, 7.179726155748598515, 1.199719254218462483 ) ) ;
#203481=CARTESIAN_POINT ( 'NONE',  ( 0.7499999999999885647, 2.847916667349487341, -1.299038105676658228 ) ) ;
#203485=CARTESIAN_POINT ( 'NONE',  ( 1.364683531249992088, 5.634375000341417916, 1.214306433183764966E-14 ) ) ;
#203487=CARTESIAN_POINT ( 'NONE',  ( -8.941766003412679353, 10.39081407785832845, -1.199719254218446718 ) ) ;
#203488=CARTESIAN_POINT ( 'NONE',  ( -4.284013352238255301, 6.981470763377843447, -1.082531754730549967 ) ) ;
#203496=CARTESIAN_POINT ( 'NONE',  ( 6.591235234537977661, 10.84152487360300299, 0.7998128361456462443 ) ) ;
#203497=CARTESIAN_POINT ( 'NONE',  ( -4.510196435976065565, 7.040407170307378060, -1.149263043085164915 ) ) ;
#203498=CARTESIAN_POINT ( 'NONE',  ( 2.859846416572967343, 6.488237919310435586, 0.2290337979853694639 ) ) ;
#203500=CARTESIAN_POINT ( 'NONE',  ( 5.734735788456138295, 8.673980272298743799, -1.082531754730537976 ) ) ;
#203502=EDGE_CURVE ( 'NONE', #105963, #177940, #207098, .T. ) ;
#203504=CARTESIAN_POINT ( 'NONE',  ( -7.263417608619167076, 9.497073181520933716, -1.599625672291263179 ) ) ;
#203506=CARTESIAN_POINT ( 'NONE',  ( 5.626797444871351139, 6.523350759560078593, 1.199719254218462483 ) ) ;
#203508=CARTESIAN_POINT ( 'NONE',  ( 0.000000000000000000, 8.600000000000017408, -0.3999999999999819811 ) ) ;
#203509=CARTESIAN_POINT ( 'NONE',  ( 2.846322183865124700, 5.408127416896231665, -1.199719254218446718 ) ) ;
#203515=DIRECTION ( 'NONE',  ( -5.578564026256490882E-16, -1.000000000000000000, -9.066213480720158442E-32 ) ) ;
#203516=CARTESIAN_POINT ( 'NONE',  ( -5.178851490740209229, 7.065079377328788546, 1.443375672974064550 ) ) ;
#203517=CARTESIAN_POINT ( 'NONE',  ( 8.242994207428692377, 12.56065097540143327, -0.7216878364870328300 ) ) ;
#203520=CARTESIAN_POINT ( 'NONE',  ( -7.705111371268023923, 7.883718109434487253, 1.040834085586084257E-14 ) ) ;
#203523=CARTESIAN_POINT ( 'NONE',  ( 3.189213936345665523, 2.817530495244580102, 2.450448857954567572 ) ) ;
#203525=CARTESIAN_POINT ( 'NONE',  ( -6.995117189646935962, 10.24838825697502109, 1.199719254218453823 ) ) ;
#203541=CARTESIAN_POINT ( 'NONE',  ( -5.859094939400033120, 9.987361195942037639, -0.7998128361456231517 ) ) ;
#203544=CARTESIAN_POINT ( 'NONE',  ( 4.690757960648221037, 7.456006139856155457, 1.082531754730558626 ) ) ;
#203549=CARTESIAN_POINT ( 'NONE',  ( -5.762378981008047241, 6.681529218386182301, 1.199719254218450271 ) ) ;
#203550=B_SPLINE_CURVE_WITH_KNOTS ( 'NONE', 1,
 ( #113551, #213088 ),
 .UNSPECIFIED., .F., .F.,
 ( 2, 2 ),
 ( 0.2265555213262060719, 0.4428258268412425536 ),
 .UNSPECIFIED. ) ;
#203551=( BOUNDED_SURFACE ( )  B_SPLINE_SURFACE ( 3, 2, ( 
 ( #193140, #111975, #44788 ),
 ( #197400, #177976, #28514 ),
 ( #94605, #131403, #95677 ),
 ( #161731, #80464, #145514 ) ),
 .UNSPECIFIED., .F., .F., .F. ) 
 B_SPLINE_SURFACE_WITH_KNOTS ( ( 4, 4 ),
 ( 3, 3 ),
 ( -4.336808689942017736E-18, 0.002003486994853882937 ),
 ( 0.000000000000000000, 1.000000000000000000 ),
 .UNSPECIFIED. ) 
 GEOMETRIC_REPRESENTATION_ITEM ( )  RATIONAL_B_SPLINE_SURFACE ( (
 ( 1.000000000000000000, 0.7779734834199527604, 1.000000000000000000),
 ( 1.000000000000000000, 0.7856061901475716036, 1.000000000000000000),
 ( 1.000000000000000000, 0.7951961705782252254, 1.000000000000000000),
 ( 1.000000000000000000, 0.8104931255419017821, 1.000000000000000000) ) ) 
 REPRESENTATION_ITEM ( '' )  SURFACE ( )  );
#203555=CARTESIAN_POINT ( 'NONE',  ( -5.422371370461663176, 8.413518134592214537, -1.199719254218446718 ) ) ;
#203556=CARTESIAN_POINT ( 'NONE',  ( 0.7499999999999885647, 3.316666666666689967, -1.299038105676658228 ) ) ;
#203562=CARTESIAN_POINT ( 'NONE',  ( -9.677822722056413696, 10.18521468535430685, 1.040834085586084257E-14 ) ) ;
#203563=CARTESIAN_POINT ( 'NONE',  ( 5.913327553854682783, 10.05063257947248800, -0.7998128361456291469 ) ) ;
#203567=CARTESIAN_POINT ( 'NONE',  ( -9.969323024750229578, 10.52529837183042716, -0.7998128361456291469 ) ) ;
#203570=CARTESIAN_POINT ( 'NONE',  ( -0.6823417656250003738, -0.9697916663252494907, -1.181850606188749264 ) ) ;
#203572=ORIENTED_EDGE ( 'NONE', *, *, #29169, .F. ) ;
#203574=CARTESIAN_POINT ( 'NONE',  ( 7.917598520700710019, 12.18102267421877727, -0.7216878364870328300 ) ) ;
#203582=CARTESIAN_POINT ( 'NONE',  ( -0.04202953795663257053, 6.478538335026032158, -3.086709765070265288 ) ) ;
#203594=CARTESIAN_POINT ( 'NONE',  ( -2.625475302540713152, 6.214804952939456228, -0.7998128361456281477 ) ) ;
#203597=CARTESIAN_POINT ( 'NONE',  ( -4.308793891044708779, 3.921347715840572956, 1.214306433183764966E-14 ) ) ;
#203601=CARTESIAN_POINT ( 'NONE',  ( -0.7500000000000006661, -1.110416665983847473, -1.299038105676652011 ) ) ;
#203606=ORIENTED_EDGE ( 'NONE', *, *, #15247, .F. ) ;
#203607=CARTESIAN_POINT ( 'NONE',  ( 1.419999999999820961, 7.176846818246208848, -4.202462424328213153 ) ) ;
#203608=CARTESIAN_POINT ( 'NONE',  ( -1.127943160727153060, 2.800000000000024691, -0.7749999999999935829 ) ) ;
#203609=CARTESIAN_POINT ( 'NONE',  ( 4.216749469050096621, 4.878294787768598262, -1.199719254218452047 ) ) ;
#203612=CARTESIAN_POINT ( 'NONE',  ( 1.499999999999821032, 10.00000000000000178, -4.154462424328206893 ) ) ;
#203613=B_SPLINE_CURVE_WITH_KNOTS ( 'NONE', 3,
 ( #73041, #207325, #140229, #120820, #23215, #187862, #119741, #39489, #204085, #186797 ),
 .UNSPECIFIED., .F., .F.,
 ( 4, 3, 3, 4 ),
 ( 0.000000000000000000, 3.125155738325145446E-05, 5.612058060597180007E-05, 8.099573230367171513E-05 ),
 .UNSPECIFIED. ) ;
#203615=CARTESIAN_POINT ( 'NONE',  ( 3.960953433486789521, 7.772862772376584850, -0.7998128361456221525 ) ) ;
#203616=CARTESIAN_POINT ( 'NONE',  ( 0.6823417656249899377, 2.155208333674753174, 1.181850606188767472 ) ) ;
#203617=CARTESIAN_POINT ( 'NONE',  ( -4.344470927813957495, 7.211826089590096522, 1.015455228366731966 ) ) ;
#203620=CARTESIAN_POINT ( 'NONE',  ( -7.648771216403934758, 12.07531685244661723, -0.7998128361456291469 ) ) ;
#203621=CARTESIAN_POINT ( 'NONE',  ( -4.812781342726871969, 6.637997537979888563, 1.443375672974064550 ) ) ;
#203623=CARTESIAN_POINT ( 'NONE',  ( -5.205440912643032547, 8.160432600470439723, 1.199719254218452047 ) ) ;
#203625=CARTESIAN_POINT ( 'NONE',  ( -1.402160292154681736E-14, -1.256249999317182953, 1.732050807568877637 ) ) ;
#203633=CARTESIAN_POINT ( 'NONE',  ( -4.894130264408866893, 6.732904613275549899, -1.443375672974051449 ) ) ;
#203639=CARTESIAN_POINT ( 'NONE',  ( -3.592547517496941900, 5.214391408544949869, -1.443375672974051449 ) ) ;
#203641=CARTESIAN_POINT ( 'NONE',  ( 7.750457368506414646, 12.19395069656619945, 0.7998128361456462443 ) ) ;
#203643=CARTESIAN_POINT ( 'NONE',  ( -1.177110729581226867, 3.120878374463987193, 0.7750000000000083489 ) ) ;
#203650=CARTESIAN_POINT ( 'NONE',  ( 4.121315508874254796, 5.831287398485175189, -1.443375672974051449 ) ) ;
#203651=CARTESIAN_POINT ( 'NONE',  ( -4.302014814237876017, 3.913438792899272212, 0.7998128361456341429 ) ) ;
#203653=CARTESIAN_POINT ( 'NONE',  ( -9.134442807305063639, 11.67993591332117376, 1.599625672291281386 ) ) ;
#203658=CARTESIAN_POINT ( 'NONE',  ( 6.817052309572890323, 6.847649204123507083, 0.7998128361456341429 ) ) ;
#203662=CARTESIAN_POINT ( 'NONE',  ( 5.181758602633668609, 4.945385036406048762, -2.420000000000000373 ) ) ;
#203663=CARTESIAN_POINT ( 'NONE',  ( 2.354312230267378236, 5.898448035287240820, -0.7998128361456281477 ) ) ;
#203674=CARTESIAN_POINT ( 'NONE',  ( 7.248805684800777804, 11.60869039890961218, 1.040834085586084257E-14 ) ) ;
#203675=CARTESIAN_POINT ( 'NONE',  ( -4.791917227426195858, 7.677988301050826969, -1.199719254218452047 ) ) ;
#203678=CARTESIAN_POINT ( 'NONE',  ( 1.252085211431710698, 2.800000000000024691, 0.7750000000000152323 ) ) ;
#203680=CIRCLE ( 'NONE', #158721, 0.08000000000000004330 ) ;
#203682=CARTESIAN_POINT ( 'NONE',  ( -0.6823417656249969321, 4.467708333674755394, -1.181850606188749264 ) ) ;
#203688=CARTESIAN_POINT ( 'NONE',  ( 4.891794496432329886, 4.601515088792824670, -0.7998128361456211532 ) ) ;
#203689=CARTESIAN_POINT ( 'NONE',  ( -5.596818484342970912, 5.424043074688562172, -0.7998128361456221525 ) ) ;
#203695=CARTESIAN_POINT ( 'NONE',  ( 4.853455804012212660, 7.645820290447483458, 1.082531754730558626 ) ) ;
#203697=CARTESIAN_POINT ( 'NONE',  ( 8.093854517234030155, 8.545177812968924869, -0.7216878364870267237 ) ) ;
#203698=CARTESIAN_POINT ( 'NONE',  ( 0.6823417656249917140, 3.655208333674754506, 1.181850606188765695 ) ) ;
#203700=CARTESIAN_POINT ( 'NONE',  ( 5.314433026432511475, 5.302519407033794430, 1.040834085586084257E-14 ) ) ;
#203707=CARTESIAN_POINT ( 'NONE',  ( -4.172014829671058855, 7.596244486910340044, 0.9145543751994407167 ) ) ;
#203713=CARTESIAN_POINT ( 'NONE',  ( -10.34217224912604571, 10.96028913360221502, 0.7998128361456462443 ) ) ;
#203715=DIRECTION ( 'NONE',  ( -0.7592566023653004592, -0.6507913734559641616, 0.000000000000000000 ) ) ;
#203721=ORIENTED_EDGE ( 'NONE', *, *, #161474, .F. ) ;
#203723=CARTESIAN_POINT ( 'NONE',  ( 3.172244755917638770, 5.684407401003788607, -1.082531754730543083 ) ) ;
#203724=CARTESIAN_POINT ( 'NONE',  ( -0.6823417656249969321, 4.030208333674754506, -1.181850606188749264 ) ) ;
#203726=CARTESIAN_POINT ( 'NONE',  ( 5.777746017718023097, 9.892454120646377191, 0.7998128361456462443 ) ) ;
#203728=CARTESIAN_POINT ( 'NONE',  ( -9.022061154889962964, 12.61315621642528129, -1.199719254218446718 ) ) ;
#203735=CARTESIAN_POINT ( 'NONE',  ( -1.500000000000011324, 4.879166666666690411, -0.8660254037844313801 ) ) ;
#203736=CARTESIAN_POINT ( 'NONE',  ( 3.486418057008484617, 7.219238166485217434, 1.040834085586084257E-14 ) ) ;
#203739=CARTESIAN_POINT ( 'NONE',  ( -0.6823417656250212460, 2.863541667008084879, 1.181850606188767472 ) ) ;
#203740=CARTESIAN_POINT ( 'NONE',  ( -0.6823417656249969321, 3.967708333674754950, -1.181850606188749264 ) ) ;
#203741=ORIENTED_EDGE ( 'NONE', *, *, #13980, .T. ) ;
#203743=CARTESIAN_POINT ( 'NONE',  ( 7.917598520700710019, 12.18102267421877727, -0.7216878364870328300 ) ) ;
#203749=CARTESIAN_POINT ( 'NONE',  ( 1.499999999999989120, 2.306250000682817713, 1.214306433183764966E-14 ) ) ;
#203751=CARTESIAN_POINT ( 'NONE',  ( -4.218558352146454915, 8.073401844146177453, 1.040834085586084257E-14 ) ) ;
#203752=CARTESIAN_POINT ( 'NONE',  ( 5.029711800545521250, 5.930713857800314237, -1.082531754730549078 ) ) ;
#203753=CARTESIAN_POINT ( 'NONE',  ( -4.905110356762790502, 4.827649200395154772, -0.06592220986076716138 ) ) ;
#203760=ORIENTED_EDGE ( 'NONE', *, *, #113143, .T. ) ;
#203762=CARTESIAN_POINT ( 'NONE',  ( 7.283754839039659146, 9.520799950344851936, -1.599625672291262513 ) ) ;
#203763=CARTESIAN_POINT ( 'NONE',  ( 3.811813743736467419, 7.598866467667865443, 1.040834085586084257E-14 ) ) ;
#203766=CARTESIAN_POINT ( 'NONE',  ( 5.301401758143367893, 6.143722458377430584, 1.199719254218462483 ) ) ;
#203773=CARTESIAN_POINT ( 'NONE',  ( 9.297140650669039275, 11.86975006391249643, 1.599625672291281386 ) ) ;
#203778=CARTESIAN_POINT ( 'NONE',  ( 5.824368567101982030, 6.018301469053008113, 0.4368841385695241275 ) ) ;
#203786=CARTESIAN_POINT ( 'NONE',  ( 6.588899466561449536, 9.670504563421618016, -1.082531754730537088 ) ) ;
#203787=CARTESIAN_POINT ( 'NONE',  ( -4.790108344329849110, 4.482881244673243337, 0.7998128361456341429 ) ) ;
#203792=CARTESIAN_POINT ( 'NONE',  ( -3.893162665418476109, 7.693773542963529444, 1.040834085586084257E-14 ) ) ;
#203794=CARTESIAN_POINT ( 'NONE',  ( -5.905025204054467736, 4.805319369744820435, 2.499999999999998668 ) ) ;
#203798=ORIENTED_EDGE ( 'NONE', *, *, #31271, .F. ) ;
#203799=CARTESIAN_POINT ( 'NONE',  ( -1.084637062511559336, 3.213621193390831188, 1.105835307554800639 ) ) ;
#203805=CARTESIAN_POINT ( 'NONE',  ( 8.048736748007069508, 12.54194330598362406, -0.7998128361456352531 ) ) ;
#203808=CARTESIAN_POINT ( 'NONE',  ( 2.250290310188348464, 5.569163095287620990, 0.7216878364870438212 ) ) ;
#203814=CARTESIAN_POINT ( 'NONE',  ( -9.327646496521984076, 11.90534021740758064, -1.443375672974059665 ) ) ;
#203818=CARTESIAN_POINT ( 'NONE',  ( 7.377608144130607393, 11.75895993479440982, -0.7998128361456291469 ) ) ;
#203823=CARTESIAN_POINT ( 'NONE',  ( -5.526920175865215334, 9.599823971818089774, 0.7998128361456481317 ) ) ;
#203824=CARTESIAN_POINT ( 'NONE',  ( 4.847203612085560387, 5.613824621309978724, -1.199719254218452047 ) ) ;
#203827=CARTESIAN_POINT ( 'NONE',  ( 9.459838494033030898, 12.05956421450382088, 1.599625672291281386 ) ) ;
#203832=CARTESIAN_POINT ( 'NONE',  ( -1.402160292154681736E-14, 2.009375000341422801, -1.575800808251660134 ) ) ;
#203834=CARTESIAN_POINT ( 'NONE',  ( 6.317736394288135493, 8.393778431468064127, 1.443375672974076540 ) ) ;
#203842=CARTESIAN_POINT ( 'NONE',  ( 8.283668667825342169, 9.726996869626816533, -1.082531754730543083 ) ) ;
#203848=CARTESIAN_POINT ( 'NONE',  ( -8.829384350997580455, 11.32403438096243775, 1.599625672291269396 ) ) ;
#203857=CARTESIAN_POINT ( 'NONE',  ( 4.864678189204997949, 4.569879397027603929, 0.7998128361456341429 ) ) ;
#203862=CARTESIAN_POINT ( 'NONE',  ( 5.880485940025228508, 7.883652901494672349, 1.599625672291267398 ) ) ;
#203866=CARTESIAN_POINT ( 'NONE',  ( 1.499999999999989120, 3.285416667349486897, 0.8660254037844524744 ) ) ;
#203872=CARTESIAN_POINT ( 'NONE',  ( -1.402160292154681736E-14, 0.5875000000000220046, -1.732050807568863648 ) ) ;
#203873=CARTESIAN_POINT ( 'NONE',  ( 7.100719765255169236, 9.307259030929609267, -1.599625672291262513 ) ) ;
#203874=CARTESIAN_POINT ( 'NONE',  ( 6.453317929980448397, 6.631218461173066459, 1.040834085586084257E-14 ) ) ;
#203878=CARTESIAN_POINT ( 'NONE',  ( 9.951321562750607086, 11.67259191370631477, -1.082531754730537088 ) ) ;
#203884=CARTESIAN_POINT ( 'NONE',  ( -5.368138756007025947, 8.350246751061767725, 1.199719254218452047 ) ) ;
#203885=CARTESIAN_POINT ( 'NONE',  ( 1.499999999999989120, 3.035416667349485564, 0.8660254037844524744 ) ) ;
#203886=CARTESIAN_POINT ( 'NONE',  ( 0.6823417656249917140, 5.405208333674749177, 1.181850606188765695 ) ) ;
#203891=CARTESIAN_POINT ( 'NONE',  ( -1.201851678989727383E-14, 3.884375000341423689, 1.575800808251672791 ) ) ;
#203900=CARTESIAN_POINT ( 'NONE',  ( -7.557780564614042795, 10.90482886110335414, -1.199719254218446718 ) ) ;
#203901=CARTESIAN_POINT ( 'NONE',  ( 6.518772930072240790, 6.499656594706071822, -0.7998128361456281477 ) ) ;
#203909=CARTESIAN_POINT ( 'NONE',  ( -6.181627972826976958, 9.299317504018391745, 1.199719254218452047 ) ) ;
#203914=CARTESIAN_POINT ( 'NONE',  ( 9.541187415715040032, 12.15447128979948310, -1.599625672291262513 ) ) ;
#203916=CARTESIAN_POINT ( 'NONE',  ( -5.590039407536138150, 5.416134151747256986, 0.000000000000000000 ) ) ;
#203917=CARTESIAN_POINT ( 'NONE',  ( -9.969323024750229578, 10.52529837183042716, -0.7998128361456291469 ) ) ;
#203920=CARTESIAN_POINT ( 'NONE',  ( -4.662544117754887196, 7.086110115384146368, -1.393066284953614620 ) ) ;
#203921=CARTESIAN_POINT ( 'NONE',  ( 0.6823417656249882723, -1.157291666325249713, 1.181850606188755259 ) ) ;
#203927=CARTESIAN_POINT ( 'NONE',  ( 6.114890974963323345, 7.092793211334054604, 1.199719254218462483 ) ) ;
#203944=CARTESIAN_POINT ( 'NONE',  ( 3.226477370372305753, 4.787309570232886280, 1.443375672974062551 ) ) ;
#203948=CARTESIAN_POINT ( 'NONE',  ( -10.29471871147821282, 10.90492667301307605, -0.7998128361456291469 ) ) ;
#203953=EDGE_CURVE ( 'NONE', #40273, #159908, #75539, .T. ) ;
#203954=CARTESIAN_POINT ( 'NONE',  ( -1.402160292154681736E-14, 1.618750000682814827, -1.732050807568863648 ) ) ;
#203955=CARTESIAN_POINT ( 'NONE',  ( 9.083072846151447166, 12.68433652289702884, 1.199719254218450271 ) ) ;
#203959=DIRECTION ( 'NONE',  ( -1.207943261119674327E-30, -2.168404344971008079E-15, -1.000000000000000000 ) ) ;
#203961=CARTESIAN_POINT ( 'NONE',  ( -0.6823417656250003738, 0.4677083336747517306, -1.181850606188749264 ) ) ;
#203963=ORIENTED_EDGE ( 'NONE', *, *, #99218, .F. ) ;
#203965=( GEOMETRIC_REPRESENTATION_CONTEXT ( 3 ) GLOBAL_UNCERTAINTY_ASSIGNED_CONTEXT ( ( #89665 ) ) GLOBAL_UNIT_ASSIGNED_CONTEXT ( ( #88563, #72270, #157831 ) ) REPRESENTATION_CONTEXT ( 'NONE', 'WORKASPACE' ) );
#203968=CARTESIAN_POINT ( 'NONE',  ( -3.255929445576174697, 6.950334786480840243, -0.7998128361456281477 ) ) ;
#203972=CARTESIAN_POINT ( 'NONE',  ( 0.6823417656249882723, 0.2385416670080825474, -1.181850606188749264 ) ) ;
#203977=CARTESIAN_POINT ( 'NONE',  ( -0.6823417656250246877, 0.05104166700808931978, 1.181850606188755259 ) ) ;
#203979=CARTESIAN_POINT ( 'NONE',  ( -7.172426956829277778, 8.326585190177668849, -1.199719254218452935 ) ) ;
#203980=CARTESIAN_POINT ( 'NONE',  ( 9.402743226277308963, 10.92862083786708816, -1.199719254218446718 ) ) ;
#203981=CARTESIAN_POINT ( 'NONE',  ( 5.138703914779377158, 5.953908307786102583, 1.199719254218462483 ) ) ;
#203985=CARTESIAN_POINT ( 'NONE',  ( 1.364683531249988757, 1.446875000341421469, 0.000000000000000000 ) ) ;
#203990=CARTESIAN_POINT ( 'NONE',  ( 7.144783764721768904, 7.437928601704619780, 1.040834085586084257E-14 ) ) ;
#203993=CARTESIAN_POINT ( 'NONE',  ( -8.376239975144482486, 8.666701480623698828, 1.040834085586084257E-14 ) ) ;
#203994=CARTESIAN_POINT ( 'NONE',  ( -5.590039407536138150, 5.416134151747256986, 0.000000000000000000 ) ) ;
#203995=CARTESIAN_POINT ( 'NONE',  ( 5.192409643909512873, 6.120528008391641350, -1.082531754730549078 ) ) ;
#203997=CARTESIAN_POINT ( 'NONE',  ( -3.440018289565379028, 5.036440642624797626, 1.599625672291267398 ) ) ;
#203998=CARTESIAN_POINT ( 'NONE',  ( 5.965224399888476192, 6.061776009399090448, 1.040834085586084257E-14 ) ) ;
#203999=CARTESIAN_POINT ( 'NONE',  ( -7.321039761255057066, 11.48503745486550365, 0.000000000000000000 ) ) ;
#204001=CARTESIAN_POINT ( 'NONE',  ( -0.7500000000000215383, 4.191666666666690411, 1.299038105676671107 ) ) ;
#204005=CARTESIAN_POINT ( 'NONE',  ( 7.293923454472069245, 11.45340176361870199, 0.7216878364870438212 ) ) ;
#204006=CONICAL_SURFACE ( 'NONE', #169406, 7.034482758620711706, 0.8621700546672336207 ) ;
#204012=DIRECTION ( 'NONE',  ( 0.000000000000000000, 8.546850786086437571E-32, 1.000000000000000000 ) ) ;
#204014=CARTESIAN_POINT ( 'NONE',  ( 8.554831740098642001, 12.92446143018304916, 0.7216878364870438212 ) ) ;
#204019=CARTESIAN_POINT ( 'NONE',  ( 8.101160479365381306, 9.410107633136481908, -1.199719254218446718 ) ) ;
#204020=CARTESIAN_POINT ( 'NONE',  ( -5.585069213825653023, 8.603332285183535433, -1.199719254218440723 ) ) ;
#204022=CARTESIAN_POINT ( 'NONE',  ( 3.714570900464274850, 6.317121236308204324, 1.082531754730558626 ) ) ;
#204024=CARTESIAN_POINT ( 'NONE',  ( -3.619663825168619731, 7.166765529431275539, 1.040834085586084257E-14 ) ) ;
#204025=CARTESIAN_POINT ( 'NONE',  ( 3.877268743828266029, 6.506935386899531437, 1.082531754730558626 ) ) ;
#204027=CARTESIAN_POINT ( 'NONE',  ( -8.853111120043687166, 9.430977182913531820, 1.040834085586084257E-14 ) ) ;
#204039=ORIENTED_EDGE ( 'NONE', *, *, #192235, .T. ) ;
#204042=CARTESIAN_POINT ( 'NONE',  ( 8.067265095331215718, 9.370563018429956870, 1.199719254218462483 ) ) ;
#204053=CARTESIAN_POINT ( 'NONE',  ( -5.391338639728555648, 9.441645512991978961, -0.7998128361456231517 ) ) ;
#204055=CARTESIAN_POINT ( 'NONE',  ( -6.078132937628113908, 5.985576603521232109, 1.040834085586084257E-14 ) ) ;
#204065=CARTESIAN_POINT ( 'NONE',  ( -3.307299406729781399, 5.945934176904983381, -1.199719254218452935 ) ) ;
#204068=CARTESIAN_POINT ( 'NONE',  ( 6.693975156845185737, 8.832723654451292816, 1.599625672291281386 ) ) ;
#204071=CARTESIAN_POINT ( 'NONE',  ( 6.046415161660691595, 6.058605959254545148, 0.4744590674741564484 ) ) ;
#204076=CARTESIAN_POINT ( 'NONE',  ( 5.219525951136835928, 7.112532914458205013, -1.443375672974051449 ) ) ;
#204077=CARTESIAN_POINT ( 'NONE',  ( -8.667740277838301921, 9.006785167099828016, -0.7998128361456291469 ) ) ;
#204080=CARTESIAN_POINT ( 'NONE',  ( -7.160677686311960777, 11.50587440067263678, -0.7998128361456291469 ) ) ;
#204081=CARTESIAN_POINT ( 'NONE',  ( -5.005985031943793295, 6.863401842066301661, -1.599625672291256295 ) ) ;
#204085=CARTESIAN_POINT ( 'NONE',  ( 4.904534058535990226, 4.831883945567478911, 0.6074287960816383558 ) ) ;
#204088=CARTESIAN_POINT ( 'NONE',  ( 6.856673000209174695, 9.022537805042615489, 1.599625672291281386 ) ) ;
#204102=ORIENTED_EDGE ( 'NONE', *, *, #109210, .T. ) ;
#204104=CARTESIAN_POINT ( 'NONE',  ( -0.7500000000000215383, 4.691666666666684193, 1.299038105676671107 ) ) ;
#204105=CARTESIAN_POINT ( 'NONE',  ( 4.147904930777053245, 6.926640621626830807, -1.199719254218452047 ) ) ;
#204106=CARTESIAN_POINT ( 'NONE',  ( 4.333802657862601215, 8.207853534148366492, 0.7998128361456462443 ) ) ;
#204108=CARTESIAN_POINT ( 'NONE',  ( -7.537970219518075332, 10.77775377520434574, -1.082531754730543971 ) ) ;
#204110=CARTESIAN_POINT ( 'NONE',  ( 7.795575138177731844, 8.197185204069915798, 1.040834085586084257E-14 ) ) ;
#204111=CARTESIAN_POINT ( 'NONE',  ( -8.473482818416664841, 11.86918514058604757, -1.082531754730543083 ) ) ;
#204114=CARTESIAN_POINT ( 'NONE',  ( 6.968000882419564945, 10.21675256520979858, 1.199719254218460707 ) ) ;
#204120=CARTESIAN_POINT ( 'NONE',  ( 1.364683531249988757, 2.384375000341422357, 1.214306433183764966E-14 ) ) ;
#204126=CARTESIAN_POINT ( 'NONE',  ( 9.206149998879153529, 10.69926207256923689, 1.199719254218453823 ) ) ;
#204129=CARTESIAN_POINT ( 'NONE',  ( -10.15235809853472126, 10.73883929124566983, -0.7998128361456291469 ) ) ;
#204135=CARTESIAN_POINT ( 'NONE',  ( 2.758194185376297902, 5.305311418659259814, 1.199719254218452047 ) ) ;
#204138=CARTESIAN_POINT ( 'NONE',  ( -9.691380875670077444, 10.20103253123691189, 0.7998128361456462443 ) ) ;
#204143=CARTESIAN_POINT ( 'NONE',  ( 5.856753424380153561, 5.998585917076054486, 0.3190708477142957245 ) ) ;
#204144=CARTESIAN_POINT ( 'NONE',  ( -0.4393598995549214958, 2.800000000000018030, -1.361929136425236386 ) ) ;
#204145=CARTESIAN_POINT ( 'NONE',  ( -5.251085567194491155, 5.020688004682002159, -0.7998128361456221525 ) ) ;
#204149=CARTESIAN_POINT ( 'NONE',  ( 7.401861798056875053, 10.72292363345333399, -1.199719254218441611 ) ) ;
#204151=CARTESIAN_POINT ( 'NONE',  ( 7.233438648090761980, 8.397765496649418182, 1.199719254218462483 ) ) ;
#204155=CARTESIAN_POINT ( 'NONE',  ( -8.676855123066022912, 10.18571440074093282, -1.082531754730543971 ) ) ;
#204163=CARTESIAN_POINT ( 'NONE',  ( -5.029675114306419559, 6.591709307070120261, -1.234896939913838754 ) ) ;
#204165=CARTESIAN_POINT ( 'NONE',  ( 6.805829924380114804, 8.002851668940699881, 1.082531754730558626 ) ) ;
#204169=CARTESIAN_POINT ( 'NONE',  ( -3.046854503059236663, 2.800000000000024691, 2.500000000000011102 ) ) ;
#204185=CARTESIAN_POINT ( 'NONE',  ( -8.283668668269720925, 8.766627655843896250, 1.056142170575426150E-14 ) ) ;
#204187=CARTESIAN_POINT ( 'NONE',  ( 6.435316467980822353, 10.65961964595298817, 1.040834085586084257E-14 ) ) ;
#204191=CARTESIAN_POINT ( 'NONE',  ( 1.499999999999989120, 1.056250000682816603, 0.000000000000000000 ) ) ;
#204193=CARTESIAN_POINT ( 'NONE',  ( -6.235860587281615075, 9.362588887548838557, -1.199719254218440723 ) ) ;
#204196=CARTESIAN_POINT ( 'NONE',  ( -7.797910906154257304, 12.24931315715533486, 0.000000000000000000 ) ) ;
#204199=EDGE_CURVE ( 'NONE', #164712, #91680, #115000, .T. ) ;
#204201=CARTESIAN_POINT ( 'NONE',  ( -0.7499999999999972244, 5.389583334016151639, -1.299038105676652899 ) ) ;
#204202=CARTESIAN_POINT ( 'NONE',  ( 6.368579470117202490, 8.453095353268645695, 1.599625672291281386 ) ) ;
#204206=CARTESIAN_POINT ( 'NONE',  ( -5.689618019229208734, 9.789638122409414223, 0.7998128361456481317 ) ) ;
#204208=CARTESIAN_POINT ( 'NONE',  ( 5.929387212421286080, 6.133046765490340668, -0.7644126115040312808 ) ) ;
#204215=CARTESIAN_POINT ( 'NONE',  ( -7.510853912290736289, 11.70648729774046792, 0.7216878364870458196 ) ) ;
#204219=CARTESIAN_POINT ( 'NONE',  ( -1.364683531250012516, 3.801041667008087099, -0.7879004041258300672 ) ) ;
#204220=TOROIDAL_SURFACE ( 'NONE', #27986, 6.909076424898650259, 0.08000000000000000167 ) ;
#204226=CARTESIAN_POINT ( 'NONE',  ( -1.364683531249997417, 4.759375000341424133, 1.214306433183764966E-14 ) ) ;
#204227=CARTESIAN_POINT ( 'NONE',  ( 3.469446951953614189E-15, 5.290451655907108197, 1.214306433183764966E-14 ) ) ;
#204230=CARTESIAN_POINT ( 'NONE',  ( 4.161989969270902812, 4.918371721313249623, 1.082531754730560403 ) ) ;
#204231=CARTESIAN_POINT ( 'NONE',  ( -1.364683531249997417, 5.321875000341417916, 1.214306433183764966E-14 ) ) ;
#204237=CARTESIAN_POINT ( 'NONE',  ( 1.364683531249988757, 0.3843750003414206362, 0.000000000000000000 ) ) ;
#204238=CARTESIAN_POINT ( 'NONE',  ( -4.446711195602264688, 4.290177271065136466, -0.7216878364870207285 ) ) ;
#204239=CARTESIAN_POINT ( 'NONE',  ( 4.527533231959700366, 7.369540306339926516, 1.199719254218462483 ) ) ;
#204242=DIRECTION ( 'NONE',  ( -5.578564026256490882E-16, -1.000000000000000000, -9.066213480720158442E-32 ) ) ;
#204245=CARTESIAN_POINT ( 'NONE',  ( 3.212919216758630014, 6.692230152952963529, 0.000000000000000000 ) ) ;
#204248=CARTESIAN_POINT ( 'NONE',  ( -7.321039761699444703, 10.52466824108257804, 1.082531754730549967 ) ) ;
#204253=CARTESIAN_POINT ( 'NONE',  ( -8.188234707649510113, 11.64035869464474082, -1.199719254218446718 ) ) ;
#204255=CARTESIAN_POINT ( 'NONE',  ( -4.677199806590235376, 7.440188293455128665, 1.082531754730560403 ) ) ;
#204257=CARTESIAN_POINT ( 'NONE',  ( -0.6823417656250003738, 2.530208333674753618, -1.181850606188749264 ) ) ;
#204274=CARTESIAN_POINT ( 'NONE',  ( 1.451998047843343409, 7.315968950353815892, -4.301760722578415574 ) ) ;
#204276=FACE_OUTER_BOUND ( 'NONE', #198726, .T. ) ;
#204279=CARTESIAN_POINT ( 'NONE',  ( -1.402160292154681736E-14, 2.509375000341417028, -1.575800808251660134 ) ) ;
#204289=CARTESIAN_POINT ( 'NONE',  ( 1.364683531249986537, 0.9052083336747533959, -0.7879004041258239610 ) ) ;
#204300=CARTESIAN_POINT ( 'NONE',  ( 6.003563092752934871, 5.898578451166879510, 0.7998128361456341429 ) ) ;
#204308=CARTESIAN_POINT ( 'NONE',  ( 6.446011968293428041, 9.607765498729298415, -1.199719254218440723 ) ) ;
#204311=CARTESIAN_POINT ( 'NONE',  ( 9.420217803396747414, 9.884675613584706255, 0.7998128361456462443 ) ) ;
#204323=CARTESIAN_POINT ( 'NONE',  ( -8.351459436338041442, 9.806086099558291025, -1.082531754730543971 ) ) ;
#204327=CARTESIAN_POINT ( 'NONE',  ( -9.806625181386236179, 10.33548422123910449, -0.7998128361456291469 ) ) ;
#204331=CARTESIAN_POINT ( 'NONE',  ( -5.274285450916075035, 6.112086766612214284, 1.199719254218450271 ) ) ;
#204334=CARTESIAN_POINT ( 'NONE',  ( 9.694243528971124846, 11.26870452434320491, 1.199719254218450271 ) ) ;
#204336=CARTESIAN_POINT ( 'NONE',  ( 3.818592820543298405, 7.606775390609172405, -0.7998128361456221525 ) ) ;
#204342=CARTESIAN_POINT ( 'NONE',  ( 2.562127843302666186, 5.932973550587659517, 0.000000000000000000 ) ) ;
#204344=CARTESIAN_POINT ( 'NONE',  ( -4.660252114795309097, 6.460046772059735432, -1.599625672291256295 ) ) ;
#204347=CARTESIAN_POINT ( 'NONE',  ( -10.15913717534155047, 10.74674821418697057, 0.7998128361456462443 ) ) ;
#204353=CARTESIAN_POINT ( 'NONE',  ( 8.107412671292035355, 10.48173408797264194, 1.443375672974076540 ) ) ;
#204355=CARTESIAN_POINT ( 'NONE',  ( -0.6823417656249969321, 4.030208333674754506, -1.181850606188749264 ) ) ;
#204358=CARTESIAN_POINT ( 'NONE',  ( 4.847203612085560387, 5.613824621309978724, -1.199719254218452047 ) ) ;
#204373=CARTESIAN_POINT ( 'NONE',  ( -1.364683531250000748, 2.071875000341422357, 1.214306433183764966E-14 ) ) ;
#204375=CARTESIAN_POINT ( 'NONE',  ( 10.38962578677386084, 11.01565159419135043, 0.000000000000000000 ) ) ;
#204378=CARTESIAN_POINT ( 'NONE',  ( -4.934804725694220906, 7.740727365743146571, -1.082531754730549967 ) ) ;
#204379=CARTESIAN_POINT ( 'NONE',  ( 2.711267533052988732, 6.106969855296372707, -0.7216878364870267237 ) ) ;
#204380=CARTESIAN_POINT ( 'NONE',  ( -6.195713011320804320, 7.291048603704809672, -1.082531754730543083 ) ) ;
#204382=ORIENTED_EDGE ( 'NONE', *, *, #211675, .F. ) ;
#204384=CARTESIAN_POINT ( 'NONE',  ( 3.798255590122797898, 7.583048621785260401, -0.7998128361456221525 ) ) ;
#204395=ADVANCED_FACE ( 'NONE', ( #112920 ), #147493, .F. ) ;
#204396=CARTESIAN_POINT ( 'NONE',  ( 6.993308306550549247, 7.053281200597435685, 1.040834085586084257E-14 ) ) ;
#204397=PRESENTATION_STYLE_ASSIGNMENT (( #138379 ) ) ;
#204399=CARTESIAN_POINT ( 'NONE',  ( -2.927671105547157371, 5.503034492191895666, 1.199719254218462483 ) ) ;
#204401=CARTESIAN_POINT ( 'NONE',  ( -6.256197817702116026, 9.386315656372753224, -1.199719254218440723 ) ) ;
#204405=CARTESIAN_POINT ( 'NONE',  ( 8.450809820019639318, 8.753699632978056755, -0.7998128361456291469 ) ) ;
#204408=CARTESIAN_POINT ( 'NONE',  ( -6.575868197828002693, 7.630599971342813426, 1.199719254218450271 ) ) ;
#204409=CARTESIAN_POINT ( 'NONE',  ( 6.941411460072420603, 7.200660912947041581, 1.040834085586084257E-14 ) ) ;
#204410=CARTESIAN_POINT ( 'NONE',  ( 5.026094266273638311, 6.779731885415203330, 1.422988838494985364 ) ) ;
#204411=CARTESIAN_POINT ( 'NONE',  ( -3.764360206088648297, 7.543504007078730922, -0.7998128361456281477 ) ) ;
#204414=CARTESIAN_POINT ( 'NONE',  ( -7.386494761346872551, 7.511998731193139989, -0.7998128361456291469 ) ) ;
#204419=CARTESIAN_POINT ( 'NONE',  ( -0.6823417656250212460, 1.301041667008083547, 1.181850606188755259 ) ) ;
#204421=CARTESIAN_POINT ( 'NONE',  ( -4.934804725694212912, 8.701096580044490381, -0.7216878364870207285 ) ) ;
#204426=CARTESIAN_POINT ( 'NONE',  ( 7.142447996300871793, 7.227277505306155092, 0.7998128361456341429 ) ) ;
#204431=CARTESIAN_POINT ( 'NONE',  ( 1.364683531249986537, 1.967708333674750731, -0.7879004041258239610 ) ) ;
#204437=CARTESIAN_POINT ( 'NONE',  ( -5.461236948206312114, 5.265864615862458464, 0.7998128361456341429 ) ) ;
#204438=CARTESIAN_POINT ( 'NONE',  ( -8.066738210006693777, 10.43428054980638997, 1.443375672974090751 ) ) ;
#204446=CARTESIAN_POINT ( 'NONE',  ( -7.578644679914719795, 9.864838098032418401, 1.443375672974090751 ) ) ;
#204451=CARTESIAN_POINT ( 'NONE',  ( -6.344852701071109102, 10.34615255131755163, 0.000000000000000000 ) ) ;
#204457=CARTESIAN_POINT ( 'NONE',  ( -1.500000000000011324, 5.452083334016153415, 0.8660254037844403729 ) ) ;
#204458=CARTESIAN_POINT ( 'NONE',  ( 4.357662274398333757, 7.395159486995275699, -1.145423081618229144 ) ) ;
#204465=CARTESIAN_POINT ( 'NONE',  ( -7.542413527904030524, 7.693903958843159252, 1.040834085586084257E-14 ) ) ;
#204468=CARTESIAN_POINT ( 'NONE',  ( 3.171717870593107058, 5.787755718078879674, -1.199719254218446718 ) ) ;
#204472=CARTESIAN_POINT ( 'NONE',  ( 5.469824908109481854, 8.468880595181346393, -1.199719254218446718 ) ) ;
#204477=CARTESIAN_POINT ( 'NONE',  ( -3.456965981804629884, 6.976951378839947537, 1.040834085586084257E-14 ) ) ;
#204489=CARTESIAN_POINT ( 'NONE',  ( -1.402160292154681736E-14, 0.4468750003414233563, -1.575800808251665908 ) ) ;
#204491=CARTESIAN_POINT ( 'NONE',  ( -9.124801077197171040, 10.60435499727357289, -1.199719254218441611 ) ) ;
#204493=CARTESIAN_POINT ( 'NONE',  ( 8.606728586576791074, 8.935604860628076906, 0.7998128361456462443 ) ) ;
#204495=CARTESIAN_POINT ( 'NONE',  ( -6.530223543276495235, 10.77034456713125188, -0.7998128361456291469 ) ) ;
#204498=CARTESIAN_POINT ( 'NONE',  ( -1.364683531250012516, 4.988541667008084879, -0.7879004041258300672 ) ) ;
#204500=CARTESIAN_POINT ( 'NONE',  ( 9.002250809793993724, 11.52571191622492464, -1.443375672974057666 ) ) ;
#204503=CARTESIAN_POINT ( 'NONE',  ( -0.7499999999999972244, 5.858333333333353821, -1.299038105676652011 ) ) ;
#204506=CARTESIAN_POINT ( 'NONE',  ( 7.171900071504736296, 9.390302721554109056, -1.443375672974058777 ) ) ;
#204509=CARTESIAN_POINT ( 'NONE',  ( -4.609409038966234995, 7.361099064560491456, -1.082531754730549967 ) ) ;
#204511=CARTESIAN_POINT ( 'NONE',  ( -1.364683531250012516, 3.030208333674755394, 0.7879004041258379498 ) ) ;
#204515=CARTESIAN_POINT ( 'NONE',  ( -7.203459687562382641, 7.298457811777897319, -0.7998128361456291469 ) ) ;
#204523=CARTESIAN_POINT ( 'NONE',  ( 7.476431642932036326, 10.80992178580769014, 1.199719254218460707 ) ) ;
#204526=CARTESIAN_POINT ( 'NONE',  ( -1.500000000000013101, 0.6708333333333583726, 0.8660254037844403729 ) ) ;
#204529=DIRECTION ( 'NONE',  ( 0.7592566023653005702, 0.6507913734559639396, 0.000000000000000000 ) ) ;
#204532=CARTESIAN_POINT ( 'NONE',  ( 5.450014563013511726, 8.341805509282339770, -1.082531754730543083 ) ) ;
#204533=AXIS2_PLACEMENT_3D ( 'NONE', #120232, #53017, #104991 ) ;
#204534=CARTESIAN_POINT ( 'NONE',  ( 0.6823417656249882723, -0.09479166632524876901, 1.181850606188755259 ) ) ;
#204542=CARTESIAN_POINT ( 'NONE',  ( 6.577677080924314801, 10.82570702772039262, 1.040834085586084257E-14 ) ) ;
#204543=CARTESIAN_POINT ( 'NONE',  ( -9.667127221743832877, 11.23706883257798772, 1.199719254218462483 ) ) ;
#204545=CARTESIAN_POINT ( 'NONE',  ( -1.402160292154681736E-14, -0.05312499965857903073, -1.575800808251665908 ) ) ;
#204546=CARTESIAN_POINT ( 'NONE',  ( -0.7500000000000006661, 1.358333333333357151, -1.299038105676652011 ) ) ;
#204548=CARTESIAN_POINT ( 'NONE',  ( 5.823390672269506574, 6.752709524857930745, -1.199719254218446718 ) ) ;
#204550=CARTESIAN_POINT ( 'NONE',  ( 1.284279953904119864, 2.827889714876734129, -0.7749999999999910294 ) ) ;
#204554=CARTESIAN_POINT ( 'NONE',  ( 1.364683531249988535, 4.655208333674755394, -0.7879004041258300672 ) ) ;
#204556=CARTESIAN_POINT ( 'NONE',  ( -7.483210719738908168, 10.81783070874899799, 1.199719254218453823 ) ) ;
#204557=CARTESIAN_POINT ( 'NONE',  ( -3.945059511896602089, 7.546393830613923548, 1.040834085586084257E-14 ) ) ;
#204565=ORIENTED_EDGE ( 'NONE', *, *, #50840, .T. ) ;
#204567=CARTESIAN_POINT ( 'NONE',  ( 6.577677080924314801, 10.82570702772039262, 1.040834085586084257E-14 ) ) ;
#204573=CARTESIAN_POINT ( 'NONE',  ( -8.518600588087975822, 8.832788862391110385, 1.040834085586084257E-14 ) ) ;
#204574=CARTESIAN_POINT ( 'NONE',  ( 4.659198344590585350, 8.587481835331020719, 0.7998128361456462443 ) ) ;
#204578=CARTESIAN_POINT ( 'NONE',  ( 4.844340958784499662, 4.546152628203684820, 0.7998128361456341429 ) ) ;
#204584=CARTESIAN_POINT ( 'NONE',  ( -5.802526556968872207, 6.832331073627524454, 1.082531754730548412 ) ) ;
#204585=CARTESIAN_POINT ( 'NONE',  ( 4.383363735919856730, 4.008345868194933104, -0.7998128361456211532 ) ) ;
#204588=CARTESIAN_POINT ( 'NONE',  ( -7.369020184227459858, 8.555943955475521889, 1.199719254218450271 ) ) ;
#204593=CARTESIAN_POINT ( 'NONE',  ( -8.483651433849100698, 10.92067931095586886, 1.599625672291269396 ) ) ;
#204599=CARTESIAN_POINT ( 'NONE',  ( 4.635998460869027227, 7.496083073400806818, -1.199719254218452047 ) ) ;
#204602=EDGE_LOOP ( 'NONE', ( #47341, #107053, #69395, #133928 ) ) ;
#204609=DIRECTION ( 'NONE',  ( 5.578564026256490882E-16, 1.000000000000000000, 9.066213480720158442E-32 ) ) ;
#204612=CARTESIAN_POINT ( 'NONE',  ( -8.016948904382338981, 8.247528564734524892, -0.7998128361456291469 ) ) ;
#204615=CARTESIAN_POINT ( 'NONE',  ( 5.504247177468179153, 7.444707678511436555, 1.443375672974062551 ) ) ;
#204618=CARTESIAN_POINT ( 'NONE',  ( 3.094265954482833703, 2.800000000000017586, -2.490342512183683965 ) ) ;
#204620=CARTESIAN_POINT ( 'NONE',  ( -4.303823697334223652, 7.108545849276850959, -1.199719254218452047 ) ) ;
#204624=CARTESIAN_POINT ( 'NONE',  ( -5.181187258716735577, 9.196468901811520880, 0.7998128361456481317 ) ) ;
#204630=CARTESIAN_POINT ( 'NONE',  ( -7.316596452869116973, 11.68777962832266049, 0.7998128361456481317 ) ) ;
#204631=CARTESIAN_POINT ( 'NONE',  ( 5.615048174354031474, 9.702639970055050966, 0.7998128361456462443 ) ) ;
#204633=CARTESIAN_POINT ( 'NONE',  ( -2.467220768007014176, 5.822248629409386922, 0.7216878364870317197 ) ) ;
#204634=CARTESIAN_POINT ( 'NONE',  ( -9.996439331977562404, 10.55693406359564790, 0.7998128361456462443 ) ) ;
#204637=CARTESIAN_POINT ( 'NONE',  ( 1.579999999999991189, 8.674529973577531194, -2.499999999999989342 ) ) ;
#204641=CARTESIAN_POINT ( 'NONE',  ( 9.734391104931951588, 11.41950637958454706, 1.082531754730548412 ) ) ;
#204662=CARTESIAN_POINT ( 'NONE',  ( -4.135400547368138113, 4.783387712472935149, 1.199719254218462483 ) ) ;
#204665=CARTESIAN_POINT ( 'NONE',  ( -3.755772246185468788, 4.340488027759846545, -1.199719254218452047 ) ) ;
#204668=ADVANCED_FACE ( 'NONE', ( #102996 ), #9915, .T. ) ;
#204670=CARTESIAN_POINT ( 'NONE',  ( -1.500000000000015099, -1.047916665983845919, 0.8660254037844403729 ) ) ;
#204678=CARTESIAN_POINT ( 'NONE',  ( 8.516493047678546091, 13.08765898893368629, -0.7998128361456352531 ) ) ;
#204679=CARTESIAN_POINT ( 'NONE',  ( -4.406036734316898240, 6.163462161501578329, -1.443375672974051449 ) ) ;
#204682=CARTESIAN_POINT ( 'NONE',  ( 8.365017589507326434, 12.70301158782650397, -0.7216878364870338292 ) ) ;
#204685=CARTESIAN_POINT ( 'NONE',  ( -1.402160292154681736E-14, 2.259375000341416140, -1.575800808251660134 ) ) ;
#204688=CARTESIAN_POINT ( 'NONE',  ( -9.508345801885592863, 9.987491611821676329, 0.7998128361456462443 ) ) ;
#204689=CARTESIAN_POINT ( 'NONE',  ( -5.382223794500845315, 6.341977850748185652, -1.082531754730543971 ) ) ;
#204691=CARTESIAN_POINT ( 'NONE',  ( -6.230135280679522936, 7.227244901336242755, 1.199719254218450271 ) ) ;
#204693=CARTESIAN_POINT ( 'NONE',  ( 0.7499999999999867883, -0.9020833326505162120, -1.299038105676652011 ) ) ;
#204701=CARTESIAN_POINT ( 'NONE',  ( -6.046573321570485327, 6.156683084694754449, 0.000000000000000000 ) ) ;
#204705=CARTESIAN_POINT ( 'NONE',  ( -3.755245360860919757, 7.324943987738961049, -0.7216878364870257245 ) ) ;
#204707=CARTESIAN_POINT ( 'NONE',  ( 10.58621901417202515, 11.24501035948919991, -0.7998128361456281477 ) ) ;
#204714=B_SPLINE_CURVE_WITH_KNOTS ( 'NONE', 3,
 ( #159870, #59162, #42946, #27735, #174019, #172937, #23446, #10403, #25588, #109055 ),
 .UNSPECIFIED., .F., .F.,
 ( 4, 3, 3, 4 ),
 ( 0.000000000000000000, 3.125151129215626700E-05, 5.612054754981304444E-05, 8.099579648775786166E-05 ),
 .UNSPECIFIED. ) ;
#204716=CARTESIAN_POINT ( 'NONE',  ( 5.043269954603521121, 4.986162489900023864, -0.7216878364870420448 ) ) ;
#204717=CARTESIAN_POINT ( 'NONE',  ( -3.741160322367112379, 6.452105245148518797, 1.199719254218464037 ) ) ;
#204718=CARTESIAN_POINT ( 'NONE',  ( -8.435144125996554720, 12.99275191363802229, 0.7998128361456341429 ) ) ;
#204722=CARTESIAN_POINT ( 'NONE',  ( 6.331821432781979730, 7.345878745455822312, -1.199719254218445830 ) ) ;
#204725=VERTEX_POINT ( 'NONE', #133987 ) ;
#204730=ORIENTED_EDGE ( 'NONE', *, *, #152121, .T. ) ;
#204739=CARTESIAN_POINT ( 'NONE',  ( 9.121938423896107651, 9.536683004167278099, -0.7998128361456221525 ) ) ;
#204740=CARTESIAN_POINT ( 'NONE',  ( -4.238895582566952314, 8.097128612970093897, 1.040834085586084257E-14 ) ) ;
#204746=CARTESIAN_POINT ( 'NONE',  ( -1.364683531250012516, 4.488541667008090208, -0.7879004041258300672 ) ) ;
#204748=CARTESIAN_POINT ( 'NONE',  ( -4.791917227426195858, 7.677988301050826969, -1.199719254218452047 ) ) ;
#204751=CARTESIAN_POINT ( 'NONE',  ( 5.331380718671758778, 7.243030143248949670, -1.599625672291256295 ) ) ;
#204752=CARTESIAN_POINT ( 'NONE',  ( -3.737243898861318137, 7.511868315313511069, 0.7998128361456341429 ) ) ;
#204758=CARTESIAN_POINT ( 'NONE',  ( 6.724481002698112775, 8.868313807946373473, -1.443375672974057666 ) ) ;
#204760=CARTESIAN_POINT ( 'NONE',  ( 5.788968402910795064, 9.697620870130524651, 0.7216878364870438212 ) ) ;
#204761=CARTESIAN_POINT ( 'NONE',  ( -1.201851678989727383E-14, 3.259375000341420581, -1.575800808251660134 ) ) ;
#204763=CARTESIAN_POINT ( 'NONE',  ( 3.497640442201256139, 7.024404915969360452, 1.040834085586084257E-14 ) ) ;
#204771=CARTESIAN_POINT ( 'NONE',  ( -5.011569529345123897, 6.785514760743092566, 1.449221747052743092 ) ) ;
#204772=CARTESIAN_POINT ( 'NONE',  ( -1.999999999999996669, 8.900000000000019895, 1.214306433183764966E-14 ) ) ;
#204778=CARTESIAN_POINT ( 'NONE',  ( -10.10098813738111545, 11.74323990082152491, -1.199719254218441611 ) ) ;
#204784=CARTESIAN_POINT ( 'NONE',  ( -3.297657676621885692, 4.870353260857385180, 1.599625672291267398 ) ) ;
#204787=EDGE_LOOP ( 'NONE', ( #188115, #189674, #66306, #183203 ) ) ;
#204790=CARTESIAN_POINT ( 'NONE',  ( -1.364683531250012516, 3.592708333674750509, 0.7879004041258379498 ) ) ;
#204792=CARTESIAN_POINT ( 'NONE',  ( 8.423693512792301163, 8.722063941212843119, 0.7998128361456481317 ) ) ;
#204793=EDGE_CURVE ( 'NONE', #210292, #196229, #61781, .T. ) ;
#204794=CARTESIAN_POINT ( 'NONE',  ( 8.283668668269706714, 8.766627655843896250, 1.040834085586084257E-14 ) ) ;
#204801=CARTESIAN_POINT ( 'NONE',  ( -0.7500000000000215383, 3.441666666666689967, 1.299038105676671107 ) ) ;
#204802=CARTESIAN_POINT ( 'NONE',  ( 6.159481859310094620, 6.080483678816896109, 1.040834085586084257E-14 ) ) ;
#204805=CARTESIAN_POINT ( 'NONE',  ( -1.201851678989727383E-14, 3.571875000341422357, 1.575800808251672791 ) ) ;
#204808=CARTESIAN_POINT ( 'NONE',  ( 7.754900677336718395, 11.99120852362745460, -0.7216878364870267237 ) ) ;
#204813=CARTESIAN_POINT ( 'NONE',  ( 0.7499999999999902300, 2.514583334016148974, 1.299038105676669330 ) ) ;
#204815=CARTESIAN_POINT ( 'NONE',  ( -4.880045225915050189, 7.780804299287790826, 1.199719254218464037 ) ) ;
#204816=CARTESIAN_POINT ( 'NONE',  ( 3.511198595814921219, 7.040222761851976152, 0.7216878364870317197 ) ) ;
#204823=EDGE_LOOP ( 'NONE', ( #57654, #43404, #8861, #188954 ) ) ;
#204824=CARTESIAN_POINT ( 'NONE',  ( 5.798083248138522272, 9.916180889470295412, 0.7998128361456462443 ) ) ;
#204825=CARTESIAN_POINT ( 'NONE',  ( 6.145923705696426431, 6.064665832934283962, 0.7998128361456341429 ) ) ;
#204827=CARTESIAN_POINT ( 'NONE',  ( 3.469446951953614189E-15, 8.900000000000019895, 1.214306433183764966E-14 ) ) ;
#204830=CARTESIAN_POINT ( 'NONE',  ( 6.505214776458575265, 6.483838748823460563, 1.040834085586084257E-14 ) ) ;
#204835=ORIENTED_EDGE ( 'NONE', *, *, #180876, .T. ) ;
#204838=CARTESIAN_POINT ( 'NONE',  ( 10.05353459973327368, 11.68787744023238417, -1.199719254218440723 ) ) ;
#204843=CARTESIAN_POINT ( 'NONE',  ( 5.150161082644886257, 6.468739049537000518, 1.195298158575591074 ) ) ;
#204851=CARTESIAN_POINT ( 'NONE',  ( 8.107412671292047790, 8.560995659369956101, 0.7216878364870458196 ) ) ;
#204852=CARTESIAN_POINT ( 'NONE',  ( -3.066115294984855133, 6.728884944124295053, 0.7998128361456341429 ) ) ;
#204856=CARTESIAN_POINT ( 'NONE',  ( -4.554649539187067830, 7.401175998105142817, 1.199719254218464037 ) ) ;
#204870=CARTESIAN_POINT ( 'NONE',  ( 10.23370702021670020, 10.83374636654133383, 0.7998128361456462443 ) ) ;
#204875=FACE_OUTER_BOUND ( 'NONE', #210976, .T. ) ;
#204880=CARTESIAN_POINT ( 'NONE',  ( -3.735435015764967837, 4.316761258935923884, -1.199719254218452047 ) ) ;
#204885=CARTESIAN_POINT ( 'NONE',  ( 7.889955328148847258, 11.29236608522730911, -1.199719254218446718 ) ) ;
#204890=CARTESIAN_POINT ( 'NONE',  ( -4.903245109636583443, 8.872203061218007392, -0.7998128361456281477 ) ) ;
#204891=CARTESIAN_POINT ( 'NONE',  ( 5.359550796103802028, 5.147230771742885125, -0.7998128361456231517 ) ) ;
#204895=CARTESIAN_POINT ( 'NONE',  ( -2.168941388506379742, 5.474256019991960542, -0.7216878364870267237 ) ) ;
#204898=CARTESIAN_POINT ( 'NONE',  ( 1.364683531249990311, 3.196875000341416140, 1.214306433183764966E-14 ) ) ;
#204901=CARTESIAN_POINT ( 'NONE',  ( 7.483737605063422116, 7.833374748769873719, -0.7216878364870257245 ) ) ;
#204905=CARTESIAN_POINT ( 'NONE',  ( 1.579999999999985860, -1.099999999999982991, 2.499999999999998668 ) ) ;
#204910=CARTESIAN_POINT ( 'NONE',  ( 8.798878505144646311, 11.28844422746735532, -1.443375672974052559 ) ) ;
#204912=ORIENTED_EDGE ( 'NONE', *, *, #156299, .T. ) ;
#204915=CARTESIAN_POINT ( 'NONE',  ( -7.492852449846775897, 11.89341162479659531, 0.000000000000000000 ) ) ;
#204924=CARTESIAN_POINT ( 'NONE',  ( 4.029797971759831121, 5.724516938518342535, -1.599625672291255185 ) ) ;
#204932=CARTESIAN_POINT ( 'NONE',  ( 4.527533231959700366, 7.369540306339926516, 1.199719254218462483 ) ) ;
#204935=CARTESIAN_POINT ( 'NONE',  ( 1.499999999999987121, 2.577083334016147198, -0.8660254037844262731 ) ) ;
#204940=CARTESIAN_POINT ( 'NONE',  ( -1.500000000000013101, 0.9208333333333594828, 0.8660254037844403729 ) ) ;
#204941=CARTESIAN_POINT ( 'NONE',  ( 8.111855979677986994, 8.358253485912799263, 1.040834085586084257E-14 ) ) ;
#204942=CARTESIAN_POINT ( 'NONE',  ( -1.364683531250000748, 0.2593750003414205252, 0.000000000000000000 ) ) ;
#204945=CARTESIAN_POINT ( 'NONE',  ( 7.944714827928033962, 12.21265836598400689, 0.7216878364870438212 ) ) ;
#204953=CARTESIAN_POINT ( 'NONE',  ( -4.394814349124112951, 8.279033840620114049, -0.7998128361456281477 ) ) ;
#204954=CARTESIAN_POINT ( 'NONE',  ( 1.499999999999989120, 2.285416667349482012, 0.8660254037844524744 ) ) ;
#204955=CARTESIAN_POINT ( 'NONE',  ( 1.364683531249990311, 5.676041667008088432, 0.7879004041258500513 ) ) ;
#204960=CARTESIAN_POINT ( 'NONE',  ( -0.6823417656250212460, 3.863541667008085767, 1.181850606188767472 ) ) ;
#204962=CARTESIAN_POINT ( 'NONE',  ( 8.235688245297327015, 11.69572115523387268, -1.199719254218446718 ) ) ;
#204970=CARTESIAN_POINT ( 'NONE',  ( -7.818248136574758256, 12.27303992597924420, 0.000000000000000000 ) ) ;
#204971=CARTESIAN_POINT ( 'NONE',  ( 7.955937213120826357, 8.176348258262782664, 0.7998128361456481317 ) ) ;
#204974=ORIENTED_EDGE ( 'NONE', *, *, #65647, .T. ) ;
#204979=CARTESIAN_POINT ( 'NONE',  ( -6.073162743917628781, 9.172774736957510555, -1.199719254218440723 ) ) ;
#204982=AXIS2_PLACEMENT_3D ( 'NONE', #164935, #52254, #67400 ) ;
#204985=CARTESIAN_POINT ( 'NONE',  ( 9.999301985278609806, 11.62460605670194447, 1.199719254218452047 ) ) ;
#204989=CARTESIAN_POINT ( 'NONE',  ( -5.928993247877788697, 5.811580298812519807, 0.7998128361456341429 ) ) ;
#204990=CARTESIAN_POINT ( 'NONE',  ( -9.820183334999905256, 10.35130206712171130, 1.040834085586084257E-14 ) ) ;
#204994=CARTESIAN_POINT ( 'NONE',  ( -3.999491622362644883, 7.816382810427971783, -0.3443157113667428271 ) ) ;
#205001=CARTESIAN_POINT ( 'NONE',  ( 5.494078562035752178, 7.432844293840273231, -1.599625672291262513 ) ) ;
#205003=CARTESIAN_POINT ( 'NONE',  ( 5.378281411895265762, 4.339595938922572671, 2.499999999999998668 ) ) ;
#205020=CARTESIAN_POINT ( 'NONE',  ( 4.365362273920252889, 4.195270195769483124, 0.7216878364870317197 ) ) ;
#205022=ORIENTED_EDGE ( 'NONE', *, *, #20455, .T. ) ;
#205025=CARTESIAN_POINT ( 'NONE',  ( 1.499999999999997113, 4.254166666666687746, 0.8660254037844477004 ) ) ;
#205030=CARTESIAN_POINT ( 'NONE',  ( 1.499999999999989120, 1.056250000682816603, 0.000000000000000000 ) ) ;
#205032=CARTESIAN_POINT ( 'NONE',  ( 5.695510712908186335, 6.192163513152999066, 0.9270467717220601811 ) ) ;
#205037=CARTESIAN_POINT ( 'NONE',  ( 1.364683531249986537, 1.155208333674754728, -0.7879004041258239610 ) ) ;
#205045=CARTESIAN_POINT ( 'NONE',  ( -3.578462479003122976, 6.262291094557191684, 1.199719254218464037 ) ) ;
#205050=CARTESIAN_POINT ( 'NONE',  ( 0.6823417656249882723, -0.09479166632524876901, 1.181850606188755259 ) ) ;
#205056=CARTESIAN_POINT ( 'NONE',  ( -1.364683531250000748, 0.009375000341420303140, 0.000000000000000000 ) ) ;
#205058=CARTESIAN_POINT ( 'NONE',  ( -7.446452682403657874, 9.710614100936176385, -1.599625672291263179 ) ) ;
#205059=CARTESIAN_POINT ( 'NONE',  ( 8.860417081730671995, 10.29590700256267155, 1.199719254218453823 ) ) ;
#205063=CARTESIAN_POINT ( 'NONE',  ( -0.6823417656250003738, 1.280208333674752508, -1.181850606188749264 ) ) ;
#205071=CARTESIAN_POINT ( 'NONE',  ( 6.561783159334121152, 8.678499657355050800, -1.443375672974057666 ) ) ;
#205074=CARTESIAN_POINT ( 'NONE',  ( -3.418627288940168096, 7.140148937072163804, -0.7998128361456281477 ) ) ;
#205075=CARTESIAN_POINT ( 'NONE',  ( 0.9486429539237137831, 3.163339070649072937, 1.028101543438981080 ) ) ;
#205079=CARTESIAN_POINT ( 'NONE',  ( 5.138177029454841893, 7.017625839162543677, 1.443375672974062551 ) ) ;
#205080=CARTESIAN_POINT ( 'NONE',  ( -9.314088342463968218, 9.968783942403868892, 0.7216878364870438212 ) ) ;
#205082=CARTESIAN_POINT ( 'NONE',  ( 1.499999999999987121, 4.045833333333359150, -0.8660254037844323793 ) ) ;
#205087=CARTESIAN_POINT ( 'NONE',  ( 9.002250809793993724, 11.52571191622492464, -1.443375672974057666 ) ) ;
#205098=DIRECTION ( 'NONE',  ( -0.7592566023653005702, -0.6507913734559640506, 0.000000000000000000 ) ) ;
#205099=CARTESIAN_POINT ( 'NONE',  ( 6.577677080924314801, 10.82570702772039262, 1.040834085586084257E-14 ) ) ;
#205101=CARTESIAN_POINT ( 'NONE',  ( -6.230135280679522936, 7.227244901336242755, 1.199719254218450271 ) ) ;
#205107=CARTESIAN_POINT ( 'NONE',  ( 5.029711800989886683, 4.970344644017389513, 1.040834085586084257E-14 ) ) ;
#205109=CARTESIAN_POINT ( 'NONE',  ( -8.514157279702033065, 9.995900250149611921, -1.082531754730543971 ) ) ;
#205131=CARTESIAN_POINT ( 'NONE',  ( 0.2871295479481039137, 7.105992221059469927, 1.980474574527469667 ) ) ;
#205135=CARTESIAN_POINT ( 'NONE',  ( -7.223796917982883592, 7.322184580601816428, -0.7998128361456291469 ) ) ;
#205146=CARTESIAN_POINT ( 'NONE',  ( -3.093231602212184850, 6.760520635889515795, -0.7998128361456281477 ) ) ;
#205149=CARTESIAN_POINT ( 'NONE',  ( 7.344766530301147789, 9.591980256816594164, 1.599625672291281386 ) ) ;
#205150=CARTESIAN_POINT ( 'NONE',  ( 0.6823417656249917140, 3.592708333674754506, 1.181850606188765695 ) ) ;
#205152=CARTESIAN_POINT ( 'NONE',  ( 6.114015800945279189, 6.016301931502064271, 0.06476946160361742033 ) ) ;
#205158=CARTESIAN_POINT ( 'NONE',  ( 5.300874872818821082, 9.128178418356554857, 0.7216878364870438212 ) ) ;
#205159=CARTESIAN_POINT ( 'NONE',  ( -7.965578943228732278, 9.251929174310385307, -1.199719254218446718 ) ) ;
#205162=CARTESIAN_POINT ( 'NONE',  ( -8.290974629956718189, 9.631557475493025322, -1.199719254218446718 ) ) ;
#205163=CARTESIAN_POINT ( 'NONE',  ( -6.901263884555985051, 8.010228272525461435, 1.199719254218450271 ) ) ;
#205171=CARTESIAN_POINT ( 'NONE',  ( 7.832860060393120882, 10.16142270859057462, 1.599625672291281386 ) ) ;
#205187=CARTESIAN_POINT ( 'NONE',  ( -1.201851678989727383E-14, 4.837500000000018119, -1.732050807568863648 ) ) ;
#205188=CARTESIAN_POINT ( 'NONE',  ( 6.010342169559767633, 5.906487374108181143, -0.7998128361456281477 ) ) ;
#205189=CARTESIAN_POINT ( 'NONE',  ( 5.147291874682557555, 9.156924287104992288, 0.7998128361456462443 ) ) ;
#205191=CARTESIAN_POINT ( 'NONE',  ( -7.863365906246054138, 11.15738207638699464, -1.082531754730543971 ) ) ;
#205193=CARTESIAN_POINT ( 'NONE',  ( 7.185458225562760148, 8.445751353653788485, -1.082531754730543083 ) ) ;
#205194=CARTESIAN_POINT ( 'NONE',  ( -7.497295758232712437, 11.69066945133944380, -0.7216878364870267237 ) ) ;
#205198=CARTESIAN_POINT ( 'NONE',  ( 7.239163954692881653, 10.53310948286200599, -1.199719254218441611 ) ) ;
#205204=CARTESIAN_POINT ( 'NONE',  ( 0.6823417656249899377, 1.842708333674752952, 1.181850606188755259 ) ) ;
#205210=CARTESIAN_POINT ( 'NONE',  ( 10.08456733046637765, 10.65975006183261087, 0.000000000000000000 ) ) ;
#205213=CARTESIAN_POINT ( 'NONE',  ( -8.910733272679575379, 11.41894145625809820, -1.599625672291263179 ) ) ;
#205215=CARTESIAN_POINT ( 'NONE',  ( -0.006768871532359390167, 8.210909518262125673, -2.038649385027042626 ) ) ;
#205219=CARTESIAN_POINT ( 'NONE',  ( 4.517891501851804215, 6.293959390292322986, -1.599625672291255185 ) ) ;
#205223=CARTESIAN_POINT ( 'NONE',  ( -9.287498920561160887, 10.79416914786490089, -1.199719254218441611 ) ) ;
#205226=CARTESIAN_POINT ( 'NONE',  ( 7.262363838414439776, 11.62450824479221900, 0.7998128361456462443 ) ) ;
#205228=CARTESIAN_POINT ( 'NONE',  ( 4.274728378101444903, 7.249864702071729283, 0.9550516446962635797 ) ) ;
#205230=CARTESIAN_POINT ( 'NONE',  ( -4.120788623549732854, 6.895004929861607401, -1.199719254218452047 ) ) ;
#205234=CARTESIAN_POINT ( 'NONE',  ( 9.264299036839600987, 9.702770385934682551, -0.7998128361456281477 ) ) ;
#205236=CARTESIAN_POINT ( 'NONE',  ( 5.750629710490689384, 9.860818428881154674, -0.7998128361456291469 ) ) ;
#205239=CARTESIAN_POINT ( 'NONE',  ( -7.849807752632384172, 12.10193344480572897, 0.000000000000000000 ) ) ;
#205247=CARTESIAN_POINT ( 'NONE',  ( -5.204229338117261072, 6.461601495962581154, -1.180324454998063377 ) ) ;
#205249=CARTESIAN_POINT ( 'NONE',  ( 6.155038550924144758, 8.203964280876741455, 1.443375672974076540 ) ) ;
#205259=DIRECTION ( 'NONE',  ( -5.578564026256490882E-16, -1.000000000000000000, -9.066213480720158442E-32 ) ) ;
#205271=AXIS2_PLACEMENT_3D ( 'NONE', #44343, #80018, #177535 ) ;
#205273=CARTESIAN_POINT ( 'NONE',  ( 7.262363838414439776, 11.62450824479221900, 0.7998128361456462443 ) ) ;
#205277=CARTESIAN_POINT ( 'NONE',  ( -0.7500000000000215383, 1.472916667349486008, 1.299038105676659116 ) ) ;
#205278=CARTESIAN_POINT ( 'NONE',  ( -2.272963308585411735, 5.803540959991587478, 0.7998128361456341429 ) ) ;
#205279=CARTESIAN_POINT ( 'NONE',  ( -5.520141099058386125, 9.591915048876776595, 0.000000000000000000 ) ) ;
#205283=CARTESIAN_POINT ( 'NONE',  ( -8.890396042259075315, 11.39521468743417998, -1.599625672291263179 ) ) ;
#205287=CARTESIAN_POINT ( 'NONE',  ( 1.499999999999991118, 5.285416667349480235, 0.8660254037844524744 ) ) ;
#205288=CARTESIAN_POINT ( 'NONE',  ( 7.293396569147545527, 10.59638086639245280, 1.199719254218460707 ) ) ;
#205291=CARTESIAN_POINT ( 'NONE',  ( -6.527360889975461156, 9.702672574024962415, 1.199719254218452047 ) ) ;
#205293=CARTESIAN_POINT ( 'NONE',  ( 0.6823417656249899377, 4.926041667008086655, -1.181850606188754593 ) ) ;
#205299=CARTESIAN_POINT ( 'NONE',  ( -9.029367117021344313, 9.636609179387466639, 0.7216878364870438212 ) ) ;
#205303=CARTESIAN_POINT ( 'NONE',  ( -1.201851678989727383E-14, 3.759375000341422801, -1.575800808251660134 ) ) ;
#205311=CARTESIAN_POINT ( 'NONE',  ( -1.364683531250012516, 4.488541667008090208, -0.7879004041258300672 ) ) ;
#205312=CARTESIAN_POINT ( 'NONE',  ( -5.434120640978981065, 5.234228924097238611, -0.7998128361456221525 ) ) ;
#205313=CARTESIAN_POINT ( 'NONE',  ( 7.284808609244363353, 7.393364887073558656, 0.7998128361456341429 ) ) ;
#205316=CARTESIAN_POINT ( 'NONE',  ( 3.456965981360264895, 6.016582164020185530, -1.082531754730543971 ) ) ;
#205317=CARTESIAN_POINT ( 'NONE',  ( -1.364683531250010295, 5.551041667008087543, -0.7879004041258300672 ) ) ;
#205322=CARTESIAN_POINT ( 'NONE',  ( -1.402160292154681736E-14, 0.9468750003414176941, -1.575800808251659024 ) ) ;
#205323=CARTESIAN_POINT ( 'NONE',  ( -4.148431816101615155, 3.942184661647709198, 0.7216878364870317197 ) ) ;
#205324=CARTESIAN_POINT ( 'NONE',  ( 5.606460214450851964, 6.499623990736163037, 1.199719254218462483 ) ) ;
#205329=CARTESIAN_POINT ( 'NONE',  ( 4.541618270897912701, 4.400902192243413502, 1.214306433183764966E-14 ) ) ;
#205332=CARTESIAN_POINT ( 'NONE',  ( -7.809133291791416909, 11.09411069285655493, 1.082531754730549967 ) ) ;
#205337=CARTESIAN_POINT ( 'NONE',  ( -8.784793466650835825, 12.33634391347959713, 1.199719254218462483 ) ) ;
#205338=CARTESIAN_POINT ( 'NONE',  ( -4.229780737339226881, 7.878568593630327577, 1.040834085586084257E-14 ) ) ;
#205340=CARTESIAN_POINT ( 'NONE',  ( -1.364683531250000748, 1.321875000341421469, 0.000000000000000000 ) ) ;
#205343=CARTESIAN_POINT ( 'NONE',  ( 3.609978820808554811, 4.211641957610042120, -7.499999999999997335 ) ) ;
#205353=CARTESIAN_POINT ( 'NONE',  ( 7.524412065460039933, 10.76193592880331984, -1.082531754730537976 ) ) ;
#205365=CARTESIAN_POINT ( 'NONE',  ( -3.904855289079262270, 2.800000000000024691, 0.7750000000000135669 ) ) ;
#205367=CARTESIAN_POINT ( 'NONE',  ( 0.6823417656249899377, 3.238541667008085323, -1.181850606188754593 ) ) ;
#205376=CARTESIAN_POINT ( 'NONE',  ( -1.364683531250012516, 1.780208333674757615, 0.7879004041258379498 ) ) ;
#205386=CARTESIAN_POINT ( 'NONE',  ( 4.873266149108180123, 7.772895376346490970, 1.199719254218462483 ) ) ;
#205397=CARTESIAN_POINT ( 'NONE',  ( 7.690499447449630210, 9.995335326823163058, 1.599625672291281386 ) ) ;
#205399=DIRECTION ( 'NONE',  ( -0.9999160831030532437, -0.01240418662286108496, 0.003736697214589113167 ) ) ;
#205409=CARTESIAN_POINT ( 'NONE',  ( -8.188761592974051595, 9.616271948966963024, -1.082531754730543971 ) ) ;
#205415=CIRCLE ( 'NONE', #94761, 1.250000000000000222 ) ;
#205416=CARTESIAN_POINT ( 'NONE',  ( -7.960608749518247151, 12.43912730774665576, 0.000000000000000000 ) ) ;
#205418=CARTESIAN_POINT ( 'NONE',  ( -4.196906876117826535, 3.977091173117547562, -0.5668149747346932221 ) ) ;
#205422=CARTESIAN_POINT ( 'NONE',  ( 9.073431116043567002, 11.60875560684942265, -1.599625672291262513 ) ) ;
#205424=CARTESIAN_POINT ( 'NONE',  ( 5.678167406024951624, 5.518950149984223508, 0.7998128361456341429 ) ) ;
#205426=ORIENTED_EDGE ( 'NONE', *, *, #151476, .F. ) ;
#205431=CARTESIAN_POINT ( 'NONE',  ( -4.381256195510448315, 8.263215994737505454, 1.040834085586084257E-14 ) ) ;
#205434=CARTESIAN_POINT ( 'NONE',  ( -2.948008335967658322, 5.526761261015804116, 1.199719254218462483 ) ) ;
#205441=CARTESIAN_POINT ( 'NONE',  ( 8.324343129110697959, 9.774450407793066731, -1.082531754730543083 ) ) ;
#205443=CARTESIAN_POINT ( 'NONE',  ( -0.6823417656249969321, 4.530208333674755394, -1.181850606188749264 ) ) ;
#205445=CARTESIAN_POINT ( 'NONE',  ( 4.476163270806094552, 8.373940915915776273, 0.7998128361456462443 ) ) ;
#205456=CARTESIAN_POINT ( 'NONE',  ( 1.445368642220961508, 8.714907460504134562, -2.589984629573225838 ) ) ;
#205461=CARTESIAN_POINT ( 'NONE',  ( 1.364683531249986537, 0.6760416670080884316, 0.7879004041258500513 ) ) ;
#205463=CARTESIAN_POINT ( 'NONE',  ( 9.297140650669039275, 11.86975006391249643, 1.599625672291281386 ) ) ;
#205465=CARTESIAN_POINT ( 'NONE',  ( -5.368665641331555882, 8.246898433986675769, 1.082531754730548412 ) ) ;
#205466=CARTESIAN_POINT ( 'NONE',  ( 4.284013352238246419, 6.021101549076499637, -1.443375672974051449 ) ) ;
#205467=CARTESIAN_POINT ( 'NONE',  ( -4.880572110795192486, 8.637825195995631589, 1.214306433183764966E-14 ) ) ;
#205472=CARTESIAN_POINT ( 'NONE',  ( 6.634017235788401301, 6.634108284708264414, 0.7998128361456341429 ) ) ;
#205482=CARTESIAN_POINT ( 'NONE',  ( 4.306686350635271054, 8.176217842383143974, -0.7998128361456221525 ) ) ;
#205484=CARTESIAN_POINT ( 'NONE',  ( -7.725448601688521322, 7.907444878258402809, 1.040834085586084257E-14 ) ) ;
#205488=CARTESIAN_POINT ( 'NONE',  ( 7.507464373665139412, 9.781794407407920389, 1.599625672291281386 ) ) ;
#205491=CARTESIAN_POINT ( 'NONE',  ( -5.930802130974132780, 9.006687355190106103, -1.199719254218440723 ) ) ;
#205492=CARTESIAN_POINT ( 'NONE',  ( 6.249945625775433555, 10.23542763013927726, -0.7216878364870267237 ) ) ;
#205493=CARTESIAN_POINT ( 'NONE',  ( 5.239055555121258756, 6.613325079961110298, 1.380154382352281495 ) ) ;
#205494=CARTESIAN_POINT ( 'NONE',  ( -5.708146366553361162, 6.618257834855742594, -1.199719254218446718 ) ) ;
#205501=CARTESIAN_POINT ( 'NONE',  ( 10.37606763316019531, 10.99983374830873650, 0.7998128361456462443 ) ) ;
#205503=CARTESIAN_POINT ( 'NONE',  ( -1.402160292154681736E-14, 1.696875000341421469, -1.575800808251659024 ) ) ;
#205505=CARTESIAN_POINT ( 'NONE',  ( -5.260200412422200600, 8.120355666925794580, -1.082531754730544860 ) ) ;
#205506=VERTEX_POINT ( 'NONE', #213071 ) ;
#205512=CARTESIAN_POINT ( 'NONE',  ( -5.803933766307007858, 6.065161521460068705, 0.5445525043519475750 ) ) ;
#205513=CARTESIAN_POINT ( 'NONE',  ( 1.364683531249988535, 1.426041667008083991, 0.7879004041258500513 ) ) ;
#205516=CARTESIAN_POINT ( 'NONE',  ( 3.036663219780971978, 6.486598156479028709, -0.7216878364870267237 ) ) ;
#205519=CARTESIAN_POINT ( 'NONE',  ( -5.284980951228653190, 5.060232619388524533, 0.000000000000000000 ) ) ;
#205521=CARTESIAN_POINT ( 'NONE',  ( -8.148087131688692253, 9.568818410800712826, -1.082531754730543083 ) ) ;
#205529=CARTESIAN_POINT ( 'NONE',  ( -8.825994812371996900, 9.399341490629888440, 0.7216878364870438212 ) ) ;
#205532=VERTEX_POINT ( 'NONE', #149151 ) ;
#205533=CARTESIAN_POINT ( 'NONE',  ( -7.659993601596720936, 8.999375959026737704, -1.082531754730543083 ) ) ;
#205536=EDGE_LOOP ( 'NONE', ( #141769, #211278, #208475, #79293 ) ) ;
#205539=CARTESIAN_POINT ( 'NONE',  ( 1.499999999999990896, 5.056250000682820378, 1.214306433183764966E-14 ) ) ;
#205540=CARTESIAN_POINT ( 'NONE',  ( 4.707942587747941943, 7.051207734045064512, -1.383178547476830111 ) ) ;
#205541=DIRECTION ( 'NONE',  ( 0.000000000000000000, 1.000000000000000000, -8.546850786086437571E-32 ) ) ;
#205546=CARTESIAN_POINT ( 'NONE',  ( -7.854251061018346469, 8.057714414143200443, -0.7998128361456291469 ) ) ;
#205549=CARTESIAN_POINT ( 'NONE',  ( 3.928111819657337911, 5.605883094398769195, 1.599625672291267398 ) ) ;
#205553=CARTESIAN_POINT ( 'NONE',  ( 7.644099680006512187, 7.812537802962739697, 1.040834085586084257E-14 ) ) ;
#205559=CARTESIAN_POINT ( 'NONE',  ( -5.585596099150191840, 7.539614753807099667, -1.443375672974052559 ) ) ;
#205566=CARTESIAN_POINT ( 'NONE',  ( 3.673896439623286714, 4.156855427197417185, -7.499999999999997335 ) ) ;
#205570=CARTESIAN_POINT ( 'NONE',  ( -0.6823417656250212460, 0.8010416670080899859, 1.181850606188755259 ) ) ;
#205572=CARTESIAN_POINT ( 'NONE',  ( -7.503547950159405566, 10.84155747757291266, 1.199719254218453823 ) ) ;
#205574=AXIS2_PLACEMENT_3D ( 'NONE', #201120, #182752, #98319 ) ;
#205575=CARTESIAN_POINT ( 'NONE',  ( 9.094822116668764167, 9.505047312402055582, 0.7998128361456462443 ) ) ;
#205577=CARTESIAN_POINT ( 'NONE',  ( -9.189729191964438826, 9.615772233580322848, 1.040834085586084257E-14 ) ) ;
#205580=CARTESIAN_POINT ( 'NONE',  ( 0.6823417656249899377, 4.426041667008086655, -1.181850606188754593 ) ) ;
#205582=CARTESIAN_POINT ( 'NONE',  ( 8.676855123066012254, 11.14608361504227574, -1.443375672974052559 ) ) ;
#205585=CARTESIAN_POINT ( 'NONE',  ( 1.364683531249986537, -0.3239583329919163424, 0.7879004041258500513 ) ) ;
#205588=CARTESIAN_POINT ( 'NONE',  ( 6.588899466117086767, 10.63087377720454363, 1.040834085586084257E-14 ) ) ;
#205591=CARTESIAN_POINT ( 'NONE',  ( -4.595850885352567694, 8.305650432979225783, 1.040834085586084257E-14 ) ) ;
#205593=CARTESIAN_POINT ( 'NONE',  ( 1.364683531249988535, 2.363541667008088432, 0.7879004041258500513 ) ) ;
#205597=CARTESIAN_POINT ( 'NONE',  ( -6.170932472514347289, 10.35117165124207972, 0.000000000000000000 ) ) ;
#205598=CARTESIAN_POINT ( 'NONE',  ( 1.364683531249988535, 4.467708333674754506, -0.7879004041258300672 ) ) ;
#205603=CARTESIAN_POINT ( 'NONE',  ( 8.606728586576791074, 8.935604860628076906, 0.7998128361456462443 ) ) ;
#205606=CARTESIAN_POINT ( 'NONE',  ( 0.7499999999999885647, 1.066666666666687968, -1.299038105676652899 ) ) ;
#205607=ADVANCED_FACE ( 'NONE', ( #129801 ), #89517, .F. ) ;
#205613=CARTESIAN_POINT ( 'NONE',  ( 8.270110514656037637, 8.750809809961280550, 0.7216878364870458196 ) ) ;
#205619=CARTESIAN_POINT ( 'NONE',  ( 9.074484886248265880, 9.481320543578137361, 0.7998128361456462443 ) ) ;
#205620=CARTESIAN_POINT ( 'NONE',  ( -4.080641063585716211, 5.783833847506671511, -1.249999999999999334 ) ) ;
#205624=CARTESIAN_POINT ( 'NONE',  ( -0.6823417656250003738, 0.2177083336747515085, -1.181850606188749264 ) ) ;
#205625=CARTESIAN_POINT ( 'NONE',  ( -0.7500000000000215383, 1.441666666666688190, 1.299038105676659116 ) ) ;
#205628=CARTESIAN_POINT ( 'NONE',  ( 4.449046963578762615, 8.342305224150557308, -0.7998128361456231517 ) ) ;
#205630=( BOUNDED_CURVE ( )  B_SPLINE_CURVE ( 2, ( #42451, #159371, #45642, #95475, #108557, #44578, #13108, #79185, #59737, #25094, #177764, #175642, #211306, #27228, #93335, #26162, #28304, #158323, #62931, #125895, #129099, #195071, #8847, #46710, #61873, #94399, #10969, #77043, #78114, #126964, #192922, #128038, #193993, #112824, #111759, #31518, #148464, #15233, #33, #99702, #162584, #84511, #165773, #66097, #133302, #114945, #16289, #14159, #150599, #113900, #67167, #80253, #197192, #137291, #178840, #147399, #1106, #71173, #48831, #180945, #17356, #100758, #2160, #132239, #82374, #163651, #199307, #149520, #198247 ),
 .UNSPECIFIED., .F., .T. ) 
 B_SPLINE_CURVE_WITH_KNOTS ( ( 3, 2, 2, 2, 2, 2, 2, 2, 2, 2, 2, 2, 2, 2, 2, 2, 2, 2, 2, 2, 2, 2, 2, 2, 2, 2, 2, 2, 2, 2, 2, 2, 2, 2, 3 ),
 ( 0.1422369605164288953, 0.1458333333333333426, 0.1499999999999999944, 0.1541666666666666741, 0.1583333333333333259, 0.1625000000000000056, 0.1666666666666666574, 0.1708333333333333370, 0.1749999999999999889, 0.1791666666666666685, 0.1833333333333333204, 0.1875000000000000000, 0.1916666666666666796, 0.1958333333333333315, 0.2000000000000000111, 0.2041666666666666630, 0.2083333333333333426, 0.2124999999999999944, 0.2166666666666666741, 0.2208333333333333259, 0.2250000000000000056, 0.2291666666666666574, 0.2333333333333333370, 0.2374999999999999889, 0.2416666666666666685, 0.2458333333333333204, 0.2500000000000000000, 0.2541666666666666519, 0.2583333333333333592, 0.2625000000000000111, 0.2666666666666666630, 0.2708333333333333148, 0.2750000000000000222, 0.2791666666666666741, 0.2794680684751273403 ),
 .UNSPECIFIED. ) 
 CURVE ( )  GEOMETRIC_REPRESENTATION_ITEM ( )  RATIONAL_B_SPLINE_CURVE ( ( 0.9683452906431684326, 0.8843625769635057310, 1.000000000000000000, 0.8660254037844387076, 1.000000000000000000, 0.8660254037844387076, 1.000000000000000000, 0.8660254037844387076, 1.000000000000000000, 0.8660254037844387076, 1.000000000000000000, 0.8660254037844387076, 1.000000000000000000, 0.8660254037844387076, 1.000000000000000000, 0.8660254037844387076, 1.000000000000000000, 0.8660254037844387076, 1.000000000000000000, 0.8660254037844387076, 1.000000000000000000, 0.8660254037844387076, 1.000000000000000000, 0.8660254037844387076, 1.000000000000000000, 0.8660254037844387076, 1.000000000000000000, 0.8660254037844387076, 1.000000000000000000, 0.8660254037844387076, 1.000000000000000000, 0.8660254037844387076, 1.000000000000000000, 0.8660254037844387076, 1.000000000000000000, 0.8660254037844387076, 1.000000000000000000, 0.8660254037844387076, 1.000000000000000000, 0.8660254037844387076, 1.000000000000000000, 0.8660254037844387076, 1.000000000000000000, 0.8660254037844387076, 1.000000000000000000, 0.8660254037844387076, 1.000000000000000000, 0.8660254037844387076, 1.000000000000000000, 0.8660254037844387076, 1.000000000000000000, 0.8660254037844387076, 1.000000000000000000, 0.8660254037844387076, 1.000000000000000000, 0.8660254037844387076, 1.000000000000000000, 0.8660254037844387076, 1.000000000000000000, 0.8660254037844387076, 1.000000000000000000, 0.8660254037844387076, 1.000000000000000000, 0.8660254037844387076, 1.000000000000000000, 0.8660254037844387076, 1.000000000000000000, 0.9903087554590821462, 0.9820195710609804784 ) ) 
 REPRESENTATION_ITEM ( '' )  );
#205633=CARTESIAN_POINT ( 'NONE',  ( -1.001543065824772872E-14, 5.571875000341416140, 1.575800808251672791 ) ) ;
#205635=CARTESIAN_POINT ( 'NONE',  ( -8.995998617867369873, 10.45408546138876993, 1.199719254218462483 ) ) ;
#205636=CARTESIAN_POINT ( 'NONE',  ( -6.249945626219832739, 6.393950773452325542, 1.040834085586084257E-14 ) ) ;
#205638=CARTESIAN_POINT ( 'NONE',  ( -1.499999999999997780, 4.931250000682820378, 1.214306433183764966E-14 ) ) ;
#205645=CARTESIAN_POINT ( 'NONE',  ( 7.263417608619159083, 9.497073181520933716, -1.599625672291262513 ) ) ;
#205649=CARTESIAN_POINT ( 'NONE',  ( 7.904040366642695048, 9.284097184913720824, 1.082531754730558626 ) ) ;
#205652=CARTESIAN_POINT ( 'NONE',  ( -8.296699936558862731, 11.76690146170562201, 1.199719254218453823 ) ) ;
#205653=CARTESIAN_POINT ( 'NONE',  ( 6.277588818327314080, 7.282607361925381717, 1.199719254218462483 ) ) ;
#205655=CARTESIAN_POINT ( 'NONE',  ( 3.267151830768944443, 4.834763107362302748, -1.443375672974058777 ) ) ;
#205657=CARTESIAN_POINT ( 'NONE',  ( 3.521367211247359741, 5.131347717920458962, -1.599625672291262513 ) ) ;
#205664=CARTESIAN_POINT ( 'NONE',  ( -4.446711195602245148, 7.171284913969171448, -1.082531754730549967 ) ) ;
#205665=CARTESIAN_POINT ( 'NONE',  ( 9.625925876022625616, 11.29296361252366765, -1.082531754730537088 ) ) ;
#205668=CARTESIAN_POINT ( 'NONE',  ( -6.124532705071231931, 8.168374127381657246, -1.599625672291263179 ) ) ;
#205673=CARTESIAN_POINT ( 'NONE',  ( -9.481229494658258261, 9.955855920056455588, -0.7998128361456291469 ) ) ;
#205674=CARTESIAN_POINT ( 'NONE',  ( 1.203941962966154744, 3.072768152887747739, 0.7750000000000065725 ) ) ;
#205676=CARTESIAN_POINT ( 'NONE',  ( -2.273105066167325550, 5.702484939155337607, -7.499999999999997335 ) ) ;
#205678=CARTESIAN_POINT ( 'NONE',  ( 4.798696304233017074, 7.685897223992134819, -1.199719254218452047 ) ) ;
#205687=FACE_OUTER_BOUND ( 'NONE', #7116, .T. ) ;
#205690=CARTESIAN_POINT ( 'NONE',  ( -5.533699252672048985, 9.607732894759390518, -0.7998128361456231517 ) ) ;
#205691=EDGE_CURVE ( 'NONE', #163734, #160319, #174432, .T. ) ;
#205694=CARTESIAN_POINT ( 'NONE',  ( 4.826339496784873617, 8.574553812983598533, -0.7216878364870257245 ) ) ;
#205696=CARTESIAN_POINT ( 'NONE',  ( -0.1099460098627005888, 6.494484681433106310, 3.110387376256865011 ) ) ;
#205698=CARTESIAN_POINT ( 'NONE',  ( 3.948449050077836642, 5.629609863222681199, 1.599625672291267398 ) ) ;
#205700=CARTESIAN_POINT ( 'NONE',  ( -5.708146366553361162, 6.618257834855742594, -1.199719254218446718 ) ) ;
#205704=CARTESIAN_POINT ( 'NONE',  ( -5.194745412330402878, 9.212286747694129474, 0.000000000000000000 ) ) ;
#205711=CARTESIAN_POINT ( 'NONE',  ( 7.800018446563675489, 7.994443030612759848, -0.7998128361456281477 ) ) ;
#205714=CARTESIAN_POINT ( 'NONE',  ( -5.704936041347759001, 6.126156357109620032, -0.7369488182252960096 ) ) ;
#205720=ORIENTED_EDGE ( 'NONE', *, *, #92993, .F. ) ;
#205722=CARTESIAN_POINT ( 'NONE',  ( 8.107412671292022921, 12.40247251657532956, 0.7216878364870438212 ) ) ;
#205742=CARTESIAN_POINT ( 'NONE',  ( -5.135841261478327979, 4.886236314679810455, 0.7998128361456341429 ) ) ;
#205745=CARTESIAN_POINT ( 'NONE',  ( -2.676845263694313637, 5.210404343363602919, -1.199719254218446718 ) ) ;
#205750=CARTESIAN_POINT ( 'NONE',  ( -1.402160292154681736E-14, -0.6312499993171797330, -1.732050807568870754 ) ) ;
#205760=CARTESIAN_POINT ( 'NONE',  ( 4.376584659113025744, 4.000436945253625254, 0.7998128361456341429 ) ) ;
#205766=CARTESIAN_POINT ( 'NONE',  ( 1.364683531249986537, 1.967708333674750731, -0.7879004041258239610 ) ) ;
#205767=EDGE_CURVE ( 'NONE', #104455, #214357, #174727, .T. ) ;
#205770=CARTESIAN_POINT ( 'NONE',  ( -9.833741488613570780, 10.36711991300432345, 0.7998128361456462443 ) ) ;
#205771=CARTESIAN_POINT ( 'NONE',  ( -4.975479186090865369, 6.827811688571220117, 1.443375672974064550 ) ) ;
#205772=B_SPLINE_CURVE_WITH_KNOTS ( 'NONE', 3,
 ( #58120, #127483, #42966, #109074, #124279, #190237 ),
 .UNSPECIFIED., .F., .F.,
 ( 4, 2, 4 ),
 ( 0.000000000000000000, 0.0006181257251340652832, 0.001236251450268130566 ),
 .UNSPECIFIED. ) ;
#205774=CARTESIAN_POINT ( 'NONE',  ( -5.018489415352746619, 9.006654751220198207, 0.7998128361456481317 ) ) ;
#205776=CARTESIAN_POINT ( 'NONE',  ( -1.001543065824772872E-14, 5.571875000341416140, 1.575800808251672791 ) ) ;
#205784=CARTESIAN_POINT ( 'NONE',  ( -4.243338890952892406, 7.894386439512932618, -0.7216878364870257245 ) ) ;
#205790=CARTESIAN_POINT ( 'NONE',  ( -4.229780737339226881, 7.878568593630327577, 1.040834085586084257E-14 ) ) ;
#205792=CARTESIAN_POINT ( 'NONE',  ( 8.374132434735052755, 12.92157160716627295, -0.7998128361456352531 ) ) ;
#205795=CARTESIAN_POINT ( 'NONE',  ( -1.499999999999997780, 3.650000000000021227, 1.214306433183764966E-14 ) ) ;
#205801=CARTESIAN_POINT ( 'NONE',  ( -2.930533758848195447, 6.570706485298192234, -0.7998128361456281477 ) ) ;
#205802=CARTESIAN_POINT ( 'NONE',  ( -10.08065090696061716, 11.71951313199760136, -1.199719254218441611 ) ) ;
#205805=VERTEX_POINT ( 'NONE', #201077 ) ;
#205807=CARTESIAN_POINT ( 'NONE',  ( 8.324343129110697959, 9.774450407793066731, -1.082531754730543083 ) ) ;
#205808=CARTESIAN_POINT ( 'NONE',  ( 6.993308306550549247, 7.053281200597435685, 1.040834085586084257E-14 ) ) ;
#205811=EDGE_LOOP ( 'NONE', ( #32001, #213585, #110748, #117206 ) ) ;
#205813=CARTESIAN_POINT ( 'NONE',  ( 5.203632029546647608, 4.965325544092860532, 1.040834085586084257E-14 ) ) ;
#205824=CARTESIAN_POINT ( 'NONE',  ( 9.206149998879153529, 10.69926207256923689, 1.199719254218453823 ) ) ;
#205825=CARTESIAN_POINT ( 'NONE',  ( -4.564291269294938225, 8.476756914152748124, 1.040834085586084257E-14 ) ) ;
#205831=CARTESIAN_POINT ( 'NONE',  ( 0.6823417656249917140, 4.592708333674755394, 1.181850606188765695 ) ) ;
#205833=CARTESIAN_POINT ( 'NONE',  ( -4.726989112658928072, 8.666571064744069020, 1.040834085586084257E-14 ) ) ;
#205836=CARTESIAN_POINT ( 'NONE',  ( 6.356075086708249167, 6.309842444114747373, -0.7998128361456281477 ) ) ;
#205837=CARTESIAN_POINT ( 'NONE',  ( -5.331380718671772101, 7.243030143248949670, -1.599625672291256295 ) ) ;
#205844=CARTESIAN_POINT ( 'NONE',  ( 7.321039761699430493, 7.643560598178549270, -0.7216878364870257245 ) ) ;
#205846=CARTESIAN_POINT ( 'NONE',  ( 7.741342523278707866, 8.133913820021057006, 0.7216878364870458196 ) ) ;
#205847=CARTESIAN_POINT ( 'NONE',  ( -1.364683531250012516, 3.551041667008086211, -0.7879004041258300672 ) ) ;
#205849=CARTESIAN_POINT ( 'NONE',  ( 5.978782553502139940, 6.077593855281705260, -0.7216878364870257245 ) ) ;
#205858=CARTESIAN_POINT ( 'NONE',  ( -4.712061673757400371, 7.041017223283659199, 1.411098259540758182 ) ) ;
#205859=CARTESIAN_POINT ( 'NONE',  ( -0.9999999999999965583, 6.120000000000022311, 1.226552901175238481E-14 ) ) ;
#205865=CARTESIAN_POINT ( 'NONE',  ( -4.243338890952916387, 4.052909582307567149, -0.7216878364870207285 ) ) ;
#205867=CARTESIAN_POINT ( 'NONE',  ( 3.277320446201373638, 4.846626492033466072, 1.599625672291267398 ) ) ;
#205870=CARTESIAN_POINT ( 'NONE',  ( -4.485049888022365927, 4.126979712314507331, 0.7998128361456341429 ) ) ;
#205875=CARTESIAN_POINT ( 'NONE',  ( 4.744990575102895569, 5.598539094783909320, -1.082531754730548412 ) ) ;
#205876=CARTESIAN_POINT ( 'NONE',  ( 1.364683531249988535, 3.217708333674748289, -0.7879004041258239610 ) ) ;
#205878=CARTESIAN_POINT ( 'NONE',  ( 7.065770611016287006, 11.39514947949436774, 1.040834085586084257E-14 ) ) ;
#205880=CARTESIAN_POINT ( 'NONE',  ( -9.938290294017125603, 11.55342575023019691, -1.199719254218441611 ) ) ;
#205882=CARTESIAN_POINT ( 'NONE',  ( -3.255929445576174697, 6.950334786480839355, -0.7998128361456282587 ) ) ;
#205887=CARTESIAN_POINT ( 'NONE',  ( 0.7499999999999885647, 3.316666666666689967, -1.299038105676658228 ) ) ;
#205888=CARTESIAN_POINT ( 'NONE',  ( 5.172599298813543633, 5.993452922492633839, -1.199719254218452047 ) ) ;
#205892=CARTESIAN_POINT ( 'NONE',  ( -1.364683531249997417, 3.509375000341423245, 1.214306433183764966E-14 ) ) ;
#205893=EDGE_CURVE ( 'NONE', #49215, #42278, #79176, .T. ) ;
#205895=CARTESIAN_POINT ( 'NONE',  ( 9.164948653157988900, 11.71552606681625619, -1.443375672974057666 ) ) ;
#205900=CARTESIAN_POINT ( 'NONE',  ( -1.499999999999997780, 2.431250000682817713, 1.214306433183764966E-14 ) ) ;
#205902=CARTESIAN_POINT ( 'NONE',  ( -6.715366157470410435, 6.729015360003925750, -0.7998128361456291469 ) ) ;
#205911=CARTESIAN_POINT ( 'NONE',  ( 4.039439701867726384, 6.800097854565950506, 1.199719254218462483 ) ) ;
#205915=CARTESIAN_POINT ( 'NONE',  ( 5.412729640353754590, 7.337937218544611895, 1.599625672291267398 ) ) ;
#205923=CARTESIAN_POINT ( 'NONE',  ( 9.511208455186636712, 11.05516360492796935, 1.199719254218453823 ) ) ;
#205928=CARTESIAN_POINT ( 'NONE',  ( 5.891030527642284298, 5.977876296848656956, -0.06656325335930267373 ) ) ;
#205940=CARTESIAN_POINT ( 'NONE',  ( 7.958272981541723468, 8.386999354661243800, 1.040834085586084257E-14 ) ) ;
#205942=CARTESIAN_POINT ( 'NONE',  ( -5.101945877444165944, 4.846691699973280976, 0.000000000000000000 ) ) ;
#205946=CARTESIAN_POINT ( 'NONE',  ( -4.855791571988752331, 8.816840600628864877, 0.7998128361456481317 ) ) ;
#205958=DIRECTION ( 'NONE',  ( 0.9055141421511273547, -0.4243160830846600673, -2.465190328815662439E-32 ) ) ;
#205959=CARTESIAN_POINT ( 'NONE',  ( 10.40996301719436090, 11.03937836301526687, 0.000000000000000000 ) ) ;
#205962=CARTESIAN_POINT ( 'NONE',  ( 4.216222584169931231, 4.021273891060765493, 1.214306433183764966E-14 ) ) ;
#205966=CARTESIAN_POINT ( 'NONE',  ( 5.327991180046136144, 5.318337252916436775, -0.7216878364870514817 ) ) ;
#205967=CARTESIAN_POINT ( 'NONE',  ( -9.246297574839990929, 11.81043314211192019, 1.443375672974076540 ) ) ;
#205969=DIRECTION ( 'NONE',  ( 1.000000000000000000, 0.000000000000000000, 0.000000000000000000 ) ) ;
#205970=CARTESIAN_POINT ( 'NONE',  ( 9.101601193475611140, 9.512956235343358102, -0.7998128361456221525 ) ) ;
#205974=CARTESIAN_POINT ( 'NONE',  ( -7.711890448074853133, 7.891627032375787998, -0.7998128361456291469 ) ) ;
#205975=CARTESIAN_POINT ( 'NONE',  ( 4.467575310902914154, 5.170924936596891008, 1.199719254218464037 ) ) ;
#205977=CARTESIAN_POINT ( 'NONE',  ( 8.204655514564224816, 12.72384853363364066, 1.040834085586084257E-14 ) ) ;
#205981=CARTESIAN_POINT ( 'NONE',  ( -1.364683531250012516, 2.592708333674753174, 0.7879004041258379498 ) ) ;
#205983=CARTESIAN_POINT ( 'NONE',  ( 5.477130870240836558, 9.333810415348903433, -0.7216878364870267237 ) ) ;
#205991=CARTESIAN_POINT ( 'NONE',  ( 8.066738210006674237, 11.39464976410773467, 1.082531754730558626 ) ) ;
#205996=CARTESIAN_POINT ( 'NONE',  ( -9.515124878692420296, 9.995400534762978850, 1.040834085586084257E-14 ) ) ;
#206005=CARTESIAN_POINT ( 'NONE',  ( 3.330499290451326200, 7.037332938835193730, -0.7998128361456291469 ) ) ;
#206011=CARTESIAN_POINT ( 'NONE',  ( 6.322179702674084467, 6.270297829408224111, 1.040834085586084257E-14 ) ) ;
#206014=CARTESIAN_POINT ( 'NONE',  ( -1.500000000000013101, 2.410416667349482456, -0.8660254037844313801 ) ) ;
#206020=CARTESIAN_POINT ( 'NONE',  ( 0.7499999999999867883, 0.3166666666666873020, -1.299038105676652899 ) ) ;
#206021=CARTESIAN_POINT ( 'NONE',  ( 8.613507663383630941, 8.943513783569379427, -0.7998128361456221525 ) ) ;
#206022=CARTESIAN_POINT ( 'NONE',  ( 0.6823417656249882723, -0.3239583329919110133, -1.181850606188749264 ) ) ;
#206025=CARTESIAN_POINT ( 'NONE',  ( 10.23604278863759909, 11.04439746293979496, 0.000000000000000000 ) ) ;
#206032=CARTESIAN_POINT ( 'NONE',  ( -4.367698041896780126, 8.247398148854895084, 0.7998128361456481317 ) ) ;
#206035=CARTESIAN_POINT ( 'NONE',  ( -1.201851678989727383E-14, 3.118750000682814161, -1.732050807568863648 ) ) ;
#206036=CARTESIAN_POINT ( 'NONE',  ( 0.6823417656249899377, 3.738541667008085767, -1.181850606188754593 ) ) ;
#206049=FACE_OUTER_BOUND ( 'NONE', #95349, .T. ) ;
#206050=CARTESIAN_POINT ( 'NONE',  ( -7.828943636887387925, 11.22118577875556156, 1.199719254218453823 ) ) ;
#206051=CARTESIAN_POINT ( 'NONE',  ( 6.446011968293428041, 9.607765498729298415, -1.199719254218440723 ) ) ;
#206058=CARTESIAN_POINT ( 'NONE',  ( -7.263417608619167076, 9.497073181520933716, -1.599625672291263179 ) ) ;
#206062=CARTESIAN_POINT ( 'NONE',  ( 2.191614386903386613, 5.708633884695917260, -0.7998128361456281477 ) ) ;
#206065=CARTESIAN_POINT ( 'NONE',  ( -3.741160322367112379, 6.452105245148518797, 1.199719254218464037 ) ) ;
#206066=CARTESIAN_POINT ( 'NONE',  ( -7.472515219426274946, 11.86968485597268064, 0.000000000000000000 ) ) ;
#206070=CARTESIAN_POINT ( 'NONE',  ( -4.613696345000219523, 7.131516869168907924, -1.371494837298018243 ) ) ;
#206077=CARTESIAN_POINT ( 'NONE',  ( 5.632522751473472589, 8.658694745772667289, -1.199719254218440723 ) ) ;
#206094=EDGE_CURVE ( 'NONE', #93282, #67678, #106819, .T. ) ;
#206097=CARTESIAN_POINT ( 'NONE',  ( 2.901081683644319842, 5.368050483351580304, 1.082531754730548412 ) ) ;
#206101=CARTESIAN_POINT ( 'NONE',  ( -8.350932551013499960, 11.83017284523606172, -1.199719254218446718 ) ) ;
#206107=CARTESIAN_POINT ( 'NONE',  ( 1.499999999999987121, 0.07708333401615156955, -0.8660254037844323793 ) ) ;
#206113=CARTESIAN_POINT ( 'NONE',  ( -2.460826785407679740, 8.202405370174460586, -2.499999999999995115 ) ) ;
#206114=CARTESIAN_POINT ( 'NONE',  ( 1.364683531249986537, 0.1552083336747499542, -0.7879004041258309554 ) ) ;
#206116=EDGE_CURVE ( 'NONE', #154752, #110280, #63436, .T. ) ;
#206122=CARTESIAN_POINT ( 'NONE',  ( -5.115504031057831469, 4.862509545855891346, 0.7998128361456341429 ) ) ;
#206123=CARTESIAN_POINT ( 'NONE',  ( -0.2123833161804513925, 7.036763569728186951, -3.929715952998865891 ) ) ;
#206125=CARTESIAN_POINT ( 'NONE',  ( -1.402160292154681736E-14, 0.08750000000001964540, -1.732050807568870754 ) ) ;
#206127=CARTESIAN_POINT ( 'NONE',  ( 1.364683531249986537, -0.8239583329919186738, 0.7879004041258500513 ) ) ;
#206132=CARTESIAN_POINT ( 'NONE',  ( 1.364683531249988757, 0.8843750003414210248, 0.000000000000000000 ) ) ;
#206134=CARTESIAN_POINT ( 'NONE',  ( -6.795661308947694934, 8.951357498570873261, -1.599625672291263179 ) ) ;
#206135=CARTESIAN_POINT ( 'NONE',  ( 9.053093885623066939, 11.58502883802551153, -1.599625672291262513 ) ) ;
#206136=CARTESIAN_POINT ( 'NONE',  ( 4.599240423533799138, 6.388866465587985211, 1.599625672291267175 ) ) ;
#206139=CARTESIAN_POINT ( 'NONE',  ( -0.6823417656250003738, 0.03020833367475134201, -1.181850606188749264 ) ) ;
#206149=CARTESIAN_POINT ( 'NONE',  ( 5.992340707560151358, 8.014150130285418783, 1.443375672974062551 ) ) ;
#206153=CARTESIAN_POINT ( 'NONE',  ( -5.928993247877788697, 5.811580298812519807, 0.7998128361456341429 ) ) ;
#206157=CARTESIAN_POINT ( 'NONE',  ( 4.148431815657221300, 7.783661518334664464, 1.040834085586084257E-14 ) ) ;
#206158=CARTESIAN_POINT ( 'NONE',  ( -7.822691444960709006, 10.14955932391940330, -1.443375672974058777 ) ) ;
#206160=CARTESIAN_POINT ( 'NONE',  ( -1.201851678989727383E-14, 3.587500000000020339, -1.732050807568863648 ) ) ;
#206164=CARTESIAN_POINT ( 'NONE',  ( 8.432808358020015049, 11.82173160345663376, 1.082531754730546636 ) ) ;
#206169=ORIENTED_EDGE ( 'NONE', *, *, #192402, .F. ) ;
#206176=CARTESIAN_POINT ( 'NONE',  ( 8.554831740098659765, 10.04335378727902395, 1.082531754730558626 ) ) ;
#206178=CARTESIAN_POINT ( 'NONE',  ( 6.903072767652295383, 11.20533532890304684, 1.040834085586084257E-14 ) ) ;
#206183=CARTESIAN_POINT ( 'NONE',  ( 4.744990575102895569, 5.598539094783909320, -1.082531754730548412 ) ) ;
#206185=CARTESIAN_POINT ( 'NONE',  ( -8.107412671292051343, 10.48173408797264194, 1.443375672974090751 ) ) ;
#206189=CARTESIAN_POINT ( 'NONE',  ( -2.428882075142555497, 5.985446187641602300, 1.040834085586084257E-14 ) ) ;
#206205=ORIENTED_EDGE ( 'NONE', *, *, #96785, .F. ) ;
#206211=CARTESIAN_POINT ( 'NONE',  ( -1.500000000000001332, 2.244000000000016648, -2.508000000000002228 ) ) ;
#206213=CARTESIAN_POINT ( 'NONE',  ( -5.738125327081750271, 7.717565519727259904, 1.599625672291269396 ) ) ;
#206217=CARTESIAN_POINT ( 'NONE',  ( 4.286349120214771879, 8.152491073559232859, -0.7998128361456221525 ) ) ;
#206227=CARTESIAN_POINT ( 'NONE',  ( -3.578462479003122976, 6.262291094557191684, 1.199719254218464037 ) ) ;
#206230=CARTESIAN_POINT ( 'NONE',  ( 6.154511665599609493, 9.267681812253174556, 1.199719254218462483 ) ) ;
#206233=CARTESIAN_POINT ( 'NONE',  ( 5.684994455280509840, 6.294486374732538359, 1.096603583888225764 ) ) ;
#206240=CARTESIAN_POINT ( 'NONE',  ( 5.111060722227499298, 8.906728576000002562, -0.7216878364870267237 ) ) ;
#206241=CARTESIAN_POINT ( 'NONE',  ( -7.374745490829552885, 10.69128794168811680, -1.199719254218446718 ) ) ;
#206245=CARTESIAN_POINT ( 'NONE',  ( -8.857554428429624593, 9.228235009456373206, 0.7998128361456462443 ) ) ;
#206246=CARTESIAN_POINT ( 'NONE',  ( -7.063961727919978451, 8.200042423116789436, 1.199719254218450271 ) ) ;
#206253=EDGE_CURVE ( 'NONE', #54971, #117563, #70621, .T. ) ;
#206254=CARTESIAN_POINT ( 'NONE',  ( 9.088043039861931405, 9.497138389460751284, 1.040834085586084257E-14 ) ) ;
#206260=CARTESIAN_POINT ( 'NONE',  ( -5.558479791478509568, 5.587240632920778438, 0.000000000000000000 ) ) ;
#206268=CARTESIAN_POINT ( 'NONE',  ( -1.201851678989727383E-14, 4.337500000000023448, -1.732050807568863648 ) ) ;
#206269=CARTESIAN_POINT ( 'NONE',  ( 4.578903193113299963, 6.365139696764064325, 1.599625672291267398 ) ) ;
#206270=CARTESIAN_POINT ( 'NONE',  ( 7.318703993278529829, 7.432909501780090800, 1.040834085586084257E-14 ) ) ;
#206273=CARTESIAN_POINT ( 'NONE',  ( -7.185458225562757484, 11.32685899655781903, 0.7216878364870458196 ) ) ;
#206275=CARTESIAN_POINT ( 'NONE',  ( 6.561783159334121152, 8.678499657355050800, -1.443375672974057666 ) ) ;
#206277=CARTESIAN_POINT ( 'NONE',  ( -9.937763408692600109, 10.69640485300394417, -0.7216878364870267237 ) ) ;
#206280=CARTESIAN_POINT ( 'NONE',  ( 7.567422294721922960, 11.98040977715095323, 0.7998128361456462443 ) ) ;
#206284=CARTESIAN_POINT ( 'NONE',  ( 1.364683531249988535, 2.905208333674754506, -0.7879004041258239610 ) ) ;
#206289=CARTESIAN_POINT ( 'NONE',  ( 1.364683531249986537, 0.1552083336747499542, -0.7879004041258309554 ) ) ;
#206291=CARTESIAN_POINT ( 'NONE',  ( 9.531545685607134999, 11.07889037375188401, 1.199719254218450271 ) ) ;
#206295=CARTESIAN_POINT ( 'NONE',  ( -8.455481356417053007, 13.01647868246193518, 0.7998128361456341429 ) ) ;
#206302=CARTESIAN_POINT ( 'NONE',  ( 4.813308228051395687, 5.574280006603454574, 1.199719254218462483 ) ) ;
#206306=CARTESIAN_POINT ( 'NONE',  ( -10.10098813738111545, 11.74323990082152491, -1.199719254218441611 ) ) ;
#206309=CARTESIAN_POINT ( 'NONE',  ( 7.587759525142423911, 12.00413654597487501, 0.7998128361456462443 ) ) ;
#206311=CARTESIAN_POINT ( 'NONE',  ( 4.959245870426344460, 6.614204113168008270, 1.243730795111185339 ) ) ;
#206313=CARTESIAN_POINT ( 'NONE',  ( -4.603156847039612920, 5.329103395422994716, 1.199719254218462483 ) ) ;
#206317=CARTESIAN_POINT ( 'NONE',  ( 8.925345196497941558, 9.307324238869423283, 1.040834085586084257E-14 ) ) ;
#206319=CARTESIAN_POINT ( 'NONE',  ( 7.558834334818744338, 8.777393797832065303, 1.199719254218462483 ) ) ;
#206321=CARTESIAN_POINT ( 'NONE',  ( -9.002250809794013264, 9.604973487622245898, -0.7216878364870267237 ) ) ;
#206328=CARTESIAN_POINT ( 'NONE',  ( -5.472563271839127275, 6.275773694203630626, -1.010060153610029321 ) ) ;
#206329=CARTESIAN_POINT ( 'NONE',  ( 0.6823417656249882723, 2.176041667008084435, -1.181850606188749264 ) ) ;
#206331=CARTESIAN_POINT ( 'NONE',  ( 4.853455804012203778, 8.606189504748821051, 0.7216878364870438212 ) ) ;
#206350=CARTESIAN_POINT ( 'NONE',  ( 8.910733272679570049, 11.41894145625809820, -1.599625672291255185 ) ) ;
#206354=CARTESIAN_POINT ( 'NONE',  ( -3.918470089549458635, 4.530302178351167441, -1.199719254218452047 ) ) ;
#206355=CARTESIAN_POINT ( 'NONE',  ( -5.696397096036042385, 9.797547045350714967, -0.7998128361456231517 ) ) ;
#206358=CARTESIAN_POINT ( 'NONE',  ( -10.47097470845587175, 11.11055866948701443, 1.040834085586084257E-14 ) ) ;
#206363=CARTESIAN_POINT ( 'NONE',  ( 6.252281394196331554, 10.44607872653774372, 1.040834085586084257E-14 ) ) ;
#206367=CARTESIAN_POINT ( 'NONE',  ( -7.202405917357668663, 9.425892875049191488, 1.599625672291295375 ) ) ;
#206369=CARTESIAN_POINT ( 'NONE',  ( 1.364683531249990311, 4.884375000341417916, 1.214306433183764966E-14 ) ) ;
#206373=CARTESIAN_POINT ( 'NONE',  ( -7.646435448427427062, 10.90429654226522693, 1.082531754730549967 ) ) ;
#206377=CARTESIAN_POINT ( 'NONE',  ( 1.364683531249990311, 2.946875000341416140, 1.214306433183764966E-14 ) ) ;
#206378=AXIS2_PLACEMENT_3D ( 'NONE', #129753, #110286, #176295 ) ;
#206384=CARTESIAN_POINT ( 'NONE',  ( -1.364683531250010295, 3.780208333674750953, 0.7879004041258379498 ) ) ;
#206385=CARTESIAN_POINT ( 'NONE',  ( -5.759516327706961647, 5.613857225279885732, -0.7998128361456221525 ) ) ;
#206386=CARTESIAN_POINT ( 'NONE',  ( 6.908042961362778733, 8.018137195466769285, 1.199719254218462483 ) ) ;
#206389=CARTESIAN_POINT ( 'NONE',  ( 3.185802909086945967, 5.700225246367978116, 1.082531754730546636 ) ) ;
#206390=CARTESIAN_POINT ( 'NONE',  ( 0.6823417656249917140, 4.155208333674755394, 1.181850606188765695 ) ) ;
#206396=CARTESIAN_POINT ( 'NONE',  ( -1.402160292154681736E-14, 1.196875000341419026, -1.575800808251659024 ) ) ;
#206398=CARTESIAN_POINT ( 'NONE',  ( -4.772106882330234612, 6.590544000850479200, -1.443375672974053447 ) ) ;
#206399=CARTESIAN_POINT ( 'NONE',  ( 5.931855901178834323, 6.879252291918818152, 1.199719254218462483 ) ) ;
#206403=CARTESIAN_POINT ( 'NONE',  ( 4.094199201646931741, 4.839282492418613302, -1.082531754730543083 ) ) ;
#206406=CARTESIAN_POINT ( 'NONE',  ( -8.297226821883391779, 11.66355314463053006, 1.082531754730549967 ) ) ;
#206412=CARTESIAN_POINT ( 'NONE',  ( -10.47097470845587175, 11.11055866948701443, 1.040834085586084257E-14 ) ) ;
#206413=CARTESIAN_POINT ( 'NONE',  ( -6.371969008298464132, 6.536311385877402458, 1.040834085586084257E-14 ) ) ;
#206415=CARTESIAN_POINT ( 'NONE',  ( 0.6823417656249882723, 0.7385416670080829915, -1.181850606188749264 ) ) ;
#206424=CARTESIAN_POINT ( 'NONE',  ( 4.175548122884573665, 3.973820352894515295, 1.214306433183764966E-14 ) ) ;
#206427=CARTESIAN_POINT ( 'NONE',  ( 8.229436053370676518, 9.663725486096376827, 1.082531754730558626 ) ) ;
#206435=ADVANCED_FACE ( 'NONE', ( #134896 ), #1637, .T. ) ;
#206437=CARTESIAN_POINT ( 'NONE',  ( -3.898132859128961236, 4.506575409527250997, -1.199719254218452047 ) ) ;
#206440=CARTESIAN_POINT ( 'NONE',  ( -0.6823417656250212460, 1.613541667008083769, 1.181850606188755259 ) ) ;
#206453=CARTESIAN_POINT ( 'NONE',  ( -0.5635687842576226902, 6.831326244322589503, -3.741768325763386915 ) ) ;
#206460=CARTESIAN_POINT ( 'NONE',  ( 4.482942347612929979, 8.381849838857084123, 1.040834085586084257E-14 ) ) ;
#206468=CARTESIAN_POINT ( 'NONE',  ( 7.039708073993665494, 9.236078724457858158, 1.599625672291281386 ) ) ;
#206471=CARTESIAN_POINT ( 'NONE',  ( 9.447334110624092673, 9.916311305349925220, -0.7998128361456281477 ) ) ;
#206474=DIRECTION ( 'NONE',  ( 1.000000000000000000, -7.387867266669436732E-31, 0.000000000000000000 ) ) ;
#206476=ORIENTED_EDGE ( 'NONE', *, *, #57396, .T. ) ;
#206478=CARTESIAN_POINT ( 'NONE',  ( -3.240035523541588081, 6.723865844199796271, 0.7216878364870096263 ) ) ;
#206483=CARTESIAN_POINT ( 'NONE',  ( -7.049876689426103127, 10.20831132343037062, -1.082531754730537976 ) ) ;
#206494=CARTESIAN_POINT ( 'NONE',  ( 4.975479186090860928, 4.907073259968533385, 0.7216878364870317197 ) ) ;
#206502=CARTESIAN_POINT ( 'NONE',  ( -5.555090253297260361, 7.504024600312024340, 1.599625672291269396 ) ) ;
#206504=CARTESIAN_POINT ( 'NONE',  ( -2.839543107058306592, 5.400218493954923815, -1.199719254218446718 ) ) ;
#206510=CARTESIAN_POINT ( 'NONE',  ( 7.592202833972727660, 11.80139437303613015, -0.7216878364870267237 ) ) ;
#206511=EDGE_LOOP ( 'NONE', ( #143011, #82172, #105522, #161971 ) ) ;
#206512=CARTESIAN_POINT ( 'NONE',  ( -1.001543065824772872E-14, 4.384375000341417916, 1.575800808251672791 ) ) ;
#206514=CARTESIAN_POINT ( 'NONE',  ( 6.308621549060418054, 6.254479983525607523, 0.7998128361456341429 ) ) ;
#206528=CARTESIAN_POINT ( 'NONE',  ( -1.364683531250014514, 1.301041667008083325, -0.7879004041258289570 ) ) ;
#206530=CARTESIAN_POINT ( 'NONE',  ( 4.701980345841006326, 4.380065246436280368, 0.7998128361456341429 ) ) ;
#206534=CARTESIAN_POINT ( 'NONE',  ( -6.738039156311804945, 6.963393225226301553, 1.040834085586084257E-14 ) ) ;
#206535=CARTESIAN_POINT ( 'NONE',  ( 4.690757960648234359, 4.574898496952131133, 0.7216878364870317197 ) ) ;
#206536=CARTESIAN_POINT ( 'NONE',  ( -5.707619481228817904, 8.642344580533519505, -1.082531754730537976 ) ) ;
#206538=ORIENTED_EDGE ( 'NONE', *, *, #164073, .F. ) ;
#206540=CARTESIAN_POINT ( 'NONE',  ( 5.229694566569264680, 7.124396299129368337, 1.599625672291267398 ) ) ;
#206545=CARTESIAN_POINT ( 'NONE',  ( -1.364683531250010295, 5.738541667008088432, -0.7879004041258300672 ) ) ;
#206550=CARTESIAN_POINT ( 'NONE',  ( 6.877010230629674759, 9.046264573866535486, 1.599625672291281386 ) ) ;
#206551=SURFACE_STYLE_FILL_AREA ( #25666 ) ;
#206555=CARTESIAN_POINT ( 'NONE',  ( -7.389357414647957256, 8.579670724299436557, 1.199719254218450271 ) ) ;
#206559=CARTESIAN_POINT ( 'NONE',  ( 8.925345196497941558, 9.307324238869423283, 1.040834085586084257E-14 ) ) ;
#206562=CARTESIAN_POINT ( 'NONE',  ( -6.388916700537716764, 8.476822122092563916, 1.599625672291283607 ) ) ;
#206564=CARTESIAN_POINT ( 'NONE',  ( 6.439759776366765998, 9.496508258194486629, 1.082531754730558626 ) ) ;
#206565=CARTESIAN_POINT ( 'NONE',  ( 4.313480937648101587, 7.206793636360196764, -1.001376897629567830 ) ) ;
#206566=CARTESIAN_POINT ( 'NONE',  ( -4.412288926243578935, 7.235088616337731260, 1.199719254218464037 ) ) ;
#206573=CARTESIAN_POINT ( 'NONE',  ( 9.185812768458653466, 10.67553530374532045, 1.199719254218453823 ) ) ;
#206574=CARTESIAN_POINT ( 'NONE',  ( -1.364683531250012516, 0.7802083336747528408, 0.7879004041258379498 ) ) ;
#206576=CARTESIAN_POINT ( 'NONE',  ( -4.921246572080546500, 8.685278734161874681, 1.214306433183764966E-14 ) ) ;
#206583=CARTESIAN_POINT ( 'NONE',  ( -5.862510748852908016, 6.029743210627831473, 0.3741650707956689081 ) ) ;
#206584=CARTESIAN_POINT ( 'NONE',  ( -1.364683531250000748, 1.571875000341421691, 0.000000000000000000 ) ) ;
#206587=CARTESIAN_POINT ( 'NONE',  ( 4.229780737783593203, 4.037091736943370535, -0.7216878364870188411 ) ) ;
#206590=CARTESIAN_POINT ( 'NONE',  ( -3.761497552787613330, 6.475832013972435242, 1.199719254218464037 ) ) ;
#206592=CARTESIAN_POINT ( 'NONE',  ( -8.988692655735990300, 9.589155641221221771, 0.7216878364870438212 ) ) ;
#206600=CARTESIAN_POINT ( 'NONE',  ( -7.280365300414089802, 10.47721470291632784, 1.082531754730549967 ) ) ;
#206606=CARTESIAN_POINT ( 'NONE',  ( -6.358410854684777291, 10.36197039720016022, -0.7216878364870267237 ) ) ;
#206611=CARTESIAN_POINT ( 'NONE',  ( 0.7499999999999902300, 5.097916667349482012, -1.299038105676658228 ) ) ;
#206613=DIRECTION ( 'NONE',  ( -0.7592566023653016805, -0.6507913734559627184, 4.115938288792108699E-15 ) ) ;
#206620=CARTESIAN_POINT ( 'NONE',  ( -5.693534442735004752, 8.729875052244421951, 1.199719254218452047 ) ) ;
#206621=CARTESIAN_POINT ( 'NONE',  ( -2.923234996448113687, 6.562191262498094702, -0.3692494997280490465 ) ) ;
#206623=CARTESIAN_POINT ( 'NONE',  ( 4.137209430464448445, 7.978494768850520558, 1.040834085586084257E-14 ) ) ;
#206625=CARTESIAN_POINT ( 'NONE',  ( 4.866817647125399660, 4.983041418240444109, 0.6113003782640200612 ) ) ;
#206627=CARTESIAN_POINT ( 'NONE',  ( 7.633404179693907388, 8.864391950186421454, -1.199719254218441611 ) ) ;
#206633=CARTESIAN_POINT ( 'NONE',  ( -6.249945626219832739, 6.393950773452325542, 1.040834085586084257E-14 ) ) ;
#206643=CARTESIAN_POINT ( 'NONE',  ( -9.501566725078754772, 9.979582688880366703, -0.7998128361456291469 ) ) ;
#206645=CARTESIAN_POINT ( 'NONE',  ( 8.067265095331215718, 9.370563018429956870, 1.199719254218462483 ) ) ;
#206647=CARTESIAN_POINT ( 'NONE',  ( -8.853638004923878313, 10.28799807962136548, 1.199719254218462483 ) ) ;
#206651=CARTESIAN_POINT ( 'NONE',  ( -1.201851678989727383E-14, 5.446875000341422357, -1.575800808251660134 ) ) ;
#206652=CARTESIAN_POINT ( 'NONE',  ( 7.619319141200051604, 11.83303006480134911, 0.7216878364870438212 ) ) ;
#206655=CARTESIAN_POINT ( 'NONE',  ( -1.500000000000011324, 5.420833333333356485, 0.8660254037844403729 ) ) ;
#206657=CARTESIAN_POINT ( 'NONE',  ( 7.090551149822722721, 11.21613407486112379, 0.7216878364870438212 ) ) ;
#206660=CARTESIAN_POINT ( 'NONE',  ( -5.043269954603569083, 7.867270132804026872, 1.082531754730560403 ) ) ;
#206663=CARTESIAN_POINT ( 'NONE',  ( 1.364683531249988757, 2.134375000341422357, 1.214306433183764966E-14 ) ) ;
#206667=CARTESIAN_POINT ( 'NONE',  ( -6.938021921891187382, 9.117444880338284818, -1.599625672291263179 ) ) ;
#206669=CARTESIAN_POINT ( 'NONE',  ( 0.6823417656249917140, 4.405208333674755394, 1.181850606188765695 ) ) ;
#206675=CARTESIAN_POINT ( 'NONE',  ( 6.584456157731144899, 10.83361595066169514, -0.7998128361456291469 ) ) ;
#206678=CARTESIAN_POINT ( 'NONE',  ( -1.402160292154681736E-14, 1.837500000000019895, -1.732050807568863648 ) ) ;
#206681=CARTESIAN_POINT ( 'NONE',  ( -0.5031024701319503079, 7.721748688245902770, -1.994341720826586561 ) ) ;
#206683=CARTESIAN_POINT ( 'NONE',  ( 6.751597309925441159, 9.860318714012938912, -1.082531754730537088 ) ) ;
#206684=VECTOR ( 'NONE', #40204, 1000.000000000000000 ) ;
#206685=CARTESIAN_POINT ( 'NONE',  ( 9.317477881089539338, 11.89347683273640932, 1.599625672291279388 ) ) ;
#206687=CARTESIAN_POINT ( 'NONE',  ( 4.715538499454675403, 4.395883092318884522, 1.214306433183764966E-14 ) ) ;
#206694=CARTESIAN_POINT ( 'NONE',  ( 8.535021395002688749, 9.916278701380017324, 1.199719254218462483 ) ) ;
#206695=CARTESIAN_POINT ( 'NONE',  ( -8.157201976916404362, 12.66848607304450702, -0.7998128361456281477 ) ) ;
#206698=CARTESIAN_POINT ( 'NONE',  ( 1.364683531249992088, 5.696875000341418804, 1.214306433183764966E-14 ) ) ;
#206700=CARTESIAN_POINT ( 'NONE',  ( -1.500000000000015099, 0.3791666666666850261, -0.8660254037844383745 ) ) ;
#206707=CARTESIAN_POINT ( 'NONE',  ( 1.364683531249990311, 4.613541667008083103, 0.7879004041258500513 ) ) ;
#206709=CARTESIAN_POINT ( 'NONE',  ( -5.395781948558855845, 9.238903340053241209, 0.7216878364870458196 ) ) ;
#206716=ORIENTED_EDGE ( 'NONE', *, *, #168698, .F. ) ;
#206717=CARTESIAN_POINT ( 'NONE',  ( 8.076906825439115423, 10.44614393447756129, -1.599625672291262513 ) ) ;
#206718=CARTESIAN_POINT ( 'NONE',  ( -1.579999999999998073, 6.280000000000042881, -2.499999999999995115 ) ) ;
#206722=( BOUNDED_CURVE ( )  B_SPLINE_CURVE ( 2, ( #192021, #209329, #48734, #159542, #157428, #91367, #60977 ),
 .UNSPECIFIED., .F., .T. ) 
 B_SPLINE_CURVE_WITH_KNOTS ( ( 3, 2, 2, 3 ),
 ( 0.2678571428571428492, 0.2738095238095239470, 0.2797619047619049337, 0.2857142857142859760 ),
 .UNSPECIFIED. ) 
 CURVE ( )  GEOMETRIC_REPRESENTATION_ITEM ( )  RATIONAL_B_SPLINE_CURVE ( ( 1.000000000000000000, 0.8660254037844387076, 1.000000000000000000, 0.8660254037844387076, 1.000000000000000000, 0.8660254037844324904, 1.000000000000006217 ) ) 
 REPRESENTATION_ITEM ( '' )  );
#206724=CARTESIAN_POINT ( 'NONE',  ( -7.621654909176601045, 12.04368116068139472, 0.7998128361456481317 ) ) ;
#206725=CARTESIAN_POINT ( 'NONE',  ( 7.145310649601935182, 8.294949498412453437, -1.199719254218446718 ) ) ;
#206727=CARTESIAN_POINT ( 'NONE',  ( 4.338245966248566177, 4.163634503485842409, 1.214306433183764966E-14 ) ) ;
#206729=CARTESIAN_POINT ( 'NONE',  ( 3.486418057008484617, 7.219238166485217434, 1.040834085586084257E-14 ) ) ;
#206736=CARTESIAN_POINT ( 'NONE',  ( -4.446711195602239819, 8.131654128270509929, -0.7216878364870267237 ) ) ;
#206737=CARTESIAN_POINT ( 'NONE',  ( 10.23604278863759909, 11.04439746293979496, 0.000000000000000000 ) ) ;
#206740=CARTESIAN_POINT ( 'NONE',  ( -7.182068686937172153, 9.402166106225269715, 1.599625672291283607 ) ) ;
#206745=CARTESIAN_POINT ( 'NONE',  ( -7.323375529675950624, 11.69568855126397011, -0.7998128361456291469 ) ) ;
#206749=CARTESIAN_POINT ( 'NONE',  ( 8.067265095331215718, 9.370563018429956870, 1.199719254218462483 ) ) ;
#206750=CARTESIAN_POINT ( 'NONE',  ( 5.015626762051672571, 7.938982758113895422, 1.199719254218462483 ) ) ;
#206760=CARTESIAN_POINT ( 'NONE',  ( -8.193204901359996128, 8.453160561208463264, 1.040834085586084257E-14 ) ) ;
#206763=CARTESIAN_POINT ( 'NONE',  ( 5.992340707560147806, 8.974519344586754599, 1.082531754730558626 ) ) ;
#206766=CARTESIAN_POINT ( 'NONE',  ( 3.734381245560244089, 6.444196322207211836, 1.199719254218462483 ) ) ;
#206768=CARTESIAN_POINT ( 'NONE',  ( -3.601662362724658895, 7.353689856487406473, -0.7998128361456281477 ) ) ;
#206771=CARTESIAN_POINT ( 'NONE',  ( 1.500000000000023981, 5.535416667349482012, 0.8660254037844334896 ) ) ;
#206777=CARTESIAN_POINT ( 'NONE',  ( -10.32861409551237486, 10.94447128771960287, 1.040834085586084257E-14 ) ) ;
#206778=CARTESIAN_POINT ( 'NONE',  ( 6.889514614038635187, 11.18951748302043114, -0.7998128361456291469 ) ) ;
#206781=CARTESIAN_POINT ( 'NONE',  ( -2.657034918598345730, 5.083329257464595408, -1.082531754730543971 ) ) ;
#206783=CARTESIAN_POINT ( 'NONE',  ( -4.885033903151685841, 6.706220529795296592, -1.250124166851230845 ) ) ;
#206788=CARTESIAN_POINT ( 'NONE',  ( 0.6823417656249882723, -1.094791666325249713, 1.181850606188755259 ) ) ;
#206792=CARTESIAN_POINT ( 'NONE',  ( 9.408995418203971894, 11.03987807840189816, 1.082531754730549967 ) ) ;
#206797=CARTESIAN_POINT ( 'NONE',  ( -5.750949863820874697, 6.097589008447164893, -0.6582294942717293873 ) ) ;
#206809=CARTESIAN_POINT ( 'NONE',  ( -2.937312835655025101, 6.578615408239493867, 1.040834085586084257E-14 ) ) ;
#206810=CARTESIAN_POINT ( 'NONE',  ( -0.7500000000000006661, 2.858333333333358706, -1.299038105676652011 ) ) ;
#206812=CARTESIAN_POINT ( 'NONE',  ( -4.406563619641430840, 5.099744630125142564, -1.199719254218446718 ) ) ;
#206817=CARTESIAN_POINT ( 'NONE',  ( 1.364683531249990311, 5.113541667008084879, 0.7879004041258500513 ) ) ;
#206820=CARTESIAN_POINT ( 'NONE',  ( -2.331639231870358930, 5.664070170583284103, -0.7216878364870267237 ) ) ;
#206822=CARTESIAN_POINT ( 'NONE',  ( -3.609978820808566802, 4.211641957610042120, -7.499999999999991118 ) ) ;
#206826=CARTESIAN_POINT ( 'NONE',  ( 4.325214697959421706, 5.004837554829479451, 1.199719254218462483 ) ) ;
#206828=DIRECTION ( 'NONE',  ( -1.207943261119674327E-30, -2.168404344971008079E-15, -1.000000000000000000 ) ) ;
#206833=CARTESIAN_POINT ( 'NONE',  ( -0.6823417656250003738, 1.530208333674752730, -1.181850606188749264 ) ) ;
#206834=DIRECTION ( 'NONE',  ( -1.000000000000000000, 5.578564026256503701E-16, 1.479114197289397135E-31 ) ) ;
#206836=CARTESIAN_POINT ( 'NONE',  ( -8.995998617867369873, 10.45408546138876993, 1.199719254218462483 ) ) ;
#206837=CARTESIAN_POINT ( 'NONE',  ( -5.002595493318215070, 7.819816594637776674, 1.082531754730560403 ) ) ;
#206840=ORIENTED_EDGE ( 'NONE', *, *, #45988, .F. ) ;
#206841=CARTESIAN_POINT ( 'NONE',  ( -1.201851678989727383E-14, 5.196875000341422357, -1.575800808251660134 ) ) ;
#206842=EDGE_CURVE ( 'NONE', #177962, #214172, #93617, .T. ) ;
#206850=CARTESIAN_POINT ( 'NONE',  ( -3.890826896997578999, 7.483122446565064756, 0.7216878364870317197 ) ) ;
#206855=CARTESIAN_POINT ( 'NONE',  ( -4.351804119862249465, 7.060559992272473551, 1.082531754730560403 ) ) ;
#206857=CARTESIAN_POINT ( 'NONE',  ( 7.913155211870404493, 12.38376484715752213, 0.7998128361456462443 ) ) ;
#206867=CARTESIAN_POINT ( 'NONE',  ( -4.790108344329849110, 4.482881244673243337, 0.7998128361456341429 ) ) ;
#206873=CARTESIAN_POINT ( 'NONE',  ( 7.890482213473377193, 11.18901776815221716, -1.082531754730543083 ) ) ;
#206874=CARTESIAN_POINT ( 'NONE',  ( 4.482942347612929979, 8.381849838857084123, 1.040834085586084257E-14 ) ) ;
#206877=VERTEX_POINT ( 'NONE', #206260 ) ;
#206878=CARTESIAN_POINT ( 'NONE',  ( 4.813308228051395687, 5.574280006603454574, 1.199719254218462483 ) ) ;
#206888=CARTESIAN_POINT ( 'NONE',  ( -4.713430959045263435, 8.650753218861462202, 0.7998128361456481317 ) ) ;
#206894=CARTESIAN_POINT ( 'NONE',  ( -1.364683531250010295, 5.030208333674757171, 0.7879004041258379498 ) ) ;
#206895=CARTESIAN_POINT ( 'NONE',  ( 9.883530794237934458, 10.63313346947350269, -0.7216878364870257245 ) ) ;
#206896=CARTESIAN_POINT ( 'NONE',  ( -5.412729640353771465, 7.337937218544611895, 1.599625672291269396 ) ) ;
#206899=CARTESIAN_POINT ( 'NONE',  ( 5.854423403002611437, 5.724582146458163656, 1.040834085586084257E-14 ) ) ;
#206900=CARTESIAN_POINT ( 'NONE',  ( -5.494078562035765501, 7.432844293840273231, -1.599625672291256295 ) ) ;
#206906=CARTESIAN_POINT ( 'NONE',  ( 6.697364695470787943, 7.876308901879812474, -1.082531754730543083 ) ) ;
#206909=CARTESIAN_POINT ( 'NONE',  ( 7.754900676892376055, 8.149731665903665601, 1.040834085586084257E-14 ) ) ;
#206910=CARTESIAN_POINT ( 'NONE',  ( -1.364683531250012516, 3.092708333674755838, 0.7879004041258379498 ) ) ;
#206912=CARTESIAN_POINT ( 'NONE',  ( 6.290620086616457662, 6.441404310581745563, 1.040834085586084257E-14 ) ) ;
#206915=CARTESIAN_POINT ( 'NONE',  ( -2.765500147507697459, 5.209872024525476597, 1.082531754730560403 ) ) ;
#206923=CARTESIAN_POINT ( 'NONE',  ( -4.014048110574687911, 7.796590492392542870, 0.4333429611983550256 ) ) ;
#206924=FACE_OUTER_BOUND ( 'NONE', #106977, .T. ) ;
#206931=CARTESIAN_POINT ( 'NONE',  ( 5.250031796989762967, 7.148123067953287446, 1.599625672291267398 ) ) ;
#206933=CARTESIAN_POINT ( 'NONE',  ( -3.972175818679615222, 4.696921878956699103, 1.082531754730558626 ) ) ;
#206940=ORIENTED_EDGE ( 'NONE', *, *, #100231, .F. ) ;
#206942=CARTESIAN_POINT ( 'NONE',  ( 4.039966587192259873, 5.736380323189513852, 1.443375672974062551 ) ) ;
#206943=CARTESIAN_POINT ( 'NONE',  ( -1.364683531250012516, 2.801041667008090652, -0.7879004041258289570 ) ) ;
#206945=CARTESIAN_POINT ( 'NONE',  ( 8.749089199520284410, 9.101692242395490240, 0.7998128361456481317 ) ) ;
#206946=CARTESIAN_POINT ( 'NONE',  ( -8.805130697071332335, 12.36007068230351358, 1.199719254218462483 ) ) ;
#206953=CARTESIAN_POINT ( 'NONE',  ( -1.500000000000011324, 2.670833333333352044, 0.8660254037844403729 ) ) ;
#206954=CARTESIAN_POINT ( 'NONE',  ( 5.666418135507635512, 8.698239360479199433, 1.199719254218462483 ) ) ;
#206958=CARTESIAN_POINT ( 'NONE',  ( 1.364683531249988535, 3.613541667008086211, 0.7879004041258500513 ) ) ;
#206960=CARTESIAN_POINT ( 'NONE',  ( 8.920901888111986366, 12.39117405523060889, 1.082531754730546636 ) ) ;
#206963=DIRECTION ( 'NONE',  ( 0.000000000000000000, 1.000000000000000000, -8.546850786086437571E-32 ) ) ;
#206965=CARTESIAN_POINT ( 'NONE',  ( -5.124618876285511604, 5.081069565195706517, 0.7216878364870705775 ) ) ;
#206966=CARTESIAN_POINT ( 'NONE',  ( -1.201851678989727383E-14, 1.743750000682815493, 1.732050807568877637 ) ) ;
#206968=CARTESIAN_POINT ( 'NONE',  ( -5.717788096661253761, 7.693838750903348789, 1.599625672291269396 ) ) ;
#206969=CARTESIAN_POINT ( 'NONE',  ( -2.480778921620681921, 5.838066475291996404, 1.040834085586084257E-14 ) ) ;
#206977=CARTESIAN_POINT ( 'NONE',  ( 5.473741331615251227, 7.409117525016355010, -1.599625672291262513 ) ) ;
#206981=CARTESIAN_POINT ( 'NONE',  ( 3.994848817520957773, 7.812407387083109001, 1.040834085586084257E-14 ) ) ;
#206987=CARTESIAN_POINT ( 'NONE',  ( 3.246287715468270108, 5.874753870433235825, 1.199719254218450271 ) ) ;
#206992=CARTESIAN_POINT ( 'NONE',  ( 5.568360837313221623, 6.179671487343128433, 0.8958872440008452953 ) ) ;
#207003=CARTESIAN_POINT ( 'NONE',  ( -4.151108609992611775, 3.976305524690391113, 0.4518923928031730042 ) ) ;
#207004=CARTESIAN_POINT ( 'NONE',  ( 7.212574532790092974, 9.437756259720353924, -1.443375672974057666 ) ) ;
#207006=CARTESIAN_POINT ( 'NONE',  ( -3.602716132929368875, 5.226254793216122074, 1.599625672291267398 ) ) ;
#207010=CARTESIAN_POINT ( 'NONE',  ( -5.904739593951539689, 6.847616600153594746, 1.199719254218450271 ) ) ;
#207033=CARTESIAN_POINT ( 'NONE',  ( -8.500599126088349777, 12.86119004717103209, 1.040834085586084257E-14 ) ) ;
#207036=CARTESIAN_POINT ( 'NONE',  ( 8.052653171512838881, 11.48218023581863001, -1.199719254218446718 ) ) ;
#207041=CARTESIAN_POINT ( 'NONE',  ( -7.446452682403657874, 9.710614100936176385, -1.599625672291263179 ) ) ;
#207042=CARTESIAN_POINT ( 'NONE',  ( 5.332434488876471868, 5.115595079977664383, 0.7998128361456341429 ) ) ;
#207046=CARTESIAN_POINT ( 'NONE',  ( -1.420000000000001039, 6.280000000000042881, -2.499999999999995115 ) ) ;
#207048=CARTESIAN_POINT ( 'NONE',  ( -1.402160292154681736E-14, 2.259375000341416140, -1.575800808251660134 ) ) ;
#207050=CARTESIAN_POINT ( 'NONE',  ( 7.782016984564065432, 8.181367358187307204, 0.7216878364870458196 ) ) ;
#207058=CARTESIAN_POINT ( 'NONE',  ( 8.053180056393003383, 12.33920113252646367, 1.040834085586084257E-14 ) ) ;
#207064=CARTESIAN_POINT ( 'NONE',  ( -7.991641480251377772, 11.41099992934688956, 1.199719254218453823 ) ) ;
#207065=CARTESIAN_POINT ( 'NONE',  ( 6.938893903907228378E-15, 10.64264068711930733, 1.214306433183764966E-14 ) ) ;
#207081=CARTESIAN_POINT ( 'NONE',  ( -0.7500000000000006661, 2.389583334016155636, -1.299038105676652011 ) ) ;
#207088=CARTESIAN_POINT ( 'NONE',  ( -1.500000000000015099, 0.6291666666666863028, -0.8660254037844313801 ) ) ;
#207089=CARTESIAN_POINT ( 'NONE',  ( 6.913768267964901071, 10.15348118167935709, -1.199719254218441611 ) ) ;
#207091=CARTESIAN_POINT ( 'NONE',  ( 1.364683531249986537, 0.1135416670080857532, 0.7879004041258500513 ) ) ;
#207094=CARTESIAN_POINT ( 'NONE',  ( 9.002250809793993724, 11.52571191622492464, -1.443375672974057666 ) ) ;
#207095=CARTESIAN_POINT ( 'NONE',  ( -6.778713617152821058, 7.971215977175476475, 1.082531754730549967 ) ) ;
#207098=CIRCLE ( 'NONE', #169069, 2.000000000000000000 ) ;
#207101=CARTESIAN_POINT ( 'NONE',  ( -7.203459687562382641, 7.298457811777897319, -0.7998128361456291469 ) ) ;
#207103=CARTESIAN_POINT ( 'NONE',  ( 1.499999999999989120, 2.556250000682817713, 1.214306433183764966E-14 ) ) ;
#207105=CARTESIAN_POINT ( 'NONE',  ( -1.364683531249997417, 3.821875000341416584, 1.214306433183764966E-14 ) ) ;
#207112=EDGE_CURVE ( 'NONE', #119686, #214172, #127721, .T. ) ;
#207120=CARTESIAN_POINT ( 'NONE',  ( -7.669108446824431269, 12.09904362127053545, -0.7998128361456291469 ) ) ;
#207121=CARTESIAN_POINT ( 'NONE',  ( 5.960781091502512119, 10.10599504006161986, 0.7998128361456462443 ) ) ;
#207122=DIRECTION ( 'NONE',  ( 0.000000000000000000, 0.8000000000040162762, -0.5999999999946449281 ) ) ;
#207128=CARTESIAN_POINT ( 'NONE',  ( -9.182950115157607840, 9.607863310639020327, 0.7998128361456462443 ) ) ;
#207134=CARTESIAN_POINT ( 'NONE',  ( 2.367870383881045981, 5.914265881169853856, 0.000000000000000000 ) ) ;
#207136=CARTESIAN_POINT ( 'NONE',  ( 0.000000000000000000, -2.856854249492362996, 0.000000000000000000 ) ) ;
#207138=CARTESIAN_POINT ( 'NONE',  ( -5.525111292768871252, 6.404716915440499037, -1.199719254218446718 ) ) ;
#207139=CARTESIAN_POINT ( 'NONE',  ( -8.402302512167102222, 10.82577223566020841, -1.599625672291263179 ) ) ;
#207150=CARTESIAN_POINT ( 'NONE',  ( 7.820355676984174664, 8.018169799436671852, -0.7998128361456281477 ) ) ;
#207169=CARTESIAN_POINT ( 'NONE',  ( 2.901081683644312736, 6.328419697652925002, 0.7216878364870338292 ) ) ;
#207173=CARTESIAN_POINT ( 'NONE',  ( -7.974166903131914452, 12.45494515362926435, -0.7998128361456281477 ) ) ;
#207176=CARTESIAN_POINT ( 'NONE',  ( 2.507895228403643539, 5.869702166538802501, -0.7216878364870267237 ) ) ;
#207186=CARTESIAN_POINT ( 'NONE',  ( -1.364683531250000748, 0.2593750003414205252, 0.000000000000000000 ) ) ;
#207191=CARTESIAN_POINT ( 'NONE',  ( -4.253507506385335368, 5.985511395581417204, 1.599625672291267398 ) ) ;
#207195=CARTESIAN_POINT ( 'NONE',  ( -1.500000000000001332, 0.1500000000000251132, 0.000000000000000000 ) ) ;
#207197=CARTESIAN_POINT ( 'NONE',  ( 1.364683531249986981, -1.053124999658580752, 0.000000000000000000 ) ) ;
#207202=CARTESIAN_POINT ( 'NONE',  ( 1.364683531249986537, 0.3635416670080869328, 0.7879004041258500513 ) ) ;
#207203=ADVANCED_FACE ( 'NONE', ( #209447 ), #202189, .T. ) ;
#207205=CARTESIAN_POINT ( 'NONE',  ( -6.028571859570855729, 10.18508426947466816, 0.000000000000000000 ) ) ;
#207206=CARTESIAN_POINT ( 'NONE',  ( 7.228468454380276853, 11.58496363008569574, 1.040834085586084257E-14 ) ) ;
#207207=CARTESIAN_POINT ( 'NONE',  ( 4.924636110261781496, 6.768494766770632332, 1.599625672291267175 ) ) ;
#207211=CARTESIAN_POINT ( 'NONE',  ( 0.6823417656249899377, 0.6552083336747518416, 1.181850606188755259 ) ) ;
#207219=CARTESIAN_POINT ( 'NONE',  ( 5.816084710582486217, 9.729256562414162701, 1.040834085586084257E-14 ) ) ;
#207222=CARTESIAN_POINT ( 'NONE',  ( -4.554649539187067830, 7.401175998105142817, 1.199719254218464037 ) ) ;
#207226=CARTESIAN_POINT ( 'NONE',  ( -2.764973262183167968, 5.313220341600567664, 1.199719254218462483 ) ) ;
#207227=CARTESIAN_POINT ( 'NONE',  ( 4.134873662043553111, 7.767843672452050541, -0.7216878364870197293 ) ) ;
#207228=CARTESIAN_POINT ( 'NONE',  ( -8.527715432871366019, 10.01171809551380143, 1.082531754730558626 ) ) ;
#207230=CARTESIAN_POINT ( 'NONE',  ( -1.499999999999997780, 3.400000000000021227, 1.214306433183764966E-14 ) ) ;
#207234=CARTESIAN_POINT ( 'NONE',  ( 8.242994207428692377, 12.56065097540143327, -0.7216878364870328300 ) ) ;
#207246=CARTESIAN_POINT ( 'NONE',  ( 9.544576953896278582, 10.23768732240824164, 0.000000000000000000 ) ) ;
#207249=CARTESIAN_POINT ( 'NONE',  ( 9.237182729612253951, 9.671134694169463586, 0.7998128361456462443 ) ) ;
#207252=CARTESIAN_POINT ( 'NONE',  ( 10.18233705906309972, 11.83814697611718714, 1.199719254218450271 ) ) ;
#207254=CARTESIAN_POINT ( 'NONE',  ( 3.660338286009610975, 6.253849852777763729, -1.082531754730543083 ) ) ;
#207256=CARTESIAN_POINT ( 'NONE',  ( -7.022760382198764084, 11.13704484596649635, 0.7216878364870458196 ) ) ;
#207276=VERTEX_POINT ( 'NONE', #22757 ) ;
#207286=CARTESIAN_POINT ( 'NONE',  ( -5.876569516519495551, 8.943415971659659292, 1.199719254218452047 ) ) ;
#207288=CARTESIAN_POINT ( 'NONE',  ( 1.217323170181688008, 2.861755683774202641, -0.7749999999999910294 ) ) ;
#207290=CARTESIAN_POINT ( 'NONE',  ( 6.959412922516382771, 7.013736585890911535, 0.7998128361456341429 ) ) ;
#207300=CARTESIAN_POINT ( 'NONE',  ( -3.716906668440817185, 7.488141546489591072, 0.7998128361456341429 ) ) ;
#207302=( BOUNDED_SURFACE ( )  B_SPLINE_SURFACE ( 1, 2, ( 
 ( #212921, #196690, #128584, #114439, #180439, #32056, #210797, #209718, #115493, #112312, #93889, #178327, #159929, #77602, #11532, #193493, #64555, #130698, #120841, #2710, #184674, #102372, #200909, #100242, #50433, #116552, #82921, #1645, #68784, #569, #70912, #83985, #34170, #135954, #182544, #3768, #166310, #36296, #152201, #134903, #69843, #66636, #198784, #20041, #17899, #16839, #201969, #18973, #150073, #168442, #67703, #133850, #199860, #51503, #148994, #117629, #35227, #33117, #183620, #54690, #52558, #101303, #118690, #119759, #21089, #99194, #86128, #167383, #53627, #185738, #151143, #169507, #137022, #103447, #85057, #37371, #87192, #165245, #153257, #203049, #4832, #132781, #140248, #8068, #122999, #171639, #142388, #39509, #105608, #138092, #90409, #73059, #92566, #56829, #55757, #75220, #60031, #23236, #191079, #74154, #91489, #174877, #121913, #172726, #187882, #206269, #57894, #188956, #208397, #40596, #58966, #124057, #204105, #42746, #170569, #26457, #157550, #190023, #88266, #106701, #41675, #24304, #156479, #89347, #107786, #108851, #173811, #155396, #38444, #158606, #25390, #207345, #9146, #205188, #141331, #154334, #125121, #186816, #139158, #10205, #76280, #6978, #104524, #22151, #5909, #71982, #211597, #192146, #144533, #30751, #114194, #47007, #62176, #28608, #48083, #97891, #79483, #178062, #110984, #128335, #210542, #163952, #43810, #95764, #77348, #180194, #11270, #109923, #93626, #145602, #80552, #78412, #147697, #63233, #194298, #13407, #212664, #31815, #175934, #161817, #61102, #129396, #14461, #29680, #15527, #81613, #196439, #94697, #179129, #64306, #126182, #45943, #213715, #195375, #112062, #113123, #96832, #162882, #176990, #27527, #193232, #44879, #143460, #146649, #12332, #159668, #130451, #209458, #127261, #160738, #198541, #69604, #167142, #184434, #53378, #148755, #51254, #325, #18727, #84811, #1399, #86949, #67460, #151959, #150900, #16589, #135711, #49132, #119513, #36051, #68537, #181240, #133606, #2461, #199611, #183376, #82671, #134665, #201737, #200668, #66395, #131485, #37124, #117379, #85883, #149829, #83737, #34982, #32868, #3529, #153017, #166067, #101053, #103203, #100000, #52318, #115250, #19799, #118447, #102131, #197490, #168200, #185499, #169265, #20851, #65338, #182298, #98944, #164998, #132543, #50187, #116308, #33926, #17654, #42493, #136777, #188715, #170321, #141080, #104277, #70667, #186575, #172481, #173568, #171397, #137852, #202806, #189777, #204941, #55517, #156237, #203873, #121673, #105360, #187639, #120598, #5658, #6742, #92323, #39266, #122753, #38203, #91241, #26206, #22988, #89106, #190834, #155160, #138924, #54455, #25139, #56592, #90171, #21909, #72820, #123816, #207089, #140000, #40351, #106457, #58718, #108602, #24068, #7814, #73907, #206021, #57657, #174630, #88019, #41428, #154090, #124868, #71738, #107536, #157301, #8891, #74970, #4593, #77091, #142137, #129143, #144289, #209207, #95518, #143218, #60847, #44621, #127010, #59782, #159413, #160484, #31560, #192968, #179936, #177811, #110736, #45690, #30495, #146393, #9957, #194038, #93377, #111805, #46757, #61922, #80296, #196187, #14202, #176736, #211349, #96579, #158365, #12091, #113941, #29427, #78158, #161566, #13154, #94445, #28349, #76034, #11015, #210282, #109679, #128082, #79231, #64049, #145348, #27271, #112868, #208152, #62974, #162626, #195118, #178883, #212407, #130194, #47829, #125939, #191897, #43559, #175682, #119252, #33666, #184178, #50996, #48871, #101874, #81361, #151707, #2203, #100798, #213465, #99740, #117116, #165812, #1146, #114989, #183119, #167941, #166884, #98684, #163692, #69343, #17395, #118189, #182037, #116049, #133344, #32609, #199349, #200416, #67208, #19542, #135453, #85619, #71, #150642, #35797, #97635, #83479, #53119, #34726, #149561, #18474, #84553, #68279, #82414, #185236, #164740, #16331, #180988, #134412, #198286, #3276, #52062, #148503, #201477, #15274, #66134, #147440, #65089, #131245, #197232, #132280, #49928, #186308, #138657, #56329, #187381, #58460, #39012, #123554, #204678, #202543, #41163, #20601, #90980, #155966, #40082, #152755 ),
 ( #55262, #154899, #4337, #189517, #124615, #137591, #121409, #8629, #71481, #171135, #86687, #205760, #22728, #122488, #102943, #105094, #7552, #24874, #172219, #88842, #153832, #173292, #74710, #188450, #6482, #21649, #72559, #106194, #140813, #169002, #23808, #54192, #157041, #136524, #70405, #120332, #89913, #57390, #203609, #170062, #37944, #73638, #139736, #87755, #107273, #5402, #206826, #36859, #104017, #92051, #191633, #192700, #63781, #27006, #212145, #210013, #142947, #77899, #62706, #178617, #42228, #13946, #46482, #93112, #29157, #128867, #190573, #44354, #146132, #144019, #110476, #61655, #11822, #126740, #175422, #108345, #43296, #109417, #141882, #94183, #76826, #96311, #60582, #59514, #78958, #174365, #159154, #194850, #127822, #95248, #30227, #125672, #176476, #10754, #193777, #45423, #28087, #25944, #160223, #112605, #111539, #207891, #162366, #158108, #80029, #161296, #177548, #9697, #12882, #145080, #211083, #75774, #208946, #149303, #200166, #133090, #130989, #195927, #101622, #132030, #150385, #214251, #148248, #33415, #97374, #1956, #151453, #16073, #65882, #167687, #164487, #49670, #179678, #84301, #115793, #884, #47564, #198040, #34479, #117938, #50734, #181782, #32358, #51820, #19289, #83221, #99494, #114734, #165551, #17144, #85371, #113675, #66951, #81100, #183932, #15010, #31299, #163431, #199088, #68017, #82157, #48619, #147189, #100551, #116860, #180732, #182861, #98422, #166624, #18216, #134158, #213214, #196979, #35544, #3025, #129939, #64843, #121163, #37693, #55014, #56081, #105941, #135215, #203362, #86442, #187132, #72301, #71229, #39833, #154648, #171965, #20357, #5152, #152507, #38761, #104842, #169821, #73376, #21408, #122238, #170887, #168754, #188197, #201230, #23556, #6230, #22480, #119006, #87518, #88591, #153583, #137344, #102696, #138407, #89663, #204426, #4091, #69093, #7298, #155715, #139481, #52871, #184984, #36610, #186058, #70162, #136273, #202293, #53945, #120082, #103770, #182481, #98079, #2646, #34109, #133788, #114379, #66576, #167320, #36228, #183555, #198723, #165182, #184611, #19977, #1580, #100181, #33055, #50369, #132718, #86061, #180374, #17836, #213902, #102307, #147886, #31998, #15718, #67641, #68719, #508, #181425, #164134, #18907, #166246, #99133, #199796, #16776, #82860, #148936, #116492, #81803, #49317, #83919, #135891, #150010, #69783, #51441, #117560, #35162, #134841, #168381, #65525, #101238, #197673, #84991, #151082, #200844, #152138, #3706, #118625, #52495, #48265, #131670, #115434, #55692, #160405, #158288, #121847, #9878, #23170, #138028, #186755, #12008, #54628, #120775, #153197, #105539, #88200, #110657, #71918, #70846, #93299, #78082, #38378, #209129, #92238, #53562, #5848, #109599, #192884, #125859, #204042, #104459, #126927, #176658, #75954, #39445, #170506, #187818, #171573, #28271, #119695, #142057, #4768, #44541, #87127, #185679, #169444, #208071, #159335, #154273, #22088, #37308, #175604, #59697, #191816, #43481, #27193, #10931, #77007, #143134, #103382, #202988, #60767, #201909, #94363, #21029, #136961, #141369, #108892, #105649, #24341, #25424, #23274, #93664, #106739, #56867, #158645, #73095, #26495, #188994, #207381, #174915, #91531, #92602, #89385, #7019, #42783, #205226, #139196, #123043, #40637, #190061, #10243, #192184, #75255, #140290, #157589, #172768, #41713, #76319, #126223, #155434, #59002, #60067, #43848, #187917, #90451, #156517, #142424, #109962, #57933, #206309, #8108, #208433, #39548, #159706, #11305, #175972, #27566, #74196, #173848, #125158, #77383, #143500, #55796, #124097, #121951, #171677, #107823, #9184, #191117, #16626, #195416, #129433, #193268, #98980, #165033, #47046, #13445, #181276, #48119, #96869, #163986, #145640, #113162, #44914, #115285, #144568, #97928, #111022, #79522, #82709, #209496, #213751, #162919, #114231, #197523, #78450, #179166, #210581, #14499, #80591, #211635, #61136, #63271, #81648, #146687, #160777, #65373, #177027, #49167, #180229, #212703, #28644, #30790, #64344, #130490, #196477, #12370, #31852, #131520, #15561, #62212, #127298, #32902, #147735, #94731, #128369, #194336 ) ),
 .UNSPECIFIED., .F., .F., .T. ) 
 B_SPLINE_SURFACE_WITH_KNOTS ( ( 2, 2 ),
 ( 3, 2, 2, 2, 2, 2, 2, 2, 2, 2, 2, 2, 2, 2, 2, 2, 2, 2, 2, 2, 2, 2, 2, 2, 2, 2, 2, 2, 2, 2, 2, 2, 2, 2, 2, 2, 2, 2, 2, 2, 2, 2, 2, 2, 2, 2, 2, 2, 2, 2, 2, 2, 2, 2, 2, 2, 2, 2, 2, 2, 2, 2, 2, 2, 2, 2, 2, 2, 2, 2, 2, 2, 2, 2, 2, 2, 2, 2, 2, 2, 2, 2, 2, 2, 2, 2, 2, 2, 2, 2, 2, 2, 2, 2, 2, 2, 2, 2, 2, 2, 2, 2, 2, 2, 2, 2, 2, 2, 2, 2, 2, 2, 2, 2, 2, 2, 2, 2, 2, 2, 2, 2, 2, 2, 2, 2, 2, 2, 2, 2, 2, 2, 2, 2, 2, 2, 2, 2, 2, 2, 2, 2, 2, 2, 2, 2, 2, 2, 2, 2, 2, 2, 2, 2, 2, 2, 2, 2, 2, 2, 2, 2, 2, 2, 2, 2, 2, 2, 2, 2, 2, 2, 2, 2, 2, 2, 2, 2, 2, 2, 2, 2, 2, 2, 2, 2, 2, 2, 2, 2, 2, 2, 2, 2, 2, 2, 2, 2, 2, 2, 2, 2, 2, 2, 2, 2, 2, 2, 2, 2, 2, 2, 2, 2, 2, 2, 2, 2, 2, 2, 2, 2, 2, 2, 2, 2, 2, 2, 2, 2, 2, 2, 2, 2, 2, 2, 2, 2, 2, 2, 3 ),
 ( 0.000000000000000000, 1.000000000000000000 ),
 ( 0.000000000000000000, 0.004166666666666666609, 0.008333333333333333218, 0.01250000000000000069, 0.01666666666666666644, 0.02083333333333333218, 0.02500000000000000139, 0.02916666666666666713, 0.03333333333333333287, 0.03749999999999999861, 0.04166666666666666435, 0.04583333333333333010, 0.05000000000000000278, 0.05416666666666666852, 0.05833333333333333426, 0.06250000000000000000, 0.06666666666666666574, 0.07083333333333333148, 0.07499999999999999722, 0.07916666666666666297, 0.08333333333333332871, 0.08749999999999999445, 0.09166666666666666019, 0.09583333333333333981, 0.1000000000000000056, 0.1041666666666666713, 0.1083333333333333370, 0.1125000000000000028, 0.1166666666666666685, 0.1208333333333333343, 0.1250000000000000000, 0.1291666666666666796, 0.1333333333333333315, 0.1375000000000000111, 0.1416666666666666630, 0.1458333333333333426, 0.1499999999999999944, 0.1541666666666666741, 0.1583333333333333259, 0.1625000000000000056, 0.1666666666666666574, 0.1708333333333333370, 0.1749999999999999889, 0.1791666666666666685, 0.1833333333333333204, 0.1875000000000000000, 0.1916666666666666796, 0.1958333333333333315, 0.2000000000000000111, 0.2041666666666666630, 0.2083333333333333426, 0.2124999999999999944, 0.2166666666666666741, 0.2208333333333333259, 0.2250000000000000056, 0.2291666666666666574, 0.2333333333333333370, 0.2374999999999999889, 0.2416666666666666685, 0.2458333333333333204, 0.2500000000000000000, 0.2541666666666666519, 0.2583333333333333592, 0.2625000000000000111, 0.2666666666666666630, 0.2708333333333333148, 0.2750000000000000222, 0.2791666666666666741, 0.2833333333333333259, 0.2874999999999999778, 0.2916666666666666852, 0.2958333333333333370, 0.2999999999999999889, 0.3041666666666666408, 0.3083333333333333481, 0.3125000000000000000, 0.3166666666666666519, 0.3208333333333333592, 0.3250000000000000111, 0.3291666666666666630, 0.3333333333333333148, 0.3375000000000000222, 0.3416666666666666741, 0.3458333333333333259, 0.3499999999999999778, 0.3541666666666666852, 0.3583333333333333370, 0.3624999999999999889, 0.3666666666666666408, 0.3708333333333333481, 0.3750000000000000000, 0.3791666666666666519, 0.3833333333333333592, 0.3875000000000000111, 0.3916666666666666630, 0.3958333333333333148, 0.4000000000000000222, 0.4041666666666666741, 0.4083333333333333259, 0.4124999999999999778, 0.4166666666666666852, 0.4208333333333333370, 0.4249999999999999889, 0.4291666666666666408, 0.4333333333333333481, 0.4375000000000000000, 0.4416666666666666519, 0.4458333333333333592, 0.4500000000000000111, 0.4541666666666666630, 0.4583333333333333148, 0.4625000000000000222, 0.4666666666666666741, 0.4708333333333333259, 0.4749999999999999778, 0.4791666666666666852, 0.4833333333333333370, 0.4874999999999999889, 0.4916666666666666408, 0.4958333333333333481, 0.5000000000000000000, 0.5041666666666666519, 0.5083333333333333037, 0.5124999999999999556, 0.5166666666666667185, 0.5208333333333333703, 0.5250000000000000222, 0.5291666666666666741, 0.5333333333333333259, 0.5374999999999999778, 0.5416666666666666297, 0.5458333333333332815, 0.5500000000000000444, 0.5541666666666666963, 0.5583333333333333481, 0.5625000000000000000, 0.5666666666666666519, 0.5708333333333333037, 0.5749999999999999556, 0.5791666666666667185, 0.5833333333333333703, 0.5875000000000000222, 0.5916666666666666741, 0.5958333333333333259, 0.5999999999999999778, 0.6041666666666666297, 0.6083333333333332815, 0.6125000000000000444, 0.6166666666666666963, 0.6208333333333333481, 0.6250000000000000000, 0.6291666666666666519, 0.6333333333333333037, 0.6374999999999999556, 0.6416666666666667185, 0.6458333333333333703, 0.6500000000000000222, 0.6541666666666666741, 0.6583333333333333259, 0.6624999999999999778, 0.6666666666666666297, 0.6708333333333332815, 0.6750000000000000444, 0.6791666666666666963, 0.6833333333333333481, 0.6875000000000000000, 0.6916666666666666519, 0.6958333333333333037, 0.6999999999999999556, 0.7041666666666667185, 0.7083333333333333703, 0.7125000000000000222, 0.7166666666666666741, 0.7208333333333333259, 0.7249999999999999778, 0.7291666666666666297, 0.7333333333333332815, 0.7375000000000000444, 0.7416666666666666963, 0.7458333333333333481, 0.7500000000000000000, 0.7541666666666666519, 0.7583333333333333037, 0.7624999999999999556, 0.7666666666666667185, 0.7708333333333333703, 0.7750000000000000222, 0.7791666666666666741, 0.7833333333333333259, 0.7874999999999999778, 0.7916666666666666297, 0.7958333333333332815, 0.8000000000000000444, 0.8041666666666666963, 0.8083333333333333481, 0.8125000000000000000, 0.8166666666666666519, 0.8208333333333333037, 0.8249999999999999556, 0.8291666666666667185, 0.8333333333333333703, 0.8375000000000000222, 0.8416666666666666741, 0.8458333333333333259, 0.8499999999999999778, 0.8541666666666666297, 0.8583333333333332815, 0.8625000000000000444, 0.8666666666666666963, 0.8708333333333333481, 0.8750000000000000000, 0.8791666666666666519, 0.8833333333333333037, 0.8874999999999999556, 0.8916666666666667185, 0.8958333333333333703, 0.9000000000000000222, 0.9041666666666666741, 0.9083333333333333259, 0.9124999999999999778, 0.9166666666666666297, 0.9208333333333332815, 0.9250000000000000444, 0.9291666666666666963, 0.9333333333333333481, 0.9375000000000000000, 0.9416666666666666519, 0.9458333333333333037, 0.9499999999999999556, 0.9541666666666667185, 0.9583333333333333703, 0.9625000000000000222, 0.9666666666666666741, 0.9708333333333333259, 0.9749999999999999778, 0.9791666666666666297, 0.9833333333333332815, 0.9875000000000000444, 0.9916666666666666963, 0.9958333333333333481, 1.000000000000000000 ),
 .UNSPECIFIED. ) 
 GEOMETRIC_REPRESENTATION_ITEM ( )  RATIONAL_B_SPLINE_SURFACE ( (
 ( 1.000000000000000000, 0.8660254037844387076, 1.000000000000000000, 0.8660254037844387076, 1.000000000000000000, 0.8660254037844387076, 1.000000000000000000, 0.8660254037844387076, 1.000000000000000000, 0.8660254037844387076, 1.000000000000000000, 0.8660254037844387076, 1.000000000000000000, 0.8660254037844387076, 1.000000000000000000, 0.8660254037844387076, 1.000000000000000000, 0.8660254037844387076, 1.000000000000000000, 0.8660254037844387076, 1.000000000000000000, 0.8660254037844387076, 1.000000000000000000, 0.8660254037844387076, 1.000000000000000000, 0.8660254037844387076, 1.000000000000000000, 0.8660254037844387076, 1.000000000000000000, 0.8660254037844387076, 1.000000000000000000, 0.8660254037844387076, 1.000000000000000000, 0.8660254037844387076, 1.000000000000000000, 0.8660254037844387076, 1.000000000000000000, 0.8660254037844387076, 1.000000000000000000, 0.8660254037844387076, 1.000000000000000000, 0.8660254037844387076, 1.000000000000000000, 0.8660254037844387076, 1.000000000000000000, 0.8660254037844387076, 1.000000000000000000, 0.8660254037844387076, 1.000000000000000000, 0.8660254037844387076, 1.000000000000000000, 0.8660254037844387076, 1.000000000000000000, 0.8660254037844387076, 1.000000000000000000, 0.8660254037844387076, 1.000000000000000000, 0.8660254037844387076, 1.000000000000000000, 0.8660254037844387076, 1.000000000000000000, 0.8660254037844387076, 1.000000000000000000, 0.8660254037844387076, 1.000000000000000000, 0.8660254037844387076, 1.000000000000000000, 0.8660254037844387076, 1.000000000000000000, 0.8660254037844387076, 1.000000000000000000, 0.8660254037844387076, 1.000000000000000000, 0.8660254037844387076, 1.000000000000000000, 0.8660254037844387076, 1.000000000000000000, 0.8660254037844387076, 1.000000000000000000, 0.8660254037844387076, 1.000000000000000000, 0.8660254037844387076, 1.000000000000000000, 0.8660254037844387076, 1.000000000000000000, 0.8660254037844387076, 1.000000000000000000, 0.8660254037844387076, 1.000000000000000000, 0.8660254037844387076, 1.000000000000000000, 0.8660254037844387076, 1.000000000000000000, 0.8660254037844387076, 1.000000000000000000, 0.8660254037844387076, 1.000000000000000000, 0.8660254037844387076, 1.000000000000000000, 0.8660254037844387076, 1.000000000000000000, 0.8660254037844387076, 1.000000000000000000, 0.8660254037844387076, 1.000000000000000000, 0.8660254037844387076, 1.000000000000000000, 0.8660254037844387076, 1.000000000000000000, 0.8660254037844387076, 1.000000000000000000, 0.8660254037844387076, 1.000000000000000000, 0.8660254037844387076, 1.000000000000000000, 0.8660254037844387076, 1.000000000000000000, 0.8660254037844387076, 1.000000000000000000, 0.8660254037844387076, 1.000000000000000000, 0.8660254037844387076, 1.000000000000000000, 0.8660254037844387076, 1.000000000000000000, 0.8660254037844387076, 1.000000000000000000, 0.8660254037844387076, 1.000000000000000000, 0.8660254037844387076, 1.000000000000000000, 0.8660254037844387076, 1.000000000000000000, 0.8660254037844387076, 1.000000000000000000, 0.8660254037844387076, 1.000000000000000000, 0.8660254037844387076, 1.000000000000000000, 0.8660254037844387076, 1.000000000000000000, 0.8660254037844387076, 1.000000000000000000, 0.8660254037844387076, 1.000000000000000000, 0.8660254037844387076, 1.000000000000000000, 0.8660254037844387076, 1.000000000000000000, 0.8660254037844387076, 1.000000000000000000, 0.8660254037844387076, 1.000000000000000000, 0.8660254037844387076, 1.000000000000000000, 0.8660254037844387076, 1.000000000000000000, 0.8660254037844387076, 1.000000000000000000, 0.8660254037844387076, 1.000000000000000000, 0.8660254037844387076, 1.000000000000000000, 0.8660254037844387076, 1.000000000000000000, 0.8660254037844387076, 1.000000000000000000, 0.8660254037844387076, 1.000000000000000000, 0.8660254037844387076, 1.000000000000000000, 0.8660254037844387076, 1.000000000000000000, 0.8660254037844387076, 1.000000000000000000, 0.8660254037844387076, 1.000000000000000000, 0.8660254037844387076, 1.000000000000000000, 0.8660254037844387076, 1.000000000000000000, 0.8660254037844387076, 1.000000000000000000, 0.8660254037844387076, 1.000000000000000000, 0.8660254037844387076, 1.000000000000000000, 0.8660254037844387076, 1.000000000000000000, 0.8660254037844387076, 1.000000000000000000, 0.8660254037844387076, 1.000000000000000000, 0.8660254037844387076, 1.000000000000000000, 0.8660254037844387076, 1.000000000000000000, 0.8660254037844387076, 1.000000000000000000, 0.8660254037844387076, 1.000000000000000000, 0.8660254037844387076, 1.000000000000000000, 0.8660254037844387076, 1.000000000000000000, 0.8660254037844387076, 1.000000000000000000, 0.8660254037844387076, 1.000000000000000000, 0.8660254037844387076, 1.000000000000000000, 0.8660254037844387076, 1.000000000000000000, 0.8660254037844387076, 1.000000000000000000, 0.8660254037844387076, 1.000000000000000000, 0.8660254037844387076, 1.000000000000000000, 0.8660254037844387076, 1.000000000000000000, 0.8660254037844387076, 1.000000000000000000, 0.8660254037844387076, 1.000000000000000000, 0.8660254037844387076, 1.000000000000000000, 0.8660254037844387076, 1.000000000000000000, 0.8660254037844387076, 1.000000000000000000, 0.8660254037844387076, 1.000000000000000000, 0.8660254037844387076, 1.000000000000000000, 0.8660254037844387076, 1.000000000000000000, 0.8660254037844387076, 1.000000000000000000, 0.8660254037844387076, 1.000000000000000000, 0.8660254037844387076, 1.000000000000000000, 0.8660254037844387076, 1.000000000000000000, 0.8660254037844387076, 1.000000000000000000, 0.8660254037844387076, 1.000000000000000000, 0.8660254037844387076, 1.000000000000000000, 0.8660254037844387076, 1.000000000000000000, 0.8660254037844387076, 1.000000000000000000, 0.8660254037844387076, 1.000000000000000000, 0.8660254037844387076, 1.000000000000000000, 0.8660254037844387076, 1.000000000000000000, 0.8660254037844387076, 1.000000000000000000, 0.8660254037844387076, 1.000000000000000000, 0.8660254037844387076, 1.000000000000000000, 0.8660254037844387076, 1.000000000000000000, 0.8660254037844387076, 1.000000000000000000, 0.8660254037844387076, 1.000000000000000000, 0.8660254037844387076, 1.000000000000000000, 0.8660254037844387076, 1.000000000000000000, 0.8660254037844387076, 1.000000000000000000, 0.8660254037844387076, 1.000000000000000000, 0.8660254037844387076, 1.000000000000000000, 0.8660254037844387076, 1.000000000000000000, 0.8660254037844387076, 1.000000000000000000, 0.8660254037844387076, 1.000000000000000000, 0.8660254037844387076, 1.000000000000000000, 0.8660254037844387076, 1.000000000000000000, 0.8660254037844387076, 1.000000000000000000, 0.8660254037844387076, 1.000000000000000000, 0.8660254037844387076, 1.000000000000000000, 0.8660254037844387076, 1.000000000000000000, 0.8660254037844387076, 1.000000000000000000, 0.8660254037844387076, 1.000000000000000000, 0.8660254037844387076, 1.000000000000000000, 0.8660254037844387076, 1.000000000000000000, 0.8660254037844387076, 1.000000000000000000, 0.8660254037844387076, 1.000000000000000000, 0.8660254037844387076, 1.000000000000000000, 0.8660254037844387076, 1.000000000000000000, 0.8660254037844387076, 1.000000000000000000, 0.8660254037844387076, 1.000000000000000000, 0.8660254037844387076, 1.000000000000000000, 0.8660254037844387076, 1.000000000000000000, 0.8660254037844387076, 1.000000000000000000, 0.8660254037844387076, 1.000000000000000000, 0.8660254037844387076, 1.000000000000000000, 0.8660254037844387076, 1.000000000000000000, 0.8660254037844387076, 1.000000000000000000, 0.8660254037844387076, 1.000000000000000000, 0.8660254037844387076, 1.000000000000000000, 0.8660254037844387076, 1.000000000000000000, 0.8660254037844387076, 1.000000000000000000, 0.8660254037844387076, 1.000000000000000000, 0.8660254037844387076, 1.000000000000000000, 0.8660254037844387076, 1.000000000000000000, 0.8660254037844387076, 1.000000000000000000, 0.8660254037844387076, 1.000000000000000000, 0.8660254037844387076, 1.000000000000000000, 0.8660254037844387076, 1.000000000000000000, 0.8660254037844387076, 1.000000000000000000, 0.8660254037844387076, 1.000000000000000000, 0.8660254037844387076, 1.000000000000000000, 0.8660254037844387076, 1.000000000000000000, 0.8660254037844387076, 1.000000000000000000, 0.8660254037844387076, 1.000000000000000000, 0.8660254037844387076, 1.000000000000000000, 0.8660254037844387076, 1.000000000000000000, 0.8660254037844387076, 1.000000000000000000, 0.8660254037844387076, 1.000000000000000000, 0.8660254037844387076, 1.000000000000000000, 0.8660254037844387076, 1.000000000000000000, 0.8660254037844387076, 1.000000000000000000, 0.8660254037844387076, 1.000000000000000000, 0.8660254037844387076, 1.000000000000000000, 0.8660254037844387076, 1.000000000000000000, 0.8660254037844387076, 1.000000000000000000, 0.8660254037844387076, 1.000000000000000000, 0.8660254037844387076, 1.000000000000000000, 0.8660254037844387076, 1.000000000000000000, 0.8660254037844387076, 1.000000000000000000, 0.8660254037844387076, 1.000000000000000000, 0.8660254037844387076, 1.000000000000000000, 0.8660254037844387076, 1.000000000000000000, 0.8660254037844387076, 1.000000000000000000, 0.8660254037844387076, 1.000000000000000000, 0.8660254037844387076, 1.000000000000000000, 0.8660254037844387076, 1.000000000000000000, 0.8660254037844387076, 1.000000000000000000, 0.8660254037844387076, 1.000000000000000000, 0.8660254037844387076, 1.000000000000000000, 0.8660254037844387076, 1.000000000000000000, 0.8660254037844387076, 1.000000000000000000, 0.8660254037844387076, 1.000000000000000000, 0.8660254037844387076, 1.000000000000000000, 0.8660254037844387076, 1.000000000000000000, 0.8660254037844387076, 1.000000000000000000, 0.8660254037844387076, 1.000000000000000000, 0.8660254037844387076, 1.000000000000000000, 0.8660254037844387076, 1.000000000000000000, 0.8660254037844387076, 1.000000000000000000, 0.8660254037844387076, 1.000000000000000000, 0.8660254037844387076, 1.000000000000000000, 0.8660254037844387076, 1.000000000000000000, 0.8660254037844387076, 1.000000000000000000, 0.8660254037844387076, 1.000000000000000000, 0.8660254037844387076, 1.000000000000000000, 0.8660254037844387076, 1.000000000000000000, 0.8660254037844387076, 1.000000000000000000, 0.8660254037844387076, 1.000000000000000000, 0.8660254037844387076, 1.000000000000000000, 0.8660254037844387076, 1.000000000000000000, 0.8660254037844387076, 1.000000000000000000, 0.8660254037844387076, 1.000000000000000000, 0.8660254037844387076, 1.000000000000000000, 0.8660254037844387076, 1.000000000000000000, 0.8660254037844387076, 1.000000000000000000, 0.8660254037844387076, 1.000000000000000000, 0.8660254037844387076, 1.000000000000000000, 0.8660254037844387076, 1.000000000000000000, 0.8660254037844387076, 1.000000000000000000, 0.8660254037844387076, 1.000000000000000000),
 ( 1.000000000000000000, 0.8660254037844387076, 1.000000000000000000, 0.8660254037844387076, 1.000000000000000000, 0.8660254037844387076, 1.000000000000000000, 0.8660254037844387076, 1.000000000000000000, 0.8660254037844387076, 1.000000000000000000, 0.8660254037844387076, 1.000000000000000000, 0.8660254037844387076, 1.000000000000000000, 0.8660254037844387076, 1.000000000000000000, 0.8660254037844387076, 1.000000000000000000, 0.8660254037844387076, 1.000000000000000000, 0.8660254037844387076, 1.000000000000000000, 0.8660254037844387076, 1.000000000000000000, 0.8660254037844387076, 1.000000000000000000, 0.8660254037844387076, 1.000000000000000000, 0.8660254037844387076, 1.000000000000000000, 0.8660254037844387076, 1.000000000000000000, 0.8660254037844387076, 1.000000000000000000, 0.8660254037844387076, 1.000000000000000000, 0.8660254037844387076, 1.000000000000000000, 0.8660254037844387076, 1.000000000000000000, 0.8660254037844387076, 1.000000000000000000, 0.8660254037844387076, 1.000000000000000000, 0.8660254037844387076, 1.000000000000000000, 0.8660254037844387076, 1.000000000000000000, 0.8660254037844387076, 1.000000000000000000, 0.8660254037844387076, 1.000000000000000000, 0.8660254037844387076, 1.000000000000000000, 0.8660254037844387076, 1.000000000000000000, 0.8660254037844387076, 1.000000000000000000, 0.8660254037844387076, 1.000000000000000000, 0.8660254037844387076, 1.000000000000000000, 0.8660254037844387076, 1.000000000000000000, 0.8660254037844387076, 1.000000000000000000, 0.8660254037844387076, 1.000000000000000000, 0.8660254037844387076, 1.000000000000000000, 0.8660254037844387076, 1.000000000000000000, 0.8660254037844387076, 1.000000000000000000, 0.8660254037844387076, 1.000000000000000000, 0.8660254037844387076, 1.000000000000000000, 0.8660254037844387076, 1.000000000000000000, 0.8660254037844387076, 1.000000000000000000, 0.8660254037844387076, 1.000000000000000000, 0.8660254037844387076, 1.000000000000000000, 0.8660254037844387076, 1.000000000000000000, 0.8660254037844387076, 1.000000000000000000, 0.8660254037844387076, 1.000000000000000000, 0.8660254037844387076, 1.000000000000000000, 0.8660254037844387076, 1.000000000000000000, 0.8660254037844387076, 1.000000000000000000, 0.8660254037844387076, 1.000000000000000000, 0.8660254037844387076, 1.000000000000000000, 0.8660254037844387076, 1.000000000000000000, 0.8660254037844387076, 1.000000000000000000, 0.8660254037844387076, 1.000000000000000000, 0.8660254037844387076, 1.000000000000000000, 0.8660254037844387076, 1.000000000000000000, 0.8660254037844387076, 1.000000000000000000, 0.8660254037844387076, 1.000000000000000000, 0.8660254037844387076, 1.000000000000000000, 0.8660254037844387076, 1.000000000000000000, 0.8660254037844387076, 1.000000000000000000, 0.8660254037844387076, 1.000000000000000000, 0.8660254037844387076, 1.000000000000000000, 0.8660254037844387076, 1.000000000000000000, 0.8660254037844387076, 1.000000000000000000, 0.8660254037844387076, 1.000000000000000000, 0.8660254037844387076, 1.000000000000000000, 0.8660254037844387076, 1.000000000000000000, 0.8660254037844387076, 1.000000000000000000, 0.8660254037844387076, 1.000000000000000000, 0.8660254037844387076, 1.000000000000000000, 0.8660254037844387076, 1.000000000000000000, 0.8660254037844387076, 1.000000000000000000, 0.8660254037844387076, 1.000000000000000000, 0.8660254037844387076, 1.000000000000000000, 0.8660254037844387076, 1.000000000000000000, 0.8660254037844387076, 1.000000000000000000, 0.8660254037844387076, 1.000000000000000000, 0.8660254037844387076, 1.000000000000000000, 0.8660254037844387076, 1.000000000000000000, 0.8660254037844387076, 1.000000000000000000, 0.8660254037844387076, 1.000000000000000000, 0.8660254037844387076, 1.000000000000000000, 0.8660254037844387076, 1.000000000000000000, 0.8660254037844387076, 1.000000000000000000, 0.8660254037844387076, 1.000000000000000000, 0.8660254037844387076, 1.000000000000000000, 0.8660254037844387076, 1.000000000000000000, 0.8660254037844387076, 1.000000000000000000, 0.8660254037844387076, 1.000000000000000000, 0.8660254037844387076, 1.000000000000000000, 0.8660254037844387076, 1.000000000000000000, 0.8660254037844387076, 1.000000000000000000, 0.8660254037844387076, 1.000000000000000000, 0.8660254037844387076, 1.000000000000000000, 0.8660254037844387076, 1.000000000000000000, 0.8660254037844387076, 1.000000000000000000, 0.8660254037844387076, 1.000000000000000000, 0.8660254037844387076, 1.000000000000000000, 0.8660254037844387076, 1.000000000000000000, 0.8660254037844387076, 1.000000000000000000, 0.8660254037844387076, 1.000000000000000000, 0.8660254037844387076, 1.000000000000000000, 0.8660254037844387076, 1.000000000000000000, 0.8660254037844387076, 1.000000000000000000, 0.8660254037844387076, 1.000000000000000000, 0.8660254037844387076, 1.000000000000000000, 0.8660254037844387076, 1.000000000000000000, 0.8660254037844387076, 1.000000000000000000, 0.8660254037844387076, 1.000000000000000000, 0.8660254037844387076, 1.000000000000000000, 0.8660254037844387076, 1.000000000000000000, 0.8660254037844387076, 1.000000000000000000, 0.8660254037844387076, 1.000000000000000000, 0.8660254037844387076, 1.000000000000000000, 0.8660254037844387076, 1.000000000000000000, 0.8660254037844387076, 1.000000000000000000, 0.8660254037844387076, 1.000000000000000000, 0.8660254037844387076, 1.000000000000000000, 0.8660254037844387076, 1.000000000000000000, 0.8660254037844387076, 1.000000000000000000, 0.8660254037844387076, 1.000000000000000000, 0.8660254037844387076, 1.000000000000000000, 0.8660254037844387076, 1.000000000000000000, 0.8660254037844387076, 1.000000000000000000, 0.8660254037844387076, 1.000000000000000000, 0.8660254037844387076, 1.000000000000000000, 0.8660254037844387076, 1.000000000000000000, 0.8660254037844387076, 1.000000000000000000, 0.8660254037844387076, 1.000000000000000000, 0.8660254037844387076, 1.000000000000000000, 0.8660254037844387076, 1.000000000000000000, 0.8660254037844387076, 1.000000000000000000, 0.8660254037844387076, 1.000000000000000000, 0.8660254037844387076, 1.000000000000000000, 0.8660254037844387076, 1.000000000000000000, 0.8660254037844387076, 1.000000000000000000, 0.8660254037844387076, 1.000000000000000000, 0.8660254037844387076, 1.000000000000000000, 0.8660254037844387076, 1.000000000000000000, 0.8660254037844387076, 1.000000000000000000, 0.8660254037844387076, 1.000000000000000000, 0.8660254037844387076, 1.000000000000000000, 0.8660254037844387076, 1.000000000000000000, 0.8660254037844387076, 1.000000000000000000, 0.8660254037844387076, 1.000000000000000000, 0.8660254037844387076, 1.000000000000000000, 0.8660254037844387076, 1.000000000000000000, 0.8660254037844387076, 1.000000000000000000, 0.8660254037844387076, 1.000000000000000000, 0.8660254037844387076, 1.000000000000000000, 0.8660254037844387076, 1.000000000000000000, 0.8660254037844387076, 1.000000000000000000, 0.8660254037844387076, 1.000000000000000000, 0.8660254037844387076, 1.000000000000000000, 0.8660254037844387076, 1.000000000000000000, 0.8660254037844387076, 1.000000000000000000, 0.8660254037844387076, 1.000000000000000000, 0.8660254037844387076, 1.000000000000000000, 0.8660254037844387076, 1.000000000000000000, 0.8660254037844387076, 1.000000000000000000, 0.8660254037844387076, 1.000000000000000000, 0.8660254037844387076, 1.000000000000000000, 0.8660254037844387076, 1.000000000000000000, 0.8660254037844387076, 1.000000000000000000, 0.8660254037844387076, 1.000000000000000000, 0.8660254037844387076, 1.000000000000000000, 0.8660254037844387076, 1.000000000000000000, 0.8660254037844387076, 1.000000000000000000, 0.8660254037844387076, 1.000000000000000000, 0.8660254037844387076, 1.000000000000000000, 0.8660254037844387076, 1.000000000000000000, 0.8660254037844387076, 1.000000000000000000, 0.8660254037844387076, 1.000000000000000000, 0.8660254037844387076, 1.000000000000000000, 0.8660254037844387076, 1.000000000000000000, 0.8660254037844387076, 1.000000000000000000, 0.8660254037844387076, 1.000000000000000000, 0.8660254037844387076, 1.000000000000000000, 0.8660254037844387076, 1.000000000000000000, 0.8660254037844387076, 1.000000000000000000, 0.8660254037844387076, 1.000000000000000000, 0.8660254037844387076, 1.000000000000000000, 0.8660254037844387076, 1.000000000000000000, 0.8660254037844387076, 1.000000000000000000, 0.8660254037844387076, 1.000000000000000000, 0.8660254037844387076, 1.000000000000000000, 0.8660254037844387076, 1.000000000000000000, 0.8660254037844387076, 1.000000000000000000, 0.8660254037844387076, 1.000000000000000000, 0.8660254037844387076, 1.000000000000000000, 0.8660254037844387076, 1.000000000000000000, 0.8660254037844387076, 1.000000000000000000, 0.8660254037844387076, 1.000000000000000000, 0.8660254037844387076, 1.000000000000000000, 0.8660254037844387076, 1.000000000000000000, 0.8660254037844387076, 1.000000000000000000, 0.8660254037844387076, 1.000000000000000000, 0.8660254037844387076, 1.000000000000000000, 0.8660254037844387076, 1.000000000000000000, 0.8660254037844387076, 1.000000000000000000, 0.8660254037844387076, 1.000000000000000000, 0.8660254037844387076, 1.000000000000000000, 0.8660254037844387076, 1.000000000000000000, 0.8660254037844387076, 1.000000000000000000, 0.8660254037844387076, 1.000000000000000000, 0.8660254037844387076, 1.000000000000000000, 0.8660254037844387076, 1.000000000000000000, 0.8660254037844387076, 1.000000000000000000, 0.8660254037844387076, 1.000000000000000000, 0.8660254037844387076, 1.000000000000000000, 0.8660254037844387076, 1.000000000000000000, 0.8660254037844387076, 1.000000000000000000, 0.8660254037844387076, 1.000000000000000000, 0.8660254037844387076, 1.000000000000000000, 0.8660254037844387076, 1.000000000000000000, 0.8660254037844387076, 1.000000000000000000, 0.8660254037844387076, 1.000000000000000000, 0.8660254037844387076, 1.000000000000000000, 0.8660254037844387076, 1.000000000000000000, 0.8660254037844387076, 1.000000000000000000, 0.8660254037844387076, 1.000000000000000000, 0.8660254037844387076, 1.000000000000000000, 0.8660254037844387076, 1.000000000000000000, 0.8660254037844387076, 1.000000000000000000, 0.8660254037844387076, 1.000000000000000000, 0.8660254037844387076, 1.000000000000000000, 0.8660254037844387076, 1.000000000000000000, 0.8660254037844387076, 1.000000000000000000, 0.8660254037844387076, 1.000000000000000000, 0.8660254037844387076, 1.000000000000000000, 0.8660254037844387076, 1.000000000000000000, 0.8660254037844387076, 1.000000000000000000, 0.8660254037844387076, 1.000000000000000000, 0.8660254037844387076, 1.000000000000000000, 0.8660254037844387076, 1.000000000000000000, 0.8660254037844387076, 1.000000000000000000, 0.8660254037844387076, 1.000000000000000000, 0.8660254037844387076, 1.000000000000000000, 0.8660254037844387076, 1.000000000000000000) ) ) 
 REPRESENTATION_ITEM ( '' )  SURFACE ( )  );
#207304=CARTESIAN_POINT ( 'NONE',  ( 7.426115451983150706, 9.686887332112256388, -1.599625672291262513 ) ) ;
#207305=CARTESIAN_POINT ( 'NONE',  ( 1.364683531249988535, 3.613541667008086211, 0.7879004041258499402 ) ) ;
#207307=CARTESIAN_POINT ( 'NONE',  ( 6.089152713731276201, 6.031799978164165132, 0.2946234760112295126 ) ) ;
#207312=B_SPLINE_CURVE_WITH_KNOTS ( 'NONE', 3,
 ( #92175, #125794, #191756, #187500 ),
 .UNSPECIFIED., .F., .F.,
 ( 4, 4 ),
 ( 6.133173666733493856E-19, 0.0003197243294386109026 ),
 .UNSPECIFIED. ) ;
#207314=CARTESIAN_POINT ( 'NONE',  ( 4.948362878863507675, 8.716914425408678113, -0.7216878364870267237 ) ) ;
#207316=CARTESIAN_POINT ( 'NONE',  ( -6.669721502918952716, 9.868759955792373972, 1.199719254218452047 ) ) ;
#207320=CARTESIAN_POINT ( 'NONE',  ( -7.862839020921525091, 11.26073039346208660, -1.199719254218446718 ) ) ;
#207321=CARTESIAN_POINT ( 'NONE',  ( -7.074657228232555717, 7.148188275893099686, 1.040834085586084257E-14 ) ) ;
#207325=CARTESIAN_POINT ( 'NONE',  ( 4.898866473728816118, 4.866114554557366745, 0.6591557868584748681 ) ) ;
#207329=CARTESIAN_POINT ( 'NONE',  ( 7.401861798056875053, 10.72292363345333399, -1.199719254218441611 ) ) ;
#207344=CARTESIAN_POINT ( 'NONE',  ( 1.499999999999990896, 4.025000000000021672, 1.214306433183764966E-14 ) ) ;
#207345=CARTESIAN_POINT ( 'NONE',  ( 5.983225862332436584, 5.874851682342960402, 0.7998128361456341429 ) ) ;
#207346=CARTESIAN_POINT ( 'NONE',  ( 5.608269097547198712, 9.694731047113750222, -0.7998128361456281477 ) ) ;
#207348=CIRCLE ( 'NONE', #110484, 0.08000000000000012657 ) ;
#207350=CARTESIAN_POINT ( 'NONE',  ( 7.619319141200072920, 7.991553207595983643, 0.7216878364870317197 ) ) ;
#207351=CARTESIAN_POINT ( 'NONE',  ( -10.11401940567025548, 10.90203684947788076, 1.040834085586084257E-14 ) ) ;
#207354=CARTESIAN_POINT ( 'NONE',  ( 7.892817981449907982, 12.36003807833360391, 0.7998128361456462443 ) ) ;
#207359=CARTESIAN_POINT ( 'NONE',  ( -1.364683531250000748, 1.009375000341421247, 0.000000000000000000 ) ) ;
#207364=CARTESIAN_POINT ( 'NONE',  ( -1.364683531250014514, -0.01145833299191483488, -0.7879004041258359514 ) ) ;
#207366=EDGE_CURVE ( 'NONE', #108613, #4315, #25093, .T. ) ;
#207367=CARTESIAN_POINT ( 'NONE',  ( 8.536830278099042602, 13.11138575775759563, -0.7998128361456352531 ) ) ;
#207370=CARTESIAN_POINT ( 'NONE',  ( -9.642873567817536795, 12.27310513391906532, 1.599625672291281386 ) ) ;
#207376=CARTESIAN_POINT ( 'NONE',  ( 4.878236342818665250, 4.585697242910212523, 1.040834085586084257E-14 ) ) ;
#207381=CARTESIAN_POINT ( 'NONE',  ( 9.271078113646423091, 9.710679308875986848, 1.040834085586084257E-14 ) ) ;
#207384=CARTESIAN_POINT ( 'NONE',  ( -4.548924232584923288, 5.265832011892554121, -1.199719254218446718 ) ) ;
#207388=CARTESIAN_POINT ( 'NONE',  ( 7.751511138711133064, 10.06651563329490529, -1.599625672291262513 ) ) ;
#207390=CARTESIAN_POINT ( 'NONE',  ( 7.938462636001388795, 9.220293482545153907, -1.199719254218441611 ) ) ;
#207393=CARTESIAN_POINT ( 'NONE',  ( -8.731087737520713432, 10.24898578427137963, 1.082531754730558626 ) ) ;
#207401=CARTESIAN_POINT ( 'NONE',  ( -6.137267537028628261, 5.996416355291856348, 0.05987573180751305790 ) ) ;
#207402=CARTESIAN_POINT ( 'NONE',  ( -1.201851678989727383E-14, 1.571875000341420581, 1.575800808251672791 ) ) ;
#207404=CARTESIAN_POINT ( 'NONE',  ( 6.995644074971448134, 7.263932296995902149, -0.7216878364870257245 ) ) ;
#207420=CARTESIAN_POINT ( 'NONE',  ( 7.587759525142423911, 12.00413654597487501, 0.7998128361456462443 ) ) ;
#207424=CARTESIAN_POINT ( 'NONE',  ( -4.081167932913447594, 4.720116328942494555, -1.199719254218452047 ) ) ;
#207425=CARTESIAN_POINT ( 'NONE',  ( -6.938021921891187382, 9.117444880338284818, -1.599625672291263179 ) ) ;
#207428=CARTESIAN_POINT ( 'NONE',  ( -8.435144125996554720, 12.99275191363802229, 0.7998128361456341429 ) ) ;
#207431=CARTESIAN_POINT ( 'NONE',  ( 1.499999999999990896, 4.056250000682819490, 1.214306433183764966E-14 ) ) ;
#207432=CARTESIAN_POINT ( 'NONE',  ( 8.613507663383630941, 8.943513783569379427, -0.7998128361456221525 ) ) ;
#207435=CIRCLE ( 'NONE', #183168, 2.750000000000000000 ) ;
#207436=CARTESIAN_POINT ( 'NONE',  ( -7.232384877886063990, 10.52520055992070525, -1.199719254218446718 ) ) ;
#207438=CARTESIAN_POINT ( 'NONE',  ( -1.364683531249997417, 4.259375000341424133, 1.214306433183764966E-14 ) ) ;
#207444=CARTESIAN_POINT ( 'NONE',  ( -8.514157279702033065, 9.995900250149611921, -1.082531754730543971 ) ) ;
#207448=CARTESIAN_POINT ( 'NONE',  ( 0.6823417656249899377, 3.238541667008085323, -1.181850606188754593 ) ) ;
#207456=CARTESIAN_POINT ( 'NONE',  ( -0.6823417656249969321, 4.467708333674755394, -1.181850606188749264 ) ) ;
#207457=CARTESIAN_POINT ( 'NONE',  ( -4.273844736805832767, 6.009238164405336313, 1.599625672291267398 ) ) ;
#207458=CARTESIAN_POINT ( 'NONE',  ( 5.341022448779654930, 8.318611059296550536, 1.199719254218462483 ) ) ;
#207461=CARTESIAN_POINT ( 'NONE',  ( -0.6823417656249969321, 4.530208333674755394, -1.181850606188749264 ) ) ;
#207466=CARTESIAN_POINT ( 'NONE',  ( -0.6823417656250246877, -0.4489583329919111243, 1.181850606188755259 ) ) ;
#207467=CARTESIAN_POINT ( 'NONE',  ( -4.202664430556263930, 5.926194473780837413, 1.443375672974064550 ) ) ;
#207468=CARTESIAN_POINT ( 'NONE',  ( 5.473741331615251227, 7.409117525016355010, -1.599625672291262513 ) ) ;
#207472=CARTESIAN_POINT ( 'NONE',  ( 2.724825686666657809, 6.122787701178987518, 0.000000000000000000 ) ) ;
#207475=CARTESIAN_POINT ( 'NONE',  ( -7.687109909268394325, 11.91211929421440097, 0.000000000000000000 ) ) ;
#207479=CARTESIAN_POINT ( 'NONE',  ( -10.30827686509187835, 10.92074451889568643, 1.040834085586084257E-14 ) ) ;
#207480=CARTESIAN_POINT ( 'NONE',  ( -4.053524740361572398, 7.672936597156388316, 0.7216878364870317197 ) ) ;
#207482=CARTESIAN_POINT ( 'NONE',  ( -1.364683531250012516, 1.092708333674754506, 0.7879004041258379498 ) ) ;
#207494=CARTESIAN_POINT ( 'NONE',  ( -0.7500000000000249800, -1.058333333333314030, 1.299038105676659116 ) ) ;
#207495=CARTESIAN_POINT ( 'NONE',  ( 7.578644679914694926, 11.78557652663510424, 0.7216878364870438212 ) ) ;
#207505=CARTESIAN_POINT ( 'NONE',  ( 4.729096653068339151, 4.411700938201493116, -0.7998128361456211532 ) ) ;
#207508=CARTESIAN_POINT ( 'NONE',  ( -4.060830702492950195, 4.696389560118578999, -1.199719254218452047 ) ) ;
#207511=CARTESIAN_POINT ( 'NONE',  ( -1.402160292154681736E-14, 1.009375000341417916, -1.575800808251659024 ) ) ;
#207524=CARTESIAN_POINT ( 'NONE',  ( -0.4579269463803092299, 6.472105396648015763, -3.262807195530565973 ) ) ;
#207531=CARTESIAN_POINT ( 'NONE',  ( 7.305145839664861640, 7.417091655897478653, 0.7998128361456341429 ) ) ;
#207540=CARTESIAN_POINT ( 'NONE',  ( 10.07100917685271035, 10.64393221595000938, 0.7998128361456462443 ) ) ;
#207542=CARTESIAN_POINT ( 'NONE',  ( 1.559074708514246010, 8.689926414953912825, -2.502785155726127808 ) ) ;
#207547=FACE_OUTER_BOUND ( 'NONE', #31465, .T. ) ;
#207550=CARTESIAN_POINT ( 'NONE',  ( -8.595506201384022660, 11.05117653974661529, 1.443375672974064550 ) ) ;
#207557=CARTESIAN_POINT ( 'NONE',  ( -4.168895032367330167, 3.976329666238523242, -0.6109567437776577403 ) ) ;
#207562=CARTESIAN_POINT ( 'NONE',  ( 2.968872451268290913, 5.447139712246216625, -1.082531754730543971 ) ) ;
#207572=CARTESIAN_POINT ( 'NONE',  ( -5.422371370461663176, 8.413518134592214537, -1.199719254218446718 ) ) ;
#207574=CARTESIAN_POINT ( 'NONE',  ( -3.623053363349869382, 5.249981562040033189, 1.599625672291267398 ) ) ;
#207580=CARTESIAN_POINT ( 'NONE',  ( -1.364683531250010740, 4.092708333674752730, 0.7879004041258379498 ) ) ;
#207582=CARTESIAN_POINT ( 'NONE',  ( 5.555090253297246150, 7.504024600312024340, 1.599625672291267398 ) ) ;
#207584=CARTESIAN_POINT ( 'NONE',  ( 1.499999999999990896, 8.627523663848661428, 2.580000000000000515 ) ) ;
#207596=CARTESIAN_POINT ( 'NONE',  ( 1.364683531249988535, 1.676041667008085101, 0.7879004041258500513 ) ) ;
#207597=CARTESIAN_POINT ( 'NONE',  ( 5.366329872910639232, 5.155139694684188534, 1.040834085586084257E-14 ) ) ;
#207599=CARTESIAN_POINT ( 'NONE',  ( -6.453317930424837812, 7.591587675992828466, 1.082531754730549967 ) ) ;
#207601=CARTESIAN_POINT ( 'NONE',  ( 3.660338286009610975, 6.253849852777763729, -1.082531754730543083 ) ) ;
#207602=CARTESIAN_POINT ( 'NONE',  ( -6.033015167956800262, 9.021972881716168402, -1.082531754730537976 ) ) ;
#207606=CARTESIAN_POINT ( 'NONE',  ( 6.311484202361478779, 7.322151976631905868, -1.199719254218446718 ) ) ;
#207612=CARTESIAN_POINT ( 'NONE',  ( 0.6823417656249917140, 5.092708333674749177, 1.181850606188765695 ) ) ;
#207617=CARTESIAN_POINT ( 'NONE',  ( 6.819914962873951936, 7.915321197229798322, -1.199719254218446718 ) ) ;
#207620=CARTESIAN_POINT ( 'NONE',  ( -8.050844288416501016, 8.287073179441051707, 1.040834085586084257E-14 ) ) ;
#207625=CARTESIAN_POINT ( 'NONE',  ( 9.413438726589914651, 9.876766690643398405, 0.000000000000000000 ) ) ;
#207627=CARTESIAN_POINT ( 'NONE',  ( -7.389357414647957256, 8.579670724299436557, 1.199719254218450271 ) ) ;
#207629=CARTESIAN_POINT ( 'NONE',  ( 8.120970824461352322, 9.537182719035495637, -1.082531754730543083 ) ) ;
#207630=CARTESIAN_POINT ( 'NONE',  ( 4.024405658984873568, 7.794362949307388710, 0.3537781459504486525 ) ) ;
#207631=CARTESIAN_POINT ( 'NONE',  ( -5.773074481320628948, 5.629675071162500544, 0.000000000000000000 ) ) ;
#207636=CARTESIAN_POINT ( 'NONE',  ( 6.647575389402066826, 6.649926130590872120, 1.040834085586084257E-14 ) ) ;
#207638=CARTESIAN_POINT ( 'NONE',  ( 9.297140650669039275, 11.86975006391249643, 1.599625672291281386 ) ) ;
#207639=CARTESIAN_POINT ( 'NONE',  ( -4.916288619803077964, 6.680904680207828683, 1.249144131323683515 ) ) ;
#207641=CARTESIAN_POINT ( 'NONE',  ( -1.402160292154681736E-14, 0.5718750003414239114, 1.575800808251672791 ) ) ;
#207643=CARTESIAN_POINT ( 'NONE',  ( -6.236387472606158333, 7.338502141871059870, -1.082531754730544860 ) ) ;
#207644=EDGE_LOOP ( 'NONE', ( #155043, #145240, #86813, #84248, #72456, #110695, #73559, #198251, #1618 ) ) ;
#207650=CARTESIAN_POINT ( 'NONE',  ( -5.512743837300482674, 6.249232958799082027, 0.9732600881407500459 ) ) ;
#207651=CARTESIAN_POINT ( 'NONE',  ( -0.6823417656250212460, 1.113541667008083325, 1.181850606188755259 ) ) ;
#207654=CARTESIAN_POINT ( 'NONE',  ( 3.931501358282940117, 4.649468341827285300, -1.082531754730543083 ) ) ;
#207660=CARTESIAN_POINT ( 'NONE',  ( -7.321039761255057066, 11.48503745486550365, 0.000000000000000000 ) ) ;
#207668=CARTESIAN_POINT ( 'NONE',  ( -7.659993601596706725, 11.88048360193076647, -0.7216878364870267237 ) ) ;
#207675=CARTESIAN_POINT ( 'NONE',  ( -8.473482818416682605, 8.988077497682020578, -0.7216878364870267237 ) ) ;
#207680=CARTESIAN_POINT ( 'NONE',  ( -1.500000000000011324, 4.702083334016148974, 0.8660254037844403729 ) ) ;
#207683=CARTESIAN_POINT ( 'NONE',  ( -1.426686711745821290, 7.396164654317650466, -4.272688476054423035 ) ) ;
#207689=CARTESIAN_POINT ( 'NONE',  ( -5.194745412330402878, 9.212286747694129474, 0.000000000000000000 ) ) ;
#207693=CARTESIAN_POINT ( 'NONE',  ( 3.988069740714122791, 7.804498464141805592, 0.7998128361456321445 ) ) ;
#207698=CARTESIAN_POINT ( 'NONE',  ( 5.445571254183207088, 9.504916896522420444, -0.7998128361456281477 ) ) ;
#207706=CARTESIAN_POINT ( 'NONE',  ( -5.910991785878175975, 6.958873840688411860, -1.082531754730544860 ) ) ;
#207715=CARTESIAN_POINT ( 'NONE',  ( -7.557780564614042795, 10.90482886110335414, -1.199719254218446718 ) ) ;
#207717=CARTESIAN_POINT ( 'NONE',  ( 8.015895134177609904, 10.37496362800581018, 1.599625672291281386 ) ) ;
#207718=CARTESIAN_POINT ( 'NONE',  ( 1.499999999999987121, -0.4958333333333110882, 0.8660254037844524744 ) ) ;
#207719=CARTESIAN_POINT ( 'NONE',  ( -6.679363233026820446, 10.94434087183997129, 0.000000000000000000 ) ) ;
#207721=CARTESIAN_POINT ( 'NONE',  ( -0.6823417656249969321, 5.467708333674756283, -1.181850606188749264 ) ) ;
#207722=CARTESIAN_POINT ( 'NONE',  ( 8.920901888111989919, 11.43080484092926241, 1.443375672974076540 ) ) ;
#207725=CARTESIAN_POINT ( 'NONE',  ( -0.7500000000000215383, 5.441666666666685082, 1.299038105676671107 ) ) ;
#207727=CARTESIAN_POINT ( 'NONE',  ( 7.415946836550712185, 10.63539316174243865, 1.082531754730558626 ) ) ;
#207730=CARTESIAN_POINT ( 'NONE',  ( -7.049876689426113785, 8.287572894827684777, -1.082531754730544860 ) ) ;
#207732=CARTESIAN_POINT ( 'NONE',  ( -1.364683531250014514, 1.738541667008085545, -0.7879004041258289570 ) ) ;
#207736=CARTESIAN_POINT ( 'NONE',  ( -7.263417608619167076, 9.497073181520933716, -1.599625672291263179 ) ) ;
#207737=CARTESIAN_POINT ( 'NONE',  ( -0.6823417656250212460, 4.363541667008085767, 1.181850606188767472 ) ) ;
#207742=CARTESIAN_POINT ( 'NONE',  ( 8.666686507633574621, 11.13422023037111330, 1.599625672291281386 ) ) ;
#207745=CARTESIAN_POINT ( 'NONE',  ( -1.500000000000013101, 1.420833333333354043, 0.8660254037844403729 ) ) ;
#207748=VERTEX_POINT ( 'NONE', #24247 ) ;
#207749=CARTESIAN_POINT ( 'NONE',  ( 7.632877294813741109, 8.007371053478589573, 1.040834085586084257E-14 ) ) ;
#207751=CARTESIAN_POINT ( 'NONE',  ( 8.561083932025322696, 12.07534945641652158, -1.199719254218446718 ) ) ;
#207756=CARTESIAN_POINT ( 'NONE',  ( 8.158255747121103241, 10.54105100977322174, 1.599625672291281386 ) ) ;
#207757=CARTESIAN_POINT ( 'NONE',  ( -9.642873567817536795, 12.27310513391906532, 1.599625672291281386 ) ) ;
#207759=CARTESIAN_POINT ( 'NONE',  ( -4.911494110671301705, 4.698710846044690470, -0.3627449832724688461 ) ) ;
#207760=CARTESIAN_POINT ( 'NONE',  ( 0.6823417656249899377, 5.488541667008087543, -1.181850606188754593 ) ) ;
#207767=CARTESIAN_POINT ( 'NONE',  ( -1.201851678989727383E-14, 3.696875000341422801, -1.575800808251660134 ) ) ;
#207769=CARTESIAN_POINT ( 'NONE',  ( -5.205967797967562483, 8.057084283395347768, 1.082531754730548412 ) ) ;
#207778=CARTESIAN_POINT ( 'NONE',  ( 9.399880572976245574, 9.860948844760784482, 0.7998128361456462443 ) ) ;
#207779=CARTESIAN_POINT ( 'NONE',  ( 2.030969412801289842, 8.463209591663510167, -2.499999999999995115 ) ) ;
#207780=AXIS2_PLACEMENT_3D ( 'NONE', #118108, #99660, #198208 ) ;
#207784=CARTESIAN_POINT ( 'NONE',  ( -9.169391961543940539, 9.592045464756413509, 1.040834085586084257E-14 ) ) ;
#207785=CARTESIAN_POINT ( 'NONE',  ( 5.120175567455225618, 9.125288595339771547, -0.7998128361456281477 ) ) ;
#207787=CARTESIAN_POINT ( 'NONE',  ( 3.999292125906905859, 5.688926785023260102, 1.443375672974062551 ) ) ;
#207789=CARTESIAN_POINT ( 'NONE',  ( 2.984766373302843778, 6.633977868828633717, -0.7998128361456291469 ) ) ;
#207796=CARTESIAN_POINT ( 'NONE',  ( -6.616015773788831211, 7.781401826584148473, 1.082531754730549967 ) ) ;
#207797=CARTESIAN_POINT ( 'NONE',  ( 2.672928840188529609, 6.270167413528593414, 0.000000000000000000 ) ) ;
#207800=CARTESIAN_POINT ( 'NONE',  ( -8.182509401047415309, 9.505014708432145909, 1.199719254218462483 ) ) ;
#207805=CARTESIAN_POINT ( 'NONE',  ( -7.621654909176601045, 12.04368116068139472, 0.7998128361456481317 ) ) ;
#207809=CARTESIAN_POINT ( 'NONE',  ( 6.259060471003163428, 10.45398764947904624, -0.7998128361456291469 ) ) ;
#207810=EDGE_CURVE ( 'NONE', #73904, #166401, #74039, .T. ) ;
#207811=CARTESIAN_POINT ( 'NONE',  ( 5.555090253297246150, 7.504024600312024340, 1.599625672291267398 ) ) ;
#207823=CARTESIAN_POINT ( 'NONE',  ( -6.672584156219988571, 10.93643194889866521, -0.7998128361456291469 ) ) ;
#207826=CARTESIAN_POINT ( 'NONE',  ( 5.314433026876846711, 9.143996264757578984, -0.7216878364870267237 ) ) ;
#207831=CARTESIAN_POINT ( 'NONE',  ( -5.436983294280064882, 6.301900917203534291, 1.199719254218450271 ) ) ;
#207843=CARTESIAN_POINT ( 'NONE',  ( -8.618179199781044630, 13.20629283305325963, 0.7998128361456341429 ) ) ;
#207844=CARTESIAN_POINT ( 'NONE',  ( 6.564118927310645724, 10.80988918183778225, -0.7998128361456291469 ) ) ;
#207848=CARTESIAN_POINT ( 'NONE',  ( -5.526577223899823643, 6.240148858909590146, -0.9599604131041916677 ) ) ;
#207855=CARTESIAN_POINT ( 'NONE',  ( 2.523789150438203510, 6.096171108819874007, 0.7998128361456462443 ) ) ;
#207859=EDGE_CURVE ( 'NONE', #162762, #59123, #203680, .T. ) ;
#207861=DIRECTION ( 'NONE',  ( 1.000000000000000000, 2.090028284309406390E-15, 0.000000000000000000 ) ) ;
#207876=CARTESIAN_POINT ( 'NONE',  ( -3.764360206088648297, 7.543504007078730922, -0.7998128361456281477 ) ) ;
#207877=CARTESIAN_POINT ( 'NONE',  ( 1.499999999999987121, 3.795833333333356929, -0.8660254037844262731 ) ) ;
#207879=CARTESIAN_POINT ( 'NONE',  ( -2.137381772448751605, 5.645362501165475777, -0.7998128361456281477 ) ) ;
#207883=CARTESIAN_POINT ( 'NONE',  ( -1.001543065824772872E-14, 4.821875000341419693, 1.575800808251672791 ) ) ;
#207886=CARTESIAN_POINT ( 'NONE',  ( -4.460269349215930212, 4.305995116947750390, 1.214306433183764966E-14 ) ) ;
#207891=CARTESIAN_POINT ( 'NONE',  ( 3.493197133815315603, 7.227147089426516402, -0.7998128361456291469 ) ) ;
#207895=CARTESIAN_POINT ( 'NONE',  ( 9.693716643646590470, 12.33242205571964512, 1.443375672974076540 ) ) ;
#207897=CARTESIAN_POINT ( 'NONE',  ( 1.364683531249988757, 1.696875000341414808, 0.000000000000000000 ) ) ;
#207900=CARTESIAN_POINT ( 'NONE',  ( -8.779068160048691283, 10.20099992726700933, -1.199719254218446718 ) ) ;
#207903=CARTESIAN_POINT ( 'NONE',  ( -6.087247782411500552, 7.164505836643929371, 1.082531754730549967 ) ) ;
#207907=CARTESIAN_POINT ( 'NONE',  ( -1.201851678989727383E-14, 5.696875000341416140, -1.575800808251660134 ) ) ;
#207915=CARTESIAN_POINT ( 'NONE',  ( -3.904385050611244079, 7.498940292447679568, 1.040834085586084257E-14 ) ) ;
#207921=CARTESIAN_POINT ( 'NONE',  ( -6.046573321570485327, 6.156683084694754449, 0.000000000000000000 ) ) ;
#207923=CARTESIAN_POINT ( 'NONE',  ( 8.778014389843965759, 12.32843499053828928, 1.199719254218450271 ) ) ;
#207927=CARTESIAN_POINT ( 'NONE',  ( 1.566031286093723995, 8.750666943143137644, -2.469538363634776079 ) ) ;
#207932=CARTESIAN_POINT ( 'NONE',  ( -4.952806187693842510, 4.672695395264567786, 0.7998128361456341429 ) ) ;
#207935=CARTESIAN_POINT ( 'NONE',  ( 1.499999999999989120, 0.7750000000000187850, 0.000000000000000000 ) ) ;
#207938=CARTESIAN_POINT ( 'NONE',  ( 9.083599731475983319, 11.62061899152058686, 1.443375672974076540 ) ) ;
#207939=CARTESIAN_POINT ( 'NONE',  ( 4.794779880727245036, 8.745660294157122649, -0.7998128361456281477 ) ) ;
#207944=LINE ( 'NONE', #13997, #97317 ) ;
#207945=CARTESIAN_POINT ( 'NONE',  ( 3.506755287428983792, 7.242964935309132990, 1.040834085586084257E-14 ) ) ;
#207954=CARTESIAN_POINT ( 'NONE',  ( -5.228640796364566690, 9.251831362400652736, -0.7998128361456231517 ) ) ;
#207959=CARTESIAN_POINT ( 'NONE',  ( -0.6823417656250212460, 5.301041667008086655, 1.181850606188767472 ) ) ;
#207960=CARTESIAN_POINT ( 'NONE',  ( 8.636180661780656465, 11.09863007687603087, -1.443375672974052559 ) ) ;
#207961=CARTESIAN_POINT ( 'NONE',  ( -5.656776405399756236, 7.622658444431597680, -1.599625672291256295 ) ) ;
#207964=CARTESIAN_POINT ( 'NONE',  ( 5.678167406024951624, 5.518950149984223508, 0.7998128361456341429 ) ) ;
#207965=CARTESIAN_POINT ( 'NONE',  ( -4.629219384062206011, 7.488174150459498968, -1.199719254218452047 ) ) ;
#207971=CARTESIAN_POINT ( 'NONE',  ( 6.643132081016124069, 7.813037518349371879, 1.082531754730558626 ) ) ;
#207974=CARTESIAN_POINT ( 'NONE',  ( 1.364683531249988535, 1.426041667008083991, 0.7879004041258500513 ) ) ;
#207976=CARTESIAN_POINT ( 'NONE',  ( 4.650083499362856365, 8.368921815991249957, 0.7216878364870438212 ) ) ;
#207979=CARTESIAN_POINT ( 'NONE',  ( -4.039966587192274083, 5.736380323189513852, 1.443375672974064550 ) ) ;
#207986=CARTESIAN_POINT ( 'NONE',  ( -3.978769281187482854, 7.845005453061479450, 0.1301786893823601021 ) ) ;
#207995=CARTESIAN_POINT ( 'NONE',  ( 7.169564303528210836, 7.258913197071374945, -0.7998128361456281477 ) ) ;
#208006=CARTESIAN_POINT ( 'NONE',  ( 4.365362273920250225, 5.155639410070820716, 1.082531754730560403 ) ) ;
#208008=CARTESIAN_POINT ( 'NONE',  ( -0.6823417656250003738, 2.280208333674753174, -1.181850606188749264 ) ) ;
#208010=CARTESIAN_POINT ( 'NONE',  ( 8.450809820019639318, 8.753699632978056755, -0.7998128361456291469 ) ) ;
#208011=CARTESIAN_POINT ( 'NONE',  ( -8.319899820280397762, 12.85830022363583147, -0.7998128361456281477 ) ) ;
#208016=CARTESIAN_POINT ( 'NONE',  ( -0.7499999999999972244, 3.608333333333359150, -1.299038105676652011 ) ) ;
#208017=CARTESIAN_POINT ( 'NONE',  ( 6.311484202361478779, 7.322151976631905868, -1.199719254218446718 ) ) ;
#208018=CARTESIAN_POINT ( 'NONE',  ( -7.039708073993679704, 9.236078724457858158, 1.599625672291283607 ) ) ;
#208022=CARTESIAN_POINT ( 'NONE',  ( -1.364683531250000748, 2.009375000341421913, 1.214306433183764966E-14 ) ) ;
#208024=CARTESIAN_POINT ( 'NONE',  ( 2.900554798319789906, 5.471398800426671372, 1.199719254218452047 ) ) ;
#208029=CARTESIAN_POINT ( 'NONE',  ( 1.499999999999987121, 0.07708333401615156955, -0.8660254037844323793 ) ) ;
#208032=CARTESIAN_POINT ( 'NONE',  ( -6.175902666224832416, 7.163973517805802160, -1.199719254218446718 ) ) ;
#208033=CARTESIAN_POINT ( 'NONE',  ( -2.819732761962335577, 5.273143408055916304, -1.082531754730543971 ) ) ;
#208040=CARTESIAN_POINT ( 'NONE',  ( 5.503720292143644777, 8.508425209887878538, 1.199719254218462483 ) ) ;
#208044=CARTESIAN_POINT ( 'NONE',  ( 4.710568305744190276, 7.583081225755162968, 1.199719254218462483 ) ) ;
#208050=CARTESIAN_POINT ( 'NONE',  ( 3.297657676621871925, 4.870353260857385180, 1.599625672291267398 ) ) ;
#208055=CARTESIAN_POINT ( 'NONE',  ( 5.891837173953166307, 5.977390820968681240, -0.04595957878574669087 ) ) ;
#208059=CARTESIAN_POINT ( 'NONE',  ( 6.471393748265519719, 5.229711127717882491, -2.419999999999995932 ) ) ;
#208064=CARTESIAN_POINT ( 'NONE',  ( -1.499999999999997780, 5.181250000682820378, 1.214306433183764966E-14 ) ) ;
#208066=CARTESIAN_POINT ( 'NONE',  ( 8.324343129110697959, 9.774450407793066731, -1.082531754730543083 ) ) ;
#208068=CARTESIAN_POINT ( 'NONE',  ( -4.446184310277715213, 7.274633231044262516, -1.199719254218452047 ) ) ;
#208069=DIRECTION ( 'NONE',  ( -7.387867266669436732E-31, -1.000000000000000000, 8.546850786086437571E-32 ) ) ;
#208071=CARTESIAN_POINT ( 'NONE',  ( 7.771848369131631351, 10.09024240211882351, -1.599625672291262513 ) ) ;
#208073=CARTESIAN_POINT ( 'NONE',  ( -6.905180308061733996, 6.950465202360470052, 0.7998128361456341429 ) ) ;
#208087=CARTESIAN_POINT ( 'NONE',  ( 8.778014389843965759, 12.32843499053828928, 1.199719254218450271 ) ) ;
#208088=CARTESIAN_POINT ( 'NONE',  ( -5.752737250900127997, 5.605948302338584099, 0.000000000000000000 ) ) ;
#208091=CARTESIAN_POINT ( 'NONE',  ( 3.172244755917638770, 5.684407401003788607, -1.082531754730543083 ) ) ;
#208097=CARTESIAN_POINT ( 'NONE',  ( -3.079673448598517549, 6.744702790006905424, 1.040834085586084257E-14 ) ) ;
#208100=CARTESIAN_POINT ( 'NONE',  ( 8.565000355531088516, 11.01558638625153286, -1.599625672291257406 ) ) ;
#208105=CARTESIAN_POINT ( 'NONE',  ( -7.335124800193271177, 8.516399340768996851, -1.199719254218452935 ) ) ;
#208106=CARTESIAN_POINT ( 'NONE',  ( 5.834086172582112262, 5.700855377634248100, 1.040834085586084257E-14 ) ) ;
#208111=CARTESIAN_POINT ( 'NONE',  ( -1.201851678989727383E-14, 2.759375000341417916, -1.575800808251660134 ) ) ;
#208114=CARTESIAN_POINT ( 'NONE',  ( 7.293923454472087897, 8.572294120714675003, 1.082531754730558626 ) ) ;
#208121=CARTESIAN_POINT ( 'NONE',  ( 9.124274191872634887, 11.66807252865000244, -1.443375672974058777 ) ) ;
#208126=CARTESIAN_POINT ( 'NONE',  ( -8.533967624797991647, 12.04371376465130439, -1.199719254218446718 ) ) ;
#208144=CARTESIAN_POINT ( 'NONE',  ( 0.7499999999999885647, 0.8479166673494853423, -1.299038105676652899 ) ) ;
#208151=CARTESIAN_POINT ( 'NONE',  ( -1.500000000000015099, 0.3791666666666850261, -0.8660254037844383745 ) ) ;
#208152=CARTESIAN_POINT ( 'NONE',  ( 7.391166297744269365, 11.77477778067701664, 1.040834085586084257E-14 ) ) ;
#208153=CARTESIAN_POINT ( 'NONE',  ( -1.364683531250000748, 0.009375000341420303140, 0.000000000000000000 ) ) ;
#208156=CARTESIAN_POINT ( 'NONE',  ( 3.521367211247359741, 5.131347717920458962, -1.599625672291262513 ) ) ;
#208157=CARTESIAN_POINT ( 'NONE',  ( -4.772106882330223954, 8.511282429453158827, -0.7216878364870267237 ) ) ;
#208161=CARTESIAN_POINT ( 'NONE',  ( -5.181187258716735577, 9.196468901811520880, 0.7998128361456481317 ) ) ;
#208164=CARTESIAN_POINT ( 'NONE',  ( -0.7500000000000215383, 2.722916667349486897, 1.299038105676671107 ) ) ;
#208170=DIRECTION ( 'NONE',  ( 0.6507913734559651608, -0.7592566023652994600, 0.000000000000000000 ) ) ;
#208176=CARTESIAN_POINT ( 'NONE',  ( -9.854078719034067291, 10.39084668182823634, 0.7998128361456462443 ) ) ;
#208178=CARTESIAN_POINT ( 'NONE',  ( 7.121056995675668411, 9.330985799753529264, -1.599625672291262513 ) ) ;
#208185=CARTESIAN_POINT ( 'NONE',  ( -9.020252271793614440, 9.418049160047695878, 0.7998128361456462443 ) ) ;
#208191=CARTESIAN_POINT ( 'NONE',  ( 9.028840231696797503, 12.62106513936658203, -1.199719254218446718 ) ) ;
#208193=EDGE_LOOP ( 'NONE', ( #79000, #173592 ) ) ;
#208195=CARTESIAN_POINT ( 'NONE',  ( -8.025536864285518490, 11.45054454405341282, -1.199719254218446718 ) ) ;
#208198=CARTESIAN_POINT ( 'NONE',  ( -5.012244793233714191, 6.784968962630095746, -1.449178643049347848 ) ) ;
#208206=CARTESIAN_POINT ( 'NONE',  ( 5.621827251160867789, 9.710548892996357040, 1.040834085586084257E-14 ) ) ;
#208209=DIRECTION ( 'NONE',  ( 0.6507913734559640506, -0.7592566023653004592, 0.000000000000000000 ) ) ;
#208211=AXIS2_PLACEMENT_3D ( 'NONE', #182977, #168862, #115910 ) ;
#208226=CARTESIAN_POINT ( 'NONE',  ( 4.378920427533921078, 4.211088041652093494, 1.214306433183764966E-14 ) ) ;
#208234=CARTESIAN_POINT ( 'NONE',  ( 9.856941372335116469, 11.45851867493453291, 1.199719254218450271 ) ) ;
#208243=CARTESIAN_POINT ( 'NONE',  ( 0.6823417656249899377, 0.5927083336747518416, 1.181850606188755259 ) ) ;
#208247=CARTESIAN_POINT ( 'NONE',  ( -4.578903193113314174, 6.365139696764064325, 1.599625672291267398 ) ) ;
#208248=DIRECTION ( 'NONE',  ( 1.000000000000000000, 0.000000000000000000, 0.000000000000000000 ) ) ;
#208250=CARTESIAN_POINT ( 'NONE',  ( 1.499999999999987566, -0.4749999999999823808, 0.000000000000000000 ) ) ;
#208252=CARTESIAN_POINT ( 'NONE',  ( -0.6823417656250003738, -0.9697916663252494907, -1.181850606188749264 ) ) ;
#208258=CARTESIAN_POINT ( 'NONE',  ( -1.001543065824772872E-14, 5.634375000341415252, 1.575800808251672791 ) ) ;
#208260=CARTESIAN_POINT ( 'NONE',  ( -7.121056995675673740, 9.330985799753529264, -1.599625672291263179 ) ) ;
#208261=CARTESIAN_POINT ( 'NONE',  ( 8.483651433849084711, 10.92067931095586886, 1.599625672291281386 ) ) ;
#208267=CARTESIAN_POINT ( 'NONE',  ( -0.6823417656250003738, 0.2802083336747515641, -1.181850606188749264 ) ) ;
#208274=CARTESIAN_POINT ( 'NONE',  ( 6.968527767744104651, 8.192665819532020777, 1.082531754730558626 ) ) ;
#208277=CARTESIAN_POINT ( 'NONE',  ( -4.229253852459088137, 7.021547696922494808, 1.199719254218464037 ) ) ;
#208281=CARTESIAN_POINT ( 'NONE',  ( -4.464712657601869417, 4.103252943490596216, 0.7998128361456341429 ) ) ;
#208282=CARTESIAN_POINT ( 'NONE',  ( 5.544921637864819175, 7.492161215640853023, -1.443375672974057666 ) ) ;
#208283=CARTESIAN_POINT ( 'NONE',  ( -9.286972035236626510, 11.85788667924133399, -1.443375672974058777 ) ) ;
#208288=CARTESIAN_POINT ( 'NONE',  ( 8.405692050792682224, 12.75046512599275772, -0.7216878364870328300 ) ) ;
#208291=DIRECTION ( 'NONE',  ( -1.207943261119674327E-30, -2.168404344971008079E-15, 1.000000000000000000 ) ) ;
#208305=CARTESIAN_POINT ( 'NONE',  ( 8.012505595552012139, 11.33137838057728786, -1.082531754730543083 ) ) ;
#208307=CARTESIAN_POINT ( 'NONE',  ( 8.613507663383630941, 8.943513783569379427, -0.7998128361456221525 ) ) ;
#208311=ADVANCED_FACE ( 'NONE', ( #145544, #81555 ), #181185, .F. ) ;
#208313=CARTESIAN_POINT ( 'NONE',  ( 5.233084105194869551, 6.167981546557892436, -1.082531754730548412 ) ) ;
#208315=CARTESIAN_POINT ( 'NONE',  ( -8.270110514656041190, 10.67154823856396817, 1.443375672974090751 ) ) ;
#208344=CARTESIAN_POINT ( 'NONE',  ( -7.700668062882072284, 10.00719871149432549, -1.443375672974059665 ) ) ;
#208348=CARTESIAN_POINT ( 'NONE',  ( 6.043183783389218355, 8.073467052085995022, 1.599625672291267398 ) ) ;
#208351=CARTESIAN_POINT ( 'NONE',  ( 2.703961570921634028, 5.242040035128820108, -1.199719254218446718 ) ) ;
#208353=CARTESIAN_POINT ( 'NONE',  ( -5.922214171070950606, 5.803671375871217286, -0.7998128361456291469 ) ) ;
#208357=CARTESIAN_POINT ( 'NONE',  ( -4.904298879841297421, 6.744767997946721216, 1.599625672291267398 ) ) ;
#208361=CARTESIAN_POINT ( 'NONE',  ( 7.507464373665139412, 9.781794407407920389, 1.599625672291281386 ) ) ;
#208364=CARTESIAN_POINT ( 'NONE',  ( 5.946581215072361815, 6.122072269273588496, 0.7275674859277461159 ) ) ;
#208365=CARTESIAN_POINT ( 'NONE',  ( 4.378920427533921078, 4.211088041652093494, 1.214306433183764966E-14 ) ) ;
#208371=CARTESIAN_POINT ( 'NONE',  ( 5.612712405933139692, 9.491988873656591608, 1.040834085586084257E-14 ) ) ;
#208372=CARTESIAN_POINT ( 'NONE',  ( -9.182950115157607840, 9.607863310639020327, 0.7998128361456462443 ) ) ;
#208375=CARTESIAN_POINT ( 'NONE',  ( -8.616370316684697883, 10.01118577667568132, -1.199719254218446718 ) ) ;
#208376=CARTESIAN_POINT ( 'NONE',  ( -5.876569516519495551, 8.943415971659659292, 1.199719254218452047 ) ) ;
#208384=CARTESIAN_POINT ( 'NONE',  ( 8.586391356156291010, 8.911878091804165791, 0.7998128361456481317 ) ) ;
#208391=CARTESIAN_POINT ( 'NONE',  ( -3.386512176934025842, 6.359426010807541552, 0.9097930222844696768 ) ) ;
#208396=CARTESIAN_POINT ( 'NONE',  ( 0.7499999999999920064, 4.233333333333352932, 1.299038105676669330 ) ) ;
#208397=CARTESIAN_POINT ( 'NONE',  ( 5.671388329218120639, 5.511041227042920099, 1.040834085586084257E-14 ) ) ;
#208398=CARTESIAN_POINT ( 'NONE',  ( 7.806797523370503811, 8.002351953554066810, 1.040834085586084257E-14 ) ) ;
#208401=CARTESIAN_POINT ( 'NONE',  ( 7.782016984564065432, 8.181367358187307204, 0.7216878364870458196 ) ) ;
#208402=CARTESIAN_POINT ( 'NONE',  ( -8.310784975052669665, 12.63974020429606249, -0.7216878364870267237 ) ) ;
#208405=CARTESIAN_POINT ( 'NONE',  ( 9.738834413317897898, 10.25639499182604730, 0.000000000000000000 ) ) ;
#208407=CARTESIAN_POINT ( 'NONE',  ( 0.7499999999999902300, 5.316666666666685082, -1.299038105676658228 ) ) ;
#208408=CARTESIAN_POINT ( 'NONE',  ( -3.277320446201389181, 4.846626492033466072, 1.599625672291267398 ) ) ;
#208409=CARTESIAN_POINT ( 'NONE',  ( -2.308604159940524703, 5.474475169625423909, -0.7811085970239580734 ) ) ;
#208410=CARTESIAN_POINT ( 'NONE',  ( 1.364683531249988757, 0.8843750003414210248, 0.000000000000000000 ) ) ;
#208415=CARTESIAN_POINT ( 'NONE',  ( -1.402160292154681736E-14, 0.1968750003414221628, -1.575800808251665908 ) ) ;
#208417=CARTESIAN_POINT ( 'NONE',  ( 8.886479618753304166, 12.45497775759917758, -1.199719254218446718 ) ) ;
#208421=CARTESIAN_POINT ( 'NONE',  ( -2.779058300676974014, 6.186059084191009916, -0.7216878364870257245 ) ) ;
#208424=CARTESIAN_POINT ( 'NONE',  ( -6.358937740009323214, 7.377514437221045718, -1.199719254218446718 ) ) ;
#208427=CARTESIAN_POINT ( 'NONE',  ( 4.325214697959421706, 5.004837554829479451, 1.199719254218462483 ) ) ;
#208433=CARTESIAN_POINT ( 'NONE',  ( 8.666686507633574621, 11.13422023037111330, 1.599625672291281386 ) ) ;
#208436=CARTESIAN_POINT ( 'NONE',  ( -6.013204822860843457, 6.974159367214481264, -1.199719254218446718 ) ) ;
#208440=CARTESIAN_POINT ( 'NONE',  ( 9.074484886248265880, 9.481320543578137361, 0.7998128361456462443 ) ) ;
#208442=CARTESIAN_POINT ( 'NONE',  ( 7.721532178182734185, 8.967207948423393304, 1.199719254218462483 ) ) ;
#208444=CARTESIAN_POINT ( 'NONE',  ( -8.649738815838677652, 13.03518635187974262, 0.7216878364870357165 ) ) ;
#208453=CARTESIAN_POINT ( 'NONE',  ( -6.123385318682658784, 6.005027156464323390, -0.2239653954101868127 ) ) ;
#208454=CARTESIAN_POINT ( 'NONE',  ( -1.364683531250012516, 1.530208333674756505, 0.7879004041258379498 ) ) ;
#208456=CARTESIAN_POINT ( 'NONE',  ( 6.860062538834778678, 8.066123052471139587, -1.082531754730543083 ) ) ;
#208469=CARTESIAN_POINT ( 'NONE',  ( 4.243338890952890630, 5.973648010910253880, -1.443375672974051449 ) ) ;
#208473=CARTESIAN_POINT ( 'NONE',  ( 9.097684769969825780, 10.57271930550834860, -1.199719254218446718 ) ) ;
#208475=ORIENTED_EDGE ( 'NONE', *, *, #141556, .F. ) ;
#208477=CARTESIAN_POINT ( 'NONE',  ( -2.923754682041362241, 6.562797562356882608, 0.7998128361456341429 ) ) ;
#208478=CARTESIAN_POINT ( 'NONE',  ( -5.533699252672048985, 9.607732894759390518, -0.7998128361456231517 ) ) ;
#208483=CARTESIAN_POINT ( 'NONE',  ( -0.7499999999999972244, 4.389583334016150751, -1.299038105676652899 ) ) ;
#208484=CARTESIAN_POINT ( 'NONE',  ( 8.274553823041976841, 8.548067636504127265, 1.040834085586084257E-14 ) ) ;
#208487=CARTESIAN_POINT ( 'NONE',  ( -8.850775351622791831, 9.220326086515070685, -0.7998128361456291469 ) ) ;
#208489=CARTESIAN_POINT ( 'NONE',  ( 0.6823417656249899377, 4.676041667008086655, -1.181850606188754593 ) ) ;
#208495=CARTESIAN_POINT ( 'NONE',  ( -7.537970219518066450, 11.73812298950569044, -0.7216878364870267237 ) ) ;
#208497=EDGE_CURVE ( 'NONE', #153422, #103797, #98886, .T. ) ;
#208500=CARTESIAN_POINT ( 'NONE',  ( 1.364683531249988535, 2.426041667008088432, 0.7879004041258500513 ) ) ;
#208507=CARTESIAN_POINT ( 'NONE',  ( 0.6823417656249899377, 3.676041667008085767, -1.181850606188754593 ) ) ;
#208509=AXIS2_PLACEMENT_3D ( 'NONE', #196788, #113480, #101414 ) ;
#208510=CARTESIAN_POINT ( 'NONE',  ( -5.057354993097396445, 5.859001232490445688, -1.199719254218446718 ) ) ;
#208511=CARTESIAN_POINT ( 'NONE',  ( 6.962275575817444384, 8.081408578997208991, -1.199719254218446718 ) ) ;
#208514=CARTESIAN_POINT ( 'NONE',  ( -1.364683531250010295, 4.592708333674755394, 0.7879004041258379498 ) ) ;
#208517=CARTESIAN_POINT ( 'NONE',  ( 1.364683531249988757, -0.8656249996585805295, 0.000000000000000000 ) ) ;
#208518=CARTESIAN_POINT ( 'NONE',  ( -3.958617665510272943, 6.601842462195195438, -1.082531754730549967 ) ) ;
#208519=EDGE_CURVE ( 'NONE', #213687, #109299, #14549, .T. ) ;
#208522=CARTESIAN_POINT ( 'NONE',  ( 3.036663219780971978, 6.486598156479028709, -0.7216878364870267237 ) ) ;
#208525=CARTESIAN_POINT ( 'NONE',  ( -9.707274797704657843, 11.38787068781932987, 1.082531754730558626 ) ) ;
#208530=CARTESIAN_POINT ( 'NONE',  ( -9.592557376868645846, 11.15007068022363157, -1.199719254218441611 ) ) ;
#208531=CARTESIAN_POINT ( 'NONE',  ( -5.870317324592812191, 7.871789516823500144, -1.443375672974051449 ) ) ;
#208533=CARTESIAN_POINT ( 'NONE',  ( -1.364683531250012516, 0.5927083336747520637, 0.7879004041258379498 ) ) ;
#208535=CARTESIAN_POINT ( 'NONE',  ( 1.436838838544731267, 7.449283400311756509, 4.203727439823562229 ) ) ;
#208539=CARTESIAN_POINT ( 'NONE',  ( -1.364683531250014514, -0.4489583329919089039, -0.7879004041258359514 ) ) ;
#208546=CARTESIAN_POINT ( 'NONE',  ( -1.402160292154681736E-14, -0.2874999999999741096, 1.732050807568877637 ) ) ;
#208547=CARTESIAN_POINT ( 'NONE',  ( 7.904040366642689719, 10.24446639921506552, 1.443375672974076540 ) ) ;
#208558=CARTESIAN_POINT ( 'NONE',  ( 1.230728480726486884, 3.226239941806479106, 0.7750000000000152323 ) ) ;
#208560=CARTESIAN_POINT ( 'NONE',  ( 1.364683531249988757, 2.196875000341415252, 1.214306433183764966E-14 ) ) ;
#208581=CARTESIAN_POINT ( 'NONE',  ( 7.156006149914539982, 7.243095351188763686, 1.040834085586084257E-14 ) ) ;
#208588=CARTESIAN_POINT ( 'NONE',  ( 6.760712154708803823, 11.03924794713562818, 1.040834085586084257E-14 ) ) ;
#208593=CARTESIAN_POINT ( 'NONE',  ( 9.745613490124728884, 10.26430391476735338, 0.7998128361456462443 ) ) ;
#208595=CARTESIAN_POINT ( 'NONE',  ( 1.500511526392835693, 8.643217832945683909, -2.569261818345971893 ) ) ;
#208602=CARTESIAN_POINT ( 'NONE',  ( -0.2652791711382684881, 7.171141847836421057, 2.094821536884128310 ) ) ;
#208606=CARTESIAN_POINT ( 'NONE',  ( -8.758204044748012507, 11.24099069033793974, 1.443375672974064550 ) ) ;
#208611=CARTESIAN_POINT ( 'NONE',  ( -9.541187415715041809, 12.15447128979948310, -1.599625672291263179 ) ) ;
#208612=CARTESIAN_POINT ( 'NONE',  ( 3.811813743736467419, 7.598866467667865443, 1.040834085586084257E-14 ) ) ;
#208618=CARTESIAN_POINT ( 'NONE',  ( 3.023105065722954787, 5.510411095776657220, 1.082531754730546636 ) ) ;
#208626=CARTESIAN_POINT ( 'NONE',  ( -4.367698041896780126, 8.247398148854895084, 0.7998128361456481317 ) ) ;
#208629=CARTESIAN_POINT ( 'NONE',  ( -4.620631424159025613, 4.285158171140619032, -0.7998128361456221525 ) ) ;
#208634=CARTESIAN_POINT ( 'NONE',  ( -0.7500000000000215383, 2.941666666666689522, 1.299038105676671107 ) ) ;
#208636=CARTESIAN_POINT ( 'NONE',  ( 1.364683531249988535, 3.426041667008085323, 0.7879004041258499402 ) ) ;
#208638=CIRCLE ( 'NONE', #77074, 0.1599999999999999756 ) ;
#208639=CARTESIAN_POINT ( 'NONE',  ( 4.150767584078112193, 7.994312614733129152, 0.7998128361456321445 ) ) ;
#208651=ORIENTED_EDGE ( 'NONE', *, *, #189189, .T. ) ;
#208653=CARTESIAN_POINT ( 'NONE',  ( 0.6823417656249882723, 1.238541667008083547, -1.181850606188749264 ) ) ;
#208655=CARTESIAN_POINT ( 'NONE',  ( 3.704402285031850539, 5.344888637335695414, -1.599625672291262513 ) ) ;
#208657=CARTESIAN_POINT ( 'NONE',  ( -5.409340102172518705, 9.254721185935849803, 0.000000000000000000 ) ) ;
#208658=CARTESIAN_POINT ( 'NONE',  ( 4.555176424511575561, 4.416720038126027426, -0.7216878364870188411 ) ) ;
#208660=CARTESIAN_POINT ( 'NONE',  ( -6.846504384776774366, 7.089935991768773427, -0.7216878364870267237 ) ) ;
#208664=CARTESIAN_POINT ( 'NONE',  ( 5.178324605415663306, 8.128796908705222535, 1.199719254218462483 ) ) ;
#208669=CARTESIAN_POINT ( 'NONE',  ( -1.364683531250010295, 4.780208333674755394, 0.7879004041258379498 ) ) ;
#208673=CARTESIAN_POINT ( 'NONE',  ( 7.630541526392844887, 7.796719957080126662, 0.7998128361456341429 ) ) ;
#208677=CARTESIAN_POINT ( 'NONE',  ( -8.037286134802835491, 8.271255333558444889, -0.7998128361456291469 ) ) ;
#208682=CARTESIAN_POINT ( 'NONE',  ( 7.781490099239519509, 11.16582331816642260, 1.199719254218460707 ) ) ;
#208684=CARTESIAN_POINT ( 'NONE',  ( -6.958359152311683893, 9.141171649162195934, -1.599625672291263179 ) ) ;
#208687=CARTESIAN_POINT ( 'NONE',  ( 6.548225005276093746, 9.623051025255367819, -1.082531754730537976 ) ) ;
#208688=CARTESIAN_POINT ( 'NONE',  ( 4.100400566228236343, 7.694619998084524681, 0.6794913885044724378 ) ) ;
#208689=CIRCLE ( 'NONE', #149812, 0.08000000000000037637 ) ;
#208690=CARTESIAN_POINT ( 'NONE',  ( -8.676855123066012254, 12.10645282934361866, -1.082531754730543971 ) ) ;
#208695=CARTESIAN_POINT ( 'NONE',  ( 4.462605117192430804, 8.358123070033169455, 1.040834085586084257E-14 ) ) ;
#208697=CARTESIAN_POINT ( 'NONE',  ( 9.887974103068218668, 10.43039129653476493, 0.7998128361456462443 ) ) ;
#208698=CARTESIAN_POINT ( 'NONE',  ( -4.552667031389123764, 6.999162803142576550, 1.172958579310765970 ) ) ;
#208699=CARTESIAN_POINT ( 'NONE',  ( 2.184835310096557404, 5.700724961754617404, 1.040834085586084257E-14 ) ) ;
#208700=CARTESIAN_POINT ( 'NONE',  ( 1.364683531249988757, 1.134375000341421247, 0.000000000000000000 ) ) ;
#208702=CARTESIAN_POINT ( 'NONE',  ( -5.043269954603569083, 7.867270132804026872, 1.082531754730560403 ) ) ;
#208708=CARTESIAN_POINT ( 'NONE',  ( -4.344470927813957495, 7.211826089590096522, 1.015455228366731966 ) ) ;
#208709=CARTESIAN_POINT ( 'NONE',  ( 1.364683531249986537, 0.6760416670080884316, 0.7879004041258500513 ) ) ;
#208713=CARTESIAN_POINT ( 'NONE',  ( 4.528060117284244512, 4.385084346360807572, 0.7216878364870317197 ) ) ;
#208718=CARTESIAN_POINT ( 'NONE',  ( -8.798878505144658746, 10.32807501316600884, -1.082531754730543083 ) ) ;
#208724=CARTESIAN_POINT ( 'NONE',  ( -8.473482818416670170, 10.90881592628469932, -1.443375672974058777 ) ) ;
#208731=CARTESIAN_POINT ( 'NONE',  ( -9.124274191872645545, 9.747334100047323702, -0.7216878364870267237 ) ) ;
#208735=CARTESIAN_POINT ( 'NONE',  ( -0.6823417656250212460, 5.113541667008086655, 1.181850606188767472 ) ) ;
#208736=CARTESIAN_POINT ( 'NONE',  ( -1.201851678989727383E-14, 3.868750000682817713, -1.732050807568863648 ) ) ;
#208737=CARTESIAN_POINT ( 'NONE',  ( 6.029390871727402512, 6.069343164222702924, -0.5281050654588164139 ) ) ;
#208743=CARTESIAN_POINT ( 'NONE',  ( -8.206763054973658100, 8.468978407091068306, 0.7998128361456602331 ) ) ;
#208747=CARTESIAN_POINT ( 'NONE',  ( 4.690231075323689325, 7.559354456931247412, 1.199719254218462483 ) ) ;
#208753=CARTESIAN_POINT ( 'NONE',  ( 5.798083248138522272, 9.916180889470295412, 0.7998128361456462443 ) ) ;
#208754=CARTESIAN_POINT ( 'NONE',  ( -4.911974738770095605, 4.719687011848955116, 0.4085689905262423482 ) ) ;
#208761=CARTESIAN_POINT ( 'NONE',  ( -4.907688418466881863, 8.669460888279271416, 0.7216878364870458196 ) ) ;
#208764=CARTESIAN_POINT ( 'NONE',  ( -5.342823980928589123, 4.390142039796948836, -2.499999999999994671 ) ) ;
#208768=CARTESIAN_POINT ( 'NONE',  ( -8.967828540435322182, 12.54988483289483980, 1.199719254218462483 ) ) ;
#208770=CARTESIAN_POINT ( 'NONE',  ( 8.097244055859613709, 10.46987070330147063, -1.599625672291262513 ) ) ;
#208771=CARTESIAN_POINT ( 'NONE',  ( 1.499999999999987121, 0.004166666666691258049, 0.8660254037844524744 ) ) ;
#208772=CARTESIAN_POINT ( 'NONE',  ( -8.701635661872465732, 9.046329781806354831, 1.040834085586084257E-14 ) ) ;
#208775=CARTESIAN_POINT ( 'NONE',  ( 0.6823417656249899377, 3.176041667008085323, -1.181850606188754593 ) ) ;
#208776=CARTESIAN_POINT ( 'NONE',  ( 2.333974999846879061, 5.874721266463329705, -0.7998128361456291469 ) ) ;
#208780=CARTESIAN_POINT ( 'NONE',  ( 1.499999999999989120, 5.004166666666691299, 0.8660254037844524744 ) ) ;
#208783=CARTESIAN_POINT ( 'NONE',  ( 8.893785580440313865, 9.478430720042945623, 1.040834085586084257E-14 ) ) ;
#208786=CARTESIAN_POINT ( 'NONE',  ( -5.422898255786193111, 8.310169817517122581, -1.082531754730544860 ) ) ;
#208788=CARTESIAN_POINT ( 'NONE',  ( 0.6823417656249899377, 2.342708333674753618, 1.181850606188767472 ) ) ;
#208793=CARTESIAN_POINT ( 'NONE',  ( -5.533699252672048985, 9.607732894759390518, -0.7998128361456231517 ) ) ;
#208794=CARTESIAN_POINT ( 'NONE',  ( 0.6823417656249899377, 4.238541667008085767, -1.181850606188754593 ) ) ;
#208798=EDGE_CURVE ( 'NONE', #116176, #27161, #38144, .T. ) ;
#208800=CARTESIAN_POINT ( 'NONE',  ( 9.610031953988080744, 10.10612545594124967, -0.7998128361456281477 ) ) ;
#208803=CARTESIAN_POINT ( 'NONE',  ( -0.7500000000000006661, 1.108333333333356929, -1.299038105676652011 ) ) ;
#208811=CARTESIAN_POINT ( 'NONE',  ( 8.076906825439115423, 10.44614393447756129, -1.599625672291262513 ) ) ;
#208812=CARTESIAN_POINT ( 'NONE',  ( -1.513761821635718485, 8.683429030108589686, 2.534756493980089509 ) ) ;
#208817=CARTESIAN_POINT ( 'NONE',  ( 1.364683531249988757, -0.8656249996585805295, 0.000000000000000000 ) ) ;
#208822=CARTESIAN_POINT ( 'NONE',  ( 7.910292558569346433, 11.31609285405122556, -1.199719254218446718 ) ) ;
#208825=CARTESIAN_POINT ( 'NONE',  ( 1.364683531249988535, 4.113541667008088432, 0.7879004041258500513 ) ) ;
#208827=CARTESIAN_POINT ( 'NONE',  ( -5.409340102172518705, 9.254721185935849803, 0.000000000000000000 ) ) ;
#208829=CARTESIAN_POINT ( 'NONE',  ( 1.499999999999990896, 5.056250000682820378, 1.214306433183764966E-14 ) ) ;
#208833=CARTESIAN_POINT ( 'NONE',  ( 4.054051625686104998, 4.688480637177271149, -1.199719254218446718 ) ) ;
#208836=CARTESIAN_POINT ( 'NONE',  ( 8.938903350111612411, 9.323142084752035430, -0.7998128361456221525 ) ) ;
#208837=CARTESIAN_POINT ( 'NONE',  ( 1.608462485350598881, 8.735270501766754236, -2.463594439587636131 ) ) ;
#208842=CARTESIAN_POINT ( 'NONE',  ( -7.147119532698295252, 11.49005655479003174, 0.000000000000000000 ) ) ;
#208843=CARTESIAN_POINT ( 'NONE',  ( 6.144869935491714230, 8.192100896205568361, -1.599625672291262513 ) ) ;
#208845=CARTESIAN_POINT ( 'NONE',  ( 5.684946482831785275, 5.526859072925533134, -0.7998128361456231517 ) ) ;
#208846=ORIENTED_EDGE ( 'NONE', *, *, #159504, .T. ) ;
#208853=CARTESIAN_POINT ( 'NONE',  ( -5.233084105194862445, 9.049089189461916760, 0.7216878364870458196 ) ) ;
#208854=CARTESIAN_POINT ( 'NONE',  ( 2.835626683552519012, 6.459981564119914310, 0.000000000000000000 ) ) ;
#208857=CARTESIAN_POINT ( 'NONE',  ( -6.659026002606323047, 10.92061410301605662, 0.000000000000000000 ) ) ;
#208863=CARTESIAN_POINT ( 'NONE',  ( -9.332089804907933939, 9.781859615347734405, 1.040834085586084257E-14 ) ) ;
#208867=CARTESIAN_POINT ( 'NONE',  ( 6.662942426112080874, 9.860851032851066122, 1.199719254218460707 ) ) ;
#208868=CARTESIAN_POINT ( 'NONE',  ( 5.311043488251262268, 7.219303374425030562, -1.599625672291256295 ) ) ;
#208869=CARTESIAN_POINT ( 'NONE',  ( -5.738979324002792204, 5.917037536912586049, -2.440165351838337049 ) ) ;
#208879=DIRECTION ( 'NONE',  ( -0.6260462619842731558, 0.7797859179643593652, 0.000000000000000000 ) ) ;
#208880=CARTESIAN_POINT ( 'NONE',  ( -8.857554428429624593, 9.228235009456373206, 0.7998128361456462443 ) ) ;
#208884=CARTESIAN_POINT ( 'NONE',  ( 6.968527767744104651, 8.192665819532020777, 1.082531754730558626 ) ) ;
#208887=CARTESIAN_POINT ( 'NONE',  ( -3.768803514918907194, 7.340761834140026032, 0.7216878364870037421 ) ) ;
#208889=CARTESIAN_POINT ( 'NONE',  ( -4.713430959045263435, 8.650753218861462202, 0.7998128361456481317 ) ) ;
#208899=CARTESIAN_POINT ( 'NONE',  ( 1.499999999999990896, 5.525000000000022560, 1.214306433183764966E-14 ) ) ;
#208900=CARTESIAN_POINT ( 'NONE',  ( 8.586391356156291010, 8.911878091804165791, 0.7998128361456481317 ) ) ;
#208904=CARTESIAN_POINT ( 'NONE',  ( -4.729598638066518035, 6.837371794175130191, -1.235194855336968045 ) ) ;
#208911=CARTESIAN_POINT ( 'NONE',  ( 4.359110081993588182, 5.044382169536003602, -1.199719254218452047 ) ) ;
#208929=CARTESIAN_POINT ( 'NONE',  ( -5.599681137644054729, 6.491715067794862293, 1.199719254218450271 ) ) ;
#208930=CARTESIAN_POINT ( 'NONE',  ( 5.788968402910812827, 6.816513227226497662, 1.082531754730558626 ) ) ;
#208931=CARTESIAN_POINT ( 'NONE',  ( -0.7500000000000215383, 3.691666666666690411, 1.299038105676671107 ) ) ;
#208934=CARTESIAN_POINT ( 'NONE',  ( -4.959585264500673496, 4.680604318205876524, 1.214306433183764966E-14 ) ) ;
#208935=CARTESIAN_POINT ( 'NONE',  ( 0.5511734105799784844, 7.507429961897218895, -1.922562588595817301 ) ) ;
#208938=CARTESIAN_POINT ( 'NONE',  ( 1.364683531249990311, 4.634375000341417916, 1.214306433183764966E-14 ) ) ;
#208941=CARTESIAN_POINT ( 'NONE',  ( -4.297571505851936813, 4.116180966356429494, 1.214306433183764966E-14 ) ) ;
#208946=CARTESIAN_POINT ( 'NONE',  ( 4.168242161197552420, 6.950367390450747251, -1.199719254218452047 ) ) ;
#208953=CARTESIAN_POINT ( 'NONE',  ( 0.6823417656249899377, 1.655208333674752730, 1.181850606188755259 ) ) ;
#208958=CARTESIAN_POINT ( 'NONE',  ( -8.459397779922852578, 11.95671561229694824, 1.199719254218453823 ) ) ;
#208959=CARTESIAN_POINT ( 'NONE',  ( -5.219525951136850139, 7.112532914458205013, -1.443375672974051449 ) ) ;
#208963=CARTESIAN_POINT ( 'NONE',  ( -1.201851678989727383E-14, 4.071875000341425022, 1.575800808251672791 ) ) ;
#208972=CARTESIAN_POINT ( 'NONE',  ( -7.199016378732087773, 7.501199984716642177, 0.7216878364870317197 ) ) ;
#208975=CARTESIAN_POINT ( 'NONE',  ( -4.406036734316898240, 6.163462161501577441, -1.443375672974051449 ) ) ;
#208983=ORIENTED_EDGE ( 'NONE', *, *, #64571, .T. ) ;
#208987=CARTESIAN_POINT ( 'NONE',  ( -2.605138072120212200, 6.191078184115536232, -0.7998128361456281477 ) ) ;
#208990=CARTESIAN_POINT ( 'NONE',  ( -0.7500000000000215383, 0.1916666666666871910, 1.299038105676659116 ) ) ;
#208992=CARTESIAN_POINT ( 'NONE',  ( 8.758204044747998296, 11.24099069033793974, 1.443375672974076540 ) ) ;
#208993=CARTESIAN_POINT ( 'NONE',  ( 7.793239369756836510, 7.986534107671458216, 0.7998128361456341429 ) ) ;
#208998=CARTESIAN_POINT ( 'NONE',  ( 3.181359600701000989, 6.863336634126477875, 0.000000000000000000 ) ) ;
#209006=CARTESIAN_POINT ( 'NONE',  ( -5.225778143063529946, 8.184159369294361497, 1.199719254218452047 ) ) ;
#209007=ORIENTED_EDGE ( 'NONE', *, *, #158430, .F. ) ;
#209012=CARTESIAN_POINT ( 'NONE',  ( -0.6823417656250212460, 3.301041667008085323, 1.181850606188767472 ) ) ;
#209013=CARTESIAN_POINT ( 'NONE',  ( 9.531018800282609504, 10.22186947652563305, 0.7216878364870458196 ) ) ;
#209014=CARTESIAN_POINT ( 'NONE',  ( -7.226659571283968297, 8.389856573708110332, 1.199719254218450271 ) ) ;
#209017=CARTESIAN_POINT ( 'NONE',  ( 5.301401758143367893, 6.143722458377430584, 1.199719254218462483 ) ) ;
#209018=CARTESIAN_POINT ( 'NONE',  ( -4.954615070790188369, 7.867802451642154082, -1.199719254218452047 ) ) ;
#209025=CARTESIAN_POINT ( 'NONE',  ( 6.317736394288122170, 10.31451686007074997, 0.7216878364870438212 ) ) ;
#209029=CARTESIAN_POINT ( 'NONE',  ( 1.364683531249990311, 2.696875000341415696, 1.214306433183764966E-14 ) ) ;
#209031=CARTESIAN_POINT ( 'NONE',  ( 4.324687812634874895, 7.989293514808604613, 0.7216878364870317197 ) ) ;
#209033=CARTESIAN_POINT ( 'NONE',  ( -4.284013352238265959, 5.060732334775157604, -1.082531754730544860 ) ) ;
#209040=CARTESIAN_POINT ( 'NONE',  ( -4.377891688998395203, 7.365737962781053305, -1.202262209786943759 ) ) ;
#209047=CARTESIAN_POINT ( 'NONE',  ( 6.226218857173709154, 8.287007971501239467, 1.599625672291281386 ) ) ;
#209058=CARTESIAN_POINT ( 'NONE',  ( 3.524756749872944628, 7.056040608253000279, -0.7216878364870267237 ) ) ;
#209059=CARTESIAN_POINT ( 'NONE',  ( -1.402160292154681736E-14, 2.009375000341422801, -1.575800808251660134 ) ) ;
#209060=CARTESIAN_POINT ( 'NONE',  ( 6.591235234537977661, 10.84152487360300299, 0.7998128361456462443 ) ) ;
#209062=CARTESIAN_POINT ( 'NONE',  ( 0.5451294715435256455, 6.857673057455659915, -3.776897409940819017 ) ) ;
#209063=CARTESIAN_POINT ( 'NONE',  ( -4.660252114795309097, 6.460046772059735432, -1.599625672291256517 ) ) ;
#209067=CARTESIAN_POINT ( 'NONE',  ( -0.7500000000000006661, 2.858333333333358706, -1.299038105676652011 ) ) ;
#209068=CARTESIAN_POINT ( 'NONE',  ( 4.937140493670735708, 8.911747675924535983, -0.7998128361456281477 ) ) ;
#209069=CARTESIAN_POINT ( 'NONE',  ( -8.362681821530818738, 8.650883634741092010, -0.7998128361456291469 ) ) ;
#209074=CARTESIAN_POINT ( 'NONE',  ( 1.364683531249988535, 2.905208333674754506, -0.7879004041258239610 ) ) ;
#209076=CARTESIAN_POINT ( 'NONE',  ( 8.568389894156670294, 12.94027927658408217, -0.7216878364870257245 ) ) ;
#209082=CARTESIAN_POINT ( 'NONE',  ( 0.7499999999999885647, 0.5145833340161540814, 1.299038105676657340 ) ) ;
#209085=CARTESIAN_POINT ( 'NONE',  ( -5.682838942422375084, 9.781729199468104596, 0.000000000000000000 ) ) ;
#209086=EDGE_CURVE ( 'NONE', #201094, #45840, #99640, .T. ) ;
#209087=CARTESIAN_POINT ( 'NONE',  ( -4.622967192579922724, 4.495809267539077503, 1.214306433183764966E-14 ) ) ;
#209095=CARTESIAN_POINT ( 'NONE',  ( 5.178324605415663306, 8.128796908705222535, 1.199719254218462483 ) ) ;
#209098=DIRECTION ( 'NONE',  ( 0.7592566023653005702, -0.6507913734559639396, 0.000000000000000000 ) ) ;
#209099=CARTESIAN_POINT ( 'NONE',  ( 6.494519276145969577, 7.535692896047149425, -1.199719254218446718 ) ) ;
#209102=CARTESIAN_POINT ( 'NONE',  ( -5.096975683733680818, 8.033889833409558534, -1.199719254218452047 ) ) ;
#209104=CARTESIAN_POINT ( 'NONE',  ( 3.948449050077836642, 5.629609863222681199, 1.599625672291267398 ) ) ;
#209109=DIRECTION ( 'NONE',  ( -0.6507913734559642727, 0.7592566023653003482, 2.775557561562893816E-17 ) ) ;
#209110=CARTESIAN_POINT ( 'NONE',  ( 4.525353972290461435, 6.990290696447242880, 1.167197606177571734 ) ) ;
#209111=ORIENTED_EDGE ( 'NONE', *, *, #19714, .F. ) ;
#209121=CARTESIAN_POINT ( 'NONE',  ( -4.151086725614978157, 2.978102892632842558, 0.7750000000000117906 ) ) ;
#209122=CARTESIAN_POINT ( 'NONE',  ( -3.551873057100300990, 5.166937871415542283, 1.443375672974064550 ) ) ;
#209124=CARTESIAN_POINT ( 'NONE',  ( 8.595506201384020883, 9.130438111143927671, 0.7216878364870438212 ) ) ;
#209126=CARTESIAN_POINT ( 'NONE',  ( -4.497554271431319250, 6.270232621468402989, -1.599625672291256295 ) ) ;
#209127=DIRECTION ( 'NONE',  ( 1.000000000000000000, 0.000000000000000000, 0.000000000000000000 ) ) ;
#209129=CARTESIAN_POINT ( 'NONE',  ( 7.446452682403650769, 9.710614100936176385, -1.599625672291262513 ) ) ;
#209131=CARTESIAN_POINT ( 'NONE',  ( -6.389970470742427189, 6.349387058821269747, -0.7998128361456291469 ) ) ;
#209139=ORIENTED_EDGE ( 'NONE', *, *, #21930, .T. ) ;
#209145=CARTESIAN_POINT ( 'NONE',  ( 10.55910270694468345, 11.21337466772398095, 0.7998128361456462443 ) ) ;
#209146=CARTESIAN_POINT ( 'NONE',  ( -4.578903193113314174, 6.365139696764064325, 1.599625672291267398 ) ) ;
#209149=CARTESIAN_POINT ( 'NONE',  ( 4.419594888374914099, 5.218910793601261311, -1.082531754730548412 ) ) ;
#209151=PLANE ( 'NONE',  #54640 ) ;
#209154=CARTESIAN_POINT ( 'NONE',  ( -4.600294193738529103, 4.261431402316699035, -0.7998128361456221525 ) ) ;
#209158=CARTESIAN_POINT ( 'NONE',  ( 9.240045382913317340, 10.73880668727576015, -1.199719254218446718 ) ) ;
#209162=CARTESIAN_POINT ( 'NONE',  ( -7.121056995675673740, 9.330985799753529264, -1.599625672291263179 ) ) ;
#209163=CARTESIAN_POINT ( 'NONE',  ( 6.322179702674084467, 6.270297829408224111, 1.040834085586084257E-14 ) ) ;
#209168=CARTESIAN_POINT ( 'NONE',  ( 0.6823417656249899377, 0.9052083336747520637, 1.181850606188755259 ) ) ;
#209171=CARTESIAN_POINT ( 'NONE',  ( 7.131225611108085616, 10.30321839872603462, 1.082531754730558626 ) ) ;
#209178=CARTESIAN_POINT ( 'NONE',  ( 7.714226216051361718, 11.94375498546120795, -0.7216878364870267237 ) ) ;
#209179=ORIENTED_EDGE ( 'NONE', *, *, #31271, .T. ) ;
#209201=CARTESIAN_POINT ( 'NONE',  ( -1.201851678989727383E-14, 1.243750000682821044, 1.732050807568877637 ) ) ;
#209207=CARTESIAN_POINT ( 'NONE',  ( 6.740374924288304648, 11.01552117831172062, 1.040834085586084257E-14 ) ) ;
#209208=CARTESIAN_POINT ( 'NONE',  ( -0.6823417656250003738, -1.032291666325242607, -1.181850606188749264 ) ) ;
#209211=CARTESIAN_POINT ( 'NONE',  ( 2.822068529938852155, 6.444163718237301275, -0.7998128361456291469 ) ) ;
#209212=CARTESIAN_POINT ( 'NONE',  ( -5.409340102172518705, 9.254721185935849803, 0.000000000000000000 ) ) ;
#209216=CARTESIAN_POINT ( 'NONE',  ( -5.371001409308059138, 9.417918744168066070, -0.7998128361456231517 ) ) ;
#209218=CARTESIAN_POINT ( 'NONE',  ( -1.500000000000013101, 1.910416667349488451, -0.8660254037844313801 ) ) ;
#209230=CARTESIAN_POINT ( 'NONE',  ( -8.154339323615371171, 11.60081407993821045, 1.199719254218453823 ) ) ;
#209231=CARTESIAN_POINT ( 'NONE',  ( 7.633404179693907388, 8.864391950186421454, -1.199719254218441611 ) ) ;
#209232=CARTESIAN_POINT ( 'NONE',  ( 1.387358672531703974, 7.315968950352358391, 4.254625267140708544 ) ) ;
#209239=CARTESIAN_POINT ( 'NONE',  ( -8.290974629956718189, 9.631557475493025322, -1.199719254218446718 ) ) ;
#209242=CARTESIAN_POINT ( 'NONE',  ( 0.9999999999999833467, 8.600000000000013856, -0.3999999999999832023 ) ) ;
#209245=CARTESIAN_POINT ( 'NONE',  ( 4.355193658487811703, 6.104145239700998538, -1.599625672291255185 ) ) ;
#209250=( BOUNDED_CURVE ( )  B_SPLINE_CURVE ( 2, ( #63818, #214284, #201259, #82191, #185016, #200196, #52899 ),
 .UNSPECIFIED., .F., .T. ) 
 B_SPLINE_CURVE_WITH_KNOTS ( ( 3, 2, 2, 3 ),
 ( 0.1071428571428572341, 0.1130952380952381098, 0.1190476190476189855, 0.1249999999999998612 ),
 .UNSPECIFIED. ) 
 CURVE ( )  GEOMETRIC_REPRESENTATION_ITEM ( )  RATIONAL_B_SPLINE_CURVE ( ( 0.9999999999999977796, 0.8660254037844409281, 1.000000000000000000, 0.8660254037844387076, 1.000000000000000000, 0.8660254037844418162, 0.9999999999999968914 ) ) 
 REPRESENTATION_ITEM ( '' )  );
#209251=CARTESIAN_POINT ( 'NONE',  ( -10.13488352141530768, 11.78278451552804817, 1.199719254218462483 ) ) ;
#209254=CARTESIAN_POINT ( 'NONE',  ( -5.989290089449875509, 6.089315518664643712, -0.6934025848366349720 ) ) ;
#209264=DIRECTION ( 'NONE',  ( 0.8660254037844385966, 0.5000000000000001110, 0.000000000000000000 ) ) ;
#209266=CIRCLE ( 'NONE', #143626, 0.08000000000000025147 ) ;
#209271=CARTESIAN_POINT ( 'NONE',  ( -0.7500000000000215383, 0.4729166673494850093, 1.299038105676659116 ) ) ;
#209282=CARTESIAN_POINT ( 'NONE',  ( 2.724825686666657809, 6.122787701178987518, 0.000000000000000000 ) ) ;
#209286=CARTESIAN_POINT ( 'NONE',  ( -8.839026081105473054, 12.39961529701003684, -1.199719254218446718 ) ) ;
#209288=CARTESIAN_POINT ( 'NONE',  ( 10.42352117080803708, 11.05519620889787724, -0.7998128361456281477 ) ) ;
#209290=CARTESIAN_POINT ( 'NONE',  ( -0.7158994178059416846, 2.800000000000024691, 1.161830092591057184 ) ) ;
#209292=LINE ( 'NONE', #145440, #15075 ) ;
#209297=CARTESIAN_POINT ( 'NONE',  ( -0.6823417656249969321, 5.780208333674756283, -1.181850606188749264 ) ) ;
#209303=CARTESIAN_POINT ( 'NONE',  ( -5.687809136132860210, 6.594531066031826150, -1.199719254218446718 ) ) ;
#209306=CARTESIAN_POINT ( 'NONE',  ( -1.500000000000015099, -0.5791666666666476226, 0.8660254037844403729 ) ) ;
#209308=CARTESIAN_POINT ( 'NONE',  ( -1.500000000000011324, 5.879166666666686858, -0.8660254037844313801 ) ) ;
#209314=CARTESIAN_POINT ( 'NONE',  ( 0.6823417656249899377, 5.738541667008087543, -1.181850606188754593 ) ) ;
#209316=CARTESIAN_POINT ( 'NONE',  ( -7.934546212495630968, 10.28005655271014795, -1.599625672291263179 ) ) ;
#209317=CARTESIAN_POINT ( 'NONE',  ( 8.540746701604824409, 12.05162268759261224, -1.199719254218446718 ) ) ;
#209323=CARTESIAN_POINT ( 'NONE',  ( -1.364683531250014514, -0.4489583329919089039, -0.7879004041258359514 ) ) ;
#209329=CARTESIAN_POINT ( 'NONE',  ( 1.499999999999989120, 3.785416667349481123, 0.8660254037844522523 ) ) ;
#209331=CARTESIAN_POINT ( 'NONE',  ( 6.466876084038451822, 10.48851316477946582, 1.040834085586084257E-14 ) ) ;
#209334=CARTESIAN_POINT ( 'NONE',  ( -6.078132937628113908, 5.985576603521232109, 1.040834085586084257E-14 ) ) ;
#209336=CARTESIAN_POINT ( 'NONE',  ( 1.499999999999989120, 5.327083334016152527, -0.8660254037844323793 ) ) ;
#209338=CARTESIAN_POINT ( 'NONE',  ( -4.223528545856940042, 4.886203710709899006, -1.199719254218446718 ) ) ;
#209340=CARTESIAN_POINT ( 'NONE',  ( 5.463572716182812705, 9.317992568947877530, 0.7216878364870438212 ) ) ;
#209341=CARTESIAN_POINT ( 'NONE',  ( -7.646435447983039424, 11.86466575604815787, 0.000000000000000000 ) ) ;
#209347=CARTESIAN_POINT ( 'NONE',  ( 10.41229878561526512, 11.25002945941372623, -0.7216878364870257245 ) ) ;
#209348=CARTESIAN_POINT ( 'NONE',  ( -1.001543065824772872E-14, 4.712500000000018119, 1.732050807568877637 ) ) ;
#209350=CARTESIAN_POINT ( 'NONE',  ( 2.535011536075336913, 5.133042487381361596, 0.9999999999999991118 ) ) ;
#209357=CARTESIAN_POINT ( 'NONE',  ( -4.559605246071192219, 3.300000000000025135, -0.7749999999999935829 ) ) ;
#209362=ORIENTED_EDGE ( 'NONE', *, *, #98529, .T. ) ;
#209364=CARTESIAN_POINT ( 'NONE',  ( 10.07778825365955733, 10.65184113889131012, -0.7998128361456281477 ) ) ;
#209367=DIRECTION ( 'NONE',  ( 5.578564026256490882E-16, 1.000000000000000000, 9.066213480720158442E-32 ) ) ;
#209371=CARTESIAN_POINT ( 'NONE',  ( -1.402160292154681736E-14, 0.3218750003414227456, 1.575800808251672791 ) ) ;
#209372=CARTESIAN_POINT ( 'NONE',  ( 6.480434237652135998, 6.662854153456708950, 0.7216878364870317197 ) ) ;
#209373=ORIENTED_EDGE ( 'NONE', *, *, #111378, .T. ) ;
#209374=CARTESIAN_POINT ( 'NONE',  ( -7.849807752632384172, 12.10193344480572897, 0.000000000000000000 ) ) ;
#209378=CARTESIAN_POINT ( 'NONE',  ( -3.358669367883384105, 4.941533567329135401, -1.599625672291262513 ) ) ;
#209387=EDGE_LOOP ( 'NONE', ( #104656, #170175, #148991, #84994, #196223 ) ) ;
#209393=CARTESIAN_POINT ( 'NONE',  ( 5.018332763094478288, 6.785885375482345161, -1.424093192218821136 ) ) ;
#209397=CARTESIAN_POINT ( 'NONE',  ( 0.5475226324602644468, 7.495867147881389414, 1.923617955668152302 ) ) ;
#209401=CARTESIAN_POINT ( 'NONE',  ( -7.158341918335454857, 10.33485409049125003, 1.082531754730549967 ) ) ;
#209405=CARTESIAN_POINT ( 'NONE',  ( 7.233438648090761980, 8.397765496649418182, 1.199719254218462483 ) ) ;
#209406=CARTESIAN_POINT ( 'NONE',  ( 3.891353782322113375, 4.498666486585943147, -1.199719254218446718 ) ) ;
#209408=CARTESIAN_POINT ( 'NONE',  ( -5.434120640978981065, 5.234228924097238611, -0.7998128361456221525 ) ) ;
#209411=VECTOR ( 'NONE', #126987, 1000.000000000000000 ) ;
#209413=CARTESIAN_POINT ( 'NONE',  ( -4.253507506385335368, 5.985511395581417204, 1.599625672291267398 ) ) ;
#209416=CARTESIAN_POINT ( 'NONE',  ( 4.222474775652216294, 7.013638773981186958, 1.199719254218462483 ) ) ;
#209418=CARTESIAN_POINT ( 'NONE',  ( 9.101601193475611140, 9.512956235343358102, -0.7998128361456221525 ) ) ;
#209421=CARTESIAN_POINT ( 'NONE',  ( 4.100400566228236343, 7.694619998084524681, 0.6794913885044724378 ) ) ;
#209422=CARTESIAN_POINT ( 'NONE',  ( 3.362058906508953449, 6.866226457661676719, -0.7216878364870267237 ) ) ;
#209429=CARTESIAN_POINT ( 'NONE',  ( 5.626270559546804328, 9.507806719539201978, 0.7216878364870438212 ) ) ;
#209430=CARTESIAN_POINT ( 'NONE',  ( -9.657485491635913633, 10.16148791653038330, 1.040834085586084257E-14 ) ) ;
#209434=CARTESIAN_POINT ( 'NONE',  ( -8.809047120577080392, 11.30030761213851953, 1.599625672291269396 ) ) ;
#209435=CARTESIAN_POINT ( 'NONE',  ( -5.540478329478883524, 9.615641817700700145, 0.000000000000000000 ) ) ;
#209436=CARTESIAN_POINT ( 'NONE',  ( -5.721177634842498527, 5.777054783512106440, 0.000000000000000000 ) ) ;
#209443=CARTESIAN_POINT ( 'NONE',  ( 8.263858322729371153, 9.599921783727809910, -1.199719254218446718 ) ) ;
#209447=FACE_OUTER_BOUND ( 'NONE', #83192, .T. ) ;
#209457=CARTESIAN_POINT ( 'NONE',  ( 0.7499999999999885647, 2.566666666666689522, -1.299038105676658228 ) ) ;
#209458=CARTESIAN_POINT ( 'NONE',  ( 5.961834861707224320, 7.978559976790334574, -1.599625672291262513 ) ) ;
#209460=EDGE_CURVE ( 'NONE', #158934, #45871, #123268, .T. ) ;
#209461=CARTESIAN_POINT ( 'NONE',  ( 7.131225611108088280, 9.342849184424693476, 1.443375672974076540 ) ) ;
#209462=CARTESIAN_POINT ( 'NONE',  ( -9.124274191872631334, 12.62844174295135069, -1.082531754730543083 ) ) ;
#209466=CARTESIAN_POINT ( 'NONE',  ( 10.07778825365955733, 10.65184113889131012, -0.7998128361456281477 ) ) ;
#209471=CARTESIAN_POINT ( 'NONE',  ( 1.364683531249986537, 0.6135416670080880985, 0.7879004041258500513 ) ) ;
#209476=CARTESIAN_POINT ( 'NONE',  ( -0.6823417656250246877, -0.9489583329919115684, 1.181850606188755259 ) ) ;
#209478=AXIS2_PLACEMENT_3D ( 'NONE', #163932, #198522, #84793 ) ;
#209479=CARTESIAN_POINT ( 'NONE',  ( 8.561083932025322696, 12.07534945641652158, -1.199719254218446718 ) ) ;
#209483=CARTESIAN_POINT ( 'NONE',  ( -2.751941993449643409, 6.154423392425789174, 0.7216878364870317197 ) ) ;
#209484=CARTESIAN_POINT ( 'NONE',  ( -4.038971567461725698, 3.986455684509185193, -0.5169845646830102392 ) ) ;
#209486=CARTESIAN_POINT ( 'NONE',  ( -5.228640796364566690, 9.251831362400652736, -0.7998128361456231517 ) ) ;
#209489=CARTESIAN_POINT ( 'NONE',  ( 3.032219910950674890, 6.689340329417765574, 0.7998128361456321445 ) ) ;
#209496=CARTESIAN_POINT ( 'NONE',  ( 10.24726517383036928, 10.84956421242393887, 0.000000000000000000 ) ) ;
#209499=CARTESIAN_POINT ( 'NONE',  ( -4.232116505760120440, 8.089219690028791376, -0.7998128361456281477 ) ) ;
#209503=CARTESIAN_POINT ( 'NONE',  ( 9.915090410295563927, 10.46202698829998567, -0.7998128361456281477 ) ) ;
#209505=CARTESIAN_POINT ( 'NONE',  ( 6.564118927310645724, 10.80988918183778225, -0.7998128361456291469 ) ) ;
#209508=CARTESIAN_POINT ( 'NONE',  ( -10.31739171031960822, 11.13930453823545186, 1.040834085586084257E-14 ) ) ;
#209511=CARTESIAN_POINT ( 'NONE',  ( -7.867809214632013770, 8.073532260025807261, 1.040834085586084257E-14 ) ) ;
#209515=CARTESIAN_POINT ( 'NONE',  ( -6.137326611691442224, 5.996379759157309586, -0.05818935505210766357 ) ) ;
#209516=CARTESIAN_POINT ( 'NONE',  ( 0.6823417656249899377, 1.342708333674752508, 1.181850606188755259 ) ) ;
#209520=CARTESIAN_POINT ( 'NONE',  ( 7.456621297836078632, 8.762108271306003004, 1.082531754730558626 ) ) ;
#209537=CARTESIAN_POINT ( 'NONE',  ( 8.585337585951586803, 11.03931315507545108, -1.599625672291255185 ) ) ;
#209541=CARTESIAN_POINT ( 'NONE',  ( -3.113568832632681360, 6.784247404713427798, -0.7998128361456281477 ) ) ;
#209542=CARTESIAN_POINT ( 'NONE',  ( -7.212047647465563038, 10.50147379109678880, -1.199719254218446718 ) ) ;
#209544=ORIENTED_EDGE ( 'NONE', *, *, #148219, .F. ) ;
#209547=CARTESIAN_POINT ( 'NONE',  ( -1.500000000000011324, 4.202083334016156080, 0.8660254037844403729 ) ) ;
#209548=CARTESIAN_POINT ( 'NONE',  ( 8.263858322729371153, 9.599921783727809910, -1.199719254218446718 ) ) ;
#209551=CARTESIAN_POINT ( 'NONE',  ( -6.906989191158078079, 10.14557225873805812, -1.199719254218440723 ) ) ;
#209553=CARTESIAN_POINT ( 'NONE',  ( -1.201851678989727383E-14, 4.071875000341425022, 1.575800808251672791 ) ) ;
#209558=CARTESIAN_POINT ( 'NONE',  ( -9.246297574839990929, 11.81043314211192019, 1.443375672974076540 ) ) ;
#209562=CARTESIAN_POINT ( 'NONE',  ( -1.364683531250012516, 3.092708333674755838, 0.7879004041258379498 ) ) ;
#209569=CARTESIAN_POINT ( 'NONE',  ( -1.201851678989727383E-14, 2.321875000341416584, 1.575800808251672791 ) ) ;
#209572=CARTESIAN_POINT ( 'NONE',  ( -3.737243898861318137, 7.511868315313511069, 0.7998128361456341429 ) ) ;
#209573=CARTESIAN_POINT ( 'NONE',  ( 5.126954644262057492, 9.133197518281081173, 0.7998128361456462443 ) ) ;
#209577=CARTESIAN_POINT ( 'NONE',  ( -1.364683531249997417, 3.571875000341423245, 1.214306433183764966E-14 ) ) ;
#209580=CARTESIAN_POINT ( 'NONE',  ( -1.402160292154681736E-14, -0.8031249996585825279, -1.575800808251665908 ) ) ;
#209581=CARTESIAN_POINT ( 'NONE',  ( -5.151735183512911043, 6.073074471262228435, 1.082531754730548412 ) ) ;
#209584=CARTESIAN_POINT ( 'NONE',  ( 4.026408433578586354, 7.641300905909586660, 1.040834085586084257E-14 ) ) ;
#209587=CARTESIAN_POINT ( 'NONE',  ( -6.665805079413154921, 10.92852302595736447, 0.7998128361456481317 ) ) ;
#209588=CARTESIAN_POINT ( 'NONE',  ( -9.002250809794006159, 10.56534270192358704, -1.082531754730543971 ) ) ;
#209590=CARTESIAN_POINT ( 'NONE',  ( -1.500000000000031530, 4.920833333333354709, 0.8660254037844287156 ) ) ;
#209594=CARTESIAN_POINT ( 'NONE',  ( -9.378489572351046633, 11.96465713920816043, -1.599625672291263179 ) ) ;
#209596=CARTESIAN_POINT ( 'NONE',  ( -6.900736999231456004, 8.113576589600553390, 1.082531754730549967 ) ) ;
#209598=CARTESIAN_POINT ( 'NONE',  ( -0.6823417656250003738, 0.2802083336747515641, -1.181850606188749264 ) ) ;
#209608=AXIS2_PLACEMENT_3D ( 'NONE', #130806, #143834, #28974 ) ;
#209611=CARTESIAN_POINT ( 'NONE',  ( 0.7499999999999867883, -0.4333333333333133641, -1.299038105676652899 ) ) ;
#209612=CARTESIAN_POINT ( 'NONE',  ( 7.239690839573049708, 11.39013037956983965, 1.040834085586084257E-14 ) ) ;
#209613=B_SPLINE_CURVE_WITH_KNOTS ( 'NONE', 3,
 ( #54189, #186305, #185233, #104014, #53116, #2200, #200413, #152752, #120329, #18471 ),
 .UNSPECIFIED., .F., .F.,
 ( 4, 3, 3, 4 ),
 ( 0.000000000000000000, 8.893179197954797545E-05, 0.0001334007970840207931, 0.0001778705873658964021 ),
 .UNSPECIFIED. ) ;
#209620=CARTESIAN_POINT ( 'NONE',  ( -1.500000000000022204, 8.627523663848661428, 2.580000000000011173 ) ) ;
#209621=CARTESIAN_POINT ( 'NONE',  ( 5.473741331615251227, 7.409117525016355010, -1.599625672291262513 ) ) ;
#209624=CARTESIAN_POINT ( 'NONE',  ( -4.765854690403601879, 5.518917546014321829, 1.199719254218462483 ) ) ;
#209627=CARTESIAN_POINT ( 'NONE',  ( -4.889337272013151825, 4.909234758358784312, -0.4031905389056227307 ) ) ;
#209628=CARTESIAN_POINT ( 'NONE',  ( -0.6823417656250003738, 1.030208333674752286, -1.181850606188749264 ) ) ;
#209630=CARTESIAN_POINT ( 'NONE',  ( -8.779068160048691283, 10.20099992726700933, -1.199719254218446718 ) ) ;
#209640=ORIENTED_EDGE ( 'NONE', *, *, #50263, .T. ) ;
#209649=CARTESIAN_POINT ( 'NONE',  ( 4.659198344590585350, 8.587481835331020719, 0.7998128361456462443 ) ) ;
#209656=CARTESIAN_POINT ( 'NONE',  ( 7.099665995050449041, 11.43469409420089455, 0.7998128361456462443 ) ) ;
#209659=CARTESIAN_POINT ( 'NONE',  ( 8.910733272679570049, 11.41894145625809820, -1.599625672291255185 ) ) ;
#209661=CARTESIAN_POINT ( 'NONE',  ( 1.525408907393396740, 8.692885148323941991, -2.521481920632477447 ) ) ;
#209667=CARTESIAN_POINT ( 'NONE',  ( -0.1368715580176214641, 8.236096389523126504, 2.000481929432245121 ) ) ;
#209672=CARTESIAN_POINT ( 'NONE',  ( -8.026063749610047537, 11.34719622697832264, -1.082531754730543971 ) ) ;
#209678=CARTESIAN_POINT ( 'NONE',  ( 5.229694566569264680, 7.124396299129368337, 1.599625672291267398 ) ) ;
#209685=CARTESIAN_POINT ( 'NONE',  ( 3.456965981360264895, 6.016582164020185530, -1.082531754730543971 ) ) ;
#209693=CARTESIAN_POINT ( 'NONE',  ( -6.067437437315529536, 7.037430750744921859, 1.199719254218450271 ) ) ;
#209696=CARTESIAN_POINT ( 'NONE',  ( -3.273404022695637572, 5.906389562198459231, 1.199719254218462483 ) ) ;
#209700=CARTESIAN_POINT ( 'NONE',  ( 0.08635228504285741291, 7.011029804986336877, -1.999717945518301399 ) ) ;
#209703=CARTESIAN_POINT ( 'NONE',  ( 5.636439174979242850, 7.598931675607687453, -1.599625672291262513 ) ) ;
#209705=CARTESIAN_POINT ( 'NONE',  ( 1.567642296063686658, 8.684662666223690763, 2.500960217906281535 ) ) ;
#209714=EDGE_CURVE ( 'NONE', #31219, #214357, #37320, .T. ) ;
#209715=ORIENTED_EDGE ( 'NONE', *, *, #51004, .F. ) ;
#209717=CARTESIAN_POINT ( 'NONE',  ( -1.364683531250000748, 1.571875000341421691, 0.000000000000000000 ) ) ;
#209718=CARTESIAN_POINT ( 'NONE',  ( 2.198393463710220264, 5.716542807637226886, 0.7998128361456462443 ) ) ;
#209719=CARTESIAN_POINT ( 'NONE',  ( 3.517450787741589036, 6.191110788085444128, -1.199719254218446718 ) ) ;
#209721=CARTESIAN_POINT ( 'NONE',  ( -7.076992996653451939, 7.358839372291564374, 0.7216878364870317197 ) ) ;
#209724=CARTESIAN_POINT ( 'NONE',  ( 3.823036129373602154, 6.443664003369091731, -1.082531754730548412 ) ) ;
#209725=CARTESIAN_POINT ( 'NONE',  ( -5.544921637864824504, 8.452530429942200385, -1.082531754730543971 ) ) ;
#209728=VERTEX_POINT ( 'NONE', #90109 ) ;
#209730=CARTESIAN_POINT ( 'NONE',  ( 5.262536180398716290, 9.291375977107183104, -0.7998128361456291469 ) ) ;
#209735=CARTESIAN_POINT ( 'NONE',  ( -1.364683531250012516, 4.488541667008090208, -0.7879004041258300672 ) ) ;
#209740=CARTESIAN_POINT ( 'NONE',  ( 7.644099680006512187, 7.812537802962739697, 1.040834085586084257E-14 ) ) ;
#209743=CARTESIAN_POINT ( 'NONE',  ( -7.015454420067433361, 10.27211502579893754, 1.199719254218453823 ) ) ;
#209748=CARTESIAN_POINT ( 'NONE',  ( 7.404724451357931336, 11.79059562655963056, 0.7998128361456462443 ) ) ;
#209751=CARTESIAN_POINT ( 'NONE',  ( -8.701635661872465732, 9.046329781806354831, 1.040834085586084257E-14 ) ) ;
#209753=CARTESIAN_POINT ( 'NONE',  ( 7.578644679914706472, 9.864838098032418401, 1.443375672974076540 ) ) ;
#209754=CARTESIAN_POINT ( 'NONE',  ( 4.022946295931974170, 7.796337852756115794, -0.3444838504574644356 ) ) ;
#209755=CARTESIAN_POINT ( 'NONE',  ( -9.490344339885977476, 11.13478515369756217, -1.082531754730539753 ) ) ;
#209759=CARTESIAN_POINT ( 'NONE',  ( 3.825371897350130723, 7.614684313550482031, 0.7998128361456321445 ) ) ;
#209761=CARTESIAN_POINT ( 'NONE',  ( 10.21336978979620191, 10.81001959771741205, 0.7998128361456462443 ) ) ;
#209762=CARTESIAN_POINT ( 'NONE',  ( -4.566676325625886435, 6.985790553628898003, 1.179912429979562249 ) ) ;
#209763=CARTESIAN_POINT ( 'NONE',  ( 2.998324526916512411, 6.649795714711241423, 0.000000000000000000 ) ) ;
#209764=CARTESIAN_POINT ( 'NONE',  ( 0.6823417656249882723, 0.1760416670080894308, -1.181850606188749264 ) ) ;
#209767=CARTESIAN_POINT ( 'NONE',  ( -6.209271165378811297, 10.18797409300986878, 0.7216878364870458196 ) ) ;
#209768=ORIENTED_EDGE ( 'NONE', *, *, #120152, .F. ) ;
#209773=CARTESIAN_POINT ( 'NONE',  ( -4.361599125657974696, 7.193191237876310318, 1.033186747995703758 ) ) ;
#209774=CARTESIAN_POINT ( 'NONE',  ( -1.364683531250014514, -0.1989583329919157317, -0.7879004041258359514 ) ) ;
#209777=CARTESIAN_POINT ( 'NONE',  ( 2.887523530030648988, 6.312601851770308414, 0.000000000000000000 ) ) ;
#209781=CARTESIAN_POINT ( 'NONE',  ( -8.419250203962027612, 11.80591375705560608, 1.082531754730549967 ) ) ;
#209787=CARTESIAN_POINT ( 'NONE',  ( -7.334597914868722590, 11.50085530074811935, -0.7216878364870267237 ) ) ;
#209788=DIRECTION ( 'NONE',  ( -5.578564026256490882E-16, -1.000000000000000000, -9.066213480720158442E-32 ) ) ;
#209790=CONICAL_SURFACE ( 'NONE', #36776, 4.000000000000000000, 0.8960553845713404852 ) ;
#209792=ADVANCED_FACE ( 'NONE', ( #175627, #204875 ), #209151, .T. ) ;
#209796=CARTESIAN_POINT ( 'NONE',  ( -8.365017589507372620, 9.821903944922480534, 1.082531754730558626 ) ) ;
#209800=CARTESIAN_POINT ( 'NONE',  ( -0.6823417656249969321, 5.530208333674756283, -1.181850606188749264 ) ) ;
#209801=CARTESIAN_POINT ( 'NONE',  ( 1.499999999999987121, 4.077083334016147198, -0.8660254037844323793 ) ) ;
#209802=CARTESIAN_POINT ( 'NONE',  ( 6.043473040404234276, 6.060458613201341826, -0.4842117992061110154 ) ) ;
#209803=DIRECTION ( 'NONE',  ( 5.578564026256490882E-16, 1.000000000000000000, 9.066213480720158442E-32 ) ) ;
#209808=CARTESIAN_POINT ( 'NONE',  ( -7.965578943228732278, 9.251929174310385307, -1.199719254218446718 ) ) ;
#209812=CARTESIAN_POINT ( 'NONE',  ( 6.322179702674084467, 6.270297829408224111, 1.040834085586084257E-14 ) ) ;
#209817=CARTESIAN_POINT ( 'NONE',  ( 6.795661308947685164, 8.951357498570873261, -1.599625672291262513 ) ) ;
#209824=CARTESIAN_POINT ( 'NONE',  ( -6.073689629242176480, 6.188318776978391611, -0.7216878364870278340 ) ) ;
#209827=CYLINDRICAL_SURFACE ( 'NONE', #206378, 1.250000000000000000 ) ;
#209833=CARTESIAN_POINT ( 'NONE',  ( -8.748035429315585532, 11.22912730566677553, -1.599625672291263179 ) ) ;
#209835=CARTESIAN_POINT ( 'NONE',  ( 7.397945374551106568, 11.78268670361832093, -0.7998128361456291469 ) ) ;
#209836=CARTESIAN_POINT ( 'NONE',  ( -0.7500000000000006661, -0.3916666666666443475, -1.299038105676652011 ) ) ;
#209837=CARTESIAN_POINT ( 'NONE',  ( -8.585337585951595685, 11.03931315507545108, -1.599625672291263179 ) ) ;
#209839=CARTESIAN_POINT ( 'NONE',  ( -1.201851678989727383E-14, 3.196875000341420137, -1.575800808251660134 ) ) ;
#209840=CARTESIAN_POINT ( 'NONE',  ( 4.207107738942202246, 3.802713871720993399, 1.214306433183764966E-14 ) ) ;
#209843=CARTESIAN_POINT ( 'NONE',  ( -1.499999999999997780, 4.650000000000022560, 1.214306433183764966E-14 ) ) ;
#209846=CARTESIAN_POINT ( 'NONE',  ( 7.727784369665023689, 11.95957283134381477, 1.040834085586084257E-14 ) ) ;
#209849=CARTESIAN_POINT ( 'NONE',  ( -7.049876689426121779, 7.327203680526343632, -0.7216878364870278340 ) ) ;
#209850=CIRCLE ( 'NONE', #78446, 2.000000000000000000 ) ;
#209851=CARTESIAN_POINT ( 'NONE',  ( 0.6823417656249899377, 1.592708333674752730, 1.181850606188755259 ) ) ;
#209855=CARTESIAN_POINT ( 'NONE',  ( -6.008234629150358330, 10.16135750065076060, 0.000000000000000000 ) ) ;
#209856=CARTESIAN_POINT ( 'NONE',  ( 1.364683531249988535, 5.217708333674750065, -0.7879004041258300672 ) ) ;
#209862=CARTESIAN_POINT ( 'NONE',  ( 8.341290820905593151, 10.75459192918846618, 1.599625672291281386 ) ) ;
#209865=CARTESIAN_POINT ( 'NONE',  ( -0.7500000000000006661, 0.6083333333333564852, -1.299038105676652011 ) ) ;
#209868=ORIENTED_EDGE ( 'NONE', *, *, #61478, .F. ) ;
#209869=CARTESIAN_POINT ( 'NONE',  ( 10.24726517383036928, 10.84956421242393887, 0.000000000000000000 ) ) ;
#209875=CARTESIAN_POINT ( 'NONE',  ( 7.889955328148847258, 11.29236608522730911, -1.199719254218446718 ) ) ;
#209876=CARTESIAN_POINT ( 'NONE',  ( -9.154780037725563702, 11.70366268214508487, 1.599625672291281386 ) ) ;
#209879=CARTESIAN_POINT ( 'NONE',  ( -1.001543065824772872E-14, 5.134375000341421469, 1.575800808251672791 ) ) ;
#209884=CARTESIAN_POINT ( 'NONE',  ( 7.639129486296027061, 10.99973593639901814, 1.199719254218460707 ) ) ;
#209887=CARTESIAN_POINT ( 'NONE',  ( 1.364683531249988535, 3.405208333674749621, -0.7879004041258239610 ) ) ;
#209889=CARTESIAN_POINT ( 'NONE',  ( -5.910991785878165317, 8.879612269291090598, -1.082531754730538864 ) ) ;
#209895=CARTESIAN_POINT ( 'NONE',  ( 4.552840656090682891, 4.206068941727564514, 1.214306433183764966E-14 ) ) ;
#209898=CARTESIAN_POINT ( 'NONE',  ( 8.372323551638698902, 9.726464550788689323, 1.199719254218462483 ) ) ;
#209899=CARTESIAN_POINT ( 'NONE',  ( 2.487170525094726248, 8.243531156566618279, -2.499999999999888534 ) ) ;
#209904=CARTESIAN_POINT ( 'NONE',  ( -8.134002093194872884, 11.57708731111429401, 1.199719254218453823 ) ) ;
#209906=CARTESIAN_POINT ( 'NONE',  ( 5.957918438201454059, 9.038323046955323292, -1.199719254218440723 ) ) ;
#209908=CARTESIAN_POINT ( 'NONE',  ( 2.846849068745292755, 6.265148313604064434, 0.000000000000000000 ) ) ;
#209910=CARTESIAN_POINT ( 'NONE',  ( 3.323720213644492993, 7.029424015893889433, 1.040834085586084257E-14 ) ) ;
#209912=VECTOR ( 'NONE', #13748, 1000.000000000000000 ) ;
#209919=CARTESIAN_POINT ( 'NONE',  ( -6.073689629242160493, 8.109057205581079231, -1.443375672974059665 ) ) ;
#209920=CARTESIAN_POINT ( 'NONE',  ( 4.695201269034174452, 4.372156323494968966, 1.214306433183764966E-14 ) ) ;
#209923=CARTESIAN_POINT ( 'NONE',  ( -7.857113714319432063, 9.125386407249497012, 1.199719254218462483 ) ) ;
#209929=CARTESIAN_POINT ( 'NONE',  ( -10.13202086811422475, 10.71511252242175161, -0.7998128361456291469 ) ) ;
#209930=CARTESIAN_POINT ( 'NONE',  ( 1.284279953904121641, 3.034610286488902187, 0.7750000000000117906 ) ) ;
#209933=CARTESIAN_POINT ( 'NONE',  ( 6.760712154708803823, 11.03924794713562818, 1.040834085586084257E-14 ) ) ;
#209934=CARTESIAN_POINT ( 'NONE',  ( 6.810273232766058449, 6.839740281182199233, 1.040834085586084257E-14 ) ) ;
#209935=CARTESIAN_POINT ( 'NONE',  ( -5.690973801496453710, 5.856266416803207697, -2.499999999999995115 ) ) ;
#209945=CARTESIAN_POINT ( 'NONE',  ( -8.345207244411405156, 9.694828859023472134, 1.199719254218462483 ) ) ;
#209949=CARTESIAN_POINT ( 'NONE',  ( 5.775410249741494972, 8.721433810464993996, -1.082531754730537088 ) ) ;
#209953=DIRECTION ( 'NONE',  ( 1.000000000000000000, 0.000000000000000000, 0.000000000000000000 ) ) ;
#209955=CARTESIAN_POINT ( 'NONE',  ( -5.605406444246153974, 8.627059054007450101, -1.199719254218440723 ) ) ;
#209963=CARTESIAN_POINT ( 'NONE',  ( -9.561524646135538319, 12.17819805862340310, -1.599625672291263179 ) ) ;
#209964=CARTESIAN_POINT ( 'NONE',  ( 6.968000882419564945, 10.21675256520979858, 1.199719254218460707 ) ) ;
#209966=CARTESIAN_POINT ( 'NONE',  ( -5.260200412422220140, 5.239248024021764039, -0.7216878364870207285 ) ) ;
#209968=CARTESIAN_POINT ( 'NONE',  ( -5.061731940678604325, 6.567192784585701659, -1.227863150880079246 ) ) ;
#209975=CARTESIAN_POINT ( 'NONE',  ( 4.518945272056516416, 4.166524327021037699, 0.7998128361456341429 ) ) ;
#209984=CARTESIAN_POINT ( 'NONE',  ( 4.704842999142070603, 5.447737239542574272, -1.199719254218452047 ) ) ;
#209988=CARTESIAN_POINT ( 'NONE',  ( 1.364683531249988535, 3.967708333674751842, -0.7879004041258239610 ) ) ;
#209993=CARTESIAN_POINT ( 'NONE',  ( 6.634017235788401301, 6.634108284708264414, 0.7998128361456341429 ) ) ;
#209997=CARTESIAN_POINT ( 'NONE',  ( -4.761938266897808525, 6.578680616179308771, 1.599625672291267398 ) ) ;
#209998=CARTESIAN_POINT ( 'NONE',  ( 4.148431815657221300, 7.783661518334664464, 1.040834085586084257E-14 ) ) ;
#209999=CARTESIAN_POINT ( 'NONE',  ( -1.499999999999997780, 3.650000000000021227, 1.214306433183764966E-14 ) ) ;
#210001=CARTESIAN_POINT ( 'NONE',  ( -2.923754682041362241, 6.562797562356882608, 0.7998128361456341429 ) ) ;
#210002=CARTESIAN_POINT ( 'NONE',  ( 0.4086240214899770073, 7.376738131363499207, -1.961326491624068913 ) ) ;
#210004=LINE ( 'NONE', #82148, #52463 ) ;
#210005=CARTESIAN_POINT ( 'NONE',  ( -1.364683531249997417, 4.509375000341424133, 1.214306433183764966E-14 ) ) ;
#210008=CARTESIAN_POINT ( 'NONE',  ( -3.145128448690310830, 6.613140923539910787, -0.7216878364870267237 ) ) ;
#210013=CARTESIAN_POINT ( 'NONE',  ( 2.869522067586683711, 6.499526178826442013, 0.7998128361456362523 ) ) ;
#210016=CARTESIAN_POINT ( 'NONE',  ( 0.1990047979249099375, 6.441647462706413307, -3.222196616944341674 ) ) ;
#210020=CARTESIAN_POINT ( 'NONE',  ( -1.402160292154681736E-14, 1.759375000341421469, -1.575800808251659024 ) ) ;
#210023=CARTESIAN_POINT ( 'NONE',  ( -9.646789991323334590, 11.21334206375407305, 1.199719254218462483 ) ) ;
#210024=CARTESIAN_POINT ( 'NONE',  ( -4.731432421044865499, 8.463828891286912182, -0.7216878364870257245 ) ) ;
#210029=CARTESIAN_POINT ( 'NONE',  ( 1.364683531249990311, 4.613541667008083103, 0.7879004041258500513 ) ) ;
#210038=CARTESIAN_POINT ( 'NONE',  ( -4.704316113817535339, 8.432193199521691440, 0.7216878364870458196 ) ) ;
#210040=ADVANCED_FACE ( 'NONE', ( #128026 ), #179882, .F. ) ;
#210045=CARTESIAN_POINT ( 'NONE',  ( -6.087247782411500552, 7.164505836643929371, 1.082531754730549967 ) ) ;
#210049=DIRECTION ( 'NONE',  ( -6.314299915563594049E-62, -8.546850786086437571E-32, -1.000000000000000000 ) ) ;
#210056=CARTESIAN_POINT ( 'NONE',  ( 4.076713200428175199, 7.699573933034834283, -0.5988845815774744841 ) ) ;
#210058=CARTESIAN_POINT ( 'NONE',  ( -6.389970470742427189, 6.349387058821269747, -0.7998128361456291469 ) ) ;
#210061=CARTESIAN_POINT ( 'NONE',  ( 0.7499999999999885647, 0.5666666666666875241, -1.299038105676652899 ) ) ;
#210063=CARTESIAN_POINT ( 'NONE',  ( 8.053180056837369705, 11.37883191874353805, -1.082531754730543083 ) ) ;
#210064=CARTESIAN_POINT ( 'NONE',  ( 6.109920781252839994, 10.27999134477033216, 1.040834085586084257E-14 ) ) ;
#210067=ORIENTED_EDGE ( 'NONE', *, *, #8236, .T. ) ;
#210069=CARTESIAN_POINT ( 'NONE',  ( 4.029797971759831121, 5.724516938518342535, -1.599625672291255185 ) ) ;
#210070=AXIS2_PLACEMENT_3D ( 'NONE', #196222, #65121, #99780 ) ;
#210071=CARTESIAN_POINT ( 'NONE',  ( -0.4545350412506695692, 7.933623023433764132, -1.993241281637189832 ) ) ;
#210078=CARTESIAN_POINT ( 'NONE',  ( 8.503988664269582998, 10.94440607977979063, 1.599625672291281386 ) ) ;
#210079=CARTESIAN_POINT ( 'NONE',  ( -6.586563698140583512, 6.578745824119123675, 1.040834085586084257E-14 ) ) ;
#210082=LINE ( 'NONE', #82218, #4245 ) ;
#210085=CARTESIAN_POINT ( 'NONE',  ( -1.201851678989727383E-14, 3.821875000341423689, 1.575800808251672791 ) ) ;
#210086=CARTESIAN_POINT ( 'NONE',  ( 8.066738210006674237, 11.39464976410773467, 1.082531754730558626 ) ) ;
#210087=CARTESIAN_POINT ( 'NONE',  ( -6.144869935491728441, 8.192100896205577243, -1.599625672291263179 ) ) ;
#210090=CARTESIAN_POINT ( 'NONE',  ( 5.795220594837462436, 8.848508896363995291, -1.199719254218440723 ) ) ;
#210091=CARTESIAN_POINT ( 'NONE',  ( -5.982172092127739482, 8.002286745614243912, -1.599625672291263179 ) ) ;
#210095=CARTESIAN_POINT ( 'NONE',  ( -0.7500000000000215383, 0.9729166673494854534, 1.299038105676659116 ) ) ;
#210098=CARTESIAN_POINT ( 'NONE',  ( 7.131225611108088280, 9.342849184424693476, 1.443375672974076540 ) ) ;
#210101=CARTESIAN_POINT ( 'NONE',  ( 0.6823417656249882723, 2.238541667008084435, -1.181850606188749264 ) ) ;
#210103=CARTESIAN_POINT ( 'NONE',  ( 4.473827502385202770, 8.163289819517311585, 1.040834085586084257E-14 ) ) ;
#210105=CARTESIAN_POINT ( 'NONE',  ( -3.470524135418306511, 5.072030796119872953, -1.443375672974053447 ) ) ;
#210113=CARTESIAN_POINT ( 'NONE',  ( -4.096253560606756494, 7.689279582349398012, -0.7399548657811344521 ) ) ;
#210120=CARTESIAN_POINT ( 'NONE',  ( 6.928380191783277908, 8.041863964290678624, 1.199719254218462483 ) ) ;
#210123=CARTESIAN_POINT ( 'NONE',  ( 2.171277156482887882, 5.684907115872006145, -0.7998128361456291469 ) ) ;
#210131=CARTESIAN_POINT ( 'NONE',  ( 4.853455804012222430, 5.725081861844796727, 1.082531754730560403 ) ) ;
#210132=CARTESIAN_POINT ( 'NONE',  ( 1.364683531249988535, 2.676041667008082214, 0.7879004041258500513 ) ) ;
#210133=CARTESIAN_POINT ( 'NONE',  ( 7.618792255875527886, 10.97600916757510170, 1.199719254218460707 ) ) ;
#210135=CARTESIAN_POINT ( 'NONE',  ( -0.9486429539237212216, 3.225839070649073825, -1.028101543438966425 ) ) ;
#210136=CARTESIAN_POINT ( 'NONE',  ( -3.744022975668146902, 7.519777238254811813, -0.7998128361456282587 ) ) ;
#210139=CARTESIAN_POINT ( 'NONE',  ( 1.499999999999989120, 2.275000000000019895, 1.214306433183764966E-14 ) ) ;
#210140=CARTESIAN_POINT ( 'NONE',  ( 6.474182045725470402, 7.511966127223233869, -1.199719254218446718 ) ) ;
#210141=CARTESIAN_POINT ( 'NONE',  ( -6.958359152311683893, 9.141171649162195934, -1.599625672291263179 ) ) ;
#210145=CARTESIAN_POINT ( 'NONE',  ( -1.364683531249997417, 2.509375000341422357, 1.214306433183764966E-14 ) ) ;
#210148=CARTESIAN_POINT ( 'NONE',  ( 2.659370686574860976, 6.254349567645977714, -0.7998128361456291469 ) ) ;
#210154=CARTESIAN_POINT ( 'NONE',  ( -1.500000000000015099, 1.160416667349484898, -0.8660254037844313801 ) ) ;
#210157=CARTESIAN_POINT ( 'NONE',  ( -5.045605722580076780, 9.038290442985410067, -0.7998128361456231517 ) ) ;
#210158=CARTESIAN_POINT ( 'NONE',  ( -3.958617665510283601, 4.681104033592509595, -1.082531754730549967 ) ) ;
#210166=CARTESIAN_POINT ( 'NONE',  ( 4.801558957534076022, 8.753569217098425170, 0.7998128361456462443 ) ) ;
#210169=CARTESIAN_POINT ( 'NONE',  ( 6.938893903907228378E-15, 10.64264068711930733, 1.214306433183764966E-14 ) ) ;
#210171=CARTESIAN_POINT ( 'NONE',  ( 7.006866460164219212, 7.069099046480051385, -0.7998128361456281477 ) ) ;
#210176=CARTESIAN_POINT ( 'NONE',  ( -4.543954038874438162, 8.453030145328826350, 1.040834085586084257E-14 ) ) ;
#210177=AXIS2_PLACEMENT_3D ( 'NONE', #183613, #138082, #153249 ) ;
#210178=CARTESIAN_POINT ( 'NONE',  ( 2.354312230267378236, 5.898448035287240820, -0.7998128361456281477 ) ) ;
#210184=CARTESIAN_POINT ( 'NONE',  ( 4.215071147998584955, 7.318223152490296535, 0.8720340548805920466 ) ) ;
#210193=CIRCLE ( 'NONE', #106515, 0.07999999999999998779 ) ;
#210197=CARTESIAN_POINT ( 'NONE',  ( 6.480434237652115570, 10.50433101066207442, 0.7216878364870438212 ) ) ;
#210199=CARTESIAN_POINT ( 'NONE',  ( -5.901876940650454095, 5.779944607047298177, -0.7998128361456291469 ) ) ;
#210204=CARTESIAN_POINT ( 'NONE',  ( -7.217017841176048165, 7.314275657660511243, 1.040834085586084257E-14 ) ) ;
#210217=CARTESIAN_POINT ( 'NONE',  ( 4.070745140982080734, 3.981847363168877774, -0.7493180678802955352 ) ) ;
#210218=CARTESIAN_POINT ( 'NONE',  ( -4.904298879841297421, 6.744767997946721216, 1.599625672291267398 ) ) ;
#210221=CARTESIAN_POINT ( 'NONE',  ( 5.029711800989886683, 4.970344644017389513, 1.040834085586084257E-14 ) ) ;
#210225=CARTESIAN_POINT ( 'NONE',  ( 1.403499169894465659, 7.376709478544011489, 4.304123474985813935 ) ) ;
#210226=CARTESIAN_POINT ( 'NONE',  ( -5.115504031057831469, 4.862509545855891346, 0.7998128361456341429 ) ) ;
#210229=CARTESIAN_POINT ( 'NONE',  ( 8.055515824813896941, 12.54985222892493368, 0.7998128361456462443 ) ) ;
#210233=CARTESIAN_POINT ( 'NONE',  ( -6.042130013184518589, 10.20090211535728031, -0.7998128361456291469 ) ) ;
#210234=CARTESIAN_POINT ( 'NONE',  ( 6.308621549060418054, 6.254479983525607523, 0.7998128361456341429 ) ) ;
#210239=CARTESIAN_POINT ( 'NONE',  ( -0.6823417656250212460, 0.8635416670080899859, 1.181850606188755259 ) ) ;
#210241=ORIENTED_EDGE ( 'NONE', *, *, #162125, .T. ) ;
#210243=CARTESIAN_POINT ( 'NONE',  ( 7.348156068926750883, 8.635565504245116486, -1.082531754730537976 ) ) ;
#210248=DIRECTION ( 'NONE',  ( -0.8660254037844382635, 0.5000000000000006661, 1.725633230170963324E-31 ) ) ;
#210251=CARTESIAN_POINT ( 'NONE',  ( 8.988692655735958326, 12.47026328412523988, -1.082531754730543083 ) ) ;
#210253=ORIENTED_EDGE ( 'NONE', *, *, #73270, .T. ) ;
#210260=CARTESIAN_POINT ( 'NONE',  ( -9.398826802771548472, 11.98838390803207865, -1.599625672291263179 ) ) ;
#210275=CARTESIAN_POINT ( 'NONE',  ( -0.7500000000000006661, 1.639583334016154970, -1.299038105676652011 ) ) ;
#210281=CARTESIAN_POINT ( 'NONE',  ( 0.000000000000000000, 3.300000000000025135, 1.561251128379126385E-14 ) ) ;
#210282=CARTESIAN_POINT ( 'NONE',  ( 8.860417081730671995, 10.29590700256267155, 1.199719254218453823 ) ) ;
#210283=AXIS2_PLACEMENT_3D ( 'NONE', #169792, #11280, #154623 ) ;
#210286=CARTESIAN_POINT ( 'NONE',  ( 3.225950485047770933, 5.851027101609320269, 1.199719254218450271 ) ) ;
#210287=CARTESIAN_POINT ( 'NONE',  ( -6.616015773788831211, 7.781401826584148473, 1.082531754730549967 ) ) ;
#210291=CARTESIAN_POINT ( 'NONE',  ( -6.181627972826976958, 9.299317504018391745, 1.199719254218452047 ) ) ;
#210292=VERTEX_POINT ( 'NONE', #82359 ) ;
#210293=CARTESIAN_POINT ( 'NONE',  ( 1.499999999999987121, 0.8270833340161471980, -0.8660254037844253849 ) ) ;
#210301=CARTESIAN_POINT ( 'NONE',  ( -4.243338890952911058, 5.013278796608906518, -1.082531754730543971 ) ) ;
#210304=ORIENTED_EDGE ( 'NONE', *, *, #107353, .F. ) ;
#210306=EDGE_CURVE ( 'NONE', #54687, #143545, #148051, .T. ) ;
#210307=CARTESIAN_POINT ( 'NONE',  ( 4.254136489245101238, 7.273159757992218921, 0.9281648423343953347 ) ) ;
#210312=CARTESIAN_POINT ( 'NONE',  ( -8.157201976916404362, 12.66848607304450702, -0.7998128361456281477 ) ) ;
#210313=CARTESIAN_POINT ( 'NONE',  ( 8.945682426918439845, 9.331051007693339727, 1.040834085586084257E-14 ) ) ;
#210317=EDGE_LOOP ( 'NONE', ( #30423, #160148, #105141, #81542 ) ) ;
#210320=CARTESIAN_POINT ( 'NONE',  ( -8.681298431451969222, 9.022603012982438386, 1.040834085586084257E-14 ) ) ;
#210326=CARTESIAN_POINT ( 'NONE',  ( 3.948449050077836642, 5.629609863222681199, 1.599625672291267398 ) ) ;
#210331=CARTESIAN_POINT ( 'NONE',  ( -8.462260433223891098, 13.02438760540324481, -0.7998128361456281477 ) ) ;
#210335=CARTESIAN_POINT ( 'NONE',  ( -5.444063778538836829, 6.456803583937833046, -1.314021404191120901 ) ) ;
#210344=EDGE_LOOP ( 'NONE', ( #59323, #182702, #208846, #202776 ) ) ;
#210353=CARTESIAN_POINT ( 'NONE',  ( -0.7500000000000006661, 0.1395833340161536928, -1.299038105676652011 ) ) ;
#210356=CARTESIAN_POINT ( 'NONE',  ( -4.326850534687610050, 7.334764357162455894, 1.087911940796560284 ) ) ;
#210357=CARTESIAN_POINT ( 'NONE',  ( 4.227444969362701421, 3.826440640544909400, 1.214306433183764966E-14 ) ) ;
#210365=CARTESIAN_POINT ( 'NONE',  ( 5.531363484695522637, 5.555604941673978558, -0.7216878364870207285 ) ) ;
#210367=ORIENTED_EDGE ( 'NONE', *, *, #105557, .T. ) ;
#210368=CARTESIAN_POINT ( 'NONE',  ( -8.597841969360544567, 13.18256606422934674, 0.7998128361456341429 ) ) ;
#210369=LINE ( 'NONE', #63066, #17711 ) ;
#210370=CARTESIAN_POINT ( 'NONE',  ( 9.236128959407556849, 11.79856975744075598, -1.599625672291262513 ) ) ;
#210379=CARTESIAN_POINT ( 'NONE',  ( 1.364683531249986537, -0.1364583329919154264, 0.7879004041258500513 ) ) ;
#210384=CARTESIAN_POINT ( 'NONE',  ( -4.771579997005698459, 7.654261532226910525, -1.199719254218452047 ) ) ;
#210387=CARTESIAN_POINT ( 'NONE',  ( 1.499999999999985123, 0.2958333333333566517, -0.8660254037844323793 ) ) ;
#210389=CARTESIAN_POINT ( 'NONE',  ( -0.6823417656250246877, -0.8864583329919115684, 1.181850606188755259 ) ) ;
#210397=CARTESIAN_POINT ( 'NONE',  ( -0.6823417656250003738, -0.7822916663252423852, -1.181850606188749264 ) ) ;
#210399=CARTESIAN_POINT ( 'NONE',  ( -6.679363233026820446, 10.94434087183997129, 0.000000000000000000 ) ) ;
#210401=CARTESIAN_POINT ( 'NONE',  ( 8.191097360950562845, 12.70803068775103739, -0.7998128361456352531 ) ) ;
#210407=CARTESIAN_POINT ( 'NONE',  ( 1.364683531249988757, -0.05312499965857975237, 0.000000000000000000 ) ) ;
#210412=B_SPLINE_CURVE_WITH_KNOTS ( 'NONE', 1,
 ( #103181, #120575 ),
 .UNSPECIFIED., .F., .F.,
 ( 2, 2 ),
 ( 0.2143153648627435515, 0.6378831769527150142 ),
 .UNSPECIFIED. ) ;
#210415=CARTESIAN_POINT ( 'NONE',  ( 8.297226821883377568, 8.782445501726501291, -0.7216878364870267237 ) ) ;
#210419=CARTESIAN_POINT ( 'NONE',  ( 0.7499999999999920064, 5.264583334016151639, 1.299038105676669330 ) ) ;
#210421=CARTESIAN_POINT ( 'NONE',  ( -3.144601563365788444, 5.756120026313656268, -1.199719254218452935 ) ) ;
#210422=CARTESIAN_POINT ( 'NONE',  ( 4.948362878863507675, 8.716914425408678113, -0.7216878364870267237 ) ) ;
#210423=CARTESIAN_POINT ( 'NONE',  ( -8.554831740098665094, 11.00372300158037042, 1.443375672974064550 ) ) ;
#210429=CARTESIAN_POINT ( 'NONE',  ( 9.571693261567954636, 12.19006144329456731, 1.443375672974076540 ) ) ;
#210431=CARTESIAN_POINT ( 'NONE',  ( 6.471393748265543699, 5.229711127717882491, 2.420000000000010587 ) ) ;
#210446=CARTESIAN_POINT ( 'NONE',  ( 7.567422294721922960, 11.98040977715095323, 0.7998128361456462443 ) ) ;
#210451=CARTESIAN_POINT ( 'NONE',  ( 1.364683531249986537, -0.5947916663252456049, -0.7879004041258309554 ) ) ;
#210452=CARTESIAN_POINT ( 'NONE',  ( 5.666945020832177882, 6.674152614801420746, 1.082531754730558626 ) ) ;
#210454=CARTESIAN_POINT ( 'NONE',  ( -7.212574532790087645, 11.35849468832304154, -0.7216878364870267237 ) ) ;
#210475=CARTESIAN_POINT ( 'NONE',  ( 4.774589472192324102, 6.991777125168484375, -1.402305405395011251 ) ) ;
#210476=CARTESIAN_POINT ( 'NONE',  ( 1.499999999999985789, -1.099999999999982991, 0.000000000000000000 ) ) ;
#210482=CARTESIAN_POINT ( 'NONE',  ( -6.724481002698115439, 10.78905223654906109, -0.7216878364870267237 ) ) ;
#210483=AXIS2_PLACEMENT_3D ( 'NONE', #95182, #12818, #209953 ) ;
#210487=CARTESIAN_POINT ( 'NONE',  ( 5.452350330990040739, 9.512825819463730070, 0.7998128361456462443 ) ) ;
#210488=CARTESIAN_POINT ( 'NONE',  ( -4.111146893441842920, 5.819424013814012753, 1.599625672291267175 ) ) ;
#210490=CARTESIAN_POINT ( 'NONE',  ( 4.162516854595432747, 4.815023404238158555, 1.199719254218464037 ) ) ;
#210492=CARTESIAN_POINT ( 'NONE',  ( -5.111587607552082524, 5.922272616020886282, 1.199719254218450271 ) ) ;
#210496=CARTESIAN_POINT ( 'NONE',  ( -3.581325132304157943, 7.329963087663487364, -0.7998128361456281477 ) ) ;
#210500=CARTESIAN_POINT ( 'NONE',  ( 4.168242161197552420, 6.950367390450747251, -1.199719254218452047 ) ) ;
#210501=CARTESIAN_POINT ( 'NONE',  ( 7.052212457402625922, 11.37933163361175382, -0.7998128361456291469 ) ) ;
#210502=FACE_OUTER_BOUND ( 'NONE', #31017, .T. ) ;
#210504=CARTESIAN_POINT ( 'NONE',  ( 4.618624277135228162, 7.133842259902017702, 1.345135577604664512 ) ) ;
#210505=CARTESIAN_POINT ( 'NONE',  ( 3.877268743828258479, 7.467304601200877023, 0.7216878364870298324 ) ) ;
#210507=CARTESIAN_POINT ( 'NONE',  ( 5.138177029454847222, 6.057256624861201644, 1.082531754730560403 ) ) ;
#210512=CARTESIAN_POINT ( 'NONE',  ( 7.090551149822735155, 9.295395646258437949, 1.443375672974076540 ) ) ;
#210513=CARTESIAN_POINT ( 'NONE',  ( -8.402302512167102222, 10.82577223566020841, -1.599625672291263179 ) ) ;
#210517=CARTESIAN_POINT ( 'NONE',  ( -7.621654909176601045, 12.04368116068139472, 0.7998128361456481317 ) ) ;
#210518=CARTESIAN_POINT ( 'NONE',  ( -7.039708073993679704, 9.236078724457858158, 1.599625672291283607 ) ) ;
#210523=CARTESIAN_POINT ( 'NONE',  ( 1.598423149420349132, 8.713846000021357341, -2.499999999999988898 ) ) ;
#210526=CARTESIAN_POINT ( 'NONE',  ( 10.22692794340986921, 10.82583744360002243, 0.000000000000000000 ) ) ;
#210532=CARTESIAN_POINT ( 'NONE',  ( 2.659370686574860976, 6.254349567645977714, -0.7998128361456291469 ) ) ;
#210535=CARTESIAN_POINT ( 'NONE',  ( 0.7499999999999902300, 5.597916667349482900, -1.299038105676658228 ) ) ;
#210539=VERTEX_POINT ( 'NONE', #150584 ) ;
#210541=CARTESIAN_POINT ( 'NONE',  ( 1.499999999999989120, 2.525000000000020339, 1.214306433183764966E-14 ) ) ;
#210542=CARTESIAN_POINT ( 'NONE',  ( 4.798696304233017074, 7.685897223992134819, -1.199719254218452047 ) ) ;
#210545=CARTESIAN_POINT ( 'NONE',  ( 5.978782553946477840, 9.919070713005490703, 1.040834085586084257E-14 ) ) ;
#210546=CARTESIAN_POINT ( 'NONE',  ( -8.446366511189330240, 12.79791866312216442, 0.7216878364870317197 ) ) ;
#210549=CARTESIAN_POINT ( 'NONE',  ( 9.240045382913317340, 10.73880668727576015, -1.199719254218446718 ) ) ;
#210552=CARTESIAN_POINT ( 'NONE',  ( -5.427341564172148303, 5.226320001155936090, 0.000000000000000000 ) ) ;
#210553=CARTESIAN_POINT ( 'NONE',  ( 0.7499999999999902300, 5.347916667349482012, -1.299038105676658228 ) ) ;
#210554=CARTESIAN_POINT ( 'NONE',  ( -1.364683531250012516, 0.5302083336747518416, 0.7879004041258379498 ) ) ;
#210560=CARTESIAN_POINT ( 'NONE',  ( -1.402160292154681736E-14, -0.1781249996585796136, 1.575800808251672791 ) ) ;
#210569=CARTESIAN_POINT ( 'NONE',  ( -6.925517538482230506, 6.974191971184389160, 0.7998128361456341429 ) ) ;
#210572=CARTESIAN_POINT ( 'NONE',  ( 3.994848817520957773, 7.812407387083109001, 1.040834085586084257E-14 ) ) ;
#210579=ORIENTED_EDGE ( 'NONE', *, *, #59736, .T. ) ;
#210581=CARTESIAN_POINT ( 'NONE',  ( 8.238550898598388628, 12.76339314834017102, 0.7998128361456462443 ) ) ;
#210584=AXIS2_PLACEMENT_3D ( 'NONE', #115103, #185351, #20706 ) ;
#210585=CARTESIAN_POINT ( 'NONE',  ( -4.394814349124112951, 8.279033840620114049, -0.7998128361456281477 ) ) ;
#210589=CARTESIAN_POINT ( 'NONE',  ( 9.077347539549325717, 10.54899253668443393, -1.199719254218446718 ) ) ;
#210591=CARTESIAN_POINT ( 'NONE',  ( 8.938903350111612411, 9.323142084752035430, -0.7998128361456221525 ) ) ;
#210594=CARTESIAN_POINT ( 'NONE',  ( -7.998947442382709383, 12.27592974951444660, 0.7216878364870478180 ) ) ;
#210597=CARTESIAN_POINT ( 'NONE',  ( -5.520141099058386125, 9.591915048876776595, 0.000000000000000000 ) ) ;
#210601=CARTESIAN_POINT ( 'NONE',  ( -6.116367690567846793, 6.009388118678342217, 0.2715307625813894177 ) ) ;
#210602=CARTESIAN_POINT ( 'NONE',  ( -1.402160292154681736E-14, 0.5718750003414239114, 1.575800808251672791 ) ) ;
#210606=CARTESIAN_POINT ( 'NONE',  ( 6.724481002698112775, 8.868313807946373473, -1.443375672974057666 ) ) ;
#210623=CARTESIAN_POINT ( 'NONE',  ( 9.911173986789782120, 11.52179005846497972, -1.199719254218440723 ) ) ;
#210627=CARTESIAN_POINT ( 'NONE',  ( -5.271422797614987665, 5.044414773505913274, -0.7998128361456221525 ) ) ;
#210628=CARTESIAN_POINT ( 'NONE',  ( -6.561256274009600986, 9.742217188731485678, -1.199719254218440723 ) ) ;
#210633=CARTESIAN_POINT ( 'NONE',  ( 0.7499999999999920064, 4.514583334016150751, 1.299038105676669330 ) ) ;
#210634=CARTESIAN_POINT ( 'NONE',  ( 8.860417081730671995, 10.29590700256267155, 1.199719254218453823 ) ) ;
#210637=CARTESIAN_POINT ( 'NONE',  ( -6.665805079413154921, 10.92852302595736447, 0.7998128361456481317 ) ) ;
#210639=CARTESIAN_POINT ( 'NONE',  ( -1.201851678989727383E-14, 3.571875000341422357, 1.575800808251672791 ) ) ;
#210645=CARTESIAN_POINT ( 'NONE',  ( -9.381879110976678149, 11.00824238663667565, 1.082531754730558626 ) ) ;
#210649=CARTESIAN_POINT ( 'NONE',  ( -1.201851678989727383E-14, 2.384375000341416584, 1.575800808251672791 ) ) ;
#210656=CARTESIAN_POINT ( 'NONE',  ( 0.6823417656249917140, 3.592708333674754506, 1.181850606188765695 ) ) ;
#210659=CARTESIAN_POINT ( 'NONE',  ( -6.437424008390261854, 6.404749519410410485, 0.7998128361456341429 ) ) ;
#210660=CARTESIAN_POINT ( 'NONE',  ( 6.103141704446003679, 10.27208242182903142, 0.7998128361456462443 ) ) ;
#210663=CARTESIAN_POINT ( 'NONE',  ( -0.6823417656250212460, 3.863541667008085767, 1.181850606188767472 ) ) ;
#210666=CARTESIAN_POINT ( 'NONE',  ( -1.402160292154681736E-14, -0.6781249996585819728, 1.575800808251672791 ) ) ;
#210667=CARTESIAN_POINT ( 'NONE',  ( -3.795919822146283540, 6.412028311603867436, -1.082531754730549967 ) ) ;
#210670=CARTESIAN_POINT ( 'NONE',  ( 4.284013352238246419, 6.021101549076499637, -1.443375672974051449 ) ) ;
#210673=CARTESIAN_POINT ( 'NONE',  ( -6.191269702934848240, 10.37489842006599616, 0.000000000000000000 ) ) ;
#210674=CARTESIAN_POINT ( 'NONE',  ( -9.991996023591624976, 10.75967623705280296, 1.040834085586084257E-14 ) ) ;
#210676=CARTESIAN_POINT ( 'NONE',  ( 0.6823417656249899377, 4.676041667008086655, -1.181850606188754593 ) ) ;
#210680=CARTESIAN_POINT ( 'NONE',  ( -7.348156068482412095, 7.675196289425353591, 1.040834085586084257E-14 ) ) ;
#210682=CARTESIAN_POINT ( 'NONE',  ( 0.6823417656249864960, -1.011458332991911568, -1.181850606188749264 ) ) ;
#210695=CARTESIAN_POINT ( 'NONE',  ( 9.124274191872634887, 11.66807252865000244, -1.443375672974058777 ) ) ;
#210705=CARTESIAN_POINT ( 'NONE',  ( 5.717788096661236885, 7.693838750903348789, 1.599625672291267398 ) ) ;
#210706=CARTESIAN_POINT ( 'NONE',  ( -4.711622075948912247, 5.455646162483875017, -1.199719254218446718 ) ) ;
#210709=CARTESIAN_POINT ( 'NONE',  ( -4.873231614920269017, 4.964772094600380825, -0.6757755802003853063 ) ) ;
#210710=CARTESIAN_POINT ( 'NONE',  ( 0.6823417656249882723, 1.488541667008083547, -1.181850606188749264 ) ) ;
#210711=DIRECTION ( 'NONE',  ( -1.000000000000000000, 8.673617379884035472E-16, 0.000000000000000000 ) ) ;
#210712=CARTESIAN_POINT ( 'NONE',  ( -9.001723924469462901, 12.58942944760136484, -1.199719254218446718 ) ) ;
#210730=CARTESIAN_POINT ( 'NONE',  ( 6.277588818327314080, 7.282607361925381717, 1.199719254218462483 ) ) ;
#210737=CARTESIAN_POINT ( 'NONE',  ( 7.639129486296027061, 10.99973593639901814, 1.199719254218460707 ) ) ;
#210738=CARTESIAN_POINT ( 'NONE',  ( 1.499999999999990674, 8.627523663848661428, 2.579999999999999627 ) ) ;
#210740=CARTESIAN_POINT ( 'NONE',  ( 9.642873567817520808, 12.27310513391906532, 1.599625672291279388 ) ) ;
#210746=CARTESIAN_POINT ( 'NONE',  ( 8.401248741962376698, 12.95320729893149370, 0.7998128361456462443 ) ) ;
#210747=CARTESIAN_POINT ( 'NONE',  ( 4.044555541517573793, 7.746237447724527492, 0.4662041258270445132 ) ) ;
#210748=CARTESIAN_POINT ( 'NONE',  ( -0.4583599637079636691, 7.954360040267954624, 1.947354497276237550 ) ) ;
#210754=CARTESIAN_POINT ( 'NONE',  ( -7.199016379176422120, 11.34267684244042584, 0.000000000000000000 ) ) ;
#210760=CARTESIAN_POINT ( 'NONE',  ( 4.690231075323689325, 7.559354456931247412, 1.199719254218462483 ) ) ;
#210766=CARTESIAN_POINT ( 'NONE',  ( 2.684151225381301575, 6.075334163012737321, 0.000000000000000000 ) ) ;
#210769=ORIENTED_EDGE ( 'NONE', *, *, #55423, .T. ) ;
#210774=CARTESIAN_POINT ( 'NONE',  ( -7.718669524881690336, 7.899535955317097624, 0.7998128361456462443 ) ) ;
#210775=DIRECTION ( 'NONE',  ( 0.000000000000000000, -0.7999999999999999334, -0.5999999999999999778 ) ) ;
#210776=CARTESIAN_POINT ( 'NONE',  ( -5.434120640978981065, 5.234228924097238611, -0.7998128361456221525 ) ) ;
#210781=CARTESIAN_POINT ( 'NONE',  ( 0.6823417656249899377, 3.488541667008085323, -1.181850606188754593 ) ) ;
#210783=CARTESIAN_POINT ( 'NONE',  ( 7.623762449586013901, 7.788811034138823253, 1.040834085586084257E-14 ) ) ;
#210796=CARTESIAN_POINT ( 'NONE',  ( -1.402160292154681736E-14, -0.3656249996585805295, 1.575800808251672791 ) ) ;
#210797=CARTESIAN_POINT ( 'NONE',  ( 2.184835310096557404, 5.700724961754617404, 1.040834085586084257E-14 ) ) ;
#210798=CARTESIAN_POINT ( 'NONE',  ( 2.517010073631369860, 6.088262185878572375, -0.7998128361456281477 ) ) ;
#210800=CARTESIAN_POINT ( 'NONE',  ( -6.399085315970142851, 8.488685506763726352, -1.443375672974059665 ) ) ;
#210801=CARTESIAN_POINT ( 'NONE',  ( 3.877268743828266029, 6.506935386899531437, 1.082531754730558626 ) ) ;
#210802=CARTESIAN_POINT ( 'NONE',  ( -7.009202228140744673, 10.16085778526412042, -1.082531754730537088 ) ) ;
#210806=CARTESIAN_POINT ( 'NONE',  ( 5.799137018343234473, 7.788745826199009237, -1.599625672291262513 ) ) ;
#210811=CARTESIAN_POINT ( 'NONE',  ( -1.364683531250010295, 5.488541667008087543, -0.7879004041258300672 ) ) ;
#210815=CARTESIAN_POINT ( 'NONE',  ( 5.770966940911189447, 9.884545197705074671, -0.7998128361456291469 ) ) ;
#210819=CARTESIAN_POINT ( 'NONE',  ( -7.069687034522070590, 10.33538640932937724, -1.199719254218440723 ) ) ;
#210824=CARTESIAN_POINT ( 'NONE',  ( 6.753933077901968396, 11.03133902419432566, 0.7998128361456462443 ) ) ;
#210827=CARTESIAN_POINT ( 'NONE',  ( -8.064402442030170093, 8.302891025323665630, 0.7998128361456602331 ) ) ;
#210831=CARTESIAN_POINT ( 'NONE',  ( 4.626207451132414938, 6.895778996938287442, -1.211788453915439989 ) ) ;
#210832=CARTESIAN_POINT ( 'NONE',  ( -10.16825202056928390, 10.96530823352674133, 0.7216878364870438212 ) ) ;
#210834=CARTESIAN_POINT ( 'NONE',  ( -1.451998047843676476, 7.315968950353781253, 4.301760722578348073 ) ) ;
#210837=CARTESIAN_POINT ( 'NONE',  ( 5.937581207780954884, 9.014596278131406848, -1.199719254218440723 ) ) ;
#210839=CARTESIAN_POINT ( 'NONE',  ( 6.419949431270806528, 7.448694743692793274, 1.199719254218462483 ) ) ;
#210840=CARTESIAN_POINT ( 'NONE',  ( -4.047283575590383542, 7.579128156381162107, 0.3715214982176785474 ) ) ;
#210841=CARTESIAN_POINT ( 'NONE',  ( 5.183294799126148433, 4.941598775268944976, 1.040834085586084257E-14 ) ) ;
#210843=CARTESIAN_POINT ( 'NONE',  ( -5.883875478650828050, 9.808345791827219884, 0.7216878364870458196 ) ) ;
#210849=CARTESIAN_POINT ( 'NONE',  ( -5.219248474292968787, 6.450796296714536915, 1.173595342525960206 ) ) ;
#210850=CARTESIAN_POINT ( 'NONE',  ( 0.6823417656249882723, 0.2385416670080825474, -1.181850606188749264 ) ) ;
#210852=CARTESIAN_POINT ( 'NONE',  ( 1.499999999999990896, 3.306250000682818602, 1.214306433183764966E-14 ) ) ;
#210853=CARTESIAN_POINT ( 'NONE',  ( 4.853455804012216213, 6.685451076146141425, 1.443375672974062551 ) ) ;
#210857=CARTESIAN_POINT ( 'NONE',  ( -8.310784975052671442, 11.67937098999472667, -1.082531754730543083 ) ) ;
#210862=CARTESIAN_POINT ( 'NONE',  ( -8.473482818416664841, 11.86918514058604757, -1.082531754730543083 ) ) ;
#210868=VERTEX_POINT ( 'NONE', #1088 ) ;
#210869=CARTESIAN_POINT ( 'NONE',  ( -7.470179451005382276, 11.65903375957422128, 0.7216878364870458196 ) ) ;
#210873=CARTESIAN_POINT ( 'NONE',  ( -1.001543065824772872E-14, 5.384375000341415252, 1.575800808251672791 ) ) ;
#210874=CARTESIAN_POINT ( 'NONE',  ( 1.499999999999990896, 4.056250000682819490, 1.214306433183764966E-14 ) ) ;
#210875=CARTESIAN_POINT ( 'NONE',  ( 5.555833580239399438, 6.383300830698137140, -1.210397860111110946 ) ) ;
#210880=CARTESIAN_POINT ( 'NONE',  ( -7.857113714319432063, 9.125386407249497012, 1.199719254218462483 ) ) ;
#210884=CARTESIAN_POINT ( 'NONE',  ( 5.341022448779654930, 8.318611059296550536, 1.199719254218462483 ) ) ;
#210889=CARTESIAN_POINT ( 'NONE',  ( 8.097244055859613709, 10.46987070330147063, -1.599625672291262513 ) ) ;
#210896=CARTESIAN_POINT ( 'NONE',  ( -7.212574532790110737, 7.517017831117667193, -0.7216878364870278340 ) ) ;
#210902=DIRECTION ( 'NONE',  ( 0.7592566023653005702, 0.6507913734559639396, 0.000000000000000000 ) ) ;
#210905=CARTESIAN_POINT ( 'NONE',  ( -10.16591625214838679, 10.75465713712827487, 1.040834085586084257E-14 ) ) ;
#210907=CARTESIAN_POINT ( 'NONE',  ( 8.772289083241844310, 10.19309100432570148, -1.199719254218446718 ) ) ;
#210908=CARTESIAN_POINT ( 'NONE',  ( -1.500000000000013101, -0.3291666666666463459, 0.8660254037844403729 ) ) ;
#210909=CARTESIAN_POINT ( 'NONE',  ( -9.016335848287868160, 10.47781223021269170, 1.199719254218462483 ) ) ;
#210912=CARTESIAN_POINT ( 'NONE',  ( -0.6823417656250212460, 4.051041667008085767, 1.181850606188767472 ) ) ;
#210913=CARTESIAN_POINT ( 'NONE',  ( 10.54788032175191326, 11.40820791823982994, 0.7216878364870317197 ) ) ;
#210918=CARTESIAN_POINT ( 'NONE',  ( 10.01911233037457905, 11.75168114260095109, 1.082531754730548412 ) ) ;
#210921=CARTESIAN_POINT ( 'NONE',  ( -5.070386261830872598, 8.859275038870594088, 0.7216878364870458196 ) ) ;
#210922=CARTESIAN_POINT ( 'NONE',  ( 1.364683531249988757, 0.6343750003414208027, 0.000000000000000000 ) ) ;
#210926=CARTESIAN_POINT ( 'NONE',  ( -8.182509401047415309, 9.505014708432145909, 1.199719254218462483 ) ) ;
#210927=CARTESIAN_POINT ( 'NONE',  ( -3.267151830768959098, 4.834763107362302748, -1.443375672974058777 ) ) ;
#210928=CARTESIAN_POINT ( 'NONE',  ( 1.364683531249988535, 3.967708333674751842, -0.7879004041258239610 ) ) ;
#210934=CARTESIAN_POINT ( 'NONE',  ( 8.422639742587595180, 10.84949900448412130, -1.599625672291268286 ) ) ;
#210944=CARTESIAN_POINT ( 'NONE',  ( -1.419999999999997708, 8.627523663848661428, -2.579999999999990301 ) ) ;
#210948=CARTESIAN_POINT ( 'NONE',  ( -1.364683531250014514, -0.7614583329919104582, -0.7879004041258359514 ) ) ;
#210952=CARTESIAN_POINT ( 'NONE',  ( 7.422199028477372451, 10.74665040227725044, -1.199719254218441611 ) ) ;
#210954=CARTESIAN_POINT ( 'NONE',  ( -1.364683531250012516, 3.280208333674756727, 0.7879004041258379498 ) ) ;
#210956=CARTESIAN_POINT ( 'NONE',  ( -6.900736999675794792, 7.153207375817628666, 1.040834085586084257E-14 ) ) ;
#210962=CARTESIAN_POINT ( 'NONE',  ( 4.701980345841006326, 4.380065246436280368, 0.7998128361456341429 ) ) ;
#210965=CARTESIAN_POINT ( 'NONE',  ( 8.028399517586572998, 12.51821653715971472, -0.7998128361456352531 ) ) ;
#210971=CARTESIAN_POINT ( 'NONE',  ( -9.809487834687324437, 11.40315621434539395, 1.199719254218462483 ) ) ;
#210972=CARTESIAN_POINT ( 'NONE',  ( 5.282873410819217241, 9.315102745931094219, -0.7998128361456281477 ) ) ;
#210974=EDGE_CURVE ( 'NONE', #6682, #60595, #138489, .T. ) ;
#210975=CARTESIAN_POINT ( 'NONE',  ( 5.671388329218120639, 5.511041227042920099, 1.040834085586084257E-14 ) ) ;
#210976=EDGE_LOOP ( 'NONE', ( #80990, #38539, #3, #60465, #113210, #16070 ) ) ;
#210984=CARTESIAN_POINT ( 'NONE',  ( -4.758548728716557541, 8.495464583570553785, 1.040834085586084257E-14 ) ) ;
#210985=CARTESIAN_POINT ( 'NONE',  ( 4.033714395265605823, 4.664753868353354704, -1.199719254218446718 ) ) ;
#210987=ADVANCED_FACE ( 'NONE', ( #165757 ), #144838, .F. ) ;
#210989=CARTESIAN_POINT ( 'NONE',  ( -7.531718027591449705, 8.745758106066849891, 1.199719254218462483 ) ) ;
#210995=CARTESIAN_POINT ( 'NONE',  ( -8.676328237741483207, 12.20980114641871062, -1.199719254218446718 ) ) ;
#211000=CARTESIAN_POINT ( 'NONE',  ( 7.476431642932036326, 10.80992178580769014, 1.199719254218460707 ) ) ;
#211001=CARTESIAN_POINT ( 'NONE',  ( 4.625302960556422427, 8.547937220624488575, 1.040834085586084257E-14 ) ) ;
#211002=CARTESIAN_POINT ( 'NONE',  ( 3.297657676621871925, 4.870353260857385180, 1.599625672291267398 ) ) ;
#211014=CARTESIAN_POINT ( 'NONE',  ( -7.263417608619167076, 9.497073181520933716, -1.599625672291263179 ) ) ;
#211018=CARTESIAN_POINT ( 'NONE',  ( 5.477130870240836558, 9.333810415348903433, -0.7216878364870267237 ) ) ;
#211019=CARTESIAN_POINT ( 'NONE',  ( 4.220665892555866883, 3.818531717603609987, -0.7998128361456211532 ) ) ;
#211022=CARTESIAN_POINT ( 'NONE',  ( -5.280010757518168063, 8.247430752824802980, -1.199719254218446718 ) ) ;
#211030=CARTESIAN_POINT ( 'NONE',  ( 0.6823417656249899377, 3.988541667008085767, -1.181850606188754593 ) ) ;
#211031=CARTESIAN_POINT ( 'NONE',  ( 3.836594282542909795, 6.459481848733281240, 1.082531754730558626 ) ) ;
#211032=CARTESIAN_POINT ( 'NONE',  ( 7.751511138711133064, 10.06651563329490529, -1.599625672291262513 ) ) ;
#211034=CARTESIAN_POINT ( 'NONE',  ( -3.795919822146289313, 5.451659097302528068, -1.443375672974053447 ) ) ;
#211035=LINE ( 'NONE', #13903, #49567 ) ;
#211036=CARTESIAN_POINT ( 'NONE',  ( -3.267151830768946663, 6.755501535964989479, -0.7216878364870257245 ) ) ;
#211043=CARTESIAN_POINT ( 'NONE',  ( 4.220665892555866883, 3.818531717603609987, -0.7998128361456211532 ) ) ;
#211050=CARTESIAN_POINT ( 'NONE',  ( 3.948449050077836642, 5.629609863222681199, 1.599625672291267398 ) ) ;
#211056=CARTESIAN_POINT ( 'NONE',  ( 1.364683531249990311, 4.446875000341417028, 1.214306433183764966E-14 ) ) ;
#211061=CARTESIAN_POINT ( 'NONE',  ( 5.660692828905515839, 6.562895374266609849, -1.199719254218445830 ) ) ;
#211066=CARTESIAN_POINT ( 'NONE',  ( -3.588104209110990706, 7.337872010604796991, 1.040834085586084257E-14 ) ) ;
#211068=CARTESIAN_POINT ( 'NONE',  ( 5.978782553502139940, 6.077593855281705260, -0.7216878364870257245 ) ) ;
#211069=CARTESIAN_POINT ( 'NONE',  ( -0.7500000000000215383, 2.941666666666689522, 1.299038105676671107 ) ) ;
#211071=CARTESIAN_POINT ( 'NONE',  ( -5.057354993097396445, 5.859001232490445688, -1.199719254218446718 ) ) ;
#211072=CARTESIAN_POINT ( 'NONE',  ( 0.1341411654174105572, 8.212692222353361160, -2.039118504324965109 ) ) ;
#211074=CARTESIAN_POINT ( 'NONE',  ( -0.6823417656249969321, 3.967708333674754950, -1.181850606188749264 ) ) ;
#211077=CARTESIAN_POINT ( 'NONE',  ( -3.470524135418294520, 6.992769224722559684, -0.7216878364870267237 ) ) ;
#211083=CARTESIAN_POINT ( 'NONE',  ( 5.192936529234042808, 6.017179691316550283, -1.199719254218452047 ) ) ;
#211086=CARTESIAN_POINT ( 'NONE',  ( 0.1914555686804124413, 7.015040164655834687, -3.986720219540934362 ) ) ;
#211087=CARTESIAN_POINT ( 'NONE',  ( -0.6823417656250212460, 4.613541667008086655, 1.181850606188767472 ) ) ;
#211091=CARTESIAN_POINT ( 'NONE',  ( 1.364683531249986537, -0.3239583329919163424, 0.7879004041258500513 ) ) ;
#211092=LINE ( 'NONE', #149312, #191343 ) ;
#211094=CARTESIAN_POINT ( 'NONE',  ( -8.839026081105473054, 12.39961529701003684, -1.199719254218446718 ) ) ;
#211095=CARTESIAN_POINT ( 'NONE',  ( -5.707619481228814351, 9.602713794834864203, -0.7216878364870207285 ) ) ;
#211099=CARTESIAN_POINT ( 'NONE',  ( -1.201851678989727383E-14, 4.196875000341417028, -1.575800808251660134 ) ) ;
#211107=CARTESIAN_POINT ( 'NONE',  ( -5.816084710138169633, 8.768887347594400694, 1.082531754730548412 ) ) ;
#211113=CARTESIAN_POINT ( 'NONE',  ( -6.548225005276122168, 6.741943382351338165, 0.7216878364870317197 ) ) ;
#211126=CARTESIAN_POINT ( 'NONE',  ( -6.254388934605767503, 6.191208599995166040, 0.7998128361456341429 ) ) ;
#211129=CARTESIAN_POINT ( 'NONE',  ( -1.500000000000013101, 0.9208333333333594828, 0.8660254037844403729 ) ) ;
#211131=CARTESIAN_POINT ( 'NONE',  ( 8.270110514656021650, 11.63191745286530576, 1.082531754730557072 ) ) ;
#211132=CARTESIAN_POINT ( 'NONE',  ( 7.983053520348166288, 8.207983950027992748, -0.7998128361456281477 ) ) ;
#211138=CARTESIAN_POINT ( 'NONE',  ( 4.761938266897790761, 6.578680616179308771, 1.599625672291267398 ) ) ;
#211140=ORIENTED_EDGE ( 'NONE', *, *, #171813, .T. ) ;
#211146=CARTESIAN_POINT ( 'NONE',  ( -4.609409038966248318, 5.440360635957812718, -1.082531754730544860 ) ) ;
#211149=CARTESIAN_POINT ( 'NONE',  ( 3.028993686180006861, 2.741750000184225211, -2.499999999999995115 ) ) ;
#211152=CARTESIAN_POINT ( 'NONE',  ( -0.6823417656250212460, 3.551041667008085323, 1.181850606188767472 ) ) ;
#211153=CARTESIAN_POINT ( 'NONE',  ( 7.741342523278692767, 11.01502146292508044, 1.082531754730558626 ) ) ;
#211154=CARTESIAN_POINT ( 'NONE',  ( -6.714312387265696458, 8.856450423275211037, 1.599625672291283607 ) ) ;
#211157=CARTESIAN_POINT ( 'NONE',  ( 4.984594031318565932, 8.967110136513669616, 0.7998128361456462443 ) ) ;
#211158=CARTESIAN_POINT ( 'NONE',  ( -7.250913225210214641, 7.353820272367037170, 0.7998128361456341429 ) ) ;
#211162=CARTESIAN_POINT ( 'NONE',  ( -1.402160292154681736E-14, 0.1187500006828157706, -1.732050807568870754 ) ) ;
#211165=CARTESIAN_POINT ( 'NONE',  ( 5.992340707560141588, 9.934888558888093968, 0.7216878364870438212 ) ) ;
#211168=CARTESIAN_POINT ( 'NONE',  ( -1.364683531249997417, 2.571875000341422357, 1.214306433183764966E-14 ) ) ;
#211170=CARTESIAN_POINT ( 'NONE',  ( 6.602457619730771832, 6.805214765881779648, 0.7216878364870317197 ) ) ;
#211173=CARTESIAN_POINT ( 'NONE',  ( -3.958617665510279160, 5.641473247893851628, -1.443375672974053447 ) ) ;
#211175=CARTESIAN_POINT ( 'NONE',  ( -1.001543065824772872E-14, 4.571875000341418804, 1.575800808251672791 ) ) ;
#211181=CARTESIAN_POINT ( 'NONE',  ( -4.418902842294746947, 7.322973332268160718, -1.241058569461401362 ) ) ;
#211187=( BOUNDED_SURFACE ( )  B_SPLINE_SURFACE ( 1, 2, ( 
 ( #112956, #177896, #15359, #178967, #144368, #13245, #95602, #161650, #27359, #79318, #145434, #30582, #63065, #96663, #114030, #162716, #14288, #80383, #31645, #97722, #163780, #59863, #150731, #16421, #213550, #157, #164831, #84640, #115080, #182127, #53211, #147529, #135540, #2291, #119342, #169087, #68368, #201565, #134501, #52147, #50014, #116138, #3365, #185329, #65173, #36952, #131328, #98776, #82501, #67294, #33756, #148588, #200504, #85703, #132371, #151791, #66224, #198373, #181076, #99833, #165899, #17483, #199440, #103032, #83569, #118275, #81452, #149651, #1232, #133433, #197322, #48962, #51083, #69435, #32694, #117208, #183205, #34811, #100886, #166973, #18564, #184260, #19632, #35886, #101962, #168028, #5488, #38032, #8713, #137677, #22814, #123639, #87847, #186395, #173378, #71569, #187468, #4423, #70493, #55344, #140899, #91064, #20686, #7636, #203698, #105183, #170152, #104102, #120421, #205847, #153918, #121496, #21738, #24962, #156047, #40166, #108430, #86777, #138743, #39098, #56413, #171219, #106280, #204761, #202634, #88928, #42314, #89996, #172301, #136609, #23890, #206910, #154982, #57480, #107356, #54284, #122574, #6567, #72647, #152848, #188536, #73721, #139818, #189602, #157124, #41248, #74798, #58540, #190653, #124695, #209029, #146217, #126827, #159233, #194934, #27095, #211168, #110560, #46571, #192784, #109498, #12971, #176562, #11911, #111625, #174450, #125759, #28171, #62793, #94267, #175505, #44442, #210101, #61741, #160307, #127908, #77984, #162450, #144107, #193860, #161388, #177638, #45509, #191721, #112690, #93202, #60664, #29246, #95338, #130023, #80112, #79047, #145163, #128955, #178701, #30315, #212235, #10834, #96400, #14026, #143034, #63868, #76908, #196014, #47650, #26026, #92136, #158191, #9782, #75854, #141962, #207974, #59601, #43377, #99570, #966, #64924, #67031, #164568, #180812, #34556, #15098, #149384, #51891, #166703, #69167, #165634, #201301, #182940, #163512, #151528, #135287, #197061, #133168, #33497, #82238, #116940, #17222, #3097, #81187, #85443, #147265, #213297, #16153, #18294, #83299, #113761, #100627, #148329, #199168, #50814, #181861, #131073, #214329, #49749, #84380, #65961, #150467, #19363, #2028, #68097, #48699, #98506, #114813, #134232, #35618, #200241, #32438, #31381, #132110, #198118, #118014, #115876, #184003, #179765, #97457, #167766, #101696, #90804, #140642, #188272, #107098, #106022, #23636, #21478, #87587, #189347, #173121, #119078, #24702, #102771, #70235, #136348, #38836, #104919, #205585, #139558, #122315, #52941, #57222, #202369, #120157, #156868, #37768, #8454, #103840, #172043, #89744, #153659, #5228, #40987, #74542, #185059, #36684, #168826, #54018, #186133, #170960, #22560, #123382, #20430, #39913, #86513, #152578, #169889, #71302, #4165, #137415, #203434, #55088, #121237, #88665, #155793, #56153, #138481, #187207, #154725 ),
 ( #6308, #72382, #204503, #7377, #73456, #45253, #213835, #43131, #65453, #59348, #75604, #25771, #109247, #9531, #141715, #110305, #32985, #191466, #61482, #49248, #175255, #10585, #207725, #206655, #190401, #60410, #131602, #197604, #42059, #115369, #76660, #125503, #11656, #26841, #181361, #147816, #126571, #124444, #192531, #92944, #158989, #99061, #142774, #208780, #95075, #44185, #157938, #165116, #176313, #27917, #108172, #174198, #94013, #16708, #82793, #58287, #193611, #160052, #77729, #143851, #209843, #91883, #177375, #127647, #111371, #28989, #161124, #15646, #81734, #22026, #148867, #52437, #34043, #184547, #167256, #168319, #118563, #116423, #67578, #170439, #3644, #19915, #198656, #86000, #120715, #117498, #185616, #20966, #119632, #169381, #68654, #38316, #104392, #134777, #36168, #100116, #102246, #199729, #1514, #69723, #50305, #152074, #87063, #201851, #441, #200785, #66510, #135827, #182414, #186688, #132652, #17766, #53496, #37249, #183489, #103319, #153135, #166178, #83854, #149944, #133723, #51375, #35098, #4708, #70783, #101169, #136896, #18843, #202923, #54567, #2584, #84928, #151016, #3120, #54043, #118038, #20453, #187229, #52963, #36707, #34579, #51915, #68121, #168850, #203456, #136372, #2050, #199191, #200264, #150491, #70258, #100651, #167791, #38858, #50839, #121257, #202391, #104942, #154747, #120180, #170982, #186156, #37790, #35641, #101720, #55111, #22581, #116966, #88687, #182964, #84403, #134257, #119101, #185083, #71325, #153680, #103864, #67054, #137440, #184025, #19386, #166729, #85465, #18320, #151551, #69190, #86536, #169913, #135311, #152602, #201325, #4188, #155815, #107120, #157960, #206678, #176333, #126592, #58309, #59371, #9553, #141738, #75628, #44208, #73480, #191487, #43156, #189368, #124465, #139580, #109268, #190424, #173143, #42081, #175276, #207745, #108196, #125529, #6330, #172065, #74563, #26862, #140663, #7399, #24724, #174220, #25795, #8477, #91904, #92966, #208803, #41010, #205606, #159012, #10606, #57244, #76682, #123404, #89769, #39934, #90827, #23658, #156889, #142798, #110328, #60432, #192553, #27940, #94035, #72403, #138503, #204526, #188294, #106042, #209865, #61503, #160074, #11676, #77751, #143872, #175786, #157405, #144387, #94547, #76135, #74005, #10059, #141185, #173669, #210387, #58820, #158458, #44727, #8997, #107637, #160585, #207195, #108704, #140098, #206125, #190934, #62029, #12192, #156334, #143313, #124973, #26305, #91344, #25244, #41525, #127110, #75072, #42598, #174733, #78263, #77193, #27378, #29528, #7920, #59884, #92419, #191996, #142238, #93479, #126033, #123915, #208250, #177914, #11117, #159518, #57755, #209306, #128184, #43661, #193075, #28453, #189883, #109777, #60953, #110835, #176840, #194145, #45793, #111914, #50034, #83589, #116159, #182145, #149671, #51100, #213569, #48981, #199458, #181096, #1252, #183223, #161670 ) ),
 .UNSPECIFIED., .F., .F., .T. ) 
 B_SPLINE_SURFACE_WITH_KNOTS ( ( 2, 2 ),
 ( 3, 2, 2, 2, 2, 2, 2, 2, 2, 2, 2, 2, 2, 2, 2, 2, 2, 2, 2, 2, 2, 2, 2, 2, 2, 2, 2, 2, 2, 2, 2, 2, 2, 2, 2, 2, 2, 2, 2, 2, 2, 2, 2, 2, 2, 2, 2, 2, 2, 2, 2, 2, 2, 2, 2, 2, 2, 2, 2, 2, 2, 2, 2, 2, 2, 2, 2, 2, 2, 2, 2, 2, 2, 2, 2, 2, 2, 2, 2, 2, 2, 2, 2, 2, 2, 2, 2, 2, 2, 2, 2, 2, 2, 2, 2, 2, 2, 2, 2, 2, 2, 2, 2, 2, 2, 2, 2, 2, 2, 2, 2, 2, 2, 2, 2, 2, 2, 2, 2, 2, 2, 2, 2, 2, 2, 2, 2, 2, 2, 2, 2, 2, 2, 2, 2, 2, 2, 2, 2, 2, 2, 2, 2, 2, 2, 2, 2, 2, 2, 2, 2, 2, 2, 2, 2, 2, 2, 2, 2, 2, 2, 2, 2, 2, 2, 2, 2, 2, 3 ),
 ( 0.000000000000000000, 1.000000000000000000 ),
 ( 0.000000000000000000, 0.005952380952380952051, 0.01190476190476190410, 0.01785714285714285615, 0.02380952380952380820, 0.02976190476190476025, 0.03571428571428571230, 0.04166666666666666435, 0.04761904761904761640, 0.05357142857142856845, 0.05952380952380952051, 0.06547619047619047949, 0.07142857142857142461, 0.07738095238095238360, 0.08333333333333332871, 0.08928571428571428770, 0.09523809523809523281, 0.1011904761904761918, 0.1071428571428571369, 0.1130952380952380959, 0.1190476190476190410, 0.1250000000000000000, 0.1309523809523809590, 0.1369047619047619180, 0.1428571428571428492, 0.1488095238095238082, 0.1547619047619047672, 0.1607142857142857262, 0.1666666666666666574, 0.1726190476190476164, 0.1785714285714285754, 0.1845238095238095344, 0.1904761904761904656, 0.1964285714285714246, 0.2023809523809523836, 0.2083333333333333426, 0.2142857142857142738, 0.2202380952380952328, 0.2261904761904761918, 0.2321428571428571508, 0.2380952380952380820, 0.2440476190476190410, 0.2500000000000000000, 0.2559523809523809312, 0.2619047619047619180, 0.2678571428571428492, 0.2738095238095238360, 0.2797619047619047672, 0.2857142857142856984, 0.2916666666666666852, 0.2976190476190476164, 0.3035714285714285476, 0.3095238095238095344, 0.3154761904761904656, 0.3214285714285714524, 0.3273809523809523836, 0.3333333333333333148, 0.3392857142857143016, 0.3452380952380952328, 0.3511904761904761640, 0.3571428571428571508, 0.3630952380952380820, 0.3690476190476190688, 0.3750000000000000000, 0.3809523809523809312, 0.3869047619047619180, 0.3928571428571428492, 0.3988095238095238360, 0.4047619047619047672, 0.4107142857142856984, 0.4166666666666666852, 0.4226190476190476164, 0.4285714285714285476, 0.4345238095238095344, 0.4404761904761904656, 0.4464285714285714524, 0.4523809523809523836, 0.4583333333333333148, 0.4642857142857143016, 0.4702380952380952328, 0.4761904761904761640, 0.4821428571428571508, 0.4880952380952380820, 0.4940476190476190688, 0.5000000000000000000, 0.5059523809523809312, 0.5119047619047618625, 0.5178571428571429047, 0.5238095238095238360, 0.5297619047619047672, 0.5357142857142856984, 0.5416666666666666297, 0.5476190476190476719, 0.5535714285714286031, 0.5595238095238095344, 0.5654761904761904656, 0.5714285714285713969, 0.5773809523809523281, 0.5833333333333333703, 0.5892857142857143016, 0.5952380952380952328, 0.6011904761904761640, 0.6071428571428570953, 0.6130952380952381375, 0.6190476190476190688, 0.6250000000000000000, 0.6309523809523809312, 0.6369047619047618625, 0.6428571428571429047, 0.6488095238095238360, 0.6547619047619047672, 0.6607142857142856984, 0.6666666666666666297, 0.6726190476190476719, 0.6785714285714286031, 0.6845238095238095344, 0.6904761904761904656, 0.6964285714285713969, 0.7023809523809523281, 0.7083333333333333703, 0.7142857142857143016, 0.7202380952380952328, 0.7261904761904761640, 0.7321428571428570953, 0.7380952380952381375, 0.7440476190476190688, 0.7500000000000000000, 0.7559523809523809312, 0.7619047619047618625, 0.7678571428571429047, 0.7738095238095238360, 0.7797619047619047672, 0.7857142857142856984, 0.7916666666666666297, 0.7976190476190476719, 0.8035714285714286031, 0.8095238095238095344, 0.8154761904761904656, 0.8214285714285713969, 0.8273809523809523281, 0.8333333333333333703, 0.8392857142857143016, 0.8452380952380952328, 0.8511904761904761640, 0.8571428571428570953, 0.8630952380952381375, 0.8690476190476190688, 0.8750000000000000000, 0.8809523809523809312, 0.8869047619047618625, 0.8928571428571429047, 0.8988095238095238360, 0.9047619047619047672, 0.9107142857142856984, 0.9166666666666666297, 0.9226190476190476719, 0.9285714285714286031, 0.9345238095238095344, 0.9404761904761904656, 0.9464285714285713969, 0.9523809523809523281, 0.9583333333333333703, 0.9642857142857143016, 0.9702380952380952328, 0.9761904761904761640, 0.9821428571428570953, 0.9880952380952381375, 0.9940476190476190688, 1.000000000000000000 ),
 .UNSPECIFIED. ) 
 GEOMETRIC_REPRESENTATION_ITEM ( )  RATIONAL_B_SPLINE_SURFACE ( (
 ( 1.000000000000000000, 0.8660254037844387076, 1.000000000000000000, 0.8660254037844387076, 1.000000000000000000, 0.8660254037844387076, 1.000000000000000000, 0.8660254037844387076, 1.000000000000000000, 0.8660254037844387076, 1.000000000000000000, 0.8660254037844387076, 1.000000000000000000, 0.8660254037844387076, 1.000000000000000000, 0.8660254037844387076, 1.000000000000000000, 0.8660254037844387076, 1.000000000000000000, 0.8660254037844387076, 1.000000000000000000, 0.8660254037844387076, 1.000000000000000000, 0.8660254037844387076, 1.000000000000000000, 0.8660254037844387076, 1.000000000000000000, 0.8660254037844387076, 1.000000000000000000, 0.8660254037844387076, 1.000000000000000000, 0.8660254037844387076, 1.000000000000000000, 0.8660254037844387076, 1.000000000000000000, 0.8660254037844387076, 1.000000000000000000, 0.8660254037844387076, 1.000000000000000000, 0.8660254037844387076, 1.000000000000000000, 0.8660254037844387076, 1.000000000000000000, 0.8660254037844387076, 1.000000000000000000, 0.8660254037844387076, 1.000000000000000000, 0.8660254037844387076, 1.000000000000000000, 0.8660254037844387076, 1.000000000000000000, 0.8660254037844387076, 1.000000000000000000, 0.8660254037844387076, 1.000000000000000000, 0.8660254037844387076, 1.000000000000000000, 0.8660254037844387076, 1.000000000000000000, 0.8660254037844387076, 1.000000000000000000, 0.8660254037844387076, 1.000000000000000000, 0.8660254037844387076, 1.000000000000000000, 0.8660254037844387076, 1.000000000000000000, 0.8660254037844387076, 1.000000000000000000, 0.8660254037844387076, 1.000000000000000000, 0.8660254037844387076, 1.000000000000000000, 0.8660254037844387076, 1.000000000000000000, 0.8660254037844387076, 1.000000000000000000, 0.8660254037844387076, 1.000000000000000000, 0.8660254037844387076, 1.000000000000000000, 0.8660254037844387076, 1.000000000000000000, 0.8660254037844387076, 1.000000000000000000, 0.8660254037844387076, 1.000000000000000000, 0.8660254037844387076, 1.000000000000000000, 0.8660254037844387076, 1.000000000000000000, 0.8660254037844387076, 1.000000000000000000, 0.8660254037844387076, 1.000000000000000000, 0.8660254037844387076, 1.000000000000000000, 0.8660254037844387076, 1.000000000000000000, 0.8660254037844387076, 1.000000000000000000, 0.8660254037844387076, 1.000000000000000000, 0.8660254037844387076, 1.000000000000000000, 0.8660254037844387076, 1.000000000000000000, 0.8660254037844387076, 1.000000000000000000, 0.8660254037844387076, 1.000000000000000000, 0.8660254037844387076, 1.000000000000000000, 0.8660254037844387076, 1.000000000000000000, 0.8660254037844387076, 1.000000000000000000, 0.8660254037844387076, 1.000000000000000000, 0.8660254037844387076, 1.000000000000000000, 0.8660254037844387076, 1.000000000000000000, 0.8660254037844387076, 1.000000000000000000, 0.8660254037844387076, 1.000000000000000000, 0.8660254037844387076, 1.000000000000000000, 0.8660254037844387076, 1.000000000000000000, 0.8660254037844387076, 1.000000000000000000, 0.8660254037844387076, 1.000000000000000000, 0.8660254037844387076, 1.000000000000000000, 0.8660254037844387076, 1.000000000000000000, 0.8660254037844387076, 1.000000000000000000, 0.8660254037844387076, 1.000000000000000000, 0.8660254037844387076, 1.000000000000000000, 0.8660254037844387076, 1.000000000000000000, 0.8660254037844387076, 1.000000000000000000, 0.8660254037844387076, 1.000000000000000000, 0.8660254037844387076, 1.000000000000000000, 0.8660254037844387076, 1.000000000000000000, 0.8660254037844387076, 1.000000000000000000, 0.8660254037844387076, 1.000000000000000000, 0.8660254037844387076, 1.000000000000000000, 0.8660254037844387076, 1.000000000000000000, 0.8660254037844387076, 1.000000000000000000, 0.8660254037844387076, 1.000000000000000000, 0.8660254037844387076, 1.000000000000000000, 0.8660254037844387076, 1.000000000000000000, 0.8660254037844387076, 1.000000000000000000, 0.8660254037844387076, 1.000000000000000000, 0.8660254037844387076, 1.000000000000000000, 0.8660254037844387076, 1.000000000000000000, 0.8660254037844387076, 1.000000000000000000, 0.8660254037844387076, 1.000000000000000000, 0.8660254037844387076, 1.000000000000000000, 0.8660254037844387076, 1.000000000000000000, 0.8660254037844387076, 1.000000000000000000, 0.8660254037844387076, 1.000000000000000000, 0.8660254037844387076, 1.000000000000000000, 0.8660254037844387076, 1.000000000000000000, 0.8660254037844387076, 1.000000000000000000, 0.8660254037844387076, 1.000000000000000000, 0.8660254037844387076, 1.000000000000000000, 0.8660254037844387076, 1.000000000000000000, 0.8660254037844387076, 1.000000000000000000, 0.8660254037844387076, 1.000000000000000000, 0.8660254037844387076, 1.000000000000000000, 0.8660254037844387076, 1.000000000000000000, 0.8660254037844387076, 1.000000000000000000, 0.8660254037844387076, 1.000000000000000000, 0.8660254037844387076, 1.000000000000000000, 0.8660254037844387076, 1.000000000000000000, 0.8660254037844387076, 1.000000000000000000, 0.8660254037844387076, 1.000000000000000000, 0.8660254037844387076, 1.000000000000000000, 0.8660254037844387076, 1.000000000000000000, 0.8660254037844387076, 1.000000000000000000, 0.8660254037844387076, 1.000000000000000000, 0.8660254037844387076, 1.000000000000000000, 0.8660254037844387076, 1.000000000000000000, 0.8660254037844387076, 1.000000000000000000, 0.8660254037844387076, 1.000000000000000000, 0.8660254037844387076, 1.000000000000000000, 0.8660254037844387076, 1.000000000000000000, 0.8660254037844387076, 1.000000000000000000, 0.8660254037844387076, 1.000000000000000000, 0.8660254037844387076, 1.000000000000000000, 0.8660254037844387076, 1.000000000000000000, 0.8660254037844387076, 1.000000000000000000, 0.8660254037844387076, 1.000000000000000000, 0.8660254037844387076, 1.000000000000000000, 0.8660254037844387076, 1.000000000000000000, 0.8660254037844387076, 1.000000000000000000, 0.8660254037844387076, 1.000000000000000000, 0.8660254037844387076, 1.000000000000000000, 0.8660254037844387076, 1.000000000000000000, 0.8660254037844387076, 1.000000000000000000, 0.8660254037844387076, 1.000000000000000000, 0.8660254037844387076, 1.000000000000000000, 0.8660254037844387076, 1.000000000000000000, 0.8660254037844387076, 1.000000000000000000, 0.8660254037844387076, 1.000000000000000000, 0.8660254037844387076, 1.000000000000000000, 0.8660254037844387076, 1.000000000000000000, 0.8660254037844387076, 1.000000000000000000, 0.8660254037844387076, 1.000000000000000000, 0.8660254037844387076, 1.000000000000000000, 0.8660254037844387076, 1.000000000000000000, 0.8660254037844387076, 1.000000000000000000, 0.8660254037844387076, 1.000000000000000000, 0.8660254037844387076, 1.000000000000000000, 0.8660254037844387076, 1.000000000000000000, 0.8660254037844387076, 1.000000000000000000, 0.8660254037844387076, 1.000000000000000000, 0.8660254037844387076, 1.000000000000000000, 0.8660254037844387076, 1.000000000000000000, 0.8660254037844387076, 1.000000000000000000, 0.8660254037844387076, 1.000000000000000000, 0.8660254037844387076, 1.000000000000000000, 0.8660254037844387076, 1.000000000000000000, 0.8660254037844387076, 1.000000000000000000, 0.8660254037844387076, 1.000000000000000000, 0.8660254037844387076, 1.000000000000000000, 0.8660254037844387076, 1.000000000000000000, 0.8660254037844387076, 1.000000000000000000, 0.8660254037844387076, 1.000000000000000000, 0.8660254037844387076, 1.000000000000000000, 0.8660254037844387076, 1.000000000000000000, 0.8660254037844387076, 1.000000000000000000, 0.8660254037844387076, 1.000000000000000000, 0.8660254037844387076, 1.000000000000000000),
 ( 1.000000000000000000, 0.8660254037844387076, 1.000000000000000000, 0.8660254037844387076, 1.000000000000000000, 0.8660254037844387076, 1.000000000000000000, 0.8660254037844387076, 1.000000000000000000, 0.8660254037844387076, 1.000000000000000000, 0.8660254037844387076, 1.000000000000000000, 0.8660254037844387076, 1.000000000000000000, 0.8660254037844387076, 1.000000000000000000, 0.8660254037844387076, 1.000000000000000000, 0.8660254037844387076, 1.000000000000000000, 0.8660254037844387076, 1.000000000000000000, 0.8660254037844387076, 1.000000000000000000, 0.8660254037844387076, 1.000000000000000000, 0.8660254037844387076, 1.000000000000000000, 0.8660254037844387076, 1.000000000000000000, 0.8660254037844387076, 1.000000000000000000, 0.8660254037844387076, 1.000000000000000000, 0.8660254037844387076, 1.000000000000000000, 0.8660254037844387076, 1.000000000000000000, 0.8660254037844387076, 1.000000000000000000, 0.8660254037844387076, 1.000000000000000000, 0.8660254037844387076, 1.000000000000000000, 0.8660254037844387076, 1.000000000000000000, 0.8660254037844387076, 1.000000000000000000, 0.8660254037844387076, 1.000000000000000000, 0.8660254037844387076, 1.000000000000000000, 0.8660254037844387076, 1.000000000000000000, 0.8660254037844387076, 1.000000000000000000, 0.8660254037844387076, 1.000000000000000000, 0.8660254037844387076, 1.000000000000000000, 0.8660254037844387076, 1.000000000000000000, 0.8660254037844387076, 1.000000000000000000, 0.8660254037844387076, 1.000000000000000000, 0.8660254037844387076, 1.000000000000000000, 0.8660254037844387076, 1.000000000000000000, 0.8660254037844387076, 1.000000000000000000, 0.8660254037844387076, 1.000000000000000000, 0.8660254037844387076, 1.000000000000000000, 0.8660254037844387076, 1.000000000000000000, 0.8660254037844387076, 1.000000000000000000, 0.8660254037844387076, 1.000000000000000000, 0.8660254037844387076, 1.000000000000000000, 0.8660254037844387076, 1.000000000000000000, 0.8660254037844387076, 1.000000000000000000, 0.8660254037844387076, 1.000000000000000000, 0.8660254037844387076, 1.000000000000000000, 0.8660254037844387076, 1.000000000000000000, 0.8660254037844387076, 1.000000000000000000, 0.8660254037844387076, 1.000000000000000000, 0.8660254037844387076, 1.000000000000000000, 0.8660254037844387076, 1.000000000000000000, 0.8660254037844387076, 1.000000000000000000, 0.8660254037844387076, 1.000000000000000000, 0.8660254037844387076, 1.000000000000000000, 0.8660254037844387076, 1.000000000000000000, 0.8660254037844387076, 1.000000000000000000, 0.8660254037844387076, 1.000000000000000000, 0.8660254037844387076, 1.000000000000000000, 0.8660254037844387076, 1.000000000000000000, 0.8660254037844387076, 1.000000000000000000, 0.8660254037844387076, 1.000000000000000000, 0.8660254037844387076, 1.000000000000000000, 0.8660254037844387076, 1.000000000000000000, 0.8660254037844387076, 1.000000000000000000, 0.8660254037844387076, 1.000000000000000000, 0.8660254037844387076, 1.000000000000000000, 0.8660254037844387076, 1.000000000000000000, 0.8660254037844387076, 1.000000000000000000, 0.8660254037844387076, 1.000000000000000000, 0.8660254037844387076, 1.000000000000000000, 0.8660254037844387076, 1.000000000000000000, 0.8660254037844387076, 1.000000000000000000, 0.8660254037844387076, 1.000000000000000000, 0.8660254037844387076, 1.000000000000000000, 0.8660254037844387076, 1.000000000000000000, 0.8660254037844387076, 1.000000000000000000, 0.8660254037844387076, 1.000000000000000000, 0.8660254037844387076, 1.000000000000000000, 0.8660254037844387076, 1.000000000000000000, 0.8660254037844387076, 1.000000000000000000, 0.8660254037844387076, 1.000000000000000000, 0.8660254037844387076, 1.000000000000000000, 0.8660254037844387076, 1.000000000000000000, 0.8660254037844387076, 1.000000000000000000, 0.8660254037844387076, 1.000000000000000000, 0.8660254037844387076, 1.000000000000000000, 0.8660254037844387076, 1.000000000000000000, 0.8660254037844387076, 1.000000000000000000, 0.8660254037844387076, 1.000000000000000000, 0.8660254037844387076, 1.000000000000000000, 0.8660254037844387076, 1.000000000000000000, 0.8660254037844387076, 1.000000000000000000, 0.8660254037844387076, 1.000000000000000000, 0.8660254037844387076, 1.000000000000000000, 0.8660254037844387076, 1.000000000000000000, 0.8660254037844387076, 1.000000000000000000, 0.8660254037844387076, 1.000000000000000000, 0.8660254037844387076, 1.000000000000000000, 0.8660254037844387076, 1.000000000000000000, 0.8660254037844387076, 1.000000000000000000, 0.8660254037844387076, 1.000000000000000000, 0.8660254037844387076, 1.000000000000000000, 0.8660254037844387076, 1.000000000000000000, 0.8660254037844387076, 1.000000000000000000, 0.8660254037844387076, 1.000000000000000000, 0.8660254037844387076, 1.000000000000000000, 0.8660254037844387076, 1.000000000000000000, 0.8660254037844387076, 1.000000000000000000, 0.8660254037844387076, 1.000000000000000000, 0.8660254037844387076, 1.000000000000000000, 0.8660254037844387076, 1.000000000000000000, 0.8660254037844387076, 1.000000000000000000, 0.8660254037844387076, 1.000000000000000000, 0.8660254037844387076, 1.000000000000000000, 0.8660254037844387076, 1.000000000000000000, 0.8660254037844387076, 1.000000000000000000, 0.8660254037844387076, 1.000000000000000000, 0.8660254037844387076, 1.000000000000000000, 0.8660254037844387076, 1.000000000000000000, 0.8660254037844387076, 1.000000000000000000, 0.8660254037844387076, 1.000000000000000000, 0.8660254037844387076, 1.000000000000000000, 0.8660254037844387076, 1.000000000000000000, 0.8660254037844387076, 1.000000000000000000, 0.8660254037844387076, 1.000000000000000000, 0.8660254037844387076, 1.000000000000000000, 0.8660254037844387076, 1.000000000000000000, 0.8660254037844387076, 1.000000000000000000, 0.8660254037844387076, 1.000000000000000000, 0.8660254037844387076, 1.000000000000000000, 0.8660254037844387076, 1.000000000000000000, 0.8660254037844387076, 1.000000000000000000, 0.8660254037844387076, 1.000000000000000000, 0.8660254037844387076, 1.000000000000000000, 0.8660254037844387076, 1.000000000000000000, 0.8660254037844387076, 1.000000000000000000, 0.8660254037844387076, 1.000000000000000000, 0.8660254037844387076, 1.000000000000000000, 0.8660254037844387076, 1.000000000000000000, 0.8660254037844387076, 1.000000000000000000, 0.8660254037844387076, 1.000000000000000000, 0.8660254037844387076, 1.000000000000000000, 0.8660254037844387076, 1.000000000000000000, 0.8660254037844387076, 1.000000000000000000, 0.8660254037844387076, 1.000000000000000000, 0.8660254037844387076, 1.000000000000000000, 0.8660254037844387076, 1.000000000000000000, 0.8660254037844387076, 1.000000000000000000, 0.8660254037844387076, 1.000000000000000000, 0.8660254037844387076, 1.000000000000000000, 0.8660254037844387076, 1.000000000000000000, 0.8660254037844387076, 1.000000000000000000, 0.8660254037844387076, 1.000000000000000000, 0.8660254037844387076, 1.000000000000000000, 0.8660254037844387076, 1.000000000000000000, 0.8660254037844387076, 1.000000000000000000, 0.8660254037844387076, 1.000000000000000000, 0.8660254037844387076, 1.000000000000000000, 0.8660254037844387076, 1.000000000000000000, 0.8660254037844387076, 1.000000000000000000, 0.8660254037844387076, 1.000000000000000000, 0.8660254037844387076, 1.000000000000000000, 0.8660254037844387076, 1.000000000000000000, 0.8660254037844387076, 1.000000000000000000, 0.8660254037844387076, 1.000000000000000000, 0.8660254037844387076, 1.000000000000000000, 0.8660254037844387076, 1.000000000000000000, 0.8660254037844387076, 1.000000000000000000) ) ) 
 REPRESENTATION_ITEM ( '' )  SURFACE ( )  );
#211189=CARTESIAN_POINT ( 'NONE',  ( 6.551614543901692400, 8.666636272683888365, 1.599625672291281386 ) ) ;
#211192=CARTESIAN_POINT ( 'NONE',  ( 4.708759422647839976, 4.387974169377582001, -0.7998128361456211532 ) ) ;
#211201=CARTESIAN_POINT ( 'NONE',  ( 6.331294547901813452, 6.488857848747989543, 1.040834085586084257E-14 ) ) ;
#211203=CARTESIAN_POINT ( 'NONE',  ( 0.6823417656249882723, 1.988541667008083991, -1.181850606188749264 ) ) ;
#211204=CARTESIAN_POINT ( 'NONE',  ( 9.264299036839600987, 9.702770385934682551, -0.7998128361456281477 ) ) ;
#211206=CARTESIAN_POINT ( 'NONE',  ( -0.1021852871783679312, 7.053056311350174745, -4.037408415133499240 ) ) ;
#211210=CARTESIAN_POINT ( 'NONE',  ( 1.499999999999987121, 1.795833333333355819, -0.8660254037844253849 ) ) ;
#211211=CARTESIAN_POINT ( 'NONE',  ( 6.972971076130050072, 7.029554431773520129, 1.040834085586084257E-14 ) ) ;
#211212=CARTESIAN_POINT ( 'NONE',  ( -7.901704598666176693, 8.113076874732334076, 0.7998128361456602331 ) ) ;
#211216=CARTESIAN_POINT ( 'NONE',  ( -1.364683531250012516, 2.238541667008087988, -0.7879004041258289570 ) ) ;
#211217=CARTESIAN_POINT ( 'NONE',  ( -0.7500000000000215383, 3.441666666666689967, 1.299038105676671107 ) ) ;
#211220=CARTESIAN_POINT ( 'NONE',  ( 9.951321562750607086, 11.67259191370631477, -1.082531754730537088 ) ) ;
#211225=CARTESIAN_POINT ( 'NONE',  ( -1.402160292154681736E-14, 0.1187500006828157706, -1.732050807568870754 ) ) ;
#211227=CARTESIAN_POINT ( 'NONE',  ( -5.585069213825653023, 8.603332285183535433, -1.199719254218440723 ) ) ;
#211235=CARTESIAN_POINT ( 'NONE',  ( 5.392392409933256303, 7.314210449720692786, 1.599625672291267398 ) ) ;
#211238=CARTESIAN_POINT ( 'NONE',  ( 6.765682348419287173, 7.852049813699357728, 1.199719254218462483 ) ) ;
#211239=VERTEX_POINT ( 'NONE', #190512 ) ;
#211244=CARTESIAN_POINT ( 'NONE',  ( -6.170932472514347289, 10.35117165124207972, 0.000000000000000000 ) ) ;
#211245=VERTEX_POINT ( 'NONE', #107212 ) ;
#211246=CARTESIAN_POINT ( 'NONE',  ( 3.785751206713845018, 5.439795712631356750, 1.599625672291267398 ) ) ;
#211253=CARTESIAN_POINT ( 'NONE',  ( 9.049177462117294013, 12.64479190819049670, -1.199719254218446718 ) ) ;
#211254=CARTESIAN_POINT ( 'NONE',  ( 4.341180335511626964, 7.176948212357606494, 1.029809165597308063 ) ) ;
#211261=CARTESIAN_POINT ( 'NONE',  ( 7.084367489069545069E-14, 8.210952333604106812, 2.038660652713624177 ) ) ;
#211262=CARTESIAN_POINT ( 'NONE',  ( -2.819732761962335577, 5.273143408055916304, -1.082531754730543971 ) ) ;
#211263=CARTESIAN_POINT ( 'NONE',  ( 8.487040972474689582, 9.964264558384387627, -1.082531754730543083 ) ) ;
#211266=CARTESIAN_POINT ( 'NONE',  ( -5.915435094264120508, 5.795762452929912101, 0.000000000000000000 ) ) ;
#211267=CARTESIAN_POINT ( 'NONE',  ( -0.4261201057540620618, 6.933630421979442460, 3.775327195640994393 ) ) ;
#211271=CARTESIAN_POINT ( 'NONE',  ( -6.018930129462987999, 9.109503353427070849, 1.199719254218452047 ) ) ;
#211278=ORIENTED_EDGE ( 'NONE', *, *, #63234, .F. ) ;
#211287=CARTESIAN_POINT ( 'NONE',  ( -5.742041750587549842, 6.657802449562273850, 1.199719254218450271 ) ) ;
#211290=CARTESIAN_POINT ( 'NONE',  ( 3.212919216758630014, 6.692230152952963529, 0.000000000000000000 ) ) ;
#211294=CARTESIAN_POINT ( 'NONE',  ( -2.435661151949389147, 5.993355110582911038, 0.7998128361456341429 ) ) ;
#211295=CARTESIAN_POINT ( 'NONE',  ( -5.251085567194491155, 5.020688004682002159, -0.7998128361456221525 ) ) ;
#211299=CARTESIAN_POINT ( 'NONE',  ( 9.673906298550626559, 11.24497775551929557, 1.199719254218452047 ) ) ;
#211302=CARTESIAN_POINT ( 'NONE',  ( -7.340850106795412167, 10.65174332698158643, 1.199719254218453823 ) ) ;
#211303=CARTESIAN_POINT ( 'NONE',  ( 6.094553744542824170, 7.069066442510145265, 1.199719254218462483 ) ) ;
#211306=CARTESIAN_POINT ( 'NONE',  ( 3.714044015139744914, 6.420469553383295391, 1.199719254218462483 ) ) ;
#211309=CARTESIAN_POINT ( 'NONE',  ( 1.364683531249988535, 1.676041667008085101, 0.7879004041258500513 ) ) ;
#211312=CARTESIAN_POINT ( 'NONE',  ( 6.643132081016105417, 10.69414516125339887, 0.7216878364870438212 ) ) ;
#211315=CARTESIAN_POINT ( 'NONE',  ( -4.067082894419624672, 6.728385229256075739, 1.082531754730560403 ) ) ;
#211335=CARTESIAN_POINT ( 'NONE',  ( 2.889785579457926801, 6.440540434672812786, -0.3822207396134719715 ) ) ;
#211342=CARTESIAN_POINT ( 'NONE',  ( 1.499999999999989120, 1.306250000682816825, 0.000000000000000000 ) ) ;
#211348=CARTESIAN_POINT ( 'NONE',  ( -1.500000000000001332, -0.5999999999999755529, 0.000000000000000000 ) ) ;
#211349=CARTESIAN_POINT ( 'NONE',  ( 8.158255747121103241, 10.54105100977322174, 1.599625672291281386 ) ) ;
#211351=CARTESIAN_POINT ( 'NONE',  ( 4.053524740805938720, 3.831459740469437936, 1.214306433183764966E-14 ) ) ;
#211353=CIRCLE ( 'NONE', #138723, 1.250000000000000222 ) ;
#211355=CARTESIAN_POINT ( 'NONE',  ( 4.304877467538922531, 4.981110786005563007, 1.199719254218464037 ) ) ;
#211356=CARTESIAN_POINT ( 'NONE',  ( -6.127922243696855453, 7.211959374810172463, 1.082531754730549967 ) ) ;
#211360=CARTESIAN_POINT ( 'NONE',  ( -7.314787569772770226, 8.492672571945082183, -1.199719254218452935 ) ) ;
#211362=ORIENTED_EDGE ( 'NONE', *, *, #206094, .F. ) ;
#211363=CARTESIAN_POINT ( 'NONE',  ( -0.7500000000000215383, 0.9729166673494854534, 1.299038105676659116 ) ) ;
#211370=CARTESIAN_POINT ( 'NONE',  ( -3.917943204224928699, 4.633650495426258509, -1.082531754730548412 ) ) ;
#211372=CARTESIAN_POINT ( 'NONE',  ( 4.532311885504772597, 6.983620743164907552, 1.170841521963662091 ) ) ;
#211377=CARTESIAN_POINT ( 'NONE',  ( -10.31505594189871111, 10.92865344183699428, -0.7998128361456291469 ) ) ;
#211378=CARTESIAN_POINT ( 'NONE',  ( 8.446893396513862839, 9.813462703143045474, -1.199719254218445830 ) ) ;
#211386=CARTESIAN_POINT ( 'NONE',  ( -6.997979842947967377, 11.31606025008131233, -0.7998128361456291469 ) ) ;
#211391=CARTESIAN_POINT ( 'NONE',  ( 3.571683402196252910, 6.254382171615883834, 1.199719254218462483 ) ) ;
#211397=CARTESIAN_POINT ( 'NONE',  ( -9.622536337397040285, 12.24937836509514710, 1.599625672291281386 ) ) ;
#211418=CARTESIAN_POINT ( 'NONE',  ( 1.499999999999987121, 0.07708333401615156955, -0.8660254037844323793 ) ) ;
#211423=CARTESIAN_POINT ( 'NONE',  ( 3.083589872104280705, 5.684939719841914929, 1.199719254218450271 ) ) ;
#211425=CARTESIAN_POINT ( 'NONE',  ( -4.243865776277440993, 4.909930479533815451, -1.199719254218446718 ) ) ;
#211431=CARTESIAN_POINT ( 'NONE',  ( 5.666945020832181434, 5.713783400500082266, 0.7216878364870317197 ) ) ;
#211434=CARTESIAN_POINT ( 'NONE',  ( -10.08065090696061716, 11.71951313199760136, -1.199719254218441611 ) ) ;
#211436=CARTESIAN_POINT ( 'NONE',  ( 8.615316546479974136, 12.13862083994696839, 1.199719254218450271 ) ) ;
#211444=CARTESIAN_POINT ( 'NONE',  ( -0.6823417656250246877, -0.9489583329919115684, 1.181850606188755259 ) ) ;
#211448=CARTESIAN_POINT ( 'NONE',  ( -4.042302355168801320, 7.867769847672247074, 0.7998128361456341429 ) ) ;
#211452=CARTESIAN_POINT ( 'NONE',  ( -0.7499999999999972244, 5.108333333333353821, -1.299038105676652011 ) ) ;
#211459=CARTESIAN_POINT ( 'NONE',  ( -1.364683531250010295, 5.592708333674750953, 0.7879004041258379498 ) ) ;
#211461=CARTESIAN_POINT ( 'NONE',  ( 6.799577732453452761, 7.891594428405881878, -1.199719254218446718 ) ) ;
#211462=CARTESIAN_POINT ( 'NONE',  ( -7.609150525767646833, 9.900428251527500834, -1.599625672291263179 ) ) ;
#211465=VECTOR ( 'NONE', #214051, 1000.000000000000000 ) ;
#211466=CARTESIAN_POINT ( 'NONE',  ( 0.000000000000000000, 8.600000000000017408, 0.4000000000000045186 ) ) ;
#211470=CARTESIAN_POINT ( 'NONE',  ( 1.499999999999989120, 5.545833333333350268, -0.8660254037844323793 ) ) ;
#211478=CARTESIAN_POINT ( 'NONE',  ( 6.453317930424781856, 10.47269531889685545, -0.7216878364870267237 ) ) ;
#211482=CARTESIAN_POINT ( 'NONE',  ( -0.7499999999999972244, 4.639583334016150751, -1.299038105676652899 ) ) ;
#211484=CARTESIAN_POINT ( 'NONE',  ( -4.600294193738529103, 4.261431402316699035, -0.7998128361456221525 ) ) ;
#211485=CARTESIAN_POINT ( 'NONE',  ( 7.280365300414074703, 7.596107060012304402, -0.7216878364870257245 ) ) ;
#211486=CARTESIAN_POINT ( 'NONE',  ( -10.10046125205659173, 10.88621900359527572, -0.7216878364870267237 ) ) ;
#211492=CARTESIAN_POINT ( 'NONE',  ( 9.788623719386617239, 11.48277776311499387, -1.082531754730537088 ) ) ;
#211496=CARTESIAN_POINT ( 'NONE',  ( 4.379447312414087357, 5.068108938359919158, -1.199719254218452047 ) ) ;
#211500=EDGE_LOOP ( 'NONE', ( #12242, #22631, #27614, #4522 ) ) ;
#211511=CARTESIAN_POINT ( 'NONE',  ( 9.023114925094663619, 10.48572115315399245, 1.199719254218453823 ) ) ;
#211514=CARTESIAN_POINT ( 'NONE',  ( 0.6823417656249882723, 0.09270833367475139752, 1.181850606188755259 ) ) ;
#211515=CARTESIAN_POINT ( 'NONE',  ( 4.012850279964918165, 7.625483060026979842, -0.7216878364870197293 ) ) ;
#211516=EDGE_CURVE ( 'NONE', #197417, #34146, #161969, .T. ) ;
#211517=CARTESIAN_POINT ( 'NONE',  ( -9.666600336863641729, 10.38004793587015584, 1.040834085586084257E-14 ) ) ;
#211522=CARTESIAN_POINT ( 'NONE',  ( -3.903858165731105778, 6.641919395739846799, 1.199719254218464037 ) ) ;
#211528=ORIENTED_EDGE ( 'NONE', *, *, #127807, .F. ) ;
#211536=CARTESIAN_POINT ( 'NONE',  ( 5.071574956294766068, 6.743279210435389359, -1.418366213760638317 ) ) ;
#211541=CARTESIAN_POINT ( 'NONE',  ( 1.500000000000007105, 10.64264068711930733, 1.214306433183764966E-14 ) ) ;
#211544=CARTESIAN_POINT ( 'NONE',  ( -8.026063749610061748, 9.426457798375635022, -1.082531754730543971 ) ) ;
#211548=CARTESIAN_POINT ( 'NONE',  ( 5.276094334012385367, 9.307193822989793475, 1.040834085586084257E-14 ) ) ;
#211549=AXIS2_PLACEMENT_3D ( 'NONE', #35139, #199772, #68697 ) ;
#211550=CARTESIAN_POINT ( 'NONE',  ( -5.122283107864663343, 4.870418468797203637, 0.000000000000000000 ) ) ;
#211551=ADVANCED_FACE ( 'NONE', ( #76764, #48556 ), #195861, .F. ) ;
#211553=CARTESIAN_POINT ( 'NONE',  ( -5.773074481320628948, 5.629675071162500544, 0.000000000000000000 ) ) ;
#211554=FACE_OUTER_BOUND ( 'NONE', #64388, .T. ) ;
#211556=CARTESIAN_POINT ( 'NONE',  ( -4.557512192488103686, 8.468847991211438497, -0.7998128361456281477 ) ) ;
#211559=CARTESIAN_POINT ( 'NONE',  ( 6.726816770674637347, 10.99970333242910669, -0.7998128361456291469 ) ) ;
#211560=CARTESIAN_POINT ( 'NONE',  ( 1.499999999999990896, 3.556250000682818602, 1.214306433183764966E-14 ) ) ;
#211562=CARTESIAN_POINT ( 'NONE',  ( 4.650497622768338779, 7.104022005431295916, 1.360104839701151480 ) ) ;
#211564=CARTESIAN_POINT ( 'NONE',  ( 4.853455804012222430, 5.725081861844796727, 1.082531754730560403 ) ) ;
#211571=CARTESIAN_POINT ( 'NONE',  ( 7.307481607641395094, 8.588111966078864512, -1.082531754730537976 ) ) ;
#211574=CARTESIAN_POINT ( 'NONE',  ( -8.109748439268576803, 12.61312361245537517, 0.7998128361456481317 ) ) ;
#211575=CARTESIAN_POINT ( 'NONE',  ( -7.552055258011950656, 8.769484874890757453, 1.199719254218462483 ) ) ;
#211580=CARTESIAN_POINT ( 'NONE',  ( 1.519536625744590363, 8.761901799250125578, -2.483436355453708444 ) ) ;
#211583=CARTESIAN_POINT ( 'NONE',  ( 9.023114925094663619, 10.48572115315399245, 1.199719254218453823 ) ) ;
#211587=CARTESIAN_POINT ( 'NONE',  ( 4.033714395265605823, 4.664753868353354704, -1.199719254218446718 ) ) ;
#211590=CARTESIAN_POINT ( 'NONE',  ( 1.499999999999989120, 5.077083334016151639, -0.8660254037844323793 ) ) ;
#211596=CARTESIAN_POINT ( 'NONE',  ( -1.499999999999997780, 3.400000000000021227, 1.214306433183764966E-14 ) ) ;
#211597=CARTESIAN_POINT ( 'NONE',  ( 5.660692828905515839, 6.562895374266609849, -1.199719254218445830 ) ) ;
#211600=CARTESIAN_POINT ( 'NONE',  ( 7.971831135155394321, 8.402817200543854170, -0.7216878364870267237 ) ) ;
#211601=CARTESIAN_POINT ( 'NONE',  ( 0.2863318758520314034, 8.150007921796387222, 2.019927845748587192 ) ) ;
#211605=CARTESIAN_POINT ( 'NONE',  ( 9.083072846151447166, 12.68433652289702884, 1.199719254218450271 ) ) ;
#211608=CARTESIAN_POINT ( 'NONE',  ( -2.903417451620861289, 6.539070793532962611, 0.7998128361456341429 ) ) ;
#211609=CARTESIAN_POINT ( 'NONE',  ( -1.201851678989727383E-14, 5.368750000682816825, -1.732050807568863648 ) ) ;
#211610=CARTESIAN_POINT ( 'NONE',  ( 1.364683531249988535, 1.363541667008083769, 0.7879004041258500513 ) ) ;
#211614=CARTESIAN_POINT ( 'NONE',  ( 4.684505768721569652, 5.424010470718658716, -1.199719254218452047 ) ) ;
#211616=CARTESIAN_POINT ( 'NONE',  ( 0.6823417656249899377, 4.988541667008086655, -1.181850606188754593 ) ) ;
#211618=CARTESIAN_POINT ( 'NONE',  ( 4.051913702378651116, 7.757429176960653372, 0.5075685776039747799 ) ) ;
#211621=EDGE_CURVE ( 'NONE', #110521, #78570, #69355, .T. ) ;
#211626=CARTESIAN_POINT ( 'NONE',  ( -7.389357414647957256, 8.579670724299436557, 1.199719254218450271 ) ) ;
#211629=CARTESIAN_POINT ( 'NONE',  ( 4.143988507271280319, 7.986403691791820414, -0.7998128361456221525 ) ) ;
#211635=CARTESIAN_POINT ( 'NONE',  ( 9.856941372335116469, 11.45851867493453291, 1.199719254218450271 ) ) ;
#211638=CARTESIAN_POINT ( 'NONE',  ( -5.850506979496850057, 6.784345216623154151, -1.199719254218446718 ) ) ;
#211643=CARTESIAN_POINT ( 'NONE',  ( 7.377608144130607393, 11.75895993479440982, -0.7998128361456291469 ) ) ;
#211645=CARTESIAN_POINT ( 'NONE',  ( 7.914208982075123799, 10.25632978388623684, -1.599625672291262513 ) ) ;
#211646=CARTESIAN_POINT ( 'NONE',  ( 4.890372329093504611, 4.905069069454044417, -0.7147567316251844938 ) ) ;
#211648=CARTESIAN_POINT ( 'NONE',  ( -10.16825202056928390, 10.96530823352674133, 0.7216878364870438212 ) ) ;
#211649=CARTESIAN_POINT ( 'NONE',  ( -5.910464900553636269, 8.982960586366182554, -1.199719254218440723 ) ) ;
#211653=CARTESIAN_POINT ( 'NONE',  ( -6.048854636777848626, 6.051613005247792998, 0.5441514604978964220 ) ) ;
#211654=CARTESIAN_POINT ( 'NONE',  ( 0.6823417656249899377, 0.8427083336747520637, 1.181850606188755259 ) ) ;
#211657=CARTESIAN_POINT ( 'NONE',  ( 8.107412671292047790, 8.560995659369956101, 0.7216878364870458196 ) ) ;
#211660=EDGE_CURVE ( 'NONE', #54687, #188383, #30160, .T. ) ;
#211661=EDGE_CURVE ( 'NONE', #73877, #3975, #177484, .T. ) ;
#211672=DIRECTION ( 'NONE',  ( 5.578564026256490882E-16, 1.000000000000000000, 9.066213480720158442E-32 ) ) ;
#211675=EDGE_CURVE ( 'NONE', #6901, #197417, #126679, .T. ) ;
#211677=CARTESIAN_POINT ( 'NONE',  ( 10.40996301719436090, 11.03937836301526687, 0.000000000000000000 ) ) ;
#211681=CARTESIAN_POINT ( 'NONE',  ( -2.462777459176719308, 6.024990802348131780, -0.7998128361456281477 ) ) ;
#211682=CARTESIAN_POINT ( 'NONE',  ( -6.832419346282942563, 10.05857410638369487, 1.199719254218453823 ) ) ;
#211688=CARTESIAN_POINT ( 'NONE',  ( 1.499999999999989120, 4.327083334016148086, -0.8660254037844323793 ) ) ;
#211689=CARTESIAN_POINT ( 'NONE',  ( 7.065770611016287006, 11.39514947949436774, 1.040834085586084257E-14 ) ) ;
#211693=CARTESIAN_POINT ( 'NONE',  ( -8.636707547105197946, 10.03491254549959777, -1.199719254218446718 ) ) ;
#211695=CARTESIAN_POINT ( 'NONE',  ( -1.364683531250012516, 2.988541667008091096, -0.7879004041258289570 ) ) ;
#211701=CARTESIAN_POINT ( 'NONE',  ( -7.863365906246048809, 12.11775129068834289, -0.7216878364870267237 ) ) ;
#211705=CARTESIAN_POINT ( 'NONE',  ( -1.201851678989727383E-14, 1.134375000341418582, 1.575800808251672791 ) ) ;
#211712=CARTESIAN_POINT ( 'NONE',  ( 1.364683531249988535, 3.113541667008083991, 0.7879004041258500513 ) ) ;
#211714=CARTESIAN_POINT ( 'NONE',  ( -4.415151579544611238, 8.302760609444034046, -0.7998128361456281477 ) ) ;
#211715=CARTESIAN_POINT ( 'NONE',  ( 6.642605195691581699, 9.837124264027149678, 1.199719254218462483 ) ) ;
#211719=CARTESIAN_POINT ( 'NONE',  ( -1.364683531250012516, 2.801041667008090652, -0.7879004041258289570 ) ) ;
#211722=CARTESIAN_POINT ( 'NONE',  ( 0.6823417656249882723, -0.3239583329919110133, -1.181850606188749264 ) ) ;
#211723=CARTESIAN_POINT ( 'NONE',  ( -5.422898255786198440, 7.349800603215774331, -1.443375672974052559 ) ) ;
#211727=CARTESIAN_POINT ( 'NONE',  ( 4.528060117284229413, 7.266191989264828344, 1.082531754730558626 ) ) ;
#211730=CARTESIAN_POINT ( 'NONE',  ( -6.679363233026820446, 10.94434087183997129, 0.000000000000000000 ) ) ;
#211731=CARTESIAN_POINT ( 'NONE',  ( -2.656508033273816238, 5.186677574539687363, -1.199719254218446718 ) ) ;
#211733=CARTESIAN_POINT ( 'NONE',  ( -1.364683531249997417, 5.759375000341418804, 1.214306433183764966E-14 ) ) ;
#211738=CARTESIAN_POINT ( 'NONE',  ( -6.358410854684789726, 8.441231968597481483, -1.443375672974058777 ) ) ;
#211740=CARTESIAN_POINT ( 'NONE',  ( -1.364683531250014514, -0.1572916663252435232, 0.7879004041258379498 ) ) ;
#211743=AXIS2_PLACEMENT_3D ( 'NONE', #203189, #116684, #199994 ) ;
#211744=CARTESIAN_POINT ( 'NONE',  ( 7.212574532790092974, 9.437756259720353924, -1.443375672974057666 ) ) ;
#211753=CARTESIAN_POINT ( 'NONE',  ( -1.500000000000015099, -0.3708333333333105331, -0.8660254037844383745 ) ) ;
#211754=CARTESIAN_POINT ( 'NONE',  ( 9.693716643646601128, 10.41168362711695750, 0.7216878364870438212 ) ) ;
#211760=CARTESIAN_POINT ( 'NONE',  ( 6.810273232766058449, 6.839740281182199233, 1.040834085586084257E-14 ) ) ;
#211762=CARTESIAN_POINT ( 'NONE',  ( -3.066115294984855133, 6.728884944124295053, 0.7998128361456341429 ) ) ;
#211766=CARTESIAN_POINT ( 'NONE',  ( 4.961921032477176752, 8.732732271291288484, 1.040834085586084257E-14 ) ) ;
#211767=CARTESIAN_POINT ( 'NONE',  ( 0.6823417656249882723, -0.01145833299191073573, -1.181850606188749264 ) ) ;
#211769=CARTESIAN_POINT ( 'NONE',  ( -9.592557376868645846, 11.15007068022363157, -1.199719254218441611 ) ) ;
#211778=EDGE_LOOP ( 'NONE', ( #131818, #75930, #192013, #175099 ) ) ;
#211784=CARTESIAN_POINT ( 'NONE',  ( 2.292764405579248876, 5.531449493117344574, 0.4111059650438048663 ) ) ;
#211788=CARTESIAN_POINT ( 'NONE',  ( 4.971035877704902184, 8.951292290631053916, 1.040834085586084257E-14 ) ) ;
#211793=AXIS2_PLACEMENT_3D ( 'NONE', #2204, #132281, #98685 ) ;
#211795=CARTESIAN_POINT ( 'NONE',  ( 8.718056468787178659, 10.12981962079525289, 1.199719254218462483 ) ) ;
#211799=CARTESIAN_POINT ( 'NONE',  ( 8.211434591371064684, 12.73175745657494851, -0.7998128361456352531 ) ) ;
#211801=CARTESIAN_POINT ( 'NONE',  ( -2.117044542028253318, 5.621635732341564662, -0.7998128361456281477 ) ) ;
#211804=CARTESIAN_POINT ( 'NONE',  ( 9.103410076571945453, 12.70806329172093818, 1.199719254218450271 ) ) ;
#211805=CARTESIAN_POINT ( 'NONE',  ( -0.006158830626143650504, 7.078243236992579845, 2.121324627965421872 ) ) ;
#211812=CARTESIAN_POINT ( 'NONE',  ( -7.687109909268394325, 11.91211929421440097, 0.000000000000000000 ) ) ;
#211816=CARTESIAN_POINT ( 'NONE',  ( 6.148786358997489820, 7.132337826040578754, -1.199719254218446718 ) ) ;
#211822=CARTESIAN_POINT ( 'NONE',  ( 5.951666246274807115, 6.045958163516475636, 0.7216878364870317197 ) ) ;
#211830=CARTESIAN_POINT ( 'NONE',  ( -7.393273838153706201, 7.519907654134449615, 0.7998128361456341429 ) ) ;
#211831=CARTESIAN_POINT ( 'NONE',  ( -3.601662362724658895, 7.353689856487406473, -0.7998128361456281477 ) ) ;
#211839=CARTESIAN_POINT ( 'NONE',  ( 7.461064606222022277, 7.598996883547496139, 1.040834085586084257E-14 ) ) ;
#211852=CARTESIAN_POINT ( 'NONE',  ( 5.463572716182826028, 5.476515711742510284, 0.7216878364870371598 ) ) ;
#211855=CARTESIAN_POINT ( 'NONE',  ( -0.6823417656250246877, -0.6364583329919113464, 1.181850606188755259 ) ) ;
#211857=CARTESIAN_POINT ( 'NONE',  ( 5.005985031943777308, 6.863401842066294556, -1.599625672291256295 ) ) ;
#211859=CARTESIAN_POINT ( 'NONE',  ( -5.883875478650828050, 9.808345791827219884, 0.7216878364870458196 ) ) ;
#211860=CARTESIAN_POINT ( 'NONE',  ( 5.233084105194869551, 6.167981546557892436, -1.082531754730548412 ) ) ;
#211861=CARTESIAN_POINT ( 'NONE',  ( -7.687109908824056426, 8.070642436490613747, 0.7216878364870438212 ) ) ;
#211863=ORIENTED_EDGE ( 'NONE', *, *, #189986, .F. ) ;
#211865=CARTESIAN_POINT ( 'NONE',  ( 4.611744806942754238, 8.532119374741881757, -0.7998128361456231517 ) ) ;
#211870=CARTESIAN_POINT ( 'NONE',  ( 1.364683531249990311, 4.863541667008084879, 0.7879004041258500513 ) ) ;
#211875=CARTESIAN_POINT ( 'NONE',  ( 6.988338112840064120, 10.24047933403371502, 1.199719254218460707 ) ) ;
#211879=CARTESIAN_POINT ( 'NONE',  ( -6.692921386640485082, 10.96015871772258521, -0.7998128361456291469 ) ) ;
#211884=CARTESIAN_POINT ( 'NONE',  ( 9.725276259704228821, 10.24057714594344048, 0.7998128361456462443 ) ) ;
#211887=CARTESIAN_POINT ( 'NONE',  ( -6.364663046611467756, 9.512858423433634414, 1.199719254218452047 ) ) ;
#211891=CARTESIAN_POINT ( 'NONE',  ( 4.708705726121224622, 6.822254573549790813, -1.234111767277449534 ) ) ;
#211892=CARTESIAN_POINT ( 'NONE',  ( -8.012505595996376684, 12.29174759539704986, 0.000000000000000000 ) ) ;
#211898=CARTESIAN_POINT ( 'NONE',  ( 4.801558957534076022, 8.753569217098425170, 0.7998128361456462443 ) ) ;
#211900=CARTESIAN_POINT ( 'NONE',  ( 6.257251587906815793, 7.258880593101466161, 1.199719254218462483 ) ) ;
#211901=CARTESIAN_POINT ( 'NONE',  ( -4.145011909418054863, 7.447386798385191575, 0.7030492056920457644 ) ) ;
#211902=CARTESIAN_POINT ( 'NONE',  ( 2.347533153460546806, 5.890539112345938300, 0.000000000000000000 ) ) ;
#211904=CARTESIAN_POINT ( 'NONE',  ( -7.388830529767770550, 7.722649827591604677, 1.040834085586084257E-14 ) ) ;
#211909=CARTESIAN_POINT ( 'NONE',  ( -4.916288619803077964, 6.680904680207828683, 1.249144131323683515 ) ) ;
#211910=CARTESIAN_POINT ( 'NONE',  ( 1.364683531249986537, 0.4260416670080872659, 0.7879004041258500513 ) ) ;
#211913=CARTESIAN_POINT ( 'NONE',  ( 3.063779527008304360, 6.518233848244248563, 0.7216878364870317197 ) ) ;
#211914=EDGE_CURVE ( 'NONE', #85368, #92250, #9180, .T. ) ;
#211919=CARTESIAN_POINT ( 'NONE',  ( -8.283668667825340393, 12.60810451253083997, 0.7216878364870458196 ) ) ;
#211925=CARTESIAN_POINT ( 'NONE',  ( -8.229436053370685400, 10.62409470039771442, 1.443375672974090751 ) ) ;
#211926=CARTESIAN_POINT ( 'NONE',  ( 1.419999999999989049, 6.200000000000045475, -2.899999999999995470 ) ) ;
#211932=CARTESIAN_POINT ( 'NONE',  ( -7.158341917891067219, 11.29522330427417565, 0.000000000000000000 ) ) ;
#211936=CARTESIAN_POINT ( 'NONE',  ( -1.364683531249997417, 5.321875000341417916, 1.214306433183764966E-14 ) ) ;
#211937=CARTESIAN_POINT ( 'NONE',  ( 1.499999999999989120, 4.577083334016148974, -0.8660254037844323793 ) ) ;
#211938=CARTESIAN_POINT ( 'NONE',  ( 5.071574956294766068, 6.743279210435389359, -1.418366213760638317 ) ) ;
#211943=CARTESIAN_POINT ( 'NONE',  ( -6.333630315878337136, 10.54098580183340772, 0.000000000000000000 ) ) ;
#211946=CARTESIAN_POINT ( 'NONE',  ( 4.961394147597008697, 7.875711374583454827, -1.199719254218452047 ) ) ;
#211947=AXIS2_PLACEMENT_3D ( 'NONE', #210476, #114136, #29616 ) ;
#211952=CARTESIAN_POINT ( 'NONE',  ( 7.422199028477372451, 10.74665040227725044, -1.199719254218441611 ) ) ;
#211957=CARTESIAN_POINT ( 'NONE',  ( -5.260200412422196159, 9.080724881227137502, -0.7216878364870207285 ) ) ;
#211960=CARTESIAN_POINT ( 'NONE',  ( -0.7500000000000006661, 3.139583334016149418, -1.299038105676652011 ) ) ;
#211966=CARTESIAN_POINT ( 'NONE',  ( -8.992082194361570302, 11.51384853155376220, 1.599625672291269396 ) ) ;
#211968=CARTESIAN_POINT ( 'NONE',  ( 9.582915646760733708, 10.07448976417602893, 0.7998128361456462443 ) ) ;
#211970=CARTESIAN_POINT ( 'NONE',  ( -8.748035429315585532, 11.22912730566677553, -1.599625672291263179 ) ) ;
#211973=CARTESIAN_POINT ( 'NONE',  ( -1.201851678989727383E-14, 3.446875000341421469, -1.575800808251660134 ) ) ;
#211974=CARTESIAN_POINT ( 'NONE',  ( 2.737856954955798727, 5.281584649835344258, 1.199719254218452047 ) ) ;
#211980=CARTESIAN_POINT ( 'NONE',  ( 8.202319746143333035, 12.51319743723517952, -0.7216878364870328300 ) ) ;
#211983=CARTESIAN_POINT ( 'NONE',  ( -6.643132081016132062, 8.773406732650713025, 1.443375672974078761 ) ) ;
#211984=CARTESIAN_POINT ( 'NONE',  ( -0.6823417656250212460, 0.8010416670080899859, 1.181850606188755259 ) ) ;
#211986=DIRECTION ( 'NONE',  ( 0.000000000000000000, 8.546850786086437571E-32, 1.000000000000000000 ) ) ;
#211988=CARTESIAN_POINT ( 'NONE',  ( -7.857113714319432063, 9.125386407249497012, 1.199719254218462483 ) ) ;
#211989=CARTESIAN_POINT ( 'NONE',  ( -4.907688418022547516, 4.827984030555475314, 1.214306433183764966E-14 ) ) ;
#211990=CARTESIAN_POINT ( 'NONE',  ( -1.364683531250012516, 3.342708333674756727, 0.7879004041258379498 ) ) ;
#212007=DIRECTION ( 'NONE',  ( 0.6507913734559640506, -0.7592566023653004592, 0.000000000000000000 ) ) ;
#212009=CARTESIAN_POINT ( 'NONE',  ( -0.6823417656249969321, 3.780208333674754506, -1.181850606188749264 ) ) ;
#212013=CARTESIAN_POINT ( 'NONE',  ( 7.151035956204054855, 10.43029348462504124, 1.199719254218460707 ) ) ;
#212015=CARTESIAN_POINT ( 'NONE',  ( 1.364683531249988535, 3.155208333674756283, -0.7879004041258239610 ) ) ;
#212017=CARTESIAN_POINT ( 'NONE',  ( -7.375272376154096143, 8.667201196010339004, -1.082531754730544860 ) ) ;
#212024=CARTESIAN_POINT ( 'NONE',  ( 2.703961570921634028, 5.242040035128820108, -1.199719254218446718 ) ) ;
#212027=CARTESIAN_POINT ( 'NONE',  ( 8.353795204314554468, 12.89784483834236184, -0.7998128361456352531 ) ) ;
#212030=CIRCLE ( 'NONE', #21848, 1.500000000000000222 ) ;
#212034=CARTESIAN_POINT ( 'NONE',  ( -10.47097470845587175, 11.11055866948701443, 1.040834085586084257E-14 ) ) ;
#212035=CARTESIAN_POINT ( 'NONE',  ( 6.421758314367153275, 10.64380180007036891, -0.7998128361456291469 ) ) ;
#212050=CARTESIAN_POINT ( 'NONE',  ( -6.155038550924159857, 8.203964280876741455, 1.443375672974078761 ) ) ;
#212051=CARTESIAN_POINT ( 'NONE',  ( 3.822509244049070887, 6.547012320444182798, -1.199719254218452047 ) ) ;
#212054=CARTESIAN_POINT ( 'NONE',  ( -7.808606406466886973, 11.19745900993164511, 1.199719254218453823 ) ) ;
#212058=CARTESIAN_POINT ( 'NONE',  ( -9.459838494033043332, 12.05956421450382088, 1.599625672291281386 ) ) ;
#212060=DIRECTION ( 'NONE',  ( -5.578564026256490882E-16, -1.000000000000000000, -9.066213480720158442E-32 ) ) ;
#212062=CARTESIAN_POINT ( 'NONE',  ( 7.560643217915098191, 11.97250085420964716, -0.7998128361456291469 ) ) ;
#212064=CARTESIAN_POINT ( 'NONE',  ( 7.334597915313080918, 9.580116872663850813, 1.040834085586084257E-14 ) ) ;
#212074=CARTESIAN_POINT ( 'NONE',  ( -7.486073373039941359, 11.88550270185529278, -0.7998128361456291469 ) ) ;
#212078=CARTESIAN_POINT ( 'NONE',  ( 6.751597309925441159, 9.860318714012938912, -1.082531754730537088 ) ) ;
#212081=CARTESIAN_POINT ( 'NONE',  ( 3.765413976293345844, 5.416068943807445635, 1.599625672291267398 ) ) ;
#212084=CARTESIAN_POINT ( 'NONE',  ( -6.413170354464012846, 7.440785820751486312, 1.199719254218450271 ) ) ;
#212094=CARTESIAN_POINT ( 'NONE',  ( -1.364683531249997417, 4.071875000341417028, 1.214306433183764966E-14 ) ) ;
#212095=CARTESIAN_POINT ( 'NONE',  ( 3.697672731465083462, 7.367968498737613281, 2.499999999999998668 ) ) ;
#212096=CARTESIAN_POINT ( 'NONE',  ( 8.269583629331492602, 11.73526576994040482, 1.199719254218450271 ) ) ;
#212098=CARTESIAN_POINT ( 'NONE',  ( -4.446711195602255806, 5.250546485366484717, -1.082531754730544860 ) ) ;
#212100=CARTESIAN_POINT ( 'NONE',  ( -5.395781948114519722, 5.397426482329451325, 0.000000000000000000 ) ) ;
#212107=CARTESIAN_POINT ( 'NONE',  ( 3.171717870593107058, 5.787755718078879674, -1.199719254218446718 ) ) ;
#212115=CARTESIAN_POINT ( 'NONE',  ( 4.493637847925535667, 7.329995691633395261, -1.199719254218452047 ) ) ;
#212119=CARTESIAN_POINT ( 'NONE',  ( 0.6823417656249917140, 3.655208333674754506, 1.181850606188765695 ) ) ;
#212124=CARTESIAN_POINT ( 'NONE',  ( 5.612185521052973414, 8.634967976948757951, -1.199719254218440723 ) ) ;
#212127=CARTESIAN_POINT ( 'NONE',  ( -5.436983294280064882, 6.301900917203534291, 1.199719254218450271 ) ) ;
#212130=CARTESIAN_POINT ( 'NONE',  ( 0.7499999999999902300, 2.483333333333351156, 1.299038105676669330 ) ) ;
#212133=CARTESIAN_POINT ( 'NONE',  ( -5.108724954250998707, 4.854600622914589714, -0.7998128361456221525 ) ) ;
#212135=CARTESIAN_POINT ( 'NONE',  ( 1.500000000000007105, 10.64264068711930733, 1.214306433183764966E-14 ) ) ;
#212137=CARTESIAN_POINT ( 'NONE',  ( 1.364683531249988535, 3.863541667008087543, 0.7879004041258500513 ) ) ;
#212139=CARTESIAN_POINT ( 'NONE',  ( -5.450014563013544588, 5.460697866378308341, 0.7216878364870317197 ) ) ;
#212145=CARTESIAN_POINT ( 'NONE',  ( 2.855963913973019963, 6.483708332943829866, 0.000000000000000000 ) ) ;
#212148=CARTESIAN_POINT ( 'NONE',  ( 0.3110919644345279678, 6.477502264753364436, -3.270003019671252176 ) ) ;
#212149=CARTESIAN_POINT ( 'NONE',  ( 0.6823417656249917140, 3.655208333674754506, 1.181850606188765695 ) ) ;
#212153=CARTESIAN_POINT ( 'NONE',  ( -1.402160292154681736E-14, 0.009375000341421267647, -1.575800808251665908 ) ) ;
#212157=CARTESIAN_POINT ( 'NONE',  ( -9.622536337397040285, 12.24937836509514710, 1.599625672291281386 ) ) ;
#212159=CARTESIAN_POINT ( 'NONE',  ( -7.022760381754429737, 7.295567988242705582, 1.040834085586084257E-14 ) ) ;
#212163=CARTESIAN_POINT ( 'NONE',  ( -1.364683531249997417, 3.759375000341423689, 1.214306433183764966E-14 ) ) ;
#212172=CARTESIAN_POINT ( 'NONE',  ( -6.114364089638801403, 8.156510742710487705, 1.443375672974078761 ) ) ;
#212177=CARTESIAN_POINT ( 'NONE',  ( -4.894130264408858899, 8.653643041878236630, -0.7216878364870207285 ) ) ;
#212190=CARTESIAN_POINT ( 'NONE',  ( -4.055860508782465068, 7.883587693554856557, 1.040834085586084257E-14 ) ) ;
#212193=CARTESIAN_POINT ( 'NONE',  ( -1.500000000000001332, 1.400000000000019229, 0.000000000000000000 ) ) ;
#212194=CARTESIAN_POINT ( 'NONE',  ( 2.184835310096557404, 5.700724961754617404, 1.040834085586084257E-14 ) ) ;
#212195=CARTESIAN_POINT ( 'NONE',  ( 5.957918438201454059, 9.038323046955323292, -1.199719254218440723 ) ) ;
#212199=CARTESIAN_POINT ( 'NONE',  ( 5.840865249388943248, 5.708764300575555062, 0.7998128361456341429 ) ) ;
#212200=CARTESIAN_POINT ( 'NONE',  ( -0.4886806171078718619, 7.337544960129616989, -1.941936010599534468 ) ) ;
#212207=CARTESIAN_POINT ( 'NONE',  ( -3.389175213736311587, 4.977123720824209840, 1.443375672974064550 ) ) ;
#212209=CARTESIAN_POINT ( 'NONE',  ( 5.378281411895256880, 4.339595938922573559, -2.499999999999995115 ) ) ;
#212214=CARTESIAN_POINT ( 'NONE',  ( 1.364683531249990311, 3.384375000341416140, 1.214306433183764966E-14 ) ) ;
#212217=CARTESIAN_POINT ( 'NONE',  ( -6.901263884555985051, 8.010228272525461435, 1.199719254218450271 ) ) ;
#212221=CARTESIAN_POINT ( 'NONE',  ( 4.794779880727245036, 8.745660294157122649, -0.7998128361456281477 ) ) ;
#212222=CARTESIAN_POINT ( 'NONE',  ( -6.684333426737305572, 7.757142738403693727, -1.199719254218446718 ) ) ;
#212224=CARTESIAN_POINT ( 'NONE',  ( -1.537272393291634565, 8.756440202903029046, 2.479668406359612831 ) ) ;
#212228=CARTESIAN_POINT ( 'NONE',  ( 0.7499999999999885647, -0.2354166659838466402, 1.299038105676657340 ) ) ;
#212231=CARTESIAN_POINT ( 'NONE',  ( 6.453317930424781856, 10.47269531889685545, -0.7216878364870267237 ) ) ;
#212235=CARTESIAN_POINT ( 'NONE',  ( 0.6823417656249882723, 1.738541667008083991, -1.181850606188749264 ) ) ;
#212237=CARTESIAN_POINT ( 'NONE',  ( 7.904040366642699489, 8.323727970612377902, 0.7216878364870458196 ) ) ;
#212240=CARTESIAN_POINT ( 'NONE',  ( -3.416291520963659512, 5.969128626890772615, 1.082531754730560403 ) ) ;
#212242=CARTESIAN_POINT ( 'NONE',  ( -1.001543065824772872E-14, 4.821875000341419693, 1.575800808251672791 ) ) ;
#212246=CARTESIAN_POINT ( 'NONE',  ( -5.391520587109122076, 6.494678753518896563, -1.342800935913717852 ) ) ;
#212252=CARTESIAN_POINT ( 'NONE',  ( 5.900823170445728572, 7.907379670318584353, 1.599625672291267398 ) ) ;
#212255=CARTESIAN_POINT ( 'NONE',  ( 4.630273154266905777, 5.360739087188218122, 1.199719254218464037 ) ) ;
#212263=CARTESIAN_POINT ( 'NONE',  ( 6.155038550924155416, 6.283225852274053835, 0.7216878364870317197 ) ) ;
#212264=CARTESIAN_POINT ( 'NONE',  ( -1.201851678989727383E-14, 1.384375000341419693, 1.575800808251672791 ) ) ;
#212267=CARTESIAN_POINT ( 'NONE',  ( 2.310781476690497271, 5.467761476598782977, -0.5169845646830224517 ) ) ;
#212270=CARTESIAN_POINT ( 'NONE',  ( -0.7500000000000215383, 2.191666666666689078, 1.299038105676671107 ) ) ;
#212271=CARTESIAN_POINT ( 'NONE',  ( 6.479907352327590964, 9.647310113435821677, 1.199719254218462483 ) ) ;
#212272=CARTESIAN_POINT ( 'NONE',  ( -7.666245793523398078, 11.03137162816423356, 1.199719254218453823 ) ) ;
#212276=CARTESIAN_POINT ( 'NONE',  ( -1.364683531250012516, 2.530208333674753174, 0.7879004041258379498 ) ) ;
#212278=CARTESIAN_POINT ( 'NONE',  ( 1.499999999999987121, 2.295833333333350268, -0.8660254037844262731 ) ) ;
#212280=CARTESIAN_POINT ( 'NONE',  ( 2.361091307074211887, 5.906356958228550447, 0.7998128361456462443 ) ) ;
#212283=CYLINDRICAL_SURFACE ( 'NONE', #114154, 1.250000000000000000 ) ;
#212286=CARTESIAN_POINT ( 'NONE',  ( 1.499999999999987121, 1.327083334016149641, -0.8660254037844253849 ) ) ;
#212289=CARTESIAN_POINT ( 'NONE',  ( -7.217017841176048165, 7.314275657660511243, 1.040834085586084257E-14 ) ) ;
#212290=CARTESIAN_POINT ( 'NONE',  ( -3.795919822146283540, 6.412028311603867436, -1.082531754730549967 ) ) ;
#212298=CARTESIAN_POINT ( 'NONE',  ( 6.799577732453452761, 7.891594428405881878, -1.199719254218446718 ) ) ;
#212299=CYLINDRICAL_SURFACE ( 'NONE', #186476, 1.500000000000000222 ) ;
#212301=CARTESIAN_POINT ( 'NONE',  ( 5.608269097547198712, 9.694731047113750222, -0.7998128361456281477 ) ) ;
#212302=CARTESIAN_POINT ( 'NONE',  ( 8.636180661780656465, 11.09863007687603087, -1.443375672974052559 ) ) ;
#212307=CARTESIAN_POINT ( 'NONE',  ( -6.449928391799210736, 8.548002428564306143, -1.599625672291263179 ) ) ;
#212308=CARTESIAN_POINT ( 'NONE',  ( 4.843287188579786573, 6.673587691474970107, -1.599625672291256295 ) ) ;
#212312=CARTESIAN_POINT ( 'NONE',  ( 4.084722907606431974, 7.479936734012107458, 0.5927516458891276541 ) ) ;
#212313=CARTESIAN_POINT ( 'NONE',  ( 9.408995418203963013, 12.00024729270324286, 1.443375672974076540 ) ) ;
#212321=CARTESIAN_POINT ( 'NONE',  ( -3.850152436600983386, 4.554561266531622188, 1.082531754730560403 ) ) ;
#212322=CARTESIAN_POINT ( 'NONE',  ( 9.097157885089661278, 9.715698408800516717, 1.040834085586084257E-14 ) ) ;
#212324=CARTESIAN_POINT ( 'NONE',  ( -3.903858165731105778, 6.641919395739846799, 1.199719254218464037 ) ) ;
#212326=CARTESIAN_POINT ( 'NONE',  ( 6.938893903907228378E-15, 10.64264068711930733, 1.214306433183764966E-14 ) ) ;
#212330=CARTESIAN_POINT ( 'NONE',  ( -5.506582945444718824, 9.576097202994168001, 0.7998128361456481317 ) ) ;
#212345=CARTESIAN_POINT ( 'NONE',  ( 1.499999999999820810, 7.388542872122566330, -4.154462424328214887 ) ) ;
#212346=CARTESIAN_POINT ( 'NONE',  ( -6.663996196316808174, 7.733415969579778171, -1.199719254218446718 ) ) ;
#212349=CARTESIAN_POINT ( 'NONE',  ( 3.877268743828276243, 4.586196958296845594, 1.082531754730560403 ) ) ;
#212354=CARTESIAN_POINT ( 'NONE',  ( -2.300079615812729905, 5.835176651756807331, -0.7998128361456281477 ) ) ;
#212357=CARTESIAN_POINT ( 'NONE',  ( 10.53876547652418338, 11.18964789890005918, 0.7998128361456462443 ) ) ;
#212360=CARTESIAN_POINT ( 'NONE',  ( -8.178592977541617515, 10.56477777859713463, 1.599625672291295375 ) ) ;
#212361=CARTESIAN_POINT ( 'NONE',  ( 4.964256800898067645, 8.943383367689749619, 0.7998128361456462443 ) ) ;
#212367=CARTESIAN_POINT ( 'NONE',  ( -0.6823417656250003738, 1.280208333674752508, -1.181850606188749264 ) ) ;
#212371=CARTESIAN_POINT ( 'NONE',  ( 6.914295153289432783, 10.05013286460426691, -1.082531754730537976 ) ) ;
#212379=CARTESIAN_POINT ( 'NONE',  ( 10.50720586046655391, 11.36075438007358507, 0.7216878364870438212 ) ) ;
#212400=CARTESIAN_POINT ( 'NONE',  ( -0.7500000000000006661, 2.139583334016155636, -1.299038105676652011 ) ) ;
#212407=CARTESIAN_POINT ( 'NONE',  ( 9.562578416340237197, 10.05076299535211781, 0.7998128361456462443 ) ) ;
#212412=CARTESIAN_POINT ( 'NONE',  ( 4.708759422647839976, 4.387974169377582001, -0.7998128361456211532 ) ) ;
#212413=CARTESIAN_POINT ( 'NONE',  ( -6.399085315970142851, 8.488685506763726352, -1.443375672974059665 ) ) ;
#212418=CARTESIAN_POINT ( 'NONE',  ( -7.528855374290365887, 7.678086112960552434, -0.7998128361456291469 ) ) ;
#212421=VERTEX_POINT ( 'NONE', #23494 ) ;
#212422=CARTESIAN_POINT ( 'NONE',  ( -1.201851678989727383E-14, 0.7437500006828187127, 1.732050807568877637 ) ) ;
#212429=CARTESIAN_POINT ( 'NONE',  ( -2.277406616971334508, 5.600798786534425311, 1.040834085586084257E-14 ) ) ;
#212433=CARTESIAN_POINT ( 'NONE',  ( 4.863282293121215183, 6.691362709583676072, 1.250037515303052738 ) ) ;
#212438=CARTESIAN_POINT ( 'NONE',  ( -9.938290294017125603, 11.55342575023019691, -1.199719254218441611 ) ) ;
#212439=CARTESIAN_POINT ( 'NONE',  ( 7.527801604085637699, 9.805521176231838609, 1.599625672291281386 ) ) ;
#212440=CARTESIAN_POINT ( 'NONE',  ( 5.029711800989886683, 4.970344644017389513, 1.040834085586084257E-14 ) ) ;
#212447=CARTESIAN_POINT ( 'NONE',  ( -9.643927338022246332, 10.14567007064778004, -0.7998128361456291469 ) ) ;
#212452=CARTESIAN_POINT ( 'NONE',  ( 3.032219910950674890, 6.689340329417765574, 0.7998128361456321445 ) ) ;
#212456=CARTESIAN_POINT ( 'NONE',  ( -8.622095623286845978, 12.14652976288826913, 1.199719254218462483 ) ) ;
#212470=CARTESIAN_POINT ( 'NONE',  ( 8.132193210098487057, 8.381980254736715708, 1.040834085586084257E-14 ) ) ;
#212472=CARTESIAN_POINT ( 'NONE',  ( -4.731959306369413198, 5.479372931307791461, -1.199719254218446718 ) ) ;
#212481=CARTESIAN_POINT ( 'NONE',  ( -1.402160292154681736E-14, 0.6187500006828180465, -1.732050807568863648 ) ) ;
#212483=EDGE_CURVE ( 'NONE', #132154, #202848, #89606, .T. ) ;
#212485=CARTESIAN_POINT ( 'NONE',  ( -1.445103857048106510, 8.688264192037884470, -2.625611233228244412 ) ) ;
#212486=CARTESIAN_POINT ( 'NONE',  ( 4.216749469050096621, 4.878294787768598262, -1.199719254218452047 ) ) ;
#212488=CARTESIAN_POINT ( 'NONE',  ( -2.839543107058306592, 5.400218493954923815, -1.199719254218446718 ) ) ;
#212495=CARTESIAN_POINT ( 'NONE',  ( 5.504247177468190699, 5.523969249908757817, 0.7216878364870317197 ) ) ;
#212498=CARTESIAN_POINT ( 'NONE',  ( -10.47097470845587175, 11.11055866948701443, 1.040834085586084257E-14 ) ) ;
#212500=CARTESIAN_POINT ( 'NONE',  ( 4.514501963226220660, 4.369266499959774563, -0.7216878364870197293 ) ) ;
#212509=CARTESIAN_POINT ( 'NONE',  ( -5.593616938499215152, 6.351546440420595019, 1.211061620805883532 ) ) ;
#212511=CARTESIAN_POINT ( 'NONE',  ( 0.6823417656249864960, -1.073958332991911568, -1.181850606188749264 ) ) ;
#212515=CARTESIAN_POINT ( 'NONE',  ( -4.880045225915050189, 7.780804299287790826, 1.199719254218464037 ) ) ;
#212519=CARTESIAN_POINT ( 'NONE',  ( -1.499999999999997780, 4.400000000000021672, 1.214306433183764966E-14 ) ) ;
#212526=CARTESIAN_POINT ( 'NONE',  ( -6.056815632531343141, 6.015240258500212711, 0.3115616189311651296 ) ) ;
#212527=CARTESIAN_POINT ( 'NONE',  ( 1.364683531249986537, -1.136458332991912235, 0.7879004041258500513 ) ) ;
#212529=CARTESIAN_POINT ( 'NONE',  ( 6.745345117998789775, 7.828323044875442172, 1.199719254218462483 ) ) ;
#212531=CARTESIAN_POINT ( 'NONE',  ( -6.855619230004478482, 11.14997286831390788, -0.7998128361456291469 ) ) ;
#212533=CARTESIAN_POINT ( 'NONE',  ( 9.728138913005292210, 11.30824913904973705, -1.199719254218440723 ) ) ;
#212535=DIRECTION ( 'NONE',  ( -1.207943261119674327E-30, -2.168404344971008079E-15, -1.000000000000000000 ) ) ;
#212539=CIRCLE ( 'NONE', #5009, 0.08000000000000030698 ) ;
#212540=CARTESIAN_POINT ( 'NONE',  ( 1.364683531249986537, -0.7822916663252464931, -0.7879004041258309554 ) ) ;
#212547=CARTESIAN_POINT ( 'NONE',  ( 6.643132081016105417, 10.69414516125339887, 0.7216878364870438212 ) ) ;
#212554=CARTESIAN_POINT ( 'NONE',  ( 1.499999999999989120, 4.785416667349486453, 0.8660254037844524744 ) ) ;
#212556=CARTESIAN_POINT ( 'NONE',  ( -3.632695093457760649, 6.325562478087638496, -1.199719254218452047 ) ) ;
#212557=CARTESIAN_POINT ( 'NONE',  ( 5.409340101728155936, 8.294351971116089572, -1.082531754730543971 ) ) ;
#212564=PLANE ( 'NONE',  #178269 ) ;
#212565=CARTESIAN_POINT ( 'NONE',  ( 3.063252641683779753, 5.661212951017999373, 1.199719254218450271 ) ) ;
#212566=CARTESIAN_POINT ( 'NONE',  ( -1.499999999999981126, 3.910416667349481123, -0.8660254037844499209 ) ) ;
#212567=CARTESIAN_POINT ( 'NONE',  ( -1.451998047843676476, 7.315968950353781253, 4.301760722578348073 ) ) ;
#212572=ORIENTED_EDGE ( 'NONE', *, *, #87068, .F. ) ;
#212574=CARTESIAN_POINT ( 'NONE',  ( -2.535011536075347571, 5.133042487381361596, -0.9999999999999956701 ) ) ;
#212581=CARTESIAN_POINT ( 'NONE',  ( 7.730120138085914583, 12.17022392774227768, 0.7998128361456462443 ) ) ;
#212585=CARTESIAN_POINT ( 'NONE',  ( -1.402160292154681736E-14, -0.05312499965857903073, -1.575800808251665908 ) ) ;
#212586=CARTESIAN_POINT ( 'NONE',  ( 3.850152436600926542, 7.435668909435648288, -0.7216878364870197293 ) ) ;
#212587=CARTESIAN_POINT ( 'NONE',  ( -9.815740026613967828, 10.55404424057886636, -0.7216878364870267237 ) ) ;
#212593=CARTESIAN_POINT ( 'NONE',  ( -4.925689880466507908, 4.641059703499347044, -0.7998128361456221525 ) ) ;
#212596=VERTEX_POINT ( 'NONE', #71163 ) ;
#212605=CARTESIAN_POINT ( 'NONE',  ( 5.555833580239399438, 6.383300830698137140, -1.210397860111110946 ) ) ;
#212613=CARTESIAN_POINT ( 'NONE',  ( -7.321039761699444703, 10.52466824108257804, 1.082531754730549967 ) ) ;
#212617=CARTESIAN_POINT ( 'NONE',  ( 6.449928391799196525, 8.548002428564306143, -1.599625672291262513 ) ) ;
#212618=CARTESIAN_POINT ( 'NONE',  ( -5.111587607552082524, 5.922272616020886282, 1.199719254218450271 ) ) ;
#212620=CARTESIAN_POINT ( 'NONE',  ( -5.738125327081750271, 7.717565519727259904, 1.599625672291269396 ) ) ;
#212623=EDGE_CURVE ( 'NONE', #189774, #109299, #106956, .T. ) ;
#212624=CARTESIAN_POINT ( 'NONE',  ( -6.715366157470410435, 6.729015360003925750, -0.7998128361456291469 ) ) ;
#212627=CARTESIAN_POINT ( 'NONE',  ( 7.540305987494599016, 11.94877408538573427, -0.7998128361456291469 ) ) ;
#212630=CARTESIAN_POINT ( 'NONE',  ( 4.350666953118342839, 7.402852620340107492, 1.136566098749042242 ) ) ;
#212631=CARTESIAN_POINT ( 'NONE',  ( 5.531363484695522637, 5.555604941673978558, -0.7216878364870207285 ) ) ;
#212638=CARTESIAN_POINT ( 'NONE',  ( 7.741342523278705201, 9.094283034322399928, 1.082531754730558626 ) ) ;
#212641=CARTESIAN_POINT ( 'NONE',  ( -10.14557902172788495, 10.73093036830436553, 1.040834085586084257E-14 ) ) ;
#212642=CARTESIAN_POINT ( 'NONE',  ( -6.744291347794091784, 9.955758108146730123, -1.199719254218440723 ) ) ;
#212643=CARTESIAN_POINT ( 'NONE',  ( -4.812781342726871969, 6.637997537979888563, 1.443375672974064550 ) ) ;
#212650=CARTESIAN_POINT ( 'NONE',  ( 9.887974103068218668, 10.43039129653476493, 0.7998128361456462443 ) ) ;
#212654=CARTESIAN_POINT ( 'NONE',  ( 4.142179624174931796, 4.791296635414242111, 1.199719254218464037 ) ) ;
#212657=CARTESIAN_POINT ( 'NONE',  ( -3.443980807556779045, 6.324176108538676289, 1.003164557157047332 ) ) ;
#212663=CARTESIAN_POINT ( 'NONE',  ( 0.7499999999999902300, 3.483333333333352044, 1.299038105676669330 ) ) ;
#212664=CARTESIAN_POINT ( 'NONE',  ( 5.015626762051672571, 7.938982758113895422, 1.199719254218462483 ) ) ;
#212667=CARTESIAN_POINT ( 'NONE',  ( 6.805829924380105034, 9.923590097543378619, 1.082531754730558626 ) ) ;
#212668=CARTESIAN_POINT ( 'NONE',  ( 0.1400748609344511231, 7.098713645440544617, 2.115199198882494080 ) ) ;
#212669=AXIS2_PLACEMENT_3D ( 'NONE', #200107, #202233, #135153 ) ;
#212672=CARTESIAN_POINT ( 'NONE',  ( 10.22692794340986921, 10.82583744360002243, 0.000000000000000000 ) ) ;
#212674=CARTESIAN_POINT ( 'NONE',  ( -3.418627288940168096, 7.140148937072163804, -0.7998128361456281477 ) ) ;
#212676=CARTESIAN_POINT ( 'NONE',  ( 0.7499999999999920064, 4.764583334016150751, 1.299038105676669330 ) ) ;
#212677=CARTESIAN_POINT ( 'NONE',  ( 1.364683531249986537, -0.1364583329919154264, 0.7879004041258500513 ) ) ;
#212681=CARTESIAN_POINT ( 'NONE',  ( 3.171717870593107058, 5.787755718078879674, -1.199719254218446718 ) ) ;
#212683=CARTESIAN_POINT ( 'NONE',  ( 0.6823417656249917140, 5.655208333674749177, 1.181850606188765695 ) ) ;
#212693=CARTESIAN_POINT ( 'NONE',  ( -5.716734326456539783, 9.821273814174633188, -0.7998128361456231517 ) ) ;
#212697=CARTESIAN_POINT ( 'NONE',  ( 5.854423403002611437, 5.724582146458163656, 1.040834085586084257E-14 ) ) ;
#212703=CARTESIAN_POINT ( 'NONE',  ( 8.940712233207955606, 12.51824914112961729, 1.199719254218450271 ) ) ;
#212706=CARTESIAN_POINT ( 'NONE',  ( -4.446184310277715213, 7.274633231044262516, -1.199719254218452047 ) ) ;
#212710=CARTESIAN_POINT ( 'NONE',  ( 9.562578416340237197, 10.05076299535211781, 0.7998128361456462443 ) ) ;
#212712=CARTESIAN_POINT ( 'NONE',  ( 9.250740883225924804, 9.686952540052077509, 1.040834085586084257E-14 ) ) ;
#212714=CARTESIAN_POINT ( 'NONE',  ( 4.175484721775176489, 3.976419294354625933, -0.06592222766770190756 ) ) ;
#212715=CARTESIAN_POINT ( 'NONE',  ( -9.490344339885973923, 12.09515436799890331, -1.443375672974059665 ) ) ;
#212716=CARTESIAN_POINT ( 'NONE',  ( -7.100719765255177229, 9.307259030929609267, -1.599625672291263179 ) ) ;
#212720=CARTESIAN_POINT ( 'NONE',  ( -4.043597078347817231, 7.757176853022865082, 0.5683662157932849457 ) ) ;
#212721=CARTESIAN_POINT ( 'NONE',  ( 1.364683531249986537, 0.8635416670080893198, 0.7879004041258500513 ) ) ;
#212725=CARTESIAN_POINT ( 'NONE',  ( 7.782016984564065432, 8.181367358187307204, 0.7216878364870458196 ) ) ;
#212728=CARTESIAN_POINT ( 'NONE',  ( 5.087333953625774008, 6.958308917361963886, 1.599625672291267398 ) ) ;
#212739=AXIS2_PLACEMENT_3D ( 'NONE', #175357, #176410, #64773 ) ;
#212747=CARTESIAN_POINT ( 'NONE',  ( 8.550388431712704573, 13.12720360364021133, 0.000000000000000000 ) ) ;
#212749=VERTEX_POINT ( 'NONE', #94936 ) ;
#212751=CARTESIAN_POINT ( 'NONE',  ( -4.355193658487827690, 6.104145239700998538, -1.599625672291256295 ) ) ;
#212752=CARTESIAN_POINT ( 'NONE',  ( -8.369460898337653276, 8.658792557682392754, 0.7998128361456462443 ) ) ;
#212758=CARTESIAN_POINT ( 'NONE',  ( -1.500000000000011324, 3.702083334016152971, 0.8660254037844403729 ) ) ;
#212759=CARTESIAN_POINT ( 'NONE',  ( 8.646349277213076334, 11.11049346154719508, 1.599625672291281386 ) ) ;
#212762=CARTESIAN_POINT ( 'NONE',  ( -7.181014916732457287, 11.52960116949655678, -0.7998128361456291469 ) ) ;
#212764=CARTESIAN_POINT ( 'NONE',  ( -1.201851678989727383E-14, 2.946875000341419248, -1.575800808251660134 ) ) ;
#212769=CARTESIAN_POINT ( 'NONE',  ( -9.978437869977959451, 10.74385839117019614, -0.7216878364870267237 ) ) ;
#212773=CARTESIAN_POINT ( 'NONE',  ( -1.364683531250012516, 2.092708333674750953, 0.7879004041258379498 ) ) ;
#212780=CARTESIAN_POINT ( 'NONE',  ( 1.364683531249988535, 2.863541667008082658, 0.7879004041258500513 ) ) ;
#212782=CARTESIAN_POINT ( 'NONE',  ( -4.089755892816631544, 7.923132308261379819, -0.7998128361456281477 ) ) ;
#212785=CARTESIAN_POINT ( 'NONE',  ( -0.6823417656250003738, 2.280208333674753174, -1.181850606188749264 ) ) ;
#212790=CARTESIAN_POINT ( 'NONE',  ( -5.761852096127856981, 5.824508321678349532, 0.000000000000000000 ) ) ;
#212793=CARTESIAN_POINT ( 'NONE',  ( 4.202664430556247055, 6.886563688082179446, 1.082531754730558626 ) ) ;
#212796=CARTESIAN_POINT ( 'NONE',  ( -6.204827856548512877, 10.39071626594860476, -0.7998128361456291469 ) ) ;
#212797=CARTESIAN_POINT ( 'NONE',  ( -8.948018195339354719, 12.42280974699582607, 1.082531754730560403 ) ) ;
#212799=CARTESIAN_POINT ( 'NONE',  ( 1.364683531249992088, 5.384375000341417916, 1.214306433183764966E-14 ) ) ;
#212805=CARTESIAN_POINT ( 'NONE',  ( -6.683806541412776525, 7.860491055478785682, -1.082531754730543083 ) ) ;
#212807=CARTESIAN_POINT ( 'NONE',  ( 1.364683531249986537, -0.07395833299191513499, 0.7879004041258500513 ) ) ;
#212810=CARTESIAN_POINT ( 'NONE',  ( 7.483737605063422116, 7.833374748769873719, -0.7216878364870257245 ) ) ;
#212816=CARTESIAN_POINT ( 'NONE',  ( 4.338245966248566177, 4.163634503485842409, 1.214306433183764966E-14 ) ) ;
#212821=CARTESIAN_POINT ( 'NONE',  ( 8.392133896734655707, 11.77427806529038357, 1.082531754730546636 ) ) ;
#212828=CARTESIAN_POINT ( 'NONE',  ( 7.284808609244363353, 7.393364887073558656, 0.7998128361456341429 ) ) ;
#212829=CARTESIAN_POINT ( 'NONE',  ( -4.939248034080176097, 4.656877549381960080, 1.214306433183764966E-14 ) ) ;
#212832=CARTESIAN_POINT ( 'NONE',  ( 4.905139262582265403, 4.827437033166341429, 0.6004564335717228474 ) ) ;
#212834=CARTESIAN_POINT ( 'NONE',  ( 4.622967192135525316, 8.337286124226029216, -0.7216878364870207285 ) ) ;
#212835=CARTESIAN_POINT ( 'NONE',  ( -1.364683531250000748, 0.3218750003414205807, 0.000000000000000000 ) ) ;
#212836=CARTESIAN_POINT ( 'NONE',  ( 6.115105756127376502, 6.015623637602188545, 0.1580619937117197227 ) ) ;
#212837=CARTESIAN_POINT ( 'NONE',  ( -9.809487834687324437, 11.40315621434539395, 1.199719254218462483 ) ) ;
#212846=CARTESIAN_POINT ( 'NONE',  ( 0.7499999999999902300, 4.566666666666691299, -1.299038105676658228 ) ) ;
#212854=CARTESIAN_POINT ( 'NONE',  ( 6.714312387265682247, 8.856450423275211037, 1.599625672291281386 ) ) ;
#212864=CARTESIAN_POINT ( 'NONE',  ( 9.317477881089539338, 11.89347683273640932, 1.599625672291279388 ) ) ;
#212870=CARTESIAN_POINT ( 'NONE',  ( 8.374132434735052755, 12.92157160716627295, -0.7998128361456352531 ) ) ;
#212873=CARTESIAN_POINT ( 'NONE',  ( -0.1081551476993485722, 7.159877756659424719, 1.998460492244615638 ) ) ;
#212881=CARTESIAN_POINT ( 'NONE',  ( -9.110716038703348119, 12.61262389758715408, 1.082531754730560403 ) ) ;
#212885=CARTESIAN_POINT ( 'NONE',  ( 6.094553744542824170, 7.069066442510145265, 1.199719254218462483 ) ) ;
#212886=CARTESIAN_POINT ( 'NONE',  ( -1.364683531250010740, 5.530208333674750953, 0.7879004041258379498 ) ) ;
#212892=CARTESIAN_POINT ( 'NONE',  ( 4.812781342726858647, 6.637997537979888563, 1.443375672974062551 ) ) ;
#212895=ORIENTED_EDGE ( 'NONE', *, *, #71271, .F. ) ;
#212899=CARTESIAN_POINT ( 'NONE',  ( -6.124532705071231931, 8.168374127381657246, -1.599625672291263179 ) ) ;
#212900=CARTESIAN_POINT ( 'NONE',  ( -4.029797971759847997, 5.724516938518342535, -1.599625672291256295 ) ) ;
#212905=CARTESIAN_POINT ( 'NONE',  ( -0.006158830626153827259, 7.078243236992583398, 2.121324627965421872 ) ) ;
#212909=CARTESIAN_POINT ( 'NONE',  ( 6.636879889089462026, 7.701780277814560982, -1.199719254218446718 ) ) ;
#212917=CARTESIAN_POINT ( 'NONE',  ( 4.487385655998878065, 6.258369236797239665, 1.443375672974062551 ) ) ;
#212920=CARTESIAN_POINT ( 'NONE',  ( -0.6823417656250003738, -0.2197916663252488800, -1.181850606188749264 ) ) ;
#212921=CARTESIAN_POINT ( 'NONE',  ( 4.207107738942202246, 3.802713871720993399, 1.214306433183764966E-14 ) ) ;
#212922=CARTESIAN_POINT ( 'NONE',  ( 3.506755287428983792, 7.242964935309132990, 1.040834085586084257E-14 ) ) ;
#212924=CARTESIAN_POINT ( 'NONE',  ( -7.890482213473404727, 8.307910125248191946, 0.7216878364870578100 ) ) ;
#212925=CARTESIAN_POINT ( 'NONE',  ( 3.524756749872944628, 7.056040608253000279, -0.7216878364870267237 ) ) ;
#212926=CARTESIAN_POINT ( 'NONE',  ( -7.822691444960716112, 8.228820895316715678, -0.7216878364870267237 ) ) ;
#212930=CARTESIAN_POINT ( 'NONE',  ( 7.396136491454752715, 8.587579647240744407, 1.199719254218462483 ) ) ;
#212932=DIRECTION ( 'NONE',  ( 1.000000000000000000, 0.000000000000000000, 0.000000000000000000 ) ) ;
#212934=CARTESIAN_POINT ( 'NONE',  ( 0.1100172516615156165, 7.047065462482140497, 3.945011421259203566 ) ) ;
#212935=CARTESIAN_POINT ( 'NONE',  ( -1.364683531250010295, 3.780208333674750953, 0.7879004041258379498 ) ) ;
#212940=CARTESIAN_POINT ( 'NONE',  ( 8.294891053462476904, 8.571794405328034827, 1.040834085586084257E-14 ) ) ;
#212943=CARTESIAN_POINT ( 'NONE',  ( -8.552495972122143186, 8.872333477097637200, 0.7998128361456462443 ) ) ;
#212949=CARTESIAN_POINT ( 'NONE',  ( 9.402743226277308963, 10.92862083786708816, -1.199719254218446718 ) ) ;
#212950=CARTESIAN_POINT ( 'NONE',  ( -3.145840728001146669, 6.444277940974754593, 0.6115128566374624652 ) ) ;
#212952=CARTESIAN_POINT ( 'NONE',  ( -7.153898609505128015, 11.49796547773133604, 0.7998128361456481317 ) ) ;
#212953=CARTESIAN_POINT ( 'NONE',  ( 7.334597915313080918, 9.580116872663850813, 1.040834085586084257E-14 ) ) ;
#212954=CARTESIAN_POINT ( 'NONE',  ( 4.968100067739229075, 6.607231601306259527, -1.242533411653036879 ) ) ;
#212955=CARTESIAN_POINT ( 'NONE',  ( -9.164948653157990677, 11.71552606681625619, -1.443375672974059665 ) ) ;
#212959=CARTESIAN_POINT ( 'NONE',  ( 4.937140493670735708, 8.911747675924535983, -0.7998128361456281477 ) ) ;
#212961=CARTESIAN_POINT ( 'NONE',  ( 5.124091990960999432, 8.065525525174782828, -1.199719254218452047 ) ) ;
#212962=CARTESIAN_POINT ( 'NONE',  ( -4.053570677780473197, 7.570253647979210854, -0.4034679714342986889 ) ) ;
#212963=CARTESIAN_POINT ( 'NONE',  ( 5.020596955762157698, 4.751784624677624080, 1.040834085586084257E-14 ) ) ;
#212965=CARTESIAN_POINT ( 'NONE',  ( -7.714226216495749355, 8.102278128774251797, 1.040834085586084257E-14 ) ) ;
#212970=CARTESIAN_POINT ( 'NONE',  ( -4.616994038156231106, 6.938643078242441753, 1.201688966319388374 ) ) ;
#212971=CARTESIAN_POINT ( 'NONE',  ( 1.364683531249986537, 0.4677083336747514530, -0.7879004041258309554 ) ) ;
#212974=CARTESIAN_POINT ( 'NONE',  ( 5.070386261830877928, 5.978167395966564435, -1.082531754730548412 ) ) ;
#212979=CARTESIAN_POINT ( 'NONE',  ( -9.625925875578284163, 10.33259439770390564, 1.040834085586084257E-14 ) ) ;
#212985=CARTESIAN_POINT ( 'NONE',  ( -10.26315909542058336, 11.07603315418659840, -0.7216878364870267237 ) ) ;
#212988=ORIENTED_EDGE ( 'NONE', *, *, #211516, .F. ) ;
#212993=CARTESIAN_POINT ( 'NONE',  ( -8.473482818416670170, 10.90881592628469932, -1.443375672974058777 ) ) ;
#212998=CARTESIAN_POINT ( 'NONE',  ( 1.364683531249988535, 4.717708333674756283, -0.7879004041258300672 ) ) ;
#212999=CARTESIAN_POINT ( 'NONE',  ( -1.499999999999997780, 3.181250000682818602, 1.214306433183764966E-14 ) ) ;
#213005=CARTESIAN_POINT ( 'NONE',  ( -8.345207244411405156, 9.694828859023472134, 1.199719254218462483 ) ) ;
#213009=CARTESIAN_POINT ( 'NONE',  ( 4.774442650306744085, 8.721933525333202653, -0.7998128361456281477 ) ) ;
#213014=CARTESIAN_POINT ( 'NONE',  ( 8.609591239877852686, 10.00327685373437347, -1.199719254218445830 ) ) ;
#213017=DIRECTION ( 'NONE',  ( -0.9829311923673912377, -0.1839735607939864959, 0.000000000000000000 ) ) ;
#213021=CARTESIAN_POINT ( 'NONE',  ( -5.572037945536512105, 9.444535336527177805, 0.000000000000000000 ) ) ;
#213024=CARTESIAN_POINT ( 'NONE',  ( -1.364683531250012516, 5.051041667008085767, -0.7879004041258300672 ) ) ;
#213034=B_SPLINE_CURVE_WITH_KNOTS ( 'NONE', 3,
 ( #186104, #152549, #206625, #173088, #156836, #174167, #38804, #137387, #203403, #104886 ),
 .UNSPECIFIED., .F., .F.,
 ( 4, 3, 3, 4 ),
 ( 0.000000000000000000, 4.390531002228115621E-05, 8.388738317900957750E-05, 0.0001586609058613872871 ),
 .UNSPECIFIED. ) ;
#213035=CARTESIAN_POINT ( 'NONE',  ( -9.989660255170729641, 10.54902514065433827, -0.7998128361456291469 ) ) ;
#213037=CARTESIAN_POINT ( 'NONE',  ( 7.736899214892750010, 12.17813285068358020, 1.040834085586084257E-14 ) ) ;
#213038=CARTESIAN_POINT ( 'NONE',  ( -1.500000000000015099, -1.079166666666641961, 0.8660254037844403729 ) ) ;
#213039=CARTESIAN_POINT ( 'NONE',  ( -7.818248136574758256, 12.27303992597924420, 0.000000000000000000 ) ) ;
#213041=CARTESIAN_POINT ( 'NONE',  ( -0.6823417656250212460, 3.051041667008084879, 1.181850606188767472 ) ) ;
#213042=AXIS2_PLACEMENT_3D ( 'NONE', #111036, #92618, #25439 ) ;
#213043=CARTESIAN_POINT ( 'NONE',  ( 3.171717870593107058, 5.787755718078879674, -1.199719254218446718 ) ) ;
#213047=DIRECTION ( 'NONE',  ( 5.578564026256490882E-16, 1.000000000000000000, 9.066213480720158442E-32 ) ) ;
#213048=CARTESIAN_POINT ( 'NONE',  ( 10.03267048398825168, 10.80712977418221676, 0.000000000000000000 ) ) ;
#213050=CARTESIAN_POINT ( 'NONE',  ( -7.049876689426106680, 9.247942109129029475, -1.443375672974059665 ) ) ;
#213051=CARTESIAN_POINT ( 'NONE',  ( 0.6823417656249882723, 0.6760416670080898749, -1.181850606188749264 ) ) ;
#213053=CARTESIAN_POINT ( 'NONE',  ( 0.006768871532346439589, 8.210909518262138107, 2.038649385027043959 ) ) ;
#213055=CARTESIAN_POINT ( 'NONE',  ( -6.835281999583978418, 11.12624609948998966, -0.7998128361456291469 ) ) ;
#213056=CARTESIAN_POINT ( 'NONE',  ( -3.104453987404957260, 6.565687385373657925, -0.7216878364870257245 ) ) ;
#213057=CARTESIAN_POINT ( 'NONE',  ( 1.364683531249990311, 2.946875000341416140, 1.214306433183764966E-14 ) ) ;
#213068=ORIENTED_EDGE ( 'NONE', *, *, #209086, .T. ) ;
#213071=CARTESIAN_POINT ( 'NONE',  ( -3.022498986271275001, 2.800000000000024691, 2.500000000000011102 ) ) ;
#213075=CARTESIAN_POINT ( 'NONE',  ( -1.364683531249997417, 4.571875000341417028, 1.214306433183764966E-14 ) ) ;
#213080=CARTESIAN_POINT ( 'NONE',  ( 7.235247531187115833, 11.59287255302699648, -0.7998128361456291469 ) ) ;
#213083=CARTESIAN_POINT ( 'NONE',  ( 0.6823417656249899377, 2.842708333674753618, 1.181850606188765695 ) ) ;
#213086=CARTESIAN_POINT ( 'NONE',  ( -6.805829924380121909, 8.963220883242035697, 1.443375672974078761 ) ) ;
#213088=CARTESIAN_POINT ( 'NONE',  ( -7.285838599102589797E-14, 7.078193277237590841, -2.121339347286493648 ) ) ;
#213092=CARTESIAN_POINT ( 'NONE',  ( 4.864678189204997949, 4.569879397027603929, 0.7998128361456341429 ) ) ;
#213095=CARTESIAN_POINT ( 'NONE',  ( 9.673906298550626559, 11.24497775551929557, 1.199719254218452047 ) ) ;
#213102=CARTESIAN_POINT ( 'NONE',  ( -4.322352044658376968, 3.937165561723182883, 0.7998128361456341429 ) ) ;
#213103=CARTESIAN_POINT ( 'NONE',  ( 8.118635056484817980, 8.366162408854107113, 0.7998128361456481317 ) ) ;
#213105=CARTESIAN_POINT ( 'NONE',  ( 3.321384445223597659, 6.818772919495430074, -0.7216878364870267237 ) ) ;
#213107=DIRECTION ( 'NONE',  ( 5.176899690512889973E-31, -0.6000000000000069722, -0.7999999999999948264 ) ) ;
#213114=CARTESIAN_POINT ( 'NONE',  ( 4.650083499807233345, 5.295740330745369207, -1.000000000000000888 ) ) ;
#213115=CIRCLE ( 'NONE', #171704, 0.08000000000000005718 ) ;
#213117=CARTESIAN_POINT ( 'NONE',  ( -7.104109303880803417, 8.350844278358124484, 1.082531754730549967 ) ) ;
#213118=CIRCLE ( 'NONE', #26367, 0.8299999999999999600 ) ;
#213119=CARTESIAN_POINT ( 'NONE',  ( 4.202137545231717120, 6.989912005157271402, 1.199719254218462483 ) ) ;
#213122=CARTESIAN_POINT ( 'NONE',  ( -7.862839020921525091, 11.26073039346208660, -1.199719254218446718 ) ) ;
#213127=CARTESIAN_POINT ( 'NONE',  ( -9.982881178363895103, 10.54111621771303753, 1.040834085586084257E-14 ) ) ;
#213129=CARTESIAN_POINT ( 'NONE',  ( 4.148431816101584957, 6.823292304551739740, -1.082531754730548412 ) ) ;
#213131=CARTESIAN_POINT ( 'NONE',  ( 9.420217803396747414, 9.884675613584706255, 0.7998128361456462443 ) ) ;
#213136=ORIENTED_EDGE ( 'NONE', *, *, #56646, .T. ) ;
#213145=CARTESIAN_POINT ( 'NONE',  ( -8.483651433849100698, 10.92067931095586886, 1.599625672291269396 ) ) ;
#213149=CARTESIAN_POINT ( 'NONE',  ( 6.480434237652115570, 10.50433101066207442, 0.7216878364870438212 ) ) ;
#213151=CARTESIAN_POINT ( 'NONE',  ( 2.900554798319789906, 5.471398800426671372, 1.199719254218452047 ) ) ;
#213154=CARTESIAN_POINT ( 'NONE',  ( -5.052384799386910430, 9.046199365926717917, 1.214306433183764966E-14 ) ) ;
#213163=CARTESIAN_POINT ( 'NONE',  ( -1.001543065824772872E-14, 4.634375000341418804, 1.575800808251672791 ) ) ;
#213164=DIRECTION ( 'NONE',  ( -5.578564026256490882E-16, -1.000000000000000000, -9.066213480720158442E-32 ) ) ;
#213165=CARTESIAN_POINT ( 'NONE',  ( 7.730120138085914583, 12.17022392774227768, 0.7998128361456462443 ) ) ;
#213168=CARTESIAN_POINT ( 'NONE',  ( -4.202664430556263930, 5.926194473780837413, 1.443375672974064550 ) ) ;
#213170=CARTESIAN_POINT ( 'NONE',  ( -3.429849674132936066, 6.945315686556313040, -0.7216878364870257245 ) ) ;
#213175=VERTEX_POINT ( 'NONE', #65572 ) ;
#213177=CARTESIAN_POINT ( 'NONE',  ( 3.822509244049070887, 6.547012320444182798, -1.199719254218452047 ) ) ;
#213187=CARTESIAN_POINT ( 'NONE',  ( 6.030679399980265920, 5.930214142932100252, -0.7998128361456281477 ) ) ;
#213192=CARTESIAN_POINT ( 'NONE',  ( 1.364683531249988535, 4.467708333674754506, -0.7879004041258300672 ) ) ;
#213197=CARTESIAN_POINT ( 'NONE',  ( 5.425234023762710578, 9.481190127698507553, -0.7998128361456291469 ) ) ;
#213199=CARTESIAN_POINT ( 'NONE',  ( -4.876128802409253282, 8.840567369452784874, 0.7998128361456481317 ) ) ;
#213200=CARTESIAN_POINT ( 'NONE',  ( -0.7500000000000006661, 2.358333333333358262, -1.299038105676652011 ) ) ;
#213203=CARTESIAN_POINT ( 'NONE',  ( -4.111146893441842920, 5.819424013814012753, 1.599625672291267398 ) ) ;
#213204=CARTESIAN_POINT ( 'NONE',  ( 0.05606965051298876818, 7.151966587341790138, -1.999903488157537046 ) ) ;
#213206=CARTESIAN_POINT ( 'NONE',  ( 1.364683531249990311, 3.134375000341423245, 1.214306433183764966E-14 ) ) ;
#213208=CARTESIAN_POINT ( 'NONE',  ( -4.284013352238262407, 6.021101549076499637, -1.443375672974053447 ) ) ;
#213211=ORIENTED_EDGE ( 'NONE', *, *, #184288, .T. ) ;
#213213=CARTESIAN_POINT ( 'NONE',  ( -4.826339496784927796, 5.693446170079573321, 1.082531754730560403 ) ) ;
#213214=CARTESIAN_POINT ( 'NONE',  ( 5.494078562035752178, 7.432844293840273231, -1.599625672291262513 ) ) ;
#213216=CARTESIAN_POINT ( 'NONE',  ( 0.2082862676862618501, 7.047992132487147288, -4.030656176649458189 ) ) ;
#213217=CARTESIAN_POINT ( 'NONE',  ( -0.6823417656249969321, 4.280208333674755394, -1.181850606188749264 ) ) ;
#213221=CARTESIAN_POINT ( 'NONE',  ( -0.6823417656250003738, -0.4697916663252491021, -1.181850606188749264 ) ) ;
#213224=CARTESIAN_POINT ( 'NONE',  ( -10.08065090696061716, 11.71951313199760136, -1.199719254218441611 ) ) ;
#213225=CARTESIAN_POINT ( 'NONE',  ( -6.846504384776765484, 8.050305206070113684, -1.082531754730543083 ) ) ;
#213229=CARTESIAN_POINT ( 'NONE',  ( -1.364683531250010295, 4.280208333674753618, 0.7879004041258379498 ) ) ;
#213237=CARTESIAN_POINT ( 'NONE',  ( -6.358410854684793279, 7.480862754296137673, -1.082531754730543083 ) ) ;
#213244=CARTESIAN_POINT ( 'NONE',  ( -5.924549939047510705, 6.974691686052601369, 1.082531754730549967 ) ) ;
#213254=ORIENTED_EDGE ( 'NONE', *, *, #101161, .F. ) ;
#213256=CARTESIAN_POINT ( 'NONE',  ( 4.041065261760094174, 7.751399574583047070, -0.4490336992654907489 ) ) ;
#213260=CARTESIAN_POINT ( 'NONE',  ( -5.576481253922474401, 5.400316305864651056, -0.7998128361456221525 ) ) ;
#213262=CARTESIAN_POINT ( 'NONE',  ( -1.500000000000015099, -0.6208333333333116988, -0.8660254037844383745 ) ) ;
#213263=CARTESIAN_POINT ( 'NONE',  ( 10.22248463502393001, 11.02857961705718282, 0.7216878364870438212 ) ) ;
#213264=CARTESIAN_POINT ( 'NONE',  ( 5.608269097547198712, 9.694731047113750222, -0.7998128361456281477 ) ) ;
#213267=CARTESIAN_POINT ( 'NONE',  ( 6.166260936116925606, 6.088392601758203071, 0.7998128361456341429 ) ) ;
#213272=CARTESIAN_POINT ( 'NONE',  ( -3.470524135418306511, 5.072030796119872953, -1.443375672974053447 ) ) ;
#213282=CARTESIAN_POINT ( 'NONE',  ( 1.364683531249988535, 3.905208333674751842, -0.7879004041258239610 ) ) ;
#213283=CARTESIAN_POINT ( 'NONE',  ( 10.50720586046655391, 11.36075438007358507, 0.7216878364870438212 ) ) ;
#213284=CARTESIAN_POINT ( 'NONE',  ( -7.250913225210214641, 7.353820272367037170, 0.7998128361456341429 ) ) ;
#213287=CARTESIAN_POINT ( 'NONE',  ( 5.656776405399742025, 7.622658444431597680, -1.599625672291262513 ) ) ;
#213288=CARTESIAN_POINT ( 'NONE',  ( -6.925517538482230506, 6.974191971184389160, 0.7998128361456341429 ) ) ;
#213291=CARTESIAN_POINT ( 'NONE',  ( -1.402160292154681736E-14, 0.8687500006828192678, -1.732050807568863648 ) ) ;
#213294=CARTESIAN_POINT ( 'NONE',  ( 6.616015773788773480, 10.66250946948817813, -0.7216878364870267237 ) ) ;
#213297=CARTESIAN_POINT ( 'NONE',  ( -0.6823417656250003738, 0.7802083336747520637, -1.181850606188749264 ) ) ;
#213299=CARTESIAN_POINT ( 'NONE',  ( 7.578644679914718019, 7.944099669429731669, 0.7216878364870317197 ) ) ;
#213303=CARTESIAN_POINT ( 'NONE',  ( -3.795919822146277767, 7.372397525905215687, -0.7216878364870267237 ) ) ;
#213305=CARTESIAN_POINT ( 'NONE',  ( 0.6823417656249917140, 4.092708333674755394, 1.181850606188765695 ) ) ;
#213309=CARTESIAN_POINT ( 'NONE',  ( -5.747250929305832479, 6.247137566976777912, -1.064685594968674209 ) ) ;
#213316=CARTESIAN_POINT ( 'NONE',  ( 6.825640269476072497, 10.05066518344239412, 1.199719254218460707 ) ) ;
#213319=CARTESIAN_POINT ( 'NONE',  ( 3.147464216666835402, 6.823792019419957278, -0.7998128361456291469 ) ) ;
#213326=CARTESIAN_POINT ( 'NONE',  ( 4.528060117284229413, 7.266191989264828344, 1.082531754730558626 ) ) ;
#213327=CARTESIAN_POINT ( 'NONE',  ( -1.364683531250000748, 0.07187500034142035865, 0.000000000000000000 ) ) ;
#213331=CARTESIAN_POINT ( 'NONE',  ( -1.402160292154681736E-14, 2.087500000000021227, -1.732050807568863648 ) ) ;
#213332=CARTESIAN_POINT ( 'NONE',  ( 6.775324078527185989, 8.927630729746953264, -1.599625672291262513 ) ) ;
#213333=CARTESIAN_POINT ( 'NONE',  ( -7.934546212495630968, 10.28005655271014795, -1.599625672291263179 ) ) ;
#213337=CARTESIAN_POINT ( 'NONE',  ( -1.364683531250012516, 0.7802083336747528408, 0.7879004041258379498 ) ) ;
#213338=ORIENTED_EDGE ( 'NONE', *, *, #42375, .F. ) ;
#213340=CARTESIAN_POINT ( 'NONE',  ( -0.7500000000000006661, 2.108333333333357817, -1.299038105676652011 ) ) ;
#213342=CARTESIAN_POINT ( 'NONE',  ( 3.985207087413062066, 6.736826471035503694, -1.199719254218452047 ) ) ;
#213349=CARTESIAN_POINT ( 'NONE',  ( -1.500000000000015099, -0.5479166659838513587, 0.8660254037844403729 ) ) ;
#213350=CARTESIAN_POINT ( 'NONE',  ( -6.826694039680798021, 7.923230120171105284, -1.199719254218446718 ) ) ;
#213352=CARTESIAN_POINT ( 'NONE',  ( -4.785665035943912571, 4.685623418130398399, 1.214306433183764966E-14 ) ) ;
#213359=CARTESIAN_POINT ( 'NONE',  ( 7.149227073107712549, 7.235186428247455837, -0.7998128361456281477 ) ) ;
#213360=CARTESIAN_POINT ( 'NONE',  ( 1.419999999999822515, 7.388542872122566330, 4.154462424328221104 ) ) ;
#213363=CARTESIAN_POINT ( 'NONE',  ( 6.819914962873951936, 7.915321197229798322, -1.199719254218446718 ) ) ;
#213364=CARTESIAN_POINT ( 'NONE',  ( 8.880227426826634129, 11.38335130276301754, 1.443375672974076540 ) ) ;
#213368=CARTESIAN_POINT ( 'NONE',  ( -5.831978632172702071, 9.955725504176825780, 0.7998128361456481317 ) ) ;
#213369=CARTESIAN_POINT ( 'NONE',  ( 5.190073875932979419, 4.949507698210251938, 0.7998128361456341429 ) ) ;
#213372=CARTESIAN_POINT ( 'NONE',  ( 4.017310073039977780, 7.571390042887482963, 0.3083681156060176232 ) ) ;
#213373=CARTESIAN_POINT ( 'NONE',  ( 9.002250809793993724, 11.52571191622492464, -1.443375672974057666 ) ) ;
#213374=EDGE_CURVE ( 'NONE', #189774, #44776, #137994, .T. ) ;
#213383=CARTESIAN_POINT ( 'NONE',  ( 9.747949258545622442, 10.47495501116581984, 0.000000000000000000 ) ) ;
#213386=CARTESIAN_POINT ( 'NONE',  ( -6.878064000834399394, 6.918829510595249310, -0.7998128361456291469 ) ) ;
#213387=CARTESIAN_POINT ( 'NONE',  ( -4.161989969270909917, 5.878740935614592544, 1.443375672974064550 ) ) ;
#213392=CARTESIAN_POINT ( 'NONE',  ( -7.393273838153706201, 7.519907654134449615, 0.7998128361456341429 ) ) ;
#213399=VERTEX_POINT ( 'NONE', #106687 ) ;
#213408=CARTESIAN_POINT ( 'NONE',  ( -5.096975683733680818, 8.033889833409558534, -1.199719254218452047 ) ) ;
#213411=CARTESIAN_POINT ( 'NONE',  ( 4.039966587192250103, 7.657118751792200584, 0.7216878364870298324 ) ) ;
#213415=CARTESIAN_POINT ( 'NONE',  ( -0.4644214298920709694, 7.369507887686579828, 4.459343850248737695 ) ) ;
#213418=CARTESIAN_POINT ( 'NONE',  ( 10.56588178375152864, 11.22128359066528169, -0.7998128361456281477 ) ) ;
#213421=CARTESIAN_POINT ( 'NONE',  ( -8.528242318195895066, 9.908369778438709474, 1.199719254218462483 ) ) ;
#213422=CARTESIAN_POINT ( 'NONE',  ( 7.298366762858032430, 7.409182732956175244, 1.040834085586084257E-14 ) ) ;
#213427=CARTESIAN_POINT ( 'NONE',  ( 5.738512597764636958, 5.917411899002901876, -2.440166504834939243 ) ) ;
#213428=CARTESIAN_POINT ( 'NONE',  ( 1.364683531249988757, 1.446875000341421469, 0.000000000000000000 ) ) ;
#213431=CARTESIAN_POINT ( 'NONE',  ( 6.941411460516762943, 11.04213777067082702, -0.7216878364870267237 ) ) ;
#213444=CARTESIAN_POINT ( 'NONE',  ( -2.493739017041104677, 8.265916556960542394, 2.456386464945204740 ) ) ;
#213446=CARTESIAN_POINT ( 'NONE',  ( -9.992522908471816123, 11.61669713376064372, 1.199719254218462483 ) ) ;
#213458=CARTESIAN_POINT ( 'NONE',  ( 1.499999999999985123, -0.1729166659838496101, -0.8660254037844323793 ) ) ;
#213462=ORIENTED_EDGE ( 'NONE', *, *, #67235, .T. ) ;
#213464=CARTESIAN_POINT ( 'NONE',  ( -1.402160292154681736E-14, -0.5374999999999753308, 1.732050807568877637 ) ) ;
#213465=CARTESIAN_POINT ( 'NONE',  ( 8.215351014876830504, 11.67199438640995801, -1.199719254218446718 ) ) ;
#213470=CARTESIAN_POINT ( 'NONE',  ( 4.009460741339333723, 5.700790169694431420, -1.599625672291256295 ) ) ;
#213471=CARTESIAN_POINT ( 'NONE',  ( -6.236387472606145010, 9.259240570473746601, -1.082531754730538864 ) ) ;
#213475=CARTESIAN_POINT ( 'NONE',  ( -7.531718027591449705, 8.745758106066849891, 1.199719254218462483 ) ) ;
#213476=CARTESIAN_POINT ( 'NONE',  ( -3.104453987404963478, 5.605318171072321221, -1.082531754730549078 ) ) ;
#213479=CARTESIAN_POINT ( 'NONE',  ( -1.201851678989727383E-14, 0.9937500006828198229, 1.732050807568877637 ) ) ;
#213487=CARTESIAN_POINT ( 'NONE',  ( -4.243338890952916387, 4.052909582307567149, -0.7216878364870207285 ) ) ;
#213489=EDGE_LOOP ( 'NONE', ( #182385, #33330, #182640, #129476, #162042 ) ) ;
#213491=CARTESIAN_POINT ( 'NONE',  ( 4.025675347721991315, 7.559696154190033823, -0.3592088497781486534 ) ) ;
#213495=CARTESIAN_POINT ( 'NONE',  ( -8.696665468161981494, 12.23352791524263239, -1.199719254218446718 ) ) ;
#213496=CARTESIAN_POINT ( 'NONE',  ( 8.471147050440139381, 8.777426401801974976, -0.7998128361456281477 ) ) ;
#213505=CARTESIAN_POINT ( 'NONE',  ( -7.147119532698295252, 11.49005655479003174, 0.000000000000000000 ) ) ;
#213508=EDGE_LOOP ( 'NONE', ( #31746, #128146, #181104, #49970 ) ) ;
#213510=CARTESIAN_POINT ( 'NONE',  ( 4.813308228051395687, 5.574280006603454574, 1.199719254218462483 ) ) ;
#213514=CARTESIAN_POINT ( 'NONE',  ( -8.448702279610222021, 13.00856975952063088, 1.040834085586084257E-14 ) ) ;
#213525=CARTESIAN_POINT ( 'NONE',  ( 6.259060471003163428, 10.45398764947904624, -0.7998128361456291469 ) ) ;
#213527=CARTESIAN_POINT ( 'NONE',  ( -3.327636637150278798, 5.969660945728899826, -1.199719254218452935 ) ) ;
#213530=CARTESIAN_POINT ( 'NONE',  ( -1.201851678989727383E-14, 2.946875000341418804, -1.575800808251660134 ) ) ;
#213533=EDGE_CURVE ( 'NONE', #199393, #13599, #85838, .T. ) ;
#213535=CARTESIAN_POINT ( 'NONE',  ( -1.500000000000001332, 0.4312500006828159926, 0.000000000000000000 ) ) ;
#213539=CARTESIAN_POINT ( 'NONE',  ( 5.151735183068521629, 5.112705256442466428, 1.040834085586084257E-14 ) ) ;
#213541=CARTESIAN_POINT ( 'NONE',  ( -3.867100128395853709, 5.534702787927018974, -1.599625672291256295 ) ) ;
#213547=CARTESIAN_POINT ( 'NONE',  ( 3.850152436600926542, 7.435668909435648288, -0.7216878364870197293 ) ) ;
#213550=CARTESIAN_POINT ( 'NONE',  ( -1.364683531249997417, 5.321875000341417916, 1.214306433183764966E-14 ) ) ;
#213552=CARTESIAN_POINT ( 'NONE',  ( 3.592547517496925913, 5.214391408544949869, -1.443375672974058777 ) ) ;
#213561=CARTESIAN_POINT ( 'NONE',  ( -6.103605818514504122, 6.017332118737867219, 0.3415998263276952551 ) ) ;
#213563=CARTESIAN_POINT ( 'NONE',  ( -0.6823417656250246877, -1.198958332991911790, 1.181850606188755259 ) ) ;
#213569=CARTESIAN_POINT ( 'NONE',  ( 1.499999999999987566, -0.9749999999999827693, 0.000000000000000000 ) ) ;
#213571=CARTESIAN_POINT ( 'NONE',  ( -1.499999999999997780, 4.900000000000022560, 1.214306433183764966E-14 ) ) ;
#213576=ORIENTED_EDGE ( 'NONE', *, *, #61445, .F. ) ;
#213579=CARTESIAN_POINT ( 'NONE',  ( -1.364683531250012516, 4.551041667008082214, -0.7879004041258300672 ) ) ;
#213581=CARTESIAN_POINT ( 'NONE',  ( 7.122110765880372618, 7.203550736482235095, 0.7998128361456341429 ) ) ;
#213582=CARTESIAN_POINT ( 'NONE',  ( -6.503107236049161521, 10.73870887536603291, 0.7998128361456481317 ) ) ;
#213584=LINE ( 'NONE', #82537, #158608 ) ;
#213585=ORIENTED_EDGE ( 'NONE', *, *, #205767, .F. ) ;
#213587=CARTESIAN_POINT ( 'NONE',  ( -1.364683531250000748, -1.178124999658580752, 0.000000000000000000 ) ) ;
#213591=CARTESIAN_POINT ( 'NONE',  ( 4.561484710689858169, 7.006108427806116978, -1.224552438206182980 ) ) ;
#213594=CARTESIAN_POINT ( 'NONE',  ( 7.944714827928050838, 9.331550723079971021, 1.082531754730558626 ) ) ;
#213598=CARTESIAN_POINT ( 'NONE',  ( -1.500000000000011324, 5.160416667349487341, -0.8660254037844313801 ) ) ;
#213600=CARTESIAN_POINT ( 'NONE',  ( -3.228813138348844536, 6.918699094715619502, 0.7998128361456341429 ) ) ;
#213601=CARTESIAN_POINT ( 'NONE',  ( 5.463572716182819811, 8.357623354646536384, 1.082531754730558626 ) ) ;
#213602=CARTESIAN_POINT ( 'NONE',  ( -10.43941509239824228, 11.28166515066052966, 1.040834085586084257E-14 ) ) ;
#213609=CARTESIAN_POINT ( 'NONE',  ( 3.714044015139744914, 6.420469553383295391, 1.199719254218462483 ) ) ;
#213610=CARTESIAN_POINT ( 'NONE',  ( -0.7499999999999972244, 3.889583334016149863, -1.299038105676652011 ) ) ;
#213613=CIRCLE ( 'NONE', #147940, 4.021913119055696484 ) ;
#213627=CARTESIAN_POINT ( 'NONE',  ( 7.892817981449907982, 12.36003807833360391, 0.7998128361456462443 ) ) ;
#213631=CARTESIAN_POINT ( 'NONE',  ( 1.364683531249988757, -0.6156249996585803075, 0.000000000000000000 ) ) ;
#213632=CARTESIAN_POINT ( 'NONE',  ( 5.585596099150174965, 7.539614753807099667, -1.443375672974057666 ) ) ;
#213633=CARTESIAN_POINT ( 'NONE',  ( -8.324343129110692630, 12.65555805069709550, 0.7216878364870338292 ) ) ;
#213640=CARTESIAN_POINT ( 'NONE',  ( -3.765413976293358278, 5.416068943807445635, 1.599625672291267398 ) ) ;
#213652=CARTESIAN_POINT ( 'NONE',  ( 5.816641468517390834, 6.206546802344954372, -0.9418049055998338748 ) ) ;
#213653=CARTESIAN_POINT ( 'NONE',  ( -1.284279953904135407, 3.128360285806111474, -0.7749999999999892530 ) ) ;
#213656=CARTESIAN_POINT ( 'NONE',  ( -3.975497760493641675, 7.849573349659754840, -7.471960471057975262E-11 ) ) ;
#213660=CARTESIAN_POINT ( 'NONE',  ( -8.514157279702027736, 10.95626946445095307, -1.443375672974059665 ) ) ;
#213664=CARTESIAN_POINT ( 'NONE',  ( 7.396136491454752715, 8.587579647240744407, 1.199719254218462483 ) ) ;
#213666=CARTESIAN_POINT ( 'NONE',  ( -4.517891501851816649, 6.293959390292322986, -1.599625672291256517 ) ) ;
#213668=CARTESIAN_POINT ( 'NONE',  ( -6.247609857798938293, 6.183299677053865295, -0.7998128361456291469 ) ) ;
#213669=CARTESIAN_POINT ( 'NONE',  ( 3.602716132929354664, 5.226254793216122074, 1.599625672291267398 ) ) ;
#213672=CARTESIAN_POINT ( 'NONE',  ( -6.230135280679522936, 7.227244901336242755, 1.199719254218450271 ) ) ;
#213675=CARTESIAN_POINT ( 'NONE',  ( 8.320953590485093088, 10.73086516036454618, 1.599625672291281386 ) ) ;
#213679=CARTESIAN_POINT ( 'NONE',  ( 4.595133766160131472, 7.156059413716462814, 1.333087067838649720 ) ) ;
#213680=CARTESIAN_POINT ( 'NONE',  ( 5.558479791922850133, 6.547609847740540445, -1.082531754730542195 ) ) ;
#213687=VERTEX_POINT ( 'NONE', #16304 ) ;
#213688=CARTESIAN_POINT ( 'NONE',  ( 7.795575137733369075, 9.157554417852841411, -1.082531754730537976 ) ) ;
#213691=CARTESIAN_POINT ( 'NONE',  ( -8.784793466650835825, 12.33634391347959713, 1.199719254218462483 ) ) ;
#213692=CARTESIAN_POINT ( 'NONE',  ( -7.888146445052511169, 8.097259028849730811, 1.040834085586084257E-14 ) ) ;
#213696=DIRECTION ( 'NONE',  ( 1.000000000000000000, -5.578564026256503701E-16, 1.972152263052529514E-31 ) ) ;
#213700=CARTESIAN_POINT ( 'NONE',  ( 8.028399517586572998, 12.51821653715971472, -0.7998128361456352531 ) ) ;
#213704=CARTESIAN_POINT ( 'NONE',  ( 3.928111819657337911, 5.605883094398769195, 1.599625672291267398 ) ) ;
#213708=CARTESIAN_POINT ( 'NONE',  ( -1.201851678989727383E-14, 3.618750000682816381, -1.732050807568863648 ) ) ;
#213714=CARTESIAN_POINT ( 'NONE',  ( -1.201851678989727383E-14, 2.837500000000024780, -1.732050807568863648 ) ) ;
#213715=CARTESIAN_POINT ( 'NONE',  ( 6.810273232766058449, 6.839740281182199233, 1.040834085586084257E-14 ) ) ;
#213717=CARTESIAN_POINT ( 'NONE',  ( 0.7499999999999902300, 4.816666666666684193, -1.299038105676658228 ) ) ;
#213718=CARTESIAN_POINT ( 'NONE',  ( 7.944714827928050838, 9.331550723079971021, 1.082531754730558626 ) ) ;
#213723=CARTESIAN_POINT ( 'NONE',  ( 10.53876547652418338, 11.18964789890005918, 0.7998128361456462443 ) ) ;
#213725=CARTESIAN_POINT ( 'NONE',  ( -4.925689880466507908, 4.641059703499347044, -0.7998128361456221525 ) ) ;
#213726=CARTESIAN_POINT ( 'NONE',  ( -1.500000000000011324, 5.452083334016153415, 0.8660254037844403729 ) ) ;
#213727=CARTESIAN_POINT ( 'NONE',  ( 0.6823417656249882723, -0.9072916663252494907, 1.181850606188755259 ) ) ;
#213731=CARTESIAN_POINT ( 'NONE',  ( 3.147464216666835402, 6.823792019419957278, -0.7998128361456291469 ) ) ;
#213733=CARTESIAN_POINT ( 'NONE',  ( 0.6823417656249899377, 4.738541667008086655, -1.181850606188754593 ) ) ;
#213741=CARTESIAN_POINT ( 'NONE',  ( -5.526920175865215334, 9.599823971818089774, 0.7998128361456481317 ) ) ;
#213743=CARTESIAN_POINT ( 'NONE',  ( 5.087333953625774008, 6.958308917361963886, 1.599625672291267398 ) ) ;
#213746=CARTESIAN_POINT ( 'NONE',  ( 0.6823417656249899377, 1.092708333674752286, 1.181850606188755259 ) ) ;
#213751=CARTESIAN_POINT ( 'NONE',  ( 10.26082332744404368, 10.86538205830655279, -0.7998128361456281477 ) ) ;
#213754=CARTESIAN_POINT ( 'NONE',  ( -6.715366157470410435, 6.729015360003925750, -0.7998128361456291469 ) ) ;
#213758=CARTESIAN_POINT ( 'NONE',  ( 7.540305987494599016, 11.94877408538573427, -0.7998128361456291469 ) ) ;
#213760=CARTESIAN_POINT ( 'NONE',  ( 9.023114925094663619, 10.48572115315399245, 1.199719254218453823 ) ) ;
#213764=CARTESIAN_POINT ( 'NONE',  ( -5.101945877444165944, 4.846691699973280976, 0.000000000000000000 ) ) ;
#213765=CARTESIAN_POINT ( 'NONE',  ( -6.235860587281615075, 9.362588887548838557, -1.199719254218440723 ) ) ;
#213768=CARTESIAN_POINT ( 'NONE',  ( -5.193604695876673283, 6.642107527433549485, 1.420026453975403724 ) ) ;
#213769=CARTESIAN_POINT ( 'NONE',  ( -0.6823417656250246877, 0.05104166700808931978, 1.181850606188755259 ) ) ;
#213773=CARTESIAN_POINT ( 'NONE',  ( 6.643132081016111634, 9.733775946952057723, 1.082531754730558626 ) ) ;
#213791=CARTESIAN_POINT ( 'NONE',  ( 8.940712233207955606, 12.51824914112961729, 1.199719254218450271 ) ) ;
#213793=ORIENTED_EDGE ( 'NONE', *, *, #181594, .T. ) ;
#213795=CARTESIAN_POINT ( 'NONE',  ( -5.168682875307782254, 7.053215992657626110, -1.599625672291256295 ) ) ;
#213796=CARTESIAN_POINT ( 'NONE',  ( -7.965578943228732278, 9.251929174310385307, -1.199719254218446718 ) ) ;
#213802=CARTESIAN_POINT ( 'NONE',  ( -1.499999999999997780, 2.681250000682818158, 1.214306433183764966E-14 ) ) ;
#213803=CARTESIAN_POINT ( 'NONE',  ( 7.716561984472250835, 12.15440608185967086, 1.040834085586084257E-14 ) ) ;
#213808=CARTESIAN_POINT ( 'NONE',  ( -7.153898609505128015, 11.49796547773133604, 0.7998128361456481317 ) ) ;
#213811=CARTESIAN_POINT ( 'NONE',  ( -1.201851678989727383E-14, 2.821875000341418804, 1.575800808251672791 ) ) ;
#213816=CARTESIAN_POINT ( 'NONE',  ( -4.189106276498259618, 6.870745841681152655, 1.082531754730560403 ) ) ;
#213818=CARTESIAN_POINT ( 'NONE',  ( -8.012505595996376684, 12.29174759539704986, 0.000000000000000000 ) ) ;
#213823=CARTESIAN_POINT ( 'NONE',  ( 1.364683531249988535, 1.926041667008086211, 0.7879004041258500513 ) ) ;
#213829=CARTESIAN_POINT ( 'NONE',  ( 1.364683531249986537, 2.155208333674751398, -0.7879004041258239610 ) ) ;
#213831=CARTESIAN_POINT ( 'NONE',  ( -6.274726165026268454, 6.214935368819085149, 0.7998128361456341429 ) ) ;
#213832=CARTESIAN_POINT ( 'NONE',  ( 8.288111976655649471, 8.563885482386732306, -0.7998128361456291469 ) ) ;
#213835=CARTESIAN_POINT ( 'NONE',  ( 1.499999999999990896, 5.775000000000023448, 1.040834085586084257E-14 ) ) ;
#213836=CARTESIAN_POINT ( 'NONE',  ( -1.402160292154681736E-14, 2.259375000341416140, -1.575800808251660134 ) ) ;
#213839=CARTESIAN_POINT ( 'NONE',  ( 1.479373551132449505, 3.300000000000025135, 0.2478989637125245671 ) ) ;
#213840=CARTESIAN_POINT ( 'NONE',  ( -4.270455198624581783, 7.926022131796578662, 1.040834085586084257E-14 ) ) ;
#213843=CARTESIAN_POINT ( 'NONE',  ( 3.714570900464269076, 7.277490450609545469, 0.7216878364870298324 ) ) ;
#213844=( BOUNDED_SURFACE ( )  B_SPLINE_SURFACE ( 3, 2, ( 
 ( #42168, #140754, #28025 ),
 ( #190511, #93054, #8568 ),
 ( #156979, #24814, #74648 ),
 ( #11761, #9634, #108285 ) ),
 .UNSPECIFIED., .F., .F., .T. ) 
 B_SPLINE_SURFACE_WITH_KNOTS ( ( 4, 4 ),
 ( 3, 3 ),
 ( 4.363913744254155347E-18, 0.0001288481725834512569 ),
 ( 0.000000000000000000, 1.000000000000000000 ),
 .UNSPECIFIED. ) 
 GEOMETRIC_REPRESENTATION_ITEM ( )  RATIONAL_B_SPLINE_SURFACE ( (
 ( 1.000000000000000000, 0.7779734834199445448, 1.000000000000000000),
 ( 1.000000000000000000, 0.8164436902882270530, 1.000000000000000000),
 ( 1.000000000000000000, 0.8496999780322816997, 1.000000000000000000),
 ( 1.000000000000000000, 0.8739472344167453777, 1.000000000000000000) ) ) 
 REPRESENTATION_ITEM ( '' )  SURFACE ( )  );
#213847=CARTESIAN_POINT ( 'NONE',  ( -7.853197290813634268, 10.18514947741448573, 1.599625672291295375 ) ) ;
#213848=CARTESIAN_POINT ( 'NONE',  ( -2.605138072120212200, 6.191078184115536232, -0.7998128361456281477 ) ) ;
#213849=CARTESIAN_POINT ( 'NONE',  ( 1.364683531249990311, 5.113541667008084879, 0.7879004041258500513 ) ) ;
#213853=CARTESIAN_POINT ( 'NONE',  ( -6.954969613686107444, 10.09758640173367894, 1.082531754730549967 ) ) ;
#213855=CARTESIAN_POINT ( 'NONE',  ( 0.6823417656249864960, -0.5114583329919111243, -1.181850606188749264 ) ) ;
#213859=CARTESIAN_POINT ( 'NONE',  ( 7.239690840017413365, 10.42976116578691403, -1.082531754730537976 ) ) ;
#213866=ORIENTED_EDGE ( 'NONE', *, *, #61776, .T. ) ;
#213867=CARTESIAN_POINT ( 'NONE',  ( 8.636180661780656465, 11.09863007687603087, -1.443375672974052559 ) ) ;
#213874=CARTESIAN_POINT ( 'NONE',  ( 7.149227073107712549, 7.235186428247455837, -0.7998128361456281477 ) ) ;
#213875=CARTESIAN_POINT ( 'NONE',  ( -3.255929445576174697, 6.950334786480840243, -0.7998128361456281477 ) ) ;
#213880=CARTESIAN_POINT ( 'NONE',  ( 6.277061933002788585, 6.425586464699131639, 0.7216878364870317197 ) ) ;
#213881=CARTESIAN_POINT ( 'NONE',  ( -0.6823417656250003738, -0.2197916663252488800, -1.181850606188749264 ) ) ;
#213883=CARTESIAN_POINT ( 'NONE',  ( -8.296699936558862731, 11.76690146170562201, 1.199719254218453823 ) ) ;
#213896=ORIENTED_EDGE ( 'NONE', *, *, #206842, .F. ) ;
#213897=CARTESIAN_POINT ( 'NONE',  ( -4.510196435976065565, 7.040407170307378060, -1.149263043085164915 ) ) ;
#213901=CARTESIAN_POINT ( 'NONE',  ( 7.806797523370503811, 8.002351953554066810, 1.040834085586084257E-14 ) ) ;
#213902=CARTESIAN_POINT ( 'NONE',  ( 7.657657833620182153, 7.828355648845348291, -0.7998128361456281477 ) ) ;
#213905=ORIENTED_EDGE ( 'NONE', *, *, #126844, .F. ) ;
#213913=CARTESIAN_POINT ( 'NONE',  ( -3.898132859128961236, 4.506575409527250997, -1.199719254218452047 ) ) ;
#213923=CARTESIAN_POINT ( 'NONE',  ( -10.16825202056928390, 10.96530823352674133, 0.7216878364870438212 ) ) ;
#213926=CARTESIAN_POINT ( 'NONE',  ( 6.531277313481192337, 8.642909503859968368, 1.599625672291281386 ) ) ;
#213928=EDGE_CURVE ( 'NONE', #9480, #137589, #189864, .T. ) ;
#213934=CARTESIAN_POINT ( 'NONE',  ( 4.650083499362875017, 5.487814173087225633, 1.082531754730560403 ) ) ;
#213935=CARTESIAN_POINT ( 'NONE',  ( -6.181627972826976958, 9.299317504018391745, 1.199719254218452047 ) ) ;
#213941=CARTESIAN_POINT ( 'NONE',  ( -7.528855374290365887, 7.678086112960552434, -0.7998128361456291469 ) ) ;
#213942=CARTESIAN_POINT ( 'NONE',  ( -3.924195396151603177, 6.665646164563756138, 1.199719254218464037 ) ) ;
#213950=CARTESIAN_POINT ( 'NONE',  ( 6.908042961362778733, 8.018137195466769285, 1.199719254218462483 ) ) ;
#213962=CARTESIAN_POINT ( 'NONE',  ( -1.402160292154681736E-14, 0.6343750003414162508, 1.575800808251672791 ) ) ;
#213964=CARTESIAN_POINT ( 'NONE',  ( 4.436542580169809291, 6.199052314996659874, 1.599625672291267398 ) ) ;
#213966=CARTESIAN_POINT ( 'NONE',  ( -8.676855123066030018, 9.225345186439589895, -0.7216878364870267237 ) ) ;
#213968=CARTESIAN_POINT ( 'NONE',  ( 3.701012746850603996, 7.261672604726938651, 1.040834085586084257E-14 ) ) ;
#213969=CARTESIAN_POINT ( 'NONE',  ( -7.998947441938374148, 8.434452891790657603, 1.040834085586084257E-14 ) ) ;
#213973=CARTESIAN_POINT ( 'NONE',  ( 5.750629710490689384, 9.860818428881154674, -0.7998128361456291469 ) ) ;
#213978=CARTESIAN_POINT ( 'NONE',  ( 1.364683531249988535, 3.405208333674749621, -0.7879004041258239610 ) ) ;
#213982=CARTESIAN_POINT ( 'NONE',  ( 6.286176778230493589, 10.48562334124426698, 0.7998128361456462443 ) ) ;
#213985=CARTESIAN_POINT ( 'NONE',  ( -7.202405917357668663, 9.425892875049191488, 1.599625672291295375 ) ) ;
#213991=CARTESIAN_POINT ( 'NONE',  ( 9.673906298550626559, 11.24497775551929557, 1.199719254218452047 ) ) ;
#213994=CARTESIAN_POINT ( 'NONE',  ( -7.492852449846775897, 11.89341162479659531, 0.000000000000000000 ) ) ;
#213998=CARTESIAN_POINT ( 'NONE',  ( 5.253083726123439767, 6.394172465367824465, -1.148862164228587890 ) ) ;
#213999=CARTESIAN_POINT ( 'NONE',  ( -4.277761160311629673, 4.949475094240346706, 1.199719254218462483 ) ) ;
#214004=CARTESIAN_POINT ( 'NONE',  ( 5.126954644262057492, 9.133197518281081173, 0.7998128361456462443 ) ) ;
#214006=CARTESIAN_POINT ( 'NONE',  ( 5.717788096661236885, 7.693838750903348789, 1.599625672291267398 ) ) ;
#214007=CARTESIAN_POINT ( 'NONE',  ( -4.014638704412293535, 7.626288086010478473, 0.05010440672792437766 ) ) ;
#214008=CARTESIAN_POINT ( 'NONE',  ( 3.521367211247359741, 5.131347717920458962, -1.599625672291262513 ) ) ;
#214010=CARTESIAN_POINT ( 'NONE',  ( -6.480434237652138663, 8.583592582059388576, 1.443375672974078761 ) ) ;
#214017=CARTESIAN_POINT ( 'NONE',  ( -4.099290701344459720, 7.507401141727952698, 0.5799236987427489609 ) ) ;
#214018=CARTESIAN_POINT ( 'NONE',  ( -1.364683531250014514, -0.6572916663252459379, 0.7879004041258379498 ) ) ;
#214021=CARTESIAN_POINT ( 'NONE',  ( 3.877268743828266029, 6.506935386899531437, 1.082531754730558626 ) ) ;
#214024=CARTESIAN_POINT ( 'NONE',  ( -10.10046125205659173, 10.88621900359527572, -0.7216878364870267237 ) ) ;
#214029=CARTESIAN_POINT ( 'NONE',  ( -10.15469386651127515, 11.90985960142705657, 1.082531754730558626 ) ) ;
#214036=CARTESIAN_POINT ( 'NONE',  ( -9.775065565328603157, 11.46695991671396087, -1.082531754730537976 ) ) ;
#214041=CARTESIAN_POINT ( 'NONE',  ( -1.500000000000013101, 2.452083334016154748, 0.8660254037844403729 ) ) ;
#214045=CARTESIAN_POINT ( 'NONE',  ( -9.481229494658258261, 9.955855920056455588, -0.7998128361456291469 ) ) ;
#214048=CARTESIAN_POINT ( 'NONE',  ( 6.257251587906815793, 7.258880593101466161, 1.199719254218462483 ) ) ;
#214051=DIRECTION ( 'NONE',  ( 1.000000000000000000, -5.578564026256504688E-16, -0.000000000000000000 ) ) ;
#214054=CARTESIAN_POINT ( 'NONE',  ( 7.958799866421889746, 9.244020251369077457, -1.199719254218441611 ) ) ;
#214060=CARTESIAN_POINT ( 'NONE',  ( -5.721177635286839092, 9.618531641235897212, 0.7216878364870458196 ) ) ;
#214063=CARTESIAN_POINT ( 'NONE',  ( -1.001543065824772872E-14, 4.884375000341420581, 1.575800808251672791 ) ) ;
#214066=ADVANCED_FACE ( 'NONE', ( #145320 ), #196554, .T. ) ;
#214071=CARTESIAN_POINT ( 'NONE',  ( -2.914639836813632812, 6.344237543017112735, 0.7216878364870317197 ) ) ;
#214073=CARTESIAN_POINT ( 'NONE',  ( 9.398826802771546696, 11.98838390803207865, -1.599625672291262513 ) ) ;
#214075=CARTESIAN_POINT ( 'NONE',  ( -9.501566725078754772, 9.979582688880366703, -0.7998128361456291469 ) ) ;
#214078=CARTESIAN_POINT ( 'NONE',  ( -1.402160292154681736E-14, 1.946875000341422579, -1.575800808251660134 ) ) ;
#214079=CARTESIAN_POINT ( 'NONE',  ( 5.169736645512481132, 4.925780929386339935, 0.7998128361456341429 ) ) ;
#214084=CARTESIAN_POINT ( 'NONE',  ( 9.531018800282605952, 11.18223869082697597, 1.082531754730548412 ) ) ;
#214086=CARTESIAN_POINT ( 'NONE',  ( -6.670248388243482651, 9.765411638717282017, 1.082531754730548412 ) ) ;
#214087=CARTESIAN_POINT ( 'NONE',  ( -1.364683531250014514, 0.9885416670080898749, -0.7879004041258289570 ) ) ;
#214089=CARTESIAN_POINT ( 'NONE',  ( 0.5050423914800099556, 7.726475908227712353, 1.936073478083413235 ) ) ;
#214091=CARTESIAN_POINT ( 'NONE',  ( -9.182950115157607840, 9.607863310639020327, 0.7998128361456462443 ) ) ;
#214092=CARTESIAN_POINT ( 'NONE',  ( -5.083944415000202888, 5.033616027029415463, 0.7216878364870317197 ) ) ;
#214093=CARTESIAN_POINT ( 'NONE',  ( 0.6823417656249917140, 3.405208333674754506, 1.181850606188765695 ) ) ;
#214115=CARTESIAN_POINT ( 'NONE',  ( -1.364683531249997417, 4.821875000341417916, 1.214306433183764966E-14 ) ) ;
#214120=CARTESIAN_POINT ( 'NONE',  ( 9.585778300061798873, 11.14216175728232550, -1.199719254218440723 ) ) ;
#214122=CARTESIAN_POINT ( 'NONE',  ( -1.201851678989727383E-14, 2.071875000341422801, 1.575800808251672791 ) ) ;
#214124=CARTESIAN_POINT ( 'NONE',  ( -7.876924059859742755, 8.292092279365579799, 1.040834085586084257E-14 ) ) ;
#214131=CARTESIAN_POINT ( 'NONE',  ( 4.704842999142070603, 5.447737239542574272, -1.199719254218452047 ) ) ;
#214133=ORIENTED_EDGE ( 'NONE', *, *, #17125, .F. ) ;
#214134=CARTESIAN_POINT ( 'NONE',  ( 9.541187415715040032, 12.15447128979948310, -1.599625672291262513 ) ) ;
#214140=EDGE_LOOP ( 'NONE', ( #4148, #50881, #46769, #118131 ) ) ;
#214142=CARTESIAN_POINT ( 'NONE',  ( -8.448702279610222021, 13.00856975952063088, 1.040834085586084257E-14 ) ) ;
#214143=CARTESIAN_POINT ( 'NONE',  ( 5.608269097547198712, 9.694731047113750222, -0.7998128361456281477 ) ) ;
#214145=CARTESIAN_POINT ( 'NONE',  ( 3.511198595814921219, 7.040222761851976152, 0.7216878364870317197 ) ) ;
#214146=CARTESIAN_POINT ( 'NONE',  ( 2.000000000000003553, 6.400000000000022560, 2.449293598294762621E-16 ) ) ;
#214153=CARTESIAN_POINT ( 'NONE',  ( -1.499999999999997113, 7.438721522839124134, -4.195160983902616714 ) ) ;
#214154=CARTESIAN_POINT ( 'NONE',  ( -7.714226216495749355, 8.102278128774251797, 1.040834085586084257E-14 ) ) ;
#214155=CARTESIAN_POINT ( 'NONE',  ( 5.229694566569264680, 7.124396299129368337, 1.599625672291267398 ) ) ;
#214158=CARTESIAN_POINT ( 'NONE',  ( -7.472515219426274946, 11.86968485597268064, 0.000000000000000000 ) ) ;
#214164=CARTESIAN_POINT ( 'NONE',  ( -7.947050595904583403, 12.42330946186405249, 0.7998128361456481317 ) ) ;
#214165=CARTESIAN_POINT ( 'NONE',  ( -0.6823417656250212460, 3.051041667008084879, 1.181850606188767472 ) ) ;
#214169=CARTESIAN_POINT ( 'NONE',  ( 8.718056468787178659, 10.12981962079525289, 1.199719254218462483 ) ) ;
#214170=CARTESIAN_POINT ( 'NONE',  ( 3.216308754939877446, 4.775446185561722956, -1.599625672291262513 ) ) ;
#214172=VERTEX_POINT ( 'NONE', #134385 ) ;
#214180=CARTESIAN_POINT ( 'NONE',  ( -7.648771216403934758, 12.07531685244661723, -0.7998128361456291469 ) ) ;
#214184=CARTESIAN_POINT ( 'NONE',  ( 8.107412671292047790, 8.560995659369956101, 0.7216878364870458196 ) ) ;
#214185=CARTESIAN_POINT ( 'NONE',  ( -1.001543065824772872E-14, 5.134375000341421469, 1.575800808251672791 ) ) ;
#214188=CARTESIAN_POINT ( 'NONE',  ( 3.171717870593107058, 5.787755718078879674, -1.199719254218446718 ) ) ;
#214191=CARTESIAN_POINT ( 'NONE',  ( -5.865874016206865882, 9.995270118883347266, 0.000000000000000000 ) ) ;
#214200=CARTESIAN_POINT ( 'NONE',  ( -1.364683531250010295, 3.842708333674751398, 0.7879004041258379498 ) ) ;
#214201=CARTESIAN_POINT ( 'NONE',  ( 5.300874872818884143, 5.286701561151147644, 0.7216878364870010776 ) ) ;
#214202=CARTESIAN_POINT ( 'NONE',  ( 7.553864141108259211, 11.96459193126834464, 1.040834085586084257E-14 ) ) ;
#214204=CARTESIAN_POINT ( 'NONE',  ( -3.307826292054310890, 5.842585859829892314, -1.082531754730549967 ) ) ;
#214207=CARTESIAN_POINT ( 'NONE',  ( -3.701012746406287413, 6.301303389907177532, 1.082531754730560403 ) ) ;
#214208=( BOUNDED_CURVE ( )  B_SPLINE_CURVE ( 2, ( #94962, #163151, #50448, #48344, #14735, #114455, #130713 ),
 .UNSPECIFIED., .F., .T. ) 
 B_SPLINE_CURVE_WITH_KNOTS ( ( 3, 2, 2, 3 ),
 ( 0.2250000000000001998, 0.2291666666666669350, 0.2333333333333336701, 0.2375000000000004052 ),
 .UNSPECIFIED. ) 
 CURVE ( )  GEOMETRIC_REPRESENTATION_ITEM ( )  RATIONAL_B_SPLINE_CURVE ( ( 0.9999999999999937828, 0.8660254037844449249, 1.000000000000000000, 0.8660254037844387076, 1.000000000000000000, 0.8660254037844252739, 1.000000000000013323 ) ) 
 REPRESENTATION_ITEM ( '' )  );
#214213=ORIENTED_EDGE ( 'NONE', *, *, #101161, .T. ) ;
#214215=CARTESIAN_POINT ( 'NONE',  ( 4.172158584703322681, 5.890604320285754980, -1.599625672291256295 ) ) ;
#214223=CARTESIAN_POINT ( 'NONE',  ( 4.761938266897790761, 6.578680616179308771, 1.599625672291267398 ) ) ;
#214228=CARTESIAN_POINT ( 'NONE',  ( -1.201851678989727383E-14, 3.384375000341421469, 1.575800808251672791 ) ) ;
#214233=CARTESIAN_POINT ( 'NONE',  ( 5.587931867126699537, 9.671004278289832001, -0.7998128361456291469 ) ) ;
#214235=EDGE_CURVE ( 'NONE', #202848, #129569, #10103, .T. ) ;
#214236=CARTESIAN_POINT ( 'NONE',  ( -6.413170354464012846, 7.440785820751486312, 1.199719254218450271 ) ) ;
#214237=CARTESIAN_POINT ( 'NONE',  ( 1.499999999999987121, 1.795833333333355819, -0.8660254037844253849 ) ) ;
#214240=CARTESIAN_POINT ( 'NONE',  ( -4.388035272317281077, 8.271124917678806199, 0.7998128361456481317 ) ) ;
#214243=CARTESIAN_POINT ( 'NONE',  ( -1.364683531250010295, 3.780208333674750953, 0.7879004041258379498 ) ) ;
#214245=CARTESIAN_POINT ( 'NONE',  ( -5.436456409399874623, 5.444880020495701523, 0.000000000000000000 ) ) ;
#214248=ORIENTED_EDGE ( 'NONE', *, *, #177361, .F. ) ;
#214251=CARTESIAN_POINT ( 'NONE',  ( 5.867981556616276073, 5.740399992340775803, -0.7998128361456281477 ) ) ;
#214254=CARTESIAN_POINT ( 'NONE',  ( -1.201851678989727383E-14, 3.009375000341419248, -1.575800808251660134 ) ) ;
#214256=CARTESIAN_POINT ( 'NONE',  ( 4.546061579283848353, 4.198160018786257552, -0.7998128361456211532 ) ) ;
#214258=CARTESIAN_POINT ( 'NONE',  ( -0.6823417656250246877, 0.6135416670080897639, 1.181850606188755259 ) ) ;
#214259=CARTESIAN_POINT ( 'NONE',  ( -4.294587207893853176, 7.385457912387431101, -1.052126661723006285 ) ) ;
#214261=CARTESIAN_POINT ( 'NONE',  ( -2.948008335967658322, 5.526761261015804116, 1.199719254218462483 ) ) ;
#214262=CARTESIAN_POINT ( 'NONE',  ( -5.707619481228817904, 8.642344580533519505, -1.082531754730537976 ) ) ;
#214266=CARTESIAN_POINT ( 'NONE',  ( 0.6823417656249899377, 3.092708333674754062, 1.181850606188765695 ) ) ;
#214274=CARTESIAN_POINT ( 'NONE',  ( -6.168596704093453731, 10.14052055484361325, 0.7216878364870458196 ) ) ;
#214280=CARTESIAN_POINT ( 'NONE',  ( -6.873620692004104527, 7.121571683533994168, 0.7216878364870317197 ) ) ;
#214284=CARTESIAN_POINT ( 'NONE',  ( -1.499999999999996669, 4.910416667349485564, -0.8660254037844395958 ) ) ;
#214285=DIRECTION ( 'NONE',  ( 5.578564026256490882E-16, 1.000000000000000000, 9.066213480720158442E-32 ) ) ;
#214291=CARTESIAN_POINT ( 'NONE',  ( -6.078132937628113908, 5.985576603521232109, 1.040834085586084257E-14 ) ) ;
#214293=CARTESIAN_POINT ( 'NONE',  ( -1.500000000000001332, -0.8499999999999757749, 0.000000000000000000 ) ) ;
#214294=CARTESIAN_POINT ( 'NONE',  ( 3.708318708537623021, 4.285125567170706695, -1.199719254218446718 ) ) ;
#214295=CARTESIAN_POINT ( 'NONE',  ( 8.633844893804129228, 8.967240552393299424, -0.7998128361456211532 ) ) ;
#214297=CARTESIAN_POINT ( 'NONE',  ( -3.253593677155282471, 6.739683690082376444, 1.040834085586084257E-14 ) ) ;
#214298=CARTESIAN_POINT ( 'NONE',  ( 4.157546660884947620, 8.002221537674429896, 1.040834085586084257E-14 ) ) ;
#214299=( BOUNDED_SURFACE ( )  B_SPLINE_SURFACE ( 3, 2, ( 
 ( #112480, #96189, #178489 ),
 ( #13826, #12757, #114613 ),
 ( #179554, #83093, #65755 ),
 ( #80977, #149172, #31175 ) ),
 .UNSPECIFIED., .F., .F., .T. ) 
 B_SPLINE_SURFACE_WITH_KNOTS ( ( 4, 4 ),
 ( 3, 3 ),
 ( 5.985662991022360223E-05, 0.0001887152224066861379 ),
 ( 0.000000000000000000, 1.000000000000000000 ),
 .UNSPECIFIED. ) 
 GEOMETRIC_REPRESENTATION_ITEM ( )  RATIONAL_B_SPLINE_SURFACE ( (
 ( 1.000000000000000000, 0.8739472344186550723, 1.000000000000000000),
 ( 1.000000000000000000, 0.8497613059194148999, 1.000000000000000000),
 ( 1.000000000000000000, 0.8164163343283504792, 1.000000000000000000),
 ( 1.000000000000000000, 0.7779734834199396598, 1.000000000000000000) ) ) 
 REPRESENTATION_ITEM ( '' )  SURFACE ( )  );
#214300=MECHANICAL_DESIGN_GEOMETRIC_PRESENTATION_REPRESENTATION('',(#41519),#203965);
#214306=CARTESIAN_POINT ( 'NONE',  ( -4.121315508874276112, 4.870918184183829602, -1.082531754730549967 ) ) ;
#214309=LINE ( 'NONE', #194911, #187502 ) ;
#214313=CARTESIAN_POINT ( 'NONE',  ( 0.6823417656249882723, 2.426041667008084435, -1.181850606188749264 ) ) ;
#214314=CARTESIAN_POINT ( 'NONE',  ( 8.202319746143333035, 12.51319743723517952, -0.7216878364870328300 ) ) ;
#214315=CARTESIAN_POINT ( 'NONE',  ( -7.714753101375940503, 8.959299025482085455, 1.199719254218462483 ) ) ;
#214318=CARTESIAN_POINT ( 'NONE',  ( 5.494078562035752178, 7.432844293840273231, -1.599625672291262513 ) ) ;
#214319=CARTESIAN_POINT ( 'NONE',  ( -5.554036483092550824, 9.631459663583308739, -0.7998128361456231517 ) ) ;
#214322=CARTESIAN_POINT ( 'NONE',  ( -1.500000000000015099, -1.089583332650509773, -0.8660254037844383745 ) ) ;
#214325=CARTESIAN_POINT ( 'NONE',  ( 8.920901888112002354, 9.510066412326583674, 0.7216878364870438212 ) ) ;
#214329=CARTESIAN_POINT ( 'NONE',  ( -1.364683531250014514, 0.5510416670080878765, -0.7879004041258289570 ) ) ;
#214331=CARTESIAN_POINT ( 'NONE',  ( 7.253248993186731219, 8.524840582548424806, 1.082531754730558626 ) ) ;
#214335=CARTESIAN_POINT ( 'NONE',  ( -3.633221978782283923, 7.182583375313884133, -0.7216878364870267237 ) ) ;
#214337=CARTESIAN_POINT ( 'NONE',  ( 1.364683531249990311, 5.134375000341417916, 1.214306433183764966E-14 ) ) ;
#214341=CARTESIAN_POINT ( 'NONE',  ( -5.512600778122673795, 6.408089294489160537, -1.271103323116394845 ) ) ;
#214348=CARTESIAN_POINT ( 'NONE',  ( 6.286176778230493589, 10.48562334124426698, 0.7998128361456462443 ) ) ;
#214351=CARTESIAN_POINT ( 'NONE',  ( 4.009460741339333723, 5.700790169694431420, -1.599625672291256295 ) ) ;
#214357=VERTEX_POINT ( 'NONE', #81075 ) ;
#214358=CARTESIAN_POINT ( 'NONE',  ( 4.690757960648221037, 7.456006139856155457, 1.082531754730558626 ) ) ;
#214359=CARTESIAN_POINT ( 'NONE',  ( 0.6823417656249882723, 1.238541667008083547, -1.181850606188749264 ) ) ;
#214362=CARTESIAN_POINT ( 'NONE',  ( 3.379006598303866848, 4.965260336153046516, -1.599625672291262513 ) ) ;
#214367=CARTESIAN_POINT ( 'NONE',  ( -1.500000000000013101, 1.170833333333352710, 0.8660254037844403729 ) ) ;
#214368=CARTESIAN_POINT ( 'NONE',  ( 5.774883364416965037, 8.824782127540085952, -1.199719254218440723 ) ) ;
#214369=CARTESIAN_POINT ( 'NONE',  ( -7.232384877886063990, 10.52520055992070525, -1.199719254218446718 ) ) ;
#214373=CARTESIAN_POINT ( 'NONE',  ( 1.364683531249986537, 1.905208333674750287, -0.7879004041258239610 ) ) ;
#214374=ORIENTED_EDGE ( 'NONE', *, *, #161432, .T. ) ;
#214375=CARTESIAN_POINT ( 'NONE',  ( 0.7499999999999902300, 2.983333333333351600, 1.299038105676669330 ) ) ;
#214377=CARTESIAN_POINT ( 'NONE',  ( 5.332434488876471868, 5.115595079977664383, 0.7998128361456341429 ) ) ;
#214385=CARTESIAN_POINT ( 'NONE',  ( 1.499999999999987566, -0.4437499993171847845, 0.000000000000000000 ) ) ;
#214387=CARTESIAN_POINT ( 'NONE',  ( -7.049349804101573191, 10.31165964050546258, -1.199719254218440723 ) ) ;
#214388=CARTESIAN_POINT ( 'NONE',  ( -4.799223189557577207, 4.701441264013013210, 0.7216878364870317197 ) ) ;
#214396=CARTESIAN_POINT ( 'NONE',  ( 6.449928391799196525, 8.548002428564306143, -1.599625672291262513 ) ) ;
#214400=CARTESIAN_POINT ( 'NONE',  ( 9.232739420781973294, 9.873876867108206667, -0.7216878364870257245 ) ) ;
#214404=CARTESIAN_POINT ( 'NONE',  ( -5.856232286098998152, 8.919689202835742847, 1.199719254218452047 ) ) ;
#214405=CARTESIAN_POINT ( 'NONE',  ( 3.669453130792974971, 7.432779085900453886, 1.040834085586084257E-14 ) ) ;
#214409=CARTESIAN_POINT ( 'NONE',  ( -2.081668171172168513E-14, 6.487495393664096888, 3.100011470320013451 ) ) ;
ENDSEC;
END-ISO-10303-21;
